#169038=CARTESIAN_POINT('Ctrl Pts',(0.232339728999104,-62.8965351787718,
40.0684393223556));
#169039=CARTESIAN_POINT('Ctrl Pts',(0.229175397308911,-62.8985027695519,
40.0715697951759));
#169040=CARTESIAN_POINT('Ctrl Pts',(0.211566610930123,-62.9094519648699,
40.0889901646418));
#169041=CARTESIAN_POINT('Ctrl Pts',(0.191177078584712,-62.9192690206957,
40.1045963098239));
#169042=CARTESIAN_POINT('Ctrl Pts',(0.168765047542055,-62.9274935913893,
40.1176634650721));
#169043=CARTESIAN_POINT('Ctrl Pts',(0.158706217640471,-62.9311848926133,
40.123528185306));
#169044=CARTESIAN_POINT('Ctrl Pts',(0.148239886921569,-62.9345557609575,
40.1288820140919));
#169045=CARTESIAN_POINT('Ctrl Pts',(0.137433186922152,-62.9375663198809,
40.1336621774101));
#169046=CARTESIAN_POINT('Ctrl Pts',(0.132736741273405,-62.9388746680683,
40.1357395717319));
#169047=CARTESIAN_POINT('Ctrl Pts',(0.127976140237891,-62.9401148076313,
40.1377083672884));
#169048=CARTESIAN_POINT('Ctrl Pts',(0.123156980417351,-62.9412833674838,
40.1395632548792));
#169049=CARTESIAN_POINT('Ctrl Pts',(0.10628992104546,-62.9453733269673,
40.146055361447));
#169050=CARTESIAN_POINT('Ctrl Pts',(0.0887055165508424,-62.9485864317704,
40.151152097463));
#169051=CARTESIAN_POINT('Ctrl Pts',(0.0706437212499514,-62.9507781643242,
40.1546258197409));
#169052=CARTESIAN_POINT('Ctrl Pts',(0.061612823599506,-62.9518740306011,
40.1563626808798));
#169053=CARTESIAN_POINT('Ctrl Pts',(0.052462578249927,-62.9527145544237,
40.1576937882008));
#169054=CARTESIAN_POINT('Ctrl Pts',(0.0432229794973055,-62.9532816790167,
40.1585906813668));
#169055=CARTESIAN_POINT('Ctrl Pts',(0.0386031801209948,-62.9535652413132,
40.1590391279498));
#169056=CARTESIAN_POINT('Ctrl Pts',(0.0339610423938992,-62.9537804539255,
40.1593790209175));
#169057=CARTESIAN_POINT('Ctrl Pts',(0.0293003156013867,-62.9539250604562,
40.1596068022931));
#169058=CARTESIAN_POINT('Ctrl Pts',(0.024639588808874,-62.9540696669868,
40.1598345836687));
#169059=CARTESIAN_POINT('Ctrl Pts',(0.0199602729505794,-62.9541436657296,
40.1599502506865));
#169060=CARTESIAN_POINT('Ctrl Pts',(0.0152661173106527,-62.9541448057648,
40.1599502534424));
#169061=CARTESIAN_POINT('',(-0.015266117311081,-62.9541448057648,40.1599502534424));
#169062=CARTESIAN_POINT('Origin',(-3.96846087890508E-17,1.55412650666996E-16,
40.1599502534424));
#169063=CARTESIAN_POINT('',(-0.318045750793257,-62.7644678366119,39.8576902534424));
#169064=CARTESIAN_POINT('Ctrl Pts',(-0.015266117311081,-62.9541448057648,
40.1599502534424));
#169065=CARTESIAN_POINT('Ctrl Pts',(-0.0190877352448612,-62.9541438736292,
40.1599502447858));
#169066=CARTESIAN_POINT('Ctrl Pts',(-0.022898872102436,-62.9540952129414,
40.1598744685927));
#169067=CARTESIAN_POINT('Ctrl Pts',(-0.0266975986405572,-62.9539999459718,
40.1597246934279));
#169068=CARTESIAN_POINT('Ctrl Pts',(-0.0486495517941837,-62.953449420412,
40.1588591777434));
#169069=CARTESIAN_POINT('Ctrl Pts',(-0.070189881249066,-62.9513443281451,
40.1555254706012));
#169070=CARTESIAN_POINT('Ctrl Pts',(-0.0909392844476108,-62.9479003565101,
40.150063182636));
#169071=CARTESIAN_POINT('Ctrl Pts',(-0.0993079960717487,-62.9465113235254,
40.1478601162465));
#169072=CARTESIAN_POINT('Ctrl Pts',(-0.107548428340522,-62.9449047668208,
40.1453112228298));
#169073=CARTESIAN_POINT('Ctrl Pts',(-0.115637319282431,-62.9430957254317,
40.1424401896328));
#169074=CARTESIAN_POINT('Ctrl Pts',(-0.118621628943688,-62.9424282989905,
40.1413809526905));
#169075=CARTESIAN_POINT('Ctrl Pts',(-0.121585194085774,-62.9417332466658,
40.1402777640512));
#169076=CARTESIAN_POINT('Ctrl Pts',(-0.124526788072995,-62.941011293136,
40.1391317641987));
#169077=CARTESIAN_POINT('Ctrl Pts',(-0.130042276799036,-62.9396576302675,
40.1369830144753));
#169078=CARTESIAN_POINT('Ctrl Pts',(-0.135480523183809,-62.938209392844,
40.134683756585));
#169079=CARTESIAN_POINT('Ctrl Pts',(-0.140833441493576,-62.9366713579026,
40.1322415082996));
#169080=CARTESIAN_POINT('Ctrl Pts',(-0.159568655577758,-62.9312882356078,
40.1236936393009));
#169081=CARTESIAN_POINT('Ctrl Pts',(-0.177258600739179,-62.9248050892389,
40.113394140767));
#169082=CARTESIAN_POINT('Ctrl Pts',(-0.193556601113859,-62.9174267595942,
40.101665321223));
#169083=CARTESIAN_POINT('Ctrl Pts',(-0.201705601301199,-62.9137375947718,
40.095800911451));
#169084=CARTESIAN_POINT('Ctrl Pts',(-0.209506615291615,-62.9098246351408,
40.0895791707949));
#169085=CARTESIAN_POINT('Ctrl Pts',(-0.216916308650606,-62.9057134946881,
40.0830403822906));
#169086=CARTESIAN_POINT('Ctrl Pts',(-0.220621155330102,-62.9036579244618,
40.0797709880385));
#169087=CARTESIAN_POINT('Ctrl Pts',(-0.224228171852759,-62.9015528091474,
40.0764223317514));
#169088=CARTESIAN_POINT('Ctrl Pts',(-0.227731941419747,-62.8994013510256,
40.0729994484778));
#169089=CARTESIAN_POINT('Ctrl Pts',(-0.231235710986736,-62.8972498929038,
40.0695765652042));
#169090=CARTESIAN_POINT('Ctrl Pts',(-0.23463611427696,-62.8950520414621,
40.0660793733488));
#169091=CARTESIAN_POINT('Ctrl Pts',(-0.237927978231146,-62.892811103745,
40.0625130768817));
#169092=CARTESIAN_POINT('Ctrl Pts',(-0.237956050936441,-62.8927919932396,
40.0624826638418));
#169093=CARTESIAN_POINT('Ctrl Pts',(-0.237984115711232,-62.8927728797351,
40.0624522459912));
#169094=CARTESIAN_POINT('Ctrl Pts',(-0.238012172553065,-62.8927537632335,
40.0624218233329));
#169095=CARTESIAN_POINT('Ctrl Pts',(-0.252341211296384,-62.8829906867849,
40.0468845275921));
#169096=CARTESIAN_POINT('Ctrl Pts',(-0.264702219189541,-62.8725309380422,
40.0302263329286));
#169097=CARTESIAN_POINT('Ctrl Pts',(-0.275152816745417,-62.8615664772848,
40.012751588482));
#169098=CARTESIAN_POINT('Ctrl Pts',(-0.285956846571237,-62.8502312057453,
39.9946858597818));
#169099=CARTESIAN_POINT('Ctrl Pts',(-0.294719332056317,-62.8383556508916,
39.9757460620621));
#169100=CARTESIAN_POINT('Ctrl Pts',(-0.301453885679313,-62.8261370346473,
39.9562444559289));
#169101=CARTESIAN_POINT('Ctrl Pts',(-0.308060333921541,-62.8141508421944,
39.9371138113796));
#169102=CARTESIAN_POINT('Ctrl Pts',(-0.312715155744977,-62.8018335935212,
39.9174410654562));
#169103=CARTESIAN_POINT('Ctrl Pts',(-0.315383336840583,-62.7893708783693,
39.8975196504379));
#169104=CARTESIAN_POINT('Ctrl Pts',(-0.317150913275331,-62.7811147664991,
39.8843224113931));
#169105=CARTESIAN_POINT('Ctrl Pts',(-0.318045664008668,-62.7727948225173,
39.871016044721));
#169106=CARTESIAN_POINT('Ctrl Pts',(-0.318045750793257,-62.7644678366119,
39.8576902534424));
#169107=CARTESIAN_POINT('',(-0.318048871877343,-62.4081695979768,39.2875012672119));
#169108=CARTESIAN_POINT('',(-0.318045750793259,-62.7644678366119,39.8576902534424));
#169109=CARTESIAN_POINT('',(-6.20712349654485,-62.0995362748658,39.2875012672119));
#169110=CARTESIAN_POINT('Origin',(5.53234440788222E-15,0.,39.2875012672119));
#169111=CARTESIAN_POINT('',(-6.24436990788081,-62.4538823482275,39.8576902534424));
#169112=CARTESIAN_POINT('',(-6.20712349654485,-62.0995362748658,39.2875012672119));
#169113=CARTESIAN_POINT('',(-6.56531752495323,-62.6108711573005,40.1599502534424));
#169114=CARTESIAN_POINT('Ctrl Pts',(-6.2443699078808,-62.4538823482275,
39.8576902534424));
#169115=CARTESIAN_POINT('Ctrl Pts',(-6.24565635961484,-62.4661208561118,
39.8773836120374));
#169116=CARTESIAN_POINT('Ctrl Pts',(-6.24887816048168,-62.4781153572978,
39.8969946442152));
#169117=CARTESIAN_POINT('Ctrl Pts',(-6.25393874389551,-62.4897034690595,
39.916252528827));
#169118=CARTESIAN_POINT('Ctrl Pts',(-6.25910101415687,-62.5015244311583,
39.9358973794102));
#169119=CARTESIAN_POINT('Ctrl Pts',(-6.26617675898623,-62.5129234357018,
39.9551762199786));
#169120=CARTESIAN_POINT('Ctrl Pts',(-6.27511683300914,-62.5237314369814,
39.9738152034297));
#169121=CARTESIAN_POINT('Ctrl Pts',(-6.28370959326059,-62.534119557209,
39.9917300792702));
#169122=CARTESIAN_POINT('Ctrl Pts',(-6.2940250923436,-62.543962460673,40.0090551158182));
#169123=CARTESIAN_POINT('Ctrl Pts',(-6.30606398948311,-62.5531007542797,
40.0255394551598));
#169124=CARTESIAN_POINT('Ctrl Pts',(-6.315311852504,-62.5601204743206,40.038202152619));
#169125=CARTESIAN_POINT('Ctrl Pts',(-6.32557753708339,-62.5667243349277,
40.0503687782142));
#169126=CARTESIAN_POINT('Ctrl Pts',(-6.33687803771711,-62.5728320301412,
40.0619155352442));
#169127=CARTESIAN_POINT('Ctrl Pts',(-6.33690765431396,-62.5728480373211,
40.0619457972351));
#169128=CARTESIAN_POINT('Ctrl Pts',(-6.33693727882117,-62.5728640408534,
40.0619760547304));
#169129=CARTESIAN_POINT('Ctrl Pts',(-6.33696691123597,-62.5728800407363,
40.0620063077269));
#169130=CARTESIAN_POINT('Ctrl Pts',(-6.34014410870348,-62.5745955535553,
40.06525004417));
#169131=CARTESIAN_POINT('Ctrl Pts',(-6.34341121944339,-62.5762674929177,
40.0684393223556));
#169132=CARTESIAN_POINT('Ctrl Pts',(-6.34676388583407,-62.5778935423007,
40.0715697951758));
#169133=CARTESIAN_POINT('Ctrl Pts',(-6.36542071199911,-62.586942137401,
40.0889901646417));
#169134=CARTESIAN_POINT('Ctrl Pts',(-6.38672471011203,-62.5945741278849,
40.1045963098237));
#169135=CARTESIAN_POINT('Ctrl Pts',(-6.40987366743906,-62.6004109483561,
40.1176634650718));
#169136=CARTESIAN_POINT('Ctrl Pts',(-6.42026324006253,-62.6030305942139,
40.1235281853058));
#169137=CARTESIAN_POINT('Ctrl Pts',(-6.43102458681472,-62.6052889671226,
40.1288820140918));
#169138=CARTESIAN_POINT('Ctrl Pts',(-6.44208677567884,-62.6071534261453,
40.1336621774101));
#169139=CARTESIAN_POINT('Ctrl Pts',(-6.44689425333237,-62.6079636948179,
40.1357395717319));
#169140=CARTESIAN_POINT('Ctrl Pts',(-6.45175840518007,-62.6086994224562,
40.1377083672884));
#169141=CARTESIAN_POINT('Ctrl Pts',(-6.45667331290448,-62.6093578414452,
40.1395632548792));
#169142=CARTESIAN_POINT('Ctrl Pts',(-6.47387548993995,-62.6116623079068,
40.146055361447));
#169143=CARTESIAN_POINT('Ctrl Pts',(-6.49169942613425,-62.6130197402063,
40.1511520974629));
#169144=CARTESIAN_POINT('Ctrl Pts',(-6.50989137546639,-62.6133114945132,
40.1546258197408));
#169145=CARTESIAN_POINT('Ctrl Pts',(-6.51898735013247,-62.6134573716666,
40.1563626808798));
#169146=CARTESIAN_POINT('Ctrl Pts',(-6.52817532814414,-62.6133368299269,
40.1576937882008));
#169147=CARTESIAN_POINT('Ctrl Pts',(-6.53742359207022,-62.6129350466932,
40.1585906813668));
#169148=CARTESIAN_POINT('Ctrl Pts',(-6.54204772403327,-62.6127341550763,
40.1590391279498));
#169149=CARTESIAN_POINT('Ctrl Pts',(-6.54668692748782,-62.6124629532086,
40.1593790209175));
#169150=CARTESIAN_POINT('Ctrl Pts',(-6.55133723782973,-62.6121195889602,
40.1596068022931));
#169151=CARTESIAN_POINT('Ctrl Pts',(-6.55598754817164,-62.6117762247118,
40.1598345836687));
#169152=CARTESIAN_POINT('Ctrl Pts',(-6.56064896522293,-62.6113606963859,
40.1599502506865));
#169153=CARTESIAN_POINT('Ctrl Pts',(-6.56531752495323,-62.6108711573005,
40.1599502534424));
#169154=CARTESIAN_POINT('',(-6.59568250079906,-62.6076796697354,40.1599502534424));
#169155=CARTESIAN_POINT('Origin',(-2.34395632424774E-17,1.54561283905546E-16,
40.1599502534424));
#169156=CARTESIAN_POINT('',(-6.87697683366585,-62.3873926810691,39.8576902534424));
#169157=CARTESIAN_POINT('Ctrl Pts',(-6.59568250079906,-62.6076796697354,
40.1599502534424));
#169158=CARTESIAN_POINT('Ctrl Pts',(-6.59948308607524,-62.6072792748563,
40.1599502447858));
#169159=CARTESIAN_POINT('Ctrl Pts',(-6.60326825869943,-62.6068325084578,
40.1598744685927));
#169160=CARTESIAN_POINT('Ctrl Pts',(-6.60703621730617,-62.6063406883232,
40.1597246934279));
#169161=CARTESIAN_POINT('Ctrl Pts',(-6.62881036976783,-62.6034985746718,
40.1588591777436));
#169162=CARTESIAN_POINT('Ctrl Pts',(-6.65001265697977,-62.5991534367857,
40.1555254706027));
#169163=CARTESIAN_POINT('Ctrl Pts',(-6.6702883997098,-62.5935594283595,
40.1500631826398));
#169164=CARTESIAN_POINT('Ctrl Pts',(-6.67846607317752,-62.5913032360762,
40.1478601162494));
#169165=CARTESIAN_POINT('Ctrl Pts',(-6.68649343259726,-62.5888441205342,
40.1453112228314));
#169166=CARTESIAN_POINT('Ctrl Pts',(-6.69434891543631,-62.586199469922,
40.1424401896328));
#169167=CARTESIAN_POINT('Ctrl Pts',(-6.69724711167674,-62.5852237544099,
40.1413809526905));
#169168=CARTESIAN_POINT('Ctrl Pts',(-6.7001217893475,-62.5842227327444,
40.1402777640511));
#169169=CARTESIAN_POINT('Ctrl Pts',(-6.70297180428205,-62.5831972538525,
40.1391317641987));
#169170=CARTESIAN_POINT('Ctrl Pts',(-6.70831558228433,-62.5812744809302,
40.1369830144753));
#169171=CARTESIAN_POINT('Ctrl Pts',(-6.71357265535406,-62.5792657255653,
40.1346837565849));
#169172=CARTESIAN_POINT('Ctrl Pts',(-6.71873548138837,-62.5771765838154,
40.1322415082996));
#169173=CARTESIAN_POINT('Ctrl Pts',(-6.73680537250844,-62.5698645876906,
40.1236936393008));
#169174=CARTESIAN_POINT('Ctrl Pts',(-6.75372073697224,-62.5615678538928,
40.113394140767));
#169175=CARTESIAN_POINT('Ctrl Pts',(-6.76915820973634,-62.5525263385764,
40.101665321223));
#169176=CARTESIAN_POINT('Ctrl Pts',(-6.77687694611839,-62.5480055809182,
40.095800911451));
#169177=CARTESIAN_POINT('Ctrl Pts',(-6.78422620968087,-62.5432986288851,
40.0895791707949));
#169178=CARTESIAN_POINT('Ctrl Pts',(-6.79116558077055,-62.5384354858298,
40.0830403822906));
#169179=CARTESIAN_POINT('Ctrl Pts',(-6.79463526631539,-62.5360039143022,
40.0797709880385));
#169180=CARTESIAN_POINT('Ctrl Pts',(-6.79800247875532,-62.5335332951358,
40.0764223317514));
#169181=CARTESIAN_POINT('Ctrl Pts',(-6.80126216569475,-62.5310273792782,
40.0729994484778));
#169182=CARTESIAN_POINT('Ctrl Pts',(-6.80452185263419,-62.5285214634206,
40.0695765652042));
#169183=CARTESIAN_POINT('Ctrl Pts',(-6.80767389012569,-62.5259802131086,
40.0660793733488));
#169184=CARTESIAN_POINT('Ctrl Pts',(-6.81071347912887,-62.5234074580024,
40.0625130768816));
#169185=CARTESIAN_POINT('Ctrl Pts',(-6.81073940045717,-62.5233855177896,
40.0624826638418));
#169186=CARTESIAN_POINT('Ctrl Pts',(-6.81076531358494,-62.5233635754231,
40.0624522459912));
#169187=CARTESIAN_POINT('Ctrl Pts',(-6.81079121850992,-62.5233416309051,
40.0624218233329));
#169188=CARTESIAN_POINT('Ctrl Pts',(-6.82402124190344,-62.5121342452095,
40.0468845275902));
#169189=CARTESIAN_POINT('Ctrl Pts',(-6.83522119344092,-62.5004397189038,
40.0302263329245));
#169190=CARTESIAN_POINT('Ctrl Pts',(-6.84446844329707,-62.4884429377054,
40.0127515884755));
#169191=CARTESIAN_POINT('Ctrl Pts',(-6.85402842900294,-62.476040433333,
39.994685859773));
#169192=CARTESIAN_POINT('Ctrl Pts',(-6.86150157917654,-62.4633140048676,
39.9757460620508));
#169193=CARTESIAN_POINT('Ctrl Pts',(-6.86692204703053,-62.450458370939,
39.9562444559149));
#169194=CARTESIAN_POINT('Ctrl Pts',(-6.8722394061801,-62.4378472782187,
39.9371138113634));
#169195=CARTESIAN_POINT('Ctrl Pts',(-6.87558122532622,-62.4251109433491,
39.9174410654378));
#169196=CARTESIAN_POINT('Ctrl Pts',(-6.87693208138238,-62.4124375993839,
39.8975196504171));
#169197=CARTESIAN_POINT('Ctrl Pts',(-6.87782697616072,-62.4040419533144,
39.8843224113792));
#169198=CARTESIAN_POINT('Ctrl Pts',(-6.87784715439656,-62.3956740599416,
39.871016044714));
#169199=CARTESIAN_POINT('Ctrl Pts',(-6.87697683366585,-62.3873926810691,
39.8576902534424));
#169200=CARTESIAN_POINT('',(-6.83973663030281,-62.0330459552232,39.2875012672119));
#169201=CARTESIAN_POINT('',(-6.87697683366585,-62.3873926810691,39.8576902534424));
#169202=CARTESIAN_POINT('',(-12.6642893210144,-61.1105274371641,39.2875012672119));
#169203=CARTESIAN_POINT('Origin',(5.53234440788222E-15,0.,39.2875012672119));
#169204=CARTESIAN_POINT('',(-12.7383709431253,-61.4590390555208,39.8576902534424));
#169205=CARTESIAN_POINT('',(-12.6642893210144,-61.1105274371641,39.2875012672119));
#169206=CARTESIAN_POINT('',(-13.0739701745327,-61.5816197022697,40.1599502534424));
#169207=CARTESIAN_POINT('Ctrl Pts',(-12.7383709431253,-61.4590390555208,
39.8576902534424));
#169208=CARTESIAN_POINT('Ctrl Pts',(-12.7409296199637,-61.4710760487551,
39.8773836120367));
#169209=CARTESIAN_POINT('Ctrl Pts',(-12.7453875382446,-61.4826680729147,
39.8969946442138));
#169210=CARTESIAN_POINT('Ctrl Pts',(-12.7516316867672,-61.4936637287798,
39.9162525288249));
#169211=CARTESIAN_POINT('Ctrl Pts',(-12.7580013045741,-61.5048803302338,
39.9358973794074));
#169212=CARTESIAN_POINT('Ctrl Pts',(-12.7662298081603,-61.5154772731038,
39.9551762199754));
#169213=CARTESIAN_POINT('Ctrl Pts',(-12.7762506512866,-61.5252915748223,
39.973815203426));
#169214=CARTESIAN_POINT('Ctrl Pts',(-12.7858821937415,-61.534724599816,
39.9917300792663));
#169215=CARTESIAN_POINT('Ctrl Pts',(-12.797170047014,-61.5434353195579,
40.0090551158141));
#169216=CARTESIAN_POINT('Ctrl Pts',(-12.8100982056025,-61.5512651452187,
40.0255394551555));
#169217=CARTESIAN_POINT('Ctrl Pts',(-12.8200291684115,-61.5572797455894,
40.0382021526163));
#169218=CARTESIAN_POINT('Ctrl Pts',(-12.8309289078987,-61.5627743733243,
40.0503687782129));
#169219=CARTESIAN_POINT('Ctrl Pts',(-12.8428059312037,-61.5676673859795,
40.0619155352442));
#169220=CARTESIAN_POINT('Ctrl Pts',(-12.8428370587636,-61.5676802096931,
40.0619457972351));
#169221=CARTESIAN_POINT('Ctrl Pts',(-12.8428681938093,-61.5676930289522,
40.0619760547305));
#169222=CARTESIAN_POINT('Ctrl Pts',(-12.8428993363378,-61.5677058437553,
40.0620063077269));
#169223=CARTESIAN_POINT('Ctrl Pts',(-12.8462384487039,-61.5690798512467,
40.06525004417));
#169224=CARTESIAN_POINT('Ctrl Pts',(-12.8496624271215,-61.5704011254854,
40.0684393223557));
#169225=CARTESIAN_POINT('Ctrl Pts',(-12.8531666956981,-61.5716678181341,
40.0715697951759));
#169226=CARTESIAN_POINT('Ctrl Pts',(-12.8726671535588,-61.5787166747155,
40.0889901646425));
#169227=CARTESIAN_POINT('Ctrl Pts',(-12.8946522063791,-61.5840799821729,
40.1045963098251));
#169228=CARTESIAN_POINT('Ctrl Pts',(-12.9182844651712,-61.5874651029952,
40.1176634650736));
#169229=CARTESIAN_POINT('Ctrl Pts',(-12.9288909501836,-61.5889843920983,
40.1235281853069));
#169230=CARTESIAN_POINT('Ctrl Pts',(-12.9398294094008,-61.5901055263651,
40.1288820140923));
#169231=CARTESIAN_POINT('Ctrl Pts',(-12.9510258874722,-61.5908034580837,
40.1336621774101));
#169232=CARTESIAN_POINT('Ctrl Pts',(-12.9558917253993,-61.5911067697685,
40.1357395717319));
#169233=CARTESIAN_POINT('Ctrl Pts',(-12.9608061353937,-61.591330024696,
40.1377083672884));
#169234=CARTESIAN_POINT('Ctrl Pts',(-12.9657629422644,-61.5914710890454,
40.1395632548792));
#169235=CARTESIAN_POINT('Ctrl Pts',(-12.9831117663121,-61.5919648142682,
40.146055361447));
#169236=CARTESIAN_POINT('Ctrl Pts',(-13.0009799514312,-61.5914517017517,
40.1511520974629));
#169237=CARTESIAN_POINT('Ctrl Pts',(-13.0191027399908,-61.5898402812905,
40.1546258197408));
#169238=CARTESIAN_POINT('Ctrl Pts',(-13.0281641342706,-61.5890345710599,
40.1563626808798));
#169239=CARTESIAN_POINT('Ctrl Pts',(-13.0372891795346,-61.5879542844383,
40.1576937882008));
#169240=CARTESIAN_POINT('Ctrl Pts',(-13.0464447827192,-61.5865879953991,
40.1585906813668));
#169241=CARTESIAN_POINT('Ctrl Pts',(-13.0510225843115,-61.5859048508795,
40.1590391279498));
#169242=CARTESIAN_POINT('Ctrl Pts',(-13.0556080254097,-61.585150205876,
40.1593790209175));
#169243=CARTESIAN_POINT('Ctrl Pts',(-13.0601969695277,-61.5843226328192,
40.1596068022931));
#169244=CARTESIAN_POINT('Ctrl Pts',(-13.0647859136458,-61.5834950597623,
40.1598345836687));
#169245=CARTESIAN_POINT('Ctrl Pts',(-13.0693783604294,-61.582594556983,
40.1599502506865));
#169246=CARTESIAN_POINT('Ctrl Pts',(-13.0739701745327,-61.5816197022697,
40.1599502534424));
#169247=CARTESIAN_POINT('',(-13.103835206573,-61.5752716937451,40.1599502534424));
#169248=CARTESIAN_POINT('Origin',(-7.37250181440781E-18,1.52016511373602E-16,
40.1599502534424));
#169249=CARTESIAN_POINT('',(-13.3605623192489,-61.3267881959112,39.8576902534424));
#169250=CARTESIAN_POINT('Ctrl Pts',(-13.103835206573,-61.5752716937451,
40.1599502534424));
#169251=CARTESIAN_POINT('Ctrl Pts',(-13.107573119184,-61.5744762229326,
40.1599502447859));
#169252=CARTESIAN_POINT('Ctrl Pts',(-13.1112908564314,-61.5736362456895,
40.1598744685927));
#169253=CARTESIAN_POINT('Ctrl Pts',(-13.1149867645638,-61.5727532608743,
40.1597246934279));
#169254=CARTESIAN_POINT('Ctrl Pts',(-13.1363445541706,-61.5676506979223,
40.1588591777434));
#169255=CARTESIAN_POINT('Ctrl Pts',(-13.1569765024517,-61.5611131206551,
40.1555254706018));
#169256=CARTESIAN_POINT('Ctrl Pts',(-13.1765564394397,-61.5534303645618,
40.1500631826374));
#169257=CARTESIAN_POINT('Ctrl Pts',(-13.1844534784414,-61.5503317322961,
40.1478601162476));
#169258=CARTESIAN_POINT('Ctrl Pts',(-13.192179815575,-61.5470470005032,
40.1453112228304));
#169259=CARTESIAN_POINT('Ctrl Pts',(-13.1997158239901,-61.5435957160156,
40.1424401896328));
#169260=CARTESIAN_POINT('Ctrl Pts',(-13.2024961535652,-61.5423224015759,
40.1413809526906));
#169261=CARTESIAN_POINT('Ctrl Pts',(-13.2052504481945,-61.5410263779725,
40.1402777640511));
#169262=CARTESIAN_POINT('Ctrl Pts',(-13.2079776587163,-61.5397086090799,
40.1391317641987));
#169263=CARTESIAN_POINT('Ctrl Pts',(-13.2130911784448,-61.5372377924062,
40.1369830144753));
#169264=CARTESIAN_POINT('Ctrl Pts',(-13.2181094806068,-61.5346905274442,
40.1346837565849));
#169265=CARTESIAN_POINT('Ctrl Pts',(-13.2230256493633,-61.5320731679598,
40.1322415082996));
#169266=CARTESIAN_POINT('Ctrl Pts',(-13.2402322400107,-61.5229124097647,
40.1236936393008));
#169267=CARTESIAN_POINT('Ctrl Pts',(-13.2561876955041,-61.5128929892897,
40.113394140767));
#169268=CARTESIAN_POINT('Ctrl Pts',(-13.2705955044755,-61.5022873490354,
40.101665321223));
#169269=CARTESIAN_POINT('Ctrl Pts',(-13.2777994089612,-61.4969845289083,
40.095800911451));
#169270=CARTESIAN_POINT('Ctrl Pts',(-13.2846164020262,-61.4915351548247,
40.0895791707949));
#169271=CARTESIAN_POINT('Ctrl Pts',(-13.2910094216448,-61.4859732907799,
40.0830403822906));
#169272=CARTESIAN_POINT('Ctrl Pts',(-13.2942059314541,-61.4831923587575,
40.0797709880385));
#169273=CARTESIAN_POINT('Ctrl Pts',(-13.2972964479272,-61.4803833043594,
40.0764223317514));
#169274=CARTESIAN_POINT('Ctrl Pts',(-13.3002763384268,-61.4775503861046,
40.0729994484778));
#169275=CARTESIAN_POINT('Ctrl Pts',(-13.3032562289264,-61.4747174678498,
40.0695765652042));
#169276=CARTESIAN_POINT('Ctrl Pts',(-13.3061253662369,-61.4718606611377,
40.0660793733488));
#169277=CARTESIAN_POINT('Ctrl Pts',(-13.3088793779158,-61.4689842762858,
40.0625130768817));
#169278=CARTESIAN_POINT('Ctrl Pts',(-13.3089028638677,-61.4689597467471,
40.0624826638418));
#169279=CARTESIAN_POINT('Ctrl Pts',(-13.3089263414387,-61.4689352159237,
40.0624522459912));
#169280=CARTESIAN_POINT('Ctrl Pts',(-13.3089498106271,-61.4689106838182,
40.0624218233329));
#169281=CARTESIAN_POINT('Ctrl Pts',(-13.3209358677635,-61.4563817793404,
40.046884527591));
#169282=CARTESIAN_POINT('Ctrl Pts',(-13.3308520539308,-61.4435806031513,
40.0302263329263));
#169283=CARTESIAN_POINT('Ctrl Pts',(-13.3387946412816,-61.4306829407593,
40.0127515884783));
#169284=CARTESIAN_POINT('Ctrl Pts',(-13.3470058416626,-61.4173490879895,
39.9946858597768));
#169285=CARTESIAN_POINT('Ctrl Pts',(-13.3531077791272,-61.4039112193281,
39.9757460620557));
#169286=CARTESIAN_POINT('Ctrl Pts',(-13.3571547734325,-61.390559416733,
39.956244455921));
#169287=CARTESIAN_POINT('Ctrl Pts',(-13.3611247853904,-61.3774615935182,
39.9371138113704));
#169288=CARTESIAN_POINT('Ctrl Pts',(-13.3631169881904,-61.3644457144043,
39.9174410654458));
#169289=CARTESIAN_POINT('Ctrl Pts',(-13.3631357189472,-61.3517005934362,
39.8975196504261));
#169290=CARTESIAN_POINT('Ctrl Pts',(-13.3631481274169,-61.3432573976163,
39.8843224113852));
#169291=CARTESIAN_POINT('Ctrl Pts',(-13.3622935120792,-61.3349332352371,
39.871016044717));
#169292=CARTESIAN_POINT('Ctrl Pts',(-13.3605623192489,-61.3267881959112,
39.8576902534424));
#169293=CARTESIAN_POINT('',(-13.2864868028998,-60.9782752797347,39.2875012672119));
#169294=CARTESIAN_POINT('',(-13.3605623192489,-61.3267881959112,39.8576902534424));
#169295=CARTESIAN_POINT('',(-18.9827025415099,-59.4519788726607,39.2875012672119));
#169296=CARTESIAN_POINT('Origin',(5.53234440788222E-15,0.,39.2875012672119));
#169297=CARTESIAN_POINT('',(-19.0928077206414,-59.7908376697911,39.8576902534424));
#169298=CARTESIAN_POINT('',(-18.9827025415099,-59.4519788726607,39.2875012672119));
#169299=CARTESIAN_POINT('',(-19.4393816709759,-59.8776671349984,40.1599502534424));
#169300=CARTESIAN_POINT('Ctrl Pts',(-19.0928077206414,-59.7908376697911,
39.8576902534424));
#169301=CARTESIAN_POINT('Ctrl Pts',(-19.0966105891856,-59.8025412685591,
39.8773836120369));
#169302=CARTESIAN_POINT('Ctrl Pts',(-19.1022557829954,-59.8136038110503,
39.8969946442141));
#169303=CARTESIAN_POINT('Ctrl Pts',(-19.1096150844294,-59.8238865403127,
39.9162525288254));
#169304=CARTESIAN_POINT('Ctrl Pts',(-19.1171222629167,-59.8343758896894,
39.9358973794081));
#169305=CARTESIAN_POINT('Ctrl Pts',(-19.1264133720529,-59.8440546685628,
39.9551762199762));
#169306=CARTESIAN_POINT('Ctrl Pts',(-19.1374051938288,-59.852767743177,
39.9738152034268));
#169307=CARTESIAN_POINT('Ctrl Pts',(-19.1479699932931,-59.8611423227411,
39.9917300792672));
#169308=CARTESIAN_POINT('Ctrl Pts',(-19.1601065286729,-59.8686254222926,
40.0090551158152));
#169309=CARTESIAN_POINT('Ctrl Pts',(-19.1737823051001,-59.875060994799,
40.0255394551566));
#169310=CARTESIAN_POINT('Ctrl Pts',(-19.1842875619894,-59.8800045782782,
40.038202152617));
#169311=CARTESIAN_POINT('Ctrl Pts',(-19.1957019365562,-59.8843297728487,
40.0503687782133));
#169312=CARTESIAN_POINT('Ctrl Pts',(-19.2080253553781,-59.8879544940744,
40.0619155352442));
#169313=CARTESIAN_POINT('Ctrl Pts',(-19.2080576528611,-59.8879639938223,
40.0619457972351));
#169314=CARTESIAN_POINT('Ctrl Pts',(-19.2080899573232,-59.8879734883576,
40.0619760547305));
#169315=CARTESIAN_POINT('Ctrl Pts',(-19.2081222687613,-59.8879829776792,
40.0620063077269));
#169316=CARTESIAN_POINT('Ctrl Pts',(-19.211586712012,-59.8890004259295,
40.06525004417));
#169317=CARTESIAN_POINT('Ctrl Pts',(-19.2151300442834,-59.8899565588874,
40.0684393223556));
#169318=CARTESIAN_POINT('Ctrl Pts',(-19.2187475215461,-59.8908500166521,
40.0715697951759));
#169319=CARTESIAN_POINT('Ctrl Pts',(-19.2388779600016,-59.8958219059657,
40.08899016464));
#169320=CARTESIAN_POINT('Ctrl Pts',(-19.2613031946851,-59.8988577688774,
40.1045963098206));
#169321=CARTESIAN_POINT('Ctrl Pts',(-19.2851598349646,-59.899754101959,
40.1176634650679));
#169322=CARTESIAN_POINT('Ctrl Pts',(-19.2958670255008,-59.9001563886589,
40.1235281853035));
#169323=CARTESIAN_POINT('Ctrl Pts',(-19.3068627531394,-59.9001280009024,
40.1288820140908));
#169324=CARTESIAN_POINT('Ctrl Pts',(-19.318070849466,-59.8996517586311,
40.1336621774101));
#169325=CARTESIAN_POINT('Ctrl Pts',(-19.3229417365282,-59.8994447901817,
40.1357395717319));
#169326=CARTESIAN_POINT('Ctrl Pts',(-19.3278525613648,-59.8991531263709,
40.1377083672884));
#169327=CARTESIAN_POINT('Ctrl Pts',(-19.3327969595686,-59.8987752905501,
40.1395632548792));
#169328=CARTESIAN_POINT('Ctrl Pts',(-19.3501023532817,-59.8974528651772,
40.146055361447));
#169329=CARTESIAN_POINT('Ctrl Pts',(-19.3678190197503,-59.8950748296129,
40.151152097463));
#169330=CARTESIAN_POINT('Ctrl Pts',(-19.3856740904735,-59.8915778894433,
40.1546258197409));
#169331=CARTESIAN_POINT('Ctrl Pts',(-19.3946016258351,-59.8898294193585,
40.1563626808798));
#169332=CARTESIAN_POINT('Ctrl Pts',(-19.4035637624458,-59.8878012237014,
40.1576937882008));
#169333=CARTESIAN_POINT('Ctrl Pts',(-19.4125263941846,-59.8854853982053,
40.1585906813668));
#169334=CARTESIAN_POINT('Ctrl Pts',(-19.417007710054,-59.8843274854573,
40.1590391279498));
#169335=CARTESIAN_POINT('Ctrl Pts',(-19.4214891497435,-59.8830976653667,
40.1593790209175));
#169336=CARTESIAN_POINT('Ctrl Pts',(-19.4259664502057,-59.881794950565,
40.1596068022931));
#169337=CARTESIAN_POINT('Ctrl Pts',(-19.4304437506678,-59.8804922357632,
40.1598345836687));
#169338=CARTESIAN_POINT('Ctrl Pts',(-19.4349169113758,-59.8791166246275,
40.1599502506865));
#169339=CARTESIAN_POINT('Ctrl Pts',(-19.4393816709759,-59.8776671349984,
40.1599502534424));
#169340=CARTESIAN_POINT('',(-19.4684195516699,-59.8682321556241,40.1599502534424));
#169341=CARTESIAN_POINT('Origin',(8.34054140790947E-18,1.4780621413155E-16,
40.1599502534424));
#169342=CARTESIAN_POINT('',(-19.6977666881848,-59.5942745858235,39.8576902534424));
#169343=CARTESIAN_POINT('Ctrl Pts',(-19.4684195516699,-59.8682321556241,
40.1599502534424));
#169344=CARTESIAN_POINT('Ctrl Pts',(-19.4720538382629,-59.8670503242229,
40.1599502447858));
#169345=CARTESIAN_POINT('Ctrl Pts',(-19.4756634078263,-59.8658263391018,
40.1598744685927));
#169346=CARTESIAN_POINT('Ctrl Pts',(-19.4792467723414,-59.8645618637723,
40.1597246934279));
#169347=CARTESIAN_POINT('Ctrl Pts',(-19.4999541986752,-59.8572547562686,
40.1588591777435));
#169348=CARTESIAN_POINT('Ctrl Pts',(-19.5197897600771,-59.848596366687,
40.1555254706027));
#169349=CARTESIAN_POINT('Ctrl Pts',(-19.5384593694314,-59.8389090368127,
40.1500631826396));
#169350=CARTESIAN_POINT('Ctrl Pts',(-19.5459892523608,-59.8350019138265,
40.1478601162493));
#169351=CARTESIAN_POINT('Ctrl Pts',(-19.553329915847,-59.8309275539895,
40.1453112228313));
#169352=CARTESIAN_POINT('Ctrl Pts',(-19.560463883758,-59.8267074486192,
40.1424401896328));
#169353=CARTESIAN_POINT('Ctrl Pts',(-19.5630958847952,-59.8251504859513,
40.1413809526906));
#169354=CARTESIAN_POINT('Ctrl Pts',(-19.5656996197547,-59.8235736599159,
40.1402777640511));
#169355=CARTESIAN_POINT('Ctrl Pts',(-19.5682741459747,-59.8219780387743,
40.1391317641987));
#169356=CARTESIAN_POINT('Ctrl Pts',(-19.5731013826371,-59.8189862491338,
40.1369830144753));
#169357=CARTESIAN_POINT('Ctrl Pts',(-19.5778259323228,-59.8159283829425,
40.134683756585));
#169358=CARTESIAN_POINT('Ctrl Pts',(-19.5824415812277,-59.812811482062,
40.1322415082996));
#169359=CARTESIAN_POINT('Ctrl Pts',(-19.5985963523948,-59.8019023289803,
40.1236936393009));
#169360=CARTESIAN_POINT('Ctrl Pts',(-19.6134170876084,-59.7902699966955,
40.113394140767));
#169361=CARTESIAN_POINT('Ctrl Pts',(-19.626637377817,-59.7782164291175,
40.101665321223));
#169362=CARTESIAN_POINT('Ctrl Pts',(-19.6332475229213,-59.7721896453284,
40.095800911451));
#169363=CARTESIAN_POINT('Ctrl Pts',(-19.6394575570863,-59.766057553677,
40.0895791707949));
#169364=CARTESIAN_POINT('Ctrl Pts',(-19.645234181973,-59.759857905589,40.0830403822906));
#169365=CARTESIAN_POINT('Ctrl Pts',(-19.6481224944163,-59.756758081545,
40.0797709880385));
#169366=CARTESIAN_POINT('Ctrl Pts',(-19.6509024545773,-59.7536413685032,
40.0764223317514));
#169367=CARTESIAN_POINT('Ctrl Pts',(-19.6535699003333,-59.7505124858964,
40.0729994484778));
#169368=CARTESIAN_POINT('Ctrl Pts',(-19.6562373460892,-59.7473836032895,
40.0695765652042));
#169369=CARTESIAN_POINT('Ctrl Pts',(-19.6587921483498,-59.7442425399496,
40.0660793733488));
#169370=CARTESIAN_POINT('Ctrl Pts',(-19.6612304091763,-59.7410940396262,
40.0625130768817));
#169371=CARTESIAN_POINT('Ctrl Pts',(-19.6612512024346,-59.7410671895124,
40.0624826638418));
#169372=CARTESIAN_POINT('Ctrl Pts',(-19.6612719872239,-59.7410403389971,
40.0624522459912));
#169373=CARTESIAN_POINT('Ctrl Pts',(-19.6612927635423,-59.7410134880828,
40.0624218233329));
#169374=CARTESIAN_POINT('Ctrl Pts',(-19.6719035326728,-59.7273003341207,
40.04688452759));
#169375=CARTESIAN_POINT('Ctrl Pts',(-19.6804273096601,-59.7135327604116,
40.0302263329241));
#169376=CARTESIAN_POINT('Ctrl Pts',(-19.686978213857,-59.6998755263127,
40.0127515884749));
#169377=CARTESIAN_POINT('Ctrl Pts',(-19.6937506652838,-59.6857564136253,
39.9946858597722));
#169378=CARTESIAN_POINT('Ctrl Pts',(-19.6984145359357,-59.6717543328675,
39.9757460620498));
#169379=CARTESIAN_POINT('Ctrl Pts',(-19.7010437169752,-59.6580526467476,
39.9562444559137));
#169380=CARTESIAN_POINT('Ctrl Pts',(-19.703622885459,-59.6446115955291,
39.937113811362));
#169381=CARTESIAN_POINT('Ctrl Pts',(-19.7042436449212,-59.6314587768652,
39.9174410654362));
#169382=CARTESIAN_POINT('Ctrl Pts',(-19.7029300451593,-59.6187815171056,
39.8975196504155));
#169383=CARTESIAN_POINT('Ctrl Pts',(-19.7020598313697,-59.6103832769599,
39.8843224113781));
#169384=CARTESIAN_POINT('Ctrl Pts',(-19.700339785803,-59.6021940468434,
39.8710160447134));
#169385=CARTESIAN_POINT('Ctrl Pts',(-19.6977666881848,-59.5942745858235,
39.8576902534424));
#169386=CARTESIAN_POINT('',(-19.5876674457081,-59.255413859757,39.2875012672119));
#169387=CARTESIAN_POINT('',(-19.6977666881848,-59.5942745858235,39.8576902534424));
#169388=CARTESIAN_POINT('',(-25.0931373005748,-57.142061986502,39.2875012672119));
#169389=CARTESIAN_POINT('Origin',(5.53234440788222E-15,0.,39.2875012672119));
#169390=CARTESIAN_POINT('',(-25.2380597013433,-57.4675553545139,39.8576902534424));
#169391=CARTESIAN_POINT('',(-25.0931373005748,-57.142061986502,39.2875012672119));
#169392=CARTESIAN_POINT('',(-25.5918112338797,-57.5176823163887,40.1599502534424));
#169393=CARTESIAN_POINT('Ctrl Pts',(-25.2380597013433,-57.4675553545139,
39.8576902534424));
#169394=CARTESIAN_POINT('Ctrl Pts',(-25.2430650965695,-57.478797331738,
39.8773836120361));
#169395=CARTESIAN_POINT('Ctrl Pts',(-25.2498357159831,-57.4892091890297,
39.8969946442126));
#169396=CARTESIAN_POINT('Ctrl Pts',(-25.2582295402814,-57.4986663319553,
39.9162525288231));
#169397=CARTESIAN_POINT('Ctrl Pts',(-25.2667920292299,-57.5083135057475,
39.9358973794049));
#169398=CARTESIAN_POINT('Ctrl Pts',(-25.2770439485794,-57.5169680778972,
39.9551762199722));
#169399=CARTESIAN_POINT('Ctrl Pts',(-25.2888863203044,-57.5244844631381,
39.9738152034221));
#169400=CARTESIAN_POINT('Ctrl Pts',(-25.3002686266233,-57.5317088436262,
39.9917300792616));
#169401=CARTESIAN_POINT('Ctrl Pts',(-25.313120873688,-57.5378823365827,
40.0090551158087));
#169402=CARTESIAN_POINT('Ctrl Pts',(-25.327394433284,-57.5428531464557,
40.0255394551494));
#169403=CARTESIAN_POINT('Ctrl Pts',(-25.3383588864627,-57.5466715501095,
40.0382021526124));
#169404=CARTESIAN_POINT('Ctrl Pts',(-25.3501628378352,-57.5497799237797,
40.0503687782111));
#169405=CARTESIAN_POINT('Ctrl Pts',(-25.3627976342212,-57.5520966403719,
40.0619155352442));
#169406=CARTESIAN_POINT('Ctrl Pts',(-25.3628307477693,-57.552102712073,
40.0619457972351));
#169407=CARTESIAN_POINT('Ctrl Pts',(-25.3628638677133,-57.5521087778605,
40.0619760547305));
#169408=CARTESIAN_POINT('Ctrl Pts',(-25.3628969940503,-57.5521148377336,
40.0620063077269));
#169409=CARTESIAN_POINT('Ctrl Pts',(-25.3664488110204,-57.5527645793669,
40.06525004417));
#169410=CARTESIAN_POINT('Ctrl Pts',(-25.3700726756556,-57.5533450954512,
40.0684393223557));
#169411=CARTESIAN_POINT('Ctrl Pts',(-25.3737637277665,-57.5538555294216,
40.0715697951759));
#169412=CARTESIAN_POINT('Ctrl Pts',(-25.3943035935255,-57.5566959784089,
40.0889901646418));
#169413=CARTESIAN_POINT('Ctrl Pts',(-25.4169233145145,-57.5573711352259,
40.1045963098239));
#169414=CARTESIAN_POINT('Ctrl Pts',(-25.4407429579447,-57.5557688601533,
40.1176634650721));
#169415=CARTESIAN_POINT('Ctrl Pts',(-25.451433543779,-57.5550497369119,
40.123528185306));
#169416=CARTESIAN_POINT('Ctrl Pts',(-25.46236606834,-57.5538721381541,40.1288820140919));
#169417=CARTESIAN_POINT('Ctrl Pts',(-25.4734629846668,-57.552226939703,
40.1336621774101));
#169418=CARTESIAN_POINT('Ctrl Pts',(-25.478285554406,-57.5515119587091,
40.1357395717319));
#169419=CARTESIAN_POINT('Ctrl Pts',(-25.4831389900605,-57.5507085716896,
40.1377083672884));
#169420=CARTESIAN_POINT('Ctrl Pts',(-25.4880168077358,-57.5498159753469,
40.1395632548792));
#169421=CARTESIAN_POINT('Ctrl Pts',(-25.5050891695995,-57.5466918881475,
40.146055361447));
#169422=CARTESIAN_POINT('Ctrl Pts',(-25.5224602099123,-57.5424749837906,
40.151152097463));
#169423=CARTESIAN_POINT('Ctrl Pts',(-25.5398519389078,-57.537130837121,
40.1546258197409));
#169424=CARTESIAN_POINT('Ctrl Pts',(-25.5485478034055,-57.5344587637861,
40.1563626808798));
#169425=CARTESIAN_POINT('Ctrl Pts',(-25.557248840319,-57.5315048804295,
40.1576937882008));
#169426=CARTESIAN_POINT('Ctrl Pts',(-25.565920304143,-57.5282648911454,
40.1585906813668));
#169427=CARTESIAN_POINT('Ctrl Pts',(-25.5702560360551,-57.5266448965033,
40.1590391279498));
#169428=CARTESIAN_POINT('Ctrl Pts',(-25.5745843747449,-57.5249533754918,
40.1593790209175));
#169429=CARTESIAN_POINT('Ctrl Pts',(-25.5789009773103,-57.5231897917612,
40.1596068022931));
#169430=CARTESIAN_POINT('Ctrl Pts',(-25.5832175798758,-57.5214262080305,
40.1598345836687));
#169431=CARTESIAN_POINT('Ctrl Pts',(-25.5875224456232,-57.5195905600218,
40.1599502506865));
#169432=CARTESIAN_POINT('Ctrl Pts',(-25.5918112338797,-57.5176823163887,
40.1599502534424));
#169433=CARTESIAN_POINT('',(-25.61970381813,-57.5052637377731,40.1599502534424));
#169434=CARTESIAN_POINT('Origin',(2.35274110347535E-17,1.4197652107703E-16,
40.1599502534424));
#169435=CARTESIAN_POINT('',(-25.8191582032623,-57.2088336324698,39.8576902534424));
#169436=CARTESIAN_POINT('Ctrl Pts',(-25.61970381813,-57.5052637377731,40.1599502534424));
#169437=CARTESIAN_POINT('Ctrl Pts',(-25.6231946607006,-57.5037084941753,
40.1599502447858));
#169438=CARTESIAN_POINT('Ctrl Pts',(-25.6266565153805,-57.5021139114132,
40.1598744685927));
#169439=CARTESIAN_POINT('Ctrl Pts',(-25.6300880761868,-57.5004817994258,
40.1597246934279));
#169440=CARTESIAN_POINT('Ctrl Pts',(-25.6499182643581,-57.4910502055668,
40.1588591777434));
#169441=CARTESIAN_POINT('Ctrl Pts',(-25.6687401163254,-57.4803658667955,
40.1555254706014));
#169442=CARTESIAN_POINT('Ctrl Pts',(-25.6862948499043,-57.4687800995496,
40.1500631826363));
#169443=CARTESIAN_POINT('Ctrl Pts',(-25.6933750777819,-57.4641072931028,
40.1478601162468));
#169444=CARTESIAN_POINT('Ctrl Pts',(-25.7002496417694,-57.4592879447641,
40.1453112228299));
#169445=CARTESIAN_POINT('Ctrl Pts',(-25.7069034079254,-57.4543452548723,
40.1424401896328));
#169446=CARTESIAN_POINT('Ctrl Pts',(-25.7093582436704,-57.4525217023851,
40.1413809526905));
#169447=CARTESIAN_POINT('Ctrl Pts',(-25.7117828918951,-57.4506813499536,
40.1402777640511));
#169448=CARTESIAN_POINT('Ctrl Pts',(-25.7141765267651,-57.4488253585221,
40.1391317641987));
#169449=CARTESIAN_POINT('Ctrl Pts',(-25.7186645921465,-57.4453453745882,
40.1369830144753));
#169450=CARTESIAN_POINT('Ctrl Pts',(-25.7230436262008,-57.4418104097895,
40.1346837565849));
#169451=CARTESIAN_POINT('Ctrl Pts',(-25.7273081852389,-57.4382281169312,
40.1322415082996));
#169452=CARTESIAN_POINT('Ctrl Pts',(-25.742234141872,-57.4256900919269,
40.1236936393009));
#169453=CARTESIAN_POINT('Ctrl Pts',(-25.7557577777295,-57.4125722940992,
40.113394140767));
#169454=CARTESIAN_POINT('Ctrl Pts',(-25.7676457049092,-57.399202860606,
40.101665321223));
#169455=CARTESIAN_POINT('Ctrl Pts',(-25.7735896684991,-57.3925181438595,
40.095800911451));
#169456=CARTESIAN_POINT('Ctrl Pts',(-25.7791247053302,-57.3857705191196,
40.0895791707949));
#169457=CARTESIAN_POINT('Ctrl Pts',(-25.7842216455739,-57.3790010116302,
40.0830403822906));
#169458=CARTESIAN_POINT('Ctrl Pts',(-25.7867701156958,-57.3756162578856,
40.0797709880385));
#169459=CARTESIAN_POINT('Ctrl Pts',(-25.7892090617194,-57.3722260335604,
40.0764223317514));
#169460=CARTESIAN_POINT('Ctrl Pts',(-25.7915348376378,-57.3688354672941,
40.0729994484778));
#169461=CARTESIAN_POINT('Ctrl Pts',(-25.7938606135562,-57.3654449010278,
40.0695765652042));
#169462=CARTESIAN_POINT('Ctrl Pts',(-25.7960730898187,-57.3620539952073,
40.0660793733488));
#169463=CARTESIAN_POINT('Ctrl Pts',(-25.7981688856969,-57.3586678750409,
40.0625130768817));
#169464=CARTESIAN_POINT('Ctrl Pts',(-25.7981867584464,-57.3586389985275,
40.0624826638418));
#169465=CARTESIAN_POINT('Ctrl Pts',(-25.7982046227313,-57.3586101225,40.0624522459912));
#169466=CARTESIAN_POINT('Ctrl Pts',(-25.7982224785501,-57.3585812469612,
40.0624218233329));
#169467=CARTESIAN_POINT('Ctrl Pts',(-25.8073417058667,-57.3438340877002,
40.0468845275903));
#169468=CARTESIAN_POINT('Ctrl Pts',(-25.8143796853889,-57.3292509568911,
40.0302263329247));
#169469=CARTESIAN_POINT('Ctrl Pts',(-25.8194671333544,-57.314983782601,
40.0127515884759));
#169470=CARTESIAN_POINT('Ctrl Pts',(-25.8247266354318,-57.3002341019502,
39.9946858597735));
#169471=CARTESIAN_POINT('Ctrl Pts',(-25.8279013409282,-57.2858212188239,
39.9757460620513));
#169472=CARTESIAN_POINT('Ctrl Pts',(-25.8290839028447,-57.2719197677207,
39.9562444559156));
#169473=CARTESIAN_POINT('Ctrl Pts',(-25.8302439699452,-57.2582827514691,
39.9371138113642));
#169474=CARTESIAN_POINT('Ctrl Pts',(-25.8294864848998,-57.2451370982896,
39.9174410654388));
#169475=CARTESIAN_POINT('Ctrl Pts',(-25.8268549466938,-57.23266659445,39.8975196504183));
#169476=CARTESIAN_POINT('Ctrl Pts',(-25.8251116448899,-57.2244053228521,
39.88432241138));
#169477=CARTESIAN_POINT('Ctrl Pts',(-25.8225450142732,-57.2164407479142,
39.8710160447144));
#169478=CARTESIAN_POINT('Ctrl Pts',(-25.8191582032623,-57.2088336324698,
39.8576902534424));
#169479=CARTESIAN_POINT('',(-25.6742415049982,-56.8833377255393,39.2875012672119));
#169480=CARTESIAN_POINT('',(-25.8191582032623,-57.2088336324698,39.8576902534424));
#169481=CARTESIAN_POINT('',(-30.9286463962981,-54.206084711474,39.2875012672119));
#169482=CARTESIAN_POINT('Origin',(5.53234440788222E-15,0.,39.2875012672119));
#169483=CARTESIAN_POINT('',(-31.1067982185537,-54.5146464769136,39.8576902534424));
#169484=CARTESIAN_POINT('',(-30.9286463962981,-54.206084711474,39.2875012672119));
#169485=CARTESIAN_POINT('',(-31.4638515574743,-54.5275217339718,40.1599502534424));
#169486=CARTESIAN_POINT('Ctrl Pts',(-31.1067982185537,-54.5146464769136,
39.8576902534424));
#169487=CARTESIAN_POINT('Ctrl Pts',(-31.1129513003034,-54.5253036631377,
39.8773836120333));
#169488=CARTESIAN_POINT('Ctrl Pts',(-31.1207731649965,-54.5349507607419,
39.896994644207));
#169489=CARTESIAN_POINT('Ctrl Pts',(-31.1301095476621,-54.5434787028934,
39.9162525288149));
#169490=CARTESIAN_POINT('Ctrl Pts',(-31.1396335346499,-54.5521780046457,
39.9358973793941));
#169491=CARTESIAN_POINT('Ctrl Pts',(-31.1507339420374,-54.559713548768,
39.9551762199589));
#169492=CARTESIAN_POINT('Ctrl Pts',(-31.1632971162072,-54.565950893546,
39.9738152034066));
#169493=CARTESIAN_POINT('Ctrl Pts',(-31.1753722224493,-54.5719459231339,
39.9917300792442));
#169494=CARTESIAN_POINT('Ctrl Pts',(-31.1887993692891,-54.576742171415,
40.0090551157898));
#169495=CARTESIAN_POINT('Ctrl Pts',(-31.2035143279466,-54.5801937574222,
40.0255394551292));
#169496=CARTESIAN_POINT('Ctrl Pts',(-31.2148178485749,-54.5828451460221,
40.0382021525994));
#169497=CARTESIAN_POINT('Ctrl Pts',(-31.2268820501958,-54.5847026428001,
40.050368778205));
#169498=CARTESIAN_POINT('Ctrl Pts',(-31.2396897946772,-54.5856859723271,
40.0619155352442));
#169499=CARTESIAN_POINT('Ctrl Pts',(-31.2397233614914,-54.5856885494584,
40.0619457972351));
#169500=CARTESIAN_POINT('Ctrl Pts',(-31.2397569340484,-54.58569112004,40.0619760547305));
#169501=CARTESIAN_POINT('Ctrl Pts',(-31.239790512345,-54.5856936840715,
40.0620063077269));
#169502=CARTESIAN_POINT('Ctrl Pts',(-31.2433907885846,-54.5859686003824,
40.06525004417));
#169503=CARTESIAN_POINT('Ctrl Pts',(-31.2470554817643,-54.5861671393375,
40.0684393223556));
#169504=CARTESIAN_POINT('Ctrl Pts',(-31.2507796687841,-54.5862889570922,
40.0715697951759));
#169505=CARTESIAN_POINT('Ctrl Pts',(-31.2715039227789,-54.5869668451993,
40.0889901646435));
#169506=CARTESIAN_POINT('Ctrl Pts',(-31.2940703036764,-54.5852738987617,
40.1045963098268));
#169507=CARTESIAN_POINT('Ctrl Pts',(-31.317591977259,-54.5811905703954,
40.1176634650757));
#169508=CARTESIAN_POINT('Ctrl Pts',(-31.328148830096,-54.5793579160778,
40.1235281853082));
#169509=CARTESIAN_POINT('Ctrl Pts',(-31.3388983725528,-54.5770440083377,
40.1288820140929));
#169510=CARTESIAN_POINT('Ctrl Pts',(-31.3497625287428,-54.5742478788458,
40.1336621774101));
#169511=CARTESIAN_POINT('Ctrl Pts',(-31.3544839440758,-54.5730327187887,
40.1357395717319));
#169512=CARTESIAN_POINT('Ctrl Pts',(-31.3592268152914,-54.5717264106368,
40.1377083672884));
#169513=CARTESIAN_POINT('Ctrl Pts',(-31.3639846100471,-54.5703288332446,
40.1395632548792));
#169514=CARTESIAN_POINT('Ctrl Pts',(-31.380636891692,-54.5654373123718,
40.146055361447));
#169515=CARTESIAN_POINT('Ctrl Pts',(-31.3974719850963,-54.559427740509,
40.1511520974629));
#169516=CARTESIAN_POINT('Ctrl Pts',(-31.4142098249418,-54.5522949389284,
40.1546258197409));
#169517=CARTESIAN_POINT('Ctrl Pts',(-31.4225787448645,-54.5487285381382,
40.1563626808798));
#169518=CARTESIAN_POINT('Ctrl Pts',(-31.4309233516994,-54.5448813304463,
40.1576937882008));
#169519=CARTESIAN_POINT('Ctrl Pts',(-31.4392086412365,-54.5407526753746,
40.1585906813668));
#169520=CARTESIAN_POINT('Ctrl Pts',(-31.443351286005,-54.5386883478388,
40.1590391279498));
#169521=CARTESIAN_POINT('Ctrl Pts',(-31.4474791015107,-54.5365536585646,
40.1593790209175));
#169522=CARTESIAN_POINT('Ctrl Pts',(-31.4515877125784,-54.5343485280975,
40.1596068022931));
#169523=CARTESIAN_POINT('Ctrl Pts',(-31.4556963236462,-54.5321433976303,
40.1598345836687));
#169524=CARTESIAN_POINT('Ctrl Pts',(-31.4597857294232,-54.5298678244923,
40.1599502506865));
#169525=CARTESIAN_POINT('Ctrl Pts',(-31.4638515574743,-54.5275217339718,
40.1599502534424));
#169526=CARTESIAN_POINT('',(-31.490293248291,-54.5122556166609,40.1599502534424));
#169527=CARTESIAN_POINT('Origin',(3.80217165444497E-17,1.34591303547096E-16,
40.1599502534424));
#169528=CARTESIAN_POINT('',(-31.6576696180587,-54.1966007261206,39.8576902534424));
#169529=CARTESIAN_POINT('Ctrl Pts',(-31.490293248291,-54.5122556166609,
40.1599502534424));
#169530=CARTESIAN_POINT('Ctrl Pts',(-31.4936024004374,-54.5103440004409,
40.1599502447858));
#169531=CARTESIAN_POINT('Ctrl Pts',(-31.4968786114295,-54.5083962906203,
40.1598744685927));
#169532=CARTESIAN_POINT('Ctrl Pts',(-31.5001207716287,-54.5064144237354,
40.1597246934279));
#169533=CARTESIAN_POINT('Ctrl Pts',(-31.5188564579439,-54.4949616780375,
40.1588591777433));
#169534=CARTESIAN_POINT('Ctrl Pts',(-31.5364583843255,-54.4823684499286,
40.1555254706007));
#169535=CARTESIAN_POINT('Ctrl Pts',(-31.5527059087924,-54.4690111814025,
40.1500631826348));
#169536=CARTESIAN_POINT('Ctrl Pts',(-31.5592589091622,-54.4636238877399,
40.1478601162456));
#169537=CARTESIAN_POINT('Ctrl Pts',(-31.5655920544915,-54.4581123526876,
40.1453112228293));
#169538=CARTESIAN_POINT('Ctrl Pts',(-31.57169271884,-54.4525012314183,40.1424401896328));
#169539=CARTESIAN_POINT('Ctrl Pts',(-31.5739434935988,-54.4504310683344,
40.1413809526906));
#169540=CARTESIAN_POINT('Ctrl Pts',(-31.5761624901353,-54.4483473527932,
40.1402777640512));
#169541=CARTESIAN_POINT('Ctrl Pts',(-31.5783490084909,-54.4462513257025,
40.1391317641987));
#169542=CARTESIAN_POINT('Ctrl Pts',(-31.5824487304078,-54.4423212749072,
40.1369830144753));
#169543=CARTESIAN_POINT('Ctrl Pts',(-31.5864342712172,-54.4383479413153,
40.134683756585));
#169544=CARTESIAN_POINT('Ctrl Pts',(-31.5903010169872,-54.4343395048293,
40.1322415082996));
#169545=CARTESIAN_POINT('Ctrl Pts',(-31.6038346271821,-54.4203099771282,
40.1236936393009));
#169546=CARTESIAN_POINT('Ctrl Pts',(-31.6159129958989,-54.4058504350956,
40.113394140767));
#169547=CARTESIAN_POINT('Ctrl Pts',(-31.6263383134319,-54.3913116139984,
40.101665321223));
#169548=CARTESIAN_POINT('Ctrl Pts',(-31.6315509721984,-54.3840422034499,
40.095800911451));
#169549=CARTESIAN_POINT('Ctrl Pts',(-31.6363503686739,-54.3767529740102,
40.0895791707949));
#169550=CARTESIAN_POINT('Ctrl Pts',(-31.6407117811307,-54.3694877752602,
40.0830403822906));
#169551=CARTESIAN_POINT('Ctrl Pts',(-31.6428924873591,-54.3658551758851,
40.0797709880385));
#169552=CARTESIAN_POINT('Ctrl Pts',(-31.6449636976424,-54.3622285842837,
40.0764223317514));
#169553=CARTESIAN_POINT('Ctrl Pts',(-31.6469223220355,-54.3586134821115,
40.0729994484778));
#169554=CARTESIAN_POINT('Ctrl Pts',(-31.6488809464287,-54.3549983799394,
40.0695765652042));
#169555=CARTESIAN_POINT('Ctrl Pts',(-31.6507268563402,-54.3513947831119,
40.0660793733488));
#169556=CARTESIAN_POINT('Ctrl Pts',(-31.6524572252919,-54.3478081421436,
40.0625130768817));
#169557=CARTESIAN_POINT('Ctrl Pts',(-31.6524719817151,-54.3477775556078,
40.0624826638418));
#169558=CARTESIAN_POINT('Ctrl Pts',(-31.6524867297707,-54.3477469704399,
40.0624522459912));
#169559=CARTESIAN_POINT('Ctrl Pts',(-31.6525014694577,-54.347716386643,
40.0624218233329));
#169560=CARTESIAN_POINT('Ctrl Pts',(-31.6600292427982,-54.3320967950452,
40.0468845275896));
#169561=CARTESIAN_POINT('Ctrl Pts',(-31.6655043152793,-54.3168578829677,
40.0302263329231));
#169562=CARTESIAN_POINT('Ctrl Pts',(-31.6690725678687,-54.3021370826328,
40.0127515884733));
#169563=CARTESIAN_POINT('Ctrl Pts',(-31.6727614963913,-54.2869184346054,
39.9946858597698));
#169564=CARTESIAN_POINT('Ctrl Pts',(-31.6744122539941,-54.2722526596734,
39.9757460620465));
#169565=CARTESIAN_POINT('Ctrl Pts',(-31.6741352403913,-54.2583037507934,
39.9562444559096));
#169566=CARTESIAN_POINT('Ctrl Pts',(-31.6738634961701,-54.2446201795118,
39.9371138113571));
#169567=CARTESIAN_POINT('Ctrl Pts',(-31.6717360657809,-54.2316257183431,
39.9174410654305));
#169568=CARTESIAN_POINT('Ctrl Pts',(-31.6678154208133,-54.2194985998727,
39.8975196504089));
#169569=CARTESIAN_POINT('Ctrl Pts',(-31.6652181309745,-54.2114648090456,
39.8843224113736));
#169570=CARTESIAN_POINT('Ctrl Pts',(-31.6618330358507,-54.2038121508387,
39.8710160447113));
#169571=CARTESIAN_POINT('Ctrl Pts',(-31.6576696180587,-54.1966007261206,
39.8576902534424));
#169572=CARTESIAN_POINT('',(-31.4795232016792,-53.8880358395969,39.2875012672119));
#169573=CARTESIAN_POINT('',(-31.6576696180587,-54.1966007261206,39.8576902534424));
#169574=CARTESIAN_POINT('',(-36.4252947698681,-50.6762142289946,39.2875012672119));
#169575=CARTESIAN_POINT('Origin',(5.53234440788222E-15,0.,39.2875012672119));
#169576=CARTESIAN_POINT('',(-36.6347241449657,-50.9644637245891,39.8576902534424));
#169577=CARTESIAN_POINT('',(-36.4252947698681,-50.6762142289946,39.2875012672119));
#169578=CARTESIAN_POINT('',(-36.991167339171,-50.93994621282,40.1599502534424));
#169579=CARTESIAN_POINT('Ctrl Pts',(-36.6347241449657,-50.9644637245891,
39.8576902534424));
#169580=CARTESIAN_POINT('Ctrl Pts',(-36.641957498789,-50.9744193574523,
39.8773836120336));
#169581=CARTESIAN_POINT('Ctrl Pts',(-36.6507449107767,-50.9831959997502,
39.8969946442077));
#169582=CARTESIAN_POINT('Ctrl Pts',(-36.6609215604495,-50.9907013072098,
39.9162525288159));
#169583=CARTESIAN_POINT('Ctrl Pts',(-36.6713026986838,-50.9983574255528,
39.9358973793952));
#169584=CARTESIAN_POINT('Ctrl Pts',(-36.6831299757253,-51.0046913806501,
39.9551762199601));
#169585=CARTESIAN_POINT('Ctrl Pts',(-36.6962763075769,-51.0095813473111,
39.9738152034078));
#169586=CARTESIAN_POINT('Ctrl Pts',(-36.7089119163533,-51.0142813432002,
39.9917300792449));
#169587=CARTESIAN_POINT('Ctrl Pts',(-36.7227668523395,-51.0176477981061,
40.0090551157899));
#169588=CARTESIAN_POINT('Ctrl Pts',(-36.7377619898945,-51.0195423439486,
40.0255394551289));
#169589=CARTESIAN_POINT('Ctrl Pts',(-36.74928073423,-51.0209976683236,40.0382021525992));
#169590=CARTESIAN_POINT('Ctrl Pts',(-36.7614730081759,-51.0215839370839,
40.0503687782048));
#169591=CARTESIAN_POINT('Ctrl Pts',(-36.7743133764174,-51.0212231059803,
40.0619155352442));
#169592=CARTESIAN_POINT('Ctrl Pts',(-36.7743470287326,-51.0212221603063,
40.0619457972351));
#169593=CARTESIAN_POINT('Ctrl Pts',(-36.7743806860745,-51.0212212075182,
40.0619760547305));
#169594=CARTESIAN_POINT('Ctrl Pts',(-36.77441434844,-51.0212202476159,40.0620063077269));
#169595=CARTESIAN_POINT('Ctrl Pts',(-36.7780236385692,-51.0211173265639,
40.06525004417));
#169596=CARTESIAN_POINT('Ctrl Pts',(-36.7816890091481,-51.0209317131554,
40.0684393223557));
#169597=CARTESIAN_POINT('Ctrl Pts',(-36.7854055281044,-51.0206635800336,
40.0715697951759));
#169598=CARTESIAN_POINT('Ctrl Pts',(-36.8060871110681,-51.0191714801764,
40.0889901646423));
#169599=CARTESIAN_POINT('Ctrl Pts',(-36.8283529098788,-51.0151289787601,
40.1045963098247));
#169600=CARTESIAN_POINT('Ctrl Pts',(-36.8513189052316,-51.0086093349016,
40.1176634650731));
#169601=CARTESIAN_POINT('Ctrl Pts',(-36.8616263619861,-51.0056832284519,
40.1235281853066));
#169602=CARTESIAN_POINT('Ctrl Pts',(-36.872075148106,-51.0022583633861,
40.1288820140922));
#169603=CARTESIAN_POINT('Ctrl Pts',(-36.8825875141943,-50.9983419378323,
40.1336621774101));
#169604=CARTESIAN_POINT('Ctrl Pts',(-36.8871560463067,-50.9966399122599,
40.1357395717319));
#169605=CARTESIAN_POINT('Ctrl Pts',(-36.8917363891939,-50.9948449951611,
40.1377083672884));
#169606=CARTESIAN_POINT('Ctrl Pts',(-36.896322033635,-50.9929577488697,
40.1395632548792));
#169607=CARTESIAN_POINT('Ctrl Pts',(-36.9123717891789,-50.9863523868499,
40.146055361447));
#169608=CARTESIAN_POINT('Ctrl Pts',(-36.9284864868683,-50.978615989608,
40.1511520974629));
#169609=CARTESIAN_POINT('Ctrl Pts',(-36.9443870542877,-50.9697726815834,
40.1546258197408));
#169610=CARTESIAN_POINT('Ctrl Pts',(-36.9523373379975,-50.9653510275711,
40.1563626808798));
#169611=CARTESIAN_POINT('Ctrl Pts',(-36.9602340894951,-50.9606526463564,
40.1576937882008));
#169612=CARTESIAN_POINT('Ctrl Pts',(-36.9680424293792,-50.9556805599062,
40.1585906813668));
#169613=CARTESIAN_POINT('Ctrl Pts',(-36.9719465993212,-50.953194516681,
40.1590391279498));
#169614=CARTESIAN_POINT('Ctrl Pts',(-36.9758286664323,-50.9506400472467,
40.1593790209175));
#169615=CARTESIAN_POINT('Ctrl Pts',(-36.9796842711996,-50.9480175299139,
40.1596068022931));
#169616=CARTESIAN_POINT('Ctrl Pts',(-36.983539875967,-50.9453950125811,
40.1598345836687));
#169617=CARTESIAN_POINT('Ctrl Pts',(-36.9873690173881,-50.9427044459692,
40.1599502506865));
#169618=CARTESIAN_POINT('Ctrl Pts',(-36.991167339171,-50.93994621282,40.1599502534424));
#169619=CARTESIAN_POINT('',(-37.0158684358562,-50.9219998155898,40.1599502534424));
#169620=CARTESIAN_POINT('Origin',(5.16646552926933E-17,1.25731475530457E-16,
40.1599502534424));
#169621=CARTESIAN_POINT('',(-37.1493329797263,-50.5905785208482,39.8576902534424));
#169622=CARTESIAN_POINT('Ctrl Pts',(-37.0158684358562,-50.9219998155898,
40.1599502534424));
#169623=CARTESIAN_POINT('Ctrl Pts',(-37.0189596418151,-50.9197527708149,
40.1599502447858));
#169624=CARTESIAN_POINT('Ctrl Pts',(-37.0220143142661,-50.9174732734521,
40.1598744685927));
#169625=CARTESIAN_POINT('Ctrl Pts',(-37.0250315520727,-50.9151633654181,
40.1597246934279));
#169626=CARTESIAN_POINT('Ctrl Pts',(-37.0424674644255,-50.9018149465641,
40.1588591777435));
#169627=CARTESIAN_POINT('Ctrl Pts',(-37.0586566148271,-50.8874508031651,
40.1555254706024));
#169628=CARTESIAN_POINT('Ctrl Pts',(-37.0734189188993,-50.8724683783931,
40.150063182639));
#169629=CARTESIAN_POINT('Ctrl Pts',(-37.0793728957238,-50.8664256218268,
40.1478601162488));
#169630=CARTESIAN_POINT('Ctrl Pts',(-37.0850952351349,-50.8602822855875,
40.145311222831));
#169631=CARTESIAN_POINT('Ctrl Pts',(-37.0905759575257,-50.8540642095544,
40.1424401896328));
#169632=CARTESIAN_POINT('Ctrl Pts',(-37.092598011339,-50.8517701170138,
40.1413809526905));
#169633=CARTESIAN_POINT('Ctrl Pts',(-37.0945870443968,-50.8494658679864,
40.1402777640511));
#169634=CARTESIAN_POINT('Ctrl Pts',(-37.0965424902854,-50.8471527697477,
40.1391317641987));
#169635=CARTESIAN_POINT('Ctrl Pts',(-37.1002089513264,-50.8428157105502,
40.1369830144753));
#169636=CARTESIAN_POINT('Ctrl Pts',(-37.1037573324719,-50.8384475408393,
40.1346837565849));
#169637=CARTESIAN_POINT('Ctrl Pts',(-37.107183900098,-50.8340568779946,
40.1322415082996));
#169638=CARTESIAN_POINT('Ctrl Pts',(-37.1191768867892,-50.8186895580381,
40.1236936393009));
#169639=CARTESIAN_POINT('Ctrl Pts',(-37.1296776552302,-50.8030466935689,
40.113394140767));
#169640=CARTESIAN_POINT('Ctrl Pts',(-37.1385261411559,-50.7874977752341,
40.101665321223));
#169641=CARTESIAN_POINT('Ctrl Pts',(-37.1429503841188,-50.7797233160668,
40.095800911451));
#169642=CARTESIAN_POINT('Ctrl Pts',(-37.1469615570465,-50.7719723442505,
40.0895791707949));
#169643=CARTESIAN_POINT('Ctrl Pts',(-37.1505396571688,-50.7642910532776,
40.0830403822906));
#169644=CARTESIAN_POINT('Ctrl Pts',(-37.1523287072299,-50.7604504077911,
40.0797709880385));
#169645=CARTESIAN_POINT('Ctrl Pts',(-37.1540094891596,-50.7566271826099,
40.0764223317514));
#169646=CARTESIAN_POINT('Ctrl Pts',(-37.1555795029288,-50.7528271523478,
40.0729994484778));
#169647=CARTESIAN_POINT('Ctrl Pts',(-37.1571495166979,-50.7490271220856,
40.0695765652042));
#169648=CARTESIAN_POINT('Ctrl Pts',(-37.1586086360832,-50.7452503160123,
40.0660793733488));
#169649=CARTESIAN_POINT('Ctrl Pts',(-37.159954619824,-50.7415024502311,
40.0625130768817));
#169650=CARTESIAN_POINT('Ctrl Pts',(-37.1599660982464,-50.7414704887852,
40.0624826638418));
#169651=CARTESIAN_POINT('Ctrl Pts',(-37.15997756849,-50.7414385295745,40.0624522459912));
#169652=CARTESIAN_POINT('Ctrl Pts',(-37.1599890305542,-50.741406572602,
40.0624218233329));
#169653=CARTESIAN_POINT('Ctrl Pts',(-37.1658428740573,-50.7250856801843,
40.0468845275916));
#169654=CARTESIAN_POINT('Ctrl Pts',(-37.1696950534569,-50.709357947551,
40.0302263329275));
#169655=CARTESIAN_POINT('Ctrl Pts',(-37.1717050161484,-50.6943448053427,
40.0127515884803));
#169656=CARTESIAN_POINT('Ctrl Pts',(-37.1737829544435,-50.6788239286339,
39.9946858597795));
#169657=CARTESIAN_POINT('Ctrl Pts',(-37.1738916781079,-50.6640659431977,
39.9757460620591));
#169658=CARTESIAN_POINT('Ctrl Pts',(-37.1721581240063,-50.6502224037077,
39.9562444559252));
#169659=CARTESIAN_POINT('Ctrl Pts',(-37.1704575457515,-50.6366421974684,
39.9371138113754));
#169660=CARTESIAN_POINT('Ctrl Pts',(-37.1669834785932,-50.6239412983478,
39.9174410654515));
#169661=CARTESIAN_POINT('Ctrl Pts',(-37.1618166822734,-50.6122904324954,
39.8975196504326));
#169662=CARTESIAN_POINT('Ctrl Pts',(-37.1583938608496,-50.6045721423254,
39.8843224113896));
#169663=CARTESIAN_POINT('Ctrl Pts',(-37.1542273890267,-50.5973152449674,
39.8710160447192));
#169664=CARTESIAN_POINT('Ctrl Pts',(-37.1493329797263,-50.5905785208482,
39.8576902534424));
#169665=CARTESIAN_POINT('',(-36.9399086546489,-50.3023253561993,39.2875012672119));
#169666=CARTESIAN_POINT('',(-37.1493329797263,-50.5905785208482,39.8576902534424));
#169667=CARTESIAN_POINT('',(-41.5228599914565,-46.5911245387428,39.2875012672119));
#169668=CARTESIAN_POINT('Origin',(5.53234440788222E-15,0.,39.2875012672119));
#169669=CARTESIAN_POINT('',(-41.7612723673365,-46.8559036426983,39.8576902534424));
#169670=CARTESIAN_POINT('',(-41.5228599914565,-46.5911245387428,39.2875012672119));
#169671=CARTESIAN_POINT('',(-42.1132001506003,-46.7942619810915,40.1599502534424));
#169672=CARTESIAN_POINT('Ctrl Pts',(-41.7612723673365,-46.8559036426983,
39.8576902534424));
#169673=CARTESIAN_POINT('Ctrl Pts',(-41.7695067430955,-46.8650486462049,
39.8773836120361));
#169674=CARTESIAN_POINT('Ctrl Pts',(-41.7791634256543,-46.8728586744677,
39.8969946442126));
#169675=CARTESIAN_POINT('Ctrl Pts',(-41.7900688448321,-46.8792591175168,
39.9162525288231));
#169676=CARTESIAN_POINT('Ctrl Pts',(-41.8011933963918,-46.8857881704164,
39.9358973794051));
#169677=CARTESIAN_POINT('Ctrl Pts',(-41.813617960967,-46.8908511403512,
39.9551762199724));
#169678=CARTESIAN_POINT('Ctrl Pts',(-41.8272034165403,-46.8943401533968,
39.9738152034225));
#169679=CARTESIAN_POINT('Ctrl Pts',(-41.8402610894803,-46.8976936214485,
39.9917300792623));
#169680=CARTESIAN_POINT('Ctrl Pts',(-41.8543920170388,-46.8995933993941,
40.0090551158097));
#169681=CARTESIAN_POINT('Ctrl Pts',(-41.8695030436303,-46.8999101480296,
40.0255394551508));
#169682=CARTESIAN_POINT('Ctrl Pts',(-41.8811108098936,-46.90015346334,40.0382021526132));
#169683=CARTESIAN_POINT('Ctrl Pts',(-41.893297575053,-46.8994620807992,
40.0503687782115));
#169684=CARTESIAN_POINT('Ctrl Pts',(-41.9060298852857,-46.897761042407,
40.0619155352442));
#169685=CARTESIAN_POINT('Ctrl Pts',(-41.9060632544001,-46.8977565842888,
40.0619457972351));
#169686=CARTESIAN_POINT('Ctrl Pts',(-41.9060966277702,-46.8977521185699,
40.0619760547305));
#169687=CARTESIAN_POINT('Ctrl Pts',(-41.9061300053926,-46.8977476452507,
40.0620063077269));
#169688=CARTESIAN_POINT('Ctrl Pts',(-41.9097087652733,-46.8972680144603,
40.06525004417));
#169689=CARTESIAN_POINT('Ctrl Pts',(-41.9133346546844,-46.8967002823075,
40.0684393223556));
#169690=CARTESIAN_POINT('Ctrl Pts',(-41.9170027866178,-46.8960451360318,
40.0715697951759));
#169691=CARTESIAN_POINT('Ctrl Pts',(-41.9374151067974,-46.8923993959692,
40.0889901646392));
#169692=CARTESIAN_POINT('Ctrl Pts',(-41.9591363747676,-46.8860516300672,
40.1045963098192));
#169693=CARTESIAN_POINT('Ctrl Pts',(-41.9812950716372,-46.8771671013007,
40.1176634650662));
#169694=CARTESIAN_POINT('Ctrl Pts',(-41.9912402016585,-46.8731796017523,
40.1235281853024));
#169695=CARTESIAN_POINT('Ctrl Pts',(-42.0012737523565,-46.8686813028981,
40.1288820140903));
#169696=CARTESIAN_POINT('Ctrl Pts',(-42.0113191526628,-46.8636874904588,
40.1336621774101));
#169697=CARTESIAN_POINT('Ctrl Pts',(-42.0156847477608,-46.8615172471195,
40.1357395717319));
#169698=CARTESIAN_POINT('Ctrl Pts',(-42.0200523791243,-46.8592533865611,
40.1377083672884));
#169699=CARTESIAN_POINT('Ctrl Pts',(-42.0244156319707,-46.8568971484358,
40.1395632548792));
#169700=CARTESIAN_POINT('Ctrl Pts',(-42.0396870169331,-46.8486503149974,
40.146055361447));
#169701=CARTESIAN_POINT('Ctrl Pts',(-42.0549047629075,-46.8392718539636,
40.151152097463));
#169702=CARTESIAN_POINT('Ctrl Pts',(-42.069793847957,-46.8288149286282,
40.1546258197409));
#169703=CARTESIAN_POINT('Ctrl Pts',(-42.0772383904817,-46.8235864659605,
40.1563626808798));
#169704=CARTESIAN_POINT('Ctrl Pts',(-42.0846007681801,-46.8180883876709,
40.1576937882008));
#169705=CARTESIAN_POINT('Ctrl Pts',(-42.0918466086054,-46.8123273450617,
40.1585906813668));
#169706=CARTESIAN_POINT('Ctrl Pts',(-42.095469528818,-46.8094468237571,
40.1590391279498));
#169707=CARTESIAN_POINT('Ctrl Pts',(-42.0990633147948,-46.8065005614642,
40.1593790209175));
#169708=CARTESIAN_POINT('Ctrl Pts',(-42.1026236704492,-46.8034893901144,
40.1596068022931));
#169709=CARTESIAN_POINT('Ctrl Pts',(-42.1061840261036,-46.8004782187647,
40.1598345836687));
#169710=CARTESIAN_POINT('Ctrl Pts',(-42.1097109502941,-46.7974021370899,
40.1599502506865));
#169711=CARTESIAN_POINT('Ctrl Pts',(-42.1132001506003,-46.7942619810915,
40.1599502534424));
#169712=CARTESIAN_POINT('',(-42.1358900227697,-46.7738319284255,40.1599502534424));
#169713=CARTESIAN_POINT('Origin',(6.43067523875937E-17,1.15494107156903E-16,
40.1599502534424));
#169714=CARTESIAN_POINT('',(-42.2339804752703,-46.4302753505423,39.8576902534424));
#169715=CARTESIAN_POINT('Ctrl Pts',(-42.1358900227697,-46.7738319284255,
40.1599502534424));
#169716=CARTESIAN_POINT('Ctrl Pts',(-42.1387294146417,-46.7712740741885,
40.1599502447858));
#169717=CARTESIAN_POINT('Ctrl Pts',(-42.141529080921,-46.7686877639337,
40.1598744685927));
#169718=CARTESIAN_POINT('Ctrl Pts',(-42.1442883388461,-46.7660751225864,
40.1597246934279));
#169719=CARTESIAN_POINT('Ctrl Pts',(-42.1602334457364,-46.750977278644,
40.1588591777436));
#169720=CARTESIAN_POINT('Ctrl Pts',(-42.1748324484421,-46.7349995965129,
40.1555254706026));
#169721=CARTESIAN_POINT('Ctrl Pts',(-42.1879477932303,-46.718556166073,
40.1500631826395));
#169722=CARTESIAN_POINT('Ctrl Pts',(-42.1932375134894,-46.7119241523112,
40.1478601162492));
#169723=CARTESIAN_POINT('Ctrl Pts',(-42.1982863518304,-46.7052163225652,
40.1453112228313));
#169724=CARTESIAN_POINT('Ctrl Pts',(-42.2030870843187,-46.6984594183137,
40.1424401896328));
#169725=CARTESIAN_POINT('Ctrl Pts',(-42.2048582631417,-46.6959665308743,
40.1413809526906));
#169726=CARTESIAN_POINT('Ctrl Pts',(-42.2065955404585,-46.6934669941952,
40.1402777640512));
#169727=CARTESIAN_POINT('Ctrl Pts',(-42.2082984896056,-46.690962167597,
40.1391317641987));
#169728=CARTESIAN_POINT('Ctrl Pts',(-42.2114915192564,-46.6862656177252,
40.1369830144753));
#169729=CARTESIAN_POINT('Ctrl Pts',(-42.2145638639316,-46.6815504704769,
40.134683756585));
#169730=CARTESIAN_POINT('Ctrl Pts',(-42.2175127112217,-46.6768256862944,
40.1322415082996));
#169731=CARTESIAN_POINT('Ctrl Pts',(-42.2278336767374,-46.6602889416557,
40.1236936393009));
#169732=CARTESIAN_POINT('Ctrl Pts',(-42.2366417962861,-46.6436341412465,
40.113394140767));
#169733=CARTESIAN_POINT('Ctrl Pts',(-42.2438165047411,-46.6272454828772,
40.101665321223));
#169734=CARTESIAN_POINT('Ctrl Pts',(-42.2474038589686,-46.6190511536926,
40.095800911451));
#169735=CARTESIAN_POINT('Ctrl Pts',(-42.2505828610986,-46.6109233607689,
40.0895791707949));
#169736=CARTESIAN_POINT('Ctrl Pts',(-42.2533384464727,-46.6029101354044,
40.0830403822907));
#169737=CARTESIAN_POINT('Ctrl Pts',(-42.2547162391598,-46.5989035227222,
40.0797709880385));
#169738=CARTESIAN_POINT('Ctrl Pts',(-42.2559881777373,-46.5949255520163,
40.0764223317514));
#169739=CARTESIAN_POINT('Ctrl Pts',(-42.2571523794831,-46.590982227591,
40.0729994484778));
#169740=CARTESIAN_POINT('Ctrl Pts',(-42.2583165812288,-46.5870389031656,
40.0695765652042));
#169741=CARTESIAN_POINT('Ctrl Pts',(-42.2593729236706,-46.5831302673241,
40.0660793733488));
#169742=CARTESIAN_POINT('Ctrl Pts',(-42.2603197753209,-46.5792622391317,
40.0625130768817));
#169743=CARTESIAN_POINT('Ctrl Pts',(-42.2603278499825,-46.5792292529522,
40.0624826638418));
#169744=CARTESIAN_POINT('Ctrl Pts',(-42.2603359167438,-46.5791962698504,
40.0624522459912));
#169745=CARTESIAN_POINT('Ctrl Pts',(-42.2603439756043,-46.5791632898296,
40.0624218233329));
#169746=CARTESIAN_POINT('Ctrl Pts',(-42.2644597533373,-46.5623199117001,
40.0468845275892));
#169747=CARTESIAN_POINT('Ctrl Pts',(-42.2666468343722,-46.5462756748365,
40.0302263329223));
#169748=CARTESIAN_POINT('Ctrl Pts',(-42.2670764855933,-46.5311346778787,
40.0127515884721));
#169749=CARTESIAN_POINT('Ctrl Pts',(-42.2675206673335,-46.5154816224575,
39.9946858597679));
#169750=CARTESIAN_POINT('Ctrl Pts',(-42.2660861658585,-46.5007931180901,
39.9757460620439));
#169751=CARTESIAN_POINT('Ctrl Pts',(-42.2629150644368,-46.4872066207025,
39.9562444559062));
#169752=CARTESIAN_POINT('Ctrl Pts',(-42.2598042840369,-46.4738785670839,
39.9371138113525));
#169753=CARTESIAN_POINT('Ctrl Pts',(-42.2550216427124,-46.4616103837176,
39.9174410654245));
#169754=CARTESIAN_POINT('Ctrl Pts',(-42.2486653035375,-46.4505634198058,
39.8975196504016));
#169755=CARTESIAN_POINT('Ctrl Pts',(-42.2444544516793,-46.4432451935069,
39.8843224113688));
#169756=CARTESIAN_POINT('Ctrl Pts',(-42.2395522518995,-46.4364635650945,
39.8710160447088));
#169757=CARTESIAN_POINT('Ctrl Pts',(-42.2339804752703,-46.4302753505423,
39.8576902534424));
#169758=CARTESIAN_POINT('',(-41.9955727382253,-46.165492069761,39.2875012672119));
#169759=CARTESIAN_POINT('',(-42.2339804752703,-46.4302753505423,39.8576902534424));
#169760=CARTESIAN_POINT('',(-46.1654920697614,-41.9955727382249,39.2875012672119));
#169761=CARTESIAN_POINT('Origin',(5.53234440788222E-15,0.,39.2875012672119));
#169762=CARTESIAN_POINT('',(-46.4302753505427,-42.2339804752699,39.8576902534424));
#169763=CARTESIAN_POINT('',(-46.1654920697614,-41.9955727382249,39.2875012672119));
#169764=CARTESIAN_POINT('',(-46.7738319284259,-42.1358900227692,40.1599502534424));
#169765=CARTESIAN_POINT('Ctrl Pts',(-46.4302753505427,-42.2339804752699,
39.8576902534424));
#169766=CARTESIAN_POINT('Ctrl Pts',(-46.4394205306938,-42.2422146548471,
39.8773836120379));
#169767=CARTESIAN_POINT('Ctrl Pts',(-46.4498406831885,-42.2489725007703,
39.8969946442163));
#169768=CARTESIAN_POINT('Ctrl Pts',(-46.4613553898164,-42.2541979548149,
39.9162525288286));
#169769=CARTESIAN_POINT('Ctrl Pts',(-46.4731014717862,-42.2595284086007,
39.9358973794123));
#169770=CARTESIAN_POINT('Ctrl Pts',(-46.4859871977651,-42.2632649224146,
39.9551762199814));
#169771=CARTESIAN_POINT('Ctrl Pts',(-46.499862931965,-42.2653147554874,
39.9738152034329));
#169772=CARTESIAN_POINT('Ctrl Pts',(-46.5131996064699,-42.2672849544035,
39.9917300792741));
#169773=CARTESIAN_POINT('Ctrl Pts',(-46.5274517041996,-42.2676972410238,
40.0090551158227));
#169774=CARTESIAN_POINT('Ctrl Pts',(-46.5425130602562,-42.2664327220881,
40.0255394551647));
#169775=CARTESIAN_POINT('Ctrl Pts',(-46.5540826713329,-42.2654613625219,
40.0382021526222));
#169776=CARTESIAN_POINT('Ctrl Pts',(-46.5661304069589,-42.263499903613,
40.0503687782157));
#169777=CARTESIAN_POINT('Ctrl Pts',(-46.5786151613303,-42.2604772948658,
40.0619155352442));
#169778=CARTESIAN_POINT('Ctrl Pts',(-46.578647881645,-42.2604693731473,
40.0619457972352));
#169779=CARTESIAN_POINT('Ctrl Pts',(-46.5786806053975,-42.260461443425,
40.0619760547305));
#169780=CARTESIAN_POINT('Ctrl Pts',(-46.5787133325846,-42.2604535056995,
40.062006307727));
#169781=CARTESIAN_POINT('Ctrl Pts',(-46.5822223525748,-42.259602420106,
40.06525004417));
#169782=CARTESIAN_POINT('Ctrl Pts',(-46.5857690348148,-42.2586587894012,
40.0684393223556));
#169783=CARTESIAN_POINT('Ctrl Pts',(-46.5893485909042,-42.2576238078913,
40.0715697951759));
#169784=CARTESIAN_POINT('Ctrl Pts',(-46.609268006654,-42.2518643711135,
40.0889901646411));
#169785=CARTESIAN_POINT('Ctrl Pts',(-46.6302067610331,-42.243280888175,
40.1045963098226));
#169786=CARTESIAN_POINT('Ctrl Pts',(-46.6513153841062,-42.2321288152531,
40.1176634650704));
#169787=CARTESIAN_POINT('Ctrl Pts',(-46.6607892264623,-42.2271236104873,
40.123528185305));
#169788=CARTESIAN_POINT('Ctrl Pts',(-46.6702976120509,-42.2216011621505,
40.1288820140914));
#169789=CARTESIAN_POINT('Ctrl Pts',(-46.6797659870608,-42.2155846760827,
40.1336621774101));
#169790=CARTESIAN_POINT('Ctrl Pts',(-46.6838808147709,-42.2129699926167,
40.1357395717319));
#169791=CARTESIAN_POINT('Ctrl Pts',(-46.6879878819276,-42.2102619919288,
40.1377083672884));
#169792=CARTESIAN_POINT('Ctrl Pts',(-46.692080938468,-42.2074625774076,
40.1395632548792));
#169793=CARTESIAN_POINT('Ctrl Pts',(-46.7064066363596,-42.1976646265836,
40.146055361447));
#169794=CARTESIAN_POINT('Ctrl Pts',(-46.7205607018097,-42.1867468541395,
40.151152097463));
#169795=CARTESIAN_POINT('Ctrl Pts',(-46.7342751765575,-42.1747908797555,
40.1546258197409));
#169796=CARTESIAN_POINT('Ctrl Pts',(-46.7411324139314,-42.1688128925635,
40.1563626808798));
#169797=CARTESIAN_POINT('Ctrl Pts',(-46.74787975408,-42.1625753552952,40.1576937882008));
#169798=CARTESIAN_POINT('Ctrl Pts',(-46.7544837081025,-42.1560884757155,
40.1585906813668));
#169799=CARTESIAN_POINT('Ctrl Pts',(-46.7577856851138,-42.1528450359257,
40.1590391279498));
#169800=CARTESIAN_POINT('Ctrl Pts',(-46.7610518156851,-42.1495392606404,
40.1593790209175));
#169801=CARTESIAN_POINT('Ctrl Pts',(-46.7642779142249,-42.1461724262971,
40.1596068022931));
#169802=CARTESIAN_POINT('Ctrl Pts',(-46.7675040127646,-42.1428055919538,
40.1598345836687));
#169803=CARTESIAN_POINT('Ctrl Pts',(-46.770690078005,-42.1393776974106,
40.1599502506865));
#169804=CARTESIAN_POINT('Ctrl Pts',(-46.773831928426,-42.1358900227693,
40.1599502534424));
#169805=CARTESIAN_POINT('',(-46.7942619810919,-42.1132001505999,40.1599502534424));
#169806=CARTESIAN_POINT('Origin',(7.58094983678529E-17,1.03991361176644E-16,
40.1599502534424));
#169807=CARTESIAN_POINT('',(-46.8559036426987,-41.761272367336,39.8576902534424));
#169808=CARTESIAN_POINT('Ctrl Pts',(-46.7942619810919,-42.1132001505999,
40.1599502534424));
#169809=CARTESIAN_POINT('Ctrl Pts',(-46.7968184499054,-42.1103595112869,
40.1599502447858));
#169810=CARTESIAN_POINT('Ctrl Pts',(-46.7993324362835,-42.1074947242965,
40.1598744685927));
#169811=CARTESIAN_POINT('Ctrl Pts',(-46.8018034833199,-42.1046079742812,
40.1597246934279));
#169812=CARTESIAN_POINT('Ctrl Pts',(-46.8160830868189,-42.0879261203894,
40.1588591777436));
#169813=CARTESIAN_POINT('Ctrl Pts',(-46.8289319920994,-42.0705099543564,
40.1555254706033));
#169814=CARTESIAN_POINT('Ctrl Pts',(-46.8402566831411,-42.0527856759149,
40.150063182641));
#169815=CARTESIAN_POINT('Ctrl Pts',(-46.8448241915534,-42.0456370666869,
40.1478601162504));
#169816=CARTESIAN_POINT('Ctrl Pts',(-46.8491442126956,-42.0384382358192,
40.1453112228319));
#169817=CARTESIAN_POINT('Ctrl Pts',(-46.8532123574521,-42.0312165334048,
40.1424401896328));
#169818=CARTESIAN_POINT('Ctrl Pts',(-46.8547132558792,-42.0285521636631,
40.1413809526905));
#169819=CARTESIAN_POINT('Ctrl Pts',(-46.8561797434811,-42.0258847247793,
40.1402777640511));
#169820=CARTESIAN_POINT('Ctrl Pts',(-46.8576115380195,-42.0232156132259,
40.1391317641987));
#169821=CARTESIAN_POINT('Ctrl Pts',(-46.860296152779,-42.0182110290632,
40.1369830144753));
#169822=CARTESIAN_POINT('Ctrl Pts',(-46.8628587997326,-42.0132005644173,
40.1346837565849));
#169823=CARTESIAN_POINT('Ctrl Pts',(-46.8652976184989,-42.0081934246213,
40.1322415082996));
#169824=CARTESIAN_POINT('Ctrl Pts',(-46.8738334841811,-41.9906684353352,
40.1236936393008));
#169825=CARTESIAN_POINT('Ctrl Pts',(-46.8808524512365,-41.9731841724646,
40.113394140767));
#169826=CARTESIAN_POINT('Ctrl Pts',(-46.8862747746135,-41.9561353316315,
40.101665321223));
#169827=CARTESIAN_POINT('Ctrl Pts',(-46.888985936302,-41.9476109112149,
40.095800911451));
#169828=CARTESIAN_POINT('Ctrl Pts',(-46.8912979378216,-41.9391953469839,
40.0895791707949));
#169829=CARTESIAN_POINT('Ctrl Pts',(-46.8932008176776,-41.9309379818018,
40.0830403822906));
#169830=CARTESIAN_POINT('Ctrl Pts',(-46.8941522576055,-41.9268092992108,
40.0797709880385));
#169831=CARTESIAN_POINT('Ctrl Pts',(-46.8950014172056,-41.9227201664598,
40.0764223317514));
#169832=CARTESIAN_POINT('Ctrl Pts',(-46.8957470516901,-41.9186767517589,
40.0729994484778));
#169833=CARTESIAN_POINT('Ctrl Pts',(-46.8964926861745,-41.9146333370579,
40.0695765652042));
#169834=CARTESIAN_POINT('Ctrl Pts',(-46.8971346781638,-41.9106356952803,
40.0660793733488));
#169835=CARTESIAN_POINT('Ctrl Pts',(-46.8976720238189,-41.9066898836032,
40.0625130768817));
#169836=CARTESIAN_POINT('Ctrl Pts',(-46.897676606252,-41.9066562340934,
40.0624826638418));
#169837=CARTESIAN_POINT('Ctrl Pts',(-46.8976811811498,-41.9066225884704,
40.0624522459912));
#169838=CARTESIAN_POINT('Ctrl Pts',(-46.8976857485122,-41.9065889467373,
40.0624218233329));
#169839=CARTESIAN_POINT('Ctrl Pts',(-46.9000183671518,-41.8894076224754,
40.0468845275905));
#169840=CARTESIAN_POINT('Ctrl Pts',(-46.9005163877045,-41.8732226654017,
40.0302263329251));
#169841=CARTESIAN_POINT('Ctrl Pts',(-46.8993610201074,-41.8581197016285,
40.0127515884765));
#169842=CARTESIAN_POINT('Ctrl Pts',(-46.8981665787455,-41.8425059656494,
39.9946858597745));
#169843=CARTESIAN_POINT('Ctrl Pts',(-46.8952045688313,-41.8280478726817,
39.9757460620529));
#169844=CARTESIAN_POINT('Ctrl Pts',(-46.8906306633432,-41.8148672739078,
39.9562444559176));
#169845=CARTESIAN_POINT('Ctrl Pts',(-46.886143763162,-41.8019373978574,
39.9371138113668));
#169846=CARTESIAN_POINT('Ctrl Pts',(-46.8801049472944,-41.7902363430322,
39.9174410654419));
#169847=CARTESIAN_POINT('Ctrl Pts',(-46.872628706651,-41.7799143139112,
39.897519650422));
#169848=CARTESIAN_POINT('Ctrl Pts',(-46.8676759593291,-41.7730763314914,
39.8843224113824));
#169849=CARTESIAN_POINT('Ctrl Pts',(-46.8620917411135,-41.7668442729553,
39.8710160447157));
#169850=CARTESIAN_POINT('Ctrl Pts',(-46.8559036426987,-41.761272367336,
39.8576902534424));
#169851=CARTESIAN_POINT('',(-46.5911245387432,-41.522859991456,39.2875012672119));
#169852=CARTESIAN_POINT('',(-46.8559036426987,-41.761272367336,39.8576902534424));
#169853=CARTESIAN_POINT('',(-50.3023253561997,-36.9399086546484,39.2875012672119));
#169854=CARTESIAN_POINT('Origin',(5.53234440788222E-15,0.,39.2875012672119));
#169855=CARTESIAN_POINT('',(-50.5905785208486,-37.1493329797258,39.8576902534424));
#169856=CARTESIAN_POINT('',(-50.3023253561997,-36.9399086546484,39.2875012672119));
#169857=CARTESIAN_POINT('',(-50.9219998155902,-37.0158684358557,40.1599502534424));
#169858=CARTESIAN_POINT('Ctrl Pts',(-50.5905785208486,-37.1493329797258,
39.8576902534424));
#169859=CARTESIAN_POINT('Ctrl Pts',(-50.6005343088827,-37.1565661199776,
39.8773836120365));
#169860=CARTESIAN_POINT('Ctrl Pts',(-50.6116037659404,-37.1621977431861,
39.8969946442134));
#169861=CARTESIAN_POINT('Ctrl Pts',(-50.6236016024807,-37.1661909570579,
39.9162525288243));
#169862=CARTESIAN_POINT('Ctrl Pts',(-50.6358405223261,-37.1702644101623,
39.9358973794066));
#169863=CARTESIAN_POINT('Ctrl Pts',(-50.6490462309955,-37.1726335298281,
39.9551762199742));
#169864=CARTESIAN_POINT('Ctrl Pts',(-50.6630602183712,-37.1732217245287,
39.9738152034244));
#169865=CARTESIAN_POINT('Ctrl Pts',(-50.6765297750414,-37.1737870683984,
39.9917300792642));
#169866=CARTESIAN_POINT('Ctrl Pts',(-50.6907468939737,-37.1727073465962,
40.0090551158116));
#169867=CARTESIAN_POINT('Ctrl Pts',(-50.7055935641233,-37.1698754144254,
40.0255394551526));
#169868=CARTESIAN_POINT('Ctrl Pts',(-50.7169982609406,-37.1677000224021,
40.0382021526144));
#169869=CARTESIAN_POINT('Ctrl Pts',(-50.7287749695284,-37.1644899772788,
40.0503687782121));
#169870=CARTESIAN_POINT('Ctrl Pts',(-50.7408753824655,-37.1601789145085,
40.0619155352442));
#169871=CARTESIAN_POINT('Ctrl Pts',(-50.7409070954898,-37.1601676159818,
40.0619457972351));
#169872=CARTESIAN_POINT('Ctrl Pts',(-50.7409388110965,-37.1601563091358,
40.0619760547305));
#169873=CARTESIAN_POINT('Ctrl Pts',(-50.7409705292823,-37.1601449939714,
40.0620063077269));
#169874=CARTESIAN_POINT('Ctrl Pts',(-50.7443713638247,-37.1589317782467,
40.06525004417));
#169875=CARTESIAN_POINT('Ctrl Pts',(-50.7477999807009,-37.1576225876054,
40.0684393223556));
#169876=CARTESIAN_POINT('Ctrl Pts',(-50.7512517425808,-37.1562191103353,
40.0715697951759));
#169877=CARTESIAN_POINT('Ctrl Pts',(-50.7704600126119,-37.148409078437,
40.0889901646418));
#169878=CARTESIAN_POINT('Ctrl Pts',(-50.7903868440233,-37.1376839208976,
40.1045963098238));
#169879=CARTESIAN_POINT('Ctrl Pts',(-50.8102141228066,-37.1243864882659,
40.1176634650719));
#169880=CARTESIAN_POINT('Ctrl Pts',(-50.8191128800998,-37.1184184163531,
40.1235281853059));
#169881=CARTESIAN_POINT('Ctrl Pts',(-50.8279919247184,-37.1119323236329,
40.1288820140919));
#169882=CARTESIAN_POINT('Ctrl Pts',(-50.8367795369357,-37.1049590818164,
40.1336621774102));
#169883=CARTESIAN_POINT('Ctrl Pts',(-50.8405985143444,-37.1019286052429,
40.135739571732));
#169884=CARTESIAN_POINT('Ctrl Pts',(-50.844400019407,-37.0988061338476,
40.1377083672884));
#169885=CARTESIAN_POINT('Ctrl Pts',(-50.8481780352575,-37.0955942139019,
40.1395632548792));
#169886=CARTESIAN_POINT('Ctrl Pts',(-50.8614010907343,-37.0843524940918,
40.146055361447));
#169887=CARTESIAN_POINT('Ctrl Pts',(-50.874336400757,-37.072015027637,40.151152097463));
#169888=CARTESIAN_POINT('Ctrl Pts',(-50.8867260065479,-37.0586909963618,
40.1546258197409));
#169889=CARTESIAN_POINT('Ctrl Pts',(-50.8929208094434,-37.0520289807242,
40.1563626808798));
#169890=CARTESIAN_POINT('Ctrl Pts',(-50.8989791867715,-37.0451203242408,
40.1576937882008));
#169891=CARTESIAN_POINT('Ctrl Pts',(-50.904868900089,-37.0379786793007,
40.1585906813668));
#169892=CARTESIAN_POINT('Ctrl Pts',(-50.9078137567478,-37.0344078568306,
40.1590391279498));
#169893=CARTESIAN_POINT('Ctrl Pts',(-50.9107164475036,-37.0307787873188,
40.1593790209175));
#169894=CARTESIAN_POINT('Ctrl Pts',(-50.913572943118,-37.0270931777236,
40.1596068022931));
#169895=CARTESIAN_POINT('Ctrl Pts',(-50.9164294387324,-37.0234075681284,
40.1598345836687));
#169896=CARTESIAN_POINT('Ctrl Pts',(-50.9192397378252,-37.0196654174467,
40.1599502506864));
#169897=CARTESIAN_POINT('Ctrl Pts',(-50.9219998155902,-37.0158684358557,
40.1599502534424));
#169898=CARTESIAN_POINT('',(-50.9399462128204,-36.9911673391705,40.1599502534424));
#169899=CARTESIAN_POINT('Origin',(8.60468667414046E-17,9.13492640817417E-17,
40.1599502534424));
#169900=CARTESIAN_POINT('',(-50.9644637245895,-36.6347241449652,39.8576902534424));
#169901=CARTESIAN_POINT('Ctrl Pts',(-50.9399462128204,-36.9911673391705,
40.1599502534424));
#169902=CARTESIAN_POINT('Ctrl Pts',(-50.9421917493682,-36.9880750374205,
40.1599502447858));
#169903=CARTESIAN_POINT('Ctrl Pts',(-50.9443925120841,-36.9849631609002,
40.1598744685927));
#169904=CARTESIAN_POINT('Ctrl Pts',(-50.9465482749233,-36.9818339300541,
40.1597246934279));
#169905=CARTESIAN_POINT('Ctrl Pts',(-50.9590059247108,-36.9637508360902,
40.1588591777435));
#169906=CARTESIAN_POINT('Ctrl Pts',(-50.969963957274,-36.94508700131,40.1555254706021));
#169907=CARTESIAN_POINT('Ctrl Pts',(-50.9793739188864,-36.9262760657652,
40.1500631826381));
#169908=CARTESIAN_POINT('Ctrl Pts',(-50.9831691728707,-36.9186891827346,
40.1478601162481));
#169909=CARTESIAN_POINT('Ctrl Pts',(-50.9867130457555,-36.9110782226479,
40.1453112228307));
#169910=CARTESIAN_POINT('Ctrl Pts',(-50.9900040313323,-36.9034708445586,
40.1424401896328));
#169911=CARTESIAN_POINT('Ctrl Pts',(-50.991218205206,-36.900664183907,40.1413809526906));
#169912=CARTESIAN_POINT('Ctrl Pts',(-50.9923978359481,-36.8978580678371,
40.1402777640512));
#169913=CARTESIAN_POINT('Ctrl Pts',(-50.9935427888372,-36.8950539146732,
40.1391317641987));
#169914=CARTESIAN_POINT('Ctrl Pts',(-50.9956895755044,-36.8897961274909,
40.1369830144753));
#169915=CARTESIAN_POINT('Ctrl Pts',(-50.9977144478401,-36.8845452411467,
40.1346837565849));
#169916=CARTESIAN_POINT('Ctrl Pts',(-50.9996165178738,-36.8793106050085,
40.1322415082996));
#169917=CARTESIAN_POINT('Ctrl Pts',(-51.0062737629917,-36.860989378525,
40.1236936393008));
#169918=CARTESIAN_POINT('Ctrl Pts',(-51.011426676282,-36.8428672144357,
40.113394140767));
#169919=CARTESIAN_POINT('Ctrl Pts',(-51.0150372064714,-36.8253449818066,
40.101665321223));
#169920=CARTESIAN_POINT('Ctrl Pts',(-51.0168424715662,-36.816583865492,
40.095800911451));
#169921=CARTESIAN_POINT('Ctrl Pts',(-51.0182621417029,-36.8079727326365,
40.0895791707949));
#169922=CARTESIAN_POINT('Ctrl Pts',(-51.0192914676908,-36.7995616970578,
40.0830403822907));
#169923=CARTESIAN_POINT('Ctrl Pts',(-51.0198061306847,-36.7953561792684,
40.0797709880385));
#169924=CARTESIAN_POINT('Ctrl Pts',(-51.0202232077371,-36.7912006858664,
40.0764223317514));
#169925=CARTESIAN_POINT('Ctrl Pts',(-51.0205421056328,-36.7871014813874,
40.0729994484778));
#169926=CARTESIAN_POINT('Ctrl Pts',(-51.0208610035285,-36.7830022769085,
40.0695765652043));
#169927=CARTESIAN_POINT('Ctrl Pts',(-51.0210816112668,-36.7789594281948,
40.0660793733488));
#169928=CARTESIAN_POINT('Ctrl Pts',(-51.0212035636552,-36.7749790641713,
40.0625130768817));
#169929=CARTESIAN_POINT('Ctrl Pts',(-51.0212046036537,-36.7749451200024,
40.0624826638418));
#169930=CARTESIAN_POINT('Ctrl Pts',(-51.0212056365645,-36.7749111804865,
40.0624522459912));
#169931=CARTESIAN_POINT('Ctrl Pts',(-51.0212066623877,-36.774877245627,
40.0624218233329));
#169932=CARTESIAN_POINT('Ctrl Pts',(-51.0217305652762,-36.7575462174171,
40.0468845275921));
#169933=CARTESIAN_POINT('Ctrl Pts',(-51.0205340689296,-36.7413978659102,
40.0302263329286));
#169934=CARTESIAN_POINT('Ctrl Pts',(-51.0178063409637,-36.7264984065536,
40.012751588482));
#169935=CARTESIAN_POINT('Ctrl Pts',(-51.0149863630493,-36.7110950573751,
39.9946858597819));
#169936=CARTESIAN_POINT('Ctrl Pts',(-51.0105292970966,-36.697025781699,
39.9757460620623));
#169937=CARTESIAN_POINT('Ctrl Pts',(-51.0046027002077,-36.6843954909367,
39.9562444559292));
#169938=CARTESIAN_POINT('Ctrl Pts',(-50.9987888396623,-36.6720054548815,
39.9371138113801));
#169939=CARTESIAN_POINT('Ctrl Pts',(-50.9915600117817,-36.6609997278017,
39.917441065457));
#169940=CARTESIAN_POINT('Ctrl Pts',(-50.9830457809264,-36.6515157237815,
39.8975196504388));
#169941=CARTESIAN_POINT('Ctrl Pts',(-50.9774054014764,-36.6452329036082,
39.8843224113937));
#169942=CARTESIAN_POINT('Ctrl Pts',(-50.9712003466883,-36.6396186946867,
39.8710160447213));
#169943=CARTESIAN_POINT('Ctrl Pts',(-50.9644637245895,-36.6347241449652,
39.8576902534424));
#169944=CARTESIAN_POINT('',(-50.676214228995,-36.4252947698676,39.2875012672119));
#169945=CARTESIAN_POINT('',(-50.9644637245895,-36.6347241449652,39.8576902534424));
#169946=CARTESIAN_POINT('',(-53.8880358395972,-31.4795232016787,39.2875012672119));
#169947=CARTESIAN_POINT('Origin',(5.53234440788222E-15,0.,39.2875012672119));
#169948=CARTESIAN_POINT('',(-54.1966007261209,-31.6576696180581,39.8576902534424));
#169949=CARTESIAN_POINT('',(-53.8880358395972,-31.4795232016787,39.2875012672119));
#169950=CARTESIAN_POINT('',(-54.5122556166612,-31.4902932482905,40.1599502534424));
#169951=CARTESIAN_POINT('Ctrl Pts',(-54.1966007261209,-31.6576696180581,
39.8576902534424));
#169952=CARTESIAN_POINT('Ctrl Pts',(-54.2072580443417,-31.6638224711871,
39.8773836120366));
#169953=CARTESIAN_POINT('Ctrl Pts',(-54.2188555266751,-31.668266170439,
39.8969946442136));
#169954=CARTESIAN_POINT('Ctrl Pts',(-54.2312050423211,-31.6709833936512,
39.9162525288247));
#169955=CARTESIAN_POINT('Ctrl Pts',(-54.2438027078763,-31.6737552164699,
39.9358973794071));
#169956=CARTESIAN_POINT('Ctrl Pts',(-54.25718371473,-31.6747309854166,39.9551762199749));
#169957=CARTESIAN_POINT('Ctrl Pts',(-54.2711824151049,-31.6738510973604,
39.9738152034253));
#169958=CARTESIAN_POINT('Ctrl Pts',(-54.2846372786604,-31.6730053921575,
39.9917300792653));
#169959=CARTESIAN_POINT('Ctrl Pts',(-54.2986636530671,-31.6704454915902,
40.0090551158128));
#169960=CARTESIAN_POINT('Ctrl Pts',(-54.3131329740864,-31.6660771734245,
40.025539455154));
#169961=CARTESIAN_POINT('Ctrl Pts',(-54.3242478043957,-31.662721582994,
40.0382021526153));
#169962=CARTESIAN_POINT('Ctrl Pts',(-54.3356244578575,-31.6582981215829,
40.0503687782125));
#169963=CARTESIAN_POINT('Ctrl Pts',(-54.3472079546995,-31.6527458376965,
40.0619155352442));
#169964=CARTESIAN_POINT('Ctrl Pts',(-54.347238312979,-31.6527312861506,
40.0619457972351));
#169965=CARTESIAN_POINT('Ctrl Pts',(-54.347268672957,-31.6527167260611,
40.0619760547305));
#169966=CARTESIAN_POINT('Ctrl Pts',(-54.3472990346306,-31.6527021574291,
40.0620063077269));
#169967=CARTESIAN_POINT('Ctrl Pts',(-54.3505544234702,-31.6511401038185,
40.06525004417));
#169968=CARTESIAN_POINT('Ctrl Pts',(-54.3538274103385,-31.6494796970074,
40.0684393223557));
#169969=CARTESIAN_POINT('Ctrl Pts',(-54.3571135597834,-31.6477231007677,
40.0715697951759));
#169970=CARTESIAN_POINT('Ctrl Pts',(-54.3754002342689,-31.6379480420931,
40.0889901646415));
#169971=CARTESIAN_POINT('Ctrl Pts',(-54.3940968201766,-31.6251987170239,
40.1045963098233));
#169972=CARTESIAN_POINT('Ctrl Pts',(-54.4124255228535,-31.6099016141378,
40.1176634650713));
#169973=CARTESIAN_POINT('Ctrl Pts',(-54.4206516984377,-31.6030360625224,
40.1235281853055));
#169974=CARTESIAN_POINT('Ctrl Pts',(-54.4288041214164,-31.5956573884072,
40.1288820140917));
#169975=CARTESIAN_POINT('Ctrl Pts',(-54.4368146919238,-31.5878037911379,
40.1336621774101));
#169976=CARTESIAN_POINT('Ctrl Pts',(-54.4402959775154,-31.5843907239923,
40.1357395717319));
#169977=CARTESIAN_POINT('Ctrl Pts',(-54.443750270399,-31.5808879923398,
40.1377083672884));
#169978=CARTESIAN_POINT('Ctrl Pts',(-54.4471718528273,-31.5772987574365,
40.1395632548792));
#169979=CARTESIAN_POINT('Ctrl Pts',(-54.4591473913264,-31.5647364352751,
40.146055361447));
#169980=CARTESIAN_POINT('Ctrl Pts',(-54.4707222239582,-31.5511144466739,
40.151152097463));
#169981=CARTESIAN_POINT('Ctrl Pts',(-54.4816512176786,-31.5365683393823,
40.1546258197409));
#169982=CARTESIAN_POINT('Ctrl Pts',(-54.4871157145388,-31.5292952857365,
40.1563626808798));
#169983=CARTESIAN_POINT('Ctrl Pts',(-54.4924187521965,-31.5217912027242,
40.1576937882008));
#169984=CARTESIAN_POINT('Ctrl Pts',(-54.4975296958774,-31.5140730377801,
40.1585906813668));
#169985=CARTESIAN_POINT('Ctrl Pts',(-54.5000851677179,-31.5102139553081,
40.1590391279498));
#169986=CARTESIAN_POINT('Ctrl Pts',(-54.5025926161709,-31.5063013524147,
40.1593790209175));
#169987=CARTESIAN_POINT('Ctrl Pts',(-54.5050482124962,-31.5023373478776,
40.1596068022931));
#169988=CARTESIAN_POINT('Ctrl Pts',(-54.5075038088216,-31.4983733433406,
40.1598345836687));
#169989=CARTESIAN_POINT('Ctrl Pts',(-54.5099075515418,-31.4943579363063,
40.1599502506865));
#169990=CARTESIAN_POINT('Ctrl Pts',(-54.5122556166612,-31.4902932482905,
40.1599502534424));
#169991=CARTESIAN_POINT('',(-54.5275217339721,-31.4638515574737,40.1599502534424));
#169992=CARTESIAN_POINT('Origin',(9.49066947580433E-17,7.77063253334978E-17,
40.1599502534424));
#169993=CARTESIAN_POINT('',(-54.514646476914,-31.1067982185532,39.8576902534424));
#169994=CARTESIAN_POINT('Ctrl Pts',(-54.5275217339721,-31.4638515574737,
40.1599502534424));
#169995=CARTESIAN_POINT('Ctrl Pts',(-54.5294317356859,-31.4605414731917,
40.1599502447858));
#169996=CARTESIAN_POINT('Ctrl Pts',(-54.5312951627229,-31.4572166015119,
40.1598744685927));
#169997=CARTESIAN_POINT('Ctrl Pts',(-54.5331120223761,-31.453879174343,
40.1597246934279));
#169998=CARTESIAN_POINT('Ctrl Pts',(-54.5436112298343,-31.4345929624664,
40.1588591777432));
#169999=CARTESIAN_POINT('Ctrl Pts',(-54.5525583311825,-31.414885943816,
40.1555254706002));
#170000=CARTESIAN_POINT('Ctrl Pts',(-54.5599504658566,-31.3951944477122,
40.1500631826335));
#170001=CARTESIAN_POINT('Ctrl Pts',(-54.5629318838159,-31.3872524143595,
40.1478601162446));
#170002=CARTESIAN_POINT('Ctrl Pts',(-54.5656607810303,-31.3793127123272,
40.1453112228287));
#170003=CARTESIAN_POINT('Ctrl Pts',(-54.5681385507009,-31.3714030065916,
40.1424401896328));
#170004=CARTESIAN_POINT('Ctrl Pts',(-54.5690526972783,-31.3684848053916,
40.1413809526906));
#170005=CARTESIAN_POINT('Ctrl Pts',(-54.5699325468791,-31.3655707565304,
40.1402777640511));
#170006=CARTESIAN_POINT('Ctrl Pts',(-54.5707781137755,-31.3626622846449,
40.1391317641987));
#170007=CARTESIAN_POINT('Ctrl Pts',(-54.5723635517064,-31.3572088998597,
40.1369830144753));
#170008=CARTESIAN_POINT('Ctrl Pts',(-54.5738284644993,-31.3517751216267,
40.134683756585));
#170009=CARTESIAN_POINT('Ctrl Pts',(-54.575172946323,-31.3463703409153,
40.1322415082996));
#170010=CARTESIAN_POINT('Ctrl Pts',(-54.5798786327061,-31.3274536084257,
40.1236936393009));
#170011=CARTESIAN_POINT('Ctrl Pts',(-54.5831090358349,-31.3088920933399,
40.113394140767));
#170012=CARTESIAN_POINT('Ctrl Pts',(-54.5848682151124,-31.2910884461622,
40.101665321223));
#170013=CARTESIAN_POINT('Ctrl Pts',(-54.5857478047512,-31.2821866225733,
40.095800911451));
#170014=CARTESIAN_POINT('Ctrl Pts',(-54.5862595893019,-31.2734742664669,
40.0895791707949));
#170015=CARTESIAN_POINT('Ctrl Pts',(-54.5864040839109,-31.2650017135574,
40.0830403822906));
#170016=CARTESIAN_POINT('Ctrl Pts',(-54.5864763312153,-31.2607654371026,
40.0797709880385));
#170017=CARTESIAN_POINT('Ctrl Pts',(-54.5864567561365,-31.256589111505,
40.0764223317514));
#170018=CARTESIAN_POINT('Ctrl Pts',(-54.5863454235314,-31.25247902899,40.0729994484778));
#170019=CARTESIAN_POINT('Ctrl Pts',(-54.5862340909262,-31.2483689464751,
40.0695765652042));
#170020=CARTESIAN_POINT('Ctrl Pts',(-54.586030897389,-31.2443251851218,
40.0660793733488));
#170021=CARTESIAN_POINT('Ctrl Pts',(-54.5857361203749,-31.2403538784532,
40.0625130768817));
#170022=CARTESIAN_POINT('Ctrl Pts',(-54.5857336065443,-31.2403200115245,
40.0624826638418));
#170023=CARTESIAN_POINT('Ctrl Pts',(-54.5857310861513,-31.2402861499643,
40.0624522459912));
#170024=CARTESIAN_POINT('Ctrl Pts',(-54.5857285591962,-31.2402522937758,
40.0624218233329));
#170025=CARTESIAN_POINT('Ctrl Pts',(-54.5844380063442,-31.2229614439868,
40.0468845275911));
#170026=CARTESIAN_POINT('Ctrl Pts',(-54.5815601021621,-31.2070266227626,
40.0302263329264));
#170027=CARTESIAN_POINT('Ctrl Pts',(-54.5772898993848,-31.1924939094151,
40.0127515884786));
#170028=CARTESIAN_POINT('Ctrl Pts',(-54.5728752811851,-31.177469709352,
39.9946858597769));
#170029=CARTESIAN_POINT('Ctrl Pts',(-54.5669719917396,-31.1639433968941,
39.9757460620557));
#170030=CARTESIAN_POINT('Ctrl Pts',(-54.5597576364835,-31.1520017942509,
39.9562444559208));
#170031=CARTESIAN_POINT('Ctrl Pts',(-54.5526805134449,-31.1402873460175,
39.9371138113699));
#170032=CARTESIAN_POINT('Ctrl Pts',(-54.5443408740998,-31.1300975277315,
39.917441065445));
#170033=CARTESIAN_POINT('Ctrl Pts',(-54.5348819367248,-31.1215554575449,
39.897519650425));
#170034=CARTESIAN_POINT('Ctrl Pts',(-54.5286157223278,-31.1158966355165,
39.8843224113845));
#170035=CARTESIAN_POINT('Ctrl Pts',(-54.5218578148503,-31.1109617866623,
39.8710160447167));
#170036=CARTESIAN_POINT('Ctrl Pts',(-54.514646476914,-31.1067982185532,
39.8576902534424));
#170037=CARTESIAN_POINT('',(-54.2060847114743,-30.9286463962975,39.2875012672119));
#170038=CARTESIAN_POINT('',(-54.514646476914,-31.1067982185532,39.8576902534424));
#170039=CARTESIAN_POINT('',(-56.8833377255396,-25.6742415049977,39.2875012672119));
#170040=CARTESIAN_POINT('Origin',(5.53234440788222E-15,0.,39.2875012672119));
#170041=CARTESIAN_POINT('',(-57.20883363247,-25.8191582032617,39.8576902534424));
#170042=CARTESIAN_POINT('',(-56.8833377255396,-25.6742415049977,39.2875012672119));
#170043=CARTESIAN_POINT('',(-57.5052637377733,-25.6197038181295,40.1599502534424));
#170044=CARTESIAN_POINT('Ctrl Pts',(-57.20883363247,-25.8191582032617,39.8576902534424));
#170045=CARTESIAN_POINT('Ctrl Pts',(-57.2200757170687,-25.8241633573214,
39.8773836120366));
#170046=CARTESIAN_POINT('Ctrl Pts',(-57.2320741602344,-25.8273704465178,
39.8969946442136));
#170047=CARTESIAN_POINT('Ctrl Pts',(-57.2446400511083,-25.8287819086044,
39.9162525288247));
#170048=CARTESIAN_POINT('Ctrl Pts',(-57.2574584397132,-25.8302217324664,
39.9358973794071));
#170049=CARTESIAN_POINT('Ctrl Pts',(-57.2708681396398,-25.8297934599654,
39.9551762199749));
#170050=CARTESIAN_POINT('Ctrl Pts',(-57.284698180323,-25.82745512939,39.9738152034254));
#170051=CARTESIAN_POINT('Ctrl Pts',(-57.2979909364631,-25.8252076408377,
39.9917300792656));
#170052=CARTESIAN_POINT('Ctrl Pts',(-57.311672890451,-25.8211956083115,
40.0090551158133));
#170053=CARTESIAN_POINT('Ctrl Pts',(-57.325606333431,-25.815338764359,40.0255394551547));
#170054=CARTESIAN_POINT('Ctrl Pts',(-57.3363095208257,-25.8108397400723,
40.0382021526157));
#170055=CARTESIAN_POINT('Ctrl Pts',(-57.3471614741657,-25.8052513267422,
40.0503687782127));
#170056=CARTESIAN_POINT('Ctrl Pts',(-57.3581011436975,-25.7985186537238,
40.0619155352442));
#170057=CARTESIAN_POINT('Ctrl Pts',(-57.3581298146204,-25.7985010085885,
40.0619457972351));
#170058=CARTESIAN_POINT('Ctrl Pts',(-57.3581584863395,-25.7984833547788,
40.0619760547305));
#170059=CARTESIAN_POINT('Ctrl Pts',(-57.358187158852,-25.7984656922963,
40.0620063077269));
#170060=CARTESIAN_POINT('Ctrl Pts',(-57.3612614352675,-25.796571914986,
40.06525004417));
#170061=CARTESIAN_POINT('Ctrl Pts',(-57.3643429325988,-25.7945784837695,
40.0684393223557));
#170062=CARTESIAN_POINT('Ctrl Pts',(-57.3674274658677,-25.7924880141963,
40.0715697951759));
#170063=CARTESIAN_POINT('Ctrl Pts',(-57.3845921921726,-25.7808550263355,
40.0889901646387));
#170064=CARTESIAN_POINT('Ctrl Pts',(-57.4018536888665,-25.7662212180126,
40.1045963098182));
#170065=CARTESIAN_POINT('Ctrl Pts',(-57.4184830023326,-25.7490920431358,
40.1176634650649));
#170066=CARTESIAN_POINT('Ctrl Pts',(-57.4259464685093,-25.7414042322357,
40.1235281853016));
#170067=CARTESIAN_POINT('Ctrl Pts',(-57.4332829501985,-25.7332138190206,
40.1288820140899));
#170068=CARTESIAN_POINT('Ctrl Pts',(-57.4404287135113,-25.7245659119508,
40.1336621774101));
#170069=CARTESIAN_POINT('Ctrl Pts',(-57.4435341655924,-25.720807648511,
40.1357395717319));
#170070=CARTESIAN_POINT('Ctrl Pts',(-57.4466034003413,-25.7169630332622,
40.1377083672884));
#170071=CARTESIAN_POINT('Ctrl Pts',(-57.4496310617744,-25.7130358078101,
40.1395632548792));
#170072=CARTESIAN_POINT('Ctrl Pts',(-57.46022787679,-25.6992905187278,40.146055361447));
#170073=CARTESIAN_POINT('Ctrl Pts',(-57.4703154157424,-25.6845332533378,
40.151152097463));
#170074=CARTESIAN_POINT('Ctrl Pts',(-57.4796640570499,-25.6689244402253,
40.1546258197409));
#170075=CARTESIAN_POINT('Ctrl Pts',(-57.4843383777036,-25.661120033669,
40.1563626808798));
#170076=CARTESIAN_POINT('Ctrl Pts',(-57.4888279745007,-25.6531027404317,
40.1576937882008));
#170077=CARTESIAN_POINT('Ctrl Pts',(-57.4931041519765,-25.6448926173139,
40.1585906813668));
#170078=CARTESIAN_POINT('Ctrl Pts',(-57.4952422407144,-25.6407875557551,
40.1590391279498));
#170079=CARTESIAN_POINT('Ctrl Pts',(-57.4973269747346,-25.6366342867762,
40.1593790209175));
#170080=CARTESIAN_POINT('Ctrl Pts',(-57.4993547677437,-25.6324353177604,
40.1596068022931));
#170081=CARTESIAN_POINT('Ctrl Pts',(-57.5013825607528,-25.6282363487447,
40.1598345836687));
#170082=CARTESIAN_POINT('Ctrl Pts',(-57.5033534111923,-25.6239916789977,
40.1599502506865));
#170083=CARTESIAN_POINT('Ctrl Pts',(-57.5052637377733,-25.6197038181295,
40.1599502534424));
#170084=CARTESIAN_POINT('',(-57.517682316389,-25.5918112338791,40.1599502534424));
#170085=CARTESIAN_POINT('Origin',(1.02291912287982E-16,6.3212019823805E-17,
40.1599502534424));
#170086=CARTESIAN_POINT('',(-57.4675553545142,-25.2380597013427,39.8576902534424));
#170087=CARTESIAN_POINT('Ctrl Pts',(-57.517682316389,-25.5918112338791,
40.1599502534424));
#170088=CARTESIAN_POINT('Ctrl Pts',(-57.5192358568902,-25.5883196330411,
40.1599502447858));
#170089=CARTESIAN_POINT('Ctrl Pts',(-57.5207415321516,-25.5848181941916,
40.1598744685927));
#170090=CARTESIAN_POINT('Ctrl Pts',(-57.5221995827244,-25.5813091362505,
40.1597246934279));
#170091=CARTESIAN_POINT('Ctrl Pts',(-57.5306253163328,-25.5610311102466,
40.1588591777435));
#170092=CARTESIAN_POINT('Ctrl Pts',(-57.5374634601467,-25.5404968219592,
40.1555254706026));
#170093=CARTESIAN_POINT('Ctrl Pts',(-57.5427567781056,-25.5201405094608,
40.1500631826394));
#170094=CARTESIAN_POINT('Ctrl Pts',(-57.5448916950062,-25.5119303403528,
40.1478601162491));
#170095=CARTESIAN_POINT('Ctrl Pts',(-57.5467757181857,-25.5037488853995,
40.1453112228312));
#170096=CARTESIAN_POINT('Ctrl Pts',(-57.5484131249909,-25.4956235123963,
40.1424401896328));
#170097=CARTESIAN_POINT('Ctrl Pts',(-57.5490172286907,-25.4926257430708,
40.1413809526906));
#170098=CARTESIAN_POINT('Ctrl Pts',(-57.549587657334,-25.4896356883475,
40.1402777640512));
#170099=CARTESIAN_POINT('Ctrl Pts',(-57.5501245740299,-25.4866547635671,
40.1391317641987));
#170100=CARTESIAN_POINT('Ctrl Pts',(-57.5511312928346,-25.4810655296038,
40.1369830144753));
#170101=CARTESIAN_POINT('Ctrl Pts',(-57.5520201961935,-25.4755083930934,
40.134683756585));
#170102=CARTESIAN_POINT('Ctrl Pts',(-57.5527923593831,-25.4699926837174,
40.1322415082996));
#170103=CARTESIAN_POINT('Ctrl Pts',(-57.5554949305467,-25.4506877009014,
40.1236936393009));
#170104=CARTESIAN_POINT('Ctrl Pts',(-57.5567674305412,-25.4318901986625,
40.113394140767));
#170105=CARTESIAN_POINT('Ctrl Pts',(-57.5566559849706,-25.4140001974204,
40.101665321223));
#170106=CARTESIAN_POINT('Ctrl Pts',(-57.5566002621852,-25.4050551967993,
40.095800911451));
#170107=CARTESIAN_POINT('Ctrl Pts',(-57.5561985539314,-25.3963370718386,
40.0895791707949));
#170108=CARTESIAN_POINT('Ctrl Pts',(-57.5554566340482,-25.387895828661,
40.0830403822906));
#170109=CARTESIAN_POINT('Ctrl Pts',(-57.5550856741066,-25.3836752070722,
40.0797709880385));
#170110=CARTESIAN_POINT('Ctrl Pts',(-57.5546296613653,-25.379523805976,
40.0764223317514));
#170111=CARTESIAN_POINT('Ctrl Pts',(-57.5540893180426,-25.3754478763493,
40.0729994484778));
#170112=CARTESIAN_POINT('Ctrl Pts',(-57.5535489747199,-25.3713719467226,
40.0695765652042));
#170113=CARTESIAN_POINT('Ctrl Pts',(-57.5529242061381,-25.3673715770253,
40.0660793733488));
#170114=CARTESIAN_POINT('Ctrl Pts',(-57.55221592936,-25.3634528381784,40.0625130768817));
#170115=CARTESIAN_POINT('Ctrl Pts',(-57.5522098892425,-25.3634194195431,
40.0624826638418));
#170116=CARTESIAN_POINT('Ctrl Pts',(-57.5522038431596,-25.3633860069329,
40.0624522459912));
#170117=CARTESIAN_POINT('Ctrl Pts',(-57.552197791112,-25.3633526003509,
40.0624218233329));
#170118=CARTESIAN_POINT('Ctrl Pts',(-57.5491069220861,-25.34629137115,40.0468845275888));
#170119=CARTESIAN_POINT('Ctrl Pts',(-57.5445791409883,-25.3307446654432,
40.0302263329214));
#170120=CARTESIAN_POINT('Ctrl Pts',(-57.5388132486341,-25.3167379215524,
40.0127515884706));
#170121=CARTESIAN_POINT('Ctrl Pts',(-57.5328523576292,-25.3022574788841,
39.9946858597662));
#170122=CARTESIAN_POINT('Ctrl Pts',(-57.5255675223644,-25.289422326754,
39.9757460620419));
#170123=CARTESIAN_POINT('Ctrl Pts',(-57.5171444507262,-25.2783002469273,
39.956244455904));
#170124=CARTESIAN_POINT('Ctrl Pts',(-57.5088816036346,-25.2673897324622,
39.9371138113505));
#170125=CARTESIAN_POINT('Ctrl Pts',(-57.4995225236582,-25.258127464752,
39.9174410654228));
#170126=CARTESIAN_POINT('Ctrl Pts',(-57.48922251386,-25.2506209171082,39.8975196504002));
#170127=CARTESIAN_POINT('Ctrl Pts',(-57.4823991184743,-25.2456480924645,
39.8843224113678));
#170128=CARTESIAN_POINT('Ctrl Pts',(-57.4751623993582,-25.2414466709153,
39.8710160447083));
#170129=CARTESIAN_POINT('Ctrl Pts',(-57.4675553545142,-25.2380597013427,
39.8576902534424));
#170130=CARTESIAN_POINT('',(-57.1420619865023,-25.0931373005743,39.2875012672119));
#170131=CARTESIAN_POINT('',(-57.4675553545142,-25.2380597013427,39.8576902534424));
#170132=CARTESIAN_POINT('',(-59.2554138597572,-19.5876674457075,39.2875012672119));
#170133=CARTESIAN_POINT('Origin',(5.53234440788222E-15,0.,39.2875012672119));
#170134=CARTESIAN_POINT('',(-59.5942745858237,-19.6977666881842,39.8576902534424));
#170135=CARTESIAN_POINT('',(-59.2554138597572,-19.5876674457075,39.2875012672119));
#170136=CARTESIAN_POINT('',(-59.8682321556243,-19.4684195516693,40.1599502534424));
#170137=CARTESIAN_POINT('Ctrl Pts',(-59.5942745858237,-19.6977666881842,
39.8576902534424));
#170138=CARTESIAN_POINT('Ctrl Pts',(-59.6059782661684,-19.7015693056588,
39.8773836120357));
#170139=CARTESIAN_POINT('Ctrl Pts',(-59.6182462127118,-19.7035046472592,
39.8969946442118));
#170140=CARTESIAN_POINT('Ctrl Pts',(-59.6308908042829,-19.7035948839463,
39.916252528822));
#170141=CARTESIAN_POINT('Ctrl Pts',(-59.6437894749888,-19.7036869338402,
39.9358973794034));
#170142=CARTESIAN_POINT('Ctrl Pts',(-59.6570809485089,-19.701859312135,
39.9551762199702));
#170143=CARTESIAN_POINT('Ctrl Pts',(-59.6705908046797,-19.6980881582803,
39.9738152034197));
#170144=CARTESIAN_POINT('Ctrl Pts',(-59.6835758151852,-19.6944635103343,
39.9917300792587));
#170145=CARTESIAN_POINT('Ctrl Pts',(-59.696763446402,-19.6890433025181,
40.0090551158054));
#170146=CARTESIAN_POINT('Ctrl Pts',(-59.7100083536245,-19.6817621015882,
40.0255394551458));
#170147=CARTESIAN_POINT('Ctrl Pts',(-59.7201826317462,-19.6761689356961,
40.03820215261));
#170148=CARTESIAN_POINT('Ctrl Pts',(-59.7303909886952,-19.6694767982716,
40.05036877821));
#170149=CARTESIAN_POINT('Ctrl Pts',(-59.7405669736108,-19.6616375006938,
40.0619155352442));
#170150=CARTESIAN_POINT('Ctrl Pts',(-59.7405936430525,-19.6616169552929,
40.0619457972351));
#170151=CARTESIAN_POINT('Ctrl Pts',(-59.7406203123794,-19.6615964011819,
40.0619760547305));
#170152=CARTESIAN_POINT('Ctrl Pts',(-59.7406469815886,-19.6615758383626,
40.0620063077269));
#170153=CARTESIAN_POINT('Ctrl Pts',(-59.7435064631642,-19.6593710859732,
40.06525004417));
#170154=CARTESIAN_POINT('Ctrl Pts',(-59.7463627094291,-19.6570664708009,
40.0684393223557));
#170155=CARTESIAN_POINT('Ctrl Pts',(-59.74921183173,-19.6546650315162,40.0715697951759));
#170156=CARTESIAN_POINT('Ctrl Pts',(-59.7650665495273,-19.6413015679142,
40.0889901646424));
#170157=CARTESIAN_POINT('Ctrl Pts',(-59.7807038364438,-19.6249436073972,
40.1045963098249));
#170158=CARTESIAN_POINT('Ctrl Pts',(-59.7954515664667,-19.6061700313457,
40.1176634650733));
#170159=CARTESIAN_POINT('Ctrl Pts',(-59.8020705519321,-19.5977441904316,
40.1235281853067));
#170160=CARTESIAN_POINT('Ctrl Pts',(-59.8085107122969,-19.5888317740044,
40.1288820140922));
#170161=CARTESIAN_POINT('Ctrl Pts',(-59.8147133779311,-19.5794843054209,
40.1336621774101));
#170162=CARTESIAN_POINT('Ctrl Pts',(-59.8174089725189,-19.5754220220077,
40.1357395717319));
#170163=CARTESIAN_POINT('Ctrl Pts',(-59.8200595219549,-19.5712776455717,
40.1377083672884));
#170164=CARTESIAN_POINT('Ctrl Pts',(-59.8226600907004,-19.5670554570747,
40.1395632548792));
#170165=CARTESIAN_POINT('Ctrl Pts',(-59.8317620813096,-19.552277797335,
40.146055361447));
#170166=CARTESIAN_POINT('Ctrl Pts',(-59.8402518053949,-19.5365469388441,
40.151152097463));
#170167=CARTESIAN_POINT('Ctrl Pts',(-59.8479176686191,-19.5200464333335,
40.1546258197409));
#170168=CARTESIAN_POINT('Ctrl Pts',(-59.8517506002312,-19.5117961805782,
40.1563626808798));
#170169=CARTESIAN_POINT('Ctrl Pts',(-59.8553775672056,-19.5033535162581,
40.1576937882008));
#170170=CARTESIAN_POINT('Ctrl Pts',(-59.858772127781,-19.4947413867936,
40.1585906813668));
#170171=CARTESIAN_POINT('Ctrl Pts',(-59.8604694080688,-19.4904353220614,
40.1590391279498));
#170172=CARTESIAN_POINT('Ctrl Pts',(-59.862108586874,-19.4860868910811,
40.1593790209175));
#170173=CARTESIAN_POINT('Ctrl Pts',(-59.8636863596423,-19.4816989623699,
40.1596068022931));
#170174=CARTESIAN_POINT('Ctrl Pts',(-59.8652641324106,-19.4773110336587,
40.1598345836687));
#170175=CARTESIAN_POINT('Ctrl Pts',(-59.8667804975193,-19.4728836066889,
40.1599502506864));
#170176=CARTESIAN_POINT('Ctrl Pts',(-59.8682321556243,-19.4684195516693,
40.1599502534424));
#170177=CARTESIAN_POINT('',(-59.8776671349986,-19.4393816709753,40.1599502534424));
#170178=CARTESIAN_POINT('Origin',(1.08121605342496E-16,4.80251501969578E-17,
40.1599502534424));
#170179=CARTESIAN_POINT('',(-59.7908376697913,-19.0928077206408,39.8576902534424));
#170180=CARTESIAN_POINT('Ctrl Pts',(-59.8776671349986,-19.4393816709753,
40.1599502534424));
#170181=CARTESIAN_POINT('Ctrl Pts',(-59.8788471933725,-19.4357468082908,
40.1599502447858));
#170182=CARTESIAN_POINT('Ctrl Pts',(-59.8799786203652,-19.4321071647684,
40.1598744685927));
#170183=CARTESIAN_POINT('Ctrl Pts',(-59.8810618871502,-19.4284649220281,
40.159724693428));
#170184=CARTESIAN_POINT('Ctrl Pts',(-59.8873218328122,-19.407417252186,
40.1588591777435));
#170185=CARTESIAN_POINT('Ctrl Pts',(-59.8919760989598,-19.3862806722135,
40.1555254706024));
#170186=CARTESIAN_POINT('Ctrl Pts',(-59.8951126055059,-19.3654825713326,
40.150063182639));
#170187=CARTESIAN_POINT('Ctrl Pts',(-59.8963776307481,-19.3570942188076,
40.1478601162488));
#170188=CARTESIAN_POINT('Ctrl Pts',(-59.897396138138,-19.3487606486732,
40.1453112228311));
#170189=CARTESIAN_POINT('Ctrl Pts',(-59.8981752423038,-19.3405086316968,
40.1424401896328));
#170190=CARTESIAN_POINT('Ctrl Pts',(-59.8984626844395,-19.337464138434,
40.1413809526905));
#170191=CARTESIAN_POINT('Ctrl Pts',(-59.8987174423897,-19.3344308375139,
40.1402777640511));
#170192=CARTESIAN_POINT('Ctrl Pts',(-59.8989398263133,-19.3314101194741,
40.1391317641987));
#170193=CARTESIAN_POINT('Ctrl Pts',(-59.8993567961701,-19.3257462731497,
40.1369830144753));
#170194=CARTESIAN_POINT('Ctrl Pts',(-59.8996599510837,-19.3201266635125,
40.1346837565849));
#170195=CARTESIAN_POINT('Ctrl Pts',(-59.8998513356577,-19.314560456738,
40.1322415082996));
#170196=CARTESIAN_POINT('Ctrl Pts',(-59.9005211816665,-19.2950787330271,
40.1236936393009));
#170197=CARTESIAN_POINT('Ctrl Pts',(-59.8998218367506,-19.2762511930034,
40.113394140767));
#170198=CARTESIAN_POINT('Ctrl Pts',(-59.8978409873528,-19.2584708442942,
40.101665321223));
#170199=CARTESIAN_POINT('Ctrl Pts',(-59.8968505626539,-19.2495806699396,
40.095800911451));
#170200=CARTESIAN_POINT('Ctrl Pts',(-59.8955397627952,-19.240952293726,
40.0895791707949));
#170201=CARTESIAN_POINT('Ctrl Pts',(-59.8939195570493,-19.2326348443071,
40.0830403822907));
#170202=CARTESIAN_POINT('Ctrl Pts',(-59.8931094541763,-19.2284761195976,
40.0797709880385));
#170203=CARTESIAN_POINT('Ctrl Pts',(-59.8922219999436,-19.2243951266221,
40.0764223317514));
#170204=CARTESIAN_POINT('Ctrl Pts',(-59.8912585660179,-19.2203980066215,
40.0729994484778));
#170205=CARTESIAN_POINT('Ctrl Pts',(-59.8902951320921,-19.2164008866209,
40.0695765652042));
#170206=CARTESIAN_POINT('Ctrl Pts',(-59.889255633561,-19.2124877374671,
40.0660793733488));
#170207=CARTESIAN_POINT('Ctrl Pts',(-59.8881416170477,-19.2086645009648,
40.0625130768817));
#170208=CARTESIAN_POINT('Ctrl Pts',(-59.8881321168199,-19.2086318967645,
40.0624826638418));
#170209=CARTESIAN_POINT('Ctrl Pts',(-59.8881226112893,-19.2085992991799,
40.0624522459912));
#170210=CARTESIAN_POINT('Ctrl Pts',(-59.8881131004568,-19.2085667082138,
40.0624218233329));
#170211=CARTESIAN_POINT('Ctrl Pts',(-59.8832557794653,-19.1919220260021,
40.0468845275897));
#170212=CARTESIAN_POINT('Ctrl Pts',(-59.8771277287702,-19.1769337687768,
40.0302263329234));
#170213=CARTESIAN_POINT('Ctrl Pts',(-59.8699293191639,-19.1636064551624,
40.0127515884738));
#170214=CARTESIAN_POINT('Ctrl Pts',(-59.8624874641246,-19.1498284206511,
39.9946858597706));
#170215=CARTESIAN_POINT('Ctrl Pts',(-59.8539008972224,-19.1378250534631,
39.9757460620477));
#170216=CARTESIAN_POINT('Ctrl Pts',(-59.8443613941402,-19.127644352288,
39.9562444559111));
#170217=CARTESIAN_POINT('Ctrl Pts',(-59.8350033524798,-19.1176573094716,
39.9371138113589));
#170218=CARTESIAN_POINT('Ctrl Pts',(-59.8247273719135,-19.1094240716805,
39.9174410654326));
#170219=CARTESIAN_POINT('Ctrl Pts',(-59.8136991387581,-19.1030352898857,
39.8975196504113));
#170220=CARTESIAN_POINT('Ctrl Pts',(-59.8063933209263,-19.098802945928,
39.8843224113753));
#170221=CARTESIAN_POINT('Ctrl Pts',(-59.7987570771745,-19.0953809833328,
39.8710160447121));
#170222=CARTESIAN_POINT('Ctrl Pts',(-59.7908376697913,-19.0928077206408,
39.8576902534424));
#170223=CARTESIAN_POINT('',(-59.4519788726609,-18.9827025415093,39.2875012672119));
#170224=CARTESIAN_POINT('',(-59.7908376697913,-19.0928077206408,39.8576902534424));
#170225=CARTESIAN_POINT('',(-60.9782752797349,-13.2864868028992,39.2875012672119));
#170226=CARTESIAN_POINT('Origin',(5.53234440788222E-15,0.,39.2875012672119));
#170227=CARTESIAN_POINT('',(-61.3267881959114,-13.3605623192483,39.8576902534424));
#170228=CARTESIAN_POINT('',(-60.9782752797349,-13.2864868028992,39.2875012672119));
#170229=CARTESIAN_POINT('',(-61.5752716937452,-13.1038352065724,40.1599502534424));
#170230=CARTESIAN_POINT('Ctrl Pts',(-61.3267881959114,-13.3605623192483,
39.8576902534424));
#170231=CARTESIAN_POINT('Ctrl Pts',(-61.3388252440322,-13.3631207378657,
39.8773836120366));
#170232=CARTESIAN_POINT('Ctrl Pts',(-61.3512282837647,-13.3637631278627,
39.8969946442137));
#170233=CARTESIAN_POINT('Ctrl Pts',(-61.363813039243,-13.3625311504981,
39.9162525288247));
#170234=CARTESIAN_POINT('Ctrl Pts',(-61.3766506715158,-13.3612744179057,
39.9358973794071));
#170235=CARTESIAN_POINT('Ctrl Pts',(-61.3896782944657,-13.3580674708013,
39.9551762199749));
#170236=CARTESIAN_POINT('Ctrl Pts',(-61.4027199493144,-13.3529048112168,
39.9738152034253));
#170237=CARTESIAN_POINT('Ctrl Pts',(-61.4152549476949,-13.3479427162771,
39.9917300792654));
#170238=CARTESIAN_POINT('Ctrl Pts',(-61.4278037696953,-13.3411737181002,
40.0090551158131));
#170239=CARTESIAN_POINT('Ctrl Pts',(-61.4402150271871,-13.3325479345514,
40.0255394551543));
#170240=CARTESIAN_POINT('Ctrl Pts',(-61.449748924511,-13.3259219069513,
40.0382021526155));
#170241=CARTESIAN_POINT('Ctrl Pts',(-61.4592018401694,-13.3181993658929,
40.0503687782126));
#170242=CARTESIAN_POINT('Ctrl Pts',(-61.4685026502439,-13.309339332744,
40.0619155352442));
#170243=CARTESIAN_POINT('Ctrl Pts',(-61.4685270260084,-13.3093161121772,
40.0619457972351));
#170244=CARTESIAN_POINT('Ctrl Pts',(-61.4685514007483,-13.30929288296,40.0619760547305));
#170245=CARTESIAN_POINT('Ctrl Pts',(-61.4685757744609,-13.3092696450946,
40.0620063077269));
#170246=CARTESIAN_POINT('Ctrl Pts',(-61.4711891321181,-13.3067780733547,
40.06525004417));
#170247=CARTESIAN_POINT('Ctrl Pts',(-61.4737888336847,-13.3041875240726,
40.0684393223557));
#170248=CARTESIAN_POINT('Ctrl Pts',(-61.4763713294375,-13.3015014257478,
40.0715697951759));
#170249=CARTESIAN_POINT('Ctrl Pts',(-61.490742331116,-13.2865538993123,
40.0889901646406));
#170250=CARTESIAN_POINT('Ctrl Pts',(-61.5045840828622,-13.2686510078457,
40.1045963098216));
#170251=CARTESIAN_POINT('Ctrl Pts',(-61.5172886502212,-13.2484387178548,
40.1176634650692));
#170252=CARTESIAN_POINT('Ctrl Pts',(-61.5229906359905,-13.2393671621978,
40.1235281853042));
#170253=CARTESIAN_POINT('Ctrl Pts',(-61.5284639152912,-13.2298303888521,
40.1288820140911));
#170254=CARTESIAN_POINT('Ctrl Pts',(-61.5336555255488,-13.2198857715702,
40.1336621774101));
#170255=CARTESIAN_POINT('Ctrl Pts',(-61.5359117291449,-13.2155639754107,
40.1357395717319));
#170256=CARTESIAN_POINT('Ctrl Pts',(-61.5381145532937,-13.2111652444432,
40.1377083672884));
#170257=CARTESIAN_POINT('Ctrl Pts',(-61.5402595369763,-13.2066943520819,
40.1395632548792));
#170258=CARTESIAN_POINT('Ctrl Pts',(-61.5477669798653,-13.1910462288175,
40.146055361447));
#170259=CARTESIAN_POINT('Ctrl Pts',(-61.5545658738899,-13.1745141278031,
40.151152097463));
#170260=CARTESIAN_POINT('Ctrl Pts',(-61.5604649702291,-13.1573027128857,
40.1546258197409));
#170261=CARTESIAN_POINT('Ctrl Pts',(-61.5634145183987,-13.148697005427,
40.1563626808798));
#170262=CARTESIAN_POINT('Ctrl Pts',(-61.5661391177411,-13.1399214696213,
40.1576937882008));
#170263=CARTESIAN_POINT('Ctrl Pts',(-61.5686148699002,-13.1310016901027,
40.1585906813668));
#170264=CARTESIAN_POINT('Ctrl Pts',(-61.5698527459798,-13.1265418003434,
40.1590391279498));
#170265=CARTESIAN_POINT('Ctrl Pts',(-61.571028410384,-13.1220458496815,
40.1593790209175));
#170266=CARTESIAN_POINT('Ctrl Pts',(-61.5721388765028,-13.11751703634,40.1596068022931));
#170267=CARTESIAN_POINT('Ctrl Pts',(-61.5732493426217,-13.1129882229985,
40.1598345836687));
#170268=CARTESIAN_POINT('Ctrl Pts',(-61.5742946087864,-13.1084265466224,
40.1599502506865));
#170269=CARTESIAN_POINT('Ctrl Pts',(-61.5752716937452,-13.1038352065724,
40.1599502534424));
#170270=CARTESIAN_POINT('',(-61.5816197022698,-13.0739701745321,40.1599502534424));
#170271=CARTESIAN_POINT('Origin',(1.12331902584552E-16,3.23121069746441E-17,
40.1599502534424));
#170272=CARTESIAN_POINT('',(-61.4590390555209,-12.7383709431247,39.8576902534424));
#170273=CARTESIAN_POINT('Ctrl Pts',(-61.5816197022698,-13.0739701745321,
40.1599502534424));
#170274=CARTESIAN_POINT('Ctrl Pts',(-61.5824133495499,-13.0702318743173,
40.1599502447858));
#170275=CARTESIAN_POINT('Ctrl Pts',(-61.5831581321229,-13.0664939028182,
40.1598744685927));
#170276=CARTESIAN_POINT('Ctrl Pts',(-61.5838547466226,-13.0627583804523,
40.1597246934279));
#170277=CARTESIAN_POINT('Ctrl Pts',(-61.5878803190634,-13.041171669447,
40.1588591777435));
#170278=CARTESIAN_POINT('Ctrl Pts',(-61.5902997144309,-13.0196643745825,
40.1555254706023));
#170279=CARTESIAN_POINT('Ctrl Pts',(-61.5912450453419,-12.9986523536645,
40.1500631826386));
#170280=CARTESIAN_POINT('Ctrl Pts',(-61.5916263190447,-12.9901777222684,
40.1478601162485));
#170281=CARTESIAN_POINT('Ctrl Pts',(-61.5917681516647,-12.9817833412915,
40.1453112228309));
#170282=CARTESIAN_POINT('Ctrl Pts',(-61.591680417163,-12.973495091167,40.1424401896328));
#170283=CARTESIAN_POINT('Ctrl Pts',(-61.5916480484584,-12.9704372300721,
40.1413809526906));
#170284=CARTESIAN_POINT('Ctrl Pts',(-61.5915843445341,-12.9673939164347,
40.1402777640511));
#170285=CARTESIAN_POINT('Ctrl Pts',(-61.5914897592007,-12.9643665007547,
40.1391317641987));
#170286=CARTESIAN_POINT('Ctrl Pts',(-61.5913124117005,-12.9586900963547,
40.1369830144753));
#170287=CARTESIAN_POINT('Ctrl Pts',(-61.5910264967403,-12.9530695832098,
40.134683756585));
#170288=CARTESIAN_POINT('Ctrl Pts',(-61.5906350058491,-12.9475138635629,
40.1322415082996));
#170289=CARTESIAN_POINT('Ctrl Pts',(-61.5892647877301,-12.9280688447991,
40.1236936393009));
#170290=CARTESIAN_POINT('Ctrl Pts',(-61.5866012600731,-12.9094175454589,
40.113394140767));
#170291=CARTESIAN_POINT('Ctrl Pts',(-61.5827727094485,-12.8919416545039,
40.101665321223));
#170292=CARTESIAN_POINT('Ctrl Pts',(-61.5808584341363,-12.8832037090263,
40.095800911451));
#170293=CARTESIAN_POINT('Ctrl Pts',(-61.5786529040703,-12.8747596158553,
40.0895791707949));
#170294=CARTESIAN_POINT('Ctrl Pts',(-61.5761721637749,-12.8666570879113,
40.0830403822907));
#170295=CARTESIAN_POINT('Ctrl Pts',(-61.5749317936272,-12.8626058239394,
40.0797709880385));
#170296=CARTESIAN_POINT('Ctrl Pts',(-61.5736226210372,-12.8586399512975,
40.0764223317514));
#170297=CARTESIAN_POINT('Ctrl Pts',(-61.5722466520922,-12.8547654342062,
40.0729994484778));
#170298=CARTESIAN_POINT('Ctrl Pts',(-61.5708706831472,-12.8508909171149,
40.0695765652042));
#170299=CARTESIAN_POINT('Ctrl Pts',(-61.5694278436302,-12.8471078617857,
40.0660793733488));
#170300=CARTESIAN_POINT('Ctrl Pts',(-61.5679202927796,-12.8434220158072,
40.0625130768817));
#170301=CARTESIAN_POINT('Ctrl Pts',(-61.5679074365281,-12.8433905832603,
40.0624826638418));
#170302=CARTESIAN_POINT('Ctrl Pts',(-61.5678945756944,-12.8433591578472,
40.0624522459912));
#170303=CARTESIAN_POINT('Ctrl Pts',(-61.5678817102796,-12.8433277395705,
40.0624218233329));
#170304=CARTESIAN_POINT('Ctrl Pts',(-61.5613111551479,-12.8272819669692,
40.0468845275905));
#170305=CARTESIAN_POINT('Ctrl Pts',(-61.5536499750613,-12.8130163727079,
40.0302263329252));
#170306=CARTESIAN_POINT('Ctrl Pts',(-61.545097915485,-12.8005145062065,
40.0127515884766));
#170307=CARTESIAN_POINT('Ctrl Pts',(-61.5362566309325,-12.7875898348815,
39.9946858597744));
#170308=CARTESIAN_POINT('Ctrl Pts',(-61.5264624086167,-12.7765497640383,
39.9757460620526));
#170309=CARTESIAN_POINT('Ctrl Pts',(-61.5159109908824,-12.767421983407,
39.9562444559172));
#170310=CARTESIAN_POINT('Ctrl Pts',(-61.5055602833158,-12.7584678323701,
39.937113811366));
#170311=CARTESIAN_POINT('Ctrl Pts',(-61.4944799879529,-12.7513538295741,
39.9174410654407));
#170312=CARTESIAN_POINT('Ctrl Pts',(-61.4828443590702,-12.7461528104584,
39.8975196504204));
#170313=CARTESIAN_POINT('Ctrl Pts',(-61.4751361628613,-12.7427073176334,
39.8843224113814));
#170314=CARTESIAN_POINT('Ctrl Pts',(-61.4671840587585,-12.7401023057311,
39.8710160447151));
#170315=CARTESIAN_POINT('Ctrl Pts',(-61.4590390555209,-12.7383709431247,
39.8576902534424));
#170316=CARTESIAN_POINT('',(-61.1105274371642,-12.6642893210138,39.2875012672119));
#170317=CARTESIAN_POINT('',(-61.4590390555209,-12.7383709431247,39.8576902534424));
#170318=CARTESIAN_POINT('',(-62.0330459552233,-6.83973663030219,39.2875012672119));
#170319=CARTESIAN_POINT('Origin',(5.53234440788222E-15,0.,39.2875012672119));
#170320=CARTESIAN_POINT('',(-62.3873926810692,-6.87697683366523,39.8576902534424));
#170321=CARTESIAN_POINT('',(-62.0330459552233,-6.83973663030219,39.2875012672119));
#170322=CARTESIAN_POINT('',(-62.6076796697355,-6.59568250079844,40.1599502534424));
#170323=CARTESIAN_POINT('Ctrl Pts',(-62.3873926810692,-6.87697683366523,
39.8576902534424));
#170324=CARTESIAN_POINT('Ctrl Pts',(-62.3996312165479,-6.87826302285553,
39.8773836120375));
#170325=CARTESIAN_POINT('Ctrl Pts',(-62.4120334591708,-6.87760542308973,
39.8969946442154));
#170326=CARTESIAN_POINT('Ctrl Pts',(-62.4244204973417,-6.87506472947493,
39.9162525288273));
#170327=CARTESIAN_POINT('Ctrl Pts',(-62.4370564393957,-6.87247298342148,
39.9358973794106));
#170328=CARTESIAN_POINT('Ctrl Pts',(-62.4496774784119,-6.8679218469014,
39.9551762199793));
#170329=CARTESIAN_POINT('Ctrl Pts',(-62.4621080448386,-6.86142424476579,
39.9738152034304));
#170330=CARTESIAN_POINT('Ctrl Pts',(-62.4740556950283,-6.85517906858289,
39.9917300792713));
#170331=CARTESIAN_POINT('Ctrl Pts',(-62.485828220292,-6.84713544260593,
40.0090551158197));
#170332=CARTESIAN_POINT('Ctrl Pts',(-62.4972698477183,-6.83725958232806,
40.0255394551615));
#170333=CARTESIAN_POINT('Ctrl Pts',(-62.5060589088708,-6.82967328916524,
40.0382021526201));
#170334=CARTESIAN_POINT('Ctrl Pts',(-62.5146528151171,-6.82100495424908,
40.0503687782148));
#170335=CARTESIAN_POINT('Ctrl Pts',(-62.5229765487298,-6.81122125790639,
40.0619155352442));
#170336=CARTESIAN_POINT('Ctrl Pts',(-62.5229983637511,-6.81119561658308,
40.0619457972351));
#170337=CARTESIAN_POINT('Ctrl Pts',(-62.5230201768492,-6.81116996676389,
40.0619760547305));
#170338=CARTESIAN_POINT('Ctrl Pts',(-62.5230419880218,-6.81114430845115,
40.0620063077269));
#170339=CARTESIAN_POINT('Ctrl Pts',(-62.5253805892672,-6.80839321554205,
40.06525004417));
#170340=CARTESIAN_POINT('Ctrl Pts',(-62.5276952632611,-6.80554511475028,
40.0684393223557));
#170341=CARTESIAN_POINT('Ctrl Pts',(-62.5299828381019,-6.80260378684076,
40.0715697951759));
#170342=CARTESIAN_POINT('Ctrl Pts',(-62.5427126719606,-6.78623596579932,
40.0889901646392));
#170343=CARTESIAN_POINT('Ctrl Pts',(-62.5546072354084,-6.76698429120816,
40.1045963098191));
#170344=CARTESIAN_POINT('Ctrl Pts',(-62.5651294462056,-6.74555473735616,
40.1176634650661));
#170345=CARTESIAN_POINT('Ctrl Pts',(-62.569851960129,-6.73593685681868,
40.1235281853023));
#170346=CARTESIAN_POINT('Ctrl Pts',(-62.5742983919715,-6.72588021343918,
40.1288820140902));
#170347=CARTESIAN_POINT('Ctrl Pts',(-62.5784220664834,-6.71544740276736,
40.1336621774101));
#170348=CARTESIAN_POINT('Ctrl Pts',(-62.580214159649,-6.71091344436472,
40.1357395717319));
#170349=CARTESIAN_POINT('Ctrl Pts',(-62.5819451239083,-6.70630855228255,
40.1377083672884));
#170350=CARTESIAN_POINT('Ctrl Pts',(-62.5836110216378,-6.70163794008936,
40.1395632548792));
#170351=CARTESIAN_POINT('Ctrl Pts',(-62.5894416636914,-6.68529079741317,
40.146055361447));
#170352=CARTESIAN_POINT('Ctrl Pts',(-62.5944752375494,-6.66813858303363,
40.151152097463));
#170353=CARTESIAN_POINT('Ctrl Pts',(-62.5985429352697,-6.65040483057297,
40.1546258197409));
#170354=CARTESIAN_POINT('Ctrl Pts',(-62.6005767841298,-6.64153795434265,
40.1563626808798));
#170355=CARTESIAN_POINT('Ctrl Pts',(-62.6023691645599,-6.63252569365801,
40.1576937882008));
#170356=CARTESIAN_POINT('Ctrl Pts',(-62.6038989834438,-6.62339599105629,
40.1585906813668));
#170357=CARTESIAN_POINT('Ctrl Pts',(-62.6046638928858,-6.61883113975543,
40.1590391279498));
#170358=CARTESIAN_POINT('Ctrl Pts',(-62.6053631620638,-6.61423692798816,
40.1593790209175));
#170359=CARTESIAN_POINT('Ctrl Pts',(-62.6059941550341,-6.6096168486431,
40.1596068022931));
#170360=CARTESIAN_POINT('Ctrl Pts',(-62.6066251480043,-6.60499676929804,
40.1598345836687));
#170361=CARTESIAN_POINT('Ctrl Pts',(-62.6071878630701,-6.60035082219649,
40.1599502506865));
#170362=CARTESIAN_POINT('Ctrl Pts',(-62.6076796697355,-6.59568250079845,
40.1599502534424));
#170363=CARTESIAN_POINT('',(-62.6108711573006,-6.56531752495261,40.1599502534424));
#170364=CARTESIAN_POINT('Origin',(1.148766751165E-16,1.62450455465728E-17,
40.1599502534424));
#170365=CARTESIAN_POINT('',(-62.4538823482276,-6.24436990788019,39.8576902534424));
#170366=CARTESIAN_POINT('Ctrl Pts',(-62.6108711573006,-6.56531752495261,
40.1599502534424));
#170367=CARTESIAN_POINT('Ctrl Pts',(-62.6112696981211,-6.56151674480702,
40.1599502447858));
#170368=CARTESIAN_POINT('Ctrl Pts',(-62.6116196762807,-6.557721399329,40.1598744685927));
#170369=CARTESIAN_POINT('Ctrl Pts',(-62.6119220062409,-6.55393352450239,
40.1597246934279));
#170370=CARTESIAN_POINT('Ctrl Pts',(-62.6136691004464,-6.53204428085628,
40.1588591777434));
#170371=CARTESIAN_POINT('Ctrl Pts',(-62.6138271176316,-6.51040190952224,
40.1555254706018));
#170372=CARTESIAN_POINT('Ctrl Pts',(-62.612570915664,-6.48940618066474,
40.1500631826375));
#170373=CARTESIAN_POINT('Ctrl Pts',(-62.6120642605129,-6.4809381202332,
40.1478601162477));
#170374=CARTESIAN_POINT('Ctrl Pts',(-62.6113278644156,-6.47257489900915,
40.1453112228304));
#170375=CARTESIAN_POINT('Ctrl Pts',(-62.610374252484,-6.46434122353989,
40.1424401896328));
#170376=CARTESIAN_POINT('Ctrl Pts',(-62.6100224275775,-6.46130349717896,
40.1413809526905));
#170377=CARTESIAN_POINT('Ctrl Pts',(-62.6096409597322,-6.45828351400542,
40.1402777640511));
#170378=CARTESIAN_POINT('Ctrl Pts',(-62.6092304414384,-6.45528256968482,
40.1391317641987));
#170379=CARTESIAN_POINT('Ctrl Pts',(-62.6084607196375,-6.4496557990837,
40.1369830144753));
#170380=CARTESIAN_POINT('Ctrl Pts',(-62.6075888673476,-6.44409596194931,
40.1346837565849));
#170381=CARTESIAN_POINT('Ctrl Pts',(-62.6066187902475,-6.43861159905725,
40.1322415082996));
#170382=CARTESIAN_POINT('Ctrl Pts',(-62.6032235203971,-6.41941632893507,
40.1236936393008));
#170383=CARTESIAN_POINT('Ctrl Pts',(-62.5986249921653,-6.40114561781709,
40.113394140767));
#170384=CARTESIAN_POINT('Ctrl Pts',(-62.5929906867159,-6.38416565413452,
40.101665321223));
#170385=CARTESIAN_POINT('Ctrl Pts',(-62.5901735339912,-6.37567567229323,
40.095800911451));
#170386=CARTESIAN_POINT('Ctrl Pts',(-62.5870974379668,-6.36750837741663,
40.0895791707949));
#170387=CARTESIAN_POINT('Ctrl Pts',(-62.5837833426318,-6.35970954393935,
40.0830403822907));
#170388=CARTESIAN_POINT('Ctrl Pts',(-62.5821262949642,-6.35581012720071,
40.0797709880385));
#170389=CARTESIAN_POINT('Ctrl Pts',(-62.580409747586,-6.35200282582317,
40.0764223317514));
#170390=CARTESIAN_POINT('Ctrl Pts',(-62.5786363190253,-6.34829336166122,
40.0729994484778));
#170391=CARTESIAN_POINT('Ctrl Pts',(-62.5768628904647,-6.34458389749927,
40.0695765652042));
#170392=CARTESIAN_POINT('Ctrl Pts',(-62.5750325180135,-6.34097238394038,
40.0660793733488));
#170393=CARTESIAN_POINT('Ctrl Pts',(-62.5731479498682,-6.33746431138553,
40.0625130768817));
#170394=CARTESIAN_POINT('Ctrl Pts',(-62.5731318784488,-6.33743439487368,
40.0624826638418));
#170395=CARTESIAN_POINT('Ctrl Pts',(-62.5731158032179,-6.33740448593541,
40.0624522459912));
#170396=CARTESIAN_POINT('Ctrl Pts',(-62.5730997241771,-6.33737458457336,
40.0624218233329));
#170397=CARTESIAN_POINT('Ctrl Pts',(-62.5648879232826,-6.32210352242532,
40.0468845275918));
#170398=CARTESIAN_POINT('Ctrl Pts',(-62.5557775512973,-6.3087168879643,
40.030226332928));
#170399=CARTESIAN_POINT('Ctrl Pts',(-62.5459655399057,-6.29717744164162,
40.012751588481));
#170400=CARTESIAN_POINT('Ctrl Pts',(-62.5358216928042,-6.28524773890675,
39.9946858597805));
#170401=CARTESIAN_POINT('Ctrl Pts',(-62.5249271226245,-6.27529192173462,
39.9757460620605));
#170402=CARTESIAN_POINT('Ctrl Pts',(-62.5134793937792,-6.26731706752176,
39.9562444559268));
#170403=CARTESIAN_POINT('Ctrl Pts',(-62.502249424825,-6.25949391181675,
39.9371138113773));
#170404=CARTESIAN_POINT('Ctrl Pts',(-62.4904862127005,-6.25357708651889,
39.9174410654536));
#170405=CARTESIAN_POINT('Ctrl Pts',(-62.4783706704757,-6.24962081353567,
39.8975196504349));
#170406=CARTESIAN_POINT('Ctrl Pts',(-62.4703445484992,-6.24699992138354,
39.8843224113911));
#170407=CARTESIAN_POINT('Ctrl Pts',(-62.4621637089609,-6.24524040122965,
39.87101604472));
#170408=CARTESIAN_POINT('Ctrl Pts',(-62.4538823482276,-6.24436990788019,
39.8576902534424));
#170409=CARTESIAN_POINT('',(-62.0995362748659,-6.20712349654422,39.2875012672119));
#170410=CARTESIAN_POINT('',(-62.4538823482276,-6.24436990788019,39.8576902534424));
#170411=CARTESIAN_POINT('',(-62.4081695979768,-0.318048871877127,39.2875012672119));
#170412=CARTESIAN_POINT('Origin',(5.53234440788222E-15,0.,39.2875012672119));
#170413=CARTESIAN_POINT('',(-62.7644678366119,-0.318045750793044,39.8576902534424));
#170414=CARTESIAN_POINT('',(-62.4081695979768,-0.318048871877129,39.2875012672119));
#170415=CARTESIAN_POINT('Ctrl Pts',(-62.7644678366119,-0.318045750793045,
39.8576902534424));
#170416=CARTESIAN_POINT('Ctrl Pts',(-62.7767737714912,-0.318045618798132,
39.8773836120357));
#170417=CARTESIAN_POINT('Ctrl Pts',(-62.7890393354372,-0.316095234070559,
39.8969946442117));
#170418=CARTESIAN_POINT('Ctrl Pts',(-62.8010929413166,-0.312273660577473,
39.9162525288219));
#170419=CARTESIAN_POINT('Ctrl Pts',(-62.8133887511246,-0.308375296775969,
39.9358973794033));
#170420=CARTESIAN_POINT('Ctrl Pts',(-62.8254649274609,-0.302529834045832,
39.9551762199702));
#170421=CARTESIAN_POINT('Ctrl Pts',(-62.8371482135769,-0.294768478449938,
39.9738152034198));
#170422=CARTESIAN_POINT('Ctrl Pts',(-62.8483776146185,-0.287308644483076,
39.9917300792591));
#170423=CARTESIAN_POINT('Ctrl Pts',(-62.8592448608937,-0.278078518358053,
40.0090551158061));
#170424=CARTESIAN_POINT('Ctrl Pts',(-62.8695915013888,-0.267060783346145,
40.0255394551467));
#170425=CARTESIAN_POINT('Ctrl Pts',(-62.8775394315818,-0.258597341632753,
40.0382021526107));
#170426=CARTESIAN_POINT('Ctrl Pts',(-62.8851801717857,-0.249078184945598,
40.0503687782103));
#170427=CARTESIAN_POINT('Ctrl Pts',(-62.8924356323738,-0.238478017627878,
40.0619155352442));
#170428=CARTESIAN_POINT('Ctrl Pts',(-62.892454647642,-0.23845023647977,
40.0619457972351));
#170429=CARTESIAN_POINT('Ctrl Pts',(-62.8924736601095,-0.238422447083347,
40.0619760547305));
#170430=CARTESIAN_POINT('Ctrl Pts',(-62.8924926697742,-0.238394649441185,
40.0620063077269));
#170431=CARTESIAN_POINT('Ctrl Pts',(-62.8945308924032,-0.23541417691252,
40.06525004417));
#170432=CARTESIAN_POINT('Ctrl Pts',(-62.8965351787718,-0.232339728999315,
40.0684393223557));
#170433=CARTESIAN_POINT('Ctrl Pts',(-62.8985027695519,-0.229175397309122,
40.0715697951759));
#170434=CARTESIAN_POINT('Ctrl Pts',(-62.9094519648694,-0.211566610931162,
40.088990164641));
#170435=CARTESIAN_POINT('Ctrl Pts',(-62.9192690206947,-0.191177078586841,
40.1045963098225));
#170436=CARTESIAN_POINT('Ctrl Pts',(-62.9274935913881,-0.168765047545427,
40.1176634650702));
#170437=CARTESIAN_POINT('Ctrl Pts',(-62.9311848926126,-0.158706217642862,
40.1235281853049));
#170438=CARTESIAN_POINT('Ctrl Pts',(-62.9345557609572,-0.148239886922884,
40.1288820140914));
#170439=CARTESIAN_POINT('Ctrl Pts',(-62.9375663198809,-0.137433186922322,
40.1336621774101));
#170440=CARTESIAN_POINT('Ctrl Pts',(-62.9388746680683,-0.132736741273575,
40.1357395717319));
#170441=CARTESIAN_POINT('Ctrl Pts',(-62.9401148076313,-0.127976140238065,
40.1377083672884));
#170442=CARTESIAN_POINT('Ctrl Pts',(-62.9412833674838,-0.123156980417526,
40.1395632548792));
#170443=CARTESIAN_POINT('Ctrl Pts',(-62.9453733269673,-0.106289921045641,
40.146055361447));
#170444=CARTESIAN_POINT('Ctrl Pts',(-62.9485864317704,-0.0887055165510291,
40.151152097463));
#170445=CARTESIAN_POINT('Ctrl Pts',(-62.9507781643242,-0.0706437212501446,
40.1546258197409));
#170446=CARTESIAN_POINT('Ctrl Pts',(-62.9518740306011,-0.0616128235997025,
40.1563626808798));
#170447=CARTESIAN_POINT('Ctrl Pts',(-62.9527145544237,-0.0524625782501274,
40.1576937882008));
#170448=CARTESIAN_POINT('Ctrl Pts',(-62.9532816790167,-0.0432229794975093,
40.1585906813668));
#170449=CARTESIAN_POINT('Ctrl Pts',(-62.9535652413132,-0.0386031801212003,
40.1590391279498));
#170450=CARTESIAN_POINT('Ctrl Pts',(-62.9537804539255,-0.0339610423941066,
40.1593790209175));
#170451=CARTESIAN_POINT('Ctrl Pts',(-62.9539250604562,-0.0293003156015957,
40.1596068022931));
#170452=CARTESIAN_POINT('Ctrl Pts',(-62.9540696669868,-0.0246395888090847,
40.1598345836687));
#170453=CARTESIAN_POINT('Ctrl Pts',(-62.9541436657296,-0.0199602729507917,
40.1599502506865));
#170454=CARTESIAN_POINT('Ctrl Pts',(-62.9541448057648,-0.0152661173108669,
40.1599502534424));
#170455=CARTESIAN_POINT('',(-62.2224557307631,-7.62005312457669E-15,38.989));
#170456=CARTESIAN_POINT('',(-62.7644678366119,0.318045750793044,39.8576902534424));
#170457=CARTESIAN_POINT('Ctrl Pts',(-62.9541448057648,0.0152661173108668,
40.1599502534424));
#170458=CARTESIAN_POINT('Ctrl Pts',(-62.9541438736292,0.0190877352446491,
40.1599502447858));
#170459=CARTESIAN_POINT('Ctrl Pts',(-62.9540952129414,0.0228988721022259,
40.1598744685927));
#170460=CARTESIAN_POINT('Ctrl Pts',(-62.9539999459718,0.0266975986403491,
40.1597246934279));
#170461=CARTESIAN_POINT('Ctrl Pts',(-62.953449420412,0.0486495517950492,
40.1588591777433));
#170462=CARTESIAN_POINT('Ctrl Pts',(-62.9513443281449,0.0701898812509633,
40.1555254706009));
#170463=CARTESIAN_POINT('Ctrl Pts',(-62.9479003565096,0.0909392844504461,
40.1500631826352));
#170464=CARTESIAN_POINT('Ctrl Pts',(-62.9465113235251,0.0993079960735539,
40.1478601162459));
#170465=CARTESIAN_POINT('Ctrl Pts',(-62.9449047668205,0.107548428341324,
40.1453112228295));
#170466=CARTESIAN_POINT('Ctrl Pts',(-62.9430957254317,0.115637319282268,
40.1424401896328));
#170467=CARTESIAN_POINT('Ctrl Pts',(-62.9424282989905,0.118621628943523,
40.1413809526906));
#170468=CARTESIAN_POINT('Ctrl Pts',(-62.9417332466658,0.121585194085607,
40.1402777640511));
#170469=CARTESIAN_POINT('Ctrl Pts',(-62.9410112931359,0.124526788072828,
40.1391317641987));
#170470=CARTESIAN_POINT('Ctrl Pts',(-62.9396576302675,0.130042276798866,
40.1369830144753));
#170471=CARTESIAN_POINT('Ctrl Pts',(-62.938209392844,0.135480523183637,
40.134683756585));
#170472=CARTESIAN_POINT('Ctrl Pts',(-62.9366713579026,0.140833441493401,
40.1322415082996));
#170473=CARTESIAN_POINT('Ctrl Pts',(-62.9312882356078,0.159568655577575,
40.1236936393009));
#170474=CARTESIAN_POINT('Ctrl Pts',(-62.9248050892389,0.177258600738988,
40.113394140767));
#170475=CARTESIAN_POINT('Ctrl Pts',(-62.9174267595942,0.193556601113662,
40.101665321223));
#170476=CARTESIAN_POINT('Ctrl Pts',(-62.9137375947718,0.201705601300999,
40.095800911451));
#170477=CARTESIAN_POINT('Ctrl Pts',(-62.9098246351408,0.209506615291412,
40.0895791707949));
#170478=CARTESIAN_POINT('Ctrl Pts',(-62.9057134946881,0.2169163086504,40.0830403822907));
#170479=CARTESIAN_POINT('Ctrl Pts',(-62.9036579244618,0.220621155329894,
40.0797709880385));
#170480=CARTESIAN_POINT('Ctrl Pts',(-62.9015528091474,0.22422817185255,
40.0764223317514));
#170481=CARTESIAN_POINT('Ctrl Pts',(-62.8994013510256,0.227731941419537,
40.0729994484778));
#170482=CARTESIAN_POINT('Ctrl Pts',(-62.8972498929038,0.231235710986524,
40.0695765652043));
#170483=CARTESIAN_POINT('Ctrl Pts',(-62.8950520414621,0.23463611427673,
40.0660793733488));
#170484=CARTESIAN_POINT('Ctrl Pts',(-62.8928111037451,0.237927978230917,
40.0625130768817));
#170485=CARTESIAN_POINT('Ctrl Pts',(-62.8927919932396,0.237956050936214,
40.0624826638418));
#170486=CARTESIAN_POINT('Ctrl Pts',(-62.8927728797351,0.237984115711007,
40.0624522459912));
#170487=CARTESIAN_POINT('Ctrl Pts',(-62.8927537632335,0.238012172552842,
40.0624218233329));
#170488=CARTESIAN_POINT('Ctrl Pts',(-62.8829906867849,0.25234121129618,
40.0468845275921));
#170489=CARTESIAN_POINT('Ctrl Pts',(-62.8725309380422,0.264702219189351,
40.0302263329286));
#170490=CARTESIAN_POINT('Ctrl Pts',(-62.8615664772848,0.275152816745237,
40.012751588482));
#170491=CARTESIAN_POINT('Ctrl Pts',(-62.8502312057452,0.285956846571069,
39.9946858597817));
#170492=CARTESIAN_POINT('Ctrl Pts',(-62.8383556508915,0.294719332056153,
39.975746062062));
#170493=CARTESIAN_POINT('Ctrl Pts',(-62.8261370346472,0.30145388567915,
39.9562444559287));
#170494=CARTESIAN_POINT('Ctrl Pts',(-62.8141508421943,0.308060333921374,
39.9371138113794));
#170495=CARTESIAN_POINT('Ctrl Pts',(-62.8018335935211,0.312715155744803,
39.9174410654561));
#170496=CARTESIAN_POINT('Ctrl Pts',(-62.7893708783692,0.315383336840398,
39.8975196504376));
#170497=CARTESIAN_POINT('Ctrl Pts',(-62.781114766499,0.317150913275127,
39.884322411393));
#170498=CARTESIAN_POINT('Ctrl Pts',(-62.7727948225173,0.318045664008455,
39.8710160447209));
#170499=CARTESIAN_POINT('Ctrl Pts',(-62.7644678366119,0.318045750793045,
39.8576902534424));
#170500=CARTESIAN_POINT('',(-62.4081695979768,0.318048871877127,39.2875012672119));
#170501=CARTESIAN_POINT('',(-62.7644678366119,0.318045750793045,39.8576902534424));
#170502=CARTESIAN_POINT('',(-62.0995362748658,6.20712349654507,39.2875012672119));
#170503=CARTESIAN_POINT('Origin',(5.53234440788222E-15,0.,39.2875012672119));
#170504=CARTESIAN_POINT('',(-62.4538823482275,6.24436990788103,39.8576902534424));
#170505=CARTESIAN_POINT('',(-62.0995362748658,6.20712349654507,39.2875012672119));
#170506=CARTESIAN_POINT('',(-62.6108711573005,6.56531752495345,40.1599502534424));
#170507=CARTESIAN_POINT('Ctrl Pts',(-62.4538823482275,6.24436990788103,
39.8576902534424));
#170508=CARTESIAN_POINT('Ctrl Pts',(-62.4661208561129,6.24565635961515,
39.8773836120393));
#170509=CARTESIAN_POINT('Ctrl Pts',(-62.4781153573,6.24887816048243,39.8969946442189));
#170510=CARTESIAN_POINT('Ctrl Pts',(-62.4897034690628,6.25393874389706,
39.9162525288325));
#170511=CARTESIAN_POINT('Ctrl Pts',(-62.5015244311627,6.25910101415925,
39.9358973794174));
#170512=CARTESIAN_POINT('Ctrl Pts',(-62.5129234357071,6.26617675898984,
39.9551762199877));
#170513=CARTESIAN_POINT('Ctrl Pts',(-62.5237314369876,6.27511683301435,
39.9738152034403));
#170514=CARTESIAN_POINT('Ctrl Pts',(-62.5341195572161,6.28370959326737,
39.9917300792824));
#170515=CARTESIAN_POINT('Ctrl Pts',(-62.5439624606807,6.29402509235232,
40.0090551158319));
#170516=CARTESIAN_POINT('Ctrl Pts',(-62.5531007542879,6.3060639894941,40.0255394551746));
#170517=CARTESIAN_POINT('Ctrl Pts',(-62.5601204743257,6.3153118525122,40.0382021526285));
#170518=CARTESIAN_POINT('Ctrl Pts',(-62.56672433493,6.32557753708801,40.0503687782188));
#170519=CARTESIAN_POINT('Ctrl Pts',(-62.5728320301412,6.33687803771732,
40.0619155352442));
#170520=CARTESIAN_POINT('Ctrl Pts',(-62.5728480373211,6.33690765431417,
40.0619457972352));
#170521=CARTESIAN_POINT('Ctrl Pts',(-62.5728640408534,6.33693727882138,
40.0619760547305));
#170522=CARTESIAN_POINT('Ctrl Pts',(-62.5728800407363,6.33696691123619,
40.062006307727));
#170523=CARTESIAN_POINT('Ctrl Pts',(-62.5745955535553,6.34014410870369,
40.06525004417));
#170524=CARTESIAN_POINT('Ctrl Pts',(-62.5762674929177,6.34341121944362,
40.0684393223557));
#170525=CARTESIAN_POINT('Ctrl Pts',(-62.5778935423007,6.3467638858343,40.0715697951759));
#170526=CARTESIAN_POINT('Ctrl Pts',(-62.586942137401,6.36542071199947,40.0889901646418));
#170527=CARTESIAN_POINT('Ctrl Pts',(-62.594574127885,6.38672471011255,40.1045963098239));
#170528=CARTESIAN_POINT('Ctrl Pts',(-62.6004109483562,6.40987366743977,
40.117663465072));
#170529=CARTESIAN_POINT('Ctrl Pts',(-62.603030594214,6.42026324006312,40.123528185306));
#170530=CARTESIAN_POINT('Ctrl Pts',(-62.6052889671226,6.43102458681517,
40.1288820140919));
#170531=CARTESIAN_POINT('Ctrl Pts',(-62.6071534261453,6.44208677567914,
40.1336621774101));
#170532=CARTESIAN_POINT('Ctrl Pts',(-62.6079636948179,6.44689425333267,
40.1357395717319));
#170533=CARTESIAN_POINT('Ctrl Pts',(-62.6086994224562,6.45175840518036,
40.1377083672884));
#170534=CARTESIAN_POINT('Ctrl Pts',(-62.6093578414452,6.45667331290478,
40.1395632548792));
#170535=CARTESIAN_POINT('Ctrl Pts',(-62.6116623079068,6.47387548994023,
40.146055361447));
#170536=CARTESIAN_POINT('Ctrl Pts',(-62.6130197402062,6.49169942613452,
40.151152097463));
#170537=CARTESIAN_POINT('Ctrl Pts',(-62.6133114945132,6.50989137546665,
40.1546258197409));
#170538=CARTESIAN_POINT('Ctrl Pts',(-62.6134573716666,6.51898735013272,
40.1563626808798));
#170539=CARTESIAN_POINT('Ctrl Pts',(-62.6133368299269,6.52817532814438,
40.1576937882008));
#170540=CARTESIAN_POINT('Ctrl Pts',(-62.6129350466932,6.53742359207046,
40.1585906813668));
#170541=CARTESIAN_POINT('Ctrl Pts',(-62.6127341550763,6.5420477240335,40.1590391279498));
#170542=CARTESIAN_POINT('Ctrl Pts',(-62.6124629532085,6.54668692748805,
40.1593790209175));
#170543=CARTESIAN_POINT('Ctrl Pts',(-62.6121195889601,6.55133723782996,
40.1596068022931));
#170544=CARTESIAN_POINT('Ctrl Pts',(-62.6117762247118,6.55598754817187,
40.1598345836687));
#170545=CARTESIAN_POINT('Ctrl Pts',(-62.6113606963859,6.56064896522315,
40.1599502506865));
#170546=CARTESIAN_POINT('Ctrl Pts',(-62.6108711573005,6.56531752495346,
40.1599502534424));
#170547=CARTESIAN_POINT('',(-62.6076796697354,6.59568250079929,40.1599502534424));
#170548=CARTESIAN_POINT('Origin',(1.14876675116497E-16,-1.62450455465748E-17,
40.1599502534424));
#170549=CARTESIAN_POINT('',(-62.3873926810691,6.87697683366608,39.8576902534424));
#170550=CARTESIAN_POINT('Ctrl Pts',(-62.6076796697354,6.59568250079929,
40.1599502534424));
#170551=CARTESIAN_POINT('Ctrl Pts',(-62.6072792748562,6.59948308607546,
40.1599502447858));
#170552=CARTESIAN_POINT('Ctrl Pts',(-62.6068325084578,6.60326825869965,
40.1598744685927));
#170553=CARTESIAN_POINT('Ctrl Pts',(-62.6063406883232,6.6070362173064,40.1597246934279));
#170554=CARTESIAN_POINT('Ctrl Pts',(-62.6034985746712,6.62881036977223,
40.1588591777434));
#170555=CARTESIAN_POINT('Ctrl Pts',(-62.5991534367841,6.65001265698812,
40.1555254706015));
#170556=CARTESIAN_POINT('Ctrl Pts',(-62.5935594283563,6.67028839972168,
40.1500631826366));
#170557=CARTESIAN_POINT('Ctrl Pts',(-62.5913032360739,6.67846607318537,
40.147860116247));
#170558=CARTESIAN_POINT('Ctrl Pts',(-62.588844120533,6.68649343260121,40.14531122283));
#170559=CARTESIAN_POINT('Ctrl Pts',(-62.586199469922,6.69434891543653,40.1424401896328));
#170560=CARTESIAN_POINT('Ctrl Pts',(-62.5852237544099,6.69724711167696,
40.1413809526905));
#170561=CARTESIAN_POINT('Ctrl Pts',(-62.5842227327444,6.70012178934772,
40.1402777640511));
#170562=CARTESIAN_POINT('Ctrl Pts',(-62.5831972538525,6.70297180428227,
40.1391317641987));
#170563=CARTESIAN_POINT('Ctrl Pts',(-62.5812744809302,6.70831558228455,
40.1369830144753));
#170564=CARTESIAN_POINT('Ctrl Pts',(-62.5792657255653,6.71357265535428,
40.1346837565849));
#170565=CARTESIAN_POINT('Ctrl Pts',(-62.5771765838154,6.71873548138859,
40.1322415082996));
#170566=CARTESIAN_POINT('Ctrl Pts',(-62.5698645876906,6.73680537250866,
40.1236936393008));
#170567=CARTESIAN_POINT('Ctrl Pts',(-62.5615678538927,6.75372073697247,
40.113394140767));
#170568=CARTESIAN_POINT('Ctrl Pts',(-62.5525263385764,6.76915820973656,
40.101665321223));
#170569=CARTESIAN_POINT('Ctrl Pts',(-62.5480055809182,6.77687694611861,
40.095800911451));
#170570=CARTESIAN_POINT('Ctrl Pts',(-62.5432986288851,6.78422620968109,
40.0895791707949));
#170571=CARTESIAN_POINT('Ctrl Pts',(-62.5384354858298,6.79116558077077,
40.0830403822906));
#170572=CARTESIAN_POINT('Ctrl Pts',(-62.5360039143022,6.79463526631561,
40.0797709880385));
#170573=CARTESIAN_POINT('Ctrl Pts',(-62.5335332951357,6.79800247875554,
40.0764223317514));
#170574=CARTESIAN_POINT('Ctrl Pts',(-62.5310273792782,6.80126216569498,
40.0729994484778));
#170575=CARTESIAN_POINT('Ctrl Pts',(-62.5285214634206,6.80452185263442,
40.0695765652042));
#170576=CARTESIAN_POINT('Ctrl Pts',(-62.5259802131085,6.80767389012592,
40.0660793733488));
#170577=CARTESIAN_POINT('Ctrl Pts',(-62.5234074580024,6.8107134791291,40.0625130768817));
#170578=CARTESIAN_POINT('Ctrl Pts',(-62.5233855177895,6.8107394004574,40.0624826638418));
#170579=CARTESIAN_POINT('Ctrl Pts',(-62.523363575423,6.81076531358517,40.0624522459912));
#170580=CARTESIAN_POINT('Ctrl Pts',(-62.5233416309051,6.81079121851015,
40.0624218233329));
#170581=CARTESIAN_POINT('Ctrl Pts',(-62.5121342452096,6.8240212419036,40.0468845275903));
#170582=CARTESIAN_POINT('Ctrl Pts',(-62.5004397189039,6.83522119344104,
40.0302263329247));
#170583=CARTESIAN_POINT('Ctrl Pts',(-62.4884429377056,6.84446844329716,
40.0127515884758));
#170584=CARTESIAN_POINT('Ctrl Pts',(-62.4760404333332,6.85402842900305,
39.9946858597733));
#170585=CARTESIAN_POINT('Ctrl Pts',(-62.4633140048678,6.86150157917666,
39.9757460620511));
#170586=CARTESIAN_POINT('Ctrl Pts',(-62.4504583709392,6.86692204703067,
39.9562444559153));
#170587=CARTESIAN_POINT('Ctrl Pts',(-62.4378472782189,6.87223940618026,
39.9371138113637));
#170588=CARTESIAN_POINT('Ctrl Pts',(-62.4251109433493,6.87558122532639,
39.9174410654381));
#170589=CARTESIAN_POINT('Ctrl Pts',(-62.4124375993841,6.87693208138258,
39.8975196504175));
#170590=CARTESIAN_POINT('Ctrl Pts',(-62.4040419533145,6.87782697616094,
39.8843224113794));
#170591=CARTESIAN_POINT('Ctrl Pts',(-62.3956740599416,6.87784715439679,
39.8710160447141));
#170592=CARTESIAN_POINT('Ctrl Pts',(-62.3873926810691,6.87697683366608,
39.8576902534424));
#170593=CARTESIAN_POINT('',(-62.0330459552232,6.83973663030303,39.2875012672119));
#170594=CARTESIAN_POINT('',(-62.3873926810691,6.87697683366608,39.8576902534424));
#170595=CARTESIAN_POINT('',(-61.110527437164,12.6642893210146,39.2875012672119));
#170596=CARTESIAN_POINT('Origin',(5.53234440788222E-15,0.,39.2875012672119));
#170597=CARTESIAN_POINT('',(-61.4590390555207,12.7383709431255,39.8576902534424));
#170598=CARTESIAN_POINT('',(-61.110527437164,12.6642893210146,39.2875012672119));
#170599=CARTESIAN_POINT('',(-61.5816197022697,13.0739701745329,40.1599502534424));
#170600=CARTESIAN_POINT('Ctrl Pts',(-61.4590390555208,12.7383709431255,
39.8576902534424));
#170601=CARTESIAN_POINT('Ctrl Pts',(-61.4710760487555,12.740929619964,39.8773836120375));
#170602=CARTESIAN_POINT('Ctrl Pts',(-61.4826680729155,12.7453875382452,
39.8969946442153));
#170603=CARTESIAN_POINT('Ctrl Pts',(-61.4936637287811,12.7516316867682,
39.9162525288271));
#170604=CARTESIAN_POINT('Ctrl Pts',(-61.5048803302354,12.7580013045755,
39.9358973794104));
#170605=CARTESIAN_POINT('Ctrl Pts',(-61.5154772731058,12.7662298081621,
39.955176219979));
#170606=CARTESIAN_POINT('Ctrl Pts',(-61.5252915748245,12.776250651289,39.9738152034302));
#170607=CARTESIAN_POINT('Ctrl Pts',(-61.5347245998185,12.7858821937447,
39.9917300792711));
#170608=CARTESIAN_POINT('Ctrl Pts',(-61.5434353195605,12.797170047018,40.0090551158196));
#170609=CARTESIAN_POINT('Ctrl Pts',(-61.5512651452214,12.8100982056074,
40.0255394551614));
#170610=CARTESIAN_POINT('Ctrl Pts',(-61.557279745591,12.8200291684151,40.0382021526201));
#170611=CARTESIAN_POINT('Ctrl Pts',(-61.562774373325,12.8309289079008,40.0503687782147));
#170612=CARTESIAN_POINT('Ctrl Pts',(-61.5676673859795,12.8428059312039,
40.0619155352442));
#170613=CARTESIAN_POINT('Ctrl Pts',(-61.5676802096931,12.8428370587639,
40.0619457972352));
#170614=CARTESIAN_POINT('Ctrl Pts',(-61.5676930289521,12.8428681938096,
40.0619760547305));
#170615=CARTESIAN_POINT('Ctrl Pts',(-61.5677058437552,12.8428993363381,
40.062006307727));
#170616=CARTESIAN_POINT('Ctrl Pts',(-61.5690798512467,12.8462384487041,
40.06525004417));
#170617=CARTESIAN_POINT('Ctrl Pts',(-61.5704011254853,12.8496624271217,
40.0684393223557));
#170618=CARTESIAN_POINT('Ctrl Pts',(-61.5716678181341,12.8531666956984,
40.0715697951759));
#170619=CARTESIAN_POINT('Ctrl Pts',(-61.5787166747147,12.8726671535572,
40.0889901646409));
#170620=CARTESIAN_POINT('Ctrl Pts',(-61.5840799821718,12.8946522063751,
40.1045963098221));
#170621=CARTESIAN_POINT('Ctrl Pts',(-61.5874651029941,12.9182844651646,
40.1176634650698));
#170622=CARTESIAN_POINT('Ctrl Pts',(-61.5889843920978,12.9288909501791,
40.1235281853046));
#170623=CARTESIAN_POINT('Ctrl Pts',(-61.5901055263649,12.9398294093986,
40.1288820140913));
#170624=CARTESIAN_POINT('Ctrl Pts',(-61.5908034580837,12.9510258874724,
40.1336621774101));
#170625=CARTESIAN_POINT('Ctrl Pts',(-61.5911067697684,12.9558917253995,
40.1357395717319));
#170626=CARTESIAN_POINT('Ctrl Pts',(-61.591330024696,12.9608061353938,40.1377083672884));
#170627=CARTESIAN_POINT('Ctrl Pts',(-61.5914710890454,12.9657629422646,
40.1395632548792));
#170628=CARTESIAN_POINT('Ctrl Pts',(-61.5919648142681,12.9831117663123,
40.146055361447));
#170629=CARTESIAN_POINT('Ctrl Pts',(-61.5914517017517,13.0009799514314,
40.151152097463));
#170630=CARTESIAN_POINT('Ctrl Pts',(-61.5898402812904,13.019102739991,40.1546258197409));
#170631=CARTESIAN_POINT('Ctrl Pts',(-61.5890345710598,13.0281641342708,
40.1563626808798));
#170632=CARTESIAN_POINT('Ctrl Pts',(-61.5879542844383,13.0372891795348,
40.1576937882008));
#170633=CARTESIAN_POINT('Ctrl Pts',(-61.5865879953991,13.0464447827194,
40.1585906813668));
#170634=CARTESIAN_POINT('Ctrl Pts',(-61.5859048508795,13.0510225843117,
40.1590391279498));
#170635=CARTESIAN_POINT('Ctrl Pts',(-61.585150205876,13.0556080254099,40.1593790209175));
#170636=CARTESIAN_POINT('Ctrl Pts',(-61.5843226328191,13.0601969695279,
40.1596068022931));
#170637=CARTESIAN_POINT('Ctrl Pts',(-61.5834950597622,13.064785913646,40.1598345836687));
#170638=CARTESIAN_POINT('Ctrl Pts',(-61.582594556983,13.0693783604296,40.1599502506865));
#170639=CARTESIAN_POINT('Ctrl Pts',(-61.5816197022697,13.0739701745329,
40.1599502534424));
#170640=CARTESIAN_POINT('',(-61.575271693745,13.1038352065732,40.1599502534424));
#170641=CARTESIAN_POINT('Origin',(1.12331902584553E-16,-3.23121069746461E-17,
40.1599502534424));
#170642=CARTESIAN_POINT('',(-61.3267881959112,13.3605623192491,39.8576902534424));
#170643=CARTESIAN_POINT('Ctrl Pts',(-61.575271693745,13.1038352065732,40.1599502534424));
#170644=CARTESIAN_POINT('Ctrl Pts',(-61.5744762229325,13.1075731191842,
40.1599502447858));
#170645=CARTESIAN_POINT('Ctrl Pts',(-61.5736362456895,13.1112908564316,
40.1598744685927));
#170646=CARTESIAN_POINT('Ctrl Pts',(-61.5727532608743,13.114986764564,40.1597246934279));
#170647=CARTESIAN_POINT('Ctrl Pts',(-61.567650697922,13.1363445541721,40.1588591777434));
#170648=CARTESIAN_POINT('Ctrl Pts',(-61.5611131206543,13.1569765024544,
40.1555254706014));
#170649=CARTESIAN_POINT('Ctrl Pts',(-61.5534303645603,13.1765564394435,
40.1500631826365));
#170650=CARTESIAN_POINT('Ctrl Pts',(-61.5503317322951,13.1844534784439,
40.1478601162469));
#170651=CARTESIAN_POINT('Ctrl Pts',(-61.5470470005027,13.1921798155763,
40.14531122283));
#170652=CARTESIAN_POINT('Ctrl Pts',(-61.5435957160156,13.1997158239902,
40.1424401896328));
#170653=CARTESIAN_POINT('Ctrl Pts',(-61.5423224015758,13.2024961535653,
40.1413809526906));
#170654=CARTESIAN_POINT('Ctrl Pts',(-61.5410263779725,13.2052504481946,
40.1402777640512));
#170655=CARTESIAN_POINT('Ctrl Pts',(-61.5397086090799,13.2079776587165,
40.1391317641987));
#170656=CARTESIAN_POINT('Ctrl Pts',(-61.5372377924062,13.213091178445,40.1369830144753));
#170657=CARTESIAN_POINT('Ctrl Pts',(-61.5346905274441,13.218109480607,40.134683756585));
#170658=CARTESIAN_POINT('Ctrl Pts',(-61.5320731679598,13.2230256493634,
40.1322415082996));
#170659=CARTESIAN_POINT('Ctrl Pts',(-61.5229124097646,13.2402322400109,
40.1236936393009));
#170660=CARTESIAN_POINT('Ctrl Pts',(-61.5128929892896,13.2561876955043,
40.113394140767));
#170661=CARTESIAN_POINT('Ctrl Pts',(-61.5022873490354,13.2705955044757,
40.101665321223));
#170662=CARTESIAN_POINT('Ctrl Pts',(-61.4969845289083,13.2777994089614,
40.095800911451));
#170663=CARTESIAN_POINT('Ctrl Pts',(-61.4915351548246,13.2846164020264,
40.0895791707949));
#170664=CARTESIAN_POINT('Ctrl Pts',(-61.4859732907798,13.291009421645,40.0830403822906));
#170665=CARTESIAN_POINT('Ctrl Pts',(-61.4831923587574,13.2942059314543,
40.0797709880385));
#170666=CARTESIAN_POINT('Ctrl Pts',(-61.4803833043594,13.2972964479274,
40.0764223317514));
#170667=CARTESIAN_POINT('Ctrl Pts',(-61.4775503861046,13.300276338427,40.0729994484778));
#170668=CARTESIAN_POINT('Ctrl Pts',(-61.4747174678497,13.3032562289267,
40.0695765652042));
#170669=CARTESIAN_POINT('Ctrl Pts',(-61.4718606611377,13.3061253662371,
40.0660793733488));
#170670=CARTESIAN_POINT('Ctrl Pts',(-61.4689842762857,13.3088793779161,
40.0625130768817));
#170671=CARTESIAN_POINT('Ctrl Pts',(-61.468959746747,13.3089028638679,40.0624826638418));
#170672=CARTESIAN_POINT('Ctrl Pts',(-61.4689352159237,13.308926341439,40.0624522459912));
#170673=CARTESIAN_POINT('Ctrl Pts',(-61.4689106838181,13.3089498106273,
40.0624218233329));
#170674=CARTESIAN_POINT('Ctrl Pts',(-61.4563817793395,13.3209358677646,
40.04688452759));
#170675=CARTESIAN_POINT('Ctrl Pts',(-61.4435806031494,13.3308520539325,
40.0302263329239));
#170676=CARTESIAN_POINT('Ctrl Pts',(-61.4306829407564,13.3387946412837,
40.0127515884746));
#170677=CARTESIAN_POINT('Ctrl Pts',(-61.4173490879857,13.347005841665,39.9946858597717));
#170678=CARTESIAN_POINT('Ctrl Pts',(-61.4039112193234,13.3531077791297,
39.9757460620491));
#170679=CARTESIAN_POINT('Ctrl Pts',(-61.3905594167273,13.3571547734346,
39.9562444559129));
#170680=CARTESIAN_POINT('Ctrl Pts',(-61.3774615935119,13.3611247853922,
39.9371138113612));
#170681=CARTESIAN_POINT('Ctrl Pts',(-61.3644457143974,13.3631169881916,
39.9174410654354));
#170682=CARTESIAN_POINT('Ctrl Pts',(-61.3517005934288,13.3631357189476,
39.8975196504146));
#170683=CARTESIAN_POINT('Ctrl Pts',(-61.3432573976115,13.3631481274168,
39.8843224113775));
#170684=CARTESIAN_POINT('Ctrl Pts',(-61.3349332352347,13.362293512079,39.8710160447132));
#170685=CARTESIAN_POINT('Ctrl Pts',(-61.3267881959112,13.3605623192491,
39.8576902534424));
#170686=CARTESIAN_POINT('',(-60.9782752797347,13.2864868029,39.2875012672119));
#170687=CARTESIAN_POINT('',(-61.3267881959112,13.3605623192491,39.8576902534424));
#170688=CARTESIAN_POINT('',(-59.4519788726606,18.9827025415101,39.2875012672119));
#170689=CARTESIAN_POINT('Origin',(5.53234440788222E-15,0.,39.2875012672119));
#170690=CARTESIAN_POINT('',(-59.790837669791,19.0928077206416,39.8576902534424));
#170691=CARTESIAN_POINT('',(-59.4519788726606,18.9827025415101,39.2875012672119));
#170692=CARTESIAN_POINT('',(-59.8776671349984,19.4393816709761,40.1599502534424));
#170693=CARTESIAN_POINT('Ctrl Pts',(-59.790837669791,19.0928077206416,39.8576902534424));
#170694=CARTESIAN_POINT('Ctrl Pts',(-59.8025412685589,19.0966105891859,
39.8773836120367));
#170695=CARTESIAN_POINT('Ctrl Pts',(-59.81360381105,19.1022557829957,39.8969946442138));
#170696=CARTESIAN_POINT('Ctrl Pts',(-59.8238865403123,19.1096150844297,
39.916252528825));
#170697=CARTESIAN_POINT('Ctrl Pts',(-59.8343758896888,19.1171222629168,
39.9358973794073));
#170698=CARTESIAN_POINT('Ctrl Pts',(-59.8440546685621,19.1264133720528,
39.9551762199751));
#170699=CARTESIAN_POINT('Ctrl Pts',(-59.8527677431762,19.1374051938284,
39.9738152034255));
#170700=CARTESIAN_POINT('Ctrl Pts',(-59.8611423227401,19.1479699932922,
39.9917300792653));
#170701=CARTESIAN_POINT('Ctrl Pts',(-59.8686254222915,19.1601065286715,
40.0090551158128));
#170702=CARTESIAN_POINT('Ctrl Pts',(-59.8750609947979,19.173782305098,40.0255394551538));
#170703=CARTESIAN_POINT('Ctrl Pts',(-59.8800045782775,19.1842875619879,
40.0382021526151));
#170704=CARTESIAN_POINT('Ctrl Pts',(-59.8843297728484,19.1957019365555,
40.0503687782124));
#170705=CARTESIAN_POINT('Ctrl Pts',(-59.8879544940743,19.2080253553783,
40.0619155352442));
#170706=CARTESIAN_POINT('Ctrl Pts',(-59.8879639938222,19.2080576528613,
40.0619457972351));
#170707=CARTESIAN_POINT('Ctrl Pts',(-59.8879734883575,19.2080899573234,
40.0619760547305));
#170708=CARTESIAN_POINT('Ctrl Pts',(-59.8879829776791,19.2081222687615,
40.0620063077269));
#170709=CARTESIAN_POINT('Ctrl Pts',(-59.8890004259295,19.2115867120122,
40.06525004417));
#170710=CARTESIAN_POINT('Ctrl Pts',(-59.8899565588874,19.2151300442836,
40.0684393223556));
#170711=CARTESIAN_POINT('Ctrl Pts',(-59.8908500166521,19.2187475215463,
40.0715697951759));
#170712=CARTESIAN_POINT('Ctrl Pts',(-59.8958219059662,19.2388779600043,
40.0889901646422));
#170713=CARTESIAN_POINT('Ctrl Pts',(-59.8988577688781,19.261303194691,40.1045963098246));
#170714=CARTESIAN_POINT('Ctrl Pts',(-59.8997541019592,19.2851598349738,
40.1176634650729));
#170715=CARTESIAN_POINT('Ctrl Pts',(-59.9001563886588,19.2958670255072,
40.1235281853065));
#170716=CARTESIAN_POINT('Ctrl Pts',(-59.9001280009022,19.3068627531428,
40.1288820140921));
#170717=CARTESIAN_POINT('Ctrl Pts',(-59.8996517586311,19.3180708494663,
40.1336621774102));
#170718=CARTESIAN_POINT('Ctrl Pts',(-59.8994447901816,19.3229417365284,
40.1357395717319));
#170719=CARTESIAN_POINT('Ctrl Pts',(-59.8991531263708,19.3278525613651,
40.1377083672884));
#170720=CARTESIAN_POINT('Ctrl Pts',(-59.89877529055,19.3327969595688,40.1395632548792));
#170721=CARTESIAN_POINT('Ctrl Pts',(-59.8974528651771,19.3501023532819,
40.146055361447));
#170722=CARTESIAN_POINT('Ctrl Pts',(-59.8950748296128,19.3678190197505,
40.151152097463));
#170723=CARTESIAN_POINT('Ctrl Pts',(-59.8915778894432,19.3856740904737,
40.1546258197409));
#170724=CARTESIAN_POINT('Ctrl Pts',(-59.8898294193584,19.3946016258353,
40.1563626808798));
#170725=CARTESIAN_POINT('Ctrl Pts',(-59.8878012237013,19.4035637624461,
40.1576937882008));
#170726=CARTESIAN_POINT('Ctrl Pts',(-59.8854853982053,19.4125263941848,
40.1585906813668));
#170727=CARTESIAN_POINT('Ctrl Pts',(-59.8843274854572,19.4170077100542,
40.1590391279498));
#170728=CARTESIAN_POINT('Ctrl Pts',(-59.8830976653666,19.4214891497437,
40.1593790209175));
#170729=CARTESIAN_POINT('Ctrl Pts',(-59.8817949505649,19.4259664502059,
40.1596068022931));
#170730=CARTESIAN_POINT('Ctrl Pts',(-59.8804922357632,19.430443750668,40.1598345836687));
#170731=CARTESIAN_POINT('Ctrl Pts',(-59.8791166246274,19.434916911376,40.1599502506865));
#170732=CARTESIAN_POINT('Ctrl Pts',(-59.8776671349984,19.4393816709761,
40.1599502534424));
#170733=CARTESIAN_POINT('',(-59.868232155624,19.4684195516701,40.1599502534424));
#170734=CARTESIAN_POINT('Origin',(1.08121605342496E-16,-4.80251501969599E-17,
40.1599502534424));
#170735=CARTESIAN_POINT('',(-59.5942745858234,19.697766688185,39.8576902534424));
#170736=CARTESIAN_POINT('Ctrl Pts',(-59.868232155624,19.4684195516701,40.1599502534424));
#170737=CARTESIAN_POINT('Ctrl Pts',(-59.8670503242228,19.4720538382631,
40.1599502447858));
#170738=CARTESIAN_POINT('Ctrl Pts',(-59.8658263391017,19.4756634078265,
40.1598744685927));
#170739=CARTESIAN_POINT('Ctrl Pts',(-59.8645618637722,19.4792467723416,
40.1597246934279));
#170740=CARTESIAN_POINT('Ctrl Pts',(-59.8572547562675,19.4999541986783,
40.1588591777434));
#170741=CARTESIAN_POINT('Ctrl Pts',(-59.8485963666845,19.5197897600828,
40.1555254706017));
#170742=CARTESIAN_POINT('Ctrl Pts',(-59.8389090368086,19.5384593694394,
40.1500631826373));
#170743=CARTESIAN_POINT('Ctrl Pts',(-59.8350019138236,19.545989252366,40.1478601162475));
#170744=CARTESIAN_POINT('Ctrl Pts',(-59.830927553988,19.5533299158496,40.1453112228304));
#170745=CARTESIAN_POINT('Ctrl Pts',(-59.8267074486192,19.5604638837582,
40.1424401896328));
#170746=CARTESIAN_POINT('Ctrl Pts',(-59.8251504859513,19.5630958847954,
40.1413809526906));
#170747=CARTESIAN_POINT('Ctrl Pts',(-59.8235736599158,19.5656996197549,
40.1402777640512));
#170748=CARTESIAN_POINT('Ctrl Pts',(-59.8219780387742,19.5682741459749,
40.1391317641987));
#170749=CARTESIAN_POINT('Ctrl Pts',(-59.8189862491337,19.5731013826373,
40.1369830144753));
#170750=CARTESIAN_POINT('Ctrl Pts',(-59.8159283829424,19.577825932323,40.134683756585));
#170751=CARTESIAN_POINT('Ctrl Pts',(-59.8128114820619,19.5824415812279,
40.1322415082996));
#170752=CARTESIAN_POINT('Ctrl Pts',(-59.8019023289802,19.5985963523949,
40.1236936393009));
#170753=CARTESIAN_POINT('Ctrl Pts',(-59.7902699966955,19.6134170876086,
40.113394140767));
#170754=CARTESIAN_POINT('Ctrl Pts',(-59.7782164291174,19.6266373778172,
40.101665321223));
#170755=CARTESIAN_POINT('Ctrl Pts',(-59.7721896453284,19.6332475229215,
40.095800911451));
#170756=CARTESIAN_POINT('Ctrl Pts',(-59.7660575536769,19.6394575570865,
40.0895791707949));
#170757=CARTESIAN_POINT('Ctrl Pts',(-59.7598579055889,19.6452341819732,
40.0830403822906));
#170758=CARTESIAN_POINT('Ctrl Pts',(-59.7567580815449,19.6481224944165,
40.0797709880385));
#170759=CARTESIAN_POINT('Ctrl Pts',(-59.7536413685032,19.6509024545775,
40.0764223317514));
#170760=CARTESIAN_POINT('Ctrl Pts',(-59.7505124858963,19.6535699003335,
40.0729994484778));
#170761=CARTESIAN_POINT('Ctrl Pts',(-59.7473836032895,19.6562373460894,
40.0695765652042));
#170762=CARTESIAN_POINT('Ctrl Pts',(-59.7442425399495,19.65879214835,40.0660793733488));
#170763=CARTESIAN_POINT('Ctrl Pts',(-59.7410940396261,19.6612304091765,
40.0625130768817));
#170764=CARTESIAN_POINT('Ctrl Pts',(-59.7410671895124,19.6612512024348,
40.0624826638418));
#170765=CARTESIAN_POINT('Ctrl Pts',(-59.741040338997,19.6612719872241,40.0624522459912));
#170766=CARTESIAN_POINT('Ctrl Pts',(-59.7410134880827,19.6612927635425,
40.0624218233329));
#170767=CARTESIAN_POINT('Ctrl Pts',(-59.7273003341234,19.6719035326708,
40.0468845275932));
#170768=CARTESIAN_POINT('Ctrl Pts',(-59.7135327604172,19.6804273096567,
40.030226332931));
#170769=CARTESIAN_POINT('Ctrl Pts',(-59.6998755263211,19.686978213853,40.0127515884857));
#170770=CARTESIAN_POINT('Ctrl Pts',(-59.6857564136365,19.6937506652793,
39.994685859787));
#170771=CARTESIAN_POINT('Ctrl Pts',(-59.6717543328814,19.6984145359315,
39.9757460620688));
#170772=CARTESIAN_POINT('Ctrl Pts',(-59.658052646764,19.7010437169722,39.9562444559372));
#170773=CARTESIAN_POINT('Ctrl Pts',(-59.6446115955477,19.7036228854571,
39.9371138113893));
#170774=CARTESIAN_POINT('Ctrl Pts',(-59.6314587768857,19.7042436449212,
39.9174410654674));
#170775=CARTESIAN_POINT('Ctrl Pts',(-59.6187815171278,19.7029300451618,
39.8975196504504));
#170776=CARTESIAN_POINT('Ctrl Pts',(-59.6103832769743,19.702059831373,39.8843224114016));
#170777=CARTESIAN_POINT('Ctrl Pts',(-59.6021940468503,19.7003397858055,
39.8710160447252));
#170778=CARTESIAN_POINT('Ctrl Pts',(-59.5942745858234,19.697766688185,39.8576902534424));
#170779=CARTESIAN_POINT('',(-59.255413859757,19.5876674457083,39.2875012672119));
#170780=CARTESIAN_POINT('',(-59.5942745858234,19.697766688185,39.8576902534424));
#170781=CARTESIAN_POINT('',(-57.1420619865019,25.093137300575,39.2875012672119));
#170782=CARTESIAN_POINT('Origin',(5.53234440788222E-15,0.,39.2875012672119));
#170783=CARTESIAN_POINT('',(-57.4675553545138,25.2380597013435,39.8576902534424));
#170784=CARTESIAN_POINT('',(-57.1420619865019,25.093137300575,39.2875012672119));
#170785=CARTESIAN_POINT('',(-57.5176823163886,25.5918112338799,40.1599502534424));
#170786=CARTESIAN_POINT('Ctrl Pts',(-57.4675553545138,25.2380597013435,
39.8576902534424));
#170787=CARTESIAN_POINT('Ctrl Pts',(-57.4787973317384,25.2430650965698,
39.8773836120369));
#170788=CARTESIAN_POINT('Ctrl Pts',(-57.4892091890305,25.2498357159837,
39.8969946442142));
#170789=CARTESIAN_POINT('Ctrl Pts',(-57.4986663319565,25.2582295402824,
39.9162525288255));
#170790=CARTESIAN_POINT('Ctrl Pts',(-57.508313505749,25.2667920292314,39.9358973794082));
#170791=CARTESIAN_POINT('Ctrl Pts',(-57.5169680778991,25.2770439485816,
39.9551762199763));
#170792=CARTESIAN_POINT('Ctrl Pts',(-57.5244844631401,25.2888863203075,
39.973815203427));
#170793=CARTESIAN_POINT('Ctrl Pts',(-57.5317088436283,25.3002686266273,
39.9917300792673));
#170794=CARTESIAN_POINT('Ctrl Pts',(-57.5378823365848,25.313120873693,40.0090551158152));
#170795=CARTESIAN_POINT('Ctrl Pts',(-57.5428531464578,25.3273944332903,
40.0255394551565));
#170796=CARTESIAN_POINT('Ctrl Pts',(-57.5466715501105,25.3383588864673,
40.0382021526169));
#170797=CARTESIAN_POINT('Ctrl Pts',(-57.54977992378,25.3501628378378,40.0503687782133));
#170798=CARTESIAN_POINT('Ctrl Pts',(-57.5520966403719,25.3627976342214,
40.0619155352442));
#170799=CARTESIAN_POINT('Ctrl Pts',(-57.5521027120729,25.3628307477695,
40.0619457972351));
#170800=CARTESIAN_POINT('Ctrl Pts',(-57.5521087778604,25.3628638677135,
40.0619760547305));
#170801=CARTESIAN_POINT('Ctrl Pts',(-57.5521148377335,25.3628969940505,
40.062006307727));
#170802=CARTESIAN_POINT('Ctrl Pts',(-57.5527645793668,25.3664488110206,
40.06525004417));
#170803=CARTESIAN_POINT('Ctrl Pts',(-57.5533450954511,25.3700726756558,
40.0684393223557));
#170804=CARTESIAN_POINT('Ctrl Pts',(-57.5538555294215,25.3737637277667,
40.0715697951759));
#170805=CARTESIAN_POINT('Ctrl Pts',(-57.5566959784093,25.3943035935289,
40.0889901646446));
#170806=CARTESIAN_POINT('Ctrl Pts',(-57.557371135226,25.4169233145218,40.1045963098288));
#170807=CARTESIAN_POINT('Ctrl Pts',(-57.5557688601525,25.4407429579562,
40.1176634650783));
#170808=CARTESIAN_POINT('Ctrl Pts',(-57.555049736911,25.4514335437868,40.1235281853097));
#170809=CARTESIAN_POINT('Ctrl Pts',(-57.5538721381535,25.4623660683441,
40.1288820140936));
#170810=CARTESIAN_POINT('Ctrl Pts',(-57.552226939703,25.473462984667,40.1336621774101));
#170811=CARTESIAN_POINT('Ctrl Pts',(-57.551511958709,25.4782855544062,40.1357395717319));
#170812=CARTESIAN_POINT('Ctrl Pts',(-57.5507085716895,25.4831389900607,
40.1377083672884));
#170813=CARTESIAN_POINT('Ctrl Pts',(-57.5498159753468,25.488016807736,40.1395632548792));
#170814=CARTESIAN_POINT('Ctrl Pts',(-57.5466918881474,25.5050891695996,
40.146055361447));
#170815=CARTESIAN_POINT('Ctrl Pts',(-57.5424749837905,25.5224602099125,
40.1511520974629));
#170816=CARTESIAN_POINT('Ctrl Pts',(-57.5371308371209,25.539851938908,40.1546258197408));
#170817=CARTESIAN_POINT('Ctrl Pts',(-57.534458763786,25.5485478034057,40.1563626808798));
#170818=CARTESIAN_POINT('Ctrl Pts',(-57.5315048804294,25.5572488403192,
40.1576937882008));
#170819=CARTESIAN_POINT('Ctrl Pts',(-57.5282648911453,25.5659203041432,
40.1585906813668));
#170820=CARTESIAN_POINT('Ctrl Pts',(-57.5266448965032,25.5702560360552,
40.1590391279498));
#170821=CARTESIAN_POINT('Ctrl Pts',(-57.5249533754917,25.5745843747451,
40.1593790209175));
#170822=CARTESIAN_POINT('Ctrl Pts',(-57.5231897917611,25.5789009773105,
40.1596068022931));
#170823=CARTESIAN_POINT('Ctrl Pts',(-57.5214262080304,25.583217579876,40.1598345836687));
#170824=CARTESIAN_POINT('Ctrl Pts',(-57.5195905600217,25.5875224456234,
40.1599502506865));
#170825=CARTESIAN_POINT('Ctrl Pts',(-57.5176823163886,25.5918112338799,
40.1599502534424));
#170826=CARTESIAN_POINT('',(-57.505263737773,25.6197038181302,40.1599502534424));
#170827=CARTESIAN_POINT('Origin',(1.02291912287982E-16,-6.32120198238069E-17,
40.1599502534424));
#170828=CARTESIAN_POINT('',(-57.2088336324697,25.8191582032625,39.8576902534424));
#170829=CARTESIAN_POINT('Ctrl Pts',(-57.505263737773,25.6197038181302,40.1599502534424));
#170830=CARTESIAN_POINT('Ctrl Pts',(-57.5037084941752,25.6231946607008,
40.1599502447858));
#170831=CARTESIAN_POINT('Ctrl Pts',(-57.5021139114131,25.6266565153807,
40.1598744685927));
#170832=CARTESIAN_POINT('Ctrl Pts',(-57.5004817994257,25.630088076187,40.1597246934279));
#170833=CARTESIAN_POINT('Ctrl Pts',(-57.4910502055662,25.6499182643595,
40.1588591777433));
#170834=CARTESIAN_POINT('Ctrl Pts',(-57.4803658667941,25.6687401163279,
40.155525470601));
#170835=CARTESIAN_POINT('Ctrl Pts',(-57.4687800995474,25.6862948499077,
40.1500631826354));
#170836=CARTESIAN_POINT('Ctrl Pts',(-57.4641072931013,25.6933750777842,
40.147860116246));
#170837=CARTESIAN_POINT('Ctrl Pts',(-57.4592879447633,25.7002496417706,
40.1453112228295));
#170838=CARTESIAN_POINT('Ctrl Pts',(-57.4543452548722,25.7069034079255,
40.1424401896328));
#170839=CARTESIAN_POINT('Ctrl Pts',(-57.452521702385,25.7093582436706,40.1413809526906));
#170840=CARTESIAN_POINT('Ctrl Pts',(-57.4506813499535,25.7117828918952,
40.1402777640512));
#170841=CARTESIAN_POINT('Ctrl Pts',(-57.4488253585221,25.7141765267653,
40.1391317641987));
#170842=CARTESIAN_POINT('Ctrl Pts',(-57.4453453745881,25.7186645921467,
40.1369830144753));
#170843=CARTESIAN_POINT('Ctrl Pts',(-57.4418104097894,25.723043626201,40.134683756585));
#170844=CARTESIAN_POINT('Ctrl Pts',(-57.4382281169311,25.727308185239,40.1322415082996));
#170845=CARTESIAN_POINT('Ctrl Pts',(-57.4256900919268,25.7422341418722,
40.1236936393009));
#170846=CARTESIAN_POINT('Ctrl Pts',(-57.4125722940991,25.7557577777296,
40.113394140767));
#170847=CARTESIAN_POINT('Ctrl Pts',(-57.399202860606,25.7676457049094,40.101665321223));
#170848=CARTESIAN_POINT('Ctrl Pts',(-57.3925181438594,25.7735896684993,
40.095800911451));
#170849=CARTESIAN_POINT('Ctrl Pts',(-57.3857705191195,25.7791247053304,
40.0895791707949));
#170850=CARTESIAN_POINT('Ctrl Pts',(-57.3790010116301,25.7842216455741,
40.0830403822906));
#170851=CARTESIAN_POINT('Ctrl Pts',(-57.3756162578855,25.786770115696,40.0797709880385));
#170852=CARTESIAN_POINT('Ctrl Pts',(-57.3722260335603,25.7892090617196,
40.0764223317514));
#170853=CARTESIAN_POINT('Ctrl Pts',(-57.368835467294,25.791534837638,40.0729994484778));
#170854=CARTESIAN_POINT('Ctrl Pts',(-57.3654449010277,25.7938606135564,
40.0695765652042));
#170855=CARTESIAN_POINT('Ctrl Pts',(-57.3620539952072,25.7960730898189,
40.0660793733488));
#170856=CARTESIAN_POINT('Ctrl Pts',(-57.3586678750408,25.7981688856971,
40.0625130768817));
#170857=CARTESIAN_POINT('Ctrl Pts',(-57.3586389985274,25.7981867584466,
40.0624826638418));
#170858=CARTESIAN_POINT('Ctrl Pts',(-57.3586101224999,25.7982046227315,
40.0624522459912));
#170859=CARTESIAN_POINT('Ctrl Pts',(-57.3585812469611,25.7982224785502,
40.0624218233329));
#170860=CARTESIAN_POINT('Ctrl Pts',(-57.3438340877015,25.807341705866,40.0468845275918));
#170861=CARTESIAN_POINT('Ctrl Pts',(-57.3292509568938,25.8143796853877,
40.0302263329279));
#170862=CARTESIAN_POINT('Ctrl Pts',(-57.3149837826051,25.819467133353,40.0127515884809));
#170863=CARTESIAN_POINT('Ctrl Pts',(-57.3002341019555,25.8247266354303,
39.9946858597802));
#170864=CARTESIAN_POINT('Ctrl Pts',(-57.2858212188304,25.8279013409269,
39.97574606206));
#170865=CARTESIAN_POINT('Ctrl Pts',(-57.2719197677283,25.8290839028441,
39.9562444559263));
#170866=CARTESIAN_POINT('Ctrl Pts',(-57.2582827514776,25.8302439699452,
39.9371138113765));
#170867=CARTESIAN_POINT('Ctrl Pts',(-57.2451370982986,25.8294864849006,
39.9174410654526));
#170868=CARTESIAN_POINT('Ctrl Pts',(-57.2326665944596,25.8268549466959,
39.8975196504337));
#170869=CARTESIAN_POINT('Ctrl Pts',(-57.2244053228583,25.8251116448919,
39.8843224113903));
#170870=CARTESIAN_POINT('Ctrl Pts',(-57.2164407479171,25.8225450142746,
39.8710160447196));
#170871=CARTESIAN_POINT('Ctrl Pts',(-57.2088336324697,25.8191582032625,
39.8576902534424));
#170872=CARTESIAN_POINT('',(-56.8833377255392,25.6742415049984,39.2875012672119));
#170873=CARTESIAN_POINT('',(-57.2088336324697,25.8191582032625,39.8576902534424));
#170874=CARTESIAN_POINT('',(-54.2060847114739,30.9286463962983,39.2875012672119));
#170875=CARTESIAN_POINT('Origin',(5.53234440788222E-15,0.,39.2875012672119));
#170876=CARTESIAN_POINT('',(-54.5146464769135,31.1067982185539,39.8576902534424));
#170877=CARTESIAN_POINT('',(-54.2060847114739,30.9286463962983,39.2875012672119));
#170878=CARTESIAN_POINT('',(-54.5275217339717,31.4638515574745,40.1599502534424));
#170879=CARTESIAN_POINT('Ctrl Pts',(-54.5146464769135,31.1067982185539,
39.8576902534424));
#170880=CARTESIAN_POINT('Ctrl Pts',(-54.5253036631391,31.1129513003049,
39.8773836120363));
#170881=CARTESIAN_POINT('Ctrl Pts',(-54.5349507607445,31.1207731649995,
39.896994644213));
#170882=CARTESIAN_POINT('Ctrl Pts',(-54.5434787028969,31.1301095476671,
39.9162525288237));
#170883=CARTESIAN_POINT('Ctrl Pts',(-54.5521780046501,31.1396335346567,
39.9358973794056));
#170884=CARTESIAN_POINT('Ctrl Pts',(-54.559713548773,31.1507339420464,39.955176219973));
#170885=CARTESIAN_POINT('Ctrl Pts',(-54.5659508935512,31.1632971162187,
39.973815203423));
#170886=CARTESIAN_POINT('Ctrl Pts',(-54.571945923139,31.175372222463,39.9917300792622));
#170887=CARTESIAN_POINT('Ctrl Pts',(-54.5767421714199,31.1887993693051,
40.0090551158092));
#170888=CARTESIAN_POINT('Ctrl Pts',(-54.5801937574264,31.2035143279653,
40.0255394551498));
#170889=CARTESIAN_POINT('Ctrl Pts',(-54.582845146024,31.2148178485882,40.0382021526126));
#170890=CARTESIAN_POINT('Ctrl Pts',(-54.5847026428005,31.2268820502029,
40.0503687782112));
#170891=CARTESIAN_POINT('Ctrl Pts',(-54.585685972327,31.2396897946774,40.0619155352442));
#170892=CARTESIAN_POINT('Ctrl Pts',(-54.5856885494583,31.2397233614916,
40.0619457972351));
#170893=CARTESIAN_POINT('Ctrl Pts',(-54.5856911200399,31.2397569340486,
40.0619760547305));
#170894=CARTESIAN_POINT('Ctrl Pts',(-54.5856936840714,31.2397905123452,
40.0620063077269));
#170895=CARTESIAN_POINT('Ctrl Pts',(-54.5859686003823,31.2433907885848,
40.06525004417));
#170896=CARTESIAN_POINT('Ctrl Pts',(-54.5861671393374,31.2470554817645,
40.0684393223557));
#170897=CARTESIAN_POINT('Ctrl Pts',(-54.5862889570921,31.2507796687843,
40.0715697951759));
#170898=CARTESIAN_POINT('Ctrl Pts',(-54.5869668451992,31.2715039227786,
40.0889901646431));
#170899=CARTESIAN_POINT('Ctrl Pts',(-54.5852738987616,31.2940703036755,
40.1045963098261));
#170900=CARTESIAN_POINT('Ctrl Pts',(-54.5811905703956,31.3175919772574,
40.1176634650748));
#170901=CARTESIAN_POINT('Ctrl Pts',(-54.5793579160779,31.328148830095,40.1235281853076));
#170902=CARTESIAN_POINT('Ctrl Pts',(-54.5770440083377,31.3388983725524,
40.1288820140926));
#170903=CARTESIAN_POINT('Ctrl Pts',(-54.5742478788457,31.349762528743,40.1336621774101));
#170904=CARTESIAN_POINT('Ctrl Pts',(-54.5730327187886,31.354483944076,40.1357395717319));
#170905=CARTESIAN_POINT('Ctrl Pts',(-54.5717264106366,31.3592268152916,
40.1377083672883));
#170906=CARTESIAN_POINT('Ctrl Pts',(-54.5703288332444,31.3639846100473,
40.1395632548791));
#170907=CARTESIAN_POINT('Ctrl Pts',(-54.5654373123716,31.3806368916922,
40.1460553614469));
#170908=CARTESIAN_POINT('Ctrl Pts',(-54.5594277405088,31.3974719850966,
40.1511520974629));
#170909=CARTESIAN_POINT('Ctrl Pts',(-54.5522949389283,31.414209824942,40.1546258197408));
#170910=CARTESIAN_POINT('Ctrl Pts',(-54.548728538138,31.4225787448647,40.1563626808798));
#170911=CARTESIAN_POINT('Ctrl Pts',(-54.5448813304462,31.4309233516996,
40.1576937882008));
#170912=CARTESIAN_POINT('Ctrl Pts',(-54.5407526753745,31.4392086412367,
40.1585906813668));
#170913=CARTESIAN_POINT('Ctrl Pts',(-54.5386883478386,31.4433512860052,
40.1590391279498));
#170914=CARTESIAN_POINT('Ctrl Pts',(-54.5365536585645,31.4474791015109,
40.1593790209175));
#170915=CARTESIAN_POINT('Ctrl Pts',(-54.5343485280974,31.4515877125786,
40.1596068022931));
#170916=CARTESIAN_POINT('Ctrl Pts',(-54.5321433976302,31.4556963236464,
40.1598345836687));
#170917=CARTESIAN_POINT('Ctrl Pts',(-54.5298678244922,31.4597857294234,
40.1599502506865));
#170918=CARTESIAN_POINT('Ctrl Pts',(-54.5275217339717,31.4638515574745,
40.1599502534424));
#170919=CARTESIAN_POINT('',(-54.5122556166608,31.4902932482912,40.1599502534424));
#170920=CARTESIAN_POINT('Origin',(9.49066947580418E-17,-7.7706325333499E-17,
40.1599502534424));
#170921=CARTESIAN_POINT('',(-54.1966007261205,31.6576696180589,39.8576902534424));
#170922=CARTESIAN_POINT('Ctrl Pts',(-54.5122556166608,31.4902932482912,
40.1599502534424));
#170923=CARTESIAN_POINT('Ctrl Pts',(-54.5103440004408,31.4936024004376,
40.1599502447858));
#170924=CARTESIAN_POINT('Ctrl Pts',(-54.5083962906202,31.4968786114297,
40.1598744685927));
#170925=CARTESIAN_POINT('Ctrl Pts',(-54.5064144237353,31.5001207716289,
40.1597246934279));
#170926=CARTESIAN_POINT('Ctrl Pts',(-54.494961678038,31.5188564579432,40.1588591777434));
#170927=CARTESIAN_POINT('Ctrl Pts',(-54.4823684499298,31.536458384324,40.1555254706011));
#170928=CARTESIAN_POINT('Ctrl Pts',(-54.4690111814043,31.5527059087901,
40.1500631826356));
#170929=CARTESIAN_POINT('Ctrl Pts',(-54.4636238877412,31.5592589091608,
40.1478601162462));
#170930=CARTESIAN_POINT('Ctrl Pts',(-54.4581123526882,31.565592054491,40.1453112228296));
#170931=CARTESIAN_POINT('Ctrl Pts',(-54.4525012314182,31.5716927188402,
40.1424401896328));
#170932=CARTESIAN_POINT('Ctrl Pts',(-54.4504310683343,31.573943493599,40.1413809526906));
#170933=CARTESIAN_POINT('Ctrl Pts',(-54.4483473527931,31.5761624901355,
40.1402777640512));
#170934=CARTESIAN_POINT('Ctrl Pts',(-54.4462513257023,31.5783490084911,
40.1391317641987));
#170935=CARTESIAN_POINT('Ctrl Pts',(-54.4423212749071,31.5824487304079,
40.1369830144753));
#170936=CARTESIAN_POINT('Ctrl Pts',(-54.4383479413152,31.5864342712174,
40.1346837565849));
#170937=CARTESIAN_POINT('Ctrl Pts',(-54.4343395048292,31.5903010169874,
40.1322415082996));
#170938=CARTESIAN_POINT('Ctrl Pts',(-54.4203099771281,31.6038346271822,
40.1236936393008));
#170939=CARTESIAN_POINT('Ctrl Pts',(-54.4058504350955,31.6159129958991,
40.113394140767));
#170940=CARTESIAN_POINT('Ctrl Pts',(-54.3913116139983,31.6263383134321,
40.101665321223));
#170941=CARTESIAN_POINT('Ctrl Pts',(-54.3840422034498,31.6315509721986,
40.095800911451));
#170942=CARTESIAN_POINT('Ctrl Pts',(-54.3767529740101,31.6363503686741,
40.0895791707949));
#170943=CARTESIAN_POINT('Ctrl Pts',(-54.36948777526,31.6407117811309,40.0830403822906));
#170944=CARTESIAN_POINT('Ctrl Pts',(-54.365855175885,31.6428924873593,40.0797709880385));
#170945=CARTESIAN_POINT('Ctrl Pts',(-54.3622285842836,31.6449636976426,
40.0764223317514));
#170946=CARTESIAN_POINT('Ctrl Pts',(-54.3586134821114,31.6469223220357,
40.0729994484778));
#170947=CARTESIAN_POINT('Ctrl Pts',(-54.3549983799392,31.6488809464288,
40.0695765652042));
#170948=CARTESIAN_POINT('Ctrl Pts',(-54.3513947831118,31.6507268563404,
40.0660793733488));
#170949=CARTESIAN_POINT('Ctrl Pts',(-54.3478081421435,31.652457225292,40.0625130768817));
#170950=CARTESIAN_POINT('Ctrl Pts',(-54.3477775556076,31.6524719817152,
40.0624826638418));
#170951=CARTESIAN_POINT('Ctrl Pts',(-54.3477469704398,31.6524867297709,
40.0624522459912));
#170952=CARTESIAN_POINT('Ctrl Pts',(-54.3477163866429,31.6525014694579,
40.0624218233329));
#170953=CARTESIAN_POINT('Ctrl Pts',(-54.3320967950451,31.6600292427984,
40.0468845275896));
#170954=CARTESIAN_POINT('Ctrl Pts',(-54.3168578829676,31.6655043152796,
40.0302263329231));
#170955=CARTESIAN_POINT('Ctrl Pts',(-54.3021370826326,31.6690725678691,
40.0127515884733));
#170956=CARTESIAN_POINT('Ctrl Pts',(-54.2869184346054,31.6727614963917,
39.9946858597701));
#170957=CARTESIAN_POINT('Ctrl Pts',(-54.2722526596735,31.6744122539946,
39.9757460620471));
#170958=CARTESIAN_POINT('Ctrl Pts',(-54.2583037507936,31.674135240392,39.9562444559105));
#170959=CARTESIAN_POINT('Ctrl Pts',(-54.2446201795125,31.6738634961709,
39.9371138113587));
#170960=CARTESIAN_POINT('Ctrl Pts',(-54.2316257183442,31.6717360657818,
39.9174410654328));
#170961=CARTESIAN_POINT('Ctrl Pts',(-54.2194985998742,31.6678154208145,
39.8975196504119));
#170962=CARTESIAN_POINT('Ctrl Pts',(-54.2114648090465,31.6652181309756,
39.8843224113757));
#170963=CARTESIAN_POINT('Ctrl Pts',(-54.203812150839,31.6618330358514,39.8710160447123));
#170964=CARTESIAN_POINT('Ctrl Pts',(-54.1966007261205,31.6576696180589,
39.8576902534424));
#170965=CARTESIAN_POINT('',(-53.8880358395968,31.4795232016794,39.2875012672119));
#170966=CARTESIAN_POINT('',(-54.1966007261205,31.6576696180589,39.8576902534424));
#170967=CARTESIAN_POINT('',(-50.6762142289945,36.4252947698683,39.2875012672119));
#170968=CARTESIAN_POINT('Origin',(5.53234440788222E-15,0.,39.2875012672119));
#170969=CARTESIAN_POINT('',(-50.964463724589,36.6347241449659,39.8576902534424));
#170970=CARTESIAN_POINT('',(-50.6762142289945,36.4252947698683,39.2875012672119));
#170971=CARTESIAN_POINT('',(-50.9399462128199,36.9911673391712,40.1599502534424));
#170972=CARTESIAN_POINT('Ctrl Pts',(-50.964463724589,36.6347241449659,39.8576902534424));
#170973=CARTESIAN_POINT('Ctrl Pts',(-50.9744193574544,36.6419574987908,
39.8773836120382));
#170974=CARTESIAN_POINT('Ctrl Pts',(-50.9831959997541,36.6507449107809,
39.8969946442167));
#170975=CARTESIAN_POINT('Ctrl Pts',(-50.9907013072149,36.6609215604566,
39.9162525288292));
#170976=CARTESIAN_POINT('Ctrl Pts',(-50.9983574255591,36.671302698694,39.9358973794129));
#170977=CARTESIAN_POINT('Ctrl Pts',(-51.0046913806569,36.6831299757391,
39.9551762199819));
#170978=CARTESIAN_POINT('Ctrl Pts',(-51.0095813473178,36.696276307595,39.9738152034334));
#170979=CARTESIAN_POINT('Ctrl Pts',(-51.0142813432067,36.7089119163756,
39.9917300792743));
#170980=CARTESIAN_POINT('Ctrl Pts',(-51.0176477981118,36.7227668523667,
40.0090551158226));
#170981=CARTESIAN_POINT('Ctrl Pts',(-51.0195423439525,36.7377619899269,
40.0255394551644));
#170982=CARTESIAN_POINT('Ctrl Pts',(-51.0209976683246,36.7492807342529,
40.0382021526219));
#170983=CARTESIAN_POINT('Ctrl Pts',(-51.0215839370835,36.761473008188,40.0503687782156));
#170984=CARTESIAN_POINT('Ctrl Pts',(-51.0212231059802,36.7743133764175,
40.0619155352442));
#170985=CARTESIAN_POINT('Ctrl Pts',(-51.0212221603062,36.7743470287327,
40.0619457972351));
#170986=CARTESIAN_POINT('Ctrl Pts',(-51.0212212075181,36.7743806860747,
40.0619760547305));
#170987=CARTESIAN_POINT('Ctrl Pts',(-51.0212202476158,36.7744143484402,
40.062006307727));
#170988=CARTESIAN_POINT('Ctrl Pts',(-51.0211173265637,36.7780236385693,
40.06525004417));
#170989=CARTESIAN_POINT('Ctrl Pts',(-51.0209317131552,36.7816890091483,
40.0684393223557));
#170990=CARTESIAN_POINT('Ctrl Pts',(-51.0206635800334,36.7854055281046,
40.0715697951759));
#170991=CARTESIAN_POINT('Ctrl Pts',(-51.0191714801765,36.8060871110647,
40.0889901646393));
#170992=CARTESIAN_POINT('Ctrl Pts',(-51.0151289787614,36.8283529098713,
40.1045963098193));
#170993=CARTESIAN_POINT('Ctrl Pts',(-51.0086093349049,36.8513189052198,
40.1176634650663));
#170994=CARTESIAN_POINT('Ctrl Pts',(-51.0056832284544,36.8616263619782,
40.1235281853025));
#170995=CARTESIAN_POINT('Ctrl Pts',(-51.0022583633875,36.8720751481021,
40.1288820140903));
#170996=CARTESIAN_POINT('Ctrl Pts',(-50.9983419378322,36.8825875141945,
40.1336621774101));
#170997=CARTESIAN_POINT('Ctrl Pts',(-50.9966399122598,36.8871560463069,
40.1357395717319));
#170998=CARTESIAN_POINT('Ctrl Pts',(-50.994844995161,36.891736389194,40.1377083672883));
#170999=CARTESIAN_POINT('Ctrl Pts',(-50.9929577488696,36.8963220336351,
40.1395632548791));
#171000=CARTESIAN_POINT('Ctrl Pts',(-50.9863523868498,36.912371789179,40.1460553614469));
#171001=CARTESIAN_POINT('Ctrl Pts',(-50.9786159896079,36.9284864868685,
40.1511520974629));
#171002=CARTESIAN_POINT('Ctrl Pts',(-50.9697726815833,36.9443870542879,
40.1546258197409));
#171003=CARTESIAN_POINT('Ctrl Pts',(-50.9653510275709,36.9523373379977,
40.1563626808798));
#171004=CARTESIAN_POINT('Ctrl Pts',(-50.9606526463563,36.9602340894953,
40.1576937882008));
#171005=CARTESIAN_POINT('Ctrl Pts',(-50.955680559906,36.9680424293794,40.1585906813668));
#171006=CARTESIAN_POINT('Ctrl Pts',(-50.9531945166809,36.9719465993214,
40.1590391279498));
#171007=CARTESIAN_POINT('Ctrl Pts',(-50.9506400472466,36.9758286664324,
40.1593790209175));
#171008=CARTESIAN_POINT('Ctrl Pts',(-50.9480175299137,36.9796842711998,
40.1596068022931));
#171009=CARTESIAN_POINT('Ctrl Pts',(-50.9453950125809,36.9835398759672,
40.1598345836687));
#171010=CARTESIAN_POINT('Ctrl Pts',(-50.9427044459691,36.9873690173883,
40.1599502506865));
#171011=CARTESIAN_POINT('Ctrl Pts',(-50.9399462128199,36.9911673391712,
40.1599502534424));
#171012=CARTESIAN_POINT('',(-50.9219998155897,37.0158684358564,40.1599502534424));
#171013=CARTESIAN_POINT('Origin',(8.60468667414046E-17,-9.13492640817437E-17,
40.1599502534424));
#171014=CARTESIAN_POINT('',(-50.5905785208481,37.1493329797265,39.8576902534424));
#171015=CARTESIAN_POINT('Ctrl Pts',(-50.9219998155897,37.0158684358564,
40.1599502534424));
#171016=CARTESIAN_POINT('Ctrl Pts',(-50.9197527708147,37.0189596418153,
40.1599502447858));
#171017=CARTESIAN_POINT('Ctrl Pts',(-50.917473273452,37.0220143142663,40.1598744685927));
#171018=CARTESIAN_POINT('Ctrl Pts',(-50.915163365418,37.0250315520728,40.1597246934279));
#171019=CARTESIAN_POINT('Ctrl Pts',(-50.9018149465622,37.0424674644279,
40.1588591777434));
#171020=CARTESIAN_POINT('Ctrl Pts',(-50.8874508031613,37.0586566148313,
40.1555254706016));
#171021=CARTESIAN_POINT('Ctrl Pts',(-50.8724683783873,37.0734189189051,
40.1500631826369));
#171022=CARTESIAN_POINT('Ctrl Pts',(-50.8664256218229,37.0793728957276,
40.1478601162472));
#171023=CARTESIAN_POINT('Ctrl Pts',(-50.8602822855854,37.0850952351368,
40.1453112228302));
#171024=CARTESIAN_POINT('Ctrl Pts',(-50.8540642095543,37.0905759575259,
40.1424401896328));
#171025=CARTESIAN_POINT('Ctrl Pts',(-50.8517701170137,37.0925980113392,
40.1413809526906));
#171026=CARTESIAN_POINT('Ctrl Pts',(-50.8494658679863,37.094587044397,40.1402777640512));
#171027=CARTESIAN_POINT('Ctrl Pts',(-50.8471527697476,37.0965424902856,
40.1391317641987));
#171028=CARTESIAN_POINT('Ctrl Pts',(-50.8428157105501,37.1002089513266,
40.1369830144753));
#171029=CARTESIAN_POINT('Ctrl Pts',(-50.8384475408392,37.1037573324721,
40.134683756585));
#171030=CARTESIAN_POINT('Ctrl Pts',(-50.8340568779945,37.1071839000981,
40.1322415082996));
#171031=CARTESIAN_POINT('Ctrl Pts',(-50.818689558038,37.1191768867893,40.1236936393009));
#171032=CARTESIAN_POINT('Ctrl Pts',(-50.8030466935688,37.1296776552303,
40.113394140767));
#171033=CARTESIAN_POINT('Ctrl Pts',(-50.787497775234,37.1385261411561,40.101665321223));
#171034=CARTESIAN_POINT('Ctrl Pts',(-50.7797233160666,37.142950384119,40.095800911451));
#171035=CARTESIAN_POINT('Ctrl Pts',(-50.7719723442504,37.1469615570466,
40.0895791707949));
#171036=CARTESIAN_POINT('Ctrl Pts',(-50.7642910532774,37.1505396571689,
40.0830403822907));
#171037=CARTESIAN_POINT('Ctrl Pts',(-50.760450407791,37.1523287072301,40.0797709880385));
#171038=CARTESIAN_POINT('Ctrl Pts',(-50.7566271826097,37.1540094891598,
40.0764223317514));
#171039=CARTESIAN_POINT('Ctrl Pts',(-50.7528271523476,37.155579502929,40.0729994484778));
#171040=CARTESIAN_POINT('Ctrl Pts',(-50.7490271220855,37.1571495166981,
40.0695765652042));
#171041=CARTESIAN_POINT('Ctrl Pts',(-50.7452503160122,37.1586086360834,
40.0660793733488));
#171042=CARTESIAN_POINT('Ctrl Pts',(-50.7415024502309,37.1599546198241,
40.0625130768817));
#171043=CARTESIAN_POINT('Ctrl Pts',(-50.7414704887851,37.1599660982465,
40.0624826638418));
#171044=CARTESIAN_POINT('Ctrl Pts',(-50.7414385295744,37.1599775684902,
40.0624522459912));
#171045=CARTESIAN_POINT('Ctrl Pts',(-50.7414065726019,37.1599890305544,
40.0624218233329));
#171046=CARTESIAN_POINT('Ctrl Pts',(-50.7250856801842,37.1658428740575,
40.0468845275916));
#171047=CARTESIAN_POINT('Ctrl Pts',(-50.7093579475509,37.1696950534571,
40.0302263329275));
#171048=CARTESIAN_POINT('Ctrl Pts',(-50.6943448053425,37.1717050161486,
40.0127515884802));
#171049=CARTESIAN_POINT('Ctrl Pts',(-50.6788239286337,37.1737829544436,
39.9946858597794));
#171050=CARTESIAN_POINT('Ctrl Pts',(-50.6640659431975,37.173891678108,39.975746062059));
#171051=CARTESIAN_POINT('Ctrl Pts',(-50.6502224037074,37.1721581240064,
39.956244455925));
#171052=CARTESIAN_POINT('Ctrl Pts',(-50.6366421974681,37.1704575457516,
39.937113811375));
#171053=CARTESIAN_POINT('Ctrl Pts',(-50.6239412983474,37.1669834785932,
39.917441065451));
#171054=CARTESIAN_POINT('Ctrl Pts',(-50.6122904324949,37.1618166822733,
39.8975196504319));
#171055=CARTESIAN_POINT('Ctrl Pts',(-50.604572142325,37.1583938608496,39.8843224113891));
#171056=CARTESIAN_POINT('Ctrl Pts',(-50.5973152449672,37.1542273890268,
39.871016044719));
#171057=CARTESIAN_POINT('Ctrl Pts',(-50.5905785208481,37.1493329797265,
39.8576902534424));
#171058=CARTESIAN_POINT('',(-50.3023253561992,36.939908654649,39.2875012672119));
#171059=CARTESIAN_POINT('',(-50.5905785208481,37.1493329797265,39.8576902534424));
#171060=CARTESIAN_POINT('',(-46.5911245387426,41.5228599914567,39.2875012672119));
#171061=CARTESIAN_POINT('Origin',(5.53234440788222E-15,0.,39.2875012672119));
#171062=CARTESIAN_POINT('',(-46.8559036426982,41.7612723673367,39.8576902534424));
#171063=CARTESIAN_POINT('',(-46.5911245387426,41.5228599914567,39.2875012672119));
#171064=CARTESIAN_POINT('',(-46.7942619810913,42.1132001506005,40.1599502534424));
#171065=CARTESIAN_POINT('Ctrl Pts',(-46.8559036426982,41.7612723673367,
39.8576902534424));
#171066=CARTESIAN_POINT('Ctrl Pts',(-46.865048646203,41.7695067430947,39.8773836120328));
#171067=CARTESIAN_POINT('Ctrl Pts',(-46.8728586744645,41.7791634256518,
39.8969946442061));
#171068=CARTESIAN_POINT('Ctrl Pts',(-46.8792591175129,41.7900688448274,
39.9162525288136));
#171069=CARTESIAN_POINT('Ctrl Pts',(-46.8857881704117,41.8011933963847,
39.9358973793919));
#171070=CARTESIAN_POINT('Ctrl Pts',(-46.8908511403464,41.8136179609569,
39.9551762199559));
#171071=CARTESIAN_POINT('Ctrl Pts',(-46.8943401533925,41.8272034165268,
39.9738152034029));
#171072=CARTESIAN_POINT('Ctrl Pts',(-46.8976936214446,41.8402610894628,
39.991730079239));
#171073=CARTESIAN_POINT('Ctrl Pts',(-46.8995933993913,41.8543920170169,
40.0090551157831));
#171074=CARTESIAN_POINT('Ctrl Pts',(-46.8999101480288,41.8695030436036,
40.0255394551213));
#171075=CARTESIAN_POINT('Ctrl Pts',(-46.9001534633409,41.8811108098749,
40.0382021525944));
#171076=CARTESIAN_POINT('Ctrl Pts',(-46.8994620808004,41.8932975750433,
40.0503687782025));
#171077=CARTESIAN_POINT('Ctrl Pts',(-46.8977610424069,41.9060298852858,
40.0619155352442));
#171078=CARTESIAN_POINT('Ctrl Pts',(-46.8977565842886,41.9060632544003,
40.0619457972351));
#171079=CARTESIAN_POINT('Ctrl Pts',(-46.8977521185698,41.9060966277703,
40.0619760547305));
#171080=CARTESIAN_POINT('Ctrl Pts',(-46.8977476452506,41.9061300053927,
40.0620063077269));
#171081=CARTESIAN_POINT('Ctrl Pts',(-46.8972680144601,41.9097087652735,
40.06525004417));
#171082=CARTESIAN_POINT('Ctrl Pts',(-46.8967002823074,41.9133346546845,
40.0684393223556));
#171083=CARTESIAN_POINT('Ctrl Pts',(-46.8960451360316,41.9170027866179,
40.0715697951759));
#171084=CARTESIAN_POINT('Ctrl Pts',(-46.8923993959675,41.9374151068061,
40.0889901646466));
#171085=CARTESIAN_POINT('Ctrl Pts',(-46.8860516300617,41.9591363747861,
40.1045963098324));
#171086=CARTESIAN_POINT('Ctrl Pts',(-46.8771671012894,41.9812950716655,
40.1176634650827));
#171087=CARTESIAN_POINT('Ctrl Pts',(-46.8731796017438,41.9912402016775,
40.1235281853125));
#171088=CARTESIAN_POINT('Ctrl Pts',(-46.8686813028933,42.0012737523661,
40.1288820140948));
#171089=CARTESIAN_POINT('Ctrl Pts',(-46.8636874904587,42.0113191526629,
40.1336621774101));
#171090=CARTESIAN_POINT('Ctrl Pts',(-46.8615172471194,42.0156847477609,
40.1357395717319));
#171091=CARTESIAN_POINT('Ctrl Pts',(-46.859253386561,42.0200523791244,40.1377083672884));
#171092=CARTESIAN_POINT('Ctrl Pts',(-46.8568971484357,42.0244156319708,
40.1395632548792));
#171093=CARTESIAN_POINT('Ctrl Pts',(-46.8486503149973,42.0396870169332,
40.146055361447));
#171094=CARTESIAN_POINT('Ctrl Pts',(-46.8392718539635,42.0549047629077,
40.1511520974629));
#171095=CARTESIAN_POINT('Ctrl Pts',(-46.8288149286281,42.0697938479571,
40.1546258197408));
#171096=CARTESIAN_POINT('Ctrl Pts',(-46.8235864659604,42.0772383904818,
40.1563626808798));
#171097=CARTESIAN_POINT('Ctrl Pts',(-46.8180883876708,42.0846007681803,
40.1576937882008));
#171098=CARTESIAN_POINT('Ctrl Pts',(-46.8123273450616,42.0918466086056,
40.1585906813668));
#171099=CARTESIAN_POINT('Ctrl Pts',(-46.809446823757,42.0954695288182,40.1590391279498));
#171100=CARTESIAN_POINT('Ctrl Pts',(-46.8065005614641,42.099063314795,40.1593790209175));
#171101=CARTESIAN_POINT('Ctrl Pts',(-46.8034893901143,42.1026236704494,
40.1596068022931));
#171102=CARTESIAN_POINT('Ctrl Pts',(-46.8004782187645,42.1061840261037,
40.1598345836687));
#171103=CARTESIAN_POINT('Ctrl Pts',(-46.7974021370897,42.1097109502942,
40.1599502506864));
#171104=CARTESIAN_POINT('Ctrl Pts',(-46.7942619810913,42.1132001506005,
40.1599502534424));
#171105=CARTESIAN_POINT('',(-46.7738319284254,42.1358900227699,40.1599502534424));
#171106=CARTESIAN_POINT('Origin',(7.58094983678529E-17,-1.03991361176645E-16,
40.1599502534424));
#171107=CARTESIAN_POINT('',(-46.4302753505421,42.2339804752705,39.8576902534424));
#171108=CARTESIAN_POINT('Ctrl Pts',(-46.7738319284254,42.1358900227699,
40.1599502534424));
#171109=CARTESIAN_POINT('Ctrl Pts',(-46.7712740741883,42.1387294146419,
40.1599502447858));
#171110=CARTESIAN_POINT('Ctrl Pts',(-46.7686877639335,42.1415290809212,
40.1598744685927));
#171111=CARTESIAN_POINT('Ctrl Pts',(-46.7660751225862,42.1442883388463,
40.1597246934279));
#171112=CARTESIAN_POINT('Ctrl Pts',(-46.7509772786444,42.1602334457359,
40.1588591777436));
#171113=CARTESIAN_POINT('Ctrl Pts',(-46.734999596514,42.1748324484411,40.1555254706029));
#171114=CARTESIAN_POINT('Ctrl Pts',(-46.7185561660749,42.1879477932289,
40.1500631826401));
#171115=CARTESIAN_POINT('Ctrl Pts',(-46.7119241523125,42.1932375134885,
40.1478601162497));
#171116=CARTESIAN_POINT('Ctrl Pts',(-46.7052163225658,42.1982863518301,
40.1453112228316));
#171117=CARTESIAN_POINT('Ctrl Pts',(-46.6984594183135,42.2030870843188,
40.1424401896328));
#171118=CARTESIAN_POINT('Ctrl Pts',(-46.6959665308742,42.2048582631419,
40.1413809526906));
#171119=CARTESIAN_POINT('Ctrl Pts',(-46.6934669941951,42.2065955404587,
40.1402777640512));
#171120=CARTESIAN_POINT('Ctrl Pts',(-46.6909621675968,42.2082984896058,
40.1391317641987));
#171121=CARTESIAN_POINT('Ctrl Pts',(-46.6862656177251,42.2114915192566,
40.1369830144753));
#171122=CARTESIAN_POINT('Ctrl Pts',(-46.6815504704768,42.2145638639317,
40.134683756585));
#171123=CARTESIAN_POINT('Ctrl Pts',(-46.6768256862943,42.2175127112219,
40.1322415082996));
#171124=CARTESIAN_POINT('Ctrl Pts',(-46.6602889416556,42.2278336767376,
40.1236936393009));
#171125=CARTESIAN_POINT('Ctrl Pts',(-46.6436341412463,42.2366417962863,
40.113394140767));
#171126=CARTESIAN_POINT('Ctrl Pts',(-46.6272454828771,42.2438165047413,
40.101665321223));
#171127=CARTESIAN_POINT('Ctrl Pts',(-46.6190511536924,42.2474038589688,
40.095800911451));
#171128=CARTESIAN_POINT('Ctrl Pts',(-46.6109233607687,42.2505828610987,
40.0895791707949));
#171129=CARTESIAN_POINT('Ctrl Pts',(-46.6029101354043,42.2533384464729,
40.0830403822906));
#171130=CARTESIAN_POINT('Ctrl Pts',(-46.598903522722,42.25471623916,40.0797709880385));
#171131=CARTESIAN_POINT('Ctrl Pts',(-46.5949255520162,42.2559881777374,
40.0764223317514));
#171132=CARTESIAN_POINT('Ctrl Pts',(-46.5909822275908,42.2571523794832,
40.0729994484778));
#171133=CARTESIAN_POINT('Ctrl Pts',(-46.5870389031655,42.258316581229,40.0695765652042));
#171134=CARTESIAN_POINT('Ctrl Pts',(-46.5831302673239,42.2593729236707,
40.0660793733488));
#171135=CARTESIAN_POINT('Ctrl Pts',(-46.5792622391316,42.2603197753211,
40.0625130768817));
#171136=CARTESIAN_POINT('Ctrl Pts',(-46.579229252952,42.2603278499826,40.0624826638418));
#171137=CARTESIAN_POINT('Ctrl Pts',(-46.5791962698503,42.260335916744,40.0624522459912));
#171138=CARTESIAN_POINT('Ctrl Pts',(-46.5791632898295,42.2603439756045,
40.0624218233329));
#171139=CARTESIAN_POINT('Ctrl Pts',(-46.5623199116986,42.2644597533378,
40.046884527588));
#171140=CARTESIAN_POINT('Ctrl Pts',(-46.5462756748339,42.2666468343728,
40.0302263329197));
#171141=CARTESIAN_POINT('Ctrl Pts',(-46.531134677875,42.2670764855937,40.012751588468));
#171142=CARTESIAN_POINT('Ctrl Pts',(-46.5154816224528,42.2675206673337,
39.9946858597626));
#171143=CARTESIAN_POINT('Ctrl Pts',(-46.5007931180847,42.2660861658582,
39.9757460620372));
#171144=CARTESIAN_POINT('Ctrl Pts',(-46.4872066206965,42.262915064436,39.9562444558982));
#171145=CARTESIAN_POINT('Ctrl Pts',(-46.4738785670777,42.2598042840354,
39.9371138113436));
#171146=CARTESIAN_POINT('Ctrl Pts',(-46.4616103837113,42.2550216427103,
39.9174410654147));
#171147=CARTESIAN_POINT('Ctrl Pts',(-46.4505634197995,42.2486653035344,
39.897519650391));
#171148=CARTESIAN_POINT('Ctrl Pts',(-46.4432451935029,42.244454451677,39.8843224113616));
#171149=CARTESIAN_POINT('Ctrl Pts',(-46.4364635650926,42.2395522518983,
39.8710160447052));
#171150=CARTESIAN_POINT('Ctrl Pts',(-46.4302753505421,42.2339804752705,
39.8576902534424));
#171151=CARTESIAN_POINT('',(-46.1654920697608,41.9955727382255,39.2875012672119));
#171152=CARTESIAN_POINT('',(-46.4302753505421,42.2339804752705,39.8576902534424));
#171153=CARTESIAN_POINT('',(-41.9955727382247,46.1654920697616,39.2875012672119));
#171154=CARTESIAN_POINT('Origin',(5.53234440788222E-15,0.,39.2875012672119));
#171155=CARTESIAN_POINT('',(-42.2339804752697,46.4302753505428,39.8576902534424));
#171156=CARTESIAN_POINT('',(-41.9955727382247,46.1654920697616,39.2875012672119));
#171157=CARTESIAN_POINT('',(-42.1358900227691,46.7738319284261,40.1599502534424));
#171158=CARTESIAN_POINT('Ctrl Pts',(-42.2339804752697,46.4302753505428,
39.8576902534424));
#171159=CARTESIAN_POINT('Ctrl Pts',(-42.2422146548469,46.4394205306943,
39.8773836120384));
#171160=CARTESIAN_POINT('Ctrl Pts',(-42.2489725007701,46.4498406831895,
39.8969946442172));
#171161=CARTESIAN_POINT('Ctrl Pts',(-42.2541979548148,46.4613553898177,
39.91625252883));
#171162=CARTESIAN_POINT('Ctrl Pts',(-42.2595284086006,46.4731014717878,
39.935897379414));
#171163=CARTESIAN_POINT('Ctrl Pts',(-42.2632649224145,46.4859871977669,
39.9551762199833));
#171164=CARTESIAN_POINT('Ctrl Pts',(-42.2653147554872,46.499862931967,39.9738152034351));
#171165=CARTESIAN_POINT('Ctrl Pts',(-42.2672849544032,46.5131996064718,
39.9917300792761));
#171166=CARTESIAN_POINT('Ctrl Pts',(-42.2676972410234,46.5274517042014,
40.0090551158245));
#171167=CARTESIAN_POINT('Ctrl Pts',(-42.2664327220877,46.5425130602579,
40.0255394551664));
#171168=CARTESIAN_POINT('Ctrl Pts',(-42.2654613625215,46.5540826713342,
40.0382021526232));
#171169=CARTESIAN_POINT('Ctrl Pts',(-42.2634999036127,46.5661304069596,
40.0503687782163));
#171170=CARTESIAN_POINT('Ctrl Pts',(-42.2604772948656,46.5786151613304,
40.0619155352442));
#171171=CARTESIAN_POINT('Ctrl Pts',(-42.2604693731471,46.5786478816451,
40.0619457972352));
#171172=CARTESIAN_POINT('Ctrl Pts',(-42.2604614434249,46.5786806053976,
40.0619760547305));
#171173=CARTESIAN_POINT('Ctrl Pts',(-42.2604535056994,46.5787133325847,
40.062006307727));
#171174=CARTESIAN_POINT('Ctrl Pts',(-42.2596024201058,46.5822223525749,
40.06525004417));
#171175=CARTESIAN_POINT('Ctrl Pts',(-42.2586587894011,46.5857690348149,
40.0684393223556));
#171176=CARTESIAN_POINT('Ctrl Pts',(-42.2576238078912,46.5893485909044,
40.0715697951759));
#171177=CARTESIAN_POINT('Ctrl Pts',(-42.2518643711132,46.609268006655,40.0889901646418));
#171178=CARTESIAN_POINT('Ctrl Pts',(-42.2432808881741,46.6302067610349,
40.1045963098239));
#171179=CARTESIAN_POINT('Ctrl Pts',(-42.2321288152516,46.651315384109,40.117663465072));
#171180=CARTESIAN_POINT('Ctrl Pts',(-42.2271236104862,46.6607892264642,
40.123528185306));
#171181=CARTESIAN_POINT('Ctrl Pts',(-42.2216011621498,46.6702976120519,
40.1288820140919));
#171182=CARTESIAN_POINT('Ctrl Pts',(-42.2155846760826,46.679765987061,40.1336621774101));
#171183=CARTESIAN_POINT('Ctrl Pts',(-42.2129699926165,46.683880814771,40.1357395717319));
#171184=CARTESIAN_POINT('Ctrl Pts',(-42.2102619919286,46.6879878819277,
40.1377083672884));
#171185=CARTESIAN_POINT('Ctrl Pts',(-42.2074625774074,46.6920809384682,
40.1395632548792));
#171186=CARTESIAN_POINT('Ctrl Pts',(-42.1976646265834,46.7064066363598,
40.146055361447));
#171187=CARTESIAN_POINT('Ctrl Pts',(-42.1867468541393,46.7205607018098,
40.151152097463));
#171188=CARTESIAN_POINT('Ctrl Pts',(-42.1747908797553,46.7342751765576,
40.1546258197409));
#171189=CARTESIAN_POINT('Ctrl Pts',(-42.1688128925634,46.7411324139316,
40.1563626808798));
#171190=CARTESIAN_POINT('Ctrl Pts',(-42.1625753552951,46.7478797540802,
40.1576937882008));
#171191=CARTESIAN_POINT('Ctrl Pts',(-42.1560884757154,46.7544837081027,
40.1585906813668));
#171192=CARTESIAN_POINT('Ctrl Pts',(-42.1528450359255,46.7577856851139,
40.1590391279498));
#171193=CARTESIAN_POINT('Ctrl Pts',(-42.1495392606402,46.7610518156853,
40.1593790209175));
#171194=CARTESIAN_POINT('Ctrl Pts',(-42.1461724262969,46.764277914225,40.1596068022931));
#171195=CARTESIAN_POINT('Ctrl Pts',(-42.1428055919536,46.7675040127647,
40.1598345836687));
#171196=CARTESIAN_POINT('Ctrl Pts',(-42.1393776974104,46.7706900780051,
40.1599502506865));
#171197=CARTESIAN_POINT('Ctrl Pts',(-42.1358900227691,46.7738319284261,
40.1599502534424));
#171198=CARTESIAN_POINT('',(-42.1132001505997,46.794261981092,40.1599502534424));
#171199=CARTESIAN_POINT('Origin',(6.43067523875891E-17,-1.15494107156905E-16,
40.1599502534424));
#171200=CARTESIAN_POINT('',(-41.7612723673359,46.8559036426989,39.8576902534424));
#171201=CARTESIAN_POINT('Ctrl Pts',(-42.1132001505997,46.794261981092,40.1599502534424));
#171202=CARTESIAN_POINT('Ctrl Pts',(-42.1103595112868,46.7968184499056,
40.1599502447859));
#171203=CARTESIAN_POINT('Ctrl Pts',(-42.1074947242963,46.7993324362836,
40.1598744685926));
#171204=CARTESIAN_POINT('Ctrl Pts',(-42.104607974281,46.80180348332,40.1597246934279));
#171205=CARTESIAN_POINT('Ctrl Pts',(-42.0879261203839,46.8160830868235,
40.1588591777433));
#171206=CARTESIAN_POINT('Ctrl Pts',(-42.0705099543453,46.8289319921076,
40.1555254706011));
#171207=CARTESIAN_POINT('Ctrl Pts',(-42.052785675898,46.8402566831519,40.1500631826359));
#171208=CARTESIAN_POINT('Ctrl Pts',(-42.0456370666755,46.8448241915603,
40.1478601162464));
#171209=CARTESIAN_POINT('Ctrl Pts',(-42.0384382358134,46.849144212699,40.1453112228297));
#171210=CARTESIAN_POINT('Ctrl Pts',(-42.0312165334047,46.8532123574523,
40.1424401896328));
#171211=CARTESIAN_POINT('Ctrl Pts',(-42.028552163663,46.8547132558793,40.1413809526906));
#171212=CARTESIAN_POINT('Ctrl Pts',(-42.0258847247792,46.8561797434812,
40.1402777640511));
#171213=CARTESIAN_POINT('Ctrl Pts',(-42.0232156132258,46.8576115380197,
40.1391317641987));
#171214=CARTESIAN_POINT('Ctrl Pts',(-42.0182110290631,46.8602961527792,
40.1369830144753));
#171215=CARTESIAN_POINT('Ctrl Pts',(-42.0132005644172,46.8628587997327,
40.1346837565849));
#171216=CARTESIAN_POINT('Ctrl Pts',(-42.0081934246212,46.8652976184991,
40.1322415082996));
#171217=CARTESIAN_POINT('Ctrl Pts',(-41.9906684353351,46.8738334841812,
40.1236936393008));
#171218=CARTESIAN_POINT('Ctrl Pts',(-41.9731841724644,46.8808524512366,
40.113394140767));
#171219=CARTESIAN_POINT('Ctrl Pts',(-41.9561353316313,46.8862747746137,
40.101665321223));
#171220=CARTESIAN_POINT('Ctrl Pts',(-41.9476109112147,46.8889859363022,
40.095800911451));
#171221=CARTESIAN_POINT('Ctrl Pts',(-41.9391953469837,46.8912979378217,
40.0895791707949));
#171222=CARTESIAN_POINT('Ctrl Pts',(-41.9309379818017,46.8932008176777,
40.0830403822906));
#171223=CARTESIAN_POINT('Ctrl Pts',(-41.9268092992106,46.8941522576057,
40.0797709880385));
#171224=CARTESIAN_POINT('Ctrl Pts',(-41.9227201664597,46.8950014172057,
40.0764223317514));
#171225=CARTESIAN_POINT('Ctrl Pts',(-41.9186767517587,46.8957470516902,
40.0729994484778));
#171226=CARTESIAN_POINT('Ctrl Pts',(-41.9146333370577,46.8964926861746,
40.0695765652042));
#171227=CARTESIAN_POINT('Ctrl Pts',(-41.9106356952802,46.897134678164,40.0660793733488));
#171228=CARTESIAN_POINT('Ctrl Pts',(-41.9066898836031,46.8976720238191,
40.0625130768817));
#171229=CARTESIAN_POINT('Ctrl Pts',(-41.9066562340933,46.8976766062522,
40.0624826638418));
#171230=CARTESIAN_POINT('Ctrl Pts',(-41.9066225884702,46.89768118115,40.0624522459912));
#171231=CARTESIAN_POINT('Ctrl Pts',(-41.9065889467371,46.8976857485123,
40.0624218233329));
#171232=CARTESIAN_POINT('Ctrl Pts',(-41.8894076224742,46.9000183671521,
40.0468845275896));
#171233=CARTESIAN_POINT('Ctrl Pts',(-41.8732226653996,46.9005163877047,
40.0302263329231));
#171234=CARTESIAN_POINT('Ctrl Pts',(-41.8581197016257,46.8993610201073,
40.0127515884734));
#171235=CARTESIAN_POINT('Ctrl Pts',(-41.8425059656456,46.898166578745,39.9946858597699));
#171236=CARTESIAN_POINT('Ctrl Pts',(-41.8280478726772,46.8952045688303,
39.9757460620467));
#171237=CARTESIAN_POINT('Ctrl Pts',(-41.8148672739026,46.8906306633413,
39.9562444559099));
#171238=CARTESIAN_POINT('Ctrl Pts',(-41.8019373978516,46.8861437631592,
39.9371138113573));
#171239=CARTESIAN_POINT('Ctrl Pts',(-41.7902363430259,46.8801049472907,
39.9174410654306));
#171240=CARTESIAN_POINT('Ctrl Pts',(-41.7799143139045,46.872628706646,39.897519650409));
#171241=CARTESIAN_POINT('Ctrl Pts',(-41.7730763314874,46.8676759593254,
39.8843224113737));
#171242=CARTESIAN_POINT('Ctrl Pts',(-41.7668442729534,46.8620917411115,
39.8710160447113));
#171243=CARTESIAN_POINT('Ctrl Pts',(-41.7612723673359,46.8559036426989,
39.8576902534424));
#171244=CARTESIAN_POINT('',(-41.5228599914559,46.5911245387433,39.2875012672119));
#171245=CARTESIAN_POINT('',(-41.7612723673359,46.8559036426989,39.8576902534424));
#171246=CARTESIAN_POINT('',(-36.9399086546482,50.3023253561999,39.2875012672119));
#171247=CARTESIAN_POINT('Origin',(5.53234440788222E-15,0.,39.2875012672119));
#171248=CARTESIAN_POINT('',(-37.1493329797256,50.5905785208487,39.8576902534424));
#171249=CARTESIAN_POINT('',(-36.9399086546482,50.3023253561999,39.2875012672119));
#171250=CARTESIAN_POINT('',(-37.0158684358555,50.9219998155903,40.1599502534424));
#171251=CARTESIAN_POINT('Ctrl Pts',(-37.1493329797256,50.5905785208487,
39.8576902534424));
#171252=CARTESIAN_POINT('Ctrl Pts',(-37.1565661199767,50.6005343088816,
39.8773836120343));
#171253=CARTESIAN_POINT('Ctrl Pts',(-37.1621977431848,50.6116037659379,
39.8969946442089));
#171254=CARTESIAN_POINT('Ctrl Pts',(-37.1661909570565,50.6236016024766,
39.9162525288178));
#171255=CARTESIAN_POINT('Ctrl Pts',(-37.1702644101608,50.6358405223205,
39.9358973793979));
#171256=CARTESIAN_POINT('Ctrl Pts',(-37.1726335298269,50.6490462309881,
39.9551762199636));
#171257=CARTESIAN_POINT('Ctrl Pts',(-37.1732217245282,50.663060218362,39.9738152034121));
#171258=CARTESIAN_POINT('Ctrl Pts',(-37.1737870683986,50.6765297750304,
39.9917300792502));
#171259=CARTESIAN_POINT('Ctrl Pts',(-37.1727073465975,50.6907468939608,
40.0090551157961));
#171260=CARTESIAN_POINT('Ctrl Pts',(-37.1698754144281,50.7055935641083,
40.0255394551359));
#171261=CARTESIAN_POINT('Ctrl Pts',(-37.1677000224047,50.7169982609304,
40.0382021526037));
#171262=CARTESIAN_POINT('Ctrl Pts',(-37.1644899772806,50.7287749695232,
40.050368778207));
#171263=CARTESIAN_POINT('Ctrl Pts',(-37.1601789145083,50.7408753824656,
40.0619155352442));
#171264=CARTESIAN_POINT('Ctrl Pts',(-37.1601676159816,50.7409070954899,
40.0619457972351));
#171265=CARTESIAN_POINT('Ctrl Pts',(-37.1601563091356,50.7409388110966,
40.0619760547305));
#171266=CARTESIAN_POINT('Ctrl Pts',(-37.1601449939713,50.7409705292825,
40.0620063077269));
#171267=CARTESIAN_POINT('Ctrl Pts',(-37.1589317782465,50.7443713638249,
40.06525004417));
#171268=CARTESIAN_POINT('Ctrl Pts',(-37.1576225876053,50.747799980701,40.0684393223557));
#171269=CARTESIAN_POINT('Ctrl Pts',(-37.1562191103351,50.7512517425809,
40.0715697951759));
#171270=CARTESIAN_POINT('Ctrl Pts',(-37.1484090784357,50.7704600126149,
40.0889901646443));
#171271=CARTESIAN_POINT('Ctrl Pts',(-37.1376839208943,50.7903868440293,
40.1045963098283));
#171272=CARTESIAN_POINT('Ctrl Pts',(-37.1243864882599,50.8102141228154,
40.1176634650776));
#171273=CARTESIAN_POINT('Ctrl Pts',(-37.1184184163487,50.8191128801057,
40.1235281853093));
#171274=CARTESIAN_POINT('Ctrl Pts',(-37.1119323236304,50.8279919247214,
40.1288820140934));
#171275=CARTESIAN_POINT('Ctrl Pts',(-37.1049590818163,50.8367795369358,
40.1336621774101));
#171276=CARTESIAN_POINT('Ctrl Pts',(-37.1019286052427,50.8405985143445,
40.1357395717319));
#171277=CARTESIAN_POINT('Ctrl Pts',(-37.0988061338475,50.8444000194071,
40.1377083672884));
#171278=CARTESIAN_POINT('Ctrl Pts',(-37.0955942139017,50.8481780352576,
40.1395632548792));
#171279=CARTESIAN_POINT('Ctrl Pts',(-37.0843524940916,50.8614010907344,
40.146055361447));
#171280=CARTESIAN_POINT('Ctrl Pts',(-37.0720150276368,50.8743364007571,
40.1511520974629));
#171281=CARTESIAN_POINT('Ctrl Pts',(-37.0586909963616,50.886726006548,40.1546258197408));
#171282=CARTESIAN_POINT('Ctrl Pts',(-37.052028980724,50.8929208094435,40.1563626808798));
#171283=CARTESIAN_POINT('Ctrl Pts',(-37.0451203242406,50.8989791867716,
40.1576937882008));
#171284=CARTESIAN_POINT('Ctrl Pts',(-37.0379786793005,50.9048689000891,
40.1585906813668));
#171285=CARTESIAN_POINT('Ctrl Pts',(-37.0344078568305,50.9078137567479,
40.1590391279498));
#171286=CARTESIAN_POINT('Ctrl Pts',(-37.0307787873186,50.9107164475037,
40.1593790209175));
#171287=CARTESIAN_POINT('Ctrl Pts',(-37.0270931777235,50.9135729431181,
40.1596068022931));
#171288=CARTESIAN_POINT('Ctrl Pts',(-37.0234075681283,50.9164294387325,
40.1598345836687));
#171289=CARTESIAN_POINT('Ctrl Pts',(-37.0196654174466,50.9192397378253,
40.1599502506865));
#171290=CARTESIAN_POINT('Ctrl Pts',(-37.0158684358555,50.9219998155903,
40.1599502534424));
#171291=CARTESIAN_POINT('',(-36.9911673391703,50.9399462128205,40.1599502534424));
#171292=CARTESIAN_POINT('Origin',(5.16646552926871E-17,-1.25731475530457E-16,
40.1599502534424));
#171293=CARTESIAN_POINT('',(-36.634724144965,50.9644637245896,39.8576902534424));
#171294=CARTESIAN_POINT('Ctrl Pts',(-36.9911673391703,50.9399462128205,
40.1599502534424));
#171295=CARTESIAN_POINT('Ctrl Pts',(-36.9880750374203,50.9421917493683,
40.1599502447858));
#171296=CARTESIAN_POINT('Ctrl Pts',(-36.9849631609,50.9443925120842,40.1598744685927));
#171297=CARTESIAN_POINT('Ctrl Pts',(-36.9818339300539,50.9465482749234,
40.1597246934279));
#171298=CARTESIAN_POINT('Ctrl Pts',(-36.9637508360915,50.9590059247098,
40.1588591777435));
#171299=CARTESIAN_POINT('Ctrl Pts',(-36.9450870013129,50.9699639572724,
40.1555254706026));
#171300=CARTESIAN_POINT('Ctrl Pts',(-36.9262760657698,50.9793739188842,
40.1500631826394));
#171301=CARTESIAN_POINT('Ctrl Pts',(-36.9186891827376,50.9831691728694,
40.1478601162492));
#171302=CARTESIAN_POINT('Ctrl Pts',(-36.9110782226493,50.9867130457549,
40.1453112228313));
#171303=CARTESIAN_POINT('Ctrl Pts',(-36.9034708445584,50.9900040313324,
40.1424401896328));
#171304=CARTESIAN_POINT('Ctrl Pts',(-36.9006641839068,50.9912182052062,
40.1413809526906));
#171305=CARTESIAN_POINT('Ctrl Pts',(-36.8978580678369,50.9923978359482,
40.1402777640512));
#171306=CARTESIAN_POINT('Ctrl Pts',(-36.895053914673,50.9935427888373,40.1391317641987));
#171307=CARTESIAN_POINT('Ctrl Pts',(-36.8897961274908,50.9956895755045,
40.1369830144753));
#171308=CARTESIAN_POINT('Ctrl Pts',(-36.8845452411465,50.9977144478402,
40.1346837565849));
#171309=CARTESIAN_POINT('Ctrl Pts',(-36.8793106050083,50.9996165178739,
40.1322415082996));
#171310=CARTESIAN_POINT('Ctrl Pts',(-36.8609893785248,51.0062737629919,
40.1236936393009));
#171311=CARTESIAN_POINT('Ctrl Pts',(-36.8428672144356,51.0114266762821,
40.113394140767));
#171312=CARTESIAN_POINT('Ctrl Pts',(-36.8253449818064,51.0150372064716,
40.101665321223));
#171313=CARTESIAN_POINT('Ctrl Pts',(-36.8165838654919,51.0168424715663,
40.095800911451));
#171314=CARTESIAN_POINT('Ctrl Pts',(-36.8079727326363,51.018262141703,40.0895791707949));
#171315=CARTESIAN_POINT('Ctrl Pts',(-36.7995616970576,51.0192914676909,
40.0830403822907));
#171316=CARTESIAN_POINT('Ctrl Pts',(-36.7953561792682,51.0198061306849,
40.0797709880385));
#171317=CARTESIAN_POINT('Ctrl Pts',(-36.7912006858663,51.0202232077372,
40.0764223317514));
#171318=CARTESIAN_POINT('Ctrl Pts',(-36.7871014813873,51.0205421056329,
40.0729994484778));
#171319=CARTESIAN_POINT('Ctrl Pts',(-36.7830022769083,51.0208610035286,
40.0695765652042));
#171320=CARTESIAN_POINT('Ctrl Pts',(-36.7789594281946,51.0210816112669,
40.0660793733488));
#171321=CARTESIAN_POINT('Ctrl Pts',(-36.7749790641711,51.0212035636554,
40.0625130768817));
#171322=CARTESIAN_POINT('Ctrl Pts',(-36.7749451200022,51.0212046036538,
40.0624826638418));
#171323=CARTESIAN_POINT('Ctrl Pts',(-36.7749111804864,51.0212056365646,
40.0624522459912));
#171324=CARTESIAN_POINT('Ctrl Pts',(-36.7748772456268,51.0212066623878,
40.0624218233329));
#171325=CARTESIAN_POINT('Ctrl Pts',(-36.7575462174132,51.0217305652765,
40.0468845275888));
#171326=CARTESIAN_POINT('Ctrl Pts',(-36.7413978659031,51.0205340689293,
40.0302263329216));
#171327=CARTESIAN_POINT('Ctrl Pts',(-36.7264984065438,51.0178063409622,
40.0127515884709));
#171328=CARTESIAN_POINT('Ctrl Pts',(-36.7110950573628,51.0149863630466,
39.9946858597669));
#171329=CARTESIAN_POINT('Ctrl Pts',(-36.6970257816846,51.0105292970922,
39.9757460620431));
#171330=CARTESIAN_POINT('Ctrl Pts',(-36.684395490921,51.0046027002009,39.9562444559056));
#171331=CARTESIAN_POINT('Ctrl Pts',(-36.6720054548649,50.9987888396535,
39.9371138113531));
#171332=CARTESIAN_POINT('Ctrl Pts',(-36.6609997277847,50.9915600117704,
39.9174410654264));
#171333=CARTESIAN_POINT('Ctrl Pts',(-36.6515157237649,50.9830457809122,
39.8975196504048));
#171334=CARTESIAN_POINT('Ctrl Pts',(-36.6452329035982,50.977405401466,39.8843224113709));
#171335=CARTESIAN_POINT('Ctrl Pts',(-36.6396186946822,50.9712003466828,
39.8710160447099));
#171336=CARTESIAN_POINT('Ctrl Pts',(-36.634724144965,50.9644637245896,39.8576902534424));
#171337=CARTESIAN_POINT('',(-36.4252947698674,50.6762142289951,39.2875012672119));
#171338=CARTESIAN_POINT('',(-36.634724144965,50.9644637245896,39.8576902534424));
#171339=CARTESIAN_POINT('',(-31.4795232016785,53.8880358395973,39.2875012672119));
#171340=CARTESIAN_POINT('Origin',(5.53234440788222E-15,0.,39.2875012672119));
#171341=CARTESIAN_POINT('',(-31.6576696180579,54.196600726121,39.8576902534424));
#171342=CARTESIAN_POINT('',(-31.4795232016785,53.8880358395973,39.2875012672119));
#171343=CARTESIAN_POINT('',(-31.4902932482903,54.5122556166614,40.1599502534424));
#171344=CARTESIAN_POINT('Ctrl Pts',(-31.6576696180579,54.196600726121,39.8576902534424));
#171345=CARTESIAN_POINT('Ctrl Pts',(-31.6638224711875,54.2072580443428,
39.8773836120385));
#171346=CARTESIAN_POINT('Ctrl Pts',(-31.6682661704396,54.2188555266773,
39.8969946442173));
#171347=CARTESIAN_POINT('Ctrl Pts',(-31.6709833936518,54.2312050423246,
39.91625252883));
#171348=CARTESIAN_POINT('Ctrl Pts',(-31.6737552164704,54.2438027078811,
39.9358973794142));
#171349=CARTESIAN_POINT('Ctrl Pts',(-31.6747309854168,54.2571837147363,
39.9551762199837));
#171350=CARTESIAN_POINT('Ctrl Pts',(-31.6738510973598,54.2711824151128,
39.9738152034356));
#171351=CARTESIAN_POINT('Ctrl Pts',(-31.6730053921561,54.2846372786697,
39.9917300792771));
#171352=CARTESIAN_POINT('Ctrl Pts',(-31.6704454915877,54.2986636530781,
40.009055115826));
#171353=CARTESIAN_POINT('Ctrl Pts',(-31.6660771734206,54.313132974099,40.0255394551682));
#171354=CARTESIAN_POINT('Ctrl Pts',(-31.6627215829905,54.3242478044044,
40.0382021526244));
#171355=CARTESIAN_POINT('Ctrl Pts',(-31.6582981215806,54.335624457862,40.0503687782168));
#171356=CARTESIAN_POINT('Ctrl Pts',(-31.6527458376963,54.3472079546997,
40.0619155352442));
#171357=CARTESIAN_POINT('Ctrl Pts',(-31.6527312861504,54.3472383129791,
40.0619457972352));
#171358=CARTESIAN_POINT('Ctrl Pts',(-31.6527167260609,54.3472686729571,
40.0619760547305));
#171359=CARTESIAN_POINT('Ctrl Pts',(-31.6527021574289,54.3472990346307,
40.0620063077269));
#171360=CARTESIAN_POINT('Ctrl Pts',(-31.6511401038183,54.3505544234703,
40.06525004417));
#171361=CARTESIAN_POINT('Ctrl Pts',(-31.6494796970072,54.3538274103386,
40.0684393223556));
#171362=CARTESIAN_POINT('Ctrl Pts',(-31.6477231007675,54.3571135597835,
40.0715697951759));
#171363=CARTESIAN_POINT('Ctrl Pts',(-31.6379480420933,54.3754002342682,
40.0889901646408));
#171364=CARTESIAN_POINT('Ctrl Pts',(-31.6251987170247,54.3940968201752,
40.104596309822));
#171365=CARTESIAN_POINT('Ctrl Pts',(-31.6099016141394,54.4124255228513,
40.1176634650697));
#171366=CARTESIAN_POINT('Ctrl Pts',(-31.6030360625235,54.4206516984363,
40.1235281853045));
#171367=CARTESIAN_POINT('Ctrl Pts',(-31.5956573884077,54.4288041214158,
40.1288820140912));
#171368=CARTESIAN_POINT('Ctrl Pts',(-31.5878037911377,54.4368146919238,
40.1336621774101));
#171369=CARTESIAN_POINT('Ctrl Pts',(-31.5843907239921,54.4402959775155,
40.1357395717319));
#171370=CARTESIAN_POINT('Ctrl Pts',(-31.5808879923396,54.4437502703991,
40.1377083672884));
#171371=CARTESIAN_POINT('Ctrl Pts',(-31.5772987574364,54.4471718528274,
40.1395632548792));
#171372=CARTESIAN_POINT('Ctrl Pts',(-31.5647364352749,54.4591473913265,
40.146055361447));
#171373=CARTESIAN_POINT('Ctrl Pts',(-31.5511144466737,54.4707222239583,
40.151152097463));
#171374=CARTESIAN_POINT('Ctrl Pts',(-31.5365683393821,54.4816512176787,
40.1546258197409));
#171375=CARTESIAN_POINT('Ctrl Pts',(-31.5292952857363,54.4871157145389,
40.1563626808798));
#171376=CARTESIAN_POINT('Ctrl Pts',(-31.521791202724,54.4924187521965,40.1576937882008));
#171377=CARTESIAN_POINT('Ctrl Pts',(-31.51407303778,54.4975296958775,40.1585906813668));
#171378=CARTESIAN_POINT('Ctrl Pts',(-31.5102139553079,54.500085167718,40.1590391279498));
#171379=CARTESIAN_POINT('Ctrl Pts',(-31.5063013524145,54.502592616171,40.1593790209175));
#171380=CARTESIAN_POINT('Ctrl Pts',(-31.5023373478775,54.5050482124963,
40.1596068022931));
#171381=CARTESIAN_POINT('Ctrl Pts',(-31.4983733433404,54.5075038088217,
40.1598345836687));
#171382=CARTESIAN_POINT('Ctrl Pts',(-31.4943579363062,54.509907551542,40.1599502506865));
#171383=CARTESIAN_POINT('Ctrl Pts',(-31.4902932482903,54.5122556166614,
40.1599502534424));
#171384=CARTESIAN_POINT('',(-31.4638515574735,54.5275217339722,40.1599502534424));
#171385=CARTESIAN_POINT('Origin',(3.80217165444466E-17,-1.34591303547096E-16,
40.1599502534424));
#171386=CARTESIAN_POINT('',(-31.106798218553,54.5146464769141,39.8576902534424));
#171387=CARTESIAN_POINT('Ctrl Pts',(-31.4638515574735,54.5275217339722,
40.1599502534424));
#171388=CARTESIAN_POINT('Ctrl Pts',(-31.4605414731915,54.529431735686,40.1599502447858));
#171389=CARTESIAN_POINT('Ctrl Pts',(-31.4572166015116,54.531295162723,40.1598744685927));
#171390=CARTESIAN_POINT('Ctrl Pts',(-31.4538791743428,54.5331120223762,
40.1597246934279));
#171391=CARTESIAN_POINT('Ctrl Pts',(-31.4345929624705,54.5436112298321,
40.1588591777434));
#171392=CARTESIAN_POINT('Ctrl Pts',(-31.4148859438247,54.5525583311786,
40.1555254706017));
#171393=CARTESIAN_POINT('Ctrl Pts',(-31.3951944477252,54.5599504658517,
40.1500631826372));
#171394=CARTESIAN_POINT('Ctrl Pts',(-31.3872524143681,54.562931883813,40.1478601162474));
#171395=CARTESIAN_POINT('Ctrl Pts',(-31.3793127123314,54.565660781029,40.1453112228303));
#171396=CARTESIAN_POINT('Ctrl Pts',(-31.3714030065914,54.568138550701,40.1424401896328));
#171397=CARTESIAN_POINT('Ctrl Pts',(-31.3684848053913,54.5690526972784,
40.1413809526905));
#171398=CARTESIAN_POINT('Ctrl Pts',(-31.3655707565302,54.5699325468792,
40.1402777640511));
#171399=CARTESIAN_POINT('Ctrl Pts',(-31.3626622846447,54.5707781137757,
40.1391317641987));
#171400=CARTESIAN_POINT('Ctrl Pts',(-31.3572088998595,54.5723635517065,
40.1369830144753));
#171401=CARTESIAN_POINT('Ctrl Pts',(-31.3517751216264,54.5738284644994,
40.1346837565849));
#171402=CARTESIAN_POINT('Ctrl Pts',(-31.3463703409151,54.5751729463231,
40.1322415082996));
#171403=CARTESIAN_POINT('Ctrl Pts',(-31.3274536084255,54.5798786327062,
40.1236936393009));
#171404=CARTESIAN_POINT('Ctrl Pts',(-31.3088920933397,54.583109035835,40.113394140767));
#171405=CARTESIAN_POINT('Ctrl Pts',(-31.291088446162,54.5848682151125,40.101665321223));
#171406=CARTESIAN_POINT('Ctrl Pts',(-31.2821866225731,54.5857478047513,
40.095800911451));
#171407=CARTESIAN_POINT('Ctrl Pts',(-31.2734742664666,54.5862595893021,
40.0895791707949));
#171408=CARTESIAN_POINT('Ctrl Pts',(-31.2650017135572,54.586404083911,40.0830403822906));
#171409=CARTESIAN_POINT('Ctrl Pts',(-31.2607654371024,54.5864763312154,
40.0797709880385));
#171410=CARTESIAN_POINT('Ctrl Pts',(-31.2565891115048,54.5864567561367,
40.0764223317514));
#171411=CARTESIAN_POINT('Ctrl Pts',(-31.2524790289898,54.5863454235315,
40.0729994484778));
#171412=CARTESIAN_POINT('Ctrl Pts',(-31.2483689464749,54.5862340909263,
40.0695765652042));
#171413=CARTESIAN_POINT('Ctrl Pts',(-31.2443251851216,54.5860308973891,
40.0660793733488));
#171414=CARTESIAN_POINT('Ctrl Pts',(-31.240353878453,54.585736120375,40.0625130768817));
#171415=CARTESIAN_POINT('Ctrl Pts',(-31.2403200115243,54.5857336065444,
40.0624826638418));
#171416=CARTESIAN_POINT('Ctrl Pts',(-31.2402861499641,54.5857310861514,
40.0624522459912));
#171417=CARTESIAN_POINT('Ctrl Pts',(-31.2402522937756,54.5857285591963,
40.0624218233329));
#171418=CARTESIAN_POINT('Ctrl Pts',(-31.2229614439845,54.5844380063441,
40.0468845275892));
#171419=CARTESIAN_POINT('Ctrl Pts',(-31.2070266227585,54.5815601021615,
40.0302263329224));
#171420=CARTESIAN_POINT('Ctrl Pts',(-31.1924939094095,54.5772898993835,
40.0127515884722));
#171421=CARTESIAN_POINT('Ctrl Pts',(-31.177469709345,54.5728752811829,39.9946858597683));
#171422=CARTESIAN_POINT('Ctrl Pts',(-31.1639433968861,54.5669719917362,
39.9757460620447));
#171423=CARTESIAN_POINT('Ctrl Pts',(-31.1520017942423,54.5597576364788,
39.9562444559074));
#171424=CARTESIAN_POINT('Ctrl Pts',(-31.1402873460085,54.5526805134389,
39.9371138113545));
#171425=CARTESIAN_POINT('Ctrl Pts',(-31.1300975277224,54.5443408740924,
39.9174410654274));
#171426=CARTESIAN_POINT('Ctrl Pts',(-31.1215554575362,54.5348819367158,
39.8975196504055));
#171427=CARTESIAN_POINT('Ctrl Pts',(-31.1158966355113,54.5286157223213,
39.8843224113713));
#171428=CARTESIAN_POINT('Ctrl Pts',(-31.11096178666,54.5218578148469,39.8710160447101));
#171429=CARTESIAN_POINT('Ctrl Pts',(-31.106798218553,54.5146464769141,39.8576902534424));
#171430=CARTESIAN_POINT('',(-30.9286463962973,54.2060847114744,39.2875012672119));
#171431=CARTESIAN_POINT('',(-31.106798218553,54.5146464769141,39.8576902534424));
#171432=CARTESIAN_POINT('',(-25.6742415049975,56.8833377255397,39.2875012672119));
#171433=CARTESIAN_POINT('Origin',(5.53234440788222E-15,0.,39.2875012672119));
#171434=CARTESIAN_POINT('',(-25.8191582032616,57.2088336324701,39.8576902534424));
#171435=CARTESIAN_POINT('',(-25.6742415049975,56.8833377255397,39.2875012672119));
#171436=CARTESIAN_POINT('',(-25.6197038181293,57.5052637377734,40.1599502534424));
#171437=CARTESIAN_POINT('Ctrl Pts',(-25.8191582032616,57.2088336324701,
39.8576902534424));
#171438=CARTESIAN_POINT('Ctrl Pts',(-25.8241633573205,57.2200757170674,
39.8773836120341));
#171439=CARTESIAN_POINT('Ctrl Pts',(-25.8273704465167,57.2320741602315,
39.8969946442087));
#171440=CARTESIAN_POINT('Ctrl Pts',(-25.8287819086036,57.2446400511037,
39.9162525288174));
#171441=CARTESIAN_POINT('Ctrl Pts',(-25.8302217324658,57.2574584397068,
39.9358973793973));
#171442=CARTESIAN_POINT('Ctrl Pts',(-25.8297934599656,57.2708681396314,
39.9551762199628));
#171443=CARTESIAN_POINT('Ctrl Pts',(-25.8274551293915,57.2846981803126,
39.9738152034111));
#171444=CARTESIAN_POINT('Ctrl Pts',(-25.8252076408405,57.2979909364506,
39.9917300792492));
#171445=CARTESIAN_POINT('Ctrl Pts',(-25.821195608316,57.3116728904364,40.0090551157951));
#171446=CARTESIAN_POINT('Ctrl Pts',(-25.8153387643658,57.3256063334144,
40.0255394551348));
#171447=CARTESIAN_POINT('Ctrl Pts',(-25.8108397400779,57.3363095208145,
40.038202152603));
#171448=CARTESIAN_POINT('Ctrl Pts',(-25.8052513267455,57.34716147416,40.0503687782067));
#171449=CARTESIAN_POINT('Ctrl Pts',(-25.7985186537236,57.3581011436976,
40.0619155352442));
#171450=CARTESIAN_POINT('Ctrl Pts',(-25.7985010085883,57.3581298146205,
40.0619457972351));
#171451=CARTESIAN_POINT('Ctrl Pts',(-25.7984833547786,57.3581584863396,
40.0619760547305));
#171452=CARTESIAN_POINT('Ctrl Pts',(-25.7984656922961,57.3581871588521,
40.0620063077269));
#171453=CARTESIAN_POINT('Ctrl Pts',(-25.7965719149858,57.3612614352675,
40.06525004417));
#171454=CARTESIAN_POINT('Ctrl Pts',(-25.7945784837693,57.3643429325989,
40.0684393223557));
#171455=CARTESIAN_POINT('Ctrl Pts',(-25.7924880141961,57.3674274658678,
40.0715697951759));
#171456=CARTESIAN_POINT('Ctrl Pts',(-25.7808550263345,57.3845921921739,
40.0889901646399));
#171457=CARTESIAN_POINT('Ctrl Pts',(-25.7662212180103,57.4018536888691,
40.1045963098205));
#171458=CARTESIAN_POINT('Ctrl Pts',(-25.7490920431318,57.4184830023364,
40.1176634650677));
#171459=CARTESIAN_POINT('Ctrl Pts',(-25.7414042322328,57.4259464685117,
40.1235281853033));
#171460=CARTESIAN_POINT('Ctrl Pts',(-25.7332138190191,57.4332829501997,
40.1288820140907));
#171461=CARTESIAN_POINT('Ctrl Pts',(-25.7245659119506,57.4404287135114,
40.1336621774101));
#171462=CARTESIAN_POINT('Ctrl Pts',(-25.7208076485109,57.4435341655925,
40.1357395717319));
#171463=CARTESIAN_POINT('Ctrl Pts',(-25.716963033262,57.4466034003414,40.1377083672884));
#171464=CARTESIAN_POINT('Ctrl Pts',(-25.7130358078099,57.4496310617744,
40.1395632548792));
#171465=CARTESIAN_POINT('Ctrl Pts',(-25.6992905187276,57.46022787679,40.146055361447));
#171466=CARTESIAN_POINT('Ctrl Pts',(-25.6845332533377,57.4703154157424,
40.1511520974629));
#171467=CARTESIAN_POINT('Ctrl Pts',(-25.6689244402251,57.4796640570499,
40.1546258197408));
#171468=CARTESIAN_POINT('Ctrl Pts',(-25.6611200336689,57.4843383777037,
40.1563626808798));
#171469=CARTESIAN_POINT('Ctrl Pts',(-25.6531027404315,57.4888279745008,
40.1576937882008));
#171470=CARTESIAN_POINT('Ctrl Pts',(-25.6448926173138,57.4931041519766,
40.1585906813668));
#171471=CARTESIAN_POINT('Ctrl Pts',(-25.6407875557549,57.4952422407145,
40.1590391279498));
#171472=CARTESIAN_POINT('Ctrl Pts',(-25.636634286776,57.4973269747347,40.1593790209175));
#171473=CARTESIAN_POINT('Ctrl Pts',(-25.6324353177602,57.4993547677438,
40.1596068022931));
#171474=CARTESIAN_POINT('Ctrl Pts',(-25.6282363487445,57.5013825607529,
40.1598345836687));
#171475=CARTESIAN_POINT('Ctrl Pts',(-25.6239916789975,57.5033534111924,
40.1599502506865));
#171476=CARTESIAN_POINT('Ctrl Pts',(-25.6197038181293,57.5052637377734,
40.1599502534424));
#171477=CARTESIAN_POINT('',(-25.5918112338789,57.5176823163891,40.1599502534424));
#171478=CARTESIAN_POINT('Origin',(2.35274110347535E-17,-1.41976521077031E-16,
40.1599502534424));
#171479=CARTESIAN_POINT('',(-25.2380597013425,57.4675553545143,39.8576902534424));
#171480=CARTESIAN_POINT('Ctrl Pts',(-25.5918112338789,57.5176823163891,
40.1599502534424));
#171481=CARTESIAN_POINT('Ctrl Pts',(-25.5883196330409,57.5192358568903,
40.1599502447858));
#171482=CARTESIAN_POINT('Ctrl Pts',(-25.5848181941914,57.5207415321517,
40.1598744685927));
#171483=CARTESIAN_POINT('Ctrl Pts',(-25.5813091362503,57.5221995827245,
40.1597246934279));
#171484=CARTESIAN_POINT('Ctrl Pts',(-25.5610311102455,57.5306253163333,
40.1588591777435));
#171485=CARTESIAN_POINT('Ctrl Pts',(-25.5404968219571,57.5374634601474,
40.1555254706023));
#171486=CARTESIAN_POINT('Ctrl Pts',(-25.5201405094577,57.5427567781065,
40.1500631826386));
#171487=CARTESIAN_POINT('Ctrl Pts',(-25.5119303403506,57.5448916950067,
40.1478601162485));
#171488=CARTESIAN_POINT('Ctrl Pts',(-25.5037488853983,57.546775718186,40.1453112228309));
#171489=CARTESIAN_POINT('Ctrl Pts',(-25.4956235123961,57.548413124991,40.1424401896328));
#171490=CARTESIAN_POINT('Ctrl Pts',(-25.4926257430706,57.5490172286908,
40.1413809526906));
#171491=CARTESIAN_POINT('Ctrl Pts',(-25.4896356883473,57.5495876573341,
40.1402777640512));
#171492=CARTESIAN_POINT('Ctrl Pts',(-25.4866547635669,57.55012457403,40.1391317641987));
#171493=CARTESIAN_POINT('Ctrl Pts',(-25.4810655296036,57.5511312928347,
40.1369830144753));
#171494=CARTESIAN_POINT('Ctrl Pts',(-25.4755083930932,57.5520201961936,
40.134683756585));
#171495=CARTESIAN_POINT('Ctrl Pts',(-25.4699926837172,57.5527923593832,
40.1322415082996));
#171496=CARTESIAN_POINT('Ctrl Pts',(-25.4506877009012,57.5554949305467,
40.1236936393009));
#171497=CARTESIAN_POINT('Ctrl Pts',(-25.4318901986623,57.5567674305413,
40.113394140767));
#171498=CARTESIAN_POINT('Ctrl Pts',(-25.4140001974202,57.5566559849707,
40.101665321223));
#171499=CARTESIAN_POINT('Ctrl Pts',(-25.4050551967992,57.5566002621853,
40.095800911451));
#171500=CARTESIAN_POINT('Ctrl Pts',(-25.3963370718384,57.5561985539315,
40.0895791707949));
#171501=CARTESIAN_POINT('Ctrl Pts',(-25.3878958286608,57.5554566340483,
40.0830403822907));
#171502=CARTESIAN_POINT('Ctrl Pts',(-25.383675207072,57.5550856741067,40.0797709880385));
#171503=CARTESIAN_POINT('Ctrl Pts',(-25.3795238059759,57.5546296613654,
40.0764223317514));
#171504=CARTESIAN_POINT('Ctrl Pts',(-25.3754478763491,57.5540893180427,
40.0729994484778));
#171505=CARTESIAN_POINT('Ctrl Pts',(-25.3713719467224,57.55354897472,40.0695765652042));
#171506=CARTESIAN_POINT('Ctrl Pts',(-25.3673715770251,57.5529242061382,
40.0660793733488));
#171507=CARTESIAN_POINT('Ctrl Pts',(-25.3634528381782,57.5522159293601,
40.0625130768817));
#171508=CARTESIAN_POINT('Ctrl Pts',(-25.363419419543,57.5522098892426,40.0624826638418));
#171509=CARTESIAN_POINT('Ctrl Pts',(-25.3633860069328,57.5522038431596,
40.0624522459912));
#171510=CARTESIAN_POINT('Ctrl Pts',(-25.3633526003507,57.5521977911121,
40.0624218233329));
#171511=CARTESIAN_POINT('Ctrl Pts',(-25.346291371152,57.5491069220866,40.0468845275908));
#171512=CARTESIAN_POINT('Ctrl Pts',(-25.3307446654471,57.5445791409896,
40.0302263329257));
#171513=CARTESIAN_POINT('Ctrl Pts',(-25.3167379215577,57.5388132486365,
40.0127515884774));
#171514=CARTESIAN_POINT('Ctrl Pts',(-25.3022574788908,57.5328523576327,
39.9946858597756));
#171515=CARTESIAN_POINT('Ctrl Pts',(-25.2894223267617,57.5255675223694,
39.9757460620541));
#171516=CARTESIAN_POINT('Ctrl Pts',(-25.2783002469356,57.5171444507329,
39.9562444559191));
#171517=CARTESIAN_POINT('Ctrl Pts',(-25.267389732471,57.5088816036429,39.9371138113683));
#171518=CARTESIAN_POINT('Ctrl Pts',(-25.2581274647609,57.4995225236683,
39.9174410654434));
#171519=CARTESIAN_POINT('Ctrl Pts',(-25.2506209171167,57.4892225138723,
39.8975196504236));
#171520=CARTESIAN_POINT('Ctrl Pts',(-25.2456480924691,57.482399118483,39.8843224113835));
#171521=CARTESIAN_POINT('Ctrl Pts',(-25.2414466709171,57.4751623993628,
39.8710160447162));
#171522=CARTESIAN_POINT('Ctrl Pts',(-25.2380597013425,57.4675553545143,
39.8576902534424));
#171523=CARTESIAN_POINT('',(-25.0931373005741,57.1420619865023,39.2875012672119));
#171524=CARTESIAN_POINT('',(-25.2380597013425,57.4675553545143,39.8576902534424));
#171525=CARTESIAN_POINT('',(-19.5876674457073,59.2554138597573,39.2875012672119));
#171526=CARTESIAN_POINT('Origin',(5.53234440788222E-15,0.,39.2875012672119));
#171527=CARTESIAN_POINT('',(-19.697766688184,59.5942745858238,39.8576902534424));
#171528=CARTESIAN_POINT('',(-19.5876674457073,59.2554138597573,39.2875012672119));
#171529=CARTESIAN_POINT('',(-19.4684195516691,59.8682321556243,40.1599502534424));
#171530=CARTESIAN_POINT('Ctrl Pts',(-19.697766688184,59.5942745858238,39.8576902534424));
#171531=CARTESIAN_POINT('Ctrl Pts',(-19.7015693056583,59.6059782661673,
39.8773836120336));
#171532=CARTESIAN_POINT('Ctrl Pts',(-19.7035046472587,59.6182462127092,
39.8969946442077));
#171533=CARTESIAN_POINT('Ctrl Pts',(-19.7035948839462,59.630890804279,39.9162525288159));
#171534=CARTESIAN_POINT('Ctrl Pts',(-19.7036869338405,59.6437894749834,
39.9358973793953));
#171535=CARTESIAN_POINT('Ctrl Pts',(-19.7018593121361,59.657080948502,39.9551762199603));
#171536=CARTESIAN_POINT('Ctrl Pts',(-19.6980881582825,59.6705908046714,
39.9738152034081));
#171537=CARTESIAN_POINT('Ctrl Pts',(-19.6944635103376,59.6835758151756,
39.9917300792457));
#171538=CARTESIAN_POINT('Ctrl Pts',(-19.6890433025229,59.696763446391,40.0090551157911));
#171539=CARTESIAN_POINT('Ctrl Pts',(-19.6817621015947,59.7100083536123,
40.0255394551304));
#171540=CARTESIAN_POINT('Ctrl Pts',(-19.6761689357012,59.7201826317381,
40.0382021526002));
#171541=CARTESIAN_POINT('Ctrl Pts',(-19.6694767982745,59.7303909886912,
40.0503687782053));
#171542=CARTESIAN_POINT('Ctrl Pts',(-19.6616375006935,59.7405669736109,
40.0619155352442));
#171543=CARTESIAN_POINT('Ctrl Pts',(-19.6616169552927,59.7405936430526,
40.0619457972351));
#171544=CARTESIAN_POINT('Ctrl Pts',(-19.6615964011817,59.7406203123794,
40.0619760547305));
#171545=CARTESIAN_POINT('Ctrl Pts',(-19.6615758383624,59.7406469815887,
40.0620063077269));
#171546=CARTESIAN_POINT('Ctrl Pts',(-19.659371085973,59.7435064631643,40.06525004417));
#171547=CARTESIAN_POINT('Ctrl Pts',(-19.6570664708007,59.7463627094292,
40.0684393223557));
#171548=CARTESIAN_POINT('Ctrl Pts',(-19.654665031516,59.7492118317301,40.0715697951759));
#171549=CARTESIAN_POINT('Ctrl Pts',(-19.6413015679145,59.7650665495268,
40.0889901646418));
#171550=CARTESIAN_POINT('Ctrl Pts',(-19.6249436073982,59.7807038364427,
40.1045963098238));
#171551=CARTESIAN_POINT('Ctrl Pts',(-19.6061700313475,59.7954515664652,
40.1176634650719));
#171552=CARTESIAN_POINT('Ctrl Pts',(-19.5977441904328,59.8020705519311,
40.1235281853059));
#171553=CARTESIAN_POINT('Ctrl Pts',(-19.588831774005,59.8085107122964,40.1288820140919));
#171554=CARTESIAN_POINT('Ctrl Pts',(-19.5794843054207,59.8147133779312,
40.1336621774101));
#171555=CARTESIAN_POINT('Ctrl Pts',(-19.5754220220075,59.817408972519,40.1357395717319));
#171556=CARTESIAN_POINT('Ctrl Pts',(-19.5712776455715,59.820059521955,40.1377083672884));
#171557=CARTESIAN_POINT('Ctrl Pts',(-19.5670554570745,59.8226600907005,
40.1395632548792));
#171558=CARTESIAN_POINT('Ctrl Pts',(-19.5522777973348,59.8317620813097,
40.146055361447));
#171559=CARTESIAN_POINT('Ctrl Pts',(-19.5365469388439,59.840251805395,40.151152097463));
#171560=CARTESIAN_POINT('Ctrl Pts',(-19.5200464333333,59.8479176686192,
40.1546258197409));
#171561=CARTESIAN_POINT('Ctrl Pts',(-19.5117961805779,59.8517506002313,
40.1563626808798));
#171562=CARTESIAN_POINT('Ctrl Pts',(-19.5033535162579,59.8553775672056,
40.1576937882008));
#171563=CARTESIAN_POINT('Ctrl Pts',(-19.4947413867934,59.8587721277811,
40.1585906813668));
#171564=CARTESIAN_POINT('Ctrl Pts',(-19.4904353220612,59.8604694080688,
40.1590391279498));
#171565=CARTESIAN_POINT('Ctrl Pts',(-19.4860868910809,59.862108586874,40.1593790209175));
#171566=CARTESIAN_POINT('Ctrl Pts',(-19.4816989623697,59.8636863596423,
40.1596068022931));
#171567=CARTESIAN_POINT('Ctrl Pts',(-19.4773110336584,59.8652641324106,
40.1598345836687));
#171568=CARTESIAN_POINT('Ctrl Pts',(-19.4728836066887,59.8667804975194,
40.1599502506865));
#171569=CARTESIAN_POINT('Ctrl Pts',(-19.4684195516691,59.8682321556243,
40.1599502534424));
#171570=CARTESIAN_POINT('',(-19.4393816709751,59.8776671349987,40.1599502534424));
#171571=CARTESIAN_POINT('Origin',(8.34054140790793E-18,-1.47806214131551E-16,
40.1599502534424));
#171572=CARTESIAN_POINT('',(-19.0928077206406,59.7908376697913,39.8576902534424));
#171573=CARTESIAN_POINT('Ctrl Pts',(-19.4393816709751,59.8776671349987,
40.1599502534424));
#171574=CARTESIAN_POINT('Ctrl Pts',(-19.4357468082906,59.8788471933726,
40.1599502447858));
#171575=CARTESIAN_POINT('Ctrl Pts',(-19.4321071647682,59.8799786203652,
40.1598744685927));
#171576=CARTESIAN_POINT('Ctrl Pts',(-19.4284649220279,59.8810618871503,
40.1597246934279));
#171577=CARTESIAN_POINT('Ctrl Pts',(-19.4074172521851,59.8873218328125,
40.1588591777435));
#171578=CARTESIAN_POINT('Ctrl Pts',(-19.3862806722119,59.8919760989602,
40.1555254706022));
#171579=CARTESIAN_POINT('Ctrl Pts',(-19.3654825713304,59.8951126055063,
40.1500631826385));
#171580=CARTESIAN_POINT('Ctrl Pts',(-19.3570942188061,59.8963776307484,
40.1478601162485));
#171581=CARTESIAN_POINT('Ctrl Pts',(-19.3487606486724,59.8973961381381,
40.1453112228309));
#171582=CARTESIAN_POINT('Ctrl Pts',(-19.3405086316967,59.8981752423038,
40.1424401896328));
#171583=CARTESIAN_POINT('Ctrl Pts',(-19.3374641384338,59.8984626844396,
40.1413809526906));
#171584=CARTESIAN_POINT('Ctrl Pts',(-19.3344308375137,59.8987174423898,
40.1402777640512));
#171585=CARTESIAN_POINT('Ctrl Pts',(-19.331410119474,59.8989398263134,40.1391317641987));
#171586=CARTESIAN_POINT('Ctrl Pts',(-19.3257462731495,59.8993567961702,
40.1369830144753));
#171587=CARTESIAN_POINT('Ctrl Pts',(-19.3201266635123,59.8996599510838,
40.134683756585));
#171588=CARTESIAN_POINT('Ctrl Pts',(-19.3145604567378,59.8998513356578,
40.1322415082996));
#171589=CARTESIAN_POINT('Ctrl Pts',(-19.295078733027,59.9005211816666,40.1236936393009));
#171590=CARTESIAN_POINT('Ctrl Pts',(-19.2762511930033,59.8998218367507,
40.113394140767));
#171591=CARTESIAN_POINT('Ctrl Pts',(-19.258470844294,59.8978409873529,40.101665321223));
#171592=CARTESIAN_POINT('Ctrl Pts',(-19.2495806699394,59.896850562654,40.095800911451));
#171593=CARTESIAN_POINT('Ctrl Pts',(-19.2409522937258,59.8955397627953,
40.0895791707949));
#171594=CARTESIAN_POINT('Ctrl Pts',(-19.2326348443069,59.8939195570494,
40.0830403822906));
#171595=CARTESIAN_POINT('Ctrl Pts',(-19.2284761195974,59.8931094541764,
40.0797709880385));
#171596=CARTESIAN_POINT('Ctrl Pts',(-19.2243951266219,59.8922219999437,
40.0764223317514));
#171597=CARTESIAN_POINT('Ctrl Pts',(-19.2203980066213,59.891258566018,40.0729994484778));
#171598=CARTESIAN_POINT('Ctrl Pts',(-19.2164008866207,59.8902951320922,
40.0695765652043));
#171599=CARTESIAN_POINT('Ctrl Pts',(-19.2124877374669,59.8892556335611,
40.0660793733488));
#171600=CARTESIAN_POINT('Ctrl Pts',(-19.2086645009646,59.8881416170477,
40.0625130768816));
#171601=CARTESIAN_POINT('Ctrl Pts',(-19.2086318967643,59.88813211682,40.0624826638418));
#171602=CARTESIAN_POINT('Ctrl Pts',(-19.2085992991797,59.8881226112893,
40.0624522459912));
#171603=CARTESIAN_POINT('Ctrl Pts',(-19.2085667082136,59.8881131004569,
40.0624218233329));
#171604=CARTESIAN_POINT('Ctrl Pts',(-19.1919220260049,59.8832557794662,
40.0468845275925));
#171605=CARTESIAN_POINT('Ctrl Pts',(-19.1769337687821,59.8771277287725,
40.0302263329295));
#171606=CARTESIAN_POINT('Ctrl Pts',(-19.1636064551696,59.8699293191679,
40.0127515884834));
#171607=CARTESIAN_POINT('Ctrl Pts',(-19.1498284206602,59.8624874641303,
39.9946858597837));
#171608=CARTESIAN_POINT('Ctrl Pts',(-19.1378250534734,59.8539008972302,
39.9757460620646));
#171609=CARTESIAN_POINT('Ctrl Pts',(-19.1276443522988,59.8443613941504,
39.956244455932));
#171610=CARTESIAN_POINT('Ctrl Pts',(-19.1176573094827,59.8350033524921,
39.9371138113831));
#171611=CARTESIAN_POINT('Ctrl Pts',(-19.1094240716913,59.8247273719282,
39.9174410654602));
#171612=CARTESIAN_POINT('Ctrl Pts',(-19.1030352898955,59.8136991387752,
39.8975196504422));
#171613=CARTESIAN_POINT('Ctrl Pts',(-19.0988029459332,59.8063933209382,
39.8843224113961));
#171614=CARTESIAN_POINT('Ctrl Pts',(-19.0953809833347,59.7987570771807,
39.8710160447225));
#171615=CARTESIAN_POINT('Ctrl Pts',(-19.0928077206406,59.7908376697913,
39.8576902534424));
#171616=CARTESIAN_POINT('',(-18.9827025415091,59.4519788726609,39.2875012672119));
#171617=CARTESIAN_POINT('',(-19.0928077206406,59.7908376697913,39.8576902534424));
#171618=CARTESIAN_POINT('',(-13.2864868028989,60.9782752797349,39.2875012672119));
#171619=CARTESIAN_POINT('Origin',(5.53234440788222E-15,0.,39.2875012672119));
#171620=CARTESIAN_POINT('',(-13.360562319248,61.3267881959114,39.8576902534424));
#171621=CARTESIAN_POINT('',(-13.2864868028989,60.9782752797349,39.2875012672119));
#171622=CARTESIAN_POINT('',(-13.1038352065721,61.5752716937453,40.1599502534424));
#171623=CARTESIAN_POINT('Ctrl Pts',(-13.360562319248,61.3267881959114,39.8576902534424));
#171624=CARTESIAN_POINT('Ctrl Pts',(-13.3631207378653,61.338825244031,39.8773836120346));
#171625=CARTESIAN_POINT('Ctrl Pts',(-13.3637631278625,61.3512282837622,
39.8969946442097));
#171626=CARTESIAN_POINT('Ctrl Pts',(-13.3625311504983,61.3638130392393,
39.9162525288189));
#171627=CARTESIAN_POINT('Ctrl Pts',(-13.3612744179065,61.3766506715107,
39.9358973793994));
#171628=CARTESIAN_POINT('Ctrl Pts',(-13.3580674708029,61.3896782944593,
39.9551762199655));
#171629=CARTESIAN_POINT('Ctrl Pts',(-13.3529048112197,61.4027199493068,
39.9738152034143));
#171630=CARTESIAN_POINT('Ctrl Pts',(-13.3479427162811,61.415254947686,39.991730079253));
#171631=CARTESIAN_POINT('Ctrl Pts',(-13.3411737181058,61.4278037696853,
40.0090551157994));
#171632=CARTESIAN_POINT('Ctrl Pts',(-13.3325479345589,61.440215027176,40.0255394551395));
#171633=CARTESIAN_POINT('Ctrl Pts',(-13.325921906957,61.4497489245037,40.038202152606));
#171634=CARTESIAN_POINT('Ctrl Pts',(-13.3181993658961,61.4592018401658,
40.0503687782081));
#171635=CARTESIAN_POINT('Ctrl Pts',(-13.3093393327438,61.468502650244,40.0619155352442));
#171636=CARTESIAN_POINT('Ctrl Pts',(-13.309316112177,61.4685270260085,40.0619457972351));
#171637=CARTESIAN_POINT('Ctrl Pts',(-13.3092928829598,61.4685514007483,
40.0619760547305));
#171638=CARTESIAN_POINT('Ctrl Pts',(-13.3092696450943,61.468575774461,40.0620063077269));
#171639=CARTESIAN_POINT('Ctrl Pts',(-13.3067780733544,61.4711891321182,
40.06525004417));
#171640=CARTESIAN_POINT('Ctrl Pts',(-13.3041875240723,61.4737888336848,
40.0684393223556));
#171641=CARTESIAN_POINT('Ctrl Pts',(-13.3015014257475,61.4763713294375,
40.0715697951759));
#171642=CARTESIAN_POINT('Ctrl Pts',(-13.2865538993096,61.4907423311184,
40.0889901646434));
#171643=CARTESIAN_POINT('Ctrl Pts',(-13.2686510078396,61.5045840828668,
40.1045963098267));
#171644=CARTESIAN_POINT('Ctrl Pts',(-13.2484387178445,61.5172886502275,
40.1176634650756));
#171645=CARTESIAN_POINT('Ctrl Pts',(-13.2393671621905,61.5229906359946,
40.1235281853082));
#171646=CARTESIAN_POINT('Ctrl Pts',(-13.2298303888482,61.5284639152932,
40.1288820140929));
#171647=CARTESIAN_POINT('Ctrl Pts',(-13.2198857715699,61.5336555255489,
40.1336621774101));
#171648=CARTESIAN_POINT('Ctrl Pts',(-13.2155639754105,61.535911729145,40.1357395717319));
#171649=CARTESIAN_POINT('Ctrl Pts',(-13.2111652444429,61.5381145532938,
40.1377083672884));
#171650=CARTESIAN_POINT('Ctrl Pts',(-13.2066943520817,61.5402595369764,
40.1395632548792));
#171651=CARTESIAN_POINT('Ctrl Pts',(-13.1910462288172,61.5477669798654,
40.146055361447));
#171652=CARTESIAN_POINT('Ctrl Pts',(-13.1745141278029,61.5545658738899,
40.1511520974629));
#171653=CARTESIAN_POINT('Ctrl Pts',(-13.1573027128854,61.5604649702291,
40.1546258197408));
#171654=CARTESIAN_POINT('Ctrl Pts',(-13.1486970054267,61.5634145183987,
40.1563626808798));
#171655=CARTESIAN_POINT('Ctrl Pts',(-13.1399214696211,61.5661391177412,
40.1576937882008));
#171656=CARTESIAN_POINT('Ctrl Pts',(-13.1310016901025,61.5686148699003,
40.1585906813668));
#171657=CARTESIAN_POINT('Ctrl Pts',(-13.1265418003432,61.5698527459798,
40.1590391279498));
#171658=CARTESIAN_POINT('Ctrl Pts',(-13.1220458496812,61.571028410384,40.1593790209175));
#171659=CARTESIAN_POINT('Ctrl Pts',(-13.1175170363398,61.5721388765029,
40.1596068022931));
#171660=CARTESIAN_POINT('Ctrl Pts',(-13.1129882229983,61.5732493426218,
40.1598345836687));
#171661=CARTESIAN_POINT('Ctrl Pts',(-13.1084265466222,61.5742946087865,
40.1599502506865));
#171662=CARTESIAN_POINT('Ctrl Pts',(-13.1038352065721,61.5752716937453,
40.1599502534424));
#171663=CARTESIAN_POINT('',(-13.0739701745318,61.5816197022699,40.1599502534424));
#171664=CARTESIAN_POINT('Origin',(-7.37250181440935E-18,-1.52016511373604E-16,
40.1599502534424));
#171665=CARTESIAN_POINT('',(-12.7383709431244,61.459039055521,39.8576902534424));
#171666=CARTESIAN_POINT('Ctrl Pts',(-13.0739701745318,61.5816197022699,
40.1599502534424));
#171667=CARTESIAN_POINT('Ctrl Pts',(-13.0702318743171,61.5824133495499,
40.1599502447858));
#171668=CARTESIAN_POINT('Ctrl Pts',(-13.0664939028179,61.5831581321229,
40.1598744685927));
#171669=CARTESIAN_POINT('Ctrl Pts',(-13.0627583804521,61.5838547466227,
40.1597246934279));
#171670=CARTESIAN_POINT('Ctrl Pts',(-13.0411716694483,61.5878803190632,
40.1588591777436));
#171671=CARTESIAN_POINT('Ctrl Pts',(-13.0196643745853,61.5902997144306,
40.1555254706027));
#171672=CARTESIAN_POINT('Ctrl Pts',(-12.9986523536687,61.5912450453417,
40.1500631826397));
#171673=CARTESIAN_POINT('Ctrl Pts',(-12.9901777222711,61.5916263190447,
40.1478601162494));
#171674=CARTESIAN_POINT('Ctrl Pts',(-12.9817833412928,61.5917681516648,
40.1453112228314));
#171675=CARTESIAN_POINT('Ctrl Pts',(-12.9734950911668,61.591680417163,40.1424401896328));
#171676=CARTESIAN_POINT('Ctrl Pts',(-12.9704372300719,61.5916480484585,
40.1413809526906));
#171677=CARTESIAN_POINT('Ctrl Pts',(-12.9673939164345,61.5915843445342,
40.1402777640511));
#171678=CARTESIAN_POINT('Ctrl Pts',(-12.9643665007545,61.5914897592007,
40.1391317641987));
#171679=CARTESIAN_POINT('Ctrl Pts',(-12.9586900963545,61.5913124117005,
40.1369830144753));
#171680=CARTESIAN_POINT('Ctrl Pts',(-12.9530695832096,61.5910264967403,
40.134683756585));
#171681=CARTESIAN_POINT('Ctrl Pts',(-12.9475138635627,61.5906350058492,
40.1322415082996));
#171682=CARTESIAN_POINT('Ctrl Pts',(-12.9280688447989,61.5892647877302,
40.1236936393009));
#171683=CARTESIAN_POINT('Ctrl Pts',(-12.9094175454587,61.5866012600731,
40.113394140767));
#171684=CARTESIAN_POINT('Ctrl Pts',(-12.8919416545036,61.5827727094486,
40.101665321223));
#171685=CARTESIAN_POINT('Ctrl Pts',(-12.8832037090261,61.5808584341363,
40.095800911451));
#171686=CARTESIAN_POINT('Ctrl Pts',(-12.8747596158551,61.5786529040703,
40.0895791707949));
#171687=CARTESIAN_POINT('Ctrl Pts',(-12.8666570879111,61.5761721637749,
40.0830403822906));
#171688=CARTESIAN_POINT('Ctrl Pts',(-12.8626058239391,61.5749317936273,
40.0797709880385));
#171689=CARTESIAN_POINT('Ctrl Pts',(-12.8586399512973,61.5736226210373,
40.0764223317514));
#171690=CARTESIAN_POINT('Ctrl Pts',(-12.854765434206,61.5722466520923,40.0729994484778));
#171691=CARTESIAN_POINT('Ctrl Pts',(-12.8508909171147,61.5708706831473,
40.0695765652042));
#171692=CARTESIAN_POINT('Ctrl Pts',(-12.8471078617854,61.5694278436303,
40.0660793733488));
#171693=CARTESIAN_POINT('Ctrl Pts',(-12.8434220158069,61.5679202927797,
40.0625130768816));
#171694=CARTESIAN_POINT('Ctrl Pts',(-12.8433905832601,61.5679074365282,
40.0624826638418));
#171695=CARTESIAN_POINT('Ctrl Pts',(-12.8433591578469,61.5678945756944,
40.0624522459912));
#171696=CARTESIAN_POINT('Ctrl Pts',(-12.8433277395702,61.5678817102797,
40.0624218233329));
#171697=CARTESIAN_POINT('Ctrl Pts',(-12.827281966969,61.561311155148,40.0468845275905));
#171698=CARTESIAN_POINT('Ctrl Pts',(-12.8130163727078,61.5536499750614,
40.0302263329252));
#171699=CARTESIAN_POINT('Ctrl Pts',(-12.8005145062063,61.5450979154851,
40.0127515884767));
#171700=CARTESIAN_POINT('Ctrl Pts',(-12.7875898348814,61.5362566309327,
39.9946858597746));
#171701=CARTESIAN_POINT('Ctrl Pts',(-12.7765497640382,61.5264624086169,
39.9757460620528));
#171702=CARTESIAN_POINT('Ctrl Pts',(-12.7674219834069,61.5159109908826,
39.9562444559174));
#171703=CARTESIAN_POINT('Ctrl Pts',(-12.75846783237,61.505560283316,39.9371138113663));
#171704=CARTESIAN_POINT('Ctrl Pts',(-12.751353829574,61.4944799879532,39.917441065441));
#171705=CARTESIAN_POINT('Ctrl Pts',(-12.7461528104583,61.4828443590704,
39.8975196504208));
#171706=CARTESIAN_POINT('Ctrl Pts',(-12.7427073176332,61.4751361628615,
39.8843224113816));
#171707=CARTESIAN_POINT('Ctrl Pts',(-12.7401023057309,61.4671840587587,
39.8710160447152));
#171708=CARTESIAN_POINT('Ctrl Pts',(-12.7383709431244,61.459039055521,39.8576902534424));
#171709=CARTESIAN_POINT('',(-12.6642893210135,61.1105274371642,39.2875012672119));
#171710=CARTESIAN_POINT('',(-12.7383709431244,61.459039055521,39.8576902534424));
#171711=CARTESIAN_POINT('',(-6.83973663030197,62.0330459552233,39.2875012672119));
#171712=CARTESIAN_POINT('Origin',(5.53234440788222E-15,0.,39.2875012672119));
#171713=CARTESIAN_POINT('',(-6.87697683366501,62.3873926810692,39.8576902534424));
#171714=CARTESIAN_POINT('',(-6.83973663030197,62.0330459552233,39.2875012672119));
#171715=CARTESIAN_POINT('',(-6.59568250079822,62.6076796697355,40.1599502534424));
#171716=CARTESIAN_POINT('Ctrl Pts',(-6.87697683366501,62.3873926810692,
39.8576902534424));
#171717=CARTESIAN_POINT('Ctrl Pts',(-6.87826302285531,62.3996312165479,
39.8773836120375));
#171718=CARTESIAN_POINT('Ctrl Pts',(-6.87760542308951,62.4120334591708,
39.8969946442153));
#171719=CARTESIAN_POINT('Ctrl Pts',(-6.87506472947472,62.4244204973417,
39.9162525288272));
#171720=CARTESIAN_POINT('Ctrl Pts',(-6.87247298342128,62.4370564393956,
39.9358973794105));
#171721=CARTESIAN_POINT('Ctrl Pts',(-6.86792184690122,62.4496774784119,
39.9551762199791));
#171722=CARTESIAN_POINT('Ctrl Pts',(-6.86142424476564,62.4621080448385,
39.9738152034302));
#171723=CARTESIAN_POINT('Ctrl Pts',(-6.85517906858276,62.4740556950282,
39.9917300792711));
#171724=CARTESIAN_POINT('Ctrl Pts',(-6.84713544260583,62.4858282202919,
40.0090551158194));
#171725=CARTESIAN_POINT('Ctrl Pts',(-6.83725958232801,62.4972698477182,
40.0255394551612));
#171726=CARTESIAN_POINT('Ctrl Pts',(-6.82967328916514,62.5060589088707,
40.0382021526199));
#171727=CARTESIAN_POINT('Ctrl Pts',(-6.82100495424893,62.5146528151171,
40.0503687782147));
#171728=CARTESIAN_POINT('Ctrl Pts',(-6.81122125790617,62.5229765487298,
40.0619155352442));
#171729=CARTESIAN_POINT('Ctrl Pts',(-6.81119561658286,62.5229983637512,
40.0619457972351));
#171730=CARTESIAN_POINT('Ctrl Pts',(-6.81116996676367,62.5230201768493,
40.0619760547305));
#171731=CARTESIAN_POINT('Ctrl Pts',(-6.81114430845093,62.5230419880218,
40.0620063077269));
#171732=CARTESIAN_POINT('Ctrl Pts',(-6.80839321554184,62.5253805892672,
40.06525004417));
#171733=CARTESIAN_POINT('Ctrl Pts',(-6.80554511475005,62.5276952632612,
40.0684393223556));
#171734=CARTESIAN_POINT('Ctrl Pts',(-6.80260378684053,62.5299828381019,
40.0715697951759));
#171735=CARTESIAN_POINT('Ctrl Pts',(-6.78623596579978,62.5427126719601,
40.0889901646384));
#171736=CARTESIAN_POINT('Ctrl Pts',(-6.76698429120954,62.5546072354075,
40.1045963098178));
#171737=CARTESIAN_POINT('Ctrl Pts',(-6.74555473735862,62.5651294462044,
40.1176634650644));
#171738=CARTESIAN_POINT('Ctrl Pts',(-6.73593685682031,62.5698519601282,
40.1235281853013));
#171739=CARTESIAN_POINT('Ctrl Pts',(-6.72588021343989,62.5742983919711,
40.1288820140898));
#171740=CARTESIAN_POINT('Ctrl Pts',(-6.71544740276709,62.5784220664834,
40.1336621774101));
#171741=CARTESIAN_POINT('Ctrl Pts',(-6.71091344436445,62.580214159649,40.1357395717319));
#171742=CARTESIAN_POINT('Ctrl Pts',(-6.70630855228228,62.5819451239083,
40.1377083672884));
#171743=CARTESIAN_POINT('Ctrl Pts',(-6.70163794008908,62.5836110216379,
40.1395632548792));
#171744=CARTESIAN_POINT('Ctrl Pts',(-6.6852907974129,62.5894416636914,40.146055361447));
#171745=CARTESIAN_POINT('Ctrl Pts',(-6.66813858303337,62.5944752375495,
40.151152097463));
#171746=CARTESIAN_POINT('Ctrl Pts',(-6.65040483057272,62.5985429352697,
40.1546258197409));
#171747=CARTESIAN_POINT('Ctrl Pts',(-6.6415379543424,62.6005767841298,40.1563626808798));
#171748=CARTESIAN_POINT('Ctrl Pts',(-6.63252569365777,62.6023691645599,
40.1576937882008));
#171749=CARTESIAN_POINT('Ctrl Pts',(-6.62339599105606,62.6038989834438,
40.1585906813668));
#171750=CARTESIAN_POINT('Ctrl Pts',(-6.6188311397552,62.6046638928858,40.1590391279498));
#171751=CARTESIAN_POINT('Ctrl Pts',(-6.61423692798793,62.6053631620638,
40.1593790209175));
#171752=CARTESIAN_POINT('Ctrl Pts',(-6.60961684864287,62.6059941550341,
40.1596068022931));
#171753=CARTESIAN_POINT('Ctrl Pts',(-6.60499676929781,62.6066251480043,
40.1598345836687));
#171754=CARTESIAN_POINT('Ctrl Pts',(-6.60035082219627,62.6071878630701,
40.1599502506865));
#171755=CARTESIAN_POINT('Ctrl Pts',(-6.59568250079822,62.6076796697355,
40.1599502534424));
#171756=CARTESIAN_POINT('',(-6.56531752495238,62.6108711573006,40.1599502534424));
#171757=CARTESIAN_POINT('Origin',(-2.34395632424767E-17,-1.54561283905549E-16,
40.1599502534424));
#171758=CARTESIAN_POINT('',(-6.24436990787996,62.4538823482276,39.8576902534424));
#171759=CARTESIAN_POINT('Ctrl Pts',(-6.56531752495238,62.6108711573006,
40.1599502534424));
#171760=CARTESIAN_POINT('Ctrl Pts',(-6.5615167448068,62.6112696981211,40.1599502447858));
#171761=CARTESIAN_POINT('Ctrl Pts',(-6.55772139932878,62.6116196762807,
40.1598744685927));
#171762=CARTESIAN_POINT('Ctrl Pts',(-6.55393352450217,62.6119220062409,
40.1597246934279));
#171763=CARTESIAN_POINT('Ctrl Pts',(-6.5320442808587,62.6136691004462,40.1588591777436));
#171764=CARTESIAN_POINT('Ctrl Pts',(-6.51040190952723,62.6138271176316,
40.1555254706026));
#171765=CARTESIAN_POINT('Ctrl Pts',(-6.48940618067211,62.6125709156645,
40.1500631826395));
#171766=CARTESIAN_POINT('Ctrl Pts',(-6.48093812023799,62.6120642605134,
40.1478601162492));
#171767=CARTESIAN_POINT('Ctrl Pts',(-6.47257489901142,62.6113278644159,
40.1453112228313));
#171768=CARTESIAN_POINT('Ctrl Pts',(-6.46434122353972,62.6103742524841,
40.1424401896328));
#171769=CARTESIAN_POINT('Ctrl Pts',(-6.4613034971788,62.6100224275775,40.1413809526906));
#171770=CARTESIAN_POINT('Ctrl Pts',(-6.45828351400525,62.6096409597322,
40.1402777640512));
#171771=CARTESIAN_POINT('Ctrl Pts',(-6.45528256968465,62.6092304414384,
40.1391317641987));
#171772=CARTESIAN_POINT('Ctrl Pts',(-6.44965579908353,62.6084607196376,
40.1369830144753));
#171773=CARTESIAN_POINT('Ctrl Pts',(-6.44409596194913,62.6075888673476,
40.134683756585));
#171774=CARTESIAN_POINT('Ctrl Pts',(-6.43861159905708,62.6066187902475,
40.1322415082996));
#171775=CARTESIAN_POINT('Ctrl Pts',(-6.41941632893489,62.6032235203971,
40.1236936393009));
#171776=CARTESIAN_POINT('Ctrl Pts',(-6.4011456178169,62.5986249921653,40.113394140767));
#171777=CARTESIAN_POINT('Ctrl Pts',(-6.38416565413432,62.5929906867159,
40.101665321223));
#171778=CARTESIAN_POINT('Ctrl Pts',(-6.37567567229303,62.5901735339912,
40.095800911451));
#171779=CARTESIAN_POINT('Ctrl Pts',(-6.36750837741642,62.5870974379669,
40.0895791707949));
#171780=CARTESIAN_POINT('Ctrl Pts',(-6.35970954393914,62.5837833426318,
40.0830403822907));
#171781=CARTESIAN_POINT('Ctrl Pts',(-6.3558101272005,62.5821262949643,40.0797709880385));
#171782=CARTESIAN_POINT('Ctrl Pts',(-6.35200282582295,62.580409747586,40.0764223317514));
#171783=CARTESIAN_POINT('Ctrl Pts',(-6.348293361661,62.5786363190253,40.0729994484778));
#171784=CARTESIAN_POINT('Ctrl Pts',(-6.34458389749904,62.5768628904647,
40.0695765652042));
#171785=CARTESIAN_POINT('Ctrl Pts',(-6.34097238394016,62.5750325180135,
40.0660793733488));
#171786=CARTESIAN_POINT('Ctrl Pts',(-6.33746431138531,62.5731479498682,
40.0625130768817));
#171787=CARTESIAN_POINT('Ctrl Pts',(-6.33743439487346,62.5731318784489,
40.0624826638418));
#171788=CARTESIAN_POINT('Ctrl Pts',(-6.33740448593519,62.5731158032179,
40.0624522459912));
#171789=CARTESIAN_POINT('Ctrl Pts',(-6.33737458457314,62.5730997241771,
40.0624218233329));
#171790=CARTESIAN_POINT('Ctrl Pts',(-6.32210352242488,62.5648879232825,
40.0468845275916));
#171791=CARTESIAN_POINT('Ctrl Pts',(-6.30871688796368,62.555777551297,40.0302263329275));
#171792=CARTESIAN_POINT('Ctrl Pts',(-6.29717744164088,62.5459655399053,
40.0127515884803));
#171793=CARTESIAN_POINT('Ctrl Pts',(-6.28524773890592,62.5358216928037,
39.9946858597795));
#171794=CARTESIAN_POINT('Ctrl Pts',(-6.27529192173375,62.5249271226238,
39.9757460620592));
#171795=CARTESIAN_POINT('Ctrl Pts',(-6.26731706752089,62.5134793937784,
39.9562444559254));
#171796=CARTESIAN_POINT('Ctrl Pts',(-6.25949391181591,62.502249424824,39.9371138113756));
#171797=CARTESIAN_POINT('Ctrl Pts',(-6.25357708651812,62.4904862126995,
39.9174410654517));
#171798=CARTESIAN_POINT('Ctrl Pts',(-6.24962081353501,62.4783706704745,
39.8975196504329));
#171799=CARTESIAN_POINT('Ctrl Pts',(-6.24699992138311,62.4703445484983,
39.8843224113898));
#171800=CARTESIAN_POINT('Ctrl Pts',(-6.24524040122936,62.4621637089605,
39.8710160447193));
#171801=CARTESIAN_POINT('Ctrl Pts',(-6.24436990787996,62.4538823482276,
39.8576902534424));
#171802=CARTESIAN_POINT('',(-6.207123496544,62.0995362748659,39.2875012672119));
#171803=CARTESIAN_POINT('',(-6.24436990787996,62.4538823482276,39.8576902534424));
#171804=CARTESIAN_POINT('',(-0.318048871876471,62.4081695979768,39.2875012672119));
#171805=CARTESIAN_POINT('Origin',(5.53234440788222E-15,0.,39.2875012672119));
#171806=CARTESIAN_POINT('',(-0.318045750792381,62.7644678366119,39.8576902534424));
#171807=CARTESIAN_POINT('',(-0.31804887187647,62.4081695979768,39.2875012672119));
#171808=CARTESIAN_POINT('Ctrl Pts',(-0.318045750792382,62.7644678366119,
39.8576902534424));
#171809=CARTESIAN_POINT('Ctrl Pts',(-0.318045618797467,62.7767737714913,
39.8773836120359));
#171810=CARTESIAN_POINT('Ctrl Pts',(-0.316095234069849,62.7890393354375,
39.8969946442122));
#171811=CARTESIAN_POINT('Ctrl Pts',(-0.312273660576672,62.8010929413171,
39.9162525288225));
#171812=CARTESIAN_POINT('Ctrl Pts',(-0.308375296775076,62.8133887511252,
39.9358973794042));
#171813=CARTESIAN_POINT('Ctrl Pts',(-0.302529834044801,62.8254649274616,
39.9551762199713));
#171814=CARTESIAN_POINT('Ctrl Pts',(-0.294768478448722,62.8371482135778,
39.9738152034211));
#171815=CARTESIAN_POINT('Ctrl Pts',(-0.287308644481687,62.8483776146195,
39.9917300792606));
#171816=CARTESIAN_POINT('Ctrl Pts',(-0.278078518356449,62.8592448608948,
40.0090551158078));
#171817=CARTESIAN_POINT('Ctrl Pts',(-0.267060783344285,62.8695915013899,
40.0255394551485));
#171818=CARTESIAN_POINT('Ctrl Pts',(-0.258597341631192,62.8775394315825,
40.0382021526118));
#171819=CARTESIAN_POINT('Ctrl Pts',(-0.249078184944433,62.8851801717861,
40.0503687782108));
#171820=CARTESIAN_POINT('Ctrl Pts',(-0.238478017627214,62.8924356323738,
40.0619155352442));
#171821=CARTESIAN_POINT('Ctrl Pts',(-0.238450236479103,62.892454647642,
40.0619457972351));
#171822=CARTESIAN_POINT('Ctrl Pts',(-0.238422447082677,62.8924736601095,
40.0619760547305));
#171823=CARTESIAN_POINT('Ctrl Pts',(-0.238394649440512,62.8924926697742,
40.0620063077269));
#171824=CARTESIAN_POINT('Ctrl Pts',(-0.235414176911847,62.8945308924032,
40.06525004417));
#171825=CARTESIAN_POINT('Ctrl Pts',(-0.232339728998654,62.8965351787718,
40.0684393223557));
#171826=CARTESIAN_POINT('Ctrl Pts',(-0.229175397308462,62.8985027695519,
40.0715697951759));
#171827=CARTESIAN_POINT('Ctrl Pts',(-0.211566610930674,62.9094519648693,
40.0889901646409));
#171828=CARTESIAN_POINT('Ctrl Pts',(-0.191177078586578,62.9192690206945,
40.1045963098222));
#171829=CARTESIAN_POINT('Ctrl Pts',(-0.168765047545422,62.9274935913879,
40.1176634650699));
#171830=CARTESIAN_POINT('Ctrl Pts',(-0.158706217642669,62.9311848926124,
40.1235281853046));
#171831=CARTESIAN_POINT('Ctrl Pts',(-0.148239886922486,62.9345557609571,
40.1288820140913));
#171832=CARTESIAN_POINT('Ctrl Pts',(-0.137433186921703,62.9375663198809,
40.1336621774101));
#171833=CARTESIAN_POINT('Ctrl Pts',(-0.132736741272955,62.9388746680683,
40.1357395717319));
#171834=CARTESIAN_POINT('Ctrl Pts',(-0.127976140237443,62.9401148076313,
40.1377083672884));
#171835=CARTESIAN_POINT('Ctrl Pts',(-0.123156980416903,62.9412833674838,
40.1395632548792));
#171836=CARTESIAN_POINT('Ctrl Pts',(-0.106289921045012,62.9453733269673,
40.146055361447));
#171837=CARTESIAN_POINT('Ctrl Pts',(-0.0887055165503932,62.9485864317703,
40.1511520974629));
#171838=CARTESIAN_POINT('Ctrl Pts',(-0.0706437212495017,62.9507781643242,
40.1546258197408));
#171839=CARTESIAN_POINT('Ctrl Pts',(-0.0616128235990559,62.9518740306011,
40.1563626808798));
#171840=CARTESIAN_POINT('Ctrl Pts',(-0.0524625782494773,62.9527145544237,
40.1576937882008));
#171841=CARTESIAN_POINT('Ctrl Pts',(-0.0432229794968555,62.9532816790167,
40.1585906813668));
#171842=CARTESIAN_POINT('Ctrl Pts',(-0.0386031801205446,62.9535652413132,
40.1590391279498));
#171843=CARTESIAN_POINT('Ctrl Pts',(-0.0339610423934489,62.9537804539255,
40.1593790209175));
#171844=CARTESIAN_POINT('Ctrl Pts',(-0.0293003156009363,62.9539250604562,
40.1596068022931));
#171845=CARTESIAN_POINT('Ctrl Pts',(-0.0246395888084235,62.9540696669868,
40.1598345836687));
#171846=CARTESIAN_POINT('Ctrl Pts',(-0.0199602729501285,62.9541436657296,
40.1599502506865));
#171847=CARTESIAN_POINT('Ctrl Pts',(-0.0152661173102018,62.9541448057648,
40.1599502534424));
#171848=CARTESIAN_POINT('',(0.318045750793707,62.7644678366119,39.8576902534424));
#171849=CARTESIAN_POINT('Ctrl Pts',(0.0152661173115319,62.9541448057648,
40.1599502534424));
#171850=CARTESIAN_POINT('Ctrl Pts',(0.0190877352453135,62.9541438736292,
40.1599502447858));
#171851=CARTESIAN_POINT('Ctrl Pts',(0.0228988721028898,62.9540952129414,
40.1598744685927));
#171852=CARTESIAN_POINT('Ctrl Pts',(0.0266975986410124,62.9539999459718,
40.1597246934279));
#171853=CARTESIAN_POINT('Ctrl Pts',(0.0486495517936765,62.953449420412,
40.1588591777434));
#171854=CARTESIAN_POINT('Ctrl Pts',(0.0701898812476337,62.9513443281453,
40.1555254706015));
#171855=CARTESIAN_POINT('Ctrl Pts',(0.0909392844453373,62.9479003565106,
40.1500631826367));
#171856=CARTESIAN_POINT('Ctrl Pts',(0.0993079960704183,62.9465113235258,
40.1478601162471));
#171857=CARTESIAN_POINT('Ctrl Pts',(0.107548428340109,62.9449047668209,
40.1453112228301));
#171858=CARTESIAN_POINT('Ctrl Pts',(0.115637319282903,62.9430957254317,
40.1424401896328));
#171859=CARTESIAN_POINT('Ctrl Pts',(0.118621628944159,62.9424282989905,
40.1413809526905));
#171860=CARTESIAN_POINT('Ctrl Pts',(0.121585194086244,62.9417332466658,
40.1402777640511));
#171861=CARTESIAN_POINT('Ctrl Pts',(0.124526788073465,62.941011293136,40.1391317641987));
#171862=CARTESIAN_POINT('Ctrl Pts',(0.130042276799505,62.9396576302675,
40.1369830144753));
#171863=CARTESIAN_POINT('Ctrl Pts',(0.135480523184277,62.938209392844,40.134683756585));
#171864=CARTESIAN_POINT('Ctrl Pts',(0.140833441494043,62.9366713579026,
40.1322415082996));
#171865=CARTESIAN_POINT('Ctrl Pts',(0.159568655578222,62.9312882356078,
40.1236936393009));
#171866=CARTESIAN_POINT('Ctrl Pts',(0.177258600739639,62.9248050892389,
40.113394140767));
#171867=CARTESIAN_POINT('Ctrl Pts',(0.193556601114317,62.9174267595942,
40.101665321223));
#171868=CARTESIAN_POINT('Ctrl Pts',(0.201705601301656,62.9137375947719,
40.095800911451));
#171869=CARTESIAN_POINT('Ctrl Pts',(0.20950661529207,62.9098246351409,40.0895791707949));
#171870=CARTESIAN_POINT('Ctrl Pts',(0.21691630865106,62.9057134946881,40.0830403822907));
#171871=CARTESIAN_POINT('Ctrl Pts',(0.220621155330555,62.9036579244618,
40.0797709880385));
#171872=CARTESIAN_POINT('Ctrl Pts',(0.224228171853212,62.9015528091475,
40.0764223317514));
#171873=CARTESIAN_POINT('Ctrl Pts',(0.227731941420199,62.8994013510256,
40.0729994484778));
#171874=CARTESIAN_POINT('Ctrl Pts',(0.231235710987187,62.8972498929038,
40.0695765652043));
#171875=CARTESIAN_POINT('Ctrl Pts',(0.234636114277394,62.8950520414621,
40.0660793733488));
#171876=CARTESIAN_POINT('Ctrl Pts',(0.237927978231581,62.8928111037451,
40.0625130768817));
#171877=CARTESIAN_POINT('Ctrl Pts',(0.237956050936881,62.8927919932396,
40.0624826638418));
#171878=CARTESIAN_POINT('Ctrl Pts',(0.237984115711677,62.8927728797351,
40.0624522459912));
#171879=CARTESIAN_POINT('Ctrl Pts',(0.238012172553515,62.8927537632335,
40.0624218233329));
#171880=CARTESIAN_POINT('Ctrl Pts',(0.252341211296938,62.8829906867849,
40.046884527592));
#171881=CARTESIAN_POINT('Ctrl Pts',(0.264702219190169,62.8725309380421,
40.0302263329284));
#171882=CARTESIAN_POINT('Ctrl Pts',(0.275152816746093,62.8615664772846,
40.0127515884816));
#171883=CARTESIAN_POINT('Ctrl Pts',(0.285956846571966,62.8502312057449,
39.9946858597813));
#171884=CARTESIAN_POINT('Ctrl Pts',(0.294719332057067,62.8383556508911,
39.9757460620614));
#171885=CARTESIAN_POINT('Ctrl Pts',(0.301453885680055,62.8261370346467,
39.956244455928));
#171886=CARTESIAN_POINT('Ctrl Pts',(0.308060333922269,62.8141508421938,
39.9371138113786));
#171887=CARTESIAN_POINT('Ctrl Pts',(0.312715155745665,62.8018335935204,
39.9174410654551));
#171888=CARTESIAN_POINT('Ctrl Pts',(0.315383336841203,62.7893708783685,
39.8975196504365));
#171889=CARTESIAN_POINT('Ctrl Pts',(0.317150913275835,62.7811147664985,
39.8843224113922));
#171890=CARTESIAN_POINT('Ctrl Pts',(0.318045664009114,62.7727948225171,
39.8710160447206));
#171891=CARTESIAN_POINT('Ctrl Pts',(0.318045750793707,62.7644678366119,
39.8576902534424));
#171892=CARTESIAN_POINT('',(0.318048871877787,62.4081695979768,39.2875012672119));
#171893=CARTESIAN_POINT('',(0.318045750793708,62.7644678366119,39.8576902534424));
#171894=CARTESIAN_POINT('',(6.20712349654526,62.0995362748658,39.2875012672119));
#171895=CARTESIAN_POINT('Origin',(5.53234440788222E-15,0.,39.2875012672119));
#171896=CARTESIAN_POINT('',(6.24436990788123,62.4538823482275,39.8576902534424));
#171897=CARTESIAN_POINT('',(6.20712349654526,62.0995362748658,39.2875012672119));
#171898=CARTESIAN_POINT('',(6.56531752495365,62.6108711573005,40.1599502534424));
#171899=CARTESIAN_POINT('Ctrl Pts',(6.24436990788122,62.4538823482275,39.8576902534424));
#171900=CARTESIAN_POINT('Ctrl Pts',(6.24565635961526,62.4661208561117,39.8773836120374));
#171901=CARTESIAN_POINT('Ctrl Pts',(6.24887816048211,62.4781153572978,39.8969946442152));
#171902=CARTESIAN_POINT('Ctrl Pts',(6.25393874389594,62.4897034690595,39.9162525288271));
#171903=CARTESIAN_POINT('Ctrl Pts',(6.2591010141573,62.5015244311583,39.9358973794102));
#171904=CARTESIAN_POINT('Ctrl Pts',(6.26617675898668,62.5129234357018,39.9551762199787));
#171905=CARTESIAN_POINT('Ctrl Pts',(6.27511683300959,62.5237314369814,39.9738152034297));
#171906=CARTESIAN_POINT('Ctrl Pts',(6.28370959326105,62.534119557209,39.9917300792702));
#171907=CARTESIAN_POINT('Ctrl Pts',(6.29402509234407,62.543962460673,40.0090551158183));
#171908=CARTESIAN_POINT('Ctrl Pts',(6.30606398948359,62.5531007542797,40.0255394551599));
#171909=CARTESIAN_POINT('Ctrl Pts',(6.31531185250446,62.5601204743206,40.038202152619));
#171910=CARTESIAN_POINT('Ctrl Pts',(6.32557753708383,62.5667243349276,40.0503687782142));
#171911=CARTESIAN_POINT('Ctrl Pts',(6.33687803771753,62.5728320301412,40.0619155352442));
#171912=CARTESIAN_POINT('Ctrl Pts',(6.33690765431437,62.5728480373211,40.0619457972351));
#171913=CARTESIAN_POINT('Ctrl Pts',(6.33693727882158,62.5728640408534,40.0619760547304));
#171914=CARTESIAN_POINT('Ctrl Pts',(6.33696691123639,62.5728800407363,40.0620063077269));
#171915=CARTESIAN_POINT('Ctrl Pts',(6.34014410870389,62.5745955535552,40.06525004417));
#171916=CARTESIAN_POINT('Ctrl Pts',(6.34341121944381,62.5762674929177,40.0684393223556));
#171917=CARTESIAN_POINT('Ctrl Pts',(6.34676388583449,62.5778935423007,40.0715697951759));
#171918=CARTESIAN_POINT('Ctrl Pts',(6.36542071199982,62.5869421374011,40.088990164642));
#171919=CARTESIAN_POINT('Ctrl Pts',(6.38672471011312,62.5945741278851,40.1045963098242));
#171920=CARTESIAN_POINT('Ctrl Pts',(6.40987366744057,62.6004109483563,40.1176634650724));
#171921=CARTESIAN_POINT('Ctrl Pts',(6.4202632400637,62.603030594214,40.1235281853061));
#171922=CARTESIAN_POINT('Ctrl Pts',(6.43102458681551,62.6052889671226,40.1288820140919));
#171923=CARTESIAN_POINT('Ctrl Pts',(6.44208677567923,62.6071534261452,40.1336621774101));
#171924=CARTESIAN_POINT('Ctrl Pts',(6.44689425333276,62.6079636948179,40.1357395717319));
#171925=CARTESIAN_POINT('Ctrl Pts',(6.45175840518046,62.6086994224562,40.1377083672883));
#171926=CARTESIAN_POINT('Ctrl Pts',(6.45667331290488,62.6093578414452,40.1395632548791));
#171927=CARTESIAN_POINT('Ctrl Pts',(6.47387548994035,62.6116623079067,40.1460553614469));
#171928=CARTESIAN_POINT('Ctrl Pts',(6.49169942613465,62.6130197402062,40.1511520974629));
#171929=CARTESIAN_POINT('Ctrl Pts',(6.5098913754668,62.6133114945131,40.1546258197408));
#171930=CARTESIAN_POINT('Ctrl Pts',(6.51898735013287,62.6134573716666,40.1563626808798));
#171931=CARTESIAN_POINT('Ctrl Pts',(6.52817532814455,62.6133368299269,40.1576937882008));
#171932=CARTESIAN_POINT('Ctrl Pts',(6.53742359207063,62.6129350466932,40.1585906813668));
#171933=CARTESIAN_POINT('Ctrl Pts',(6.54204772403368,62.6127341550763,40.1590391279498));
#171934=CARTESIAN_POINT('Ctrl Pts',(6.54668692748823,62.6124629532085,40.1593790209175));
#171935=CARTESIAN_POINT('Ctrl Pts',(6.55133723783015,62.6121195889601,40.1596068022931));
#171936=CARTESIAN_POINT('Ctrl Pts',(6.55598754817206,62.6117762247117,40.1598345836687));
#171937=CARTESIAN_POINT('Ctrl Pts',(6.56064896522335,62.6113606963859,40.1599502506865));
#171938=CARTESIAN_POINT('Ctrl Pts',(6.56531752495365,62.6108711573005,40.1599502534424));
#171939=CARTESIAN_POINT('',(6.59568250079948,62.6076796697353,40.1599502534424));
#171940=CARTESIAN_POINT('Origin',(5.63895492999586E-15,5.54032330042594E-15,
40.1599502534424));
#171941=CARTESIAN_POINT('',(6.87697683366627,62.387392681069,39.8576902534424));
#171942=CARTESIAN_POINT('Ctrl Pts',(6.59568250079949,62.6076796697354,40.1599502534424));
#171943=CARTESIAN_POINT('Ctrl Pts',(6.59948308607566,62.6072792748562,40.1599502447858));
#171944=CARTESIAN_POINT('Ctrl Pts',(6.60326825869985,62.6068325084577,40.1598744685927));
#171945=CARTESIAN_POINT('Ctrl Pts',(6.60703621730659,62.6063406883232,40.1597246934279));
#171946=CARTESIAN_POINT('Ctrl Pts',(6.62881036977204,62.6034985746713,40.1588591777434));
#171947=CARTESIAN_POINT('Ctrl Pts',(6.65001265698756,62.5991534367842,40.1555254706016));
#171948=CARTESIAN_POINT('Ctrl Pts',(6.67028839972079,62.5935594283565,40.1500631826369));
#171949=CARTESIAN_POINT('Ctrl Pts',(6.67846607318486,62.5913032360741,40.1478601162472));
#171950=CARTESIAN_POINT('Ctrl Pts',(6.68649343260107,62.588844120533,40.1453112228302));
#171951=CARTESIAN_POINT('Ctrl Pts',(6.69434891543673,62.586199469922,40.1424401896328));
#171952=CARTESIAN_POINT('Ctrl Pts',(6.69724711167717,62.5852237544098,40.1413809526905));
#171953=CARTESIAN_POINT('Ctrl Pts',(6.70012178934792,62.5842227327444,40.1402777640511));
#171954=CARTESIAN_POINT('Ctrl Pts',(6.70297180428247,62.5831972538525,40.1391317641987));
#171955=CARTESIAN_POINT('Ctrl Pts',(6.70831558228476,62.5812744809302,40.1369830144753));
#171956=CARTESIAN_POINT('Ctrl Pts',(6.71357265535449,62.5792657255653,40.1346837565849));
#171957=CARTESIAN_POINT('Ctrl Pts',(6.7187354813888,62.5771765838154,40.1322415082996));
#171958=CARTESIAN_POINT('Ctrl Pts',(6.73680537250886,62.5698645876905,40.1236936393009));
#171959=CARTESIAN_POINT('Ctrl Pts',(6.75372073697266,62.5615678538927,40.113394140767));
#171960=CARTESIAN_POINT('Ctrl Pts',(6.76915820973676,62.5525263385763,40.101665321223));
#171961=CARTESIAN_POINT('Ctrl Pts',(6.7768769461188,62.5480055809181,40.095800911451));
#171962=CARTESIAN_POINT('Ctrl Pts',(6.78422620968128,62.5432986288851,40.0895791707949));
#171963=CARTESIAN_POINT('Ctrl Pts',(6.79116558077096,62.5384354858298,40.0830403822906));
#171964=CARTESIAN_POINT('Ctrl Pts',(6.7946352663158,62.5360039143022,40.0797709880385));
#171965=CARTESIAN_POINT('Ctrl Pts',(6.79800247875573,62.5335332951357,40.0764223317514));
#171966=CARTESIAN_POINT('Ctrl Pts',(6.80126216569517,62.5310273792781,40.0729994484778));
#171967=CARTESIAN_POINT('Ctrl Pts',(6.8045218526346,62.5285214634205,40.0695765652042));
#171968=CARTESIAN_POINT('Ctrl Pts',(6.80767389012611,62.5259802131085,40.0660793733488));
#171969=CARTESIAN_POINT('Ctrl Pts',(6.81071347912929,62.5234074580024,40.0625130768817));
#171970=CARTESIAN_POINT('Ctrl Pts',(6.8107394004576,62.5233855177895,40.0624826638418));
#171971=CARTESIAN_POINT('Ctrl Pts',(6.81076531358536,62.523363575423,40.0624522459912));
#171972=CARTESIAN_POINT('Ctrl Pts',(6.81079121851035,62.5233416309051,40.0624218233329));
#171973=CARTESIAN_POINT('Ctrl Pts',(6.82402124190388,62.5121342452095,40.0468845275902));
#171974=CARTESIAN_POINT('Ctrl Pts',(6.83522119344137,62.5004397189038,40.0302263329244));
#171975=CARTESIAN_POINT('Ctrl Pts',(6.84446844329752,62.4884429377053,40.0127515884755));
#171976=CARTESIAN_POINT('Ctrl Pts',(6.85402842900344,62.4760404333329,39.9946858597728));
#171977=CARTESIAN_POINT('Ctrl Pts',(6.86150157917705,62.4633140048674,39.9757460620505));
#171978=CARTESIAN_POINT('Ctrl Pts',(6.86692204703104,62.4504583709387,39.9562444559146));
#171979=CARTESIAN_POINT('Ctrl Pts',(6.87223940618061,62.4378472782183,39.9371138113629));
#171980=CARTESIAN_POINT('Ctrl Pts',(6.87558122532671,62.4251109433487,39.9174410654371));
#171981=CARTESIAN_POINT('Ctrl Pts',(6.87693208138284,62.4124375993835,39.8975196504164));
#171982=CARTESIAN_POINT('Ctrl Pts',(6.87782697616113,62.404041953314,39.8843224113787));
#171983=CARTESIAN_POINT('Ctrl Pts',(6.87784715439695,62.3956740599414,39.8710160447138));
#171984=CARTESIAN_POINT('Ctrl Pts',(6.87697683366627,62.3873926810691,39.8576902534424));
#171985=CARTESIAN_POINT('',(6.83973663030322,62.0330459552232,39.2875012672119));
#171986=CARTESIAN_POINT('',(6.87697683366627,62.387392681069,39.8576902534424));
#171987=CARTESIAN_POINT('',(12.6642893210148,61.110527437164,39.2875012672119));
#171988=CARTESIAN_POINT('Origin',(5.53234440788222E-15,0.,39.2875012672119));
#171989=CARTESIAN_POINT('',(12.7383709431257,61.4590390555207,39.8576902534424));
#171990=CARTESIAN_POINT('',(12.6642893210148,61.110527437164,39.2875012672119));
#171991=CARTESIAN_POINT('',(13.0739701745332,61.5816197022696,40.1599502534424));
#171992=CARTESIAN_POINT('Ctrl Pts',(12.7383709431257,61.4590390555207,39.8576902534424));
#171993=CARTESIAN_POINT('Ctrl Pts',(12.7409296199642,61.4710760487551,39.8773836120368));
#171994=CARTESIAN_POINT('Ctrl Pts',(12.7453875382452,61.4826680729147,39.896994644214));
#171995=CARTESIAN_POINT('Ctrl Pts',(12.7516316867679,61.4936637287799,39.9162525288252));
#171996=CARTESIAN_POINT('Ctrl Pts',(12.7580013045749,61.5048803302339,39.9358973794079));
#171997=CARTESIAN_POINT('Ctrl Pts',(12.7662298081611,61.515477273104,39.9551762199759));
#171998=CARTESIAN_POINT('Ctrl Pts',(12.7762506512874,61.5252915748225,39.9738152034265));
#171999=CARTESIAN_POINT('Ctrl Pts',(12.7858821937424,61.5347245998162,39.9917300792667));
#172000=CARTESIAN_POINT('Ctrl Pts',(12.7971700470149,61.543435319558,40.0090551158146));
#172001=CARTESIAN_POINT('Ctrl Pts',(12.8100982056033,61.5512651452188,40.025539455156));
#172002=CARTESIAN_POINT('Ctrl Pts',(12.8200291684122,61.5572797455894,40.0382021526165));
#172003=CARTESIAN_POINT('Ctrl Pts',(12.8309289078993,61.5627743733242,40.050368778213));
#172004=CARTESIAN_POINT('Ctrl Pts',(12.8428059312041,61.5676673859794,40.0619155352442));
#172005=CARTESIAN_POINT('Ctrl Pts',(12.8428370587641,61.567680209693,40.0619457972351));
#172006=CARTESIAN_POINT('Ctrl Pts',(12.8428681938098,61.5676930289521,40.0619760547304));
#172007=CARTESIAN_POINT('Ctrl Pts',(12.8428993363383,61.5677058437551,40.0620063077269));
#172008=CARTESIAN_POINT('Ctrl Pts',(12.8462384487043,61.5690798512466,40.06525004417));
#172009=CARTESIAN_POINT('Ctrl Pts',(12.849662427122,61.5704011254853,40.0684393223556));
#172010=CARTESIAN_POINT('Ctrl Pts',(12.8531666956986,61.571667818134,40.0715697951759));
#172011=CARTESIAN_POINT('Ctrl Pts',(12.8726671535569,61.5787166747145,40.0889901646404));
#172012=CARTESIAN_POINT('Ctrl Pts',(12.8946522063743,61.5840799821715,40.1045963098214));
#172013=CARTESIAN_POINT('Ctrl Pts',(12.9182844651632,61.5874651029938,40.1176634650689));
#172014=CARTESIAN_POINT('Ctrl Pts',(12.9288909501782,61.5889843920976,40.123528185304));
#172015=CARTESIAN_POINT('Ctrl Pts',(12.9398294093983,61.5901055263648,40.128882014091));
#172016=CARTESIAN_POINT('Ctrl Pts',(12.9510258874727,61.5908034580836,40.1336621774101));
#172017=CARTESIAN_POINT('Ctrl Pts',(12.9558917253998,61.5911067697684,40.1357395717319));
#172018=CARTESIAN_POINT('Ctrl Pts',(12.9608061353941,61.591330024696,40.1377083672884));
#172019=CARTESIAN_POINT('Ctrl Pts',(12.9657629422649,61.5914710890453,40.1395632548792));
#172020=CARTESIAN_POINT('Ctrl Pts',(12.9831117663125,61.5919648142681,40.146055361447));
#172021=CARTESIAN_POINT('Ctrl Pts',(13.0009799514316,61.5914517017516,40.1511520974629));
#172022=CARTESIAN_POINT('Ctrl Pts',(13.0191027399912,61.5898402812904,40.1546258197408));
#172023=CARTESIAN_POINT('Ctrl Pts',(13.028164134271,61.5890345710598,40.1563626808798));
#172024=CARTESIAN_POINT('Ctrl Pts',(13.037289179535,61.5879542844382,40.1576937882008));
#172025=CARTESIAN_POINT('Ctrl Pts',(13.0464447827196,61.586587995399,40.1585906813668));
#172026=CARTESIAN_POINT('Ctrl Pts',(13.051022584312,61.5859048508794,40.1590391279498));
#172027=CARTESIAN_POINT('Ctrl Pts',(13.0556080254101,61.5851502058759,40.1593790209175));
#172028=CARTESIAN_POINT('Ctrl Pts',(13.0601969695282,61.5843226328191,40.1596068022931));
#172029=CARTESIAN_POINT('Ctrl Pts',(13.0647859136462,61.5834950597622,40.1598345836687));
#172030=CARTESIAN_POINT('Ctrl Pts',(13.0693783604298,61.582594556983,40.1599502506865));
#172031=CARTESIAN_POINT('Ctrl Pts',(13.0739701745332,61.5816197022696,40.1599502534424));
#172032=CARTESIAN_POINT('',(13.1038352065734,61.575271693745,40.1599502534424));
#172033=CARTESIAN_POINT('Origin',(5.62288786856779E-15,5.54286807295788E-15,
40.1599502534424));
#172034=CARTESIAN_POINT('',(13.3605623192493,61.3267881959111,39.8576902534424));
#172035=CARTESIAN_POINT('Ctrl Pts',(13.1038352065734,61.575271693745,40.1599502534424));
#172036=CARTESIAN_POINT('Ctrl Pts',(13.1075731191844,61.5744762229325,40.1599502447858));
#172037=CARTESIAN_POINT('Ctrl Pts',(13.1112908564318,61.5736362456894,40.1598744685927));
#172038=CARTESIAN_POINT('Ctrl Pts',(13.1149867645642,61.5727532608742,40.1597246934279));
#172039=CARTESIAN_POINT('Ctrl Pts',(13.1363445541734,61.5676506979217,40.1588591777433));
#172040=CARTESIAN_POINT('Ctrl Pts',(13.1569765024567,61.5611131206536,40.1555254706011));
#172041=CARTESIAN_POINT('Ctrl Pts',(13.1765564394468,61.5534303645591,40.1500631826356));
#172042=CARTESIAN_POINT('Ctrl Pts',(13.1844534784461,61.5503317322942,40.1478601162462));
#172043=CARTESIAN_POINT('Ctrl Pts',(13.1921798155775,61.5470470005022,40.1453112228296));
#172044=CARTESIAN_POINT('Ctrl Pts',(13.1997158239904,61.5435957160156,40.1424401896328));
#172045=CARTESIAN_POINT('Ctrl Pts',(13.2024961535655,61.5423224015758,40.1413809526906));
#172046=CARTESIAN_POINT('Ctrl Pts',(13.2052504481948,61.5410263779725,40.1402777640512));
#172047=CARTESIAN_POINT('Ctrl Pts',(13.2079776587167,61.5397086090799,40.1391317641987));
#172048=CARTESIAN_POINT('Ctrl Pts',(13.2130911784452,61.5372377924062,40.1369830144753));
#172049=CARTESIAN_POINT('Ctrl Pts',(13.2181094806072,61.5346905274441,40.134683756585));
#172050=CARTESIAN_POINT('Ctrl Pts',(13.2230256493636,61.5320731679598,40.1322415082996));
#172051=CARTESIAN_POINT('Ctrl Pts',(13.2402322400111,61.5229124097646,40.1236936393009));
#172052=CARTESIAN_POINT('Ctrl Pts',(13.2561876955045,61.5128929892896,40.113394140767));
#172053=CARTESIAN_POINT('Ctrl Pts',(13.2705955044759,61.5022873490354,40.101665321223));
#172054=CARTESIAN_POINT('Ctrl Pts',(13.2777994089616,61.4969845289083,40.095800911451));
#172055=CARTESIAN_POINT('Ctrl Pts',(13.2846164020267,61.4915351548246,40.0895791707949));
#172056=CARTESIAN_POINT('Ctrl Pts',(13.2910094216452,61.4859732907798,40.0830403822906));
#172057=CARTESIAN_POINT('Ctrl Pts',(13.2942059314545,61.4831923587574,40.0797709880385));
#172058=CARTESIAN_POINT('Ctrl Pts',(13.2972964479276,61.4803833043593,40.0764223317514));
#172059=CARTESIAN_POINT('Ctrl Pts',(13.3002763384272,61.4775503861045,40.0729994484778));
#172060=CARTESIAN_POINT('Ctrl Pts',(13.3032562289269,61.4747174678497,40.0695765652042));
#172061=CARTESIAN_POINT('Ctrl Pts',(13.3061253662373,61.4718606611376,40.0660793733488));
#172062=CARTESIAN_POINT('Ctrl Pts',(13.3088793779163,61.4689842762857,40.0625130768816));
#172063=CARTESIAN_POINT('Ctrl Pts',(13.3089028638681,61.468959746747,40.0624826638418));
#172064=CARTESIAN_POINT('Ctrl Pts',(13.3089263414392,61.4689352159237,40.0624522459912));
#172065=CARTESIAN_POINT('Ctrl Pts',(13.3089498106276,61.4689106838181,40.0624218233329));
#172066=CARTESIAN_POINT('Ctrl Pts',(13.320935867764,61.4563817793403,40.046884527591));
#172067=CARTESIAN_POINT('Ctrl Pts',(13.3308520539314,61.443580603151,40.0302263329261));
#172068=CARTESIAN_POINT('Ctrl Pts',(13.3387946412822,61.430682940759,40.0127515884781));
#172069=CARTESIAN_POINT('Ctrl Pts',(13.3470058416633,61.4173490879891,39.9946858597764));
#172070=CARTESIAN_POINT('Ctrl Pts',(13.3531077791279,61.4039112193276,39.9757460620551));
#172071=CARTESIAN_POINT('Ctrl Pts',(13.3571547734332,61.3905594167323,39.9562444559201));
#172072=CARTESIAN_POINT('Ctrl Pts',(13.361124785391,61.3774615935173,39.9371138113694));
#172073=CARTESIAN_POINT('Ctrl Pts',(13.3631169881909,61.3644457144034,39.9174410654445));
#172074=CARTESIAN_POINT('Ctrl Pts',(13.3631357189476,61.3517005934352,39.8975196504246));
#172075=CARTESIAN_POINT('Ctrl Pts',(13.3631481274173,61.3432573976156,39.8843224113842));
#172076=CARTESIAN_POINT('Ctrl Pts',(13.3622935120796,61.3349332352367,39.8710160447165));
#172077=CARTESIAN_POINT('Ctrl Pts',(13.3605623192493,61.3267881959111,39.8576902534424));
#172078=CARTESIAN_POINT('',(13.2864868029002,60.9782752797346,39.2875012672119));
#172079=CARTESIAN_POINT('',(13.3605623192493,61.3267881959111,39.8576902534424));
#172080=CARTESIAN_POINT('',(18.9827025415103,59.4519788726605,39.2875012672119));
#172081=CARTESIAN_POINT('Origin',(5.53234440788222E-15,0.,39.2875012672119));
#172082=CARTESIAN_POINT('',(19.0928077206418,59.7908376697909,39.8576902534424));
#172083=CARTESIAN_POINT('',(18.9827025415103,59.4519788726606,39.2875012672119));
#172084=CARTESIAN_POINT('',(19.4393816709763,59.8776671349983,40.1599502534424));
#172085=CARTESIAN_POINT('Ctrl Pts',(19.0928077206418,59.7908376697909,39.8576902534424));
#172086=CARTESIAN_POINT('Ctrl Pts',(19.0966105891856,59.8025412685583,39.8773836120355));
#172087=CARTESIAN_POINT('Ctrl Pts',(19.1022557829948,59.8136038110487,39.8969946442114));
#172088=CARTESIAN_POINT('Ctrl Pts',(19.1096150844281,59.8238865403105,39.9162525288214));
#172089=CARTESIAN_POINT('Ctrl Pts',(19.1171222629146,59.8343758896866,39.9358973794029));
#172090=CARTESIAN_POINT('Ctrl Pts',(19.1264133720499,59.8440546685596,39.9551762199699));
#172091=CARTESIAN_POINT('Ctrl Pts',(19.1374051938247,59.8527677431735,39.9738152034195));
#172092=CARTESIAN_POINT('Ctrl Pts',(19.147969993288,59.8611423227373,39.991730079259));
#172093=CARTESIAN_POINT('Ctrl Pts',(19.1601065286666,59.8686254222887,40.0090551158061));
#172094=CARTESIAN_POINT('Ctrl Pts',(19.1737823050924,59.8750609947952,40.0255394551469));
#172095=CARTESIAN_POINT('Ctrl Pts',(19.1842875619839,59.8800045782759,40.0382021526108));
#172096=CARTESIAN_POINT('Ctrl Pts',(19.1957019365535,59.8843297728477,40.0503687782103));
#172097=CARTESIAN_POINT('Ctrl Pts',(19.2080253553785,59.8879544940742,40.0619155352442));
#172098=CARTESIAN_POINT('Ctrl Pts',(19.2080576528615,59.8879639938221,40.0619457972351));
#172099=CARTESIAN_POINT('Ctrl Pts',(19.2080899573236,59.8879734883575,40.0619760547305));
#172100=CARTESIAN_POINT('Ctrl Pts',(19.2081222687617,59.8879829776791,40.0620063077269));
#172101=CARTESIAN_POINT('Ctrl Pts',(19.2115867120124,59.8890004259294,40.06525004417));
#172102=CARTESIAN_POINT('Ctrl Pts',(19.2151300442838,59.8899565588873,40.0684393223556));
#172103=CARTESIAN_POINT('Ctrl Pts',(19.2187475215465,59.890850016652,40.0715697951759));
#172104=CARTESIAN_POINT('Ctrl Pts',(19.2388779600064,59.8958219059666,40.0889901646438));
#172105=CARTESIAN_POINT('Ctrl Pts',(19.2613031946953,59.8988577688785,40.1045963098274));
#172106=CARTESIAN_POINT('Ctrl Pts',(19.2851598349806,59.8997541019594,40.1176634650765));
#172107=CARTESIAN_POINT('Ctrl Pts',(19.2958670255119,59.9001563886587,40.1235281853086));
#172108=CARTESIAN_POINT('Ctrl Pts',(19.3068627531452,59.9001280009021,40.1288820140931));
#172109=CARTESIAN_POINT('Ctrl Pts',(19.3180708494664,59.899651758631,40.1336621774101));
#172110=CARTESIAN_POINT('Ctrl Pts',(19.3229417365285,59.8994447901816,40.1357395717319));
#172111=CARTESIAN_POINT('Ctrl Pts',(19.3278525613652,59.8991531263707,40.1377083672884));
#172112=CARTESIAN_POINT('Ctrl Pts',(19.332796959569,59.8987752905499,40.1395632548792));
#172113=CARTESIAN_POINT('Ctrl Pts',(19.3501023532821,59.8974528651771,40.146055361447));
#172114=CARTESIAN_POINT('Ctrl Pts',(19.3678190197507,59.8950748296128,40.1511520974629));
#172115=CARTESIAN_POINT('Ctrl Pts',(19.3856740904739,59.8915778894432,40.1546258197408));
#172116=CARTESIAN_POINT('Ctrl Pts',(19.3946016258354,59.8898294193584,40.1563626808798));
#172117=CARTESIAN_POINT('Ctrl Pts',(19.4035637624462,59.8878012237013,40.1576937882008));
#172118=CARTESIAN_POINT('Ctrl Pts',(19.412526394185,59.8854853982052,40.1585906813668));
#172119=CARTESIAN_POINT('Ctrl Pts',(19.4170077100544,59.8843274854572,40.1590391279498));
#172120=CARTESIAN_POINT('Ctrl Pts',(19.4214891497439,59.8830976653666,40.1593790209175));
#172121=CARTESIAN_POINT('Ctrl Pts',(19.4259664502061,59.8817949505648,40.1596068022931));
#172122=CARTESIAN_POINT('Ctrl Pts',(19.4304437506682,59.8804922357631,40.1598345836687));
#172123=CARTESIAN_POINT('Ctrl Pts',(19.4349169113761,59.8791166246274,40.1599502506865));
#172124=CARTESIAN_POINT('Ctrl Pts',(19.4393816709763,59.8776671349983,40.1599502534424));
#172125=CARTESIAN_POINT('',(19.4684195516703,59.868232155624,40.1599502534424));
#172126=CARTESIAN_POINT('Origin',(5.60717482534548E-15,5.54707837019994E-15,
40.1599502534424));
#172127=CARTESIAN_POINT('',(19.6977666881852,59.5942745858234,39.8576902534424));
#172128=CARTESIAN_POINT('Ctrl Pts',(19.4684195516703,59.868232155624,40.1599502534424));
#172129=CARTESIAN_POINT('Ctrl Pts',(19.4720538382633,59.8670503242228,40.1599502447858));
#172130=CARTESIAN_POINT('Ctrl Pts',(19.4756634078267,59.8658263391016,40.1598744685927));
#172131=CARTESIAN_POINT('Ctrl Pts',(19.4792467723418,59.8645618637721,40.1597246934279));
#172132=CARTESIAN_POINT('Ctrl Pts',(19.4999541986819,59.8572547562663,40.1588591777433));
#172133=CARTESIAN_POINT('Ctrl Pts',(19.5197897600895,59.8485963666816,40.1555254706007));
#172134=CARTESIAN_POINT('Ctrl Pts',(19.5384593694488,59.8389090368037,40.1500631826346));
#172135=CARTESIAN_POINT('Ctrl Pts',(19.5459892523722,59.8350019138202,40.1478601162455));
#172136=CARTESIAN_POINT('Ctrl Pts',(19.5533299158528,59.8309275539862,40.1453112228292));
#172137=CARTESIAN_POINT('Ctrl Pts',(19.5604638837584,59.8267074486191,40.1424401896328));
#172138=CARTESIAN_POINT('Ctrl Pts',(19.5630958847956,59.8251504859512,40.1413809526905));
#172139=CARTESIAN_POINT('Ctrl Pts',(19.5656996197551,59.8235736599158,40.1402777640511));
#172140=CARTESIAN_POINT('Ctrl Pts',(19.5682741459751,59.8219780387742,40.1391317641987));
#172141=CARTESIAN_POINT('Ctrl Pts',(19.5731013826375,59.8189862491337,40.1369830144753));
#172142=CARTESIAN_POINT('Ctrl Pts',(19.5778259323232,59.8159283829423,40.1346837565849));
#172143=CARTESIAN_POINT('Ctrl Pts',(19.5824415812281,59.8128114820619,40.1322415082996));
#172144=CARTESIAN_POINT('Ctrl Pts',(19.5985963523951,59.8019023289801,40.1236936393009));
#172145=CARTESIAN_POINT('Ctrl Pts',(19.6134170876088,59.7902699966954,40.113394140767));
#172146=CARTESIAN_POINT('Ctrl Pts',(19.6266373778174,59.7782164291174,40.101665321223));
#172147=CARTESIAN_POINT('Ctrl Pts',(19.6332475229217,59.7721896453283,40.095800911451));
#172148=CARTESIAN_POINT('Ctrl Pts',(19.6394575570867,59.7660575536769,40.0895791707949));
#172149=CARTESIAN_POINT('Ctrl Pts',(19.6452341819734,59.7598579055889,40.0830403822906));
#172150=CARTESIAN_POINT('Ctrl Pts',(19.6481224944167,59.7567580815449,40.0797709880385));
#172151=CARTESIAN_POINT('Ctrl Pts',(19.6509024545777,59.7536413685031,40.0764223317514));
#172152=CARTESIAN_POINT('Ctrl Pts',(19.6535699003337,59.7505124858963,40.0729994484778));
#172153=CARTESIAN_POINT('Ctrl Pts',(19.6562373460896,59.7473836032894,40.0695765652042));
#172154=CARTESIAN_POINT('Ctrl Pts',(19.6587921483502,59.7442425399495,40.0660793733488));
#172155=CARTESIAN_POINT('Ctrl Pts',(19.6612304091767,59.7410940396261,40.0625130768816));
#172156=CARTESIAN_POINT('Ctrl Pts',(19.661251202435,59.7410671895123,40.0624826638418));
#172157=CARTESIAN_POINT('Ctrl Pts',(19.6612719872243,59.741040338997,40.0624522459912));
#172158=CARTESIAN_POINT('Ctrl Pts',(19.6612927635427,59.7410134880826,40.0624218233329));
#172159=CARTESIAN_POINT('Ctrl Pts',(19.6719035326713,59.7273003341229,40.0468845275927));
#172160=CARTESIAN_POINT('Ctrl Pts',(19.6804273096575,59.7135327604163,40.0302263329299));
#172161=CARTESIAN_POINT('Ctrl Pts',(19.6869782138539,59.6998755263197,40.0127515884841));
#172162=CARTESIAN_POINT('Ctrl Pts',(19.6937506652803,59.6857564136346,39.9946858597846));
#172163=CARTESIAN_POINT('Ctrl Pts',(19.6984145359325,59.671754332879,39.9757460620657));
#172164=CARTESIAN_POINT('Ctrl Pts',(19.7010437169729,59.6580526467613,39.9562444559333));
#172165=CARTESIAN_POINT('Ctrl Pts',(19.7036228854577,59.6446115955445,39.9371138113848));
#172166=CARTESIAN_POINT('Ctrl Pts',(19.7042436449215,59.6314587768822,39.9174410654622));
#172167=CARTESIAN_POINT('Ctrl Pts',(19.7029300451616,59.618781517124,39.8975196504446));
#172168=CARTESIAN_POINT('Ctrl Pts',(19.7020598313727,59.6103832769719,39.8843224113977));
#172169=CARTESIAN_POINT('Ctrl Pts',(19.7003397858053,59.6021940468491,39.8710160447233));
#172170=CARTESIAN_POINT('Ctrl Pts',(19.6977666881852,59.5942745858234,39.8576902534424));
#172171=CARTESIAN_POINT('',(19.5876674457085,59.2554138597569,39.2875012672119));
#172172=CARTESIAN_POINT('',(19.6977666881852,59.5942745858234,39.8576902534424));
#172173=CARTESIAN_POINT('',(25.0931373005752,57.1420619865018,39.2875012672119));
#172174=CARTESIAN_POINT('Origin',(5.53234440788222E-15,0.,39.2875012672119));
#172175=CARTESIAN_POINT('',(25.2380597013437,57.4675553545137,39.8576902534424));
#172176=CARTESIAN_POINT('',(25.0931373005752,57.1420619865019,39.2875012672119));
#172177=CARTESIAN_POINT('',(25.5918112338801,57.5176823163886,40.1599502534424));
#172178=CARTESIAN_POINT('Ctrl Pts',(25.2380597013437,57.4675553545137,39.8576902534424));
#172179=CARTESIAN_POINT('Ctrl Pts',(25.24306509657,57.4787973317381,39.8773836120366));
#172180=CARTESIAN_POINT('Ctrl Pts',(25.2498357159838,57.4892091890301,39.8969946442136));
#172181=CARTESIAN_POINT('Ctrl Pts',(25.2582295402824,57.498666331956,39.9162525288247));
#172182=CARTESIAN_POINT('Ctrl Pts',(25.2667920292312,57.5083135057483,39.9358973794071));
#172183=CARTESIAN_POINT('Ctrl Pts',(25.2770439485812,57.5169680778983,39.9551762199749));
#172184=CARTESIAN_POINT('Ctrl Pts',(25.2888863203068,57.5244844631393,39.9738152034253));
#172185=CARTESIAN_POINT('Ctrl Pts',(25.3002686266262,57.5317088436274,39.9917300792652));
#172186=CARTESIAN_POINT('Ctrl Pts',(25.3131208736915,57.5378823365839,40.0090551158128));
#172187=CARTESIAN_POINT('Ctrl Pts',(25.3273944332882,57.5428531464569,40.0255394551538));
#172188=CARTESIAN_POINT('Ctrl Pts',(25.3383588864659,57.54667155011,40.0382021526152));
#172189=CARTESIAN_POINT('Ctrl Pts',(25.3501628378371,57.5497799237798,40.0503687782124));
#172190=CARTESIAN_POINT('Ctrl Pts',(25.3627976342216,57.5520966403718,40.0619155352442));
#172191=CARTESIAN_POINT('Ctrl Pts',(25.3628307477697,57.5521027120728,40.0619457972351));
#172192=CARTESIAN_POINT('Ctrl Pts',(25.3628638677137,57.5521087778603,40.0619760547305));
#172193=CARTESIAN_POINT('Ctrl Pts',(25.3628969940507,57.5521148377334,40.0620063077269));
#172194=CARTESIAN_POINT('Ctrl Pts',(25.3664488110208,57.5527645793667,40.06525004417));
#172195=CARTESIAN_POINT('Ctrl Pts',(25.370072675656,57.553345095451,40.0684393223556));
#172196=CARTESIAN_POINT('Ctrl Pts',(25.3737637277669,57.5538555294214,40.0715697951759));
#172197=CARTESIAN_POINT('Ctrl Pts',(25.3943035935321,57.5566959784096,40.0889901646471));
#172198=CARTESIAN_POINT('Ctrl Pts',(25.4169233145287,57.5573711352261,40.1045963098334));
#172199=CARTESIAN_POINT('Ctrl Pts',(25.4407429579668,57.5557688601517,40.117663465084));
#172200=CARTESIAN_POINT('Ctrl Pts',(25.4514335437942,57.5550497369101,40.1235281853132));
#172201=CARTESIAN_POINT('Ctrl Pts',(25.462366068348,57.5538721381528,40.1288820140951));
#172202=CARTESIAN_POINT('Ctrl Pts',(25.4734629846673,57.5522269397028,40.1336621774101));
#172203=CARTESIAN_POINT('Ctrl Pts',(25.4782855544065,57.5515119587089,40.1357395717319));
#172204=CARTESIAN_POINT('Ctrl Pts',(25.483138990061,57.5507085716893,40.1377083672884));
#172205=CARTESIAN_POINT('Ctrl Pts',(25.4880168077363,57.5498159753467,40.1395632548792));
#172206=CARTESIAN_POINT('Ctrl Pts',(25.5050891695999,57.5466918881473,40.146055361447));
#172207=CARTESIAN_POINT('Ctrl Pts',(25.5224602099128,57.5424749837905,40.1511520974629));
#172208=CARTESIAN_POINT('Ctrl Pts',(25.5398519389082,57.5371308371208,40.1546258197408));
#172209=CARTESIAN_POINT('Ctrl Pts',(25.5485478034059,57.5344587637859,40.1563626808798));
#172210=CARTESIAN_POINT('Ctrl Pts',(25.5572488403194,57.5315048804294,40.1576937882008));
#172211=CARTESIAN_POINT('Ctrl Pts',(25.5659203041434,57.5282648911452,40.1585906813668));
#172212=CARTESIAN_POINT('Ctrl Pts',(25.5702560360555,57.5266448965031,40.1590391279498));
#172213=CARTESIAN_POINT('Ctrl Pts',(25.5745843747453,57.5249533754917,40.1593790209175));
#172214=CARTESIAN_POINT('Ctrl Pts',(25.5789009773107,57.523189791761,40.1596068022931));
#172215=CARTESIAN_POINT('Ctrl Pts',(25.5832175798762,57.5214262080303,40.1598345836687));
#172216=CARTESIAN_POINT('Ctrl Pts',(25.5875224456236,57.5195905600216,40.1599502506864));
#172217=CARTESIAN_POINT('Ctrl Pts',(25.5918112338801,57.5176823163886,40.1599502534424));
#172218=CARTESIAN_POINT('',(25.6197038181304,57.5052637377729,40.1599502534424));
#172219=CARTESIAN_POINT('Origin',(5.59198795571863E-15,5.55290806325446E-15,
40.1599502534424));
#172220=CARTESIAN_POINT('',(25.8191582032627,57.2088336324696,39.8576902534424));
#172221=CARTESIAN_POINT('Ctrl Pts',(25.6197038181304,57.5052637377729,40.1599502534424));
#172222=CARTESIAN_POINT('Ctrl Pts',(25.623194660701,57.5037084941751,40.1599502447858));
#172223=CARTESIAN_POINT('Ctrl Pts',(25.6266565153809,57.502113911413,40.1598744685927));
#172224=CARTESIAN_POINT('Ctrl Pts',(25.6300880761872,57.5004817994256,40.1597246934279));
#172225=CARTESIAN_POINT('Ctrl Pts',(25.6499182643587,57.4910502055666,40.1588591777434));
#172226=CARTESIAN_POINT('Ctrl Pts',(25.6687401163261,57.4803658667952,40.1555254706013));
#172227=CARTESIAN_POINT('Ctrl Pts',(25.6862948499051,57.4687800995491,40.1500631826362));
#172228=CARTESIAN_POINT('Ctrl Pts',(25.6933750777826,57.4641072931025,40.1478601162467));
#172229=CARTESIAN_POINT('Ctrl Pts',(25.7002496417699,57.4592879447638,40.1453112228299));
#172230=CARTESIAN_POINT('Ctrl Pts',(25.7069034079257,57.4543452548722,40.1424401896328));
#172231=CARTESIAN_POINT('Ctrl Pts',(25.7093582436707,57.4525217023849,40.1413809526906));
#172232=CARTESIAN_POINT('Ctrl Pts',(25.7117828918954,57.4506813499534,40.1402777640512));
#172233=CARTESIAN_POINT('Ctrl Pts',(25.7141765267655,57.448825358522,40.1391317641987));
#172234=CARTESIAN_POINT('Ctrl Pts',(25.7186645921469,57.445345374588,40.1369830144753));
#172235=CARTESIAN_POINT('Ctrl Pts',(25.7230436262012,57.4418104097894,40.1346837565849));
#172236=CARTESIAN_POINT('Ctrl Pts',(25.7273081852392,57.438228116931,40.1322415082996));
#172237=CARTESIAN_POINT('Ctrl Pts',(25.7422341418723,57.4256900919268,40.1236936393008));
#172238=CARTESIAN_POINT('Ctrl Pts',(25.7557577777298,57.412572294099,40.113394140767));
#172239=CARTESIAN_POINT('Ctrl Pts',(25.7676457049096,57.3992028606059,40.101665321223));
#172240=CARTESIAN_POINT('Ctrl Pts',(25.7735896684995,57.3925181438593,40.095800911451));
#172241=CARTESIAN_POINT('Ctrl Pts',(25.7791247053306,57.3857705191194,40.0895791707949));
#172242=CARTESIAN_POINT('Ctrl Pts',(25.7842216455743,57.3790010116301,40.0830403822906));
#172243=CARTESIAN_POINT('Ctrl Pts',(25.7867701156962,57.3756162578854,40.0797709880385));
#172244=CARTESIAN_POINT('Ctrl Pts',(25.7892090617198,57.3722260335602,40.0764223317514));
#172245=CARTESIAN_POINT('Ctrl Pts',(25.7915348376382,57.3688354672939,40.0729994484778));
#172246=CARTESIAN_POINT('Ctrl Pts',(25.7938606135566,57.3654449010277,40.0695765652042));
#172247=CARTESIAN_POINT('Ctrl Pts',(25.7960730898191,57.3620539952071,40.0660793733488));
#172248=CARTESIAN_POINT('Ctrl Pts',(25.7981688856973,57.3586678750407,40.0625130768817));
#172249=CARTESIAN_POINT('Ctrl Pts',(25.7981867584468,57.3586389985273,40.0624826638418));
#172250=CARTESIAN_POINT('Ctrl Pts',(25.7982046227317,57.3586101224998,40.0624522459912));
#172251=CARTESIAN_POINT('Ctrl Pts',(25.7982224785504,57.358581246961,40.0624218233329));
#172252=CARTESIAN_POINT('Ctrl Pts',(25.8073417058668,57.3438340877005,40.0468845275908));
#172253=CARTESIAN_POINT('Ctrl Pts',(25.8143796853889,57.3292509568918,40.0302263329258));
#172254=CARTESIAN_POINT('Ctrl Pts',(25.8194671333542,57.3149837826022,40.0127515884775));
#172255=CARTESIAN_POINT('Ctrl Pts',(25.8247266354315,57.3002341019519,39.9946858597757));
#172256=CARTESIAN_POINT('Ctrl Pts',(25.827901340928,57.285821218826,39.9757460620543));
#172257=CARTESIAN_POINT('Ctrl Pts',(25.8290839028447,57.2719197677231,39.9562444559192));
#172258=CARTESIAN_POINT('Ctrl Pts',(25.8302439699455,57.2582827514719,39.9371138113683));
#172259=CARTESIAN_POINT('Ctrl Pts',(25.8294864849003,57.2451370982925,39.9174410654434));
#172260=CARTESIAN_POINT('Ctrl Pts',(25.8268549466948,57.2326665944531,39.8975196504234));
#172261=CARTESIAN_POINT('Ctrl Pts',(25.8251116448908,57.224405322854,39.8843224113834));
#172262=CARTESIAN_POINT('Ctrl Pts',(25.8225450142739,57.216440747915,39.8710160447161));
#172263=CARTESIAN_POINT('Ctrl Pts',(25.8191582032627,57.2088336324696,39.8576902534424));
#172264=CARTESIAN_POINT('',(25.6742415049986,56.8833377255391,39.2875012672119));
#172265=CARTESIAN_POINT('',(25.8191582032627,57.2088336324696,39.8576902534424));
#172266=CARTESIAN_POINT('',(30.9286463962985,54.2060847114738,39.2875012672119));
#172267=CARTESIAN_POINT('Origin',(5.53234440788222E-15,0.,39.2875012672119));
#172268=CARTESIAN_POINT('',(31.1067982185541,54.5146464769134,39.8576902534424));
#172269=CARTESIAN_POINT('',(30.9286463962985,54.2060847114738,39.2875012672119));
#172270=CARTESIAN_POINT('',(31.4638515574747,54.5275217339716,40.1599502534424));
#172271=CARTESIAN_POINT('Ctrl Pts',(31.1067982185541,54.5146464769134,39.8576902534424));
#172272=CARTESIAN_POINT('Ctrl Pts',(31.1129513003045,54.5253036631383,39.8773836120348));
#172273=CARTESIAN_POINT('Ctrl Pts',(31.1207731649983,54.5349507607431,39.8969946442101));
#172274=CARTESIAN_POINT('Ctrl Pts',(31.130109547665,54.5434787028951,39.9162525288194));
#172275=CARTESIAN_POINT('Ctrl Pts',(31.1396335346537,54.5521780046478,39.9358973794001));
#172276=CARTESIAN_POINT('Ctrl Pts',(31.1507339420424,54.5597135487704,39.9551762199662));
#172277=CARTESIAN_POINT('Ctrl Pts',(31.1632971162134,54.5659508935486,39.9738152034151));
#172278=CARTESIAN_POINT('Ctrl Pts',(31.1753722224568,54.5719459231365,39.9917300792537));
#172279=CARTESIAN_POINT('Ctrl Pts',(31.1887993692979,54.5767421714175,40.0090551158002));
#172280=CARTESIAN_POINT('Ctrl Pts',(31.203514327957,54.5801937574243,40.0255394551403));
#172281=CARTESIAN_POINT('Ctrl Pts',(31.2148178485824,54.582845146023,40.0382021526065));
#172282=CARTESIAN_POINT('Ctrl Pts',(31.2268820502,54.5847026428002,40.0503687782083));
#172283=CARTESIAN_POINT('Ctrl Pts',(31.2396897946776,54.5856859723269,40.0619155352442));
#172284=CARTESIAN_POINT('Ctrl Pts',(31.2397233614918,54.5856885494582,40.0619457972351));
#172285=CARTESIAN_POINT('Ctrl Pts',(31.2397569340488,54.5856911200398,40.0619760547304));
#172286=CARTESIAN_POINT('Ctrl Pts',(31.2397905123454,54.5856936840712,40.0620063077269));
#172287=CARTESIAN_POINT('Ctrl Pts',(31.243390788585,54.5859686003822,40.06525004417));
#172288=CARTESIAN_POINT('Ctrl Pts',(31.2470554817647,54.5861671393373,40.0684393223556));
#172289=CARTESIAN_POINT('Ctrl Pts',(31.2507796687845,54.586288957092,40.0715697951759));
#172290=CARTESIAN_POINT('Ctrl Pts',(31.2715039227771,54.586966845199,40.0889901646416));
#172291=CARTESIAN_POINT('Ctrl Pts',(31.294070303672,54.5852738987618,40.1045963098235));
#172292=CARTESIAN_POINT('Ctrl Pts',(31.3175919772518,54.5811905703965,40.1176634650715));
#172293=CARTESIAN_POINT('Ctrl Pts',(31.3281488300912,54.5793579160787,40.1235281853056));
#172294=CARTESIAN_POINT('Ctrl Pts',(31.3388983725506,54.5770440083381,40.1288820140917));
#172295=CARTESIAN_POINT('Ctrl Pts',(31.3497625287432,54.5742478788456,40.1336621774101));
#172296=CARTESIAN_POINT('Ctrl Pts',(31.3544839440762,54.5730327187885,40.1357395717319));
#172297=CARTESIAN_POINT('Ctrl Pts',(31.3592268152918,54.5717264106366,40.1377083672883));
#172298=CARTESIAN_POINT('Ctrl Pts',(31.3639846100475,54.5703288332443,40.1395632548791));
#172299=CARTESIAN_POINT('Ctrl Pts',(31.3806368916924,54.5654373123716,40.1460553614469));
#172300=CARTESIAN_POINT('Ctrl Pts',(31.3974719850968,54.5594277405088,40.1511520974629));
#172301=CARTESIAN_POINT('Ctrl Pts',(31.4142098249422,54.5522949389282,40.1546258197409));
#172302=CARTESIAN_POINT('Ctrl Pts',(31.4225787448649,54.548728538138,40.1563626808798));
#172303=CARTESIAN_POINT('Ctrl Pts',(31.4309233516999,54.5448813304461,40.1576937882008));
#172304=CARTESIAN_POINT('Ctrl Pts',(31.4392086412369,54.5407526753744,40.1585906813668));
#172305=CARTESIAN_POINT('Ctrl Pts',(31.4433512860054,54.5386883478385,40.1590391279498));
#172306=CARTESIAN_POINT('Ctrl Pts',(31.4474791015111,54.5365536585644,40.1593790209175));
#172307=CARTESIAN_POINT('Ctrl Pts',(31.4515877125788,54.5343485280973,40.1596068022931));
#172308=CARTESIAN_POINT('Ctrl Pts',(31.4556963236466,54.5321433976301,40.1598345836687));
#172309=CARTESIAN_POINT('Ctrl Pts',(31.4597857294236,54.529867824492,40.1599502506864));
#172310=CARTESIAN_POINT('Ctrl Pts',(31.4638515574747,54.5275217339716,40.1599502534424));
#172311=CARTESIAN_POINT('',(31.4902932482914,54.5122556166607,40.1599502534424));
#172312=CARTESIAN_POINT('Origin',(5.57749365020894E-15,5.56029328078439E-15,
40.1599502534424));
#172313=CARTESIAN_POINT('',(31.6576696180591,54.1966007261204,39.8576902534424));
#172314=CARTESIAN_POINT('Ctrl Pts',(31.4902932482914,54.5122556166607,40.1599502534424));
#172315=CARTESIAN_POINT('Ctrl Pts',(31.4936024004378,54.5103440004407,40.1599502447858));
#172316=CARTESIAN_POINT('Ctrl Pts',(31.4968786114299,54.5083962906201,40.1598744685927));
#172317=CARTESIAN_POINT('Ctrl Pts',(31.5001207716291,54.5064144237352,40.1597246934279));
#172318=CARTESIAN_POINT('Ctrl Pts',(31.5188564579433,54.4949616780379,40.1588591777433));
#172319=CARTESIAN_POINT('Ctrl Pts',(31.536458384324,54.4823684499298,40.1555254706011));
#172320=CARTESIAN_POINT('Ctrl Pts',(31.5527059087901,54.4690111814044,40.1500631826357));
#172321=CARTESIAN_POINT('Ctrl Pts',(31.5592589091609,54.4636238877412,40.1478601162463));
#172322=CARTESIAN_POINT('Ctrl Pts',(31.5655920544911,54.4581123526882,40.1453112228296));
#172323=CARTESIAN_POINT('Ctrl Pts',(31.5716927188405,54.4525012314181,40.1424401896328));
#172324=CARTESIAN_POINT('Ctrl Pts',(31.5739434935993,54.4504310683342,40.1413809526905));
#172325=CARTESIAN_POINT('Ctrl Pts',(31.5761624901357,54.448347352793,40.1402777640511));
#172326=CARTESIAN_POINT('Ctrl Pts',(31.5783490084914,54.4462513257022,40.1391317641987));
#172327=CARTESIAN_POINT('Ctrl Pts',(31.5824487304082,54.442321274907,40.1369830144753));
#172328=CARTESIAN_POINT('Ctrl Pts',(31.5864342712177,54.4383479413151,40.134683756585));
#172329=CARTESIAN_POINT('Ctrl Pts',(31.5903010169876,54.4343395048291,40.1322415082996));
#172330=CARTESIAN_POINT('Ctrl Pts',(31.6038346271825,54.420309977128,40.1236936393009));
#172331=CARTESIAN_POINT('Ctrl Pts',(31.6159129958993,54.4058504350953,40.113394140767));
#172332=CARTESIAN_POINT('Ctrl Pts',(31.6263383134323,54.3913116139982,40.101665321223));
#172333=CARTESIAN_POINT('Ctrl Pts',(31.6315509721988,54.3840422034496,40.095800911451));
#172334=CARTESIAN_POINT('Ctrl Pts',(31.6363503686743,54.37675297401,40.0895791707949));
#172335=CARTESIAN_POINT('Ctrl Pts',(31.6407117811311,54.3694877752599,40.0830403822906));
#172336=CARTESIAN_POINT('Ctrl Pts',(31.6428924873595,54.3658551758849,40.0797709880385));
#172337=CARTESIAN_POINT('Ctrl Pts',(31.6449636976428,54.3622285842835,40.0764223317514));
#172338=CARTESIAN_POINT('Ctrl Pts',(31.6469223220359,54.3586134821113,40.0729994484778));
#172339=CARTESIAN_POINT('Ctrl Pts',(31.648880946429,54.3549983799391,40.0695765652042));
#172340=CARTESIAN_POINT('Ctrl Pts',(31.6507268563406,54.3513947831117,40.0660793733488));
#172341=CARTESIAN_POINT('Ctrl Pts',(31.6524572252922,54.3478081421434,40.0625130768817));
#172342=CARTESIAN_POINT('Ctrl Pts',(31.6524719817154,54.3477775556075,40.0624826638418));
#172343=CARTESIAN_POINT('Ctrl Pts',(31.6524867297711,54.3477469704397,40.0624522459912));
#172344=CARTESIAN_POINT('Ctrl Pts',(31.6525014694581,54.3477163866428,40.0624218233329));
#172345=CARTESIAN_POINT('Ctrl Pts',(31.660029242797,54.3320967950481,40.0468845275927));
#172346=CARTESIAN_POINT('Ctrl Pts',(31.6655043152774,54.3168578829737,40.0302263329298));
#172347=CARTESIAN_POINT('Ctrl Pts',(31.6690725678669,54.3021370826415,40.0127515884839));
#172348=CARTESIAN_POINT('Ctrl Pts',(31.6727614963895,54.286918434617,39.9946858597844));
#172349=CARTESIAN_POINT('Ctrl Pts',(31.6744122539932,54.2722526596876,39.9757460620654));
#172350=CARTESIAN_POINT('Ctrl Pts',(31.674135240392,54.2583037508099,39.956244455933));
#172351=CARTESIAN_POINT('Ctrl Pts',(31.6738634961724,54.2446201795303,39.9371138113845));
#172352=CARTESIAN_POINT('Ctrl Pts',(31.6717360657854,54.2316257183632,39.9174410654619));
#172353=CARTESIAN_POINT('Ctrl Pts',(31.6678154208207,54.219498599894,39.8975196504443));
#172354=CARTESIAN_POINT('Ctrl Pts',(31.665218130981,54.2114648090591,39.8843224113974));
#172355=CARTESIAN_POINT('Ctrl Pts',(31.6618330358548,54.2038121508449,39.8710160447231));
#172356=CARTESIAN_POINT('Ctrl Pts',(31.6576696180591,54.1966007261204,39.8576902534424));
#172357=CARTESIAN_POINT('',(31.4795232016796,53.8880358395967,39.2875012672119));
#172358=CARTESIAN_POINT('',(31.6576696180591,54.1966007261204,39.8576902534424));
#172359=CARTESIAN_POINT('',(36.4252947698685,50.6762142289944,39.2875012672119));
#172360=CARTESIAN_POINT('Origin',(5.53234440788222E-15,0.,39.2875012672119));
#172361=CARTESIAN_POINT('',(36.634724144966,50.9644637245889,39.8576902534424));
#172362=CARTESIAN_POINT('',(36.4252947698685,50.6762142289944,39.2875012672119));
#172363=CARTESIAN_POINT('',(36.9911673391713,50.9399462128198,40.1599502534424));
#172364=CARTESIAN_POINT('Ctrl Pts',(36.634724144966,50.9644637245889,39.8576902534424));
#172365=CARTESIAN_POINT('Ctrl Pts',(36.6419574987908,50.9744193574547,39.8773836120385));
#172366=CARTESIAN_POINT('Ctrl Pts',(36.6507449107808,50.9831959997547,39.8969946442174));
#172367=CARTESIAN_POINT('Ctrl Pts',(36.6609215604567,50.9907013072156,39.9162525288302));
#172368=CARTESIAN_POINT('Ctrl Pts',(36.6713026986945,50.9983574255601,39.9358973794146));
#172369=CARTESIAN_POINT('Ctrl Pts',(36.6831299757402,51.004691380658,39.9551762199843));
#172370=CARTESIAN_POINT('Ctrl Pts',(36.6962763075968,51.0095813473188,39.9738152034364));
#172371=CARTESIAN_POINT('Ctrl Pts',(36.7089119163785,51.0142813432078,39.9917300792784));
#172372=CARTESIAN_POINT('Ctrl Pts',(36.7227668523708,51.0176477981128,40.0090551158278));
#172373=CARTESIAN_POINT('Ctrl Pts',(36.7377619899324,51.0195423439532,40.0255394551704));
#172374=CARTESIAN_POINT('Ctrl Pts',(36.7492807342569,51.0209976683247,40.0382021526258));
#172375=CARTESIAN_POINT('Ctrl Pts',(36.7614730081902,51.0215839370833,40.0503687782175));
#172376=CARTESIAN_POINT('Ctrl Pts',(36.7743133764177,51.0212231059801,40.0619155352442));
#172377=CARTESIAN_POINT('Ctrl Pts',(36.7743470287329,51.0212221603061,40.0619457972352));
#172378=CARTESIAN_POINT('Ctrl Pts',(36.7743806860749,51.021221207518,40.0619760547305));
#172379=CARTESIAN_POINT('Ctrl Pts',(36.7744143484403,51.0212202476157,40.062006307727));
#172380=CARTESIAN_POINT('Ctrl Pts',(36.7780236385695,51.0211173265636,40.06525004417));
#172381=CARTESIAN_POINT('Ctrl Pts',(36.7816890091485,51.0209317131551,40.0684393223556));
#172382=CARTESIAN_POINT('Ctrl Pts',(36.7854055281047,51.0206635800333,40.0715697951759));
#172383=CARTESIAN_POINT('Ctrl Pts',(36.8060871110678,51.0191714801762,40.0889901646418));
#172384=CARTESIAN_POINT('Ctrl Pts',(36.8283529098778,51.0151289787602,40.1045963098238));
#172385=CARTESIAN_POINT('Ctrl Pts',(36.8513189052297,51.008609334902,40.1176634650719));
#172386=CARTESIAN_POINT('Ctrl Pts',(36.861626361985,51.0056832284521,40.1235281853059));
#172387=CARTESIAN_POINT('Ctrl Pts',(36.8720751481056,51.0022583633862,40.1288820140918));
#172388=CARTESIAN_POINT('Ctrl Pts',(36.8825875141947,50.9983419378321,40.1336621774101));
#172389=CARTESIAN_POINT('Ctrl Pts',(36.8871560463071,50.9966399122597,40.1357395717319));
#172390=CARTESIAN_POINT('Ctrl Pts',(36.8917363891942,50.9948449951609,40.1377083672884));
#172391=CARTESIAN_POINT('Ctrl Pts',(36.8963220336353,50.9929577488695,40.1395632548792));
#172392=CARTESIAN_POINT('Ctrl Pts',(36.9123717891792,50.9863523868496,40.146055361447));
#172393=CARTESIAN_POINT('Ctrl Pts',(36.9284864868686,50.9786159896077,40.1511520974629));
#172394=CARTESIAN_POINT('Ctrl Pts',(36.9443870542881,50.9697726815831,40.1546258197408));
#172395=CARTESIAN_POINT('Ctrl Pts',(36.9523373379978,50.9653510275708,40.1563626808798));
#172396=CARTESIAN_POINT('Ctrl Pts',(36.9602340894955,50.9606526463562,40.1576937882008));
#172397=CARTESIAN_POINT('Ctrl Pts',(36.9680424293795,50.9556805599059,40.1585906813668));
#172398=CARTESIAN_POINT('Ctrl Pts',(36.9719465993215,50.9531945166808,40.1590391279498));
#172399=CARTESIAN_POINT('Ctrl Pts',(36.9758286664326,50.9506400472465,40.1593790209175));
#172400=CARTESIAN_POINT('Ctrl Pts',(36.9796842712,50.9480175299136,40.1596068022931));
#172401=CARTESIAN_POINT('Ctrl Pts',(36.9835398759674,50.9453950125808,40.1598345836687));
#172402=CARTESIAN_POINT('Ctrl Pts',(36.9873690173885,50.942704445969,40.1599502506864));
#172403=CARTESIAN_POINT('Ctrl Pts',(36.9911673391713,50.9399462128198,40.1599502534424));
#172404=CARTESIAN_POINT('',(37.0158684358566,50.9219998155896,40.1599502534424));
#172405=CARTESIAN_POINT('Origin',(5.56385071146069E-15,5.56915310880103E-15,
40.1599502534424));
#172406=CARTESIAN_POINT('',(37.1493329797267,50.590578520848,39.8576902534424));
#172407=CARTESIAN_POINT('Ctrl Pts',(37.0158684358566,50.9219998155896,40.1599502534424));
#172408=CARTESIAN_POINT('Ctrl Pts',(37.0189596418154,50.9197527708146,40.1599502447858));
#172409=CARTESIAN_POINT('Ctrl Pts',(37.0220143142664,50.9174732734519,40.1598744685927));
#172410=CARTESIAN_POINT('Ctrl Pts',(37.025031552073,50.9151633654179,40.1597246934279));
#172411=CARTESIAN_POINT('Ctrl Pts',(37.0424674644282,50.901814946562,40.1588591777434));
#172412=CARTESIAN_POINT('Ctrl Pts',(37.0586566148318,50.8874508031609,40.1555254706015));
#172413=CARTESIAN_POINT('Ctrl Pts',(37.0734189189057,50.8724683783868,40.1500631826367));
#172414=CARTESIAN_POINT('Ctrl Pts',(37.079372895728,50.8664256218225,40.1478601162471));
#172415=CARTESIAN_POINT('Ctrl Pts',(37.085095235137,50.8602822855852,40.1453112228301));
#172416=CARTESIAN_POINT('Ctrl Pts',(37.090575957526,50.8540642095543,40.1424401896328));
#172417=CARTESIAN_POINT('Ctrl Pts',(37.0925980113393,50.8517701170137,40.1413809526906));
#172418=CARTESIAN_POINT('Ctrl Pts',(37.0945870443971,50.8494658679862,40.1402777640511));
#172419=CARTESIAN_POINT('Ctrl Pts',(37.0965424902857,50.8471527697475,40.1391317641987));
#172420=CARTESIAN_POINT('Ctrl Pts',(37.1002089513267,50.84281571055,40.1369830144753));
#172421=CARTESIAN_POINT('Ctrl Pts',(37.1037573324722,50.8384475408391,40.1346837565849));
#172422=CARTESIAN_POINT('Ctrl Pts',(37.1071839000983,50.8340568779944,40.1322415082996));
#172423=CARTESIAN_POINT('Ctrl Pts',(37.1191768867895,50.8186895580379,40.1236936393008));
#172424=CARTESIAN_POINT('Ctrl Pts',(37.1296776552305,50.8030466935687,40.113394140767));
#172425=CARTESIAN_POINT('Ctrl Pts',(37.1385261411562,50.7874977752339,40.101665321223));
#172426=CARTESIAN_POINT('Ctrl Pts',(37.1429503841191,50.7797233160665,40.095800911451));
#172427=CARTESIAN_POINT('Ctrl Pts',(37.1469615570468,50.7719723442503,40.0895791707949));
#172428=CARTESIAN_POINT('Ctrl Pts',(37.1505396571691,50.7642910532773,40.0830403822906));
#172429=CARTESIAN_POINT('Ctrl Pts',(37.1523287072303,50.7604504077909,40.0797709880385));
#172430=CARTESIAN_POINT('Ctrl Pts',(37.1540094891599,50.7566271826096,40.0764223317514));
#172431=CARTESIAN_POINT('Ctrl Pts',(37.1555795029291,50.7528271523475,40.0729994484778));
#172432=CARTESIAN_POINT('Ctrl Pts',(37.1571495166982,50.7490271220854,40.0695765652042));
#172433=CARTESIAN_POINT('Ctrl Pts',(37.1586086360836,50.7452503160121,40.0660793733488));
#172434=CARTESIAN_POINT('Ctrl Pts',(37.1599546198243,50.7415024502308,40.0625130768817));
#172435=CARTESIAN_POINT('Ctrl Pts',(37.1599660982467,50.741470488785,40.0624826638418));
#172436=CARTESIAN_POINT('Ctrl Pts',(37.1599775684904,50.7414385295743,40.0624522459912));
#172437=CARTESIAN_POINT('Ctrl Pts',(37.1599890305545,50.7414065726018,40.0624218233329));
#172438=CARTESIAN_POINT('Ctrl Pts',(37.1658428740582,50.7250856801826,40.0468845275902));
#172439=CARTESIAN_POINT('Ctrl Pts',(37.1696950534579,50.709357947548,40.0302263329246));
#172440=CARTESIAN_POINT('Ctrl Pts',(37.1717050161492,50.6943448053385,40.0127515884756));
#172441=CARTESIAN_POINT('Ctrl Pts',(37.1737829544441,50.6788239286284,39.9946858597729));
#172442=CARTESIAN_POINT('Ctrl Pts',(37.1738916781079,50.664065943191,39.9757460620504));
#172443=CARTESIAN_POINT('Ctrl Pts',(37.1721581240054,50.6502224036999,39.9562444559144));
#172444=CARTESIAN_POINT('Ctrl Pts',(37.1704575457498,50.6366421974596,39.9371138113623));
#172445=CARTESIAN_POINT('Ctrl Pts',(37.1669834785902,50.6239412983381,39.9174410654362));
#172446=CARTESIAN_POINT('Ctrl Pts',(37.1618166822689,50.612290432485,39.897519650415));
#172447=CARTESIAN_POINT('Ctrl Pts',(37.158393860846,50.6045721423189,39.8843224113778));
#172448=CARTESIAN_POINT('Ctrl Pts',(37.1542273890247,50.5973152449643,39.8710160447133));
#172449=CARTESIAN_POINT('Ctrl Pts',(37.1493329797266,50.590578520848,39.8576902534424));
#172450=CARTESIAN_POINT('',(36.9399086546492,50.3023253561991,39.2875012672119));
#172451=CARTESIAN_POINT('',(37.1493329797266,50.590578520848,39.8576902534424));
#172452=CARTESIAN_POINT('',(41.5228599914568,46.5911245387425,39.2875012672119));
#172453=CARTESIAN_POINT('Origin',(5.53234440788222E-15,0.,39.2875012672119));
#172454=CARTESIAN_POINT('',(41.7612723673368,46.855903642698,39.8576902534424));
#172455=CARTESIAN_POINT('',(41.5228599914568,46.5911245387425,39.2875012672119));
#172456=CARTESIAN_POINT('',(42.1132001506006,46.7942619810912,40.1599502534424));
#172457=CARTESIAN_POINT('Ctrl Pts',(41.7612723673368,46.855903642698,39.8576902534424));
#172458=CARTESIAN_POINT('Ctrl Pts',(41.7695067430961,46.8650486462045,39.8773836120362));
#172459=CARTESIAN_POINT('Ctrl Pts',(41.779163425655,46.8728586744673,39.8969946442129));
#172460=CARTESIAN_POINT('Ctrl Pts',(41.7900688448329,46.8792591175164,39.9162525288236));
#172461=CARTESIAN_POINT('Ctrl Pts',(41.8011933963927,46.885788170416,39.9358973794055));
#172462=CARTESIAN_POINT('Ctrl Pts',(41.8136179609679,46.8908511403508,39.9551762199728));
#172463=CARTESIAN_POINT('Ctrl Pts',(41.8272034165412,46.8943401533964,39.9738152034229));
#172464=CARTESIAN_POINT('Ctrl Pts',(41.8402610894808,46.897693621448,39.9917300792622));
#172465=CARTESIAN_POINT('Ctrl Pts',(41.8543920170388,46.8995933993937,40.0090551158092));
#172466=CARTESIAN_POINT('Ctrl Pts',(41.8695030436299,46.8999101480293,40.0255394551499));
#172467=CARTESIAN_POINT('Ctrl Pts',(41.8811108098934,46.9001534633397,40.0382021526126));
#172468=CARTESIAN_POINT('Ctrl Pts',(41.893297575053,46.899462080799,40.0503687782112));
#172469=CARTESIAN_POINT('Ctrl Pts',(41.906029885286,46.8977610424068,40.0619155352442));
#172470=CARTESIAN_POINT('Ctrl Pts',(41.9060632544005,46.8977565842885,40.0619457972351));
#172471=CARTESIAN_POINT('Ctrl Pts',(41.9060966277705,46.8977521185696,40.0619760547305));
#172472=CARTESIAN_POINT('Ctrl Pts',(41.9061300053929,46.8977476452504,40.0620063077269));
#172473=CARTESIAN_POINT('Ctrl Pts',(41.9097087652737,46.89726801446,40.06525004417));
#172474=CARTESIAN_POINT('Ctrl Pts',(41.9133346546847,46.8967002823072,40.0684393223556));
#172475=CARTESIAN_POINT('Ctrl Pts',(41.9170027866181,46.8960451360315,40.0715697951759));
#172476=CARTESIAN_POINT('Ctrl Pts',(41.9374151068048,46.8923993959677,40.0889901646453));
#172477=CARTESIAN_POINT('Ctrl Pts',(41.959136374783,46.8860516300625,40.10459630983));
#172478=CARTESIAN_POINT('Ctrl Pts',(41.9812950716606,46.8771671012912,40.1176634650798));
#172479=CARTESIAN_POINT('Ctrl Pts',(41.9912402016744,46.8731796017451,40.1235281853107));
#172480=CARTESIAN_POINT('Ctrl Pts',(42.0012737523646,46.8686813028939,40.128882014094));
#172481=CARTESIAN_POINT('Ctrl Pts',(42.0113191526632,46.8636874904585,40.1336621774102));
#172482=CARTESIAN_POINT('Ctrl Pts',(42.0156847477611,46.8615172471192,40.135739571732));
#172483=CARTESIAN_POINT('Ctrl Pts',(42.0200523791246,46.8592533865608,40.1377083672884));
#172484=CARTESIAN_POINT('Ctrl Pts',(42.024415631971,46.8568971484355,40.1395632548792));
#172485=CARTESIAN_POINT('Ctrl Pts',(42.0396870169335,46.8486503149971,40.146055361447));
#172486=CARTESIAN_POINT('Ctrl Pts',(42.0549047629079,46.8392718539633,40.151152097463));
#172487=CARTESIAN_POINT('Ctrl Pts',(42.0697938479573,46.8288149286279,40.1546258197409));
#172488=CARTESIAN_POINT('Ctrl Pts',(42.077238390482,46.8235864659602,40.1563626808798));
#172489=CARTESIAN_POINT('Ctrl Pts',(42.0846007681805,46.8180883876706,40.1576937882008));
#172490=CARTESIAN_POINT('Ctrl Pts',(42.0918466086057,46.8123273450614,40.1585906813668));
#172491=CARTESIAN_POINT('Ctrl Pts',(42.0954695288184,46.8094468237568,40.1590391279498));
#172492=CARTESIAN_POINT('Ctrl Pts',(42.0990633147952,46.8065005614639,40.1593790209175));
#172493=CARTESIAN_POINT('Ctrl Pts',(42.1026236704495,46.8034893901141,40.1596068022931));
#172494=CARTESIAN_POINT('Ctrl Pts',(42.1061840261039,46.8004782187644,40.1598345836687));
#172495=CARTESIAN_POINT('Ctrl Pts',(42.1097109502944,46.7974021370896,40.1599502506864));
#172496=CARTESIAN_POINT('Ctrl Pts',(42.1132001506006,46.7942619810912,40.1599502534424));
#172497=CARTESIAN_POINT('',(42.1358900227701,46.7738319284252,40.1599502534424));
#172498=CARTESIAN_POINT('Origin',(5.55120861436579E-15,5.57939047717458E-15,
40.1599502534424));
#172499=CARTESIAN_POINT('',(42.2339804752707,46.430275350542,39.8576902534424));
#172500=CARTESIAN_POINT('Ctrl Pts',(42.1358900227701,46.7738319284252,40.1599502534424));
#172501=CARTESIAN_POINT('Ctrl Pts',(42.138729414642,46.7712740741881,40.1599502447857));
#172502=CARTESIAN_POINT('Ctrl Pts',(42.1415290809214,46.7686877639334,40.1598744685927));
#172503=CARTESIAN_POINT('Ctrl Pts',(42.1442883388465,46.766075122586,40.1597246934279));
#172504=CARTESIAN_POINT('Ctrl Pts',(42.1602334457308,46.7509772786493,40.1588591777438));
#172505=CARTESIAN_POINT('Ctrl Pts',(42.1748324484317,46.7349995965244,40.1555254706051));
#172506=CARTESIAN_POINT('Ctrl Pts',(42.1879477932161,46.718556166091,40.1500631826455));
#172507=CARTESIAN_POINT('Ctrl Pts',(42.1932375134805,46.7119241523232,40.1478601162538));
#172508=CARTESIAN_POINT('Ctrl Pts',(42.1982863518264,46.705216322571,40.1453112228339));
#172509=CARTESIAN_POINT('Ctrl Pts',(42.2030870843191,46.6984594183133,40.1424401896328));
#172510=CARTESIAN_POINT('Ctrl Pts',(42.2048582631421,46.6959665308739,40.1413809526905));
#172511=CARTESIAN_POINT('Ctrl Pts',(42.2065955404589,46.6934669941948,40.1402777640511));
#172512=CARTESIAN_POINT('Ctrl Pts',(42.208298489606,46.6909621675966,40.1391317641986));
#172513=CARTESIAN_POINT('Ctrl Pts',(42.2114915192568,46.6862656177249,40.1369830144753));
#172514=CARTESIAN_POINT('Ctrl Pts',(42.214563863932,46.6815504704765,40.1346837565849));
#172515=CARTESIAN_POINT('Ctrl Pts',(42.2175127112221,46.676825686294,40.1322415082996));
#172516=CARTESIAN_POINT('Ctrl Pts',(42.2278336767378,46.6602889416554,40.1236936393008));
#172517=CARTESIAN_POINT('Ctrl Pts',(42.2366417962865,46.6436341412461,40.113394140767));
#172518=CARTESIAN_POINT('Ctrl Pts',(42.2438165047415,46.6272454828769,40.101665321223));
#172519=CARTESIAN_POINT('Ctrl Pts',(42.247403858969,46.6190511536923,40.095800911451));
#172520=CARTESIAN_POINT('Ctrl Pts',(42.2505828610989,46.6109233607685,40.0895791707949));
#172521=CARTESIAN_POINT('Ctrl Pts',(42.253338446473,46.6029101354041,40.0830403822906));
#172522=CARTESIAN_POINT('Ctrl Pts',(42.2547162391601,46.5989035227218,40.0797709880385));
#172523=CARTESIAN_POINT('Ctrl Pts',(42.2559881777376,46.594925552016,40.0764223317514));
#172524=CARTESIAN_POINT('Ctrl Pts',(42.2571523794834,46.5909822275907,40.0729994484778));
#172525=CARTESIAN_POINT('Ctrl Pts',(42.2583165812292,46.5870389031653,40.0695765652042));
#172526=CARTESIAN_POINT('Ctrl Pts',(42.2593729236709,46.5831302673238,40.0660793733488));
#172527=CARTESIAN_POINT('Ctrl Pts',(42.2603197753212,46.5792622391315,40.0625130768816));
#172528=CARTESIAN_POINT('Ctrl Pts',(42.2603278499828,46.5792292529519,40.0624826638418));
#172529=CARTESIAN_POINT('Ctrl Pts',(42.2603359167441,46.5791962698501,40.0624522459912));
#172530=CARTESIAN_POINT('Ctrl Pts',(42.2603439756046,46.5791632898293,40.0624218233329));
#172531=CARTESIAN_POINT('Ctrl Pts',(42.2644597533381,46.5623199116979,40.0468845275875));
#172532=CARTESIAN_POINT('Ctrl Pts',(42.2666468343731,46.5462756748327,40.0302263329187));
#172533=CARTESIAN_POINT('Ctrl Pts',(42.267076485594,46.5311346778733,40.0127515884664));
#172534=CARTESIAN_POINT('Ctrl Pts',(42.2675206673339,46.515481622451,39.9946858597607));
#172535=CARTESIAN_POINT('Ctrl Pts',(42.2660861658584,46.5007931180827,39.975746062035));
#172536=CARTESIAN_POINT('Ctrl Pts',(42.2629150644359,46.4872066206944,39.9562444558956));
#172537=CARTESIAN_POINT('Ctrl Pts',(42.2598042840353,46.4738785670757,39.937113811341));
#172538=CARTESIAN_POINT('Ctrl Pts',(42.25502164271,46.4616103837094,39.9174410654122));
#172539=CARTESIAN_POINT('Ctrl Pts',(42.248665303534,46.4505634197978,39.8975196503884));
#172540=CARTESIAN_POINT('Ctrl Pts',(42.2444544516767,46.4432451935018,39.8843224113599));
#172541=CARTESIAN_POINT('Ctrl Pts',(42.2395522518982,46.4364635650919,39.8710160447043));
#172542=CARTESIAN_POINT('Ctrl Pts',(42.2339804752707,46.430275350542,39.8576902534424));
#172543=CARTESIAN_POINT('',(41.9955727382256,46.1654920697607,39.2875012672119));
#172544=CARTESIAN_POINT('',(42.2339804752707,46.430275350542,39.8576902534424));
#172545=CARTESIAN_POINT('',(46.1654920697617,41.9955727382246,39.2875012672119));
#172546=CARTESIAN_POINT('Origin',(5.53234440788222E-15,0.,39.2875012672119));
#172547=CARTESIAN_POINT('',(46.430275350543,42.2339804752696,39.8576902534424));
#172548=CARTESIAN_POINT('',(46.1654920697617,41.9955727382246,39.2875012672119));
#172549=CARTESIAN_POINT('',(46.7738319284262,42.1358900227689,40.1599502534424));
#172550=CARTESIAN_POINT('Ctrl Pts',(46.430275350543,42.2339804752696,39.8576902534424));
#172551=CARTESIAN_POINT('Ctrl Pts',(46.4394205306927,42.2422146548452,39.8773836120346));
#172552=CARTESIAN_POINT('Ctrl Pts',(46.4498406831856,42.2489725007674,39.8969946442096));
#172553=CARTESIAN_POINT('Ctrl Pts',(46.4613553898112,42.2541979548116,39.9162525288188));
#172554=CARTESIAN_POINT('Ctrl Pts',(46.4731014717785,42.2595284085969,39.935897379399));
#172555=CARTESIAN_POINT('Ctrl Pts',(46.4859871977545,42.2632649224109,39.9551762199648));
#172556=CARTESIAN_POINT('Ctrl Pts',(46.4998629319511,42.2653147554846,39.9738152034134));
#172557=CARTESIAN_POINT('Ctrl Pts',(46.5131996064525,42.2672849544014,39.9917300792513));
#172558=CARTESIAN_POINT('Ctrl Pts',(46.5274517041783,42.2676972410233,40.009055115797));
#172559=CARTESIAN_POINT('Ctrl Pts',(46.5425130602309,42.2664327220898,40.0255394551366));
#172560=CARTESIAN_POINT('Ctrl Pts',(46.5540826713154,42.2654613625244,40.0382021526041));
#172561=CARTESIAN_POINT('Ctrl Pts',(46.56613040695,42.2634999036149,40.0503687782072));
#172562=CARTESIAN_POINT('Ctrl Pts',(46.5786151613306,42.2604772948654,40.0619155352442));
#172563=CARTESIAN_POINT('Ctrl Pts',(46.5786478816453,42.260469373147,40.0619457972351));
#172564=CARTESIAN_POINT('Ctrl Pts',(46.5786806053978,42.2604614434247,40.0619760547305));
#172565=CARTESIAN_POINT('Ctrl Pts',(46.5787133325848,42.2604535056992,40.0620063077269));
#172566=CARTESIAN_POINT('Ctrl Pts',(46.5822223525751,42.2596024201057,40.06525004417));
#172567=CARTESIAN_POINT('Ctrl Pts',(46.5857690348151,42.2586587894009,40.0684393223556));
#172568=CARTESIAN_POINT('Ctrl Pts',(46.5893485909045,42.257623807891,40.0715697951758));
#172569=CARTESIAN_POINT('Ctrl Pts',(46.6092680066565,42.2518643711126,40.088990164643));
#172570=CARTESIAN_POINT('Ctrl Pts',(46.630206761038,42.2432808881728,40.104596309826));
#172571=CARTESIAN_POINT('Ctrl Pts',(46.6513153841135,42.2321288152491,40.1176634650747));
#172572=CARTESIAN_POINT('Ctrl Pts',(46.6607892264673,42.2271236104843,40.1235281853076));
#172573=CARTESIAN_POINT('Ctrl Pts',(46.6702976120535,42.2216011621487,40.1288820140926));
#172574=CARTESIAN_POINT('Ctrl Pts',(46.6797659870611,42.2155846760824,40.1336621774101));
#172575=CARTESIAN_POINT('Ctrl Pts',(46.6838808147711,42.2129699926164,40.1357395717319));
#172576=CARTESIAN_POINT('Ctrl Pts',(46.6879878819278,42.2102619919285,40.1377083672883));
#172577=CARTESIAN_POINT('Ctrl Pts',(46.6920809384683,42.2074625774073,40.1395632548791));
#172578=CARTESIAN_POINT('Ctrl Pts',(46.7064066363599,42.1976646265833,40.1460553614469));
#172579=CARTESIAN_POINT('Ctrl Pts',(46.72056070181,42.1867468541392,40.1511520974629));
#172580=CARTESIAN_POINT('Ctrl Pts',(46.7342751765578,42.1747908797552,40.1546258197408));
#172581=CARTESIAN_POINT('Ctrl Pts',(46.7411324139317,42.1688128925632,40.1563626808798));
#172582=CARTESIAN_POINT('Ctrl Pts',(46.7478797540803,42.1625753552949,40.1576937882008));
#172583=CARTESIAN_POINT('Ctrl Pts',(46.7544837081028,42.1560884757152,40.1585906813668));
#172584=CARTESIAN_POINT('Ctrl Pts',(46.7577856851141,42.1528450359254,40.1590391279498));
#172585=CARTESIAN_POINT('Ctrl Pts',(46.7610518156854,42.1495392606401,40.1593790209175));
#172586=CARTESIAN_POINT('Ctrl Pts',(46.7642779142251,42.1461724262968,40.1596068022931));
#172587=CARTESIAN_POINT('Ctrl Pts',(46.7675040127649,42.1428055919535,40.1598345836686));
#172588=CARTESIAN_POINT('Ctrl Pts',(46.7706900780053,42.1393776974103,40.1599502506865));
#172589=CARTESIAN_POINT('Ctrl Pts',(46.7738319284262,42.1358900227689,40.1599502534424));
#172590=CARTESIAN_POINT('',(46.7942619810922,42.1132001505995,40.1599502534424));
#172591=CARTESIAN_POINT('Origin',(5.53970586838553E-15,5.59089322315484E-15,
40.1599502534424));
#172592=CARTESIAN_POINT('',(46.855903642699,41.7612723673357,39.8576902534424));
#172593=CARTESIAN_POINT('Ctrl Pts',(46.7942619810922,42.1132001505995,40.1599502534424));
#172594=CARTESIAN_POINT('Ctrl Pts',(46.7968184499057,42.1103595112866,40.1599502447858));
#172595=CARTESIAN_POINT('Ctrl Pts',(46.7993324362838,42.1074947242962,40.1598744685927));
#172596=CARTESIAN_POINT('Ctrl Pts',(46.8018034833201,42.1046079742808,40.1597246934279));
#172597=CARTESIAN_POINT('Ctrl Pts',(46.8160830868243,42.087926120383,40.1588591777433));
#172598=CARTESIAN_POINT('Ctrl Pts',(46.828931992109,42.0705099543436,40.1555254706008));
#172599=CARTESIAN_POINT('Ctrl Pts',(46.8402566831536,42.0527856758954,40.1500631826351));
#172600=CARTESIAN_POINT('Ctrl Pts',(46.8448241915615,42.0456370666737,40.1478601162458));
#172601=CARTESIAN_POINT('Ctrl Pts',(46.8491442126995,42.0384382358125,40.1453112228294));
#172602=CARTESIAN_POINT('Ctrl Pts',(46.8532123574524,42.0312165334046,40.1424401896328));
#172603=CARTESIAN_POINT('Ctrl Pts',(46.8547132558794,42.0285521636629,40.1413809526906));
#172604=CARTESIAN_POINT('Ctrl Pts',(46.8561797434814,42.0258847247791,40.1402777640512));
#172605=CARTESIAN_POINT('Ctrl Pts',(46.8576115380198,42.0232156132257,40.1391317641987));
#172606=CARTESIAN_POINT('Ctrl Pts',(46.8602961527793,42.018211029063,40.1369830144753));
#172607=CARTESIAN_POINT('Ctrl Pts',(46.8628587997329,42.0132005644171,40.134683756585));
#172608=CARTESIAN_POINT('Ctrl Pts',(46.8652976184992,42.0081934246211,40.1322415082996));
#172609=CARTESIAN_POINT('Ctrl Pts',(46.8738334841813,41.990668435335,40.1236936393009));
#172610=CARTESIAN_POINT('Ctrl Pts',(46.8808524512367,41.9731841724643,40.113394140767));
#172611=CARTESIAN_POINT('Ctrl Pts',(46.8862747746138,41.9561353316312,40.101665321223));
#172612=CARTESIAN_POINT('Ctrl Pts',(46.8889859363023,41.9476109112146,40.095800911451));
#172613=CARTESIAN_POINT('Ctrl Pts',(46.8912979378218,41.9391953469836,40.0895791707949));
#172614=CARTESIAN_POINT('Ctrl Pts',(46.8932008176778,41.9309379818015,40.0830403822906));
#172615=CARTESIAN_POINT('Ctrl Pts',(46.8941522576058,41.9268092992105,40.0797709880385));
#172616=CARTESIAN_POINT('Ctrl Pts',(46.8950014172059,41.9227201664596,40.0764223317514));
#172617=CARTESIAN_POINT('Ctrl Pts',(46.8957470516903,41.9186767517586,40.0729994484778));
#172618=CARTESIAN_POINT('Ctrl Pts',(46.8964926861748,41.9146333370576,40.0695765652042));
#172619=CARTESIAN_POINT('Ctrl Pts',(46.8971346781641,41.91063569528,40.0660793733488));
#172620=CARTESIAN_POINT('Ctrl Pts',(46.8976720238192,41.9066898836029,40.0625130768817));
#172621=CARTESIAN_POINT('Ctrl Pts',(46.8976766062523,41.9066562340931,40.0624826638418));
#172622=CARTESIAN_POINT('Ctrl Pts',(46.8976811811501,41.9066225884701,40.0624522459912));
#172623=CARTESIAN_POINT('Ctrl Pts',(46.8976857485125,41.906588946737,40.0624218233329));
#172624=CARTESIAN_POINT('Ctrl Pts',(46.9000183671521,41.889407622475,40.0468845275904));
#172625=CARTESIAN_POINT('Ctrl Pts',(46.9005163877048,41.8732226654012,40.030226332925));
#172626=CARTESIAN_POINT('Ctrl Pts',(46.8993610201077,41.858119701628,40.0127515884763));
#172627=CARTESIAN_POINT('Ctrl Pts',(46.8981665787457,41.8425059656487,39.994685859774));
#172628=CARTESIAN_POINT('Ctrl Pts',(46.8952045688315,41.8280478726808,39.9757460620521));
#172629=CARTESIAN_POINT('Ctrl Pts',(46.8906306633432,41.8148672739068,39.9562444559166));
#172630=CARTESIAN_POINT('Ctrl Pts',(46.8861437631619,41.8019373978563,39.9371138113654));
#172631=CARTESIAN_POINT('Ctrl Pts',(46.8801049472942,41.7902363430309,39.9174410654402));
#172632=CARTESIAN_POINT('Ctrl Pts',(46.8726287066505,41.7799143139099,39.8975196504199));
#172633=CARTESIAN_POINT('Ctrl Pts',(46.8676759593288,41.7730763314905,39.8843224113811));
#172634=CARTESIAN_POINT('Ctrl Pts',(46.8620917411135,41.7668442729547,39.871016044715));
#172635=CARTESIAN_POINT('Ctrl Pts',(46.855903642699,41.7612723673357,39.8576902534424));
#172636=CARTESIAN_POINT('',(46.5911245387435,41.5228599914557,39.2875012672119));
#172637=CARTESIAN_POINT('',(46.855903642699,41.7612723673357,39.8576902534424));
#172638=CARTESIAN_POINT('',(50.3023253562,36.939908654648,39.2875012672119));
#172639=CARTESIAN_POINT('Origin',(5.53234440788222E-15,0.,39.2875012672119));
#172640=CARTESIAN_POINT('',(50.5905785208489,37.1493329797255,39.8576902534424));
#172641=CARTESIAN_POINT('',(50.3023253562,36.939908654648,39.2875012672119));
#172642=CARTESIAN_POINT('',(50.9219998155904,37.0158684358554,40.1599502534424));
#172643=CARTESIAN_POINT('Ctrl Pts',(50.5905785208489,37.1493329797255,39.8576902534424));
#172644=CARTESIAN_POINT('Ctrl Pts',(50.6005343088819,37.1565661199767,39.8773836120345));
#172645=CARTESIAN_POINT('Ctrl Pts',(50.6116037659383,37.1621977431848,39.8969946442095));
#172646=CARTESIAN_POINT('Ctrl Pts',(50.6236016024772,37.1661909570565,39.9162525288185));
#172647=CARTESIAN_POINT('Ctrl Pts',(50.6358405223212,37.1702644101609,39.9358973793989));
#172648=CARTESIAN_POINT('Ctrl Pts',(50.6490462309891,37.1726335298269,39.9551762199648));
#172649=CARTESIAN_POINT('Ctrl Pts',(50.6630602183632,37.1732217245281,39.9738152034136));
#172650=CARTESIAN_POINT('Ctrl Pts',(50.6765297750321,37.1737870683984,39.9917300792521));
#172651=CARTESIAN_POINT('Ctrl Pts',(50.690746893963,37.1727073465971,40.0090551157985));
#172652=CARTESIAN_POINT('Ctrl Pts',(50.7055935641109,37.1698754144274,40.0255394551386));
#172653=CARTESIAN_POINT('Ctrl Pts',(50.7169982609322,37.1677000224041,40.0382021526055));
#172654=CARTESIAN_POINT('Ctrl Pts',(50.7287749695242,37.1644899772801,40.0503687782078));
#172655=CARTESIAN_POINT('Ctrl Pts',(50.7408753824657,37.1601789145081,40.0619155352442));
#172656=CARTESIAN_POINT('Ctrl Pts',(50.7409070954901,37.1601676159814,40.0619457972351));
#172657=CARTESIAN_POINT('Ctrl Pts',(50.7409388110967,37.1601563091354,40.0619760547305));
#172658=CARTESIAN_POINT('Ctrl Pts',(50.7409705292826,37.1601449939711,40.0620063077269));
#172659=CARTESIAN_POINT('Ctrl Pts',(50.744371363825,37.1589317782463,40.06525004417));
#172660=CARTESIAN_POINT('Ctrl Pts',(50.7477999807011,37.1576225876051,40.0684393223556));
#172661=CARTESIAN_POINT('Ctrl Pts',(50.751251742581,37.1562191103349,40.0715697951759));
#172662=CARTESIAN_POINT('Ctrl Pts',(50.7704600126123,37.1484090784366,40.0889901646418));
#172663=CARTESIAN_POINT('Ctrl Pts',(50.7903868440238,37.1376839208971,40.1045963098239));
#172664=CARTESIAN_POINT('Ctrl Pts',(50.8102141228071,37.1243864882653,40.117663465072));
#172665=CARTESIAN_POINT('Ctrl Pts',(50.8191128801002,37.1184184163527,40.1235281853059));
#172666=CARTESIAN_POINT('Ctrl Pts',(50.8279919247187,37.1119323236325,40.1288820140919));
#172667=CARTESIAN_POINT('Ctrl Pts',(50.8367795369359,37.1049590818162,40.1336621774101));
#172668=CARTESIAN_POINT('Ctrl Pts',(50.8405985143445,37.1019286052426,40.1357395717319));
#172669=CARTESIAN_POINT('Ctrl Pts',(50.8444000194072,37.0988061338473,40.1377083672883));
#172670=CARTESIAN_POINT('Ctrl Pts',(50.8481780352577,37.0955942139016,40.1395632548791));
#172671=CARTESIAN_POINT('Ctrl Pts',(50.8614010907345,37.0843524940915,40.1460553614469));
#172672=CARTESIAN_POINT('Ctrl Pts',(50.8743364007572,37.0720150276367,40.1511520974629));
#172673=CARTESIAN_POINT('Ctrl Pts',(50.8867260065482,37.0586909963615,40.1546258197408));
#172674=CARTESIAN_POINT('Ctrl Pts',(50.8929208094437,37.0520289807239,40.1563626808798));
#172675=CARTESIAN_POINT('Ctrl Pts',(50.8989791867717,37.0451203242405,40.1576937882008));
#172676=CARTESIAN_POINT('Ctrl Pts',(50.9048689000892,37.0379786793004,40.1585906813668));
#172677=CARTESIAN_POINT('Ctrl Pts',(50.907813756748,37.0344078568303,40.1590391279498));
#172678=CARTESIAN_POINT('Ctrl Pts',(50.9107164475038,37.0307787873185,40.1593790209175));
#172679=CARTESIAN_POINT('Ctrl Pts',(50.9135729431182,37.0270931777233,40.1596068022931));
#172680=CARTESIAN_POINT('Ctrl Pts',(50.9164294387326,37.0234075681281,40.1598345836687));
#172681=CARTESIAN_POINT('Ctrl Pts',(50.9192397378254,37.0196654174464,40.1599502506864));
#172682=CARTESIAN_POINT('Ctrl Pts',(50.9219998155904,37.0158684358554,40.1599502534424));
#172683=CARTESIAN_POINT('',(50.9399462128206,36.9911673391701,40.1599502534424));
#172684=CARTESIAN_POINT('Origin',(5.52946850001198E-15,5.60353532024975E-15,
40.1599502534424));
#172685=CARTESIAN_POINT('',(50.9644637245897,36.6347241449648,39.8576902534424));
#172686=CARTESIAN_POINT('Ctrl Pts',(50.9399462128206,36.9911673391701,40.1599502534424));
#172687=CARTESIAN_POINT('Ctrl Pts',(50.9421917493684,36.9880750374201,40.1599502447858));
#172688=CARTESIAN_POINT('Ctrl Pts',(50.9443925120844,36.9849631608998,40.1598744685927));
#172689=CARTESIAN_POINT('Ctrl Pts',(50.9465482749236,36.9818339300537,40.1597246934279));
#172690=CARTESIAN_POINT('Ctrl Pts',(50.9590059247076,36.9637508360949,40.1588591777437));
#172691=CARTESIAN_POINT('Ctrl Pts',(50.9699639572682,36.94508700132,40.1555254706039));
#172692=CARTESIAN_POINT('Ctrl Pts',(50.9793739188788,36.9262760657806,40.1500631826426));
#172693=CARTESIAN_POINT('Ctrl Pts',(50.9831691728661,36.9186891827448,40.1478601162516));
#172694=CARTESIAN_POINT('Ctrl Pts',(50.9867130457535,36.9110782226527,40.1453112228326));
#172695=CARTESIAN_POINT('Ctrl Pts',(50.9900040313326,36.9034708445582,40.1424401896328));
#172696=CARTESIAN_POINT('Ctrl Pts',(50.9912182052063,36.9006641839067,40.1413809526905));
#172697=CARTESIAN_POINT('Ctrl Pts',(50.9923978359483,36.8978580678368,40.1402777640511));
#172698=CARTESIAN_POINT('Ctrl Pts',(50.9935427888375,36.8950539146729,40.1391317641987));
#172699=CARTESIAN_POINT('Ctrl Pts',(50.9956895755046,36.8897961274906,40.1369830144753));
#172700=CARTESIAN_POINT('Ctrl Pts',(50.9977144478404,36.8845452411463,40.1346837565849));
#172701=CARTESIAN_POINT('Ctrl Pts',(50.9996165178741,36.8793106050082,40.1322415082996));
#172702=CARTESIAN_POINT('Ctrl Pts',(51.006273762992,36.8609893785247,40.1236936393009));
#172703=CARTESIAN_POINT('Ctrl Pts',(51.0114266762823,36.8428672144354,40.113394140767));
#172704=CARTESIAN_POINT('Ctrl Pts',(51.0150372064717,36.8253449818063,40.101665321223));
#172705=CARTESIAN_POINT('Ctrl Pts',(51.0168424715664,36.8165838654917,40.095800911451));
#172706=CARTESIAN_POINT('Ctrl Pts',(51.0182621417031,36.8079727326361,40.0895791707949));
#172707=CARTESIAN_POINT('Ctrl Pts',(51.019291467691,36.7995616970574,40.0830403822906));
#172708=CARTESIAN_POINT('Ctrl Pts',(51.019806130685,36.795356179268,40.0797709880385));
#172709=CARTESIAN_POINT('Ctrl Pts',(51.0202232077374,36.7912006858661,40.0764223317514));
#172710=CARTESIAN_POINT('Ctrl Pts',(51.0205421056331,36.7871014813871,40.0729994484778));
#172711=CARTESIAN_POINT('Ctrl Pts',(51.0208610035287,36.7830022769081,40.0695765652042));
#172712=CARTESIAN_POINT('Ctrl Pts',(51.0210816112671,36.7789594281944,40.0660793733488));
#172713=CARTESIAN_POINT('Ctrl Pts',(51.0212035636555,36.7749790641709,40.0625130768816));
#172714=CARTESIAN_POINT('Ctrl Pts',(51.021204603654,36.774945120002,40.0624826638418));
#172715=CARTESIAN_POINT('Ctrl Pts',(51.0212056365647,36.7749111804862,40.0624522459912));
#172716=CARTESIAN_POINT('Ctrl Pts',(51.021206662388,36.7748772456266,40.0624218233329));
#172717=CARTESIAN_POINT('Ctrl Pts',(51.0217305652767,36.7575462174121,40.0468845275879));
#172718=CARTESIAN_POINT('Ctrl Pts',(51.0205340689293,36.7413978659011,40.0302263329196));
#172719=CARTESIAN_POINT('Ctrl Pts',(51.017806340962,36.726498406541,40.0127515884679));
#172720=CARTESIAN_POINT('Ctrl Pts',(51.0149863630461,36.7110950573594,39.994685859763));
#172721=CARTESIAN_POINT('Ctrl Pts',(51.0105292970913,36.6970257816808,39.9757460620383));
#172722=CARTESIAN_POINT('Ctrl Pts',(51.0046027001994,36.6843954909168,39.9562444558998));
#172723=CARTESIAN_POINT('Ctrl Pts',(50.9987888396517,36.6720054548607,39.9371138113467));
#172724=CARTESIAN_POINT('Ctrl Pts',(50.9915600117681,36.6609997277806,39.9174410654195));
#172725=CARTESIAN_POINT('Ctrl Pts',(50.9830457809093,36.651515723761,39.8975196503974));
#172726=CARTESIAN_POINT('Ctrl Pts',(50.977405401464,36.6452329035958,39.8843224113659));
#172727=CARTESIAN_POINT('Ctrl Pts',(50.9712003466817,36.639618694681,39.8710160447074));
#172728=CARTESIAN_POINT('Ctrl Pts',(50.9644637245897,36.6347241449648,39.8576902534424));
#172729=CARTESIAN_POINT('',(50.6762142289952,36.4252947698673,39.2875012672119));
#172730=CARTESIAN_POINT('',(50.9644637245897,36.6347241449648,39.8576902534424));
#172731=CARTESIAN_POINT('',(53.8880358395974,31.4795232016783,39.2875012672119));
#172732=CARTESIAN_POINT('Origin',(5.53234440788222E-15,0.,39.2875012672119));
#172733=CARTESIAN_POINT('',(54.1966007261211,31.6576696180577,39.8576902534424));
#172734=CARTESIAN_POINT('',(53.8880358395974,31.4795232016783,39.2875012672119));
#172735=CARTESIAN_POINT('',(54.5122556166615,31.4902932482901,40.1599502534424));
#172736=CARTESIAN_POINT('Ctrl Pts',(54.1966007261211,31.6576696180577,39.8576902534424));
#172737=CARTESIAN_POINT('Ctrl Pts',(54.207258044343,31.6638224711873,39.8773836120385));
#172738=CARTESIAN_POINT('Ctrl Pts',(54.2188555266776,31.6682661704395,39.8969946442175));
#172739=CARTESIAN_POINT('Ctrl Pts',(54.231205042325,31.6709833936517,39.9162525288304));
#172740=CARTESIAN_POINT('Ctrl Pts',(54.2438027078816,31.6737552164703,39.9358973794147));
#172741=CARTESIAN_POINT('Ctrl Pts',(54.2571837147368,31.6747309854166,39.9551762199842));
#172742=CARTESIAN_POINT('Ctrl Pts',(54.2711824151134,31.6738510973596,39.9738152034363));
#172743=CARTESIAN_POINT('Ctrl Pts',(54.2846372786704,31.6730053921559,39.9917300792778));
#172744=CARTESIAN_POINT('Ctrl Pts',(54.2986636530789,31.6704454915874,40.0090551158268));
#172745=CARTESIAN_POINT('Ctrl Pts',(54.3131329740999,31.6660771734201,40.0255394551691));
#172746=CARTESIAN_POINT('Ctrl Pts',(54.324247804405,31.6627215829901,40.038202152625));
#172747=CARTESIAN_POINT('Ctrl Pts',(54.3356244578624,31.6582981215803,40.0503687782171));
#172748=CARTESIAN_POINT('Ctrl Pts',(54.3472079546998,31.6527458376961,40.0619155352442));
#172749=CARTESIAN_POINT('Ctrl Pts',(54.3472383129792,31.6527312861502,40.0619457972351));
#172750=CARTESIAN_POINT('Ctrl Pts',(54.3472686729572,31.6527167260607,40.0619760547305));
#172751=CARTESIAN_POINT('Ctrl Pts',(54.3472990346308,31.6527021574288,40.0620063077269));
#172752=CARTESIAN_POINT('Ctrl Pts',(54.3505544234704,31.6511401038181,40.06525004417));
#172753=CARTESIAN_POINT('Ctrl Pts',(54.3538274103387,31.649479697007,40.0684393223556));
#172754=CARTESIAN_POINT('Ctrl Pts',(54.3571135597836,31.6477231007673,40.0715697951759));
#172755=CARTESIAN_POINT('Ctrl Pts',(54.3754002342679,31.6379480420934,40.0889901646403));
#172756=CARTESIAN_POINT('Ctrl Pts',(54.3940968201743,31.6251987170252,40.1045963098211));
#172757=CARTESIAN_POINT('Ctrl Pts',(54.4124255228499,31.6099016141405,40.1176634650686));
#172758=CARTESIAN_POINT('Ctrl Pts',(54.4206516984354,31.6030360625242,40.1235281853038));
#172759=CARTESIAN_POINT('Ctrl Pts',(54.4288041214155,31.595657388408,40.1288820140909));
#172760=CARTESIAN_POINT('Ctrl Pts',(54.436814691924,31.5878037911375,40.1336621774101));
#172761=CARTESIAN_POINT('Ctrl Pts',(54.4402959775156,31.5843907239919,40.1357395717319));
#172762=CARTESIAN_POINT('Ctrl Pts',(54.4437502703992,31.5808879923394,40.1377083672884));
#172763=CARTESIAN_POINT('Ctrl Pts',(54.4471718528276,31.5772987574361,40.1395632548792));
#172764=CARTESIAN_POINT('Ctrl Pts',(54.4591473913267,31.5647364352747,40.146055361447));
#172765=CARTESIAN_POINT('Ctrl Pts',(54.4707222239585,31.5511144466735,40.151152097463));
#172766=CARTESIAN_POINT('Ctrl Pts',(54.4816512176788,31.5365683393819,40.1546258197409));
#172767=CARTESIAN_POINT('Ctrl Pts',(54.487115714539,31.5292952857361,40.1563626808798));
#172768=CARTESIAN_POINT('Ctrl Pts',(54.4924187521967,31.5217912027238,40.1576937882008));
#172769=CARTESIAN_POINT('Ctrl Pts',(54.4975296958776,31.5140730377798,40.1585906813668));
#172770=CARTESIAN_POINT('Ctrl Pts',(54.5000851677181,31.5102139553077,40.1590391279498));
#172771=CARTESIAN_POINT('Ctrl Pts',(54.5025926161711,31.5063013524143,40.1593790209175));
#172772=CARTESIAN_POINT('Ctrl Pts',(54.5050482124964,31.5023373478773,40.1596068022931));
#172773=CARTESIAN_POINT('Ctrl Pts',(54.5075038088218,31.4983733433402,40.1598345836687));
#172774=CARTESIAN_POINT('Ctrl Pts',(54.5099075515421,31.494357936306,40.1599502506865));
#172775=CARTESIAN_POINT('Ctrl Pts',(54.5122556166615,31.4902932482901,40.1599502534424));
#172776=CARTESIAN_POINT('',(54.5275217339723,31.4638515574734,40.1599502534424));
#172777=CARTESIAN_POINT('Origin',(5.52060867199534E-15,5.61717825899799E-15,
40.1599502534424));
#172778=CARTESIAN_POINT('',(54.5146464769142,31.1067982185528,39.8576902534424));
#172779=CARTESIAN_POINT('Ctrl Pts',(54.5275217339724,31.4638515574734,40.1599502534424));
#172780=CARTESIAN_POINT('Ctrl Pts',(54.5294317356861,31.4605414731913,40.1599502447858));
#172781=CARTESIAN_POINT('Ctrl Pts',(54.5312951627231,31.4572166015115,40.1598744685927));
#172782=CARTESIAN_POINT('Ctrl Pts',(54.5331120223763,31.4538791743426,40.1597246934279));
#172783=CARTESIAN_POINT('Ctrl Pts',(54.543611229832,31.4345929624707,40.1588591777434));
#172784=CARTESIAN_POINT('Ctrl Pts',(54.5525583311783,31.4148859438253,40.1555254706018));
#172785=CARTESIAN_POINT('Ctrl Pts',(54.5599504658514,31.3951944477263,40.1500631826375));
#172786=CARTESIAN_POINT('Ctrl Pts',(54.5629318838128,31.3872524143687,40.1478601162477));
#172787=CARTESIAN_POINT('Ctrl Pts',(54.565660781029,31.3793127123316,40.1453112228304));
#172788=CARTESIAN_POINT('Ctrl Pts',(54.5681385507011,31.3714030065912,40.1424401896328));
#172789=CARTESIAN_POINT('Ctrl Pts',(54.5690526972785,31.3684848053912,40.1413809526905));
#172790=CARTESIAN_POINT('Ctrl Pts',(54.5699325468794,31.36557075653,40.1402777640511));
#172791=CARTESIAN_POINT('Ctrl Pts',(54.5707781137758,31.3626622846446,40.1391317641987));
#172792=CARTESIAN_POINT('Ctrl Pts',(54.5723635517066,31.3572088998593,40.1369830144753));
#172793=CARTESIAN_POINT('Ctrl Pts',(54.5738284644995,31.3517751216263,40.1346837565849));
#172794=CARTESIAN_POINT('Ctrl Pts',(54.5751729463232,31.3463703409149,40.1322415082996));
#172795=CARTESIAN_POINT('Ctrl Pts',(54.5798786327064,31.3274536084253,40.1236936393008));
#172796=CARTESIAN_POINT('Ctrl Pts',(54.5831090358351,31.3088920933395,40.113394140767));
#172797=CARTESIAN_POINT('Ctrl Pts',(54.5848682151126,31.2910884461618,40.101665321223));
#172798=CARTESIAN_POINT('Ctrl Pts',(54.5857478047514,31.282186622573,40.095800911451));
#172799=CARTESIAN_POINT('Ctrl Pts',(54.5862595893022,31.2734742664665,40.0895791707949));
#172800=CARTESIAN_POINT('Ctrl Pts',(54.5864040839111,31.265001713557,40.0830403822906));
#172801=CARTESIAN_POINT('Ctrl Pts',(54.5864763312156,31.2607654371022,40.0797709880385));
#172802=CARTESIAN_POINT('Ctrl Pts',(54.5864567561368,31.2565891115046,40.0764223317514));
#172803=CARTESIAN_POINT('Ctrl Pts',(54.5863454235316,31.2524790289897,40.0729994484778));
#172804=CARTESIAN_POINT('Ctrl Pts',(54.5862340909265,31.2483689464747,40.0695765652042));
#172805=CARTESIAN_POINT('Ctrl Pts',(54.5860308973893,31.2443251851214,40.0660793733488));
#172806=CARTESIAN_POINT('Ctrl Pts',(54.5857361203751,31.2403538784528,40.0625130768817));
#172807=CARTESIAN_POINT('Ctrl Pts',(54.5857336065446,31.2403200115241,40.0624826638418));
#172808=CARTESIAN_POINT('Ctrl Pts',(54.5857310861515,31.2402861499639,40.0624522459912));
#172809=CARTESIAN_POINT('Ctrl Pts',(54.5857285591964,31.2402522937754,40.0624218233329));
#172810=CARTESIAN_POINT('Ctrl Pts',(54.5844380063443,31.2229614439847,40.0468845275895));
#172811=CARTESIAN_POINT('Ctrl Pts',(54.5815601021618,31.207026622759,40.030226332923));
#172812=CARTESIAN_POINT('Ctrl Pts',(54.5772898993838,31.1924939094102,40.0127515884733));
#172813=CARTESIAN_POINT('Ctrl Pts',(54.5728752811835,31.1774697093461,39.9946858597698));
#172814=CARTESIAN_POINT('Ctrl Pts',(54.566971991737,31.1639433968874,39.9757460620467));
#172815=CARTESIAN_POINT('Ctrl Pts',(54.5597576364798,31.1520017942437,39.9562444559099));
#172816=CARTESIAN_POINT('Ctrl Pts',(54.5526805134402,31.14028734601,39.9371138113575));
#172817=CARTESIAN_POINT('Ctrl Pts',(54.544340874094,31.130097527724,39.9174410654309));
#172818=CARTESIAN_POINT('Ctrl Pts',(54.5348819367177,31.1215554575377,39.8975196504094));
#172819=CARTESIAN_POINT('Ctrl Pts',(54.5286157223228,31.1158966355121,39.884322411374));
#172820=CARTESIAN_POINT('Ctrl Pts',(54.5218578148477,31.1109617866602,39.8710160447114));
#172821=CARTESIAN_POINT('Ctrl Pts',(54.5146464769142,31.1067982185528,39.8576902534424));
#172822=CARTESIAN_POINT('',(54.2060847114746,30.9286463962971,39.2875012672119));
#172823=CARTESIAN_POINT('',(54.5146464769142,31.1067982185528,39.8576902534424));
#172824=CARTESIAN_POINT('',(56.8833377255397,25.6742415049973,39.2875012672119));
#172825=CARTESIAN_POINT('Origin',(5.53234440788222E-15,0.,39.2875012672119));
#172826=CARTESIAN_POINT('',(57.2088336324702,25.8191582032614,39.8576902534424));
#172827=CARTESIAN_POINT('',(56.8833377255398,25.6742415049973,39.2875012672119));
#172828=CARTESIAN_POINT('',(57.5052637377735,25.6197038181291,40.1599502534424));
#172829=CARTESIAN_POINT('Ctrl Pts',(57.2088336324702,25.8191582032614,39.8576902534424));
#172830=CARTESIAN_POINT('Ctrl Pts',(57.2200757170675,25.8241633573202,39.8773836120341));
#172831=CARTESIAN_POINT('Ctrl Pts',(57.2320741602317,25.8273704465163,39.8969946442086));
#172832=CARTESIAN_POINT('Ctrl Pts',(57.2446400511038,25.8287819086031,39.9162525288172));
#172833=CARTESIAN_POINT('Ctrl Pts',(57.2574584397068,25.8302217324653,39.935897379397));
#172834=CARTESIAN_POINT('Ctrl Pts',(57.2708681396313,25.8297934599651,39.9551762199623));
#172835=CARTESIAN_POINT('Ctrl Pts',(57.2846981803123,25.8274551293912,39.9738152034104));
#172836=CARTESIAN_POINT('Ctrl Pts',(57.29799093645,25.8252076408403,39.9917300792482));
#172837=CARTESIAN_POINT('Ctrl Pts',(57.3116728904355,25.821195608316,40.0090551157937));
#172838=CARTESIAN_POINT('Ctrl Pts',(57.3256063334131,25.8153387643661,40.0255394551332));
#172839=CARTESIAN_POINT('Ctrl Pts',(57.3363095208137,25.8108397400781,40.0382021526019));
#172840=CARTESIAN_POINT('Ctrl Pts',(57.3471614741597,25.8052513267456,40.0503687782061));
#172841=CARTESIAN_POINT('Ctrl Pts',(57.3581011436977,25.7985186537234,40.0619155352442));
#172842=CARTESIAN_POINT('Ctrl Pts',(57.3581298146206,25.7985010085881,40.0619457972351));
#172843=CARTESIAN_POINT('Ctrl Pts',(57.3581584863397,25.7984833547784,40.0619760547304));
#172844=CARTESIAN_POINT('Ctrl Pts',(57.3581871588522,25.7984656922959,40.0620063077269));
#172845=CARTESIAN_POINT('Ctrl Pts',(57.3612614352676,25.7965719149857,40.06525004417));
#172846=CARTESIAN_POINT('Ctrl Pts',(57.364342932599,25.7945784837691,40.0684393223556));
#172847=CARTESIAN_POINT('Ctrl Pts',(57.3674274658679,25.7924880141959,40.0715697951759));
#172848=CARTESIAN_POINT('Ctrl Pts',(57.3845921921748,25.7808550263338,40.0889901646407));
#172849=CARTESIAN_POINT('Ctrl Pts',(57.4018536888708,25.7662212180087,40.104596309822));
#172850=CARTESIAN_POINT('Ctrl Pts',(57.4184830023389,25.7490920431292,40.1176634650696));
#172851=CARTESIAN_POINT('Ctrl Pts',(57.4259464685134,25.7414042322309,40.1235281853045));
#172852=CARTESIAN_POINT('Ctrl Pts',(57.4332829502005,25.733213819018,40.1288820140912));
#172853=CARTESIAN_POINT('Ctrl Pts',(57.4404287135114,25.7245659119504,40.1336621774101));
#172854=CARTESIAN_POINT('Ctrl Pts',(57.4435341655926,25.7208076485107,40.1357395717319));
#172855=CARTESIAN_POINT('Ctrl Pts',(57.4466034003415,25.7169630332619,40.1377083672884));
#172856=CARTESIAN_POINT('Ctrl Pts',(57.4496310617745,25.7130358078098,40.1395632548792));
#172857=CARTESIAN_POINT('Ctrl Pts',(57.4602278767901,25.6992905187274,40.146055361447));
#172858=CARTESIAN_POINT('Ctrl Pts',(57.4703154157425,25.6845332533375,40.1511520974629));
#172859=CARTESIAN_POINT('Ctrl Pts',(57.4796640570501,25.668924440225,40.1546258197408));
#172860=CARTESIAN_POINT('Ctrl Pts',(57.4843383777038,25.6611200336687,40.1563626808798));
#172861=CARTESIAN_POINT('Ctrl Pts',(57.4888279745008,25.6531027404313,40.1576937882008));
#172862=CARTESIAN_POINT('Ctrl Pts',(57.4931041519767,25.6448926173136,40.1585906813668));
#172863=CARTESIAN_POINT('Ctrl Pts',(57.4952422407146,25.6407875557547,40.1590391279498));
#172864=CARTESIAN_POINT('Ctrl Pts',(57.4973269747348,25.6366342867758,40.1593790209175));
#172865=CARTESIAN_POINT('Ctrl Pts',(57.4993547677439,25.63243531776,40.1596068022931));
#172866=CARTESIAN_POINT('Ctrl Pts',(57.501382560753,25.6282363487443,40.1598345836687));
#172867=CARTESIAN_POINT('Ctrl Pts',(57.5033534111924,25.6239916789973,40.1599502506864));
#172868=CARTESIAN_POINT('Ctrl Pts',(57.5052637377735,25.6197038181291,40.1599502534424));
#172869=CARTESIAN_POINT('',(57.5176823163891,25.5918112338787,40.1599502534424));
#172870=CARTESIAN_POINT('Origin',(5.5132234544654E-15,5.63167256450768E-15,
40.1599502534424));
#172871=CARTESIAN_POINT('',(57.4675553545144,25.2380597013423,39.8576902534424));
#172872=CARTESIAN_POINT('Ctrl Pts',(57.5176823163891,25.5918112338787,40.1599502534424));
#172873=CARTESIAN_POINT('Ctrl Pts',(57.5192358568904,25.5883196330407,40.1599502447858));
#172874=CARTESIAN_POINT('Ctrl Pts',(57.5207415321518,25.5848181941912,40.1598744685927));
#172875=CARTESIAN_POINT('Ctrl Pts',(57.5221995827245,25.5813091362501,40.1597246934279));
#172876=CARTESIAN_POINT('Ctrl Pts',(57.530625316332,25.5610311102486,40.1588591777436));
#172877=CARTESIAN_POINT('Ctrl Pts',(57.5374634601452,25.5404968219637,40.1555254706034));
#172878=CARTESIAN_POINT('Ctrl Pts',(57.5427567781039,25.5201405094677,40.1500631826413));
#172879=CARTESIAN_POINT('Ctrl Pts',(57.5448916950053,25.5119303403572,40.1478601162506));
#172880=CARTESIAN_POINT('Ctrl Pts',(57.5467757181854,25.5037488854015,40.1453112228321));
#172881=CARTESIAN_POINT('Ctrl Pts',(57.548413124991,25.4956235123959,40.1424401896328));
#172882=CARTESIAN_POINT('Ctrl Pts',(57.5490172286909,25.4926257430704,40.1413809526905));
#172883=CARTESIAN_POINT('Ctrl Pts',(57.5495876573342,25.4896356883471,40.1402777640512));
#172884=CARTESIAN_POINT('Ctrl Pts',(57.5501245740301,25.4866547635667,40.1391317641987));
#172885=CARTESIAN_POINT('Ctrl Pts',(57.5511312928348,25.4810655296034,40.1369830144753));
#172886=CARTESIAN_POINT('Ctrl Pts',(57.5520201961937,25.475508393093,40.1346837565849));
#172887=CARTESIAN_POINT('Ctrl Pts',(57.5527923593833,25.469992683717,40.1322415082996));
#172888=CARTESIAN_POINT('Ctrl Pts',(57.5554949305468,25.450687700901,40.1236936393008));
#172889=CARTESIAN_POINT('Ctrl Pts',(57.5567674305414,25.4318901986622,40.113394140767));
#172890=CARTESIAN_POINT('Ctrl Pts',(57.5566559849708,25.41400019742,40.101665321223));
#172891=CARTESIAN_POINT('Ctrl Pts',(57.5566002621854,25.405055196799,40.095800911451));
#172892=CARTESIAN_POINT('Ctrl Pts',(57.5561985539316,25.3963370718382,40.0895791707949));
#172893=CARTESIAN_POINT('Ctrl Pts',(57.5554566340484,25.3878958286606,40.0830403822906));
#172894=CARTESIAN_POINT('Ctrl Pts',(57.5550856741068,25.3836752070718,40.0797709880385));
#172895=CARTESIAN_POINT('Ctrl Pts',(57.5546296613655,25.3795238059757,40.0764223317514));
#172896=CARTESIAN_POINT('Ctrl Pts',(57.5540893180428,25.3754478763489,40.0729994484778));
#172897=CARTESIAN_POINT('Ctrl Pts',(57.5535489747201,25.3713719467222,40.0695765652042));
#172898=CARTESIAN_POINT('Ctrl Pts',(57.5529242061383,25.3673715770249,40.0660793733488));
#172899=CARTESIAN_POINT('Ctrl Pts',(57.5522159293602,25.363452838178,40.0625130768817));
#172900=CARTESIAN_POINT('Ctrl Pts',(57.5522098892427,25.3634194195428,40.0624826638418));
#172901=CARTESIAN_POINT('Ctrl Pts',(57.5522038431597,25.3633860069326,40.0624522459912));
#172902=CARTESIAN_POINT('Ctrl Pts',(57.5521977911122,25.3633526003505,40.0624218233329));
#172903=CARTESIAN_POINT('Ctrl Pts',(57.549106922086,25.3462913711479,40.0468845275872));
#172904=CARTESIAN_POINT('Ctrl Pts',(57.5445791409876,25.3307446654397,40.030226332918));
#172905=CARTESIAN_POINT('Ctrl Pts',(57.5388132486326,25.3167379215479,40.0127515884654));
#172906=CARTESIAN_POINT('Ctrl Pts',(57.5328523576269,25.3022574788784,39.994685859759));
#172907=CARTESIAN_POINT('Ctrl Pts',(57.525567522361,25.2894223267475,39.9757460620327));
#172908=CARTESIAN_POINT('Ctrl Pts',(57.5171444507216,25.2783002469205,39.9562444558927));
#172909=CARTESIAN_POINT('Ctrl Pts',(57.5088816036288,25.2673897324551,39.9371138113373));
#172910=CARTESIAN_POINT('Ctrl Pts',(57.499522523651,25.258127464745,39.9174410654078));
#172911=CARTESIAN_POINT('Ctrl Pts',(57.4892225138515,25.2506209171015,39.8975196503834));
#172912=CARTESIAN_POINT('Ctrl Pts',(57.4823991184684,25.2456480924605,39.8843224113565));
#172913=CARTESIAN_POINT('Ctrl Pts',(57.4751623993551,25.2414466709135,39.8710160447026));
#172914=CARTESIAN_POINT('Ctrl Pts',(57.4675553545144,25.2380597013423,39.8576902534424));
#172915=CARTESIAN_POINT('',(57.1420619865024,25.0931373005739,39.2875012672119));
#172916=CARTESIAN_POINT('',(57.4675553545144,25.2380597013423,39.8576902534424));
#172917=CARTESIAN_POINT('',(59.2554138597574,19.5876674457071,39.2875012672119));
#172918=CARTESIAN_POINT('Origin',(5.53234440788222E-15,0.,39.2875012672119));
#172919=CARTESIAN_POINT('',(59.5942745858238,19.6977666881838,39.8576902534424));
#172920=CARTESIAN_POINT('',(59.2554138597574,19.5876674457071,39.2875012672119));
#172921=CARTESIAN_POINT('',(59.8682321556244,19.4684195516689,40.1599502534424));
#172922=CARTESIAN_POINT('Ctrl Pts',(59.5942745858238,19.6977666881838,39.8576902534424));
#172923=CARTESIAN_POINT('Ctrl Pts',(59.6059782661682,19.7015693056585,39.877383612035));
#172924=CARTESIAN_POINT('Ctrl Pts',(59.618246212711,19.7035046472589,39.8969946442105));
#172925=CARTESIAN_POINT('Ctrl Pts',(59.6308908042817,19.7035948839462,39.91625252882));
#172926=CARTESIAN_POINT('Ctrl Pts',(59.6437894749872,19.7036869338402,39.9358973794009));
#172927=CARTESIAN_POINT('Ctrl Pts',(59.657080948507,19.7018593121352,39.9551762199673));
#172928=CARTESIAN_POINT('Ctrl Pts',(59.6705908046774,19.6980881582808,39.9738152034164));
#172929=CARTESIAN_POINT('Ctrl Pts',(59.6835758151828,19.6944635103349,39.9917300792554));
#172930=CARTESIAN_POINT('Ctrl Pts',(59.6967634463995,19.689043302519,40.009055115802));
#172931=CARTESIAN_POINT('Ctrl Pts',(59.710008353622,19.6817621015893,40.0255394551424));
#172932=CARTESIAN_POINT('Ctrl Pts',(59.7201826317446,19.6761689356968,40.0382021526078));
#172933=CARTESIAN_POINT('Ctrl Pts',(59.7303909886945,19.6694767982719,40.0503687782089));
#172934=CARTESIAN_POINT('Ctrl Pts',(59.740566973611,19.6616375006933,40.0619155352442));
#172935=CARTESIAN_POINT('Ctrl Pts',(59.7405936430527,19.6616169552925,40.0619457972351));
#172936=CARTESIAN_POINT('Ctrl Pts',(59.7406203123795,19.6615964011814,40.0619760547304));
#172937=CARTESIAN_POINT('Ctrl Pts',(59.7406469815888,19.6615758383622,40.0620063077269));
#172938=CARTESIAN_POINT('Ctrl Pts',(59.7435064631644,19.6593710859728,40.06525004417));
#172939=CARTESIAN_POINT('Ctrl Pts',(59.7463627094293,19.6570664708005,40.0684393223556));
#172940=CARTESIAN_POINT('Ctrl Pts',(59.7492118317302,19.6546650315158,40.0715697951759));
#172941=CARTESIAN_POINT('Ctrl Pts',(59.7650665495264,19.6413015679147,40.0889901646412));
#172942=CARTESIAN_POINT('Ctrl Pts',(59.7807038364419,19.6249436073989,40.1045963098228));
#172943=CARTESIAN_POINT('Ctrl Pts',(59.795451566464,19.606170031349,40.1176634650707));
#172944=CARTESIAN_POINT('Ctrl Pts',(59.8020705519303,19.5977441904338,40.1235281853051));
#172945=CARTESIAN_POINT('Ctrl Pts',(59.8085107122961,19.5888317740054,40.1288820140915));
#172946=CARTESIAN_POINT('Ctrl Pts',(59.8147133779312,19.5794843054205,40.1336621774101));
#172947=CARTESIAN_POINT('Ctrl Pts',(59.817408972519,19.5754220220073,40.1357395717319));
#172948=CARTESIAN_POINT('Ctrl Pts',(59.820059521955,19.5712776455713,40.1377083672884));
#172949=CARTESIAN_POINT('Ctrl Pts',(59.8226600907005,19.5670554570743,40.1395632548792));
#172950=CARTESIAN_POINT('Ctrl Pts',(59.8317620813098,19.5522777973346,40.146055361447));
#172951=CARTESIAN_POINT('Ctrl Pts',(59.8402518053951,19.5365469388437,40.1511520974629));
#172952=CARTESIAN_POINT('Ctrl Pts',(59.8479176686193,19.5200464333331,40.1546258197408));
#172953=CARTESIAN_POINT('Ctrl Pts',(59.8517506002314,19.5117961805777,40.1563626808798));
#172954=CARTESIAN_POINT('Ctrl Pts',(59.8553775672057,19.5033535162577,40.1576937882008));
#172955=CARTESIAN_POINT('Ctrl Pts',(59.8587721277812,19.4947413867932,40.1585906813668));
#172956=CARTESIAN_POINT('Ctrl Pts',(59.8604694080689,19.490435322061,40.1590391279498));
#172957=CARTESIAN_POINT('Ctrl Pts',(59.8621085868741,19.4860868910807,40.1593790209175));
#172958=CARTESIAN_POINT('Ctrl Pts',(59.8636863596424,19.4816989623695,40.1596068022931));
#172959=CARTESIAN_POINT('Ctrl Pts',(59.8652641324107,19.4773110336582,40.1598345836686));
#172960=CARTESIAN_POINT('Ctrl Pts',(59.8667804975195,19.4728836066885,40.1599502506864));
#172961=CARTESIAN_POINT('Ctrl Pts',(59.8682321556244,19.4684195516689,40.1599502534424));
#172962=CARTESIAN_POINT('',(59.8776671349988,19.4393816709748,40.1599502534424));
#172963=CARTESIAN_POINT('Origin',(5.50739376141089E-15,5.64685943413453E-15,
40.1599502534424));
#172964=CARTESIAN_POINT('',(59.7908376697914,19.0928077206404,39.8576902534424));
#172965=CARTESIAN_POINT('Ctrl Pts',(59.8776671349988,19.4393816709748,40.1599502534424));
#172966=CARTESIAN_POINT('Ctrl Pts',(59.8788471933727,19.4357468082904,40.1599502447858));
#172967=CARTESIAN_POINT('Ctrl Pts',(59.8799786203653,19.432107164768,40.1598744685927));
#172968=CARTESIAN_POINT('Ctrl Pts',(59.8810618871504,19.4284649220277,40.1597246934279));
#172969=CARTESIAN_POINT('Ctrl Pts',(59.8873218328124,19.4074172521853,40.1588591777435));
#172970=CARTESIAN_POINT('Ctrl Pts',(59.8919760989601,19.3862806722125,40.1555254706023));
#172971=CARTESIAN_POINT('Ctrl Pts',(59.8951126055062,19.3654825713314,40.1500631826388));
#172972=CARTESIAN_POINT('Ctrl Pts',(59.8963776307484,19.3570942188066,40.1478601162487));
#172973=CARTESIAN_POINT('Ctrl Pts',(59.8973961381381,19.3487606486725,40.1453112228309));
#172974=CARTESIAN_POINT('Ctrl Pts',(59.8981752423039,19.3405086316964,40.1424401896328));
#172975=CARTESIAN_POINT('Ctrl Pts',(59.8984626844396,19.3374641384336,40.1413809526905));
#172976=CARTESIAN_POINT('Ctrl Pts',(59.8987174423899,19.3344308375134,40.1402777640511));
#172977=CARTESIAN_POINT('Ctrl Pts',(59.8989398263135,19.3314101194737,40.1391317641986));
#172978=CARTESIAN_POINT('Ctrl Pts',(59.8993567961703,19.3257462731493,40.1369830144753));
#172979=CARTESIAN_POINT('Ctrl Pts',(59.8996599510839,19.320126663512,40.1346837565849));
#172980=CARTESIAN_POINT('Ctrl Pts',(59.8998513356578,19.3145604567375,40.1322415082996));
#172981=CARTESIAN_POINT('Ctrl Pts',(59.9005211816666,19.2950787330267,40.1236936393008));
#172982=CARTESIAN_POINT('Ctrl Pts',(59.8998218367508,19.276251193003,40.113394140767));
#172983=CARTESIAN_POINT('Ctrl Pts',(59.8978409873529,19.2584708442938,40.101665321223));
#172984=CARTESIAN_POINT('Ctrl Pts',(59.896850562654,19.2495806699392,40.095800911451));
#172985=CARTESIAN_POINT('Ctrl Pts',(59.8955397627954,19.2409522937256,40.0895791707949));
#172986=CARTESIAN_POINT('Ctrl Pts',(59.8939195570494,19.2326348443066,40.0830403822906));
#172987=CARTESIAN_POINT('Ctrl Pts',(59.8931094541765,19.2284761195972,40.0797709880385));
#172988=CARTESIAN_POINT('Ctrl Pts',(59.8922219999437,19.2243951266217,40.0764223317514));
#172989=CARTESIAN_POINT('Ctrl Pts',(59.891258566018,19.2203980066211,40.0729994484778));
#172990=CARTESIAN_POINT('Ctrl Pts',(59.8902951320923,19.2164008866205,40.0695765652042));
#172991=CARTESIAN_POINT('Ctrl Pts',(59.8892556335612,19.2124877374667,40.0660793733488));
#172992=CARTESIAN_POINT('Ctrl Pts',(59.8881416170478,19.2086645009644,40.0625130768817));
#172993=CARTESIAN_POINT('Ctrl Pts',(59.8881321168201,19.2086318967641,40.0624826638418));
#172994=CARTESIAN_POINT('Ctrl Pts',(59.8881226112894,19.2085992991795,40.0624522459912));
#172995=CARTESIAN_POINT('Ctrl Pts',(59.888113100457,19.2085667082134,40.0624218233329));
#172996=CARTESIAN_POINT('Ctrl Pts',(59.883255779466,19.1919220260038,40.0468845275916));
#172997=CARTESIAN_POINT('Ctrl Pts',(59.8771277287718,19.1769337687802,40.0302263329276));
#172998=CARTESIAN_POINT('Ctrl Pts',(59.8699293191667,19.1636064551671,40.0127515884804));
#172999=CARTESIAN_POINT('Ctrl Pts',(59.8624874641286,19.1498284206571,39.9946858597795));
#173000=CARTESIAN_POINT('Ctrl Pts',(59.8539008972278,19.1378250534699,39.9757460620591));
#173001=CARTESIAN_POINT('Ctrl Pts',(59.8443613941471,19.1276443522951,39.9562444559251));
#173002=CARTESIAN_POINT('Ctrl Pts',(59.8350033524881,19.1176573094789,39.937113811375));
#173003=CARTESIAN_POINT('Ctrl Pts',(59.8247273719232,19.1094240716875,39.9174410654508));
#173004=CARTESIAN_POINT('Ctrl Pts',(59.8136991387694,19.103035289892,39.8975196504315));
#173005=CARTESIAN_POINT('Ctrl Pts',(59.8063933209342,19.0988029459312,39.8843224113889));
#173006=CARTESIAN_POINT('Ctrl Pts',(59.7987570771787,19.0953809833338,39.8710160447189));
#173007=CARTESIAN_POINT('Ctrl Pts',(59.7908376697914,19.0928077206404,39.8576902534424));
#173008=CARTESIAN_POINT('',(59.451978872661,18.9827025415089,39.2875012672119));
#173009=CARTESIAN_POINT('',(59.7908376697914,19.0928077206404,39.8576902534424));
#173010=CARTESIAN_POINT('',(60.978275279735,13.2864868028988,39.2875012672119));
#173011=CARTESIAN_POINT('Origin',(5.53234440788222E-15,0.,39.2875012672119));
#173012=CARTESIAN_POINT('',(61.3267881959115,13.3605623192479,39.8576902534424));
#173013=CARTESIAN_POINT('',(60.978275279735,13.2864868028988,39.2875012672119));
#173014=CARTESIAN_POINT('',(61.5752716937453,13.103835206572,40.1599502534424));
#173015=CARTESIAN_POINT('Ctrl Pts',(61.3267881959115,13.3605623192479,39.8576902534424));
#173016=CARTESIAN_POINT('Ctrl Pts',(61.3388252440299,13.3631207378648,39.8773836120328));
#173017=CARTESIAN_POINT('Ctrl Pts',(61.35122828376,13.363763127862,39.896994644206));
#173018=CARTESIAN_POINT('Ctrl Pts',(61.3638130392359,13.3625311504982,39.9162525288135));
#173019=CARTESIAN_POINT('Ctrl Pts',(61.376650671506,13.3612744179069,39.9358973793921));
#173020=CARTESIAN_POINT('Ctrl Pts',(61.3896782944532,13.3580674708042,39.9551762199564));
#173021=CARTESIAN_POINT('Ctrl Pts',(61.4027199492994,13.3529048112222,39.9738152034036));
#173022=CARTESIAN_POINT('Ctrl Pts',(61.4152549476772,13.347942716285,39.9917300792404));
#173023=CARTESIAN_POINT('Ctrl Pts',(61.427803769675,13.3411737181114,40.0090551157852));
#173024=CARTESIAN_POINT('Ctrl Pts',(61.4402150271644,13.3325479345667,40.025539455124));
#173025=CARTESIAN_POINT('Ctrl Pts',(61.4497489244961,13.3259219069631,40.0382021525961));
#173026=CARTESIAN_POINT('Ctrl Pts',(61.4592018401621,13.3181993658996,40.0503687782034));
#173027=CARTESIAN_POINT('Ctrl Pts',(61.468502650244,13.3093393327436,40.0619155352442));
#173028=CARTESIAN_POINT('Ctrl Pts',(61.4685270260085,13.3093161121768,40.0619457972351));
#173029=CARTESIAN_POINT('Ctrl Pts',(61.4685514007484,13.3092928829596,40.0619760547305));
#173030=CARTESIAN_POINT('Ctrl Pts',(61.468575774461,13.3092696450942,40.0620063077269));
#173031=CARTESIAN_POINT('Ctrl Pts',(61.4711891321182,13.3067780733542,40.06525004417));
#173032=CARTESIAN_POINT('Ctrl Pts',(61.4737888336848,13.3041875240722,40.0684393223556));
#173033=CARTESIAN_POINT('Ctrl Pts',(61.4763713294376,13.3015014257474,40.0715697951759));
#173034=CARTESIAN_POINT('Ctrl Pts',(61.4907423311191,13.2865538993088,40.0889901646442));
#173035=CARTESIAN_POINT('Ctrl Pts',(61.504584082868,13.2686510078378,40.1045963098281));
#173036=CARTESIAN_POINT('Ctrl Pts',(61.5172886502292,13.2484387178417,40.1176634650774));
#173037=CARTESIAN_POINT('Ctrl Pts',(61.5229906359957,13.2393671621885,40.1235281853092));
#173038=CARTESIAN_POINT('Ctrl Pts',(61.5284639152937,13.229830388847,40.1288820140933));
#173039=CARTESIAN_POINT('Ctrl Pts',(61.5336555255489,13.2198857715698,40.1336621774101));
#173040=CARTESIAN_POINT('Ctrl Pts',(61.535911729145,13.2155639754103,40.1357395717319));
#173041=CARTESIAN_POINT('Ctrl Pts',(61.5381145532938,13.2111652444428,40.1377083672884));
#173042=CARTESIAN_POINT('Ctrl Pts',(61.5402595369764,13.2066943520815,40.1395632548792));
#173043=CARTESIAN_POINT('Ctrl Pts',(61.5477669798654,13.1910462288171,40.146055361447));
#173044=CARTESIAN_POINT('Ctrl Pts',(61.5545658738899,13.1745141278027,40.1511520974629));
#173045=CARTESIAN_POINT('Ctrl Pts',(61.5604649702291,13.1573027128853,40.1546258197408));
#173046=CARTESIAN_POINT('Ctrl Pts',(61.5634145183987,13.1486970054266,40.1563626808798));
#173047=CARTESIAN_POINT('Ctrl Pts',(61.5661391177413,13.1399214696209,40.1576937882008));
#173048=CARTESIAN_POINT('Ctrl Pts',(61.5686148699003,13.1310016901023,40.1585906813668));
#173049=CARTESIAN_POINT('Ctrl Pts',(61.5698527459799,13.126541800343,40.1590391279498));
#173050=CARTESIAN_POINT('Ctrl Pts',(61.5710284103841,13.1220458496811,40.1593790209175));
#173051=CARTESIAN_POINT('Ctrl Pts',(61.5721388765029,13.1175170363396,40.1596068022931));
#173052=CARTESIAN_POINT('Ctrl Pts',(61.5732493426218,13.1129882229981,40.1598345836687));
#173053=CARTESIAN_POINT('Ctrl Pts',(61.5742946087865,13.108426546622,40.1599502506865));
#173054=CARTESIAN_POINT('Ctrl Pts',(61.5752716937453,13.103835206572,40.1599502534424));
#173055=CARTESIAN_POINT('',(61.5816197022699,13.0739701745317,40.1599502534424));
#173056=CARTESIAN_POINT('Origin',(5.50318346416883E-15,5.66257247735684E-15,
40.1599502534424));
#173057=CARTESIAN_POINT('',(61.459039055521,12.7383709431243,39.8576902534424));
#173058=CARTESIAN_POINT('Ctrl Pts',(61.5816197022699,13.0739701745317,40.1599502534424));
#173059=CARTESIAN_POINT('Ctrl Pts',(61.58241334955,13.070231874317,40.1599502447858));
#173060=CARTESIAN_POINT('Ctrl Pts',(61.5831581321229,13.0664939028178,40.1598744685927));
#173061=CARTESIAN_POINT('Ctrl Pts',(61.5838547466227,13.0627583804519,40.1597246934279));
#173062=CARTESIAN_POINT('Ctrl Pts',(61.5878803190637,13.041171669446,40.1588591777435));
#173063=CARTESIAN_POINT('Ctrl Pts',(61.5902997144311,13.0196643745808,40.155525470602));
#173064=CARTESIAN_POINT('Ctrl Pts',(61.5912450453421,12.9986523536622,40.150063182638));
#173065=CARTESIAN_POINT('Ctrl Pts',(61.5916263190448,12.9901777222667,40.1478601162481));
#173066=CARTESIAN_POINT('Ctrl Pts',(61.5917681516648,12.9817833412905,40.1453112228306));
#173067=CARTESIAN_POINT('Ctrl Pts',(61.5916804171631,12.9734950911666,40.1424401896328));
#173068=CARTESIAN_POINT('Ctrl Pts',(61.5916480484585,12.9704372300717,40.1413809526905));
#173069=CARTESIAN_POINT('Ctrl Pts',(61.5915843445342,12.9673939164343,40.1402777640511));
#173070=CARTESIAN_POINT('Ctrl Pts',(61.5914897592008,12.9643665007543,40.1391317641987));
#173071=CARTESIAN_POINT('Ctrl Pts',(61.5913124117006,12.9586900963543,40.1369830144753));
#173072=CARTESIAN_POINT('Ctrl Pts',(61.5910264967404,12.9530695832094,40.134683756585));
#173073=CARTESIAN_POINT('Ctrl Pts',(61.5906350058492,12.9475138635626,40.1322415082996));
#173074=CARTESIAN_POINT('Ctrl Pts',(61.5892647877302,12.9280688447987,40.1236936393009));
#173075=CARTESIAN_POINT('Ctrl Pts',(61.5866012600732,12.9094175454586,40.113394140767));
#173076=CARTESIAN_POINT('Ctrl Pts',(61.5827727094486,12.8919416545035,40.101665321223));
#173077=CARTESIAN_POINT('Ctrl Pts',(61.5808584341364,12.8832037090259,40.095800911451));
#173078=CARTESIAN_POINT('Ctrl Pts',(61.5786529040704,12.8747596158549,40.0895791707949));
#173079=CARTESIAN_POINT('Ctrl Pts',(61.576172163775,12.8666570879109,40.0830403822906));
#173080=CARTESIAN_POINT('Ctrl Pts',(61.5749317936273,12.862605823939,40.0797709880385));
#173081=CARTESIAN_POINT('Ctrl Pts',(61.5736226210374,12.8586399512971,40.0764223317514));
#173082=CARTESIAN_POINT('Ctrl Pts',(61.5722466520923,12.8547654342058,40.0729994484778));
#173083=CARTESIAN_POINT('Ctrl Pts',(61.5708706831473,12.8508909171145,40.0695765652042));
#173084=CARTESIAN_POINT('Ctrl Pts',(61.5694278436303,12.8471078617853,40.0660793733488));
#173085=CARTESIAN_POINT('Ctrl Pts',(61.5679202927797,12.8434220158068,40.0625130768817));
#173086=CARTESIAN_POINT('Ctrl Pts',(61.5679074365282,12.8433905832599,40.0624826638418));
#173087=CARTESIAN_POINT('Ctrl Pts',(61.5678945756945,12.8433591578468,40.0624522459912));
#173088=CARTESIAN_POINT('Ctrl Pts',(61.5678817102797,12.8433277395701,40.0624218233329));
#173089=CARTESIAN_POINT('Ctrl Pts',(61.5613111551481,12.8272819669691,40.0468845275908));
#173090=CARTESIAN_POINT('Ctrl Pts',(61.5536499750617,12.813016372708,40.0302263329257));
#173091=CARTESIAN_POINT('Ctrl Pts',(61.5450979154855,12.8005145062067,40.0127515884775));
#173092=CARTESIAN_POINT('Ctrl Pts',(61.5362566309333,12.7875898348819,39.9946858597757));
#173093=CARTESIAN_POINT('Ctrl Pts',(61.5264624086177,12.7765497640387,39.9757460620543));
#173094=CARTESIAN_POINT('Ctrl Pts',(61.5159109908837,12.7674219834074,39.9562444559193));
#173095=CARTESIAN_POINT('Ctrl Pts',(61.5055602833174,12.7584678323706,39.9371138113686));
#173096=CARTESIAN_POINT('Ctrl Pts',(61.4944799879548,12.7513538295746,39.9174410654438));
#173097=CARTESIAN_POINT('Ctrl Pts',(61.4828443590724,12.7461528104588,39.897519650424));
#173098=CARTESIAN_POINT('Ctrl Pts',(61.4751361628629,12.7427073176333,39.8843224113838));
#173099=CARTESIAN_POINT('Ctrl Pts',(61.4671840587594,12.7401023057308,39.8710160447164));
#173100=CARTESIAN_POINT('Ctrl Pts',(61.459039055521,12.7383709431243,39.8576902534424));
#173101=CARTESIAN_POINT('',(61.1105274371643,12.6642893210133,39.2875012672119));
#173102=CARTESIAN_POINT('',(61.459039055521,12.7383709431243,39.8576902534424));
#173103=CARTESIAN_POINT('',(62.0330459552233,6.83973663030176,39.2875012672119));
#173104=CARTESIAN_POINT('Origin',(5.53234440788222E-15,0.,39.2875012672119));
#173105=CARTESIAN_POINT('',(62.3873926810692,6.8769768336648,39.8576902534424));
#173106=CARTESIAN_POINT('',(62.0330459552233,6.83973663030176,39.2875012672119));
#173107=CARTESIAN_POINT('',(62.6076796697355,6.59568250079801,40.1599502534424));
#173108=CARTESIAN_POINT('Ctrl Pts',(62.3873926810692,6.8769768336648,39.8576902534424));
#173109=CARTESIAN_POINT('Ctrl Pts',(62.3996312165469,6.87826302285496,39.8773836120357));
#173110=CARTESIAN_POINT('Ctrl Pts',(62.4120334591686,6.87760542308938,39.8969946442118));
#173111=CARTESIAN_POINT('Ctrl Pts',(62.4244204973384,6.87506472947515,39.9162525288219));
#173112=CARTESIAN_POINT('Ctrl Pts',(62.4370564393911,6.87247298342229,39.9358973794034));
#173113=CARTESIAN_POINT('Ctrl Pts',(62.4496774784062,6.86792184690318,39.9551762199703));
#173114=CARTESIAN_POINT('Ctrl Pts',(62.4621080448317,6.86142424476893,39.97381520342));
#173115=CARTESIAN_POINT('Ctrl Pts',(62.4740556950203,6.85517906858736,39.9917300792593));
#173116=CARTESIAN_POINT('Ctrl Pts',(62.4858282202829,6.8471354426121,40.0090551158062));
#173117=CARTESIAN_POINT('Ctrl Pts',(62.4972698477083,6.83725958233632,40.0255394551469));
#173118=CARTESIAN_POINT('Ctrl Pts',(62.5060589088643,6.82967328917143,40.0382021526107));
#173119=CARTESIAN_POINT('Ctrl Pts',(62.514652815114,6.82100495425239,40.0503687782103));
#173120=CARTESIAN_POINT('Ctrl Pts',(62.5229765487298,6.81122125790595,40.0619155352442));
#173121=CARTESIAN_POINT('Ctrl Pts',(62.5229983637512,6.81119561658265,40.0619457972351));
#173122=CARTESIAN_POINT('Ctrl Pts',(62.5230201768493,6.81116996676345,40.0619760547305));
#173123=CARTESIAN_POINT('Ctrl Pts',(62.5230419880218,6.81114430845071,40.0620063077269));
#173124=CARTESIAN_POINT('Ctrl Pts',(62.5253805892672,6.80839321554162,40.06525004417));
#173125=CARTESIAN_POINT('Ctrl Pts',(62.5276952632612,6.80554511474983,40.0684393223556));
#173126=CARTESIAN_POINT('Ctrl Pts',(62.5299828381019,6.80260378684031,40.0715697951759));
#173127=CARTESIAN_POINT('Ctrl Pts',(62.5427126719621,6.78623596579693,40.0889901646412));
#173128=CARTESIAN_POINT('Ctrl Pts',(62.5546072354113,6.76698429120314,40.1045963098228));
#173129=CARTESIAN_POINT('Ctrl Pts',(62.5651294462094,6.74555473734808,40.1176634650707));
#173130=CARTESIAN_POINT('Ctrl Pts',(62.5698519601314,6.7359368568129,40.1235281853051));
#173131=CARTESIAN_POINT('Ctrl Pts',(62.5742983919726,6.72588021343593,40.1288820140915));
#173132=CARTESIAN_POINT('Ctrl Pts',(62.5784220664835,6.71544740276686,40.1336621774101));
#173133=CARTESIAN_POINT('Ctrl Pts',(62.5802141596491,6.71091344436422,40.1357395717319));
#173134=CARTESIAN_POINT('Ctrl Pts',(62.5819451239083,6.70630855228205,40.1377083672884));
#173135=CARTESIAN_POINT('Ctrl Pts',(62.5836110216379,6.70163794008886,40.1395632548791));
#173136=CARTESIAN_POINT('Ctrl Pts',(62.5894416636914,6.68529079741268,40.1460553614469));
#173137=CARTESIAN_POINT('Ctrl Pts',(62.5944752375495,6.66813858303315,40.1511520974629));
#173138=CARTESIAN_POINT('Ctrl Pts',(62.5985429352697,6.6504048305725,40.1546258197408));
#173139=CARTESIAN_POINT('Ctrl Pts',(62.6005767841298,6.64153795434218,40.1563626808798));
#173140=CARTESIAN_POINT('Ctrl Pts',(62.6023691645599,6.63252569365755,40.1576937882008));
#173141=CARTESIAN_POINT('Ctrl Pts',(62.6038989834439,6.62339599105584,40.1585906813668));
#173142=CARTESIAN_POINT('Ctrl Pts',(62.6046638928858,6.61883113975498,40.1590391279498));
#173143=CARTESIAN_POINT('Ctrl Pts',(62.6053631620638,6.61423692798771,40.1593790209175));
#173144=CARTESIAN_POINT('Ctrl Pts',(62.6059941550341,6.60961684864265,40.1596068022931));
#173145=CARTESIAN_POINT('Ctrl Pts',(62.6066251480044,6.6049967692976,40.1598345836687));
#173146=CARTESIAN_POINT('Ctrl Pts',(62.6071878630701,6.60035082219605,40.1599502506865));
#173147=CARTESIAN_POINT('Ctrl Pts',(62.6076796697355,6.59568250079801,40.1599502534424));
#173148=CARTESIAN_POINT('',(62.6108711573006,6.56531752495217,40.1599502534424));
#173149=CARTESIAN_POINT('Origin',(5.50063869163689E-15,5.67863953878492E-15,
40.1599502534424));
#173150=CARTESIAN_POINT('',(62.4538823482276,6.24436990787975,39.8576902534424));
#173151=CARTESIAN_POINT('Ctrl Pts',(62.6108711573006,6.56531752495217,40.1599502534424));
#173152=CARTESIAN_POINT('Ctrl Pts',(62.6112696981211,6.56151674480659,40.1599502447858));
#173153=CARTESIAN_POINT('Ctrl Pts',(62.6116196762807,6.55772139932857,40.1598744685927));
#173154=CARTESIAN_POINT('Ctrl Pts',(62.6119220062409,6.55393352450196,40.1597246934279));
#173155=CARTESIAN_POINT('Ctrl Pts',(62.6136691004464,6.53204428085642,40.1588591777434));
#173156=CARTESIAN_POINT('Ctrl Pts',(62.6138271176316,6.51040190952294,40.155525470602));
#173157=CARTESIAN_POINT('Ctrl Pts',(62.6125709156641,6.48940618066597,40.150063182638));
#173158=CARTESIAN_POINT('Ctrl Pts',(62.6120642605131,6.48093812023388,40.147860116248));
#173159=CARTESIAN_POINT('Ctrl Pts',(62.6113278644157,6.47257489900929,40.1453112228306));
#173160=CARTESIAN_POINT('Ctrl Pts',(62.6103742524841,6.46434122353952,40.1424401896328));
#173161=CARTESIAN_POINT('Ctrl Pts',(62.6100224275775,6.46130349717859,40.1413809526906));
#173162=CARTESIAN_POINT('Ctrl Pts',(62.6096409597323,6.45828351400505,40.1402777640512));
#173163=CARTESIAN_POINT('Ctrl Pts',(62.6092304414385,6.45528256968445,40.1391317641987));
#173164=CARTESIAN_POINT('Ctrl Pts',(62.6084607196376,6.44965579908332,40.1369830144753));
#173165=CARTESIAN_POINT('Ctrl Pts',(62.6075888673476,6.44409596194893,40.134683756585));
#173166=CARTESIAN_POINT('Ctrl Pts',(62.6066187902475,6.43861159905687,40.1322415082996));
#173167=CARTESIAN_POINT('Ctrl Pts',(62.6032235203971,6.41941632893468,40.1236936393009));
#173168=CARTESIAN_POINT('Ctrl Pts',(62.5986249921653,6.40114561781669,40.113394140767));
#173169=CARTESIAN_POINT('Ctrl Pts',(62.592990686716,6.38416565413411,40.101665321223));
#173170=CARTESIAN_POINT('Ctrl Pts',(62.5901735339913,6.37567567229282,40.095800911451));
#173171=CARTESIAN_POINT('Ctrl Pts',(62.5870974379669,6.36750837741621,40.0895791707949));
#173172=CARTESIAN_POINT('Ctrl Pts',(62.5837833426318,6.35970954393893,40.0830403822906));
#173173=CARTESIAN_POINT('Ctrl Pts',(62.5821262949643,6.35581012720029,40.0797709880385));
#173174=CARTESIAN_POINT('Ctrl Pts',(62.580409747586,6.35200282582274,40.0764223317514));
#173175=CARTESIAN_POINT('Ctrl Pts',(62.5786363190254,6.34829336166079,40.0729994484778));
#173176=CARTESIAN_POINT('Ctrl Pts',(62.5768628904648,6.34458389749884,40.0695765652042));
#173177=CARTESIAN_POINT('Ctrl Pts',(62.5750325180136,6.34097238393994,40.0660793733488));
#173178=CARTESIAN_POINT('Ctrl Pts',(62.5731479498683,6.33746431138509,40.0625130768817));
#173179=CARTESIAN_POINT('Ctrl Pts',(62.5731318784489,6.33743439487324,40.0624826638418));
#173180=CARTESIAN_POINT('Ctrl Pts',(62.573115803218,6.33740448593497,40.0624522459912));
#173181=CARTESIAN_POINT('Ctrl Pts',(62.5730997241772,6.33737458457292,40.0624218233329));
#173182=CARTESIAN_POINT('Ctrl Pts',(62.5648879232826,6.32210352242476,40.0468845275917));
#173183=CARTESIAN_POINT('Ctrl Pts',(62.5557775512972,6.30871688796365,40.0302263329277));
#173184=CARTESIAN_POINT('Ctrl Pts',(62.5459655399055,6.2971774416409,40.0127515884806));
#173185=CARTESIAN_POINT('Ctrl Pts',(62.535821692804,6.28524773890599,39.99468585978));
#173186=CARTESIAN_POINT('Ctrl Pts',(62.5249271226242,6.27529192173385,39.9757460620598));
#173187=CARTESIAN_POINT('Ctrl Pts',(62.5134793937788,6.26731706752099,39.9562444559261));
#173188=CARTESIAN_POINT('Ctrl Pts',(62.5022494248245,6.25949391181599,39.9371138113764));
#173189=CARTESIAN_POINT('Ctrl Pts',(62.4904862127,6.25357708651817,39.9174410654527));
#173190=CARTESIAN_POINT('Ctrl Pts',(62.4783706704752,6.24962081353501,39.8975196504339));
#173191=CARTESIAN_POINT('Ctrl Pts',(62.4703445484988,6.24699992138299,39.8843224113905));
#173192=CARTESIAN_POINT('Ctrl Pts',(62.4621637089607,6.24524040122917,39.8710160447197));
#173193=CARTESIAN_POINT('Ctrl Pts',(62.4538823482276,6.24436990787975,39.8576902534424));
#173194=CARTESIAN_POINT('',(62.099536274866,6.20712349654379,39.2875012672119));
#173195=CARTESIAN_POINT('',(62.4538823482276,6.24436990787975,39.8576902534424));
#173196=CARTESIAN_POINT('',(62.4081695979768,0.318048871877121,39.2875012672119));
#173197=CARTESIAN_POINT('Origin',(5.53234440788222E-15,0.,39.2875012672119));
#173198=CARTESIAN_POINT('',(62.7644678366119,0.318045750793045,39.8576902534424));
#173199=CARTESIAN_POINT('',(62.4081695979768,0.318048871877129,39.2875012672119));
#173200=CARTESIAN_POINT('Ctrl Pts',(62.7644678366119,0.318045750793045,
39.8576902534424));
#173201=CARTESIAN_POINT('Ctrl Pts',(62.77677377149,0.318045618798131,39.8773836120337));
#173202=CARTESIAN_POINT('Ctrl Pts',(62.7890393354348,0.316095234070915,
39.8969946442079));
#173203=CARTESIAN_POINT('Ctrl Pts',(62.8010929413131,0.312273660578547,
39.9162525288162));
#173204=CARTESIAN_POINT('Ctrl Pts',(62.8133887511199,0.308375296777785,
39.9358973793958));
#173205=CARTESIAN_POINT('Ctrl Pts',(62.8254649274551,0.302529834048776,
39.9551762199609));
#173206=CARTESIAN_POINT('Ctrl Pts',(62.8371482135701,0.294768478454403,
39.9738152034089));
#173207=CARTESIAN_POINT('Ctrl Pts',(62.8483776146108,0.287308644488986,
39.9917300792467));
#173208=CARTESIAN_POINT('Ctrl Pts',(62.8592448608851,0.278078518365762,
40.0090551157924));
#173209=CARTESIAN_POINT('Ctrl Pts',(62.8695915013795,0.267060783356013,
40.0255394551319));
#173210=CARTESIAN_POINT('Ctrl Pts',(62.8775394315759,0.258597341640156,
40.0382021526012));
#173211=CARTESIAN_POINT('Ctrl Pts',(62.8851801717829,0.24907818494972,40.0503687782058));
#173212=CARTESIAN_POINT('Ctrl Pts',(62.8924356323738,0.238478017627863,
40.0619155352442));
#173213=CARTESIAN_POINT('Ctrl Pts',(62.892454647642,0.238450236479755,40.0619457972351));
#173214=CARTESIAN_POINT('Ctrl Pts',(62.8924736601095,0.238422447083332,
40.0619760547304));
#173215=CARTESIAN_POINT('Ctrl Pts',(62.8924926697742,0.238394649441168,
40.0620063077269));
#173216=CARTESIAN_POINT('Ctrl Pts',(62.8945308924032,0.235414176912503,
40.06525004417));
#173217=CARTESIAN_POINT('Ctrl Pts',(62.8965351787718,0.232339728999319,
40.0684393223556));
#173218=CARTESIAN_POINT('Ctrl Pts',(62.8985027695519,0.229175397309127,
40.0715697951759));
#173219=CARTESIAN_POINT('Ctrl Pts',(62.9094519648687,0.211566610932373,
40.0889901646398));
#173220=CARTESIAN_POINT('Ctrl Pts',(62.9192690206934,0.191177078589634,
40.1045963098203));
#173221=CARTESIAN_POINT('Ctrl Pts',(62.9274935913864,0.168765047550033,
40.1176634650675));
#173222=CARTESIAN_POINT('Ctrl Pts',(62.9311848926116,0.158706217646069,
40.1235281853032));
#173223=CARTESIAN_POINT('Ctrl Pts',(62.9345557609568,0.14823988692456,40.1288820140906));
#173224=CARTESIAN_POINT('Ctrl Pts',(62.9375663198809,0.137433186922361,
40.1336621774101));
#173225=CARTESIAN_POINT('Ctrl Pts',(62.9388746680683,0.132736741273613,
40.1357395717319));
#173226=CARTESIAN_POINT('Ctrl Pts',(62.9401148076313,0.127976140238101,
40.1377083672884));
#173227=CARTESIAN_POINT('Ctrl Pts',(62.9412833674838,0.123156980417561,
40.1395632548791));
#173228=CARTESIAN_POINT('Ctrl Pts',(62.9453733269673,0.106289921045671,
40.1460553614469));
#173229=CARTESIAN_POINT('Ctrl Pts',(62.9485864317704,0.0887055165510538,
40.151152097463));
#173230=CARTESIAN_POINT('Ctrl Pts',(62.9507781643242,0.0706437212501634,
40.1546258197409));
#173231=CARTESIAN_POINT('Ctrl Pts',(62.9518740306011,0.0616128235997182,
40.1563626808798));
#173232=CARTESIAN_POINT('Ctrl Pts',(62.9527145544238,0.05246257825014,40.1576937882008));
#173233=CARTESIAN_POINT('Ctrl Pts',(62.9532816790167,0.0432229794975189,
40.1585906813668));
#173234=CARTESIAN_POINT('Ctrl Pts',(62.9535652413132,0.0386031801212083,
40.1590391279498));
#173235=CARTESIAN_POINT('Ctrl Pts',(62.9537804539255,0.0339610423941129,
40.1593790209175));
#173236=CARTESIAN_POINT('Ctrl Pts',(62.9539250604562,0.0293003156016006,
40.1596068022931));
#173237=CARTESIAN_POINT('Ctrl Pts',(62.9540696669868,0.024639588809088,
40.1598345836686));
#173238=CARTESIAN_POINT('Ctrl Pts',(62.9541436657296,0.0199602729507933,
40.1599502506865));
#173239=CARTESIAN_POINT('Ctrl Pts',(62.9541448057648,0.0152661173108668,
40.1599502534424));
#173240=CARTESIAN_POINT('Origin',(5.71385722241845E-15,0.,40.5765));
#173241=CARTESIAN_POINT('',(-59.1088767419348,-0.316922544675689,39.8576902534424));
#173242=CARTESIAN_POINT('Ctrl Pts',(-58.9208513795073,-0.0152121934559198,
40.1599502534424));
#173243=CARTESIAN_POINT('Ctrl Pts',(-58.9208504012364,-0.0190220008285423,
40.1599502448875));
#173244=CARTESIAN_POINT('Ctrl Pts',(-58.9208964366351,-0.0228214099817212,
40.1598743450437));
#173245=CARTESIAN_POINT('Ctrl Pts',(-58.9209883940807,-0.0266084895330029,
40.1597243308499));
#173246=CARTESIAN_POINT('Ctrl Pts',(-58.9215313038856,-0.048967120813079,
40.1588386583938));
#173247=CARTESIAN_POINT('Ctrl Pts',(-58.9236732325286,-0.0708986527603139,
40.1553722553618));
#173248=CARTESIAN_POINT('Ctrl Pts',(-58.9271900305696,-0.0919988953507848,
40.1496902177788));
#173249=CARTESIAN_POINT('Ctrl Pts',(-58.9285037892487,-0.0998812435867534,
40.1475675976844));
#173250=CARTESIAN_POINT('Ctrl Pts',(-58.9300091878196,-0.107647933246467,
40.1451361443096));
#173251=CARTESIAN_POINT('Ctrl Pts',(-58.9316938830317,-0.115279202946911,
40.1424159447501));
#173252=CARTESIAN_POINT('Ctrl Pts',(-58.933008366749,-0.121233502390215,
40.1402935085949));
#173253=CARTESIAN_POINT('Ctrl Pts',(-58.9344322364591,-0.127104908280006,
40.1379949176048));
#173254=CARTESIAN_POINT('Ctrl Pts',(-58.9359598525093,-0.132883578273067,
40.1355293609261));
#173255=CARTESIAN_POINT('Ctrl Pts',(-58.9413065086849,-0.153108923248783,
40.1268999125509));
#173256=CARTESIAN_POINT('Ctrl Pts',(-58.9479240485795,-0.172198253417716,
40.1162251288835));
#173257=CARTESIAN_POINT('Ctrl Pts',(-58.9555707636545,-0.189729578870775,
40.1038990521418));
#173258=CARTESIAN_POINT('Ctrl Pts',(-58.959394121192,-0.198495241597304,
40.097736013771));
#173259=CARTESIAN_POINT('Ctrl Pts',(-58.9634747743348,-0.20687140316055,
40.0911601532641));
#173260=CARTESIAN_POINT('Ctrl Pts',(-58.9677825146336,-0.214805314863214,
40.084220729064));
#173261=CARTESIAN_POINT('Ctrl Pts',(-58.9720718502312,-0.222705329147628,
40.0773109533618));
#173262=CARTESIAN_POINT('Ctrl Pts',(-58.9765861722458,-0.230167055079178,
40.0700409753048));
#173263=CARTESIAN_POINT('Ctrl Pts',(-58.9812961520165,-0.237137844566648,
40.0624586415899));
#173264=CARTESIAN_POINT('Ctrl Pts',(-58.9813163616197,-0.237167754862791,
40.062426107277));
#173265=CARTESIAN_POINT('Ctrl Pts',(-58.9813365744745,-0.2371976565367,
40.0623935677889));
#173266=CARTESIAN_POINT('Ctrl Pts',(-58.9813567905789,-0.237227549587953,
40.0623610231289));
#173267=CARTESIAN_POINT('Ctrl Pts',(-58.9908903168209,-0.251324537972149,
40.0470135870235));
#173268=CARTESIAN_POINT('Ctrl Pts',(-59.0011093202327,-0.263501580512048,
40.0305755292096));
#173269=CARTESIAN_POINT('Ctrl Pts',(-59.0118294103842,-0.273820596508944,
40.0133447567344));
#173270=CARTESIAN_POINT('Ctrl Pts',(-59.0229394763222,-0.284514998003796,
39.9954871626604));
#173271=CARTESIAN_POINT('Ctrl Pts',(-59.034588573655,-0.293214009568305,
39.9767767954325));
#173272=CARTESIAN_POINT('Ctrl Pts',(-59.0465875206388,-0.299936893972227,
39.9575197577489));
#173273=CARTESIAN_POINT('Ctrl Pts',(-59.0584152157261,-0.306563827731033,
39.9385375612016));
#173274=CARTESIAN_POINT('Ctrl Pts',(-59.0705837677952,-0.311270560393244,
39.9190226977119));
#173275=CARTESIAN_POINT('Ctrl Pts',(-59.0829139906028,-0.314027284735643,
39.8992655451885));
#173276=CARTESIAN_POINT('Ctrl Pts',(-59.0915108413207,-0.315949321994157,
39.8854905069345));
#173277=CARTESIAN_POINT('Ctrl Pts',(-59.100186339707,-0.316922445687725,
39.8715976051485));
#173278=CARTESIAN_POINT('Ctrl Pts',(-59.1088767419348,-0.316922544675689,
39.8576902534424));
#173279=CARTESIAN_POINT('',(-59.4651754363832,-0.316925998273048,39.2875012672119));
#173280=CARTESIAN_POINT('',(-59.1088767419348,-0.316922544675689,39.8576902534424));
#173281=CARTESIAN_POINT('',(-59.1725467709678,-5.90061356181218,39.2875012672119));
#173282=CARTESIAN_POINT('Origin',(5.53234440788222E-15,0.,39.2875012672119));
#173283=CARTESIAN_POINT('',(-58.8181995570485,-5.86337364149541,39.8576902534424));
#173284=CARTESIAN_POINT('',(-59.1725467709678,-5.90061356181218,39.2875012672119));
#173285=CARTESIAN_POINT('',(-58.5996668978649,-6.14377718965283,40.1599502534424));
#173286=CARTESIAN_POINT('Ctrl Pts',(-58.8181995570485,-5.86337364149541,
39.8576902534424));
#173287=CARTESIAN_POINT('Ctrl Pts',(-58.8060365798455,-5.86209540502828,
39.8772619994052));
#173288=CARTESIAN_POINT('Ctrl Pts',(-58.7937272422247,-5.86273454612488,
39.8967644650367));
#173289=CARTESIAN_POINT('Ctrl Pts',(-58.7814443761802,-5.86523378400431,
39.9159282836043));
#173290=CARTESIAN_POINT('Ctrl Pts',(-58.7689396367198,-5.86777816724666,
39.9354382707185));
#173291=CARTESIAN_POINT('Ctrl Pts',(-58.7564614161384,-5.87225032431021,
39.9545987622356));
#173292=CARTESIAN_POINT('Ctrl Pts',(-58.7441787427588,-5.87864135443934,
39.9731387498235));
#173293=CARTESIAN_POINT('Ctrl Pts',(-58.7324160859241,-5.88476180492315,
39.9908938024065));
#173294=CARTESIAN_POINT('Ctrl Pts',(-58.7208319573121,-5.89264238981923,
40.0080810366197));
#173295=CARTESIAN_POINT('Ctrl Pts',(-58.709575439463,-5.90232005415971,
40.024454274256));
#173296=CARTESIAN_POINT('Ctrl Pts',(-58.7006223753283,-5.91001735013313,
40.0374770090498));
#173297=CARTESIAN_POINT('Ctrl Pts',(-58.6918764318948,-5.91885232406574,
40.0499848770044));
#173298=CARTESIAN_POINT('Ctrl Pts',(-58.6834178317481,-5.92886364759513,
40.0618424270193));
#173299=CARTESIAN_POINT('Ctrl Pts',(-58.6833947425173,-5.92889097525637,
40.0618747942791));
#173300=CARTESIAN_POINT('Ctrl Pts',(-58.683371655605,-5.92891831167191,
40.0619071564124));
#173301=CARTESIAN_POINT('Ctrl Pts',(-58.6833485710132,-5.9289456568414,
40.0619395134161));
#173302=CARTESIAN_POINT('Ctrl Pts',(-58.6787531612542,-5.9343892124318,
40.0683807661799));
#173303=CARTESIAN_POINT('Ctrl Pts',(-58.6742527563956,-5.94021607194738,
40.0746073439084));
#173304=CARTESIAN_POINT('Ctrl Pts',(-58.6698707672381,-5.94639317576837,
40.0805869293669));
#173305=CARTESIAN_POINT('Ctrl Pts',(-58.6611744062938,-5.95865206607742,
40.092453830807));
#173306=CARTESIAN_POINT('Ctrl Pts',(-58.6529445485198,-5.97229179622479,
40.1033475319609));
#173307=CARTESIAN_POINT('Ctrl Pts',(-58.6453649253901,-5.98706231729999,
40.1130129263075));
#173308=CARTESIAN_POINT('Ctrl Pts',(-58.6396802080428,-5.99814020810639,
40.1202619720674));
#173309=CARTESIAN_POINT('Ctrl Pts',(-58.6343612468744,-6.0098541687323,
40.1268200947266));
#173310=CARTESIAN_POINT('Ctrl Pts',(-58.6294855649109,-6.02209871088753,
40.1325796782703));
#173311=CARTESIAN_POINT('Ctrl Pts',(-58.6276571841746,-6.02669041419573,
40.1347395220992));
#173312=CARTESIAN_POINT('Ctrl Pts',(-58.6258911397672,-6.03135673055,40.1367870714852));
#173313=CARTESIAN_POINT('Ctrl Pts',(-58.624191520627,-6.0360920971711,40.1387166518767));
#173314=CARTESIAN_POINT('Ctrl Pts',(-58.6182428536363,-6.05266588034495,
40.1454701832469));
#173315=CARTESIAN_POINT('Ctrl Pts',(-58.6131078911177,-6.07008552874929,
40.1507785912492));
#173316=CARTESIAN_POINT('Ctrl Pts',(-58.608961992561,-6.08811254303222,
40.1543986087265));
#173317=CARTESIAN_POINT('Ctrl Pts',(-58.6068890432827,-6.09712605017368,
40.1562086174652));
#173318=CARTESIAN_POINT('Ctrl Pts',(-58.6050633610079,-6.10629139889362,
40.1575965292115));
#173319=CARTESIAN_POINT('Ctrl Pts',(-58.6035068699781,-6.11557877725374,
40.1585319382567));
#173320=CARTESIAN_POINT('Ctrl Pts',(-58.6027286244632,-6.1202224664338,
40.1589996427793));
#173321=CARTESIAN_POINT('Ctrl Pts',(-58.6020176767849,-6.12489666302693,
40.159354221642));
#173322=CARTESIAN_POINT('Ctrl Pts',(-58.6013767677628,-6.1295976405732,
40.159591874311));
#173323=CARTESIAN_POINT('Ctrl Pts',(-58.6007358587407,-6.13429861811947,
40.1598295269801));
#173324=CARTESIAN_POINT('Ctrl Pts',(-58.600164990065,-6.13902637679605,
40.1599502506896));
#173325=CARTESIAN_POINT('Ctrl Pts',(-58.5996668978649,-6.14377718965283,
40.1599502534424));
#173326=CARTESIAN_POINT('',(-58.5964866834551,-6.17403490858981,40.1599502534424));
#173327=CARTESIAN_POINT('Origin',(3.34731138317026E-16,-7.12196207432512E-18,
40.1599502534424));
#173328=CARTESIAN_POINT('',(-58.7519447039089,-6.49374646112701,39.8576902534424));
#173329=CARTESIAN_POINT('Ctrl Pts',(-58.5964866834551,-6.17403490858982,
40.1599502534424));
#173330=CARTESIAN_POINT('Ctrl Pts',(-58.5960874772333,-6.17782374318187,
40.1599502448875));
#173331=CARTESIAN_POINT('Ctrl Pts',(-58.5957361140451,-6.18160715078365,
40.1598743450437));
#173332=CARTESIAN_POINT('Ctrl Pts',(-58.5954317101325,-6.18538309648738,
40.1597243308499));
#173333=CARTESIAN_POINT('Ctrl Pts',(-58.5936345324521,-6.20767599437444,
40.1588386583938));
#173334=CARTESIAN_POINT('Ctrl Pts',(-58.5934722580544,-6.22971127560536,
40.1553722553615));
#173335=CARTESIAN_POINT('Ctrl Pts',(-58.5947642147754,-6.25106353435488,
40.149690217778));
#173336=CARTESIAN_POINT('Ctrl Pts',(-58.5952468467989,-6.25904002743736,
40.1475675976838));
#173337=CARTESIAN_POINT('Ctrl Pts',(-58.595932158504,-6.26692152735676,
40.1451361443093));
#173338=CARTESIAN_POINT('Ctrl Pts',(-58.5968099398848,-6.27468709076401,
40.1424159447501));
#173339=CARTESIAN_POINT('Ctrl Pts',(-58.5974948289521,-6.28074617289492,
40.1402935085949));
#173340=CARTESIAN_POINT('Ctrl Pts',(-58.5982971695201,-6.2867342495216,
40.1379949176048));
#173341=CARTESIAN_POINT('Ctrl Pts',(-58.5992123816356,-6.292640942714,40.1355293609261));
#173342=CARTESIAN_POINT('Ctrl Pts',(-58.6024156240399,-6.31331436888738,
40.1268999125509));
#173343=CARTESIAN_POINT('Ctrl Pts',(-58.6070015340112,-6.33299084698409,
40.1162251288835));
#173344=CARTESIAN_POINT('Ctrl Pts',(-58.6127738370723,-6.35122543337782,
40.1038990521418));
#173345=CARTESIAN_POINT('Ctrl Pts',(-58.6156599886028,-6.36034272657469,
40.097736013771));
#173346=CARTESIAN_POINT('Ctrl Pts',(-58.6188427402045,-6.36909954705062,
40.0911601532641));
#173347=CARTESIAN_POINT('Ctrl Pts',(-58.6222975626532,-6.37744027742843,
40.084220729064));
#173348=CARTESIAN_POINT('Ctrl Pts',(-58.6257376244687,-6.38574537226646,
40.0773109533619));
#173349=CARTESIAN_POINT('Ctrl Pts',(-58.6294472538099,-6.3936380972255,
40.0700409753048));
#173350=CARTESIAN_POINT('Ctrl Pts',(-58.6334027859057,-6.40106302694625,
40.0624586415899));
#173351=CARTESIAN_POINT('Ctrl Pts',(-58.6334197583214,-6.40109488586943,
40.0624261072769));
#173352=CARTESIAN_POINT('Ctrl Pts',(-58.633436734872,-6.40112673655749,
40.0623935677889));
#173353=CARTESIAN_POINT('Ctrl Pts',(-58.6334537155557,-6.4011585790098,
40.0623610231289));
#173354=CARTESIAN_POINT('Ctrl Pts',(-58.6414614796112,-6.41617486746464,
40.0470135870231));
#173355=CARTESIAN_POINT('Ctrl Pts',(-58.6503516547095,-6.42935337961447,
40.0305755292087));
#173356=CARTESIAN_POINT('Ctrl Pts',(-58.6599343882012,-6.44073642151188,
40.013344756733));
#173357=CARTESIAN_POINT('Ctrl Pts',(-58.6698657226821,-6.45253355607591,
39.9954871626584));
#173358=CARTESIAN_POINT('Ctrl Pts',(-58.6805417107304,-6.46240257578764,
39.9767767954299));
#173359=CARTESIAN_POINT('Ctrl Pts',(-58.691772193452,-6.47034286301642,
39.9575197577457));
#173360=CARTESIAN_POINT('Ctrl Pts',(-58.7028423919865,-6.47816982453019,
39.9385375611978));
#173361=CARTESIAN_POINT('Ctrl Pts',(-58.7144522959223,-6.48412273326628,
39.9190226977075));
#173362=CARTESIAN_POINT('Ctrl Pts',(-58.7264268163205,-6.48815321522591,
39.8992655451835));
#173363=CARTESIAN_POINT('Ctrl Pts',(-58.7347756649887,-6.49096333895714,
39.8854905069312));
#173364=CARTESIAN_POINT('Ctrl Pts',(-58.7433019189619,-6.49283796829136,
39.8715976051468));
#173365=CARTESIAN_POINT('Ctrl Pts',(-58.7519447039089,-6.49374646112702,
39.8576902534424));
#173366=CARTESIAN_POINT('',(-59.1062911958297,-6.53099325080016,39.2875012672119));
#173367=CARTESIAN_POINT('',(-58.7519447039089,-6.49374646112701,39.8576902534424));
#173368=CARTESIAN_POINT('',(-58.2316113004782,-12.0535047649318,39.2875012672119));
#173369=CARTESIAN_POINT('Origin',(5.53234440788222E-15,0.,39.2875012672119));
#173370=CARTESIAN_POINT('',(-57.8830978693156,-11.9794294790609,39.8576902534424));
#173371=CARTESIAN_POINT('',(-58.2316113004781,-12.0535047649318,39.2875012672119));
#173372=CARTESIAN_POINT('',(-57.6364522029208,-12.2354540642041,40.1599502534424));
#173373=CARTESIAN_POINT('Ctrl Pts',(-57.8830978693156,-11.9794294790609,
39.8576902534424));
#173374=CARTESIAN_POINT('Ctrl Pts',(-57.8711351342687,-11.9768868675911,
39.877261999404));
#173375=CARTESIAN_POINT('Ctrl Pts',(-57.8588264200515,-11.9762358312605,
39.8967644650343));
#173376=CARTESIAN_POINT('Ctrl Pts',(-57.8463495993382,-11.9774374689408,
39.9159282836008));
#173377=CARTESIAN_POINT('Ctrl Pts',(-57.8336474016795,-11.9786608125859,
39.9354382707139));
#173378=CARTESIAN_POINT('Ctrl Pts',(-57.8207700703914,-11.9818041414829,
39.95459876223));
#173379=CARTESIAN_POINT('Ctrl Pts',(-57.8078866382244,-11.9868762719064,
39.973138749817));
#173380=CARTESIAN_POINT('Ctrl Pts',(-57.7955486571718,-11.9917336614785,
39.9908938023992));
#173381=CARTESIAN_POINT('Ctrl Pts',(-57.7832042422001,-11.998360204543,
40.0080810366116));
#173382=CARTESIAN_POINT('Ctrl Pts',(-57.7709977973527,-12.006808227112,
40.0244542742473));
#173383=CARTESIAN_POINT('Ctrl Pts',(-57.7612891925185,-12.0135275064582,
40.0374770090442));
#173384=CARTESIAN_POINT('Ctrl Pts',(-57.7516676540278,-12.0213998814537,
40.0499848770018));
#173385=CARTESIAN_POINT('Ctrl Pts',(-57.7422089227118,-12.0304721974326,
40.0618424270193));
#173386=CARTESIAN_POINT('Ctrl Pts',(-57.7421831034479,-12.0304969619082,
40.0618747942791));
#173387=CARTESIAN_POINT('Ctrl Pts',(-57.7421572855746,-12.0305217353326,
40.0619071564124));
#173388=CARTESIAN_POINT('Ctrl Pts',(-57.7421314690941,-12.0305465177055,
40.0619395134162));
#173389=CARTESIAN_POINT('Ctrl Pts',(-57.7369922269699,-12.0354799018086,
40.0683807661799));
#173390=CARTESIAN_POINT('Ctrl Pts',(-57.7319074031292,-12.0408044207741,
40.0746073439084));
#173391=CARTESIAN_POINT('Ctrl Pts',(-57.726903735797,-12.0464896431813,
40.0805869293669));
#173392=CARTESIAN_POINT('Ctrl Pts',(-57.7169736114625,-12.0577723607611,
40.092453830807));
#173393=CARTESIAN_POINT('Ctrl Pts',(-57.7073630976788,-12.0704771166535,
40.1033475319609));
#173394=CARTESIAN_POINT('Ctrl Pts',(-57.698281056648,-12.0843744369109,
40.1130129263075));
#173395=CARTESIAN_POINT('Ctrl Pts',(-57.6914695258749,-12.094797427104,
40.1202619720674));
#173396=CARTESIAN_POINT('Ctrl Pts',(-57.6849552602293,-12.1058912345908,
40.1268200947266));
#173397=CARTESIAN_POINT('Ctrl Pts',(-57.6788263845868,-12.1175590523199,
40.1325796782703));
#173398=CARTESIAN_POINT('Ctrl Pts',(-57.6765280562209,-12.1219344839683,
40.1347395220992));
#173399=CARTESIAN_POINT('Ctrl Pts',(-57.674283923512,-12.1263906358454,
40.1367870714852));
#173400=CARTESIAN_POINT('Ctrl Pts',(-57.6720986344674,-12.1309224030558,
40.1387166518767));
#173401=CARTESIAN_POINT('Ctrl Pts',(-57.6644501228112,-12.1467835882923,
40.1454701832469));
#173402=CARTESIAN_POINT('Ctrl Pts',(-57.6575224410761,-12.163571060299,
40.1507785912492));
#173403=CARTESIAN_POINT('Ctrl Pts',(-57.6515149180852,-12.1810659563065,
40.1543986087265));
#173404=CARTESIAN_POINT('Ctrl Pts',(-57.6485111565898,-12.1898134043102,
40.1562086174652));
#173405=CARTESIAN_POINT('Ctrl Pts',(-57.6457374357765,-12.1987377085283,
40.1575965292115));
#173406=CARTESIAN_POINT('Ctrl Pts',(-57.6432186759796,-12.2078115120426,
40.1585319382567));
#173407=CARTESIAN_POINT('Ctrl Pts',(-57.6419592960812,-12.2123484137997,
40.1589996427793));
#173408=CARTESIAN_POINT('Ctrl Pts',(-57.6407636564618,-12.2169226903865,
40.159354221642));
#173409=CARTESIAN_POINT('Ctrl Pts',(-57.6396348724476,-12.2215309222508,
40.1595918743111));
#173410=CARTESIAN_POINT('Ctrl Pts',(-57.6385060884334,-12.226139154115,
40.1598295269801));
#173411=CARTESIAN_POINT('Ctrl Pts',(-57.637444161687,-12.2307813416095,
40.1599502506896));
#173412=CARTESIAN_POINT('Ctrl Pts',(-57.6364522029208,-12.2354540642041,
40.1599502534424));
#173413=CARTESIAN_POINT('',(-57.6301266171958,-12.2652136052657,40.1599502534424));
#173414=CARTESIAN_POINT('Origin',(3.35846787602729E-16,-1.41658944417981E-17,
40.1599502534424));
#173415=CARTESIAN_POINT('',(-57.7513140650721,-12.5994235324468,39.8576902534424));
#173416=CARTESIAN_POINT('Ctrl Pts',(-57.6301266171958,-12.2652136052657,
40.1599502534424));
#173417=CARTESIAN_POINT('Ctrl Pts',(-57.62933355681,-12.2689399558126,40.1599502448875));
#173418=CARTESIAN_POINT('Ctrl Pts',(-57.6285886446436,-12.2726659100575,
40.1598743450437));
#173419=CARTESIAN_POINT('Ctrl Pts',(-57.6278912144856,-12.2763893518624,
40.1597243308499));
#173420=CARTESIAN_POINT('Ctrl Pts',(-57.6237736395752,-12.2983722706985,
40.1588386583939));
#173421=CARTESIAN_POINT('Ctrl Pts',(-57.621308940049,-12.3202698780571,
40.1553722553623));
#173422=CARTESIAN_POINT('Ctrl Pts',(-57.6203619005013,-12.3416402131472,
40.1496902177801));
#173423=CARTESIAN_POINT('Ctrl Pts',(-57.6200081180517,-12.3496234589524,
40.1475675976854));
#173424=CARTESIAN_POINT('Ctrl Pts',(-57.6198658344726,-12.3575334177726,
40.1451361443101));
#173425=CARTESIAN_POINT('Ctrl Pts',(-57.6199270848658,-12.3653481937524,
40.1424159447501));
#173426=CARTESIAN_POINT('Ctrl Pts',(-57.6199748754952,-12.3714456739991,
40.1402935085949));
#173427=CARTESIAN_POINT('Ctrl Pts',(-57.6201468963099,-12.3774848147421,
40.1379949176048));
#173428=CARTESIAN_POINT('Ctrl Pts',(-57.6204396772352,-12.3834548161672,
40.1355293609261));
#173429=CARTESIAN_POINT('Ctrl Pts',(-57.6214644104741,-12.4043498211549,
40.1268999125509));
#173430=CARTESIAN_POINT('Ctrl Pts',(-57.6239684463328,-12.4243978675678,
40.1162251288835));
#173431=CARTESIAN_POINT('Ctrl Pts',(-57.6278030948197,-12.4431359329578,
40.1038990521418));
#173432=CARTESIAN_POINT('Ctrl Pts',(-57.6297204190631,-12.4525049656528,
40.097736013771));
#173433=CARTESIAN_POINT('Ctrl Pts',(-57.631970398231,-12.4615465034838,
40.0911601532641));
#173434=CARTESIAN_POINT('Ctrl Pts',(-57.634534451072,-12.4702026697494,
40.084220729064));
#173435=CARTESIAN_POINT('Ctrl Pts',(-57.6370875490682,-12.478821852784,
40.0773109533619));
#173436=CARTESIAN_POINT('Ctrl Pts',(-57.6399518422608,-12.4870591024242,
40.0700409753048));
#173437=CARTESIAN_POINT('Ctrl Pts',(-57.6431095890443,-12.4948568232945,
40.0624586415899));
#173438=CARTESIAN_POINT('Ctrl Pts',(-57.643123138319,-12.4948902817916,
40.062426107277));
#173439=CARTESIAN_POINT('Ctrl Pts',(-57.6431366925668,-12.4949237325311,
40.0623935677889));
#173440=CARTESIAN_POINT('Ctrl Pts',(-57.643150251786,-12.4949571755119,
40.0623610231289));
#173441=CARTESIAN_POINT('Ctrl Pts',(-57.6495445189164,-12.5107282424396,
40.0470135870218));
#173442=CARTESIAN_POINT('Ctrl Pts',(-57.6570084630829,-12.5247638376633,
40.0305755292059));
#173443=CARTESIAN_POINT('Ctrl Pts',(-57.6653488494819,-12.5370861904728,
40.0133447567286));
#173444=CARTESIAN_POINT('Ctrl Pts',(-57.6739926427273,-12.5498568062315,
39.9954871626524));
#173445=CARTESIAN_POINT('Ctrl Pts',(-57.6835785531326,-12.5607877070457,
39.9767767954222));
#173446=CARTESIAN_POINT('Ctrl Pts',(-57.693917528074,-12.569858401651,39.9575197577362));
#173447=CARTESIAN_POINT('Ctrl Pts',(-57.7041089426444,-12.5787996370916,
39.9385375611868));
#173448=CARTESIAN_POINT('Ctrl Pts',(-57.7150329979106,-12.5859335005876,
39.919022697695));
#173449=CARTESIAN_POINT('Ctrl Pts',(-57.7265206205487,-12.5911935813604,
39.8992655451695));
#173450=CARTESIAN_POINT('Ctrl Pts',(-57.7345299954327,-12.5948610032592,
39.8854905069218));
#173451=CARTESIAN_POINT('Ctrl Pts',(-57.7428135895682,-12.5976165994018,
39.8715976051421));
#173452=CARTESIAN_POINT('Ctrl Pts',(-57.7513140650721,-12.5994235324468,
39.8576902534424));
#173453=CARTESIAN_POINT('',(-58.0998260601481,-12.6735055745737,39.2875012672119));
#173454=CARTESIAN_POINT('',(-57.7513140650721,-12.5994235324468,39.8576902534424));
#173455=CARTESIAN_POINT('',(-56.6526781108324,-18.0743352474888,39.2875012672119));
#173456=CARTESIAN_POINT('Origin',(5.53234440788222E-15,0.,39.2875012672119));
#173457=CARTESIAN_POINT('',(-56.3138168485096,-17.9642361803969,39.8576902534424));
#173458=CARTESIAN_POINT('',(-56.6526781108324,-18.0743352474888,39.2875012672119));
#173459=CARTESIAN_POINT('',(-56.0417604764384,-18.1930767435946,40.1599502534424));
#173460=CARTESIAN_POINT('Ctrl Pts',(-56.3138168485096,-17.9642361803969,
39.8576902534424));
#173461=CARTESIAN_POINT('Ctrl Pts',(-56.3021854218462,-17.960457051308,
39.8772619994045));
#173462=CARTESIAN_POINT('Ctrl Pts',(-56.2900121878802,-17.9585229704407,
39.8967644650352));
#173463=CARTESIAN_POINT('Ctrl Pts',(-56.2774781111558,-17.9584138425286,
39.9159282836022));
#173464=CARTESIAN_POINT('Ctrl Pts',(-56.2647176232334,-17.9583027433679,
39.9354382707156));
#173465=CARTESIAN_POINT('Ctrl Pts',(-56.2515822679742,-17.9600828051299,
39.9545987622319));
#173466=CARTESIAN_POINT('Ctrl Pts',(-56.2382392305977,-17.9637804645263,
39.9731387498191));
#173467=CARTESIAN_POINT('Ctrl Pts',(-56.2254611028288,-17.967321574611,
39.9908938024012));
#173468=CARTESIAN_POINT('Ctrl Pts',(-56.2124916494907,-17.9726214740523,
40.0080810366136));
#173469=CARTESIAN_POINT('Ctrl Pts',(-56.1994690140086,-17.979747296548,
40.0244542742491));
#173470=CARTESIAN_POINT('Ctrl Pts',(-56.1891112379837,-17.9854149414348,
40.0374770090454));
#173471=CARTESIAN_POINT('Ctrl Pts',(-56.1787195200275,-17.9922384661035,
40.0499848770023));
#173472=CARTESIAN_POINT('Ctrl Pts',(-56.1683642893843,-18.0002723763369,
40.0618424270193));
#173473=CARTESIAN_POINT('Ctrl Pts',(-56.1683360229684,-18.0002943063021,
40.0618747942791));
#173474=CARTESIAN_POINT('Ctrl Pts',(-56.1683077570002,-18.0003162453124,
40.0619071564124));
#173475=CARTESIAN_POINT('Ctrl Pts',(-56.1682794914817,-18.0003381933678,
40.0619395134161));
#173476=CARTESIAN_POINT('Ctrl Pts',(-56.1626527236046,-18.004707354795,
40.0683807661799));
#173477=CARTESIAN_POINT('Ctrl Pts',(-56.1570391911758,-18.0094711966665,
40.0746073439084));
#173478=CARTESIAN_POINT('Ctrl Pts',(-56.1514686668952,-18.0146022491736,
40.0805869293669));
#173479=CARTESIAN_POINT('Ctrl Pts',(-56.1404135756907,-18.0247851782092,
40.092453830807));
#173480=CARTESIAN_POINT('Ctrl Pts',(-56.1295277006975,-18.0364157638825,
40.1033475319609));
#173481=CARTESIAN_POINT('Ctrl Pts',(-56.1190427465077,-18.0492876213731,
40.1130129263075));
#173482=CARTESIAN_POINT('Ctrl Pts',(-56.1111790308653,-18.0589415144911,
40.1202619720674));
#173483=CARTESIAN_POINT('Ctrl Pts',(-56.1035408324002,-18.0692936227625,
40.1268200947266));
#173484=CARTESIAN_POINT('Ctrl Pts',(-56.0962259123228,-18.0802568810128,
40.1325796782703));
#173485=CARTESIAN_POINT('Ctrl Pts',(-56.0934828172938,-18.0843681028567,
40.1347395220992));
#173486=CARTESIAN_POINT('Ctrl Pts',(-56.0907851834709,-18.0885652677241,
40.1367870714852));
#173487=CARTESIAN_POINT('Ctrl Pts',(-56.0881381670059,-18.0928437845339,
40.1387166518767));
#173488=CARTESIAN_POINT('Ctrl Pts',(-56.0788736093784,-18.1078185933684,
40.1454701832469));
#173489=CARTESIAN_POINT('Ctrl Pts',(-56.0702291095578,-18.1237899619212,
40.1507785912492));
#173490=CARTESIAN_POINT('Ctrl Pts',(-56.0624257818118,-18.1405610619115,
40.1543986087265));
#173491=CARTESIAN_POINT('Ctrl Pts',(-56.0585241179387,-18.1489466119067,
40.1562086174652));
#173492=CARTESIAN_POINT('Ctrl Pts',(-56.0548327480526,-18.1575320950784,
40.1575965292115));
#173493=CARTESIAN_POINT('Ctrl Pts',(-56.0513793155481,-18.1662929092567,
40.1585319382567));
#173494=CARTESIAN_POINT('Ctrl Pts',(-56.0496525992959,-18.1706733163458,
40.1589996427793));
#173495=CARTESIAN_POINT('Ctrl Pts',(-56.0479853674132,-18.1750975561949,
40.159354221642));
#173496=CARTESIAN_POINT('Ctrl Pts',(-56.0463810756008,-18.1795625536244,
40.159591874311));
#173497=CARTESIAN_POINT('Ctrl Pts',(-56.0447767837884,-18.1840275510539,
40.1598295269801));
#173498=CARTESIAN_POINT('Ctrl Pts',(-56.0432354336628,-18.1885333065887,
40.1599502506896));
#173499=CARTESIAN_POINT('Ctrl Pts',(-56.0417604764384,-18.1930767435946,
40.1599502534424));
#173500=CARTESIAN_POINT('',(-56.0323588238392,-18.2220120550214,40.1599502534424));
#173501=CARTESIAN_POINT('Origin',(3.37692616670652E-16,-2.10546223053625E-17,
40.1599502534424));
#173502=CARTESIAN_POINT('',(-56.1179479440989,-18.5670586829462,39.8576902534424));
#173503=CARTESIAN_POINT('Ctrl Pts',(-56.0323588238392,-18.2220120550214,
40.1599502534424));
#173504=CARTESIAN_POINT('Ctrl Pts',(-56.0311805982249,-18.2256350948466,
40.1599502448875));
#173505=CARTESIAN_POINT('Ctrl Pts',(-56.0300502984939,-18.2292627734003,
40.1598743450437));
#173506=CARTESIAN_POINT('Ctrl Pts',(-56.0289674832814,-18.2328929164988,
40.1597243308499));
#173507=CARTESIAN_POINT('Ctrl Pts',(-56.0225746241534,-18.2543250068264,
40.1588386583939));
#173508=CARTESIAN_POINT('Ctrl Pts',(-56.0178345032628,-18.2758450255457,
40.1553722553627));
#173509=CARTESIAN_POINT('Ctrl Pts',(-56.0146588434103,-18.2969992991145,
40.149690217781));
#173510=CARTESIAN_POINT('Ctrl Pts',(-56.0134725226018,-18.3049018315292,
40.1475675976861));
#173511=CARTESIAN_POINT('Ctrl Pts',(-56.0125042026269,-18.3127535860847,
40.1451361443106));
#173512=CARTESIAN_POINT('Ctrl Pts',(-56.01174825096,-18.3205319543145,40.1424159447501));
#173513=CARTESIAN_POINT('Ctrl Pts',(-56.0111584195474,-18.3266010274075,
40.1402935085949));
#173514=CARTESIAN_POINT('Ctrl Pts',(-56.0106982359127,-18.332625066177,
40.1379949176048));
#173515=CARTESIAN_POINT('Ctrl Pts',(-56.0103653778789,-18.3385929672498,
40.1355293609261));
#173516=CARTESIAN_POINT('Ctrl Pts',(-56.0092003747605,-18.3594806210046,
40.1268999125509));
#173517=CARTESIAN_POINT('Ctrl Pts',(-56.0095951017657,-18.3796805851419,
40.1162251288835));
#173518=CARTESIAN_POINT('Ctrl Pts',(-56.0114500824671,-18.3987168313627,
40.1038990521418));
#173519=CARTESIAN_POINT('Ctrl Pts',(-56.0123775728178,-18.408234954473,
40.097736013771));
#173520=CARTESIAN_POINT('Ctrl Pts',(-56.0136701283094,-18.4174621486786,
40.0911601532641));
#173521=CARTESIAN_POINT('Ctrl Pts',(-56.0153153192431,-18.4263389120628,
40.084220729064));
#173522=CARTESIAN_POINT('Ctrl Pts',(-56.016953481144,-18.4351777497211,
40.0773109533618));
#173523=CARTESIAN_POINT('Ctrl Pts',(-56.0189410563924,-18.4436692750117,
40.0700409753048));
#173524=CARTESIAN_POINT('Ctrl Pts',(-56.0212664209291,-18.4517543535697,
40.0624586415899));
#173525=CARTESIAN_POINT('Ctrl Pts',(-56.0212763986141,-18.4517890450626,
40.0624261072769));
#173526=CARTESIAN_POINT('Ctrl Pts',(-56.021286382056,-18.4518237293601,
40.0623935677888));
#173527=CARTESIAN_POINT('Ctrl Pts',(-56.021296371253,-18.4518584064611,
40.0623610231288));
#173528=CARTESIAN_POINT('Ctrl Pts',(-56.0260070845288,-18.4682114607502,
40.0470135870224));
#173529=CARTESIAN_POINT('Ctrl Pts',(-56.031963021228,-18.4829503621277,
40.0305755292074));
#173530=CARTESIAN_POINT('Ctrl Pts',(-56.0389696815142,-18.4960770195721,
40.0133447567309));
#173531=CARTESIAN_POINT('Ctrl Pts',(-56.0462312303151,-18.5096811989857,
39.9954871626557));
#173532=CARTESIAN_POINT('Ctrl Pts',(-56.0546220378354,-18.5215542196648,
39.9767767954265));
#173533=CARTESIAN_POINT('Ctrl Pts',(-56.0639562290217,-18.5316559412182,
39.9575197577416));
#173534=CARTESIAN_POINT('Ctrl Pts',(-56.0731572003559,-18.5416134885389,
39.9385375611932));
#173535=CARTESIAN_POINT('Ctrl Pts',(-56.0832757207152,-18.5498501466939,
39.9190226977025));
#173536=CARTESIAN_POINT('Ctrl Pts',(-56.094150584794,-18.5562821957351,
39.899265545178));
#173537=CARTESIAN_POINT('Ctrl Pts',(-56.1017327335105,-18.5607667347627,
39.8854905069275));
#173538=CARTESIAN_POINT('Ctrl Pts',(-56.109682911022,-18.5643731068275,
39.8715976051449));
#173539=CARTESIAN_POINT('Ctrl Pts',(-56.1179479440989,-18.5670586829462,
39.8576902534424));
#173540=CARTESIAN_POINT('',(-56.4568070719812,-18.6771643191707,39.2875012672119));
#173541=CARTESIAN_POINT('',(-56.1179479440989,-18.5670586829462,39.8576902534424));
#173542=CARTESIAN_POINT('',(-54.4530463244694,-23.8971395307765,39.2875012672119));
#173543=CARTESIAN_POINT('Origin',(5.53234440788222E-15,0.,39.2875012672119));
#173544=CARTESIAN_POINT('',(-54.1275498658875,-23.7522229508825,39.8576902534424));
#173545=CARTESIAN_POINT('',(-54.4530463244694,-23.8971395307765,39.2875012672119));
#173546=CARTESIAN_POINT('',(-53.8330634946839,-23.9513722670362,40.1599502534424));
#173547=CARTESIAN_POINT('Ctrl Pts',(-54.1275498658875,-23.7522229508825,
39.8576902534424));
#173548=CARTESIAN_POINT('Ctrl Pts',(-54.1163771839516,-23.747248709103,
39.8772619994063));
#173549=CARTESIAN_POINT('Ctrl Pts',(-54.1044728027347,-23.7440527738934,
39.8967644650387));
#173550=CARTESIAN_POINT('Ctrl Pts',(-54.0920187959658,-23.7426340760171,
39.9159282836073));
#173551=CARTESIAN_POINT('Ctrl Pts',(-54.0793398243547,-23.7411897512764,
39.9354382707224));
#173552=CARTESIAN_POINT('Ctrl Pts',(-54.0660903588241,-23.7415870431746,
39.9545987622403));
#173553=CARTESIAN_POINT('Ctrl Pts',(-54.0524339053468,-23.7438697192145,
39.9731387498289));
#173554=CARTESIAN_POINT('Ctrl Pts',(-54.0393556307021,-23.7460557526693,
39.9908938024123));
#173555=CARTESIAN_POINT('Ctrl Pts',(-54.0259032350411,-23.7499709416813,
40.0080810366259));
#173556=CARTESIAN_POINT('Ctrl Pts',(-54.0122070876424,-23.7556964921025,
40.0244542742624));
#173557=CARTESIAN_POINT('Ctrl Pts',(-54.0013136223915,-23.7602504066262,
40.0374770090539));
#173558=CARTESIAN_POINT('Ctrl Pts',(-53.9902655788097,-23.7659503210025,
40.0499848770064));
#173559=CARTESIAN_POINT('Ctrl Pts',(-53.9791273029165,-23.7728578042868,
40.0618424270193));
#173560=CARTESIAN_POINT('Ctrl Pts',(-53.9790968990413,-23.7728766594724,
40.0618747942791));
#173561=CARTESIAN_POINT('Ctrl Pts',(-53.979066494666,-23.7728955237003,
40.0619071564124));
#173562=CARTESIAN_POINT('Ctrl Pts',(-53.9790360897925,-23.7729143969707,
40.0619395134162));
#173563=CARTESIAN_POINT('Ctrl Pts',(-53.9729834442088,-23.7766714662751,
40.0683807661799));
#173564=CARTESIAN_POINT('Ctrl Pts',(-53.966902706228,-23.7808224374041,
40.0746073439084));
#173565=CARTESIAN_POINT('Ctrl Pts',(-53.9608263568287,-23.7853431031261,
40.0805869293669));
#173566=CARTESIAN_POINT('Ctrl Pts',(-53.9487674206469,-23.794314677316,
40.092453830807));
#173567=CARTESIAN_POINT('Ctrl Pts',(-53.9367254523686,-23.8047436656398,
40.1033475319609));
#173568=CARTESIAN_POINT('Ctrl Pts',(-53.924952460372,-23.8164490335994,
40.1130129263075));
#173569=CARTESIAN_POINT('Ctrl Pts',(-53.9161227163745,-23.8252280595691,
40.1202619720674));
#173570=CARTESIAN_POINT('Ctrl Pts',(-53.9074442707905,-23.8347250487605,
40.1268200947266));
#173571=CARTESIAN_POINT('Ctrl Pts',(-53.8990234500734,-23.8448636317804,
40.1325796782703));
#173572=CARTESIAN_POINT('Ctrl Pts',(-53.8958656423045,-23.8486656004128,
40.1347395220992));
#173573=CARTESIAN_POINT('Ctrl Pts',(-53.8927440632083,-23.852557793254,
40.1367870714852));
#173574=CARTESIAN_POINT('Ctrl Pts',(-53.8896643205893,-23.8565361833377,
40.1387166518767));
#173575=CARTESIAN_POINT('Ctrl Pts',(-53.8788852214227,-23.8704605486309,
40.1454701832469));
#173576=CARTESIAN_POINT('Ctrl Pts',(-53.8686186144654,-23.8854408280736,
40.1507785912492));
#173577=CARTESIAN_POINT('Ctrl Pts',(-53.8591049768559,-23.9013043843658,
40.1543986087265));
#173578=CARTESIAN_POINT('Ctrl Pts',(-53.8543481580512,-23.9092361625119,
40.1562086174652));
#173579=CARTESIAN_POINT('Ctrl Pts',(-53.8497795825132,-23.9173887602869,
40.1575965292115));
#173580=CARTESIAN_POINT('Ctrl Pts',(-53.8454293138303,-23.9257405998158,
40.1585319382567));
#173581=CARTESIAN_POINT('Ctrl Pts',(-53.8432541794888,-23.9299165195802,
40.1589996427793));
#173582=CARTESIAN_POINT('Ctrl Pts',(-53.8411336218843,-23.9341422497938,
40.159354221642));
#173583=CARTESIAN_POINT('Ctrl Pts',(-53.8390713992305,-23.9384150933425,
40.1595918743111));
#173584=CARTESIAN_POINT('Ctrl Pts',(-53.8370091765767,-23.9426879368912,
40.1598295269801));
#173585=CARTESIAN_POINT('Ctrl Pts',(-53.8350052904264,-23.9470078944656,
40.1599502506896));
#173586=CARTESIAN_POINT('Ctrl Pts',(-53.8330634946839,-23.9513722670362,
40.1599502534424));
#173587=CARTESIAN_POINT('',(-53.8206887816837,-23.9791663275011,40.1599502534424));
#173588=CARTESIAN_POINT('Origin',(3.40248402231255E-16,-2.77126713209864E-17,
40.1599502534424));
#173589=CARTESIAN_POINT('',(-53.8697418420146,-24.3312692531085,39.8576902534424));
#173590=CARTESIAN_POINT('Ctrl Pts',(-53.8206887816837,-23.9791663275011,
40.1599502534424));
#173591=CARTESIAN_POINT('Ctrl Pts',(-53.8191382997273,-23.9826463618222,
40.1599502448875));
#173592=CARTESIAN_POINT('Ctrl Pts',(-53.817634996232,-23.9861360190793,
40.1598743450437));
#173593=CARTESIAN_POINT('Ctrl Pts',(-53.816178659515,-23.9896330908639,
40.1597243308499));
#173594=CARTESIAN_POINT('Ctrl Pts',(-53.8075805576699,-24.010279538222,
40.1588386583938));
#173595=CARTESIAN_POINT('Ctrl Pts',(-53.8006169491702,-24.0311861904791,
40.1553722553612));
#173596=CARTESIAN_POINT('Ctrl Pts',(-53.7952474622065,-24.0518926318839,
40.1496902177775));
#173597=CARTESIAN_POINT('Ctrl Pts',(-53.7932416006197,-24.0596278691038,
40.1475675976834));
#173598=CARTESIAN_POINT('Ctrl Pts',(-53.7914578533664,-24.0673353939229,
40.145136144309));
#173599=CARTESIAN_POINT('Ctrl Pts',(-53.7898929820049,-24.0749921329674,
40.1424159447501));
#173600=CARTESIAN_POINT('Ctrl Pts',(-53.7886719908666,-24.0809663048718,
40.1402935085949));
#173601=CARTESIAN_POINT('Ctrl Pts',(-53.7875846446508,-24.0869092410385,
40.1379949176048));
#173602=CARTESIAN_POINT('Ctrl Pts',(-53.78662979452,-24.092809656186,40.1355293609262));
#173603=CARTESIAN_POINT('Ctrl Pts',(-53.7832878190623,-24.1134611092024,
40.1268999125509));
#173604=CARTESIAN_POINT('Ctrl Pts',(-53.7815689125023,-24.1335916760299,
40.1162251288835));
#173605=CARTESIAN_POINT('Ctrl Pts',(-53.7814239018616,-24.1527175379841,
40.1038990521418));
#173606=CARTESIAN_POINT('Ctrl Pts',(-53.7813513965412,-24.1622804689613,
40.097736013771));
#173607=CARTESIAN_POINT('Ctrl Pts',(-53.7816723668479,-24.1715922244707,
40.0911601532641));
#173608=CARTESIAN_POINT('Ctrl Pts',(-53.7823806708182,-24.1805923292964,
40.0842207290641));
#173609=CARTESIAN_POINT('Ctrl Pts',(-53.7830859485794,-24.1895539814232,
40.0773109533619));
#173610=CARTESIAN_POINT('Ctrl Pts',(-53.7841750295932,-24.1982067474361,
40.0700409753048));
#173611=CARTESIAN_POINT('Ctrl Pts',(-53.7856425347026,-24.2064906018695,
40.0624586415899));
#173612=CARTESIAN_POINT('Ctrl Pts',(-53.7856488314803,-24.2065261462708,
40.0624261072769));
#173613=CARTESIAN_POINT('Ctrl Pts',(-53.7856551347355,-24.2065616841179,
40.0623935677889));
#173614=CARTESIAN_POINT('Ctrl Pts',(-53.7856614444665,-24.2065972154095,
40.0623610231288));
#173615=CARTESIAN_POINT('Ctrl Pts',(-53.7886369923274,-24.2233530895747,
40.0470135870235));
#173616=CARTESIAN_POINT('Ctrl Pts',(-53.7930196670706,-24.2386338146178,
40.0305755292097));
#173617=CARTESIAN_POINT('Ctrl Pts',(-53.7986158348076,-24.2524209582908,
40.0133447567345));
#173618=CARTESIAN_POINT('Ctrl Pts',(-53.8044155801157,-24.2667096511226,
39.9954871626604));
#173619=CARTESIAN_POINT('Ctrl Pts',(-53.8115193533079,-24.2793947083673,
39.9767767954325));
#173620=CARTESIAN_POINT('Ctrl Pts',(-53.8197464933872,-24.2904167802934,
39.9575197577489));
#173621=CARTESIAN_POINT('Ctrl Pts',(-53.8278562137176,-24.3012815425221,
39.9385375612015));
#173622=CARTESIAN_POINT('Ctrl Pts',(-53.8370583385436,-24.3105307527857,
39.9190226977117));
#173623=CARTESIAN_POINT('Ctrl Pts',(-53.8472012967764,-24.3180642992198,
39.8992655451882));
#173624=CARTESIAN_POINT('Ctrl Pts',(-53.8542731477173,-24.3233168218288,
39.8854905069344));
#173625=CARTESIAN_POINT('Ctrl Pts',(-53.8618028047964,-24.3277344576494,
39.8715976051484));
#173626=CARTESIAN_POINT('Ctrl Pts',(-53.8697418420146,-24.3312692531085,
39.8576902534424));
#173627=CARTESIAN_POINT('',(-54.1952354911873,-24.4761921430389,39.2875012672119));
#173628=CARTESIAN_POINT('',(-53.8697418420146,-24.3312692531085,39.8576902534424));
#173629=CARTESIAN_POINT('',(-51.6568155675429,-29.4581217525671,39.2875012672119));
#173630=CARTESIAN_POINT('Origin',(5.53234440788222E-15,0.,39.2875012672119));
#173631=CARTESIAN_POINT('',(-51.3482501200167,-29.279975396246,39.8576902534424));
#173632=CARTESIAN_POINT('',(-51.6568155675429,-29.4581217525671,39.2875012672119));
#173633=CARTESIAN_POINT('',(-51.0345602039888,-29.4472515437732,40.1599502534424));
#173634=CARTESIAN_POINT('Ctrl Pts',(-51.3482501200167,-29.2799753962459,
39.8576902534424));
#173635=CARTESIAN_POINT('Ctrl Pts',(-51.3376585930521,-29.2738605406108,
39.8772619994035));
#173636=CARTESIAN_POINT('Ctrl Pts',(-51.326153491479,-29.2694377663943,
39.8967644650332));
#173637=CARTESIAN_POINT('Ctrl Pts',(-51.3139160033731,-29.2667250421043,
39.9159282835992));
#173638=CARTESIAN_POINT('Ctrl Pts',(-51.3014574615426,-29.2639633161072,
39.9354382707117));
#173639=CARTESIAN_POINT('Ctrl Pts',(-51.288239049661,-29.2629734853272,
39.9545987622272));
#173640=CARTESIAN_POINT('Ctrl Pts',(-51.2744188030484,-29.2638161685322,
39.9731387498136));
#173641=CARTESIAN_POINT('Ctrl Pts',(-51.2611836698449,-29.2646231747151,
39.9908938023951));
#173642=CARTESIAN_POINT('Ctrl Pts',(-51.2473957191261,-29.2671107576648,
40.0080810366069));
#173643=CARTESIAN_POINT('Ctrl Pts',(-51.2331761176712,-29.2713733056795,
40.024454274242));
#173644=CARTESIAN_POINT('Ctrl Pts',(-51.2218663142702,-29.2747635962011,
40.0374770090408));
#173645=CARTESIAN_POINT('Ctrl Pts',(-51.2102829897306,-29.2792774508342,
40.0499848770002));
#173646=CARTESIAN_POINT('Ctrl Pts',(-51.1984837018592,-29.2849828273427,
40.0618424270193));
#173647=CARTESIAN_POINT('Ctrl Pts',(-51.1984514936361,-29.2849984011672,
40.0618747942791));
#173648=CARTESIAN_POINT('Ctrl Pts',(-51.1984192839704,-29.2850139839323,
40.0619071564124));
#173649=CARTESIAN_POINT('Ctrl Pts',(-51.198387072864,-29.2850295756383,
40.0619395134161));
#173650=CARTESIAN_POINT('Ctrl Pts',(-51.1919748636254,-29.2881333895824,
40.0683807661799));
#173651=CARTESIAN_POINT('Ctrl Pts',(-51.1854935419303,-29.2916260110605,
40.0746073439084));
#173652=CARTESIAN_POINT('Ctrl Pts',(-51.1789779411679,-29.2954867606376,
40.0805869293669));
#173653=CARTESIAN_POINT('Ctrl Pts',(-51.1660472802371,-29.3031486855377,
40.092453830807));
#173654=CARTESIAN_POINT('Ctrl Pts',(-51.152981152998,-29.3122618143334,
40.1033475319609));
#173655=CARTESIAN_POINT('Ctrl Pts',(-51.1400491105586,-29.3226724463011,
40.1130129263075));
#173656=CARTESIAN_POINT('Ctrl Pts',(-51.1303500787291,-29.3304804202768,
40.1202619720674));
#173657=CARTESIAN_POINT('Ctrl Pts',(-51.1207264688922,-29.3390182393874,
40.1268200947266));
#173658=CARTESIAN_POINT('Ctrl Pts',(-51.1112920078093,-29.3482210667396,
40.1325796782703));
#173659=CARTESIAN_POINT('Ctrl Pts',(-51.1077540849032,-29.3516721269967,
40.1347395220992));
#173660=CARTESIAN_POINT('Ctrl Pts',(-51.1042427612074,-29.3552167041323,
40.1367870714852));
#173661=CARTESIAN_POINT('Ctrl Pts',(-51.100764034739,-29.3588513794157,
40.1387166518767));
#173662=CARTESIAN_POINT('Ctrl Pts',(-51.0885884920994,-29.3715727429076,
40.1454701832469));
#173663=CARTESIAN_POINT('Ctrl Pts',(-51.0768122610998,-29.3853978061639,
40.1507785912492));
#173664=CARTESIAN_POINT('Ctrl Pts',(-51.0656925470314,-29.4001800143155,
40.1543986087265));
#173665=CARTESIAN_POINT('Ctrl Pts',(-51.0601326899972,-29.4075711183913,
40.1562086174652));
#173666=CARTESIAN_POINT('Ctrl Pts',(-51.0547369630769,-29.4152015092023,
40.1575965292115));
#173667=CARTESIAN_POINT('Ctrl Pts',(-51.0495375206696,-29.4230528695802,
40.1585319382567));
#173668=CARTESIAN_POINT('Ctrl Pts',(-51.046937799466,-29.4269785497691,
40.1589996427793));
#173669=CARTESIAN_POINT('Ctrl Pts',(-51.0443871494124,-29.4309594723628,
40.159354221642));
#173670=CARTESIAN_POINT('Ctrl Pts',(-51.0418895900602,-29.4349933478625,
40.159591874311));
#173671=CARTESIAN_POINT('Ctrl Pts',(-51.039392030708,-29.4390272233622,
40.1598295269801));
#173672=CARTESIAN_POINT('Ctrl Pts',(-51.0369475635291,-29.4431140526173,
40.1599502506895));
#173673=CARTESIAN_POINT('Ctrl Pts',(-51.0345602039888,-29.4472515437732,
40.1599502534424));
#173674=CARTESIAN_POINT('',(-51.0193480105329,-29.4735998357335,40.1599502534424));
#173675=CARTESIAN_POINT('Origin',(3.434861425631E-16,-3.40670945103686E-17,
40.1599502534424));
#173676=CARTESIAN_POINT('',(-51.031327575341,-29.8289013456883,39.8576902534424));
#173677=CARTESIAN_POINT('Ctrl Pts',(-51.0193480105329,-29.4735998357335,
40.1599502534424));
#173678=CARTESIAN_POINT('Ctrl Pts',(-51.0174422596392,-29.4768987365662,
40.1599502448875));
#173679=CARTESIAN_POINT('Ctrl Pts',(-51.0155824228873,-29.4802121391116,
40.1598743450437));
#173680=CARTESIAN_POINT('Ctrl Pts',(-51.0137685205956,-29.483537824932,
40.1597243308499));
#173681=CARTESIAN_POINT('Ctrl Pts',(-51.0030593786376,-29.5031724225186,
40.1588386583938));
#173682=CARTESIAN_POINT('Ctrl Pts',(-50.9939485772813,-29.5232366506522,
40.1553722553611));
#173683=CARTESIAN_POINT('Ctrl Pts',(-50.9864440924291,-29.5432683957839,
40.1496902177772));
#173684=CARTESIAN_POINT('Ctrl Pts',(-50.9836406667025,-29.5507515889354,
40.1475675976832));
#173685=CARTESIAN_POINT('Ctrl Pts',(-50.9810610352785,-29.5582304387676,
40.1451361443089));
#173686=CARTESIAN_POINT('Ctrl Pts',(-50.9787043892801,-29.5656816597956,
40.1424159447501));
#173687=CARTESIAN_POINT('Ctrl Pts',(-50.9768656158505,-29.5714954762339,
40.1402935085949));
#173688=CARTESIAN_POINT('Ctrl Pts',(-50.9751630202463,-29.5772921977454,
40.1379949176048));
#173689=CARTESIAN_POINT('Ctrl Pts',(-50.9735966395564,-29.5830604807846,
40.1355293609261));
#173690=CARTESIAN_POINT('Ctrl Pts',(-50.9681143071419,-29.6032494714217,
40.1268999125509));
#173691=CARTESIAN_POINT('Ctrl Pts',(-50.9643005997168,-29.6230900862365,
40.1162251288835));
#173692=CARTESIAN_POINT('Ctrl Pts',(-50.9621571865007,-29.6420960169784,
40.1038990521418));
#173693=CARTESIAN_POINT('Ctrl Pts',(-50.9610854798927,-29.6515989823493,
40.0977360137709));
#173694=CARTESIAN_POINT('Ctrl Pts',(-50.9604313483968,-29.6608932776207,
40.0911601532641));
#173695=CARTESIAN_POINT('Ctrl Pts',(-50.9601950050771,-29.669918116856,
40.084220729064));
#173696=CARTESIAN_POINT('Ctrl Pts',(-50.9599596715278,-29.6789043977153,
40.0773109533619));
#173697=CARTESIAN_POINT('Ctrl Pts',(-50.9601383261075,-29.6876236029354,
40.0700409753048));
#173698=CARTESIAN_POINT('Ctrl Pts',(-50.9607318934965,-29.6960154736014,
40.0624586415899));
#173699=CARTESIAN_POINT('Ctrl Pts',(-50.9607344403782,-29.6960514814793,
40.0624261072769));
#173700=CARTESIAN_POINT('Ctrl Pts',(-50.960736994387,-29.6960874835159,
40.0623935677889));
#173701=CARTESIAN_POINT('Ctrl Pts',(-50.9607395555213,-29.6961234797099,
40.0623610231289));
#173702=CARTESIAN_POINT('Ctrl Pts',(-50.9619473372424,-29.7130985928884,
40.0470135870235));
#173703=CARTESIAN_POINT('Ctrl Pts',(-50.9647087325285,-29.7287537227769,
40.0305755292096));
#173704=CARTESIAN_POINT('Ctrl Pts',(-50.9688330949321,-29.743050297848,
40.0133447567344));
#173705=CARTESIAN_POINT('Ctrl Pts',(-50.9731074935248,-29.7578669541898,
39.9954871626603));
#173706=CARTESIAN_POINT('Ctrl Pts',(-50.9788464019639,-29.7712250678589,
39.9767767954323));
#173707=CARTESIAN_POINT('Ctrl Pts',(-50.9858763526686,-29.7830467300313,
39.9575197577486));
#173708=CARTESIAN_POINT('Ctrl Pts',(-50.992805970203,-29.7946996705593,
39.9385375612012));
#173709=CARTESIAN_POINT('Ctrl Pts',(-51.0009908790911,-29.8048600966482,
39.9190226977114));
#173710=CARTESIAN_POINT('Ctrl Pts',(-51.0102908031057,-29.8134126013638,
39.8992655451879));
#173711=CARTESIAN_POINT('Ctrl Pts',(-51.0167748755906,-29.8193755598155,
39.8854905069341));
#173712=CARTESIAN_POINT('Ctrl Pts',(-51.0238015157368,-29.8245560588483,
39.8715976051482));
#173713=CARTESIAN_POINT('Ctrl Pts',(-51.0313275753411,-29.8289013456882,
39.8576902534424));
#173714=CARTESIAN_POINT('',(-51.3398895692699,-30.0070536838155,39.2875012672119));
#173715=CARTESIAN_POINT('',(-51.031327575341,-29.8289013456883,39.8576902534424));
#173716=CARTESIAN_POINT('',(-48.2946219293748,-34.6963546279283,39.2875012672119));
#173717=CARTESIAN_POINT('Origin',(5.53234440788222E-15,0.,39.2875012672119));
#173718=CARTESIAN_POINT('',(-48.0063682005189,-34.4869303039394,39.8576902534424));
#173719=CARTESIAN_POINT('',(-48.2946219293748,-34.6963546279283,39.2875012672119));
#173720=CARTESIAN_POINT('',(-47.6769115920306,-34.6205005703632,40.1599502534424));
#173721=CARTESIAN_POINT('Ctrl Pts',(-48.0063682005189,-34.4869303039394,
39.8576902534424));
#173722=CARTESIAN_POINT('Ctrl Pts',(-47.9964738715087,-34.4797418300851,
39.8772619994058));
#173723=CARTESIAN_POINT('Ctrl Pts',(-47.9854941018767,-34.4741406737008,
39.8967644650379));
#173724=CARTESIAN_POINT('Ctrl Pts',(-47.9736072089107,-34.4701636441721,
39.9159282836061));
#173725=CARTESIAN_POINT('Ctrl Pts',(-47.9615055952487,-34.4661147749668,
39.9354382707209));
#173726=CARTESIAN_POINT('Ctrl Pts',(-47.9484630606988,-34.4637486663029,
39.9545987622386));
#173727=CARTESIAN_POINT('Ctrl Pts',(-47.9346304384606,-34.4631421240615,
39.9731387498271));
#173728=CARTESIAN_POINT('Ctrl Pts',(-47.9213834535833,-34.462561261246,
39.9908938024107));
#173729=CARTESIAN_POINT('Ctrl Pts',(-47.9074110114758,-34.463593983657,
40.0080810366245));
#173730=CARTESIAN_POINT('Ctrl Pts',(-47.8928237488894,-34.4663468279011,
40.0244542742612));
#173731=CARTESIAN_POINT('Ctrl Pts',(-47.8812215199217,-34.4685363496872,
40.0374770090531));
#173732=CARTESIAN_POINT('Ctrl Pts',(-47.8692298237635,-34.4718146898375,
40.049984877006));
#173733=CARTESIAN_POINT('Ctrl Pts',(-47.8568987993929,-34.4762554502655,
40.0618424270192));
#173734=CARTESIAN_POINT('Ctrl Pts',(-47.8568651397019,-34.476267572099,
40.0618747942791));
#173735=CARTESIAN_POINT('Ctrl Pts',(-47.8568314776416,-34.4762797026732,
40.0619071564124));
#173736=CARTESIAN_POINT('Ctrl Pts',(-47.8567978132139,-34.4762918419887,
40.0619395134162));
#173737=CARTESIAN_POINT('Ctrl Pts',(-47.8500962938266,-34.4787083945374,
40.0683807661799));
#173738=CARTESIAN_POINT('Ctrl Pts',(-47.843285399134,-34.4815044004729,
40.0746073439084));
#173739=CARTESIAN_POINT('Ctrl Pts',(-47.836401933294,-34.4846629347249,
40.0805869293669));
#173740=CARTESIAN_POINT('Ctrl Pts',(-47.8227412186412,-34.4909312646827,
40.092453830807));
#173741=CARTESIAN_POINT('Ctrl Pts',(-47.8087940876657,-34.4986286886041,
40.1033475319609));
#173742=CARTESIAN_POINT('Ctrl Pts',(-47.7948446809467,-34.5076305235174,
40.1130129263075));
#173743=CARTESIAN_POINT('Ctrl Pts',(-47.7843826259074,-34.5143818997025,
40.1202619720674));
#173744=CARTESIAN_POINT('Ctrl Pts',(-47.7739192901009,-34.5218670065993,
40.1268200947266));
#173745=CARTESIAN_POINT('Ctrl Pts',(-47.763574554582,-34.5300332501816,
40.1325796782703));
#173746=CARTESIAN_POINT('Ctrl Pts',(-47.7596952787625,-34.533095591525,
40.1347395220992));
#173747=CARTESIAN_POINT('Ctrl Pts',(-47.7558326812644,-34.5362537178262,
40.1367870714852));
#173748=CARTESIAN_POINT('Ctrl Pts',(-47.7519930846017,-34.5395048560462,
40.1387166518767));
#173749=CARTESIAN_POINT('Ctrl Pts',(-47.7385544962822,-34.5508838398163,
40.1454701832469));
#173750=CARTESIAN_POINT('Ctrl Pts',(-47.7253976640914,-34.5634022166001,
40.1507785912492));
#173751=CARTESIAN_POINT('Ctrl Pts',(-47.7127937034783,-34.5769411196452,
40.1543986087265));
#173752=CARTESIAN_POINT('Ctrl Pts',(-47.7064917231718,-34.5837105711677,
40.1562086174652));
#173753=CARTESIAN_POINT('Ctrl Pts',(-47.7003279615826,-34.5907351548563,
40.1575965292115));
#173754=CARTESIAN_POINT('Ctrl Pts',(-47.69433631163,-34.5980000149358,40.1585319382567));
#173755=CARTESIAN_POINT('Ctrl Pts',(-47.6913404866536,-34.6016324449756,
40.1589996427793));
#173756=CARTESIAN_POINT('Ctrl Pts',(-47.6883876896069,-34.6053249441283,
40.159354221642));
#173757=CARTESIAN_POINT('Ctrl Pts',(-47.6854821573391,-34.609075655595,
40.159591874311));
#173758=CARTESIAN_POINT('Ctrl Pts',(-47.6825766250713,-34.6128263670616,
40.1598295269801));
#173759=CARTESIAN_POINT('Ctrl Pts',(-47.6797183589577,-34.6166352918407,
40.1599502506896));
#173760=CARTESIAN_POINT('Ctrl Pts',(-47.6769115920305,-34.6205005703632,
40.1599502534424));
#173761=CARTESIAN_POINT('',(-47.6590285860937,-34.6451144164183,40.1599502534424));
#173762=CARTESIAN_POINT('Origin',(3.4737036430558E-16,-4.00482714832972E-17,
40.1599502534424));
#173763=CARTESIAN_POINT('',(-47.6338034047601,-34.9997217530258,39.8576902534424));
#173764=CARTESIAN_POINT('Ctrl Pts',(-47.6590285860937,-34.6451144164183,
40.1599502534424));
#173765=CARTESIAN_POINT('Ctrl Pts',(-47.6567884460683,-34.6481960403149,
40.1599502448875));
#173766=CARTESIAN_POINT('Ctrl Pts',(-47.6545924528205,-34.6512968858168,
40.1598743450437));
#173767=CARTESIAN_POINT('Ctrl Pts',(-47.6524408584472,-34.6544147487632,
40.1597243308499));
#173768=CARTESIAN_POINT('Ctrl Pts',(-47.6397380079794,-34.6728223758142,
40.1588386583939));
#173769=CARTESIAN_POINT('Ctrl Pts',(-47.6285798336148,-34.6918243519377,
40.1553722553626));
#173770=CARTESIAN_POINT('Ctrl Pts',(-47.619022571582,-34.7109619288003,
40.1496902177808));
#173771=CARTESIAN_POINT('Ctrl Pts',(-47.6154522966321,-34.7181110904577,
40.1475675976859));
#173772=CARTESIAN_POINT('Ctrl Pts',(-47.6121050440169,-34.7252793254635,
40.1451361443104));
#173773=CARTESIAN_POINT('Ctrl Pts',(-47.6089824432867,-34.7324433913424,
40.1424159447501));
#173774=CARTESIAN_POINT('Ctrl Pts',(-47.6065460335523,-34.738033154925,
40.1402935085949));
#173775=CARTESIAN_POINT('Ctrl Pts',(-47.6042468425534,-34.7436201516875,
40.1379949176048));
#173776=CARTESIAN_POINT('Ctrl Pts',(-47.602086092899,-34.7491931041022,
40.1355293609261));
#173777=CARTESIAN_POINT('Ctrl Pts',(-47.5945234691089,-34.7686984375538,
40.1268999125509));
#173778=CARTESIAN_POINT('Ctrl Pts',(-47.5886567445952,-34.7880317224282,
40.1162251288835));
#173779=CARTESIAN_POINT('Ctrl Pts',(-47.5845384124876,-34.8067094890032,
40.1038990521418));
#173780=CARTESIAN_POINT('Ctrl Pts',(-47.5824792464338,-34.8160483722907,
40.097736013771));
#173781=CARTESIAN_POINT('Ctrl Pts',(-47.5808571799368,-34.8252233770801,
40.0911601532641));
#173782=CARTESIAN_POINT('Ctrl Pts',(-47.5796787787541,-34.8341740726978,
40.0842207290641));
#173783=CARTESIAN_POINT('Ctrl Pts',(-47.5785054122578,-34.8430865267161,
40.0773109533619));
#173784=CARTESIAN_POINT('Ctrl Pts',(-47.5777716830264,-34.8517766417063,
40.0700409753048));
#173785=CARTESIAN_POINT('Ctrl Pts',(-47.5774848094465,-34.8601845855137,
40.0624586415899));
#173786=CARTESIAN_POINT('Ctrl Pts',(-47.577483578528,-34.8602206623583,
40.0624261072769));
#173787=CARTESIAN_POINT('Ctrl Pts',(-47.5774823553081,-34.8602567341386,
40.0623935677888));
#173788=CARTESIAN_POINT('Ctrl Pts',(-47.5774811397854,-34.8602928008531,
40.0623610231288));
#173789=CARTESIAN_POINT('Ctrl Pts',(-47.5769079226575,-34.8773011701534,
40.047013587023));
#173790=CARTESIAN_POINT('Ctrl Pts',(-47.5780177840619,-34.8931591840084,
40.0305755292085));
#173791=CARTESIAN_POINT('Ctrl Pts',(-47.5806251537548,-34.9078085542098,
40.0133447567327));
#173792=CARTESIAN_POINT('Ctrl Pts',(-47.5833273744267,-34.9229908396747,
39.9954871626579));
#173793=CARTESIAN_POINT('Ctrl Pts',(-47.5876385414313,-34.9368756554797,
39.9767767954292));
#173794=CARTESIAN_POINT('Ctrl Pts',(-47.5933942811507,-34.949367387294,
39.9575197577448));
#173795=CARTESIAN_POINT('Ctrl Pts',(-47.5990678735498,-34.9616808340667,
39.9385375611966));
#173796=CARTESIAN_POINT('Ctrl Pts',(-47.6061458909259,-34.9726411562266,
39.9190226977059));
#173797=CARTESIAN_POINT('Ctrl Pts',(-47.6145008888092,-34.9821189161924,
39.8992655451816));
#173798=CARTESIAN_POINT('Ctrl Pts',(-47.6203261419824,-34.9887269790652,
39.8854905069299));
#173799=CARTESIAN_POINT('Ctrl Pts',(-47.6267727798548,-34.9946135826776,
39.8715976051461));
#173800=CARTESIAN_POINT('Ctrl Pts',(-47.6338034047601,-34.9997217530258,
39.8576902534424));
#173801=CARTESIAN_POINT('',(-47.9220530736689,-35.2091516650525,39.2875012672119));
#173802=CARTESIAN_POINT('',(-47.6338034047601,-34.9997217530258,39.8576902534424));
#173803=CARTESIAN_POINT('',(-44.4033023070491,-39.5544469813068,39.2875012672119));
#173804=CARTESIAN_POINT('Origin',(5.53234440788222E-15,0.,39.2875012672119));
#173805=CARTESIAN_POINT('',(-44.1385184650378,-39.3160391863688,39.8576902534424));
#173806=CARTESIAN_POINT('',(-44.4033023070491,-39.5544469813068,39.2875012672119));
#173807=CARTESIAN_POINT('',(-43.7969047596348,-39.4144401478987,40.1599502534424));
#173808=CARTESIAN_POINT('Ctrl Pts',(-44.1385184650378,-39.3160391863687,
39.8576902534424));
#173809=CARTESIAN_POINT('Ctrl Pts',(-44.1294297383233,-39.3078558527208,
39.8772619994037));
#173810=CARTESIAN_POINT('Ctrl Pts',(-44.1190955972887,-39.3011376816112,
39.8967644650337));
#173811=CARTESIAN_POINT('Ctrl Pts',(-44.1076895347526,-39.2959399200119,
39.9159282835999));
#173812=CARTESIAN_POINT('Ctrl Pts',(-44.096077437074,-39.2906482678568,
39.9354382707126));
#173813=CARTESIAN_POINT('Ctrl Pts',(-44.0833536765974,-39.2869318048901,
39.9545987622283));
#173814=CARTESIAN_POINT('Ctrl Pts',(-44.0696602318415,-39.2848826826045,
39.9731387498149));
#173815=CARTESIAN_POINT('Ctrl Pts',(-44.0565465320329,-39.2829203148436,
39.9908938023966));
#173816=CARTESIAN_POINT('Ctrl Pts',(-44.042542683541,-39.2824868619907,
40.0080810366086));
#173817=CARTESIAN_POINT('Ctrl Pts',(-44.0277475809293,-39.2836998417232,
40.0244542742438));
#173818=CARTESIAN_POINT('Ctrl Pts',(-44.0159800428336,-39.2846646059149,
40.037477009042));
#173819=CARTESIAN_POINT('Ctrl Pts',(-44.0037113585784,-39.2866715134039,
40.0499848770007));
#173820=CARTESIAN_POINT('Ctrl Pts',(-43.9909836989806,-39.289799003855,
40.0618424270193));
#173821=CARTESIAN_POINT('Ctrl Pts',(-43.9909489566042,-39.289807540888,
40.0618747942791));
#173822=CARTESIAN_POINT('Ctrl Pts',(-43.990914210958,-39.2898160863662,
40.0619071564124));
#173823=CARTESIAN_POINT('Ctrl Pts',(-43.9908794620435,-39.2898246402904,
40.0619395134161));
#173824=CARTESIAN_POINT('Ctrl Pts',(-43.9839620557563,-39.2915274551883,
40.0683807661799));
#173825=CARTESIAN_POINT('Ctrl Pts',(-43.9768962096537,-39.293596211955,
40.0746073439084));
#173826=CARTESIAN_POINT('Ctrl Pts',(-43.9697202954283,-39.2960179253197,
40.0805869293669));
#173827=CARTESIAN_POINT('Ctrl Pts',(-43.955479196702,-39.3008239832003,
40.092453830807));
#173828=CARTESIAN_POINT('Ctrl Pts',(-43.9408038696757,-39.3070213676602,
40.1033475319609));
#173829=CARTESIAN_POINT('Ctrl Pts',(-43.9259899312961,-39.3145157795322,
40.1130129263075));
#173830=CARTESIAN_POINT('Ctrl Pts',(-43.9148794775114,-39.3201365884362,
40.1202619720674));
#173831=CARTESIAN_POINT('Ctrl Pts',(-43.9036910542319,-39.3264869747217,
40.1268200947266));
#173832=CARTESIAN_POINT('Ctrl Pts',(-43.8925493833643,-39.3335271634606,
40.1325796782703));
#173833=CARTESIAN_POINT('Ctrl Pts',(-43.888371256789,-39.3361672342377,
40.1347395220992));
#173834=CARTESIAN_POINT('Ctrl Pts',(-43.8841997049151,-39.3389043086119,
40.1367870714852));
#173835=CARTESIAN_POINT('Ctrl Pts',(-43.8800413054826,-39.3417362896178,
40.1387166518767));
#173836=CARTESIAN_POINT('Ctrl Pts',(-43.865486907469,-39.3516482231386,
40.1454701832469));
#173837=CARTESIAN_POINT('Ctrl Pts',(-43.8510936230937,-39.3627227594942,
40.1507785912492));
#173838=CARTESIAN_POINT('Ctrl Pts',(-43.8371435075661,-39.3748700223779,
40.1543986087265));
#173839=CARTESIAN_POINT('Ctrl Pts',(-43.8301684498022,-39.3809436538197,
40.1562086174652));
#173840=CARTESIAN_POINT('Ctrl Pts',(-43.8233041850059,-39.387285467577,
40.1575965292115));
#173841=CARTESIAN_POINT('Ctrl Pts',(-43.8165859732786,-39.3938842320308,
40.1585319382567));
#173842=CARTESIAN_POINT('Ctrl Pts',(-43.813226867415,-39.3971836142578,
40.1589996427793));
#173843=CARTESIAN_POINT('Ctrl Pts',(-43.8099042748374,-39.4005472341762,
40.159354221642));
#173844=CARTESIAN_POINT('Ctrl Pts',(-43.8066226032736,-39.4039736880301,
40.159591874311));
#173845=CARTESIAN_POINT('Ctrl Pts',(-43.8033409317098,-39.4074001418839,
40.1598295269801));
#173846=CARTESIAN_POINT('Ctrl Pts',(-43.8001001824232,-39.4108894308101,
40.1599502506895));
#173847=CARTESIAN_POINT('Ctrl Pts',(-43.7969047596348,-39.4144401478987,
40.1599502534424));
#173848=CARTESIAN_POINT('',(-43.7765468711724,-39.4370498736006,40.1599502534424));
#173849=CARTESIAN_POINT('Origin',(3.51858511112454E-16,-4.55906712132145E-17,
40.1599502534424));
#173850=CARTESIAN_POINT('',(-43.7143933160625,-39.7870778846745,39.8576902534424));
#173851=CARTESIAN_POINT('Ctrl Pts',(-43.7765468711724,-39.4370498736006,
40.1599502534424));
#173852=CARTESIAN_POINT('Ctrl Pts',(-43.7739968854581,-39.4398804576446,
40.1599502448875));
#173853=CARTESIAN_POINT('Ctrl Pts',(-43.771488795476,-39.4427347725909,
40.1598743450437));
#173854=CARTESIAN_POINT('Ctrl Pts',(-43.7690230823394,-39.4456106527045,
40.1597243308499));
#173855=CARTESIAN_POINT('Ctrl Pts',(-43.7544656984485,-39.4625896314089,
40.158838658394));
#173856=CARTESIAN_POINT('Ctrl Pts',(-43.7413824023679,-39.4803211658986,
40.155372255363));
#173857=CARTESIAN_POINT('Ctrl Pts',(-43.7298770745169,-39.4983548991982,
40.1496902177819));
#173858=CARTESIAN_POINT('Ctrl Pts',(-43.7255790670243,-39.5050917016472,
40.1475675976867));
#173859=CARTESIAN_POINT('Ctrl Pts',(-43.721500866419,-39.5118707851407,
40.1451361443109));
#173860=CARTESIAN_POINT('Ctrl Pts',(-43.7176465228246,-39.5186692048625,
40.1424159447501));
#173861=CARTESIAN_POINT('Ctrl Pts',(-43.7146391706004,-39.5239736729699,
40.1402935085949));
#173862=CARTESIAN_POINT('Ctrl Pts',(-43.7117685746243,-39.5292897326777,
40.1379949176048));
#173863=CARTESIAN_POINT('Ctrl Pts',(-43.7090371296309,-39.5346062960351,
40.1355293609261));
#173864=CARTESIAN_POINT('Ctrl Pts',(-43.699477072154,-39.5532142677861,
40.1268999125509));
#173865=CARTESIAN_POINT('Ctrl Pts',(-43.6916216076132,-39.5718284032053,
40.1162251288835));
#173866=CARTESIAN_POINT('Ctrl Pts',(-43.6855734779224,-39.5899733680943,
40.1038990521418));
#173867=CARTESIAN_POINT('Ctrl Pts',(-43.682549413077,-39.5990458505388,
40.097736013771));
#173868=CARTESIAN_POINT('Ctrl Pts',(-43.6799771832789,-39.6080010415737,
40.0911601532641));
#173869=CARTESIAN_POINT('Ctrl Pts',(-43.677869635043,-39.6167795278795,
40.084220729064));
#173870=CARTESIAN_POINT('Ctrl Pts',(-43.6757710912487,-39.6255205083455,
40.0773109533619));
#173871=CARTESIAN_POINT('Ctrl Pts',(-43.6741330170974,-39.6340863223875,
40.0700409753048));
#173872=CARTESIAN_POINT('Ctrl Pts',(-43.6729688455955,-39.6424182201445,
40.0624586415899));
#173873=CARTESIAN_POINT('Ctrl Pts',(-43.672963850363,-39.6424539706904,
40.0624261072769));
#173874=CARTESIAN_POINT('Ctrl Pts',(-43.6729588633162,-39.6424897170044,
40.0623935677889));
#173875=CARTESIAN_POINT('Ctrl Pts',(-43.6729538844541,-39.6425254590849,
40.0623610231289));
#173876=CARTESIAN_POINT('Ctrl Pts',(-43.6706059487639,-39.6593807372529,
40.0470135870232));
#173877=CARTESIAN_POINT('Ctrl Pts',(-43.6700521164126,-39.6752678913557,
40.0305755292089));
#173878=CARTESIAN_POINT('Ctrl Pts',(-43.6711139265064,-39.6901095551213,
40.0133447567333));
#173879=CARTESIAN_POINT('Ctrl Pts',(-43.6722143631621,-39.7054911294118,
39.995487162659));
#173880=CARTESIAN_POINT('Ctrl Pts',(-43.6750505546837,-39.7197505224047,
39.9767767954308));
#173881=CARTESIAN_POINT('Ctrl Pts',(-43.6794690223284,-39.7327754618328,
39.9575197577469));
#173882=CARTESIAN_POINT('Ctrl Pts',(-43.6838244285256,-39.74561450615,39.9385375611994));
#173883=CARTESIAN_POINT('Ctrl Pts',(-43.6897180061492,-39.7572546407973,
39.9190226977096));
#173884=CARTESIAN_POINT('Ctrl Pts',(-43.6970365387951,-39.7675538156914,
39.899265545186));
#173885=CARTESIAN_POINT('Ctrl Pts',(-43.7021391499651,-39.7747345836676,
39.8854905069329));
#173886=CARTESIAN_POINT('Ctrl Pts',(-43.7079351548518,-39.7812627970003,
39.8715976051476));
#173887=CARTESIAN_POINT('Ctrl Pts',(-43.7143933160625,-39.7870778846745,
39.8576902534424));
#173888=CARTESIAN_POINT('',(-43.9791725362585,-40.0254908126586,39.2875012672119));
#173889=CARTESIAN_POINT('',(-43.7143933160625,-39.7870778846745,39.8576902534424));
#173890=CARTESIAN_POINT('',(-40.025490812659,-43.9791725362581,39.2875012672119));
#173891=CARTESIAN_POINT('Origin',(5.53234440788222E-15,0.,39.2875012672119));
#173892=CARTESIAN_POINT('',(-39.7870778846749,-43.7143933160621,39.8576902534424));
#173893=CARTESIAN_POINT('',(-40.025490812659,-43.9791725362581,39.2875012672119));
#173894=CARTESIAN_POINT('',(-39.437049873601,-43.776546871172,40.1599502534424));
#173895=CARTESIAN_POINT('Ctrl Pts',(-39.7870778846749,-43.7143933160621,
39.8576902534424));
#173896=CARTESIAN_POINT('Ctrl Pts',(-39.778894338246,-43.7053047809342,
39.8772619994065));
#173897=CARTESIAN_POINT('Ctrl Pts',(-39.7693190488178,-43.6975432007863,
39.8967644650393));
#173898=CARTESIAN_POINT('Ctrl Pts',(-39.7585187839162,-43.6911816548796,
39.9159282836082));
#173899=CARTESIAN_POINT('Ctrl Pts',(-39.7475234267896,-43.6847051962224,
39.9354382707237));
#173900=CARTESIAN_POINT('Ctrl Pts',(-39.7352578445645,-43.6796790972989,
39.9545987622422));
#173901=CARTESIAN_POINT('Ctrl Pts',(-39.7218536055326,-43.6762098455828,
39.9731387498312));
#173902=CARTESIAN_POINT('Ctrl Pts',(-39.7090168672273,-43.6728874729895,
39.9908938024155));
#173903=CARTESIAN_POINT('Ctrl Pts',(-39.69513504144,-43.6709925938748,40.0080810366299));
#173904=CARTESIAN_POINT('Ctrl Pts',(-39.6802941970377,-43.670652419439,
40.0244542742671));
#173905=CARTESIAN_POINT('Ctrl Pts',(-39.6684902774348,-43.6703818558793,
40.0374770090569));
#173906=CARTESIAN_POINT('Ctrl Pts',(-39.6560790233668,-43.6710953426078,
40.0499848770078));
#173907=CARTESIAN_POINT('Ctrl Pts',(-39.643094175457,-43.6728752976392,
40.0618424270193));
#173908=CARTESIAN_POINT('Ctrl Pts',(-39.6430587310401,-43.6728801563383,
40.0618747942791));
#173909=CARTESIAN_POINT('Ctrl Pts',(-39.6430232824884,-43.6728850230944,
40.0619071564124));
#173910=CARTESIAN_POINT('Ctrl Pts',(-39.6429878298037,-43.6728898979087,
40.0619395134161));
#173911=CARTESIAN_POINT('Ctrl Pts',(-39.6359303251673,-43.6738603187594,
40.0683807661799));
#173912=CARTESIAN_POINT('Ctrl Pts',(-39.6286869425433,-43.6751791606253,
40.0746073439084));
#173913=CARTESIAN_POINT('Ctrl Pts',(-39.6212972007503,-43.6768375203043,
40.0805869293669));
#173914=CARTESIAN_POINT('Ctrl Pts',(-39.6066317464083,-43.6801286499318,
40.092453830807));
#173915=CARTESIAN_POINT('Ctrl Pts',(-39.5913890092851,-43.6847580950892,
40.1033475319609));
#173916=CARTESIAN_POINT('Ctrl Pts',(-39.5758728438539,-43.6906629735751,
40.1130129263075));
#173917=CARTESIAN_POINT('Ctrl Pts',(-39.5642357197805,-43.6950916324395,
40.1202619720674));
#173918=CARTESIAN_POINT('Ctrl Pts',(-39.5524447917348,-43.7002377219526,
40.1268200947266));
#173919=CARTESIAN_POINT('Ctrl Pts',(-39.540628255996,-43.706074722067,40.1325796782703));
#173920=CARTESIAN_POINT('Ctrl Pts',(-39.5361970550939,-43.7082635971098,
40.1347395220992));
#173921=CARTESIAN_POINT('Ctrl Pts',(-39.5317622532395,-43.7105496315974,
40.1367870714852));
#173922=CARTESIAN_POINT('Ctrl Pts',(-39.5273306113316,-43.7129314276128,
40.1387166518767));
#173923=CARTESIAN_POINT('Ctrl Pts',(-39.5118198646542,-43.7212677136665,
40.1454701832469));
#173924=CARTESIAN_POINT('Ctrl Pts',(-39.4963478239301,-43.7307770746561,
40.1507785912492));
#173925=CARTESIAN_POINT('Ctrl Pts',(-39.4812043938728,-43.7413996094241,
40.1543986087265));
#173926=CARTESIAN_POINT('Ctrl Pts',(-39.4736326788442,-43.7467108768082,
40.1562086174652));
#173927=CARTESIAN_POINT('Ctrl Pts',(-39.4661431171622,-43.7523004383955,
40.1575965292115));
#173928=CARTESIAN_POINT('Ctrl Pts',(-39.4587719497939,-43.7581608097795,
40.1585319382567));
#173929=CARTESIAN_POINT('Ctrl Pts',(-39.4550863661098,-43.7610909954715,
40.1589996427793));
#173930=CARTESIAN_POINT('Ctrl Pts',(-39.4514303810208,-43.7640888836318,
40.159354221642));
#173931=CARTESIAN_POINT('Ctrl Pts',(-39.4478085248414,-43.7671535389275,
40.159591874311));
#173932=CARTESIAN_POINT('Ctrl Pts',(-39.4441866686621,-43.7702181942231,
40.1598295269801));
#173933=CARTESIAN_POINT('Ctrl Pts',(-39.4405989425298,-43.7733496179167,
40.1599502506895));
#173934=CARTESIAN_POINT('Ctrl Pts',(-39.437049873601,-43.776546871172,40.1599502534424));
#173935=CARTESIAN_POINT('',(-39.4144401478992,-43.7969047596345,40.1599502534424));
#173936=CARTESIAN_POINT('Origin',(3.56901409908097E-16,-5.06335700088594E-17,
40.1599502534424));
#173937=CARTESIAN_POINT('',(-39.3160391863692,-44.1385184650374,39.8576902534424));
#173938=CARTESIAN_POINT('Ctrl Pts',(-39.4144401478992,-43.7969047596345,
40.1599502534424));
#173939=CARTESIAN_POINT('Ctrl Pts',(-39.4116082546731,-43.7994532913549,
40.1599502448875));
#173940=CARTESIAN_POINT('Ctrl Pts',(-39.4088155471153,-43.8020298032736,
40.1598743450437));
#173941=CARTESIAN_POINT('Ctrl Pts',(-39.4060627300845,-43.80463219181,40.1597243308499));
#173942=CARTESIAN_POINT('Ctrl Pts',(-39.3898103065094,-43.8199964969294,
40.1588386583938));
#173943=CARTESIAN_POINT('Ctrl Pts',(-39.3749452320384,-43.8362633193889,
40.1553722553611));
#173944=CARTESIAN_POINT('Ctrl Pts',(-39.3616178931456,-43.8529956277758,
40.1496902177772));
#173945=CARTESIAN_POINT('Ctrl Pts',(-39.3566392429844,-43.8592462611932,
40.1475675976832));
#173946=CARTESIAN_POINT('Ctrl Pts',(-39.3518747760124,-43.8655619201113,
40.1451361443089));
#173947=CARTESIAN_POINT('Ctrl Pts',(-39.3473309185527,-43.871920208761,
40.1424159447501));
#173948=CARTESIAN_POINT('Ctrl Pts',(-39.3437855730188,-43.8768812645307,
40.1402935085949));
#173949=CARTESIAN_POINT('Ctrl Pts',(-39.3403750229161,-43.8818681433211,
40.1379949176048));
#173950=CARTESIAN_POINT('Ctrl Pts',(-39.3371028088665,-43.8868700682405,
40.1355293609261));
#173951=CARTESIAN_POINT('Ctrl Pts',(-39.3256500596931,-43.9043768054584,
40.1268999125509));
#173952=CARTESIAN_POINT('Ctrl Pts',(-39.3158919212385,-43.9220678510595,
40.1162251288835));
#173953=CARTESIAN_POINT('Ctrl Pts',(-39.3079802585391,-43.93948121423,40.1038990521418));
#173954=CARTESIAN_POINT('Ctrl Pts',(-39.3040244271894,-43.9481878958153,
40.097736013771));
#173955=CARTESIAN_POINT('Ctrl Pts',(-39.3005302159781,-43.9568251581487,
40.0911601532641));
#173956=CARTESIAN_POINT('Ctrl Pts',(-39.2975166114287,-43.9653352562097,
40.084220729064));
#173957=CARTESIAN_POINT('Ctrl Pts',(-39.2945158824213,-43.9738089951121,
40.0773109533619));
#173958=CARTESIAN_POINT('Ctrl Pts',(-39.2919914104331,-43.9821566593549,
40.0700409753048));
#173959=CARTESIAN_POINT('Ctrl Pts',(-39.2899626959158,-43.9903212250461,
40.0624586415899));
#173960=CARTESIAN_POINT('Ctrl Pts',(-39.2899539910981,-43.9903562576028,
40.0624261072769));
#173961=CARTESIAN_POINT('Ctrl Pts',(-39.2899452948636,-43.9903912868064,
40.0623935677888));
#173962=CARTESIAN_POINT('Ctrl Pts',(-39.2899366072115,-43.9904263126553,
40.0623610231288));
#173963=CARTESIAN_POINT('Ctrl Pts',(-39.2858396774348,-44.0069438297326,
40.0470135870265));
#173964=CARTESIAN_POINT('Ctrl Pts',(-39.2836282192311,-44.022686061095,
40.0305755292161));
#173965=CARTESIAN_POINT('Ctrl Pts',(-39.2831328363118,-44.0375574100482,
40.0133447567446));
#173966=CARTESIAN_POINT('Ctrl Pts',(-39.2826194323365,-44.052969749415,
39.9954871626743));
#173967=CARTESIAN_POINT('Ctrl Pts',(-39.2839495744662,-44.0674474907,39.9767767954504));
#173968=CARTESIAN_POINT('Ctrl Pts',(-39.2869823603782,-44.0808629337781,
39.9575197577708));
#173969=CARTESIAN_POINT('Ctrl Pts',(-39.2899718616304,-44.0940869083826,
39.9385375612269));
#173970=CARTESIAN_POINT('Ctrl Pts',(-39.2946164282299,-44.1062793237656,
39.9190226977407));
#173971=CARTESIAN_POINT('Ctrl Pts',(-39.3008183122606,-44.1172870736725,
39.8992655452207));
#173972=CARTESIAN_POINT('Ctrl Pts',(-39.3051423761534,-44.124961872762,
39.8854905069562));
#173973=CARTESIAN_POINT('Ctrl Pts',(-39.310224245815,-44.1320601713495,
39.8715976051593));
#173974=CARTESIAN_POINT('Ctrl Pts',(-39.3160391863692,-44.1385184650374,
39.8576902534424));
#173975=CARTESIAN_POINT('',(-39.5544469813073,-44.4033023070487,39.2875012672119));
#173976=CARTESIAN_POINT('',(-39.3160391863692,-44.1385184650374,39.8576902534424));
#173977=CARTESIAN_POINT('',(-35.209151665053,-47.9220530736685,39.2875012672119));
#173978=CARTESIAN_POINT('Origin',(5.53234440788222E-15,0.,39.2875012672119));
#173979=CARTESIAN_POINT('',(-34.9997217530263,-47.6338034047598,39.8576902534424));
#173980=CARTESIAN_POINT('',(-35.209151665053,-47.9220530736685,39.2875012672119));
#173981=CARTESIAN_POINT('',(-34.6451144164188,-47.6590285860934,40.1599502534424));
#173982=CARTESIAN_POINT('Ctrl Pts',(-34.9997217530263,-47.6338034047598,
39.8576902534424));
#173983=CARTESIAN_POINT('Ctrl Pts',(-34.9925330475314,-47.6239092440462,
39.8772619994059));
#173984=CARTESIAN_POINT('Ctrl Pts',(-34.9838215185863,-47.6151892923575,
39.8967644650381));
#173985=CARTESIAN_POINT('Ctrl Pts',(-34.9737453812839,-47.6077336605719,
39.9159282836064));
#173986=CARTESIAN_POINT('Ctrl Pts',(-34.9634872321454,-47.6001433528495,
39.9354382707214));
#173987=CARTESIAN_POINT('Ctrl Pts',(-34.9518142124603,-47.5938626849608,
39.9545987622393));
#173988=CARTESIAN_POINT('Ctrl Pts',(-34.9388460388034,-47.5890113136614,
39.9731387498278));
#173989=CARTESIAN_POINT('Ctrl Pts',(-34.9264269039957,-47.5843653368443,
39.9908938024117));
#173990=CARTESIAN_POINT('Ctrl Pts',(-34.9128191931051,-47.5810297921587,
40.0080810366257));
#173991=CARTESIAN_POINT('Ctrl Pts',(-34.8980952063128,-47.5791401905748,
40.0244542742626));
#173992=CARTESIAN_POINT('Ctrl Pts',(-34.8863842314085,-47.5776372636136,
40.037477009054));
#173993=CARTESIAN_POINT('Ctrl Pts',(-34.8739663878163,-47.577049512472,
40.0499848770064));
#173994=CARTESIAN_POINT('Ctrl Pts',(-34.8608666162964,-47.5774624305258,
40.0618424270193));
#173995=CARTESIAN_POINT('Ctrl Pts',(-34.8608308581753,-47.5774635576579,
40.0618747942791));
#173996=CARTESIAN_POINT('Ctrl Pts',(-34.8607950951,-47.5774646923709,40.0619071564124));
#173997=CARTESIAN_POINT('Ctrl Pts',(-34.8607593270719,-47.5774658346658,
40.0619395134162));
#173998=CARTESIAN_POINT('Ctrl Pts',(-34.8536390475841,-47.5776932293353,
40.0683807661799));
#173999=CARTESIAN_POINT('Ctrl Pts',(-34.8462974884545,-47.578247706793,
40.0746073439084));
#174000=CARTESIAN_POINT('Ctrl Pts',(-34.8387748826515,-47.5791245434505,
40.0805869293669));
#174001=CARTESIAN_POINT('Ctrl Pts',(-34.8238457504804,-47.5808646865201,
40.092453830807));
#174002=CARTESIAN_POINT('Ctrl Pts',(-34.808202605878,-47.583875471205,40.1033475319609));
#174003=CARTESIAN_POINT('Ctrl Pts',(-34.7921542117506,-47.5881261212204,
40.1130129263075));
#174004=CARTESIAN_POINT('Ctrl Pts',(-34.780117916155,-47.5913141087319,
40.1202619720674));
#174005=CARTESIAN_POINT('Ctrl Pts',(-34.7678536672182,-47.5951995198392,
40.1268200947267));
#174006=CARTESIAN_POINT('Ctrl Pts',(-34.7554917310465,-47.5997693799342,
40.1325796782703));
#174007=CARTESIAN_POINT('Ctrl Pts',(-34.7508560049821,-47.6014830774699,
40.1347395220992));
#174008=CARTESIAN_POINT('Ctrl Pts',(-34.7462065417643,-47.6032930257986,
40.1367870714852));
#174009=CARTESIAN_POINT('Ctrl Pts',(-34.7415502113773,-47.6051985413678,
40.1387166518767));
#174010=CARTESIAN_POINT('Ctrl Pts',(-34.7252530550225,-47.6118678458599,
40.1454701832469));
#174011=CARTESIAN_POINT('Ctrl Pts',(-34.7088717728655,-47.6197078449345,
40.1507785912492));
#174012=CARTESIAN_POINT('Ctrl Pts',(-34.6927009428672,-47.6286892688732,
40.1543986087265));
#174013=CARTESIAN_POINT('Ctrl Pts',(-34.684615527868,-47.6331799808425,
40.1562086174652));
#174014=CARTESIAN_POINT('Ctrl Pts',(-34.6765827265055,-47.6379560498535,
40.1575965292115));
#174015=CARTESIAN_POINT('Ctrl Pts',(-34.6686393635484,-47.6430138207123,
40.1585319382567));
#174016=CARTESIAN_POINT('Ctrl Pts',(-34.6646676820698,-47.6455427061418,
40.1589996427793));
#174017=CARTESIAN_POINT('Ctrl Pts',(-34.6607183602073,-47.6481420170541,
40.159354221642));
#174018=CARTESIAN_POINT('Ctrl Pts',(-34.6567960012265,-47.6508112967867,
40.1595918743111));
#174019=CARTESIAN_POINT('Ctrl Pts',(-34.6528736422457,-47.6534805765194,
40.1598295269801));
#174020=CARTESIAN_POINT('Ctrl Pts',(-34.6489782471461,-47.656219826447,
40.1599502506896));
#174021=CARTESIAN_POINT('Ctrl Pts',(-34.6451144164188,-47.6590285860934,
40.1599502534424));
#174022=CARTESIAN_POINT('',(-34.6205005703637,-47.6769115920302,40.1599502534424));
#174023=CARTESIAN_POINT('Origin',(3.62443809638014E-16,-5.51217168157313E-17,
40.1599502534424));
#174024=CARTESIAN_POINT('',(-34.4869303039399,-48.0063682005185,39.8576902534424));
#174025=CARTESIAN_POINT('Ctrl Pts',(-34.6205005703637,-47.6769115920302,
40.1599502534424));
#174026=CARTESIAN_POINT('Ctrl Pts',(-34.6174177964407,-47.6791501491801,
40.1599502448875));
#174027=CARTESIAN_POINT('Ctrl Pts',(-34.6143710687956,-47.6814206292677,
40.1598743450437));
#174028=CARTESIAN_POINT('Ctrl Pts',(-34.61136130831,-47.6837210139134,40.1597243308499));
#174029=CARTESIAN_POINT('Ctrl Pts',(-34.5935919100082,-47.6973023109013,
40.1588386583937));
#174030=CARTESIAN_POINT('Ctrl Pts',(-34.5771079220164,-47.7119261986147,
40.155372255361));
#174031=CARTESIAN_POINT('Ctrl Pts',(-34.5621045891978,-47.7271737594119,
40.1496902177769));
#174032=CARTESIAN_POINT('Ctrl Pts',(-34.5564998434977,-47.7328697405547,
40.147567597683));
#174033=CARTESIAN_POINT('Ctrl Pts',(-34.5511013106533,-47.7386527792213,
40.1451361443088));
#174034=CARTESIAN_POINT('Ctrl Pts',(-34.5459177227788,-47.7445012740628,
40.1424159447501));
#174035=CARTESIAN_POINT('Ctrl Pts',(-34.5418732274829,-47.7490645631294,
40.1402935085949));
#174036=CARTESIAN_POINT('Ctrl Pts',(-34.537960089954,-47.7536676237149,
40.1379949176048));
#174037=CARTESIAN_POINT('Ctrl Pts',(-34.5341829579102,-47.7583001080602,
40.1355293609261));
#174038=CARTESIAN_POINT('Ctrl Pts',(-34.5209629957568,-47.7745138032686,
40.1268999125509));
#174039=CARTESIAN_POINT('Ctrl Pts',(-34.5094090955954,-47.7910879322537,
40.1162251288835));
#174040=CARTESIAN_POINT('Ctrl Pts',(-34.4997205817196,-47.807578909255,
40.1038990521418));
#174041=CARTESIAN_POINT('Ctrl Pts',(-34.4948763247817,-47.8158243977557,
40.097736013771));
#174042=CARTESIAN_POINT('Ctrl Pts',(-34.4904984154664,-47.824049099734,
40.0911601532641));
#174043=CARTESIAN_POINT('Ctrl Pts',(-34.4866117722854,-47.832197571135,
40.084220729064));
#174044=CARTESIAN_POINT('Ctrl Pts',(-34.4827417346799,-47.8403112284173,
40.0773109533619));
#174045=CARTESIAN_POINT('Ctrl Pts',(-34.4793585234982,-47.8483492841043,
40.0700409753048));
#174046=CARTESIAN_POINT('Ctrl Pts',(-34.4764874929864,-47.8562570650396,
40.0624586415899));
#174047=CARTESIAN_POINT('Ctrl Pts',(-34.4764751739553,-47.856290995783,
40.062426107277));
#174048=CARTESIAN_POINT('Ctrl Pts',(-34.4764628638109,-47.856324924089,
40.0623935677889));
#174049=CARTESIAN_POINT('Ctrl Pts',(-34.4764505625524,-47.8563588499556,
40.0623610231289));
#174050=CARTESIAN_POINT('Ctrl Pts',(-34.4706495255073,-47.872357636576,
40.0470135870232));
#174051=CARTESIAN_POINT('Ctrl Pts',(-34.4668046706499,-47.8877824700235,
40.030575529209));
#174052=CARTESIAN_POINT('Ctrl Pts',(-34.4647575222376,-47.9025205705587,
40.0133447567334));
#174053=CARTESIAN_POINT('Ctrl Pts',(-34.462635902594,-47.9177948141924,
39.9954871626587));
#174054=CARTESIAN_POINT('Ctrl Pts',(-34.462445422019,-47.9323322826113,
39.9767767954302));
#174055=CARTESIAN_POINT('Ctrl Pts',(-34.4640592983654,-47.9459912469416,
39.9575197577459));
#174056=CARTESIAN_POINT('Ctrl Pts',(-34.4656501410751,-47.9594552672033,
39.9385375611976));
#174057=CARTESIAN_POINT('Ctrl Pts',(-34.4689948098118,-47.9720663806699,
39.919022697707));
#174058=CARTESIAN_POINT('Ctrl Pts',(-34.4740120960943,-47.9836621023791,
39.8992655451827));
#174059=CARTESIAN_POINT('Ctrl Pts',(-34.4775102373562,-47.9917468458617,
39.8854905069307));
#174060=CARTESIAN_POINT('Ctrl Pts',(-34.4818222937577,-47.9993374592455,
39.8715976051465));
#174061=CARTESIAN_POINT('Ctrl Pts',(-34.4869303039399,-48.0063682005185,
39.8576902534424));
#174062=CARTESIAN_POINT('',(-34.6963546279287,-48.2946219293745,39.2875012672119));
#174063=CARTESIAN_POINT('',(-34.4869303039399,-48.0063682005185,39.8576902534424));
#174064=CARTESIAN_POINT('',(-30.007053683816,-51.3398895692696,39.2875012672119));
#174065=CARTESIAN_POINT('Origin',(5.53234440788222E-15,0.,39.2875012672119));
#174066=CARTESIAN_POINT('',(-29.8289013456888,-51.0313275753407,39.8576902534424));
#174067=CARTESIAN_POINT('',(-30.007053683816,-51.3398895692696,39.2875012672119));
#174068=CARTESIAN_POINT('',(-29.473599835734,-51.0193480105326,40.1599502534424));
#174069=CARTESIAN_POINT('Ctrl Pts',(-29.8289013456888,-51.0313275753407,
39.8576902534424));
#174070=CARTESIAN_POINT('Ctrl Pts',(-29.822786242089,-51.0207361915361,
39.877261999407));
#174071=CARTESIAN_POINT('Ctrl Pts',(-29.8150339189602,-51.0111534059212,
39.8967644650402));
#174072=CARTESIAN_POINT('Ctrl Pts',(-29.8057923055248,-51.0026853737185,
39.9159282836095));
#174073=CARTESIAN_POINT('Ctrl Pts',(-29.7963837548019,-50.9940643779303,
39.9354382707254));
#174074=CARTESIAN_POINT('Ctrl Pts',(-29.7854311897019,-50.9865979533879,
39.9545987622442));
#174075=CARTESIAN_POINT('Ctrl Pts',(-29.7730411634431,-50.9804176151442,
39.9731387498335));
#174076=CARTESIAN_POINT('Ctrl Pts',(-29.7611756987718,-50.9744989363977,
39.9908938024178));
#174077=CARTESIAN_POINT('Ctrl Pts',(-29.7479911917047,-50.969759271067,
40.0080810366322));
#174078=CARTESIAN_POINT('Ctrl Pts',(-29.7335453816016,-50.966340945206,
40.0244542742694));
#174079=CARTESIAN_POINT('Ctrl Pts',(-29.7220556592906,-50.9636221212266,
40.0374770090583));
#174080=CARTESIAN_POINT('Ctrl Pts',(-29.7097672786705,-50.9617395717399,
40.0499848770085));
#174081=CARTESIAN_POINT('Ctrl Pts',(-29.6966961073823,-50.9607809287994,
40.0618424270193));
#174082=CARTESIAN_POINT('Ctrl Pts',(-29.6966604273306,-50.9607783120156,
40.0618747942791));
#174083=CARTESIAN_POINT('Ctrl Pts',(-29.6966247415593,-50.9607757022531,
40.0619071564124));
#174084=CARTESIAN_POINT('Ctrl Pts',(-29.6965890500698,-50.9607730995134,
40.0619395134161));
#174085=CARTESIAN_POINT('Ctrl Pts',(-29.6894840070028,-50.9602549766183,
40.0683807661799));
#174086=CARTESIAN_POINT('Ctrl Pts',(-29.6821247070256,-50.9600390146966,
40.0746073439084));
#174087=CARTESIAN_POINT('Ctrl Pts',(-29.6745516564559,-50.9601247215269,
40.0805869293669));
#174088=CARTESIAN_POINT('Ctrl Pts',(-29.6595224131521,-50.9602948126669,
40.092453830807));
#174089=CARTESIAN_POINT('Ctrl Pts',(-29.6436502506361,-50.9616539500923,
40.1033475319609));
#174090=CARTESIAN_POINT('Ctrl Pts',(-29.6272454573769,-50.9642038006261,
40.1130129263075));
#174091=CARTESIAN_POINT('Ctrl Pts',(-29.6149418624325,-50.9661161885264,
40.1202619720674));
#174092=CARTESIAN_POINT('Ctrl Pts',(-29.6023386622824,-50.9686983518506,
40.1268200947266));
#174093=CARTESIAN_POINT('Ctrl Pts',(-29.5895667656375,-50.9719510035828,
40.1325796782703));
#174094=CARTESIAN_POINT('Ctrl Pts',(-29.5847773043956,-50.9731707479824,
40.1347395220992));
#174095=CARTESIAN_POINT('Ctrl Pts',(-29.5799641203064,-50.9744847799796,
40.1367870714852));
#174096=CARTESIAN_POINT('Ctrl Pts',(-29.5751341171702,-50.9758931378753,
40.1387166518767));
#174097=CARTESIAN_POINT('Ctrl Pts',(-29.5582291061935,-50.9808223905103,
40.1454701832469));
#174098=CARTESIAN_POINT('Ctrl Pts',(-29.5411180593589,-50.9869071309994,
40.1507785912492));
#174099=CARTESIAN_POINT('Ctrl Pts',(-29.524097000417,-50.9941490417485,
40.1543986087265));
#174100=CARTESIAN_POINT('Ctrl Pts',(-29.5155864709461,-50.997769997123,
40.1562086174652));
#174101=CARTESIAN_POINT('Ctrl Pts',(-29.5070984389558,-51.0016802459461,
40.1575965292115));
#174102=CARTESIAN_POINT('Ctrl Pts',(-29.4986699095566,-51.0058800022839,
40.1585319382567));
#174103=CARTESIAN_POINT('Ctrl Pts',(-29.494455644857,-51.0079798804528,
40.1589996427793));
#174104=CARTESIAN_POINT('Ctrl Pts',(-29.4902562558177,-51.0101521355227,
40.159354221642));
#174105=CARTESIAN_POINT('Ctrl Pts',(-29.4860763682213,-51.012396794505,
40.1595918743111));
#174106=CARTESIAN_POINT('Ctrl Pts',(-29.481896480625,-51.0146414534874,
40.1598295269801));
#174107=CARTESIAN_POINT('Ctrl Pts',(-29.4777360953218,-51.0169585178537,
40.1599502506895));
#174108=CARTESIAN_POINT('Ctrl Pts',(-29.473599835734,-51.0193480105326,
40.1599502534424));
#174109=CARTESIAN_POINT('',(-29.4472515437738,-51.0345602039885,40.1599502534424));
#174110=CARTESIAN_POINT('Origin',(3.68424986610942E-16,-5.90059385582098E-17,
40.1599502534424));
#174111=CARTESIAN_POINT('',(-29.2799753962465,-51.3482501200164,39.8576902534424));
#174112=CARTESIAN_POINT('Ctrl Pts',(-29.4472515437738,-51.0345602039885,
40.1599502534424));
#174113=CARTESIAN_POINT('Ctrl Pts',(-29.4439516646701,-51.0364642604674,
40.1599502448875));
#174114=CARTESIAN_POINT('Ctrl Pts',(-29.4406842975234,-51.0384038328687,
40.1598743450437));
#174115=CARTESIAN_POINT('Ctrl Pts',(-29.4374505691487,-51.0403770101283,
40.1597243308499));
#174116=CARTESIAN_POINT('Ctrl Pts',(-29.4183588813689,-51.0520264994513,
40.1588386583938));
#174117=CARTESIAN_POINT('Ctrl Pts',(-29.4004365818804,-51.0648472300426,
40.1553722553618));
#174118=CARTESIAN_POINT('Ctrl Pts',(-29.3839216347917,-51.0784429877812,
40.149690217779));
#174119=CARTESIAN_POINT('Ctrl Pts',(-29.3777522003172,-51.0835219102899,
40.1475675976845));
#174120=CARTESIAN_POINT('Ctrl Pts',(-29.3717787490539,-51.088708968525,
40.1451361443097));
#174121=CARTESIAN_POINT('Ctrl Pts',(-29.3660122232361,-51.0939835922267,
40.1424159447501));
#174122=CARTESIAN_POINT('Ctrl Pts',(-29.3615128905151,-51.0980991182404,
40.1402935085949));
#174123=CARTESIAN_POINT('Ctrl Pts',(-29.3571400387136,-51.102267928526,
40.1379949176048));
#174124=CARTESIAN_POINT('Ctrl Pts',(-29.3528993717246,-51.1064802178292,
40.1355293609261));
#174125=CARTESIAN_POINT('Ctrl Pts',(-29.3380570372632,-51.1212232303904,
40.1268999125509));
#174126=CARTESIAN_POINT('Ctrl Pts',(-29.3248339623429,-51.1364988531342,
40.1162251288835));
#174127=CARTESIAN_POINT('Ctrl Pts',(-29.3134747466761,-51.1518867653712,
40.1038990521418));
#174128=CARTESIAN_POINT('Ctrl Pts',(-29.3077951388427,-51.1595807214897,
40.097736013771));
#174129=CARTESIAN_POINT('Ctrl Pts',(-29.3025814967141,-51.167302751557,
40.0911601532641));
#174130=CARTESIAN_POINT('Ctrl Pts',(-29.2978643977776,-51.17500031994,40.084220729064));
#174131=CARTESIAN_POINT('Ctrl Pts',(-29.2931674525158,-51.1826650006751,
40.0773109533619));
#174132=CARTESIAN_POINT('Ctrl Pts',(-29.2889625693103,-51.1903053811864,
40.0700409753048));
#174133=CARTESIAN_POINT('Ctrl Pts',(-29.2852806784151,-51.1978697380628,
40.0624586415899));
#174134=CARTESIAN_POINT('Ctrl Pts',(-29.2852648801404,-51.1979021952407,
40.0624261072769));
#174135=CARTESIAN_POINT('Ctrl Pts',(-29.2852490909586,-51.1979346509234,
40.0623935677888));
#174136=CARTESIAN_POINT('Ctrl Pts',(-29.285233310869,-51.197967105109,40.0623610231288));
#174137=CARTESIAN_POINT('Ctrl Pts',(-29.2777917239326,-51.2132718752139,
40.0470135870239));
#174138=CARTESIAN_POINT('Ctrl Pts',(-29.2723555974561,-51.2282103130394,
40.0305755292105));
#174139=CARTESIAN_POINT('Ctrl Pts',(-29.2687791125364,-51.2426536914396,
40.0133447567357));
#174140=CARTESIAN_POINT('Ctrl Pts',(-29.2650725221326,-51.2576224915267,
39.9954871626622));
#174141=CARTESIAN_POINT('Ctrl Pts',(-29.2633635057962,-51.27206041153,39.976776795435));
#174142=CARTESIAN_POINT('Ctrl Pts',(-29.2635407906074,-51.2858132466382,
39.957519757752));
#174143=CARTESIAN_POINT('Ctrl Pts',(-29.2637155451665,-51.2993697979311,
39.9385375612053));
#174144=CARTESIAN_POINT('Ctrl Pts',(-29.2657236711464,-51.312261439481,
39.9190226977163));
#174145=CARTESIAN_POINT('Ctrl Pts',(-29.2695013892381,-51.3243180878377,
39.8992655451936));
#174146=CARTESIAN_POINT('Ctrl Pts',(-29.2721352815043,-51.3327241975823,
39.885490506938));
#174147=CARTESIAN_POINT('Ctrl Pts',(-29.2756302808581,-51.3407239614232,
39.8715976051502));
#174148=CARTESIAN_POINT('Ctrl Pts',(-29.2799753962465,-51.3482501200164,
39.8576902534424));
#174149=CARTESIAN_POINT('',(-29.4581217525676,-51.6568155675426,39.2875012672119));
#174150=CARTESIAN_POINT('',(-29.2799753962465,-51.3482501200164,39.8576902534424));
#174151=CARTESIAN_POINT('',(-24.4761921430394,-54.1952354911871,39.2875012672119));
#174152=CARTESIAN_POINT('Origin',(5.53234440788222E-15,0.,39.2875012672119));
#174153=CARTESIAN_POINT('',(-24.331269253109,-53.8697418420144,39.8576902534424));
#174154=CARTESIAN_POINT('',(-24.4761921430394,-54.1952354911871,39.2875012672119));
#174155=CARTESIAN_POINT('',(-23.9791663275016,-53.8206887816835,40.1599502534424));
#174156=CARTESIAN_POINT('Ctrl Pts',(-24.331269253109,-53.8697418420144,
39.8576902534424));
#174157=CARTESIAN_POINT('Ctrl Pts',(-24.3262947497604,-53.858569276538,
39.877261999404));
#174158=CARTESIAN_POINT('Ctrl Pts',(-24.3195865685243,-53.8482286480035,
39.8967644650344));
#174159=CARTESIAN_POINT('Ctrl Pts',(-24.311280732009,-53.8388409929178,
39.9159282836009));
#174160=CARTESIAN_POINT('Ctrl Pts',(-24.3028248617547,-53.8292837624991,
39.935438270714));
#174161=CARTESIAN_POINT('Ctrl Pts',(-24.2927127498381,-53.8207133850136,
39.95459876223));
#174162=CARTESIAN_POINT('Ctrl Pts',(-24.2810366187012,-53.8132717929053,
39.973138749817));
#174163=CARTESIAN_POINT('Ctrl Pts',(-24.2698548246833,-53.8061452585126,
39.990893802399));
#174164=CARTESIAN_POINT('Ctrl Pts',(-24.2572379736618,-53.8000534013019,
40.0080810366113));
#174165=CARTESIAN_POINT('Ctrl Pts',(-24.2432286115706,-53.7951438030566,
40.0244542742468));
#174166=CARTESIAN_POINT('Ctrl Pts',(-24.2320860256476,-53.7912388700597,
40.0374770090439));
#174167=CARTESIAN_POINT('Ctrl Pts',(-24.2200617420608,-53.7880821478315,
40.0499848770016));
#174168=CARTESIAN_POINT('Ctrl Pts',(-24.2071623814825,-53.7857624469882,
40.0618424270193));
#174169=CARTESIAN_POINT('Ctrl Pts',(-24.2071271704182,-53.7857561149584,
40.0618747942791));
#174170=CARTESIAN_POINT('Ctrl Pts',(-24.2070919529318,-53.7857497893136,
40.0619071564124));
#174171=CARTESIAN_POINT('Ctrl Pts',(-24.2070567290244,-53.7857434700554,
40.0619395134162));
#174172=CARTESIAN_POINT('Ctrl Pts',(-24.2000447667167,-53.7844855062585,
40.0683807661799));
#174173=CARTESIAN_POINT('Ctrl Pts',(-24.1927483559227,-53.7835014710815,
40.0746073439084));
#174174=CARTESIAN_POINT('Ctrl Pts',(-24.1852078325131,-53.7827951090624,
40.0805869293669));
#174175=CARTESIAN_POINT('Ctrl Pts',(-24.1702431416111,-53.7813932847187,
40.092453830807));
#174176=CARTESIAN_POINT('Ctrl Pts',(-24.1543158599158,-53.7810858838906,
40.1033475319609));
#174177=CARTESIAN_POINT('Ctrl Pts',(-24.1377344018726,-53.7819069982468,
40.1130129263075));
#174178=CARTESIAN_POINT('Ctrl Pts',(-24.1252983083403,-53.7825228340139,
40.1202619720675));
#174179=CARTESIAN_POINT('Ctrl Pts',(-24.1124942402751,-53.7837734588333,
40.1268200947266));
#174180=CARTESIAN_POINT('Ctrl Pts',(-24.0994523147292,-53.7856732654697,
40.1325796782703));
#174181=CARTESIAN_POINT('Ctrl Pts',(-24.0945615926495,-53.7863856929583,
40.1347395220992));
#174182=CARTESIAN_POINT('Ctrl Pts',(-24.089637421941,-53.7871894118145,
40.1367870714852));
#174183=CARTESIAN_POINT('Ctrl Pts',(-24.0846866645808,-53.7880851817729,
40.1387166518767));
#174184=CARTESIAN_POINT('Ctrl Pts',(-24.06735901382,-53.7912203766272,40.1454701832469));
#174185=CARTESIAN_POINT('Ctrl Pts',(-24.0497056745176,-53.7954831928408,
40.1507785912492));
#174186=CARTESIAN_POINT('Ctrl Pts',(-24.0320208729158,-53.8009062465107,
40.1543986087265));
#174187=CARTESIAN_POINT('Ctrl Pts',(-24.023178472115,-53.8036177733456,
40.1562086174652));
#174188=CARTESIAN_POINT('Ctrl Pts',(-24.0143282061515,-53.8066193604763,
40.1575965292115));
#174189=CARTESIAN_POINT('Ctrl Pts',(-24.0055068550422,-53.8099150888838,
40.1585319382567));
#174190=CARTESIAN_POINT('Ctrl Pts',(-24.0010961794876,-53.8115629530876,
40.1589996427793));
#174191=CARTESIAN_POINT('Ctrl Pts',(-23.9966927326565,-53.8132843526339,
40.159354221642));
#174192=CARTESIAN_POINT('Ctrl Pts',(-23.9923011121677,-53.8150797979124,
40.159591874311));
#174193=CARTESIAN_POINT('Ctrl Pts',(-23.987909491679,-53.8168752431909,
40.1598295269801));
#174194=CARTESIAN_POINT('Ctrl Pts',(-23.9835296982243,-53.8187447357539,
40.1599502506895));
#174195=CARTESIAN_POINT('Ctrl Pts',(-23.9791663275016,-53.8206887816835,
40.1599502534424));
#174196=CARTESIAN_POINT('',(-23.9513722670367,-53.8330634946837,40.1599502534424));
#174197=CARTESIAN_POINT('Origin',(3.74779409800327E-16,-6.22436788900567E-17,
40.1599502534424));
#174198=CARTESIAN_POINT('',(-23.752222950883,-54.1275498658872,39.8576902534424));
#174199=CARTESIAN_POINT('Ctrl Pts',(-23.9513722670367,-53.8330634946837,
40.1599502534424));
#174200=CARTESIAN_POINT('Ctrl Pts',(-23.9478914369183,-53.8346121892502,
40.1599502448875));
#174201=CARTESIAN_POINT('Ctrl Pts',(-23.9444392282283,-53.8361996036042,
40.1598743450437));
#174202=CARTESIAN_POINT('Ctrl Pts',(-23.9410169613692,-53.8378239549347,
40.1597243308499));
#174203=CARTESIAN_POINT('Ctrl Pts',(-23.920812156637,-53.8474140023509,
40.1588386583939));
#174204=CARTESIAN_POINT('Ctrl Pts',(-23.9016479061145,-53.8582911092143,
40.1553722553622));
#174205=CARTESIAN_POINT('Ctrl Pts',(-23.8838022859714,-53.8700861059286,
40.1496902177798));
#174206=CARTESIAN_POINT('Ctrl Pts',(-23.8771357563386,-53.874492324064,
40.1475675976852));
#174207=CARTESIAN_POINT('Ctrl Pts',(-23.8706528330392,-53.8790265713711,
40.1451361443101));
#174208=CARTESIAN_POINT('Ctrl Pts',(-23.8643665485424,-53.8836695340508,
40.1424159447502));
#174209=CARTESIAN_POINT('Ctrl Pts',(-23.8594616740271,-53.8872922064473,
40.1402935085949));
#174210=CARTESIAN_POINT('Ctrl Pts',(-23.8546770178326,-53.890981092075,
40.1379949176048));
#174211=CARTESIAN_POINT('Ctrl Pts',(-23.8500192775334,-53.8947270356131,
40.1355293609261));
#174212=CARTESIAN_POINT('Ctrl Pts',(-23.8337171864861,-53.9078378379964,
40.1268999125509));
#174213=CARTESIAN_POINT('Ctrl Pts',(-23.818969811583,-53.9216475915793,
40.1162251288835));
#174214=CARTESIAN_POINT('Ctrl Pts',(-23.806064348069,-53.9357638458655,
40.1038990521418));
#174215=CARTESIAN_POINT('Ctrl Pts',(-23.7996116163121,-53.9428219730085,
40.097736013771));
#174216=CARTESIAN_POINT('Ctrl Pts',(-23.7936193631243,-53.9499567269874,
40.0911601532641));
#174217=CARTESIAN_POINT('Ctrl Pts',(-23.7881234899554,-53.9571190561825,
40.084220729064));
#174218=CARTESIAN_POINT('Ctrl Pts',(-23.7826510977526,-53.9642507845243,
40.0773109533619));
#174219=CARTESIAN_POINT('Ctrl Pts',(-23.7776706121036,-53.971409780252,
40.0700409753048));
#174220=CARTESIAN_POINT('Ctrl Pts',(-23.773218200392,-53.9785478363928,
40.0624586415899));
#174221=CARTESIAN_POINT('Ctrl Pts',(-23.773199095963,-53.9785784643975,
40.0624261072769));
#174222=CARTESIAN_POINT('Ctrl Pts',(-23.7731800007333,-53.9786090918657,
40.0623935677888));
#174223=CARTESIAN_POINT('Ctrl Pts',(-23.7731609147026,-53.9786397187953,
40.0623610231288));
#174224=CARTESIAN_POINT('Ctrl Pts',(-23.7641603094579,-53.9930827901221,
40.0470135870232));
#174225=CARTESIAN_POINT('Ctrl Pts',(-23.7571924707012,-54.0073711636762,
40.030575529209));
#174226=CARTESIAN_POINT('Ctrl Pts',(-23.7521258339916,-54.0213615752664,
40.0133447567334));
#174227=CARTESIAN_POINT('Ctrl Pts',(-23.7468748830077,-54.0358609305021,
39.9954871626591));
#174228=CARTESIAN_POINT('Ctrl Pts',(-23.743666055251,-54.0500411172181,
39.976776795431));
#174229=CARTESIAN_POINT('Ctrl Pts',(-23.7424048061582,-54.0637371441659,
39.9575197577471));
#174230=CARTESIAN_POINT('Ctrl Pts',(-23.74116155792,-54.0772376980782,39.9385375611998));
#174231=CARTESIAN_POINT('Ctrl Pts',(-23.7418111396959,-54.0902686241898,
39.9190226977101));
#174232=CARTESIAN_POINT('Ctrl Pts',(-23.7443079001282,-54.1026541040323,
39.8992655451867));
#174233=CARTESIAN_POINT('Ctrl Pts',(-23.7460486859234,-54.1112894809377,
39.8854905069334));
#174234=CARTESIAN_POINT('Ctrl Pts',(-23.748688336284,-54.1196107481453,
39.8715976051479));
#174235=CARTESIAN_POINT('Ctrl Pts',(-23.7522229508831,-54.1275498658872,
39.8576902534424));
#174236=CARTESIAN_POINT('',(-23.8971395307771,-54.4530463244691,39.2875012672119));
#174237=CARTESIAN_POINT('',(-23.752222950883,-54.1275498658872,39.8576902534424));
#174238=CARTESIAN_POINT('',(-18.6771643191712,-56.456807071981,39.2875012672119));
#174239=CARTESIAN_POINT('Origin',(5.53234440788222E-15,0.,39.2875012672119));
#174240=CARTESIAN_POINT('',(-18.5670586829468,-56.1179479440987,39.8576902534424));
#174241=CARTESIAN_POINT('',(-18.6771643191712,-56.456807071981,39.2875012672119));
#174242=CARTESIAN_POINT('',(-18.2220120550219,-56.032358823839,40.1599502534424));
#174243=CARTESIAN_POINT('Ctrl Pts',(-18.5670586829468,-56.1179479440987,
39.8576902534424));
#174244=CARTESIAN_POINT('Ctrl Pts',(-18.5632792815475,-56.1063166059131,
39.8772619994065));
#174245=CARTESIAN_POINT('Ctrl Pts',(-18.557688738439,-56.0953314285464,
39.8967644650392));
#174246=CARTESIAN_POINT('Ctrl Pts',(-18.5504096793237,-56.0851270036894,
39.915928283608));
#174247=CARTESIAN_POINT('Ctrl Pts',(-18.5429991338188,-56.0747382496545,
39.9354382707233));
#174248=CARTESIAN_POINT('Ctrl Pts',(-18.5338382654958,-56.0651578180738,
39.9545987622416));
#174249=CARTESIAN_POINT('Ctrl Pts',(-18.5230039556122,-56.0565365037404,
39.9731387498305));
#174250=CARTESIAN_POINT('Ctrl Pts',(-18.5126283423185,-56.048280193503,
39.9908938024142));
#174251=CARTESIAN_POINT('Ctrl Pts',(-18.5007173801975,-56.0409028880747,
40.0080810366281));
#174252=CARTESIAN_POINT('Ctrl Pts',(-18.4872979556147,-56.0345558080315,
40.0244542742649));
#174253=CARTESIAN_POINT('Ctrl Pts',(-18.4766245865927,-56.0295075492857,
40.0374770090555));
#174254=CARTESIAN_POINT('Ctrl Pts',(-18.464996140618,-56.0251112400294,
40.0499848770071));
#174255=CARTESIAN_POINT('Ctrl Pts',(-18.4524099188568,-56.0214558964133,
40.0618424270193));
#174256=CARTESIAN_POINT('Ctrl Pts',(-18.4523755625598,-56.0214459185126,
40.0618747942791));
#174257=CARTESIAN_POINT('Ctrl Pts',(-18.4523411992083,-56.0214359462906,
40.0619071564124));
#174258=CARTESIAN_POINT('Ctrl Pts',(-18.4523068288036,-56.0214259797491,
40.0619395134162));
#174259=CARTESIAN_POINT('Ctrl Pts',(-18.4454647717816,-56.0194419575649,
40.0683807661799));
#174260=CARTESIAN_POINT('Ctrl Pts',(-18.4383111911741,-56.0177006304279,
40.0746073439084));
#174261=CARTESIAN_POINT('Ctrl Pts',(-18.4308858104772,-56.0162099386097,
40.0805869293669));
#174262=CARTESIAN_POINT('Ctrl Pts',(-18.4161496282621,-56.0132515574632,
40.092453830807));
#174263=CARTESIAN_POINT('Ctrl Pts',(-18.4003417300186,-56.0112809863293,
40.1033475319609));
#174264=CARTESIAN_POINT('Ctrl Pts',(-18.3837652771157,-56.0103643682071,
40.1130129263075));
#174265=CARTESIAN_POINT('Ctrl Pts',(-18.3713329374386,-56.0096769046155,
40.1202619720674));
#174266=CARTESIAN_POINT('Ctrl Pts',(-18.3584682855075,-56.0095822888228,
40.1268200947266));
#174267=CARTESIAN_POINT('Ctrl Pts',(-18.3452992211262,-56.0101084356843,
40.1325796782703));
#174268=CARTESIAN_POINT('Ctrl Pts',(-18.3403608219831,-56.0103057407574,
40.1347395220992));
#174269=CARTESIAN_POINT('Ctrl Pts',(-18.3353796149,-56.0105903407606,40.1367870714852));
#174270=CARTESIAN_POINT('Ctrl Pts',(-18.3303623448495,-56.0109637085385,
40.1387166518767));
#174271=CARTESIAN_POINT('Ctrl Pts',(-18.3128018996725,-56.0122704957613,
40.1454701832469));
#174272=CARTESIAN_POINT('Ctrl Pts',(-18.2947996815818,-56.0146646833928,
40.1507785912492));
#174273=CARTESIAN_POINT('Ctrl Pts',(-18.2766448957073,-56.0182094638726,
40.1543986087265));
#174274=CARTESIAN_POINT('Ctrl Pts',(-18.2675675027701,-56.0199818541126,
40.1562086174652));
#174275=CARTESIAN_POINT('Ctrl Pts',(-18.2584519681994,-56.0220418935342,
40.1575965292115));
#174276=CARTESIAN_POINT('Ctrl Pts',(-18.2493344439487,-56.0243974853213,
40.1585319382567));
#174277=CARTESIAN_POINT('Ctrl Pts',(-18.2447756818233,-56.0255752812148,
40.1589996427793));
#174278=CARTESIAN_POINT('Ctrl Pts',(-18.2402164222855,-56.026826965224,
40.159354221642));
#174279=CARTESIAN_POINT('Ctrl Pts',(-18.2356611844174,-56.0281535255244,
40.159591874311));
#174280=CARTESIAN_POINT('Ctrl Pts',(-18.2311059465494,-56.0294800858249,
40.1598295269801));
#174281=CARTESIAN_POINT('Ctrl Pts',(-18.2265547308768,-56.0308815240328,
40.1599502506895));
#174282=CARTESIAN_POINT('Ctrl Pts',(-18.2220120550219,-56.032358823839,
40.1599502534424));
#174283=CARTESIAN_POINT('',(-18.1930767435952,-56.0417604764382,40.1599502534424));
#174284=CARTESIAN_POINT('Origin',(3.81437458815951E-16,-6.47994644506575E-17,
40.1599502534424));
#174285=CARTESIAN_POINT('',(-17.9642361803975,-56.3138168485094,39.8576902534424));
#174286=CARTESIAN_POINT('Ctrl Pts',(-18.1930767435952,-56.0417604764382,
40.1599502534424));
#174287=CARTESIAN_POINT('Ctrl Pts',(-18.1894530991653,-56.0429368412708,
40.1599502448875));
#174288=CARTESIAN_POINT('Ctrl Pts',(-18.1858538720526,-56.0441547055336,
40.1598743450437));
#174289=CARTESIAN_POINT('Ctrl Pts',(-18.1822805617811,-56.0454124342019,
40.1597243308499));
#174290=CARTESIAN_POINT('Ctrl Pts',(-18.1611840081625,-56.0528379691462,
40.1588386583938));
#174291=CARTESIAN_POINT('Ctrl Pts',(-18.1409877741429,-56.0616522804241,
40.1553722553617));
#174292=CARTESIAN_POINT('Ctrl Pts',(-18.122007001292,-56.0715172876635,
40.1496902177785));
#174293=CARTESIAN_POINT('Ctrl Pts',(-18.1149164163972,-56.0752025259765,
40.1475675976842));
#174294=CARTESIAN_POINT('Ctrl Pts',(-18.1079950493283,-56.0790342841916,
40.1451361443095));
#174295=CARTESIAN_POINT('Ctrl Pts',(-18.1012578800032,-56.082994716577,
40.1424159447502));
#174296=CARTESIAN_POINT('Ctrl Pts',(-18.0960012025252,-56.0860848445995,
40.1402935085949));
#174297=CARTESIAN_POINT('Ctrl Pts',(-18.0908571636321,-56.0892533893665,
40.1379949176048));
#174298=CARTESIAN_POINT('Ctrl Pts',(-18.0858333812,-56.0924919457981,40.1355293609261));
#174299=CARTESIAN_POINT('Ctrl Pts',(-18.0682501426879,-56.1038268933089,
40.1268999125509));
#174300=CARTESIAN_POINT('Ctrl Pts',(-18.0521400431274,-56.116019475181,
40.1162251288835));
#174301=CARTESIAN_POINT('Ctrl Pts',(-18.0378297267253,-56.1287094108802,
40.1038990521418));
#174302=CARTESIAN_POINT('Ctrl Pts',(-18.0306745685242,-56.1350543787299,
40.097736013771));
#174303=CARTESIAN_POINT('Ctrl Pts',(-18.0239693566573,-56.1415236867628,
40.0911601532641));
#174304=CARTESIAN_POINT('Ctrl Pts',(-18.0177549231924,-56.1480723047925,
40.0842207290641));
#174305=CARTESIAN_POINT('Ctrl Pts',(-18.0115670407226,-56.1545929440328,
40.0773109533619));
#174306=CARTESIAN_POINT('Ctrl Pts',(-18.0058655198732,-56.1611921195216,
40.0700409753048));
#174307=CARTESIAN_POINT('Ctrl Pts',(-18.0006913688997,-56.16782566889,40.0624586415899));
#174308=CARTESIAN_POINT('Ctrl Pts',(-18.0006691676285,-56.1678541321547,
40.0624261072769));
#174309=CARTESIAN_POINT('Ctrl Pts',(-18.0006469755623,-56.1678825958473,
40.0623935677888));
#174310=CARTESIAN_POINT('Ctrl Pts',(-18.000624792701,-56.167911059966,40.0623610231288));
#174311=CARTESIAN_POINT('Ctrl Pts',(-17.9901637816642,-56.1813341912006,
40.047013587025));
#174312=CARTESIAN_POINT('Ctrl Pts',(-17.9817405717279,-56.1948159540701,
40.0305755292129));
#174313=CARTESIAN_POINT('Ctrl Pts',(-17.9752392943607,-56.2082001169709,
40.0133447567395));
#174314=CARTESIAN_POINT('Ctrl Pts',(-17.9685015133149,-56.222071169383,
39.9954871626674));
#174315=CARTESIAN_POINT('Ctrl Pts',(-17.963828030726,-56.2358382617167,
39.9767767954415));
#174316=CARTESIAN_POINT('Ctrl Pts',(-17.9611420662374,-56.2493274239651,
39.9575197577599));
#174317=CARTESIAN_POINT('Ctrl Pts',(-17.9584944364888,-56.2626240656018,
39.9385375612143));
#174318=CARTESIAN_POINT('Ctrl Pts',(-17.9577783571054,-56.2756515067207,
39.9190226977264));
#174319=CARTESIAN_POINT('Ctrl Pts',(-17.9589668048467,-56.2882301201392,
39.8992655452047));
#174320=CARTESIAN_POINT('Ctrl Pts',(-17.959795411757,-56.2970001532144,
39.8854905069454));
#174321=CARTESIAN_POINT('Ctrl Pts',(-17.9615507925633,-56.3055517542492,
39.8715976051539));
#174322=CARTESIAN_POINT('Ctrl Pts',(-17.9642361803975,-56.3138168485094,
39.8576902534424));
#174323=CARTESIAN_POINT('',(-18.0743352474894,-56.6526781108323,39.2875012672119));
#174324=CARTESIAN_POINT('',(-17.9642361803975,-56.3138168485094,39.8576902534424));
#174325=CARTESIAN_POINT('',(-12.6735055745743,-58.0998260601479,39.2875012672119));
#174326=CARTESIAN_POINT('Origin',(5.53234440788222E-15,0.,39.2875012672119));
#174327=CARTESIAN_POINT('',(-12.5994235324474,-57.751314065072,39.8576902534424));
#174328=CARTESIAN_POINT('',(-12.6735055745743,-58.0998260601479,39.2875012672119));
#174329=CARTESIAN_POINT('',(-12.2652136052663,-57.6301266171957,40.1599502534424));
#174330=CARTESIAN_POINT('Ctrl Pts',(-12.5994235324474,-57.751314065072,
39.8576902534424));
#174331=CARTESIAN_POINT('Ctrl Pts',(-12.5968806409107,-57.7393513895537,
39.8772619994062));
#174332=CARTESIAN_POINT('Ctrl Pts',(-12.5924689870913,-57.7278420192582,
39.8967644650387));
#174333=CARTESIAN_POINT('Ctrl Pts',(-12.5862964562724,-57.716932626445,
39.9159282836073));
#174334=CARTESIAN_POINT('Ctrl Pts',(-12.5800124270059,-57.7058261701582,
39.9354382707225));
#174335=CARTESIAN_POINT('Ctrl Pts',(-12.5719031706688,-57.6953406496962,
39.9545987622405));
#174336=CARTESIAN_POINT('Ctrl Pts',(-12.5620293850071,-57.6856340700621,
39.9731387498292));
#174337=CARTESIAN_POINT('Ctrl Pts',(-12.5525736298301,-57.676338441843,
39.990893802413));
#174338=CARTESIAN_POINT('Ctrl Pts',(-12.5414990556053,-57.6677565154992,
40.0080810366269));
#174339=CARTESIAN_POINT('Ctrl Pts',(-12.5288165945578,-57.660041493595,
40.0244542742637));
#174340=CARTESIAN_POINT('Ctrl Pts',(-12.5187293820967,-57.6539052188769,
40.0374770090547));
#174341=CARTESIAN_POINT('Ctrl Pts',(-12.507624177416,-57.6483174894745,
40.0499848770067));
#174342=CARTESIAN_POINT('Ctrl Pts',(-12.495488991745,-57.643366551794,40.0618424270193));
#174343=CARTESIAN_POINT('Ctrl Pts',(-12.49545586663,-57.6433530373423,40.0618747942791));
#174344=CARTESIAN_POINT('Ctrl Pts',(-12.4954227339057,-57.643339527801,
40.0619071564124));
#174345=CARTESIAN_POINT('Ctrl Pts',(-12.4953895935729,-57.6433260231716,
40.0619395134161));
#174346=CARTESIAN_POINT('Ctrl Pts',(-12.4887924048451,-57.6406376799625,
40.0683807661799));
#174347=CARTESIAN_POINT('Ctrl Pts',(-12.4818600305505,-57.6381581392099,
40.0746073439084));
#174348=CARTESIAN_POINT('Ctrl Pts',(-12.4746311465908,-57.635899449924,
40.0805869293669));
#174349=CARTESIAN_POINT('Ctrl Pts',(-12.4602849257588,-57.6314169246176,
40.092453830807));
#174350=CARTESIAN_POINT('Ctrl Pts',(-12.4447696056082,-57.6278047731677,
40.1033475319609));
#174351=CARTESIAN_POINT('Ctrl Pts',(-12.4283797729326,-57.6251604652271,
40.1130129263075));
#174352=CARTESIAN_POINT('Ctrl Pts',(-12.4160873984258,-57.6231772342717,
40.1202619720674));
#174353=CARTESIAN_POINT('Ctrl Pts',(-12.4033031104474,-57.6217384144974,
40.1268200947266));
#174354=CARTESIAN_POINT('Ctrl Pts',(-12.3901511902558,-57.6208851370089,
40.1325796782703));
#174355=CARTESIAN_POINT('Ctrl Pts',(-12.3852192201839,-57.6205651579507,
40.1347395220992));
#174356=CARTESIAN_POINT('Ctrl Pts',(-12.3802355518734,-57.6203275209637,
40.1367870714852));
#174357=CARTESIAN_POINT('Ctrl Pts',(-12.3752067393931,-57.6201743958657,
40.1387166518767));
#174358=CARTESIAN_POINT('Ctrl Pts',(-12.3576058957119,-57.6196384580227,
40.1454701832469));
#174359=CARTESIAN_POINT('Ctrl Pts',(-12.3394520349016,-57.6201377858514,
40.1507785912492));
#174360=CARTESIAN_POINT('Ctrl Pts',(-12.3210261723876,-57.6217654557844,
40.1543986087265));
#174361=CARTESIAN_POINT('Ctrl Pts',(-12.3118132411305,-57.622579290751,
40.1562086174652));
#174362=CARTESIAN_POINT('Ctrl Pts',(-12.302532309657,-57.6236752122406,
40.1575965292115));
#174363=CARTESIAN_POINT('Ctrl Pts',(-12.2932185057685,-57.6250648590507,
40.1585319382567));
#174364=CARTESIAN_POINT('Ctrl Pts',(-12.2885616038243,-57.6257596824557,
40.1589996427793));
#174365=CARTESIAN_POINT('Ctrl Pts',(-12.2838964837812,-57.6265279372158,
40.159354221642));
#174366=CARTESIAN_POINT('Ctrl Pts',(-12.2792275366732,-57.6273710784659,
40.159591874311));
#174367=CARTESIAN_POINT('Ctrl Pts',(-12.2745585895652,-57.6282142197161,
40.1598295269801));
#174368=CARTESIAN_POINT('Ctrl Pts',(-12.2698858157461,-57.6291322491186,
40.1599502506895));
#174369=CARTESIAN_POINT('Ctrl Pts',(-12.2652136052663,-57.6301266171957,
40.1599502534424));
#174370=CARTESIAN_POINT('',(-12.2354540642047,-57.6364522029206,40.1599502534424));
#174371=CARTESIAN_POINT('Origin',(3.88326186679512E-16,-6.6645293518578E-17,
40.1599502534424));
#174372=CARTESIAN_POINT('',(-11.9794294790614,-57.8830978693155,39.8576902534424));
#174373=CARTESIAN_POINT('Ctrl Pts',(-12.2354540642047,-57.6364522029206,
40.1599502534424));
#174374=CARTESIAN_POINT('Ctrl Pts',(-12.2317273068699,-57.6372433495199,
40.1599502448875));
#174375=CARTESIAN_POINT('Ctrl Pts',(-12.2280204952201,-57.6380783205158,
40.1598743450437));
#174376=CARTESIAN_POINT('Ctrl Pts',(-12.2243352914712,-57.6389556465833,
40.1597243308499));
#174377=CARTESIAN_POINT('Ctrl Pts',(-12.2025781272236,-57.6441353133404,
40.1588386583938));
#174378=CARTESIAN_POINT('Ctrl Pts',(-12.181571183874,-57.6507902575932,
40.1553722553615));
#174379=CARTESIAN_POINT('Ctrl Pts',(-12.1616632156355,-57.6586171922733,
40.1496902177781));
#174380=CARTESIAN_POINT('Ctrl Pts',(-12.1542262614095,-57.6615410745223,
40.1475675976839));
#174381=CARTESIAN_POINT('Ctrl Pts',(-12.1469422825162,-57.6646283621014,
40.1451361443093));
#174382=CARTESIAN_POINT('Ctrl Pts',(-12.139828042199,-57.6678628728673,
40.1424159447501));
#174383=CARTESIAN_POINT('Ctrl Pts',(-12.1342771550167,-57.6703866004265,
40.1402935085949));
#174384=CARTESIAN_POINT('Ctrl Pts',(-12.1288300925916,-57.6730000890932,
40.1379949176048));
#174385=CARTESIAN_POINT('Ctrl Pts',(-12.1234953096383,-57.6756957761164,
40.1355293609261));
#174386=CARTESIAN_POINT('Ctrl Pts',(-12.104823569302,-57.6851306806978,
40.1268999125509));
#174387=CARTESIAN_POINT('Ctrl Pts',(-12.0875272507062,-57.6955725063805,
40.1162251288835));
#174388=CARTESIAN_POINT('Ctrl Pts',(-12.071968868237,-57.7066970899019,
40.1038990521418));
#174389=CARTESIAN_POINT('Ctrl Pts',(-12.0641896770024,-57.7122593816626,
40.097736013771));
#174390=CARTESIAN_POINT('Ctrl Pts',(-12.0568449701605,-57.7179923646568,
40.0911601532641));
#174391=CARTESIAN_POINT('Ctrl Pts',(-12.0499800630333,-57.7238555234916,
40.084220729064));
#174392=CARTESIAN_POINT('Ctrl Pts',(-12.0431444860318,-57.7296936321424,
40.0773109533618));
#174393=CARTESIAN_POINT('Ctrl Pts',(-12.0367843970375,-57.7356606854448,
40.0700409753047));
#174394=CARTESIAN_POINT('Ctrl Pts',(-12.0309451958829,-57.7417170494856,
40.0624586415899));
#174395=CARTESIAN_POINT('Ctrl Pts',(-12.0309201410113,-57.7417430361608,
40.0624261072769));
#174396=CARTESIAN_POINT('Ctrl Pts',(-12.0308950952495,-57.7417690242238,
40.0623935677888));
#174397=CARTESIAN_POINT('Ctrl Pts',(-12.0308700585976,-57.7417950136726,
40.0623610231288));
#174398=CARTESIAN_POINT('Ctrl Pts',(-12.0190632547924,-57.7540511381832,
40.0470135870234));
#174399=CARTESIAN_POINT('Ctrl Pts',(-12.0092769601257,-57.7665785813561,
40.0305755292095));
#174400=CARTESIAN_POINT('Ctrl Pts',(-12.0014122714555,-57.7792098558809,
40.0133447567342));
#174401=CARTESIAN_POINT('Ctrl Pts',(-11.9932614808863,-57.7923006313193,
39.9954871626601));
#174402=CARTESIAN_POINT('Ctrl Pts',(-11.9871745471187,-57.805503794129,
39.9767767954322));
#174403=CARTESIAN_POINT('Ctrl Pts',(-11.9830932952244,-57.8186383015961,
39.9575197577485));
#174404=CARTESIAN_POINT('Ctrl Pts',(-11.9790702919521,-57.8315853501706,
39.9385375612013));
#174405=CARTESIAN_POINT('Ctrl Pts',(-11.9769963969268,-57.8444665749274,
39.9190226977116));
#174406=CARTESIAN_POINT('Ctrl Pts',(-11.9768635110975,-57.8571005080023,
39.8992655451883));
#174407=CARTESIAN_POINT('Ctrl Pts',(-11.9767708607331,-57.8659091109221,
39.8854905069344));
#174408=CARTESIAN_POINT('Ctrl Pts',(-11.9776227396652,-57.8745973526463,
39.8715976051484));
#174409=CARTESIAN_POINT('Ctrl Pts',(-11.9794294790615,-57.8830978693155,
39.8576902534424));
#174410=CARTESIAN_POINT('',(-12.0535047649324,-58.2316113004781,39.2875012672119));
#174411=CARTESIAN_POINT('',(-11.9794294790614,-57.8830978693155,39.8576902534424));
#174412=CARTESIAN_POINT('',(-6.53099325080075,-59.1062911958296,39.2875012672119));
#174413=CARTESIAN_POINT('Origin',(5.53234440788222E-15,0.,39.2875012672119));
#174414=CARTESIAN_POINT('',(-6.4937464611276,-58.7519447039088,39.8576902534424));
#174415=CARTESIAN_POINT('',(-6.53099325080075,-59.1062911958296,39.2875012672119));
#174416=CARTESIAN_POINT('',(-6.1740349085904,-58.5964866834551,40.1599502534424));
#174417=CARTESIAN_POINT('Ctrl Pts',(-6.4937464611276,-58.7519447039088,
39.8576902534424));
#174418=CARTESIAN_POINT('Ctrl Pts',(-6.49246793990533,-58.739781756634,
39.8772619994064));
#174419=CARTESIAN_POINT('Ctrl Pts',(-6.48928351037725,-58.7278742924789,
39.8967644650391));
#174420=CARTESIAN_POINT('Ctrl Pts',(-6.48428513539387,-58.7163794572999,
39.915928283608));
#174421=CARTESIAN_POINT('Ctrl Pts',(-6.47919647150502,-58.7046769834202,
39.9354382707233));
#174422=CARTESIAN_POINT('Ctrl Pts',(-6.47222767386294,-58.6934012556331,
39.9545987622416));
#174423=CARTESIAN_POINT('Ctrl Pts',(-6.46342259168479,-58.682715758016,
39.9731387498305));
#174424=CARTESIAN_POINT('Ctrl Pts',(-6.45499029385669,-58.6724826566631,
39.9908938024145));
#174425=CARTESIAN_POINT('Ctrl Pts',(-6.44487344288068,-58.6627901347846,
40.0080810366285));
#174426=CARTESIAN_POINT('Ctrl Pts',(-6.43306689706524,-58.6537916984138,
40.0244542742654));
#174427=CARTESIAN_POINT('Ctrl Pts',(-6.42367635877621,-58.6466346380338,
40.0374770090558));
#174428=CARTESIAN_POINT('Ctrl Pts',(-6.41321606633668,-58.6399167088185,
40.0499848770073));
#174429=CARTESIAN_POINT('Ctrl Pts',(-6.40166487239057,-58.6337244205833,
40.0618424270192));
#174430=CARTESIAN_POINT('Ctrl Pts',(-6.40163334138329,-58.6337075176478,
40.0618747942791));
#174431=CARTESIAN_POINT('Ctrl Pts',(-6.40160180229505,-58.6336906188004,
40.0619071564124));
#174432=CARTESIAN_POINT('Ctrl Pts',(-6.40157025512661,-58.6336737240427,
40.0619395134161));
#174433=CARTESIAN_POINT('Ctrl Pts',(-6.3952902148734,-58.6303105138594,
40.0683807661799));
#174434=CARTESIAN_POINT('Ctrl Pts',(-6.38865499943491,-58.6271199258587,
40.0746073439084));
#174435=CARTESIAN_POINT('Ctrl Pts',(-6.38170181337804,-58.6241179857776,
40.0805869293668));
#174436=CARTESIAN_POINT('Ctrl Pts',(-6.36790273412669,-58.6181604277965,
40.092453830807));
#174437=CARTESIAN_POINT('Ctrl Pts',(-6.35284998116341,-58.6129462715178,
40.1033475319609));
#174438=CARTESIAN_POINT('Ctrl Pts',(-6.33682633915145,-58.60860324535,40.1130129263075));
#174439=CARTESIAN_POINT('Ctrl Pts',(-6.32480860764249,-58.6053459757241,
40.1202619720674));
#174440=CARTESIAN_POINT('Ctrl Pts',(-6.31224475095125,-58.6025787159788,
40.1268200947266));
#174441=CARTESIAN_POINT('Ctrl Pts',(-6.2992540701391,-58.600355362827,40.1325796782703));
#174442=CARTESIAN_POINT('Ctrl Pts',(-6.29438256483455,-58.5995216053951,
40.1347395220992));
#174443=CARTESIAN_POINT('Ctrl Pts',(-6.28945103740957,-58.5987643350184,
40.1367870714852));
#174444=CARTESIAN_POINT('Ctrl Pts',(-6.28446577922136,-58.598086394715,
40.1387166518767));
#174445=CARTESIAN_POINT('Ctrl Pts',(-6.26701737556263,-58.5957136036534,
40.1454701832469));
#174446=CARTESIAN_POINT('Ctrl Pts',(-6.24891076953076,-58.5943126009392,
40.1507785912492));
#174447=CARTESIAN_POINT('Ctrl Pts',(-6.23041570798265,-58.5940053272331,
40.1543986087265));
#174448=CARTESIAN_POINT('Ctrl Pts',(-6.2211681772086,-58.59385169038,40.1562086174652));
#174449=CARTESIAN_POINT('Ctrl Pts',(-6.21182353265963,-58.5939714867925,
40.1575965292115));
#174450=CARTESIAN_POINT('Ctrl Pts',(-6.20241549311782,-58.5943799633642,
40.1585319382567));
#174451=CARTESIAN_POINT('Ctrl Pts',(-6.19771147334692,-58.5945842016501,
40.1589996427793));
#174452=CARTESIAN_POINT('Ctrl Pts',(-6.19299160483011,-58.5948606100012,
40.159354221642));
#174453=CARTESIAN_POINT('Ctrl Pts',(-6.18826010244368,-58.5952110945691,
40.159591874311));
#174454=CARTESIAN_POINT('Ctrl Pts',(-6.18352860005725,-58.595561579137,
40.1598295269801));
#174455=CARTESIAN_POINT('Ctrl Pts',(-6.17878546397932,-58.5959861416118,
40.1599502506895));
#174456=CARTESIAN_POINT('Ctrl Pts',(-6.1740349085904,-58.5964866834551,
40.1599502534424));
#174457=CARTESIAN_POINT('',(-6.14377718965342,-58.5996668978648,40.1599502534424));
#174458=CARTESIAN_POINT('Origin',(3.95370119046986E-16,-6.77609428042844E-17,
40.1599502534424));
#174459=CARTESIAN_POINT('',(-5.86337364149601,-58.8181995570485,39.8576902534424));
#174460=CARTESIAN_POINT('Ctrl Pts',(-6.14377718965342,-58.5996668978648,
40.1599502534424));
#174461=CARTESIAN_POINT('Ctrl Pts',(-6.13998815054705,-58.600064158263,
40.1599502448875));
#174462=CARTESIAN_POINT('Ctrl Pts',(-6.13621436696423,-58.6005070878751,
40.1598743450437));
#174463=CARTESIAN_POINT('Ctrl Pts',(-6.13245764560146,-58.6009943991739,
40.1597243308499));
#174464=CARTESIAN_POINT('Ctrl Pts',(-6.11027824676966,-58.6038714482307,
40.1588386583938));
#174465=CARTESIAN_POINT('Ctrl Pts',(-6.08869075055779,-58.6082941124963,
40.1553722553615));
#174466=CARTESIAN_POINT('Ctrl Pts',(-6.06807370279808,-58.6139972210825,
40.1496902177781));
#174467=CARTESIAN_POINT('Ctrl Pts',(-6.06037186006718,-58.616127712602,
40.1475675976838));
#174468=CARTESIAN_POINT('Ctrl Pts',(-6.05280507414612,-58.6184367045765,
40.1451361443093));
#174469=CARTESIAN_POINT('Ctrl Pts',(-6.04539170794196,-58.6209098557463,
40.1424159447501));
#174470=CARTESIAN_POINT('Ctrl Pts',(-6.03960742773698,-58.6228395323549,
40.1402935085949));
#174471=CARTESIAN_POINT('Ctrl Pts',(-6.03391702093568,-58.6248693309927,
40.1379949176048));
#174472=CARTESIAN_POINT('Ctrl Pts',(-6.02832968645966,-58.6269926140964,
40.1355293609261));
#174473=CARTESIAN_POINT('Ctrl Pts',(-6.00877401579359,-58.6344241049594,
40.1268999125508));
#174474=CARTESIAN_POINT('Ctrl Pts',(-5.99048098024847,-58.6430007716254,
40.1162251288835));
#174475=CARTESIAN_POINT('Ctrl Pts',(-5.97384499260642,-58.6524381197038,
40.1038990521418));
#174476=CARTESIAN_POINT('Ctrl Pts',(-5.96552699878539,-58.657156793743,
40.0977360137709));
#174477=CARTESIAN_POINT('Ctrl Pts',(-5.95762326711375,-58.6620906399372,
40.0911601532641));
#174478=CARTESIAN_POINT('Ctrl Pts',(-5.95018309968312,-58.667204101582,
40.084220729064));
#174479=CARTESIAN_POINT('Ctrl Pts',(-5.942774720162,-58.6722957161033,40.0773109533618));
#174480=CARTESIAN_POINT('Ctrl Pts',(-5.93582574548873,-58.6775652709344,
40.0700409753047));
#174481=CARTESIAN_POINT('Ctrl Pts',(-5.92938546966289,-58.682978094856,
40.0624586415899));
#174482=CARTESIAN_POINT('Ctrl Pts',(-5.92935783569725,-58.6830013202262,
40.0624261072769));
#174483=CARTESIAN_POINT('Ctrl Pts',(-5.92933021064649,-58.6830245479289,
40.0623935677888));
#174484=CARTESIAN_POINT('Ctrl Pts',(-5.92930259451082,-58.6830477779621,
40.0623610231288));
#174485=CARTESIAN_POINT('Ctrl Pts',(-5.91627935575207,-58.6940026150819,
40.047013587024));
#174486=CARTESIAN_POINT('Ctrl Pts',(-5.90523719704842,-58.7054384852672,
40.0305755292109));
#174487=CARTESIAN_POINT('Ctrl Pts',(-5.89609526425068,-58.7171784805273,
40.0133447567363));
#174488=CARTESIAN_POINT('Ctrl Pts',(-5.88662076592572,-58.729345553715,
39.995487162663));
#174489=CARTESIAN_POINT('Ctrl Pts',(-5.87918707069946,-58.741840130384,
39.976776795436));
#174490=CARTESIAN_POINT('Ctrl Pts',(-5.87375524644868,-58.7544760786557,
39.9575197577532));
#174491=CARTESIAN_POINT('Ctrl Pts',(-5.86840094651777,-58.7669316835932,
39.9385375612066));
#174492=CARTESIAN_POINT('Ctrl Pts',(-5.86499195787729,-58.7795255625926,
39.9190226977177));
#174493=CARTESIAN_POINT('Ctrl Pts',(-5.86353919440072,-58.7920763953083,
39.8992655451951));
#174494=CARTESIAN_POINT('Ctrl Pts',(-5.86252630185744,-58.8008270591809,
39.885490506939));
#174495=CARTESIAN_POINT('Ctrl Pts',(-5.86246534555152,-58.8095567514049,
39.8715976051507));
#174496=CARTESIAN_POINT('Ctrl Pts',(-5.86337364149604,-58.8181995570485,
39.8576902534424));
#174497=CARTESIAN_POINT('',(-5.90061356181277,-59.1725467709677,39.2875012672119));
#174498=CARTESIAN_POINT('',(-5.863373641496,-58.8181995570485,39.8576902534424));
#174499=CARTESIAN_POINT('',(-0.316925998273249,-59.4651754363832,39.2875012672119));
#174500=CARTESIAN_POINT('Origin',(5.53234440788222E-15,0.,39.2875012672119));
#174501=CARTESIAN_POINT('',(-0.316922544675889,-59.1088767419348,39.8576902534424));
#174502=CARTESIAN_POINT('',(-0.316925998273249,-59.4651754363832,39.2875012672119));
#174503=CARTESIAN_POINT('',(-0.0152121934561199,-58.9208513795073,40.1599502534424));
#174504=CARTESIAN_POINT('Ctrl Pts',(-0.316922544675889,-59.1088767419348,
39.8576902534424));
#174505=CARTESIAN_POINT('Ctrl Pts',(-0.316922401514067,-59.0966467826991,
39.8772619994066));
#174506=CARTESIAN_POINT('Ctrl Pts',(-0.31500008555365,-59.0844716853535,
39.8967644650393));
#174507=CARTESIAN_POINT('Ctrl Pts',(-0.311230629648154,-59.0725173476285,
39.9159282836083));
#174508=CARTESIAN_POINT('Ctrl Pts',(-0.307393083603557,-59.0603470709087,
39.9354382707237));
#174509=CARTESIAN_POINT('Ctrl Pts',(-0.30164109626188,-59.0484046750299,
39.954598762242));
#174510=CARTESIAN_POINT('Ctrl Pts',(-0.294001187890306,-59.0368573319776,
39.973138749831));
#174511=CARTESIAN_POINT('Ctrl Pts',(-0.286684733430826,-59.0257988734909,
39.990893802415));
#174512=CARTESIAN_POINT('Ctrl Pts',(-0.2776364480401,-59.0151019493757,
40.0080810366291));
#174513=CARTESIAN_POINT('Ctrl Pts',(-0.266835172443557,-59.0049186872903,
40.024454274266));
#174514=CARTESIAN_POINT('Ctrl Pts',(-0.258244193028963,-58.9968192554994,
40.0374770090562));
#174515=CARTESIAN_POINT('Ctrl Pts',(-0.248543417983242,-58.9890447295094,
40.0499848770074));
#174516=CARTESIAN_POINT('Ctrl Pts',(-0.237702773059699,-58.981678934725,
40.0618424270193));
#174517=CARTESIAN_POINT('Ctrl Pts',(-0.23767318162044,-58.9816588284979,
40.0618747942791));
#174518=CARTESIAN_POINT('Ctrl Pts',(-0.23764358171718,-58.9816387254916,
40.0619071564124));
#174519=CARTESIAN_POINT('Ctrl Pts',(-0.237613973350494,-58.9816186257082,
40.0619395134161));
#174520=CARTESIAN_POINT('Ctrl Pts',(-0.231719887006989,-58.9776173965852,
40.0683807661799));
#174521=CARTESIAN_POINT('Ctrl Pts',(-0.225454527233562,-58.9737507180862,
40.0746073439084));
#174522=CARTESIAN_POINT('Ctrl Pts',(-0.218853219640932,-58.9700384170936,
40.0805869293669));
#174523=CARTESIAN_POINT('Ctrl Pts',(-0.205752467570129,-58.9626710986899,
40.092453830807));
#174524=CARTESIAN_POINT('Ctrl Pts',(-0.191327202905632,-58.9559120649696,
40.1033475319609));
#174525=CARTESIAN_POINT('Ctrl Pts',(-0.17584530993245,-58.9499179036781,
40.1130129263075));
#174526=CARTESIAN_POINT('Ctrl Pts',(-0.164233890202564,-58.9454222827095,
40.1202619720674));
#174527=CARTESIAN_POINT('Ctrl Pts',(-0.152028117041501,-58.9413569016699,
40.1268200947266));
#174528=CARTESIAN_POINT('Ctrl Pts',(-0.139341004226341,-58.9377878323772,
40.1325796782703));
#174529=CARTESIAN_POINT('Ctrl Pts',(-0.134583336920656,-58.9364494313924,
40.1347395220992));
#174530=CARTESIAN_POINT('Ctrl Pts',(-0.129757981227665,-58.9351808244388,
40.1367870714852));
#174531=CARTESIAN_POINT('Ctrl Pts',(-0.124870896863519,-58.933985496586,
40.1387166518767));
#174532=CARTESIAN_POINT('Ctrl Pts',(-0.10776610158901,-58.9298018491012,
40.1454701832469));
#174533=CARTESIAN_POINT('Ctrl Pts',(-0.089905130100263,-58.9265158655229,
40.1507785912492));
#174534=CARTESIAN_POINT('Ctrl Pts',(-0.0715435052827867,-58.9242770147326,
40.1543986087265));
#174535=CARTESIAN_POINT('Ctrl Pts',(-0.0623626928740485,-58.9231575893375,
40.1562086174652));
#174536=CARTESIAN_POINT('Ctrl Pts',(-0.0530567171307724,-58.9222999481582,
40.1575965292115));
#174537=CARTESIAN_POINT('Ctrl Pts',(-0.0436575183856271,-58.9217227791368,
40.1585319382567));
#174538=CARTESIAN_POINT('Ctrl Pts',(-0.0389579190130544,-58.9214341946262,
40.1589996427793));
#174539=CARTESIAN_POINT('Ctrl Pts',(-0.0342350138896586,-58.9212157281805,
40.159354221642));
#174540=CARTESIAN_POINT('Ctrl Pts',(-0.0294927955550829,-58.9210697160839,
40.159591874311));
#174541=CARTESIAN_POINT('Ctrl Pts',(-0.0247505772205073,-58.9209237039872,
40.1598295269801));
#174542=CARTESIAN_POINT('Ctrl Pts',(-0.0199890456752399,-58.9208501479391,
40.1599502506895));
#174543=CARTESIAN_POINT('Ctrl Pts',(-0.0152121934561203,-58.9208513795073,
40.1599502534424));
#174544=CARTESIAN_POINT('',(0.0152121934557198,-58.9208513795073,40.1599502534424));
#174545=CARTESIAN_POINT('Origin',(4.02492081121313E-16,-6.81341890207372E-17,
40.1599502534424));
#174546=CARTESIAN_POINT('',(0.316922544675488,-59.1088767419348,39.8576902534424));
#174547=CARTESIAN_POINT('Ctrl Pts',(0.0152121934557198,-58.9208513795073,
40.1599502534424));
#174548=CARTESIAN_POINT('Ctrl Pts',(0.0190220008283426,-58.9208504012364,
40.1599502448875));
#174549=CARTESIAN_POINT('Ctrl Pts',(0.0228214099815219,-58.9208964366351,
40.1598743450437));
#174550=CARTESIAN_POINT('Ctrl Pts',(0.0266084895328039,-58.9209883940807,
40.1597243308499));
#174551=CARTESIAN_POINT('Ctrl Pts',(0.0489671208138393,-58.9215313038857,
40.1588386583938));
#174552=CARTESIAN_POINT('Ctrl Pts',(0.0708986527619951,-58.9236732325288,
40.1553722553614));
#174553=CARTESIAN_POINT('Ctrl Pts',(0.0919988953533014,-58.9271900305701,
40.149690217778));
#174554=CARTESIAN_POINT('Ctrl Pts',(0.0998812435883289,-58.9285037892491,
40.1475675976838));
#174555=CARTESIAN_POINT('Ctrl Pts',(0.107647933247126,-58.9300091878198,
40.1451361443093));
#174556=CARTESIAN_POINT('Ctrl Pts',(0.115279202946685,-58.9316938830317,
40.1424159447501));
#174557=CARTESIAN_POINT('Ctrl Pts',(0.12123350238999,-58.933008366749,40.1402935085949));
#174558=CARTESIAN_POINT('Ctrl Pts',(0.127104908279783,-58.9344322364591,
40.1379949176048));
#174559=CARTESIAN_POINT('Ctrl Pts',(0.132883578272846,-58.9359598525093,
40.1355293609261));
#174560=CARTESIAN_POINT('Ctrl Pts',(0.153108923248566,-58.9413065086849,
40.1268999125509));
#174561=CARTESIAN_POINT('Ctrl Pts',(0.172198253417505,-58.9479240485795,
40.1162251288835));
#174562=CARTESIAN_POINT('Ctrl Pts',(0.189729578870567,-58.9555707636545,
40.1038990521418));
#174563=CARTESIAN_POINT('Ctrl Pts',(0.198495241597098,-58.959394121192,
40.097736013771));
#174564=CARTESIAN_POINT('Ctrl Pts',(0.206871403160346,-58.9634747743348,
40.0911601532641));
#174565=CARTESIAN_POINT('Ctrl Pts',(0.214805314863011,-58.9677825146336,
40.0842207290641));
#174566=CARTESIAN_POINT('Ctrl Pts',(0.222705329147431,-58.9720718502312,
40.0773109533619));
#174567=CARTESIAN_POINT('Ctrl Pts',(0.230167055078978,-58.9765861722458,
40.0700409753048));
#174568=CARTESIAN_POINT('Ctrl Pts',(0.237137844566452,-58.9812961520165,
40.0624586415899));
#174569=CARTESIAN_POINT('Ctrl Pts',(0.237167754862592,-58.9813163616197,
40.0624261072769));
#174570=CARTESIAN_POINT('Ctrl Pts',(0.237197656536499,-58.9813365744745,
40.0623935677888));
#174571=CARTESIAN_POINT('Ctrl Pts',(0.237227549587748,-58.9813567905789,
40.0623610231288));
#174572=CARTESIAN_POINT('Ctrl Pts',(0.251324537972111,-58.990890316821,
40.0470135870233));
#174573=CARTESIAN_POINT('Ctrl Pts',(0.263501580512134,-59.0011093202329,
40.0305755292092));
#174574=CARTESIAN_POINT('Ctrl Pts',(0.273820596509111,-59.0118294103846,
40.0133447567338));
#174575=CARTESIAN_POINT('Ctrl Pts',(0.284514998004039,-59.0229394763227,
39.9954871626595));
#174576=CARTESIAN_POINT('Ctrl Pts',(0.29321400956858,-59.0345885736557,
39.9767767954314));
#174577=CARTESIAN_POINT('Ctrl Pts',(0.299936893972488,-59.0465875206396,
39.9575197577476));
#174578=CARTESIAN_POINT('Ctrl Pts',(0.306563827731274,-59.058415215727,
39.9385375612));
#174579=CARTESIAN_POINT('Ctrl Pts',(0.311270560393424,-59.0705837677963,
39.9190226977101));
#174580=CARTESIAN_POINT('Ctrl Pts',(0.314027284735721,-59.082913990604,
39.8992655451865));
#174581=CARTESIAN_POINT('Ctrl Pts',(0.315949321994053,-59.0915108413215,
39.8854905069332));
#174582=CARTESIAN_POINT('Ctrl Pts',(0.316922445687527,-59.1001863397074,
39.8715976051478));
#174583=CARTESIAN_POINT('Ctrl Pts',(0.316922544675488,-59.1088767419348,
39.8576902534424));
#174584=CARTESIAN_POINT('',(0.316925998272844,-59.4651754363832,39.2875012672119));
#174585=CARTESIAN_POINT('',(0.316922544675488,-59.1088767419348,39.8576902534424));
#174586=CARTESIAN_POINT('',(5.90061356181238,-59.1725467709678,39.2875012672119));
#174587=CARTESIAN_POINT('Origin',(5.53234440788222E-15,0.,39.2875012672119));
#174588=CARTESIAN_POINT('',(5.86337364149561,-58.8181995570485,39.8576902534424));
#174589=CARTESIAN_POINT('',(5.90061356181238,-59.1725467709677,39.2875012672119));
#174590=CARTESIAN_POINT('',(6.14377718965303,-58.5996668978649,40.1599502534424));
#174591=CARTESIAN_POINT('Ctrl Pts',(5.86337364149561,-58.8181995570485,
39.8576902534424));
#174592=CARTESIAN_POINT('Ctrl Pts',(5.86209540502861,-58.8060365798462,
39.8772619994041));
#174593=CARTESIAN_POINT('Ctrl Pts',(5.8627345461251,-58.7937272422261,39.8967644650344));
#174594=CARTESIAN_POINT('Ctrl Pts',(5.86523378400419,-58.7814443761823,
39.915928283601));
#174595=CARTESIAN_POINT('Ctrl Pts',(5.86777816724618,-58.7689396367226,
39.935438270714));
#174596=CARTESIAN_POINT('Ctrl Pts',(5.87225032430913,-58.756461416142,39.9545987622301));
#174597=CARTESIAN_POINT('Ctrl Pts',(5.8786413544374,-58.7441787427631,39.973138749817));
#174598=CARTESIAN_POINT('Ctrl Pts',(5.88476180492035,-58.7324160859292,
39.9908938023989));
#174599=CARTESIAN_POINT('Ctrl Pts',(5.8926423898153,-58.7208319573178,40.0080810366112));
#174600=CARTESIAN_POINT('Ctrl Pts',(5.90232005415442,-58.7095754394694,
40.0244542742466));
#174601=CARTESIAN_POINT('Ctrl Pts',(5.91001735012912,-58.7006223753325,
40.0374770090438));
#174602=CARTESIAN_POINT('Ctrl Pts',(5.91885232406354,-58.6918764318968,
40.0499848770016));
#174603=CARTESIAN_POINT('Ctrl Pts',(5.92886364759533,-58.683417831748,40.0618424270192));
#174604=CARTESIAN_POINT('Ctrl Pts',(5.92889097525656,-58.6833947425173,
40.0618747942791));
#174605=CARTESIAN_POINT('Ctrl Pts',(5.92891831167211,-58.683371655605,40.0619071564124));
#174606=CARTESIAN_POINT('Ctrl Pts',(5.92894565684159,-58.6833485710132,
40.0619395134162));
#174607=CARTESIAN_POINT('Ctrl Pts',(5.93438921243199,-58.6787531612542,
40.0683807661799));
#174608=CARTESIAN_POINT('Ctrl Pts',(5.94021607194758,-58.6742527563956,
40.0746073439084));
#174609=CARTESIAN_POINT('Ctrl Pts',(5.94639317576857,-58.6698707672381,
40.0805869293669));
#174610=CARTESIAN_POINT('Ctrl Pts',(5.95865206607762,-58.6611744062938,
40.092453830807));
#174611=CARTESIAN_POINT('Ctrl Pts',(5.97229179622499,-58.6529445485198,
40.1033475319609));
#174612=CARTESIAN_POINT('Ctrl Pts',(5.98706231730019,-58.6453649253901,
40.1130129263075));
#174613=CARTESIAN_POINT('Ctrl Pts',(5.99814020810659,-58.6396802080428,
40.1202619720674));
#174614=CARTESIAN_POINT('Ctrl Pts',(6.0098541687325,-58.6343612468744,40.1268200947266));
#174615=CARTESIAN_POINT('Ctrl Pts',(6.02209871088773,-58.6294855649109,
40.1325796782703));
#174616=CARTESIAN_POINT('Ctrl Pts',(6.02669041419593,-58.6276571841746,
40.1347395220992));
#174617=CARTESIAN_POINT('Ctrl Pts',(6.0313567305502,-58.6258911397672,40.1367870714852));
#174618=CARTESIAN_POINT('Ctrl Pts',(6.0360920971713,-58.624191520627,40.1387166518767));
#174619=CARTESIAN_POINT('Ctrl Pts',(6.05266588034515,-58.6182428536363,
40.1454701832469));
#174620=CARTESIAN_POINT('Ctrl Pts',(6.07008552874949,-58.6131078911177,
40.1507785912492));
#174621=CARTESIAN_POINT('Ctrl Pts',(6.08811254303242,-58.608961992561,40.1543986087265));
#174622=CARTESIAN_POINT('Ctrl Pts',(6.09712605017388,-58.6068890432827,
40.1562086174652));
#174623=CARTESIAN_POINT('Ctrl Pts',(6.10629139889382,-58.6050633610079,
40.1575965292115));
#174624=CARTESIAN_POINT('Ctrl Pts',(6.11557877725394,-58.6035068699781,
40.1585319382567));
#174625=CARTESIAN_POINT('Ctrl Pts',(6.120222466434,-58.6027286244632,40.1589996427793));
#174626=CARTESIAN_POINT('Ctrl Pts',(6.12489666302713,-58.6020176767849,
40.159354221642));
#174627=CARTESIAN_POINT('Ctrl Pts',(6.1295976405734,-58.6013767677628,40.159591874311));
#174628=CARTESIAN_POINT('Ctrl Pts',(6.13429861811967,-58.6007358587407,
40.1598295269801));
#174629=CARTESIAN_POINT('Ctrl Pts',(6.13902637679625,-58.6001649900651,
40.1599502506895));
#174630=CARTESIAN_POINT('Ctrl Pts',(6.14377718965303,-58.5996668978649,
40.1599502534424));
#174631=CARTESIAN_POINT('',(6.17403490859001,-58.5964866834551,40.1599502534424));
#174632=CARTESIAN_POINT('Origin',(5.66232193761676E-15,5.18494695161684E-15,
40.1599502534424));
#174633=CARTESIAN_POINT('',(6.4937464611272,-58.7519447039089,39.8576902534424));
#174634=CARTESIAN_POINT('Ctrl Pts',(6.17403490859001,-58.5964866834551,
40.1599502534424));
#174635=CARTESIAN_POINT('Ctrl Pts',(6.17782374318207,-58.5960874772333,
40.1599502448875));
#174636=CARTESIAN_POINT('Ctrl Pts',(6.18160715078385,-58.5957361140451,
40.1598743450437));
#174637=CARTESIAN_POINT('Ctrl Pts',(6.18538309648758,-58.5954317101325,
40.1597243308499));
#174638=CARTESIAN_POINT('Ctrl Pts',(6.20767599437374,-58.5936345324522,
40.1588386583938));
#174639=CARTESIAN_POINT('Ctrl Pts',(6.22971127560378,-58.5934722580544,
40.1553722553617));
#174640=CARTESIAN_POINT('Ctrl Pts',(6.25106353435248,-58.5947642147752,
40.1496902177787));
#174641=CARTESIAN_POINT('Ctrl Pts',(6.25904002743583,-58.5952468467988,
40.1475675976843));
#174642=CARTESIAN_POINT('Ctrl Pts',(6.26692152735609,-58.5959321585039,
40.1451361443095));
#174643=CARTESIAN_POINT('Ctrl Pts',(6.27468709076417,-58.5968099398848,
40.1424159447501));
#174644=CARTESIAN_POINT('Ctrl Pts',(6.28074617289508,-58.5974948289521,
40.1402935085949));
#174645=CARTESIAN_POINT('Ctrl Pts',(6.28673424952176,-58.5982971695201,
40.1379949176048));
#174646=CARTESIAN_POINT('Ctrl Pts',(6.29264094271416,-58.5992123816356,
40.1355293609261));
#174647=CARTESIAN_POINT('Ctrl Pts',(6.31331436888755,-58.6024156240399,
40.1268999125509));
#174648=CARTESIAN_POINT('Ctrl Pts',(6.33299084698427,-58.6070015340112,
40.1162251288835));
#174649=CARTESIAN_POINT('Ctrl Pts',(6.35122543337801,-58.6127738370723,
40.1038990521418));
#174650=CARTESIAN_POINT('Ctrl Pts',(6.36034272657487,-58.6156599886028,
40.097736013771));
#174651=CARTESIAN_POINT('Ctrl Pts',(6.36909954705081,-58.6188427402045,
40.0911601532641));
#174652=CARTESIAN_POINT('Ctrl Pts',(6.37744027742862,-58.6222975626532,
40.084220729064));
#174653=CARTESIAN_POINT('Ctrl Pts',(6.38574537226665,-58.6257376244687,
40.0773109533618));
#174654=CARTESIAN_POINT('Ctrl Pts',(6.39363809722571,-58.6294472538099,
40.0700409753047));
#174655=CARTESIAN_POINT('Ctrl Pts',(6.40106302694645,-58.6334027859057,
40.0624586415899));
#174656=CARTESIAN_POINT('Ctrl Pts',(6.40109488586963,-58.6334197583214,
40.0624261072769));
#174657=CARTESIAN_POINT('Ctrl Pts',(6.40112673655769,-58.633436734872,40.0623935677888));
#174658=CARTESIAN_POINT('Ctrl Pts',(6.40115857901001,-58.6334537155557,
40.0623610231288));
#174659=CARTESIAN_POINT('Ctrl Pts',(6.41617486746476,-58.6414614796111,
40.0470135870231));
#174660=CARTESIAN_POINT('Ctrl Pts',(6.42935337961453,-58.6503516547094,
40.0305755292089));
#174661=CARTESIAN_POINT('Ctrl Pts',(6.4407364215119,-58.659934388201,40.0133447567333));
#174662=CARTESIAN_POINT('Ctrl Pts',(6.45253355607587,-58.6698657226818,
39.9954871626588));
#174663=CARTESIAN_POINT('Ctrl Pts',(6.46240257578758,-58.68054171073,39.9767767954305));
#174664=CARTESIAN_POINT('Ctrl Pts',(6.47034286301635,-58.6917721934516,
39.9575197577464));
#174665=CARTESIAN_POINT('Ctrl Pts',(6.47816982453009,-58.7028423919859,
39.9385375611987));
#174666=CARTESIAN_POINT('Ctrl Pts',(6.48412273326619,-58.7144522959216,
39.9190226977086));
#174667=CARTESIAN_POINT('Ctrl Pts',(6.48815321522585,-58.7264268163197,
39.8992655451849));
#174668=CARTESIAN_POINT('Ctrl Pts',(6.49096333895723,-58.7347756649882,
39.8854905069321));
#174669=CARTESIAN_POINT('Ctrl Pts',(6.49283796829152,-58.7433019189616,
39.8715976051472));
#174670=CARTESIAN_POINT('Ctrl Pts',(6.49374646112718,-58.7519447039089,
39.8576902534424));
#174671=CARTESIAN_POINT('',(6.53099325080036,-59.1062911958297,39.2875012672119));
#174672=CARTESIAN_POINT('',(6.49374646112721,-58.7519447039089,39.8576902534424));
#174673=CARTESIAN_POINT('',(12.053504764932,-58.2316113004781,39.2875012672119));
#174674=CARTESIAN_POINT('Origin',(5.53234440788222E-15,0.,39.2875012672119));
#174675=CARTESIAN_POINT('',(11.9794294790611,-57.8830978693156,39.8576902534424));
#174676=CARTESIAN_POINT('',(12.053504764932,-58.2316113004781,39.2875012672119));
#174677=CARTESIAN_POINT('',(12.2354540642043,-57.6364522029207,40.1599502534424));
#174678=CARTESIAN_POINT('Ctrl Pts',(11.9794294790611,-57.8830978693156,
39.8576902534424));
#174679=CARTESIAN_POINT('Ctrl Pts',(11.9768868675911,-57.8711351342675,
39.877261999406));
#174680=CARTESIAN_POINT('Ctrl Pts',(11.9762358312606,-57.858826420049,39.8967644650382));
#174681=CARTESIAN_POINT('Ctrl Pts',(11.9774374689414,-57.8463495993344,
39.9159282836066));
#174682=CARTESIAN_POINT('Ctrl Pts',(11.978660812587,-57.8336474016744,39.9354382707216));
#174683=CARTESIAN_POINT('Ctrl Pts',(11.9818041414849,-57.820770070385,39.9545987622394));
#174684=CARTESIAN_POINT('Ctrl Pts',(11.9868762719096,-57.8078866382167,
39.973138749828));
#174685=CARTESIAN_POINT('Ctrl Pts',(11.9917336614829,-57.7955486571629,
39.9908938024116));
#174686=CARTESIAN_POINT('Ctrl Pts',(11.9983602045489,-57.7832042421901,
40.0080810366254));
#174687=CARTESIAN_POINT('Ctrl Pts',(12.0068082271198,-57.7709977973416,
40.0244542742621));
#174688=CARTESIAN_POINT('Ctrl Pts',(12.0135275064643,-57.7612891925112,
40.0374770090537));
#174689=CARTESIAN_POINT('Ctrl Pts',(12.0213998814573,-57.7516676540242,
40.0499848770063));
#174690=CARTESIAN_POINT('Ctrl Pts',(12.0304721974328,-57.7422089227118,
40.0618424270193));
#174691=CARTESIAN_POINT('Ctrl Pts',(12.0304969619084,-57.7421831034478,
40.0618747942791));
#174692=CARTESIAN_POINT('Ctrl Pts',(12.0305217353328,-57.7421572855745,
40.0619071564124));
#174693=CARTESIAN_POINT('Ctrl Pts',(12.0305465177056,-57.742131469094,40.0619395134162));
#174694=CARTESIAN_POINT('Ctrl Pts',(12.0354799018087,-57.7369922269699,
40.0683807661799));
#174695=CARTESIAN_POINT('Ctrl Pts',(12.0408044207743,-57.7319074031292,
40.0746073439084));
#174696=CARTESIAN_POINT('Ctrl Pts',(12.0464896431815,-57.7269037357969,
40.0805869293669));
#174697=CARTESIAN_POINT('Ctrl Pts',(12.0577723607613,-57.7169736114624,
40.092453830807));
#174698=CARTESIAN_POINT('Ctrl Pts',(12.0704771166537,-57.7073630976788,
40.1033475319609));
#174699=CARTESIAN_POINT('Ctrl Pts',(12.0843744369111,-57.698281056648,40.1130129263075));
#174700=CARTESIAN_POINT('Ctrl Pts',(12.0947974271042,-57.6914695258749,
40.1202619720674));
#174701=CARTESIAN_POINT('Ctrl Pts',(12.105891234591,-57.6849552602293,40.1268200947266));
#174702=CARTESIAN_POINT('Ctrl Pts',(12.1175590523201,-57.6788263845868,
40.1325796782703));
#174703=CARTESIAN_POINT('Ctrl Pts',(12.1219344839685,-57.6765280562208,
40.1347395220992));
#174704=CARTESIAN_POINT('Ctrl Pts',(12.1263906358456,-57.6742839235119,
40.1367870714852));
#174705=CARTESIAN_POINT('Ctrl Pts',(12.130922403056,-57.6720986344673,40.1387166518767));
#174706=CARTESIAN_POINT('Ctrl Pts',(12.1467835882925,-57.6644501228111,
40.1454701832469));
#174707=CARTESIAN_POINT('Ctrl Pts',(12.1635710602992,-57.657522441076,40.1507785912492));
#174708=CARTESIAN_POINT('Ctrl Pts',(12.1810659563067,-57.6515149180852,
40.1543986087265));
#174709=CARTESIAN_POINT('Ctrl Pts',(12.1898134043104,-57.6485111565898,
40.1562086174652));
#174710=CARTESIAN_POINT('Ctrl Pts',(12.1987377085285,-57.6457374357764,
40.1575965292115));
#174711=CARTESIAN_POINT('Ctrl Pts',(12.2078115120428,-57.6432186759796,
40.1585319382567));
#174712=CARTESIAN_POINT('Ctrl Pts',(12.2123484137999,-57.6419592960811,
40.1589996427793));
#174713=CARTESIAN_POINT('Ctrl Pts',(12.2169226903867,-57.6407636564617,
40.159354221642));
#174714=CARTESIAN_POINT('Ctrl Pts',(12.221530922251,-57.6396348724475,40.159591874311));
#174715=CARTESIAN_POINT('Ctrl Pts',(12.2261391541152,-57.6385060884334,
40.1598295269801));
#174716=CARTESIAN_POINT('Ctrl Pts',(12.2307813416097,-57.6374441616869,
40.1599502506895));
#174717=CARTESIAN_POINT('Ctrl Pts',(12.2354540642043,-57.6364522029207,
40.1599502534424));
#174718=CARTESIAN_POINT('',(12.2652136052659,-57.6301266171958,40.1599502534424));
#174719=CARTESIAN_POINT('Origin',(5.66936586998423E-15,5.18606260090255E-15,
40.1599502534424));
#174720=CARTESIAN_POINT('',(12.599423532447,-57.751314065072,39.8576902534424));
#174721=CARTESIAN_POINT('Ctrl Pts',(12.2652136052659,-57.6301266171958,
40.1599502534424));
#174722=CARTESIAN_POINT('Ctrl Pts',(12.2689399558127,-57.6293335568099,
40.1599502448875));
#174723=CARTESIAN_POINT('Ctrl Pts',(12.2726659100577,-57.6285886446436,
40.1598743450437));
#174724=CARTESIAN_POINT('Ctrl Pts',(12.2763893518626,-57.6278912144856,
40.1597243308499));
#174725=CARTESIAN_POINT('Ctrl Pts',(12.2983722707009,-57.6237736395748,
40.1588386583938));
#174726=CARTESIAN_POINT('Ctrl Pts',(12.3202698780618,-57.6213089400485,
40.1553722553616));
#174727=CARTESIAN_POINT('Ctrl Pts',(12.341640213154,-57.6203619005009,40.1496902177784));
#174728=CARTESIAN_POINT('Ctrl Pts',(12.349623458957,-57.6200081180515,40.1475675976841));
#174729=CARTESIAN_POINT('Ctrl Pts',(12.357533417775,-57.6198658344726,40.1451361443094));
#174730=CARTESIAN_POINT('Ctrl Pts',(12.3653481937526,-57.6199270848658,
40.1424159447501));
#174731=CARTESIAN_POINT('Ctrl Pts',(12.3714456739993,-57.6199748754952,
40.1402935085949));
#174732=CARTESIAN_POINT('Ctrl Pts',(12.3774848147423,-57.6201468963098,
40.1379949176048));
#174733=CARTESIAN_POINT('Ctrl Pts',(12.3834548161673,-57.6204396772352,
40.1355293609261));
#174734=CARTESIAN_POINT('Ctrl Pts',(12.404349821155,-57.621464410474,40.1268999125509));
#174735=CARTESIAN_POINT('Ctrl Pts',(12.4243978675679,-57.6239684463327,
40.1162251288835));
#174736=CARTESIAN_POINT('Ctrl Pts',(12.443135932958,-57.6278030948196,40.1038990521418));
#174737=CARTESIAN_POINT('Ctrl Pts',(12.452504965653,-57.6297204190631,40.097736013771));
#174738=CARTESIAN_POINT('Ctrl Pts',(12.461546503484,-57.631970398231,40.0911601532641));
#174739=CARTESIAN_POINT('Ctrl Pts',(12.4702026697495,-57.6345344510719,
40.084220729064));
#174740=CARTESIAN_POINT('Ctrl Pts',(12.4788218527842,-57.6370875490681,
40.0773109533619));
#174741=CARTESIAN_POINT('Ctrl Pts',(12.4870591024244,-57.6399518422607,
40.0700409753048));
#174742=CARTESIAN_POINT('Ctrl Pts',(12.4948568232946,-57.6431095890442,
40.0624586415899));
#174743=CARTESIAN_POINT('Ctrl Pts',(12.4948902817918,-57.6431231383189,
40.0624261072769));
#174744=CARTESIAN_POINT('Ctrl Pts',(12.4949237325312,-57.6431366925668,
40.0623935677889));
#174745=CARTESIAN_POINT('Ctrl Pts',(12.494957175512,-57.6431502517859,40.0623610231289));
#174746=CARTESIAN_POINT('Ctrl Pts',(12.5107282424386,-57.6495445189159,
40.0470135870229));
#174747=CARTESIAN_POINT('Ctrl Pts',(12.5247638376614,-57.6570084630818,
40.0305755292084));
#174748=CARTESIAN_POINT('Ctrl Pts',(12.5370861904701,-57.66534884948,40.0133447567324));
#174749=CARTESIAN_POINT('Ctrl Pts',(12.5498568062282,-57.6739926427246,
39.9954871626576));
#174750=CARTESIAN_POINT('Ctrl Pts',(12.560787707042,-57.683578553129,39.976776795429));
#174751=CARTESIAN_POINT('Ctrl Pts',(12.5698584016472,-57.6939175280694,
39.9575197577446));
#174752=CARTESIAN_POINT('Ctrl Pts',(12.5787996370877,-57.7041089426389,
39.9385375611966));
#174753=CARTESIAN_POINT('Ctrl Pts',(12.5859335005839,-57.7150329979042,
39.9190226977063));
#174754=CARTESIAN_POINT('Ctrl Pts',(12.5911935813571,-57.7265206205413,
39.8992655451822));
#174755=CARTESIAN_POINT('Ctrl Pts',(12.5948610032577,-57.7345299954275,
39.8854905069303));
#174756=CARTESIAN_POINT('Ctrl Pts',(12.5976165994014,-57.7428135895655,
39.8715976051464));
#174757=CARTESIAN_POINT('Ctrl Pts',(12.599423532447,-57.751314065072,39.8576902534424));
#174758=CARTESIAN_POINT('',(12.6735055745739,-58.099826060148,39.2875012672119));
#174759=CARTESIAN_POINT('',(12.599423532447,-57.751314065072,39.8576902534424));
#174760=CARTESIAN_POINT('',(18.074335247489,-56.6526781108324,39.2875012672119));
#174761=CARTESIAN_POINT('Origin',(5.53234440788222E-15,0.,39.2875012672119));
#174762=CARTESIAN_POINT('',(17.9642361803971,-56.3138168485095,39.8576902534424));
#174763=CARTESIAN_POINT('',(18.074335247489,-56.6526781108324,39.2875012672119));
#174764=CARTESIAN_POINT('',(18.1930767435948,-56.0417604764384,40.1599502534424));
#174765=CARTESIAN_POINT('Ctrl Pts',(17.9642361803971,-56.3138168485095,
39.8576902534424));
#174766=CARTESIAN_POINT('Ctrl Pts',(17.9604570513081,-56.3021854218454,
39.8772619994058));
#174767=CARTESIAN_POINT('Ctrl Pts',(17.9585229704408,-56.2900121878784,
39.8967644650379));
#174768=CARTESIAN_POINT('Ctrl Pts',(17.958413842529,-56.2774781111531,39.9159282836061));
#174769=CARTESIAN_POINT('Ctrl Pts',(17.9583027433685,-56.2647176232298,
39.9354382707207));
#174770=CARTESIAN_POINT('Ctrl Pts',(17.960082805131,-56.2515822679697,39.9545987622382));
#174771=CARTESIAN_POINT('Ctrl Pts',(17.9637804645281,-56.2382392305924,
39.9731387498264));
#174772=CARTESIAN_POINT('Ctrl Pts',(17.9673215746134,-56.2254611028227,
39.9908938024093));
#174773=CARTESIAN_POINT('Ctrl Pts',(17.9726214740556,-56.2124916494839,
40.0080810366224));
#174774=CARTESIAN_POINT('Ctrl Pts',(17.9797472965523,-56.1994690140011,
40.0244542742585));
#174775=CARTESIAN_POINT('Ctrl Pts',(17.9854149414383,-56.1891112379787,
40.0374770090514));
#174776=CARTESIAN_POINT('Ctrl Pts',(17.9922384661056,-56.178719520025,40.0499848770052));
#174777=CARTESIAN_POINT('Ctrl Pts',(18.0002723763371,-56.1683642893843,
40.0618424270193));
#174778=CARTESIAN_POINT('Ctrl Pts',(18.0002943063023,-56.1683360229683,
40.0618747942791));
#174779=CARTESIAN_POINT('Ctrl Pts',(18.0003162453126,-56.1683077570001,
40.0619071564124));
#174780=CARTESIAN_POINT('Ctrl Pts',(18.000338193368,-56.1682794914816,40.0619395134161));
#174781=CARTESIAN_POINT('Ctrl Pts',(18.0047073547952,-56.1626527236046,
40.0683807661799));
#174782=CARTESIAN_POINT('Ctrl Pts',(18.0094711966667,-56.1570391911758,
40.0746073439084));
#174783=CARTESIAN_POINT('Ctrl Pts',(18.0146022491738,-56.1514686668951,
40.0805869293669));
#174784=CARTESIAN_POINT('Ctrl Pts',(18.0247851782094,-56.1404135756907,
40.092453830807));
#174785=CARTESIAN_POINT('Ctrl Pts',(18.0364157638827,-56.1295277006974,
40.1033475319609));
#174786=CARTESIAN_POINT('Ctrl Pts',(18.0492876213734,-56.1190427465076,
40.1130129263075));
#174787=CARTESIAN_POINT('Ctrl Pts',(18.0589415144913,-56.1111790308653,
40.1202619720674));
#174788=CARTESIAN_POINT('Ctrl Pts',(18.0692936227627,-56.1035408324001,
40.1268200947266));
#174789=CARTESIAN_POINT('Ctrl Pts',(18.080256881013,-56.0962259123227,40.1325796782703));
#174790=CARTESIAN_POINT('Ctrl Pts',(18.0843681028569,-56.0934828172937,
40.1347395220992));
#174791=CARTESIAN_POINT('Ctrl Pts',(18.0885652677243,-56.0907851834708,
40.1367870714852));
#174792=CARTESIAN_POINT('Ctrl Pts',(18.0928437845341,-56.0881381670059,
40.1387166518767));
#174793=CARTESIAN_POINT('Ctrl Pts',(18.1078185933686,-56.0788736093784,
40.1454701832469));
#174794=CARTESIAN_POINT('Ctrl Pts',(18.1237899619214,-56.0702291095577,
40.1507785912492));
#174795=CARTESIAN_POINT('Ctrl Pts',(18.1405610619117,-56.0624257818117,
40.1543986087265));
#174796=CARTESIAN_POINT('Ctrl Pts',(18.1489466119069,-56.0585241179387,
40.1562086174652));
#174797=CARTESIAN_POINT('Ctrl Pts',(18.1575320950786,-56.0548327480525,
40.1575965292115));
#174798=CARTESIAN_POINT('Ctrl Pts',(18.1662929092569,-56.0513793155481,
40.1585319382567));
#174799=CARTESIAN_POINT('Ctrl Pts',(18.170673316346,-56.0496525992958,40.1589996427793));
#174800=CARTESIAN_POINT('Ctrl Pts',(18.1750975561951,-56.0479853674131,
40.159354221642));
#174801=CARTESIAN_POINT('Ctrl Pts',(18.1795625536246,-56.0463810756007,
40.1595918743111));
#174802=CARTESIAN_POINT('Ctrl Pts',(18.1840275510542,-56.0447767837883,
40.1598295269801));
#174803=CARTESIAN_POINT('Ctrl Pts',(18.1885333065889,-56.0432354336628,
40.1599502506895));
#174804=CARTESIAN_POINT('Ctrl Pts',(18.1930767435948,-56.0417604764383,
40.1599502534424));
#174805=CARTESIAN_POINT('',(18.2220120550216,-56.0323588238392,40.1599502534424));
#174806=CARTESIAN_POINT('Origin',(5.6762545978478E-15,5.18790842997046E-15,
40.1599502534424));
#174807=CARTESIAN_POINT('',(18.5670586829464,-56.1179479440989,39.8576902534424));
#174808=CARTESIAN_POINT('Ctrl Pts',(18.2220120550216,-56.0323588238392,
40.1599502534424));
#174809=CARTESIAN_POINT('Ctrl Pts',(18.2256350948468,-56.0311805982248,
40.1599502448875));
#174810=CARTESIAN_POINT('Ctrl Pts',(18.2292627734005,-56.0300502984938,
40.1598743450437));
#174811=CARTESIAN_POINT('Ctrl Pts',(18.232892916499,-56.0289674832813,40.1597243308499));
#174812=CARTESIAN_POINT('Ctrl Pts',(18.2543250068277,-56.022574624153,40.1588386583939));
#174813=CARTESIAN_POINT('Ctrl Pts',(18.2758450255481,-56.0178345032623,
40.1553722553623));
#174814=CARTESIAN_POINT('Ctrl Pts',(18.296999299118,-56.0146588434098,40.1496902177801));
#174815=CARTESIAN_POINT('Ctrl Pts',(18.3049018315316,-56.0134725226015,
40.1475675976854));
#174816=CARTESIAN_POINT('Ctrl Pts',(18.3127535860859,-56.0125042026268,
40.1451361443102));
#174817=CARTESIAN_POINT('Ctrl Pts',(18.3205319543147,-56.01174825096,40.1424159447501));
#174818=CARTESIAN_POINT('Ctrl Pts',(18.3266010274077,-56.0111584195473,
40.1402935085949));
#174819=CARTESIAN_POINT('Ctrl Pts',(18.3326250661772,-56.0106982359126,
40.1379949176048));
#174820=CARTESIAN_POINT('Ctrl Pts',(18.33859296725,-56.0103653778788,40.1355293609261));
#174821=CARTESIAN_POINT('Ctrl Pts',(18.3594806210048,-56.0092003747604,
40.1268999125509));
#174822=CARTESIAN_POINT('Ctrl Pts',(18.3796805851421,-56.0095951017656,
40.1162251288835));
#174823=CARTESIAN_POINT('Ctrl Pts',(18.3987168313629,-56.011450082467,40.1038990521418));
#174824=CARTESIAN_POINT('Ctrl Pts',(18.4082349544732,-56.0123775728178,
40.097736013771));
#174825=CARTESIAN_POINT('Ctrl Pts',(18.4174621486788,-56.0136701283093,
40.0911601532641));
#174826=CARTESIAN_POINT('Ctrl Pts',(18.426338912063,-56.015315319243,40.0842207290641));
#174827=CARTESIAN_POINT('Ctrl Pts',(18.4351777497213,-56.016953481144,40.0773109533619));
#174828=CARTESIAN_POINT('Ctrl Pts',(18.4436692750118,-56.0189410563924,
40.0700409753047));
#174829=CARTESIAN_POINT('Ctrl Pts',(18.4517543535699,-56.0212664209291,
40.0624586415899));
#174830=CARTESIAN_POINT('Ctrl Pts',(18.4517890450628,-56.0212763986141,
40.0624261072769));
#174831=CARTESIAN_POINT('Ctrl Pts',(18.4518237293603,-56.021286382056,40.0623935677888));
#174832=CARTESIAN_POINT('Ctrl Pts',(18.4518584064613,-56.0212963712529,
40.0623610231288));
#174833=CARTESIAN_POINT('Ctrl Pts',(18.4682114607472,-56.0260070845278,
40.0470135870254));
#174834=CARTESIAN_POINT('Ctrl Pts',(18.4829503621221,-56.0319630212257,
40.0305755292138));
#174835=CARTESIAN_POINT('Ctrl Pts',(18.4960770195644,-56.0389696815101,
40.013344756741));
#174836=CARTESIAN_POINT('Ctrl Pts',(18.5096811989761,-56.0462312303092,
39.9954871626695));
#174837=CARTESIAN_POINT('Ctrl Pts',(18.5215542196539,-56.0546220378273,
39.9767767954443));
#174838=CARTESIAN_POINT('Ctrl Pts',(18.5316559412067,-56.0639562290112,
39.9575197577634));
#174839=CARTESIAN_POINT('Ctrl Pts',(18.5416134885271,-56.0731572003431,
39.9385375612185));
#174840=CARTESIAN_POINT('Ctrl Pts',(18.5498501466824,-56.0832757207001,
39.9190226977313));
#174841=CARTESIAN_POINT('Ctrl Pts',(18.5562821957245,-56.0941505847762,
39.8992655452103));
#174842=CARTESIAN_POINT('Ctrl Pts',(18.5607667347571,-56.101732733498,39.8854905069492));
#174843=CARTESIAN_POINT('Ctrl Pts',(18.5643731068255,-56.1096829110155,
39.8715976051558));
#174844=CARTESIAN_POINT('Ctrl Pts',(18.5670586829464,-56.1179479440989,
39.8576902534424));
#174845=CARTESIAN_POINT('',(18.6771643191709,-56.4568070719812,39.2875012672119));
#174846=CARTESIAN_POINT('',(18.5670586829464,-56.1179479440989,39.8576902534424));
#174847=CARTESIAN_POINT('',(23.8971395307767,-54.4530463244693,39.2875012672119));
#174848=CARTESIAN_POINT('Origin',(5.53234440788222E-15,0.,39.2875012672119));
#174849=CARTESIAN_POINT('',(23.7522229508827,-54.1275498658874,39.8576902534424));
#174850=CARTESIAN_POINT('',(23.8971395307767,-54.4530463244693,39.2875012672119));
#174851=CARTESIAN_POINT('',(23.9513722670364,-53.8330634946838,40.1599502534424));
#174852=CARTESIAN_POINT('Ctrl Pts',(23.7522229508827,-54.1275498658874,
39.8576902534424));
#174853=CARTESIAN_POINT('Ctrl Pts',(23.7472487091037,-54.116377183953,39.8772619994037));
#174854=CARTESIAN_POINT('Ctrl Pts',(23.7440527738942,-54.1044728027377,
39.8967644650337));
#174855=CARTESIAN_POINT('Ctrl Pts',(23.7426340760177,-54.0920187959705,
39.9159282836));
#174856=CARTESIAN_POINT('Ctrl Pts',(23.7411897512766,-54.0793398243611,
39.9354382707127));
#174857=CARTESIAN_POINT('Ctrl Pts',(23.7415870431742,-54.0660903588324,
39.9545987622285));
#174858=CARTESIAN_POINT('Ctrl Pts',(23.7438697192129,-54.0524339053569,
39.9731387498152));
#174859=CARTESIAN_POINT('Ctrl Pts',(23.7460557526666,-54.0393556307138,
39.990893802397));
#174860=CARTESIAN_POINT('Ctrl Pts',(23.7499709416771,-54.0259032350543,
40.0080810366091));
#174861=CARTESIAN_POINT('Ctrl Pts',(23.7556964920965,-54.0122070876573,
40.0244542742445));
#174862=CARTESIAN_POINT('Ctrl Pts',(23.7602504066211,-54.0013136224016,
40.0374770090424));
#174863=CARTESIAN_POINT('Ctrl Pts',(23.7659503209996,-53.9902655788147,
40.0499848770009));
#174864=CARTESIAN_POINT('Ctrl Pts',(23.772857804287,-53.9791273029164,40.0618424270192));
#174865=CARTESIAN_POINT('Ctrl Pts',(23.7728766594726,-53.9790968990413,
40.0618747942791));
#174866=CARTESIAN_POINT('Ctrl Pts',(23.7728955237005,-53.9790664946659,
40.0619071564124));
#174867=CARTESIAN_POINT('Ctrl Pts',(23.772914396971,-53.9790360897924,40.0619395134161));
#174868=CARTESIAN_POINT('Ctrl Pts',(23.7766714662754,-53.9729834442088,
40.0683807661799));
#174869=CARTESIAN_POINT('Ctrl Pts',(23.7808224374043,-53.9669027062279,
40.0746073439084));
#174870=CARTESIAN_POINT('Ctrl Pts',(23.7853431031263,-53.9608263568286,
40.0805869293668));
#174871=CARTESIAN_POINT('Ctrl Pts',(23.7943146773162,-53.9487674206468,
40.092453830807));
#174872=CARTESIAN_POINT('Ctrl Pts',(23.8047436656399,-53.9367254523685,
40.1033475319609));
#174873=CARTESIAN_POINT('Ctrl Pts',(23.8164490335995,-53.9249524603719,
40.1130129263075));
#174874=CARTESIAN_POINT('Ctrl Pts',(23.8252280595692,-53.9161227163744,
40.1202619720674));
#174875=CARTESIAN_POINT('Ctrl Pts',(23.8347250487607,-53.9074442707905,
40.1268200947266));
#174876=CARTESIAN_POINT('Ctrl Pts',(23.8448636317806,-53.8990234500734,
40.1325796782703));
#174877=CARTESIAN_POINT('Ctrl Pts',(23.848665600413,-53.8958656423044,40.1347395220992));
#174878=CARTESIAN_POINT('Ctrl Pts',(23.8525577932542,-53.8927440632082,
40.1367870714852));
#174879=CARTESIAN_POINT('Ctrl Pts',(23.8565361833379,-53.8896643205892,
40.1387166518767));
#174880=CARTESIAN_POINT('Ctrl Pts',(23.8704605486311,-53.8788852214226,
40.1454701832469));
#174881=CARTESIAN_POINT('Ctrl Pts',(23.8854408280738,-53.8686186144653,
40.1507785912492));
#174882=CARTESIAN_POINT('Ctrl Pts',(23.901304384366,-53.8591049768559,40.1543986087265));
#174883=CARTESIAN_POINT('Ctrl Pts',(23.9092361625121,-53.8543481580511,
40.1562086174652));
#174884=CARTESIAN_POINT('Ctrl Pts',(23.9173887602871,-53.8497795825131,
40.1575965292115));
#174885=CARTESIAN_POINT('Ctrl Pts',(23.9257405998159,-53.8454293138302,
40.1585319382567));
#174886=CARTESIAN_POINT('Ctrl Pts',(23.9299165195804,-53.8432541794887,
40.1589996427793));
#174887=CARTESIAN_POINT('Ctrl Pts',(23.934142249794,-53.8411336218842,40.159354221642));
#174888=CARTESIAN_POINT('Ctrl Pts',(23.9384150933427,-53.8390713992304,
40.159591874311));
#174889=CARTESIAN_POINT('Ctrl Pts',(23.9426879368913,-53.8370091765766,
40.1598295269801));
#174890=CARTESIAN_POINT('Ctrl Pts',(23.9470078944659,-53.8350052904264,
40.1599502506895));
#174891=CARTESIAN_POINT('Ctrl Pts',(23.9513722670364,-53.8330634946838,
40.1599502534424));
#174892=CARTESIAN_POINT('',(23.9791663275012,-53.8206887816837,40.1599502534424));
#174893=CARTESIAN_POINT('Origin',(5.68291264686342E-15,5.19046421553107E-15,
40.1599502534424));
#174894=CARTESIAN_POINT('',(24.3312692531087,-53.8697418420146,39.8576902534424));
#174895=CARTESIAN_POINT('Ctrl Pts',(23.9791663275012,-53.8206887816837,
40.1599502534424));
#174896=CARTESIAN_POINT('Ctrl Pts',(23.9826463618224,-53.8191382997272,
40.1599502448875));
#174897=CARTESIAN_POINT('Ctrl Pts',(23.9861360190795,-53.8176349962319,
40.1598743450437));
#174898=CARTESIAN_POINT('Ctrl Pts',(23.9896330908641,-53.8161786595149,
40.1597243308499));
#174899=CARTESIAN_POINT('Ctrl Pts',(24.0102795382215,-53.8075805576701,
40.1588386583938));
#174900=CARTESIAN_POINT('Ctrl Pts',(24.0311861904778,-53.8006169491706,
40.1553722553615));
#174901=CARTESIAN_POINT('Ctrl Pts',(24.0518926318819,-53.795247462207,40.1496902177781));
#174902=CARTESIAN_POINT('Ctrl Pts',(24.0596278691025,-53.7932416006199,
40.1475675976838));
#174903=CARTESIAN_POINT('Ctrl Pts',(24.0673353939224,-53.7914578533665,
40.1451361443093));
#174904=CARTESIAN_POINT('Ctrl Pts',(24.0749921329677,-53.7898929820048,
40.1424159447501));
#174905=CARTESIAN_POINT('Ctrl Pts',(24.0809663048721,-53.7886719908665,
40.1402935085949));
#174906=CARTESIAN_POINT('Ctrl Pts',(24.0869092410388,-53.7875846446507,
40.1379949176048));
#174907=CARTESIAN_POINT('Ctrl Pts',(24.0928096561863,-53.7866297945199,
40.1355293609261));
#174908=CARTESIAN_POINT('Ctrl Pts',(24.1134611092026,-53.7832878190622,
40.1268999125509));
#174909=CARTESIAN_POINT('Ctrl Pts',(24.1335916760301,-53.7815689125023,
40.1162251288835));
#174910=CARTESIAN_POINT('Ctrl Pts',(24.1527175379843,-53.7814239018615,
40.1038990521418));
#174911=CARTESIAN_POINT('Ctrl Pts',(24.1622804689615,-53.7813513965411,
40.0977360137709));
#174912=CARTESIAN_POINT('Ctrl Pts',(24.1715922244709,-53.7816723668478,
40.0911601532641));
#174913=CARTESIAN_POINT('Ctrl Pts',(24.1805923292966,-53.7823806708181,
40.084220729064));
#174914=CARTESIAN_POINT('Ctrl Pts',(24.1895539814234,-53.7830859485793,
40.0773109533618));
#174915=CARTESIAN_POINT('Ctrl Pts',(24.1982067474363,-53.7841750295931,
40.0700409753047));
#174916=CARTESIAN_POINT('Ctrl Pts',(24.2064906018697,-53.7856425347025,
40.0624586415899));
#174917=CARTESIAN_POINT('Ctrl Pts',(24.206526146271,-53.7856488314803,40.0624261072769));
#174918=CARTESIAN_POINT('Ctrl Pts',(24.2065616841181,-53.7856551347355,
40.0623935677888));
#174919=CARTESIAN_POINT('Ctrl Pts',(24.2065972154097,-53.7856614444665,
40.0623610231288));
#174920=CARTESIAN_POINT('Ctrl Pts',(24.2233530895738,-53.7886369923271,
40.0470135870244));
#174921=CARTESIAN_POINT('Ctrl Pts',(24.2386338146162,-53.79301966707,40.0305755292117));
#174922=CARTESIAN_POINT('Ctrl Pts',(24.2524209582886,-53.7986158348064,
40.0133447567377));
#174923=CARTESIAN_POINT('Ctrl Pts',(24.2667096511195,-53.8044155801139,
39.9954871626651));
#174924=CARTESIAN_POINT('Ctrl Pts',(24.2793947083637,-53.8115193533052,
39.9767767954389));
#174925=CARTESIAN_POINT('Ctrl Pts',(24.2904167802894,-53.8197464933835,
39.9575197577569));
#174926=CARTESIAN_POINT('Ctrl Pts',(24.3012815425175,-53.8278562137128,
39.9385375612115));
#174927=CARTESIAN_POINT('Ctrl Pts',(24.3105307527809,-53.8370583385375,
39.9190226977238));
#174928=CARTESIAN_POINT('Ctrl Pts',(24.318064299215,-53.8472012967688,39.8992655452024));
#174929=CARTESIAN_POINT('Ctrl Pts',(24.3233168218262,-53.8542731477119,
39.8854905069439));
#174930=CARTESIAN_POINT('Ctrl Pts',(24.3277344576485,-53.8618028047936,
39.8715976051531));
#174931=CARTESIAN_POINT('Ctrl Pts',(24.3312692531087,-53.8697418420146,
39.8576902534424));
#174932=CARTESIAN_POINT('',(24.4761921430391,-54.1952354911873,39.2875012672119));
#174933=CARTESIAN_POINT('',(24.3312692531087,-53.8697418420146,39.8576902534424));
#174934=CARTESIAN_POINT('',(29.4581217525673,-51.6568155675428,39.2875012672119));
#174935=CARTESIAN_POINT('Origin',(5.53234440788222E-15,0.,39.2875012672119));
#174936=CARTESIAN_POINT('',(29.2799753962461,-51.3482501200166,39.8576902534424));
#174937=CARTESIAN_POINT('',(29.4581217525673,-51.6568155675428,39.2875012672119));
#174938=CARTESIAN_POINT('',(29.4472515437734,-51.0345602039887,40.1599502534424));
#174939=CARTESIAN_POINT('Ctrl Pts',(29.2799753962461,-51.3482501200166,
39.8576902534424));
#174940=CARTESIAN_POINT('Ctrl Pts',(29.273860540611,-51.337658593052,39.8772619994036));
#174941=CARTESIAN_POINT('Ctrl Pts',(29.2694377663945,-51.3261534914788,
39.8967644650335));
#174942=CARTESIAN_POINT('Ctrl Pts',(29.2667250421045,-51.3139160033728,
39.9159282835996));
#174943=CARTESIAN_POINT('Ctrl Pts',(29.2639633161073,-51.3014574615422,
39.9354382707121));
#174944=CARTESIAN_POINT('Ctrl Pts',(29.2629734853274,-51.2882390496606,
39.9545987622277));
#174945=CARTESIAN_POINT('Ctrl Pts',(29.2638161685324,-51.2744188030479,
39.9731387498142));
#174946=CARTESIAN_POINT('Ctrl Pts',(29.2646231747154,-51.2611836698443,
39.9908938023957));
#174947=CARTESIAN_POINT('Ctrl Pts',(29.2671107576651,-51.2473957191255,
40.0080810366075));
#174948=CARTESIAN_POINT('Ctrl Pts',(29.2713733056799,-51.2331761176706,
40.0244542742427));
#174949=CARTESIAN_POINT('Ctrl Pts',(29.2747635962015,-51.2218663142697,
40.0374770090412));
#174950=CARTESIAN_POINT('Ctrl Pts',(29.2792774508344,-51.2102829897303,
40.0499848770004));
#174951=CARTESIAN_POINT('Ctrl Pts',(29.2849828273429,-51.1984837018591,
40.0618424270193));
#174952=CARTESIAN_POINT('Ctrl Pts',(29.2849984011674,-51.1984514936361,
40.0618747942791));
#174953=CARTESIAN_POINT('Ctrl Pts',(29.2850139839325,-51.1984192839703,
40.0619071564124));
#174954=CARTESIAN_POINT('Ctrl Pts',(29.2850295756385,-51.1983870728639,
40.0619395134161));
#174955=CARTESIAN_POINT('Ctrl Pts',(29.2881333895826,-51.1919748636253,
40.0683807661799));
#174956=CARTESIAN_POINT('Ctrl Pts',(29.2916260110607,-51.1854935419302,
40.0746073439084));
#174957=CARTESIAN_POINT('Ctrl Pts',(29.2954867606378,-51.1789779411678,
40.0805869293669));
#174958=CARTESIAN_POINT('Ctrl Pts',(29.3031486855379,-51.166047280237,40.092453830807));
#174959=CARTESIAN_POINT('Ctrl Pts',(29.3122618143336,-51.1529811529979,
40.1033475319609));
#174960=CARTESIAN_POINT('Ctrl Pts',(29.3226724463013,-51.1400491105585,
40.1130129263075));
#174961=CARTESIAN_POINT('Ctrl Pts',(29.330480420277,-51.130350078729,40.1202619720674));
#174962=CARTESIAN_POINT('Ctrl Pts',(29.3390182393876,-51.1207264688921,
40.1268200947266));
#174963=CARTESIAN_POINT('Ctrl Pts',(29.3482210667398,-51.1112920078092,
40.1325796782703));
#174964=CARTESIAN_POINT('Ctrl Pts',(29.3516721269969,-51.1077540849031,
40.1347395220992));
#174965=CARTESIAN_POINT('Ctrl Pts',(29.3552167041325,-51.1042427612073,
40.1367870714852));
#174966=CARTESIAN_POINT('Ctrl Pts',(29.3588513794159,-51.1007640347389,
40.1387166518767));
#174967=CARTESIAN_POINT('Ctrl Pts',(29.3715727429078,-51.0885884920993,
40.1454701832469));
#174968=CARTESIAN_POINT('Ctrl Pts',(29.3853978061641,-51.0768122610997,
40.1507785912492));
#174969=CARTESIAN_POINT('Ctrl Pts',(29.4001800143157,-51.0656925470313,
40.1543986087265));
#174970=CARTESIAN_POINT('Ctrl Pts',(29.4075711183915,-51.0601326899971,
40.1562086174652));
#174971=CARTESIAN_POINT('Ctrl Pts',(29.4152015092025,-51.0547369630768,
40.1575965292115));
#174972=CARTESIAN_POINT('Ctrl Pts',(29.4230528695803,-51.0495375206695,
40.1585319382567));
#174973=CARTESIAN_POINT('Ctrl Pts',(29.4269785497693,-51.0469377994658,
40.1589996427793));
#174974=CARTESIAN_POINT('Ctrl Pts',(29.430959472363,-51.0443871494123,40.159354221642));
#174975=CARTESIAN_POINT('Ctrl Pts',(29.4349933478627,-51.0418895900601,
40.159591874311));
#174976=CARTESIAN_POINT('Ctrl Pts',(29.4390272233624,-51.0393920307079,
40.1598295269801));
#174977=CARTESIAN_POINT('Ctrl Pts',(29.4431140526175,-51.036947563529,40.1599502506895));
#174978=CARTESIAN_POINT('Ctrl Pts',(29.4472515437734,-51.0345602039887,
40.1599502534424));
#174979=CARTESIAN_POINT('',(29.4735998357337,-51.0193480105328,40.1599502534424));
#174980=CARTESIAN_POINT('Origin',(5.68926707005281E-15,5.19370195586291E-15,
40.1599502534424));
#174981=CARTESIAN_POINT('',(29.8289013456884,-51.0313275753409,39.8576902534424));
#174982=CARTESIAN_POINT('Ctrl Pts',(29.4735998357337,-51.0193480105328,
40.1599502534424));
#174983=CARTESIAN_POINT('Ctrl Pts',(29.4768987365664,-51.0174422596391,
40.1599502448875));
#174984=CARTESIAN_POINT('Ctrl Pts',(29.4802121391118,-51.0155824228872,
40.1598743450437));
#174985=CARTESIAN_POINT('Ctrl Pts',(29.4835378249322,-51.0137685205955,
40.1597243308499));
#174986=CARTESIAN_POINT('Ctrl Pts',(29.5031724225184,-51.0030593786378,
40.1588386583938));
#174987=CARTESIAN_POINT('Ctrl Pts',(29.5232366506516,-50.9939485772816,
40.1553722553613));
#174988=CARTESIAN_POINT('Ctrl Pts',(29.5432683957828,-50.9864440924295,
40.1496902177776));
#174989=CARTESIAN_POINT('Ctrl Pts',(29.5507515889348,-50.9836406667027,
40.1475675976835));
#174990=CARTESIAN_POINT('Ctrl Pts',(29.5582304387674,-50.9810610352785,
40.1451361443091));
#174991=CARTESIAN_POINT('Ctrl Pts',(29.5656816597957,-50.9787043892801,
40.1424159447501));
#174992=CARTESIAN_POINT('Ctrl Pts',(29.571495476234,-50.9768656158505,40.1402935085949));
#174993=CARTESIAN_POINT('Ctrl Pts',(29.5772921977456,-50.9751630202462,
40.1379949176048));
#174994=CARTESIAN_POINT('Ctrl Pts',(29.5830604807847,-50.9735966395564,
40.1355293609261));
#174995=CARTESIAN_POINT('Ctrl Pts',(29.6032494714218,-50.9681143071419,
40.1268999125509));
#174996=CARTESIAN_POINT('Ctrl Pts',(29.6230900862367,-50.9643005997167,
40.1162251288835));
#174997=CARTESIAN_POINT('Ctrl Pts',(29.6420960169785,-50.9621571865006,
40.1038990521418));
#174998=CARTESIAN_POINT('Ctrl Pts',(29.6515989823495,-50.9610854798926,
40.097736013771));
#174999=CARTESIAN_POINT('Ctrl Pts',(29.6608932776208,-50.9604313483967,
40.0911601532641));
#175000=CARTESIAN_POINT('Ctrl Pts',(29.6699181168562,-50.960195005077,40.084220729064));
#175001=CARTESIAN_POINT('Ctrl Pts',(29.6789043977155,-50.9599596715277,
40.0773109533618));
#175002=CARTESIAN_POINT('Ctrl Pts',(29.6876236029356,-50.9601383261074,
40.0700409753048));
#175003=CARTESIAN_POINT('Ctrl Pts',(29.6960154736015,-50.9607318934964,
40.0624586415899));
#175004=CARTESIAN_POINT('Ctrl Pts',(29.6960514814794,-50.9607344403781,
40.0624261072769));
#175005=CARTESIAN_POINT('Ctrl Pts',(29.6960874835161,-50.9607369943869,
40.0623935677888));
#175006=CARTESIAN_POINT('Ctrl Pts',(29.69612347971,-50.9607395555212,40.0623610231288));
#175007=CARTESIAN_POINT('Ctrl Pts',(29.7130985928867,-50.9619473372422,
40.0470135870252));
#175008=CARTESIAN_POINT('Ctrl Pts',(29.7287537227735,-50.9647087325278,
40.0305755292133));
#175009=CARTESIAN_POINT('Ctrl Pts',(29.7430502978434,-50.9688330949306,
40.0133447567401));
#175010=CARTESIAN_POINT('Ctrl Pts',(29.7578669541839,-50.9731074935224,
39.9954871626683));
#175011=CARTESIAN_POINT('Ctrl Pts',(29.7712250678519,-50.9788464019604,
39.9767767954429));
#175012=CARTESIAN_POINT('Ctrl Pts',(29.7830467300236,-50.9858763526636,
39.9575197577617));
#175013=CARTESIAN_POINT('Ctrl Pts',(29.794699670551,-50.9928059701967,39.9385375612167));
#175014=CARTESIAN_POINT('Ctrl Pts',(29.8048600966396,-51.0009908790831,
39.9190226977294));
#175015=CARTESIAN_POINT('Ctrl Pts',(29.8134126013553,-51.0102908030958,
39.8992655452084));
#175016=CARTESIAN_POINT('Ctrl Pts',(29.8193755598108,-51.0167748755835,
39.8854905069479));
#175017=CARTESIAN_POINT('Ctrl Pts',(29.8245560588464,-51.0238015157329,
39.8715976051552));
#175018=CARTESIAN_POINT('Ctrl Pts',(29.8289013456884,-51.0313275753409,
39.8576902534424));
#175019=CARTESIAN_POINT('',(30.0070536838157,-51.3398895692698,39.2875012672119));
#175020=CARTESIAN_POINT('',(29.8289013456884,-51.0313275753409,39.8576902534424));
#175021=CARTESIAN_POINT('',(34.6963546279284,-48.2946219293747,39.2875012672119));
#175022=CARTESIAN_POINT('Origin',(5.53234440788222E-15,0.,39.2875012672119));
#175023=CARTESIAN_POINT('',(34.4869303039396,-48.0063682005188,39.8576902534424));
#175024=CARTESIAN_POINT('',(34.6963546279284,-48.2946219293747,39.2875012672119));
#175025=CARTESIAN_POINT('',(34.6205005703634,-47.6769115920305,40.1599502534424));
#175026=CARTESIAN_POINT('Ctrl Pts',(34.4869303039396,-48.0063682005188,
39.8576902534424));
#175027=CARTESIAN_POINT('Ctrl Pts',(34.4797418300849,-47.9964738715081,
39.8772619994068));
#175028=CARTESIAN_POINT('Ctrl Pts',(34.4741406737004,-47.9854941018754,
39.8967644650398));
#175029=CARTESIAN_POINT('Ctrl Pts',(34.4701636441718,-47.9736072089088,
39.9159282836089));
#175030=CARTESIAN_POINT('Ctrl Pts',(34.4661147749664,-47.9615055952461,
39.9354382707247));
#175031=CARTESIAN_POINT('Ctrl Pts',(34.4637486663026,-47.9484630606955,
39.9545987622433));
#175032=CARTESIAN_POINT('Ctrl Pts',(34.4631421240615,-47.9346304384564,
39.9731387498325));
#175033=CARTESIAN_POINT('Ctrl Pts',(34.4625612612463,-47.9213834535785,
39.9908938024167));
#175034=CARTESIAN_POINT('Ctrl Pts',(34.4635939836577,-47.9074110114703,
40.0080810366309));
#175035=CARTESIAN_POINT('Ctrl Pts',(34.4663468279024,-47.8928237488832,
40.024454274268));
#175036=CARTESIAN_POINT('Ctrl Pts',(34.4685363496885,-47.8812215199175,
40.0374770090575));
#175037=CARTESIAN_POINT('Ctrl Pts',(34.4718146898385,-47.8692298237612,
40.0499848770081));
#175038=CARTESIAN_POINT('Ctrl Pts',(34.4762554502657,-47.8568987993928,
40.0618424270193));
#175039=CARTESIAN_POINT('Ctrl Pts',(34.4762675720991,-47.8568651397018,
40.0618747942791));
#175040=CARTESIAN_POINT('Ctrl Pts',(34.4762797026733,-47.8568314776415,
40.0619071564124));
#175041=CARTESIAN_POINT('Ctrl Pts',(34.4762918419889,-47.8567978132139,
40.0619395134161));
#175042=CARTESIAN_POINT('Ctrl Pts',(34.4787083945375,-47.8500962938265,
40.0683807661799));
#175043=CARTESIAN_POINT('Ctrl Pts',(34.4815044004731,-47.8432853991339,
40.0746073439084));
#175044=CARTESIAN_POINT('Ctrl Pts',(34.4846629347251,-47.8364019332939,
40.0805869293669));
#175045=CARTESIAN_POINT('Ctrl Pts',(34.4909312646828,-47.8227412186411,
40.092453830807));
#175046=CARTESIAN_POINT('Ctrl Pts',(34.4986286886042,-47.8087940876656,
40.1033475319609));
#175047=CARTESIAN_POINT('Ctrl Pts',(34.5076305235176,-47.7948446809466,
40.1130129263075));
#175048=CARTESIAN_POINT('Ctrl Pts',(34.5143818997026,-47.7843826259073,
40.1202619720674));
#175049=CARTESIAN_POINT('Ctrl Pts',(34.5218670065994,-47.7739192901008,
40.1268200947266));
#175050=CARTESIAN_POINT('Ctrl Pts',(34.5300332501818,-47.763574554582,40.1325796782703));
#175051=CARTESIAN_POINT('Ctrl Pts',(34.5330955915252,-47.7596952787624,
40.1347395220992));
#175052=CARTESIAN_POINT('Ctrl Pts',(34.5362537178264,-47.7558326812643,
40.1367870714852));
#175053=CARTESIAN_POINT('Ctrl Pts',(34.5395048560464,-47.7519930846016,
40.1387166518767));
#175054=CARTESIAN_POINT('Ctrl Pts',(34.5508838398164,-47.7385544962821,
40.1454701832469));
#175055=CARTESIAN_POINT('Ctrl Pts',(34.5634022166003,-47.7253976640913,
40.1507785912492));
#175056=CARTESIAN_POINT('Ctrl Pts',(34.5769411196453,-47.7127937034783,
40.1543986087265));
#175057=CARTESIAN_POINT('Ctrl Pts',(34.5837105711679,-47.7064917231718,
40.1562086174652));
#175058=CARTESIAN_POINT('Ctrl Pts',(34.5907351548565,-47.7003279615825,
40.1575965292115));
#175059=CARTESIAN_POINT('Ctrl Pts',(34.598000014936,-47.6943363116299,40.1585319382567));
#175060=CARTESIAN_POINT('Ctrl Pts',(34.6016324449757,-47.6913404866536,
40.1589996427793));
#175061=CARTESIAN_POINT('Ctrl Pts',(34.6053249441285,-47.6883876896068,
40.159354221642));
#175062=CARTESIAN_POINT('Ctrl Pts',(34.6090756555951,-47.685482157339,40.159591874311));
#175063=CARTESIAN_POINT('Ctrl Pts',(34.6128263670618,-47.6825766250712,
40.1598295269801));
#175064=CARTESIAN_POINT('Ctrl Pts',(34.6166352918409,-47.6797183589577,
40.1599502506895));
#175065=CARTESIAN_POINT('Ctrl Pts',(34.6205005703634,-47.6769115920305,
40.1599502534424));
#175066=CARTESIAN_POINT('',(34.6451144164185,-47.6590285860936,40.1599502534424));
#175067=CARTESIAN_POINT('Origin',(5.69524824702573E-15,5.19758617760539E-15,
40.1599502534424));
#175068=CARTESIAN_POINT('',(34.9997217530259,-47.63380340476,39.8576902534424));
#175069=CARTESIAN_POINT('Ctrl Pts',(34.6451144164185,-47.6590285860936,
40.1599502534424));
#175070=CARTESIAN_POINT('Ctrl Pts',(34.648196040315,-47.6567884460682,40.1599502448875));
#175071=CARTESIAN_POINT('Ctrl Pts',(34.651296885817,-47.6545924528204,40.1598743450437));
#175072=CARTESIAN_POINT('Ctrl Pts',(34.6544147487634,-47.6524408584472,
40.1597243308499));
#175073=CARTESIAN_POINT('Ctrl Pts',(34.6728223758152,-47.6397380079788,
40.1588386583939));
#175074=CARTESIAN_POINT('Ctrl Pts',(34.6918243519396,-47.6285798336136,
40.1553722553623));
#175075=CARTESIAN_POINT('Ctrl Pts',(34.7109619288031,-47.6190225715805,
40.14969021778));
#175076=CARTESIAN_POINT('Ctrl Pts',(34.7181110904596,-47.6154522966311,
40.1475675976853));
#175077=CARTESIAN_POINT('Ctrl Pts',(34.7252793254645,-47.6121050440165,
40.1451361443101));
#175078=CARTESIAN_POINT('Ctrl Pts',(34.7324433913425,-47.6089824432866,
40.1424159447501));
#175079=CARTESIAN_POINT('Ctrl Pts',(34.7380331549251,-47.6065460335523,
40.1402935085949));
#175080=CARTESIAN_POINT('Ctrl Pts',(34.7436201516876,-47.6042468425533,
40.1379949176048));
#175081=CARTESIAN_POINT('Ctrl Pts',(34.7491931041024,-47.6020860928989,
40.1355293609261));
#175082=CARTESIAN_POINT('Ctrl Pts',(34.7686984375539,-47.5945234691088,
40.1268999125509));
#175083=CARTESIAN_POINT('Ctrl Pts',(34.7880317224283,-47.5886567445951,
40.1162251288835));
#175084=CARTESIAN_POINT('Ctrl Pts',(34.8067094890034,-47.5845384124875,
40.1038990521418));
#175085=CARTESIAN_POINT('Ctrl Pts',(34.8160483722909,-47.5824792464336,
40.097736013771));
#175086=CARTESIAN_POINT('Ctrl Pts',(34.8252233770802,-47.5808571799366,
40.0911601532641));
#175087=CARTESIAN_POINT('Ctrl Pts',(34.8341740726979,-47.5796787787539,
40.084220729064));
#175088=CARTESIAN_POINT('Ctrl Pts',(34.8430865267162,-47.5785054122577,
40.0773109533618));
#175089=CARTESIAN_POINT('Ctrl Pts',(34.8517766417065,-47.5777716830263,
40.0700409753048));
#175090=CARTESIAN_POINT('Ctrl Pts',(34.8601845855138,-47.5774848094464,
40.0624586415899));
#175091=CARTESIAN_POINT('Ctrl Pts',(34.8602206623585,-47.5774835785279,
40.0624261072769));
#175092=CARTESIAN_POINT('Ctrl Pts',(34.8602567341388,-47.577482355308,40.0623935677889));
#175093=CARTESIAN_POINT('Ctrl Pts',(34.8602928008533,-47.5774811397853,
40.0623610231288));
#175094=CARTESIAN_POINT('Ctrl Pts',(34.8773011701546,-47.5769079226574,
40.047013587022));
#175095=CARTESIAN_POINT('Ctrl Pts',(34.8931591840106,-47.5780177840619,
40.0305755292066));
#175096=CARTESIAN_POINT('Ctrl Pts',(34.9078085542128,-47.580625153755,40.0133447567296));
#175097=CARTESIAN_POINT('Ctrl Pts',(34.9229908396783,-47.5833273744273,
39.9954871626538));
#175098=CARTESIAN_POINT('Ctrl Pts',(34.9368756554839,-47.5876385414323,
39.976776795424));
#175099=CARTESIAN_POINT('Ctrl Pts',(34.9493673872986,-47.5933942811523,
39.9575197577385));
#175100=CARTESIAN_POINT('Ctrl Pts',(34.9616808340714,-47.5990678735518,
39.9385375611895));
#175101=CARTESIAN_POINT('Ctrl Pts',(34.9726411562313,-47.6061458909284,
39.9190226976982));
#175102=CARTESIAN_POINT('Ctrl Pts',(34.9821189161968,-47.6145008888124,
39.8992655451732));
#175103=CARTESIAN_POINT('Ctrl Pts',(34.9887269790679,-47.6203261419847,
39.8854905069243));
#175104=CARTESIAN_POINT('Ctrl Pts',(34.9946135826789,-47.626772779856,39.8715976051433));
#175105=CARTESIAN_POINT('Ctrl Pts',(34.9997217530259,-47.6338034047601,
39.8576902534424));
#175106=CARTESIAN_POINT('',(35.2091516650527,-47.9220530736688,39.2875012672119));
#175107=CARTESIAN_POINT('',(34.9997217530259,-47.63380340476,39.8576902534424));
#175108=CARTESIAN_POINT('',(39.554446981307,-44.403302307049,39.2875012672119));
#175109=CARTESIAN_POINT('Origin',(5.53234440788222E-15,0.,39.2875012672119));
#175110=CARTESIAN_POINT('',(39.3160391863689,-44.1385184650376,39.8576902534424));
#175111=CARTESIAN_POINT('',(39.554446981307,-44.403302307049,39.2875012672119));
#175112=CARTESIAN_POINT('',(39.4144401478989,-43.7969047596347,40.1599502534424));
#175113=CARTESIAN_POINT('Ctrl Pts',(39.3160391863689,-44.1385184650377,
39.8576902534424));
#175114=CARTESIAN_POINT('Ctrl Pts',(39.3078558527209,-44.1294297383233,
39.8772619994037));
#175115=CARTESIAN_POINT('Ctrl Pts',(39.3011376816113,-44.1190955972887,
39.8967644650336));
#175116=CARTESIAN_POINT('Ctrl Pts',(39.2959399200121,-44.1076895347526,
39.9159282835998));
#175117=CARTESIAN_POINT('Ctrl Pts',(39.2906482678569,-44.0960774370739,
39.9354382707125));
#175118=CARTESIAN_POINT('Ctrl Pts',(39.2869318048902,-44.0833536765974,
39.9545987622282));
#175119=CARTESIAN_POINT('Ctrl Pts',(39.2848826826046,-44.0696602318415,
39.9731387498148));
#175120=CARTESIAN_POINT('Ctrl Pts',(39.2829203148437,-44.0565465320328,
39.9908938023966));
#175121=CARTESIAN_POINT('Ctrl Pts',(39.2824868619908,-44.0425426835408,
40.0080810366086));
#175122=CARTESIAN_POINT('Ctrl Pts',(39.2836998417234,-44.0277475809291,
40.0244542742439));
#175123=CARTESIAN_POINT('Ctrl Pts',(39.284664605915,-44.0159800428334,40.037477009042));
#175124=CARTESIAN_POINT('Ctrl Pts',(39.286671513404,-44.0037113585782,40.0499848770007));
#175125=CARTESIAN_POINT('Ctrl Pts',(39.2897990038552,-43.9909836989804,
40.0618424270192));
#175126=CARTESIAN_POINT('Ctrl Pts',(39.2898075408882,-43.9909489566041,
40.0618747942791));
#175127=CARTESIAN_POINT('Ctrl Pts',(39.2898160863664,-43.9909142109578,
40.0619071564124));
#175128=CARTESIAN_POINT('Ctrl Pts',(39.2898246402906,-43.9908794620434,
40.0619395134161));
#175129=CARTESIAN_POINT('Ctrl Pts',(39.2915274551884,-43.9839620557562,
40.0683807661799));
#175130=CARTESIAN_POINT('Ctrl Pts',(39.2935962119552,-43.9768962096536,
40.0746073439084));
#175131=CARTESIAN_POINT('Ctrl Pts',(39.2960179253199,-43.9697202954281,
40.0805869293669));
#175132=CARTESIAN_POINT('Ctrl Pts',(39.3008239832004,-43.9554791967018,
40.092453830807));
#175133=CARTESIAN_POINT('Ctrl Pts',(39.3070213676603,-43.9408038696755,
40.1033475319609));
#175134=CARTESIAN_POINT('Ctrl Pts',(39.3145157795323,-43.925989931296,40.1130129263075));
#175135=CARTESIAN_POINT('Ctrl Pts',(39.3201365884364,-43.9148794775113,
40.1202619720674));
#175136=CARTESIAN_POINT('Ctrl Pts',(39.3264869747219,-43.9036910542318,
40.1268200947266));
#175137=CARTESIAN_POINT('Ctrl Pts',(39.3335271634607,-43.8925493833642,
40.1325796782703));
#175138=CARTESIAN_POINT('Ctrl Pts',(39.3361672342378,-43.8883712567889,
40.1347395220992));
#175139=CARTESIAN_POINT('Ctrl Pts',(39.338904308612,-43.8841997049149,40.1367870714852));
#175140=CARTESIAN_POINT('Ctrl Pts',(39.341736289618,-43.8800413054825,40.1387166518767));
#175141=CARTESIAN_POINT('Ctrl Pts',(39.3516482231388,-43.8654869074688,
40.1454701832469));
#175142=CARTESIAN_POINT('Ctrl Pts',(39.3627227594944,-43.8510936230936,
40.1507785912492));
#175143=CARTESIAN_POINT('Ctrl Pts',(39.374870022378,-43.8371435075659,40.1543986087265));
#175144=CARTESIAN_POINT('Ctrl Pts',(39.3809436538198,-43.8301684498021,
40.1562086174652));
#175145=CARTESIAN_POINT('Ctrl Pts',(39.3872854675771,-43.8233041850057,
40.1575965292115));
#175146=CARTESIAN_POINT('Ctrl Pts',(39.393884232031,-43.8165859732785,40.1585319382567));
#175147=CARTESIAN_POINT('Ctrl Pts',(39.3971836142579,-43.8132268674149,
40.1589996427793));
#175148=CARTESIAN_POINT('Ctrl Pts',(39.4005472341764,-43.8099042748372,
40.159354221642));
#175149=CARTESIAN_POINT('Ctrl Pts',(39.4039736880302,-43.8066226032735,
40.1595918743111));
#175150=CARTESIAN_POINT('Ctrl Pts',(39.4074001418841,-43.8033409317097,
40.1598295269801));
#175151=CARTESIAN_POINT('Ctrl Pts',(39.4108894308102,-43.8001001824231,
40.1599502506895));
#175152=CARTESIAN_POINT('Ctrl Pts',(39.4144401478989,-43.7969047596347,
40.1599502534424));
#175153=CARTESIAN_POINT('',(39.4370498736007,-43.7765468711723,40.1599502534424));
#175154=CARTESIAN_POINT('Origin',(5.70079064675565E-15,5.20207432441226E-15,
40.1599502534424));
#175155=CARTESIAN_POINT('',(39.7870778846746,-43.7143933160624,39.8576902534424));
#175156=CARTESIAN_POINT('Ctrl Pts',(39.4370498736007,-43.7765468711723,
40.1599502534424));
#175157=CARTESIAN_POINT('Ctrl Pts',(39.4398804576448,-43.773996885458,40.1599502448875));
#175158=CARTESIAN_POINT('Ctrl Pts',(39.4427347725911,-43.7714887954758,
40.1598743450437));
#175159=CARTESIAN_POINT('Ctrl Pts',(39.4456106527046,-43.7690230823392,
40.1597243308499));
#175160=CARTESIAN_POINT('Ctrl Pts',(39.4625896314128,-43.7544656984451,
40.1588386583938));
#175161=CARTESIAN_POINT('Ctrl Pts',(39.4803211659066,-43.741382402362,40.1553722553615));
#175162=CARTESIAN_POINT('Ctrl Pts',(39.4983548992104,-43.7298770745092,
40.1496902177781));
#175163=CARTESIAN_POINT('Ctrl Pts',(39.5050917016554,-43.7255790670193,
40.1475675976838));
#175164=CARTESIAN_POINT('Ctrl Pts',(39.5118707851449,-43.7215008664166,
40.1451361443093));
#175165=CARTESIAN_POINT('Ctrl Pts',(39.5186692048627,-43.7176465228244,
40.1424159447501));
#175166=CARTESIAN_POINT('Ctrl Pts',(39.5239736729701,-43.7146391706002,
40.1402935085949));
#175167=CARTESIAN_POINT('Ctrl Pts',(39.5292897326779,-43.7117685746242,
40.1379949176048));
#175168=CARTESIAN_POINT('Ctrl Pts',(39.5346062960353,-43.7090371296308,
40.1355293609261));
#175169=CARTESIAN_POINT('Ctrl Pts',(39.5532142677863,-43.6994770721539,
40.1268999125508));
#175170=CARTESIAN_POINT('Ctrl Pts',(39.5718284032055,-43.691621607613,40.1162251288835));
#175171=CARTESIAN_POINT('Ctrl Pts',(39.5899733680945,-43.6855734779223,
40.1038990521418));
#175172=CARTESIAN_POINT('Ctrl Pts',(39.599045850539,-43.6825494130769,40.0977360137709));
#175173=CARTESIAN_POINT('Ctrl Pts',(39.6080010415738,-43.6799771832788,
40.0911601532641));
#175174=CARTESIAN_POINT('Ctrl Pts',(39.6167795278797,-43.6778696350429,
40.084220729064));
#175175=CARTESIAN_POINT('Ctrl Pts',(39.6255205083456,-43.6757710912486,
40.0773109533618));
#175176=CARTESIAN_POINT('Ctrl Pts',(39.6340863223877,-43.6741330170972,
40.0700409753048));
#175177=CARTESIAN_POINT('Ctrl Pts',(39.6424182201447,-43.6729688455953,
40.0624586415899));
#175178=CARTESIAN_POINT('Ctrl Pts',(39.6424539706906,-43.6729638503628,
40.0624261072769));
#175179=CARTESIAN_POINT('Ctrl Pts',(39.6424897170046,-43.6729588633161,
40.0623935677889));
#175180=CARTESIAN_POINT('Ctrl Pts',(39.6425254590851,-43.6729538844539,
40.0623610231289));
#175181=CARTESIAN_POINT('Ctrl Pts',(39.6593807372547,-43.6706059487636,
40.0470135870217));
#175182=CARTESIAN_POINT('Ctrl Pts',(39.6752678913589,-43.6700521164124,
40.0305755292057));
#175183=CARTESIAN_POINT('Ctrl Pts',(39.6901095551258,-43.6711139265066,
40.0133447567283));
#175184=CARTESIAN_POINT('Ctrl Pts',(39.7054911294178,-43.6722143631629,
39.9954871626517));
#175185=CARTESIAN_POINT('Ctrl Pts',(39.7197505224119,-43.6750505546854,
39.9767767954212));
#175186=CARTESIAN_POINT('Ctrl Pts',(39.7327754618409,-43.6794690223312,
39.9575197577348));
#175187=CARTESIAN_POINT('Ctrl Pts',(39.7456145061592,-43.6838244285297,
39.9385375611848));
#175188=CARTESIAN_POINT('Ctrl Pts',(39.7572546408072,-43.6897180061549,
39.9190226976923));
#175189=CARTESIAN_POINT('Ctrl Pts',(39.7675538157017,-43.6970365388026,
39.8992655451661));
#175190=CARTESIAN_POINT('Ctrl Pts',(39.7747345836738,-43.7021391499707,
39.8854905069195));
#175191=CARTESIAN_POINT('Ctrl Pts',(39.7812627970031,-43.707935154855,39.8715976051409));
#175192=CARTESIAN_POINT('Ctrl Pts',(39.7870778846746,-43.7143933160624,
39.8576902534424));
#175193=CARTESIAN_POINT('',(40.0254908126588,-43.9791725362583,39.2875012672119));
#175194=CARTESIAN_POINT('',(39.7870778846746,-43.7143933160624,39.8576902534424));
#175195=CARTESIAN_POINT('',(43.9791725362582,-40.0254908126589,39.2875012672119));
#175196=CARTESIAN_POINT('Origin',(5.53234440788222E-15,0.,39.2875012672119));
#175197=CARTESIAN_POINT('',(43.7143933160623,-39.7870778846748,39.8576902534424));
#175198=CARTESIAN_POINT('',(43.9791725362582,-40.0254908126589,39.2875012672119));
#175199=CARTESIAN_POINT('',(43.7765468711722,-39.4370498736009,40.1599502534424));
#175200=CARTESIAN_POINT('Ctrl Pts',(43.7143933160623,-39.7870778846748,
39.8576902534424));
#175201=CARTESIAN_POINT('Ctrl Pts',(43.7053047809348,-39.7788943382461,
39.8772619994057));
#175202=CARTESIAN_POINT('Ctrl Pts',(43.6975432007873,-39.7693190488183,
39.8967644650376));
#175203=CARTESIAN_POINT('Ctrl Pts',(43.6911816548807,-39.7585187839172,
39.9159282836057));
#175204=CARTESIAN_POINT('Ctrl Pts',(43.6847051962237,-39.7475234267912,
39.9354382707203));
#175205=CARTESIAN_POINT('Ctrl Pts',(43.6796790973003,-39.735257844567,39.9545987622378));
#175206=CARTESIAN_POINT('Ctrl Pts',(43.6762098455841,-39.7218536055359,
39.9731387498261));
#175207=CARTESIAN_POINT('Ctrl Pts',(43.6728874729907,-39.7090168672317,
39.9908938024093));
#175208=CARTESIAN_POINT('Ctrl Pts',(43.6709925938757,-39.6951350414458,
40.0080810366227));
#175209=CARTESIAN_POINT('Ctrl Pts',(43.6706524194394,-39.6802941970447,
40.024454274259));
#175210=CARTESIAN_POINT('Ctrl Pts',(43.6703818558792,-39.6684902774397,
40.0374770090517));
#175211=CARTESIAN_POINT('Ctrl Pts',(43.6710953426076,-39.6560790233694,
40.0499848770053));
#175212=CARTESIAN_POINT('Ctrl Pts',(43.6728752976393,-39.6430941754569,
40.0618424270193));
#175213=CARTESIAN_POINT('Ctrl Pts',(43.6728801563384,-39.64305873104,40.0618747942791));
#175214=CARTESIAN_POINT('Ctrl Pts',(43.6728850230945,-39.6430232824883,
40.0619071564124));
#175215=CARTESIAN_POINT('Ctrl Pts',(43.6728898979088,-39.6429878298035,
40.0619395134161));
#175216=CARTESIAN_POINT('Ctrl Pts',(43.6738603187595,-39.6359303251672,
40.0683807661799));
#175217=CARTESIAN_POINT('Ctrl Pts',(43.6751791606254,-39.6286869425432,
40.0746073439084));
#175218=CARTESIAN_POINT('Ctrl Pts',(43.6768375203044,-39.6212972007502,
40.0805869293669));
#175219=CARTESIAN_POINT('Ctrl Pts',(43.6801286499319,-39.6066317464081,
40.092453830807));
#175220=CARTESIAN_POINT('Ctrl Pts',(43.6847580950893,-39.5913890092849,
40.1033475319609));
#175221=CARTESIAN_POINT('Ctrl Pts',(43.6906629735752,-39.5758728438537,
40.1130129263075));
#175222=CARTESIAN_POINT('Ctrl Pts',(43.6950916324396,-39.5642357197803,
40.1202619720674));
#175223=CARTESIAN_POINT('Ctrl Pts',(43.7002377219528,-39.5524447917346,
40.1268200947266));
#175224=CARTESIAN_POINT('Ctrl Pts',(43.7060747220671,-39.5406282559958,
40.1325796782703));
#175225=CARTESIAN_POINT('Ctrl Pts',(43.70826359711,-39.5361970550938,40.1347395220992));
#175226=CARTESIAN_POINT('Ctrl Pts',(43.7105496315975,-39.5317622532393,
40.1367870714852));
#175227=CARTESIAN_POINT('Ctrl Pts',(43.7129314276129,-39.5273306113315,
40.1387166518767));
#175228=CARTESIAN_POINT('Ctrl Pts',(43.7212677136666,-39.5118198646541,
40.1454701832469));
#175229=CARTESIAN_POINT('Ctrl Pts',(43.7307770746562,-39.49634782393,40.1507785912491));
#175230=CARTESIAN_POINT('Ctrl Pts',(43.7413996094243,-39.4812043938727,
40.1543986087265));
#175231=CARTESIAN_POINT('Ctrl Pts',(43.7467108768083,-39.473632678844,40.1562086174652));
#175232=CARTESIAN_POINT('Ctrl Pts',(43.7523004383956,-39.4661431171621,
40.1575965292115));
#175233=CARTESIAN_POINT('Ctrl Pts',(43.7581608097796,-39.4587719497938,
40.1585319382567));
#175234=CARTESIAN_POINT('Ctrl Pts',(43.7610909954716,-39.4550863661096,
40.1589996427793));
#175235=CARTESIAN_POINT('Ctrl Pts',(43.764088883632,-39.4514303810207,40.159354221642));
#175236=CARTESIAN_POINT('Ctrl Pts',(43.7671535389276,-39.4478085248413,
40.159591874311));
#175237=CARTESIAN_POINT('Ctrl Pts',(43.7702181942232,-39.4441866686619,
40.1598295269801));
#175238=CARTESIAN_POINT('Ctrl Pts',(43.7733496179168,-39.4405989425296,
40.1599502506895));
#175239=CARTESIAN_POINT('Ctrl Pts',(43.7765468711722,-39.4370498736009,
40.1599502534424));
#175240=CARTESIAN_POINT('',(43.7969047596346,-39.414440147899,40.1599502534424));
#175241=CARTESIAN_POINT('Origin',(5.7058335455513E-15,5.20711722320791E-15,
40.1599502534424));
#175242=CARTESIAN_POINT('',(44.1385184650375,-39.3160391863691,39.8576902534424));
#175243=CARTESIAN_POINT('Ctrl Pts',(43.7969047596346,-39.414440147899,40.1599502534424));
#175244=CARTESIAN_POINT('Ctrl Pts',(43.799453291355,-39.411608254673,40.1599502448875));
#175245=CARTESIAN_POINT('Ctrl Pts',(43.8020298032738,-39.4088155471152,
40.1598743450437));
#175246=CARTESIAN_POINT('Ctrl Pts',(43.8046321918101,-39.4060627300843,
40.1597243308499));
#175247=CARTESIAN_POINT('Ctrl Pts',(43.8199964969274,-39.3898103065115,
40.1588386583939));
#175248=CARTESIAN_POINT('Ctrl Pts',(43.8362633193845,-39.3749452320424,
40.1553722553621));
#175249=CARTESIAN_POINT('Ctrl Pts',(43.8529956277689,-39.3616178931511,
40.1496902177795));
#175250=CARTESIAN_POINT('Ctrl Pts',(43.8592462611886,-39.3566392429878,
40.147567597685));
#175251=CARTESIAN_POINT('Ctrl Pts',(43.865561920109,-39.351874776014,40.1451361443099));
#175252=CARTESIAN_POINT('Ctrl Pts',(43.8719202087611,-39.3473309185525,
40.1424159447501));
#175253=CARTESIAN_POINT('Ctrl Pts',(43.8768812645308,-39.3437855730187,
40.1402935085949));
#175254=CARTESIAN_POINT('Ctrl Pts',(43.8818681433212,-39.3403750229159,
40.1379949176048));
#175255=CARTESIAN_POINT('Ctrl Pts',(43.8868700682406,-39.3371028088664,
40.1355293609261));
#175256=CARTESIAN_POINT('Ctrl Pts',(43.9043768054585,-39.325650059693,40.1268999125508));
#175257=CARTESIAN_POINT('Ctrl Pts',(43.9220678510596,-39.3158919212384,
40.1162251288835));
#175258=CARTESIAN_POINT('Ctrl Pts',(43.9394812142301,-39.307980258539,40.1038990521418));
#175259=CARTESIAN_POINT('Ctrl Pts',(43.9481878958154,-39.3040244271893,
40.0977360137709));
#175260=CARTESIAN_POINT('Ctrl Pts',(43.9568251581488,-39.300530215978,40.0911601532641));
#175261=CARTESIAN_POINT('Ctrl Pts',(43.9653352562098,-39.2975166114285,
40.084220729064));
#175262=CARTESIAN_POINT('Ctrl Pts',(43.9738089951123,-39.2945158824212,
40.0773109533618));
#175263=CARTESIAN_POINT('Ctrl Pts',(43.982156659355,-39.2919914104329,40.0700409753048));
#175264=CARTESIAN_POINT('Ctrl Pts',(43.9903212250463,-39.2899626959157,
40.0624586415899));
#175265=CARTESIAN_POINT('Ctrl Pts',(43.9903562576029,-39.2899539910979,
40.0624261072769));
#175266=CARTESIAN_POINT('Ctrl Pts',(43.9903912868066,-39.2899452948635,
40.0623935677889));
#175267=CARTESIAN_POINT('Ctrl Pts',(43.9904263126554,-39.2899366072113,
40.0623610231288));
#175268=CARTESIAN_POINT('Ctrl Pts',(44.006943829738,-39.2858396774333,40.0470135870217));
#175269=CARTESIAN_POINT('Ctrl Pts',(44.0226860611052,-39.2836282192294,
40.0305755292057));
#175270=CARTESIAN_POINT('Ctrl Pts',(44.0375574100625,-39.283132836311,40.0133447567283));
#175271=CARTESIAN_POINT('Ctrl Pts',(44.0529697494336,-39.2826194323366,
39.995487162652));
#175272=CARTESIAN_POINT('Ctrl Pts',(44.0674474907222,-39.2839495744683,
39.9767767954217));
#175273=CARTESIAN_POINT('Ctrl Pts',(44.080862933803,-39.2869823603832,39.9575197577357));
#175274=CARTESIAN_POINT('Ctrl Pts',(44.0940869084097,-39.2899718616383,
39.9385375611862));
#175275=CARTESIAN_POINT('Ctrl Pts',(44.1062793237942,-39.2946164282413,
39.9190226976944));
#175276=CARTESIAN_POINT('Ctrl Pts',(44.1172870737017,-39.3008183122765,
39.8992655451689));
#175277=CARTESIAN_POINT('Ctrl Pts',(44.1249618727802,-39.3051423761658,
39.8854905069213));
#175278=CARTESIAN_POINT('Ctrl Pts',(44.1320601713578,-39.310224245822,39.8715976051418));
#175279=CARTESIAN_POINT('Ctrl Pts',(44.1385184650375,-39.3160391863691,
39.8576902534424));
#175280=CARTESIAN_POINT('',(44.4033023070489,-39.5544469813072,39.2875012672119));
#175281=CARTESIAN_POINT('',(44.1385184650375,-39.3160391863691,39.8576902534424));
#175282=CARTESIAN_POINT('',(47.9220530736687,-35.2091516650529,39.2875012672119));
#175283=CARTESIAN_POINT('Origin',(5.53234440788222E-15,0.,39.2875012672119));
#175284=CARTESIAN_POINT('',(47.6338034047599,-34.9997217530261,39.8576902534424));
#175285=CARTESIAN_POINT('',(47.9220530736687,-35.2091516650529,39.2875012672119));
#175286=CARTESIAN_POINT('',(47.6590285860935,-34.6451144164186,40.1599502534424));
#175287=CARTESIAN_POINT('Ctrl Pts',(47.6338034047599,-34.9997217530261,
39.8576902534424));
#175288=CARTESIAN_POINT('Ctrl Pts',(47.6239092440476,-34.9925330475317,
39.8772619994039));
#175289=CARTESIAN_POINT('Ctrl Pts',(47.6151892923597,-34.9838215185875,
39.8967644650341));
#175290=CARTESIAN_POINT('Ctrl Pts',(47.6077336605747,-34.9737453812864,
39.9159282836005));
#175291=CARTESIAN_POINT('Ctrl Pts',(47.600143352853,-34.9634872321492,39.9354382707132));
#175292=CARTESIAN_POINT('Ctrl Pts',(47.5938626849646,-34.951814212466,39.954598762229));
#175293=CARTESIAN_POINT('Ctrl Pts',(47.589011313665,-34.9388460388113,39.9731387498156));
#175294=CARTESIAN_POINT('Ctrl Pts',(47.584365336848,-34.9264269040061,39.990893802397));
#175295=CARTESIAN_POINT('Ctrl Pts',(47.581029792162,-34.9128191931185,40.0080810366088));
#175296=CARTESIAN_POINT('Ctrl Pts',(47.5791401905773,-34.8980952063294,
40.0244542742438));
#175297=CARTESIAN_POINT('Ctrl Pts',(47.5776372636143,-34.8863842314202,
40.037477009042));
#175298=CARTESIAN_POINT('Ctrl Pts',(47.5770495124719,-34.8739663878225,
40.0499848770007));
#175299=CARTESIAN_POINT('Ctrl Pts',(47.5774624305259,-34.8608666162962,
40.0618424270193));
#175300=CARTESIAN_POINT('Ctrl Pts',(47.5774635576581,-34.8608308581752,
40.0618747942791));
#175301=CARTESIAN_POINT('Ctrl Pts',(47.577464692371,-34.8607950950998,40.0619071564124));
#175302=CARTESIAN_POINT('Ctrl Pts',(47.5774658346659,-34.8607593270717,
40.0619395134161));
#175303=CARTESIAN_POINT('Ctrl Pts',(47.5776932293355,-34.853639047584,40.0683807661799));
#175304=CARTESIAN_POINT('Ctrl Pts',(47.5782477067931,-34.8462974884544,
40.0746073439084));
#175305=CARTESIAN_POINT('Ctrl Pts',(47.5791245434507,-34.8387748826513,
40.0805869293668));
#175306=CARTESIAN_POINT('Ctrl Pts',(47.5808646865202,-34.8238457504803,
40.092453830807));
#175307=CARTESIAN_POINT('Ctrl Pts',(47.5838754712052,-34.8082026058778,
40.1033475319609));
#175308=CARTESIAN_POINT('Ctrl Pts',(47.5881261212205,-34.7921542117504,
40.1130129263075));
#175309=CARTESIAN_POINT('Ctrl Pts',(47.591314108732,-34.7801179161549,40.1202619720674));
#175310=CARTESIAN_POINT('Ctrl Pts',(47.5951995198393,-34.7678536672181,
40.1268200947266));
#175311=CARTESIAN_POINT('Ctrl Pts',(47.5997693799344,-34.7554917310464,
40.1325796782703));
#175312=CARTESIAN_POINT('Ctrl Pts',(47.60148307747,-34.750856004982,40.1347395220992));
#175313=CARTESIAN_POINT('Ctrl Pts',(47.6032930257987,-34.7462065417642,
40.1367870714852));
#175314=CARTESIAN_POINT('Ctrl Pts',(47.6051985413679,-34.7415502113771,
40.1387166518767));
#175315=CARTESIAN_POINT('Ctrl Pts',(47.6118678458601,-34.7252530550223,
40.1454701832469));
#175316=CARTESIAN_POINT('Ctrl Pts',(47.6197078449347,-34.7088717728653,
40.1507785912492));
#175317=CARTESIAN_POINT('Ctrl Pts',(47.6286892688733,-34.692700942867,40.1543986087265));
#175318=CARTESIAN_POINT('Ctrl Pts',(47.6331799808426,-34.6846155278679,
40.1562086174652));
#175319=CARTESIAN_POINT('Ctrl Pts',(47.6379560498536,-34.6765827265054,
40.1575965292115));
#175320=CARTESIAN_POINT('Ctrl Pts',(47.6430138207125,-34.6686393635482,
40.1585319382567));
#175321=CARTESIAN_POINT('Ctrl Pts',(47.6455427061419,-34.6646676820696,
40.1589996427793));
#175322=CARTESIAN_POINT('Ctrl Pts',(47.6481420170542,-34.6607183602071,
40.159354221642));
#175323=CARTESIAN_POINT('Ctrl Pts',(47.6508112967868,-34.6567960012263,
40.159591874311));
#175324=CARTESIAN_POINT('Ctrl Pts',(47.6534805765195,-34.6528736422456,
40.1598295269801));
#175325=CARTESIAN_POINT('Ctrl Pts',(47.6562198264472,-34.6489782471459,
40.1599502506895));
#175326=CARTESIAN_POINT('Ctrl Pts',(47.6590285860935,-34.6451144164186,
40.1599502534424));
#175327=CARTESIAN_POINT('',(47.6769115920304,-34.6205005703635,40.1599502534424));
#175328=CARTESIAN_POINT('Origin',(5.71032169235817E-15,5.21265962293783E-15,
40.1599502534424));
#175329=CARTESIAN_POINT('',(48.0063682005187,-34.4869303039397,39.8576902534424));
#175330=CARTESIAN_POINT('Ctrl Pts',(47.6769115920304,-34.6205005703635,
40.1599502534424));
#175331=CARTESIAN_POINT('Ctrl Pts',(47.6791501491803,-34.6174177964406,
40.1599502448875));
#175332=CARTESIAN_POINT('Ctrl Pts',(47.6814206292678,-34.6143710687955,
40.1598743450437));
#175333=CARTESIAN_POINT('Ctrl Pts',(47.6837210139136,-34.6113613083098,
40.1597243308499));
#175334=CARTESIAN_POINT('Ctrl Pts',(47.6973023109009,-34.5935919100088,
40.1588386583938));
#175335=CARTESIAN_POINT('Ctrl Pts',(47.7119261986137,-34.5771079220176,
40.1553722553613));
#175336=CARTESIAN_POINT('Ctrl Pts',(47.7271737594101,-34.5621045891995,
40.1496902177776));
#175337=CARTESIAN_POINT('Ctrl Pts',(47.7328697405536,-34.5564998434987,
40.1475675976835));
#175338=CARTESIAN_POINT('Ctrl Pts',(47.7386527792208,-34.5511013106537,
40.1451361443091));
#175339=CARTESIAN_POINT('Ctrl Pts',(47.7445012740629,-34.5459177227786,
40.1424159447501));
#175340=CARTESIAN_POINT('Ctrl Pts',(47.7490645631296,-34.5418732274828,
40.1402935085949));
#175341=CARTESIAN_POINT('Ctrl Pts',(47.7536676237151,-34.5379600899538,
40.1379949176048));
#175342=CARTESIAN_POINT('Ctrl Pts',(47.7583001080603,-34.53418295791,40.1355293609261));
#175343=CARTESIAN_POINT('Ctrl Pts',(47.7745138032687,-34.5209629957567,
40.1268999125509));
#175344=CARTESIAN_POINT('Ctrl Pts',(47.7910879322539,-34.5094090955953,
40.1162251288835));
#175345=CARTESIAN_POINT('Ctrl Pts',(47.8075789092552,-34.4997205817194,
40.1038990521418));
#175346=CARTESIAN_POINT('Ctrl Pts',(47.8158243977558,-34.4948763247815,
40.0977360137709));
#175347=CARTESIAN_POINT('Ctrl Pts',(47.8240490997342,-34.4904984154663,
40.0911601532641));
#175348=CARTESIAN_POINT('Ctrl Pts',(47.8321975711351,-34.4866117722853,
40.084220729064));
#175349=CARTESIAN_POINT('Ctrl Pts',(47.8403112284174,-34.4827417346798,
40.0773109533618));
#175350=CARTESIAN_POINT('Ctrl Pts',(47.8483492841045,-34.479358523498,40.0700409753047));
#175351=CARTESIAN_POINT('Ctrl Pts',(47.8562570650397,-34.4764874929863,
40.0624586415899));
#175352=CARTESIAN_POINT('Ctrl Pts',(47.8562909957831,-34.4764751739551,
40.0624261072769));
#175353=CARTESIAN_POINT('Ctrl Pts',(47.8563249240891,-34.4764628638107,
40.0623935677888));
#175354=CARTESIAN_POINT('Ctrl Pts',(47.8563588499558,-34.4764505625523,
40.0623610231288));
#175355=CARTESIAN_POINT('Ctrl Pts',(47.8723576365755,-34.4706495255074,
40.0470135870237));
#175356=CARTESIAN_POINT('Ctrl Pts',(47.8877824700225,-34.4668046706501,
40.0305755292102));
#175357=CARTESIAN_POINT('Ctrl Pts',(47.9025205705571,-34.4647575222378,
40.0133447567353));
#175358=CARTESIAN_POINT('Ctrl Pts',(47.9177948141903,-34.4626359025942,
39.9954871626613));
#175359=CARTESIAN_POINT('Ctrl Pts',(47.9323322826087,-34.462445422019,39.9767767954335));
#175360=CARTESIAN_POINT('Ctrl Pts',(47.9459912469386,-34.464059298365,39.95751975775));
#175361=CARTESIAN_POINT('Ctrl Pts',(47.9594552672001,-34.4656501410745,
39.9385375612023));
#175362=CARTESIAN_POINT('Ctrl Pts',(47.9720663806666,-34.4689948098108,
39.9190226977123));
#175363=CARTESIAN_POINT('Ctrl Pts',(47.9836621023758,-34.4740120960928,
39.8992655451885));
#175364=CARTESIAN_POINT('Ctrl Pts',(47.9917468458596,-34.4775102373549,
39.8854905069345));
#175365=CARTESIAN_POINT('Ctrl Pts',(47.9993374592446,-34.4818222937569,
39.8715976051484));
#175366=CARTESIAN_POINT('Ctrl Pts',(48.0063682005187,-34.4869303039397,
39.8576902534424));
#175367=CARTESIAN_POINT('',(48.2946219293746,-34.6963546279286,39.2875012672119));
#175368=CARTESIAN_POINT('',(48.0063682005187,-34.4869303039397,39.8576902534424));
#175369=CARTESIAN_POINT('',(51.3398895692697,-30.0070536838158,39.2875012672119));
#175370=CARTESIAN_POINT('Origin',(5.53234440788222E-15,0.,39.2875012672119));
#175371=CARTESIAN_POINT('',(51.0313275753408,-29.8289013456886,39.8576902534424));
#175372=CARTESIAN_POINT('',(51.3398895692697,-30.0070536838158,39.2875012672119));
#175373=CARTESIAN_POINT('',(51.0193480105327,-29.4735998357338,40.1599502534424));
#175374=CARTESIAN_POINT('Ctrl Pts',(51.0313275753408,-29.8289013456886,
39.8576902534424));
#175375=CARTESIAN_POINT('Ctrl Pts',(51.0207361915351,-29.8227862420882,
39.8772619994089));
#175376=CARTESIAN_POINT('Ctrl Pts',(51.0111534059195,-29.8150339189585,
39.8967644650441));
#175377=CARTESIAN_POINT('Ctrl Pts',(51.0026853737161,-29.8057923055218,
39.9159282836152));
#175378=CARTESIAN_POINT('Ctrl Pts',(50.9940643779273,-29.7963837547977,
39.935438270733));
#175379=CARTESIAN_POINT('Ctrl Pts',(50.9865979533845,-29.7854311896963,
39.9545987622535));
#175380=CARTESIAN_POINT('Ctrl Pts',(50.9804176151407,-29.7730411634356,
39.9731387498444));
#175381=CARTESIAN_POINT('Ctrl Pts',(50.9744989363941,-29.7611756987626,
39.9908938024301));
#175382=CARTESIAN_POINT('Ctrl Pts',(50.9697592710636,-29.7479911916937,
40.0080810366458));
#175383=CARTESIAN_POINT('Ctrl Pts',(50.9663409452031,-29.7335453815885,
40.024454274284));
#175384=CARTESIAN_POINT('Ctrl Pts',(50.9636221212252,-29.7220556592812,
40.0374770090677));
#175385=CARTESIAN_POINT('Ctrl Pts',(50.9617395717397,-29.7097672786655,
40.0499848770129));
#175386=CARTESIAN_POINT('Ctrl Pts',(50.9607809287995,-29.6966961073821,
40.0618424270193));
#175387=CARTESIAN_POINT('Ctrl Pts',(50.9607783120157,-29.6966604273304,
40.0618747942791));
#175388=CARTESIAN_POINT('Ctrl Pts',(50.9607757022532,-29.6966247415591,
40.0619071564124));
#175389=CARTESIAN_POINT('Ctrl Pts',(50.9607730995135,-29.6965890500697,
40.0619395134161));
#175390=CARTESIAN_POINT('Ctrl Pts',(50.9602549766184,-29.6894840070026,
40.0683807661799));
#175391=CARTESIAN_POINT('Ctrl Pts',(50.9600390146967,-29.6821247070255,
40.0746073439084));
#175392=CARTESIAN_POINT('Ctrl Pts',(50.960124721527,-29.6745516564558,40.0805869293669));
#175393=CARTESIAN_POINT('Ctrl Pts',(50.960294812667,-29.6595224131519,40.092453830807));
#175394=CARTESIAN_POINT('Ctrl Pts',(50.9616539500924,-29.643650250636,40.1033475319609));
#175395=CARTESIAN_POINT('Ctrl Pts',(50.9642038006262,-29.6272454573768,
40.1130129263075));
#175396=CARTESIAN_POINT('Ctrl Pts',(50.9661161885265,-29.6149418624324,
40.1202619720674));
#175397=CARTESIAN_POINT('Ctrl Pts',(50.9686983518507,-29.6023386622823,
40.1268200947266));
#175398=CARTESIAN_POINT('Ctrl Pts',(50.9719510035829,-29.5895667656373,
40.1325796782703));
#175399=CARTESIAN_POINT('Ctrl Pts',(50.9731707479825,-29.5847773043955,
40.1347395220992));
#175400=CARTESIAN_POINT('Ctrl Pts',(50.9744847799797,-29.5799641203062,
40.1367870714852));
#175401=CARTESIAN_POINT('Ctrl Pts',(50.9758931378754,-29.57513411717,40.1387166518767));
#175402=CARTESIAN_POINT('Ctrl Pts',(50.9808223905104,-29.5582291061934,
40.1454701832469));
#175403=CARTESIAN_POINT('Ctrl Pts',(50.9869071309995,-29.5411180593587,
40.1507785912492));
#175404=CARTESIAN_POINT('Ctrl Pts',(50.9941490417486,-29.5240970004169,
40.1543986087265));
#175405=CARTESIAN_POINT('Ctrl Pts',(50.9977699971231,-29.515586470946,40.1562086174652));
#175406=CARTESIAN_POINT('Ctrl Pts',(51.0016802459462,-29.5070984389556,
40.1575965292115));
#175407=CARTESIAN_POINT('Ctrl Pts',(51.005880002284,-29.4986699095565,40.1585319382567));
#175408=CARTESIAN_POINT('Ctrl Pts',(51.0079798804529,-29.4944556448569,
40.1589996427793));
#175409=CARTESIAN_POINT('Ctrl Pts',(51.0101521355228,-29.4902562558175,
40.159354221642));
#175410=CARTESIAN_POINT('Ctrl Pts',(51.0123967945051,-29.4860763682211,
40.159591874311));
#175411=CARTESIAN_POINT('Ctrl Pts',(51.0146414534875,-29.4818964806248,
40.1598295269801));
#175412=CARTESIAN_POINT('Ctrl Pts',(51.0169585178538,-29.4777360953216,
40.1599502506895));
#175413=CARTESIAN_POINT('Ctrl Pts',(51.0193480105327,-29.4735998357338,
40.1599502534424));
#175414=CARTESIAN_POINT('',(51.0345602039887,-29.4472515437736,40.1599502534424));
#175415=CARTESIAN_POINT('Origin',(5.71420591410065E-15,5.21864079991075E-15,
40.1599502534424));
#175416=CARTESIAN_POINT('',(51.3482501200165,-29.2799753962463,39.8576902534424));
#175417=CARTESIAN_POINT('Ctrl Pts',(51.0345602039887,-29.4472515437736,
40.1599502534424));
#175418=CARTESIAN_POINT('Ctrl Pts',(51.0364642604675,-29.4439516646699,
40.1599502448875));
#175419=CARTESIAN_POINT('Ctrl Pts',(51.0384038328688,-29.4406842975233,
40.1598743450437));
#175420=CARTESIAN_POINT('Ctrl Pts',(51.0403770101285,-29.4374505691485,
40.1597243308499));
#175421=CARTESIAN_POINT('Ctrl Pts',(51.0520264994549,-29.4183588813631,
40.1588386583936));
#175422=CARTESIAN_POINT('Ctrl Pts',(51.0648472300504,-29.4004365818696,
40.1553722553598));
#175423=CARTESIAN_POINT('Ctrl Pts',(51.0784429877935,-29.3839216347767,
40.1496902177739));
#175424=CARTESIAN_POINT('Ctrl Pts',(51.0835219102983,-29.3777522003075,
40.1475675976806));
#175425=CARTESIAN_POINT('Ctrl Pts',(51.0887089685294,-29.371778749049,40.1451361443075));
#175426=CARTESIAN_POINT('Ctrl Pts',(51.0939835922269,-29.3660122232358,
40.1424159447501));
#175427=CARTESIAN_POINT('Ctrl Pts',(51.0980991182406,-29.3615128905148,
40.1402935085949));
#175428=CARTESIAN_POINT('Ctrl Pts',(51.1022679285261,-29.3571400387134,
40.1379949176048));
#175429=CARTESIAN_POINT('Ctrl Pts',(51.1064802178293,-29.3528993717244,
40.1355293609261));
#175430=CARTESIAN_POINT('Ctrl Pts',(51.1212232303906,-29.3380570372629,
40.1268999125508));
#175431=CARTESIAN_POINT('Ctrl Pts',(51.1364988531343,-29.3248339623427,
40.1162251288835));
#175432=CARTESIAN_POINT('Ctrl Pts',(51.1518867653713,-29.3134747466759,
40.1038990521418));
#175433=CARTESIAN_POINT('Ctrl Pts',(51.1595807214898,-29.3077951388425,
40.0977360137709));
#175434=CARTESIAN_POINT('Ctrl Pts',(51.1673027515571,-29.3025814967139,
40.0911601532641));
#175435=CARTESIAN_POINT('Ctrl Pts',(51.1750003199402,-29.2978643977774,
40.084220729064));
#175436=CARTESIAN_POINT('Ctrl Pts',(51.1826650006752,-29.2931674525157,
40.0773109533619));
#175437=CARTESIAN_POINT('Ctrl Pts',(51.1903053811865,-29.2889625693101,
40.0700409753048));
#175438=CARTESIAN_POINT('Ctrl Pts',(51.1978697380629,-29.2852806784149,
40.0624586415899));
#175439=CARTESIAN_POINT('Ctrl Pts',(51.1979021952408,-29.2852648801402,
40.0624261072769));
#175440=CARTESIAN_POINT('Ctrl Pts',(51.1979346509235,-29.2852490909584,
40.0623935677889));
#175441=CARTESIAN_POINT('Ctrl Pts',(51.1979671051091,-29.2852333108688,
40.0623610231288));
#175442=CARTESIAN_POINT('Ctrl Pts',(51.2132718752132,-29.2777917239328,
40.0470135870247));
#175443=CARTESIAN_POINT('Ctrl Pts',(51.228210313038,-29.2723555974564,40.0305755292122));
#175444=CARTESIAN_POINT('Ctrl Pts',(51.2426536914375,-29.2687791125368,
40.0133447567384));
#175445=CARTESIAN_POINT('Ctrl Pts',(51.2576224915239,-29.265072522133,39.995487162666));
#175446=CARTESIAN_POINT('Ctrl Pts',(51.2720604115264,-29.2633635057963,
39.9767767954398));
#175447=CARTESIAN_POINT('Ctrl Pts',(51.2858132466341,-29.263540790607,39.9575197577579));
#175448=CARTESIAN_POINT('Ctrl Pts',(51.2993697979264,-29.2637155451657,
39.9385375612124));
#175449=CARTESIAN_POINT('Ctrl Pts',(51.3122614394758,-29.265723671145,39.9190226977245));
#175450=CARTESIAN_POINT('Ctrl Pts',(51.3243180878321,-29.269501389236,39.899265545203));
#175451=CARTESIAN_POINT('Ctrl Pts',(51.3327241975788,-29.2721352815024,
39.8854905069443));
#175452=CARTESIAN_POINT('Ctrl Pts',(51.3407239614216,-29.2756302808569,
39.8715976051533));
#175453=CARTESIAN_POINT('Ctrl Pts',(51.3482501200165,-29.2799753962463,
39.8576902534424));
#175454=CARTESIAN_POINT('',(51.6568155675427,-29.4581217525674,39.2875012672119));
#175455=CARTESIAN_POINT('',(51.3482501200165,-29.2799753962463,39.8576902534424));
#175456=CARTESIAN_POINT('',(54.1952354911872,-24.4761921430393,39.2875012672119));
#175457=CARTESIAN_POINT('Origin',(5.53234440788222E-15,0.,39.2875012672119));
#175458=CARTESIAN_POINT('',(53.8697418420145,-24.3312692531089,39.8576902534424));
#175459=CARTESIAN_POINT('',(54.1952354911872,-24.4761921430393,39.2875012672119));
#175460=CARTESIAN_POINT('',(53.8206887816836,-23.9791663275014,40.1599502534424));
#175461=CARTESIAN_POINT('Ctrl Pts',(53.8697418420145,-24.3312692531089,
39.8576902534424));
#175462=CARTESIAN_POINT('Ctrl Pts',(53.8585692765391,-24.3262947497603,
39.8772619994026));
#175463=CARTESIAN_POINT('Ctrl Pts',(53.8482286480054,-24.3195865685246,
39.8967644650314));
#175464=CARTESIAN_POINT('Ctrl Pts',(53.8388409929203,-24.3112807320101,
39.9159282835966));
#175465=CARTESIAN_POINT('Ctrl Pts',(53.8292837625023,-24.3028248617567,
39.9354382707079));
#175466=CARTESIAN_POINT('Ctrl Pts',(53.8207133850174,-24.2927127498415,
39.9545987622223));
#175467=CARTESIAN_POINT('Ctrl Pts',(53.8132717929093,-24.2810366187063,
39.9731387498077));
#175468=CARTESIAN_POINT('Ctrl Pts',(53.8061452585171,-24.2698548246904,
39.9908938023878));
#175469=CARTESIAN_POINT('Ctrl Pts',(53.8000534013066,-24.2572379736713,
40.0080810365982));
#175470=CARTESIAN_POINT('Ctrl Pts',(53.7951438030611,-24.2432286115827,
40.0244542742322));
#175471=CARTESIAN_POINT('Ctrl Pts',(53.7912388700622,-24.2320860256563,
40.0374770090346));
#175472=CARTESIAN_POINT('Ctrl Pts',(53.7880821478325,-24.2200617420654,
40.0499848769972));
#175473=CARTESIAN_POINT('Ctrl Pts',(53.7857624469883,-24.2071623814823,
40.0618424270193));
#175474=CARTESIAN_POINT('Ctrl Pts',(53.7857561149585,-24.207127170418,40.0618747942791));
#175475=CARTESIAN_POINT('Ctrl Pts',(53.7857497893137,-24.2070919529316,
40.0619071564124));
#175476=CARTESIAN_POINT('Ctrl Pts',(53.7857434700555,-24.2070567290242,
40.0619395134162));
#175477=CARTESIAN_POINT('Ctrl Pts',(53.7844855062586,-24.2000447667165,
40.0683807661799));
#175478=CARTESIAN_POINT('Ctrl Pts',(53.7835014710816,-24.1927483559225,
40.0746073439084));
#175479=CARTESIAN_POINT('Ctrl Pts',(53.7827951090625,-24.1852078325129,
40.0805869293669));
#175480=CARTESIAN_POINT('Ctrl Pts',(53.7813932847188,-24.1702431416109,
40.092453830807));
#175481=CARTESIAN_POINT('Ctrl Pts',(53.7810858838907,-24.1543158599156,
40.1033475319609));
#175482=CARTESIAN_POINT('Ctrl Pts',(53.7819069982469,-24.1377344018724,
40.1130129263075));
#175483=CARTESIAN_POINT('Ctrl Pts',(53.782522834014,-24.1252983083401,40.1202619720674));
#175484=CARTESIAN_POINT('Ctrl Pts',(53.7837734588334,-24.1124942402749,
40.1268200947266));
#175485=CARTESIAN_POINT('Ctrl Pts',(53.7856732654698,-24.099452314729,40.1325796782703));
#175486=CARTESIAN_POINT('Ctrl Pts',(53.7863856929585,-24.0945615926493,
40.1347395220992));
#175487=CARTESIAN_POINT('Ctrl Pts',(53.7871894118146,-24.0896374219408,
40.1367870714852));
#175488=CARTESIAN_POINT('Ctrl Pts',(53.788085181773,-24.0846866645806,40.1387166518767));
#175489=CARTESIAN_POINT('Ctrl Pts',(53.7912203766273,-24.0673590138199,
40.1454701832468));
#175490=CARTESIAN_POINT('Ctrl Pts',(53.7954831928409,-24.0497056745174,
40.1507785912492));
#175491=CARTESIAN_POINT('Ctrl Pts',(53.8009062465108,-24.0320208729156,
40.1543986087265));
#175492=CARTESIAN_POINT('Ctrl Pts',(53.8036177733457,-24.0231784721148,
40.1562086174652));
#175493=CARTESIAN_POINT('Ctrl Pts',(53.8066193604764,-24.0143282061514,
40.1575965292115));
#175494=CARTESIAN_POINT('Ctrl Pts',(53.8099150888839,-24.005506855042,40.1585319382567));
#175495=CARTESIAN_POINT('Ctrl Pts',(53.8115629530877,-24.0010961794874,
40.1589996427793));
#175496=CARTESIAN_POINT('Ctrl Pts',(53.813284352634,-23.9966927326563,40.159354221642));
#175497=CARTESIAN_POINT('Ctrl Pts',(53.8150797979125,-23.9923011121675,
40.159591874311));
#175498=CARTESIAN_POINT('Ctrl Pts',(53.816875243191,-23.9879094916788,40.1598295269801));
#175499=CARTESIAN_POINT('Ctrl Pts',(53.818744735754,-23.9835296982241,40.1599502506895));
#175500=CARTESIAN_POINT('Ctrl Pts',(53.8206887816836,-23.9791663275014,
40.1599502534424));
#175501=CARTESIAN_POINT('',(53.8330634946837,-23.9513722670365,40.1599502534424));
#175502=CARTESIAN_POINT('Origin',(5.71744365443249E-15,5.22499522310014E-15,
40.1599502534424));
#175503=CARTESIAN_POINT('',(54.1275498658873,-23.7522229508829,39.8576902534424));
#175504=CARTESIAN_POINT('Ctrl Pts',(53.8330634946837,-23.9513722670365,
40.1599502534424));
#175505=CARTESIAN_POINT('Ctrl Pts',(53.8346121892503,-23.9478914369182,
40.1599502448875));
#175506=CARTESIAN_POINT('Ctrl Pts',(53.8361996036043,-23.9444392282281,
40.1598743450437));
#175507=CARTESIAN_POINT('Ctrl Pts',(53.8378239549348,-23.941016961369,40.1597243308498));
#175508=CARTESIAN_POINT('Ctrl Pts',(53.8474140023521,-23.9208121566345,
40.1588386583938));
#175509=CARTESIAN_POINT('Ctrl Pts',(53.8582911092169,-23.90164790611,40.1553722553614));
#175510=CARTESIAN_POINT('Ctrl Pts',(53.8700861059327,-23.8838022859651,
40.1496902177779));
#175511=CARTESIAN_POINT('Ctrl Pts',(53.8744923240669,-23.8771357563345,
40.1475675976837));
#175512=CARTESIAN_POINT('Ctrl Pts',(53.8790265713726,-23.8706528330371,
40.1451361443092));
#175513=CARTESIAN_POINT('Ctrl Pts',(53.8836695340509,-23.8643665485423,
40.1424159447501));
#175514=CARTESIAN_POINT('Ctrl Pts',(53.8872922064474,-23.8594616740269,
40.1402935085949));
#175515=CARTESIAN_POINT('Ctrl Pts',(53.8909810920751,-23.8546770178324,
40.1379949176048));
#175516=CARTESIAN_POINT('Ctrl Pts',(53.8947270356132,-23.8500192775332,
40.1355293609261));
#175517=CARTESIAN_POINT('Ctrl Pts',(53.9078378379964,-23.8337171864859,
40.1268999125509));
#175518=CARTESIAN_POINT('Ctrl Pts',(53.9216475915794,-23.8189698115828,
40.1162251288835));
#175519=CARTESIAN_POINT('Ctrl Pts',(53.9357638458656,-23.8060643480688,
40.1038990521418));
#175520=CARTESIAN_POINT('Ctrl Pts',(53.9428219730086,-23.7996116163119,
40.097736013771));
#175521=CARTESIAN_POINT('Ctrl Pts',(53.9499567269876,-23.7936193631242,
40.0911601532641));
#175522=CARTESIAN_POINT('Ctrl Pts',(53.9571190561826,-23.7881234899552,
40.084220729064));
#175523=CARTESIAN_POINT('Ctrl Pts',(53.9642507845244,-23.7826510977524,
40.0773109533618));
#175524=CARTESIAN_POINT('Ctrl Pts',(53.9714097802521,-23.7776706121034,
40.0700409753047));
#175525=CARTESIAN_POINT('Ctrl Pts',(53.9785478363929,-23.7732182003918,
40.0624586415899));
#175526=CARTESIAN_POINT('Ctrl Pts',(53.9785784643976,-23.7731990959628,
40.0624261072769));
#175527=CARTESIAN_POINT('Ctrl Pts',(53.9786090918658,-23.7731800007332,
40.0623935677888));
#175528=CARTESIAN_POINT('Ctrl Pts',(53.9786397187954,-23.7731609147024,
40.0623610231288));
#175529=CARTESIAN_POINT('Ctrl Pts',(53.9930827901212,-23.7641603094583,
40.0470135870242));
#175530=CARTESIAN_POINT('Ctrl Pts',(54.0073711636744,-23.757192470702,40.0305755292112));
#175531=CARTESIAN_POINT('Ctrl Pts',(54.0213615752636,-23.7521258339925,
40.0133447567369));
#175532=CARTESIAN_POINT('Ctrl Pts',(54.0358609304984,-23.7468748830087,
39.9954871626638));
#175533=CARTESIAN_POINT('Ctrl Pts',(54.0500411172136,-23.7436660552518,
39.976776795437));
#175534=CARTESIAN_POINT('Ctrl Pts',(54.0637371441607,-23.7424048061586,
39.9575197577545));
#175535=CARTESIAN_POINT('Ctrl Pts',(54.0772376980724,-23.74116155792,39.9385375612083));
#175536=CARTESIAN_POINT('Ctrl Pts',(54.0902686241836,-23.7418111396953,
39.9190226977197));
#175537=CARTESIAN_POINT('Ctrl Pts',(54.1026541040257,-23.7443079001268,
39.8992655451974));
#175538=CARTESIAN_POINT('Ctrl Pts',(54.1112894809334,-23.7460486859219,
39.8854905069405));
#175539=CARTESIAN_POINT('Ctrl Pts',(54.1196107481433,-23.7486883362829,
39.8715976051514));
#175540=CARTESIAN_POINT('Ctrl Pts',(54.1275498658873,-23.7522229508829,
39.8576902534424));
#175541=CARTESIAN_POINT('',(54.4530463244692,-23.8971395307769,39.2875012672119));
#175542=CARTESIAN_POINT('',(54.1275498658873,-23.7522229508828,39.8576902534424));
#175543=CARTESIAN_POINT('',(56.4568070719811,-18.6771643191711,39.2875012672119));
#175544=CARTESIAN_POINT('Origin',(5.53234440788222E-15,0.,39.2875012672119));
#175545=CARTESIAN_POINT('',(56.1179479440988,-18.5670586829466,39.8576902534424));
#175546=CARTESIAN_POINT('',(56.4568070719811,-18.677164319171,39.2875012672119));
#175547=CARTESIAN_POINT('',(56.0323588238391,-18.2220120550218,40.1599502534424));
#175548=CARTESIAN_POINT('Ctrl Pts',(56.1179479440988,-18.5670586829466,
39.8576902534424));
#175549=CARTESIAN_POINT('Ctrl Pts',(56.1063166059129,-18.563279281547,39.877261999407));
#175550=CARTESIAN_POINT('Ctrl Pts',(56.095331428546,-18.5576887384383,39.8967644650402));
#175551=CARTESIAN_POINT('Ctrl Pts',(56.0851270036887,-18.5504096793227,
39.9159282836095));
#175552=CARTESIAN_POINT('Ctrl Pts',(56.0747382496537,-18.5429991338175,
39.9354382707253));
#175553=CARTESIAN_POINT('Ctrl Pts',(56.0651578180728,-18.5338382654942,
39.9545987622439));
#175554=CARTESIAN_POINT('Ctrl Pts',(56.0565365037393,-18.5230039556103,
39.9731387498331));
#175555=CARTESIAN_POINT('Ctrl Pts',(56.0482801935019,-18.5126283423164,
39.990893802417));
#175556=CARTESIAN_POINT('Ctrl Pts',(56.0409028880736,-18.5007173801951,
40.008081036631));
#175557=CARTESIAN_POINT('Ctrl Pts',(56.0345558080305,-18.4872979556121,
40.0244542742679));
#175558=CARTESIAN_POINT('Ctrl Pts',(56.0295075492851,-18.4766245865907,
40.0374770090574));
#175559=CARTESIAN_POINT('Ctrl Pts',(56.0251112400292,-18.4649961406168,
40.049984877008));
#175560=CARTESIAN_POINT('Ctrl Pts',(56.0214558964133,-18.4524099188566,
40.0618424270193));
#175561=CARTESIAN_POINT('Ctrl Pts',(56.0214459185126,-18.4523755625596,
40.0618747942791));
#175562=CARTESIAN_POINT('Ctrl Pts',(56.0214359462907,-18.4523411992081,
40.0619071564124));
#175563=CARTESIAN_POINT('Ctrl Pts',(56.0214259797492,-18.4523068288034,
40.0619395134161));
#175564=CARTESIAN_POINT('Ctrl Pts',(56.019441957565,-18.4454647717814,40.0683807661799));
#175565=CARTESIAN_POINT('Ctrl Pts',(56.017700630428,-18.438311191174,40.0746073439084));
#175566=CARTESIAN_POINT('Ctrl Pts',(56.0162099386098,-18.430885810477,40.0805869293668));
#175567=CARTESIAN_POINT('Ctrl Pts',(56.0132515574632,-18.4161496282619,
40.092453830807));
#175568=CARTESIAN_POINT('Ctrl Pts',(56.0112809863294,-18.4003417300184,
40.1033475319609));
#175569=CARTESIAN_POINT('Ctrl Pts',(56.0103643682072,-18.3837652771156,
40.1130129263075));
#175570=CARTESIAN_POINT('Ctrl Pts',(56.0096769046155,-18.3713329374384,
40.1202619720674));
#175571=CARTESIAN_POINT('Ctrl Pts',(56.0095822888229,-18.3584682855073,
40.1268200947266));
#175572=CARTESIAN_POINT('Ctrl Pts',(56.0101084356844,-18.345299221126,40.1325796782703));
#175573=CARTESIAN_POINT('Ctrl Pts',(56.0103057407575,-18.340360821983,40.1347395220992));
#175574=CARTESIAN_POINT('Ctrl Pts',(56.0105903407606,-18.3353796148998,
40.1367870714852));
#175575=CARTESIAN_POINT('Ctrl Pts',(56.0109637085386,-18.3303623448493,
40.1387166518767));
#175576=CARTESIAN_POINT('Ctrl Pts',(56.0122704957614,-18.3128018996723,
40.1454701832469));
#175577=CARTESIAN_POINT('Ctrl Pts',(56.0146646833929,-18.2947996815816,
40.1507785912491));
#175578=CARTESIAN_POINT('Ctrl Pts',(56.0182094638727,-18.2766448957071,
40.1543986087265));
#175579=CARTESIAN_POINT('Ctrl Pts',(56.0199818541126,-18.2675675027699,
40.1562086174652));
#175580=CARTESIAN_POINT('Ctrl Pts',(56.0220418935343,-18.2584519681993,
40.1575965292115));
#175581=CARTESIAN_POINT('Ctrl Pts',(56.0243974853213,-18.2493344439485,
40.1585319382567));
#175582=CARTESIAN_POINT('Ctrl Pts',(56.0255752812149,-18.2447756818231,
40.1589996427793));
#175583=CARTESIAN_POINT('Ctrl Pts',(56.0268269652241,-18.2402164222853,
40.159354221642));
#175584=CARTESIAN_POINT('Ctrl Pts',(56.0281535255245,-18.2356611844172,
40.159591874311));
#175585=CARTESIAN_POINT('Ctrl Pts',(56.029480085825,-18.2311059465492,40.1598295269801));
#175586=CARTESIAN_POINT('Ctrl Pts',(56.0308815240329,-18.2265547308766,
40.1599502506895));
#175587=CARTESIAN_POINT('Ctrl Pts',(56.0323588238391,-18.2220120550218,
40.1599502534424));
#175588=CARTESIAN_POINT('',(56.0417604764383,-18.193076743595,40.1599502534424));
#175589=CARTESIAN_POINT('Origin',(5.71999943999309E-15,5.23165327211576E-15,
40.1599502534424));
#175590=CARTESIAN_POINT('',(56.3138168485095,-17.9642361803973,39.8576902534424));
#175591=CARTESIAN_POINT('Ctrl Pts',(56.0417604764383,-18.193076743595,40.1599502534424));
#175592=CARTESIAN_POINT('Ctrl Pts',(56.0429368412708,-18.1894530991651,
40.1599502448875));
#175593=CARTESIAN_POINT('Ctrl Pts',(56.0441547055336,-18.1858538720524,
40.1598743450437));
#175594=CARTESIAN_POINT('Ctrl Pts',(56.0454124342019,-18.1822805617809,
40.1597243308499));
#175595=CARTESIAN_POINT('Ctrl Pts',(56.0528379691473,-18.1611840081594,
40.1588386583937));
#175596=CARTESIAN_POINT('Ctrl Pts',(56.0616522804266,-18.1409877741371,
40.1553722553607));
#175597=CARTESIAN_POINT('Ctrl Pts',(56.0715172876677,-18.1220070012839,
40.1496902177761));
#175598=CARTESIAN_POINT('Ctrl Pts',(56.0752025259794,-18.1149164163918,
40.1475675976823));
#175599=CARTESIAN_POINT('Ctrl Pts',(56.0790342841932,-18.1079950493255,
40.1451361443084));
#175600=CARTESIAN_POINT('Ctrl Pts',(56.0829947165771,-18.101257880003,40.1424159447501));
#175601=CARTESIAN_POINT('Ctrl Pts',(56.0860848445996,-18.096001202525,40.1402935085949));
#175602=CARTESIAN_POINT('Ctrl Pts',(56.0892533893665,-18.0908571636319,
40.1379949176048));
#175603=CARTESIAN_POINT('Ctrl Pts',(56.0924919457982,-18.0858333811998,
40.1355293609261));
#175604=CARTESIAN_POINT('Ctrl Pts',(56.103826893309,-18.0682501426877,40.1268999125509));
#175605=CARTESIAN_POINT('Ctrl Pts',(56.1160194751811,-18.0521400431272,
40.1162251288835));
#175606=CARTESIAN_POINT('Ctrl Pts',(56.1287094108803,-18.0378297267251,
40.1038990521418));
#175607=CARTESIAN_POINT('Ctrl Pts',(56.13505437873,-18.0306745685241,40.097736013771));
#175608=CARTESIAN_POINT('Ctrl Pts',(56.1415236867628,-18.0239693566571,
40.0911601532641));
#175609=CARTESIAN_POINT('Ctrl Pts',(56.1480723047925,-18.0177549231922,
40.084220729064));
#175610=CARTESIAN_POINT('Ctrl Pts',(56.1545929440329,-18.0115670407224,
40.0773109533618));
#175611=CARTESIAN_POINT('Ctrl Pts',(56.1611921195217,-18.005865519873,40.0700409753047));
#175612=CARTESIAN_POINT('Ctrl Pts',(56.1678256688901,-18.0006913688995,
40.0624586415899));
#175613=CARTESIAN_POINT('Ctrl Pts',(56.1678541321547,-18.0006691676283,
40.0624261072769));
#175614=CARTESIAN_POINT('Ctrl Pts',(56.1678825958474,-18.0006469755621,
40.0623935677888));
#175615=CARTESIAN_POINT('Ctrl Pts',(56.167911059966,-18.0006247927008,40.0623610231288));
#175616=CARTESIAN_POINT('Ctrl Pts',(56.1813341912004,-17.9901637816641,
40.0470135870252));
#175617=CARTESIAN_POINT('Ctrl Pts',(56.1948159540698,-17.9817405717279,
40.0305755292134));
#175618=CARTESIAN_POINT('Ctrl Pts',(56.2082001169704,-17.9752392943607,
40.0133447567403));
#175619=CARTESIAN_POINT('Ctrl Pts',(56.2220711693822,-17.9685015133149,
39.9954871626685));
#175620=CARTESIAN_POINT('Ctrl Pts',(56.2358382617157,-17.963828030726,39.9767767954431));
#175621=CARTESIAN_POINT('Ctrl Pts',(56.2493274239639,-17.9611420662373,
39.957519757762));
#175622=CARTESIAN_POINT('Ctrl Pts',(56.2626240656001,-17.9584944364886,
39.938537561217));
#175623=CARTESIAN_POINT('Ctrl Pts',(56.2756515067187,-17.9577783571049,
39.9190226977296));
#175624=CARTESIAN_POINT('Ctrl Pts',(56.2882301201368,-17.9589668048461,
39.8992655452086));
#175625=CARTESIAN_POINT('Ctrl Pts',(56.2970001532129,-17.9597954117562,
39.885490506948));
#175626=CARTESIAN_POINT('Ctrl Pts',(56.3055517542485,-17.9615507925628,
39.8715976051552));
#175627=CARTESIAN_POINT('Ctrl Pts',(56.3138168485095,-17.9642361803973,
39.8576902534424));
#175628=CARTESIAN_POINT('',(56.6526781108323,-18.0743352474892,39.2875012672119));
#175629=CARTESIAN_POINT('',(56.3138168485095,-17.9642361803973,39.8576902534424));
#175630=CARTESIAN_POINT('',(58.099826060148,-12.6735055745741,39.2875012672119));
#175631=CARTESIAN_POINT('Origin',(5.53234440788222E-15,0.,39.2875012672119));
#175632=CARTESIAN_POINT('',(57.751314065072,-12.5994235324472,39.8576902534424));
#175633=CARTESIAN_POINT('',(58.099826060148,-12.6735055745741,39.2875012672119));
#175634=CARTESIAN_POINT('',(57.6301266171957,-12.2652136052661,40.1599502534424));
#175635=CARTESIAN_POINT('Ctrl Pts',(57.751314065072,-12.5994235324472,39.8576902534424));
#175636=CARTESIAN_POINT('Ctrl Pts',(57.7393513895544,-12.5968806409106,
39.8772619994052));
#175637=CARTESIAN_POINT('Ctrl Pts',(57.7278420192595,-12.5924689870915,
39.8967644650367));
#175638=CARTESIAN_POINT('Ctrl Pts',(57.7169326264468,-12.5862964562731,
39.9159282836043));
#175639=CARTESIAN_POINT('Ctrl Pts',(57.7058261701605,-12.580012427007,39.9354382707184));
#175640=CARTESIAN_POINT('Ctrl Pts',(57.695340649699,-12.5719031706707,39.9545987622355));
#175641=CARTESIAN_POINT('Ctrl Pts',(57.6856340700653,-12.5620293850099,
39.9731387498233));
#175642=CARTESIAN_POINT('Ctrl Pts',(57.6763384418466,-12.5525736298339,
39.9908938024062));
#175643=CARTESIAN_POINT('Ctrl Pts',(57.667756515503,-12.5414990556102,40.0080810366192));
#175644=CARTESIAN_POINT('Ctrl Pts',(57.660041493599,-12.528816594564,40.0244542742554));
#175645=CARTESIAN_POINT('Ctrl Pts',(57.6539052188793,-12.5187293821012,
40.0374770090494));
#175646=CARTESIAN_POINT('Ctrl Pts',(57.6483174894756,-12.5076241774183,
40.0499848770042));
#175647=CARTESIAN_POINT('Ctrl Pts',(57.643366551794,-12.4954889917448,40.0618424270193));
#175648=CARTESIAN_POINT('Ctrl Pts',(57.6433530373424,-12.4954558666298,
40.0618747942791));
#175649=CARTESIAN_POINT('Ctrl Pts',(57.643339527801,-12.4954227339055,40.0619071564124));
#175650=CARTESIAN_POINT('Ctrl Pts',(57.6433260231716,-12.4953895935727,
40.0619395134161));
#175651=CARTESIAN_POINT('Ctrl Pts',(57.6406376799625,-12.4887924048449,
40.0683807661799));
#175652=CARTESIAN_POINT('Ctrl Pts',(57.63815813921,-12.4818600305503,40.0746073439084));
#175653=CARTESIAN_POINT('Ctrl Pts',(57.6358994499241,-12.4746311465906,
40.0805869293669));
#175654=CARTESIAN_POINT('Ctrl Pts',(57.6314169246176,-12.4602849257587,
40.092453830807));
#175655=CARTESIAN_POINT('Ctrl Pts',(57.6278047731677,-12.444769605608,40.1033475319609));
#175656=CARTESIAN_POINT('Ctrl Pts',(57.6251604652272,-12.4283797729324,
40.1130129263075));
#175657=CARTESIAN_POINT('Ctrl Pts',(57.6231772342717,-12.4160873984256,
40.1202619720674));
#175658=CARTESIAN_POINT('Ctrl Pts',(57.6217384144975,-12.4033031104472,
40.1268200947266));
#175659=CARTESIAN_POINT('Ctrl Pts',(57.620885137009,-12.3901511902556,40.1325796782703));
#175660=CARTESIAN_POINT('Ctrl Pts',(57.6205651579508,-12.3852192201837,
40.1347395220992));
#175661=CARTESIAN_POINT('Ctrl Pts',(57.6203275209637,-12.3802355518732,
40.1367870714852));
#175662=CARTESIAN_POINT('Ctrl Pts',(57.6201743958657,-12.3752067393928,
40.1387166518767));
#175663=CARTESIAN_POINT('Ctrl Pts',(57.6196384580227,-12.3576058957117,
40.1454701832469));
#175664=CARTESIAN_POINT('Ctrl Pts',(57.6201377858514,-12.3394520349014,
40.1507785912492));
#175665=CARTESIAN_POINT('Ctrl Pts',(57.6217654557845,-12.3210261723874,
40.1543986087265));
#175666=CARTESIAN_POINT('Ctrl Pts',(57.622579290751,-12.3118132411303,40.1562086174652));
#175667=CARTESIAN_POINT('Ctrl Pts',(57.6236752122407,-12.3025323096568,
40.1575965292115));
#175668=CARTESIAN_POINT('Ctrl Pts',(57.6250648590507,-12.2932185057683,
40.1585319382567));
#175669=CARTESIAN_POINT('Ctrl Pts',(57.6257596824557,-12.2885616038241,
40.1589996427793));
#175670=CARTESIAN_POINT('Ctrl Pts',(57.6265279372158,-12.2838964837811,
40.159354221642));
#175671=CARTESIAN_POINT('Ctrl Pts',(57.627371078466,-12.279227536673,40.159591874311));
#175672=CARTESIAN_POINT('Ctrl Pts',(57.6282142197162,-12.274558589565,40.1598295269801));
#175673=CARTESIAN_POINT('Ctrl Pts',(57.6291322491186,-12.2698858157459,
40.1599502506895));
#175674=CARTESIAN_POINT('Ctrl Pts',(57.6301266171957,-12.2652136052661,
40.1599502534424));
#175675=CARTESIAN_POINT('',(57.6364522029207,-12.2354540642045,40.1599502534424));
#175676=CARTESIAN_POINT('Origin',(5.72184526906101E-15,5.23854199997932E-15,
40.1599502534424));
#175677=CARTESIAN_POINT('',(57.8830978693156,-11.9794294790612,39.8576902534424));
#175678=CARTESIAN_POINT('Ctrl Pts',(57.6364522029207,-12.2354540642045,
40.1599502534424));
#175679=CARTESIAN_POINT('Ctrl Pts',(57.6372433495199,-12.2317273068698,
40.1599502448874));
#175680=CARTESIAN_POINT('Ctrl Pts',(57.6380783205158,-12.2280204952199,
40.1598743450437));
#175681=CARTESIAN_POINT('Ctrl Pts',(57.6389556465834,-12.2243352914711,
40.1597243308498));
#175682=CARTESIAN_POINT('Ctrl Pts',(57.6441353133399,-12.2025781272258,
40.1588386583939));
#175683=CARTESIAN_POINT('Ctrl Pts',(57.6507902575918,-12.1815711838785,
40.1553722553622));
#175684=CARTESIAN_POINT('Ctrl Pts',(57.6586171922707,-12.161663215642,40.14969021778));
#175685=CARTESIAN_POINT('Ctrl Pts',(57.6615410745205,-12.1542262614136,
40.1475675976853));
#175686=CARTESIAN_POINT('Ctrl Pts',(57.6646283621005,-12.1469422825181,
40.1451361443101));
#175687=CARTESIAN_POINT('Ctrl Pts',(57.6678628728673,-12.1398280421987,
40.1424159447501));
#175688=CARTESIAN_POINT('Ctrl Pts',(57.6703866004265,-12.1342771550164,
40.1402935085949));
#175689=CARTESIAN_POINT('Ctrl Pts',(57.6730000890933,-12.1288300925913,
40.1379949176047));
#175690=CARTESIAN_POINT('Ctrl Pts',(57.6756957761165,-12.1234953096381,
40.1355293609261));
#175691=CARTESIAN_POINT('Ctrl Pts',(57.6851306806979,-12.1048235693018,
40.1268999125508));
#175692=CARTESIAN_POINT('Ctrl Pts',(57.6955725063806,-12.087527250706,40.1162251288835));
#175693=CARTESIAN_POINT('Ctrl Pts',(57.7066970899019,-12.0719688682368,
40.1038990521418));
#175694=CARTESIAN_POINT('Ctrl Pts',(57.7122593816626,-12.0641896770022,
40.0977360137709));
#175695=CARTESIAN_POINT('Ctrl Pts',(57.7179923646568,-12.0568449701604,
40.0911601532641));
#175696=CARTESIAN_POINT('Ctrl Pts',(57.7238555234916,-12.0499800630331,
40.084220729064));
#175697=CARTESIAN_POINT('Ctrl Pts',(57.7296936321425,-12.0431444860316,
40.0773109533618));
#175698=CARTESIAN_POINT('Ctrl Pts',(57.7356606854448,-12.0367843970373,
40.0700409753048));
#175699=CARTESIAN_POINT('Ctrl Pts',(57.7417170494857,-12.0309451958827,
40.0624586415899));
#175700=CARTESIAN_POINT('Ctrl Pts',(57.7417430361609,-12.0309201410111,
40.0624261072769));
#175701=CARTESIAN_POINT('Ctrl Pts',(57.7417690242238,-12.0308950952493,
40.0623935677888));
#175702=CARTESIAN_POINT('Ctrl Pts',(57.7417950136727,-12.0308700585974,
40.0623610231288));
#175703=CARTESIAN_POINT('Ctrl Pts',(57.7540511381846,-12.0190632547909,
40.0470135870217));
#175704=CARTESIAN_POINT('Ctrl Pts',(57.7665785813589,-12.0092769601233,
40.0305755292058));
#175705=CARTESIAN_POINT('Ctrl Pts',(57.7792098558853,-12.0014122714526,
40.0133447567283));
#175706=CARTESIAN_POINT('Ctrl Pts',(57.7923006313251,-11.993261480883,39.9954871626521));
#175707=CARTESIAN_POINT('Ctrl Pts',(57.8055037941362,-11.9871745471154,
39.9767767954219));
#175708=CARTESIAN_POINT('Ctrl Pts',(57.8186383016047,-11.9830932952215,
39.9575197577359));
#175709=CARTESIAN_POINT('Ctrl Pts',(57.8315853501805,-11.9790702919497,
39.9385375611865));
#175710=CARTESIAN_POINT('Ctrl Pts',(57.8444665749385,-11.9769963969252,
39.9190226976948));
#175711=CARTESIAN_POINT('Ctrl Pts',(57.8571005080145,-11.9768635110972,
39.8992655451694));
#175712=CARTESIAN_POINT('Ctrl Pts',(57.8659091109301,-11.9767708607337,
39.8854905069217));
#175713=CARTESIAN_POINT('Ctrl Pts',(57.8745973526502,-11.9776227396658,
39.871597605142));
#175714=CARTESIAN_POINT('Ctrl Pts',(57.8830978693156,-11.9794294790612,
39.8576902534424));
#175715=CARTESIAN_POINT('',(58.2316113004781,-12.0535047649322,39.2875012672119));
#175716=CARTESIAN_POINT('',(57.8830978693156,-11.9794294790612,39.8576902534424));
#175717=CARTESIAN_POINT('',(59.1062911958296,-6.53099325080055,39.2875012672119));
#175718=CARTESIAN_POINT('Origin',(5.53234440788222E-15,0.,39.2875012672119));
#175719=CARTESIAN_POINT('',(58.7519447039088,-6.4937464611274,39.8576902534424));
#175720=CARTESIAN_POINT('',(59.1062911958296,-6.53099325080055,39.2875012672119));
#175721=CARTESIAN_POINT('',(58.5964866834551,-6.1740349085902,40.1599502534424));
#175722=CARTESIAN_POINT('Ctrl Pts',(58.7519447039088,-6.49374646112741,
39.8576902534424));
#175723=CARTESIAN_POINT('Ctrl Pts',(58.7397817566352,-6.49246793990524,
39.8772619994045));
#175724=CARTESIAN_POINT('Ctrl Pts',(58.7278742924813,-6.48928351037763,
39.8967644650353));
#175725=CARTESIAN_POINT('Ctrl Pts',(58.7163794573033,-6.48428513539508,
39.9159282836023));
#175726=CARTESIAN_POINT('Ctrl Pts',(58.7046769834247,-6.47919647150708,
39.9354382707158));
#175727=CARTESIAN_POINT('Ctrl Pts',(58.6934012556386,-6.47222767386624,
39.9545987622323));
#175728=CARTESIAN_POINT('Ctrl Pts',(58.6827157580223,-6.4634225916897,39.9731387498196));
#175729=CARTESIAN_POINT('Ctrl Pts',(58.6724826566703,-6.4549902938632,39.9908938024019));
#175730=CARTESIAN_POINT('Ctrl Pts',(58.6627901347925,-6.44487344288915,
40.0080810366144));
#175731=CARTESIAN_POINT('Ctrl Pts',(58.6537916984223,-6.43306689707603,
40.0244542742501));
#175732=CARTESIAN_POINT('Ctrl Pts',(58.6466346380391,-6.42367635878418,
40.037477009046));
#175733=CARTESIAN_POINT('Ctrl Pts',(58.639916708821,-6.413216066341,40.0499848770026));
#175734=CARTESIAN_POINT('Ctrl Pts',(58.6337244205833,-6.40166487239037,
40.0618424270193));
#175735=CARTESIAN_POINT('Ctrl Pts',(58.6337075176478,-6.40163334138309,
40.0618747942791));
#175736=CARTESIAN_POINT('Ctrl Pts',(58.6336906188004,-6.40160180229485,
40.0619071564124));
#175737=CARTESIAN_POINT('Ctrl Pts',(58.6336737240427,-6.40157025512642,
40.0619395134161));
#175738=CARTESIAN_POINT('Ctrl Pts',(58.6303105138594,-6.39529021487321,
40.0683807661799));
#175739=CARTESIAN_POINT('Ctrl Pts',(58.6271199258587,-6.38865499943471,
40.0746073439084));
#175740=CARTESIAN_POINT('Ctrl Pts',(58.6241179857776,-6.38170181337784,
40.0805869293669));
#175741=CARTESIAN_POINT('Ctrl Pts',(58.6181604277966,-6.36790273412649,
40.092453830807));
#175742=CARTESIAN_POINT('Ctrl Pts',(58.6129462715178,-6.35284998116321,
40.1033475319609));
#175743=CARTESIAN_POINT('Ctrl Pts',(58.60860324535,-6.33682633915125,40.1130129263075));
#175744=CARTESIAN_POINT('Ctrl Pts',(58.6053459757242,-6.32480860764228,
40.1202619720674));
#175745=CARTESIAN_POINT('Ctrl Pts',(58.6025787159788,-6.31224475095104,
40.1268200947266));
#175746=CARTESIAN_POINT('Ctrl Pts',(58.600355362827,-6.2992540701389,40.1325796782703));
#175747=CARTESIAN_POINT('Ctrl Pts',(58.5995216053951,-6.29438256483434,
40.1347395220992));
#175748=CARTESIAN_POINT('Ctrl Pts',(58.5987643350184,-6.28945103740937,
40.1367870714852));
#175749=CARTESIAN_POINT('Ctrl Pts',(58.5980863947151,-6.28446577922116,
40.1387166518766));
#175750=CARTESIAN_POINT('Ctrl Pts',(58.5957136036535,-6.26701737556243,
40.1454701832468));
#175751=CARTESIAN_POINT('Ctrl Pts',(58.5943126009392,-6.24891076953056,
40.1507785912491));
#175752=CARTESIAN_POINT('Ctrl Pts',(58.5940053272331,-6.23041570798245,
40.1543986087265));
#175753=CARTESIAN_POINT('Ctrl Pts',(58.59385169038,-6.2211681772084,40.1562086174652));
#175754=CARTESIAN_POINT('Ctrl Pts',(58.5939714867925,-6.21182353265943,
40.1575965292115));
#175755=CARTESIAN_POINT('Ctrl Pts',(58.5943799633642,-6.20241549311763,
40.1585319382567));
#175756=CARTESIAN_POINT('Ctrl Pts',(58.5945842016501,-6.19771147334672,
40.1589996427793));
#175757=CARTESIAN_POINT('Ctrl Pts',(58.5948606100012,-6.19299160482992,
40.159354221642));
#175758=CARTESIAN_POINT('Ctrl Pts',(58.5952110945691,-6.18826010244349,
40.159591874311));
#175759=CARTESIAN_POINT('Ctrl Pts',(58.595561579137,-6.18352860005705,40.1598295269801));
#175760=CARTESIAN_POINT('Ctrl Pts',(58.5959861416119,-6.17878546397913,
40.1599502506895));
#175761=CARTESIAN_POINT('Ctrl Pts',(58.5964866834551,-6.1740349085902,40.1599502534424));
#175762=CARTESIAN_POINT('',(58.5996668978648,-6.14377718965322,40.1599502534424));
#175763=CARTESIAN_POINT('Origin',(5.72296091834672E-15,5.2455859323468E-15,
40.1599502534424));
#175764=CARTESIAN_POINT('',(58.8181995570485,-5.86337364149581,39.8576902534424));
#175765=CARTESIAN_POINT('Ctrl Pts',(58.5996668978648,-6.14377718965322,
40.1599502534424));
#175766=CARTESIAN_POINT('Ctrl Pts',(58.600064158263,-6.13998815054686,40.1599502448875));
#175767=CARTESIAN_POINT('Ctrl Pts',(58.6005070878751,-6.13621436696404,
40.1598743450437));
#175768=CARTESIAN_POINT('Ctrl Pts',(58.600994399174,-6.13245764560126,40.1597243308498));
#175769=CARTESIAN_POINT('Ctrl Pts',(58.6038714482307,-6.11027824676979,
40.1588386583938));
#175770=CARTESIAN_POINT('Ctrl Pts',(58.6082941124962,-6.08869075055824,
40.1553722553616));
#175771=CARTESIAN_POINT('Ctrl Pts',(58.6139972210823,-6.0680737027988,40.1496902177783));
#175772=CARTESIAN_POINT('Ctrl Pts',(58.6161277126018,-6.06037186006759,
40.147567597684));
#175773=CARTESIAN_POINT('Ctrl Pts',(58.6184367045765,-6.05280507414621,
40.1451361443094));
#175774=CARTESIAN_POINT('Ctrl Pts',(58.6209098557463,-6.04539170794176,
40.1424159447501));
#175775=CARTESIAN_POINT('Ctrl Pts',(58.6228395323549,-6.03960742773678,
40.1402935085949));
#175776=CARTESIAN_POINT('Ctrl Pts',(58.6248693309927,-6.03391702093548,
40.1379949176048));
#175777=CARTESIAN_POINT('Ctrl Pts',(58.6269926140964,-6.02832968645946,
40.1355293609261));
#175778=CARTESIAN_POINT('Ctrl Pts',(58.6344241049594,-6.0087740157934,40.1268999125508));
#175779=CARTESIAN_POINT('Ctrl Pts',(58.6430007716254,-5.99048098024828,
40.1162251288835));
#175780=CARTESIAN_POINT('Ctrl Pts',(58.6524381197038,-5.97384499260622,
40.1038990521418));
#175781=CARTESIAN_POINT('Ctrl Pts',(58.657156793743,-5.9655269987852,40.0977360137709));
#175782=CARTESIAN_POINT('Ctrl Pts',(58.6620906399372,-5.95762326711356,
40.0911601532641));
#175783=CARTESIAN_POINT('Ctrl Pts',(58.667204101582,-5.95018309968293,40.084220729064));
#175784=CARTESIAN_POINT('Ctrl Pts',(58.6722957161033,-5.94277472016181,
40.0773109533618));
#175785=CARTESIAN_POINT('Ctrl Pts',(58.6775652709345,-5.93582574548853,
40.0700409753048));
#175786=CARTESIAN_POINT('Ctrl Pts',(58.682978094856,-5.92938546966269,40.0624586415899));
#175787=CARTESIAN_POINT('Ctrl Pts',(58.6830013202262,-5.92935783569705,
40.0624261072769));
#175788=CARTESIAN_POINT('Ctrl Pts',(58.6830245479289,-5.92933021064629,
40.0623935677888));
#175789=CARTESIAN_POINT('Ctrl Pts',(58.6830477779621,-5.92930259451062,
40.0623610231288));
#175790=CARTESIAN_POINT('Ctrl Pts',(58.6940026150818,-5.91627935575194,
40.0470135870241));
#175791=CARTESIAN_POINT('Ctrl Pts',(58.7054384852671,-5.90523719704834,
40.030575529211));
#175792=CARTESIAN_POINT('Ctrl Pts',(58.7171784805271,-5.89609526425064,
40.0133447567366));
#175793=CARTESIAN_POINT('Ctrl Pts',(58.7293455537148,-5.8866207659257,39.9954871626633));
#175794=CARTESIAN_POINT('Ctrl Pts',(58.7418401303837,-5.87918707069946,
39.9767767954363));
#175795=CARTESIAN_POINT('Ctrl Pts',(58.7544760786554,-5.87375524644868,
39.9575197577536));
#175796=CARTESIAN_POINT('Ctrl Pts',(58.7669316835929,-5.86840094651774,
39.938537561207));
#175797=CARTESIAN_POINT('Ctrl Pts',(58.7795255625923,-5.86499195787722,
39.9190226977181));
#175798=CARTESIAN_POINT('Ctrl Pts',(58.792076395308,-5.86353919440062,39.8992655451955));
#175799=CARTESIAN_POINT('Ctrl Pts',(58.8008270591807,-5.86252630185729,
39.8854905069393));
#175800=CARTESIAN_POINT('Ctrl Pts',(58.8095567514049,-5.86246534555135,
39.8715976051508));
#175801=CARTESIAN_POINT('Ctrl Pts',(58.8181995570485,-5.86337364149584,
39.8576902534424));
#175802=CARTESIAN_POINT('',(59.1725467709677,-5.90061356181257,39.2875012672119));
#175803=CARTESIAN_POINT('',(58.8181995570485,-5.8633736414958,39.8576902534424));
#175804=CARTESIAN_POINT('',(59.4651754363832,-0.316925998273047,39.2875012672119));
#175805=CARTESIAN_POINT('Origin',(5.53234440788222E-15,0.,39.2875012672119));
#175806=CARTESIAN_POINT('',(59.1088767419348,-0.316922544675689,39.8576902534424));
#175807=CARTESIAN_POINT('',(59.4651754363832,-0.316925998273047,39.2875012672119));
#175808=CARTESIAN_POINT('',(58.9208513795073,-0.0152121934559198,40.1599502534424));
#175809=CARTESIAN_POINT('Ctrl Pts',(59.1088767419348,-0.316922544675689,
39.8576902534424));
#175810=CARTESIAN_POINT('Ctrl Pts',(59.0966467826998,-0.316922401513862,
39.8772619994055));
#175811=CARTESIAN_POINT('Ctrl Pts',(59.0844716853548,-0.315000085553629,
39.8967644650373));
#175812=CARTESIAN_POINT('Ctrl Pts',(59.0725173476303,-0.311230629648508,
39.9159282836053));
#175813=CARTESIAN_POINT('Ctrl Pts',(59.0603470709112,-0.307393083604294,
39.9354382707198));
#175814=CARTESIAN_POINT('Ctrl Pts',(59.0484046750329,-0.301641096263203,
39.9545987622372));
#175815=CARTESIAN_POINT('Ctrl Pts',(59.0368573319812,-0.294001187892417,
39.9731387498253));
#175816=CARTESIAN_POINT('Ctrl Pts',(59.0257988734949,-0.286684733433703,
39.9908938024085));
#175817=CARTESIAN_POINT('Ctrl Pts',(59.0151019493803,-0.277636448043934,
40.0080810366218));
#175818=CARTESIAN_POINT('Ctrl Pts',(59.0049186872952,-0.266835172448542,
40.0244542742581));
#175819=CARTESIAN_POINT('Ctrl Pts',(58.9968192555025,-0.258244193032669,
40.0374770090511));
#175820=CARTESIAN_POINT('Ctrl Pts',(58.9890447295109,-0.248543417985227,
40.049984877005));
#175821=CARTESIAN_POINT('Ctrl Pts',(58.981678934725,-0.237702773059495,
40.0618424270192));
#175822=CARTESIAN_POINT('Ctrl Pts',(58.9816588284979,-0.237673181620236,
40.0618747942791));
#175823=CARTESIAN_POINT('Ctrl Pts',(58.9816387254916,-0.237643581716976,
40.0619071564124));
#175824=CARTESIAN_POINT('Ctrl Pts',(58.9816186257082,-0.237613973350289,
40.0619395134161));
#175825=CARTESIAN_POINT('Ctrl Pts',(58.9776173965852,-0.231719887006783,
40.0683807661799));
#175826=CARTESIAN_POINT('Ctrl Pts',(58.9737507180862,-0.225454527233356,
40.0746073439084));
#175827=CARTESIAN_POINT('Ctrl Pts',(58.9700384170936,-0.218853219640725,
40.0805869293669));
#175828=CARTESIAN_POINT('Ctrl Pts',(58.9626710986899,-0.205752467569922,
40.092453830807));
#175829=CARTESIAN_POINT('Ctrl Pts',(58.9559120649696,-0.191327202905425,
40.1033475319609));
#175830=CARTESIAN_POINT('Ctrl Pts',(58.9499179036781,-0.175845309932244,
40.1130129263075));
#175831=CARTESIAN_POINT('Ctrl Pts',(58.9454222827095,-0.164233890202358,
40.1202619720674));
#175832=CARTESIAN_POINT('Ctrl Pts',(58.9413569016699,-0.152028117041295,
40.1268200947266));
#175833=CARTESIAN_POINT('Ctrl Pts',(58.9377878323772,-0.139341004226136,
40.1325796782703));
#175834=CARTESIAN_POINT('Ctrl Pts',(58.9364494313924,-0.134583336920451,
40.1347395220992));
#175835=CARTESIAN_POINT('Ctrl Pts',(58.9351808244388,-0.12975798122746,
40.1367870714852));
#175836=CARTESIAN_POINT('Ctrl Pts',(58.933985496586,-0.124870896863315,
40.1387166518767));
#175837=CARTESIAN_POINT('Ctrl Pts',(58.9298018491012,-0.107766101588806,
40.1454701832469));
#175838=CARTESIAN_POINT('Ctrl Pts',(58.9265158655229,-0.0899051301000603,
40.1507785912492));
#175839=CARTESIAN_POINT('Ctrl Pts',(58.9242770147326,-0.0715435052825847,
40.1543986087265));
#175840=CARTESIAN_POINT('Ctrl Pts',(58.9231575893375,-0.0623626928738469,
40.1562086174652));
#175841=CARTESIAN_POINT('Ctrl Pts',(58.9222999481582,-0.0530567171305711,
40.1575965292115));
#175842=CARTESIAN_POINT('Ctrl Pts',(58.9217227791368,-0.043657518385426,
40.1585319382567));
#175843=CARTESIAN_POINT('Ctrl Pts',(58.9214341946262,-0.0389579190128535,
40.1589996427793));
#175844=CARTESIAN_POINT('Ctrl Pts',(58.9212157281805,-0.0342350138894578,
40.159354221642));
#175845=CARTESIAN_POINT('Ctrl Pts',(58.9210697160839,-0.0294927955548823,
40.159591874311));
#175846=CARTESIAN_POINT('Ctrl Pts',(58.9209237039872,-0.0247505772203069,
40.1598295269801));
#175847=CARTESIAN_POINT('Ctrl Pts',(58.9208501479391,-0.0199890456750397,
40.1599502506895));
#175848=CARTESIAN_POINT('Ctrl Pts',(58.9208513795073,-0.0152121934559204,
40.1599502534424));
#175849=CARTESIAN_POINT('',(58.9208533432504,-7.21572344498422E-15,40.1599502534424));
#175850=CARTESIAN_POINT('Origin',(4.7062627014205E-16,0.,40.1599502534424));
#175851=CARTESIAN_POINT('',(58.6605641730809,-7.18384721507414E-15,40.5765));
#175852=CARTESIAN_POINT('',(58.9208513795073,0.0152121934559198,40.1599502534424));
#175853=CARTESIAN_POINT('Origin',(4.7062627014205E-16,0.,40.1599502534424));
#175854=CARTESIAN_POINT('',(59.1088767419348,0.316922544675676,39.8576902534424));
#175855=CARTESIAN_POINT('Ctrl Pts',(58.9208513795073,0.0152121934559198,
40.1599502534424));
#175856=CARTESIAN_POINT('Ctrl Pts',(58.9208504012364,0.0190220008285439,
40.1599502448875));
#175857=CARTESIAN_POINT('Ctrl Pts',(58.9208964366351,0.0228214099817244,
40.1598743450437));
#175858=CARTESIAN_POINT('Ctrl Pts',(58.9209883940807,0.0266084895330077,
40.1597243308498));
#175859=CARTESIAN_POINT('Ctrl Pts',(58.9215313038857,0.0489671208154066,
40.1588386583937));
#175860=CARTESIAN_POINT('Ctrl Pts',(58.9236732325291,0.0708986527648728,
40.155372255361));
#175861=CARTESIAN_POINT('Ctrl Pts',(58.9271900305707,0.0919988953573648,
40.149690217777));
#175862=CARTESIAN_POINT('Ctrl Pts',(58.9285037892496,0.0998812435910838,
40.147567597683));
#175863=CARTESIAN_POINT('Ctrl Pts',(58.93000918782,0.107647933248606,40.1451361443088));
#175864=CARTESIAN_POINT('Ctrl Pts',(58.9316938830317,0.115279202946934,
40.1424159447501));
#175865=CARTESIAN_POINT('Ctrl Pts',(58.933008366749,0.121233502390237,40.1402935085949));
#175866=CARTESIAN_POINT('Ctrl Pts',(58.9344322364591,0.127104908280027,
40.1379949176047));
#175867=CARTESIAN_POINT('Ctrl Pts',(58.9359598525093,0.132883578273087,
40.1355293609261));
#175868=CARTESIAN_POINT('Ctrl Pts',(58.9413065086849,0.153108923248799,
40.1268999125508));
#175869=CARTESIAN_POINT('Ctrl Pts',(58.9479240485795,0.172198253417729,
40.1162251288835));
#175870=CARTESIAN_POINT('Ctrl Pts',(58.9555707636545,0.189729578870784,
40.1038990521418));
#175871=CARTESIAN_POINT('Ctrl Pts',(58.959394121192,0.198495241597312,40.0977360137709));
#175872=CARTESIAN_POINT('Ctrl Pts',(58.9634747743348,0.206871403160556,
40.0911601532641));
#175873=CARTESIAN_POINT('Ctrl Pts',(58.9677825146337,0.214805314863219,
40.084220729064));
#175874=CARTESIAN_POINT('Ctrl Pts',(58.9720718502312,0.222705329147635,
40.0773109533618));
#175875=CARTESIAN_POINT('Ctrl Pts',(58.9765861722458,0.230167055079184,
40.0700409753048));
#175876=CARTESIAN_POINT('Ctrl Pts',(58.9812961520165,0.237137844566655,
40.0624586415899));
#175877=CARTESIAN_POINT('Ctrl Pts',(58.9813163616197,0.237167754862796,
40.0624261072769));
#175878=CARTESIAN_POINT('Ctrl Pts',(58.9813365744745,0.237197656536702,
40.0623935677888));
#175879=CARTESIAN_POINT('Ctrl Pts',(58.9813567905789,0.237227549587952,
40.0623610231288));
#175880=CARTESIAN_POINT('Ctrl Pts',(58.9908903168209,0.251324537972177,
40.0470135870234));
#175881=CARTESIAN_POINT('Ctrl Pts',(59.0011093202327,0.263501580512099,
40.0305755292095));
#175882=CARTESIAN_POINT('Ctrl Pts',(59.0118294103843,0.27382059650901,40.0133447567343));
#175883=CARTESIAN_POINT('Ctrl Pts',(59.0229394763223,0.284514998003889,
39.9954871626602));
#175884=CARTESIAN_POINT('Ctrl Pts',(59.0345885736552,0.293214009568411,
39.9767767954322));
#175885=CARTESIAN_POINT('Ctrl Pts',(59.046587520639,0.299936893972332,39.9575197577486));
#175886=CARTESIAN_POINT('Ctrl Pts',(59.0584152157263,0.306563827731132,
39.9385375612012));
#175887=CARTESIAN_POINT('Ctrl Pts',(59.0705837677954,0.311270560393325,
39.9190226977114));
#175888=CARTESIAN_POINT('Ctrl Pts',(59.0829139906031,0.314027284735693,
39.899265545188));
#175889=CARTESIAN_POINT('Ctrl Pts',(59.0915108413209,0.315949321994159,
39.8854905069342));
#175890=CARTESIAN_POINT('Ctrl Pts',(59.1001863397071,0.316922445687698,
39.8715976051483));
#175891=CARTESIAN_POINT('Ctrl Pts',(59.1088767419348,0.316922544675652,
39.8576902534424));
#175892=CARTESIAN_POINT('',(59.4651754363832,0.316925998273047,39.2875012672119));
#175893=CARTESIAN_POINT('',(59.1088767419348,0.316922544675689,39.8576902534424));
#175894=CARTESIAN_POINT('',(59.1725467709678,5.90061356181176,39.2875012672119));
#175895=CARTESIAN_POINT('Origin',(5.53234440788222E-15,0.,39.2875012672119));
#175896=CARTESIAN_POINT('',(58.8181995570486,5.863373641495,39.8576902534424));
#175897=CARTESIAN_POINT('',(59.1725467709678,5.90061356181176,39.2875012672119));
#175898=CARTESIAN_POINT('',(58.5996668978649,6.14377718965242,40.1599502534424));
#175899=CARTESIAN_POINT('Ctrl Pts',(58.8181995570486,5.863373641495,39.8576902534424));
#175900=CARTESIAN_POINT('Ctrl Pts',(58.806036579845,5.86209540502784,39.877261999406));
#175901=CARTESIAN_POINT('Ctrl Pts',(58.7937272422237,5.86273454612455,39.8967644650383));
#175902=CARTESIAN_POINT('Ctrl Pts',(58.7814443761786,5.86523378400424,39.9159282836067));
#175903=CARTESIAN_POINT('Ctrl Pts',(58.7689396367178,5.86777816724686,39.9354382707217));
#175904=CARTESIAN_POINT('Ctrl Pts',(58.7564614161358,5.87225032431083,39.9545987622396));
#175905=CARTESIAN_POINT('Ctrl Pts',(58.7441787427557,5.87864135444053,39.9731387498282));
#175906=CARTESIAN_POINT('Ctrl Pts',(58.7324160859207,5.88476180492487,39.9908938024117));
#175907=CARTESIAN_POINT('Ctrl Pts',(58.7208319573083,5.8926423898216,40.0080810366254));
#175908=CARTESIAN_POINT('Ctrl Pts',(58.7095754394589,5.90232005416288,40.024454274262));
#175909=CARTESIAN_POINT('Ctrl Pts',(58.7006223753257,5.91001735013546,40.0374770090537));
#175910=CARTESIAN_POINT('Ctrl Pts',(58.6918764318935,5.91885232406688,40.0499848770062));
#175911=CARTESIAN_POINT('Ctrl Pts',(58.6834178317481,5.92886364759471,40.0618424270193));
#175912=CARTESIAN_POINT('Ctrl Pts',(58.6833947425173,5.92889097525594,40.0618747942791));
#175913=CARTESIAN_POINT('Ctrl Pts',(58.6833716556051,5.92891831167149,40.0619071564124));
#175914=CARTESIAN_POINT('Ctrl Pts',(58.6833485710133,5.92894565684097,40.0619395134161));
#175915=CARTESIAN_POINT('Ctrl Pts',(58.6787531612542,5.93438921243137,40.0683807661799));
#175916=CARTESIAN_POINT('Ctrl Pts',(58.6742527563957,5.94021607194697,40.0746073439084));
#175917=CARTESIAN_POINT('Ctrl Pts',(58.6698707672382,5.94639317576796,40.0805869293669));
#175918=CARTESIAN_POINT('Ctrl Pts',(58.6611744062939,5.95865206607701,40.092453830807));
#175919=CARTESIAN_POINT('Ctrl Pts',(58.6529445485199,5.97229179622438,40.1033475319609));
#175920=CARTESIAN_POINT('Ctrl Pts',(58.6453649253902,5.98706231729958,40.1130129263075));
#175921=CARTESIAN_POINT('Ctrl Pts',(58.6396802080429,5.99814020810598,40.1202619720674));
#175922=CARTESIAN_POINT('Ctrl Pts',(58.6343612468745,6.00985416873189,40.1268200947266));
#175923=CARTESIAN_POINT('Ctrl Pts',(58.629485564911,6.02209871088711,40.1325796782703));
#175924=CARTESIAN_POINT('Ctrl Pts',(58.6276571841746,6.02669041419532,40.1347395220992));
#175925=CARTESIAN_POINT('Ctrl Pts',(58.6258911397673,6.03135673054958,40.1367870714852));
#175926=CARTESIAN_POINT('Ctrl Pts',(58.6241915206271,6.03609209717068,40.1387166518767));
#175927=CARTESIAN_POINT('Ctrl Pts',(58.6182428536364,6.05266588034453,40.1454701832469));
#175928=CARTESIAN_POINT('Ctrl Pts',(58.6131078911178,6.07008552874888,40.1507785912492));
#175929=CARTESIAN_POINT('Ctrl Pts',(58.6089619925611,6.0881125430318,40.1543986087265));
#175930=CARTESIAN_POINT('Ctrl Pts',(58.6068890432828,6.09712605017327,40.1562086174652));
#175931=CARTESIAN_POINT('Ctrl Pts',(58.6050633610079,6.10629139889321,40.1575965292115));
#175932=CARTESIAN_POINT('Ctrl Pts',(58.6035068699781,6.11557877725333,40.1585319382567));
#175933=CARTESIAN_POINT('Ctrl Pts',(58.6027286244632,6.12022246643339,40.1589996427793));
#175934=CARTESIAN_POINT('Ctrl Pts',(58.6020176767849,6.12489666302651,40.159354221642));
#175935=CARTESIAN_POINT('Ctrl Pts',(58.6013767677628,6.12959764057279,40.159591874311));
#175936=CARTESIAN_POINT('Ctrl Pts',(58.6007358587407,6.13429861811906,40.1598295269801));
#175937=CARTESIAN_POINT('Ctrl Pts',(58.6001649900651,6.13902637679564,40.1599502506895));
#175938=CARTESIAN_POINT('Ctrl Pts',(58.5996668978649,6.14377718965242,40.1599502534424));
#175939=CARTESIAN_POINT('',(58.5964866834552,6.17403490858941,40.1599502534424));
#175940=CARTESIAN_POINT('Origin',(5.72296091834672E-15,5.25982985649545E-15,
40.1599502534424));
#175941=CARTESIAN_POINT('',(58.7519447039089,6.49374646112659,39.8576902534424));
#175942=CARTESIAN_POINT('Ctrl Pts',(58.5964866834552,6.17403490858941,40.1599502534424));
#175943=CARTESIAN_POINT('Ctrl Pts',(58.5960874772333,6.17782374318146,40.1599502448875));
#175944=CARTESIAN_POINT('Ctrl Pts',(58.5957361140452,6.18160715078324,40.1598743450437));
#175945=CARTESIAN_POINT('Ctrl Pts',(58.5954317101325,6.18538309648697,40.1597243308499));
#175946=CARTESIAN_POINT('Ctrl Pts',(58.5936345324522,6.20767599437318,40.1588386583938));
#175947=CARTESIAN_POINT('Ctrl Pts',(58.5934722580545,6.22971127560327,40.1553722553617));
#175948=CARTESIAN_POINT('Ctrl Pts',(58.5947642147753,6.25106353435202,40.1496902177787));
#175949=CARTESIAN_POINT('Ctrl Pts',(58.5952468467988,6.25904002743534,40.1475675976843));
#175950=CARTESIAN_POINT('Ctrl Pts',(58.595932158504,6.26692152735556,40.1451361443095));
#175951=CARTESIAN_POINT('Ctrl Pts',(58.5968099398849,6.27468709076361,40.1424159447501));
#175952=CARTESIAN_POINT('Ctrl Pts',(58.5974948289522,6.28074617289452,40.1402935085949));
#175953=CARTESIAN_POINT('Ctrl Pts',(58.5982971695202,6.2867342495212,40.1379949176048));
#175954=CARTESIAN_POINT('Ctrl Pts',(58.5992123816357,6.29264094271359,40.1355293609261));
#175955=CARTESIAN_POINT('Ctrl Pts',(58.6024156240399,6.31331436888697,40.1268999125508));
#175956=CARTESIAN_POINT('Ctrl Pts',(58.6070015340113,6.33299084698369,40.1162251288835));
#175957=CARTESIAN_POINT('Ctrl Pts',(58.6127738370723,6.35122543337742,40.1038990521418));
#175958=CARTESIAN_POINT('Ctrl Pts',(58.6156599886029,6.36034272657428,40.097736013771));
#175959=CARTESIAN_POINT('Ctrl Pts',(58.6188427402045,6.36909954705021,40.0911601532641));
#175960=CARTESIAN_POINT('Ctrl Pts',(58.6222975626533,6.37744027742802,40.084220729064));
#175961=CARTESIAN_POINT('Ctrl Pts',(58.6257376244687,6.38574537226605,40.0773109533618));
#175962=CARTESIAN_POINT('Ctrl Pts',(58.62944725381,6.3936380972251,40.0700409753048));
#175963=CARTESIAN_POINT('Ctrl Pts',(58.6334027859058,6.40106302694584,40.0624586415899));
#175964=CARTESIAN_POINT('Ctrl Pts',(58.6334197583214,6.40109488586902,40.0624261072769));
#175965=CARTESIAN_POINT('Ctrl Pts',(58.6334367348721,6.40112673655708,40.0623935677888));
#175966=CARTESIAN_POINT('Ctrl Pts',(58.6334537155558,6.40115857900939,40.0623610231288));
#175967=CARTESIAN_POINT('Ctrl Pts',(58.6414614796113,6.41617486746432,40.047013587023));
#175968=CARTESIAN_POINT('Ctrl Pts',(58.6503516547097,6.42935337961424,40.0305755292085));
#175969=CARTESIAN_POINT('Ctrl Pts',(58.6599343882014,6.44073642151171,40.0133447567327));
#175970=CARTESIAN_POINT('Ctrl Pts',(58.6698657226823,6.45253355607577,39.995487162658));
#175971=CARTESIAN_POINT('Ctrl Pts',(58.6805417107307,6.46240257578753,39.9767767954295));
#175972=CARTESIAN_POINT('Ctrl Pts',(58.6917721934523,6.47034286301631,39.9575197577452));
#175973=CARTESIAN_POINT('Ctrl Pts',(58.7028423919867,6.47816982453002,39.9385375611974));
#175974=CARTESIAN_POINT('Ctrl Pts',(58.7144522959225,6.48412273326606,39.9190226977072));
#175975=CARTESIAN_POINT('Ctrl Pts',(58.7264268163207,6.48815321522562,39.8992655451833));
#175976=CARTESIAN_POINT('Ctrl Pts',(58.7347756649889,6.49096333895681,39.885490506931));
#175977=CARTESIAN_POINT('Ctrl Pts',(58.743301918962,6.49283796829098,39.8715976051467));
#175978=CARTESIAN_POINT('Ctrl Pts',(58.7519447039089,6.49374646112657,39.8576902534424));
#175979=CARTESIAN_POINT('',(59.1062911958297,6.53099325079975,39.2875012672119));
#175980=CARTESIAN_POINT('',(58.7519447039089,6.49374646112661,39.8576902534424));
#175981=CARTESIAN_POINT('',(58.2316113004783,12.0535047649314,39.2875012672119));
#175982=CARTESIAN_POINT('Origin',(5.53234440788222E-15,0.,39.2875012672119));
#175983=CARTESIAN_POINT('',(57.8830978693157,11.9794294790605,39.8576902534424));
#175984=CARTESIAN_POINT('',(58.2316113004783,12.0535047649314,39.2875012672119));
#175985=CARTESIAN_POINT('',(57.6364522029208,12.2354540642037,40.1599502534424));
#175986=CARTESIAN_POINT('Ctrl Pts',(57.8830978693157,11.9794294790605,39.8576902534424));
#175987=CARTESIAN_POINT('Ctrl Pts',(57.8711351342687,11.9768868675908,39.8772619994041));
#175988=CARTESIAN_POINT('Ctrl Pts',(57.8588264200514,11.9762358312602,39.8967644650345));
#175989=CARTESIAN_POINT('Ctrl Pts',(57.8463495993381,11.9774374689406,39.9159282836011));
#175990=CARTESIAN_POINT('Ctrl Pts',(57.8336474016793,11.9786608125857,39.9354382707143));
#175991=CARTESIAN_POINT('Ctrl Pts',(57.8207700703912,11.9818041414828,39.9545987622304));
#175992=CARTESIAN_POINT('Ctrl Pts',(57.8078866382242,11.9868762719063,39.9731387498174));
#175993=CARTESIAN_POINT('Ctrl Pts',(57.7955486571716,11.9917336614784,39.9908938023995));
#175994=CARTESIAN_POINT('Ctrl Pts',(57.7832042422,11.9983602045428,40.0080810366118));
#175995=CARTESIAN_POINT('Ctrl Pts',(57.7709977973527,12.0068082271118,40.0244542742474));
#175996=CARTESIAN_POINT('Ctrl Pts',(57.7612891925185,12.0135275064579,40.0374770090443));
#175997=CARTESIAN_POINT('Ctrl Pts',(57.7516676540279,12.0213998814534,40.0499848770018));
#175998=CARTESIAN_POINT('Ctrl Pts',(57.7422089227119,12.0304721974322,40.0618424270192));
#175999=CARTESIAN_POINT('Ctrl Pts',(57.7421831034479,12.0304969619079,40.0618747942791));
#176000=CARTESIAN_POINT('Ctrl Pts',(57.7421572855747,12.0305217353322,40.0619071564124));
#176001=CARTESIAN_POINT('Ctrl Pts',(57.7421314690942,12.0305465177051,40.0619395134161));
#176002=CARTESIAN_POINT('Ctrl Pts',(57.73699222697,12.0354799018082,40.0683807661799));
#176003=CARTESIAN_POINT('Ctrl Pts',(57.7319074031293,12.0408044207737,40.0746073439084));
#176004=CARTESIAN_POINT('Ctrl Pts',(57.726903735797,12.046489643181,40.0805869293669));
#176005=CARTESIAN_POINT('Ctrl Pts',(57.7169736114626,12.0577723607607,40.092453830807));
#176006=CARTESIAN_POINT('Ctrl Pts',(57.7073630976789,12.0704771166532,40.1033475319609));
#176007=CARTESIAN_POINT('Ctrl Pts',(57.6982810566481,12.0843744369106,40.1130129263075));
#176008=CARTESIAN_POINT('Ctrl Pts',(57.691469525875,12.0947974271036,40.1202619720674));
#176009=CARTESIAN_POINT('Ctrl Pts',(57.6849552602294,12.1058912345904,40.1268200947266));
#176010=CARTESIAN_POINT('Ctrl Pts',(57.6788263845869,12.1175590523195,40.1325796782703));
#176011=CARTESIAN_POINT('Ctrl Pts',(57.676528056221,12.1219344839679,40.1347395220992));
#176012=CARTESIAN_POINT('Ctrl Pts',(57.6742839235121,12.126390635845,40.1367870714852));
#176013=CARTESIAN_POINT('Ctrl Pts',(57.6720986344674,12.1309224030554,40.1387166518767));
#176014=CARTESIAN_POINT('Ctrl Pts',(57.6644501228112,12.1467835882919,40.1454701832469));
#176015=CARTESIAN_POINT('Ctrl Pts',(57.6575224410762,12.1635710602986,40.1507785912492));
#176016=CARTESIAN_POINT('Ctrl Pts',(57.6515149180853,12.1810659563061,40.1543986087265));
#176017=CARTESIAN_POINT('Ctrl Pts',(57.6485111565899,12.1898134043099,40.1562086174652));
#176018=CARTESIAN_POINT('Ctrl Pts',(57.6457374357766,12.1987377085279,40.1575965292115));
#176019=CARTESIAN_POINT('Ctrl Pts',(57.6432186759797,12.2078115120422,40.1585319382567));
#176020=CARTESIAN_POINT('Ctrl Pts',(57.6419592960813,12.2123484137993,40.1589996427793));
#176021=CARTESIAN_POINT('Ctrl Pts',(57.6407636564618,12.2169226903862,40.159354221642));
#176022=CARTESIAN_POINT('Ctrl Pts',(57.6396348724477,12.2215309222504,40.159591874311));
#176023=CARTESIAN_POINT('Ctrl Pts',(57.6385060884335,12.2261391541146,40.1598295269801));
#176024=CARTESIAN_POINT('Ctrl Pts',(57.6374441616871,12.2307813416091,40.1599502506895));
#176025=CARTESIAN_POINT('Ctrl Pts',(57.6364522029208,12.2354540642037,40.1599502534424));
#176026=CARTESIAN_POINT('',(57.6301266171959,12.2652136052653,40.1599502534424));
#176027=CARTESIAN_POINT('Origin',(5.72184526906101E-15,5.26687378886292E-15,
40.1599502534424));
#176028=CARTESIAN_POINT('',(57.7513140650722,12.5994235324464,39.8576902534424));
#176029=CARTESIAN_POINT('Ctrl Pts',(57.6301266171959,12.2652136052653,40.1599502534424));
#176030=CARTESIAN_POINT('Ctrl Pts',(57.6293335568101,12.2689399558122,40.1599502448875));
#176031=CARTESIAN_POINT('Ctrl Pts',(57.6285886446437,12.2726659100571,40.1598743450437));
#176032=CARTESIAN_POINT('Ctrl Pts',(57.6278912144857,12.276389351862,40.1597243308498));
#176033=CARTESIAN_POINT('Ctrl Pts',(57.6237736395748,12.2983722707006,40.1588386583938));
#176034=CARTESIAN_POINT('Ctrl Pts',(57.6213089400485,12.3202698780618,40.1553722553615));
#176035=CARTESIAN_POINT('Ctrl Pts',(57.620361900501,12.3416402131543,40.1496902177781));
#176036=CARTESIAN_POINT('Ctrl Pts',(57.6200081180517,12.349623458957,40.1475675976839));
#176037=CARTESIAN_POINT('Ctrl Pts',(57.6198658344727,12.3575334177747,40.1451361443093));
#176038=CARTESIAN_POINT('Ctrl Pts',(57.6199270848659,12.365348193752,40.1424159447501));
#176039=CARTESIAN_POINT('Ctrl Pts',(57.6199748754953,12.3714456739988,40.1402935085949));
#176040=CARTESIAN_POINT('Ctrl Pts',(57.62014689631,12.3774848147417,40.1379949176047));
#176041=CARTESIAN_POINT('Ctrl Pts',(57.6204396772353,12.3834548161668,40.1355293609261));
#176042=CARTESIAN_POINT('Ctrl Pts',(57.6214644104742,12.4043498211545,40.1268999125508));
#176043=CARTESIAN_POINT('Ctrl Pts',(57.6239684463329,12.4243978675674,40.1162251288835));
#176044=CARTESIAN_POINT('Ctrl Pts',(57.6278030948198,12.4431359329574,40.1038990521418));
#176045=CARTESIAN_POINT('Ctrl Pts',(57.6297204190632,12.4525049656524,40.0977360137709));
#176046=CARTESIAN_POINT('Ctrl Pts',(57.6319703982311,12.4615465034834,40.0911601532641));
#176047=CARTESIAN_POINT('Ctrl Pts',(57.6345344510721,12.470202669749,40.084220729064));
#176048=CARTESIAN_POINT('Ctrl Pts',(57.6370875490682,12.4788218527836,40.0773109533618));
#176049=CARTESIAN_POINT('Ctrl Pts',(57.6399518422609,12.4870591024238,40.0700409753048));
#176050=CARTESIAN_POINT('Ctrl Pts',(57.6431095890444,12.4948568232941,40.0624586415899));
#176051=CARTESIAN_POINT('Ctrl Pts',(57.6431231383191,12.4948902817913,40.0624261072769));
#176052=CARTESIAN_POINT('Ctrl Pts',(57.6431366925669,12.4949237325307,40.0623935677888));
#176053=CARTESIAN_POINT('Ctrl Pts',(57.6431502517861,12.4949571755115,40.0623610231288));
#176054=CARTESIAN_POINT('Ctrl Pts',(57.6495445189161,12.5107282424382,40.0470135870228));
#176055=CARTESIAN_POINT('Ctrl Pts',(57.657008463082,12.524763837661,40.0305755292082));
#176056=CARTESIAN_POINT('Ctrl Pts',(57.6653488494803,12.5370861904698,40.0133447567321));
#176057=CARTESIAN_POINT('Ctrl Pts',(57.673992642725,12.549856806228,39.9954871626571));
#176058=CARTESIAN_POINT('Ctrl Pts',(57.6835785531295,12.5607877070418,39.9767767954283));
#176059=CARTESIAN_POINT('Ctrl Pts',(57.69391752807,12.569858401647,39.9575197577437));
#176060=CARTESIAN_POINT('Ctrl Pts',(57.7041089426397,12.5787996370875,39.9385375611954));
#176061=CARTESIAN_POINT('Ctrl Pts',(57.7150329979052,12.5859335005837,39.9190226977048));
#176062=CARTESIAN_POINT('Ctrl Pts',(57.7265206205425,12.591193581357,39.8992655451805));
#176063=CARTESIAN_POINT('Ctrl Pts',(57.7345299954284,12.5948610032573,39.8854905069291));
#176064=CARTESIAN_POINT('Ctrl Pts',(57.742813589566,12.5976165994009,39.8715976051458));
#176065=CARTESIAN_POINT('Ctrl Pts',(57.7513140650722,12.5994235324464,39.8576902534424));
#176066=CARTESIAN_POINT('',(58.0998260601482,12.6735055745733,39.2875012672119));
#176067=CARTESIAN_POINT('',(57.7513140650722,12.5994235324464,39.8576902534424));
#176068=CARTESIAN_POINT('',(56.6526781108326,18.0743352474884,39.2875012672119));
#176069=CARTESIAN_POINT('Origin',(5.53234440788222E-15,0.,39.2875012672119));
#176070=CARTESIAN_POINT('',(56.3138168485097,17.9642361803965,39.8576902534424));
#176071=CARTESIAN_POINT('',(56.6526781108326,18.0743352474884,39.2875012672119));
#176072=CARTESIAN_POINT('',(56.0417604764386,18.1930767435942,40.1599502534424));
#176073=CARTESIAN_POINT('Ctrl Pts',(56.3138168485097,17.9642361803965,39.8576902534424));
#176074=CARTESIAN_POINT('Ctrl Pts',(56.302185421847,17.9604570513077,39.8772619994036));
#176075=CARTESIAN_POINT('Ctrl Pts',(56.2900121878815,17.9585229704403,39.8967644650334));
#176076=CARTESIAN_POINT('Ctrl Pts',(56.2774781111578,17.9584138425281,39.9159282835995));
#176077=CARTESIAN_POINT('Ctrl Pts',(56.2647176232359,17.9583027433672,39.935438270712));
#176078=CARTESIAN_POINT('Ctrl Pts',(56.2515822679773,17.9600828051289,39.9545987622276));
#176079=CARTESIAN_POINT('Ctrl Pts',(56.2382392306015,17.9637804645249,39.9731387498141));
#176080=CARTESIAN_POINT('Ctrl Pts',(56.225461102833,17.9673215746091,39.9908938023957));
#176081=CARTESIAN_POINT('Ctrl Pts',(56.2124916494954,17.9726214740499,40.0080810366076));
#176082=CARTESIAN_POINT('Ctrl Pts',(56.1994690140138,17.9797472965448,40.0244542742428));
#176083=CARTESIAN_POINT('Ctrl Pts',(56.1891112379872,17.9854149414322,40.0374770090413));
#176084=CARTESIAN_POINT('Ctrl Pts',(56.1787195200293,17.9922384661018,40.0499848770004));
#176085=CARTESIAN_POINT('Ctrl Pts',(56.1683642893845,18.0002723763365,40.0618424270192));
#176086=CARTESIAN_POINT('Ctrl Pts',(56.1683360229685,18.0002943063017,40.0618747942791));
#176087=CARTESIAN_POINT('Ctrl Pts',(56.1683077570003,18.000316245312,40.0619071564124));
#176088=CARTESIAN_POINT('Ctrl Pts',(56.1682794914818,18.0003381933675,40.0619395134161));
#176089=CARTESIAN_POINT('Ctrl Pts',(56.1626527236048,18.0047073547947,40.0683807661799));
#176090=CARTESIAN_POINT('Ctrl Pts',(56.157039191176,18.0094711966661,40.0746073439084));
#176091=CARTESIAN_POINT('Ctrl Pts',(56.1514686668953,18.0146022491732,40.0805869293669));
#176092=CARTESIAN_POINT('Ctrl Pts',(56.1404135756909,18.0247851782088,40.092453830807));
#176093=CARTESIAN_POINT('Ctrl Pts',(56.1295277006976,18.0364157638821,40.1033475319609));
#176094=CARTESIAN_POINT('Ctrl Pts',(56.1190427465078,18.0492876213728,40.1130129263075));
#176095=CARTESIAN_POINT('Ctrl Pts',(56.1111790308655,18.0589415144907,40.1202619720674));
#176096=CARTESIAN_POINT('Ctrl Pts',(56.1035408324003,18.0692936227621,40.1268200947266));
#176097=CARTESIAN_POINT('Ctrl Pts',(56.096225912323,18.0802568810124,40.1325796782703));
#176098=CARTESIAN_POINT('Ctrl Pts',(56.0934828172939,18.0843681028563,40.1347395220992));
#176099=CARTESIAN_POINT('Ctrl Pts',(56.090785183471,18.0885652677237,40.1367870714852));
#176100=CARTESIAN_POINT('Ctrl Pts',(56.088138167006,18.0928437845335,40.1387166518767));
#176101=CARTESIAN_POINT('Ctrl Pts',(56.0788736093786,18.107818593368,40.1454701832469));
#176102=CARTESIAN_POINT('Ctrl Pts',(56.0702291095579,18.1237899619208,40.1507785912492));
#176103=CARTESIAN_POINT('Ctrl Pts',(56.0624257818119,18.1405610619111,40.1543986087265));
#176104=CARTESIAN_POINT('Ctrl Pts',(56.0585241179389,18.1489466119063,40.1562086174652));
#176105=CARTESIAN_POINT('Ctrl Pts',(56.0548327480527,18.157532095078,40.1575965292115));
#176106=CARTESIAN_POINT('Ctrl Pts',(56.0513793155483,18.1662929092563,40.1585319382567));
#176107=CARTESIAN_POINT('Ctrl Pts',(56.049652599296,18.1706733163454,40.1589996427793));
#176108=CARTESIAN_POINT('Ctrl Pts',(56.0479853674133,18.1750975561945,40.159354221642));
#176109=CARTESIAN_POINT('Ctrl Pts',(56.0463810756009,18.179562553624,40.159591874311));
#176110=CARTESIAN_POINT('Ctrl Pts',(56.0447767837886,18.1840275510536,40.1598295269801));
#176111=CARTESIAN_POINT('Ctrl Pts',(56.043235433663,18.1885333065883,40.1599502506895));
#176112=CARTESIAN_POINT('Ctrl Pts',(56.0417604764386,18.1930767435942,40.1599502534424));
#176113=CARTESIAN_POINT('',(56.0323588238394,18.222012055021,40.1599502534424));
#176114=CARTESIAN_POINT('Origin',(5.71999943999309E-15,5.27376251672649E-15,
40.1599502534424));
#176115=CARTESIAN_POINT('',(56.1179479440991,18.5670586829459,39.8576902534424));
#176116=CARTESIAN_POINT('Ctrl Pts',(56.0323588238394,18.222012055021,40.1599502534424));
#176117=CARTESIAN_POINT('Ctrl Pts',(56.031180598225,18.2256350948462,40.1599502448875));
#176118=CARTESIAN_POINT('Ctrl Pts',(56.030050298494,18.2292627734,40.1598743450437));
#176119=CARTESIAN_POINT('Ctrl Pts',(56.0289674832815,18.2328929164984,40.1597243308499));
#176120=CARTESIAN_POINT('Ctrl Pts',(56.0225746241526,18.2543250068291,40.1588386583938));
#176121=CARTESIAN_POINT('Ctrl Pts',(56.0178345032616,18.2758450255515,40.1553722553616));
#176122=CARTESIAN_POINT('Ctrl Pts',(56.0146588434091,18.2969992991233,40.1496902177785));
#176123=CARTESIAN_POINT('Ctrl Pts',(56.0134725226012,18.3049018315349,40.1475675976842));
#176124=CARTESIAN_POINT('Ctrl Pts',(56.0125042026268,18.3127535860873,40.1451361443095));
#176125=CARTESIAN_POINT('Ctrl Pts',(56.0117482509602,18.3205319543142,40.1424159447501));
#176126=CARTESIAN_POINT('Ctrl Pts',(56.0111584195475,18.3266010274072,40.1402935085949));
#176127=CARTESIAN_POINT('Ctrl Pts',(56.0106982359128,18.3326250661767,40.1379949176047));
#176128=CARTESIAN_POINT('Ctrl Pts',(56.010365377879,18.3385929672495,40.1355293609261));
#176129=CARTESIAN_POINT('Ctrl Pts',(56.0092003747606,18.3594806210043,40.1268999125508));
#176130=CARTESIAN_POINT('Ctrl Pts',(56.0095951017658,18.3796805851416,40.1162251288835));
#176131=CARTESIAN_POINT('Ctrl Pts',(56.0114500824673,18.3987168313623,40.1038990521418));
#176132=CARTESIAN_POINT('Ctrl Pts',(56.012377572818,18.4082349544727,40.0977360137709));
#176133=CARTESIAN_POINT('Ctrl Pts',(56.0136701283095,18.4174621486782,40.0911601532641));
#176134=CARTESIAN_POINT('Ctrl Pts',(56.0153153192432,18.4263389120624,40.084220729064));
#176135=CARTESIAN_POINT('Ctrl Pts',(56.0169534811442,18.4351777497207,40.0773109533618));
#176136=CARTESIAN_POINT('Ctrl Pts',(56.0189410563926,18.4436692750113,40.0700409753048));
#176137=CARTESIAN_POINT('Ctrl Pts',(56.0212664209293,18.4517543535694,40.0624586415899));
#176138=CARTESIAN_POINT('Ctrl Pts',(56.0212763986143,18.4517890450622,40.0624261072769));
#176139=CARTESIAN_POINT('Ctrl Pts',(56.0212863820562,18.4518237293597,40.0623935677888));
#176140=CARTESIAN_POINT('Ctrl Pts',(56.0212963712531,18.4518584064607,40.0623610231288));
#176141=CARTESIAN_POINT('Ctrl Pts',(56.0260070845284,18.4682114607482,40.047013587024));
#176142=CARTESIAN_POINT('Ctrl Pts',(56.031963021227,18.4829503621244,40.0305755292107));
#176143=CARTESIAN_POINT('Ctrl Pts',(56.0389696815123,18.4960770195677,40.0133447567361));
#176144=CARTESIAN_POINT('Ctrl Pts',(56.0462312303122,18.5096811989804,39.9954871626627));
#176145=CARTESIAN_POINT('Ctrl Pts',(56.0546220378314,18.5215542196589,39.9767767954356));
#176146=CARTESIAN_POINT('Ctrl Pts',(56.0639562290165,18.531655941212,39.9575197577527));
#176147=CARTESIAN_POINT('Ctrl Pts',(56.0731572003495,18.5416134885325,39.9385375612061));
#176148=CARTESIAN_POINT('Ctrl Pts',(56.0832757207076,18.5498501466877,39.9190226977172));
#176149=CARTESIAN_POINT('Ctrl Pts',(56.0941505847851,18.5562821957293,39.8992655451945));
#176150=CARTESIAN_POINT('Ctrl Pts',(56.1017327335043,18.5607667347594,39.8854905069386));
#176151=CARTESIAN_POINT('Ctrl Pts',(56.1096829110188,18.564373106826,39.8715976051505));
#176152=CARTESIAN_POINT('Ctrl Pts',(56.1179479440991,18.5670586829458,39.8576902534424));
#176153=CARTESIAN_POINT('',(56.4568070719814,18.6771643191703,39.2875012672119));
#176154=CARTESIAN_POINT('',(56.1179479440991,18.5670586829459,39.8576902534424));
#176155=CARTESIAN_POINT('',(54.4530463244696,23.8971395307762,39.2875012672119));
#176156=CARTESIAN_POINT('Origin',(5.53234440788222E-15,0.,39.2875012672119));
#176157=CARTESIAN_POINT('',(54.1275498658877,23.7522229508821,39.8576902534424));
#176158=CARTESIAN_POINT('',(54.4530463244695,23.8971395307762,39.2875012672119));
#176159=CARTESIAN_POINT('',(53.8330634946841,23.9513722670358,40.1599502534424));
#176160=CARTESIAN_POINT('Ctrl Pts',(54.1275498658877,23.7522229508821,39.8576902534424));
#176161=CARTESIAN_POINT('Ctrl Pts',(54.1163771839515,23.7472487091024,39.8772619994067));
#176162=CARTESIAN_POINT('Ctrl Pts',(54.1044728027344,23.7440527738927,39.8967644650396));
#176163=CARTESIAN_POINT('Ctrl Pts',(54.0920187959652,23.7426340760165,39.9159282836086));
#176164=CARTESIAN_POINT('Ctrl Pts',(54.0793398243537,23.7411897512758,39.9354382707242));
#176165=CARTESIAN_POINT('Ctrl Pts',(54.0660903588227,23.7415870431742,39.9545987622426));
#176166=CARTESIAN_POINT('Ctrl Pts',(54.052433905345,23.7438697192144,39.9731387498317));
#176167=CARTESIAN_POINT('Ctrl Pts',(54.0393556306996,23.7460557526694,39.9908938024159));
#176168=CARTESIAN_POINT('Ctrl Pts',(54.0259032350379,23.7499709416819,40.0080810366301));
#176169=CARTESIAN_POINT('Ctrl Pts',(54.0122070876386,23.7556964921038,40.0244542742672));
#176170=CARTESIAN_POINT('Ctrl Pts',(54.001313622389,23.7602504066272,40.0374770090569));
#176171=CARTESIAN_POINT('Ctrl Pts',(53.9902655788085,23.765950321003,40.0499848770078));
#176172=CARTESIAN_POINT('Ctrl Pts',(53.9791273029166,23.7728578042865,40.0618424270193));
#176173=CARTESIAN_POINT('Ctrl Pts',(53.9790968990415,23.7728766594721,40.0618747942791));
#176174=CARTESIAN_POINT('Ctrl Pts',(53.9790664946662,23.7728955236999,40.0619071564124));
#176175=CARTESIAN_POINT('Ctrl Pts',(53.9790360897926,23.7729143969704,40.0619395134161));
#176176=CARTESIAN_POINT('Ctrl Pts',(53.972983444209,23.7766714662748,40.0683807661799));
#176177=CARTESIAN_POINT('Ctrl Pts',(53.9669027062282,23.7808224374038,40.0746073439084));
#176178=CARTESIAN_POINT('Ctrl Pts',(53.9608263568289,23.7853431031257,40.0805869293668));
#176179=CARTESIAN_POINT('Ctrl Pts',(53.9487674206471,23.7943146773157,40.092453830807));
#176180=CARTESIAN_POINT('Ctrl Pts',(53.9367254523687,23.8047436656394,40.1033475319609));
#176181=CARTESIAN_POINT('Ctrl Pts',(53.9249524603721,23.816449033599,40.1130129263075));
#176182=CARTESIAN_POINT('Ctrl Pts',(53.9161227163747,23.8252280595687,40.1202619720674));
#176183=CARTESIAN_POINT('Ctrl Pts',(53.9074442707907,23.8347250487601,40.1268200947266));
#176184=CARTESIAN_POINT('Ctrl Pts',(53.8990234500736,23.84486363178,40.1325796782703));
#176185=CARTESIAN_POINT('Ctrl Pts',(53.8958656423047,23.8486656004125,40.1347395220992));
#176186=CARTESIAN_POINT('Ctrl Pts',(53.8927440632084,23.8525577932536,40.1367870714852));
#176187=CARTESIAN_POINT('Ctrl Pts',(53.8896643205894,23.8565361833374,40.1387166518767));
#176188=CARTESIAN_POINT('Ctrl Pts',(53.8788852214228,23.8704605486305,40.1454701832469));
#176189=CARTESIAN_POINT('Ctrl Pts',(53.8686186144656,23.8854408280733,40.1507785912491));
#176190=CARTESIAN_POINT('Ctrl Pts',(53.8591049768561,23.9013043843655,40.1543986087265));
#176191=CARTESIAN_POINT('Ctrl Pts',(53.8543481580514,23.9092361625115,40.1562086174652));
#176192=CARTESIAN_POINT('Ctrl Pts',(53.8497795825134,23.9173887602865,40.1575965292115));
#176193=CARTESIAN_POINT('Ctrl Pts',(53.8454293138304,23.9257405998154,40.1585319382567));
#176194=CARTESIAN_POINT('Ctrl Pts',(53.843254179489,23.9299165195798,40.1589996427793));
#176195=CARTESIAN_POINT('Ctrl Pts',(53.8411336218844,23.9341422497935,40.159354221642));
#176196=CARTESIAN_POINT('Ctrl Pts',(53.8390713992307,23.9384150933421,40.159591874311));
#176197=CARTESIAN_POINT('Ctrl Pts',(53.8370091765769,23.9426879368908,40.1598295269801));
#176198=CARTESIAN_POINT('Ctrl Pts',(53.8350052904266,23.9470078944653,40.1599502506895));
#176199=CARTESIAN_POINT('Ctrl Pts',(53.8330634946841,23.9513722670358,40.1599502534424));
#176200=CARTESIAN_POINT('',(53.8206887816839,23.9791663275007,40.1599502534424));
#176201=CARTESIAN_POINT('Origin',(5.71744365443249E-15,5.28042056574211E-15,
40.1599502534424));
#176202=CARTESIAN_POINT('',(53.8697418420148,24.3312692531081,39.8576902534424));
#176203=CARTESIAN_POINT('Ctrl Pts',(53.8206887816839,23.9791663275007,40.1599502534424));
#176204=CARTESIAN_POINT('Ctrl Pts',(53.8191382997274,23.9826463618218,40.1599502448875));
#176205=CARTESIAN_POINT('Ctrl Pts',(53.8176349962322,23.986136019079,40.1598743450437));
#176206=CARTESIAN_POINT('Ctrl Pts',(53.8161786595152,23.9896330908635,40.1597243308499));
#176207=CARTESIAN_POINT('Ctrl Pts',(53.8075805576712,24.010279538219,40.1588386583939));
#176208=CARTESIAN_POINT('Ctrl Pts',(53.8006169491721,24.0311861904735,40.1553722553621));
#176209=CARTESIAN_POINT('Ctrl Pts',(53.7952474622087,24.0518926318757,40.1496902177796));
#176210=CARTESIAN_POINT('Ctrl Pts',(53.7932416006211,24.0596278690982,40.147567597685));
#176211=CARTESIAN_POINT('Ctrl Pts',(53.7914578533671,24.06733539392,40.1451361443099));
#176212=CARTESIAN_POINT('Ctrl Pts',(53.7898929820051,24.0749921329672,40.1424159447501));
#176213=CARTESIAN_POINT('Ctrl Pts',(53.7886719908667,24.0809663048716,40.1402935085949));
#176214=CARTESIAN_POINT('Ctrl Pts',(53.7875846446509,24.0869092410382,40.1379949176048));
#176215=CARTESIAN_POINT('Ctrl Pts',(53.7866297945202,24.0928096561858,40.1355293609261));
#176216=CARTESIAN_POINT('Ctrl Pts',(53.7832878190625,24.1134611092021,40.1268999125508));
#176217=CARTESIAN_POINT('Ctrl Pts',(53.7815689125025,24.1335916760296,40.1162251288835));
#176218=CARTESIAN_POINT('Ctrl Pts',(53.7814239018617,24.1527175379838,40.1038990521418));
#176219=CARTESIAN_POINT('Ctrl Pts',(53.7813513965413,24.1622804689609,40.0977360137709));
#176220=CARTESIAN_POINT('Ctrl Pts',(53.7816723668481,24.1715922244704,40.0911601532641));
#176221=CARTESIAN_POINT('Ctrl Pts',(53.7823806708184,24.1805923292961,40.084220729064));
#176222=CARTESIAN_POINT('Ctrl Pts',(53.7830859485795,24.1895539814229,40.0773109533618));
#176223=CARTESIAN_POINT('Ctrl Pts',(53.7841750295933,24.1982067474358,40.0700409753048));
#176224=CARTESIAN_POINT('Ctrl Pts',(53.7856425347027,24.2064906018692,40.0624586415899));
#176225=CARTESIAN_POINT('Ctrl Pts',(53.7856488314805,24.2065261462705,40.0624261072769));
#176226=CARTESIAN_POINT('Ctrl Pts',(53.7856551347357,24.2065616841176,40.0623935677888));
#176227=CARTESIAN_POINT('Ctrl Pts',(53.7856614444667,24.2065972154092,40.0623610231288));
#176228=CARTESIAN_POINT('Ctrl Pts',(53.7886369923277,24.2233530895755,40.0470135870225));
#176229=CARTESIAN_POINT('Ctrl Pts',(53.7930196670713,24.2386338146195,40.0305755292075));
#176230=CARTESIAN_POINT('Ctrl Pts',(53.7986158348088,24.2524209582933,40.013344756731));
#176231=CARTESIAN_POINT('Ctrl Pts',(53.8044155801174,24.2667096511258,39.9954871626558));
#176232=CARTESIAN_POINT('Ctrl Pts',(53.8115193533103,24.279394708371,39.9767767954267));
#176233=CARTESIAN_POINT('Ctrl Pts',(53.8197464933903,24.2904167802974,39.9575197577417));
#176234=CARTESIAN_POINT('Ctrl Pts',(53.8278562137214,24.3012815425261,39.9385375611934));
#176235=CARTESIAN_POINT('Ctrl Pts',(53.837058338548,24.3105307527896,39.9190226977027));
#176236=CARTESIAN_POINT('Ctrl Pts',(53.8472012967816,24.3180642992234,39.8992655451783));
#176237=CARTESIAN_POINT('Ctrl Pts',(53.8542731477211,24.3233168218307,39.8854905069277));
#176238=CARTESIAN_POINT('Ctrl Pts',(53.8618028047985,24.32773445765,39.871597605145));
#176239=CARTESIAN_POINT('Ctrl Pts',(53.8697418420148,24.3312692531081,39.8576902534424));
#176240=CARTESIAN_POINT('',(54.1952354911875,24.4761921430385,39.2875012672119));
#176241=CARTESIAN_POINT('',(53.8697418420148,24.3312692531081,39.8576902534424));
#176242=CARTESIAN_POINT('',(51.6568155675431,29.4581217525667,39.2875012672119));
#176243=CARTESIAN_POINT('Origin',(5.53234440788222E-15,0.,39.2875012672119));
#176244=CARTESIAN_POINT('',(51.3482501200169,29.2799753962456,39.8576902534424));
#176245=CARTESIAN_POINT('',(51.6568155675431,29.4581217525667,39.2875012672119));
#176246=CARTESIAN_POINT('',(51.0345602039891,29.4472515437729,40.1599502534424));
#176247=CARTESIAN_POINT('Ctrl Pts',(51.3482501200169,29.2799753962456,39.8576902534424));
#176248=CARTESIAN_POINT('Ctrl Pts',(51.3376585930516,29.2738605406101,39.8772619994048));
#176249=CARTESIAN_POINT('Ctrl Pts',(51.3261534914777,29.2694377663934,39.8967644650358));
#176250=CARTESIAN_POINT('Ctrl Pts',(51.3139160033709,29.2667250421034,39.915928283603));
#176251=CARTESIAN_POINT('Ctrl Pts',(51.3014574615395,29.2639633161063,39.9354382707168));
#176252=CARTESIAN_POINT('Ctrl Pts',(51.2882390496569,29.2629734853266,39.9545987622334));
#176253=CARTESIAN_POINT('Ctrl Pts',(51.2744188030431,29.2638161685321,39.9731387498209));
#176254=CARTESIAN_POINT('Ctrl Pts',(51.2611836698386,29.2646231747156,39.9908938024034));
#176255=CARTESIAN_POINT('Ctrl Pts',(51.2473957191187,29.267110757666,40.0080810366162));
#176256=CARTESIAN_POINT('Ctrl Pts',(51.2331761176627,29.2713733056818,40.0244542742521));
#176257=CARTESIAN_POINT('Ctrl Pts',(51.2218663142644,29.2747635962031,40.0374770090473));
#176258=CARTESIAN_POINT('Ctrl Pts',(51.2102829897278,29.2792774508353,40.0499848770032));
#176259=CARTESIAN_POINT('Ctrl Pts',(51.1984837018595,29.2849828273423,40.0618424270193));
#176260=CARTESIAN_POINT('Ctrl Pts',(51.1984514936364,29.2849984011669,40.0618747942791));
#176261=CARTESIAN_POINT('Ctrl Pts',(51.1984192839706,29.2850139839319,40.0619071564124));
#176262=CARTESIAN_POINT('Ctrl Pts',(51.1983870728642,29.2850295756379,40.0619395134161));
#176263=CARTESIAN_POINT('Ctrl Pts',(51.1919748636256,29.288133389582,40.0683807661799));
#176264=CARTESIAN_POINT('Ctrl Pts',(51.1854935419305,29.2916260110601,40.0746073439084));
#176265=CARTESIAN_POINT('Ctrl Pts',(51.1789779411681,29.2954867606373,40.0805869293669));
#176266=CARTESIAN_POINT('Ctrl Pts',(51.1660472802373,29.3031486855374,40.092453830807));
#176267=CARTESIAN_POINT('Ctrl Pts',(51.1529811529982,29.312261814333,40.1033475319609));
#176268=CARTESIAN_POINT('Ctrl Pts',(51.1400491105588,29.3226724463007,40.1130129263075));
#176269=CARTESIAN_POINT('Ctrl Pts',(51.1303500787293,29.3304804202765,40.1202619720674));
#176270=CARTESIAN_POINT('Ctrl Pts',(51.1207264688924,29.339018239387,40.1268200947266));
#176271=CARTESIAN_POINT('Ctrl Pts',(51.1112920078095,29.3482210667393,40.1325796782703));
#176272=CARTESIAN_POINT('Ctrl Pts',(51.1077540849034,29.3516721269964,40.1347395220992));
#176273=CARTESIAN_POINT('Ctrl Pts',(51.1042427612076,29.355216704132,40.1367870714852));
#176274=CARTESIAN_POINT('Ctrl Pts',(51.1007640347392,29.3588513794154,40.1387166518767));
#176275=CARTESIAN_POINT('Ctrl Pts',(51.0885884920996,29.3715727429072,40.1454701832469));
#176276=CARTESIAN_POINT('Ctrl Pts',(51.0768122611,29.3853978061636,40.1507785912491));
#176277=CARTESIAN_POINT('Ctrl Pts',(51.0656925470316,29.4001800143151,40.1543986087265));
#176278=CARTESIAN_POINT('Ctrl Pts',(51.0601326899974,29.4075711183909,40.1562086174652));
#176279=CARTESIAN_POINT('Ctrl Pts',(51.0547369630771,29.4152015092019,40.1575965292115));
#176280=CARTESIAN_POINT('Ctrl Pts',(51.0495375206698,29.4230528695798,40.1585319382567));
#176281=CARTESIAN_POINT('Ctrl Pts',(51.0469377994662,29.4269785497687,40.1589996427792));
#176282=CARTESIAN_POINT('Ctrl Pts',(51.0443871494127,29.4309594723624,40.159354221642));
#176283=CARTESIAN_POINT('Ctrl Pts',(51.0418895900604,29.4349933478621,40.159591874311));
#176284=CARTESIAN_POINT('Ctrl Pts',(51.0393920307082,29.4390272233619,40.1598295269801));
#176285=CARTESIAN_POINT('Ctrl Pts',(51.0369475635293,29.4431140526169,40.1599502506895));
#176286=CARTESIAN_POINT('Ctrl Pts',(51.0345602039891,29.4472515437729,40.1599502534424));
#176287=CARTESIAN_POINT('',(51.0193480105331,29.4735998357331,40.1599502534424));
#176288=CARTESIAN_POINT('Origin',(5.71420591410065E-15,5.28677498893149E-15,
40.1599502534424));
#176289=CARTESIAN_POINT('',(51.0313275753413,29.8289013456879,39.8576902534424));
#176290=CARTESIAN_POINT('Ctrl Pts',(51.0193480105331,29.4735998357331,40.1599502534424));
#176291=CARTESIAN_POINT('Ctrl Pts',(51.0174422596394,29.4768987365659,40.1599502448875));
#176292=CARTESIAN_POINT('Ctrl Pts',(51.0155824228875,29.4802121391113,40.1598743450437));
#176293=CARTESIAN_POINT('Ctrl Pts',(51.0137685205959,29.4835378249316,40.1597243308499));
#176294=CARTESIAN_POINT('Ctrl Pts',(51.0030593786379,29.5031724225183,40.1588386583937));
#176295=CARTESIAN_POINT('Ctrl Pts',(50.9939485772815,29.5232366506519,40.1553722553611));
#176296=CARTESIAN_POINT('Ctrl Pts',(50.9864440924293,29.5432683957836,40.1496902177772));
#176297=CARTESIAN_POINT('Ctrl Pts',(50.9836406667027,29.5507515889351,40.1475675976832));
#176298=CARTESIAN_POINT('Ctrl Pts',(50.9810610352787,29.5582304387673,40.1451361443089));
#176299=CARTESIAN_POINT('Ctrl Pts',(50.9787043892804,29.5656816597952,40.1424159447501));
#176300=CARTESIAN_POINT('Ctrl Pts',(50.9768656158508,29.5714954762335,40.1402935085949));
#176301=CARTESIAN_POINT('Ctrl Pts',(50.9751630202465,29.5772921977451,40.1379949176048));
#176302=CARTESIAN_POINT('Ctrl Pts',(50.9735966395567,29.5830604807842,40.1355293609261));
#176303=CARTESIAN_POINT('Ctrl Pts',(50.9681143071422,29.6032494714213,40.1268999125509));
#176304=CARTESIAN_POINT('Ctrl Pts',(50.964300599717,29.6230900862361,40.1162251288835));
#176305=CARTESIAN_POINT('Ctrl Pts',(50.9621571865009,29.642096016978,40.1038990521418));
#176306=CARTESIAN_POINT('Ctrl Pts',(50.9610854798929,29.6515989823489,40.0977360137709));
#176307=CARTESIAN_POINT('Ctrl Pts',(50.960431348397,29.6608932776203,40.0911601532641));
#176308=CARTESIAN_POINT('Ctrl Pts',(50.9601950050774,29.6699181168556,40.084220729064));
#176309=CARTESIAN_POINT('Ctrl Pts',(50.959959671528,29.678904397715,40.0773109533618));
#176310=CARTESIAN_POINT('Ctrl Pts',(50.9601383261077,29.6876236029351,40.0700409753048));
#176311=CARTESIAN_POINT('Ctrl Pts',(50.9607318934967,29.696015473601,40.0624586415899));
#176312=CARTESIAN_POINT('Ctrl Pts',(50.9607344403784,29.6960514814789,40.0624261072769));
#176313=CARTESIAN_POINT('Ctrl Pts',(50.9607369943872,29.6960874835155,40.0623935677888));
#176314=CARTESIAN_POINT('Ctrl Pts',(50.9607395555215,29.6961234797095,40.0623610231288));
#176315=CARTESIAN_POINT('Ctrl Pts',(50.9619473372426,29.7130985928882,40.0470135870233));
#176316=CARTESIAN_POINT('Ctrl Pts',(50.9647087325287,29.7287537227769,40.0305755292093));
#176317=CARTESIAN_POINT('Ctrl Pts',(50.9688330949324,29.7430502978482,40.0133447567338));
#176318=CARTESIAN_POINT('Ctrl Pts',(50.9731074935251,29.7578669541901,39.9954871626596));
#176319=CARTESIAN_POINT('Ctrl Pts',(50.9788464019642,29.7712250678592,39.9767767954316));
#176320=CARTESIAN_POINT('Ctrl Pts',(50.9858763526689,29.7830467300316,39.9575197577479));
#176321=CARTESIAN_POINT('Ctrl Pts',(50.9928059702033,29.7946996705595,39.9385375612006));
#176322=CARTESIAN_POINT('Ctrl Pts',(51.0009908790913,29.8048600966483,39.919022697711));
#176323=CARTESIAN_POINT('Ctrl Pts',(51.0102908031059,29.8134126013637,39.8992655451877));
#176324=CARTESIAN_POINT('Ctrl Pts',(51.0167748755908,29.8193755598154,39.885490506934));
#176325=CARTESIAN_POINT('Ctrl Pts',(51.023801515737,29.8245560588481,39.8715976051482));
#176326=CARTESIAN_POINT('Ctrl Pts',(51.0313275753413,29.8289013456879,39.8576902534424));
#176327=CARTESIAN_POINT('',(51.3398895692701,30.0070536838151,39.2875012672119));
#176328=CARTESIAN_POINT('',(51.0313275753413,29.8289013456879,39.8576902534424));
#176329=CARTESIAN_POINT('',(48.2946219293751,34.6963546279279,39.2875012672119));
#176330=CARTESIAN_POINT('Origin',(5.53234440788222E-15,0.,39.2875012672119));
#176331=CARTESIAN_POINT('',(48.0063682005191,34.4869303039391,39.8576902534424));
#176332=CARTESIAN_POINT('',(48.2946219293751,34.6963546279279,39.2875012672119));
#176333=CARTESIAN_POINT('',(47.6769115920308,34.6205005703629,40.1599502534424));
#176334=CARTESIAN_POINT('Ctrl Pts',(48.0063682005191,34.4869303039391,39.8576902534424));
#176335=CARTESIAN_POINT('Ctrl Pts',(47.9964738715094,34.4797418300848,39.8772619994052));
#176336=CARTESIAN_POINT('Ctrl Pts',(47.9854941018778,34.4741406737006,39.8967644650366));
#176337=CARTESIAN_POINT('Ctrl Pts',(47.9736072089122,34.470163644172,39.9159282836043));
#176338=CARTESIAN_POINT('Ctrl Pts',(47.9615055952506,34.4661147749665,39.9354382707186));
#176339=CARTESIAN_POINT('Ctrl Pts',(47.9484630607011,34.4637486663026,39.954598762236));
#176340=CARTESIAN_POINT('Ctrl Pts',(47.9346304384632,34.4631421240611,39.973138749824));
#176341=CARTESIAN_POINT('Ctrl Pts',(47.9213834535862,34.4625612612454,39.9908938024074));
#176342=CARTESIAN_POINT('Ctrl Pts',(47.907411011479,34.4635939836562,40.008081036621));
#176343=CARTESIAN_POINT('Ctrl Pts',(47.8928237488929,34.4663468279001,40.0244542742576));
#176344=CARTESIAN_POINT('Ctrl Pts',(47.8812215199242,34.4685363496862,40.0374770090508));
#176345=CARTESIAN_POINT('Ctrl Pts',(47.8692298237649,34.4718146898368,40.0499848770049));
#176346=CARTESIAN_POINT('Ctrl Pts',(47.8568987993932,34.4762554502652,40.0618424270193));
#176347=CARTESIAN_POINT('Ctrl Pts',(47.8568651397022,34.4762675720986,40.0618747942791));
#176348=CARTESIAN_POINT('Ctrl Pts',(47.8568314776419,34.4762797026728,40.0619071564124));
#176349=CARTESIAN_POINT('Ctrl Pts',(47.8567978132142,34.4762918419884,40.0619395134162));
#176350=CARTESIAN_POINT('Ctrl Pts',(47.8500962938269,34.4787083945371,40.0683807661799));
#176351=CARTESIAN_POINT('Ctrl Pts',(47.8432853991343,34.4815044004726,40.0746073439084));
#176352=CARTESIAN_POINT('Ctrl Pts',(47.8364019332942,34.4846629347246,40.0805869293669));
#176353=CARTESIAN_POINT('Ctrl Pts',(47.8227412186415,34.4909312646823,40.092453830807));
#176354=CARTESIAN_POINT('Ctrl Pts',(47.808794087666,34.4986286886037,40.1033475319609));
#176355=CARTESIAN_POINT('Ctrl Pts',(47.7948446809469,34.5076305235171,40.1130129263075));
#176356=CARTESIAN_POINT('Ctrl Pts',(47.7843826259076,34.5143818997022,40.1202619720674));
#176357=CARTESIAN_POINT('Ctrl Pts',(47.7739192901011,34.5218670065989,40.1268200947266));
#176358=CARTESIAN_POINT('Ctrl Pts',(47.7635745545823,34.5300332501813,40.1325796782703));
#176359=CARTESIAN_POINT('Ctrl Pts',(47.7596952787628,34.5330955915247,40.1347395220992));
#176360=CARTESIAN_POINT('Ctrl Pts',(47.7558326812647,34.5362537178259,40.1367870714852));
#176361=CARTESIAN_POINT('Ctrl Pts',(47.751993084602,34.5395048560459,40.1387166518767));
#176362=CARTESIAN_POINT('Ctrl Pts',(47.7385544962824,34.5508838398159,40.1454701832469));
#176363=CARTESIAN_POINT('Ctrl Pts',(47.7253976640916,34.5634022165997,40.1507785912491));
#176364=CARTESIAN_POINT('Ctrl Pts',(47.7127937034786,34.5769411196448,40.1543986087265));
#176365=CARTESIAN_POINT('Ctrl Pts',(47.7064917231721,34.5837105711674,40.1562086174652));
#176366=CARTESIAN_POINT('Ctrl Pts',(47.7003279615829,34.590735154856,40.1575965292115));
#176367=CARTESIAN_POINT('Ctrl Pts',(47.6943363116302,34.5980000149355,40.1585319382567));
#176368=CARTESIAN_POINT('Ctrl Pts',(47.6913404866539,34.6016324449753,40.1589996427793));
#176369=CARTESIAN_POINT('Ctrl Pts',(47.6883876896072,34.605324944128,40.159354221642));
#176370=CARTESIAN_POINT('Ctrl Pts',(47.6854821573394,34.6090756555947,40.159591874311));
#176371=CARTESIAN_POINT('Ctrl Pts',(47.6825766250716,34.6128263670613,40.1598295269801));
#176372=CARTESIAN_POINT('Ctrl Pts',(47.679718358958,34.6166352918404,40.1599502506895));
#176373=CARTESIAN_POINT('Ctrl Pts',(47.6769115920308,34.6205005703629,40.1599502534424));
#176374=CARTESIAN_POINT('',(47.659028586094,34.645114416418,40.1599502534424));
#176375=CARTESIAN_POINT('Origin',(5.71032169235817E-15,5.29275616590442E-15,
40.1599502534424));
#176376=CARTESIAN_POINT('',(47.6338034047604,34.9997217530255,39.8576902534424));
#176377=CARTESIAN_POINT('Ctrl Pts',(47.659028586094,34.645114416418,40.1599502534424));
#176378=CARTESIAN_POINT('Ctrl Pts',(47.6567884460685,34.6481960403145,40.1599502448875));
#176379=CARTESIAN_POINT('Ctrl Pts',(47.6545924528207,34.6512968858165,40.1598743450437));
#176380=CARTESIAN_POINT('Ctrl Pts',(47.6524408584475,34.6544147487629,40.1597243308499));
#176381=CARTESIAN_POINT('Ctrl Pts',(47.6397380079776,34.6728223758169,40.1588386583938));
#176382=CARTESIAN_POINT('Ctrl Pts',(47.6285798336113,34.6918243519436,40.1553722553614));
#176383=CARTESIAN_POINT('Ctrl Pts',(47.6190225715775,34.7109619288094,40.149690217778));
#176384=CARTESIAN_POINT('Ctrl Pts',(47.6154522966294,34.7181110904637,40.1475675976838));
#176385=CARTESIAN_POINT('Ctrl Pts',(47.6121050440158,34.7252793254663,40.1451361443092));
#176386=CARTESIAN_POINT('Ctrl Pts',(47.608982443287,34.732443391342,40.1424159447501));
#176387=CARTESIAN_POINT('Ctrl Pts',(47.6065460335526,34.7380331549247,40.1402935085949));
#176388=CARTESIAN_POINT('Ctrl Pts',(47.6042468425536,34.7436201516872,40.1379949176048));
#176389=CARTESIAN_POINT('Ctrl Pts',(47.6020860928993,34.7491931041019,40.1355293609261));
#176390=CARTESIAN_POINT('Ctrl Pts',(47.5945234691092,34.7686984375535,40.1268999125509));
#176391=CARTESIAN_POINT('Ctrl Pts',(47.5886567445954,34.7880317224279,40.1162251288835));
#176392=CARTESIAN_POINT('Ctrl Pts',(47.5845384124878,34.8067094890029,40.1038990521418));
#176393=CARTESIAN_POINT('Ctrl Pts',(47.582479246434,34.8160483722904,40.097736013771));
#176394=CARTESIAN_POINT('Ctrl Pts',(47.580857179937,34.8252233770798,40.0911601532641));
#176395=CARTESIAN_POINT('Ctrl Pts',(47.5796787787543,34.8341740726974,40.084220729064));
#176396=CARTESIAN_POINT('Ctrl Pts',(47.578505412258,34.8430865267157,40.0773109533619));
#176397=CARTESIAN_POINT('Ctrl Pts',(47.5777716830267,34.851776641706,40.0700409753047));
#176398=CARTESIAN_POINT('Ctrl Pts',(47.5774848094468,34.8601845855133,40.0624586415899));
#176399=CARTESIAN_POINT('Ctrl Pts',(47.5774835785283,34.860220662358,40.0624261072769));
#176400=CARTESIAN_POINT('Ctrl Pts',(47.5774823553084,34.8602567341383,40.0623935677888));
#176401=CARTESIAN_POINT('Ctrl Pts',(47.5774811397857,34.8602928008528,40.0623610231288));
#176402=CARTESIAN_POINT('Ctrl Pts',(47.5769079226579,34.8773011701495,40.0470135870261));
#176403=CARTESIAN_POINT('Ctrl Pts',(47.5780177840617,34.8931591840015,40.0305755292153));
#176404=CARTESIAN_POINT('Ctrl Pts',(47.5806251537534,34.9078085542004,40.0133447567433));
#176405=CARTESIAN_POINT('Ctrl Pts',(47.5833273744242,34.9229908396626,39.9954871626726));
#176406=CARTESIAN_POINT('Ctrl Pts',(47.587638541427,34.9368756554655,39.9767767954483));
#176407=CARTESIAN_POINT('Ctrl Pts',(47.593394281144,34.9493673872784,39.9575197577683));
#176408=CARTESIAN_POINT('Ctrl Pts',(47.5990678735408,34.96168083405,39.938537561224));
#176409=CARTESIAN_POINT('Ctrl Pts',(47.6061458909142,34.9726411562093,39.9190226977374));
#176410=CARTESIAN_POINT('Ctrl Pts',(47.6145008887944,34.982118916175,39.8992655452171));
#176411=CARTESIAN_POINT('Ctrl Pts',(47.6203261419715,34.9887269790548,39.8854905069538));
#176412=CARTESIAN_POINT('Ctrl Pts',(47.626772779849,34.9946135826729,39.8715976051581));
#176413=CARTESIAN_POINT('Ctrl Pts',(47.6338034047604,34.9997217530255,39.8576902534424));
#176414=CARTESIAN_POINT('',(47.9220530736691,35.2091516650522,39.2875012672119));
#176415=CARTESIAN_POINT('',(47.6338034047604,34.9997217530255,39.8576902534424));
#176416=CARTESIAN_POINT('',(44.4033023070494,39.5544469813066,39.2875012672119));
#176417=CARTESIAN_POINT('Origin',(5.53234440788222E-15,0.,39.2875012672119));
#176418=CARTESIAN_POINT('',(44.1385184650381,39.3160391863685,39.8576902534424));
#176419=CARTESIAN_POINT('',(44.4033023070494,39.5544469813066,39.2875012672119));
#176420=CARTESIAN_POINT('',(43.7969047596351,39.4144401478985,40.1599502534424));
#176421=CARTESIAN_POINT('Ctrl Pts',(44.1385184650381,39.3160391863685,39.8576902534424));
#176422=CARTESIAN_POINT('Ctrl Pts',(44.1294297383225,39.3078558527197,39.877261999406));
#176423=CARTESIAN_POINT('Ctrl Pts',(44.1190955972865,39.3011376816095,39.8967644650382));
#176424=CARTESIAN_POINT('Ctrl Pts',(44.1076895347488,39.29593992001,39.9159282836065));
#176425=CARTESIAN_POINT('Ctrl Pts',(44.0960774370686,39.2906482678547,39.9354382707213));
#176426=CARTESIAN_POINT('Ctrl Pts',(44.0833536765903,39.286931804888,39.954598762239));
#176427=CARTESIAN_POINT('Ctrl Pts',(44.0696602318325,39.2848826826029,39.9731387498273));
#176428=CARTESIAN_POINT('Ctrl Pts',(44.0565465320223,39.2829203148425,39.9908938024105));
#176429=CARTESIAN_POINT('Ctrl Pts',(44.0425426835285,39.2824868619904,40.0080810366238));
#176430=CARTESIAN_POINT('Ctrl Pts',(44.0277475809149,39.2836998417242,40.0244542742601));
#176431=CARTESIAN_POINT('Ctrl Pts',(44.0159800428236,39.2846646059163,40.0374770090524));
#176432=CARTESIAN_POINT('Ctrl Pts',(44.0037113585733,39.2866715134049,40.0499848770057));
#176433=CARTESIAN_POINT('Ctrl Pts',(43.9909836989809,39.2897990038547,40.0618424270193));
#176434=CARTESIAN_POINT('Ctrl Pts',(43.9909489566045,39.2898075408878,40.0618747942791));
#176435=CARTESIAN_POINT('Ctrl Pts',(43.9909142109582,39.2898160863659,40.0619071564124));
#176436=CARTESIAN_POINT('Ctrl Pts',(43.9908794620438,39.2898246402901,40.0619395134161));
#176437=CARTESIAN_POINT('Ctrl Pts',(43.9839620557566,39.291527455188,40.0683807661799));
#176438=CARTESIAN_POINT('Ctrl Pts',(43.976896209654,39.2935962119547,40.0746073439084));
#176439=CARTESIAN_POINT('Ctrl Pts',(43.9697202954285,39.2960179253194,40.0805869293669));
#176440=CARTESIAN_POINT('Ctrl Pts',(43.9554791967022,39.3008239832,40.092453830807));
#176441=CARTESIAN_POINT('Ctrl Pts',(43.9408038696759,39.3070213676599,40.1033475319609));
#176442=CARTESIAN_POINT('Ctrl Pts',(43.9259899312964,39.3145157795319,40.1130129263075));
#176443=CARTESIAN_POINT('Ctrl Pts',(43.9148794775117,39.3201365884359,40.1202619720674));
#176444=CARTESIAN_POINT('Ctrl Pts',(43.9036910542322,39.3264869747214,40.1268200947266));
#176445=CARTESIAN_POINT('Ctrl Pts',(43.8925493833646,39.3335271634603,40.1325796782703));
#176446=CARTESIAN_POINT('Ctrl Pts',(43.8883712567893,39.3361672342374,40.1347395220992));
#176447=CARTESIAN_POINT('Ctrl Pts',(43.8841997049153,39.3389043086116,40.1367870714852));
#176448=CARTESIAN_POINT('Ctrl Pts',(43.8800413054829,39.3417362896176,40.1387166518767));
#176449=CARTESIAN_POINT('Ctrl Pts',(43.8654869074692,39.3516482231383,40.1454701832469));
#176450=CARTESIAN_POINT('Ctrl Pts',(43.851093623094,39.362722759494,40.1507785912492));
#176451=CARTESIAN_POINT('Ctrl Pts',(43.8371435075663,39.3748700223776,40.1543986087265));
#176452=CARTESIAN_POINT('Ctrl Pts',(43.8301684498025,39.3809436538194,40.1562086174652));
#176453=CARTESIAN_POINT('Ctrl Pts',(43.8233041850061,39.3872854675767,40.1575965292115));
#176454=CARTESIAN_POINT('Ctrl Pts',(43.8165859732789,39.3938842320306,40.1585319382567));
#176455=CARTESIAN_POINT('Ctrl Pts',(43.8132268674153,39.3971836142575,40.1589996427793));
#176456=CARTESIAN_POINT('Ctrl Pts',(43.8099042748376,39.4005472341759,40.159354221642));
#176457=CARTESIAN_POINT('Ctrl Pts',(43.8066226032738,39.4039736880298,40.159591874311));
#176458=CARTESIAN_POINT('Ctrl Pts',(43.8033409317101,39.4074001418836,40.1598295269801));
#176459=CARTESIAN_POINT('Ctrl Pts',(43.8001001824235,39.4108894308098,40.1599502506895));
#176460=CARTESIAN_POINT('Ctrl Pts',(43.7969047596351,39.4144401478985,40.1599502534424));
#176461=CARTESIAN_POINT('',(43.7765468711727,39.4370498736003,40.1599502534424));
#176462=CARTESIAN_POINT('Origin',(5.7058335455513E-15,5.29829856563434E-15,
40.1599502534424));
#176463=CARTESIAN_POINT('',(43.7143933160628,39.7870778846742,39.8576902534424));
#176464=CARTESIAN_POINT('Ctrl Pts',(43.7765468711727,39.4370498736003,40.1599502534424));
#176465=CARTESIAN_POINT('Ctrl Pts',(43.7739968854584,39.4398804576443,40.1599502448875));
#176466=CARTESIAN_POINT('Ctrl Pts',(43.7714887954763,39.4427347725906,40.1598743450437));
#176467=CARTESIAN_POINT('Ctrl Pts',(43.7690230823397,39.4456106527042,40.1597243308499));
#176468=CARTESIAN_POINT('Ctrl Pts',(43.7544656984424,39.4625896314159,40.1588386583936));
#176469=CARTESIAN_POINT('Ctrl Pts',(43.7413824023569,39.4803211659136,40.15537225536));
#176470=CARTESIAN_POINT('Ctrl Pts',(43.7298770745023,39.4983548992213,40.1496902177745));
#176471=CARTESIAN_POINT('Ctrl Pts',(43.7255790670151,39.5050917016626,40.1475675976811));
#176472=CARTESIAN_POINT('Ctrl Pts',(43.7215008664148,39.5118707851483,40.1451361443077));
#176473=CARTESIAN_POINT('Ctrl Pts',(43.7176465228248,39.5186692048623,40.1424159447501));
#176474=CARTESIAN_POINT('Ctrl Pts',(43.7146391706006,39.5239736729698,40.1402935085948));
#176475=CARTESIAN_POINT('Ctrl Pts',(43.7117685746245,39.5292897326775,40.1379949176047));
#176476=CARTESIAN_POINT('Ctrl Pts',(43.7090371296311,39.534606296035,40.1355293609261));
#176477=CARTESIAN_POINT('Ctrl Pts',(43.6994770721542,39.5532142677859,40.1268999125508));
#176478=CARTESIAN_POINT('Ctrl Pts',(43.6916216076134,39.5718284032051,40.1162251288835));
#176479=CARTESIAN_POINT('Ctrl Pts',(43.6855734779227,39.5899733680941,40.1038990521418));
#176480=CARTESIAN_POINT('Ctrl Pts',(43.6825494130773,39.5990458505386,40.0977360137709));
#176481=CARTESIAN_POINT('Ctrl Pts',(43.6799771832791,39.6080010415734,40.0911601532641));
#176482=CARTESIAN_POINT('Ctrl Pts',(43.6778696350433,39.6167795278792,40.084220729064));
#176483=CARTESIAN_POINT('Ctrl Pts',(43.675771091249,39.6255205083452,40.0773109533618));
#176484=CARTESIAN_POINT('Ctrl Pts',(43.6741330170976,39.6340863223872,40.0700409753048));
#176485=CARTESIAN_POINT('Ctrl Pts',(43.6729688455957,39.6424182201442,40.0624586415899));
#176486=CARTESIAN_POINT('Ctrl Pts',(43.6729638503632,39.6424539706901,40.0624261072769));
#176487=CARTESIAN_POINT('Ctrl Pts',(43.6729588633165,39.6424897170041,40.0623935677889));
#176488=CARTESIAN_POINT('Ctrl Pts',(43.6729538844543,39.6425254590847,40.0623610231289));
#176489=CARTESIAN_POINT('Ctrl Pts',(43.6706059487643,39.6593807372514,40.0470135870242));
#176490=CARTESIAN_POINT('Ctrl Pts',(43.670052116413,39.6752678913532,40.0305755292112));
#176491=CARTESIAN_POINT('Ctrl Pts',(43.6711139265065,39.690109555118,40.0133447567368));
#176492=CARTESIAN_POINT('Ctrl Pts',(43.672214363162,39.7054911294078,39.9954871626635));
#176493=CARTESIAN_POINT('Ctrl Pts',(43.6750505546831,39.7197505224001,39.9767767954365));
#176494=CARTESIAN_POINT('Ctrl Pts',(43.6794690223272,39.7327754618278,39.9575197577537));
#176495=CARTESIAN_POINT('Ctrl Pts',(43.6838244285239,39.7456145061448,39.938537561207));
#176496=CARTESIAN_POINT('Ctrl Pts',(43.6897180061469,39.7572546407921,39.919022697718));
#176497=CARTESIAN_POINT('Ctrl Pts',(43.697036538792,39.7675538156862,39.8992655451953));
#176498=CARTESIAN_POINT('Ctrl Pts',(43.7021391499628,39.7747345836643,39.8854905069391));
#176499=CARTESIAN_POINT('Ctrl Pts',(43.7079351548507,39.7812627969986,39.8715976051507));
#176500=CARTESIAN_POINT('Ctrl Pts',(43.7143933160628,39.7870778846742,39.8576902534424));
#176501=CARTESIAN_POINT('',(43.9791725362587,40.0254908126583,39.2875012672119));
#176502=CARTESIAN_POINT('',(43.7143933160628,39.7870778846742,39.8576902534424));
#176503=CARTESIAN_POINT('',(40.0254908126594,43.9791725362578,39.2875012672119));
#176504=CARTESIAN_POINT('Origin',(5.53234440788222E-15,0.,39.2875012672119));
#176505=CARTESIAN_POINT('',(39.7870778846752,43.7143933160618,39.8576902534424));
#176506=CARTESIAN_POINT('',(40.0254908126594,43.9791725362578,39.2875012672119));
#176507=CARTESIAN_POINT('',(39.4370498736014,43.7765468711718,40.1599502534424));
#176508=CARTESIAN_POINT('Ctrl Pts',(39.7870778846752,43.7143933160618,39.8576902534424));
#176509=CARTESIAN_POINT('Ctrl Pts',(39.7788943382462,43.7053047809343,39.8772619994062));
#176510=CARTESIAN_POINT('Ctrl Pts',(39.7693190488181,43.6975432007866,39.8967644650386));
#176511=CARTESIAN_POINT('Ctrl Pts',(39.7585187839167,43.69118165488,39.9159282836071));
#176512=CARTESIAN_POINT('Ctrl Pts',(39.7475234267904,43.684705196223,39.9354382707221));
#176513=CARTESIAN_POINT('Ctrl Pts',(39.7352578445659,43.6796790972996,39.9545987622399));
#176514=CARTESIAN_POINT('Ctrl Pts',(39.7218536055345,43.6762098455834,39.9731387498284));
#176515=CARTESIAN_POINT('Ctrl Pts',(39.7090168672302,43.67288747299,39.9908938024117));
#176516=CARTESIAN_POINT('Ctrl Pts',(39.6951350414442,43.6709925938752,40.008081036625));
#176517=CARTESIAN_POINT('Ctrl Pts',(39.680294197043,43.670652419439,40.0244542742614));
#176518=CARTESIAN_POINT('Ctrl Pts',(39.6684902774386,43.6703818558789,40.0374770090532));
#176519=CARTESIAN_POINT('Ctrl Pts',(39.656079023369,43.6710953426073,40.049984877006));
#176520=CARTESIAN_POINT('Ctrl Pts',(39.6430941754573,43.6728752976389,40.0618424270193));
#176521=CARTESIAN_POINT('Ctrl Pts',(39.6430587310404,43.672880156338,40.0618747942791));
#176522=CARTESIAN_POINT('Ctrl Pts',(39.6430232824887,43.6728850230941,40.0619071564124));
#176523=CARTESIAN_POINT('Ctrl Pts',(39.642987829804,43.6728898979084,40.0619395134161));
#176524=CARTESIAN_POINT('Ctrl Pts',(39.6359303251676,43.6738603187591,40.0683807661799));
#176525=CARTESIAN_POINT('Ctrl Pts',(39.6286869425436,43.675179160625,40.0746073439084));
#176526=CARTESIAN_POINT('Ctrl Pts',(39.6212972007506,43.676837520304,40.0805869293668));
#176527=CARTESIAN_POINT('Ctrl Pts',(39.6066317464086,43.6801286499315,40.092453830807));
#176528=CARTESIAN_POINT('Ctrl Pts',(39.5913890092854,43.6847580950889,40.1033475319609));
#176529=CARTESIAN_POINT('Ctrl Pts',(39.5758728438542,43.6906629735748,40.1130129263075));
#176530=CARTESIAN_POINT('Ctrl Pts',(39.5642357197808,43.6950916324392,40.1202619720674));
#176531=CARTESIAN_POINT('Ctrl Pts',(39.5524447917351,43.7002377219523,40.1268200947266));
#176532=CARTESIAN_POINT('Ctrl Pts',(39.5406282559963,43.7060747220667,40.1325796782703));
#176533=CARTESIAN_POINT('Ctrl Pts',(39.5361970550943,43.7082635971095,40.1347395220992));
#176534=CARTESIAN_POINT('Ctrl Pts',(39.5317622532398,43.7105496315971,40.1367870714852));
#176535=CARTESIAN_POINT('Ctrl Pts',(39.527330611332,43.7129314276125,40.1387166518767));
#176536=CARTESIAN_POINT('Ctrl Pts',(39.5118198646546,43.7212677136662,40.1454701832469));
#176537=CARTESIAN_POINT('Ctrl Pts',(39.4963478239305,43.7307770746558,40.1507785912492));
#176538=CARTESIAN_POINT('Ctrl Pts',(39.4812043938732,43.7413996094238,40.1543986087265));
#176539=CARTESIAN_POINT('Ctrl Pts',(39.4736326788445,43.7467108768079,40.1562086174652));
#176540=CARTESIAN_POINT('Ctrl Pts',(39.4661431171625,43.7523004383952,40.1575965292115));
#176541=CARTESIAN_POINT('Ctrl Pts',(39.4587719497942,43.7581608097792,40.1585319382567));
#176542=CARTESIAN_POINT('Ctrl Pts',(39.4550863661101,43.7610909954712,40.1589996427793));
#176543=CARTESIAN_POINT('Ctrl Pts',(39.4514303810211,43.7640888836316,40.159354221642));
#176544=CARTESIAN_POINT('Ctrl Pts',(39.4478085248418,43.7671535389272,40.159591874311));
#176545=CARTESIAN_POINT('Ctrl Pts',(39.4441866686624,43.7702181942228,40.1598295269801));
#176546=CARTESIAN_POINT('Ctrl Pts',(39.4405989425301,43.7733496179164,40.1599502506895));
#176547=CARTESIAN_POINT('Ctrl Pts',(39.4370498736014,43.7765468711718,40.1599502534424));
#176548=CARTESIAN_POINT('',(39.4144401478995,43.7969047596342,40.1599502534424));
#176549=CARTESIAN_POINT('Origin',(5.70079064675565E-15,5.30334146442998E-15,
40.1599502534424));
#176550=CARTESIAN_POINT('',(39.3160391863695,44.1385184650371,39.8576902534424));
#176551=CARTESIAN_POINT('Ctrl Pts',(39.4144401478995,43.7969047596342,40.1599502534424));
#176552=CARTESIAN_POINT('Ctrl Pts',(39.4116082546735,43.7994532913546,40.1599502448875));
#176553=CARTESIAN_POINT('Ctrl Pts',(39.4088155471156,43.8020298032734,40.1598743450437));
#176554=CARTESIAN_POINT('Ctrl Pts',(39.4060627300848,43.8046321918097,40.1597243308499));
#176555=CARTESIAN_POINT('Ctrl Pts',(39.3898103065136,43.8199964969255,40.1588386583939));
#176556=CARTESIAN_POINT('Ctrl Pts',(39.3749452320458,43.8362633193808,40.1553722553627));
#176557=CARTESIAN_POINT('Ctrl Pts',(39.3616178931555,43.8529956277635,40.1496902177812));
#176558=CARTESIAN_POINT('Ctrl Pts',(39.3566392429908,43.8592462611849,40.1475675976862));
#176559=CARTESIAN_POINT('Ctrl Pts',(39.3518747760156,43.865561920107,40.1451361443106));
#176560=CARTESIAN_POINT('Ctrl Pts',(39.347330918553,43.8719202087608,40.1424159447501));
#176561=CARTESIAN_POINT('Ctrl Pts',(39.3437855730191,43.8768812645304,40.1402935085949));
#176562=CARTESIAN_POINT('Ctrl Pts',(39.3403750229164,43.8818681433209,40.1379949176048));
#176563=CARTESIAN_POINT('Ctrl Pts',(39.3371028088668,43.8868700682403,40.1355293609261));
#176564=CARTESIAN_POINT('Ctrl Pts',(39.3256500596934,43.9043768054582,40.1268999125508));
#176565=CARTESIAN_POINT('Ctrl Pts',(39.3158919212388,43.9220678510592,40.1162251288835));
#176566=CARTESIAN_POINT('Ctrl Pts',(39.3079802585394,43.9394812142298,40.1038990521418));
#176567=CARTESIAN_POINT('Ctrl Pts',(39.3040244271897,43.948187895815,40.0977360137709));
#176568=CARTESIAN_POINT('Ctrl Pts',(39.3005302159784,43.9568251581485,40.0911601532641));
#176569=CARTESIAN_POINT('Ctrl Pts',(39.297516611429,43.9653352562094,40.084220729064));
#176570=CARTESIAN_POINT('Ctrl Pts',(39.2945158824216,43.9738089951119,40.0773109533619));
#176571=CARTESIAN_POINT('Ctrl Pts',(39.2919914104334,43.9821566593546,40.0700409753047));
#176572=CARTESIAN_POINT('Ctrl Pts',(39.2899626959162,43.9903212250458,40.0624586415899));
#176573=CARTESIAN_POINT('Ctrl Pts',(39.2899539910984,43.9903562576025,40.0624261072769));
#176574=CARTESIAN_POINT('Ctrl Pts',(39.289945294864,43.9903912868061,40.0623935677888));
#176575=CARTESIAN_POINT('Ctrl Pts',(39.2899366072118,43.990426312655,40.0623610231288));
#176576=CARTESIAN_POINT('Ctrl Pts',(39.2858396774346,44.0069438297345,40.0470135870245));
#176577=CARTESIAN_POINT('Ctrl Pts',(39.2836282192308,44.0226860610988,40.0305755292119));
#176578=CARTESIAN_POINT('Ctrl Pts',(39.2831328363119,44.0375574100537,40.013344756738));
#176579=CARTESIAN_POINT('Ctrl Pts',(39.282619432337,44.0529697494221,39.9954871626652));
#176580=CARTESIAN_POINT('Ctrl Pts',(39.2839495744675,44.0674474907085,39.9767767954388));
#176581=CARTESIAN_POINT('Ctrl Pts',(39.2869823603807,44.0808629337877,39.9575197577567));
#176582=CARTESIAN_POINT('Ctrl Pts',(39.2899718616341,44.094086908393,39.9385375612105));
#176583=CARTESIAN_POINT('Ctrl Pts',(39.294616428235,44.1062793237767,39.919022697722));
#176584=CARTESIAN_POINT('Ctrl Pts',(39.3008183122675,44.1172870736838,39.8992655451998));
#176585=CARTESIAN_POINT('Ctrl Pts',(39.3051423761588,44.1249618727689,39.8854905069421));
#176586=CARTESIAN_POINT('Ctrl Pts',(39.3102242458182,44.1320601713525,39.8715976051522));
#176587=CARTESIAN_POINT('Ctrl Pts',(39.3160391863696,44.1385184650371,39.8576902534424));
#176588=CARTESIAN_POINT('',(39.5544469813076,44.4033023070484,39.2875012672119));
#176589=CARTESIAN_POINT('',(39.3160391863695,44.1385184650371,39.8576902534424));
#176590=CARTESIAN_POINT('',(35.2091516650533,47.9220530736683,39.2875012672119));
#176591=CARTESIAN_POINT('Origin',(5.53234440788222E-15,0.,39.2875012672119));
#176592=CARTESIAN_POINT('',(34.9997217530266,47.6338034047596,39.8576902534424));
#176593=CARTESIAN_POINT('',(35.2091516650533,47.9220530736683,39.2875012672119));
#176594=CARTESIAN_POINT('',(34.6451144164191,47.6590285860932,40.1599502534424));
#176595=CARTESIAN_POINT('Ctrl Pts',(34.9997217530266,47.6338034047596,39.8576902534424));
#176596=CARTESIAN_POINT('Ctrl Pts',(34.9925330475319,47.6239092440465,39.8772619994051));
#176597=CARTESIAN_POINT('Ctrl Pts',(34.9838215185872,47.6151892923581,39.8967644650364));
#176598=CARTESIAN_POINT('Ctrl Pts',(34.9737453812853,47.6077336605728,39.915928283604));
#176599=CARTESIAN_POINT('Ctrl Pts',(34.9634872321473,47.6001433528506,39.9354382707181));
#176600=CARTESIAN_POINT('Ctrl Pts',(34.951814212463,47.5938626849621,39.9545987622351));
#176601=CARTESIAN_POINT('Ctrl Pts',(34.9388460388069,47.5890113136625,39.9731387498229));
#176602=CARTESIAN_POINT('Ctrl Pts',(34.9264269040003,47.5843653368455,39.9908938024059));
#176603=CARTESIAN_POINT('Ctrl Pts',(34.9128191931108,47.5810297921597,40.008081036619));
#176604=CARTESIAN_POINT('Ctrl Pts',(34.8980952063197,47.5791401905755,40.0244542742552));
#176605=CARTESIAN_POINT('Ctrl Pts',(34.8863842314135,47.5776372636136,40.0374770090492));
#176606=CARTESIAN_POINT('Ctrl Pts',(34.8739663878191,47.5770495124717,40.0499848770041));
#176607=CARTESIAN_POINT('Ctrl Pts',(34.8608666162967,47.5774624305256,40.0618424270192));
#176608=CARTESIAN_POINT('Ctrl Pts',(34.8608308581757,47.5774635576577,40.0618747942791));
#176609=CARTESIAN_POINT('Ctrl Pts',(34.8607950951003,47.5774646923706,40.0619071564124));
#176610=CARTESIAN_POINT('Ctrl Pts',(34.8607593270722,47.5774658346655,40.0619395134161));
#176611=CARTESIAN_POINT('Ctrl Pts',(34.8536390475845,47.5776932293351,40.0683807661799));
#176612=CARTESIAN_POINT('Ctrl Pts',(34.8462974884548,47.5782477067928,40.0746073439084));
#176613=CARTESIAN_POINT('Ctrl Pts',(34.8387748826518,47.5791245434503,40.0805869293669));
#176614=CARTESIAN_POINT('Ctrl Pts',(34.8238457504807,47.5808646865199,40.092453830807));
#176615=CARTESIAN_POINT('Ctrl Pts',(34.8082026058783,47.5838754712048,40.1033475319609));
#176616=CARTESIAN_POINT('Ctrl Pts',(34.7921542117509,47.5881261212202,40.1130129263075));
#176617=CARTESIAN_POINT('Ctrl Pts',(34.7801179161553,47.5913141087317,40.1202619720674));
#176618=CARTESIAN_POINT('Ctrl Pts',(34.7678536672185,47.595199519839,40.1268200947266));
#176619=CARTESIAN_POINT('Ctrl Pts',(34.7554917310469,47.599769379934,40.1325796782703));
#176620=CARTESIAN_POINT('Ctrl Pts',(34.7508560049825,47.6014830774696,40.1347395220992));
#176621=CARTESIAN_POINT('Ctrl Pts',(34.7462065417646,47.6032930257984,40.1367870714852));
#176622=CARTESIAN_POINT('Ctrl Pts',(34.7415502113776,47.6051985413675,40.1387166518767));
#176623=CARTESIAN_POINT('Ctrl Pts',(34.7252530550228,47.6118678458597,40.1454701832469));
#176624=CARTESIAN_POINT('Ctrl Pts',(34.7088717728658,47.6197078449343,40.1507785912492));
#176625=CARTESIAN_POINT('Ctrl Pts',(34.6927009428675,47.628689268873,40.1543986087265));
#176626=CARTESIAN_POINT('Ctrl Pts',(34.6846155278684,47.6331799808423,40.1562086174652));
#176627=CARTESIAN_POINT('Ctrl Pts',(34.6765827265058,47.6379560498532,40.1575965292115));
#176628=CARTESIAN_POINT('Ctrl Pts',(34.6686393635487,47.6430138207121,40.1585319382567));
#176629=CARTESIAN_POINT('Ctrl Pts',(34.6646676820701,47.6455427061416,40.1589996427793));
#176630=CARTESIAN_POINT('Ctrl Pts',(34.6607183602076,47.6481420170538,40.159354221642));
#176631=CARTESIAN_POINT('Ctrl Pts',(34.6567960012268,47.6508112967865,40.159591874311));
#176632=CARTESIAN_POINT('Ctrl Pts',(34.6528736422461,47.6534805765192,40.1598295269801));
#176633=CARTESIAN_POINT('Ctrl Pts',(34.6489782471464,47.6562198264468,40.1599502506894));
#176634=CARTESIAN_POINT('Ctrl Pts',(34.6451144164191,47.6590285860932,40.1599502534424));
#176635=CARTESIAN_POINT('',(34.620500570364,47.67691159203,40.1599502534424));
#176636=CARTESIAN_POINT('Origin',(5.69524824702573E-15,5.30782961123685E-15,
40.1599502534424));
#176637=CARTESIAN_POINT('',(34.4869303039402,48.0063682005183,39.8576902534424));
#176638=CARTESIAN_POINT('Ctrl Pts',(34.620500570364,47.67691159203,40.1599502534424));
#176639=CARTESIAN_POINT('Ctrl Pts',(34.617417796441,47.6791501491799,40.1599502448875));
#176640=CARTESIAN_POINT('Ctrl Pts',(34.614371068796,47.6814206292675,40.1598743450437));
#176641=CARTESIAN_POINT('Ctrl Pts',(34.6113613083103,47.6837210139132,40.1597243308499));
#176642=CARTESIAN_POINT('Ctrl Pts',(34.5935919100098,47.6973023109002,40.1588386583938));
#176643=CARTESIAN_POINT('Ctrl Pts',(34.5771079220191,47.7119261986124,40.1553722553615));
#176644=CARTESIAN_POINT('Ctrl Pts',(34.5621045892013,47.7271737594084,40.1496902177782));
#176645=CARTESIAN_POINT('Ctrl Pts',(34.5564998435001,47.7328697405523,40.1475675976839));
#176646=CARTESIAN_POINT('Ctrl Pts',(34.5511013106546,47.73865277922,40.1451361443093));
#176647=CARTESIAN_POINT('Ctrl Pts',(34.5459177227791,47.7445012740626,40.1424159447501));
#176648=CARTESIAN_POINT('Ctrl Pts',(34.5418732274832,47.7490645631293,40.1402935085949));
#176649=CARTESIAN_POINT('Ctrl Pts',(34.5379600899543,47.7536676237148,40.1379949176048));
#176650=CARTESIAN_POINT('Ctrl Pts',(34.5341829579105,47.75830010806,40.1355293609261));
#176651=CARTESIAN_POINT('Ctrl Pts',(34.5209629957571,47.7745138032684,40.1268999125509));
#176652=CARTESIAN_POINT('Ctrl Pts',(34.5094090955958,47.7910879322535,40.1162251288835));
#176653=CARTESIAN_POINT('Ctrl Pts',(34.4997205817199,47.8075789092548,40.1038990521418));
#176654=CARTESIAN_POINT('Ctrl Pts',(34.494876324782,47.8158243977555,40.097736013771));
#176655=CARTESIAN_POINT('Ctrl Pts',(34.4904984154667,47.8240490997338,40.0911601532641));
#176656=CARTESIAN_POINT('Ctrl Pts',(34.4866117722857,47.8321975711347,40.084220729064));
#176657=CARTESIAN_POINT('Ctrl Pts',(34.4827417346802,47.840311228417,40.0773109533618));
#176658=CARTESIAN_POINT('Ctrl Pts',(34.4793585234985,47.8483492841041,40.0700409753047));
#176659=CARTESIAN_POINT('Ctrl Pts',(34.4764874929868,47.8562570650393,40.0624586415899));
#176660=CARTESIAN_POINT('Ctrl Pts',(34.4764751739556,47.8562909957828,40.0624261072769));
#176661=CARTESIAN_POINT('Ctrl Pts',(34.4764628638112,47.8563249240887,40.0623935677888));
#176662=CARTESIAN_POINT('Ctrl Pts',(34.4764505625528,47.8563588499554,40.0623610231288));
#176663=CARTESIAN_POINT('Ctrl Pts',(34.4706495255091,47.8723576365719,40.0470135870269));
#176664=CARTESIAN_POINT('Ctrl Pts',(34.4668046706522,47.8877824700158,40.0305755292169));
#176665=CARTESIAN_POINT('Ctrl Pts',(34.4647575222394,47.9025205705478,40.0133447567459));
#176666=CARTESIAN_POINT('Ctrl Pts',(34.4626359025954,47.9177948141779,39.9954871626762));
#176667=CARTESIAN_POINT('Ctrl Pts',(34.462445422019,47.9323322825936,39.9767767954531));
#176668=CARTESIAN_POINT('Ctrl Pts',(34.4640592983631,47.9459912469213,39.9575197577743));
#176669=CARTESIAN_POINT('Ctrl Pts',(34.4656501410707,47.9594552671806,39.9385375612313));
#176670=CARTESIAN_POINT('Ctrl Pts',(34.4689948098043,47.9720663806451,39.9190226977461));
#176671=CARTESIAN_POINT('Ctrl Pts',(34.4740120960831,47.983662102353,39.8992655452271));
#176672=CARTESIAN_POINT('Ctrl Pts',(34.477510237347,47.9917468458453,39.8854905069605));
#176673=CARTESIAN_POINT('Ctrl Pts',(34.4818222937524,47.9993374592379,39.8715976051615));
#176674=CARTESIAN_POINT('Ctrl Pts',(34.4869303039402,48.0063682005183,39.8576902534424));
#176675=CARTESIAN_POINT('',(34.6963546279291,48.2946219293742,39.2875012672119));
#176676=CARTESIAN_POINT('',(34.4869303039402,48.0063682005183,39.8576902534424));
#176677=CARTESIAN_POINT('',(30.0070536838164,51.3398895692693,39.2875012672119));
#176678=CARTESIAN_POINT('Origin',(5.53234440788222E-15,0.,39.2875012672119));
#176679=CARTESIAN_POINT('',(29.8289013456892,51.0313275753405,39.8576902534424));
#176680=CARTESIAN_POINT('',(30.0070536838164,51.3398895692693,39.2875012672119));
#176681=CARTESIAN_POINT('',(29.4735998357344,51.0193480105324,40.1599502534424));
#176682=CARTESIAN_POINT('Ctrl Pts',(29.8289013456892,51.0313275753405,39.8576902534424));
#176683=CARTESIAN_POINT('Ctrl Pts',(29.82278624209,51.020736191537,39.8772619994049));
#176684=CARTESIAN_POINT('Ctrl Pts',(29.8150339189622,51.0111534059232,39.896764465036));
#176685=CARTESIAN_POINT('Ctrl Pts',(29.8057923055281,51.0026853737211,39.9159282836033));
#176686=CARTESIAN_POINT('Ctrl Pts',(29.7963837548065,50.9940643779337,39.935438270717));
#176687=CARTESIAN_POINT('Ctrl Pts',(29.7854311897083,50.9865979533917,39.9545987622337));
#176688=CARTESIAN_POINT('Ctrl Pts',(29.7730411634515,50.9804176151481,39.9731387498212));
#176689=CARTESIAN_POINT('Ctrl Pts',(29.7611756987822,50.9744989364018,39.9908938024036));
#176690=CARTESIAN_POINT('Ctrl Pts',(29.7479911917175,50.969759271071,40.0080810366163));
#176691=CARTESIAN_POINT('Ctrl Pts',(29.7335453816171,50.9663409452095,40.0244542742521));
#176692=CARTESIAN_POINT('Ctrl Pts',(29.7220556593017,50.963622121228,40.0374770090473));
#176693=CARTESIAN_POINT('Ctrl Pts',(29.7097672786766,50.9617395717401,40.0499848770032));
#176694=CARTESIAN_POINT('Ctrl Pts',(29.6966961073826,50.9607809287992,40.0618424270192));
#176695=CARTESIAN_POINT('Ctrl Pts',(29.6966604273309,50.9607783120154,40.0618747942791));
#176696=CARTESIAN_POINT('Ctrl Pts',(29.6966247415596,50.9607757022529,40.0619071564124));
#176697=CARTESIAN_POINT('Ctrl Pts',(29.6965890500702,50.9607730995132,40.0619395134161));
#176698=CARTESIAN_POINT('Ctrl Pts',(29.6894840070031,50.9602549766181,40.0683807661799));
#176699=CARTESIAN_POINT('Ctrl Pts',(29.682124707026,50.9600390146964,40.0746073439084));
#176700=CARTESIAN_POINT('Ctrl Pts',(29.6745516564563,50.9601247215267,40.0805869293668));
#176701=CARTESIAN_POINT('Ctrl Pts',(29.6595224131525,50.9602948126666,40.092453830807));
#176702=CARTESIAN_POINT('Ctrl Pts',(29.6436502506365,50.9616539500921,40.1033475319609));
#176703=CARTESIAN_POINT('Ctrl Pts',(29.6272454573773,50.9642038006258,40.1130129263075));
#176704=CARTESIAN_POINT('Ctrl Pts',(29.6149418624329,50.9661161885262,40.1202619720674));
#176705=CARTESIAN_POINT('Ctrl Pts',(29.6023386622828,50.9686983518504,40.1268200947266));
#176706=CARTESIAN_POINT('Ctrl Pts',(29.5895667656379,50.9719510035826,40.1325796782703));
#176707=CARTESIAN_POINT('Ctrl Pts',(29.584777304396,50.9731707479822,40.1347395220992));
#176708=CARTESIAN_POINT('Ctrl Pts',(29.5799641203068,50.9744847799794,40.1367870714852));
#176709=CARTESIAN_POINT('Ctrl Pts',(29.5751341171706,50.9758931378751,40.1387166518767));
#176710=CARTESIAN_POINT('Ctrl Pts',(29.5582291061939,50.9808223905101,40.1454701832469));
#176711=CARTESIAN_POINT('Ctrl Pts',(29.5411180593592,50.9869071309992,40.1507785912492));
#176712=CARTESIAN_POINT('Ctrl Pts',(29.5240970004174,50.9941490417483,40.1543986087265));
#176713=CARTESIAN_POINT('Ctrl Pts',(29.5155864709465,50.9977699971228,40.1562086174652));
#176714=CARTESIAN_POINT('Ctrl Pts',(29.5070984389562,51.0016802459459,40.1575965292115));
#176715=CARTESIAN_POINT('Ctrl Pts',(29.498669909557,51.0058800022837,40.1585319382567));
#176716=CARTESIAN_POINT('Ctrl Pts',(29.4944556448574,51.0079798804526,40.1589996427793));
#176717=CARTESIAN_POINT('Ctrl Pts',(29.490256255818,51.0101521355225,40.159354221642));
#176718=CARTESIAN_POINT('Ctrl Pts',(29.4860763682217,51.0123967945048,40.159591874311));
#176719=CARTESIAN_POINT('Ctrl Pts',(29.4818964806253,51.0146414534872,40.1598295269801));
#176720=CARTESIAN_POINT('Ctrl Pts',(29.4777360953222,51.0169585178535,40.1599502506895));
#176721=CARTESIAN_POINT('Ctrl Pts',(29.4735998357344,51.0193480105324,40.1599502534424));
#176722=CARTESIAN_POINT('',(29.4472515437741,51.0345602039883,40.1599502534424));
#176723=CARTESIAN_POINT('Origin',(5.68926707005281E-15,5.31171383297933E-15,
40.1599502534424));
#176724=CARTESIAN_POINT('',(29.2799753962469,51.3482501200162,39.8576902534424));
#176725=CARTESIAN_POINT('Ctrl Pts',(29.4472515437741,51.0345602039883,40.1599502534424));
#176726=CARTESIAN_POINT('Ctrl Pts',(29.4439516646705,51.0364642604672,40.1599502448875));
#176727=CARTESIAN_POINT('Ctrl Pts',(29.4406842975238,51.0384038328685,40.1598743450437));
#176728=CARTESIAN_POINT('Ctrl Pts',(29.4374505691491,51.0403770101281,40.1597243308499));
#176729=CARTESIAN_POINT('Ctrl Pts',(29.4183588813694,51.052026499451,40.1588386583938));
#176730=CARTESIAN_POINT('Ctrl Pts',(29.4004365818809,51.0648472300424,40.1553722553619));
#176731=CARTESIAN_POINT('Ctrl Pts',(29.3839216347922,51.0784429877809,40.149690217779));
#176732=CARTESIAN_POINT('Ctrl Pts',(29.3777522003177,51.0835219102896,40.1475675976846));
#176733=CARTESIAN_POINT('Ctrl Pts',(29.3717787490543,51.0887089685248,40.1451361443097));
#176734=CARTESIAN_POINT('Ctrl Pts',(29.3660122232364,51.0939835922265,40.1424159447501));
#176735=CARTESIAN_POINT('Ctrl Pts',(29.3615128905155,51.0980991182402,40.1402935085949));
#176736=CARTESIAN_POINT('Ctrl Pts',(29.357140038714,51.1022679285257,40.1379949176048));
#176737=CARTESIAN_POINT('Ctrl Pts',(29.352899371725,51.1064802178289,40.1355293609261));
#176738=CARTESIAN_POINT('Ctrl Pts',(29.3380570372635,51.1212232303902,40.1268999125509));
#176739=CARTESIAN_POINT('Ctrl Pts',(29.3248339623433,51.136498853134,40.1162251288835));
#176740=CARTESIAN_POINT('Ctrl Pts',(29.3134747466765,51.151886765371,40.1038990521418));
#176741=CARTESIAN_POINT('Ctrl Pts',(29.307795138843,51.1595807214895,40.097736013771));
#176742=CARTESIAN_POINT('Ctrl Pts',(29.3025814967144,51.1673027515568,40.0911601532641));
#176743=CARTESIAN_POINT('Ctrl Pts',(29.297864397778,51.1750003199398,40.084220729064));
#176744=CARTESIAN_POINT('Ctrl Pts',(29.2931674525162,51.1826650006749,40.0773109533618));
#176745=CARTESIAN_POINT('Ctrl Pts',(29.2889625693107,51.1903053811861,40.0700409753048));
#176746=CARTESIAN_POINT('Ctrl Pts',(29.2852806784154,51.1978697380626,40.0624586415899));
#176747=CARTESIAN_POINT('Ctrl Pts',(29.2852648801407,51.1979021952405,40.0624261072769));
#176748=CARTESIAN_POINT('Ctrl Pts',(29.2852490909589,51.1979346509232,40.0623935677889));
#176749=CARTESIAN_POINT('Ctrl Pts',(29.2852333108693,51.1979671051088,40.0623610231288));
#176750=CARTESIAN_POINT('Ctrl Pts',(29.2777917239323,51.2132718752149,40.0470135870226));
#176751=CARTESIAN_POINT('Ctrl Pts',(29.2723555974555,51.2282103130417,40.0305755292077));
#176752=CARTESIAN_POINT('Ctrl Pts',(29.2687791125359,51.242653691443,40.0133447567315));
#176753=CARTESIAN_POINT('Ctrl Pts',(29.2650725221321,51.2576224915312,39.9954871626564));
#176754=CARTESIAN_POINT('Ctrl Pts',(29.263363505796,51.2720604115355,39.9767767954275));
#176755=CARTESIAN_POINT('Ctrl Pts',(29.2635407906077,51.2858132466446,39.9575197577428));
#176756=CARTESIAN_POINT('Ctrl Pts',(29.2637155451674,51.2993697979382,39.9385375611947));
#176757=CARTESIAN_POINT('Ctrl Pts',(29.2657236711482,51.3122614394886,39.9190226977042));
#176758=CARTESIAN_POINT('Ctrl Pts',(29.2695013892409,51.3243180878457,39.8992655451801));
#176759=CARTESIAN_POINT('Ctrl Pts',(29.2721352815069,51.3327241975874,39.8854905069289));
#176760=CARTESIAN_POINT('Ctrl Pts',(29.2756302808599,51.3407239614254,39.8715976051456));
#176761=CARTESIAN_POINT('Ctrl Pts',(29.2799753962468,51.3482501200162,39.8576902534424));
#176762=CARTESIAN_POINT('',(29.458121752568,51.6568155675424,39.2875012672119));
#176763=CARTESIAN_POINT('',(29.2799753962469,51.3482501200162,39.8576902534424));
#176764=CARTESIAN_POINT('',(24.4761921430398,54.1952354911869,39.2875012672119));
#176765=CARTESIAN_POINT('Origin',(5.53234440788222E-15,0.,39.2875012672119));
#176766=CARTESIAN_POINT('',(24.3312692531094,53.8697418420142,39.8576902534424));
#176767=CARTESIAN_POINT('',(24.4761921430398,54.1952354911869,39.2875012672119));
#176768=CARTESIAN_POINT('',(23.979166327502,53.8206887816833,40.1599502534424));
#176769=CARTESIAN_POINT('Ctrl Pts',(24.3312692531094,53.8697418420142,39.8576902534424));
#176770=CARTESIAN_POINT('Ctrl Pts',(24.3262947497605,53.8585692765376,39.8772619994046));
#176771=CARTESIAN_POINT('Ctrl Pts',(24.3195865685239,53.8482286480028,39.8967644650355));
#176772=CARTESIAN_POINT('Ctrl Pts',(24.3112807320083,53.8388409929169,39.9159282836026));
#176773=CARTESIAN_POINT('Ctrl Pts',(24.3028248617536,53.8292837624981,39.9354382707161));
#176774=CARTESIAN_POINT('Ctrl Pts',(24.2927127498367,53.8207133850125,39.9545987622325));
#176775=CARTESIAN_POINT('Ctrl Pts',(24.2810366186995,53.8132717929041,39.9731387498198));
#176776=CARTESIAN_POINT('Ctrl Pts',(24.2698548246814,53.8061452585114,39.9908938024019));
#176777=CARTESIAN_POINT('Ctrl Pts',(24.2572379736598,53.8000534013008,40.0080810366143));
#176778=CARTESIAN_POINT('Ctrl Pts',(24.2432286115683,53.7951438030556,40.0244542742498));
#176779=CARTESIAN_POINT('Ctrl Pts',(24.2320860256461,53.791238870059,40.0374770090458));
#176780=CARTESIAN_POINT('Ctrl Pts',(24.2200617420602,53.7880821478312,40.0499848770025));
#176781=CARTESIAN_POINT('Ctrl Pts',(24.2071623814828,53.785762446988,40.0618424270193));
#176782=CARTESIAN_POINT('Ctrl Pts',(24.2071271704186,53.7857561149582,40.0618747942791));
#176783=CARTESIAN_POINT('Ctrl Pts',(24.2070919529321,53.7857497893135,40.0619071564124));
#176784=CARTESIAN_POINT('Ctrl Pts',(24.2070567290248,53.7857434700553,40.0619395134161));
#176785=CARTESIAN_POINT('Ctrl Pts',(24.2000447667171,53.7844855062584,40.0683807661799));
#176786=CARTESIAN_POINT('Ctrl Pts',(24.192748355923,53.7835014710813,40.0746073439084));
#176787=CARTESIAN_POINT('Ctrl Pts',(24.1852078325135,53.7827951090623,40.0805869293669));
#176788=CARTESIAN_POINT('Ctrl Pts',(24.1702431416115,53.7813932847186,40.092453830807));
#176789=CARTESIAN_POINT('Ctrl Pts',(24.1543158599161,53.7810858838905,40.1033475319609));
#176790=CARTESIAN_POINT('Ctrl Pts',(24.137734401873,53.7819069982466,40.1130129263075));
#176791=CARTESIAN_POINT('Ctrl Pts',(24.1252983083407,53.7825228340137,40.1202619720674));
#176792=CARTESIAN_POINT('Ctrl Pts',(24.1124942402755,53.7837734588331,40.1268200947266));
#176793=CARTESIAN_POINT('Ctrl Pts',(24.0994523147296,53.7856732654695,40.1325796782703));
#176794=CARTESIAN_POINT('Ctrl Pts',(24.0945615926499,53.7863856929582,40.1347395220992));
#176795=CARTESIAN_POINT('Ctrl Pts',(24.0896374219413,53.7871894118144,40.1367870714852));
#176796=CARTESIAN_POINT('Ctrl Pts',(24.0846866645811,53.7880851817728,40.1387166518767));
#176797=CARTESIAN_POINT('Ctrl Pts',(24.0673590138204,53.7912203766271,40.1454701832469));
#176798=CARTESIAN_POINT('Ctrl Pts',(24.0497056745179,53.7954831928406,40.1507785912491));
#176799=CARTESIAN_POINT('Ctrl Pts',(24.0320208729162,53.8009062465105,40.1543986087265));
#176800=CARTESIAN_POINT('Ctrl Pts',(24.0231784721154,53.8036177733455,40.1562086174652));
#176801=CARTESIAN_POINT('Ctrl Pts',(24.0143282061519,53.8066193604762,40.1575965292115));
#176802=CARTESIAN_POINT('Ctrl Pts',(24.0055068550426,53.8099150888837,40.1585319382567));
#176803=CARTESIAN_POINT('Ctrl Pts',(24.0010961794879,53.8115629530874,40.1589996427793));
#176804=CARTESIAN_POINT('Ctrl Pts',(23.9966927326568,53.8132843526338,40.159354221642));
#176805=CARTESIAN_POINT('Ctrl Pts',(23.9923011121681,53.8150797979123,40.159591874311));
#176806=CARTESIAN_POINT('Ctrl Pts',(23.9879094916794,53.8168752431908,40.1598295269801));
#176807=CARTESIAN_POINT('Ctrl Pts',(23.9835296982247,53.8187447357538,40.1599502506895));
#176808=CARTESIAN_POINT('Ctrl Pts',(23.979166327502,53.8206887816833,40.1599502534424));
#176809=CARTESIAN_POINT('',(23.9513722670371,53.8330634946835,40.1599502534424));
#176810=CARTESIAN_POINT('Origin',(5.68291264686342E-15,5.31495157331118E-15,
40.1599502534424));
#176811=CARTESIAN_POINT('',(23.7522229508834,54.1275498658871,39.8576902534424));
#176812=CARTESIAN_POINT('Ctrl Pts',(23.9513722670371,53.8330634946835,40.1599502534424));
#176813=CARTESIAN_POINT('Ctrl Pts',(23.9478914369187,53.8346121892501,40.1599502448875));
#176814=CARTESIAN_POINT('Ctrl Pts',(23.9444392282286,53.8361996036041,40.1598743450437));
#176815=CARTESIAN_POINT('Ctrl Pts',(23.9410169613696,53.8378239549346,40.1597243308499));
#176816=CARTESIAN_POINT('Ctrl Pts',(23.9208121566336,53.8474140023525,40.1588386583937));
#176817=CARTESIAN_POINT('Ctrl Pts',(23.9016479061078,53.8582911092182,40.1553722553609));
#176818=CARTESIAN_POINT('Ctrl Pts',(23.8838022859618,53.8700861059349,40.1496902177767));
#176819=CARTESIAN_POINT('Ctrl Pts',(23.8771357563326,53.8744923240684,40.1475675976828));
#176820=CARTESIAN_POINT('Ctrl Pts',(23.8706528330364,53.8790265713733,40.1451361443087));
#176821=CARTESIAN_POINT('Ctrl Pts',(23.8643665485428,53.8836695340507,40.1424159447501));
#176822=CARTESIAN_POINT('Ctrl Pts',(23.8594616740274,53.8872922064472,40.1402935085949));
#176823=CARTESIAN_POINT('Ctrl Pts',(23.8546770178329,53.8909810920749,40.1379949176048));
#176824=CARTESIAN_POINT('Ctrl Pts',(23.8500192775337,53.894727035613,40.1355293609261));
#176825=CARTESIAN_POINT('Ctrl Pts',(23.8337171864864,53.9078378379962,40.1268999125508));
#176826=CARTESIAN_POINT('Ctrl Pts',(23.8189698115833,53.9216475915792,40.1162251288835));
#176827=CARTESIAN_POINT('Ctrl Pts',(23.8060643480694,53.9357638458653,40.1038990521418));
#176828=CARTESIAN_POINT('Ctrl Pts',(23.7996116163124,53.9428219730084,40.0977360137709));
#176829=CARTESIAN_POINT('Ctrl Pts',(23.7936193631247,53.9499567269873,40.0911601532641));
#176830=CARTESIAN_POINT('Ctrl Pts',(23.7881234899558,53.9571190561824,40.084220729064));
#176831=CARTESIAN_POINT('Ctrl Pts',(23.7826510977529,53.9642507845242,40.0773109533618));
#176832=CARTESIAN_POINT('Ctrl Pts',(23.7776706121039,53.9714097802518,40.0700409753047));
#176833=CARTESIAN_POINT('Ctrl Pts',(23.7732182003924,53.9785478363927,40.0624586415899));
#176834=CARTESIAN_POINT('Ctrl Pts',(23.7731990959634,53.9785784643974,40.0624261072769));
#176835=CARTESIAN_POINT('Ctrl Pts',(23.7731800007337,53.9786090918655,40.0623935677888));
#176836=CARTESIAN_POINT('Ctrl Pts',(23.7731609147029,53.9786397187951,40.0623610231288));
#176837=CARTESIAN_POINT('Ctrl Pts',(23.7641603094588,53.9930827901211,40.0470135870241));
#176838=CARTESIAN_POINT('Ctrl Pts',(23.7571924707025,54.0073711636743,40.0305755292109));
#176839=CARTESIAN_POINT('Ctrl Pts',(23.7521258339929,54.0213615752637,40.0133447567365));
#176840=CARTESIAN_POINT('Ctrl Pts',(23.7468748830091,54.0358609304986,39.9954871626633));
#176841=CARTESIAN_POINT('Ctrl Pts',(23.7436660552522,54.0500411172139,39.9767767954363));
#176842=CARTESIAN_POINT('Ctrl Pts',(23.7424048061591,54.0637371441611,39.9575197577536));
#176843=CARTESIAN_POINT('Ctrl Pts',(23.7411615579205,54.0772376980728,39.9385375612074));
#176844=CARTESIAN_POINT('Ctrl Pts',(23.7418111396958,54.090268624184,39.9190226977187));
#176845=CARTESIAN_POINT('Ctrl Pts',(23.7443079001274,54.1026541040261,39.8992655451964));
#176846=CARTESIAN_POINT('Ctrl Pts',(23.7460486859225,54.1112894809336,39.8854905069398));
#176847=CARTESIAN_POINT('Ctrl Pts',(23.7486883362836,54.1196107481433,39.8715976051511));
#176848=CARTESIAN_POINT('Ctrl Pts',(23.7522229508834,54.1275498658871,39.8576902534424));
#176849=CARTESIAN_POINT('',(23.8971395307774,54.453046324469,39.2875012672119));
#176850=CARTESIAN_POINT('',(23.7522229508834,54.1275498658871,39.8576902534424));
#176851=CARTESIAN_POINT('',(18.6771643191716,56.4568070719809,39.2875012672119));
#176852=CARTESIAN_POINT('Origin',(5.53234440788222E-15,0.,39.2875012672119));
#176853=CARTESIAN_POINT('',(18.5670586829472,56.1179479440986,39.8576902534424));
#176854=CARTESIAN_POINT('',(18.6771643191716,56.4568070719809,39.2875012672119));
#176855=CARTESIAN_POINT('',(18.2220120550223,56.0323588238389,40.1599502534424));
#176856=CARTESIAN_POINT('Ctrl Pts',(18.5670586829472,56.1179479440986,39.8576902534424));
#176857=CARTESIAN_POINT('Ctrl Pts',(18.5632792815478,56.106316605913,39.8772619994065));
#176858=CARTESIAN_POINT('Ctrl Pts',(18.5576887384393,56.0953314285463,39.8967644650392));
#176859=CARTESIAN_POINT('Ctrl Pts',(18.5504096793239,56.0851270036893,39.915928283608));
#176860=CARTESIAN_POINT('Ctrl Pts',(18.5429991338191,56.0747382496544,39.9354382707233));
#176861=CARTESIAN_POINT('Ctrl Pts',(18.5338382654961,56.0651578180737,39.9545987622415));
#176862=CARTESIAN_POINT('Ctrl Pts',(18.5230039556125,56.0565365037403,39.9731387498304));
#176863=CARTESIAN_POINT('Ctrl Pts',(18.512628342319,56.048280193503,39.990893802414));
#176864=CARTESIAN_POINT('Ctrl Pts',(18.5007173801981,56.0409028880748,40.0080810366277));
#176865=CARTESIAN_POINT('Ctrl Pts',(18.4872979556155,56.0345558080316,40.0244542742644));
#176866=CARTESIAN_POINT('Ctrl Pts',(18.4766245865934,56.0295075492857,40.0374770090551));
#176867=CARTESIAN_POINT('Ctrl Pts',(18.4649961406185,56.0251112400293,40.049984877007));
#176868=CARTESIAN_POINT('Ctrl Pts',(18.4524099188571,56.0214558964132,40.0618424270193));
#176869=CARTESIAN_POINT('Ctrl Pts',(18.4523755625601,56.0214459185124,40.0618747942791));
#176870=CARTESIAN_POINT('Ctrl Pts',(18.4523411992087,56.0214359462905,40.0619071564124));
#176871=CARTESIAN_POINT('Ctrl Pts',(18.4523068288039,56.021425979749,40.0619395134162));
#176872=CARTESIAN_POINT('Ctrl Pts',(18.445464771782,56.0194419575648,40.0683807661799));
#176873=CARTESIAN_POINT('Ctrl Pts',(18.4383111911745,56.0177006304278,40.0746073439084));
#176874=CARTESIAN_POINT('Ctrl Pts',(18.4308858104775,56.0162099386096,40.0805869293669));
#176875=CARTESIAN_POINT('Ctrl Pts',(18.4161496282625,56.0132515574631,40.092453830807));
#176876=CARTESIAN_POINT('Ctrl Pts',(18.4003417300189,56.0112809863292,40.1033475319609));
#176877=CARTESIAN_POINT('Ctrl Pts',(18.3837652771161,56.010364368207,40.1130129263075));
#176878=CARTESIAN_POINT('Ctrl Pts',(18.371332937439,56.0096769046154,40.1202619720674));
#176879=CARTESIAN_POINT('Ctrl Pts',(18.3584682855079,56.0095822888227,40.1268200947266));
#176880=CARTESIAN_POINT('Ctrl Pts',(18.3452992211265,56.0101084356842,40.1325796782703));
#176881=CARTESIAN_POINT('Ctrl Pts',(18.3403608219835,56.0103057407573,40.1347395220992));
#176882=CARTESIAN_POINT('Ctrl Pts',(18.3353796149004,56.0105903407604,40.1367870714852));
#176883=CARTESIAN_POINT('Ctrl Pts',(18.3303623448498,56.0109637085384,40.1387166518767));
#176884=CARTESIAN_POINT('Ctrl Pts',(18.3128018996728,56.0122704957612,40.1454701832468));
#176885=CARTESIAN_POINT('Ctrl Pts',(18.2947996815822,56.0146646833927,40.1507785912492));
#176886=CARTESIAN_POINT('Ctrl Pts',(18.2766448957077,56.0182094638725,40.1543986087265));
#176887=CARTESIAN_POINT('Ctrl Pts',(18.2675675027704,56.0199818541124,40.1562086174652));
#176888=CARTESIAN_POINT('Ctrl Pts',(18.2584519681998,56.0220418935341,40.1575965292115));
#176889=CARTESIAN_POINT('Ctrl Pts',(18.2493344439491,56.0243974853212,40.1585319382567));
#176890=CARTESIAN_POINT('Ctrl Pts',(18.2447756818237,56.0255752812147,40.1589996427793));
#176891=CARTESIAN_POINT('Ctrl Pts',(18.2402164222858,56.0268269652239,40.159354221642));
#176892=CARTESIAN_POINT('Ctrl Pts',(18.2356611844178,56.0281535255243,40.159591874311));
#176893=CARTESIAN_POINT('Ctrl Pts',(18.2311059465498,56.0294800858248,40.1598295269801));
#176894=CARTESIAN_POINT('Ctrl Pts',(18.2265547308772,56.0308815240327,40.1599502506895));
#176895=CARTESIAN_POINT('Ctrl Pts',(18.2220120550223,56.0323588238389,40.1599502534424));
#176896=CARTESIAN_POINT('',(18.1930767435955,56.0417604764381,40.1599502534424));
#176897=CARTESIAN_POINT('Origin',(5.6762545978478E-15,5.31750735887178E-15,
40.1599502534424));
#176898=CARTESIAN_POINT('',(17.9642361803979,56.3138168485093,39.8576902534424));
#176899=CARTESIAN_POINT('Ctrl Pts',(18.1930767435955,56.0417604764381,40.1599502534424));
#176900=CARTESIAN_POINT('Ctrl Pts',(18.1894530991656,56.0429368412706,40.1599502448875));
#176901=CARTESIAN_POINT('Ctrl Pts',(18.185853872053,56.0441547055335,40.1598743450437));
#176902=CARTESIAN_POINT('Ctrl Pts',(18.1822805617814,56.0454124342017,40.1597243308498));
#176903=CARTESIAN_POINT('Ctrl Pts',(18.1611840081625,56.0528379691462,40.1588386583938));
#176904=CARTESIAN_POINT('Ctrl Pts',(18.1409877741425,56.0616522804243,40.1553722553615));
#176905=CARTESIAN_POINT('Ctrl Pts',(18.1220070012914,56.071517287664,40.1496902177782));
#176906=CARTESIAN_POINT('Ctrl Pts',(18.1149164163968,56.0752025259768,40.1475675976839));
#176907=CARTESIAN_POINT('Ctrl Pts',(18.1079950493283,56.0790342841917,40.1451361443093));
#176908=CARTESIAN_POINT('Ctrl Pts',(18.1012578800035,56.0829947165769,40.1424159447501));
#176909=CARTESIAN_POINT('Ctrl Pts',(18.0960012025255,56.0860848445994,40.1402935085949));
#176910=CARTESIAN_POINT('Ctrl Pts',(18.0908571636324,56.0892533893664,40.1379949176048));
#176911=CARTESIAN_POINT('Ctrl Pts',(18.0858333812004,56.0924919457981,40.1355293609261));
#176912=CARTESIAN_POINT('Ctrl Pts',(18.0682501426882,56.1038268933088,40.1268999125509));
#176913=CARTESIAN_POINT('Ctrl Pts',(18.0521400431277,56.1160194751809,40.1162251288835));
#176914=CARTESIAN_POINT('Ctrl Pts',(18.0378297267256,56.1287094108802,40.1038990521418));
#176915=CARTESIAN_POINT('Ctrl Pts',(18.0306745685246,56.1350543787298,40.0977360137709));
#176916=CARTESIAN_POINT('Ctrl Pts',(18.0239693566576,56.1415236867627,40.0911601532641));
#176917=CARTESIAN_POINT('Ctrl Pts',(18.0177549231928,56.1480723047924,40.084220729064));
#176918=CARTESIAN_POINT('Ctrl Pts',(18.011567040723,56.1545929440327,40.0773109533618));
#176919=CARTESIAN_POINT('Ctrl Pts',(18.0058655198736,56.1611921195215,40.0700409753047));
#176920=CARTESIAN_POINT('Ctrl Pts',(18.0006913689001,56.1678256688899,40.0624586415899));
#176921=CARTESIAN_POINT('Ctrl Pts',(18.0006691676289,56.1678541321546,40.0624261072769));
#176922=CARTESIAN_POINT('Ctrl Pts',(18.0006469755627,56.1678825958472,40.0623935677888));
#176923=CARTESIAN_POINT('Ctrl Pts',(18.0006247927013,56.1679110599659,40.0623610231288));
#176924=CARTESIAN_POINT('Ctrl Pts',(17.9901637816636,56.1813341912017,40.0470135870236));
#176925=CARTESIAN_POINT('Ctrl Pts',(17.9817405717267,56.1948159540725,40.0305755292099));
#176926=CARTESIAN_POINT('Ctrl Pts',(17.9752392943591,56.2082001169745,40.0133447567349));
#176927=CARTESIAN_POINT('Ctrl Pts',(17.9685015133131,56.2220711693878,39.995487162661));
#176928=CARTESIAN_POINT('Ctrl Pts',(17.9638280307243,56.2358382617226,39.9767767954334));
#176929=CARTESIAN_POINT('Ctrl Pts',(17.9611420662362,56.2493274239721,39.95751975775));
#176930=CARTESIAN_POINT('Ctrl Pts',(17.958494436488,56.2626240656095,39.938537561203));
#176931=CARTESIAN_POINT('Ctrl Pts',(17.9577783571053,56.2756515067291,39.9190226977136));
#176932=CARTESIAN_POINT('Ctrl Pts',(17.9589668048477,56.2882301201481,39.8992655451906));
#176933=CARTESIAN_POINT('Ctrl Pts',(17.9597954117583,56.2970001532202,39.8854905069359));
#176934=CARTESIAN_POINT('Ctrl Pts',(17.9615507925645,56.305551754252,39.8715976051492));
#176935=CARTESIAN_POINT('Ctrl Pts',(17.9642361803979,56.3138168485093,39.8576902534424));
#176936=CARTESIAN_POINT('',(18.0743352474898,56.6526781108321,39.2875012672119));
#176937=CARTESIAN_POINT('',(17.9642361803979,56.3138168485093,39.8576902534424));
#176938=CARTESIAN_POINT('',(12.6735055745747,58.0998260601478,39.2875012672119));
#176939=CARTESIAN_POINT('Origin',(5.53234440788222E-15,0.,39.2875012672119));
#176940=CARTESIAN_POINT('',(12.5994235324478,57.7513140650719,39.8576902534424));
#176941=CARTESIAN_POINT('',(12.6735055745747,58.0998260601478,39.2875012672119));
#176942=CARTESIAN_POINT('',(12.2652136052667,57.6301266171956,40.1599502534424));
#176943=CARTESIAN_POINT('Ctrl Pts',(12.5994235324478,57.7513140650719,39.8576902534424));
#176944=CARTESIAN_POINT('Ctrl Pts',(12.5968806409115,57.739351389555,39.8772619994039));
#176945=CARTESIAN_POINT('Ctrl Pts',(12.5924689870928,57.7278420192608,39.8967644650342));
#176946=CARTESIAN_POINT('Ctrl Pts',(12.5862964562751,57.7169326264487,39.9159282836006));
#176947=CARTESIAN_POINT('Ctrl Pts',(12.5800124270096,57.7058261701631,39.9354382707136));
#176948=CARTESIAN_POINT('Ctrl Pts',(12.571903170674,57.695340649702,39.9545987622296));
#176949=CARTESIAN_POINT('Ctrl Pts',(12.5620293850143,57.6856340700687,39.9731387498165));
#176950=CARTESIAN_POINT('Ctrl Pts',(12.5525736298391,57.6763384418503,39.9908938023985));
#176951=CARTESIAN_POINT('Ctrl Pts',(12.5414990556166,57.6677565155071,40.0080810366108));
#176952=CARTESIAN_POINT('Ctrl Pts',(12.5288165945717,57.6600414936031,40.0244542742463));
#176953=CARTESIAN_POINT('Ctrl Pts',(12.518729382107,57.6539052188818,40.0374770090436));
#176954=CARTESIAN_POINT('Ctrl Pts',(12.5076241774218,57.6483174894766,40.0499848770015));
#176955=CARTESIAN_POINT('Ctrl Pts',(12.4954889917454,57.6433665517939,40.0618424270192));
#176956=CARTESIAN_POINT('Ctrl Pts',(12.4954558666304,57.6433530373422,40.0618747942791));
#176957=CARTESIAN_POINT('Ctrl Pts',(12.4954227339061,57.6433395278008,40.0619071564124));
#176958=CARTESIAN_POINT('Ctrl Pts',(12.4953895935733,57.6433260231715,40.0619395134161));
#176959=CARTESIAN_POINT('Ctrl Pts',(12.4887924048456,57.6406376799624,40.0683807661799));
#176960=CARTESIAN_POINT('Ctrl Pts',(12.4818600305509,57.6381581392098,40.0746073439084));
#176961=CARTESIAN_POINT('Ctrl Pts',(12.4746311465912,57.6358994499239,40.0805869293669));
#176962=CARTESIAN_POINT('Ctrl Pts',(12.4602849257593,57.6314169246175,40.092453830807));
#176963=CARTESIAN_POINT('Ctrl Pts',(12.4447696056087,57.6278047731676,40.1033475319609));
#176964=CARTESIAN_POINT('Ctrl Pts',(12.428379772933,57.625160465227,40.1130129263075));
#176965=CARTESIAN_POINT('Ctrl Pts',(12.4160873984262,57.6231772342716,40.1202619720674));
#176966=CARTESIAN_POINT('Ctrl Pts',(12.4033031104478,57.6217384144973,40.1268200947266));
#176967=CARTESIAN_POINT('Ctrl Pts',(12.3901511902562,57.6208851370088,40.1325796782703));
#176968=CARTESIAN_POINT('Ctrl Pts',(12.3852192201843,57.6205651579506,40.1347395220992));
#176969=CARTESIAN_POINT('Ctrl Pts',(12.3802355518738,57.6203275209636,40.1367870714852));
#176970=CARTESIAN_POINT('Ctrl Pts',(12.3752067393935,57.6201743958656,40.1387166518767));
#176971=CARTESIAN_POINT('Ctrl Pts',(12.3576058957123,57.6196384580226,40.1454701832469));
#176972=CARTESIAN_POINT('Ctrl Pts',(12.339452034902,57.6201377858513,40.1507785912492));
#176973=CARTESIAN_POINT('Ctrl Pts',(12.321026172388,57.6217654557844,40.1543986087265));
#176974=CARTESIAN_POINT('Ctrl Pts',(12.3118132411309,57.6225792907509,40.1562086174652));
#176975=CARTESIAN_POINT('Ctrl Pts',(12.3025323096575,57.6236752122406,40.1575965292115));
#176976=CARTESIAN_POINT('Ctrl Pts',(12.293218505769,57.6250648590506,40.1585319382567));
#176977=CARTESIAN_POINT('Ctrl Pts',(12.2885616038247,57.6257596824556,40.1589996427793));
#176978=CARTESIAN_POINT('Ctrl Pts',(12.2838964837817,57.6265279372157,40.159354221642));
#176979=CARTESIAN_POINT('Ctrl Pts',(12.2792275366736,57.6273710784659,40.159591874311));
#176980=CARTESIAN_POINT('Ctrl Pts',(12.2745585895656,57.628214219716,40.1598295269801));
#176981=CARTESIAN_POINT('Ctrl Pts',(12.2698858157465,57.6291322491185,40.1599502506895));
#176982=CARTESIAN_POINT('Ctrl Pts',(12.2652136052667,57.6301266171956,40.1599502534424));
#176983=CARTESIAN_POINT('',(12.2354540642051,57.6364522029206,40.1599502534424));
#176984=CARTESIAN_POINT('Origin',(5.66936586998424E-15,5.3193531879397E-15,
40.1599502534424));
#176985=CARTESIAN_POINT('',(11.9794294790618,57.8830978693155,39.8576902534424));
#176986=CARTESIAN_POINT('Ctrl Pts',(12.2354540642051,57.6364522029206,40.1599502534424));
#176987=CARTESIAN_POINT('Ctrl Pts',(12.2317273068703,57.6372433495198,40.1599502448875));
#176988=CARTESIAN_POINT('Ctrl Pts',(12.2280204952205,57.6380783205157,40.1598743450437));
#176989=CARTESIAN_POINT('Ctrl Pts',(12.2243352914717,57.6389556465833,40.1597243308499));
#176990=CARTESIAN_POINT('Ctrl Pts',(12.202578127225,57.6441353133401,40.1588386583938));
#176991=CARTESIAN_POINT('Ctrl Pts',(12.1815711838763,57.6507902575925,40.1553722553618));
#176992=CARTESIAN_POINT('Ctrl Pts',(12.1616632156387,57.6586171922721,40.1496902177789));
#176993=CARTESIAN_POINT('Ctrl Pts',(12.1542262614116,57.6615410745215,40.1475675976844));
#176994=CARTESIAN_POINT('Ctrl Pts',(12.1469422825174,57.664628362101,40.1451361443096));
#176995=CARTESIAN_POINT('Ctrl Pts',(12.1398280421993,57.6678628728672,40.1424159447501));
#176996=CARTESIAN_POINT('Ctrl Pts',(12.134277155017,57.6703866004264,40.1402935085949));
#176997=CARTESIAN_POINT('Ctrl Pts',(12.1288300925919,57.6730000890931,40.1379949176047));
#176998=CARTESIAN_POINT('Ctrl Pts',(12.1234953096386,57.6756957761164,40.1355293609261));
#176999=CARTESIAN_POINT('Ctrl Pts',(12.1048235693023,57.6851306806978,40.1268999125508));
#177000=CARTESIAN_POINT('Ctrl Pts',(12.0875272507065,57.6955725063805,40.1162251288835));
#177001=CARTESIAN_POINT('Ctrl Pts',(12.0719688682374,57.7066970899018,40.1038990521418));
#177002=CARTESIAN_POINT('Ctrl Pts',(12.0641896770028,57.7122593816625,40.0977360137709));
#177003=CARTESIAN_POINT('Ctrl Pts',(12.0568449701609,57.7179923646567,40.0911601532641));
#177004=CARTESIAN_POINT('Ctrl Pts',(12.0499800630337,57.7238555234915,40.084220729064));
#177005=CARTESIAN_POINT('Ctrl Pts',(12.0431444860322,57.7296936321424,40.0773109533619));
#177006=CARTESIAN_POINT('Ctrl Pts',(12.0367843970379,57.7356606854447,40.0700409753048));
#177007=CARTESIAN_POINT('Ctrl Pts',(12.0309451958833,57.7417170494856,40.0624586415899));
#177008=CARTESIAN_POINT('Ctrl Pts',(12.0309201410117,57.7417430361607,40.0624261072769));
#177009=CARTESIAN_POINT('Ctrl Pts',(12.0308950952499,57.7417690242237,40.0623935677889));
#177010=CARTESIAN_POINT('Ctrl Pts',(12.030870058598,57.7417950136726,40.0623610231289));
#177011=CARTESIAN_POINT('Ctrl Pts',(12.0190632547928,57.7540511381831,40.0470135870234));
#177012=CARTESIAN_POINT('Ctrl Pts',(12.0092769601261,57.766578581356,40.0305755292094));
#177013=CARTESIAN_POINT('Ctrl Pts',(12.0014122714559,57.7792098558809,40.0133447567341));
#177014=CARTESIAN_POINT('Ctrl Pts',(11.9932614808867,57.7923006313193,39.99548716266));
#177015=CARTESIAN_POINT('Ctrl Pts',(11.9871745471191,57.805503794129,39.976776795432));
#177016=CARTESIAN_POINT('Ctrl Pts',(11.9830932952248,57.8186383015961,39.9575197577483));
#177017=CARTESIAN_POINT('Ctrl Pts',(11.9790702919525,57.8315853501707,39.9385375612009));
#177018=CARTESIAN_POINT('Ctrl Pts',(11.9769963969272,57.8444665749276,39.9190226977112));
#177019=CARTESIAN_POINT('Ctrl Pts',(11.976863511098,57.8571005080025,39.8992655451878));
#177020=CARTESIAN_POINT('Ctrl Pts',(11.9767708607335,57.8659091109222,39.8854905069341));
#177021=CARTESIAN_POINT('Ctrl Pts',(11.9776227396656,57.8745973526463,39.8715976051482));
#177022=CARTESIAN_POINT('Ctrl Pts',(11.9794294790618,57.8830978693154,39.8576902534424));
#177023=CARTESIAN_POINT('',(12.0535047649328,58.231611300478,39.2875012672119));
#177024=CARTESIAN_POINT('',(11.9794294790618,57.8830978693155,39.8576902534424));
#177025=CARTESIAN_POINT('',(6.53099325080115,59.1062911958296,39.2875012672119));
#177026=CARTESIAN_POINT('Origin',(5.53234440788222E-15,0.,39.2875012672119));
#177027=CARTESIAN_POINT('',(6.493746461128,58.7519447039088,39.8576902534424));
#177028=CARTESIAN_POINT('',(6.53099325080115,59.1062911958296,39.2875012672119));
#177029=CARTESIAN_POINT('',(6.17403490859079,58.596486683455,40.1599502534424));
#177030=CARTESIAN_POINT('Ctrl Pts',(6.493746461128,58.7519447039088,39.8576902534424));
#177031=CARTESIAN_POINT('Ctrl Pts',(6.49246793990594,58.7397817566363,39.8772619994027));
#177032=CARTESIAN_POINT('Ctrl Pts',(6.48928351037877,58.7278742924834,39.8967644650317));
#177033=CARTESIAN_POINT('Ctrl Pts',(6.484285135397,58.7163794573064,39.915928283597));
#177034=CARTESIAN_POINT('Ctrl Pts',(6.47919647150981,58.7046769834289,39.9354382707087));
#177035=CARTESIAN_POINT('Ctrl Pts',(6.47222767387013,58.6934012556437,39.9545987622235));
#177036=CARTESIAN_POINT('Ctrl Pts',(6.4634225916951,58.6827157580282,39.9731387498093));
#177037=CARTESIAN_POINT('Ctrl Pts',(6.45499029387005,58.672482656677,39.9908938023901));
#177038=CARTESIAN_POINT('Ctrl Pts',(6.4448734428978,58.6627901347998,40.0080810366013));
#177039=CARTESIAN_POINT('Ctrl Pts',(6.4330668970868,58.65379169843,40.024454274236));
#177040=CARTESIAN_POINT('Ctrl Pts',(6.42367635879233,58.6466346380439,40.0374770090369));
#177041=CARTESIAN_POINT('Ctrl Pts',(6.41321606634576,58.6399167088232,40.0499848769983));
#177042=CARTESIAN_POINT('Ctrl Pts',(6.40166487239094,58.6337244205832,40.0618424270192));
#177043=CARTESIAN_POINT('Ctrl Pts',(6.40163334138366,58.6337075176478,40.0618747942791));
#177044=CARTESIAN_POINT('Ctrl Pts',(6.40160180229542,58.6336906188003,40.0619071564124));
#177045=CARTESIAN_POINT('Ctrl Pts',(6.40157025512699,58.6336737240427,40.0619395134161));
#177046=CARTESIAN_POINT('Ctrl Pts',(6.39529021487377,58.6303105138593,40.0683807661799));
#177047=CARTESIAN_POINT('Ctrl Pts',(6.38865499943531,58.6271199258587,40.0746073439084));
#177048=CARTESIAN_POINT('Ctrl Pts',(6.38170181337843,58.6241179857776,40.0805869293669));
#177049=CARTESIAN_POINT('Ctrl Pts',(6.36790273412708,58.6181604277965,40.092453830807));
#177050=CARTESIAN_POINT('Ctrl Pts',(6.3528499811638,58.6129462715177,40.1033475319609));
#177051=CARTESIAN_POINT('Ctrl Pts',(6.33682633915184,58.6086032453499,40.1130129263075));
#177052=CARTESIAN_POINT('Ctrl Pts',(6.32480860764288,58.6053459757241,40.1202619720674));
#177053=CARTESIAN_POINT('Ctrl Pts',(6.31224475095164,58.6025787159787,40.1268200947266));
#177054=CARTESIAN_POINT('Ctrl Pts',(6.29925407013949,58.6003553628269,40.1325796782703));
#177055=CARTESIAN_POINT('Ctrl Pts',(6.29438256483494,58.599521605395,40.1347395220992));
#177056=CARTESIAN_POINT('Ctrl Pts',(6.28945103740996,58.5987643350183,40.1367870714852));
#177057=CARTESIAN_POINT('Ctrl Pts',(6.28446577922175,58.598086394715,40.1387166518767));
#177058=CARTESIAN_POINT('Ctrl Pts',(6.26701737556302,58.5957136036534,40.1454701832469));
#177059=CARTESIAN_POINT('Ctrl Pts',(6.24891076953115,58.5943126009391,40.1507785912491));
#177060=CARTESIAN_POINT('Ctrl Pts',(6.23041570798304,58.594005327233,40.1543986087265));
#177061=CARTESIAN_POINT('Ctrl Pts',(6.22116817720899,58.59385169038,40.1562086174652));
#177062=CARTESIAN_POINT('Ctrl Pts',(6.21182353266002,58.5939714867924,40.1575965292115));
#177063=CARTESIAN_POINT('Ctrl Pts',(6.20241549311822,58.5943799633642,40.1585319382567));
#177064=CARTESIAN_POINT('Ctrl Pts',(6.19771147334731,58.59458420165,40.1589996427793));
#177065=CARTESIAN_POINT('Ctrl Pts',(6.19299160483051,58.5948606100011,40.159354221642));
#177066=CARTESIAN_POINT('Ctrl Pts',(6.18826010244408,58.595211094569,40.159591874311));
#177067=CARTESIAN_POINT('Ctrl Pts',(6.18352860005764,58.5955615791369,40.1598295269801));
#177068=CARTESIAN_POINT('Ctrl Pts',(6.17878546397972,58.5959861416118,40.1599502506895));
#177069=CARTESIAN_POINT('Ctrl Pts',(6.17403490859079,58.596486683455,40.1599502534424));
#177070=CARTESIAN_POINT('',(6.14377718965381,58.5996668978648,40.1599502534424));
#177071=CARTESIAN_POINT('Origin',(5.66232193761676E-15,5.32046883722541E-15,
40.1599502534424));
#177072=CARTESIAN_POINT('',(5.86337364149639,58.8181995570484,39.8576902534424));
#177073=CARTESIAN_POINT('Ctrl Pts',(6.14377718965381,58.5996668978648,40.1599502534424));
#177074=CARTESIAN_POINT('Ctrl Pts',(6.13998815054745,58.6000641582629,40.1599502448875));
#177075=CARTESIAN_POINT('Ctrl Pts',(6.13621436696463,58.600507087875,40.1598743450437));
#177076=CARTESIAN_POINT('Ctrl Pts',(6.13245764560186,58.6009943991739,40.1597243308499));
#177077=CARTESIAN_POINT('Ctrl Pts',(6.11027824677019,58.6038714482306,40.1588386583938));
#177078=CARTESIAN_POINT('Ctrl Pts',(6.08869075055846,58.6082941124962,40.1553722553615));
#177079=CARTESIAN_POINT('Ctrl Pts',(6.06807370279885,58.6139972210824,40.1496902177782));
#177080=CARTESIAN_POINT('Ctrl Pts',(6.06037186006783,58.6161277126019,40.1475675976839));
#177081=CARTESIAN_POINT('Ctrl Pts',(6.05280507414665,58.6184367045764,40.1451361443093));
#177082=CARTESIAN_POINT('Ctrl Pts',(6.04539170794238,58.6209098557462,40.1424159447501));
#177083=CARTESIAN_POINT('Ctrl Pts',(6.0396074277374,58.6228395323549,40.1402935085949));
#177084=CARTESIAN_POINT('Ctrl Pts',(6.0339170209361,58.6248693309926,40.1379949176048));
#177085=CARTESIAN_POINT('Ctrl Pts',(6.02832968646008,58.6269926140963,40.1355293609261));
#177086=CARTESIAN_POINT('Ctrl Pts',(6.00877401579401,58.6344241049593,40.1268999125508));
#177087=CARTESIAN_POINT('Ctrl Pts',(5.99048098024888,58.6430007716254,40.1162251288835));
#177088=CARTESIAN_POINT('Ctrl Pts',(5.97384499260683,58.6524381197038,40.1038990521418));
#177089=CARTESIAN_POINT('Ctrl Pts',(5.9655269987858,58.657156793743,40.097736013771));
#177090=CARTESIAN_POINT('Ctrl Pts',(5.95762326711415,58.6620906399372,40.0911601532641));
#177091=CARTESIAN_POINT('Ctrl Pts',(5.95018309968352,58.6672041015819,40.084220729064));
#177092=CARTESIAN_POINT('Ctrl Pts',(5.9427747201624,58.6722957161032,40.0773109533618));
#177093=CARTESIAN_POINT('Ctrl Pts',(5.93582574548912,58.6775652709344,40.0700409753048));
#177094=CARTESIAN_POINT('Ctrl Pts',(5.92938546966327,58.682978094856,40.0624586415899));
#177095=CARTESIAN_POINT('Ctrl Pts',(5.92935783569764,58.6830013202262,40.0624261072769));
#177096=CARTESIAN_POINT('Ctrl Pts',(5.92933021064688,58.6830245479289,40.0623935677889));
#177097=CARTESIAN_POINT('Ctrl Pts',(5.92930259451122,58.683047777962,40.0623610231289));
#177098=CARTESIAN_POINT('Ctrl Pts',(5.91627935575158,58.6940026150826,40.047013587023));
#177099=CARTESIAN_POINT('Ctrl Pts',(5.90523719704731,58.7054384852687,40.0305755292086));
#177100=CARTESIAN_POINT('Ctrl Pts',(5.8960952642492,58.7171784805296,40.0133447567329));
#177101=CARTESIAN_POINT('Ctrl Pts',(5.88662076592385,58.7293455537182,39.9954871626582));
#177102=CARTESIAN_POINT('Ctrl Pts',(5.87918707069749,58.7418401303881,39.9767767954297));
#177103=CARTESIAN_POINT('Ctrl Pts',(5.87375524644688,58.7544760786607,39.9575197577455));
#177104=CARTESIAN_POINT('Ctrl Pts',(5.86840094651616,58.766931683599,39.9385375611976));
#177105=CARTESIAN_POINT('Ctrl Pts',(5.86499195787612,58.7795255625992,39.9190226977074));
#177106=CARTESIAN_POINT('Ctrl Pts',(5.86353919440024,58.7920763953157,39.8992655451834));
#177107=CARTESIAN_POINT('Ctrl Pts',(5.86252630185778,58.8008270591857,39.8854905069311));
#177108=CARTESIAN_POINT('Ctrl Pts',(5.86246534555215,58.8095567514073,39.8715976051467));
#177109=CARTESIAN_POINT('Ctrl Pts',(5.86337364149639,58.8181995570484,39.8576902534424));
#177110=CARTESIAN_POINT('',(5.90061356181316,59.1725467709677,39.2875012672119));
#177111=CARTESIAN_POINT('',(5.86337364149639,58.8181995570484,39.8576902534424));
#177112=CARTESIAN_POINT('',(0.316925998273675,59.4651754363832,39.2875012672119));
#177113=CARTESIAN_POINT('Origin',(5.53234440788222E-15,0.,39.2875012672119));
#177114=CARTESIAN_POINT('',(0.316922544676313,59.1088767419348,39.8576902534424));
#177115=CARTESIAN_POINT('',(0.316925998273675,59.4651754363832,39.2875012672119));
#177116=CARTESIAN_POINT('Ctrl Pts',(0.316922544676314,59.1088767419348,
39.8576902534424));
#177117=CARTESIAN_POINT('Ctrl Pts',(0.316922401514489,59.0966467826992,
39.8772619994065));
#177118=CARTESIAN_POINT('Ctrl Pts',(0.31500008555408,59.0844716853536,39.8967644650393));
#177119=CARTESIAN_POINT('Ctrl Pts',(0.311230629648603,59.0725173476285,
39.9159282836081));
#177120=CARTESIAN_POINT('Ctrl Pts',(0.307393083604025,59.0603470709089,
39.9354382707235));
#177121=CARTESIAN_POINT('Ctrl Pts',(0.301641096262377,59.04840467503,39.9545987622418));
#177122=CARTESIAN_POINT('Ctrl Pts',(0.294001187890843,59.0368573319778,
39.9731387498307));
#177123=CARTESIAN_POINT('Ctrl Pts',(0.2866847334314,59.0257988734911,39.9908938024147));
#177124=CARTESIAN_POINT('Ctrl Pts',(0.27763644804072,59.0151019493759,40.0080810366287));
#177125=CARTESIAN_POINT('Ctrl Pts',(0.266835172444231,59.0049186872905,
40.0244542742656));
#177126=CARTESIAN_POINT('Ctrl Pts',(0.258244193029575,58.9968192554995,
40.0374770090559));
#177127=CARTESIAN_POINT('Ctrl Pts',(0.24854341798377,58.9890447295094,40.0499848770073));
#177128=CARTESIAN_POINT('Ctrl Pts',(0.237702773060119,58.981678934725,40.0618424270193));
#177129=CARTESIAN_POINT('Ctrl Pts',(0.237673181620862,58.9816588284979,
40.0618747942791));
#177130=CARTESIAN_POINT('Ctrl Pts',(0.237643581717602,58.9816387254916,
40.0619071564124));
#177131=CARTESIAN_POINT('Ctrl Pts',(0.237613973350917,58.9816186257082,
40.0619395134161));
#177132=CARTESIAN_POINT('Ctrl Pts',(0.231719887007412,58.9776173965852,
40.0683807661799));
#177133=CARTESIAN_POINT('Ctrl Pts',(0.225454527233989,58.9737507180862,
40.0746073439084));
#177134=CARTESIAN_POINT('Ctrl Pts',(0.218853219641359,58.9700384170936,
40.0805869293669));
#177135=CARTESIAN_POINT('Ctrl Pts',(0.205752467570556,58.9626710986899,
40.092453830807));
#177136=CARTESIAN_POINT('Ctrl Pts',(0.191327202906059,58.9559120649696,
40.1033475319609));
#177137=CARTESIAN_POINT('Ctrl Pts',(0.175845309932877,58.9499179036781,
40.1130129263075));
#177138=CARTESIAN_POINT('Ctrl Pts',(0.16423389020299,58.9454222827095,40.1202619720674));
#177139=CARTESIAN_POINT('Ctrl Pts',(0.152028117041927,58.9413569016699,
40.1268200947266));
#177140=CARTESIAN_POINT('Ctrl Pts',(0.139341004226766,58.9377878323772,
40.1325796782703));
#177141=CARTESIAN_POINT('Ctrl Pts',(0.134583336921081,58.9364494313924,
40.1347395220992));
#177142=CARTESIAN_POINT('Ctrl Pts',(0.12975798122809,58.9351808244388,40.1367870714852));
#177143=CARTESIAN_POINT('Ctrl Pts',(0.124870896863944,58.933985496586,40.1387166518767));
#177144=CARTESIAN_POINT('Ctrl Pts',(0.107766101589435,58.9298018491012,
40.1454701832469));
#177145=CARTESIAN_POINT('Ctrl Pts',(0.0899051301006875,58.9265158655229,
40.1507785912492));
#177146=CARTESIAN_POINT('Ctrl Pts',(0.0715435052832107,58.9242770147326,
40.1543986087265));
#177147=CARTESIAN_POINT('Ctrl Pts',(0.0623626928744723,58.9231575893375,
40.1562086174652));
#177148=CARTESIAN_POINT('Ctrl Pts',(0.053056717131196,58.9222999481582,
40.1575965292115));
#177149=CARTESIAN_POINT('Ctrl Pts',(0.0436575183860504,58.9217227791369,
40.1585319382567));
#177150=CARTESIAN_POINT('Ctrl Pts',(0.0389579190134777,58.9214341946262,
40.1589996427793));
#177151=CARTESIAN_POINT('Ctrl Pts',(0.0342350138900817,58.9212157281805,
40.159354221642));
#177152=CARTESIAN_POINT('Ctrl Pts',(0.029492795555506,58.9210697160839,
40.159591874311));
#177153=CARTESIAN_POINT('Ctrl Pts',(0.0247505772209303,58.9209237039872,
40.1598295269801));
#177154=CARTESIAN_POINT('Ctrl Pts',(0.0199890456756627,58.9208501479391,
40.1599502506895));
#177155=CARTESIAN_POINT('Ctrl Pts',(0.0152121934565431,58.9208513795073,
40.1599502534424));
#177156=CARTESIAN_POINT('',(-0.316922544675064,59.1088767419348,39.8576902534424));
#177157=CARTESIAN_POINT('Ctrl Pts',(-0.015212193455297,58.9208513795073,
40.1599502534424));
#177158=CARTESIAN_POINT('Ctrl Pts',(-0.0190220008279198,58.9208504012364,
40.1599502448875));
#177159=CARTESIAN_POINT('Ctrl Pts',(-0.0228214099810991,58.9208964366351,
40.1598743450437));
#177160=CARTESIAN_POINT('Ctrl Pts',(-0.0266084895323811,58.9209883940807,
40.1597243308499));
#177161=CARTESIAN_POINT('Ctrl Pts',(-0.0489671208125404,58.9215313038856,
40.1588386583938));
#177162=CARTESIAN_POINT('Ctrl Pts',(-0.0708986527598547,58.9236732325286,
40.1553722553617));
#177163=CARTESIAN_POINT('Ctrl Pts',(-0.0919988953503987,58.9271900305696,
40.1496902177787));
#177164=CARTESIAN_POINT('Ctrl Pts',(-0.0998812435862781,58.9285037892488,
40.1475675976843));
#177165=CARTESIAN_POINT('Ctrl Pts',(-0.107647933245904,58.9300091878196,
40.1451361443095));
#177166=CARTESIAN_POINT('Ctrl Pts',(-0.115279202946265,58.9316938830317,
40.1424159447501));
#177167=CARTESIAN_POINT('Ctrl Pts',(-0.12123350238957,58.933008366749,40.1402935085949));
#177168=CARTESIAN_POINT('Ctrl Pts',(-0.127104908279362,58.9344322364591,
40.1379949176048));
#177169=CARTESIAN_POINT('Ctrl Pts',(-0.132883578272425,58.9359598525093,
40.1355293609261));
#177170=CARTESIAN_POINT('Ctrl Pts',(-0.153108923248145,58.9413065086849,
40.1268999125509));
#177171=CARTESIAN_POINT('Ctrl Pts',(-0.172198253417083,58.9479240485795,
40.1162251288835));
#177172=CARTESIAN_POINT('Ctrl Pts',(-0.189729578870145,58.9555707636545,
40.1038990521418));
#177173=CARTESIAN_POINT('Ctrl Pts',(-0.198495241596676,58.959394121192,
40.097736013771));
#177174=CARTESIAN_POINT('Ctrl Pts',(-0.206871403159924,58.9634747743348,
40.0911601532641));
#177175=CARTESIAN_POINT('Ctrl Pts',(-0.214805314862589,58.9677825146336,
40.084220729064));
#177176=CARTESIAN_POINT('Ctrl Pts',(-0.222705329147007,58.9720718502312,
40.0773109533618));
#177177=CARTESIAN_POINT('Ctrl Pts',(-0.230167055078556,58.9765861722458,
40.0700409753047));
#177178=CARTESIAN_POINT('Ctrl Pts',(-0.237137844566028,58.9812961520165,
40.0624586415899));
#177179=CARTESIAN_POINT('Ctrl Pts',(-0.23716775486217,58.9813163616197,
40.0624261072769));
#177180=CARTESIAN_POINT('Ctrl Pts',(-0.237197656536078,58.9813365744745,
40.0623935677888));
#177181=CARTESIAN_POINT('Ctrl Pts',(-0.237227549587329,58.9813567905789,
40.0623610231288));
#177182=CARTESIAN_POINT('Ctrl Pts',(-0.251324537971654,58.990890316821,
40.0470135870233));
#177183=CARTESIAN_POINT('Ctrl Pts',(-0.263501580511648,59.0011093202329,
40.0305755292093));
#177184=CARTESIAN_POINT('Ctrl Pts',(-0.273820596508607,59.0118294103845,
40.0133447567339));
#177185=CARTESIAN_POINT('Ctrl Pts',(-0.284514998003514,59.0229394763226,
39.9954871626597));
#177186=CARTESIAN_POINT('Ctrl Pts',(-0.293214009568045,59.0345885736555,
39.9767767954317));
#177187=CARTESIAN_POINT('Ctrl Pts',(-0.299936893971955,59.0465875206394,
39.9575197577479));
#177188=CARTESIAN_POINT('Ctrl Pts',(-0.306563827730748,59.0584152157268,
39.9385375612004));
#177189=CARTESIAN_POINT('Ctrl Pts',(-0.311270560392914,59.070583767796,
39.9190226977105));
#177190=CARTESIAN_POINT('Ctrl Pts',(-0.314027284735234,59.0829139906038,
39.899265545187));
#177191=CARTESIAN_POINT('Ctrl Pts',(-0.315949321993608,59.0915108413214,
39.8854905069335));
#177192=CARTESIAN_POINT('Ctrl Pts',(-0.316922445687103,59.1001863397073,
39.8715976051479));
#177193=CARTESIAN_POINT('Ctrl Pts',(-0.316922544675064,59.1088767419348,
39.8576902534424));
#177194=CARTESIAN_POINT('',(-0.316925998272418,59.4651754363832,39.2875012672119));
#177195=CARTESIAN_POINT('',(-0.316922544675064,59.1088767419348,39.8576902534424));
#177196=CARTESIAN_POINT('',(-5.90061356181196,59.1725467709678,39.2875012672119));
#177197=CARTESIAN_POINT('Origin',(5.53234440788222E-15,0.,39.2875012672119));
#177198=CARTESIAN_POINT('',(-5.8633736414952,58.8181995570485,39.8576902534424));
#177199=CARTESIAN_POINT('',(-5.90061356181196,59.1725467709678,39.2875012672119));
#177200=CARTESIAN_POINT('',(-6.14377718965262,58.5996668978649,40.1599502534424));
#177201=CARTESIAN_POINT('Ctrl Pts',(-5.8633736414952,58.8181995570485,39.8576902534424));
#177202=CARTESIAN_POINT('Ctrl Pts',(-5.86209540502807,58.8060365798455,
39.8772619994052));
#177203=CARTESIAN_POINT('Ctrl Pts',(-5.86273454612467,58.7937272422247,
39.8967644650367));
#177204=CARTESIAN_POINT('Ctrl Pts',(-5.8652337840041,58.7814443761802,39.9159282836043));
#177205=CARTESIAN_POINT('Ctrl Pts',(-5.86777816724645,58.7689396367198,
39.9354382707185));
#177206=CARTESIAN_POINT('Ctrl Pts',(-5.87225032431001,58.7564614161383,
39.9545987622357));
#177207=CARTESIAN_POINT('Ctrl Pts',(-5.87864135443915,58.7441787427587,
39.9731387498236));
#177208=CARTESIAN_POINT('Ctrl Pts',(-5.88476180492296,58.7324160859241,
39.9908938024066));
#177209=CARTESIAN_POINT('Ctrl Pts',(-5.89264238981903,58.7208319573121,
40.0080810366197));
#177210=CARTESIAN_POINT('Ctrl Pts',(-5.9023200541595,58.709575439463,40.024454274256));
#177211=CARTESIAN_POINT('Ctrl Pts',(-5.91001735013293,58.7006223753283,
40.0374770090498));
#177212=CARTESIAN_POINT('Ctrl Pts',(-5.91885232406554,58.6918764318948,
40.0499848770044));
#177213=CARTESIAN_POINT('Ctrl Pts',(-5.92886364759493,58.6834178317481,
40.0618424270193));
#177214=CARTESIAN_POINT('Ctrl Pts',(-5.92889097525616,58.6833947425173,
40.0618747942791));
#177215=CARTESIAN_POINT('Ctrl Pts',(-5.9289183116717,58.683371655605,40.0619071564124));
#177216=CARTESIAN_POINT('Ctrl Pts',(-5.92894565684118,58.6833485710132,
40.0619395134161));
#177217=CARTESIAN_POINT('Ctrl Pts',(-5.93438921243158,58.6787531612542,
40.0683807661799));
#177218=CARTESIAN_POINT('Ctrl Pts',(-5.94021607194716,58.6742527563957,
40.0746073439084));
#177219=CARTESIAN_POINT('Ctrl Pts',(-5.94639317576815,58.6698707672381,
40.0805869293669));
#177220=CARTESIAN_POINT('Ctrl Pts',(-5.95865206607721,58.6611744062939,
40.092453830807));
#177221=CARTESIAN_POINT('Ctrl Pts',(-5.97229179622457,58.6529445485199,
40.1033475319609));
#177222=CARTESIAN_POINT('Ctrl Pts',(-5.98706231729977,58.6453649253901,
40.1130129263075));
#177223=CARTESIAN_POINT('Ctrl Pts',(-5.99814020810617,58.6396802080428,
40.1202619720675));
#177224=CARTESIAN_POINT('Ctrl Pts',(-6.00985416873208,58.6343612468744,
40.1268200947266));
#177225=CARTESIAN_POINT('Ctrl Pts',(-6.02209871088731,58.6294855649109,
40.1325796782703));
#177226=CARTESIAN_POINT('Ctrl Pts',(-6.02669041419551,58.6276571841746,
40.1347395220992));
#177227=CARTESIAN_POINT('Ctrl Pts',(-6.03135673054978,58.6258911397673,
40.1367870714852));
#177228=CARTESIAN_POINT('Ctrl Pts',(-6.03609209717088,58.6241915206271,
40.1387166518767));
#177229=CARTESIAN_POINT('Ctrl Pts',(-6.05266588034473,58.6182428536364,
40.1454701832469));
#177230=CARTESIAN_POINT('Ctrl Pts',(-6.07008552874908,58.6131078911177,
40.1507785912492));
#177231=CARTESIAN_POINT('Ctrl Pts',(-6.088112543032,58.6089619925611,40.1543986087265));
#177232=CARTESIAN_POINT('Ctrl Pts',(-6.09712605017347,58.6068890432828,
40.1562086174652));
#177233=CARTESIAN_POINT('Ctrl Pts',(-6.10629139889341,58.6050633610079,
40.1575965292115));
#177234=CARTESIAN_POINT('Ctrl Pts',(-6.11557877725353,58.6035068699781,
40.1585319382567));
#177235=CARTESIAN_POINT('Ctrl Pts',(-6.12022246643359,58.6027286244632,
40.1589996427793));
#177236=CARTESIAN_POINT('Ctrl Pts',(-6.12489666302671,58.6020176767849,
40.159354221642));
#177237=CARTESIAN_POINT('Ctrl Pts',(-6.12959764057299,58.6013767677628,
40.159591874311));
#177238=CARTESIAN_POINT('Ctrl Pts',(-6.13429861811926,58.6007358587407,
40.1598295269801));
#177239=CARTESIAN_POINT('Ctrl Pts',(-6.13902637679584,58.6001649900651,
40.1599502506895));
#177240=CARTESIAN_POINT('Ctrl Pts',(-6.14377718965262,58.5996668978649,
40.1599502534424));
#177241=CARTESIAN_POINT('',(-6.17403490858961,58.5964866834551,40.1599502534424));
#177242=CARTESIAN_POINT('Origin',(3.95370119046988E-16,6.77609428042844E-17,
40.1599502534424));
#177243=CARTESIAN_POINT('',(-6.49374646112681,58.7519447039089,39.8576902534424));
#177244=CARTESIAN_POINT('Ctrl Pts',(-6.17403490858961,58.5964866834551,
40.1599502534424));
#177245=CARTESIAN_POINT('Ctrl Pts',(-6.17782374318166,58.5960874772333,
40.1599502448875));
#177246=CARTESIAN_POINT('Ctrl Pts',(-6.18160715078344,58.5957361140451,
40.1598743450437));
#177247=CARTESIAN_POINT('Ctrl Pts',(-6.18538309648717,58.5954317101325,
40.1597243308499));
#177248=CARTESIAN_POINT('Ctrl Pts',(-6.20767599437464,58.5936345324521,
40.1588386583938));
#177249=CARTESIAN_POINT('Ctrl Pts',(-6.22971127560594,58.5934722580544,
40.1553722553613));
#177250=CARTESIAN_POINT('Ctrl Pts',(-6.25106353435582,58.5947642147755,
40.1496902177777));
#177251=CARTESIAN_POINT('Ctrl Pts',(-6.2590400274379,58.595246846799,40.1475675976836));
#177252=CARTESIAN_POINT('Ctrl Pts',(-6.26692152735692,58.5959321585041,
40.1451361443091));
#177253=CARTESIAN_POINT('Ctrl Pts',(-6.2746870907638,58.5968099398849,40.1424159447501));
#177254=CARTESIAN_POINT('Ctrl Pts',(-6.2807461728947,58.5974948289522,40.1402935085949));
#177255=CARTESIAN_POINT('Ctrl Pts',(-6.28673424952138,58.5982971695202,
40.1379949176048));
#177256=CARTESIAN_POINT('Ctrl Pts',(-6.29264094271378,58.5992123816357,
40.1355293609261));
#177257=CARTESIAN_POINT('Ctrl Pts',(-6.31331436888716,58.6024156240399,
40.1268999125509));
#177258=CARTESIAN_POINT('Ctrl Pts',(-6.33299084698388,58.6070015340112,
40.1162251288835));
#177259=CARTESIAN_POINT('Ctrl Pts',(-6.35122543337761,58.6127738370723,
40.1038990521418));
#177260=CARTESIAN_POINT('Ctrl Pts',(-6.36034272657447,58.6156599886029,
40.097736013771));
#177261=CARTESIAN_POINT('Ctrl Pts',(-6.36909954705041,58.6188427402045,
40.0911601532641));
#177262=CARTESIAN_POINT('Ctrl Pts',(-6.37744027742822,58.6222975626533,
40.084220729064));
#177263=CARTESIAN_POINT('Ctrl Pts',(-6.38574537226625,58.6257376244687,
40.0773109533618));
#177264=CARTESIAN_POINT('Ctrl Pts',(-6.3936380972253,58.62944725381,40.0700409753048));
#177265=CARTESIAN_POINT('Ctrl Pts',(-6.40106302694604,58.6334027859058,
40.0624586415899));
#177266=CARTESIAN_POINT('Ctrl Pts',(-6.40109488586922,58.6334197583214,
40.0624261072769));
#177267=CARTESIAN_POINT('Ctrl Pts',(-6.40112673655728,58.633436734872,40.0623935677888));
#177268=CARTESIAN_POINT('Ctrl Pts',(-6.40115857900959,58.6334537155558,
40.0623610231288));
#177269=CARTESIAN_POINT('Ctrl Pts',(-6.41617486746443,58.6414614796112,
40.0470135870231));
#177270=CARTESIAN_POINT('Ctrl Pts',(-6.42935337961428,58.6503516547095,
40.0305755292087));
#177271=CARTESIAN_POINT('Ctrl Pts',(-6.44073642151171,58.6599343882012,
40.013344756733));
#177272=CARTESIAN_POINT('Ctrl Pts',(-6.45253355607573,58.6698657226821,
39.9954871626584));
#177273=CARTESIAN_POINT('Ctrl Pts',(-6.46240257578747,58.6805417107303,
39.97677679543));
#177274=CARTESIAN_POINT('Ctrl Pts',(-6.47034286301626,58.6917721934519,
39.9575197577459));
#177275=CARTESIAN_POINT('Ctrl Pts',(-6.47816982452998,58.7028423919863,
39.9385375611982));
#177276=CARTESIAN_POINT('Ctrl Pts',(-6.48412273326605,58.714452295922,39.9190226977081));
#177277=CARTESIAN_POINT('Ctrl Pts',(-6.48815321522567,58.7264268163201,
39.8992655451843));
#177278=CARTESIAN_POINT('Ctrl Pts',(-6.49096333895696,58.7347756649885,
39.8854905069317));
#177279=CARTESIAN_POINT('Ctrl Pts',(-6.4928379682912,58.7433019189617,39.871597605147));
#177280=CARTESIAN_POINT('Ctrl Pts',(-6.49374646112681,58.7519447039089,
39.8576902534424));
#177281=CARTESIAN_POINT('',(-6.53099325079995,59.1062911958297,39.2875012672119));
#177282=CARTESIAN_POINT('',(-6.49374646112681,58.7519447039089,39.8576902534424));
#177283=CARTESIAN_POINT('',(-12.0535047649316,58.2316113004782,39.2875012672119));
#177284=CARTESIAN_POINT('Origin',(5.53234440788222E-15,0.,39.2875012672119));
#177285=CARTESIAN_POINT('',(-11.9794294790606,57.8830978693157,39.8576902534424));
#177286=CARTESIAN_POINT('',(-12.0535047649316,58.2316113004782,39.2875012672119));
#177287=CARTESIAN_POINT('',(-12.2354540642039,57.6364522029208,40.1599502534424));
#177288=CARTESIAN_POINT('Ctrl Pts',(-11.9794294790606,57.8830978693157,
39.8576902534424));
#177289=CARTESIAN_POINT('Ctrl Pts',(-11.9768868675907,57.8711351342676,
39.877261999406));
#177290=CARTESIAN_POINT('Ctrl Pts',(-11.9762358312602,57.858826420049,39.8967644650382));
#177291=CARTESIAN_POINT('Ctrl Pts',(-11.9774374689411,57.8463495993345,
39.9159282836066));
#177292=CARTESIAN_POINT('Ctrl Pts',(-11.9786608125867,57.8336474016745,
39.9354382707215));
#177293=CARTESIAN_POINT('Ctrl Pts',(-11.9818041414845,57.8207700703852,
39.9545987622393));
#177294=CARTESIAN_POINT('Ctrl Pts',(-11.9868762719092,57.8078866382169,
39.9731387498279));
#177295=CARTESIAN_POINT('Ctrl Pts',(-11.9917336614825,57.7955486571631,
39.9908938024114));
#177296=CARTESIAN_POINT('Ctrl Pts',(-11.9983602045484,57.7832042421904,
40.0080810366251));
#177297=CARTESIAN_POINT('Ctrl Pts',(-12.0068082271193,57.770997797342,40.0244542742617));
#177298=CARTESIAN_POINT('Ctrl Pts',(-12.0135275064638,57.7612891925114,
40.0374770090534));
#177299=CARTESIAN_POINT('Ctrl Pts',(-12.0213998814569,57.7516676540244,
40.0499848770061));
#177300=CARTESIAN_POINT('Ctrl Pts',(-12.0304721974324,57.7422089227119,
40.0618424270193));
#177301=CARTESIAN_POINT('Ctrl Pts',(-12.030496961908,57.7421831034479,40.0618747942791));
#177302=CARTESIAN_POINT('Ctrl Pts',(-12.0305217353323,57.7421572855746,
40.0619071564124));
#177303=CARTESIAN_POINT('Ctrl Pts',(-12.0305465177052,57.7421314690941,
40.0619395134161));
#177304=CARTESIAN_POINT('Ctrl Pts',(-12.0354799018083,57.73699222697,40.0683807661799));
#177305=CARTESIAN_POINT('Ctrl Pts',(-12.0408044207739,57.7319074031293,
40.0746073439084));
#177306=CARTESIAN_POINT('Ctrl Pts',(-12.0464896431811,57.726903735797,40.0805869293669));
#177307=CARTESIAN_POINT('Ctrl Pts',(-12.0577723607609,57.7169736114625,
40.092453830807));
#177308=CARTESIAN_POINT('Ctrl Pts',(-12.0704771166533,57.7073630976789,
40.1033475319609));
#177309=CARTESIAN_POINT('Ctrl Pts',(-12.0843744369107,57.698281056648,40.1130129263075));
#177310=CARTESIAN_POINT('Ctrl Pts',(-12.0947974271037,57.6914695258749,
40.1202619720674));
#177311=CARTESIAN_POINT('Ctrl Pts',(-12.1058912345906,57.6849552602294,
40.1268200947266));
#177312=CARTESIAN_POINT('Ctrl Pts',(-12.1175590523197,57.6788263845869,
40.1325796782703));
#177313=CARTESIAN_POINT('Ctrl Pts',(-12.1219344839681,57.6765280562209,
40.1347395220992));
#177314=CARTESIAN_POINT('Ctrl Pts',(-12.1263906358452,57.674283923512,40.1367870714852));
#177315=CARTESIAN_POINT('Ctrl Pts',(-12.1309224030556,57.6720986344674,
40.1387166518767));
#177316=CARTESIAN_POINT('Ctrl Pts',(-12.146783588292,57.6644501228112,40.1454701832469));
#177317=CARTESIAN_POINT('Ctrl Pts',(-12.1635710602988,57.6575224410761,
40.1507785912492));
#177318=CARTESIAN_POINT('Ctrl Pts',(-12.1810659563062,57.6515149180853,
40.1543986087265));
#177319=CARTESIAN_POINT('Ctrl Pts',(-12.18981340431,57.6485111565899,40.1562086174652));
#177320=CARTESIAN_POINT('Ctrl Pts',(-12.1987377085281,57.6457374357765,
40.1575965292115));
#177321=CARTESIAN_POINT('Ctrl Pts',(-12.2078115120423,57.6432186759797,
40.1585319382567));
#177322=CARTESIAN_POINT('Ctrl Pts',(-12.2123484137995,57.6419592960812,
40.1589996427793));
#177323=CARTESIAN_POINT('Ctrl Pts',(-12.2169226903863,57.6407636564618,
40.159354221642));
#177324=CARTESIAN_POINT('Ctrl Pts',(-12.2215309222505,57.6396348724476,
40.159591874311));
#177325=CARTESIAN_POINT('Ctrl Pts',(-12.2261391541148,57.6385060884334,
40.1598295269801));
#177326=CARTESIAN_POINT('Ctrl Pts',(-12.2307813416093,57.637444161687,40.1599502506895));
#177327=CARTESIAN_POINT('Ctrl Pts',(-12.2354540642039,57.6364522029208,
40.1599502534424));
#177328=CARTESIAN_POINT('',(-12.2652136052655,57.6301266171959,40.1599502534424));
#177329=CARTESIAN_POINT('Origin',(3.88326186679512E-16,6.66452935185788E-17,
40.1599502534424));
#177330=CARTESIAN_POINT('',(-12.5994235324466,57.7513140650721,39.8576902534424));
#177331=CARTESIAN_POINT('Ctrl Pts',(-12.2652136052655,57.6301266171959,
40.1599502534424));
#177332=CARTESIAN_POINT('Ctrl Pts',(-12.2689399558123,57.62933355681,40.1599502448875));
#177333=CARTESIAN_POINT('Ctrl Pts',(-12.2726659100573,57.6285886446436,
40.1598743450437));
#177334=CARTESIAN_POINT('Ctrl Pts',(-12.2763893518622,57.6278912144857,
40.1597243308499));
#177335=CARTESIAN_POINT('Ctrl Pts',(-12.2983722706983,57.6237736395753,
40.1588386583939));
#177336=CARTESIAN_POINT('Ctrl Pts',(-12.3202698780569,57.6213089400491,
40.1553722553623));
#177337=CARTESIAN_POINT('Ctrl Pts',(-12.3416402131471,57.6203619005013,
40.1496902177801));
#177338=CARTESIAN_POINT('Ctrl Pts',(-12.3496234589522,57.6200081180517,
40.1475675976854));
#177339=CARTESIAN_POINT('Ctrl Pts',(-12.3575334177724,57.6198658344726,
40.1451361443101));
#177340=CARTESIAN_POINT('Ctrl Pts',(-12.3653481937521,57.6199270848659,
40.1424159447501));
#177341=CARTESIAN_POINT('Ctrl Pts',(-12.3714456739989,57.6199748754953,
40.1402935085949));
#177342=CARTESIAN_POINT('Ctrl Pts',(-12.3774848147418,57.6201468963099,
40.1379949176048));
#177343=CARTESIAN_POINT('Ctrl Pts',(-12.3834548161669,57.6204396772353,
40.1355293609261));
#177344=CARTESIAN_POINT('Ctrl Pts',(-12.4043498211546,57.6214644104741,
40.1268999125509));
#177345=CARTESIAN_POINT('Ctrl Pts',(-12.4243978675675,57.6239684463328,
40.1162251288835));
#177346=CARTESIAN_POINT('Ctrl Pts',(-12.4431359329575,57.6278030948197,
40.1038990521418));
#177347=CARTESIAN_POINT('Ctrl Pts',(-12.4525049656526,57.6297204190632,
40.0977360137709));
#177348=CARTESIAN_POINT('Ctrl Pts',(-12.4615465034836,57.6319703982311,
40.0911601532641));
#177349=CARTESIAN_POINT('Ctrl Pts',(-12.4702026697491,57.634534451072,40.084220729064));
#177350=CARTESIAN_POINT('Ctrl Pts',(-12.4788218527838,57.6370875490682,
40.0773109533618));
#177351=CARTESIAN_POINT('Ctrl Pts',(-12.487059102424,57.6399518422609,40.0700409753047));
#177352=CARTESIAN_POINT('Ctrl Pts',(-12.4948568232942,57.6431095890444,
40.0624586415899));
#177353=CARTESIAN_POINT('Ctrl Pts',(-12.4948902817914,57.6431231383191,
40.0624261072769));
#177354=CARTESIAN_POINT('Ctrl Pts',(-12.4949237325308,57.6431366925669,
40.0623935677888));
#177355=CARTESIAN_POINT('Ctrl Pts',(-12.4949571755116,57.6431502517861,
40.0623610231288));
#177356=CARTESIAN_POINT('Ctrl Pts',(-12.5107282424363,57.6495445189153,
40.0470135870247));
#177357=CARTESIAN_POINT('Ctrl Pts',(-12.5247638376576,57.6570084630801,
40.0305755292122));
#177358=CARTESIAN_POINT('Ctrl Pts',(-12.5370861904653,57.6653488494772,
40.0133447567385));
#177359=CARTESIAN_POINT('Ctrl Pts',(-12.5498568062223,57.6739926427205,
39.995487162666));
#177360=CARTESIAN_POINT('Ctrl Pts',(-12.5607877070354,57.6835785531235,
39.9767767954399));
#177361=CARTESIAN_POINT('Ctrl Pts',(-12.5698584016403,57.6939175280623,
39.9575197577581));
#177362=CARTESIAN_POINT('Ctrl Pts',(-12.5787996370807,57.7041089426304,
39.9385375612124));
#177363=CARTESIAN_POINT('Ctrl Pts',(-12.5859335005772,57.715032997894,39.9190226977244));
#177364=CARTESIAN_POINT('Ctrl Pts',(-12.5911935813512,57.7265206205295,
39.8992655452027));
#177365=CARTESIAN_POINT('Ctrl Pts',(-12.5948610032545,57.7345299954194,
39.8854905069441));
#177366=CARTESIAN_POINT('Ctrl Pts',(-12.5976165994001,57.7428135895614,
39.8715976051532));
#177367=CARTESIAN_POINT('Ctrl Pts',(-12.5994235324466,57.7513140650721,
39.8576902534424));
#177368=CARTESIAN_POINT('',(-12.6735055745735,58.0998260601481,39.2875012672119));
#177369=CARTESIAN_POINT('',(-12.5994235324466,57.7513140650721,39.8576902534424));
#177370=CARTESIAN_POINT('',(-18.0743352474886,56.6526781108325,39.2875012672119));
#177371=CARTESIAN_POINT('Origin',(5.53234440788222E-15,0.,39.2875012672119));
#177372=CARTESIAN_POINT('',(-17.9642361803967,56.3138168485097,39.8576902534424));
#177373=CARTESIAN_POINT('',(-18.0743352474886,56.6526781108325,39.2875012672119));
#177374=CARTESIAN_POINT('',(-18.1930767435944,56.0417604764385,40.1599502534424));
#177375=CARTESIAN_POINT('Ctrl Pts',(-17.9642361803967,56.3138168485097,
39.8576902534424));
#177376=CARTESIAN_POINT('Ctrl Pts',(-17.9604570513079,56.3021854218463,
39.8772619994045));
#177377=CARTESIAN_POINT('Ctrl Pts',(-17.9585229704406,56.2900121878802,
39.8967644650353));
#177378=CARTESIAN_POINT('Ctrl Pts',(-17.9584138425285,56.2774781111558,
39.9159282836022));
#177379=CARTESIAN_POINT('Ctrl Pts',(-17.9583027433679,56.2647176232334,
39.9354382707156));
#177380=CARTESIAN_POINT('Ctrl Pts',(-17.9600828051299,56.2515822679742,
39.9545987622319));
#177381=CARTESIAN_POINT('Ctrl Pts',(-17.9637804645262,56.2382392305978,
39.973138749819));
#177382=CARTESIAN_POINT('Ctrl Pts',(-17.9673215746108,56.225461102829,39.990893802401));
#177383=CARTESIAN_POINT('Ctrl Pts',(-17.9726214740521,56.212491649491,40.0080810366132));
#177384=CARTESIAN_POINT('Ctrl Pts',(-17.9797472965476,56.199469014009,40.0244542742487));
#177385=CARTESIAN_POINT('Ctrl Pts',(-17.9854149414345,56.189111237984,40.0374770090451));
#177386=CARTESIAN_POINT('Ctrl Pts',(-17.9922384661032,56.1787195200277,
40.0499848770022));
#177387=CARTESIAN_POINT('Ctrl Pts',(-18.0002723763367,56.1683642893844,
40.0618424270193));
#177388=CARTESIAN_POINT('Ctrl Pts',(-18.0002943063019,56.1683360229685,
40.0618747942791));
#177389=CARTESIAN_POINT('Ctrl Pts',(-18.0003162453122,56.1683077570002,
40.0619071564124));
#177390=CARTESIAN_POINT('Ctrl Pts',(-18.0003381933676,56.1682794914817,
40.0619395134161));
#177391=CARTESIAN_POINT('Ctrl Pts',(-18.0047073547949,56.1626527236047,
40.0683807661799));
#177392=CARTESIAN_POINT('Ctrl Pts',(-18.0094711966663,56.1570391911759,
40.0746073439084));
#177393=CARTESIAN_POINT('Ctrl Pts',(-18.0146022491734,56.1514686668952,
40.0805869293669));
#177394=CARTESIAN_POINT('Ctrl Pts',(-18.024785178209,56.1404135756908,40.092453830807));
#177395=CARTESIAN_POINT('Ctrl Pts',(-18.0364157638823,56.1295277006976,
40.1033475319609));
#177396=CARTESIAN_POINT('Ctrl Pts',(-18.049287621373,56.1190427465077,40.1130129263075));
#177397=CARTESIAN_POINT('Ctrl Pts',(-18.0589415144909,56.1111790308654,
40.1202619720674));
#177398=CARTESIAN_POINT('Ctrl Pts',(-18.0692936227623,56.1035408324002,
40.1268200947266));
#177399=CARTESIAN_POINT('Ctrl Pts',(-18.0802568810126,56.0962259123229,
40.1325796782703));
#177400=CARTESIAN_POINT('Ctrl Pts',(-18.0843681028565,56.0934828172939,
40.1347395220992));
#177401=CARTESIAN_POINT('Ctrl Pts',(-18.0885652677239,56.0907851834709,
40.1367870714852));
#177402=CARTESIAN_POINT('Ctrl Pts',(-18.0928437845337,56.088138167006,40.1387166518767));
#177403=CARTESIAN_POINT('Ctrl Pts',(-18.1078185933682,56.0788736093785,
40.1454701832469));
#177404=CARTESIAN_POINT('Ctrl Pts',(-18.1237899619209,56.0702291095579,
40.1507785912491));
#177405=CARTESIAN_POINT('Ctrl Pts',(-18.1405610619113,56.0624257818118,
40.1543986087265));
#177406=CARTESIAN_POINT('Ctrl Pts',(-18.1489466119065,56.0585241179388,
40.1562086174652));
#177407=CARTESIAN_POINT('Ctrl Pts',(-18.1575320950781,56.0548327480527,
40.1575965292115));
#177408=CARTESIAN_POINT('Ctrl Pts',(-18.1662929092565,56.0513793155482,
40.1585319382567));
#177409=CARTESIAN_POINT('Ctrl Pts',(-18.1706733163456,56.0496525992959,
40.1589996427793));
#177410=CARTESIAN_POINT('Ctrl Pts',(-18.1750975561947,56.0479853674133,
40.159354221642));
#177411=CARTESIAN_POINT('Ctrl Pts',(-18.1795625536242,56.0463810756009,
40.1595918743111));
#177412=CARTESIAN_POINT('Ctrl Pts',(-18.1840275510537,56.0447767837885,
40.1598295269801));
#177413=CARTESIAN_POINT('Ctrl Pts',(-18.1885333065885,56.0432354336629,
40.1599502506895));
#177414=CARTESIAN_POINT('Ctrl Pts',(-18.1930767435944,56.0417604764385,
40.1599502534424));
#177415=CARTESIAN_POINT('',(-18.2220120550212,56.0323588238393,40.1599502534424));
#177416=CARTESIAN_POINT('Origin',(3.81437458815951E-16,6.47994644506575E-17,
40.1599502534424));
#177417=CARTESIAN_POINT('',(-18.567058682946,56.117947944099,39.8576902534424));
#177418=CARTESIAN_POINT('Ctrl Pts',(-18.2220120550212,56.0323588238393,
40.1599502534424));
#177419=CARTESIAN_POINT('Ctrl Pts',(-18.2256350948464,56.0311805982249,
40.1599502448875));
#177420=CARTESIAN_POINT('Ctrl Pts',(-18.2292627734001,56.0300502984939,
40.1598743450437));
#177421=CARTESIAN_POINT('Ctrl Pts',(-18.2328929164986,56.0289674832814,
40.1597243308499));
#177422=CARTESIAN_POINT('Ctrl Pts',(-18.2543250068315,56.0225746241519,
40.1588386583937));
#177423=CARTESIAN_POINT('Ctrl Pts',(-18.2758450255561,56.0178345032605,
40.155372255361));
#177424=CARTESIAN_POINT('Ctrl Pts',(-18.2969992991299,56.014658843408,40.1496902177768));
#177425=CARTESIAN_POINT('Ctrl Pts',(-18.3049018315393,56.0134725226006,
40.1475675976829));
#177426=CARTESIAN_POINT('Ctrl Pts',(-18.3127535860896,56.0125042026265,
40.1451361443088));
#177427=CARTESIAN_POINT('Ctrl Pts',(-18.3205319543143,56.0117482509601,
40.1424159447501));
#177428=CARTESIAN_POINT('Ctrl Pts',(-18.3266010274073,56.0111584195474,
40.1402935085949));
#177429=CARTESIAN_POINT('Ctrl Pts',(-18.3326250661768,56.0106982359128,
40.1379949176048));
#177430=CARTESIAN_POINT('Ctrl Pts',(-18.3385929672496,56.0103653778789,
40.1355293609261));
#177431=CARTESIAN_POINT('Ctrl Pts',(-18.3594806210044,56.0092003747605,
40.1268999125509));
#177432=CARTESIAN_POINT('Ctrl Pts',(-18.3796805851417,56.0095951017657,
40.1162251288835));
#177433=CARTESIAN_POINT('Ctrl Pts',(-18.3987168313625,56.0114500824672,
40.1038990521418));
#177434=CARTESIAN_POINT('Ctrl Pts',(-18.4082349544728,56.0123775728179,
40.097736013771));
#177435=CARTESIAN_POINT('Ctrl Pts',(-18.4174621486784,56.0136701283094,
40.0911601532641));
#177436=CARTESIAN_POINT('Ctrl Pts',(-18.4263389120626,56.0153153192431,
40.0842207290641));
#177437=CARTESIAN_POINT('Ctrl Pts',(-18.4351777497209,56.0169534811441,
40.0773109533619));
#177438=CARTESIAN_POINT('Ctrl Pts',(-18.4436692750114,56.0189410563925,
40.0700409753048));
#177439=CARTESIAN_POINT('Ctrl Pts',(-18.4517543535695,56.0212664209292,
40.0624586415899));
#177440=CARTESIAN_POINT('Ctrl Pts',(-18.4517890450624,56.0212763986142,
40.0624261072769));
#177441=CARTESIAN_POINT('Ctrl Pts',(-18.4518237293599,56.0212863820561,
40.0623935677888));
#177442=CARTESIAN_POINT('Ctrl Pts',(-18.4518584064609,56.021296371253,40.0623610231288));
#177443=CARTESIAN_POINT('Ctrl Pts',(-18.4682114607453,56.0260070845275,
40.0470135870268));
#177444=CARTESIAN_POINT('Ctrl Pts',(-18.482950362119,56.0319630212247,40.0305755292168));
#177445=CARTESIAN_POINT('Ctrl Pts',(-18.4960770195605,56.0389696815083,
40.0133447567458));
#177446=CARTESIAN_POINT('Ctrl Pts',(-18.5096811989713,56.0462312303064,
39.9954871626761));
#177447=CARTESIAN_POINT('Ctrl Pts',(-18.5215542196485,56.0546220378234,
39.976776795453));
#177448=CARTESIAN_POINT('Ctrl Pts',(-18.531655941201,56.063956229006,39.9575197577742));
#177449=CARTESIAN_POINT('Ctrl Pts',(-18.541613488521,56.0731572003366,39.9385375612315));
#177450=CARTESIAN_POINT('Ctrl Pts',(-18.5498501466764,56.0832757206921,
39.9190226977465));
#177451=CARTESIAN_POINT('Ctrl Pts',(-18.5562821957188,56.0941505847667,
39.8992655452277));
#177452=CARTESIAN_POINT('Ctrl Pts',(-18.5607667347539,56.1017327334914,
39.8854905069609));
#177453=CARTESIAN_POINT('Ctrl Pts',(-18.5643731068241,56.1096829110121,
39.8715976051617));
#177454=CARTESIAN_POINT('Ctrl Pts',(-18.567058682946,56.117947944099,39.8576902534424));
#177455=CARTESIAN_POINT('',(-18.6771643191705,56.4568070719813,39.2875012672119));
#177456=CARTESIAN_POINT('',(-18.567058682946,56.117947944099,39.8576902534424));
#177457=CARTESIAN_POINT('',(-23.8971395307763,54.4530463244695,39.2875012672119));
#177458=CARTESIAN_POINT('Origin',(5.53234440788222E-15,0.,39.2875012672119));
#177459=CARTESIAN_POINT('',(-23.7522229508823,54.1275498658876,39.8576902534424));
#177460=CARTESIAN_POINT('',(-23.8971395307763,54.4530463244694,39.2875012672119));
#177461=CARTESIAN_POINT('',(-23.951372267036,53.833063494684,40.1599502534424));
#177462=CARTESIAN_POINT('Ctrl Pts',(-23.7522229508823,54.1275498658876,
39.8576902534424));
#177463=CARTESIAN_POINT('Ctrl Pts',(-23.7472487091031,54.1163771839524,
39.8772619994049));
#177464=CARTESIAN_POINT('Ctrl Pts',(-23.7440527738935,54.1044728027364,
39.8967644650361));
#177465=CARTESIAN_POINT('Ctrl Pts',(-23.7426340760171,54.0920187959684,
39.9159282836035));
#177466=CARTESIAN_POINT('Ctrl Pts',(-23.7411897512762,54.0793398243582,
39.9354382707173));
#177467=CARTESIAN_POINT('Ctrl Pts',(-23.7415870431741,54.0660903588286,
39.9545987622342));
#177468=CARTESIAN_POINT('Ctrl Pts',(-23.7438697192134,54.0524339053522,
39.9731387498218));
#177469=CARTESIAN_POINT('Ctrl Pts',(-23.7460557526676,54.0393556307082,
39.9908938024045));
#177470=CARTESIAN_POINT('Ctrl Pts',(-23.7499709416789,54.0259032350479,
40.0080810366174));
#177471=CARTESIAN_POINT('Ctrl Pts',(-23.7556964920992,54.01220708765,40.0244542742534));
#177472=CARTESIAN_POINT('Ctrl Pts',(-23.7602504066234,54.0013136223967,
40.0374770090481));
#177473=CARTESIAN_POINT('Ctrl Pts',(-23.7659503210008,53.9902655788123,
40.0499848770036));
#177474=CARTESIAN_POINT('Ctrl Pts',(-23.7728578042866,53.9791273029165,
40.0618424270192));
#177475=CARTESIAN_POINT('Ctrl Pts',(-23.7728766594722,53.9790968990414,
40.0618747942791));
#177476=CARTESIAN_POINT('Ctrl Pts',(-23.7728955237001,53.9790664946661,
40.0619071564124));
#177477=CARTESIAN_POINT('Ctrl Pts',(-23.7729143969706,53.9790360897925,
40.0619395134161));
#177478=CARTESIAN_POINT('Ctrl Pts',(-23.776671466275,53.9729834442089,40.0683807661799));
#177479=CARTESIAN_POINT('Ctrl Pts',(-23.780822437404,53.966902706228,40.0746073439084));
#177480=CARTESIAN_POINT('Ctrl Pts',(-23.7853431031259,53.9608263568287,
40.0805869293669));
#177481=CARTESIAN_POINT('Ctrl Pts',(-23.7943146773159,53.9487674206469,
40.092453830807));
#177482=CARTESIAN_POINT('Ctrl Pts',(-23.8047436656396,53.9367254523686,
40.1033475319609));
#177483=CARTESIAN_POINT('Ctrl Pts',(-23.8164490335992,53.924952460372,40.1130129263075));
#177484=CARTESIAN_POINT('Ctrl Pts',(-23.8252280595689,53.9161227163746,
40.1202619720674));
#177485=CARTESIAN_POINT('Ctrl Pts',(-23.8347250487603,53.9074442707906,
40.1268200947266));
#177486=CARTESIAN_POINT('Ctrl Pts',(-23.8448636317802,53.8990234500735,
40.1325796782703));
#177487=CARTESIAN_POINT('Ctrl Pts',(-23.8486656004127,53.8958656423046,
40.1347395220992));
#177488=CARTESIAN_POINT('Ctrl Pts',(-23.8525577932538,53.8927440632083,
40.1367870714852));
#177489=CARTESIAN_POINT('Ctrl Pts',(-23.8565361833376,53.8896643205893,
40.1387166518767));
#177490=CARTESIAN_POINT('Ctrl Pts',(-23.8704605486307,53.8788852214227,
40.1454701832469));
#177491=CARTESIAN_POINT('Ctrl Pts',(-23.8854408280735,53.8686186144655,
40.1507785912492));
#177492=CARTESIAN_POINT('Ctrl Pts',(-23.9013043843657,53.859104976856,40.1543986087265));
#177493=CARTESIAN_POINT('Ctrl Pts',(-23.9092361625117,53.8543481580513,
40.1562086174652));
#177494=CARTESIAN_POINT('Ctrl Pts',(-23.9173887602867,53.8497795825133,
40.1575965292115));
#177495=CARTESIAN_POINT('Ctrl Pts',(-23.9257405998156,53.8454293138304,
40.1585319382567));
#177496=CARTESIAN_POINT('Ctrl Pts',(-23.92991651958,53.8432541794889,40.1589996427793));
#177497=CARTESIAN_POINT('Ctrl Pts',(-23.9341422497936,53.8411336218844,
40.159354221642));
#177498=CARTESIAN_POINT('Ctrl Pts',(-23.9384150933423,53.8390713992306,
40.1595918743111));
#177499=CARTESIAN_POINT('Ctrl Pts',(-23.942687936891,53.8370091765768,40.1598295269801));
#177500=CARTESIAN_POINT('Ctrl Pts',(-23.9470078944655,53.8350052904266,
40.1599502506895));
#177501=CARTESIAN_POINT('Ctrl Pts',(-23.951372267036,53.833063494684,40.1599502534424));
#177502=CARTESIAN_POINT('',(-23.9791663275009,53.8206887816838,40.1599502534424));
#177503=CARTESIAN_POINT('Origin',(3.74779409800327E-16,6.22436788900575E-17,
40.1599502534424));
#177504=CARTESIAN_POINT('',(-24.3312692531083,53.8697418420147,39.8576902534424));
#177505=CARTESIAN_POINT('Ctrl Pts',(-23.9791663275009,53.8206887816838,
40.1599502534424));
#177506=CARTESIAN_POINT('Ctrl Pts',(-23.982646361822,53.8191382997274,40.1599502448875));
#177507=CARTESIAN_POINT('Ctrl Pts',(-23.9861360190791,53.8176349962321,
40.1598743450437));
#177508=CARTESIAN_POINT('Ctrl Pts',(-23.9896330908637,53.8161786595151,
40.1597243308499));
#177509=CARTESIAN_POINT('Ctrl Pts',(-24.0102795382188,53.8075805576713,
40.1588386583939));
#177510=CARTESIAN_POINT('Ctrl Pts',(-24.0311861904727,53.8006169491723,
40.1553722553623));
#177511=CARTESIAN_POINT('Ctrl Pts',(-24.0518926318745,53.7952474622089,
40.14969021778));
#177512=CARTESIAN_POINT('Ctrl Pts',(-24.0596278690975,53.7932416006212,
40.1475675976853));
#177513=CARTESIAN_POINT('Ctrl Pts',(-24.0673353939197,53.7914578533671,
40.1451361443101));
#177514=CARTESIAN_POINT('Ctrl Pts',(-24.0749921329673,53.789892982005,40.1424159447501));
#177515=CARTESIAN_POINT('Ctrl Pts',(-24.0809663048717,53.7886719908666,
40.1402935085949));
#177516=CARTESIAN_POINT('Ctrl Pts',(-24.0869092410384,53.7875846446508,
40.1379949176048));
#177517=CARTESIAN_POINT('Ctrl Pts',(-24.0928096561859,53.7866297945201,
40.1355293609261));
#177518=CARTESIAN_POINT('Ctrl Pts',(-24.1134611092023,53.7832878190624,
40.1268999125509));
#177519=CARTESIAN_POINT('Ctrl Pts',(-24.1335916760297,53.7815689125024,
40.1162251288835));
#177520=CARTESIAN_POINT('Ctrl Pts',(-24.152717537984,53.7814239018616,40.1038990521418));
#177521=CARTESIAN_POINT('Ctrl Pts',(-24.1622804689611,53.7813513965412,
40.097736013771));
#177522=CARTESIAN_POINT('Ctrl Pts',(-24.1715922244705,53.781672366848,40.0911601532641));
#177523=CARTESIAN_POINT('Ctrl Pts',(-24.1805923292962,53.7823806708183,
40.084220729064));
#177524=CARTESIAN_POINT('Ctrl Pts',(-24.1895539814231,53.7830859485794,
40.0773109533619));
#177525=CARTESIAN_POINT('Ctrl Pts',(-24.198206747436,53.7841750295932,40.0700409753048));
#177526=CARTESIAN_POINT('Ctrl Pts',(-24.2064906018693,53.7856425347026,
40.0624586415899));
#177527=CARTESIAN_POINT('Ctrl Pts',(-24.2065261462707,53.7856488314804,
40.062426107277));
#177528=CARTESIAN_POINT('Ctrl Pts',(-24.2065616841178,53.7856551347356,
40.0623935677889));
#177529=CARTESIAN_POINT('Ctrl Pts',(-24.2065972154094,53.7856614444666,
40.0623610231289));
#177530=CARTESIAN_POINT('Ctrl Pts',(-24.2233530895771,53.7886369923279,
40.0470135870212));
#177531=CARTESIAN_POINT('Ctrl Pts',(-24.2386338146223,53.793019667072,40.0305755292047));
#177532=CARTESIAN_POINT('Ctrl Pts',(-24.252420958297,53.7986158348102,40.0133447567266));
#177533=CARTESIAN_POINT('Ctrl Pts',(-24.2667096511305,53.8044155801195,
39.9954871626496));
#177534=CARTESIAN_POINT('Ctrl Pts',(-24.2793947083764,53.8115193533133,
39.9767767954186));
#177535=CARTESIAN_POINT('Ctrl Pts',(-24.2904167803032,53.8197464933945,
39.9575197577317));
#177536=CARTESIAN_POINT('Ctrl Pts',(-24.3012815425323,53.8278562137268,
39.9385375611815));
#177537=CARTESIAN_POINT('Ctrl Pts',(-24.3105307527959,53.8370583385547,
39.9190226976888));
#177538=CARTESIAN_POINT('Ctrl Pts',(-24.3180642992295,53.8472012967897,
39.8992655451625));
#177539=CARTESIAN_POINT('Ctrl Pts',(-24.3233168218341,53.8542731477268,
39.885490506917));
#177540=CARTESIAN_POINT('Ctrl Pts',(-24.3277344576514,53.8618028048015,
39.8715976051397));
#177541=CARTESIAN_POINT('Ctrl Pts',(-24.3312692531083,53.8697418420147,
39.8576902534424));
#177542=CARTESIAN_POINT('',(-24.4761921430387,54.1952354911874,39.2875012672119));
#177543=CARTESIAN_POINT('',(-24.3312692531083,53.8697418420147,39.8576902534424));
#177544=CARTESIAN_POINT('',(-29.4581217525669,51.656815567543,39.2875012672119));
#177545=CARTESIAN_POINT('Origin',(5.53234440788222E-15,0.,39.2875012672119));
#177546=CARTESIAN_POINT('',(-29.2799753962458,51.3482501200168,39.8576902534424));
#177547=CARTESIAN_POINT('',(-29.4581217525669,51.656815567543,39.2875012672119));
#177548=CARTESIAN_POINT('',(-29.4472515437731,51.0345602039889,40.1599502534424));
#177549=CARTESIAN_POINT('Ctrl Pts',(-29.2799753962458,51.3482501200168,
39.8576902534424));
#177550=CARTESIAN_POINT('Ctrl Pts',(-29.2738605406099,51.3376585930511,
39.8772619994057));
#177551=CARTESIAN_POINT('Ctrl Pts',(-29.269437766393,51.3261534914766,39.8967644650376));
#177552=CARTESIAN_POINT('Ctrl Pts',(-29.266725042103,51.3139160033692,39.9159282836057));
#177553=CARTESIAN_POINT('Ctrl Pts',(-29.2639633161059,51.3014574615371,
39.9354382707205));
#177554=CARTESIAN_POINT('Ctrl Pts',(-29.2629734853264,51.2882390496537,
39.9545987622381));
#177555=CARTESIAN_POINT('Ctrl Pts',(-29.2638161685324,51.2744188030391,
39.9731387498264));
#177556=CARTESIAN_POINT('Ctrl Pts',(-29.2646231747162,51.2611836698336,
39.99089380241));
#177557=CARTESIAN_POINT('Ctrl Pts',(-29.2671107576673,51.2473957191126,
40.0080810366237));
#177558=CARTESIAN_POINT('Ctrl Pts',(-29.271373305684,51.2331761176555,40.0244542742603));
#177559=CARTESIAN_POINT('Ctrl Pts',(-29.2747635962052,51.2218663142594,
40.0374770090526));
#177560=CARTESIAN_POINT('Ctrl Pts',(-29.2792774508366,51.2102829897252,
40.0499848770057));
#177561=CARTESIAN_POINT('Ctrl Pts',(-29.2849828273425,51.1984837018593,
40.0618424270193));
#177562=CARTESIAN_POINT('Ctrl Pts',(-29.2849984011671,51.1984514936363,
40.0618747942791));
#177563=CARTESIAN_POINT('Ctrl Pts',(-29.2850139839321,51.1984192839705,
40.0619071564124));
#177564=CARTESIAN_POINT('Ctrl Pts',(-29.2850295756381,51.1983870728641,
40.0619395134162));
#177565=CARTESIAN_POINT('Ctrl Pts',(-29.2881333895822,51.1919748636255,
40.0683807661799));
#177566=CARTESIAN_POINT('Ctrl Pts',(-29.2916260110603,51.1854935419304,
40.0746073439084));
#177567=CARTESIAN_POINT('Ctrl Pts',(-29.2954867606374,51.178977941168,40.0805869293669));
#177568=CARTESIAN_POINT('Ctrl Pts',(-29.3031486855376,51.1660472802372,
40.092453830807));
#177569=CARTESIAN_POINT('Ctrl Pts',(-29.3122618143332,51.1529811529981,
40.1033475319609));
#177570=CARTESIAN_POINT('Ctrl Pts',(-29.3226724463009,51.1400491105587,
40.1130129263075));
#177571=CARTESIAN_POINT('Ctrl Pts',(-29.3304804202767,51.1303500787292,
40.1202619720674));
#177572=CARTESIAN_POINT('Ctrl Pts',(-29.3390182393872,51.1207264688923,
40.1268200947266));
#177573=CARTESIAN_POINT('Ctrl Pts',(-29.3482210667394,51.1112920078094,
40.1325796782703));
#177574=CARTESIAN_POINT('Ctrl Pts',(-29.3516721269965,51.1077540849033,
40.1347395220992));
#177575=CARTESIAN_POINT('Ctrl Pts',(-29.3552167041322,51.1042427612075,
40.1367870714852));
#177576=CARTESIAN_POINT('Ctrl Pts',(-29.3588513794155,51.1007640347391,
40.1387166518767));
#177577=CARTESIAN_POINT('Ctrl Pts',(-29.3715727429074,51.0885884920995,
40.1454701832469));
#177578=CARTESIAN_POINT('Ctrl Pts',(-29.3853978061637,51.0768122610999,
40.1507785912492));
#177579=CARTESIAN_POINT('Ctrl Pts',(-29.4001800143153,51.0656925470315,
40.1543986087265));
#177580=CARTESIAN_POINT('Ctrl Pts',(-29.4075711183911,51.0601326899973,
40.1562086174652));
#177581=CARTESIAN_POINT('Ctrl Pts',(-29.4152015092021,51.054736963077,40.1575965292115));
#177582=CARTESIAN_POINT('Ctrl Pts',(-29.42305286958,51.0495375206697,40.1585319382567));
#177583=CARTESIAN_POINT('Ctrl Pts',(-29.4269785497689,51.0469377994661,
40.1589996427793));
#177584=CARTESIAN_POINT('Ctrl Pts',(-29.4309594723626,51.0443871494125,
40.159354221642));
#177585=CARTESIAN_POINT('Ctrl Pts',(-29.4349933478623,51.0418895900603,
40.1595918743111));
#177586=CARTESIAN_POINT('Ctrl Pts',(-29.439027223362,51.0393920307081,40.1598295269801));
#177587=CARTESIAN_POINT('Ctrl Pts',(-29.4431140526171,51.0369475635292,
40.1599502506895));
#177588=CARTESIAN_POINT('Ctrl Pts',(-29.4472515437731,51.034560203989,40.1599502534424));
#177589=CARTESIAN_POINT('',(-29.4735998357333,51.019348010533,40.1599502534424));
#177590=CARTESIAN_POINT('Origin',(3.68424986610945E-16,5.90059385582091E-17,
40.1599502534424));
#177591=CARTESIAN_POINT('',(-29.8289013456881,51.0313275753412,39.8576902534424));
#177592=CARTESIAN_POINT('Ctrl Pts',(-29.4735998357333,51.019348010533,40.1599502534424));
#177593=CARTESIAN_POINT('Ctrl Pts',(-29.476898736566,51.0174422596393,40.1599502448875));
#177594=CARTESIAN_POINT('Ctrl Pts',(-29.4802121391114,51.0155824228874,
40.1598743450438));
#177595=CARTESIAN_POINT('Ctrl Pts',(-29.4835378249318,51.0137685205958,
40.1597243308499));
#177596=CARTESIAN_POINT('Ctrl Pts',(-29.5031724225167,51.0030593786387,
40.1588386583938));
#177597=CARTESIAN_POINT('Ctrl Pts',(-29.5232366506486,50.9939485772829,
40.1553722553617));
#177598=CARTESIAN_POINT('Ctrl Pts',(-29.5432683957785,50.9864440924311,
40.1496902177787));
#177599=CARTESIAN_POINT('Ctrl Pts',(-29.5507515889318,50.9836406667038,
40.1475675976843));
#177600=CARTESIAN_POINT('Ctrl Pts',(-29.5582304387657,50.9810610352791,
40.1451361443096));
#177601=CARTESIAN_POINT('Ctrl Pts',(-29.5656816597953,50.9787043892803,
40.1424159447501));
#177602=CARTESIAN_POINT('Ctrl Pts',(-29.5714954762336,50.9768656158507,
40.1402935085949));
#177603=CARTESIAN_POINT('Ctrl Pts',(-29.5772921977452,50.9751630202464,
40.1379949176048));
#177604=CARTESIAN_POINT('Ctrl Pts',(-29.5830604807844,50.9735966395566,
40.1355293609262));
#177605=CARTESIAN_POINT('Ctrl Pts',(-29.6032494714214,50.9681143071421,
40.1268999125509));
#177606=CARTESIAN_POINT('Ctrl Pts',(-29.6230900862363,50.9643005997169,
40.1162251288835));
#177607=CARTESIAN_POINT('Ctrl Pts',(-29.6420960169782,50.9621571865008,
40.1038990521418));
#177608=CARTESIAN_POINT('Ctrl Pts',(-29.6515989823491,50.9610854798928,
40.097736013771));
#177609=CARTESIAN_POINT('Ctrl Pts',(-29.6608932776205,50.9604313483969,
40.0911601532641));
#177610=CARTESIAN_POINT('Ctrl Pts',(-29.6699181168558,50.9601950050772,
40.084220729064));
#177611=CARTESIAN_POINT('Ctrl Pts',(-29.6789043977152,50.9599596715279,
40.0773109533619));
#177612=CARTESIAN_POINT('Ctrl Pts',(-29.6876236029352,50.9601383261076,
40.0700409753048));
#177613=CARTESIAN_POINT('Ctrl Pts',(-29.6960154736012,50.9607318934966,
40.0624586415899));
#177614=CARTESIAN_POINT('Ctrl Pts',(-29.6960514814791,50.9607344403783,
40.0624261072769));
#177615=CARTESIAN_POINT('Ctrl Pts',(-29.6960874835157,50.9607369943871,
40.0623935677888));
#177616=CARTESIAN_POINT('Ctrl Pts',(-29.6961234797097,50.9607395555214,
40.0623610231288));
#177617=CARTESIAN_POINT('Ctrl Pts',(-29.7130985928884,50.9619473372425,
40.0470135870233));
#177618=CARTESIAN_POINT('Ctrl Pts',(-29.728753722777,50.9647087325286,40.0305755292094));
#177619=CARTESIAN_POINT('Ctrl Pts',(-29.7430502978482,50.9688330949322,
40.013344756734));
#177620=CARTESIAN_POINT('Ctrl Pts',(-29.7578669541901,50.9731074935248,
39.9954871626599));
#177621=CARTESIAN_POINT('Ctrl Pts',(-29.7712250678592,50.9788464019639,
39.9767767954321));
#177622=CARTESIAN_POINT('Ctrl Pts',(-29.7830467300316,50.9858763526685,
39.9575197577485));
#177623=CARTESIAN_POINT('Ctrl Pts',(-29.7946996705594,50.9928059702028,
39.9385375612016));
#177624=CARTESIAN_POINT('Ctrl Pts',(-29.804860096648,51.0009908790906,39.9190226977123));
#177625=CARTESIAN_POINT('Ctrl Pts',(-29.8134126013634,51.010290803105,39.8992655451893));
#177626=CARTESIAN_POINT('Ctrl Pts',(-29.8193755598153,51.0167748755901,
39.8854905069351));
#177627=CARTESIAN_POINT('Ctrl Pts',(-29.8245560588482,51.0238015157365,
39.8715976051487));
#177628=CARTESIAN_POINT('Ctrl Pts',(-29.8289013456881,51.0313275753412,
39.8576902534424));
#177629=CARTESIAN_POINT('',(-30.0070536838153,51.33988956927,39.2875012672119));
#177630=CARTESIAN_POINT('',(-29.8289013456881,51.0313275753412,39.8576902534424));
#177631=CARTESIAN_POINT('',(-34.6963546279281,48.2946219293749,39.2875012672119));
#177632=CARTESIAN_POINT('Origin',(5.53234440788222E-15,0.,39.2875012672119));
#177633=CARTESIAN_POINT('',(-34.4869303039392,48.006368200519,39.8576902534424));
#177634=CARTESIAN_POINT('',(-34.6963546279281,48.2946219293749,39.2875012672119));
#177635=CARTESIAN_POINT('',(-34.620500570363,47.6769115920307,40.1599502534424));
#177636=CARTESIAN_POINT('Ctrl Pts',(-34.4869303039393,48.006368200519,39.8576902534424));
#177637=CARTESIAN_POINT('Ctrl Pts',(-34.4797418300853,47.9964738715094,
39.8772619994048));
#177638=CARTESIAN_POINT('Ctrl Pts',(-34.4741406737012,47.9854941018779,
39.8967644650359));
#177639=CARTESIAN_POINT('Ctrl Pts',(-34.4701636441726,47.9736072089126,
39.9159282836032));
#177640=CARTESIAN_POINT('Ctrl Pts',(-34.4661147749673,47.9615055952513,
39.935438270717));
#177641=CARTESIAN_POINT('Ctrl Pts',(-34.4637486663033,47.9484630607023,
39.9545987622339));
#177642=CARTESIAN_POINT('Ctrl Pts',(-34.4631421240615,47.9346304384649,
39.9731387498215));
#177643=CARTESIAN_POINT('Ctrl Pts',(-34.4625612612457,47.9213834535885,
39.9908938024042));
#177644=CARTESIAN_POINT('Ctrl Pts',(-34.4635939836562,47.907411011482,40.0080810366171));
#177645=CARTESIAN_POINT('Ctrl Pts',(-34.4663468278996,47.8928237488966,
40.0244542742532));
#177646=CARTESIAN_POINT('Ctrl Pts',(-34.4685363496856,47.8812215199268,
40.037477009048));
#177647=CARTESIAN_POINT('Ctrl Pts',(-34.4718146898364,47.8692298237661,
40.0499848770036));
#177648=CARTESIAN_POINT('Ctrl Pts',(-34.4762554502654,47.8568987993931,
40.0618424270193));
#177649=CARTESIAN_POINT('Ctrl Pts',(-34.4762675720988,47.856865139702,40.0618747942791));
#177650=CARTESIAN_POINT('Ctrl Pts',(-34.476279702673,47.8568314776417,40.0619071564124));
#177651=CARTESIAN_POINT('Ctrl Pts',(-34.4762918419885,47.8567978132141,
40.0619395134161));
#177652=CARTESIAN_POINT('Ctrl Pts',(-34.4787083945372,47.8500962938268,
40.0683807661799));
#177653=CARTESIAN_POINT('Ctrl Pts',(-34.4815044004727,47.8432853991342,
40.0746073439084));
#177654=CARTESIAN_POINT('Ctrl Pts',(-34.4846629347248,47.8364019332941,
40.0805869293668));
#177655=CARTESIAN_POINT('Ctrl Pts',(-34.4909312646825,47.8227412186414,
40.092453830807));
#177656=CARTESIAN_POINT('Ctrl Pts',(-34.4986286886039,47.8087940876659,
40.1033475319609));
#177657=CARTESIAN_POINT('Ctrl Pts',(-34.5076305235172,47.7948446809468,
40.1130129263075));
#177658=CARTESIAN_POINT('Ctrl Pts',(-34.5143818997023,47.7843826259075,
40.1202619720674));
#177659=CARTESIAN_POINT('Ctrl Pts',(-34.5218670065991,47.773919290101,40.1268200947266));
#177660=CARTESIAN_POINT('Ctrl Pts',(-34.5300332501814,47.7635745545822,
40.1325796782703));
#177661=CARTESIAN_POINT('Ctrl Pts',(-34.5330955915248,47.7596952787626,
40.1347395220992));
#177662=CARTESIAN_POINT('Ctrl Pts',(-34.5362537178261,47.7558326812646,
40.1367870714852));
#177663=CARTESIAN_POINT('Ctrl Pts',(-34.5395048560461,47.7519930846018,
40.1387166518767));
#177664=CARTESIAN_POINT('Ctrl Pts',(-34.5508838398161,47.7385544962823,
40.1454701832469));
#177665=CARTESIAN_POINT('Ctrl Pts',(-34.5634022165999,47.7253976640915,
40.1507785912492));
#177666=CARTESIAN_POINT('Ctrl Pts',(-34.576941119645,47.7127937034785,40.1543986087265));
#177667=CARTESIAN_POINT('Ctrl Pts',(-34.5837105711675,47.706491723172,40.1562086174652));
#177668=CARTESIAN_POINT('Ctrl Pts',(-34.5907351548561,47.7003279615827,
40.1575965292115));
#177669=CARTESIAN_POINT('Ctrl Pts',(-34.5980000149356,47.6943363116301,
40.1585319382567));
#177670=CARTESIAN_POINT('Ctrl Pts',(-34.6016324449754,47.6913404866538,
40.1589996427793));
#177671=CARTESIAN_POINT('Ctrl Pts',(-34.6053249441282,47.688387689607,40.159354221642));
#177672=CARTESIAN_POINT('Ctrl Pts',(-34.6090756555948,47.6854821573393,
40.159591874311));
#177673=CARTESIAN_POINT('Ctrl Pts',(-34.6128263670615,47.6825766250715,
40.1598295269801));
#177674=CARTESIAN_POINT('Ctrl Pts',(-34.6166352918406,47.6797183589579,
40.1599502506895));
#177675=CARTESIAN_POINT('Ctrl Pts',(-34.620500570363,47.6769115920307,40.1599502534424));
#177676=CARTESIAN_POINT('',(-34.6451144164181,47.6590285860939,40.1599502534424));
#177677=CARTESIAN_POINT('Origin',(3.62443809638016E-16,5.51217168157321E-17,
40.1599502534424));
#177678=CARTESIAN_POINT('',(-34.9997217530256,47.6338034047603,39.8576902534424));
#177679=CARTESIAN_POINT('Ctrl Pts',(-34.6451144164181,47.6590285860939,
40.1599502534424));
#177680=CARTESIAN_POINT('Ctrl Pts',(-34.6481960403147,47.6567884460684,
40.1599502448875));
#177681=CARTESIAN_POINT('Ctrl Pts',(-34.6512968858166,47.6545924528206,
40.1598743450437));
#177682=CARTESIAN_POINT('Ctrl Pts',(-34.654414748763,47.6524408584474,40.1597243308499));
#177683=CARTESIAN_POINT('Ctrl Pts',(-34.672822375821,47.6397380079748,40.1588386583936));
#177684=CARTESIAN_POINT('Ctrl Pts',(-34.6918243519518,47.6285798336065,
40.15537225536));
#177685=CARTESIAN_POINT('Ctrl Pts',(-34.7109619288217,47.6190225715713,
40.1496902177744));
#177686=CARTESIAN_POINT('Ctrl Pts',(-34.718111090472,47.6154522966254,40.147567597681));
#177687=CARTESIAN_POINT('Ctrl Pts',(-34.7252793254705,47.6121050440139,
40.1451361443077));
#177688=CARTESIAN_POINT('Ctrl Pts',(-34.7324433913422,47.6089824432868,
40.1424159447501));
#177689=CARTESIAN_POINT('Ctrl Pts',(-34.7380331549248,47.6065460335525,
40.1402935085949));
#177690=CARTESIAN_POINT('Ctrl Pts',(-34.7436201516873,47.6042468425535,
40.1379949176048));
#177691=CARTESIAN_POINT('Ctrl Pts',(-34.7491931041021,47.6020860928991,
40.1355293609261));
#177692=CARTESIAN_POINT('Ctrl Pts',(-34.7686984375536,47.594523469109,40.1268999125509));
#177693=CARTESIAN_POINT('Ctrl Pts',(-34.788031722428,47.5886567445953,40.1162251288835));
#177694=CARTESIAN_POINT('Ctrl Pts',(-34.806709489003,47.5845384124877,40.1038990521418));
#177695=CARTESIAN_POINT('Ctrl Pts',(-34.8160483722906,47.5824792464339,
40.097736013771));
#177696=CARTESIAN_POINT('Ctrl Pts',(-34.8252233770799,47.5808571799369,
40.0911601532641));
#177697=CARTESIAN_POINT('Ctrl Pts',(-34.8341740726976,47.5796787787542,
40.084220729064));
#177698=CARTESIAN_POINT('Ctrl Pts',(-34.8430865267159,47.5785054122579,
40.0773109533619));
#177699=CARTESIAN_POINT('Ctrl Pts',(-34.8517766417061,47.5777716830265,
40.0700409753048));
#177700=CARTESIAN_POINT('Ctrl Pts',(-34.8601845855135,47.5774848094466,
40.0624586415899));
#177701=CARTESIAN_POINT('Ctrl Pts',(-34.8602206623581,47.5774835785281,
40.0624261072769));
#177702=CARTESIAN_POINT('Ctrl Pts',(-34.8602567341385,47.5774823553082,
40.0623935677889));
#177703=CARTESIAN_POINT('Ctrl Pts',(-34.8602928008529,47.5774811397856,
40.0623610231288));
#177704=CARTESIAN_POINT('Ctrl Pts',(-34.8773011701497,47.5769079226578,
40.0470135870262));
#177705=CARTESIAN_POINT('Ctrl Pts',(-34.8931591840017,47.5780177840616,
40.0305755292153));
#177706=CARTESIAN_POINT('Ctrl Pts',(-34.9078085542006,47.5806251537532,
40.0133447567434));
#177707=CARTESIAN_POINT('Ctrl Pts',(-34.9229908396628,47.583327374424,39.9954871626726));
#177708=CARTESIAN_POINT('Ctrl Pts',(-34.9368756554658,47.5876385414267,
39.9767767954483));
#177709=CARTESIAN_POINT('Ctrl Pts',(-34.9493673872787,47.5933942811437,
39.9575197577683));
#177710=CARTESIAN_POINT('Ctrl Pts',(-34.9616808340502,47.5990678735405,
39.9385375612242));
#177711=CARTESIAN_POINT('Ctrl Pts',(-34.9726411562094,47.6061458909138,
39.9190226977378));
#177712=CARTESIAN_POINT('Ctrl Pts',(-34.9821189161751,47.6145008887939,
39.8992655452176));
#177713=CARTESIAN_POINT('Ctrl Pts',(-34.9887269790549,47.6203261419712,
39.8854905069541));
#177714=CARTESIAN_POINT('Ctrl Pts',(-34.9946135826731,47.6267727798487,
39.8715976051582));
#177715=CARTESIAN_POINT('Ctrl Pts',(-34.9997217530256,47.6338034047603,
39.8576902534424));
#177716=CARTESIAN_POINT('',(-35.2091516650524,47.922053073669,39.2875012672119));
#177717=CARTESIAN_POINT('',(-34.9997217530256,47.6338034047603,39.8576902534424));
#177718=CARTESIAN_POINT('',(-39.5544469813067,44.4033023070493,39.2875012672119));
#177719=CARTESIAN_POINT('Origin',(5.53234440788222E-15,0.,39.2875012672119));
#177720=CARTESIAN_POINT('',(-39.3160391863686,44.1385184650379,39.8576902534424));
#177721=CARTESIAN_POINT('',(-39.5544469813067,44.4033023070493,39.2875012672119));
#177722=CARTESIAN_POINT('',(-39.4144401478986,43.796904759635,40.1599502534424));
#177723=CARTESIAN_POINT('Ctrl Pts',(-39.3160391863686,44.1385184650379,
39.8576902534424));
#177724=CARTESIAN_POINT('Ctrl Pts',(-39.3078558527195,44.1294297383223,
39.8772619994063));
#177725=CARTESIAN_POINT('Ctrl Pts',(-39.3011376816091,44.1190955972862,
39.8967644650388));
#177726=CARTESIAN_POINT('Ctrl Pts',(-39.2959399200096,44.1076895347483,
39.9159282836075));
#177727=CARTESIAN_POINT('Ctrl Pts',(-39.2906482678542,44.0960774370678,
39.9354382707228));
#177728=CARTESIAN_POINT('Ctrl Pts',(-39.2869318048875,44.0833536765891,
39.9545987622409));
#177729=CARTESIAN_POINT('Ctrl Pts',(-39.2848826826026,44.0696602318308,
39.9731387498297));
#177730=CARTESIAN_POINT('Ctrl Pts',(-39.2829203148423,44.0565465320198,
39.9908938024137));
#177731=CARTESIAN_POINT('Ctrl Pts',(-39.2824868619904,44.0425426835252,
40.0080810366277));
#177732=CARTESIAN_POINT('Ctrl Pts',(-39.2836998417246,44.0277475809106,
40.0244542742647));
#177733=CARTESIAN_POINT('Ctrl Pts',(-39.2846646059168,44.0159800428206,
40.0374770090554));
#177734=CARTESIAN_POINT('Ctrl Pts',(-39.2866715134054,44.0037113585717,
40.049984877007));
#177735=CARTESIAN_POINT('Ctrl Pts',(-39.2897990038549,43.9909836989807,
40.0618424270193));
#177736=CARTESIAN_POINT('Ctrl Pts',(-39.2898075408879,43.9909489566044,
40.0618747942791));
#177737=CARTESIAN_POINT('Ctrl Pts',(-39.2898160863661,43.9909142109581,
40.0619071564124));
#177738=CARTESIAN_POINT('Ctrl Pts',(-39.2898246402903,43.9908794620437,
40.0619395134162));
#177739=CARTESIAN_POINT('Ctrl Pts',(-39.2915274551881,43.9839620557564,
40.0683807661799));
#177740=CARTESIAN_POINT('Ctrl Pts',(-39.2935962119549,43.9768962096539,
40.0746073439084));
#177741=CARTESIAN_POINT('Ctrl Pts',(-39.2960179253196,43.9697202954284,
40.0805869293669));
#177742=CARTESIAN_POINT('Ctrl Pts',(-39.3008239832001,43.9554791967021,
40.092453830807));
#177743=CARTESIAN_POINT('Ctrl Pts',(-39.30702136766,43.9408038696758,40.1033475319609));
#177744=CARTESIAN_POINT('Ctrl Pts',(-39.314515779532,43.9259899312962,40.1130129263075));
#177745=CARTESIAN_POINT('Ctrl Pts',(-39.320136588436,43.9148794775116,40.1202619720674));
#177746=CARTESIAN_POINT('Ctrl Pts',(-39.3264869747216,43.9036910542321,
40.1268200947266));
#177747=CARTESIAN_POINT('Ctrl Pts',(-39.3335271634604,43.8925493833645,
40.1325796782703));
#177748=CARTESIAN_POINT('Ctrl Pts',(-39.3361672342375,43.8883712567891,
40.1347395220992));
#177749=CARTESIAN_POINT('Ctrl Pts',(-39.3389043086117,43.8841997049152,
40.1367870714852));
#177750=CARTESIAN_POINT('Ctrl Pts',(-39.3417362896176,43.8800413054828,
40.1387166518767));
#177751=CARTESIAN_POINT('Ctrl Pts',(-39.3516482231384,43.8654869074691,
40.1454701832469));
#177752=CARTESIAN_POINT('Ctrl Pts',(-39.3627227594941,43.8510936230939,
40.1507785912492));
#177753=CARTESIAN_POINT('Ctrl Pts',(-39.3748700223777,43.8371435075662,
40.1543986087265));
#177754=CARTESIAN_POINT('Ctrl Pts',(-39.3809436538195,43.8301684498024,
40.1562086174652));
#177755=CARTESIAN_POINT('Ctrl Pts',(-39.3872854675768,43.823304185006,40.1575965292115));
#177756=CARTESIAN_POINT('Ctrl Pts',(-39.3938842320307,43.8165859732788,
40.1585319382567));
#177757=CARTESIAN_POINT('Ctrl Pts',(-39.3971836142576,43.8132268674151,
40.1589996427793));
#177758=CARTESIAN_POINT('Ctrl Pts',(-39.400547234176,43.8099042748375,40.159354221642));
#177759=CARTESIAN_POINT('Ctrl Pts',(-39.4039736880299,43.8066226032737,
40.1595918743111));
#177760=CARTESIAN_POINT('Ctrl Pts',(-39.4074001418838,43.8033409317099,
40.1598295269801));
#177761=CARTESIAN_POINT('Ctrl Pts',(-39.4108894308099,43.8001001824233,
40.1599502506895));
#177762=CARTESIAN_POINT('Ctrl Pts',(-39.4144401478986,43.796904759635,40.1599502534424));
#177763=CARTESIAN_POINT('',(-39.4370498736004,43.7765468711726,40.1599502534424));
#177764=CARTESIAN_POINT('Origin',(3.56901409908096E-16,5.06335700088602E-17,
40.1599502534424));
#177765=CARTESIAN_POINT('',(-39.7870778846743,43.7143933160627,39.8576902534424));
#177766=CARTESIAN_POINT('Ctrl Pts',(-39.4370498736004,43.7765468711726,
40.1599502534424));
#177767=CARTESIAN_POINT('Ctrl Pts',(-39.4398804576445,43.7739968854583,
40.1599502448875));
#177768=CARTESIAN_POINT('Ctrl Pts',(-39.4427347725908,43.7714887954761,
40.1598743450437));
#177769=CARTESIAN_POINT('Ctrl Pts',(-39.4456106527043,43.7690230823395,
40.1597243308499));
#177770=CARTESIAN_POINT('Ctrl Pts',(-39.4625896314139,43.7544656984441,
40.1588386583937));
#177771=CARTESIAN_POINT('Ctrl Pts',(-39.4803211659092,43.7413824023601,
40.1553722553609));
#177772=CARTESIAN_POINT('Ctrl Pts',(-39.4983548992145,43.7298770745066,
40.1496902177767));
#177773=CARTESIAN_POINT('Ctrl Pts',(-39.505091701658,43.7255790670178,40.1475675976828));
#177774=CARTESIAN_POINT('Ctrl Pts',(-39.511870785146,43.721500866416,40.1451361443087));
#177775=CARTESIAN_POINT('Ctrl Pts',(-39.5186692048623,43.7176465228247,
40.1424159447502));
#177776=CARTESIAN_POINT('Ctrl Pts',(-39.5239736729698,43.7146391706005,
40.1402935085949));
#177777=CARTESIAN_POINT('Ctrl Pts',(-39.5292897326775,43.7117685746245,
40.1379949176048));
#177778=CARTESIAN_POINT('Ctrl Pts',(-39.534606296035,43.7090371296311,40.1355293609261));
#177779=CARTESIAN_POINT('Ctrl Pts',(-39.5532142677859,43.6994770721542,
40.1268999125509));
#177780=CARTESIAN_POINT('Ctrl Pts',(-39.5718284032051,43.6916216076133,
40.1162251288835));
#177781=CARTESIAN_POINT('Ctrl Pts',(-39.5899733680941,43.6855734779225,
40.1038990521418));
#177782=CARTESIAN_POINT('Ctrl Pts',(-39.5990458505387,43.6825494130771,
40.097736013771));
#177783=CARTESIAN_POINT('Ctrl Pts',(-39.6080010415735,43.679977183279,40.0911601532641));
#177784=CARTESIAN_POINT('Ctrl Pts',(-39.6167795278793,43.6778696350432,
40.084220729064));
#177785=CARTESIAN_POINT('Ctrl Pts',(-39.6255205083453,43.6757710912489,
40.0773109533619));
#177786=CARTESIAN_POINT('Ctrl Pts',(-39.6340863223874,43.6741330170974,
40.0700409753048));
#177787=CARTESIAN_POINT('Ctrl Pts',(-39.6424182201444,43.6729688455956,
40.0624586415899));
#177788=CARTESIAN_POINT('Ctrl Pts',(-39.6424539706902,43.6729638503631,
40.0624261072769));
#177789=CARTESIAN_POINT('Ctrl Pts',(-39.6424897170043,43.6729588633163,
40.0623935677889));
#177790=CARTESIAN_POINT('Ctrl Pts',(-39.6425254590848,43.6729538844542,
40.0623610231289));
#177791=CARTESIAN_POINT('Ctrl Pts',(-39.6593807372525,43.6706059487641,
40.0470135870233));
#177792=CARTESIAN_POINT('Ctrl Pts',(-39.6752678913551,43.6700521164128,
40.0305755292093));
#177793=CARTESIAN_POINT('Ctrl Pts',(-39.6901095551207,43.6711139265065,
40.0133447567339));
#177794=CARTESIAN_POINT('Ctrl Pts',(-39.7054911294111,43.6722143631623,
39.9954871626596));
#177795=CARTESIAN_POINT('Ctrl Pts',(-39.719750522404,43.6750505546838,39.9767767954314));
#177796=CARTESIAN_POINT('Ctrl Pts',(-39.7327754618321,43.6794690223284,
39.9575197577475));
#177797=CARTESIAN_POINT('Ctrl Pts',(-39.7456145061495,43.6838244285257,
39.9385375611999));
#177798=CARTESIAN_POINT('Ctrl Pts',(-39.7572546407969,43.6897180061494,
39.9190226977099));
#177799=CARTESIAN_POINT('Ctrl Pts',(-39.7675538156911,43.6970365387953,
39.8992655451861));
#177800=CARTESIAN_POINT('Ctrl Pts',(-39.7747345836673,43.7021391499652,
39.885490506933));
#177801=CARTESIAN_POINT('Ctrl Pts',(-39.7812627970001,43.707935154852,39.8715976051477));
#177802=CARTESIAN_POINT('Ctrl Pts',(-39.7870778846743,43.7143933160627,
39.8576902534424));
#177803=CARTESIAN_POINT('',(-40.0254908126585,43.9791725362586,39.2875012672119));
#177804=CARTESIAN_POINT('',(-39.7870778846743,43.7143933160627,39.8576902534424));
#177805=CARTESIAN_POINT('',(-43.9791725362579,40.0254908126592,39.2875012672119));
#177806=CARTESIAN_POINT('Origin',(5.53234440788222E-15,0.,39.2875012672119));
#177807=CARTESIAN_POINT('',(-43.714393316062,39.7870778846751,39.8576902534424));
#177808=CARTESIAN_POINT('',(-43.9791725362579,40.0254908126592,39.2875012672119));
#177809=CARTESIAN_POINT('',(-43.7765468711719,39.4370498736012,40.1599502534424));
#177810=CARTESIAN_POINT('Ctrl Pts',(-43.714393316062,39.7870778846751,39.8576902534424));
#177811=CARTESIAN_POINT('Ctrl Pts',(-43.7053047809354,39.7788943382471,
39.8772619994039));
#177812=CARTESIAN_POINT('Ctrl Pts',(-43.6975432007884,39.7693190488203,
39.896764465034));
#177813=CARTESIAN_POINT('Ctrl Pts',(-43.6911816548822,39.7585187839205,
39.9159282836004));
#177814=CARTESIAN_POINT('Ctrl Pts',(-43.6847051962256,39.7475234267957,
39.9354382707133));
#177815=CARTESIAN_POINT('Ctrl Pts',(-43.6796790973022,39.7352578445729,
39.9545987622292));
#177816=CARTESIAN_POINT('Ctrl Pts',(-43.6762098455857,39.7218536055436,
39.9731387498159));
#177817=CARTESIAN_POINT('Ctrl Pts',(-43.6728874729921,39.7090168672409,
39.9908938023977));
#177818=CARTESIAN_POINT('Ctrl Pts',(-43.6709925938766,39.6951350414567,
40.0080810366098));
#177819=CARTESIAN_POINT('Ctrl Pts',(-43.6706524194394,39.6802941970576,
40.0244542742451));
#177820=CARTESIAN_POINT('Ctrl Pts',(-43.6703818558784,39.6684902774488,
40.0374770090428));
#177821=CARTESIAN_POINT('Ctrl Pts',(-43.6710953426067,39.6560790233743,
40.0499848770011));
#177822=CARTESIAN_POINT('Ctrl Pts',(-43.6728752976391,39.6430941754572,
40.0618424270193));
#177823=CARTESIAN_POINT('Ctrl Pts',(-43.6728801563381,39.6430587310403,
40.0618747942791));
#177824=CARTESIAN_POINT('Ctrl Pts',(-43.6728850230943,39.6430232824886,
40.0619071564124));
#177825=CARTESIAN_POINT('Ctrl Pts',(-43.6728898979086,39.6429878298038,
40.0619395134161));
#177826=CARTESIAN_POINT('Ctrl Pts',(-43.6738603187593,39.6359303251675,
40.0683807661799));
#177827=CARTESIAN_POINT('Ctrl Pts',(-43.6751791606252,39.6286869425435,
40.0746073439084));
#177828=CARTESIAN_POINT('Ctrl Pts',(-43.6768375203041,39.6212972007505,
40.0805869293669));
#177829=CARTESIAN_POINT('Ctrl Pts',(-43.6801286499317,39.6066317464085,
40.092453830807));
#177830=CARTESIAN_POINT('Ctrl Pts',(-43.684758095089,39.5913890092852,40.1033475319609));
#177831=CARTESIAN_POINT('Ctrl Pts',(-43.6906629735749,39.575872843854,40.1130129263075));
#177832=CARTESIAN_POINT('Ctrl Pts',(-43.6950916324393,39.5642357197806,
40.1202619720674));
#177833=CARTESIAN_POINT('Ctrl Pts',(-43.7002377219525,39.5524447917349,
40.1268200947266));
#177834=CARTESIAN_POINT('Ctrl Pts',(-43.7060747220668,39.5406282559961,
40.1325796782703));
#177835=CARTESIAN_POINT('Ctrl Pts',(-43.7082635971097,39.5361970550941,
40.1347395220992));
#177836=CARTESIAN_POINT('Ctrl Pts',(-43.7105496315973,39.5317622532396,
40.1367870714852));
#177837=CARTESIAN_POINT('Ctrl Pts',(-43.7129314276126,39.5273306113318,
40.1387166518767));
#177838=CARTESIAN_POINT('Ctrl Pts',(-43.7212677136663,39.5118198646544,
40.1454701832469));
#177839=CARTESIAN_POINT('Ctrl Pts',(-43.7307770746559,39.4963478239303,
40.1507785912492));
#177840=CARTESIAN_POINT('Ctrl Pts',(-43.741399609424,39.481204393873,40.1543986087265));
#177841=CARTESIAN_POINT('Ctrl Pts',(-43.746710876808,39.4736326788443,40.1562086174652));
#177842=CARTESIAN_POINT('Ctrl Pts',(-43.7523004383954,39.4661431171624,
40.1575965292115));
#177843=CARTESIAN_POINT('Ctrl Pts',(-43.7581608097794,39.4587719497941,
40.1585319382567));
#177844=CARTESIAN_POINT('Ctrl Pts',(-43.7610909954714,39.4550863661099,
40.1589996427793));
#177845=CARTESIAN_POINT('Ctrl Pts',(-43.7640888836317,39.451430381021,40.159354221642));
#177846=CARTESIAN_POINT('Ctrl Pts',(-43.7671535389273,39.4478085248416,
40.159591874311));
#177847=CARTESIAN_POINT('Ctrl Pts',(-43.7702181942229,39.4441866686622,
40.1598295269801));
#177848=CARTESIAN_POINT('Ctrl Pts',(-43.7733496179165,39.4405989425299,
40.1599502506895));
#177849=CARTESIAN_POINT('Ctrl Pts',(-43.7765468711719,39.4370498736012,
40.1599502534424));
#177850=CARTESIAN_POINT('',(-43.7969047596343,39.4144401478993,40.1599502534424));
#177851=CARTESIAN_POINT('Origin',(3.51858511112452E-16,4.55906712132165E-17,
40.1599502534424));
#177852=CARTESIAN_POINT('',(-44.1385184650372,39.3160391863694,39.8576902534424));
#177853=CARTESIAN_POINT('Ctrl Pts',(-43.7969047596343,39.4144401478993,
40.1599502534424));
#177854=CARTESIAN_POINT('Ctrl Pts',(-43.7994532913547,39.4116082546733,
40.1599502448875));
#177855=CARTESIAN_POINT('Ctrl Pts',(-43.8020298032735,39.4088155471155,
40.1598743450437));
#177856=CARTESIAN_POINT('Ctrl Pts',(-43.8046321918099,39.4060627300846,
40.1597243308499));
#177857=CARTESIAN_POINT('Ctrl Pts',(-43.8199964969272,39.3898103065117,
40.1588386583939));
#177858=CARTESIAN_POINT('Ctrl Pts',(-43.8362633193843,39.3749452320426,
40.1553722553621));
#177859=CARTESIAN_POINT('Ctrl Pts',(-43.8529956277688,39.3616178931512,
40.1496902177795));
#177860=CARTESIAN_POINT('Ctrl Pts',(-43.8592462611885,39.356639242988,40.1475675976849));
#177861=CARTESIAN_POINT('Ctrl Pts',(-43.8655619201088,39.3518747760142,
40.1451361443099));
#177862=CARTESIAN_POINT('Ctrl Pts',(-43.8719202087609,39.3473309185528,
40.1424159447501));
#177863=CARTESIAN_POINT('Ctrl Pts',(-43.8768812645305,39.343785573019,40.1402935085949));
#177864=CARTESIAN_POINT('Ctrl Pts',(-43.881868143321,39.3403750229162,40.1379949176048));
#177865=CARTESIAN_POINT('Ctrl Pts',(-43.8868700682404,39.3371028088667,
40.1355293609261));
#177866=CARTESIAN_POINT('Ctrl Pts',(-43.9043768054583,39.3256500596932,
40.1268999125509));
#177867=CARTESIAN_POINT('Ctrl Pts',(-43.9220678510593,39.3158919212387,
40.1162251288835));
#177868=CARTESIAN_POINT('Ctrl Pts',(-43.9394812142299,39.3079802585393,
40.1038990521418));
#177869=CARTESIAN_POINT('Ctrl Pts',(-43.9481878958152,39.3040244271896,
40.097736013771));
#177870=CARTESIAN_POINT('Ctrl Pts',(-43.9568251581486,39.3005302159783,
40.0911601532641));
#177871=CARTESIAN_POINT('Ctrl Pts',(-43.9653352562096,39.2975166114288,
40.084220729064));
#177872=CARTESIAN_POINT('Ctrl Pts',(-43.973808995112,39.2945158824214,40.0773109533619));
#177873=CARTESIAN_POINT('Ctrl Pts',(-43.9821566593547,39.2919914104332,
40.0700409753048));
#177874=CARTESIAN_POINT('Ctrl Pts',(-43.990321225046,39.289962695916,40.0624586415899));
#177875=CARTESIAN_POINT('Ctrl Pts',(-43.9903562576026,39.2899539910983,
40.0624261072769));
#177876=CARTESIAN_POINT('Ctrl Pts',(-43.9903912868063,39.2899452948638,
40.0623935677888));
#177877=CARTESIAN_POINT('Ctrl Pts',(-43.9904263126551,39.2899366072116,
40.0623610231288));
#177878=CARTESIAN_POINT('Ctrl Pts',(-44.0069438297354,39.2858396774342,
40.0470135870238));
#177879=CARTESIAN_POINT('Ctrl Pts',(-44.0226860611005,39.2836282192304,
40.0305755292104));
#177880=CARTESIAN_POINT('Ctrl Pts',(-44.037557410056,39.2831328363114,40.0133447567356));
#177881=CARTESIAN_POINT('Ctrl Pts',(-44.052969749425,39.2826194323366,39.9954871626623));
#177882=CARTESIAN_POINT('Ctrl Pts',(-44.0674474907118,39.2839495744672,
39.9767767954353));
#177883=CARTESIAN_POINT('Ctrl Pts',(-44.0808629337912,39.2869823603807,
39.9575197577525));
#177884=CARTESIAN_POINT('Ctrl Pts',(-44.0940869083964,39.2899718616342,
39.9385375612064));
#177885=CARTESIAN_POINT('Ctrl Pts',(-44.1062793237798,39.2946164282353,
39.919022697718));
#177886=CARTESIAN_POINT('Ctrl Pts',(-44.1172870736866,39.3008183122681,
39.8992655451958));
#177887=CARTESIAN_POINT('Ctrl Pts',(-44.1249618727708,39.3051423761592,
39.8854905069395));
#177888=CARTESIAN_POINT('Ctrl Pts',(-44.1320601713535,39.3102242458184,
39.8715976051509));
#177889=CARTESIAN_POINT('Ctrl Pts',(-44.1385184650372,39.3160391863694,
39.8576902534424));
#177890=CARTESIAN_POINT('',(-44.4033023070486,39.5544469813075,39.2875012672119));
#177891=CARTESIAN_POINT('',(-44.1385184650372,39.3160391863694,39.8576902534424));
#177892=CARTESIAN_POINT('',(-47.9220530736684,35.2091516650532,39.2875012672119));
#177893=CARTESIAN_POINT('Origin',(5.53234440788222E-15,0.,39.2875012672119));
#177894=CARTESIAN_POINT('',(-47.6338034047597,34.9997217530264,39.8576902534424));
#177895=CARTESIAN_POINT('',(-47.9220530736684,35.2091516650532,39.2875012672119));
#177896=CARTESIAN_POINT('',(-47.6590285860933,34.645114416419,40.1599502534424));
#177897=CARTESIAN_POINT('Ctrl Pts',(-47.6338034047597,34.9997217530264,
39.8576902534424));
#177898=CARTESIAN_POINT('Ctrl Pts',(-47.6239092440465,34.9925330475316,
39.8772619994054));
#177899=CARTESIAN_POINT('Ctrl Pts',(-47.615189292358,34.9838215185866,39.8967644650371));
#177900=CARTESIAN_POINT('Ctrl Pts',(-47.6077336605726,34.9737453812845,
39.9159282836049));
#177901=CARTESIAN_POINT('Ctrl Pts',(-47.6001433528505,34.9634872321464,
39.9354382707192));
#177902=CARTESIAN_POINT('Ctrl Pts',(-47.5938626849619,34.9518142124619,
39.9545987622365));
#177903=CARTESIAN_POINT('Ctrl Pts',(-47.5890113136624,34.9388460388056,
39.9731387498244));
#177904=CARTESIAN_POINT('Ctrl Pts',(-47.5843653368453,34.9264269039989,
39.9908938024073));
#177905=CARTESIAN_POINT('Ctrl Pts',(-47.5810297921596,34.9128191931094,
40.0080810366204));
#177906=CARTESIAN_POINT('Ctrl Pts',(-47.5791401905755,34.8980952063184,
40.0244542742565));
#177907=CARTESIAN_POINT('Ctrl Pts',(-47.5776372636137,34.8863842314125,
40.0374770090501));
#177908=CARTESIAN_POINT('Ctrl Pts',(-47.5770495124718,34.8739663878185,
40.0499848770046));
#177909=CARTESIAN_POINT('Ctrl Pts',(-47.5774624305257,34.8608666162966,
40.0618424270193));
#177910=CARTESIAN_POINT('Ctrl Pts',(-47.5774635576578,34.8608308581755,
40.0618747942791));
#177911=CARTESIAN_POINT('Ctrl Pts',(-47.5774646923707,34.8607950951002,
40.0619071564124));
#177912=CARTESIAN_POINT('Ctrl Pts',(-47.5774658346656,34.860759327072,40.0619395134161));
#177913=CARTESIAN_POINT('Ctrl Pts',(-47.5776932293352,34.8536390475843,
40.0683807661799));
#177914=CARTESIAN_POINT('Ctrl Pts',(-47.5782477067929,34.8462974884547,
40.0746073439084));
#177915=CARTESIAN_POINT('Ctrl Pts',(-47.5791245434504,34.8387748826516,
40.0805869293669));
#177916=CARTESIAN_POINT('Ctrl Pts',(-47.58086468652,34.8238457504806,40.092453830807));
#177917=CARTESIAN_POINT('Ctrl Pts',(-47.5838754712049,34.8082026058781,
40.1033475319609));
#177918=CARTESIAN_POINT('Ctrl Pts',(-47.5881261212203,34.7921542117507,
40.1130129263075));
#177919=CARTESIAN_POINT('Ctrl Pts',(-47.5913141087318,34.7801179161552,
40.1202619720674));
#177920=CARTESIAN_POINT('Ctrl Pts',(-47.5951995198391,34.7678536672184,
40.1268200947266));
#177921=CARTESIAN_POINT('Ctrl Pts',(-47.5997693799341,34.7554917310467,
40.1325796782703));
#177922=CARTESIAN_POINT('Ctrl Pts',(-47.6014830774698,34.7508560049823,
40.1347395220992));
#177923=CARTESIAN_POINT('Ctrl Pts',(-47.6032930257985,34.7462065417645,
40.1367870714852));
#177924=CARTESIAN_POINT('Ctrl Pts',(-47.6051985413677,34.7415502113774,
40.1387166518767));
#177925=CARTESIAN_POINT('Ctrl Pts',(-47.6118678458598,34.7252530550227,
40.1454701832469));
#177926=CARTESIAN_POINT('Ctrl Pts',(-47.6197078449344,34.7088717728656,
40.1507785912492));
#177927=CARTESIAN_POINT('Ctrl Pts',(-47.6286892688731,34.6927009428673,
40.1543986087265));
#177928=CARTESIAN_POINT('Ctrl Pts',(-47.6331799808424,34.6846155278682,
40.1562086174652));
#177929=CARTESIAN_POINT('Ctrl Pts',(-47.6379560498533,34.6765827265057,
40.1575965292115));
#177930=CARTESIAN_POINT('Ctrl Pts',(-47.6430138207122,34.6686393635485,
40.1585319382567));
#177931=CARTESIAN_POINT('Ctrl Pts',(-47.6455427061417,34.66466768207,40.1589996427793));
#177932=CARTESIAN_POINT('Ctrl Pts',(-47.6481420170539,34.6607183602074,
40.159354221642));
#177933=CARTESIAN_POINT('Ctrl Pts',(-47.6508112967866,34.6567960012267,
40.159591874311));
#177934=CARTESIAN_POINT('Ctrl Pts',(-47.6534805765192,34.6528736422459,
40.1598295269801));
#177935=CARTESIAN_POINT('Ctrl Pts',(-47.6562198264469,34.6489782471462,
40.1599502506895));
#177936=CARTESIAN_POINT('Ctrl Pts',(-47.6590285860933,34.645114416419,40.1599502534424));
#177937=CARTESIAN_POINT('',(-47.6769115920301,34.6205005703638,40.1599502534424));
#177938=CARTESIAN_POINT('Origin',(3.4737036430558E-16,4.0048271483298E-17,
40.1599502534424));
#177939=CARTESIAN_POINT('',(-48.0063682005184,34.4869303039401,39.8576902534424));
#177940=CARTESIAN_POINT('Ctrl Pts',(-47.6769115920301,34.6205005703638,
40.1599502534424));
#177941=CARTESIAN_POINT('Ctrl Pts',(-47.67915014918,34.6174177964409,40.1599502448875));
#177942=CARTESIAN_POINT('Ctrl Pts',(-47.6814206292676,34.6143710687958,
40.1598743450437));
#177943=CARTESIAN_POINT('Ctrl Pts',(-47.6837210139133,34.6113613083102,
40.1597243308499));
#177944=CARTESIAN_POINT('Ctrl Pts',(-47.6973023108995,34.5935919100107,
40.1588386583939));
#177945=CARTESIAN_POINT('Ctrl Pts',(-47.7119261986107,34.5771079220209,
40.1553722553619));
#177946=CARTESIAN_POINT('Ctrl Pts',(-47.7271737594057,34.5621045892039,
40.1496902177792));
#177947=CARTESIAN_POINT('Ctrl Pts',(-47.7328697405506,34.5564998435016,
40.1475675976847));
#177948=CARTESIAN_POINT('Ctrl Pts',(-47.7386527792192,34.5511013106553,
40.1451361443098));
#177949=CARTESIAN_POINT('Ctrl Pts',(-47.7445012740627,34.5459177227789,
40.1424159447501));
#177950=CARTESIAN_POINT('Ctrl Pts',(-47.7490645631294,34.5418732274831,
40.1402935085949));
#177951=CARTESIAN_POINT('Ctrl Pts',(-47.7536676237148,34.5379600899542,
40.1379949176048));
#177952=CARTESIAN_POINT('Ctrl Pts',(-47.7583001080601,34.5341829579103,
40.1355293609261));
#177953=CARTESIAN_POINT('Ctrl Pts',(-47.7745138032685,34.520962995757,40.1268999125509));
#177954=CARTESIAN_POINT('Ctrl Pts',(-47.7910879322536,34.5094090955956,
40.1162251288835));
#177955=CARTESIAN_POINT('Ctrl Pts',(-47.8075789092549,34.4997205817197,
40.1038990521418));
#177956=CARTESIAN_POINT('Ctrl Pts',(-47.8158243977556,34.4948763247818,
40.0977360137709));
#177957=CARTESIAN_POINT('Ctrl Pts',(-47.8240490997339,34.4904984154666,
40.0911601532641));
#177958=CARTESIAN_POINT('Ctrl Pts',(-47.8321975711348,34.4866117722856,
40.084220729064));
#177959=CARTESIAN_POINT('Ctrl Pts',(-47.8403112284171,34.4827417346801,
40.0773109533618));
#177960=CARTESIAN_POINT('Ctrl Pts',(-47.8483492841042,34.4793585234984,
40.0700409753048));
#177961=CARTESIAN_POINT('Ctrl Pts',(-47.8562570650395,34.4764874929866,
40.0624586415899));
#177962=CARTESIAN_POINT('Ctrl Pts',(-47.8562909957829,34.4764751739554,
40.0624261072769));
#177963=CARTESIAN_POINT('Ctrl Pts',(-47.8563249240888,34.4764628638111,
40.0623935677888));
#177964=CARTESIAN_POINT('Ctrl Pts',(-47.8563588499555,34.4764505625526,
40.0623610231288));
#177965=CARTESIAN_POINT('Ctrl Pts',(-47.8723576365755,34.4706495255077,
40.0470135870235));
#177966=CARTESIAN_POINT('Ctrl Pts',(-47.8877824700227,34.4668046706503,
40.0305755292097));
#177967=CARTESIAN_POINT('Ctrl Pts',(-47.9025205705575,34.464757522238,40.0133447567346));
#177968=CARTESIAN_POINT('Ctrl Pts',(-47.9177948141909,34.4626359025944,
39.9954871626604));
#177969=CARTESIAN_POINT('Ctrl Pts',(-47.9323322826094,34.4624454220193,
39.9767767954324));
#177970=CARTESIAN_POINT('Ctrl Pts',(-47.9459912469394,34.4640592983654,
39.9575197577486));
#177971=CARTESIAN_POINT('Ctrl Pts',(-47.959455267201,34.465650141075,39.9385375612008));
#177972=CARTESIAN_POINT('Ctrl Pts',(-47.9720663806674,34.4689948098114,
39.9190226977106));
#177973=CARTESIAN_POINT('Ctrl Pts',(-47.9836621023766,34.4740120960936,
39.8992655451867));
#177974=CARTESIAN_POINT('Ctrl Pts',(-47.9917468458601,34.4775102373556,
39.8854905069333));
#177975=CARTESIAN_POINT('Ctrl Pts',(-47.9993374592447,34.4818222937574,
39.8715976051478));
#177976=CARTESIAN_POINT('Ctrl Pts',(-48.0063682005184,34.4869303039401,
39.8576902534424));
#177977=CARTESIAN_POINT('',(-48.2946219293743,34.6963546279289,39.2875012672119));
#177978=CARTESIAN_POINT('',(-48.0063682005184,34.4869303039401,39.8576902534424));
#177979=CARTESIAN_POINT('',(-51.3398895692695,30.0070536838162,39.2875012672119));
#177980=CARTESIAN_POINT('Origin',(5.53234440788222E-15,0.,39.2875012672119));
#177981=CARTESIAN_POINT('',(-51.0313275753406,29.828901345689,39.8576902534424));
#177982=CARTESIAN_POINT('',(-51.3398895692695,30.0070536838162,39.2875012672119));
#177983=CARTESIAN_POINT('',(-51.0193480105325,29.4735998357342,40.1599502534424));
#177984=CARTESIAN_POINT('Ctrl Pts',(-51.0313275753406,29.828901345689,39.8576902534424));
#177985=CARTESIAN_POINT('Ctrl Pts',(-51.020736191538,29.8227862420905,39.8772619994031));
#177986=CARTESIAN_POINT('Ctrl Pts',(-51.0111534059249,29.8150339189635,
39.8967644650325));
#177987=CARTESIAN_POINT('Ctrl Pts',(-51.0026853737234,29.8057923055305,
39.9159282835982));
#177988=CARTESIAN_POINT('Ctrl Pts',(-50.9940643779364,29.79638375481,39.9354382707104));
#177989=CARTESIAN_POINT('Ctrl Pts',(-50.9865979533948,29.7854311897131,
39.9545987622257));
#177990=CARTESIAN_POINT('Ctrl Pts',(-50.9804176151513,29.7730411634577,
39.9731387498119));
#177991=CARTESIAN_POINT('Ctrl Pts',(-50.974498936405,29.7611756987897,39.9908938023933));
#177992=CARTESIAN_POINT('Ctrl Pts',(-50.969759271074,29.7479911917264,40.0080810366051));
#177993=CARTESIAN_POINT('Ctrl Pts',(-50.966340945212,29.7335453816275,40.0244542742402));
#177994=CARTESIAN_POINT('Ctrl Pts',(-50.9636221212293,29.7220556593091,
40.0374770090397));
#177995=CARTESIAN_POINT('Ctrl Pts',(-50.9617395717405,29.7097672786805,
40.0499848769996));
#177996=CARTESIAN_POINT('Ctrl Pts',(-50.9607809287993,29.6966961073824,
40.0618424270193));
#177997=CARTESIAN_POINT('Ctrl Pts',(-50.9607783120155,29.6966604273307,
40.0618747942791));
#177998=CARTESIAN_POINT('Ctrl Pts',(-50.960775702253,29.6966247415594,40.0619071564124));
#177999=CARTESIAN_POINT('Ctrl Pts',(-50.9607730995133,29.69658905007,40.0619395134161));
#178000=CARTESIAN_POINT('Ctrl Pts',(-50.9602549766182,29.6894840070029,
40.0683807661799));
#178001=CARTESIAN_POINT('Ctrl Pts',(-50.9600390146965,29.6821247070258,
40.0746073439084));
#178002=CARTESIAN_POINT('Ctrl Pts',(-50.9601247215268,29.6745516564561,
40.0805869293669));
#178003=CARTESIAN_POINT('Ctrl Pts',(-50.9602948126668,29.6595224131522,
40.092453830807));
#178004=CARTESIAN_POINT('Ctrl Pts',(-50.9616539500922,29.6436502506363,
40.1033475319609));
#178005=CARTESIAN_POINT('Ctrl Pts',(-50.964203800626,29.6272454573771,40.1130129263075));
#178006=CARTESIAN_POINT('Ctrl Pts',(-50.9661161885263,29.6149418624327,
40.1202619720674));
#178007=CARTESIAN_POINT('Ctrl Pts',(-50.9686983518505,29.6023386622826,
40.1268200947266));
#178008=CARTESIAN_POINT('Ctrl Pts',(-50.9719510035827,29.5895667656377,
40.1325796782703));
#178009=CARTESIAN_POINT('Ctrl Pts',(-50.9731707479823,29.5847773043958,
40.1347395220992));
#178010=CARTESIAN_POINT('Ctrl Pts',(-50.9744847799795,29.5799641203066,
40.1367870714852));
#178011=CARTESIAN_POINT('Ctrl Pts',(-50.9758931378752,29.5751341171704,
40.1387166518767));
#178012=CARTESIAN_POINT('Ctrl Pts',(-50.9808223905102,29.5582291061937,
40.1454701832469));
#178013=CARTESIAN_POINT('Ctrl Pts',(-50.9869071309993,29.541118059359,40.1507785912492));
#178014=CARTESIAN_POINT('Ctrl Pts',(-50.9941490417484,29.5240970004172,
40.1543986087265));
#178015=CARTESIAN_POINT('Ctrl Pts',(-50.9977699971229,29.5155864709463,
40.1562086174652));
#178016=CARTESIAN_POINT('Ctrl Pts',(-51.001680245946,29.507098438956,40.1575965292115));
#178017=CARTESIAN_POINT('Ctrl Pts',(-51.0058800022838,29.4986699095568,
40.1585319382567));
#178018=CARTESIAN_POINT('Ctrl Pts',(-51.0079798804527,29.4944556448572,
40.1589996427793));
#178019=CARTESIAN_POINT('Ctrl Pts',(-51.0101521355226,29.4902562558179,
40.159354221642));
#178020=CARTESIAN_POINT('Ctrl Pts',(-51.0123967945049,29.4860763682215,
40.159591874311));
#178021=CARTESIAN_POINT('Ctrl Pts',(-51.0146414534873,29.4818964806251,
40.1598295269801));
#178022=CARTESIAN_POINT('Ctrl Pts',(-51.0169585178536,29.477736095322,40.1599502506896));
#178023=CARTESIAN_POINT('Ctrl Pts',(-51.0193480105325,29.4735998357342,
40.1599502534424));
#178024=CARTESIAN_POINT('',(-51.0345602039884,29.447251543774,40.1599502534424));
#178025=CARTESIAN_POINT('Origin',(3.43486142563102E-16,3.40670945103694E-17,
40.1599502534424));
#178026=CARTESIAN_POINT('',(-51.3482501200163,29.2799753962467,39.8576902534424));
#178027=CARTESIAN_POINT('Ctrl Pts',(-51.0345602039884,29.447251543774,40.1599502534424));
#178028=CARTESIAN_POINT('Ctrl Pts',(-51.0364642604673,29.4439516646703,
40.1599502448875));
#178029=CARTESIAN_POINT('Ctrl Pts',(-51.0384038328686,29.4406842975236,
40.1598743450437));
#178030=CARTESIAN_POINT('Ctrl Pts',(-51.0403770101282,29.4374505691489,
40.1597243308499));
#178031=CARTESIAN_POINT('Ctrl Pts',(-51.0520264994498,29.4183588813712,
40.158838658394));
#178032=CARTESIAN_POINT('Ctrl Pts',(-51.0648472300397,29.4004365818846,
40.1553722553626));
#178033=CARTESIAN_POINT('Ctrl Pts',(-51.0784429877766,29.3839216347975,
40.1496902177808));
#178034=CARTESIAN_POINT('Ctrl Pts',(-51.0835219102867,29.377752200321,40.1475675976859));
#178035=CARTESIAN_POINT('Ctrl Pts',(-51.0887089685234,29.3717787490558,
40.1451361443104));
#178036=CARTESIAN_POINT('Ctrl Pts',(-51.0939835922267,29.3660122232363,
40.14241594475));
#178037=CARTESIAN_POINT('Ctrl Pts',(-51.0980991182404,29.3615128905153,
40.1402935085948));
#178038=CARTESIAN_POINT('Ctrl Pts',(-51.1022679285259,29.3571400387138,
40.1379949176048));
#178039=CARTESIAN_POINT('Ctrl Pts',(-51.1064802178291,29.3528993717248,
40.1355293609261));
#178040=CARTESIAN_POINT('Ctrl Pts',(-51.1212232303903,29.3380570372633,
40.1268999125509));
#178041=CARTESIAN_POINT('Ctrl Pts',(-51.1364988531341,29.3248339623431,
40.1162251288835));
#178042=CARTESIAN_POINT('Ctrl Pts',(-51.1518867653711,29.3134747466763,
40.1038990521418));
#178043=CARTESIAN_POINT('Ctrl Pts',(-51.1595807214896,29.3077951388428,
40.0977360137709));
#178044=CARTESIAN_POINT('Ctrl Pts',(-51.1673027515569,29.3025814967143,
40.0911601532641));
#178045=CARTESIAN_POINT('Ctrl Pts',(-51.1750003199399,29.2978643977778,
40.084220729064));
#178046=CARTESIAN_POINT('Ctrl Pts',(-51.182665000675,29.293167452516,40.0773109533618));
#178047=CARTESIAN_POINT('Ctrl Pts',(-51.1903053811862,29.2889625693105,
40.0700409753047));
#178048=CARTESIAN_POINT('Ctrl Pts',(-51.1978697380627,29.2852806784153,
40.0624586415899));
#178049=CARTESIAN_POINT('Ctrl Pts',(-51.1979021952406,29.2852648801406,
40.0624261072769));
#178050=CARTESIAN_POINT('Ctrl Pts',(-51.1979346509233,29.2852490909588,
40.0623935677888));
#178051=CARTESIAN_POINT('Ctrl Pts',(-51.1979671051088,29.2852333108692,
40.0623610231288));
#178052=CARTESIAN_POINT('Ctrl Pts',(-51.2132718752125,29.2777917239334,
40.0470135870251));
#178053=CARTESIAN_POINT('Ctrl Pts',(-51.228210313037,29.2723555974571,40.030575529213));
#178054=CARTESIAN_POINT('Ctrl Pts',(-51.2426536914361,29.2687791125375,
40.0133447567398));
#178055=CARTESIAN_POINT('Ctrl Pts',(-51.2576224915221,29.2650725221337,
39.9954871626678));
#178056=CARTESIAN_POINT('Ctrl Pts',(-51.2720604115243,29.2633635057969,
39.9767767954423));
#178057=CARTESIAN_POINT('Ctrl Pts',(-51.2858132466317,29.2635407906075,
39.957519757761));
#178058=CARTESIAN_POINT('Ctrl Pts',(-51.2993697979237,29.263715545166,39.9385375612159));
#178059=CARTESIAN_POINT('Ctrl Pts',(-51.312261439473,29.265723671145,39.9190226977285));
#178060=CARTESIAN_POINT('Ctrl Pts',(-51.3243180878291,29.2695013892356,
39.8992655452074));
#178061=CARTESIAN_POINT('Ctrl Pts',(-51.3327241975769,29.2721352815021,
39.8854905069473));
#178062=CARTESIAN_POINT('Ctrl Pts',(-51.3407239614206,29.2756302808568,
39.8715976051548));
#178063=CARTESIAN_POINT('Ctrl Pts',(-51.3482501200163,29.2799753962467,
39.8576902534424));
#178064=CARTESIAN_POINT('',(-51.6568155675425,29.4581217525678,39.2875012672119));
#178065=CARTESIAN_POINT('',(-51.3482501200163,29.2799753962467,39.8576902534424));
#178066=CARTESIAN_POINT('',(-54.195235491187,24.4761921430396,39.2875012672119));
#178067=CARTESIAN_POINT('Origin',(5.53234440788222E-15,0.,39.2875012672119));
#178068=CARTESIAN_POINT('',(-53.8697418420143,24.3312692531092,39.8576902534424));
#178069=CARTESIAN_POINT('',(-54.195235491187,24.4761921430396,39.2875012672119));
#178070=CARTESIAN_POINT('',(-53.8206887816834,23.9791663275018,40.1599502534424));
#178071=CARTESIAN_POINT('Ctrl Pts',(-53.8697418420143,24.3312692531092,
39.8576902534424));
#178072=CARTESIAN_POINT('Ctrl Pts',(-53.8585692765373,24.3262947497602,
39.8772619994052));
#178073=CARTESIAN_POINT('Ctrl Pts',(-53.8482286480022,24.3195865685235,
39.8967644650367));
#178074=CARTESIAN_POINT('Ctrl Pts',(-53.838840992916,24.3112807320075,39.9159282836044));
#178075=CARTESIAN_POINT('Ctrl Pts',(-53.8292837624968,24.3028248617525,
39.9354382707186));
#178076=CARTESIAN_POINT('Ctrl Pts',(-53.8207133850111,24.2927127498351,
39.9545987622357));
#178077=CARTESIAN_POINT('Ctrl Pts',(-53.8132717929025,24.2810366186971,
39.9731387498236));
#178078=CARTESIAN_POINT('Ctrl Pts',(-53.8061452585097,24.2698548246783,
39.9908938024065));
#178079=CARTESIAN_POINT('Ctrl Pts',(-53.800053401299,24.2572379736556,40.0080810366196));
#178080=CARTESIAN_POINT('Ctrl Pts',(-53.7951438030538,24.2432286115631,
40.0244542742558));
#178081=CARTESIAN_POINT('Ctrl Pts',(-53.7912388700581,24.2320860256422,
40.0374770090497));
#178082=CARTESIAN_POINT('Ctrl Pts',(-53.7880821478309,24.220061742058,40.0499848770043));
#178083=CARTESIAN_POINT('Ctrl Pts',(-53.7857624469881,24.2071623814826,
40.0618424270193));
#178084=CARTESIAN_POINT('Ctrl Pts',(-53.7857561149583,24.2071271704184,
40.0618747942791));
#178085=CARTESIAN_POINT('Ctrl Pts',(-53.7857497893135,24.207091952932,40.0619071564124));
#178086=CARTESIAN_POINT('Ctrl Pts',(-53.7857434700554,24.2070567290246,
40.0619395134161));
#178087=CARTESIAN_POINT('Ctrl Pts',(-53.7844855062584,24.2000447667169,
40.0683807661799));
#178088=CARTESIAN_POINT('Ctrl Pts',(-53.7835014710814,24.1927483559228,
40.0746073439084));
#178089=CARTESIAN_POINT('Ctrl Pts',(-53.7827951090624,24.1852078325133,
40.0805869293669));
#178090=CARTESIAN_POINT('Ctrl Pts',(-53.7813932847187,24.1702431416113,
40.092453830807));
#178091=CARTESIAN_POINT('Ctrl Pts',(-53.7810858838905,24.1543158599159,
40.1033475319609));
#178092=CARTESIAN_POINT('Ctrl Pts',(-53.7819069982467,24.1377344018728,
40.1130129263075));
#178093=CARTESIAN_POINT('Ctrl Pts',(-53.7825228340138,24.1252983083405,
40.1202619720674));
#178094=CARTESIAN_POINT('Ctrl Pts',(-53.7837734588332,24.1124942402753,
40.1268200947266));
#178095=CARTESIAN_POINT('Ctrl Pts',(-53.7856732654696,24.0994523147294,
40.1325796782703));
#178096=CARTESIAN_POINT('Ctrl Pts',(-53.7863856929583,24.0945615926497,
40.1347395220992));
#178097=CARTESIAN_POINT('Ctrl Pts',(-53.7871894118144,24.0896374219411,
40.1367870714852));
#178098=CARTESIAN_POINT('Ctrl Pts',(-53.7880851817728,24.0846866645809,
40.1387166518767));
#178099=CARTESIAN_POINT('Ctrl Pts',(-53.7912203766271,24.0673590138202,
40.1454701832469));
#178100=CARTESIAN_POINT('Ctrl Pts',(-53.7954831928407,24.0497056745177,
40.1507785912492));
#178101=CARTESIAN_POINT('Ctrl Pts',(-53.8009062465106,24.032020872916,40.1543986087265));
#178102=CARTESIAN_POINT('Ctrl Pts',(-53.8036177733455,24.0231784721152,
40.1562086174652));
#178103=CARTESIAN_POINT('Ctrl Pts',(-53.8066193604763,24.0143282061517,
40.1575965292115));
#178104=CARTESIAN_POINT('Ctrl Pts',(-53.8099150888837,24.0055068550424,
40.1585319382567));
#178105=CARTESIAN_POINT('Ctrl Pts',(-53.8115629530875,24.0010961794877,
40.1589996427793));
#178106=CARTESIAN_POINT('Ctrl Pts',(-53.8132843526339,23.9966927326566,
40.159354221642));
#178107=CARTESIAN_POINT('Ctrl Pts',(-53.8150797979123,23.9923011121679,
40.159591874311));
#178108=CARTESIAN_POINT('Ctrl Pts',(-53.8168752431908,23.9879094916792,
40.1598295269801));
#178109=CARTESIAN_POINT('Ctrl Pts',(-53.8187447357538,23.9835296982245,
40.1599502506895));
#178110=CARTESIAN_POINT('Ctrl Pts',(-53.8206887816834,23.9791663275018,
40.1599502534424));
#178111=CARTESIAN_POINT('',(-53.8330634946836,23.9513722670369,40.1599502534424));
#178112=CARTESIAN_POINT('Origin',(3.40248402231257E-16,2.77126713209872E-17,
40.1599502534424));
#178113=CARTESIAN_POINT('',(-54.1275498658872,23.7522229508832,39.8576902534424));
#178114=CARTESIAN_POINT('Ctrl Pts',(-53.8330634946836,23.9513722670369,
40.1599502534424));
#178115=CARTESIAN_POINT('Ctrl Pts',(-53.8346121892501,23.9478914369185,
40.1599502448875));
#178116=CARTESIAN_POINT('Ctrl Pts',(-53.8361996036041,23.9444392282284,
40.1598743450437));
#178117=CARTESIAN_POINT('Ctrl Pts',(-53.8378239549346,23.9410169613694,
40.1597243308499));
#178118=CARTESIAN_POINT('Ctrl Pts',(-53.8474140023496,23.9208121566398,
40.158838658394));
#178119=CARTESIAN_POINT('Ctrl Pts',(-53.8582911092114,23.9016479061198,
40.1553722553631));
#178120=CARTESIAN_POINT('Ctrl Pts',(-53.8700861059238,23.8838022859786,
40.1496902177821));
#178121=CARTESIAN_POINT('Ctrl Pts',(-53.8744923240608,23.8771357563434,
40.1475675976869));
#178122=CARTESIAN_POINT('Ctrl Pts',(-53.8790265713694,23.8706528330416,
40.145136144311));
#178123=CARTESIAN_POINT('Ctrl Pts',(-53.8836695340507,23.8643665485426,
40.1424159447501));
#178124=CARTESIAN_POINT('Ctrl Pts',(-53.8872922064473,23.8594616740273,
40.1402935085949));
#178125=CARTESIAN_POINT('Ctrl Pts',(-53.8909810920749,23.8546770178327,
40.1379949176048));
#178126=CARTESIAN_POINT('Ctrl Pts',(-53.894727035613,23.8500192775335,40.1355293609261));
#178127=CARTESIAN_POINT('Ctrl Pts',(-53.9078378379963,23.8337171864862,
40.1268999125509));
#178128=CARTESIAN_POINT('Ctrl Pts',(-53.9216475915793,23.8189698115831,
40.1162251288835));
#178129=CARTESIAN_POINT('Ctrl Pts',(-53.9357638458654,23.8060643480692,
40.1038990521418));
#178130=CARTESIAN_POINT('Ctrl Pts',(-53.9428219730085,23.7996116163122,
40.097736013771));
#178131=CARTESIAN_POINT('Ctrl Pts',(-53.9499567269874,23.7936193631245,
40.0911601532641));
#178132=CARTESIAN_POINT('Ctrl Pts',(-53.9571190561825,23.7881234899556,
40.084220729064));
#178133=CARTESIAN_POINT('Ctrl Pts',(-53.9642507845243,23.7826510977527,
40.0773109533619));
#178134=CARTESIAN_POINT('Ctrl Pts',(-53.9714097802519,23.7776706121038,
40.0700409753048));
#178135=CARTESIAN_POINT('Ctrl Pts',(-53.9785478363928,23.7732182003922,
40.0624586415899));
#178136=CARTESIAN_POINT('Ctrl Pts',(-53.9785784643974,23.7731990959632,
40.0624261072769));
#178137=CARTESIAN_POINT('Ctrl Pts',(-53.9786090918656,23.7731800007335,
40.0623935677888));
#178138=CARTESIAN_POINT('Ctrl Pts',(-53.9786397187952,23.7731609147028,
40.0623610231288));
#178139=CARTESIAN_POINT('Ctrl Pts',(-53.9930827901223,23.764160309458,40.0470135870229));
#178140=CARTESIAN_POINT('Ctrl Pts',(-54.0073711636766,23.7571924707013,
40.0305755292085));
#178141=CARTESIAN_POINT('Ctrl Pts',(-54.0213615752669,23.7521258339916,
40.0133447567326));
#178142=CARTESIAN_POINT('Ctrl Pts',(-54.0358609305028,23.7468748830077,
39.995487162658));
#178143=CARTESIAN_POINT('Ctrl Pts',(-54.050041117219,23.7436660552511,39.9767767954295));
#178144=CARTESIAN_POINT('Ctrl Pts',(-54.0637371441671,23.7424048061585,
39.9575197577452));
#178145=CARTESIAN_POINT('Ctrl Pts',(-54.0772376980797,23.7411615579204,
39.9385375611974));
#178146=CARTESIAN_POINT('Ctrl Pts',(-54.0902686241916,23.7418111396964,
39.9190226977072));
#178147=CARTESIAN_POINT('Ctrl Pts',(-54.1026541040343,23.744307900129,39.8992655451833));
#178148=CARTESIAN_POINT('Ctrl Pts',(-54.1112894809389,23.7460486859241,
39.885490506931));
#178149=CARTESIAN_POINT('Ctrl Pts',(-54.1196107481458,23.7486883362846,
39.8715976051467));
#178150=CARTESIAN_POINT('Ctrl Pts',(-54.1275498658872,23.7522229508832,
39.8576902534424));
#178151=CARTESIAN_POINT('',(-54.4530463244691,23.8971395307772,39.2875012672119));
#178152=CARTESIAN_POINT('',(-54.1275498658872,23.7522229508832,39.8576902534424));
#178153=CARTESIAN_POINT('',(-56.456807071981,18.6771643191714,39.2875012672119));
#178154=CARTESIAN_POINT('Origin',(5.53234440788222E-15,0.,39.2875012672119));
#178155=CARTESIAN_POINT('',(-56.1179479440987,18.567058682947,39.8576902534424));
#178156=CARTESIAN_POINT('',(-56.456807071981,18.6771643191714,39.2875012672119));
#178157=CARTESIAN_POINT('',(-56.032358823839,18.2220120550221,40.1599502534424));
#178158=CARTESIAN_POINT('Ctrl Pts',(-56.1179479440987,18.567058682947,39.8576902534424));
#178159=CARTESIAN_POINT('Ctrl Pts',(-56.1063166059142,18.563279281548,39.8772619994045));
#178160=CARTESIAN_POINT('Ctrl Pts',(-56.0953314285486,18.5576887384402,
39.8967644650353));
#178161=CARTESIAN_POINT('Ctrl Pts',(-56.0851270036924,18.5504096793259,
39.9159282836023));
#178162=CARTESIAN_POINT('Ctrl Pts',(-56.0747382496585,18.5429991338221,
39.9354382707157));
#178163=CARTESIAN_POINT('Ctrl Pts',(-56.0651578180785,18.5338382655006,
39.9545987622321));
#178164=CARTESIAN_POINT('Ctrl Pts',(-56.0565365037455,18.5230039556188,
39.9731387498193));
#178165=CARTESIAN_POINT('Ctrl Pts',(-56.0482801935087,18.5126283423269,
39.9908938024014));
#178166=CARTESIAN_POINT('Ctrl Pts',(-56.0409028880807,18.500717380208,40.0080810366137));
#178167=CARTESIAN_POINT('Ctrl Pts',(-56.0345558080376,18.4872979556277,
40.0244542742492));
#178168=CARTESIAN_POINT('Ctrl Pts',(-56.0295075492892,18.4766245866022,
40.0374770090455));
#178169=CARTESIAN_POINT('Ctrl Pts',(-56.0251112400308,18.4649961406232,
40.0499848770024));
#178170=CARTESIAN_POINT('Ctrl Pts',(-56.0214558964132,18.452409918857,40.0618424270193));
#178171=CARTESIAN_POINT('Ctrl Pts',(-56.0214459185125,18.45237556256,40.0618747942791));
#178172=CARTESIAN_POINT('Ctrl Pts',(-56.0214359462906,18.4523411992085,
40.0619071564124));
#178173=CARTESIAN_POINT('Ctrl Pts',(-56.021425979749,18.4523068288038,40.0619395134161));
#178174=CARTESIAN_POINT('Ctrl Pts',(-56.0194419575649,18.4454647717818,
40.0683807661799));
#178175=CARTESIAN_POINT('Ctrl Pts',(-56.0177006304278,18.4383111911743,
40.0746073439084));
#178176=CARTESIAN_POINT('Ctrl Pts',(-56.0162099386096,18.4308858104773,
40.0805869293669));
#178177=CARTESIAN_POINT('Ctrl Pts',(-56.0132515574631,18.4161496282623,
40.092453830807));
#178178=CARTESIAN_POINT('Ctrl Pts',(-56.0112809863292,18.4003417300187,
40.1033475319609));
#178179=CARTESIAN_POINT('Ctrl Pts',(-56.010364368207,18.3837652771159,40.1130129263075));
#178180=CARTESIAN_POINT('Ctrl Pts',(-56.0096769046154,18.3713329374388,
40.1202619720674));
#178181=CARTESIAN_POINT('Ctrl Pts',(-56.0095822888227,18.3584682855077,
40.1268200947267));
#178182=CARTESIAN_POINT('Ctrl Pts',(-56.0101084356843,18.3452992211263,
40.1325796782703));
#178183=CARTESIAN_POINT('Ctrl Pts',(-56.0103057407573,18.3403608219833,
40.1347395220992));
#178184=CARTESIAN_POINT('Ctrl Pts',(-56.0105903407605,18.3353796149002,
40.1367870714852));
#178185=CARTESIAN_POINT('Ctrl Pts',(-56.0109637085384,18.3303623448496,
40.1387166518767));
#178186=CARTESIAN_POINT('Ctrl Pts',(-56.0122704957612,18.3128018996726,
40.1454701832469));
#178187=CARTESIAN_POINT('Ctrl Pts',(-56.0146646833927,18.294799681582,40.1507785912492));
#178188=CARTESIAN_POINT('Ctrl Pts',(-56.0182094638726,18.2766448957075,
40.1543986087265));
#178189=CARTESIAN_POINT('Ctrl Pts',(-56.0199818541125,18.2675675027702,
40.1562086174652));
#178190=CARTESIAN_POINT('Ctrl Pts',(-56.0220418935342,18.2584519681996,
40.1575965292115));
#178191=CARTESIAN_POINT('Ctrl Pts',(-56.0243974853212,18.2493344439489,
40.1585319382567));
#178192=CARTESIAN_POINT('Ctrl Pts',(-56.0255752812147,18.2447756818235,
40.1589996427793));
#178193=CARTESIAN_POINT('Ctrl Pts',(-56.0268269652239,18.2402164222857,
40.159354221642));
#178194=CARTESIAN_POINT('Ctrl Pts',(-56.0281535255244,18.2356611844176,
40.1595918743111));
#178195=CARTESIAN_POINT('Ctrl Pts',(-56.0294800858248,18.2311059465496,
40.1598295269801));
#178196=CARTESIAN_POINT('Ctrl Pts',(-56.0308815240327,18.226554730877,40.1599502506896));
#178197=CARTESIAN_POINT('Ctrl Pts',(-56.032358823839,18.2220120550221,40.1599502534424));
#178198=CARTESIAN_POINT('',(-56.0417604764382,18.1930767435953,40.1599502534424));
#178199=CARTESIAN_POINT('Origin',(3.37692616670652E-16,2.10546223053637E-17,
40.1599502534424));
#178200=CARTESIAN_POINT('',(-56.3138168485094,17.9642361803977,39.8576902534424));
#178201=CARTESIAN_POINT('Ctrl Pts',(-56.0417604764382,18.1930767435953,
40.1599502534424));
#178202=CARTESIAN_POINT('Ctrl Pts',(-56.0429368412707,18.1894530991654,
40.1599502448875));
#178203=CARTESIAN_POINT('Ctrl Pts',(-56.0441547055335,18.1858538720528,
40.1598743450437));
#178204=CARTESIAN_POINT('Ctrl Pts',(-56.0454124342018,18.1822805617813,
40.1597243308499));
#178205=CARTESIAN_POINT('Ctrl Pts',(-56.0528379691453,18.1611840081651,
40.1588386583939));
#178206=CARTESIAN_POINT('Ctrl Pts',(-56.0616522804221,18.1409877741476,
40.1553722553624));
#178207=CARTESIAN_POINT('Ctrl Pts',(-56.0715172876601,18.1220070012986,
40.1496902177804));
#178208=CARTESIAN_POINT('Ctrl Pts',(-56.0752025259741,18.1149164164015,
40.1475675976856));
#178209=CARTESIAN_POINT('Ctrl Pts',(-56.0790342841904,18.1079950493304,
40.1451361443103));
#178210=CARTESIAN_POINT('Ctrl Pts',(-56.082994716577,18.1012578800034,40.1424159447501));
#178211=CARTESIAN_POINT('Ctrl Pts',(-56.0860848445995,18.0960012025253,
40.1402935085949));
#178212=CARTESIAN_POINT('Ctrl Pts',(-56.0892533893664,18.0908571636322,
40.1379949176048));
#178213=CARTESIAN_POINT('Ctrl Pts',(-56.0924919457981,18.0858333812002,
40.1355293609261));
#178214=CARTESIAN_POINT('Ctrl Pts',(-56.1038268933089,18.068250142688,40.1268999125509));
#178215=CARTESIAN_POINT('Ctrl Pts',(-56.1160194751809,18.0521400431276,
40.1162251288835));
#178216=CARTESIAN_POINT('Ctrl Pts',(-56.1287094108802,18.0378297267255,
40.1038990521418));
#178217=CARTESIAN_POINT('Ctrl Pts',(-56.1350543787298,18.0306745685244,
40.097736013771));
#178218=CARTESIAN_POINT('Ctrl Pts',(-56.1415236867627,18.0239693566574,
40.0911601532641));
#178219=CARTESIAN_POINT('Ctrl Pts',(-56.1480723047924,18.0177549231926,
40.084220729064));
#178220=CARTESIAN_POINT('Ctrl Pts',(-56.1545929440328,18.0115670407228,
40.0773109533618));
#178221=CARTESIAN_POINT('Ctrl Pts',(-56.1611921195216,18.0058655198734,
40.0700409753047));
#178222=CARTESIAN_POINT('Ctrl Pts',(-56.1678256688899,18.0006913688999,
40.0624586415899));
#178223=CARTESIAN_POINT('Ctrl Pts',(-56.1678541321546,18.0006691676287,
40.0624261072769));
#178224=CARTESIAN_POINT('Ctrl Pts',(-56.1678825958473,18.0006469755625,
40.0623935677888));
#178225=CARTESIAN_POINT('Ctrl Pts',(-56.1679110599659,18.0006247927011,
40.0623610231288));
#178226=CARTESIAN_POINT('Ctrl Pts',(-56.1813341912027,17.9901637816626,
40.0470135870225));
#178227=CARTESIAN_POINT('Ctrl Pts',(-56.1948159540745,17.9817405717252,
40.0305755292076));
#178228=CARTESIAN_POINT('Ctrl Pts',(-56.2082001169775,17.9752392943574,
40.0133447567312));
#178229=CARTESIAN_POINT('Ctrl Pts',(-56.2220711693916,17.9685015133111,
39.9954871626562));
#178230=CARTESIAN_POINT('Ctrl Pts',(-56.2358382617272,17.9638280307224,
39.9767767954273));
#178231=CARTESIAN_POINT('Ctrl Pts',(-56.2493274239774,17.9611420662345,
39.9575197577427));
#178232=CARTESIAN_POINT('Ctrl Pts',(-56.2626240656151,17.9584944364867,
39.938537561195));
#178233=CARTESIAN_POINT('Ctrl Pts',(-56.275651506735,17.9577783571046,39.9190226977049));
#178234=CARTESIAN_POINT('Ctrl Pts',(-56.2882301201542,17.9589668048477,
39.8992655451812));
#178235=CARTESIAN_POINT('Ctrl Pts',(-56.2970001532242,17.9597954117587,
39.8854905069296));
#178236=CARTESIAN_POINT('Ctrl Pts',(-56.3055517542539,17.9615507925648,
39.871597605146));
#178237=CARTESIAN_POINT('Ctrl Pts',(-56.3138168485093,17.9642361803977,
39.8576902534424));
#178238=CARTESIAN_POINT('',(-56.6526781108322,18.0743352474896,39.2875012672119));
#178239=CARTESIAN_POINT('',(-56.3138168485094,17.9642361803977,39.8576902534424));
#178240=CARTESIAN_POINT('',(-58.0998260601479,12.6735055745745,39.2875012672119));
#178241=CARTESIAN_POINT('Origin',(5.53234440788222E-15,0.,39.2875012672119));
#178242=CARTESIAN_POINT('',(-57.7513140650719,12.5994235324476,39.8576902534424));
#178243=CARTESIAN_POINT('',(-58.0998260601479,12.6735055745745,39.2875012672119));
#178244=CARTESIAN_POINT('',(-57.6301266171956,12.2652136052665,40.1599502534424));
#178245=CARTESIAN_POINT('Ctrl Pts',(-57.7513140650719,12.5994235324476,
39.8576902534424));
#178246=CARTESIAN_POINT('Ctrl Pts',(-57.7393513895531,12.5968806409109,
39.8772619994072));
#178247=CARTESIAN_POINT('Ctrl Pts',(-57.727842019257,12.5924689870912,39.8967644650405));
#178248=CARTESIAN_POINT('Ctrl Pts',(-57.7169326264434,12.5862964562719,
39.91592828361));
#178249=CARTESIAN_POINT('Ctrl Pts',(-57.7058261701561,12.5800124270049,
39.9354382707261));
#178250=CARTESIAN_POINT('Ctrl Pts',(-57.6953406496936,12.5719031706671,
39.9545987622451));
#178251=CARTESIAN_POINT('Ctrl Pts',(-57.6856340700592,12.5620293850045,
39.9731387498347));
#178252=CARTESIAN_POINT('Ctrl Pts',(-57.6763384418397,12.5525736298267,
39.9908938024193));
#178253=CARTESIAN_POINT('Ctrl Pts',(-57.6677565154956,12.5414990556008,
40.008081036634));
#178254=CARTESIAN_POINT('Ctrl Pts',(-57.6600414935913,12.5288165945521,
40.0244542742715));
#178255=CARTESIAN_POINT('Ctrl Pts',(-57.6539052188746,12.5187293820925,
40.0374770090597));
#178256=CARTESIAN_POINT('Ctrl Pts',(-57.6483174894735,12.5076241774138,
40.0499848770091));
#178257=CARTESIAN_POINT('Ctrl Pts',(-57.6433665517939,12.4954889917452,
40.0618424270193));
#178258=CARTESIAN_POINT('Ctrl Pts',(-57.6433530373423,12.4954558666302,
40.0618747942791));
#178259=CARTESIAN_POINT('Ctrl Pts',(-57.6433395278009,12.4954227339059,
40.0619071564124));
#178260=CARTESIAN_POINT('Ctrl Pts',(-57.6433260231715,12.4953895935731,
40.0619395134162));
#178261=CARTESIAN_POINT('Ctrl Pts',(-57.6406376799624,12.4887924048454,
40.0683807661799));
#178262=CARTESIAN_POINT('Ctrl Pts',(-57.6381581392099,12.4818600305507,
40.0746073439084));
#178263=CARTESIAN_POINT('Ctrl Pts',(-57.635899449924,12.474631146591,40.0805869293669));
#178264=CARTESIAN_POINT('Ctrl Pts',(-57.6314169246175,12.460284925759,40.092453830807));
#178265=CARTESIAN_POINT('Ctrl Pts',(-57.6278047731676,12.4447696056084,
40.1033475319609));
#178266=CARTESIAN_POINT('Ctrl Pts',(-57.6251604652271,12.4283797729328,
40.1130129263075));
#178267=CARTESIAN_POINT('Ctrl Pts',(-57.6231772342716,12.416087398426,40.1202619720674));
#178268=CARTESIAN_POINT('Ctrl Pts',(-57.6217384144973,12.4033031104476,
40.1268200947266));
#178269=CARTESIAN_POINT('Ctrl Pts',(-57.6208851370088,12.390151190256,40.1325796782703));
#178270=CARTESIAN_POINT('Ctrl Pts',(-57.6205651579507,12.3852192201841,
40.1347395220992));
#178271=CARTESIAN_POINT('Ctrl Pts',(-57.6203275209636,12.3802355518736,
40.1367870714852));
#178272=CARTESIAN_POINT('Ctrl Pts',(-57.6201743958656,12.3752067393933,
40.1387166518767));
#178273=CARTESIAN_POINT('Ctrl Pts',(-57.6196384580226,12.3576058957121,
40.1454701832469));
#178274=CARTESIAN_POINT('Ctrl Pts',(-57.6201377858513,12.3394520349018,
40.1507785912492));
#178275=CARTESIAN_POINT('Ctrl Pts',(-57.6217654557844,12.3210261723878,
40.1543986087265));
#178276=CARTESIAN_POINT('Ctrl Pts',(-57.6225792907509,12.3118132411307,
40.1562086174652));
#178277=CARTESIAN_POINT('Ctrl Pts',(-57.6236752122406,12.3025323096572,
40.1575965292115));
#178278=CARTESIAN_POINT('Ctrl Pts',(-57.6250648590506,12.2932185057687,
40.1585319382567));
#178279=CARTESIAN_POINT('Ctrl Pts',(-57.6257596824556,12.2885616038245,
40.1589996427793));
#178280=CARTESIAN_POINT('Ctrl Pts',(-57.6265279372157,12.2838964837814,
40.159354221642));
#178281=CARTESIAN_POINT('Ctrl Pts',(-57.6273710784659,12.2792275366734,
40.159591874311));
#178282=CARTESIAN_POINT('Ctrl Pts',(-57.6282142197161,12.2745585895654,
40.1598295269801));
#178283=CARTESIAN_POINT('Ctrl Pts',(-57.6291322491185,12.2698858157463,
40.1599502506896));
#178284=CARTESIAN_POINT('Ctrl Pts',(-57.6301266171956,12.2652136052665,
40.1599502534424));
#178285=CARTESIAN_POINT('',(-57.6364522029206,12.2354540642049,40.1599502534424));
#178286=CARTESIAN_POINT('Origin',(3.35846787602732E-16,1.4165894441799E-17,
40.1599502534424));
#178287=CARTESIAN_POINT('',(-57.8830978693155,11.9794294790617,39.8576902534424));
#178288=CARTESIAN_POINT('Ctrl Pts',(-57.6364522029206,12.2354540642049,
40.1599502534424));
#178289=CARTESIAN_POINT('Ctrl Pts',(-57.6372433495198,12.2317273068701,
40.1599502448875));
#178290=CARTESIAN_POINT('Ctrl Pts',(-57.6380783205157,12.2280204952203,
40.1598743450438));
#178291=CARTESIAN_POINT('Ctrl Pts',(-57.6389556465833,12.2243352914715,
40.1597243308499));
#178292=CARTESIAN_POINT('Ctrl Pts',(-57.6441353133406,12.2025781272228,
40.1588386583938));
#178293=CARTESIAN_POINT('Ctrl Pts',(-57.6507902575938,12.1815711838723,
40.1553722553612));
#178294=CARTESIAN_POINT('Ctrl Pts',(-57.6586171922743,12.161663215633,40.1496902177773));
#178295=CARTESIAN_POINT('Ctrl Pts',(-57.661541074523,12.1542262614079,40.1475675976833));
#178296=CARTESIAN_POINT('Ctrl Pts',(-57.6646283621018,12.1469422825155,
40.145136144309));
#178297=CARTESIAN_POINT('Ctrl Pts',(-57.6678628728672,12.1398280421991,
40.1424159447501));
#178298=CARTESIAN_POINT('Ctrl Pts',(-57.6703866004264,12.1342771550168,
40.1402935085949));
#178299=CARTESIAN_POINT('Ctrl Pts',(-57.6730000890932,12.1288300925917,
40.1379949176048));
#178300=CARTESIAN_POINT('Ctrl Pts',(-57.6756957761164,12.1234953096385,
40.1355293609261));
#178301=CARTESIAN_POINT('Ctrl Pts',(-57.6851306806978,12.1048235693021,
40.1268999125508));
#178302=CARTESIAN_POINT('Ctrl Pts',(-57.6955725063805,12.0875272507063,
40.1162251288835));
#178303=CARTESIAN_POINT('Ctrl Pts',(-57.7066970899018,12.0719688682372,
40.1038990521418));
#178304=CARTESIAN_POINT('Ctrl Pts',(-57.7122593816625,12.0641896770026,
40.097736013771));
#178305=CARTESIAN_POINT('Ctrl Pts',(-57.7179923646568,12.0568449701607,
40.0911601532641));
#178306=CARTESIAN_POINT('Ctrl Pts',(-57.7238555234915,12.0499800630335,
40.084220729064));
#178307=CARTESIAN_POINT('Ctrl Pts',(-57.7296936321424,12.043144486032,40.0773109533618));
#178308=CARTESIAN_POINT('Ctrl Pts',(-57.7356606854447,12.0367843970377,
40.0700409753048));
#178309=CARTESIAN_POINT('Ctrl Pts',(-57.7417170494856,12.0309451958831,
40.0624586415899));
#178310=CARTESIAN_POINT('Ctrl Pts',(-57.7417430361607,12.0309201410115,
40.0624261072769));
#178311=CARTESIAN_POINT('Ctrl Pts',(-57.7417690242238,12.0308950952497,
40.0623935677889));
#178312=CARTESIAN_POINT('Ctrl Pts',(-57.7417950136726,12.0308700585978,
40.0623610231289));
#178313=CARTESIAN_POINT('Ctrl Pts',(-57.7540511381833,12.0190632547925,
40.0470135870233));
#178314=CARTESIAN_POINT('Ctrl Pts',(-57.7665785813563,12.0092769601257,
40.0305755292092));
#178315=CARTESIAN_POINT('Ctrl Pts',(-57.7792098558813,12.0014122714555,
40.0133447567337));
#178316=CARTESIAN_POINT('Ctrl Pts',(-57.7923006313198,11.9932614808862,
39.9954871626594));
#178317=CARTESIAN_POINT('Ctrl Pts',(-57.8055037941296,11.9871745471185,
39.9767767954313));
#178318=CARTESIAN_POINT('Ctrl Pts',(-57.8186383015968,11.9830932952243,
39.9575197577474));
#178319=CARTESIAN_POINT('Ctrl Pts',(-57.8315853501714,11.9790702919521,
39.9385375612));
#178320=CARTESIAN_POINT('Ctrl Pts',(-57.8444665749283,11.9769963969268,
39.9190226977102));
#178321=CARTESIAN_POINT('Ctrl Pts',(-57.8571005080032,11.9768635110977,
39.8992655451868));
#178322=CARTESIAN_POINT('Ctrl Pts',(-57.8659091109227,11.9767708607333,
39.8854905069334));
#178323=CARTESIAN_POINT('Ctrl Pts',(-57.8745973526466,11.9776227396654,
39.8715976051479));
#178324=CARTESIAN_POINT('Ctrl Pts',(-57.8830978693155,11.9794294790617,
39.8576902534424));
#178325=CARTESIAN_POINT('',(-58.231611300478,12.0535047649326,39.2875012672119));
#178326=CARTESIAN_POINT('',(-57.8830978693155,11.9794294790616,39.8576902534424));
#178327=CARTESIAN_POINT('',(-59.1062911958296,6.53099325080096,39.2875012672119));
#178328=CARTESIAN_POINT('Origin',(5.53234440788222E-15,0.,39.2875012672119));
#178329=CARTESIAN_POINT('',(-58.7519447039088,6.49374646112781,39.8576902534424));
#178330=CARTESIAN_POINT('',(-59.1062911958296,6.53099325080096,39.2875012672119));
#178331=CARTESIAN_POINT('',(-58.596486683455,6.17403490859061,40.1599502534424));
#178332=CARTESIAN_POINT('Ctrl Pts',(-58.7519447039088,6.49374646112781,
39.8576902534424));
#178333=CARTESIAN_POINT('Ctrl Pts',(-58.7397817566348,6.4924679399056,39.8772619994052));
#178334=CARTESIAN_POINT('Ctrl Pts',(-58.7278742924804,6.48928351037781,
39.8967644650367));
#178335=CARTESIAN_POINT('Ctrl Pts',(-58.716379457302,6.48428513539496,39.9159282836043));
#178336=CARTESIAN_POINT('Ctrl Pts',(-58.7046769834231,6.47919647150667,
39.9354382707185));
#178337=CARTESIAN_POINT('Ctrl Pts',(-58.6934012556367,6.47222767386539,
39.9545987622356));
#178338=CARTESIAN_POINT('Ctrl Pts',(-58.6827157580201,6.4634225916883,39.9731387498234));
#178339=CARTESIAN_POINT('Ctrl Pts',(-58.6724826566677,6.45499029386124,
39.9908938024063));
#178340=CARTESIAN_POINT('Ctrl Pts',(-58.6627901347897,6.44487344288651,
40.0080810366194));
#178341=CARTESIAN_POINT('Ctrl Pts',(-58.6537916984193,6.43306689707259,
40.0244542742555));
#178342=CARTESIAN_POINT('Ctrl Pts',(-58.6466346380372,6.42367635878173,
40.0374770090495));
#178343=CARTESIAN_POINT('Ctrl Pts',(-58.6399167088201,6.41321606633983,
40.0499848770043));
#178344=CARTESIAN_POINT('Ctrl Pts',(-58.6337244205832,6.40166487239078,
40.0618424270193));
#178345=CARTESIAN_POINT('Ctrl Pts',(-58.6337075176478,6.4016333413835,40.0618747942791));
#178346=CARTESIAN_POINT('Ctrl Pts',(-58.6336906188003,6.40160180229526,
40.0619071564124));
#178347=CARTESIAN_POINT('Ctrl Pts',(-58.6336737240427,6.40157025512682,
40.0619395134162));
#178348=CARTESIAN_POINT('Ctrl Pts',(-58.6303105138593,6.39529021487361,
40.0683807661799));
#178349=CARTESIAN_POINT('Ctrl Pts',(-58.6271199258587,6.38865499943512,
40.0746073439084));
#178350=CARTESIAN_POINT('Ctrl Pts',(-58.6241179857776,6.38170181337825,
40.0805869293669));
#178351=CARTESIAN_POINT('Ctrl Pts',(-58.6181604277965,6.3679027341269,40.092453830807));
#178352=CARTESIAN_POINT('Ctrl Pts',(-58.6129462715177,6.35284998116362,
40.1033475319609));
#178353=CARTESIAN_POINT('Ctrl Pts',(-58.6086032453499,6.33682633915166,
40.1130129263075));
#178354=CARTESIAN_POINT('Ctrl Pts',(-58.6053459757241,6.3248086076427,40.1202619720674));
#178355=CARTESIAN_POINT('Ctrl Pts',(-58.6025787159787,6.31224475095145,
40.1268200947266));
#178356=CARTESIAN_POINT('Ctrl Pts',(-58.600355362827,6.29925407013931,40.1325796782703));
#178357=CARTESIAN_POINT('Ctrl Pts',(-58.599521605395,6.29438256483475,40.1347395220992));
#178358=CARTESIAN_POINT('Ctrl Pts',(-58.5987643350183,6.28945103740978,
40.1367870714852));
#178359=CARTESIAN_POINT('Ctrl Pts',(-58.598086394715,6.28446577922157,40.1387166518767));
#178360=CARTESIAN_POINT('Ctrl Pts',(-58.5957136036534,6.26701737556284,
40.1454701832469));
#178361=CARTESIAN_POINT('Ctrl Pts',(-58.5943126009392,6.24891076953097,
40.1507785912492));
#178362=CARTESIAN_POINT('Ctrl Pts',(-58.594005327233,6.23041570798286,40.1543986087265));
#178363=CARTESIAN_POINT('Ctrl Pts',(-58.59385169038,6.22116817720881,40.1562086174652));
#178364=CARTESIAN_POINT('Ctrl Pts',(-58.5939714867924,6.21182353265984,
40.1575965292115));
#178365=CARTESIAN_POINT('Ctrl Pts',(-58.5943799633642,6.20241549311804,
40.1585319382567));
#178366=CARTESIAN_POINT('Ctrl Pts',(-58.5945842016501,6.19771147334713,
40.1589996427793));
#178367=CARTESIAN_POINT('Ctrl Pts',(-58.5948606100011,6.19299160483032,
40.159354221642));
#178368=CARTESIAN_POINT('Ctrl Pts',(-58.595211094569,6.18826010244389,40.159591874311));
#178369=CARTESIAN_POINT('Ctrl Pts',(-58.5955615791369,6.18352860005746,
40.1598295269801));
#178370=CARTESIAN_POINT('Ctrl Pts',(-58.5959861416118,6.17878546397953,
40.1599502506895));
#178371=CARTESIAN_POINT('Ctrl Pts',(-58.596486683455,6.17403490859061,40.1599502534424));
#178372=CARTESIAN_POINT('',(-58.5996668978648,6.14377718965363,40.1599502534424));
#178373=CARTESIAN_POINT('Origin',(3.34731138317027E-16,7.12196207432608E-18,
40.1599502534424));
#178374=CARTESIAN_POINT('',(-58.8181995570484,5.86337364149622,39.8576902534424));
#178375=CARTESIAN_POINT('Ctrl Pts',(-58.5996668978648,6.14377718965363,
40.1599502534424));
#178376=CARTESIAN_POINT('Ctrl Pts',(-58.600064158263,6.13998815054726,40.1599502448875));
#178377=CARTESIAN_POINT('Ctrl Pts',(-58.600507087875,6.13621436696444,40.1598743450437));
#178378=CARTESIAN_POINT('Ctrl Pts',(-58.6009943991739,6.13245764560167,
40.1597243308499));
#178379=CARTESIAN_POINT('Ctrl Pts',(-58.6038714482307,6.11027824676932,
40.1588386583938));
#178380=CARTESIAN_POINT('Ctrl Pts',(-58.6082941124965,6.08869075055693,
40.1553722553613));
#178381=CARTESIAN_POINT('Ctrl Pts',(-58.6139972210829,6.06807370279675,
40.1496902177777));
#178382=CARTESIAN_POINT('Ctrl Pts',(-58.6161277126023,6.0603718600664,40.1475675976835));
#178383=CARTESIAN_POINT('Ctrl Pts',(-58.6184367045766,6.05280507414586,
40.1451361443091));
#178384=CARTESIAN_POINT('Ctrl Pts',(-58.6209098557462,6.04539170794222,
40.1424159447501));
#178385=CARTESIAN_POINT('Ctrl Pts',(-58.6228395323549,6.03960742773723,
40.1402935085949));
#178386=CARTESIAN_POINT('Ctrl Pts',(-58.6248693309926,6.03391702093593,
40.1379949176048));
#178387=CARTESIAN_POINT('Ctrl Pts',(-58.6269926140963,6.02832968645991,
40.1355293609261));
#178388=CARTESIAN_POINT('Ctrl Pts',(-58.6344241049593,6.00877401579383,
40.1268999125509));
#178389=CARTESIAN_POINT('Ctrl Pts',(-58.6430007716254,5.9904809802487,40.1162251288835));
#178390=CARTESIAN_POINT('Ctrl Pts',(-58.6524381197038,5.97384499260664,
40.1038990521418));
#178391=CARTESIAN_POINT('Ctrl Pts',(-58.657156793743,5.96552699878561,40.097736013771));
#178392=CARTESIAN_POINT('Ctrl Pts',(-58.6620906399372,5.95762326711397,
40.0911601532641));
#178393=CARTESIAN_POINT('Ctrl Pts',(-58.6672041015819,5.95018309968334,
40.084220729064));
#178394=CARTESIAN_POINT('Ctrl Pts',(-58.6722957161032,5.94277472016222,
40.0773109533619));
#178395=CARTESIAN_POINT('Ctrl Pts',(-58.6775652709344,5.93582574548894,
40.0700409753048));
#178396=CARTESIAN_POINT('Ctrl Pts',(-58.682978094856,5.9293854696631,40.0624586415899));
#178397=CARTESIAN_POINT('Ctrl Pts',(-58.6830013202262,5.92935783569746,
40.0624261072769));
#178398=CARTESIAN_POINT('Ctrl Pts',(-58.6830245479289,5.9293302106467,40.0623935677888));
#178399=CARTESIAN_POINT('Ctrl Pts',(-58.683047777962,5.92930259451103,40.0623610231288));
#178400=CARTESIAN_POINT('Ctrl Pts',(-58.6940026150817,5.91627935575239,
40.0470135870242));
#178401=CARTESIAN_POINT('Ctrl Pts',(-58.7054384852669,5.90523719704883,
40.0305755292111));
#178402=CARTESIAN_POINT('Ctrl Pts',(-58.7171784805269,5.89609526425114,
40.0133447567368));
#178403=CARTESIAN_POINT('Ctrl Pts',(-58.7293455537145,5.88662076592623,
39.9954871626637));
#178404=CARTESIAN_POINT('Ctrl Pts',(-58.7418401303834,5.87918707069999,
39.9767767954368));
#178405=CARTESIAN_POINT('Ctrl Pts',(-58.754476078655,5.87375524644919,39.9575197577541));
#178406=CARTESIAN_POINT('Ctrl Pts',(-58.7669316835925,5.86840094651825,
39.9385375612077));
#178407=CARTESIAN_POINT('Ctrl Pts',(-58.7795255625917,5.86499195787771,
39.919022697719));
#178408=CARTESIAN_POINT('Ctrl Pts',(-58.7920763953073,5.86353919440106,
39.8992655451965));
#178409=CARTESIAN_POINT('Ctrl Pts',(-58.8008270591802,5.86252630185767,
39.8854905069399));
#178410=CARTESIAN_POINT('Ctrl Pts',(-58.8095567514046,5.86246534555171,
39.8715976051512));
#178411=CARTESIAN_POINT('Ctrl Pts',(-58.8181995570484,5.86337364149624,
39.8576902534424));
#178412=CARTESIAN_POINT('',(-59.1725467709677,5.90061356181298,39.2875012672119));
#178413=CARTESIAN_POINT('',(-58.8181995570484,5.8633736414962,39.8576902534424));
#178414=CARTESIAN_POINT('',(-59.4651754363832,0.316925998273044,39.2875012672119));
#178415=CARTESIAN_POINT('Origin',(5.53234440788222E-15,0.,39.2875012672119));
#178416=CARTESIAN_POINT('',(-59.1088767419348,0.316922544675689,39.8576902534424));
#178417=CARTESIAN_POINT('',(-59.4651754363832,0.316925998273047,39.2875012672119));
#178418=CARTESIAN_POINT('Ctrl Pts',(-59.1088767419348,0.316922544675689,
39.8576902534424));
#178419=CARTESIAN_POINT('Ctrl Pts',(-59.096646782701,0.316922401513864,
39.8772619994035));
#178420=CARTESIAN_POINT('Ctrl Pts',(-59.0844716853573,0.315000085554014,
39.8967644650332));
#178421=CARTESIAN_POINT('Ctrl Pts',(-59.0725173476341,0.311230629649666,
39.9159282835992));
#178422=CARTESIAN_POINT('Ctrl Pts',(-59.0603470709162,0.307393083606243,
39.9354382707117));
#178423=CARTESIAN_POINT('Ctrl Pts',(-59.0484046750391,0.30164109626635,
39.9545987622272));
#178424=CARTESIAN_POINT('Ctrl Pts',(-59.0368573319885,0.294001187897179,
39.9731387498136));
#178425=CARTESIAN_POINT('Ctrl Pts',(-59.0257988735033,0.286684733440014,
39.9908938023951));
#178426=CARTESIAN_POINT('Ctrl Pts',(-59.0151019493895,0.27763644805218,
40.0080810366069));
#178427=CARTESIAN_POINT('Ctrl Pts',(-59.0049186873052,0.266835172459114,
40.0244542742421));
#178428=CARTESIAN_POINT('Ctrl Pts',(-58.9968192555089,0.258244193040634,
40.0374770090409));
#178429=CARTESIAN_POINT('Ctrl Pts',(-58.9890447295139,0.248543417989683,
40.0499848770002));
#178430=CARTESIAN_POINT('Ctrl Pts',(-58.981678934725,0.23770277305949,40.0618424270193));
#178431=CARTESIAN_POINT('Ctrl Pts',(-58.9816588284979,0.23767318162023,
40.0618747942791));
#178432=CARTESIAN_POINT('Ctrl Pts',(-58.9816387254916,0.237643581716968,
40.0619071564124));
#178433=CARTESIAN_POINT('Ctrl Pts',(-58.9816186257082,0.23761397335028,
40.0619395134162));
#178434=CARTESIAN_POINT('Ctrl Pts',(-58.9776173965852,0.231719887006775,
40.0683807661799));
#178435=CARTESIAN_POINT('Ctrl Pts',(-58.9737507180862,0.22545452723336,
40.0746073439084));
#178436=CARTESIAN_POINT('Ctrl Pts',(-58.9700384170936,0.218853219640731,
40.0805869293669));
#178437=CARTESIAN_POINT('Ctrl Pts',(-58.9626710986899,0.205752467569928,
40.092453830807));
#178438=CARTESIAN_POINT('Ctrl Pts',(-58.9559120649696,0.191327202905431,
40.1033475319609));
#178439=CARTESIAN_POINT('Ctrl Pts',(-58.9499179036781,0.175845309932249,
40.1130129263075));
#178440=CARTESIAN_POINT('Ctrl Pts',(-58.9454222827095,0.164233890202363,
40.1202619720674));
#178441=CARTESIAN_POINT('Ctrl Pts',(-58.9413569016699,0.1520281170413,40.1268200947267));
#178442=CARTESIAN_POINT('Ctrl Pts',(-58.9377878323772,0.139341004226139,
40.1325796782703));
#178443=CARTESIAN_POINT('Ctrl Pts',(-58.9364494313924,0.134583336920454,
40.1347395220992));
#178444=CARTESIAN_POINT('Ctrl Pts',(-58.9351808244388,0.129757981227463,
40.1367870714852));
#178445=CARTESIAN_POINT('Ctrl Pts',(-58.933985496586,0.124870896863318,
40.1387166518767));
#178446=CARTESIAN_POINT('Ctrl Pts',(-58.9298018491012,0.107766101588809,
40.1454701832469));
#178447=CARTESIAN_POINT('Ctrl Pts',(-58.9265158655229,0.089905130100062,
40.1507785912492));
#178448=CARTESIAN_POINT('Ctrl Pts',(-58.9242770147326,0.0715435052825858,
40.1543986087265));
#178449=CARTESIAN_POINT('Ctrl Pts',(-58.9231575893375,0.0623626928738478,
40.1562086174652));
#178450=CARTESIAN_POINT('Ctrl Pts',(-58.9222999481582,0.0530567171305718,
40.1575965292115));
#178451=CARTESIAN_POINT('Ctrl Pts',(-58.9217227791368,0.0436575183854266,
40.1585319382567));
#178452=CARTESIAN_POINT('Ctrl Pts',(-58.9214341946262,0.038957919012854,
40.1589996427793));
#178453=CARTESIAN_POINT('Ctrl Pts',(-58.9212157281805,0.034235013889458,
40.159354221642));
#178454=CARTESIAN_POINT('Ctrl Pts',(-58.9210697160839,0.0294927955548825,
40.1595918743111));
#178455=CARTESIAN_POINT('Ctrl Pts',(-58.9209237039872,0.024750577220307,
40.1598295269801));
#178456=CARTESIAN_POINT('Ctrl Pts',(-58.9208501479391,0.0199890456750398,
40.1599502506895));
#178457=CARTESIAN_POINT('Ctrl Pts',(-58.9208513795073,0.0152121934559205,
40.1599502534424));
#178458=CARTESIAN_POINT('Origin',(5.49031038273072E-15,0.,38.989));
#178459=CARTESIAN_POINT('',(56.875,6.96517867015057E-15,38.989));
#178460=CARTESIAN_POINT('',(-56.875,-6.96517867015057E-15,38.989));
#178461=CARTESIAN_POINT('Origin',(5.49031038273072E-15,0.,38.989));
#178462=CARTESIAN_POINT('',(-56.875,-6.96517867015057E-15,38.989));
#178463=CARTESIAN_POINT('Origin',(5.49031038273072E-15,0.,38.989));
#178464=CARTESIAN_POINT('Origin',(0.,0.,0.));
#178465=CARTESIAN_POINT('',(56.875,-6.96517867015057E-15,38.6715));
#178466=CARTESIAN_POINT('',(56.875,-6.96517867015057E-15,-8.00896157936366E-15));
#178467=CARTESIAN_POINT('Origin',(5.44560101479317E-15,0.,38.6715));
#178468=CARTESIAN_POINT('Origin',(60.4792282238308,0.,38.989));
#178469=CARTESIAN_POINT('',(60.1802756340597,6.00595296980781,38.989));
#178470=CARTESIAN_POINT('',(60.1803330762808,6.00537737563911,38.9889999997818));
#178471=CARTESIAN_POINT('Origin',(5.49031038273072E-15,0.,38.989));
#178472=CARTESIAN_POINT('',(59.7081718144893,5.95633285891129,38.989));
#178473=CARTESIAN_POINT('',(59.70870646733,5.95638905318924,38.989));
#178474=CARTESIAN_POINT('',(60.0036905223731,0.3175,38.989));
#178475=CARTESIAN_POINT('Origin',(5.49031038273072E-15,0.,38.989));
#178476=CARTESIAN_POINT('',(60.4783948217626,0.317500000025261,38.989));
#178477=CARTESIAN_POINT('',(60.4792282238308,0.3175,38.989));
#178478=CARTESIAN_POINT('',(60.4783917836883,0.318078445377853,38.9889999995776));
#178479=CARTESIAN_POINT('Origin',(5.49031038273072E-15,0.,38.989));
#178480=CARTESIAN_POINT('Origin',(5.49031038273072E-15,0.,38.989));
#178481=CARTESIAN_POINT('Origin',(5.49031038273072E-15,0.,38.989));
#178482=CARTESIAN_POINT('',(60.6410923272405,0.318076890623366,39.2708017080178));
#178483=CARTESIAN_POINT('',(60.3421421673489,6.02238575973002,39.2708017078546));
#178484=CARTESIAN_POINT('Origin',(5.52999282761009E-15,0.,39.2708017080178));
#178485=CARTESIAN_POINT('',(60.3421421670676,6.02238575970194,39.2708017080178));
#178486=CARTESIAN_POINT('',(60.4783917829566,0.318078445374005,38.989));
#178487=CARTESIAN_POINT('Origin',(60.71525,0.,39.3978017080178));
#178488=CARTESIAN_POINT('',(61.0122769227456,0.3175,39.3978017080178));
#178489=CARTESIAN_POINT('',(60.7112330730305,6.06175884541488,39.3978017080178));
#178490=CARTESIAN_POINT('Origin',(5.5478765747851E-15,0.,39.3978017080178));
#178491=CARTESIAN_POINT('',(60.5608532912344,6.04595329344978,39.3978017080178));
#178492=CARTESIAN_POINT('',(60.561380412237,6.04600869609965,39.3978017080178));
#178493=CARTESIAN_POINT('',(60.8610688070707,0.3175,39.3978017080178));
#178494=CARTESIAN_POINT('Origin',(5.5478765747851E-15,0.,39.3978017080178));
#178495=CARTESIAN_POINT('',(60.71525,0.3175,39.3978017080178));
#178496=CARTESIAN_POINT('Origin',(5.5478765747851E-15,0.,39.3978017080178));
#178497=CARTESIAN_POINT('',(61.0917542093525,6.10232411256005,38.9890000005754));
#178498=CARTESIAN_POINT('',(61.0918106390013,6.1017591594455,38.989));
#178499=CARTESIAN_POINT('Origin',(5.49031038273072E-15,0.,38.989));
#178500=CARTESIAN_POINT('',(60.9299448846691,6.08531878138237,39.2708017080178));
#178501=CARTESIAN_POINT('',(61.0917542096815,6.10232411260841,38.989));
#178502=CARTESIAN_POINT('',(61.2322532923707,0.316930737397327,39.2708017081757));
#178503=CARTESIAN_POINT('Origin',(5.52999282761008E-15,0.,39.2708017080178));
#178504=CARTESIAN_POINT('',(61.3949537495049,0.31693224325326,38.9890000005756));
#178505=CARTESIAN_POINT('',(61.2322532920972,0.316930737395914,39.2708017080178));
#178506=CARTESIAN_POINT('',(61.3949508163454,0.3175,38.989));
#178507=CARTESIAN_POINT('Origin',(5.49031038273072E-15,0.,38.989));
#178508=CARTESIAN_POINT('Origin',(5.49031038273072E-15,0.,38.989));
#178509=CARTESIAN_POINT('Origin',(62.2224557307631,0.,38.989));
#178510=CARTESIAN_POINT('',(61.8696548221181,0.3175,38.989));
#178511=CARTESIAN_POINT('',(61.5639141665613,6.15137923967592,38.989));
#178512=CARTESIAN_POINT('Origin',(5.49031038273072E-15,0.,38.989));
#178513=CARTESIAN_POINT('',(61.0923331762718,6.10181408032572,38.989));
#178514=CARTESIAN_POINT('',(62.2224557307631,0.3175,38.989));
#178515=CARTESIAN_POINT('Origin',(5.57972911860581E-15,0.,39.624));
#178516=CARTESIAN_POINT('Origin',(59.7081714060831,5.95632779542214,39.6240070731883));
#178517=CARTESIAN_POINT('Origin',(60.0036895869254,0.317504993060516,39.6240070731883));
#178518=CARTESIAN_POINT('Origin',(5.57972911860581E-15,0.,39.624));
#178519=CARTESIAN_POINT('Origin',(61.6018378049617,6.15533145331002,39.555211759881));
#178520=CARTESIAN_POINT('Origin',(61.9077842377873,0.31753353701155,39.5552135207987));
#178521=CARTESIAN_POINT('Origin',(5.51210908043506E-15,0.,39.1438017080178));
#178522=CARTESIAN_POINT('Origin',(60.7269085901936,6.06344346747426,39.1712173702614));
#178523=CARTESIAN_POINT('Origin',(61.0281367271395,0.31746290747849,39.1711625381338));
#178524=CARTESIAN_POINT('Origin',(5.51210908043507E-15,0.,39.1438017080178));
#178525=CARTESIAN_POINT('Origin',(60.5450849487961,6.04425010054726,39.1711627526728));
#178526=CARTESIAN_POINT('Origin',(60.845302880269,0.317545368445466,39.171217585939));
#178527=CARTESIAN_POINT('Origin',(60.4792282238308,0.,38.989));
#178528=CARTESIAN_POINT('',(58.7584778814678,12.1649068885784,38.989));
#178529=CARTESIAN_POINT('',(59.6417962403144,6.58785426247015,38.989));
#178530=CARTESIAN_POINT('Origin',(5.49031038273072E-15,0.,38.989));
#178531=CARTESIAN_POINT('',(60.1139000598801,6.637474373417,38.989));
#178532=CARTESIAN_POINT('',(59.7852323155142,6.60293000146354,38.989));
#178533=CARTESIAN_POINT('',(60.1138365744453,6.63804933242023,38.9889999995773));
#178534=CARTESIAN_POINT('Origin',(5.49031038273072E-15,0.,38.989));
#178535=CARTESIAN_POINT('',(59.2229260464988,12.2630370254216,38.9889999997818));
#178536=CARTESIAN_POINT('Origin',(5.49031038273072E-15,0.,38.989));
#178537=CARTESIAN_POINT('',(59.2228087529784,12.2636034620781,38.989));
#178538=CARTESIAN_POINT('Origin',(5.49031038273072E-15,0.,38.989));
#178539=CARTESIAN_POINT('',(58.7590037315227,12.165018661458,38.989));
#178540=CARTESIAN_POINT('Origin',(5.49031038273072E-15,0.,38.989));
#178541=CARTESIAN_POINT('',(60.275645989912,6.65505462397314,39.2708017080178));
#178542=CARTESIAN_POINT('',(60.1138365737176,6.63804933233988,38.989));
#178543=CARTESIAN_POINT('',(59.3820708701841,12.2968658914369,39.2708017078546));
#178544=CARTESIAN_POINT('Origin',(5.52999282761009E-15,0.,39.2708017080178));
#178545=CARTESIAN_POINT('',(59.3820708699072,12.2968658913796,39.2708017080178));
#178546=CARTESIAN_POINT('Origin',(60.71525,0.,39.3978017080178));
#178547=CARTESIAN_POINT('',(59.5971203935661,12.3431658574203,39.3978017080178));
#178548=CARTESIAN_POINT('',(60.4944777170595,6.67747469700864,39.3978017080178));
#178549=CARTESIAN_POINT('Origin',(5.5478765747851E-15,0.,39.3978017080178));
#178550=CARTESIAN_POINT('',(60.6448574988555,6.69328024897373,39.3978017080178));
#178551=CARTESIAN_POINT('',(60.0186752706393,6.62746584474012,39.3978017080178));
#178552=CARTESIAN_POINT('',(59.7450242491249,12.3746037924156,39.3978017080178));
#178553=CARTESIAN_POINT('Origin',(5.5478765747851E-15,0.,39.3978017080178));
#178554=CARTESIAN_POINT('',(59.5976388357908,12.343276055717,39.3978017080178));
#178555=CARTESIAN_POINT('Origin',(5.5478765747851E-15,0.,39.3978017080178));
#178556=CARTESIAN_POINT('',(59.9600752506739,12.4208962741579,39.2708017080178));
#178557=CARTESIAN_POINT('',(60.8636883190564,6.71570789672327,39.2708017081757));
#178558=CARTESIAN_POINT('Origin',(5.52999282761008E-15,0.,39.2708017080178));
#178559=CARTESIAN_POINT('',(61.025497328658,6.73271622308714,38.9890000005756));
#178560=CARTESIAN_POINT('',(60.8636883187846,6.71570789669327,39.2708017080178));
#178561=CARTESIAN_POINT('',(61.0254350648263,6.73328056300436,38.989));
#178562=CARTESIAN_POINT('Origin',(5.49031038273072E-15,0.,38.989));
#178563=CARTESIAN_POINT('',(60.119335800013,12.4541661686658,38.989));
#178564=CARTESIAN_POINT('Origin',(5.49031038273072E-15,0.,38.989));
#178565=CARTESIAN_POINT('',(60.1192206258109,12.4547221284036,38.9890000005754));
#178566=CARTESIAN_POINT('Origin',(5.49031038273072E-15,0.,38.989));
#178567=CARTESIAN_POINT('',(60.1192206261331,12.4547221284861,38.989));
#178568=CARTESIAN_POINT('Origin',(62.2224557307631,0.,38.989));
#178569=CARTESIAN_POINT('',(61.4975385923863,6.78290064323477,38.989));
#178570=CARTESIAN_POINT('',(61.5094129706999,6.78414869068668,38.989));
#178571=CARTESIAN_POINT('',(60.5836663843183,12.5528626811439,38.989));
#178572=CARTESIAN_POINT('Origin',(5.49031038273072E-15,0.,38.989));
#178573=CARTESIAN_POINT('',(60.1198497339745,12.4542754087016,38.989));
#178574=CARTESIAN_POINT('Origin',(5.57972911860581E-15,0.,39.624));
#178575=CARTESIAN_POINT('Origin',(59.6417947880742,6.58785913039734,39.6240070731883));
#178576=CARTESIAN_POINT('Origin',(58.7584780045776,12.1649018101376,39.6240070731883));
#178577=CARTESIAN_POINT('Origin',(5.57972911860581E-15,0.,39.624));
#178578=CARTESIAN_POINT('Origin',(61.535455625554,6.78691960575244,39.5552135207993));
#178579=CARTESIAN_POINT('Origin',(60.6209691542404,12.5607573437818,39.5552117598835));
#178580=CARTESIAN_POINT('Origin',(5.51210908043506E-15,0.,39.1438017080178));
#178581=CARTESIAN_POINT('Origin',(60.6606342988042,6.69490116062979,39.1711625381311));
#178582=CARTESIAN_POINT('Origin',(59.7604378032078,12.3779177236587,39.1712173702578));
#178583=CARTESIAN_POINT('Origin',(5.51210908043507E-15,0.,39.1438017080178));
#178584=CARTESIAN_POINT('Origin',(60.4787934153619,6.67587182882045,39.1712175859371));
#178585=CARTESIAN_POINT('Origin',(59.5816164638931,12.3398237541811,39.1711627526761));
#178586=CARTESIAN_POINT('Origin',(60.4792282238308,0.,38.989));
#178587=CARTESIAN_POINT('',(57.1650137687749,18.2401996527038,38.989));
#178588=CARTESIAN_POINT('',(58.6264539577985,12.7860306150444,38.989));
#178589=CARTESIAN_POINT('Origin',(5.49031038273072E-15,0.,38.989));
#178590=CARTESIAN_POINT('',(59.0907848292992,12.8847271885936,38.989));
#178591=CARTESIAN_POINT('',(57.7988642628865,12.6101209950203,38.989));
#178592=CARTESIAN_POINT('',(59.0906615920642,12.8852923618765,38.9889999995768));
#178593=CARTESIAN_POINT('Origin',(5.49031038273072E-15,0.,38.989));
#178594=CARTESIAN_POINT('',(57.6166602457575,18.386340275348,38.9889999997818));
#178595=CARTESIAN_POINT('Origin',(5.49031038273072E-15,0.,38.989));
#178596=CARTESIAN_POINT('',(57.6164843860299,18.3868913484938,38.989));
#178597=CARTESIAN_POINT('Origin',(5.49031038273072E-15,0.,38.989));
#178598=CARTESIAN_POINT('',(57.1655250547209,18.240365779578,38.989));
#178599=CARTESIAN_POINT('Origin',(5.49031038273072E-15,0.,38.989));
#178600=CARTESIAN_POINT('',(59.2498070616281,12.9191181862038,39.2708017080178));
#178601=CARTESIAN_POINT('',(59.0906615913479,12.8852923617204,38.989));
#178602=CARTESIAN_POINT('',(57.7713971780683,18.4366189871525,39.2708017078546));
#178603=CARTESIAN_POINT('Origin',(5.52999282761009E-15,0.,39.2708017080178));
#178604=CARTESIAN_POINT('',(57.771397177799,18.4366189870665,39.2708017080178));
#178605=CARTESIAN_POINT('Origin',(60.71525,0.,39.3978017080178));
#178606=CARTESIAN_POINT('',(57.9804289733666,18.5051441132834,39.3978017080178));
#178607=CARTESIAN_POINT('',(59.4650964698968,12.9642895838863,39.3978017080178));
#178608=CARTESIAN_POINT('Origin',(5.5478765747851E-15,0.,39.3978017080178));
#178609=CARTESIAN_POINT('',(59.6130003254557,12.9957275188816,39.3978017080178));
#178610=CARTESIAN_POINT('',(58.0246834617332,12.6581203474863,39.3978017080178));
#178611=CARTESIAN_POINT('',(58.1242364370959,18.5518699907143,39.3978017080178));
#178612=CARTESIAN_POINT('Origin',(5.5478765747851E-15,0.,39.3978017080178));
#178613=CARTESIAN_POINT('',(57.9809330566519,18.5053078998713,39.3978017080178));
#178614=CARTESIAN_POINT('Origin',(5.5478765747851E-15,0.,39.3978017080178));
#178615=CARTESIAN_POINT('',(58.3332704847798,18.620387828114,39.2708017080178));
#178616=CARTESIAN_POINT('',(59.8282880399729,13.0409063549813,39.2708017081757));
#178617=CARTESIAN_POINT('Origin',(5.52999282761008E-15,0.,39.2708017080178));
#178618=CARTESIAN_POINT('',(59.9874327886719,13.0747351550703,38.9890000005756));
#178619=CARTESIAN_POINT('',(59.8282880397057,13.0409063549231,39.2708017080178));
#178620=CARTESIAN_POINT('',(59.9873118763437,13.0752898951317,38.989));
#178621=CARTESIAN_POINT('Origin',(5.49031038273072E-15,0.,38.989));
#178622=CARTESIAN_POINT('',(58.48818093722,18.6701227271403,38.989));
#178623=CARTESIAN_POINT('Origin',(5.49031038273072E-15,0.,38.989));
#178624=CARTESIAN_POINT('',(58.4880082803372,18.6706636022901,38.9890000005754));
#178625=CARTESIAN_POINT('Origin',(5.49031038273072E-15,0.,38.989));
#178626=CARTESIAN_POINT('',(58.488008280649,18.6706636024058,38.989));
#178627=CARTESIAN_POINT('Origin',(62.2224557307631,0.,38.989));
#178628=CARTESIAN_POINT('',(60.4516424606491,13.1739864076099,38.989));
#178629=CARTESIAN_POINT('',(59.4667368016504,12.9646382471638,38.989));
#178630=CARTESIAN_POINT('',(58.9396512752216,18.8168143322219,38.989));
#178631=CARTESIAN_POINT('Origin',(5.49031038273072E-15,0.,38.989));
#178632=CARTESIAN_POINT('',(58.4886806371044,18.6702850894749,38.989));
#178633=CARTESIAN_POINT('Origin',(5.57972911860581E-15,0.,39.624));
#178634=CARTESIAN_POINT('Origin',(58.626452004677,12.7860353045041,39.6240070731883));
#178635=CARTESIAN_POINT('Origin',(57.165014422052,18.2401946149516,39.6240070731883));
#178636=CARTESIAN_POINT('Origin',(5.57972911860581E-15,0.,39.624));
#178637=CARTESIAN_POINT('Origin',(60.4889316843632,13.1819467630385,39.5552135208047));
#178638=CARTESIAN_POINT('Origin',(58.975924479715,18.8285649482875,39.5552117598805));
#178639=CARTESIAN_POINT('Origin',(5.51210908043506E-15,0.,39.1438017080178));
#178640=CARTESIAN_POINT('Origin',(59.6285212670419,12.9989886756685,39.1711625381368));
#178641=CARTESIAN_POINT('Origin',(58.1392191539782,18.5567769230176,39.1712173702607));
#178642=CARTESIAN_POINT('Origin',(5.51210908043507E-15,0.,39.1438017080178));
#178643=CARTESIAN_POINT('Origin',(59.4496656337923,12.9610560404236,39.1712175859393));
#178644=CARTESIAN_POINT('Origin',(57.9653593207591,18.5001997164918,39.1711627526745));
#178645=CARTESIAN_POINT('Origin',(60.4792282238308,0.,38.989));
#178646=CARTESIAN_POINT('',(54.9452378026832,24.115648972427,38.989));
#178647=CARTESIAN_POINT('',(56.9687879773468,18.8441205405512,38.989));
#178648=CARTESIAN_POINT('Origin',(5.49031038273072E-15,0.,38.989));
#178649=CARTESIAN_POINT('',(57.4202585945868,18.9908122363895,38.989));
#178650=CARTESIAN_POINT('',(54.6058629360818,18.0763596539223,38.989));
#178651=CARTESIAN_POINT('',(57.4200769557624,18.9913614317948,38.9889999995774));
#178652=CARTESIAN_POINT('Origin',(5.49031038273072E-15,0.,38.989));
#178653=CARTESIAN_POINT('',(55.3791342583023,24.3081989336286,38.9889999997818));
#178654=CARTESIAN_POINT('Origin',(5.49031038273072E-15,0.,38.989));
#178655=CARTESIAN_POINT('',(55.3789017591236,24.308728605591,38.989));
#178656=CARTESIAN_POINT('Origin',(5.49031038273072E-15,0.,38.989));
#178657=CARTESIAN_POINT('',(54.9457289227643,24.1158676331751,38.989));
#178658=CARTESIAN_POINT('Origin',(5.49031038273072E-15,0.,38.989));
#178659=CARTESIAN_POINT('',(57.5748148483578,19.041637186087,39.2708017080178));
#178660=CARTESIAN_POINT('',(57.4200769550675,18.991361431565,38.989));
#178661=CARTESIAN_POINT('',(55.5277679690275,24.3743766271344,39.2708017078546));
#178662=CARTESIAN_POINT('Origin',(5.52999282761009E-15,0.,39.2708017080178));
#178663=CARTESIAN_POINT('',(55.5277679687686,24.3743766270207,39.2708017080178));
#178664=CARTESIAN_POINT('Origin',(60.71525,0.,39.3978017080178));
#178665=CARTESIAN_POINT('',(55.7284918401501,24.464376137791,39.3978017080178));
#178666=CARTESIAN_POINT('',(57.7842031819385,19.1090650011308,39.3978017080178));
#178667=CARTESIAN_POINT('Origin',(5.5478765747851E-15,0.,39.3978017080178));
#178668=CARTESIAN_POINT('',(57.9280106456678,19.1557908785618,39.3978017080178));
#178669=CARTESIAN_POINT('',(54.8193466381482,18.1457247135484,39.3978017080178));
#178670=CARTESIAN_POINT('',(55.8666273273836,24.5258780191664,39.3978017080178));
#178671=CARTESIAN_POINT('Origin',(5.5478765747851E-15,0.,39.3978017080178));
#178672=CARTESIAN_POINT('',(55.7289760416541,24.4645917181901,39.3978017080178));
#178673=CARTESIAN_POINT('Origin',(5.5478765747851E-15,0.,39.3978017080178));
#178674=CARTESIAN_POINT('',(56.0673542004329,24.6158705164587,39.2708017080178));
#178675=CARTESIAN_POINT('',(58.1373965172492,19.2232259142291,39.2708017081757));
#178676=CARTESIAN_POINT('Origin',(5.52999282761008E-15,0.,39.2708017080178));
#178677=CARTESIAN_POINT('',(58.2921333818759,19.2735045526302,38.9890000005756));
#178678=CARTESIAN_POINT('',(58.1373965169896,19.2232259141432,39.2708017080178));
#178679=CARTESIAN_POINT('',(58.2919551457919,19.2740436149877,38.989));
#178680=CARTESIAN_POINT('Origin',(5.49031038273072E-15,0.,38.989));
#178681=CARTESIAN_POINT('',(56.2162173246401,24.6815255140419,38.989));
#178682=CARTESIAN_POINT('Origin',(5.49031038273072E-15,0.,38.989));
#178683=CARTESIAN_POINT('',(56.2159890767415,24.6820453786625,38.9890000005754));
#178684=CARTESIAN_POINT('Origin',(5.49031038273072E-15,0.,38.989));
#178685=CARTESIAN_POINT('',(56.2159890770395,24.6820453788101,38.989));
#178686=CARTESIAN_POINT('Origin',(62.2224557307631,0.,38.989));
#178687=CARTESIAN_POINT('',(58.7434254837935,19.4207352200693,38.989));
#178688=CARTESIAN_POINT('',(56.182627028633,18.588681363905,38.989));
#178689=CARTESIAN_POINT('',(56.6498810128385,24.8746050278046,38.989));
#178690=CARTESIAN_POINT('Origin',(5.49031038273072E-15,0.,38.989));
#178691=CARTESIAN_POINT('',(56.2166973156309,24.6817392197998,38.989));
#178692=CARTESIAN_POINT('Origin',(5.57972911860581E-15,0.,39.624));
#178693=CARTESIAN_POINT('Origin',(56.9687855447427,18.8441250001648,39.6240070731883));
#178694=CARTESIAN_POINT('Origin',(54.94523897897,24.1156440305582,39.6240070731883));
#178695=CARTESIAN_POINT('Origin',(5.57972911860581E-15,0.,39.624));
#178696=CARTESIAN_POINT('Origin',(58.77967834952,19.4325497530897,39.5552135208021));
#178697=CARTESIAN_POINT('Origin',(56.6847272350833,24.8900828550895,39.555211759879));
#178698=CARTESIAN_POINT('Origin',(5.51210908043506E-15,0.,39.1438017080178));
#178699=CARTESIAN_POINT('Origin',(57.9431056782062,19.1606565505636,39.1711625381395));
#178700=CARTESIAN_POINT('Origin',(55.8810150532815,24.5323241911521,39.171217370259));
#178701=CARTESIAN_POINT('Origin',(5.51210908043507E-15,0.,39.1438017080178));
#178702=CARTESIAN_POINT('Origin',(57.7691948748958,19.1042362097737,39.1712175859413));
#178703=CARTESIAN_POINT('Origin',(55.7140215708744,24.4578836192922,39.1711627526757));
#178704=CARTESIAN_POINT('Origin',(60.4792282238308,0.,38.989));
#178705=CARTESIAN_POINT('',(52.123470313195,29.7268821954843,38.989));
#178706=CARTESIAN_POINT('',(54.68696003433,24.6957503380301,38.989));
#178707=CARTESIAN_POINT('Origin',(5.49031038273072E-15,0.,38.989));
#178708=CARTESIAN_POINT('',(55.1206239907505,24.8888299712405,38.989));
#178709=CARTESIAN_POINT('',(50.3447265545032,22.7624634345041,38.989));
#178710=CARTESIAN_POINT('',(55.1203859404108,24.8893571716688,38.9889999995774));
#178711=CARTESIAN_POINT('Origin',(5.49031038273072E-15,0.,38.989));
#178712=CARTESIAN_POINT('',(52.5348628870842,29.9637318775748,38.9889999997818));
#178713=CARTESIAN_POINT('Origin',(5.49031038273072E-15,0.,38.989));
#178714=CARTESIAN_POINT('',(52.5345762957642,29.9642343451569,38.989));
#178715=CARTESIAN_POINT('Origin',(5.49031038273072E-15,0.,38.989));
#178716=CARTESIAN_POINT('',(52.123935886597,29.7271509944133,38.989));
#178717=CARTESIAN_POINT('Origin',(5.49031038273072E-15,0.,38.989));
#178718=CARTESIAN_POINT('',(55.2690209153043,24.9555320242408,39.2708017080178));
#178719=CARTESIAN_POINT('',(55.1203859397437,24.8893571713676,38.989));
#178720=CARTESIAN_POINT('',(52.6757649141856,30.0450834961231,39.2708017078546));
#178721=CARTESIAN_POINT('Origin',(5.52999282761009E-15,0.,39.2708017080178));
#178722=CARTESIAN_POINT('',(52.67576491394,30.045083495983,39.2708017080178));
#178723=CARTESIAN_POINT('Origin',(60.71525,0.,39.3978017080178));
#178724=CARTESIAN_POINT('',(52.8659816883963,30.1555713378331,39.3978017080178));
#178725=CARTESIAN_POINT('',(55.470214071797,25.0444775033941,39.3978017080178));
#178726=CARTESIAN_POINT('Origin',(5.5478765747851E-15,0.,39.3978017080178));
#178727=CARTESIAN_POINT('',(55.6083495590305,25.1059793847695,39.3978017080178));
#178728=CARTESIAN_POINT('',(50.5417021396889,22.8501626153342,39.3978017080178));
#178729=CARTESIAN_POINT('',(52.9969317578291,30.2311753956706,39.3978017080178));
#178730=CARTESIAN_POINT('Origin',(5.5478765747851E-15,0.,39.3978017080178));
#178731=CARTESIAN_POINT('',(52.866440703106,30.1558363500993,39.3978017080178));
#178732=CARTESIAN_POINT('Origin',(5.5478765747851E-15,0.,39.3978017080178));
#178733=CARTESIAN_POINT('',(53.1871522506179,30.3416565762229,39.2708017080178));
#178734=CARTESIAN_POINT('',(55.8095395122503,25.1949317876419,39.2708017081757));
#178735=CARTESIAN_POINT('Origin',(5.52999282761008E-15,0.,39.2708017080178));
#178736=CARTESIAN_POINT('',(55.9581731633348,25.2611094010714,38.9890000005756));
#178737=CARTESIAN_POINT('',(55.809539512001,25.1949317875294,39.2708017080178));
#178738=CARTESIAN_POINT('',(55.9579395562869,25.261626879645,38.989));
#178739=CARTESIAN_POINT('Origin',(5.49031038273072E-15,0.,38.989));
#178740=CARTESIAN_POINT('',(53.3283370710516,30.4225123424704,38.989));
#178741=CARTESIAN_POINT('Origin',(5.49031038273072E-15,0.,38.989));
#178742=CARTESIAN_POINT('',(53.328055732869,30.4230055008161,38.9890000005754));
#178743=CARTESIAN_POINT('Origin',(5.49031038273072E-15,0.,38.989));
#178744=CARTESIAN_POINT('',(53.32805573315,30.4230055009941,38.989));
#178745=CARTESIAN_POINT('Origin',(62.2224557307631,0.,38.989));
#178746=CARTESIAN_POINT('',(56.3916032444854,25.4547063934076,38.989));
#178747=CARTESIAN_POINT('',(51.7995637473369,23.4101986852074,38.989));
#178748=CARTESIAN_POINT('',(53.7394427993291,30.6598643453568,38.989));
#178749=CARTESIAN_POINT('Origin',(5.49031038273072E-15,0.,38.989));
#178750=CARTESIAN_POINT('',(53.3287920942672,30.4227750502464,38.989));
#178751=CARTESIAN_POINT('Origin',(5.57972911860581E-15,0.,39.624));
#178752=CARTESIAN_POINT('Origin',(54.6869571488954,24.6957545189371,39.6240070731883));
#178753=CARTESIAN_POINT('Origin',(52.1234719996039,29.7268774036431,39.6240070731883));
#178754=CARTESIAN_POINT('Origin',(5.57972911860581E-15,0.,39.624));
#178755=CARTESIAN_POINT('Origin',(56.4264225582409,25.4702456615226,39.5552135207995));
#178756=CARTESIAN_POINT('Origin',(53.7724802568187,30.6788998055464,39.5552117598838));
#178757=CARTESIAN_POINT('Origin',(5.51210908043506E-15,0.,39.1438017080178));
#178758=CARTESIAN_POINT('Origin',(55.6228532981798,25.1123962626632,39.1711625381312));
#178759=CARTESIAN_POINT('Origin',(53.0105668578091,30.2390901817305,39.1712173702627));
#178760=CARTESIAN_POINT('Origin',(5.51210908043507E-15,0.,39.1438017080178));
#178761=CARTESIAN_POINT('Origin',(55.4557927279734,25.03810636939,39.1712175859376));
#178762=CARTESIAN_POINT('Origin',(52.8522693417516,30.1476018310223,39.1711627526727));
#178763=CARTESIAN_POINT('Origin',(60.4792282238308,0.,38.989));
#178764=CARTESIAN_POINT('',(48.7306271754181,35.0124214764579,38.989));
#178765=CARTESIAN_POINT('',(51.805970313195,30.2768083268874,38.989));
#178766=CARTESIAN_POINT('Origin',(5.49031038273072E-15,0.,38.989));
#178767=CARTESIAN_POINT('',(52.2170762957395,30.5141604766041,38.989));
#178768=CARTESIAN_POINT('',(45.2006711678738,26.4632370872583,38.989));
#178769=CARTESIAN_POINT('',(52.2167844420139,30.5146599059371,38.9889999995774));
#178770=CARTESIAN_POINT('Origin',(5.49031038273072E-15,0.,38.989));
#178771=CARTESIAN_POINT('',(49.1150085644485,35.2909759047562,38.9889999997818));
#178772=CARTESIAN_POINT('Origin',(5.49031038273072E-15,0.,38.989));
#178773=CARTESIAN_POINT('',(49.1146710209415,35.2914456628181,38.989));
#178774=CARTESIAN_POINT('Origin',(5.49031038273072E-15,0.,38.989));
#178775=CARTESIAN_POINT('',(48.7310621012213,35.0127374685504,38.989));
#178776=CARTESIAN_POINT('Origin',(5.49031038273072E-15,0.,38.989));
#178777=CARTESIAN_POINT('',(52.3576880233166,30.5960088312562,39.2708017080178));
#178778=CARTESIAN_POINT('',(52.2167844413819,30.5146599055678,38.989));
#178779=CARTESIAN_POINT('',(49.2466351558313,35.3866101429904,39.2708017078546));
#178780=CARTESIAN_POINT('Origin',(5.52999282761009E-15,0.,39.2708017080178));
#178781=CARTESIAN_POINT('',(49.2466351556017,35.3866101428254,39.2708017080178));
#178782=CARTESIAN_POINT('Origin',(60.71525,0.,39.3978017080178));
#178783=CARTESIAN_POINT('',(49.4242607783465,35.516375787839,39.3978017080178));
#178784=CARTESIAN_POINT('',(52.5484816883963,30.7054974692362,39.3978017080178));
#178785=CARTESIAN_POINT('Origin',(5.5478765747851E-15,0.,39.3978017080178));
#178786=CARTESIAN_POINT('',(52.6794317578291,30.7811015270737,39.3978017080178));
#178787=CARTESIAN_POINT('',(45.3776875000007,26.5654375142627,39.3978017080178));
#178788=CARTESIAN_POINT('',(49.5465907136149,35.6052536882596,39.3978017080178));
#178789=CARTESIAN_POINT('Origin',(5.5478765747851E-15,0.,39.3978017080178));
#178790=CARTESIAN_POINT('',(49.4246895772007,35.5166873284425,39.3978017080178));
#178791=CARTESIAN_POINT('Origin',(5.5478765747851E-15,0.,39.3978017080178));
#178792=CARTESIAN_POINT('',(49.7242207306179,35.7350130971383,39.2708017080178));
#178793=CARTESIAN_POINT('',(52.8702215134581,30.8905967160109,39.2708017081757));
#178794=CARTESIAN_POINT('Origin',(5.52999282761008E-15,0.,39.2708017080178));
#178795=CARTESIAN_POINT('',(53.0111234896157,30.9719482486875,38.9890000005756));
#178796=CARTESIAN_POINT('',(52.870221513222,30.8905967158729,39.2708017080178));
#178797=CARTESIAN_POINT('',(53.0108370710516,30.9724384738736,38.989));
#178798=CARTESIAN_POINT('Origin',(5.49031038273072E-15,0.,38.989));
#178799=CARTESIAN_POINT('',(49.8561803968407,35.8301837593549,38.989));
#178800=CARTESIAN_POINT('Origin',(5.49031038273072E-15,0.,38.989));
#178801=CARTESIAN_POINT('',(49.8558490507741,35.8306448082797,38.9890000005754));
#178802=CARTESIAN_POINT('Origin',(5.49031038273072E-15,0.,38.989));
#178803=CARTESIAN_POINT('',(49.8558490510349,35.830644808486,38.989));
#178804=CARTESIAN_POINT('Origin',(62.2224557307631,0.,38.989));
#178805=CARTESIAN_POINT('',(53.4219427993291,31.2097904767599,38.989));
#178806=CARTESIAN_POINT('',(46.508091798073,27.2180767400479,38.989));
#178807=CARTESIAN_POINT('',(50.2402240048087,36.1092077731522,38.989));
#178808=CARTESIAN_POINT('Origin',(5.49031038273072E-15,0.,38.989));
#178809=CARTESIAN_POINT('',(49.8566054669514,35.8304925908676,38.989));
#178810=CARTESIAN_POINT('Origin',(5.57972911860581E-15,0.,39.624));
#178811=CARTESIAN_POINT('Origin',(51.8059670065433,30.2768121832809,39.6240070731883));
#178812=CARTESIAN_POINT('Origin',(48.7306293534724,35.0124168871446,39.6240070731883));
#178813=CARTESIAN_POINT('Origin',(5.57972911860581E-15,0.,39.624));
#178814=CARTESIAN_POINT('Origin',(53.454947073427,31.2288842284962,39.5552135207965));
#178815=CARTESIAN_POINT('Origin',(50.271090732248,36.1315923097651,39.5552117598796));
#178816=CARTESIAN_POINT('Origin',(5.51210908043506E-15,0.,39.1438017080178));
#178817=CARTESIAN_POINT('Origin',(52.6931852975962,30.7889993062059,39.1711625381385));
#178818=CARTESIAN_POINT('Origin',(49.5593237986654,35.6145503723399,39.1712173702604));
#178819=CARTESIAN_POINT('Origin',(5.51210908043507E-15,0.,39.1438017080178));
#178820=CARTESIAN_POINT('Origin',(52.5348053110498,30.6976537960598,39.1712175859399));
#178821=CARTESIAN_POINT('Origin',(49.4114565896725,35.507016608296,39.171162752673));
#178822=CARTESIAN_POINT('Origin',(60.4792282238308,0.,38.989));
#178823=CARTESIAN_POINT('',(44.8038810887679,39.9143573409152,38.989));
#178824=CARTESIAN_POINT('',(48.3573835402124,35.526147267886,38.989));
#178825=CARTESIAN_POINT('Origin',(5.49031038273072E-15,0.,38.989));
#178826=CARTESIAN_POINT('',(48.7414273857065,35.8051714542874,38.989));
#178827=CARTESIAN_POINT('',(39.3975469582356,29.0164449471018,38.989));
#178828=CARTESIAN_POINT('',(48.7410849262056,35.805637640673,38.9889999995773));
#178829=CARTESIAN_POINT('Origin',(5.49031038273072E-15,0.,38.989));
#178830=CARTESIAN_POINT('',(45.1570399300043,40.2315646148137,38.9889999997818));
#178831=CARTESIAN_POINT('Origin',(5.49031038273072E-15,0.,38.989));
#178832=CARTESIAN_POINT('',(45.1566551325076,40.2319965165876,38.989));
#178833=CARTESIAN_POINT('Origin',(5.49031038273072E-15,0.,38.989));
#178834=CARTESIAN_POINT('',(44.8042806018342,39.9147170640958,38.989));
#178835=CARTESIAN_POINT('Origin',(5.49031038273072E-15,0.,38.989));
#178836=CARTESIAN_POINT('',(48.8727133447948,35.9012693628899,39.2708017080178));
#178837=CARTESIAN_POINT('',(48.7410849256156,35.8056376402395,38.989));
#178838=CARTESIAN_POINT('',(45.2779489571888,40.3404336840068,39.2708017078546));
#178839=CARTESIAN_POINT('Origin',(5.52999282761009E-15,0.,39.2708017080178));
#178840=CARTESIAN_POINT('',(45.2779489569777,40.3404336838187,39.2708017080178));
#178841=CARTESIAN_POINT('Origin',(60.71525,0.,39.3978017080178));
#178842=CARTESIAN_POINT('',(45.4410373245177,40.4880553924338,39.3978017080178));
#178843=CARTESIAN_POINT('',(49.0510171431408,36.0301015792671,39.3978017080178));
#178844=CARTESIAN_POINT('Origin',(5.5478765747851E-15,0.,39.3978017080178));
#178845=CARTESIAN_POINT('',(49.1733470784092,36.1189794796877,39.3978017080178));
#178846=CARTESIAN_POINT('',(39.5520252162596,29.1286799712085,39.3978017080178));
#178847=CARTESIAN_POINT('',(45.5534068532516,40.5892333705617,39.3978017080178));
#178848=CARTESIAN_POINT('Origin',(5.5478765747851E-15,0.,39.3978017080178));
#178849=CARTESIAN_POINT('',(45.4414312095063,40.4884100480706,39.3978017080178));
#178850=CARTESIAN_POINT('Origin',(5.5478765747851E-15,0.,39.3978017080178));
#178851=CARTESIAN_POINT('',(45.7165002428312,40.7368493365292,39.2708017080178));
#178852=CARTESIAN_POINT('',(49.3516463039594,36.2478178024864,39.2708017081757));
#178853=CARTESIAN_POINT('Origin',(5.52999282761008E-15,0.,39.2708017080178));
#178854=CARTESIAN_POINT('',(49.4832728536536,36.3434519499941,38.9890000005756));
#178855=CARTESIAN_POINT('',(49.351646303739,36.2478178023245,39.2708017080178));
#178856=CARTESIAN_POINT('',(49.482936761635,36.343909550783,38.989));
#178857=CARTESIAN_POINT('Origin',(5.49031038273072E-15,0.,38.989));
#178858=CARTESIAN_POINT('',(45.8377889771256,40.8452921850238,38.989));
#178859=CARTESIAN_POINT('Origin',(5.49031038273072E-15,0.,38.989));
#178860=CARTESIAN_POINT('',(45.8374112534718,40.8457160731792,38.9890000005754));
#178861=CARTESIAN_POINT('Origin',(5.49031038273072E-15,0.,38.989));
#178862=CARTESIAN_POINT('',(45.8374112537096,40.8457160734117,38.989));
#178863=CARTESIAN_POINT('Origin',(62.2224557307631,0.,38.989));
#178864=CARTESIAN_POINT('',(49.866980369603,36.6229335645803,38.989));
#178865=CARTESIAN_POINT('',(40.5385041740537,29.8453988870283,38.989));
#178866=CARTESIAN_POINT('',(46.190562802649,41.1629311642475,38.989));
#178867=CARTESIAN_POINT('Origin',(5.49031038273072E-15,0.,38.989));
#178868=CARTESIAN_POINT('',(45.8381794369742,40.8456437566507,38.989));
#178869=CARTESIAN_POINT('Origin',(5.57972911860581E-15,0.,39.624));
#178870=CARTESIAN_POINT('Origin',(48.3573798485719,35.5261507575145,39.6240070731883));
#178871=CARTESIAN_POINT('Origin',(44.8038837346046,39.9143530044112,39.6240070731883));
#178872=CARTESIAN_POINT('Origin',(5.57972911860581E-15,0.,39.624));
#178873=CARTESIAN_POINT('Origin',(49.8978080023047,36.6453726047993,39.5552135208004));
#178874=CARTESIAN_POINT('Origin',(46.2189206177148,41.1884195276092,39.5552117598801));
#178875=CARTESIAN_POINT('Origin',(5.51210908043506E-15,0.,39.1438017080178));
#178876=CARTESIAN_POINT('Origin',(49.18619973213,36.1282716303355,39.1711625381374));
#178877=CARTESIAN_POINT('Origin',(45.5650984170279,40.5998100962455,39.1712173702563));
#178878=CARTESIAN_POINT('Origin',(5.51210908043507E-15,0.,39.1438017080178));
#178879=CARTESIAN_POINT('Origin',(49.0382355735257,36.0208713038458,39.1712175859374));
#178880=CARTESIAN_POINT('Origin',(45.4292815791832,40.4774090812886,39.1711627526757));
#178881=CARTESIAN_POINT('Origin',(60.4792282238308,0.,38.989));
#178882=CARTESIAN_POINT('',(40.3862543050944,44.3789831537291,38.989));
#178883=CARTESIAN_POINT('',(44.37898315373,40.3862543050933,38.989));
#178884=CARTESIAN_POINT('Origin',(5.49031038273072E-15,0.,38.989));
#178885=CARTESIAN_POINT('',(44.7317571974364,40.7038934808038,38.989));
#178886=CARTESIAN_POINT('',(33.1880655373225,30.3099068238763,38.989));
#178887=CARTESIAN_POINT('',(44.731367884218,40.7043213166062,38.9889999995773));
#178888=CARTESIAN_POINT('Origin',(5.49031038273072E-15,0.,38.989));
#178889=CARTESIAN_POINT('',(40.7043213163689,44.7313678839551,38.9889999997818));
#178890=CARTESIAN_POINT('Origin',(5.49031038273072E-15,0.,38.989));
#178891=CARTESIAN_POINT('',(40.7038934808044,44.7317571974349,38.989));
#178892=CARTESIAN_POINT('Origin',(5.49031038273072E-15,0.,38.989));
#178893=CARTESIAN_POINT('',(40.386614028275,44.3793826667954,38.989));
#178894=CARTESIAN_POINT('Origin',(5.49031038273072E-15,0.,38.989));
#178895=CARTESIAN_POINT('',(44.8522789915946,40.8131880745601,39.2708017080178));
#178896=CARTESIAN_POINT('',(44.7313678836765,40.7043213161134,38.989));
#178897=CARTESIAN_POINT('',(40.8131880747515,44.8522789918028,39.2708017078546));
#178898=CARTESIAN_POINT('Origin',(5.52999282761009E-15,0.,39.2708017080178));
#178899=CARTESIAN_POINT('',(40.8131880745612,44.8522789915937,39.2708017080178));
#178900=CARTESIAN_POINT('Origin',(60.71525,0.,39.3978017080178));
#178901=CARTESIAN_POINT('',(40.959952356613,45.0161393894788,39.3978017080178));
#178902=CARTESIAN_POINT('',(45.0161393894798,40.959952356612,39.3978017080178));
#178903=CARTESIAN_POINT('Origin',(5.5478765747851E-15,0.,39.3978017080178));
#178904=CARTESIAN_POINT('',(45.1285089182138,41.0611303347399,39.3978017080178));
#178905=CARTESIAN_POINT('',(33.3184119221875,30.4272712359683,39.3978017080178));
#178906=CARTESIAN_POINT('',(41.0611303347409,45.1285089182128,39.3978017080178));
#178907=CARTESIAN_POINT('Origin',(5.5478765747851E-15,0.,39.3978017080178));
#178908=CARTESIAN_POINT('',(40.9603070122498,45.0165332744675,39.3978017080178));
#178909=CARTESIAN_POINT('Origin',(5.5478765747851E-15,0.,39.3978017080178));
#178910=CARTESIAN_POINT('',(41.2079002115913,45.2923641298552,39.2708017080178));
#178911=CARTESIAN_POINT('',(45.2923641300585,41.2079002117742,39.2708017081757));
#178912=CARTESIAN_POINT('Origin',(5.52999282761008E-15,0.,39.2708017080178));
#178913=CARTESIAN_POINT('',(45.4132731252663,41.3167691863804,38.9890000005756));
#178914=CARTESIAN_POINT('',(45.2923641298562,41.2079002115902,39.2708017080178));
#178915=CARTESIAN_POINT('',(45.4128910420877,41.317189149202,38.989));
#178916=CARTESIAN_POINT('Origin',(5.49031038273072E-15,0.,38.989));
#178917=CARTESIAN_POINT('',(41.3171891492031,45.4128910420867,38.989));
#178918=CARTESIAN_POINT('Origin',(5.49031038273072E-15,0.,38.989));
#178919=CARTESIAN_POINT('',(41.3167691863815,45.4132731252654,38.9890000005754));
#178920=CARTESIAN_POINT('Origin',(5.49031038273072E-15,0.,38.989));
#178921=CARTESIAN_POINT('',(41.3167691865937,45.4132731255215,38.989));
#178922=CARTESIAN_POINT('Origin',(62.2224557307631,0.,38.989));
#178923=CARTESIAN_POINT('',(45.7656648676111,41.6348281284257,38.989));
#178924=CARTESIAN_POINT('',(34.1507877370015,31.1767457860025,38.989));
#178925=CARTESIAN_POINT('',(41.6348281284267,45.7656648676101,38.989));
#178926=CARTESIAN_POINT('Origin',(5.49031038273072E-15,0.,38.989));
#178927=CARTESIAN_POINT('',(41.3175407208299,45.4132815019354,38.989));
#178928=CARTESIAN_POINT('Origin',(5.57972911860581E-15,0.,39.624));
#178929=CARTESIAN_POINT('Origin',(44.3789791175472,40.3862573897239,39.6240070731883));
#178930=CARTESIAN_POINT('Origin',(40.386257389725,44.3789791175462,39.6240070731883));
#178931=CARTESIAN_POINT('Origin',(5.57972911860581E-15,0.,39.624));
#178932=CARTESIAN_POINT('Origin',(45.7939781049223,41.6603666103081,39.5552135208011));
#178933=CARTESIAN_POINT('Origin',(41.6603663369573,45.7939778018841,39.5552117598806));
#178934=CARTESIAN_POINT('Origin',(5.51210908043506E-15,0.,39.1438017080178));
#178935=CARTESIAN_POINT('Origin',(45.1403198695228,41.0717150501545,39.1711625381326));
#178936=CARTESIAN_POINT('Origin',(41.0716522820274,45.1402498046835,39.1712173702617));
#178937=CARTESIAN_POINT('Origin',(5.51210908043507E-15,0.,39.1438017080178));
#178938=CARTESIAN_POINT('Origin',(45.0043926651423,40.949436607778,39.171217585939));
#178939=CARTESIAN_POINT('Origin',(40.9493738530264,45.0043225899457,39.1711627526739));
#178940=CARTESIAN_POINT('Origin',(60.4792282238308,0.,38.989));
#178941=CARTESIAN_POINT('',(35.5261472678871,48.3573835402115,38.989));
#178942=CARTESIAN_POINT('',(39.9143573409162,44.803881088767,38.989));
#178943=CARTESIAN_POINT('Origin',(5.49031038273072E-15,0.,38.989));
#178944=CARTESIAN_POINT('',(40.2319965165892,45.1566551325071,38.989));
#178945=CARTESIAN_POINT('',(26.8427652369017,30.2864073093063,38.989));
#178946=CARTESIAN_POINT('',(40.2315646150503,45.1570399302677,38.9889999995773));
#178947=CARTESIAN_POINT('Origin',(5.49031038273072E-15,0.,38.989));
#178948=CARTESIAN_POINT('',(35.8056376404645,48.7410849259194,38.9889999997818));
#178949=CARTESIAN_POINT('Origin',(5.49031038273072E-15,0.,38.989));
#178950=CARTESIAN_POINT('',(35.8051714542882,48.7414273857052,38.989));
#178951=CARTESIAN_POINT('Origin',(5.49031038273072E-15,0.,38.989));
#178952=CARTESIAN_POINT('',(35.5264632599797,48.3578184660147,38.989));
#178953=CARTESIAN_POINT('Origin',(5.49031038273072E-15,0.,38.989));
#178954=CARTESIAN_POINT('',(40.3404336838198,45.2779489569768,39.2708017080178));
#178955=CARTESIAN_POINT('',(40.2315646145633,45.1570399297211,38.989));
#178956=CARTESIAN_POINT('',(35.9012693630584,48.8727133450218,39.2708017078546));
#178957=CARTESIAN_POINT('Origin',(5.52999282761009E-15,0.,39.2708017080178));
#178958=CARTESIAN_POINT('',(35.901269362891,48.8727133447939,39.2708017080178));
#178959=CARTESIAN_POINT('Origin',(60.71525,0.,39.3978017080178));
#178960=CARTESIAN_POINT('',(36.0301015792682,49.0510171431399,39.3978017080178));
#178961=CARTESIAN_POINT('',(40.4880553924349,45.4410373245167,39.3978017080178));
#178962=CARTESIAN_POINT('Origin',(5.5478765747851E-15,0.,39.3978017080178));
#178963=CARTESIAN_POINT('',(40.5892333705628,45.5534068532507,39.3978017080178));
#178964=CARTESIAN_POINT('',(26.948440628206,30.4037717213983,39.3978017080178));
#178965=CARTESIAN_POINT('',(36.1189794796889,49.1733470784083,39.3978017080178));
#178966=CARTESIAN_POINT('Origin',(5.5478765747851E-15,0.,39.3978017080178));
#178967=CARTESIAN_POINT('',(36.0304131198717,49.0514459419941,39.3978017080178));
#178968=CARTESIAN_POINT('Origin',(5.5478765747851E-15,0.,39.3978017080178));
#178969=CARTESIAN_POINT('',(36.2478178023256,49.3516463037381,39.2708017080178));
#178970=CARTESIAN_POINT('',(40.7368493367122,45.7165002430344,39.2708017081757));
#178971=CARTESIAN_POINT('Origin',(5.52999282761008E-15,0.,39.2708017080178));
#178972=CARTESIAN_POINT('',(40.8457160731802,45.8374112534707,38.9890000005756));
#178973=CARTESIAN_POINT('',(40.7368493365303,45.7165002428302,39.2708017080178));
#178974=CARTESIAN_POINT('',(40.8452921850249,45.8377889771246,38.989));
#178975=CARTESIAN_POINT('Origin',(5.49031038273072E-15,0.,38.989));
#178976=CARTESIAN_POINT('',(36.3439095507841,49.4829367616342,38.989));
#178977=CARTESIAN_POINT('Origin',(5.49031038273072E-15,0.,38.989));
#178978=CARTESIAN_POINT('',(36.3434519499953,49.4832728536528,38.9890000005754));
#178979=CARTESIAN_POINT('Origin',(5.49031038273072E-15,0.,38.989));
#178980=CARTESIAN_POINT('',(36.3434519501796,49.4832728539297,38.989));
#178981=CARTESIAN_POINT('Origin',(62.2224557307631,0.,38.989));
#178982=CARTESIAN_POINT('',(41.1629311642486,46.190562802648,38.989));
#178983=CARTESIAN_POINT('',(27.6232705441551,31.1532462714325,38.989));
#178984=CARTESIAN_POINT('',(36.6229335645815,49.8669803696022,38.989));
#178985=CARTESIAN_POINT('Origin',(5.49031038273072E-15,0.,38.989));
#178986=CARTESIAN_POINT('',(36.3442183822969,49.4833618317448,38.989));
#178987=CARTESIAN_POINT('Origin',(5.57972911860581E-15,0.,39.624));
#178988=CARTESIAN_POINT('Origin',(39.9143530044124,44.8038837346035,39.6240070731883));
#178989=CARTESIAN_POINT('Origin',(35.5261507575157,48.357379848571,39.6240070731883));
#178990=CARTESIAN_POINT('Origin',(5.57972911860581E-15,0.,39.624));
#178991=CARTESIAN_POINT('Origin',(41.1884198004163,46.2189209212438,39.5552135207988));
#178992=CARTESIAN_POINT('Origin',(36.6453723646245,49.8978076723501,39.5552117598822));
#178993=CARTESIAN_POINT('Origin',(5.51210908043506E-15,0.,39.1438017080178));
#178994=CARTESIAN_POINT('Origin',(40.5998732162095,45.5651681650781,39.1711625381354));
#178995=CARTESIAN_POINT('Origin',(36.1282165298278,49.1861234900562,39.1712173702643));
#178996=CARTESIAN_POINT('Origin',(5.51210908043507E-15,0.,39.1438017080178));
#178997=CARTESIAN_POINT('Origin',(40.4774722129479,45.4293513150122,39.1712175859383));
#178998=CARTESIAN_POINT('Origin',(36.0208162177228,49.0381593225517,39.1711627526726));
#178999=CARTESIAN_POINT('Origin',(60.4792282238308,0.,38.989));
#179000=CARTESIAN_POINT('',(30.2768083268887,51.8059703131943,38.989));
#179001=CARTESIAN_POINT('',(35.012421476459,48.7306271754172,38.989));
#179002=CARTESIAN_POINT('Origin',(5.49031038273072E-15,0.,38.989));
#179003=CARTESIAN_POINT('',(35.2914456628196,49.1146710209411,38.989));
#179004=CARTESIAN_POINT('',(20.6381965522797,28.9462038689911,38.989));
#179005=CARTESIAN_POINT('',(35.2909759049641,49.1150085647353,38.9889999995772));
#179006=CARTESIAN_POINT('Origin',(5.49031038273072E-15,0.,38.989));
#179007=CARTESIAN_POINT('',(30.5146599057598,52.2167844417075,38.9889999997818));
#179008=CARTESIAN_POINT('Origin',(5.49031038273072E-15,0.,38.989));
#179009=CARTESIAN_POINT('',(30.5141604766051,52.2170762957381,38.989));
#179010=CARTESIAN_POINT('Origin',(5.49031038273072E-15,0.,38.989));
#179011=CARTESIAN_POINT('',(30.2770771258177,51.8064358865963,38.989));
#179012=CARTESIAN_POINT('Origin',(5.49031038273072E-15,0.,38.989));
#179013=CARTESIAN_POINT('',(35.3866101428265,49.2466351556009,39.2708017080178));
#179014=CARTESIAN_POINT('',(35.2909759045368,49.1150085641407,38.989));
#179015=CARTESIAN_POINT('',(30.5960088314001,52.35768802356,39.2708017078546));
#179016=CARTESIAN_POINT('Origin',(5.52999282761009E-15,0.,39.2708017080178));
#179017=CARTESIAN_POINT('',(30.5960088312575,52.3576880233159,39.2708017080178));
#179018=CARTESIAN_POINT('Origin',(60.71525,0.,39.3978017080178));
#179019=CARTESIAN_POINT('',(30.7054974692375,52.5484816883955,39.3978017080178));
#179020=CARTESIAN_POINT('',(35.5163757878401,49.4242607783457,39.3978017080178));
#179021=CARTESIAN_POINT('Origin',(5.5478765747851E-15,0.,39.3978017080178));
#179022=CARTESIAN_POINT('',(35.6052536882608,49.5465907136141,39.3978017080178));
#179023=CARTESIAN_POINT('',(20.7197400704249,29.0584388930977,39.3978017080178));
#179024=CARTESIAN_POINT('',(30.781101527075,52.6794317578284,39.3978017080178));
#179025=CARTESIAN_POINT('Origin',(5.5478765747851E-15,0.,39.3978017080178));
#179026=CARTESIAN_POINT('',(30.7057624815037,52.5489407031053,39.3978017080178));
#179027=CARTESIAN_POINT('Origin',(5.5478765747851E-15,0.,39.3978017080178));
#179028=CARTESIAN_POINT('',(30.8905967158742,52.8702215132212,39.2708017080178));
#179029=CARTESIAN_POINT('',(35.7350130972991,49.7242207308392,39.2708017081757));
#179030=CARTESIAN_POINT('Origin',(5.52999282761008E-15,0.,39.2708017080178));
#179031=CARTESIAN_POINT('',(35.8306448082808,49.8558490507732,38.9890000005756));
#179032=CARTESIAN_POINT('',(35.7350130971395,49.7242207306171,39.2708017080178));
#179033=CARTESIAN_POINT('',(35.8301837593561,49.8561803968399,38.989));
#179034=CARTESIAN_POINT('Origin',(5.49031038273072E-15,0.,38.989));
#179035=CARTESIAN_POINT('',(30.9724384738749,53.0108370710509,38.989));
#179036=CARTESIAN_POINT('Origin',(5.49031038273072E-15,0.,38.989));
#179037=CARTESIAN_POINT('',(30.9719482486888,53.011123489615,38.9890000005754));
#179038=CARTESIAN_POINT('Origin',(5.49031038273072E-15,0.,38.989));
#179039=CARTESIAN_POINT('',(30.9719482488431,53.0111234899096,38.989));
#179040=CARTESIAN_POINT('Origin',(62.2224557307631,0.,38.989));
#179041=CARTESIAN_POINT('',(36.1092077731534,50.2402240048079,38.989));
#179042=CARTESIAN_POINT('',(21.2404668433939,29.7751578089176,38.989));
#179043=CARTESIAN_POINT('',(31.2097904767612,53.4219427993283,38.989));
#179044=CARTESIAN_POINT('Origin',(5.49031038273072E-15,0.,38.989));
#179045=CARTESIAN_POINT('',(30.9727011816508,53.0112920942664,38.989));
#179046=CARTESIAN_POINT('Origin',(5.57972911860581E-15,0.,39.624));
#179047=CARTESIAN_POINT('Origin',(35.0124168871459,48.7306293534715,39.6240070731883));
#179048=CARTESIAN_POINT('Origin',(30.2768121832823,51.8059670065424,39.6240070731883));
#179049=CARTESIAN_POINT('Origin',(5.57972911860581E-15,0.,39.624));
#179050=CARTESIAN_POINT('Origin',(36.131592549347,50.2710910626322,39.5552135207999));
#179051=CARTESIAN_POINT('Origin',(31.22888402413,53.4549467201701,39.5552117598832));
#179052=CARTESIAN_POINT('Origin',(5.51210908043506E-15,0.,39.1438017080178));
#179053=CARTESIAN_POINT('Origin',(35.6146058558682,49.5593997624593,39.1711625381345));
#179054=CARTESIAN_POINT('Origin',(30.7889524770109,52.6931037136121,39.1712173702631));
#179055=CARTESIAN_POINT('Origin',(5.51210908043507E-15,0.,39.1438017080178));
#179056=CARTESIAN_POINT('Origin',(35.5070721047336,49.411532542537,39.1712175859357));
#179057=CARTESIAN_POINT('Origin',(30.6976069821061,52.5347237197182,39.1711627526718));
#179058=CARTESIAN_POINT('Origin',(60.4792282238308,0.,38.989));
#179059=CARTESIAN_POINT('',(24.6957503380314,54.6869600343295,38.989));
#179060=CARTESIAN_POINT('',(29.7268821954856,52.1234703131943,38.989));
#179061=CARTESIAN_POINT('Origin',(5.49031038273072E-15,0.,38.989));
#179062=CARTESIAN_POINT('',(29.9642343451585,52.534576295764,38.989));
#179063=CARTESIAN_POINT('',(14.8448439902567,26.3470240215575,38.989));
#179064=CARTESIAN_POINT('',(29.9637318777514,52.534862887391,38.9889999995774));
#179065=CARTESIAN_POINT('Origin',(5.49031038273072E-15,0.,38.989));
#179066=CARTESIAN_POINT('',(24.8893571715245,55.1203859400877,38.9889999997818));
#179067=CARTESIAN_POINT('Origin',(5.49031038273072E-15,0.,38.989));
#179068=CARTESIAN_POINT('',(24.8888299712416,55.1206239907494,38.989));
#179069=CARTESIAN_POINT('Origin',(5.49031038273072E-15,0.,38.989));
#179070=CARTESIAN_POINT('',(24.6959689987794,54.6874511544106,38.989));
#179071=CARTESIAN_POINT('Origin',(5.49031038273072E-15,0.,38.989));
#179072=CARTESIAN_POINT('',(30.0450834959843,52.6757649139392,39.2708017080178));
#179073=CARTESIAN_POINT('',(29.9637318773888,52.5348628867551,38.989));
#179074=CARTESIAN_POINT('',(24.9555320243585,55.2690209155614,39.2708017078546));
#179075=CARTESIAN_POINT('Origin',(5.52999282761009E-15,0.,39.2708017080178));
#179076=CARTESIAN_POINT('',(24.9555320242422,55.2690209153037,39.2708017080178));
#179077=CARTESIAN_POINT('Origin',(60.71525,0.,39.3978017080178));
#179078=CARTESIAN_POINT('',(25.0444775033954,55.4702140717964,39.3978017080178));
#179079=CARTESIAN_POINT('',(30.1555713378344,52.8659816883956,39.3978017080178));
#179080=CARTESIAN_POINT('Origin',(5.5478765747851E-15,0.,39.3978017080178));
#179081=CARTESIAN_POINT('',(30.2311753956719,52.9969317578284,39.3978017080178));
#179082=CARTESIAN_POINT('',(14.9038494342991,26.4492244485619,39.3978017080178));
#179083=CARTESIAN_POINT('',(25.1059793847708,55.6083495590299,39.3978017080178));
#179084=CARTESIAN_POINT('Origin',(5.5478765747851E-15,0.,39.3978017080178));
#179085=CARTESIAN_POINT('',(25.0446930837944,55.4706982733004,39.3978017080178));
#179086=CARTESIAN_POINT('Origin',(5.5478765747851E-15,0.,39.3978017080178));
#179087=CARTESIAN_POINT('',(25.1949317875307,55.8095395120004,39.2708017080178));
#179088=CARTESIAN_POINT('',(30.3416565763598,53.1871522508547,39.2708017081757));
#179089=CARTESIAN_POINT('Origin',(5.52999282761008E-15,0.,39.2708017080178));
#179090=CARTESIAN_POINT('',(30.4230055008174,53.3280557328682,38.9890000005756));
#179091=CARTESIAN_POINT('',(30.3416565762242,53.1871522506171,39.2708017080178));
#179092=CARTESIAN_POINT('',(30.4225123424717,53.3283370710509,38.989));
#179093=CARTESIAN_POINT('Origin',(5.49031038273072E-15,0.,38.989));
#179094=CARTESIAN_POINT('',(25.2616268796463,55.9579395562863,38.989));
#179095=CARTESIAN_POINT('Origin',(5.49031038273072E-15,0.,38.989));
#179096=CARTESIAN_POINT('',(25.2611094010728,55.9581731633343,38.9890000005754));
#179097=CARTESIAN_POINT('Origin',(5.49031038273072E-15,0.,38.989));
#179098=CARTESIAN_POINT('',(25.2611094011954,55.9581731636434,38.989));
#179099=CARTESIAN_POINT('Origin',(62.2224557307631,0.,38.989));
#179100=CARTESIAN_POINT('',(30.6598643453581,53.7394427993283,38.989));
#179101=CARTESIAN_POINT('',(15.2806508669898,27.1018636743471,38.989));
#179102=CARTESIAN_POINT('',(25.454706393409,56.3916032444848,38.989));
#179103=CARTESIAN_POINT('Origin',(5.49031038273072E-15,0.,38.989));
#179104=CARTESIAN_POINT('',(25.2618405854041,55.9584195472772,38.989));
#179105=CARTESIAN_POINT('Origin',(5.57972911860581E-15,0.,39.624));
#179106=CARTESIAN_POINT('Origin',(29.7268774036444,52.1234719996031,39.6240070731883));
#179107=CARTESIAN_POINT('Origin',(24.6957545189384,54.6869571488947,39.6240070731883));
#179108=CARTESIAN_POINT('Origin',(5.57972911860581E-15,0.,39.624));
#179109=CARTESIAN_POINT('Origin',(30.6789000092884,53.7724806104368,39.5552135207961));
#179110=CARTESIAN_POINT('Origin',(25.4702454952004,56.4264221855602,39.5552117598815));
#179111=CARTESIAN_POINT('Origin',(5.51210908043506E-15,0.,39.1438017080178));
#179112=CARTESIAN_POINT('Origin',(30.2391374209353,53.0106482050728,39.1711625381366));
#179113=CARTESIAN_POINT('Origin',(25.112358217853,55.6227672661399,39.1712173702603));
#179114=CARTESIAN_POINT('Origin',(5.51210908043507E-15,0.,39.1438017080178));
#179115=CARTESIAN_POINT('Origin',(30.1476490842099,52.8523506794944,39.1712175859362));
#179116=CARTESIAN_POINT('Origin',(25.038068340494,55.4557066902169,39.171162752677));
#179117=CARTESIAN_POINT('Origin',(60.4792282238308,0.,38.989));
#179118=CARTESIAN_POINT('',(18.8441205405526,56.9687879773464,38.989));
#179119=CARTESIAN_POINT('',(24.1156489724283,54.9452378026826,38.989));
#179120=CARTESIAN_POINT('Origin',(5.49031038273072E-15,0.,38.989));
#179121=CARTESIAN_POINT('',(24.3087286055926,55.3789017591236,38.989));
#179122=CARTESIAN_POINT('',(9.71531210235053,22.6015516358801,38.989));
#179123=CARTESIAN_POINT('',(24.3081989337721,55.3791342586255,38.9889999995776));
#179124=CARTESIAN_POINT('Origin',(5.49031038273072E-15,0.,38.989));
#179125=CARTESIAN_POINT('',(18.9913614316851,57.4200769554259,38.9889999997818));
#179126=CARTESIAN_POINT('Origin',(5.49031038273072E-15,0.,38.989));
#179127=CARTESIAN_POINT('',(18.9908122363906,57.4202585945858,38.989));
#179128=CARTESIAN_POINT('Origin',(5.49031038273072E-15,0.,38.989));
#179129=CARTESIAN_POINT('',(18.8442866674268,56.9692992632924,38.989));
#179130=CARTESIAN_POINT('Origin',(5.49031038273072E-15,0.,38.989));
#179131=CARTESIAN_POINT('',(24.374376627022,55.527767968768,39.2708017080178));
#179132=CARTESIAN_POINT('',(24.308198933478,55.3791342579555,38.989));
#179133=CARTESIAN_POINT('',(19.0416371861772,57.5748148486258,39.2708017078546));
#179134=CARTESIAN_POINT('Origin',(5.52999282761009E-15,0.,39.2708017080178));
#179135=CARTESIAN_POINT('',(19.0416371860884,57.5748148483574,39.2708017080178));
#179136=CARTESIAN_POINT('Origin',(60.71525,0.,39.3978017080178));
#179137=CARTESIAN_POINT('',(19.1090650011322,57.7842031819381,39.3978017080178));
#179138=CARTESIAN_POINT('',(24.4643761377923,55.7284918401495,39.3978017080178));
#179139=CARTESIAN_POINT('Origin',(5.5478765747851E-15,0.,39.3978017080178));
#179140=CARTESIAN_POINT('',(24.5258780191677,55.866627327383,39.3978017080178));
#179141=CARTESIAN_POINT('',(9.75435829333414,22.6892508167102,39.3978017080178));
#179142=CARTESIAN_POINT('',(19.1557908785631,57.9280106456674,39.3978017080178));
#179143=CARTESIAN_POINT('Origin',(5.5478765747851E-15,0.,39.3978017080178));
#179144=CARTESIAN_POINT('',(19.1092287877201,57.7847072652234,39.3978017080178));
#179145=CARTESIAN_POINT('Origin',(5.5478765747851E-15,0.,39.3978017080178));
#179146=CARTESIAN_POINT('',(19.2232259141446,58.1373965169891,39.2708017080178));
#179147=CARTESIAN_POINT('',(24.6158705165699,56.0673542006827,39.2708017081757));
#179148=CARTESIAN_POINT('Origin',(5.52999282761008E-15,0.,39.2708017080178));
#179149=CARTESIAN_POINT('',(24.6820453786638,56.2159890767408,38.9890000005756));
#179150=CARTESIAN_POINT('',(24.61587051646,56.0673542004323,39.2708017080178));
#179151=CARTESIAN_POINT('',(24.6815255140433,56.2162173246395,38.989));
#179152=CARTESIAN_POINT('Origin',(5.49031038273072E-15,0.,38.989));
#179153=CARTESIAN_POINT('',(19.2740436149891,58.2919551457914,38.989));
#179154=CARTESIAN_POINT('Origin',(5.49031038273072E-15,0.,38.989));
#179155=CARTESIAN_POINT('',(19.2735045526316,58.2921333818755,38.9890000005754));
#179156=CARTESIAN_POINT('Origin',(5.49031038273072E-15,0.,38.989));
#179157=CARTESIAN_POINT('',(19.2735045527213,58.2921333821957,38.989));
#179158=CARTESIAN_POINT('Origin',(62.2224557307631,0.,38.989));
#179159=CARTESIAN_POINT('',(24.8746050278059,56.6498810128379,38.989));
#179160=CARTESIAN_POINT('',(10.0037024164492,23.2492868865834,38.989));
#179161=CARTESIAN_POINT('',(19.4207352200707,58.743425483793,38.989));
#179162=CARTESIAN_POINT('Origin',(5.49031038273072E-15,0.,38.989));
#179163=CARTESIAN_POINT('',(19.2742059773237,58.2924548456759,38.989));
#179164=CARTESIAN_POINT('Origin',(5.57972911860581E-15,0.,39.624));
#179165=CARTESIAN_POINT('Origin',(24.1156440305597,54.9452389789693,39.6240070731883));
#179166=CARTESIAN_POINT('Origin',(18.8441250001663,56.9687855447422,39.6240070731883));
#179167=CARTESIAN_POINT('Origin',(5.57972911860581E-15,0.,39.624));
#179168=CARTESIAN_POINT('Origin',(24.8900830207503,56.6847276080573,39.5552135207989));
#179169=CARTESIAN_POINT('Origin',(19.4325496266321,58.7796779614968,39.5552117598826));
#179170=CARTESIAN_POINT('Origin',(5.51210908043506E-15,0.,39.1438017080178));
#179171=CARTESIAN_POINT('Origin',(24.5323626684704,55.8811008927563,39.1711625381296));
#179172=CARTESIAN_POINT('Origin',(19.1606277069624,57.9430161406894,39.1712173702622));
#179173=CARTESIAN_POINT('Origin',(5.51210908043507E-15,0.,39.1438017080178));
#179174=CARTESIAN_POINT('Origin',(24.4579221115139,55.7141074023442,39.1712175859374));
#179175=CARTESIAN_POINT('Origin',(19.1042073826023,57.769105333365,39.171162752673));
#179176=CARTESIAN_POINT('Origin',(60.4792282238308,0.,38.989));
#179177=CARTESIAN_POINT('',(12.7860306150458,58.6264539577982,38.989));
#179178=CARTESIAN_POINT('',(18.2401996527051,57.1650137687745,38.989));
#179179=CARTESIAN_POINT('Origin',(5.49031038273072E-15,0.,38.989));
#179180=CARTESIAN_POINT('',(18.3868913484954,57.6164843860301,38.989));
#179181=CARTESIAN_POINT('',(5.47329194811204,17.8725121057138,38.989));
#179182=CARTESIAN_POINT('',(18.3863402754571,57.6166602460946,38.9889999995772));
#179183=CARTESIAN_POINT('Origin',(5.49031038273072E-15,0.,38.989));
#179184=CARTESIAN_POINT('',(12.8852923618023,59.0906615917169,38.9889999997818));
#179185=CARTESIAN_POINT('Origin',(5.49031038273072E-15,0.,38.989));
#179186=CARTESIAN_POINT('',(12.8847271885949,59.0907848292983,38.989));
#179187=CARTESIAN_POINT('Origin',(5.49031038273072E-15,0.,38.989));
#179188=CARTESIAN_POINT('',(12.7861423879254,58.6269798078531,38.989));
#179189=CARTESIAN_POINT('Origin',(5.49031038273072E-15,0.,38.989));
#179190=CARTESIAN_POINT('',(18.4366189870679,57.7713971777985,39.2708017080178));
#179191=CARTESIAN_POINT('',(18.3863402752344,57.6166602453969,38.989));
#179192=CARTESIAN_POINT('',(12.9191181862654,59.249807061904,39.2708017078546));
#179193=CARTESIAN_POINT('Origin',(5.52999282761009E-15,0.,39.2708017080178));
#179194=CARTESIAN_POINT('',(12.9191181862052,59.2498070616278,39.2708017080178));
#179195=CARTESIAN_POINT('Origin',(60.71525,0.,39.3978017080178));
#179196=CARTESIAN_POINT('',(12.9642895838877,59.4650964698965,39.3978017080178));
#179197=CARTESIAN_POINT('',(18.5051441132848,57.9804289733662,39.3978017080178));
#179198=CARTESIAN_POINT('Origin',(5.5478765747851E-15,0.,39.3978017080178));
#179199=CARTESIAN_POINT('',(18.5518699907157,58.1242364370955,39.3978017080178));
#179200=CARTESIAN_POINT('',(5.49583002221492,17.9418771653399,39.3978017080178));
#179201=CARTESIAN_POINT('',(12.995727518883,59.6130003254554,39.3978017080178));
#179202=CARTESIAN_POINT('Origin',(5.5478765747851E-15,0.,39.3978017080178));
#179203=CARTESIAN_POINT('',(12.9643997821844,59.4656149121212,39.3978017080178));
#179204=CARTESIAN_POINT('Origin',(5.5478765747851E-15,0.,39.3978017080178));
#179205=CARTESIAN_POINT('',(13.0409063549245,59.8282880397053,39.2708017080178));
#179206=CARTESIAN_POINT('',(18.6203878281985,58.3332704850399,39.2708017081757));
#179207=CARTESIAN_POINT('Origin',(5.52999282761008E-15,0.,39.2708017080178));
#179208=CARTESIAN_POINT('',(18.6706636022915,58.4880082803367,38.9890000005756));
#179209=CARTESIAN_POINT('',(18.6203878281154,58.3332704847794,39.2708017080178));
#179210=CARTESIAN_POINT('',(18.6701227271417,58.4881809372196,38.989));
#179211=CARTESIAN_POINT('Origin',(5.49031038273072E-15,0.,38.989));
#179212=CARTESIAN_POINT('',(13.0752898951332,59.9873118763434,38.989));
#179213=CARTESIAN_POINT('Origin',(5.49031038273072E-15,0.,38.989));
#179214=CARTESIAN_POINT('',(13.0747351550717,59.9874327886717,38.9890000005754));
#179215=CARTESIAN_POINT('Origin',(5.49031038273072E-15,0.,38.989));
#179216=CARTESIAN_POINT('',(13.0747351551274,59.9874327889996,38.989));
#179217=CARTESIAN_POINT('Origin',(62.2224557307631,0.,38.989));
#179218=CARTESIAN_POINT('',(18.8168143322233,58.9396512752211,38.989));
#179219=CARTESIAN_POINT('',(5.63975536249314,18.3848338156965,38.989));
#179220=CARTESIAN_POINT('',(13.1739864076113,60.4516424606487,38.989));
#179221=CARTESIAN_POINT('Origin',(5.49031038273072E-15,0.,38.989));
#179222=CARTESIAN_POINT('',(13.075399135169,59.9878258103049,38.989));
#179223=CARTESIAN_POINT('Origin',(5.57972911860581E-15,0.,39.624));
#179224=CARTESIAN_POINT('Origin',(18.2401946149532,57.1650144220515,39.6240070731883));
#179225=CARTESIAN_POINT('Origin',(12.7860353045056,58.6264520046766,39.6240070731883));
#179226=CARTESIAN_POINT('Origin',(5.57972911860581E-15,0.,39.624));
#179227=CARTESIAN_POINT('Origin',(18.8285650740585,58.9759248679615,39.5552135207994));
#179228=CARTESIAN_POINT('Origin',(13.1819466778345,60.4889312852505,39.555211759879));
#179229=CARTESIAN_POINT('Origin',(5.51210908043506E-15,0.,39.1438017080178));
#179230=CARTESIAN_POINT('Origin',(18.5568062168849,58.1393085451912,39.1711625381331));
#179231=CARTESIAN_POINT('Origin',(12.9989693492948,59.6284292050442,39.1712173702602));
#179232=CARTESIAN_POINT('Origin',(5.51210908043507E-15,0.,39.1438017080178));
#179233=CARTESIAN_POINT('Origin',(18.5002290260147,57.9654487055675,39.1712175859381));
#179234=CARTESIAN_POINT('Origin',(12.9610367308112,59.4495735695181,39.1711627526717));
#179235=CARTESIAN_POINT('Origin',(60.4792282238308,0.,38.989));
#179236=CARTESIAN_POINT('',(6.58785426247156,59.6417962403142,38.989));
#179237=CARTESIAN_POINT('',(12.1649068885798,58.7584778814675,38.989));
#179238=CARTESIAN_POINT('Origin',(5.49031038273072E-15,0.,38.989));
#179239=CARTESIAN_POINT('',(12.2636034620796,59.2228087529787,38.989));
#179240=CARTESIAN_POINT('',(2.30379013587727,12.3655710936233,38.989));
#179241=CARTESIAN_POINT('',(12.2630370254948,59.2229260468454,38.9889999995773));
#179242=CARTESIAN_POINT('Origin',(5.49031038273072E-15,0.,38.989));
#179243=CARTESIAN_POINT('',(6.63804933238279,60.1138365740932,38.9889999997818));
#179244=CARTESIAN_POINT('Origin',(5.49031038273072E-15,0.,38.989));
#179245=CARTESIAN_POINT('',(6.63747437341838,60.1139000598793,38.989));
#179246=CARTESIAN_POINT('Origin',(5.49031038273072E-15,0.,38.989));
#179247=CARTESIAN_POINT('',(6.58791045674951,59.6423308931549,38.989));
#179248=CARTESIAN_POINT('Origin',(5.49031038273072E-15,0.,38.989));
#179249=CARTESIAN_POINT('',(12.296865891381,59.3820708699069,39.2708017080178));
#179250=CARTESIAN_POINT('',(12.2630370253463,59.2229260461284,38.989));
#179251=CARTESIAN_POINT('',(6.65505462400558,60.2756459901928,39.2708017078546));
#179252=CARTESIAN_POINT('Origin',(5.52999282761009E-15,0.,39.2708017080178));
#179253=CARTESIAN_POINT('',(6.65505462397456,60.2756459899118,39.2708017080178));
#179254=CARTESIAN_POINT('Origin',(60.71525,0.,39.3978017080178));
#179255=CARTESIAN_POINT('',(6.67747469701007,60.4944777170593,39.3978017080178));
#179256=CARTESIAN_POINT('',(12.3431658574217,59.5971203935658,39.3978017080178));
#179257=CARTESIAN_POINT('Origin',(5.5478765747851E-15,0.,39.3978017080178));
#179258=CARTESIAN_POINT('',(12.3746037924171,59.7450242491246,39.3978017080178));
#179259=CARTESIAN_POINT('',(2.31399271319981,12.4135704460892,39.3978017080178));
#179260=CARTESIAN_POINT('',(6.69328024897516,60.6448574988554,39.3978017080178));
#179261=CARTESIAN_POINT('Origin',(5.5478765747851E-15,0.,39.3978017080178));
#179262=CARTESIAN_POINT('',(6.67753009965994,60.4950048380619,39.3978017080178));
#179263=CARTESIAN_POINT('Origin',(5.5478765747851E-15,0.,39.3978017080178));
#179264=CARTESIAN_POINT('',(6.71570789669471,60.8636883187844,39.2708017080178));
#179265=CARTESIAN_POINT('',(12.4208962742148,59.9600752509413,39.2708017081757));
#179266=CARTESIAN_POINT('Origin',(5.52999282761008E-15,0.,39.2708017080178));
#179267=CARTESIAN_POINT('',(12.454722128405,60.1192206258105,38.9890000005756));
#179268=CARTESIAN_POINT('',(12.4208962741593,59.9600752506736,39.2708017080178));
#179269=CARTESIAN_POINT('',(12.4541661686672,60.1193358000127,38.989));
#179270=CARTESIAN_POINT('Origin',(5.49031038273072E-15,0.,38.989));
#179271=CARTESIAN_POINT('',(6.7332805630058,61.0254350648261,38.989));
#179272=CARTESIAN_POINT('Origin',(5.49031038273072E-15,0.,38.989));
#179273=CARTESIAN_POINT('',(6.73271622308859,61.0254973286579,38.9890000005754));
#179274=CARTESIAN_POINT('Origin',(5.49031038273072E-15,0.,38.989));
#179275=CARTESIAN_POINT('',(6.7327162231097,61.0254973289898,38.989));
#179276=CARTESIAN_POINT('Origin',(62.2224557307631,0.,38.989));
#179277=CARTESIAN_POINT('',(12.5528626811454,60.583666384318,38.989));
#179278=CARTESIAN_POINT('',(2.3791451040456,12.7200883457668,38.989));
#179279=CARTESIAN_POINT('',(6.78290064323623,61.4975385923861,38.989));
#179280=CARTESIAN_POINT('Origin',(5.49031038273072E-15,0.,38.989));
#179281=CARTESIAN_POINT('',(6.73333548388602,61.0259576020967,38.989));
#179282=CARTESIAN_POINT('Origin',(5.57972911860581E-15,0.,39.624));
#179283=CARTESIAN_POINT('Origin',(12.1649018101392,58.7584780045773,39.6240070731883));
#179284=CARTESIAN_POINT('Origin',(6.58785913039885,59.6417947880741,39.6240070731883));
#179285=CARTESIAN_POINT('Origin',(5.57972911860581E-15,0.,39.624));
#179286=CARTESIAN_POINT('Origin',(12.5607574282786,60.6209695535089,39.5552135207989));
#179287=CARTESIAN_POINT('Origin',(6.78691956273318,61.5354552197195,39.5552117598775));
#179288=CARTESIAN_POINT('Origin',(5.51210908043506E-15,0.,39.1438017080178));
#179289=CARTESIAN_POINT('Origin',(12.3779375131252,59.7605297667703,39.1711625381316));
#179290=CARTESIAN_POINT('Origin',(6.69489156322753,60.6605407209802,39.1712173702623));
#179291=CARTESIAN_POINT('Origin',(5.51210908043507E-15,0.,39.1438017080178));
#179292=CARTESIAN_POINT('Origin',(12.3398435598877,59.5817084227229,39.171217585937));
#179293=CARTESIAN_POINT('Origin',(6.67586224832399,60.4786998370191,39.1711627526734));
#179294=CARTESIAN_POINT('Origin',(60.4792282238308,0.,38.989));
#179295=CARTESIAN_POINT('',(0.317500000000634,60.0036905223731,38.989));
#179296=CARTESIAN_POINT('',(5.95633285891271,59.7081718144892,38.989));
#179297=CARTESIAN_POINT('Origin',(5.49031038273072E-15,0.,38.989));
#179298=CARTESIAN_POINT('',(6.00595296980932,60.1802756340602,38.989));
#179299=CARTESIAN_POINT('',(0.34504741944992,6.32035708677299,38.989));
#179300=CARTESIAN_POINT('',(6.00537737567573,60.1803330766332,38.9889999995772));
#179301=CARTESIAN_POINT('Origin',(5.49031038273072E-15,0.,38.989));
#179302=CARTESIAN_POINT('',(0.31807844537663,60.4783917833346,38.9889999997818));
#179303=CARTESIAN_POINT('Origin',(5.49031038273072E-15,0.,38.989));
#179304=CARTESIAN_POINT('',(0.317500000025924,60.478394821762,38.989));
#179305=CARTESIAN_POINT('Origin',(5.49031038273072E-15,0.,38.989));
#179306=CARTESIAN_POINT('',(0.317500000000634,60.004228120231,38.989));
#179307=CARTESIAN_POINT('Origin',(5.49031038273072E-15,0.,38.989));
#179308=CARTESIAN_POINT('',(6.02238575970337,60.3421421670675,39.2708017080178));
#179309=CARTESIAN_POINT('',(6.00537737560301,60.1803330759045,38.989));
#179310=CARTESIAN_POINT('',(0.318076890625489,60.6410923275232,39.2708017078546));
#179311=CARTESIAN_POINT('Origin',(5.52999282761009E-15,0.,39.2708017080178));
#179312=CARTESIAN_POINT('',(0.318076890624007,60.6410923272405,39.2708017080178));
#179313=CARTESIAN_POINT('Origin',(60.71525,0.,39.3978017080178));
#179314=CARTESIAN_POINT('',(0.317500000000643,60.8610688070707,39.3978017080178));
#179315=CARTESIAN_POINT('',(6.04595329345123,60.5608532912343,39.3978017080178));
#179316=CARTESIAN_POINT('Origin',(5.5478765747851E-15,0.,39.3978017080178));
#179317=CARTESIAN_POINT('',(6.06175884541631,60.7112330730303,39.3978017080178));
#179318=CARTESIAN_POINT('',(0.347626240494121,6.34489293004957,39.3978017080178));
#179319=CARTESIAN_POINT('',(0.317500000000645,61.0122769227456,39.3978017080178));
#179320=CARTESIAN_POINT('Origin',(5.5478765747851E-15,0.,39.3978017080178));
#179321=CARTESIAN_POINT('',(0.317500000000643,60.8615988316031,39.3978017080178));
#179322=CARTESIAN_POINT('Origin',(5.5478765747851E-15,0.,39.3978017080178));
#179323=CARTESIAN_POINT('',(0.316930737396561,61.2322532920972,39.2708017080178));
#179324=CARTESIAN_POINT('',(6.08531878141099,60.9299448849411,39.2708017081757));
#179325=CARTESIAN_POINT('Origin',(5.52999282761008E-15,0.,39.2708017080178));
#179326=CARTESIAN_POINT('',(6.10232411256148,61.0917542093523,38.9890000005756));
#179327=CARTESIAN_POINT('',(6.08531878138382,60.929944884669,39.2708017080178));
#179328=CARTESIAN_POINT('',(6.10175915944695,61.0918106390011,38.989));
#179329=CARTESIAN_POINT('Origin',(5.49031038273072E-15,0.,38.989));
#179330=CARTESIAN_POINT('',(0.317500000000649,61.3949508163454,38.989));
#179331=CARTESIAN_POINT('Origin',(5.49031038273072E-15,0.,38.989));
#179332=CARTESIAN_POINT('',(0.316932243253905,61.394953749505,38.9890000005754));
#179333=CARTESIAN_POINT('Origin',(5.49031038273072E-15,0.,38.989));
#179334=CARTESIAN_POINT('',(0.316932243240209,61.3949537498373,38.989));
#179335=CARTESIAN_POINT('Origin',(62.2224557307631,0.,38.989));
#179336=CARTESIAN_POINT('',(6.15137923967738,61.5639141665611,38.989));
#179337=CARTESIAN_POINT('',(0.364094271196581,6.50157577599617,38.989));
#179338=CARTESIAN_POINT('',(0.317500000000654,61.8696548221181,38.989));
#179339=CARTESIAN_POINT('Origin',(5.49031038273072E-15,0.,38.989));
#179340=CARTESIAN_POINT('',(0.317500000000649,61.3954762318973,38.989));
#179341=CARTESIAN_POINT('Origin',(5.57972911860581E-15,0.,39.624));
#179342=CARTESIAN_POINT('Origin',(5.95632779542376,59.7081714060829,39.6240070731883));
#179343=CARTESIAN_POINT('Origin',(0.317504993061332,60.0036895869254,39.6240070731883));
#179344=CARTESIAN_POINT('Origin',(5.57972911860581E-15,0.,39.624));
#179345=CARTESIAN_POINT('Origin',(6.15533149561049,61.6018382108738,39.5552135207989));
#179346=CARTESIAN_POINT('Origin',(0.31753353664925,61.907783829676,39.5552117598823));
#179347=CARTESIAN_POINT('Origin',(5.51210908043506E-15,0.,39.1438017080178));
#179348=CARTESIAN_POINT('Origin',(6.06345353572217,60.7270021185324,39.1711625381353));
#179349=CARTESIAN_POINT('Origin',(0.317463144197165,61.0280426587396,39.1712173702592));
#179350=CARTESIAN_POINT('Origin',(5.51210908043507E-15,0.,39.1438017080178));
#179351=CARTESIAN_POINT('Origin',(6.04426018543824,60.545178474123,39.1712175859392));
#179352=CARTESIAN_POINT('Origin',(0.317545622031397,60.845208813123,39.1711627526774));
#179353=CARTESIAN_POINT('Origin',(60.4792282238308,0.,38.989));
#179354=CARTESIAN_POINT('',(-5.9563328589115,59.7081718144893,38.989));
#179355=CARTESIAN_POINT('',(-0.317499999999366,60.0036905223731,38.989));
#179356=CARTESIAN_POINT('Origin',(5.49031038273072E-15,0.,38.989));
#179357=CARTESIAN_POINT('',(-0.317500000024619,60.4783948217626,38.989));
#179358=CARTESIAN_POINT('',(-0.317499999999991,6.36811926168668E-13,38.989));
#179359=CARTESIAN_POINT('',(-0.318078445377217,60.4783917836887,38.9889999995774));
#179360=CARTESIAN_POINT('Origin',(5.49031038273072E-15,0.,38.989));
#179361=CARTESIAN_POINT('',(-6.00537737563932,60.1803330762807,38.9889999997818));
#179362=CARTESIAN_POINT('Origin',(5.49031038273072E-15,0.,38.989));
#179363=CARTESIAN_POINT('',(-6.00595296980802,60.1802756340597,38.989));
#179364=CARTESIAN_POINT('Origin',(5.49031038273072E-15,0.,38.989));
#179365=CARTESIAN_POINT('',(-5.95638905318945,59.7087064673299,38.989));
#179366=CARTESIAN_POINT('Origin',(5.49031038273072E-15,0.,38.989));
#179367=CARTESIAN_POINT('',(-0.318076890622726,60.6410923272405,39.2708017080178));
#179368=CARTESIAN_POINT('',(-0.318078445373366,60.4783917829566,38.989));
#179369=CARTESIAN_POINT('',(-6.02238575973022,60.3421421673489,39.2708017078546));
#179370=CARTESIAN_POINT('Origin',(5.52999282761009E-15,0.,39.2708017080178));
#179371=CARTESIAN_POINT('',(-6.02238575970214,60.3421421670676,39.2708017080178));
#179372=CARTESIAN_POINT('Origin',(60.71525,0.,39.3978017080178));
#179373=CARTESIAN_POINT('',(-6.04595329344999,60.5608532912344,39.3978017080178));
#179374=CARTESIAN_POINT('',(-0.317499999999354,60.8610688070707,39.3978017080178));
#179375=CARTESIAN_POINT('Origin',(5.5478765747851E-15,0.,39.3978017080178));
#179376=CARTESIAN_POINT('',(-0.317499999999355,61.0122769227456,39.3978017080178));
#179377=CARTESIAN_POINT('',(-0.317499999999991,6.39284123049835E-13,39.3978017080178));
#179378=CARTESIAN_POINT('',(-6.06175884541508,60.7112330730304,39.3978017080178));
#179379=CARTESIAN_POINT('Origin',(5.5478765747851E-15,0.,39.3978017080178));
#179380=CARTESIAN_POINT('',(-6.04600869609986,60.561380412237,39.3978017080178));
#179381=CARTESIAN_POINT('Origin',(5.5478765747851E-15,0.,39.3978017080178));
#179382=CARTESIAN_POINT('',(-6.08531878138258,60.9299448846691,39.2708017080178));
#179383=CARTESIAN_POINT('',(-0.316930737396683,61.2322532923707,39.2708017081757));
#179384=CARTESIAN_POINT('Origin',(5.52999282761008E-15,0.,39.2708017080178));
#179385=CARTESIAN_POINT('',(-0.316932243252611,61.3949537495049,38.9890000005756));
#179386=CARTESIAN_POINT('',(-0.316930737395267,61.2322532920972,39.2708017080178));
#179387=CARTESIAN_POINT('',(-0.317499999999355,61.3949508163454,38.989));
#179388=CARTESIAN_POINT('Origin',(5.49031038273072E-15,0.,38.989));
#179389=CARTESIAN_POINT('',(-6.10175915944571,61.0918106390012,38.989));
#179390=CARTESIAN_POINT('Origin',(5.49031038273072E-15,0.,38.989));
#179391=CARTESIAN_POINT('',(-6.10232411256026,61.0917542093525,38.9890000005754));
#179392=CARTESIAN_POINT('Origin',(5.49031038273072E-15,0.,38.989));
#179393=CARTESIAN_POINT('',(-6.10232411260861,61.0917542096815,38.989));
#179394=CARTESIAN_POINT('Origin',(62.2224557307631,0.,38.989));
#179395=CARTESIAN_POINT('',(-0.317499999999346,61.8696548221181,38.989));
#179396=CARTESIAN_POINT('',(-0.317499999999998,6.55071265098105E-13,38.989));
#179397=CARTESIAN_POINT('',(-6.15137923967613,61.5639141665612,38.989));
#179398=CARTESIAN_POINT('Origin',(5.49031038273072E-15,0.,38.989));
#179399=CARTESIAN_POINT('',(-6.10181408032593,61.0923331762718,38.989));
#179400=CARTESIAN_POINT('Origin',(5.57972911860581E-15,0.,39.624));
#179401=CARTESIAN_POINT('Origin',(-0.317504993059919,60.0036895869254,39.6240070731883));
#179402=CARTESIAN_POINT('Origin',(-5.95632779542241,59.7081714060831,39.6240070731883));
#179403=CARTESIAN_POINT('Origin',(5.57972911860581E-15,0.,39.624));
#179404=CARTESIAN_POINT('Origin',(-0.317533537010864,61.9077842377891,39.5552135207949));
#179405=CARTESIAN_POINT('Origin',(-6.15533145331129,61.6018378049591,39.5552117598854));
#179406=CARTESIAN_POINT('Origin',(5.51210908043506E-15,0.,39.1438017080178));
#179407=CARTESIAN_POINT('Origin',(-0.317462907477851,61.0281367271385,39.1711625381323));
#179408=CARTESIAN_POINT('Origin',(-6.06344346747441,60.7269085901931,39.1712173702603));
#179409=CARTESIAN_POINT('Origin',(5.51210908043507E-15,0.,39.1438017080178));
#179410=CARTESIAN_POINT('Origin',(-0.317545368444817,60.8453028802704,39.1712175859369));
#179411=CARTESIAN_POINT('Origin',(-6.04425010054706,60.5450849487948,39.1711627526752));
#179412=CARTESIAN_POINT('Origin',(60.4792282238308,0.,38.989));
#179413=CARTESIAN_POINT('',(-12.1649068885786,58.7584778814678,38.989));
#179414=CARTESIAN_POINT('',(-6.58785426247035,59.6417962403143,38.989));
#179415=CARTESIAN_POINT('Origin',(5.49031038273072E-15,0.,38.989));
#179416=CARTESIAN_POINT('',(-6.63747437341721,60.1139000598801,38.989));
#179417=CARTESIAN_POINT('',(0.345047419449671,-6.32035708677179,38.989));
#179418=CARTESIAN_POINT('',(-6.6380493324205,60.1138365744458,38.988999999577));
#179419=CARTESIAN_POINT('Origin',(5.49031038273072E-15,0.,38.989));
#179420=CARTESIAN_POINT('',(-12.2630370254217,59.2229260464988,38.9889999997818));
#179421=CARTESIAN_POINT('Origin',(5.49031038273072E-15,0.,38.989));
#179422=CARTESIAN_POINT('',(-12.2636034620782,59.2228087529783,38.989));
#179423=CARTESIAN_POINT('Origin',(5.49031038273072E-15,0.,38.989));
#179424=CARTESIAN_POINT('',(-12.1650186614582,58.7590037315227,38.989));
#179425=CARTESIAN_POINT('Origin',(5.49031038273072E-15,0.,38.989));
#179426=CARTESIAN_POINT('',(-6.65505462397334,60.275645989912,39.2708017080178));
#179427=CARTESIAN_POINT('',(-6.63804933234009,60.1138365737176,38.989));
#179428=CARTESIAN_POINT('',(-12.296865891437,59.3820708701841,39.2708017078546));
#179429=CARTESIAN_POINT('Origin',(5.52999282761009E-15,0.,39.2708017080178));
#179430=CARTESIAN_POINT('',(-12.2968658913797,59.3820708699072,39.2708017080178));
#179431=CARTESIAN_POINT('Origin',(60.71525,0.,39.3978017080178));
#179432=CARTESIAN_POINT('',(-12.3431658574205,59.597120393566,39.3978017080178));
#179433=CARTESIAN_POINT('',(-6.67747469700884,60.4944777170594,39.3978017080178));
#179434=CARTESIAN_POINT('Origin',(5.5478765747851E-15,0.,39.3978017080178));
#179435=CARTESIAN_POINT('',(-6.69328024897394,60.6448574988555,39.3978017080178));
#179436=CARTESIAN_POINT('',(0.347626240493851,-6.34489293004837,39.3978017080178));
#179437=CARTESIAN_POINT('',(-12.3746037924158,59.7450242491249,39.3978017080178));
#179438=CARTESIAN_POINT('Origin',(5.5478765747851E-15,0.,39.3978017080178));
#179439=CARTESIAN_POINT('',(-12.3432760557172,59.5976388357908,39.3978017080178));
#179440=CARTESIAN_POINT('Origin',(5.5478765747851E-15,0.,39.3978017080178));
#179441=CARTESIAN_POINT('',(-12.420896274158,59.9600752506738,39.2708017080178));
#179442=CARTESIAN_POINT('',(-6.71570789672347,60.8636883190564,39.2708017081757));
#179443=CARTESIAN_POINT('Origin',(5.52999282761008E-15,0.,39.2708017080178));
#179444=CARTESIAN_POINT('',(-6.73271622308735,61.0254973286579,38.9890000005756));
#179445=CARTESIAN_POINT('',(-6.71570789669348,60.8636883187845,39.2708017080178));
#179446=CARTESIAN_POINT('',(-6.73328056300457,61.0254350648263,38.989));
#179447=CARTESIAN_POINT('Origin',(5.49031038273072E-15,0.,38.989));
#179448=CARTESIAN_POINT('',(-12.4541661686659,60.119335800013,38.989));
#179449=CARTESIAN_POINT('Origin',(5.49031038273072E-15,0.,38.989));
#179450=CARTESIAN_POINT('',(-12.4547221284037,60.1192206258109,38.9890000005754));
#179451=CARTESIAN_POINT('Origin',(5.49031038273072E-15,0.,38.989));
#179452=CARTESIAN_POINT('',(-12.4547221284862,60.119220626133,38.989));
#179453=CARTESIAN_POINT('Origin',(62.2224557307631,0.,38.989));
#179454=CARTESIAN_POINT('',(-6.78290064323498,61.4975385923863,38.989));
#179455=CARTESIAN_POINT('',(0.364094271196325,-6.50157577599494,38.989));
#179456=CARTESIAN_POINT('',(-12.5528626811441,60.5836663843183,38.989));
#179457=CARTESIAN_POINT('Origin',(5.49031038273072E-15,0.,38.989));
#179458=CARTESIAN_POINT('',(-12.4542754087017,60.1198497339745,38.989));
#179459=CARTESIAN_POINT('Origin',(5.57972911860581E-15,0.,39.624));
#179460=CARTESIAN_POINT('Origin',(-6.58785913039747,59.6417947880742,39.6240070731883));
#179461=CARTESIAN_POINT('Origin',(-12.1649018101377,58.7584780045776,39.6240070731883));
#179462=CARTESIAN_POINT('Origin',(5.57972911860581E-15,0.,39.624));
#179463=CARTESIAN_POINT('Origin',(-6.78691960575238,61.5354556255527,39.5552135208018));
#179464=CARTESIAN_POINT('Origin',(-12.5607573437817,60.620969154241,39.5552117598825));
#179465=CARTESIAN_POINT('Origin',(5.51210908043506E-15,0.,39.1438017080178));
#179466=CARTESIAN_POINT('Origin',(-6.69490116062997,60.6606342988039,39.1711625381309));
#179467=CARTESIAN_POINT('Origin',(-12.3779177236594,59.7604378032104,39.1712173702625));
#179468=CARTESIAN_POINT('Origin',(5.51210908043507E-15,0.,39.1438017080178));
#179469=CARTESIAN_POINT('Origin',(-6.67587182882098,60.4787934153615,39.1712175859378));
#179470=CARTESIAN_POINT('Origin',(-12.3398237541834,59.5816164638937,39.1711627526742));
#179471=CARTESIAN_POINT('Origin',(60.4792282238308,0.,38.989));
#179472=CARTESIAN_POINT('',(-18.240199652704,57.1650137687749,38.989));
#179473=CARTESIAN_POINT('',(-12.7860306150445,58.6264539577985,38.989));
#179474=CARTESIAN_POINT('Origin',(5.49031038273072E-15,0.,38.989));
#179475=CARTESIAN_POINT('',(-12.8847271885938,59.0907848292992,38.989));
#179476=CARTESIAN_POINT('',(2.30379013587678,-12.3655710936221,38.989));
#179477=CARTESIAN_POINT('',(-12.8852923618764,59.0906615920626,38.9889999995776));
#179478=CARTESIAN_POINT('Origin',(5.49031038273072E-15,0.,38.989));
#179479=CARTESIAN_POINT('',(-18.3863402753482,57.6166602457574,38.9889999997818));
#179480=CARTESIAN_POINT('Origin',(5.49031038273072E-15,0.,38.989));
#179481=CARTESIAN_POINT('',(-18.386891348494,57.6164843860299,38.989));
#179482=CARTESIAN_POINT('Origin',(5.49031038273072E-15,0.,38.989));
#179483=CARTESIAN_POINT('',(-18.2403657795782,57.1655250547208,38.989));
#179484=CARTESIAN_POINT('Origin',(5.49031038273072E-15,0.,38.989));
#179485=CARTESIAN_POINT('',(-12.9191181862039,59.2498070616281,39.2708017080178));
#179486=CARTESIAN_POINT('',(-12.8852923617205,59.0906615913479,38.989));
#179487=CARTESIAN_POINT('',(-18.4366189871527,57.7713971780682,39.2708017078546));
#179488=CARTESIAN_POINT('Origin',(5.52999282761009E-15,0.,39.2708017080178));
#179489=CARTESIAN_POINT('',(-18.4366189870667,57.7713971777989,39.2708017080178));
#179490=CARTESIAN_POINT('Origin',(60.71525,0.,39.3978017080178));
#179491=CARTESIAN_POINT('',(-18.5051441132836,57.9804289733665,39.3978017080178));
#179492=CARTESIAN_POINT('',(-12.9642895838864,59.4650964698968,39.3978017080178));
#179493=CARTESIAN_POINT('Origin',(5.5478765747851E-15,0.,39.3978017080178));
#179494=CARTESIAN_POINT('',(-12.9957275188818,59.6130003254556,39.3978017080178));
#179495=CARTESIAN_POINT('',(2.31399271319931,-12.4135704460881,39.3978017080178));
#179496=CARTESIAN_POINT('',(-18.5518699907145,58.1242364370958,39.3978017080178));
#179497=CARTESIAN_POINT('Origin',(5.5478765747851E-15,0.,39.3978017080178));
#179498=CARTESIAN_POINT('',(-18.5053078998715,57.9809330566519,39.3978017080178));
#179499=CARTESIAN_POINT('Origin',(5.5478765747851E-15,0.,39.3978017080178));
#179500=CARTESIAN_POINT('',(-18.6203878281142,58.3332704847798,39.2708017080178));
#179501=CARTESIAN_POINT('',(-13.0409063549815,59.8282880399728,39.2708017081757));
#179502=CARTESIAN_POINT('Origin',(5.52999282761008E-15,0.,39.2708017080178));
#179503=CARTESIAN_POINT('',(-13.0747351550704,59.9874327886719,38.9890000005756));
#179504=CARTESIAN_POINT('',(-13.0409063549232,59.8282880397056,39.2708017080178));
#179505=CARTESIAN_POINT('',(-13.0752898951319,59.9873118763437,38.989));
#179506=CARTESIAN_POINT('Origin',(5.49031038273072E-15,0.,38.989));
#179507=CARTESIAN_POINT('',(-18.6701227271405,58.4881809372199,38.989));
#179508=CARTESIAN_POINT('Origin',(5.49031038273072E-15,0.,38.989));
#179509=CARTESIAN_POINT('',(-18.6706636022903,58.4880082803371,38.9890000005754));
#179510=CARTESIAN_POINT('Origin',(5.49031038273072E-15,0.,38.989));
#179511=CARTESIAN_POINT('',(-18.670663602406,58.4880082806489,38.989));
#179512=CARTESIAN_POINT('Origin',(62.2224557307631,0.,38.989));
#179513=CARTESIAN_POINT('',(-13.1739864076101,60.451642460649,38.989));
#179514=CARTESIAN_POINT('',(2.3791451040451,-12.7200883457656,38.989));
#179515=CARTESIAN_POINT('',(-18.8168143322221,58.9396512752215,38.989));
#179516=CARTESIAN_POINT('Origin',(5.49031038273072E-15,0.,38.989));
#179517=CARTESIAN_POINT('',(-18.6702850894751,58.4886806371044,38.989));
#179518=CARTESIAN_POINT('Origin',(5.57972911860581E-15,0.,39.624));
#179519=CARTESIAN_POINT('Origin',(-12.7860353045041,58.626452004677,39.6240070731883));
#179520=CARTESIAN_POINT('Origin',(-18.2401946149518,57.1650144220519,39.6240070731883));
#179521=CARTESIAN_POINT('Origin',(5.57972911860581E-15,0.,39.624));
#179522=CARTESIAN_POINT('Origin',(-13.1819467630411,60.4889316843654,39.5552135207998));
#179523=CARTESIAN_POINT('Origin',(-18.8285649482859,58.9759244797165,39.5552117598789));
#179524=CARTESIAN_POINT('Origin',(5.51210908043506E-15,0.,39.1438017080178));
#179525=CARTESIAN_POINT('Origin',(-12.9989886756678,59.6285212670377,39.1711625381293));
#179526=CARTESIAN_POINT('Origin',(-18.5567769230181,58.1392191539792,39.1712173702626));
#179527=CARTESIAN_POINT('Origin',(5.51210908043507E-15,0.,39.1438017080178));
#179528=CARTESIAN_POINT('Origin',(-12.9610560404226,59.4496656337912,39.1712175859416));
#179529=CARTESIAN_POINT('Origin',(-18.5001997164926,57.9653593207583,39.1711627526753));
#179530=CARTESIAN_POINT('Origin',(60.4792282238308,0.,38.989));
#179531=CARTESIAN_POINT('',(-24.1156489724272,54.9452378026831,38.989));
#179532=CARTESIAN_POINT('',(-18.8441205405514,56.9687879773468,38.989));
#179533=CARTESIAN_POINT('Origin',(5.49031038273072E-15,0.,38.989));
#179534=CARTESIAN_POINT('',(-18.9908122363897,57.4202585945868,38.989));
#179535=CARTESIAN_POINT('',(5.47329194811131,-17.8725121057128,38.989));
#179536=CARTESIAN_POINT('',(-18.9913614317952,57.4200769557627,38.9889999995772));
#179537=CARTESIAN_POINT('Origin',(5.49031038273072E-15,0.,38.989));
#179538=CARTESIAN_POINT('',(-24.3081989336288,55.3791342583022,38.9889999997818));
#179539=CARTESIAN_POINT('Origin',(5.49031038273072E-15,0.,38.989));
#179540=CARTESIAN_POINT('',(-24.3087286055912,55.3789017591235,38.989));
#179541=CARTESIAN_POINT('Origin',(5.49031038273072E-15,0.,38.989));
#179542=CARTESIAN_POINT('',(-24.1158676331753,54.9457289227642,38.989));
#179543=CARTESIAN_POINT('Origin',(5.49031038273072E-15,0.,38.989));
#179544=CARTESIAN_POINT('',(-19.0416371860872,57.5748148483578,39.2708017080178));
#179545=CARTESIAN_POINT('',(-18.9913614315652,57.4200769550674,38.989));
#179546=CARTESIAN_POINT('',(-24.3743766271346,55.5277679690274,39.2708017078546));
#179547=CARTESIAN_POINT('Origin',(5.52999282761009E-15,0.,39.2708017080178));
#179548=CARTESIAN_POINT('',(-24.3743766270209,55.5277679687685,39.2708017080178));
#179549=CARTESIAN_POINT('Origin',(60.71525,0.,39.3978017080178));
#179550=CARTESIAN_POINT('',(-24.4643761377912,55.72849184015,39.3978017080178));
#179551=CARTESIAN_POINT('',(-19.109065001131,57.7842031819385,39.3978017080178));
#179552=CARTESIAN_POINT('Origin',(5.5478765747851E-15,0.,39.3978017080178));
#179553=CARTESIAN_POINT('',(-19.155790878562,57.9280106456677,39.3978017080178));
#179554=CARTESIAN_POINT('',(5.4958300222142,-17.9418771653389,39.3978017080178));
#179555=CARTESIAN_POINT('',(-24.5258780191666,55.8666273273835,39.3978017080178));
#179556=CARTESIAN_POINT('Origin',(5.5478765747851E-15,0.,39.3978017080178));
#179557=CARTESIAN_POINT('',(-24.4645917181903,55.7289760416541,39.3978017080178));
#179558=CARTESIAN_POINT('Origin',(5.5478765747851E-15,0.,39.3978017080178));
#179559=CARTESIAN_POINT('',(-24.6158705164589,56.0673542004328,39.2708017080178));
#179560=CARTESIAN_POINT('',(-19.2232259142293,58.1373965172492,39.2708017081757));
#179561=CARTESIAN_POINT('Origin',(5.52999282761008E-15,0.,39.2708017080178));
#179562=CARTESIAN_POINT('',(-19.2735045526304,58.2921333818758,38.9890000005756));
#179563=CARTESIAN_POINT('',(-19.2232259141434,58.1373965169895,39.2708017080178));
#179564=CARTESIAN_POINT('',(-19.2740436149879,58.2919551457918,38.989));
#179565=CARTESIAN_POINT('Origin',(5.49031038273072E-15,0.,38.989));
#179566=CARTESIAN_POINT('',(-24.6815255140421,56.21621732464,38.989));
#179567=CARTESIAN_POINT('Origin',(5.49031038273072E-15,0.,38.989));
#179568=CARTESIAN_POINT('',(-24.6820453786627,56.2159890767414,38.9890000005754));
#179569=CARTESIAN_POINT('Origin',(5.49031038273072E-15,0.,38.989));
#179570=CARTESIAN_POINT('',(-24.6820453788103,56.2159890770394,38.989));
#179571=CARTESIAN_POINT('Origin',(62.2224557307631,0.,38.989));
#179572=CARTESIAN_POINT('',(-19.4207352200695,58.7434254837934,38.989));
#179573=CARTESIAN_POINT('',(5.6397553624924,-18.3848338156955,38.989));
#179574=CARTESIAN_POINT('',(-24.8746050278048,56.6498810128384,38.989));
#179575=CARTESIAN_POINT('Origin',(5.49031038273072E-15,0.,38.989));
#179576=CARTESIAN_POINT('',(-24.6817392197999,56.2166973156308,38.989));
#179577=CARTESIAN_POINT('Origin',(5.57972911860581E-15,0.,39.624));
#179578=CARTESIAN_POINT('Origin',(-18.8441250001649,56.9687855447426,39.6240070731883));
#179579=CARTESIAN_POINT('Origin',(-24.1156440305584,54.9452389789698,39.6240070731883));
#179580=CARTESIAN_POINT('Origin',(5.57972911860581E-15,0.,39.624));
#179581=CARTESIAN_POINT('Origin',(-19.4325497530907,58.7796783495197,39.5552135208017));
#179582=CARTESIAN_POINT('Origin',(-24.8900828550914,56.6847272350837,39.5552117598772));
#179583=CARTESIAN_POINT('Origin',(5.51210908043506E-15,0.,39.1438017080178));
#179584=CARTESIAN_POINT('Origin',(-19.1606565505623,57.9431056782018,39.1711625381312));
#179585=CARTESIAN_POINT('Origin',(-24.5323241911529,55.8810150532827,39.1712173702612));
#179586=CARTESIAN_POINT('Origin',(5.51210908043507E-15,0.,39.1438017080178));
#179587=CARTESIAN_POINT('Origin',(-19.1042362097708,57.7691948748993,39.1712175859379));
#179588=CARTESIAN_POINT('Origin',(-24.4578836192968,55.7140215708741,39.171162752673));
#179589=CARTESIAN_POINT('Origin',(60.4792282238308,0.,38.989));
#179590=CARTESIAN_POINT('',(-29.7268821954845,52.1234703131949,38.989));
#179591=CARTESIAN_POINT('',(-24.6957503380303,54.6869600343299,38.989));
#179592=CARTESIAN_POINT('Origin',(5.49031038273072E-15,0.,38.989));
#179593=CARTESIAN_POINT('',(-24.8888299712407,55.1206239907504,38.989));
#179594=CARTESIAN_POINT('',(9.71531210234964,-22.6015516358793,38.989));
#179595=CARTESIAN_POINT('',(-24.8893571716693,55.1203859404114,38.988999999577));
#179596=CARTESIAN_POINT('Origin',(5.49031038273072E-15,0.,38.989));
#179597=CARTESIAN_POINT('',(-29.963731877575,52.5348628870841,38.9889999997818));
#179598=CARTESIAN_POINT('Origin',(5.49031038273072E-15,0.,38.989));
#179599=CARTESIAN_POINT('',(-29.964234345157,52.5345762957641,38.989));
#179600=CARTESIAN_POINT('Origin',(5.49031038273072E-15,0.,38.989));
#179601=CARTESIAN_POINT('',(-29.7271509944135,52.1239358865969,38.989));
#179602=CARTESIAN_POINT('Origin',(5.49031038273072E-15,0.,38.989));
#179603=CARTESIAN_POINT('',(-24.955532024241,55.2690209153042,39.2708017080178));
#179604=CARTESIAN_POINT('',(-24.8893571713678,55.1203859397437,38.989));
#179605=CARTESIAN_POINT('',(-30.0450834961232,52.6757649141855,39.2708017078546));
#179606=CARTESIAN_POINT('Origin',(5.52999282761009E-15,0.,39.2708017080178));
#179607=CARTESIAN_POINT('',(-30.0450834959832,52.6757649139399,39.2708017080178));
#179608=CARTESIAN_POINT('Origin',(60.71525,0.,39.3978017080178));
#179609=CARTESIAN_POINT('',(-30.1555713378333,52.8659816883962,39.3978017080178));
#179610=CARTESIAN_POINT('',(-25.0444775033943,55.4702140717969,39.3978017080178));
#179611=CARTESIAN_POINT('Origin',(5.5478765747851E-15,0.,39.3978017080178));
#179612=CARTESIAN_POINT('',(-25.1059793847697,55.6083495590304,39.3978017080178));
#179613=CARTESIAN_POINT('',(9.75435829333326,-22.6892508167094,39.3978017080178));
#179614=CARTESIAN_POINT('',(-30.2311753956707,52.996931757829,39.3978017080178));
#179615=CARTESIAN_POINT('Origin',(5.5478765747851E-15,0.,39.3978017080178));
#179616=CARTESIAN_POINT('',(-30.1558363500995,52.8664407031059,39.3978017080178));
#179617=CARTESIAN_POINT('Origin',(5.5478765747851E-15,0.,39.3978017080178));
#179618=CARTESIAN_POINT('',(-30.3416565762231,53.1871522506178,39.2708017080178));
#179619=CARTESIAN_POINT('',(-25.1949317876421,55.8095395122502,39.2708017081757));
#179620=CARTESIAN_POINT('Origin',(5.52999282761008E-15,0.,39.2708017080178));
#179621=CARTESIAN_POINT('',(-25.2611094010716,55.9581731633347,38.9890000005756));
#179622=CARTESIAN_POINT('',(-25.1949317875296,55.8095395120009,39.2708017080178));
#179623=CARTESIAN_POINT('',(-25.2616268796452,55.9579395562868,38.989));
#179624=CARTESIAN_POINT('Origin',(5.49031038273072E-15,0.,38.989));
#179625=CARTESIAN_POINT('',(-30.4225123424706,53.3283370710515,38.989));
#179626=CARTESIAN_POINT('Origin',(5.49031038273072E-15,0.,38.989));
#179627=CARTESIAN_POINT('',(-30.4230055008163,53.3280557328689,38.9890000005754));
#179628=CARTESIAN_POINT('Origin',(5.49031038273072E-15,0.,38.989));
#179629=CARTESIAN_POINT('',(-30.4230055009943,53.3280557331498,38.989));
#179630=CARTESIAN_POINT('Origin',(62.2224557307631,0.,38.989));
#179631=CARTESIAN_POINT('',(-25.4547063934078,56.3916032444853,38.989));
#179632=CARTESIAN_POINT('',(10.0037024164483,-23.2492868865826,38.989));
#179633=CARTESIAN_POINT('',(-30.659864345357,53.7394427993289,38.989));
#179634=CARTESIAN_POINT('Origin',(5.49031038273072E-15,0.,38.989));
#179635=CARTESIAN_POINT('',(-30.4227750502466,53.328792094267,38.989));
#179636=CARTESIAN_POINT('Origin',(5.57972911860581E-15,0.,39.624));
#179637=CARTESIAN_POINT('Origin',(-24.6957545189371,54.6869571488953,39.6240070731883));
#179638=CARTESIAN_POINT('Origin',(-29.7268774036432,52.1234719996038,39.6240070731883));
#179639=CARTESIAN_POINT('Origin',(5.57972911860581E-15,0.,39.624));
#179640=CARTESIAN_POINT('Origin',(-25.4702456615205,56.4264225582429,39.5552135207977));
#179641=CARTESIAN_POINT('Origin',(-30.6788998055462,53.7724802568187,39.5552117598843));
#179642=CARTESIAN_POINT('Origin',(5.51210908043506E-15,0.,39.1438017080178));
#179643=CARTESIAN_POINT('Origin',(-25.112396262664,55.6228532981809,39.1711625381333));
#179644=CARTESIAN_POINT('Origin',(-30.2390901817291,53.0105668578062,39.1712173702566));
#179645=CARTESIAN_POINT('Origin',(5.51210908043507E-15,0.,39.1438017080178));
#179646=CARTESIAN_POINT('Origin',(-25.0381063693886,55.4557927279736,39.171217585938));
#179647=CARTESIAN_POINT('Origin',(-30.147601831023,52.8522693417483,39.1711627526774));
#179648=CARTESIAN_POINT('Origin',(60.4792282238308,0.,38.989));
#179649=CARTESIAN_POINT('',(-35.0124214764581,48.7306271754179,38.989));
#179650=CARTESIAN_POINT('',(-30.2768083268876,51.8059703131949,38.989));
#179651=CARTESIAN_POINT('Origin',(5.49031038273072E-15,0.,38.989));
#179652=CARTESIAN_POINT('',(-30.5141604766043,52.2170762957393,38.989));
#179653=CARTESIAN_POINT('',(14.8448439902557,-26.3470240215568,38.989));
#179654=CARTESIAN_POINT('',(-30.5146599059373,52.2167844420138,38.9889999995774));
#179655=CARTESIAN_POINT('Origin',(5.49031038273072E-15,0.,38.989));
#179656=CARTESIAN_POINT('',(-35.2909759047564,49.1150085644483,38.9889999997818));
#179657=CARTESIAN_POINT('Origin',(5.49031038273072E-15,0.,38.989));
#179658=CARTESIAN_POINT('',(-35.2914456628182,49.1146710209413,38.989));
#179659=CARTESIAN_POINT('Origin',(5.49031038273072E-15,0.,38.989));
#179660=CARTESIAN_POINT('',(-35.0127374685506,48.7310621012212,38.989));
#179661=CARTESIAN_POINT('Origin',(5.49031038273072E-15,0.,38.989));
#179662=CARTESIAN_POINT('',(-30.5960088312564,52.3576880233165,39.2708017080178));
#179663=CARTESIAN_POINT('',(-30.514659905568,52.2167844413818,38.989));
#179664=CARTESIAN_POINT('',(-35.3866101429905,49.2466351558312,39.2708017078546));
#179665=CARTESIAN_POINT('Origin',(5.52999282761009E-15,0.,39.2708017080178));
#179666=CARTESIAN_POINT('',(-35.3866101428255,49.2466351556016,39.2708017080178));
#179667=CARTESIAN_POINT('Origin',(60.71525,0.,39.3978017080178));
#179668=CARTESIAN_POINT('',(-35.5163757878391,49.4242607783464,39.3978017080178));
#179669=CARTESIAN_POINT('',(-30.7054974692364,52.5484816883962,39.3978017080178));
#179670=CARTESIAN_POINT('Origin',(5.5478765747851E-15,0.,39.3978017080178));
#179671=CARTESIAN_POINT('',(-30.7811015270739,52.679431757829,39.3978017080178));
#179672=CARTESIAN_POINT('',(14.903849434298,-26.4492244485613,39.3978017080178));
#179673=CARTESIAN_POINT('',(-35.6052536882598,49.5465907136148,39.3978017080178));
#179674=CARTESIAN_POINT('Origin',(5.5478765747851E-15,0.,39.3978017080178));
#179675=CARTESIAN_POINT('',(-35.5166873284426,49.4246895772005,39.3978017080178));
#179676=CARTESIAN_POINT('Origin',(5.5478765747851E-15,0.,39.3978017080178));
#179677=CARTESIAN_POINT('',(-35.7350130971385,49.7242207306178,39.2708017080178));
#179678=CARTESIAN_POINT('',(-30.8905967160111,52.870221513458,39.2708017081757));
#179679=CARTESIAN_POINT('Origin',(5.52999282761008E-15,0.,39.2708017080178));
#179680=CARTESIAN_POINT('',(-30.9719482486877,53.0111234896156,38.9890000005756));
#179681=CARTESIAN_POINT('',(-30.8905967158731,52.8702215132219,39.2708017080178));
#179682=CARTESIAN_POINT('',(-30.9724384738737,53.0108370710515,38.989));
#179683=CARTESIAN_POINT('Origin',(5.49031038273072E-15,0.,38.989));
#179684=CARTESIAN_POINT('',(-35.830183759355,49.8561803968406,38.989));
#179685=CARTESIAN_POINT('Origin',(5.49031038273072E-15,0.,38.989));
#179686=CARTESIAN_POINT('',(-35.8306448082798,49.855849050774,38.9890000005754));
#179687=CARTESIAN_POINT('Origin',(5.49031038273072E-15,0.,38.989));
#179688=CARTESIAN_POINT('',(-35.8306448084862,49.8558490510348,38.989));
#179689=CARTESIAN_POINT('Origin',(62.2224557307631,0.,38.989));
#179690=CARTESIAN_POINT('',(-31.2097904767601,53.4219427993289,38.989));
#179691=CARTESIAN_POINT('',(15.2806508669887,-27.1018636743464,38.989));
#179692=CARTESIAN_POINT('',(-36.1092077731524,50.2402240048086,38.989));
#179693=CARTESIAN_POINT('Origin',(5.49031038273072E-15,0.,38.989));
#179694=CARTESIAN_POINT('',(-35.8304925908678,49.8566054669512,38.989));
#179695=CARTESIAN_POINT('Origin',(5.57972911860581E-15,0.,39.624));
#179696=CARTESIAN_POINT('Origin',(-30.2768121832811,51.8059670065432,39.6240070731883));
#179697=CARTESIAN_POINT('Origin',(-35.0124168871447,48.7306293534723,39.6240070731883));
#179698=CARTESIAN_POINT('Origin',(5.57972911860581E-15,0.,39.624));
#179699=CARTESIAN_POINT('Origin',(-31.2288842284945,53.4549470734247,39.5552135208013));
#179700=CARTESIAN_POINT('Origin',(-36.1315923097633,50.2710907322474,39.5552117598819));
#179701=CARTESIAN_POINT('Origin',(5.51210908043506E-15,0.,39.1438017080178));
#179702=CARTESIAN_POINT('Origin',(-30.7889993062062,52.6931852975962,39.1711625381386));
#179703=CARTESIAN_POINT('Origin',(-35.614550372342,49.5593237986677,39.1712173702654));
#179704=CARTESIAN_POINT('Origin',(5.51210908043507E-15,0.,39.1438017080178));
#179705=CARTESIAN_POINT('Origin',(-30.6976537960621,52.5348053110493,39.1712175859384));
#179706=CARTESIAN_POINT('Origin',(-35.5070166083006,49.4114565896685,39.1711627526738));
#179707=CARTESIAN_POINT('Origin',(60.4792282238308,0.,38.989));
#179708=CARTESIAN_POINT('',(-39.9143573409153,44.8038810887678,38.989));
#179709=CARTESIAN_POINT('',(-35.5261472678861,48.3573835402122,38.989));
#179710=CARTESIAN_POINT('Origin',(5.49031038273072E-15,0.,38.989));
#179711=CARTESIAN_POINT('',(-35.8051714542876,48.7414273857064,38.989));
#179712=CARTESIAN_POINT('',(20.6381965522785,-28.9462038689907,38.989));
#179713=CARTESIAN_POINT('',(-35.8056376406732,48.7410849262056,38.9889999995772));
#179714=CARTESIAN_POINT('Origin',(5.49031038273072E-15,0.,38.989));
#179715=CARTESIAN_POINT('',(-40.2315646148138,45.1570399300041,38.9889999997818));
#179716=CARTESIAN_POINT('Origin',(5.49031038273072E-15,0.,38.989));
#179717=CARTESIAN_POINT('',(-40.2319965165878,45.1566551325075,38.989));
#179718=CARTESIAN_POINT('Origin',(5.49031038273072E-15,0.,38.989));
#179719=CARTESIAN_POINT('',(-39.914717064096,44.8042806018341,38.989));
#179720=CARTESIAN_POINT('Origin',(5.49031038273072E-15,0.,38.989));
#179721=CARTESIAN_POINT('',(-35.90126936289,48.8727133447947,39.2708017080178));
#179722=CARTESIAN_POINT('',(-35.8056376402397,48.7410849256154,38.989));
#179723=CARTESIAN_POINT('',(-40.3404336840069,45.2779489571887,39.2708017078546));
#179724=CARTESIAN_POINT('Origin',(5.52999282761009E-15,0.,39.2708017080178));
#179725=CARTESIAN_POINT('',(-40.3404336838189,45.2779489569776,39.2708017080178));
#179726=CARTESIAN_POINT('Origin',(60.71525,0.,39.3978017080178));
#179727=CARTESIAN_POINT('',(-40.4880553924339,45.4410373245175,39.3978017080178));
#179728=CARTESIAN_POINT('',(-36.0301015792672,49.0510171431407,39.3978017080178));
#179729=CARTESIAN_POINT('Origin',(5.5478765747851E-15,0.,39.3978017080178));
#179730=CARTESIAN_POINT('',(-36.1189794796879,49.1733470784091,39.3978017080178));
#179731=CARTESIAN_POINT('',(20.7197400704237,-29.0584388930974,39.3978017080178));
#179732=CARTESIAN_POINT('',(-40.5892333705619,45.5534068532515,39.3978017080178));
#179733=CARTESIAN_POINT('Origin',(5.5478765747851E-15,0.,39.3978017080178));
#179734=CARTESIAN_POINT('',(-40.4884100480707,45.4414312095062,39.3978017080178));
#179735=CARTESIAN_POINT('Origin',(5.5478765747851E-15,0.,39.3978017080178));
#179736=CARTESIAN_POINT('',(-40.7368493365293,45.716500242831,39.2708017080178));
#179737=CARTESIAN_POINT('',(-36.2478178024865,49.3516463039592,39.2708017081757));
#179738=CARTESIAN_POINT('Origin',(5.52999282761008E-15,0.,39.2708017080178));
#179739=CARTESIAN_POINT('',(-36.3434519499943,49.4832728536535,38.9890000005756));
#179740=CARTESIAN_POINT('',(-36.2478178023246,49.3516463037388,39.2708017080178));
#179741=CARTESIAN_POINT('',(-36.3439095507831,49.4829367616349,38.989));
#179742=CARTESIAN_POINT('Origin',(5.49031038273072E-15,0.,38.989));
#179743=CARTESIAN_POINT('',(-40.845292185024,45.8377889771254,38.989));
#179744=CARTESIAN_POINT('Origin',(5.49031038273072E-15,0.,38.989));
#179745=CARTESIAN_POINT('',(-40.8457160731793,45.8374112534716,38.9890000005754));
#179746=CARTESIAN_POINT('Origin',(5.49031038273072E-15,0.,38.989));
#179747=CARTESIAN_POINT('',(-40.8457160734119,45.8374112537094,38.989));
#179748=CARTESIAN_POINT('Origin',(62.2224557307631,0.,38.989));
#179749=CARTESIAN_POINT('',(-36.6229335645805,49.8669803696029,38.989));
#179750=CARTESIAN_POINT('',(21.2404668433927,-29.7751578089171,38.989));
#179751=CARTESIAN_POINT('',(-41.1629311642477,46.1905628026488,38.989));
#179752=CARTESIAN_POINT('Origin',(5.49031038273072E-15,0.,38.989));
#179753=CARTESIAN_POINT('',(-40.8456437566508,45.8381794369741,38.989));
#179754=CARTESIAN_POINT('Origin',(5.57972911860581E-15,0.,39.624));
#179755=CARTESIAN_POINT('Origin',(-35.5261507575146,48.3573798485718,39.6240070731883));
#179756=CARTESIAN_POINT('Origin',(-39.9143530044114,44.8038837346044,39.6240070731883));
#179757=CARTESIAN_POINT('Origin',(5.57972911860581E-15,0.,39.624));
#179758=CARTESIAN_POINT('Origin',(-36.6453726048013,49.8978080023008,39.555213520804));
#179759=CARTESIAN_POINT('Origin',(-41.1884195276088,46.218920617714,39.5552117598819));
#179760=CARTESIAN_POINT('Origin',(5.51210908043506E-15,0.,39.1438017080178));
#179761=CARTESIAN_POINT('Origin',(-36.1282716303341,49.1861997321277,39.1711625381329));
#179762=CARTESIAN_POINT('Origin',(-40.5998100962482,45.5650984170306,39.1712173702632));
#179763=CARTESIAN_POINT('Origin',(5.51210908043507E-15,0.,39.1438017080178));
#179764=CARTESIAN_POINT('Origin',(-36.0208713038459,49.0382355735241,39.1712175859398));
#179765=CARTESIAN_POINT('Origin',(-40.4774090812904,45.4292815791817,39.1711627526756));
#179766=CARTESIAN_POINT('Origin',(60.4792282238308,0.,38.989));
#179767=CARTESIAN_POINT('',(-44.3789831537292,40.3862543050942,38.989));
#179768=CARTESIAN_POINT('',(-40.3862543050934,44.3789831537299,38.989));
#179769=CARTESIAN_POINT('Origin',(5.49031038273072E-15,0.,38.989));
#179770=CARTESIAN_POINT('',(-40.7038934808039,44.7317571974363,38.989));
#179771=CARTESIAN_POINT('',(26.8427652369004,-30.2864073093061,38.989));
#179772=CARTESIAN_POINT('',(-40.7043213166062,44.7313678842177,38.9889999995774));
#179773=CARTESIAN_POINT('Origin',(5.49031038273072E-15,0.,38.989));
#179774=CARTESIAN_POINT('',(-44.7313678839552,40.7043213163687,38.9889999997818));
#179775=CARTESIAN_POINT('Origin',(5.49031038273072E-15,0.,38.989));
#179776=CARTESIAN_POINT('',(-44.7317571974351,40.7038934808043,38.989));
#179777=CARTESIAN_POINT('Origin',(5.49031038273072E-15,0.,38.989));
#179778=CARTESIAN_POINT('',(-44.3793826667955,40.3866140282749,38.989));
#179779=CARTESIAN_POINT('Origin',(5.49031038273072E-15,0.,38.989));
#179780=CARTESIAN_POINT('',(-40.8131880745603,44.8522789915945,39.2708017080178));
#179781=CARTESIAN_POINT('',(-40.7043213161135,44.7313678836763,38.989));
#179782=CARTESIAN_POINT('',(-44.8522789918029,40.8131880747513,39.2708017078546));
#179783=CARTESIAN_POINT('Origin',(5.52999282761009E-15,0.,39.2708017080178));
#179784=CARTESIAN_POINT('',(-44.8522789915938,40.813188074561,39.2708017080178));
#179785=CARTESIAN_POINT('Origin',(60.71525,0.,39.3978017080178));
#179786=CARTESIAN_POINT('',(-45.016139389479,40.9599523566129,39.3978017080178));
#179787=CARTESIAN_POINT('',(-40.9599523566121,45.0161393894797,39.3978017080178));
#179788=CARTESIAN_POINT('Origin',(5.5478765747851E-15,0.,39.3978017080178));
#179789=CARTESIAN_POINT('',(-41.06113033474,45.1285089182136,39.3978017080178));
#179790=CARTESIAN_POINT('',(26.9484406282047,-30.4037717213982,39.3978017080178));
#179791=CARTESIAN_POINT('',(-45.1285089182129,41.0611303347408,39.3978017080178));
#179792=CARTESIAN_POINT('Origin',(5.5478765747851E-15,0.,39.3978017080178));
#179793=CARTESIAN_POINT('',(-45.0165332744676,40.9603070122496,39.3978017080178));
#179794=CARTESIAN_POINT('Origin',(5.5478765747851E-15,0.,39.3978017080178));
#179795=CARTESIAN_POINT('',(-45.2923641298554,41.2079002115911,39.2708017080178));
#179796=CARTESIAN_POINT('',(-41.2079002117744,45.2923641300583,39.2708017081757));
#179797=CARTESIAN_POINT('Origin',(5.52999282761008E-15,0.,39.2708017080178));
#179798=CARTESIAN_POINT('',(-41.3167691863805,45.4132731252661,38.9890000005756));
#179799=CARTESIAN_POINT('',(-41.2079002115903,45.2923641298561,39.2708017080178));
#179800=CARTESIAN_POINT('',(-41.3171891492021,45.4128910420876,38.989));
#179801=CARTESIAN_POINT('Origin',(5.49031038273072E-15,0.,38.989));
#179802=CARTESIAN_POINT('',(-45.4128910420869,41.3171891492029,38.989));
#179803=CARTESIAN_POINT('Origin',(5.49031038273072E-15,0.,38.989));
#179804=CARTESIAN_POINT('',(-45.4132731252655,41.3167691863813,38.9890000005754));
#179805=CARTESIAN_POINT('Origin',(5.49031038273072E-15,0.,38.989));
#179806=CARTESIAN_POINT('',(-45.4132731255216,41.3167691865935,38.989));
#179807=CARTESIAN_POINT('Origin',(62.2224557307631,0.,38.989));
#179808=CARTESIAN_POINT('',(-41.6348281284258,45.765664867611,38.989));
#179809=CARTESIAN_POINT('',(27.6232705441538,-31.1532462714324,38.989));
#179810=CARTESIAN_POINT('',(-45.7656648676103,41.6348281284266,38.989));
#179811=CARTESIAN_POINT('Origin',(5.49031038273072E-15,0.,38.989));
#179812=CARTESIAN_POINT('',(-45.4132815019355,41.3175407208297,38.989));
#179813=CARTESIAN_POINT('Origin',(5.57972911860581E-15,0.,39.624));
#179814=CARTESIAN_POINT('Origin',(-40.3862573897239,44.3789791175472,39.6240070731883));
#179815=CARTESIAN_POINT('Origin',(-44.3789791175464,40.3862573897248,39.6240070731883));
#179816=CARTESIAN_POINT('Origin',(5.57972911860581E-15,0.,39.624));
#179817=CARTESIAN_POINT('Origin',(-41.6603666103049,45.7939781049238,39.5552135208033));
#179818=CARTESIAN_POINT('Origin',(-45.7939778018808,41.6603663369617,39.5552117598793));
#179819=CARTESIAN_POINT('Origin',(5.51210908043506E-15,0.,39.1438017080178));
#179820=CARTESIAN_POINT('Origin',(-41.0717150501544,45.1403198695223,39.1711625381314));
#179821=CARTESIAN_POINT('Origin',(-45.1402498046847,41.0716522820281,39.1712173702639));
#179822=CARTESIAN_POINT('Origin',(5.51210908043507E-15,0.,39.1438017080178));
#179823=CARTESIAN_POINT('Origin',(-40.9494366077754,45.0043926651436,39.1712175859396));
#179824=CARTESIAN_POINT('Origin',(-45.0043225899482,40.9493738530245,39.1711627526731));
#179825=CARTESIAN_POINT('Origin',(60.4792282238308,0.,38.989));
#179826=CARTESIAN_POINT('',(-48.3573835402116,35.526147267887,38.989));
#179827=CARTESIAN_POINT('',(-44.8038810887671,39.9143573409161,38.989));
#179828=CARTESIAN_POINT('Origin',(5.49031038273072E-15,0.,38.989));
#179829=CARTESIAN_POINT('',(-45.1566551325072,40.231996516589,38.989));
#179830=CARTESIAN_POINT('',(33.1880655373213,-30.3099068238764,38.989));
#179831=CARTESIAN_POINT('',(-45.1570399302679,40.2315646150502,38.9889999995773));
#179832=CARTESIAN_POINT('Origin',(5.49031038273072E-15,0.,38.989));
#179833=CARTESIAN_POINT('',(-48.7410849259195,35.8056376404643,38.9889999997818));
#179834=CARTESIAN_POINT('Origin',(5.49031038273072E-15,0.,38.989));
#179835=CARTESIAN_POINT('',(-48.7414273857053,35.8051714542881,38.989));
#179836=CARTESIAN_POINT('Origin',(5.49031038273072E-15,0.,38.989));
#179837=CARTESIAN_POINT('',(-48.3578184660148,35.5264632599795,38.989));
#179838=CARTESIAN_POINT('Origin',(5.49031038273072E-15,0.,38.989));
#179839=CARTESIAN_POINT('',(-45.2779489569769,40.3404336838196,39.2708017080178));
#179840=CARTESIAN_POINT('',(-45.1570399297212,40.2315646145632,38.989));
#179841=CARTESIAN_POINT('',(-48.8727133450219,35.9012693630583,39.2708017078546));
#179842=CARTESIAN_POINT('Origin',(5.52999282761009E-15,0.,39.2708017080178));
#179843=CARTESIAN_POINT('',(-48.8727133447941,35.9012693628909,39.2708017080178));
#179844=CARTESIAN_POINT('Origin',(60.71525,0.,39.3978017080178));
#179845=CARTESIAN_POINT('',(-49.05101714314,36.0301015792681,39.3978017080178));
#179846=CARTESIAN_POINT('',(-45.4410373245168,40.4880553924347,39.3978017080178));
#179847=CARTESIAN_POINT('Origin',(5.5478765747851E-15,0.,39.3978017080178));
#179848=CARTESIAN_POINT('',(-45.5534068532508,40.5892333705626,39.3978017080178));
#179849=CARTESIAN_POINT('',(33.3184119221863,-30.4272712359684,39.3978017080178));
#179850=CARTESIAN_POINT('',(-49.1733470784084,36.1189794796887,39.3978017080178));
#179851=CARTESIAN_POINT('Origin',(5.5478765747851E-15,0.,39.3978017080178));
#179852=CARTESIAN_POINT('',(-49.0514459419942,36.0304131198716,39.3978017080178));
#179853=CARTESIAN_POINT('Origin',(5.5478765747851E-15,0.,39.3978017080178));
#179854=CARTESIAN_POINT('',(-49.3516463037382,36.2478178023255,39.2708017080178));
#179855=CARTESIAN_POINT('',(-45.7165002430345,40.736849336712,39.2708017081757));
#179856=CARTESIAN_POINT('Origin',(5.52999282761008E-15,0.,39.2708017080178));
#179857=CARTESIAN_POINT('',(-45.8374112534709,40.84571607318,38.9890000005756));
#179858=CARTESIAN_POINT('',(-45.7165002428303,40.7368493365301,39.2708017080178));
#179859=CARTESIAN_POINT('',(-45.8377889771247,40.8452921850248,38.989));
#179860=CARTESIAN_POINT('Origin',(5.49031038273072E-15,0.,38.989));
#179861=CARTESIAN_POINT('',(-49.4829367616343,36.343909550784,38.989));
#179862=CARTESIAN_POINT('Origin',(5.49031038273072E-15,0.,38.989));
#179863=CARTESIAN_POINT('',(-49.4832728536529,36.3434519499952,38.9890000005754));
#179864=CARTESIAN_POINT('Origin',(5.49031038273072E-15,0.,38.989));
#179865=CARTESIAN_POINT('',(-49.4832728539298,36.3434519501794,38.989));
#179866=CARTESIAN_POINT('Origin',(62.2224557307631,0.,38.989));
#179867=CARTESIAN_POINT('',(-46.1905628026481,41.1629311642484,38.989));
#179868=CARTESIAN_POINT('',(34.1507877370002,-31.1767457860026,38.989));
#179869=CARTESIAN_POINT('',(-49.8669803696023,36.6229335645814,38.989));
#179870=CARTESIAN_POINT('Origin',(5.49031038273072E-15,0.,38.989));
#179871=CARTESIAN_POINT('',(-49.4833618317449,36.3442183822967,38.989));
#179872=CARTESIAN_POINT('Origin',(5.57972911860581E-15,0.,39.624));
#179873=CARTESIAN_POINT('Origin',(-44.8038837346036,39.9143530044123,39.6240070731883));
#179874=CARTESIAN_POINT('Origin',(-48.3573798485711,35.5261507575156,39.6240070731883));
#179875=CARTESIAN_POINT('Origin',(5.57972911860581E-15,0.,39.624));
#179876=CARTESIAN_POINT('Origin',(-46.2189209212417,41.1884198004172,39.5552135208006));
#179877=CARTESIAN_POINT('Origin',(-49.897807672349,36.6453723646258,39.5552117598824));
#179878=CARTESIAN_POINT('Origin',(5.51210908043506E-15,0.,39.1438017080178));
#179879=CARTESIAN_POINT('Origin',(-45.5651681650772,40.5998732162083,39.1711625381327));
#179880=CARTESIAN_POINT('Origin',(-49.1861234900541,36.1282165298261,39.1712173702595));
#179881=CARTESIAN_POINT('Origin',(5.51210908043507E-15,0.,39.1438017080178));
#179882=CARTESIAN_POINT('Origin',(-45.4293513150125,40.4774722129461,39.1712175859399));
#179883=CARTESIAN_POINT('Origin',(-49.0381593225488,36.0208162177226,39.171162752677));
#179884=CARTESIAN_POINT('Origin',(60.4792282238308,0.,38.989));
#179885=CARTESIAN_POINT('',(-51.8059703131944,30.2768083268885,38.989));
#179886=CARTESIAN_POINT('',(-48.7306271754173,35.0124214764589,38.989));
#179887=CARTESIAN_POINT('Origin',(5.49031038273072E-15,0.,38.989));
#179888=CARTESIAN_POINT('',(-49.1146710209412,35.2914456628195,38.989));
#179889=CARTESIAN_POINT('',(39.3975469582344,-29.0164449471022,38.989));
#179890=CARTESIAN_POINT('',(-49.115008564735,35.2909759049636,38.9889999995775));
#179891=CARTESIAN_POINT('Origin',(5.49031038273072E-15,0.,38.989));
#179892=CARTESIAN_POINT('',(-52.2167844417076,30.5146599057596,38.9889999997818));
#179893=CARTESIAN_POINT('Origin',(5.49031038273072E-15,0.,38.989));
#179894=CARTESIAN_POINT('',(-52.2170762957382,30.5141604766049,38.989));
#179895=CARTESIAN_POINT('Origin',(5.49031038273072E-15,0.,38.989));
#179896=CARTESIAN_POINT('',(-51.8064358865964,30.2770771258175,38.989));
#179897=CARTESIAN_POINT('Origin',(5.49031038273072E-15,0.,38.989));
#179898=CARTESIAN_POINT('',(-49.246635155601,35.3866101428264,39.2708017080178));
#179899=CARTESIAN_POINT('',(-49.1150085641408,35.2909759045367,38.989));
#179900=CARTESIAN_POINT('',(-52.3576880235601,30.5960088313999,39.2708017078546));
#179901=CARTESIAN_POINT('Origin',(5.52999282761009E-15,0.,39.2708017080178));
#179902=CARTESIAN_POINT('',(-52.357688023316,30.5960088312573,39.2708017080178));
#179903=CARTESIAN_POINT('Origin',(60.71525,0.,39.3978017080178));
#179904=CARTESIAN_POINT('',(-52.5484816883957,30.7054974692373,39.3978017080178));
#179905=CARTESIAN_POINT('',(-49.4242607783458,35.51637578784,39.3978017080178));
#179906=CARTESIAN_POINT('Origin',(5.5478765747851E-15,0.,39.3978017080178));
#179907=CARTESIAN_POINT('',(-49.5465907136142,35.6052536882606,39.3978017080178));
#179908=CARTESIAN_POINT('',(39.5520252162584,-29.1286799712089,39.3978017080178));
#179909=CARTESIAN_POINT('',(-52.6794317578285,30.7811015270748,39.3978017080178));
#179910=CARTESIAN_POINT('Origin',(5.5478765747851E-15,0.,39.3978017080178));
#179911=CARTESIAN_POINT('',(-52.5489407031054,30.7057624815036,39.3978017080178));
#179912=CARTESIAN_POINT('Origin',(5.5478765747851E-15,0.,39.3978017080178));
#179913=CARTESIAN_POINT('',(-52.8702215132213,30.8905967158741,39.2708017080178));
#179914=CARTESIAN_POINT('',(-49.7242207308393,35.7350130972989,39.2708017081757));
#179915=CARTESIAN_POINT('Origin',(5.52999282761008E-15,0.,39.2708017080178));
#179916=CARTESIAN_POINT('',(-49.8558490507733,35.8306448082806,38.9890000005756));
#179917=CARTESIAN_POINT('',(-49.7242207306172,35.7350130971393,39.2708017080178));
#179918=CARTESIAN_POINT('',(-49.85618039684,35.8301837593559,38.989));
#179919=CARTESIAN_POINT('Origin',(5.49031038273072E-15,0.,38.989));
#179920=CARTESIAN_POINT('',(-53.010837071051,30.9724384738747,38.989));
#179921=CARTESIAN_POINT('Origin',(5.49031038273072E-15,0.,38.989));
#179922=CARTESIAN_POINT('',(-53.0111234896151,30.9719482486886,38.9890000005754));
#179923=CARTESIAN_POINT('Origin',(5.49031038273072E-15,0.,38.989));
#179924=CARTESIAN_POINT('',(-53.0111234899097,30.9719482488429,38.989));
#179925=CARTESIAN_POINT('Origin',(62.2224557307631,0.,38.989));
#179926=CARTESIAN_POINT('',(-50.240224004808,36.1092077731533,38.989));
#179927=CARTESIAN_POINT('',(40.5385041740525,-29.8453988870287,38.989));
#179928=CARTESIAN_POINT('',(-53.4219427993284,31.209790476761,38.989));
#179929=CARTESIAN_POINT('Origin',(5.49031038273072E-15,0.,38.989));
#179930=CARTESIAN_POINT('',(-53.0112920942665,30.9727011816506,38.989));
#179931=CARTESIAN_POINT('Origin',(5.57972911860581E-15,0.,39.624));
#179932=CARTESIAN_POINT('Origin',(-48.7306293534716,35.0124168871457,39.6240070731883));
#179933=CARTESIAN_POINT('Origin',(-51.8059670065426,30.2768121832821,39.6240070731883));
#179934=CARTESIAN_POINT('Origin',(5.57972911860581E-15,0.,39.624));
#179935=CARTESIAN_POINT('Origin',(-50.2710910626268,36.1315925493537,39.5552135208003));
#179936=CARTESIAN_POINT('Origin',(-53.4549467201713,31.2288840241332,39.5552117598781));
#179937=CARTESIAN_POINT('Origin',(5.51210908043506E-15,0.,39.1438017080178));
#179938=CARTESIAN_POINT('Origin',(-49.5593997624591,35.6146058558679,39.1711625381343));
#179939=CARTESIAN_POINT('Origin',(-52.6931037136118,30.7889524770105,39.171217370262));
#179940=CARTESIAN_POINT('Origin',(5.51210908043507E-15,0.,39.1438017080178));
#179941=CARTESIAN_POINT('Origin',(-49.4115325425356,35.5070721047332,39.1712175859377));
#179942=CARTESIAN_POINT('Origin',(-52.5347237197191,30.697606982104,39.1711627526724));
#179943=CARTESIAN_POINT('Origin',(60.4792282238308,0.,38.989));
#179944=CARTESIAN_POINT('',(-54.6869600343295,24.6957503380312,38.989));
#179945=CARTESIAN_POINT('',(-52.1234703131944,29.7268821954854,38.989));
#179946=CARTESIAN_POINT('Origin',(5.49031038273072E-15,0.,38.989));
#179947=CARTESIAN_POINT('',(-52.5345762957641,29.9642343451583,38.989));
#179948=CARTESIAN_POINT('',(45.2006711678726,-26.4632370872589,38.989));
#179949=CARTESIAN_POINT('',(-52.5348628873914,29.9637318777514,38.9889999995772));
#179950=CARTESIAN_POINT('Origin',(5.49031038273072E-15,0.,38.989));
#179951=CARTESIAN_POINT('',(-55.1203859400878,24.8893571715243,38.9889999997818));
#179952=CARTESIAN_POINT('Origin',(5.49031038273072E-15,0.,38.989));
#179953=CARTESIAN_POINT('',(-55.1206239907494,24.8888299712414,38.989));
#179954=CARTESIAN_POINT('Origin',(5.49031038273072E-15,0.,38.989));
#179955=CARTESIAN_POINT('',(-54.6874511544107,24.6959689987792,38.989));
#179956=CARTESIAN_POINT('Origin',(5.49031038273072E-15,0.,38.989));
#179957=CARTESIAN_POINT('',(-52.6757649139393,30.0450834959841,39.2708017080178));
#179958=CARTESIAN_POINT('',(-52.5348628867552,29.9637318773886,38.989));
#179959=CARTESIAN_POINT('',(-55.2690209155615,24.9555320243583,39.2708017078546));
#179960=CARTESIAN_POINT('Origin',(5.52999282761009E-15,0.,39.2708017080178));
#179961=CARTESIAN_POINT('',(-55.2690209153038,24.9555320242419,39.2708017080178));
#179962=CARTESIAN_POINT('Origin',(60.71525,0.,39.3978017080178));
#179963=CARTESIAN_POINT('',(-55.4702140717965,25.0444775033952,39.3978017080178));
#179964=CARTESIAN_POINT('',(-52.8659816883957,30.1555713378342,39.3978017080178));
#179965=CARTESIAN_POINT('Origin',(5.5478765747851E-15,0.,39.3978017080178));
#179966=CARTESIAN_POINT('',(-52.9969317578285,30.2311753956717,39.3978017080178));
#179967=CARTESIAN_POINT('',(45.3776874999996,-26.5654375142634,39.3978017080178));
#179968=CARTESIAN_POINT('',(-55.6083495590299,25.1059793847706,39.3978017080178));
#179969=CARTESIAN_POINT('Origin',(5.5478765747851E-15,0.,39.3978017080178));
#179970=CARTESIAN_POINT('',(-55.4706982733005,25.0446930837942,39.3978017080178));
#179971=CARTESIAN_POINT('Origin',(5.5478765747851E-15,0.,39.3978017080178));
#179972=CARTESIAN_POINT('',(-55.8095395120005,25.1949317875305,39.2708017080178));
#179973=CARTESIAN_POINT('',(-53.1871522508548,30.3416565763596,39.2708017081757));
#179974=CARTESIAN_POINT('Origin',(5.52999282761008E-15,0.,39.2708017080178));
#179975=CARTESIAN_POINT('',(-53.3280557328683,30.4230055008172,38.9890000005756));
#179976=CARTESIAN_POINT('',(-53.1871522506172,30.3416565762241,39.2708017080178));
#179977=CARTESIAN_POINT('',(-53.328337071051,30.4225123424716,38.989));
#179978=CARTESIAN_POINT('Origin',(5.49031038273072E-15,0.,38.989));
#179979=CARTESIAN_POINT('',(-55.9579395562864,25.2616268796461,38.989));
#179980=CARTESIAN_POINT('Origin',(5.49031038273072E-15,0.,38.989));
#179981=CARTESIAN_POINT('',(-55.9581731633343,25.2611094010726,38.9890000005754));
#179982=CARTESIAN_POINT('Origin',(5.49031038273072E-15,0.,38.989));
#179983=CARTESIAN_POINT('',(-55.9581731636435,25.2611094011952,38.989));
#179984=CARTESIAN_POINT('Origin',(62.2224557307631,0.,38.989));
#179985=CARTESIAN_POINT('',(-53.7394427993284,30.6598643453579,38.989));
#179986=CARTESIAN_POINT('',(46.5080917980719,-27.2180767400485,38.989));
#179987=CARTESIAN_POINT('',(-56.3916032444849,25.4547063934088,38.989));
#179988=CARTESIAN_POINT('Origin',(5.49031038273072E-15,0.,38.989));
#179989=CARTESIAN_POINT('',(-55.9584195472773,25.2618405854039,38.989));
#179990=CARTESIAN_POINT('Origin',(5.57972911860581E-15,0.,39.624));
#179991=CARTESIAN_POINT('Origin',(-52.1234719996032,29.7268774036442,39.6240070731883));
#179992=CARTESIAN_POINT('Origin',(-54.6869571488948,24.6957545189383,39.6240070731883));
#179993=CARTESIAN_POINT('Origin',(5.57972911860581E-15,0.,39.624));
#179994=CARTESIAN_POINT('Origin',(-53.7724806104361,30.6789000092871,39.5552135207983));
#179995=CARTESIAN_POINT('Origin',(-56.4264221855586,25.4702454951994,39.5552117598846));
#179996=CARTESIAN_POINT('Origin',(5.51210908043506E-15,0.,39.1438017080178));
#179997=CARTESIAN_POINT('Origin',(-53.0106482050727,30.239137420935,39.1711625381359));
#179998=CARTESIAN_POINT('Origin',(-55.6227672661403,25.112358217853,39.1712173702612));
#179999=CARTESIAN_POINT('Origin',(5.51210908043507E-15,0.,39.1438017080178));
#180000=CARTESIAN_POINT('Origin',(-52.8523506794951,30.1476490842054,39.1712175859386));
#180001=CARTESIAN_POINT('Origin',(-55.4557066902174,25.0380683404998,39.1711627526719));
#180002=CARTESIAN_POINT('Origin',(60.4792282238308,0.,38.989));
#180003=CARTESIAN_POINT('',(-56.9687879773465,18.8441205405524,38.989));
#180004=CARTESIAN_POINT('',(-54.9452378026827,24.1156489724281,38.989));
#180005=CARTESIAN_POINT('Origin',(5.49031038273072E-15,0.,38.989));
#180006=CARTESIAN_POINT('',(-55.3789017591237,24.3087286055924,38.989));
#180007=CARTESIAN_POINT('',(50.3447265545023,-22.7624634345049,38.989));
#180008=CARTESIAN_POINT('',(-55.3791342586262,24.3081989337722,38.9889999995772));
#180009=CARTESIAN_POINT('Origin',(5.49031038273072E-15,0.,38.989));
#180010=CARTESIAN_POINT('',(-57.420076955426,18.9913614316849,38.9889999997818));
#180011=CARTESIAN_POINT('Origin',(5.49031038273072E-15,0.,38.989));
#180012=CARTESIAN_POINT('',(-57.4202585945858,18.9908122363905,38.989));
#180013=CARTESIAN_POINT('Origin',(5.49031038273072E-15,0.,38.989));
#180014=CARTESIAN_POINT('',(-56.9692992632924,18.8442866674266,38.989));
#180015=CARTESIAN_POINT('Origin',(5.49031038273072E-15,0.,38.989));
#180016=CARTESIAN_POINT('',(-55.5277679687681,24.3743766270218,39.2708017080178));
#180017=CARTESIAN_POINT('',(-55.3791342579556,24.3081989334778,38.989));
#180018=CARTESIAN_POINT('',(-57.5748148486259,19.041637186177,39.2708017078546));
#180019=CARTESIAN_POINT('Origin',(5.52999282761009E-15,0.,39.2708017080178));
#180020=CARTESIAN_POINT('',(-57.5748148483574,19.0416371860882,39.2708017080178));
#180021=CARTESIAN_POINT('Origin',(60.71525,0.,39.3978017080178));
#180022=CARTESIAN_POINT('',(-57.7842031819381,19.109065001132,39.3978017080178));
#180023=CARTESIAN_POINT('',(-55.7284918401496,24.4643761377921,39.3978017080178));
#180024=CARTESIAN_POINT('Origin',(5.5478765747851E-15,0.,39.3978017080178));
#180025=CARTESIAN_POINT('',(-55.8666273273831,24.5258780191675,39.3978017080178));
#180026=CARTESIAN_POINT('',(50.541702139688,-22.850162615335,39.3978017080178));
#180027=CARTESIAN_POINT('',(-57.9280106456674,19.1557908785629,39.3978017080178));
#180028=CARTESIAN_POINT('Origin',(5.5478765747851E-15,0.,39.3978017080178));
#180029=CARTESIAN_POINT('',(-57.7847072652235,19.1092287877199,39.3978017080178));
#180030=CARTESIAN_POINT('Origin',(5.5478765747851E-15,0.,39.3978017080178));
#180031=CARTESIAN_POINT('',(-58.1373965169892,19.2232259141444,39.2708017080178));
#180032=CARTESIAN_POINT('',(-56.0673542006828,24.6158705165698,39.2708017081757));
#180033=CARTESIAN_POINT('Origin',(5.52999282761008E-15,0.,39.2708017080178));
#180034=CARTESIAN_POINT('',(-56.2159890767409,24.6820453786636,38.9890000005756));
#180035=CARTESIAN_POINT('',(-56.0673542004324,24.6158705164598,39.2708017080178));
#180036=CARTESIAN_POINT('',(-56.2162173246396,24.6815255140431,38.989));
#180037=CARTESIAN_POINT('Origin',(5.49031038273072E-15,0.,38.989));
#180038=CARTESIAN_POINT('',(-58.2919551457915,19.2740436149889,38.989));
#180039=CARTESIAN_POINT('Origin',(5.49031038273072E-15,0.,38.989));
#180040=CARTESIAN_POINT('',(-58.2921333818755,19.2735045526314,38.9890000005754));
#180041=CARTESIAN_POINT('Origin',(5.49031038273072E-15,0.,38.989));
#180042=CARTESIAN_POINT('',(-58.2921333821958,19.2735045527211,38.989));
#180043=CARTESIAN_POINT('Origin',(62.2224557307631,0.,38.989));
#180044=CARTESIAN_POINT('',(-56.649881012838,24.8746050278057,38.989));
#180045=CARTESIAN_POINT('',(51.799563747336,-23.4101986852082,38.989));
#180046=CARTESIAN_POINT('',(-58.7434254837931,19.4207352200705,38.989));
#180047=CARTESIAN_POINT('Origin',(5.49031038273072E-15,0.,38.989));
#180048=CARTESIAN_POINT('',(-58.2924548456759,19.2742059773236,38.989));
#180049=CARTESIAN_POINT('Origin',(5.57972911860581E-15,0.,39.624));
#180050=CARTESIAN_POINT('Origin',(-54.9452389789694,24.1156440305594,39.6240070731884));
#180051=CARTESIAN_POINT('Origin',(-56.9687855447422,18.8441250001661,39.6240070731883));
#180052=CARTESIAN_POINT('Origin',(5.57972911860581E-15,0.,39.624));
#180053=CARTESIAN_POINT('Origin',(-56.6847276080567,24.8900830207528,39.5552135207981));
#180054=CARTESIAN_POINT('Origin',(-58.7796779614985,19.4325496266337,39.5552117598791));
#180055=CARTESIAN_POINT('Origin',(5.51210908043506E-15,0.,39.1438017080178));
#180056=CARTESIAN_POINT('Origin',(-55.8811008927611,24.5323626684723,39.1711625381393));
#180057=CARTESIAN_POINT('Origin',(-57.94301614069,19.1606277069624,39.171217370263));
#180058=CARTESIAN_POINT('Origin',(5.51210908043507E-15,0.,39.1438017080178));
#180059=CARTESIAN_POINT('Origin',(-55.7141074023455,24.4579221115113,39.1712175859368));
#180060=CARTESIAN_POINT('Origin',(-57.7691053333631,19.1042073826016,39.1711627526768));
#180061=CARTESIAN_POINT('Origin',(60.4792282238308,0.,38.989));
#180062=CARTESIAN_POINT('',(-58.6264539577983,12.7860306150456,38.989));
#180063=CARTESIAN_POINT('',(-57.1650137687745,18.240199652705,38.989));
#180064=CARTESIAN_POINT('Origin',(5.49031038273072E-15,0.,38.989));
#180065=CARTESIAN_POINT('',(-57.6164843860301,18.3868913484952,38.989));
#180066=CARTESIAN_POINT('',(54.6058629360811,-18.0763596539233,38.989));
#180067=CARTESIAN_POINT('',(-57.616660246095,18.386340275457,38.988999999577));
#180068=CARTESIAN_POINT('Origin',(5.49031038273072E-15,0.,38.989));
#180069=CARTESIAN_POINT('',(-59.090661591717,12.8852923618021,38.9889999997818));
#180070=CARTESIAN_POINT('Origin',(5.49031038273072E-15,0.,38.989));
#180071=CARTESIAN_POINT('',(-59.0907848292983,12.8847271885947,38.989));
#180072=CARTESIAN_POINT('Origin',(5.49031038273072E-15,0.,38.989));
#180073=CARTESIAN_POINT('',(-58.6269798078532,12.7861423879252,38.989));
#180074=CARTESIAN_POINT('Origin',(5.49031038273072E-15,0.,38.989));
#180075=CARTESIAN_POINT('',(-57.7713971777986,18.4366189870677,39.2708017080178));
#180076=CARTESIAN_POINT('',(-57.616660245397,18.3863402752342,38.989));
#180077=CARTESIAN_POINT('',(-59.2498070619041,12.9191181862652,39.2708017078546));
#180078=CARTESIAN_POINT('Origin',(5.52999282761009E-15,0.,39.2708017080178));
#180079=CARTESIAN_POINT('',(-59.2498070616278,12.919118186205,39.2708017080178));
#180080=CARTESIAN_POINT('Origin',(60.71525,0.,39.3978017080178));
#180081=CARTESIAN_POINT('',(-59.4650964698965,12.9642895838875,39.3978017080178));
#180082=CARTESIAN_POINT('',(-57.9804289733662,18.5051441132846,39.3978017080178));
#180083=CARTESIAN_POINT('Origin',(5.5478765747851E-15,0.,39.3978017080178));
#180084=CARTESIAN_POINT('',(-58.1242364370955,18.5518699907155,39.3978017080178));
#180085=CARTESIAN_POINT('',(54.8193466381475,-18.1457247135494,39.3978017080178));
#180086=CARTESIAN_POINT('',(-59.6130003254554,12.9957275188828,39.3978017080178));
#180087=CARTESIAN_POINT('Origin',(5.5478765747851E-15,0.,39.3978017080178));
#180088=CARTESIAN_POINT('',(-59.4656149121213,12.9643997821842,39.3978017080178));
#180089=CARTESIAN_POINT('Origin',(5.5478765747851E-15,0.,39.3978017080178));
#180090=CARTESIAN_POINT('',(-59.8282880397054,13.0409063549243,39.2708017080178));
#180091=CARTESIAN_POINT('',(-58.33327048504,18.6203878281983,39.2708017081757));
#180092=CARTESIAN_POINT('Origin',(5.52999282761008E-15,0.,39.2708017080178));
#180093=CARTESIAN_POINT('',(-58.4880082803367,18.6706636022913,38.9890000005756));
#180094=CARTESIAN_POINT('',(-58.3332704847794,18.6203878281152,39.2708017080178));
#180095=CARTESIAN_POINT('',(-58.4881809372196,18.6701227271415,38.989));
#180096=CARTESIAN_POINT('Origin',(5.49031038273072E-15,0.,38.989));
#180097=CARTESIAN_POINT('',(-59.9873118763435,13.075289895133,38.989));
#180098=CARTESIAN_POINT('Origin',(5.49031038273072E-15,0.,38.989));
#180099=CARTESIAN_POINT('',(-59.9874327886717,13.0747351550715,38.9890000005754));
#180100=CARTESIAN_POINT('Origin',(5.49031038273072E-15,0.,38.989));
#180101=CARTESIAN_POINT('',(-59.9874327889996,13.0747351551272,38.989));
#180102=CARTESIAN_POINT('Origin',(62.2224557307631,0.,38.989));
#180103=CARTESIAN_POINT('',(-58.9396512752212,18.8168143322231,38.989));
#180104=CARTESIAN_POINT('',(56.1826270286323,-18.588681363906,38.989));
#180105=CARTESIAN_POINT('',(-60.4516424606488,13.1739864076111,38.989));
#180106=CARTESIAN_POINT('Origin',(5.49031038273072E-15,0.,38.989));
#180107=CARTESIAN_POINT('',(-59.987825810305,13.0753991351687,38.989));
#180108=CARTESIAN_POINT('Origin',(5.57972911860581E-15,0.,39.624));
#180109=CARTESIAN_POINT('Origin',(-57.1650144220515,18.2401946149529,39.6240070731884));
#180110=CARTESIAN_POINT('Origin',(-58.6264520046767,12.7860353045054,39.6240070731884));
#180111=CARTESIAN_POINT('Origin',(5.57972911860581E-15,0.,39.624));
#180112=CARTESIAN_POINT('Origin',(-58.9759248679604,18.8285650740589,39.5552135208012));
#180113=CARTESIAN_POINT('Origin',(-60.4889312852515,13.1819466778347,39.5552117598777));
#180114=CARTESIAN_POINT('Origin',(5.51210908043506E-15,0.,39.1438017080178));
#180115=CARTESIAN_POINT('Origin',(-58.1393085451906,18.5568062168846,39.1711625381322));
#180116=CARTESIAN_POINT('Origin',(-59.6284292050461,12.998969349295,39.171217370263));
#180117=CARTESIAN_POINT('Origin',(5.51210908043507E-15,0.,39.1438017080178));
#180118=CARTESIAN_POINT('Origin',(-57.9654487055671,18.5002290260152,39.1712175859384));
#180119=CARTESIAN_POINT('Origin',(-59.4495735695152,12.9610367308092,39.1711627526779));
#180120=CARTESIAN_POINT('Origin',(60.4792282238308,0.,38.989));
#180121=CARTESIAN_POINT('',(-59.6417962403142,6.58785426247137,38.989));
#180122=CARTESIAN_POINT('',(-58.7584778814675,12.1649068885796,38.989));
#180123=CARTESIAN_POINT('Origin',(5.49031038273072E-15,0.,38.989));
#180124=CARTESIAN_POINT('',(-59.2228087529787,12.2636034620794,38.989));
#180125=CARTESIAN_POINT('',(57.7988642628859,-12.6101209950214,38.989));
#180126=CARTESIAN_POINT('',(-59.2229260468456,12.2630370254946,38.9889999995771));
#180127=CARTESIAN_POINT('Origin',(5.49031038273072E-15,0.,38.989));
#180128=CARTESIAN_POINT('',(-60.1138365740932,6.6380493323826,38.9889999997818));
#180129=CARTESIAN_POINT('Origin',(5.49031038273072E-15,0.,38.989));
#180130=CARTESIAN_POINT('',(-60.1139000598793,6.63747437341819,38.989));
#180131=CARTESIAN_POINT('Origin',(5.49031038273072E-15,0.,38.989));
#180132=CARTESIAN_POINT('',(-59.6423308931549,6.58791045674932,38.989));
#180133=CARTESIAN_POINT('Origin',(5.49031038273072E-15,0.,38.989));
#180134=CARTESIAN_POINT('',(-59.382070869907,12.2968658913807,39.2708017080178));
#180135=CARTESIAN_POINT('',(-59.2229260461284,12.2630370253461,38.989));
#180136=CARTESIAN_POINT('',(-60.2756459901929,6.6550546240054,39.2708017078546));
#180137=CARTESIAN_POINT('Origin',(5.52999282761009E-15,0.,39.2708017080178));
#180138=CARTESIAN_POINT('',(-60.2756459899118,6.65505462397437,39.2708017080178));
#180139=CARTESIAN_POINT('Origin',(60.71525,0.,39.3978017080178));
#180140=CARTESIAN_POINT('',(-60.4944777170593,6.67747469700988,39.3978017080178));
#180141=CARTESIAN_POINT('',(-59.5971203935658,12.3431658574215,39.3978017080178));
#180142=CARTESIAN_POINT('Origin',(5.5478765747851E-15,0.,39.3978017080178));
#180143=CARTESIAN_POINT('',(-59.7450242491247,12.3746037924168,39.3978017080178));
#180144=CARTESIAN_POINT('',(58.0246834617327,-12.6581203474874,39.3978017080178));
#180145=CARTESIAN_POINT('',(-60.6448574988554,6.69328024897497,39.3978017080178));
#180146=CARTESIAN_POINT('Origin',(5.5478765747851E-15,0.,39.3978017080178));
#180147=CARTESIAN_POINT('',(-60.4950048380619,6.67753009965975,39.3978017080178));
#180148=CARTESIAN_POINT('Origin',(5.5478765747851E-15,0.,39.3978017080178));
#180149=CARTESIAN_POINT('',(-60.8636883187844,6.71570789669452,39.2708017080178));
#180150=CARTESIAN_POINT('',(-59.9600752509414,12.4208962742145,39.2708017081757));
#180151=CARTESIAN_POINT('Origin',(5.52999282761008E-15,0.,39.2708017080178));
#180152=CARTESIAN_POINT('',(-60.1192206258105,12.4547221284048,38.9890000005756));
#180153=CARTESIAN_POINT('',(-59.9600752506736,12.4208962741591,39.2708017080178));
#180154=CARTESIAN_POINT('',(-60.1193358000127,12.454166168667,38.989));
#180155=CARTESIAN_POINT('Origin',(5.49031038273072E-15,0.,38.989));
#180156=CARTESIAN_POINT('',(-61.0254350648262,6.73328056300561,38.989));
#180157=CARTESIAN_POINT('Origin',(5.49031038273072E-15,0.,38.989));
#180158=CARTESIAN_POINT('',(-61.0254973286579,6.7327162230884,38.9890000005754));
#180159=CARTESIAN_POINT('Origin',(5.49031038273072E-15,0.,38.989));
#180160=CARTESIAN_POINT('',(-61.0254973289898,6.73271622310951,38.989));
#180161=CARTESIAN_POINT('Origin',(62.2224557307631,0.,38.989));
#180162=CARTESIAN_POINT('',(-60.5836663843181,12.5528626811452,38.989));
#180163=CARTESIAN_POINT('',(59.4667368016499,-12.964638247165,38.989));
#180164=CARTESIAN_POINT('',(-61.4975385923862,6.78290064323603,38.989));
#180165=CARTESIAN_POINT('Origin',(5.49031038273072E-15,0.,38.989));
#180166=CARTESIAN_POINT('',(-61.0259576020967,6.73333548388583,38.989));
#180167=CARTESIAN_POINT('Origin',(5.57972911860581E-15,0.,39.624));
#180168=CARTESIAN_POINT('Origin',(-58.7584780045773,12.1649018101389,39.6240070731883));
#180169=CARTESIAN_POINT('Origin',(-59.6417947880741,6.58785913039868,39.6240070731883));
#180170=CARTESIAN_POINT('Origin',(5.57972911860581E-15,0.,39.624));
#180171=CARTESIAN_POINT('Origin',(-60.620969553508,12.5607574282799,39.5552135208001));
#180172=CARTESIAN_POINT('Origin',(-61.5354552197157,6.78691956273326,39.5552117598845));
#180173=CARTESIAN_POINT('Origin',(5.51210908043506E-15,0.,39.1438017080178));
#180174=CARTESIAN_POINT('Origin',(-59.7605297667705,12.3779375131251,39.1711625381321));
#180175=CARTESIAN_POINT('Origin',(-60.6605407209825,6.6948915632276,39.1712173702665));
#180176=CARTESIAN_POINT('Origin',(5.51210908043507E-15,0.,39.1438017080178));
#180177=CARTESIAN_POINT('Origin',(-59.5817084227212,12.339843559887,39.17121758594));
#180178=CARTESIAN_POINT('Origin',(-60.4786998370186,6.67586224832373,39.1711627526745));
#180179=CARTESIAN_POINT('Origin',(60.4792282238308,0.,38.989));
#180180=CARTESIAN_POINT('',(-60.003690522373,0.3175,38.989));
#180181=CARTESIAN_POINT('',(-59.7081718144892,5.95633285891252,38.989));
#180182=CARTESIAN_POINT('Origin',(5.49031038273072E-15,0.,38.989));
#180183=CARTESIAN_POINT('',(-60.1802756340603,6.00595296980914,38.989));
#180184=CARTESIAN_POINT('',(59.785232315514,-6.60293000146475,38.989));
#180185=CARTESIAN_POINT('',(-60.1803330766331,6.00537737567553,38.9889999995772));
#180186=CARTESIAN_POINT('Origin',(5.49031038273072E-15,0.,38.989));
#180187=CARTESIAN_POINT('',(-60.4783917833346,0.318078445375988,38.9889999997818));
#180188=CARTESIAN_POINT('Origin',(5.49031038273072E-15,0.,38.989));
#180189=CARTESIAN_POINT('',(-60.478394821762,0.317500000025284,38.989));
#180190=CARTESIAN_POINT('Origin',(5.49031038273072E-15,0.,38.989));
#180191=CARTESIAN_POINT('',(-60.004228120231,0.3175,38.989));
#180192=CARTESIAN_POINT('Origin',(5.49031038273072E-15,0.,38.989));
#180193=CARTESIAN_POINT('',(-60.3421421670675,6.02238575970318,39.2708017080178));
#180194=CARTESIAN_POINT('',(-60.1803330759045,6.00537737560282,38.989));
#180195=CARTESIAN_POINT('',(-60.6410923275232,0.31807689062485,39.2708017078546));
#180196=CARTESIAN_POINT('Origin',(5.52999282761009E-15,0.,39.2708017080178));
#180197=CARTESIAN_POINT('',(-60.6410923272405,0.318076890623367,39.2708017080178));
#180198=CARTESIAN_POINT('Origin',(60.71525,0.,39.3978017080178));
#180199=CARTESIAN_POINT('',(-60.8610688070707,0.3175,39.3978017080178));
#180200=CARTESIAN_POINT('',(-60.5608532912343,6.04595329345103,39.3978017080178));
#180201=CARTESIAN_POINT('Origin',(5.5478765747851E-15,0.,39.3978017080178));
#180202=CARTESIAN_POINT('',(-60.7112330730303,6.06175884541612,39.3978017080178));
#180203=CARTESIAN_POINT('',(60.0186752706391,-6.62746584474133,39.3978017080178));
#180204=CARTESIAN_POINT('',(-61.0122769227456,0.3175,39.3978017080178));
#180205=CARTESIAN_POINT('Origin',(5.5478765747851E-15,0.,39.3978017080178));
#180206=CARTESIAN_POINT('',(-60.8615988316031,0.3175,39.3978017080178));
#180207=CARTESIAN_POINT('Origin',(5.5478765747851E-15,0.,39.3978017080178));
#180208=CARTESIAN_POINT('',(-61.2322532920972,0.316930737395914,39.2708017080178));
#180209=CARTESIAN_POINT('',(-60.9299448849411,6.0853187814108,39.2708017081757));
#180210=CARTESIAN_POINT('Origin',(5.52999282761008E-15,0.,39.2708017080178));
#180211=CARTESIAN_POINT('',(-61.0917542093523,6.10232411256129,38.9890000005756));
#180212=CARTESIAN_POINT('',(-60.929944884669,6.08531878138362,39.2708017080178));
#180213=CARTESIAN_POINT('',(-61.0918106390011,6.10175915944675,38.989));
#180214=CARTESIAN_POINT('Origin',(5.49031038273072E-15,0.,38.989));
#180215=CARTESIAN_POINT('',(-61.3949508163453,0.3175,38.989));
#180216=CARTESIAN_POINT('Origin',(5.49031038273072E-15,0.,38.989));
#180217=CARTESIAN_POINT('',(-61.394953749505,0.316932243253257,38.9890000005754));
#180218=CARTESIAN_POINT('Origin',(5.49031038273072E-15,0.,38.989));
#180219=CARTESIAN_POINT('',(-61.3949537498373,0.31693224323956,38.989));
#180220=CARTESIAN_POINT('Origin',(62.2224557307631,0.,38.989));
#180221=CARTESIAN_POINT('',(-61.5639141665611,6.15137923967718,38.989));
#180222=CARTESIAN_POINT('',(61.5094129706996,-6.78414869068793,38.989));
#180223=CARTESIAN_POINT('',(-61.8696548221181,0.3175,38.989));
#180224=CARTESIAN_POINT('Origin',(5.49031038273072E-15,0.,38.989));
#180225=CARTESIAN_POINT('',(-61.3954762318973,0.3175,38.989));
#180226=CARTESIAN_POINT('Origin',(5.57972911860581E-15,0.,39.624));
#180227=CARTESIAN_POINT('Origin',(-59.7081714060829,5.95632779542356,39.6240070731883));
#180228=CARTESIAN_POINT('Origin',(-60.0036895869254,0.317504993060722,39.6240070731883));
#180229=CARTESIAN_POINT('Origin',(5.57972911860581E-15,0.,39.624));
#180230=CARTESIAN_POINT('Origin',(-61.6018382108737,6.15533149561012,39.5552135207994));
#180231=CARTESIAN_POINT('Origin',(-61.9077838296762,0.317533536648604,39.5552117598821));
#180232=CARTESIAN_POINT('Origin',(5.51210908043506E-15,0.,39.1438017080178));
#180233=CARTESIAN_POINT('Origin',(-60.7270021185293,6.06345353572164,39.17116253813));
#180234=CARTESIAN_POINT('Origin',(-61.0280426587373,0.317463144196525,39.1712173702556));
#180235=CARTESIAN_POINT('Origin',(5.51210908043507E-15,0.,39.1438017080178));
#180236=CARTESIAN_POINT('Origin',(-60.5451784741237,6.04426018543771,39.1712175859386));
#180237=CARTESIAN_POINT('Origin',(-60.8452088131251,0.317545622030734,39.1711627526739));
#180238=CARTESIAN_POINT('Origin',(60.4792282238308,0.,38.989));
#180239=CARTESIAN_POINT('',(-59.7081718144893,-5.95633285891171,38.989));
#180240=CARTESIAN_POINT('',(-60.003690522373,-0.3175,38.989));
#180241=CARTESIAN_POINT('Origin',(5.49031038273072E-15,0.,38.989));
#180242=CARTESIAN_POINT('',(-60.4783948217626,-0.317500000025261,38.989));
#180243=CARTESIAN_POINT('',(60.4792282238308,-0.3175,38.989));
#180244=CARTESIAN_POINT('',(-60.4783917836889,-0.318078445377852,38.9889999995772));
#180245=CARTESIAN_POINT('Origin',(5.49031038273072E-15,0.,38.989));
#180246=CARTESIAN_POINT('',(-60.1803330762807,-6.00537737563954,38.9889999997818));
#180247=CARTESIAN_POINT('Origin',(5.49031038273072E-15,0.,38.989));
#180248=CARTESIAN_POINT('',(-60.1802756340597,-6.00595296980823,38.989));
#180249=CARTESIAN_POINT('Origin',(5.49031038273072E-15,0.,38.989));
#180250=CARTESIAN_POINT('',(-59.7087064673299,-5.95638905318966,38.989));
#180251=CARTESIAN_POINT('Origin',(5.49031038273072E-15,0.,38.989));
#180252=CARTESIAN_POINT('',(-60.6410923272405,-0.318076890623366,39.2708017080178));
#180253=CARTESIAN_POINT('',(-60.4783917829566,-0.318078445374005,38.989));
#180254=CARTESIAN_POINT('',(-60.3421421673489,-6.02238575973044,39.2708017078546));
#180255=CARTESIAN_POINT('Origin',(5.52999282761009E-15,0.,39.2708017080178));
#180256=CARTESIAN_POINT('',(-60.3421421670675,-6.02238575970236,39.2708017080178));
#180257=CARTESIAN_POINT('Origin',(60.71525,0.,39.3978017080178));
#180258=CARTESIAN_POINT('',(-60.5608532912344,-6.04595329345021,39.3978017080178));
#180259=CARTESIAN_POINT('',(-60.8610688070707,-0.3175,39.3978017080178));
#180260=CARTESIAN_POINT('Origin',(5.5478765747851E-15,0.,39.3978017080178));
#180261=CARTESIAN_POINT('',(-61.0122769227456,-0.3175,39.3978017080178));
#180262=CARTESIAN_POINT('',(60.71525,-0.3175,39.3978017080178));
#180263=CARTESIAN_POINT('',(-60.7112330730304,-6.0617588454153,39.3978017080178));
#180264=CARTESIAN_POINT('Origin',(5.5478765747851E-15,0.,39.3978017080178));
#180265=CARTESIAN_POINT('',(-60.5613804122369,-6.04600869610007,39.3978017080178));
#180266=CARTESIAN_POINT('Origin',(5.5478765747851E-15,0.,39.3978017080178));
#180267=CARTESIAN_POINT('',(-60.9299448846691,-6.0853187813828,39.2708017080178));
#180268=CARTESIAN_POINT('',(-61.2322532923707,-0.31693073739733,39.2708017081757));
#180269=CARTESIAN_POINT('Origin',(5.52999282761008E-15,0.,39.2708017080178));
#180270=CARTESIAN_POINT('',(-61.3949537495049,-0.31693224325326,38.9890000005756));
#180271=CARTESIAN_POINT('',(-61.2322532920972,-0.316930737395914,39.2708017080178));
#180272=CARTESIAN_POINT('',(-61.3949508163453,-0.3175,38.989));
#180273=CARTESIAN_POINT('Origin',(5.49031038273072E-15,0.,38.989));
#180274=CARTESIAN_POINT('',(-61.0918106390012,-6.10175915944593,38.989));
#180275=CARTESIAN_POINT('Origin',(5.49031038273072E-15,0.,38.989));
#180276=CARTESIAN_POINT('',(-61.0917542093524,-6.10232411256048,38.9890000005754));
#180277=CARTESIAN_POINT('Origin',(5.49031038273072E-15,0.,38.989));
#180278=CARTESIAN_POINT('',(-61.0917542096815,-6.10232411260883,38.989));
#180279=CARTESIAN_POINT('Origin',(62.2224557307631,0.,38.989));
#180280=CARTESIAN_POINT('',(-61.8696548221181,-0.3175,38.989));
#180281=CARTESIAN_POINT('',(62.2224557307631,-0.3175,38.989));
#180282=CARTESIAN_POINT('',(-61.5639141665612,-6.15137923967635,38.989));
#180283=CARTESIAN_POINT('Origin',(5.49031038273072E-15,0.,38.989));
#180284=CARTESIAN_POINT('',(-61.0923331762718,-6.10181408032615,38.989));
#180285=CARTESIAN_POINT('Origin',(5.57972911860581E-15,0.,39.624));
#180286=CARTESIAN_POINT('Origin',(-60.0036895869254,-0.317504993060547,
39.6240070731883));
#180287=CARTESIAN_POINT('Origin',(-59.708171406083,-5.95632779542259,39.6240070731883));
#180288=CARTESIAN_POINT('Origin',(5.57972911860581E-15,0.,39.624));
#180289=CARTESIAN_POINT('Origin',(-61.9077842377874,-0.317533537011564,
39.5552135207981));
#180290=CARTESIAN_POINT('Origin',(-61.6018378049611,-6.15533145331103,39.5552117598819));
#180291=CARTESIAN_POINT('Origin',(5.51210908043506E-15,0.,39.1438017080178));
#180292=CARTESIAN_POINT('Origin',(-61.028136727137,-0.317462907478496,39.1711625381301));
#180293=CARTESIAN_POINT('Origin',(-60.726908590193,-6.0634434674746,39.1712173702598));
#180294=CARTESIAN_POINT('Origin',(5.51210908043507E-15,0.,39.1438017080178));
#180295=CARTESIAN_POINT('Origin',(-60.845302880271,-0.31754536844547,39.1712175859354));
#180296=CARTESIAN_POINT('Origin',(-60.5450849487951,-6.04425010054802,39.1711627526745));
#180297=CARTESIAN_POINT('Origin',(60.4792282238308,0.,38.989));
#180298=CARTESIAN_POINT('',(-58.7584778814677,-12.1649068885788,38.989));
#180299=CARTESIAN_POINT('',(-59.6417962403143,-6.58785426247057,38.989));
#180300=CARTESIAN_POINT('Origin',(5.49031038273072E-15,0.,38.989));
#180301=CARTESIAN_POINT('',(-60.1139000598801,-6.63747437341743,38.989));
#180302=CARTESIAN_POINT('',(59.8516078896891,5.9714085979051,38.989));
#180303=CARTESIAN_POINT('',(-60.1138365744455,-6.63804933242069,38.9889999995772));
#180304=CARTESIAN_POINT('Origin',(5.49031038273072E-15,0.,38.989));
#180305=CARTESIAN_POINT('',(-59.2229260464987,-12.2630370254219,38.9889999997818));
#180306=CARTESIAN_POINT('Origin',(5.49031038273072E-15,0.,38.989));
#180307=CARTESIAN_POINT('',(-59.2228087529783,-12.2636034620785,38.989));
#180308=CARTESIAN_POINT('Origin',(5.49031038273072E-15,0.,38.989));
#180309=CARTESIAN_POINT('',(-58.7590037315226,-12.1650186614584,38.989));
#180310=CARTESIAN_POINT('Origin',(5.49031038273072E-15,0.,38.989));
#180311=CARTESIAN_POINT('',(-60.2756459899119,-6.65505462397356,39.2708017080178));
#180312=CARTESIAN_POINT('',(-60.1138365737176,-6.6380493323403,38.989));
#180313=CARTESIAN_POINT('',(-59.382070870184,-12.2968658914373,39.2708017078546));
#180314=CARTESIAN_POINT('Origin',(5.52999282761009E-15,0.,39.2708017080178));
#180315=CARTESIAN_POINT('',(-59.3820708699071,-12.2968658913799,39.2708017080178));
#180316=CARTESIAN_POINT('Origin',(60.71525,0.,39.3978017080178));
#180317=CARTESIAN_POINT('',(-59.597120393566,-12.3431658574207,39.3978017080178));
#180318=CARTESIAN_POINT('',(-60.4944777170594,-6.67747469700906,39.3978017080178));
#180319=CARTESIAN_POINT('Origin',(5.5478765747851E-15,0.,39.3978017080178));
#180320=CARTESIAN_POINT('',(-60.6448574988555,-6.69328024897415,39.3978017080178));
#180321=CARTESIAN_POINT('',(60.0850508448142,5.99594444118168,39.3978017080178));
#180322=CARTESIAN_POINT('',(-59.7450242491248,-12.374603792416,39.3978017080178));
#180323=CARTESIAN_POINT('Origin',(5.5478765747851E-15,0.,39.3978017080178));
#180324=CARTESIAN_POINT('',(-59.5976388357907,-12.3432760557174,39.3978017080178));
#180325=CARTESIAN_POINT('Origin',(5.5478765747851E-15,0.,39.3978017080178));
#180326=CARTESIAN_POINT('',(-59.9600752506738,-12.4208962741583,39.2708017080178));
#180327=CARTESIAN_POINT('',(-60.8636883190563,-6.71570789672369,39.2708017081757));
#180328=CARTESIAN_POINT('Origin',(5.52999282761008E-15,0.,39.2708017080178));
#180329=CARTESIAN_POINT('',(-61.0254973286579,-6.73271622308757,38.9890000005756));
#180330=CARTESIAN_POINT('',(-60.8636883187845,-6.7157078966937,39.2708017080178));
#180331=CARTESIAN_POINT('',(-61.0254350648263,-6.73328056300478,38.989));
#180332=CARTESIAN_POINT('Origin',(5.49031038273072E-15,0.,38.989));
#180333=CARTESIAN_POINT('',(-60.1193358000129,-12.4541661686662,38.989));
#180334=CARTESIAN_POINT('Origin',(5.49031038273072E-15,0.,38.989));
#180335=CARTESIAN_POINT('',(-60.1192206258108,-12.454722128404,38.9890000005754));
#180336=CARTESIAN_POINT('Origin',(5.49031038273072E-15,0.,38.989));
#180337=CARTESIAN_POINT('',(-60.119220626133,-12.4547221284865,38.989));
#180338=CARTESIAN_POINT('Origin',(62.2224557307631,0.,38.989));
#180339=CARTESIAN_POINT('',(-61.4975385923863,-6.7829006432352,38.989));
#180340=CARTESIAN_POINT('',(61.5757885448748,6.15262728712825,38.989));
#180341=CARTESIAN_POINT('',(-60.5836663843182,-12.5528626811443,38.989));
#180342=CARTESIAN_POINT('Origin',(5.49031038273072E-15,0.,38.989));
#180343=CARTESIAN_POINT('',(-60.1198497339744,-12.454275408702,38.989));
#180344=CARTESIAN_POINT('Origin',(5.57972911860581E-15,0.,39.624));
#180345=CARTESIAN_POINT('Origin',(-59.6417947880742,-6.58785913039772,39.6240070731883));
#180346=CARTESIAN_POINT('Origin',(-58.7584780045775,-12.1649018101379,39.6240070731883));
#180347=CARTESIAN_POINT('Origin',(5.57972911860581E-15,0.,39.624));
#180348=CARTESIAN_POINT('Origin',(-61.5354556255515,-6.78691960575365,39.555213520804));
#180349=CARTESIAN_POINT('Origin',(-60.620969154242,-12.5607573437815,39.555211759881));
#180350=CARTESIAN_POINT('Origin',(5.51210908043506E-15,0.,39.1438017080178));
#180351=CARTESIAN_POINT('Origin',(-60.6606342988047,-6.69490116063027,39.1711625381324));
#180352=CARTESIAN_POINT('Origin',(-59.7604378032096,-12.3779177236595,39.171217370261));
#180353=CARTESIAN_POINT('Origin',(5.51210908043507E-15,0.,39.1438017080178));
#180354=CARTESIAN_POINT('Origin',(-60.478793415361,-6.67587182882111,39.1712175859386));
#180355=CARTESIAN_POINT('Origin',(-59.5816164638925,-12.3398237541832,39.1711627526759));
#180356=CARTESIAN_POINT('Origin',(60.4792282238308,0.,38.989));
#180357=CARTESIAN_POINT('',(-57.1650137687748,-18.2401996527042,38.989));
#180358=CARTESIAN_POINT('',(-58.6264539577984,-12.7860306150448,38.989));
#180359=CARTESIAN_POINT('Origin',(5.49031038273072E-15,0.,38.989));
#180360=CARTESIAN_POINT('',(-59.0907848292991,-12.884727188594,38.989));
#180361=CARTESIAN_POINT('',(57.9308881865556,11.9889972685547,38.989));
#180362=CARTESIAN_POINT('',(-59.0906615920626,-12.8852923618766,38.9889999995776));
#180363=CARTESIAN_POINT('Origin',(5.49031038273072E-15,0.,38.989));
#180364=CARTESIAN_POINT('',(-57.6166602457573,-18.3863402753484,38.9889999997818));
#180365=CARTESIAN_POINT('Origin',(5.49031038273072E-15,0.,38.989));
#180366=CARTESIAN_POINT('',(-57.6164843860298,-18.3868913484942,38.989));
#180367=CARTESIAN_POINT('Origin',(5.49031038273072E-15,0.,38.989));
#180368=CARTESIAN_POINT('',(-57.1655250547207,-18.2403657795784,38.989));
#180369=CARTESIAN_POINT('Origin',(5.49031038273072E-15,0.,38.989));
#180370=CARTESIAN_POINT('',(-59.249807061628,-12.9191181862042,39.2708017080178));
#180371=CARTESIAN_POINT('',(-59.0906615913478,-12.8852923617207,38.989));
#180372=CARTESIAN_POINT('',(-57.7713971780681,-18.4366189871529,39.2708017078546));
#180373=CARTESIAN_POINT('Origin',(5.52999282761009E-15,0.,39.2708017080178));
#180374=CARTESIAN_POINT('',(-57.7713971777988,-18.4366189870669,39.2708017080178));
#180375=CARTESIAN_POINT('Origin',(60.71525,0.,39.3978017080178));
#180376=CARTESIAN_POINT('',(-57.9804289733665,-18.5051441132838,39.3978017080178));
#180377=CARTESIAN_POINT('',(-59.4650964698967,-12.9642895838867,39.3978017080178));
#180378=CARTESIAN_POINT('Origin',(5.5478765747851E-15,0.,39.3978017080178));
#180379=CARTESIAN_POINT('',(-59.6130003254556,-12.995727518882,39.3978017080178));
#180380=CARTESIAN_POINT('',(58.1567073854023,12.0369966210207,39.3978017080178));
#180381=CARTESIAN_POINT('',(-58.1242364370958,-18.5518699907147,39.3978017080178));
#180382=CARTESIAN_POINT('Origin',(5.5478765747851E-15,0.,39.3978017080178));
#180383=CARTESIAN_POINT('',(-57.9809330566518,-18.5053078998717,39.3978017080178));
#180384=CARTESIAN_POINT('Origin',(5.5478765747851E-15,0.,39.3978017080178));
#180385=CARTESIAN_POINT('',(-58.3332704847797,-18.6203878281144,39.2708017080178));
#180386=CARTESIAN_POINT('',(-59.8282880399728,-13.0409063549817,39.2708017081757));
#180387=CARTESIAN_POINT('Origin',(5.52999282761008E-15,0.,39.2708017080178));
#180388=CARTESIAN_POINT('',(-59.9874327886718,-13.0747351550707,38.9890000005756));
#180389=CARTESIAN_POINT('',(-59.8282880397056,-13.0409063549235,39.2708017080178));
#180390=CARTESIAN_POINT('',(-59.9873118763436,-13.0752898951321,38.989));
#180391=CARTESIAN_POINT('Origin',(5.49031038273072E-15,0.,38.989));
#180392=CARTESIAN_POINT('',(-58.4881809372199,-18.6701227271407,38.989));
#180393=CARTESIAN_POINT('Origin',(5.49031038273072E-15,0.,38.989));
#180394=CARTESIAN_POINT('',(-58.488008280337,-18.6706636022905,38.9890000005754));
#180395=CARTESIAN_POINT('Origin',(5.49031038273072E-15,0.,38.989));
#180396=CARTESIAN_POINT('',(-58.4880082806488,-18.6706636024062,38.989));
#180397=CARTESIAN_POINT('Origin',(62.2224557307631,0.,38.989));
#180398=CARTESIAN_POINT('',(-60.451642460649,-13.1739864076103,38.989));
#180399=CARTESIAN_POINT('',(59.5987607253196,12.3435145206982,38.989));
#180400=CARTESIAN_POINT('',(-58.9396512752214,-18.8168143322223,38.989));
#180401=CARTESIAN_POINT('Origin',(5.49031038273072E-15,0.,38.989));
#180402=CARTESIAN_POINT('',(-58.4886806371043,-18.6702850894754,38.989));
#180403=CARTESIAN_POINT('Origin',(5.57972911860581E-15,0.,39.624));
#180404=CARTESIAN_POINT('Origin',(-58.6264520046769,-12.7860353045044,39.6240070731883));
#180405=CARTESIAN_POINT('Origin',(-57.1650144220518,-18.240194614952,39.6240070731883));
#180406=CARTESIAN_POINT('Origin',(5.57972911860581E-15,0.,39.624));
#180407=CARTESIAN_POINT('Origin',(-60.488931684366,-13.1819467630401,39.5552135207985));
#180408=CARTESIAN_POINT('Origin',(-58.9759244797144,-18.8285649482878,39.5552117598814));
#180409=CARTESIAN_POINT('Origin',(5.51210908043506E-15,0.,39.1438017080178));
#180410=CARTESIAN_POINT('Origin',(-59.6285212670397,-12.9989886756685,39.1711625381335));
#180411=CARTESIAN_POINT('Origin',(-58.139219153978,-18.556776923018,39.171217370261));
#180412=CARTESIAN_POINT('Origin',(5.51210908043507E-15,0.,39.1438017080178));
#180413=CARTESIAN_POINT('Origin',(-59.4496656337937,-12.9610560404249,39.1712175859361));
#180414=CARTESIAN_POINT('Origin',(-57.9653593207593,-18.5001997164937,39.1711627526731));
#180415=CARTESIAN_POINT('Origin',(60.4792282238308,0.,38.989));
#180416=CARTESIAN_POINT('',(-54.945237802683,-24.1156489724274,38.989));
#180417=CARTESIAN_POINT('',(-56.9687879773467,-18.8441205405516,38.989));
#180418=CARTESIAN_POINT('Origin',(5.49031038273072E-15,0.,38.989));
#180419=CARTESIAN_POINT('',(-57.4202585945867,-18.9908122363899,38.989));
#180420=CARTESIAN_POINT('',(54.8020887275097,17.4724387660752,38.989));
#180421=CARTESIAN_POINT('',(-57.4200769557628,-18.9913614317954,38.9889999995771));
#180422=CARTESIAN_POINT('Origin',(5.49031038273072E-15,0.,38.989));
#180423=CARTESIAN_POINT('',(-55.3791342583021,-24.308198933629,38.9889999997818));
#180424=CARTESIAN_POINT('Origin',(5.49031038273072E-15,0.,38.989));
#180425=CARTESIAN_POINT('',(-55.3789017591235,-24.3087286055914,38.989));
#180426=CARTESIAN_POINT('Origin',(5.49031038273072E-15,0.,38.989));
#180427=CARTESIAN_POINT('',(-54.9457289227642,-24.1158676331754,38.989));
#180428=CARTESIAN_POINT('Origin',(5.49031038273072E-15,0.,38.989));
#180429=CARTESIAN_POINT('',(-57.5748148483577,-19.0416371860875,39.2708017080178));
#180430=CARTESIAN_POINT('',(-57.4200769550674,-18.9913614315654,38.989));
#180431=CARTESIAN_POINT('',(-55.5277679690273,-24.3743766271347,39.2708017078546));
#180432=CARTESIAN_POINT('Origin',(5.52999282761009E-15,0.,39.2708017080178));
#180433=CARTESIAN_POINT('',(-55.5277679687684,-24.3743766270211,39.2708017080178));
#180434=CARTESIAN_POINT('Origin',(60.71525,0.,39.3978017080178));
#180435=CARTESIAN_POINT('',(-55.7284918401499,-24.4643761377914,39.3978017080178));
#180436=CARTESIAN_POINT('',(-57.7842031819384,-19.1090650011312,39.3978017080178));
#180437=CARTESIAN_POINT('Origin',(5.5478765747851E-15,0.,39.3978017080178));
#180438=CARTESIAN_POINT('',(-57.9280106456677,-19.1557908785622,39.3978017080178));
#180439=CARTESIAN_POINT('',(55.0155724295761,17.5418038257013,39.3978017080178));
#180440=CARTESIAN_POINT('',(-55.8666273273834,-24.5258780191668,39.3978017080178));
#180441=CARTESIAN_POINT('Origin',(5.5478765747851E-15,0.,39.3978017080178));
#180442=CARTESIAN_POINT('',(-55.728976041654,-24.4645917181904,39.3978017080178));
#180443=CARTESIAN_POINT('Origin',(5.5478765747851E-15,0.,39.3978017080178));
#180444=CARTESIAN_POINT('',(-56.0673542004327,-24.6158705164591,39.2708017080178));
#180445=CARTESIAN_POINT('',(-58.1373965172491,-19.2232259142295,39.2708017081757));
#180446=CARTESIAN_POINT('Origin',(5.52999282761008E-15,0.,39.2708017080178));
#180447=CARTESIAN_POINT('',(-58.2921333818757,-19.2735045526306,38.9890000005756));
#180448=CARTESIAN_POINT('',(-58.1373965169894,-19.2232259141436,39.2708017080178));
#180449=CARTESIAN_POINT('',(-58.2919551457918,-19.2740436149881,38.989));
#180450=CARTESIAN_POINT('Origin',(5.49031038273072E-15,0.,38.989));
#180451=CARTESIAN_POINT('',(-56.2162173246399,-24.6815255140423,38.989));
#180452=CARTESIAN_POINT('Origin',(5.49031038273072E-15,0.,38.989));
#180453=CARTESIAN_POINT('',(-56.2159890767413,-24.6820453786628,38.9890000005754));
#180454=CARTESIAN_POINT('Origin',(5.49031038273072E-15,0.,38.989));
#180455=CARTESIAN_POINT('',(-56.2159890770393,-24.6820453788105,38.989));
#180456=CARTESIAN_POINT('Origin',(62.2224557307631,0.,38.989));
#180457=CARTESIAN_POINT('',(-58.7434254837933,-19.4207352200698,38.989));
#180458=CARTESIAN_POINT('',(56.3788528200609,17.9847604760579,38.989));
#180459=CARTESIAN_POINT('',(-56.6498810128383,-24.8746050278049,38.989));
#180460=CARTESIAN_POINT('Origin',(5.49031038273072E-15,0.,38.989));
#180461=CARTESIAN_POINT('',(-56.2166973156307,-24.6817392198001,38.989));
#180462=CARTESIAN_POINT('Origin',(5.57972911860581E-15,0.,39.624));
#180463=CARTESIAN_POINT('Origin',(-56.9687855447425,-18.8441250001651,39.6240070731883));
#180464=CARTESIAN_POINT('Origin',(-54.9452389789698,-24.1156440305586,39.6240070731883));
#180465=CARTESIAN_POINT('Origin',(5.57972911860581E-15,0.,39.624));
#180466=CARTESIAN_POINT('Origin',(-58.7796783495205,-19.4325497530928,39.5552135207989));
#180467=CARTESIAN_POINT('Origin',(-56.6847272350812,-24.8900828550894,39.5552117598828));
#180468=CARTESIAN_POINT('Origin',(5.51210908043506E-15,0.,39.1438017080178));
#180469=CARTESIAN_POINT('Origin',(-57.9431056782044,-19.1606565505634,39.1711625381365));
#180470=CARTESIAN_POINT('Origin',(-55.8810150532827,-24.5323241911531,39.1712173702617));
#180471=CARTESIAN_POINT('Origin',(5.51210908043507E-15,0.,39.1438017080178));
#180472=CARTESIAN_POINT('Origin',(-57.7691948748979,-19.1042362097727,39.171217585939));
#180473=CARTESIAN_POINT('Origin',(-55.7140215708744,-24.4578836192969,39.1711627526724));
#180474=CARTESIAN_POINT('Origin',(60.4792282238308,0.,38.989));
#180475=CARTESIAN_POINT('',(-52.1234703131948,-29.7268821954847,38.989));
#180476=CARTESIAN_POINT('',(-54.6869600343299,-24.6957503380304,38.989));
#180477=CARTESIAN_POINT('Origin',(5.49031038273072E-15,0.,38.989));
#180478=CARTESIAN_POINT('',(-55.1206239907504,-24.8888299712409,38.989));
#180479=CARTESIAN_POINT('',(50.603004322856,22.1823620689013,38.989));
#180480=CARTESIAN_POINT('',(-55.1203859404106,-24.8893571716692,38.9889999995774));
#180481=CARTESIAN_POINT('Origin',(5.49031038273072E-15,0.,38.989));
#180482=CARTESIAN_POINT('',(-52.534862887084,-29.9637318775751,38.9889999997818));
#180483=CARTESIAN_POINT('Origin',(5.49031038273072E-15,0.,38.989));
#180484=CARTESIAN_POINT('',(-52.5345762957639,-29.9642343451572,38.989));
#180485=CARTESIAN_POINT('Origin',(5.49031038273072E-15,0.,38.989));
#180486=CARTESIAN_POINT('',(-52.1239358865968,-29.7271509944136,38.989));
#180487=CARTESIAN_POINT('Origin',(5.49031038273072E-15,0.,38.989));
#180488=CARTESIAN_POINT('',(-55.2690209153042,-24.9555320242412,39.2708017080178));
#180489=CARTESIAN_POINT('',(-55.1203859397436,-24.889357171368,38.989));
#180490=CARTESIAN_POINT('',(-52.6757649141853,-30.0450834961234,39.2708017078546));
#180491=CARTESIAN_POINT('Origin',(5.52999282761009E-15,0.,39.2708017080178));
#180492=CARTESIAN_POINT('',(-52.6757649139398,-30.0450834959834,39.2708017080178));
#180493=CARTESIAN_POINT('Origin',(60.71525,0.,39.3978017080178));
#180494=CARTESIAN_POINT('',(-52.8659816883961,-30.1555713378335,39.3978017080178));
#180495=CARTESIAN_POINT('',(-55.4702140717968,-25.0444775033944,39.3978017080178));
#180496=CARTESIAN_POINT('Origin',(5.5478765747851E-15,0.,39.3978017080178));
#180497=CARTESIAN_POINT('',(-55.6083495590303,-25.1059793847698,39.3978017080178));
#180498=CARTESIAN_POINT('',(50.7999799080417,22.2700612497314,39.3978017080178));
#180499=CARTESIAN_POINT('',(-52.9969317578289,-30.2311753956709,39.3978017080178));
#180500=CARTESIAN_POINT('Origin',(5.5478765747851E-15,0.,39.3978017080178));
#180501=CARTESIAN_POINT('',(-52.8664407031058,-30.1558363500997,39.3978017080178));
#180502=CARTESIAN_POINT('Origin',(5.5478765747851E-15,0.,39.3978017080178));
#180503=CARTESIAN_POINT('',(-53.1871522506177,-30.3416565762233,39.2708017080178));
#180504=CARTESIAN_POINT('',(-55.8095395122501,-25.1949317876423,39.2708017081757));
#180505=CARTESIAN_POINT('Origin',(5.52999282761008E-15,0.,39.2708017080178));
#180506=CARTESIAN_POINT('',(-55.9581731633346,-25.2611094010718,38.9890000005756));
#180507=CARTESIAN_POINT('',(-55.8095395120008,-25.1949317875298,39.2708017080178));
#180508=CARTESIAN_POINT('',(-55.9579395562868,-25.2616268796454,38.989));
#180509=CARTESIAN_POINT('Origin',(5.49031038273072E-15,0.,38.989));
#180510=CARTESIAN_POINT('',(-53.3283370710514,-30.4225123424708,38.989));
#180511=CARTESIAN_POINT('Origin',(5.49031038273072E-15,0.,38.989));
#180512=CARTESIAN_POINT('',(-53.3280557328688,-30.4230055008165,38.9890000005754));
#180513=CARTESIAN_POINT('Origin',(5.49031038273072E-15,0.,38.989));
#180514=CARTESIAN_POINT('',(-53.3280557331497,-30.4230055009945,38.989));
#180515=CARTESIAN_POINT('Origin',(62.2224557307631,0.,38.989));
#180516=CARTESIAN_POINT('',(-56.3916032444852,-25.454706393408,38.989));
#180517=CARTESIAN_POINT('',(52.0578415156897,22.8300973196046,38.989));
#180518=CARTESIAN_POINT('',(-53.7394427993288,-30.6598643453572,38.989));
#180519=CARTESIAN_POINT('Origin',(5.49031038273072E-15,0.,38.989));
#180520=CARTESIAN_POINT('',(-53.3287920942669,-30.4227750502468,38.989));
#180521=CARTESIAN_POINT('Origin',(5.57972911860581E-15,0.,39.624));
#180522=CARTESIAN_POINT('Origin',(-54.6869571488952,-24.6957545189373,39.6240070731883));
#180523=CARTESIAN_POINT('Origin',(-52.1234719996037,-29.7268774036434,39.6240070731883));
#180524=CARTESIAN_POINT('Origin',(5.57972911860581E-15,0.,39.624));
#180525=CARTESIAN_POINT('Origin',(-56.4264225582403,-25.4702456615252,39.5552135207993));
#180526=CARTESIAN_POINT('Origin',(-53.7724802568185,-30.6788998055495,39.5552117598812));
#180527=CARTESIAN_POINT('Origin',(5.51210908043506E-15,0.,39.1438017080178));
#180528=CARTESIAN_POINT('Origin',(-55.6228532981808,-25.1123962626642,39.1711625381337));
#180529=CARTESIAN_POINT('Origin',(-53.0105668578087,-30.2390901817308,39.1712173702625));
#180530=CARTESIAN_POINT('Origin',(5.51210908043507E-15,0.,39.1438017080178));
#180531=CARTESIAN_POINT('Origin',(-55.4557927279719,-25.0381063693876,39.1712175859413));
#180532=CARTESIAN_POINT('Origin',(-52.852269341752,-30.1476018310227,39.1711627526721));
#180533=CARTESIAN_POINT('Origin',(60.4792282238308,0.,38.989));
#180534=CARTESIAN_POINT('',(-48.7306271754178,-35.0124214764582,38.989));
#180535=CARTESIAN_POINT('',(-51.8059703131948,-30.2768083268878,38.989));
#180536=CARTESIAN_POINT('Origin',(5.49031038273072E-15,0.,38.989));
#180537=CARTESIAN_POINT('',(-52.2170762957392,-30.5141604766044,38.989));
#180538=CARTESIAN_POINT('',(45.5181711678734,25.9133109558554,38.989));
#180539=CARTESIAN_POINT('',(-52.2167844420139,-30.5146599059376,38.9889999995773));
#180540=CARTESIAN_POINT('Origin',(5.49031038273072E-15,0.,38.989));
#180541=CARTESIAN_POINT('',(-49.1150085644482,-35.2909759047566,38.9889999997818));
#180542=CARTESIAN_POINT('Origin',(5.49031038273072E-15,0.,38.989));
#180543=CARTESIAN_POINT('',(-49.1146710209412,-35.2914456628184,38.989));
#180544=CARTESIAN_POINT('Origin',(5.49031038273072E-15,0.,38.989));
#180545=CARTESIAN_POINT('',(-48.731062101221,-35.0127374685508,38.989));
#180546=CARTESIAN_POINT('Origin',(5.49031038273072E-15,0.,38.989));
#180547=CARTESIAN_POINT('',(-52.3576880233164,-30.5960088312566,39.2708017080178));
#180548=CARTESIAN_POINT('',(-52.2167844413817,-30.5146599055682,38.989));
#180549=CARTESIAN_POINT('',(-49.2466351558311,-35.3866101429907,39.2708017078546));
#180550=CARTESIAN_POINT('Origin',(5.52999282761009E-15,0.,39.2708017080178));
#180551=CARTESIAN_POINT('',(-49.2466351556015,-35.3866101428257,39.2708017080178));
#180552=CARTESIAN_POINT('Origin',(60.71525,0.,39.3978017080178));
#180553=CARTESIAN_POINT('',(-49.4242607783462,-35.5163757878393,39.3978017080178));
#180554=CARTESIAN_POINT('',(-52.5484816883961,-30.7054974692366,39.3978017080178));
#180555=CARTESIAN_POINT('Origin',(5.5478765747851E-15,0.,39.3978017080178));
#180556=CARTESIAN_POINT('',(-52.6794317578289,-30.781101527074,39.3978017080178));
#180557=CARTESIAN_POINT('',(45.6951875000003,26.0155113828598,39.3978017080178));
#180558=CARTESIAN_POINT('',(-49.5465907136146,-35.6052536882599,39.3978017080178));
#180559=CARTESIAN_POINT('Origin',(5.5478765747851E-15,0.,39.3978017080178));
#180560=CARTESIAN_POINT('',(-49.4246895772004,-35.5166873284428,39.3978017080178));
#180561=CARTESIAN_POINT('Origin',(5.5478765747851E-15,0.,39.3978017080178));
#180562=CARTESIAN_POINT('',(-49.7242207306177,-35.7350130971387,39.2708017080178));
#180563=CARTESIAN_POINT('',(-52.8702215134579,-30.8905967160113,39.2708017081757));
#180564=CARTESIAN_POINT('Origin',(5.52999282761008E-15,0.,39.2708017080178));
#180565=CARTESIAN_POINT('',(-53.0111234896155,-30.9719482486879,38.9890000005756));
#180566=CARTESIAN_POINT('',(-52.8702215132218,-30.8905967158733,39.2708017080178));
#180567=CARTESIAN_POINT('',(-53.0108370710514,-30.9724384738739,38.989));
#180568=CARTESIAN_POINT('Origin',(5.49031038273072E-15,0.,38.989));
#180569=CARTESIAN_POINT('',(-49.8561803968405,-35.8301837593552,38.989));
#180570=CARTESIAN_POINT('Origin',(5.49031038273072E-15,0.,38.989));
#180571=CARTESIAN_POINT('',(-49.8558490507739,-35.83064480828,38.9890000005754));
#180572=CARTESIAN_POINT('Origin',(5.49031038273072E-15,0.,38.989));
#180573=CARTESIAN_POINT('',(-49.8558490510346,-35.8306448084864,38.989));
#180574=CARTESIAN_POINT('Origin',(62.2224557307631,0.,38.989));
#180575=CARTESIAN_POINT('',(-53.4219427993288,-31.2097904767603,38.989));
#180576=CARTESIAN_POINT('',(46.8255917980726,26.668150608645,38.989));
#180577=CARTESIAN_POINT('',(-50.2402240048085,-36.1092077731526,38.989));
#180578=CARTESIAN_POINT('Origin',(5.49031038273072E-15,0.,38.989));
#180579=CARTESIAN_POINT('',(-49.8566054669511,-35.830492590868,38.989));
#180580=CARTESIAN_POINT('Origin',(5.57972911860581E-15,0.,39.624));
#180581=CARTESIAN_POINT('Origin',(-51.8059670065431,-30.2768121832812,39.6240070731883));
#180582=CARTESIAN_POINT('Origin',(-48.7306293534723,-35.0124168871448,39.6240070731883));
#180583=CARTESIAN_POINT('Origin',(5.57972911860581E-15,0.,39.624));
#180584=CARTESIAN_POINT('Origin',(-53.4549470734238,-31.2288842284974,39.5552135208002));
#180585=CARTESIAN_POINT('Origin',(-50.2710907322476,-36.1315923097635,39.5552117598819));
#180586=CARTESIAN_POINT('Origin',(5.51210908043506E-15,0.,39.1438017080178));
#180587=CARTESIAN_POINT('Origin',(-52.6931852975955,-30.788999306206,39.1711625381373));
#180588=CARTESIAN_POINT('Origin',(-49.559323798665,-35.6145503723402,39.1712173702594));
#180589=CARTESIAN_POINT('Origin',(5.51210908043507E-15,0.,39.1438017080178));
#180590=CARTESIAN_POINT('Origin',(-52.5348053110496,-30.6976537960616,39.1712175859388));
#180591=CARTESIAN_POINT('Origin',(-49.4114565896704,-35.5070166082983,39.1711627526735));
#180592=CARTESIAN_POINT('Origin',(60.4792282238308,0.,38.989));
#180593=CARTESIAN_POINT('',(-44.8038810887676,-39.9143573409155,38.989));
#180594=CARTESIAN_POINT('',(-48.3573835402121,-35.5261472678863,38.989));
#180595=CARTESIAN_POINT('Origin',(5.49031038273072E-15,0.,38.989));
#180596=CARTESIAN_POINT('',(-48.7414273857063,-35.8051714542878,38.989));
#180597=CARTESIAN_POINT('',(39.7707905934409,28.5027191556738,38.989));
#180598=CARTESIAN_POINT('',(-48.7410849262056,-35.8056376406735,38.9889999995771));
#180599=CARTESIAN_POINT('Origin',(5.49031038273072E-15,0.,38.989));
#180600=CARTESIAN_POINT('',(-45.157039930004,-40.231564614814,38.9889999997818));
#180601=CARTESIAN_POINT('Origin',(5.49031038273072E-15,0.,38.989));
#180602=CARTESIAN_POINT('',(-45.1566551325073,-40.231996516588,38.989));
#180603=CARTESIAN_POINT('Origin',(5.49031038273072E-15,0.,38.989));
#180604=CARTESIAN_POINT('',(-44.804280601834,-39.9147170640961,38.989));
#180605=CARTESIAN_POINT('Origin',(5.49031038273072E-15,0.,38.989));
#180606=CARTESIAN_POINT('',(-48.8727133447945,-35.9012693628902,39.2708017080178));
#180607=CARTESIAN_POINT('',(-48.7410849256153,-35.8056376402399,38.989));
#180608=CARTESIAN_POINT('',(-45.2779489571886,-40.3404336840071,39.2708017078546));
#180609=CARTESIAN_POINT('Origin',(5.52999282761009E-15,0.,39.2708017080178));
#180610=CARTESIAN_POINT('',(-45.2779489569775,-40.340433683819,39.2708017080178));
#180611=CARTESIAN_POINT('Origin',(60.71525,0.,39.3978017080178));
#180612=CARTESIAN_POINT('',(-45.4410373245174,-40.4880553924341,39.3978017080178));
#180613=CARTESIAN_POINT('',(-49.0510171431405,-36.0301015792674,39.3978017080178));
#180614=CARTESIAN_POINT('Origin',(5.5478765747851E-15,0.,39.3978017080178));
#180615=CARTESIAN_POINT('',(-49.1733470784089,-36.118979479688,39.3978017080178));
#180616=CARTESIAN_POINT('',(39.9252688514649,28.6149541797805,39.3978017080178));
#180617=CARTESIAN_POINT('',(-45.5534068532513,-40.589233370562,39.3978017080178));
#180618=CARTESIAN_POINT('Origin',(5.5478765747851E-15,0.,39.3978017080178));
#180619=CARTESIAN_POINT('',(-45.441431209506,-40.4884100480709,39.3978017080178));
#180620=CARTESIAN_POINT('Origin',(5.5478765747851E-15,0.,39.3978017080178));
#180621=CARTESIAN_POINT('',(-45.7165002428309,-40.7368493365295,39.2708017080178));
#180622=CARTESIAN_POINT('',(-49.3516463039591,-36.2478178024867,39.2708017081757));
#180623=CARTESIAN_POINT('Origin',(5.52999282761008E-15,0.,39.2708017080178));
#180624=CARTESIAN_POINT('',(-49.4832728536533,-36.3434519499945,38.9890000005756));
#180625=CARTESIAN_POINT('',(-49.3516463037387,-36.2478178023248,39.2708017080178));
#180626=CARTESIAN_POINT('',(-49.4829367616348,-36.3439095507833,38.989));
#180627=CARTESIAN_POINT('Origin',(5.49031038273072E-15,0.,38.989));
#180628=CARTESIAN_POINT('',(-45.8377889771253,-40.8452921850241,38.989));
#180629=CARTESIAN_POINT('Origin',(5.49031038273072E-15,0.,38.989));
#180630=CARTESIAN_POINT('',(-45.8374112534715,-40.8457160731795,38.9890000005754));
#180631=CARTESIAN_POINT('Origin',(5.49031038273072E-15,0.,38.989));
#180632=CARTESIAN_POINT('',(-45.8374112537093,-40.845716073412,38.989));
#180633=CARTESIAN_POINT('Origin',(62.2224557307631,0.,38.989));
#180634=CARTESIAN_POINT('',(-49.8669803696028,-36.6229335645807,38.989));
#180635=CARTESIAN_POINT('',(40.911747809259,29.3316730956003,38.989));
#180636=CARTESIAN_POINT('',(-46.1905628026487,-41.1629311642478,38.989));
#180637=CARTESIAN_POINT('Origin',(5.49031038273072E-15,0.,38.989));
#180638=CARTESIAN_POINT('',(-45.838179436974,-40.845643756651,38.989));
#180639=CARTESIAN_POINT('Origin',(5.57972911860581E-15,0.,39.624));
#180640=CARTESIAN_POINT('Origin',(-48.3573798485717,-35.5261507575148,39.6240070731883));
#180641=CARTESIAN_POINT('Origin',(-44.8038837346043,-39.9143530044115,39.6240070731883));
#180642=CARTESIAN_POINT('Origin',(5.57972911860581E-15,0.,39.624));
#180643=CARTESIAN_POINT('Origin',(-49.8978080023051,-36.6453726047975,39.5552135208017));
#180644=CARTESIAN_POINT('Origin',(-46.2189206177146,-41.188419527607,39.5552117598829));
#180645=CARTESIAN_POINT('Origin',(5.51210908043506E-15,0.,39.1438017080178));
#180646=CARTESIAN_POINT('Origin',(-49.1861997321292,-36.1282716303355,39.1711625381366));
#180647=CARTESIAN_POINT('Origin',(-45.5650984170296,-40.5998100962475,39.1712173702608));
#180648=CARTESIAN_POINT('Origin',(5.51210908043507E-15,0.,39.1438017080178));
#180649=CARTESIAN_POINT('Origin',(-49.0382355735267,-36.0208713038452,39.1712175859367));
#180650=CARTESIAN_POINT('Origin',(-45.4292815791796,-40.4774090812932,39.1711627526754));
#180651=CARTESIAN_POINT('Origin',(60.4792282238308,0.,38.989));
#180652=CARTESIAN_POINT('',(-40.386254305094,-44.3789831537294,38.989));
#180653=CARTESIAN_POINT('',(-44.3789831537298,-40.3862543050936,38.989));
#180654=CARTESIAN_POINT('Origin',(5.49031038273072E-15,0.,38.989));
#180655=CARTESIAN_POINT('',(-44.7317571974361,-40.7038934808041,38.989));
#180656=CARTESIAN_POINT('',(33.61296347236,29.8380098596982,38.989));
#180657=CARTESIAN_POINT('',(-44.7313678842178,-40.7043213166066,38.9889999995772));
#180658=CARTESIAN_POINT('Origin',(5.49031038273072E-15,0.,38.989));
#180659=CARTESIAN_POINT('',(-40.7043213163686,-44.7313678839554,38.9889999997818));
#180660=CARTESIAN_POINT('Origin',(5.49031038273072E-15,0.,38.989));
#180661=CARTESIAN_POINT('',(-40.7038934808041,-44.7317571974352,38.989));
#180662=CARTESIAN_POINT('Origin',(5.49031038273072E-15,0.,38.989));
#180663=CARTESIAN_POINT('',(-40.3866140282747,-44.3793826667957,38.989));
#180664=CARTESIAN_POINT('Origin',(5.49031038273072E-15,0.,38.989));
#180665=CARTESIAN_POINT('',(-44.8522789915944,-40.8131880745604,39.2708017080178));
#180666=CARTESIAN_POINT('',(-44.7313678836762,-40.7043213161137,38.989));
#180667=CARTESIAN_POINT('',(-40.8131880747511,-44.8522789918031,39.2708017078546));
#180668=CARTESIAN_POINT('Origin',(5.52999282761009E-15,0.,39.2708017080178));
#180669=CARTESIAN_POINT('',(-40.8131880745609,-44.8522789915939,39.2708017080178));
#180670=CARTESIAN_POINT('Origin',(60.71525,0.,39.3978017080178));
#180671=CARTESIAN_POINT('',(-40.9599523566127,-45.0161393894791,39.3978017080178));
#180672=CARTESIAN_POINT('',(-45.0161393894795,-40.9599523566123,39.3978017080178));
#180673=CARTESIAN_POINT('Origin',(5.5478765747851E-15,0.,39.3978017080178));
#180674=CARTESIAN_POINT('',(-45.1285089182135,-41.0611303347402,39.3978017080178));
#180675=CARTESIAN_POINT('',(33.743309857225,29.9553742717902,39.3978017080178));
#180676=CARTESIAN_POINT('',(-41.0611303347406,-45.1285089182131,39.3978017080178));
#180677=CARTESIAN_POINT('Origin',(5.5478765747851E-15,0.,39.3978017080178));
#180678=CARTESIAN_POINT('',(-40.9603070122495,-45.0165332744677,39.3978017080178));
#180679=CARTESIAN_POINT('Origin',(5.5478765747851E-15,0.,39.3978017080178));
#180680=CARTESIAN_POINT('',(-41.2079002115909,-45.2923641298555,39.2708017080178));
#180681=CARTESIAN_POINT('',(-45.2923641300582,-41.2079002117745,39.2708017081757));
#180682=CARTESIAN_POINT('Origin',(5.52999282761008E-15,0.,39.2708017080178));
#180683=CARTESIAN_POINT('',(-45.413273125266,-41.3167691863806,38.9890000005756));
#180684=CARTESIAN_POINT('',(-45.2923641298559,-41.2079002115905,39.2708017080178));
#180685=CARTESIAN_POINT('',(-45.4128910420874,-41.3171891492023,38.989));
#180686=CARTESIAN_POINT('Origin',(5.49031038273072E-15,0.,38.989));
#180687=CARTESIAN_POINT('',(-41.3171891492027,-45.412891042087,38.989));
#180688=CARTESIAN_POINT('Origin',(5.49031038273072E-15,0.,38.989));
#180689=CARTESIAN_POINT('',(-41.3167691863812,-45.4132731252656,38.9890000005754));
#180690=CARTESIAN_POINT('Origin',(5.49031038273072E-15,0.,38.989));
#180691=CARTESIAN_POINT('',(-41.3167691865933,-45.4132731255218,38.989));
#180692=CARTESIAN_POINT('Origin',(62.2224557307631,0.,38.989));
#180693=CARTESIAN_POINT('',(-45.7656648676108,-41.634828128426,38.989));
#180694=CARTESIAN_POINT('',(34.5756856720389,30.7048488218244,38.989));
#180695=CARTESIAN_POINT('',(-41.6348281284264,-45.7656648676104,38.989));
#180696=CARTESIAN_POINT('Origin',(5.49031038273072E-15,0.,38.989));
#180697=CARTESIAN_POINT('',(-41.3175407208296,-45.4132815019357,38.989));
#180698=CARTESIAN_POINT('Origin',(5.57972911860581E-15,0.,39.624));
#180699=CARTESIAN_POINT('Origin',(-44.378979117547,-40.386257389724,39.6240070731883));
#180700=CARTESIAN_POINT('Origin',(-40.3862573897246,-44.3789791175465,39.6240070731883));
#180701=CARTESIAN_POINT('Origin',(5.57972911860581E-15,0.,39.624));
#180702=CARTESIAN_POINT('Origin',(-45.7939781049219,-41.6603666103106,39.5552135207989));
#180703=CARTESIAN_POINT('Origin',(-41.6603663369578,-45.7939778018852,39.5552117598784));
#180704=CARTESIAN_POINT('Origin',(5.51210908043506E-15,0.,39.1438017080178));
#180705=CARTESIAN_POINT('Origin',(-45.1403198695221,-41.0717150501546,39.1711625381318));
#180706=CARTESIAN_POINT('Origin',(-41.0716522820273,-45.1402498046841,39.1712173702621));
#180707=CARTESIAN_POINT('Origin',(5.51210908043507E-15,0.,39.1438017080178));
#180708=CARTESIAN_POINT('Origin',(-45.0043926651424,-40.9494366077789,39.1712175859375));
#180709=CARTESIAN_POINT('Origin',(-40.9493738530243,-45.0043225899483,39.1711627526731));
#180710=CARTESIAN_POINT('Origin',(60.4792282238308,0.,38.989));
#180711=CARTESIAN_POINT('',(-35.5261472678868,-48.3573835402117,38.989));
#180712=CARTESIAN_POINT('',(-39.9143573409159,-44.8038810887672,38.989));
#180713=CARTESIAN_POINT('Origin',(5.49031038273072E-15,0.,38.989));
#180714=CARTESIAN_POINT('',(-40.2319965165888,-45.1566551325074,38.989));
#180715=CARTESIAN_POINT('',(27.3146622010794,29.8615093742684,38.989));
#180716=CARTESIAN_POINT('',(-40.2315646150499,-45.1570399302679,38.9889999995774));
#180717=CARTESIAN_POINT('Origin',(5.49031038273072E-15,0.,38.989));
#180718=CARTESIAN_POINT('',(-35.8056376404641,-48.7410849259196,38.9889999997818));
#180719=CARTESIAN_POINT('Origin',(5.49031038273072E-15,0.,38.989));
#180720=CARTESIAN_POINT('',(-35.8051714542879,-48.7414273857054,38.989));
#180721=CARTESIAN_POINT('Origin',(5.49031038273072E-15,0.,38.989));
#180722=CARTESIAN_POINT('',(-35.5264632599794,-48.357818466015,38.989));
#180723=CARTESIAN_POINT('Origin',(5.49031038273072E-15,0.,38.989));
#180724=CARTESIAN_POINT('',(-40.3404336838195,-45.2779489569771,39.2708017080178));
#180725=CARTESIAN_POINT('',(-40.231564614563,-45.1570399297214,38.989));
#180726=CARTESIAN_POINT('',(-35.9012693630581,-48.872713345022,39.2708017078546));
#180727=CARTESIAN_POINT('Origin',(5.52999282761009E-15,0.,39.2708017080178));
#180728=CARTESIAN_POINT('',(-35.9012693628907,-48.8727133447942,39.2708017080178));
#180729=CARTESIAN_POINT('Origin',(60.71525,0.,39.3978017080178));
#180730=CARTESIAN_POINT('',(-36.0301015792679,-49.0510171431402,39.3978017080178));
#180731=CARTESIAN_POINT('',(-40.4880553924345,-45.441037324517,39.3978017080178));
#180732=CARTESIAN_POINT('Origin',(5.5478765747851E-15,0.,39.3978017080178));
#180733=CARTESIAN_POINT('',(-40.5892333705625,-45.5534068532509,39.3978017080178));
#180734=CARTESIAN_POINT('',(27.4203375923837,29.9788737863604,39.3978017080178));
#180735=CARTESIAN_POINT('',(-36.1189794796885,-49.1733470784086,39.3978017080178));
#180736=CARTESIAN_POINT('Origin',(5.5478765747851E-15,0.,39.3978017080178));
#180737=CARTESIAN_POINT('',(-36.0304131198714,-49.0514459419943,39.3978017080178));
#180738=CARTESIAN_POINT('Origin',(5.5478765747851E-15,0.,39.3978017080178));
#180739=CARTESIAN_POINT('',(-36.2478178023253,-49.3516463037383,39.2708017080178));
#180740=CARTESIAN_POINT('',(-40.7368493367119,-45.7165002430347,39.2708017081757));
#180741=CARTESIAN_POINT('Origin',(5.52999282761008E-15,0.,39.2708017080178));
#180742=CARTESIAN_POINT('',(-40.8457160731799,-45.837411253471,38.9890000005756));
#180743=CARTESIAN_POINT('',(-40.7368493365299,-45.7165002428305,39.2708017080178));
#180744=CARTESIAN_POINT('',(-40.8452921850246,-45.8377889771249,38.989));
#180745=CARTESIAN_POINT('Origin',(5.49031038273072E-15,0.,38.989));
#180746=CARTESIAN_POINT('',(-36.3439095507838,-49.4829367616344,38.989));
#180747=CARTESIAN_POINT('Origin',(5.49031038273072E-15,0.,38.989));
#180748=CARTESIAN_POINT('',(-36.343451949995,-49.483272853653,38.9890000005754));
#180749=CARTESIAN_POINT('Origin',(5.49031038273072E-15,0.,38.989));
#180750=CARTESIAN_POINT('',(-36.3434519501792,-49.4832728539299,38.989));
#180751=CARTESIAN_POINT('Origin',(62.2224557307631,0.,38.989));
#180752=CARTESIAN_POINT('',(-41.1629311642483,-46.1905628026483,38.989));
#180753=CARTESIAN_POINT('',(28.0951675083328,30.7283483363946,38.989));
#180754=CARTESIAN_POINT('',(-36.6229335645812,-49.8669803696024,38.989));
#180755=CARTESIAN_POINT('Origin',(5.49031038273072E-15,0.,38.989));
#180756=CARTESIAN_POINT('',(-36.3442183822966,-49.483361831745,38.989));
#180757=CARTESIAN_POINT('Origin',(5.57972911860581E-15,0.,39.624));
#180758=CARTESIAN_POINT('Origin',(-39.9143530044121,-44.8038837346038,39.6240070731883));
#180759=CARTESIAN_POINT('Origin',(-35.5261507575154,-48.3573798485712,39.6240070731883));
#180760=CARTESIAN_POINT('Origin',(5.57972911860581E-15,0.,39.624));
#180761=CARTESIAN_POINT('Origin',(-41.1884198004145,-46.2189209212423,39.555213520803));
#180762=CARTESIAN_POINT('Origin',(-36.6453723646293,-49.8978076723474,39.5552117598808));
#180763=CARTESIAN_POINT('Origin',(5.51210908043506E-15,0.,39.1438017080178));
#180764=CARTESIAN_POINT('Origin',(-40.5998732162091,-45.5651681650783,39.1711625381351));
#180765=CARTESIAN_POINT('Origin',(-36.1282165298269,-49.1861234900555,39.1712173702626));
#180766=CARTESIAN_POINT('Origin',(5.51210908043507E-15,0.,39.1438017080178));
#180767=CARTESIAN_POINT('Origin',(-40.4774722129479,-45.4293513150148,39.1712175859345));
#180768=CARTESIAN_POINT('Origin',(-36.0208162177223,-49.03815932255,39.1711627526757));
#180769=CARTESIAN_POINT('Origin',(60.4792282238308,0.,38.989));
#180770=CARTESIAN_POINT('',(-30.2768083268883,-51.8059703131945,38.989));
#180771=CARTESIAN_POINT('',(-35.0124214764587,-48.7306271754175,38.989));
#180772=CARTESIAN_POINT('Origin',(5.49031038273072E-15,0.,38.989));
#180773=CARTESIAN_POINT('',(-35.2914456628193,-49.1146710209414,38.989));
#180774=CARTESIAN_POINT('',(21.1519223437074,28.5729602337852,38.989));
#180775=CARTESIAN_POINT('',(-35.2909759049637,-49.1150085647354,38.9889999995773));
#180776=CARTESIAN_POINT('Origin',(5.49031038273072E-15,0.,38.989));
#180777=CARTESIAN_POINT('',(-30.5146599057594,-52.2167844417077,38.9889999997818));
#180778=CARTESIAN_POINT('Origin',(5.49031038273072E-15,0.,38.989));
#180779=CARTESIAN_POINT('',(-30.5141604766047,-52.2170762957384,38.989));
#180780=CARTESIAN_POINT('Origin',(5.49031038273072E-15,0.,38.989));
#180781=CARTESIAN_POINT('',(-30.2770771258173,-51.8064358865965,38.989));
#180782=CARTESIAN_POINT('Origin',(5.49031038273072E-15,0.,38.989));
#180783=CARTESIAN_POINT('',(-35.3866101428262,-49.2466351556011,39.2708017080178));
#180784=CARTESIAN_POINT('',(-35.2909759045365,-49.1150085641409,38.989));
#180785=CARTESIAN_POINT('',(-30.5960088313997,-52.3576880235602,39.2708017078546));
#180786=CARTESIAN_POINT('Origin',(5.52999282761009E-15,0.,39.2708017080178));
#180787=CARTESIAN_POINT('',(-30.5960088312571,-52.3576880233161,39.2708017080178));
#180788=CARTESIAN_POINT('Origin',(60.71525,0.,39.3978017080178));
#180789=CARTESIAN_POINT('',(-30.7054974692372,-52.5484816883958,39.3978017080178));
#180790=CARTESIAN_POINT('',(-35.5163757878398,-49.4242607783459,39.3978017080178));
#180791=CARTESIAN_POINT('Origin',(5.5478765747851E-15,0.,39.3978017080178));
#180792=CARTESIAN_POINT('',(-35.6052536882604,-49.5465907136143,39.3978017080178));
#180793=CARTESIAN_POINT('',(21.2334658618526,28.6851952578919,39.3978017080178));
#180794=CARTESIAN_POINT('',(-30.7811015270746,-52.6794317578286,39.3978017080178));
#180795=CARTESIAN_POINT('Origin',(5.5478765747851E-15,0.,39.3978017080178));
#180796=CARTESIAN_POINT('',(-30.7057624815034,-52.5489407031055,39.3978017080178));
#180797=CARTESIAN_POINT('Origin',(5.5478765747851E-15,0.,39.3978017080178));
#180798=CARTESIAN_POINT('',(-30.8905967158739,-52.8702215132214,39.2708017080178));
#180799=CARTESIAN_POINT('',(-35.7350130972987,-49.7242207308394,39.2708017081757));
#180800=CARTESIAN_POINT('Origin',(5.52999282761008E-15,0.,39.2708017080178));
#180801=CARTESIAN_POINT('',(-35.8306448082804,-49.8558490507735,38.9890000005756));
#180802=CARTESIAN_POINT('',(-35.7350130971392,-49.7242207306173,39.2708017080178));
#180803=CARTESIAN_POINT('',(-35.8301837593557,-49.8561803968401,38.989));
#180804=CARTESIAN_POINT('Origin',(5.49031038273072E-15,0.,38.989));
#180805=CARTESIAN_POINT('',(-30.9724384738745,-53.0108370710511,38.989));
#180806=CARTESIAN_POINT('Origin',(5.49031038273072E-15,0.,38.989));
#180807=CARTESIAN_POINT('',(-30.9719482486884,-53.0111234896152,38.9890000005754));
#180808=CARTESIAN_POINT('Origin',(5.49031038273072E-15,0.,38.989));
#180809=CARTESIAN_POINT('',(-30.9719482488427,-53.0111234899098,38.989));
#180810=CARTESIAN_POINT('Origin',(62.2224557307631,0.,38.989));
#180811=CARTESIAN_POINT('',(-36.1092077731531,-50.2402240048081,38.989));
#180812=CARTESIAN_POINT('',(21.7541926348216,29.4019141737117,38.989));
#180813=CARTESIAN_POINT('',(-31.2097904767608,-53.4219427993285,38.989));
#180814=CARTESIAN_POINT('Origin',(5.49031038273072E-15,0.,38.989));
#180815=CARTESIAN_POINT('',(-30.9727011816504,-53.0112920942666,38.989));
#180816=CARTESIAN_POINT('Origin',(5.57972911860581E-15,0.,39.624));
#180817=CARTESIAN_POINT('Origin',(-35.0124168871455,-48.7306293534718,39.6240070731883));
#180818=CARTESIAN_POINT('Origin',(-30.276812183282,-51.8059670065426,39.6240070731883));
#180819=CARTESIAN_POINT('Origin',(5.57972911860581E-15,0.,39.624));
#180820=CARTESIAN_POINT('Origin',(-36.1315925493512,-50.2710910626307,39.5552135207972));
#180821=CARTESIAN_POINT('Origin',(-31.2288840241297,-53.4549467201703,39.5552117598825));
#180822=CARTESIAN_POINT('Origin',(5.51210908043506E-15,0.,39.1438017080178));
#180823=CARTESIAN_POINT('Origin',(-35.6146058558682,-49.55939976246,39.171162538136));
#180824=CARTESIAN_POINT('Origin',(-30.7889524770111,-52.6931037136134,39.1712173702653));
#180825=CARTESIAN_POINT('Origin',(5.51210908043507E-15,0.,39.1438017080178));
#180826=CARTESIAN_POINT('Origin',(-35.5070721047369,-49.4115325425342,39.171217585936));
#180827=CARTESIAN_POINT('Origin',(-30.6976069821036,-52.534723719719,39.1711627526727));
#180828=CARTESIAN_POINT('Origin',(60.4792282238308,0.,38.989));
#180829=CARTESIAN_POINT('',(-24.695750338031,-54.6869600343296,38.989));
#180830=CARTESIAN_POINT('',(-29.7268821954852,-52.1234703131945,38.989));
#180831=CARTESIAN_POINT('Origin',(5.49031038273072E-15,0.,38.989));
#180832=CARTESIAN_POINT('',(-29.9642343451581,-52.5345762957642,38.989));
#180833=CARTESIAN_POINT('',(15.3947701216595,26.0295240215573,38.989));
#180834=CARTESIAN_POINT('',(-29.9637318777512,-52.5348628873915,38.9889999995772));
#180835=CARTESIAN_POINT('Origin',(5.49031038273072E-15,0.,38.989));
#180836=CARTESIAN_POINT('',(-24.8893571715241,-55.1203859400878,38.9889999997818));
#180837=CARTESIAN_POINT('Origin',(5.49031038273072E-15,0.,38.989));
#180838=CARTESIAN_POINT('',(-24.8888299712412,-55.1206239907495,38.989));
#180839=CARTESIAN_POINT('Origin',(5.49031038273072E-15,0.,38.989));
#180840=CARTESIAN_POINT('',(-24.6959689987791,-54.6874511544108,38.989));
#180841=CARTESIAN_POINT('Origin',(5.49031038273072E-15,0.,38.989));
#180842=CARTESIAN_POINT('',(-30.0450834959839,-52.6757649139395,39.2708017080178));
#180843=CARTESIAN_POINT('',(-29.9637318773884,-52.5348628867553,38.989));
#180844=CARTESIAN_POINT('',(-24.9555320243581,-55.2690209155616,39.2708017078546));
#180845=CARTESIAN_POINT('Origin',(5.52999282761009E-15,0.,39.2708017080178));
#180846=CARTESIAN_POINT('',(-24.9555320242418,-55.2690209153039,39.2708017080178));
#180847=CARTESIAN_POINT('Origin',(60.71525,0.,39.3978017080178));
#180848=CARTESIAN_POINT('',(-25.044477503395,-55.4702140717966,39.3978017080178));
#180849=CARTESIAN_POINT('',(-30.155571337834,-52.8659816883958,39.3978017080178));
#180850=CARTESIAN_POINT('Origin',(5.5478765747851E-15,0.,39.3978017080178));
#180851=CARTESIAN_POINT('',(-30.2311753956715,-52.9969317578286,39.3978017080178));
#180852=CARTESIAN_POINT('',(15.4537755657018,26.1317244485617,39.3978017080178));
#180853=CARTESIAN_POINT('',(-25.1059793847704,-55.60834955903,39.3978017080178));
#180854=CARTESIAN_POINT('Origin',(5.5478765747851E-15,0.,39.3978017080178));
#180855=CARTESIAN_POINT('',(-25.0446930837941,-55.4706982733006,39.3978017080178));
#180856=CARTESIAN_POINT('Origin',(5.5478765747851E-15,0.,39.3978017080178));
#180857=CARTESIAN_POINT('',(-25.1949317875303,-55.8095395120006,39.2708017080178));
#180858=CARTESIAN_POINT('',(-30.3416565763594,-53.1871522508549,39.2708017081757));
#180859=CARTESIAN_POINT('Origin',(5.52999282761008E-15,0.,39.2708017080178));
#180860=CARTESIAN_POINT('',(-30.423005500817,-53.3280557328684,38.9890000005756));
#180861=CARTESIAN_POINT('',(-30.3416565762239,-53.1871522506173,39.2708017080178));
#180862=CARTESIAN_POINT('',(-30.4225123424714,-53.3283370710511,38.989));
#180863=CARTESIAN_POINT('Origin',(5.49031038273072E-15,0.,38.989));
#180864=CARTESIAN_POINT('',(-25.2616268796459,-55.9579395562865,38.989));
#180865=CARTESIAN_POINT('Origin',(5.49031038273072E-15,0.,38.989));
#180866=CARTESIAN_POINT('',(-25.2611094010724,-55.9581731633344,38.9890000005754));
#180867=CARTESIAN_POINT('Origin',(5.49031038273072E-15,0.,38.989));
#180868=CARTESIAN_POINT('',(-25.261109401195,-55.9581731636436,38.989));
#180869=CARTESIAN_POINT('Origin',(62.2224557307631,0.,38.989));
#180870=CARTESIAN_POINT('',(-30.6598643453577,-53.7394427993285,38.989));
#180871=CARTESIAN_POINT('',(15.8305769983926,26.7843636743469,38.989));
#180872=CARTESIAN_POINT('',(-25.4547063934086,-56.3916032444849,38.989));
#180873=CARTESIAN_POINT('Origin',(5.49031038273072E-15,0.,38.989));
#180874=CARTESIAN_POINT('',(-25.2618405854037,-55.9584195472774,38.989));
#180875=CARTESIAN_POINT('Origin',(5.57972911860581E-15,0.,39.624));
#180876=CARTESIAN_POINT('Origin',(-29.7268774036441,-52.1234719996033,39.6240070731883));
#180877=CARTESIAN_POINT('Origin',(-24.6957545189381,-54.6869571488949,39.6240070731883));
#180878=CARTESIAN_POINT('Origin',(5.57972911860581E-15,0.,39.624));
#180879=CARTESIAN_POINT('Origin',(-30.6789000092878,-53.7724806104346,39.5552135207999));
#180880=CARTESIAN_POINT('Origin',(-25.4702454952,-56.4264221855589,39.5552117598839));
#180881=CARTESIAN_POINT('Origin',(5.51210908043506E-15,0.,39.1438017080178));
#180882=CARTESIAN_POINT('Origin',(-30.2391374209327,-53.0106482050692,39.1711625381285));
#180883=CARTESIAN_POINT('Origin',(-25.1123582178529,-55.6227672661409,39.1712173702621));
#180884=CARTESIAN_POINT('Origin',(5.51210908043507E-15,0.,39.1438017080178));
#180885=CARTESIAN_POINT('Origin',(-30.1476490842061,-52.8523506794962,39.1712175859364));
#180886=CARTESIAN_POINT('Origin',(-25.0380683404975,-55.4557066902184,39.1711627526722));
#180887=CARTESIAN_POINT('Origin',(60.4792282238308,0.,38.989));
#180888=CARTESIAN_POINT('',(-18.8441205405522,-56.9687879773465,38.989));
#180889=CARTESIAN_POINT('',(-24.1156489724279,-54.9452378026827,38.989));
#180890=CARTESIAN_POINT('Origin',(5.49031038273072E-15,0.,38.989));
#180891=CARTESIAN_POINT('',(-24.3087286055922,-55.3789017591238,38.989));
#180892=CARTESIAN_POINT('',(10.2954134679533,22.3432738675267,38.989));
#180893=CARTESIAN_POINT('',(-24.3081989337718,-55.3791342586258,38.9889999995775));
#180894=CARTESIAN_POINT('Origin',(5.49031038273072E-15,0.,38.989));
#180895=CARTESIAN_POINT('',(-18.9913614316847,-57.420076955426,38.9889999997818));
#180896=CARTESIAN_POINT('Origin',(5.49031038273072E-15,0.,38.989));
#180897=CARTESIAN_POINT('',(-18.9908122363903,-57.4202585945859,38.989));
#180898=CARTESIAN_POINT('Origin',(5.49031038273072E-15,0.,38.989));
#180899=CARTESIAN_POINT('',(-18.8442866674264,-56.9692992632925,38.989));
#180900=CARTESIAN_POINT('Origin',(5.49031038273072E-15,0.,38.989));
#180901=CARTESIAN_POINT('',(-24.3743766270217,-55.5277679687682,39.2708017080178));
#180902=CARTESIAN_POINT('',(-24.3081989334776,-55.3791342579557,38.989));
#180903=CARTESIAN_POINT('',(-19.0416371861768,-57.5748148486259,39.2708017078546));
#180904=CARTESIAN_POINT('Origin',(5.52999282761009E-15,0.,39.2708017080178));
#180905=CARTESIAN_POINT('',(-19.041637186088,-57.5748148483575,39.2708017080178));
#180906=CARTESIAN_POINT('Origin',(60.71525,0.,39.3978017080178));
#180907=CARTESIAN_POINT('',(-19.1090650011318,-57.7842031819382,39.3978017080178));
#180908=CARTESIAN_POINT('',(-24.464376137792,-55.7284918401497,39.3978017080178));
#180909=CARTESIAN_POINT('Origin',(5.5478765747851E-15,0.,39.3978017080178));
#180910=CARTESIAN_POINT('',(-24.5258780191674,-55.8666273273832,39.3978017080178));
#180911=CARTESIAN_POINT('',(10.3344596589369,22.4309730483568,39.3978017080178));
#180912=CARTESIAN_POINT('',(-19.1557908785628,-57.9280106456675,39.3978017080178));
#180913=CARTESIAN_POINT('Origin',(5.5478765747851E-15,0.,39.3978017080178));
#180914=CARTESIAN_POINT('',(-19.1092287877198,-57.7847072652235,39.3978017080178));
#180915=CARTESIAN_POINT('Origin',(5.5478765747851E-15,0.,39.3978017080178));
#180916=CARTESIAN_POINT('',(-19.2232259141442,-58.1373965169892,39.2708017080178));
#180917=CARTESIAN_POINT('',(-24.6158705165696,-56.0673542006829,39.2708017081757));
#180918=CARTESIAN_POINT('Origin',(5.52999282761008E-15,0.,39.2708017080178));
#180919=CARTESIAN_POINT('',(-24.6820453786634,-56.215989076741,38.9890000005756));
#180920=CARTESIAN_POINT('',(-24.6158705164596,-56.0673542004325,39.2708017080178));
#180921=CARTESIAN_POINT('',(-24.6815255140429,-56.2162173246396,38.989));
#180922=CARTESIAN_POINT('Origin',(5.49031038273072E-15,0.,38.989));
#180923=CARTESIAN_POINT('',(-19.2740436149887,-58.2919551457916,38.989));
#180924=CARTESIAN_POINT('Origin',(5.49031038273072E-15,0.,38.989));
#180925=CARTESIAN_POINT('',(-19.2735045526312,-58.2921333818756,38.9890000005754));
#180926=CARTESIAN_POINT('Origin',(5.49031038273072E-15,0.,38.989));
#180927=CARTESIAN_POINT('',(-19.2735045527209,-58.2921333821958,38.989));
#180928=CARTESIAN_POINT('Origin',(62.2224557307631,0.,38.989));
#180929=CARTESIAN_POINT('',(-24.8746050278055,-56.6498810128381,38.989));
#180930=CARTESIAN_POINT('',(10.5838037820519,22.99100911823,38.989));
#180931=CARTESIAN_POINT('',(-19.4207352200703,-58.7434254837931,38.989));
#180932=CARTESIAN_POINT('Origin',(5.49031038273072E-15,0.,38.989));
#180933=CARTESIAN_POINT('',(-19.2742059773234,-58.292454845676,38.989));
#180934=CARTESIAN_POINT('Origin',(5.57972911860581E-15,0.,39.624));
#180935=CARTESIAN_POINT('Origin',(-24.1156440305593,-54.9452389789695,39.6240070731883));
#180936=CARTESIAN_POINT('Origin',(-18.844125000166,-56.9687855447423,39.6240070731883));
#180937=CARTESIAN_POINT('Origin',(5.57972911860581E-15,0.,39.624));
#180938=CARTESIAN_POINT('Origin',(-24.8900830207539,-56.6847276080563,39.5552135207985));
#180939=CARTESIAN_POINT('Origin',(-19.432549626632,-58.779677961498,39.5552117598806));
#180940=CARTESIAN_POINT('Origin',(5.51210908043506E-15,0.,39.1438017080178));
#180941=CARTESIAN_POINT('Origin',(-24.5323626684707,-55.8811008927581,39.171162538133));
#180942=CARTESIAN_POINT('Origin',(-19.1606277069624,-57.9430161406907,39.1712173702639));
#180943=CARTESIAN_POINT('Origin',(5.51210908043507E-15,0.,39.1438017080178));
#180944=CARTESIAN_POINT('Origin',(-24.4579221115101,-55.7141074023459,39.1712175859372));
#180945=CARTESIAN_POINT('Origin',(-19.1042073826023,-57.7691053333654,39.1711627526724));
#180946=CARTESIAN_POINT('Origin',(60.4792282238308,0.,38.989));
#180947=CARTESIAN_POINT('',(-12.7860306150453,-58.6264539577983,38.989));
#180948=CARTESIAN_POINT('',(-18.2401996527048,-57.1650137687746,38.989));
#180949=CARTESIAN_POINT('Origin',(5.49031038273072E-15,0.,38.989));
#180950=CARTESIAN_POINT('',(-18.386891348495,-57.6164843860302,38.989));
#180951=CARTESIAN_POINT('',(6.07721283595923,17.6762863142854,38.989));
#180952=CARTESIAN_POINT('',(-18.3863402754567,-57.6166602460949,38.988999999577));
#180953=CARTESIAN_POINT('Origin',(5.49031038273072E-15,0.,38.989));
#180954=CARTESIAN_POINT('',(-12.8852923618019,-59.090661591717,38.9889999997818));
#180955=CARTESIAN_POINT('Origin',(5.49031038273072E-15,0.,38.989));
#180956=CARTESIAN_POINT('',(-12.8847271885945,-59.0907848292984,38.989));
#180957=CARTESIAN_POINT('Origin',(5.49031038273072E-15,0.,38.989));
#180958=CARTESIAN_POINT('',(-12.786142387925,-58.6269798078532,38.989));
#180959=CARTESIAN_POINT('Origin',(5.49031038273072E-15,0.,38.989));
#180960=CARTESIAN_POINT('',(-18.4366189870675,-57.7713971777986,39.2708017080178));
#180961=CARTESIAN_POINT('',(-18.386340275234,-57.616660245397,38.989));
#180962=CARTESIAN_POINT('',(-12.919118186265,-59.2498070619041,39.2708017078546));
#180963=CARTESIAN_POINT('Origin',(5.52999282761009E-15,0.,39.2708017080178));
#180964=CARTESIAN_POINT('',(-12.9191181862048,-59.2498070616279,39.2708017080178));
#180965=CARTESIAN_POINT('Origin',(60.71525,0.,39.3978017080178));
#180966=CARTESIAN_POINT('',(-12.9642895838873,-59.4650964698966,39.3978017080178));
#180967=CARTESIAN_POINT('',(-18.5051441132844,-57.9804289733663,39.3978017080178));
#180968=CARTESIAN_POINT('Origin',(5.5478765747851E-15,0.,39.3978017080178));
#180969=CARTESIAN_POINT('',(-18.5518699907153,-58.1242364370956,39.3978017080178));
#180970=CARTESIAN_POINT('',(6.0997509100621,17.7456513739115,39.3978017080178));
#180971=CARTESIAN_POINT('',(-12.9957275188826,-59.6130003254554,39.3978017080178));
#180972=CARTESIAN_POINT('Origin',(5.5478765747851E-15,0.,39.3978017080178));
#180973=CARTESIAN_POINT('',(-12.964399782184,-59.4656149121213,39.3978017080178));
#180974=CARTESIAN_POINT('Origin',(5.5478765747851E-15,0.,39.3978017080178));
#180975=CARTESIAN_POINT('',(-13.0409063549241,-59.8282880397054,39.2708017080178));
#180976=CARTESIAN_POINT('',(-18.6203878281982,-58.33327048504,39.2708017081757));
#180977=CARTESIAN_POINT('Origin',(5.52999282761008E-15,0.,39.2708017080178));
#180978=CARTESIAN_POINT('',(-18.6706636022911,-58.4880082803368,38.9890000005756));
#180979=CARTESIAN_POINT('',(-18.620387828115,-58.3332704847795,39.2708017080178));
#180980=CARTESIAN_POINT('',(-18.6701227271413,-58.4881809372197,38.989));
#180981=CARTESIAN_POINT('Origin',(5.49031038273072E-15,0.,38.989));
#180982=CARTESIAN_POINT('',(-13.0752898951327,-59.9873118763435,38.989));
#180983=CARTESIAN_POINT('Origin',(5.49031038273072E-15,0.,38.989));
#180984=CARTESIAN_POINT('',(-13.0747351550713,-59.9874327886718,38.9890000005754));
#180985=CARTESIAN_POINT('Origin',(5.49031038273072E-15,0.,38.989));
#180986=CARTESIAN_POINT('',(-13.074735155127,-59.9874327889997,38.989));
#180987=CARTESIAN_POINT('Origin',(62.2224557307631,0.,38.989));
#180988=CARTESIAN_POINT('',(-18.8168143322229,-58.9396512752212,38.989));
#180989=CARTESIAN_POINT('',(6.24367625034032,18.1886080242681,38.989));
#180990=CARTESIAN_POINT('',(-13.1739864076109,-60.4516424606488,38.989));
#180991=CARTESIAN_POINT('Origin',(5.49031038273072E-15,0.,38.989));
#180992=CARTESIAN_POINT('',(-13.0753991351685,-59.987825810305,38.989));
#180993=CARTESIAN_POINT('Origin',(5.57972911860581E-15,0.,39.624));
#180994=CARTESIAN_POINT('Origin',(-18.2401946149528,-57.1650144220516,39.6240070731883));
#180995=CARTESIAN_POINT('Origin',(-12.7860353045052,-58.6264520046767,39.6240070731883));
#180996=CARTESIAN_POINT('Origin',(5.57972911860581E-15,0.,39.624));
#180997=CARTESIAN_POINT('Origin',(-18.8285650740579,-58.9759248679608,39.5552135208012));
#180998=CARTESIAN_POINT('Origin',(-13.1819466778331,-60.488931285249,39.5552117598823));
#180999=CARTESIAN_POINT('Origin',(5.51210908043506E-15,0.,39.1438017080178));
#181000=CARTESIAN_POINT('Origin',(-18.5568062168851,-58.139308545193,39.1711625381365));
#181001=CARTESIAN_POINT('Origin',(-12.9989693492948,-59.6284292050461,39.1712173702627));
#181002=CARTESIAN_POINT('Origin',(5.51210908043507E-15,0.,39.1438017080178));
#181003=CARTESIAN_POINT('Origin',(-18.5002290260138,-57.9654487055683,39.1712175859374));
#181004=CARTESIAN_POINT('Origin',(-12.961036730811,-59.4495735695164,39.1711627526749));
#181005=CARTESIAN_POINT('Origin',(60.4792282238308,0.,38.989));
#181006=CARTESIAN_POINT('',(-6.58785426247116,-59.6417962403142,38.989));
#181007=CARTESIAN_POINT('',(-12.1649068885794,-58.7584778814676,38.989));
#181008=CARTESIAN_POINT('Origin',(5.49031038273072E-15,0.,38.989));
#181009=CARTESIAN_POINT('',(-12.2636034620792,-59.2228087529788,38.989));
#181010=CARTESIAN_POINT('',(2.92491386234308,12.2335471699536,38.989));
#181011=CARTESIAN_POINT('',(-12.2630370254944,-59.2229260468456,38.9889999995772));
#181012=CARTESIAN_POINT('Origin',(5.49031038273072E-15,0.,38.989));
#181013=CARTESIAN_POINT('',(-6.63804933238239,-60.1138365740932,38.9889999997818));
#181014=CARTESIAN_POINT('Origin',(5.49031038273072E-15,0.,38.989));
#181015=CARTESIAN_POINT('',(-6.63747437341798,-60.1139000598793,38.989));
#181016=CARTESIAN_POINT('Origin',(5.49031038273072E-15,0.,38.989));
#181017=CARTESIAN_POINT('',(-6.58791045674911,-59.6423308931549,38.989));
#181018=CARTESIAN_POINT('Origin',(5.49031038273072E-15,0.,38.989));
#181019=CARTESIAN_POINT('',(-12.2968658913805,-59.382070869907,39.2708017080178));
#181020=CARTESIAN_POINT('',(-12.2630370253459,-59.2229260461285,38.989));
#181021=CARTESIAN_POINT('',(-6.65505462400518,-60.2756459901929,39.2708017078546));
#181022=CARTESIAN_POINT('Origin',(5.52999282761009E-15,0.,39.2708017080178));
#181023=CARTESIAN_POINT('',(-6.65505462397415,-60.2756459899119,39.2708017080178));
#181024=CARTESIAN_POINT('Origin',(60.71525,0.,39.3978017080178));
#181025=CARTESIAN_POINT('',(-6.67747469700966,-60.4944777170594,39.3978017080178));
#181026=CARTESIAN_POINT('',(-12.3431658574213,-59.5971203935659,39.3978017080178));
#181027=CARTESIAN_POINT('Origin',(5.5478765747851E-15,0.,39.3978017080178));
#181028=CARTESIAN_POINT('',(-12.3746037924166,-59.7450242491247,39.3978017080178));
#181029=CARTESIAN_POINT('',(2.93511643966565,12.2815465224196,39.3978017080178));
#181030=CARTESIAN_POINT('',(-6.69328024897475,-60.6448574988554,39.3978017080178));
#181031=CARTESIAN_POINT('Origin',(5.5478765747851E-15,0.,39.3978017080178));
#181032=CARTESIAN_POINT('',(-6.67753009965953,-60.4950048380619,39.3978017080178));
#181033=CARTESIAN_POINT('Origin',(5.5478765747851E-15,0.,39.3978017080178));
#181034=CARTESIAN_POINT('',(-6.7157078966943,-60.8636883187844,39.2708017080178));
#181035=CARTESIAN_POINT('',(-12.4208962742143,-59.9600752509414,39.2708017081757));
#181036=CARTESIAN_POINT('Origin',(5.52999282761008E-15,0.,39.2708017080178));
#181037=CARTESIAN_POINT('',(-12.4547221284046,-60.1192206258106,38.9890000005756));
#181038=CARTESIAN_POINT('',(-12.4208962741589,-59.9600752506736,39.2708017080178));
#181039=CARTESIAN_POINT('',(-12.4541661686668,-60.1193358000128,38.989));
#181040=CARTESIAN_POINT('Origin',(5.49031038273072E-15,0.,38.989));
#181041=CARTESIAN_POINT('',(-6.73328056300539,-61.0254350648262,38.989));
#181042=CARTESIAN_POINT('Origin',(5.49031038273072E-15,0.,38.989));
#181043=CARTESIAN_POINT('',(-6.73271622308818,-61.0254973286579,38.9890000005754));
#181044=CARTESIAN_POINT('Origin',(5.49031038273072E-15,0.,38.989));
#181045=CARTESIAN_POINT('',(-6.73271622310929,-61.0254973289898,38.989));
#181046=CARTESIAN_POINT('Origin',(62.2224557307631,0.,38.989));
#181047=CARTESIAN_POINT('',(-12.5528626811449,-60.5836663843181,38.989));
#181048=CARTESIAN_POINT('',(3.00026883051142,12.5880644220972,38.989));
#181049=CARTESIAN_POINT('',(-6.78290064323581,-61.4975385923862,38.989));
#181050=CARTESIAN_POINT('Origin',(5.49031038273072E-15,0.,38.989));
#181051=CARTESIAN_POINT('',(-6.73333548388561,-61.0259576020968,38.989));
#181052=CARTESIAN_POINT('Origin',(5.57972911860581E-15,0.,39.624));
#181053=CARTESIAN_POINT('Origin',(-12.1649018101387,-58.7584780045774,39.6240070731883));
#181054=CARTESIAN_POINT('Origin',(-6.58785913039844,-59.6417947880741,39.6240070731883));
#181055=CARTESIAN_POINT('Origin',(5.57972911860581E-15,0.,39.624));
#181056=CARTESIAN_POINT('Origin',(-12.560757428279,-60.6209695535074,39.5552135208015));
#181057=CARTESIAN_POINT('Origin',(-6.78691956273258,-61.5354552197177,39.5552117598811));
#181058=CARTESIAN_POINT('Origin',(5.51210908043506E-15,0.,39.1438017080178));
#181059=CARTESIAN_POINT('Origin',(-12.3779375131254,-59.7605297667732,39.1711625381368));
#181060=CARTESIAN_POINT('Origin',(-6.69489156322713,-60.6605407209803,39.1712173702631));
#181061=CARTESIAN_POINT('Origin',(5.51210908043507E-15,0.,39.1438017080178));
#181062=CARTESIAN_POINT('Origin',(-12.3398435598864,-59.581708422721,39.1712175859406));
#181063=CARTESIAN_POINT('Origin',(-6.67586224832375,-60.4786998370192,39.1711627526733));
#181064=CARTESIAN_POINT('Origin',(60.4792282238308,0.,38.989));
#181065=CARTESIAN_POINT('',(-0.317500000000204,-60.0036905223731,38.989));
#181066=CARTESIAN_POINT('',(-5.9563328589123,-59.7081718144892,38.989));
#181067=CARTESIAN_POINT('Origin',(5.49031038273072E-15,0.,38.989));
#181068=CARTESIAN_POINT('',(-6.00595296980892,-60.1802756340603,38.989));
#181069=CARTESIAN_POINT('',(0.9765688230087,6.25398151259764,38.989));
#181070=CARTESIAN_POINT('',(-6.00537737567531,-60.1803330766331,38.9889999995773));
#181071=CARTESIAN_POINT('Origin',(5.49031038273072E-15,0.,38.989));
#181072=CARTESIAN_POINT('',(-0.3180784453762,-60.4783917833346,38.9889999997818));
#181073=CARTESIAN_POINT('Origin',(5.49031038273072E-15,0.,38.989));
#181074=CARTESIAN_POINT('',(-0.31750000002549,-60.478394821762,38.989));
#181075=CARTESIAN_POINT('Origin',(5.49031038273072E-15,0.,38.989));
#181076=CARTESIAN_POINT('',(-0.317500000000204,-60.004228120231,38.989));
#181077=CARTESIAN_POINT('Origin',(5.49031038273072E-15,0.,38.989));
#181078=CARTESIAN_POINT('',(-6.02238575970296,-60.3421421670675,39.2708017080178));
#181079=CARTESIAN_POINT('',(-6.0053773756026,-60.1803330759045,38.989));
#181080=CARTESIAN_POINT('',(-0.318076890625054,-60.6410923275232,39.2708017078546));
#181081=CARTESIAN_POINT('Origin',(5.52999282761009E-15,0.,39.2708017080178));
#181082=CARTESIAN_POINT('',(-0.318076890623573,-60.6410923272405,39.2708017080178));
#181083=CARTESIAN_POINT('Origin',(60.71525,0.,39.3978017080178));
#181084=CARTESIAN_POINT('',(-0.317500000000207,-60.8610688070707,39.3978017080178));
#181085=CARTESIAN_POINT('',(-6.04595329345081,-60.5608532912343,39.3978017080178));
#181086=CARTESIAN_POINT('Origin',(5.5478765747851E-15,0.,39.3978017080178));
#181087=CARTESIAN_POINT('',(-6.0617588454159,-60.7112330730304,39.3978017080178));
#181088=CARTESIAN_POINT('',(0.97914764405288,6.27851735587422,39.3978017080178));
#181089=CARTESIAN_POINT('',(-0.317500000000208,-61.0122769227456,39.3978017080178));
#181090=CARTESIAN_POINT('Origin',(5.5478765747851E-15,0.,39.3978017080178));
#181091=CARTESIAN_POINT('',(-0.317500000000207,-60.8615988316031,39.3978017080178));
#181092=CARTESIAN_POINT('Origin',(5.5478765747851E-15,0.,39.3978017080178));
#181093=CARTESIAN_POINT('',(-0.316930737396123,-61.2322532920972,39.2708017080178));
#181094=CARTESIAN_POINT('',(-6.08531878141059,-60.9299448849411,39.2708017081757));
#181095=CARTESIAN_POINT('Origin',(5.52999282761008E-15,0.,39.2708017080178));
#181096=CARTESIAN_POINT('',(-6.10232411256107,-61.0917542093523,38.9890000005756));
#181097=CARTESIAN_POINT('',(-6.08531878138341,-60.929944884669,39.2708017080178));
#181098=CARTESIAN_POINT('',(-6.10175915944654,-61.0918106390012,38.989));
#181099=CARTESIAN_POINT('Origin',(5.49031038273072E-15,0.,38.989));
#181100=CARTESIAN_POINT('',(-0.317500000000209,-61.3949508163454,38.989));
#181101=CARTESIAN_POINT('Origin',(5.49031038273072E-15,0.,38.989));
#181102=CARTESIAN_POINT('',(-0.316932243253465,-61.394953749505,38.9890000005754));
#181103=CARTESIAN_POINT('Origin',(5.49031038273072E-15,0.,38.989));
#181104=CARTESIAN_POINT('',(-0.316932243239769,-61.3949537498373,38.989));
#181105=CARTESIAN_POINT('Origin',(62.2224557307631,0.,38.989));
#181106=CARTESIAN_POINT('',(-6.15137923967696,-61.5639141665612,38.989));
#181107=CARTESIAN_POINT('',(0.995615674755347,6.43520020182081,38.989));
#181108=CARTESIAN_POINT('',(-0.317500000000211,-61.8696548221181,38.989));
#181109=CARTESIAN_POINT('Origin',(5.49031038273072E-15,0.,38.989));
#181110=CARTESIAN_POINT('',(-0.317500000000209,-61.3954762318973,38.989));
#181111=CARTESIAN_POINT('Origin',(5.57972911860581E-15,0.,39.624));
#181112=CARTESIAN_POINT('Origin',(-5.95632779542335,-59.708171406083,39.6240070731883));
#181113=CARTESIAN_POINT('Origin',(-0.317504993060902,-60.0036895869254,
39.6240070731883));
#181114=CARTESIAN_POINT('Origin',(5.57972911860581E-15,0.,39.624));
#181115=CARTESIAN_POINT('Origin',(-6.15533149561007,-61.6018382108724,39.5552135208017));
#181116=CARTESIAN_POINT('Origin',(-0.317533536648827,-61.9077838296766,
39.5552117598813));
#181117=CARTESIAN_POINT('Origin',(5.51210908043506E-15,0.,39.1438017080178));
#181118=CARTESIAN_POINT('Origin',(-6.06345353572162,-60.7270021185312,39.1711625381328));
#181119=CARTESIAN_POINT('Origin',(-0.317463144196724,-61.0280426587412,
39.1712173702625));
#181120=CARTESIAN_POINT('Origin',(5.51210908043507E-15,0.,39.1438017080178));
#181121=CARTESIAN_POINT('Origin',(-6.04426018543789,-60.5451784741235,39.1712175859388));
#181122=CARTESIAN_POINT('Origin',(-0.317545622030958,-60.8452088131237,
39.171162752676));
#181123=CARTESIAN_POINT('Origin',(60.4792282238308,0.,38.989));
#181124=CARTESIAN_POINT('',(5.95633285891191,-59.7081718144893,38.989));
#181125=CARTESIAN_POINT('',(0.317499999999796,-60.0036905223731,38.989));
#181126=CARTESIAN_POINT('Origin',(5.49031038273072E-15,0.,38.989));
#181127=CARTESIAN_POINT('',(0.317500000025055,-60.4783948217626,38.989));
#181128=CARTESIAN_POINT('',(0.317500000000005,2.10053551406057E-13,38.989));
#181129=CARTESIAN_POINT('',(0.318078445377651,-60.4783917836887,38.9889999995774));
#181130=CARTESIAN_POINT('Origin',(5.49031038273072E-15,0.,38.989));
#181131=CARTESIAN_POINT('',(6.00537737563974,-60.1803330762807,38.9889999997818));
#181132=CARTESIAN_POINT('Origin',(5.49031038273072E-15,0.,38.989));
#181133=CARTESIAN_POINT('',(6.00595296980844,-60.1802756340597,38.989));
#181134=CARTESIAN_POINT('Origin',(5.49031038273072E-15,0.,38.989));
#181135=CARTESIAN_POINT('',(5.95638905318986,-59.7087064673299,38.989));
#181136=CARTESIAN_POINT('Origin',(5.49031038273072E-15,0.,38.989));
#181137=CARTESIAN_POINT('',(0.31807689062316,-60.6410923272405,39.2708017080178));
#181138=CARTESIAN_POINT('',(0.318078445373799,-60.4783917829566,38.989));
#181139=CARTESIAN_POINT('',(6.02238575973065,-60.3421421673489,39.2708017078546));
#181140=CARTESIAN_POINT('Origin',(5.52999282761009E-15,0.,39.2708017080178));
#181141=CARTESIAN_POINT('',(6.02238575970257,-60.3421421670675,39.2708017080178));
#181142=CARTESIAN_POINT('Origin',(60.71525,0.,39.3978017080178));
#181143=CARTESIAN_POINT('',(6.04595329345041,-60.5608532912344,39.3978017080178));
#181144=CARTESIAN_POINT('',(0.317499999999793,-60.8610688070707,39.3978017080178));
#181145=CARTESIAN_POINT('Origin',(5.5478765747851E-15,0.,39.3978017080178));
#181146=CARTESIAN_POINT('',(0.317499999999792,-61.0122769227456,39.3978017080178));
#181147=CARTESIAN_POINT('',(0.317500000000005,2.10877617033113E-13,39.3978017080178));
#181148=CARTESIAN_POINT('',(6.0617588454155,-60.7112330730304,39.3978017080178));
#181149=CARTESIAN_POINT('Origin',(5.5478765747851E-15,0.,39.3978017080178));
#181150=CARTESIAN_POINT('',(6.04600869610028,-60.5613804122369,39.3978017080178));
#181151=CARTESIAN_POINT('Origin',(5.5478765747851E-15,0.,39.3978017080178));
#181152=CARTESIAN_POINT('',(6.08531878138301,-60.929944884669,39.2708017080178));
#181153=CARTESIAN_POINT('',(0.316930737397122,-61.2322532923707,39.2708017081757));
#181154=CARTESIAN_POINT('Origin',(5.52999282761008E-15,0.,39.2708017080178));
#181155=CARTESIAN_POINT('',(0.316932243253051,-61.3949537495049,38.9890000005756));
#181156=CARTESIAN_POINT('',(0.316930737395706,-61.2322532920972,39.2708017080178));
#181157=CARTESIAN_POINT('',(0.317499999999791,-61.3949508163454,38.989));
#181158=CARTESIAN_POINT('Origin',(5.49031038273072E-15,0.,38.989));
#181159=CARTESIAN_POINT('',(6.10175915944613,-61.0918106390012,38.989));
#181160=CARTESIAN_POINT('Origin',(5.49031038273072E-15,0.,38.989));
#181161=CARTESIAN_POINT('',(6.10232411256069,-61.0917542093524,38.9890000005754));
#181162=CARTESIAN_POINT('Origin',(5.49031038273072E-15,0.,38.989));
#181163=CARTESIAN_POINT('',(6.10232411260904,-61.0917542096815,38.989));
#181164=CARTESIAN_POINT('Origin',(62.2224557307631,0.,38.989));
#181165=CARTESIAN_POINT('',(0.31749999999979,-61.8696548221181,38.989));
#181166=CARTESIAN_POINT('',(0.317500000000005,2.1613999771587E-13,38.989));
#181167=CARTESIAN_POINT('',(6.15137923967656,-61.5639141665612,38.989));
#181168=CARTESIAN_POINT('Origin',(5.49031038273072E-15,0.,38.989));
#181169=CARTESIAN_POINT('',(6.10181408032636,-61.0923331762718,38.989));
#181170=CARTESIAN_POINT('Origin',(5.57972911860581E-15,0.,39.624));
#181171=CARTESIAN_POINT('Origin',(0.317504993060349,-60.0036895869254,39.6240070731883));
#181172=CARTESIAN_POINT('Origin',(5.95632779542281,-59.708171406083,39.6240070731883));
#181173=CARTESIAN_POINT('Origin',(5.57972911860581E-15,0.,39.624));
#181174=CARTESIAN_POINT('Origin',(0.31753353701135,-61.9077842377855,39.5552135208018));
#181175=CARTESIAN_POINT('Origin',(6.15533145331131,-61.6018378049618,39.5552117598803));
#181176=CARTESIAN_POINT('Origin',(5.51210908043506E-15,0.,39.1438017080178));
#181177=CARTESIAN_POINT('Origin',(0.317462907478285,-61.0281367271401,39.1711625381349));
#181178=CARTESIAN_POINT('Origin',(6.06344346747477,-60.7269085901925,39.1712173702593));
#181179=CARTESIAN_POINT('Origin',(5.51210908043507E-15,0.,39.1438017080178));
#181180=CARTESIAN_POINT('Origin',(0.317545368445239,-60.8453028802699,39.1712175859377));
#181181=CARTESIAN_POINT('Origin',(6.04425010054675,-60.5450849487952,39.1711627526747));
#181182=CARTESIAN_POINT('Origin',(60.4792282238308,0.,38.989));
#181183=CARTESIAN_POINT('',(12.164906888579,-58.7584778814677,38.989));
#181184=CARTESIAN_POINT('',(6.58785426247077,-59.6417962403143,38.989));
#181185=CARTESIAN_POINT('Origin',(5.49031038273072E-15,0.,38.989));
#181186=CARTESIAN_POINT('',(6.63747437341763,-60.1139000598801,38.989));
#181187=CARTESIAN_POINT('',(0.976568823008617,-6.25398151259724,38.989));
#181188=CARTESIAN_POINT('',(6.63804933242089,-60.1138365744455,38.9889999995772));
#181189=CARTESIAN_POINT('Origin',(5.49031038273072E-15,0.,38.989));
#181190=CARTESIAN_POINT('',(12.2630370254221,-59.2229260464987,38.9889999997818));
#181191=CARTESIAN_POINT('Origin',(5.49031038273072E-15,0.,38.989));
#181192=CARTESIAN_POINT('',(12.2636034620787,-59.2228087529783,38.989));
#181193=CARTESIAN_POINT('Origin',(5.49031038273072E-15,0.,38.989));
#181194=CARTESIAN_POINT('',(12.1650186614586,-58.7590037315226,38.989));
#181195=CARTESIAN_POINT('Origin',(5.49031038273072E-15,0.,38.989));
#181196=CARTESIAN_POINT('',(6.65505462397376,-60.2756459899119,39.2708017080178));
#181197=CARTESIAN_POINT('',(6.6380493323405,-60.1138365737175,38.989));
#181198=CARTESIAN_POINT('',(12.2968658914375,-59.382070870184,39.2708017078546));
#181199=CARTESIAN_POINT('Origin',(5.52999282761009E-15,0.,39.2708017080178));
#181200=CARTESIAN_POINT('',(12.2968658913801,-59.3820708699071,39.2708017080178));
#181201=CARTESIAN_POINT('Origin',(60.71525,0.,39.3978017080178));
#181202=CARTESIAN_POINT('',(12.3431658574209,-59.5971203935659,39.3978017080178));
#181203=CARTESIAN_POINT('',(6.67747469700926,-60.4944777170594,39.3978017080178));
#181204=CARTESIAN_POINT('Origin',(5.5478765747851E-15,0.,39.3978017080178));
#181205=CARTESIAN_POINT('',(6.69328024897435,-60.6448574988554,39.3978017080178));
#181206=CARTESIAN_POINT('',(0.979147644052797,-6.27851735587382,39.3978017080178));
#181207=CARTESIAN_POINT('',(12.3746037924162,-59.7450242491248,39.3978017080178));
#181208=CARTESIAN_POINT('Origin',(5.5478765747851E-15,0.,39.3978017080178));
#181209=CARTESIAN_POINT('',(12.3432760557176,-59.5976388357907,39.3978017080178));
#181210=CARTESIAN_POINT('Origin',(5.5478765747851E-15,0.,39.3978017080178));
#181211=CARTESIAN_POINT('',(12.4208962741585,-59.9600752506737,39.2708017080178));
#181212=CARTESIAN_POINT('',(6.7157078967239,-60.8636883190563,39.2708017081757));
#181213=CARTESIAN_POINT('Origin',(5.52999282761008E-15,0.,39.2708017080178));
#181214=CARTESIAN_POINT('',(6.73271622308777,-61.0254973286579,38.9890000005756));
#181215=CARTESIAN_POINT('',(6.7157078966939,-60.8636883187845,39.2708017080178));
#181216=CARTESIAN_POINT('',(6.73328056300499,-61.0254350648262,38.989));
#181217=CARTESIAN_POINT('Origin',(5.49031038273072E-15,0.,38.989));
#181218=CARTESIAN_POINT('',(12.4541661686664,-60.1193358000129,38.989));
#181219=CARTESIAN_POINT('Origin',(5.49031038273072E-15,0.,38.989));
#181220=CARTESIAN_POINT('',(12.4547221284042,-60.1192206258107,38.9890000005754));
#181221=CARTESIAN_POINT('Origin',(5.49031038273072E-15,0.,38.989));
#181222=CARTESIAN_POINT('',(12.4547221284867,-60.1192206261329,38.989));
#181223=CARTESIAN_POINT('Origin',(62.2224557307631,0.,38.989));
#181224=CARTESIAN_POINT('',(6.78290064323541,-61.4975385923862,38.989));
#181225=CARTESIAN_POINT('',(0.995615674755264,-6.4352002018204,38.989));
#181226=CARTESIAN_POINT('',(12.5528626811445,-60.5836663843182,38.989));
#181227=CARTESIAN_POINT('Origin',(5.49031038273072E-15,0.,38.989));
#181228=CARTESIAN_POINT('',(12.4542754087022,-60.1198497339744,38.989));
#181229=CARTESIAN_POINT('Origin',(5.57972911860581E-15,0.,39.624));
#181230=CARTESIAN_POINT('Origin',(6.5878591303979,-59.6417947880742,39.6240070731883));
#181231=CARTESIAN_POINT('Origin',(12.1649018101382,-58.7584780045775,39.6240070731883));
#181232=CARTESIAN_POINT('Origin',(5.57972911860581E-15,0.,39.624));
#181233=CARTESIAN_POINT('Origin',(6.78691960575346,-61.5354556255537,39.5552135208006));
#181234=CARTESIAN_POINT('Origin',(12.5607573437828,-60.6209691542412,39.5552117598815));
#181235=CARTESIAN_POINT('Origin',(5.51210908043506E-15,0.,39.1438017080178));
#181236=CARTESIAN_POINT('Origin',(6.69490116063052,-60.6606342988051,39.1711625381332));
#181237=CARTESIAN_POINT('Origin',(12.3779177236596,-59.7604378032094,39.1712173702605));
#181238=CARTESIAN_POINT('Origin',(5.51210908043507E-15,0.,39.1438017080178));
#181239=CARTESIAN_POINT('Origin',(6.67587182882202,-60.4787934153613,39.1712175859376));
#181240=CARTESIAN_POINT('Origin',(12.3398237541815,-59.5816164638928,39.171162752676));
#181241=CARTESIAN_POINT('Origin',(60.4792282238308,0.,38.989));
#181242=CARTESIAN_POINT('',(18.2401996527044,-57.1650137687747,38.989));
#181243=CARTESIAN_POINT('',(12.786030615045,-58.6264539577984,38.989));
#181244=CARTESIAN_POINT('Origin',(5.49031038273072E-15,0.,38.989));
#181245=CARTESIAN_POINT('',(12.8847271885942,-59.0907848292991,38.989));
#181246=CARTESIAN_POINT('',(2.92491386234291,-12.2335471699533,38.989));
#181247=CARTESIAN_POINT('',(12.885292361877,-59.0906615920632,38.9889999995772));
#181248=CARTESIAN_POINT('Origin',(5.49031038273072E-15,0.,38.989));
#181249=CARTESIAN_POINT('',(18.3863402753486,-57.6166602457573,38.9889999997818));
#181250=CARTESIAN_POINT('Origin',(5.49031038273072E-15,0.,38.989));
#181251=CARTESIAN_POINT('',(18.3868913484944,-57.6164843860297,38.989));
#181252=CARTESIAN_POINT('Origin',(5.49031038273072E-15,0.,38.989));
#181253=CARTESIAN_POINT('',(18.2403657795786,-57.1655250547207,38.989));
#181254=CARTESIAN_POINT('Origin',(5.49031038273072E-15,0.,38.989));
#181255=CARTESIAN_POINT('',(12.9191181862044,-59.249807061628,39.2708017080178));
#181256=CARTESIAN_POINT('',(12.8852923617209,-59.0906615913478,38.989));
#181257=CARTESIAN_POINT('',(18.4366189871531,-57.7713971780681,39.2708017078546));
#181258=CARTESIAN_POINT('Origin',(5.52999282761009E-15,0.,39.2708017080178));
#181259=CARTESIAN_POINT('',(18.4366189870671,-57.7713971777987,39.2708017080178));
#181260=CARTESIAN_POINT('Origin',(60.71525,0.,39.3978017080178));
#181261=CARTESIAN_POINT('',(18.505144113284,-57.9804289733664,39.3978017080178));
#181262=CARTESIAN_POINT('',(12.9642895838869,-59.4650964698967,39.3978017080178));
#181263=CARTESIAN_POINT('Origin',(5.5478765747851E-15,0.,39.3978017080178));
#181264=CARTESIAN_POINT('',(12.9957275188822,-59.6130003254555,39.3978017080178));
#181265=CARTESIAN_POINT('',(2.93511643966547,-12.2815465224192,39.3978017080178));
#181266=CARTESIAN_POINT('',(18.5518699907149,-58.1242364370957,39.3978017080178));
#181267=CARTESIAN_POINT('Origin',(5.5478765747851E-15,0.,39.3978017080178));
#181268=CARTESIAN_POINT('',(18.505307899872,-57.9809330566518,39.3978017080178));
#181269=CARTESIAN_POINT('Origin',(5.5478765747851E-15,0.,39.3978017080178));
#181270=CARTESIAN_POINT('',(18.6203878281146,-58.3332704847796,39.2708017080178));
#181271=CARTESIAN_POINT('',(13.0409063549819,-59.8282880399727,39.2708017081757));
#181272=CARTESIAN_POINT('Origin',(5.52999282761008E-15,0.,39.2708017080178));
#181273=CARTESIAN_POINT('',(13.0747351550709,-59.9874327886718,38.9890000005756));
#181274=CARTESIAN_POINT('',(13.0409063549237,-59.8282880397055,39.2708017080178));
#181275=CARTESIAN_POINT('',(13.0752898951324,-59.9873118763436,38.989));
#181276=CARTESIAN_POINT('Origin',(5.49031038273072E-15,0.,38.989));
#181277=CARTESIAN_POINT('',(18.6701227271409,-58.4881809372198,38.989));
#181278=CARTESIAN_POINT('Origin',(5.49031038273072E-15,0.,38.989));
#181279=CARTESIAN_POINT('',(18.6706636022907,-58.488008280337,38.9890000005754));
#181280=CARTESIAN_POINT('Origin',(5.49031038273072E-15,0.,38.989));
#181281=CARTESIAN_POINT('',(18.6706636024065,-58.4880082806488,38.989));
#181282=CARTESIAN_POINT('Origin',(62.2224557307631,0.,38.989));
#181283=CARTESIAN_POINT('',(13.1739864076105,-60.4516424606489,38.989));
#181284=CARTESIAN_POINT('',(3.00026883051124,-12.5880644220968,38.989));
#181285=CARTESIAN_POINT('',(18.8168143322225,-58.9396512752214,38.989));
#181286=CARTESIAN_POINT('Origin',(5.49031038273072E-15,0.,38.989));
#181287=CARTESIAN_POINT('',(18.6702850894756,-58.4886806371042,38.989));
#181288=CARTESIAN_POINT('Origin',(5.57972911860581E-15,0.,39.624));
#181289=CARTESIAN_POINT('Origin',(12.7860353045047,-58.6264520046768,39.6240070731883));
#181290=CARTESIAN_POINT('Origin',(18.2401946149522,-57.1650144220518,39.6240070731883));
#181291=CARTESIAN_POINT('Origin',(5.57972911860581E-15,0.,39.624));
#181292=CARTESIAN_POINT('Origin',(13.18194676304,-60.4889316843658,39.5552135207995));
#181293=CARTESIAN_POINT('Origin',(18.8285649482889,-58.9759244797131,39.5552117598831));
#181294=CARTESIAN_POINT('Origin',(5.51210908043506E-15,0.,39.1438017080178));
#181295=CARTESIAN_POINT('Origin',(12.9989886756685,-59.6285212670386,39.1711625381305));
#181296=CARTESIAN_POINT('Origin',(18.5567769230188,-58.1392191539798,39.1712173702638));
#181297=CARTESIAN_POINT('Origin',(5.51210908043507E-15,0.,39.1438017080178));
#181298=CARTESIAN_POINT('Origin',(12.9610560404262,-59.4496656337931,39.171217585937));
#181299=CARTESIAN_POINT('Origin',(18.5001997164958,-57.9653593207584,39.1711627526739));
#181300=CARTESIAN_POINT('Origin',(60.4792282238308,0.,38.989));
#181301=CARTESIAN_POINT('',(24.1156489724276,-54.9452378026829,38.989));
#181302=CARTESIAN_POINT('',(18.8441205405518,-56.9687879773467,38.989));
#181303=CARTESIAN_POINT('Origin',(5.49031038273072E-15,0.,38.989));
#181304=CARTESIAN_POINT('',(18.9908122363901,-57.4202585945866,38.989));
#181305=CARTESIAN_POINT('',(6.07721283595898,-17.676286314285,38.989));
#181306=CARTESIAN_POINT('',(18.9913614317957,-57.4200769557629,38.988999999577));
#181307=CARTESIAN_POINT('Origin',(5.49031038273072E-15,0.,38.989));
#181308=CARTESIAN_POINT('',(24.3081989336292,-55.379134258302,38.9889999997818));
#181309=CARTESIAN_POINT('Origin',(5.49031038273072E-15,0.,38.989));
#181310=CARTESIAN_POINT('',(24.3087286055916,-55.3789017591234,38.989));
#181311=CARTESIAN_POINT('Origin',(5.49031038273072E-15,0.,38.989));
#181312=CARTESIAN_POINT('',(24.1158676331756,-54.9457289227641,38.989));
#181313=CARTESIAN_POINT('Origin',(5.49031038273072E-15,0.,38.989));
#181314=CARTESIAN_POINT('',(19.0416371860877,-57.5748148483576,39.2708017080178));
#181315=CARTESIAN_POINT('',(18.9913614315656,-57.4200769550673,38.989));
#181316=CARTESIAN_POINT('',(24.3743766271349,-55.5277679690272,39.2708017078546));
#181317=CARTESIAN_POINT('Origin',(5.52999282761009E-15,0.,39.2708017080178));
#181318=CARTESIAN_POINT('',(24.3743766270213,-55.5277679687684,39.2708017080178));
#181319=CARTESIAN_POINT('Origin',(60.71525,0.,39.3978017080178));
#181320=CARTESIAN_POINT('',(24.4643761377916,-55.7284918401499,39.3978017080178));
#181321=CARTESIAN_POINT('',(19.1090650011314,-57.7842031819383,39.3978017080178));
#181322=CARTESIAN_POINT('Origin',(5.5478765747851E-15,0.,39.3978017080178));
#181323=CARTESIAN_POINT('',(19.1557908785624,-57.9280106456676,39.3978017080178));
#181324=CARTESIAN_POINT('',(6.09975091006187,-17.7456513739111,39.3978017080178));
#181325=CARTESIAN_POINT('',(24.525878019167,-55.8666273273833,39.3978017080178));
#181326=CARTESIAN_POINT('Origin',(5.5478765747851E-15,0.,39.3978017080178));
#181327=CARTESIAN_POINT('',(24.4645917181906,-55.7289760416539,39.3978017080178));
#181328=CARTESIAN_POINT('Origin',(5.5478765747851E-15,0.,39.3978017080178));
#181329=CARTESIAN_POINT('',(24.6158705164593,-56.0673542004326,39.2708017080178));
#181330=CARTESIAN_POINT('',(19.2232259142297,-58.137396517249,39.2708017081757));
#181331=CARTESIAN_POINT('Origin',(5.52999282761008E-15,0.,39.2708017080178));
#181332=CARTESIAN_POINT('',(19.2735045526308,-58.2921333818756,38.9890000005756));
#181333=CARTESIAN_POINT('',(19.2232259141438,-58.1373965169894,39.2708017080178));
#181334=CARTESIAN_POINT('',(19.2740436149883,-58.2919551457917,38.989));
#181335=CARTESIAN_POINT('Origin',(5.49031038273072E-15,0.,38.989));
#181336=CARTESIAN_POINT('',(24.6815255140425,-56.2162173246398,38.989));
#181337=CARTESIAN_POINT('Origin',(5.49031038273072E-15,0.,38.989));
#181338=CARTESIAN_POINT('',(24.6820453786631,-56.2159890767412,38.9890000005754));
#181339=CARTESIAN_POINT('Origin',(5.49031038273072E-15,0.,38.989));
#181340=CARTESIAN_POINT('',(24.6820453788107,-56.2159890770392,38.989));
#181341=CARTESIAN_POINT('Origin',(62.2224557307631,0.,38.989));
#181342=CARTESIAN_POINT('',(19.42073522007,-58.7434254837933,38.989));
#181343=CARTESIAN_POINT('',(6.24367625034007,-18.1886080242677,38.989));
#181344=CARTESIAN_POINT('',(24.8746050278051,-56.6498810128382,38.989));
#181345=CARTESIAN_POINT('Origin',(5.49031038273072E-15,0.,38.989));
#181346=CARTESIAN_POINT('',(24.6817392198003,-56.2166973156307,38.989));
#181347=CARTESIAN_POINT('Origin',(5.57972911860581E-15,0.,39.624));
#181348=CARTESIAN_POINT('Origin',(18.8441250001654,-56.9687855447425,39.6240070731883));
#181349=CARTESIAN_POINT('Origin',(24.1156440305588,-54.9452389789697,39.6240070731883));
#181350=CARTESIAN_POINT('Origin',(5.57972911860581E-15,0.,39.624));
#181351=CARTESIAN_POINT('Origin',(19.4325497530937,-58.7796783495198,39.5552135207998));
#181352=CARTESIAN_POINT('Origin',(24.890082855091,-56.6847272350816,39.5552117598808));
#181353=CARTESIAN_POINT('Origin',(5.51210908043506E-15,0.,39.1438017080178));
#181354=CARTESIAN_POINT('Origin',(19.1606565505633,-57.9431056782032,39.1711625381345));
#181355=CARTESIAN_POINT('Origin',(24.5323241911535,-55.8810150532832,39.1712173702631));
#181356=CARTESIAN_POINT('Origin',(5.51210908043507E-15,0.,39.1438017080178));
#181357=CARTESIAN_POINT('Origin',(19.1042362097731,-57.7691948748978,39.1712175859387));
#181358=CARTESIAN_POINT('Origin',(24.457883619298,-55.7140215708725,39.1711627526749));
#181359=CARTESIAN_POINT('Origin',(60.4792282238308,0.,38.989));
#181360=CARTESIAN_POINT('',(29.7268821954849,-52.1234703131947,38.989));
#181361=CARTESIAN_POINT('',(24.6957503380306,-54.6869600343298,38.989));
#181362=CARTESIAN_POINT('Origin',(5.49031038273072E-15,0.,38.989));
#181363=CARTESIAN_POINT('',(24.8888299712411,-55.1206239907503,38.989));
#181364=CARTESIAN_POINT('',(10.295413467953,-22.3432738675264,38.989));
#181365=CARTESIAN_POINT('',(24.8893571716697,-55.1203859404113,38.988999999577));
#181366=CARTESIAN_POINT('Origin',(5.49031038273072E-15,0.,38.989));
#181367=CARTESIAN_POINT('',(29.9637318775753,-52.5348628870839,38.9889999997818));
#181368=CARTESIAN_POINT('Origin',(5.49031038273072E-15,0.,38.989));
#181369=CARTESIAN_POINT('',(29.9642343451574,-52.5345762957638,38.989));
#181370=CARTESIAN_POINT('Origin',(5.49031038273072E-15,0.,38.989));
#181371=CARTESIAN_POINT('',(29.7271509944138,-52.1239358865967,38.989));
#181372=CARTESIAN_POINT('Origin',(5.49031038273072E-15,0.,38.989));
#181373=CARTESIAN_POINT('',(24.9555320242414,-55.2690209153041,39.2708017080178));
#181374=CARTESIAN_POINT('',(24.8893571713682,-55.1203859397435,38.989));
#181375=CARTESIAN_POINT('',(30.0450834961236,-52.6757649141852,39.2708017078546));
#181376=CARTESIAN_POINT('Origin',(5.52999282761009E-15,0.,39.2708017080178));
#181377=CARTESIAN_POINT('',(30.0450834959836,-52.6757649139397,39.2708017080178));
#181378=CARTESIAN_POINT('Origin',(60.71525,0.,39.3978017080178));
#181379=CARTESIAN_POINT('',(30.1555713378337,-52.865981688396,39.3978017080178));
#181380=CARTESIAN_POINT('',(25.0444775033946,-55.4702140717967,39.3978017080178));
#181381=CARTESIAN_POINT('Origin',(5.5478765747851E-15,0.,39.3978017080178));
#181382=CARTESIAN_POINT('',(25.1059793847701,-55.6083495590302,39.3978017080178));
#181383=CARTESIAN_POINT('',(10.3344596589366,-22.4309730483565,39.3978017080178));
#181384=CARTESIAN_POINT('',(30.2311753956711,-52.9969317578288,39.3978017080178));
#181385=CARTESIAN_POINT('Origin',(5.5478765747851E-15,0.,39.3978017080178));
#181386=CARTESIAN_POINT('',(30.1558363500999,-52.8664407031057,39.3978017080178));
#181387=CARTESIAN_POINT('Origin',(5.5478765747851E-15,0.,39.3978017080178));
#181388=CARTESIAN_POINT('',(30.3416565762235,-53.1871522506176,39.2708017080178));
#181389=CARTESIAN_POINT('',(25.1949317876425,-55.80953951225,39.2708017081757));
#181390=CARTESIAN_POINT('Origin',(5.52999282761008E-15,0.,39.2708017080178));
#181391=CARTESIAN_POINT('',(25.261109401072,-55.9581731633345,38.9890000005756));
#181392=CARTESIAN_POINT('',(25.19493178753,-55.8095395120007,39.2708017080178));
#181393=CARTESIAN_POINT('',(25.2616268796456,-55.9579395562867,38.989));
#181394=CARTESIAN_POINT('Origin',(5.49031038273072E-15,0.,38.989));
#181395=CARTESIAN_POINT('',(30.422512342471,-53.3283370710513,38.989));
#181396=CARTESIAN_POINT('Origin',(5.49031038273072E-15,0.,38.989));
#181397=CARTESIAN_POINT('',(30.4230055008167,-53.3280557328687,38.9890000005754));
#181398=CARTESIAN_POINT('Origin',(5.49031038273072E-15,0.,38.989));
#181399=CARTESIAN_POINT('',(30.4230055009947,-53.3280557331496,38.989));
#181400=CARTESIAN_POINT('Origin',(62.2224557307631,0.,38.989));
#181401=CARTESIAN_POINT('',(25.4547063934082,-56.3916032444851,38.989));
#181402=CARTESIAN_POINT('',(10.5838037820516,-22.9910091182297,38.989));
#181403=CARTESIAN_POINT('',(30.6598643453574,-53.7394427993287,38.989));
#181404=CARTESIAN_POINT('Origin',(5.49031038273072E-15,0.,38.989));
#181405=CARTESIAN_POINT('',(30.422775050247,-53.3287920942668,38.989));
#181406=CARTESIAN_POINT('Origin',(5.57972911860581E-15,0.,39.624));
#181407=CARTESIAN_POINT('Origin',(24.6957545189376,-54.6869571488951,39.6240070731884));
#181408=CARTESIAN_POINT('Origin',(29.7268774036436,-52.1234719996036,39.6240070731883));
#181409=CARTESIAN_POINT('Origin',(5.57972911860581E-15,0.,39.624));
#181410=CARTESIAN_POINT('Origin',(25.470245661519,-56.4264225582401,39.5552135208038));
#181411=CARTESIAN_POINT('Origin',(30.6788998055465,-53.7724802568205,39.5552117598807));
#181412=CARTESIAN_POINT('Origin',(5.51210908043506E-15,0.,39.1438017080178));
#181413=CARTESIAN_POINT('Origin',(25.1123962626642,-55.6228532981804,39.1711625381332));
#181414=CARTESIAN_POINT('Origin',(30.2390901817301,-53.0105668578071,39.1712173702593));
#181415=CARTESIAN_POINT('Origin',(5.51210908043507E-15,0.,39.1438017080178));
#181416=CARTESIAN_POINT('Origin',(25.0381063693916,-55.4557927279735,39.1712175859357));
#181417=CARTESIAN_POINT('Origin',(30.1476018310217,-52.8522693417523,39.1711627526723));
#181418=CARTESIAN_POINT('Origin',(60.4792282238308,0.,38.989));
#181419=CARTESIAN_POINT('',(35.0124214764584,-48.7306271754177,38.989));
#181420=CARTESIAN_POINT('',(30.276808326888,-51.8059703131947,38.989));
#181421=CARTESIAN_POINT('Origin',(5.49031038273072E-15,0.,38.989));
#181422=CARTESIAN_POINT('',(30.5141604766046,-52.2170762957391,38.989));
#181423=CARTESIAN_POINT('',(15.3947701216591,-26.0295240215571,38.989));
#181424=CARTESIAN_POINT('',(30.5146599059377,-52.2167844420135,38.9889999995774));
#181425=CARTESIAN_POINT('Origin',(5.49031038273072E-15,0.,38.989));
#181426=CARTESIAN_POINT('',(35.2909759047567,-49.1150085644481,38.9889999997818));
#181427=CARTESIAN_POINT('Origin',(5.49031038273072E-15,0.,38.989));
#181428=CARTESIAN_POINT('',(35.2914456628186,-49.1146710209411,38.989));
#181429=CARTESIAN_POINT('Origin',(5.49031038273072E-15,0.,38.989));
#181430=CARTESIAN_POINT('',(35.012737468551,-48.7310621012209,38.989));
#181431=CARTESIAN_POINT('Origin',(5.49031038273072E-15,0.,38.989));
#181432=CARTESIAN_POINT('',(30.5960088312567,-52.3576880233163,39.2708017080178));
#181433=CARTESIAN_POINT('',(30.5146599055683,-52.2167844413816,38.989));
#181434=CARTESIAN_POINT('',(35.3866101429909,-49.246635155831,39.2708017078546));
#181435=CARTESIAN_POINT('Origin',(5.52999282761009E-15,0.,39.2708017080178));
#181436=CARTESIAN_POINT('',(35.3866101428259,-49.2466351556014,39.2708017080178));
#181437=CARTESIAN_POINT('Origin',(60.71525,0.,39.3978017080178));
#181438=CARTESIAN_POINT('',(35.5163757878395,-49.4242607783461,39.3978017080178));
#181439=CARTESIAN_POINT('',(30.7054974692368,-52.548481688396,39.3978017080178));
#181440=CARTESIAN_POINT('Origin',(5.5478765747851E-15,0.,39.3978017080178));
#181441=CARTESIAN_POINT('',(30.7811015270742,-52.6794317578288,39.3978017080178));
#181442=CARTESIAN_POINT('',(15.4537755657014,-26.1317244485615,39.3978017080178));
#181443=CARTESIAN_POINT('',(35.6052536882601,-49.5465907136145,39.3978017080178));
#181444=CARTESIAN_POINT('Origin',(5.5478765747851E-15,0.,39.3978017080178));
#181445=CARTESIAN_POINT('',(35.516687328443,-49.4246895772003,39.3978017080178));
#181446=CARTESIAN_POINT('Origin',(5.5478765747851E-15,0.,39.3978017080178));
#181447=CARTESIAN_POINT('',(35.7350130971388,-49.7242207306176,39.2708017080178));
#181448=CARTESIAN_POINT('',(30.8905967160115,-52.8702215134578,39.2708017081757));
#181449=CARTESIAN_POINT('Origin',(5.52999282761008E-15,0.,39.2708017080178));
#181450=CARTESIAN_POINT('',(30.971948248688,-53.0111234896154,38.9890000005756));
#181451=CARTESIAN_POINT('',(30.8905967158735,-52.8702215132217,39.2708017080178));
#181452=CARTESIAN_POINT('',(30.9724384738741,-53.0108370710513,38.989));
#181453=CARTESIAN_POINT('Origin',(5.49031038273072E-15,0.,38.989));
#181454=CARTESIAN_POINT('',(35.8301837593554,-49.8561803968404,38.989));
#181455=CARTESIAN_POINT('Origin',(5.49031038273072E-15,0.,38.989));
#181456=CARTESIAN_POINT('',(35.8306448082802,-49.8558490507737,38.9890000005754));
#181457=CARTESIAN_POINT('Origin',(5.49031038273072E-15,0.,38.989));
#181458=CARTESIAN_POINT('',(35.8306448084866,-49.8558490510345,38.989));
#181459=CARTESIAN_POINT('Origin',(62.2224557307631,0.,38.989));
#181460=CARTESIAN_POINT('',(31.2097904767605,-53.4219427993287,38.989));
#181461=CARTESIAN_POINT('',(15.8305769983922,-26.7843636743467,38.989));
#181462=CARTESIAN_POINT('',(36.1092077731528,-50.2402240048084,38.989));
#181463=CARTESIAN_POINT('Origin',(5.49031038273072E-15,0.,38.989));
#181464=CARTESIAN_POINT('',(35.8304925908681,-49.856605466951,38.989));
#181465=CARTESIAN_POINT('Origin',(5.57972911860581E-15,0.,39.624));
#181466=CARTESIAN_POINT('Origin',(30.2768121832815,-51.8059670065429,39.6240070731883));
#181467=CARTESIAN_POINT('Origin',(35.012416887145,-48.7306293534722,39.6240070731883));
#181468=CARTESIAN_POINT('Origin',(5.57972911860581E-15,0.,39.624));
#181469=CARTESIAN_POINT('Origin',(31.2288842284956,-53.4549470734246,39.5552135208005));
#181470=CARTESIAN_POINT('Origin',(36.1315923097622,-50.2710907322489,39.5552117598816));
#181471=CARTESIAN_POINT('Origin',(5.51210908043506E-15,0.,39.1438017080178));
#181472=CARTESIAN_POINT('Origin',(30.7889993062059,-52.6931852975948,39.1711625381365));
#181473=CARTESIAN_POINT('Origin',(35.6145503723398,-49.5593237986641,39.1712173702577));
#181474=CARTESIAN_POINT('Origin',(5.51210908043507E-15,0.,39.1438017080178));
#181475=CARTESIAN_POINT('Origin',(30.6976537960619,-52.5348053110497,39.171217585938));
#181476=CARTESIAN_POINT('Origin',(35.5070166083004,-49.4114565896691,39.1711627526733));
#181477=CARTESIAN_POINT('Origin',(60.4792282238308,0.,38.989));
#181478=CARTESIAN_POINT('',(39.9143573409156,-44.8038810887675,38.989));
#181479=CARTESIAN_POINT('',(35.5261472678865,-48.357383540212,38.989));
#181480=CARTESIAN_POINT('Origin',(5.49031038273072E-15,0.,38.989));
#181481=CARTESIAN_POINT('',(35.8051714542879,-48.7414273857062,38.989));
#181482=CARTESIAN_POINT('',(21.151922343707,-28.5729602337851,38.989));
#181483=CARTESIAN_POINT('',(35.8056376406738,-48.7410849262057,38.988999999577));
#181484=CARTESIAN_POINT('Origin',(5.49031038273072E-15,0.,38.989));
#181485=CARTESIAN_POINT('',(40.2315646148142,-45.1570399300039,38.9889999997818));
#181486=CARTESIAN_POINT('Origin',(5.49031038273072E-15,0.,38.989));
#181487=CARTESIAN_POINT('',(40.2319965165881,-45.1566551325072,38.989));
#181488=CARTESIAN_POINT('Origin',(5.49031038273072E-15,0.,38.989));
#181489=CARTESIAN_POINT('',(39.9147170640963,-44.8042806018338,38.989));
#181490=CARTESIAN_POINT('Origin',(5.49031038273072E-15,0.,38.989));
#181491=CARTESIAN_POINT('',(35.9012693628904,-48.8727133447944,39.2708017080178));
#181492=CARTESIAN_POINT('',(35.80563764024,-48.7410849256152,38.989));
#181493=CARTESIAN_POINT('',(40.3404336840073,-45.2779489571884,39.2708017078546));
#181494=CARTESIAN_POINT('Origin',(5.52999282761009E-15,0.,39.2708017080178));
#181495=CARTESIAN_POINT('',(40.3404336838192,-45.2779489569773,39.2708017080178));
#181496=CARTESIAN_POINT('Origin',(60.71525,0.,39.3978017080178));
#181497=CARTESIAN_POINT('',(40.4880553924343,-45.4410373245173,39.3978017080178));
#181498=CARTESIAN_POINT('',(36.0301015792676,-49.0510171431404,39.3978017080178));
#181499=CARTESIAN_POINT('Origin',(5.5478765747851E-15,0.,39.3978017080178));
#181500=CARTESIAN_POINT('',(36.1189794796882,-49.1733470784088,39.3978017080178));
#181501=CARTESIAN_POINT('',(21.2334658618522,-28.6851952578918,39.3978017080178));
#181502=CARTESIAN_POINT('',(40.5892333705622,-45.5534068532512,39.3978017080178));
#181503=CARTESIAN_POINT('Origin',(5.5478765747851E-15,0.,39.3978017080178));
#181504=CARTESIAN_POINT('',(40.488410048071,-45.4414312095059,39.3978017080178));
#181505=CARTESIAN_POINT('Origin',(5.5478765747851E-15,0.,39.3978017080178));
#181506=CARTESIAN_POINT('',(40.7368493365296,-45.7165002428308,39.2708017080178));
#181507=CARTESIAN_POINT('',(36.2478178024869,-49.351646303959,39.2708017081757));
#181508=CARTESIAN_POINT('Origin',(5.52999282761008E-15,0.,39.2708017080178));
#181509=CARTESIAN_POINT('',(36.3434519499946,-49.4832728536532,38.9890000005756));
#181510=CARTESIAN_POINT('',(36.247817802325,-49.3516463037386,39.2708017080178));
#181511=CARTESIAN_POINT('',(36.3439095507835,-49.4829367616347,38.989));
#181512=CARTESIAN_POINT('Origin',(5.49031038273072E-15,0.,38.989));
#181513=CARTESIAN_POINT('',(40.8452921850243,-45.8377889771252,38.989));
#181514=CARTESIAN_POINT('Origin',(5.49031038273072E-15,0.,38.989));
#181515=CARTESIAN_POINT('',(40.8457160731797,-45.8374112534714,38.9890000005754));
#181516=CARTESIAN_POINT('Origin',(5.49031038273072E-15,0.,38.989));
#181517=CARTESIAN_POINT('',(40.8457160734122,-45.8374112537091,38.989));
#181518=CARTESIAN_POINT('Origin',(62.2224557307631,0.,38.989));
#181519=CARTESIAN_POINT('',(36.6229335645808,-49.8669803696027,38.989));
#181520=CARTESIAN_POINT('',(21.7541926348211,-29.4019141737116,38.989));
#181521=CARTESIAN_POINT('',(41.162931164248,-46.1905628026486,38.989));
#181522=CARTESIAN_POINT('Origin',(5.49031038273072E-15,0.,38.989));
#181523=CARTESIAN_POINT('',(40.8456437566512,-45.8381794369738,38.989));
#181524=CARTESIAN_POINT('Origin',(5.57972911860581E-15,0.,39.624));
#181525=CARTESIAN_POINT('Origin',(35.5261507575148,-48.3573798485716,39.6240070731883));
#181526=CARTESIAN_POINT('Origin',(39.9143530044118,-44.8038837346041,39.6240070731883));
#181527=CARTESIAN_POINT('Origin',(5.57972911860581E-15,0.,39.624));
#181528=CARTESIAN_POINT('Origin',(36.6453726047983,-49.8978080023045,39.5552135208014));
#181529=CARTESIAN_POINT('Origin',(41.188419527604,-46.2189206177181,39.5552117598817));
#181530=CARTESIAN_POINT('Origin',(5.51210908043506E-15,0.,39.1438017080178));
#181531=CARTESIAN_POINT('Origin',(36.128271630334,-49.1861997321268,39.1711625381318));
#181532=CARTESIAN_POINT('Origin',(40.5998100962481,-45.5650984170299,39.171217370262));
#181533=CARTESIAN_POINT('Origin',(5.51210908043507E-15,0.,39.1438017080178));
#181534=CARTESIAN_POINT('Origin',(36.0208713038458,-49.0382355735244,39.1712175859395));
#181535=CARTESIAN_POINT('Origin',(40.4774090812916,-45.4292815791814,39.171162752675));
#181536=CARTESIAN_POINT('Origin',(60.4792282238308,0.,38.989));
#181537=CARTESIAN_POINT('',(44.3789831537295,-40.3862543050939,38.989));
#181538=CARTESIAN_POINT('',(40.3862543050938,-44.3789831537296,38.989));
#181539=CARTESIAN_POINT('Origin',(5.49031038273072E-15,0.,38.989));
#181540=CARTESIAN_POINT('',(40.7038934808042,-44.731757197436,38.989));
#181541=CARTESIAN_POINT('',(27.314662201079,-29.8615093742683,38.989));
#181542=CARTESIAN_POINT('',(40.7043213166065,-44.7313678842174,38.9889999995774));
#181543=CARTESIAN_POINT('Origin',(5.49031038273072E-15,0.,38.989));
#181544=CARTESIAN_POINT('',(44.7313678839555,-40.7043213163684,38.9889999997818));
#181545=CARTESIAN_POINT('Origin',(5.49031038273072E-15,0.,38.989));
#181546=CARTESIAN_POINT('',(44.7317571974354,-40.703893480804,38.989));
#181547=CARTESIAN_POINT('Origin',(5.49031038273072E-15,0.,38.989));
#181548=CARTESIAN_POINT('',(44.3793826667958,-40.3866140282746,38.989));
#181549=CARTESIAN_POINT('Origin',(5.49031038273072E-15,0.,38.989));
#181550=CARTESIAN_POINT('',(40.8131880745606,-44.8522789915942,39.2708017080178));
#181551=CARTESIAN_POINT('',(40.7043213161139,-44.7313678836761,38.989));
#181552=CARTESIAN_POINT('',(44.8522789918032,-40.813188074751,39.2708017078546));
#181553=CARTESIAN_POINT('Origin',(5.52999282761009E-15,0.,39.2708017080178));
#181554=CARTESIAN_POINT('',(44.8522789915941,-40.8131880745607,39.2708017080178));
#181555=CARTESIAN_POINT('Origin',(60.71525,0.,39.3978017080178));
#181556=CARTESIAN_POINT('',(45.0161393894793,-40.9599523566126,39.3978017080178));
#181557=CARTESIAN_POINT('',(40.9599523566124,-45.0161393894794,39.3978017080178));
#181558=CARTESIAN_POINT('Origin',(5.5478765747851E-15,0.,39.3978017080178));
#181559=CARTESIAN_POINT('',(41.0611303347403,-45.1285089182133,39.3978017080178));
#181560=CARTESIAN_POINT('',(27.4203375923833,-29.9788737863603,39.3978017080178));
#181561=CARTESIAN_POINT('',(45.1285089182132,-41.0611303347405,39.3978017080178));
#181562=CARTESIAN_POINT('Origin',(5.5478765747851E-15,0.,39.3978017080178));
#181563=CARTESIAN_POINT('',(45.0165332744679,-40.9603070122493,39.3978017080178));
#181564=CARTESIAN_POINT('Origin',(5.5478765747851E-15,0.,39.3978017080178));
#181565=CARTESIAN_POINT('',(45.2923641298556,-41.2079002115908,39.2708017080178));
#181566=CARTESIAN_POINT('',(41.2079002117747,-45.2923641300581,39.2708017081757));
#181567=CARTESIAN_POINT('Origin',(5.52999282761008E-15,0.,39.2708017080178));
#181568=CARTESIAN_POINT('',(41.3167691863808,-45.4132731252659,38.9890000005756));
#181569=CARTESIAN_POINT('',(41.2079002115907,-45.2923641298558,39.2708017080178));
#181570=CARTESIAN_POINT('',(41.3171891492024,-45.4128910420873,38.989));
#181571=CARTESIAN_POINT('Origin',(5.49031038273072E-15,0.,38.989));
#181572=CARTESIAN_POINT('',(45.4128910420872,-41.3171891492026,38.989));
#181573=CARTESIAN_POINT('Origin',(5.49031038273072E-15,0.,38.989));
#181574=CARTESIAN_POINT('',(45.4132731252658,-41.316769186381,38.9890000005754));
#181575=CARTESIAN_POINT('Origin',(5.49031038273072E-15,0.,38.989));
#181576=CARTESIAN_POINT('',(45.4132731255219,-41.3167691865932,38.989));
#181577=CARTESIAN_POINT('Origin',(62.2224557307631,0.,38.989));
#181578=CARTESIAN_POINT('',(41.6348281284261,-45.7656648676107,38.989));
#181579=CARTESIAN_POINT('',(28.0951675083324,-30.7283483363945,38.989));
#181580=CARTESIAN_POINT('',(45.7656648676106,-41.6348281284263,38.989));
#181581=CARTESIAN_POINT('Origin',(5.49031038273072E-15,0.,38.989));
#181582=CARTESIAN_POINT('',(45.4132815019358,-41.3175407208294,38.989));
#181583=CARTESIAN_POINT('Origin',(5.57972911860581E-15,0.,39.624));
#181584=CARTESIAN_POINT('Origin',(40.3862573897243,-44.3789791175468,39.6240070731883));
#181585=CARTESIAN_POINT('Origin',(44.3789791175466,-40.3862573897245,39.6240070731883));
#181586=CARTESIAN_POINT('Origin',(5.57972911860581E-15,0.,39.624));
#181587=CARTESIAN_POINT('Origin',(41.6603666103054,-45.7939781049239,39.5552135208022));
#181588=CARTESIAN_POINT('Origin',(45.793977801882,-41.6603663369584,39.5552117598818));
#181589=CARTESIAN_POINT('Origin',(5.51210908043506E-15,0.,39.1438017080178));
#181590=CARTESIAN_POINT('Origin',(41.0717150501549,-45.1403198695223,39.1711625381316));
#181591=CARTESIAN_POINT('Origin',(45.1402498046834,-41.0716522820265,39.1712173702609));
#181592=CARTESIAN_POINT('Origin',(5.51210908043507E-15,0.,39.1438017080178));
#181593=CARTESIAN_POINT('Origin',(40.9494366077774,-45.0043926651421,39.1712175859395));
#181594=CARTESIAN_POINT('Origin',(45.0043225899499,-40.9493738530219,39.171162752674));
#181595=CARTESIAN_POINT('Origin',(60.4792282238308,0.,38.989));
#181596=CARTESIAN_POINT('',(48.3573835402119,-35.5261472678866,38.989));
#181597=CARTESIAN_POINT('',(44.8038810887674,-39.9143573409157,38.989));
#181598=CARTESIAN_POINT('Origin',(5.49031038273072E-15,0.,38.989));
#181599=CARTESIAN_POINT('',(45.1566551325075,-40.2319965165887,38.989));
#181600=CARTESIAN_POINT('',(33.6129634723596,-29.8380098596982,38.989));
#181601=CARTESIAN_POINT('',(45.1570399302684,-40.2315646150501,38.9889999995771));
#181602=CARTESIAN_POINT('Origin',(5.49031038273072E-15,0.,38.989));
#181603=CARTESIAN_POINT('',(48.7410849259197,-35.805637640464,38.9889999997818));
#181604=CARTESIAN_POINT('Origin',(5.49031038273072E-15,0.,38.989));
#181605=CARTESIAN_POINT('',(48.7414273857055,-35.8051714542877,38.989));
#181606=CARTESIAN_POINT('Origin',(5.49031038273072E-15,0.,38.989));
#181607=CARTESIAN_POINT('',(48.3578184660151,-35.5264632599792,38.989));
#181608=CARTESIAN_POINT('Origin',(5.49031038273072E-15,0.,38.989));
#181609=CARTESIAN_POINT('',(45.2779489569772,-40.3404336838193,39.2708017080178));
#181610=CARTESIAN_POINT('',(45.1570399297215,-40.2315646145628,38.989));
#181611=CARTESIAN_POINT('',(48.8727133450222,-35.9012693630579,39.2708017078546));
#181612=CARTESIAN_POINT('Origin',(5.52999282761009E-15,0.,39.2708017080178));
#181613=CARTESIAN_POINT('',(48.8727133447943,-35.9012693628905,39.2708017080178));
#181614=CARTESIAN_POINT('Origin',(60.71525,0.,39.3978017080178));
#181615=CARTESIAN_POINT('',(49.0510171431403,-36.0301015792677,39.3978017080178));
#181616=CARTESIAN_POINT('',(45.4410373245171,-40.4880553924344,39.3978017080178));
#181617=CARTESIAN_POINT('Origin',(5.5478765747851E-15,0.,39.3978017080178));
#181618=CARTESIAN_POINT('',(45.5534068532511,-40.5892333705623,39.3978017080178));
#181619=CARTESIAN_POINT('',(33.7433098572246,-29.9553742717902,39.3978017080178));
#181620=CARTESIAN_POINT('',(49.1733470784087,-36.1189794796884,39.3978017080178));
#181621=CARTESIAN_POINT('Origin',(5.5478765747851E-15,0.,39.3978017080178));
#181622=CARTESIAN_POINT('',(49.0514459419945,-36.0304131198712,39.3978017080178));
#181623=CARTESIAN_POINT('Origin',(5.5478765747851E-15,0.,39.3978017080178));
#181624=CARTESIAN_POINT('',(49.3516463037384,-36.2478178023251,39.2708017080178));
#181625=CARTESIAN_POINT('',(45.7165002430348,-40.7368493367117,39.2708017081757));
#181626=CARTESIAN_POINT('Origin',(5.52999282761008E-15,0.,39.2708017080178));
#181627=CARTESIAN_POINT('',(45.8374112534712,-40.8457160731798,38.9890000005756));
#181628=CARTESIAN_POINT('',(45.7165002428306,-40.7368493365298,39.2708017080178));
#181629=CARTESIAN_POINT('',(45.8377889771251,-40.8452921850244,38.989));
#181630=CARTESIAN_POINT('Origin',(5.49031038273072E-15,0.,38.989));
#181631=CARTESIAN_POINT('',(49.4829367616345,-36.3439095507836,38.989));
#181632=CARTESIAN_POINT('Origin',(5.49031038273072E-15,0.,38.989));
#181633=CARTESIAN_POINT('',(49.4832728536532,-36.3434519499948,38.9890000005754));
#181634=CARTESIAN_POINT('Origin',(5.49031038273072E-15,0.,38.989));
#181635=CARTESIAN_POINT('',(49.48327285393,-36.3434519501791,38.989));
#181636=CARTESIAN_POINT('Origin',(62.2224557307631,0.,38.989));
#181637=CARTESIAN_POINT('',(46.1905628026484,-41.1629311642481,38.989));
#181638=CARTESIAN_POINT('',(34.5756856720385,-30.7048488218244,38.989));
#181639=CARTESIAN_POINT('',(49.8669803696025,-36.622933564581,38.989));
#181640=CARTESIAN_POINT('Origin',(5.49031038273072E-15,0.,38.989));
#181641=CARTESIAN_POINT('',(49.4833618317452,-36.3442183822964,38.989));
#181642=CARTESIAN_POINT('Origin',(5.57972911860581E-15,0.,39.624));
#181643=CARTESIAN_POINT('Origin',(44.803883734604,-39.9143530044119,39.6240070731883));
#181644=CARTESIAN_POINT('Origin',(48.3573798485713,-35.5261507575154,39.6240070731883));
#181645=CARTESIAN_POINT('Origin',(5.57972911860581E-15,0.,39.624));
#181646=CARTESIAN_POINT('Origin',(46.2189209212412,-41.1884198004176,39.5552135208008));
#181647=CARTESIAN_POINT('Origin',(49.8978076723516,-36.6453723646222,39.5552117598824));
#181648=CARTESIAN_POINT('Origin',(5.51210908043506E-15,0.,39.1438017080178));
#181649=CARTESIAN_POINT('Origin',(45.5651681650756,-40.5998732162064,39.1711625381287));
#181650=CARTESIAN_POINT('Origin',(49.1861234900558,-36.1282165298268,39.1712173702623));
#181651=CARTESIAN_POINT('Origin',(5.51210908043507E-15,0.,39.1438017080178));
#181652=CARTESIAN_POINT('Origin',(45.4293513150133,-40.4774722129475,39.1712175859372));
#181653=CARTESIAN_POINT('Origin',(49.0381593225499,-36.0208162177252,39.1711627526725));
#181654=CARTESIAN_POINT('Origin',(60.4792282238308,0.,38.989));
#181655=CARTESIAN_POINT('',(51.8059703131946,-30.2768083268882,38.989));
#181656=CARTESIAN_POINT('',(48.7306271754176,-35.0124214764585,38.989));
#181657=CARTESIAN_POINT('Origin',(5.49031038273072E-15,0.,38.989));
#181658=CARTESIAN_POINT('',(49.1146710209415,-35.2914456628191,38.989));
#181659=CARTESIAN_POINT('',(39.7707905934405,-28.502719155674,38.989));
#181660=CARTESIAN_POINT('',(49.1150085647358,-35.2909759049637,38.9889999995772));
#181661=CARTESIAN_POINT('Origin',(5.49031038273072E-15,0.,38.989));
#181662=CARTESIAN_POINT('',(52.2167844417078,-30.5146599057592,38.9889999997818));
#181663=CARTESIAN_POINT('Origin',(5.49031038273072E-15,0.,38.989));
#181664=CARTESIAN_POINT('',(52.2170762957385,-30.5141604766045,38.989));
#181665=CARTESIAN_POINT('Origin',(5.49031038273072E-15,0.,38.989));
#181666=CARTESIAN_POINT('',(51.8064358865966,-30.2770771258171,38.989));
#181667=CARTESIAN_POINT('Origin',(5.49031038273072E-15,0.,38.989));
#181668=CARTESIAN_POINT('',(49.2466351556012,-35.386610142826,39.2708017080178));
#181669=CARTESIAN_POINT('',(49.115008564141,-35.2909759045363,38.989));
#181670=CARTESIAN_POINT('',(52.3576880235603,-30.5960088313996,39.2708017078546));
#181671=CARTESIAN_POINT('Origin',(5.52999282761009E-15,0.,39.2708017080178));
#181672=CARTESIAN_POINT('',(52.3576880233162,-30.5960088312569,39.2708017080178));
#181673=CARTESIAN_POINT('Origin',(60.71525,0.,39.3978017080178));
#181674=CARTESIAN_POINT('',(52.5484816883959,-30.705497469237,39.3978017080178));
#181675=CARTESIAN_POINT('',(49.424260778346,-35.5163757878396,39.3978017080178));
#181676=CARTESIAN_POINT('Origin',(5.5478765747851E-15,0.,39.3978017080178));
#181677=CARTESIAN_POINT('',(49.5465907136144,-35.6052536882603,39.3978017080178));
#181678=CARTESIAN_POINT('',(39.9252688514646,-28.6149541797807,39.3978017080178));
#181679=CARTESIAN_POINT('',(52.6794317578287,-30.7811015270744,39.3978017080178));
#181680=CARTESIAN_POINT('Origin',(5.5478765747851E-15,0.,39.3978017080178));
#181681=CARTESIAN_POINT('',(52.5489407031056,-30.7057624815032,39.3978017080178));
#181682=CARTESIAN_POINT('Origin',(5.5478765747851E-15,0.,39.3978017080178));
#181683=CARTESIAN_POINT('',(52.8702215132216,-30.8905967158737,39.2708017080178));
#181684=CARTESIAN_POINT('',(49.7242207308395,-35.7350130972986,39.2708017081757));
#181685=CARTESIAN_POINT('Origin',(5.52999282761008E-15,0.,39.2708017080178));
#181686=CARTESIAN_POINT('',(49.8558490507736,-35.8306448082803,38.9890000005756));
#181687=CARTESIAN_POINT('',(49.7242207306174,-35.735013097139,39.2708017080178));
#181688=CARTESIAN_POINT('',(49.8561803968403,-35.8301837593555,38.989));
#181689=CARTESIAN_POINT('Origin',(5.49031038273072E-15,0.,38.989));
#181690=CARTESIAN_POINT('',(53.0108370710512,-30.9724384738743,38.989));
#181691=CARTESIAN_POINT('Origin',(5.49031038273072E-15,0.,38.989));
#181692=CARTESIAN_POINT('',(53.0111234896153,-30.9719482486883,38.9890000005754));
#181693=CARTESIAN_POINT('Origin',(5.49031038273072E-15,0.,38.989));
#181694=CARTESIAN_POINT('',(53.01112348991,-30.9719482488426,38.989));
#181695=CARTESIAN_POINT('Origin',(62.2224557307631,0.,38.989));
#181696=CARTESIAN_POINT('',(50.2402240048083,-36.1092077731529,38.989));
#181697=CARTESIAN_POINT('',(40.9117478092586,-29.3316730956005,38.989));
#181698=CARTESIAN_POINT('',(53.4219427993286,-31.2097904767607,38.989));
#181699=CARTESIAN_POINT('Origin',(5.49031038273072E-15,0.,38.989));
#181700=CARTESIAN_POINT('',(53.0112920942667,-30.9727011816503,38.989));
#181701=CARTESIAN_POINT('Origin',(5.57972911860581E-15,0.,39.624));
#181702=CARTESIAN_POINT('Origin',(48.7306293534718,-35.0124168871455,39.6240070731883));
#181703=CARTESIAN_POINT('Origin',(51.8059670065428,-30.2768121832818,39.6240070731883));
#181704=CARTESIAN_POINT('Origin',(5.57972911860581E-15,0.,39.624));
#181705=CARTESIAN_POINT('Origin',(50.2710910626291,-36.1315925493507,39.5552135208));
#181706=CARTESIAN_POINT('Origin',(53.4549467201732,-31.2288840241294,39.5552117598782));
#181707=CARTESIAN_POINT('Origin',(5.51210908043506E-15,0.,39.1438017080178));
#181708=CARTESIAN_POINT('Origin',(49.5593997624581,-35.6146058558666,39.1711625381308));
#181709=CARTESIAN_POINT('Origin',(52.6931037136124,-30.7889524770104,39.1712173702627));
#181710=CARTESIAN_POINT('Origin',(5.51210908043507E-15,0.,39.1438017080178));
#181711=CARTESIAN_POINT('Origin',(49.4115325425387,-35.507072104731,39.171217585936));
#181712=CARTESIAN_POINT('Origin',(52.5347237197204,-30.6976069821028,39.1711627526715));
#181713=CARTESIAN_POINT('Origin',(60.4792282238308,0.,38.989));
#181714=CARTESIAN_POINT('',(54.6869600343297,-24.6957503380308,38.989));
#181715=CARTESIAN_POINT('',(52.1234703131946,-29.726882195485,38.989));
#181716=CARTESIAN_POINT('Origin',(5.49031038273072E-15,0.,38.989));
#181717=CARTESIAN_POINT('',(52.5345762957643,-29.9642343451579,38.989));
#181718=CARTESIAN_POINT('',(45.518171167873,-25.9133109558556,38.989));
#181719=CARTESIAN_POINT('',(52.5348628873914,-29.9637318777509,38.9889999995773));
#181720=CARTESIAN_POINT('Origin',(5.49031038273072E-15,0.,38.989));
#181721=CARTESIAN_POINT('',(55.1203859400879,-24.8893571715239,38.9889999997818));
#181722=CARTESIAN_POINT('Origin',(5.49031038273072E-15,0.,38.989));
#181723=CARTESIAN_POINT('',(55.1206239907496,-24.888829971241,38.989));
#181724=CARTESIAN_POINT('Origin',(5.49031038273072E-15,0.,38.989));
#181725=CARTESIAN_POINT('',(54.6874511544109,-24.6959689987789,38.989));
#181726=CARTESIAN_POINT('Origin',(5.49031038273072E-15,0.,38.989));
#181727=CARTESIAN_POINT('',(52.6757649139395,-30.0450834959837,39.2708017080178));
#181728=CARTESIAN_POINT('',(52.5348628867555,-29.9637318773882,38.989));
#181729=CARTESIAN_POINT('',(55.2690209155617,-24.9555320243579,39.2708017078546));
#181730=CARTESIAN_POINT('Origin',(5.52999282761009E-15,0.,39.2708017080178));
#181731=CARTESIAN_POINT('',(55.269020915304,-24.9555320242416,39.2708017080178));
#181732=CARTESIAN_POINT('Origin',(60.71525,0.,39.3978017080178));
#181733=CARTESIAN_POINT('',(55.4702140717966,-25.0444775033948,39.3978017080178));
#181734=CARTESIAN_POINT('',(52.8659816883959,-30.1555713378339,39.3978017080178));
#181735=CARTESIAN_POINT('Origin',(5.5478765747851E-15,0.,39.3978017080178));
#181736=CARTESIAN_POINT('',(52.9969317578287,-30.2311753956713,39.3978017080178));
#181737=CARTESIAN_POINT('',(45.6951875,-26.0155113828601,39.3978017080178));
#181738=CARTESIAN_POINT('',(55.6083495590301,-25.1059793847702,39.3978017080178));
#181739=CARTESIAN_POINT('Origin',(5.5478765747851E-15,0.,39.3978017080178));
#181740=CARTESIAN_POINT('',(55.4706982733007,-25.0446930837939,39.3978017080178));
#181741=CARTESIAN_POINT('Origin',(5.5478765747851E-15,0.,39.3978017080178));
#181742=CARTESIAN_POINT('',(55.8095395120007,-25.1949317875302,39.2708017080178));
#181743=CARTESIAN_POINT('',(53.187152250855,-30.3416565763592,39.2708017081757));
#181744=CARTESIAN_POINT('Origin',(5.52999282761008E-15,0.,39.2708017080178));
#181745=CARTESIAN_POINT('',(53.3280557328685,-30.4230055008168,38.9890000005756));
#181746=CARTESIAN_POINT('',(53.1871522506175,-30.3416565762237,39.2708017080178));
#181747=CARTESIAN_POINT('',(53.3283370710512,-30.4225123424712,38.989));
#181748=CARTESIAN_POINT('Origin',(5.49031038273072E-15,0.,38.989));
#181749=CARTESIAN_POINT('',(55.9579395562866,-25.2616268796457,38.989));
#181750=CARTESIAN_POINT('Origin',(5.49031038273072E-15,0.,38.989));
#181751=CARTESIAN_POINT('',(55.9581731633345,-25.2611094010722,38.9890000005754));
#181752=CARTESIAN_POINT('Origin',(5.49031038273072E-15,0.,38.989));
#181753=CARTESIAN_POINT('',(55.9581731636437,-25.2611094011949,38.989));
#181754=CARTESIAN_POINT('Origin',(62.2224557307631,0.,38.989));
#181755=CARTESIAN_POINT('',(53.7394427993286,-30.6598643453575,38.989));
#181756=CARTESIAN_POINT('',(46.8255917980722,-26.6681506086452,38.989));
#181757=CARTESIAN_POINT('',(56.391603244485,-25.4547063934084,38.989));
#181758=CARTESIAN_POINT('Origin',(5.49031038273072E-15,0.,38.989));
#181759=CARTESIAN_POINT('',(55.9584195472775,-25.2618405854036,38.989));
#181760=CARTESIAN_POINT('Origin',(5.57972911860581E-15,0.,39.624));
#181761=CARTESIAN_POINT('Origin',(52.1234719996035,-29.7268774036438,39.6240070731883));
#181762=CARTESIAN_POINT('Origin',(54.6869571488949,-24.695754518938,39.6240070731883));
#181763=CARTESIAN_POINT('Origin',(5.57972911860581E-15,0.,39.624));
#181764=CARTESIAN_POINT('Origin',(53.7724806104346,-30.6789000092877,39.5552135208009));
#181765=CARTESIAN_POINT('Origin',(56.4264221855611,-25.4702454951992,39.5552117598807));
#181766=CARTESIAN_POINT('Origin',(5.51210908043506E-15,0.,39.1438017080178));
#181767=CARTESIAN_POINT('Origin',(53.0106482050716,-30.2391374209339,39.1711625381337));
#181768=CARTESIAN_POINT('Origin',(55.6227672661409,-25.1123582178528,39.1712173702621));
#181769=CARTESIAN_POINT('Origin',(5.51210908043507E-15,0.,39.1438017080178));
#181770=CARTESIAN_POINT('Origin',(52.852350679497,-30.1476490842092,39.1712175859328));
#181771=CARTESIAN_POINT('Origin',(55.4557066902172,-25.038068340499,39.1711627526733));
#181772=CARTESIAN_POINT('Origin',(60.4792282238308,0.,38.989));
#181773=CARTESIAN_POINT('',(56.9687879773466,-18.844120540552,38.989));
#181774=CARTESIAN_POINT('',(54.9452378026828,-24.1156489724277,38.989));
#181775=CARTESIAN_POINT('Origin',(5.49031038273072E-15,0.,38.989));
#181776=CARTESIAN_POINT('',(55.3789017591239,-24.308728605592,38.989));
#181777=CARTESIAN_POINT('',(50.6030043228557,-22.1823620689016,38.989));
#181778=CARTESIAN_POINT('',(55.3791342586264,-24.3081989337718,38.9889999995772));
#181779=CARTESIAN_POINT('Origin',(5.49031038273072E-15,0.,38.989));
#181780=CARTESIAN_POINT('',(57.4200769554261,-18.9913614316845,38.9889999997818));
#181781=CARTESIAN_POINT('Origin',(5.49031038273072E-15,0.,38.989));
#181782=CARTESIAN_POINT('',(57.420258594586,-18.9908122363901,38.989));
#181783=CARTESIAN_POINT('Origin',(5.49031038273072E-15,0.,38.989));
#181784=CARTESIAN_POINT('',(56.9692992632926,-18.8442866674262,38.989));
#181785=CARTESIAN_POINT('Origin',(5.49031038273072E-15,0.,38.989));
#181786=CARTESIAN_POINT('',(55.5277679687683,-24.3743766270215,39.2708017080178));
#181787=CARTESIAN_POINT('',(55.3791342579558,-24.3081989334774,38.989));
#181788=CARTESIAN_POINT('',(57.574814848626,-19.0416371861766,39.2708017078546));
#181789=CARTESIAN_POINT('Origin',(5.52999282761009E-15,0.,39.2708017080178));
#181790=CARTESIAN_POINT('',(57.5748148483576,-19.0416371860878,39.2708017080178));
#181791=CARTESIAN_POINT('Origin',(60.71525,0.,39.3978017080178));
#181792=CARTESIAN_POINT('',(57.7842031819382,-19.1090650011316,39.3978017080178));
#181793=CARTESIAN_POINT('',(55.7284918401498,-24.4643761377918,39.3978017080178));
#181794=CARTESIAN_POINT('Origin',(5.5478765747851E-15,0.,39.3978017080178));
#181795=CARTESIAN_POINT('',(55.8666273273833,-24.5258780191672,39.3978017080178));
#181796=CARTESIAN_POINT('',(50.7999799080414,-22.2700612497317,39.3978017080178));
#181797=CARTESIAN_POINT('',(57.9280106456676,-19.1557908785626,39.3978017080178));
#181798=CARTESIAN_POINT('Origin',(5.5478765747851E-15,0.,39.3978017080178));
#181799=CARTESIAN_POINT('',(57.7847072652236,-19.1092287877196,39.3978017080178));
#181800=CARTESIAN_POINT('Origin',(5.5478765747851E-15,0.,39.3978017080178));
#181801=CARTESIAN_POINT('',(58.1373965169893,-19.223225914144,39.2708017080178));
#181802=CARTESIAN_POINT('',(56.067354200683,-24.6158705165694,39.2708017081757));
#181803=CARTESIAN_POINT('Origin',(5.52999282761008E-15,0.,39.2708017080178));
#181804=CARTESIAN_POINT('',(56.2159890767411,-24.6820453786632,38.9890000005756));
#181805=CARTESIAN_POINT('',(56.0673542004326,-24.6158705164594,39.2708017080178));
#181806=CARTESIAN_POINT('',(56.2162173246397,-24.6815255140427,38.989));
#181807=CARTESIAN_POINT('Origin',(5.49031038273072E-15,0.,38.989));
#181808=CARTESIAN_POINT('',(58.2919551457916,-19.2740436149885,38.989));
#181809=CARTESIAN_POINT('Origin',(5.49031038273072E-15,0.,38.989));
#181810=CARTESIAN_POINT('',(58.2921333818757,-19.273504552631,38.9890000005754));
#181811=CARTESIAN_POINT('Origin',(5.49031038273072E-15,0.,38.989));
#181812=CARTESIAN_POINT('',(58.2921333821959,-19.2735045527207,38.989));
#181813=CARTESIAN_POINT('Origin',(62.2224557307631,0.,38.989));
#181814=CARTESIAN_POINT('',(56.6498810128382,-24.8746050278053,38.989));
#181815=CARTESIAN_POINT('',(52.0578415156894,-22.8300973196049,38.989));
#181816=CARTESIAN_POINT('',(58.7434254837932,-19.4207352200701,38.989));
#181817=CARTESIAN_POINT('Origin',(5.49031038273072E-15,0.,38.989));
#181818=CARTESIAN_POINT('',(58.2924548456761,-19.2742059773232,38.989));
#181819=CARTESIAN_POINT('Origin',(5.57972911860581E-15,0.,39.624));
#181820=CARTESIAN_POINT('Origin',(54.9452389789695,-24.1156440305593,39.6240070731883));
#181821=CARTESIAN_POINT('Origin',(56.9687855447424,-18.8441250001657,39.6240070731883));
#181822=CARTESIAN_POINT('Origin',(5.57972911860581E-15,0.,39.624));
#181823=CARTESIAN_POINT('Origin',(56.6847276080575,-24.8900830207517,39.5552135207979));
#181824=CARTESIAN_POINT('Origin',(58.7796779614986,-19.4325496266341,39.5552117598785));
#181825=CARTESIAN_POINT('Origin',(5.51210908043506E-15,0.,39.1438017080178));
#181826=CARTESIAN_POINT('Origin',(55.881100892759,-24.5323626684708,39.1711625381347));
#181827=CARTESIAN_POINT('Origin',(57.9430161406909,-19.1606277069622,39.1712173702642));
#181828=CARTESIAN_POINT('Origin',(5.51210908043507E-15,0.,39.1438017080178));
#181829=CARTESIAN_POINT('Origin',(55.7141074023426,-24.4579221115153,39.1712175859392));
#181830=CARTESIAN_POINT('Origin',(57.7691053333641,-19.1042073825995,39.1711627526757));
#181831=CARTESIAN_POINT('Origin',(60.4792282238308,0.,38.989));
#181832=CARTESIAN_POINT('',(58.6264539577984,-12.7860306150452,38.989));
#181833=CARTESIAN_POINT('',(57.1650137687747,-18.2401996527046,38.989));
#181834=CARTESIAN_POINT('Origin',(5.49031038273072E-15,0.,38.989));
#181835=CARTESIAN_POINT('',(57.6164843860303,-18.3868913484948,38.989));
#181836=CARTESIAN_POINT('',(54.8020887275094,-17.4724387660755,38.989));
#181837=CARTESIAN_POINT('',(57.6166602460947,-18.3863402754565,38.9889999995772));
#181838=CARTESIAN_POINT('Origin',(5.49031038273072E-15,0.,38.989));
#181839=CARTESIAN_POINT('',(59.0906615917171,-12.8852923618017,38.9889999997818));
#181840=CARTESIAN_POINT('Origin',(5.49031038273072E-15,0.,38.989));
#181841=CARTESIAN_POINT('',(59.0907848292984,-12.8847271885943,38.989));
#181842=CARTESIAN_POINT('Origin',(5.49031038273072E-15,0.,38.989));
#181843=CARTESIAN_POINT('',(58.6269798078533,-12.7861423879248,38.989));
#181844=CARTESIAN_POINT('Origin',(5.49031038273072E-15,0.,38.989));
#181845=CARTESIAN_POINT('',(57.7713971777987,-18.4366189870673,39.2708017080178));
#181846=CARTESIAN_POINT('',(57.6166602453971,-18.3863402752338,38.989));
#181847=CARTESIAN_POINT('',(59.2498070619042,-12.9191181862648,39.2708017078546));
#181848=CARTESIAN_POINT('Origin',(5.52999282761009E-15,0.,39.2708017080178));
#181849=CARTESIAN_POINT('',(59.249807061628,-12.9191181862046,39.2708017080178));
#181850=CARTESIAN_POINT('Origin',(60.71525,0.,39.3978017080178));
#181851=CARTESIAN_POINT('',(59.4650964698966,-12.9642895838871,39.3978017080178));
#181852=CARTESIAN_POINT('',(57.9804289733663,-18.5051441132842,39.3978017080178));
#181853=CARTESIAN_POINT('Origin',(5.5478765747851E-15,0.,39.3978017080178));
#181854=CARTESIAN_POINT('',(58.1242364370956,-18.5518699907151,39.3978017080178));
#181855=CARTESIAN_POINT('',(55.0155724295758,-17.5418038257016,39.3978017080178));
#181856=CARTESIAN_POINT('',(59.6130003254555,-12.9957275188824,39.3978017080178));
#181857=CARTESIAN_POINT('Origin',(5.5478765747851E-15,0.,39.3978017080178));
#181858=CARTESIAN_POINT('',(59.4656149121214,-12.9643997821838,39.3978017080178));
#181859=CARTESIAN_POINT('Origin',(5.5478765747851E-15,0.,39.3978017080178));
#181860=CARTESIAN_POINT('',(59.8282880397055,-13.0409063549239,39.2708017080178));
#181861=CARTESIAN_POINT('',(58.3332704850401,-18.620387828198,39.2708017081757));
#181862=CARTESIAN_POINT('Origin',(5.52999282761008E-15,0.,39.2708017080178));
#181863=CARTESIAN_POINT('',(58.4880082803368,-18.6706636022909,38.9890000005756));
#181864=CARTESIAN_POINT('',(58.3332704847796,-18.6203878281148,39.2708017080178));
#181865=CARTESIAN_POINT('',(58.4881809372197,-18.6701227271411,38.989));
#181866=CARTESIAN_POINT('Origin',(5.49031038273072E-15,0.,38.989));
#181867=CARTESIAN_POINT('',(59.9873118763436,-13.0752898951325,38.989));
#181868=CARTESIAN_POINT('Origin',(5.49031038273072E-15,0.,38.989));
#181869=CARTESIAN_POINT('',(59.9874327886718,-13.0747351550711,38.9890000005754));
#181870=CARTESIAN_POINT('Origin',(5.49031038273072E-15,0.,38.989));
#181871=CARTESIAN_POINT('',(59.9874327889997,-13.0747351551268,38.989));
#181872=CARTESIAN_POINT('Origin',(62.2224557307631,0.,38.989));
#181873=CARTESIAN_POINT('',(58.9396512752213,-18.8168143322227,38.989));
#181874=CARTESIAN_POINT('',(56.3788528200606,-17.9847604760582,38.989));
#181875=CARTESIAN_POINT('',(60.4516424606489,-13.1739864076107,38.989));
#181876=CARTESIAN_POINT('Origin',(5.49031038273072E-15,0.,38.989));
#181877=CARTESIAN_POINT('',(59.9878258103051,-13.0753991351683,38.989));
#181878=CARTESIAN_POINT('Origin',(5.57972911860581E-15,0.,39.624));
#181879=CARTESIAN_POINT('Origin',(57.1650144220517,-18.2401946149524,39.6240070731883));
#181880=CARTESIAN_POINT('Origin',(58.6264520046768,-12.786035304505,39.6240070731883));
#181881=CARTESIAN_POINT('Origin',(5.57972911860581E-15,0.,39.624));
#181882=CARTESIAN_POINT('Origin',(58.9759248679598,-18.828565074058,39.5552135208021));
#181883=CARTESIAN_POINT('Origin',(60.4889312852489,-13.1819466778325,39.5552117598828));
#181884=CARTESIAN_POINT('Origin',(5.51210908043506E-15,0.,39.1438017080178));
#181885=CARTESIAN_POINT('Origin',(58.1393085451921,-18.5568062168846,39.171162538134));
#181886=CARTESIAN_POINT('Origin',(59.6284292050448,-12.9989693492943,39.1712173702605));
#181887=CARTESIAN_POINT('Origin',(5.51210908043507E-15,0.,39.1438017080178));
#181888=CARTESIAN_POINT('Origin',(57.9654487055673,-18.5002290260163,39.1712175859376));
#181889=CARTESIAN_POINT('Origin',(59.4495735695174,-12.9610367308101,39.1711627526733));
#181890=CARTESIAN_POINT('Origin',(60.4792282238308,0.,38.989));
#181891=CARTESIAN_POINT('',(59.6417962403143,-6.58785426247096,38.989));
#181892=CARTESIAN_POINT('',(58.7584778814676,-12.1649068885792,38.989));
#181893=CARTESIAN_POINT('Origin',(5.49031038273072E-15,0.,38.989));
#181894=CARTESIAN_POINT('',(59.2228087529788,-12.263603462079,38.989));
#181895=CARTESIAN_POINT('',(57.9308881865554,-11.9889972685551,38.989));
#181896=CARTESIAN_POINT('',(59.2229260468457,-12.2630370254942,38.9889999995772));
#181897=CARTESIAN_POINT('Origin',(5.49031038273072E-15,0.,38.989));
#181898=CARTESIAN_POINT('',(60.1138365740932,-6.63804933238219,38.9889999997818));
#181899=CARTESIAN_POINT('Origin',(5.49031038273072E-15,0.,38.989));
#181900=CARTESIAN_POINT('',(60.1139000598794,-6.63747437341778,38.989));
#181901=CARTESIAN_POINT('Origin',(5.49031038273072E-15,0.,38.989));
#181902=CARTESIAN_POINT('',(59.6423308931549,-6.58791045674891,38.989));
#181903=CARTESIAN_POINT('Origin',(5.49031038273072E-15,0.,38.989));
#181904=CARTESIAN_POINT('',(59.3820708699071,-12.2968658913803,39.2708017080178));
#181905=CARTESIAN_POINT('',(59.2229260461285,-12.2630370253457,38.989));
#181906=CARTESIAN_POINT('',(60.2756459901929,-6.65505462400498,39.2708017078546));
#181907=CARTESIAN_POINT('Origin',(5.52999282761009E-15,0.,39.2708017080178));
#181908=CARTESIAN_POINT('',(60.2756459899119,-6.65505462397395,39.2708017080178));
#181909=CARTESIAN_POINT('Origin',(60.71525,0.,39.3978017080178));
#181910=CARTESIAN_POINT('',(60.4944777170594,-6.67747469700946,39.3978017080178));
#181911=CARTESIAN_POINT('',(59.5971203935659,-12.3431658574211,39.3978017080178));
#181912=CARTESIAN_POINT('Origin',(5.5478765747851E-15,0.,39.3978017080178));
#181913=CARTESIAN_POINT('',(59.7450242491248,-12.3746037924164,39.3978017080178));
#181914=CARTESIAN_POINT('',(58.1567073854021,-12.036996621021,39.3978017080178));
#181915=CARTESIAN_POINT('',(60.6448574988554,-6.69328024897455,39.3978017080178));
#181916=CARTESIAN_POINT('Origin',(5.5478765747851E-15,0.,39.3978017080178));
#181917=CARTESIAN_POINT('',(60.495004838062,-6.67753009965933,39.3978017080178));
#181918=CARTESIAN_POINT('Origin',(5.5478765747851E-15,0.,39.3978017080178));
#181919=CARTESIAN_POINT('',(60.8636883187845,-6.7157078966941,39.2708017080178));
#181920=CARTESIAN_POINT('',(59.9600752509415,-12.4208962742141,39.2708017081757));
#181921=CARTESIAN_POINT('Origin',(5.52999282761008E-15,0.,39.2708017080178));
#181922=CARTESIAN_POINT('',(60.1192206258106,-12.4547221284044,38.9890000005756));
#181923=CARTESIAN_POINT('',(59.9600752506737,-12.4208962741587,39.2708017080178));
#181924=CARTESIAN_POINT('',(60.1193358000128,-12.4541661686666,38.989));
#181925=CARTESIAN_POINT('Origin',(5.49031038273072E-15,0.,38.989));
#181926=CARTESIAN_POINT('',(61.0254350648262,-6.73328056300519,38.989));
#181927=CARTESIAN_POINT('Origin',(5.49031038273072E-15,0.,38.989));
#181928=CARTESIAN_POINT('',(61.025497328658,-6.73271622308798,38.9890000005754));
#181929=CARTESIAN_POINT('Origin',(5.49031038273072E-15,0.,38.989));
#181930=CARTESIAN_POINT('',(61.0254973289899,-6.73271622310909,38.989));
#181931=CARTESIAN_POINT('Origin',(62.2224557307631,0.,38.989));
#181932=CARTESIAN_POINT('',(60.5836663843182,-12.5528626811448,38.989));
#181933=CARTESIAN_POINT('',(59.5987607253194,-12.3435145206986,38.989));
#181934=CARTESIAN_POINT('',(61.4975385923862,-6.78290064323561,38.989));
#181935=CARTESIAN_POINT('Origin',(5.49031038273072E-15,0.,38.989));
#181936=CARTESIAN_POINT('',(61.0259576020968,-6.73333548388541,38.989));
#181937=CARTESIAN_POINT('Origin',(5.57972911860581E-15,0.,39.624));
#181938=CARTESIAN_POINT('Origin',(58.7584780045774,-12.1649018101385,39.6240070731883));
#181939=CARTESIAN_POINT('Origin',(59.6417947880741,-6.58785913039828,39.6240070731883));
#181940=CARTESIAN_POINT('Origin',(5.57972911860581E-15,0.,39.624));
#181941=CARTESIAN_POINT('Origin',(60.6209695535084,-12.5607574282778,39.5552135208006));
#181942=CARTESIAN_POINT('Origin',(61.5354552197178,-6.78691956273256,39.5552117598807));
#181943=CARTESIAN_POINT('Origin',(5.51210908043506E-15,0.,39.1438017080178));
#181944=CARTESIAN_POINT('Origin',(59.760529766771,-12.3779375131248,39.1711625381325));
#181945=CARTESIAN_POINT('Origin',(60.6605407209802,-6.69489156322693,39.1712173702618));
#181946=CARTESIAN_POINT('Origin',(5.51210908043507E-15,0.,39.1438017080178));
#181947=CARTESIAN_POINT('Origin',(59.5817084227223,-12.3398435598876,39.1712175859377));
#181948=CARTESIAN_POINT('Origin',(60.4786998370193,-6.67586224832376,39.1711627526732));
#181949=CARTESIAN_POINT('Origin',(57.8669800961561,0.,40.5765));
#181950=CARTESIAN_POINT('Origin',(60.4792282238308,0.,38.989));
#181951=CARTESIAN_POINT('',(60.0036905223731,-0.3175,38.989));
#181952=CARTESIAN_POINT('',(59.7081718144892,-5.95633285891211,38.989));
#181953=CARTESIAN_POINT('Origin',(5.49031038273072E-15,0.,38.989));
#181954=CARTESIAN_POINT('',(60.1802756340603,-6.00595296980872,38.989));
#181955=CARTESIAN_POINT('',(59.851607889689,-5.97140859790549,38.989));
#181956=CARTESIAN_POINT('',(60.1803330766335,-6.00537737567514,38.988999999577));
#181957=CARTESIAN_POINT('Origin',(5.49031038273072E-15,0.,38.989));
#181958=CARTESIAN_POINT('',(60.4783917833346,-0.318078445375993,38.9889999997818));
#181959=CARTESIAN_POINT('Origin',(5.49031038273072E-15,0.,38.989));
#181960=CARTESIAN_POINT('',(60.478394821762,-0.317500000025285,38.989));
#181961=CARTESIAN_POINT('Origin',(5.49031038273072E-15,0.,38.989));
#181962=CARTESIAN_POINT('',(60.004228120231,-0.3175,38.989));
#181963=CARTESIAN_POINT('Origin',(5.49031038273072E-15,0.,38.989));
#181964=CARTESIAN_POINT('',(60.3421421670675,-6.02238575970276,39.2708017080178));
#181965=CARTESIAN_POINT('',(60.1803330759045,-6.0053773756024,38.989));
#181966=CARTESIAN_POINT('',(60.6410923275233,-0.318076890624849,39.2708017078546));
#181967=CARTESIAN_POINT('Origin',(5.52999282761009E-15,0.,39.2708017080178));
#181968=CARTESIAN_POINT('',(60.6410923272405,-0.318076890623366,39.2708017080178));
#181969=CARTESIAN_POINT('Origin',(60.71525,0.,39.3978017080178));
#181970=CARTESIAN_POINT('',(60.8610688070707,-0.3175,39.3978017080178));
#181971=CARTESIAN_POINT('',(60.5608532912343,-6.04595329345061,39.3978017080178));
#181972=CARTESIAN_POINT('Origin',(5.5478765747851E-15,0.,39.3978017080178));
#181973=CARTESIAN_POINT('',(60.7112330730304,-6.0617588454157,39.3978017080178));
#181974=CARTESIAN_POINT('',(60.0850508448141,-5.99594444118207,39.3978017080178));
#181975=CARTESIAN_POINT('',(61.0122769227456,-0.3175,39.3978017080178));
#181976=CARTESIAN_POINT('Origin',(5.5478765747851E-15,0.,39.3978017080178));
#181977=CARTESIAN_POINT('',(60.8615988316031,-0.3175,39.3978017080178));
#181978=CARTESIAN_POINT('Origin',(5.5478765747851E-15,0.,39.3978017080178));
#181979=CARTESIAN_POINT('',(61.2322532920972,-0.316930737395914,39.2708017080178));
#181980=CARTESIAN_POINT('',(60.9299448849412,-6.08531878141038,39.2708017081757));
#181981=CARTESIAN_POINT('Origin',(5.52999282761008E-15,0.,39.2708017080178));
#181982=CARTESIAN_POINT('',(61.0917542093523,-6.10232411256087,38.9890000005756));
#181983=CARTESIAN_POINT('',(60.929944884669,-6.0853187813832,39.2708017080178));
#181984=CARTESIAN_POINT('',(61.0918106390012,-6.10175915944633,38.989));
#181985=CARTESIAN_POINT('Origin',(5.49031038273072E-15,0.,38.989));
#181986=CARTESIAN_POINT('',(61.3949508163454,-0.3175,38.989));
#181987=CARTESIAN_POINT('Origin',(5.49031038273072E-15,0.,38.989));
#181988=CARTESIAN_POINT('',(61.394953749505,-0.316932243253256,38.9890000005754));
#181989=CARTESIAN_POINT('Origin',(5.49031038273072E-15,0.,38.989));
#181990=CARTESIAN_POINT('',(61.3949537498373,-0.31693224323956,38.989));
#181991=CARTESIAN_POINT('Origin',(62.2224557307631,0.,38.989));
#181992=CARTESIAN_POINT('',(61.5639141665612,-6.15137923967676,38.989));
#181993=CARTESIAN_POINT('',(61.5757885448747,-6.15262728712865,38.989));
#181994=CARTESIAN_POINT('',(61.8696548221181,-0.3175,38.989));
#181995=CARTESIAN_POINT('Origin',(5.49031038273072E-15,0.,38.989));
#181996=CARTESIAN_POINT('',(61.3954762318973,-0.3175,38.989));
#181997=CARTESIAN_POINT('Origin',(63.2144358269191,0.,40.5765));
#181998=CARTESIAN_POINT('Origin',(65.,0.,38.6715));
#181999=CARTESIAN_POINT('Origin',(5.57972911860581E-15,0.,39.624));
#182000=CARTESIAN_POINT('Origin',(59.708171406083,-5.95632779542302,39.6240070731883));
#182001=CARTESIAN_POINT('Origin',(60.0036895869254,-0.317504993060752,39.6240070731883));
#182002=CARTESIAN_POINT('Origin',(5.57972911860581E-15,0.,39.624));
#182003=CARTESIAN_POINT('Origin',(61.6018382108738,-6.15533149560949,39.5552135207993));
#182004=CARTESIAN_POINT('Origin',(61.9077838296774,-0.317533536648587,39.55521175988));
#182005=CARTESIAN_POINT('Origin',(5.51210908043506E-15,0.,39.1438017080178));
#182006=CARTESIAN_POINT('Origin',(60.7270021185297,-6.06345353572125,39.1711625381299));
#182007=CARTESIAN_POINT('Origin',(61.0280426587402,-0.317463144196517,39.1712173702601));
#182008=CARTESIAN_POINT('Origin',(5.51210908043507E-15,0.,39.1438017080178));
#182009=CARTESIAN_POINT('Origin',(60.5451784741259,-6.04426018543854,39.1712175859343));
#182010=CARTESIAN_POINT('Origin',(60.8452088131256,-0.317545622030759,39.1711627526726));
#182011=CARTESIAN_POINT('Origin',(58.2637721346185,0.1905,40.10025));
#182012=CARTESIAN_POINT('',(59.0285534841296,-0.01524,40.10025));
#182013=CARTESIAN_POINT('',(62.8464427007196,-0.01524,40.10025));
#182014=CARTESIAN_POINT('',(58.2637721346185,-0.01524,40.10025));
#182015=CARTESIAN_POINT('',(62.8464427007196,0.01524,40.10025));
#182016=CARTESIAN_POINT('Origin',(-1.95097259456047E-16,0.,40.10025));
#182017=CARTESIAN_POINT('',(59.0285534841296,0.01524,40.10025));
#182018=CARTESIAN_POINT('',(58.9578504383728,0.01524,40.10025));
#182019=CARTESIAN_POINT('Origin',(4.7062627014205E-16,0.,40.10025));
#182020=CARTESIAN_POINT('Origin',(0.,0.1905,0.));
#182021=CARTESIAN_POINT('',(60.0036905223731,0.1905,39.116));
#182022=CARTESIAN_POINT('',(59.5728760150042,0.1905,39.3548010137695));
#182023=CARTESIAN_POINT('Origin',(59.9654595002501,0.1905,39.5550297832849));
#182024=CARTESIAN_POINT('',(59.2165773020941,0.190499999468626,39.92499));
#182025=CARTESIAN_POINT('',(59.5728760150042,0.1905,39.3548010137695));
#182026=CARTESIAN_POINT('',(62.6567671111299,0.190499999999999,39.92499));
#182027=CARTESIAN_POINT('',(62.9165533988763,0.1905,39.92499));
#182028=CARTESIAN_POINT('',(62.3004688883555,0.190500000605232,39.3548010137695));
#182029=CARTESIAN_POINT('',(62.6567671111299,0.1905,39.92499));
#182030=CARTESIAN_POINT('',(61.8696548221181,0.1905,39.116));
#182031=CARTESIAN_POINT('Origin',(61.907885967377,0.1905,39.5550293907185));
#182032=CARTESIAN_POINT('',(61.4682752798284,0.190500000711878,39.116));
#182033=CARTESIAN_POINT('',(5.50819412990574E-15,0.1905,39.116));
#182034=CARTESIAN_POINT('',(61.3422370451705,0.1905,39.3343017080178));
#182035=CARTESIAN_POINT('',(61.4682752798284,0.1905,39.116));
#182036=CARTESIAN_POINT('',(61.0122769227456,0.1905,39.5248017080178));
#182037=CARTESIAN_POINT('Origin',(61.0417043405058,0.190499486622398,39.1947747614266));
#182038=CARTESIAN_POINT('',(60.8610688070707,0.1905,39.5248017080178));
#182039=CARTESIAN_POINT('',(5.56576032196012E-15,0.1905,39.5248017080178));
#182040=CARTESIAN_POINT('',(60.5311086139135,0.1905,39.3343017080178));
#182041=CARTESIAN_POINT('Origin',(60.831638480741,0.190499486573503,39.19477289119));
#182042=CARTESIAN_POINT('',(60.4050703266283,0.1905,39.116));
#182043=CARTESIAN_POINT('',(60.5311086139135,0.1905,39.3343017080178));
#182044=CARTESIAN_POINT('',(5.50819412990574E-15,0.1905,39.116));
#182045=CARTESIAN_POINT('Origin',(0.,-0.1905,0.));
#182046=CARTESIAN_POINT('',(61.8696548221181,-0.1905,39.116));
#182047=CARTESIAN_POINT('',(62.3004688883555,-0.190500000000001,39.3548010137695));
#182048=CARTESIAN_POINT('Origin',(61.9078859670888,-0.1905,39.5550293912443));
#182049=CARTESIAN_POINT('',(62.6567671111299,-0.19050000045281,39.92499));
#182050=CARTESIAN_POINT('',(62.3004688883555,-0.1905,39.3548010137695));
#182051=CARTESIAN_POINT('',(59.2165773020941,-0.1905,39.92499));
#182052=CARTESIAN_POINT('',(0.,-0.1905,39.92499));
#182053=CARTESIAN_POINT('',(59.5728760150042,-0.190499999293268,39.3548010137695));
#182054=CARTESIAN_POINT('',(59.2165773020941,-0.1905,39.92499));
#182055=CARTESIAN_POINT('',(60.0036905223731,-0.1905,39.116));
#182056=CARTESIAN_POINT('Origin',(59.9654594999459,-0.1905,39.5550297827296));
#182057=CARTESIAN_POINT('',(60.4050703266283,-0.190499999258369,39.116));
#182058=CARTESIAN_POINT('',(60.4789282006569,-0.1905,39.116));
#182059=CARTESIAN_POINT('',(60.5311086139135,-0.1905,39.3343017080178));
#182060=CARTESIAN_POINT('',(60.4050703266283,-0.1905,39.116));
#182061=CARTESIAN_POINT('',(60.8610688070707,-0.1905,39.5248017080178));
#182062=CARTESIAN_POINT('Origin',(60.8316414495909,-0.190499486502558,39.1947745585603));
#182063=CARTESIAN_POINT('',(61.0122769227456,-0.1905,39.5248017080178));
#182064=CARTESIAN_POINT('',(61.0128056337175,-0.1905,39.5248017080178));
#182065=CARTESIAN_POINT('',(61.3422370451705,-0.1905,39.3343017080178));
#182066=CARTESIAN_POINT('Origin',(61.0417071743798,-0.190499486688097,39.1947728594227));
#182067=CARTESIAN_POINT('',(61.4682752798284,-0.1905,39.116));
#182068=CARTESIAN_POINT('',(61.3422370451705,-0.1905,39.3343017080178));
#182069=CARTESIAN_POINT('',(61.8701762063762,-0.1905,39.116));
#182070=CARTESIAN_POINT('Origin',(58.2637721346185,-0.01524,39.92499));
#182071=CARTESIAN_POINT('Ctrl Pts',(62.6567671111299,-0.1905,39.92499));
#182072=CARTESIAN_POINT('Ctrl Pts',(62.6673774406538,-0.1905,39.9348354642021));
#182073=CARTESIAN_POINT('Ctrl Pts',(62.6779562874465,-0.189662809673067,
39.9446440828463));
#182074=CARTESIAN_POINT('Ctrl Pts',(62.6884465439476,-0.1880036041151,39.9543641760338));
#182075=CARTESIAN_POINT('Ctrl Pts',(62.6985959295776,-0.186398312857848,
39.963768424072));
#182076=CARTESIAN_POINT('Ctrl Pts',(62.7086636500152,-0.184023290311169,
39.9730909636405));
#182077=CARTESIAN_POINT('Ctrl Pts',(62.718593962217,-0.180846261210442,
39.982280897715));
#182078=CARTESIAN_POINT('Ctrl Pts',(62.7279874260866,-0.177840987311337,
39.990974009466));
#182079=CARTESIAN_POINT('Ctrl Pts',(62.7372588214087,-0.174117798730811,
39.9995492765012));
#182080=CARTESIAN_POINT('Ctrl Pts',(62.7463424082318,-0.169611579426027,
40.0079462328706));
#182081=CARTESIAN_POINT('Ctrl Pts',(62.7547090486376,-0.165461025548246,
40.0156804369701));
#182082=CARTESIAN_POINT('Ctrl Pts',(62.7629168328863,-0.16064587058751,
40.0232638017434));
#182083=CARTESIAN_POINT('Ctrl Pts',(62.7708892610819,-0.155086395961918,
40.0306257269979));
#182084=CARTESIAN_POINT('Ctrl Pts',(62.7732017594462,-0.153473803704847,
40.032761141666));
#182085=CARTESIAN_POINT('Ctrl Pts',(62.7754942590279,-0.151798403770304,
40.0348777427275));
#182086=CARTESIAN_POINT('Ctrl Pts',(62.7777643638145,-0.150057792857652,
40.0369733168701));
#182087=CARTESIAN_POINT('Ctrl Pts',(62.780225303358,-0.148170858717032,
40.039245053974));
#182088=CARTESIAN_POINT('Ctrl Pts',(62.7826571567198,-0.14621076955376,
40.041487875195));
#182089=CARTESIAN_POINT('Ctrl Pts',(62.7850565204094,-0.144175421826142,
40.0436985701601));
#182090=CARTESIAN_POINT('Ctrl Pts',(62.791641592883,-0.138589394016614,
40.0497658398386));
#182091=CARTESIAN_POINT('Ctrl Pts',(62.7979456687653,-0.132410786669041,
40.0555581699984));
#182092=CARTESIAN_POINT('Ctrl Pts',(62.8038680995981,-0.125664597436735,
40.0609828468885));
#182093=CARTESIAN_POINT('Ctrl Pts',(62.8092868022738,-0.119492200548398,
40.0659461317304));
#182094=CARTESIAN_POINT('Ctrl Pts',(62.8143744518938,-0.112844347460372,
40.0706039980705));
#182095=CARTESIAN_POINT('Ctrl Pts',(62.8190433630432,-0.10570804383351,
40.0748843180602));
#182096=CARTESIAN_POINT('Ctrl Pts',(62.8213367169482,-0.102202714803632,
40.0769867972569));
#182097=CARTESIAN_POINT('Ctrl Pts',(62.8235285419787,-0.0985794274533726,
40.0789976708174));
#182098=CARTESIAN_POINT('Ctrl Pts',(62.8256051102647,-0.0948363533472265,
40.08090504915));
#182099=CARTESIAN_POINT('Ctrl Pts',(62.825999118871,-0.0941261414936272,
40.0812669556105));
#182100=CARTESIAN_POINT('Ctrl Pts',(62.8263888407139,-0.0934111032312788,
40.0816253922032));
#182101=CARTESIAN_POINT('Ctrl Pts',(62.826774159152,-0.0926913160160826,
40.0819801989139));
#182102=CARTESIAN_POINT('Ctrl Pts',(62.8271474363889,-0.0919940221513613,
40.0823239179149));
#182103=CARTESIAN_POINT('Ctrl Pts',(62.8275165811343,-0.0912922715310412,
40.0826642303498));
#182104=CARTESIAN_POINT('Ctrl Pts',(62.8278814873655,-0.0905861384169516,
40.0830009916099));
#182105=CARTESIAN_POINT('Ctrl Pts',(62.8318581602824,-0.0828908452418622,
40.0866709464312));
#182106=CARTESIAN_POINT('Ctrl Pts',(62.8353337180912,-0.0746698316630608,
40.0899175831877));
#182107=CARTESIAN_POINT('Ctrl Pts',(62.8381654210186,-0.0660491922297058,
40.0925642067062));
#182108=CARTESIAN_POINT('Ctrl Pts',(62.8393612667489,-0.0624086426654192,
40.0936818922527));
#182109=CARTESIAN_POINT('Ctrl Pts',(62.8404425512865,-0.0586971697057385,
40.094693009479));
#182110=CARTESIAN_POINT('Ctrl Pts',(62.8414000604479,-0.0549254519864779,
40.0955863397546));
#182111=CARTESIAN_POINT('Ctrl Pts',(62.8430124819501,-0.0485739735922166,
40.0970906856166));
#182112=CARTESIAN_POINT('Ctrl Pts',(62.8442717146911,-0.0420529246952733,
40.0982599215483));
#182113=CARTESIAN_POINT('Ctrl Pts',(62.8451307298764,-0.0354197192407095,
40.0990497370453));
#182114=CARTESIAN_POINT('Ctrl Pts',(62.8453454836727,-0.0337614178770686,
40.0992471909196));
#182115=CARTESIAN_POINT('Ctrl Pts',(62.8455349903695,-0.0320960919385888,
40.0994209989363));
#182116=CARTESIAN_POINT('Ctrl Pts',(62.8456982067485,-0.0304246312365872,
40.0995705982975));
#182117=CARTESIAN_POINT('Ctrl Pts',(62.845943031317,-0.0279174401835849,
40.0997949973393));
#182118=CARTESIAN_POINT('Ctrl Pts',(62.8461286892223,-0.0253964615339684,
40.0999649129781));
#182119=CARTESIAN_POINT('Ctrl Pts',(62.846253337618,-0.0228647168031114,
40.1000786629733));
#182120=CARTESIAN_POINT('Ctrl Pts',(62.8463779860137,-0.0203329720722545,
40.1001924129685));
#182121=CARTESIAN_POINT('Ctrl Pts',(62.8464416340693,-0.0177904683741538,
40.10025));
#182122=CARTESIAN_POINT('Ctrl Pts',(62.8464427007196,-0.01524,40.10025));
#182123=CARTESIAN_POINT('Ctrl Pts',(59.0285534841296,-0.0152400000000003,
40.10025));
#182124=CARTESIAN_POINT('Ctrl Pts',(59.0285496414744,-0.0238699985092282,
40.10025));
#182125=CARTESIAN_POINT('Ctrl Pts',(59.0292582026622,-0.0324255116353481,
40.0995786334241));
#182126=CARTESIAN_POINT('Ctrl Pts',(59.0305954788489,-0.0407807192225228,
40.0983063763366));
#182127=CARTESIAN_POINT('Ctrl Pts',(59.0314592220531,-0.0461773260301675,
40.0974846287993));
#182128=CARTESIAN_POINT('Ctrl Pts',(59.0325843328198,-0.051490526840898,
40.0964130309338));
#182129=CARTESIAN_POINT('Ctrl Pts',(59.0339399880044,-0.0566895722962414,
40.0951176960923));
#182130=CARTESIAN_POINT('Ctrl Pts',(59.0357368312949,-0.0635806092274516,
40.0934008039614));
#182131=CARTESIAN_POINT('Ctrl Pts',(59.0379438906768,-0.0702685278901257,
40.0912909372156));
#182132=CARTESIAN_POINT('Ctrl Pts',(59.0405007795597,-0.0766865040604523,
40.0888630467851));
#182133=CARTESIAN_POINT('Ctrl Pts',(59.0417792240012,-0.0798954921456156,
40.0876491015699));
#182134=CARTESIAN_POINT('Ctrl Pts',(59.0431451240706,-0.0830371938949207,
40.0863558569271));
#182135=CARTESIAN_POINT('Ctrl Pts',(59.0445909239228,-0.0861046703637865,
40.0849936342771));
#182136=CARTESIAN_POINT('Ctrl Pts',(59.0453138238489,-0.0876384085982195,
40.0843125229521));
#182137=CARTESIAN_POINT('Ctrl Pts',(59.0460566986719,-0.0891536069436217,
40.0836141747074));
#182138=CARTESIAN_POINT('Ctrl Pts',(59.0468186034776,-0.0906495011920565,
40.0828999161609));
#182139=CARTESIAN_POINT('Ctrl Pts',(59.047009079679,-0.0910234747541652,
40.0827213515243));
#182140=CARTESIAN_POINT('Ctrl Pts',(59.0472007452523,-0.0913962421596992,
40.0825417925842));
#182141=CARTESIAN_POINT('Ctrl Pts',(59.0473935854286,-0.0917677921727011,
40.082361260236));
#182142=CARTESIAN_POINT('Ctrl Pts',(59.0479721059574,-0.0928824422117066,
40.0818196631917));
#182143=CARTESIAN_POINT('Ctrl Pts',(59.0485611979309,-0.0939861339737851,
40.0812693052021));
#182144=CARTESIAN_POINT('Ctrl Pts',(59.0491604624443,-0.0950785796749054,
40.0807107531874));
#182145=CARTESIAN_POINT('Ctrl Pts',(59.0533816042977,-0.102773626133362,
40.0767763849181));
#182146=CARTESIAN_POINT('Ctrl Pts',(59.0580834293368,-0.109958823466688,
40.0724140586135));
#182147=CARTESIAN_POINT('Ctrl Pts',(59.0631465696374,-0.116642428647161,
40.0677221223765));
#182148=CARTESIAN_POINT('Ctrl Pts',(59.0656021872118,-0.119883969937114,
40.0654465383718));
#182149=CARTESIAN_POINT('Ctrl Pts',(59.068143371512,-0.123007567718246,
40.0630928000678));
#182150=CARTESIAN_POINT('Ctrl Pts',(59.0707593633743,-0.126014035556417,
40.0606689262479));
#182151=CARTESIAN_POINT('Ctrl Pts',(59.0747642641416,-0.130616727761041,
40.0569581447805));
#182152=CARTESIAN_POINT('Ctrl Pts',(59.0789414743143,-0.134943070277262,
40.0530843804605));
#182153=CARTESIAN_POINT('Ctrl Pts',(59.0832455674828,-0.138985142830725,
40.0490800251457));
#182154=CARTESIAN_POINT('Ctrl Pts',(59.0852444106167,-0.140862302235466,
40.0472203818218));
#182155=CARTESIAN_POINT('Ctrl Pts',(59.0872703932642,-0.142678271527114,
40.0453323608818));
#182156=CARTESIAN_POINT('Ctrl Pts',(59.0893195943183,-0.144431197308738,
40.0434201572162));
#182157=CARTESIAN_POINT('Ctrl Pts',(59.0894766575049,-0.144565552163021,
40.0432735943397));
#182158=CARTESIAN_POINT('Ctrl Pts',(59.0896338466134,-0.144699568925786,
40.0431268995707));
#182159=CARTESIAN_POINT('Ctrl Pts',(59.0897911602042,-0.144833247843074,
40.0429800745037));
#182160=CARTESIAN_POINT('Ctrl Pts',(59.0920009418701,-0.146711033602081,
40.0409176249753));
#182161=CARTESIAN_POINT('Ctrl Pts',(59.0942367399983,-0.148520654544882,
40.0388310783332));
#182162=CARTESIAN_POINT('Ctrl Pts',(59.0964928714566,-0.150262619641264,
40.036725739981));
#182163=CARTESIAN_POINT('Ctrl Pts',(59.1045829576263,-0.156508996678761,
40.0291763710718));
#182164=CARTESIAN_POINT('Ctrl Pts',(59.1129958342949,-0.161935290145609,
40.0213310894596));
#182165=CARTESIAN_POINT('Ctrl Pts',(59.1216309196484,-0.166622470787464,
40.0132837551322));
#182166=CARTESIAN_POINT('Ctrl Pts',(59.1311200109807,-0.171773211443903,
40.0044405431327));
#182167=CARTESIAN_POINT('Ctrl Pts',(59.1408779306737,-0.176031864362409,
39.9953528710602));
#182168=CARTESIAN_POINT('Ctrl Pts',(59.15080876581,-0.179468536017301,39.9861103629556));
#182169=CARTESIAN_POINT('Ctrl Pts',(59.1615315754581,-0.183179278917837,
39.9761307737552));
#182170=CARTESIAN_POINT('Ctrl Pts',(59.1724570142855,-0.185932239424911,
39.9659696936003));
#182171=CARTESIAN_POINT('Ctrl Pts',(59.1834936683149,-0.187766286100047,
39.9557128217493));
#182172=CARTESIAN_POINT('Ctrl Pts',(59.1944377361562,-0.189584947007891,
39.9455419945152));
#182173=CARTESIAN_POINT('Ctrl Pts',(59.205492595812,-0.1905,39.9352756289336));
#182174=CARTESIAN_POINT('Ctrl Pts',(59.2165773020941,-0.1905,39.92499));
#182175=CARTESIAN_POINT('Origin',(0.,0.01524,39.92499));
#182176=CARTESIAN_POINT('Ctrl Pts',(62.8464427007196,0.01524,40.10025));
#182177=CARTESIAN_POINT('Ctrl Pts',(62.8464391086779,0.0238289333903777,
40.10025));
#182178=CARTESIAN_POINT('Ctrl Pts',(62.8457180711405,0.0323412407623314,
40.0995859581842));
#182179=CARTESIAN_POINT('Ctrl Pts',(62.8443658068291,0.0406531130499672,
40.0983275959622));
#182180=CARTESIAN_POINT('Ctrl Pts',(62.843501774309,0.0459640037532213,
40.0975235624069));
#182181=CARTESIAN_POINT('Ctrl Pts',(62.8423809556999,0.0511932363888995,
40.0964777059491));
#182182=CARTESIAN_POINT('Ctrl Pts',(62.841033859251,0.0563116129573394,
40.0952149915961));
#182183=CARTESIAN_POINT('Ctrl Pts',(62.8391953428955,0.0632971699621427,
40.0934916398701));
#182184=CARTESIAN_POINT('Ctrl Pts',(62.8369299537504,0.0700734120983113,
40.0913643921631));
#182185=CARTESIAN_POINT('Ctrl Pts',(62.8343031482014,0.0765705776094334,
40.0889118607713));
#182186=CARTESIAN_POINT('Ctrl Pts',(62.8329897454269,0.0798191603649944,
40.0876855950754));
#182187=CARTESIAN_POINT('Ctrl Pts',(62.8315859904681,0.0829981827952882,
40.0863782327527));
#182188=CARTESIAN_POINT('Ctrl Pts',(62.8301000734874,0.0861004173278454,
40.0850006373334));
#182189=CARTESIAN_POINT('Ctrl Pts',(62.8293571149971,0.0876515345941241,
40.0843118396238));
#182190=CARTESIAN_POINT('Ctrl Pts',(62.8285936160519,0.0891834722996921,
40.0836054919165));
#182191=CARTESIAN_POINT('Ctrl Pts',(62.82781060087,0.090695436427861,40.0828829920418));
#182192=CARTESIAN_POINT('Ctrl Pts',(62.8276148470746,0.0910734274599033,
40.0827023670731));
#182193=CARTESIAN_POINT('Ctrl Pts',(62.8274178735164,0.0914501705143267,
40.0825207326933));
#182194=CARTESIAN_POINT('Ctrl Pts',(62.8272196962038,0.0918256539328356,
40.0823381109275));
#182195=CARTESIAN_POINT('Ctrl Pts',(62.8266251642659,0.0929521041883625,
40.0817902456303));
#182196=CARTESIAN_POINT('Ctrl Pts',(62.826019798519,0.0940672158686514,
40.0812334935553));
#182197=CARTESIAN_POINT('Ctrl Pts',(62.8254040313373,0.0951706907488451,
40.0806684524227));
#182198=CARTESIAN_POINT('Ctrl Pts',(62.8211486980557,0.102796386827344,
40.0767636676138));
#182199=CARTESIAN_POINT('Ctrl Pts',(62.8164204928787,0.109916699411088,
40.0724404510891));
#182200=CARTESIAN_POINT('Ctrl Pts',(62.81133770774,0.116542502759262,40.0677949937414));
#182201=CARTESIAN_POINT('Ctrl Pts',(62.8088115774778,0.119835508836132,
40.0654862141909));
#182202=CARTESIAN_POINT('Ctrl Pts',(62.8061972539434,0.123006400629168,
40.0630972003218));
#182203=CARTESIAN_POINT('Ctrl Pts',(62.8035061084565,0.126056303769965,
40.0606363359906));
#182204=CARTESIAN_POINT('Ctrl Pts',(62.7975690395531,0.132784845643283,
40.0552073017123));
#182205=CARTESIAN_POINT('Ctrl Pts',(62.7912680187377,0.138932019324687,
40.0494204304519));
#182206=CARTESIAN_POINT('Ctrl Pts',(62.7847385034067,0.14444511341317,40.0434049749851));
#182207=CARTESIAN_POINT('Ctrl Pts',(62.7823531891148,0.146459116207466,
40.0412074532442));
#182208=CARTESIAN_POINT('Ctrl Pts',(62.7799396422115,0.148396130390979,
40.0389814735788));
#182209=CARTESIAN_POINT('Ctrl Pts',(62.7775029828616,0.150257579786486,
40.0367321210016));
#182210=CARTESIAN_POINT('Ctrl Pts',(62.769318501945,0.156509991333365,40.0291767837143));
#182211=CARTESIAN_POINT('Ctrl Pts',(62.7608162581029,0.161942805717658,
40.0213235332581));
#182212=CARTESIAN_POINT('Ctrl Pts',(62.7520965944507,0.166635979460955,
40.0132649215866));
#182213=CARTESIAN_POINT('Ctrl Pts',(62.7425126511848,0.171794333347845,
40.0044075527543));
#182214=CARTESIAN_POINT('Ctrl Pts',(62.7326655363519,0.176059615357,39.9953016253733));
#182215=CARTESIAN_POINT('Ctrl Pts',(62.7226511116323,0.179500292056221,
39.9860353422374));
#182216=CARTESIAN_POINT('Ctrl Pts',(62.7118651471253,0.183206048282561,
39.9760551582714));
#182217=CARTESIAN_POINT('Ctrl Pts',(62.7008840239684,0.185955767118701,
39.9658879738179));
#182218=CARTESIAN_POINT('Ctrl Pts',(62.6897991274298,0.187785458034746,
39.9556174643281));
#182219=CARTESIAN_POINT('Ctrl Pts',(62.6788639144199,0.189590441945929,
39.9454856413922));
#182220=CARTESIAN_POINT('Ctrl Pts',(62.6678262782743,0.1905,39.9352519465122));
#182221=CARTESIAN_POINT('Ctrl Pts',(62.6567671111299,0.1905,39.92499));
#182222=CARTESIAN_POINT('Ctrl Pts',(59.2165773020941,0.1905,39.92499));
#182223=CARTESIAN_POINT('Ctrl Pts',(59.2059936184293,0.1905,39.9348107241722));
#182224=CARTESIAN_POINT('Ctrl Pts',(59.1954479901463,0.18966522548866,39.9446038383169));
#182225=CARTESIAN_POINT('Ctrl Pts',(59.1849969778462,0.188008762314096,
39.9543158069384));
#182226=CARTESIAN_POINT('Ctrl Pts',(59.17490560595,0.186409301377007,39.9636935671391));
#182227=CARTESIAN_POINT('Ctrl Pts',(59.1649012152151,0.184043455438166,
39.9729968320987));
#182228=CARTESIAN_POINT('Ctrl Pts',(59.1550396955537,0.18087742372664,39.9821731151334));
#182229=CARTESIAN_POINT('Ctrl Pts',(59.1457174710368,0.177884532219491,
39.9908475764351));
#182230=CARTESIAN_POINT('Ctrl Pts',(59.1365220583453,0.174176304386962,
39.9994093733845));
#182231=CARTESIAN_POINT('Ctrl Pts',(59.1275197082956,0.169686797572386,
40.0077966115841));
#182232=CARTESIAN_POINT('Ctrl Pts',(59.1192286949255,0.165552037113266,
40.0155211172595));
#182233=CARTESIAN_POINT('Ctrl Pts',(59.1111009786088,0.160754293903562,
40.0230979941021));
#182234=CARTESIAN_POINT('Ctrl Pts',(59.1032135992724,0.155213515013196,
40.0304554104748));
#182235=CARTESIAN_POINT('Ctrl Pts',(59.1008617419714,0.153561366595946,
40.0326492435181));
#182236=CARTESIAN_POINT('Ctrl Pts',(59.098531460358,0.151842962927709,40.0348233715061));
#182237=CARTESIAN_POINT('Ctrl Pts',(59.096225375957,0.150055686180142,40.0369753512356));
#182238=CARTESIAN_POINT('Ctrl Pts',(59.093942854056,0.148286670996707,40.0391053430352));
#182239=CARTESIAN_POINT('Ctrl Pts',(59.0916862380348,0.146452235168901,
40.041211089324));
#182240=CARTESIAN_POINT('Ctrl Pts',(59.0894604907299,0.144552116609965,
40.0432881154904));
#182241=CARTESIAN_POINT('Ctrl Pts',(59.0893057166152,0.144419986081416,
40.043432547828));
#182242=CARTESIAN_POINT('Ctrl Pts',(59.0891510807051,0.144287542502095,
40.0435768364421));
#182243=CARTESIAN_POINT('Ctrl Pts',(59.0889965840074,0.144154785043939,
40.0437209807855));
#182244=CARTESIAN_POINT('Ctrl Pts',(59.0822228828154,0.138334211749542,
40.050040796842));
#182245=CARTESIAN_POINT('Ctrl Pts',(59.0757535782846,0.131883990154185,
40.0560490279344));
#182246=CARTESIAN_POINT('Ctrl Pts',(59.0697047694308,0.124808417215433,
40.0616647108614));
#182247=CARTESIAN_POINT('Ctrl Pts',(59.0640662283033,0.118212753510261,
40.0668995033484));
#182248=CARTESIAN_POINT('Ctrl Pts',(59.0587927761314,0.111072931137642,
40.071793326748));
#182249=CARTESIAN_POINT('Ctrl Pts',(59.05400766547,0.103389544768602,40.076246030307));
#182250=CARTESIAN_POINT('Ctrl Pts',(59.0522572100838,0.100578862632908,
40.0778748868746));
#182251=CARTESIAN_POINT('Ctrl Pts',(59.0505724231958,0.0976954648439348,
40.0794443522247));
#182252=CARTESIAN_POINT('Ctrl Pts',(59.048960544286,0.094739558525343,40.0809482021492));
#182253=CARTESIAN_POINT('Ctrl Pts',(59.0485729412563,0.0940287618038469,
40.0813098278168));
#182254=CARTESIAN_POINT('Ctrl Pts',(59.0481896206934,0.0933131922167491,
40.0816679525672));
#182255=CARTESIAN_POINT('Ctrl Pts',(59.0478106940136,0.092592927197163,
40.082022419258));
#182256=CARTESIAN_POINT('Ctrl Pts',(59.0474436087926,0.0918951704594389,
40.0823658088648));
#182257=CARTESIAN_POINT('Ctrl Pts',(59.0470806471271,0.0911930071934228,
40.0827057654616));
#182258=CARTESIAN_POINT('Ctrl Pts',(59.0467219102889,0.0904865115878245,
40.0830421470151));
#182259=CARTESIAN_POINT('Ctrl Pts',(59.0427915336441,0.0827460357498801,
40.0867275956806));
#182260=CARTESIAN_POINT('Ctrl Pts',(59.039366072413,0.0744802459943286,
40.0899823432031));
#182261=CARTESIAN_POINT('Ctrl Pts',(59.036584160269,0.0658168714608708,
40.0926299529356));
#182262=CARTESIAN_POINT('Ctrl Pts',(59.0354304183829,0.0622239118143531,
40.0937279956084));
#182263=CARTESIAN_POINT('Ctrl Pts',(59.0343871039217,0.0585629032864951,
40.0947220371802));
#182264=CARTESIAN_POINT('Ctrl Pts',(59.0334626554262,0.0548440714999742,
40.0956014538692));
#182265=CARTESIAN_POINT('Ctrl Pts',(59.0318859121828,0.048501216358407,
40.097101390674));
#182266=CARTESIAN_POINT('Ctrl Pts',(59.0306571138137,0.0419914004944189,
40.0982667904316));
#182267=CARTESIAN_POINT('Ctrl Pts',(59.0298212958157,0.0353717968088257,
40.0990539325582));
#182268=CARTESIAN_POINT('Ctrl Pts',(59.0294033868167,0.032061994966029,
40.0994475036216));
#182269=CARTESIAN_POINT('Ctrl Pts',(59.0290851681639,0.0287246785546796,
40.0997467259952));
#182270=CARTESIAN_POINT('Ctrl Pts',(59.0288723192866,0.0253670368748701,
40.0999473488896));
#182271=CARTESIAN_POINT('Ctrl Pts',(59.0286594704093,0.0220093951950606,
40.100147971784));
#182272=CARTESIAN_POINT('Ctrl Pts',(59.0285519740191,0.0186314705080073,
40.10025));
#182273=CARTESIAN_POINT('Ctrl Pts',(59.0285534841296,0.01524,40.10025));
#182274=CARTESIAN_POINT('Origin',(61.4240753804089,-0.317499999706107,39.1925554495083));
#182275=CARTESIAN_POINT('Origin',(61.4683012396072,-0.317551690012947,39.116037328526));
#182276=CARTESIAN_POINT('Origin',(61.3422370451705,-0.3175,39.3343017080178));
#182277=CARTESIAN_POINT('Ctrl Pts',(61.2322532920972,-0.316930737395914,
39.2708017080178));
#182278=CARTESIAN_POINT('Ctrl Pts',(61.2327440814646,-0.190499999999994,
39.2710850691866));
#182279=CARTESIAN_POINT('Ctrl Pts',(61.3422370451705,-0.1905,39.3343017080178));
#182280=CARTESIAN_POINT('Ctrl Pts',(61.1872475084174,-0.317046579199636,
39.3487519293518));
#182281=CARTESIAN_POINT('Ctrl Pts',(61.1875064541762,-0.190500000001215,
39.3492068662928));
#182282=CARTESIAN_POINT('Ctrl Pts',(61.2747290395312,-0.1905,39.451227124874));
#182283=CARTESIAN_POINT('Ctrl Pts',(61.1019842137032,-0.31726659691349,
39.3978017080178));
#182284=CARTESIAN_POINT('Ctrl Pts',(61.1018997758106,-0.190499999999995,
39.3980347781183));
#182285=CARTESIAN_POINT('Ctrl Pts',(61.146836207171,-0.1905,39.5248015355195));
#182286=CARTESIAN_POINT('Ctrl Pts',(61.0122769227456,-0.3175,39.3978017080178));
#182287=CARTESIAN_POINT('Ctrl Pts',(61.0122769227456,-0.1905,39.3978017080178));
#182288=CARTESIAN_POINT('Ctrl Pts',(61.0122769227456,-0.1905,39.5248017080178));
#182289=CARTESIAN_POINT('Origin',(61.0122769227456,-0.3175,39.5248017080178));
#182290=CARTESIAN_POINT('Origin',(5.50819412990574E-15,-0.3175,39.116));
#182291=CARTESIAN_POINT('Origin',(61.8696548221181,-0.3175,39.116));
#182292=CARTESIAN_POINT('Origin',(5.56576032196012E-15,-0.3175,39.5248017080178));
#182293=CARTESIAN_POINT('Origin',(60.8610688070707,-0.3175,39.5248017080178));
#182294=CARTESIAN_POINT('Ctrl Pts',(62.4081695979768,-0.318048871877129,
39.2875012672119));
#182295=CARTESIAN_POINT('Ctrl Pts',(62.4086377819835,-0.190309034175017,
39.287208709576));
#182296=CARTESIAN_POINT('Ctrl Pts',(62.3003077603769,-0.190500142125054,
39.3549016990126));
#182297=CARTESIAN_POINT('Ctrl Pts',(62.2931881445371,-0.31793248988995,
39.103493917393));
#182298=CARTESIAN_POINT('Ctrl Pts',(62.2934975005738,-0.190309294367355,
39.1031692336349));
#182299=CARTESIAN_POINT('Ctrl Pts',(62.208356400327,-0.190500141995468,
39.2077507202312));
#182300=CARTESIAN_POINT('Ctrl Pts',(62.0866281564672,-0.317722686167412,
38.989));
#182301=CARTESIAN_POINT('Ctrl Pts',(62.0868143053088,-0.190309769569384,
38.9887769311152));
#182302=CARTESIAN_POINT('Ctrl Pts',(62.0431695205371,-0.190500141761867,
39.1161898712897));
#182303=CARTESIAN_POINT('Ctrl Pts',(61.8696548221181,-0.3175,38.989));
#182304=CARTESIAN_POINT('Ctrl Pts',(61.8696548221181,-0.190310267888658,
38.989));
#182305=CARTESIAN_POINT('Ctrl Pts',(61.8696548221181,-0.190500141513915,
39.116189590386));
#182306=CARTESIAN_POINT('Origin',(62.3004688883555,-0.3175,39.3548010137695));
#182307=CARTESIAN_POINT('Ctrl Pts',(60.8610688070707,-0.3175,39.3978017080178));
#182308=CARTESIAN_POINT('Ctrl Pts',(60.8610688070707,-0.1905,39.3978017080178));
#182309=CARTESIAN_POINT('Ctrl Pts',(60.8610688070707,-0.1905,39.5248017080178));
#182310=CARTESIAN_POINT('Ctrl Pts',(60.7710583184321,-0.317734773760269,
39.3978017080178));
#182311=CARTESIAN_POINT('Ctrl Pts',(60.7709717342408,-0.190499999999991,
39.3975666025021));
#182312=CARTESIAN_POINT('Ctrl Pts',(60.7260547307352,-0.1905,39.5248015517177));
#182313=CARTESIAN_POINT('Ctrl Pts',(60.6859465754578,-0.31795861791903,
39.3484894016716));
#182314=CARTESIAN_POINT('Ctrl Pts',(60.6862105562579,-0.190500000001618,
39.3480259000038));
#182315=CARTESIAN_POINT('Ctrl Pts',(60.5983892955417,-0.1905,39.4508333188945));
#182316=CARTESIAN_POINT('Ctrl Pts',(60.6410923272405,-0.318076890623366,
39.2708017080178));
#182317=CARTESIAN_POINT('Ctrl Pts',(60.6415942020421,-0.1905,39.27051194648));
#182318=CARTESIAN_POINT('Ctrl Pts',(60.5311086139135,-0.1905,39.3343017080178));
#182319=CARTESIAN_POINT('Origin',(60.5311086139135,-0.3175,39.3343017080178));
#182320=CARTESIAN_POINT('Origin',(62.4786179998489,-0.31749999997796,39.6398955068184));
#182321=CARTESIAN_POINT('Origin',(62.6567671111299,-0.3175,39.92499));
#182322=CARTESIAN_POINT('Origin',(60.4497583458782,-0.317499999994971,39.1934008539952));
#182323=CARTESIAN_POINT('Origin',(60.4050521322801,-0.317550804320654,39.1160402713849));
#182324=CARTESIAN_POINT('Ctrl Pts',(62.9541448057648,-0.0152661173108668,
40.1599502534424));
#182325=CARTESIAN_POINT('Ctrl Pts',(62.9168399481843,-0.0152570710386341,
40.10025));
#182326=CARTESIAN_POINT('Ctrl Pts',(62.8464427007196,-0.01524,40.10025));
#182327=CARTESIAN_POINT('Ctrl Pts',(62.9541233134297,-0.103381504925241,
40.1599500538463));
#182328=CARTESIAN_POINT('Ctrl Pts',(62.9168211560341,-0.0794415635236045,
40.100244835349));
#182329=CARTESIAN_POINT('Ctrl Pts',(62.8464212442881,-0.0662446030559618,
40.10025));
#182330=CARTESIAN_POINT('Ctrl Pts',(62.9290872705826,-0.184683583687744,
40.1202442001037));
#182331=CARTESIAN_POINT('Ctrl Pts',(62.8936771137448,-0.138547994784254,
40.0633873868017));
#182332=CARTESIAN_POINT('Ctrl Pts',(62.8213855864655,-0.113305567451532,
40.0772271723538));
#182333=CARTESIAN_POINT('Ctrl Pts',(62.8564203507742,-0.291340992631754,
40.0045995998164));
#182334=CARTESIAN_POINT('Ctrl Pts',(62.8329175802742,-0.201910351191398,
39.9663485808314));
#182335=CARTESIAN_POINT('Ctrl Pts',(62.7487193609389,-0.175042741957872,
40.0101727202466));
#182336=CARTESIAN_POINT('Ctrl Pts',(62.8099434033761,-0.318045276842621,
39.9304654349858));
#182337=CARTESIAN_POINT('Ctrl Pts',(62.7947175425014,-0.205831635642736,
39.905190016294));
#182338=CARTESIAN_POINT('Ctrl Pts',(62.7022409210439,-0.190500000000001,
39.9671857458183));
#182339=CARTESIAN_POINT('Ctrl Pts',(62.7644678366119,-0.318045750793045,
39.8576902534424));
#182340=CARTESIAN_POINT('Ctrl Pts',(62.7649326510148,-0.1905,39.8573998014387));
#182341=CARTESIAN_POINT('Ctrl Pts',(62.6567671111299,-0.1905,39.92499));
#182342=CARTESIAN_POINT('Origin',(62.8464427007196,-0.01524,40.22725));
#182343=CARTESIAN_POINT('Origin',(5.50819412990574E-15,-0.3175,39.116));
#182344=CARTESIAN_POINT('Origin',(60.0036905223731,-0.3175,39.116));
#182345=CARTESIAN_POINT('Origin',(-1.95097259456047E-16,0.,40.22725));
#182346=CARTESIAN_POINT('Origin',(62.8464427007196,0.01524,40.22725));
#182347=CARTESIAN_POINT('Ctrl Pts',(60.0036905223731,-0.3175,38.989));
#182348=CARTESIAN_POINT('Ctrl Pts',(60.0036905223731,-0.19030974826532,
38.989));
#182349=CARTESIAN_POINT('Ctrl Pts',(60.003690522373,-0.190500142289529,
39.116190109232));
#182350=CARTESIAN_POINT('Ctrl Pts',(59.7867137603524,-0.317270385524412,
38.989));
#182351=CARTESIAN_POINT('Ctrl Pts',(59.7869045527967,-0.190310262476384,
38.9892298989766));
#182352=CARTESIAN_POINT('Ctrl Pts',(59.8301727552493,-0.190500142032462,
39.1161900493206));
#182353=CARTESIAN_POINT('Ctrl Pts',(59.5801552670728,-0.317049440713614,
39.1034966344368));
#182354=CARTESIAN_POINT('Ctrl Pts',(59.5804765271874,-0.190310761082376,
39.1038314102564));
#182355=CARTESIAN_POINT('Ctrl Pts',(59.6649871046552,-0.190500141785105,
39.2077528789596));
#182356=CARTESIAN_POINT('Ctrl Pts',(59.4651754363832,-0.316925998273047,
39.2875012672119));
#182357=CARTESIAN_POINT('Ctrl Pts',(59.4656607446594,-0.190311035335061,
39.2878045257868));
#182358=CARTESIAN_POINT('Ctrl Pts',(59.5730368716576,-0.190500141646902,
39.3549015295898));
#182359=CARTESIAN_POINT('Origin',(59.5728760150042,-0.3175,39.3548010137695));
#182360=CARTESIAN_POINT('Ctrl Pts',(62.7644678366119,0.318045750793045,
39.8576902534424));
#182361=CARTESIAN_POINT('Ctrl Pts',(62.7649326510148,0.1905,39.8573998014387));
#182362=CARTESIAN_POINT('Ctrl Pts',(62.6567671111299,0.1905,39.92499));
#182363=CARTESIAN_POINT('Ctrl Pts',(62.8099640589334,0.318045262795179,
39.9304984902489));
#182364=CARTESIAN_POINT('Ctrl Pts',(62.7947344577637,0.205840330723205,
39.9052171569779));
#182365=CARTESIAN_POINT('Ctrl Pts',(62.7022616416345,0.1905,39.9672049726594));
#182366=CARTESIAN_POINT('Ctrl Pts',(62.8562601188215,0.29133411785554,40.0043437678664));
#182367=CARTESIAN_POINT('Ctrl Pts',(62.8328016940825,0.201836550627893,
39.9661628577643));
#182368=CARTESIAN_POINT('Ctrl Pts',(62.7485591297232,0.175038734052128,
40.0100243556235));
#182369=CARTESIAN_POINT('Ctrl Pts',(62.928611257107,0.18562218956026,40.1194874821985));
#182370=CARTESIAN_POINT('Ctrl Pts',(62.8932808767899,0.139140155999965,
40.062755148314));
#182371=CARTESIAN_POINT('Ctrl Pts',(62.8209095783125,0.113848895265745,
40.0767884282377));
#182372=CARTESIAN_POINT('Ctrl Pts',(62.9541233349674,0.103673266462929,
40.1599502015391));
#182373=CARTESIAN_POINT('Ctrl Pts',(62.9168211653022,0.0796882264537865,
40.1002449453869));
#182374=CARTESIAN_POINT('Ctrl Pts',(62.8464212664863,0.0664134143651042,
40.10025));
#182375=CARTESIAN_POINT('Ctrl Pts',(62.9541448057648,0.0152661173108668,
40.1599502534424));
#182376=CARTESIAN_POINT('Ctrl Pts',(62.9168399481843,0.0152570710386341,
40.10025));
#182377=CARTESIAN_POINT('Ctrl Pts',(62.8464427007196,0.01524,40.10025));
#182378=CARTESIAN_POINT('Origin',(62.6567671111299,0.3175,39.92499));
#182379=CARTESIAN_POINT('Origin',(59.3947266586252,-0.317499999970944,39.6398955069323));
#182380=CARTESIAN_POINT('Origin',(59.2165773020941,-0.3175,39.92499));
#182381=CARTESIAN_POINT('Origin',(62.478617999835,0.317499999978368,39.6398955068271));
#182382=CARTESIAN_POINT('Origin',(62.3004688883555,0.3175,39.3548010137695));
#182383=CARTESIAN_POINT('Ctrl Pts',(59.1088767419348,-0.316922544675689,
39.8576902534424));
#182384=CARTESIAN_POINT('Ctrl Pts',(59.1093642282367,-0.1905,39.8579948730703));
#182385=CARTESIAN_POINT('Ctrl Pts',(59.2165773020941,-0.1905,39.92499));
#182386=CARTESIAN_POINT('Ctrl Pts',(59.0634407053229,-0.316922012809157,
39.9304020711231));
#182387=CARTESIAN_POINT('Ctrl Pts',(59.0793536643045,-0.2056949737408,39.9058915297385));
#182388=CARTESIAN_POINT('Ctrl Pts',(59.1711393827295,-0.1905,39.9671523786035));
#182389=CARTESIAN_POINT('Ctrl Pts',(59.0174076205276,-0.290332993455009,
40.0043257306693));
#182390=CARTESIAN_POINT('Ctrl Pts',(59.0412846811395,-0.201480151665877,
39.9667894847835));
#182391=CARTESIAN_POINT('Ctrl Pts',(59.1251084688121,-0.175054909459681,
40.01001389752));
#182392=CARTESIAN_POINT('Ctrl Pts',(58.9458296250062,-0.184894967401558,
40.1195533054857));
#182393=CARTESIAN_POINT('Ctrl Pts',(58.9812445774292,-0.138672156931214,
40.0630813209236));
#182394=CARTESIAN_POINT('Ctrl Pts',(59.0535312451933,-0.113807322597802,
40.076826594242));
#182395=CARTESIAN_POINT('Ctrl Pts',(58.9208287018091,-0.103171606455737,
40.1599502027518));
#182396=CARTESIAN_POINT('Ctrl Pts',(58.9581363848263,-0.0793367652458399,
40.1002552791541));
#182397=CARTESIAN_POINT('Ctrl Pts',(59.0285307646513,-0.0663350652343413,
40.10025));
#182398=CARTESIAN_POINT('Ctrl Pts',(58.9208513795073,-0.0152121934559204,
40.1599502534424));
#182399=CARTESIAN_POINT('Ctrl Pts',(58.9581562369413,-0.0152218248291072,
40.10025));
#182400=CARTESIAN_POINT('Ctrl Pts',(59.0285534841296,-0.0152400000000003,
40.10025));
#182401=CARTESIAN_POINT('Origin',(59.0285534841296,-0.01524,40.22725));
#182402=CARTESIAN_POINT('Ctrl Pts',(61.8696548221181,0.3175,38.989));
#182403=CARTESIAN_POINT('Ctrl Pts',(61.8696548221181,0.190310256931022,
38.989));
#182404=CARTESIAN_POINT('Ctrl Pts',(61.8696548221181,0.190500141530249,
39.1161896013273));
#182405=CARTESIAN_POINT('Ctrl Pts',(62.0866315324121,0.31772268963223,38.989));
#182406=CARTESIAN_POINT('Ctrl Pts',(62.0868176889525,0.19030975857524,38.9887769275436));
#182407=CARTESIAN_POINT('Ctrl Pts',(62.0431722165642,0.190500141778233,
39.116189882183));
#182408=CARTESIAN_POINT('Ctrl Pts',(62.2931898887681,0.317932491655691,
39.1034967087243));
#182409=CARTESIAN_POINT('Ctrl Pts',(62.2934992458059,0.190309283351463,
39.1031720232722));
#182410=CARTESIAN_POINT('Ctrl Pts',(62.2083577878531,0.190500142011856,
39.2077529615015));
#182411=CARTESIAN_POINT('Ctrl Pts',(62.4081695979768,0.318048871877129,
39.2875012672119));
#182412=CARTESIAN_POINT('Ctrl Pts',(62.4086377820239,0.190309023146095,
39.2872087095507));
#182413=CARTESIAN_POINT('Ctrl Pts',(62.3003077510782,0.190500142141459,
39.3549017048231));
#182414=CARTESIAN_POINT('Origin',(61.8696548221181,0.3175,39.116));
#182415=CARTESIAN_POINT('Origin',(4.7062627014205E-16,0.,40.22725));
#182416=CARTESIAN_POINT('Origin',(59.0285534841296,0.01524,40.22725));
#182417=CARTESIAN_POINT('Origin',(62.2224557307631,0.3175,39.116));
#182418=CARTESIAN_POINT('Origin',(61.4683012396074,0.317551690013413,39.1160373285266));
#182419=CARTESIAN_POINT('Ctrl Pts',(58.9208513795073,0.0152121934559198,
40.1599502534424));
#182420=CARTESIAN_POINT('Ctrl Pts',(58.9581562369414,0.0152218248291069,
40.10025));
#182421=CARTESIAN_POINT('Ctrl Pts',(59.0285534841296,0.01524,40.10025));
#182422=CARTESIAN_POINT('Ctrl Pts',(58.9208288705618,0.102871702177323,
40.1599500566037));
#182423=CARTESIAN_POINT('Ctrl Pts',(58.9581365422943,0.0790852439333523,
40.1002551305372));
#182424=CARTESIAN_POINT('Ctrl Pts',(59.0285309330218,0.0661608181924836,
40.10025));
#182425=CARTESIAN_POINT('Ctrl Pts',(58.9453619764183,0.183955833237606,
40.1203070619046));
#182426=CARTESIAN_POINT('Ctrl Pts',(58.9808530699761,0.138075936736041,
40.0637098684499));
#182427=CARTESIAN_POINT('Ctrl Pts',(59.0530636028226,0.113261762368195,
40.0772636213362));
#182428=CARTESIAN_POINT('Ctrl Pts',(59.0172303255294,0.290319860890557,
40.0046102245801));
#182429=CARTESIAN_POINT('Ctrl Pts',(59.0411528690721,0.201541405841854,
39.9670001894012));
#182430=CARTESIAN_POINT('Ctrl Pts',(59.1249311745757,0.17504730955115,40.0101788811209));
#182431=CARTESIAN_POINT('Ctrl Pts',(59.0634600627912,0.316922027357347,
39.9303710930186));
#182432=CARTESIAN_POINT('Ctrl Pts',(59.0793694364691,0.20568700036727,39.9058663574113));
#182433=CARTESIAN_POINT('Ctrl Pts',(59.1711586818658,0.1905,39.9671344706364));
#182434=CARTESIAN_POINT('Ctrl Pts',(59.1088767419348,0.316922544675689,
39.8576902534424));
#182435=CARTESIAN_POINT('Ctrl Pts',(59.1093642282367,0.1905,39.8579948730703));
#182436=CARTESIAN_POINT('Ctrl Pts',(59.2165773020941,0.1905,39.92499));
#182437=CARTESIAN_POINT('Origin',(59.2165773020941,0.3175,39.92499));
#182438=CARTESIAN_POINT('Origin',(61.4240753793296,0.317499999995729,39.1925554488852));
#182439=CARTESIAN_POINT('Origin',(61.3422370451705,0.3175,39.3343017080178));
#182440=CARTESIAN_POINT('Origin',(59.3947266586076,0.317499999969843,39.6398955069213));
#182441=CARTESIAN_POINT('Origin',(59.5728760150042,0.3175,39.3548010137695));
#182442=CARTESIAN_POINT('Ctrl Pts',(61.0122769227456,0.3175,39.3978017080178));
#182443=CARTESIAN_POINT('Ctrl Pts',(61.0122769227456,0.1905,39.3978017080178));
#182444=CARTESIAN_POINT('Ctrl Pts',(61.0122769227456,0.1905,39.5248017080178));
#182445=CARTESIAN_POINT('Ctrl Pts',(61.1022873990971,0.317265808076389,
39.3978017080178));
#182446=CARTESIAN_POINT('Ctrl Pts',(61.1022028716714,0.190499999999991,
39.3980355775177));
#182447=CARTESIAN_POINT('Ctrl Pts',(61.1472909869841,0.1905,39.5248015517192));
#182448=CARTESIAN_POINT('Ctrl Pts',(61.1873990841185,0.317046189129096,
39.3484893995498));
#182449=CARTESIAN_POINT('Ctrl Pts',(61.1876587562312,0.190500000001213,
39.3489438303423));
#182450=CARTESIAN_POINT('Ctrl Pts',(61.2749563897832,0.1905,39.4508333155592));
#182451=CARTESIAN_POINT('Ctrl Pts',(61.2322532920972,0.316930737395914,
39.2708017080178));
#182452=CARTESIAN_POINT('Ctrl Pts',(61.2327440814646,0.190499999999994,
39.2710850691866));
#182453=CARTESIAN_POINT('Ctrl Pts',(61.3422370451705,0.1905,39.3343017080178));
#182454=CARTESIAN_POINT('Origin',(61.0122769227456,0.3175,39.5248017080178));
#182455=CARTESIAN_POINT('Ctrl Pts',(59.4651754363832,0.316925998273047,
39.2875012672119));
#182456=CARTESIAN_POINT('Ctrl Pts',(59.4656607446034,0.190311049925411,
39.2878045257518));
#182457=CARTESIAN_POINT('Ctrl Pts',(59.5730368592467,0.190500141625045,
39.3549015218345));
#182458=CARTESIAN_POINT('Ctrl Pts',(59.5801570044831,0.317049442579172,
39.1034938540228));
#182459=CARTESIAN_POINT('Ctrl Pts',(59.5804782634901,0.190310775688126,
39.1038286278819));
#182460=CARTESIAN_POINT('Ctrl Pts',(59.6649884842725,0.190500141763232,
39.2077506434032));
#182461=CARTESIAN_POINT('Ctrl Pts',(59.7867171285936,0.317270389088827,
38.989));
#182462=CARTESIAN_POINT('Ctrl Pts',(59.7869079131798,0.190310277118492,
38.9892298954611));
#182463=CARTESIAN_POINT('Ctrl Pts',(59.8301754438916,0.19050014201055,39.1161900347286));
#182464=CARTESIAN_POINT('Ctrl Pts',(60.0036905223731,0.3175,38.989));
#182465=CARTESIAN_POINT('Ctrl Pts',(60.0036905223731,0.190309762955091,
38.989));
#182466=CARTESIAN_POINT('Ctrl Pts',(60.0036905223731,0.190500142267573,
39.1161900945642));
#182467=CARTESIAN_POINT('Origin',(60.0036905223731,0.3175,39.116));
#182468=CARTESIAN_POINT('Origin',(60.71525,0.3175,39.5248017080178));
#182469=CARTESIAN_POINT('Origin',(60.8610688070707,0.3175,39.5248017080178));
#182470=CARTESIAN_POINT('Origin',(60.4792282238308,0.3175,39.116));
#182471=CARTESIAN_POINT('Origin',(60.4050521322803,0.317550804320378,39.1160402713846));
#182472=CARTESIAN_POINT('Ctrl Pts',(60.6410923272405,0.318076890623366,
39.2708017080178));
#182473=CARTESIAN_POINT('Ctrl Pts',(60.6415942020421,0.1905,39.27051194648));
#182474=CARTESIAN_POINT('Ctrl Pts',(60.5311086139135,0.1905,39.3343017080178));
#182475=CARTESIAN_POINT('Ctrl Pts',(60.6860981505083,0.317958218318763,
39.3487519301186));
#182476=CARTESIAN_POINT('Ctrl Pts',(60.6863613750282,0.190499999999993,
39.3482879463987));
#182477=CARTESIAN_POINT('Ctrl Pts',(60.5986166446955,0.1905,39.451227126164));
#182478=CARTESIAN_POINT('Ctrl Pts',(60.771361502534,0.317733982967541,39.3978017080178));
#182479=CARTESIAN_POINT('Ctrl Pts',(60.7712750141994,0.190499999999998,
39.3975673827397));
#182480=CARTESIAN_POINT('Ctrl Pts',(60.7265095085051,0.1905,39.524801535518));
#182481=CARTESIAN_POINT('Ctrl Pts',(60.8610688070707,0.3175,39.3978017080178));
#182482=CARTESIAN_POINT('Ctrl Pts',(60.8610688070707,0.1905,39.3978017080178));
#182483=CARTESIAN_POINT('Ctrl Pts',(60.8610688070707,0.1905,39.5248017080178));
#182484=CARTESIAN_POINT('Origin',(60.5311086139135,0.3175,39.3343017080178));
#182485=CARTESIAN_POINT('Origin',(60.449758346987,0.317500000300332,39.193400853355));
#182486=CARTESIAN_POINT('Origin',(57.9645097668785,-5.90076614434076,40.10025));
#182487=CARTESIAN_POINT('',(58.7035958781039,-6.18532049829399,40.10025));
#182488=CARTESIAN_POINT('',(62.5005702980931,-6.58439859103029,40.10025));
#182489=CARTESIAN_POINT('',(57.9430040808458,-6.10537907909383,40.10025));
#182490=CARTESIAN_POINT('',(62.5037563256535,-6.55408556365946,40.10025));
#182491=CARTESIAN_POINT('Origin',(5.50059263827931E-15,5.71025087946725E-15,
40.10025));
#182492=CARTESIAN_POINT('',(58.7067819056643,-6.15500747092316,40.10025));
#182493=CARTESIAN_POINT('',(58.63646617859,-6.14761699020186,40.10025));
#182494=CARTESIAN_POINT('Origin',(5.72291486498914E-15,5.24470718193599E-15,
40.10025));
#182495=CARTESIAN_POINT('Origin',(0.019912672252488,0.189456421067656,-2.80404091450791E-18));
#182496=CARTESIAN_POINT('',(59.6948966996543,-6.08263713962388,39.116));
#182497=CARTESIAN_POINT('',(59.2664422392336,-6.0376047612152,39.3548010137695));
#182498=CARTESIAN_POINT('Origin',(59.6568751110691,-6.07864090963206,39.555029783282));
#182499=CARTESIAN_POINT('',(58.9120953678975,-6.00036140481896,39.92499));
#182500=CARTESIAN_POINT('',(59.2664422392336,-6.0376047612152,39.3548010137695));
#182501=CARTESIAN_POINT('',(62.3334394572619,-6.35995915837802,39.92499));
#182502=CARTESIAN_POINT('',(62.5918026085422,-6.38711421981416,39.92499));
#182503=CARTESIAN_POINT('',(61.9790930734951,-6.32271585208485,39.3548010137695));
#182504=CARTESIAN_POINT('',(62.3334394572619,-6.35995915837802,39.92499));
#182505=CARTESIAN_POINT('',(61.5506390517262,-6.27768352038853,39.116));
#182506=CARTESIAN_POINT('Origin',(61.5886607627709,-6.28167976325137,39.5550293907194));
#182507=CARTESIAN_POINT('',(61.1514583086406,-6.23572793293807,39.116));
#182508=CARTESIAN_POINT('',(0.0199126722524935,0.189456421067656,39.116));
#182509=CARTESIAN_POINT('',(61.0261105245454,-6.22255335066416,39.3343017080178));
#182510=CARTESIAN_POINT('',(61.1514583085662,-6.23572793364592,39.116));
#182511=CARTESIAN_POINT('',(60.6979579581954,-6.18806312612747,39.5248017080178));
#182512=CARTESIAN_POINT('Origin',(60.7272241158256,-6.19113963944979,39.1947747614368));
#182513=CARTESIAN_POINT('',(60.5475781763993,-6.17225757416238,39.5248017080178));
#182514=CARTESIAN_POINT('',(0.0199126722524936,0.189456421067656,39.5248017080178));
#182515=CARTESIAN_POINT('',(60.2194255397045,-6.13776734223215,39.3343017080178));
#182516=CARTESIAN_POINT('Origin',(60.5183090188078,-6.16918177799145,39.1947728911918));
#182517=CARTESIAN_POINT('',(60.0940777033447,-6.12459275374935,39.116));
#182518=CARTESIAN_POINT('',(60.2194255397045,-6.13776734223215,39.3343017080178));
#182519=CARTESIAN_POINT('',(0.0199126722524935,0.189456421067656,39.116));
#182520=CARTESIAN_POINT('Origin',(-0.019912672252488,-0.189456421067656,
2.80404091450791E-18));
#182521=CARTESIAN_POINT('',(61.5108137072212,-6.65659636252384,39.116));
#182522=CARTESIAN_POINT('',(61.9392677289269,-6.70162869482172,39.3548010137695));
#182523=CARTESIAN_POINT('Origin',(61.5488354179797,-6.66059260535659,39.5550293912439));
#182524=CARTESIAN_POINT('',(62.2936141127097,-6.73887200096311,39.92499));
#182525=CARTESIAN_POINT('',(61.9392677289269,-6.70162869482172,39.3548010137695));
#182526=CARTESIAN_POINT('',(58.872270023448,-6.37927424642578,39.92499));
#182527=CARTESIAN_POINT('',(-0.019912672252488,-0.189456421067656,39.92499));
#182528=CARTESIAN_POINT('',(59.2266168948024,-6.41651760264851,39.3548010137695));
#182529=CARTESIAN_POINT('',(58.872270023448,-6.37927424642578,39.92499));
#182530=CARTESIAN_POINT('',(59.6550713551493,-6.46154998175919,39.116));
#182531=CARTESIAN_POINT('Origin',(59.6170497662622,-6.45755375173563,39.5550297827282));
#182532=CARTESIAN_POINT('',(60.0542523589173,-6.50350559514667,39.116));
#182533=CARTESIAN_POINT('',(60.1277056317065,-6.51122584595708,39.116));
#182534=CARTESIAN_POINT('',(60.1796001951995,-6.51668018436746,39.3343017080178));
#182535=CARTESIAN_POINT('',(60.0542523588397,-6.50350559588466,39.116));
#182536=CARTESIAN_POINT('',(60.5077528318944,-6.55117041629769,39.5248017080178));
#182537=CARTESIAN_POINT('Origin',(60.4784867342332,-6.54809390915787,39.1947745585596));
#182538=CARTESIAN_POINT('',(60.6581326136904,-6.56697596826278,39.5248017080178));
#182539=CARTESIAN_POINT('',(60.6586584283283,-6.56703123360819,39.5248017080178));
#182540=CARTESIAN_POINT('',(60.9862851800404,-6.60146619279947,39.3343017080178));
#182541=CARTESIAN_POINT('Origin',(60.6874016969799,-6.57005175673948,39.194772859418));
#182542=CARTESIAN_POINT('',(61.1116329640613,-6.61464077578123,39.116));
#182543=CARTESIAN_POINT('',(60.9862851800404,-6.60146619279947,39.3343017080178));
#182544=CARTESIAN_POINT('',(61.5113322352818,-6.65665086201911,39.116));
#182545=CARTESIAN_POINT('Origin',(57.030176100279,-11.9273822599894,40.10025));
#182546=CARTESIAN_POINT('',(57.7354693911204,-12.2876333308471,40.10025));
#182547=CARTESIAN_POINT('',(61.4699285681954,-13.0814171332233,40.10025));
#182548=CARTESIAN_POINT('',(56.9874003490102,-12.1286263473644,40.10025));
#182549=CARTESIAN_POINT('',(61.4762657165316,-13.0516031943529,40.10025));
#182550=CARTESIAN_POINT('Origin',(5.50299975530876E-15,5.72544881825791E-15,
40.10025));
#182551=CARTESIAN_POINT('',(57.7418065394566,-12.2578193919768,40.10025));
#182552=CARTESIAN_POINT('',(57.672648524885,-12.2431194021875,40.10025));
#182553=CARTESIAN_POINT('Origin',(5.72166156020094E-15,5.2367941269311E-15,
40.10025));
#182554=CARTESIAN_POINT('Origin',(0.0396071771007832,0.18633711793979,-5.57736016997319E-18));
#182555=CARTESIAN_POINT('',(58.7320730967338,-12.2891316338724,39.116));
#182556=CARTESIAN_POINT('',(58.3106729199896,-12.1995602612165,39.3548010137695));
#182557=CARTESIAN_POINT('Origin',(58.6946775141703,-12.281182957421,39.5550297832841));
#182558=CARTESIAN_POINT('',(57.9621601887016,-12.1254815938991,39.92499));
#182559=CARTESIAN_POINT('',(58.3106729199896,-12.1995602612165,39.3548010137695));
#182560=CARTESIAN_POINT('',(61.3271735965893,-12.8407372733098,39.92499));
#182561=CARTESIAN_POINT('',(61.581282930652,-12.8947498796465,39.92499));
#182562=CARTESIAN_POINT('',(60.9786613449626,-12.7666587067855,39.3548010137695));
#182563=CARTESIAN_POINT('',(61.3271735965893,-12.8407372733098,39.92499));
#182564=CARTESIAN_POINT('',(60.5572615995843,-12.6770874264379,39.116));
#182565=CARTESIAN_POINT('Origin',(60.5946573025927,-12.6850361284907,39.5550293907183));
#182566=CARTESIAN_POINT('',(60.164653163458,-12.5936359264446,39.116));
#182567=CARTESIAN_POINT('',(0.0396071771007887,0.18633711793979,39.116));
#182568=CARTESIAN_POINT('',(60.0413691664787,-12.5674311046654,39.3343017080178));
#182569=CARTESIAN_POINT('',(60.16465316331,-12.5936359271408,39.116));
#182570=CARTESIAN_POINT('',(59.7186194643909,-12.4988285377096,39.5248017080178));
#182571=CARTESIAN_POINT('Origin',(59.7474037157358,-12.5049473440525,39.1947747614341));
#182572=CARTESIAN_POINT('',(59.5707156088321,-12.4673906027143,39.5248017080178));
#182573=CARTESIAN_POINT('',(0.0396071771007888,0.18633711793979,39.5248017080178));
#182574=CARTESIAN_POINT('',(59.2479658375576,-12.3987880210524,39.3343017080178));
#182575=CARTESIAN_POINT('Origin',(59.5419282989939,-12.4612721960121,39.1947728911945));
#182576=CARTESIAN_POINT('',(59.124681789249,-12.3725831876352,39.116));
#182577=CARTESIAN_POINT('',(59.2479658375576,-12.3987880210524,39.3343017080178));
#182578=CARTESIAN_POINT('',(0.0396071771007887,0.18633711793979,39.116));
#182579=CARTESIAN_POINT('Origin',(-0.0396071771007832,-0.18633711793979,
5.57736016997319E-18));
#182580=CARTESIAN_POINT('',(60.4780472453827,-13.0497616623175,39.116));
#182581=CARTESIAN_POINT('',(60.8994469906352,-13.139332943257,39.3548010137695));
#182582=CARTESIAN_POINT('Origin',(60.5154429481078,-13.05771036431,39.5550293912467));
#182583=CARTESIAN_POINT('',(61.2479592422937,-13.213411509632,39.92499));
#182584=CARTESIAN_POINT('',(60.8994469906352,-13.139332943257,39.3548010137695));
#182585=CARTESIAN_POINT('',(57.8829458346105,-12.4981558292588,39.92499));
#182586=CARTESIAN_POINT('',(-0.0396071771007831,-0.186337117939789,39.92499));
#182587=CARTESIAN_POINT('',(58.2314585659349,-12.5722344964053,39.3548010137695));
#182588=CARTESIAN_POINT('',(57.8829458346105,-12.4981558292588,39.92499));
#182589=CARTESIAN_POINT('',(58.6528587425322,-12.661805869752,39.116));
#182590=CARTESIAN_POINT('Origin',(58.6154631596733,-12.6538571932378,39.5550297827333));
#182591=CARTESIAN_POINT('',(59.0454674352017,-12.7452574227892,39.116));
#182592=CARTESIAN_POINT('',(59.1177113373238,-12.7606133389842,39.116));
#182593=CARTESIAN_POINT('',(59.1687514833561,-12.771462256932,39.3343017080178));
#182594=CARTESIAN_POINT('',(59.0454674350475,-12.7452574235148,39.116));
#182595=CARTESIAN_POINT('',(59.4915012546305,-12.8400648385939,39.5248017080178));
#182596=CARTESIAN_POINT('Origin',(59.4627170622795,-12.833946044668,39.1947745585571));
#182597=CARTESIAN_POINT('',(59.6394051101893,-12.8715027735892,39.5248017080178));
#182598=CARTESIAN_POINT('',(59.639922267558,-12.8716126987813,39.5248017080178));
#182599=CARTESIAN_POINT('',(59.9621548122771,-12.940105340545,39.3343017080178));
#182600=CARTESIAN_POINT('Origin',(59.6681923469408,-12.8776211648735,39.1947728594281));
#182601=CARTESIAN_POINT('',(60.0854388091085,-12.9663101630204,39.116));
#182602=CARTESIAN_POINT('',(59.9621548122771,-12.940105340545,39.3343017080178));
#182603=CARTESIAN_POINT('',(60.4785572361439,-13.0498700642002,39.116));
#182604=CARTESIAN_POINT('Origin',(55.4710078899933,-17.8233194796324,40.10025));
#182605=CARTESIAN_POINT('',(56.1347810195642,-18.2553202812749,40.10025));
#182606=CARTESIAN_POINT('',(59.7658094374951,-19.4351129318421,40.10025));
#182607=CARTESIAN_POINT('',(55.4074307335706,-18.018989847295,40.10025));
#182608=CARTESIAN_POINT('',(59.7752282754837,-19.4061247292254,40.10025));
#182609=CARTESIAN_POINT('Origin',(5.50698230308588E-15,5.74031188890569E-15,
40.10025));
#182610=CARTESIAN_POINT('',(56.1441998575527,-18.2263320786583,40.10025));
#182611=CARTESIAN_POINT('',(56.0769572651639,-18.2044836359653,40.10025));
#182612=CARTESIAN_POINT('Origin',(5.71958798166808E-15,5.229055426493E-15,
40.10025));
#182613=CARTESIAN_POINT('Origin',(0.0588677374284276,0.181176266354227,
-8.28957270027859E-18));
#182614=CARTESIAN_POINT('',(57.1257686104891,-18.3609838302741,39.116));
#182615=CARTESIAN_POINT('',(56.7160396659414,-18.2278548260738,39.3548010137695));
#182616=CARTESIAN_POINT('Origin',(57.0894087477753,-18.349169794726,39.5550297832868));
#182617=CARTESIAN_POINT('',(56.3771794531165,-18.1177524692162,39.92499));
#182618=CARTESIAN_POINT('',(56.7160396659414,-18.2278548260738,39.3548010137695));
#182619=CARTESIAN_POINT('',(59.6489943884564,-19.1808295835782,39.92499));
#182620=CARTESIAN_POINT('',(59.8960658302617,-19.2611079613975,39.92499));
#182621=CARTESIAN_POINT('',(59.3101346421293,-19.0707273771,39.3548010137695));
#182622=CARTESIAN_POINT('',(59.6489943884564,-19.1808295835782,39.92499));
#182623=CARTESIAN_POINT('',(58.9004061169357,-18.9375985097922,39.116));
#182624=CARTESIAN_POINT('Origin',(58.9367660967592,-18.9494125833915,39.5550293907195));
#182625=CARTESIAN_POINT('',(58.5186714879536,-18.8135654093531,39.116));
#182626=CARTESIAN_POINT('',(0.0588677374284331,0.181176266354227,39.116));
#182627=CARTESIAN_POINT('',(58.3988020033598,-18.77461745358,39.3343017080178));
#182628=CARTESIAN_POINT('',(58.5186714877335,-18.8135654100303,39.116));
#182629=CARTESIAN_POINT('',(58.08499127881,-18.6726541682846,39.5248017080178));
#182630=CARTESIAN_POINT('Origin',(58.1129782575897,-18.6817482287253,39.1947747614326));
#182631=CARTESIAN_POINT('',(57.9411838150807,-18.6259282908537,39.5248017080178));
#182632=CARTESIAN_POINT('',(0.0588677374284332,0.181176266354227,39.5248017080178));
#182633=CARTESIAN_POINT('',(57.6273730232605,-18.5239649837008,39.3343017080178));
#182634=CARTESIAN_POINT('Origin',(57.9131937527906,-18.6168343081654,39.1947728911901));
#182635=CARTESIAN_POINT('',(57.5075034888353,-18.4850170109878,39.116));
#182636=CARTESIAN_POINT('',(57.6273730232605,-18.5239649837008,39.3343017080178));
#182637=CARTESIAN_POINT('',(0.0588677374284331,0.181176266354227,39.116));
#182638=CARTESIAN_POINT('Origin',(-0.0588677374284276,-0.181176266354227,
8.28957270027859E-18));
#182639=CARTESIAN_POINT('',(58.7826706420788,-19.2999510425007,39.116));
#182640=CARTESIAN_POINT('',(59.1923991670855,-19.4330799103838,39.3548010137695));
#182641=CARTESIAN_POINT('Origin',(58.8190306216277,-19.3117651160107,39.5550293912458));
#182642=CARTESIAN_POINT('',(59.5312589134599,-19.5431821167165,39.92499));
#182643=CARTESIAN_POINT('',(59.1923991670855,-19.4330799103838,39.3548010137695));
#182644=CARTESIAN_POINT('',(56.2594439784239,-18.4801050014191,39.92499));
#182645=CARTESIAN_POINT('',(-0.0588677374284273,-0.181176266354225,39.92499));
#182646=CARTESIAN_POINT('',(56.5983041913028,-18.5902073581106,39.3548010137695));
#182647=CARTESIAN_POINT('',(56.2594439784239,-18.4801050014191,39.92499));
#182648=CARTESIAN_POINT('',(57.0080331356322,-18.7233363629825,39.116));
#182649=CARTESIAN_POINT('Origin',(56.9716732726282,-18.7115223273402,39.5550297827295));
#182650=CARTESIAN_POINT('',(57.3897680142076,-18.8473695429909,39.116));
#182651=CARTESIAN_POINT('',(57.460011026353,-18.8701928819395,39.116));
#182652=CARTESIAN_POINT('',(57.5096375484037,-18.8863175164093,39.3343017080178));
#182653=CARTESIAN_POINT('',(57.3897680139784,-18.8473695436963,39.116));
#182654=CARTESIAN_POINT('',(57.8234483402239,-18.9882808235621,39.5248017080178));
#182655=CARTESIAN_POINT('Origin',(57.7954614188153,-18.9791867816364,39.194774558559));
#182656=CARTESIAN_POINT('',(57.9672558039532,-19.0350067009931,39.5248017080178));
#182657=CARTESIAN_POINT('',(57.9677586379683,-19.0351700816685,39.5248017080178));
#182658=CARTESIAN_POINT('',(58.281066528503,-19.1369699862884,39.3343017080178));
#182659=CARTESIAN_POINT('Origin',(57.995245795169,-19.0441006607084,39.1947728594241));
#182660=CARTESIAN_POINT('',(58.4009360128767,-19.1759179427387,39.116));
#182661=CARTESIAN_POINT('',(58.281066528503,-19.1369699862884,39.3343017080178));
#182662=CARTESIAN_POINT('',(58.783166507975,-19.300112159097,39.116));
#182663=CARTESIAN_POINT('Origin',(53.3040877092102,-23.5239806812872,40.10025));
#182664=CARTESIAN_POINT('',(53.9190682401995,-24.0229981225297,40.10025));
#182665=CARTESIAN_POINT('',(57.4068835917979,-25.5758735661209,40.10025));
#182666=CARTESIAN_POINT('',(53.2204057122638,-23.7119335237426,40.10025));
#182667=CARTESIAN_POINT('',(57.4192809246789,-25.5480287005719,40.10025));
#182668=CARTESIAN_POINT('Origin',(5.51249664798382E-15,5.75467724849828E-15,
40.10025));
#182669=CARTESIAN_POINT('',(53.9314655730804,-23.9951532569808,40.10025));
#182670=CARTESIAN_POINT('',(53.8668751267878,-23.9663957374944,40.10025));
#182671=CARTESIAN_POINT('Origin',(5.71671684795091E-15,5.22157586744312E-15,
40.10025));
#182672=CARTESIAN_POINT('Origin',(0.0774833305059401,0.174030409680915,
-1.09109629373751E-17));
#182673=CARTESIAN_POINT('',(54.8935822490122,-24.2316692455484,39.116));
#182674=CARTESIAN_POINT('',(54.5000136127188,-24.0564411990328,39.3548010137695));
#182675=CARTESIAN_POINT('Origin',(54.8586564724101,-24.2161192879484,39.5550297832837));
#182676=CARTESIAN_POINT('',(54.1745185417599,-23.9115214570969,39.92499));
#182677=CARTESIAN_POINT('',(54.5000136127188,-24.0564411990328,39.3548010137695));
#182678=CARTESIAN_POINT('',(57.317288315449,-25.3107727110823,39.92499));
#182679=CARTESIAN_POINT('',(57.5546148985775,-25.4164373136774,39.92499));
#182680=CARTESIAN_POINT('',(56.9917936927132,-25.1658531674647,39.3548010137695));
#182681=CARTESIAN_POINT('',(57.317288315449,-25.3107727110823,39.92499));
#182682=CARTESIAN_POINT('',(56.5982254591675,-24.9906253009259,39.116));
#182683=CARTESIAN_POINT('Origin',(56.6331513482598,-25.0061753086097,39.5550293907183));
#182684=CARTESIAN_POINT('',(56.2315470018076,-24.8273695326456,39.116));
#182685=CARTESIAN_POINT('',(0.0774833305059456,0.174030409680915,39.116));
#182686=CARTESIAN_POINT('',(56.1164053447571,-24.7761051648318,39.3343017080178));
#182687=CARTESIAN_POINT('',(56.2315470015181,-24.8273695332957,39.116));
#182688=CARTESIAN_POINT('',(55.8149717737126,-24.6418982922878,39.5248017080178));
#182689=CARTESIAN_POINT('Origin',(55.8418548487303,-24.6538679703967,39.1947747614298));
#182690=CARTESIAN_POINT('',(55.6768362864792,-24.5803964109124,39.5248017080178));
#182691=CARTESIAN_POINT('',(0.0774833305059457,0.174030409680915,39.5248017080178));
#182692=CARTESIAN_POINT('',(55.3754026508175,-24.4461895095989,39.3343017080178));
#182693=CARTESIAN_POINT('Origin',(55.6499501367123,-24.568426487814,39.1947728911939));
#182694=CARTESIAN_POINT('',(55.260260945979,-24.3949251197295,39.116));
#182695=CARTESIAN_POINT('',(55.3754026508175,-24.4461895095989,39.3343017080178));
#182696=CARTESIAN_POINT('',(0.0774833305059456,0.174030409680915,39.116));
#182697=CARTESIAN_POINT('Origin',(-0.0774833305059401,-0.174030409680915,
1.09109629373751E-17));
#182698=CARTESIAN_POINT('',(56.4432587981556,-25.3386861202878,39.116));
#182699=CARTESIAN_POINT('',(56.8368270314553,-25.513913987379,39.3548010137695));
#182700=CARTESIAN_POINT('Origin',(56.4781846869833,-25.3542361278537,39.5550293912457));
#182701=CARTESIAN_POINT('',(57.1623216542531,-25.6588335308574,39.92499));
#182702=CARTESIAN_POINT('',(56.8368270314553,-25.513913987379,39.3548010137695));
#182703=CARTESIAN_POINT('',(54.0195518809641,-24.2595822759734,39.92499));
#182704=CARTESIAN_POINT('',(-0.0774833305059396,-0.174030409680913,39.92499));
#182705=CARTESIAN_POINT('',(54.3450469519941,-24.4045020177498,39.3548010137695));
#182706=CARTESIAN_POINT('',(54.0195518809641,-24.2595822759734,39.92499));
#182707=CARTESIAN_POINT('',(54.7386155880003,-24.5797300649102,39.116));
#182708=CARTESIAN_POINT('Origin',(54.703689811123,-24.5641801071878,39.5550297827337));
#182709=CARTESIAN_POINT('',(55.1052942852688,-24.7429859384138,39.116));
#182710=CARTESIAN_POINT('',(55.1727668102971,-24.7730266428385,39.116));
#182711=CARTESIAN_POINT('',(55.2204359898056,-24.7942503289608,39.3343017080178));
#182712=CARTESIAN_POINT('',(55.1052942849672,-24.7429859390914,39.116));
#182713=CARTESIAN_POINT('',(55.5218696254673,-24.9284572302742,39.5248017080178));
#182714=CARTESIAN_POINT('Origin',(55.49498660557,-24.9164875765753,39.194774558559));
#182715=CARTESIAN_POINT('',(55.6600051127008,-24.9899591116496,39.5248017080178));
#182716=CARTESIAN_POINT('',(55.6604881142076,-24.9901741577755,39.5248017080178));
#182717=CARTESIAN_POINT('',(55.9614386837453,-25.1241659841936,39.3343017080178));
#182718=CARTESIAN_POINT('Origin',(55.6868911941832,-25.0019290044714,39.1947728594271));
#182719=CARTESIAN_POINT('',(56.0765803405063,-25.1754303526576,39.116));
#182720=CARTESIAN_POINT('',(55.9614386837453,-25.1241659841936,39.3343017080178));
#182721=CARTESIAN_POINT('',(56.4437351063763,-25.3388981863707,39.116));
#182722=CARTESIAN_POINT('Origin',(50.5531567888875,-28.9669082278884,40.10025));
#182723=CARTESIAN_POINT('',(51.1126068659047,-29.5274749692186,40.10025));
#182724=CARTESIAN_POINT('',(54.4189959163063,-31.4364195775136,40.10025));
#182725=CARTESIAN_POINT('',(50.4502867888875,-29.145084294463,40.10025));
#182726=CARTESIAN_POINT('',(54.4342359163063,-31.4100231232062,40.10025));
#182727=CARTESIAN_POINT('Origin',(5.51948237368594E-15,5.76838750714983E-15,
40.10025));
#182728=CARTESIAN_POINT('',(51.1278468659047,-29.5010785149112,40.10025));
#182729=CARTESIAN_POINT('',(51.0666162321543,-29.4657269920328,40.10025));
#182730=CARTESIAN_POINT('Origin',(5.71307961579125E-15,5.2144373973956E-15,
40.10025));
#182731=CARTESIAN_POINT('Origin',(0.0952500000000002,0.164977839420935,
-1.3412810381264E-17));
#182732=CARTESIAN_POINT('',(52.0599703131946,-29.8368674217657,39.116));
#182733=CARTESIAN_POINT('',(51.6868740054943,-29.6214601680812,39.3548010137695));
#182734=CARTESIAN_POINT('Origin',(52.0268612768236,-29.8177519107043,39.5550297832855));
#182735=CARTESIAN_POINT('',(51.3783102685129,-29.4433108120862,39.92499));
#182736=CARTESIAN_POINT('',(51.6868740054943,-29.6214601680812,39.3548010137695));
#182737=CARTESIAN_POINT('',(54.3576020372438,-31.1634057161441,39.92499));
#182738=CARTESIAN_POINT('',(54.582583561987,-31.2932988600173,39.92499));
#182739=CARTESIAN_POINT('',(54.0490387253005,-30.9852566042327,39.3548010137695));
#182740=CARTESIAN_POINT('',(54.3576020372438,-31.1634057161441,39.92499));
#182741=CARTESIAN_POINT('',(53.6759427993286,-30.7698495716382,39.116));
#182742=CARTESIAN_POINT('Origin',(53.7090519423387,-30.7889651442676,39.5550293907189));
#182743=CARTESIAN_POINT('',(53.3283379195023,-30.5691597998769,39.116));
#182744=CARTESIAN_POINT('',(0.0952500000000057,0.164977839420935,39.116));
#182745=CARTESIAN_POINT('',(53.2191856060845,-30.5061406831644,39.3343017080178));
#182746=CARTESIAN_POINT('',(53.3283379191464,-30.5691598004933,39.116));
#182747=CARTESIAN_POINT('',(52.9334317578287,-30.3411606219519,39.5248017080178));
#182748=CARTESIAN_POINT('Origin',(52.958916392489,-30.3558747754306,39.1947747614273));
#182749=CARTESIAN_POINT('',(52.8024816883959,-30.2655565641145,39.5248017080178));
#182750=CARTESIAN_POINT('',(0.0952500000000058,0.164977839420935,39.5248017080178));
#182751=CARTESIAN_POINT('',(52.5167277788841,-30.1005764675359,39.3343017080178));
#182752=CARTESIAN_POINT('Origin',(52.7769940214392,-30.2508418455899,39.1947728911908));
#182753=CARTESIAN_POINT('',(52.4075754202456,-30.0375573238933,39.116));
#182754=CARTESIAN_POINT('',(52.5167277788841,-30.1005764675359,39.3343017080178));
#182755=CARTESIAN_POINT('',(0.0952500000000057,0.164977839420935,39.116));
#182756=CARTESIAN_POINT('Origin',(-0.0952500000000002,-0.164977839420935,
1.3412810381264E-17));
#182757=CARTESIAN_POINT('',(53.4854427993286,-31.09980525048,39.116));
#182758=CARTESIAN_POINT('',(53.8585387249979,-31.3152122835987,39.3548010137695));
#182759=CARTESIAN_POINT('Origin',(53.518551942088,-31.1189208229648,39.5550293912464));
#182760=CARTESIAN_POINT('',(54.1671020370176,-31.4933613953777,39.92499));
#182761=CARTESIAN_POINT('',(53.8585387249979,-31.3152122835987,39.3548010137695));
#182762=CARTESIAN_POINT('',(51.1878102687785,-29.7732664904681,39.92499));
#182763=CARTESIAN_POINT('',(-0.0952499999999994,-0.164977839420933,39.92499));
#182764=CARTESIAN_POINT('',(51.4963740058478,-29.9514158463108,39.3548010137695));
#182765=CARTESIAN_POINT('',(51.1878102687785,-29.7732664904681,39.92499));
#182766=CARTESIAN_POINT('',(51.8694703131946,-30.1668231006075,39.116));
#182767=CARTESIAN_POINT('Origin',(51.8363612765606,-30.1477075893943,39.5550297827308));
#182768=CARTESIAN_POINT('',(52.2170754206164,-30.3675130020929,39.116));
#182769=CARTESIAN_POINT('',(52.2810382154239,-30.4044419397494,39.116));
#182770=CARTESIAN_POINT('',(52.3262277788841,-30.4305321463777,39.3343017080178));
#182771=CARTESIAN_POINT('',(52.2170754202456,-30.3675130027351,39.116));
#182772=CARTESIAN_POINT('',(52.6119816883959,-30.5955122429563,39.5248017080178));
#182773=CARTESIAN_POINT('Origin',(52.5864971060027,-30.5807981195157,39.1947745585563));
#182774=CARTESIAN_POINT('',(52.7429317578287,-30.6711163007938,39.5248017080178));
#182775=CARTESIAN_POINT('',(52.7433896349617,-30.6713806562798,39.5248017080178));
#182776=CARTESIAN_POINT('',(53.0286856060845,-30.8360963620063,39.3343017080178));
#182777=CARTESIAN_POINT('Origin',(52.7684193600401,-30.68583098207,39.1947728594247));
#182778=CARTESIAN_POINT('',(53.1378379191464,-30.8991154793352,39.116));
#182779=CARTESIAN_POINT('',(53.0286856060845,-30.8360963620063,39.3343017080178));
#182780=CARTESIAN_POINT('',(53.4858943313413,-31.1000659426091,39.116));
#182781=CARTESIAN_POINT('Origin',(47.2483549038575,-34.0924682662295,40.10025));
#182782=CARTESIAN_POINT('',(47.7461450747864,-34.7084426211232,40.10025));
#182783=CARTESIAN_POINT('',(50.8348823336486,-36.9525415975213,40.10025));
#182784=CARTESIAN_POINT('',(47.1274239660509,-34.2589154226522,40.10025));
#182785=CARTESIAN_POINT('',(50.8527980281384,-36.9278827595327,40.10025));
#182786=CARTESIAN_POINT('Origin',(5.52786294311959E-15,5.78129245239752E-15,
40.10025));
#182787=CARTESIAN_POINT('',(47.7640607692763,-34.6837837831347,40.10025));
#182788=CARTESIAN_POINT('',(47.706860803705,-34.6422255755467,40.10025));
#182789=CARTESIAN_POINT('Origin',(5.70871613546578E-15,5.20771822692212E-15,
40.10025));
#182790=CARTESIAN_POINT('Origin',(0.111973090561716,0.154117737428427,-1.57677042678047E-17));
#182791=CARTESIAN_POINT('',(48.6559784483765,-35.1151666347442,39.116));
#182792=CARTESIAN_POINT('',(48.3074421904918,-34.8619402208391,39.3548010137695));
#182793=CARTESIAN_POINT('Origin',(48.6250489017663,-35.09269500376,39.5550297832842));
#182794=CARTESIAN_POINT('',(48.019190476361,-34.6525130924099,39.92499));
#182795=CARTESIAN_POINT('',(48.3074421904918,-34.8619402208391,39.3548010137695));
#182796=CARTESIAN_POINT('',(50.8023624960591,-36.6746059268179,39.92499));
#182797=CARTESIAN_POINT('',(51.0125340177515,-36.827304475503,39.92499));
#182798=CARTESIAN_POINT('',(50.5141111791244,-36.4651790855637,39.3548010137695));
#182799=CARTESIAN_POINT('',(50.8023624960591,-36.6746059268179,39.92499));
#182800=CARTESIAN_POINT('',(50.1655752777671,-36.2119529314385,39.116));
#182801=CARTESIAN_POINT('Origin',(50.196504923995,-36.2344246347993,39.5550293907212));
#182802=CARTESIAN_POINT('',(49.8408524072787,-35.976027955333,39.116));
#182803=CARTESIAN_POINT('',(0.111973090561722,0.154117737428427,39.116));
#182804=CARTESIAN_POINT('',(49.7388853330811,-35.9019445403519,39.3343017080178));
#182805=CARTESIAN_POINT('',(49.8408524068603,-35.9760279559088,39.116));
#182806=CARTESIAN_POINT('',(49.4719419865733,-35.7079988465459,39.5248017080178));
#182807=CARTESIAN_POINT('Origin',(49.4957489658851,-35.7252962640489,39.1947747614236));
#182808=CARTESIAN_POINT('',(49.3496120513049,-35.6191209461253,39.5248017080178));
#182809=CARTESIAN_POINT('',(0.111973090561722,0.154117737428427,39.5248017080178));
#182810=CARTESIAN_POINT('',(49.0826686475734,-35.4251752107439,39.3343017080178));
#182811=CARTESIAN_POINT('Origin',(49.3258021153687,-35.6018226497085,39.1947728911923));
#182812=CARTESIAN_POINT('',(48.9807015312178,-35.3510917642534,39.116));
#182813=CARTESIAN_POINT('',(49.0826686475734,-35.4251752107439,39.3343017080178));
#182814=CARTESIAN_POINT('',(0.111973090561722,0.154117737428427,39.116));
#182815=CARTESIAN_POINT('Origin',(-0.111973090561716,-0.154117737428427,
1.57677042678047E-17));
#182816=CARTESIAN_POINT('',(49.9416290966437,-36.5201884062954,39.116));
#182817=CARTESIAN_POINT('',(50.2901649976455,-36.7734145609099,39.3548010137695));
#182818=CARTESIAN_POINT('Origin',(49.9725587426391,-36.5426601094872,39.5550293912449));
#182819=CARTESIAN_POINT('',(50.5784163146695,-36.9828414020411,39.92499));
#182820=CARTESIAN_POINT('',(50.2901649976455,-36.7734145609099,39.3548010137695));
#182821=CARTESIAN_POINT('',(47.7952442955502,-34.9607485668366,39.92499));
#182822=CARTESIAN_POINT('',(-0.111973090561715,-0.154117737428424,39.92499));
#182823=CARTESIAN_POINT('',(48.0834960097836,-35.1701756951243,39.3548010137695));
#182824=CARTESIAN_POINT('',(47.7952442955502,-34.9607485668366,39.92499));
#182825=CARTESIAN_POINT('',(48.432032267253,-35.423402109601,39.116));
#182826=CARTESIAN_POINT('Origin',(48.4011027203971,-35.4009304784382,39.5550297827298));
#182827=CARTESIAN_POINT('',(48.7567553505303,-35.6593272385103,39.116));
#182828=CARTESIAN_POINT('',(48.8165076253519,-35.7027398082299,39.116));
#182829=CARTESIAN_POINT('',(48.85872246645,-35.7334106856007,39.3343017080178));
#182830=CARTESIAN_POINT('',(48.7567553500944,-35.6593272391103,39.116));
#182831=CARTESIAN_POINT('',(49.1256658701815,-35.9273564209821,39.5248017080178));
#182832=CARTESIAN_POINT('Origin',(49.1018589397078,-35.910059038814,39.1947745585581));
#182833=CARTESIAN_POINT('',(49.2479958054498,-36.0162343214027,39.5248017080178));
#182834=CARTESIAN_POINT('',(49.2484235416113,-36.0165450899148,39.5248017080178));
#182835=CARTESIAN_POINT('',(49.5149391519577,-36.2101800152087,39.3343017080178));
#182836=CARTESIAN_POINT('Origin',(49.2718056808862,-36.0335325740054,39.1947728594183));
#182837=CARTESIAN_POINT('',(49.6169062257369,-36.2842634307656,39.116));
#182838=CARTESIAN_POINT('',(49.5149391519577,-36.2101800152087,39.3343017080178));
#182839=CARTESIAN_POINT('',(49.9420509053691,-36.5204948682731,39.116));
#182840=CARTESIAN_POINT('Origin',(43.425890155147,-38.8445040879382,40.10025));
#182841=CARTESIAN_POINT('',(43.8565665267056,-39.5091373124623,40.10025));
#182842=CARTESIAN_POINT('',(46.6938111422604,-42.0638038389701,40.10025));
#182843=CARTESIAN_POINT('',(43.2882232241948,-38.997398704332,40.10025));
#182844=CARTESIAN_POINT('',(46.7142062431422,-42.0411527846896,40.10025));
#182845=CARTESIAN_POINT('Origin',(5.5375465370123E-15,5.79325069496066E-15,
40.10025));
#182846=CARTESIAN_POINT('',(43.8769616275874,-39.4864862581817,40.10025));
#182847=CARTESIAN_POINT('',(43.8244190249878,-39.4391766863031,40.10025));
#182848=CARTESIAN_POINT('Origin',(5.70367421417806E-15,5.20149197266044E-15,
40.10025));
#182849=CARTESIAN_POINT('Origin',(0.127469380511363,0.141569089253443,-1.79498438867831E-17));
#182850=CARTESIAN_POINT('',(44.7189015017598,-40.0087367337514,39.116));
#182851=CARTESIAN_POINT('',(44.398743929868,-39.7204655612074,39.3548010137695));
#182852=CARTESIAN_POINT('Origin',(44.6904903154964,-39.9831551867365,39.5550297832852));
#182853=CARTESIAN_POINT('',(44.1339623846891,-39.482055187788,39.92499));
#182854=CARTESIAN_POINT('',(44.398743929868,-39.7204655612074,39.3548010137695));
#182855=CARTESIAN_POINT('',(46.6905216402897,-41.7839914803027,39.92499));
#182856=CARTESIAN_POINT('',(46.8835804757584,-41.9578224365462,39.92499));
#182857=CARTESIAN_POINT('',(46.425740460113,-41.5455814340034,39.3548010137695));
#182858=CARTESIAN_POINT('',(46.6905216402897,-41.7839914803027,39.92499));
#182859=CARTESIAN_POINT('',(46.1055832156409,-41.2573105570837,39.116));
#182860=CARTESIAN_POINT('Origin',(46.1339944934108,-41.2828921864915,39.5550293907218));
#182861=CARTESIAN_POINT('',(45.8073000862121,-40.9887352200425,39.116));
#182862=CARTESIAN_POINT('',(0.127469380511368,0.141569089253443,39.116));
#182863=CARTESIAN_POINT('',(45.7136354238375,-40.9043991801904,39.3343017080178));
#182864=CARTESIAN_POINT('',(45.8073000857358,-40.9887352205714,39.116));
#182865=CARTESIAN_POINT('',(45.4684272662435,-40.6836127633979,39.5248017080178));
#182866=CARTESIAN_POINT('Origin',(45.4902957559679,-40.7033039308062,39.1947747614394));
#182867=CARTESIAN_POINT('',(45.3560577375095,-40.58243478527,39.5248017080178));
#182868=CARTESIAN_POINT('',(0.127469380511368,0.141569089253443,39.5248017080178));
#182869=CARTESIAN_POINT('',(45.1108495273512,-40.3616483211485,39.3343017080178));
#182870=CARTESIAN_POINT('Origin',(45.3341863992353,-40.5627424347171,39.1947728911915));
#182871=CARTESIAN_POINT('',(45.0171848263432,-40.2773122455529,39.116));
#182872=CARTESIAN_POINT('',(45.1108495273512,-40.3616483211485,39.3343017080178));
#182873=CARTESIAN_POINT('',(0.127469380511368,0.141569089253443,39.116));
#182874=CARTESIAN_POINT('Origin',(-0.127469380511363,-0.141569089253443,
1.79498438867831E-17));
#182875=CARTESIAN_POINT('',(45.8506444546181,-41.5404487355906,39.116));
#182876=CARTESIAN_POINT('',(46.1708016986853,-41.82871961296,39.3548010137695));
#182877=CARTESIAN_POINT('Origin',(45.8790557321746,-41.5660303648061,39.5550293912458));
#182878=CARTESIAN_POINT('',(46.4355828789645,-42.0671296591456,39.92499));
#182879=CARTESIAN_POINT('',(46.1708016986853,-41.82871961296,39.3548010137695));
#182880=CARTESIAN_POINT('',(43.8790236240219,-39.7651933658999,39.92499));
#182881=CARTESIAN_POINT('',(-0.127469380511361,-0.14156908925344,39.92499));
#182882=CARTESIAN_POINT('',(44.1438051693183,-40.003603739189,39.3548010137695));
#182883=CARTESIAN_POINT('',(43.8790236240219,-39.7651933658999,39.92499));
#182884=CARTESIAN_POINT('',(44.4639627407371,-40.2918749122583,39.116));
#182885=CARTESIAN_POINT('Origin',(44.4355515542499,-40.2662933650419,39.5550297827353));
#182886=CARTESIAN_POINT('',(44.7622460658165,-40.5604504235089,39.116));
#182887=CARTESIAN_POINT('',(44.8171331622256,-40.6098709880929,39.116));
#182888=CARTESIAN_POINT('',(44.8559107663285,-40.6447864996553,39.3343017080178));
#182889=CARTESIAN_POINT('',(44.7622460653205,-40.5604504240598,39.116));
#182890=CARTESIAN_POINT('',(45.1011189764868,-40.8655729637769,39.5248017080178));
#182891=CARTESIAN_POINT('Origin',(45.0792505316454,-40.8458818366201,39.1947745585599));
#182892=CARTESIAN_POINT('',(45.2134885052208,-40.9667509419048,39.5248017080178));
#182893=CARTESIAN_POINT('',(45.2138814140438,-40.9671047185981,39.5248017080178));
#182894=CARTESIAN_POINT('',(45.4586966628148,-41.1875373586973,39.3343017080178));
#182895=CARTESIAN_POINT('Origin',(45.2353597879066,-40.9864432425598,39.1947728594184));
#182896=CARTESIAN_POINT('',(45.5523613247131,-41.2718733990783,39.116));
#182897=CARTESIAN_POINT('',(45.4586966628148,-41.1875373586973,39.3343017080178));
#182898=CARTESIAN_POINT('',(45.8510319186316,-41.5407976097554,39.116));
#182899=CARTESIAN_POINT('Origin',(39.127642266445,-43.1709513941244,40.10025));
#182900=CARTESIAN_POINT('',(39.4864862581816,-43.8769616275875,40.10025));
#182901=CARTESIAN_POINT('',(42.0411527846894,-46.7142062431423,40.10025));
#182902=CARTESIAN_POINT('',(38.9747476500513,-43.3086183250767,40.10025));
#182903=CARTESIAN_POINT('',(42.06380383897,-46.6938111422605,40.10025));
#182904=CARTESIAN_POINT('Origin',(5.54842705988296E-15,5.80413121783132E-15,
40.10025));
#182905=CARTESIAN_POINT('',(39.5091373124621,-43.8565665267057,40.10025));
#182906=CARTESIAN_POINT('',(39.4618277405835,-43.804023924106,40.10025));
#182907=CARTESIAN_POINT('Origin',(5.69800909227282E-15,5.1958268507552E-15,
40.10025));
#182908=CARTESIAN_POINT('Origin',(0.141569089253444,0.127469380511362,-1.99353212598916E-17));
#182909=CARTESIAN_POINT('',(40.2918749122581,-44.4639627407372,39.116));
#182910=CARTESIAN_POINT('',(40.0036037397142,-44.1438051688454,39.3548010137695));
#182911=CARTESIAN_POINT('Origin',(40.2662933652425,-44.4355515544729,39.5550297832825));
#182912=CARTESIAN_POINT('',(39.7651933655048,-43.8790236243778,39.92499));
#182913=CARTESIAN_POINT('',(40.0036037397142,-44.1438051688454,39.3548010137695));
#182914=CARTESIAN_POINT('',(42.0671296588095,-46.4355828792671,39.92499));
#182915=CARTESIAN_POINT('',(42.240960615053,-46.6286417147358,39.92499));
#182916=CARTESIAN_POINT('',(41.8287196134096,-46.1708016982805,39.3548010137695));
#182917=CARTESIAN_POINT('',(42.0671296588095,-46.4355828792671,39.92499));
#182918=CARTESIAN_POINT('',(41.5404487355905,-45.8506444546183,39.116));
#182919=CARTESIAN_POINT('Origin',(41.5660303649986,-45.8790557323886,39.5550293907208));
#182920=CARTESIAN_POINT('',(41.2718733996072,-45.5523613242369,39.116));
#182921=CARTESIAN_POINT('',(0.141569089253449,0.127469380511362,39.116));
#182922=CARTESIAN_POINT('',(41.1875373586971,-45.4586966628149,39.3343017080178));
#182923=CARTESIAN_POINT('',(41.2718733990782,-45.5523613247132,39.116));
#182924=CARTESIAN_POINT('',(40.9667509419047,-45.2134885052209,39.5248017080178));
#182925=CARTESIAN_POINT('Origin',(40.9864413462789,-45.2353576819716,39.1947747614227));
#182926=CARTESIAN_POINT('',(40.8655729637768,-45.101118976487,39.5248017080178));
#182927=CARTESIAN_POINT('',(0.141569089253449,0.127469380511362,39.5248017080178));
#182928=CARTESIAN_POINT('',(40.6447864996552,-44.8559107663286,39.3343017080178));
#182929=CARTESIAN_POINT('Origin',(40.8458798501228,-45.0792483253108,39.1947728911931));
#182930=CARTESIAN_POINT('',(40.5604504240596,-44.7622460653206,39.116));
#182931=CARTESIAN_POINT('',(40.6447864996552,-44.8559107663286,39.3343017080178));
#182932=CARTESIAN_POINT('',(0.141569089253449,0.127469380511362,39.116));
#182933=CARTESIAN_POINT('Origin',(-0.141569089253444,-0.127469380511362,
1.99353212598916E-17));
#182934=CARTESIAN_POINT('',(41.2573105570836,-46.105583215641,39.116));
#182935=CARTESIAN_POINT('',(41.5455814344529,-46.4257404597082,39.3548010137695));
#182936=CARTESIAN_POINT('Origin',(41.2828921862997,-46.1339944931981,39.555029391244));
#182937=CARTESIAN_POINT('',(41.7839914799665,-46.6905216405924,39.92499));
#182938=CARTESIAN_POINT('',(41.5455814344529,-46.4257404597082,39.3548010137695));
#182939=CARTESIAN_POINT('',(39.4820551873929,-44.1339623850448,39.92499));
#182940=CARTESIAN_POINT('',(-0.141569089253442,-0.127469380511358,39.92499));
#182941=CARTESIAN_POINT('',(39.7204655617324,-44.3987439293954,39.3548010137695));
#182942=CARTESIAN_POINT('',(39.4820551873929,-44.1339623850448,39.92499));
#182943=CARTESIAN_POINT('',(40.0087367337512,-44.7189015017599,39.116));
#182944=CARTESIAN_POINT('Origin',(39.9831551865335,-44.6904903152712,39.5550297827315));
#182945=CARTESIAN_POINT('',(40.2773122461036,-45.0171848258473,39.116));
#182946=CARTESIAN_POINT('',(40.3267328095859,-45.0720719232484,39.116));
#182947=CARTESIAN_POINT('',(40.3616483211483,-45.1108495273513,39.3343017080178));
#182948=CARTESIAN_POINT('',(40.2773122455527,-45.0171848263433,39.116));
#182949=CARTESIAN_POINT('',(40.5824347852699,-45.3560577375097,39.5248017080178));
#182950=CARTESIAN_POINT('Origin',(40.5627444213182,-45.3341886054734,39.1947745585617));
#182951=CARTESIAN_POINT('',(40.6836127633978,-45.4684272662437,39.5248017080178));
#182952=CARTESIAN_POINT('',(40.6839665400911,-45.4688201750666,39.5248017080178));
#182953=CARTESIAN_POINT('',(40.9043991801903,-45.7136354238376,39.3343017080178));
#182954=CARTESIAN_POINT('Origin',(40.7033058269822,-45.4902978619832,39.1947728594174));
#182955=CARTESIAN_POINT('',(40.9887352205713,-45.807300085736,39.116));
#182956=CARTESIAN_POINT('',(40.9043991801903,-45.7136354238376,39.3343017080178));
#182957=CARTESIAN_POINT('',(41.2576594312484,-46.1059706796545,39.116));
#182958=CARTESIAN_POINT('Origin',(34.4007037410862,-47.0244087227342,40.10025));
#182959=CARTESIAN_POINT('',(34.6837837831345,-47.7640607692764,40.10025));
#182960=CARTESIAN_POINT('',(36.9278827595326,-50.8527980281386,40.10025));
#182961=CARTESIAN_POINT('',(34.2342565846635,-47.1453396605409,40.10025));
#182962=CARTESIAN_POINT('',(36.9525415975211,-50.8348823336487,40.10025));
#182963=CARTESIAN_POINT('Origin',(5.5603853024461E-15,5.81381481172403E-15,
40.10025));
#182964=CARTESIAN_POINT('',(34.7084426211231,-47.7461450747865,40.10025));
#182965=CARTESIAN_POINT('',(34.6668844135351,-47.6889451092152,40.10025));
#182966=CARTESIAN_POINT('Origin',(5.69178283801114E-15,5.19078492946748E-15,
40.10025));
#182967=CARTESIAN_POINT('Origin',(0.154117737428428,0.111973090561716,-2.17023830815426E-17));
#182968=CARTESIAN_POINT('',(35.4234021096009,-48.4320322672531,39.116));
#182969=CARTESIAN_POINT('',(35.1701756956958,-48.0834960093684,39.3548010137695));
#182970=CARTESIAN_POINT('Origin',(35.4009304786184,-48.4011027206453,39.5550297832894));
#182971=CARTESIAN_POINT('',(34.9607485664066,-47.7952442958626,39.92499));
#182972=CARTESIAN_POINT('',(35.1701756956958,-48.0834960093684,39.3548010137695));
#182973=CARTESIAN_POINT('',(36.9828414016746,-50.5784163149358,39.92499));
#182974=CARTESIAN_POINT('',(37.1355399503597,-50.7885878366282,39.92499));
#182975=CARTESIAN_POINT('',(36.7734145613992,-50.29016499729,39.3548010137695));
#182976=CARTESIAN_POINT('',(36.9828414016746,-50.5784163149357,39.92499));
#182977=CARTESIAN_POINT('',(36.5201884062952,-49.9416290966438,39.116));
#182978=CARTESIAN_POINT('Origin',(36.5426601096567,-49.9725587428728,39.5550293907182));
#182979=CARTESIAN_POINT('',(36.284263431341,-49.6169062253189,39.116));
#182980=CARTESIAN_POINT('',(0.154117737428433,0.111973090561716,39.116));
#182981=CARTESIAN_POINT('',(36.2101800152086,-49.5149391519578,39.3343017080178));
#182982=CARTESIAN_POINT('',(36.2842634307655,-49.616906225737,39.116));
#182983=CARTESIAN_POINT('',(36.0162343214026,-49.24799580545,39.5248017080178));
#182984=CARTESIAN_POINT('Origin',(36.0335309082456,-49.2718033882767,39.1947747614309));
#182985=CARTESIAN_POINT('',(35.927356420982,-49.1256658701816,39.5248017080178));
#182986=CARTESIAN_POINT('',(0.154117737428433,0.111973090561716,39.5248017080178));
#182987=CARTESIAN_POINT('',(35.7334106856005,-48.8587224664501,39.3343017080178));
#182988=CARTESIAN_POINT('Origin',(35.9100572938238,-49.1018565378146,39.1947728911917));
#182989=CARTESIAN_POINT('',(35.6593272391101,-48.7567553500945,39.116));
#182990=CARTESIAN_POINT('',(35.7334106856005,-48.8587224664501,39.3343017080178));
#182991=CARTESIAN_POINT('',(0.154117737428433,0.111973090561716,39.116));
#182992=CARTESIAN_POINT('Origin',(-0.154117737428428,-0.111973090561716,
2.17023830815426E-17));
#182993=CARTESIAN_POINT('',(36.2119529314384,-50.1655752777672,39.116));
#182994=CARTESIAN_POINT('',(36.4651790860528,-50.514111178769,39.3548010137695));
#182995=CARTESIAN_POINT('Origin',(36.2344246346305,-50.196504923763,39.5550293912442));
#182996=CARTESIAN_POINT('',(36.6746059264518,-50.802362496325,39.92499));
#182997=CARTESIAN_POINT('',(36.4651790860528,-50.514111178769,39.3548010137695));
#182998=CARTESIAN_POINT('',(34.6525130919796,-48.0191904766737,39.92499));
#182999=CARTESIAN_POINT('',(-0.154117737428425,-0.111973090561711,39.92499));
#183000=CARTESIAN_POINT('',(34.8619402214101,-48.3074421900769,39.3548010137695));
#183001=CARTESIAN_POINT('',(34.6525130919796,-48.0191904766737,39.92499));
#183002=CARTESIAN_POINT('',(35.115166634744,-48.6559784483766,39.116));
#183003=CARTESIAN_POINT('Origin',(35.0926950035817,-48.6250489015213,39.5550297827311));
#183004=CARTESIAN_POINT('',(35.3510917648534,-48.9807015307819,39.116));
#183005=CARTESIAN_POINT('',(35.3945043333729,-49.0404538064755,39.116));
#183006=CARTESIAN_POINT('',(35.4251752107437,-49.0826686475735,39.3343017080178));
#183007=CARTESIAN_POINT('',(35.3510917642532,-48.9807015312179,39.116));
#183008=CARTESIAN_POINT('',(35.6191209461251,-49.349612051305,39.5248017080178));
#183009=CARTESIAN_POINT('Origin',(35.6018243948131,-49.3258045171787,39.1947745585585));
#183010=CARTESIAN_POINT('',(35.7079988465457,-49.4719419865734,39.5248017080178));
#183011=CARTESIAN_POINT('',(35.7083096150578,-49.4723697227348,39.5248017080178));
#183012=CARTESIAN_POINT('',(35.9019445403517,-49.7388853330812,39.3343017080178));
#183013=CARTESIAN_POINT('Origin',(35.7252979297061,-49.4957512585778,39.1947728594245));
#183014=CARTESIAN_POINT('',(35.9760279559086,-49.8408524068605,39.116));
#183015=CARTESIAN_POINT('',(35.9019445403517,-49.7388853330812,39.3343017080178));
#183016=CARTESIAN_POINT('',(36.2122593934161,-50.1659970864927,39.116));
#183017=CARTESIAN_POINT('Origin',(29.2968639067301,-50.3626567888876,40.10025));
#183018=CARTESIAN_POINT('',(29.501078514911,-51.1278468659048,40.10025));
#183019=CARTESIAN_POINT('',(31.410023123206,-54.4342359163064,40.10025));
#183020=CARTESIAN_POINT('',(29.1186878401555,-50.4655267888876,40.10025));
#183021=CARTESIAN_POINT('',(31.4364195775134,-54.4189959163064,40.10025));
#183022=CARTESIAN_POINT('Origin',(5.57329024769379E-15,5.82219538115768E-15,
40.10025));
#183023=CARTESIAN_POINT('',(29.5274749692184,-51.1126068659048,40.10025));
#183024=CARTESIAN_POINT('',(29.49212344634,-51.0513762321545,40.10025));
#183025=CARTESIAN_POINT('Origin',(5.68506366753766E-15,5.18642144914201E-15,
40.10025));
#183026=CARTESIAN_POINT('Origin',(0.164977839420936,0.0952499999999996,
-2.32316690526365E-17));
#183027=CARTESIAN_POINT('',(30.1668231006074,-51.8694703131947,39.116));
#183028=CARTESIAN_POINT('',(29.9514158469229,-51.4963740054944,39.3548010137695));
#183029=CARTESIAN_POINT('Origin',(30.1477075895458,-51.8363612768235,39.5550297832851));
#183030=CARTESIAN_POINT('',(29.7732664900074,-51.1878102690444,39.92499));
#183031=CARTESIAN_POINT('',(29.9514158469229,-51.4963740054944,39.3548010137695));
#183032=CARTESIAN_POINT('',(31.4933613949858,-54.1671020372439,39.92499));
#183033=CARTESIAN_POINT('',(31.623254538859,-54.3920835619871,39.92499));
#183034=CARTESIAN_POINT('',(31.3152122841232,-53.8585387246951,39.3548010137695));
#183035=CARTESIAN_POINT('',(31.4933613949858,-54.1671020372439,39.92499));
#183036=CARTESIAN_POINT('',(31.0998052504799,-53.4854427993287,39.116));
#183037=CARTESIAN_POINT('Origin',(31.1189208231087,-53.5185519423377,39.5550293907207));
#183038=CARTESIAN_POINT('',(30.8991154799516,-53.1378379187905,39.116));
#183039=CARTESIAN_POINT('',(0.164977839420941,0.0952499999999996,39.116));
#183040=CARTESIAN_POINT('',(30.8360963620061,-53.0286856060847,39.3343017080178));
#183041=CARTESIAN_POINT('',(30.899115479335,-53.1378379191465,39.116));
#183042=CARTESIAN_POINT('',(30.6711163007936,-52.7429317578288,39.5248017080178));
#183043=CARTESIAN_POINT('Origin',(30.6858295650754,-52.7684169058653,39.1947747614259));
#183044=CARTESIAN_POINT('',(30.5955122429562,-52.611981688396,39.5248017080178));
#183045=CARTESIAN_POINT('',(0.164977839420941,0.0952499999999996,39.5248017080178));
#183046=CARTESIAN_POINT('',(30.4305321463776,-52.3262277788842,39.3343017080178));
#183047=CARTESIAN_POINT('Origin',(30.5807966351526,-52.5864945348689,39.1947728911841));
#183048=CARTESIAN_POINT('',(30.367513002735,-52.2170754202457,39.116));
#183049=CARTESIAN_POINT('',(30.4305321463776,-52.3262277788842,39.3343017080178));
#183050=CARTESIAN_POINT('',(0.164977839420941,0.0952499999999996,39.116));
#183051=CARTESIAN_POINT('Origin',(-0.164977839420936,-0.0952499999999996,
2.32316690526365E-17));
#183052=CARTESIAN_POINT('',(30.769849571638,-53.6759427993287,39.116));
#183053=CARTESIAN_POINT('',(30.9852566047567,-54.0490387249979,39.3548010137695));
#183054=CARTESIAN_POINT('Origin',(30.788965144123,-53.7090519420886,39.555029391245));
#183055=CARTESIAN_POINT('',(31.163405715752,-54.3576020374702,39.92499));
#183056=CARTESIAN_POINT('',(30.9852566047567,-54.0490387249979,39.3548010137695));
#183057=CARTESIAN_POINT('',(29.443310811626,-51.3783102687785,39.92499));
#183058=CARTESIAN_POINT('',(-0.164977839420933,-0.0952499999999948,39.92499));
#183059=CARTESIAN_POINT('',(29.6214601686927,-51.6868740051412,39.3548010137695));
#183060=CARTESIAN_POINT('',(29.443310811626,-51.3783102687785,39.92499));
#183061=CARTESIAN_POINT('',(29.8368674217655,-52.0599703131947,39.116));
#183062=CARTESIAN_POINT('Origin',(29.8177519105517,-52.0268612765597,39.5550297827289));
#183063=CARTESIAN_POINT('',(30.0375573245355,-52.4075754198748,39.116));
#183064=CARTESIAN_POINT('',(30.0744862609074,-52.471538215424,39.116));
#183065=CARTESIAN_POINT('',(30.1005764675357,-52.5167277788842,39.3343017080178));
#183066=CARTESIAN_POINT('',(30.0375573238931,-52.4075754202457,39.116));
#183067=CARTESIAN_POINT('',(30.2655565641143,-52.802481688396,39.5248017080178));
#183068=CARTESIAN_POINT('Origin',(30.2508433300769,-52.7769965925048,39.1947745585576));
#183069=CARTESIAN_POINT('',(30.3411606219517,-52.9334317578288,39.5248017080178));
#183070=CARTESIAN_POINT('',(30.3414249774377,-52.9338896349618,39.5248017080178));
#183071=CARTESIAN_POINT('',(30.5061406831642,-53.2191856060846,39.3343017080178));
#183072=CARTESIAN_POINT('Origin',(30.3558761923092,-52.9589188467264,39.1947728594198));
#183073=CARTESIAN_POINT('',(30.5691598004931,-53.3283379191465,39.116));
#183074=CARTESIAN_POINT('',(30.5061406831642,-53.2191856060846,39.3343017080178));
#183075=CARTESIAN_POINT('',(30.770110263767,-53.6763943313414,39.116));
#183076=CARTESIAN_POINT('Origin',(23.8720415006489,-53.1491210481984,40.10025));
#183077=CARTESIAN_POINT('',(23.9951532569806,-53.9314655730805,40.10025));
#183078=CARTESIAN_POINT('',(25.5480287005717,-57.4192809246789,40.10025));
#183079=CARTESIAN_POINT('',(23.6840886581935,-53.2328030451448,40.10025));
#183080=CARTESIAN_POINT('',(25.5758735661207,-57.406883591798,40.10025));
#183081=CARTESIAN_POINT('Origin',(5.58700050634535E-15,5.8291811068598E-15,
40.10025));
#183082=CARTESIAN_POINT('',(24.0229981225296,-53.9190682401995,40.10025));
#183083=CARTESIAN_POINT('',(23.9942406030432,-53.8544777939069,40.10025));
#183084=CARTESIAN_POINT('Origin',(5.67792519749014E-15,5.18278421698235E-15,
40.10025));
#183085=CARTESIAN_POINT('Origin',(0.174030409680916,0.0774833305059395,
-2.45064239960505E-17));
#183086=CARTESIAN_POINT('',(24.57973006491,-54.7386155880004,39.116));
#183087=CARTESIAN_POINT('',(24.4045020183944,-54.345046951707,39.3548010137695));
#183088=CARTESIAN_POINT('Origin',(24.5641801073104,-54.7036898113989,39.5550297832849));
#183089=CARTESIAN_POINT('',(24.2595822754874,-54.0195518811805,39.92499));
#183090=CARTESIAN_POINT('',(24.4045020183944,-54.345046951707,39.3548010137695));
#183091=CARTESIAN_POINT('',(25.658833530444,-57.1623216544372,39.92499));
#183092=CARTESIAN_POINT('',(25.764498133039,-57.3996482375657,39.92499));
#183093=CARTESIAN_POINT('',(25.5139139879314,-56.8368270312094,39.3548010137695));
#183094=CARTESIAN_POINT('',(25.658833530444,-57.1623216544372,39.92499));
#183095=CARTESIAN_POINT('',(25.3386861202876,-56.4432587981557,39.116));
#183096=CARTESIAN_POINT('Origin',(25.3542361279706,-56.4781846872463,39.5550293907214));
#183097=CARTESIAN_POINT('',(25.1754303533075,-56.0765803402169,39.116));
#183098=CARTESIAN_POINT('',(0.174030409680921,0.0774833305059395,39.116));
#183099=CARTESIAN_POINT('',(25.1241659841934,-55.9614386837454,39.3343017080178));
#183100=CARTESIAN_POINT('',(25.1754303526574,-56.0765803405064,39.116));
#183101=CARTESIAN_POINT('',(24.9899591116494,-55.6600051127008,39.5248017080178));
#183102=CARTESIAN_POINT('Origin',(25.0019278517687,-55.6868886053327,39.1947747614216));
#183103=CARTESIAN_POINT('',(24.928457230274,-55.5218696254673,39.5248017080178));
#183104=CARTESIAN_POINT('',(0.174030409680921,0.0774833305059395,39.5248017080178));
#183105=CARTESIAN_POINT('',(24.7942503289606,-55.2204359898057,39.3343017080178));
#183106=CARTESIAN_POINT('Origin',(24.9164863690992,-55.4949838933603,39.1947728911913));
#183107=CARTESIAN_POINT('',(24.7429859390912,-55.1052942849672,39.116));
#183108=CARTESIAN_POINT('',(24.7942503289606,-55.2204359898057,39.3343017080178));
#183109=CARTESIAN_POINT('',(0.174030409680921,0.0774833305059395,39.116));
#183110=CARTESIAN_POINT('Origin',(-0.174030409680916,-0.0774833305059395,
2.45064239960505E-17));
#183111=CARTESIAN_POINT('',(24.9906253009257,-56.5982254591676,39.116));
#183112=CARTESIAN_POINT('',(25.165853168017,-56.9917936924673,39.3548010137695));
#183113=CARTESIAN_POINT('Origin',(25.006175308492,-56.6331513479958,39.5550293912451));
#183114=CARTESIAN_POINT('',(25.3107727106685,-57.3172883156332,39.92499));
#183115=CARTESIAN_POINT('',(25.165853168017,-56.9917936924673,39.3548010137695));
#183116=CARTESIAN_POINT('',(23.9115214566113,-54.174518541976,39.92499));
#183117=CARTESIAN_POINT('',(-0.174030409680912,-0.0774833305059344,39.92499));
#183118=CARTESIAN_POINT('',(24.0564411996773,-54.5000136124319,39.3548010137695));
#183119=CARTESIAN_POINT('',(23.9115214566113,-54.174518541976,39.92499));
#183120=CARTESIAN_POINT('',(24.2316692455482,-54.8935822490123,39.116));
#183121=CARTESIAN_POINT('Origin',(24.2161192878248,-54.8586564721328,39.5550297827294));
#183122=CARTESIAN_POINT('',(24.3949251204072,-55.2602609456773,39.116));
#183123=CARTESIAN_POINT('',(24.4249658234765,-55.3277334713091,39.116));
#183124=CARTESIAN_POINT('',(24.4461895095988,-55.3754026508175,39.3343017080178));
#183125=CARTESIAN_POINT('',(24.3949251197294,-55.2602609459791,39.116));
#183126=CARTESIAN_POINT('',(24.5803964109122,-55.6768362864792,39.5248017080178));
#183127=CARTESIAN_POINT('Origin',(24.5684276954197,-55.6499528488653,39.1947745585593));
#183128=CARTESIAN_POINT('',(24.6418982922876,-55.8149717737127,39.5248017080178));
#183129=CARTESIAN_POINT('',(24.6421133384135,-55.8154547752195,39.5248017080178));
#183130=CARTESIAN_POINT('',(24.7761051648316,-56.1164053447572,39.3343017080178));
#183131=CARTESIAN_POINT('Origin',(24.6538691229762,-55.8418574376282,39.194772859424));
#183132=CARTESIAN_POINT('',(24.8273695332956,-56.2315470015182,39.116));
#183133=CARTESIAN_POINT('',(24.7761051648316,-56.1164053447572,39.3343017080178));
#183134=CARTESIAN_POINT('',(24.9908373670086,-56.5987017673883,39.116));
#183135=CARTESIAN_POINT('Origin',(18.1856720123407,-55.3532724151365,40.10025));
#183136=CARTESIAN_POINT('',(18.2263320786581,-56.1441998575528,40.10025));
#183137=CARTESIAN_POINT('',(19.4061247292252,-59.7752282754837,40.10025));
#183138=CARTESIAN_POINT('',(17.9900016446781,-55.4168495715592,40.10025));
#183139=CARTESIAN_POINT('',(19.4351129318419,-59.7658094374952,40.10025));
#183140=CARTESIAN_POINT('Origin',(5.60136586593794E-15,5.83469545175774E-15,
40.10025));
#183141=CARTESIAN_POINT('',(18.2553202812748,-56.1347810195642,40.10025));
#183142=CARTESIAN_POINT('',(18.2334718385819,-56.0675384271753,40.10025));
#183143=CARTESIAN_POINT('Origin',(5.67044563844026E-15,5.17991308326517E-15,
40.10025));
#183144=CARTESIAN_POINT('Origin',(0.181176266354227,0.058867737428427,-2.55126814298648E-17));
#183145=CARTESIAN_POINT('',(18.7233363629823,-57.0080331356323,39.116));
#183146=CARTESIAN_POINT('',(18.5902073587821,-56.5983041910846,39.3548010137695));
#183147=CARTESIAN_POINT('Origin',(18.7115223274341,-56.9716732729178,39.5550297832854));
#183148=CARTESIAN_POINT('',(18.4801050009135,-56.2594439785882,39.92499));
#183149=CARTESIAN_POINT('',(18.5902073587821,-56.5983041910846,39.3548010137695));
#183150=CARTESIAN_POINT('',(19.5431821162865,-59.5312589135996,39.92499));
#183151=CARTESIAN_POINT('',(19.6234604941057,-59.778330355405,39.92499));
#183152=CARTESIAN_POINT('',(19.4330799109586,-59.1923991668987,39.3548010137695));
#183153=CARTESIAN_POINT('',(19.5431821162865,-59.5312589135996,39.92499));
#183154=CARTESIAN_POINT('',(19.2999510425005,-58.7826706420789,39.116));
#183155=CARTESIAN_POINT('Origin',(19.3117651160996,-58.8190306219019,39.5550293907203));
#183156=CARTESIAN_POINT('',(19.1759179434156,-58.4009360126567,39.116));
#183157=CARTESIAN_POINT('',(0.181176266354232,0.058867737428427,39.116));
#183158=CARTESIAN_POINT('',(19.1369699862882,-58.281066528503,39.3343017080178));
#183159=CARTESIAN_POINT('',(19.1759179427385,-58.4009360128767,39.116));
#183160=CARTESIAN_POINT('',(19.0350067009929,-57.9672558039532,39.5248017080178));
#183161=CARTESIAN_POINT('Origin',(19.0440997849305,-57.9952431000151,39.1947747614281));
#183162=CARTESIAN_POINT('',(18.9882808235619,-57.8234483402239,39.5248017080178));
#183163=CARTESIAN_POINT('',(0.181176266354233,0.058867737428427,39.5248017080178));
#183164=CARTESIAN_POINT('',(18.8863175164091,-57.5096375484037,39.3343017080178));
#183165=CARTESIAN_POINT('Origin',(18.9791858642777,-57.7954585952468,39.1947728911937));
#183166=CARTESIAN_POINT('',(18.8473695436961,-57.3897680139785,39.116));
#183167=CARTESIAN_POINT('',(18.8863175164091,-57.5096375484037,39.3343017080178));
#183168=CARTESIAN_POINT('',(0.181176266354232,0.058867737428427,39.116));
#183169=CARTESIAN_POINT('Origin',(-0.181176266354227,-0.058867737428427,
2.55126814298648E-17));
#183170=CARTESIAN_POINT('',(18.937598509792,-58.9004061169357,39.116));
#183171=CARTESIAN_POINT('',(19.0707273776751,-59.3101346419424,39.3548010137695));
#183172=CARTESIAN_POINT('Origin',(18.9494125833023,-58.9367660964853,39.5550293912449));
#183173=CARTESIAN_POINT('',(19.1808295831476,-59.6489943885963,39.92499));
#183174=CARTESIAN_POINT('',(19.0707273776751,-59.3101346419424,39.3548010137695));
#183175=CARTESIAN_POINT('',(18.1177524687105,-56.3771794532808,39.92499));
#183176=CARTESIAN_POINT('',(-0.181176266354223,-0.0588677374284217,39.92499));
#183177=CARTESIAN_POINT('',(18.2278548267459,-56.716039665723,39.3548010137695));
#183178=CARTESIAN_POINT('',(18.1177524687105,-56.3771794532808,39.92499));
#183179=CARTESIAN_POINT('',(18.3609838302739,-57.1257686104891,39.116));
#183180=CARTESIAN_POINT('Origin',(18.3491697946315,-57.0894087474849,39.5550297827295));
#183181=CARTESIAN_POINT('',(18.4850170116927,-57.5075034886062,39.116));
#183182=CARTESIAN_POINT('',(18.5078403492309,-57.5777465012099,39.116));
#183183=CARTESIAN_POINT('',(18.5239649837007,-57.6273730232606,39.3343017080178));
#183184=CARTESIAN_POINT('',(18.4850170109876,-57.5075034888353,39.116));
#183185=CARTESIAN_POINT('',(18.6259282908535,-57.9411838150808,39.5248017080178));
#183186=CARTESIAN_POINT('Origin',(18.6168352256581,-57.9131965763138,39.1947745585583));
#183187=CARTESIAN_POINT('',(18.6726541682844,-58.0849912788101,39.5248017080178));
#183188=CARTESIAN_POINT('',(18.6728175489599,-58.0854941128252,39.5248017080178));
#183189=CARTESIAN_POINT('',(18.7746174535798,-58.3988020033599,39.3343017080178));
#183190=CARTESIAN_POINT('Origin',(18.6817491043777,-58.1129809527839,39.1947728594284));
#183191=CARTESIAN_POINT('',(18.8135654100301,-58.5186714877336,39.116));
#183192=CARTESIAN_POINT('',(18.7746174535798,-58.3988020033599,39.3343017080178));
#183193=CARTESIAN_POINT('',(18.9377596263884,-58.9009019828319,39.116));
#183194=CARTESIAN_POINT('Origin',(12.3000564958688,-56.9509617460775,40.10025));
#183195=CARTESIAN_POINT('',(12.2578193919766,-57.7418065394566,40.10025));
#183196=CARTESIAN_POINT('',(13.0516031943527,-61.4762657165316,40.10025));
#183197=CARTESIAN_POINT('',(12.0988124084938,-56.9937374973463,40.10025));
#183198=CARTESIAN_POINT('',(13.0814171332231,-61.4699285681955,40.10025));
#183199=CARTESIAN_POINT('Origin',(5.61622893658571E-15,5.83867799953487E-15,
40.10025));
#183200=CARTESIAN_POINT('',(12.2876333308469,-57.7354693911205,40.10025));
#183201=CARTESIAN_POINT('',(12.2729333410577,-57.6663113765489,40.10025));
#183202=CARTESIAN_POINT('Origin',(5.66270693800216E-15,5.17783950473232E-15,
40.10025));
#183203=CARTESIAN_POINT('Origin',(0.18633711793979,0.0396071771007826,-2.62394165870617E-17));
#183204=CARTESIAN_POINT('',(12.6618058697518,-58.6528587425323,39.116));
#183205=CARTESIAN_POINT('',(12.5722344970959,-58.2314585657881,39.3548010137695));
#183206=CARTESIAN_POINT('Origin',(12.6538571933006,-58.6154631599697,39.5550297832864));
#183207=CARTESIAN_POINT('',(12.4981558287384,-57.8829458347211,39.92499));
#183208=CARTESIAN_POINT('',(12.5722344970959,-58.2314585657881,39.3548010137695));
#183209=CARTESIAN_POINT('',(13.2134115091892,-61.2479592423878,39.92499));
#183210=CARTESIAN_POINT('',(13.2674241155258,-61.5020685764505,39.92499));
#183211=CARTESIAN_POINT('',(13.1393329438488,-60.8994469905094,39.3548010137695));
#183212=CARTESIAN_POINT('',(13.2134115091892,-61.2479592423878,39.92499));
#183213=CARTESIAN_POINT('',(13.0497616623173,-60.4780472453828,39.116));
#183214=CARTESIAN_POINT('Origin',(13.0577103643698,-60.5154429483902,39.5550293907202));
#183215=CARTESIAN_POINT('',(12.9663101637164,-60.0854388089605,39.116));
#183216=CARTESIAN_POINT('',(0.186337117939796,0.0396071771007826,39.116));
#183217=CARTESIAN_POINT('',(12.9401053405448,-59.9621548122772,39.3343017080178));
#183218=CARTESIAN_POINT('',(12.9663101630202,-60.0854388091085,39.116));
#183219=CARTESIAN_POINT('',(12.871502773589,-59.6394051101894,39.5248017080178));
#183220=CARTESIAN_POINT('Origin',(12.8776205756134,-59.6681895750072,39.1947747614316));
#183221=CARTESIAN_POINT('',(12.8400648385937,-59.4915012546305,39.5248017080178));
#183222=CARTESIAN_POINT('',(0.186337117939796,0.0396071771007826,39.5248017080178));
#183223=CARTESIAN_POINT('',(12.7714622569318,-59.1687514833561,39.3343017080178));
#183224=CARTESIAN_POINT('Origin',(12.833945427478,-59.4627141582885,39.1947728911924));
#183225=CARTESIAN_POINT('',(12.7452574235146,-59.0454674350475,39.116));
#183226=CARTESIAN_POINT('',(12.7714622569318,-59.1687514833561,39.3343017080178));
#183227=CARTESIAN_POINT('',(0.186337117939796,0.0396071771007826,39.116));
#183228=CARTESIAN_POINT('Origin',(-0.18633711793979,-0.0396071771007826,
2.62394165870617E-17));
#183229=CARTESIAN_POINT('',(12.6770874264377,-60.5572615995844,39.116));
#183230=CARTESIAN_POINT('',(12.7666587073772,-60.9786613448368,39.3548010137695));
#183231=CARTESIAN_POINT('Origin',(12.6850361284303,-60.5946573023097,39.5550293912463));
#183232=CARTESIAN_POINT('',(12.840737272867,-61.3271735966835,39.92499));
#183233=CARTESIAN_POINT('',(12.7666587073772,-60.9786613448368,39.3548010137695));
#183234=CARTESIAN_POINT('',(12.125481593379,-57.9621601888121,39.92499));
#183235=CARTESIAN_POINT('',(-0.186337117939786,-0.0396071771007771,39.92499));
#183236=CARTESIAN_POINT('',(12.1995602619083,-58.3106729198425,39.3548010137695));
#183237=CARTESIAN_POINT('',(12.125481593379,-57.9621601888121,39.92499));
#183238=CARTESIAN_POINT('',(12.2891316338722,-58.7320730967338,39.116));
#183239=CARTESIAN_POINT('Origin',(12.281182957358,-58.6946775138747,39.5550297827326));
#183240=CARTESIAN_POINT('',(12.3725831883602,-59.1246817890949,39.116));
#183241=CARTESIAN_POINT('',(12.3879391031045,-59.1969256915254,39.116));
#183242=CARTESIAN_POINT('',(12.3987880210522,-59.2479658375577,39.3343017080178));
#183243=CARTESIAN_POINT('',(12.372583187635,-59.1246817892491,39.116));
#183244=CARTESIAN_POINT('',(12.4673906027141,-59.5707156088321,39.5248017080178));
#183245=CARTESIAN_POINT('Origin',(12.4612728133404,-59.5419312029551,39.1947745585607));
#183246=CARTESIAN_POINT('',(12.4988285377094,-59.7186194643909,39.5248017080178));
#183247=CARTESIAN_POINT('',(12.4989384629016,-59.7191366217596,39.5248017080178));
#183248=CARTESIAN_POINT('',(12.5674311046652,-60.0413691664788,39.3343017080178));
#183249=CARTESIAN_POINT('Origin',(12.5049479331829,-59.7474064876936,39.1947728594244));
#183250=CARTESIAN_POINT('',(12.5936359271406,-60.1646531633101,39.116));
#183251=CARTESIAN_POINT('',(12.5674311046652,-60.0413691664788,39.3343017080178));
#183252=CARTESIAN_POINT('',(12.6771958283204,-60.5577715903455,39.116));
#183253=CARTESIAN_POINT('Origin',(6.27967898647588,-57.9246844223735,40.10025));
#183254=CARTESIAN_POINT('',(6.15500747092297,-58.7067819056643,40.10025));
#183255=CARTESIAN_POINT('',(6.55408556365926,-62.5037563256535,40.10025));
#183256=CARTESIAN_POINT('',(6.07506605172282,-57.9461901084062,40.10025));
#183257=CARTESIAN_POINT('',(6.58439859103008,-62.5005702980931,40.10025));
#183258=CARTESIAN_POINT('Origin',(5.63142687537637E-15,5.84108511656431E-15,
40.10025));
#183259=CARTESIAN_POINT('',(6.1853204982938,-58.7035958781039,40.10025));
#183260=CARTESIAN_POINT('',(6.1779300175725,-58.6332801510296,40.10025));
#183261=CARTESIAN_POINT('Origin',(5.65479388299727E-15,5.17658619994411E-15,
40.10025));
#183262=CARTESIAN_POINT('Origin',(0.189456421067656,0.0199126722524874,
-2.66786672051798E-17));
#183263=CARTESIAN_POINT('',(6.46154998175899,-59.6550713551493,39.116));
#183264=CARTESIAN_POINT('',(6.41651760335031,-59.2266168947286,39.3548010137695));
#183265=CARTESIAN_POINT('Origin',(6.45755375176722,-59.6170497665647,39.5550297832833));
#183266=CARTESIAN_POINT('',(6.37927424589724,-58.8722700235036,39.92499));
#183267=CARTESIAN_POINT('',(6.41651760335031,-59.2266168947286,39.3548010137695));
#183268=CARTESIAN_POINT('',(6.73887200051313,-62.2936141127569,39.92499));
#183269=CARTESIAN_POINT('',(6.76602706194927,-62.5519772640372,39.92499));
#183270=CARTESIAN_POINT('',(6.70162869542395,-61.9392677288636,39.3548010137695));
#183271=CARTESIAN_POINT('',(6.73887200051313,-62.2936141127569,39.92499));
#183272=CARTESIAN_POINT('',(6.65659636252364,-61.5108137072212,39.116));
#183273=CARTESIAN_POINT('Origin',(6.66059260538629,-61.5488354182641,39.5550293907226));
#183274=CARTESIAN_POINT('',(6.61464077648889,-61.1116329639869,39.116));
#183275=CARTESIAN_POINT('',(0.189456421067662,0.0199126722524874,39.116));
#183276=CARTESIAN_POINT('',(6.60146619279927,-60.9862851800404,39.3343017080178));
#183277=CARTESIAN_POINT('',(6.61464077578103,-61.1116329640613,39.116));
#183278=CARTESIAN_POINT('',(6.56697596826259,-60.6581326136904,39.5248017080178));
#183279=CARTESIAN_POINT('Origin',(6.57005146045377,-60.68739887864,39.1947747614269));
#183280=CARTESIAN_POINT('',(6.55117041629749,-60.5077528318944,39.5248017080178));
#183281=CARTESIAN_POINT('',(0.189456421067662,0.0199126722524874,39.5248017080178));
#183282=CARTESIAN_POINT('',(6.51668018436727,-60.1796001951995,39.3343017080178));
#183283=CARTESIAN_POINT('Origin',(6.54809359889865,-60.478483781637,39.1947728911937));
#183284=CARTESIAN_POINT('',(6.50350559588446,-60.0542523588397,39.116));
#183285=CARTESIAN_POINT('',(6.51668018436727,-60.1796001951995,39.3343017080178));
#183286=CARTESIAN_POINT('',(0.189456421067662,0.0199126722524874,39.116));
#183287=CARTESIAN_POINT('Origin',(-0.189456421067656,-0.0199126722524874,
2.66786672051798E-17));
#183288=CARTESIAN_POINT('',(6.27768352038833,-61.5506390517262,39.116));
#183289=CARTESIAN_POINT('',(6.32271585268621,-61.9790930734319,39.3548010137695));
#183290=CARTESIAN_POINT('Origin',(6.2816797632211,-61.5886607624848,39.555029391244));
#183291=CARTESIAN_POINT('',(6.35995915792839,-62.3334394573092,39.92499));
#183292=CARTESIAN_POINT('',(6.32271585268621,-61.9790930734319,39.3548010137695));
#183293=CARTESIAN_POINT('',(6.00036140429027,-58.912095367953,39.92499));
#183294=CARTESIAN_POINT('',(-0.189456421067651,-0.0199126722524818,39.92499));
#183295=CARTESIAN_POINT('',(6.03760476191764,-59.2664422391598,39.3548010137695));
#183296=CARTESIAN_POINT('',(6.00036140429027,-58.912095367953,39.92499));
#183297=CARTESIAN_POINT('',(6.08263713962368,-59.6948966996543,39.116));
#183298=CARTESIAN_POINT('Origin',(6.07864090960028,-59.6568751107687,39.5550297827311));
#183299=CARTESIAN_POINT('',(6.12459275448592,-60.0940777032673,39.116));
#183300=CARTESIAN_POINT('',(6.13231300382157,-60.1675309762115,39.116));
#183301=CARTESIAN_POINT('',(6.13776734223196,-60.2194255397045,39.3343017080178));
#183302=CARTESIAN_POINT('',(6.12459275374915,-60.0940777033447,39.116));
#183303=CARTESIAN_POINT('',(6.17225757416218,-60.5475781763994,39.5248017080178));
#183304=CARTESIAN_POINT('Origin',(6.16918208839128,-60.5183119713882,39.194774558559));
#183305=CARTESIAN_POINT('',(6.18806312612727,-60.6979579581954,39.5248017080178));
#183306=CARTESIAN_POINT('',(6.18811839147268,-60.6984837728333,39.5248017080178));
#183307=CARTESIAN_POINT('',(6.22255335066396,-61.0261105245454,39.3343017080178));
#183308=CARTESIAN_POINT('Origin',(6.19113993560417,-60.7272269341768,39.1947728594245));
#183309=CARTESIAN_POINT('',(6.23572793364572,-61.1514583085662,39.116));
#183310=CARTESIAN_POINT('',(6.22255335066396,-61.0261105245454,39.3343017080178));
#183311=CARTESIAN_POINT('',(6.2777380198836,-61.5511575797868,39.116));
#183312=CARTESIAN_POINT('Origin',(0.190499999999802,-58.2637721346185,40.10025));
#183313=CARTESIAN_POINT('',(-0.0152400000002005,-59.0285534841296,40.10025));
#183314=CARTESIAN_POINT('',(-0.0152400000002138,-62.8464427007196,40.10025));
#183315=CARTESIAN_POINT('',(-0.0152400000001978,-58.2637721346185,40.10025));
#183316=CARTESIAN_POINT('',(0.0152399999997862,-62.8464427007196,40.10025));
#183317=CARTESIAN_POINT('Origin',(-4.80914138193527E-17,1.47005845636695E-16,
40.10025));
#183318=CARTESIAN_POINT('',(0.0152399999997995,-59.0285534841296,40.10025));
#183319=CARTESIAN_POINT('',(0.0152399999997998,-58.9578504383728,40.10025));
#183320=CARTESIAN_POINT('Origin',(3.94085276091011E-16,-7.6540994051039E-17,
40.10025));
#183321=CARTESIAN_POINT('Origin',(0.1905,-6.65127195049617E-16,-2.68256207625279E-17));
#183322=CARTESIAN_POINT('',(0.190499999999796,-60.0036905223731,39.116));
#183323=CARTESIAN_POINT('',(0.190499999999797,-59.5728760150042,39.3548010137695));
#183324=CARTESIAN_POINT('Origin',(0.190499999999796,-59.9654595002498,39.5550297832847));
#183325=CARTESIAN_POINT('',(0.190499999468434,-59.2165773020941,39.92499));
#183326=CARTESIAN_POINT('',(0.190499999999798,-59.5728760150042,39.3548010137695));
#183327=CARTESIAN_POINT('',(0.190499999999788,-62.6567671111299,39.92499));
#183328=CARTESIAN_POINT('',(0.190499999999786,-62.9165533988763,39.92499));
#183329=CARTESIAN_POINT('',(0.19050000060545,-62.3004688883555,39.3548010137695));
#183330=CARTESIAN_POINT('',(0.190499999999787,-62.6567671111299,39.92499));
#183331=CARTESIAN_POINT('',(0.19049999999979,-61.8696548221181,39.116));
#183332=CARTESIAN_POINT('Origin',(0.190499999999789,-61.9078859673761,39.5550293907201));
#183333=CARTESIAN_POINT('',(0.190500000711669,-61.4682752798284,39.116));
#183334=CARTESIAN_POINT('',(0.190500000000006,-6.65127195049617E-16,39.116));
#183335=CARTESIAN_POINT('',(0.190499999999791,-61.3422370451705,39.3343017080178));
#183336=CARTESIAN_POINT('',(0.190499999999791,-61.4682752798284,39.116));
#183337=CARTESIAN_POINT('',(0.190499999999793,-61.0122769227456,39.5248017080178));
#183338=CARTESIAN_POINT('Origin',(0.19049948662219,-61.0417043405089,39.1947747614312));
#183339=CARTESIAN_POINT('',(0.190499999999793,-60.8610688070707,39.5248017080178));
#183340=CARTESIAN_POINT('',(0.190500000000006,-6.65127195049617E-16,39.5248017080178));
#183341=CARTESIAN_POINT('',(0.190499999999794,-60.5311086139135,39.3343017080178));
#183342=CARTESIAN_POINT('Origin',(0.190499486573297,-60.8316384807416,39.1947728911891));
#183343=CARTESIAN_POINT('',(0.190499999999795,-60.4050703266283,39.116));
#183344=CARTESIAN_POINT('',(0.190499999999794,-60.5311086139135,39.3343017080178));
#183345=CARTESIAN_POINT('',(0.190500000000006,-6.65127195049617E-16,39.116));
#183346=CARTESIAN_POINT('Origin',(-0.1905,6.65127195049617E-16,2.68256207625279E-17));
#183347=CARTESIAN_POINT('',(-0.190500000000211,-61.8696548221181,39.116));
#183348=CARTESIAN_POINT('',(-0.190500000000213,-62.3004688883554,39.3548010137695));
#183349=CARTESIAN_POINT('Origin',(-0.190500000000211,-61.9078859670887,
39.5550293912444));
#183350=CARTESIAN_POINT('',(-0.190500000452744,-62.6567671111299,39.92499));
#183351=CARTESIAN_POINT('',(-0.190500000000212,-62.3004688883554,39.3548010137695));
#183352=CARTESIAN_POINT('',(-0.190500000000201,-59.2165773020941,39.92499));
#183353=CARTESIAN_POINT('',(-0.190499999999994,6.28724079446023E-15,39.92499));
#183354=CARTESIAN_POINT('',(-0.190499999294014,-59.5728760150042,39.3548010137695));
#183355=CARTESIAN_POINT('',(-0.190500000000201,-59.2165773020941,39.92499));
#183356=CARTESIAN_POINT('',(-0.190500000000204,-60.0036905223731,39.116));
#183357=CARTESIAN_POINT('Origin',(-0.190500000000204,-59.9654594999465,
39.5550297827309));
#183358=CARTESIAN_POINT('',(-0.190499999258436,-60.4050703266283,39.116));
#183359=CARTESIAN_POINT('',(-0.190500000000206,-60.4789282006569,39.116));
#183360=CARTESIAN_POINT('',(-0.190500000000206,-60.5311086139135,39.3343017080178));
#183361=CARTESIAN_POINT('',(-0.190500000000205,-60.4050703266283,39.116));
#183362=CARTESIAN_POINT('',(-0.190500000000207,-60.8610688070707,39.5248017080178));
#183363=CARTESIAN_POINT('Origin',(-0.190499486502767,-60.8316414495905,
39.1947745585607));
#183364=CARTESIAN_POINT('',(-0.190500000000207,-61.0122769227456,39.5248017080178));
#183365=CARTESIAN_POINT('',(-0.190500000000207,-61.0128056337175,39.5248017080178));
#183366=CARTESIAN_POINT('',(-0.190500000000209,-61.3422370451705,39.3343017080178));
#183367=CARTESIAN_POINT('Origin',(-0.190499486688308,-61.0417071743813,
39.1947728594259));
#183368=CARTESIAN_POINT('',(-0.190500000000209,-61.4682752798284,39.116));
#183369=CARTESIAN_POINT('',(-0.190500000000209,-61.3422370451705,39.3343017080178));
#183370=CARTESIAN_POINT('',(-0.190500000000211,-61.8701762063762,39.116));
#183371=CARTESIAN_POINT('Origin',(-5.90076614434095,-57.9645097668785,40.10025));
#183372=CARTESIAN_POINT('',(-6.18532049829418,-58.7035958781039,40.10025));
#183373=CARTESIAN_POINT('',(-6.58439859103049,-62.5005702980931,40.10025));
#183374=CARTESIAN_POINT('',(-6.10537907909402,-57.9430040808458,40.10025));
#183375=CARTESIAN_POINT('',(-6.55408556365967,-62.5037563256534,40.10025));
#183376=CARTESIAN_POINT('Origin',(-3.27251186835855E-17,1.46200532232821E-16,
40.10025));
#183377=CARTESIAN_POINT('',(-6.15500747092336,-58.7067819056643,40.10025));
#183378=CARTESIAN_POINT('',(-6.14761699020206,-58.6364661785899,40.10025));
#183379=CARTESIAN_POINT('Origin',(3.86084563605877E-16,-7.61216944770112E-17,
40.10025));
#183380=CARTESIAN_POINT('Origin',(0.189456421067656,-0.0199126722524887,
-2.66786672051798E-17));
#183381=CARTESIAN_POINT('',(-6.08263713962407,-59.6948966996542,39.116));
#183382=CARTESIAN_POINT('',(-6.03760476121539,-59.2664422392336,39.3548010137695));
#183383=CARTESIAN_POINT('Origin',(-6.07864090963236,-59.6568751110701,39.5550297832838));
#183384=CARTESIAN_POINT('',(-6.0003614048196,-58.9120953678974,39.92499));
#183385=CARTESIAN_POINT('',(-6.03760476121539,-59.2664422392336,39.3548010137695));
#183386=CARTESIAN_POINT('',(-6.35995915837823,-62.3334394572619,39.92499));
#183387=CARTESIAN_POINT('',(-6.38711421981437,-62.5918026085421,39.92499));
#183388=CARTESIAN_POINT('',(-6.32271585208497,-61.9790930734951,39.3548010137695));
#183389=CARTESIAN_POINT('',(-6.35995915837823,-62.3334394572619,39.92499));
#183390=CARTESIAN_POINT('',(-6.27768352038873,-61.5506390517262,39.116));
#183391=CARTESIAN_POINT('Origin',(-6.28167976325141,-61.5886607627694,39.5550293907224));
#183392=CARTESIAN_POINT('',(-6.23572793293811,-61.1514583086406,39.116));
#183393=CARTESIAN_POINT('',(0.189456421067662,-0.0199126722524887,39.116));
#183394=CARTESIAN_POINT('',(-6.22255335066436,-61.0261105245454,39.3343017080178));
#183395=CARTESIAN_POINT('',(-6.23572793364612,-61.1514583085662,39.116));
#183396=CARTESIAN_POINT('',(-6.18806312612767,-60.6979579581954,39.5248017080178));
#183397=CARTESIAN_POINT('Origin',(-6.19113963945004,-60.7272241158261,39.1947747614376));
#183398=CARTESIAN_POINT('',(-6.17225757416258,-60.5475781763993,39.5248017080178));
#183399=CARTESIAN_POINT('',(0.189456421067662,-0.0199126722524887,39.5248017080178));
#183400=CARTESIAN_POINT('',(-6.13776734223235,-60.2194255397045,39.3343017080178));
#183401=CARTESIAN_POINT('Origin',(-6.16918177799152,-60.5183090188066,39.1947728911941));
#183402=CARTESIAN_POINT('',(-6.12459275374954,-60.0940777033447,39.116));
#183403=CARTESIAN_POINT('',(-6.13776734223235,-60.2194255397045,39.3343017080178));
#183404=CARTESIAN_POINT('',(0.189456421067662,-0.0199126722524887,39.116));
#183405=CARTESIAN_POINT('Origin',(-0.189456421067656,0.0199126722524887,
2.66786672051798E-17));
#183406=CARTESIAN_POINT('',(-6.65659636252404,-61.5108137072212,39.116));
#183407=CARTESIAN_POINT('',(-6.70162869482193,-61.9392677289269,39.3548010137695));
#183408=CARTESIAN_POINT('Origin',(-6.6605926053566,-61.5488354179777,39.5550293912481));
#183409=CARTESIAN_POINT('',(-6.73887200096381,-62.2936141127096,39.92499));
#183410=CARTESIAN_POINT('',(-6.70162869482193,-61.9392677289269,39.3548010137695));
#183411=CARTESIAN_POINT('',(-6.37927424642597,-58.872270023448,39.92499));
#183412=CARTESIAN_POINT('',(-0.18945642106765,0.0199126722524943,39.92499));
#183413=CARTESIAN_POINT('',(-6.41651760264748,-59.2266168948025,39.3548010137695));
#183414=CARTESIAN_POINT('',(-6.37927424642597,-58.872270023448,39.92499));
#183415=CARTESIAN_POINT('',(-6.46154998175939,-59.6550713551492,39.116));
#183416=CARTESIAN_POINT('Origin',(-6.45755375173582,-59.6170497662621,39.5550297827283));
#183417=CARTESIAN_POINT('',(-6.5035055951475,-60.0542523589172,39.116));
#183418=CARTESIAN_POINT('',(-6.51122584595728,-60.1277056317065,39.116));
#183419=CARTESIAN_POINT('',(-6.51668018436767,-60.1796001951995,39.3343017080178));
#183420=CARTESIAN_POINT('',(-6.50350559588486,-60.0542523588397,39.116));
#183421=CARTESIAN_POINT('',(-6.55117041629789,-60.5077528318944,39.5248017080178));
#183422=CARTESIAN_POINT('Origin',(-6.54809390915818,-60.4784867342341,39.1947745585578));
#183423=CARTESIAN_POINT('',(-6.56697596826298,-60.6581326136904,39.5248017080178));
#183424=CARTESIAN_POINT('',(-6.5670312336084,-60.6586584283283,39.5248017080178));
#183425=CARTESIAN_POINT('',(-6.60146619279967,-60.9862851800404,39.3343017080178));
#183426=CARTESIAN_POINT('Origin',(-6.57005175673992,-60.687401696982,39.1947728594215));
#183427=CARTESIAN_POINT('',(-6.61464077578143,-61.1116329640612,39.116));
#183428=CARTESIAN_POINT('',(-6.60146619279967,-60.9862851800404,39.3343017080178));
#183429=CARTESIAN_POINT('',(-6.65665086201932,-61.5113322352818,39.116));
#183430=CARTESIAN_POINT('Origin',(-11.9273822599896,-57.030176100279,40.10025));
#183431=CARTESIAN_POINT('',(-12.2876333308473,-57.7354693911204,40.10025));
#183432=CARTESIAN_POINT('',(-13.0814171332235,-61.4699285681954,40.10025));
#183433=CARTESIAN_POINT('',(-12.1286263473646,-56.9874003490101,40.10025));
#183434=CARTESIAN_POINT('',(-13.0516031943531,-61.4762657165315,40.10025));
#183435=CARTESIAN_POINT('Origin',(-1.75271798929331E-17,1.43793415203377E-16,
40.10025));
#183436=CARTESIAN_POINT('',(-12.257819391977,-57.7418065394565,40.10025));
#183437=CARTESIAN_POINT('',(-12.2431194021877,-57.672648524885,40.10025));
#183438=CARTESIAN_POINT('Origin',(3.78171508600985E-16,-7.48683896888047E-17,
40.10025));
#183439=CARTESIAN_POINT('Origin',(0.18633711793979,-0.0396071771007839,
-2.62394165870617E-17));
#183440=CARTESIAN_POINT('',(-12.2891316338726,-58.7320730967337,39.116));
#183441=CARTESIAN_POINT('',(-12.1995602612167,-58.3106729199896,39.3548010137695));
#183442=CARTESIAN_POINT('Origin',(-12.281182957421,-58.6946775141692,39.5550297832827));
#183443=CARTESIAN_POINT('',(-12.1254815938996,-57.9621601887015,39.92499));
#183444=CARTESIAN_POINT('',(-12.1995602612167,-58.3106729199896,39.3548010137695));
#183445=CARTESIAN_POINT('',(-12.84073727331,-61.3271735965893,39.92499));
#183446=CARTESIAN_POINT('',(-12.8947498796467,-61.581282930652,39.92499));
#183447=CARTESIAN_POINT('',(-12.7666587067853,-60.9786613449626,39.3548010137695));
#183448=CARTESIAN_POINT('',(-12.84073727331,-61.3271735965893,39.92499));
#183449=CARTESIAN_POINT('',(-12.6770874264381,-60.5572615995843,39.116));
#183450=CARTESIAN_POINT('Origin',(-12.6850361284907,-60.5946573025919,39.5550293907204));
#183451=CARTESIAN_POINT('',(-12.5936359264447,-60.164653163458,39.116));
#183452=CARTESIAN_POINT('',(0.186337117939795,-0.0396071771007839,39.116));
#183453=CARTESIAN_POINT('',(-12.5674311046656,-60.0413691664787,39.3343017080178));
#183454=CARTESIAN_POINT('',(-12.593635927141,-60.16465316331,39.116));
#183455=CARTESIAN_POINT('',(-12.4988285377098,-59.7186194643909,39.5248017080178));
#183456=CARTESIAN_POINT('Origin',(-12.5049473440529,-59.7474037157365,39.1947747614353));
#183457=CARTESIAN_POINT('',(-12.4673906027145,-59.570715608832,39.5248017080178));
#183458=CARTESIAN_POINT('',(0.186337117939795,-0.0396071771007839,39.5248017080178));
#183459=CARTESIAN_POINT('',(-12.3987880210526,-59.2479658375576,39.3343017080178));
#183460=CARTESIAN_POINT('Origin',(-12.4612721960127,-59.5419282989955,39.1947728911913));
#183461=CARTESIAN_POINT('',(-12.3725831876354,-59.124681789249,39.116));
#183462=CARTESIAN_POINT('',(-12.3987880210526,-59.2479658375576,39.3343017080178));
#183463=CARTESIAN_POINT('',(0.186337117939795,-0.0396071771007839,39.116));
#183464=CARTESIAN_POINT('Origin',(-0.18633711793979,0.0396071771007839,
2.62394165870617E-17));
#183465=CARTESIAN_POINT('',(-13.0497616623177,-60.4780472453827,39.116));
#183466=CARTESIAN_POINT('',(-13.1393329432572,-60.8994469906352,39.3548010137695));
#183467=CARTESIAN_POINT('Origin',(-13.0577103643103,-60.5154429481083,39.5550293912458));
#183468=CARTESIAN_POINT('',(-13.2134115096323,-61.2479592422936,39.92499));
#183469=CARTESIAN_POINT('',(-13.1393329432572,-60.8994469906352,39.3548010137695));
#183470=CARTESIAN_POINT('',(-12.4981558292589,-57.8829458346105,39.92499));
#183471=CARTESIAN_POINT('',(-0.186337117939783,0.0396071771007894,39.92499));
#183472=CARTESIAN_POINT('',(-12.5722344964058,-58.2314585659347,39.3548010137695));
#183473=CARTESIAN_POINT('',(-12.4981558292589,-57.8829458346105,39.92499));
#183474=CARTESIAN_POINT('',(-12.6618058697522,-58.6528587425322,39.116));
#183475=CARTESIAN_POINT('Origin',(-12.6538571932377,-58.6154631596715,39.5550297827294));
#183476=CARTESIAN_POINT('',(-12.7452574227898,-59.0454674352015,39.116));
#183477=CARTESIAN_POINT('',(-12.7606133389844,-59.1177113373238,39.116));
#183478=CARTESIAN_POINT('',(-12.7714622569322,-59.168751483356,39.3343017080178));
#183479=CARTESIAN_POINT('',(-12.745257423515,-59.0454674350474,39.116));
#183480=CARTESIAN_POINT('',(-12.8400648385941,-59.4915012546304,39.5248017080178));
#183481=CARTESIAN_POINT('Origin',(-12.8339460446676,-59.4627170622764,39.1947745585626));
#183482=CARTESIAN_POINT('',(-12.8715027735894,-59.6394051101893,39.5248017080178));
#183483=CARTESIAN_POINT('',(-12.8716126987815,-59.639922267558,39.5248017080178));
#183484=CARTESIAN_POINT('',(-12.9401053405452,-59.9621548122771,39.3343017080178));
#183485=CARTESIAN_POINT('Origin',(-12.8776211648735,-59.6681923469399,39.1947728594259));
#183486=CARTESIAN_POINT('',(-12.9663101630206,-60.0854388091084,39.116));
#183487=CARTESIAN_POINT('',(-12.9401053405452,-59.9621548122771,39.3343017080178));
#183488=CARTESIAN_POINT('',(-13.0498700642004,-60.4785572361438,39.116));
#183489=CARTESIAN_POINT('Origin',(-17.8233194796326,-55.4710078899933,40.10025));
#183490=CARTESIAN_POINT('',(-18.2553202812751,-56.1347810195641,40.10025));
#183491=CARTESIAN_POINT('',(-19.4351129318423,-59.765809437495,40.10025));
#183492=CARTESIAN_POINT('',(-18.0189898472952,-55.4074307335706,40.10025));
#183493=CARTESIAN_POINT('',(-19.4061247292256,-59.7752282754836,40.10025));
#183494=CARTESIAN_POINT('Origin',(-2.66410924515271E-18,1.39810867426259E-16,
40.10025));
#183495=CARTESIAN_POINT('',(-18.2263320786585,-56.1441998575527,40.10025));
#183496=CARTESIAN_POINT('',(-18.2044836359655,-56.0769572651638,40.10025));
#183497=CARTESIAN_POINT('Origin',(3.70432808162889E-16,-7.27948111559479E-17,
40.10025));
#183498=CARTESIAN_POINT('Origin',(0.181176266354227,-0.0588677374284282,
-2.55126814298647E-17));
#183499=CARTESIAN_POINT('',(-18.3609838302743,-57.125768610489,39.116));
#183500=CARTESIAN_POINT('',(-18.227854826074,-56.7160396659413,39.3548010137695));
#183501=CARTESIAN_POINT('Origin',(-18.3491697947259,-57.0894087477742,39.5550297832844));
#183502=CARTESIAN_POINT('',(-18.1177524692165,-56.3771794531163,39.92499));
#183503=CARTESIAN_POINT('',(-18.227854826074,-56.7160396659413,39.3548010137695));
#183504=CARTESIAN_POINT('',(-19.1808295835784,-59.6489943884563,39.92499));
#183505=CARTESIAN_POINT('',(-19.2611079613977,-59.8960658302617,39.92499));
#183506=CARTESIAN_POINT('',(-19.0707273770997,-59.3101346421294,39.3548010137695));
#183507=CARTESIAN_POINT('',(-19.1808295835784,-59.6489943884563,39.92499));
#183508=CARTESIAN_POINT('',(-18.9375985097924,-58.9004061169356,39.116));
#183509=CARTESIAN_POINT('Origin',(-18.9494125833914,-58.936766096758,39.5550293907216));
#183510=CARTESIAN_POINT('',(-18.8135654093534,-58.5186714879534,39.116));
#183511=CARTESIAN_POINT('',(0.181176266354232,-0.0588677374284282,39.116));
#183512=CARTESIAN_POINT('',(-18.7746174535802,-58.3988020033598,39.3343017080178));
#183513=CARTESIAN_POINT('',(-18.8135654100305,-58.5186714877335,39.116));
#183514=CARTESIAN_POINT('',(-18.6726541682848,-58.08499127881,39.5248017080178));
#183515=CARTESIAN_POINT('Origin',(-18.6817482287253,-58.1129782575888,39.1947747614318));
#183516=CARTESIAN_POINT('',(-18.6259282908539,-57.9411838150807,39.5248017080178));
#183517=CARTESIAN_POINT('',(0.181176266354232,-0.0588677374284282,39.5248017080178));
#183518=CARTESIAN_POINT('',(-18.523964983701,-57.6273730232604,39.3343017080178));
#183519=CARTESIAN_POINT('Origin',(-18.6168343081655,-57.9131937527902,39.1947728911903));
#183520=CARTESIAN_POINT('',(-18.485017010988,-57.5075034888352,39.116));
#183521=CARTESIAN_POINT('',(-18.523964983701,-57.6273730232604,39.3343017080178));
#183522=CARTESIAN_POINT('',(0.181176266354232,-0.0588677374284282,39.116));
#183523=CARTESIAN_POINT('Origin',(-0.181176266354227,0.0588677374284282,
2.55126814298647E-17));
#183524=CARTESIAN_POINT('',(-19.2999510425009,-58.7826706420788,39.116));
#183525=CARTESIAN_POINT('',(-19.433079910384,-59.1923991670854,39.3548010137695));
#183526=CARTESIAN_POINT('Origin',(-19.311765116011,-58.8190306216278,39.555029391246));
#183527=CARTESIAN_POINT('',(-19.5431821167168,-59.5312589134598,39.92499));
#183528=CARTESIAN_POINT('',(-19.433079910384,-59.1923991670854,39.3548010137695));
#183529=CARTESIAN_POINT('',(-18.4801050014193,-56.2594439784238,39.92499));
#183530=CARTESIAN_POINT('',(-0.181176266354219,0.0588677374284336,39.92499));
#183531=CARTESIAN_POINT('',(-18.5902073581106,-56.5983041913028,39.3548010137695));
#183532=CARTESIAN_POINT('',(-18.4801050014193,-56.2594439784238,39.92499));
#183533=CARTESIAN_POINT('',(-18.7233363629827,-57.0080331356321,39.116));
#183534=CARTESIAN_POINT('Origin',(-18.7115223273411,-56.9716732726305,39.555029782734));
#183535=CARTESIAN_POINT('',(-18.8473695429908,-57.3897680142076,39.116));
#183536=CARTESIAN_POINT('',(-18.8701928819397,-57.4600110263529,39.116));
#183537=CARTESIAN_POINT('',(-18.8863175164095,-57.5096375484036,39.3343017080178));
#183538=CARTESIAN_POINT('',(-18.8473695436964,-57.3897680139783,39.116));
#183539=CARTESIAN_POINT('',(-18.9882808235623,-57.8234483402238,39.5248017080178));
#183540=CARTESIAN_POINT('Origin',(-18.9791867816365,-57.7954614188148,39.19477455856));
#183541=CARTESIAN_POINT('',(-19.0350067009933,-57.9672558039531,39.5248017080178));
#183542=CARTESIAN_POINT('',(-19.0351700816687,-57.9677586379682,39.5248017080178));
#183543=CARTESIAN_POINT('',(-19.1369699862886,-58.2810665285029,39.3343017080178));
#183544=CARTESIAN_POINT('Origin',(-19.0441006607084,-57.9952457951681,39.1947728594225));
#183545=CARTESIAN_POINT('',(-19.1759179427389,-58.4009360128766,39.116));
#183546=CARTESIAN_POINT('',(-19.1369699862886,-58.2810665285029,39.3343017080178));
#183547=CARTESIAN_POINT('',(-19.3001121590972,-58.7831665079749,39.116));
#183548=CARTESIAN_POINT('Origin',(-23.5239806812874,-53.3040877092101,40.10025));
#183549=CARTESIAN_POINT('',(-24.0229981225299,-53.9190682401994,40.10025));
#183550=CARTESIAN_POINT('',(-25.5758735661211,-57.4068835917978,40.10025));
#183551=CARTESIAN_POINT('',(-23.7119335237428,-53.2204057122637,40.10025));
#183552=CARTESIAN_POINT('',(-25.5480287005721,-57.4192809246788,40.10025));
#183553=CARTESIAN_POINT('Origin',(1.17012503474363E-17,1.34296522528312E-16,
40.10025));
#183554=CARTESIAN_POINT('',(-23.995153256981,-53.9314655730803,40.10025));
#183555=CARTESIAN_POINT('',(-23.9663957374946,-53.8668751267877,40.10025));
#183556=CARTESIAN_POINT('Origin',(3.62953249113008E-16,-6.99236774387749E-17,
40.10025));
#183557=CARTESIAN_POINT('Origin',(0.174030409680915,-0.0774833305059407,
-2.45064239960504E-17));
#183558=CARTESIAN_POINT('',(-24.2316692455485,-54.8935822490121,39.116));
#183559=CARTESIAN_POINT('',(-24.056441199033,-54.5000136127188,39.3548010137695));
#183560=CARTESIAN_POINT('Origin',(-24.2161192879494,-54.8586564724117,39.5550297832871));
#183561=CARTESIAN_POINT('',(-23.9115214570974,-54.1745185417596,39.92499));
#183562=CARTESIAN_POINT('',(-24.056441199033,-54.5000136127187,39.3548010137695));
#183563=CARTESIAN_POINT('',(-25.3107727110825,-57.3172883154489,39.92499));
#183564=CARTESIAN_POINT('',(-25.4164373136776,-57.5546148985774,39.92499));
#183565=CARTESIAN_POINT('',(-25.1658531674643,-56.9917936927134,39.3548010137695));
#183566=CARTESIAN_POINT('',(-25.3107727110825,-57.3172883154489,39.92499));
#183567=CARTESIAN_POINT('',(-24.9906253009261,-56.5982254591674,39.116));
#183568=CARTESIAN_POINT('Origin',(-25.0061753086093,-56.6331513482585,39.5550293907201));
#183569=CARTESIAN_POINT('',(-24.8273695326456,-56.2315470018076,39.116));
#183570=CARTESIAN_POINT('',(0.174030409680921,-0.0774833305059407,39.116));
#183571=CARTESIAN_POINT('',(-24.776105164832,-56.1164053447571,39.3343017080178));
#183572=CARTESIAN_POINT('',(-24.8273695332959,-56.2315470015181,39.116));
#183573=CARTESIAN_POINT('',(-24.641898292288,-55.8149717737125,39.5248017080178));
#183574=CARTESIAN_POINT('Origin',(-24.6538679703959,-55.841854848728,39.1947747614267));
#183575=CARTESIAN_POINT('',(-24.5803964109126,-55.6768362864791,39.5248017080178));
#183576=CARTESIAN_POINT('',(0.174030409680921,-0.0774833305059407,39.5248017080178));
#183577=CARTESIAN_POINT('',(-24.4461895095991,-55.3754026508174,39.3343017080178));
#183578=CARTESIAN_POINT('Origin',(-24.568426487815,-55.6499501367141,39.1947728911901));
#183579=CARTESIAN_POINT('',(-24.3949251197297,-55.2602609459789,39.116));
#183580=CARTESIAN_POINT('',(-24.4461895095991,-55.3754026508174,39.3343017080178));
#183581=CARTESIAN_POINT('',(0.174030409680921,-0.0774833305059407,39.116));
#183582=CARTESIAN_POINT('Origin',(-0.174030409680915,0.0774833305059407,
2.45064239960504E-17));
#183583=CARTESIAN_POINT('',(-25.338686120288,-56.4432587981556,39.116));
#183584=CARTESIAN_POINT('',(-25.5139139873792,-56.8368270314553,39.3548010137695));
#183585=CARTESIAN_POINT('Origin',(-25.3542361278543,-56.4781846869842,39.5550293912438));
#183586=CARTESIAN_POINT('',(-25.6588335308579,-57.1623216542529,39.92499));
#183587=CARTESIAN_POINT('',(-25.5139139873792,-56.8368270314553,39.3548010137695));
#183588=CARTESIAN_POINT('',(-24.2595822759735,-54.019551880964,39.92499));
#183589=CARTESIAN_POINT('',(-0.174030409680907,0.0774833305059458,39.92499));
#183590=CARTESIAN_POINT('',(-24.4045020177493,-54.3450469519942,39.3548010137695));
#183591=CARTESIAN_POINT('',(-24.2595822759735,-54.019551880964,39.92499));
#183592=CARTESIAN_POINT('',(-24.5797300649104,-54.7386155880002,39.116));
#183593=CARTESIAN_POINT('Origin',(-24.5641801071868,-54.7036898111204,39.5550297827287));
#183594=CARTESIAN_POINT('',(-24.742985938414,-55.1052942852688,39.116));
#183595=CARTESIAN_POINT('',(-24.7730266428387,-55.172766810297,39.116));
#183596=CARTESIAN_POINT('',(-24.794250328961,-55.2204359898055,39.3343017080178));
#183597=CARTESIAN_POINT('',(-24.7429859390916,-55.1052942849671,39.116));
#183598=CARTESIAN_POINT('',(-24.9284572302744,-55.5218696254672,39.5248017080178));
#183599=CARTESIAN_POINT('Origin',(-24.9164875765753,-55.4949866055695,39.1947745585593));
#183600=CARTESIAN_POINT('',(-24.9899591116498,-55.6600051127007,39.5248017080178));
#183601=CARTESIAN_POINT('',(-24.9901741577757,-55.6604881142075,39.5248017080178));
#183602=CARTESIAN_POINT('',(-25.1241659841938,-55.9614386837452,39.3343017080178));
#183603=CARTESIAN_POINT('Origin',(-25.001929004471,-55.686891194182,39.1947728594246));
#183604=CARTESIAN_POINT('',(-25.1754303526578,-56.0765803405062,39.116));
#183605=CARTESIAN_POINT('',(-25.1241659841938,-55.9614386837452,39.3343017080178));
#183606=CARTESIAN_POINT('',(-25.3388981863709,-56.4437351063763,39.116));
#183607=CARTESIAN_POINT('Origin',(-28.9669082278886,-50.5531567888874,40.10025));
#183608=CARTESIAN_POINT('',(-29.5274749692187,-51.1126068659046,40.10025));
#183609=CARTESIAN_POINT('',(-31.4364195775137,-54.4189959163062,40.10025));
#183610=CARTESIAN_POINT('',(-29.1450842944632,-50.4502867888874,40.10025));
#183611=CARTESIAN_POINT('',(-31.4100231232064,-54.4342359163062,40.10025));
#183612=CARTESIAN_POINT('Origin',(2.54115089989956E-17,1.27310796826192E-16,
40.10025));
#183613=CARTESIAN_POINT('',(-29.5010785149114,-51.1278468659046,40.10025));
#183614=CARTESIAN_POINT('',(-29.465726992033,-51.0666162321542,40.10025));
#183615=CARTESIAN_POINT('Origin',(3.55814779065492E-16,-6.62864452791125E-17,
40.10025));
#183616=CARTESIAN_POINT('Origin',(0.164977839420935,-0.0952500000000008,
-2.32316690526364E-17));
#183617=CARTESIAN_POINT('',(-29.8368674217658,-52.0599703131945,39.116));
#183618=CARTESIAN_POINT('',(-29.6214601680814,-51.6868740054942,39.3548010137695));
#183619=CARTESIAN_POINT('Origin',(-29.8177519107039,-52.0268612768225,39.5550297832829));
#183620=CARTESIAN_POINT('',(-29.4433108120869,-51.3783102685125,39.92499));
#183621=CARTESIAN_POINT('',(-29.6214601680814,-51.6868740054942,39.3548010137695));
#183622=CARTESIAN_POINT('',(-31.1634057161443,-54.3576020372437,39.92499));
#183623=CARTESIAN_POINT('',(-31.2932988600175,-54.5825835619869,39.92499));
#183624=CARTESIAN_POINT('',(-30.9852566042328,-54.0490387253004,39.3548010137695));
#183625=CARTESIAN_POINT('',(-31.1634057161443,-54.3576020372437,39.92499));
#183626=CARTESIAN_POINT('',(-30.7698495716383,-53.6759427993285,39.116));
#183627=CARTESIAN_POINT('Origin',(-30.7889651442679,-53.7090519423387,39.555029390718));
#183628=CARTESIAN_POINT('',(-30.5691597998771,-53.3283379195022,39.116));
#183629=CARTESIAN_POINT('',(0.164977839420941,-0.0952500000000008,39.116));
#183630=CARTESIAN_POINT('',(-30.5061406831646,-53.2191856060844,39.3343017080178));
#183631=CARTESIAN_POINT('',(-30.5691598004935,-53.3283379191463,39.116));
#183632=CARTESIAN_POINT('',(-30.3411606219521,-52.9334317578286,39.5248017080178));
#183633=CARTESIAN_POINT('Origin',(-30.3558747754319,-52.9589163924907,39.1947747614318));
#183634=CARTESIAN_POINT('',(-30.2655565641147,-52.8024816883958,39.5248017080178));
#183635=CARTESIAN_POINT('',(0.164977839420941,-0.0952500000000008,39.5248017080178));
#183636=CARTESIAN_POINT('',(-30.100576467536,-52.516727778884,39.3343017080178));
#183637=CARTESIAN_POINT('Origin',(-30.250841845589,-52.7769940214372,39.1947728911941));
#183638=CARTESIAN_POINT('',(-30.0375573238934,-52.4075754202455,39.116));
#183639=CARTESIAN_POINT('',(-30.100576467536,-52.516727778884,39.3343017080178));
#183640=CARTESIAN_POINT('',(0.164977839420941,-0.0952500000000008,39.116));
#183641=CARTESIAN_POINT('Origin',(-0.164977839420935,0.0952500000000008,
2.32316690526364E-17));
#183642=CARTESIAN_POINT('',(-31.0998052504802,-53.4854427993285,39.116));
#183643=CARTESIAN_POINT('',(-31.3152122835989,-53.8585387249978,39.3548010137695));
#183644=CARTESIAN_POINT('Origin',(-31.1189208229653,-53.5185519420886,39.5550293912447));
#183645=CARTESIAN_POINT('',(-31.493361395377,-54.167102037018,39.92499));
#183646=CARTESIAN_POINT('',(-31.3152122835989,-53.8585387249977,39.3548010137695));
#183647=CARTESIAN_POINT('',(-29.7732664904682,-51.1878102687783,39.92499));
#183648=CARTESIAN_POINT('',(-0.164977839420927,0.0952500000000056,39.92499));
#183649=CARTESIAN_POINT('',(-29.951415846311,-51.4963740058477,39.3548010137695));
#183650=CARTESIAN_POINT('',(-29.7732664904682,-51.1878102687783,39.92499));
#183651=CARTESIAN_POINT('',(-30.1668231006077,-51.8694703131945,39.116));
#183652=CARTESIAN_POINT('Origin',(-30.1477075893945,-51.8363612765607,39.5550297827313));
#183653=CARTESIAN_POINT('',(-30.3675130020931,-52.2170754206163,39.116));
#183654=CARTESIAN_POINT('',(-30.4044419397496,-52.2810382154238,39.116));
#183655=CARTESIAN_POINT('',(-30.4305321463779,-52.326227778884,39.3343017080178));
#183656=CARTESIAN_POINT('',(-30.3675130027353,-52.2170754202455,39.116));
#183657=CARTESIAN_POINT('',(-30.5955122429565,-52.6119816883958,39.5248017080178));
#183658=CARTESIAN_POINT('Origin',(-30.5807981195149,-52.5864971060008,39.1947745585599));
#183659=CARTESIAN_POINT('',(-30.671116300794,-52.7429317578286,39.5248017080178));
#183660=CARTESIAN_POINT('',(-30.6713806562799,-52.7433896349616,39.5248017080178));
#183661=CARTESIAN_POINT('',(-30.8360963620065,-53.0286856060844,39.3343017080178));
#183662=CARTESIAN_POINT('Origin',(-30.6858309820702,-52.7684193600399,39.1947728594235));
#183663=CARTESIAN_POINT('',(-30.8991154793354,-53.1378379191463,39.116));
#183664=CARTESIAN_POINT('',(-30.8360963620065,-53.0286856060844,39.3343017080178));
#183665=CARTESIAN_POINT('',(-31.1000659426093,-53.4858943313412,39.116));
#183666=CARTESIAN_POINT('Origin',(-34.0924682662297,-47.2483549038574,40.10025));
#183667=CARTESIAN_POINT('',(-34.7084426211234,-47.7461450747863,40.10025));
#183668=CARTESIAN_POINT('',(-36.9525415975215,-50.8348823336484,40.10025));
#183669=CARTESIAN_POINT('',(-34.2589154226524,-47.1274239660508,40.10025));
#183670=CARTESIAN_POINT('',(-36.9278827595329,-50.8527980281383,40.10025));
#183671=CARTESIAN_POINT('Origin',(3.83164542466812E-17,1.18930227392546E-16,
40.10025));
#183672=CARTESIAN_POINT('',(-34.6837837831348,-47.7640607692762,40.10025));
#183673=CARTESIAN_POINT('',(-34.6422255755468,-47.7068608037048,40.10025));
#183674=CARTESIAN_POINT('Origin',(3.49095608592005E-16,-6.19229649536416E-17,
40.10025));
#183675=CARTESIAN_POINT('Origin',(0.154117737428427,-0.111973090561717,
-2.17023830815425E-17));
#183676=CARTESIAN_POINT('',(-35.1151666347443,-48.6559784483763,39.116));
#183677=CARTESIAN_POINT('',(-34.8619402208392,-48.3074421904916,39.3548010137695));
#183678=CARTESIAN_POINT('Origin',(-35.0926950037607,-48.6250489017669,39.5550297832855));
#183679=CARTESIAN_POINT('',(-34.65251309241,-48.019190476361,39.92499));
#183680=CARTESIAN_POINT('',(-34.8619402208392,-48.3074421904916,39.3548010137695));
#183681=CARTESIAN_POINT('',(-36.674605926818,-50.8023624960589,39.92499));
#183682=CARTESIAN_POINT('',(-36.8273044755032,-51.0125340177513,39.92499));
#183683=CARTESIAN_POINT('',(-36.4651790855633,-50.5141111791247,39.3548010137695));
#183684=CARTESIAN_POINT('',(-36.674605926818,-50.8023624960589,39.92499));
#183685=CARTESIAN_POINT('',(-36.2119529314387,-50.165575277767,39.116));
#183686=CARTESIAN_POINT('Origin',(-36.2344246347989,-50.1965049239941,39.5550293907223));
#183687=CARTESIAN_POINT('',(-35.9760279553332,-49.8408524072785,39.116));
#183688=CARTESIAN_POINT('',(0.154117737428432,-0.111973090561717,39.116));
#183689=CARTESIAN_POINT('',(-35.9019445403521,-49.738885333081,39.3343017080178));
#183690=CARTESIAN_POINT('',(-35.9760279559089,-49.8408524068602,39.116));
#183691=CARTESIAN_POINT('',(-35.7079988465461,-49.4719419865731,39.5248017080178));
#183692=CARTESIAN_POINT('Origin',(-35.7252962640503,-49.4957489658867,39.1947747614277));
#183693=CARTESIAN_POINT('',(-35.6191209461254,-49.3496120513048,39.5248017080178));
#183694=CARTESIAN_POINT('',(0.154117737428432,-0.111973090561717,39.5248017080178));
#183695=CARTESIAN_POINT('',(-35.425175210744,-49.0826686475733,39.3343017080178));
#183696=CARTESIAN_POINT('Origin',(-35.6018226497073,-49.3258021153664,39.1947728911967));
#183697=CARTESIAN_POINT('',(-35.3510917642536,-48.9807015312177,39.116));
#183698=CARTESIAN_POINT('',(-35.425175210744,-49.0826686475733,39.3343017080178));
#183699=CARTESIAN_POINT('',(0.154117737428432,-0.111973090561717,39.116));
#183700=CARTESIAN_POINT('Origin',(-0.154117737428427,0.111973090561717,
2.17023830815425E-17));
#183701=CARTESIAN_POINT('',(-36.5201884062956,-49.9416290966435,39.116));
#183702=CARTESIAN_POINT('',(-36.7734145609101,-50.2901649976454,39.3548010137695));
#183703=CARTESIAN_POINT('Origin',(-36.5426601094875,-49.9725587426392,39.5550293912446));
#183704=CARTESIAN_POINT('',(-36.9828414020407,-50.5784163146697,39.92499));
#183705=CARTESIAN_POINT('',(-36.7734145609101,-50.2901649976454,39.3548010137695));
#183706=CARTESIAN_POINT('',(-34.9607485668368,-47.79524429555,39.92499));
#183707=CARTESIAN_POINT('',(-0.154117737428418,0.111973090561721,39.92499));
#183708=CARTESIAN_POINT('',(-35.1701756951245,-48.0834960097835,39.3548010137695));
#183709=CARTESIAN_POINT('',(-34.9607485668368,-47.79524429555,39.92499));
#183710=CARTESIAN_POINT('',(-35.4234021096012,-48.4320322672529,39.116));
#183711=CARTESIAN_POINT('Origin',(-35.4009304784381,-48.4011027203966,39.555029782729));
#183712=CARTESIAN_POINT('',(-35.6593272385104,-48.7567553505302,39.116));
#183713=CARTESIAN_POINT('',(-35.7027398082301,-48.8165076253518,39.116));
#183714=CARTESIAN_POINT('',(-35.7334106856009,-48.8587224664499,39.3343017080178));
#183715=CARTESIAN_POINT('',(-35.6593272391104,-48.7567553500942,39.116));
#183716=CARTESIAN_POINT('',(-35.9273564209823,-49.1256658701813,39.5248017080178));
#183717=CARTESIAN_POINT('Origin',(-35.910059038814,-49.1018589397074,39.1947745585586));
#183718=CARTESIAN_POINT('',(-36.0162343214029,-49.2479958054497,39.5248017080178));
#183719=CARTESIAN_POINT('',(-36.0165450899149,-49.2484235416111,39.5248017080178));
#183720=CARTESIAN_POINT('',(-36.2101800152089,-49.5149391519575,39.3343017080178));
#183721=CARTESIAN_POINT('Origin',(-36.0335325740062,-49.2718056808869,39.1947728594212));
#183722=CARTESIAN_POINT('',(-36.2842634307658,-49.6169062257368,39.116));
#183723=CARTESIAN_POINT('',(-36.2101800152089,-49.5149391519575,39.3343017080178));
#183724=CARTESIAN_POINT('',(-36.5204948682733,-49.942050905369,39.116));
#183725=CARTESIAN_POINT('Origin',(-38.8445040879384,-43.4258901551469,40.10025));
#183726=CARTESIAN_POINT('',(-39.5091373124624,-43.8565665267054,40.10025));
#183727=CARTESIAN_POINT('',(-42.0638038389703,-46.6938111422602,40.10025));
#183728=CARTESIAN_POINT('',(-38.9973987043321,-43.2882232241946,40.10025));
#183729=CARTESIAN_POINT('',(-42.0411527846897,-46.7142062431421,40.10025));
#183730=CARTESIAN_POINT('Origin',(5.02746968098277E-17,1.09246633499838E-16,
40.10025));
#183731=CARTESIAN_POINT('',(-39.4864862581819,-43.8769616275872,40.10025));
#183732=CARTESIAN_POINT('',(-39.4391766863032,-43.8244190249876,40.10025));
#183733=CARTESIAN_POINT('Origin',(3.42869354330331E-16,-5.68810436659251E-17,
40.10025));
#183734=CARTESIAN_POINT('Origin',(0.141569089253443,-0.127469380511363,
-1.99353212598915E-17));
#183735=CARTESIAN_POINT('',(-40.0087367337515,-44.7189015017597,39.116));
#183736=CARTESIAN_POINT('',(-39.7204655612076,-44.3987439298679,39.3548010137695));
#183737=CARTESIAN_POINT('Origin',(-39.9831551867361,-44.6904903154957,39.5550297832831));
#183738=CARTESIAN_POINT('',(-39.4820551877882,-44.1339623846889,39.92499));
#183739=CARTESIAN_POINT('',(-39.7204655612076,-44.3987439298679,39.3548010137695));
#183740=CARTESIAN_POINT('',(-41.7839914803029,-46.6905216402895,39.92499));
#183741=CARTESIAN_POINT('',(-41.9578224365464,-46.8835804757583,39.92499));
#183742=CARTESIAN_POINT('',(-41.5455814340034,-46.4257404601129,39.3548010137695));
#183743=CARTESIAN_POINT('',(-41.7839914803029,-46.6905216402895,39.92499));
#183744=CARTESIAN_POINT('',(-41.2573105570839,-46.1055832156407,39.116));
#183745=CARTESIAN_POINT('Origin',(-41.2828921864909,-46.1339944934099,39.5550293907235));
#183746=CARTESIAN_POINT('',(-40.9887352200426,-45.807300086212,39.116));
#183747=CARTESIAN_POINT('',(0.141569089253448,-0.127469380511363,39.116));
#183748=CARTESIAN_POINT('',(-40.9043991801906,-45.7136354238374,39.3343017080178));
#183749=CARTESIAN_POINT('',(-40.9887352205716,-45.8073000857357,39.116));
#183750=CARTESIAN_POINT('',(-40.6836127633981,-45.4684272662434,39.5248017080178));
#183751=CARTESIAN_POINT('Origin',(-40.7033039308042,-45.4902957559654,39.1947747614341));
#183752=CARTESIAN_POINT('',(-40.5824347852702,-45.3560577375094,39.5248017080178));
#183753=CARTESIAN_POINT('',(0.141569089253449,-0.127469380511363,39.5248017080178));
#183754=CARTESIAN_POINT('',(-40.3616483211486,-45.1108495273511,39.3343017080178));
#183755=CARTESIAN_POINT('Origin',(-40.5627424347164,-45.334186399234,39.1947728911947));
#183756=CARTESIAN_POINT('',(-40.277312245553,-45.0171848263431,39.116));
#183757=CARTESIAN_POINT('',(-40.3616483211486,-45.1108495273511,39.3343017080178));
#183758=CARTESIAN_POINT('',(0.141569089253448,-0.127469380511363,39.116));
#183759=CARTESIAN_POINT('Origin',(-0.141569089253443,0.127469380511363,
1.99353212598915E-17));
#183760=CARTESIAN_POINT('',(-41.5404487355908,-45.850644454618,39.116));
#183761=CARTESIAN_POINT('',(-41.8287196129601,-46.1708016986852,39.3548010137695));
#183762=CARTESIAN_POINT('Origin',(-41.5660303648068,-45.8790557321751,39.5550293912439));
#183763=CARTESIAN_POINT('',(-42.0671296591461,-46.435582878964,39.92499));
#183764=CARTESIAN_POINT('',(-41.8287196129601,-46.1708016986852,39.3548010137695));
#183765=CARTESIAN_POINT('',(-39.7651933659001,-43.8790236240218,39.92499));
#183766=CARTESIAN_POINT('',(-0.141569089253434,0.127469380511367,39.92499));
#183767=CARTESIAN_POINT('',(-40.0036037391898,-44.1438051693176,39.3548010137695));
#183768=CARTESIAN_POINT('',(-39.7651933659001,-43.8790236240218,39.92499));
#183769=CARTESIAN_POINT('',(-40.2918749122584,-44.4639627407369,39.116));
#183770=CARTESIAN_POINT('Origin',(-40.2662933650397,-44.4355515542471,39.555029782729));
#183771=CARTESIAN_POINT('',(-40.560450423509,-44.7622460658163,39.116));
#183772=CARTESIAN_POINT('',(-40.609870988093,-44.8171331622254,39.116));
#183773=CARTESIAN_POINT('',(-40.6447864996555,-44.8559107663283,39.3343017080178));
#183774=CARTESIAN_POINT('',(-40.5604504240599,-44.7622460653203,39.116));
#183775=CARTESIAN_POINT('',(-40.8655729637771,-45.1011189764867,39.5248017080178));
#183776=CARTESIAN_POINT('Origin',(-40.8458818366203,-45.0792505316452,39.1947745585594));
#183777=CARTESIAN_POINT('',(-40.966750941905,-45.2134885052207,39.5248017080178));
#183778=CARTESIAN_POINT('',(-40.9671047185982,-45.2138814140436,39.5248017080178));
#183779=CARTESIAN_POINT('',(-41.1875373586974,-45.4586966628146,39.3343017080178));
#183780=CARTESIAN_POINT('Origin',(-40.9864432425609,-45.2353597879075,39.1947728594213));
#183781=CARTESIAN_POINT('',(-41.2718733990785,-45.5523613247129,39.116));
#183782=CARTESIAN_POINT('',(-41.1875373586974,-45.4586966628146,39.3343017080178));
#183783=CARTESIAN_POINT('',(-41.5407976097556,-45.8510319186315,39.116));
#183784=CARTESIAN_POINT('Origin',(-43.1709513941246,-39.1276422664448,40.10025));
#183785=CARTESIAN_POINT('',(-43.8769616275876,-39.4864862581814,40.10025));
#183786=CARTESIAN_POINT('',(-46.7142062431425,-42.0411527846893,40.10025));
#183787=CARTESIAN_POINT('',(-43.3086183250768,-38.9747476500511,40.10025));
#183788=CARTESIAN_POINT('',(-46.6938111422606,-42.0638038389698,40.10025));
#183789=CARTESIAN_POINT('Origin',(6.11552196804858E-17,9.83661106291779E-17,
40.10025));
#183790=CARTESIAN_POINT('',(-43.8565665267058,-39.509137312462,40.10025));
#183791=CARTESIAN_POINT('',(-43.8040239241062,-39.4618277405834,40.10025));
#183792=CARTESIAN_POINT('Origin',(3.37204232425085E-16,-5.1215921760681E-17,
40.10025));
#183793=CARTESIAN_POINT('Origin',(0.127469380511362,-0.141569089253444,
-1.7949843886783E-17));
#183794=CARTESIAN_POINT('',(-44.4639627407373,-40.291874912258,39.116));
#183795=CARTESIAN_POINT('',(-44.1438051688456,-40.003603739714,39.3548010137695));
#183796=CARTESIAN_POINT('Origin',(-44.4355515544744,-40.2662933652435,39.5550297832866));
#183797=CARTESIAN_POINT('',(-43.8790236243775,-39.7651933655051,39.92499));
#183798=CARTESIAN_POINT('',(-44.1438051688456,-40.003603739714,39.3548010137695));
#183799=CARTESIAN_POINT('',(-46.4355828792672,-42.0671296588093,39.92499));
#183800=CARTESIAN_POINT('',(-46.6286417147359,-42.2409606150528,39.92499));
#183801=CARTESIAN_POINT('',(-46.1708016982804,-41.8287196134097,39.3548010137695));
#183802=CARTESIAN_POINT('',(-46.4355828792672,-42.0671296588093,39.92499));
#183803=CARTESIAN_POINT('',(-45.8506444546184,-41.5404487355903,39.116));
#183804=CARTESIAN_POINT('Origin',(-45.8790557323879,-41.5660303649976,39.5550293907227));
#183805=CARTESIAN_POINT('',(-45.552361324237,-41.271873399607,39.116));
#183806=CARTESIAN_POINT('',(0.127469380511367,-0.141569089253444,39.116));
#183807=CARTESIAN_POINT('',(-45.458696662815,-41.187537358697,39.3343017080178));
#183808=CARTESIAN_POINT('',(-45.5523613247134,-41.271873399078,39.116));
#183809=CARTESIAN_POINT('',(-45.2134885052211,-40.9667509419045,39.5248017080178));
#183810=CARTESIAN_POINT('Origin',(-45.2353576819754,-40.986441346282,39.1947747614315));
#183811=CARTESIAN_POINT('',(-45.1011189764871,-40.8655729637766,39.5248017080178));
#183812=CARTESIAN_POINT('',(0.127469380511367,-0.141569089253444,39.5248017080178));
#183813=CARTESIAN_POINT('',(-44.8559107663287,-40.644786499655,39.3343017080178));
#183814=CARTESIAN_POINT('Origin',(-45.0792483253096,-40.8458798501216,39.1947728911967));
#183815=CARTESIAN_POINT('',(-44.7622460653207,-40.5604504240595,39.116));
#183816=CARTESIAN_POINT('',(-44.8559107663287,-40.644786499655,39.3343017080178));
#183817=CARTESIAN_POINT('',(0.127469380511367,-0.141569089253444,39.116));
#183818=CARTESIAN_POINT('Origin',(-0.127469380511362,0.141569089253444,
1.7949843886783E-17));
#183819=CARTESIAN_POINT('',(-46.1055832156411,-41.2573105570834,39.116));
#183820=CARTESIAN_POINT('',(-46.4257404597083,-41.5455814344528,39.3548010137695));
#183821=CARTESIAN_POINT('Origin',(-46.1339944931974,-41.2828921862988,39.5550293912464));
#183822=CARTESIAN_POINT('',(-46.6905216405927,-41.7839914799662,39.92499));
#183823=CARTESIAN_POINT('',(-46.4257404597083,-41.5455814344528,39.3548010137695));
#183824=CARTESIAN_POINT('',(-44.1339623850449,-39.4820551873928,39.92499));
#183825=CARTESIAN_POINT('',(-0.127469380511352,0.141569089253448,39.92499));
#183826=CARTESIAN_POINT('',(-44.3987439293951,-39.7204655617327,39.3548010137695));
#183827=CARTESIAN_POINT('',(-44.1339623850449,-39.4820551873928,39.92499));
#183828=CARTESIAN_POINT('',(-44.7189015017601,-40.0087367337511,39.116));
#183829=CARTESIAN_POINT('Origin',(-44.6904903152715,-39.9831551865335,39.5550297827315));
#183830=CARTESIAN_POINT('',(-45.0171848258473,-40.2773122461036,39.116));
#183831=CARTESIAN_POINT('',(-45.0720719232486,-40.3267328095857,39.116));
#183832=CARTESIAN_POINT('',(-45.1108495273515,-40.3616483211481,39.3343017080178));
#183833=CARTESIAN_POINT('',(-45.0171848263434,-40.2773122455526,39.116));
#183834=CARTESIAN_POINT('',(-45.3560577375098,-40.5824347852697,39.5248017080178));
#183835=CARTESIAN_POINT('Origin',(-45.3341886054736,-40.562744421318,39.1947745585619));
#183836=CARTESIAN_POINT('',(-45.4684272662438,-40.6836127633977,39.5248017080178));
#183837=CARTESIAN_POINT('',(-45.4688201750668,-40.6839665400909,39.5248017080178));
#183838=CARTESIAN_POINT('',(-45.7136354238378,-40.9043991801901,39.3343017080178));
#183839=CARTESIAN_POINT('Origin',(-45.4902978619858,-40.7033058269843,39.1947728594229));
#183840=CARTESIAN_POINT('',(-45.8073000857361,-40.9887352205711,39.116));
#183841=CARTESIAN_POINT('',(-45.7136354238378,-40.9043991801901,39.3343017080178));
#183842=CARTESIAN_POINT('',(-46.1059706796546,-41.2576594312482,39.116));
#183843=CARTESIAN_POINT('Origin',(-47.0244087227343,-34.4007037410861,40.10025));
#183844=CARTESIAN_POINT('',(-47.7640607692765,-34.6837837831344,40.10025));
#183845=CARTESIAN_POINT('',(-50.8527980281387,-36.9278827595324,40.10025));
#183846=CARTESIAN_POINT('',(-47.145339660541,-34.2342565846634,40.10025));
#183847=CARTESIAN_POINT('',(-50.8348823336488,-36.9525415975209,40.10025));
#183848=CARTESIAN_POINT('Origin',(7.08388135731919E-17,8.64078680660324E-17,
40.10025));
#183849=CARTESIAN_POINT('',(-47.7461450747866,-34.7084426211229,40.10025));
#183850=CARTESIAN_POINT('',(-47.6889451092153,-34.6668844135349,40.10025));
#183851=CARTESIAN_POINT('Origin',(3.32162311137368E-16,-4.49896674990063E-17,
40.10025));
#183852=CARTESIAN_POINT('Origin',(0.111973090561715,-0.154117737428428,
-1.57677042678046E-17));
#183853=CARTESIAN_POINT('',(-48.4320322672532,-35.4234021096007,39.116));
#183854=CARTESIAN_POINT('',(-48.0834960093685,-35.1701756956956,39.3548010137695));
#183855=CARTESIAN_POINT('Origin',(-48.401102720643,-35.4009304786164,39.555029783284));
#183856=CARTESIAN_POINT('',(-47.7952442958628,-34.9607485664063,39.92499));
#183857=CARTESIAN_POINT('',(-48.0834960093685,-35.1701756956956,39.3548010137695));
#183858=CARTESIAN_POINT('',(-50.5784163149358,-36.9828414016744,39.92499));
#183859=CARTESIAN_POINT('',(-50.7885878366283,-37.1355399503595,39.92499));
#183860=CARTESIAN_POINT('',(-50.2901649972901,-36.773414561399,39.3548010137695));
#183861=CARTESIAN_POINT('',(-50.5784163149359,-36.9828414016744,39.92499));
#183862=CARTESIAN_POINT('',(-49.9416290966439,-36.5201884062951,39.116));
#183863=CARTESIAN_POINT('Origin',(-49.9725587428701,-36.5426601096545,39.555029390725));
#183864=CARTESIAN_POINT('',(-49.6169062253186,-36.2842634313414,39.116));
#183865=CARTESIAN_POINT('',(0.111973090561721,-0.154117737428428,39.116));
#183866=CARTESIAN_POINT('',(-49.5149391519579,-36.2101800152084,39.3343017080178));
#183867=CARTESIAN_POINT('',(-49.6169062257371,-36.2842634307653,39.116));
#183868=CARTESIAN_POINT('',(-49.2479958054501,-36.0162343214024,39.5248017080178));
#183869=CARTESIAN_POINT('Origin',(-49.2718033882782,-36.0335309082465,39.1947747614342));
#183870=CARTESIAN_POINT('',(-49.1256658701817,-35.9273564209818,39.5248017080178));
#183871=CARTESIAN_POINT('',(0.111973090561721,-0.154117737428428,39.5248017080178));
#183872=CARTESIAN_POINT('',(-48.8587224664502,-35.7334106856004,39.3343017080178));
#183873=CARTESIAN_POINT('Origin',(-49.1018565378149,-35.9100572938239,39.1947728911913));
#183874=CARTESIAN_POINT('',(-48.7567553500946,-35.6593272391099,39.116));
#183875=CARTESIAN_POINT('',(-48.8587224664502,-35.7334106856004,39.3343017080178));
#183876=CARTESIAN_POINT('',(0.111973090561721,-0.154117737428428,39.116));
#183877=CARTESIAN_POINT('Origin',(-0.111973090561715,0.154117737428428,
1.57677042678046E-17));
#183878=CARTESIAN_POINT('',(-50.1655752777673,-36.2119529314382,39.116));
#183879=CARTESIAN_POINT('',(-50.5141111787691,-36.4651790860527,39.3548010137695));
#183880=CARTESIAN_POINT('Origin',(-50.1965049237625,-36.2344246346299,39.5550293912453));
#183881=CARTESIAN_POINT('',(-50.8023624963252,-36.6746059264515,39.92499));
#183882=CARTESIAN_POINT('',(-50.5141111787691,-36.4651790860527,39.3548010137695));
#183883=CARTESIAN_POINT('',(-48.0191904766738,-34.6525130919795,39.92499));
#183884=CARTESIAN_POINT('',(-0.111973090561705,0.154117737428431,39.92499));
#183885=CARTESIAN_POINT('',(-48.3074421900765,-34.8619402214106,39.3548010137695));
#183886=CARTESIAN_POINT('',(-48.0191904766738,-34.6525130919795,39.92499));
#183887=CARTESIAN_POINT('',(-48.6559784483767,-35.1151666347439,39.116));
#183888=CARTESIAN_POINT('Origin',(-48.625048901522,-35.092695003582,39.555029782732));
#183889=CARTESIAN_POINT('',(-48.9807015307823,-35.3510917648528,39.116));
#183890=CARTESIAN_POINT('',(-49.0404538064756,-35.3945043333728,39.116));
#183891=CARTESIAN_POINT('',(-49.0826686475736,-35.4251752107435,39.3343017080178));
#183892=CARTESIAN_POINT('',(-48.980701531218,-35.3510917642531,39.116));
#183893=CARTESIAN_POINT('',(-49.3496120513051,-35.6191209461249,39.5248017080178));
#183894=CARTESIAN_POINT('Origin',(-49.325804517179,-35.6018243948132,39.1947745585582));
#183895=CARTESIAN_POINT('',(-49.4719419865735,-35.7079988465456,39.5248017080178));
#183896=CARTESIAN_POINT('',(-49.4723697227349,-35.7083096150576,39.5248017080178));
#183897=CARTESIAN_POINT('',(-49.7388853330813,-35.9019445403516,39.3343017080178));
#183898=CARTESIAN_POINT('Origin',(-49.4957512585773,-35.7252979297056,39.1947728594226));
#183899=CARTESIAN_POINT('',(-49.8408524068606,-35.9760279559084,39.116));
#183900=CARTESIAN_POINT('',(-49.7388853330813,-35.9019445403516,39.3343017080178));
#183901=CARTESIAN_POINT('',(-50.1659970864927,-36.2122593934159,39.116));
#183902=CARTESIAN_POINT('Origin',(-50.3626567888877,-29.2968639067299,40.10025));
#183903=CARTESIAN_POINT('',(-51.1278468659049,-29.5010785149108,40.10025));
#183904=CARTESIAN_POINT('',(-54.4342359163065,-31.4100231232058,40.10025));
#183905=CARTESIAN_POINT('',(-50.4655267888877,-29.1186878401553,40.10025));
#183906=CARTESIAN_POINT('',(-54.4189959163065,-31.4364195775132,40.10025));
#183907=CARTESIAN_POINT('Origin',(7.92193830068373E-17,7.35029228183466E-17,
40.10025));
#183908=CARTESIAN_POINT('',(-51.1126068659049,-29.5274749692182,40.10025));
#183909=CARTESIAN_POINT('',(-51.0513762321546,-29.4921234463398,40.10025));
#183910=CARTESIAN_POINT('Origin',(3.27798830811897E-16,-3.82704970255191E-17,
40.10025));
#183911=CARTESIAN_POINT('Origin',(0.095249999999999,-0.164977839420936,
-1.34128103812638E-17));
#183912=CARTESIAN_POINT('',(-51.8694703131948,-30.1668231006072,39.116));
#183913=CARTESIAN_POINT('',(-51.4963740054945,-29.9514158469227,39.3548010137695));
#183914=CARTESIAN_POINT('Origin',(-51.8363612768256,-30.1477075895468,39.5550297832895));
#183915=CARTESIAN_POINT('',(-51.1878102690446,-29.7732664900071,39.92499));
#183916=CARTESIAN_POINT('',(-51.4963740054945,-29.9514158469227,39.3548010137695));
#183917=CARTESIAN_POINT('',(-54.167102037244,-31.4933613949856,39.92499));
#183918=CARTESIAN_POINT('',(-54.3920835619873,-31.6232545388588,39.92499));
#183919=CARTESIAN_POINT('',(-53.8585387246954,-31.3152122841226,39.3548010137695));
#183920=CARTESIAN_POINT('',(-54.167102037244,-31.4933613949856,39.92499));
#183921=CARTESIAN_POINT('',(-53.4854427993288,-31.0998052504797,39.116));
#183922=CARTESIAN_POINT('Origin',(-53.5185519423378,-31.1189208231085,39.5550293907208));
#183923=CARTESIAN_POINT('',(-53.1378379187909,-30.8991154799509,39.116));
#183924=CARTESIAN_POINT('',(0.0952500000000046,-0.164977839420936,39.116));
#183925=CARTESIAN_POINT('',(-53.0286856060847,-30.8360963620059,39.3343017080178));
#183926=CARTESIAN_POINT('',(-53.1378379191466,-30.8991154793348,39.116));
#183927=CARTESIAN_POINT('',(-52.7429317578289,-30.6711163007934,39.5248017080178));
#183928=CARTESIAN_POINT('Origin',(-52.7684169058718,-30.685829565079,39.194774761439));
#183929=CARTESIAN_POINT('',(-52.6119816883961,-30.595512242956,39.5248017080178));
#183930=CARTESIAN_POINT('',(0.0952500000000046,-0.164977839420936,39.5248017080178));
#183931=CARTESIAN_POINT('',(-52.3262277788843,-30.4305321463774,39.3343017080178));
#183932=CARTESIAN_POINT('Origin',(-52.5864945348662,-30.5807966351507,39.1947728911897));
#183933=CARTESIAN_POINT('',(-52.2170754202458,-30.3675130027348,39.116));
#183934=CARTESIAN_POINT('',(-52.3262277788843,-30.4305321463774,39.3343017080178));
#183935=CARTESIAN_POINT('',(0.0952500000000046,-0.164977839420936,39.116));
#183936=CARTESIAN_POINT('Origin',(-0.095249999999999,0.164977839420936,
1.34128103812638E-17));
#183937=CARTESIAN_POINT('',(-53.6759427993288,-30.7698495716378,39.116));
#183938=CARTESIAN_POINT('',(-54.0490387249981,-30.9852566047565,39.3548010137695));
#183939=CARTESIAN_POINT('Origin',(-53.7090519420885,-30.7889651441227,39.555029391246));
#183940=CARTESIAN_POINT('',(-54.3576020374704,-31.1634057157515,39.92499));
#183941=CARTESIAN_POINT('',(-54.0490387249981,-30.9852566047565,39.3548010137695));
#183942=CARTESIAN_POINT('',(-51.3783102687787,-29.4433108116258,39.92499));
#183943=CARTESIAN_POINT('',(-0.0952499999999886,0.164977839420939,39.92499));
#183944=CARTESIAN_POINT('',(-51.6868740051412,-29.6214601686927,39.3548010137695));
#183945=CARTESIAN_POINT('',(-51.3783102687787,-29.4433108116258,39.92499));
#183946=CARTESIAN_POINT('',(-52.0599703131948,-29.8368674217653,39.116));
#183947=CARTESIAN_POINT('Origin',(-52.0268612765596,-29.8177519105513,39.5550297827285));
#183948=CARTESIAN_POINT('',(-52.407575419875,-30.0375573245352,39.116));
#183949=CARTESIAN_POINT('',(-52.4715382154241,-30.0744862609072,39.116));
#183950=CARTESIAN_POINT('',(-52.5167277788843,-30.1005764675355,39.3343017080178));
#183951=CARTESIAN_POINT('',(-52.4075754202458,-30.0375573238929,39.116));
#183952=CARTESIAN_POINT('',(-52.8024816883961,-30.2655565641141,39.5248017080178));
#183953=CARTESIAN_POINT('Origin',(-52.7769965925041,-30.2508433300763,39.1947745585587));
#183954=CARTESIAN_POINT('',(-52.9334317578289,-30.3411606219516,39.5248017080178));
#183955=CARTESIAN_POINT('',(-52.9338896349619,-30.3414249774375,39.5248017080178));
#183956=CARTESIAN_POINT('',(-53.2191856060847,-30.506140683164,39.3343017080178));
#183957=CARTESIAN_POINT('Origin',(-52.9589188467305,-30.3558761923113,39.1947728594283));
#183958=CARTESIAN_POINT('',(-53.3283379191466,-30.569159800493,39.116));
#183959=CARTESIAN_POINT('',(-53.2191856060847,-30.506140683164,39.3343017080178));
#183960=CARTESIAN_POINT('',(-53.6763943313415,-30.7701102637668,39.116));
#183961=CARTESIAN_POINT('Origin',(-53.1491210481985,-23.8720415006487,40.10025));
#183962=CARTESIAN_POINT('',(-53.9314655730806,-23.9951532569804,40.10025));
#183963=CARTESIAN_POINT('',(-57.419280924679,-25.5480287005715,40.10025));
#183964=CARTESIAN_POINT('',(-53.2328030451449,-23.6840886581933,40.10025));
#183965=CARTESIAN_POINT('',(-57.4068835917981,-25.5758735661205,40.10025));
#183966=CARTESIAN_POINT('Origin',(8.62051087089598E-17,5.97926641667876E-17,
40.10025));
#183967=CARTESIAN_POINT('',(-53.9190682401996,-24.0229981225294,40.10025));
#183968=CARTESIAN_POINT('',(-53.854477793907,-23.994240603043,40.10025));
#183969=CARTESIAN_POINT('Origin',(3.24161598652235E-16,-3.1132026978004E-17,
40.10025));
#183970=CARTESIAN_POINT('Origin',(0.0774833305059389,-0.174030409680916,
-1.0910962937375E-17));
#183971=CARTESIAN_POINT('',(-54.7386155880005,-24.5797300649098,39.116));
#183972=CARTESIAN_POINT('',(-54.3450469517071,-24.4045020183943,39.3548010137695));
#183973=CARTESIAN_POINT('Origin',(-54.7036898113999,-24.5641801073105,39.5550297832868));
#183974=CARTESIAN_POINT('',(-54.0195518811807,-24.2595822754869,39.92499));
#183975=CARTESIAN_POINT('',(-54.3450469517071,-24.4045020183942,39.3548010137695));
#183976=CARTESIAN_POINT('',(-57.1623216544372,-25.6588335304438,39.92499));
#183977=CARTESIAN_POINT('',(-57.3996482375658,-25.7644981330389,39.92499));
#183978=CARTESIAN_POINT('',(-56.8368270312096,-25.5139139879309,39.3548010137695));
#183979=CARTESIAN_POINT('',(-57.1623216544372,-25.6588335304438,39.92499));
#183980=CARTESIAN_POINT('',(-56.4432587981558,-25.3386861202874,39.116));
#183981=CARTESIAN_POINT('Origin',(-56.4781846872462,-25.3542361279703,39.5550293907216));
#183982=CARTESIAN_POINT('',(-56.0765803402172,-25.1754303533067,39.116));
#183983=CARTESIAN_POINT('',(0.0774833305059444,-0.174030409680916,39.116));
#183984=CARTESIAN_POINT('',(-55.9614386837454,-25.1241659841932,39.3343017080178));
#183985=CARTESIAN_POINT('',(-56.0765803405064,-25.1754303526572,39.116));
#183986=CARTESIAN_POINT('',(-55.6600051127009,-24.9899591116492,39.5248017080178));
#183987=CARTESIAN_POINT('Origin',(-55.6868886053382,-25.0019278517709,39.194774761431));
#183988=CARTESIAN_POINT('',(-55.5218696254674,-24.9284572302738,39.5248017080178));
#183989=CARTESIAN_POINT('',(0.0774833305059445,-0.174030409680916,39.5248017080178));
#183990=CARTESIAN_POINT('',(-55.2204359898058,-24.7942503289604,39.3343017080178));
#183991=CARTESIAN_POINT('Origin',(-55.4949838933598,-24.9164863690987,39.1947728911928));
#183992=CARTESIAN_POINT('',(-55.1052942849673,-24.742985939091,39.116));
#183993=CARTESIAN_POINT('',(-55.2204359898058,-24.7942503289604,39.3343017080178));
#183994=CARTESIAN_POINT('',(0.0774833305059444,-0.174030409680916,39.116));
#183995=CARTESIAN_POINT('Origin',(-0.0774833305059389,0.174030409680916,
1.0910962937375E-17));
#183996=CARTESIAN_POINT('',(-56.5982254591677,-24.9906253009256,39.116));
#183997=CARTESIAN_POINT('',(-56.9917936924674,-25.1658531680168,39.3548010137695));
#183998=CARTESIAN_POINT('Origin',(-56.633151347996,-25.0061753084918,39.5550293912444));
#183999=CARTESIAN_POINT('',(-57.3172883156331,-25.3107727106687,39.92499));
#184000=CARTESIAN_POINT('',(-56.9917936924674,-25.1658531680168,39.3548010137695));
#184001=CARTESIAN_POINT('',(-54.1745185419761,-23.9115214566112,39.92499));
#184002=CARTESIAN_POINT('',(-0.0774833305059281,0.174030409680918,39.92499));
#184003=CARTESIAN_POINT('',(-54.5000136124315,-24.0564411996782,39.3548010137695));
#184004=CARTESIAN_POINT('',(-54.1745185419761,-23.9115214566111,39.92499));
#184005=CARTESIAN_POINT('',(-54.8935822490124,-24.231669245548,39.116));
#184006=CARTESIAN_POINT('Origin',(-54.858656472134,-24.2161192878251,39.5550297827315));
#184007=CARTESIAN_POINT('',(-55.2602609456776,-24.3949251204066,39.116));
#184008=CARTESIAN_POINT('',(-55.3277334713091,-24.4249658234763,39.116));
#184009=CARTESIAN_POINT('',(-55.3754026508176,-24.4461895095986,39.3343017080178));
#184010=CARTESIAN_POINT('',(-55.2602609459792,-24.3949251197292,39.116));
#184011=CARTESIAN_POINT('',(-55.6768362864793,-24.580396410912,39.5248017080178));
#184012=CARTESIAN_POINT('Origin',(-55.6499528488661,-24.5684276954198,39.1947745585575));
#184013=CARTESIAN_POINT('',(-55.8149717737128,-24.6418982922874,39.5248017080178));
#184014=CARTESIAN_POINT('',(-55.8154547752196,-24.6421133384133,39.5248017080178));
#184015=CARTESIAN_POINT('',(-56.1164053447573,-24.7761051648314,39.3343017080178));
#184016=CARTESIAN_POINT('Origin',(-55.8418574376333,-24.6538691229782,39.1947728594331));
#184017=CARTESIAN_POINT('',(-56.2315470015183,-24.8273695332954,39.116));
#184018=CARTESIAN_POINT('',(-56.1164053447573,-24.7761051648314,39.3343017080178));
#184019=CARTESIAN_POINT('',(-56.5987017673884,-24.9908373670084,39.116));
#184020=CARTESIAN_POINT('Origin',(-55.3532724151366,-18.1856720123405,40.10025));
#184021=CARTESIAN_POINT('',(-56.1441998575528,-18.2263320786579,40.10025));
#184022=CARTESIAN_POINT('',(-59.7752282754838,-19.406124729225,40.10025));
#184023=CARTESIAN_POINT('',(-55.4168495715593,-17.9900016446779,40.10025));
#184024=CARTESIAN_POINT('',(-59.7658094374952,-19.4351129318417,40.10025));
#184025=CARTESIAN_POINT('Origin',(9.17194536069053E-17,4.54273045741979E-17,
40.10025));
#184026=CARTESIAN_POINT('',(-56.1347810195643,-18.2553202812746,40.10025));
#184027=CARTESIAN_POINT('',(-56.0675384271754,-18.2334718385816,40.10025));
#184028=CARTESIAN_POINT('Origin',(3.21290464935061E-16,-2.36524679281224E-17,
40.10025));
#184029=CARTESIAN_POINT('Origin',(0.0588677374284264,-0.181176266354227,
-8.28957270027842E-18));
#184030=CARTESIAN_POINT('',(-57.0080331356323,-18.7233363629821,39.116));
#184031=CARTESIAN_POINT('',(-56.5983041910847,-18.5902073587819,39.3548010137695));
#184032=CARTESIAN_POINT('Origin',(-56.9716732729182,-18.711522327434,39.5550297832862));
#184033=CARTESIAN_POINT('',(-56.2594439785882,-18.4801050009132,39.92499));
#184034=CARTESIAN_POINT('',(-56.5983041910847,-18.5902073587819,39.3548010137695));
#184035=CARTESIAN_POINT('',(-59.5312589135997,-19.5431821162863,39.92499));
#184036=CARTESIAN_POINT('',(-59.778330355405,-19.6234604941055,39.92499));
#184037=CARTESIAN_POINT('',(-59.1923991668986,-19.4330799109589,39.3548010137695));
#184038=CARTESIAN_POINT('',(-59.5312589135997,-19.5431821162863,39.92499));
#184039=CARTESIAN_POINT('',(-58.7826706420789,-19.2999510425003,39.116));
#184040=CARTESIAN_POINT('Origin',(-58.8190306219019,-19.3117651160994,39.5550293907208));
#184041=CARTESIAN_POINT('',(-58.4009360126569,-19.1759179434153,39.116));
#184042=CARTESIAN_POINT('',(0.0588677374284319,-0.181176266354227,39.116));
#184043=CARTESIAN_POINT('',(-58.2810665285031,-19.136969986288,39.3343017080178));
#184044=CARTESIAN_POINT('',(-58.4009360128768,-19.1759179427383,39.116));
#184045=CARTESIAN_POINT('',(-57.9672558039533,-19.0350067009927,39.5248017080178));
#184046=CARTESIAN_POINT('Origin',(-57.9952431000167,-19.0440997849308,39.1947747614299));
#184047=CARTESIAN_POINT('',(-57.823448340224,-18.9882808235617,39.5248017080178));
#184048=CARTESIAN_POINT('',(0.0588677374284319,-0.181176266354227,39.5248017080178));
#184049=CARTESIAN_POINT('',(-57.5096375484038,-18.8863175164089,39.3343017080178));
#184050=CARTESIAN_POINT('Origin',(-57.7954585952486,-18.9791858642781,39.1947728911906));
#184051=CARTESIAN_POINT('',(-57.3897680139785,-18.8473695436959,39.116));
#184052=CARTESIAN_POINT('',(-57.5096375484038,-18.8863175164089,39.3343017080178));
#184053=CARTESIAN_POINT('',(0.0588677374284319,-0.181176266354227,39.116));
#184054=CARTESIAN_POINT('Origin',(-0.0588677374284264,0.181176266354227,
8.28957270027842E-18));
#184055=CARTESIAN_POINT('',(-58.9004061169358,-18.9375985097918,39.116));
#184056=CARTESIAN_POINT('',(-59.3101346419425,-19.0707273776749,39.3548010137695));
#184057=CARTESIAN_POINT('Origin',(-58.9367660964857,-18.9494125833022,39.555029391244));
#184058=CARTESIAN_POINT('',(-59.6489943885963,-19.1808295831477,39.92499));
#184059=CARTESIAN_POINT('',(-59.3101346419425,-19.0707273776749,39.3548010137695));
#184060=CARTESIAN_POINT('',(-56.3771794532808,-18.1177524687103,39.92499));
#184061=CARTESIAN_POINT('',(-0.0588677374284154,0.181176266354229,39.92499));
#184062=CARTESIAN_POINT('',(-56.7160396657231,-18.2278548267456,39.3548010137695));
#184063=CARTESIAN_POINT('',(-56.3771794532808,-18.1177524687103,39.92499));
#184064=CARTESIAN_POINT('',(-57.1257686104892,-18.3609838302737,39.116));
#184065=CARTESIAN_POINT('Origin',(-57.0894087474847,-18.3491697946312,39.555029782729));
#184066=CARTESIAN_POINT('',(-57.5075034886062,-18.4850170116927,39.116));
#184067=CARTESIAN_POINT('',(-57.57774650121,-18.5078403492306,39.116));
#184068=CARTESIAN_POINT('',(-57.6273730232606,-18.5239649837004,39.3343017080178));
#184069=CARTESIAN_POINT('',(-57.5075034888354,-18.4850170109874,39.116));
#184070=CARTESIAN_POINT('',(-57.9411838150808,-18.6259282908533,39.5248017080178));
#184071=CARTESIAN_POINT('Origin',(-57.913196576314,-18.6168352256579,39.1947745585584));
#184072=CARTESIAN_POINT('',(-58.0849912788101,-18.6726541682842,39.5248017080178));
#184073=CARTESIAN_POINT('',(-58.0854941128252,-18.6728175489597,39.5248017080178));
#184074=CARTESIAN_POINT('',(-58.3988020033599,-18.7746174535796,39.3343017080178));
#184075=CARTESIAN_POINT('Origin',(-58.1129809527835,-18.6817491043774,39.1947728594267));
#184076=CARTESIAN_POINT('',(-58.5186714877337,-18.8135654100299,39.116));
#184077=CARTESIAN_POINT('',(-58.3988020033599,-18.7746174535796,39.3343017080178));
#184078=CARTESIAN_POINT('',(-58.900901982832,-18.9377596263882,39.116));
#184079=CARTESIAN_POINT('Origin',(-56.9509617460775,-12.3000564958686,40.10025));
#184080=CARTESIAN_POINT('',(-57.7418065394567,-12.2578193919764,40.10025));
#184081=CARTESIAN_POINT('',(-61.4762657165316,-13.0516031943525,40.10025));
#184082=CARTESIAN_POINT('',(-56.9937374973464,-12.0988124084936,40.10025));
#184083=CARTESIAN_POINT('',(-61.4699285681955,-13.0814171332228,40.10025));
#184084=CARTESIAN_POINT('Origin',(9.57020013840216E-17,3.05642339264188E-17,
40.10025));
#184085=CARTESIAN_POINT('',(-57.7354693911205,-12.2876333308468,40.10025));
#184086=CARTESIAN_POINT('',(-57.6663113765489,-12.2729333410575,40.10025));
#184087=CARTESIAN_POINT('Origin',(3.19216886402203E-16,-1.59137674900232E-17,
40.10025));
#184088=CARTESIAN_POINT('Origin',(0.039607177100782,-0.18633711793979,-5.57736016997301E-18));
#184089=CARTESIAN_POINT('',(-58.6528587425323,-12.6618058697516,39.116));
#184090=CARTESIAN_POINT('',(-58.2314585657881,-12.5722344970957,39.3548010137695));
#184091=CARTESIAN_POINT('Origin',(-58.6154631599693,-12.6538571933003,39.5550297832852));
#184092=CARTESIAN_POINT('',(-57.882945834721,-12.4981558287388,39.92499));
#184093=CARTESIAN_POINT('',(-58.2314585657881,-12.5722344970957,39.3548010137695));
#184094=CARTESIAN_POINT('',(-61.2479592423879,-13.213411509189,39.92499));
#184095=CARTESIAN_POINT('',(-61.5020685764505,-13.2674241155256,39.92499));
#184096=CARTESIAN_POINT('',(-60.8994469905094,-13.1393329438486,39.3548010137695));
#184097=CARTESIAN_POINT('',(-61.2479592423878,-13.213411509189,39.92499));
#184098=CARTESIAN_POINT('',(-60.4780472453828,-13.0497616623171,39.116));
#184099=CARTESIAN_POINT('Origin',(-60.5154429483886,-13.0577103643693,39.5550293907236));
#184100=CARTESIAN_POINT('',(-60.0854388089606,-12.966310163716,39.116));
#184101=CARTESIAN_POINT('',(0.0396071771007875,-0.18633711793979,39.116));
#184102=CARTESIAN_POINT('',(-59.9621548122772,-12.9401053405446,39.3343017080178));
#184103=CARTESIAN_POINT('',(-60.0854388091086,-12.96631016302,39.116));
#184104=CARTESIAN_POINT('',(-59.6394051101894,-12.8715027735888,39.5248017080178));
#184105=CARTESIAN_POINT('Origin',(-59.6681895750049,-12.8776205756127,39.1947747614269));
#184106=CARTESIAN_POINT('',(-59.4915012546306,-12.8400648385935,39.5248017080178));
#184107=CARTESIAN_POINT('',(0.0396071771007876,-0.18633711793979,39.5248017080178));
#184108=CARTESIAN_POINT('',(-59.1687514833561,-12.7714622569316,39.3343017080178));
#184109=CARTESIAN_POINT('Origin',(-59.4627141582876,-12.8339454274776,39.1947728911936));
#184110=CARTESIAN_POINT('',(-59.0454674350475,-12.7452574235144,39.116));
#184111=CARTESIAN_POINT('',(-59.1687514833561,-12.7714622569316,39.3343017080178));
#184112=CARTESIAN_POINT('',(0.0396071771007875,-0.18633711793979,39.116));
#184113=CARTESIAN_POINT('Origin',(-0.039607177100782,0.18633711793979,5.57736016997301E-18));
#184114=CARTESIAN_POINT('',(-60.5572615995844,-12.6770874264375,39.116));
#184115=CARTESIAN_POINT('',(-60.9786613448368,-12.766658707377,39.3548010137695));
#184116=CARTESIAN_POINT('Origin',(-60.5946573023114,-12.6850361284304,39.5550293912429));
#184117=CARTESIAN_POINT('',(-61.3271735966834,-12.8407372728674,39.92499));
#184118=CARTESIAN_POINT('',(-60.9786613448368,-12.766658707377,39.3548010137695));
#184119=CARTESIAN_POINT('',(-57.9621601888121,-12.1254815933788,39.92499));
#184120=CARTESIAN_POINT('',(-0.0396071771007709,0.186337117939791,39.92499));
#184121=CARTESIAN_POINT('',(-58.3106729198427,-12.1995602619073,39.3548010137695));
#184122=CARTESIAN_POINT('',(-57.9621601888121,-12.1254815933788,39.92499));
#184123=CARTESIAN_POINT('',(-58.7320730967339,-12.289131633872,39.116));
#184124=CARTESIAN_POINT('Origin',(-58.6946775138732,-12.2811829573575,39.5550297827297));
#184125=CARTESIAN_POINT('',(-59.1246817890949,-12.3725831883604,39.116));
#184126=CARTESIAN_POINT('',(-59.1969256915255,-12.3879391031043,39.116));
#184127=CARTESIAN_POINT('',(-59.2479658375577,-12.398788021052,39.3343017080178));
#184128=CARTESIAN_POINT('',(-59.1246817892491,-12.3725831876348,39.116));
#184129=CARTESIAN_POINT('',(-59.5707156088321,-12.4673906027139,39.5248017080178));
#184130=CARTESIAN_POINT('Origin',(-59.5419312029551,-12.4612728133403,39.19477455856));
#184131=CARTESIAN_POINT('',(-59.718619464391,-12.4988285377092,39.5248017080178));
#184132=CARTESIAN_POINT('',(-59.7191366217597,-12.4989384629014,39.5248017080178));
#184133=CARTESIAN_POINT('',(-60.0413691664788,-12.567431104665,39.3343017080178));
#184134=CARTESIAN_POINT('Origin',(-59.7474064876957,-12.5049479331832,39.1947728594283));
#184135=CARTESIAN_POINT('',(-60.1646531633101,-12.5936359271404,39.116));
#184136=CARTESIAN_POINT('',(-60.0413691664788,-12.567431104665,39.3343017080178));
#184137=CARTESIAN_POINT('',(-60.5577715903455,-12.6771958283202,39.116));
#184138=CARTESIAN_POINT('Origin',(-57.9246844223735,-6.27967898647569,40.10025));
#184139=CARTESIAN_POINT('',(-58.7067819056643,-6.15500747092277,40.10025));
#184140=CARTESIAN_POINT('',(-62.5037563256535,-6.55408556365905,40.10025));
#184141=CARTESIAN_POINT('',(-57.9461901084062,-6.07506605172262,40.10025));
#184142=CARTESIAN_POINT('',(-62.5005702980931,-6.58439859102987,40.10025));
#184143=CARTESIAN_POINT('Origin',(9.81091184134694E-17,1.53662951357646E-17,
40.10025));
#184144=CARTESIAN_POINT('',(-58.7035958781039,-6.1853204982936,40.10025));
#184145=CARTESIAN_POINT('',(-58.6332801510296,-6.1779300175723,40.10025));
#184146=CARTESIAN_POINT('Origin',(3.17963581613999E-16,-8.00071248513326E-18,
40.10025));
#184147=CARTESIAN_POINT('Origin',(0.0199126722524868,-0.189456421067656,
-2.80404091450773E-18));
#184148=CARTESIAN_POINT('',(-59.6550713551493,-6.46154998175879,39.116));
#184149=CARTESIAN_POINT('',(-59.2266168947286,-6.41651760335012,39.3548010137695));
#184150=CARTESIAN_POINT('Origin',(-59.6170497665656,-6.45755375176711,39.5550297832845));
#184151=CARTESIAN_POINT('',(-58.8722700235037,-6.3792742458964,39.92499));
#184152=CARTESIAN_POINT('',(-59.2266168947286,-6.41651760335012,39.3548010137695));
#184153=CARTESIAN_POINT('',(-62.293614112757,-6.73887200051292,39.92499));
#184154=CARTESIAN_POINT('',(-62.5519772640372,-6.76602706194906,39.92499));
#184155=CARTESIAN_POINT('',(-61.9392677288637,-6.70162869542303,39.3548010137695));
#184156=CARTESIAN_POINT('',(-62.293614112757,-6.73887200051292,39.92499));
#184157=CARTESIAN_POINT('',(-61.5108137072212,-6.65659636252343,39.116));
#184158=CARTESIAN_POINT('Origin',(-61.5488354182644,-6.66059260538611,39.5550293907221));
#184159=CARTESIAN_POINT('',(-61.1116329639869,-6.61464077648877,39.116));
#184160=CARTESIAN_POINT('',(0.0199126722524923,-0.189456421067656,39.116));
#184161=CARTESIAN_POINT('',(-60.9862851800405,-6.60146619279907,39.3343017080178));
#184162=CARTESIAN_POINT('',(-61.1116329640613,-6.61464077578082,39.116));
#184163=CARTESIAN_POINT('',(-60.6581326136904,-6.56697596826238,39.5248017080178));
#184164=CARTESIAN_POINT('Origin',(-60.6873988786444,-6.57005146045401,39.1947747614342));
#184165=CARTESIAN_POINT('',(-60.5077528318944,-6.55117041629729,39.5248017080178));
#184166=CARTESIAN_POINT('',(0.0199126722524923,-0.189456421067656,39.5248017080178));
#184167=CARTESIAN_POINT('',(-60.1796001951996,-6.51668018436707,39.3343017080178));
#184168=CARTESIAN_POINT('Origin',(-60.4784837816391,-6.54809359889867,39.1947728911901));
#184169=CARTESIAN_POINT('',(-60.0542523588397,-6.50350559588426,39.116));
#184170=CARTESIAN_POINT('',(-60.1796001951996,-6.51668018436707,39.3343017080178));
#184171=CARTESIAN_POINT('',(0.0199126722524923,-0.189456421067656,39.116));
#184172=CARTESIAN_POINT('Origin',(-0.0199126722524868,0.189456421067656,
2.80404091450773E-18));
#184173=CARTESIAN_POINT('',(-61.5506390517262,-6.27768352038812,39.116));
#184174=CARTESIAN_POINT('',(-61.9790930734319,-6.322715852686,39.3548010137695));
#184175=CARTESIAN_POINT('Origin',(-61.5886607624846,-6.28167976322088,39.555029391244));
#184176=CARTESIAN_POINT('',(-62.3334394573092,-6.35995915792788,39.92499));
#184177=CARTESIAN_POINT('',(-61.9790930734319,-6.322715852686,39.3548010137695));
#184178=CARTESIAN_POINT('',(-58.9120953679531,-6.00036140429008,39.92499));
#184179=CARTESIAN_POINT('',(-0.0199126722524756,0.189456421067657,39.92499));
#184180=CARTESIAN_POINT('',(-59.2664422391598,-6.03760476191742,39.3548010137695));
#184181=CARTESIAN_POINT('',(-58.912095367953,-6.00036140429008,39.92499));
#184182=CARTESIAN_POINT('',(-59.6948966996543,-6.08263713962348,39.116));
#184183=CARTESIAN_POINT('Origin',(-59.6568751107679,-6.07864090959999,39.5550297827291));
#184184=CARTESIAN_POINT('',(-60.0940777032672,-6.12459275448644,39.116));
#184185=CARTESIAN_POINT('',(-60.1675309762115,-6.13231300382137,39.116));
#184186=CARTESIAN_POINT('',(-60.2194255397045,-6.13776734223176,39.3343017080178));
#184187=CARTESIAN_POINT('',(-60.0940777033447,-6.12459275374895,39.116));
#184188=CARTESIAN_POINT('',(-60.5475781763994,-6.17225757416198,39.5248017080178));
#184189=CARTESIAN_POINT('Origin',(-60.5183119713893,-6.16918208839119,39.1947745585571));
#184190=CARTESIAN_POINT('',(-60.6979579581954,-6.18806312612707,39.5248017080178));
#184191=CARTESIAN_POINT('',(-60.6984837728333,-6.18811839147248,39.5248017080178));
#184192=CARTESIAN_POINT('',(-61.0261105245454,-6.22255335066375,39.3343017080178));
#184193=CARTESIAN_POINT('Origin',(-60.7272269341776,-6.19113993560405,39.1947728594259));
#184194=CARTESIAN_POINT('',(-61.1514583085663,-6.23572793364551,39.116));
#184195=CARTESIAN_POINT('',(-61.0261105245454,-6.22255335066375,39.3343017080178));
#184196=CARTESIAN_POINT('',(-61.5511575797868,-6.27773801988339,39.116));
#184197=CARTESIAN_POINT('Origin',(-58.2637721346185,-0.1905,40.10025));
#184198=CARTESIAN_POINT('',(-58.2637721346185,0.01524,40.10025));
#184199=CARTESIAN_POINT('',(-58.9578504383728,-0.01524,40.10025));
#184200=CARTESIAN_POINT('Origin',(0.,-0.1905,0.));
#184201=CARTESIAN_POINT('',(-60.0036905223731,-0.1905,39.116));
#184202=CARTESIAN_POINT('',(-59.5728760150042,-0.1905,39.3548010137695));
#184203=CARTESIAN_POINT('Origin',(-59.9654595002513,-0.1905,39.5550297832875));
#184204=CARTESIAN_POINT('',(-59.2165773020941,-0.190499999468477,39.92499));
#184205=CARTESIAN_POINT('',(-59.5728760150042,-0.1905,39.3548010137695));
#184206=CARTESIAN_POINT('',(-62.6567671111299,-0.190499999999999,39.92499));
#184207=CARTESIAN_POINT('',(-62.9165533988763,-0.1905,39.92499));
#184208=CARTESIAN_POINT('',(-62.3004688883554,-0.190500000605399,39.3548010137695));
#184209=CARTESIAN_POINT('',(-62.6567671111299,-0.1905,39.92499));
#184210=CARTESIAN_POINT('',(-61.8696548221181,-0.1905,39.116));
#184211=CARTESIAN_POINT('Origin',(-61.9078859673759,-0.1905,39.5550293907204));
#184212=CARTESIAN_POINT('',(-61.4682752798284,-0.190500000712027,39.116));
#184213=CARTESIAN_POINT('',(5.50819412990574E-15,-0.1905,39.116));
#184214=CARTESIAN_POINT('',(-61.3422370451705,-0.1905,39.3343017080178));
#184215=CARTESIAN_POINT('',(-61.4682752798284,-0.1905,39.116));
#184216=CARTESIAN_POINT('',(-61.0122769227456,-0.1905,39.5248017080178));
#184217=CARTESIAN_POINT('Origin',(-61.04170434051,-0.190499486622401,39.1947747614337));
#184218=CARTESIAN_POINT('',(-60.8610688070707,-0.1905,39.5248017080178));
#184219=CARTESIAN_POINT('',(5.56576032196012E-15,-0.1905,39.5248017080178));
#184220=CARTESIAN_POINT('',(-60.5311086139135,-0.1905,39.3343017080178));
#184221=CARTESIAN_POINT('Origin',(-60.8316384807414,-0.190499486573508,
39.1947728911889));
#184222=CARTESIAN_POINT('',(-60.4050703266282,-0.1905,39.116));
#184223=CARTESIAN_POINT('',(-60.5311086139135,-0.1905,39.3343017080178));
#184224=CARTESIAN_POINT('',(5.50819412990574E-15,-0.1905,39.116));
#184225=CARTESIAN_POINT('Origin',(0.,0.1905,0.));
#184226=CARTESIAN_POINT('',(-61.8696548221181,0.1905,39.116));
#184227=CARTESIAN_POINT('',(-62.3004688883554,0.190500000000001,39.3548010137695));
#184228=CARTESIAN_POINT('Origin',(-61.9078859670881,0.1905,39.5550293912456));
#184229=CARTESIAN_POINT('',(-62.6567671111299,0.190500000452307,39.92499));
#184230=CARTESIAN_POINT('',(-62.3004688883554,0.1905,39.3548010137695));
#184231=CARTESIAN_POINT('',(-59.2165773020941,0.1905,39.92499));
#184232=CARTESIAN_POINT('',(1.12442271988212E-14,0.1905,39.92499));
#184233=CARTESIAN_POINT('',(-59.5728760150042,0.190499999293399,39.3548010137695));
#184234=CARTESIAN_POINT('',(-59.2165773020941,0.1905,39.92499));
#184235=CARTESIAN_POINT('',(-60.003690522373,0.1905,39.116));
#184236=CARTESIAN_POINT('Origin',(-59.9654594999476,0.1905,39.5550297827329));
#184237=CARTESIAN_POINT('',(-60.4050703266283,0.190499999257743,39.116));
#184238=CARTESIAN_POINT('',(-60.4789282006568,0.1905,39.116));
#184239=CARTESIAN_POINT('',(-60.5311086139135,0.1905,39.3343017080178));
#184240=CARTESIAN_POINT('',(-60.4050703266282,0.1905,39.116));
#184241=CARTESIAN_POINT('',(-60.8610688070707,0.1905,39.5248017080178));
#184242=CARTESIAN_POINT('Origin',(-60.8316414495934,0.190499486502559,39.1947745585556));
#184243=CARTESIAN_POINT('',(-61.0122769227456,0.1905,39.5248017080178));
#184244=CARTESIAN_POINT('',(-61.0128056337175,0.1905,39.5248017080178));
#184245=CARTESIAN_POINT('',(-61.3422370451705,0.1905,39.3343017080178));
#184246=CARTESIAN_POINT('Origin',(-61.0417071743819,0.190499486688105,39.1947728594266));
#184247=CARTESIAN_POINT('',(-61.4682752798284,0.1905,39.116));
#184248=CARTESIAN_POINT('',(-61.3422370451705,0.1905,39.3343017080178));
#184249=CARTESIAN_POINT('',(-61.8701762063762,0.1905,39.116));
#184250=CARTESIAN_POINT('Origin',(-57.9645097668784,5.90076614434116,40.10025));
#184251=CARTESIAN_POINT('',(-58.7035958781038,6.18532049829439,40.10025));
#184252=CARTESIAN_POINT('',(-62.500570298093,6.58439859103072,40.10025));
#184253=CARTESIAN_POINT('',(-57.9430040808457,6.10537907909423,40.10025));
#184254=CARTESIAN_POINT('',(-62.5037563256534,6.55408556365989,40.10025));
#184255=CARTESIAN_POINT('Origin',(9.81091184134687E-17,-1.53662951357666E-17,
40.10025));
#184256=CARTESIAN_POINT('',(-58.7067819056642,6.15500747092357,40.10025));
#184257=CARTESIAN_POINT('',(-58.6364661785899,6.14761699020227,40.10025));
#184258=CARTESIAN_POINT('Origin',(3.17963581613999E-16,8.00071248513429E-18,
40.10025));
#184259=CARTESIAN_POINT('Origin',(-0.0199126722524893,-0.189456421067656,
2.8040409145081E-18));
#184260=CARTESIAN_POINT('',(-59.6948966996542,6.08263713962429,39.116));
#184261=CARTESIAN_POINT('',(-59.2664422392335,6.03760476121561,39.3548010137695));
#184262=CARTESIAN_POINT('Origin',(-59.6568751110713,6.0786409096327,39.5550297832861));
#184263=CARTESIAN_POINT('',(-58.9120953678974,6.00036140481904,39.92499));
#184264=CARTESIAN_POINT('',(-59.2664422392335,6.03760476121561,39.3548010137695));
#184265=CARTESIAN_POINT('',(-62.3334394572618,6.35995915837845,39.92499));
#184266=CARTESIAN_POINT('',(-62.5918026085421,6.38711421981459,39.92499));
#184267=CARTESIAN_POINT('',(-61.9790930734951,6.322715852085,39.3548010137695));
#184268=CARTESIAN_POINT('',(-62.3334394572618,6.35995915837845,39.92499));
#184269=CARTESIAN_POINT('',(-61.5506390517261,6.27768352038895,39.116));
#184270=CARTESIAN_POINT('Origin',(-61.5886607627699,6.2816797632517,39.5550293907212));
#184271=CARTESIAN_POINT('',(-61.1514583086406,6.23572793293842,39.116));
#184272=CARTESIAN_POINT('',(-0.0199126722524838,-0.189456421067656,39.116));
#184273=CARTESIAN_POINT('',(-61.0261105245453,6.22255335066458,39.3343017080178));
#184274=CARTESIAN_POINT('',(-61.1514583085662,6.23572793364634,39.116));
#184275=CARTESIAN_POINT('',(-60.6979579581953,6.18806312612789,39.5248017080178));
#184276=CARTESIAN_POINT('Origin',(-60.7272241158223,6.19113963944987,39.1947747614314));
#184277=CARTESIAN_POINT('',(-60.5475781763993,6.1722575741628,39.5248017080178));
#184278=CARTESIAN_POINT('',(-0.0199126722524838,-0.189456421067656,39.5248017080178));
#184279=CARTESIAN_POINT('',(-60.2194255397045,6.13776734223257,39.3343017080178));
#184280=CARTESIAN_POINT('Origin',(-60.518309018805,6.16918177799158,39.1947728911969));
#184281=CARTESIAN_POINT('',(-60.0940777033446,6.12459275374976,39.116));
#184282=CARTESIAN_POINT('',(-60.2194255397045,6.13776734223257,39.3343017080178));
#184283=CARTESIAN_POINT('',(-0.0199126722524838,-0.189456421067656,39.116));
#184284=CARTESIAN_POINT('Origin',(0.0199126722524893,0.189456421067656,
-2.8040409145081E-18));
#184285=CARTESIAN_POINT('',(-61.5108137072212,6.65659636252426,39.116));
#184286=CARTESIAN_POINT('',(-61.9392677289269,6.70162869482215,39.3548010137695));
#184287=CARTESIAN_POINT('Origin',(-61.5488354179797,6.66059260535702,39.555029391244));
#184288=CARTESIAN_POINT('',(-62.2936141127096,6.73887200096387,39.92499));
#184289=CARTESIAN_POINT('',(-61.9392677289269,6.70162869482215,39.3548010137695));
#184290=CARTESIAN_POINT('',(-58.872270023448,6.37927424642618,39.92499));
#184291=CARTESIAN_POINT('',(0.0199126722525006,0.189456421067655,39.92499));
#184292=CARTESIAN_POINT('',(-59.2266168948024,6.4165176026483,39.3548010137695));
#184293=CARTESIAN_POINT('',(-58.872270023448,6.37927424642618,39.92499));
#184294=CARTESIAN_POINT('',(-59.6550713551492,6.4615499817596,39.116));
#184295=CARTESIAN_POINT('Origin',(-59.6170497662618,6.457553751736,39.5550297827272));
#184296=CARTESIAN_POINT('',(-60.0542523589172,6.50350559514732,39.116));
#184297=CARTESIAN_POINT('',(-60.1277056317064,6.5112258459575,39.116));
#184298=CARTESIAN_POINT('',(-60.1796001951995,6.51668018436788,39.3343017080178));
#184299=CARTESIAN_POINT('',(-60.0542523588397,6.50350559588507,39.116));
#184300=CARTESIAN_POINT('',(-60.5077528318943,6.55117041629811,39.5248017080178));
#184301=CARTESIAN_POINT('Origin',(-60.4784867342325,6.54809390915823,39.1947745585609));
#184302=CARTESIAN_POINT('',(-60.6581326136904,6.5669759682632,39.5248017080178));
#184303=CARTESIAN_POINT('',(-60.6586584283283,6.56703123360861,39.5248017080178));
#184304=CARTESIAN_POINT('',(-60.9862851800404,6.60146619279989,39.3343017080178));
#184305=CARTESIAN_POINT('Origin',(-60.6874016969804,6.57005175673997,39.1947728594192));
#184306=CARTESIAN_POINT('',(-61.1116329640612,6.61464077578165,39.116));
#184307=CARTESIAN_POINT('',(-60.9862851800404,6.60146619279989,39.3343017080178));
#184308=CARTESIAN_POINT('',(-61.5113322352818,6.65665086201954,39.116));
#184309=CARTESIAN_POINT('Origin',(-57.0301761002789,11.9273822599898,40.10025));
#184310=CARTESIAN_POINT('',(-57.7354693911204,12.2876333308475,40.10025));
#184311=CARTESIAN_POINT('',(-61.4699285681953,13.0814171332237,40.10025));
#184312=CARTESIAN_POINT('',(-56.9874003490101,12.1286263473648,40.10025));
#184313=CARTESIAN_POINT('',(-61.4762657165315,13.0516031943533,40.10025));
#184314=CARTESIAN_POINT('Origin',(9.5702001384024E-17,-3.05642339264207E-17,
40.10025));
#184315=CARTESIAN_POINT('',(-57.7418065394565,12.2578193919772,40.10025));
#184316=CARTESIAN_POINT('',(-57.6726485248849,12.2431194021879,40.10025));
#184317=CARTESIAN_POINT('Origin',(3.19216886402205E-16,1.59137674900242E-17,
40.10025));
#184318=CARTESIAN_POINT('Origin',(-0.0396071771007845,-0.18633711793979,
5.57736016997337E-18));
#184319=CARTESIAN_POINT('',(-58.7320730967337,12.2891316338728,39.116));
#184320=CARTESIAN_POINT('',(-58.3106729199895,12.1995602612169,39.3548010137695));
#184321=CARTESIAN_POINT('Origin',(-58.6946775141716,12.2811829574217,39.5550297832871));
#184322=CARTESIAN_POINT('',(-57.9621601887014,12.1254815938998,39.92499));
#184323=CARTESIAN_POINT('',(-58.3106729199895,12.1995602612169,39.3548010137695));
#184324=CARTESIAN_POINT('',(-61.3271735965892,12.8407372733103,39.92499));
#184325=CARTESIAN_POINT('',(-61.5812829306519,12.8947498796469,39.92499));
#184326=CARTESIAN_POINT('',(-60.9786613449624,12.7666587067861,39.3548010137695));
#184327=CARTESIAN_POINT('',(-61.3271735965892,12.8407372733103,39.92499));
#184328=CARTESIAN_POINT('',(-60.5572615995842,12.6770874264384,39.116));
#184329=CARTESIAN_POINT('Origin',(-60.594657302592,12.6850361284909,39.5550293907194));
#184330=CARTESIAN_POINT('',(-60.164653163458,12.5936359264449,39.116));
#184331=CARTESIAN_POINT('',(-0.039607177100779,-0.18633711793979,39.116));
#184332=CARTESIAN_POINT('',(-60.0413691664786,12.5674311046659,39.3343017080178));
#184333=CARTESIAN_POINT('',(-60.1646531633099,12.5936359271413,39.116));
#184334=CARTESIAN_POINT('',(-59.7186194643908,12.49882853771,39.5248017080178));
#184335=CARTESIAN_POINT('Origin',(-59.7474037157301,12.5049473440517,39.1947747614238));
#184336=CARTESIAN_POINT('',(-59.570715608832,12.4673906027147,39.5248017080178));
#184337=CARTESIAN_POINT('',(-0.0396071771007789,-0.18633711793979,39.5248017080178));
#184338=CARTESIAN_POINT('',(-59.2479658375575,12.3987880210528,39.3343017080178));
#184339=CARTESIAN_POINT('Origin',(-59.5419282989946,12.4612721960127,39.1947728911921));
#184340=CARTESIAN_POINT('',(-59.1246817892489,12.3725831876356,39.116));
#184341=CARTESIAN_POINT('',(-59.2479658375575,12.3987880210528,39.3343017080178));
#184342=CARTESIAN_POINT('',(-0.039607177100779,-0.18633711793979,39.116));
#184343=CARTESIAN_POINT('Origin',(0.0396071771007845,0.18633711793979,-5.57736016997337E-18));
#184344=CARTESIAN_POINT('',(-60.4780472453826,13.0497616623179,39.116));
#184345=CARTESIAN_POINT('',(-60.8994469906351,13.1393329432574,39.3548010137695));
#184346=CARTESIAN_POINT('Origin',(-60.5154429481093,13.0577103643107,39.5550293912437));
#184347=CARTESIAN_POINT('',(-61.2479592422936,13.2134115096323,39.92499));
#184348=CARTESIAN_POINT('',(-60.8994469906351,13.1393329432574,39.3548010137695));
#184349=CARTESIAN_POINT('',(-57.8829458346104,12.4981558292591,39.92499));
#184350=CARTESIAN_POINT('',(0.0396071771007956,0.186337117939789,39.92499));
#184351=CARTESIAN_POINT('',(-58.2314585659347,12.5722344964058,39.3548010137695));
#184352=CARTESIAN_POINT('',(-57.8829458346104,12.4981558292591,39.92499));
#184353=CARTESIAN_POINT('',(-58.6528587425321,12.6618058697524,39.116));
#184354=CARTESIAN_POINT('Origin',(-58.6154631596727,12.6538571932381,39.555029782732));
#184355=CARTESIAN_POINT('',(-59.0454674352016,12.7452574227896,39.116));
#184356=CARTESIAN_POINT('',(-59.1177113373237,12.7606133389847,39.116));
#184357=CARTESIAN_POINT('',(-59.168751483356,12.7714622569324,39.3343017080178));
#184358=CARTESIAN_POINT('',(-59.0454674350473,12.7452574235152,39.116));
#184359=CARTESIAN_POINT('',(-59.4915012546304,12.8400648385943,39.5248017080178));
#184360=CARTESIAN_POINT('Origin',(-59.4627170622777,12.8339460446681,39.1947745585593));
#184361=CARTESIAN_POINT('',(-59.6394051101892,12.8715027735896,39.5248017080178));
#184362=CARTESIAN_POINT('',(-59.6399222675579,12.8716126987817,39.5248017080178));
#184363=CARTESIAN_POINT('',(-59.962154812277,12.9401053405454,39.3343017080178));
#184364=CARTESIAN_POINT('Origin',(-59.6681923469416,12.8776211648741,39.19477285943));
#184365=CARTESIAN_POINT('',(-60.0854388091084,12.9663101630208,39.116));
#184366=CARTESIAN_POINT('',(-59.962154812277,12.9401053405454,39.3343017080178));
#184367=CARTESIAN_POINT('',(-60.4785572361438,13.0498700642006,39.116));
#184368=CARTESIAN_POINT('Origin',(-55.4710078899932,17.8233194796328,40.10025));
#184369=CARTESIAN_POINT('',(-56.1347810195641,18.2553202812753,40.10025));
#184370=CARTESIAN_POINT('',(-59.765809437495,19.4351129318425,40.10025));
#184371=CARTESIAN_POINT('',(-55.4074307335705,18.0189898472954,40.10025));
#184372=CARTESIAN_POINT('',(-59.7752282754835,19.4061247292258,40.10025));
#184373=CARTESIAN_POINT('Origin',(9.1719453606903E-17,-4.54273045741998E-17,
40.10025));
#184374=CARTESIAN_POINT('',(-56.1441998575526,18.2263320786586,40.10025));
#184375=CARTESIAN_POINT('',(-56.0769572651637,18.2044836359657,40.10025));
#184376=CARTESIAN_POINT('Origin',(3.2129046493506E-16,2.36524679281234E-17,
40.10025));
#184377=CARTESIAN_POINT('Origin',(-0.0588677374284288,-0.181176266354226,
8.28957270027876E-18));
#184378=CARTESIAN_POINT('',(-57.1257686104889,18.3609838302744,39.116));
#184379=CARTESIAN_POINT('',(-56.7160396659413,18.2278548260742,39.3548010137695));
#184380=CARTESIAN_POINT('Origin',(-57.0894087477764,18.3491697947268,39.5550297832891));
#184381=CARTESIAN_POINT('',(-56.3771794531162,18.1177524692168,39.92499));
#184382=CARTESIAN_POINT('',(-56.7160396659413,18.2278548260742,39.3548010137695));
#184383=CARTESIAN_POINT('',(-59.6489943884562,19.1808295835786,39.92499));
#184384=CARTESIAN_POINT('',(-59.8960658302616,19.2611079613979,39.92499));
#184385=CARTESIAN_POINT('',(-59.3101346421292,19.0707273771002,39.3548010137695));
#184386=CARTESIAN_POINT('',(-59.6489943884562,19.1808295835786,39.92499));
#184387=CARTESIAN_POINT('',(-58.9004061169356,18.9375985097926,39.116));
#184388=CARTESIAN_POINT('Origin',(-58.9367660967581,18.9494125833916,39.5550293907212));
#184389=CARTESIAN_POINT('',(-58.5186714879534,18.8135654093536,39.116));
#184390=CARTESIAN_POINT('',(-0.0588677374284233,-0.181176266354226,39.116));
#184391=CARTESIAN_POINT('',(-58.3988020033597,18.7746174535804,39.3343017080178));
#184392=CARTESIAN_POINT('',(-58.5186714877334,18.8135654100307,39.116));
#184393=CARTESIAN_POINT('',(-58.0849912788099,18.672654168285,39.5248017080178));
#184394=CARTESIAN_POINT('Origin',(-58.1129782575873,18.681748228725,39.1947747614283));
#184395=CARTESIAN_POINT('',(-57.9411838150806,18.6259282908541,39.5248017080178));
#184396=CARTESIAN_POINT('',(-0.0588677374284233,-0.181176266354226,39.5248017080178));
#184397=CARTESIAN_POINT('',(-57.6273730232604,18.5239649837012,39.3343017080178));
#184398=CARTESIAN_POINT('Origin',(-57.9131937527875,18.6168343081648,39.1947728911954));
#184399=CARTESIAN_POINT('',(-57.5075034888351,18.4850170109882,39.116));
#184400=CARTESIAN_POINT('',(-57.6273730232604,18.5239649837012,39.3343017080178));
#184401=CARTESIAN_POINT('',(-0.0588677374284233,-0.181176266354226,39.116));
#184402=CARTESIAN_POINT('Origin',(0.0588677374284288,0.181176266354226,
-8.28957270027876E-18));
#184403=CARTESIAN_POINT('',(-58.7826706420787,19.2999510425011,39.116));
#184404=CARTESIAN_POINT('',(-59.1923991670854,19.4330799103842,39.3548010137695));
#184405=CARTESIAN_POINT('Origin',(-58.8190306216277,19.3117651160112,39.5550293912458));
#184406=CARTESIAN_POINT('',(-59.5312589134596,19.5431821167172,39.92499));
#184407=CARTESIAN_POINT('',(-59.1923991670854,19.4330799103842,39.3548010137695));
#184408=CARTESIAN_POINT('',(-56.2594439784237,18.4801050014195,39.92499));
#184409=CARTESIAN_POINT('',(0.0588677374284398,0.181176266354225,39.92499));
#184410=CARTESIAN_POINT('',(-56.5983041913027,18.5902073581107,39.3548010137695));
#184411=CARTESIAN_POINT('',(-56.2594439784237,18.4801050014195,39.92499));
#184412=CARTESIAN_POINT('',(-57.0080331356321,18.7233363629829,39.116));
#184413=CARTESIAN_POINT('Origin',(-56.9716732726289,18.7115223273408,39.5550297827311));
#184414=CARTESIAN_POINT('',(-57.3897680142075,18.847369542991,39.116));
#184415=CARTESIAN_POINT('',(-57.4600110263529,18.8701928819399,39.116));
#184416=CARTESIAN_POINT('',(-57.5096375484035,18.8863175164097,39.3343017080178));
#184417=CARTESIAN_POINT('',(-57.3897680139783,18.8473695436966,39.116));
#184418=CARTESIAN_POINT('',(-57.8234483402237,18.9882808235625,39.5248017080178));
#184419=CARTESIAN_POINT('Origin',(-57.7954614188134,18.9791867816362,39.1947745585618));
#184420=CARTESIAN_POINT('',(-57.967255803953,19.0350067009935,39.5248017080178));
#184421=CARTESIAN_POINT('',(-57.9677586379681,19.0351700816689,39.5248017080178));
#184422=CARTESIAN_POINT('',(-58.2810665285028,19.1369699862888,39.3343017080178));
#184423=CARTESIAN_POINT('Origin',(-57.9952457951704,19.0441006607093,39.1947728594272));
#184424=CARTESIAN_POINT('',(-58.4009360128765,19.1759179427391,39.116));
#184425=CARTESIAN_POINT('',(-58.2810665285028,19.1369699862888,39.3343017080178));
#184426=CARTESIAN_POINT('',(-58.7831665079749,19.3001121590974,39.116));
#184427=CARTESIAN_POINT('Origin',(-53.30408770921,23.5239806812876,40.10025));
#184428=CARTESIAN_POINT('',(-53.9190682401993,24.0229981225301,40.10025));
#184429=CARTESIAN_POINT('',(-57.4068835917977,25.5758735661212,40.10025));
#184430=CARTESIAN_POINT('',(-53.2204057122636,23.7119335237429,40.10025));
#184431=CARTESIAN_POINT('',(-57.4192809246787,25.5480287005723,40.10025));
#184432=CARTESIAN_POINT('Origin',(8.62051087089599E-17,-5.97926641667894E-17,
40.10025));
#184433=CARTESIAN_POINT('',(-53.9314655730802,23.9951532569811,40.10025));
#184434=CARTESIAN_POINT('',(-53.8668751267876,23.9663957374948,40.10025));
#184435=CARTESIAN_POINT('Origin',(3.24161598652236E-16,3.1132026978005E-17,
40.10025));
#184436=CARTESIAN_POINT('Origin',(-0.0774833305059413,-0.174030409680915,
1.09109629373753E-17));
#184437=CARTESIAN_POINT('',(-54.893582249012,24.2316692455487,39.116));
#184438=CARTESIAN_POINT('',(-54.5000136127187,24.0564411990331,39.3548010137695));
#184439=CARTESIAN_POINT('Origin',(-54.8586564724104,24.216119287949,39.5550297832847));
#184440=CARTESIAN_POINT('',(-54.1745185417597,23.9115214570974,39.92499));
#184441=CARTESIAN_POINT('',(-54.5000136127187,24.0564411990331,39.3548010137695));
#184442=CARTESIAN_POINT('',(-57.3172883154488,25.3107727110827,39.92499));
#184443=CARTESIAN_POINT('',(-57.5546148985774,25.4164373136778,39.92499));
#184444=CARTESIAN_POINT('',(-56.991793692713,25.1658531674651,39.3548010137695));
#184445=CARTESIAN_POINT('',(-57.3172883154488,25.3107727110827,39.92499));
#184446=CARTESIAN_POINT('',(-56.5982254591674,24.9906253009263,39.116));
#184447=CARTESIAN_POINT('Origin',(-56.6331513482564,25.0061753086086,39.5550293907245));
#184448=CARTESIAN_POINT('',(-56.2315470018074,24.8273695326461,39.116));
#184449=CARTESIAN_POINT('',(-0.0774833305059357,-0.174030409680915,39.116));
#184450=CARTESIAN_POINT('',(-56.116405344757,24.7761051648322,39.3343017080178));
#184451=CARTESIAN_POINT('',(-56.231547001518,24.8273695332961,39.116));
#184452=CARTESIAN_POINT('',(-55.8149717737125,24.6418982922882,39.5248017080178));
#184453=CARTESIAN_POINT('Origin',(-55.8418548487323,24.653867970398,39.1947747614342));
#184454=CARTESIAN_POINT('',(-55.676836286479,24.5803964109127,39.5248017080178));
#184455=CARTESIAN_POINT('',(-0.0774833305059357,-0.174030409680915,39.5248017080178));
#184456=CARTESIAN_POINT('',(-55.3754026508173,24.4461895095993,39.3343017080178));
#184457=CARTESIAN_POINT('Origin',(-55.6499501367158,24.5684264878159,39.1947728911866));
#184458=CARTESIAN_POINT('',(-55.2602609459789,24.3949251197299,39.116));
#184459=CARTESIAN_POINT('',(-55.3754026508173,24.4461895095993,39.3343017080178));
#184460=CARTESIAN_POINT('',(-0.0774833305059357,-0.174030409680915,39.116));
#184461=CARTESIAN_POINT('Origin',(0.0774833305059413,0.174030409680915,
-1.09109629373753E-17));
#184462=CARTESIAN_POINT('',(-56.4432587981555,25.3386861202881,39.116));
#184463=CARTESIAN_POINT('',(-56.8368270314552,25.5139139873794,39.3548010137695));
#184464=CARTESIAN_POINT('Origin',(-56.4781846869828,25.354236127854,39.5550293912465));
#184465=CARTESIAN_POINT('',(-57.162321654253,25.6588335308577,39.92499));
#184466=CARTESIAN_POINT('',(-56.8368270314552,25.5139139873794,39.3548010137695));
#184467=CARTESIAN_POINT('',(-54.0195518809639,24.2595822759737,39.92499));
#184468=CARTESIAN_POINT('',(0.077483330505952,0.174030409680913,39.92499));
#184469=CARTESIAN_POINT('',(-54.3450469519945,24.4045020177487,39.3548010137695));
#184470=CARTESIAN_POINT('',(-54.0195518809639,24.2595822759737,39.92499));
#184471=CARTESIAN_POINT('',(-54.7386155880002,24.5797300649105,39.116));
#184472=CARTESIAN_POINT('Origin',(-54.7036898111205,24.564180107187,39.5550297827293));
#184473=CARTESIAN_POINT('',(-55.1052942852684,24.7429859384148,39.116));
#184474=CARTESIAN_POINT('',(-55.1727668102969,24.7730266428388,39.116));
#184475=CARTESIAN_POINT('',(-55.2204359898054,24.7942503289612,39.3343017080178));
#184476=CARTESIAN_POINT('',(-55.105294284967,24.7429859390917,39.116));
#184477=CARTESIAN_POINT('',(-55.5218696254671,24.9284572302746,39.5248017080178));
#184478=CARTESIAN_POINT('Origin',(-55.4949866055697,24.9164875765756,39.1947745585588));
#184479=CARTESIAN_POINT('',(-55.6600051127006,24.98995911165,39.5248017080178));
#184480=CARTESIAN_POINT('',(-55.6604881142074,24.9901741577759,39.5248017080178));
#184481=CARTESIAN_POINT('',(-55.9614386837451,25.124165984194,39.3343017080178));
#184482=CARTESIAN_POINT('Origin',(-55.6868911941801,25.0019290044704,39.1947728594209));
#184483=CARTESIAN_POINT('',(-56.0765803405061,25.1754303526579,39.116));
#184484=CARTESIAN_POINT('',(-55.9614386837451,25.124165984194,39.3343017080178));
#184485=CARTESIAN_POINT('',(-56.4437351063762,25.338898186371,39.116));
#184486=CARTESIAN_POINT('Origin',(-50.5531567888873,28.9669082278887,40.10025));
#184487=CARTESIAN_POINT('',(-51.1126068659045,29.5274749692189,40.10025));
#184488=CARTESIAN_POINT('',(-54.4189959163061,31.4364195775139,40.10025));
#184489=CARTESIAN_POINT('',(-50.4502867888873,29.1450842944633,40.10025));
#184490=CARTESIAN_POINT('',(-54.434235916306,31.4100231232066,40.10025));
#184491=CARTESIAN_POINT('Origin',(7.92193830068374E-17,-7.35029228183484E-17,
40.10025));
#184492=CARTESIAN_POINT('',(-51.1278468659044,29.5010785149116,40.10025));
#184493=CARTESIAN_POINT('',(-51.0666162321541,29.4657269920332,40.10025));
#184494=CARTESIAN_POINT('Origin',(3.27798830811898E-16,3.82704970255201E-17,
40.10025));
#184495=CARTESIAN_POINT('Origin',(-0.0952500000000014,-0.164977839420935,
1.34128103812642E-17));
#184496=CARTESIAN_POINT('',(-52.0599703131944,29.836867421766,39.116));
#184497=CARTESIAN_POINT('',(-51.686874005494,29.6214601680816,39.3548010137695));
#184498=CARTESIAN_POINT('Origin',(-52.0268612768248,29.8177519107055,39.5550297832886));
#184499=CARTESIAN_POINT('',(-51.3783102685123,29.4433108120871,39.92499));
#184500=CARTESIAN_POINT('',(-51.686874005494,29.6214601680816,39.3548010137695));
#184501=CARTESIAN_POINT('',(-54.3576020372436,31.1634057161445,39.92499));
#184502=CARTESIAN_POINT('',(-54.5825835619868,31.2932988600177,39.92499));
#184503=CARTESIAN_POINT('',(-54.0490387253,30.9852566042336,39.3548010137695));
#184504=CARTESIAN_POINT('',(-54.3576020372436,31.1634057161445,39.92499));
#184505=CARTESIAN_POINT('',(-53.6759427993284,30.7698495716385,39.116));
#184506=CARTESIAN_POINT('Origin',(-53.7090519423364,30.7889651442668,39.5550293907229));
#184507=CARTESIAN_POINT('',(-53.328337919502,30.5691597998774,39.116));
#184508=CARTESIAN_POINT('',(-0.0952499999999959,-0.164977839420935,39.116));
#184509=CARTESIAN_POINT('',(-53.2191856060843,30.5061406831648,39.3343017080178));
#184510=CARTESIAN_POINT('',(-53.3283379191462,30.5691598004937,39.116));
#184511=CARTESIAN_POINT('',(-52.9334317578285,30.3411606219523,39.5248017080178));
#184512=CARTESIAN_POINT('Origin',(-52.958916392492,30.3558747754329,39.1947747614341));
#184513=CARTESIAN_POINT('',(-52.8024816883957,30.2655565641149,39.5248017080178));
#184514=CARTESIAN_POINT('',(-0.0952499999999958,-0.164977839420935,39.5248017080178));
#184515=CARTESIAN_POINT('',(-52.5167277788839,30.1005764675362,39.3343017080178));
#184516=CARTESIAN_POINT('Origin',(-52.7769940214391,30.2508418455903,39.1947728911909));
#184517=CARTESIAN_POINT('',(-52.4075754202454,30.0375573238936,39.116));
#184518=CARTESIAN_POINT('',(-52.5167277788839,30.1005764675362,39.3343017080178));
#184519=CARTESIAN_POINT('',(-0.0952499999999959,-0.164977839420935,39.116));
#184520=CARTESIAN_POINT('Origin',(0.0952500000000014,0.164977839420935,
-1.34128103812642E-17));
#184521=CARTESIAN_POINT('',(-53.4854427993284,31.0998052504804,39.116));
#184522=CARTESIAN_POINT('',(-53.8585387249976,31.3152122835991,39.3548010137695));
#184523=CARTESIAN_POINT('Origin',(-53.5185519420879,31.1189208229652,39.5550293912461));
#184524=CARTESIAN_POINT('',(-54.1671020370176,31.4933613953778,39.92499));
#184525=CARTESIAN_POINT('',(-53.8585387249976,31.3152122835991,39.3548010137695));
#184526=CARTESIAN_POINT('',(-51.1878102687783,29.7732664904684,39.92499));
#184527=CARTESIAN_POINT('',(0.0952500000000119,0.164977839420932,39.92499));
#184528=CARTESIAN_POINT('',(-51.4963740058469,29.9514158463123,39.3548010137695));
#184529=CARTESIAN_POINT('',(-51.1878102687783,29.7732664904684,39.92499));
#184530=CARTESIAN_POINT('',(-51.8694703131944,30.1668231006079,39.116));
#184531=CARTESIAN_POINT('Origin',(-51.8363612765597,30.1477075893942,39.5550297827294));
#184532=CARTESIAN_POINT('',(-52.2170754206163,30.3675130020931,39.116));
#184533=CARTESIAN_POINT('',(-52.2810382154237,30.4044419397498,39.116));
#184534=CARTESIAN_POINT('',(-52.3262277788839,30.4305321463781,39.3343017080178));
#184535=CARTESIAN_POINT('',(-52.2170754202454,30.3675130027355,39.116));
#184536=CARTESIAN_POINT('',(-52.6119816883956,30.5955122429567,39.5248017080178));
#184537=CARTESIAN_POINT('Origin',(-52.5864971060013,30.5807981195153,39.1947745585587));
#184538=CARTESIAN_POINT('',(-52.7429317578285,30.6711163007942,39.5248017080178));
#184539=CARTESIAN_POINT('',(-52.7433896349615,30.6713806562801,39.5248017080178));
#184540=CARTESIAN_POINT('',(-53.0286856060843,30.8360963620066,39.3343017080178));
#184541=CARTESIAN_POINT('Origin',(-52.7684193600402,30.6858309820706,39.1947728594246));
#184542=CARTESIAN_POINT('',(-53.1378379191462,30.8991154793356,39.116));
#184543=CARTESIAN_POINT('',(-53.0286856060843,30.8360963620066,39.3343017080178));
#184544=CARTESIAN_POINT('',(-53.4858943313411,31.1000659426095,39.116));
#184545=CARTESIAN_POINT('Origin',(-47.2483549038573,34.0924682662299,40.10025));
#184546=CARTESIAN_POINT('',(-47.7461450747862,34.7084426211235,40.10025));
#184547=CARTESIAN_POINT('',(-50.8348823336483,36.9525415975216,40.10025));
#184548=CARTESIAN_POINT('',(-47.1274239660506,34.2589154226526,40.10025));
#184549=CARTESIAN_POINT('',(-50.8527980281382,36.9278827595331,40.10025));
#184550=CARTESIAN_POINT('Origin',(7.08388135731921E-17,-8.6407868066034E-17,
40.10025));
#184551=CARTESIAN_POINT('',(-47.764060769276,34.683783783135,40.10025));
#184552=CARTESIAN_POINT('',(-47.7068608037047,34.642225575547,40.10025));
#184553=CARTESIAN_POINT('Origin',(3.32162311137369E-16,4.49896674990071E-17,
40.10025));
#184554=CARTESIAN_POINT('Origin',(-0.111973090561717,-0.154117737428427,
1.57677042678049E-17));
#184555=CARTESIAN_POINT('',(-48.6559784483762,35.1151666347445,39.116));
#184556=CARTESIAN_POINT('',(-48.3074421904915,34.8619402208394,39.3548010137695));
#184557=CARTESIAN_POINT('Origin',(-48.6250489017688,35.0926950037622,39.5550297832907));
#184558=CARTESIAN_POINT('',(-48.0191904763611,34.6525130924099,39.92499));
#184559=CARTESIAN_POINT('',(-48.3074421904915,34.8619402208394,39.3548010137695));
#184560=CARTESIAN_POINT('',(-50.8023624960588,36.6746059268182,39.92499));
#184561=CARTESIAN_POINT('',(-51.0125340177512,36.8273044755034,39.92499));
#184562=CARTESIAN_POINT('',(-50.5141111791242,36.465179085564,39.3548010137695));
#184563=CARTESIAN_POINT('',(-50.8023624960588,36.6746059268182,39.92499));
#184564=CARTESIAN_POINT('',(-50.1655752777668,36.2119529314389,39.116));
#184565=CARTESIAN_POINT('Origin',(-50.1965049239947,36.2344246347996,39.5550293907213));
#184566=CARTESIAN_POINT('',(-49.8408524072783,35.9760279553334,39.116));
#184567=CARTESIAN_POINT('',(-0.111973090561712,-0.154117737428427,39.116));
#184568=CARTESIAN_POINT('',(-49.7388853330808,35.9019445403522,39.3343017080178));
#184569=CARTESIAN_POINT('',(-49.8408524068601,35.9760279559091,39.116));
#184570=CARTESIAN_POINT('',(-49.471941986573,35.7079988465462,39.5248017080178));
#184571=CARTESIAN_POINT('Origin',(-49.4957489658884,35.7252962640518,39.1947747614325));
#184572=CARTESIAN_POINT('',(-49.3496120513046,35.6191209461256,39.5248017080178));
#184573=CARTESIAN_POINT('',(-0.111973090561712,-0.154117737428427,39.5248017080178));
#184574=CARTESIAN_POINT('',(-49.0826686475732,35.4251752107442,39.3343017080178));
#184575=CARTESIAN_POINT('Origin',(-49.3258021153708,35.6018226497106,39.1947728911869));
#184576=CARTESIAN_POINT('',(-48.9807015312175,35.3510917642538,39.116));
#184577=CARTESIAN_POINT('',(-49.0826686475732,35.4251752107442,39.3343017080178));
#184578=CARTESIAN_POINT('',(-0.111973090561712,-0.154117737428427,39.116));
#184579=CARTESIAN_POINT('Origin',(0.111973090561717,0.154117737428427,-1.57677042678049E-17));
#184580=CARTESIAN_POINT('',(-49.9416290966434,36.5201884062957,39.116));
#184581=CARTESIAN_POINT('',(-50.2901649976452,36.7734145609102,39.3548010137695));
#184582=CARTESIAN_POINT('Origin',(-49.9725587426391,36.5426601094878,39.5550293912443));
#184583=CARTESIAN_POINT('',(-50.5784163146694,36.9828414020412,39.92499));
#184584=CARTESIAN_POINT('',(-50.2901649976452,36.7734145609102,39.3548010137695));
#184585=CARTESIAN_POINT('',(-47.7952442955499,34.960748566837,39.92499));
#184586=CARTESIAN_POINT('',(0.111973090561728,0.154117737428423,39.92499));
#184587=CARTESIAN_POINT('',(-48.0834960097837,35.1701756951242,39.3548010137695));
#184588=CARTESIAN_POINT('',(-47.7952442955499,34.960748566837,39.92499));
#184589=CARTESIAN_POINT('',(-48.4320322672528,35.4234021096014,39.116));
#184590=CARTESIAN_POINT('Origin',(-48.4011027203979,35.4009304784394,39.5550297827317));
#184591=CARTESIAN_POINT('',(-48.7567553505297,35.659327238511,39.116));
#184592=CARTESIAN_POINT('',(-48.8165076253516,35.7027398082303,39.116));
#184593=CARTESIAN_POINT('',(-48.8587224664497,35.733410685601,39.3343017080178));
#184594=CARTESIAN_POINT('',(-48.7567553500941,35.6593272391106,39.116));
#184595=CARTESIAN_POINT('',(-49.1256658701812,35.9273564209824,39.5248017080178));
#184596=CARTESIAN_POINT('Origin',(-49.101858939706,35.9100590388132,39.1947745585612));
#184597=CARTESIAN_POINT('',(-49.2479958054496,36.0162343214031,39.5248017080178));
#184598=CARTESIAN_POINT('',(-49.248423541611,36.0165450899151,39.5248017080178));
#184599=CARTESIAN_POINT('',(-49.5149391519574,36.2101800152091,39.3343017080178));
#184600=CARTESIAN_POINT('Origin',(-49.2718056808913,36.0335325740096,39.1947728594319));
#184601=CARTESIAN_POINT('',(-49.6169062257367,36.284263430766,39.116));
#184602=CARTESIAN_POINT('',(-49.5149391519574,36.2101800152091,39.3343017080178));
#184603=CARTESIAN_POINT('',(-49.9420509053688,36.5204948682734,39.116));
#184604=CARTESIAN_POINT('Origin',(-43.4258901551468,38.8445040879385,40.10025));
#184605=CARTESIAN_POINT('',(-43.8565665267053,39.5091373124626,40.10025));
#184606=CARTESIAN_POINT('',(-46.6938111422601,42.0638038389704,40.10025));
#184607=CARTESIAN_POINT('',(-43.2882232241945,38.9973987043323,40.10025));
#184608=CARTESIAN_POINT('',(-46.7142062431419,42.0411527846899,40.10025));
#184609=CARTESIAN_POINT('Origin',(6.11552196804844E-17,-9.83661106291793E-17,
40.10025));
#184610=CARTESIAN_POINT('',(-43.8769616275871,39.486486258182,40.10025));
#184611=CARTESIAN_POINT('',(-43.8244190249875,39.4391766863034,40.10025));
#184612=CARTESIAN_POINT('Origin',(3.37204232425086E-16,5.12159217606818E-17,
40.10025));
#184613=CARTESIAN_POINT('Origin',(-0.127469380511364,-0.141569089253443,
1.79498438867833E-17));
#184614=CARTESIAN_POINT('',(-44.7189015017595,40.0087367337517,39.116));
#184615=CARTESIAN_POINT('',(-44.3987439298677,39.7204655612078,39.3548010137695));
#184616=CARTESIAN_POINT('Origin',(-44.6904903154964,39.9831551867371,39.5550297832859));
#184617=CARTESIAN_POINT('',(-44.1339623846887,39.4820551877883,39.92499));
#184618=CARTESIAN_POINT('',(-44.3987439298677,39.7204655612078,39.3548010137695));
#184619=CARTESIAN_POINT('',(-46.6905216402894,41.7839914803031,39.92499));
#184620=CARTESIAN_POINT('',(-46.8835804757581,41.9578224365465,39.92499));
#184621=CARTESIAN_POINT('',(-46.425740460113,41.5455814340033,39.3548010137695));
#184622=CARTESIAN_POINT('',(-46.6905216402894,41.7839914803031,39.92499));
#184623=CARTESIAN_POINT('',(-46.1055832156406,41.2573105570841,39.116));
#184624=CARTESIAN_POINT('Origin',(-46.1339944934112,41.2828921864924,39.5550293907205));
#184625=CARTESIAN_POINT('',(-45.8073000862117,40.9887352200428,39.116));
#184626=CARTESIAN_POINT('',(-0.127469380511358,-0.141569089253443,39.116));
#184627=CARTESIAN_POINT('',(-45.7136354238372,40.9043991801907,39.3343017080178));
#184628=CARTESIAN_POINT('',(-45.8073000857355,40.9887352205717,39.116));
#184629=CARTESIAN_POINT('',(-45.4684272662432,40.6836127633983,39.5248017080178));
#184630=CARTESIAN_POINT('Origin',(-45.4902957559641,40.7033039308033,39.1947747614306));
#184631=CARTESIAN_POINT('',(-45.3560577375092,40.5824347852704,39.5248017080178));
#184632=CARTESIAN_POINT('',(-0.127469380511358,-0.141569089253443,39.5248017080178));
#184633=CARTESIAN_POINT('',(-45.1108495273509,40.3616483211488,39.3343017080178));
#184634=CARTESIAN_POINT('Origin',(-45.3341863992356,40.562742434718,39.1947728911902));
#184635=CARTESIAN_POINT('',(-45.0171848263429,40.2773122455532,39.116));
#184636=CARTESIAN_POINT('',(-45.1108495273509,40.3616483211488,39.3343017080178));
#184637=CARTESIAN_POINT('',(-0.127469380511358,-0.141569089253443,39.116));
#184638=CARTESIAN_POINT('Origin',(0.127469380511364,0.141569089253443,-1.79498438867833E-17));
#184639=CARTESIAN_POINT('',(-45.8506444546178,41.5404487355909,39.116));
#184640=CARTESIAN_POINT('',(-46.170801698685,41.8287196129603,39.3548010137695));
#184641=CARTESIAN_POINT('Origin',(-45.8790557321747,41.5660303648068,39.5550293912447));
#184642=CARTESIAN_POINT('',(-46.4355828789641,42.067129659146,39.92499));
#184643=CARTESIAN_POINT('',(-46.170801698685,41.8287196129603,39.3548010137695));
#184644=CARTESIAN_POINT('',(-43.8790236240217,39.7651933659003,39.92499));
#184645=CARTESIAN_POINT('',(0.127469380511373,0.141569089253439,39.92499));
#184646=CARTESIAN_POINT('',(-44.1438051693171,40.0036037391903,39.3548010137695));
#184647=CARTESIAN_POINT('',(-43.8790236240217,39.7651933659002,39.92499));
#184648=CARTESIAN_POINT('',(-44.4639627407368,40.2918749122586,39.116));
#184649=CARTESIAN_POINT('Origin',(-44.4355515542491,40.2662933650416,39.555029782734));
#184650=CARTESIAN_POINT('',(-44.7622460658166,40.5604504235087,39.116));
#184651=CARTESIAN_POINT('',(-44.8171331622253,40.6098709880932,39.116));
#184652=CARTESIAN_POINT('',(-44.8559107663282,40.6447864996556,39.3343017080178));
#184653=CARTESIAN_POINT('',(-44.7622460653202,40.5604504240601,39.116));
#184654=CARTESIAN_POINT('',(-45.1011189764865,40.8655729637772,39.5248017080178));
#184655=CARTESIAN_POINT('Origin',(-45.0792505316453,40.8458818366207,39.194774558559));
#184656=CARTESIAN_POINT('',(-45.2134885052205,40.9667509419051,39.5248017080178));
#184657=CARTESIAN_POINT('',(-45.2138814140435,40.9671047185984,39.5248017080178));
#184658=CARTESIAN_POINT('',(-45.4586966628145,41.1875373586976,39.3343017080178));
#184659=CARTESIAN_POINT('Origin',(-45.2353597879103,40.9864432425637,39.1947728594292));
#184660=CARTESIAN_POINT('',(-45.5523613247128,41.2718733990786,39.116));
#184661=CARTESIAN_POINT('',(-45.4586966628145,41.1875373586976,39.3343017080178));
#184662=CARTESIAN_POINT('',(-45.8510319186313,41.5407976097557,39.116));
#184663=CARTESIAN_POINT('Origin',(-39.1276422664447,43.1709513941247,40.10025));
#184664=CARTESIAN_POINT('',(-39.4864862581813,43.8769616275878,40.10025));
#184665=CARTESIAN_POINT('',(-42.0411527846891,46.7142062431426,40.10025));
#184666=CARTESIAN_POINT('',(-38.974747650051,43.308618325077,40.10025));
#184667=CARTESIAN_POINT('',(-42.0638038389696,46.6938111422608,40.10025));
#184668=CARTESIAN_POINT('Origin',(5.02746968098233E-17,-1.09246633499839E-16,
40.10025));
#184669=CARTESIAN_POINT('',(-39.5091373124618,43.856566526706,40.10025));
#184670=CARTESIAN_POINT('',(-39.4618277405832,43.8040239241063,40.10025));
#184671=CARTESIAN_POINT('Origin',(3.4286935433033E-16,5.68810436659258E-17,
40.10025));
#184672=CARTESIAN_POINT('Origin',(-0.141569089253445,-0.127469380511361,
1.99353212598918E-17));
#184673=CARTESIAN_POINT('',(-40.2918749122578,44.4639627407375,39.116));
#184674=CARTESIAN_POINT('',(-40.0036037397139,44.1438051688457,39.3548010137695));
#184675=CARTESIAN_POINT('Origin',(-40.2662933652429,44.435551554474,39.5550297832848));
#184676=CARTESIAN_POINT('',(-39.765193365504,43.8790236243784,39.92499));
#184677=CARTESIAN_POINT('',(-40.0036037397139,44.1438051688457,39.3548010137695));
#184678=CARTESIAN_POINT('',(-42.0671296588092,46.4355828792674,39.92499));
#184679=CARTESIAN_POINT('',(-42.2409606150526,46.6286417147361,39.92499));
#184680=CARTESIAN_POINT('',(-41.8287196134094,46.1708016982806,39.3548010137695));
#184681=CARTESIAN_POINT('',(-42.0671296588092,46.4355828792674,39.92499));
#184682=CARTESIAN_POINT('',(-41.5404487355902,45.8506444546186,39.116));
#184683=CARTESIAN_POINT('Origin',(-41.5660303649983,45.8790557323889,39.5550293907209));
#184684=CARTESIAN_POINT('',(-41.2718733996071,45.552361324237,39.116));
#184685=CARTESIAN_POINT('',(-0.141569089253439,-0.127469380511361,39.116));
#184686=CARTESIAN_POINT('',(-41.1875373586968,45.4586966628152,39.3343017080178));
#184687=CARTESIAN_POINT('',(-41.2718733990778,45.5523613247135,39.116));
#184688=CARTESIAN_POINT('',(-40.9667509419044,45.2134885052212,39.5248017080178));
#184689=CARTESIAN_POINT('Origin',(-40.9864413462806,45.2353576819744,39.1947747614277));
#184690=CARTESIAN_POINT('',(-40.8655729637765,45.1011189764872,39.5248017080178));
#184691=CARTESIAN_POINT('',(-0.141569089253439,-0.127469380511361,39.5248017080178));
#184692=CARTESIAN_POINT('',(-40.6447864996549,44.8559107663289,39.3343017080178));
#184693=CARTESIAN_POINT('Origin',(-40.8458798501211,45.0792483253095,39.1947728911976));
#184694=CARTESIAN_POINT('',(-40.5604504240593,44.7622460653209,39.116));
#184695=CARTESIAN_POINT('',(-40.6447864996549,44.8559107663289,39.3343017080178));
#184696=CARTESIAN_POINT('',(-0.141569089253439,-0.127469380511361,39.116));
#184697=CARTESIAN_POINT('Origin',(0.141569089253445,0.127469380511361,-1.99353212598918E-17));
#184698=CARTESIAN_POINT('',(-41.2573105570833,46.1055832156413,39.116));
#184699=CARTESIAN_POINT('',(-41.5455814344526,46.4257404597085,39.3548010137695));
#184700=CARTESIAN_POINT('Origin',(-41.2828921862987,46.1339944931977,39.5550293912461));
#184701=CARTESIAN_POINT('',(-41.7839914799654,46.6905216405934,39.92499));
#184702=CARTESIAN_POINT('',(-41.5455814344526,46.4257404597085,39.3548010137695));
#184703=CARTESIAN_POINT('',(-39.4820551873926,44.1339623850451,39.92499));
#184704=CARTESIAN_POINT('',(0.141569089253454,0.127469380511357,39.92499));
#184705=CARTESIAN_POINT('',(-39.7204655617323,44.3987439293954,39.3548010137695));
#184706=CARTESIAN_POINT('',(-39.4820551873926,44.1339623850451,39.92499));
#184707=CARTESIAN_POINT('',(-40.0087367337509,44.7189015017602,39.116));
#184708=CARTESIAN_POINT('Origin',(-39.9831551865335,44.6904903152718,39.5550297827328));
#184709=CARTESIAN_POINT('',(-40.2773122461034,45.0171848258474,39.116));
#184710=CARTESIAN_POINT('',(-40.3267328095855,45.0720719232487,39.116));
#184711=CARTESIAN_POINT('',(-40.361648321148,45.1108495273516,39.3343017080178));
#184712=CARTESIAN_POINT('',(-40.2773122455524,45.0171848263436,39.116));
#184713=CARTESIAN_POINT('',(-40.5824347852696,45.3560577375099,39.5248017080178));
#184714=CARTESIAN_POINT('Origin',(-40.5627444213194,45.3341886054756,39.1947745585574));
#184715=CARTESIAN_POINT('',(-40.6836127633975,45.4684272662439,39.5248017080178));
#184716=CARTESIAN_POINT('',(-40.6839665400907,45.4688201750669,39.5248017080178));
#184717=CARTESIAN_POINT('',(-40.9043991801899,45.7136354238379,39.3343017080178));
#184718=CARTESIAN_POINT('Origin',(-40.7033058269857,45.4902978619877,39.1947728594267));
#184719=CARTESIAN_POINT('',(-40.988735220571,45.8073000857362,39.116));
#184720=CARTESIAN_POINT('',(-40.9043991801899,45.7136354238379,39.3343017080178));
#184721=CARTESIAN_POINT('',(-41.2576594312481,46.1059706796548,39.116));
#184722=CARTESIAN_POINT('Origin',(-34.4007037410859,47.0244087227344,40.10025));
#184723=CARTESIAN_POINT('',(-34.6837837831342,47.7640607692766,40.10025));
#184724=CARTESIAN_POINT('',(-36.9278827595322,50.8527980281388,40.10025));
#184725=CARTESIAN_POINT('',(-34.2342565846632,47.1453396605411,40.10025));
#184726=CARTESIAN_POINT('',(-36.9525415975208,50.8348823336489,40.10025));
#184727=CARTESIAN_POINT('Origin',(3.83164542466798E-17,-1.18930227392547E-16,
40.10025));
#184728=CARTESIAN_POINT('',(-34.7084426211227,47.7461450747867,40.10025));
#184729=CARTESIAN_POINT('',(-34.6668844135347,47.6889451092154,40.10025));
#184730=CARTESIAN_POINT('Origin',(3.49095608592005E-16,6.19229649536422E-17,
40.10025));
#184731=CARTESIAN_POINT('Origin',(-0.154117737428428,-0.111973090561715,
2.17023830815427E-17));
#184732=CARTESIAN_POINT('',(-35.4234021096005,48.4320322672534,39.116));
#184733=CARTESIAN_POINT('',(-35.1701756956954,48.0834960093687,39.3548010137695));
#184734=CARTESIAN_POINT('Origin',(-35.400930478617,48.4011027206441,39.5550297832863));
#184735=CARTESIAN_POINT('',(-34.9607485664064,47.7952442958627,39.92499));
#184736=CARTESIAN_POINT('',(-35.1701756956954,48.0834960093687,39.3548010137695));
#184737=CARTESIAN_POINT('',(-36.9828414016742,50.578416314936,39.92499));
#184738=CARTESIAN_POINT('',(-37.1355399503593,50.7885878366284,39.92499));
#184739=CARTESIAN_POINT('',(-36.7734145613992,50.29016499729,39.3548010137695));
#184740=CARTESIAN_POINT('',(-36.9828414016742,50.578416314936,39.92499));
#184741=CARTESIAN_POINT('',(-36.5201884062949,49.941629096644,39.116));
#184742=CARTESIAN_POINT('Origin',(-36.5426601096559,49.9725587428724,39.5550293907199));
#184743=CARTESIAN_POINT('',(-36.2842634313413,49.6169062253187,39.116));
#184744=CARTESIAN_POINT('',(-0.154117737428423,-0.111973090561715,39.116));
#184745=CARTESIAN_POINT('',(-36.2101800152082,49.514939151958,39.3343017080178));
#184746=CARTESIAN_POINT('',(-36.2842634307651,49.6169062257373,39.116));
#184747=CARTESIAN_POINT('',(-36.0162343214022,49.2479958054502,39.5248017080178));
#184748=CARTESIAN_POINT('Origin',(-36.0335309082442,49.2718033882756,39.194774761429));
#184749=CARTESIAN_POINT('',(-35.9273564209816,49.1256658701818,39.5248017080178));
#184750=CARTESIAN_POINT('',(-0.154117737428423,-0.111973090561715,39.5248017080178));
#184751=CARTESIAN_POINT('',(-35.7334106856002,48.8587224664504,39.3343017080178));
#184752=CARTESIAN_POINT('Origin',(-35.910057293824,49.1018565378156,39.1947728911897));
#184753=CARTESIAN_POINT('',(-35.6593272391098,48.7567553500947,39.116));
#184754=CARTESIAN_POINT('',(-35.7334106856002,48.8587224664504,39.3343017080178));
#184755=CARTESIAN_POINT('',(-0.154117737428423,-0.111973090561715,39.116));
#184756=CARTESIAN_POINT('Origin',(0.154117737428428,0.111973090561715,-2.17023830815427E-17));
#184757=CARTESIAN_POINT('',(-36.211952931438,50.1655752777675,39.116));
#184758=CARTESIAN_POINT('',(-36.4651790860525,50.5141111787693,39.3548010137695));
#184759=CARTESIAN_POINT('Origin',(-36.2344246346303,50.1965049237634,39.5550293912439));
#184760=CARTESIAN_POINT('',(-36.6746059264512,50.8023624963254,39.92499));
#184761=CARTESIAN_POINT('',(-36.4651790860525,50.5141111787693,39.3548010137695));
#184762=CARTESIAN_POINT('',(-34.6525130919793,48.0191904766739,39.92499));
#184763=CARTESIAN_POINT('',(0.154117737428437,0.11197309056171,39.92499));
#184764=CARTESIAN_POINT('',(-34.8619402214104,48.3074421900766,39.3548010137695));
#184765=CARTESIAN_POINT('',(-34.6525130919793,48.0191904766739,39.92499));
#184766=CARTESIAN_POINT('',(-35.1151666347437,48.6559784483768,39.116));
#184767=CARTESIAN_POINT('Origin',(-35.0926950035808,48.6250489015207,39.5550297827299));
#184768=CARTESIAN_POINT('',(-35.3510917648529,48.9807015307823,39.116));
#184769=CARTESIAN_POINT('',(-35.3945043333726,49.0404538064757,39.116));
#184770=CARTESIAN_POINT('',(-35.4251752107434,49.0826686475738,39.3343017080178));
#184771=CARTESIAN_POINT('',(-35.3510917642529,48.9807015312181,39.116));
#184772=CARTESIAN_POINT('',(-35.6191209461248,49.3496120513052,39.5248017080178));
#184773=CARTESIAN_POINT('Origin',(-35.6018243948127,49.3258045171787,39.1947745585588));
#184774=CARTESIAN_POINT('',(-35.7079988465454,49.4719419865736,39.5248017080178));
#184775=CARTESIAN_POINT('',(-35.7083096150574,49.472369722735,39.5248017080178));
#184776=CARTESIAN_POINT('',(-35.9019445403514,49.7388853330814,39.3343017080178));
#184777=CARTESIAN_POINT('Origin',(-35.7252979297055,49.4957512585776,39.1947728594227));
#184778=CARTESIAN_POINT('',(-35.9760279559083,49.8408524068607,39.116));
#184779=CARTESIAN_POINT('',(-35.9019445403514,49.7388853330814,39.3343017080178));
#184780=CARTESIAN_POINT('',(-36.2122593934157,50.1659970864929,39.116));
#184781=CARTESIAN_POINT('Origin',(-29.2968639067297,50.3626567888878,40.10025));
#184782=CARTESIAN_POINT('',(-29.5010785149107,51.127846865905,40.10025));
#184783=CARTESIAN_POINT('',(-31.4100231232056,54.4342359163066,40.10025));
#184784=CARTESIAN_POINT('',(-29.1186878401551,50.4655267888878,40.10025));
#184785=CARTESIAN_POINT('',(-31.436419577513,54.4189959163066,40.10025));
#184786=CARTESIAN_POINT('Origin',(2.54115089989943E-17,-1.27310796826193E-16,
40.10025));
#184787=CARTESIAN_POINT('',(-29.527474969218,51.112606865905,40.10025));
#184788=CARTESIAN_POINT('',(-29.4921234463396,51.0513762321547,40.10025));
#184789=CARTESIAN_POINT('Origin',(3.55814779065493E-16,6.6286445279113E-17,
40.10025));
#184790=CARTESIAN_POINT('Origin',(-0.164977839420936,-0.0952499999999985,
2.32316690526366E-17));
#184791=CARTESIAN_POINT('',(-30.166823100607,51.8694703131949,39.116));
#184792=CARTESIAN_POINT('',(-29.9514158469225,51.4963740054946,39.3548010137695));
#184793=CARTESIAN_POINT('Origin',(-30.1477075895458,51.8363612768244,39.5550297832863));
#184794=CARTESIAN_POINT('',(-29.7732664900073,51.1878102690445,39.92499));
#184795=CARTESIAN_POINT('',(-29.9514158469225,51.4963740054946,39.3548010137695));
#184796=CARTESIAN_POINT('',(-31.4933613949854,54.1671020372441,39.92499));
#184797=CARTESIAN_POINT('',(-31.6232545388586,54.3920835619874,39.92499));
#184798=CARTESIAN_POINT('',(-31.3152122841225,53.8585387246954,39.3548010137695));
#184799=CARTESIAN_POINT('',(-31.4933613949854,54.1671020372441,39.92499));
#184800=CARTESIAN_POINT('',(-31.0998052504795,53.4854427993289,39.116));
#184801=CARTESIAN_POINT('Origin',(-31.118920823109,53.5185519423391,39.5550293907184));
#184802=CARTESIAN_POINT('',(-30.8991154799509,53.1378379187909,39.116));
#184803=CARTESIAN_POINT('',(-0.164977839420931,-0.0952499999999985,39.116));
#184804=CARTESIAN_POINT('',(-30.8360963620057,53.0286856060848,39.3343017080178));
#184805=CARTESIAN_POINT('',(-30.8991154793346,53.1378379191467,39.116));
#184806=CARTESIAN_POINT('',(-30.6711163007932,52.742931757829,39.5248017080178));
#184807=CARTESIAN_POINT('Origin',(-30.6858295650774,52.7684169058696,39.1947747614331));
#184808=CARTESIAN_POINT('',(-30.5955122429558,52.6119816883962,39.5248017080178));
#184809=CARTESIAN_POINT('',(-0.164977839420931,-0.0952499999999985,39.5248017080178));
#184810=CARTESIAN_POINT('',(-30.4305321463772,52.3262277788844,39.3343017080178));
#184811=CARTESIAN_POINT('Origin',(-30.5807966351501,52.5864945348654,39.1947728911916));
#184812=CARTESIAN_POINT('',(-30.3675130027346,52.2170754202459,39.116));
#184813=CARTESIAN_POINT('',(-30.4305321463772,52.3262277788844,39.3343017080178));
#184814=CARTESIAN_POINT('',(-0.164977839420931,-0.0952499999999985,39.116));
#184815=CARTESIAN_POINT('Origin',(0.164977839420936,0.0952499999999985,
-2.32316690526366E-17));
#184816=CARTESIAN_POINT('',(-30.7698495716376,53.6759427993289,39.116));
#184817=CARTESIAN_POINT('',(-30.9852566047563,54.0490387249982,39.3548010137695));
#184818=CARTESIAN_POINT('Origin',(-30.788965144123,53.7090519420896,39.5550293912436));
#184819=CARTESIAN_POINT('',(-31.1634057157511,54.3576020374707,39.92499));
#184820=CARTESIAN_POINT('',(-30.9852566047563,54.0490387249982,39.3548010137695));
#184821=CARTESIAN_POINT('',(-29.4433108116256,51.3783102687788,39.92499));
#184822=CARTESIAN_POINT('',(0.164977839420945,0.0952499999999936,39.92499));
#184823=CARTESIAN_POINT('',(-29.6214601686921,51.6868740051415,39.3548010137695));
#184824=CARTESIAN_POINT('',(-29.4433108116256,51.3783102687788,39.92499));
#184825=CARTESIAN_POINT('',(-29.8368674217651,52.0599703131949,39.116));
#184826=CARTESIAN_POINT('Origin',(-29.8177519105508,52.026861276559,39.5550297827274));
#184827=CARTESIAN_POINT('',(-30.0375573245351,52.407575419875,39.116));
#184828=CARTESIAN_POINT('',(-30.074486260907,52.4715382154242,39.116));
#184829=CARTESIAN_POINT('',(-30.1005764675353,52.5167277788844,39.3343017080178));
#184830=CARTESIAN_POINT('',(-30.0375573238927,52.4075754202459,39.116));
#184831=CARTESIAN_POINT('',(-30.2655565641139,52.8024816883962,39.5248017080178));
#184832=CARTESIAN_POINT('Origin',(-30.2508433300758,52.7769965925036,39.1947745585601));
#184833=CARTESIAN_POINT('',(-30.3411606219514,52.933431757829,39.5248017080178));
#184834=CARTESIAN_POINT('',(-30.3414249774373,52.933889634962,39.5248017080178));
#184835=CARTESIAN_POINT('',(-30.5061406831638,53.2191856060848,39.3343017080178));
#184836=CARTESIAN_POINT('Origin',(-30.3558761923107,52.9589188467299,39.1947728594266));
#184837=CARTESIAN_POINT('',(-30.5691598004928,53.3283379191467,39.116));
#184838=CARTESIAN_POINT('',(-30.5061406831638,53.2191856060848,39.3343017080178));
#184839=CARTESIAN_POINT('',(-30.7701102637667,53.6763943313416,39.116));
#184840=CARTESIAN_POINT('Origin',(-23.8720415006485,53.1491210481985,40.10025));
#184841=CARTESIAN_POINT('',(-23.9951532569802,53.9314655730806,40.10025));
#184842=CARTESIAN_POINT('',(-25.5480287005713,57.4192809246791,40.10025));
#184843=CARTESIAN_POINT('',(-23.6840886581931,53.232803045145,40.10025));
#184844=CARTESIAN_POINT('',(-25.5758735661203,57.4068835917982,40.10025));
#184845=CARTESIAN_POINT('Origin',(1.17012503474357E-17,-1.34296522528313E-16,
40.10025));
#184846=CARTESIAN_POINT('',(-24.0229981225292,53.9190682401997,40.10025));
#184847=CARTESIAN_POINT('',(-23.9942406030429,53.8544777939071,40.10025));
#184848=CARTESIAN_POINT('Origin',(3.6295324911301E-16,6.99236774387753E-17,
40.10025));
#184849=CARTESIAN_POINT('Origin',(-0.174030409680916,-0.0774833305059384,
2.45064239960505E-17));
#184850=CARTESIAN_POINT('',(-24.5797300649096,54.7386155880006,39.116));
#184851=CARTESIAN_POINT('',(-24.4045020183941,54.3450469517072,39.3548010137695));
#184852=CARTESIAN_POINT('Origin',(-24.5641801073101,54.7036898113994,39.5550297832858));
#184853=CARTESIAN_POINT('',(-24.2595822754869,54.0195518811807,39.92499));
#184854=CARTESIAN_POINT('',(-24.4045020183941,54.3450469517072,39.3548010137695));
#184855=CARTESIAN_POINT('',(-25.6588335304436,57.1623216544373,39.92499));
#184856=CARTESIAN_POINT('',(-25.7644981330387,57.3996482375659,39.92499));
#184857=CARTESIAN_POINT('',(-25.5139139879313,56.8368270312094,39.3548010137695));
#184858=CARTESIAN_POINT('',(-25.6588335304436,57.1623216544373,39.92499));
#184859=CARTESIAN_POINT('',(-25.3386861202872,56.4432587981559,39.116));
#184860=CARTESIAN_POINT('Origin',(-25.3542361279707,56.4781846872474,39.5550293907191));
#184861=CARTESIAN_POINT('',(-25.1754303533072,56.076580340217,39.116));
#184862=CARTESIAN_POINT('',(-0.174030409680911,-0.0774833305059384,39.116));
#184863=CARTESIAN_POINT('',(-25.1241659841931,55.9614386837455,39.3343017080178));
#184864=CARTESIAN_POINT('',(-25.175430352657,56.0765803405065,39.116));
#184865=CARTESIAN_POINT('',(-24.9899591116491,55.660005112701,39.5248017080178));
#184866=CARTESIAN_POINT('Origin',(-25.00192785177,55.6868886053366,39.1947747614285));
#184867=CARTESIAN_POINT('',(-24.9284572302736,55.5218696254675,39.5248017080178));
#184868=CARTESIAN_POINT('',(-0.174030409680911,-0.0774833305059384,39.5248017080178));
#184869=CARTESIAN_POINT('',(-24.7942503289602,55.2204359898058,39.3343017080178));
#184870=CARTESIAN_POINT('Origin',(-24.9164863690984,55.4949838933597,39.1947728911931));
#184871=CARTESIAN_POINT('',(-24.7429859390908,55.1052942849674,39.116));
#184872=CARTESIAN_POINT('',(-24.7942503289602,55.2204359898058,39.3343017080178));
#184873=CARTESIAN_POINT('',(-0.174030409680911,-0.0774833305059384,39.116));
#184874=CARTESIAN_POINT('Origin',(0.174030409680916,0.0774833305059384,
-2.45064239960505E-17));
#184875=CARTESIAN_POINT('',(-24.9906253009254,56.5982254591678,39.116));
#184876=CARTESIAN_POINT('',(-25.1658531680166,56.9917936924675,39.3548010137695));
#184877=CARTESIAN_POINT('Origin',(-25.0061753084915,56.6331513479959,39.5550293912447));
#184878=CARTESIAN_POINT('',(-25.3107727106682,57.3172883156333,39.92499));
#184879=CARTESIAN_POINT('',(-25.1658531680166,56.9917936924675,39.3548010137695));
#184880=CARTESIAN_POINT('',(-23.911521456611,54.1745185419762,39.92499));
#184881=CARTESIAN_POINT('',(0.174030409680924,0.0774833305059332,39.92499));
#184882=CARTESIAN_POINT('',(-24.0564411996771,54.500013612432,39.3548010137695));
#184883=CARTESIAN_POINT('',(-23.911521456611,54.1745185419762,39.92499));
#184884=CARTESIAN_POINT('',(-24.2316692455478,54.8935822490125,39.116));
#184885=CARTESIAN_POINT('Origin',(-24.216119287825,54.8586564721344,39.5550297827321));
#184886=CARTESIAN_POINT('',(-24.3949251204065,55.2602609456776,39.116));
#184887=CARTESIAN_POINT('',(-24.4249658234761,55.3277334713092,39.116));
#184888=CARTESIAN_POINT('',(-24.4461895095984,55.3754026508177,39.3343017080178));
#184889=CARTESIAN_POINT('',(-24.394925119729,55.2602609459793,39.116));
#184890=CARTESIAN_POINT('',(-24.5803964109118,55.6768362864794,39.5248017080178));
#184891=CARTESIAN_POINT('Origin',(-24.5684276954195,55.649952848866,39.1947745585588));
#184892=CARTESIAN_POINT('',(-24.6418982922872,55.8149717737129,39.5248017080178));
#184893=CARTESIAN_POINT('',(-24.6421133384131,55.8154547752197,39.5248017080178));
#184894=CARTESIAN_POINT('',(-24.7761051648312,56.1164053447574,39.3343017080178));
#184895=CARTESIAN_POINT('Origin',(-24.653869122976,55.8418574376289,39.1947728594248));
#184896=CARTESIAN_POINT('',(-24.8273695332952,56.2315470015184,39.116));
#184897=CARTESIAN_POINT('',(-24.7761051648312,56.1164053447574,39.3343017080178));
#184898=CARTESIAN_POINT('',(-24.9908373670083,56.5987017673885,39.116));
#184899=CARTESIAN_POINT('Origin',(-18.1856720123403,55.3532724151367,40.10025));
#184900=CARTESIAN_POINT('',(-18.2263320786577,56.1441998575529,40.10025));
#184901=CARTESIAN_POINT('',(-19.4061247292248,59.7752282754838,40.10025));
#184902=CARTESIAN_POINT('',(-17.9900016446778,55.4168495715594,40.10025));
#184903=CARTESIAN_POINT('',(-19.4351129318415,59.7658094374953,40.10025));
#184904=CARTESIAN_POINT('Origin',(-2.66410924515479E-18,-1.3981086742626E-16,
40.10025));
#184905=CARTESIAN_POINT('',(-18.2553202812744,56.1347810195644,40.10025));
#184906=CARTESIAN_POINT('',(-18.2334718385814,56.0675384271755,40.10025));
#184907=CARTESIAN_POINT('Origin',(3.7043280816289E-16,7.27948111559483E-17,
40.10025));
#184908=CARTESIAN_POINT('Origin',(-0.181176266354227,-0.0588677374284257,
2.55126814298649E-17));
#184909=CARTESIAN_POINT('',(-18.7233363629819,57.0080331356324,39.116));
#184910=CARTESIAN_POINT('',(-18.5902073587817,56.5983041910847,39.3548010137695));
#184911=CARTESIAN_POINT('Origin',(-18.7115223274338,56.9716732729184,39.5550297832861));
#184912=CARTESIAN_POINT('',(-18.4801050009129,56.2594439785883,39.92499));
#184913=CARTESIAN_POINT('',(-18.5902073587817,56.5983041910847,39.3548010137695));
#184914=CARTESIAN_POINT('',(-19.5431821162861,59.5312589135997,39.92499));
#184915=CARTESIAN_POINT('',(-19.6234604941053,59.7783303554051,39.92499));
#184916=CARTESIAN_POINT('',(-19.4330799109589,59.1923991668986,39.3548010137695));
#184917=CARTESIAN_POINT('',(-19.5431821162861,59.5312589135997,39.92499));
#184918=CARTESIAN_POINT('',(-19.2999510425001,58.782670642079,39.116));
#184919=CARTESIAN_POINT('Origin',(-19.3117651160997,58.8190306219038,39.5550293907171));
#184920=CARTESIAN_POINT('',(-19.1759179434146,58.4009360126571,39.116));
#184921=CARTESIAN_POINT('',(-0.181176266354222,-0.0588677374284257,39.116));
#184922=CARTESIAN_POINT('',(-19.1369699862878,58.2810665285032,39.3343017080178));
#184923=CARTESIAN_POINT('',(-19.1759179427381,58.4009360128769,39.116));
#184924=CARTESIAN_POINT('',(-19.0350067009925,57.9672558039534,39.5248017080178));
#184925=CARTESIAN_POINT('Origin',(-19.0440997849299,57.9952431000144,39.1947747614259));
#184926=CARTESIAN_POINT('',(-18.9882808235615,57.8234483402241,39.5248017080178));
#184927=CARTESIAN_POINT('',(-0.181176266354222,-0.0588677374284257,39.5248017080178));
#184928=CARTESIAN_POINT('',(-18.8863175164087,57.5096375484038,39.3343017080178));
#184929=CARTESIAN_POINT('Origin',(-18.9791858642783,57.79545859525,39.1947728911881));
#184930=CARTESIAN_POINT('',(-18.8473695436957,57.3897680139786,39.116));
#184931=CARTESIAN_POINT('',(-18.8863175164087,57.5096375484038,39.3343017080178));
#184932=CARTESIAN_POINT('',(-0.181176266354222,-0.0588677374284257,39.116));
#184933=CARTESIAN_POINT('Origin',(0.181176266354227,0.0588677374284257,
-2.55126814298649E-17));
#184934=CARTESIAN_POINT('',(-18.9375985097916,58.9004061169359,39.116));
#184935=CARTESIAN_POINT('',(-19.0707273776747,59.3101346419425,39.3548010137695));
#184936=CARTESIAN_POINT('Origin',(-18.9494125833019,58.9367660964855,39.5550293912448));
#184937=CARTESIAN_POINT('',(-19.1808295831467,59.6489943885966,39.92499));
#184938=CARTESIAN_POINT('',(-19.0707273776747,59.3101346419425,39.3548010137695));
#184939=CARTESIAN_POINT('',(-18.1177524687101,56.3771794532809,39.92499));
#184940=CARTESIAN_POINT('',(0.181176266354235,0.0588677374284204,39.92499));
#184941=CARTESIAN_POINT('',(-18.2278548267452,56.7160396657232,39.3548010137695));
#184942=CARTESIAN_POINT('',(-18.1177524687101,56.3771794532809,39.92499));
#184943=CARTESIAN_POINT('',(-18.3609838302735,57.1257686104892,39.116));
#184944=CARTESIAN_POINT('Origin',(-18.3491697946313,57.0894087474858,39.5550297827304));
#184945=CARTESIAN_POINT('',(-18.4850170116926,57.5075034886062,39.116));
#184946=CARTESIAN_POINT('',(-18.5078403492304,57.57774650121,39.116));
#184947=CARTESIAN_POINT('',(-18.5239649837002,57.6273730232607,39.3343017080178));
#184948=CARTESIAN_POINT('',(-18.4850170109872,57.5075034888354,39.116));
#184949=CARTESIAN_POINT('',(-18.6259282908531,57.9411838150809,39.5248017080178));
#184950=CARTESIAN_POINT('Origin',(-18.6168352256568,57.9131965763112,39.1947745585637));
#184951=CARTESIAN_POINT('',(-18.672654168284,58.0849912788102,39.5248017080178));
#184952=CARTESIAN_POINT('',(-18.6728175489595,58.0854941128253,39.5248017080178));
#184953=CARTESIAN_POINT('',(-18.7746174535794,58.39880200336,39.3343017080178));
#184954=CARTESIAN_POINT('Origin',(-18.6817491043762,58.1129809527805,39.1947728594212));
#184955=CARTESIAN_POINT('',(-18.8135654100297,58.5186714877337,39.116));
#184956=CARTESIAN_POINT('',(-18.7746174535794,58.39880200336,39.3343017080178));
#184957=CARTESIAN_POINT('',(-18.937759626388,58.900901982832,39.116));
#184958=CARTESIAN_POINT('Origin',(-12.3000564958684,56.9509617460776,40.10025));
#184959=CARTESIAN_POINT('',(-12.2578193919762,57.7418065394567,40.10025));
#184960=CARTESIAN_POINT('',(-13.0516031943522,61.4762657165317,40.10025));
#184961=CARTESIAN_POINT('',(-12.0988124084934,56.9937374973464,40.10025));
#184962=CARTESIAN_POINT('',(-13.0814171332226,61.4699285681956,40.10025));
#184963=CARTESIAN_POINT('Origin',(-1.75271798929367E-17,-1.43793415203377E-16,
40.10025));
#184964=CARTESIAN_POINT('',(-12.2876333308465,57.7354693911206,40.10025));
#184965=CARTESIAN_POINT('',(-12.2729333410573,57.666311376549,40.10025));
#184966=CARTESIAN_POINT('Origin',(3.78171508600986E-16,7.48683896888049E-17,
40.10025));
#184967=CARTESIAN_POINT('Origin',(-0.18633711793979,-0.0396071771007813,
2.62394165870617E-17));
#184968=CARTESIAN_POINT('',(-12.6618058697513,58.6528587425324,39.116));
#184969=CARTESIAN_POINT('',(-12.5722344970954,58.2314585657882,39.3548010137695));
#184970=CARTESIAN_POINT('Origin',(-12.6538571933003,58.6154631599705,39.5550297832875));
#184971=CARTESIAN_POINT('',(-12.498155828738,57.8829458347212,39.92499));
#184972=CARTESIAN_POINT('',(-12.5722344970954,58.2314585657882,39.3548010137695));
#184973=CARTESIAN_POINT('',(-13.2134115091888,61.2479592423879,39.92499));
#184974=CARTESIAN_POINT('',(-13.2674241155254,61.5020685764506,39.92499));
#184975=CARTESIAN_POINT('',(-13.1393329438483,60.8994469905095,39.3548010137695));
#184976=CARTESIAN_POINT('',(-13.2134115091888,61.2479592423879,39.92499));
#184977=CARTESIAN_POINT('',(-13.0497616623169,60.4780472453829,39.116));
#184978=CARTESIAN_POINT('Origin',(-13.0577103643692,60.5154429483896,39.5550293907215));
#184979=CARTESIAN_POINT('',(-12.9663101637159,60.0854388089606,39.116));
#184980=CARTESIAN_POINT('',(-0.186337117939785,-0.0396071771007813,39.116));
#184981=CARTESIAN_POINT('',(-12.9401053405444,59.9621548122773,39.3343017080178));
#184982=CARTESIAN_POINT('',(-12.9663101630198,60.0854388091086,39.116));
#184983=CARTESIAN_POINT('',(-12.8715027735886,59.6394051101895,39.5248017080178));
#184984=CARTESIAN_POINT('Origin',(-12.8776205756126,59.6681895750056,39.1947747614283));
#184985=CARTESIAN_POINT('',(-12.8400648385932,59.4915012546306,39.5248017080178));
#184986=CARTESIAN_POINT('',(-0.186337117939785,-0.0396071771007813,39.5248017080178));
#184987=CARTESIAN_POINT('',(-12.7714622569314,59.1687514833562,39.3343017080178));
#184988=CARTESIAN_POINT('Origin',(-12.833945427478,59.4627141582908,39.1947728911885));
#184989=CARTESIAN_POINT('',(-12.7452574235141,59.0454674350476,39.116));
#184990=CARTESIAN_POINT('',(-12.7714622569314,59.1687514833562,39.3343017080178));
#184991=CARTESIAN_POINT('',(-0.186337117939785,-0.0396071771007813,39.116));
#184992=CARTESIAN_POINT('Origin',(0.18633711793979,0.0396071771007813,-2.62394165870617E-17));
#184993=CARTESIAN_POINT('',(-12.6770874264373,60.5572615995844,39.116));
#184994=CARTESIAN_POINT('',(-12.7666587073768,60.9786613448369,39.3548010137695));
#184995=CARTESIAN_POINT('Origin',(-12.6850361284299,60.5946573023103,39.5550293912455));
#184996=CARTESIAN_POINT('',(-12.8407372728669,61.3271735966835,39.92499));
#184997=CARTESIAN_POINT('',(-12.7666587073768,60.9786613448369,39.3548010137695));
#184998=CARTESIAN_POINT('',(-12.1254815933786,57.9621601888122,39.92499));
#184999=CARTESIAN_POINT('',(0.186337117939797,0.0396071771007757,39.92499));
#185000=CARTESIAN_POINT('',(-12.1995602619069,58.3106729198428,39.3548010137695));
#185001=CARTESIAN_POINT('',(-12.1254815933786,57.9621601888122,39.92499));
#185002=CARTESIAN_POINT('',(-12.2891316338718,58.7320730967339,39.116));
#185003=CARTESIAN_POINT('Origin',(-12.2811829573572,58.694677513873,39.5550297827296));
#185004=CARTESIAN_POINT('',(-12.3725831883604,59.1246817890949,39.116));
#185005=CARTESIAN_POINT('',(-12.387939103104,59.1969256915255,39.116));
#185006=CARTESIAN_POINT('',(-12.3987880210518,59.2479658375578,39.3343017080178));
#185007=CARTESIAN_POINT('',(-12.3725831876346,59.1246817892491,39.116));
#185008=CARTESIAN_POINT('',(-12.4673906027137,59.5707156088322,39.5248017080178));
#185009=CARTESIAN_POINT('Origin',(-12.4612728133405,59.5419312029573,39.1947745585561));
#185010=CARTESIAN_POINT('',(-12.498828537709,59.718619464391,39.5248017080178));
#185011=CARTESIAN_POINT('',(-12.4989384629011,59.7191366217597,39.5248017080178));
#185012=CARTESIAN_POINT('',(-12.5674311046648,60.0413691664788,39.3343017080178));
#185013=CARTESIAN_POINT('Origin',(-12.5049479331823,59.7474064876929,39.1947728594233));
#185014=CARTESIAN_POINT('',(-12.5936359271402,60.1646531633102,39.116));
#185015=CARTESIAN_POINT('',(-12.5674311046648,60.0413691664788,39.3343017080178));
#185016=CARTESIAN_POINT('',(-12.67719582832,60.5577715903456,39.116));
#185017=CARTESIAN_POINT('Origin',(-6.27967898647548,57.9246844223736,40.10025));
#185018=CARTESIAN_POINT('',(-6.15500747092256,58.7067819056644,40.10025));
#185019=CARTESIAN_POINT('',(-6.55408556365883,62.5037563256535,40.10025));
#185020=CARTESIAN_POINT('',(-6.07506605172241,57.9461901084062,40.10025));
#185021=CARTESIAN_POINT('',(-6.58439859102965,62.5005702980932,40.10025));
#185022=CARTESIAN_POINT('Origin',(-3.27251186835868E-17,-1.46200532232821E-16,
40.10025));
#185023=CARTESIAN_POINT('',(-6.18532049829339,58.7035958781039,40.10025));
#185024=CARTESIAN_POINT('',(-6.17793001757209,58.6332801510296,40.10025));
#185025=CARTESIAN_POINT('Origin',(3.86084563605879E-16,7.61216944770113E-17,
40.10025));
#185026=CARTESIAN_POINT('Origin',(-0.189456421067656,-0.0199126722524861,
2.66786672051798E-17));
#185027=CARTESIAN_POINT('',(-6.46154998175858,59.6550713551493,39.116));
#185028=CARTESIAN_POINT('',(-6.41651760334991,59.2266168947287,39.3548010137695));
#185029=CARTESIAN_POINT('Origin',(-6.45755375176684,59.617049766565,39.5550297832836));
#185030=CARTESIAN_POINT('',(-6.37927424589634,58.8722700235037,39.92499));
#185031=CARTESIAN_POINT('',(-6.4165176033499,59.2266168947287,39.3548010137695));
#185032=CARTESIAN_POINT('',(-6.7388720005127,62.293614112757,39.92499));
#185033=CARTESIAN_POINT('',(-6.76602706194884,62.5519772640373,39.92499));
#185034=CARTESIAN_POINT('',(-6.70162869542298,61.9392677288637,39.3548010137695));
#185035=CARTESIAN_POINT('',(-6.7388720005127,62.293614112757,39.92499));
#185036=CARTESIAN_POINT('',(-6.65659636252321,61.5108137072213,39.116));
#185037=CARTESIAN_POINT('Origin',(-6.66059260538601,61.5488354182655,39.55502939072));
#185038=CARTESIAN_POINT('',(-6.61464077648821,61.1116329639869,39.116));
#185039=CARTESIAN_POINT('',(-0.189456421067651,-0.0199126722524861,39.116));
#185040=CARTESIAN_POINT('',(-6.60146619279885,60.9862851800405,39.3343017080178));
#185041=CARTESIAN_POINT('',(-6.6146407757806,61.1116329640613,39.116));
#185042=CARTESIAN_POINT('',(-6.56697596826216,60.6581326136905,39.5248017080178));
#185043=CARTESIAN_POINT('Origin',(-6.57005146045362,60.6873988786426,39.1947747614312));
#185044=CARTESIAN_POINT('',(-6.55117041629707,60.5077528318944,39.5248017080178));
#185045=CARTESIAN_POINT('',(-0.189456421067651,-0.0199126722524861,39.5248017080178));
#185046=CARTESIAN_POINT('',(-6.51668018436685,60.1796001951996,39.3343017080178));
#185047=CARTESIAN_POINT('Origin',(-6.54809359889826,60.4784837816373,39.1947728911934));
#185048=CARTESIAN_POINT('',(-6.50350559588404,60.0542523588398,39.116));
#185049=CARTESIAN_POINT('',(-6.51668018436685,60.1796001951996,39.3343017080178));
#185050=CARTESIAN_POINT('',(-0.189456421067651,-0.0199126722524861,39.116));
#185051=CARTESIAN_POINT('Origin',(0.189456421067656,0.0199126722524861,
-2.66786672051798E-17));
#185052=CARTESIAN_POINT('',(-6.2776835203879,61.5506390517263,39.116));
#185053=CARTESIAN_POINT('',(-6.32271585268577,61.979093073432,39.3548010137695));
#185054=CARTESIAN_POINT('Origin',(-6.28167976322052,61.5886607624834,39.5550293912467));
#185055=CARTESIAN_POINT('',(-6.35995915792738,62.3334394573093,39.92499));
#185056=CARTESIAN_POINT('',(-6.32271585268577,61.979093073432,39.3548010137695));
#185057=CARTESIAN_POINT('',(-6.00036140428986,58.9120953679531,39.92499));
#185058=CARTESIAN_POINT('',(0.189456421067662,0.0199126722524805,39.92499));
#185059=CARTESIAN_POINT('',(-6.03760476191729,59.2664422391598,39.3548010137695));
#185060=CARTESIAN_POINT('',(-6.00036140428986,58.9120953679531,39.92499));
#185061=CARTESIAN_POINT('',(-6.08263713962327,59.6948966996543,39.116));
#185062=CARTESIAN_POINT('Origin',(-6.07864090959991,59.6568751107691,39.5550297827311));
#185063=CARTESIAN_POINT('',(-6.12459275448616,60.0940777032672,39.116));
#185064=CARTESIAN_POINT('',(-6.13231300382116,60.1675309762115,39.116));
#185065=CARTESIAN_POINT('',(-6.13776734223154,60.2194255397046,39.3343017080178));
#185066=CARTESIAN_POINT('',(-6.12459275374873,60.0940777033447,39.116));
#185067=CARTESIAN_POINT('',(-6.17225757416176,60.5475781763994,39.5248017080178));
#185068=CARTESIAN_POINT('Origin',(-6.16918208839087,60.5183119713883,39.1947745585589));
#185069=CARTESIAN_POINT('',(-6.18806312612685,60.6979579581955,39.5248017080178));
#185070=CARTESIAN_POINT('',(-6.18811839147226,60.6984837728334,39.5248017080178));
#185071=CARTESIAN_POINT('',(-6.22255335066353,61.0261105245455,39.3343017080178));
#185072=CARTESIAN_POINT('Origin',(-6.19113993560366,60.7272269341761,39.1947728594228));
#185073=CARTESIAN_POINT('',(-6.23572793364529,61.1514583085663,39.116));
#185074=CARTESIAN_POINT('',(-6.22255335066353,61.0261105245455,39.3343017080178));
#185075=CARTESIAN_POINT('',(-6.27773801988317,61.5511575797869,39.116));
#185076=CARTESIAN_POINT('Origin',(-0.190499999999384,58.2637721346185,40.10025));
#185077=CARTESIAN_POINT('',(0.0152400000006159,58.2637721346185,40.10025));
#185078=CARTESIAN_POINT('',(-0.0152399999993768,58.9578504383728,40.10025));
#185079=CARTESIAN_POINT('Origin',(-0.1905,1.99538158514885E-15,2.68256207625279E-17));
#185080=CARTESIAN_POINT('',(-0.190499999999366,60.0036905223731,39.116));
#185081=CARTESIAN_POINT('',(-0.19049999999937,59.5728760150042,39.3548010137695));
#185082=CARTESIAN_POINT('Origin',(-0.190499999999367,59.9654595002486,39.5550297832821));
#185083=CARTESIAN_POINT('',(-0.190499999467978,59.2165773020941,39.92499));
#185084=CARTESIAN_POINT('',(-0.19049999999937,59.5728760150042,39.3548010137695));
#185085=CARTESIAN_POINT('',(-0.190499999999337,62.6567671111299,39.92499));
#185086=CARTESIAN_POINT('',(-0.190499999999335,62.9165533988763,39.92499));
#185087=CARTESIAN_POINT('',(-0.190500000605309,62.3004688883555,39.3548010137695));
#185088=CARTESIAN_POINT('',(-0.190499999999338,62.6567671111299,39.92499));
#185089=CARTESIAN_POINT('',(-0.190499999999346,61.8696548221181,39.116));
#185090=CARTESIAN_POINT('Origin',(-0.190499999999346,61.9078859673755,39.5550293907214));
#185091=CARTESIAN_POINT('',(-0.190500000711194,61.4682752798284,39.116));
#185092=CARTESIAN_POINT('',(-0.190499999999995,1.99538158514885E-15,39.116));
#185093=CARTESIAN_POINT('',(-0.190499999999352,61.3422370451705,39.3343017080178));
#185094=CARTESIAN_POINT('',(-0.190499999999351,61.4682752798284,39.116));
#185095=CARTESIAN_POINT('',(-0.190499999999355,61.0122769227456,39.5248017080178));
#185096=CARTESIAN_POINT('Origin',(-0.190499486621753,61.0417043405088,39.1947747614311));
#185097=CARTESIAN_POINT('',(-0.190499999999357,60.8610688070707,39.5248017080178));
#185098=CARTESIAN_POINT('',(-0.190499999999994,1.99538158514885E-15,39.5248017080178));
#185099=CARTESIAN_POINT('',(-0.19049999999936,60.5311086139135,39.3343017080178));
#185100=CARTESIAN_POINT('Origin',(-0.190499486572862,60.831638480743,39.1947728911869));
#185101=CARTESIAN_POINT('',(-0.190499999999362,60.4050703266283,39.116));
#185102=CARTESIAN_POINT('',(-0.19049999999936,60.5311086139135,39.3343017080178));
#185103=CARTESIAN_POINT('',(-0.190499999999995,1.99538158514885E-15,39.116));
#185104=CARTESIAN_POINT('Origin',(0.1905,-1.99538158514885E-15,-2.68256207625279E-17));
#185105=CARTESIAN_POINT('',(0.190500000000654,61.8696548221181,39.116));
#185106=CARTESIAN_POINT('',(0.190500000000659,62.3004688883554,39.3548010137695));
#185107=CARTESIAN_POINT('Origin',(0.190500000000654,61.9078859670887,39.5550293912442));
#185108=CARTESIAN_POINT('',(0.190500000452942,62.6567671111299,39.92499));
#185109=CARTESIAN_POINT('',(0.190500000000658,62.3004688883554,39.3548010137695));
#185110=CARTESIAN_POINT('',(0.190500000000626,59.2165773020941,39.92499));
#185111=CARTESIAN_POINT('',(0.190500000000006,-7.61749518455946E-15,39.92499));
#185112=CARTESIAN_POINT('',(0.190499999294509,59.5728760150042,39.3548010137695));
#185113=CARTESIAN_POINT('',(0.190500000000626,59.2165773020941,39.92499));
#185114=CARTESIAN_POINT('',(0.190500000000634,60.0036905223731,39.116));
#185115=CARTESIAN_POINT('Origin',(0.190500000000634,59.9654594999465,39.5550297827309));
#185116=CARTESIAN_POINT('',(0.190499999259078,60.4050703266283,39.116));
#185117=CARTESIAN_POINT('',(0.190500000000639,60.4789282006569,39.116));
#185118=CARTESIAN_POINT('',(0.19050000000064,60.5311086139135,39.3343017080178));
#185119=CARTESIAN_POINT('',(0.190500000000638,60.4050703266283,39.116));
#185120=CARTESIAN_POINT('',(0.190500000000643,60.8610688070707,39.5248017080178));
#185121=CARTESIAN_POINT('Origin',(0.190499486503203,60.8316414495916,39.1947745585591));
#185122=CARTESIAN_POINT('',(0.190500000000645,61.0122769227456,39.5248017080178));
#185123=CARTESIAN_POINT('',(0.190500000000645,61.0128056337175,39.5248017080178));
#185124=CARTESIAN_POINT('',(0.190500000000648,61.3422370451705,39.3343017080178));
#185125=CARTESIAN_POINT('Origin',(0.190499486688745,61.0417071743813,39.1947728594256));
#185126=CARTESIAN_POINT('',(0.190500000000649,61.4682752798284,39.116));
#185127=CARTESIAN_POINT('',(0.190500000000648,61.3422370451705,39.3343017080178));
#185128=CARTESIAN_POINT('',(0.190500000000654,61.8701762063762,39.116));
#185129=CARTESIAN_POINT('Origin',(5.90076614434134,57.9645097668784,40.10025));
#185130=CARTESIAN_POINT('',(6.18532049829458,58.7035958781038,40.10025));
#185131=CARTESIAN_POINT('',(6.58439859103091,62.500570298093,40.10025));
#185132=CARTESIAN_POINT('',(6.10537907909441,57.9430040808457,40.10025));
#185133=CARTESIAN_POINT('',(6.55408556366009,62.5037563256534,40.10025));
#185134=CARTESIAN_POINT('Origin',(5.63142687537637E-15,5.54868405209867E-15,
40.10025));
#185135=CARTESIAN_POINT('',(6.15500747092375,58.7067819056642,40.10025));
#185136=CARTESIAN_POINT('',(6.14761699020245,58.6364661785899,40.10025));
#185137=CARTESIAN_POINT('Origin',(5.65479388299727E-15,5.32882958889813E-15,
40.10025));
#185138=CARTESIAN_POINT('Origin',(-0.189456421067656,0.0199126722524899,
2.66786672051798E-17));
#185139=CARTESIAN_POINT('',(6.08263713962448,59.6948966996542,39.116));
#185140=CARTESIAN_POINT('',(6.03760476121579,59.2664422392335,39.3548010137695));
#185141=CARTESIAN_POINT('Origin',(6.07864090963279,59.6568751110704,39.5550297832848));
#185142=CARTESIAN_POINT('',(6.00036140481959,58.9120953678974,39.92499));
#185143=CARTESIAN_POINT('',(6.03760476121579,59.2664422392335,39.3548010137695));
#185144=CARTESIAN_POINT('',(6.35995915837865,62.3334394572618,39.92499));
#185145=CARTESIAN_POINT('',(6.38711421981479,62.5918026085421,39.92499));
#185146=CARTESIAN_POINT('',(6.32271585208515,61.9790930734951,39.3548010137695));
#185147=CARTESIAN_POINT('',(6.35995915837864,62.3334394572618,39.92499));
#185148=CARTESIAN_POINT('',(6.27768352038914,61.5506390517261,39.116));
#185149=CARTESIAN_POINT('Origin',(6.28167976325196,61.5886607627705,39.5550293907198));
#185150=CARTESIAN_POINT('',(6.23572793293866,61.1514583086406,39.116));
#185151=CARTESIAN_POINT('',(-0.18945642106765,0.0199126722524899,39.116));
#185152=CARTESIAN_POINT('',(6.22255335066477,61.0261105245453,39.3343017080178));
#185153=CARTESIAN_POINT('',(6.23572793364653,61.1514583085662,39.116));
#185154=CARTESIAN_POINT('',(6.18806312612808,60.6979579581953,39.5248017080178));
#185155=CARTESIAN_POINT('Origin',(6.19113963945,60.7272241158218,39.1947747614305));
#185156=CARTESIAN_POINT('',(6.17225757416298,60.5475781763993,39.5248017080178));
#185157=CARTESIAN_POINT('',(-0.18945642106765,0.0199126722524899,39.5248017080178));
#185158=CARTESIAN_POINT('',(6.13776734223276,60.2194255397044,39.3343017080178));
#185159=CARTESIAN_POINT('Origin',(6.16918177799204,60.5183090188076,39.1947728911921));
#185160=CARTESIAN_POINT('',(6.12459275374995,60.0940777033446,39.116));
#185161=CARTESIAN_POINT('',(6.13776734223276,60.2194255397044,39.3343017080178));
#185162=CARTESIAN_POINT('',(-0.18945642106765,0.0199126722524899,39.116));
#185163=CARTESIAN_POINT('Origin',(0.189456421067656,-0.0199126722524899,
-2.66786672051798E-17));
#185164=CARTESIAN_POINT('',(6.65659636252446,61.5108137072211,39.116));
#185165=CARTESIAN_POINT('',(6.70162869482234,61.9392677289268,39.3548010137695));
#185166=CARTESIAN_POINT('Origin',(6.66059260535715,61.548835417979,39.5550293912451));
#185167=CARTESIAN_POINT('',(6.73887200096445,62.2936141127095,39.92499));
#185168=CARTESIAN_POINT('',(6.70162869482234,61.9392677289269,39.3548010137695));
#185169=CARTESIAN_POINT('',(6.37927424642637,58.872270023448,39.92499));
#185170=CARTESIAN_POINT('',(0.189456421067661,-0.0199126722524955,39.92499));
#185171=CARTESIAN_POINT('',(6.41651760264858,59.2266168948024,39.3548010137695));
#185172=CARTESIAN_POINT('',(6.37927424642637,58.872270023448,39.92499));
#185173=CARTESIAN_POINT('',(6.46154998175979,59.6550713551492,39.116));
#185174=CARTESIAN_POINT('Origin',(6.45755375173627,59.6170497662626,39.555029782729));
#185175=CARTESIAN_POINT('',(6.50350559514777,60.0542523589171,39.116));
#185176=CARTESIAN_POINT('',(6.51122584595768,60.1277056317064,39.116));
#185177=CARTESIAN_POINT('',(6.51668018436807,60.1796001951995,39.3343017080178));
#185178=CARTESIAN_POINT('',(6.50350559588526,60.0542523588396,39.116));
#185179=CARTESIAN_POINT('',(6.5511704162983,60.5077528318943,39.5248017080178));
#185180=CARTESIAN_POINT('Origin',(6.54809390915835,60.4784867342318,39.1947745585617));
#185181=CARTESIAN_POINT('',(6.56697596826339,60.6581326136904,39.5248017080178));
#185182=CARTESIAN_POINT('',(6.5670312336088,60.6586584283283,39.5248017080178));
#185183=CARTESIAN_POINT('',(6.60146619280008,60.9862851800404,39.3343017080178));
#185184=CARTESIAN_POINT('Origin',(6.57005175674075,60.6874016969861,39.1947728594294));
#185185=CARTESIAN_POINT('',(6.61464077578184,61.1116329640612,39.116));
#185186=CARTESIAN_POINT('',(6.60146619280008,60.9862851800404,39.3343017080178));
#185187=CARTESIAN_POINT('',(6.65665086201973,61.5113322352818,39.116));
#185188=CARTESIAN_POINT('Origin',(11.92738225999,57.0301761002789,40.10025));
#185189=CARTESIAN_POINT('',(12.2876333308477,57.7354693911203,40.10025));
#185190=CARTESIAN_POINT('',(13.0814171332239,61.4699285681953,40.10025));
#185191=CARTESIAN_POINT('',(12.128626347365,56.9874003490101,40.10025));
#185192=CARTESIAN_POINT('',(13.0516031943535,61.4762657165314,40.10025));
#185193=CARTESIAN_POINT('Origin',(5.61622893658571E-15,5.55109116912811E-15,
40.10025));
#185194=CARTESIAN_POINT('',(12.2578193919774,57.7418065394565,40.10025));
#185195=CARTESIAN_POINT('',(12.2431194021881,57.6726485248849,40.10025));
#185196=CARTESIAN_POINT('Origin',(5.66270693800216E-15,5.32757628410993E-15,
40.10025));
#185197=CARTESIAN_POINT('Origin',(-0.18633711793979,0.0396071771007852,
2.62394165870616E-17));
#185198=CARTESIAN_POINT('',(12.289131633873,58.7320730967337,39.116));
#185199=CARTESIAN_POINT('',(12.1995602612171,58.3106729199895,39.3548010137695));
#185200=CARTESIAN_POINT('Origin',(12.2811829574215,58.6946775141693,39.5550297832828));
#185201=CARTESIAN_POINT('',(12.1254815939001,57.9621601887014,39.92499));
#185202=CARTESIAN_POINT('',(12.1995602612171,58.3106729199895,39.3548010137695));
#185203=CARTESIAN_POINT('',(12.8407372733105,61.3271735965892,39.92499));
#185204=CARTESIAN_POINT('',(12.8947498796471,61.5812829306519,39.92499));
#185205=CARTESIAN_POINT('',(12.7666587067863,60.9786613449624,39.3548010137695));
#185206=CARTESIAN_POINT('',(12.8407372733105,61.3271735965892,39.92499));
#185207=CARTESIAN_POINT('',(12.6770874264386,60.5572615995842,39.116));
#185208=CARTESIAN_POINT('Origin',(12.685036128491,60.5946573025912,39.5550293907214));
#185209=CARTESIAN_POINT('',(12.5936359264456,60.1646531634578,39.116));
#185210=CARTESIAN_POINT('',(-0.186337117939784,0.0396071771007852,39.116));
#185211=CARTESIAN_POINT('',(12.5674311046661,60.0413691664786,39.3343017080178));
#185212=CARTESIAN_POINT('',(12.5936359271415,60.1646531633099,39.116));
#185213=CARTESIAN_POINT('',(12.4988285377103,59.7186194643908,39.5248017080178));
#185214=CARTESIAN_POINT('Origin',(12.5049473440533,59.7474037157363,39.1947747614349));
#185215=CARTESIAN_POINT('',(12.4673906027149,59.5707156088319,39.5248017080178));
#185216=CARTESIAN_POINT('',(-0.186337117939784,0.0396071771007852,39.5248017080178));
#185217=CARTESIAN_POINT('',(12.398788021053,59.2479658375575,39.3343017080178));
#185218=CARTESIAN_POINT('Origin',(12.4612721960133,59.5419282989966,39.1947728911891));
#185219=CARTESIAN_POINT('',(12.3725831876358,59.1246817892489,39.116));
#185220=CARTESIAN_POINT('',(12.398788021053,59.2479658375575,39.3343017080178));
#185221=CARTESIAN_POINT('',(-0.186337117939784,0.0396071771007852,39.116));
#185222=CARTESIAN_POINT('Origin',(0.18633711793979,-0.0396071771007852,
-2.62394165870616E-17));
#185223=CARTESIAN_POINT('',(13.0497616623182,60.4780472453826,39.116));
#185224=CARTESIAN_POINT('',(13.1393329432576,60.8994469906351,39.3548010137695));
#185225=CARTESIAN_POINT('Origin',(13.0577103643107,60.5154429481081,39.555029391246));
#185226=CARTESIAN_POINT('',(13.2134115096326,61.2479592422935,39.92499));
#185227=CARTESIAN_POINT('',(13.1393329432576,60.8994469906351,39.3548010137695));
#185228=CARTESIAN_POINT('',(12.4981558292594,57.8829458346104,39.92499));
#185229=CARTESIAN_POINT('',(0.186337117939794,-0.0396071771007907,39.92499));
#185230=CARTESIAN_POINT('',(12.5722344964052,58.2314585659349,39.3548010137695));
#185231=CARTESIAN_POINT('',(12.4981558292594,57.8829458346104,39.92499));
#185232=CARTESIAN_POINT('',(12.6618058697526,58.6528587425321,39.116));
#185233=CARTESIAN_POINT('Origin',(12.6538571932381,58.6154631596714,39.5550297827299));
#185234=CARTESIAN_POINT('',(12.74525742279,59.0454674352015,39.116));
#185235=CARTESIAN_POINT('',(12.7606133389849,59.1177113373237,39.116));
#185236=CARTESIAN_POINT('',(12.7714622569326,59.1687514833559,39.3343017080178));
#185237=CARTESIAN_POINT('',(12.7452574235154,59.0454674350473,39.116));
#185238=CARTESIAN_POINT('',(12.8400648385945,59.4915012546304,39.5248017080178));
#185239=CARTESIAN_POINT('Origin',(12.8339460446679,59.4627170622758,39.1947745585633));
#185240=CARTESIAN_POINT('',(12.8715027735898,59.6394051101892,39.5248017080178));
#185241=CARTESIAN_POINT('',(12.871612698782,59.6399222675579,39.5248017080178));
#185242=CARTESIAN_POINT('',(12.9401053405456,59.962154812277,39.3343017080178));
#185243=CARTESIAN_POINT('Origin',(12.8776211648729,59.668192346935,39.1947728594185));
#185244=CARTESIAN_POINT('',(12.966310163021,60.0854388091083,39.116));
#185245=CARTESIAN_POINT('',(12.9401053405456,59.962154812277,39.3343017080178));
#185246=CARTESIAN_POINT('',(13.0498700642008,60.4785572361437,39.116));
#185247=CARTESIAN_POINT('Origin',(17.823319479633,55.4710078899932,40.10025));
#185248=CARTESIAN_POINT('',(18.2553202812755,56.134781019564,40.10025));
#185249=CARTESIAN_POINT('',(19.4351129318427,59.7658094374949,40.10025));
#185250=CARTESIAN_POINT('',(18.0189898472955,55.4074307335705,40.10025));
#185251=CARTESIAN_POINT('',(19.406124729226,59.7752282754835,40.10025));
#185252=CARTESIAN_POINT('Origin',(5.60136586593793E-15,5.55507371690523E-15,
40.10025));
#185253=CARTESIAN_POINT('',(18.2263320786588,56.1441998575526,40.10025));
#185254=CARTESIAN_POINT('',(18.2044836359659,56.0769572651636,40.10025));
#185255=CARTESIAN_POINT('Origin',(5.67044563844026E-15,5.32550270557707E-15,
40.10025));
#185256=CARTESIAN_POINT('Origin',(-0.181176266354226,0.0588677374284294,
2.55126814298647E-17));
#185257=CARTESIAN_POINT('',(18.3609838302746,57.1257686104889,39.116));
#185258=CARTESIAN_POINT('',(18.2278548260744,56.7160396659412,39.3548010137695));
#185259=CARTESIAN_POINT('Origin',(18.3491697947263,57.0894087477743,39.5550297832854));
#185260=CARTESIAN_POINT('',(18.1177524692166,56.3771794531163,39.92499));
#185261=CARTESIAN_POINT('',(18.2278548260744,56.7160396659412,39.3548010137695));
#185262=CARTESIAN_POINT('',(19.1808295835788,59.6489943884562,39.92499));
#185263=CARTESIAN_POINT('',(19.261107961398,59.8960658302615,39.92499));
#185264=CARTESIAN_POINT('',(19.0707273771003,59.3101346421292,39.3548010137695));
#185265=CARTESIAN_POINT('',(19.1808295835788,59.6489943884562,39.92499));
#185266=CARTESIAN_POINT('',(18.9375985097928,58.9004061169355,39.116));
#185267=CARTESIAN_POINT('Origin',(18.9494125833917,58.9367660967579,39.555029390722));
#185268=CARTESIAN_POINT('',(18.8135654093542,58.5186714879532,39.116));
#185269=CARTESIAN_POINT('',(-0.181176266354221,0.0588677374284294,39.116));
#185270=CARTESIAN_POINT('',(18.7746174535806,58.3988020033596,39.3343017080178));
#185271=CARTESIAN_POINT('',(18.8135654100308,58.5186714877334,39.116));
#185272=CARTESIAN_POINT('',(18.6726541682852,58.0849912788098,39.5248017080178));
#185273=CARTESIAN_POINT('Origin',(18.6817482287252,58.1129782575874,39.1947747614284));
#185274=CARTESIAN_POINT('',(18.6259282908542,57.9411838150805,39.5248017080178));
#185275=CARTESIAN_POINT('',(-0.181176266354221,0.0588677374284294,39.5248017080178));
#185276=CARTESIAN_POINT('',(18.5239649837014,57.6273730232603,39.3343017080178));
#185277=CARTESIAN_POINT('Origin',(18.6168343081661,57.913193752791,39.1947728911888));
#185278=CARTESIAN_POINT('',(18.4850170109884,57.5075034888351,39.116));
#185279=CARTESIAN_POINT('',(18.5239649837014,57.6273730232603,39.3343017080178));
#185280=CARTESIAN_POINT('',(-0.181176266354221,0.0588677374284294,39.116));
#185281=CARTESIAN_POINT('Origin',(0.181176266354226,-0.0588677374284294,
-2.55126814298647E-17));
#185282=CARTESIAN_POINT('',(19.2999510425012,58.7826706420786,39.116));
#185283=CARTESIAN_POINT('',(19.4330799103844,59.1923991670853,39.3548010137695));
#185284=CARTESIAN_POINT('Origin',(19.3117651160114,58.8190306216277,39.5550293912458));
#185285=CARTESIAN_POINT('',(19.5431821167173,59.5312589134596,39.92499));
#185286=CARTESIAN_POINT('',(19.4330799103844,59.1923991670853,39.3548010137695));
#185287=CARTESIAN_POINT('',(18.4801050014197,56.2594439784237,39.92499));
#185288=CARTESIAN_POINT('',(0.18117626635423,-0.0588677374284347,39.92499));
#185289=CARTESIAN_POINT('',(18.5902073581112,56.5983041913026,39.3548010137695));
#185290=CARTESIAN_POINT('',(18.4801050014197,56.2594439784237,39.92499));
#185291=CARTESIAN_POINT('',(18.7233363629831,57.008033135632,39.116));
#185292=CARTESIAN_POINT('Origin',(18.7115223273417,56.9716732726309,39.5550297827351));
#185293=CARTESIAN_POINT('',(18.8473695429913,57.3897680142074,39.116));
#185294=CARTESIAN_POINT('',(18.8701928819401,57.4600110263528,39.116));
#185295=CARTESIAN_POINT('',(18.8863175164099,57.5096375484035,39.3343017080178));
#185296=CARTESIAN_POINT('',(18.8473695436968,57.3897680139782,39.116));
#185297=CARTESIAN_POINT('',(18.9882808235627,57.8234483402237,39.5248017080178));
#185298=CARTESIAN_POINT('Origin',(18.979186781637,57.7954614188152,39.1947745585588));
#185299=CARTESIAN_POINT('',(19.0350067009936,57.967255803953,39.5248017080178));
#185300=CARTESIAN_POINT('',(19.0351700816691,57.9677586379681,39.5248017080178));
#185301=CARTESIAN_POINT('',(19.136969986289,58.2810665285028,39.3343017080178));
#185302=CARTESIAN_POINT('Origin',(19.0441006607092,57.9952457951693,39.1947728594247));
#185303=CARTESIAN_POINT('',(19.1759179427393,58.4009360128765,39.116));
#185304=CARTESIAN_POINT('',(19.136969986289,58.2810665285028,39.3343017080178));
#185305=CARTESIAN_POINT('',(19.3001121590976,58.7831665079748,39.116));
#185306=CARTESIAN_POINT('Origin',(23.5239806812878,53.30408770921,40.10025));
#185307=CARTESIAN_POINT('',(24.0229981225303,53.9190682401992,40.10025));
#185308=CARTESIAN_POINT('',(25.5758735661215,57.4068835917977,40.10025));
#185309=CARTESIAN_POINT('',(23.7119335237431,53.2204057122635,40.10025));
#185310=CARTESIAN_POINT('',(25.5480287005725,57.4192809246786,40.10025));
#185311=CARTESIAN_POINT('Origin',(5.58700050634534E-15,5.56058806180318E-15,
40.10025));
#185312=CARTESIAN_POINT('',(23.9951532569813,53.9314655730802,40.10025));
#185313=CARTESIAN_POINT('',(23.966395737495,53.8668751267876,40.10025));
#185314=CARTESIAN_POINT('Origin',(5.67792519749014E-15,5.3226315718599E-15,
40.10025));
#185315=CARTESIAN_POINT('Origin',(-0.174030409680915,0.0774833305059419,
2.45064239960503E-17));
#185316=CARTESIAN_POINT('',(24.2316692455489,54.893582249012,39.116));
#185317=CARTESIAN_POINT('',(24.0564411990333,54.5000136127186,39.3548010137695));
#185318=CARTESIAN_POINT('Origin',(24.216119287949,54.8586564724098,39.5550297832835));
#185319=CARTESIAN_POINT('',(23.9115214570975,54.1745185417596,39.92499));
#185320=CARTESIAN_POINT('',(24.0564411990333,54.5000136127186,39.3548010137695));
#185321=CARTESIAN_POINT('',(25.3107727110829,57.3172883154487,39.92499));
#185322=CARTESIAN_POINT('',(25.416437313678,57.5546148985773,39.92499));
#185323=CARTESIAN_POINT('',(25.1658531674639,56.9917936927136,39.3548010137695));
#185324=CARTESIAN_POINT('',(25.3107727110829,57.3172883154487,39.92499));
#185325=CARTESIAN_POINT('',(24.9906253009265,56.5982254591673,39.116));
#185326=CARTESIAN_POINT('Origin',(25.0061753086094,56.6331513482574,39.5550293907218));
#185327=CARTESIAN_POINT('',(24.827369532646,56.2315470018075,39.116));
#185328=CARTESIAN_POINT('',(-0.174030409680909,0.0774833305059419,39.116));
#185329=CARTESIAN_POINT('',(24.7761051648324,56.1164053447569,39.3343017080178));
#185330=CARTESIAN_POINT('',(24.8273695332963,56.2315470015179,39.116));
#185331=CARTESIAN_POINT('',(24.6418982922884,55.8149717737124,39.5248017080178));
#185332=CARTESIAN_POINT('Origin',(24.6538679703961,55.8418548487275,39.1947747614258));
#185333=CARTESIAN_POINT('',(24.5803964109129,55.6768362864789,39.5248017080178));
#185334=CARTESIAN_POINT('',(-0.174030409680909,0.0774833305059419,39.5248017080178));
#185335=CARTESIAN_POINT('',(24.4461895095995,55.3754026508172,39.3343017080178));
#185336=CARTESIAN_POINT('Origin',(24.5684264878148,55.6499501367125,39.1947728911925));
#185337=CARTESIAN_POINT('',(24.3949251197301,55.2602609459788,39.116));
#185338=CARTESIAN_POINT('',(24.4461895095995,55.3754026508172,39.3343017080178));
#185339=CARTESIAN_POINT('',(-0.174030409680909,0.0774833305059419,39.116));
#185340=CARTESIAN_POINT('Origin',(0.174030409680915,-0.0774833305059419,
-2.45064239960503E-17));
#185341=CARTESIAN_POINT('',(25.3386861202883,56.4432587981554,39.116));
#185342=CARTESIAN_POINT('',(25.5139139873796,56.8368270314551,39.3548010137695));
#185343=CARTESIAN_POINT('Origin',(25.3542361278548,56.4781846869841,39.5550293912436));
#185344=CARTESIAN_POINT('',(25.6588335308583,57.1623216542527,39.92499));
#185345=CARTESIAN_POINT('',(25.5139139873796,56.8368270314551,39.3548010137695));
#185346=CARTESIAN_POINT('',(24.2595822759739,54.0195518809638,39.92499));
#185347=CARTESIAN_POINT('',(0.174030409680918,-0.077483330505947,39.92499));
#185348=CARTESIAN_POINT('',(24.4045020177506,54.3450469519937,39.3548010137695));
#185349=CARTESIAN_POINT('',(24.2595822759739,54.0195518809638,39.92499));
#185350=CARTESIAN_POINT('',(24.5797300649108,54.7386155880001,39.116));
#185351=CARTESIAN_POINT('Origin',(24.5641801071874,54.7036898111209,39.5550297827301));
#185352=CARTESIAN_POINT('',(24.7429859384139,55.1052942852688,39.116));
#185353=CARTESIAN_POINT('',(24.773026642839,55.1727668102968,39.116));
#185354=CARTESIAN_POINT('',(24.7942503289613,55.2204359898053,39.3343017080178));
#185355=CARTESIAN_POINT('',(24.7429859390919,55.1052942849669,39.116));
#185356=CARTESIAN_POINT('',(24.9284572302748,55.521869625467,39.5248017080178));
#185357=CARTESIAN_POINT('Origin',(24.9164875765758,55.4949866055697,39.1947745585588));
#185358=CARTESIAN_POINT('',(24.9899591116502,55.6600051127005,39.5248017080178));
#185359=CARTESIAN_POINT('',(24.9901741577761,55.6604881142073,39.5248017080178));
#185360=CARTESIAN_POINT('',(25.1241659841942,55.961438683745,39.3343017080178));
#185361=CARTESIAN_POINT('Origin',(25.0019290044727,55.6868911941847,39.1947728594294));
#185362=CARTESIAN_POINT('',(25.1754303526582,56.076580340506,39.116));
#185363=CARTESIAN_POINT('',(25.1241659841942,55.961438683745,39.3343017080178));
#185364=CARTESIAN_POINT('',(25.3388981863712,56.4437351063761,39.116));
#185365=CARTESIAN_POINT('Origin',(28.9669082278889,50.5531567888872,40.10025));
#185366=CARTESIAN_POINT('',(29.5274749692191,51.1126068659043,40.10025));
#185367=CARTESIAN_POINT('',(31.4364195775141,54.4189959163059,40.10025));
#185368=CARTESIAN_POINT('',(29.1450842944635,50.4502867888872,40.10025));
#185369=CARTESIAN_POINT('',(31.4100231232068,54.4342359163059,40.10025));
#185370=CARTESIAN_POINT('Origin',(5.57329024769379E-15,5.5675737875053E-15,
40.10025));
#185371=CARTESIAN_POINT('',(29.5010785149117,51.1278468659043,40.10025));
#185372=CARTESIAN_POINT('',(29.4657269920333,51.0666162321541,40.10025));
#185373=CARTESIAN_POINT('Origin',(5.68506366753766E-15,5.31899433970023E-15,
40.10025));
#185374=CARTESIAN_POINT('Origin',(-0.164977839420934,0.0952500000000019,
2.32316690526363E-17));
#185375=CARTESIAN_POINT('',(29.8368674217662,52.0599703131943,39.116));
#185376=CARTESIAN_POINT('',(29.6214601680818,51.6868740054939,39.3548010137695));
#185377=CARTESIAN_POINT('Origin',(29.817751910705,52.0268612768237,39.5550297832864));
#185378=CARTESIAN_POINT('',(29.4433108120868,51.3783102685125,39.92499));
#185379=CARTESIAN_POINT('',(29.6214601680818,51.6868740054939,39.3548010137695));
#185380=CARTESIAN_POINT('',(31.1634057161447,54.3576020372435,39.92499));
#185381=CARTESIAN_POINT('',(31.2932988600179,54.5825835619867,39.92499));
#185382=CARTESIAN_POINT('',(30.9852566042334,54.0490387253001,39.3548010137695));
#185383=CARTESIAN_POINT('',(31.1634057161447,54.3576020372435,39.92499));
#185384=CARTESIAN_POINT('',(30.7698495716387,53.6759427993283,39.116));
#185385=CARTESIAN_POINT('Origin',(30.788965144268,53.709051942338,39.555029390719));
#185386=CARTESIAN_POINT('',(30.5691597998772,53.3283379195021,39.116));
#185387=CARTESIAN_POINT('',(-0.164977839420929,0.0952500000000019,39.116));
#185388=CARTESIAN_POINT('',(30.506140683165,53.2191856060842,39.3343017080178));
#185389=CARTESIAN_POINT('',(30.5691598004939,53.3283379191461,39.116));
#185390=CARTESIAN_POINT('',(30.3411606219525,52.9334317578284,39.5248017080178));
#185391=CARTESIAN_POINT('Origin',(30.3558747754311,52.9589163924886,39.1947747614277));
#185392=CARTESIAN_POINT('',(30.265556564115,52.8024816883956,39.5248017080178));
#185393=CARTESIAN_POINT('',(-0.164977839420929,0.0952500000000019,39.5248017080178));
#185394=CARTESIAN_POINT('',(30.1005764675364,52.5167277788838,39.3343017080178));
#185395=CARTESIAN_POINT('Origin',(30.2508418455894,52.776994021437,39.1947728911944));
#185396=CARTESIAN_POINT('',(30.0375573238938,52.4075754202453,39.116));
#185397=CARTESIAN_POINT('',(30.1005764675364,52.5167277788838,39.3343017080178));
#185398=CARTESIAN_POINT('',(-0.164977839420929,0.0952500000000019,39.116));
#185399=CARTESIAN_POINT('Origin',(0.164977839420934,-0.0952500000000019,
-2.32316690526363E-17));
#185400=CARTESIAN_POINT('',(31.0998052504806,53.4854427993283,39.116));
#185401=CARTESIAN_POINT('',(31.3152122835993,53.8585387249975,39.3548010137695));
#185402=CARTESIAN_POINT('Origin',(31.1189208229657,53.5185519420882,39.5550293912452));
#185403=CARTESIAN_POINT('',(31.4933613953778,54.1671020370175,39.92499));
#185404=CARTESIAN_POINT('',(31.3152122835993,53.8585387249975,39.3548010137695));
#185405=CARTESIAN_POINT('',(29.7732664904686,51.1878102687781,39.92499));
#185406=CARTESIAN_POINT('',(0.164977839420937,-0.0952500000000068,39.92499));
#185407=CARTESIAN_POINT('',(29.9514158463121,51.496374005847,39.3548010137695));
#185408=CARTESIAN_POINT('',(29.7732664904686,51.1878102687781,39.92499));
#185409=CARTESIAN_POINT('',(30.1668231006081,51.8694703131943,39.116));
#185410=CARTESIAN_POINT('Origin',(30.1477075893947,51.83636127656,39.5550297827307));
#185411=CARTESIAN_POINT('',(30.3675130020937,52.2170754206159,39.116));
#185412=CARTESIAN_POINT('',(30.40444193975,52.2810382154236,39.116));
#185413=CARTESIAN_POINT('',(30.4305321463783,52.3262277788838,39.3343017080178));
#185414=CARTESIAN_POINT('',(30.3675130027357,52.2170754202453,39.116));
#185415=CARTESIAN_POINT('',(30.5955122429569,52.6119816883956,39.5248017080178));
#185416=CARTESIAN_POINT('Origin',(30.5807981195143,52.5864971059991,39.1947745585629));
#185417=CARTESIAN_POINT('',(30.6711163007943,52.7429317578284,39.5248017080178));
#185418=CARTESIAN_POINT('',(30.6713806562803,52.7433896349613,39.5248017080178));
#185419=CARTESIAN_POINT('',(30.8360963620068,53.0286856060842,39.3343017080178));
#185420=CARTESIAN_POINT('Origin',(30.6858309820708,52.7684193600401,39.1947728594248));
#185421=CARTESIAN_POINT('',(30.8991154793358,53.1378379191461,39.116));
#185422=CARTESIAN_POINT('',(30.8360963620068,53.0286856060842,39.3343017080178));
#185423=CARTESIAN_POINT('',(31.1000659426097,53.4858943313409,39.116));
#185424=CARTESIAN_POINT('Origin',(34.09246826623,47.2483549038572,40.10025));
#185425=CARTESIAN_POINT('',(34.7084426211237,47.7461450747861,40.10025));
#185426=CARTESIAN_POINT('',(36.9525415975218,50.8348823336482,40.10025));
#185427=CARTESIAN_POINT('',(34.2589154226527,47.1274239660506,40.10025));
#185428=CARTESIAN_POINT('',(36.9278827595333,50.8527980281381,40.10025));
#185429=CARTESIAN_POINT('Origin',(5.5603853024461E-15,5.57595435693894E-15,
40.10025));
#185430=CARTESIAN_POINT('',(34.6837837831351,47.7640607692759,40.10025));
#185431=CARTESIAN_POINT('',(34.6422255755471,47.7068608037046,40.10025));
#185432=CARTESIAN_POINT('Origin',(5.69178283801114E-15,5.31463085937477E-15,
40.10025));
#185433=CARTESIAN_POINT('Origin',(-0.154117737428426,0.111973090561718,
2.17023830815424E-17));
#185434=CARTESIAN_POINT('',(35.1151666347447,48.6559784483761,39.116));
#185435=CARTESIAN_POINT('',(34.8619402208396,48.3074421904914,39.3548010137695));
#185436=CARTESIAN_POINT('Origin',(35.0926950037606,48.6250489017661,39.5550297832849));
#185437=CARTESIAN_POINT('',(34.65251309241,48.019190476361,39.92499));
#185438=CARTESIAN_POINT('',(34.8619402208396,48.3074421904914,39.3548010137695));
#185439=CARTESIAN_POINT('',(36.6746059268184,50.8023624960587,39.92499));
#185440=CARTESIAN_POINT('',(36.8273044755035,51.0125340177511,39.92499));
#185441=CARTESIAN_POINT('',(36.4651790855635,50.5141111791246,39.3548010137695));
#185442=CARTESIAN_POINT('',(36.6746059268184,50.8023624960587,39.92499));
#185443=CARTESIAN_POINT('',(36.2119529314391,50.1655752777668,39.116));
#185444=CARTESIAN_POINT('Origin',(36.2344246347994,50.1965049239941,39.555029390722));
#185445=CARTESIAN_POINT('',(35.9760279553336,49.8408524072782,39.116));
#185446=CARTESIAN_POINT('',(-0.154117737428421,0.111973090561718,39.116));
#185447=CARTESIAN_POINT('',(35.9019445403524,49.7388853330807,39.3343017080178));
#185448=CARTESIAN_POINT('',(35.9760279559093,49.84085240686,39.116));
#185449=CARTESIAN_POINT('',(35.7079988465464,49.4719419865729,39.5248017080178));
#185450=CARTESIAN_POINT('Origin',(35.7252962640545,49.4957489658917,39.194774761439));
#185451=CARTESIAN_POINT('',(35.6191209461258,49.3496120513045,39.5248017080178));
#185452=CARTESIAN_POINT('',(-0.154117737428421,0.111973090561718,39.5248017080178));
#185453=CARTESIAN_POINT('',(35.4251752107443,49.0826686475731,39.3343017080178));
#185454=CARTESIAN_POINT('Origin',(35.6018226497084,49.3258021153674,39.1947728911938));
#185455=CARTESIAN_POINT('',(35.3510917642539,48.9807015312174,39.116));
#185456=CARTESIAN_POINT('',(35.4251752107443,49.0826686475731,39.3343017080178));
#185457=CARTESIAN_POINT('',(-0.154117737428421,0.111973090561718,39.116));
#185458=CARTESIAN_POINT('Origin',(0.154117737428426,-0.111973090561718,
-2.17023830815424E-17));
#185459=CARTESIAN_POINT('',(36.5201884062959,49.9416290966433,39.116));
#185460=CARTESIAN_POINT('',(36.7734145609104,50.2901649976451,39.3548010137695));
#185461=CARTESIAN_POINT('Origin',(36.5426601094884,49.9725587426398,39.5550293912424));
#185462=CARTESIAN_POINT('',(36.9828414020408,50.5784163146696,39.92499));
#185463=CARTESIAN_POINT('',(36.7734145609104,50.2901649976451,39.3548010137695));
#185464=CARTESIAN_POINT('',(34.9607485668371,47.7952442955498,39.92499));
#185465=CARTESIAN_POINT('',(0.154117737428429,-0.111973090561722,39.92499));
#185466=CARTESIAN_POINT('',(35.1701756951245,48.0834960097835,39.3548010137695));
#185467=CARTESIAN_POINT('',(34.9607485668371,47.7952442955498,39.92499));
#185468=CARTESIAN_POINT('',(35.4234021096015,48.4320322672527,39.116));
#185469=CARTESIAN_POINT('Origin',(35.4009304784386,48.4011027203966,39.5550297827295));
#185470=CARTESIAN_POINT('',(35.6593272385114,48.7567553505295,39.116));
#185471=CARTESIAN_POINT('',(35.7027398082304,48.8165076253515,39.116));
#185472=CARTESIAN_POINT('',(35.7334106856012,48.8587224664496,39.3343017080178));
#185473=CARTESIAN_POINT('',(35.6593272391108,48.756755350094,39.116));
#185474=CARTESIAN_POINT('',(35.9273564209826,49.1256658701811,39.5248017080178));
#185475=CARTESIAN_POINT('Origin',(35.9100590388139,49.1018589397066,39.1947745585602));
#185476=CARTESIAN_POINT('',(36.0162343214032,49.2479958054495,39.5248017080178));
#185477=CARTESIAN_POINT('',(36.0165450899153,49.2484235416109,39.5248017080178));
#185478=CARTESIAN_POINT('',(36.2101800152092,49.5149391519573,39.3343017080178));
#185479=CARTESIAN_POINT('Origin',(36.0335325740085,49.2718056808895,39.194772859428));
#185480=CARTESIAN_POINT('',(36.2842634307661,49.6169062257365,39.116));
#185481=CARTESIAN_POINT('',(36.2101800152092,49.5149391519573,39.3343017080178));
#185482=CARTESIAN_POINT('',(36.5204948682736,49.9420509053687,39.116));
#185483=CARTESIAN_POINT('Origin',(38.8445040879387,43.4258901551466,40.10025));
#185484=CARTESIAN_POINT('',(39.5091373124628,43.8565665267052,40.10025));
#185485=CARTESIAN_POINT('',(42.0638038389706,46.6938111422599,40.10025));
#185486=CARTESIAN_POINT('',(38.9973987043324,43.2882232241943,40.10025));
#185487=CARTESIAN_POINT('',(42.04115278469,46.7142062431418,40.10025));
#185488=CARTESIAN_POINT('Origin',(5.54842705988295E-15,5.58563795083165E-15,
40.10025));
#185489=CARTESIAN_POINT('',(39.4864862581822,43.876961627587,40.10025));
#185490=CARTESIAN_POINT('',(39.4391766863035,43.8244190249873,40.10025));
#185491=CARTESIAN_POINT('Origin',(5.69800909227282E-15,5.30958893808705E-15,
40.10025));
#185492=CARTESIAN_POINT('Origin',(-0.141569089253442,0.127469380511364,
1.99353212598914E-17));
#185493=CARTESIAN_POINT('',(40.0087367337519,44.7189015017594,39.116));
#185494=CARTESIAN_POINT('',(39.7204655612079,44.3987439298676,39.3548010137695));
#185495=CARTESIAN_POINT('Origin',(39.9831551867375,44.6904903154966,39.5550297832865));
#185496=CARTESIAN_POINT('',(39.4820551877886,44.1339623846886,39.92499));
#185497=CARTESIAN_POINT('',(39.7204655612079,44.3987439298676,39.3548010137695));
#185498=CARTESIAN_POINT('',(41.7839914803032,46.6905216402892,39.92499));
#185499=CARTESIAN_POINT('',(41.9578224365467,46.883580475758,39.92499));
#185500=CARTESIAN_POINT('',(41.5455814340041,46.4257404601123,39.3548010137695));
#185501=CARTESIAN_POINT('',(41.7839914803032,46.6905216402892,39.92499));
#185502=CARTESIAN_POINT('',(41.2573105570842,46.1055832156404,39.116));
#185503=CARTESIAN_POINT('Origin',(41.2828921864919,46.1339944934103,39.5550293907218));
#185504=CARTESIAN_POINT('',(40.988735220043,45.8073000862116,39.116));
#185505=CARTESIAN_POINT('',(-0.141569089253437,0.127469380511364,39.116));
#185506=CARTESIAN_POINT('',(40.9043991801909,45.7136354238371,39.3343017080178));
#185507=CARTESIAN_POINT('',(40.9887352205719,45.8073000857354,39.116));
#185508=CARTESIAN_POINT('',(40.6836127633984,45.4684272662431,39.5248017080178));
#185509=CARTESIAN_POINT('Origin',(40.7033039308025,45.4902957559628,39.194774761428));
#185510=CARTESIAN_POINT('',(40.5824347852705,45.3560577375091,39.5248017080178));
#185511=CARTESIAN_POINT('',(-0.141569089253437,0.127469380511364,39.5248017080178));
#185512=CARTESIAN_POINT('',(40.3616483211489,45.1108495273508,39.3343017080178));
#185513=CARTESIAN_POINT('Origin',(40.5627424347173,45.3341863992345,39.1947728911927));
#185514=CARTESIAN_POINT('',(40.2773122455534,45.0171848263428,39.116));
#185515=CARTESIAN_POINT('',(40.3616483211489,45.1108495273508,39.3343017080178));
#185516=CARTESIAN_POINT('',(-0.141569089253437,0.127469380511364,39.116));
#185517=CARTESIAN_POINT('Origin',(0.141569089253442,-0.127469380511364,
-1.99353212598914E-17));
#185518=CARTESIAN_POINT('',(41.5404487355911,45.8506444546177,39.116));
#185519=CARTESIAN_POINT('',(41.8287196129605,46.1708016986849,39.3548010137695));
#185520=CARTESIAN_POINT('Origin',(41.566030364806,45.8790557321734,39.5550293912477));
#185521=CARTESIAN_POINT('',(42.0671296591463,46.4355828789639,39.92499));
#185522=CARTESIAN_POINT('',(41.8287196129605,46.1708016986849,39.3548010137695));
#185523=CARTESIAN_POINT('',(39.7651933659004,43.8790236240215,39.92499));
#185524=CARTESIAN_POINT('',(0.141569089253444,-0.127469380511368,39.92499));
#185525=CARTESIAN_POINT('',(40.0036037391898,44.1438051693176,39.3548010137695));
#185526=CARTESIAN_POINT('',(39.7651933659004,43.8790236240215,39.92499));
#185527=CARTESIAN_POINT('',(40.2918749122587,44.4639627407367,39.116));
#185528=CARTESIAN_POINT('Origin',(40.2662933650396,44.4355515542463,39.5550297827278));
#185529=CARTESIAN_POINT('',(40.5604504235094,44.762246065816,39.116));
#185530=CARTESIAN_POINT('',(40.6098709880934,44.8171331622252,39.116));
#185531=CARTESIAN_POINT('',(40.6447864996558,44.8559107663281,39.3343017080178));
#185532=CARTESIAN_POINT('',(40.5604504240602,44.76224606532,39.116));
#185533=CARTESIAN_POINT('',(40.8655729637774,45.1011189764864,39.5248017080178));
#185534=CARTESIAN_POINT('Origin',(40.8458818366199,45.079250531644,39.1947745585614));
#185535=CARTESIAN_POINT('',(40.9667509419053,45.2134885052204,39.5248017080178));
#185536=CARTESIAN_POINT('',(40.9671047185986,45.2138814140433,39.5248017080178));
#185537=CARTESIAN_POINT('',(41.1875373586978,45.4586966628144,39.3343017080178));
#185538=CARTESIAN_POINT('Origin',(40.9864432425615,45.2353597879075,39.194772859423));
#185539=CARTESIAN_POINT('',(41.2718733990788,45.5523613247127,39.116));
#185540=CARTESIAN_POINT('',(41.1875373586978,45.4586966628144,39.3343017080178));
#185541=CARTESIAN_POINT('',(41.5407976097559,45.8510319186312,39.116));
#185542=CARTESIAN_POINT('Origin',(43.1709513941248,39.1276422664446,40.10025));
#185543=CARTESIAN_POINT('',(43.8769616275879,39.4864862581812,40.10025));
#185544=CARTESIAN_POINT('',(46.7142062431428,42.041152784689,40.10025));
#185545=CARTESIAN_POINT('',(43.3086183250771,38.9747476500508,40.10025));
#185546=CARTESIAN_POINT('',(46.6938111422609,42.0638038389695,40.10025));
#185547=CARTESIAN_POINT('Origin',(5.5375465370123E-15,5.59651847370231E-15,
40.10025));
#185548=CARTESIAN_POINT('',(43.8565665267061,39.5091373124617,40.10025));
#185549=CARTESIAN_POINT('',(43.8040239241064,39.461827740583,40.10025));
#185550=CARTESIAN_POINT('Origin',(5.70367421417806E-15,5.3039238161818E-15,
40.10025));
#185551=CARTESIAN_POINT('Origin',(-0.127469380511361,0.141569089253445,
1.79498438867829E-17));
#185552=CARTESIAN_POINT('',(44.4639627407376,40.2918749122577,39.116));
#185553=CARTESIAN_POINT('',(44.1438051688458,40.0036037397138,39.3548010137695));
#185554=CARTESIAN_POINT('Origin',(44.4355515544746,40.2662933652431,39.5550297832857));
#185555=CARTESIAN_POINT('',(43.8790236243778,39.7651933655047,39.92499));
#185556=CARTESIAN_POINT('',(44.1438051688458,40.0036037397138,39.3548010137695));
#185557=CARTESIAN_POINT('',(46.4355828792675,42.067129658809,39.92499));
#185558=CARTESIAN_POINT('',(46.6286417147362,42.2409606150525,39.92499));
#185559=CARTESIAN_POINT('',(46.1708016982805,41.8287196134095,39.3548010137695));
#185560=CARTESIAN_POINT('',(46.4355828792675,42.067129658809,39.92499));
#185561=CARTESIAN_POINT('',(45.8506444546187,41.54044873559,39.116));
#185562=CARTESIAN_POINT('Origin',(45.8790557323893,41.5660303649984,39.5550293907199));
#185563=CARTESIAN_POINT('',(45.5523613242375,41.2718733996065,39.116));
#185564=CARTESIAN_POINT('',(-0.127469380511355,0.141569089253445,39.116));
#185565=CARTESIAN_POINT('',(45.4586966628153,41.1875373586967,39.3343017080178));
#185566=CARTESIAN_POINT('',(45.5523613247136,41.2718733990777,39.116));
#185567=CARTESIAN_POINT('',(45.2134885052213,40.9667509419042,39.5248017080178));
#185568=CARTESIAN_POINT('Origin',(45.2353576819756,40.9864413462816,39.1947747614304));
#185569=CARTESIAN_POINT('',(45.1011189764874,40.8655729637763,39.5248017080178));
#185570=CARTESIAN_POINT('',(-0.127469380511355,0.141569089253445,39.5248017080178));
#185571=CARTESIAN_POINT('',(44.855910766329,40.6447864996547,39.3343017080178));
#185572=CARTESIAN_POINT('Origin',(45.0792483253111,40.8458798501223,39.1947728911937));
#185573=CARTESIAN_POINT('',(44.762246065321,40.5604504240592,39.116));
#185574=CARTESIAN_POINT('',(44.855910766329,40.6447864996547,39.3343017080178));
#185575=CARTESIAN_POINT('',(-0.127469380511355,0.141569089253445,39.116));
#185576=CARTESIAN_POINT('Origin',(0.127469380511361,-0.141569089253445,
-1.79498438867829E-17));
#185577=CARTESIAN_POINT('',(46.1055832156414,41.2573105570831,39.116));
#185578=CARTESIAN_POINT('',(46.4257404597086,41.5455814344525,39.3548010137695));
#185579=CARTESIAN_POINT('Origin',(46.1339944931977,41.2828921862985,39.5550293912464));
#185580=CARTESIAN_POINT('',(46.690521640593,41.7839914799658,39.92499));
#185581=CARTESIAN_POINT('',(46.4257404597086,41.5455814344525,39.3548010137695));
#185582=CARTESIAN_POINT('',(44.1339623850452,39.4820551873925,39.92499));
#185583=CARTESIAN_POINT('',(0.127469380511362,-0.141569089253449,39.92499));
#185584=CARTESIAN_POINT('',(44.3987439293955,39.7204655617323,39.3548010137695));
#185585=CARTESIAN_POINT('',(44.1339623850452,39.4820551873925,39.92499));
#185586=CARTESIAN_POINT('',(44.7189015017603,40.0087367337508,39.116));
#185587=CARTESIAN_POINT('Origin',(44.6904903152708,39.9831551865323,39.5550297827294));
#185588=CARTESIAN_POINT('',(45.0171848258473,40.2773122461036,39.116));
#185589=CARTESIAN_POINT('',(45.0720719232488,40.3267328095854,39.116));
#185590=CARTESIAN_POINT('',(45.1108495273517,40.3616483211478,39.3343017080178));
#185591=CARTESIAN_POINT('',(45.0171848263437,40.2773122455523,39.116));
#185592=CARTESIAN_POINT('',(45.3560577375101,40.5824347852694,39.5248017080178));
#185593=CARTESIAN_POINT('Origin',(45.3341886054765,40.5627444213201,39.1947745585557));
#185594=CARTESIAN_POINT('',(45.4684272662441,40.6836127633974,39.5248017080178));
#185595=CARTESIAN_POINT('',(45.468820175067,40.6839665400906,39.5248017080178));
#185596=CARTESIAN_POINT('',(45.7136354238381,40.9043991801898,39.3343017080178));
#185597=CARTESIAN_POINT('Origin',(45.4902978619848,40.7033058269827,39.1947728594193));
#185598=CARTESIAN_POINT('',(45.8073000857364,40.9887352205708,39.116));
#185599=CARTESIAN_POINT('',(45.7136354238381,40.9043991801898,39.3343017080178));
#185600=CARTESIAN_POINT('',(46.1059706796549,41.2576594312479,39.116));
#185601=CARTESIAN_POINT('Origin',(47.0244087227346,34.4007037410858,40.10025));
#185602=CARTESIAN_POINT('',(47.7640607692767,34.683783783134,40.10025));
#185603=CARTESIAN_POINT('',(50.8527980281389,36.9278827595321,40.10025));
#185604=CARTESIAN_POINT('',(47.1453396605412,34.2342565846631,40.10025));
#185605=CARTESIAN_POINT('',(50.8348823336491,36.9525415975206,40.10025));
#185606=CARTESIAN_POINT('Origin',(5.52786294311959E-15,5.60847671626546E-15,
40.10025));
#185607=CARTESIAN_POINT('',(47.7461450747869,34.7084426211226,40.10025));
#185608=CARTESIAN_POINT('',(47.6889451092156,34.6668844135346,40.10025));
#185609=CARTESIAN_POINT('Origin',(5.70871613546578E-15,5.29769756192013E-15,
40.10025));
#185610=CARTESIAN_POINT('Origin',(-0.111973090561714,0.154117737428429,
1.57677042678044E-17));
#185611=CARTESIAN_POINT('',(48.4320322672535,35.4234021096004,39.116));
#185612=CARTESIAN_POINT('',(48.0834960093688,35.1701756956953,39.3548010137695));
#185613=CARTESIAN_POINT('Origin',(48.4011027206445,35.400930478617,39.555029783287));
#185614=CARTESIAN_POINT('',(47.795244295863,34.960748566406,39.92499));
#185615=CARTESIAN_POINT('',(48.0834960093688,35.1701756956953,39.3548010137695));
#185616=CARTESIAN_POINT('',(50.5784163149361,36.982841401674,39.92499));
#185617=CARTESIAN_POINT('',(50.7885878366285,37.1355399503592,39.92499));
#185618=CARTESIAN_POINT('',(50.2901649972898,36.7734145613995,39.3548010137695));
#185619=CARTESIAN_POINT('',(50.5784163149361,36.982841401674,39.92499));
#185620=CARTESIAN_POINT('',(49.9416290966442,36.5201884062947,39.116));
#185621=CARTESIAN_POINT('Origin',(49.9725587428723,36.5426601096556,39.5550293907206));
#185622=CARTESIAN_POINT('',(49.6169062253194,36.2842634313403,39.116));
#185623=CARTESIAN_POINT('',(-0.111973090561709,0.154117737428429,39.116));
#185624=CARTESIAN_POINT('',(49.5149391519582,36.2101800152081,39.3343017080178));
#185625=CARTESIAN_POINT('',(49.6169062257374,36.284263430765,39.116));
#185626=CARTESIAN_POINT('',(49.2479958054503,36.0162343214021,39.5248017080178));
#185627=CARTESIAN_POINT('Origin',(49.271803388278,36.0335309082458,39.1947747614336));
#185628=CARTESIAN_POINT('',(49.1256658701819,35.9273564209815,39.5248017080178));
#185629=CARTESIAN_POINT('',(-0.111973090561709,0.154117737428429,39.5248017080178));
#185630=CARTESIAN_POINT('',(48.8587224664505,35.7334106856,39.3343017080178));
#185631=CARTESIAN_POINT('Origin',(49.1018565378157,35.9100572938239,39.1947728911905));
#185632=CARTESIAN_POINT('',(48.7567553500948,35.6593272391096,39.116));
#185633=CARTESIAN_POINT('',(48.8587224664505,35.7334106856,39.3343017080178));
#185634=CARTESIAN_POINT('',(-0.111973090561709,0.154117737428429,39.116));
#185635=CARTESIAN_POINT('Origin',(0.111973090561714,-0.154117737428429,
-1.57677042678044E-17));
#185636=CARTESIAN_POINT('',(50.1655752777676,36.2119529314379,39.116));
#185637=CARTESIAN_POINT('',(50.5141111787694,36.4651790860523,39.3548010137695));
#185638=CARTESIAN_POINT('Origin',(50.1965049237639,36.2344246346304,39.5550293912429));
#185639=CARTESIAN_POINT('',(50.8023624963257,36.6746059264508,39.92499));
#185640=CARTESIAN_POINT('',(50.5141111787694,36.4651790860523,39.3548010137695));
#185641=CARTESIAN_POINT('',(48.0191904766741,34.6525130919791,39.92499));
#185642=CARTESIAN_POINT('',(0.111973090561715,-0.154117737428432,39.92499));
#185643=CARTESIAN_POINT('',(48.3074421900769,34.8619402214101,39.3548010137695));
#185644=CARTESIAN_POINT('',(48.0191904766741,34.6525130919791,39.92499));
#185645=CARTESIAN_POINT('',(48.6559784483769,35.1151666347435,39.116));
#185646=CARTESIAN_POINT('Origin',(48.6250489015221,35.0926950035815,39.5550297827322));
#185647=CARTESIAN_POINT('',(48.9807015307826,35.3510917648525,39.116));
#185648=CARTESIAN_POINT('',(49.0404538064758,35.3945043333724,39.116));
#185649=CARTESIAN_POINT('',(49.0826686475739,35.4251752107432,39.3343017080178));
#185650=CARTESIAN_POINT('',(48.9807015312183,35.3510917642528,39.116));
#185651=CARTESIAN_POINT('',(49.3496120513054,35.6191209461246,39.5248017080178));
#185652=CARTESIAN_POINT('Origin',(49.3258045171785,35.6018243948122,39.1947745585601));
#185653=CARTESIAN_POINT('',(49.4719419865737,35.7079988465452,39.5248017080178));
#185654=CARTESIAN_POINT('',(49.4723697227352,35.7083096150572,39.5248017080178));
#185655=CARTESIAN_POINT('',(49.7388853330816,35.9019445403512,39.3343017080178));
#185656=CARTESIAN_POINT('Origin',(49.4957512585809,35.7252979297077,39.194772859431));
#185657=CARTESIAN_POINT('',(49.8408524068608,35.9760279559081,39.116));
#185658=CARTESIAN_POINT('',(49.7388853330816,35.9019445403512,39.3343017080178));
#185659=CARTESIAN_POINT('',(50.165997086493,36.2122593934156,39.116));
#185660=CARTESIAN_POINT('Origin',(50.3626567888879,29.2968639067295,40.10025));
#185661=CARTESIAN_POINT('',(51.1278468659051,29.5010785149105,40.10025));
#185662=CARTESIAN_POINT('',(54.4342359163067,31.4100231232054,40.10025));
#185663=CARTESIAN_POINT('',(50.4655267888879,29.1186878401549,40.10025));
#185664=CARTESIAN_POINT('',(54.4189959163067,31.4364195775128,40.10025));
#185665=CARTESIAN_POINT('Origin',(5.51948237368594E-15,5.62138166151314E-15,
40.10025));
#185666=CARTESIAN_POINT('',(51.1126068659051,29.5274749692178,40.10025));
#185667=CARTESIAN_POINT('',(51.0513762321548,29.4921234463394,40.10025));
#185668=CARTESIAN_POINT('Origin',(5.71307961579125E-15,5.29097839144664E-15,
40.10025));
#185669=CARTESIAN_POINT('Origin',(-0.0952499999999979,0.164977839420937,
1.34128103812637E-17));
#185670=CARTESIAN_POINT('',(51.869470313195,30.1668231006068,39.116));
#185671=CARTESIAN_POINT('',(51.4963740054947,29.9514158469224,39.3548010137695));
#185672=CARTESIAN_POINT('Origin',(51.836361276822,30.1477075895442,39.5550297832805));
#185673=CARTESIAN_POINT('',(51.1878102690448,29.7732664900068,39.92499));
#185674=CARTESIAN_POINT('',(51.4963740054947,29.9514158469224,39.3548010137695));
#185675=CARTESIAN_POINT('',(54.1671020372442,31.4933613949852,39.92499));
#185676=CARTESIAN_POINT('',(54.3920835619875,31.6232545388584,39.92499));
#185677=CARTESIAN_POINT('',(53.8585387246958,31.315212284122,39.3548010137695));
#185678=CARTESIAN_POINT('',(54.1671020372442,31.4933613949852,39.92499));
#185679=CARTESIAN_POINT('',(53.4854427993291,31.0998052504793,39.116));
#185680=CARTESIAN_POINT('Origin',(53.5185519423382,31.1189208231082,39.5550293907202));
#185681=CARTESIAN_POINT('',(53.137837918791,30.8991154799507,39.116));
#185682=CARTESIAN_POINT('',(-0.0952499999999924,0.164977839420937,39.116));
#185683=CARTESIAN_POINT('',(53.028685606085,30.8360963620055,39.3343017080178));
#185684=CARTESIAN_POINT('',(53.1378379191468,30.8991154793345,39.116));
#185685=CARTESIAN_POINT('',(52.7429317578291,30.671116300793,39.5248017080178));
#185686=CARTESIAN_POINT('Origin',(52.7684169058672,30.6858295650758,39.1947747614281));
#185687=CARTESIAN_POINT('',(52.6119816883963,30.5955122429556,39.5248017080178));
#185688=CARTESIAN_POINT('',(-0.0952499999999923,0.164977839420937,39.5248017080178));
#185689=CARTESIAN_POINT('',(52.3262277788845,30.430532146377,39.3343017080178));
#185690=CARTESIAN_POINT('Origin',(52.5864945348652,30.5807966351497,39.1947728911925));
#185691=CARTESIAN_POINT('',(52.217075420246,30.3675130027344,39.116));
#185692=CARTESIAN_POINT('',(52.3262277788845,30.430532146377,39.3343017080178));
#185693=CARTESIAN_POINT('',(-0.0952499999999924,0.164977839420937,39.116));
#185694=CARTESIAN_POINT('Origin',(0.0952499999999979,-0.164977839420937,
-1.34128103812637E-17));
#185695=CARTESIAN_POINT('',(53.675942799329,30.7698495716374,39.116));
#185696=CARTESIAN_POINT('',(54.0490387249983,30.9852566047561,39.3548010137695));
#185697=CARTESIAN_POINT('Origin',(53.7090519420883,30.7889651441222,39.5550293912471));
#185698=CARTESIAN_POINT('',(54.3576020374704,31.1634057157515,39.92499));
#185699=CARTESIAN_POINT('',(54.0490387249983,30.9852566047561,39.3548010137695));
#185700=CARTESIAN_POINT('',(51.3783102687789,29.4433108116255,39.92499));
#185701=CARTESIAN_POINT('',(0.0952499999999987,-0.16497783942094,39.92499));
#185702=CARTESIAN_POINT('',(51.6868740051415,29.6214601686922,39.3548010137695));
#185703=CARTESIAN_POINT('',(51.3783102687789,29.4433108116255,39.92499));
#185704=CARTESIAN_POINT('',(52.059970313195,29.8368674217649,39.116));
#185705=CARTESIAN_POINT('Origin',(52.0268612765588,29.8177519105504,39.5550297827267));
#185706=CARTESIAN_POINT('',(52.4075754198752,30.0375573245348,39.116));
#185707=CARTESIAN_POINT('',(52.4715382154243,30.0744862609068,39.116));
#185708=CARTESIAN_POINT('',(52.5167277788845,30.1005764675351,39.3343017080178));
#185709=CARTESIAN_POINT('',(52.407575420246,30.0375573238925,39.116));
#185710=CARTESIAN_POINT('',(52.8024816883963,30.2655565641137,39.5248017080178));
#185711=CARTESIAN_POINT('Origin',(52.7769965925056,30.2508433300767,39.1947745585566));
#185712=CARTESIAN_POINT('',(52.9334317578291,30.3411606219512,39.5248017080178));
#185713=CARTESIAN_POINT('',(52.9338896349621,30.3414249774371,39.5248017080178));
#185714=CARTESIAN_POINT('',(53.219185606085,30.5061406831637,39.3343017080178));
#185715=CARTESIAN_POINT('Origin',(52.9589188467291,30.3558761923099,39.1947728594246));
#185716=CARTESIAN_POINT('',(53.3283379191468,30.5691598004926,39.116));
#185717=CARTESIAN_POINT('',(53.219185606085,30.5061406831637,39.3343017080178));
#185718=CARTESIAN_POINT('',(53.6763943313417,30.7701102637665,39.116));
#185719=CARTESIAN_POINT('Origin',(53.1491210481986,23.8720415006483,40.10025));
#185720=CARTESIAN_POINT('',(53.9314655730807,23.9951532569801,40.10025));
#185721=CARTESIAN_POINT('',(57.4192809246792,25.5480287005711,40.10025));
#185722=CARTESIAN_POINT('',(53.2328030451451,23.6840886581929,40.10025));
#185723=CARTESIAN_POINT('',(57.4068835917983,25.5758735661201,40.10025));
#185724=CARTESIAN_POINT('Origin',(5.51249664798382E-15,5.6350919201647E-15,
40.10025));
#185725=CARTESIAN_POINT('',(53.9190682401998,24.022998122529,40.10025));
#185726=CARTESIAN_POINT('',(53.8544777939072,23.9942406030427,40.10025));
#185727=CARTESIAN_POINT('Origin',(5.71671684795091E-15,5.28383992139913E-15,
40.10025));
#185728=CARTESIAN_POINT('Origin',(-0.0774833305059378,0.174030409680916,
1.09109629373748E-17));
#185729=CARTESIAN_POINT('',(54.7386155880007,24.5797300649095,39.116));
#185730=CARTESIAN_POINT('',(54.3450469517073,24.4045020183939,39.3548010137695));
#185731=CARTESIAN_POINT('Origin',(54.7036898113993,24.5641801073098,39.5550297832851));
#185732=CARTESIAN_POINT('',(54.0195518811806,24.259582275487,39.92499));
#185733=CARTESIAN_POINT('',(54.3450469517073,24.4045020183939,39.3548010137695));
#185734=CARTESIAN_POINT('',(57.1623216544374,25.6588335304434,39.92499));
#185735=CARTESIAN_POINT('',(57.399648237566,25.7644981330385,39.92499));
#185736=CARTESIAN_POINT('',(56.8368270312096,25.5139139879309,39.3548010137695));
#185737=CARTESIAN_POINT('',(57.1623216544374,25.6588335304434,39.92499));
#185738=CARTESIAN_POINT('',(56.443258798156,25.338686120287,39.116));
#185739=CARTESIAN_POINT('Origin',(56.4781846872468,25.3542361279702,39.5550293907207));
#185740=CARTESIAN_POINT('',(56.0765803402173,25.1754303533066,39.116));
#185741=CARTESIAN_POINT('',(-0.0774833305059323,0.174030409680916,39.116));
#185742=CARTESIAN_POINT('',(55.9614386837456,25.1241659841929,39.3343017080178));
#185743=CARTESIAN_POINT('',(56.0765803405066,25.1754303526568,39.116));
#185744=CARTESIAN_POINT('',(55.6600051127011,24.9899591116489,39.5248017080178));
#185745=CARTESIAN_POINT('Origin',(55.6868886053399,25.0019278517712,39.1947747614349));
#185746=CARTESIAN_POINT('',(55.5218696254676,24.9284572302735,39.5248017080178));
#185747=CARTESIAN_POINT('',(-0.0774833305059322,0.174030409680916,39.5248017080178));
#185748=CARTESIAN_POINT('',(55.2204359898059,24.79425032896,39.3343017080178));
#185749=CARTESIAN_POINT('Origin',(55.4949838933612,24.9164863690989,39.1947728911908));
#185750=CARTESIAN_POINT('',(55.1052942849675,24.7429859390906,39.116));
#185751=CARTESIAN_POINT('',(55.2204359898059,24.79425032896,39.3343017080178));
#185752=CARTESIAN_POINT('',(-0.0774833305059323,0.174030409680916,39.116));
#185753=CARTESIAN_POINT('Origin',(0.0774833305059378,-0.174030409680916,
-1.09109629373748E-17));
#185754=CARTESIAN_POINT('',(56.5982254591679,24.9906253009252,39.116));
#185755=CARTESIAN_POINT('',(56.9917936924676,25.1658531680164,39.3548010137695));
#185756=CARTESIAN_POINT('Origin',(56.633151347996,25.0061753084914,39.5550293912448));
#185757=CARTESIAN_POINT('',(57.317288315633,25.3107727106689,39.92499));
#185758=CARTESIAN_POINT('',(56.9917936924676,25.1658531680164,39.3548010137695));
#185759=CARTESIAN_POINT('',(54.1745185419763,23.9115214566108,39.92499));
#185760=CARTESIAN_POINT('',(0.0774833305059383,-0.174030409680919,39.92499));
#185761=CARTESIAN_POINT('',(54.5000136124317,24.0564411996777,39.3548010137695));
#185762=CARTESIAN_POINT('',(54.1745185419763,23.9115214566108,39.92499));
#185763=CARTESIAN_POINT('',(54.8935822490125,24.2316692455476,39.116));
#185764=CARTESIAN_POINT('Origin',(54.858656472133,24.2161192878242,39.5550297827294));
#185765=CARTESIAN_POINT('',(55.2602609456778,24.3949251204062,39.116));
#185766=CARTESIAN_POINT('',(55.3277334713093,24.4249658234759,39.116));
#185767=CARTESIAN_POINT('',(55.3754026508178,24.4461895095982,39.3343017080178));
#185768=CARTESIAN_POINT('',(55.2602609459794,24.3949251197288,39.116));
#185769=CARTESIAN_POINT('',(55.6768362864795,24.5803964109116,39.5248017080178));
#185770=CARTESIAN_POINT('Origin',(55.6499528488663,24.5684276954194,39.1947745585578));
#185771=CARTESIAN_POINT('',(55.814971773713,24.641898292287,39.5248017080178));
#185772=CARTESIAN_POINT('',(55.8154547752198,24.6421133384129,39.5248017080178));
#185773=CARTESIAN_POINT('',(56.1164053447575,24.776105164831,39.3343017080178));
#185774=CARTESIAN_POINT('Origin',(55.8418574376285,24.6538691229756,39.1947728594241));
#185775=CARTESIAN_POINT('',(56.2315470015185,24.827369533295,39.116));
#185776=CARTESIAN_POINT('',(56.1164053447575,24.776105164831,39.3343017080178));
#185777=CARTESIAN_POINT('',(56.5987017673886,24.9908373670081,39.116));
#185778=CARTESIAN_POINT('Origin',(55.3532724151367,18.1856720123401,40.10025));
#185779=CARTESIAN_POINT('',(56.144199857553,18.2263320786575,40.10025));
#185780=CARTESIAN_POINT('',(59.7752282754839,19.4061247292246,40.10025));
#185781=CARTESIAN_POINT('',(55.4168495715594,17.9900016446776,40.10025));
#185782=CARTESIAN_POINT('',(59.7658094374954,19.4351129318413,40.10025));
#185783=CARTESIAN_POINT('Origin',(5.50698230308587E-15,5.64945727975729E-15,
40.10025));
#185784=CARTESIAN_POINT('',(56.1347810195644,18.2553202812742,40.10025));
#185785=CARTESIAN_POINT('',(56.0675384271755,18.2334718385813,40.10025));
#185786=CARTESIAN_POINT('Origin',(5.71958798166808E-15,5.27636036234925E-15,
40.10025));
#185787=CARTESIAN_POINT('Origin',(-0.0588677374284251,0.181176266354228,
8.28957270027824E-18));
#185788=CARTESIAN_POINT('',(57.0080331356325,18.7233363629817,39.116));
#185789=CARTESIAN_POINT('',(56.5983041910848,18.5902073587815,39.3548010137695));
#185790=CARTESIAN_POINT('Origin',(56.9716732729192,18.7115223274338,39.5550297832882));
#185791=CARTESIAN_POINT('',(56.2594439785883,18.4801050009129,39.92499));
#185792=CARTESIAN_POINT('',(56.5983041910848,18.5902073587815,39.3548010137695));
#185793=CARTESIAN_POINT('',(59.5312589135998,19.5431821162859,39.92499));
#185794=CARTESIAN_POINT('',(59.7783303554051,19.6234604941051,39.92499));
#185795=CARTESIAN_POINT('',(59.1923991668989,19.433079910958,39.3548010137695));
#185796=CARTESIAN_POINT('',(59.5312589135998,19.5431821162859,39.92499));
#185797=CARTESIAN_POINT('',(58.7826706420791,19.2999510424999,39.116));
#185798=CARTESIAN_POINT('Origin',(58.8190306219008,19.3117651160986,39.5550293907231));
#185799=CARTESIAN_POINT('',(58.4009360126571,19.1759179434146,39.116));
#185800=CARTESIAN_POINT('',(-0.0588677374284196,0.181176266354228,39.116));
#185801=CARTESIAN_POINT('',(58.2810665285032,19.1369699862876,39.3343017080178));
#185802=CARTESIAN_POINT('',(58.4009360128769,19.1759179427379,39.116));
#185803=CARTESIAN_POINT('',(57.9672558039534,19.0350067009923,39.5248017080178));
#185804=CARTESIAN_POINT('Origin',(57.9952431000171,19.0440997849305,39.1947747614319));
#185805=CARTESIAN_POINT('',(57.8234483402241,18.9882808235613,39.5248017080178));
#185806=CARTESIAN_POINT('',(-0.0588677374284196,0.181176266354228,39.5248017080178));
#185807=CARTESIAN_POINT('',(57.5096375484039,18.8863175164085,39.3343017080178));
#185808=CARTESIAN_POINT('Origin',(57.7954585952484,18.9791858642776,39.1947728911916));
#185809=CARTESIAN_POINT('',(57.3897680139787,18.8473695436955,39.116));
#185810=CARTESIAN_POINT('',(57.5096375484039,18.8863175164085,39.3343017080178));
#185811=CARTESIAN_POINT('',(-0.0588677374284196,0.181176266354228,39.116));
#185812=CARTESIAN_POINT('Origin',(0.0588677374284251,-0.181176266354228,
-8.28957270027824E-18));
#185813=CARTESIAN_POINT('',(58.9004061169359,18.9375985097914,39.116));
#185814=CARTESIAN_POINT('',(59.3101346419426,19.0707273776745,39.3548010137695));
#185815=CARTESIAN_POINT('Origin',(58.9367660964832,18.949412583301,39.5550293912495));
#185816=CARTESIAN_POINT('',(59.6489943885965,19.180829583147,39.92499));
#185817=CARTESIAN_POINT('',(59.3101346419426,19.0707273776745,39.3548010137695));
#185818=CARTESIAN_POINT('',(56.377179453281,18.1177524687099,39.92499));
#185819=CARTESIAN_POINT('',(0.0588677374284254,-0.181176266354229,39.92499));
#185820=CARTESIAN_POINT('',(56.7160396657233,18.2278548267449,39.3548010137695));
#185821=CARTESIAN_POINT('',(56.377179453281,18.1177524687099,39.92499));
#185822=CARTESIAN_POINT('',(57.1257686104893,18.3609838302733,39.116));
#185823=CARTESIAN_POINT('Origin',(57.0894087474837,18.3491697946304,39.5550297827266));
#185824=CARTESIAN_POINT('',(57.5075034886064,18.4850170116922,39.116));
#185825=CARTESIAN_POINT('',(57.5777465012101,18.5078403492302,39.116));
#185826=CARTESIAN_POINT('',(57.6273730232608,18.5239649837,39.3343017080178));
#185827=CARTESIAN_POINT('',(57.5075034888355,18.485017010987,39.116));
#185828=CARTESIAN_POINT('',(57.941183815081,18.6259282908529,39.5248017080178));
#185829=CARTESIAN_POINT('Origin',(57.9131965763113,18.6168352256566,39.194774558563));
#185830=CARTESIAN_POINT('',(58.0849912788103,18.6726541682838,39.5248017080178));
#185831=CARTESIAN_POINT('',(58.0854941128254,18.6728175489593,39.5248017080178));
#185832=CARTESIAN_POINT('',(58.3988020033601,18.7746174535792,39.3343017080178));
#185833=CARTESIAN_POINT('Origin',(58.1129809527781,18.6817491043752,39.1947728594169));
#185834=CARTESIAN_POINT('',(58.5186714877338,18.8135654100295,39.116));
#185835=CARTESIAN_POINT('',(58.3988020033601,18.7746174535792,39.3343017080178));
#185836=CARTESIAN_POINT('',(58.9009019828321,18.9377596263878,39.116));
#185837=CARTESIAN_POINT('Origin',(56.9509617460776,12.3000564958682,40.10025));
#185838=CARTESIAN_POINT('',(57.7418065394567,12.257819391976,40.10025));
#185839=CARTESIAN_POINT('',(61.4762657165317,13.0516031943521,40.10025));
#185840=CARTESIAN_POINT('',(56.9937374973465,12.0988124084933,40.10025));
#185841=CARTESIAN_POINT('',(61.4699285681956,13.0814171332224,40.10025));
#185842=CARTESIAN_POINT('Origin',(5.50299975530876E-15,5.66432035040507E-15,
40.10025));
#185843=CARTESIAN_POINT('',(57.7354693911206,12.2876333308464,40.10025));
#185844=CARTESIAN_POINT('',(57.666311376549,12.2729333410571,40.10025));
#185845=CARTESIAN_POINT('Origin',(5.72166156020094E-15,5.26862166191115E-15,
40.10025));
#185846=CARTESIAN_POINT('Origin',(-0.0396071771007808,0.18633711793979,
5.57736016997284E-18));
#185847=CARTESIAN_POINT('',(58.6528587425324,12.6618058697512,39.116));
#185848=CARTESIAN_POINT('',(58.2314585657882,12.5722344970953,39.3548010137695));
#185849=CARTESIAN_POINT('Origin',(58.6154631599691,12.6538571932999,39.5550297832851));
#185850=CARTESIAN_POINT('',(57.8829458347212,12.4981558287379,39.92499));
#185851=CARTESIAN_POINT('',(58.2314585657882,12.5722344970953,39.3548010137695));
#185852=CARTESIAN_POINT('',(61.2479592423879,13.2134115091886,39.92499));
#185853=CARTESIAN_POINT('',(61.5020685764506,13.2674241155252,39.92499));
#185854=CARTESIAN_POINT('',(60.8994469905094,13.1393329438488,39.3548010137695));
#185855=CARTESIAN_POINT('',(61.2479592423879,13.2134115091886,39.92499));
#185856=CARTESIAN_POINT('',(60.4780472453829,13.0497616623167,39.116));
#185857=CARTESIAN_POINT('Origin',(60.5154429483898,13.0577103643691,39.5550293907213));
#185858=CARTESIAN_POINT('',(60.0854388089607,12.9663101637158,39.116));
#185859=CARTESIAN_POINT('',(-0.0396071771007753,0.18633711793979,39.116));
#185860=CARTESIAN_POINT('',(59.9621548122773,12.9401053405442,39.3343017080178));
#185861=CARTESIAN_POINT('',(60.0854388091086,12.9663101630196,39.116));
#185862=CARTESIAN_POINT('',(59.6394051101895,12.8715027735884,39.5248017080178));
#185863=CARTESIAN_POINT('Origin',(59.6681895750054,12.8776205756125,39.1947747614281));
#185864=CARTESIAN_POINT('',(59.4915012546306,12.8400648385931,39.5248017080178));
#185865=CARTESIAN_POINT('',(-0.0396071771007752,0.18633711793979,39.5248017080178));
#185866=CARTESIAN_POINT('',(59.1687514833562,12.7714622569312,39.3343017080178));
#185867=CARTESIAN_POINT('Origin',(59.4627141582885,12.8339454274774,39.194772891192));
#185868=CARTESIAN_POINT('',(59.0454674350476,12.745257423514,39.116));
#185869=CARTESIAN_POINT('',(59.1687514833562,12.7714622569312,39.3343017080178));
#185870=CARTESIAN_POINT('',(-0.0396071771007753,0.18633711793979,39.116));
#185871=CARTESIAN_POINT('Origin',(0.0396071771007808,-0.18633711793979,
-5.57736016997284E-18));
#185872=CARTESIAN_POINT('',(60.5572615995845,12.6770874264371,39.116));
#185873=CARTESIAN_POINT('',(60.9786613448369,12.7666587073766,39.3548010137695));
#185874=CARTESIAN_POINT('Origin',(60.5946573023102,12.6850361284297,39.5550293912459));
#185875=CARTESIAN_POINT('',(61.3271735966836,12.8407372728665,39.92499));
#185876=CARTESIAN_POINT('',(60.9786613448369,12.7666587073766,39.3548010137695));
#185877=CARTESIAN_POINT('',(57.9621601888122,12.1254815933784,39.92499));
#185878=CARTESIAN_POINT('',(0.0396071771007809,-0.186337117939792,39.92499));
#185879=CARTESIAN_POINT('',(58.3106729198429,12.1995602619065,39.3548010137695));
#185880=CARTESIAN_POINT('',(57.9621601888122,12.1254815933784,39.92499));
#185881=CARTESIAN_POINT('',(58.7320730967339,12.2891316338716,39.116));
#185882=CARTESIAN_POINT('Origin',(58.6946775138724,12.2811829573569,39.5550297827283));
#185883=CARTESIAN_POINT('',(59.124681789095,12.3725831883596,39.116));
#185884=CARTESIAN_POINT('',(59.1969256915255,12.3879391031039,39.116));
#185885=CARTESIAN_POINT('',(59.2479658375578,12.3987880210516,39.3343017080178));
#185886=CARTESIAN_POINT('',(59.1246817892492,12.3725831876344,39.116));
#185887=CARTESIAN_POINT('',(59.5707156088322,12.4673906027135,39.5248017080178));
#185888=CARTESIAN_POINT('Origin',(59.5419312029547,12.4612728133398,39.1947745585609));
#185889=CARTESIAN_POINT('',(59.7186194643911,12.4988285377088,39.5248017080178));
#185890=CARTESIAN_POINT('',(59.7191366217598,12.498938462901,39.5248017080178));
#185891=CARTESIAN_POINT('',(60.0413691664789,12.5674311046646,39.3343017080178));
#185892=CARTESIAN_POINT('Origin',(59.7474064876886,12.5049479331813,39.1947728594153));
#185893=CARTESIAN_POINT('',(60.1646531633102,12.59363592714,39.116));
#185894=CARTESIAN_POINT('',(60.0413691664789,12.5674311046646,39.3343017080178));
#185895=CARTESIAN_POINT('',(60.5577715903456,12.6771958283198,39.116));
#185896=CARTESIAN_POINT('Origin',(57.9246844223736,6.27967898647528,40.10025));
#185897=CARTESIAN_POINT('',(58.7067819056644,6.15500747092236,40.10025));
#185898=CARTESIAN_POINT('',(62.5037563256536,6.55408556365861,40.10025));
#185899=CARTESIAN_POINT('',(57.9461901084063,6.07506605172221,40.10025));
#185900=CARTESIAN_POINT('',(62.5005702980932,6.58439859102944,40.10025));
#185901=CARTESIAN_POINT('Origin',(5.50059263827931E-15,5.67951828919572E-15,
40.10025));
#185902=CARTESIAN_POINT('',(58.703595878104,6.18532049829319,40.10025));
#185903=CARTESIAN_POINT('',(58.6332801510296,6.17793001757189,40.10025));
#185904=CARTESIAN_POINT('Origin',(5.72291486498914E-15,5.26070860690626E-15,
40.10025));
#185905=CARTESIAN_POINT('Origin',(-0.0199126722524855,0.189456421067656,
2.80404091450755E-18));
#185906=CARTESIAN_POINT('',(59.6550713551494,6.46154998175838,39.116));
#185907=CARTESIAN_POINT('',(59.2266168947287,6.4165176033497,39.3548010137695));
#185908=CARTESIAN_POINT('Origin',(59.6170497665651,6.45755375176664,39.5550297832836));
#185909=CARTESIAN_POINT('',(58.8722700235037,6.37927424589616,39.92499));
#185910=CARTESIAN_POINT('',(59.2266168947287,6.4165176033497,39.3548010137695));
#185911=CARTESIAN_POINT('',(62.293614112757,6.73887200051248,39.92499));
#185912=CARTESIAN_POINT('',(62.5519772640373,6.76602706194862,39.92499));
#185913=CARTESIAN_POINT('',(61.9392677288637,6.70162869542306,39.3548010137695));
#185914=CARTESIAN_POINT('',(62.293614112757,6.73887200051248,39.92499));
#185915=CARTESIAN_POINT('',(61.5108137072213,6.656596362523,39.116));
#185916=CARTESIAN_POINT('Origin',(61.5488354182638,6.66059260538561,39.5550293907231));
#185917=CARTESIAN_POINT('',(61.1116329639869,6.61464077648856,39.116));
#185918=CARTESIAN_POINT('',(-0.0199126722524799,0.189456421067656,39.116));
#185919=CARTESIAN_POINT('',(60.9862851800405,6.60146619279864,39.3343017080178));
#185920=CARTESIAN_POINT('',(61.1116329640613,6.6146407757804,39.116));
#185921=CARTESIAN_POINT('',(60.6581326136905,6.56697596826196,39.5248017080178));
#185922=CARTESIAN_POINT('Origin',(60.6873988786453,6.57005146045368,39.1947747614359));
#185923=CARTESIAN_POINT('',(60.5077528318945,6.55117041629687,39.5248017080178));
#185924=CARTESIAN_POINT('',(-0.0199126722524799,0.189456421067656,39.5248017080178));
#185925=CARTESIAN_POINT('',(60.1796001951996,6.51668018436665,39.3343017080178));
#185926=CARTESIAN_POINT('Origin',(60.4784837816392,6.54809359889824,39.1947728911902));
#185927=CARTESIAN_POINT('',(60.0542523588398,6.50350559588384,39.116));
#185928=CARTESIAN_POINT('',(60.1796001951996,6.51668018436665,39.3343017080178));
#185929=CARTESIAN_POINT('',(-0.0199126722524799,0.189456421067656,39.116));
#185930=CARTESIAN_POINT('Origin',(0.0199126722524855,-0.189456421067656,
-2.80404091450755E-18));
#185931=CARTESIAN_POINT('',(61.5506390517263,6.27768352038769,39.116));
#185932=CARTESIAN_POINT('',(61.979093073432,6.32271585268557,39.3548010137695));
#185933=CARTESIAN_POINT('Origin',(61.5886607624852,6.2816797632205,39.5550293912434));
#185934=CARTESIAN_POINT('',(62.3334394573093,6.35995915792716,39.92499));
#185935=CARTESIAN_POINT('',(61.979093073432,6.32271585268557,39.3548010137695));
#185936=CARTESIAN_POINT('',(58.9120953679531,6.00036140428966,39.92499));
#185937=CARTESIAN_POINT('',(0.0199126722524855,-0.189456421067657,39.92499));
#185938=CARTESIAN_POINT('',(59.2664422391598,6.03760476191703,39.3548010137695));
#185939=CARTESIAN_POINT('',(58.9120953679531,6.00036140428966,39.92499));
#185940=CARTESIAN_POINT('',(59.6948966996543,6.08263713962306,39.116));
#185941=CARTESIAN_POINT('Origin',(59.6568751107691,6.0786409095997,39.5550297827316));
#185942=CARTESIAN_POINT('',(60.0940777032672,6.12459275448621,39.116));
#185943=CARTESIAN_POINT('',(60.1675309762116,6.13231300382095,39.116));
#185944=CARTESIAN_POINT('',(60.2194255397046,6.13776734223133,39.3343017080178));
#185945=CARTESIAN_POINT('',(60.0940777033448,6.12459275374853,39.116));
#185946=CARTESIAN_POINT('',(60.5475781763994,6.17225757416155,39.5248017080178));
#185947=CARTESIAN_POINT('Origin',(60.5183119713874,6.16918208839056,39.1947745585607));
#185948=CARTESIAN_POINT('',(60.6979579581955,6.18806312612664,39.5248017080178));
#185949=CARTESIAN_POINT('',(60.6984837728334,6.18811839147206,39.5248017080178));
#185950=CARTESIAN_POINT('',(61.0261105245455,6.22255335066333,39.3343017080178));
#185951=CARTESIAN_POINT('Origin',(60.7272269341789,6.19113993560376,39.194772859427));
#185952=CARTESIAN_POINT('',(61.1514583085663,6.23572793364508,39.116));
#185953=CARTESIAN_POINT('',(61.0261105245455,6.22255335066333,39.3343017080178));
#185954=CARTESIAN_POINT('',(61.5511575797869,6.27773801988296,39.116));
#185955=CARTESIAN_POINT('Origin',(57.9430040808458,-6.10537907909383,39.92499));
#185956=CARTESIAN_POINT('Ctrl Pts',(62.2936141127569,-6.73887200051333,
39.92499));
#185957=CARTESIAN_POINT('Ctrl Pts',(62.3041663177862,-6.7399810819533,39.9348354642028));
#185958=CARTESIAN_POINT('Ctrl Pts',(62.3147747227683,-6.74025426844094,
39.9446440828477));
#185959=CARTESIAN_POINT('Ctrl Pts',(62.3253809467545,-6.73970068257582,
39.9543641760359));
#185960=CARTESIAN_POINT('Ctrl Pts',(62.3356425316169,-6.73916508495494,
39.9637684240747));
#185961=CARTESIAN_POINT('Ctrl Pts',(62.3459033574861,-6.737855436376,39.9730909636437));
#185962=CARTESIAN_POINT('Ctrl Pts',(62.3561113603689,-6.73573381164702,
39.9822808977187));
#185963=CARTESIAN_POINT('Ctrl Pts',(62.3657675025234,-6.73372688529553,
39.99097400947));
#185964=CARTESIAN_POINT('Ctrl Pts',(62.3753772873532,-6.73099321743661,
39.9995492765056));
#185965=CARTESIAN_POINT('Ctrl Pts',(62.3848821415168,-6.72746117704375,
40.0079462328753));
#185966=CARTESIAN_POINT('Ctrl Pts',(62.3936367996101,-6.72420791239824,
40.0156804369753));
#185967=CARTESIAN_POINT('Ctrl Pts',(62.4023029415068,-6.72027708243395,
40.0232638017489));
#185968=CARTESIAN_POINT('Ctrl Pts',(62.4108128192462,-6.71558140885914,
40.0306257270037));
#185969=CARTESIAN_POINT('Ctrl Pts',(62.4132812112908,-6.71421937245263,
40.0327611416698));
#185970=CARTESIAN_POINT('Ctrl Pts',(62.4157362792982,-6.71279278199377,
40.0348777427294));
#185971=CARTESIAN_POINT('Ctrl Pts',(62.4181758915949,-6.71129899689598,
40.0369733168701));
#185972=CARTESIAN_POINT('Ctrl Pts',(62.4208205881801,-6.70967963780669,
40.039245053974));
#185973=CARTESIAN_POINT('Ctrl Pts',(62.4234440047029,-6.70798448411175,
40.041487875195));
#185974=CARTESIAN_POINT('Ctrl Pts',(62.4260429761973,-6.70621108803123,
40.04369857016));
#185975=CARTESIAN_POINT('Ctrl Pts',(62.4331758738576,-6.70134398857268,
40.0497658398386));
#185976=CARTESIAN_POINT('Ctrl Pts',(62.4400912556838,-6.69585818364696,
40.0555581699984));
#185977=CARTESIAN_POINT('Ctrl Pts',(62.4466864116142,-6.6897680133389,40.0609828468886));
#185978=CARTESIAN_POINT('Ctrl Pts',(62.4527206212313,-6.68419583814993,
40.0659461317306));
#185979=CARTESIAN_POINT('Ctrl Pts',(62.4584752900418,-6.67811620689287,
40.0706039980709));
#185980=CARTESIAN_POINT('Ctrl Pts',(62.4638645712592,-6.67150703079124,
40.0748843180607));
#185981=CARTESIAN_POINT('Ctrl Pts',(62.466511768588,-6.66826062508022,40.0769867972572));
#185982=CARTESIAN_POINT('Ctrl Pts',(62.4690703232302,-6.66488629457962,
40.0789976708176));
#185983=CARTESIAN_POINT('Ctrl Pts',(62.4715267736418,-6.66138078591716,
40.08090504915));
#185984=CARTESIAN_POINT('Ctrl Pts',(62.4719928611813,-6.66071564979253,
40.0812669556105));
#185985=CARTESIAN_POINT('Ctrl Pts',(62.472455189938,-6.66004526560994,40.0816253922033));
#185986=CARTESIAN_POINT('Ctrl Pts',(62.4729136358129,-6.65936969820862,
40.081980198914));
#185987=CARTESIAN_POINT('Ctrl Pts',(62.4733577552542,-6.6587152422886,40.082323917915));
#185988=CARTESIAN_POINT('Ctrl Pts',(62.4737982306999,-6.65805592206456,
40.0826642303499));
#185989=CARTESIAN_POINT('Ctrl Pts',(62.4742349489459,-6.65739180030914,
40.08300099161));
#185990=CARTESIAN_POINT('Ctrl Pts',(62.4789942144022,-6.65015433826465,
40.086670946431));
#185991=CARTESIAN_POINT('Ctrl Pts',(62.4833100626573,-6.64234165497574,
40.0899175831873));
#185992=CARTESIAN_POINT('Ctrl Pts',(62.4870273554119,-6.63406423386325,
40.0925642067057));
#185993=CARTESIAN_POINT('Ctrl Pts',(62.4885971912258,-6.63056862752634,
40.0936818922524));
#185994=CARTESIAN_POINT('Ctrl Pts',(62.4900605069388,-6.62699051141436,
40.0946930094789));
#185995=CARTESIAN_POINT('Ctrl Pts',(62.4914070226221,-6.62333954252002,
40.0955863397546));
#185996=CARTESIAN_POINT('Ctrl Pts',(62.4936745213867,-6.61719140213073,
40.0970906856167));
#185997=CARTESIAN_POINT('Ctrl Pts',(62.4956084911391,-6.61083770188526,
40.0982599215483));
#185998=CARTESIAN_POINT('Ctrl Pts',(62.4971561593216,-6.6043306253614,40.0990497370454));
#185999=CARTESIAN_POINT('Ctrl Pts',(62.4975430763672,-6.60270385623043,
40.0992471909196));
#186000=CARTESIAN_POINT('Ctrl Pts',(62.4979056188877,-6.60106746196549,
40.0994209989363));
#186001=CARTESIAN_POINT('Ctrl Pts',(62.4982426563689,-6.59942221845739,
40.0995705982975));
#186002=CARTESIAN_POINT('Ctrl Pts',(62.4987482125908,-6.59695435319524,
40.0997949973393));
#186003=CARTESIAN_POINT('Ctrl Pts',(62.4991963674669,-6.59446659126598,
40.0999649129781));
#186004=CARTESIAN_POINT('Ctrl Pts',(62.4995849724118,-6.59196174500292,
40.1000786629733));
#186005=CARTESIAN_POINT('Ctrl Pts',(62.4999735773567,-6.58945689873986,
40.1001924129685));
#186006=CARTESIAN_POINT('Ctrl Pts',(62.5003026407462,-6.5869349761765,40.10025));
#186007=CARTESIAN_POINT('Ctrl Pts',(62.5005702980931,-6.58439859103029,
40.10025));
#186008=CARTESIAN_POINT('Ctrl Pts',(58.7035958781039,-6.18532049829399,
40.10025));
#186009=CARTESIAN_POINT('Ctrl Pts',(58.7026899760169,-6.19390281910185,
40.10025));
#186010=CARTESIAN_POINT('Ctrl Pts',(58.7025003609928,-6.20248552904425,
40.099578633424));
#186011=CARTESIAN_POINT('Ctrl Pts',(58.7029569544314,-6.21093474935507,
40.0983063763365));
#186012=CARTESIAN_POINT('Ctrl Pts',(58.7032518669435,-6.21639207873545,
40.0974846287991));
#186013=CARTESIAN_POINT('Ctrl Pts',(58.7038154335199,-6.22179377937535,
40.0964130309337));
#186014=CARTESIAN_POINT('Ctrl Pts',(58.7046202140516,-6.22710604846857,
40.0951176960923));
#186015=CARTESIAN_POINT('Ctrl Pts',(58.7056869045458,-6.23414715684634,
40.0934008039614));
#186016=CARTESIAN_POINT('Ctrl Pts',(58.7071827955652,-6.24102913891637,
40.0912909372156));
#186017=CARTESIAN_POINT('Ctrl Pts',(58.7090548163569,-6.24767922440741,
40.0888630467851));
#186018=CARTESIAN_POINT('Ctrl Pts',(58.7099908267528,-6.25100426715293,
40.0876491015699));
#186019=CARTESIAN_POINT('Ctrl Pts',(58.7110208470228,-6.25427153376657,
40.0863558569271));
#186020=CARTESIAN_POINT('Ctrl Pts',(58.7121380880307,-6.25747333351513,
40.0849936342771));
#186021=CARTESIAN_POINT('Ctrl Pts',(58.7126967085347,-6.25907423338942,
40.0843125229521));
#186022=CARTESIAN_POINT('Ctrl Pts',(58.7132771324571,-6.26065878288339,
40.0836141747074));
#186023=CARTESIAN_POINT('Ctrl Pts',(58.7138784999415,-6.26222612320511,
40.0828999161609));
#186024=CARTESIAN_POINT('Ctrl Pts',(58.7140288418127,-6.26261795828554,
40.0827213515243));
#186025=CARTESIAN_POINT('Ctrl Pts',(58.7141804926178,-6.26300871814006,
40.0825417925841));
#186026=CARTESIAN_POINT('Ctrl Pts',(58.7143334388436,-6.2633983900505,40.082361260236));
#186027=CARTESIAN_POINT('Ctrl Pts',(58.7147922775208,-6.26456740578181,
40.0818196631917));
#186028=CARTESIAN_POINT('Ctrl Pts',(58.715262775183,-6.26572662828366,40.0812693052021));
#186029=CARTESIAN_POINT('Ctrl Pts',(58.7157445651924,-6.26687572965161,
40.0807107531874));
#186030=CARTESIAN_POINT('Ctrl Pts',(58.7191382318078,-6.27496985131128,
40.0767763849182));
#186031=CARTESIAN_POINT('Ctrl Pts',(58.7230632421217,-6.28260716192743,
40.0724140586138));
#186032=CARTESIAN_POINT('Ctrl Pts',(58.7274000190312,-6.2897833958941,40.067722122377));
#186033=CARTESIAN_POINT('Ctrl Pts',(58.729503351146,-6.2932638616134,40.0654465383722));
#186034=CARTESIAN_POINT('Ctrl Pts',(58.731704109697,-6.29663597408912,40.063092800068));
#186035=CARTESIAN_POINT('Ctrl Pts',(58.7339915094194,-6.29989941779144,
40.0606689262479));
#186036=CARTESIAN_POINT('Ctrl Pts',(58.7374933585782,-6.30489552208934,
40.0569581447805));
#186037=CARTESIAN_POINT('Ctrl Pts',(58.7411954596217,-6.30963480180868,
40.0530843804605));
#186038=CARTESIAN_POINT('Ctrl Pts',(58.745053462885,-6.31410463171043,40.0490800251458));
#186039=CARTESIAN_POINT('Ctrl Pts',(58.7468451395591,-6.31618044384063,
40.0472203818218));
#186040=CARTESIAN_POINT('Ctrl Pts',(58.7486702031823,-6.31819823791525,
40.0453323608818));
#186041=CARTESIAN_POINT('Ctrl Pts',(58.7505249478605,-6.32015576082315,
40.0434201572162));
#186042=CARTESIAN_POINT('Ctrl Pts',(58.750667106732,-6.32030579724101,40.0432735943397));
#186043=CARTESIAN_POINT('Ctrl Pts',(58.7508094261759,-6.32045551058188,
40.0431268995707));
#186044=CARTESIAN_POINT('Ctrl Pts',(58.7509519047346,-6.32060490093997,
40.0429800745037));
#186045=CARTESIAN_POINT('Ctrl Pts',(58.7529532989256,-6.32270338507381,
40.0409176249753));
#186046=CARTESIAN_POINT('Ctrl Pts',(58.7549876922215,-6.32473679726626,
40.0388310783332));
#186047=CARTESIAN_POINT('Ctrl Pts',(58.757049379421,-6.32670504964984,40.036725739981));
#186048=CARTESIAN_POINT('Ctrl Pts',(58.7644422230598,-6.33376285265574,
40.0291763710714));
#186049=CARTESIAN_POINT('Ctrl Pts',(58.7722418109928,-6.34003880538934,
40.0213310894588));
#186050=CARTESIAN_POINT('Ctrl Pts',(58.7803396486561,-6.34560292136761,
40.013283755131));
#186051=CARTESIAN_POINT('Ctrl Pts',(58.7892383587482,-6.35171732586278,
40.004440543131));
#186052=CARTESIAN_POINT('Ctrl Pts',(58.7984976730914,-6.35697262978531,
39.9953528710581));
#186053=CARTESIAN_POINT('Ctrl Pts',(58.8080148760673,-6.36142852992911,
39.9861103629531));
#186054=CARTESIAN_POINT('Ctrl Pts',(58.8182910667897,-6.36623978380624,
39.9761307737523));
#186055=CARTESIAN_POINT('Ctrl Pts',(58.8288688921894,-6.37011968263873,
39.9659696935969));
#186056=CARTESIAN_POINT('Ctrl Pts',(58.8396533761932,-6.37309732669947,
39.9557128217455));
#186057=CARTESIAN_POINT('Ctrl Pts',(58.8503473894546,-6.37604999138532,
39.9455419945126));
#186058=CARTESIAN_POINT('Ctrl Pts',(58.861246040348,-6.37811557911247,39.9352756289323));
#186059=CARTESIAN_POINT('Ctrl Pts',(58.872270023448,-6.37927424642578,39.92499));
#186060=CARTESIAN_POINT('Origin',(0.00159301378019908,0.0151565136854131,
39.92499));
#186061=CARTESIAN_POINT('Ctrl Pts',(62.5037563256535,-6.55408556365946,
40.10025));
#186062=CARTESIAN_POINT('Ctrl Pts',(62.5046505412978,-6.54554330587368,
40.10025));
#186063=CARTESIAN_POINT('Ctrl Pts',(62.5048232320879,-6.53700226086583,
40.0995859581841));
#186064=CARTESIAN_POINT('Ctrl Pts',(62.5043472028589,-6.52859457177331,
40.0983275959619));
#186065=CARTESIAN_POINT('Ctrl Pts',(62.5040430428431,-6.52322245869402,
40.0975235624066));
#186066=CARTESIAN_POINT('Ctrl Pts',(62.5034749678471,-6.5179047148956,40.0964777059489));
#186067=CARTESIAN_POINT('Ctrl Pts',(62.5026702669707,-6.5126735674084,40.095214991596));
#186068=CARTESIAN_POINT('Ctrl Pts',(62.5015720117389,-6.50553410072647,
40.0934916398701));
#186069=CARTESIAN_POINT('Ctrl Pts',(62.5000273428098,-6.49855818190772,
40.091364392163));
#186070=CARTESIAN_POINT('Ctrl Pts',(62.4980940659029,-6.49182203260176,
40.0889118607712));
#186071=CARTESIAN_POINT('Ctrl Pts',(62.4971274274495,-6.48845395794878,
40.0876855950754));
#186072=CARTESIAN_POINT('Ctrl Pts',(62.4960636607366,-6.48514561818735,
40.0863782327526));
#186073=CARTESIAN_POINT('Ctrl Pts',(62.494910155573,-6.48190505740164,40.0850006373333));
#186074=CARTESIAN_POINT('Ctrl Pts',(62.4943334029912,-6.48028477700878,
40.0843118396237));
#186075=CARTESIAN_POINT('Ctrl Pts',(62.4937342176673,-6.47868142404681,
40.0836054919164));
#186076=CARTESIAN_POINT('Ctrl Pts',(62.4931135352114,-6.47709589524266,
40.0828829920417));
#186077=CARTESIAN_POINT('Ctrl Pts',(62.4929583645974,-6.47669951304162,
40.0827023670731));
#186078=CARTESIAN_POINT('Ctrl Pts',(62.4928018504535,-6.47630424448174,
40.0825207326932));
#186079=CARTESIAN_POINT('Ctrl Pts',(62.4926440074816,-6.47591010283074,
40.0823381109275));
#186080=CARTESIAN_POINT('Ctrl Pts',(62.4921704785661,-6.47472767787775,
40.0817902456303));
#186081=CARTESIAN_POINT('Ctrl Pts',(62.4916849899864,-6.47355539694469,
40.0812334935553));
#186082=CARTESIAN_POINT('Ctrl Pts',(62.4911879405752,-6.47239360181811,
40.0806684524227));
#186083=CARTESIAN_POINT('Ctrl Pts',(62.4877530207469,-6.46436487665163,
40.0767636676136));
#186084=CARTESIAN_POINT('Ctrl Pts',(62.4837949925046,-6.45678933786372,
40.0724404510887));
#186085=CARTESIAN_POINT('Ctrl Pts',(62.4794326364364,-6.4496685356396,40.0677949937407));
#186086=CARTESIAN_POINT('Ctrl Pts',(62.4772645574451,-6.4461295164806,40.0654862141904));
#186087=CARTESIAN_POINT('Ctrl Pts',(62.474996003895,-6.44270272394338,40.0630972003215));
#186088=CARTESIAN_POINT('Ctrl Pts',(62.4726384024734,-6.43938822718924,
40.0606363359906));
#186089=CARTESIAN_POINT('Ctrl Pts',(62.4674371815967,-6.43207595228354,
40.0552073017123));
#186090=CARTESIAN_POINT('Ctrl Pts',(62.461813233051,-6.4253038174399,40.0494204304519));
#186091=CARTESIAN_POINT('Ctrl Pts',(62.4558957623411,-6.41913840445425,
40.0434049749851));
#186092=CARTESIAN_POINT('Ctrl Pts',(62.4537340356675,-6.41688610134064,
40.0412074532442));
#186093=CARTESIAN_POINT('Ctrl Pts',(62.4515361835425,-6.41470741397467,
40.0389814735788));
#186094=CARTESIAN_POINT('Ctrl Pts',(62.4493074469123,-6.41260146153638,
40.0367321210017));
#186095=CARTESIAN_POINT('Ctrl Pts',(62.4418213564087,-6.4055277901409,40.029176783714));
#186096=CARTESIAN_POINT('Ctrl Pts',(62.4339335724863,-6.39923601079879,
40.0213235332573));
#186097=CARTESIAN_POINT('Ctrl Pts',(62.4257522463025,-6.39365709371028,
40.0132649215854));
#186098=CARTESIAN_POINT('Ctrl Pts',(62.4167599996848,-6.38752520296383,
40.0044075527527));
#186099=CARTESIAN_POINT('Ctrl Pts',(62.4074126717505,-6.38225398283454,
39.9953016253712));
#186100=CARTESIAN_POINT('Ctrl Pts',(62.3978127557447,-6.37778536209576,
39.9860353422349));
#186101=CARTESIAN_POINT('Ctrl Pts',(62.3874732348828,-6.3729724660949,39.9760551582683));
#186102=CARTESIAN_POINT('Ctrl Pts',(62.3768396913512,-6.36908997057771,
39.9658879738141));
#186103=CARTESIAN_POINT('Ctrl Pts',(62.3660067738148,-6.36611161569942,
39.9556174643237));
#186104=CARTESIAN_POINT('Ctrl Pts',(62.3553201372421,-6.36317347866826,
39.9454856413893));
#186105=CARTESIAN_POINT('Ctrl Pts',(62.3444380411296,-6.36111515612444,
39.9352519465108));
#186106=CARTESIAN_POINT('Ctrl Pts',(62.3334394572619,-6.35995915837802,
39.92499));
#186107=CARTESIAN_POINT('Ctrl Pts',(58.912095367953,-6.00036140429046,39.92499));
#186108=CARTESIAN_POINT('Ctrl Pts',(58.9015696628156,-5.99925510810136,
39.9348107241714));
#186109=CARTESIAN_POINT('Ctrl Pts',(58.8909945468917,-5.99898299131194,
39.9446038383152));
#186110=CARTESIAN_POINT('Ctrl Pts',(58.8804276387814,-5.99953795195244,
39.9543158069359));
#186111=CARTESIAN_POINT('Ctrl Pts',(58.8702243592831,-6.00007381527843,
39.963693567136));
#186112=CARTESIAN_POINT('Ctrl Pts',(58.8600274754076,-6.00138095727599,
39.9729968320952));
#186113=CARTESIAN_POINT('Ctrl Pts',(58.8498890377538,-6.00349883563849,
39.9821731151294));
#186114=CARTESIAN_POINT('Ctrl Pts',(58.8403050390087,-6.00550089396953,
39.9908475764307));
#186115=CARTESIAN_POINT('Ctrl Pts',(58.8307723843936,-6.00822762538385,
39.9994093733799));
#186116=CARTESIAN_POINT('Ctrl Pts',(58.8213500689115,-6.0117515363934,40.0077966115792));
#186117=CARTESIAN_POINT('Ctrl Pts',(58.8126722744237,-6.01499699931519,
40.0155211172544));
#186118=CARTESIAN_POINT('Ctrl Pts',(58.8040875818627,-6.01891888228866,
40.0230979940969));
#186119=CARTESIAN_POINT('Ctrl Pts',(58.7956642413131,-6.02360485257075,
40.0304554104694));
#186120=CARTESIAN_POINT('Ctrl Pts',(58.7931525711953,-6.02500211431762,
40.0326492435145));
#186121=CARTESIAN_POINT('Ctrl Pts',(58.7906554330116,-6.02646752363586,
40.0348233715043));
#186122=CARTESIAN_POINT('Ctrl Pts',(58.7881751602884,-6.02800395803705,
40.0369753512356));
#186123=CARTESIAN_POINT('Ctrl Pts',(58.7857202298425,-6.02952469386352,
40.0391053430352));
#186124=CARTESIAN_POINT('Ctrl Pts',(58.783284225042,-6.03111319985504,40.041211089324));
#186125=CARTESIAN_POINT('Ctrl Pts',(58.7808720541407,-6.0327702554203,40.0432881154904));
#186126=CARTESIAN_POINT('Ctrl Pts',(58.7807043164937,-6.03288548382362,
40.043432547828));
#186127=CARTESIAN_POINT('Ctrl Pts',(58.7805366835715,-6.0330010380091,40.0435768364421));
#186128=CARTESIAN_POINT('Ctrl Pts',(58.7803691562898,-6.03311691890562,
40.0437209807855));
#186129=CARTESIAN_POINT('Ctrl Pts',(58.7730241465597,-6.03819756191435,
40.0500407968421));
#186130=CARTESIAN_POINT('Ctrl Pts',(58.7659160498048,-6.04393622206,40.0560490279346));
#186131=CARTESIAN_POINT('Ctrl Pts',(58.7591607781928,-6.05034076157591,
40.0616647108616));
#186132=CARTESIAN_POINT('Ctrl Pts',(58.7528636909919,-6.05631090550629,
40.0668995033488));
#186133=CARTESIAN_POINT('Ctrl Pts',(58.746872812682,-6.06286038933354,40.0717933267486));
#186134=CARTESIAN_POINT('Ctrl Pts',(58.7413107827875,-6.07000150504443,
40.0762460303077));
#186135=CARTESIAN_POINT('Ctrl Pts',(58.739276120295,-6.07261381755741,40.0778748868751));
#186136=CARTESIAN_POINT('Ctrl Pts',(58.7372991657062,-6.07530531160687,
40.0794443522249));
#186137=CARTESIAN_POINT('Ctrl Pts',(58.735387140493,-6.07807653793555,40.0809482021492));
#186138=CARTESIAN_POINT('Ctrl Pts',(58.7349273623043,-6.07874292528918,
40.0813098278168));
#186139=CARTESIAN_POINT('Ctrl Pts',(58.7344713442223,-6.07941450700183,
40.0816679525672));
#186140=CARTESIAN_POINT('Ctrl Pts',(58.7340192051468,-6.08009121771075,
40.082022419258));
#186141=CARTESIAN_POINT('Ctrl Pts',(58.7335811954175,-6.08074678121001,
40.0823658088648));
#186142=CARTESIAN_POINT('Ctrl Pts',(58.7331468260468,-6.08140715812707,
40.0827057654616));
#186143=CARTESIAN_POINT('Ctrl Pts',(58.7327162055066,-6.08207228526541,
40.0830421470151));
#186144=CARTESIAN_POINT('Ctrl Pts',(58.7279982598321,-6.08935952173594,
40.0867275956805));
#186145=CARTESIAN_POINT('Ctrl Pts',(58.7237275533352,-6.09722197243172,
40.089982343203));
#186146=CARTESIAN_POINT('Ctrl Pts',(58.7200553115704,-6.1055470990915,40.0926299529354));
#186147=CARTESIAN_POINT('Ctrl Pts',(58.7185323234526,-6.10899977726292,
40.0937279956083));
#186148=CARTESIAN_POINT('Ctrl Pts',(58.7171120447816,-6.11253167434582,
40.0947220371802));
#186149=CARTESIAN_POINT('Ctrl Pts',(58.7158039367398,-6.11613350280225,
40.0956014538692));
#186150=CARTESIAN_POINT('Ctrl Pts',(58.7135728221602,-6.12227679657149,
40.097101390674));
#186151=CARTESIAN_POINT('Ctrl Pts',(58.7116702942288,-6.12862250657786,
40.0982667904316));
#186152=CARTESIAN_POINT('Ctrl Pts',(58.7101471179289,-6.13511848061099,
40.0990539325582));
#186153=CARTESIAN_POINT('Ctrl Pts',(58.7093855297789,-6.13836646762756,
40.0994475036216));
#186154=CARTESIAN_POINT('Ctrl Pts',(58.7087202098052,-6.14165223896364,
40.0997467259952));
#186155=CARTESIAN_POINT('Ctrl Pts',(58.7081575578112,-6.14496923836494,
40.0999473488896));
#186156=CARTESIAN_POINT('Ctrl Pts',(58.7075949058173,-6.14828623776625,
40.100147971784));
#186157=CARTESIAN_POINT('Ctrl Pts',(58.7071349090267,-6.15163442139592,
40.10025));
#186158=CARTESIAN_POINT('Ctrl Pts',(58.7067819056643,-6.15500747092316,
40.10025));
#186159=CARTESIAN_POINT('Origin',(56.9874003490102,-12.1286263473644,39.92499));
#186160=CARTESIAN_POINT('Ctrl Pts',(61.2479592423878,-13.2134115091894,
39.92499));
#186161=CARTESIAN_POINT('Ctrl Pts',(61.2583377107546,-13.2156175207409,
39.9348354642018));
#186162=CARTESIAN_POINT('Ctrl Pts',(61.2688594460198,-13.2169980909548,
39.9446440828459));
#186163=CARTESIAN_POINT('Ctrl Pts',(61.2794654334802,-13.2175561899854,
39.9543641760333));
#186164=CARTESIAN_POINT('Ctrl Pts',(61.2897267895027,-13.2180961541208,
39.9637684240714));
#186165=CARTESIAN_POINT('Ctrl Pts',(61.3000683010468,-13.2178662282939,
39.9730909636398));
#186166=CARTESIAN_POINT('Ctrl Pts',(61.3104421535935,-13.2168232529018,
39.9822808977143));
#186167=CARTESIAN_POINT('Ctrl Pts',(61.3202551793177,-13.2158366624037,
39.9909740094652));
#186168=CARTESIAN_POINT('Ctrl Pts',(61.3300980668405,-13.2141224659043,
39.9995492765004));
#186169=CARTESIAN_POINT('Ctrl Pts',(61.3399200511722,-13.211603302198,40.0079462328697));
#186170=CARTESIAN_POINT('Ctrl Pts',(61.3489668090858,-13.2092829702341,
40.0156804369693));
#186171=CARTESIAN_POINT('Ctrl Pts',(61.3579963605654,-13.2062795322631,
40.0232638017425));
#186172=CARTESIAN_POINT('Ctrl Pts',(61.3669504518463,-13.2024991065229,
40.030625726997));
#186173=CARTESIAN_POINT('Ctrl Pts',(61.3695476933562,-13.2014025487205,
40.0327611416654));
#186174=CARTESIAN_POINT('Ctrl Pts',(61.3721384315552,-13.2002403977584,
40.0348777427272));
#186175=CARTESIAN_POINT('Ctrl Pts',(61.374720822464,-13.1990098046947,40.0369733168701));
#186176=CARTESIAN_POINT('Ctrl Pts',(61.3775203002416,-13.1976757626938,
40.039245053974));
#186177=CARTESIAN_POINT('Ctrl Pts',(61.3803065372249,-13.1962641169258,
40.041487875195));
#186178=CARTESIAN_POINT('Ctrl Pts',(61.3830766416486,-13.194772102191,40.0436985701601));
#186179=CARTESIAN_POINT('Ctrl Pts',(61.3906792149762,-13.1906772560436,
40.0497658398386));
#186180=CARTESIAN_POINT('Ctrl Pts',(61.3981301363758,-13.1859443571664,
40.0555581699984));
#186181=CARTESIAN_POINT('Ctrl Pts',(61.4053257594953,-13.1805769309629,
40.0609828468885));
#186182=CARTESIAN_POINT('Ctrl Pts',(61.41190936399,-13.1756660273912,40.0659461317304));
#186183=CARTESIAN_POINT('Ctrl Pts',(61.418268002635,-13.1702212276779,40.0706039980705));
#186184=CARTESIAN_POINT('Ctrl Pts',(61.4243186078271,-13.1642115906185,
40.0748843180601));
#186185=CARTESIAN_POINT('Ctrl Pts',(61.4272906453324,-13.1612596765262,
40.0769867972569));
#186186=CARTESIAN_POINT('Ctrl Pts',(61.4301878975266,-13.1581712727458,
40.0789976708174));
#186187=CARTESIAN_POINT('Ctrl Pts',(61.4329973166796,-13.154941736613,40.0809050491499));
#186188=CARTESIAN_POINT('Ctrl Pts',(61.4335303765997,-13.1543289635879,
40.0812669556104));
#186189=CARTESIAN_POINT('Ctrl Pts',(61.4340602468995,-13.1537105783544,
40.0816253922032));
#186190=CARTESIAN_POINT('Ctrl Pts',(61.4345867973822,-13.1530866324248,
40.0819801989139));
#186191=CARTESIAN_POINT('Ctrl Pts',(61.4350968931623,-13.1524821848055,
40.0823239179149));
#186192=CARTESIAN_POINT('Ctrl Pts',(61.4356038733673,-13.1518725186281,
40.0826642303498));
#186193=CARTESIAN_POINT('Ctrl Pts',(61.4361076188515,-13.1512576844883,
40.0830009916099));
#186194=CARTESIAN_POINT('Ctrl Pts',(61.4415973333395,-13.1445573487221,
40.0866709464312));
#186195=CARTESIAN_POINT('Ctrl Pts',(61.4467061867047,-13.137238593115,40.0899175831877));
#186196=CARTESIAN_POINT('Ctrl Pts',(61.4512683418496,-13.1293950794801,
40.0925642067061));
#186197=CARTESIAN_POINT('Ctrl Pts',(61.453194968297,-13.1260827149661,40.0936818922527));
#186198=CARTESIAN_POINT('Ctrl Pts',(61.4550242827916,-13.1226771582918,
40.094693009479));
#186199=CARTESIAN_POINT('Ctrl Pts',(61.4567450522889,-13.1191869390028,
40.0955863397545));
#186200=CARTESIAN_POINT('Ctrl Pts',(61.4596427851248,-13.1133094969312,
40.0970906856166));
#186201=CARTESIAN_POINT('Ctrl Pts',(61.4622303029113,-13.1071927578067,
40.0982599215483));
#186202=CARTESIAN_POINT('Ctrl Pts',(61.4644496675152,-13.1008831031057,
40.0990497370453));
#186203=CARTESIAN_POINT('Ctrl Pts',(61.4650045086662,-13.0993056894304,
40.0992471909196));
#186204=CARTESIAN_POINT('Ctrl Pts',(61.4655361149186,-13.097716155517,40.0994209989363));
#186205=CARTESIAN_POINT('Ctrl Pts',(61.4660432808488,-13.096115154835,40.0995705982975));
#186206=CARTESIAN_POINT('Ctrl Pts',(61.4668040297442,-13.0937136538119,
40.0997949973393));
#186207=CARTESIAN_POINT('Ctrl Pts',(61.4675097715123,-13.0912863650433,
40.0999649129781));
#186208=CARTESIAN_POINT('Ctrl Pts',(61.4681580753693,-13.0888358608678,
40.1000786629733));
#186209=CARTESIAN_POINT('Ctrl Pts',(61.4688063792262,-13.0863853566924,
40.1001924129685));
#186210=CARTESIAN_POINT('Ctrl Pts',(61.4693972526619,-13.0839116459751,
40.10025));
#186211=CARTESIAN_POINT('Ctrl Pts',(61.4699285681954,-13.0814171332233,
40.10025));
#186212=CARTESIAN_POINT('Ctrl Pts',(57.7354693911205,-12.2876333308471,
40.10025));
#186213=CARTESIAN_POINT('Ctrl Pts',(57.7336713548546,-12.2960739442505,
40.10025));
#186214=CARTESIAN_POINT('Ctrl Pts',(57.7325856410805,-12.3045898170426,
40.0995786334241));
#186215=CARTESIAN_POINT('Ctrl Pts',(57.7321565492375,-12.3130404786508,
40.0983063763366));
#186216=CARTESIAN_POINT('Ctrl Pts',(57.7318793999343,-12.3184987389617,
40.0974846287992));
#186217=CARTESIAN_POINT('Ctrl Pts',(57.7318752477672,-12.3239297572686,
40.0964130309338));
#186218=CARTESIAN_POINT('Ctrl Pts',(57.7321203363021,-12.3292970476683,
40.0951176960924));
#186219=CARTESIAN_POINT('Ctrl Pts',(57.7324451871157,-12.3364110836358,
40.0934008039614));
#186220=CARTESIAN_POINT('Ctrl Pts',(57.7332135204776,-12.3434117286774,
40.0912909372157));
#186221=CARTESIAN_POINT('Ctrl Pts',(57.7343801629266,-12.3502210637609,
40.0888630467851));
#186222=CARTESIAN_POINT('Ctrl Pts',(57.7349634841511,-12.3536257313026,
40.0876491015699));
#186223=CARTESIAN_POINT('Ctrl Pts',(57.735646339504,-12.3569827659239,40.0863558569271));
#186224=CARTESIAN_POINT('Ctrl Pts',(57.7364227809414,-12.3602838093641,
40.0849936342771));
#186225=CARTESIAN_POINT('Ctrl Pts',(57.7368110016602,-12.3619343310841,
40.0843125229521));
#186226=CARTESIAN_POINT('Ctrl Pts',(57.737222615436,-12.3635708710708,40.0836141747074));
#186227=CARTESIAN_POINT('Ctrl Pts',(57.7376568568912,-12.3651924853573,
40.0828999161609));
#186228=CARTESIAN_POINT('Ctrl Pts',(57.737765417255,-12.3655978889289,40.0827213515243));
#186229=CARTESIAN_POINT('Ctrl Pts',(57.7378753917741,-12.3660023599857,
40.0825417925842));
#186230=CARTESIAN_POINT('Ctrl Pts',(57.7379867683384,-12.3664058844666,
40.0823612602361));
#186231=CARTESIAN_POINT('Ctrl Pts',(57.7383208980314,-12.3676164579092,
40.0818196631917));
#186232=CARTESIAN_POINT('Ctrl Pts',(57.7386676465115,-12.3688185104665,
40.0812693052021));
#186233=CARTESIAN_POINT('Ctrl Pts',(57.7390266834247,-12.3700116777062,
40.0807107531875));
#186234=CARTESIAN_POINT('Ctrl Pts',(57.7415556930806,-12.3784161936765,
40.0767763849183));
#186235=CARTESIAN_POINT('Ctrl Pts',(57.7446608854351,-12.3864219416023,
40.072414058614));
#186236=CARTESIAN_POINT('Ctrl Pts',(57.7482237843182,-12.3940121800342,
40.0677221223773));
#186237=CARTESIAN_POINT('Ctrl Pts',(57.7499517864266,-12.397693437472,40.0654465383724));
#186238=CARTESIAN_POINT('Ctrl Pts',(57.751788007257,-12.4012771190722,40.0630928000681));
#186239=CARTESIAN_POINT('Ctrl Pts',(57.7537217536093,-12.4047617836665,
40.0606689262479));
#186240=CARTESIAN_POINT('Ctrl Pts',(57.7566821841674,-12.4100965616934,
40.0569581447806));
#186241=CARTESIAN_POINT('Ctrl Pts',(57.759868615088,-12.4151968540755,40.0530843804605));
#186242=CARTESIAN_POINT('Ctrl Pts',(57.7632382593551,-12.4200454689338,
40.0490800251457));
#186243=CARTESIAN_POINT('Ctrl Pts',(57.7648031395849,-12.4222971907574,
40.0472203818218));
#186244=CARTESIAN_POINT('Ctrl Pts',(57.7664072884048,-12.4244947022408,
40.0453323608818));
#186245=CARTESIAN_POINT('Ctrl Pts',(57.7680472557362,-12.4266353752444,
40.0434201572162));
#186246=CARTESIAN_POINT('Ctrl Pts',(57.7681729527704,-12.4267994493954,
40.0432735943397));
#186247=CARTESIAN_POINT('Ctrl Pts',(57.768298843268,-12.4269632190237,40.0431268995707));
#186248=CARTESIAN_POINT('Ctrl Pts',(57.7684249257697,-12.4271266840706,
40.0429800745037));
#186249=CARTESIAN_POINT('Ctrl Pts',(57.7701960047922,-12.4294228751479,
40.0409176249753));
#186250=CARTESIAN_POINT('Ctrl Pts',(57.7720067040171,-12.4316578001005,
40.0388310783333));
#186251=CARTESIAN_POINT('Ctrl Pts',(57.7738513586814,-12.4338307751863,
40.036725739981));
#186252=CARTESIAN_POINT('Ctrl Pts',(57.7804659622464,-12.4416226773929,
40.0291763710721));
#186253=CARTESIAN_POINT('Ctrl Pts',(57.7875668075252,-12.4486795287409,
40.0213310894602));
#186254=CARTESIAN_POINT('Ctrl Pts',(57.7950386758931,-12.4550596184359,
40.0132837551331));
#186255=CARTESIAN_POINT('Ctrl Pts',(57.8032495086137,-12.462070696074,40.004440543134));
#186256=CARTESIAN_POINT('Ctrl Pts',(57.8119087706201,-12.4682650727906,
39.995352871062));
#186257=CARTESIAN_POINT('Ctrl Pts',(57.820908068967,-12.4736913816486,39.9861103629579));
#186258=CARTESIAN_POINT('Ctrl Pts',(57.830625052666,-12.4795504333977,39.9761307737582));
#186259=CARTESIAN_POINT('Ctrl Pts',(57.8407393717675,-12.484514761572,39.9659696936041));
#186260=CARTESIAN_POINT('Ctrl Pts',(57.8511535286804,-12.4886033793272,
39.9557128217538));
#186261=CARTESIAN_POINT('Ctrl Pts',(57.8614803215187,-12.4926576977809,
39.9455419945182));
#186262=CARTESIAN_POINT('Ctrl Pts',(57.8721033557542,-12.4958511892331,
39.9352756289351));
#186263=CARTESIAN_POINT('Ctrl Pts',(57.8829458346105,-12.4981558292588,
39.92499));
#186264=CARTESIAN_POINT('Origin',(0.00316857416806278,0.0149069694351844,
39.92499));
#186265=CARTESIAN_POINT('Ctrl Pts',(61.4762657165316,-13.0516031943529,
40.10025));
#186266=CARTESIAN_POINT('Ctrl Pts',(61.4780479426482,-13.0432012029365,
40.10025));
#186267=CARTESIAN_POINT('Ctrl Pts',(61.4791124697294,-13.03472499777,40.0995859581842));
#186268=CARTESIAN_POINT('Ctrl Pts',(61.4795178910588,-13.0263136082746,
40.098327595962));
#186269=CARTESIAN_POINT('Ctrl Pts',(61.4797769359881,-13.0209391308135,
40.0975235624068));
#186270=CARTESIAN_POINT('Ctrl Pts',(61.4797678285537,-13.0155911381655,
40.096477705949));
#186271=CARTESIAN_POINT('Ctrl Pts',(61.4795143397209,-13.0103045333053,
40.0952149915961));
#186272=CARTESIAN_POINT('Ctrl Pts',(61.479168378327,-13.0030893784372,40.0934916398701));
#186273=CARTESIAN_POINT('Ctrl Pts',(61.4783613533299,-12.9959902125622,
40.0913643921631));
#186274=CARTESIAN_POINT('Ctrl Pts',(61.4771427864515,-12.9890888821228,
40.0889118607713));
#186275=CARTESIAN_POINT('Ctrl Pts',(61.4765335030122,-12.9856382169031,
40.0876855950754));
#186276=CARTESIAN_POINT('Ctrl Pts',(61.4758213793959,-12.9822368066732,
40.0863782327526));
#186277=CARTESIAN_POINT('Ctrl Pts',(61.4750129240934,-12.9788934238964,
40.0850006373334));
#186278=CARTESIAN_POINT('Ctrl Pts',(61.4746086964421,-12.977221732508,40.0843118396237));
#186279=CARTESIAN_POINT('Ctrl Pts',(61.4741803895393,-12.9755645309602,
40.0836054919164));
#186280=CARTESIAN_POINT('Ctrl Pts',(61.4737288401362,-12.9739228088655,
40.0828829920418));
#186281=CARTESIAN_POINT('Ctrl Pts',(61.4736159527854,-12.9735123783418,
40.0827023670731));
#186282=CARTESIAN_POINT('Ctrl Pts',(61.4735016128575,-12.9731029149215,
40.0825207326933));
#186283=CARTESIAN_POINT('Ctrl Pts',(61.4733858335871,-12.9726944333364,
40.0823381109275));
#186284=CARTESIAN_POINT('Ctrl Pts',(61.4730384957757,-12.9714689885812,
40.0817902456303));
#186285=CARTESIAN_POINT('Ctrl Pts',(61.4726782034777,-12.9702523821505,
40.0812334935553));
#186286=CARTESIAN_POINT('Ctrl Pts',(61.4723053176144,-12.9690449956481,
40.0806684524227));
#186287=CARTESIAN_POINT('Ctrl Pts',(61.46972844494,-12.9607012057873,40.0767636676137));
#186288=CARTESIAN_POINT('Ctrl Pts',(61.4665839586187,-12.952753439984,40.0724404510889));
#186289=CARTESIAN_POINT('Ctrl Pts',(61.4629898265073,-12.9452156558837,
40.0677949937411));
#186290=CARTESIAN_POINT('Ctrl Pts',(61.4612035527136,-12.9414693978765,
40.0654862141907));
#186291=CARTESIAN_POINT('Ctrl Pts',(61.459305623895,-12.9378242492507,40.0630972003217));
#186292=CARTESIAN_POINT('Ctrl Pts',(61.4573073969127,-12.9342814732027,
40.0606363359906));
#186293=CARTESIAN_POINT('Ctrl Pts',(61.4528990097271,-12.9264655800787,
40.0552073017123));
#186294=CARTESIAN_POINT('Ctrl Pts',(61.4480137506082,-12.9191426809994,
40.0494204304519));
#186295=CARTESIAN_POINT('Ctrl Pts',(61.4427731575668,-12.9123924986714,
40.0434049749851));
#186296=CARTESIAN_POINT('Ctrl Pts',(61.4408587028414,-12.9099265719427,
40.0412074532442));
#186297=CARTESIAN_POINT('Ctrl Pts',(61.4389006256227,-12.907530081549,40.0389814735788));
#186298=CARTESIAN_POINT('Ctrl Pts',(61.436904230217,-12.9052026993235,40.0367321210016));
#186299=CARTESIAN_POINT('Ctrl Pts',(61.4301985493013,-12.8973852687041,
40.0291767837142));
#186300=CARTESIAN_POINT('Ctrl Pts',(61.4230116455107,-12.8903034584557,
40.0213235332578));
#186301=CARTESIAN_POINT('Ctrl Pts',(61.415458293118,-12.8838999218055,40.0132649215862));
#186302=CARTESIAN_POINT('Ctrl Pts',(61.407156264085,-12.876861676478,40.0044075527538));
#186303=CARTESIAN_POINT('Ctrl Pts',(61.3984111343311,-12.8706422708196,
39.9953016253726));
#186304=CARTESIAN_POINT('Ctrl Pts',(61.3893309057287,-12.8651946651852,
39.9860353422365));
#186305=CARTESIAN_POINT('Ctrl Pts',(61.3795511104669,-12.8593273605057,
39.9760551582702));
#186306=CARTESIAN_POINT('Ctrl Pts',(61.3693816498897,-12.8543546257407,
39.9658879738164));
#186307=CARTESIAN_POINT('Ctrl Pts',(61.3589193990679,-12.8502602383793,
39.9556174643262));
#186308=CARTESIAN_POINT('Ctrl Pts',(61.3485984239564,-12.8462211390713,
39.945485641391));
#186309=CARTESIAN_POINT('Ctrl Pts',(61.3379910943966,-12.8430366034496,
39.9352519465116));
#186310=CARTESIAN_POINT('Ctrl Pts',(61.3271735965893,-12.8407372733098,
39.92499));
#186311=CARTESIAN_POINT('Ctrl Pts',(57.9621601888121,-12.1254815933792,
39.92499));
#186312=CARTESIAN_POINT('Ctrl Pts',(57.9518077840279,-12.1232811218132,
39.9348107241727));
#186313=CARTESIAN_POINT('Ctrl Pts',(57.9413190436441,-12.1219050950916,
39.9446038383178));
#186314=CARTESIAN_POINT('Ctrl Pts',(57.9307520129777,-12.1213524729335,
39.9543158069397));
#186315=CARTESIAN_POINT('Ctrl Pts',(57.9205486151411,-12.120818867618,39.9636935671407));
#186316=CARTESIAN_POINT('Ctrl Pts',(57.9102709573172,-12.1210529843536,
39.9729968321007));
#186317=CARTESIAN_POINT('Ctrl Pts',(57.899966680514,-12.1220995054494,39.9821731151357));
#186318=CARTESIAN_POINT('Ctrl Pts',(57.8902259118354,-12.123088795635,39.9908475764376));
#186319=CARTESIAN_POINT('Ctrl Pts',(57.8804604570545,-12.1248041559921,
39.9994093733873));
#186320=CARTESIAN_POINT('Ctrl Pts',(57.8707214089994,-12.1273238624914,
40.007796611587));
#186321=CARTESIAN_POINT('Ctrl Pts',(57.8617519091254,-12.129644469906,40.0155211172626));
#186322=CARTESIAN_POINT('Ctrl Pts',(57.8528042960076,-12.1326475236739,
40.0230979941055));
#186323=CARTESIAN_POINT('Ctrl Pts',(57.8439372821258,-12.1364273448781,
40.0304554104783));
#186324=CARTESIAN_POINT('Ctrl Pts',(57.8412933175801,-12.13755441126,40.0326492435204));
#186325=CARTESIAN_POINT('Ctrl Pts',(57.8386566820001,-12.1387507708942,
40.0348233715072));
#186326=CARTESIAN_POINT('Ctrl Pts',(57.8360293953471,-12.140019529449,40.0369753512355));
#186327=CARTESIAN_POINT('Ctrl Pts',(57.8334289530881,-12.1412753244186,
40.0391053430352));
#186328=CARTESIAN_POINT('Ctrl Pts',(57.8308402488866,-12.1426004965698,
40.041211089324));
#186329=CARTESIAN_POINT('Ctrl Pts',(57.8282680826381,-12.1439963340938,
40.0432881154904));
#186330=CARTESIAN_POINT('Ctrl Pts',(57.8280892192276,-12.1440933979054,
40.0434325478279));
#186331=CARTESIAN_POINT('Ctrl Pts',(57.8279104259146,-12.1441907966612,
40.0435768364421));
#186332=CARTESIAN_POINT('Ctrl Pts',(57.8277317035128,-12.1442885313808,
40.0437209807855));
#186333=CARTESIAN_POINT('Ctrl Pts',(57.8198958587084,-12.1485735795158,
40.0500407968421));
#186334=CARTESIAN_POINT('Ctrl Pts',(57.8122268475249,-12.1535378042502,
40.0560490279347));
#186335=CARTESIAN_POINT('Ctrl Pts',(57.8048391253239,-12.159201140868,40.0616647108618));
#186336=CARTESIAN_POINT('Ctrl Pts',(57.797952484255,-12.1644803548773,40.0668995033491));
#186337=CARTESIAN_POINT('Ctrl Pts',(57.7913098171235,-12.1703677426436,
40.071793326749));
#186338=CARTESIAN_POINT('Ctrl Pts',(57.7850318067593,-12.1768883481381,
40.0762460303082));
#186339=CARTESIAN_POINT('Ctrl Pts',(57.7827352293485,-12.179273669986,40.0778748868754));
#186340=CARTESIAN_POINT('Ctrl Pts',(57.7804877669872,-12.1817437717241,
40.0794443522251));
#186341=CARTESIAN_POINT('Ctrl Pts',(57.7782965440188,-12.1842999559275,
40.0809482021492));
#186342=CARTESIAN_POINT('Ctrl Pts',(57.7777696280971,-12.184914632834,40.0813098278169));
#186343=CARTESIAN_POINT('Ctrl Pts',(57.7772459087255,-12.1855348686824,
40.0816679525672));
#186344=CARTESIAN_POINT('Ctrl Pts',(57.7767255109847,-12.1861606108965,
40.0820224192581));
#186345=CARTESIAN_POINT('Ctrl Pts',(57.7762213756734,-12.1867667986664,
40.0823658088648));
#186346=CARTESIAN_POINT('Ctrl Pts',(57.7757203576392,-12.1873781540068,
40.0827057654617));
#186347=CARTESIAN_POINT('Ctrl Pts',(57.7752225713658,-12.1879946254058,
40.0830421470151));
#186348=CARTESIAN_POINT('Ctrl Pts',(57.7697687474619,-12.1947487820209,
40.0867275956804));
#186349=CARTESIAN_POINT('Ctrl Pts',(57.7646995864536,-12.2021217510015,
40.0899823432026));
#186350=CARTESIAN_POINT('Ctrl Pts',(57.7601772489173,-12.2100174179573,
40.092629952935));
#186351=CARTESIAN_POINT('Ctrl Pts',(57.7583017007441,-12.2132919863894,
40.0937279956081));
#186352=CARTESIAN_POINT('Ctrl Pts',(57.7565200187335,-12.2166560758241,
40.0947220371801));
#186353=CARTESIAN_POINT('Ctrl Pts',(57.7548425830507,-12.2201014385646,
40.0956014538693));
#186354=CARTESIAN_POINT('Ctrl Pts',(57.7519815416931,-12.2259778637494,
40.097101390674));
#186355=CARTESIAN_POINT('Ctrl Pts',(57.7494261286934,-12.2320899429714,
40.0982667904316));
#186356=CARTESIAN_POINT('Ctrl Pts',(57.7472322823296,-12.2383911161012,
40.0990539325583));
#186357=CARTESIAN_POINT('Ctrl Pts',(57.7461353591478,-12.2415417026661,
40.0994475036216));
#186358=CARTESIAN_POINT('Ctrl Pts',(57.745130227238,-12.2447399293285,40.0997467259952));
#186359=CARTESIAN_POINT('Ctrl Pts',(57.7442239366604,-12.2479799447118,
40.0999473488896));
#186360=CARTESIAN_POINT('Ctrl Pts',(57.7433176460829,-12.251219960095,40.100147971784));
#186361=CARTESIAN_POINT('Ctrl Pts',(57.7425101887133,-12.2545017192668,
40.10025));
#186362=CARTESIAN_POINT('Ctrl Pts',(57.7418065394566,-12.2578193919768,
40.10025));
#186363=CARTESIAN_POINT('Origin',(55.4074307335706,-18.018989847295,39.92499));
#186364=CARTESIAN_POINT('Ctrl Pts',(59.5312589135995,-19.5431821162867,
39.92499));
#186365=CARTESIAN_POINT('Ctrl Pts',(59.5413499366334,-19.5464608884255,
39.9348354642019));
#186366=CARTESIAN_POINT('Ctrl Pts',(59.551669723849,-19.5489337165495,39.9446440828461));
#186367=CARTESIAN_POINT('Ctrl Pts',(59.5621592733664,-19.5505973858259,
39.9543641760335));
#186368=CARTESIAN_POINT('Ctrl Pts',(59.5723079749857,-19.5522069957573,
39.9637684240717));
#186369=CARTESIAN_POINT('Ctrl Pts',(59.582616868441,-19.5530593117978,39.9730909636402));
#186370=CARTESIAN_POINT('Ctrl Pts',(59.5930429125531,-19.5531064127989,
39.9822808977148));
#186371=CARTESIAN_POINT('Ctrl Pts',(59.6029053082843,-19.5531509674456,
39.9909740094658));
#186372=CARTESIAN_POINT('Ctrl Pts',(59.6128734577652,-19.5524750234008,
39.999549276501));
#186373=CARTESIAN_POINT('Ctrl Pts',(59.6229049605502,-19.5509963368653,
40.0079462328704));
#186374=CARTESIAN_POINT('Ctrl Pts',(59.6321447001119,-19.5496343596248,
40.01568043697));
#186375=CARTESIAN_POINT('Ctrl Pts',(59.6414387315194,-19.5475912199415,
40.0232638017433));
#186376=CARTESIAN_POINT('Ctrl Pts',(59.6507389334447,-19.5447674611705,
40.0306257269978));
#186377=CARTESIAN_POINT('Ctrl Pts',(59.6534365684955,-19.5439483960903,
40.032761141666));
#186378=CARTESIAN_POINT('Ctrl Pts',(59.6561345922133,-19.5430634173955,
40.0348777427275));
#186379=CARTESIAN_POINT('Ctrl Pts',(59.658831468516,-19.5421094990028,40.0369733168701));
#186380=CARTESIAN_POINT('Ctrl Pts',(59.6617550558218,-19.5410753901336,
40.039245053974));
#186381=CARTESIAN_POINT('Ctrl Pts',(59.6646735866702,-19.539962718579,40.041487875195));
#186382=CARTESIAN_POINT('Ctrl Pts',(59.6675844741795,-19.5387684320155,
40.0436985701601));
#186383=CARTESIAN_POINT('Ctrl Pts',(59.6755734277899,-19.5354907031706,
40.0497658398386));
#186384=CARTESIAN_POINT('Ctrl Pts',(59.683478254909,-19.5315625649725,40.0555581699984));
#186385=CARTESIAN_POINT('Ctrl Pts',(59.6911955084649,-19.5269766895183,
40.0609828468885));
#186386=CARTESIAN_POINT('Ctrl Pts',(59.6982563764893,-19.5227808624506,
40.0659461317306));
#186387=CARTESIAN_POINT('Ctrl Pts',(59.7051493183936,-19.5180305486456,
40.0706039980709));
#186388=CARTESIAN_POINT('Ctrl Pts',(59.7117949558642,-19.5126862934691,
40.0748843180607));
#186389=CARTESIAN_POINT('Ctrl Pts',(59.7150592712806,-19.5100612127845,
40.0769867972572));
#186390=CARTESIAN_POINT('Ctrl Pts',(59.7182634781249,-19.5072925729229,
40.0789976708176));
#186391=CARTESIAN_POINT('Ctrl Pts',(59.7213950854346,-19.5043743927939,
40.0809050491499));
#186392=CARTESIAN_POINT('Ctrl Pts',(59.7219892774193,-19.5038206965379,
40.0812669556104));
#186393=CARTESIAN_POINT('Ctrl Pts',(59.7225808838923,-19.5032610854116,
40.0816253922032));
#186394=CARTESIAN_POINT('Ctrl Pts',(59.7231697699856,-19.5026955970359,
40.0819801989139));
#186395=CARTESIAN_POINT('Ctrl Pts',(59.7237402533884,-19.5021477801719,
40.0823239179149));
#186396=CARTESIAN_POINT('Ctrl Pts',(59.7243081837714,-19.5015944476713,
40.0826642303498));
#186397=CARTESIAN_POINT('Ctrl Pts',(59.724873437353,-19.5010356373986,40.0830009916099));
#186398=CARTESIAN_POINT('Ctrl Pts',(59.7310334544115,-19.4949458381921,
40.0866709464311));
#186399=CARTESIAN_POINT('Ctrl Pts',(59.7368793392201,-19.4882011960854,
40.0899175831876));
#186400=CARTESIAN_POINT('Ctrl Pts',(59.7422363728286,-19.4808775251054,
40.092564206706));
#186401=CARTESIAN_POINT('Ctrl Pts',(59.7444986813872,-19.4777846933726,
40.0936818922526));
#186402=CARTESIAN_POINT('Ctrl Pts',(59.7466739523114,-19.474589008127,40.094693009479));
#186403=CARTESIAN_POINT('Ctrl Pts',(59.7487501225121,-19.4712977780155,
40.0955863397545));
#186404=CARTESIAN_POINT('Ctrl Pts',(59.7522463412521,-19.4657554287468,
40.0970906856166));
#186405=CARTESIAN_POINT('Ctrl Pts',(59.7554590576862,-19.4599426670171,
40.0982599215483));
#186406=CARTESIAN_POINT('Ctrl Pts',(59.758325802888,-19.4538995640362,40.0990497370453));
#186407=CARTESIAN_POINT('Ctrl Pts',(59.7590424891885,-19.4523887882909,
40.0992471909196));
#186408=CARTESIAN_POINT('Ctrl Pts',(59.7597373347835,-19.4508635299952,
40.0994209989363));
#186409=CARTESIAN_POINT('Ctrl Pts',(59.7604090725467,-19.4493243130378,
40.0995705982975));
#186410=CARTESIAN_POINT('Ctrl Pts',(59.7614166791915,-19.4470154876015,
40.0997949973393));
#186411=CARTESIAN_POINT('Ctrl Pts',(59.7623722755974,-19.4446752658773,
40.0999649129781));
#186412=CARTESIAN_POINT('Ctrl Pts',(59.7632731754137,-19.442305952026,40.1000786629733));
#186413=CARTESIAN_POINT('Ctrl Pts',(59.76417407523,-19.4399366381748,40.1001924129685));
#186414=CARTESIAN_POINT('Ctrl Pts',(59.7650202849791,-19.4375382417959,
40.10025));
#186415=CARTESIAN_POINT('Ctrl Pts',(59.7658094374951,-19.4351129318421,
40.10025));
#186416=CARTESIAN_POINT('Ctrl Pts',(56.1347810195642,-18.2553202812749,
40.10025));
#186417=CARTESIAN_POINT('Ctrl Pts',(56.1321105487811,-18.2635267101472,
40.10025));
#186418=CARTESIAN_POINT('Ctrl Pts',(56.1301406315643,-18.2718824441048,
40.0995786334241));
#186419=CARTESIAN_POINT('Ctrl Pts',(56.1288305556598,-18.2802419597937,
40.0983063763366));
#186420=CARTESIAN_POINT('Ctrl Pts',(56.1279843810471,-18.2856413491926,
40.0974846287992));
#186421=CARTESIAN_POINT('Ctrl Pts',(56.1274125556283,-18.2910421817933,
40.0964130309338));
#186422=CARTESIAN_POINT('Ctrl Pts',(56.1270952669252,-18.2964056883424,
40.0951176960924));
#186423=CARTESIAN_POINT('Ctrl Pts',(56.1266747189247,-18.3035147090328,
40.0934008039614));
#186424=CARTESIAN_POINT('Ctrl Pts',(56.1267070766081,-18.3105573165141,
40.0912909372156));
#186425=CARTESIAN_POINT('Ctrl Pts',(56.1271555587355,-18.3174512966899,
40.0888630467851));
#186426=CARTESIAN_POINT('Ctrl Pts',(56.1273797997992,-18.3208982867778,
40.0876491015699));
#186427=CARTESIAN_POINT('Ctrl Pts',(56.127708008729,-18.3243083090328,40.0863558569271));
#186428=CARTESIAN_POINT('Ctrl Pts',(56.128135143741,-18.3276724292419,40.0849936342771));
#186429=CARTESIAN_POINT('Ctrl Pts',(56.128348711247,-18.3293544893464,40.0843125229521));
#186430=CARTESIAN_POINT('Ctrl Pts',(56.1285870051495,-18.3310250895513,
40.0836141747074));
#186431=CARTESIAN_POINT('Ctrl Pts',(56.1288493629352,-18.332683211057,40.0828999161609));
#186432=CARTESIAN_POINT('Ctrl Pts',(56.1289149523817,-18.3330977414334,
40.0827213515243));
#186433=CARTESIAN_POINT('Ctrl Pts',(56.1289820457108,-18.3335114922229,
40.0825417925842));
#186434=CARTESIAN_POINT('Ctrl Pts',(56.1290506323488,-18.3339244481756,
40.082361260236));
#186435=CARTESIAN_POINT('Ctrl Pts',(56.1292563922628,-18.3351633160336,
40.0818196631917));
#186436=CARTESIAN_POINT('Ctrl Pts',(56.1294755925119,-18.336395028707,40.0812693052021));
#186437=CARTESIAN_POINT('Ctrl Pts',(56.1297079426452,-18.3376191892285,
40.0807107531874));
#186438=CARTESIAN_POINT('Ctrl Pts',(56.1313445869829,-18.3462420178743,
40.0767763849181));
#186439=CARTESIAN_POINT('Ctrl Pts',(56.1335959402409,-18.3545284904606,
40.0724140586136));
#186440=CARTESIAN_POINT('Ctrl Pts',(56.1363459252322,-18.3624495731175,
40.0677221223766));
#186441=CARTESIAN_POINT('Ctrl Pts',(56.1376796649813,-18.3662912896464,
40.0654465383719));
#186442=CARTESIAN_POINT('Ctrl Pts',(56.1391312300712,-18.3700472768051,
40.0630928000678));
#186443=CARTESIAN_POINT('Ctrl Pts',(56.1406901365234,-18.3737149835763,
40.0606689262479));
#186444=CARTESIAN_POINT('Ctrl Pts',(56.1430767133842,-18.3793299863879,
40.0569581447805));
#186445=CARTESIAN_POINT('Ctrl Pts',(56.1457125629779,-18.3847354115622,
40.0530843804605));
#186446=CARTESIAN_POINT('Ctrl Pts',(56.1485569297209,-18.3899096889379,
40.0490800251457));
#186447=CARTESIAN_POINT('Ctrl Pts',(56.1498778683512,-18.3923126501193,
40.0472203818218));
#186448=CARTESIAN_POINT('Ctrl Pts',(56.1512435269776,-18.3946658026159,
40.0453323608818));
#186449=CARTESIAN_POINT('Ctrl Pts',(56.152650749137,-18.3969661720538,40.0434201572162));
#186450=CARTESIAN_POINT('Ctrl Pts',(56.1527586071708,-18.3971424863073,
40.0432735943397));
#186451=CARTESIAN_POINT('Ctrl Pts',(56.1528666894395,-18.3973185179286,
40.0431268995707));
#186452=CARTESIAN_POINT('Ctrl Pts',(56.1529749944979,-18.397494266707,40.0429800745037));
#186453=CARTESIAN_POINT('Ctrl Pts',(56.1544963540395,-18.399963007178,40.0409176249753));
#186454=CARTESIAN_POINT('Ctrl Pts',(56.1560635207938,-18.4023749585853,
40.0388310783332));
#186455=CARTESIAN_POINT('Ctrl Pts',(56.1576709325004,-18.4047288488035,
40.036725739981));
#186456=CARTESIAN_POINT('Ctrl Pts',(56.1634348250117,-18.4131694805007,
40.0291763710717));
#186457=CARTESIAN_POINT('Ctrl Pts',(56.1697591292905,-18.4209299141239,
40.0213310894594));
#186458=CARTESIAN_POINT('Ctrl Pts',(56.1765231650107,-18.4280560759386,
40.0132837551319));
#186459=CARTESIAN_POINT('Ctrl Pts',(56.1839561607595,-18.4358870118863,
40.0044405431325));
#186460=CARTESIAN_POINT('Ctrl Pts',(56.1919204977438,-18.4429525945098,
39.9953528710602));
#186461=CARTESIAN_POINT('Ctrl Pts',(56.2003032932669,-18.4492898603069,
39.9861103629557));
#186462=CARTESIAN_POINT('Ctrl Pts',(56.209354608637,-18.456132516931,39.9761307737561));
#186463=CARTESIAN_POINT('Ctrl Pts',(56.218894606845,-18.4621268842287,39.9659696936019));
#186464=CARTESIAN_POINT('Ctrl Pts',(56.2288243369859,-18.4672816799262,
39.9557128217517));
#186465=CARTESIAN_POINT('Ctrl Pts',(56.2386707668943,-18.4723932321846,
39.9455419945168));
#186466=CARTESIAN_POINT('Ctrl Pts',(56.2489017962821,-18.4766796388,39.9352756289344));
#186467=CARTESIAN_POINT('Ctrl Pts',(56.2594439784239,-18.4801050014191,
39.92499));
#186468=CARTESIAN_POINT('Origin',(0.00470941899427448,0.0144941013083399,
39.92499));
#186469=CARTESIAN_POINT('Ctrl Pts',(59.7752282754837,-19.4061247292254,
40.10025));
#186470=CARTESIAN_POINT('Ctrl Pts',(59.7778789856303,-19.3979550581542,
40.10025));
#186471=CARTESIAN_POINT('Ctrl Pts',(59.7798236858211,-19.3896365599065,
40.0995859581841));
#186472=CARTESIAN_POINT('Ctrl Pts',(59.781106115828,-19.3813136269513,40.098327595962));
#186473=CARTESIAN_POINT('Ctrl Pts',(59.7819255275519,-19.3759956690085,
40.0975235624068));
#186474=CARTESIAN_POINT('Ctrl Pts',(59.7824754874621,-19.3706760212377,
40.096477705949));
#186475=CARTESIAN_POINT('Ctrl Pts',(59.7827759879495,-19.365391880154,40.0952149915961));
#186476=CARTESIAN_POINT('Ctrl Pts',(59.783186110819,-19.3581800878463,40.0934916398701));
#186477=CARTESIAN_POINT('Ctrl Pts',(59.7831255716887,-19.351035454862,40.0913643921631));
#186478=CARTESIAN_POINT('Ctrl Pts',(59.7826350657124,-19.3440445557096,
40.0889118607713));
#186479=CARTESIAN_POINT('Ctrl Pts',(59.7823898127243,-19.3405491061334,
40.0876855950754));
#186480=CARTESIAN_POINT('Ctrl Pts',(59.7820371343799,-19.3370918919974,
40.0863782327527));
#186481=CARTESIAN_POINT('Ctrl Pts',(59.7815825865439,-19.3336823180309,
40.0850006373334));
#186482=CARTESIAN_POINT('Ctrl Pts',(59.7813553126259,-19.3319775310477,
40.0843118396238));
#186483=CARTESIAN_POINT('Ctrl Pts',(59.7811025767643,-19.330284637561,40.0836054919165));
#186484=CARTESIAN_POINT('Ctrl Pts',(59.7808251076837,-19.3286047092264,
40.0828829920418));
#186485=CARTESIAN_POINT('Ctrl Pts',(59.7807557404135,-19.3281847271428,
40.0827023670731));
#186486=CARTESIAN_POINT('Ctrl Pts',(59.7806848274338,-19.327765555029,40.0825207326933));
#186487=CARTESIAN_POINT('Ctrl Pts',(59.7806123803667,-19.3273472089195,
40.0823381109276));
#186488=CARTESIAN_POINT('Ctrl Pts',(59.7803950391653,-19.3260921705912,
40.0817902456304));
#186489=CARTESIAN_POINT('Ctrl Pts',(59.7801638905868,-19.3248445680577,
40.0812334935553));
#186490=CARTESIAN_POINT('Ctrl Pts',(59.7799192536869,-19.3236048185586,
40.0806684524227));
#186491=CARTESIAN_POINT('Ctrl Pts',(59.7782286609226,-19.3150373803107,
40.0767636676136));
#186492=CARTESIAN_POINT('Ctrl Pts',(59.7759321681721,-19.3068044648769,
40.0724404510887));
#186493=CARTESIAN_POINT('Ctrl Pts',(59.7731456380808,-19.29893228444,40.0677949937407));
#186494=CARTESIAN_POINT('Ctrl Pts',(59.7717607402744,-19.2950198323717,
40.0654862141904));
#186495=CARTESIAN_POINT('Ctrl Pts',(59.7702542302928,-19.291196264669,40.0630972003215));
#186496=CARTESIAN_POINT('Ctrl Pts',(59.7686372707431,-19.2874640247234,
40.0606363359906));
#186497=CARTESIAN_POINT('Ctrl Pts',(59.7650700164611,-19.2792301459417,
40.0552073017123));
#186498=CARTESIAN_POINT('Ctrl Pts',(59.7609769706902,-19.2714367138414,
40.0494204304519));
#186499=CARTESIAN_POINT('Ctrl Pts',(59.7564706723513,-19.2641757185812,
40.0434049749851));
#186500=CARTESIAN_POINT('Ctrl Pts',(59.7548244647406,-19.2615231854467,
40.0412074532442));
#186501=CARTESIAN_POINT('Ctrl Pts',(59.7531276155319,-19.2589351484755,
40.0389814735788));
#186502=CARTESIAN_POINT('Ctrl Pts',(59.7513854342766,-19.2564118357496,
40.0367321210016));
#186503=CARTESIAN_POINT('Ctrl Pts',(59.7455336317916,-19.2479362953112,
40.0291767837137));
#186504=CARTESIAN_POINT('Ctrl Pts',(59.7391263493539,-19.2401420439511,
40.0213235332568));
#186505=CARTESIAN_POINT('Ctrl Pts',(59.7322837268611,-19.2329840462261,
40.0132649215847));
#186506=CARTESIAN_POINT('Ctrl Pts',(59.7247628741796,-19.2251165588058,
40.0044075527517));
#186507=CARTESIAN_POINT('Ctrl Pts',(59.7167157560769,-19.2180171087279,
39.9953016253699));
#186508=CARTESIAN_POINT('Ctrl Pts',(59.7082546997619,-19.2116502033051,
39.9860353422333));
#186509=CARTESIAN_POINT('Ctrl Pts',(59.6991417795831,-19.2047927733646,
39.9760551582665));
#186510=CARTESIAN_POINT('Ctrl Pts',(59.6895478206977,-19.1987842816745,
39.9658879738121));
#186511=CARTESIAN_POINT('Ctrl Pts',(59.6795708631988,-19.1936187207947,
39.9556174643214));
#186512=CARTESIAN_POINT('Ctrl Pts',(59.6697286283139,-19.1885229124285,
39.9454856413877));
#186513=CARTESIAN_POINT('Ctrl Pts',(59.6595122814314,-19.1842470541687,
39.93525194651));
#186514=CARTESIAN_POINT('Ctrl Pts',(59.6489943884564,-19.1808295835782,
39.92499));
#186515=CARTESIAN_POINT('Ctrl Pts',(56.3771794532807,-18.1177524687107,
39.92499));
#186516=CARTESIAN_POINT('Ctrl Pts',(56.3671137719651,-18.1144819305952,
39.934810724172));
#186517=CARTESIAN_POINT('Ctrl Pts',(56.3568263239579,-18.1120170699781,
39.9446038383165));
#186518=CARTESIAN_POINT('Ctrl Pts',(56.3463749453368,-18.1103629196652,
39.9543158069377));
#186519=CARTESIAN_POINT('Ctrl Pts',(56.3362832197254,-18.1087656919994,
39.9636935671382));
#186520=CARTESIAN_POINT('Ctrl Pts',(56.3260373921244,-18.1079242184406,
39.9729968320977));
#186521=CARTESIAN_POINT('Ctrl Pts',(56.3156801719865,-18.1078879163649,
39.9821731151321));
#186522=CARTESIAN_POINT('Ctrl Pts',(56.3058893552755,-18.1078535995342,
39.9908475764337));
#186523=CARTESIAN_POINT('Ctrl Pts',(56.2959980926961,-18.1085387949861,
39.9994093733829));
#186524=CARTESIAN_POINT('Ctrl Pts',(56.2860490151176,-18.1100266905422,
40.0077966115823));
#186525=CARTESIAN_POINT('Ctrl Pts',(56.276886081576,-18.1113970173881,40.0155211172575));
#186526=CARTESIAN_POINT('Ctrl Pts',(56.2676735798242,-18.1134483398637,
40.0230979941));
#186527=CARTESIAN_POINT('Ctrl Pts',(56.2584600414709,-18.1162805994765,
40.0304554104726));
#186528=CARTESIAN_POINT('Ctrl Pts',(56.2557127503202,-18.1171251221205,
40.0326492435166));
#186529=CARTESIAN_POINT('Ctrl Pts',(56.2529655048694,-18.1180393245068,
40.0348233715053));
#186530=CARTESIAN_POINT('Ctrl Pts',(56.2502199893831,-18.119026506434,40.0369753512355));
#186531=CARTESIAN_POINT('Ctrl Pts',(56.2475025263006,-18.1200036017942,
40.0391053430352));
#186532=CARTESIAN_POINT('Ctrl Pts',(56.244789485083,-18.1210509212416,40.041211089324));
#186533=CARTESIAN_POINT('Ctrl Pts',(56.242085504679,-18.1221702476364,40.0432881154904));
#186534=CARTESIAN_POINT('Ctrl Pts',(56.2418974751699,-18.1222480834049,
40.0434325478279));
#186535=CARTESIAN_POINT('Ctrl Pts',(56.2417094803631,-18.1223262596099,
40.0435768364421));
#186536=CARTESIAN_POINT('Ctrl Pts',(56.2415215209613,-18.1224047773504,
40.0437209807855));
#186537=CARTESIAN_POINT('Ctrl Pts',(56.2332806922381,-18.1258472827275,
40.050040796842));
#186538=CARTESIAN_POINT('Ctrl Pts',(56.2251347899176,-18.1299826829656,
40.0560490279345));
#186539=CARTESIAN_POINT('Ctrl Pts',(56.2171955585583,-18.1348427679841,
40.0616647108616));
#186540=CARTESIAN_POINT('Ctrl Pts',(56.2097948151022,-18.1393732118985,
40.0668995033488));
#186541=CARTESIAN_POINT('Ctrl Pts',(56.2025731376006,-18.1445340001513,
40.0717933267485));
#186542=CARTESIAN_POINT('Ctrl Pts',(56.1956479299622,-18.1503626543107,
40.0762460303077));
#186543=CARTESIAN_POINT('Ctrl Pts',(56.1931145994154,-18.1524948514086,
40.0778748868751));
#186544=CARTESIAN_POINT('Ctrl Pts',(56.190621252949,-18.1547164978842,40.0794443522248));
#186545=CARTESIAN_POINT('Ctrl Pts',(56.1881748397225,-18.1570296338737,
40.0809482021491));
#186546=CARTESIAN_POINT('Ctrl Pts',(56.1875865590689,-18.1575858658042,
40.0813098278168));
#186547=CARTESIAN_POINT('Ctrl Pts',(56.1870008763867,-18.1581479603547,
40.0816679525671));
#186548=CARTESIAN_POINT('Ctrl Pts',(56.1864179215672,-18.1587158783113,
40.082022419258));
#186549=CARTESIAN_POINT('Ctrl Pts',(56.1858531840858,-18.1592660488318,
40.0823658088647));
#186550=CARTESIAN_POINT('Ctrl Pts',(56.1852910066466,-18.1598216844585,
40.0827057654616));
#186551=CARTESIAN_POINT('Ctrl Pts',(56.1847315084904,-18.1603827459285,
40.083042147015));
#186552=CARTESIAN_POINT('Ctrl Pts',(56.1786015595925,-18.1665298227358,
40.0867275956805));
#186553=CARTESIAN_POINT('Ctrl Pts',(56.1727894828609,-18.1733325302111,
40.089982343203));
#186554=CARTESIAN_POINT('Ctrl Pts',(56.1674665972292,-18.1807122308848,
40.0926299529355));
#186555=CARTESIAN_POINT('Ctrl Pts',(56.1652590378994,-18.1837728127196,
40.0937279956083));
#186556=CARTESIAN_POINT('Ctrl Pts',(56.1631354730308,-18.1869322368372,
40.0947220371802));
#186557=CARTESIAN_POINT('Ctrl Pts',(56.1611070880438,-18.1901833857453,
40.0956014538692));
#186558=CARTESIAN_POINT('Ctrl Pts',(56.1576474660761,-18.1957285590017,
40.097101390674));
#186559=CARTESIAN_POINT('Ctrl Pts',(56.1544671656478,-18.2015400422203,
40.0982667904316));
#186560=CARTESIAN_POINT('Ctrl Pts',(56.1516266854597,-18.2075773774753,
40.0990539325582));
#186561=CARTESIAN_POINT('Ctrl Pts',(56.1502064453657,-18.2105960451028,
40.0994475036216));
#186562=CARTESIAN_POINT('Ctrl Pts',(56.1488725139556,-18.2136716866511,
40.0997467259952));
#186563=CARTESIAN_POINT('Ctrl Pts',(56.1476325143037,-18.2167992197297,
40.0999473488896));
#186564=CARTESIAN_POINT('Ctrl Pts',(56.1463925146518,-18.2199267528083,
40.100147971784));
#186565=CARTESIAN_POINT('Ctrl Pts',(56.1452464433752,-18.223106131882,40.10025));
#186566=CARTESIAN_POINT('Ctrl Pts',(56.1441998575527,-18.2263320786583,
40.10025));
#186567=CARTESIAN_POINT('Origin',(53.2204057122638,-23.7119335237426,39.92499));
#186568=CARTESIAN_POINT('Ctrl Pts',(57.1623216544371,-25.6588335304441,
39.92499));
#186569=CARTESIAN_POINT('Ctrl Pts',(57.172014672778,-25.6631491402567,39.9348354642022));
#186570=CARTESIAN_POINT('Ctrl Pts',(57.182019446196,-25.6666871334685,39.9446440828466));
#186571=CARTESIAN_POINT('Ctrl Pts',(57.192277632071,-25.669438145482,39.9543641760343));
#186572=CARTESIAN_POINT('Ctrl Pts',(57.2022024879886,-25.6720997659862,
39.9637684240727));
#186573=CARTESIAN_POINT('Ctrl Pts',(57.2123658169611,-25.6740249857411,
39.9730909636413));
#186574=CARTESIAN_POINT('Ctrl Pts',(57.2227298227177,-25.6751616470869,
39.982280897716));
#186575=CARTESIAN_POINT('Ctrl Pts',(57.2325335339847,-25.6762368587286,
39.9909740094672));
#186576=CARTESIAN_POINT('Ctrl Pts',(57.2425177322922,-25.6766065729228,
39.9995492765025));
#186577=CARTESIAN_POINT('Ctrl Pts',(57.2526488462867,-25.6761845643571,
40.0079462328721));
#186578=CARTESIAN_POINT('Ctrl Pts',(57.2619803349765,-25.6757958639477,
40.0156804369718));
#186579=CARTESIAN_POINT('Ctrl Pts',(57.2714370189591,-25.6747354076178,
40.0232638017452));
#186580=CARTESIAN_POINT('Ctrl Pts',(57.2809814365703,-25.6728992535079,
40.0306257269999));
#186581=CARTESIAN_POINT('Ctrl Pts',(57.2837499093073,-25.6723666549984,
40.0327611416673));
#186582=CARTESIAN_POINT('Ctrl Pts',(57.2865256584311,-25.6717685445827,
40.0348777427281));
#186583=CARTESIAN_POINT('Ctrl Pts',(57.289307472586,-25.6711017521905,40.0369733168701));
#186584=CARTESIAN_POINT('Ctrl Pts',(57.2923231379855,-25.6703789063662,
40.039245053974));
#186585=CARTESIAN_POINT('Ctrl Pts',(57.2953419866643,-25.6695773996874,
40.041487875195));
#186586=CARTESIAN_POINT('Ctrl Pts',(57.2983617649664,-25.6686939261487,
40.0436985701601));
#186587=CARTESIAN_POINT('Ctrl Pts',(57.3066495702123,-25.6662692260894,
40.0497658398386));
#186588=CARTESIAN_POINT('Ctrl Pts',(57.3149216961106,-25.6631888860745,
40.0555581699984));
#186589=CARTESIAN_POINT('Ctrl Pts',(57.323076028258,-25.6594348051807,40.0609828468885));
#186590=CARTESIAN_POINT('Ctrl Pts',(57.3305367994639,-25.6560000249767,
40.0659461317305));
#186591=CARTESIAN_POINT('Ctrl Pts',(57.3378885241132,-25.6519962425126,
40.0706039980707));
#186592=CARTESIAN_POINT('Ctrl Pts',(57.3450563828671,-25.6473759219975,
40.0748843180604));
#186593=CARTESIAN_POINT('Ctrl Pts',(57.3485772116722,-25.6451064356535,
40.076986797257));
#186594=CARTESIAN_POINT('Ctrl Pts',(57.3520532672064,-25.6426878935081,
40.0789976708175));
#186595=CARTESIAN_POINT('Ctrl Pts',(57.3554727521281,-25.6401130415747,
40.08090504915));
#186596=CARTESIAN_POINT('Ctrl Pts',(57.3561215660858,-25.6396244884997,
40.0812669556105));
#186597=CARTESIAN_POINT('Ctrl Pts',(57.3567684269677,-25.6391297826973,
40.0816253922032));
#186598=CARTESIAN_POINT('Ctrl Pts',(57.3574131967122,-25.6386289474844,
40.0819801989139));
#186599=CARTESIAN_POINT('Ctrl Pts',(57.3580378174021,-25.6381437633719,
40.0823239179149));
#186600=CARTESIAN_POINT('Ctrl Pts',(57.3586604755991,-25.6376528269749,
40.0826642303498));
#186601=CARTESIAN_POINT('Ctrl Pts',(57.3592810442415,-25.6371561630115,
40.0830009916099));
#186602=CARTESIAN_POINT('Ctrl Pts',(57.3660438734345,-25.6317436214793,
40.086670946431));
#186603=CARTESIAN_POINT('Ctrl Pts',(57.3725627409489,-25.6256469885834,
40.0899175831874));
#186604=CARTESIAN_POINT('Ctrl Pts',(57.3786559602396,-25.6189233999304,
40.0925642067058));
#186605=CARTESIAN_POINT('Ctrl Pts',(57.3812291645836,-25.6160839866903,
40.0936818922525));
#186606=CARTESIAN_POINT('Ctrl Pts',(57.3837265592141,-25.6131331854695,
40.0946930094789));
#186607=CARTESIAN_POINT('Ctrl Pts',(57.3861353831632,-25.6100770039412,
40.0955863397546));
#186608=CARTESIAN_POINT('Ctrl Pts',(57.390191782503,-25.6049304706139,40.0970906856166));
#186609=CARTESIAN_POINT('Ctrl Pts',(57.3939944983914,-25.5994853721129,
40.0982599215483));
#186610=CARTESIAN_POINT('Ctrl Pts',(57.3974772155311,-25.593775030353,40.0990497370453));
#186611=CARTESIAN_POINT('Ctrl Pts',(57.398347894816,-25.592347444913,40.0992471909196));
#186612=CARTESIAN_POINT('Ctrl Pts',(57.3991983668799,-25.5909031732841,
40.0994209989363));
#186613=CARTESIAN_POINT('Ctrl Pts',(57.4000273167765,-25.5894426040343,
40.0995705982975));
#186614=CARTESIAN_POINT('Ctrl Pts',(57.4012707416215,-25.5872517501595,
40.0997949973393));
#186615=CARTESIAN_POINT('Ctrl Pts',(57.4024657229508,-25.5850242354385,
40.0999649129781));
#186616=CARTESIAN_POINT('Ctrl Pts',(57.4036093482795,-25.5827620706098,
40.1000786629733));
#186617=CARTESIAN_POINT('Ctrl Pts',(57.4047529736082,-25.5804999057811,
40.1001924129685));
#186618=CARTESIAN_POINT('Ctrl Pts',(57.4058452484196,-25.5782031010731,
40.10025));
#186619=CARTESIAN_POINT('Ctrl Pts',(57.4068835917979,-25.5758735661209,
40.10025));
#186620=CARTESIAN_POINT('Ctrl Pts',(53.9190682401995,-24.0229981225297,
40.10025));
#186621=CARTESIAN_POINT('Ctrl Pts',(53.9155545931359,-24.0308804555185,
40.10025));
#186622=CARTESIAN_POINT('Ctrl Pts',(53.9127220553017,-24.0389845034715,
40.0995786334241));
#186623=CARTESIAN_POINT('Ctrl Pts',(53.9105453488015,-24.0471612846374,
40.0983063763367));
#186624=CARTESIAN_POINT('Ctrl Pts',(53.9091394197453,-24.0524426462847,
40.0974846287993));
#186625=CARTESIAN_POINT('Ctrl Pts',(53.9080061861138,-24.0577541205273,
40.0964130309338));
#186626=CARTESIAN_POINT('Ctrl Pts',(53.9071299964541,-24.0630550795261,
40.0951176960923));
#186627=CARTESIAN_POINT('Ctrl Pts',(53.9059686572515,-24.0700811970212,
40.0934008039614));
#186628=CARTESIAN_POINT('Ctrl Pts',(53.9052646847386,-24.0770886066606,
40.0912909372156));
#186629=CARTESIAN_POINT('Ctrl Pts',(53.9049900928805,-24.0839917000392,
40.0888630467851));
#186630=CARTESIAN_POINT('Ctrl Pts',(53.9048527969514,-24.0874432467286,
40.0876491015698));
#186631=CARTESIAN_POINT('Ctrl Pts',(53.9048227635323,-24.0908688956999,
40.0863558569271));
#186632=CARTESIAN_POINT('Ctrl Pts',(53.9048959123383,-24.0942592346729,
40.0849936342771));
#186633=CARTESIAN_POINT('Ctrl Pts',(53.9049324867413,-24.0959544041594,
40.0843125229521));
#186634=CARTESIAN_POINT('Ctrl Pts',(53.9049948499728,-24.097640761137,40.0836141747074));
#186635=CARTESIAN_POINT('Ctrl Pts',(53.9050824496422,-24.0993172231358,
40.0828999161609));
#186636=CARTESIAN_POINT('Ctrl Pts',(53.9051043495595,-24.0997363386355,
40.0827213515243));
#186637=CARTESIAN_POINT('Ctrl Pts',(53.9051278266102,-24.1001548360174,
40.0825417925841));
#186638=CARTESIAN_POINT('Ctrl Pts',(53.9051528718723,-24.10057269901,40.082361260236));
#186639=CARTESIAN_POINT('Ctrl Pts',(53.9052280076585,-24.1018262879879,
40.0818196631917));
#186640=CARTESIAN_POINT('Ctrl Pts',(53.9053172580728,-24.1030741658756,
40.0812693052021));
#186641=CARTESIAN_POINT('Ctrl Pts',(53.9054203757497,-24.10431590752,40.0807107531874));
#186642=CARTESIAN_POINT('Ctrl Pts',(53.9061467233511,-24.1130625753258,
40.0767763849181));
#186643=CARTESIAN_POINT('Ctrl Pts',(53.907519571215,-24.1215389842446,40.0724140586136));
#186644=CARTESIAN_POINT('Ctrl Pts',(53.9094265129032,-24.1297041260871,
40.0677221223766));
#186645=CARTESIAN_POINT('Ctrl Pts',(53.9103513775613,-24.1336642110573,
40.0654465383719));
#186646=CARTESIAN_POINT('Ctrl Pts',(53.91140238326,-24.1375513523935,40.0630928000678));
#186647=CARTESIAN_POINT('Ctrl Pts',(53.9125693701071,-24.1413619171791,
40.0606689262478));
#186648=CARTESIAN_POINT('Ctrl Pts',(53.914355945435,-24.1471956256295,40.0569581447805));
#186649=CARTESIAN_POINT('Ctrl Pts',(53.916412334782,-24.1528469606265,40.0530843804605));
#186650=CARTESIAN_POINT('Ctrl Pts',(53.9187002605239,-24.158290210054,40.0490800251457));
#186651=CARTESIAN_POINT('Ctrl Pts',(53.9197627850745,-24.1608180832477,
40.0472203818218));
#186652=CARTESIAN_POINT('Ctrl Pts',(53.9208749910658,-24.1633010951263,
40.0453323608818));
#186653=CARTESIAN_POINT('Ctrl Pts',(53.9220340502327,-24.1657359576695,
40.0434201572162));
#186654=CARTESIAN_POINT('Ctrl Pts',(53.9221228875509,-24.1659225802895,
40.0432735943397));
#186655=CARTESIAN_POINT('Ctrl Pts',(53.9222119774187,-24.1661089452647,
40.0431268995707));
#186656=CARTESIAN_POINT('Ctrl Pts',(53.922301318421,-24.1662950522343,40.0429800745037));
#186657=CARTESIAN_POINT('Ctrl Pts',(53.9235562901482,-24.1689092940616,
40.0409176249753));
#186658=CARTESIAN_POINT('Ctrl Pts',(53.9248627542249,-24.1714718460792,
40.0388310783332));
#186659=CARTESIAN_POINT('Ctrl Pts',(53.9262153118348,-24.173980861716,40.036725739981));
#186660=CARTESIAN_POINT('Ctrl Pts',(53.9310653428793,-24.1829777455759,
40.029176371072));
#186661=CARTESIAN_POINT('Ctrl Pts',(53.9365438157564,-24.191356736539,40.02133108946));
#186662=CARTESIAN_POINT('Ctrl Pts',(53.9425259106375,-24.1991508947526,
40.0132837551329));
#186663=CARTESIAN_POINT('Ctrl Pts',(53.9490996319571,-24.2077158916369,
40.0044405431337));
#186664=CARTESIAN_POINT('Ctrl Pts',(53.9562817849761,-24.2155752681652,
39.9953528710616));
#186665=CARTESIAN_POINT('Ctrl Pts',(53.9639562340128,-24.222754058491,39.9861103629574));
#186666=CARTESIAN_POINT('Ctrl Pts',(53.9722427129487,-24.2305053504125,
39.9761307737578));
#186667=CARTESIAN_POINT('Ctrl Pts',(53.9811038680463,-24.2374640812912,
39.9659696936037));
#186668=CARTESIAN_POINT('Ctrl Pts',(53.9904403792137,-24.2436285779109,
39.9557128217535));
#186669=CARTESIAN_POINT('Ctrl Pts',(53.9996985666468,-24.2497413607387,
39.945541994518));
#186670=CARTESIAN_POINT('Ctrl Pts',(54.0094254978893,-24.25507371975,39.935275628935));
#186671=CARTESIAN_POINT('Ctrl Pts',(54.0195518809641,-24.2595822759734,
39.92499));
#186672=CARTESIAN_POINT('Origin',(0.00619866644047569,0.0139224327744755,
39.92499));
#186673=CARTESIAN_POINT('Ctrl Pts',(57.4192809246789,-25.5480287005719,
40.10025));
#186674=CARTESIAN_POINT('Ctrl Pts',(57.4227710771202,-25.5401808584722,
40.10025));
#186675=CARTESIAN_POINT('Ctrl Pts',(57.4255746438784,-25.5321112063511,
40.0995859581842));
#186676=CARTESIAN_POINT('Ctrl Pts',(57.4277200319911,-25.5239679177318,
40.0983275959622));
#186677=CARTESIAN_POINT('Ctrl Pts',(57.4290908328636,-25.5187647439669,
40.0975235624069));
#186678=CARTESIAN_POINT('Ctrl Pts',(57.4301938346425,-25.5135317242469,
40.0964777059491));
#186679=CARTESIAN_POINT('Ctrl Pts',(57.4310450321041,-25.5083079410947,
40.0952149915961));
#186680=CARTESIAN_POINT('Ctrl Pts',(57.4322067458449,-25.5011785252532,
40.0934916398701));
#186681=CARTESIAN_POINT('Ctrl Pts',(57.4328933558607,-25.4940667032537,
40.0913643921631));
#186682=CARTESIAN_POINT('Ctrl Pts',(57.4331362848728,-25.4870628291424,
40.0889118607713));
#186683=CARTESIAN_POINT('Ctrl Pts',(57.4332577493788,-25.4835608920868,
40.0876855950755));
#186684=CARTESIAN_POINT('Ctrl Pts',(57.4332683803241,-25.4800857520062,
40.0863782327527));
#186685=CARTESIAN_POINT('Ctrl Pts',(57.4331727200758,-25.4766473428559,
40.0850006373334));
#186686=CARTESIAN_POINT('Ctrl Pts',(57.4331248899517,-25.4749281382807,
40.0843118396238));
#186687=CARTESIAN_POINT('Ctrl Pts',(57.4330504941582,-25.4732181005505,
40.0836054919165));
#186688=CARTESIAN_POINT('Ctrl Pts',(57.4329501454094,-25.4715183716225,
40.0828829920418));
#186689=CARTESIAN_POINT('Ctrl Pts',(57.4329250582223,-25.4710934393905,
40.0827023670731));
#186690=CARTESIAN_POINT('Ctrl Pts',(57.4328983491282,-25.4706691511206,
40.0825207326933));
#186691=CARTESIAN_POINT('Ctrl Pts',(57.4328700280096,-25.4702455239743,
40.0823381109276));
#186692=CARTESIAN_POINT('Ctrl Pts',(57.4327850646539,-25.4689746425355,
40.0817902456304));
#186693=CARTESIAN_POINT('Ctrl Pts',(57.4326855923071,-25.4677097128935,
40.0812334935553));
#186694=CARTESIAN_POINT('Ctrl Pts',(57.4325718846637,-25.4664511833527,
40.0806684524227));
#186695=CARTESIAN_POINT('Ctrl Pts',(57.4317860942977,-25.4577539633646,
40.0767636676138));
#186696=CARTESIAN_POINT('Ctrl Pts',(57.4303627559733,-25.4493260998452,
40.0724404510891));
#186697=CARTESIAN_POINT('Ctrl Pts',(57.4284143577092,-25.4412057723284,
40.0677949937413));
#186698=CARTESIAN_POINT('Ctrl Pts',(57.4274460091201,-25.4371699918422,
40.0654862141908));
#186699=CARTESIAN_POINT('Ctrl Pts',(57.4263474236139,-25.4332098968697,
40.0630972003217));
#186700=CARTESIAN_POINT('Ctrl Pts',(57.4251294472437,-25.4293290842279,
40.0606363359906));
#186701=CARTESIAN_POINT('Ctrl Pts',(57.4224424094497,-25.4207674318875,
40.0552073017123));
#186702=CARTESIAN_POINT('Ctrl Pts',(57.4191864212928,-25.4125888532391,
40.0494204304519));
#186703=CARTESIAN_POINT('Ctrl Pts',(57.4154637896041,-25.4048965980304,
40.0434049749851));
#186704=CARTESIAN_POINT('Ctrl Pts',(57.4141038653033,-25.4020865201982,
40.0412074532442));
#186705=CARTESIAN_POINT('Ctrl Pts',(57.4126868351396,-25.3993352917241,
40.0389814735788));
#186706=CARTESIAN_POINT('Ctrl Pts',(57.4112179557371,-25.3966436944399,
40.0367321210016));
#186707=CARTESIAN_POINT('Ctrl Pts',(57.4062841452561,-25.3876029039781,
40.029176783714));
#186708=CARTESIAN_POINT('Ctrl Pts',(57.4007266836992,-25.3791816069558,
40.0213235332574));
#186709=CARTESIAN_POINT('Ctrl Pts',(57.3946697603108,-25.3713475726777,
40.0132649215856));
#186710=CARTESIAN_POINT('Ctrl Pts',(57.3880124840173,-25.3627370410036,
40.0044075527529));
#186711=CARTESIAN_POINT('Ctrl Pts',(57.3807515434765,-25.3548353295672,
39.9953016253715));
#186712=CARTESIAN_POINT('Ctrl Pts',(57.373002360553,-25.3476188815044,39.9860353422352));
#186713=CARTESIAN_POINT('Ctrl Pts',(57.3646561585183,-25.3398464577404,
39.9760551582687));
#186714=CARTESIAN_POINT('Ctrl Pts',(57.3557428147466,-25.3328680394176,
39.9658879738145));
#186715=CARTESIAN_POINT('Ctrl Pts',(57.3463604602058,-25.3266878999853,
39.955617464324));
#186716=CARTESIAN_POINT('Ctrl Pts',(57.3371047991303,-25.3205912133023,
39.9454856413896));
#186717=CARTESIAN_POINT('Ctrl Pts',(57.3273913673573,-25.3152708796011,
39.9352519465109));
#186718=CARTESIAN_POINT('Ctrl Pts',(57.317288315449,-25.3107727110823,39.92499));
#186719=CARTESIAN_POINT('Ctrl Pts',(54.1745185419759,-23.9115214566115,
39.92499));
#186720=CARTESIAN_POINT('Ctrl Pts',(54.1648498658388,-23.9072166846463,
39.9348107241722));
#186721=CARTESIAN_POINT('Ctrl Pts',(54.1548764216404,-23.9036899956623,
39.9446038383169));
#186722=CARTESIAN_POINT('Ctrl Pts',(54.1446552025549,-23.9009524404116,
39.9543158069384));
#186723=CARTESIAN_POINT('Ctrl Pts',(54.1347857162254,-23.8983090899562,
39.9636935671391));
#186724=CARTESIAN_POINT('Ctrl Pts',(54.1246839742778,-23.8964012454636,
39.9729968320988));
#186725=CARTESIAN_POINT('Ctrl Pts',(54.1143872866754,-23.8952825179497,
39.9821731151335));
#186726=CARTESIAN_POINT('Ctrl Pts',(54.1046536921683,-23.8942249700853,
39.9908475764352));
#186727=CARTESIAN_POINT('Ctrl Pts',(54.0947449925324,-23.8938724934877,
39.9994093733846));
#186728=CARTESIAN_POINT('Ctrl Pts',(54.0846948896055,-23.8943122764062,
40.0077966115842));
#186729=CARTESIAN_POINT('Ctrl Pts',(54.075438913413,-23.8947173090963,40.0155211172595));
#186730=CARTESIAN_POINT('Ctrl Pts',(54.0660624571234,-23.8957944255619,
40.0230979941022));
#186731=CARTESIAN_POINT('Ctrl Pts',(54.0566033397521,-23.8976480927551,
40.0304554104749));
#186732=CARTESIAN_POINT('Ctrl Pts',(54.0537828218966,-23.8982008188934,
40.0326492435181));
#186733=CARTESIAN_POINT('Ctrl Pts',(54.0509550659742,-23.898822847838,40.0348233715061));
#186734=CARTESIAN_POINT('Ctrl Pts',(54.0481214021002,-23.8995176373644,
40.0369753512356));
#186735=CARTESIAN_POINT('Ctrl Pts',(54.0453166912883,-23.9002053278539,
40.0391053430352));
#186736=CARTESIAN_POINT('Ctrl Pts',(54.042509037702,-23.9009633199466,40.041211089324));
#186737=CARTESIAN_POINT('Ctrl Pts',(54.0397028685177,-23.901793871638,40.0432881154904));
#186738=CARTESIAN_POINT('Ctrl Pts',(54.0395077330006,-23.9018516265783,
40.043432547828));
#186739=CARTESIAN_POINT('Ctrl Pts',(54.0393125964105,-23.9019097237176,
40.0435768364421));
#186740=CARTESIAN_POINT('Ctrl Pts',(54.0391174593312,-23.9019681642223,
40.0437209807855));
#186741=CARTESIAN_POINT('Ctrl Pts',(54.0305619349334,-23.9045304100322,
40.0500407968419));
#186742=CARTESIAN_POINT('Ctrl Pts',(54.0220283896864,-23.9077916774635,
40.0560490279343));
#186743=CARTESIAN_POINT('Ctrl Pts',(54.0136246330491,-23.9117952627741,
40.0616647108612));
#186744=CARTESIAN_POINT('Ctrl Pts',(54.0057908713001,-23.9155273001019,
40.0668995033481));
#186745=CARTESIAN_POINT('Ctrl Pts',(53.9980693056387,-23.9199049461648,
40.0717933267476));
#186746=CARTESIAN_POINT('Ctrl Pts',(53.9905727747505,-23.9249777890342,
40.0762460303065));
#186747=CARTESIAN_POINT('Ctrl Pts',(53.9878304467668,-23.9268335005847,
40.0778748868743));
#186748=CARTESIAN_POINT('Ctrl Pts',(53.9851185338205,-23.9287823509744,
40.0794443522245));
#186749=CARTESIAN_POINT('Ctrl Pts',(53.9824437337507,-23.9308270955484,
40.0809482021492));
#186750=CARTESIAN_POINT('Ctrl Pts',(53.9818005336912,-23.9313187883095,
40.0813098278168));
#186751=CARTESIAN_POINT('Ctrl Pts',(53.9811593045604,-23.9318165831365,
40.0816679525672));
#186752=CARTESIAN_POINT('Ctrl Pts',(53.9805201796371,-23.9323204546077,
40.0820224192581));
#186753=CARTESIAN_POINT('Ctrl Pts',(53.9799010273676,-23.9328085800954,
40.0823658088648));
#186754=CARTESIAN_POINT('Ctrl Pts',(53.9792838498571,-23.9333024083482,
40.0827057654617));
#186755=CARTESIAN_POINT('Ctrl Pts',(53.9786687697971,-23.9338019127823,
40.0830421470151));
#186756=CARTESIAN_POINT('Ctrl Pts',(53.9719298569081,-23.9392745611217,
40.0867275956808));
#186757=CARTESIAN_POINT('Ctrl Pts',(53.9654385427823,-23.9454324752048,
40.0899823432033));
#186758=CARTESIAN_POINT('Ctrl Pts',(53.9593734277039,-23.9522153560512,
40.0926299529359));
#186759=CARTESIAN_POINT('Ctrl Pts',(53.9568580436995,-23.9550284189139,
40.0937279956086));
#186760=CARTESIAN_POINT('Ctrl Pts',(53.9544158621939,-23.957948562403,40.0947220371803));
#186761=CARTESIAN_POINT('Ctrl Pts',(53.9520587513132,-23.9609698772113,
40.0956014538692));
#186762=CARTESIAN_POINT('Ctrl Pts',(53.9480384530775,-23.9661230444605,
40.097101390674));
#186763=CARTESIAN_POINT('Ctrl Pts',(53.9442681092575,-23.9715702598495,
40.0982667904316));
#186764=CARTESIAN_POINT('Ctrl Pts',(53.9408121161403,-23.9772776109211,
40.0990539325582));
#186765=CARTESIAN_POINT('Ctrl Pts',(53.9390841195817,-23.9801312864569,
40.0994475036216));
#186766=CARTESIAN_POINT('Ctrl Pts',(53.9374360035029,-23.9830506455186,
40.0997467259952));
#186767=CARTESIAN_POINT('Ctrl Pts',(53.9358758804724,-23.9860314303857,
40.0999473488896));
#186768=CARTESIAN_POINT('Ctrl Pts',(53.9343157574419,-23.9890122152529,
40.100147971784));
#186769=CARTESIAN_POINT('Ctrl Pts',(53.9328436288553,-23.9920543802862,
40.10025));
#186770=CARTESIAN_POINT('Ctrl Pts',(53.9314655730804,-23.9951532569808,
40.10025));
#186771=CARTESIAN_POINT('Origin',(50.4502867888875,-29.145084294463,39.92499));
#186772=CARTESIAN_POINT('Ctrl Pts',(54.1671020372438,-31.493361394986,39.92499));
#186773=CARTESIAN_POINT('Ctrl Pts',(54.176290852154,-31.4986665597479,39.9348354642018));
#186774=CARTESIAN_POINT('Ctrl Pts',(54.1858709973826,-31.5032309550533,
39.9446440828458));
#186775=CARTESIAN_POINT('Ctrl Pts',(54.1957854287835,-31.5070391691405,
39.9543641760331));
#186776=CARTESIAN_POINT('Ctrl Pts',(54.2053777002004,-31.5107236389463,
39.9637684240711));
#186777=CARTESIAN_POINT('Ctrl Pts',(54.2152841131307,-31.513700669305,39.9730909636394));
#186778=CARTESIAN_POINT('Ctrl Pts',(54.2254725303152,-31.5159144374962,
39.9822808977138));
#186779=CARTESIAN_POINT('Ctrl Pts',(54.2351101456051,-31.518008525889,39.9909740094647));
#186780=CARTESIAN_POINT('Ctrl Pts',(54.2450010037726,-31.5194198476563,
39.9995492764997));
#186781=CARTESIAN_POINT('Ctrl Pts',(54.255120730371,-31.520059140675,40.007946232869));
#186782=CARTESIAN_POINT('Ctrl Pts',(54.2644417304454,-31.52064797578,40.0156804369684));
#186783=CARTESIAN_POINT('Ctrl Pts',(54.2739574575936,-31.5205818213852,
40.0232638017416));
#186784=CARTESIAN_POINT('Ctrl Pts',(54.2836415202534,-31.5197533892257,
40.030625726996));
#186785=CARTESIAN_POINT('Ctrl Pts',(54.2864504987124,-31.5195130925472,
40.0327611416647));
#186786=CARTESIAN_POINT('Ctrl Pts',(54.2892735615563,-31.5192084034332,
40.0348777427268));
#186787=CARTESIAN_POINT('Ctrl Pts',(54.292109835428,-31.5188360425579,40.03697331687));
#186788=CARTESIAN_POINT('Ctrl Pts',(54.2951845386601,-31.5184323794286,
40.039245053974));
#186789=CARTESIAN_POINT('Ctrl Pts',(54.2982706300314,-31.5179508191004,
40.041487875195));
#186790=CARTESIAN_POINT('Ctrl Pts',(54.3013662138033,-31.5173878381076,
40.04369857016));
#186791=CARTESIAN_POINT('Ctrl Pts',(54.3098620677559,-31.515842732355,40.0497658398386));
#186792=CARTESIAN_POINT('Ctrl Pts',(54.3184108612912,-31.5136439393732,
40.0555581699984));
#186793=CARTESIAN_POINT('Ctrl Pts',(54.3269129314607,-31.5107627835357,
40.0609828468885));
#186794=CARTESIAN_POINT('Ctrl Pts',(54.3346918640778,-31.5081266823659,
40.0659461317305));
#186795=CARTESIAN_POINT('Ctrl Pts',(54.3424218244385,-31.504913297521,40.0706039980708));
#186796=CARTESIAN_POINT('Ctrl Pts',(54.3500333719155,-31.5010675328656,
40.0748843180606));
#186797=CARTESIAN_POINT('Ctrl Pts',(54.3537721391719,-31.4991785058297,
40.0769867972571));
#186798=CARTESIAN_POINT('Ctrl Pts',(54.3574819590038,-31.4971365594545,
40.0789976708176));
#186799=CARTESIAN_POINT('Ctrl Pts',(54.3611518569451,-31.4949332463334,
40.08090504915));
#186800=CARTESIAN_POINT('Ctrl Pts',(54.3618481843341,-31.4945151891293,
40.0812669556105));
#186801=CARTESIAN_POINT('Ctrl Pts',(54.3625432124818,-31.4940908087509,
40.0816253922033));
#186802=CARTESIAN_POINT('Ctrl Pts',(54.3632368016453,-31.4936601139562,
40.081980198914));
#186803=CARTESIAN_POINT('Ctrl Pts',(54.3639087161475,-31.4932428783739,
40.0823239179149));
#186804=CARTESIAN_POINT('Ctrl Pts',(54.3645792801848,-31.4928197168823,
40.0826642303499));
#186805=CARTESIAN_POINT('Ctrl Pts',(54.365248364808,-31.4923906407827,40.08300099161));
#186806=CARTESIAN_POINT('Ctrl Pts',(54.372539911164,-31.487714657862,40.0866709464311));
#186807=CARTESIAN_POINT('Ctrl Pts',(54.379660339308,-31.4823328301624,40.0899175831876));
#186808=CARTESIAN_POINT('Ctrl Pts',(54.3864229856957,-31.4762829888801,
40.092564206706));
#186809=CARTESIAN_POINT('Ctrl Pts',(54.3892788932594,-31.4737281033387,
40.0936818922527));
#186810=CARTESIAN_POINT('Ctrl Pts',(54.3920710496176,-31.4710545157388,
40.094693009479));
#186811=CARTESIAN_POINT('Ctrl Pts',(54.3947861357355,-31.4682668669586,
40.0955863397546));
#186812=CARTESIAN_POINT('Ctrl Pts',(54.3993582729152,-31.4635725360687,
40.0970906856166));
#186813=CARTESIAN_POINT('Ctrl Pts',(54.4037093249067,-31.4585547584352,
40.0982599215483));
#186814=CARTESIAN_POINT('Ctrl Pts',(54.4077698566065,-31.4532397415955,
40.0990497370454));
#186815=CARTESIAN_POINT('Ctrl Pts',(54.4087849895314,-31.4519109873856,
40.0992471909196));
#186816=CARTESIAN_POINT('Ctrl Pts',(54.4097817701143,-31.4505635261657,
40.0994209989363));
#186817=CARTESIAN_POINT('Ctrl Pts',(54.4107588499958,-31.4491976069258,
40.0995705982975));
#186818=CARTESIAN_POINT('Ctrl Pts',(54.4122244698181,-31.4471487280661,
40.0997949973393));
#186819=CARTESIAN_POINT('Ctrl Pts',(54.4136457436054,-31.4450583254658,
40.0999649129781));
#186820=CARTESIAN_POINT('Ctrl Pts',(54.4150195646481,-31.4429280944108,
40.1000786629733));
#186821=CARTESIAN_POINT('Ctrl Pts',(54.4163933856907,-31.4407978633559,
40.1001924129685));
#186822=CARTESIAN_POINT('Ctrl Pts',(54.4177197583729,-31.4386278145919,
40.10025));
#186823=CARTESIAN_POINT('Ctrl Pts',(54.4189959163063,-31.4364195775136,
40.10025));
#186824=CARTESIAN_POINT('Ctrl Pts',(51.1126068659047,-29.5274749692186,
40.10025));
#186825=CARTESIAN_POINT('Ctrl Pts',(51.1082885388132,-29.5349468458343,
40.10025));
#186826=CARTESIAN_POINT('Ctrl Pts',(51.104624414239,-29.5427104181375,40.0995786334242));
#186827=CARTESIAN_POINT('Ctrl Pts',(51.101604925595,-29.5506148782549,40.0983063763368));
#186828=CARTESIAN_POINT('Ctrl Pts',(51.0996546457482,-29.555720348447,40.0974846287994));
#186829=CARTESIAN_POINT('Ctrl Pts',(51.0979724198488,-29.5608842707082,
40.0964130309339));
#186830=CARTESIAN_POINT('Ctrl Pts',(51.0965469289497,-29.5660646037405,
40.0951176960924));
#186831=CARTESIAN_POINT('Ctrl Pts',(51.0946575224202,-29.5729308384266,
40.0934008039615));
#186832=CARTESIAN_POINT('Ctrl Pts',(51.0932249325813,-29.5798262755779,
40.0912909372157));
#186833=CARTESIAN_POINT('Ctrl Pts',(51.0922302752234,-29.5866628504238,
40.0888630467852));
#186834=CARTESIAN_POINT('Ctrl Pts',(51.0917329465444,-29.5900811378467,
40.08764910157));
#186835=CARTESIAN_POINT('Ctrl Pts',(51.0913449998289,-29.5934848814074,
40.0863558569272));
#186836=CARTESIAN_POINT('Ctrl Pts',(51.0910633609953,-29.596864293881,40.0849936342772));
#186837=CARTESIAN_POINT('Ctrl Pts',(51.0909225415785,-29.5985540001179,
40.0843125229522));
#186838=CARTESIAN_POINT('Ctrl Pts',(51.0908082908743,-29.6002376377882,
40.0836141747075));
#186839=CARTESIAN_POINT('Ctrl Pts',(51.0907201726671,-29.6019140726116,
40.082899916161));
#186840=CARTESIAN_POINT('Ctrl Pts',(51.0906981431153,-29.6023331813174,
40.0827213515244));
#186841=CARTESIAN_POINT('Ctrl Pts',(51.090677746668,-29.602751840147,40.0825417925842));
#186842=CARTESIAN_POINT('Ctrl Pts',(51.090658976153,-29.6031700319852,40.0823612602361));
#186843=CARTESIAN_POINT('Ctrl Pts',(51.0906026646081,-29.6044246074997,
40.0818196631918));
#186844=CARTESIAN_POINT('Ctrl Pts',(51.0905609873413,-29.6056749785904,
40.0812693052022));
#186845=CARTESIAN_POINT('Ctrl Pts',(51.0905337427829,-29.6069206965765,
40.0807107531875));
#186846=CARTESIAN_POINT('Ctrl Pts',(51.0903418356317,-29.6156953732194,
40.0767763849182));
#186847=CARTESIAN_POINT('Ctrl Pts',(51.0908211368931,-29.6242688491608,
40.0724140586136));
#186848=CARTESIAN_POINT('Ctrl Pts',(51.0918641424261,-29.6325885911862,
40.0677221223766));
#186849=CARTESIAN_POINT('Ctrl Pts',(51.0923699989825,-29.6366236570779,
40.0654465383719));
#186850=CARTESIAN_POINT('Ctrl Pts',(51.0930089302516,-29.6405993642578,
40.0630928000679));
#186851=CARTESIAN_POINT('Ctrl Pts',(51.0937712117414,-29.6445110377125,
40.0606689262479));
#186852=CARTESIAN_POINT('Ctrl Pts',(51.0949382114433,-29.6504995364712,
40.0569581447805));
#186853=CARTESIAN_POINT('Ctrl Pts',(51.0963926103116,-29.656334864082,40.0530843804605));
#186854=CARTESIAN_POINT('Ctrl Pts',(51.098099028059,-29.6619874481815,40.0490800251457));
#186855=CARTESIAN_POINT('Ctrl Pts',(51.0988914972888,-29.6646125374799,
40.0472203818218));
#186856=CARTESIAN_POINT('Ctrl Pts',(51.0997380650833,-29.6671982043427,
40.0453323608818));
#186857=CARTESIAN_POINT('Ctrl Pts',(51.1006362623629,-29.6697408831276,
40.0434201572162));
#186858=CARTESIAN_POINT('Ctrl Pts',(51.1007051056453,-29.6699357694378,
40.0432735943397));
#186859=CARTESIAN_POINT('Ctrl Pts',(51.1007742270251,-29.6701304259131,
40.0431268995707));
#186860=CARTESIAN_POINT('Ctrl Pts',(51.1008436251324,-29.6703248520469,
40.0429800745037));
#186861=CARTESIAN_POINT('Ctrl Pts',(51.1018184593124,-29.67305595305,40.0409176249753));
#186862=CARTESIAN_POINT('Ctrl Pts',(51.1028499068178,-29.6757410298218,
40.0388310783332));
#186863=CARTESIAN_POINT('Ctrl Pts',(51.1039327914267,-29.6783776815769,
40.036725739981));
#186864=CARTESIAN_POINT('Ctrl Pts',(51.10781582305,-29.6878322458584,40.0291763710714));
#186865=CARTESIAN_POINT('Ctrl Pts',(51.1123884412308,-29.6967379921839,
40.0213310894586));
#186866=CARTESIAN_POINT('Ctrl Pts',(51.1175230541902,-29.705114752369,40.0132837551307));
#186867=CARTESIAN_POINT('Ctrl Pts',(51.1231654780149,-29.7143199702922,
40.0044405431309));
#186868=CARTESIAN_POINT('Ctrl Pts',(51.129486757898,-29.7228870317522,39.9953528710581));
#186869=CARTESIAN_POINT('Ctrl Pts',(51.1363687775798,-29.7308286942781,
39.9861103629531));
#186870=CARTESIAN_POINT('Ctrl Pts',(51.1437996316847,-29.7394036967207,
39.9761307737529));
#186871=CARTESIAN_POINT('Ctrl Pts',(51.1518848590033,-29.747250549869,39.9659696935981));
#186872=CARTESIAN_POINT('Ctrl Pts',(51.160525858428,-29.7543572078959,39.9557128217472));
#186873=CARTESIAN_POINT('Ctrl Pts',(51.1690943687448,-29.761404248363,39.9455419945137));
#186874=CARTESIAN_POINT('Ctrl Pts',(51.1782106315453,-29.7677241373274,
39.9352756289329));
#186875=CARTESIAN_POINT('Ctrl Pts',(51.1878102687784,-29.7732664904681,
39.92499));
#186876=CARTESIAN_POINT('Origin',(0.00762000000000077,0.0131982271536777,
39.92499));
#186877=CARTESIAN_POINT('Ctrl Pts',(54.4342359163063,-31.4100231232062,
40.10025));
#186878=CARTESIAN_POINT('Ctrl Pts',(54.4385272722023,-31.4025830926774,
40.10025));
#186879=CARTESIAN_POINT('Ctrl Pts',(54.442158989064,-31.3948506994793,40.0995859581841));
#186880=CARTESIAN_POINT('Ctrl Pts',(54.4451438299616,-31.386976274769,40.0983275959619));
#186881=CARTESIAN_POINT('Ctrl Pts',(54.4470510012009,-31.3819448922437,
40.0975235624067));
#186882=CARTESIAN_POINT('Ctrl Pts',(54.4486949601301,-31.3768558346348,
40.096477705949));
#186883=CARTESIAN_POINT('Ctrl Pts',(54.4500875286681,-31.3717496422764,
40.0952149915961));
#186884=CARTESIAN_POINT('Ctrl Pts',(54.4519881053013,-31.3647807142729,
40.0934916398701));
#186885=CARTESIAN_POINT('Ctrl Pts',(54.4534143418203,-31.3577796218683,
40.0913643921631));
#186886=CARTESIAN_POINT('Ctrl Pts',(54.4543880442396,-31.3508395087086,
40.0889118607713));
#186887=CARTESIAN_POINT('Ctrl Pts',(54.4548748954493,-31.3473694521287,
40.0876855950755));
#186888=CARTESIAN_POINT('Ctrl Pts',(54.4552487192094,-31.3439144604654,
40.0863782327527));
#186889=CARTESIAN_POINT('Ctrl Pts',(54.4555129946225,-31.3404848880614,
40.0850006373334));
#186890=CARTESIAN_POINT('Ctrl Pts',(54.4556451323291,-31.3387701018594,
40.0843118396238));
#186891=CARTESIAN_POINT('Ctrl Pts',(54.4557498916996,-31.3370616554168,
40.0836054919165));
#186892=CARTESIAN_POINT('Ctrl Pts',(54.4558277627246,-31.3353607484812,
40.0828829920418));
#186893=CARTESIAN_POINT('Ctrl Pts',(54.4558472304808,-31.3349355217473,
40.0827023670731));
#186894=CARTESIAN_POINT('Ctrl Pts',(54.4558650179028,-31.3345107659124,
40.0825207326933));
#186895=CARTESIAN_POINT('Ctrl Pts',(54.4558811330249,-31.334086499077,40.0823381109276));
#186896=CARTESIAN_POINT('Ctrl Pts',(54.4559294783911,-31.3328136985707,
40.0817902456304));
#186897=CARTESIAN_POINT('Ctrl Pts',(54.4559627721159,-31.331545300654,40.0812334935553));
#186898=CARTESIAN_POINT('Ctrl Pts',(54.4559812395338,-31.3302817797845,
40.0806684524227));
#186899=CARTESIAN_POINT('Ctrl Pts',(54.4561088608496,-31.3215500666178,
40.0767636676136));
#186900=CARTESIAN_POINT('Ctrl Pts',(54.4555742713438,-31.3130195924484,
40.0724404510887));
#186901=CARTESIAN_POINT('Ctrl Pts',(54.4544853519657,-31.3047400858587,
40.0677949937407));
#186902=CARTESIAN_POINT('Ctrl Pts',(54.4539441620239,-31.3006251938107,
40.0654862141904));
#186903=CARTESIAN_POINT('Ctrl Pts',(54.4532655373259,-31.2965719591984,
40.0630972003215));
#186904=CARTESIAN_POINT('Ctrl Pts',(54.4524598885395,-31.2925850928564,
40.0606363359906));
#186905=CARTESIAN_POINT('Ctrl Pts',(54.4506825069818,-31.283789470212,40.0552073017124));
#186906=CARTESIAN_POINT('Ctrl Pts',(54.4482992497266,-31.2753153512347,
40.0494204304519));
#186907=CARTESIAN_POINT('Ctrl Pts',(54.4454010706198,-31.2672761140351,
40.0434049749851));
#186908=CARTESIAN_POINT('Ctrl Pts',(54.4443423292441,-31.264339279306,40.0412074532442));
#186909=CARTESIAN_POINT('Ctrl Pts',(54.4432206434044,-31.2614550023639,
40.0389814735788));
#186910=CARTESIAN_POINT('Ctrl Pts',(54.4420411592048,-31.2586246102246,
40.0367321210016));
#186911=CARTESIAN_POINT('Ctrl Pts',(54.4380793965876,-31.2491176225317,
40.0291767837142));
#186912=CARTESIAN_POINT('Ctrl Pts',(54.4334326446233,-31.2401615453397,
40.021323533258));
#186913=CARTESIAN_POINT('Ctrl Pts',(54.4282277812596,-31.2317373058274,
40.0132649215865));
#186914=CARTESIAN_POINT('Ctrl Pts',(54.4225070198661,-31.2224780686866,
40.0044075527541));
#186915=CARTESIAN_POINT('Ctrl Pts',(54.4161118092713,-31.2138606686957,
39.995301625373));
#186916=CARTESIAN_POINT('Ctrl Pts',(54.4091594014093,-31.2058737429081,
39.9860353422371));
#186917=CARTESIAN_POINT('Ctrl Pts',(54.4016713602548,-31.1972714816222,
39.9760551582709));
#186918=CARTESIAN_POINT('Ctrl Pts',(54.3935362880566,-31.1893995936782,
39.9658879738171));
#186919=CARTESIAN_POINT('Ctrl Pts',(54.3848513315137,-31.1822725865945,
39.9556174643271));
#186920=CARTESIAN_POINT('Ctrl Pts',(54.3762836512073,-31.1752418181694,
39.9454856413916));
#186921=CARTESIAN_POINT('Ctrl Pts',(54.3671795569349,-31.1689352997159,
39.9352519465119));
#186922=CARTESIAN_POINT('Ctrl Pts',(54.3576020372438,-31.1634057161441,
39.92499));
#186923=CARTESIAN_POINT('Ctrl Pts',(51.3783102687785,-29.4433108116262,
39.92499));
#186924=CARTESIAN_POINT('Ctrl Pts',(51.3691445298583,-29.4380189697933,
39.9348107241731));
#186925=CARTESIAN_POINT('Ctrl Pts',(51.3595943606098,-29.4334690915847,
39.9446038383186));
#186926=CARTESIAN_POINT('Ctrl Pts',(51.3497152868745,-29.4296781246241,
39.954315806941));
#186927=CARTESIAN_POINT('Ctrl Pts',(51.3401761719842,-29.4260176124798,
39.9636935671422));
#186928=CARTESIAN_POINT('Ctrl Pts',(51.3303291924883,-29.4230642997968,
39.9729968321024));
#186929=CARTESIAN_POINT('Ctrl Pts',(51.3202058500852,-29.4208754038575,
39.9821731151375));
#186930=CARTESIAN_POINT('Ctrl Pts',(51.3106361210799,-29.4188062116752,
39.9908475764395));
#186931=CARTESIAN_POINT('Ctrl Pts',(51.300818546174,-29.4174199248356,39.9994093733891));
#186932=CARTESIAN_POINT('Ctrl Pts',(51.2907775289294,-29.4168067767629,
40.0077966115889));
#186933=CARTESIAN_POINT('Ctrl Pts',(51.281529920498,-29.4162420776743,40.0155211172644));
#186934=CARTESIAN_POINT('Ctrl Pts',(51.2720922400877,-29.4163331870167,
40.0230979941072));
#186935=CARTESIAN_POINT('Ctrl Pts',(51.2624911797676,-29.4171879526248,
40.03045541048));
#186936=CARTESIAN_POINT('Ctrl Pts',(51.2596283373925,-29.4174428264743,
40.0326492435215));
#186937=CARTESIAN_POINT('Ctrl Pts',(51.2567510524854,-29.4177658668981,
40.0348233715077));
#186938=CARTESIAN_POINT('Ctrl Pts',(51.2538602864394,-29.4181606517643,
40.0369753512356));
#186939=CARTESIAN_POINT('Ctrl Pts',(51.2509990568967,-29.4185514029023,
40.0391053430352));
#186940=CARTESIAN_POINT('Ctrl Pts',(51.2481275521818,-29.4190117629202,
40.041211089324));
#186941=CARTESIAN_POINT('Ctrl Pts',(51.2452499391939,-29.41954444021,40.0432881154904));
#186942=CARTESIAN_POINT('Ctrl Pts',(51.2450498356145,-29.4195814815469,
40.043432547828));
#186943=CARTESIAN_POINT('Ctrl Pts',(51.2448496951983,-29.4196188630961,
40.0435768364421));
#186944=CARTESIAN_POINT('Ctrl Pts',(51.2446495184043,-29.4196565860786,
40.0437209807855));
#186945=CARTESIAN_POINT('Ctrl Pts',(51.2358730344471,-29.4213104998201,
40.050040796842));
#186946=CARTESIAN_POINT('Ctrl Pts',(51.2270453415809,-29.4236619033164,
40.0560490279344));
#186947=CARTESIAN_POINT('Ctrl Pts',(51.2182691329815,-29.4267651248008,
40.0616647108614));
#186948=CARTESIAN_POINT('Ctrl Pts',(51.2100881812722,-29.4296578665605,
40.0668995033484));
#186949=CARTESIAN_POINT('Ctrl Pts',(51.2019513265394,-29.4332044080278,
40.071793326748));
#186950=CARTESIAN_POINT('Ctrl Pts',(51.1939656059621,-29.4374658604798,
40.0762460303071));
#186951=CARTESIAN_POINT('Ctrl Pts',(51.1910443260617,-29.4390247549181,
40.0778748868747));
#186952=CARTESIAN_POINT('Ctrl Pts',(51.1881435589222,-29.4406794572086,
40.0794443522247));
#186953=CARTESIAN_POINT('Ctrl Pts',(51.1852696776793,-29.4424334077168,
40.0809482021492));
#186954=CARTESIAN_POINT('Ctrl Pts',(51.1845786052483,-29.4428551742197,
40.0813098278168));
#186955=CARTESIAN_POINT('Ctrl Pts',(51.1838888551095,-29.4432832153789,
40.0816679525672));
#186956=CARTESIAN_POINT('Ctrl Pts',(51.1832005624688,-29.4437175198434,
40.082022419258));
#186957=CARTESIAN_POINT('Ctrl Pts',(51.1825337789732,-29.4441382522934,
40.0823658088648));
#186958=CARTESIAN_POINT('Ctrl Pts',(51.1818683633172,-29.4445648626866,
40.0827057654616));
#186959=CARTESIAN_POINT('Ctrl Pts',(51.1812044402993,-29.4449973374096,
40.0830421470151));
#186960=CARTESIAN_POINT('Ctrl Pts',(51.1739303963596,-29.4497355978002,
40.0867275956805));
#186961=CARTESIAN_POINT('Ctrl Pts',(51.1668309650361,-29.4551812510951,
40.089982343203));
#186962=CARTESIAN_POINT('Ctrl Pts',(51.1600900711817,-29.4612929974515,
40.0926299529354));
#186963=CARTESIAN_POINT('Ctrl Pts',(51.1572944215756,-29.4638277208372,
40.0937279956083));
#186964=CARTESIAN_POINT('Ctrl Pts',(51.1545603804839,-29.4664765899953,
40.0947220371802));
#186965=CARTESIAN_POINT('Ctrl Pts',(51.151900368709,-29.4692349685472,40.0956014538692));
#186966=CARTESIAN_POINT('Ctrl Pts',(51.1473634414341,-29.4739396706106,
40.097101390674));
#186967=CARTESIAN_POINT('Ctrl Pts',(51.1430443628984,-29.4789629373382,
40.0982667904316));
#186968=CARTESIAN_POINT('Ctrl Pts',(51.1390107214365,-29.484277773294,40.0990539325582));
#186969=CARTESIAN_POINT('Ctrl Pts',(51.1369939007055,-29.4869351912719,
40.0994475036216));
#186970=CARTESIAN_POINT('Ctrl Pts',(51.1350496570625,-29.4896662827381,
40.0997467259952));
#186971=CARTESIAN_POINT('Ctrl Pts',(51.1331865036877,-29.492467661291,40.0999473488896));
#186972=CARTESIAN_POINT('Ctrl Pts',(51.1313233503129,-29.4952690398439,
40.100147971784));
#186973=CARTESIAN_POINT('Ctrl Pts',(51.1295412933646,-29.4981406602398,
40.10025));
#186974=CARTESIAN_POINT('Ctrl Pts',(51.1278468659047,-29.5010785149112,
40.10025));
#186975=CARTESIAN_POINT('Origin',(47.1274239660509,-34.2589154226522,39.92499));
#186976=CARTESIAN_POINT('Ctrl Pts',(50.5784163149356,-36.9828414016747,
39.92499));
#186977=CARTESIAN_POINT('Ctrl Pts',(50.5870002518364,-36.9890779968908,
39.9348354642022));
#186978=CARTESIAN_POINT('Ctrl Pts',(50.5960508068002,-36.9946187858199,
39.9446440828466));
#186979=CARTESIAN_POINT('Ctrl Pts',(50.6055128591424,-36.9994424783904,
39.9543641760342));
#186980=CARTESIAN_POINT('Ctrl Pts',(50.6146674511263,-37.0041094296755,
39.9637684240726));
#186981=CARTESIAN_POINT('Ctrl Pts',(50.6242084112817,-37.0081056536706,
39.9730909636412));
#186982=CARTESIAN_POINT('Ctrl Pts',(50.6341096134641,-37.0113722741994,
39.9822808977158));
#186983=CARTESIAN_POINT('Ctrl Pts',(50.6434755410477,-37.0144622960727,
39.9909740094668));
#186984=CARTESIAN_POINT('Ctrl Pts',(50.6531646927642,-37.0168997626763,
39.9995492765021));
#186985=CARTESIAN_POINT('Ctrl Pts',(50.663162158125,-37.0185933530509,40.0079462328715));
#186986=CARTESIAN_POINT('Ctrl Pts',(50.6723705467575,-37.0201532722694,
40.0156804369711));
#186987=CARTESIAN_POINT('Ctrl Pts',(50.6818410607745,-37.021082144611,40.0232638017444));
#186988=CARTESIAN_POINT('Ctrl Pts',(50.6915586678667,-37.0212705108774,
40.0306257269989));
#186989=CARTESIAN_POINT('Ctrl Pts',(50.6943773762892,-37.021325148771,40.0327611416667));
#186990=CARTESIAN_POINT('Ctrl Pts',(50.6972168227831,-37.0213172191965,
40.0348777427279));
#186991=CARTESIAN_POINT('Ctrl Pts',(50.7000764815586,-37.0212433695024,
40.0369733168701));
#186992=CARTESIAN_POINT('Ctrl Pts',(50.7031765355313,-37.0211633116858,
40.0392450539741));
#186993=CARTESIAN_POINT('Ctrl Pts',(50.7062960577322,-37.0210069737841,
40.041487875195));
#186994=CARTESIAN_POINT('Ctrl Pts',(50.7094335311103,-37.0207706534746,
40.0436985701601));
#186995=CARTESIAN_POINT('Ctrl Pts',(50.718044351416,-37.0201220705309,40.0497658398386));
#186996=CARTESIAN_POINT('Ctrl Pts',(50.7267761502172,-37.0188289150181,
40.0555581699984));
#186997=CARTESIAN_POINT('Ctrl Pts',(50.7355328079489,-37.0168522507831,
40.0609828468885));
#186998=CARTESIAN_POINT('Ctrl Pts',(50.7435446743638,-37.0150437103237,
40.0659461317307));
#186999=CARTESIAN_POINT('Ctrl Pts',(50.7515681793728,-37.0126559296146,
40.0706039980711));
#187000=CARTESIAN_POINT('Ctrl Pts',(50.7595400218662,-37.0096268558211,
40.0748843180609));
#187001=CARTESIAN_POINT('Ctrl Pts',(50.7634557648571,-37.0081389846688,
40.0769867972574));
#187002=CARTESIAN_POINT('Ctrl Pts',(50.7673587034243,-37.0064960060557,
40.0789976708176));
#187003=CARTESIAN_POINT('Ctrl Pts',(50.771238806215,-37.0046883717067,40.0809050491499));
#187004=CARTESIAN_POINT('Ctrl Pts',(50.7719750179269,-37.0043453906956,
40.0812669556104));
#187005=CARTESIAN_POINT('Ctrl Pts',(50.7727105984664,-37.0039959853415,
40.0816253922032));
#187006=CARTESIAN_POINT('Ctrl Pts',(50.7734454079409,-37.0036401497474,
40.0819801989139));
#187007=CARTESIAN_POINT('Ctrl Pts',(50.7741572546194,-37.0032954340157,
40.0823239179149));
#187008=CARTESIAN_POINT('Ctrl Pts',(50.7748683776572,-37.0029446836753,
40.0826642303498));
#187009=CARTESIAN_POINT('Ctrl Pts',(50.7755786476302,-37.0025878964869,
40.0830009916099));
#187010=CARTESIAN_POINT('Ctrl Pts',(50.7833190234413,-36.9986997032254,
40.0866709464311));
#187011=CARTESIAN_POINT('Ctrl Pts',(50.790962999314,-36.9940916451527,40.0899175831876));
#187012=CARTESIAN_POINT('Ctrl Pts',(50.7983209798294,-36.9887818345684,
40.092564206706));
#187013=CARTESIAN_POINT('Ctrl Pts',(50.8014283006921,-36.9865394685863,
40.0936818922526));
#187014=CARTESIAN_POINT('Ctrl Pts',(50.8044846273289,-36.9841723869924,
40.094693009479));
#187015=CARTESIAN_POINT('Ctrl Pts',(50.807476228564,-36.9816838130234,40.0955863397545));
#187016=CARTESIAN_POINT('Ctrl Pts',(50.8125140102918,-36.9774931166426,
40.0970906856166));
#187017=CARTESIAN_POINT('Ctrl Pts',(50.8173657273503,-36.9729576356982,
40.0982599215483));
#187018=CARTESIAN_POINT('Ctrl Pts',(50.8219595855749,-36.9680961762154,
40.0990497370453));
#187019=CARTESIAN_POINT('Ctrl Pts',(50.8231080501311,-36.9668808113447,
40.0992471909196));
#187020=CARTESIAN_POINT('Ctrl Pts',(50.8242402182962,-36.9656449236009,
40.0994209989363));
#187021=CARTESIAN_POINT('Ctrl Pts',(50.8253547230711,-36.9643886196681,
40.0995705982975));
#187022=CARTESIAN_POINT('Ctrl Pts',(50.8270264802333,-36.9625041637689,
40.0997949973393));
#187023=CARTESIAN_POINT('Ctrl Pts',(50.8286584747055,-36.9605737761776,
40.0999649129781));
#187024=CARTESIAN_POINT('Ctrl Pts',(50.8302474395913,-36.9585988181537,
40.1000786629733));
#187025=CARTESIAN_POINT('Ctrl Pts',(50.8318364044772,-36.9566238601298,
40.1001924129685));
#187026=CARTESIAN_POINT('Ctrl Pts',(50.833382343015,-36.9546043428193,40.10025));
#187027=CARTESIAN_POINT('Ctrl Pts',(50.83488233365,-36.9525415975223,40.10025));
#187028=CARTESIAN_POINT('Ctrl Pts',(47.7461450747864,-34.7084426211232,
40.10025));
#187029=CARTESIAN_POINT('Ctrl Pts',(47.7410693801618,-34.7154221779228,
40.10025));
#187030=CARTESIAN_POINT('Ctrl Pts',(47.7366138137628,-34.7227602152543,
40.099578633424));
#187031=CARTESIAN_POINT('Ctrl Pts',(47.7327846251243,-34.7303057514049,
40.0983063763365));
#187032=CARTESIAN_POINT('Ctrl Pts',(47.7303113621615,-34.7351793935412,
40.0974846287991));
#187033=CARTESIAN_POINT('Ctrl Pts',(47.7280985748135,-34.7401391868071,
40.0964130309337));
#187034=CARTESIAN_POINT('Ctrl Pts',(47.7261394006518,-34.7451421370594,
40.0951176960923));
#187035=CARTESIAN_POINT('Ctrl Pts',(47.7235426275288,-34.7517732610324,
40.0934008039614));
#187036=CARTESIAN_POINT('Ctrl Pts',(47.721397116118,-34.7584811778432,40.0912909372156));
#187037=CARTESIAN_POINT('Ctrl Pts',(47.7196932909345,-34.7651763312116,
40.0888630467851));
#187038=CARTESIAN_POINT('Ctrl Pts',(47.7188413783428,-34.7685239078958,
40.0876491015699));
#187039=CARTESIAN_POINT('Ctrl Pts',(47.7180997687562,-34.7718684539192,
40.0863558569271));
#187040=CARTESIAN_POINT('Ctrl Pts',(47.717466427977,-34.7751999143432,40.0849936342771));
#187041=CARTESIAN_POINT('Ctrl Pts',(47.7171497575873,-34.7768656445553,
40.0843125229521));
#187042=CARTESIAN_POINT('Ctrl Pts',(47.716860144702,-34.7785281166318,40.0836141747074));
#187043=CARTESIAN_POINT('Ctrl Pts',(47.7165972740597,-34.780186156909,40.0828999161609));
#187044=CARTESIAN_POINT('Ctrl Pts',(47.7165315563991,-34.7806006669783,
40.0827213515243));
#187045=CARTESIAN_POINT('Ctrl Pts',(47.7164675099217,-34.7810149003417,
40.0825417925842));
#187046=CARTESIAN_POINT('Ctrl Pts',(47.7164051292834,-34.7814288392281,
40.0823612602361));
#187047=CARTESIAN_POINT('Ctrl Pts',(47.7162179873684,-34.7826706558875,
40.0818196631917));
#187048=CARTESIAN_POINT('Ctrl Pts',(47.7160458390454,-34.7839098208538,
40.0812693052021));
#187049=CARTESIAN_POINT('Ctrl Pts',(47.7158885307488,-34.7851458668347,
40.0807107531874));
#187050=CARTESIAN_POINT('Ctrl Pts',(47.7147804714199,-34.7938524151211,
40.0767763849181));
#187051=CARTESIAN_POINT('Ctrl Pts',(47.7143609747538,-34.8024290252884,
40.0724140586137));
#187052=CARTESIAN_POINT('Ctrl Pts',(47.7145286167446,-34.8108122146619,
40.0677221223768));
#187053=CARTESIAN_POINT('Ctrl Pts',(47.714609922929,-34.8148780524491,40.065446538372));
#187054=CARTESIAN_POINT('Ctrl Pts',(47.7148297795039,-34.8188987667928,
40.0630928000679));
#187055=CARTESIAN_POINT('Ctrl Pts',(47.7151790039209,-34.8228686918039,
40.0606689262479));
#187056=CARTESIAN_POINT('Ctrl Pts',(47.7157136421037,-34.8289463696253,
40.0569581447805));
#187057=CARTESIAN_POINT('Ctrl Pts',(47.7165501157951,-34.8349017567796,
40.0530843804605));
#187058=CARTESIAN_POINT('Ctrl Pts',(47.7176563296782,-34.8407017446568,
40.0490800251457));
#187059=CARTESIAN_POINT('Ctrl Pts',(47.7181700611282,-34.8433952890321,
40.0472203818218));
#187060=CARTESIAN_POINT('Ctrl Pts',(47.7187417155521,-34.8460552817719,
40.0453323608818));
#187061=CARTESIAN_POINT('Ctrl Pts',(47.719369210107,-34.8486779186777,40.0434201572162));
#187062=CARTESIAN_POINT('Ctrl Pts',(47.7194173050922,-34.8488789334628,
40.0432735943397));
#187063=CARTESIAN_POINT('Ctrl Pts',(47.7194657006756,-34.8490797487412,
40.0431268995707));
#187064=CARTESIAN_POINT('Ctrl Pts',(47.7195143955479,-34.8492803638658,
40.0429800745037));
#187065=CARTESIAN_POINT('Ctrl Pts',(47.7201984116934,-34.8520984015307,
40.0409176249753));
#187066=CARTESIAN_POINT('Ctrl Pts',(47.7209435418727,-34.8548765847936,
40.0388310783332));
#187067=CARTESIAN_POINT('Ctrl Pts',(47.7217448891703,-34.8576119849586,
40.036725739981));
#187068=CARTESIAN_POINT('Ctrl Pts',(47.7246183780646,-34.8674206434752,
40.0291763710721));
#187069=CARTESIAN_POINT('Ctrl Pts',(47.7282350429864,-34.8767555719411,
40.0213310894601));
#187070=CARTESIAN_POINT('Ctrl Pts',(47.732465918129,-34.8856231565589,40.013283755133));
#187071=CARTESIAN_POINT('Ctrl Pts',(47.7371152248815,-34.8953677412259,
40.004440543134));
#187072=CARTESIAN_POINT('Ctrl Pts',(47.7425063743623,-34.9045486250982,
39.995352871062));
#187073=CARTESIAN_POINT('Ctrl Pts',(47.7485205638398,-34.9131661493068,
39.9861103629579));
#187074=CARTESIAN_POINT('Ctrl Pts',(47.7550143791198,-34.9224709127486,
39.9761307737586));
#187075=CARTESIAN_POINT('Ctrl Pts',(47.7622350952152,-34.9311199164006,
39.9659696936047));
#187076=CARTESIAN_POINT('Ctrl Pts',(47.7700859102973,-34.9390908738019,
39.9557128217548));
#187077=CARTESIAN_POINT('Ctrl Pts',(47.7778708651091,-34.9469949630621,
39.9455419945188));
#187078=CARTESIAN_POINT('Ctrl Pts',(47.7862765797886,-34.9542331399568,
39.9352756289355));
#187079=CARTESIAN_POINT('Ctrl Pts',(47.7952442955502,-34.9607485668366,
39.92499));
#187080=CARTESIAN_POINT('Origin',(0.00895784724493838,0.0123294189942775,
39.92499));
#187081=CARTESIAN_POINT('Ctrl Pts',(50.8527980281385,-36.9278827595327,
40.10025));
#187082=CARTESIAN_POINT('Ctrl Pts',(50.8578435704958,-36.9209320551068,
40.10025));
#187083=CARTESIAN_POINT('Ctrl Pts',(50.8622636476109,-36.9136216385502,
40.0995859581841));
#187084=CARTESIAN_POINT('Ctrl Pts',(50.8660552387518,-36.9061023515945,
40.0983275959619));
#187085=CARTESIAN_POINT('Ctrl Pts',(50.868477884991,-36.9012978851879,40.0975235624066));
#187086=CARTESIAN_POINT('Ctrl Pts',(50.8706447895124,-36.8964085464697,
40.0964777059489));
#187087=CARTESIAN_POINT('Ctrl Pts',(50.8725634718546,-36.8914758894166,
40.095214991596));
#187088=CARTESIAN_POINT('Ctrl Pts',(50.875182088265,-36.8847438022847,40.09349163987));
#187089=CARTESIAN_POINT('Ctrl Pts',(50.8773323251414,-36.8779301449084,
40.091364392163));
#187090=CARTESIAN_POINT('Ctrl Pts',(50.8790261328804,-36.8711298300322,
40.0889118607712));
#187091=CARTESIAN_POINT('Ctrl Pts',(50.87987303675,-36.8677296725942,40.0876855950753));
#187092=CARTESIAN_POINT('Ctrl Pts',(50.8806059576336,-36.86433268296,40.0863782327526));
#187093=CARTESIAN_POINT('Ctrl Pts',(50.8812272732514,-36.8609495224152,
40.0850006373333));
#187094=CARTESIAN_POINT('Ctrl Pts',(50.8815379310603,-36.8592579421429,
40.0843118396237));
#187095=CARTESIAN_POINT('Ctrl Pts',(50.8818206978293,-36.8575698050846,
40.0836054919164));
#187096=CARTESIAN_POINT('Ctrl Pts',(50.8820759354568,-36.8558863556338,
40.0828829920417));
#187097=CARTESIAN_POINT('Ctrl Pts',(50.8821397448637,-36.8554654932711,
40.082702367073));
#187098=CARTESIAN_POINT('Ctrl Pts',(50.882201833919,-36.855044923585,40.0825207326932));
#187099=CARTESIAN_POINT('Ctrl Pts',(50.8822622087211,-36.8546246654166,
40.0823381109275));
#187100=CARTESIAN_POINT('Ctrl Pts',(50.8824433331273,-36.8533638909115,
40.0817902456303));
#187101=CARTESIAN_POINT('Ctrl Pts',(50.8826090281505,-36.8521059215532,
40.0812334935552));
#187102=CARTESIAN_POINT('Ctrl Pts',(50.8827594682968,-36.850851252754,40.0806684524226));
#187103=CARTESIAN_POINT('Ctrl Pts',(50.8837991030487,-36.842180712886,40.0767636676137));
#187104=CARTESIAN_POINT('Ctrl Pts',(50.884159119436,-36.8336410897275,40.072440451089));
#187105=CARTESIAN_POINT('Ctrl Pts',(50.8839416093727,-36.8252931160723,
40.0677949937412));
#187106=CARTESIAN_POINT('Ctrl Pts',(50.8838335074683,-36.8211441960801,
40.0654862141907));
#187107=CARTESIAN_POINT('Ctrl Pts',(50.8835822787327,-36.8170422299141,
40.0630972003217));
#187108=CARTESIAN_POINT('Ctrl Pts',(50.8831977843866,-36.8129929908131,
40.0606363359906));
#187109=CARTESIAN_POINT('Ctrl Pts',(50.8823495324296,-36.804059764547,40.0552073017123));
#187110=CARTESIAN_POINT('Ctrl Pts',(50.8808651175412,-36.7953829494616,
40.0494204304519));
#187111=CARTESIAN_POINT('Ctrl Pts',(50.8788231440731,-36.7870848098363,
40.0434049749851));
#187112=CARTESIAN_POINT('Ctrl Pts',(50.8780771854145,-36.7840533947861,
40.0412074532442));
#187113=CARTESIAN_POINT('Ctrl Pts',(50.8772631333235,-36.7810676701177,
40.0389814735788));
#187114=CARTESIAN_POINT('Ctrl Pts',(50.8763859670025,-36.7781294934919,
40.0367321210017));
#187115=CARTESIAN_POINT('Ctrl Pts',(50.8734396581493,-36.7682604691142,
40.0291767837144));
#187116=CARTESIAN_POINT('Ctrl Pts',(50.8697545265642,-36.7588677364083,
40.0213235332583));
#187117=CARTESIAN_POINT('Ctrl Pts',(50.8654587487971,-36.7499455893927,
40.0132649215869));
#187118=CARTESIAN_POINT('Ctrl Pts',(50.8607371801626,-36.7401390929248,
40.0044075527547));
#187119=CARTESIAN_POINT('Ctrl Pts',(50.8552777667792,-36.7309004184172,
39.9953016253738));
#187120=CARTESIAN_POINT('Ctrl Pts',(50.8491983060139,-36.7222305213351,
39.986035342238));
#187121=CARTESIAN_POINT('Ctrl Pts',(50.8426504662856,-36.7128926707021,
39.9760551582722));
#187122=CARTESIAN_POINT('Ctrl Pts',(50.8353827952143,-36.7042135591887,
39.9658879738187));
#187123=CARTESIAN_POINT('Ctrl Pts',(50.8274903908706,-36.6962177694347,
39.955617464329));
#187124=CARTESIAN_POINT('Ctrl Pts',(50.819704560632,-36.6883299498379,39.9454856413929));
#187125=CARTESIAN_POINT('Ctrl Pts',(50.8113095502226,-36.6811063421681,
39.9352519465126));
#187126=CARTESIAN_POINT('Ctrl Pts',(50.8023624960591,-36.6746059268179,
39.92499));
#187127=CARTESIAN_POINT('Ctrl Pts',(48.0191904766736,-34.6525130919798,
39.92499));
#187128=CARTESIAN_POINT('Ctrl Pts',(48.0106280967258,-34.6462921588067,
39.9348107241721));
#187129=CARTESIAN_POINT('Ctrl Pts',(48.0016058360818,-34.640768940792,39.9446038383167));
#187130=CARTESIAN_POINT('Ctrl Pts',(47.9921771448978,-34.6359660967493,
39.9543158069381));
#187131=CARTESIAN_POINT('Ctrl Pts',(47.9830729139868,-34.6313285282533,
39.9636935671387));
#187132=CARTESIAN_POINT('Ctrl Pts',(47.9735885825119,-34.6273621044917,
39.9729968320983));
#187133=CARTESIAN_POINT('Ctrl Pts',(47.9637494987672,-34.6241270221289,
39.9821731151329));
#187134=CARTESIAN_POINT('Ctrl Pts',(47.9544484832181,-34.6210688561309,
39.9908475764345));
#187135=CARTESIAN_POINT('Ctrl Pts',(47.9448295964483,-34.6186639474976,
39.9994093733839));
#187136=CARTESIAN_POINT('Ctrl Pts',(47.9349076763732,-34.6170045862117,
40.0077966115834));
#187137=CARTESIAN_POINT('Ctrl Pts',(47.9257697544367,-34.6154763423053,
40.0155211172588));
#187138=CARTESIAN_POINT('Ctrl Pts',(47.9163742511081,-34.6145804463108,
40.0230979941014));
#187139=CARTESIAN_POINT('Ctrl Pts',(47.906736439066,-34.614426945342,40.0304554104741));
#187140=CARTESIAN_POINT('Ctrl Pts',(47.9038626380665,-34.6143811744517,
40.0326492435176));
#187141=CARTESIAN_POINT('Ctrl Pts',(47.9009673483056,-34.6144016870564,
40.0348233715058));
#187142=CARTESIAN_POINT('Ctrl Pts',(47.8980511519205,-34.6144921419175,
40.0369753512355));
#187143=CARTESIAN_POINT('Ctrl Pts',(47.8951647518766,-34.6145816725527,
40.0391053430351));
#187144=CARTESIAN_POINT('Ctrl Pts',(47.8922608568399,-34.6147393566952,
40.041211089324));
#187145=CARTESIAN_POINT('Ctrl Pts',(47.8893433277785,-34.6149683234595,
40.0432881154904));
#187146=CARTESIAN_POINT('Ctrl Pts',(47.8891404485133,-34.6149842453605,
40.043432547828));
#187147=CARTESIAN_POINT('Ctrl Pts',(47.8889374970514,-34.6150005017596,
40.0435768364421));
#187148=CARTESIAN_POINT('Ctrl Pts',(47.8887344737214,-34.6150170939189,
40.0437209807855));
#187149=CARTESIAN_POINT('Ctrl Pts',(47.8798331871998,-34.615744554967,40.050040796842));
#187150=CARTESIAN_POINT('Ctrl Pts',(47.8708080647647,-34.6171603320593,
40.0560490279345));
#187151=CARTESIAN_POINT('Ctrl Pts',(47.8617555581812,-34.6193291901736,
40.0616647108616));
#187152=CARTESIAN_POINT('Ctrl Pts',(47.8533170487304,-34.6213509428811,
40.0668995033487));
#187153=CARTESIAN_POINT('Ctrl Pts',(47.8448540540096,-34.6240275231021,
40.0717933267483));
#187154=CARTESIAN_POINT('Ctrl Pts',(47.836466636969,-34.6274308957718,40.0762460303074));
#187155=CARTESIAN_POINT('Ctrl Pts',(47.8333984113058,-34.6286758935245,
40.0778748868749));
#187156=CARTESIAN_POINT('Ctrl Pts',(47.8303405713848,-34.6300183184511,
40.0794443522248));
#187157=CARTESIAN_POINT('Ctrl Pts',(47.827299095813,-34.6314622582449,40.0809482021492));
#187158=CARTESIAN_POINT('Ctrl Pts',(47.8265677225446,-34.6318094775275,
40.0813098278168));
#187159=CARTESIAN_POINT('Ctrl Pts',(47.8258370084447,-34.6321630753104,
40.0816679525672));
#187160=CARTESIAN_POINT('Ctrl Pts',(47.8251070891649,-34.6325230544376,
40.082022419258));
#187161=CARTESIAN_POINT('Ctrl Pts',(47.8243999798625,-34.6328717842171,
40.0823658088648));
#187162=CARTESIAN_POINT('Ctrl Pts',(47.8236936164943,-34.633226502718,40.0827057654617));
#187163=CARTESIAN_POINT('Ctrl Pts',(47.822988124598,-34.6335872094465,40.0830421470151));
#187164=CARTESIAN_POINT('Ctrl Pts',(47.8152586455547,-34.6375391685162,
40.0867275956807));
#187165=CARTESIAN_POINT('Ctrl Pts',(47.8076288798881,-34.6422128973065,
40.0899823432032));
#187166=CARTESIAN_POINT('Ctrl Pts',(47.8002860619008,-34.6475865476014,
40.0926299529357));
#187167=CARTESIAN_POINT('Ctrl Pts',(47.7972407764157,-34.6498151605499,
40.0937279956085));
#187168=CARTESIAN_POINT('Ctrl Pts',(47.794244830465,-34.6521637338115,40.0947220371803));
#187169=CARTESIAN_POINT('Ctrl Pts',(47.7913110614419,-34.6546289547338,
40.0956014538692));
#187170=CARTESIAN_POINT('Ctrl Pts',(47.7863072126526,-34.6588336459111,
40.097101390674));
#187171=CARTESIAN_POINT('Ctrl Pts',(47.7814867201294,-34.6633779280159,
40.0982667904316));
#187172=CARTESIAN_POINT('Ctrl Pts',(47.7769196237425,-34.6682420184009,
40.0990539325582));
#187173=CARTESIAN_POINT('Ctrl Pts',(47.774636075549,-34.6706740635933,40.0994475036216));
#187174=CARTESIAN_POINT('Ctrl Pts',(47.7724170058821,-34.6731869650546,
40.0997467259952));
#187175=CARTESIAN_POINT('Ctrl Pts',(47.7702712352612,-34.6757782448035,
40.0999473488896));
#187176=CARTESIAN_POINT('Ctrl Pts',(47.7681254646404,-34.6783695245524,
40.100147971784));
#187177=CARTESIAN_POINT('Ctrl Pts',(47.7660530039194,-34.681039138237,40.10025));
#187178=CARTESIAN_POINT('Ctrl Pts',(47.7640607692763,-34.6837837831347,
40.10025));
#187179=CARTESIAN_POINT('Origin',(43.2882232241948,-38.997398704332,39.92499));
#187180=CARTESIAN_POINT('Ctrl Pts',(46.435582879267,-42.0671296588096,39.92499));
#187181=CARTESIAN_POINT('Ctrl Pts',(46.4434678907493,-42.0742293550377,
39.9348354642017));
#187182=CARTESIAN_POINT('Ctrl Pts',(46.4518896956739,-42.0806858315473,
39.9446440828457));
#187183=CARTESIAN_POINT('Ctrl Pts',(46.4607957007316,-42.0864721532159,
39.9543641760331));
#187184=CARTESIAN_POINT('Ctrl Pts',(46.4694123136567,-42.0920704538855,
39.9637684240712));
#187185=CARTESIAN_POINT('Ctrl Pts',(46.4784832882808,-42.0970420880505,
39.9730909636396));
#187186=CARTESIAN_POINT('Ctrl Pts',(46.4879887958175,-42.1013257711388,
39.9822808977141));
#187187=CARTESIAN_POINT('Ctrl Pts',(46.4969804206317,-42.1053778715664,
39.9909740094651));
#187188=CARTESIAN_POINT('Ctrl Pts',(46.5063617095226,-42.1088147776121,
39.9995492765003));
#187189=CARTESIAN_POINT('Ctrl Pts',(46.5161273793226,-42.1115441100121,
40.0079462328696));
#187190=CARTESIAN_POINT('Ctrl Pts',(46.5251222674796,-42.1140580225429,
40.0156804369692));
#187191=CARTESIAN_POINT('Ctrl Pts',(46.5344438074312,-42.1159717447011,
40.0232638017425));
#187192=CARTESIAN_POINT('Ctrl Pts',(46.5440884908184,-42.1171748456134,
40.030625726997));
#187193=CARTESIAN_POINT('Ctrl Pts',(46.5468860468469,-42.1175238194548,
40.0327611416654));
#187194=CARTESIAN_POINT('Ctrl Pts',(46.5497107674229,-42.117812736298,40.0348777427272));
#187195=CARTESIAN_POINT('Ctrl Pts',(46.5525624800842,-42.1180382068975,
40.0369733168701));
#187196=CARTESIAN_POINT('Ctrl Pts',(46.5556539199574,-42.1182826315239,
40.039245053974));
#187197=CARTESIAN_POINT('Ctrl Pts',(46.5587726948499,-42.1184532289193,
40.041487875195));
#187198=CARTESIAN_POINT('Ctrl Pts',(46.5619176830194,-42.118546158468,40.0436985701601));
#187199=CARTESIAN_POINT('Ctrl Pts',(46.5705491277288,-42.1188012043435,
40.0497658398386));
#187200=CARTESIAN_POINT('Ctrl Pts',(46.5793682643811,-42.1184278543821,
40.0555581699984));
#187201=CARTESIAN_POINT('Ctrl Pts',(46.5882835699004,-42.1173773384967,
40.0609828468885));
#187202=CARTESIAN_POINT('Ctrl Pts',(46.5964405904276,-42.1164161734954,
40.0659461317306));
#187203=CARTESIAN_POINT('Ctrl Pts',(46.6046697328848,-42.1148801579475,
40.070603998071));
#187204=CARTESIAN_POINT('Ctrl Pts',(46.6129145292195,-42.1127009621825,
40.0748843180608));
#187205=CARTESIAN_POINT('Ctrl Pts',(46.6169643462458,-42.1116305483415,
40.0769867972573));
#187206=CARTESIAN_POINT('Ctrl Pts',(46.6210176421369,-42.1104045383077,
40.0789976708176));
#187207=CARTESIAN_POINT('Ctrl Pts',(46.6250654385592,-42.1090123875508,
40.08090504915));
#187208=CARTESIAN_POINT('Ctrl Pts',(46.6258334685044,-42.1087482405044,
40.0812669556105));
#187209=CARTESIAN_POINT('Ctrl Pts',(46.6266015422614,-42.1084776383328,
40.0816253922032));
#187210=CARTESIAN_POINT('Ctrl Pts',(46.6273695213206,-42.1082005605485,
40.0819801989139));
#187211=CARTESIAN_POINT('Ctrl Pts',(46.6281135010342,-42.107932141445,40.0823239179149));
#187212=CARTESIAN_POINT('Ctrl Pts',(46.6288573918596,-42.10765764515,40.0826642303498));
#187213=CARTESIAN_POINT('Ctrl Pts',(46.6296010653159,-42.107377055908,40.0830009916099));
#187214=CARTESIAN_POINT('Ctrl Pts',(46.6377054654047,-42.1043192521647,
40.086670946431));
#187215=CARTESIAN_POINT('Ctrl Pts',(46.6457892400063,-42.1005354505678,
40.0899175831874));
#187216=CARTESIAN_POINT('Ctrl Pts',(46.6536619390749,-42.0960238460778,
40.0925642067057));
#187217=CARTESIAN_POINT('Ctrl Pts',(46.6569866287793,-42.0941185674855,
40.0936818922525));
#187218=CARTESIAN_POINT('Ctrl Pts',(46.6602736399407,-42.0920839261387,
40.0946930094789));
#187219=CARTESIAN_POINT('Ctrl Pts',(46.6635089796843,-42.0899216923179,
40.0955863397546));
#187220=CARTESIAN_POINT('Ctrl Pts',(46.6689572109695,-42.0862805445926,
40.0970906856166));
#187221=CARTESIAN_POINT('Ctrl Pts',(46.6742564366675,-42.0822770520157,
40.0982599215483));
#187222=CARTESIAN_POINT('Ctrl Pts',(46.679333290145,-42.0779224130572,40.0990497370454));
#187223=CARTESIAN_POINT('Ctrl Pts',(46.6806025035144,-42.0768337533176,
40.0992471909196));
#187224=CARTESIAN_POINT('Ctrl Pts',(46.6818576549905,-42.0757229796946,
40.0994209989363));
#187225=CARTESIAN_POINT('Ctrl Pts',(46.683097373911,-42.0745900553976,40.0995705982975));
#187226=CARTESIAN_POINT('Ctrl Pts',(46.6849569522919,-42.0728906689521,
40.0997949973393));
#187227=CARTESIAN_POINT('Ctrl Pts',(46.686781786976,-42.0711414461003,40.0999649129781));
#187228=CARTESIAN_POINT('Ctrl Pts',(46.6885684866733,-42.0693433991608,
40.1000786629733));
#187229=CARTESIAN_POINT('Ctrl Pts',(46.6903551863705,-42.0675453522213,
40.1001924129685));
#187230=CARTESIAN_POINT('Ctrl Pts',(46.692103753135,-42.0656984926165,40.10025));
#187231=CARTESIAN_POINT('Ctrl Pts',(46.6938111422604,-42.0638038389701,
40.10025));
#187232=CARTESIAN_POINT('Ctrl Pts',(43.8565665267056,-39.5091373124623,
40.10025));
#187233=CARTESIAN_POINT('Ctrl Pts',(43.8507890749204,-39.5155480799606,
40.10025));
#187234=CARTESIAN_POINT('Ctrl Pts',(43.8455908828145,-39.5223801852474,
40.099578633424));
#187235=CARTESIAN_POINT('Ctrl Pts',(43.8409939475736,-39.5294841269579,
40.0983063763364));
#187236=CARTESIAN_POINT('Ctrl Pts',(43.8380247990813,-39.5340725443955,
40.097484628799));
#187237=CARTESIAN_POINT('Ctrl Pts',(43.8353056940458,-39.5387738681337,
40.0964130309337));
#187238=CARTESIAN_POINT('Ctrl Pts',(43.8328343017437,-39.5435446222363,
40.0951176960924));
#187239=CARTESIAN_POINT('Ctrl Pts',(43.8295586128169,-39.5498679835144,
40.0934008039614));
#187240=CARTESIAN_POINT('Ctrl Pts',(43.8267236865061,-39.5563148866443,
40.0912909372156));
#187241=CARTESIAN_POINT('Ctrl Pts',(43.8243293609623,-39.562795265034,40.0888630467851));
#187242=CARTESIAN_POINT('Ctrl Pts',(43.8231321981904,-39.5660354542288,
40.0876491015699));
#187243=CARTESIAN_POINT('Ctrl Pts',(43.8220450509626,-39.5692841591686,
40.0863558569271));
#187244=CARTESIAN_POINT('Ctrl Pts',(43.8210669472518,-39.5725311673655,
40.0849936342771));
#187245=CARTESIAN_POINT('Ctrl Pts',(43.8205778953964,-39.574154671464,40.0843125229521));
#187246=CARTESIAN_POINT('Ctrl Pts',(43.8201160933895,-39.5757777635547,
40.0836141747074));
#187247=CARTESIAN_POINT('Ctrl Pts',(43.8196813503779,-39.5773992434495,
40.0828999161609));
#187248=CARTESIAN_POINT('Ctrl Pts',(43.8195726646249,-39.5778046134232,
40.0827213515243));
#187249=CARTESIAN_POINT('Ctrl Pts',(43.8194656698239,-39.578209882893,40.0825417925842));
#187250=CARTESIAN_POINT('Ctrl Pts',(43.8193603625175,-39.5786150336267,
40.0823612602361));
#187251=CARTESIAN_POINT('Ctrl Pts',(43.8190444405985,-39.5798304858276,
40.0818196631917));
#187252=CARTESIAN_POINT('Ctrl Pts',(43.8187437073123,-39.581044868119,40.0812693052021));
#187253=CARTESIAN_POINT('Ctrl Pts',(43.8184580587802,-39.5822576997161,
40.0807107531875));
#187254=CARTESIAN_POINT('Ctrl Pts',(43.8164459874034,-39.5908007288813,
40.0767763849181));
#187255=CARTESIAN_POINT('Ctrl Pts',(43.8151322889031,-39.5992865061389,
40.0724140586137));
#187256=CARTESIAN_POINT('Ctrl Pts',(43.8144227306311,-39.6076412948836,
40.0677221223767));
#187257=CARTESIAN_POINT('Ctrl Pts',(43.8140785956359,-39.6116933583964,
40.065446538372));
#187258=CARTESIAN_POINT('Ctrl Pts',(43.8138769687219,-39.6157150281161,
40.0630928000679));
#187259=CARTESIAN_POINT('Ctrl Pts',(43.8138093098903,-39.6196997093542,
40.0606689262479));
#187260=CARTESIAN_POINT('Ctrl Pts',(43.8137057289464,-39.6257999779282,
40.0569581447806));
#187261=CARTESIAN_POINT('Ctrl Pts',(43.8139151128799,-39.6318101761581,
40.0530843804606));
#187262=CARTESIAN_POINT('Ctrl Pts',(43.8144090029878,-39.637694021932,40.0490800251458));
#187263=CARTESIAN_POINT('Ctrl Pts',(43.8146383681089,-39.6404265103485,
40.0472203818218));
#187264=CARTESIAN_POINT('Ctrl Pts',(43.8149288459967,-39.6431316855282,
40.0453323608818));
#187265=CARTESIAN_POINT('Ctrl Pts',(43.8152787628653,-39.6458055463961,
40.0434201572162));
#187266=CARTESIAN_POINT('Ctrl Pts',(43.8153055826145,-39.6460104872961,
40.0432735943397));
#187267=CARTESIAN_POINT('Ctrl Pts',(43.8153327221694,-39.6462152612034,
40.0431268995707));
#187268=CARTESIAN_POINT('Ctrl Pts',(43.8153601802954,-39.6464198673375,
40.0429800745037));
#187269=CARTESIAN_POINT('Ctrl Pts',(43.8157458841823,-39.6492939666537,
40.0409176249753));
#187270=CARTESIAN_POINT('Ctrl Pts',(43.8161965332334,-39.6521348180506,
40.0388310783332));
#187271=CARTESIAN_POINT('Ctrl Pts',(43.816707563491,-39.6549389970088,40.036725739981));
#187272=CARTESIAN_POINT('Ctrl Pts',(43.8185400271111,-39.664994284047,40.0291763710714));
#187273=CARTESIAN_POINT('Ctrl Pts',(43.8211611138372,-39.6746561192254,
40.0213310894587));
#187274=CARTESIAN_POINT('Ctrl Pts',(43.8244418968104,-39.6839173731645,
40.0132837551308));
#187275=CARTESIAN_POINT('Ctrl Pts',(43.8280471477141,-39.694094560868,40.004440543131));
#187276=CARTESIAN_POINT('Ctrl Pts',(43.8324491002319,-39.7037886794691,
39.9953528710582));
#187277=CARTESIAN_POINT('Ctrl Pts',(43.8375295667881,-39.7129876499629,
39.9861103629532));
#187278=CARTESIAN_POINT('Ctrl Pts',(43.8430151956457,-39.7229202294697,
39.9761307737529));
#187279=CARTESIAN_POINT('Ctrl Pts',(43.8492922888431,-39.7322766233325,
39.965969693598));
#187280=CARTESIAN_POINT('Ctrl Pts',(43.8562669044119,-39.7410245486315,
39.9557128217471));
#187281=CARTESIAN_POINT('Ctrl Pts',(43.8631830101214,-39.7496990878244,
39.9455419945137));
#187282=CARTESIAN_POINT('Ctrl Pts',(43.870786081907,-39.7577762496646,39.9352756289329));
#187283=CARTESIAN_POINT('Ctrl Pts',(43.8790236240219,-39.7651933658999,
39.92499));
#187284=CARTESIAN_POINT('Origin',(0.0101975504409105,0.0113255271402792,
39.92499));
#187285=CARTESIAN_POINT('Ctrl Pts',(46.7142062431422,-42.0411527846896,
40.10025));
#187286=CARTESIAN_POINT('Ctrl Pts',(46.7199506919422,-42.0347675597394,
40.10025));
#187287=CARTESIAN_POINT('Ctrl Pts',(46.7251107020204,-42.0279592142787,
40.0995859581842));
#187288=CARTESIAN_POINT('Ctrl Pts',(46.7296675019384,-42.0208774479599,
40.0983275959623));
#187289=CARTESIAN_POINT('Ctrl Pts',(46.7325790801588,-42.0163525364107,
40.097523562407));
#187290=CARTESIAN_POINT('Ctrl Pts',(46.7352451892137,-42.0117164852004,
40.0964777059492));
#187291=CARTESIAN_POINT('Ctrl Pts',(46.7376689638752,-42.0070114066747,
40.0952149915961));
#187292=CARTESIAN_POINT('Ctrl Pts',(46.7409769299535,-42.0005899185698,
40.0934916398701));
#187293=CARTESIAN_POINT('Ctrl Pts',(46.743827608742,-41.9940383480778,40.091364392163));
#187294=CARTESIAN_POINT('Ctrl Pts',(46.7462229640888,-41.9874523371581,
40.0889118607713));
#187295=CARTESIAN_POINT('Ctrl Pts',(46.7474206417622,-41.9841593316983,
40.0876855950754));
#187296=CARTESIAN_POINT('Ctrl Pts',(46.7485046297347,-41.9808575622224,
40.0863782327526));
#187297=CARTESIAN_POINT('Ctrl Pts',(46.7494761782933,-41.9775578801518,
40.0850006373333));
#187298=CARTESIAN_POINT('Ctrl Pts',(46.7499619525726,-41.9759080391166,
40.0843118396237));
#187299=CARTESIAN_POINT('Ctrl Pts',(46.7504196286881,-41.9742587070256,
40.0836054919164));
#187300=CARTESIAN_POINT('Ctrl Pts',(46.7508494364812,-41.972611159284,40.0828829920417));
#187301=CARTESIAN_POINT('Ctrl Pts',(46.7509568884295,-41.9721992723486,
40.0827023670731));
#187302=CARTESIAN_POINT('Ctrl Pts',(46.7510625988575,-41.9717874966607,
40.0825207326932));
#187303=CARTESIAN_POINT('Ctrl Pts',(46.7511665718606,-41.9713758515958,
40.0823381109275));
#187304=CARTESIAN_POINT('Ctrl Pts',(46.7514784908699,-41.9701409164012,
40.0817902456303));
#187305=CARTESIAN_POINT('Ctrl Pts',(46.7517747718024,-41.9689071581769,
40.0812334935553));
#187306=CARTESIAN_POINT('Ctrl Pts',(46.7520555364232,-41.9676750878619,
40.0806684524227));
#187307=CARTESIAN_POINT('Ctrl Pts',(46.7539957941553,-41.9591607175417,
40.0767636676138));
#187308=CARTESIAN_POINT('Ctrl Pts',(46.7552464720207,-41.9507055072923,
40.0724404510892));
#187309=CARTESIAN_POINT('Ctrl Pts',(46.7559027543579,-41.9423805287177,
40.0677949937415));
#187310=CARTESIAN_POINT('Ctrl Pts',(46.7562289248781,-41.9382430372173,
40.065486214191));
#187311=CARTESIAN_POINT('Ctrl Pts',(46.7564078446195,-41.9341372814972,
40.0630972003218));
#187312=CARTESIAN_POINT('Ctrl Pts',(46.7564487173143,-41.9300700339484,
40.0606363359906));
#187313=CARTESIAN_POINT('Ctrl Pts',(46.7565388885838,-41.9210970783569,
40.0552073017123));
#187314=CARTESIAN_POINT('Ctrl Pts',(46.7559695796225,-41.9123126321654,
40.0494204304519));
#187315=CARTESIAN_POINT('Ctrl Pts',(46.7548061840817,-41.9038465062684,
40.0434049749851));
#187316=CARTESIAN_POINT('Ctrl Pts',(46.7543811810194,-41.9007537237148,
40.0412074532442));
#187317=CARTESIAN_POINT('Ctrl Pts',(46.7538836816023,-41.8976992635446,
40.0389814735788));
#187318=CARTESIAN_POINT('Ctrl Pts',(46.7533184435777,-41.8946854937102,
40.0367321210017));
#187319=CARTESIAN_POINT('Ctrl Pts',(46.7514198688647,-41.8845625597432,
40.0291767837139));
#187320=CARTESIAN_POINT('Ctrl Pts',(46.7487367327314,-41.8748360802677,
40.0213235332573));
#187321=CARTESIAN_POINT('Ctrl Pts',(46.7453971060007,-41.8655137786579,
40.0132649215853));
#187322=CARTESIAN_POINT('Ctrl Pts',(46.7417264606188,-41.8552674648896,
40.0044075527525));
#187323=CARTESIAN_POINT('Ctrl Pts',(46.7372626589216,-41.8455087367158,
39.995301625371));
#187324=CARTESIAN_POINT('Ctrl Pts',(46.7321227530968,-41.8362508575454,
39.9860353422346));
#187325=CARTESIAN_POINT('Ctrl Pts',(46.726586854296,-41.8262797250103,39.9760551582681));
#187326=CARTESIAN_POINT('Ctrl Pts',(46.7202662104757,-41.8168884800889,
39.965887973814));
#187327=CARTESIAN_POINT('Ctrl Pts',(46.7132528291638,-41.80811151121,39.9556174643237));
#187328=CARTESIAN_POINT('Ctrl Pts',(46.7063341521798,-41.7994530610458,
39.9454856413893));
#187329=CARTESIAN_POINT('Ctrl Pts',(46.6987402031259,-41.7913915075188,
39.9352519465107));
#187330=CARTESIAN_POINT('Ctrl Pts',(46.6905216402897,-41.7839914803027,
39.92499));
#187331=CARTESIAN_POINT('Ctrl Pts',(44.1339623850447,-39.4820551873931,
39.92499));
#187332=CARTESIAN_POINT('Ctrl Pts',(44.1260971752941,-39.4749733207244,
39.9348107241729));
#187333=CARTESIAN_POINT('Ctrl Pts',(44.1177016730286,-39.4685372764351,
39.9446038383183));
#187334=CARTESIAN_POINT('Ctrl Pts',(44.1088266671078,-39.4627751762741,
39.9543158069405));
#187335=CARTESIAN_POINT('Ctrl Pts',(44.100257068034,-39.457211361597,39.9636935671416));
#187336=CARTESIAN_POINT('Ctrl Pts',(44.0912392968991,-39.4522752837255,
39.9729968321017));
#187337=CARTESIAN_POINT('Ctrl Pts',(44.0817922708719,-39.4480294591785,
39.9821731151368));
#187338=CARTESIAN_POINT('Ctrl Pts',(44.0728618726509,-39.4440158252717,
39.9908475764388));
#187339=CARTESIAN_POINT('Ctrl Pts',(44.0635470605524,-39.4406186435271,
39.9994093733886));
#187340=CARTESIAN_POINT('Ctrl Pts',(44.0538529442782,-39.4379312493381,
40.0077966115884));
#187341=CARTESIAN_POINT('Ctrl Pts',(44.0449248258207,-39.4354562043743,
40.015521117264));
#187342=CARTESIAN_POINT('Ctrl Pts',(44.0356744386734,-39.4335831186675,
40.0230979941068));
#187343=CARTESIAN_POINT('Ctrl Pts',(44.0261054687939,-39.4324230329113,
40.0304554104797));
#187344=CARTESIAN_POINT('Ctrl Pts',(44.0232521951402,-39.432077118757,40.0326492435213));
#187345=CARTESIAN_POINT('Ctrl Pts',(44.020370621931,-39.4317948788024,40.0348233715076));
#187346=CARTESIAN_POINT('Ctrl Pts',(44.0174609456696,-39.4315800126157,
40.0369753512355));
#187347=CARTESIAN_POINT('Ctrl Pts',(44.0145809991274,-39.4313673418318,
40.0391053430352));
#187348=CARTESIAN_POINT('Ctrl Pts',(44.0116765294504,-39.4312206224783,
40.041211089324));
#187349=CARTESIAN_POINT('Ctrl Pts',(44.0087510493745,-39.4311433701095,
40.0432881154904));
#187350=CARTESIAN_POINT('Ctrl Pts',(44.0085476172113,-39.4311379981308,
40.043432547828));
#187351=CARTESIAN_POINT('Ctrl Pts',(44.0083440782824,-39.4311329512712,
40.0435768364421));
#187352=CARTESIAN_POINT('Ctrl Pts',(44.0081404327825,-39.4311282308202,
40.0437209807855));
#187353=CARTESIAN_POINT('Ctrl Pts',(43.9992118680544,-39.4309212689594,
40.050040796842));
#187354=CARTESIAN_POINT('Ctrl Pts',(43.9900881971805,-39.4313859080977,
40.0560490279345));
#187355=CARTESIAN_POINT('Ctrl Pts',(43.9808585737696,-39.4325966403784,
40.0616647108615));
#187356=CARTESIAN_POINT('Ctrl Pts',(43.9722549606529,-39.4337252532879,
40.0668995033487));
#187357=CARTESIAN_POINT('Ctrl Pts',(43.9635585482853,-39.4355025470896,
40.0717933267483));
#187358=CARTESIAN_POINT('Ctrl Pts',(43.9548613290778,-39.4380105519136,
40.0762460303074));
#187359=CARTESIAN_POINT('Ctrl Pts',(43.9516797737739,-39.4389280125248,
40.0778748868749));
#187360=CARTESIAN_POINT('Ctrl Pts',(43.9484983634053,-39.4399434521994,
40.0794443522248));
#187361=CARTESIAN_POINT('Ctrl Pts',(43.9453226165472,-39.4410615611723,
40.0809482021492));
#187362=CARTESIAN_POINT('Ctrl Pts',(43.9445589555201,-39.4413304290276,
40.0813098278169));
#187363=CARTESIAN_POINT('Ctrl Pts',(43.9437952833156,-39.4416057093429,
40.0816679525673));
#187364=CARTESIAN_POINT('Ctrl Pts',(43.943031734545,-39.4418874191261,40.0820224192581));
#187365=CARTESIAN_POINT('Ctrl Pts',(43.9422920466734,-39.4421603254786,
40.0823658088649));
#187366=CARTESIAN_POINT('Ctrl Pts',(43.9415524746579,-39.4424392657171,
40.0827057654617));
#187367=CARTESIAN_POINT('Ctrl Pts',(43.9408131433999,-39.4427242524725,
40.0830421470151));
#187368=CARTESIAN_POINT('Ctrl Pts',(43.9327129150435,-39.4458466117306,
40.0867275956805));
#187369=CARTESIAN_POINT('Ctrl Pts',(43.9246364083438,-39.4496972096651,
40.0899823432029));
#187370=CARTESIAN_POINT('Ctrl Pts',(43.9167721156746,-39.4542738890609,
40.0926299529354));
#187371=CARTESIAN_POINT('Ctrl Pts',(43.9135105590949,-39.4561719744227,
40.0937279956083));
#187372=CARTESIAN_POINT('Ctrl Pts',(43.9102855324952,-39.4581945203283,
40.0947220371802));
#187373=CARTESIAN_POINT('Ctrl Pts',(43.9071101492109,-39.4603395741451,
40.0956014538693));
#187374=CARTESIAN_POINT('Ctrl Pts',(43.9016942021215,-39.4639981869597,
40.097101390674));
#187375=CARTESIAN_POINT('Ctrl Pts',(43.8964251099356,-39.4680136963361,
40.0982667904316));
#187376=CARTESIAN_POINT('Ctrl Pts',(43.8913745966875,-39.472373749158,40.0990539325583));
#187377=CARTESIAN_POINT('Ctrl Pts',(43.8888493400634,-39.474553775569,40.0994475036216));
#187378=CARTESIAN_POINT('Ctrl Pts',(43.8863797569642,-39.476820955151,40.0997467259952));
#187379=CARTESIAN_POINT('Ctrl Pts',(43.8839748786093,-39.4791737454928,
40.0999473488896));
#187380=CARTESIAN_POINT('Ctrl Pts',(43.8815700002543,-39.4815265358346,
40.100147971784));
#187381=CARTESIAN_POINT('Ctrl Pts',(43.879229842074,-39.4839648939618,40.10025));
#187382=CARTESIAN_POINT('Ctrl Pts',(43.8769616275874,-39.4864862581817,
40.10025));
#187383=CARTESIAN_POINT('Origin',(38.9747476500513,-43.3086183250767,39.92499));
#187384=CARTESIAN_POINT('Ctrl Pts',(41.7839914803026,-46.6905216402898,
39.92499));
#187385=CARTESIAN_POINT('Ctrl Pts',(41.7910911765308,-46.6984066517723,
39.9348354642023));
#187386=CARTESIAN_POINT('Ctrl Pts',(41.7987919603593,-46.7057080773549,
39.9446440828467));
#187387=CARTESIAN_POINT('Ctrl Pts',(41.8070443420777,-46.7123936319706,
39.9543641760345));
#187388=CARTESIAN_POINT('Ctrl Pts',(41.81502857053,-46.7188619458711,39.9637684240729));
#187389=CARTESIAN_POINT('Ctrl Pts',(41.8235301761271,-46.7247545199419,
39.9730909636415));
#187390=CARTESIAN_POINT('Ctrl Pts',(41.8325358446889,-46.7300083326616,
39.9822808977162));
#187391=CARTESIAN_POINT('Ctrl Pts',(41.8410546526111,-46.7349781159832,
39.9909740094673));
#187392=CARTESIAN_POINT('Ctrl Pts',(41.8500252953129,-46.7393768060093,
39.9995492765025));
#187393=CARTESIAN_POINT('Ctrl Pts',(41.8594521748307,-46.7431119772979,
40.007946232872));
#187394=CARTESIAN_POINT('Ctrl Pts',(41.868135012636,-46.746552340189,40.0156804369717));
#187395=CARTESIAN_POINT('Ctrl Pts',(41.8772054497804,-46.7494299450235,
40.0232638017451));
#187396=CARTESIAN_POINT('Ctrl Pts',(41.8866715402936,-46.7516345991562,
40.0306257269996));
#187397=CARTESIAN_POINT('Ctrl Pts',(41.8894172933171,-46.7522740855146,
40.0327611416671));
#187398=CARTESIAN_POINT('Ctrl Pts',(41.8921963397434,-46.7528566833418,
40.034877742728));
#187399=CARTESIAN_POINT('Ctrl Pts',(41.8950088623279,-46.7533790039317,
40.03697331687));
#187400=CARTESIAN_POINT('Ctrl Pts',(41.8980578176395,-46.7539452330336,
40.039245053974));
#187401=CARTESIAN_POINT('Ctrl Pts',(41.9011416752732,-46.7544408966254,
40.041487875195));
#187402=CARTESIAN_POINT('Ctrl Pts',(41.9042597210856,-46.7548620578767,
40.04369857016));
#187403=CARTESIAN_POINT('Ctrl Pts',(41.9128172222843,-46.7560179382354,
40.0497658398386));
#187404=CARTESIAN_POINT('Ctrl Pts',(41.921627072481,-46.7565684843259,40.0555581699984));
#187405=CARTESIAN_POINT('Ctrl Pts',(41.9306033478349,-46.7564556264619,
40.0609828468885));
#187406=CARTESIAN_POINT('Ctrl Pts',(41.9388161524506,-46.7563523676436,
40.0659461317305));
#187407=CARTESIAN_POINT('Ctrl Pts',(41.9471607721489,-46.7556849461647,
40.0706039980708));
#187408=CARTESIAN_POINT('Ctrl Pts',(41.9555881906109,-46.7543795041529,
40.0748843180606));
#187409=CARTESIAN_POINT('Ctrl Pts',(41.9597277110299,-46.7537382753012,
40.0769867972572));
#187410=CARTESIAN_POINT('Ctrl Pts',(41.9638869554869,-46.7529426662693,
40.0789976708176));
#187411=CARTESIAN_POINT('Ctrl Pts',(41.9680580970364,-46.7519812517995,
40.08090504915));
#187412=CARTESIAN_POINT('Ctrl Pts',(41.968849530518,-46.7517988327682,40.0812669556105));
#187413=CARTESIAN_POINT('Ctrl Pts',(41.9696416823158,-46.7516099985531,
40.0816253922033));
#187414=CARTESIAN_POINT('Ctrl Pts',(41.9704344168203,-46.7514147143008,
40.081980198914));
#187415=CARTESIAN_POINT('Ctrl Pts',(41.9712023783716,-46.7512255326814,
40.0823239179149));
#187416=CARTESIAN_POINT('Ctrl Pts',(41.9719708867612,-46.7510302978707,
40.0826642303499));
#187417=CARTESIAN_POINT('Ctrl Pts',(41.9727398158587,-46.7508289807694,
40.08300099161));
#187418=CARTESIAN_POINT('Ctrl Pts',(41.9811194467227,-46.7486350684818,
40.0866709464313));
#187419=CARTESIAN_POINT('Ctrl Pts',(41.9895544525281,-46.7457169794821,
40.0899175831879));
#187420=CARTESIAN_POINT('Ctrl Pts',(41.9978556152123,-46.7420530111686,
40.0925642067063));
#187421=CARTESIAN_POINT('Ctrl Pts',(42.0013612477613,-46.7405056945977,
40.0936818922528));
#187422=CARTESIAN_POINT('Ctrl Pts',(42.0048429302643,-46.7388257854547,
40.0946930094791));
#187423=CARTESIAN_POINT('Ctrl Pts',(42.0082865614562,-46.737013581669,40.0955863397546));
#187424=CARTESIAN_POINT('Ctrl Pts',(42.0140855503365,-46.7339618757756,
40.0970906856166));
#187425=CARTESIAN_POINT('Ctrl Pts',(42.0197742252486,-46.7305342346687,
40.0982599215483));
#187426=CARTESIAN_POINT('Ctrl Pts',(42.0252784509104,-46.7267341265709,
40.0990497370453));
#187427=CARTESIAN_POINT('Ctrl Pts',(42.0266545073258,-46.7257840995464,
40.0992471909196));
#187428=CARTESIAN_POINT('Ctrl Pts',(42.0280188904106,-46.7248106099125,
40.0994209989363));
#187429=CARTESIAN_POINT('Ctrl Pts',(42.029370240857,-46.7238134778069,40.0995705982975));
#187430=CARTESIAN_POINT('Ctrl Pts',(42.0313972665264,-46.7223177796486,
40.0997949973393));
#187431=CARTESIAN_POINT('Ctrl Pts',(42.0333949481518,-46.7207688863878,
40.0999649129781));
#187432=CARTESIAN_POINT('Ctrl Pts',(42.0353598072045,-46.7191674503111,
40.1000786629733));
#187433=CARTESIAN_POINT('Ctrl Pts',(42.0373246662573,-46.7175660142344,
40.1001924129685));
#187434=CARTESIAN_POINT('Ctrl Pts',(42.0392567035862,-46.7159120469163,
40.10025));
#187435=CARTESIAN_POINT('Ctrl Pts',(42.0411527846894,-46.7142062431423,
40.10025));
#187436=CARTESIAN_POINT('Ctrl Pts',(39.4864862581816,-43.8769616275875,
40.10025));
#187437=CARTESIAN_POINT('Ctrl Pts',(39.4800703482066,-43.8827333680742,
40.10025));
#187438=CARTESIAN_POINT('Ctrl Pts',(39.4741864828742,-43.8889846873409,
40.0995786334239));
#187439=CARTESIAN_POINT('Ctrl Pts',(39.4688721660153,-43.8955692023392,
40.0983063763362));
#187440=CARTESIAN_POINT('Ctrl Pts',(39.4654396626057,-43.8998221234167,
40.0974846287989));
#187441=CARTESIAN_POINT('Ctrl Pts',(39.4622440309667,-43.9042134689405,
40.0964130309336));
#187442=CARTESIAN_POINT('Ctrl Pts',(39.4592874976153,-43.9086997575132,
40.0951176960923));
#187443=CARTESIAN_POINT('Ctrl Pts',(39.4553687820182,-43.914646076027,40.0934008039614));
#187444=CARTESIAN_POINT('Ctrl Pts',(39.4518755008533,-43.9207613318563,
40.0912909372156));
#187445=CARTESIAN_POINT('Ctrl Pts',(39.4488169076809,-43.9269559348854,
40.0888630467851));
#187446=CARTESIAN_POINT('Ctrl Pts',(39.4472876110947,-43.9300532363999,
40.0876491015698));
#187447=CARTESIAN_POINT('Ctrl Pts',(39.4458668372382,-43.9331705067652,
40.0863558569271));
#187448=CARTESIAN_POINT('Ctrl Pts',(39.4445546869049,-43.9362974878336,
40.084993634277));
#187449=CARTESIAN_POINT('Ctrl Pts',(39.4438986117382,-43.9378609783679,
40.084312522952));
#187450=CARTESIAN_POINT('Ctrl Pts',(39.443269680209,-43.9394269075361,40.0836141747073));
#187451=CARTESIAN_POINT('Ctrl Pts',(39.4426678279634,-43.9409940617755,
40.0828999161609));
#187452=CARTESIAN_POINT('Ctrl Pts',(39.442517364902,-43.9413858503353,40.0827213515242));
#187453=CARTESIAN_POINT('Ctrl Pts',(39.4423685940348,-43.9417777156945,
40.0825417925841));
#187454=CARTESIAN_POINT('Ctrl Pts',(39.4422215138293,-43.9421696393591,
40.082361260236));
#187455=CARTESIAN_POINT('Ctrl Pts',(39.4417802732128,-43.943345410353,40.0818196631917));
#187456=CARTESIAN_POINT('Ctrl Pts',(39.4413542498604,-43.9445217049429,
40.0812693052021));
#187457=CARTESIAN_POINT('Ctrl Pts',(39.4409433907177,-43.9456980341195,
40.0807107531874));
#187458=CARTESIAN_POINT('Ctrl Pts',(39.4380493519682,-43.9539839449479,
40.0767763849181));
#187459=CARTESIAN_POINT('Ctrl Pts',(39.4358558447894,-43.9622859173443,
40.0724140586137));
#187460=CARTESIAN_POINT('Ctrl Pts',(39.4342768603234,-43.9705207686462,
40.0677221223768));
#187461=CARTESIAN_POINT('Ctrl Pts',(39.4335110545637,-43.974514662629,40.0654465383721));
#187462=CARTESIAN_POINT('Ctrl Pts',(39.4328901532274,-43.9784932254699,
40.0630928000679));
#187463=CARTESIAN_POINT('Ctrl Pts',(39.4324063524315,-43.9824490059336,
40.0606689262479));
#187464=CARTESIAN_POINT('Ctrl Pts',(39.4316656872153,-43.9885050294412,
40.0569581447805));
#187465=CARTESIAN_POINT('Ctrl Pts',(39.4312456873368,-43.9945041897572,
40.0530843804605));
#187466=CARTESIAN_POINT('Ctrl Pts',(39.4311218425061,-44.0004074287823,
40.0490800251457));
#187467=CARTESIAN_POINT('Ctrl Pts',(39.4310643283261,-44.0031489235249,
40.0472203818218));
#187468=CARTESIAN_POINT('Ctrl Pts',(39.4310704471411,-44.0058696426791,
40.0453323608818));
#187469=CARTESIAN_POINT('Ctrl Pts',(39.431138952561,-44.0085654321301,40.0434201572162));
#187470=CARTESIAN_POINT('Ctrl Pts',(39.4311442032315,-44.0087720537695,
40.0432735943397));
#187471=CARTESIAN_POINT('Ctrl Pts',(39.4311497894112,-44.0089785427599,
40.0431268995707));
#187472=CARTESIAN_POINT('Ctrl Pts',(39.431155709954,-44.0091848981958,40.0429800745037));
#187473=CARTESIAN_POINT('Ctrl Pts',(39.4312388757299,-44.0120835699299,
40.0409176249753));
#187474=CARTESIAN_POINT('Ctrl Pts',(39.4313901062474,-44.0149559644984,
40.0388310783332));
#187475=CARTESIAN_POINT('Ctrl Pts',(39.4316052205105,-44.0177981990784,
40.036725739981));
#187476=CARTESIAN_POINT('Ctrl Pts',(39.4323765820013,-44.027989946807,40.0291763710723));
#187477=CARTESIAN_POINT('Ctrl Pts',(39.4339733733562,-44.0378728316078,
40.0213310894606));
#187478=CARTESIAN_POINT('Ctrl Pts',(39.4362681192145,-44.0474262866303,
40.0132837551337));
#187479=CARTESIAN_POINT('Ctrl Pts',(39.4387898143851,-44.0579245739704,
40.0044405431347));
#187480=CARTESIAN_POINT('Ctrl Pts',(39.4421543412257,-44.0680257165067,
39.9953528710629));
#187481=CARTESIAN_POINT('Ctrl Pts',(39.4462454222045,-44.0777053474387,
39.9861103629589));
#187482=CARTESIAN_POINT('Ctrl Pts',(39.4506627629405,-44.0881569195897,
39.9761307737593));
#187483=CARTESIAN_POINT('Ctrl Pts',(39.4559274600916,-44.0981181930531,
39.9659696936053));
#187484=CARTESIAN_POINT('Ctrl Pts',(39.4619494607974,-44.107547242149,39.9557128217551));
#187485=CARTESIAN_POINT('Ctrl Pts',(39.4679209431059,-44.1168971912129,
39.9455419945191));
#187486=CARTESIAN_POINT('Ctrl Pts',(39.4746380711556,-44.1257248429277,
39.9352756289356));
#187487=CARTESIAN_POINT('Ctrl Pts',(39.4820551873929,-44.1339623850448,
39.92499));
#187488=CARTESIAN_POINT('Origin',(0.0113255271402773,0.0101975504409131,
39.92499));
#187489=CARTESIAN_POINT('Ctrl Pts',(42.06380383897,-46.6938111422605,40.10025));
#187490=CARTESIAN_POINT('Ctrl Pts',(42.0701842568307,-46.6880613546455,
40.10025));
#187491=CARTESIAN_POINT('Ctrl Pts',(42.0760276657227,-46.6818296739369,
40.0995859581841));
#187492=CARTESIAN_POINT('Ctrl Pts',(42.0812997491649,-46.6752630175671,
40.0983275959619));
#187493=CARTESIAN_POINT('Ctrl Pts',(42.0846683595052,-46.6710672367544,
40.0975235624067));
#187494=CARTESIAN_POINT('Ctrl Pts',(42.0878044626438,-46.6667352666009,
40.096477705949));
#187495=CARTESIAN_POINT('Ctrl Pts',(42.0907067742416,-46.662309316429,40.0952149915961));
#187496=CARTESIAN_POINT('Ctrl Pts',(42.094667847219,-46.6562687825185,40.0934916398701));
#187497=CARTESIAN_POINT('Ctrl Pts',(42.0981877352864,-46.6500510792882,
40.091364392163));
#187498=CARTESIAN_POINT('Ctrl Pts',(42.1012583942265,-46.6437515300389,
40.0889118607713));
#187499=CARTESIAN_POINT('Ctrl Pts',(42.1027937236965,-46.6406017554142,
40.0876855950754));
#187500=CARTESIAN_POINT('Ctrl Pts',(42.1042169023589,-46.6374313809739,
40.0863782327526));
#187501=CARTESIAN_POINT('Ctrl Pts',(42.1055280393689,-46.6342513293848,
40.0850006373333));
#187502=CARTESIAN_POINT('Ctrl Pts',(42.1061836078739,-46.6326613035902,
40.0843118396237));
#187503=CARTESIAN_POINT('Ctrl Pts',(42.1068111789406,-46.6310688468941,
40.0836054919164));
#187504=CARTESIAN_POINT('Ctrl Pts',(42.1074108478353,-46.6294752517395,
40.0828829920417));
#187505=CARTESIAN_POINT('Ctrl Pts',(42.107560765059,-46.6290768529508,40.0827023670731));
#187506=CARTESIAN_POINT('Ctrl Pts',(42.1077089386741,-46.6286783827619,
40.0825207326932));
#187507=CARTESIAN_POINT('Ctrl Pts',(42.1078553707282,-46.62827986087,40.0823381109275));
#187508=CARTESIAN_POINT('Ctrl Pts',(42.1082946668907,-46.6270842951943,
40.0817902456303));
#187509=CARTESIAN_POINT('Ctrl Pts',(42.1087182876164,-46.6258882654171,
40.0812334935553));
#187510=CARTESIAN_POINT('Ctrl Pts',(42.109126300596,-46.6246922924066,40.0806684524226));
#187511=CARTESIAN_POINT('Ctrl Pts',(42.1119459234384,-46.6164273768569,
40.0767636676138));
#187512=CARTESIAN_POINT('Ctrl Pts',(42.1140735600937,-46.6081492165691,
40.0724404510891));
#187513=CARTESIAN_POINT('Ctrl Pts',(42.1155964444647,-46.5999384432823,
40.0677949937414));
#187514=CARTESIAN_POINT('Ctrl Pts',(42.116353313817,-46.5958577114966,40.0654862141909));
#187515=CARTESIAN_POINT('Ctrl Pts',(42.1169604217533,-46.5917931497416,
40.0630972003217));
#187516=CARTESIAN_POINT('Ctrl Pts',(42.1174262136791,-46.5877524553605,
40.0606363359906));
#187517=CARTESIAN_POINT('Ctrl Pts',(42.11845382024,-46.5788380800229,40.0552073017123));
#187518=CARTESIAN_POINT('Ctrl Pts',(42.1188058546738,-46.5700422469559,
40.0494204304519));
#187519=CARTESIAN_POINT('Ctrl Pts',(42.1185337834653,-46.5615008914344,
40.0434049749851));
#187520=CARTESIAN_POINT('Ctrl Pts',(42.1184343924218,-46.5583806265502,
40.0412074532442));
#187521=CARTESIAN_POINT('Ctrl Pts',(42.1182588963863,-46.5552908961828,
40.0389814735788));
#187522=CARTESIAN_POINT('Ctrl Pts',(42.1180117795242,-46.5522345526328,
40.0367321210017));
#187523=CARTESIAN_POINT('Ctrl Pts',(42.1171817401335,-46.5419686180608,
40.0291767837144));
#187524=CARTESIAN_POINT('Ctrl Pts',(42.1155299964534,-46.5320149571613,
40.0213235332582));
#187525=CARTESIAN_POINT('Ctrl Pts',(42.1131831104089,-46.5223946380456,
40.0132649215868));
#187526=CARTESIAN_POINT('Ctrl Pts',(42.110603604639,-46.5118207677355,40.0044075527545));
#187527=CARTESIAN_POINT('Ctrl Pts',(42.1071843209742,-46.5016489045644,
39.9953016253735));
#187528=CARTESIAN_POINT('Ctrl Pts',(42.1030402839743,-46.4919044745678,
39.9860353422377));
#187529=CARTESIAN_POINT('Ctrl Pts',(42.0985769785676,-46.4814093059457,
39.9760551582716));
#187530=CARTESIAN_POINT('Ctrl Pts',(42.0932726122956,-46.4714088200615,
39.9658879738179));
#187531=CARTESIAN_POINT('Ctrl Pts',(42.0872150940898,-46.4619468343658,
39.955617464328));
#187532=CARTESIAN_POINT('Ctrl Pts',(42.0812393728316,-46.4526126174232,
39.9454856413922));
#187533=CARTESIAN_POINT('Ctrl Pts',(42.0745296860263,-46.4438014421041,
39.9352519465123));
#187534=CARTESIAN_POINT('Ctrl Pts',(42.0671296588095,-46.4355828792671,
39.92499));
#187535=CARTESIAN_POINT('Ctrl Pts',(39.7651933658998,-43.8790236240221,
39.92499));
#187536=CARTESIAN_POINT('Ctrl Pts',(39.7581114992314,-43.8711584142718,
39.9348107241725));
#187537=CARTESIAN_POINT('Ctrl Pts',(39.7504347382251,-43.8638800583566,
39.9446038383176));
#187538=CARTESIAN_POINT('Ctrl Pts',(39.7422106539907,-43.857221832853,39.9543158069394));
#187539=CARTESIAN_POINT('Ctrl Pts',(39.7342695770756,-43.850792730313,39.9636935671402));
#187540=CARTESIAN_POINT('Ctrl Pts',(39.7258171668693,-43.8449410790338,
39.9729968321001));
#187541=CARTESIAN_POINT('Ctrl Pts',(39.7168657021547,-43.8397310304449,
39.982173115135));
#187542=CARTESIAN_POINT('Ctrl Pts',(39.7084037645741,-43.8348059028422,
39.9908475764368));
#187543=CARTESIAN_POINT('Ctrl Pts',(39.6994950821784,-43.8304536682204,
39.9994093733864));
#187544=CARTESIAN_POINT('Ctrl Pts',(39.6901349804726,-43.826767684781,40.0077966115861));
#187545=CARTESIAN_POINT('Ctrl Pts',(39.6815144838289,-43.8233729558702,
40.0155211172616));
#187546=CARTESIAN_POINT('Ctrl Pts',(39.6725105620411,-43.8205432023696,
40.0230979941044));
#187547=CARTESIAN_POINT('Ctrl Pts',(39.6631152739614,-43.818389241968,40.0304554104772));
#187548=CARTESIAN_POINT('Ctrl Pts',(39.6603137887132,-43.8177469744569,
40.0326492435197));
#187549=CARTESIAN_POINT('Ctrl Pts',(39.6574775031712,-43.8171650742227,
40.0348233715068));
#187550=CARTESIAN_POINT('Ctrl Pts',(39.654606226052,-43.8166472411071,40.0369753512356));
#187551=CARTESIAN_POINT('Ctrl Pts',(39.6517642863086,-43.8161346989696,
40.0391053430352));
#187552=CARTESIAN_POINT('Ctrl Pts',(39.6488910639689,-43.8156851836082,
40.041211089324));
#187553=CARTESIAN_POINT('Ctrl Pts',(39.6459896850503,-43.8153025584992,
40.0432881154904));
#187554=CARTESIAN_POINT('Ctrl Pts',(39.6457879288345,-43.8152759514975,
40.043432547828));
#187555=CARTESIAN_POINT('Ctrl Pts',(39.6455860324536,-43.8152496566736,
40.0435768364421));
#187556=CARTESIAN_POINT('Ctrl Pts',(39.6453839959665,-43.8152236753306,
40.0437209807855));
#187557=CARTESIAN_POINT('Ctrl Pts',(39.6365259762555,-43.8140845580783,
40.050040796842));
#187558=CARTESIAN_POINT('Ctrl Pts',(39.6274037177903,-43.813592968579,40.0560490279344));
#187559=CARTESIAN_POINT('Ctrl Pts',(39.6180980992375,-43.8138323099899,
40.0616647108614));
#187560=CARTESIAN_POINT('Ctrl Pts',(39.6094236454408,-43.8140554177821,
40.0668995033484));
#187561=CARTESIAN_POINT('Ctrl Pts',(39.6005890951404,-43.8149139527617,
40.071793326748));
#187562=CARTESIAN_POINT('Ctrl Pts',(39.5916773623197,-43.8164991115143,
40.076246030307));
#187563=CARTESIAN_POINT('Ctrl Pts',(39.5884173351606,-43.8170789830936,
40.0778748868747));
#187564=CARTESIAN_POINT('Ctrl Pts',(39.5851472105419,-43.8177563121466,
40.0794443522247));
#187565=CARTESIAN_POINT('Ctrl Pts',(39.5818719865444,-43.8185363400628,
40.0809482021492));
#187566=CARTESIAN_POINT('Ctrl Pts',(39.5810844045886,-43.8187239107182,
40.0813098278168));
#187567=CARTESIAN_POINT('Ctrl Pts',(39.580296141232,-43.8189178575371,40.0816679525672));
#187568=CARTESIAN_POINT('Ctrl Pts',(39.5795073285707,-43.8191182115051,
40.0820224192581));
#187569=CARTESIAN_POINT('Ctrl Pts',(39.5787431663051,-43.8193123044115,
40.0823658088648));
#187570=CARTESIAN_POINT('Ctrl Pts',(39.577978488548,-43.8195124102599,40.0827057654617));
#187571=CARTESIAN_POINT('Ctrl Pts',(39.5772134181964,-43.8197185546679,
40.0830421470151));
#187572=CARTESIAN_POINT('Ctrl Pts',(39.5688311883231,-43.8219771048931,
40.0867275956807));
#187573=CARTESIAN_POINT('Ctrl Pts',(39.560396428487,-43.8249623840155,40.0899823432032));
#187574=CARTESIAN_POINT('Ctrl Pts',(39.5520968239715,-43.8286919494555,
40.0926299529357));
#187575=CARTESIAN_POINT('Ctrl Pts',(39.5486547305943,-43.8302387114098,
40.0937279956085));
#187576=CARTESIAN_POINT('Ctrl Pts',(39.5452359574128,-43.8319130705227,
40.0947220371803));
#187577=CARTESIAN_POINT('Ctrl Pts',(39.5418537500316,-43.8337144555751,
40.0956014538692));
#187578=CARTESIAN_POINT('Ctrl Pts',(39.5360850428918,-43.8367869054995,
40.097101390674));
#187579=CARTESIAN_POINT('Ctrl Pts',(39.5304250803199,-43.8402296473864,
40.0982667904316));
#187580=CARTESIAN_POINT('Ctrl Pts',(39.5249464846904,-43.8440378929941,
40.0990539325582));
#187581=CARTESIAN_POINT('Ctrl Pts',(39.5222071868757,-43.845942015798,40.0994475036216));
#187582=CARTESIAN_POINT('Ctrl Pts',(39.5195141476135,-43.8479386338067,
40.0997467259952));
#187583=CARTESIAN_POINT('Ctrl Pts',(39.516876509875,-43.8500271570781,40.0999473488896));
#187584=CARTESIAN_POINT('Ctrl Pts',(39.5142388721366,-43.8521156803494,
40.100147971784));
#187585=CARTESIAN_POINT('Ctrl Pts',(39.5116566557598,-43.8542960677574,
40.10025));
#187586=CARTESIAN_POINT('Ctrl Pts',(39.5091373124622,-43.8565665267057,
40.10025));
#187587=CARTESIAN_POINT('Origin',(34.2342565846635,-47.1453396605409,39.92499));
#187588=CARTESIAN_POINT('Ctrl Pts',(36.6746059268177,-50.8023624960592,
39.92499));
#187589=CARTESIAN_POINT('Ctrl Pts',(36.6808425220337,-50.8109464329598,
39.9348354642014));
#187590=CARTESIAN_POINT('Ctrl Pts',(36.6877379133665,-50.8190128116683,
39.944644082845));
#187591=CARTESIAN_POINT('Ctrl Pts',(36.6952462569238,-50.8265243508952,
39.9543641760321));
#187592=CARTESIAN_POINT('Ctrl Pts',(36.7025106240248,-50.8337918098256,
39.96376842407));
#187593=CARTESIAN_POINT('Ctrl Pts',(36.7103497152241,-50.8405407635272,
39.9730909636382));
#187594=CARTESIAN_POINT('Ctrl Pts',(36.7187568768207,-50.8467071440062,
39.9822808977125));
#187595=CARTESIAN_POINT('Ctrl Pts',(36.726709534008,-50.8525401602356,39.9909740094633));
#187596=CARTESIAN_POINT('Ctrl Pts',(36.735171246281,-50.8578524412735,39.9995492764984));
#187597=CARTESIAN_POINT('Ctrl Pts',(36.7441560526511,-50.8625525281322,
40.0079462328676));
#187598=CARTESIAN_POINT('Ctrl Pts',(36.7524317091156,-50.8668816480481,
40.0156804369671));
#187599=CARTESIAN_POINT('Ctrl Pts',(36.7611516658444,-50.870691607918,40.0232638017403));
#187600=CARTESIAN_POINT('Ctrl Pts',(36.7703354510142,-50.8738736606193,
40.0306257269946));
#187601=CARTESIAN_POINT('Ctrl Pts',(36.772999317991,-50.8747966531494,40.0327611416638));
#187602=CARTESIAN_POINT('Ctrl Pts',(36.7757022424567,-50.8756665488978,
40.0348777427264));
#187603=CARTESIAN_POINT('Ctrl Pts',(36.7784447603818,-50.8764799968252,
40.0369733168701));
#187604=CARTESIAN_POINT('Ctrl Pts',(36.7814178261393,-50.8773618266782,
40.039245053974));
#187605=CARTESIAN_POINT('Ctrl Pts',(36.7844329791247,-50.8781771258723,
40.041487875195));
#187606=CARTESIAN_POINT('Ctrl Pts',(36.7874899206174,-50.8789219044953,
40.0436985701601));
#187607=CARTESIAN_POINT('Ctrl Pts',(36.7958797205316,-50.8809659552704,
40.0497658398386));
#187608=CARTESIAN_POINT('Ctrl Pts',(36.8045837617103,-50.8824343655144,
40.0555581699984));
#187609=CARTESIAN_POINT('Ctrl Pts',(36.8135226609478,-50.8832604021662,
40.0609828468885));
#187610=CARTESIAN_POINT('Ctrl Pts',(36.8217012684462,-50.8840161808561,
40.0659461317306));
#187611=CARTESIAN_POINT('Ctrl Pts',(36.8300699399865,-50.8842246658555,
40.070603998071));
#187612=CARTESIAN_POINT('Ctrl Pts',(36.838587648016,-50.8838072802927,40.0748843180608));
#187613=CARTESIAN_POINT('Ctrl Pts',(36.8427715183753,-50.8836022618678,
40.0769867972572));
#187614=CARTESIAN_POINT('Ctrl Pts',(36.8469911418452,-50.8832457706969,
40.0789976708176));
#187615=CARTESIAN_POINT('Ctrl Pts',(36.8512399286217,-50.8827256259725,
40.0809050491499));
#187616=CARTESIAN_POINT('Ctrl Pts',(36.8520460945289,-50.8826269335773,
40.0812669556104));
#187617=CARTESIAN_POINT('Ctrl Pts',(36.8528536453866,-50.8825219362259,
40.0816253922032));
#187618=CARTESIAN_POINT('Ctrl Pts',(36.8536624499713,-50.8824105850807,
40.0819801989139));
#187619=CARTESIAN_POINT('Ctrl Pts',(36.8544459794128,-50.8823027136588,
40.0823239179148));
#187620=CARTESIAN_POINT('Ctrl Pts',(36.8552306854278,-50.8821888793657,
40.0826642303498));
#187621=CARTESIAN_POINT('Ctrl Pts',(36.8560164456186,-50.8820690400775,
40.0830009916099));
#187622=CARTESIAN_POINT('Ctrl Pts',(36.8645794982679,-50.8807630562079,
40.0866709464313));
#187623=CARTESIAN_POINT('Ctrl Pts',(36.8732733195879,-50.8787426509996,
40.0899175831879));
#187624=CARTESIAN_POINT('Ctrl Pts',(36.8819119966118,-50.8759664620665,
40.0925642067064));
#187625=CARTESIAN_POINT('Ctrl Pts',(36.8855601635621,-50.8747940602409,
40.0936818922528));
#187626=CARTESIAN_POINT('Ctrl Pts',(36.8891983713651,-50.8734872887376,
40.0946930094791));
#187627=CARTESIAN_POINT('Ctrl Pts',(36.8928125648617,-50.8720449698704,
40.0955863397545));
#187628=CARTESIAN_POINT('Ctrl Pts',(36.8988987764016,-50.8696161409374,
40.0970906856166));
#187629=CARTESIAN_POINT('Ctrl Pts',(36.9049145742147,-50.8668019052537,
40.0982599215483));
#187630=CARTESIAN_POINT('Ctrl Pts',(36.9107858666119,-50.8635979627951,
40.0990497370453));
#187631=CARTESIAN_POINT('Ctrl Pts',(36.9122536897111,-50.8627969771804,
40.0992471909196));
#187632=CARTESIAN_POINT('Ctrl Pts',(36.9137123559381,-50.8619714372918,
40.0994209989363));
#187633=CARTESIAN_POINT('Ctrl Pts',(36.915160532232,-50.8611210221658,40.0995705982975));
#187634=CARTESIAN_POINT('Ctrl Pts',(36.9173327966728,-50.8598453994767,
40.0997949973393));
#187635=CARTESIAN_POINT('Ctrl Pts',(36.9194814382215,-50.8585138058057,
40.0999649129781));
#187636=CARTESIAN_POINT('Ctrl Pts',(36.921602929223,-50.8571265262608,40.1000786629733));
#187637=CARTESIAN_POINT('Ctrl Pts',(36.9237244202244,-50.855739246716,40.1001924129685));
#187638=CARTESIAN_POINT('Ctrl Pts',(36.9258187603139,-50.8542962928985,
40.10025));
#187639=CARTESIAN_POINT('Ctrl Pts',(36.9278827595336,-50.85279802814,40.10025));
#187640=CARTESIAN_POINT('Ctrl Pts',(34.6837837831345,-47.7640607692764,
40.10025));
#187641=CARTESIAN_POINT('Ctrl Pts',(34.6767997090229,-47.7691302463542,
40.10025));
#187642=CARTESIAN_POINT('Ctrl Pts',(34.6702946353246,-47.7747322888382,
40.0995786334241));
#187643=CARTESIAN_POINT('Ctrl Pts',(34.6643211616157,-47.7807252357992,
40.0983063763366));
#187644=CARTESIAN_POINT('Ctrl Pts',(34.6604629105137,-47.7845960646239,
40.0974846287992));
#187645=CARTESIAN_POINT('Ctrl Pts',(34.6568257642793,-47.7886293194336,
40.0964130309338));
#187646=CARTESIAN_POINT('Ctrl Pts',(34.6534164822763,-47.7927819897609,
40.0951176960924));
#187647=CARTESIAN_POINT('Ctrl Pts',(34.6488976742769,-47.7982861164003,
40.0934008039614));
#187648=CARTESIAN_POINT('Ctrl Pts',(34.6447843113774,-47.8040027249063,
40.0912909372156));
#187649=CARTESIAN_POINT('Ctrl Pts',(34.6410949611633,-47.8098436832078,
40.0888630467851));
#187650=CARTESIAN_POINT('Ctrl Pts',(34.6392502860562,-47.8127641623586,
40.0876491015699));
#187651=CARTESIAN_POINT('Ctrl Pts',(34.6375114518666,-47.8157158446827,
40.0863558569271));
#187652=CARTESIAN_POINT('Ctrl Pts',(34.6358796311044,-47.8186885387637,
40.0849936342771));
#187653=CARTESIAN_POINT('Ctrl Pts',(34.6350637207232,-47.8201748858042,
40.0843125229521));
#187654=CARTESIAN_POINT('Ctrl Pts',(34.6342745503772,-47.8216664954025,
40.0836141747074));
#187655=CARTESIAN_POINT('Ctrl Pts',(34.6335121829169,-47.8231621539166,
40.0828999161609));
#187656=CARTESIAN_POINT('Ctrl Pts',(34.6333215910518,-47.8235360685451,
40.0827213515243));
#187657=CARTESIAN_POINT('Ctrl Pts',(34.6331326740831,-47.8239102364346,
40.0825417925842));
#187658=CARTESIAN_POINT('Ctrl Pts',(34.63294543242,-47.8242846390326,40.0823612602361));
#187659=CARTESIAN_POINT('Ctrl Pts',(34.6323837074307,-47.8254078468264,
40.0818196631917));
#187660=CARTESIAN_POINT('Ctrl Pts',(34.6318370616129,-47.8265331659851,
40.0812693052022));
#187661=CARTESIAN_POINT('Ctrl Pts',(34.6313054933184,-47.8276601046326,
40.0807107531875));
#187662=CARTESIAN_POINT('Ctrl Pts',(34.6275611948903,-47.8355981149514,
40.0767763849182));
#187663=CARTESIAN_POINT('Ctrl Pts',(34.6245119115567,-47.8436253243398,
40.0724140586137));
#187664=CARTESIAN_POINT('Ctrl Pts',(34.622080800581,-47.851650015445,40.0677221223768));
#187665=CARTESIAN_POINT('Ctrl Pts',(34.6209017143849,-47.8555419819595,
40.0654465383721));
#187666=CARTESIAN_POINT('Ctrl Pts',(34.6198683413513,-47.8594338479542,
40.0630928000679));
#187667=CARTESIAN_POINT('Ctrl Pts',(34.618973699214,-47.8633173872849,40.0606689262479));
#187668=CARTESIAN_POINT('Ctrl Pts',(34.6176040646085,-47.8692628146652,
40.0569581447805));
#187669=CARTESIAN_POINT('Ctrl Pts',(34.6165592825246,-47.8751852090113,
40.0530843804605));
#187670=CARTESIAN_POINT('Ctrl Pts',(34.6158190596252,-47.8810431641656,
40.0490800251457));
#187671=CARTESIAN_POINT('Ctrl Pts',(34.6154752962814,-47.8837636288443,
40.0472203818218));
#187672=CARTESIAN_POINT('Ctrl Pts',(34.6151969889848,-47.8864700832047,
40.0453323608818));
#187673=CARTESIAN_POINT('Ctrl Pts',(34.6149833323962,-47.8891582656052,
40.0434201572162));
#187674=CARTESIAN_POINT('Ctrl Pts',(34.6149669564605,-47.8893643041942,
40.0432735943397));
#187675=CARTESIAN_POINT('Ctrl Pts',(34.6149509280617,-47.889570245931,40.0431268995707));
#187676=CARTESIAN_POINT('Ctrl Pts',(34.6149352461545,-47.8897760897956,
40.0429800745037));
#187677=CARTESIAN_POINT('Ctrl Pts',(34.6147149626377,-47.8926675754933,
40.0409176249753));
#187678=CARTESIAN_POINT('Ctrl Pts',(34.6145651177085,-47.8955400426774,
40.0388310783332));
#187679=CARTESIAN_POINT('Ctrl Pts',(34.6144819591403,-47.8983891927623,
40.036725739981));
#187680=CARTESIAN_POINT('Ctrl Pts',(34.614183767304,-47.9086057382627,40.0291763710716));
#187681=CARTESIAN_POINT('Ctrl Pts',(34.614738768508,-47.9186013937339,40.0213310894592));
#187682=CARTESIAN_POINT('Ctrl Pts',(34.6160223355362,-47.928342380189,40.0132837551316));
#187683=CARTESIAN_POINT('Ctrl Pts',(34.6174328467544,-47.9390467457341,
40.0044405431322));
#187684=CARTESIAN_POINT('Ctrl Pts',(34.6197230854587,-47.9494442419753,
39.9953528710599));
#187685=CARTESIAN_POINT('Ctrl Pts',(34.6227799581218,-47.9594984812844,
39.9861103629555));
#187686=CARTESIAN_POINT('Ctrl Pts',(34.6260806134275,-47.9703545364682,
39.976130773756));
#187687=CARTESIAN_POINT('Ctrl Pts',(34.6302752334096,-47.9808115517359,
39.9659696936021));
#187688=CARTESIAN_POINT('Ctrl Pts',(34.6352786409534,-47.9908184179935,
39.9557128217521));
#187689=CARTESIAN_POINT('Ctrl Pts',(34.6402400750495,-48.0007413369263,
39.945541994517));
#187690=CARTESIAN_POINT('Ctrl Pts',(34.6459976651004,-48.010222760913,39.9352756289345));
#187691=CARTESIAN_POINT('Ctrl Pts',(34.6525130919796,-48.0191904766737,
39.92499));
#187692=CARTESIAN_POINT('Origin',(0.0123294189942765,0.0089578472449418,
39.92499));
#187693=CARTESIAN_POINT('Ctrl Pts',(36.9525415975211,-50.8348823336487,
40.10025));
#187694=CARTESIAN_POINT('Ctrl Pts',(36.959488079248,-50.8298309792464,40.10025));
#187695=CARTESIAN_POINT('Ctrl Pts',(36.9659508653421,-50.8242442388892,
40.0995859581843));
#187696=CARTESIAN_POINT('Ctrl Pts',(36.9718804702581,-50.8182646381311,
40.0983275959624));
#187697=CARTESIAN_POINT('Ctrl Pts',(36.9756692055198,-50.8144439579064,
40.0975235624071));
#187698=CARTESIAN_POINT('Ctrl Pts',(36.9792409429411,-50.8104635307797,
40.0964777059492));
#187699=CARTESIAN_POINT('Ctrl Pts',(36.9825899931427,-50.8063652005965,
40.0952149915962));
#187700=CARTESIAN_POINT('Ctrl Pts',(36.9871607746749,-50.800771802234,40.0934916398702));
#187701=CARTESIAN_POINT('Ctrl Pts',(36.9913113073909,-50.7949560887231,
40.0913643921631));
#187702=CARTESIAN_POINT('Ctrl Pts',(36.9950236271423,-50.7890120203239,
40.0889118607714));
#187703=CARTESIAN_POINT('Ctrl Pts',(36.996879787018,-50.7860399861243,40.0876855950755));
#187704=CARTESIAN_POINT('Ctrl Pts',(36.998626563727,-50.7830357420055,40.0863782327527));
#187705=CARTESIAN_POINT('Ctrl Pts',(37.000262924097,-50.7800101622085,40.0850006373335));
#187706=CARTESIAN_POINT('Ctrl Pts',(37.0010811042821,-50.77849737231,40.0843118396238));
#187707=CARTESIAN_POINT('Ctrl Pts',(37.0018716945001,-50.7769792382974,
40.0836054919165));
#187708=CARTESIAN_POINT('Ctrl Pts',(37.0026346543984,-50.7754570554919,
40.0828829920418));
#187709=CARTESIAN_POINT('Ctrl Pts',(37.002825394373,-50.7750765097905,40.0827023670732));
#187710=CARTESIAN_POINT('Ctrl Pts',(37.003014407754,-50.7746957108232,40.0825207326934));
#187711=CARTESIAN_POINT('Ctrl Pts',(37.0032016945189,-50.7743146783935,
40.0823381109276));
#187712=CARTESIAN_POINT('Ctrl Pts',(37.0037635548139,-50.7731715811044,
40.0817902456304));
#187713=CARTESIAN_POINT('Ctrl Pts',(37.0043098740556,-50.7720263837271,
40.0812334935554));
#187714=CARTESIAN_POINT('Ctrl Pts',(37.0048406651183,-50.7708796113516,
40.0806684524228));
#187715=CARTESIAN_POINT('Ctrl Pts',(37.0085087606932,-50.7629547027167,
40.0767636676139));
#187716=CARTESIAN_POINT('Ctrl Pts',(37.0114900453058,-50.7549442896472,
40.0724404510892));
#187717=CARTESIAN_POINT('Ctrl Pts',(37.0138628466708,-50.7469376805987,
40.0677949937416));
#187718=CARTESIAN_POINT('Ctrl Pts',(37.0150421224361,-50.7429584178789,
40.065486214191));
#187719=CARTESIAN_POINT('Ctrl Pts',(37.0160707669657,-50.7389795822781,
40.0630972003218));
#187720=CARTESIAN_POINT('Ctrl Pts',(37.0169563748089,-50.7350097117577,
40.0606363359906));
#187721=CARTESIAN_POINT('Ctrl Pts',(37.0189101579885,-50.7262515844356,
40.0552073017124));
#187722=CARTESIAN_POINT('Ctrl Pts',(37.0201796788544,-50.7175407334808,
40.049420430452));
#187723=CARTESIAN_POINT('Ctrl Pts',(37.0208019128475,-50.7090177292133,
40.0434049749851));
#187724=CARTESIAN_POINT('Ctrl Pts',(37.0210292227719,-50.7059041682736,
40.0412074532442));
#187725=CARTESIAN_POINT('Ctrl Pts',(37.0211776528892,-50.7028130194416,
40.0389814735788));
#187726=CARTESIAN_POINT('Ctrl Pts',(37.0212513646537,-50.6997475881155,
40.0367321210016));
#187727=CARTESIAN_POINT('Ctrl Pts',(37.0214989546705,-50.6894511286651,
40.0291767837141));
#187728=CARTESIAN_POINT('Ctrl Pts',(37.0208967002929,-50.6793793407328,
40.0213235332578));
#187729=CARTESIAN_POINT('Ctrl Pts',(37.019568267909,-50.6695664063399,40.0132649215862));
#187730=CARTESIAN_POINT('Ctrl Pts',(37.0181081633559,-50.6587808290235,
40.0044075527537));
#187731=CARTESIAN_POINT('Ctrl Pts',(37.0157708601105,-50.648307275916,39.9953016253725));
#187732=CARTESIAN_POINT('Ctrl Pts',(37.0126680948718,-50.638183057107,39.9860353422364));
#187733=CARTESIAN_POINT('Ctrl Pts',(37.0093262837667,-50.6272788396614,
39.9760551582701));
#187734=CARTESIAN_POINT('Ctrl Pts',(37.0050963107894,-50.6167786802299,
39.9658879738162));
#187735=CARTESIAN_POINT('Ctrl Pts',(37.0000610231261,-50.6067353452124,
39.9556174643261));
#187736=CARTESIAN_POINT('Ctrl Pts',(36.9950937288471,-50.5968276291274,
39.9454856413909));
#187737=CARTESIAN_POINT('Ctrl Pts',(36.9893418170241,-50.5873633690984,
39.9352519465116));
#187738=CARTESIAN_POINT('Ctrl Pts',(36.9828414016746,-50.5784163149358,
39.92499));
#187739=CARTESIAN_POINT('Ctrl Pts',(34.9607485668365,-47.7952442955503,
39.92499));
#187740=CARTESIAN_POINT('Ctrl Pts',(34.9545276336626,-47.7866819156013,
39.9348107241734));
#187741=CARTESIAN_POINT('Ctrl Pts',(34.9476537221147,-47.7786409912499,
39.9446038383192));
#187742=CARTESIAN_POINT('Ctrl Pts',(34.9401706643534,-47.7711595893149,
39.9543158069418));
#187743=CARTESIAN_POINT('Ctrl Pts',(34.9329451136968,-47.7639356375043,
39.9636935671432));
#187744=CARTESIAN_POINT('Ctrl Pts',(34.9251506707932,-47.757232524733,39.9729968321037));
#187745=CARTESIAN_POINT('Ctrl Pts',(34.9167928415108,-47.7511153344846,
39.982173115139));
#187746=CARTESIAN_POINT('Ctrl Pts',(34.9088920753289,-47.7453326739146,
39.9908475764412));
#187747=CARTESIAN_POINT('Ctrl Pts',(34.9004871280237,-47.7400730704088,
39.9994093733912));
#187748=CARTESIAN_POINT('Ctrl Pts',(34.8915635921182,-47.735428882125,40.0077966115912));
#187749=CARTESIAN_POINT('Ctrl Pts',(34.8833451652528,-47.7311516626277,
40.015521117267));
#187750=CARTESIAN_POINT('Ctrl Pts',(34.8746863576748,-47.7273962447052,
40.02309799411));
#187751=CARTESIAN_POINT('Ctrl Pts',(34.8655676881364,-47.7242720088992,
40.030455410483));
#187752=CARTESIAN_POINT('Ctrl Pts',(34.8628486849558,-47.7233404248499,
40.0326492435235));
#187753=CARTESIAN_POINT('Ctrl Pts',(34.8600887620223,-47.7224652397578,
40.0348233715087));
#187754=CARTESIAN_POINT('Ctrl Pts',(34.857287342362,-47.721650113202,40.0369753512355));
#187755=CARTESIAN_POINT('Ctrl Pts',(34.8545145463038,-47.7208433152299,
40.0391053430351));
#187756=CARTESIAN_POINT('Ctrl Pts',(34.8517040509267,-47.7200959288448,
40.0412110893239));
#187757=CARTESIAN_POINT('Ctrl Pts',(34.84885856128,-47.7194121231166,40.0432881154903));
#187758=CARTESIAN_POINT('Ctrl Pts',(34.8486606914949,-47.7193645726035,
40.0434325478279));
#187759=CARTESIAN_POINT('Ctrl Pts',(34.848462649681,-47.719317317907,40.0435768364421));
#187760=CARTESIAN_POINT('Ctrl Pts',(34.8482644357608,-47.719270360329,40.0437209807855));
#187761=CARTESIAN_POINT('Ctrl Pts',(34.8395740113844,-47.7172115680922,
40.050040796842));
#187762=CARTESIAN_POINT('Ctrl Pts',(34.8305531107003,-47.7157691359127,
40.0560490279346));
#187763=CARTESIAN_POINT('Ctrl Pts',(34.8212734513095,-47.7150344641792,
40.0616647108616));
#187764=CARTESIAN_POINT('Ctrl Pts',(34.8126231959634,-47.7143496224385,
40.0668995033488));
#187765=CARTESIAN_POINT('Ctrl Pts',(34.8037473009116,-47.7142799923071,
40.0717933267485));
#187766=CARTESIAN_POINT('Ctrl Pts',(34.794718693287,-47.7149249376575,40.0762460303076));
#187767=CARTESIAN_POINT('Ctrl Pts',(34.7914159118131,-47.7151608670105,
40.077874886875));
#187768=CARTESIAN_POINT('Ctrl Pts',(34.7880929011146,-47.715492664483,40.0794443522248));
#187769=CARTESIAN_POINT('Ctrl Pts',(34.7847540840179,-47.7159260651933,
40.0809482021492));
#187770=CARTESIAN_POINT('Ctrl Pts',(34.7839512100461,-47.7160302835855,
40.0813098278168));
#187771=CARTESIAN_POINT('Ctrl Pts',(34.7831469919157,-47.7161407719861,
40.0816679525672));
#187772=CARTESIAN_POINT('Ctrl Pts',(34.7823415577603,-47.7162575750188,
40.082022419258));
#187773=CARTESIAN_POINT('Ctrl Pts',(34.7815612934223,-47.7163707279567,
40.0823658088648));
#187774=CARTESIAN_POINT('Ctrl Pts',(34.7807798878931,-47.7164898070134,
40.0827057654616));
#187775=CARTESIAN_POINT('Ctrl Pts',(34.7799974607188,-47.7166148505126,
40.0830421470151));
#187776=CARTESIAN_POINT('Ctrl Pts',(34.7714250667942,-47.7179848465559,
40.0867275956804));
#187777=CARTESIAN_POINT('Ctrl Pts',(34.7627244668166,-47.720072099523,40.0899823432026));
#187778=CARTESIAN_POINT('Ctrl Pts',(34.7540804826596,-47.7229136891072,
40.092629952935));
#187779=CARTESIAN_POINT('Ctrl Pts',(34.7504955647793,-47.7240921810067,
40.0937279956081));
#187780=CARTESIAN_POINT('Ctrl Pts',(34.7469205018093,-47.7254000086985,
40.0947220371801));
#187781=CARTESIAN_POINT('Ctrl Pts',(34.7433685265021,-47.7268379886353,
40.0956014538692));
#187782=CARTESIAN_POINT('Ctrl Pts',(34.7373102624745,-47.7292906132652,
40.097101390674));
#187783=CARTESIAN_POINT('Ctrl Pts',(34.7313214412509,-47.732122868262,40.0982667904316));
#187784=CARTESIAN_POINT('Ctrl Pts',(34.7254747878805,-47.73533758272,40.0990539325582));
#187785=CARTESIAN_POINT('Ctrl Pts',(34.7225514611953,-47.736944939949,40.0994475036216));
#187786=CARTESIAN_POINT('Ctrl Pts',(34.7196644712718,-47.7386491210197,
40.0997467259952));
#187787=CARTESIAN_POINT('Ctrl Pts',(34.7168229726608,-47.7404504949226,
40.0999473488896));
#187788=CARTESIAN_POINT('Ctrl Pts',(34.7139814740497,-47.7422518688254,
40.100147971784));
#187789=CARTESIAN_POINT('Ctrl Pts',(34.7111854907792,-47.7441503967332,
40.10025));
#187790=CARTESIAN_POINT('Ctrl Pts',(34.7084426211231,-47.7461450747865,
40.10025));
#187791=CARTESIAN_POINT('Origin',(29.1186878401555,-50.4655267888876,39.92499));
#187792=CARTESIAN_POINT('Ctrl Pts',(31.1634057161439,-54.3576020372439,
39.92499));
#187793=CARTESIAN_POINT('Ctrl Pts',(31.1687108809057,-54.3667908521538,
39.934835464201));
#187794=CARTESIAN_POINT('Ctrl Pts',(31.1747253323926,-54.3755338070552,
39.9446440828443));
#187795=CARTESIAN_POINT('Ctrl Pts',(31.1814073748059,-54.3837890328978,
39.954364176031));
#187796=CARTESIAN_POINT('Ctrl Pts',(31.1878722906298,-54.3917760130574,
39.9637684240687));
#187797=CARTESIAN_POINT('Ctrl Pts',(31.194962980708,-54.3993074034408,39.9730909636366));
#187798=CARTESIAN_POINT('Ctrl Pts',(31.202679524718,-54.4063187915244,39.9822808977107));
#187799=CARTESIAN_POINT('Ctrl Pts',(31.2099789001941,-54.4129511329151,
39.9909740094612));
#187800=CARTESIAN_POINT('Ctrl Pts',(31.2178389737483,-54.4191188025021,
39.9995492764961));
#187801=CARTESIAN_POINT('Ctrl Pts',(31.226283267552,-54.4247323097957,40.0079462328652));
#187802=CARTESIAN_POINT('Ctrl Pts',(31.234061072852,-54.4299027559923,40.0156804369644));
#187803=CARTESIAN_POINT('Ctrl Pts',(31.2423350114947,-54.43460332818,40.0232638017373));
#187804=CARTESIAN_POINT('Ctrl Pts',(31.251135871849,-54.4387279162144,40.0306257269915));
#187805=CARTESIAN_POINT('Ctrl Pts',(31.2536886668942,-54.4399243024168,
40.0327611416618));
#187806=CARTESIAN_POINT('Ctrl Pts',(31.2562858555923,-54.4410719653266,
40.0348777427254));
#187807=CARTESIAN_POINT('Ctrl Pts',(31.2589283212566,-54.4421676282858,
40.03697331687));
#187808=CARTESIAN_POINT('Ctrl Pts',(31.2617929239294,-54.4433553973773,
40.039245053974));
#187809=CARTESIAN_POINT('Ctrl Pts',(31.2647063376194,-54.4444813995853,
40.041487875195));
#187810=CARTESIAN_POINT('Ctrl Pts',(31.2676686823018,-54.4455416356296,
40.04369857016));
#187811=CARTESIAN_POINT('Ctrl Pts',(31.2757988605279,-54.4484514617727,
40.0497658398386));
#187812=CARTESIAN_POINT('Ctrl Pts',(31.2843017293921,-54.4508216479603,
40.0555581699984));
#187813=CARTESIAN_POINT('Ctrl Pts',(31.2931053160624,-54.4525775288975,
40.0609828468885));
#187814=CARTESIAN_POINT('Ctrl Pts',(31.3011601199077,-54.4541840646261,
40.0659461317304));
#187815=CARTESIAN_POINT('Ctrl Pts',(31.3094611543726,-54.4552661718985,
40.0706039980705));
#187816=CARTESIAN_POINT('Ctrl Pts',(31.3179758301772,-54.4557414157485,
40.0748843180601));
#187817=CARTESIAN_POINT('Ctrl Pts',(31.3221582111182,-54.4559748539752,
40.0769867972569));
#187818=CARTESIAN_POINT('Ctrl Pts',(31.3263919825241,-54.4560613864571,
40.0789976708174));
#187819=CARTESIAN_POINT('Ctrl Pts',(31.3306718639313,-54.4559882102924,
40.08090504915));
#187820=CARTESIAN_POINT('Ctrl Pts',(31.3314839297417,-54.4559743258279,
40.0812669556105));
#187821=CARTESIAN_POINT('Ctrl Pts',(31.332298031963,-54.4559543157131,40.0816253922032));
#187822=CARTESIAN_POINT('Ctrl Pts',(31.3331140451957,-54.4559281176615,
40.0819801989139));
#187823=CARTESIAN_POINT('Ctrl Pts',(31.3339045580149,-54.4559027382989,
40.0823239179149));
#187824=CARTESIAN_POINT('Ctrl Pts',(31.334696864252,-54.4558715517159,40.0826642303498));
#187825=CARTESIAN_POINT('Ctrl Pts',(31.3354908465828,-54.4558345032251,
40.0830009916099));
#187826=CARTESIAN_POINT('Ctrl Pts',(31.3441435024208,-54.4554307564062,
40.0866709464313));
#187827=CARTESIAN_POINT('Ctrl Pts',(31.3530008879296,-54.4543301709715,
40.0899175831879));
#187828=CARTESIAN_POINT('Ctrl Pts',(31.3618824321397,-54.4524721779258,
40.0925642067064));
#187829=CARTESIAN_POINT('Ctrl Pts',(31.3656331634109,-54.4516875359251,
40.0936818922529));
#187830=CARTESIAN_POINT('Ctrl Pts',(31.369388035548,-54.4507682193235,40.0946930094791));
#187831=CARTESIAN_POINT('Ctrl Pts',(31.3731331934892,-54.4497115877221,
40.0955863397546));
#187832=CARTESIAN_POINT('Ctrl Pts',(31.3794399458813,-54.4479322465076,
40.0970906856166));
#187833=CARTESIAN_POINT('Ctrl Pts',(31.3857169562559,-54.4457622496021,
40.0982599215483));
#187834=CARTESIAN_POINT('Ctrl Pts',(31.3918909882807,-54.4431895758475,
40.0990497370454));
#187835=CARTESIAN_POINT('Ctrl Pts',(31.393434496287,-54.4425464074089,40.0992471909196));
#187836=CARTESIAN_POINT('Ctrl Pts',(31.3949714642036,-54.4418778620532,
40.0994209989363));
#187837=CARTESIAN_POINT('Ctrl Pts',(31.3965005998225,-54.4411834812328,
40.0995705982975));
#187838=CARTESIAN_POINT('Ctrl Pts',(31.3987943032508,-54.4401419100021,
40.0997949973393));
#187839=CARTESIAN_POINT('Ctrl Pts',(31.4010703637564,-54.4390422051396,
40.0999649129781));
#187840=CARTESIAN_POINT('Ctrl Pts',(31.4033252432071,-54.4378842814514,
40.1000786629733));
#187841=CARTESIAN_POINT('Ctrl Pts',(31.4055801226577,-54.4367263577632,
40.1001924129685));
#187842=CARTESIAN_POINT('Ctrl Pts',(31.4078138194781,-54.4355102267487,
40.10025));
#187843=CARTESIAN_POINT('Ctrl Pts',(31.4100231232069,-54.4342359163079,
40.10025));
#187844=CARTESIAN_POINT('Ctrl Pts',(29.501078514911,-51.1278468659048,40.10025));
#187845=CARTESIAN_POINT('Ctrl Pts',(29.4936027956392,-51.1321585373227,
40.10025));
#187846=CARTESIAN_POINT('Ctrl Pts',(29.4865477845229,-51.137049925875,40.099578633424));
#187847=CARTESIAN_POINT('Ctrl Pts',(29.4799806005914,-51.1423856448187,
40.0983063763363));
#187848=CARTESIAN_POINT('Ctrl Pts',(29.4757388736044,-51.1458319717793,
40.097484628799));
#187849=CARTESIAN_POINT('Ctrl Pts',(29.4717000621108,-51.1494629466902,
40.0964130309336));
#187850=CARTESIAN_POINT('Ctrl Pts',(29.4678753842638,-51.153236501246,40.0951176960923));
#187851=CARTESIAN_POINT('Ctrl Pts',(29.4628059928682,-51.1582381316478,
40.0934008039613));
#187852=CARTESIAN_POINT('Ctrl Pts',(29.4581176150989,-51.1634934604716,
40.0912909372156));
#187853=CARTESIAN_POINT('Ctrl Pts',(29.453837929136,-51.168916779284,40.0888630467851));
#187854=CARTESIAN_POINT('Ctrl Pts',(29.4516980861545,-51.1716284386902,
40.0876491015698));
#187855=CARTESIAN_POINT('Ctrl Pts',(29.4496602426632,-51.174382193724,40.0863558569271));
#187856=CARTESIAN_POINT('Ctrl Pts',(29.4477266300417,-51.1771680313592,
40.084993634277));
#187857=CARTESIAN_POINT('Ctrl Pts',(29.446759823731,-51.1785609501768,40.084312522952));
#187858=CARTESIAN_POINT('Ctrl Pts',(29.4458190608836,-51.179961897818,40.0836141747074));
#187859=CARTESIAN_POINT('Ctrl Pts',(29.4449045308659,-51.1813696738592,
40.0828999161609));
#187860=CARTESIAN_POINT('Ctrl Pts',(29.4446758983615,-51.1817216178695,
40.0827213515243));
#187861=CARTESIAN_POINT('Ctrl Pts',(29.4444489051053,-51.1820739888278,
40.0825417925841));
#187862=CARTESIAN_POINT('Ctrl Pts',(29.4442235534434,-51.1824267683258,
40.082361260236));
#187863=CARTESIAN_POINT('Ctrl Pts',(29.4435474984577,-51.1834851068199,
40.0818196631917));
#187864=CARTESIAN_POINT('Ctrl Pts',(29.4428862193406,-51.1845471213152,
40.0812693052021));
#187865=CARTESIAN_POINT('Ctrl Pts',(29.4422397658678,-51.185612322458,40.0807107531874));
#187866=CARTESIAN_POINT('Ctrl Pts',(29.4376862310784,-51.1931154617649,
40.0767763849182));
#187867=CARTESIAN_POINT('Ctrl Pts',(29.4338145801762,-51.2007799603592,
40.0724140586139));
#187868=CARTESIAN_POINT('Ctrl Pts',(29.4305579784515,-51.2085065710724,
40.0677221223771));
#187869=CARTESIAN_POINT('Ctrl Pts',(29.428978530134,-51.2122539689191,40.0654465383722));
#187870=CARTESIAN_POINT('Ctrl Pts',(29.4275440072543,-51.2160164979697,
40.063092800068));
#187871=CARTESIAN_POINT('Ctrl Pts',(29.4262483256618,-51.2197852472979,
40.0606689262479));
#187872=CARTESIAN_POINT('Ctrl Pts',(29.4242647276705,-51.2255549392044,
40.0569581447805));
#187873=CARTESIAN_POINT('Ctrl Pts',(29.4226066102323,-51.231335680589,40.0530843804605));
#187874=CARTESIAN_POINT('Ctrl Pts',(29.4212581193013,-51.2370841708899,
40.0490800251457));
#187875=CARTESIAN_POINT('Ctrl Pts',(29.4206318731367,-51.2397537995244,
40.0472203818218));
#187876=CARTESIAN_POINT('Ctrl Pts',(29.4200721889214,-51.2424163366105,
40.0453323608818));
#187877=CARTESIAN_POINT('Ctrl Pts',(29.4195787111907,-51.2450674596717,
40.0434201572162));
#187878=CARTESIAN_POINT('Ctrl Pts',(29.419540888067,-51.2452706578084,40.0432735943397));
#187879=CARTESIAN_POINT('Ctrl Pts',(29.4195034207002,-51.2454737959509,
40.0431268995707));
#187880=CARTESIAN_POINT('Ctrl Pts',(29.4194663081573,-51.2456768729756,
40.0429800745037));
#187881=CARTESIAN_POINT('Ctrl Pts',(29.4189449888201,-51.2485294929146,
40.0409176249753));
#187882=CARTESIAN_POINT('Ctrl Pts',(29.4184957101765,-51.2513705613628,
40.0388310783332));
#187883=CARTESIAN_POINT('Ctrl Pts',(29.4181151898796,-51.2541954110681,
40.036725739981));
#187884=CARTESIAN_POINT('Ctrl Pts',(29.4167507117685,-51.2643248197279,
40.0291763710723));
#187885=CARTESIAN_POINT('Ctrl Pts',(29.4162578421121,-51.2743237313746,
40.0213310894606));
#187886=CARTESIAN_POINT('Ctrl Pts',(29.4165161672808,-51.2841455249748,
40.0132837551338));
#187887=CARTESIAN_POINT('Ctrl Pts',(29.4168000406901,-51.2949386894547,
40.0044405431351));
#187888=CARTESIAN_POINT('Ctrl Pts',(29.4179908989229,-51.3055186222551,
39.9953528710635));
#187889=CARTESIAN_POINT('Ctrl Pts',(29.419980071533,-51.3158373135905,39.9861103629598));
#187890=CARTESIAN_POINT('Ctrl Pts',(29.4221278787377,-51.3269789105944,
39.976130773761));
#187891=CARTESIAN_POINT('Ctrl Pts',(29.4252064644159,-51.3378170984186,
39.9659696936077));
#187892=CARTESIAN_POINT('Ctrl Pts',(29.4291364604171,-51.3482921445171,
39.9557128217582));
#187893=CARTESIAN_POINT('Ctrl Pts',(29.4330334877913,-51.3586793157456,
39.9455419945212));
#187894=CARTESIAN_POINT('Ctrl Pts',(29.4377684584833,-51.3687106315419,
39.9352756289366));
#187895=CARTESIAN_POINT('Ctrl Pts',(29.443310811626,-51.3783102687785,39.92499));
#187896=CARTESIAN_POINT('Origin',(0.0131982271536777,0.00762000000000484,
39.92499));
#187897=CARTESIAN_POINT('Ctrl Pts',(31.4364195775134,-54.4189959163064,
40.10025));
#187898=CARTESIAN_POINT('Ctrl Pts',(31.4438560160002,-54.4146983388117,
40.10025));
#187899=CARTESIAN_POINT('Ctrl Pts',(31.4508673716606,-54.4098177483011,
40.0995859581842));
#187900=CARTESIAN_POINT('Ctrl Pts',(31.4573895320591,-54.4044907169108,
40.098327595962));
#187901=CARTESIAN_POINT('Ctrl Pts',(31.4615568820646,-54.4010869974472,
40.0975235624068));
#187902=CARTESIAN_POINT('Ctrl Pts',(31.4655251210647,-54.397501723741,40.096477705949));
#187903=CARTESIAN_POINT('Ctrl Pts',(31.4692842169746,-54.3937759157108,
40.095214991596));
#187904=CARTESIAN_POINT('Ctrl Pts',(31.4744146286225,-54.3886909353393,
40.09349163987));
#187905=CARTESIAN_POINT('Ctrl Pts',(31.4791503318821,-54.3833409297221,
40.091364392163));
#187906=CARTESIAN_POINT('Ctrl Pts',(31.4834636394928,-54.3778174666303,
40.0889118607712));
#187907=CARTESIAN_POINT('Ctrl Pts',(31.4856202932981,-54.3750557350844,
40.0876855950753));
#187908=CARTESIAN_POINT('Ctrl Pts',(31.4876715300026,-54.3722505364142,
40.0863782327526));
#187909=CARTESIAN_POINT('Ctrl Pts',(31.4896151854259,-54.3694125772948,
40.0850006373333));
#187910=CARTESIAN_POINT('Ctrl Pts',(31.4905870131376,-54.3679935977351,
40.0843118396237));
#187911=CARTESIAN_POINT('Ctrl Pts',(31.4915319606351,-54.3665664194,40.0836054919164));
#187912=CARTESIAN_POINT('Ctrl Pts',(31.4924498523887,-54.3651323262969,
40.0828829920417));
#187913=CARTESIAN_POINT('Ctrl Pts',(31.4926793253271,-54.3647738030211,
40.082702367073));
#187914=CARTESIAN_POINT('Ctrl Pts',(31.4929071076039,-54.3644148473886,
40.0825207326932));
#187915=CARTESIAN_POINT('Ctrl Pts',(31.4931331971267,-54.3640554790922,
40.0823381109275));
#187916=CARTESIAN_POINT('Ctrl Pts',(31.4938114656951,-54.3629773742029,
40.0817902456303));
#187917=CARTESIAN_POINT('Ctrl Pts',(31.4944744978649,-54.3618955562473,
40.0812334935552));
#187918=CARTESIAN_POINT('Ctrl Pts',(31.4951222515527,-54.360810548785,40.0806684524226));
#187919=CARTESIAN_POINT('Ctrl Pts',(31.4995986314374,-54.3533124740225,
40.0767636676138));
#187920=CARTESIAN_POINT('Ctrl Pts',(31.5034009004292,-54.3456575719331,
40.0724404510892));
#187921=CARTESIAN_POINT('Ctrl Pts',(31.5065976218799,-54.337942849207,40.0677949937415));
#187922=CARTESIAN_POINT('Ctrl Pts',(31.5081863836662,-54.3341086531882,
40.065486214191));
#187923=CARTESIAN_POINT('Ctrl Pts',(31.5096252947445,-54.330259136697,40.0630972003218));
#187924=CARTESIAN_POINT('Ctrl Pts',(31.5109210156001,-54.3264035847696,
40.0606363359906));
#187925=CARTESIAN_POINT('Ctrl Pts',(31.5137795693411,-54.3178976613386,
40.0552073017123));
#187926=CARTESIAN_POINT('Ctrl Pts',(31.515952667503,-54.309367230402,40.0494204304519));
#187927=CARTESIAN_POINT('Ctrl Pts',(31.5174623893716,-54.3009559572067,
40.0434049749851));
#187928=CARTESIAN_POINT('Ctrl Pts',(31.5180139098087,-54.2978832130367,
40.0412074532442));
#187929=CARTESIAN_POINT('Ctrl Pts',(31.5184846398474,-54.2948245130134,
40.0389814735788));
#187930=CARTESIAN_POINT('Ctrl Pts',(31.5188783726369,-54.2917835794183,
40.0367321210017));
#187931=CARTESIAN_POINT('Ctrl Pts',(31.520200879413,-54.2815694052536,40.029176783714));
#187932=CARTESIAN_POINT('Ctrl Pts',(31.5206547127627,-54.2714898389044,
40.0213235332575));
#187933=CARTESIAN_POINT('Ctrl Pts',(31.5203592886225,-54.2615918017969,
40.0132649215857));
#187934=CARTESIAN_POINT('Ctrl Pts',(31.5200345824972,-54.2507126865161,
40.004407552753));
#187935=CARTESIAN_POINT('Ctrl Pts',(31.5188048676547,-54.2400521939116,
39.9953016253716));
#187936=CARTESIAN_POINT('Ctrl Pts',(31.5167773687224,-54.2296591093501,
39.9860353422353));
#187937=CARTESIAN_POINT('Ctrl Pts',(31.5145936655009,-54.218465311969,39.9760551582688));
#187938=CARTESIAN_POINT('Ctrl Pts',(31.5114844302874,-54.2075805209344,
39.9658879738147));
#187939=CARTESIAN_POINT('Ctrl Pts',(31.5075265408321,-54.1970658734754,
39.9556174643242));
#187940=CARTESIAN_POINT('Ctrl Pts',(31.5036220962481,-54.1866932092591,
39.9454856413897));
#187941=CARTESIAN_POINT('Ctrl Pts',(31.498890978557,-54.1766795569339,39.935251946511));
#187942=CARTESIAN_POINT('Ctrl Pts',(31.4933613949858,-54.1671020372439,
39.92499));
#187943=CARTESIAN_POINT('Ctrl Pts',(29.7732664904679,-51.1878102687786,
39.92499));
#187944=CARTESIAN_POINT('Ctrl Pts',(29.7679746486359,-51.1786445298599,
39.9348107241715));
#187945=CARTESIAN_POINT('Ctrl Pts',(29.7619788985616,-51.1699291351242,
39.9446038383154));
#187946=CARTESIAN_POINT('Ctrl Pts',(29.7553188532225,-51.1617065245649,
39.9543158069362));
#187947=CARTESIAN_POINT('Ctrl Pts',(29.748887993471,-51.1537668706126,39.9636935671364));
#187948=CARTESIAN_POINT('Ctrl Pts',(29.7418369154195,-51.1462857370565,
39.9729968320956));
#187949=CARTESIAN_POINT('Ctrl Pts',(29.7341642916979,-51.1393284263657,
39.9821731151299));
#187950=CARTESIAN_POINT('Ctrl Pts',(29.7269112593639,-51.132751588868,39.9908475764313));
#187951=CARTESIAN_POINT('Ctrl Pts',(29.7191021335126,-51.1266422417952,
39.9994093733805));
#187952=CARTESIAN_POINT('Ctrl Pts',(29.7107129315363,-51.1210907313657,
40.0077966115799));
#187953=CARTESIAN_POINT('Ctrl Pts',(29.7029866172554,-51.1159778833935,
40.0155211172552));
#187954=CARTESIAN_POINT('Ctrl Pts',(29.694767791597,-51.1113379461933,40.0230979940978));
#187955=CARTESIAN_POINT('Ctrl Pts',(29.6860256466534,-51.1072776647637,
40.0304554104705));
#187956=CARTESIAN_POINT('Ctrl Pts',(29.683418915501,-51.1060669708027,40.0326492435152));
#187957=CARTESIAN_POINT('Ctrl Pts',(29.6807655934619,-51.1049080895608,
40.0348233715046));
#187958=CARTESIAN_POINT('Ctrl Pts',(29.6780647241927,-51.1038046002594,
40.0369753512356));
#187959=CARTESIAN_POINT('Ctrl Pts',(29.6753914511536,-51.1027123859001,
40.0391053430352));
#187960=CARTESIAN_POINT('Ctrl Pts',(29.6726744751146,-51.101675317013,40.041211089324));
#187961=CARTESIAN_POINT('Ctrl Pts',(29.6699160505199,-51.1006978225841,
40.0432881154904));
#187962=CARTESIAN_POINT('Ctrl Pts',(29.6697242350682,-51.1006298495331,
40.0434325478279));
#187963=CARTESIAN_POINT('Ctrl Pts',(29.6695322176089,-51.1005621526963,
40.0435768364421));
#187964=CARTESIAN_POINT('Ctrl Pts',(29.6693399979287,-51.1004947333604,
40.0437209807855));
#187965=CARTESIAN_POINT('Ctrl Pts',(29.6609123829953,-51.0975388226977,
40.0500407968418));
#187966=CARTESIAN_POINT('Ctrl Pts',(29.6520916749685,-51.095161351427,40.0560490279341));
#187967=CARTESIAN_POINT('Ctrl Pts',(29.6429396446305,-51.0934607157664,
40.061664710861));
#187968=CARTESIAN_POINT('Ctrl Pts',(29.6344083617435,-51.0918754277622,
40.0668995033479));
#187969=CARTESIAN_POINT('Ctrl Pts',(29.6255883681047,-51.0908783954021,
40.0717933267473));
#187970=CARTESIAN_POINT('Ctrl Pts',(29.6165418049916,-51.0905760611938,
40.0762460303063));
#187971=CARTESIAN_POINT('Ctrl Pts',(29.6132324551666,-51.090465463429,40.0778748868741));
#187972=CARTESIAN_POINT('Ctrl Pts',(29.6098929659876,-51.0904480940785,
40.0794443522244));
#187973=CARTESIAN_POINT('Ctrl Pts',(29.6065271365691,-51.0905301191541,
40.0809482021491));
#187974=CARTESIAN_POINT('Ctrl Pts',(29.6057177670366,-51.0905498434446,
40.0813098278168));
#187975=CARTESIAN_POINT('Ctrl Pts',(29.6049064053145,-51.0905756628929,
40.0816679525671));
#187976=CARTESIAN_POINT('Ctrl Pts',(29.6040931741702,-51.0906076352718,
40.082022419258));
#187977=CARTESIAN_POINT('Ctrl Pts',(29.6033053564991,-51.0906386085138,
40.0823658088647));
#187978=CARTESIAN_POINT('Ctrl Pts',(29.6025157844404,-51.0906753561239,
40.0827057654616));
#187979=CARTESIAN_POINT('Ctrl Pts',(29.6017245728792,-51.0907179287116,
40.083042147015));
#187980=CARTESIAN_POINT('Ctrl Pts',(29.5930559358432,-51.0911843606098,
40.0867275956808));
#187981=CARTESIAN_POINT('Ctrl Pts',(29.5841848213163,-51.0923507190418,
40.0899823432035));
#187982=CARTESIAN_POINT('Ctrl Pts',(29.5752911628152,-51.094273199721,40.0926299529361));
#187983=CARTESIAN_POINT('Ctrl Pts',(29.5716026975442,-51.0950705097614,
40.0937279956087));
#187984=CARTESIAN_POINT('Ctrl Pts',(29.5679105139256,-51.0959974771976,
40.0947220371803));
#187985=CARTESIAN_POINT('Ctrl Pts',(29.5642276868789,-51.0970562972091,
40.0956014538692));
#187986=CARTESIAN_POINT('Ctrl Pts',(29.5579462415721,-51.0988622250758,
40.097101390674));
#187987=CARTESIAN_POINT('Ctrl Pts',(29.5516941764754,-51.1010529624041,
40.0982667904316));
#187988=CARTESIAN_POINT('Ctrl Pts',(29.5455435225216,-51.1036389246275,
40.0990539325582));
#187989=CARTESIAN_POINT('Ctrl Pts',(29.5424681955447,-51.1049319057392,
40.0994475036216));
#187990=CARTESIAN_POINT('Ctrl Pts',(29.5394188854256,-51.1063249785076,
40.0997467259952));
#187991=CARTESIAN_POINT('Ctrl Pts',(29.5364046579954,-51.1078194668127,
40.0999473488896));
#187992=CARTESIAN_POINT('Ctrl Pts',(29.5333904305653,-51.1093139551177,
40.100147971784));
#187993=CARTESIAN_POINT('Ctrl Pts',(29.5304113137792,-51.1109098228567,
40.10025));
#187994=CARTESIAN_POINT('Ctrl Pts',(29.5274749692184,-51.1126068659048,
40.10025));
#187995=CARTESIAN_POINT('Origin',(23.6840886581935,-53.2328030451448,39.92499));
#187996=CARTESIAN_POINT('Ctrl Pts',(25.3107727110821,-57.317288315449,39.92499));
#187997=CARTESIAN_POINT('Ctrl Pts',(25.3150883208945,-57.3269813337896,
39.9348354642016));
#187998=CARTESIAN_POINT('Ctrl Pts',(25.3201559369468,-57.3363050752407,
39.9446440828455));
#187999=CARTESIAN_POINT('Ctrl Pts',(25.3259384683616,-57.3452135417177,
39.9543641760326));
#188000=CARTESIAN_POINT('Ctrl Pts',(25.3315331019382,-57.3538325360806,
39.9637684240707));
#188001=CARTESIAN_POINT('Ctrl Pts',(25.3377977038115,-57.3620638476571,
39.9730909636389));
#188002=CARTESIAN_POINT('Ctrl Pts',(25.3447390861647,-57.3698434251105,
39.9822808977133));
#188003=CARTESIAN_POINT('Ctrl Pts',(25.3513052064451,-57.3772024263426,
39.9909740094641));
#188004=CARTESIAN_POINT('Ctrl Pts',(25.3584775246705,-57.3841579102003,
39.9995492764992));
#188005=CARTESIAN_POINT('Ctrl Pts',(25.3662887884588,-57.3906233351686,
40.0079462328685));
#188006=CARTESIAN_POINT('Ctrl Pts',(25.3734835273328,-57.3965784591557,
40.015680436968));
#188007=CARTESIAN_POINT('Ctrl Pts',(25.3812207968871,-57.4021181432088,
40.0232638017412));
#188008=CARTESIAN_POINT('Ctrl Pts',(25.3895423083593,-57.4071400767268,
40.0306257269956));
#188009=CARTESIAN_POINT('Ctrl Pts',(25.3919560625135,-57.4085967487426,
40.0327611416645));
#188010=CARTESIAN_POINT('Ctrl Pts',(25.3944190600984,-57.4100096047774,
40.0348777427267));
#188011=CARTESIAN_POINT('Ctrl Pts',(25.3969325220924,-57.4113754784546,
40.0369733168701));
#188012=CARTESIAN_POINT('Ctrl Pts',(25.3996572764942,-57.4128561733381,
40.039245053974));
#188013=CARTESIAN_POINT('Ctrl Pts',(25.4024370309187,-57.414280541844,40.041487875195));
#188014=CARTESIAN_POINT('Ctrl Pts',(25.4052723227226,-57.4156446191417,
40.04369857016));
#188015=CARTESIAN_POINT('Ctrl Pts',(25.4130538033266,-57.4193883399888,
40.0497658398386));
#188016=CARTESIAN_POINT('Ctrl Pts',(25.4212623406656,-57.4226343338643,
40.0555581699984));
#188017=CARTESIAN_POINT('Ctrl Pts',(25.4298341608309,-57.4253008212879,
40.0609828468885));
#188018=CARTESIAN_POINT('Ctrl Pts',(25.4376769109071,-57.4277405125134,
40.0659461317303));
#188019=CARTESIAN_POINT('Ctrl Pts',(25.4458193604262,-57.4296843862652,
40.0706039980704));
#188020=CARTESIAN_POINT('Ctrl Pts',(25.4542377154365,-57.4310470526567,
40.07488431806));
#188021=CARTESIAN_POINT('Ctrl Pts',(25.4583727839181,-57.4317163899369,
40.0769867972567));
#188022=CARTESIAN_POINT('Ctrl Pts',(25.4625743171739,-57.4322449980037,
40.0789976708173));
#188023=CARTESIAN_POINT('Ctrl Pts',(25.4668384019351,-57.4326195921322,
40.0809050491499));
#188024=CARTESIAN_POINT('Ctrl Pts',(25.4676474704857,-57.4326906677195,
40.0812669556104));
#188025=CARTESIAN_POINT('Ctrl Pts',(25.4684592045965,-57.4327558640763,
40.0816253922032));
#188026=CARTESIAN_POINT('Ctrl Pts',(25.4692734860654,-57.4328151061496,
40.0819801989139));
#188027=CARTESIAN_POINT('Ctrl Pts',(25.4700623212384,-57.432872496908,40.0823239179149));
#188028=CARTESIAN_POINT('Ctrl Pts',(25.4708535470246,-57.4329242997218,
40.0826642303498));
#188029=CARTESIAN_POINT('Ctrl Pts',(25.471647052459,-57.4329704479394,40.0830009916099));
#188030=CARTESIAN_POINT('Ctrl Pts',(25.4802945111775,-57.4334733617057,
40.0866709464313));
#188031=CARTESIAN_POINT('Ctrl Pts',(25.489218417506,-57.4333046542889,40.089917583188));
#188032=CARTESIAN_POINT('Ctrl Pts',(25.4982455208455,-57.4323852136912,
40.0925642067065));
#188033=CARTESIAN_POINT('Ctrl Pts',(25.5020577226409,-57.4319969282174,
40.0936818922529));
#188034=CARTESIAN_POINT('Ctrl Pts',(25.505888119947,-57.4314751387427,40.0946930094791));
#188035=CARTESIAN_POINT('Ctrl Pts',(25.5097232095986,-57.4308157710841,
40.0955863397545));
#188036=CARTESIAN_POINT('Ctrl Pts',(25.5161814047441,-57.4297054124226,
40.0970906856166));
#188037=CARTESIAN_POINT('Ctrl Pts',(25.5226508554408,-57.4282034292356,
40.0982599215483));
#188038=CARTESIAN_POINT('Ctrl Pts',(25.5290599831064,-57.426290210937,40.0990497370453));
#188039=CARTESIAN_POINT('Ctrl Pts',(25.5306622650228,-57.4258119063624,
40.0992471909196));
#188040=CARTESIAN_POINT('Ctrl Pts',(25.532260695287,-57.4253076802625,40.0994209989363));
#188041=CARTESIAN_POINT('Ctrl Pts',(25.5338540367011,-57.4247769415292,
40.0995705982975));
#188042=CARTESIAN_POINT('Ctrl Pts',(25.5362440488221,-57.4239808334292,
40.0997949973393));
#188043=CARTESIAN_POINT('Ctrl Pts',(25.5386225912894,-57.423125065972,40.0999649129781));
#188044=CARTESIAN_POINT('Ctrl Pts',(25.5409861542582,-57.4222091845947,
40.1000786629733));
#188045=CARTESIAN_POINT('Ctrl Pts',(25.543349717227,-57.4212933032174,40.1001924129685));
#188046=CARTESIAN_POINT('Ctrl Pts',(25.5456982979279,-57.4203173191901,
40.10025));
#188047=CARTESIAN_POINT('Ctrl Pts',(25.5480287005717,-57.419280924679,40.10025));
#188048=CARTESIAN_POINT('Ctrl Pts',(23.9951532569806,-53.9314655730805,
40.10025));
#188049=CARTESIAN_POINT('Ctrl Pts',(23.9872677980943,-53.9349721992637,
40.10025));
#188050=CARTESIAN_POINT('Ctrl Pts',(23.9797401457389,-53.939099342807,40.0995786334241));
#188051=CARTESIAN_POINT('Ctrl Pts',(23.972651203027,-53.9437193744793,40.0983063763366));
#188052=CARTESIAN_POINT('Ctrl Pts',(23.9680724734026,-53.9467034408969,
40.0974846287992));
#188053=CARTESIAN_POINT('Ctrl Pts',(23.9636762467129,-53.9498923541889,
40.0964130309338));
#188054=CARTESIAN_POINT('Ctrl Pts',(23.9594780769922,-53.9532454491205,
40.0951176960924));
#188055=CARTESIAN_POINT('Ctrl Pts',(23.9539136435133,-53.9576897843753,
40.0934008039614));
#188056=CARTESIAN_POINT('Ctrl Pts',(23.948701617722,-53.9624262550345,40.0912909372156));
#188057=CARTESIAN_POINT('Ctrl Pts',(23.9438784851453,-53.967372515342,40.0888630467851));
#188058=CARTESIAN_POINT('Ctrl Pts',(23.9414669188569,-53.9698456454958,
40.0876491015699));
#188059=CARTESIAN_POINT('Ctrl Pts',(23.9391523931036,-53.9723713025228,
40.0863558569271));
#188060=CARTESIAN_POINT('Ctrl Pts',(23.9369381736874,-53.9749397614922,
40.0849936342771));
#188061=CARTESIAN_POINT('Ctrl Pts',(23.9358310639794,-53.9762239909768,
40.0843125229521));
#188062=CARTESIAN_POINT('Ctrl Pts',(23.9347490158252,-53.9775189275856,
40.0836141747074));
#188063=CARTESIAN_POINT('Ctrl Pts',(23.9336923430325,-53.978823397265,40.0828999161609));
#188064=CARTESIAN_POINT('Ctrl Pts',(23.9334281748343,-53.9791495146848,
40.0827213515243));
#188065=CARTESIAN_POINT('Ctrl Pts',(23.9331655922761,-53.9794762280618,
40.0825417925842));
#188066=CARTESIAN_POINT('Ctrl Pts',(23.9329045996154,-53.979803519334,40.082361260236));
#188067=CARTESIAN_POINT('Ctrl Pts',(23.9321216216332,-53.9807853931503,
40.0818196631917));
#188068=CARTESIAN_POINT('Ctrl Pts',(23.9313529543291,-53.9817724673292,
40.0812693052021));
#188069=CARTESIAN_POINT('Ctrl Pts',(23.9305986983576,-53.9827642604005,
40.0807107531874));
#188070=CARTESIAN_POINT('Ctrl Pts',(23.9252858166868,-53.9897503227312,
40.0767763849182));
#188071=CARTESIAN_POINT('Ctrl Pts',(23.9206342168336,-53.9969681366812,
40.0724140586139));
#188072=CARTESIAN_POINT('Ctrl Pts',(23.9165878043697,-54.0043120126387,
40.0677221223771));
#188073=CARTESIAN_POINT('Ctrl Pts',(23.9146252986972,-54.0078737845424,
40.0654465383723));
#188074=CARTESIAN_POINT('Ctrl Pts',(23.9128053429043,-54.0114657535931,
40.063092800068));
#188075=CARTESIAN_POINT('Ctrl Pts',(23.9111228176154,-54.0150784217125,
40.0606689262479));
#188076=CARTESIAN_POINT('Ctrl Pts',(23.9085469889529,-54.0206091641932,
40.0569581447806));
#188077=CARTESIAN_POINT('Ctrl Pts',(23.906293702842,-54.0261849176039,40.0530843804606));
#188078=CARTESIAN_POINT('Ctrl Pts',(23.9043517182282,-54.0317609613887,
40.0490800251458));
#188079=CARTESIAN_POINT('Ctrl Pts',(23.903449850527,-54.034350504969,40.0472203818218));
#188080=CARTESIAN_POINT('Ctrl Pts',(23.9026149214104,-54.0369399534675,
40.0453323608818));
#188081=CARTESIAN_POINT('Ctrl Pts',(23.9018470291827,-54.0395249709303,
40.0434201572162));
#188082=CARTESIAN_POINT('Ctrl Pts',(23.9017881732692,-54.0397231023333,
40.0432735943397));
#188083=CARTESIAN_POINT('Ctrl Pts',(23.9017296774346,-54.0399212112576,
40.0431268995707));
#188084=CARTESIAN_POINT('Ctrl Pts',(23.9016715408688,-54.040119296488,40.0429800745037));
#188085=CARTESIAN_POINT('Ctrl Pts',(23.9008548973949,-54.0429017967673,
40.0409176249753));
#188086=CARTESIAN_POINT('Ctrl Pts',(23.9001111074278,-54.045680339139,40.0388310783332));
#188087=CARTESIAN_POINT('Ctrl Pts',(23.8994373944623,-54.0484499388202,
40.036725739981));
#188088=CARTESIAN_POINT('Ctrl Pts',(23.8970215795839,-54.0583812307199,
40.029176371072));
#188089=CARTESIAN_POINT('Ctrl Pts',(23.8954862390503,-54.068273848375,40.02133108946));
#188090=CARTESIAN_POINT('Ctrl Pts',(23.8947164920951,-54.0780688394955,
40.0132837551328));
#188091=CARTESIAN_POINT('Ctrl Pts',(23.8938706175193,-54.0888325507427,
40.0044405431337));
#188092=CARTESIAN_POINT('Ctrl Pts',(23.8939490479891,-54.0994790041457,
39.9953528710617));
#188093=CARTESIAN_POINT('Ctrl Pts',(23.8948487267555,-54.1099490937668,
39.9861103629577));
#188094=CARTESIAN_POINT('Ctrl Pts',(23.8958201540346,-54.1212541629234,
39.9761307737585));
#188095=CARTESIAN_POINT('Ctrl Pts',(23.8977489757806,-54.132354777851,39.9659696936048));
#188096=CARTESIAN_POINT('Ctrl Pts',(23.9005625023815,-54.1431832369939,
39.955712821755));
#188097=CARTESIAN_POINT('Ctrl Pts',(23.9033524263857,-54.153920856493,39.945541994519));
#188098=CARTESIAN_POINT('Ctrl Pts',(23.9070129003878,-54.1643921589007,
39.9352756289355));
#188099=CARTESIAN_POINT('Ctrl Pts',(23.9115214566113,-54.174518541976,39.92499));
#188100=CARTESIAN_POINT('Origin',(0.0139224327744766,0.00619866644048029,
39.92499));
#188101=CARTESIAN_POINT('Ctrl Pts',(25.5758735661207,-57.406883591798,40.10025));
#188102=CARTESIAN_POINT('Ctrl Pts',(25.5837184861912,-57.4033868763695,
40.10025));
#188103=CARTESIAN_POINT('Ctrl Pts',(25.591201593538,-57.3992659084767,40.0995859581841));
#188104=CARTESIAN_POINT('Ctrl Pts',(25.5982448512649,-57.394649810525,40.0983275959618));
#188105=CARTESIAN_POINT('Ctrl Pts',(25.6027451576555,-57.391700343685,40.0975235624066));
#188106=CARTESIAN_POINT('Ctrl Pts',(25.6070664213775,-57.3885495044081,
40.0964777059489));
#188107=CARTESIAN_POINT('Ctrl Pts',(25.611194377554,-57.3852370392633,40.0952149915961));
#188108=CARTESIAN_POINT('Ctrl Pts',(25.6168282094542,-57.3807161889917,
40.0934916398701));
#188109=CARTESIAN_POINT('Ctrl Pts',(25.6220971979014,-57.3758905070493,
40.0913643921631));
#188110=CARTESIAN_POINT('Ctrl Pts',(25.6269642358707,-57.3708481654824,
40.0889118607713));
#188111=CARTESIAN_POINT('Ctrl Pts',(25.6293977548553,-57.3683269946989,
40.0876855950754));
#188112=CARTESIAN_POINT('Ctrl Pts',(25.6317309777765,-57.3657515758211,
40.0863782327527));
#188113=CARTESIAN_POINT('Ctrl Pts',(25.6339606331577,-57.3631323306532,
40.0850006373334));
#188114=CARTESIAN_POINT('Ctrl Pts',(25.6350754608483,-57.3618227080692,
40.0843118396237));
#188115=CARTESIAN_POINT('Ctrl Pts',(25.6361644125826,-57.3605021218762,
40.0836054919164));
#188116=CARTESIAN_POINT('Ctrl Pts',(25.6372271795775,-57.3591718306995,
40.0828829920417));
#188117=CARTESIAN_POINT('Ctrl Pts',(25.6374928713262,-57.3588392579054,
40.0827023670731));
#188118=CARTESIAN_POINT('Ctrl Pts',(25.6377569268685,-57.3585060784008,
40.0825207326933));
#188119=CARTESIAN_POINT('Ctrl Pts',(25.638019342065,-57.3581723115519,40.0823381109275));
#188120=CARTESIAN_POINT('Ctrl Pts',(25.6388065876546,-57.3571710110051,
40.0817902456303));
#188121=CARTESIAN_POINT('Ctrl Pts',(25.6395790684331,-57.3561644250953,
40.0812334935553));
#188122=CARTESIAN_POINT('Ctrl Pts',(25.6403366878211,-57.355153070115,40.0806684524227));
#188123=CARTESIAN_POINT('Ctrl Pts',(25.6455723078611,-57.3481639797005,
40.0767636676137));
#188124=CARTESIAN_POINT('Ctrl Pts',(25.6501539027776,-57.3409484573,40.0724404510888));
#188125=CARTESIAN_POINT('Ctrl Pts',(25.6541395203649,-57.3336101450126,
40.0677949937409));
#188126=CARTESIAN_POINT('Ctrl Pts',(25.6561203613654,-57.3299630239491,
40.0654862141906));
#188127=CARTESIAN_POINT('Ctrl Pts',(25.6579537739812,-57.3262850026762,
40.0630972003216));
#188128=CARTESIAN_POINT('Ctrl Pts',(25.6596454116602,-57.3225860115759,
40.0606363359906));
#188129=CARTESIAN_POINT('Ctrl Pts',(25.6633774170497,-57.3144254847132,
40.0552073017123));
#188130=CARTESIAN_POINT('Ctrl Pts',(25.6664302835893,-57.3061689349812,
40.0494204304519));
#188131=CARTESIAN_POINT('Ctrl Pts',(25.6688109525047,-57.2979615485274,
40.0434049749851));
#188132=CARTESIAN_POINT('Ctrl Pts',(25.6696806408813,-57.2949632867552,
40.0412074532442));
#188133=CARTESIAN_POINT('Ctrl Pts',(25.6704685134247,-57.2919705472983,
40.0389814735788));
#188134=CARTESIAN_POINT('Ctrl Pts',(25.6711779534203,-57.288987428539,40.0367321210017));
#188135=CARTESIAN_POINT('Ctrl Pts',(25.673560887295,-57.2789674482903,40.029176783714));
#188136=CARTESIAN_POINT('Ctrl Pts',(25.6750658360791,-57.268990537363,40.0213235332575));
#188137=CARTESIAN_POINT('Ctrl Pts',(25.6758066569115,-57.2591158425071,
40.0132649215858));
#188138=CARTESIAN_POINT('Ctrl Pts',(25.6766209067623,-57.248262383126,40.0044075527531));
#188139=CARTESIAN_POINT('Ctrl Pts',(25.676512253336,-57.2375317496128,39.9953016253718));
#188140=CARTESIAN_POINT('Ctrl Pts',(25.6755822344129,-57.2269836681084,
39.9860353422355));
#188141=CARTESIAN_POINT('Ctrl Pts',(25.6745805641845,-57.2156229323787,
39.9760551582691));
#188142=CARTESIAN_POINT('Ctrl Pts',(25.6726261321667,-57.2044727657896,
39.9658879738151));
#188143=CARTESIAN_POINT('Ctrl Pts',(25.6697890043847,-57.1936020065669,
39.9556174643248));
#188144=CARTESIAN_POINT('Ctrl Pts',(25.6669901874071,-57.1828780392979,
39.94548564139));
#188145=CARTESIAN_POINT('Ctrl Pts',(25.6633316989628,-57.1724247063458,
39.9352519465111));
#188146=CARTESIAN_POINT('Ctrl Pts',(25.658833530444,-57.1623216544372,39.92499));
#188147=CARTESIAN_POINT('Ctrl Pts',(24.2595822759732,-54.0195518809642,
39.92499));
#188148=CARTESIAN_POINT('Ctrl Pts',(24.2552775040085,-54.0098832048283,
39.9348107241709));
#188149=CARTESIAN_POINT('Ctrl Pts',(24.2502256060993,-54.000588827396,39.9446038383143));
#188150=CARTESIAN_POINT('Ctrl Pts',(24.2444615420317,-53.9917150968536,
39.9543158069345));
#188151=CARTESIAN_POINT('Ctrl Pts',(24.2388958310295,-53.9831467292694,
39.9636935671344));
#188152=CARTESIAN_POINT('Ctrl Pts',(24.2326653709158,-53.9749695397927,
39.9729968320933));
#188153=CARTESIAN_POINT('Ctrl Pts',(24.2257620156251,-53.9672483344113,
39.9821731151272));
#188154=CARTESIAN_POINT('Ctrl Pts',(24.2192361828782,-53.9599493771937,
39.9908475764284));
#188155=CARTESIAN_POINT('Ctrl Pts',(24.2121084368968,-53.9530572218387,
39.9994093733774));
#188156=CARTESIAN_POINT('Ctrl Pts',(24.2043454827012,-53.9466592127736,
40.0077966115766));
#188157=CARTESIAN_POINT('Ctrl Pts',(24.1971959321202,-53.9407667537592,
40.0155211172517));
#188158=CARTESIAN_POINT('Ctrl Pts',(24.1895071355543,-53.9352931334045,
40.0230979940941));
#188159=CARTESIAN_POINT('Ctrl Pts',(24.1812372959741,-53.9303412916448,
40.0304554104666));
#188160=CARTESIAN_POINT('Ctrl Pts',(24.1787713967456,-53.9288647523895,
40.0326492435127));
#188161=CARTESIAN_POINT('Ctrl Pts',(24.1762537459562,-53.9274348719442,
40.0348233715034));
#188162=CARTESIAN_POINT('Ctrl Pts',(24.1736830183708,-53.9260551099576,
40.0369753512355));
#188163=CARTESIAN_POINT('Ctrl Pts',(24.1711385572897,-53.9246894457402,
40.0391053430352));
#188164=CARTESIAN_POINT('Ctrl Pts',(24.1685448683467,-53.923374056695,40.041211089324));
#188165=CARTESIAN_POINT('Ctrl Pts',(24.1659037306811,-53.9221135831988,
40.0432881154904));
#188166=CARTESIAN_POINT('Ctrl Pts',(24.1657200711331,-53.922025932337,40.043432547828));
#188167=CARTESIAN_POINT('Ctrl Pts',(24.1655361818118,-53.9219385350606,
40.0435768364421));
#188168=CARTESIAN_POINT('Ctrl Pts',(24.1653520623708,-53.9218513926271,
40.0437209807855));
#188169=CARTESIAN_POINT('Ctrl Pts',(24.1572795915928,-53.9180307491142,
40.0500407968419));
#188170=CARTESIAN_POINT('Ctrl Pts',(24.1487557177458,-53.9147442868248,
40.0560490279343));
#188171=CARTESIAN_POINT('Ctrl Pts',(24.1398315880196,-53.9120963197573,
40.0616647108613));
#188172=CARTESIAN_POINT('Ctrl Pts',(24.1315127481117,-53.9096279542368,
40.0668995033482));
#188173=CARTESIAN_POINT('Ctrl Pts',(24.1228452895811,-53.9077144433431,
40.0717933267478));
#188174=CARTESIAN_POINT('Ctrl Pts',(24.1138798870173,-53.9064681420132,
40.0762460303068));
#188175=CARTESIAN_POINT('Ctrl Pts',(24.1106002267716,-53.906012228863,40.0778748868745));
#188176=CARTESIAN_POINT('Ctrl Pts',(24.1072808472556,-53.9056458829916,
40.0794443522246));
#188177=CARTESIAN_POINT('Ctrl Pts',(24.103924882248,-53.9053756337486,40.0809482021492));
#188178=CARTESIAN_POINT('Ctrl Pts',(24.1031178847767,-53.9053106478339,
40.0813098278168));
#188179=CARTESIAN_POINT('Ctrl Pts',(24.1023082689118,-53.9052515154466,
40.0816679525672));
#188180=CARTESIAN_POINT('Ctrl Pts',(24.1014961507091,-53.9051983068757,
40.0820224192581));
#188181=CARTESIAN_POINT('Ctrl Pts',(24.1007094112003,-53.9051467610726,
40.0823658088648));
#188182=CARTESIAN_POINT('Ctrl Pts',(24.0999203233287,-53.9051007746215,
40.0827057654617));
#188183=CARTESIAN_POINT('Ctrl Pts',(24.0991289960601,-53.9050604098635,
40.0830421470151));
#188184=CARTESIAN_POINT('Ctrl Pts',(24.0904590913157,-53.9046181672909,
40.0867275956807));
#188185=CARTESIAN_POINT('Ctrl Pts',(24.0815146560285,-53.9048508523204,
40.0899823432031));
#188186=CARTESIAN_POINT('Ctrl Pts',(24.0724687639687,-53.9058331609932,
40.0926299529357));
#188187=CARTESIAN_POINT('Ctrl Pts',(24.0687171629025,-53.9062405536792,
40.0937279956085));
#188188=CARTESIAN_POINT('Ctrl Pts',(24.0649483109699,-53.9067765048111,
40.0947220371803));
#188189=CARTESIAN_POINT('Ctrl Pts',(24.0611749820059,-53.9074445642442,
40.0956014538692));
#188190=CARTESIAN_POINT('Ctrl Pts',(24.0547391762491,-53.9085840092241,
40.097101390674));
#188191=CARTESIAN_POINT('Ctrl Pts',(24.0482923662128,-53.9101092267073,
40.0982667904316));
#188192=CARTESIAN_POINT('Ctrl Pts',(24.0419050995277,-53.9120381043533,
40.0990539325582));
#188193=CARTESIAN_POINT('Ctrl Pts',(24.0387114661851,-53.9130025431763,
40.0994475036216));
#188194=CARTESIAN_POINT('Ctrl Pts',(24.0355332447502,-53.9140692448455,
40.0997467259952));
#188195=CARTESIAN_POINT('Ctrl Pts',(24.0323793130074,-53.915240473626,40.0999473488896));
#188196=CARTESIAN_POINT('Ctrl Pts',(24.0292253812646,-53.9164117024065,
40.100147971784));
#188197=CARTESIAN_POINT('Ctrl Pts',(24.0260957707896,-53.9176874253154,
40.10025));
#188198=CARTESIAN_POINT('Ctrl Pts',(24.0229981225296,-53.9190682401995,
40.10025));
#188199=CARTESIAN_POINT('Origin',(17.9900016446781,-55.4168495715592,39.92499));
#188200=CARTESIAN_POINT('Ctrl Pts',(19.180829583578,-59.6489943884565,39.92499));
#188201=CARTESIAN_POINT('Ctrl Pts',(19.1841083557168,-59.65908541149,39.9348354642015));
#188202=CARTESIAN_POINT('Ctrl Pts',(19.1881736144723,-59.6688877866282,
39.9446440828453));
#188203=CARTESIAN_POINT('Ctrl Pts',(19.192993280264,-59.6783518907163,39.9543641760323));
#188204=CARTESIAN_POINT('Ctrl Pts',(19.1976563356167,-59.6875084677765,
39.9637684240702));
#188205=CARTESIAN_POINT('Ctrl Pts',(19.2030262129956,-59.6963495165736,
39.9730909636384));
#188206=CARTESIAN_POINT('Ctrl Pts',(19.2091163824538,-59.704812048718,39.9822808977126));
#188207=CARTESIAN_POINT('Ctrl Pts',(19.2148773077502,-59.7128170830339,
39.9909740094633));
#188208=CARTESIAN_POINT('Ctrl Pts',(19.2212832892268,-59.7204841754253,
39.9995492764982));
#188209=CARTESIAN_POINT('Ctrl Pts',(19.2283759411582,-59.727730681519,40.0079462328674));
#188210=CARTESIAN_POINT('Ctrl Pts',(19.2349087865407,-59.7344052377118,
40.0156804369667));
#188211=CARTESIAN_POINT('Ctrl Pts',(19.2420246158616,-59.7407233396923,
40.0232638017398));
#188212=CARTESIAN_POINT('Ctrl Pts',(19.2497756062298,-59.7465875973392,
40.030625726994));
#188213=CARTESIAN_POINT('Ctrl Pts',(19.2520238738993,-59.7482885955661,
40.0327611416634));
#188214=CARTESIAN_POINT('Ctrl Pts',(19.2543256952561,-59.7499511651806,
40.0348777427262));
#188215=CARTESIAN_POINT('Ctrl Pts',(19.2566826155664,-59.751572284779,40.03697331687));
#188216=CARTESIAN_POINT('Ctrl Pts',(19.2592376687177,-59.7533296826513,
40.039245053974));
#188217=CARTESIAN_POINT('Ctrl Pts',(19.2618533083056,-59.7550368117758,
40.041487875195));
#188218=CARTESIAN_POINT('Ctrl Pts',(19.2645304831806,-59.7566897852104,
40.0436985701601));
#188219=CARTESIAN_POINT('Ctrl Pts',(19.2718780106326,-59.7612263837725,
40.0497658398386));
#188220=CARTESIAN_POINT('Ctrl Pts',(19.2797022819936,-59.7653126215476,
40.0555581699984));
#188221=CARTESIAN_POINT('Ctrl Pts',(19.2879484209985,-59.7688605008634,
40.0609828468886));
#188222=CARTESIAN_POINT('Ctrl Pts',(19.2954931904948,-59.7721066178186,
40.0659461317306));
#188223=CARTESIAN_POINT('Ctrl Pts',(19.3033878446878,-59.7748909605621,
40.0706039980708));
#188224=CARTESIAN_POINT('Ctrl Pts',(19.3116176456451,-59.777126119837,40.0748843180606));
#188225=CARTESIAN_POINT('Ctrl Pts',(19.3156600969912,-59.7782240227714,
40.0769867972572));
#188226=CARTESIAN_POINT('Ctrl Pts',(19.3197833592189,-59.7791889148824,
40.0789976708176));
#188227=CARTESIAN_POINT('Ctrl Pts',(19.3239849291286,-59.7800071751723,
40.08090504915));
#188228=CARTESIAN_POINT('Ctrl Pts',(19.3247821360952,-59.7801624320923,
40.0812669556105));
#188229=CARTESIAN_POINT('Ctrl Pts',(19.3255826085666,-59.7803121206159,
40.0816253922033));
#188230=CARTESIAN_POINT('Ctrl Pts',(19.3263862368335,-59.7804561537455,
40.0819801989139));
#188231=CARTESIAN_POINT('Ctrl Pts',(19.3271647517172,-59.7805956858397,
40.0823239179149));
#188232=CARTESIAN_POINT('Ctrl Pts',(19.3279462282172,-59.7807299104878,
40.0826642303498));
#188233=CARTESIAN_POINT('Ctrl Pts',(19.3287305629435,-59.7808587498043,
40.0830009916099));
#188234=CARTESIAN_POINT('Ctrl Pts',(19.3372780811747,-59.7822628141273,
40.0866709464312));
#188235=CARTESIAN_POINT('Ctrl Pts',(19.3461707361371,-59.7830278331223,
40.0899175831877));
#188236=CARTESIAN_POINT('Ctrl Pts',(19.3552444957723,-59.7830570185563,
40.0925642067061));
#188237=CARTESIAN_POINT('Ctrl Pts',(19.3590764008117,-59.7830693437464,
40.0936818922527));
#188238=CARTESIAN_POINT('Ctrl Pts',(19.3629403566531,-59.7829507982331,
40.094693009479));
#188239=CARTESIAN_POINT('Ctrl Pts',(19.3668233599709,-59.7826959186872,
40.0955863397546));
#188240=CARTESIAN_POINT('Ctrl Pts',(19.3733622405322,-59.7822667079007,
40.0970906856167));
#188241=CARTESIAN_POINT('Ctrl Pts',(19.3799532508955,-59.7814491944743,
40.0982599215483));
#188242=CARTESIAN_POINT('Ctrl Pts',(19.3865272544576,-59.7802163932509,
40.0990497370454));
#188243=CARTESIAN_POINT('Ctrl Pts',(19.3881707553481,-59.7799081929451,
40.0992471909196));
#188244=CARTESIAN_POINT('Ctrl Pts',(19.3898131352235,-59.7795738105078,
40.0994209989363));
#188245=CARTESIAN_POINT('Ctrl Pts',(19.3914532254508,-59.7792125287463,
40.0995705982975));
#188246=CARTESIAN_POINT('Ctrl Pts',(19.3939133607917,-59.778670606104,40.0997949973393));
#188247=CARTESIAN_POINT('Ctrl Pts',(19.3963683254117,-59.7780681520195,
40.0999649129781));
#188248=CARTESIAN_POINT('Ctrl Pts',(19.3988146762082,-59.7774043475413,
40.1000786629733));
#188249=CARTESIAN_POINT('Ctrl Pts',(19.4012610270047,-59.7767405430631,
40.1001924129685));
#188250=CARTESIAN_POINT('Ctrl Pts',(19.4036987600453,-59.7760153991102,
40.10025));
#188251=CARTESIAN_POINT('Ctrl Pts',(19.4061247292252,-59.7752282754837,
40.10025));
#188252=CARTESIAN_POINT('Ctrl Pts',(18.2263320786581,-56.1441998575528,
40.10025));
#188253=CARTESIAN_POINT('Ctrl Pts',(18.2181232748944,-56.1468630191713,
40.10025));
#188254=CARTESIAN_POINT('Ctrl Pts',(18.2102054558341,-56.1501806998577,
40.0995786334241));
#188255=CARTESIAN_POINT('Ctrl Pts',(18.2026724222811,-56.1540344262252,
40.0983063763366));
#188256=CARTESIAN_POINT('Ctrl Pts',(18.1978068555398,-56.1565235380435,
40.0974846287993));
#188257=CARTESIAN_POINT('Ctrl Pts',(18.1931013796339,-56.1592354513147,
40.0964130309338));
#188258=CARTESIAN_POINT('Ctrl Pts',(18.1885757140657,-56.162131349412,40.0951176960924));
#188259=CARTESIAN_POINT('Ctrl Pts',(18.1825772036012,-56.1659696964527,
40.0934008039614));
#188260=CARTESIAN_POINT('Ctrl Pts',(18.1768986338332,-56.1701354151836,
40.0912909372157));
#188261=CARTESIAN_POINT('Ctrl Pts',(18.1715848978926,-56.1745504247233,
40.0888630467852));
#188262=CARTESIAN_POINT('Ctrl Pts',(18.1689280299222,-56.1767579294931,
40.0876491015699));
#188263=CARTESIAN_POINT('Ctrl Pts',(18.1663621803353,-56.1790278168865,
40.0863558569272));
#188264=CARTESIAN_POINT('Ctrl Pts',(18.1638916135758,-56.1813507566159,
40.0849936342771));
#188265=CARTESIAN_POINT('Ctrl Pts',(18.1626563301961,-56.1825122264807,
40.0843125229521));
#188266=CARTESIAN_POINT('Ctrl Pts',(18.1614448518812,-56.1836869644604,
40.0836141747074));
#188267=CARTESIAN_POINT('Ctrl Pts',(18.1602576134416,-56.1848738357352,
40.082899916161));
#188268=CARTESIAN_POINT('Ctrl Pts',(18.1599608038317,-56.1851705535539,
40.0827213515244));
#188269=CARTESIAN_POINT('Ctrl Pts',(18.159665508881,-56.1854680298096,40.0825417925842));
#188270=CARTESIAN_POINT('Ctrl Pts',(18.1593717347116,-56.1857662469842,
40.0823612602361));
#188271=CARTESIAN_POINT('Ctrl Pts',(18.1584904122037,-56.1866608985078,
40.0818196631918));
#188272=CARTESIAN_POINT('Ctrl Pts',(18.1576227783924,-56.1875622177789,
40.0812693052022));
#188273=CARTESIAN_POINT('Ctrl Pts',(18.1567689837085,-56.1884697364865,
40.0807107531875));
#188274=CARTESIAN_POINT('Ctrl Pts',(18.1507549641993,-56.1948621810804,
40.0767763849182));
#188275=CARTESIAN_POINT('Ctrl Pts',(18.1453743792963,-56.2015542305062,
40.0724140586136));
#188276=CARTESIAN_POINT('Ctrl Pts',(18.1405824894349,-56.2084349106665,
40.0677221223766));
#188277=CARTESIAN_POINT('Ctrl Pts',(18.1382584280304,-56.2117720331087,
40.0654465383719));
#188278=CARTESIAN_POINT('Ctrl Pts',(18.1360729791409,-56.2151540877946,
40.0630928000678));
#188279=CARTESIAN_POINT('Ctrl Pts',(18.134022044255,-56.2185710935569,40.0606689262479));
#188280=CARTESIAN_POINT('Ctrl Pts',(18.1308822062392,-56.2238022906399,
40.0569581447806));
#188281=CARTESIAN_POINT('Ctrl Pts',(18.1280584389298,-56.2291119669555,
40.0530843804606));
#188282=CARTESIAN_POINT('Ctrl Pts',(18.125544237423,-56.2344544719217,40.0490800251458));
#188283=CARTESIAN_POINT('Ctrl Pts',(18.1243766292364,-56.2369355588664,
40.0472203818218));
#188284=CARTESIAN_POINT('Ctrl Pts',(18.1232756028766,-56.2394235482376,
40.0453323608818));
#188285=CARTESIAN_POINT('Ctrl Pts',(18.12224170934,-56.2419141381097,40.0434201572162));
#188286=CARTESIAN_POINT('Ctrl Pts',(18.1221624654742,-56.24210503201,40.0432735943397));
#188287=CARTESIAN_POINT('Ctrl Pts',(18.1220835820645,-56.2422959411932,
40.0431268995707));
#188288=CARTESIAN_POINT('Ctrl Pts',(18.1220050584321,-56.2424868643661,
40.0429800745037));
#188289=CARTESIAN_POINT('Ctrl Pts',(18.1209020381385,-56.2451687593303,
40.0409176249753));
#188290=CARTESIAN_POINT('Ctrl Pts',(18.1198718859664,-56.247854333334,40.0388310783332));
#188291=CARTESIAN_POINT('Ctrl Pts',(18.1189123616725,-56.2505383386774,
40.036725739981));
#188292=CARTESIAN_POINT('Ctrl Pts',(18.1154716782,-56.2601627045047,40.0291763710716));
#188293=CARTESIAN_POINT('Ctrl Pts',(18.1129106883011,-56.2698406425792,
40.021331089459));
#188294=CARTESIAN_POINT('Ctrl Pts',(18.1111213027307,-56.2795015152478,
40.0132837551313));
#188295=CARTESIAN_POINT('Ctrl Pts',(18.1091549477485,-56.2901178437901,
40.0044405431314));
#188296=CARTESIAN_POINT('Ctrl Pts',(18.1081200911546,-56.300714173025,39.9953528710584));
#188297=CARTESIAN_POINT('Ctrl Pts',(18.1079204190084,-56.3112209484395,
39.9861103629534));
#188298=CARTESIAN_POINT('Ctrl Pts',(18.1077048232014,-56.3225656290471,
39.9761307737524));
#188299=CARTESIAN_POINT('Ctrl Pts',(18.108462748441,-56.3338070504196,39.9659696935968));
#188300=CARTESIAN_POINT('Ctrl Pts',(18.1101289800559,-56.3448702837441,
39.9557128217451));
#188301=CARTESIAN_POINT('Ctrl Pts',(18.1117812336992,-56.3558407079052,
39.9455419945123));
#188302=CARTESIAN_POINT('Ctrl Pts',(18.1143271060921,-56.3666372711414,
39.9352756289322));
#188303=CARTESIAN_POINT('Ctrl Pts',(18.1177524687105,-56.3771794532808,
39.92499));
#188304=CARTESIAN_POINT('Origin',(0.014494101308342,0.00470941899427951,
39.92499));
#188305=CARTESIAN_POINT('Ctrl Pts',(19.4351129318419,-59.7658094374952,
40.10025));
#188306=CARTESIAN_POINT('Ctrl Pts',(19.4432803829091,-59.7631518948793,
40.10025));
#188307=CARTESIAN_POINT('Ctrl Pts',(19.4511532554515,-59.7598356997914,
40.0995859581842));
#188308=CARTESIAN_POINT('Ctrl Pts',(19.4586404431003,-59.7559811102142,
40.0983275959621));
#188309=CARTESIAN_POINT('Ctrl Pts',(19.4634243995784,-59.7535182109732,
40.0975235624068));
#188310=CARTESIAN_POINT('Ctrl Pts',(19.4680513433538,-59.7508363273795,
40.096477705949));
#188311=CARTESIAN_POINT('Ctrl Pts',(19.4725029330461,-59.7479734971806,
40.0952149915961));
#188312=CARTESIAN_POINT('Ctrl Pts',(19.4785784597572,-59.7440663083907,
40.0934916398701));
#188313=CARTESIAN_POINT('Ctrl Pts',(19.4843230052521,-59.7398178213043,
40.091364392163));
#188314=CARTESIAN_POINT('Ctrl Pts',(19.4896904492933,-59.7353118462116,
40.0889118607713));
#188315=CARTESIAN_POINT('Ctrl Pts',(19.4923741713139,-59.7330588586653,
40.0876855950754));
#188316=CARTESIAN_POINT('Ctrl Pts',(19.4949638171735,-59.730741436408,40.0863782327527));
#188317=CARTESIAN_POINT('Ctrl Pts',(19.4974550439415,-59.7283696021898,
40.0850006373334));
#188318=CARTESIAN_POINT('Ctrl Pts',(19.4987006573255,-59.7271836850807,
40.0843118396238));
#188319=CARTESIAN_POINT('Ctrl Pts',(19.4999216825137,-59.7259841596484,
40.0836054919165));
#188320=CARTESIAN_POINT('Ctrl Pts',(19.5011176808521,-59.7247722453468,
40.0828829920418));
#188321=CARTESIAN_POINT('Ctrl Pts',(19.5014166804367,-59.7244692667714,
40.0827023670731));
#188322=CARTESIAN_POINT('Ctrl Pts',(19.5017141161967,-59.724165513779,40.0825207326933));
#188323=CARTESIAN_POINT('Ctrl Pts',(19.5020099819911,-59.723861005197,40.0823381109275));
#188324=CARTESIAN_POINT('Ctrl Pts',(19.5028975793744,-59.7229474794511,
40.0817902456303));
#188325=CARTESIAN_POINT('Ctrl Pts',(19.5037710453008,-59.7220271539529,
40.0812334935553));
#188326=CARTESIAN_POINT('Ctrl Pts',(19.5046302297524,-59.7211005320714,
40.0806684524227));
#188327=CARTESIAN_POINT('Ctrl Pts',(19.5105677273986,-59.7146969999425,
40.0767636676137));
#188328=CARTESIAN_POINT('Ctrl Pts',(19.515878451327,-59.7079999120046,40.0724404510888));
#188329=CARTESIAN_POINT('Ctrl Pts',(19.5206092977905,-59.7011184102413,
40.0677949937409));
#188330=CARTESIAN_POINT('Ctrl Pts',(19.5229605154969,-59.6976983227544,
40.0654862141905));
#188331=CARTESIAN_POINT('Ctrl Pts',(19.5251683423981,-59.6942320938701,
40.0630972003216));
#188332=CARTESIAN_POINT('Ctrl Pts',(19.5272373629643,-59.6907301905171,
40.0606363359906));
#188333=CARTESIAN_POINT('Ctrl Pts',(19.5318019313701,-59.6830044686627,
40.0552073017123));
#188334=CARTESIAN_POINT('Ctrl Pts',(19.5357011184427,-59.6751122606219,
40.0494204304519));
#188335=CARTESIAN_POINT('Ctrl Pts',(19.5389266512982,-59.6671986827532,
40.0434049749851));
#188336=CARTESIAN_POINT('Ctrl Pts',(19.5401049791265,-59.6643077529623,
40.0412074532442));
#188337=CARTESIAN_POINT('Ctrl Pts',(19.541201362078,-59.6614137631514,40.0389814735788));
#188338=CARTESIAN_POINT('Ctrl Pts',(19.5422187365067,-59.6585211429014,
40.0367321210016));
#188339=CARTESIAN_POINT('Ctrl Pts',(19.5456359895575,-59.6488051375696,
40.0291767837145));
#188340=CARTESIAN_POINT('Ctrl Pts',(19.5481755652419,-59.6390401911886,
40.0213235332585));
#188341=CARTESIAN_POINT('Ctrl Pts',(19.5499445144588,-59.6292970278081,
40.0132649215873));
#188342=CARTESIAN_POINT('Ctrl Pts',(19.551888799194,-59.6185881370994,40.0044075527552));
#188343=CARTESIAN_POINT('Ctrl Pts',(19.5529023976137,-59.6079049297443,
39.9953016253744));
#188344=CARTESIAN_POINT('Ctrl Pts',(19.5530800481818,-59.5973174182857,
39.9860353422388));
#188345=CARTESIAN_POINT('Ctrl Pts',(19.5532713854553,-59.5859142148059,
39.9760551582729));
#188346=CARTESIAN_POINT('Ctrl Pts',(19.5524931697996,-59.5746208362211,
39.9658879738195));
#188347=CARTESIAN_POINT('Ctrl Pts',(19.5508078878569,-59.5635130675483,
39.9556174643298));
#188348=CARTESIAN_POINT('Ctrl Pts',(19.5491453629103,-59.5525552912546,
39.9454856413934));
#188349=CARTESIAN_POINT('Ctrl Pts',(19.5465995868778,-59.5417768065773,
39.9352519465128));
#188350=CARTESIAN_POINT('Ctrl Pts',(19.5431821162865,-59.5312589135996,
39.92499));
#188351=CARTESIAN_POINT('Ctrl Pts',(18.4801050014189,-56.2594439784239,
39.92499));
#188352=CARTESIAN_POINT('Ctrl Pts',(18.4768344633035,-56.2493782971082,
39.9348107241721));
#188353=CARTESIAN_POINT('Ctrl Pts',(18.472781767209,-56.2396067681217,39.9446038383168));
#188354=CARTESIAN_POINT('Ctrl Pts',(18.4679768367038,-56.2301791400435,
39.9543158069382));
#188355=CARTESIAN_POINT('Ctrl Pts',(18.4633372535446,-56.2210759356547,
39.9636935671387));
#188356=CARTESIAN_POINT('Ctrl Pts',(18.4579956735925,-56.2122922812559,
39.9729968320983));
#188357=CARTESIAN_POINT('Ctrl Pts',(18.4519372213368,-56.203891776325,39.9821731151329));
#188358=CARTESIAN_POINT('Ctrl Pts',(18.4462100865654,-56.19595066829,39.9908475764345));
#188359=CARTESIAN_POINT('Ctrl Pts',(18.4398418135294,-56.188351216549,39.9994093733838));
#188360=CARTESIAN_POINT('Ctrl Pts',(18.4327901596639,-56.1811768067744,
40.0077966115833));
#188361=CARTESIAN_POINT('Ctrl Pts',(18.4262957047542,-56.1745692957318,
40.0155211172585));
#188362=CARTESIAN_POINT('Ctrl Pts',(18.4192211773439,-56.1683219623526,
40.0230979941011));
#188363=CARTESIAN_POINT('Ctrl Pts',(18.4115142492191,-56.1625328136775,
40.0304554104737));
#188364=CARTESIAN_POINT('Ctrl Pts',(18.4092161988262,-56.1608066064038,
40.0326492435173));
#188365=CARTESIAN_POINT('Ctrl Pts',(18.4068618031993,-56.159121392827,40.0348233715057));
#188366=CARTESIAN_POINT('Ctrl Pts',(18.4044493827314,-56.1574804751187,
40.0369753512355));
#188367=CARTESIAN_POINT('Ctrl Pts',(18.4020616112563,-56.1558563235461,
40.0391053430352));
#188368=CARTESIAN_POINT('Ctrl Pts',(18.3996196264082,-56.1542770260203,
40.041211089324));
#188369=CARTESIAN_POINT('Ctrl Pts',(18.3971247125286,-56.1527473834684,
40.0432881154904));
#188370=CARTESIAN_POINT('Ctrl Pts',(18.3969512210967,-56.1526410151168,
40.043432547828));
#188371=CARTESIAN_POINT('Ctrl Pts',(18.3967774746434,-56.1525348749437,
40.0435768364421));
#188372=CARTESIAN_POINT('Ctrl Pts',(18.3966034726925,-56.1524289641633,
40.0437209807855));
#188373=CARTESIAN_POINT('Ctrl Pts',(18.3889745897491,-56.1477854475702,
40.050040796842));
#188374=CARTESIAN_POINT('Ctrl Pts',(18.3808409394275,-56.1436260014307,
40.0560490279344));
#188375=CARTESIAN_POINT('Ctrl Pts',(18.3722424849459,-56.1400597146375,
40.0616647108614));
#188376=CARTESIAN_POINT('Ctrl Pts',(18.3642272309678,-56.1367353155297,
40.0668995033486));
#188377=CARTESIAN_POINT('Ctrl Pts',(18.3558072700349,-56.1339262909283,
40.0717933267482));
#188378=CARTESIAN_POINT('Ctrl Pts',(18.3470212548469,-56.1317496772149,
40.0762460303073));
#188379=CARTESIAN_POINT('Ctrl Pts',(18.3438072168245,-56.1309534437592,
40.0778748868748));
#188380=CARTESIAN_POINT('Ctrl Pts',(18.3405443147881,-56.1302421351291,
40.0794443522247));
#188381=CARTESIAN_POINT('Ctrl Pts',(18.3372349828464,-56.1296225724748,
40.0809482021492));
#188382=CARTESIAN_POINT('Ctrl Pts',(18.3364391990694,-56.1294735883542,
40.0813098278168));
#188383=CARTESIAN_POINT('Ctrl Pts',(18.3356401993826,-56.1293301519981,
40.0816679525672));
#188384=CARTESIAN_POINT('Ctrl Pts',(18.3348380918585,-56.1291923454416,
40.082022419258));
#188385=CARTESIAN_POINT('Ctrl Pts',(18.3340610501946,-56.1290588453399,
40.0823658088648));
#188386=CARTESIAN_POINT('Ctrl Pts',(18.333281091922,-56.1289306286648,40.0827057654616));
#188387=CARTESIAN_POINT('Ctrl Pts',(18.3324983188931,-56.1288077688058,
40.0830421470151));
#188388=CARTESIAN_POINT('Ctrl Pts',(18.3239221357307,-56.1274616970648,
40.0867275956806));
#188389=CARTESIAN_POINT('Ctrl Pts',(18.3150023767873,-56.126758159346,40.0899823432031));
#188390=CARTESIAN_POINT('Ctrl Pts',(18.3059033598548,-56.1267895336331,
40.0926299529356));
#188391=CARTESIAN_POINT('Ctrl Pts',(18.3021297263203,-56.1268025454852,
40.0937279956084));
#188392=CARTESIAN_POINT('Ctrl Pts',(18.2983254984047,-56.1269416083199,
40.0947220371802));
#188393=CARTESIAN_POINT('Ctrl Pts',(18.2945030089056,-56.1272115877755,
40.0956014538692));
#188394=CARTESIAN_POINT('Ctrl Pts',(18.2879833547333,-56.1276720658709,
40.097101390674));
#188395=CARTESIAN_POINT('Ctrl Pts',(18.2814124323572,-56.1285150529071,
40.0982667904316));
#188396=CARTESIAN_POINT('Ctrl Pts',(18.2748585331712,-56.1297657127887,
40.0990539325582));
#188397=CARTESIAN_POINT('Ctrl Pts',(18.2715815835782,-56.1303910427295,
40.0994475036216));
#188398=CARTESIAN_POINT('Ctrl Pts',(18.2683092720866,-56.1311196862928,
40.0997467259952));
#188399=CARTESIAN_POINT('Ctrl Pts',(18.2650501911673,-56.1319548233211,
40.0999473488896));
#188400=CARTESIAN_POINT('Ctrl Pts',(18.261791110248,-56.1327899603494,40.100147971784));
#188401=CARTESIAN_POINT('Ctrl Pts',(18.2585452947514,-56.1337315613409,
40.10025));
#188402=CARTESIAN_POINT('Ctrl Pts',(18.2553202812748,-56.1347810195642,
40.10025));
#188403=CARTESIAN_POINT('Origin',(12.0988124084938,-56.9937374973463,39.92499));
#188404=CARTESIAN_POINT('Ctrl Pts',(12.8407372733096,-61.3271735965894,
39.92499));
#188405=CARTESIAN_POINT('Ctrl Pts',(12.8429432848611,-61.3375520649562,
39.9348354642019));
#188406=CARTESIAN_POINT('Ctrl Pts',(12.8459616464943,-61.3477256769086,
39.944644082846));
#188407=CARTESIAN_POINT('Ctrl Pts',(12.8497656413962,-61.3576417279031,
39.9543641760335));
#188408=CARTESIAN_POINT('Ctrl Pts',(12.853446029115,-61.3672355662866,39.9637684240717));
#188409=CARTESIAN_POINT('Ctrl Pts',(12.8578623484995,-61.3765894879239,
39.9730909636401));
#188410=CARTESIAN_POINT('Ctrl Pts',(12.8630345798921,-61.3856422574865,
39.9822808977146));
#188411=CARTESIAN_POINT('Ctrl Pts',(12.8679271923017,-61.3942056200553,
39.9909740094656));
#188412=CARTESIAN_POINT('Ctrl Pts',(12.8734966517565,-61.4025003187121,
39.9995492765008));
#188413=CARTESIAN_POINT('Ctrl Pts',(12.8797929832529,-61.4104485116943,
40.0079462328702));
#188414=CARTESIAN_POINT('Ctrl Pts',(12.8855923599233,-61.4177693722588,
40.0156804369697));
#188415=CARTESIAN_POINT('Ctrl Pts',(12.8920087864963,-61.4247966697195,
40.023263801743));
#188416=CARTESIAN_POINT('Ctrl Pts',(12.8991043342887,-61.4314390014616,
40.0306257269974));
#188417=CARTESIAN_POINT('Ctrl Pts',(12.901162482981,-61.4333656894057,40.0327611416657));
#188418=CARTESIAN_POINT('Ctrl Pts',(12.9032779088716,-61.4352597571381,
40.0348777427274));
#188419=CARTESIAN_POINT('Ctrl Pts',(12.9054524645843,-61.4371183613309,
40.0369733168701));
#188420=CARTESIAN_POINT('Ctrl Pts',(12.9078098227881,-61.4391332077732,
40.039245053974));
#188421=CARTESIAN_POINT('Ctrl Pts',(12.9102326900447,-61.4411043938523,
40.041487875195));
#188422=CARTESIAN_POINT('Ctrl Pts',(12.9127224163027,-61.4430281531012,
40.0436985701601));
#188423=CARTESIAN_POINT('Ctrl Pts',(12.9195554895544,-61.448307925455,40.0497658398386));
#188424=CARTESIAN_POINT('Ctrl Pts',(12.926909770583,-61.4531896374536,40.0555581699984));
#188425=CARTESIAN_POINT('Ctrl Pts',(12.9347398820029,-61.4575800373534,
40.0609828468886));
#188426=CARTESIAN_POINT('Ctrl Pts',(12.9419040088455,-61.4615970149013,
40.0659461317305));
#188427=CARTESIAN_POINT('Ctrl Pts',(12.9494643722285,-61.4651913207947,
40.0706039980707));
#188428=CARTESIAN_POINT('Ctrl Pts',(12.9574154517107,-61.4682744840803,
40.0748843180604));
#188429=CARTESIAN_POINT('Ctrl Pts',(12.961320995979,-61.4697889238146,40.076986797257));
#188430=CARTESIAN_POINT('Ctrl Pts',(12.9653208118553,-61.47117952841,40.0789976708175));
#188431=CARTESIAN_POINT('Ctrl Pts',(12.9694138336349,-61.4724324898304,
40.08090504915));
#188432=CARTESIAN_POINT('Ctrl Pts',(12.970190444651,-61.4726702270559,40.0812669556105));
#188433=CARTESIAN_POINT('Ctrl Pts',(12.9709708853391,-61.4729027677274,
40.0816253922033));
#188434=CARTESIAN_POINT('Ctrl Pts',(12.9717550556846,-61.4731300138562,
40.0819801989139));
#188435=CARTESIAN_POINT('Ctrl Pts',(12.9725147207069,-61.4733501585435,
40.0823239179149));
#188436=CARTESIAN_POINT('Ctrl Pts',(12.9732778859006,-61.4735653344326,
40.0826642303498));
#188437=CARTESIAN_POINT('Ctrl Pts',(12.9740444565835,-61.4737754532574,
40.0830009916099));
#188438=CARTESIAN_POINT('Ctrl Pts',(12.9823983859298,-61.4760652849147,
40.0866709464313));
#188439=CARTESIAN_POINT('Ctrl Pts',(12.9911623597382,-61.4777556486132,
40.0899175831878));
#188440=CARTESIAN_POINT('Ctrl Pts',(13.0001833616604,-61.478733140317,40.0925642067063));
#188441=CARTESIAN_POINT('Ctrl Pts',(13.0039929867896,-61.4791459411335,
40.0936818922528));
#188442=CARTESIAN_POINT('Ctrl Pts',(13.0078481668567,-61.4794319383911,
40.0946930094791));
#188443=CARTESIAN_POINT('Ctrl Pts',(13.011736540843,-61.4795843394718,40.0955863397546));
#188444=CARTESIAN_POINT('Ctrl Pts',(13.0182844654763,-61.4798409790834,
40.0970906856166));
#188445=CARTESIAN_POINT('Ctrl Pts',(13.0249248230174,-61.4797168922658,
40.0982599215483));
#188446=CARTESIAN_POINT('Ctrl Pts',(13.0315916763176,-61.4791780149467,
40.0990497370454));
#188447=CARTESIAN_POINT('Ctrl Pts',(13.0332583896426,-61.4790432956169,
40.0992471909196));
#188448=CARTESIAN_POINT('Ctrl Pts',(13.0349267248715,-61.4788824204061,
40.0994209989363));
#188449=CARTESIAN_POINT('Ctrl Pts',(13.0365955947403,-61.4786945538949,
40.0995705982975));
#188450=CARTESIAN_POINT('Ctrl Pts',(13.0390988995433,-61.4784127541282,
40.0997949973393));
#188451=CARTESIAN_POINT('Ctrl Pts',(13.04160338921,-61.4780702140292,40.0999649129781));
#188452=CARTESIAN_POINT('Ctrl Pts',(13.0441057251028,-61.4776657592307,
40.1000786629733));
#188453=CARTESIAN_POINT('Ctrl Pts',(13.0466080609957,-61.4772613044321,
40.1001924129685));
#188454=CARTESIAN_POINT('Ctrl Pts',(13.0491082380627,-61.4767949453822,
40.10025));
#188455=CARTESIAN_POINT('Ctrl Pts',(13.0516031943527,-61.4762657165316,
40.10025));
#188456=CARTESIAN_POINT('Ctrl Pts',(12.2578193919766,-57.7418065394566,
40.10025));
#188457=CARTESIAN_POINT('Ctrl Pts',(12.2493771807071,-57.7435970583545,
40.10025));
#188458=CARTESIAN_POINT('Ctrl Pts',(12.2411559442239,-57.7460689269803,
40.099578633424));
#188459=CARTESIAN_POINT('Ctrl Pts',(12.2332613533216,-57.7491141258107,
40.0983063763365));
#188460=CARTESIAN_POINT('Ctrl Pts',(12.228162257631,-57.7510810117995,40.0974846287991));
#188461=CARTESIAN_POINT('Ctrl Pts',(12.223199086688,-57.7532862127606,40.0964130309337));
#188462=CARTESIAN_POINT('Ctrl Pts',(12.2183955094117,-57.7556931859579,
40.0951176960924));
#188463=CARTESIAN_POINT('Ctrl Pts',(12.2120286428976,-57.7588834910511,
40.0934008039614));
#188464=CARTESIAN_POINT('Ctrl Pts',(12.2059457447516,-57.7624328173675,
40.0912909372156));
#188465=CARTESIAN_POINT('Ctrl Pts',(12.2001996238499,-57.7662682043709,
40.0888630467851));
#188466=CARTESIAN_POINT('Ctrl Pts',(12.1973265633991,-57.7681858978726,
40.0876491015699));
#188467=CARTESIAN_POINT('Ctrl Pts',(12.1945375019637,-57.770175146271,40.0863558569271));
#188468=CARTESIAN_POINT('Ctrl Pts',(12.1918376559072,-57.7722271161468,
40.0849936342771));
#188469=CARTESIAN_POINT('Ctrl Pts',(12.190487732879,-57.7732531010847,40.0843125229521));
#188470=CARTESIAN_POINT('Ctrl Pts',(12.1891600976133,-57.7742947697603,
40.0836141747074));
#188471=CARTESIAN_POINT('Ctrl Pts',(12.1878553011596,-57.7753510390204,
40.082899916161));
#188472=CARTESIAN_POINT('Ctrl Pts',(12.1875291020462,-57.7756151063355,
40.0827213515243));
#188473=CARTESIAN_POINT('Ctrl Pts',(12.1872043300163,-57.7758800862577,
40.0825417925842));
#188474=CARTESIAN_POINT('Ctrl Pts',(12.1868809929896,-57.7761459620049,
40.0823612602361));
#188475=CARTESIAN_POINT('Ctrl Pts',(12.1859109819096,-57.7769435892465,
40.0818196631917));
#188476=CARTESIAN_POINT('Ctrl Pts',(12.1849538875689,-57.7777492785674,
40.0812693052022));
#188477=CARTESIAN_POINT('Ctrl Pts',(12.1840099085256,-57.7785625799462,
40.0807107531875));
#188478=CARTESIAN_POINT('Ctrl Pts',(12.1773606420347,-57.7842913698425,
40.0767763849181));
#188479=CARTESIAN_POINT('Ctrl Pts',(12.1713100228962,-57.7903843352499,
40.0724140586136));
#188480=CARTESIAN_POINT('Ctrl Pts',(12.1658251565855,-57.7967264334409,
40.0677221223767));
#188481=CARTESIAN_POINT('Ctrl Pts',(12.1631650023518,-57.7998023442101,
40.065446538372));
#188482=CARTESIAN_POINT('Ctrl Pts',(12.1606380046011,-57.8029374300326,
40.0630928000679));
#188483=CARTESIAN_POINT('Ctrl Pts',(12.1582411305897,-57.8061213360079,
40.0606689262479));
#188484=CARTESIAN_POINT('Ctrl Pts',(12.1545716839429,-57.8109956736032,
40.0569581447806));
#188485=CARTESIAN_POINT('Ctrl Pts',(12.1512083732206,-57.815981098899,40.0530843804605));
#188486=CARTESIAN_POINT('Ctrl Pts',(12.1481495009385,-57.8210315314441,
40.0490800251457));
#188487=CARTESIAN_POINT('Ctrl Pts',(12.1467289448262,-57.8233769784455,
40.0472203818218));
#188488=CARTESIAN_POINT('Ctrl Pts',(12.1453738842984,-57.8257362497572,
40.0453323608818));
#188489=CARTESIAN_POINT('Ctrl Pts',(12.1440853170069,-57.8281051246148,
40.0434201572162));
#188490=CARTESIAN_POINT('Ctrl Pts',(12.1439865534012,-57.8282866895388,
40.0432735943397));
#188491=CARTESIAN_POINT('Ctrl Pts',(12.1438881466795,-57.8284683073399,
40.0431268995708));
#188492=CARTESIAN_POINT('Ctrl Pts',(12.143790096302,-57.8286499766611,40.0429800745037));
#188493=CARTESIAN_POINT('Ctrl Pts',(12.1424127841096,-57.8312018829079,
40.0409176249753));
#188494=CARTESIAN_POINT('Ctrl Pts',(12.1411075562953,-57.8337650648327,
40.0388310783332));
#188495=CARTESIAN_POINT('Ctrl Pts',(12.1398727334219,-57.836334069314,40.036725739981));
#188496=CARTESIAN_POINT('Ctrl Pts',(12.1354448782036,-57.8455460625025,
40.0291763710714));
#188497=CARTESIAN_POINT('Ctrl Pts',(12.1318862976808,-57.8549032874812,
40.0213310894588));
#188498=CARTESIAN_POINT('Ctrl Pts',(12.1290968783779,-57.8643241951548,
40.0132837551309));
#188499=CARTESIAN_POINT('Ctrl Pts',(12.126031586786,-57.874676826274,40.004440543131));
#188500=CARTESIAN_POINT('Ctrl Pts',(12.1238947812336,-57.8851069357391,
39.9953528710581));
#188501=CARTESIAN_POINT('Ctrl Pts',(12.1225979458244,-57.895535282516,39.986110362953));
#188502=CARTESIAN_POINT('Ctrl Pts',(12.1211976890437,-57.9067952798775,
39.9761307737522));
#188503=CARTESIAN_POINT('Ctrl Pts',(12.1207764137885,-57.9180543443278,
39.9659696935969));
#188504=CARTESIAN_POINT('Ctrl Pts',(12.1212770948341,-57.9292311407324,
39.9557128217455));
#188505=CARTESIAN_POINT('Ctrl Pts',(12.12177357568,-57.9403141752966,39.9455419945126));
#188506=CARTESIAN_POINT('Ctrl Pts',(12.1231769533539,-57.9513177099587,
39.9352756289323));
#188507=CARTESIAN_POINT('Ctrl Pts',(12.125481593379,-57.9621601888121,39.92499));
#188508=CARTESIAN_POINT('Origin',(0.0149069694351876,0.0031685741680681,
39.92499));
#188509=CARTESIAN_POINT('Ctrl Pts',(13.0814171332231,-61.4699285681955,
40.10025));
#188510=CARTESIAN_POINT('Ctrl Pts',(13.0898176309848,-61.4681393149849,
40.10025));
#188511=CARTESIAN_POINT('Ctrl Pts',(13.0979940118843,-61.465664225629,40.0995859581841));
#188512=CARTESIAN_POINT('Ctrl Pts',(13.1058430982611,-61.4626133761158,
40.0983275959619));
#188513=CARTESIAN_POINT('Ctrl Pts',(13.1108582907976,-61.4606640285135,
40.0975235624067));
#188514=CARTESIAN_POINT('Ctrl Pts',(13.1157402208612,-61.4584804838814,
40.0964777059489));
#188515=CARTESIAN_POINT('Ctrl Pts',(13.1204666715205,-61.4560986543956,
40.0952149915961));
#188516=CARTESIAN_POINT('Ctrl Pts',(13.1269173283004,-61.4528479350654,
40.0934916398701));
#188517=CARTESIAN_POINT('Ctrl Pts',(13.1330744924004,-61.4492231901485,
40.0913643921631));
#188518=CARTESIAN_POINT('Ctrl Pts',(13.1388835356735,-61.4453029499362,
40.0889118607713));
#188519=CARTESIAN_POINT('Ctrl Pts',(13.1417880573101,-61.44334282983,40.0876855950754));
#188520=CARTESIAN_POINT('Ctrl Pts',(13.144605753406,-61.4413087943564,40.0863782327527));
#188521=CARTESIAN_POINT('Ctrl Pts',(13.147331257159,-61.4392103573999,40.0850006373334));
#188522=CARTESIAN_POINT('Ctrl Pts',(13.1486940090356,-61.4381611389217,
40.0843118396237));
#188523=CARTESIAN_POINT('Ctrl Pts',(13.1500337298701,-61.4370958165017,
40.0836054919165));
#188524=CARTESIAN_POINT('Ctrl Pts',(13.1513498559441,-61.4360155570619,
40.0828829920418));
#188525=CARTESIAN_POINT('Ctrl Pts',(13.1516788874626,-61.4357454922019,
40.0827023670731));
#188526=CARTESIAN_POINT('Ctrl Pts',(13.1520064446718,-61.4354744937031,
40.0825207326933));
#188527=CARTESIAN_POINT('Ctrl Pts',(13.1523325194966,-61.4352025796478,
40.0823381109275));
#188528=CARTESIAN_POINT('Ctrl Pts',(13.1533107439709,-61.434386837482,40.0817902456303));
#188529=CARTESIAN_POINT('Ctrl Pts',(13.1542756251696,-61.4335628556742,
40.0812334935553));
#188530=CARTESIAN_POINT('Ctrl Pts',(13.1552269612802,-61.4327311191547,
40.0806684524227));
#188531=CARTESIAN_POINT('Ctrl Pts',(13.161801284066,-61.4269833037494,40.0767636676136));
#188532=CARTESIAN_POINT('Ctrl Pts',(13.1677829516036,-61.420878024971,40.0724404510887));
#188533=CARTESIAN_POINT('Ctrl Pts',(13.1732071947995,-61.4145287289051,
40.0677949937408));
#188534=CARTESIAN_POINT('Ctrl Pts',(13.1759030287785,-61.411373146189,40.0654862141905));
#188535=CARTESIAN_POINT('Ctrl Pts',(13.1784610805514,-61.4081566864224,
40.0630972003215));
#188536=CARTESIAN_POINT('Ctrl Pts',(13.1808848153825,-61.4048902384027,
40.0606363359906));
#188537=CARTESIAN_POINT('Ctrl Pts',(13.1862319364381,-61.3976839661818,
40.0552073017124));
#188538=CARTESIAN_POINT('Ctrl Pts',(13.1909347237342,-61.3902425685152,
40.0494204304519));
#188539=CARTESIAN_POINT('Ctrl Pts',(13.1949697809168,-61.3827095020466,
40.0434049749851));
#188540=CARTESIAN_POINT('Ctrl Pts',(13.1964438381903,-61.3799575778687,
40.0412074532442));
#188541=CARTESIAN_POINT('Ctrl Pts',(13.197836719349,-61.3771940448619,40.0389814735788));
#188542=CARTESIAN_POINT('Ctrl Pts',(13.1991508816437,-61.3744236152738,
40.0367321210017));
#188543=CARTESIAN_POINT('Ctrl Pts',(13.2035650137315,-61.3651180354449,
40.0291767837139));
#188544=CARTESIAN_POINT('Ctrl Pts',(13.207111392194,-61.3556720404047,40.0213235332572));
#188545=CARTESIAN_POINT('Ctrl Pts',(13.2098890888176,-61.346167156635,40.0132649215853));
#188546=CARTESIAN_POINT('Ctrl Pts',(13.2129421064467,-61.3357201634447,
40.0044075527525));
#188547=CARTESIAN_POINT('Ctrl Pts',(13.2150668515158,-61.3252014297016,
39.9953016253709));
#188548=CARTESIAN_POINT('Ctrl Pts',(13.2163502251979,-61.3146904872786,
39.9860353422345));
#188549=CARTESIAN_POINT('Ctrl Pts',(13.2177324736417,-61.3033697519309,
39.9760551582678));
#188550=CARTESIAN_POINT('Ctrl Pts',(13.2181390006411,-61.2920568939682,
39.9658879738135));
#188551=CARTESIAN_POINT('Ctrl Pts',(13.2176240288384,-61.280833814882,39.9556174643229));
#188552=CARTESIAN_POINT('Ctrl Pts',(13.217116010894,-61.2697622852581,39.9454856413888));
#188553=CARTESIAN_POINT('Ctrl Pts',(13.2157108393287,-61.2587767401938,
39.9352519465106));
#188554=CARTESIAN_POINT('Ctrl Pts',(13.2134115091892,-61.2479592423878,
39.92499));
#188555=CARTESIAN_POINT('Ctrl Pts',(12.4981558292586,-57.8829458346106,
39.92499));
#188556=CARTESIAN_POINT('Ctrl Pts',(12.4959553576927,-57.8725934298269,
39.9348107241722));
#188557=CARTESIAN_POINT('Ctrl Pts',(12.4929462656002,-57.8624518082037,
39.944603838317));
#188558=CARTESIAN_POINT('Ctrl Pts',(12.4891531124823,-57.8525735736565,
39.9543158069385));
#188559=CARTESIAN_POINT('Ctrl Pts',(12.4854904894106,-57.8430352690759,
39.9636935671392));
#188560=CARTESIAN_POINT('Ctrl Pts',(12.4810963130884,-57.8337413853111,
39.9729968320989));
#188561=CARTESIAN_POINT('Ctrl Pts',(12.4759491415391,-57.8247536185209,
39.9821731151335));
#188562=CARTESIAN_POINT('Ctrl Pts',(12.4710834524306,-57.8162573641099,
39.9908475764353));
#188563=CARTESIAN_POINT('Ctrl Pts',(12.4655444244727,-57.8080338771665,
39.9994093733848));
#188564=CARTESIAN_POINT('Ctrl Pts',(12.4592813303333,-57.8001616710171,
40.0077966115844));
#188565=CARTESIAN_POINT('Ctrl Pts',(12.4535131257022,-57.7929115012196,
40.0155211172599));
#188566=CARTESIAN_POINT('Ctrl Pts',(12.4471303774507,-57.7859589019078,
40.0230979941026));
#188567=CARTESIAN_POINT('Ctrl Pts',(12.4400707994989,-57.7793958734413,
40.0304554104753));
#188568=CARTESIAN_POINT('Ctrl Pts',(12.4379657758606,-57.7774389108361,
40.0326492435184));
#188569=CARTESIAN_POINT('Ctrl Pts',(12.4358004306453,-57.7755168276793,
40.0348233715062));
#188570=CARTESIAN_POINT('Ctrl Pts',(12.433572748276,-57.7736327324861,40.0369753512356));
#188571=CARTESIAN_POINT('Ctrl Pts',(12.4313678273309,-57.7717678881028,
40.0391053430352));
#188572=CARTESIAN_POINT('Ctrl Pts',(12.4291043014747,-57.7699419852106,
40.041211089324));
#188573=CARTESIAN_POINT('Ctrl Pts',(12.4267829461797,-57.7681599326868,
40.0432881154904));
#188574=CARTESIAN_POINT('Ctrl Pts',(12.4266215236723,-57.7680360122395,
40.043432547828));
#188575=CARTESIAN_POINT('Ctrl Pts',(12.4264598236895,-57.7679122920635,
40.0435768364421));
#188576=CARTESIAN_POINT('Ctrl Pts',(12.4262978456307,-57.7677887733169,
40.0437209807855));
#188577=CARTESIAN_POINT('Ctrl Pts',(12.4191961341598,-57.762373258983,40.0500407968421));
#188578=CARTESIAN_POINT('Ctrl Pts',(12.4115418213385,-57.7573864007557,
40.0560490279346));
#188579=CARTESIAN_POINT('Ctrl Pts',(12.4033632485683,-57.7529408672212,
40.0616647108617));
#188580=CARTESIAN_POINT('Ctrl Pts',(12.39573939732,-57.7487968573386,40.0668995033489));
#188581=CARTESIAN_POINT('Ctrl Pts',(12.3876591848388,-57.7451230952906,
40.0717933267486));
#188582=CARTESIAN_POINT('Ctrl Pts',(12.3791488184477,-57.742040016629,40.0762460303077));
#188583=CARTESIAN_POINT('Ctrl Pts',(12.3760356163216,-57.7409121865683,
40.0778748868751));
#188584=CARTESIAN_POINT('Ctrl Pts',(12.3728649408022,-57.7398637084257,
40.0794443522249));
#188585=CARTESIAN_POINT('Ctrl Pts',(12.3696384996596,-57.7389016204182,
40.0809482021492));
#188586=CARTESIAN_POINT('Ctrl Pts',(12.3688626483506,-57.7386702703929,
40.0813098278168));
#188587=CARTESIAN_POINT('Ctrl Pts',(12.3680830188495,-57.7384441015868,
40.0816679525672));
#188588=CARTESIAN_POINT('Ctrl Pts',(12.367299710062,-57.7382232068821,40.082022419258));
#188589=CARTESIAN_POINT('Ctrl Pts',(12.3665408796741,-57.738009215137,40.0823658088648));
#188590=CARTESIAN_POINT('Ctrl Pts',(12.3657785963866,-57.7378001730065,
40.0827057654617));
#188591=CARTESIAN_POINT('Ctrl Pts',(12.3650129538224,-57.7375961641249,
40.0830421470151));
#188592=CARTESIAN_POINT('Ctrl Pts',(12.3566244546994,-57.7353610110591,
40.0867275956806));
#188593=CARTESIAN_POINT('Ctrl Pts',(12.3478270988457,-57.7337289586985,
40.0899823432029));
#188594=CARTESIAN_POINT('Ctrl Pts',(12.3387746477742,-57.7328090548568,
40.0926299529354));
#188595=CARTESIAN_POINT('Ctrl Pts',(12.3350203264899,-57.7324275433142,
40.0937279956083));
#188596=CARTESIAN_POINT('Ctrl Pts',(12.3312224025082,-57.7321681942502,
40.0947220371802));
#188597=CARTESIAN_POINT('Ctrl Pts',(12.3273926324687,-57.7320371357769,
40.0956014538693));
#188598=CARTESIAN_POINT('Ctrl Pts',(12.3208605605765,-57.7318136018935,
40.097101390674));
#188599=CARTESIAN_POINT('Ctrl Pts',(12.3142375182613,-57.7319651225402,
40.0982667904316));
#188600=CARTESIAN_POINT('Ctrl Pts',(12.3075887924653,-57.7325238621659,
40.0990539325582));
#188601=CARTESIAN_POINT('Ctrl Pts',(12.3042644295673,-57.7328032319787,
40.0994475036216));
#188602=CARTESIAN_POINT('Ctrl Pts',(12.3009338801485,-57.7331858342648,
40.0997467259952));
#188603=CARTESIAN_POINT('Ctrl Pts',(12.2976053572253,-57.7336757296049,
40.0999473488896));
#188604=CARTESIAN_POINT('Ctrl Pts',(12.294276834302,-57.734165624945,40.100147971784));
#188605=CARTESIAN_POINT('Ctrl Pts',(12.2909503756177,-57.7347627876418,
40.10025));
#188606=CARTESIAN_POINT('Ctrl Pts',(12.2876333308469,-57.7354693911205,
40.10025));
#188607=CARTESIAN_POINT('Origin',(6.07506605172281,-57.9461901084062,39.92499));
#188608=CARTESIAN_POINT('Ctrl Pts',(6.35995915837782,-62.3334394572619,
39.92499));
#188609=CARTESIAN_POINT('Ctrl Pts',(6.36106823981771,-62.3439916622904,
39.934835464202));
#188610=CARTESIAN_POINT('Ctrl Pts',(6.3630066345268,-62.3544250468352,39.9446440828461));
#188611=CARTESIAN_POINT('Ctrl Pts',(6.36575328117442,-62.3646844024062,
39.9543641760336));
#188612=CARTESIAN_POINT('Ctrl Pts',(6.36841067816121,-62.3746103900116,
39.9637684240718));
#188613=CARTESIAN_POINT('Ctrl Pts',(6.37182505343178,-62.384374700966,39.9730909636402));
#188614=CARTESIAN_POINT('Ctrl Pts',(6.37602267870886,-62.3939185239089,
39.9822808977147));
#188615=CARTESIAN_POINT('Ctrl Pts',(6.3799933737461,-62.4029463927381,39.9909740094656));
#188616=CARTESIAN_POINT('Ctrl Pts',(6.38466529101533,-62.4117778192058,
39.9995492765008));
#188617=CARTESIAN_POINT('Ctrl Pts',(6.39009631815078,-62.4203406170107,
40.0079462328701));
#188618=CARTESIAN_POINT('Ctrl Pts',(6.39509868692439,-62.4282275730663,
40.0156804369695));
#188619=CARTESIAN_POINT('Ctrl Pts',(6.4007454110367,-62.4358870734656,40.0232638017428));
#188620=CARTESIAN_POINT('Ctrl Pts',(6.40710777594629,-62.4432347045261,
40.0306257269972));
#188621=CARTESIAN_POINT('Ctrl Pts',(6.40895325615476,-62.4453659729922,
40.0327611416655));
#188622=CARTESIAN_POINT('Ctrl Pts',(6.41085910953167,-62.447470787041,40.0348777427273));
#188623=CARTESIAN_POINT('Ctrl Pts',(6.41282747576063,-62.4495465125725,
40.0369733168701));
#188624=CARTESIAN_POINT('Ctrl Pts',(6.41496131130727,-62.4517967325056,
40.039245053974));
#188625=CARTESIAN_POINT('Ctrl Pts',(6.41716486079182,-62.4540103788122,
40.041487875195));
#188626=CARTESIAN_POINT('Ctrl Pts',(6.41943986047092,-62.4561838467662,
40.04369857016));
#188627=CARTESIAN_POINT('Ctrl Pts',(6.4256836149418,-62.4621489466211,40.0497658398386));
#188628=CARTESIAN_POINT('Ctrl Pts',(6.43248733059615,-62.4677726477849,
40.0555581699984));
#188629=CARTESIAN_POINT('Ctrl Pts',(6.43981562609174,-62.4729574661286,
40.0609828468885));
#188630=CARTESIAN_POINT('Ctrl Pts',(6.4465206186082,-62.477701293423,40.0659461317308));
#188631=CARTESIAN_POINT('Ctrl Pts',(6.45366385825844,-62.482066182499,40.0706039980712));
#188632=CARTESIAN_POINT('Ctrl Pts',(6.46124910257559,-62.4859635700134,
40.0748843180612));
#188633=CARTESIAN_POINT('Ctrl Pts',(6.46497494980514,-62.4878779540286,
40.0769867972575));
#188634=CARTESIAN_POINT('Ctrl Pts',(6.46880749650979,-62.4896790353533,
40.0789976708177));
#188635=CARTESIAN_POINT('Ctrl Pts',(6.47274712615552,-62.4913529701965,
40.08090504915));
#188636=CARTESIAN_POINT('Ctrl Pts',(6.4734946325084,-62.4916705830287,40.0812669556104));
#188637=CARTESIAN_POINT('Ctrl Pts',(6.47424649074167,-62.4919834280838,
40.0816253922032));
#188638=CARTESIAN_POINT('Ctrl Pts',(6.47500261163139,-62.4922913974557,
40.0819801989139));
#188639=CARTESIAN_POINT('Ctrl Pts',(6.47573510374331,-62.4925897427847,
40.0823239179149));
#188640=CARTESIAN_POINT('Ctrl Pts',(6.47647159623326,-62.4928835124027,
40.0826642303498));
#188641=CARTESIAN_POINT('Ctrl Pts',(6.47721200416385,-62.4931726086301,
40.0830009916099));
#188642=CARTESIAN_POINT('Ctrl Pts',(6.4852808172263,-62.4963231197465,40.086670946431));
#188643=CARTESIAN_POINT('Ctrl Pts',(6.49382008994887,-62.49892030817,40.0899175831874));
#188644=CARTESIAN_POINT('Ctrl Pts',(6.5026894981724,-62.5008353965401,40.0925642067058));
#188645=CARTESIAN_POINT('Ctrl Pts',(6.50643510434215,-62.5016441502511,
40.0936818922525));
#188646=CARTESIAN_POINT('Ctrl Pts',(6.51023927047611,-62.5023315568339,
40.0946930094789));
#188647=CARTESIAN_POINT('Ctrl Pts',(6.5140904132927,-62.502889568803,40.0955863397546));
#188648=CARTESIAN_POINT('Ctrl Pts',(6.52057564156552,-62.5038292470155,
40.0970906856166));
#188649=CARTESIAN_POINT('Ctrl Pts',(6.52719259313763,-62.5043999463277,
40.0982599215483));
#188650=CARTESIAN_POINT('Ctrl Pts',(6.53387925273587,-62.5045608969643,
40.0990497370454));
#188651=CARTESIAN_POINT('Ctrl Pts',(6.53555091763542,-62.5046011346235,
40.0992471909196));
#188652=CARTESIAN_POINT('Ctrl Pts',(6.53722692958795,-62.5046155292216,
40.0994209989363));
#188653=CARTESIAN_POINT('Ctrl Pts',(6.53890629461062,-62.5046031362657,
40.0995705982975));
#188654=CARTESIAN_POINT('Ctrl Pts',(6.54142534214462,-62.5045845468319,
40.0997949973393));
#188655=CARTESIAN_POINT('Ctrl Pts',(6.54395191714495,-62.5045056736597,
40.0999649129781));
#188656=CARTESIAN_POINT('Ctrl Pts',(6.54648282201853,-62.5043649998325,
40.1000786629733));
#188657=CARTESIAN_POINT('Ctrl Pts',(6.54901372689211,-62.5042243260053,
40.1001924129685));
#188658=CARTESIAN_POINT('Ctrl Pts',(6.5515489555224,-62.5040218613861,40.10025));
#188659=CARTESIAN_POINT('Ctrl Pts',(6.55408556365926,-62.5037563256535,
40.10025));
#188660=CARTESIAN_POINT('Ctrl Pts',(6.15500747092297,-58.7067819056643,
40.10025));
#188661=CARTESIAN_POINT('Ctrl Pts',(6.14642434678156,-58.7076801645418,
40.10025));
#188662=CARTESIAN_POINT('Ctrl Pts',(6.13798976646346,-58.7092791387968,
40.0995786334241));
#188663=CARTESIAN_POINT('Ctrl Pts',(6.1298201130023,-58.7114824462541,40.0983063763366));
#188664=CARTESIAN_POINT('Ctrl Pts',(6.12454335512134,-58.7129055567991,
40.0974846287992));
#188665=CARTESIAN_POINT('Ctrl Pts',(6.11937686668017,-58.714579884807,40.0964130309338));
#188666=CARTESIAN_POINT('Ctrl Pts',(6.11434800669312,-58.7164715618025,
40.0951176960923));
#188667=CARTESIAN_POINT('Ctrl Pts',(6.10768254085112,-58.7189788712981,
40.0934008039614));
#188668=CARTESIAN_POINT('Ctrl Pts',(6.10126195983219,-58.7218729180381,
40.0912909372156));
#188669=CARTESIAN_POINT('Ctrl Pts',(6.09514640967252,-58.7250866612026,
40.0888630467851));
#188670=CARTESIAN_POINT('Ctrl Pts',(6.09208863459269,-58.7266935327848,
40.0876491015699));
#188671=CARTESIAN_POINT('Ctrl Pts',(6.08910691884952,-58.7283803475666,
40.0863558569271));
#188672=CARTESIAN_POINT('Ctrl Pts',(6.08620737357445,-58.7301388657774,
40.0849936342771));
#188673=CARTESIAN_POINT('Ctrl Pts',(6.08475760093692,-58.7310181248827,
40.0843125229521));
#188674=CARTESIAN_POINT('Ctrl Pts',(6.08332835457024,-58.7319153115143,
40.0836141747074));
#188675=CARTESIAN_POINT('Ctrl Pts',(6.08192029572551,-58.7328294060527,
40.0828999161609));
#188676=CARTESIAN_POINT('Ctrl Pts',(6.08156828101433,-58.7330579296873,
40.0827213515243));
#188677=CARTESIAN_POINT('Ctrl Pts',(6.08121759017549,-58.7332875101006,
40.0825417925841));
#188678=CARTESIAN_POINT('Ctrl Pts',(6.08086823283962,-58.7335181314301,
40.082361260236));
#188679=CARTESIAN_POINT('Ctrl Pts',(6.079820160832,-58.7342099954187,40.0818196631917));
#188680=CARTESIAN_POINT('Ctrl Pts',(6.07878409208759,-58.7349112274885,
40.0812693052021));
#188681=CARTESIAN_POINT('Ctrl Pts',(6.077760271117,-58.7356214008386,40.0807107531875));
#188682=CARTESIAN_POINT('Ctrl Pts',(6.07054860839961,-58.7406237702161,
40.0767763849182));
#188683=CARTESIAN_POINT('Ctrl Pts',(6.0638942468752,-58.746050895801,40.0724140586138));
#188684=CARTESIAN_POINT('Ctrl Pts',(6.05777649745833,-58.7517849266677,
40.067722122377));
#188685=CARTESIAN_POINT('Ctrl Pts',(6.05480939560192,-58.7545659254419,
40.0654465383722));
#188686=CARTESIAN_POINT('Ctrl Pts',(6.05196853530582,-58.7574196937447,
40.063092800068));
#188687=CARTESIAN_POINT('Ctrl Pts',(6.04925198282213,-58.7603356163931,
40.0606689262479));
#188688=CARTESIAN_POINT('Ctrl Pts',(6.04509313076973,-58.7647996902381,
40.0569581447805));
#188689=CARTESIAN_POINT('Ctrl Pts',(6.04122712577058,-58.7694062431511,
40.0530843804605));
#188690=CARTESIAN_POINT('Ctrl Pts',(6.03765709635815,-58.7741092696793,
40.0490800251457));
#188691=CARTESIAN_POINT('Ctrl Pts',(6.03599915623013,-58.7762933795292,
40.0472203818218));
#188692=CARTESIAN_POINT('Ctrl Pts',(6.03440490786102,-58.7784980841112,
40.0453323608818));
#188693=CARTESIAN_POINT('Ctrl Pts',(6.03287578462736,-58.7807192900657,
40.0434201572162));
#188694=CARTESIAN_POINT('Ctrl Pts',(6.03275858335655,-58.7808895367501,
40.0432735943397));
#188695=CARTESIAN_POINT('Ctrl Pts',(6.03264173148759,-58.7810598733265,
40.0431268995707));
#188696=CARTESIAN_POINT('Ctrl Pts',(6.03252522862529,-58.7812302983888,
40.0429800745037));
#188697=CARTESIAN_POINT('Ctrl Pts',(6.03088871465485,-58.7836242566993,
40.0409176249753));
#188698=CARTESIAN_POINT('Ctrl Pts',(6.02932271154744,-58.7860369637877,
40.0388310783332));
#188699=CARTESIAN_POINT('Ctrl Pts',(6.02782611907238,-58.7884628208563,
40.036725739981));
#188700=CARTESIAN_POINT('Ctrl Pts',(6.02245960461748,-58.7971615128793,
40.0291763710726));
#188701=CARTESIAN_POINT('Ctrl Pts',(6.01794242202427,-58.8060955050456,
40.0213310894612));
#188702=CARTESIAN_POINT('Ctrl Pts',(6.01418353045086,-58.8151732302866,
40.0132837551347));
#188703=CARTESIAN_POINT('Ctrl Pts',(6.01005288622599,-58.8251487383876,
40.0044405431366));
#188704=CARTESIAN_POINT('Ctrl Pts',(6.00683754300419,-58.8352983536189,
39.9953528710656));
#188705=CARTESIAN_POINT('Ctrl Pts',(6.00445775273193,-58.8455340166064,
39.9861103629626));
#188706=CARTESIAN_POINT('Ctrl Pts',(6.00188817648396,-58.8565859638311,
39.9761307737652));
#188707=CARTESIAN_POINT('Ctrl Pts',(6.00029231631344,-58.8677393146896,
39.9659696936133));
#188708=CARTESIAN_POINT('Ctrl Pts',(5.99962196122237,-58.8789072188508,
39.9557128217654));
#188709=CARTESIAN_POINT('Ctrl Pts',(5.99895722972124,-58.889981435779,39.945541994526));
#188710=CARTESIAN_POINT('Ctrl Pts',(5.99920273697621,-58.9010713848459,
39.935275628939));
#188711=CARTESIAN_POINT('Ctrl Pts',(6.00036140429027,-58.912095367953,39.92499));
#188712=CARTESIAN_POINT('Origin',(0.0151565136854175,0.00159301378020458,
39.92499));
#188713=CARTESIAN_POINT('Ctrl Pts',(6.58439859103009,-62.5005702980931,
40.10025));
#188714=CARTESIAN_POINT('Ctrl Pts',(6.59294009787482,-62.4996689377205,
40.10025));
#188715=CARTESIAN_POINT('Ctrl Pts',(6.60133040499131,-62.4980620716935,
40.0995859581841));
#188716=CARTESIAN_POINT('Ctrl Pts',(6.60945539386312,-62.4958483879901,
40.0983275959618));
#188717=CARTESIAN_POINT('Ctrl Pts',(6.6146468749591,-62.4944339494868,40.0975235624066));
#188718=CARTESIAN_POINT('Ctrl Pts',(6.61973030386369,-62.4927726671881,
40.0964777059489));
#188719=CARTESIAN_POINT('Ctrl Pts',(6.62467983150736,-62.4908979342377,
40.0952149915961));
#188720=CARTESIAN_POINT('Ctrl Pts',(6.63143494361066,-62.4883392999283,
40.0934916398701));
#188721=CARTESIAN_POINT('Ctrl Pts',(6.63793726713738,-62.4853780106448,
40.0913643921631));
#188722=CARTESIAN_POINT('Ctrl Pts',(6.64412426454869,-62.4820864562849,
40.0889118607713));
#188723=CARTESIAN_POINT('Ctrl Pts',(6.64721776325435,-62.480440679105,40.0876855950754));
#188724=CARTESIAN_POINT('Ctrl Pts',(6.6502326383185,-62.4787123157334,40.0863782327526));
#188725=CARTESIAN_POINT('Ctrl Pts',(6.65316255786718,-62.476910266953,40.0850006373334));
#188726=CARTESIAN_POINT('Ctrl Pts',(6.65462751764151,-62.4760092425629,
40.0843118396237));
#188727=CARTESIAN_POINT('Ctrl Pts',(6.65607125586061,-62.4750897950506,
40.0836054919164));
#188728=CARTESIAN_POINT('Ctrl Pts',(6.6574930899174,-62.474153026021,40.0828829920417));
#188729=CARTESIAN_POINT('Ctrl Pts',(6.6578485484316,-62.4739188337636,40.0827023670731));
#188730=CARTESIAN_POINT('Ctrl Pts',(6.65820263830482,-62.4736835588747,
40.0825207326932));
#188731=CARTESIAN_POINT('Ctrl Pts',(6.65855534961594,-62.4734472184934,
40.0823381109275));
#188732=CARTESIAN_POINT('Ctrl Pts',(6.65961348354927,-62.4727381973495,
40.0817902456303));
#188733=CARTESIAN_POINT('Ctrl Pts',(6.66065920857986,-62.4720195869492,
40.0812334935553));
#188734=CARTESIAN_POINT('Ctrl Pts',(6.66169227331197,-62.471291848471,40.0806684524227));
#188735=CARTESIAN_POINT('Ctrl Pts',(6.66883139158116,-62.4662627240578,
40.0767636676136));
#188736=CARTESIAN_POINT('Ctrl Pts',(6.67541846632667,-62.4608161451508,
40.0724404510887));
#188737=CARTESIAN_POINT('Ctrl Pts',(6.6814766771114,-62.4550686189988,40.0677949937407));
#188738=CARTESIAN_POINT('Ctrl Pts',(6.68448759124181,-62.452212114278,40.0654862141904));
#188739=CARTESIAN_POINT('Ctrl Pts',(6.68736784133602,-62.4492806638353,
40.0630972003215));
#188740=CARTESIAN_POINT('Ctrl Pts',(6.69011973548588,-62.4462854590369,
40.0606363359906));
#188741=CARTESIAN_POINT('Ctrl Pts',(6.69619082501401,-62.4396775898761,
40.0552073017123));
#188742=CARTESIAN_POINT('Ctrl Pts',(6.70164568781197,-62.4327685320937,
40.0494204304519));
#188743=CARTESIAN_POINT('Ctrl Pts',(6.70644606039073,-62.4256985108779,
40.0434049749851));
#188744=CARTESIAN_POINT('Ctrl Pts',(6.70819969702964,-62.42311574297,40.0412074532442));
#188745=CARTESIAN_POINT('Ctrl Pts',(6.70987381569794,-62.4205129446132,
40.0389814735788));
#188746=CARTESIAN_POINT('Ctrl Pts',(6.71147036762154,-62.4178950590935,
40.0367321210017));
#188747=CARTESIAN_POINT('Ctrl Pts',(6.71683301659107,-62.4091018586486,
40.0291767837141));
#188748=CARTESIAN_POINT('Ctrl Pts',(6.72134734296672,-62.4000783072487,
40.0213235332576));
#188749=CARTESIAN_POINT('Ctrl Pts',(6.7251033539715,-62.3909158405868,40.0132649215857));
#188750=CARTESIAN_POINT('Ctrl Pts',(6.7292316549945,-62.3808452043598,40.0044075527531));
#188751=CARTESIAN_POINT('Ctrl Pts',(6.73244426756144,-62.3706061896782,
39.9953016253718));
#188752=CARTESIAN_POINT('Ctrl Pts',(6.73481930344724,-62.3602869763768,
39.9860353422356));
#188753=CARTESIAN_POINT('Ctrl Pts',(6.7373773188584,-62.3491727415083,39.9760551582693));
#188754=CARTESIAN_POINT('Ctrl Pts',(6.73896413451842,-62.3379643502084,
39.9658879738155));
#188755=CARTESIAN_POINT('Ctrl Pts',(6.7396251149954,-62.326748923113,39.9556174643255));
#188756=CARTESIAN_POINT('Ctrl Pts',(6.74027717000425,-62.3156849421506,
39.9454856413905));
#188757=CARTESIAN_POINT('Ctrl Pts',(6.74002799825967,-62.3046126966258,
39.9352519465113));
#188758=CARTESIAN_POINT('Ctrl Pts',(6.73887200051313,-62.2936141127569,
39.92499));
#188759=CARTESIAN_POINT('Ctrl Pts',(6.37927424642559,-58.8722700234481,
39.92499));
#188760=CARTESIAN_POINT('Ctrl Pts',(6.37816795023629,-58.8617443183088,
39.9348107241731));
#188761=CARTESIAN_POINT('Ctrl Pts',(6.37623543038822,-58.8513437177768,
39.9446038383187));
#188762=CARTESIAN_POINT('Ctrl Pts',(6.37349561323655,-58.8411231047648,
39.9543158069411));
#188763=CARTESIAN_POINT('Ctrl Pts',(6.37085007871699,-58.8312542036531,
39.9636935671423));
#188764=CARTESIAN_POINT('Ctrl Pts',(6.36745144953993,-58.8215519162572,
39.9729968321024));
#188765=CARTESIAN_POINT('Ctrl Pts',(6.36327195218524,-58.8120753594613,
39.9821731151375));
#188766=CARTESIAN_POINT('Ctrl Pts',(6.35932101824761,-58.8031170454156,
39.9908475764394));
#188767=CARTESIAN_POINT('Ctrl Pts',(6.354671922117,-58.7943596215135,39.9994093733891));
#188768=CARTESIAN_POINT('Ctrl Pts',(6.34926600747357,-58.7858758685273,
40.0077966115888));
#188769=CARTESIAN_POINT('Ctrl Pts',(6.34428725077805,-58.7780624743528,
40.0155211172641));
#188770=CARTESIAN_POINT('Ctrl Pts',(6.33866621241084,-58.7704807832414,
40.0230979941068));
#188771=CARTESIAN_POINT('Ctrl Pts',(6.33233133084537,-58.7632157808971,
40.0304554104795));
#188772=CARTESIAN_POINT('Ctrl Pts',(6.33044239704174,-58.7610495038531,
40.0326492435212));
#188773=CARTESIAN_POINT('Ctrl Pts',(6.3284898262139,-58.7589116098624,40.0348233715076));
#188774=CARTESIAN_POINT('Ctrl Pts',(6.32647128889818,-58.7568049797264,
40.0369753512356));
#188775=CARTESIAN_POINT('Ctrl Pts',(6.32447337605832,-58.7547198741578,
40.0391053430352));
#188776=CARTESIAN_POINT('Ctrl Pts',(6.32241310885704,-58.7526673708734,
40.041211089324));
#188777=CARTESIAN_POINT('Ctrl Pts',(6.32029074540098,-58.7506524329181,
40.0432881154904));
#188778=CARTESIAN_POINT('Ctrl Pts',(6.32014316039693,-58.7505123180733,
40.043432547828));
#188779=CARTESIAN_POINT('Ctrl Pts',(6.31999527850335,-58.7503723733987,
40.0435768364421));
#188780=CARTESIAN_POINT('Ctrl Pts',(6.31984709900205,-58.7502325999832,
40.0437209807855));
#188781=CARTESIAN_POINT('Ctrl Pts',(6.31335036684093,-58.7441044214168,
40.050040796842));
#188782=CARTESIAN_POINT('Ctrl Pts',(6.30625925377334,-58.7383447881642,
40.0560490279344));
#188783=CARTESIAN_POINT('Ctrl Pts',(6.29859016886937,-58.7330687140843,
40.0616647108614));
#188784=CARTESIAN_POINT('Ctrl Pts',(6.29144124886088,-58.7281504960662,
40.0668995033485));
#188785=CARTESIAN_POINT('Ctrl Pts',(6.28378931333054,-58.7236522470777,
40.0717933267481));
#188786=CARTESIAN_POINT('Ctrl Pts',(6.27564783709185,-58.719696482323,40.0762460303072));
#188787=CARTESIAN_POINT('Ctrl Pts',(6.27266957975555,-58.718249412399,40.0778748868748));
#188788=CARTESIAN_POINT('Ctrl Pts',(6.26962586933712,-58.7168752520897,
40.0794443522247));
#188789=CARTESIAN_POINT('Ctrl Pts',(6.26651766855732,-58.7155811795664,
40.0809482021492));
#188790=CARTESIAN_POINT('Ctrl Pts',(6.26577025010559,-58.7152699983557,
40.0813098278168));
#188791=CARTESIAN_POINT('Ctrl Pts',(6.26501853257419,-58.7149635750523,
40.0816679525672));
#188792=CARTESIAN_POINT('Ctrl Pts',(6.26426260461821,-58.7146620123681,
40.082022419258));
#188793=CARTESIAN_POINT('Ctrl Pts',(6.26353029941086,-58.7143698735178,
40.0823658088648));
#188794=CARTESIAN_POINT('Ctrl Pts',(6.26279404284355,-58.7140822962414,
40.0827057654616));
#188795=CARTESIAN_POINT('Ctrl Pts',(6.26205391928439,-58.7137993735012,
40.0830421470151));
#188796=CARTESIAN_POINT('Ctrl Pts',(6.25394501035227,-58.7106996279152,
40.0867275956806));
#188797=CARTESIAN_POINT('Ctrl Pts',(6.24536644325941,-58.7081569420199,
40.0899823432031));
#188798=CARTESIAN_POINT('Ctrl Pts',(6.23645973859677,-58.7062958387084,
40.0926299529356));
#188799=CARTESIAN_POINT('Ctrl Pts',(6.23276586269276,-58.7055239836916,
40.0937279956084));
#188800=CARTESIAN_POINT('Ctrl Pts',(6.22901585349531,-58.7048690642115,
40.0947220371802));
#188801=CARTESIAN_POINT('Ctrl Pts',(6.22522076267779,-58.7043384037134,
40.0956014538692));
#188802=CARTESIAN_POINT('Ctrl Pts',(6.21874783981215,-58.7034333069351,
40.097101390674));
#188803=CARTESIAN_POINT('Ctrl Pts',(6.21214524099542,-58.7028917011005,
40.0982667904316));
#188804=CARTESIAN_POINT('Ctrl Pts',(6.20547453342054,-58.7027523988018,
40.0990539325582));
#188805=CARTESIAN_POINT('Ctrl Pts',(6.2021391796331,-58.7026827476525,40.0994475036216));
#188806=CARTESIAN_POINT('Ctrl Pts',(6.19878688248348,-58.7027151167906,
40.0997467259952));
#188807=CARTESIAN_POINT('Ctrl Pts',(6.19542538555006,-58.7028544030467,
40.0999473488896));
#188808=CARTESIAN_POINT('Ctrl Pts',(6.19206388861663,-58.7029936893028,
40.100147971784));
#188809=CARTESIAN_POINT('Ctrl Pts',(6.18869323212197,-58.7032398710655,
40.10025));
#188810=CARTESIAN_POINT('Ctrl Pts',(6.1853204982938,-58.7035958781039,40.10025));
#188811=CARTESIAN_POINT('Origin',(-0.0152400000001978,-58.2637721346185,
39.92499));
#188812=CARTESIAN_POINT('Ctrl Pts',(-0.190500000000213,-62.6567671111299,
39.92499));
#188813=CARTESIAN_POINT('Ctrl Pts',(-0.190500000000213,-62.6673774406538,
39.9348354642013));
#188814=CARTESIAN_POINT('Ctrl Pts',(-0.189662809673347,-62.6779562874462,
39.9446440828448));
#188815=CARTESIAN_POINT('Ctrl Pts',(-0.188003604115532,-62.6884465439468,
39.9543641760318));
#188816=CARTESIAN_POINT('Ctrl Pts',(-0.186398312858405,-62.6985959295766,
39.9637684240697));
#188817=CARTESIAN_POINT('Ctrl Pts',(-0.18402329031191,-62.7086636500137,
39.9730909636378));
#188818=CARTESIAN_POINT('Ctrl Pts',(-0.18084626121144,-62.7185939622152,
39.9822808977121));
#188819=CARTESIAN_POINT('Ctrl Pts',(-0.177840987312561,-62.7279874260843,
39.9909740094629));
#188820=CARTESIAN_POINT('Ctrl Pts',(-0.174117798732319,-62.7372588214061,
39.9995492764979));
#188821=CARTESIAN_POINT('Ctrl Pts',(-0.169611579427885,-62.7463424082288,
40.0079462328672));
#188822=CARTESIAN_POINT('Ctrl Pts',(-0.165461025550434,-62.7547090486342,
40.0156804369666));
#188823=CARTESIAN_POINT('Ctrl Pts',(-0.160645870590088,-62.7629168328826,
40.0232638017397));
#188824=CARTESIAN_POINT('Ctrl Pts',(-0.155086395964948,-62.7708892610779,
40.0306257269941));
#188825=CARTESIAN_POINT('Ctrl Pts',(-0.153473803707011,-62.7732017594436,
40.0327611416635));
#188826=CARTESIAN_POINT('Ctrl Pts',(-0.15179840377153,-62.7754942590266,
40.0348777427262));
#188827=CARTESIAN_POINT('Ctrl Pts',(-0.150057792857863,-62.7777643638146,
40.0369733168701));
#188828=CARTESIAN_POINT('Ctrl Pts',(-0.148170858717248,-62.7802253033581,
40.039245053974));
#188829=CARTESIAN_POINT('Ctrl Pts',(-0.146210769553979,-62.7826571567199,
40.041487875195));
#188830=CARTESIAN_POINT('Ctrl Pts',(-0.144175421826364,-62.7850565204095,
40.0436985701601));
#188831=CARTESIAN_POINT('Ctrl Pts',(-0.138589394016836,-62.791641592883,
40.0497658398386));
#188832=CARTESIAN_POINT('Ctrl Pts',(-0.13241078666925,-62.7979456687653,
40.0555581699984));
#188833=CARTESIAN_POINT('Ctrl Pts',(-0.125664597436941,-62.8038680995981,
40.0609828468886));
#188834=CARTESIAN_POINT('Ctrl Pts',(-0.119492200548591,-62.8092868022738,
40.0659461317304));
#188835=CARTESIAN_POINT('Ctrl Pts',(-0.11284434746055,-62.8143744518938,
40.0706039980706));
#188836=CARTESIAN_POINT('Ctrl Pts',(-0.105708043833672,-62.8190433630433,
40.0748843180602));
#188837=CARTESIAN_POINT('Ctrl Pts',(-0.102202714803807,-62.8213367169483,
40.0769867972569));
#188838=CARTESIAN_POINT('Ctrl Pts',(-0.0985794274535627,-62.8235285419788,
40.0789976708174));
#188839=CARTESIAN_POINT('Ctrl Pts',(-0.0948363533474329,-62.8256051102648,
40.08090504915));
#188840=CARTESIAN_POINT('Ctrl Pts',(-0.0941261414938337,-62.825999118871,
40.0812669556105));
#188841=CARTESIAN_POINT('Ctrl Pts',(-0.0934111032314831,-62.8263888407139,
40.0816253922032));
#188842=CARTESIAN_POINT('Ctrl Pts',(-0.0926913160162872,-62.826774159152,
40.0819801989139));
#188843=CARTESIAN_POINT('Ctrl Pts',(-0.0919940221515661,-62.8271474363889,
40.0823239179149));
#188844=CARTESIAN_POINT('Ctrl Pts',(-0.0912922715312453,-62.8275165811343,
40.0826642303498));
#188845=CARTESIAN_POINT('Ctrl Pts',(-0.0905861384171559,-62.8278814873655,
40.0830009916099));
#188846=CARTESIAN_POINT('Ctrl Pts',(-0.0828908452419125,-62.8318581602825,
40.0866709464313));
#188847=CARTESIAN_POINT('Ctrl Pts',(-0.0746698316629355,-62.8353337180914,
40.0899175831879));
#188848=CARTESIAN_POINT('Ctrl Pts',(-0.0660491922293915,-62.8381654210188,
40.0925642067063));
#188849=CARTESIAN_POINT('Ctrl Pts',(-0.0624086426652736,-62.839361266749,
40.0936818922528));
#188850=CARTESIAN_POINT('Ctrl Pts',(-0.0586971697057687,-62.8404425512865,
40.0946930094791));
#188851=CARTESIAN_POINT('Ctrl Pts',(-0.0549254519866895,-62.8414000604479,
40.0955863397546));
#188852=CARTESIAN_POINT('Ctrl Pts',(-0.0485739735924287,-62.8430124819501,
40.0970906856166));
#188853=CARTESIAN_POINT('Ctrl Pts',(-0.0420529246954846,-62.8442717146911,
40.0982599215483));
#188854=CARTESIAN_POINT('Ctrl Pts',(-0.0354197192409226,-62.8451307298764,
40.0990497370454));
#188855=CARTESIAN_POINT('Ctrl Pts',(-0.033761417877282,-62.8453454836727,
40.0992471909196));
#188856=CARTESIAN_POINT('Ctrl Pts',(-0.0320960919388051,-62.8455349903695,
40.0994209989363));
#188857=CARTESIAN_POINT('Ctrl Pts',(-0.0304246312368034,-62.8456982067485,
40.0995705982975));
#188858=CARTESIAN_POINT('Ctrl Pts',(-0.027917440183801,-62.845943031317,
40.0997949973393));
#188859=CARTESIAN_POINT('Ctrl Pts',(-0.0253964615341821,-62.8461286892223,
40.0999649129781));
#188860=CARTESIAN_POINT('Ctrl Pts',(-0.0228647168033253,-62.846253337618,
40.1000786629733));
#188861=CARTESIAN_POINT('Ctrl Pts',(-0.0203329720724685,-62.8463779860137,
40.1001924129685));
#188862=CARTESIAN_POINT('Ctrl Pts',(-0.0177904683743677,-62.8464416340693,
40.10025));
#188863=CARTESIAN_POINT('Ctrl Pts',(-0.0152400000002138,-62.8464427007196,
40.10025));
#188864=CARTESIAN_POINT('Ctrl Pts',(-0.0152400000002007,-59.0285534841296,
40.10025));
#188865=CARTESIAN_POINT('Ctrl Pts',(-0.0238699985093192,-59.0285496414744,
40.10025));
#188866=CARTESIAN_POINT('Ctrl Pts',(-0.0324255116353325,-59.0292582026621,
40.0995786334241));
#188867=CARTESIAN_POINT('Ctrl Pts',(-0.0407807192224094,-59.0305954788489,
40.0983063763367));
#188868=CARTESIAN_POINT('Ctrl Pts',(-0.046177326030172,-59.0314592220531,
40.0974846287994));
#188869=CARTESIAN_POINT('Ctrl Pts',(-0.0514905268410185,-59.0325843328198,
40.0964130309339));
#188870=CARTESIAN_POINT('Ctrl Pts',(-0.0566895722964741,-59.0339399880044,
40.0951176960924));
#188871=CARTESIAN_POINT('Ctrl Pts',(-0.063580609227685,-59.0357368312948,
40.0934008039614));
#188872=CARTESIAN_POINT('Ctrl Pts',(-0.0702685278903685,-59.0379438906768,
40.0912909372157));
#188873=CARTESIAN_POINT('Ctrl Pts',(-0.0766865040606948,-59.0405007795597,
40.0888630467852));
#188874=CARTESIAN_POINT('Ctrl Pts',(-0.079895492145858,-59.0417792240012,
40.0876491015699));
#188875=CARTESIAN_POINT('Ctrl Pts',(-0.0830371938951596,-59.0431451240706,
40.0863558569272));
#188876=CARTESIAN_POINT('Ctrl Pts',(-0.086104670364025,-59.0445909239228,
40.0849936342771));
#188877=CARTESIAN_POINT('Ctrl Pts',(-0.0876384085984576,-59.0453138238489,
40.0843125229521));
#188878=CARTESIAN_POINT('Ctrl Pts',(-0.0891536069438513,-59.0460566986719,
40.0836141747075));
#188879=CARTESIAN_POINT('Ctrl Pts',(-0.0906495011922853,-59.0468186034776,
40.082899916161));
#188880=CARTESIAN_POINT('Ctrl Pts',(-0.0910234747543938,-59.047009079679,
40.0827213515244));
#188881=CARTESIAN_POINT('Ctrl Pts',(-0.0913962421599235,-59.0472007452523,
40.0825417925842));
#188882=CARTESIAN_POINT('Ctrl Pts',(-0.0917677921729251,-59.0473935854286,
40.0823612602361));
#188883=CARTESIAN_POINT('Ctrl Pts',(-0.09288244221193,-59.0479721059574,
40.0818196631918));
#188884=CARTESIAN_POINT('Ctrl Pts',(-0.0939861339740177,-59.0485611979309,
40.0812693052022));
#188885=CARTESIAN_POINT('Ctrl Pts',(-0.0950785796751375,-59.0491604624443,
40.0807107531875));
#188886=CARTESIAN_POINT('Ctrl Pts',(-0.102773626133571,-59.0533816042977,
40.0767763849181));
#188887=CARTESIAN_POINT('Ctrl Pts',(-0.109958823466872,-59.0580834293368,
40.0724140586136));
#188888=CARTESIAN_POINT('Ctrl Pts',(-0.116642428647321,-59.0631465696374,
40.0677221223766));
#188889=CARTESIAN_POINT('Ctrl Pts',(-0.119883969937292,-59.0656021872118,
40.0654465383719));
#188890=CARTESIAN_POINT('Ctrl Pts',(-0.123007567718441,-59.068143371512,
40.0630928000678));
#188891=CARTESIAN_POINT('Ctrl Pts',(-0.126014035556628,-59.0707593633743,
40.0606689262479));
#188892=CARTESIAN_POINT('Ctrl Pts',(-0.130616727761249,-59.0747642641417,
40.0569581447806));
#188893=CARTESIAN_POINT('Ctrl Pts',(-0.13494307027746,-59.0789414743144,
40.0530843804606));
#188894=CARTESIAN_POINT('Ctrl Pts',(-0.138985142830921,-59.0832455674828,
40.0490800251458));
#188895=CARTESIAN_POINT('Ctrl Pts',(-0.140862302235661,-59.0852444106167,
40.0472203818218));
#188896=CARTESIAN_POINT('Ctrl Pts',(-0.142678271527312,-59.0872703932642,
40.0453323608818));
#188897=CARTESIAN_POINT('Ctrl Pts',(-0.144431197308936,-59.0893195943183,
40.0434201572162));
#188898=CARTESIAN_POINT('Ctrl Pts',(-0.144565552163221,-59.0894766575049,
40.0432735943397));
#188899=CARTESIAN_POINT('Ctrl Pts',(-0.144699568925986,-59.0896338466134,
40.0431268995707));
#188900=CARTESIAN_POINT('Ctrl Pts',(-0.144833247843275,-59.0897911602042,
40.0429800745037));
#188901=CARTESIAN_POINT('Ctrl Pts',(-0.146711033602282,-59.0920009418701,
40.0409176249753));
#188902=CARTESIAN_POINT('Ctrl Pts',(-0.148520654545084,-59.0942367399983,
40.0388310783332));
#188903=CARTESIAN_POINT('Ctrl Pts',(-0.150262619641468,-59.0964928714566,
40.036725739981));
#188904=CARTESIAN_POINT('Ctrl Pts',(-0.15650899667944,-59.1045829576269,
40.0291763710713));
#188905=CARTESIAN_POINT('Ctrl Pts',(-0.161935290146647,-59.1129958342961,
40.0213310894585));
#188906=CARTESIAN_POINT('Ctrl Pts',(-0.166622470788754,-59.1216309196503,
40.0132837551304));
#188907=CARTESIAN_POINT('Ctrl Pts',(-0.171773211445404,-59.1311200109833,
40.0044405431303));
#188908=CARTESIAN_POINT('Ctrl Pts',(-0.176031864364012,-59.1408779306769,
39.9953528710572));
#188909=CARTESIAN_POINT('Ctrl Pts',(-0.179468536018904,-59.1508087658139,
39.9861103629519));
#188910=CARTESIAN_POINT('Ctrl Pts',(-0.18317927891942,-59.1615315754626,
39.976130773751));
#188911=CARTESIAN_POINT('Ctrl Pts',(-0.185932239426363,-59.1724570142908,
39.9659696935954));
#188912=CARTESIAN_POINT('Ctrl Pts',(-0.187766286101261,-59.1834936683209,
39.9557128217438));
#188913=CARTESIAN_POINT('Ctrl Pts',(-0.189584947008437,-59.1944377361602,
39.9455419945115));
#188914=CARTESIAN_POINT('Ctrl Pts',(-0.190500000000201,-59.205492595814,
39.9352756289317));
#188915=CARTESIAN_POINT('Ctrl Pts',(-0.190500000000201,-59.2165773020941,
39.92499));
#188916=CARTESIAN_POINT('Origin',(0.0152400000000056,5.56890342380664E-15,
39.92499));
#188917=CARTESIAN_POINT('Ctrl Pts',(0.0152399999997863,-62.8464427007196,
40.10025));
#188918=CARTESIAN_POINT('Ctrl Pts',(0.0238289333903676,-62.8464391086779,
40.10025));
#188919=CARTESIAN_POINT('Ctrl Pts',(0.0323412407625178,-62.8457180711405,
40.0995859581842));
#188920=CARTESIAN_POINT('Ctrl Pts',(0.0406531130503384,-62.844365806829,
40.0983275959621));
#188921=CARTESIAN_POINT('Ctrl Pts',(0.0459640037534202,-62.8435017743089,
40.0975235624068));
#188922=CARTESIAN_POINT('Ctrl Pts',(0.0511932363889303,-62.8423809556998,
40.096477705949));
#188923=CARTESIAN_POINT('Ctrl Pts',(0.0563116129572096,-62.841033859251,
40.0952149915961));
#188924=CARTESIAN_POINT('Ctrl Pts',(0.0632971699619951,-62.8391953428955,
40.0934916398701));
#188925=CARTESIAN_POINT('Ctrl Pts',(0.0700734120981451,-62.8369299537504,
40.091364392163));
#188926=CARTESIAN_POINT('Ctrl Pts',(0.0765705776092501,-62.8343031482014,
40.0889118607713));
#188927=CARTESIAN_POINT('Ctrl Pts',(0.0798191603648026,-62.8329897454269,
40.0876855950754));
#188928=CARTESIAN_POINT('Ctrl Pts',(0.0829981827950912,-62.8315859904681,
40.0863782327526));
#188929=CARTESIAN_POINT('Ctrl Pts',(0.0861004173276405,-62.8301000734874,
40.0850006373334));
#188930=CARTESIAN_POINT('Ctrl Pts',(0.0876515345939151,-62.8293571149971,
40.0843118396237));
#188931=CARTESIAN_POINT('Ctrl Pts',(0.0891834722994834,-62.8285936160519,
40.0836054919164));
#188932=CARTESIAN_POINT('Ctrl Pts',(0.0906954364276482,-62.82781060087,
40.0828829920418));
#188933=CARTESIAN_POINT('Ctrl Pts',(0.0910734274596893,-62.8276148470746,
40.0827023670731));
#188934=CARTESIAN_POINT('Ctrl Pts',(0.091450170514115,-62.8274178735164,
40.0825207326933));
#188935=CARTESIAN_POINT('Ctrl Pts',(0.091825653932623,-62.8272196962038,
40.0823381109275));
#188936=CARTESIAN_POINT('Ctrl Pts',(0.092952104188147,-62.8266251642659,
40.0817902456303));
#188937=CARTESIAN_POINT('Ctrl Pts',(0.0940672158684322,-62.826019798519,
40.0812334935553));
#188938=CARTESIAN_POINT('Ctrl Pts',(0.0951706907486232,-62.8254040313373,
40.0806684524227));
#188939=CARTESIAN_POINT('Ctrl Pts',(0.102796386827374,-62.8211486980556,
40.0767636676137));
#188940=CARTESIAN_POINT('Ctrl Pts',(0.109916699411343,-62.8164204928784,
40.0724404510888));
#188941=CARTESIAN_POINT('Ctrl Pts',(0.116542502759708,-62.8113377077395,
40.0677949937409));
#188942=CARTESIAN_POINT('Ctrl Pts',(0.119835508836344,-62.8088115774775,
40.0654862141906));
#188943=CARTESIAN_POINT('Ctrl Pts',(0.123006400629162,-62.8061972539432,
40.0630972003216));
#188944=CARTESIAN_POINT('Ctrl Pts',(0.126056303769755,-62.8035061084565,
40.0606363359906));
#188945=CARTESIAN_POINT('Ctrl Pts',(0.13278484564307,-62.7975690395532,
40.0552073017123));
#188946=CARTESIAN_POINT('Ctrl Pts',(0.138932019324476,-62.7912680187378,
40.0494204304519));
#188947=CARTESIAN_POINT('Ctrl Pts',(0.144445113412955,-62.7847385034067,
40.0434049749851));
#188948=CARTESIAN_POINT('Ctrl Pts',(0.146459116207252,-62.7823531891148,
40.0412074532442));
#188949=CARTESIAN_POINT('Ctrl Pts',(0.148396130390766,-62.7799396422114,
40.0389814735788));
#188950=CARTESIAN_POINT('Ctrl Pts',(0.150257579786274,-62.7775029828616,
40.0367321210016));
#188951=CARTESIAN_POINT('Ctrl Pts',(0.156509991333158,-62.7693185019449,
40.0291767837143));
#188952=CARTESIAN_POINT('Ctrl Pts',(0.161942805717456,-62.7608162581028,
40.0213235332582));
#188953=CARTESIAN_POINT('Ctrl Pts',(0.166635979460758,-62.7520965944505,
40.0132649215867));
#188954=CARTESIAN_POINT('Ctrl Pts',(0.171794333347662,-62.7425126511844,
40.0044075527545));
#188955=CARTESIAN_POINT('Ctrl Pts',(0.176059615356826,-62.7326655363514,
39.9953016253735));
#188956=CARTESIAN_POINT('Ctrl Pts',(0.179500292056051,-62.7226511116317,
39.9860353422376));
#188957=CARTESIAN_POINT('Ctrl Pts',(0.183206048282415,-62.7118651471246,
39.9760551582716));
#188958=CARTESIAN_POINT('Ctrl Pts',(0.185955767118563,-62.7008840239675,
39.9658879738179));
#188959=CARTESIAN_POINT('Ctrl Pts',(0.1877854580346,-62.6897991274289,39.955617464328));
#188960=CARTESIAN_POINT('Ctrl Pts',(0.18959044194574,-62.6788639144192,
39.9454856413922));
#188961=CARTESIAN_POINT('Ctrl Pts',(0.190499999999787,-62.6678262782739,
39.9352519465123));
#188962=CARTESIAN_POINT('Ctrl Pts',(0.190499999999787,-62.6567671111299,
39.92499));
#188963=CARTESIAN_POINT('Ctrl Pts',(0.190499999999799,-59.2165773020941,
39.92499));
#188964=CARTESIAN_POINT('Ctrl Pts',(0.190499999999799,-59.2059936184294,
39.9348107241721));
#188965=CARTESIAN_POINT('Ctrl Pts',(0.189665225488479,-59.1954479901466,
39.9446038383166));
#188966=CARTESIAN_POINT('Ctrl Pts',(0.18800876231396,-59.1849969778467,
39.954315806938));
#188967=CARTESIAN_POINT('Ctrl Pts',(0.186409301376905,-59.1749056059505,
39.9636935671386));
#188968=CARTESIAN_POINT('Ctrl Pts',(0.184043455438109,-59.1649012152157,
39.9729968320982));
#188969=CARTESIAN_POINT('Ctrl Pts',(0.180877423726644,-59.1550396955543,
39.9821731151328));
#188970=CARTESIAN_POINT('Ctrl Pts',(0.177884532219545,-59.1457174710375,
39.9908475764344));
#188971=CARTESIAN_POINT('Ctrl Pts',(0.174176304387074,-59.136522058346,
39.9994093733838));
#188972=CARTESIAN_POINT('Ctrl Pts',(0.169686797572568,-59.1275197082963,
40.0077966115833));
#188973=CARTESIAN_POINT('Ctrl Pts',(0.16555203711349,-59.1192286949263,
40.0155211172587));
#188974=CARTESIAN_POINT('Ctrl Pts',(0.160754293903832,-59.1111009786095,
40.0230979941014));
#188975=CARTESIAN_POINT('Ctrl Pts',(0.155213515013513,-59.1032135992732,
40.0304554104741));
#188976=CARTESIAN_POINT('Ctrl Pts',(0.153561366596104,-59.1008617419719,
40.0326492435176));
#188977=CARTESIAN_POINT('Ctrl Pts',(0.151842962927694,-59.0985314603582,
40.0348233715058));
#188978=CARTESIAN_POINT('Ctrl Pts',(0.150055686179939,-59.096225375957,
40.0369753512356));
#188979=CARTESIAN_POINT('Ctrl Pts',(0.148286670996504,-59.0939428540559,
40.0391053430352));
#188980=CARTESIAN_POINT('Ctrl Pts',(0.146452235168709,-59.0916862380348,
40.041211089324));
#188981=CARTESIAN_POINT('Ctrl Pts',(0.144552116609772,-59.0894604907299,
40.0432881154904));
#188982=CARTESIAN_POINT('Ctrl Pts',(0.144419986081224,-59.0893057166152,
40.043432547828));
#188983=CARTESIAN_POINT('Ctrl Pts',(0.144287542501902,-59.0891510807051,
40.0435768364421));
#188984=CARTESIAN_POINT('Ctrl Pts',(0.144154785043746,-59.0889965840074,
40.0437209807855));
#188985=CARTESIAN_POINT('Ctrl Pts',(0.138334211749301,-59.0822228828153,
40.050040796842));
#188986=CARTESIAN_POINT('Ctrl Pts',(0.131883990153885,-59.0757535782845,
40.0560490279345));
#188987=CARTESIAN_POINT('Ctrl Pts',(0.124808417215064,-59.0697047694307,
40.0616647108615));
#188988=CARTESIAN_POINT('Ctrl Pts',(0.118212753509824,-59.0640662283031,
40.0668995033486));
#188989=CARTESIAN_POINT('Ctrl Pts',(0.111072931137127,-59.0587927761312,
40.0717933267482));
#188990=CARTESIAN_POINT('Ctrl Pts',(0.103389544768,-59.0540076654697,40.0762460303072));
#188991=CARTESIAN_POINT('Ctrl Pts',(0.100578862632434,-59.0522572100837,
40.0778748868748));
#188992=CARTESIAN_POINT('Ctrl Pts',(0.0976954648435965,-59.0505724231957,
40.0794443522248));
#188993=CARTESIAN_POINT('Ctrl Pts',(0.094739558525147,-59.048960544286,
40.0809482021492));
#188994=CARTESIAN_POINT('Ctrl Pts',(0.0940287618036509,-59.0485729412563,
40.0813098278168));
#188995=CARTESIAN_POINT('Ctrl Pts',(0.0933131922165579,-59.0481896206935,
40.0816679525672));
#188996=CARTESIAN_POINT('Ctrl Pts',(0.0925929271969717,-59.0478106940136,
40.082022419258));
#188997=CARTESIAN_POINT('Ctrl Pts',(0.0918951704592475,-59.0474436087926,
40.0823658088648));
#188998=CARTESIAN_POINT('Ctrl Pts',(0.091193007193228,-59.0470806471271,
40.0827057654616));
#188999=CARTESIAN_POINT('Ctrl Pts',(0.0904865115876297,-59.0467219102889,
40.0830421470151));
#189000=CARTESIAN_POINT('Ctrl Pts',(0.0827460357497242,-59.0427915336441,
40.0867275956806));
#189001=CARTESIAN_POINT('Ctrl Pts',(0.0744802459942153,-59.039366072413,
40.0899823432031));
#189002=CARTESIAN_POINT('Ctrl Pts',(0.0658168714608038,-59.036584160269,
40.0926299529356));
#189003=CARTESIAN_POINT('Ctrl Pts',(0.0622239118142435,-59.035430418383,
40.0937279956084));
#189004=CARTESIAN_POINT('Ctrl Pts',(0.0585629032863412,-59.0343871039217,
40.0947220371802));
#189005=CARTESIAN_POINT('Ctrl Pts',(0.0548440714997746,-59.0334626554262,
40.0956014538692));
#189006=CARTESIAN_POINT('Ctrl Pts',(0.0485012163582068,-59.0318859121827,
40.097101390674));
#189007=CARTESIAN_POINT('Ctrl Pts',(0.0419914004942192,-59.0306571138137,
40.0982667904316));
#189008=CARTESIAN_POINT('Ctrl Pts',(0.0353717968086245,-59.0298212958157,
40.0990539325582));
#189009=CARTESIAN_POINT('Ctrl Pts',(0.0320619949658271,-59.0294033868167,
40.0994475036216));
#189010=CARTESIAN_POINT('Ctrl Pts',(0.0287246785544799,-59.0290851681639,
40.0997467259952));
#189011=CARTESIAN_POINT('Ctrl Pts',(0.0253670368746702,-59.0288723192866,
40.0999473488896));
#189012=CARTESIAN_POINT('Ctrl Pts',(0.0220093951948606,-59.0286594704093,
40.100147971784));
#189013=CARTESIAN_POINT('Ctrl Pts',(0.0186314705078069,-59.0285519740191,
40.10025));
#189014=CARTESIAN_POINT('Ctrl Pts',(0.0152399999997995,-59.0285534841296,
40.10025));
#189015=CARTESIAN_POINT('Origin',(-6.10537907909402,-57.9430040808458,39.92499));
#189016=CARTESIAN_POINT('Ctrl Pts',(-6.73887200051354,-62.2936141127569,
39.92499));
#189017=CARTESIAN_POINT('Ctrl Pts',(-6.73998108195343,-62.3041663177855,
39.9348354642016));
#189018=CARTESIAN_POINT('Ctrl Pts',(-6.74025426844112,-62.3147747227668,
39.9446440828455));
#189019=CARTESIAN_POINT('Ctrl Pts',(-6.7397006825762,-62.3253809467521,
39.9543641760327));
#189020=CARTESIAN_POINT('Ctrl Pts',(-6.7391650849555,-62.3356425316138,
39.9637684240707));
#189021=CARTESIAN_POINT('Ctrl Pts',(-6.73785543637686,-62.3459033574821,
39.973090963639));
#189022=CARTESIAN_POINT('Ctrl Pts',(-6.73573381164832,-62.3561113603641,
39.9822808977133));
#189023=CARTESIAN_POINT('Ctrl Pts',(-6.73372688529723,-62.3657675025179,
39.9909740094642));
#189024=CARTESIAN_POINT('Ctrl Pts',(-6.73099321743882,-62.375377287347,
39.9995492764993));
#189025=CARTESIAN_POINT('Ctrl Pts',(-6.72746117704663,-62.3848821415098,
40.0079462328686));
#189026=CARTESIAN_POINT('Ctrl Pts',(-6.72420791240176,-62.3936367996024,
40.0156804369681));
#189027=CARTESIAN_POINT('Ctrl Pts',(-6.72027708243827,-62.4023029414984,
40.0232638017413));
#189028=CARTESIAN_POINT('Ctrl Pts',(-6.7155814088644,-62.4108128192372,
40.0306257269957));
#189029=CARTESIAN_POINT('Ctrl Pts',(-6.71421937245637,-62.4132812112848,
40.0327611416645));
#189030=CARTESIAN_POINT('Ctrl Pts',(-6.71279278199583,-62.4157362792952,
40.0348777427268));
#189031=CARTESIAN_POINT('Ctrl Pts',(-6.7112989968962,-62.418175891595,40.03697331687));
#189032=CARTESIAN_POINT('Ctrl Pts',(-6.70967963780691,-62.4208205881801,
40.039245053974));
#189033=CARTESIAN_POINT('Ctrl Pts',(-6.70798448411196,-62.4234440047029,
40.041487875195));
#189034=CARTESIAN_POINT('Ctrl Pts',(-6.70621108803145,-62.4260429761973,
40.0436985701601));
#189035=CARTESIAN_POINT('Ctrl Pts',(-6.7013439885729,-62.4331758738575,
40.0497658398386));
#189036=CARTESIAN_POINT('Ctrl Pts',(-6.69585818364715,-62.4400912556837,
40.0555581699984));
#189037=CARTESIAN_POINT('Ctrl Pts',(-6.68976801333909,-62.4466864116141,
40.0609828468885));
#189038=CARTESIAN_POINT('Ctrl Pts',(-6.68419583815052,-62.4527206212308,
40.0659461317302));
#189039=CARTESIAN_POINT('Ctrl Pts',(-6.67811620689394,-62.458475290041,
40.0706039980702));
#189040=CARTESIAN_POINT('Ctrl Pts',(-6.67150703079287,-62.463864571258,
40.0748843180598));
#189041=CARTESIAN_POINT('Ctrl Pts',(-6.6682606250814,-62.4665117685873,
40.0769867972566));
#189042=CARTESIAN_POINT('Ctrl Pts',(-6.66488629458032,-62.4690703232298,
40.0789976708173));
#189043=CARTESIAN_POINT('Ctrl Pts',(-6.66138078591733,-62.4715267736418,
40.08090504915));
#189044=CARTESIAN_POINT('Ctrl Pts',(-6.6607156497927,-62.4719928611813,
40.0812669556105));
#189045=CARTESIAN_POINT('Ctrl Pts',(-6.66004526561012,-62.472455189938,
40.0816253922033));
#189046=CARTESIAN_POINT('Ctrl Pts',(-6.65936969820881,-62.4729136358129,
40.0819801989139));
#189047=CARTESIAN_POINT('Ctrl Pts',(-6.65871524228878,-62.4733577552541,
40.0823239179149));
#189048=CARTESIAN_POINT('Ctrl Pts',(-6.65805592206474,-62.4737982306999,
40.0826642303498));
#189049=CARTESIAN_POINT('Ctrl Pts',(-6.65739180030931,-62.4742349489459,
40.0830009916099));
#189050=CARTESIAN_POINT('Ctrl Pts',(-6.65015433826397,-62.4789942144027,
40.0866709464314));
#189051=CARTESIAN_POINT('Ctrl Pts',(-6.64234165497406,-62.4833100626583,
40.0899175831881));
#189052=CARTESIAN_POINT('Ctrl Pts',(-6.63406423386048,-62.4870273554132,
40.0925642067066));
#189053=CARTESIAN_POINT('Ctrl Pts',(-6.63056862752451,-62.4885971912266,
40.093681892253));
#189054=CARTESIAN_POINT('Ctrl Pts',(-6.62699051141353,-62.4900605069391,
40.0946930094792));
#189055=CARTESIAN_POINT('Ctrl Pts',(-6.62333954252022,-62.491407022622,
40.0955863397546));
#189056=CARTESIAN_POINT('Ctrl Pts',(-6.61719140213093,-62.4936745213866,
40.0970906856166));
#189057=CARTESIAN_POINT('Ctrl Pts',(-6.61083770188548,-62.4956084911391,
40.0982599215483));
#189058=CARTESIAN_POINT('Ctrl Pts',(-6.60433062536177,-62.4971561593225,
40.0990497370453));
#189059=CARTESIAN_POINT('Ctrl Pts',(-6.60270385623084,-62.4975430763684,
40.0992471909196));
#189060=CARTESIAN_POINT('Ctrl Pts',(-6.60106746196587,-62.4979056188888,
40.0994209989363));
#189061=CARTESIAN_POINT('Ctrl Pts',(-6.59942221845775,-62.4982426563699,
40.0995705982975));
#189062=CARTESIAN_POINT('Ctrl Pts',(-6.59695435319557,-62.4987482125917,
40.0997949973393));
#189063=CARTESIAN_POINT('Ctrl Pts',(-6.59446659126629,-62.4991963674676,
40.0999649129781));
#189064=CARTESIAN_POINT('Ctrl Pts',(-6.5919617450032,-62.4995849724124,
40.1000786629733));
#189065=CARTESIAN_POINT('Ctrl Pts',(-6.58945689874012,-62.4999735773571,
40.1001924129685));
#189066=CARTESIAN_POINT('Ctrl Pts',(-6.58693497617671,-62.5003026407462,
40.10025));
#189067=CARTESIAN_POINT('Ctrl Pts',(-6.5843985910305,-62.5005702980931,
40.10025));
#189068=CARTESIAN_POINT('Ctrl Pts',(-6.18532049829418,-58.7035958781039,
40.10025));
#189069=CARTESIAN_POINT('Ctrl Pts',(-6.19390281910169,-58.702689976017,
40.10025));
#189070=CARTESIAN_POINT('Ctrl Pts',(-6.20248552904374,-58.7025003609928,
40.0995786334241));
#189071=CARTESIAN_POINT('Ctrl Pts',(-6.21093474935423,-58.7029569544313,
40.0983063763367));
#189072=CARTESIAN_POINT('Ctrl Pts',(-6.21639207873495,-58.7032518669434,
40.0974846287993));
#189073=CARTESIAN_POINT('Ctrl Pts',(-6.2217937793752,-58.7038154335198,
40.0964130309338));
#189074=CARTESIAN_POINT('Ctrl Pts',(-6.22710604846875,-58.7046202140516,
40.0951176960924));
#189075=CARTESIAN_POINT('Ctrl Pts',(-6.23414715684653,-58.7056869045457,
40.0934008039614));
#189076=CARTESIAN_POINT('Ctrl Pts',(-6.24102913891656,-58.7071827955652,
40.0912909372156));
#189077=CARTESIAN_POINT('Ctrl Pts',(-6.2476792244076,-58.7090548163569,
40.0888630467851));
#189078=CARTESIAN_POINT('Ctrl Pts',(-6.25100426715312,-58.7099908267528,
40.0876491015699));
#189079=CARTESIAN_POINT('Ctrl Pts',(-6.25427153376677,-58.7110208470228,
40.0863558569271));
#189080=CARTESIAN_POINT('Ctrl Pts',(-6.25747333351534,-58.7121380880307,
40.0849936342771));
#189081=CARTESIAN_POINT('Ctrl Pts',(-6.25907423338962,-58.7126967085347,
40.0843125229521));
#189082=CARTESIAN_POINT('Ctrl Pts',(-6.2606587828836,-58.7132771324571,
40.0836141747074));
#189083=CARTESIAN_POINT('Ctrl Pts',(-6.26222612320532,-58.7138784999415,
40.0828999161609));
#189084=CARTESIAN_POINT('Ctrl Pts',(-6.26261795828575,-58.7140288418126,
40.0827213515243));
#189085=CARTESIAN_POINT('Ctrl Pts',(-6.26300871814027,-58.7141804926178,
40.0825417925842));
#189086=CARTESIAN_POINT('Ctrl Pts',(-6.26339839005071,-58.7143334388435,
40.082361260236));
#189087=CARTESIAN_POINT('Ctrl Pts',(-6.26456740578202,-58.7147922775207,
40.0818196631917));
#189088=CARTESIAN_POINT('Ctrl Pts',(-6.26572662828387,-58.715262775183,
40.0812693052021));
#189089=CARTESIAN_POINT('Ctrl Pts',(-6.26687572965181,-58.7157445651924,
40.0807107531875));
#189090=CARTESIAN_POINT('Ctrl Pts',(-6.27496985131161,-58.7191382318078,
40.0767763849182));
#189091=CARTESIAN_POINT('Ctrl Pts',(-6.28260716192787,-58.7230632421218,
40.0724140586137));
#189092=CARTESIAN_POINT('Ctrl Pts',(-6.28978339589464,-58.7274000190313,
40.0677221223768));
#189093=CARTESIAN_POINT('Ctrl Pts',(-6.29326386161383,-58.7295033511461,
40.0654465383721));
#189094=CARTESIAN_POINT('Ctrl Pts',(-6.29663597408943,-58.731704109697,
40.0630928000679));
#189095=CARTESIAN_POINT('Ctrl Pts',(-6.29989941779165,-58.7339915094193,
40.0606689262479));
#189096=CARTESIAN_POINT('Ctrl Pts',(-6.30489552208954,-58.7374933585782,
40.0569581447805));
#189097=CARTESIAN_POINT('Ctrl Pts',(-6.30963480180889,-58.7411954596217,
40.0530843804605));
#189098=CARTESIAN_POINT('Ctrl Pts',(-6.31410463171063,-58.745053462885,
40.0490800251457));
#189099=CARTESIAN_POINT('Ctrl Pts',(-6.31618044384084,-58.7468451395592,
40.0472203818218));
#189100=CARTESIAN_POINT('Ctrl Pts',(-6.31819823791544,-58.7486702031823,
40.0453323608818));
#189101=CARTESIAN_POINT('Ctrl Pts',(-6.32015576082334,-58.7505249478605,
40.0434201572162));
#189102=CARTESIAN_POINT('Ctrl Pts',(-6.3203057972412,-58.750667106732,40.0432735943397));
#189103=CARTESIAN_POINT('Ctrl Pts',(-6.32045551058208,-58.7508094261759,
40.0431268995707));
#189104=CARTESIAN_POINT('Ctrl Pts',(-6.32060490094018,-58.7509519047346,
40.0429800745037));
#189105=CARTESIAN_POINT('Ctrl Pts',(-6.32270338507402,-58.7529532989256,
40.0409176249753));
#189106=CARTESIAN_POINT('Ctrl Pts',(-6.32473679726646,-58.7549876922215,
40.0388310783332));
#189107=CARTESIAN_POINT('Ctrl Pts',(-6.32670504965004,-58.757049379421,
40.036725739981));
#189108=CARTESIAN_POINT('Ctrl Pts',(-6.33376285265555,-58.7644422230594,
40.0291763710718));
#189109=CARTESIAN_POINT('Ctrl Pts',(-6.34003880538882,-58.772241810992,
40.0213310894596));
#189110=CARTESIAN_POINT('Ctrl Pts',(-6.34560292136685,-58.7803396486548,
40.0132837551322));
#189111=CARTESIAN_POINT('Ctrl Pts',(-6.35171732586152,-58.7892383587461,
40.0044405431331));
#189112=CARTESIAN_POINT('Ctrl Pts',(-6.35697262978372,-58.7984976730883,
39.995352871061));
#189113=CARTESIAN_POINT('Ctrl Pts',(-6.36142852992733,-58.8080148760634,
39.9861103629568));
#189114=CARTESIAN_POINT('Ctrl Pts',(-6.36623978380391,-58.818291066784,
39.9761307737578));
#189115=CARTESIAN_POINT('Ctrl Pts',(-6.37011968263616,-58.8288688921818,
39.9659696936042));
#189116=CARTESIAN_POINT('Ctrl Pts',(-6.37309732669698,-58.8396533761837,
39.9557128217545));
#189117=CARTESIAN_POINT('Ctrl Pts',(-6.37604999138425,-58.8503473894481,
39.9455419945187));
#189118=CARTESIAN_POINT('Ctrl Pts',(-6.37811557911233,-58.8612460403448,
39.9352756289354));
#189119=CARTESIAN_POINT('Ctrl Pts',(-6.37927424642597,-58.872270023448,
39.92499));
#189120=CARTESIAN_POINT('Origin',(0.0151565136854187,-0.0015930137801935,
39.92499));
#189121=CARTESIAN_POINT('Ctrl Pts',(-6.55408556365967,-62.5037563256534,
40.10025));
#189122=CARTESIAN_POINT('Ctrl Pts',(-6.54554330587437,-62.5046505412977,
40.10025));
#189123=CARTESIAN_POINT('Ctrl Pts',(-6.537002260867,-62.5048232320878,40.0995859581842));
#189124=CARTESIAN_POINT('Ctrl Pts',(-6.52859457177493,-62.5043472028589,
40.0983275959621));
#189125=CARTESIAN_POINT('Ctrl Pts',(-6.52322245869524,-62.5040430428431,
40.0975235624068));
#189126=CARTESIAN_POINT('Ctrl Pts',(-6.51790471489642,-62.5034749678471,
40.0964777059491));
#189127=CARTESIAN_POINT('Ctrl Pts',(-6.51267356740883,-62.5026702669707,
40.0952149915961));
#189128=CARTESIAN_POINT('Ctrl Pts',(-6.50553410072686,-62.5015720117389,
40.0934916398701));
#189129=CARTESIAN_POINT('Ctrl Pts',(-6.49855818190806,-62.5000273428098,
40.0913643921631));
#189130=CARTESIAN_POINT('Ctrl Pts',(-6.49182203260206,-62.4980940659029,
40.0889118607713));
#189131=CARTESIAN_POINT('Ctrl Pts',(-6.48845395794906,-62.4971274274495,
40.0876855950754));
#189132=CARTESIAN_POINT('Ctrl Pts',(-6.48514561818761,-62.4960636607365,
40.0863782327526));
#189133=CARTESIAN_POINT('Ctrl Pts',(-6.48190505740188,-62.494910155573,
40.0850006373334));
#189134=CARTESIAN_POINT('Ctrl Pts',(-6.48028477700901,-62.4943334029912,
40.0843118396237));
#189135=CARTESIAN_POINT('Ctrl Pts',(-6.47868142404705,-62.4937342176673,
40.0836054919164));
#189136=CARTESIAN_POINT('Ctrl Pts',(-6.47709589524289,-62.4931135352113,
40.0828829920417));
#189137=CARTESIAN_POINT('Ctrl Pts',(-6.47669951304185,-62.4929583645973,
40.0827023670731));
#189138=CARTESIAN_POINT('Ctrl Pts',(-6.47630424448195,-62.4928018504535,
40.0825207326933));
#189139=CARTESIAN_POINT('Ctrl Pts',(-6.47591010283095,-62.4926440074817,
40.0823381109275));
#189140=CARTESIAN_POINT('Ctrl Pts',(-6.47472767787796,-62.4921704785661,
40.0817902456303));
#189141=CARTESIAN_POINT('Ctrl Pts',(-6.47355539694489,-62.4916849899864,
40.0812334935553));
#189142=CARTESIAN_POINT('Ctrl Pts',(-6.47239360181831,-62.4911879405752,
40.0806684524227));
#189143=CARTESIAN_POINT('Ctrl Pts',(-6.46436487665219,-62.487753020747,
40.0767636676138));
#189144=CARTESIAN_POINT('Ctrl Pts',(-6.45678933786461,-62.483794992505,
40.0724404510891));
#189145=CARTESIAN_POINT('Ctrl Pts',(-6.44966853564077,-62.479432636437,
40.0677949937413));
#189146=CARTESIAN_POINT('Ctrl Pts',(-6.44612951648143,-62.4772645574455,
40.0654862141908));
#189147=CARTESIAN_POINT('Ctrl Pts',(-6.44270272394389,-62.4749960038953,
40.0630972003217));
#189148=CARTESIAN_POINT('Ctrl Pts',(-6.43938822718945,-62.4726384024734,
40.0606363359906));
#189149=CARTESIAN_POINT('Ctrl Pts',(-6.43207595228375,-62.4674371815967,
40.0552073017123));
#189150=CARTESIAN_POINT('Ctrl Pts',(-6.42530381744011,-62.461813233051,
40.0494204304519));
#189151=CARTESIAN_POINT('Ctrl Pts',(-6.41913840445446,-62.455895762341,
40.0434049749851));
#189152=CARTESIAN_POINT('Ctrl Pts',(-6.41688610134085,-62.4537340356674,
40.0412074532442));
#189153=CARTESIAN_POINT('Ctrl Pts',(-6.41470741397488,-62.4515361835425,
40.0389814735788));
#189154=CARTESIAN_POINT('Ctrl Pts',(-6.41260146153659,-62.4493074469123,
40.0367321210017));
#189155=CARTESIAN_POINT('Ctrl Pts',(-6.40552779014119,-62.4418213564088,
40.029176783714));
#189156=CARTESIAN_POINT('Ctrl Pts',(-6.39923601079914,-62.4339335724864,
40.0213235332575));
#189157=CARTESIAN_POINT('Ctrl Pts',(-6.39365709371068,-62.4257522463028,
40.0132649215856));
#189158=CARTESIAN_POINT('Ctrl Pts',(-6.3875252029643,-62.4167599996853,
40.004407552753));
#189159=CARTESIAN_POINT('Ctrl Pts',(-6.38225398283504,-62.4074126717511,
39.9953016253716));
#189160=CARTESIAN_POINT('Ctrl Pts',(-6.37778536209628,-62.3978127557455,
39.9860353422353));
#189161=CARTESIAN_POINT('Ctrl Pts',(-6.37297246609546,-62.3874732348838,
39.9760551582689));
#189162=CARTESIAN_POINT('Ctrl Pts',(-6.36908997057829,-62.3768396913524,
39.9658879738149));
#189163=CARTESIAN_POINT('Ctrl Pts',(-6.36611161569997,-62.3660067738162,
39.9556174643246));
#189164=CARTESIAN_POINT('Ctrl Pts',(-6.36317347866863,-62.355320137243,
39.9454856413899));
#189165=CARTESIAN_POINT('Ctrl Pts',(-6.3611151561247,-62.3444380411301,
39.9352519465111));
#189166=CARTESIAN_POINT('Ctrl Pts',(-6.35995915837823,-62.3334394572619,
39.92499));
#189167=CARTESIAN_POINT('Ctrl Pts',(-6.00036140429066,-58.912095367953,
39.92499));
#189168=CARTESIAN_POINT('Ctrl Pts',(-5.99925510810146,-58.9015696628146,
39.9348107241723));
#189169=CARTESIAN_POINT('Ctrl Pts',(-5.99898299131207,-58.8909945468898,
39.9446038383171));
#189170=CARTESIAN_POINT('Ctrl Pts',(-5.99953795195275,-58.8804276387785,
39.9543158069386));
#189171=CARTESIAN_POINT('Ctrl Pts',(-6.00007381527891,-58.8702243592796,
39.9636935671393));
#189172=CARTESIAN_POINT('Ctrl Pts',(-6.00138095727672,-58.8600274754035,
39.972996832099));
#189173=CARTESIAN_POINT('Ctrl Pts',(-6.00349883563959,-58.8498890377491,
39.9821731151337));
#189174=CARTESIAN_POINT('Ctrl Pts',(-6.00550089397094,-58.8403050390036,
39.9908475764353));
#189175=CARTESIAN_POINT('Ctrl Pts',(-6.00822762538565,-58.8307723843882,
39.9994093733847));
#189176=CARTESIAN_POINT('Ctrl Pts',(-6.01175153639566,-58.8213500689059,
40.0077966115843));
#189177=CARTESIAN_POINT('Ctrl Pts',(-6.01499699931784,-58.8126722744178,
40.0155211172596));
#189178=CARTESIAN_POINT('Ctrl Pts',(-6.01891888229176,-58.8040875818567,
40.0230979941022));
#189179=CARTESIAN_POINT('Ctrl Pts',(-6.02360485257435,-58.795664241307,
40.0304554104749));
#189180=CARTESIAN_POINT('Ctrl Pts',(-6.0250021143202,-58.7931525711912,
40.0326492435181));
#189181=CARTESIAN_POINT('Ctrl Pts',(-6.0264675236373,-58.7906554330095,
40.0348233715061));
#189182=CARTESIAN_POINT('Ctrl Pts',(-6.02800395803724,-58.7881751602884,
40.0369753512356));
#189183=CARTESIAN_POINT('Ctrl Pts',(-6.02952469386371,-58.7857202298425,
40.0391053430352));
#189184=CARTESIAN_POINT('Ctrl Pts',(-6.03111319985524,-58.783284225042,
40.041211089324));
#189185=CARTESIAN_POINT('Ctrl Pts',(-6.03277025542049,-58.7808720541407,
40.0432881154904));
#189186=CARTESIAN_POINT('Ctrl Pts',(-6.03288548382381,-58.7807043164937,
40.043432547828));
#189187=CARTESIAN_POINT('Ctrl Pts',(-6.0330010380093,-58.7805366835715,
40.0435768364421));
#189188=CARTESIAN_POINT('Ctrl Pts',(-6.03311691890582,-58.7803691562898,
40.0437209807855));
#189189=CARTESIAN_POINT('Ctrl Pts',(-6.03819756191453,-58.7730241465597,
40.050040796842));
#189190=CARTESIAN_POINT('Ctrl Pts',(-6.04393622206017,-58.7659160498048,
40.0560490279345));
#189191=CARTESIAN_POINT('Ctrl Pts',(-6.05034076157606,-58.7591607781928,
40.0616647108616));
#189192=CARTESIAN_POINT('Ctrl Pts',(-6.05631090550637,-58.752863690992,
40.0668995033488));
#189193=CARTESIAN_POINT('Ctrl Pts',(-6.06286038933353,-58.7468728126822,
40.0717933267484));
#189194=CARTESIAN_POINT('Ctrl Pts',(-6.07000150504434,-58.7413107827877,
40.0762460303076));
#189195=CARTESIAN_POINT('Ctrl Pts',(-6.0726138175574,-58.7392761202951,
40.077874886875));
#189196=CARTESIAN_POINT('Ctrl Pts',(-6.07530531160696,-58.7372991657063,
40.0794443522248));
#189197=CARTESIAN_POINT('Ctrl Pts',(-6.07807653793574,-58.735387140493,
40.0809482021492));
#189198=CARTESIAN_POINT('Ctrl Pts',(-6.07874292528937,-58.7349273623043,
40.0813098278168));
#189199=CARTESIAN_POINT('Ctrl Pts',(-6.07941450700203,-58.7344713442223,
40.0816679525672));
#189200=CARTESIAN_POINT('Ctrl Pts',(-6.08009121771094,-58.7340192051468,
40.082022419258));
#189201=CARTESIAN_POINT('Ctrl Pts',(-6.08074678121021,-58.7335811954175,
40.0823658088648));
#189202=CARTESIAN_POINT('Ctrl Pts',(-6.08140715812726,-58.7331468260468,
40.0827057654617));
#189203=CARTESIAN_POINT('Ctrl Pts',(-6.0820722852656,-58.7327162055066,
40.0830421470151));
#189204=CARTESIAN_POINT('Ctrl Pts',(-6.0893595217361,-58.7279982598321,
40.0867275956805));
#189205=CARTESIAN_POINT('Ctrl Pts',(-6.09722197243183,-58.7237275533352,
40.0899823432029));
#189206=CARTESIAN_POINT('Ctrl Pts',(-6.10554709909155,-58.7200553115704,
40.0926299529354));
#189207=CARTESIAN_POINT('Ctrl Pts',(-6.10899977726302,-58.7185323234526,
40.0937279956083));
#189208=CARTESIAN_POINT('Ctrl Pts',(-6.11253167434596,-58.7171120447816,
40.0947220371802));
#189209=CARTESIAN_POINT('Ctrl Pts',(-6.11613350280244,-58.7158039367398,
40.0956014538692));
#189210=CARTESIAN_POINT('Ctrl Pts',(-6.12227679657168,-58.7135728221602,
40.097101390674));
#189211=CARTESIAN_POINT('Ctrl Pts',(-6.12862250657806,-58.7116702942288,
40.0982667904316));
#189212=CARTESIAN_POINT('Ctrl Pts',(-6.13511848061117,-58.7101471179287,
40.0990539325582));
#189213=CARTESIAN_POINT('Ctrl Pts',(-6.13836646762773,-58.7093855297787,
40.0994475036216));
#189214=CARTESIAN_POINT('Ctrl Pts',(-6.14165223896381,-58.708720209805,
40.0997467259952));
#189215=CARTESIAN_POINT('Ctrl Pts',(-6.14496923836512,-58.7081575578111,
40.0999473488896));
#189216=CARTESIAN_POINT('Ctrl Pts',(-6.14828623776643,-58.7075949058171,
40.100147971784));
#189217=CARTESIAN_POINT('Ctrl Pts',(-6.15163442139611,-58.7071349090267,
40.10025));
#189218=CARTESIAN_POINT('Ctrl Pts',(-6.15500747092336,-58.7067819056643,
40.10025));
#189219=CARTESIAN_POINT('Origin',(-12.1286263473646,-56.9874003490101,39.92499));
#189220=CARTESIAN_POINT('Ctrl Pts',(-13.2134115091896,-61.2479592423877,
39.92499));
#189221=CARTESIAN_POINT('Ctrl Pts',(-13.215617520741,-61.2583377107544,
39.9348354642017));
#189222=CARTESIAN_POINT('Ctrl Pts',(-13.216998090955,-61.2688594460194,
39.9446440828456));
#189223=CARTESIAN_POINT('Ctrl Pts',(-13.2175561899856,-61.2794654334797,
39.9543641760328));
#189224=CARTESIAN_POINT('Ctrl Pts',(-13.218096154121,-61.289726789502,39.9637684240708));
#189225=CARTESIAN_POINT('Ctrl Pts',(-13.2178662282942,-61.300068301046,
39.9730909636391));
#189226=CARTESIAN_POINT('Ctrl Pts',(-13.2168232529022,-61.3104421535926,
39.9822808977134));
#189227=CARTESIAN_POINT('Ctrl Pts',(-13.2158366624041,-61.3202551793167,
39.9909740094642));
#189228=CARTESIAN_POINT('Ctrl Pts',(-13.2141224659048,-61.3300980668392,
39.9995492764992));
#189229=CARTESIAN_POINT('Ctrl Pts',(-13.2116033021987,-61.3399200511708,
40.0079462328684));
#189230=CARTESIAN_POINT('Ctrl Pts',(-13.2092829702348,-61.3489668090842,
40.0156804369678));
#189231=CARTESIAN_POINT('Ctrl Pts',(-13.2062795322641,-61.3579963605636,
40.0232638017409));
#189232=CARTESIAN_POINT('Ctrl Pts',(-13.202499106524,-61.3669504518443,
40.0306257269953));
#189233=CARTESIAN_POINT('Ctrl Pts',(-13.2014025487214,-61.3695476933549,
40.0327611416642));
#189234=CARTESIAN_POINT('Ctrl Pts',(-13.2002403977589,-61.3721384315545,
40.0348777427266));
#189235=CARTESIAN_POINT('Ctrl Pts',(-13.1990098046949,-61.374720822464,
40.03697331687));
#189236=CARTESIAN_POINT('Ctrl Pts',(-13.197675762694,-61.3775203002416,
40.039245053974));
#189237=CARTESIAN_POINT('Ctrl Pts',(-13.196264116926,-61.3803065372249,
40.041487875195));
#189238=CARTESIAN_POINT('Ctrl Pts',(-13.1947721021912,-61.3830766416486,
40.0436985701601));
#189239=CARTESIAN_POINT('Ctrl Pts',(-13.1906772560438,-61.3906792149761,
40.0497658398386));
#189240=CARTESIAN_POINT('Ctrl Pts',(-13.1859443571666,-61.3981301363758,
40.0555581699984));
#189241=CARTESIAN_POINT('Ctrl Pts',(-13.1805769309631,-61.4053257594952,
40.0609828468885));
#189242=CARTESIAN_POINT('Ctrl Pts',(-13.1756660273915,-61.4119093639898,
40.0659461317303));
#189243=CARTESIAN_POINT('Ctrl Pts',(-13.1702212276784,-61.4182680026346,
40.0706039980703));
#189244=CARTESIAN_POINT('Ctrl Pts',(-13.1642115906192,-61.4243186078266,
40.0748843180598));
#189245=CARTESIAN_POINT('Ctrl Pts',(-13.1612596765267,-61.4272906453321,
40.0769867972567));
#189246=CARTESIAN_POINT('Ctrl Pts',(-13.1581712727462,-61.4301878975264,
40.0789976708173));
#189247=CARTESIAN_POINT('Ctrl Pts',(-13.1549417366132,-61.4329973166795,
40.08090504915));
#189248=CARTESIAN_POINT('Ctrl Pts',(-13.1543289635881,-61.4335303765997,
40.0812669556105));
#189249=CARTESIAN_POINT('Ctrl Pts',(-13.1537105783546,-61.4340602468994,
40.0816253922032));
#189250=CARTESIAN_POINT('Ctrl Pts',(-13.153086632425,-61.4345867973821,
40.0819801989139));
#189251=CARTESIAN_POINT('Ctrl Pts',(-13.1524821848057,-61.4350968931622,
40.0823239179149));
#189252=CARTESIAN_POINT('Ctrl Pts',(-13.1518725186283,-61.4356038733672,
40.0826642303498));
#189253=CARTESIAN_POINT('Ctrl Pts',(-13.1512576844885,-61.4361076188515,
40.0830009916099));
#189254=CARTESIAN_POINT('Ctrl Pts',(-13.1445573487221,-61.4415973333396,
40.0866709464313));
#189255=CARTESIAN_POINT('Ctrl Pts',(-13.1372385931148,-61.446706186705,
40.0899175831879));
#189256=CARTESIAN_POINT('Ctrl Pts',(-13.1293950794796,-61.45126834185,40.0925642067064));
#189257=CARTESIAN_POINT('Ctrl Pts',(-13.1260827149658,-61.4531949682972,
40.0936818922529));
#189258=CARTESIAN_POINT('Ctrl Pts',(-13.1226771582918,-61.4550242827917,
40.0946930094791));
#189259=CARTESIAN_POINT('Ctrl Pts',(-13.119186939003,-61.4567450522888,
40.0955863397546));
#189260=CARTESIAN_POINT('Ctrl Pts',(-13.1133094969314,-61.4596427851248,
40.0970906856166));
#189261=CARTESIAN_POINT('Ctrl Pts',(-13.1071927578069,-61.4622303029112,
40.0982599215483));
#189262=CARTESIAN_POINT('Ctrl Pts',(-13.100883103106,-61.4644496675157,
40.0990497370454));
#189263=CARTESIAN_POINT('Ctrl Pts',(-13.0993056894308,-61.4650045086668,
40.0992471909196));
#189264=CARTESIAN_POINT('Ctrl Pts',(-13.0977161555174,-61.4655361149191,
40.0994209989363));
#189265=CARTESIAN_POINT('Ctrl Pts',(-13.0961151548353,-61.4660432808493,
40.0995705982975));
#189266=CARTESIAN_POINT('Ctrl Pts',(-13.0937136538122,-61.4668040297446,
40.0997949973393));
#189267=CARTESIAN_POINT('Ctrl Pts',(-13.0912863650436,-61.4675097715127,
40.0999649129781));
#189268=CARTESIAN_POINT('Ctrl Pts',(-13.0888358608681,-61.4681580753695,
40.1000786629733));
#189269=CARTESIAN_POINT('Ctrl Pts',(-13.0863853566926,-61.4688063792264,
40.1001924129685));
#189270=CARTESIAN_POINT('Ctrl Pts',(-13.0839116459753,-61.4693972526618,
40.10025));
#189271=CARTESIAN_POINT('Ctrl Pts',(-13.0814171332235,-61.4699285681954,
40.10025));
#189272=CARTESIAN_POINT('Ctrl Pts',(-12.2876333308473,-57.7354693911204,
40.10025));
#189273=CARTESIAN_POINT('Ctrl Pts',(-12.2960739442508,-57.7336713548546,
40.10025));
#189274=CARTESIAN_POINT('Ctrl Pts',(-12.3045898170431,-57.7325856410804,
40.099578633424));
#189275=CARTESIAN_POINT('Ctrl Pts',(-12.3130404786515,-57.7321565492375,
40.0983063763365));
#189276=CARTESIAN_POINT('Ctrl Pts',(-12.3184987389622,-57.7318793999343,
40.0974846287991));
#189277=CARTESIAN_POINT('Ctrl Pts',(-12.323929757269,-57.7318752477671,
40.0964130309337));
#189278=CARTESIAN_POINT('Ctrl Pts',(-12.3292970476685,-57.7321203363021,
40.0951176960924));
#189279=CARTESIAN_POINT('Ctrl Pts',(-12.336411083636,-57.7324451871157,
40.0934008039614));
#189280=CARTESIAN_POINT('Ctrl Pts',(-12.3434117286777,-57.7332135204776,
40.0912909372156));
#189281=CARTESIAN_POINT('Ctrl Pts',(-12.3502210637611,-57.7343801629266,
40.0888630467851));
#189282=CARTESIAN_POINT('Ctrl Pts',(-12.3536257313028,-57.734963484151,
40.0876491015699));
#189283=CARTESIAN_POINT('Ctrl Pts',(-12.3569827659241,-57.735646339504,
40.0863558569271));
#189284=CARTESIAN_POINT('Ctrl Pts',(-12.3602838093643,-57.7364227809414,
40.0849936342771));
#189285=CARTESIAN_POINT('Ctrl Pts',(-12.3619343310843,-57.7368110016601,
40.0843125229521));
#189286=CARTESIAN_POINT('Ctrl Pts',(-12.363570871071,-57.7372226154359,
40.0836141747074));
#189287=CARTESIAN_POINT('Ctrl Pts',(-12.3651924853575,-57.7376568568911,
40.0828999161609));
#189288=CARTESIAN_POINT('Ctrl Pts',(-12.3655978889291,-57.7377654172549,
40.0827213515243));
#189289=CARTESIAN_POINT('Ctrl Pts',(-12.3660023599859,-57.737875391774,
40.0825417925842));
#189290=CARTESIAN_POINT('Ctrl Pts',(-12.3664058844668,-57.7379867683383,
40.0823612602361));
#189291=CARTESIAN_POINT('Ctrl Pts',(-12.3676164579094,-57.7383208980313,
40.0818196631917));
#189292=CARTESIAN_POINT('Ctrl Pts',(-12.3688185104667,-57.7386676465115,
40.0812693052021));
#189293=CARTESIAN_POINT('Ctrl Pts',(-12.3700116777064,-57.7390266834246,
40.0807107531875));
#189294=CARTESIAN_POINT('Ctrl Pts',(-12.3784161936772,-57.7415556930807,
40.0767763849181));
#189295=CARTESIAN_POINT('Ctrl Pts',(-12.3864219416033,-57.7446608854354,
40.0724140586136));
#189296=CARTESIAN_POINT('Ctrl Pts',(-12.3940121800356,-57.7482237843187,
40.0677221223766));
#189297=CARTESIAN_POINT('Ctrl Pts',(-12.3976934374729,-57.749951786427,
40.0654465383719));
#189298=CARTESIAN_POINT('Ctrl Pts',(-12.4012771190728,-57.7517880072572,
40.0630928000678));
#189299=CARTESIAN_POINT('Ctrl Pts',(-12.4047617836667,-57.7537217536092,
40.0606689262479));
#189300=CARTESIAN_POINT('Ctrl Pts',(-12.4100965616936,-57.7566821841674,
40.0569581447805));
#189301=CARTESIAN_POINT('Ctrl Pts',(-12.4151968540757,-57.759868615088,
40.0530843804605));
#189302=CARTESIAN_POINT('Ctrl Pts',(-12.420045468934,-57.763238259355,40.0490800251457));
#189303=CARTESIAN_POINT('Ctrl Pts',(-12.4222971907576,-57.7648031395849,
40.0472203818218));
#189304=CARTESIAN_POINT('Ctrl Pts',(-12.424494702241,-57.7664072884047,
40.0453323608818));
#189305=CARTESIAN_POINT('Ctrl Pts',(-12.4266353752445,-57.7680472557362,
40.0434201572162));
#189306=CARTESIAN_POINT('Ctrl Pts',(-12.4267994493956,-57.7681729527703,
40.0432735943397));
#189307=CARTESIAN_POINT('Ctrl Pts',(-12.4269632190239,-57.7682988432679,
40.0431268995707));
#189308=CARTESIAN_POINT('Ctrl Pts',(-12.4271266840708,-57.7684249257696,
40.0429800745037));
#189309=CARTESIAN_POINT('Ctrl Pts',(-12.4294228751481,-57.7701960047921,
40.0409176249753));
#189310=CARTESIAN_POINT('Ctrl Pts',(-12.4316578001007,-57.772006704017,
40.0388310783332));
#189311=CARTESIAN_POINT('Ctrl Pts',(-12.4338307751865,-57.7738513586813,
40.036725739981));
#189312=CARTESIAN_POINT('Ctrl Pts',(-12.4416226773931,-57.7804659622463,
40.0291763710721));
#189313=CARTESIAN_POINT('Ctrl Pts',(-12.448679528741,-57.7875668075251,
40.0213310894602));
#189314=CARTESIAN_POINT('Ctrl Pts',(-12.455059618436,-57.7950386758929,
40.0132837551332));
#189315=CARTESIAN_POINT('Ctrl Pts',(-12.4620706960738,-57.8032495086132,
40.0044405431344));
#189316=CARTESIAN_POINT('Ctrl Pts',(-12.4682650727902,-57.8119087706193,
39.9953528710627));
#189317=CARTESIAN_POINT('Ctrl Pts',(-12.4736913816481,-57.8209080689657,
39.986110362959));
#189318=CARTESIAN_POINT('Ctrl Pts',(-12.4795504333966,-57.8306250526638,
39.9761307737604));
#189319=CARTESIAN_POINT('Ctrl Pts',(-12.4845147615706,-57.8407393717642,
39.9659696936073));
#189320=CARTESIAN_POINT('Ctrl Pts',(-12.4886033793256,-57.851153528676,
39.9557128217581));
#189321=CARTESIAN_POINT('Ctrl Pts',(-12.4926576977801,-57.8614803215156,
39.9455419945211));
#189322=CARTESIAN_POINT('Ctrl Pts',(-12.4958511892329,-57.8721033557526,
39.9352756289366));
#189323=CARTESIAN_POINT('Ctrl Pts',(-12.4981558292589,-57.8829458346105,
39.92499));
#189324=CARTESIAN_POINT('Origin',(0.0149069694351899,-0.0031685741680572,
39.92499));
#189325=CARTESIAN_POINT('Ctrl Pts',(-13.0516031943531,-61.4762657165315,
40.10025));
#189326=CARTESIAN_POINT('Ctrl Pts',(-13.0432012029365,-61.4780479426482,
40.10025));
#189327=CARTESIAN_POINT('Ctrl Pts',(-13.0347249977698,-61.4791124697294,
40.0995859581841));
#189328=CARTESIAN_POINT('Ctrl Pts',(-13.0263136082741,-61.4795178910588,
40.0983275959619));
#189329=CARTESIAN_POINT('Ctrl Pts',(-13.0209391308134,-61.479776935988,
40.0975235624067));
#189330=CARTESIAN_POINT('Ctrl Pts',(-13.0155911381655,-61.4797678285536,
40.096477705949));
#189331=CARTESIAN_POINT('Ctrl Pts',(-13.0103045333056,-61.4795143397208,
40.0952149915961));
#189332=CARTESIAN_POINT('Ctrl Pts',(-13.0030893784375,-61.4791683783269,
40.0934916398701));
#189333=CARTESIAN_POINT('Ctrl Pts',(-12.9959902125625,-61.4783613533298,
40.0913643921631));
#189334=CARTESIAN_POINT('Ctrl Pts',(-12.989088882123,-61.4771427864514,
40.0889118607713));
#189335=CARTESIAN_POINT('Ctrl Pts',(-12.9856382169033,-61.4765335030122,
40.0876855950754));
#189336=CARTESIAN_POINT('Ctrl Pts',(-12.9822368066734,-61.4758213793959,
40.0863782327526));
#189337=CARTESIAN_POINT('Ctrl Pts',(-12.9788934238966,-61.4750129240933,
40.0850006373334));
#189338=CARTESIAN_POINT('Ctrl Pts',(-12.9772217325082,-61.4746086964421,
40.0843118396237));
#189339=CARTESIAN_POINT('Ctrl Pts',(-12.9755645309605,-61.4741803895393,
40.0836054919164));
#189340=CARTESIAN_POINT('Ctrl Pts',(-12.9739228088657,-61.4737288401361,
40.0828829920418));
#189341=CARTESIAN_POINT('Ctrl Pts',(-12.973512378342,-61.4736159527853,
40.0827023670731));
#189342=CARTESIAN_POINT('Ctrl Pts',(-12.9731029149217,-61.4735016128574,
40.0825207326933));
#189343=CARTESIAN_POINT('Ctrl Pts',(-12.9726944333366,-61.473385833587,
40.0823381109275));
#189344=CARTESIAN_POINT('Ctrl Pts',(-12.9714689885814,-61.4730384957757,
40.0817902456303));
#189345=CARTESIAN_POINT('Ctrl Pts',(-12.9702523821507,-61.4726782034777,
40.0812334935553));
#189346=CARTESIAN_POINT('Ctrl Pts',(-12.9690449956483,-61.4723053176143,
40.0806684524227));
#189347=CARTESIAN_POINT('Ctrl Pts',(-12.9607012057876,-61.46972844494,40.0767636676138));
#189348=CARTESIAN_POINT('Ctrl Pts',(-12.9527534399845,-61.4665839586187,
40.0724404510891));
#189349=CARTESIAN_POINT('Ctrl Pts',(-12.9452156558843,-61.4629898265075,
40.0677949937414));
#189350=CARTESIAN_POINT('Ctrl Pts',(-12.9414693978769,-61.4612035527137,
40.0654862141909));
#189351=CARTESIAN_POINT('Ctrl Pts',(-12.937824249251,-61.459305623895,40.0630972003217));
#189352=CARTESIAN_POINT('Ctrl Pts',(-12.9342814732029,-61.4573073969127,
40.0606363359906));
#189353=CARTESIAN_POINT('Ctrl Pts',(-12.9264655800789,-61.4528990097271,
40.0552073017123));
#189354=CARTESIAN_POINT('Ctrl Pts',(-12.9191426809995,-61.4480137506082,
40.0494204304519));
#189355=CARTESIAN_POINT('Ctrl Pts',(-12.9123924986716,-61.4427731575667,
40.0434049749851));
#189356=CARTESIAN_POINT('Ctrl Pts',(-12.9099265719429,-61.4408587028413,
40.0412074532442));
#189357=CARTESIAN_POINT('Ctrl Pts',(-12.9075300815492,-61.4389006256226,
40.0389814735788));
#189358=CARTESIAN_POINT('Ctrl Pts',(-12.9052026993237,-61.4369042302169,
40.0367321210016));
#189359=CARTESIAN_POINT('Ctrl Pts',(-12.8973852687043,-61.4301985493013,
40.0291767837142));
#189360=CARTESIAN_POINT('Ctrl Pts',(-12.8903034584561,-61.4230116455107,
40.0213235332579));
#189361=CARTESIAN_POINT('Ctrl Pts',(-12.8838999218058,-61.4154582931182,
40.0132649215863));
#189362=CARTESIAN_POINT('Ctrl Pts',(-12.8768616764785,-61.4071562640854,
40.0044075527539));
#189363=CARTESIAN_POINT('Ctrl Pts',(-12.8706422708201,-61.3984111343316,
39.9953016253727));
#189364=CARTESIAN_POINT('Ctrl Pts',(-12.8651946651858,-61.3893309057294,
39.9860353422367));
#189365=CARTESIAN_POINT('Ctrl Pts',(-12.8593273605064,-61.379551110468,
39.9760551582706));
#189366=CARTESIAN_POINT('Ctrl Pts',(-12.8543546257415,-61.3693816498911,
39.9658879738169));
#189367=CARTESIAN_POINT('Ctrl Pts',(-12.85026023838,-61.3589193990694,39.955617464327));
#189368=CARTESIAN_POINT('Ctrl Pts',(-12.8462211390718,-61.3485984239575,
39.9454856413915));
#189369=CARTESIAN_POINT('Ctrl Pts',(-12.84303660345,-61.3379910943973,39.9352519465118));
#189370=CARTESIAN_POINT('Ctrl Pts',(-12.84073727331,-61.3271735965893,39.92499));
#189371=CARTESIAN_POINT('Ctrl Pts',(-12.1254815933794,-57.962160188812,
39.92499));
#189372=CARTESIAN_POINT('Ctrl Pts',(-12.1232811218133,-57.9518077840272,
39.9348107241733));
#189373=CARTESIAN_POINT('Ctrl Pts',(-12.1219050950916,-57.9413190436427,
39.944603838319));
#189374=CARTESIAN_POINT('Ctrl Pts',(-12.1213524729335,-57.9307520129756,
39.9543158069416));
#189375=CARTESIAN_POINT('Ctrl Pts',(-12.1208188676181,-57.9205486151387,
39.9636935671429));
#189376=CARTESIAN_POINT('Ctrl Pts',(-12.1210529843538,-57.9102709573144,
39.9729968321032));
#189377=CARTESIAN_POINT('Ctrl Pts',(-12.1220995054498,-57.899966680511,
39.9821731151384));
#189378=CARTESIAN_POINT('Ctrl Pts',(-12.1230887956356,-57.8902259118322,
39.9908475764405));
#189379=CARTESIAN_POINT('Ctrl Pts',(-12.1248041559929,-57.8804604570511,
39.9994093733903));
#189380=CARTESIAN_POINT('Ctrl Pts',(-12.1273238624924,-57.8707214089959,
40.0077966115901));
#189381=CARTESIAN_POINT('Ctrl Pts',(-12.1296444699072,-57.8617519091218,
40.0155211172656));
#189382=CARTESIAN_POINT('Ctrl Pts',(-12.1326475236753,-57.852804296004,
40.0230979941085));
#189383=CARTESIAN_POINT('Ctrl Pts',(-12.1364273448798,-57.8439372821223,
40.0304554104812));
#189384=CARTESIAN_POINT('Ctrl Pts',(-12.1375544112612,-57.8412933175777,
40.0326492435223));
#189385=CARTESIAN_POINT('Ctrl Pts',(-12.138750770895,-57.8386566819989,
40.0348233715081));
#189386=CARTESIAN_POINT('Ctrl Pts',(-12.1400195294492,-57.8360293953471,
40.0369753512356));
#189387=CARTESIAN_POINT('Ctrl Pts',(-12.1412753244188,-57.833428953088,
40.0391053430352));
#189388=CARTESIAN_POINT('Ctrl Pts',(-12.14260049657,-57.8308402488865,40.041211089324));
#189389=CARTESIAN_POINT('Ctrl Pts',(-12.143996334094,-57.8282680826381,
40.0432881154904));
#189390=CARTESIAN_POINT('Ctrl Pts',(-12.1440933979056,-57.8280892192275,
40.0434325478279));
#189391=CARTESIAN_POINT('Ctrl Pts',(-12.1441907966614,-57.8279104259145,
40.0435768364421));
#189392=CARTESIAN_POINT('Ctrl Pts',(-12.144288531381,-57.8277317035128,
40.0437209807855));
#189393=CARTESIAN_POINT('Ctrl Pts',(-12.1485735795159,-57.8198958587084,
40.0500407968421));
#189394=CARTESIAN_POINT('Ctrl Pts',(-12.1535378042503,-57.812226847525,
40.0560490279346));
#189395=CARTESIAN_POINT('Ctrl Pts',(-12.1592011408681,-57.804839125324,
40.0616647108617));
#189396=CARTESIAN_POINT('Ctrl Pts',(-12.1644803548773,-57.7979524842552,
40.066899503349));
#189397=CARTESIAN_POINT('Ctrl Pts',(-12.1703677426436,-57.7913098171238,
40.0717933267487));
#189398=CARTESIAN_POINT('Ctrl Pts',(-12.176888348138,-57.7850318067596,
40.0762460303079));
#189399=CARTESIAN_POINT('Ctrl Pts',(-12.179273669986,-57.7827352293487,
40.0778748868752));
#189400=CARTESIAN_POINT('Ctrl Pts',(-12.1817437717242,-57.7804877669872,
40.0794443522249));
#189401=CARTESIAN_POINT('Ctrl Pts',(-12.1842999559277,-57.7782965440188,
40.0809482021492));
#189402=CARTESIAN_POINT('Ctrl Pts',(-12.1849146328342,-57.7777696280971,
40.0813098278168));
#189403=CARTESIAN_POINT('Ctrl Pts',(-12.1855348686826,-57.7772459087254,
40.0816679525672));
#189404=CARTESIAN_POINT('Ctrl Pts',(-12.1861606108967,-57.7767255109847,
40.082022419258));
#189405=CARTESIAN_POINT('Ctrl Pts',(-12.1867667986667,-57.7762213756733,
40.0823658088648));
#189406=CARTESIAN_POINT('Ctrl Pts',(-12.1873781540071,-57.7757203576392,
40.0827057654616));
#189407=CARTESIAN_POINT('Ctrl Pts',(-12.187994625406,-57.7752225713657,
40.0830421470151));
#189408=CARTESIAN_POINT('Ctrl Pts',(-12.1947487820215,-57.7697687474616,
40.0867275956805));
#189409=CARTESIAN_POINT('Ctrl Pts',(-12.2021217510025,-57.764699586453,
40.0899823432029));
#189410=CARTESIAN_POINT('Ctrl Pts',(-12.2100174179588,-57.7601772489165,
40.0926299529354));
#189411=CARTESIAN_POINT('Ctrl Pts',(-12.2132919863905,-57.7583017007436,
40.0937279956083));
#189412=CARTESIAN_POINT('Ctrl Pts',(-12.2166560758248,-57.7565200187332,
40.0947220371802));
#189413=CARTESIAN_POINT('Ctrl Pts',(-12.2201014385647,-57.7548425830506,
40.0956014538692));
#189414=CARTESIAN_POINT('Ctrl Pts',(-12.2259778637495,-57.751981541693,
40.097101390674));
#189415=CARTESIAN_POINT('Ctrl Pts',(-12.2320899429716,-57.7494261286934,
40.0982667904316));
#189416=CARTESIAN_POINT('Ctrl Pts',(-12.2383911161013,-57.7472322823295,
40.0990539325582));
#189417=CARTESIAN_POINT('Ctrl Pts',(-12.2415417026662,-57.7461353591476,
40.0994475036216));
#189418=CARTESIAN_POINT('Ctrl Pts',(-12.2447399293287,-57.7451302272379,
40.0997467259952));
#189419=CARTESIAN_POINT('Ctrl Pts',(-12.2479799447119,-57.7442239366603,
40.0999473488896));
#189420=CARTESIAN_POINT('Ctrl Pts',(-12.2512199600952,-57.7433176460828,
40.100147971784));
#189421=CARTESIAN_POINT('Ctrl Pts',(-12.254501719267,-57.7425101887132,
40.10025));
#189422=CARTESIAN_POINT('Ctrl Pts',(-12.257819391977,-57.7418065394565,
40.10025));
#189423=CARTESIAN_POINT('Origin',(-18.0189898472952,-55.4074307335706,39.92499));
#189424=CARTESIAN_POINT('Ctrl Pts',(-19.5431821162869,-59.5312589135995,
39.92499));
#189425=CARTESIAN_POINT('Ctrl Pts',(-19.5464608884256,-59.5413499366329,
39.934835464202));
#189426=CARTESIAN_POINT('Ctrl Pts',(-19.5489337165496,-59.5516697238483,
39.9446440828461));
#189427=CARTESIAN_POINT('Ctrl Pts',(-19.550597385826,-59.5621592733656,
39.9543641760334));
#189428=CARTESIAN_POINT('Ctrl Pts',(-19.5522069957574,-59.5723079749847,
39.9637684240715));
#189429=CARTESIAN_POINT('Ctrl Pts',(-19.5530593117978,-59.5826168684398,
39.9730909636398));
#189430=CARTESIAN_POINT('Ctrl Pts',(-19.553106412799,-59.5930429125518,
39.9822808977141));
#189431=CARTESIAN_POINT('Ctrl Pts',(-19.5531509674458,-59.6029053082829,
39.9909740094649));
#189432=CARTESIAN_POINT('Ctrl Pts',(-19.5524750234012,-59.6128734577637,
39.9995492764999));
#189433=CARTESIAN_POINT('Ctrl Pts',(-19.5509963368659,-59.6229049605484,
40.0079462328691));
#189434=CARTESIAN_POINT('Ctrl Pts',(-19.5496343596255,-59.6321447001099,
40.0156804369684));
#189435=CARTESIAN_POINT('Ctrl Pts',(-19.5475912199423,-59.6414387315172,
40.0232638017415));
#189436=CARTESIAN_POINT('Ctrl Pts',(-19.5447674611716,-59.6507389334421,
40.0306257269958));
#189437=CARTESIAN_POINT('Ctrl Pts',(-19.5439483960912,-59.6534365684937,
40.0327611416646));
#189438=CARTESIAN_POINT('Ctrl Pts',(-19.5430634173961,-59.6561345922125,
40.0348777427268));
#189439=CARTESIAN_POINT('Ctrl Pts',(-19.542109499003,-59.658831468516,40.0369733168701));
#189440=CARTESIAN_POINT('Ctrl Pts',(-19.5410753901339,-59.6617550558218,
40.039245053974));
#189441=CARTESIAN_POINT('Ctrl Pts',(-19.5399627185792,-59.6646735866702,
40.041487875195));
#189442=CARTESIAN_POINT('Ctrl Pts',(-19.5387684320157,-59.6675844741794,
40.0436985701601));
#189443=CARTESIAN_POINT('Ctrl Pts',(-19.5354907031708,-59.6755734277898,
40.0497658398386));
#189444=CARTESIAN_POINT('Ctrl Pts',(-19.5315625649727,-59.6834782549089,
40.0555581699984));
#189445=CARTESIAN_POINT('Ctrl Pts',(-19.5269766895185,-59.6911955084648,
40.0609828468886));
#189446=CARTESIAN_POINT('Ctrl Pts',(-19.5227808624509,-59.698256376489,
40.0659461317305));
#189447=CARTESIAN_POINT('Ctrl Pts',(-19.518030548646,-59.7051493183932,
40.0706039980707));
#189448=CARTESIAN_POINT('Ctrl Pts',(-19.5126862934697,-59.7117949558637,
40.0748843180604));
#189449=CARTESIAN_POINT('Ctrl Pts',(-19.510061212785,-59.7150592712802,
40.076986797257));
#189450=CARTESIAN_POINT('Ctrl Pts',(-19.5072925729233,-59.7182634781247,
40.0789976708175));
#189451=CARTESIAN_POINT('Ctrl Pts',(-19.5043743927941,-59.7213950854345,
40.08090504915));
#189452=CARTESIAN_POINT('Ctrl Pts',(-19.5038206965381,-59.7219892774193,
40.0812669556105));
#189453=CARTESIAN_POINT('Ctrl Pts',(-19.5032610854118,-59.7225808838922,
40.0816253922033));
#189454=CARTESIAN_POINT('Ctrl Pts',(-19.5026955970361,-59.7231697699855,
40.0819801989139));
#189455=CARTESIAN_POINT('Ctrl Pts',(-19.5021477801721,-59.7237402533883,
40.0823239179149));
#189456=CARTESIAN_POINT('Ctrl Pts',(-19.5015944476715,-59.7243081837713,
40.0826642303498));
#189457=CARTESIAN_POINT('Ctrl Pts',(-19.5010356373988,-59.7248734373529,
40.0830009916099));
#189458=CARTESIAN_POINT('Ctrl Pts',(-19.4949458381922,-59.7310334544116,
40.0866709464312));
#189459=CARTESIAN_POINT('Ctrl Pts',(-19.4882011960853,-59.7368793392203,
40.0899175831878));
#189460=CARTESIAN_POINT('Ctrl Pts',(-19.4808775251051,-59.7422363728289,
40.0925642067062));
#189461=CARTESIAN_POINT('Ctrl Pts',(-19.4777846933724,-59.7444986813873,
40.0936818922528));
#189462=CARTESIAN_POINT('Ctrl Pts',(-19.474589008127,-59.7466739523114,
40.0946930094791));
#189463=CARTESIAN_POINT('Ctrl Pts',(-19.4712977780157,-59.748750122512,
40.0955863397546));
#189464=CARTESIAN_POINT('Ctrl Pts',(-19.465755428747,-59.752246341252,40.0970906856166));
#189465=CARTESIAN_POINT('Ctrl Pts',(-19.4599426670173,-59.7554590576861,
40.0982599215483));
#189466=CARTESIAN_POINT('Ctrl Pts',(-19.4538995640365,-59.7583258028883,
40.0990497370454));
#189467=CARTESIAN_POINT('Ctrl Pts',(-19.4523887882913,-59.7590424891888,
40.0992471909196));
#189468=CARTESIAN_POINT('Ctrl Pts',(-19.4508635299956,-59.7597373347838,
40.0994209989363));
#189469=CARTESIAN_POINT('Ctrl Pts',(-19.4493243130381,-59.760409072547,
40.0995705982975));
#189470=CARTESIAN_POINT('Ctrl Pts',(-19.4470154876019,-59.7614166791918,
40.0997949973393));
#189471=CARTESIAN_POINT('Ctrl Pts',(-19.4446752658776,-59.7623722755976,
40.0999649129781));
#189472=CARTESIAN_POINT('Ctrl Pts',(-19.4423059520263,-59.7632731754138,
40.1000786629733));
#189473=CARTESIAN_POINT('Ctrl Pts',(-19.439936638175,-59.7641740752301,
40.1001924129685));
#189474=CARTESIAN_POINT('Ctrl Pts',(-19.4375382417961,-59.765020284979,
40.10025));
#189475=CARTESIAN_POINT('Ctrl Pts',(-19.4351129318423,-59.765809437495,
40.10025));
#189476=CARTESIAN_POINT('Ctrl Pts',(-18.2553202812751,-56.1347810195641,
40.10025));
#189477=CARTESIAN_POINT('Ctrl Pts',(-18.263526710147,-56.1321105487811,
40.10025));
#189478=CARTESIAN_POINT('Ctrl Pts',(-18.2718824441042,-56.1301406315644,
40.0995786334241));
#189479=CARTESIAN_POINT('Ctrl Pts',(-18.2802419597926,-56.1288305556599,
40.0983063763368));
#189480=CARTESIAN_POINT('Ctrl Pts',(-18.285641349192,-56.1279843810471,
40.0974846287994));
#189481=CARTESIAN_POINT('Ctrl Pts',(-18.2910421817931,-56.1274125556282,
40.0964130309339));
#189482=CARTESIAN_POINT('Ctrl Pts',(-18.2964056883426,-56.1270952669252,
40.0951176960924));
#189483=CARTESIAN_POINT('Ctrl Pts',(-18.3035147090331,-56.1266747189247,
40.0934008039614));
#189484=CARTESIAN_POINT('Ctrl Pts',(-18.3105573165143,-56.126707076608,
40.0912909372157));
#189485=CARTESIAN_POINT('Ctrl Pts',(-18.3174512966901,-56.1271555587354,
40.0888630467852));
#189486=CARTESIAN_POINT('Ctrl Pts',(-18.320898286778,-56.1273797997991,
40.0876491015699));
#189487=CARTESIAN_POINT('Ctrl Pts',(-18.324308309033,-56.1277080087289,
40.0863558569272));
#189488=CARTESIAN_POINT('Ctrl Pts',(-18.3276724292421,-56.1281351437409,
40.0849936342772));
#189489=CARTESIAN_POINT('Ctrl Pts',(-18.3293544893467,-56.1283487112469,
40.0843125229521));
#189490=CARTESIAN_POINT('Ctrl Pts',(-18.3310250895515,-56.1285870051495,
40.0836141747075));
#189491=CARTESIAN_POINT('Ctrl Pts',(-18.3326832110572,-56.1288493629352,
40.082899916161));
#189492=CARTESIAN_POINT('Ctrl Pts',(-18.3330977414337,-56.1289149523816,
40.0827213515244));
#189493=CARTESIAN_POINT('Ctrl Pts',(-18.3335114922231,-56.1289820457108,
40.0825417925842));
#189494=CARTESIAN_POINT('Ctrl Pts',(-18.3339244481758,-56.1290506323488,
40.0823612602361));
#189495=CARTESIAN_POINT('Ctrl Pts',(-18.3351633160338,-56.1292563922627,
40.0818196631918));
#189496=CARTESIAN_POINT('Ctrl Pts',(-18.3363950287072,-56.1294755925118,
40.0812693052022));
#189497=CARTESIAN_POINT('Ctrl Pts',(-18.3376191892287,-56.1297079426452,
40.0807107531875));
#189498=CARTESIAN_POINT('Ctrl Pts',(-18.3462420178744,-56.1313445869828,
40.0767763849182));
#189499=CARTESIAN_POINT('Ctrl Pts',(-18.3545284904607,-56.1335959402408,
40.0724140586137));
#189500=CARTESIAN_POINT('Ctrl Pts',(-18.3624495731176,-56.136345925232,
40.0677221223768));
#189501=CARTESIAN_POINT('Ctrl Pts',(-18.3662912896465,-56.1376796649811,
40.065446538372));
#189502=CARTESIAN_POINT('Ctrl Pts',(-18.3700472768053,-56.1391312300711,
40.0630928000679));
#189503=CARTESIAN_POINT('Ctrl Pts',(-18.3737149835765,-56.1406901365233,
40.0606689262479));
#189504=CARTESIAN_POINT('Ctrl Pts',(-18.3793299863881,-56.1430767133841,
40.0569581447806));
#189505=CARTESIAN_POINT('Ctrl Pts',(-18.3847354115624,-56.1457125629778,
40.0530843804605));
#189506=CARTESIAN_POINT('Ctrl Pts',(-18.3899096889381,-56.1485569297209,
40.0490800251457));
#189507=CARTESIAN_POINT('Ctrl Pts',(-18.3923126501195,-56.1498778683512,
40.0472203818218));
#189508=CARTESIAN_POINT('Ctrl Pts',(-18.3946658026161,-56.1512435269776,
40.0453323608818));
#189509=CARTESIAN_POINT('Ctrl Pts',(-18.3969661720539,-56.1526507491369,
40.0434201572162));
#189510=CARTESIAN_POINT('Ctrl Pts',(-18.3971424863074,-56.1527586071707,
40.0432735943397));
#189511=CARTESIAN_POINT('Ctrl Pts',(-18.3973185179288,-56.1528666894394,
40.0431268995707));
#189512=CARTESIAN_POINT('Ctrl Pts',(-18.3974942667072,-56.1529749944978,
40.0429800745037));
#189513=CARTESIAN_POINT('Ctrl Pts',(-18.3999630071782,-56.1544963540395,
40.0409176249753));
#189514=CARTESIAN_POINT('Ctrl Pts',(-18.4023749585854,-56.1560635207937,
40.0388310783332));
#189515=CARTESIAN_POINT('Ctrl Pts',(-18.4047288488037,-56.1576709325003,
40.036725739981));
#189516=CARTESIAN_POINT('Ctrl Pts',(-18.413169480501,-56.1634348250117,
40.0291763710717));
#189517=CARTESIAN_POINT('Ctrl Pts',(-18.4209299141243,-56.1697591292906,
40.0213310894593));
#189518=CARTESIAN_POINT('Ctrl Pts',(-18.428056075939,-56.1765231650109,
40.0132837551317));
#189519=CARTESIAN_POINT('Ctrl Pts',(-18.4358870118869,-56.1839561607598,
40.0044405431321));
#189520=CARTESIAN_POINT('Ctrl Pts',(-18.4429525945105,-56.1919204977443,
39.9953528710596));
#189521=CARTESIAN_POINT('Ctrl Pts',(-18.4492898603077,-56.2003032932675,
39.986110362955));
#189522=CARTESIAN_POINT('Ctrl Pts',(-18.456132516932,-56.2093546086381,
39.9761307737549));
#189523=CARTESIAN_POINT('Ctrl Pts',(-18.4621268842299,-56.2188946068466,
39.9659696936003));
#189524=CARTESIAN_POINT('Ctrl Pts',(-18.4672816799275,-56.2288243369879,
39.9557128217496));
#189525=CARTESIAN_POINT('Ctrl Pts',(-18.4723932321854,-56.2386707668957,
39.9455419945154));
#189526=CARTESIAN_POINT('Ctrl Pts',(-18.4766796388004,-56.2489017962828,
39.9352756289337));
#189527=CARTESIAN_POINT('Ctrl Pts',(-18.4801050014193,-56.2594439784238,
39.92499));
#189528=CARTESIAN_POINT('Origin',(0.0144941013083455,-0.00470941899426891,
39.92499));
#189529=CARTESIAN_POINT('Ctrl Pts',(-19.4061247292256,-59.7752282754836,
40.10025));
#189530=CARTESIAN_POINT('Ctrl Pts',(-19.3979550581547,-59.7778789856301,
40.10025));
#189531=CARTESIAN_POINT('Ctrl Pts',(-19.3896365599073,-59.7798236858209,
40.0995859581842));
#189532=CARTESIAN_POINT('Ctrl Pts',(-19.3813136269524,-59.7811061158278,
40.0983275959622));
#189533=CARTESIAN_POINT('Ctrl Pts',(-19.3759956690093,-59.7819255275518,
40.0975235624069));
#189534=CARTESIAN_POINT('Ctrl Pts',(-19.3706760212382,-59.782475487462,
40.0964777059491));
#189535=CARTESIAN_POINT('Ctrl Pts',(-19.3653918801542,-59.7827759879494,
40.0952149915962));
#189536=CARTESIAN_POINT('Ctrl Pts',(-19.3581800878465,-59.7831861108189,
40.0934916398702));
#189537=CARTESIAN_POINT('Ctrl Pts',(-19.3510354548622,-59.7831255716886,
40.0913643921631));
#189538=CARTESIAN_POINT('Ctrl Pts',(-19.3440445557098,-59.7826350657123,
40.0889118607714));
#189539=CARTESIAN_POINT('Ctrl Pts',(-19.3405491061336,-59.7823898127242,
40.0876855950755));
#189540=CARTESIAN_POINT('Ctrl Pts',(-19.3370918919976,-59.7820371343798,
40.0863782327527));
#189541=CARTESIAN_POINT('Ctrl Pts',(-19.3336823180311,-59.7815825865438,
40.0850006373335));
#189542=CARTESIAN_POINT('Ctrl Pts',(-19.3319775310479,-59.7813553126258,
40.0843118396238));
#189543=CARTESIAN_POINT('Ctrl Pts',(-19.3302846375612,-59.7811025767642,
40.0836054919165));
#189544=CARTESIAN_POINT('Ctrl Pts',(-19.3286047092266,-59.7808251076836,
40.0828829920418));
#189545=CARTESIAN_POINT('Ctrl Pts',(-19.328184727143,-59.7807557404134,
40.0827023670732));
#189546=CARTESIAN_POINT('Ctrl Pts',(-19.3277655550292,-59.7806848274337,
40.0825207326934));
#189547=CARTESIAN_POINT('Ctrl Pts',(-19.3273472089197,-59.7806123803666,
40.0823381109276));
#189548=CARTESIAN_POINT('Ctrl Pts',(-19.3260921705914,-59.7803950391652,
40.0817902456304));
#189549=CARTESIAN_POINT('Ctrl Pts',(-19.3248445680579,-59.7801638905867,
40.0812334935554));
#189550=CARTESIAN_POINT('Ctrl Pts',(-19.3236048185588,-59.7799192536868,
40.0806684524228));
#189551=CARTESIAN_POINT('Ctrl Pts',(-19.3150373803109,-59.7782286609225,
40.0767636676137));
#189552=CARTESIAN_POINT('Ctrl Pts',(-19.306804464877,-59.775932168172,40.0724404510887));
#189553=CARTESIAN_POINT('Ctrl Pts',(-19.2989322844401,-59.7731456380807,
40.0677949937407));
#189554=CARTESIAN_POINT('Ctrl Pts',(-19.2950198323719,-59.7717607402743,
40.0654862141904));
#189555=CARTESIAN_POINT('Ctrl Pts',(-19.2911962646691,-59.7702542302927,
40.0630972003216));
#189556=CARTESIAN_POINT('Ctrl Pts',(-19.2874640247236,-59.768637270743,
40.0606363359906));
#189557=CARTESIAN_POINT('Ctrl Pts',(-19.2792301459419,-59.765070016461,
40.0552073017124));
#189558=CARTESIAN_POINT('Ctrl Pts',(-19.2714367138416,-59.7609769706901,
40.0494204304519));
#189559=CARTESIAN_POINT('Ctrl Pts',(-19.2641757185814,-59.7564706723512,
40.0434049749851));
#189560=CARTESIAN_POINT('Ctrl Pts',(-19.2615231854469,-59.7548244647406,
40.0412074532442));
#189561=CARTESIAN_POINT('Ctrl Pts',(-19.2589351484757,-59.7531276155318,
40.0389814735788));
#189562=CARTESIAN_POINT('Ctrl Pts',(-19.2564118357498,-59.7513854342765,
40.0367321210017));
#189563=CARTESIAN_POINT('Ctrl Pts',(-19.2479362953114,-59.7455336317915,
40.0291767837137));
#189564=CARTESIAN_POINT('Ctrl Pts',(-19.2401420439511,-59.7391263493538,
40.0213235332567));
#189565=CARTESIAN_POINT('Ctrl Pts',(-19.2329840462261,-59.7322837268608,
40.0132649215845));
#189566=CARTESIAN_POINT('Ctrl Pts',(-19.2251165588057,-59.7247628741792,
40.0044075527515));
#189567=CARTESIAN_POINT('Ctrl Pts',(-19.2180171087277,-59.7167157560764,
39.9953016253696));
#189568=CARTESIAN_POINT('Ctrl Pts',(-19.2116502033049,-59.7082546997612,
39.986035342233));
#189569=CARTESIAN_POINT('Ctrl Pts',(-19.2047927733642,-59.6991417795822,
39.976055158266));
#189570=CARTESIAN_POINT('Ctrl Pts',(-19.1987842816741,-59.6895478206965,
39.9658879738114));
#189571=CARTESIAN_POINT('Ctrl Pts',(-19.1936187207943,-59.6795708631975,
39.9556174643205));
#189572=CARTESIAN_POINT('Ctrl Pts',(-19.1885229124283,-59.6697286283129,
39.9454856413872));
#189573=CARTESIAN_POINT('Ctrl Pts',(-19.1842470541687,-59.6595122814308,
39.9352519465097));
#189574=CARTESIAN_POINT('Ctrl Pts',(-19.1808295835784,-59.6489943884563,
39.92499));
#189575=CARTESIAN_POINT('Ctrl Pts',(-18.1177524687109,-56.3771794532806,
39.92499));
#189576=CARTESIAN_POINT('Ctrl Pts',(-18.1144819305953,-56.3671137719645,
39.9348107241725));
#189577=CARTESIAN_POINT('Ctrl Pts',(-18.112017069978,-56.3568263239568,
39.9446038383174));
#189578=CARTESIAN_POINT('Ctrl Pts',(-18.1103629196651,-56.3463749453352,
39.9543158069392));
#189579=CARTESIAN_POINT('Ctrl Pts',(-18.1087656919994,-56.3362832197235,
39.9636935671399));
#189580=CARTESIAN_POINT('Ctrl Pts',(-18.1079242184407,-56.3260373921222,
39.9729968320996));
#189581=CARTESIAN_POINT('Ctrl Pts',(-18.107887916365,-56.315680171984,39.9821731151343));
#189582=CARTESIAN_POINT('Ctrl Pts',(-18.1078535995344,-56.305889355273,
39.9908475764359));
#189583=CARTESIAN_POINT('Ctrl Pts',(-18.1085387949865,-56.2959980926935,
39.9994093733852));
#189584=CARTESIAN_POINT('Ctrl Pts',(-18.1100266905428,-56.2860490151148,
40.0077966115846));
#189585=CARTESIAN_POINT('Ctrl Pts',(-18.1113970173888,-56.2768860815733,
40.0155211172598));
#189586=CARTESIAN_POINT('Ctrl Pts',(-18.1134483398646,-56.2676735798215,
40.0230979941022));
#189587=CARTESIAN_POINT('Ctrl Pts',(-18.1162805994775,-56.2584600414683,
40.0304554104747));
#189588=CARTESIAN_POINT('Ctrl Pts',(-18.1171251221212,-56.2557127503185,
40.032649243518));
#189589=CARTESIAN_POINT('Ctrl Pts',(-18.1180393245073,-56.2529655048685,
40.034823371506));
#189590=CARTESIAN_POINT('Ctrl Pts',(-18.1190265064342,-56.2502199893831,
40.0369753512356));
#189591=CARTESIAN_POINT('Ctrl Pts',(-18.1200036017944,-56.2475025263005,
40.0391053430352));
#189592=CARTESIAN_POINT('Ctrl Pts',(-18.1210509212418,-56.2447894850829,
40.041211089324));
#189593=CARTESIAN_POINT('Ctrl Pts',(-18.1221702476366,-56.242085504679,
40.0432881154904));
#189594=CARTESIAN_POINT('Ctrl Pts',(-18.1222480834051,-56.2418974751698,
40.043432547828));
#189595=CARTESIAN_POINT('Ctrl Pts',(-18.12232625961,-56.241709480363,40.0435768364421));
#189596=CARTESIAN_POINT('Ctrl Pts',(-18.1224047773506,-56.2415215209613,
40.0437209807855));
#189597=CARTESIAN_POINT('Ctrl Pts',(-18.1258472827276,-56.2332806922381,
40.050040796842));
#189598=CARTESIAN_POINT('Ctrl Pts',(-18.1299826829657,-56.2251347899177,
40.0560490279345));
#189599=CARTESIAN_POINT('Ctrl Pts',(-18.1348427679841,-56.2171955585584,
40.0616647108615));
#189600=CARTESIAN_POINT('Ctrl Pts',(-18.1393732118983,-56.2097948151026,
40.0668995033485));
#189601=CARTESIAN_POINT('Ctrl Pts',(-18.1445340001509,-56.2025731376012,
40.0717933267481));
#189602=CARTESIAN_POINT('Ctrl Pts',(-18.15036265431,-56.1956479299631,40.0762460303071));
#189603=CARTESIAN_POINT('Ctrl Pts',(-18.1524948514082,-56.193114599416,
40.0778748868747));
#189604=CARTESIAN_POINT('Ctrl Pts',(-18.1547164978841,-56.1906212529492,
40.0794443522247));
#189605=CARTESIAN_POINT('Ctrl Pts',(-18.1570296338739,-56.1881748397224,
40.0809482021492));
#189606=CARTESIAN_POINT('Ctrl Pts',(-18.1575858658044,-56.1875865590688,
40.0813098278168));
#189607=CARTESIAN_POINT('Ctrl Pts',(-18.1581479603548,-56.1870008763867,
40.0816679525672));
#189608=CARTESIAN_POINT('Ctrl Pts',(-18.1587158783115,-56.1864179215671,
40.082022419258));
#189609=CARTESIAN_POINT('Ctrl Pts',(-18.159266048832,-56.1858531840857,
40.0823658088648));
#189610=CARTESIAN_POINT('Ctrl Pts',(-18.1598216844587,-56.1852910066465,
40.0827057654616));
#189611=CARTESIAN_POINT('Ctrl Pts',(-18.1603827459286,-56.1847315084904,
40.0830421470151));
#189612=CARTESIAN_POINT('Ctrl Pts',(-18.166529822736,-56.1786015595924,
40.0867275956806));
#189613=CARTESIAN_POINT('Ctrl Pts',(-18.1733325302114,-56.1727894828607,
40.0899823432031));
#189614=CARTESIAN_POINT('Ctrl Pts',(-18.1807122308852,-56.1674665972289,
40.0926299529356));
#189615=CARTESIAN_POINT('Ctrl Pts',(-18.1837728127199,-56.1652590378992,
40.0937279956085));
#189616=CARTESIAN_POINT('Ctrl Pts',(-18.1869322368375,-56.1631354730306,
40.0947220371803));
#189617=CARTESIAN_POINT('Ctrl Pts',(-18.1901833857455,-56.1611070880438,
40.0956014538692));
#189618=CARTESIAN_POINT('Ctrl Pts',(-18.1957285590018,-56.157647466076,
40.097101390674));
#189619=CARTESIAN_POINT('Ctrl Pts',(-18.2015400422205,-56.1544671656477,
40.0982667904316));
#189620=CARTESIAN_POINT('Ctrl Pts',(-18.2075773774753,-56.1516266854593,
40.0990539325582));
#189621=CARTESIAN_POINT('Ctrl Pts',(-18.2105960451028,-56.1502064453651,
40.0994475036216));
#189622=CARTESIAN_POINT('Ctrl Pts',(-18.2136716866511,-56.1488725139551,
40.0997467259952));
#189623=CARTESIAN_POINT('Ctrl Pts',(-18.2167992197297,-56.1476325143033,
40.0999473488896));
#189624=CARTESIAN_POINT('Ctrl Pts',(-18.2199267528084,-56.1463925146515,
40.100147971784));
#189625=CARTESIAN_POINT('Ctrl Pts',(-18.2231061318822,-56.1452464433751,
40.10025));
#189626=CARTESIAN_POINT('Ctrl Pts',(-18.2263320786585,-56.1441998575527,
40.10025));
#189627=CARTESIAN_POINT('Origin',(-23.7119335237428,-53.2204057122637,39.92499));
#189628=CARTESIAN_POINT('Ctrl Pts',(-25.6588335304443,-57.162321654437,
39.92499));
#189629=CARTESIAN_POINT('Ctrl Pts',(-25.6631491402569,-57.1720146727778,
39.9348354642018));
#189630=CARTESIAN_POINT('Ctrl Pts',(-25.6666871334687,-57.1820194461957,
39.9446440828459));
#189631=CARTESIAN_POINT('Ctrl Pts',(-25.6694381454821,-57.1922776320705,
39.9543641760333));
#189632=CARTESIAN_POINT('Ctrl Pts',(-25.6720997659863,-57.2022024879878,
39.9637684240715));
#189633=CARTESIAN_POINT('Ctrl Pts',(-25.6740249857412,-57.2123658169602,
39.97309096364));
#189634=CARTESIAN_POINT('Ctrl Pts',(-25.6751616470871,-57.2227298227164,
39.9822808977145));
#189635=CARTESIAN_POINT('Ctrl Pts',(-25.6762368587287,-57.2325335339832,
39.9909740094656));
#189636=CARTESIAN_POINT('Ctrl Pts',(-25.676606572923,-57.2425177322905,
39.9995492765009));
#189637=CARTESIAN_POINT('Ctrl Pts',(-25.6761845643574,-57.2526488462847,
40.0079462328703));
#189638=CARTESIAN_POINT('Ctrl Pts',(-25.6757958639481,-57.2619803349743,
40.01568043697));
#189639=CARTESIAN_POINT('Ctrl Pts',(-25.6747354076183,-57.2714370189567,
40.0232638017433));
#189640=CARTESIAN_POINT('Ctrl Pts',(-25.6728992535086,-57.2809814365677,
40.0306257269979));
#189641=CARTESIAN_POINT('Ctrl Pts',(-25.672366654999,-57.2837499093055,
40.032761141666));
#189642=CARTESIAN_POINT('Ctrl Pts',(-25.6717685445831,-57.2865256584302,
40.0348777427275));
#189643=CARTESIAN_POINT('Ctrl Pts',(-25.6711017521907,-57.2893074725859,
40.0369733168701));
#189644=CARTESIAN_POINT('Ctrl Pts',(-25.6703789063664,-57.2923231379855,
40.039245053974));
#189645=CARTESIAN_POINT('Ctrl Pts',(-25.6695773996876,-57.2953419866642,
40.041487875195));
#189646=CARTESIAN_POINT('Ctrl Pts',(-25.6686939261489,-57.2983617649663,
40.0436985701601));
#189647=CARTESIAN_POINT('Ctrl Pts',(-25.6662692260896,-57.3066495702122,
40.0497658398386));
#189648=CARTESIAN_POINT('Ctrl Pts',(-25.6631888860747,-57.3149216961105,
40.0555581699984));
#189649=CARTESIAN_POINT('Ctrl Pts',(-25.6594348051809,-57.3230760282579,
40.0609828468886));
#189650=CARTESIAN_POINT('Ctrl Pts',(-25.656000024977,-57.3305367994636,
40.0659461317303));
#189651=CARTESIAN_POINT('Ctrl Pts',(-25.651996242513,-57.3378885241126,
40.0706039980704));
#189652=CARTESIAN_POINT('Ctrl Pts',(-25.6473759219982,-57.3450563828663,
40.07488431806));
#189653=CARTESIAN_POINT('Ctrl Pts',(-25.645106435654,-57.3485772116716,
40.0769867972568));
#189654=CARTESIAN_POINT('Ctrl Pts',(-25.6426878935085,-57.352053267206,
40.0789976708174));
#189655=CARTESIAN_POINT('Ctrl Pts',(-25.6401130415749,-57.355472752128,
40.08090504915));
#189656=CARTESIAN_POINT('Ctrl Pts',(-25.6396244884999,-57.3561215660857,
40.0812669556105));
#189657=CARTESIAN_POINT('Ctrl Pts',(-25.6391297826974,-57.3567684269676,
40.0816253922032));
#189658=CARTESIAN_POINT('Ctrl Pts',(-25.6386289474846,-57.3574131967121,
40.0819801989139));
#189659=CARTESIAN_POINT('Ctrl Pts',(-25.6381437633721,-57.3580378174021,
40.0823239179149));
#189660=CARTESIAN_POINT('Ctrl Pts',(-25.637652826975,-57.358660475599,40.0826642303498));
#189661=CARTESIAN_POINT('Ctrl Pts',(-25.6371561630117,-57.3592810442414,
40.0830009916099));
#189662=CARTESIAN_POINT('Ctrl Pts',(-25.6317436214791,-57.3660438734349,
40.0866709464313));
#189663=CARTESIAN_POINT('Ctrl Pts',(-25.6256469885827,-57.3725627409497,
40.0899175831879));
#189664=CARTESIAN_POINT('Ctrl Pts',(-25.6189233999291,-57.3786559602408,
40.0925642067064));
#189665=CARTESIAN_POINT('Ctrl Pts',(-25.6160839866894,-57.3812291645843,
40.0936818922529));
#189666=CARTESIAN_POINT('Ctrl Pts',(-25.6131331854691,-57.3837265592144,
40.0946930094791));
#189667=CARTESIAN_POINT('Ctrl Pts',(-25.6100770039414,-57.3861353831631,
40.0955863397546));
#189668=CARTESIAN_POINT('Ctrl Pts',(-25.6049304706141,-57.3901917825029,
40.0970906856166));
#189669=CARTESIAN_POINT('Ctrl Pts',(-25.5994853721131,-57.3939944983913,
40.0982599215483));
#189670=CARTESIAN_POINT('Ctrl Pts',(-25.5937750303535,-57.3974772155317,
40.0990497370454));
#189671=CARTESIAN_POINT('Ctrl Pts',(-25.5923474449136,-57.3983478948168,
40.0992471909196));
#189672=CARTESIAN_POINT('Ctrl Pts',(-25.5909031732847,-57.3991983668806,
40.0994209989363));
#189673=CARTESIAN_POINT('Ctrl Pts',(-25.5894426040348,-57.4000273167772,
40.0995705982975));
#189674=CARTESIAN_POINT('Ctrl Pts',(-25.58725175016,-57.4012707416221,40.0997949973393));
#189675=CARTESIAN_POINT('Ctrl Pts',(-25.585024235439,-57.4024657229512,
40.0999649129781));
#189676=CARTESIAN_POINT('Ctrl Pts',(-25.5827620706102,-57.4036093482798,
40.1000786629733));
#189677=CARTESIAN_POINT('Ctrl Pts',(-25.5804999057814,-57.4047529736084,
40.1001924129685));
#189678=CARTESIAN_POINT('Ctrl Pts',(-25.578203101074,-57.4058452484211,
40.10025));
#189679=CARTESIAN_POINT('Ctrl Pts',(-25.5758735661218,-57.4068835917994,
40.10025));
#189680=CARTESIAN_POINT('Ctrl Pts',(-24.0229981225299,-53.9190682401994,
40.10025));
#189681=CARTESIAN_POINT('Ctrl Pts',(-24.0308804555189,-53.9155545931357,
40.10025));
#189682=CARTESIAN_POINT('Ctrl Pts',(-24.0389845034721,-53.9127220553015,
40.0995786334241));
#189683=CARTESIAN_POINT('Ctrl Pts',(-24.0471612846382,-53.9105453488013,
40.0983063763366));
#189684=CARTESIAN_POINT('Ctrl Pts',(-24.0524426462853,-53.9091394197452,
40.0974846287992));
#189685=CARTESIAN_POINT('Ctrl Pts',(-24.0577541205276,-53.9080061861137,
40.0964130309338));
#189686=CARTESIAN_POINT('Ctrl Pts',(-24.0630550795263,-53.9071299964541,
40.0951176960924));
#189687=CARTESIAN_POINT('Ctrl Pts',(-24.0700811970213,-53.9059686572514,
40.0934008039614));
#189688=CARTESIAN_POINT('Ctrl Pts',(-24.0770886066608,-53.9052646847385,
40.0912909372156));
#189689=CARTESIAN_POINT('Ctrl Pts',(-24.0839917000394,-53.9049900928804,
40.0888630467851));
#189690=CARTESIAN_POINT('Ctrl Pts',(-24.0874432467287,-53.9048527969513,
40.0876491015699));
#189691=CARTESIAN_POINT('Ctrl Pts',(-24.0908688957001,-53.9048227635322,
40.0863558569271));
#189692=CARTESIAN_POINT('Ctrl Pts',(-24.0942592346731,-53.9048959123382,
40.0849936342771));
#189693=CARTESIAN_POINT('Ctrl Pts',(-24.0959544041596,-53.9049324867412,
40.0843125229521));
#189694=CARTESIAN_POINT('Ctrl Pts',(-24.0976407611372,-53.9049948499727,
40.0836141747074));
#189695=CARTESIAN_POINT('Ctrl Pts',(-24.099317223136,-53.9050824496421,
40.0828999161609));
#189696=CARTESIAN_POINT('Ctrl Pts',(-24.0997363386357,-53.9051043495594,
40.0827213515243));
#189697=CARTESIAN_POINT('Ctrl Pts',(-24.1001548360176,-53.9051278266101,
40.0825417925842));
#189698=CARTESIAN_POINT('Ctrl Pts',(-24.1005726990102,-53.9051528718722,
40.082361260236));
#189699=CARTESIAN_POINT('Ctrl Pts',(-24.1018262879881,-53.9052280076584,
40.0818196631917));
#189700=CARTESIAN_POINT('Ctrl Pts',(-24.1030741658758,-53.9053172580726,
40.0812693052021));
#189701=CARTESIAN_POINT('Ctrl Pts',(-24.1043159075202,-53.9054203757496,
40.0807107531875));
#189702=CARTESIAN_POINT('Ctrl Pts',(-24.1130625753257,-53.9061467233509,
40.0767763849182));
#189703=CARTESIAN_POINT('Ctrl Pts',(-24.1215389842443,-53.9075195712148,
40.0724140586139));
#189704=CARTESIAN_POINT('Ctrl Pts',(-24.1297041260866,-53.9094265129029,
40.067722122377));
#189705=CARTESIAN_POINT('Ctrl Pts',(-24.133664211057,-53.9103513775611,
40.0654465383722));
#189706=CARTESIAN_POINT('Ctrl Pts',(-24.1375513523935,-53.9114023832599,
40.063092800068));
#189707=CARTESIAN_POINT('Ctrl Pts',(-24.1413619171793,-53.912569370107,
40.0606689262479));
#189708=CARTESIAN_POINT('Ctrl Pts',(-24.1471956256297,-53.9143559454349,
40.0569581447806));
#189709=CARTESIAN_POINT('Ctrl Pts',(-24.1528469606267,-53.9164123347819,
40.0530843804605));
#189710=CARTESIAN_POINT('Ctrl Pts',(-24.1582902100542,-53.9187002605238,
40.0490800251458));
#189711=CARTESIAN_POINT('Ctrl Pts',(-24.1608180832479,-53.9197627850744,
40.0472203818218));
#189712=CARTESIAN_POINT('Ctrl Pts',(-24.1633010951265,-53.9208749910657,
40.0453323608818));
#189713=CARTESIAN_POINT('Ctrl Pts',(-24.1657359576696,-53.9220340502326,
40.0434201572162));
#189714=CARTESIAN_POINT('Ctrl Pts',(-24.1659225802897,-53.9221228875508,
40.0432735943397));
#189715=CARTESIAN_POINT('Ctrl Pts',(-24.1661089452649,-53.9222119774186,
40.0431268995707));
#189716=CARTESIAN_POINT('Ctrl Pts',(-24.1662950522344,-53.9223013184209,
40.0429800745037));
#189717=CARTESIAN_POINT('Ctrl Pts',(-24.1689092940617,-53.9235562901481,
40.0409176249753));
#189718=CARTESIAN_POINT('Ctrl Pts',(-24.1714718460793,-53.9248627542249,
40.0388310783332));
#189719=CARTESIAN_POINT('Ctrl Pts',(-24.1739808617162,-53.9262153118347,
40.036725739981));
#189720=CARTESIAN_POINT('Ctrl Pts',(-24.1829777455758,-53.9310653428791,
40.0291763710723));
#189721=CARTESIAN_POINT('Ctrl Pts',(-24.1913567365385,-53.936543815756,
40.0213310894606));
#189722=CARTESIAN_POINT('Ctrl Pts',(-24.199150894752,-53.9425259106368,
40.0132837551337));
#189723=CARTESIAN_POINT('Ctrl Pts',(-24.2077158916356,-53.9490996319559,
40.0044405431351));
#189724=CARTESIAN_POINT('Ctrl Pts',(-24.2155752681635,-53.9562817849744,
39.9953528710637));
#189725=CARTESIAN_POINT('Ctrl Pts',(-24.222754058489,-53.9639562340105,
39.9861103629602));
#189726=CARTESIAN_POINT('Ctrl Pts',(-24.2305053504095,-53.9722427129451,
39.9761307737619));
#189727=CARTESIAN_POINT('Ctrl Pts',(-24.2374640812876,-53.9811038680413,
39.9659696936093));
#189728=CARTESIAN_POINT('Ctrl Pts',(-24.2436285779068,-53.9904403792073,
39.9557128217605));
#189729=CARTESIAN_POINT('Ctrl Pts',(-24.2497413607364,-53.9996985666423,
39.9455419945227));
#189730=CARTESIAN_POINT('Ctrl Pts',(-24.2550737197492,-54.0094254978869,
39.9352756289374));
#189731=CARTESIAN_POINT('Ctrl Pts',(-24.2595822759735,-54.019551880964,
39.92499));
#189732=CARTESIAN_POINT('Origin',(0.0139224327744811,-0.00619866644047012,
39.92499));
#189733=CARTESIAN_POINT('Ctrl Pts',(-25.5480287005721,-57.4192809246788,
40.10025));
#189734=CARTESIAN_POINT('Ctrl Pts',(-25.5401808584716,-57.4227710771205,
40.10025));
#189735=CARTESIAN_POINT('Ctrl Pts',(-25.5321112063496,-57.4255746438789,
40.0995859581841));
#189736=CARTESIAN_POINT('Ctrl Pts',(-25.5239679177294,-57.4277200319917,
40.0983275959618));
#189737=CARTESIAN_POINT('Ctrl Pts',(-25.5187647439654,-57.4290908328638,
40.0975235624066));
#189738=CARTESIAN_POINT('Ctrl Pts',(-25.5135317242463,-57.4301938346426,
40.0964777059489));
#189739=CARTESIAN_POINT('Ctrl Pts',(-25.5083079410949,-57.431045032104,
40.0952149915961));
#189740=CARTESIAN_POINT('Ctrl Pts',(-25.5011785252534,-57.4322067458447,
40.0934916398701));
#189741=CARTESIAN_POINT('Ctrl Pts',(-25.4940667032539,-57.4328933558606,
40.091364392163));
#189742=CARTESIAN_POINT('Ctrl Pts',(-25.4870628291426,-57.4331362848727,
40.0889118607713));
#189743=CARTESIAN_POINT('Ctrl Pts',(-25.483560892087,-57.4332577493787,
40.0876855950754));
#189744=CARTESIAN_POINT('Ctrl Pts',(-25.4800857520064,-57.433268380324,
40.0863782327527));
#189745=CARTESIAN_POINT('Ctrl Pts',(-25.4766473428561,-57.4331727200757,
40.0850006373334));
#189746=CARTESIAN_POINT('Ctrl Pts',(-25.4749281382809,-57.4331248899516,
40.0843118396238));
#189747=CARTESIAN_POINT('Ctrl Pts',(-25.4732181005507,-57.4330504941581,
40.0836054919165));
#189748=CARTESIAN_POINT('Ctrl Pts',(-25.4715183716227,-57.4329501454093,
40.0828829920418));
#189749=CARTESIAN_POINT('Ctrl Pts',(-25.4710934393907,-57.4329250582221,
40.0827023670731));
#189750=CARTESIAN_POINT('Ctrl Pts',(-25.4706691511208,-57.4328983491281,
40.0825207326933));
#189751=CARTESIAN_POINT('Ctrl Pts',(-25.4702455239745,-57.4328700280095,
40.0823381109276));
#189752=CARTESIAN_POINT('Ctrl Pts',(-25.4689746425358,-57.4327850646537,
40.0817902456304));
#189753=CARTESIAN_POINT('Ctrl Pts',(-25.4677097128937,-57.432685592307,
40.0812334935553));
#189754=CARTESIAN_POINT('Ctrl Pts',(-25.4664511833529,-57.4325718846636,
40.0806684524227));
#189755=CARTESIAN_POINT('Ctrl Pts',(-25.4577539633643,-57.4317860942975,
40.0767636676136));
#189756=CARTESIAN_POINT('Ctrl Pts',(-25.4493260998444,-57.430362755973,
40.0724404510885));
#189757=CARTESIAN_POINT('Ctrl Pts',(-25.4412057723272,-57.4284143577087,
40.0677949937404));
#189758=CARTESIAN_POINT('Ctrl Pts',(-25.4371699918414,-57.4274460091197,
40.0654862141902));
#189759=CARTESIAN_POINT('Ctrl Pts',(-25.4332098968694,-57.4263474236137,
40.0630972003214));
#189760=CARTESIAN_POINT('Ctrl Pts',(-25.4293290842281,-57.4251294472436,
40.0606363359906));
#189761=CARTESIAN_POINT('Ctrl Pts',(-25.4207674318877,-57.4224424094496,
40.0552073017123));
#189762=CARTESIAN_POINT('Ctrl Pts',(-25.4125888532393,-57.4191864212928,
40.0494204304519));
#189763=CARTESIAN_POINT('Ctrl Pts',(-25.4048965980306,-57.415463789604,
40.0434049749851));
#189764=CARTESIAN_POINT('Ctrl Pts',(-25.4020865201984,-57.4141038653032,
40.0412074532442));
#189765=CARTESIAN_POINT('Ctrl Pts',(-25.3993352917243,-57.4126868351394,
40.0389814735788));
#189766=CARTESIAN_POINT('Ctrl Pts',(-25.3966436944401,-57.411217955737,
40.0367321210016));
#189767=CARTESIAN_POINT('Ctrl Pts',(-25.3876029039784,-57.4062841452559,
40.029176783714));
#189768=CARTESIAN_POINT('Ctrl Pts',(-25.3791816069561,-57.400726683699,
40.0213235332575));
#189769=CARTESIAN_POINT('Ctrl Pts',(-25.3713475726781,-57.3946697603108,
40.0132649215857));
#189770=CARTESIAN_POINT('Ctrl Pts',(-25.3627370410041,-57.3880124840173,
40.0044075527531));
#189771=CARTESIAN_POINT('Ctrl Pts',(-25.3548353295677,-57.3807515434767,
39.9953016253717));
#189772=CARTESIAN_POINT('Ctrl Pts',(-25.347618881505,-57.3730023605534,
39.9860353422355));
#189773=CARTESIAN_POINT('Ctrl Pts',(-25.3398464577412,-57.3646561585189,
39.9760551582691));
#189774=CARTESIAN_POINT('Ctrl Pts',(-25.3328680394184,-57.3557428147474,
39.9658879738151));
#189775=CARTESIAN_POINT('Ctrl Pts',(-25.3266878999862,-57.3463604602068,
39.9556174643249));
#189776=CARTESIAN_POINT('Ctrl Pts',(-25.3205912133029,-57.337104799131,
39.9454856413901));
#189777=CARTESIAN_POINT('Ctrl Pts',(-25.3152708796015,-57.3273913673577,
39.9352519465112));
#189778=CARTESIAN_POINT('Ctrl Pts',(-25.3107727110825,-57.3172883154489,
39.92499));
#189779=CARTESIAN_POINT('Ctrl Pts',(-23.9115214566117,-54.1745185419759,
39.92499));
#189780=CARTESIAN_POINT('Ctrl Pts',(-23.9072166846462,-54.1648498658381,
39.9348107241728));
#189781=CARTESIAN_POINT('Ctrl Pts',(-23.903689995662,-54.1548764216391,
39.9446038383182));
#189782=CARTESIAN_POINT('Ctrl Pts',(-23.9009524404112,-54.1446552025529,
39.9543158069403));
#189783=CARTESIAN_POINT('Ctrl Pts',(-23.8983090899558,-54.134785716223,
39.9636935671413));
#189784=CARTESIAN_POINT('Ctrl Pts',(-23.8964012454632,-54.124683974275,
39.9729968321014));
#189785=CARTESIAN_POINT('Ctrl Pts',(-23.8952825179495,-54.1143872866722,
39.9821731151364));
#189786=CARTESIAN_POINT('Ctrl Pts',(-23.8942249700852,-54.1046536921647,
39.9908475764383));
#189787=CARTESIAN_POINT('Ctrl Pts',(-23.8938724934878,-54.0947449925285,
39.9994093733879));
#189788=CARTESIAN_POINT('Ctrl Pts',(-23.8943122764065,-54.0846948896014,
40.0077966115876));
#189789=CARTESIAN_POINT('Ctrl Pts',(-23.8947173090968,-54.0754389134087,
40.015521117263));
#189790=CARTESIAN_POINT('Ctrl Pts',(-23.8957944255627,-54.0660624571189,
40.0230979941058));
#189791=CARTESIAN_POINT('Ctrl Pts',(-23.8976480927561,-54.0566033397473,
40.0304554104785));
#189792=CARTESIAN_POINT('Ctrl Pts',(-23.8982008188942,-54.0537828218934,
40.0326492435205));
#189793=CARTESIAN_POINT('Ctrl Pts',(-23.8988228478386,-54.0509550659726,
40.0348233715073));
#189794=CARTESIAN_POINT('Ctrl Pts',(-23.8995176373646,-54.0481214021002,
40.0369753512356));
#189795=CARTESIAN_POINT('Ctrl Pts',(-23.9002053278541,-54.0453166912882,
40.0391053430352));
#189796=CARTESIAN_POINT('Ctrl Pts',(-23.9009633199468,-54.0425090377019,
40.041211089324));
#189797=CARTESIAN_POINT('Ctrl Pts',(-23.9017938716382,-54.0397028685176,
40.0432881154904));
#189798=CARTESIAN_POINT('Ctrl Pts',(-23.9018516265785,-54.0395077330005,
40.043432547828));
#189799=CARTESIAN_POINT('Ctrl Pts',(-23.9019097237178,-54.0393125964103,
40.0435768364421));
#189800=CARTESIAN_POINT('Ctrl Pts',(-23.9019681642225,-54.0391174593311,
40.0437209807855));
#189801=CARTESIAN_POINT('Ctrl Pts',(-23.9045304100324,-54.0305619349332,
40.050040796842));
#189802=CARTESIAN_POINT('Ctrl Pts',(-23.9077916774637,-54.0220283896862,
40.0560490279344));
#189803=CARTESIAN_POINT('Ctrl Pts',(-23.9117952627744,-54.0136246330487,
40.0616647108614));
#189804=CARTESIAN_POINT('Ctrl Pts',(-23.9155273001023,-54.0057908712996,
40.0668995033484));
#189805=CARTESIAN_POINT('Ctrl Pts',(-23.9199049461654,-53.9980693056379,
40.0717933267479));
#189806=CARTESIAN_POINT('Ctrl Pts',(-23.9249777890349,-53.9905727747497,
40.076246030307));
#189807=CARTESIAN_POINT('Ctrl Pts',(-23.9268335005852,-53.9878304467662,
40.0778748868746));
#189808=CARTESIAN_POINT('Ctrl Pts',(-23.9287823509748,-53.9851185338202,
40.0794443522247));
#189809=CARTESIAN_POINT('Ctrl Pts',(-23.9308270955486,-53.9824437337506,
40.0809482021492));
#189810=CARTESIAN_POINT('Ctrl Pts',(-23.9313187883097,-53.9818005336911,
40.0813098278168));
#189811=CARTESIAN_POINT('Ctrl Pts',(-23.9318165831366,-53.9811593045603,
40.0816679525672));
#189812=CARTESIAN_POINT('Ctrl Pts',(-23.9323204546079,-53.980520179637,
40.082022419258));
#189813=CARTESIAN_POINT('Ctrl Pts',(-23.9328085800956,-53.9799010273675,
40.0823658088648));
#189814=CARTESIAN_POINT('Ctrl Pts',(-23.9333024083484,-53.979283849857,
40.0827057654616));
#189815=CARTESIAN_POINT('Ctrl Pts',(-23.9338019127824,-53.978668769797,
40.0830421470151));
#189816=CARTESIAN_POINT('Ctrl Pts',(-23.9392745611216,-53.9719298569083,
40.0867275956806));
#189817=CARTESIAN_POINT('Ctrl Pts',(-23.9454324752044,-53.9654385427828,
40.089982343203));
#189818=CARTESIAN_POINT('Ctrl Pts',(-23.9522153560504,-53.9593734277047,
40.0926299529355));
#189819=CARTESIAN_POINT('Ctrl Pts',(-23.9550284189133,-53.9568580437,40.0937279956084));
#189820=CARTESIAN_POINT('Ctrl Pts',(-23.9579485624028,-53.954415862194,
40.0947220371802));
#189821=CARTESIAN_POINT('Ctrl Pts',(-23.9609698772114,-53.9520587513131,
40.0956014538692));
#189822=CARTESIAN_POINT('Ctrl Pts',(-23.9661230444607,-53.9480384530774,
40.097101390674));
#189823=CARTESIAN_POINT('Ctrl Pts',(-23.9715702598497,-53.9442681092574,
40.0982667904316));
#189824=CARTESIAN_POINT('Ctrl Pts',(-23.9772776109213,-53.9408121161403,
40.0990539325582));
#189825=CARTESIAN_POINT('Ctrl Pts',(-23.9801312864571,-53.9390841195818,
40.0994475036216));
#189826=CARTESIAN_POINT('Ctrl Pts',(-23.9830506455188,-53.937436003503,
40.0997467259952));
#189827=CARTESIAN_POINT('Ctrl Pts',(-23.986031430386,-53.9358758804725,
40.0999473488896));
#189828=CARTESIAN_POINT('Ctrl Pts',(-23.9890122152531,-53.934315757442,
40.100147971784));
#189829=CARTESIAN_POINT('Ctrl Pts',(-23.9920543802864,-53.9328436288552,
40.10025));
#189830=CARTESIAN_POINT('Ctrl Pts',(-23.995153256981,-53.9314655730803,
40.10025));
#189831=CARTESIAN_POINT('Origin',(-29.1450842944632,-50.4502867888874,39.92499));
#189832=CARTESIAN_POINT('Ctrl Pts',(-31.4933613949861,-54.1671020372437,
39.92499));
#189833=CARTESIAN_POINT('Ctrl Pts',(-31.4986665597482,-54.1762908521541,
39.9348354642018));
#189834=CARTESIAN_POINT('Ctrl Pts',(-31.5032309550537,-54.1858709973829,
39.9446440828459));
#189835=CARTESIAN_POINT('Ctrl Pts',(-31.5070391691409,-54.195785428784,
39.9543641760333));
#189836=CARTESIAN_POINT('Ctrl Pts',(-31.5107236389468,-54.2053777002011,
39.9637684240715));
#189837=CARTESIAN_POINT('Ctrl Pts',(-31.5137006693055,-54.2152841131315,
39.97309096364));
#189838=CARTESIAN_POINT('Ctrl Pts',(-31.5159144374966,-54.2254725303162,
39.9822808977146));
#189839=CARTESIAN_POINT('Ctrl Pts',(-31.5180085258894,-54.2351101456063,
39.9909740094657));
#189840=CARTESIAN_POINT('Ctrl Pts',(-31.5194198476566,-54.245001003774,
39.999549276501));
#189841=CARTESIAN_POINT('Ctrl Pts',(-31.5200591406751,-54.2551207303727,
40.0079462328705));
#189842=CARTESIAN_POINT('Ctrl Pts',(-31.5206479757801,-54.2644417304473,
40.0156804369702));
#189843=CARTESIAN_POINT('Ctrl Pts',(-31.5205818213852,-54.2739574575959,
40.0232638017436));
#189844=CARTESIAN_POINT('Ctrl Pts',(-31.5197533892255,-54.283641520256,
40.0306257269981));
#189845=CARTESIAN_POINT('Ctrl Pts',(-31.5195130925471,-54.2864504987141,
40.0327611416661));
#189846=CARTESIAN_POINT('Ctrl Pts',(-31.5192084034331,-54.2892735615571,
40.0348777427276));
#189847=CARTESIAN_POINT('Ctrl Pts',(-31.518836042558,-54.2921098354278,
40.0369733168701));
#189848=CARTESIAN_POINT('Ctrl Pts',(-31.5184323794287,-54.29518453866,40.039245053974));
#189849=CARTESIAN_POINT('Ctrl Pts',(-31.5179508191006,-54.2982706300313,
40.041487875195));
#189850=CARTESIAN_POINT('Ctrl Pts',(-31.5173878381078,-54.3013662138032,
40.0436985701601));
#189851=CARTESIAN_POINT('Ctrl Pts',(-31.5158427323552,-54.3098620677558,
40.0497658398386));
#189852=CARTESIAN_POINT('Ctrl Pts',(-31.5136439393734,-54.3184108612911,
40.0555581699984));
#189853=CARTESIAN_POINT('Ctrl Pts',(-31.5107627835359,-54.3269129314606,
40.0609828468886));
#189854=CARTESIAN_POINT('Ctrl Pts',(-31.508126682366,-54.3346918640779,
40.0659461317307));
#189855=CARTESIAN_POINT('Ctrl Pts',(-31.504913297521,-54.3424218244388,
40.0706039980711));
#189856=CARTESIAN_POINT('Ctrl Pts',(-31.5010675328654,-54.350033371916,
40.0748843180609));
#189857=CARTESIAN_POINT('Ctrl Pts',(-31.4991785058296,-54.3537721391722,
40.0769867972573));
#189858=CARTESIAN_POINT('Ctrl Pts',(-31.4971365594545,-54.3574819590039,
40.0789976708176));
#189859=CARTESIAN_POINT('Ctrl Pts',(-31.4949332463336,-54.361151856945,
40.08090504915));
#189860=CARTESIAN_POINT('Ctrl Pts',(-31.4945151891294,-54.361848184334,
40.0812669556105));
#189861=CARTESIAN_POINT('Ctrl Pts',(-31.494090808751,-54.3625432124816,
40.0816253922033));
#189862=CARTESIAN_POINT('Ctrl Pts',(-31.4936601139564,-54.3632368016452,
40.0819801989139));
#189863=CARTESIAN_POINT('Ctrl Pts',(-31.4932428783741,-54.3639087161473,
40.0823239179149));
#189864=CARTESIAN_POINT('Ctrl Pts',(-31.4928197168825,-54.3645792801847,
40.0826642303498));
#189865=CARTESIAN_POINT('Ctrl Pts',(-31.4923906407828,-54.3652483648079,
40.0830009916099));
#189866=CARTESIAN_POINT('Ctrl Pts',(-31.4877146578622,-54.372539911164,
40.0866709464311));
#189867=CARTESIAN_POINT('Ctrl Pts',(-31.4823328301626,-54.379660339308,
40.0899175831876));
#189868=CARTESIAN_POINT('Ctrl Pts',(-31.4762829888802,-54.3864229856956,
40.092564206706));
#189869=CARTESIAN_POINT('Ctrl Pts',(-31.4737281033389,-54.3892788932593,
40.0936818922527));
#189870=CARTESIAN_POINT('Ctrl Pts',(-31.471054515739,-54.3920710496175,
40.094693009479));
#189871=CARTESIAN_POINT('Ctrl Pts',(-31.4682668669588,-54.3947861357354,
40.0955863397546));
#189872=CARTESIAN_POINT('Ctrl Pts',(-31.4635725360689,-54.3993582729151,
40.0970906856166));
#189873=CARTESIAN_POINT('Ctrl Pts',(-31.4585547584353,-54.4037093249066,
40.0982599215483));
#189874=CARTESIAN_POINT('Ctrl Pts',(-31.4532397415957,-54.4077698566064,
40.0990497370454));
#189875=CARTESIAN_POINT('Ctrl Pts',(-31.4519109873858,-54.4087849895313,
40.0992471909196));
#189876=CARTESIAN_POINT('Ctrl Pts',(-31.4505635261659,-54.4097817701142,
40.0994209989363));
#189877=CARTESIAN_POINT('Ctrl Pts',(-31.449197606926,-54.4107588499957,
40.0995705982975));
#189878=CARTESIAN_POINT('Ctrl Pts',(-31.4471487280663,-54.412224469818,
40.0997949973393));
#189879=CARTESIAN_POINT('Ctrl Pts',(-31.445058325466,-54.4136457436053,
40.0999649129781));
#189880=CARTESIAN_POINT('Ctrl Pts',(-31.442928094411,-54.4150195646479,
40.1000786629733));
#189881=CARTESIAN_POINT('Ctrl Pts',(-31.4407978633561,-54.4163933856906,
40.1001924129685));
#189882=CARTESIAN_POINT('Ctrl Pts',(-31.438627814593,-54.4177197583743,
40.10025));
#189883=CARTESIAN_POINT('Ctrl Pts',(-31.4364195775146,-54.4189959163077,
40.10025));
#189884=CARTESIAN_POINT('Ctrl Pts',(-29.5274749692187,-51.1126068659045,
40.10025));
#189885=CARTESIAN_POINT('Ctrl Pts',(-29.5349468458348,-51.1082885388128,
40.10025));
#189886=CARTESIAN_POINT('Ctrl Pts',(-29.5427104181385,-51.1046244142385,
40.0995786334241));
#189887=CARTESIAN_POINT('Ctrl Pts',(-29.5506148782564,-51.1016049255944,
40.0983063763366));
#189888=CARTESIAN_POINT('Ctrl Pts',(-29.555720348448,-51.0996546457479,
40.0974846287992));
#189889=CARTESIAN_POINT('Ctrl Pts',(-29.5608842707087,-51.0979724198486,
40.0964130309338));
#189890=CARTESIAN_POINT('Ctrl Pts',(-29.5660646037406,-51.0965469289496,
40.0951176960924));
#189891=CARTESIAN_POINT('Ctrl Pts',(-29.5729308384267,-51.0946575224201,
40.0934008039614));
#189892=CARTESIAN_POINT('Ctrl Pts',(-29.579826275578,-51.0932249325812,
40.0912909372156));
#189893=CARTESIAN_POINT('Ctrl Pts',(-29.5866628504239,-51.0922302752233,
40.0888630467851));
#189894=CARTESIAN_POINT('Ctrl Pts',(-29.5900811378468,-51.0917329465443,
40.0876491015699));
#189895=CARTESIAN_POINT('Ctrl Pts',(-29.5934848814075,-51.0913449998288,
40.0863558569271));
#189896=CARTESIAN_POINT('Ctrl Pts',(-29.5968642938812,-51.0910633609952,
40.0849936342771));
#189897=CARTESIAN_POINT('Ctrl Pts',(-29.598554000118,-51.0909225415784,
40.0843125229521));
#189898=CARTESIAN_POINT('Ctrl Pts',(-29.6002376377884,-51.0908082908742,
40.0836141747074));
#189899=CARTESIAN_POINT('Ctrl Pts',(-29.6019140726117,-51.090720172667,
40.0828999161609));
#189900=CARTESIAN_POINT('Ctrl Pts',(-29.6023331813176,-51.0906981431152,
40.0827213515243));
#189901=CARTESIAN_POINT('Ctrl Pts',(-29.6027518401471,-51.0906777466679,
40.0825417925842));
#189902=CARTESIAN_POINT('Ctrl Pts',(-29.6031700319853,-51.0906589761529,
40.0823612602361));
#189903=CARTESIAN_POINT('Ctrl Pts',(-29.6044246074998,-51.090602664608,
40.0818196631917));
#189904=CARTESIAN_POINT('Ctrl Pts',(-29.6056749785905,-51.0905609873412,
40.0812693052022));
#189905=CARTESIAN_POINT('Ctrl Pts',(-29.6069206965766,-51.0905337427829,
40.0807107531875));
#189906=CARTESIAN_POINT('Ctrl Pts',(-29.6156953732195,-51.0903418356316,
40.0767763849181));
#189907=CARTESIAN_POINT('Ctrl Pts',(-29.6242688491609,-51.090821136893,
40.0724140586136));
#189908=CARTESIAN_POINT('Ctrl Pts',(-29.6325885911862,-51.091864142426,
40.0677221223767));
#189909=CARTESIAN_POINT('Ctrl Pts',(-29.636623657078,-51.0923699989824,
40.065446538372));
#189910=CARTESIAN_POINT('Ctrl Pts',(-29.6405993642579,-51.0930089302515,
40.0630928000679));
#189911=CARTESIAN_POINT('Ctrl Pts',(-29.6445110377126,-51.0937712117413,
40.0606689262479));
#189912=CARTESIAN_POINT('Ctrl Pts',(-29.6504995364713,-51.0949382114431,
40.0569581447805));
#189913=CARTESIAN_POINT('Ctrl Pts',(-29.6563348640822,-51.0963926103115,
40.0530843804606));
#189914=CARTESIAN_POINT('Ctrl Pts',(-29.6619874481817,-51.098099028059,
40.0490800251458));
#189915=CARTESIAN_POINT('Ctrl Pts',(-29.66461253748,-51.0988914972887,40.0472203818218));
#189916=CARTESIAN_POINT('Ctrl Pts',(-29.6671982043428,-51.0997380650832,
40.0453323608819));
#189917=CARTESIAN_POINT('Ctrl Pts',(-29.6697408831278,-51.1006362623628,
40.0434201572162));
#189918=CARTESIAN_POINT('Ctrl Pts',(-29.669935769438,-51.1007051056452,
40.0432735943397));
#189919=CARTESIAN_POINT('Ctrl Pts',(-29.6701304259133,-51.1007742270249,
40.0431268995707));
#189920=CARTESIAN_POINT('Ctrl Pts',(-29.670324852047,-51.1008436251323,
40.0429800745037));
#189921=CARTESIAN_POINT('Ctrl Pts',(-29.6730559530502,-51.1018184593123,
40.0409176249753));
#189922=CARTESIAN_POINT('Ctrl Pts',(-29.675741029822,-51.1028499068177,
40.0388310783332));
#189923=CARTESIAN_POINT('Ctrl Pts',(-29.6783776815771,-51.1039327914266,
40.036725739981));
#189924=CARTESIAN_POINT('Ctrl Pts',(-29.687832245858,-51.1078158230496,
40.0291763710718));
#189925=CARTESIAN_POINT('Ctrl Pts',(-29.6967379921829,-51.1123884412301,
40.0213310894596));
#189926=CARTESIAN_POINT('Ctrl Pts',(-29.7051147523676,-51.1175230541891,
40.0132837551322));
#189927=CARTESIAN_POINT('Ctrl Pts',(-29.7143199702903,-51.1231654780134,
40.004440543133));
#189928=CARTESIAN_POINT('Ctrl Pts',(-29.7228870317498,-51.129486757896,
39.9953528710608));
#189929=CARTESIAN_POINT('Ctrl Pts',(-29.7308286942753,-51.1363687775772,
39.9861103629565));
#189930=CARTESIAN_POINT('Ctrl Pts',(-29.7394036967174,-51.1437996316814,
39.9761307737571));
#189931=CARTESIAN_POINT('Ctrl Pts',(-29.7472505498652,-51.151884858999,
39.9659696936032));
#189932=CARTESIAN_POINT('Ctrl Pts',(-29.7543572078919,-51.1605258584228,
39.9557128217532));
#189933=CARTESIAN_POINT('Ctrl Pts',(-29.7614042483606,-51.169094368741,
39.9455419945178));
#189934=CARTESIAN_POINT('Ctrl Pts',(-29.7677241373264,-51.1782106315433,
39.9352756289349));
#189935=CARTESIAN_POINT('Ctrl Pts',(-29.7732664904682,-51.1878102687783,
39.92499));
#189936=CARTESIAN_POINT('Origin',(0.0131982271536832,-0.00761999999999517,
39.92499));
#189937=CARTESIAN_POINT('Ctrl Pts',(-31.4100231232064,-54.4342359163062,
40.10025));
#189938=CARTESIAN_POINT('Ctrl Pts',(-31.402583092678,-54.438527272202,40.10025));
#189939=CARTESIAN_POINT('Ctrl Pts',(-31.3948506994802,-54.4421589890635,
40.0995859581842));
#189940=CARTESIAN_POINT('Ctrl Pts',(-31.3869762747703,-54.4451438299611,
40.0983275959621));
#189941=CARTESIAN_POINT('Ctrl Pts',(-31.3819448922446,-54.4470510012005,
40.0975235624068));
#189942=CARTESIAN_POINT('Ctrl Pts',(-31.3768558346353,-54.4486949601299,
40.096477705949));
#189943=CARTESIAN_POINT('Ctrl Pts',(-31.3717496422765,-54.450087528668,
40.0952149915961));
#189944=CARTESIAN_POINT('Ctrl Pts',(-31.364780714273,-54.4519881053012,
40.0934916398701));
#189945=CARTESIAN_POINT('Ctrl Pts',(-31.3577796218684,-54.4534143418202,
40.091364392163));
#189946=CARTESIAN_POINT('Ctrl Pts',(-31.3508395087087,-54.4543880442395,
40.0889118607713));
#189947=CARTESIAN_POINT('Ctrl Pts',(-31.3473694521288,-54.4548748954491,
40.0876855950754));
#189948=CARTESIAN_POINT('Ctrl Pts',(-31.3439144604656,-54.4552487192093,
40.0863782327526));
#189949=CARTESIAN_POINT('Ctrl Pts',(-31.3404848880616,-54.4555129946224,
40.0850006373334));
#189950=CARTESIAN_POINT('Ctrl Pts',(-31.3387701018596,-54.455645132329,
40.0843118396237));
#189951=CARTESIAN_POINT('Ctrl Pts',(-31.337061655417,-54.4557498916995,
40.0836054919164));
#189952=CARTESIAN_POINT('Ctrl Pts',(-31.3353607484814,-54.4558277627245,
40.0828829920417));
#189953=CARTESIAN_POINT('Ctrl Pts',(-31.3349355217475,-54.4558472304807,
40.0827023670731));
#189954=CARTESIAN_POINT('Ctrl Pts',(-31.3345107659126,-54.4558650179027,
40.0825207326933));
#189955=CARTESIAN_POINT('Ctrl Pts',(-31.3340864990772,-54.4558811330248,
40.0823381109275));
#189956=CARTESIAN_POINT('Ctrl Pts',(-31.3328136985709,-54.455929478391,
40.0817902456303));
#189957=CARTESIAN_POINT('Ctrl Pts',(-31.3315453006542,-54.4559627721157,
40.0812334935553));
#189958=CARTESIAN_POINT('Ctrl Pts',(-31.3302817797847,-54.4559812395336,
40.0806684524227));
#189959=CARTESIAN_POINT('Ctrl Pts',(-31.321550066618,-54.4561088608495,
40.0767636676136));
#189960=CARTESIAN_POINT('Ctrl Pts',(-31.3130195924487,-54.4555742713437,
40.0724404510887));
#189961=CARTESIAN_POINT('Ctrl Pts',(-31.304740085859,-54.4544853519656,
40.0677949937408));
#189962=CARTESIAN_POINT('Ctrl Pts',(-31.3006251938109,-54.4539441620238,
40.0654862141905));
#189963=CARTESIAN_POINT('Ctrl Pts',(-31.2965719591987,-54.4532655373258,
40.0630972003215));
#189964=CARTESIAN_POINT('Ctrl Pts',(-31.2925850928566,-54.4524598885394,
40.0606363359906));
#189965=CARTESIAN_POINT('Ctrl Pts',(-31.2837894702122,-54.4506825069817,
40.0552073017123));
#189966=CARTESIAN_POINT('Ctrl Pts',(-31.2753153512349,-54.4482992497265,
40.0494204304519));
#189967=CARTESIAN_POINT('Ctrl Pts',(-31.2672761140353,-54.4454010706196,
40.0434049749851));
#189968=CARTESIAN_POINT('Ctrl Pts',(-31.2643392793061,-54.444342329244,
40.0412074532442));
#189969=CARTESIAN_POINT('Ctrl Pts',(-31.2614550023641,-54.4432206434042,
40.0389814735788));
#189970=CARTESIAN_POINT('Ctrl Pts',(-31.2586246102248,-54.4420411592046,
40.0367321210016));
#189971=CARTESIAN_POINT('Ctrl Pts',(-31.2491176225321,-54.4380793965875,
40.0291767837144));
#189972=CARTESIAN_POINT('Ctrl Pts',(-31.2401615453402,-54.4334326446233,
40.0213235332584));
#189973=CARTESIAN_POINT('Ctrl Pts',(-31.2317373058281,-54.4282277812596,
40.0132649215871));
#189974=CARTESIAN_POINT('Ctrl Pts',(-31.2224780686874,-54.4225070198663,
40.0044075527549));
#189975=CARTESIAN_POINT('Ctrl Pts',(-31.2138606686968,-54.4161118092716,
39.995301625374));
#189976=CARTESIAN_POINT('Ctrl Pts',(-31.2058737429093,-54.4091594014098,
39.9860353422383));
#189977=CARTESIAN_POINT('Ctrl Pts',(-31.1972714816235,-54.4016713602556,
39.9760551582724));
#189978=CARTESIAN_POINT('Ctrl Pts',(-31.1893995936796,-54.3935362880577,
39.9658879738188));
#189979=CARTESIAN_POINT('Ctrl Pts',(-31.182272586596,-54.3848513315151,
39.9556174643291));
#189980=CARTESIAN_POINT('Ctrl Pts',(-31.1752418181704,-54.3762836512082,
39.9454856413929));
#189981=CARTESIAN_POINT('Ctrl Pts',(-31.1689352997164,-54.3671795569354,
39.9352519465126));
#189982=CARTESIAN_POINT('Ctrl Pts',(-31.1634057161443,-54.3576020372437,
39.92499));
#189983=CARTESIAN_POINT('Ctrl Pts',(-29.4433108116264,-51.3783102687783,
39.92499));
#189984=CARTESIAN_POINT('Ctrl Pts',(-29.4380189697943,-51.3691445298596,
39.9348107241716));
#189985=CARTESIAN_POINT('Ctrl Pts',(-29.4334690915863,-51.3595943606125,
39.9446038383157));
#189986=CARTESIAN_POINT('Ctrl Pts',(-29.429678124626,-51.3497152868788,
39.9543158069366));
#189987=CARTESIAN_POINT('Ctrl Pts',(-29.4260176124818,-51.3401761719895,
39.9636935671369));
#189988=CARTESIAN_POINT('Ctrl Pts',(-29.4230642997988,-51.3303291924946,
39.9729968320963));
#189989=CARTESIAN_POINT('Ctrl Pts',(-29.4208754038594,-51.3202058500926,
39.9821731151306));
#189990=CARTESIAN_POINT('Ctrl Pts',(-29.4188062116769,-51.3106361210879,
39.9908475764321));
#189991=CARTESIAN_POINT('Ctrl Pts',(-29.4174199248369,-51.3008185461827,
39.9994093733814));
#189992=CARTESIAN_POINT('Ctrl Pts',(-29.4168067767638,-51.2907775289389,
40.0077966115808));
#189993=CARTESIAN_POINT('Ctrl Pts',(-29.4162420776747,-51.281529920508,
40.0155211172561));
#189994=CARTESIAN_POINT('Ctrl Pts',(-29.4163331870166,-51.2720922400983,
40.0230979940988));
#189995=CARTESIAN_POINT('Ctrl Pts',(-29.4171879526239,-51.2624911797787,
40.0304554104714));
#189996=CARTESIAN_POINT('Ctrl Pts',(-29.4174428264736,-51.2596283373998,
40.0326492435158));
#189997=CARTESIAN_POINT('Ctrl Pts',(-29.4177658668977,-51.2567510524891,
40.0348233715049));
#189998=CARTESIAN_POINT('Ctrl Pts',(-29.4181606517644,-51.2538602864393,
40.0369753512355));
#189999=CARTESIAN_POINT('Ctrl Pts',(-29.4185514029024,-51.2509990568965,
40.0391053430352));
#190000=CARTESIAN_POINT('Ctrl Pts',(-29.4190117629203,-51.2481275521817,
40.041211089324));
#190001=CARTESIAN_POINT('Ctrl Pts',(-29.4195444402101,-51.2452499391938,
40.0432881154904));
#190002=CARTESIAN_POINT('Ctrl Pts',(-29.4195814815471,-51.2450498356144,
40.043432547828));
#190003=CARTESIAN_POINT('Ctrl Pts',(-29.4196188630963,-51.2448496951982,
40.0435768364421));
#190004=CARTESIAN_POINT('Ctrl Pts',(-29.4196565860788,-51.2446495184042,
40.0437209807855));
#190005=CARTESIAN_POINT('Ctrl Pts',(-29.4213104998203,-51.235873034447,
40.050040796842));
#190006=CARTESIAN_POINT('Ctrl Pts',(-29.4236619033165,-51.2270453415808,
40.0560490279344));
#190007=CARTESIAN_POINT('Ctrl Pts',(-29.426765124801,-51.2182691329814,
40.0616647108614));
#190008=CARTESIAN_POINT('Ctrl Pts',(-29.4296578665607,-51.2100881812721,
40.0668995033484));
#190009=CARTESIAN_POINT('Ctrl Pts',(-29.4332044080279,-51.2019513265394,
40.071793326748));
#190010=CARTESIAN_POINT('Ctrl Pts',(-29.4374658604799,-51.1939656059622,
40.076246030307));
#190011=CARTESIAN_POINT('Ctrl Pts',(-29.4390247549183,-51.1910443260617,
40.0778748868747));
#190012=CARTESIAN_POINT('Ctrl Pts',(-29.4406794572087,-51.1881435589222,
40.0794443522247));
#190013=CARTESIAN_POINT('Ctrl Pts',(-29.4424334077169,-51.1852696776792,
40.0809482021492));
#190014=CARTESIAN_POINT('Ctrl Pts',(-29.4428551742199,-51.1845786052482,
40.0813098278169));
#190015=CARTESIAN_POINT('Ctrl Pts',(-29.443283215379,-51.1838888551094,
40.0816679525672));
#190016=CARTESIAN_POINT('Ctrl Pts',(-29.4437175198435,-51.1832005624687,
40.0820224192581));
#190017=CARTESIAN_POINT('Ctrl Pts',(-29.4441382522935,-51.1825337789731,
40.0823658088648));
#190018=CARTESIAN_POINT('Ctrl Pts',(-29.4445648626868,-51.1818683633171,
40.0827057654617));
#190019=CARTESIAN_POINT('Ctrl Pts',(-29.4449973374098,-51.1812044402992,
40.0830421470151));
#190020=CARTESIAN_POINT('Ctrl Pts',(-29.4497355978005,-51.1739303963594,
40.0867275956807));
#190021=CARTESIAN_POINT('Ctrl Pts',(-29.4551812510955,-51.1668309650357,
40.0899823432031));
#190022=CARTESIAN_POINT('Ctrl Pts',(-29.461292997452,-51.1600900711811,
40.0926299529356));
#190023=CARTESIAN_POINT('Ctrl Pts',(-29.4638277208377,-51.1572944215752,
40.0937279956085));
#190024=CARTESIAN_POINT('Ctrl Pts',(-29.4664765899956,-51.1545603804837,
40.0947220371803));
#190025=CARTESIAN_POINT('Ctrl Pts',(-29.4692349685474,-51.1519003687089,
40.0956014538693));
#190026=CARTESIAN_POINT('Ctrl Pts',(-29.4739396706108,-51.147363441434,
40.097101390674));
#190027=CARTESIAN_POINT('Ctrl Pts',(-29.4789629373384,-51.1430443628983,
40.0982667904316));
#190028=CARTESIAN_POINT('Ctrl Pts',(-29.4842777732941,-51.1390107214363,
40.0990539325583));
#190029=CARTESIAN_POINT('Ctrl Pts',(-29.486935191272,-51.1369939007053,
40.0994475036216));
#190030=CARTESIAN_POINT('Ctrl Pts',(-29.4896662827383,-51.1350496570623,
40.0997467259952));
#190031=CARTESIAN_POINT('Ctrl Pts',(-29.4924676612911,-51.1331865036875,
40.0999473488896));
#190032=CARTESIAN_POINT('Ctrl Pts',(-29.495269039844,-51.1313233503127,
40.100147971784));
#190033=CARTESIAN_POINT('Ctrl Pts',(-29.49814066024,-51.1295412933645,40.10025));
#190034=CARTESIAN_POINT('Ctrl Pts',(-29.5010785149114,-51.1278468659046,
40.10025));
#190035=CARTESIAN_POINT('Origin',(-34.2589154226524,-47.1274239660508,39.92499));
#190036=CARTESIAN_POINT('Ctrl Pts',(-36.9828414016749,-50.5784163149355,
39.92499));
#190037=CARTESIAN_POINT('Ctrl Pts',(-36.989077996891,-50.5870002518363,
39.9348354642021));
#190038=CARTESIAN_POINT('Ctrl Pts',(-36.99461878582,-50.5960508068,39.9446440828464));
#190039=CARTESIAN_POINT('Ctrl Pts',(-36.9994424783905,-50.6055128591422,
39.9543641760339));
#190040=CARTESIAN_POINT('Ctrl Pts',(-37.0041094296757,-50.6146674511261,
39.9637684240722));
#190041=CARTESIAN_POINT('Ctrl Pts',(-37.0081056536708,-50.6242084112815,
39.9730909636407));
#190042=CARTESIAN_POINT('Ctrl Pts',(-37.0113722741996,-50.6341096134638,
39.9822808977153));
#190043=CARTESIAN_POINT('Ctrl Pts',(-37.0144622960729,-50.6434755410473,
39.9909740094663));
#190044=CARTESIAN_POINT('Ctrl Pts',(-37.0168997626766,-50.6531646927637,
39.9995492765015));
#190045=CARTESIAN_POINT('Ctrl Pts',(-37.0185933530511,-50.6631621581244,
40.0079462328709));
#190046=CARTESIAN_POINT('Ctrl Pts',(-37.0201532722697,-50.6723705467568,
40.0156804369705));
#190047=CARTESIAN_POINT('Ctrl Pts',(-37.0210821446113,-50.6818410607736,
40.0232638017438));
#190048=CARTESIAN_POINT('Ctrl Pts',(-37.0212705108777,-50.6915586678658,
40.0306257269983));
#190049=CARTESIAN_POINT('Ctrl Pts',(-37.0213251487712,-50.6943773762885,
40.0327611416662));
#190050=CARTESIAN_POINT('Ctrl Pts',(-37.0213172191968,-50.6972168227827,
40.0348777427276));
#190051=CARTESIAN_POINT('Ctrl Pts',(-37.0212433695026,-50.7000764815584,
40.0369733168701));
#190052=CARTESIAN_POINT('Ctrl Pts',(-37.021163311686,-50.7031765355312,
40.0392450539741));
#190053=CARTESIAN_POINT('Ctrl Pts',(-37.0210069737843,-50.706296057732,
40.041487875195));
#190054=CARTESIAN_POINT('Ctrl Pts',(-37.0207706534748,-50.7094335311102,
40.0436985701601));
#190055=CARTESIAN_POINT('Ctrl Pts',(-37.0201220705311,-50.7180443514158,
40.0497658398386));
#190056=CARTESIAN_POINT('Ctrl Pts',(-37.0188289150183,-50.7267761502171,
40.0555581699984));
#190057=CARTESIAN_POINT('Ctrl Pts',(-37.0168522507833,-50.7355328079488,
40.0609828468885));
#190058=CARTESIAN_POINT('Ctrl Pts',(-37.015043710324,-50.743544674363,40.0659461317303));
#190059=CARTESIAN_POINT('Ctrl Pts',(-37.0126559296152,-50.7515681793715,
40.0706039980704));
#190060=CARTESIAN_POINT('Ctrl Pts',(-37.009626855822,-50.7595400218642,
40.07488431806));
#190061=CARTESIAN_POINT('Ctrl Pts',(-37.0081389846695,-50.7634557648558,
40.0769867972568));
#190062=CARTESIAN_POINT('Ctrl Pts',(-37.0064960060562,-50.7673587034236,
40.0789976708174));
#190063=CARTESIAN_POINT('Ctrl Pts',(-37.0046883717069,-50.7712388062148,
40.08090504915));
#190064=CARTESIAN_POINT('Ctrl Pts',(-37.0043453906958,-50.7719750179268,
40.0812669556105));
#190065=CARTESIAN_POINT('Ctrl Pts',(-37.0039959853417,-50.7727105984662,
40.0816253922032));
#190066=CARTESIAN_POINT('Ctrl Pts',(-37.0036401497476,-50.7734454079408,
40.0819801989139));
#190067=CARTESIAN_POINT('Ctrl Pts',(-37.0032954340158,-50.7741572546192,
40.0823239179149));
#190068=CARTESIAN_POINT('Ctrl Pts',(-37.0029446836755,-50.774868377657,
40.0826642303498));
#190069=CARTESIAN_POINT('Ctrl Pts',(-37.0025878964871,-50.77557864763,40.0830009916099));
#190070=CARTESIAN_POINT('Ctrl Pts',(-36.9986997032254,-50.7833190234415,
40.0866709464313));
#190071=CARTESIAN_POINT('Ctrl Pts',(-36.9940916451525,-50.7909629993145,
40.0899175831879));
#190072=CARTESIAN_POINT('Ctrl Pts',(-36.988781834568,-50.7983209798302,
40.0925642067064));
#190073=CARTESIAN_POINT('Ctrl Pts',(-36.986539468586,-50.8014283006926,
40.0936818922529));
#190074=CARTESIAN_POINT('Ctrl Pts',(-36.9841723869923,-50.804484627329,
40.0946930094791));
#190075=CARTESIAN_POINT('Ctrl Pts',(-36.9816838130236,-50.8074762285638,
40.0955863397546));
#190076=CARTESIAN_POINT('Ctrl Pts',(-36.9774931166428,-50.8125140102917,
40.0970906856166));
#190077=CARTESIAN_POINT('Ctrl Pts',(-36.9729576356984,-50.8173657273501,
40.0982599215483));
#190078=CARTESIAN_POINT('Ctrl Pts',(-36.9680961762159,-50.8219595855752,
40.0990497370454));
#190079=CARTESIAN_POINT('Ctrl Pts',(-36.9668808113453,-50.8231080501314,
40.0992471909196));
#190080=CARTESIAN_POINT('Ctrl Pts',(-36.9656449236015,-50.8242402182965,
40.0994209989363));
#190081=CARTESIAN_POINT('Ctrl Pts',(-36.9643886196686,-50.8253547230713,
40.0995705982975));
#190082=CARTESIAN_POINT('Ctrl Pts',(-36.9625041637694,-50.8270264802335,
40.0997949973393));
#190083=CARTESIAN_POINT('Ctrl Pts',(-36.9605737761781,-50.8286584747056,
40.0999649129781));
#190084=CARTESIAN_POINT('Ctrl Pts',(-36.9585988181541,-50.8302474395914,
40.1000786629733));
#190085=CARTESIAN_POINT('Ctrl Pts',(-36.9566238601301,-50.8318364044772,
40.1001924129685));
#190086=CARTESIAN_POINT('Ctrl Pts',(-36.9546043428195,-50.8333823430148,
40.10025));
#190087=CARTESIAN_POINT('Ctrl Pts',(-36.9525415975225,-50.8348823336498,
40.10025));
#190088=CARTESIAN_POINT('Ctrl Pts',(-34.7084426211234,-47.7461450747863,
40.10025));
#190089=CARTESIAN_POINT('Ctrl Pts',(-34.7154221779228,-47.7410693801618,
40.10025));
#190090=CARTESIAN_POINT('Ctrl Pts',(-34.722760215254,-47.7366138137629,
40.0995786334241));
#190091=CARTESIAN_POINT('Ctrl Pts',(-34.7303057514044,-47.7327846251246,
40.0983063763366));
#190092=CARTESIAN_POINT('Ctrl Pts',(-34.7351793935409,-47.7303113621616,
40.0974846287993));
#190093=CARTESIAN_POINT('Ctrl Pts',(-34.7401391868071,-47.7280985748135,
40.0964130309338));
#190094=CARTESIAN_POINT('Ctrl Pts',(-34.7451421370596,-47.7261394006517,
40.0951176960924));
#190095=CARTESIAN_POINT('Ctrl Pts',(-34.7517732610326,-47.7235426275287,
40.0934008039614));
#190096=CARTESIAN_POINT('Ctrl Pts',(-34.7584811778434,-47.7213971161179,
40.0912909372156));
#190097=CARTESIAN_POINT('Ctrl Pts',(-34.7651763312118,-47.7196932909344,
40.0888630467851));
#190098=CARTESIAN_POINT('Ctrl Pts',(-34.768523907896,-47.7188413783427,
40.0876491015699));
#190099=CARTESIAN_POINT('Ctrl Pts',(-34.7718684539193,-47.718099768756,
40.0863558569271));
#190100=CARTESIAN_POINT('Ctrl Pts',(-34.7751999143434,-47.7174664279768,
40.0849936342771));
#190101=CARTESIAN_POINT('Ctrl Pts',(-34.7768656445554,-47.7171497575872,
40.0843125229521));
#190102=CARTESIAN_POINT('Ctrl Pts',(-34.7785281166319,-47.7168601447019,
40.0836141747074));
#190103=CARTESIAN_POINT('Ctrl Pts',(-34.7801861569092,-47.7165972740596,
40.0828999161609));
#190104=CARTESIAN_POINT('Ctrl Pts',(-34.7806006669785,-47.716531556399,
40.0827213515243));
#190105=CARTESIAN_POINT('Ctrl Pts',(-34.7810149003418,-47.7164675099216,
40.0825417925842));
#190106=CARTESIAN_POINT('Ctrl Pts',(-34.7814288392283,-47.7164051292833,
40.0823612602361));
#190107=CARTESIAN_POINT('Ctrl Pts',(-34.7826706558876,-47.7162179873683,
40.0818196631917));
#190108=CARTESIAN_POINT('Ctrl Pts',(-34.783909820854,-47.7160458390453,
40.0812693052022));
#190109=CARTESIAN_POINT('Ctrl Pts',(-34.7851458668348,-47.7158885307487,
40.0807107531875));
#190110=CARTESIAN_POINT('Ctrl Pts',(-34.7938524151213,-47.7147804714198,
40.0767763849182));
#190111=CARTESIAN_POINT('Ctrl Pts',(-34.8024290252887,-47.7143609747537,
40.0724140586137));
#190112=CARTESIAN_POINT('Ctrl Pts',(-34.8108122146622,-47.7145286167445,
40.0677221223767));
#190113=CARTESIAN_POINT('Ctrl Pts',(-34.8148780524494,-47.7146099229289,
40.065446538372));
#190114=CARTESIAN_POINT('Ctrl Pts',(-34.818898766793,-47.7148297795038,
40.0630928000679));
#190115=CARTESIAN_POINT('Ctrl Pts',(-34.8228686918041,-47.7151790039208,
40.0606689262479));
#190116=CARTESIAN_POINT('Ctrl Pts',(-34.8289463696254,-47.7157136421036,
40.0569581447806));
#190117=CARTESIAN_POINT('Ctrl Pts',(-34.8349017567798,-47.716550115795,
40.0530843804606));
#190118=CARTESIAN_POINT('Ctrl Pts',(-34.8407017446569,-47.717656329678,
40.0490800251458));
#190119=CARTESIAN_POINT('Ctrl Pts',(-34.8433952890323,-47.7181700611281,
40.0472203818218));
#190120=CARTESIAN_POINT('Ctrl Pts',(-34.8460552817721,-47.718741715552,
40.0453323608819));
#190121=CARTESIAN_POINT('Ctrl Pts',(-34.8486779186779,-47.7193692101069,
40.0434201572162));
#190122=CARTESIAN_POINT('Ctrl Pts',(-34.848878933463,-47.7194173050921,
40.0432735943397));
#190123=CARTESIAN_POINT('Ctrl Pts',(-34.8490797487414,-47.7194657006755,
40.0431268995707));
#190124=CARTESIAN_POINT('Ctrl Pts',(-34.849280363866,-47.7195143955478,
40.0429800745037));
#190125=CARTESIAN_POINT('Ctrl Pts',(-34.8520984015308,-47.7201984116933,
40.0409176249753));
#190126=CARTESIAN_POINT('Ctrl Pts',(-34.8548765847938,-47.7209435418726,
40.0388310783332));
#190127=CARTESIAN_POINT('Ctrl Pts',(-34.8576119849588,-47.7217448891702,
40.036725739981));
#190128=CARTESIAN_POINT('Ctrl Pts',(-34.8674206434757,-47.7246183780645,
40.0291763710718));
#190129=CARTESIAN_POINT('Ctrl Pts',(-34.8767555719421,-47.7282350429866,
40.0213310894595));
#190130=CARTESIAN_POINT('Ctrl Pts',(-34.8856231565602,-47.7324659181293,
40.0132837551321));
#190131=CARTESIAN_POINT('Ctrl Pts',(-34.8953677412278,-47.7371152248822,
40.0044405431325));
#190132=CARTESIAN_POINT('Ctrl Pts',(-34.9045486251006,-47.7425063743635,
39.9953528710599));
#190133=CARTESIAN_POINT('Ctrl Pts',(-34.9131661493096,-47.7485205638414,
39.9861103629552));
#190134=CARTESIAN_POINT('Ctrl Pts',(-34.9224709127524,-47.7550143791224,
39.9761307737546));
#190135=CARTESIAN_POINT('Ctrl Pts',(-34.9311199164051,-47.7622350952187,
39.9659696935995));
#190136=CARTESIAN_POINT('Ctrl Pts',(-34.939090873807,-47.7700859103021,
39.9557128217484));
#190137=CARTESIAN_POINT('Ctrl Pts',(-34.9469949630654,-47.7778708651125,
39.9455419945145));
#190138=CARTESIAN_POINT('Ctrl Pts',(-34.9542331399583,-47.7862765797904,
39.9352756289333));
#190139=CARTESIAN_POINT('Ctrl Pts',(-34.9607485668368,-47.79524429555,39.92499));
#190140=CARTESIAN_POINT('Origin',(0.0123294189942831,-0.00895784724493279,
39.92499));
#190141=CARTESIAN_POINT('Ctrl Pts',(-36.9278827595329,-50.8527980281383,
40.10025));
#190142=CARTESIAN_POINT('Ctrl Pts',(-36.920932055107,-50.8578435704956,
40.10025));
#190143=CARTESIAN_POINT('Ctrl Pts',(-36.9136216385504,-50.8622636476107,
40.0995859581841));
#190144=CARTESIAN_POINT('Ctrl Pts',(-36.9061023515947,-50.8660552387517,
40.0983275959619));
#190145=CARTESIAN_POINT('Ctrl Pts',(-36.9012978851881,-50.8684778849908,
40.0975235624067));
#190146=CARTESIAN_POINT('Ctrl Pts',(-36.8964085464699,-50.8706447895123,
40.0964777059489));
#190147=CARTESIAN_POINT('Ctrl Pts',(-36.8914758894168,-50.8725634718545,
40.0952149915961));
#190148=CARTESIAN_POINT('Ctrl Pts',(-36.8847438022849,-50.8751820882649,
40.0934916398701));
#190149=CARTESIAN_POINT('Ctrl Pts',(-36.8779301449085,-50.8773323251413,
40.091364392163));
#190150=CARTESIAN_POINT('Ctrl Pts',(-36.8711298300324,-50.8790261328804,
40.0889118607712));
#190151=CARTESIAN_POINT('Ctrl Pts',(-36.8677296725944,-50.8798730367499,
40.0876855950754));
#190152=CARTESIAN_POINT('Ctrl Pts',(-36.8643326829601,-50.8806059576335,
40.0863782327526));
#190153=CARTESIAN_POINT('Ctrl Pts',(-36.8609495224154,-50.8812272732513,
40.0850006373333));
#190154=CARTESIAN_POINT('Ctrl Pts',(-36.8592579421431,-50.8815379310602,
40.0843118396237));
#190155=CARTESIAN_POINT('Ctrl Pts',(-36.8575698050848,-50.8818206978292,
40.0836054919164));
#190156=CARTESIAN_POINT('Ctrl Pts',(-36.855886355634,-50.8820759354567,
40.0828829920417));
#190157=CARTESIAN_POINT('Ctrl Pts',(-36.8554654932713,-50.8821397448636,
40.082702367073));
#190158=CARTESIAN_POINT('Ctrl Pts',(-36.8550449235852,-50.8822018339189,
40.0825207326932));
#190159=CARTESIAN_POINT('Ctrl Pts',(-36.8546246654168,-50.8822622087209,
40.0823381109275));
#190160=CARTESIAN_POINT('Ctrl Pts',(-36.8533638909117,-50.8824433331272,
40.0817902456303));
#190161=CARTESIAN_POINT('Ctrl Pts',(-36.8521059215534,-50.8826090281504,
40.0812334935553));
#190162=CARTESIAN_POINT('Ctrl Pts',(-36.8508512527542,-50.8827594682966,
40.0806684524226));
#190163=CARTESIAN_POINT('Ctrl Pts',(-36.8421807128861,-50.8837991030486,
40.0767636676137));
#190164=CARTESIAN_POINT('Ctrl Pts',(-36.8336410897277,-50.8841591194359,
40.072440451089));
#190165=CARTESIAN_POINT('Ctrl Pts',(-36.8252931160724,-50.8839416093726,
40.0677949937412));
#190166=CARTESIAN_POINT('Ctrl Pts',(-36.8211441960803,-50.8838335074682,
40.0654862141908));
#190167=CARTESIAN_POINT('Ctrl Pts',(-36.8170422299142,-50.8835822787326,
40.0630972003217));
#190168=CARTESIAN_POINT('Ctrl Pts',(-36.8129929908133,-50.8831977843865,
40.0606363359906));
#190169=CARTESIAN_POINT('Ctrl Pts',(-36.8040597645471,-50.8823495324294,
40.0552073017123));
#190170=CARTESIAN_POINT('Ctrl Pts',(-36.7953829494618,-50.8808651175411,
40.0494204304519));
#190171=CARTESIAN_POINT('Ctrl Pts',(-36.7870848098364,-50.878823144073,
40.0434049749851));
#190172=CARTESIAN_POINT('Ctrl Pts',(-36.7840533947862,-50.8780771854144,
40.0412074532442));
#190173=CARTESIAN_POINT('Ctrl Pts',(-36.7810676701179,-50.8772631333234,
40.0389814735788));
#190174=CARTESIAN_POINT('Ctrl Pts',(-36.7781294934921,-50.8763859670025,
40.0367321210016));
#190175=CARTESIAN_POINT('Ctrl Pts',(-36.7682604691151,-50.8734396581495,
40.0291767837149));
#190176=CARTESIAN_POINT('Ctrl Pts',(-36.7588677364097,-50.8697545265647,
40.0213235332593));
#190177=CARTESIAN_POINT('Ctrl Pts',(-36.7499455893946,-50.8654587487979,
40.0132649215884));
#190178=CARTESIAN_POINT('Ctrl Pts',(-36.7401390929271,-50.8607371801638,
40.0044075527568));
#190179=CARTESIAN_POINT('Ctrl Pts',(-36.7309004184199,-50.8552777667807,
39.9953016253764));
#190180=CARTESIAN_POINT('Ctrl Pts',(-36.7222305213381,-50.8491983060158,
39.9860353422412));
#190181=CARTESIAN_POINT('Ctrl Pts',(-36.7128926707054,-50.8426504662879,
39.9760551582758));
#190182=CARTESIAN_POINT('Ctrl Pts',(-36.7042135591923,-50.835382795217,
39.9658879738229));
#190183=CARTESIAN_POINT('Ctrl Pts',(-36.6962177694384,-50.8274903908739,
39.9556174643338));
#190184=CARTESIAN_POINT('Ctrl Pts',(-36.6883299498402,-50.8197045606343,
39.9454856413961));
#190185=CARTESIAN_POINT('Ctrl Pts',(-36.6811063421692,-50.8113095502238,
39.9352519465142));
#190186=CARTESIAN_POINT('Ctrl Pts',(-36.674605926818,-50.8023624960589,
39.92499));
#190187=CARTESIAN_POINT('Ctrl Pts',(-34.6525130919799,-48.0191904766735,
39.92499));
#190188=CARTESIAN_POINT('Ctrl Pts',(-34.6462921588072,-48.0106280967261,
39.9348107241715));
#190189=CARTESIAN_POINT('Ctrl Pts',(-34.6407689407928,-48.0016058360827,
39.9446038383155));
#190190=CARTESIAN_POINT('Ctrl Pts',(-34.6359660967504,-47.9921771448993,
39.9543158069363));
#190191=CARTESIAN_POINT('Ctrl Pts',(-34.6313285282544,-47.9830729139886,
39.9636935671366));
#190192=CARTESIAN_POINT('Ctrl Pts',(-34.6273621044928,-47.9735885825141,
39.972996832096));
#190193=CARTESIAN_POINT('Ctrl Pts',(-34.62412702213,-47.9637494987697,39.9821731151303));
#190194=CARTESIAN_POINT('Ctrl Pts',(-34.6210688561319,-47.9544484832207,
39.990847576432));
#190195=CARTESIAN_POINT('Ctrl Pts',(-34.6186639474984,-47.944829596451,
39.9994093733814));
#190196=CARTESIAN_POINT('Ctrl Pts',(-34.6170045862124,-47.934907676376,
40.007796611581));
#190197=CARTESIAN_POINT('Ctrl Pts',(-34.6154763423058,-47.9257697544393,
40.0155211172565));
#190198=CARTESIAN_POINT('Ctrl Pts',(-34.6145804463111,-47.9163742511105,
40.0230979940994));
#190199=CARTESIAN_POINT('Ctrl Pts',(-34.6144269453422,-47.9067364390682,
40.0304554104723));
#190200=CARTESIAN_POINT('Ctrl Pts',(-34.6143811744519,-47.903862638068,
40.0326492435164));
#190201=CARTESIAN_POINT('Ctrl Pts',(-34.6144016870566,-47.9009673483063,
40.0348233715052));
#190202=CARTESIAN_POINT('Ctrl Pts',(-34.6144921419176,-47.8980511519204,
40.0369753512356));
#190203=CARTESIAN_POINT('Ctrl Pts',(-34.6145816725529,-47.8951647518765,
40.0391053430352));
#190204=CARTESIAN_POINT('Ctrl Pts',(-34.6147393566953,-47.8922608568397,
40.041211089324));
#190205=CARTESIAN_POINT('Ctrl Pts',(-34.6149683234597,-47.8893433277783,
40.0432881154904));
#190206=CARTESIAN_POINT('Ctrl Pts',(-34.6149842453607,-47.8891404485132,
40.043432547828));
#190207=CARTESIAN_POINT('Ctrl Pts',(-34.6150005017597,-47.8889374970513,
40.0435768364421));
#190208=CARTESIAN_POINT('Ctrl Pts',(-34.6150170939191,-47.8887344737213,
40.0437209807855));
#190209=CARTESIAN_POINT('Ctrl Pts',(-34.6157445549671,-47.8798331871998,
40.0500407968419));
#190210=CARTESIAN_POINT('Ctrl Pts',(-34.6171603320595,-47.8708080647648,
40.0560490279343));
#190211=CARTESIAN_POINT('Ctrl Pts',(-34.6193291901737,-47.8617555581815,
40.0616647108613));
#190212=CARTESIAN_POINT('Ctrl Pts',(-34.6213509428811,-47.8533170487309,
40.0668995033483));
#190213=CARTESIAN_POINT('Ctrl Pts',(-34.6240275231021,-47.8448540540103,
40.0717933267478));
#190214=CARTESIAN_POINT('Ctrl Pts',(-34.6274308957715,-47.8364666369699,
40.0762460303069));
#190215=CARTESIAN_POINT('Ctrl Pts',(-34.6286758935244,-47.8333984113063,
40.0778748868745));
#190216=CARTESIAN_POINT('Ctrl Pts',(-34.6300183184512,-47.830340571385,
40.0794443522246));
#190217=CARTESIAN_POINT('Ctrl Pts',(-34.6314622582451,-47.8272990958128,
40.0809482021492));
#190218=CARTESIAN_POINT('Ctrl Pts',(-34.6318094775277,-47.8265677225445,
40.0813098278168));
#190219=CARTESIAN_POINT('Ctrl Pts',(-34.6321630753106,-47.8258370084446,
40.0816679525672));
#190220=CARTESIAN_POINT('Ctrl Pts',(-34.6325230544378,-47.8251070891647,
40.082022419258));
#190221=CARTESIAN_POINT('Ctrl Pts',(-34.6328717842173,-47.8243999798624,
40.0823658088648));
#190222=CARTESIAN_POINT('Ctrl Pts',(-34.6332265027182,-47.8236936164942,
40.0827057654616));
#190223=CARTESIAN_POINT('Ctrl Pts',(-34.6335872094466,-47.8229881245978,
40.0830421470151));
#190224=CARTESIAN_POINT('Ctrl Pts',(-34.6375391685163,-47.8152586455546,
40.0867275956806));
#190225=CARTESIAN_POINT('Ctrl Pts',(-34.6422128973066,-47.8076288798881,
40.0899823432031));
#190226=CARTESIAN_POINT('Ctrl Pts',(-34.6475865476014,-47.8002860619008,
40.0926299529356));
#190227=CARTESIAN_POINT('Ctrl Pts',(-34.6498151605499,-47.7972407764157,
40.0937279956084));
#190228=CARTESIAN_POINT('Ctrl Pts',(-34.6521637338117,-47.7942448304649,
40.0947220371802));
#190229=CARTESIAN_POINT('Ctrl Pts',(-34.654628954734,-47.7913110614418,
40.0956014538692));
#190230=CARTESIAN_POINT('Ctrl Pts',(-34.6588336459112,-47.7863072126524,
40.097101390674));
#190231=CARTESIAN_POINT('Ctrl Pts',(-34.6633779280161,-47.7814867201292,
40.0982667904316));
#190232=CARTESIAN_POINT('Ctrl Pts',(-34.6682420184009,-47.7769196237422,
40.0990539325582));
#190233=CARTESIAN_POINT('Ctrl Pts',(-34.6706740635933,-47.7746360755486,
40.0994475036216));
#190234=CARTESIAN_POINT('Ctrl Pts',(-34.6731869650545,-47.7724170058818,
40.0997467259952));
#190235=CARTESIAN_POINT('Ctrl Pts',(-34.6757782448035,-47.7702712352609,
40.0999473488896));
#190236=CARTESIAN_POINT('Ctrl Pts',(-34.6783695245525,-47.7681254646401,
40.100147971784));
#190237=CARTESIAN_POINT('Ctrl Pts',(-34.6810391382372,-47.7660530039192,
40.10025));
#190238=CARTESIAN_POINT('Ctrl Pts',(-34.6837837831348,-47.7640607692761,
40.10025));
#190239=CARTESIAN_POINT('Origin',(-38.9973987043321,-43.2882232241946,39.92499));
#190240=CARTESIAN_POINT('Ctrl Pts',(-42.0671296588098,-46.4355828792668,
39.92499));
#190241=CARTESIAN_POINT('Ctrl Pts',(-42.0742293550381,-46.4434678907494,
39.9348354642022));
#190242=CARTESIAN_POINT('Ctrl Pts',(-42.0806858315479,-46.4518896956744,
39.9446440828466));
#190243=CARTESIAN_POINT('Ctrl Pts',(-42.0864721532166,-46.4607957007324,
39.9543641760343));
#190244=CARTESIAN_POINT('Ctrl Pts',(-42.0920704538863,-46.4694123136578,
39.9637684240728));
#190245=CARTESIAN_POINT('Ctrl Pts',(-42.0970420880514,-46.4784832882822,
39.9730909636415));
#190246=CARTESIAN_POINT('Ctrl Pts',(-42.1013257711398,-46.4879887958193,
39.9822808977163));
#190247=CARTESIAN_POINT('Ctrl Pts',(-42.1053778715674,-46.4969804206339,
39.9909740094675));
#190248=CARTESIAN_POINT('Ctrl Pts',(-42.1088147776131,-46.5063617095252,
39.999549276503));
#190249=CARTESIAN_POINT('Ctrl Pts',(-42.1115441100131,-46.5161273793256,
40.0079462328726));
#190250=CARTESIAN_POINT('Ctrl Pts',(-42.1140580225438,-46.5251222674832,
40.0156804369724));
#190251=CARTESIAN_POINT('Ctrl Pts',(-42.115971744702,-46.5344438074352,
40.023263801746));
#190252=CARTESIAN_POINT('Ctrl Pts',(-42.1171748456141,-46.544088490823,
40.0306257270007));
#190253=CARTESIAN_POINT('Ctrl Pts',(-42.1175238194552,-46.5468860468499,
40.0327611416679));
#190254=CARTESIAN_POINT('Ctrl Pts',(-42.1178127362982,-46.5497107674243,
40.0348777427284));
#190255=CARTESIAN_POINT('Ctrl Pts',(-42.1180382068977,-46.552562480084,
40.0369733168701));
#190256=CARTESIAN_POINT('Ctrl Pts',(-42.118282631524,-46.5556539199572,
40.039245053974));
#190257=CARTESIAN_POINT('Ctrl Pts',(-42.1184532289194,-46.5587726948497,
40.041487875195));
#190258=CARTESIAN_POINT('Ctrl Pts',(-42.1185461584681,-46.5619176830192,
40.0436985701601));
#190259=CARTESIAN_POINT('Ctrl Pts',(-42.1188012043436,-46.5705491277287,
40.0497658398386));
#190260=CARTESIAN_POINT('Ctrl Pts',(-42.1184278543823,-46.579368264381,
40.0555581699984));
#190261=CARTESIAN_POINT('Ctrl Pts',(-42.1173773384969,-46.5882835699002,
40.0609828468886));
#190262=CARTESIAN_POINT('Ctrl Pts',(-42.1164161734956,-46.5964405904272,
40.0659461317305));
#190263=CARTESIAN_POINT('Ctrl Pts',(-42.1148801579478,-46.604669732884,
40.0706039980707));
#190264=CARTESIAN_POINT('Ctrl Pts',(-42.1127009621828,-46.6129145292184,
40.0748843180604));
#190265=CARTESIAN_POINT('Ctrl Pts',(-42.1116305483418,-46.616964346245,
40.076986797257));
#190266=CARTESIAN_POINT('Ctrl Pts',(-42.1104045383079,-46.6210176421364,
40.0789976708175));
#190267=CARTESIAN_POINT('Ctrl Pts',(-42.109012387551,-46.6250654385591,
40.08090504915));
#190268=CARTESIAN_POINT('Ctrl Pts',(-42.1087482405046,-46.6258334685042,
40.0812669556105));
#190269=CARTESIAN_POINT('Ctrl Pts',(-42.108477638333,-46.6266015422612,
40.0816253922033));
#190270=CARTESIAN_POINT('Ctrl Pts',(-42.1082005605487,-46.6273695213204,
40.0819801989139));
#190271=CARTESIAN_POINT('Ctrl Pts',(-42.1079321414451,-46.628113501034,
40.0823239179149));
#190272=CARTESIAN_POINT('Ctrl Pts',(-42.1076576451502,-46.6288573918595,
40.0826642303498));
#190273=CARTESIAN_POINT('Ctrl Pts',(-42.1073770559081,-46.6296010653158,
40.0830009916099));
#190274=CARTESIAN_POINT('Ctrl Pts',(-42.1043192521647,-46.6377054654049,
40.0866709464312));
#190275=CARTESIAN_POINT('Ctrl Pts',(-42.1005354505675,-46.645789240007,
40.0899175831877));
#190276=CARTESIAN_POINT('Ctrl Pts',(-42.0960238460772,-46.6536619390761,
40.0925642067062));
#190277=CARTESIAN_POINT('Ctrl Pts',(-42.0941185674852,-46.65698662878,40.0936818922527));
#190278=CARTESIAN_POINT('Ctrl Pts',(-42.0920839261385,-46.660273639941,
40.094693009479));
#190279=CARTESIAN_POINT('Ctrl Pts',(-42.0899216923181,-46.6635089796842,
40.0955863397546));
#190280=CARTESIAN_POINT('Ctrl Pts',(-42.0862805445927,-46.6689572109693,
40.0970906856166));
#190281=CARTESIAN_POINT('Ctrl Pts',(-42.0822770520158,-46.6742564366674,
40.0982599215483));
#190282=CARTESIAN_POINT('Ctrl Pts',(-42.0779224130575,-46.679333290145,
40.0990497370454));
#190283=CARTESIAN_POINT('Ctrl Pts',(-42.0768337533179,-46.6806025035144,
40.0992471909196));
#190284=CARTESIAN_POINT('Ctrl Pts',(-42.0757229796949,-46.6818576549905,
40.0994209989363));
#190285=CARTESIAN_POINT('Ctrl Pts',(-42.0745900553979,-46.6830973739111,
40.0995705982975));
#190286=CARTESIAN_POINT('Ctrl Pts',(-42.0728906689524,-46.6849569522919,
40.0997949973393));
#190287=CARTESIAN_POINT('Ctrl Pts',(-42.0711414461006,-46.686781786976,
40.0999649129781));
#190288=CARTESIAN_POINT('Ctrl Pts',(-42.0693433991611,-46.6885684866732,
40.1000786629733));
#190289=CARTESIAN_POINT('Ctrl Pts',(-42.0675453522215,-46.6903551863704,
40.1001924129685));
#190290=CARTESIAN_POINT('Ctrl Pts',(-42.0656984926178,-46.6921037531361,
40.10025));
#190291=CARTESIAN_POINT('Ctrl Pts',(-42.0638038389714,-46.6938111422615,
40.10025));
#190292=CARTESIAN_POINT('Ctrl Pts',(-39.5091373124624,-43.8565665267054,
40.10025));
#190293=CARTESIAN_POINT('Ctrl Pts',(-39.5155480799606,-43.8507890749204,
40.10025));
#190294=CARTESIAN_POINT('Ctrl Pts',(-39.5223801852472,-43.8455908828145,
40.099578633424));
#190295=CARTESIAN_POINT('Ctrl Pts',(-39.5294841269576,-43.8409939475737,
40.0983063763364));
#190296=CARTESIAN_POINT('Ctrl Pts',(-39.5340725443954,-43.8380247990812,
40.0974846287991));
#190297=CARTESIAN_POINT('Ctrl Pts',(-39.5387738681337,-43.8353056940457,
40.0964130309337));
#190298=CARTESIAN_POINT('Ctrl Pts',(-39.5435446222366,-43.8328343017435,
40.0951176960924));
#190299=CARTESIAN_POINT('Ctrl Pts',(-39.5498679835146,-43.8295586128167,
40.0934008039614));
#190300=CARTESIAN_POINT('Ctrl Pts',(-39.5563148866445,-43.826723686506,
40.0912909372156));
#190301=CARTESIAN_POINT('Ctrl Pts',(-39.5627952650342,-43.8243293609622,
40.0888630467851));
#190302=CARTESIAN_POINT('Ctrl Pts',(-39.566035454229,-43.8231321981903,
40.0876491015699));
#190303=CARTESIAN_POINT('Ctrl Pts',(-39.5692841591688,-43.8220450509624,
40.0863558569271));
#190304=CARTESIAN_POINT('Ctrl Pts',(-39.5725311673657,-43.8210669472517,
40.0849936342771));
#190305=CARTESIAN_POINT('Ctrl Pts',(-39.5741546714642,-43.8205778953963,
40.0843125229521));
#190306=CARTESIAN_POINT('Ctrl Pts',(-39.5757777635549,-43.8201160933894,
40.0836141747074));
#190307=CARTESIAN_POINT('Ctrl Pts',(-39.5773992434497,-43.8196813503777,
40.082899916161));
#190308=CARTESIAN_POINT('Ctrl Pts',(-39.5778046134234,-43.8195726646248,
40.0827213515243));
#190309=CARTESIAN_POINT('Ctrl Pts',(-39.5782098828931,-43.8194656698237,
40.0825417925842));
#190310=CARTESIAN_POINT('Ctrl Pts',(-39.5786150336268,-43.8193603625174,
40.0823612602361));
#190311=CARTESIAN_POINT('Ctrl Pts',(-39.5798304858278,-43.8190444405983,
40.0818196631917));
#190312=CARTESIAN_POINT('Ctrl Pts',(-39.5810448681191,-43.8187437073122,
40.0812693052022));
#190313=CARTESIAN_POINT('Ctrl Pts',(-39.5822576997163,-43.81845805878,40.0807107531875));
#190314=CARTESIAN_POINT('Ctrl Pts',(-39.5908007288818,-43.8164459874032,
40.076776384918));
#190315=CARTESIAN_POINT('Ctrl Pts',(-39.5992865061397,-43.8151322889028,
40.0724140586133));
#190316=CARTESIAN_POINT('Ctrl Pts',(-39.6076412948847,-43.8144227306309,
40.0677221223761));
#190317=CARTESIAN_POINT('Ctrl Pts',(-39.6116933583972,-43.8140785956357,
40.0654465383716));
#190318=CARTESIAN_POINT('Ctrl Pts',(-39.6157150281166,-43.8138769687218,
40.0630928000677));
#190319=CARTESIAN_POINT('Ctrl Pts',(-39.6196997093544,-43.8138093098902,
40.0606689262479));
#190320=CARTESIAN_POINT('Ctrl Pts',(-39.6257999779283,-43.8137057289462,
40.0569581447806));
#190321=CARTESIAN_POINT('Ctrl Pts',(-39.6318101761582,-43.8139151128798,
40.0530843804606));
#190322=CARTESIAN_POINT('Ctrl Pts',(-39.6376940219322,-43.8144090029876,
40.0490800251458));
#190323=CARTESIAN_POINT('Ctrl Pts',(-39.6404265103486,-43.8146383681088,
40.0472203818218));
#190324=CARTESIAN_POINT('Ctrl Pts',(-39.6431316855283,-43.8149288459965,
40.0453323608818));
#190325=CARTESIAN_POINT('Ctrl Pts',(-39.6458055463963,-43.8152787628651,
40.0434201572162));
#190326=CARTESIAN_POINT('Ctrl Pts',(-39.6460104872963,-43.8153055826144,
40.0432735943397));
#190327=CARTESIAN_POINT('Ctrl Pts',(-39.6462152612035,-43.8153327221692,
40.0431268995707));
#190328=CARTESIAN_POINT('Ctrl Pts',(-39.6464198673376,-43.8153601802952,
40.0429800745037));
#190329=CARTESIAN_POINT('Ctrl Pts',(-39.6492939666538,-43.8157458841822,
40.0409176249753));
#190330=CARTESIAN_POINT('Ctrl Pts',(-39.6521348180507,-43.8161965332332,
40.0388310783333));
#190331=CARTESIAN_POINT('Ctrl Pts',(-39.654938997009,-43.8167075634908,
40.036725739981));
#190332=CARTESIAN_POINT('Ctrl Pts',(-39.6649942840467,-43.8185400271109,
40.0291763710718));
#190333=CARTESIAN_POINT('Ctrl Pts',(-39.6746561192247,-43.8211611138368,
40.0213310894594));
#190334=CARTESIAN_POINT('Ctrl Pts',(-39.6839173731634,-43.8244418968099,
40.0132837551319));
#190335=CARTESIAN_POINT('Ctrl Pts',(-39.6940945608669,-43.8280471477135,
40.0044405431322));
#190336=CARTESIAN_POINT('Ctrl Pts',(-39.7037886794679,-43.8324491002312,
39.9953528710595));
#190337=CARTESIAN_POINT('Ctrl Pts',(-39.7129876499617,-43.8375295667873,
39.9861103629547));
#190338=CARTESIAN_POINT('Ctrl Pts',(-39.7229202294689,-43.843015195645,
39.9761307737539));
#190339=CARTESIAN_POINT('Ctrl Pts',(-39.7322766233322,-43.8492922888427,
39.9659696935986));
#190340=CARTESIAN_POINT('Ctrl Pts',(-39.7410245486316,-43.8562669044117,
39.9557128217472));
#190341=CARTESIAN_POINT('Ctrl Pts',(-39.7496990878245,-43.8631830101212,
39.9455419945137));
#190342=CARTESIAN_POINT('Ctrl Pts',(-39.7577762496647,-43.8707860819069,
39.9352756289329));
#190343=CARTESIAN_POINT('Ctrl Pts',(-39.7651933659001,-43.8790236240218,
39.92499));
#190344=CARTESIAN_POINT('Origin',(0.0113255271402848,-0.0101975504409049,
39.92499));
#190345=CARTESIAN_POINT('Ctrl Pts',(-42.0411527846897,-46.714206243142,
40.10025));
#190346=CARTESIAN_POINT('Ctrl Pts',(-42.0347675597394,-46.7199506919421,
40.10025));
#190347=CARTESIAN_POINT('Ctrl Pts',(-42.0279592142787,-46.7251107020204,
40.0995859581842));
#190348=CARTESIAN_POINT('Ctrl Pts',(-42.0208774479597,-46.7296675019384,
40.0983275959623));
#190349=CARTESIAN_POINT('Ctrl Pts',(-42.0163525364106,-46.7325790801588,
40.097523562407));
#190350=CARTESIAN_POINT('Ctrl Pts',(-42.0117164852005,-46.7352451892135,
40.0964777059492));
#190351=CARTESIAN_POINT('Ctrl Pts',(-42.0070114066749,-46.737668963875,
40.0952149915962));
#190352=CARTESIAN_POINT('Ctrl Pts',(-42.00058991857,-46.7409769299533,40.0934916398702));
#190353=CARTESIAN_POINT('Ctrl Pts',(-41.994038348078,-46.7438276087418,
40.0913643921631));
#190354=CARTESIAN_POINT('Ctrl Pts',(-41.9874523371583,-46.7462229640886,
40.0889118607714));
#190355=CARTESIAN_POINT('Ctrl Pts',(-41.9841593316985,-46.747420641762,
40.0876855950755));
#190356=CARTESIAN_POINT('Ctrl Pts',(-41.9808575622225,-46.7485046297345,
40.0863782327527));
#190357=CARTESIAN_POINT('Ctrl Pts',(-41.977557880152,-46.7494761782931,
40.0850006373334));
#190358=CARTESIAN_POINT('Ctrl Pts',(-41.9759080391167,-46.7499619525724,
40.0843118396238));
#190359=CARTESIAN_POINT('Ctrl Pts',(-41.9742587070257,-46.7504196286879,
40.0836054919165));
#190360=CARTESIAN_POINT('Ctrl Pts',(-41.9726111592841,-46.7508494364811,
40.0828829920418));
#190361=CARTESIAN_POINT('Ctrl Pts',(-41.9721992723487,-46.7509568884294,
40.0827023670732));
#190362=CARTESIAN_POINT('Ctrl Pts',(-41.9717874966609,-46.7510625988573,
40.0825207326933));
#190363=CARTESIAN_POINT('Ctrl Pts',(-41.971375851596,-46.7511665718604,
40.0823381109276));
#190364=CARTESIAN_POINT('Ctrl Pts',(-41.9701409164013,-46.7514784908697,
40.0817902456304));
#190365=CARTESIAN_POINT('Ctrl Pts',(-41.968907158177,-46.7517747718022,
40.0812334935554));
#190366=CARTESIAN_POINT('Ctrl Pts',(-41.9676750878621,-46.7520555364231,
40.0806684524227));
#190367=CARTESIAN_POINT('Ctrl Pts',(-41.9591607175413,-46.7539957941552,
40.0767636676137));
#190368=CARTESIAN_POINT('Ctrl Pts',(-41.9507055072913,-46.7552464720207,
40.0724404510887));
#190369=CARTESIAN_POINT('Ctrl Pts',(-41.9423805287162,-46.7559027543579,
40.0677949937407));
#190370=CARTESIAN_POINT('Ctrl Pts',(-41.9382430372163,-46.756228924878,
40.0654862141904));
#190371=CARTESIAN_POINT('Ctrl Pts',(-41.9341372814968,-46.7564078446194,
40.0630972003215));
#190372=CARTESIAN_POINT('Ctrl Pts',(-41.9300700339485,-46.7564487173141,
40.0606363359906));
#190373=CARTESIAN_POINT('Ctrl Pts',(-41.9210970783571,-46.7565388885837,
40.0552073017124));
#190374=CARTESIAN_POINT('Ctrl Pts',(-41.9123126321655,-46.7559695796223,
40.0494204304519));
#190375=CARTESIAN_POINT('Ctrl Pts',(-41.9038465062686,-46.7548061840815,
40.0434049749851));
#190376=CARTESIAN_POINT('Ctrl Pts',(-41.900753723715,-46.7543811810193,
40.0412074532442));
#190377=CARTESIAN_POINT('Ctrl Pts',(-41.8976992635448,-46.7538836816022,
40.0389814735788));
#190378=CARTESIAN_POINT('Ctrl Pts',(-41.8946854937103,-46.7533184435776,
40.0367321210016));
#190379=CARTESIAN_POINT('Ctrl Pts',(-41.8845625597436,-46.7514198688647,
40.029176783714));
#190380=CARTESIAN_POINT('Ctrl Pts',(-41.8748360802682,-46.7487367327316,
40.0213235332574));
#190381=CARTESIAN_POINT('Ctrl Pts',(-41.8655137786585,-46.7453971060009,
40.0132649215856));
#190382=CARTESIAN_POINT('Ctrl Pts',(-41.8552674648902,-46.741726460619,
40.0044075527529));
#190383=CARTESIAN_POINT('Ctrl Pts',(-41.8455087367165,-46.7372626589218,
39.9953016253715));
#190384=CARTESIAN_POINT('Ctrl Pts',(-41.836250857546,-46.732122753097,39.9860353422352));
#190385=CARTESIAN_POINT('Ctrl Pts',(-41.8262797250108,-46.7265868542962,
39.9760551582687));
#190386=CARTESIAN_POINT('Ctrl Pts',(-41.8168884800893,-46.7202662104758,
39.9658879738146));
#190387=CARTESIAN_POINT('Ctrl Pts',(-41.8081115112103,-46.7132528291638,
39.9556174643242));
#190388=CARTESIAN_POINT('Ctrl Pts',(-41.799453061046,-46.7063341521797,
39.9454856413897));
#190389=CARTESIAN_POINT('Ctrl Pts',(-41.791391507519,-46.6987402031258,
39.9352519465109));
#190390=CARTESIAN_POINT('Ctrl Pts',(-41.7839914803029,-46.6905216402895,
39.92499));
#190391=CARTESIAN_POINT('Ctrl Pts',(-39.4820551873932,-44.1339623850445,
39.92499));
#190392=CARTESIAN_POINT('Ctrl Pts',(-39.4749733207259,-44.1260971752955,
39.934810724171));
#190393=CARTESIAN_POINT('Ctrl Pts',(-39.4685372764378,-44.1177016730317,
39.9446038383145));
#190394=CARTESIAN_POINT('Ctrl Pts',(-39.4627751762777,-44.1088266671127,
39.9543158069348));
#190395=CARTESIAN_POINT('Ctrl Pts',(-39.4572113616012,-44.1002570680403,
39.9636935671346));
#190396=CARTESIAN_POINT('Ctrl Pts',(-39.45227528373,-44.091239296907,39.9729968320934));
#190397=CARTESIAN_POINT('Ctrl Pts',(-39.4480294591832,-44.0817922708815,
39.9821731151272));
#190398=CARTESIAN_POINT('Ctrl Pts',(-39.4440158252765,-44.0728618726619,
39.9908475764281));
#190399=CARTESIAN_POINT('Ctrl Pts',(-39.4406186435318,-44.0635470605651,
39.9994093733768));
#190400=CARTESIAN_POINT('Ctrl Pts',(-39.4379312493424,-44.0538529442926,
40.0077966115757));
#190401=CARTESIAN_POINT('Ctrl Pts',(-39.4354562043783,-44.0449248258367,
40.0155211172504));
#190402=CARTESIAN_POINT('Ctrl Pts',(-39.4335831186709,-44.0356744386912,
40.0230979940924));
#190403=CARTESIAN_POINT('Ctrl Pts',(-39.4324230329139,-44.0261054688135,
40.0304554104645));
#190404=CARTESIAN_POINT('Ctrl Pts',(-39.4320771187584,-44.0232521951534,
40.0326492435113));
#190405=CARTESIAN_POINT('Ctrl Pts',(-39.431794878803,-44.0203706219375,
40.0348233715027));
#190406=CARTESIAN_POINT('Ctrl Pts',(-39.4315800126158,-44.0174609456694,
40.0369753512356));
#190407=CARTESIAN_POINT('Ctrl Pts',(-39.4313673418319,-44.0145809991273,
40.0391053430352));
#190408=CARTESIAN_POINT('Ctrl Pts',(-39.4312206224785,-44.0116765294503,
40.041211089324));
#190409=CARTESIAN_POINT('Ctrl Pts',(-39.4311433701096,-44.0087510493743,
40.0432881154904));
#190410=CARTESIAN_POINT('Ctrl Pts',(-39.431137998131,-44.0085476172112,
40.043432547828));
#190411=CARTESIAN_POINT('Ctrl Pts',(-39.4311329512713,-44.0083440782822,
40.0435768364421));
#190412=CARTESIAN_POINT('Ctrl Pts',(-39.4311282308204,-44.0081404327823,
40.0437209807855));
#190413=CARTESIAN_POINT('Ctrl Pts',(-39.4309212689595,-43.9992118680545,
40.0500407968419));
#190414=CARTESIAN_POINT('Ctrl Pts',(-39.4313859080978,-43.9900881971809,
40.0560490279341));
#190415=CARTESIAN_POINT('Ctrl Pts',(-39.4325966403785,-43.9808585737702,
40.061664710861));
#190416=CARTESIAN_POINT('Ctrl Pts',(-39.4337252532878,-43.9722549606539,
40.0668995033479));
#190417=CARTESIAN_POINT('Ctrl Pts',(-39.4355025470894,-43.9635585482867,
40.0717933267474));
#190418=CARTESIAN_POINT('Ctrl Pts',(-39.4380105519132,-43.9548613290796,
40.0762460303063));
#190419=CARTESIAN_POINT('Ctrl Pts',(-39.4389280125246,-43.951679773775,
40.0778748868742));
#190420=CARTESIAN_POINT('Ctrl Pts',(-39.4399434521993,-43.9484983634058,
40.0794443522244));
#190421=CARTESIAN_POINT('Ctrl Pts',(-39.4410615611725,-43.945322616547,
40.0809482021491));
#190422=CARTESIAN_POINT('Ctrl Pts',(-39.4413304290278,-43.9445589555199,
40.0813098278168));
#190423=CARTESIAN_POINT('Ctrl Pts',(-39.441605709343,-43.9437952833154,
40.0816679525671));
#190424=CARTESIAN_POINT('Ctrl Pts',(-39.4418874191263,-43.9430317345448,
40.082022419258));
#190425=CARTESIAN_POINT('Ctrl Pts',(-39.4421603254788,-43.9422920466732,
40.0823658088647));
#190426=CARTESIAN_POINT('Ctrl Pts',(-39.4424392657172,-43.9415524746577,
40.0827057654616));
#190427=CARTESIAN_POINT('Ctrl Pts',(-39.4427242524727,-43.9408131433997,
40.083042147015));
#190428=CARTESIAN_POINT('Ctrl Pts',(-39.4458466117312,-43.9327129150422,
40.086727595681));
#190429=CARTESIAN_POINT('Ctrl Pts',(-39.4496972096663,-43.9246364083414,
40.0899823432037));
#190430=CARTESIAN_POINT('Ctrl Pts',(-39.4542738890629,-43.9167721156712,
40.0926299529364));
#190431=CARTESIAN_POINT('Ctrl Pts',(-39.4561719744242,-43.9135105590926,
40.0937279956089));
#190432=CARTESIAN_POINT('Ctrl Pts',(-39.4581945203291,-43.9102855324941,
40.0947220371804));
#190433=CARTESIAN_POINT('Ctrl Pts',(-39.4603395741452,-43.9071101492107,
40.0956014538692));
#190434=CARTESIAN_POINT('Ctrl Pts',(-39.4639981869599,-43.9016942021213,
40.097101390674));
#190435=CARTESIAN_POINT('Ctrl Pts',(-39.4680136963363,-43.8964251099355,
40.0982667904316));
#190436=CARTESIAN_POINT('Ctrl Pts',(-39.472373749158,-43.8913745966872,
40.0990539325582));
#190437=CARTESIAN_POINT('Ctrl Pts',(-39.4745537755689,-43.888849340063,
40.0994475036216));
#190438=CARTESIAN_POINT('Ctrl Pts',(-39.4768209551509,-43.8863797569639,
40.0997467259952));
#190439=CARTESIAN_POINT('Ctrl Pts',(-39.4791737454928,-43.883974878609,
40.0999473488896));
#190440=CARTESIAN_POINT('Ctrl Pts',(-39.4815265358346,-43.8815700002541,
40.100147971784));
#190441=CARTESIAN_POINT('Ctrl Pts',(-39.4839648939619,-43.8792298420739,
40.10025));
#190442=CARTESIAN_POINT('Ctrl Pts',(-39.4864862581819,-43.8769616275872,
40.10025));
#190443=CARTESIAN_POINT('Origin',(-43.3086183250768,-38.9747476500511,39.92499));
#190444=CARTESIAN_POINT('Ctrl Pts',(-46.6905216402899,-41.7839914803024,
39.92499));
#190445=CARTESIAN_POINT('Ctrl Pts',(-46.6984066517724,-41.7910911765306,
39.9348354642025));
#190446=CARTESIAN_POINT('Ctrl Pts',(-46.705708077355,-41.7987919603592,
39.944644082847));
#190447=CARTESIAN_POINT('Ctrl Pts',(-46.7123936319708,-41.8070443420777,
39.9543641760349));
#190448=CARTESIAN_POINT('Ctrl Pts',(-46.7188619458713,-41.81502857053,39.9637684240734));
#190449=CARTESIAN_POINT('Ctrl Pts',(-46.7247545199422,-41.8235301761272,
39.9730909636421));
#190450=CARTESIAN_POINT('Ctrl Pts',(-46.7300083326618,-41.8325358446891,
39.9822808977169));
#190451=CARTESIAN_POINT('Ctrl Pts',(-46.7349781159835,-41.8410546526115,
39.9909740094681));
#190452=CARTESIAN_POINT('Ctrl Pts',(-46.7393768060097,-41.8500252953134,
39.9995492765035));
#190453=CARTESIAN_POINT('Ctrl Pts',(-46.7431119772982,-41.8594521748314,
40.007946232873));
#190454=CARTESIAN_POINT('Ctrl Pts',(-46.7465523401894,-41.8681350126368,
40.0156804369727));
#190455=CARTESIAN_POINT('Ctrl Pts',(-46.7494299450239,-41.8772054497814,
40.0232638017462));
#190456=CARTESIAN_POINT('Ctrl Pts',(-46.7516345991566,-41.8866715402948,
40.0306257270008));
#190457=CARTESIAN_POINT('Ctrl Pts',(-46.7522740855148,-41.8894172933178,
40.0327611416679));
#190458=CARTESIAN_POINT('Ctrl Pts',(-46.752856683342,-41.8921963397437,
40.0348777427285));
#190459=CARTESIAN_POINT('Ctrl Pts',(-46.7533790039318,-41.8950088623277,
40.0369733168701));
#190460=CARTESIAN_POINT('Ctrl Pts',(-46.7539452330337,-41.8980578176393,
40.0392450539741));
#190461=CARTESIAN_POINT('Ctrl Pts',(-46.7544408966255,-41.9011416752731,
40.0414878751951));
#190462=CARTESIAN_POINT('Ctrl Pts',(-46.7548620578768,-41.9042597210854,
40.0436985701601));
#190463=CARTESIAN_POINT('Ctrl Pts',(-46.7560179382356,-41.9128172222842,
40.0497658398386));
#190464=CARTESIAN_POINT('Ctrl Pts',(-46.756568484326,-41.9216270724808,
40.0555581699984));
#190465=CARTESIAN_POINT('Ctrl Pts',(-46.756455626462,-41.9306033478348,
40.0609828468886));
#190466=CARTESIAN_POINT('Ctrl Pts',(-46.7563523676437,-41.9388161524504,
40.0659461317305));
#190467=CARTESIAN_POINT('Ctrl Pts',(-46.7556849461648,-41.9471607721487,
40.0706039980708));
#190468=CARTESIAN_POINT('Ctrl Pts',(-46.754379504153,-41.9555881906108,
40.0748843180606));
#190469=CARTESIAN_POINT('Ctrl Pts',(-46.7537382753013,-41.9597277110297,
40.0769867972571));
#190470=CARTESIAN_POINT('Ctrl Pts',(-46.7529426662694,-41.9638869554867,
40.0789976708176));
#190471=CARTESIAN_POINT('Ctrl Pts',(-46.7519812517997,-41.9680580970362,
40.08090504915));
#190472=CARTESIAN_POINT('Ctrl Pts',(-46.7517988327683,-41.9688495305178,
40.0812669556105));
#190473=CARTESIAN_POINT('Ctrl Pts',(-46.7516099985532,-41.9696416823156,
40.0816253922033));
#190474=CARTESIAN_POINT('Ctrl Pts',(-46.7514147143009,-41.9704344168201,
40.0819801989139));
#190475=CARTESIAN_POINT('Ctrl Pts',(-46.7512255326815,-41.9712023783714,
40.0823239179149));
#190476=CARTESIAN_POINT('Ctrl Pts',(-46.7510302978708,-41.971970886761,
40.0826642303498));
#190477=CARTESIAN_POINT('Ctrl Pts',(-46.7508289807695,-41.9727398158586,
40.0830009916099));
#190478=CARTESIAN_POINT('Ctrl Pts',(-46.7486350684819,-41.9811194467225,
40.0866709464313));
#190479=CARTESIAN_POINT('Ctrl Pts',(-46.7457169794822,-41.9895544525281,
40.0899175831879));
#190480=CARTESIAN_POINT('Ctrl Pts',(-46.7420530111687,-41.9978556152123,
40.0925642067064));
#190481=CARTESIAN_POINT('Ctrl Pts',(-46.7405056945978,-42.0013612477613,
40.0936818922529));
#190482=CARTESIAN_POINT('Ctrl Pts',(-46.7388257854549,-42.0048429302643,
40.0946930094791));
#190483=CARTESIAN_POINT('Ctrl Pts',(-46.7370135816691,-42.0082865614561,
40.0955863397546));
#190484=CARTESIAN_POINT('Ctrl Pts',(-46.7339618757758,-42.0140855503364,
40.0970906856166));
#190485=CARTESIAN_POINT('Ctrl Pts',(-46.7305342346688,-42.0197742252484,
40.0982599215483));
#190486=CARTESIAN_POINT('Ctrl Pts',(-46.7267341265708,-42.02527845091,40.0990497370454));
#190487=CARTESIAN_POINT('Ctrl Pts',(-46.7257840995463,-42.0266545073254,
40.0992471909196));
#190488=CARTESIAN_POINT('Ctrl Pts',(-46.7248106099124,-42.0280188904103,
40.0994209989363));
#190489=CARTESIAN_POINT('Ctrl Pts',(-46.7238134778068,-42.0293702408566,
40.0995705982975));
#190490=CARTESIAN_POINT('Ctrl Pts',(-46.7223177796485,-42.0313972665261,
40.0997949973393));
#190491=CARTESIAN_POINT('Ctrl Pts',(-46.7207688863877,-42.0333949481515,
40.0999649129781));
#190492=CARTESIAN_POINT('Ctrl Pts',(-46.7191674503111,-42.0353598072042,
40.1000786629733));
#190493=CARTESIAN_POINT('Ctrl Pts',(-46.7175660142345,-42.037324666257,
40.1001924129685));
#190494=CARTESIAN_POINT('Ctrl Pts',(-46.7159120469165,-42.039256703586,
40.10025));
#190495=CARTESIAN_POINT('Ctrl Pts',(-46.7142062431425,-42.0411527846892,
40.10025));
#190496=CARTESIAN_POINT('Ctrl Pts',(-43.8769616275876,-39.4864862581814,
40.10025));
#190497=CARTESIAN_POINT('Ctrl Pts',(-43.8827333680735,-39.4800703482075,
40.10025));
#190498=CARTESIAN_POINT('Ctrl Pts',(-43.8889846873392,-39.4741864828759,
40.0995786334241));
#190499=CARTESIAN_POINT('Ctrl Pts',(-43.8955692023364,-39.4688721660176,
40.0983063763368));
#190500=CARTESIAN_POINT('Ctrl Pts',(-43.8998221234149,-39.465439662607,
40.0974846287994));
#190501=CARTESIAN_POINT('Ctrl Pts',(-43.9042134689397,-39.4622440309671,
40.0964130309339));
#190502=CARTESIAN_POINT('Ctrl Pts',(-43.9086997575136,-39.4592874976151,
40.0951176960923));
#190503=CARTESIAN_POINT('Ctrl Pts',(-43.9146460760273,-39.4553687820179,
40.0934008039614));
#190504=CARTESIAN_POINT('Ctrl Pts',(-43.9207613318565,-39.4518755008531,
40.0912909372156));
#190505=CARTESIAN_POINT('Ctrl Pts',(-43.9269559348856,-39.4488169076807,
40.0888630467851));
#190506=CARTESIAN_POINT('Ctrl Pts',(-43.9300532364002,-39.4472876110945,
40.0876491015699));
#190507=CARTESIAN_POINT('Ctrl Pts',(-43.9331705067654,-39.445866837238,
40.0863558569271));
#190508=CARTESIAN_POINT('Ctrl Pts',(-43.9362974878338,-39.4445546869046,
40.0849936342771));
#190509=CARTESIAN_POINT('Ctrl Pts',(-43.937860978368,-39.443898611738,40.0843125229521));
#190510=CARTESIAN_POINT('Ctrl Pts',(-43.9394269075363,-39.4432696802088,
40.0836141747074));
#190511=CARTESIAN_POINT('Ctrl Pts',(-43.9409940617757,-39.4426678279632,
40.082899916161));
#190512=CARTESIAN_POINT('Ctrl Pts',(-43.9413858503355,-39.4425173649018,
40.0827213515243));
#190513=CARTESIAN_POINT('Ctrl Pts',(-43.9417777156946,-39.4423685940346,
40.0825417925842));
#190514=CARTESIAN_POINT('Ctrl Pts',(-43.9421696393592,-39.4422215138291,
40.0823612602361));
#190515=CARTESIAN_POINT('Ctrl Pts',(-43.9433454103532,-39.4417802732126,
40.0818196631917));
#190516=CARTESIAN_POINT('Ctrl Pts',(-43.944521704943,-39.4413542498602,
40.0812693052022));
#190517=CARTESIAN_POINT('Ctrl Pts',(-43.9456980341197,-39.4409433907175,
40.0807107531875));
#190518=CARTESIAN_POINT('Ctrl Pts',(-43.9539839449482,-39.438049351968,
40.0767763849181));
#190519=CARTESIAN_POINT('Ctrl Pts',(-43.9622859173447,-39.4358558447891,
40.0724140586136));
#190520=CARTESIAN_POINT('Ctrl Pts',(-43.9705207686468,-39.4342768603232,
40.0677221223766));
#190521=CARTESIAN_POINT('Ctrl Pts',(-43.9745146626295,-39.4335110545635,
40.0654465383719));
#190522=CARTESIAN_POINT('Ctrl Pts',(-43.9784932254702,-39.4328901532272,
40.0630928000678));
#190523=CARTESIAN_POINT('Ctrl Pts',(-43.9824490059338,-39.4324063524313,
40.0606689262479));
#190524=CARTESIAN_POINT('Ctrl Pts',(-43.9885050294413,-39.4316656872151,
40.0569581447805));
#190525=CARTESIAN_POINT('Ctrl Pts',(-43.9945041897573,-39.4312456873366,
40.0530843804606));
#190526=CARTESIAN_POINT('Ctrl Pts',(-44.0004074287824,-39.431121842506,
40.0490800251458));
#190527=CARTESIAN_POINT('Ctrl Pts',(-44.003148923525,-39.4310643283259,
40.0472203818218));
#190528=CARTESIAN_POINT('Ctrl Pts',(-44.0058696426793,-39.431070447141,
40.0453323608819));
#190529=CARTESIAN_POINT('Ctrl Pts',(-44.0085654321302,-39.4311389525609,
40.0434201572162));
#190530=CARTESIAN_POINT('Ctrl Pts',(-44.0087720537697,-39.4311442032314,
40.0432735943397));
#190531=CARTESIAN_POINT('Ctrl Pts',(-44.00897854276,-39.4311497894111,40.0431268995707));
#190532=CARTESIAN_POINT('Ctrl Pts',(-44.009184898196,-39.4311557099538,
40.0429800745037));
#190533=CARTESIAN_POINT('Ctrl Pts',(-44.01208356993,-39.4312388757297,40.0409176249753));
#190534=CARTESIAN_POINT('Ctrl Pts',(-44.0149559644985,-39.4313901062472,
40.0388310783332));
#190535=CARTESIAN_POINT('Ctrl Pts',(-44.0177981990785,-39.4316052205103,
40.036725739981));
#190536=CARTESIAN_POINT('Ctrl Pts',(-44.0279899468075,-39.4323765820012,
40.029176371072));
#190537=CARTESIAN_POINT('Ctrl Pts',(-44.0378728316086,-39.4339733733562,
40.02133108946));
#190538=CARTESIAN_POINT('Ctrl Pts',(-44.0474262866314,-39.4362681192145,
40.0132837551329));
#190539=CARTESIAN_POINT('Ctrl Pts',(-44.0579245739715,-39.4387898143852,
40.0044405431339));
#190540=CARTESIAN_POINT('Ctrl Pts',(-44.0680257165077,-39.4421543412259,
39.995352871062));
#190541=CARTESIAN_POINT('Ctrl Pts',(-44.0777053474396,-39.4462454222047,
39.986110362958));
#190542=CARTESIAN_POINT('Ctrl Pts',(-44.08815691959,-39.4506627629405,39.9761307737591));
#190543=CARTESIAN_POINT('Ctrl Pts',(-44.0981181930529,-39.4559274600913,
39.9659696936056));
#190544=CARTESIAN_POINT('Ctrl Pts',(-44.1075472421482,-39.4619494607967,
39.955712821756));
#190545=CARTESIAN_POINT('Ctrl Pts',(-44.1168971912124,-39.4679209431054,
39.9455419945197));
#190546=CARTESIAN_POINT('Ctrl Pts',(-44.1257248429276,-39.4746380711552,
39.9352756289359));
#190547=CARTESIAN_POINT('Ctrl Pts',(-44.1339623850449,-39.4820551873928,
39.92499));
#190548=CARTESIAN_POINT('Origin',(0.0101975504409187,-0.0113255271402718,
39.92499));
#190549=CARTESIAN_POINT('Ctrl Pts',(-46.6938111422607,-42.0638038389698,
40.10025));
#190550=CARTESIAN_POINT('Ctrl Pts',(-46.6880613546458,-42.0701842568303,
40.10025));
#190551=CARTESIAN_POINT('Ctrl Pts',(-46.6818296739374,-42.0760276657222,
40.0995859581842));
#190552=CARTESIAN_POINT('Ctrl Pts',(-46.6752630175678,-42.0812997491642,
40.0983275959621));
#190553=CARTESIAN_POINT('Ctrl Pts',(-46.671067236755,-42.0846683595048,
40.0975235624068));
#190554=CARTESIAN_POINT('Ctrl Pts',(-46.6667352666012,-42.0878044626436,
40.096477705949));
#190555=CARTESIAN_POINT('Ctrl Pts',(-46.6623093164291,-42.0907067742415,
40.0952149915961));
#190556=CARTESIAN_POINT('Ctrl Pts',(-46.6562687825186,-42.0946678472189,
40.0934916398701));
#190557=CARTESIAN_POINT('Ctrl Pts',(-46.6500510792883,-42.0981877352863,
40.0913643921631));
#190558=CARTESIAN_POINT('Ctrl Pts',(-46.643751530039,-42.1012583942263,
40.0889118607713));
#190559=CARTESIAN_POINT('Ctrl Pts',(-46.6406017554143,-42.1027937236964,
40.0876855950754));
#190560=CARTESIAN_POINT('Ctrl Pts',(-46.637431380974,-42.1042169023588,
40.0863782327527));
#190561=CARTESIAN_POINT('Ctrl Pts',(-46.6342513293849,-42.1055280393688,
40.0850006373334));
#190562=CARTESIAN_POINT('Ctrl Pts',(-46.6326613035904,-42.1061836078738,
40.0843118396238));
#190563=CARTESIAN_POINT('Ctrl Pts',(-46.6310688468942,-42.1068111789405,
40.0836054919165));
#190564=CARTESIAN_POINT('Ctrl Pts',(-46.6294752517396,-42.1074108478352,
40.0828829920418));
#190565=CARTESIAN_POINT('Ctrl Pts',(-46.629076852951,-42.1075607650589,
40.0827023670731));
#190566=CARTESIAN_POINT('Ctrl Pts',(-46.628678382762,-42.1077089386739,
40.0825207326933));
#190567=CARTESIAN_POINT('Ctrl Pts',(-46.6282798608701,-42.1078553707281,
40.0823381109276));
#190568=CARTESIAN_POINT('Ctrl Pts',(-46.6270842951944,-42.1082946668906,
40.0817902456304));
#190569=CARTESIAN_POINT('Ctrl Pts',(-46.6258882654173,-42.1087182876163,
40.0812334935553));
#190570=CARTESIAN_POINT('Ctrl Pts',(-46.6246922924068,-42.1091263005959,
40.0806684524227));
#190571=CARTESIAN_POINT('Ctrl Pts',(-46.6164273768568,-42.1119459234384,
40.0767636676137));
#190572=CARTESIAN_POINT('Ctrl Pts',(-46.6081492165687,-42.1140735600937,
40.0724404510889));
#190573=CARTESIAN_POINT('Ctrl Pts',(-46.5999384432817,-42.1155964444647,
40.067794993741));
#190574=CARTESIAN_POINT('Ctrl Pts',(-46.5958577114962,-42.1163533138169,
40.0654862141906));
#190575=CARTESIAN_POINT('Ctrl Pts',(-46.5917931497415,-42.1169604217532,
40.0630972003216));
#190576=CARTESIAN_POINT('Ctrl Pts',(-46.5877524553607,-42.117426213679,
40.0606363359906));
#190577=CARTESIAN_POINT('Ctrl Pts',(-46.578838080023,-42.1184538202399,
40.0552073017124));
#190578=CARTESIAN_POINT('Ctrl Pts',(-46.570042246956,-42.1188058546736,
40.0494204304519));
#190579=CARTESIAN_POINT('Ctrl Pts',(-46.5615008914345,-42.1185337834651,
40.0434049749851));
#190580=CARTESIAN_POINT('Ctrl Pts',(-46.5583806265503,-42.1184343924217,
40.0412074532442));
#190581=CARTESIAN_POINT('Ctrl Pts',(-46.5552908961829,-42.1182588963861,
40.0389814735788));
#190582=CARTESIAN_POINT('Ctrl Pts',(-46.5522345526329,-42.118011779524,
40.0367321210017));
#190583=CARTESIAN_POINT('Ctrl Pts',(-46.5419686180598,-42.1171817401332,
40.0291767837136));
#190584=CARTESIAN_POINT('Ctrl Pts',(-46.5320149571592,-42.1155299964529,
40.0213235332566));
#190585=CARTESIAN_POINT('Ctrl Pts',(-46.5223946380425,-42.1131831104079,
40.0132649215844));
#190586=CARTESIAN_POINT('Ctrl Pts',(-46.5118207677315,-42.1106036046376,
40.0044075527513));
#190587=CARTESIAN_POINT('Ctrl Pts',(-46.5016489045595,-42.1071843209722,
39.9953016253694));
#190588=CARTESIAN_POINT('Ctrl Pts',(-46.4919044745621,-42.1030402839717,
39.9860353422326));
#190589=CARTESIAN_POINT('Ctrl Pts',(-46.4814093059391,-42.0985769785641,
39.9760551582655));
#190590=CARTESIAN_POINT('Ctrl Pts',(-46.471408820054,-42.0932726122912,
39.9658879738107));
#190591=CARTESIAN_POINT('Ctrl Pts',(-46.4619468343577,-42.0872150940844,
39.9556174643197));
#190592=CARTESIAN_POINT('Ctrl Pts',(-46.4526126174182,-42.0812393728275,
39.9454856413867));
#190593=CARTESIAN_POINT('Ctrl Pts',(-46.4438014421018,-42.0745296860239,
39.9352519465095));
#190594=CARTESIAN_POINT('Ctrl Pts',(-46.4355828792672,-42.0671296588093,
39.92499));
#190595=CARTESIAN_POINT('Ctrl Pts',(-43.8790236240222,-39.7651933658996,
39.92499));
#190596=CARTESIAN_POINT('Ctrl Pts',(-43.8711584142706,-39.7581114992301,
39.9348107241742));
#190597=CARTESIAN_POINT('Ctrl Pts',(-43.8638800583542,-39.7504347382225,
39.9446038383209));
#190598=CARTESIAN_POINT('Ctrl Pts',(-43.8572218328498,-39.7422106539865,
39.9543158069443));
#190599=CARTESIAN_POINT('Ctrl Pts',(-43.8507927303092,-39.7342695770704,
39.9636935671462));
#190600=CARTESIAN_POINT('Ctrl Pts',(-43.8449410790297,-39.725817166863,
39.972996832107));
#190601=CARTESIAN_POINT('Ctrl Pts',(-43.8397310304406,-39.7168657021472,
39.9821731151428));
#190602=CARTESIAN_POINT('Ctrl Pts',(-43.8348059028379,-39.7084037645658,
39.9908475764451));
#190603=CARTESIAN_POINT('Ctrl Pts',(-43.8304536682163,-39.6994950821693,
39.9994093733951));
#190604=CARTESIAN_POINT('Ctrl Pts',(-43.8267676847771,-39.6901349804625,
40.0077966115952));
#190605=CARTESIAN_POINT('Ctrl Pts',(-43.8233729558667,-39.6815144838182,
40.0155211172709));
#190606=CARTESIAN_POINT('Ctrl Pts',(-43.8205432023665,-39.6725105620296,
40.0230979941138));
#190607=CARTESIAN_POINT('Ctrl Pts',(-43.8183892419653,-39.6631152739492,
40.0304554104866));
#190608=CARTESIAN_POINT('Ctrl Pts',(-43.8177469744554,-39.660313788705,
40.0326492435259));
#190609=CARTESIAN_POINT('Ctrl Pts',(-43.8171650742221,-39.6574775031669,
40.0348233715099));
#190610=CARTESIAN_POINT('Ctrl Pts',(-43.8166472411072,-39.6546062260519,
40.0369753512356));
#190611=CARTESIAN_POINT('Ctrl Pts',(-43.8161346989697,-39.6517642863084,
40.0391053430352));
#190612=CARTESIAN_POINT('Ctrl Pts',(-43.8156851836083,-39.6488910639687,
40.041211089324));
#190613=CARTESIAN_POINT('Ctrl Pts',(-43.8153025584994,-39.6459896850502,
40.0432881154904));
#190614=CARTESIAN_POINT('Ctrl Pts',(-43.8152759514976,-39.6457879288344,
40.043432547828));
#190615=CARTESIAN_POINT('Ctrl Pts',(-43.8152496566737,-39.6455860324534,
40.0435768364421));
#190616=CARTESIAN_POINT('Ctrl Pts',(-43.8152236753307,-39.6453839959663,
40.0437209807855));
#190617=CARTESIAN_POINT('Ctrl Pts',(-43.8140845580784,-39.6365259762553,
40.050040796842));
#190618=CARTESIAN_POINT('Ctrl Pts',(-43.8135929685791,-39.62740371779,40.0560490279345));
#190619=CARTESIAN_POINT('Ctrl Pts',(-43.81383230999,-39.6180980992371,40.0616647108616));
#190620=CARTESIAN_POINT('Ctrl Pts',(-43.8140554177822,-39.6094236454403,
40.0668995033487));
#190621=CARTESIAN_POINT('Ctrl Pts',(-43.8149139527618,-39.6005890951398,
40.0717933267483));
#190622=CARTESIAN_POINT('Ctrl Pts',(-43.8164991115145,-39.591677362319,
40.0762460303074));
#190623=CARTESIAN_POINT('Ctrl Pts',(-43.8170789830938,-39.5884173351601,
40.0778748868749));
#190624=CARTESIAN_POINT('Ctrl Pts',(-43.8177563121467,-39.5851472105416,
40.0794443522248));
#190625=CARTESIAN_POINT('Ctrl Pts',(-43.8185363400629,-39.5818719865443,
40.0809482021492));
#190626=CARTESIAN_POINT('Ctrl Pts',(-43.8187239107183,-39.5810844045885,
40.0813098278169));
#190627=CARTESIAN_POINT('Ctrl Pts',(-43.8189178575372,-39.5802961412319,
40.0816679525673));
#190628=CARTESIAN_POINT('Ctrl Pts',(-43.8191182115052,-39.5795073285706,
40.0820224192581));
#190629=CARTESIAN_POINT('Ctrl Pts',(-43.8193123044117,-39.578743166305,
40.0823658088649));
#190630=CARTESIAN_POINT('Ctrl Pts',(-43.81951241026,-39.5779784885478,40.0827057654617));
#190631=CARTESIAN_POINT('Ctrl Pts',(-43.819718554668,-39.5772134181963,
40.0830421470152));
#190632=CARTESIAN_POINT('Ctrl Pts',(-43.8219771048932,-39.5688311883232,
40.0867275956806));
#190633=CARTESIAN_POINT('Ctrl Pts',(-43.8249623840155,-39.5603964284874,
40.089982343203));
#190634=CARTESIAN_POINT('Ctrl Pts',(-43.8286919494553,-39.552096823972,
40.0926299529355));
#190635=CARTESIAN_POINT('Ctrl Pts',(-43.8302387114097,-39.5486547305946,
40.0937279956084));
#190636=CARTESIAN_POINT('Ctrl Pts',(-43.8319130705227,-39.5452359574129,
40.0947220371802));
#190637=CARTESIAN_POINT('Ctrl Pts',(-43.8337144555752,-39.5418537500314,
40.0956014538693));
#190638=CARTESIAN_POINT('Ctrl Pts',(-43.8367869054997,-39.5360850428917,
40.097101390674));
#190639=CARTESIAN_POINT('Ctrl Pts',(-43.8402296473865,-39.5304250803198,
40.0982667904316));
#190640=CARTESIAN_POINT('Ctrl Pts',(-43.8440378929943,-39.5249464846903,
40.0990539325583));
#190641=CARTESIAN_POINT('Ctrl Pts',(-43.8459420157982,-39.5222071868756,
40.0994475036216));
#190642=CARTESIAN_POINT('Ctrl Pts',(-43.8479386338069,-39.5195141476134,
40.0997467259952));
#190643=CARTESIAN_POINT('Ctrl Pts',(-43.8500271570783,-39.5168765098749,
40.0999473488896));
#190644=CARTESIAN_POINT('Ctrl Pts',(-43.8521156803496,-39.5142388721364,
40.100147971784));
#190645=CARTESIAN_POINT('Ctrl Pts',(-43.8542960677575,-39.5116566557596,
40.10025));
#190646=CARTESIAN_POINT('Ctrl Pts',(-43.8565665267058,-39.509137312462,
40.10025));
#190647=CARTESIAN_POINT('Origin',(-47.145339660541,-34.2342565846634,39.92499));
#190648=CARTESIAN_POINT('Ctrl Pts',(-50.8023624960593,-36.6746059268175,
39.92499));
#190649=CARTESIAN_POINT('Ctrl Pts',(-50.8109464329598,-36.6808425220335,
39.9348354642014));
#190650=CARTESIAN_POINT('Ctrl Pts',(-50.8190128116682,-36.6877379133662,
39.944644082845));
#190651=CARTESIAN_POINT('Ctrl Pts',(-50.8265243508951,-36.6952462569234,
39.954364176032));
#190652=CARTESIAN_POINT('Ctrl Pts',(-50.8337918098254,-36.7025106240243,
39.9637684240698));
#190653=CARTESIAN_POINT('Ctrl Pts',(-50.840540763527,-36.7103497152236,
39.9730909636379));
#190654=CARTESIAN_POINT('Ctrl Pts',(-50.8467071440061,-36.7187568768201,
39.9822808977121));
#190655=CARTESIAN_POINT('Ctrl Pts',(-50.8525401602354,-36.7267095340072,
39.9909740094627));
#190656=CARTESIAN_POINT('Ctrl Pts',(-50.8578524412734,-36.7351712462802,
39.9995492764976));
#190657=CARTESIAN_POINT('Ctrl Pts',(-50.8625525281321,-36.74415605265,40.0079462328667));
#190658=CARTESIAN_POINT('Ctrl Pts',(-50.8668816480479,-36.7524317091144,
40.015680436966));
#190659=CARTESIAN_POINT('Ctrl Pts',(-50.8706916079178,-36.7611516658429,
40.023263801739));
#190660=CARTESIAN_POINT('Ctrl Pts',(-50.8738736606191,-36.7703354510124,
40.0306257269932));
#190661=CARTESIAN_POINT('Ctrl Pts',(-50.8747966531493,-36.7729993179897,
40.0327611416629));
#190662=CARTESIAN_POINT('Ctrl Pts',(-50.8756665488979,-36.775702242456,
40.034877742726));
#190663=CARTESIAN_POINT('Ctrl Pts',(-50.8764799968255,-36.7784447603817,
40.03697331687));
#190664=CARTESIAN_POINT('Ctrl Pts',(-50.8773618266784,-36.7814178261391,
40.039245053974));
#190665=CARTESIAN_POINT('Ctrl Pts',(-50.8781771258725,-36.7844329791245,
40.041487875195));
#190666=CARTESIAN_POINT('Ctrl Pts',(-50.8789219044955,-36.7874899206173,
40.0436985701601));
#190667=CARTESIAN_POINT('Ctrl Pts',(-50.8809659552704,-36.7958797205314,
40.0497658398386));
#190668=CARTESIAN_POINT('Ctrl Pts',(-50.8824343655145,-36.8045837617102,
40.0555581699984));
#190669=CARTESIAN_POINT('Ctrl Pts',(-50.8832604021663,-36.8135226609476,
40.0609828468886));
#190670=CARTESIAN_POINT('Ctrl Pts',(-50.8840161808562,-36.8217012684457,
40.0659461317305));
#190671=CARTESIAN_POINT('Ctrl Pts',(-50.8842246658556,-36.8300699399856,
40.0706039980707));
#190672=CARTESIAN_POINT('Ctrl Pts',(-50.8838072802929,-36.8385876480148,
40.0748843180603));
#190673=CARTESIAN_POINT('Ctrl Pts',(-50.883602261868,-36.8427715183744,
40.076986797257));
#190674=CARTESIAN_POINT('Ctrl Pts',(-50.8832457706971,-36.8469911418447,
40.0789976708175));
#190675=CARTESIAN_POINT('Ctrl Pts',(-50.8827256259726,-36.8512399286215,
40.08090504915));
#190676=CARTESIAN_POINT('Ctrl Pts',(-50.8826269335774,-36.8520460945287,
40.0812669556105));
#190677=CARTESIAN_POINT('Ctrl Pts',(-50.882521936226,-36.8528536453864,
40.0816253922033));
#190678=CARTESIAN_POINT('Ctrl Pts',(-50.8824105850808,-36.8536624499711,
40.0819801989139));
#190679=CARTESIAN_POINT('Ctrl Pts',(-50.8823027136589,-36.8544459794126,
40.0823239179149));
#190680=CARTESIAN_POINT('Ctrl Pts',(-50.8821888793659,-36.8552306854276,
40.0826642303498));
#190681=CARTESIAN_POINT('Ctrl Pts',(-50.8820690400776,-36.8560164456183,
40.0830009916099));
#190682=CARTESIAN_POINT('Ctrl Pts',(-50.8807630562081,-36.8645794982677,
40.0866709464313));
#190683=CARTESIAN_POINT('Ctrl Pts',(-50.8787426509998,-36.8732733195876,
40.0899175831879));
#190684=CARTESIAN_POINT('Ctrl Pts',(-50.8759664620667,-36.8819119966114,
40.0925642067064));
#190685=CARTESIAN_POINT('Ctrl Pts',(-50.874794060241,-36.8855601635618,
40.0936818922529));
#190686=CARTESIAN_POINT('Ctrl Pts',(-50.8734872887378,-36.8891983713649,
40.0946930094791));
#190687=CARTESIAN_POINT('Ctrl Pts',(-50.8720449698705,-36.8928125648615,
40.0955863397546));
#190688=CARTESIAN_POINT('Ctrl Pts',(-50.8696161409376,-36.8988987764014,
40.0970906856166));
#190689=CARTESIAN_POINT('Ctrl Pts',(-50.8668019052538,-36.9049145742146,
40.0982599215483));
#190690=CARTESIAN_POINT('Ctrl Pts',(-50.8635979627954,-36.9107858666119,
40.0990497370454));
#190691=CARTESIAN_POINT('Ctrl Pts',(-50.8627969771808,-36.9122536897112,
40.0992471909196));
#190692=CARTESIAN_POINT('Ctrl Pts',(-50.8619714372922,-36.9137123559381,
40.0994209989363));
#190693=CARTESIAN_POINT('Ctrl Pts',(-50.8611210221662,-36.915160532232,
40.0995705982975));
#190694=CARTESIAN_POINT('Ctrl Pts',(-50.8598453994771,-36.9173327966728,
40.0997949973393));
#190695=CARTESIAN_POINT('Ctrl Pts',(-50.858513805806,-36.9194814382215,
40.0999649129781));
#190696=CARTESIAN_POINT('Ctrl Pts',(-50.8571265262611,-36.9216029292229,
40.1000786629733));
#190697=CARTESIAN_POINT('Ctrl Pts',(-50.8557392467162,-36.9237244202243,
40.1001924129685));
#190698=CARTESIAN_POINT('Ctrl Pts',(-50.8542962928986,-36.9258187603138,
40.10025));
#190699=CARTESIAN_POINT('Ctrl Pts',(-50.8527980281401,-36.9278827595334,
40.10025));
#190700=CARTESIAN_POINT('Ctrl Pts',(-47.7640607692765,-34.6837837831344,
40.10025));
#190701=CARTESIAN_POINT('Ctrl Pts',(-47.7691302463542,-34.6767997090229,
40.10025));
#190702=CARTESIAN_POINT('Ctrl Pts',(-47.7747322888379,-34.6702946353247,
40.0995786334241));
#190703=CARTESIAN_POINT('Ctrl Pts',(-47.7807252357988,-34.664321161616,
40.0983063763367));
#190704=CARTESIAN_POINT('Ctrl Pts',(-47.7845960646237,-34.6604629105138,
40.0974846287993));
#190705=CARTESIAN_POINT('Ctrl Pts',(-47.7886293194335,-34.6568257642794,
40.0964130309339));
#190706=CARTESIAN_POINT('Ctrl Pts',(-47.7927819897609,-34.6534164822762,
40.0951176960924));
#190707=CARTESIAN_POINT('Ctrl Pts',(-47.7982861164003,-34.6488976742768,
40.0934008039615));
#190708=CARTESIAN_POINT('Ctrl Pts',(-47.8040027249064,-34.6447843113773,
40.0912909372157));
#190709=CARTESIAN_POINT('Ctrl Pts',(-47.8098436832079,-34.6410949611631,
40.0888630467852));
#190710=CARTESIAN_POINT('Ctrl Pts',(-47.8127641623586,-34.639250286056,
40.0876491015699));
#190711=CARTESIAN_POINT('Ctrl Pts',(-47.8157158446827,-34.6375114518665,
40.0863558569272));
#190712=CARTESIAN_POINT('Ctrl Pts',(-47.8186885387638,-34.6358796311042,
40.0849936342772));
#190713=CARTESIAN_POINT('Ctrl Pts',(-47.8201748858043,-34.6350637207231,
40.0843125229522));
#190714=CARTESIAN_POINT('Ctrl Pts',(-47.8216664954025,-34.634274550377,
40.0836141747075));
#190715=CARTESIAN_POINT('Ctrl Pts',(-47.8231621539167,-34.6335121829167,
40.082899916161));
#190716=CARTESIAN_POINT('Ctrl Pts',(-47.8235360685452,-34.6333215910516,
40.0827213515244));
#190717=CARTESIAN_POINT('Ctrl Pts',(-47.8239102364347,-34.6331326740829,
40.0825417925842));
#190718=CARTESIAN_POINT('Ctrl Pts',(-47.8242846390327,-34.6329454324198,
40.0823612602361));
#190719=CARTESIAN_POINT('Ctrl Pts',(-47.8254078468265,-34.6323837074305,
40.0818196631918));
#190720=CARTESIAN_POINT('Ctrl Pts',(-47.8265331659852,-34.6318370616127,
40.0812693052022));
#190721=CARTESIAN_POINT('Ctrl Pts',(-47.8276601046327,-34.6313054933183,
40.0807107531875));
#190722=CARTESIAN_POINT('Ctrl Pts',(-47.8355981149517,-34.6275611948901,
40.0767763849182));
#190723=CARTESIAN_POINT('Ctrl Pts',(-47.8436253243402,-34.6245119115564,
40.0724140586137));
#190724=CARTESIAN_POINT('Ctrl Pts',(-47.8516500154454,-34.6220808005807,
40.0677221223767));
#190725=CARTESIAN_POINT('Ctrl Pts',(-47.8555419819598,-34.6209017143847,
40.065446538372));
#190726=CARTESIAN_POINT('Ctrl Pts',(-47.8594338479544,-34.6198683413511,
40.0630928000679));
#190727=CARTESIAN_POINT('Ctrl Pts',(-47.863317387285,-34.6189736992138,
40.0606689262479));
#190728=CARTESIAN_POINT('Ctrl Pts',(-47.8692628146652,-34.6176040646083,
40.0569581447806));
#190729=CARTESIAN_POINT('Ctrl Pts',(-47.8751852090114,-34.6165592825244,
40.0530843804605));
#190730=CARTESIAN_POINT('Ctrl Pts',(-47.8810431641657,-34.6158190596251,
40.0490800251457));
#190731=CARTESIAN_POINT('Ctrl Pts',(-47.8837636288444,-34.6154752962812,
40.0472203818218));
#190732=CARTESIAN_POINT('Ctrl Pts',(-47.8864700832048,-34.6151969889846,
40.0453323608819));
#190733=CARTESIAN_POINT('Ctrl Pts',(-47.8891582656053,-34.614983332396,
40.0434201572162));
#190734=CARTESIAN_POINT('Ctrl Pts',(-47.8893643041943,-34.6149669564604,
40.0432735943397));
#190735=CARTESIAN_POINT('Ctrl Pts',(-47.8895702459311,-34.6149509280615,
40.0431268995707));
#190736=CARTESIAN_POINT('Ctrl Pts',(-47.8897760897957,-34.6149352461543,
40.0429800745037));
#190737=CARTESIAN_POINT('Ctrl Pts',(-47.8926675754934,-34.6147149626375,
40.0409176249753));
#190738=CARTESIAN_POINT('Ctrl Pts',(-47.8955400426775,-34.6145651177083,
40.0388310783332));
#190739=CARTESIAN_POINT('Ctrl Pts',(-47.8983891927624,-34.6144819591401,
40.036725739981));
#190740=CARTESIAN_POINT('Ctrl Pts',(-47.9086057382628,-34.6141837673038,
40.0291763710717));
#190741=CARTESIAN_POINT('Ctrl Pts',(-47.9186013937339,-34.6147387685079,
40.0213310894592));
#190742=CARTESIAN_POINT('Ctrl Pts',(-47.9283423801891,-34.616022335536,
40.0132837551316));
#190743=CARTESIAN_POINT('Ctrl Pts',(-47.9390467457342,-34.6174328467542,
40.0044405431322));
#190744=CARTESIAN_POINT('Ctrl Pts',(-47.9494442419754,-34.6197230854585,
39.9953528710599));
#190745=CARTESIAN_POINT('Ctrl Pts',(-47.9594984812846,-34.6227799581216,
39.9861103629555));
#190746=CARTESIAN_POINT('Ctrl Pts',(-47.9703545364684,-34.6260806134274,
39.9761307737559));
#190747=CARTESIAN_POINT('Ctrl Pts',(-47.9808115517362,-34.6302752334095,
39.9659696936019));
#190748=CARTESIAN_POINT('Ctrl Pts',(-47.9908184179939,-34.6352786409534,
39.9557128217518));
#190749=CARTESIAN_POINT('Ctrl Pts',(-48.0007413369265,-34.6402400750494,
39.9455419945169));
#190750=CARTESIAN_POINT('Ctrl Pts',(-48.0102227609131,-34.6459976651003,
39.9352756289345));
#190751=CARTESIAN_POINT('Ctrl Pts',(-48.0191904766738,-34.6525130919795,
39.92499));
#190752=CARTESIAN_POINT('Origin',(0.00895784724494739,-0.0123294189942709,
39.92499));
#190753=CARTESIAN_POINT('Ctrl Pts',(-50.8348823336488,-36.952541597521,
40.10025));
#190754=CARTESIAN_POINT('Ctrl Pts',(-50.8298309792457,-36.9594880792489,
40.10025));
#190755=CARTESIAN_POINT('Ctrl Pts',(-50.8242442388875,-36.965950865344,
40.0995859581841));
#190756=CARTESIAN_POINT('Ctrl Pts',(-50.8182646381283,-36.9718804702608,
40.0983275959618));
#190757=CARTESIAN_POINT('Ctrl Pts',(-50.8144439579046,-36.9756692055214,
40.0975235624066));
#190758=CARTESIAN_POINT('Ctrl Pts',(-50.8104635307789,-36.9792409429416,
40.0964777059489));
#190759=CARTESIAN_POINT('Ctrl Pts',(-50.8063652005968,-36.9825899931424,
40.0952149915962));
#190760=CARTESIAN_POINT('Ctrl Pts',(-50.8007718022343,-36.9871607746747,
40.0934916398702));
#190761=CARTESIAN_POINT('Ctrl Pts',(-50.7949560887234,-36.9913113073907,
40.0913643921631));
#190762=CARTESIAN_POINT('Ctrl Pts',(-50.7890120203241,-36.9950236271421,
40.0889118607714));
#190763=CARTESIAN_POINT('Ctrl Pts',(-50.7860399861245,-36.9968797870178,
40.0876855950755));
#190764=CARTESIAN_POINT('Ctrl Pts',(-50.7830357420057,-36.9986265637268,
40.0863782327527));
#190765=CARTESIAN_POINT('Ctrl Pts',(-50.7800101622087,-37.0002629240968,
40.0850006373334));
#190766=CARTESIAN_POINT('Ctrl Pts',(-50.7784973723102,-37.0010811042819,
40.0843118396238));
#190767=CARTESIAN_POINT('Ctrl Pts',(-50.7769792382976,-37.0018716944999,
40.0836054919165));
#190768=CARTESIAN_POINT('Ctrl Pts',(-50.775457055492,-37.0026346543982,
40.0828829920418));
#190769=CARTESIAN_POINT('Ctrl Pts',(-50.7750765097907,-37.0028253943728,
40.0827023670731));
#190770=CARTESIAN_POINT('Ctrl Pts',(-50.7746957108234,-37.0030144077538,
40.0825207326933));
#190771=CARTESIAN_POINT('Ctrl Pts',(-50.7743146783937,-37.0032016945188,
40.0823381109276));
#190772=CARTESIAN_POINT('Ctrl Pts',(-50.7731715811046,-37.0037635548137,
40.0817902456304));
#190773=CARTESIAN_POINT('Ctrl Pts',(-50.7720263837272,-37.0043098740554,
40.0812334935553));
#190774=CARTESIAN_POINT('Ctrl Pts',(-50.7708796113517,-37.0048406651181,
40.0806684524227));
#190775=CARTESIAN_POINT('Ctrl Pts',(-50.7629547027167,-37.0085087606931,
40.0767636676138));
#190776=CARTESIAN_POINT('Ctrl Pts',(-50.754944289647,-37.0114900453058,
40.072440451089));
#190777=CARTESIAN_POINT('Ctrl Pts',(-50.7469376805983,-37.0138628466708,
40.0677949937412));
#190778=CARTESIAN_POINT('Ctrl Pts',(-50.7429584178786,-37.015042122436,
40.0654862141907));
#190779=CARTESIAN_POINT('Ctrl Pts',(-50.738979582278,-37.0160707669656,
40.0630972003217));
#190780=CARTESIAN_POINT('Ctrl Pts',(-50.7350097117579,-37.0169563748087,
40.0606363359906));
#190781=CARTESIAN_POINT('Ctrl Pts',(-50.7262515844357,-37.0189101579884,
40.0552073017124));
#190782=CARTESIAN_POINT('Ctrl Pts',(-50.717540733481,-37.0201796788543,
40.0494204304519));
#190783=CARTESIAN_POINT('Ctrl Pts',(-50.7090177292134,-37.0208019128473,
40.0434049749852));
#190784=CARTESIAN_POINT('Ctrl Pts',(-50.7059041682737,-37.0210292227717,
40.0412074532442));
#190785=CARTESIAN_POINT('Ctrl Pts',(-50.7028130194416,-37.021177652889,
40.0389814735788));
#190786=CARTESIAN_POINT('Ctrl Pts',(-50.6997475881155,-37.0212513646534,
40.0367321210017));
#190787=CARTESIAN_POINT('Ctrl Pts',(-50.6894511286645,-37.0214989546702,
40.0291767837139));
#190788=CARTESIAN_POINT('Ctrl Pts',(-50.6793793407317,-37.0208967002924,
40.0213235332571));
#190789=CARTESIAN_POINT('Ctrl Pts',(-50.6695664063384,-37.0195682679084,
40.0132649215851));
#190790=CARTESIAN_POINT('Ctrl Pts',(-50.6587808290217,-37.0181081633552,
40.0044075527522));
#190791=CARTESIAN_POINT('Ctrl Pts',(-50.6483072759139,-37.0157708601097,
39.9953016253706));
#190792=CARTESIAN_POINT('Ctrl Pts',(-50.6381830571046,-37.0126680948708,
39.9860353422341));
#190793=CARTESIAN_POINT('Ctrl Pts',(-50.6272788396587,-37.0093262837655,
39.9760551582674));
#190794=CARTESIAN_POINT('Ctrl Pts',(-50.6167786802271,-37.005096310788,
39.9658879738132));
#190795=CARTESIAN_POINT('Ctrl Pts',(-50.6067353452094,-37.0000610231244,
39.9556174643228));
#190796=CARTESIAN_POINT('Ctrl Pts',(-50.5968276291256,-36.9950937288458,
39.9454856413887));
#190797=CARTESIAN_POINT('Ctrl Pts',(-50.5873633690976,-36.9893418170233,
39.9352519465104));
#190798=CARTESIAN_POINT('Ctrl Pts',(-50.5784163149359,-36.9828414016744,
39.92499));
#190799=CARTESIAN_POINT('Ctrl Pts',(-47.7952442955504,-34.9607485668363,
39.92499));
#190800=CARTESIAN_POINT('Ctrl Pts',(-47.7866819156022,-34.954527633663,
39.9348107241725));
#190801=CARTESIAN_POINT('Ctrl Pts',(-47.7786409912514,-34.9476537221158,
39.9446038383174));
#190802=CARTESIAN_POINT('Ctrl Pts',(-47.7711595893171,-34.9401706643553,
39.9543158069391));
#190803=CARTESIAN_POINT('Ctrl Pts',(-47.7639356375068,-34.9329451136992,
39.96369356714));
#190804=CARTESIAN_POINT('Ctrl Pts',(-47.7572325247358,-34.9251506707962,
39.9729968320999));
#190805=CARTESIAN_POINT('Ctrl Pts',(-47.7511153344876,-34.9167928415144,
39.9821731151347));
#190806=CARTESIAN_POINT('Ctrl Pts',(-47.7453326739177,-34.908892075333,
39.9908475764366));
#190807=CARTESIAN_POINT('Ctrl Pts',(-47.7400730704119,-34.9004871280284,
39.9994093733862));
#190808=CARTESIAN_POINT('Ctrl Pts',(-47.7354288821281,-34.8915635921236,
40.0077966115859));
#190809=CARTESIAN_POINT('Ctrl Pts',(-47.7311516626307,-34.8833451652587,
40.0155211172615));
#190810=CARTESIAN_POINT('Ctrl Pts',(-47.727396244708,-34.8746863576813,
40.0230979941043));
#190811=CARTESIAN_POINT('Ctrl Pts',(-47.7242720089018,-34.8655676881434,
40.0304554104772));
#190812=CARTESIAN_POINT('Ctrl Pts',(-47.7233404248515,-34.8628486849605,
40.0326492435196));
#190813=CARTESIAN_POINT('Ctrl Pts',(-47.7224652397586,-34.8600887620247,
40.0348233715068));
#190814=CARTESIAN_POINT('Ctrl Pts',(-47.7216501132021,-34.8572873423618,
40.0369753512356));
#190815=CARTESIAN_POINT('Ctrl Pts',(-47.72084331523,-34.8545145463036,40.0391053430352));
#190816=CARTESIAN_POINT('Ctrl Pts',(-47.720095928845,-34.8517040509265,
40.041211089324));
#190817=CARTESIAN_POINT('Ctrl Pts',(-47.7194121231167,-34.8488585612799,
40.0432881154904));
#190818=CARTESIAN_POINT('Ctrl Pts',(-47.7193645726037,-34.8486606914947,
40.043432547828));
#190819=CARTESIAN_POINT('Ctrl Pts',(-47.7193173179071,-34.8484626496808,
40.0435768364421));
#190820=CARTESIAN_POINT('Ctrl Pts',(-47.7192703603292,-34.8482644357606,
40.0437209807855));
#190821=CARTESIAN_POINT('Ctrl Pts',(-47.7172115680923,-34.8395740113842,
40.0500407968421));
#190822=CARTESIAN_POINT('Ctrl Pts',(-47.7157691359129,-34.8305531107002,
40.0560490279346));
#190823=CARTESIAN_POINT('Ctrl Pts',(-47.7150344641794,-34.8212734513095,
40.0616647108616));
#190824=CARTESIAN_POINT('Ctrl Pts',(-47.7143496224387,-34.8126231959632,
40.0668995033489));
#190825=CARTESIAN_POINT('Ctrl Pts',(-47.7142799923072,-34.8037473009113,
40.0717933267486));
#190826=CARTESIAN_POINT('Ctrl Pts',(-47.7149249376577,-34.7947186932867,
40.0762460303077));
#190827=CARTESIAN_POINT('Ctrl Pts',(-47.7151608670106,-34.7914159118128,
40.0778748868751));
#190828=CARTESIAN_POINT('Ctrl Pts',(-47.7154926644831,-34.7880929011144,
40.0794443522249));
#190829=CARTESIAN_POINT('Ctrl Pts',(-47.7159260651934,-34.7847540840178,
40.0809482021492));
#190830=CARTESIAN_POINT('Ctrl Pts',(-47.7160302835856,-34.7839512100459,
40.0813098278169));
#190831=CARTESIAN_POINT('Ctrl Pts',(-47.7161407719862,-34.7831469919156,
40.0816679525672));
#190832=CARTESIAN_POINT('Ctrl Pts',(-47.7162575750189,-34.7823415577602,
40.0820224192581));
#190833=CARTESIAN_POINT('Ctrl Pts',(-47.7163707279568,-34.7815612934222,
40.0823658088648));
#190834=CARTESIAN_POINT('Ctrl Pts',(-47.7164898070135,-34.780779887893,
40.0827057654617));
#190835=CARTESIAN_POINT('Ctrl Pts',(-47.7166148505127,-34.7799974607187,
40.0830421470151));
#190836=CARTESIAN_POINT('Ctrl Pts',(-47.717984846556,-34.7714250667938,
40.0867275956805));
#190837=CARTESIAN_POINT('Ctrl Pts',(-47.7200720995232,-34.7627244668161,
40.0899823432028));
#190838=CARTESIAN_POINT('Ctrl Pts',(-47.7229136891075,-34.7540804826588,
40.0926299529353));
#190839=CARTESIAN_POINT('Ctrl Pts',(-47.724092181007,-34.7504955647788,
40.0937279956083));
#190840=CARTESIAN_POINT('Ctrl Pts',(-47.7254000086987,-34.7469205018089,
40.0947220371802));
#190841=CARTESIAN_POINT('Ctrl Pts',(-47.7268379886354,-34.7433685265019,
40.0956014538693));
#190842=CARTESIAN_POINT('Ctrl Pts',(-47.7292906132653,-34.7373102624744,
40.097101390674));
#190843=CARTESIAN_POINT('Ctrl Pts',(-47.7321228682622,-34.7313214412508,
40.0982667904316));
#190844=CARTESIAN_POINT('Ctrl Pts',(-47.7353375827202,-34.7254747878805,
40.0990539325583));
#190845=CARTESIAN_POINT('Ctrl Pts',(-47.7369449399493,-34.7225514611953,
40.0994475036216));
#190846=CARTESIAN_POINT('Ctrl Pts',(-47.73864912102,-34.7196644712718,40.0997467259952));
#190847=CARTESIAN_POINT('Ctrl Pts',(-47.7404504949228,-34.7168229726607,
40.0999473488896));
#190848=CARTESIAN_POINT('Ctrl Pts',(-47.7422518688256,-34.7139814740496,
40.100147971784));
#190849=CARTESIAN_POINT('Ctrl Pts',(-47.7441503967333,-34.7111854907791,
40.10025));
#190850=CARTESIAN_POINT('Ctrl Pts',(-47.7461450747866,-34.7084426211229,
40.10025));
#190851=CARTESIAN_POINT('Origin',(-50.4655267888877,-29.1186878401553,39.92499));
#190852=CARTESIAN_POINT('Ctrl Pts',(-54.357602037244,-31.1634057161437,
39.92499));
#190853=CARTESIAN_POINT('Ctrl Pts',(-54.3667908521539,-31.1687108809055,
39.9348354642015));
#190854=CARTESIAN_POINT('Ctrl Pts',(-54.3755338070554,-31.1747253323925,
39.9446440828451));
#190855=CARTESIAN_POINT('Ctrl Pts',(-54.3837890328982,-31.1814073748059,
39.9543641760321));
#190856=CARTESIAN_POINT('Ctrl Pts',(-54.3917760130578,-31.18787229063,39.96376842407));
#190857=CARTESIAN_POINT('Ctrl Pts',(-54.3993074034413,-31.1949629807083,
39.9730909636381));
#190858=CARTESIAN_POINT('Ctrl Pts',(-54.406318791525,-31.2026795247186,
39.9822808977123));
#190859=CARTESIAN_POINT('Ctrl Pts',(-54.4129511329158,-31.2099789001949,
39.9909740094629));
#190860=CARTESIAN_POINT('Ctrl Pts',(-54.4191188025029,-31.2178389737493,
39.9995492764979));
#190861=CARTESIAN_POINT('Ctrl Pts',(-54.4247323097967,-31.2262832675533,
40.007946232867));
#190862=CARTESIAN_POINT('Ctrl Pts',(-54.4299027559934,-31.2340610728536,
40.0156804369663));
#190863=CARTESIAN_POINT('Ctrl Pts',(-54.4346033281811,-31.2423350114965,
40.0232638017393));
#190864=CARTESIAN_POINT('Ctrl Pts',(-54.4387279162155,-31.2511358718512,
40.0306257269936));
#190865=CARTESIAN_POINT('Ctrl Pts',(-54.4399243024176,-31.2536886668955,
40.0327611416631));
#190866=CARTESIAN_POINT('Ctrl Pts',(-54.441071965327,-31.2562858555929,
40.0348777427261));
#190867=CARTESIAN_POINT('Ctrl Pts',(-54.4421676282859,-31.2589283212564,
40.0369733168701));
#190868=CARTESIAN_POINT('Ctrl Pts',(-54.4433553973774,-31.2617929239292,
40.039245053974));
#190869=CARTESIAN_POINT('Ctrl Pts',(-54.4444813995853,-31.2647063376192,
40.041487875195));
#190870=CARTESIAN_POINT('Ctrl Pts',(-54.4455416356296,-31.2676686823016,
40.0436985701601));
#190871=CARTESIAN_POINT('Ctrl Pts',(-54.4484514617727,-31.2757988605277,
40.0497658398386));
#190872=CARTESIAN_POINT('Ctrl Pts',(-54.4508216479604,-31.2843017293919,
40.0555581699984));
#190873=CARTESIAN_POINT('Ctrl Pts',(-54.4525775288976,-31.2931053160622,
40.0609828468886));
#190874=CARTESIAN_POINT('Ctrl Pts',(-54.4541840646262,-31.3011601199077,
40.0659461317305));
#190875=CARTESIAN_POINT('Ctrl Pts',(-54.4552661718987,-31.3094611543727,
40.0706039980707));
#190876=CARTESIAN_POINT('Ctrl Pts',(-54.4557414157486,-31.3179758301776,
40.0748843180604));
#190877=CARTESIAN_POINT('Ctrl Pts',(-54.4559748539753,-31.3221582111184,
40.076986797257));
#190878=CARTESIAN_POINT('Ctrl Pts',(-54.4560613864572,-31.3263919825241,
40.0789976708175));
#190879=CARTESIAN_POINT('Ctrl Pts',(-54.4559882102925,-31.3306718639311,
40.08090504915));
#190880=CARTESIAN_POINT('Ctrl Pts',(-54.455974325828,-31.3314839297415,
40.0812669556105));
#190881=CARTESIAN_POINT('Ctrl Pts',(-54.4559543157132,-31.3322980319628,
40.0816253922032));
#190882=CARTESIAN_POINT('Ctrl Pts',(-54.4559281176616,-31.3331140451956,
40.0819801989139));
#190883=CARTESIAN_POINT('Ctrl Pts',(-54.455902738299,-31.3339045580148,
40.0823239179149));
#190884=CARTESIAN_POINT('Ctrl Pts',(-54.4558715517161,-31.3346968642518,
40.0826642303498));
#190885=CARTESIAN_POINT('Ctrl Pts',(-54.4558345032252,-31.3354908465826,
40.0830009916099));
#190886=CARTESIAN_POINT('Ctrl Pts',(-54.4554307564063,-31.3441435024201,
40.0866709464311));
#190887=CARTESIAN_POINT('Ctrl Pts',(-54.4543301709717,-31.3530008879284,
40.0899175831876));
#190888=CARTESIAN_POINT('Ctrl Pts',(-54.4524721779261,-31.361882432138,
40.092564206706));
#190889=CARTESIAN_POINT('Ctrl Pts',(-54.4516875359254,-31.3656331634098,
40.0936818922526));
#190890=CARTESIAN_POINT('Ctrl Pts',(-54.4507682193238,-31.3693880355473,
40.094693009479));
#190891=CARTESIAN_POINT('Ctrl Pts',(-54.4497115877222,-31.373133193489,
40.0955863397546));
#190892=CARTESIAN_POINT('Ctrl Pts',(-54.4479322465077,-31.3794399458811,
40.0970906856166));
#190893=CARTESIAN_POINT('Ctrl Pts',(-54.4457622496022,-31.3857169562557,
40.0982599215483));
#190894=CARTESIAN_POINT('Ctrl Pts',(-54.4431895758471,-31.3918909882803,
40.0990497370454));
#190895=CARTESIAN_POINT('Ctrl Pts',(-54.4425464074084,-31.3934344962864,
40.0992471909196));
#190896=CARTESIAN_POINT('Ctrl Pts',(-54.4418778620528,-31.3949714642032,
40.0994209989363));
#190897=CARTESIAN_POINT('Ctrl Pts',(-54.4411834812323,-31.396500599822,
40.0995705982975));
#190898=CARTESIAN_POINT('Ctrl Pts',(-54.4401419100017,-31.3987943032504,
40.0997949973393));
#190899=CARTESIAN_POINT('Ctrl Pts',(-54.4390422051394,-31.401070363756,
40.0999649129781));
#190900=CARTESIAN_POINT('Ctrl Pts',(-54.4378842814512,-31.4033252432067,
40.1000786629733));
#190901=CARTESIAN_POINT('Ctrl Pts',(-54.4367263577631,-31.4055801226574,
40.1001924129685));
#190902=CARTESIAN_POINT('Ctrl Pts',(-54.4355102267488,-31.407813819478,
40.10025));
#190903=CARTESIAN_POINT('Ctrl Pts',(-54.434235916308,-31.4100231232067,
40.10025));
#190904=CARTESIAN_POINT('Ctrl Pts',(-51.1278468659049,-29.5010785149108,
40.10025));
#190905=CARTESIAN_POINT('Ctrl Pts',(-51.1321585373226,-29.4936027956393,
40.10025));
#190906=CARTESIAN_POINT('Ctrl Pts',(-51.1370499258746,-29.4865477845233,
40.099578633424));
#190907=CARTESIAN_POINT('Ctrl Pts',(-51.142385644818,-29.4799806005921,
40.0983063763365));
#190908=CARTESIAN_POINT('Ctrl Pts',(-51.1458319717788,-29.4757388736048,
40.0974846287991));
#190909=CARTESIAN_POINT('Ctrl Pts',(-51.1494629466901,-29.4717000621109,
40.0964130309337));
#190910=CARTESIAN_POINT('Ctrl Pts',(-51.1532365012461,-29.4678753842637,
40.0951176960923));
#190911=CARTESIAN_POINT('Ctrl Pts',(-51.1582381316479,-29.462805992868,
40.0934008039614));
#190912=CARTESIAN_POINT('Ctrl Pts',(-51.1634934604717,-29.4581176150987,
40.0912909372156));
#190913=CARTESIAN_POINT('Ctrl Pts',(-51.1689167792841,-29.4538379291358,
40.0888630467851));
#190914=CARTESIAN_POINT('Ctrl Pts',(-51.1716284386903,-29.4516980861543,
40.0876491015698));
#190915=CARTESIAN_POINT('Ctrl Pts',(-51.174382193724,-29.449660242663,40.0863558569271));
#190916=CARTESIAN_POINT('Ctrl Pts',(-51.1771680313593,-29.4477266300416,
40.0849936342771));
#190917=CARTESIAN_POINT('Ctrl Pts',(-51.1785609501769,-29.4467598237308,
40.084312522952));
#190918=CARTESIAN_POINT('Ctrl Pts',(-51.1799618978181,-29.4458190608834,
40.0836141747074));
#190919=CARTESIAN_POINT('Ctrl Pts',(-51.1813696738593,-29.4449045308658,
40.0828999161609));
#190920=CARTESIAN_POINT('Ctrl Pts',(-51.1817216178696,-29.4446758983613,
40.0827213515243));
#190921=CARTESIAN_POINT('Ctrl Pts',(-51.1820739888279,-29.4444489051051,
40.0825417925841));
#190922=CARTESIAN_POINT('Ctrl Pts',(-51.182426768326,-29.4442235534432,
40.082361260236));
#190923=CARTESIAN_POINT('Ctrl Pts',(-51.1834851068201,-29.4435474984575,
40.0818196631917));
#190924=CARTESIAN_POINT('Ctrl Pts',(-51.1845471213153,-29.4428862193404,
40.0812693052021));
#190925=CARTESIAN_POINT('Ctrl Pts',(-51.1856123224581,-29.4422397658677,
40.0807107531874));
#190926=CARTESIAN_POINT('Ctrl Pts',(-51.1931154617649,-29.4376862310782,
40.0767763849183));
#190927=CARTESIAN_POINT('Ctrl Pts',(-51.2007799603592,-29.4338145801761,
40.072414058614));
#190928=CARTESIAN_POINT('Ctrl Pts',(-51.2085065710723,-29.4305579784514,
40.0677221223772));
#190929=CARTESIAN_POINT('Ctrl Pts',(-51.212253968919,-29.4289785301338,
40.0654465383723));
#190930=CARTESIAN_POINT('Ctrl Pts',(-51.2160164979697,-29.4275440072541,
40.0630928000681));
#190931=CARTESIAN_POINT('Ctrl Pts',(-51.219785247298,-29.4262483256616,
40.0606689262479));
#190932=CARTESIAN_POINT('Ctrl Pts',(-51.2255549392045,-29.4242647276703,
40.0569581447806));
#190933=CARTESIAN_POINT('Ctrl Pts',(-51.2313356805891,-29.4226066102321,
40.0530843804606));
#190934=CARTESIAN_POINT('Ctrl Pts',(-51.23708417089,-29.4212581193011,40.0490800251458));
#190935=CARTESIAN_POINT('Ctrl Pts',(-51.2397537995245,-29.4206318731365,
40.0472203818218));
#190936=CARTESIAN_POINT('Ctrl Pts',(-51.2424163366106,-29.4200721889212,
40.0453323608819));
#190937=CARTESIAN_POINT('Ctrl Pts',(-51.2450674596718,-29.4195787111905,
40.0434201572162));
#190938=CARTESIAN_POINT('Ctrl Pts',(-51.2452706578085,-29.4195408880668,
40.0432735943397));
#190939=CARTESIAN_POINT('Ctrl Pts',(-51.245473795951,-29.4195034207,40.0431268995707));
#190940=CARTESIAN_POINT('Ctrl Pts',(-51.2456768729757,-29.4194663081571,
40.0429800745037));
#190941=CARTESIAN_POINT('Ctrl Pts',(-51.2485294929147,-29.4189449888199,
40.0409176249753));
#190942=CARTESIAN_POINT('Ctrl Pts',(-51.2513705613629,-29.4184957101763,
40.0388310783332));
#190943=CARTESIAN_POINT('Ctrl Pts',(-51.2541954110682,-29.4181151898794,
40.036725739981));
#190944=CARTESIAN_POINT('Ctrl Pts',(-51.2643248197284,-29.4167507117682,
40.0291763710721));
#190945=CARTESIAN_POINT('Ctrl Pts',(-51.2743237313754,-29.4162578421119,
40.0213310894601));
#190946=CARTESIAN_POINT('Ctrl Pts',(-51.284145524976,-29.4165161672806,
40.0132837551329));
#190947=CARTESIAN_POINT('Ctrl Pts',(-51.2949386894566,-29.4168000406899,
40.0044405431337));
#190948=CARTESIAN_POINT('Ctrl Pts',(-51.3055186222576,-29.417990898923,
39.9953528710615));
#190949=CARTESIAN_POINT('Ctrl Pts',(-51.3158373135936,-29.4199800715334,
39.9861103629572));
#190950=CARTESIAN_POINT('Ctrl Pts',(-51.3269789105987,-29.4221278787384,
39.9761307737573));
#190951=CARTESIAN_POINT('Ctrl Pts',(-51.3378170984239,-29.4252064644172,
39.9659696936028));
#190952=CARTESIAN_POINT('Ctrl Pts',(-51.3482921445234,-29.4291364604192,
39.9557128217522));
#190953=CARTESIAN_POINT('Ctrl Pts',(-51.3586793157496,-29.4330334877929,
39.9455419945171));
#190954=CARTESIAN_POINT('Ctrl Pts',(-51.3687106315439,-29.4377684584842,
39.9352756289346));
#190955=CARTESIAN_POINT('Ctrl Pts',(-51.3783102687786,-29.4433108116258,
39.92499));
#190956=CARTESIAN_POINT('Origin',(0.00762000000001041,-0.0131982271536721,
39.92499));
#190957=CARTESIAN_POINT('Ctrl Pts',(-54.4189959163065,-31.4364195775132,
40.10025));
#190958=CARTESIAN_POINT('Ctrl Pts',(-54.4146983388119,-31.4438560159999,
40.10025));
#190959=CARTESIAN_POINT('Ctrl Pts',(-54.4098177483014,-31.4508673716601,
40.0995859581842));
#190960=CARTESIAN_POINT('Ctrl Pts',(-54.4044907169112,-31.4573895320586,
40.0983275959621));
#190961=CARTESIAN_POINT('Ctrl Pts',(-54.4010869974475,-31.4615568820642,
40.0975235624069));
#190962=CARTESIAN_POINT('Ctrl Pts',(-54.3975017237412,-31.4655251210644,
40.0964777059491));
#190963=CARTESIAN_POINT('Ctrl Pts',(-54.393775915711,-31.4692842169743,
40.0952149915961));
#190964=CARTESIAN_POINT('Ctrl Pts',(-54.3886909353394,-31.4744146286223,
40.0934916398701));
#190965=CARTESIAN_POINT('Ctrl Pts',(-54.3833409297223,-31.4791503318818,
40.091364392163));
#190966=CARTESIAN_POINT('Ctrl Pts',(-54.3778174666304,-31.4834636394926,
40.0889118607713));
#190967=CARTESIAN_POINT('Ctrl Pts',(-54.3750557350845,-31.4856202932979,
40.0876855950754));
#190968=CARTESIAN_POINT('Ctrl Pts',(-54.3722505364144,-31.4876715300024,
40.0863782327526));
#190969=CARTESIAN_POINT('Ctrl Pts',(-54.3694125772949,-31.4896151854257,
40.0850006373334));
#190970=CARTESIAN_POINT('Ctrl Pts',(-54.3679935977352,-31.4905870131374,
40.0843118396237));
#190971=CARTESIAN_POINT('Ctrl Pts',(-54.3665664194001,-31.4915319606349,
40.0836054919164));
#190972=CARTESIAN_POINT('Ctrl Pts',(-54.365132326297,-31.4924498523885,
40.0828829920417));
#190973=CARTESIAN_POINT('Ctrl Pts',(-54.3647738030212,-31.4926793253269,
40.0827023670731));
#190974=CARTESIAN_POINT('Ctrl Pts',(-54.3644148473887,-31.4929071076037,
40.0825207326933));
#190975=CARTESIAN_POINT('Ctrl Pts',(-54.3640554790923,-31.4931331971265,
40.0823381109275));
#190976=CARTESIAN_POINT('Ctrl Pts',(-54.362977374203,-31.493811465695,40.0817902456303));
#190977=CARTESIAN_POINT('Ctrl Pts',(-54.3618955562474,-31.4944744978647,
40.0812334935553));
#190978=CARTESIAN_POINT('Ctrl Pts',(-54.3608105487851,-31.4951222515525,
40.0806684524227));
#190979=CARTESIAN_POINT('Ctrl Pts',(-54.3533124740222,-31.4995986314374,
40.0767636676137));
#190980=CARTESIAN_POINT('Ctrl Pts',(-54.3456575719325,-31.5034009004294,
40.0724404510888));
#190981=CARTESIAN_POINT('Ctrl Pts',(-54.3379428492061,-31.5065976218801,
40.0677949937409));
#190982=CARTESIAN_POINT('Ctrl Pts',(-54.3341086531876,-31.5081863836663,
40.0654862141906));
#190983=CARTESIAN_POINT('Ctrl Pts',(-54.3302591366968,-31.5096252947444,
40.0630972003216));
#190984=CARTESIAN_POINT('Ctrl Pts',(-54.3264035847697,-31.5109210155999,
40.0606363359906));
#190985=CARTESIAN_POINT('Ctrl Pts',(-54.3178976613387,-31.5137795693409,
40.0552073017123));
#190986=CARTESIAN_POINT('Ctrl Pts',(-54.3093672304021,-31.5159526675028,
40.0494204304519));
#190987=CARTESIAN_POINT('Ctrl Pts',(-54.3009559572068,-31.5174623893714,
40.0434049749851));
#190988=CARTESIAN_POINT('Ctrl Pts',(-54.2978832130368,-31.5180139098085,
40.0412074532442));
#190989=CARTESIAN_POINT('Ctrl Pts',(-54.2948245130135,-31.5184846398473,
40.0389814735788));
#190990=CARTESIAN_POINT('Ctrl Pts',(-54.2917835794184,-31.5188783726367,
40.0367321210017));
#190991=CARTESIAN_POINT('Ctrl Pts',(-54.2815694052539,-31.5202008794129,
40.0291767837141));
#190992=CARTESIAN_POINT('Ctrl Pts',(-54.2714898389049,-31.5206547127626,
40.0213235332576));
#190993=CARTESIAN_POINT('Ctrl Pts',(-54.2615918017975,-31.5203592886225,
40.0132649215858));
#190994=CARTESIAN_POINT('Ctrl Pts',(-54.250712686517,-31.5200345824972,
40.0044075527532));
#190995=CARTESIAN_POINT('Ctrl Pts',(-54.2400521939127,-31.5188048676548,
39.9953016253719));
#190996=CARTESIAN_POINT('Ctrl Pts',(-54.2296591093513,-31.5167773687226,
39.9860353422357));
#190997=CARTESIAN_POINT('Ctrl Pts',(-54.2184653119704,-31.5145936655011,
39.9760551582693));
#190998=CARTESIAN_POINT('Ctrl Pts',(-54.207580520936,-31.5114844302878,
39.9658879738153));
#190999=CARTESIAN_POINT('Ctrl Pts',(-54.197065873477,-31.5075265408326,
39.9556174643251));
#191000=CARTESIAN_POINT('Ctrl Pts',(-54.1866932092603,-31.5036220962484,
39.9454856413903));
#191001=CARTESIAN_POINT('Ctrl Pts',(-54.1766795569346,-31.4988909785571,
39.9352519465112));
#191002=CARTESIAN_POINT('Ctrl Pts',(-54.167102037244,-31.4933613949856,
39.92499));
#191003=CARTESIAN_POINT('Ctrl Pts',(-51.1878102687787,-29.7732664904677,
39.92499));
#191004=CARTESIAN_POINT('Ctrl Pts',(-51.1786445298599,-29.7679746486356,
39.9348107241716));
#191005=CARTESIAN_POINT('Ctrl Pts',(-51.1699291351241,-29.7619788985613,
39.9446038383157));
#191006=CARTESIAN_POINT('Ctrl Pts',(-51.1617065245647,-29.7553188532221,
39.9543158069366));
#191007=CARTESIAN_POINT('Ctrl Pts',(-51.1537668706124,-29.7488879934705,
39.9636935671368));
#191008=CARTESIAN_POINT('Ctrl Pts',(-51.1462857370563,-29.741836915419,
39.9729968320961));
#191009=CARTESIAN_POINT('Ctrl Pts',(-51.1393284263655,-29.7341642916973,
39.9821731151303));
#191010=CARTESIAN_POINT('Ctrl Pts',(-51.1327515888678,-29.7269112593634,
39.9908475764318));
#191011=CARTESIAN_POINT('Ctrl Pts',(-51.126642241795,-29.719102133512,39.9994093733809));
#191012=CARTESIAN_POINT('Ctrl Pts',(-51.1210907313655,-29.7107129315358,
40.0077966115803));
#191013=CARTESIAN_POINT('Ctrl Pts',(-51.1159778833935,-29.702986617255,
40.0155211172554));
#191014=CARTESIAN_POINT('Ctrl Pts',(-51.1113379461932,-29.6947677915966,
40.023097994098));
#191015=CARTESIAN_POINT('Ctrl Pts',(-51.1072776647637,-29.6860256466531,
40.0304554104705));
#191016=CARTESIAN_POINT('Ctrl Pts',(-51.1060669708027,-29.6834189155008,
40.0326492435153));
#191017=CARTESIAN_POINT('Ctrl Pts',(-51.1049080895609,-29.6807655934617,
40.0348233715046));
#191018=CARTESIAN_POINT('Ctrl Pts',(-51.1038046002594,-29.6780647241925,
40.0369753512356));
#191019=CARTESIAN_POINT('Ctrl Pts',(-51.1027123859001,-29.6753914511534,
40.0391053430352));
#191020=CARTESIAN_POINT('Ctrl Pts',(-51.1016753170131,-29.6726744751144,
40.041211089324));
#191021=CARTESIAN_POINT('Ctrl Pts',(-51.1006978225842,-29.6699160505197,
40.0432881154904));
#191022=CARTESIAN_POINT('Ctrl Pts',(-51.1006298495333,-29.669724235068,
40.043432547828));
#191023=CARTESIAN_POINT('Ctrl Pts',(-51.1005621526964,-29.6695322176087,
40.0435768364421));
#191024=CARTESIAN_POINT('Ctrl Pts',(-51.1004947333605,-29.6693399979285,
40.0437209807855));
#191025=CARTESIAN_POINT('Ctrl Pts',(-51.0975388226978,-29.660912382995,
40.050040796842));
#191026=CARTESIAN_POINT('Ctrl Pts',(-51.095161351427,-29.652091674968,40.0560490279343));
#191027=CARTESIAN_POINT('Ctrl Pts',(-51.0934607157664,-29.6429396446298,
40.0616647108613));
#191028=CARTESIAN_POINT('Ctrl Pts',(-51.0918754277622,-29.6344083617426,
40.0668995033484));
#191029=CARTESIAN_POINT('Ctrl Pts',(-51.090878395402,-29.6255883681034,
40.071793326748));
#191030=CARTESIAN_POINT('Ctrl Pts',(-51.0905760611938,-29.61654180499,40.076246030307));
#191031=CARTESIAN_POINT('Ctrl Pts',(-51.0904654634291,-29.6132324551655,
40.0778748868746));
#191032=CARTESIAN_POINT('Ctrl Pts',(-51.0904480940785,-29.609892965987,
40.0794443522246));
#191033=CARTESIAN_POINT('Ctrl Pts',(-51.0905301191541,-29.606527136569,
40.0809482021492));
#191034=CARTESIAN_POINT('Ctrl Pts',(-51.0905498434446,-29.6057177670364,
40.0813098278168));
#191035=CARTESIAN_POINT('Ctrl Pts',(-51.090575662893,-29.6049064053144,
40.0816679525672));
#191036=CARTESIAN_POINT('Ctrl Pts',(-51.0906076352719,-29.60409317417,40.082022419258));
#191037=CARTESIAN_POINT('Ctrl Pts',(-51.0906386085139,-29.603305356499,
40.0823658088648));
#191038=CARTESIAN_POINT('Ctrl Pts',(-51.090675356124,-29.6025157844402,
40.0827057654616));
#191039=CARTESIAN_POINT('Ctrl Pts',(-51.0907179287116,-29.601724572879,
40.0830421470151));
#191040=CARTESIAN_POINT('Ctrl Pts',(-51.0911843606098,-29.5930559358435,
40.0867275956807));
#191041=CARTESIAN_POINT('Ctrl Pts',(-51.0923507190418,-29.5841848213171,
40.0899823432032));
#191042=CARTESIAN_POINT('Ctrl Pts',(-51.0942731997207,-29.5752911628165,
40.0926299529357));
#191043=CARTESIAN_POINT('Ctrl Pts',(-51.0950705097613,-29.571602697545,
40.0937279956085));
#191044=CARTESIAN_POINT('Ctrl Pts',(-51.0959974771976,-29.5679105139259,
40.0947220371803));
#191045=CARTESIAN_POINT('Ctrl Pts',(-51.0970562972092,-29.5642276868787,
40.0956014538692));
#191046=CARTESIAN_POINT('Ctrl Pts',(-51.0988622250759,-29.5579462415719,
40.097101390674));
#191047=CARTESIAN_POINT('Ctrl Pts',(-51.1010529624042,-29.5516941764752,
40.0982667904316));
#191048=CARTESIAN_POINT('Ctrl Pts',(-51.1036389246278,-29.5455435225215,
40.0990539325582));
#191049=CARTESIAN_POINT('Ctrl Pts',(-51.1049319057396,-29.5424681955446,
40.0994475036216));
#191050=CARTESIAN_POINT('Ctrl Pts',(-51.106324978508,-29.5394188854256,
40.0997467259952));
#191051=CARTESIAN_POINT('Ctrl Pts',(-51.107819466813,-29.5364046579954,
40.0999473488896));
#191052=CARTESIAN_POINT('Ctrl Pts',(-51.109313955118,-29.5333904305652,
40.100147971784));
#191053=CARTESIAN_POINT('Ctrl Pts',(-51.1109098228568,-29.530411313779,
40.10025));
#191054=CARTESIAN_POINT('Ctrl Pts',(-51.1126068659049,-29.5274749692182,
40.10025));
#191055=CARTESIAN_POINT('Origin',(-53.2328030451449,-23.6840886581933,39.92499));
#191056=CARTESIAN_POINT('Ctrl Pts',(-57.3172883154491,-25.3107727110819,
39.92499));
#191057=CARTESIAN_POINT('Ctrl Pts',(-57.3269813337899,-25.3150883208945,
39.9348354642018));
#191058=CARTESIAN_POINT('Ctrl Pts',(-57.3363050752413,-25.3201559369469,
39.9446440828457));
#191059=CARTESIAN_POINT('Ctrl Pts',(-57.3452135417184,-25.3259384683618,
39.9543641760331));
#191060=CARTESIAN_POINT('Ctrl Pts',(-57.3538325360815,-25.3315331019385,
39.9637684240712));
#191061=CARTESIAN_POINT('Ctrl Pts',(-57.3620638476581,-25.3377977038119,
39.9730909636396));
#191062=CARTESIAN_POINT('Ctrl Pts',(-57.3698434251116,-25.3447390861652,
39.9822808977141));
#191063=CARTESIAN_POINT('Ctrl Pts',(-57.3772024263438,-25.3513052064458,
39.990974009465));
#191064=CARTESIAN_POINT('Ctrl Pts',(-57.3841579102015,-25.3584775246713,
39.9995492765002));
#191065=CARTESIAN_POINT('Ctrl Pts',(-57.3906233351697,-25.3662887884596,
40.0079462328695));
#191066=CARTESIAN_POINT('Ctrl Pts',(-57.3965784591569,-25.3734835273337,
40.015680436969));
#191067=CARTESIAN_POINT('Ctrl Pts',(-57.4021181432099,-25.3812207968882,
40.0232638017423));
#191068=CARTESIAN_POINT('Ctrl Pts',(-57.4071400767278,-25.3895423083605,
40.0306257269968));
#191069=CARTESIAN_POINT('Ctrl Pts',(-57.4085967487433,-25.3919560625142,
40.0327611416652));
#191070=CARTESIAN_POINT('Ctrl Pts',(-57.4100096047778,-25.3944190600986,
40.0348777427271));
#191071=CARTESIAN_POINT('Ctrl Pts',(-57.4113754784548,-25.3969325220922,
40.0369733168701));
#191072=CARTESIAN_POINT('Ctrl Pts',(-57.4128561733382,-25.399657276494,
40.039245053974));
#191073=CARTESIAN_POINT('Ctrl Pts',(-57.4142805418441,-25.4024370309185,
40.041487875195));
#191074=CARTESIAN_POINT('Ctrl Pts',(-57.4156446191418,-25.4052723227224,
40.0436985701601));
#191075=CARTESIAN_POINT('Ctrl Pts',(-57.4193883399888,-25.4130538033264,
40.0497658398386));
#191076=CARTESIAN_POINT('Ctrl Pts',(-57.4226343338644,-25.4212623406654,
40.0555581699984));
#191077=CARTESIAN_POINT('Ctrl Pts',(-57.425300821288,-25.4298341608307,
40.0609828468886));
#191078=CARTESIAN_POINT('Ctrl Pts',(-57.4277405125136,-25.4376769109069,
40.0659461317304));
#191079=CARTESIAN_POINT('Ctrl Pts',(-57.4296843862653,-25.445819360426,
40.0706039980705));
#191080=CARTESIAN_POINT('Ctrl Pts',(-57.4310470526568,-25.4542377154364,
40.0748843180601));
#191081=CARTESIAN_POINT('Ctrl Pts',(-57.431716389937,-25.4583727839179,
40.0769867972569));
#191082=CARTESIAN_POINT('Ctrl Pts',(-57.4322449980039,-25.4625743171737,
40.0789976708174));
#191083=CARTESIAN_POINT('Ctrl Pts',(-57.4326195921323,-25.4668384019348,
40.08090504915));
#191084=CARTESIAN_POINT('Ctrl Pts',(-57.4326906677196,-25.4676474704855,
40.0812669556105));
#191085=CARTESIAN_POINT('Ctrl Pts',(-57.4327558640765,-25.4684592045962,
40.0816253922033));
#191086=CARTESIAN_POINT('Ctrl Pts',(-57.4328151061497,-25.4692734860652,
40.081980198914));
#191087=CARTESIAN_POINT('Ctrl Pts',(-57.4328724969081,-25.4700623212382,
40.082323917915));
#191088=CARTESIAN_POINT('Ctrl Pts',(-57.4329242997219,-25.4708535470243,
40.0826642303499));
#191089=CARTESIAN_POINT('Ctrl Pts',(-57.4329704479395,-25.4716470524587,
40.08300099161));
#191090=CARTESIAN_POINT('Ctrl Pts',(-57.4334733617057,-25.4802945111766,
40.0866709464311));
#191091=CARTESIAN_POINT('Ctrl Pts',(-57.433304654289,-25.4892184175044,
40.0899175831876));
#191092=CARTESIAN_POINT('Ctrl Pts',(-57.4323852136915,-25.4982455208433,
40.0925642067059));
#191093=CARTESIAN_POINT('Ctrl Pts',(-57.4319969282177,-25.5020577226393,
40.0936818922526));
#191094=CARTESIAN_POINT('Ctrl Pts',(-57.4314751387429,-25.5058881199461,
40.094693009479));
#191095=CARTESIAN_POINT('Ctrl Pts',(-57.4308157710842,-25.5097232095984,
40.0955863397546));
#191096=CARTESIAN_POINT('Ctrl Pts',(-57.4297054124227,-25.5161814047439,
40.0970906856167));
#191097=CARTESIAN_POINT('Ctrl Pts',(-57.4282034292357,-25.5226508554406,
40.0982599215483));
#191098=CARTESIAN_POINT('Ctrl Pts',(-57.426290210937,-25.5290599831061,
40.0990497370454));
#191099=CARTESIAN_POINT('Ctrl Pts',(-57.4258119063623,-25.5306622650225,
40.0992471909196));
#191100=CARTESIAN_POINT('Ctrl Pts',(-57.4253076802625,-25.5322606952868,
40.0994209989363));
#191101=CARTESIAN_POINT('Ctrl Pts',(-57.4247769415292,-25.5338540367008,
40.0995705982975));
#191102=CARTESIAN_POINT('Ctrl Pts',(-57.4239808334292,-25.5362440488219,
40.0997949973393));
#191103=CARTESIAN_POINT('Ctrl Pts',(-57.423125065972,-25.5386225912892,
40.0999649129781));
#191104=CARTESIAN_POINT('Ctrl Pts',(-57.4222091845947,-25.540986154258,
40.1000786629733));
#191105=CARTESIAN_POINT('Ctrl Pts',(-57.4212933032174,-25.5433497172268,
40.1001924129685));
#191106=CARTESIAN_POINT('Ctrl Pts',(-57.4203173191918,-25.5456982979284,
40.10025));
#191107=CARTESIAN_POINT('Ctrl Pts',(-57.4192809246806,-25.5480287005722,
40.10025));
#191108=CARTESIAN_POINT('Ctrl Pts',(-53.9314655730806,-23.9951532569804,
40.10025));
#191109=CARTESIAN_POINT('Ctrl Pts',(-53.9349721992636,-23.9872677980944,
40.10025));
#191110=CARTESIAN_POINT('Ctrl Pts',(-53.9390993428067,-23.9797401457394,
40.0995786334242));
#191111=CARTESIAN_POINT('Ctrl Pts',(-53.9437193744788,-23.9726512030277,
40.0983063763368));
#191112=CARTESIAN_POINT('Ctrl Pts',(-53.9467034408966,-23.968072473403,
40.0974846287994));
#191113=CARTESIAN_POINT('Ctrl Pts',(-53.9498923541887,-23.963676246713,
40.0964130309339));
#191114=CARTESIAN_POINT('Ctrl Pts',(-53.9532454491206,-23.9594780769919,
40.0951176960924));
#191115=CARTESIAN_POINT('Ctrl Pts',(-53.9576897843754,-23.953913643513,
40.0934008039614));
#191116=CARTESIAN_POINT('Ctrl Pts',(-53.9624262550345,-23.9487016177218,
40.0912909372157));
#191117=CARTESIAN_POINT('Ctrl Pts',(-53.9673725153421,-23.943878485145,
40.0888630467852));
#191118=CARTESIAN_POINT('Ctrl Pts',(-53.9698456454959,-23.9414669188567,
40.0876491015699));
#191119=CARTESIAN_POINT('Ctrl Pts',(-53.9723713025229,-23.9391523931033,
40.0863558569271));
#191120=CARTESIAN_POINT('Ctrl Pts',(-53.9749397614923,-23.9369381736872,
40.0849936342771));
#191121=CARTESIAN_POINT('Ctrl Pts',(-53.9762239909769,-23.9358310639792,
40.0843125229521));
#191122=CARTESIAN_POINT('Ctrl Pts',(-53.9775189275856,-23.934749015825,
40.0836141747074));
#191123=CARTESIAN_POINT('Ctrl Pts',(-53.978823397265,-23.9336923430323,
40.082899916161));
#191124=CARTESIAN_POINT('Ctrl Pts',(-53.9791495146849,-23.9334281748341,
40.0827213515243));
#191125=CARTESIAN_POINT('Ctrl Pts',(-53.9794762280619,-23.9331655922759,
40.0825417925842));
#191126=CARTESIAN_POINT('Ctrl Pts',(-53.979803519334,-23.9329045996151,
40.0823612602361));
#191127=CARTESIAN_POINT('Ctrl Pts',(-53.9807853931504,-23.932121621633,
40.0818196631917));
#191128=CARTESIAN_POINT('Ctrl Pts',(-53.9817724673293,-23.9313529543289,
40.0812693052022));
#191129=CARTESIAN_POINT('Ctrl Pts',(-53.9827642604006,-23.9305986983574,
40.0807107531875));
#191130=CARTESIAN_POINT('Ctrl Pts',(-53.9897503227313,-23.9252858166865,
40.0767763849183));
#191131=CARTESIAN_POINT('Ctrl Pts',(-53.9969681366814,-23.9206342168333,
40.0724140586139));
#191132=CARTESIAN_POINT('Ctrl Pts',(-54.0043120126389,-23.9165878043694,
40.0677221223771));
#191133=CARTESIAN_POINT('Ctrl Pts',(-54.0078737845426,-23.9146252986969,
40.0654465383722));
#191134=CARTESIAN_POINT('Ctrl Pts',(-54.0114657535932,-23.912805342904,
40.063092800068));
#191135=CARTESIAN_POINT('Ctrl Pts',(-54.0150784217125,-23.9111228176151,
40.0606689262479));
#191136=CARTESIAN_POINT('Ctrl Pts',(-54.0206091641933,-23.9085469889526,
40.0569581447805));
#191137=CARTESIAN_POINT('Ctrl Pts',(-54.026184917604,-23.9062937028418,
40.0530843804606));
#191138=CARTESIAN_POINT('Ctrl Pts',(-54.0317609613888,-23.904351718228,
40.0490800251458));
#191139=CARTESIAN_POINT('Ctrl Pts',(-54.0343505049691,-23.9034498505268,
40.0472203818218));
#191140=CARTESIAN_POINT('Ctrl Pts',(-54.0369399534675,-23.9026149214102,
40.0453323608819));
#191141=CARTESIAN_POINT('Ctrl Pts',(-54.0395249709303,-23.9018470291825,
40.0434201572162));
#191142=CARTESIAN_POINT('Ctrl Pts',(-54.0397231023334,-23.9017881732689,
40.0432735943397));
#191143=CARTESIAN_POINT('Ctrl Pts',(-54.0399212112576,-23.9017296774344,
40.0431268995707));
#191144=CARTESIAN_POINT('Ctrl Pts',(-54.040119296488,-23.9016715408685,
40.0429800745037));
#191145=CARTESIAN_POINT('Ctrl Pts',(-54.0429017967674,-23.9008548973947,
40.0409176249753));
#191146=CARTESIAN_POINT('Ctrl Pts',(-54.0456803391391,-23.9001111074276,
40.0388310783332));
#191147=CARTESIAN_POINT('Ctrl Pts',(-54.0484499388203,-23.8994373944621,
40.036725739981));
#191148=CARTESIAN_POINT('Ctrl Pts',(-54.0583812307206,-23.8970215795835,
40.0291763710715));
#191149=CARTESIAN_POINT('Ctrl Pts',(-54.0682738483764,-23.8954862390498,
40.0213310894589));
#191150=CARTESIAN_POINT('Ctrl Pts',(-54.0780688394977,-23.8947164920947,
40.0132837551311));
#191151=CARTESIAN_POINT('Ctrl Pts',(-54.0888325507459,-23.8938706175189,
40.0044405431312));
#191152=CARTESIAN_POINT('Ctrl Pts',(-54.0994790041498,-23.8939490479889,
39.9953528710584));
#191153=CARTESIAN_POINT('Ctrl Pts',(-54.1099490937719,-23.8948487267556,
39.9861103629534));
#191154=CARTESIAN_POINT('Ctrl Pts',(-54.1212541629301,-23.8958201540352,
39.9761307737527));
#191155=CARTESIAN_POINT('Ctrl Pts',(-54.1323547778592,-23.8977489757819,
39.9659696935974));
#191156=CARTESIAN_POINT('Ctrl Pts',(-54.1431832370035,-23.9005625023838,
39.955712821746));
#191157=CARTESIAN_POINT('Ctrl Pts',(-54.1539208564994,-23.9033524263876,
39.9455419945129));
#191158=CARTESIAN_POINT('Ctrl Pts',(-54.1643921589038,-23.907012900389,
39.9352756289325));
#191159=CARTESIAN_POINT('Ctrl Pts',(-54.1745185419761,-23.9115214566111,
39.92499));
#191160=CARTESIAN_POINT('Origin',(0.00619866644048587,-0.013922432774471,
39.92499));
#191161=CARTESIAN_POINT('Ctrl Pts',(-57.4068835917981,-25.5758735661205,
40.10025));
#191162=CARTESIAN_POINT('Ctrl Pts',(-57.4033868763699,-25.5837184861902,
40.10025));
#191163=CARTESIAN_POINT('Ctrl Pts',(-57.3992659084775,-25.5912015935365,
40.0995859581842));
#191164=CARTESIAN_POINT('Ctrl Pts',(-57.3946498105264,-25.5982448512628,
40.0983275959622));
#191165=CARTESIAN_POINT('Ctrl Pts',(-57.391700343686,-25.602745157654,40.0975235624069));
#191166=CARTESIAN_POINT('Ctrl Pts',(-57.3885495044088,-25.6070664213767,
40.0964777059491));
#191167=CARTESIAN_POINT('Ctrl Pts',(-57.3852370392634,-25.6111943775537,
40.0952149915962));
#191168=CARTESIAN_POINT('Ctrl Pts',(-57.3807161889919,-25.6168282094539,
40.0934916398702));
#191169=CARTESIAN_POINT('Ctrl Pts',(-57.3758905070495,-25.6220971979012,
40.0913643921631));
#191170=CARTESIAN_POINT('Ctrl Pts',(-57.3708481654825,-25.6269642358704,
40.0889118607713));
#191171=CARTESIAN_POINT('Ctrl Pts',(-57.368326994699,-25.629397754855,40.0876855950754));
#191172=CARTESIAN_POINT('Ctrl Pts',(-57.3657515758212,-25.6317309777763,
40.0863782327527));
#191173=CARTESIAN_POINT('Ctrl Pts',(-57.3631323306533,-25.6339606331575,
40.0850006373334));
#191174=CARTESIAN_POINT('Ctrl Pts',(-57.3618227080694,-25.6350754608481,
40.0843118396238));
#191175=CARTESIAN_POINT('Ctrl Pts',(-57.3605021218763,-25.6361644125824,
40.0836054919165));
#191176=CARTESIAN_POINT('Ctrl Pts',(-57.3591718306997,-25.6372271795773,
40.0828829920418));
#191177=CARTESIAN_POINT('Ctrl Pts',(-57.3588392579055,-25.637492871326,
40.0827023670731));
#191178=CARTESIAN_POINT('Ctrl Pts',(-57.3585060784009,-25.6377569268682,
40.0825207326933));
#191179=CARTESIAN_POINT('Ctrl Pts',(-57.358172311552,-25.6380193420648,
40.0823381109276));
#191180=CARTESIAN_POINT('Ctrl Pts',(-57.3571710110052,-25.6388065876544,
40.0817902456304));
#191181=CARTESIAN_POINT('Ctrl Pts',(-57.3561644250954,-25.6395790684329,
40.0812334935553));
#191182=CARTESIAN_POINT('Ctrl Pts',(-57.3551530701151,-25.6403366878209,
40.0806684524227));
#191183=CARTESIAN_POINT('Ctrl Pts',(-57.3481639797007,-25.6455723078608,
40.0767636676138));
#191184=CARTESIAN_POINT('Ctrl Pts',(-57.3409484573003,-25.6501539027773,
40.072440451089));
#191185=CARTESIAN_POINT('Ctrl Pts',(-57.3336101450131,-25.6541395203645,
40.0677949937412));
#191186=CARTESIAN_POINT('Ctrl Pts',(-57.3299630239495,-25.6561203613651,
40.0654862141907));
#191187=CARTESIAN_POINT('Ctrl Pts',(-57.3262850026764,-25.6579537739809,
40.0630972003217));
#191188=CARTESIAN_POINT('Ctrl Pts',(-57.322586011576,-25.6596454116601,
40.0606363359906));
#191189=CARTESIAN_POINT('Ctrl Pts',(-57.3144254847133,-25.6633774170495,
40.0552073017124));
#191190=CARTESIAN_POINT('Ctrl Pts',(-57.3061689349813,-25.6664302835891,
40.0494204304519));
#191191=CARTESIAN_POINT('Ctrl Pts',(-57.2979615485275,-25.6688109525045,
40.0434049749851));
#191192=CARTESIAN_POINT('Ctrl Pts',(-57.2949632867553,-25.6696806408811,
40.0412074532442));
#191193=CARTESIAN_POINT('Ctrl Pts',(-57.2919705472984,-25.6704685134245,
40.0389814735788));
#191194=CARTESIAN_POINT('Ctrl Pts',(-57.2889874285391,-25.6711779534201,
40.0367321210017));
#191195=CARTESIAN_POINT('Ctrl Pts',(-57.2789674482897,-25.6735608872949,
40.0291767837137));
#191196=CARTESIAN_POINT('Ctrl Pts',(-57.2689905373618,-25.675065836079,
40.0213235332567));
#191197=CARTESIAN_POINT('Ctrl Pts',(-57.2591158425054,-25.6758066569113,
40.0132649215845));
#191198=CARTESIAN_POINT('Ctrl Pts',(-57.2482623831237,-25.6766209067621,
40.0044075527514));
#191199=CARTESIAN_POINT('Ctrl Pts',(-57.2375317496099,-25.6765122533357,
39.9953016253696));
#191200=CARTESIAN_POINT('Ctrl Pts',(-57.226983668105,-25.6755822344123,
39.9860353422328));
#191201=CARTESIAN_POINT('Ctrl Pts',(-57.2156229323747,-25.6745805641837,
39.9760551582659));
#191202=CARTESIAN_POINT('Ctrl Pts',(-57.204472765785,-25.6726261321656,
39.9658879738112));
#191203=CARTESIAN_POINT('Ctrl Pts',(-57.1936020065619,-25.6697890043832,
39.9556174643203));
#191204=CARTESIAN_POINT('Ctrl Pts',(-57.1828780392947,-25.6669901874057,
39.9454856413871));
#191205=CARTESIAN_POINT('Ctrl Pts',(-57.1724247063442,-25.6633316989619,
39.9352519465097));
#191206=CARTESIAN_POINT('Ctrl Pts',(-57.1623216544372,-25.6588335304438,
39.92499));
#191207=CARTESIAN_POINT('Ctrl Pts',(-54.0195518809642,-24.259582275973,
39.92499));
#191208=CARTESIAN_POINT('Ctrl Pts',(-54.009883204825,-24.2552775040068,
39.9348107241744));
#191209=CARTESIAN_POINT('Ctrl Pts',(-54.0005888273895,-24.2502256060956,
39.9446038383213));
#191210=CARTESIAN_POINT('Ctrl Pts',(-53.9917150968443,-24.2444615420256,
39.9543158069449));
#191211=CARTESIAN_POINT('Ctrl Pts',(-53.9831467292584,-24.2388958310217,
39.9636935671468));
#191212=CARTESIAN_POINT('Ctrl Pts',(-53.9749695397803,-24.232665370906,
39.9729968321077));
#191213=CARTESIAN_POINT('Ctrl Pts',(-53.9672483343977,-24.2257620156131,
39.9821731151436));
#191214=CARTESIAN_POINT('Ctrl Pts',(-53.9599493771797,-24.2192361828646,
39.9908475764458));
#191215=CARTESIAN_POINT('Ctrl Pts',(-53.9530572218243,-24.2121084368813,
39.9994093733958));
#191216=CARTESIAN_POINT('Ctrl Pts',(-53.9466592127591,-24.2043454826836,
40.0077966115958));
#191217=CARTESIAN_POINT('Ctrl Pts',(-53.9407667537449,-24.197195932101,
40.0155211172713));
#191218=CARTESIAN_POINT('Ctrl Pts',(-53.9352931333904,-24.1895071355333,
40.0230979941141));
#191219=CARTESIAN_POINT('Ctrl Pts',(-53.9303412916313,-24.1812372959513,
40.0304554104869));
#191220=CARTESIAN_POINT('Ctrl Pts',(-53.9288647523808,-24.17877139673,40.0326492435261));
#191221=CARTESIAN_POINT('Ctrl Pts',(-53.9274348719401,-24.1762537459482,
40.03482337151));
#191222=CARTESIAN_POINT('Ctrl Pts',(-53.9260551099577,-24.1736830183707,
40.0369753512355));
#191223=CARTESIAN_POINT('Ctrl Pts',(-53.9246894457403,-24.1711385572896,
40.0391053430352));
#191224=CARTESIAN_POINT('Ctrl Pts',(-53.923374056695,-24.1685448683466,
40.041211089324));
#191225=CARTESIAN_POINT('Ctrl Pts',(-53.9221135831989,-24.1659037306809,
40.0432881154904));
#191226=CARTESIAN_POINT('Ctrl Pts',(-53.9220259323371,-24.1657200711329,
40.043432547828));
#191227=CARTESIAN_POINT('Ctrl Pts',(-53.9219385350607,-24.1655361818117,
40.0435768364421));
#191228=CARTESIAN_POINT('Ctrl Pts',(-53.9218513926272,-24.1653520623706,
40.0437209807855));
#191229=CARTESIAN_POINT('Ctrl Pts',(-53.9180307491142,-24.1572795915924,
40.0500407968421));
#191230=CARTESIAN_POINT('Ctrl Pts',(-53.9147442868247,-24.1487557177452,
40.0560490279346));
#191231=CARTESIAN_POINT('Ctrl Pts',(-53.9120963197572,-24.1398315880188,
40.0616647108617));
#191232=CARTESIAN_POINT('Ctrl Pts',(-53.9096279542366,-24.1315127481104,
40.0668995033489));
#191233=CARTESIAN_POINT('Ctrl Pts',(-53.9077144433429,-24.1228452895794,
40.0717933267486));
#191234=CARTESIAN_POINT('Ctrl Pts',(-53.906468142013,-24.1138798870151,
40.0762460303077));
#191235=CARTESIAN_POINT('Ctrl Pts',(-53.9060122288629,-24.1106002267701,
40.0778748868751));
#191236=CARTESIAN_POINT('Ctrl Pts',(-53.9056458829917,-24.1072808472547,
40.0794443522249));
#191237=CARTESIAN_POINT('Ctrl Pts',(-53.9053756337487,-24.1039248822478,
40.0809482021492));
#191238=CARTESIAN_POINT('Ctrl Pts',(-53.905310647834,-24.1031178847765,
40.0813098278169));
#191239=CARTESIAN_POINT('Ctrl Pts',(-53.9052515154467,-24.1023082689116,
40.0816679525672));
#191240=CARTESIAN_POINT('Ctrl Pts',(-53.9051983068758,-24.101496150709,
40.0820224192581));
#191241=CARTESIAN_POINT('Ctrl Pts',(-53.9051467610727,-24.1007094112001,
40.0823658088648));
#191242=CARTESIAN_POINT('Ctrl Pts',(-53.9051007746215,-24.0999203233285,
40.0827057654617));
#191243=CARTESIAN_POINT('Ctrl Pts',(-53.9050604098635,-24.0991289960599,
40.0830421470151));
#191244=CARTESIAN_POINT('Ctrl Pts',(-53.904618167291,-24.090459091316,40.0867275956805));
#191245=CARTESIAN_POINT('Ctrl Pts',(-53.9048508523205,-24.0815146560292,
40.0899823432028));
#191246=CARTESIAN_POINT('Ctrl Pts',(-53.9058331609931,-24.0724687639699,
40.0926299529353));
#191247=CARTESIAN_POINT('Ctrl Pts',(-53.9062405536792,-24.0687171629032,
40.0937279956083));
#191248=CARTESIAN_POINT('Ctrl Pts',(-53.9067765048111,-24.0649483109702,
40.0947220371802));
#191249=CARTESIAN_POINT('Ctrl Pts',(-53.9074445642443,-24.0611749820058,
40.0956014538693));
#191250=CARTESIAN_POINT('Ctrl Pts',(-53.9085840092242,-24.0547391762489,
40.097101390674));
#191251=CARTESIAN_POINT('Ctrl Pts',(-53.9101092267074,-24.0482923662126,
40.0982667904316));
#191252=CARTESIAN_POINT('Ctrl Pts',(-53.9120381043537,-24.0419050995276,
40.0990539325583));
#191253=CARTESIAN_POINT('Ctrl Pts',(-53.9130025431769,-24.0387114661851,
40.0994475036216));
#191254=CARTESIAN_POINT('Ctrl Pts',(-53.9140692448461,-24.0355332447502,
40.0997467259952));
#191255=CARTESIAN_POINT('Ctrl Pts',(-53.9152404736265,-24.0323793130073,
40.0999473488896));
#191256=CARTESIAN_POINT('Ctrl Pts',(-53.9164117024069,-24.0292253812645,
40.100147971784));
#191257=CARTESIAN_POINT('Ctrl Pts',(-53.9176874253155,-24.0260957707894,
40.10025));
#191258=CARTESIAN_POINT('Ctrl Pts',(-53.9190682401996,-24.0229981225294,
40.10025));
#191259=CARTESIAN_POINT('Origin',(-55.4168495715593,-17.9900016446779,39.92499));
#191260=CARTESIAN_POINT('Ctrl Pts',(-59.6489943884565,-19.1808295835778,
39.92499));
#191261=CARTESIAN_POINT('Ctrl Pts',(-59.6590854114904,-19.1841083557167,
39.934835464202));
#191262=CARTESIAN_POINT('Ctrl Pts',(-59.668887786629,-19.1881736144724,
39.9446440828463));
#191263=CARTESIAN_POINT('Ctrl Pts',(-59.6783518907174,-19.1929932802643,
39.9543641760338));
#191264=CARTESIAN_POINT('Ctrl Pts',(-59.6875084677779,-19.1976563356173,
39.9637684240721));
#191265=CARTESIAN_POINT('Ctrl Pts',(-59.6963495165753,-19.2030262129965,
39.9730909636406));
#191266=CARTESIAN_POINT('Ctrl Pts',(-59.70481204872,-19.2091163824551,39.9822808977152));
#191267=CARTESIAN_POINT('Ctrl Pts',(-59.7128170830362,-19.2148773077518,
39.9909740094662));
#191268=CARTESIAN_POINT('Ctrl Pts',(-59.7204841754278,-19.2212832892289,
39.9995492765015));
#191269=CARTESIAN_POINT('Ctrl Pts',(-59.7277306815217,-19.2283759411608,
40.0079462328709));
#191270=CARTESIAN_POINT('Ctrl Pts',(-59.7344052377148,-19.2349087865438,
40.0156804369706));
#191271=CARTESIAN_POINT('Ctrl Pts',(-59.7407233396955,-19.2420246158653,
40.0232638017439));
#191272=CARTESIAN_POINT('Ctrl Pts',(-59.7465875973425,-19.2497756062341,
40.0306257269984));
#191273=CARTESIAN_POINT('Ctrl Pts',(-59.7482885955682,-19.2520238739022,
40.0327611416664));
#191274=CARTESIAN_POINT('Ctrl Pts',(-59.7499511651817,-19.2543256952574,
40.0348777427277));
#191275=CARTESIAN_POINT('Ctrl Pts',(-59.751572284779,-19.2566826155661,
40.0369733168701));
#191276=CARTESIAN_POINT('Ctrl Pts',(-59.7533296826513,-19.2592376687175,
40.039245053974));
#191277=CARTESIAN_POINT('Ctrl Pts',(-59.7550368117758,-19.2618533083053,
40.041487875195));
#191278=CARTESIAN_POINT('Ctrl Pts',(-59.7566897852105,-19.2645304831804,
40.0436985701601));
#191279=CARTESIAN_POINT('Ctrl Pts',(-59.7612263837726,-19.2718780106324,
40.0497658398386));
#191280=CARTESIAN_POINT('Ctrl Pts',(-59.7653126215477,-19.2797022819934,
40.0555581699984));
#191281=CARTESIAN_POINT('Ctrl Pts',(-59.7688605008635,-19.2879484209983,
40.0609828468886));
#191282=CARTESIAN_POINT('Ctrl Pts',(-59.7721066178186,-19.2954931904946,
40.0659461317305));
#191283=CARTESIAN_POINT('Ctrl Pts',(-59.7748909605621,-19.3033878446875,
40.0706039980708));
#191284=CARTESIAN_POINT('Ctrl Pts',(-59.7771261198371,-19.3116176456448,
40.0748843180605));
#191285=CARTESIAN_POINT('Ctrl Pts',(-59.7782240227714,-19.3156600969909,
40.0769867972571));
#191286=CARTESIAN_POINT('Ctrl Pts',(-59.7791889148824,-19.3197833592187,
40.0789976708175));
#191287=CARTESIAN_POINT('Ctrl Pts',(-59.7800071751723,-19.3239849291284,
40.08090504915));
#191288=CARTESIAN_POINT('Ctrl Pts',(-59.7801624320924,-19.324782136095,
40.0812669556105));
#191289=CARTESIAN_POINT('Ctrl Pts',(-59.780312120616,-19.3255826085664,
40.0816253922032));
#191290=CARTESIAN_POINT('Ctrl Pts',(-59.7804561537455,-19.3263862368333,
40.0819801989139));
#191291=CARTESIAN_POINT('Ctrl Pts',(-59.7805956858398,-19.327164751717,
40.0823239179149));
#191292=CARTESIAN_POINT('Ctrl Pts',(-59.7807299104879,-19.327946228217,
40.0826642303498));
#191293=CARTESIAN_POINT('Ctrl Pts',(-59.7808587498044,-19.3287305629433,
40.0830009916099));
#191294=CARTESIAN_POINT('Ctrl Pts',(-59.7822628141274,-19.3372780811746,
40.0866709464312));
#191295=CARTESIAN_POINT('Ctrl Pts',(-59.7830278331223,-19.3461707361371,
40.0899175831877));
#191296=CARTESIAN_POINT('Ctrl Pts',(-59.7830570185564,-19.3552444957724,
40.0925642067062));
#191297=CARTESIAN_POINT('Ctrl Pts',(-59.7830693437464,-19.3590764008118,
40.0936818922527));
#191298=CARTESIAN_POINT('Ctrl Pts',(-59.7829507982331,-19.362940356653,
40.0946930094791));
#191299=CARTESIAN_POINT('Ctrl Pts',(-59.7826959186873,-19.3668233599707,
40.0955863397546));
#191300=CARTESIAN_POINT('Ctrl Pts',(-59.7822667079008,-19.373362240532,
40.0970906856166));
#191301=CARTESIAN_POINT('Ctrl Pts',(-59.7814491944743,-19.3799532508953,
40.0982599215483));
#191302=CARTESIAN_POINT('Ctrl Pts',(-59.780216393251,-19.3865272544574,
40.0990497370454));
#191303=CARTESIAN_POINT('Ctrl Pts',(-59.7799081929452,-19.3881707553479,
40.0992471909196));
#191304=CARTESIAN_POINT('Ctrl Pts',(-59.7795738105079,-19.3898131352233,
40.0994209989363));
#191305=CARTESIAN_POINT('Ctrl Pts',(-59.7792125287464,-19.3914532254506,
40.0995705982975));
#191306=CARTESIAN_POINT('Ctrl Pts',(-59.7786706061041,-19.3939133607915,
40.0997949973393));
#191307=CARTESIAN_POINT('Ctrl Pts',(-59.7780681520196,-19.3963683254115,
40.0999649129781));
#191308=CARTESIAN_POINT('Ctrl Pts',(-59.7774043475413,-19.398814676208,
40.1000786629733));
#191309=CARTESIAN_POINT('Ctrl Pts',(-59.7767405430631,-19.4012610270045,
40.1001924129685));
#191310=CARTESIAN_POINT('Ctrl Pts',(-59.7760153991102,-19.4036987600451,
40.10025));
#191311=CARTESIAN_POINT('Ctrl Pts',(-59.7752282754838,-19.406124729225,
40.10025));
#191312=CARTESIAN_POINT('Ctrl Pts',(-56.1441998575528,-18.2263320786579,
40.10025));
#191313=CARTESIAN_POINT('Ctrl Pts',(-56.1468630191714,-18.2181232748941,
40.10025));
#191314=CARTESIAN_POINT('Ctrl Pts',(-56.1501806998579,-18.2102054558337,
40.0995786334241));
#191315=CARTESIAN_POINT('Ctrl Pts',(-56.1540344262254,-18.2026724222806,
40.0983063763366));
#191316=CARTESIAN_POINT('Ctrl Pts',(-56.1565235380436,-18.1978068555394,
40.0974846287992));
#191317=CARTESIAN_POINT('Ctrl Pts',(-56.1592354513148,-18.1931013796336,
40.0964130309338));
#191318=CARTESIAN_POINT('Ctrl Pts',(-56.1621313494121,-18.1885757140655,
40.0951176960924));
#191319=CARTESIAN_POINT('Ctrl Pts',(-56.1659696964528,-18.182577203601,
40.0934008039614));
#191320=CARTESIAN_POINT('Ctrl Pts',(-56.1701354151837,-18.176898633833,
40.0912909372157));
#191321=CARTESIAN_POINT('Ctrl Pts',(-56.1745504247234,-18.1715848978924,
40.0888630467852));
#191322=CARTESIAN_POINT('Ctrl Pts',(-56.1767579294932,-18.168928029922,
40.0876491015699));
#191323=CARTESIAN_POINT('Ctrl Pts',(-56.1790278168866,-18.1663621803351,
40.0863558569271));
#191324=CARTESIAN_POINT('Ctrl Pts',(-56.181350756616,-18.1638916135756,
40.0849936342771));
#191325=CARTESIAN_POINT('Ctrl Pts',(-56.1825122264807,-18.1626563301959,
40.0843125229521));
#191326=CARTESIAN_POINT('Ctrl Pts',(-56.1836869644605,-18.161444851881,
40.0836141747074));
#191327=CARTESIAN_POINT('Ctrl Pts',(-56.1848738357353,-18.1602576134414,
40.082899916161));
#191328=CARTESIAN_POINT('Ctrl Pts',(-56.185170553554,-18.1599608038315,
40.0827213515244));
#191329=CARTESIAN_POINT('Ctrl Pts',(-56.1854680298097,-18.1596655088808,
40.0825417925842));
#191330=CARTESIAN_POINT('Ctrl Pts',(-56.1857662469842,-18.1593717347115,
40.0823612602361));
#191331=CARTESIAN_POINT('Ctrl Pts',(-56.1866608985078,-18.1584904122035,
40.0818196631918));
#191332=CARTESIAN_POINT('Ctrl Pts',(-56.187562217779,-18.1576227783922,
40.0812693052022));
#191333=CARTESIAN_POINT('Ctrl Pts',(-56.1884697364865,-18.1567689837083,
40.0807107531875));
#191334=CARTESIAN_POINT('Ctrl Pts',(-56.1948621810804,-18.1507549641992,
40.0767763849182));
#191335=CARTESIAN_POINT('Ctrl Pts',(-56.2015542305061,-18.1453743792963,
40.0724140586137));
#191336=CARTESIAN_POINT('Ctrl Pts',(-56.2084349106663,-18.1405824894349,
40.0677221223768));
#191337=CARTESIAN_POINT('Ctrl Pts',(-56.2117720331086,-18.1382584280303,
40.0654465383721));
#191338=CARTESIAN_POINT('Ctrl Pts',(-56.2151540877945,-18.1360729791408,
40.0630928000679));
#191339=CARTESIAN_POINT('Ctrl Pts',(-56.2185710935569,-18.1340220442548,
40.0606689262479));
#191340=CARTESIAN_POINT('Ctrl Pts',(-56.2238022906399,-18.130882206239,
40.0569581447806));
#191341=CARTESIAN_POINT('Ctrl Pts',(-56.2291119669556,-18.1280584389296,
40.0530843804606));
#191342=CARTESIAN_POINT('Ctrl Pts',(-56.2344544719217,-18.1255442374228,
40.0490800251458));
#191343=CARTESIAN_POINT('Ctrl Pts',(-56.2369355588664,-18.1243766292362,
40.0472203818218));
#191344=CARTESIAN_POINT('Ctrl Pts',(-56.2394235482376,-18.1232756028764,
40.0453323608819));
#191345=CARTESIAN_POINT('Ctrl Pts',(-56.2419141381098,-18.1222417093398,
40.0434201572162));
#191346=CARTESIAN_POINT('Ctrl Pts',(-56.2421050320101,-18.122162465474,
40.0432735943397));
#191347=CARTESIAN_POINT('Ctrl Pts',(-56.2422959411932,-18.1220835820643,
40.0431268995708));
#191348=CARTESIAN_POINT('Ctrl Pts',(-56.2424868643661,-18.1220050584319,
40.0429800745037));
#191349=CARTESIAN_POINT('Ctrl Pts',(-56.2451687593304,-18.1209020381383,
40.0409176249753));
#191350=CARTESIAN_POINT('Ctrl Pts',(-56.247854333334,-18.1198718859662,
40.0388310783333));
#191351=CARTESIAN_POINT('Ctrl Pts',(-56.2505383386774,-18.1189123616723,
40.036725739981));
#191352=CARTESIAN_POINT('Ctrl Pts',(-56.2601627045042,-18.1154716782,40.029176371072));
#191353=CARTESIAN_POINT('Ctrl Pts',(-56.2698406425781,-18.1129106883012,
40.0213310894599));
#191354=CARTESIAN_POINT('Ctrl Pts',(-56.2795015152461,-18.1111213027308,
40.0132837551327));
#191355=CARTESIAN_POINT('Ctrl Pts',(-56.2901178437879,-18.1091549477487,
40.0044405431333));
#191356=CARTESIAN_POINT('Ctrl Pts',(-56.3007141730221,-18.1081200911547,
39.9953528710609));
#191357=CARTESIAN_POINT('Ctrl Pts',(-56.3112209484361,-18.1079204190084,
39.9861103629564));
#191358=CARTESIAN_POINT('Ctrl Pts',(-56.3225656290429,-18.1077048232012,
39.9761307737561));
#191359=CARTESIAN_POINT('Ctrl Pts',(-56.3338070504147,-18.1084627484405,
39.9659696936013));
#191360=CARTESIAN_POINT('Ctrl Pts',(-56.3448702837385,-18.1101289800549,
39.9557128217503));
#191361=CARTESIAN_POINT('Ctrl Pts',(-56.3558407079016,-18.1117812336981,
39.9455419945158));
#191362=CARTESIAN_POINT('Ctrl Pts',(-56.3666372711396,-18.1143271060913,
39.9352756289339));
#191363=CARTESIAN_POINT('Ctrl Pts',(-56.3771794532808,-18.1177524687103,
39.92499));
#191364=CARTESIAN_POINT('Origin',(0.00470941899428508,-0.0144941013083364,
39.92499));
#191365=CARTESIAN_POINT('Ctrl Pts',(-59.7658094374952,-19.4351129318417,
40.10025));
#191366=CARTESIAN_POINT('Ctrl Pts',(-59.7631518948791,-19.4432803829096,
40.10025));
#191367=CARTESIAN_POINT('Ctrl Pts',(-59.7598356997909,-19.4511532554527,
40.0995859581841));
#191368=CARTESIAN_POINT('Ctrl Pts',(-59.7559811102133,-19.4586404431021,
40.0983275959617));
#191369=CARTESIAN_POINT('Ctrl Pts',(-59.7535182109725,-19.4634243995794,
40.0975235624065));
#191370=CARTESIAN_POINT('Ctrl Pts',(-59.7508363273792,-19.4680513433541,
40.0964777059489));
#191371=CARTESIAN_POINT('Ctrl Pts',(-59.7479734971807,-19.4725029330458,
40.0952149915961));
#191372=CARTESIAN_POINT('Ctrl Pts',(-59.7440663083908,-19.4785784597569,
40.0934916398701));
#191373=CARTESIAN_POINT('Ctrl Pts',(-59.7398178213043,-19.4843230052518,
40.0913643921631));
#191374=CARTESIAN_POINT('Ctrl Pts',(-59.7353118462117,-19.489690449293,
40.0889118607713));
#191375=CARTESIAN_POINT('Ctrl Pts',(-59.7330588586654,-19.4923741713137,
40.0876855950754));
#191376=CARTESIAN_POINT('Ctrl Pts',(-59.7307414364081,-19.4949638171732,
40.0863782327527));
#191377=CARTESIAN_POINT('Ctrl Pts',(-59.7283696021899,-19.4974550439412,
40.0850006373334));
#191378=CARTESIAN_POINT('Ctrl Pts',(-59.7271836850807,-19.4987006573253,
40.0843118396237));
#191379=CARTESIAN_POINT('Ctrl Pts',(-59.7259841596484,-19.4999216825135,
40.0836054919164));
#191380=CARTESIAN_POINT('Ctrl Pts',(-59.7247722453468,-19.5011176808519,
40.0828829920418));
#191381=CARTESIAN_POINT('Ctrl Pts',(-59.7244692667714,-19.5014166804365,
40.0827023670731));
#191382=CARTESIAN_POINT('Ctrl Pts',(-59.7241655137791,-19.5017141161965,
40.0825207326933));
#191383=CARTESIAN_POINT('Ctrl Pts',(-59.7238610051971,-19.5020099819909,
40.0823381109275));
#191384=CARTESIAN_POINT('Ctrl Pts',(-59.7229474794512,-19.5028975793742,
40.0817902456303));
#191385=CARTESIAN_POINT('Ctrl Pts',(-59.722027153953,-19.5037710453005,
40.0812334935553));
#191386=CARTESIAN_POINT('Ctrl Pts',(-59.7211005320715,-19.5046302297522,
40.0806684524227));
#191387=CARTESIAN_POINT('Ctrl Pts',(-59.7146969999426,-19.5105677273984,
40.0767636676136));
#191388=CARTESIAN_POINT('Ctrl Pts',(-59.7079999120046,-19.5158784513269,
40.0724404510887));
#191389=CARTESIAN_POINT('Ctrl Pts',(-59.7011184102413,-19.5206092977904,
40.0677949937408));
#191390=CARTESIAN_POINT('Ctrl Pts',(-59.6976983227544,-19.5229605154967,
40.0654862141905));
#191391=CARTESIAN_POINT('Ctrl Pts',(-59.6942320938702,-19.5251683423979,
40.0630972003216));
#191392=CARTESIAN_POINT('Ctrl Pts',(-59.6907301905172,-19.527237362964,
40.0606363359906));
#191393=CARTESIAN_POINT('Ctrl Pts',(-59.6830044686627,-19.5318019313699,
40.0552073017124));
#191394=CARTESIAN_POINT('Ctrl Pts',(-59.675112260622,-19.5357011184425,
40.0494204304519));
#191395=CARTESIAN_POINT('Ctrl Pts',(-59.6671986827532,-19.538926651298,
40.0434049749851));
#191396=CARTESIAN_POINT('Ctrl Pts',(-59.6643077529623,-19.5401049791262,
40.0412074532442));
#191397=CARTESIAN_POINT('Ctrl Pts',(-59.6614137631514,-19.5412013620777,
40.0389814735788));
#191398=CARTESIAN_POINT('Ctrl Pts',(-59.6585211429014,-19.5422187365065,
40.0367321210017));
#191399=CARTESIAN_POINT('Ctrl Pts',(-59.6488051375686,-19.5456359895575,
40.0291767837139));
#191400=CARTESIAN_POINT('Ctrl Pts',(-59.6390401911867,-19.5481755652421,
40.0213235332572));
#191401=CARTESIAN_POINT('Ctrl Pts',(-59.6292970278053,-19.549944514459,
40.0132649215852));
#191402=CARTESIAN_POINT('Ctrl Pts',(-59.6185881370957,-19.5518887991941,
40.0044075527524));
#191403=CARTESIAN_POINT('Ctrl Pts',(-59.6079049297397,-19.5529023976137,
39.9953016253709));
#191404=CARTESIAN_POINT('Ctrl Pts',(-59.5973174182803,-19.5530800481815,
39.9860353422344));
#191405=CARTESIAN_POINT('Ctrl Pts',(-59.5859142147997,-19.5532713854548,
39.9760551582678));
#191406=CARTESIAN_POINT('Ctrl Pts',(-59.5746208362142,-19.5524931697987,
39.9658879738135));
#191407=CARTESIAN_POINT('Ctrl Pts',(-59.5635130675406,-19.5508078878555,
39.9556174643229));
#191408=CARTESIAN_POINT('Ctrl Pts',(-59.5525552912495,-19.5491453629089,
39.9454856413888));
#191409=CARTESIAN_POINT('Ctrl Pts',(-59.5417768065749,-19.5465995868768,
39.9352519465105));
#191410=CARTESIAN_POINT('Ctrl Pts',(-59.5312589135997,-19.5431821162863,
39.92499));
#191411=CARTESIAN_POINT('Ctrl Pts',(-56.259443978424,-18.4801050014187,
39.92499));
#191412=CARTESIAN_POINT('Ctrl Pts',(-56.2493782971083,-18.4768344633033,
39.934810724172));
#191413=CARTESIAN_POINT('Ctrl Pts',(-56.2396067681219,-18.4727817672089,
39.9446038383166));
#191414=CARTESIAN_POINT('Ctrl Pts',(-56.2301791400438,-18.4679768367037,
39.9543158069379));
#191415=CARTESIAN_POINT('Ctrl Pts',(-56.221075935655,-18.4633372535445,
39.9636935671385));
#191416=CARTESIAN_POINT('Ctrl Pts',(-56.2122922812561,-18.4579956735924,
39.9729968320981));
#191417=CARTESIAN_POINT('Ctrl Pts',(-56.2038917763252,-18.4519372213367,
39.9821731151327));
#191418=CARTESIAN_POINT('Ctrl Pts',(-56.1959506682901,-18.4462100865652,
39.9908475764345));
#191419=CARTESIAN_POINT('Ctrl Pts',(-56.1883512165489,-18.4398418135292,
39.9994093733839));
#191420=CARTESIAN_POINT('Ctrl Pts',(-56.1811768067742,-18.4327901596635,
40.0077966115835));
#191421=CARTESIAN_POINT('Ctrl Pts',(-56.1745692957314,-18.4262957047536,
40.015521117259));
#191422=CARTESIAN_POINT('Ctrl Pts',(-56.1683219623521,-18.419221177343,
40.0230979941019));
#191423=CARTESIAN_POINT('Ctrl Pts',(-56.1625328136768,-18.4115142492179,
40.0304554104747));
#191424=CARTESIAN_POINT('Ctrl Pts',(-56.1608066064034,-18.4092161988253,
40.032649243518));
#191425=CARTESIAN_POINT('Ctrl Pts',(-56.1591213928268,-18.4068618031988,
40.034823371506));
#191426=CARTESIAN_POINT('Ctrl Pts',(-56.1574804751188,-18.4044493827312,
40.0369753512356));
#191427=CARTESIAN_POINT('Ctrl Pts',(-56.1558563235462,-18.4020616112561,
40.0391053430352));
#191428=CARTESIAN_POINT('Ctrl Pts',(-56.1542770260204,-18.399619626408,
40.041211089324));
#191429=CARTESIAN_POINT('Ctrl Pts',(-56.1527473834685,-18.3971247125284,
40.0432881154904));
#191430=CARTESIAN_POINT('Ctrl Pts',(-56.1526410151169,-18.3969512210965,
40.043432547828));
#191431=CARTESIAN_POINT('Ctrl Pts',(-56.1525348749437,-18.3967774746432,
40.0435768364421));
#191432=CARTESIAN_POINT('Ctrl Pts',(-56.1524289641634,-18.3966034726923,
40.0437209807855));
#191433=CARTESIAN_POINT('Ctrl Pts',(-56.1477854475702,-18.3889745897489,
40.050040796842));
#191434=CARTESIAN_POINT('Ctrl Pts',(-56.1436260014306,-18.3808409394271,
40.0560490279345));
#191435=CARTESIAN_POINT('Ctrl Pts',(-56.1400597146374,-18.3722424849456,
40.0616647108616));
#191436=CARTESIAN_POINT('Ctrl Pts',(-56.1367353155297,-18.3642272309674,
40.0668995033487));
#191437=CARTESIAN_POINT('Ctrl Pts',(-56.1339262909282,-18.3558072700344,
40.0717933267484));
#191438=CARTESIAN_POINT('Ctrl Pts',(-56.1317496772148,-18.3470212548463,
40.0762460303075));
#191439=CARTESIAN_POINT('Ctrl Pts',(-56.1309534437592,-18.343807216824,
40.077874886875));
#191440=CARTESIAN_POINT('Ctrl Pts',(-56.1302421351291,-18.3405443147878,
40.0794443522248));
#191441=CARTESIAN_POINT('Ctrl Pts',(-56.1296225724748,-18.3372349828462,
40.0809482021492));
#191442=CARTESIAN_POINT('Ctrl Pts',(-56.1294735883542,-18.3364391990693,
40.0813098278168));
#191443=CARTESIAN_POINT('Ctrl Pts',(-56.1293301519981,-18.3356401993824,
40.0816679525672));
#191444=CARTESIAN_POINT('Ctrl Pts',(-56.1291923454416,-18.3348380918583,
40.0820224192581));
#191445=CARTESIAN_POINT('Ctrl Pts',(-56.12905884534,-18.3340610501944,40.0823658088648));
#191446=CARTESIAN_POINT('Ctrl Pts',(-56.1289306286648,-18.3332810919218,
40.0827057654617));
#191447=CARTESIAN_POINT('Ctrl Pts',(-56.1288077688059,-18.3324983188929,
40.0830421470151));
#191448=CARTESIAN_POINT('Ctrl Pts',(-56.1274616970649,-18.3239221357306,
40.0867275956806));
#191449=CARTESIAN_POINT('Ctrl Pts',(-56.126758159346,-18.3150023767874,
40.089982343203));
#191450=CARTESIAN_POINT('Ctrl Pts',(-56.1267895336332,-18.3059033598551,
40.0926299529355));
#191451=CARTESIAN_POINT('Ctrl Pts',(-56.1268025454852,-18.3021297263204,
40.0937279956084));
#191452=CARTESIAN_POINT('Ctrl Pts',(-56.1269416083199,-18.2983254984046,
40.0947220371802));
#191453=CARTESIAN_POINT('Ctrl Pts',(-56.1272115877755,-18.2945030089054,
40.0956014538692));
#191454=CARTESIAN_POINT('Ctrl Pts',(-56.127672065871,-18.2879833547331,
40.097101390674));
#191455=CARTESIAN_POINT('Ctrl Pts',(-56.1285150529071,-18.2814124323571,
40.0982667904316));
#191456=CARTESIAN_POINT('Ctrl Pts',(-56.1297657127887,-18.274858533171,
40.0990539325583));
#191457=CARTESIAN_POINT('Ctrl Pts',(-56.1303910427295,-18.271581583578,
40.0994475036216));
#191458=CARTESIAN_POINT('Ctrl Pts',(-56.1311196862928,-18.2683092720864,
40.0997467259952));
#191459=CARTESIAN_POINT('Ctrl Pts',(-56.1319548233211,-18.2650501911671,
40.0999473488896));
#191460=CARTESIAN_POINT('Ctrl Pts',(-56.1327899603494,-18.2617911102478,
40.100147971784));
#191461=CARTESIAN_POINT('Ctrl Pts',(-56.1337315613409,-18.2585452947512,
40.10025));
#191462=CARTESIAN_POINT('Ctrl Pts',(-56.1347810195643,-18.2553202812746,
40.10025));
#191463=CARTESIAN_POINT('Origin',(-56.9937374973464,-12.0988124084936,39.92499));
#191464=CARTESIAN_POINT('Ctrl Pts',(-61.3271735965894,-12.8407372733094,
39.92499));
#191465=CARTESIAN_POINT('Ctrl Pts',(-61.3375520649564,-12.8429432848609,
39.9348354642022));
#191466=CARTESIAN_POINT('Ctrl Pts',(-61.347725676909,-12.8459616464942,
39.9446440828466));
#191467=CARTESIAN_POINT('Ctrl Pts',(-61.3576417279037,-12.8497656413962,
39.9543641760342));
#191468=CARTESIAN_POINT('Ctrl Pts',(-61.3672355662873,-12.8534460291151,
39.9637684240726));
#191469=CARTESIAN_POINT('Ctrl Pts',(-61.3765894879248,-12.8578623484998,
39.9730909636412));
#191470=CARTESIAN_POINT('Ctrl Pts',(-61.3856422574875,-12.8630345798924,
39.9822808977158));
#191471=CARTESIAN_POINT('Ctrl Pts',(-61.3942056200565,-12.8679271923022,
39.9909740094669));
#191472=CARTESIAN_POINT('Ctrl Pts',(-61.4025003187134,-12.8734966517571,
39.9995492765022));
#191473=CARTESIAN_POINT('Ctrl Pts',(-61.4104485116956,-12.8797929832537,
40.0079462328716));
#191474=CARTESIAN_POINT('Ctrl Pts',(-61.4177693722602,-12.8855923599243,
40.0156804369713));
#191475=CARTESIAN_POINT('Ctrl Pts',(-61.4247966697211,-12.8920087864975,
40.0232638017446));
#191476=CARTESIAN_POINT('Ctrl Pts',(-61.4314390014632,-12.8991043342901,
40.0306257269992));
#191477=CARTESIAN_POINT('Ctrl Pts',(-61.4333656894068,-12.9011624829819,
40.0327611416669));
#191478=CARTESIAN_POINT('Ctrl Pts',(-61.4352597571387,-12.9032779088719,
40.0348777427279));
#191479=CARTESIAN_POINT('Ctrl Pts',(-61.4371183613309,-12.905452464584,
40.0369733168701));
#191480=CARTESIAN_POINT('Ctrl Pts',(-61.4391332077732,-12.9078098227879,
40.039245053974));
#191481=CARTESIAN_POINT('Ctrl Pts',(-61.4411043938524,-12.9102326900445,
40.041487875195));
#191482=CARTESIAN_POINT('Ctrl Pts',(-61.4430281531012,-12.9127224163025,
40.0436985701601));
#191483=CARTESIAN_POINT('Ctrl Pts',(-61.448307925455,-12.9195554895542,
40.0497658398386));
#191484=CARTESIAN_POINT('Ctrl Pts',(-61.4531896374536,-12.9269097705828,
40.0555581699984));
#191485=CARTESIAN_POINT('Ctrl Pts',(-61.4575800373534,-12.9347398820027,
40.0609828468886));
#191486=CARTESIAN_POINT('Ctrl Pts',(-61.4615970149013,-12.9419040088453,
40.0659461317306));
#191487=CARTESIAN_POINT('Ctrl Pts',(-61.4651913207948,-12.9494643722284,
40.0706039980708));
#191488=CARTESIAN_POINT('Ctrl Pts',(-61.4682744840804,-12.9574154517107,
40.0748843180606));
#191489=CARTESIAN_POINT('Ctrl Pts',(-61.4697889238147,-12.9613209959789,
40.0769867972571));
#191490=CARTESIAN_POINT('Ctrl Pts',(-61.4711795284101,-12.9653208118552,
40.0789976708176));
#191491=CARTESIAN_POINT('Ctrl Pts',(-61.4724324898305,-12.9694138336347,
40.08090504915));
#191492=CARTESIAN_POINT('Ctrl Pts',(-61.472670227056,-12.9701904446508,
40.0812669556105));
#191493=CARTESIAN_POINT('Ctrl Pts',(-61.4729027677275,-12.9709708853389,
40.0816253922033));
#191494=CARTESIAN_POINT('Ctrl Pts',(-61.4731300138563,-12.9717550556844,
40.081980198914));
#191495=CARTESIAN_POINT('Ctrl Pts',(-61.4733501585436,-12.9725147207067,
40.0823239179149));
#191496=CARTESIAN_POINT('Ctrl Pts',(-61.4735653344326,-12.9732778859004,
40.0826642303499));
#191497=CARTESIAN_POINT('Ctrl Pts',(-61.4737754532574,-12.9740444565833,
40.08300099161));
#191498=CARTESIAN_POINT('Ctrl Pts',(-61.4760652849146,-12.9823983859292,
40.0866709464311));
#191499=CARTESIAN_POINT('Ctrl Pts',(-61.477755648613,-12.9911623597372,
40.0899175831876));
#191500=CARTESIAN_POINT('Ctrl Pts',(-61.4787331403169,-13.0001833616589,
40.0925642067059));
#191501=CARTESIAN_POINT('Ctrl Pts',(-61.4791459411335,-13.0039929867886,
40.0936818922526));
#191502=CARTESIAN_POINT('Ctrl Pts',(-61.4794319383912,-13.007848166856,
40.094693009479));
#191503=CARTESIAN_POINT('Ctrl Pts',(-61.4795843394718,-13.0117365408428,
40.0955863397546));
#191504=CARTESIAN_POINT('Ctrl Pts',(-61.4798409790835,-13.0182844654761,
40.0970906856167));
#191505=CARTESIAN_POINT('Ctrl Pts',(-61.4797168922658,-13.0249248230172,
40.0982599215483));
#191506=CARTESIAN_POINT('Ctrl Pts',(-61.4791780149462,-13.0315916763173,
40.0990497370454));
#191507=CARTESIAN_POINT('Ctrl Pts',(-61.4790432956163,-13.0332583896423,
40.0992471909196));
#191508=CARTESIAN_POINT('Ctrl Pts',(-61.4788824204055,-13.0349267248713,
40.0994209989363));
#191509=CARTESIAN_POINT('Ctrl Pts',(-61.4786945538944,-13.03659559474,40.0995705982975));
#191510=CARTESIAN_POINT('Ctrl Pts',(-61.4784127541277,-13.039098899543,
40.0997949973393));
#191511=CARTESIAN_POINT('Ctrl Pts',(-61.4780702140288,-13.0416033892097,
40.0999649129781));
#191512=CARTESIAN_POINT('Ctrl Pts',(-61.4776657592304,-13.0441057251026,
40.1000786629733));
#191513=CARTESIAN_POINT('Ctrl Pts',(-61.477261304432,-13.0466080609954,
40.1001924129685));
#191514=CARTESIAN_POINT('Ctrl Pts',(-61.4767949453822,-13.0491082380625,
40.10025));
#191515=CARTESIAN_POINT('Ctrl Pts',(-61.4762657165316,-13.0516031943525,
40.10025));
#191516=CARTESIAN_POINT('Ctrl Pts',(-57.7418065394566,-12.2578193919764,
40.10025));
#191517=CARTESIAN_POINT('Ctrl Pts',(-57.7435970583545,-12.2493771807074,
40.10025));
#191518=CARTESIAN_POINT('Ctrl Pts',(-57.7460689269801,-12.2411559442247,
40.0995786334241));
#191519=CARTESIAN_POINT('Ctrl Pts',(-57.7491141258102,-12.2332613533229,
40.0983063763367));
#191520=CARTESIAN_POINT('Ctrl Pts',(-57.7510810117991,-12.2281622576318,
40.0974846287993));
#191521=CARTESIAN_POINT('Ctrl Pts',(-57.7532862127604,-12.2231990866883,
40.0964130309338));
#191522=CARTESIAN_POINT('Ctrl Pts',(-57.7556931859579,-12.2183955094115,
40.0951176960923));
#191523=CARTESIAN_POINT('Ctrl Pts',(-57.7588834910512,-12.2120286428973,
40.0934008039614));
#191524=CARTESIAN_POINT('Ctrl Pts',(-57.7624328173676,-12.2059457447514,
40.0912909372156));
#191525=CARTESIAN_POINT('Ctrl Pts',(-57.7662682043709,-12.2001996238497,
40.0888630467851));
#191526=CARTESIAN_POINT('Ctrl Pts',(-57.7681858978726,-12.1973265633989,
40.0876491015699));
#191527=CARTESIAN_POINT('Ctrl Pts',(-57.7701751462711,-12.1945375019635,
40.0863558569271));
#191528=CARTESIAN_POINT('Ctrl Pts',(-57.7722271161468,-12.191837655907,
40.0849936342771));
#191529=CARTESIAN_POINT('Ctrl Pts',(-57.7732531010847,-12.1904877328788,
40.0843125229521));
#191530=CARTESIAN_POINT('Ctrl Pts',(-57.7742947697604,-12.1891600976131,
40.0836141747074));
#191531=CARTESIAN_POINT('Ctrl Pts',(-57.7753510390205,-12.1878553011595,
40.0828999161609));
#191532=CARTESIAN_POINT('Ctrl Pts',(-57.7756151063355,-12.187529102046,
40.0827213515243));
#191533=CARTESIAN_POINT('Ctrl Pts',(-57.7758800862578,-12.1872043300161,
40.0825417925841));
#191534=CARTESIAN_POINT('Ctrl Pts',(-57.776145962005,-12.1868809929894,
40.082361260236));
#191535=CARTESIAN_POINT('Ctrl Pts',(-57.7769435892465,-12.1859109819095,
40.0818196631917));
#191536=CARTESIAN_POINT('Ctrl Pts',(-57.7777492785674,-12.1849538875687,
40.0812693052021));
#191537=CARTESIAN_POINT('Ctrl Pts',(-57.7785625799463,-12.1840099085254,
40.0807107531875));
#191538=CARTESIAN_POINT('Ctrl Pts',(-57.7842913698424,-12.1773606420347,
40.0767763849182));
#191539=CARTESIAN_POINT('Ctrl Pts',(-57.7903843352498,-12.1713100228962,
40.0724140586138));
#191540=CARTESIAN_POINT('Ctrl Pts',(-57.7967264334407,-12.1658251565856,
40.0677221223769));
#191541=CARTESIAN_POINT('Ctrl Pts',(-57.79980234421,-12.1631650023519,40.0654465383721));
#191542=CARTESIAN_POINT('Ctrl Pts',(-57.8029374300325,-12.160638004601,
40.0630928000679));
#191543=CARTESIAN_POINT('Ctrl Pts',(-57.806121336008,-12.1582411305895,
40.0606689262479));
#191544=CARTESIAN_POINT('Ctrl Pts',(-57.8109956736033,-12.1545716839427,
40.0569581447805));
#191545=CARTESIAN_POINT('Ctrl Pts',(-57.8159810988991,-12.1512083732204,
40.0530843804606));
#191546=CARTESIAN_POINT('Ctrl Pts',(-57.8210315314441,-12.1481495009383,
40.0490800251458));
#191547=CARTESIAN_POINT('Ctrl Pts',(-57.8233769784455,-12.146728944826,
40.0472203818218));
#191548=CARTESIAN_POINT('Ctrl Pts',(-57.8257362497572,-12.1453738842982,
40.0453323608818));
#191549=CARTESIAN_POINT('Ctrl Pts',(-57.8281051246149,-12.1440853170067,
40.0434201572162));
#191550=CARTESIAN_POINT('Ctrl Pts',(-57.8282866895389,-12.143986553401,
40.0432735943397));
#191551=CARTESIAN_POINT('Ctrl Pts',(-57.82846830734,-12.1438881466793,40.0431268995708));
#191552=CARTESIAN_POINT('Ctrl Pts',(-57.8286499766611,-12.1437900963018,
40.0429800745037));
#191553=CARTESIAN_POINT('Ctrl Pts',(-57.8312018829079,-12.1424127841094,
40.0409176249753));
#191554=CARTESIAN_POINT('Ctrl Pts',(-57.8337650648327,-12.1411075562951,
40.0388310783332));
#191555=CARTESIAN_POINT('Ctrl Pts',(-57.8363340693141,-12.1398727334217,
40.036725739981));
#191556=CARTESIAN_POINT('Ctrl Pts',(-57.845546062502,-12.1354448782037,
40.0291763710719));
#191557=CARTESIAN_POINT('Ctrl Pts',(-57.8549032874802,-12.131886297681,
40.0213310894597));
#191558=CARTESIAN_POINT('Ctrl Pts',(-57.8643241951532,-12.1290968783782,
40.0132837551324));
#191559=CARTESIAN_POINT('Ctrl Pts',(-57.8746768262719,-12.1260315867863,
40.0044405431328));
#191560=CARTESIAN_POINT('Ctrl Pts',(-57.8851069357366,-12.1238947812339,
39.9953528710603));
#191561=CARTESIAN_POINT('Ctrl Pts',(-57.895535282513,-12.1225979458246,
39.9861103629557));
#191562=CARTESIAN_POINT('Ctrl Pts',(-57.9067952798742,-12.1211976890437,
39.9761307737553));
#191563=CARTESIAN_POINT('Ctrl Pts',(-57.9180543443241,-12.1207764137884,
39.9659696936003));
#191564=CARTESIAN_POINT('Ctrl Pts',(-57.9292311407285,-12.1212770948337,
39.9557128217492));
#191565=CARTESIAN_POINT('Ctrl Pts',(-57.940314175294,-12.1217735756794,
39.9455419945151));
#191566=CARTESIAN_POINT('Ctrl Pts',(-57.9513177099575,-12.1231769533535,
39.9352756289336));
#191567=CARTESIAN_POINT('Ctrl Pts',(-57.9621601888121,-12.1254815933788,
39.92499));
#191568=CARTESIAN_POINT('Origin',(0.00316857416807368,-0.0149069694351821,
39.92499));
#191569=CARTESIAN_POINT('Ctrl Pts',(-61.4699285681955,-13.0814171332229,
40.10025));
#191570=CARTESIAN_POINT('Ctrl Pts',(-61.4681393149849,-13.0898176309845,
40.10025));
#191571=CARTESIAN_POINT('Ctrl Pts',(-61.465664225629,-13.097994011884,40.0995859581841));
#191572=CARTESIAN_POINT('Ctrl Pts',(-61.4626133761159,-13.1058430982607,
40.098327595962));
#191573=CARTESIAN_POINT('Ctrl Pts',(-61.4606640285136,-13.1108582907972,
40.0975235624067));
#191574=CARTESIAN_POINT('Ctrl Pts',(-61.4584804838815,-13.1157402208609,
40.096477705949));
#191575=CARTESIAN_POINT('Ctrl Pts',(-61.4560986543957,-13.1204666715201,
40.0952149915962));
#191576=CARTESIAN_POINT('Ctrl Pts',(-61.4528479350655,-13.1269173283001,
40.0934916398702));
#191577=CARTESIAN_POINT('Ctrl Pts',(-61.4492231901485,-13.1330744924001,
40.0913643921631));
#191578=CARTESIAN_POINT('Ctrl Pts',(-61.4453029499362,-13.1388835356733,
40.0889118607714));
#191579=CARTESIAN_POINT('Ctrl Pts',(-61.44334282983,-13.1417880573098,40.0876855950755));
#191580=CARTESIAN_POINT('Ctrl Pts',(-61.4413087943565,-13.1446057534057,
40.0863782327527));
#191581=CARTESIAN_POINT('Ctrl Pts',(-61.4392103574,-13.1473312571588,40.0850006373334));
#191582=CARTESIAN_POINT('Ctrl Pts',(-61.4381611389217,-13.1486940090354,
40.0843118396238));
#191583=CARTESIAN_POINT('Ctrl Pts',(-61.4370958165018,-13.1500337298699,
40.0836054919165));
#191584=CARTESIAN_POINT('Ctrl Pts',(-61.4360155570619,-13.1513498559439,
40.0828829920418));
#191585=CARTESIAN_POINT('Ctrl Pts',(-61.4357454922019,-13.1516788874624,
40.0827023670731));
#191586=CARTESIAN_POINT('Ctrl Pts',(-61.4354744937032,-13.1520064446716,
40.0825207326933));
#191587=CARTESIAN_POINT('Ctrl Pts',(-61.4352025796479,-13.1523325194964,
40.0823381109276));
#191588=CARTESIAN_POINT('Ctrl Pts',(-61.4343868374821,-13.1533107439708,
40.0817902456304));
#191589=CARTESIAN_POINT('Ctrl Pts',(-61.4335628556743,-13.1542756251694,
40.0812334935554));
#191590=CARTESIAN_POINT('Ctrl Pts',(-61.4327311191547,-13.15522696128,40.0806684524227));
#191591=CARTESIAN_POINT('Ctrl Pts',(-61.4269833037494,-13.1618012840659,
40.0767636676136));
#191592=CARTESIAN_POINT('Ctrl Pts',(-61.4208780249709,-13.1677829516035,
40.0724404510887));
#191593=CARTESIAN_POINT('Ctrl Pts',(-61.414528728905,-13.1732071947995,
40.0677949937407));
#191594=CARTESIAN_POINT('Ctrl Pts',(-61.4113731461889,-13.1759030287784,
40.0654862141904));
#191595=CARTESIAN_POINT('Ctrl Pts',(-61.4081566864224,-13.1784610805513,
40.0630972003215));
#191596=CARTESIAN_POINT('Ctrl Pts',(-61.4048902384027,-13.1808848153823,
40.0606363359906));
#191597=CARTESIAN_POINT('Ctrl Pts',(-61.3976839661818,-13.1862319364379,
40.0552073017124));
#191598=CARTESIAN_POINT('Ctrl Pts',(-61.3902425685153,-13.190934723734,
40.0494204304519));
#191599=CARTESIAN_POINT('Ctrl Pts',(-61.3827095020467,-13.1949697809166,
40.0434049749851));
#191600=CARTESIAN_POINT('Ctrl Pts',(-61.3799575778688,-13.1964438381902,
40.0412074532442));
#191601=CARTESIAN_POINT('Ctrl Pts',(-61.377194044862,-13.1978367193488,
40.0389814735788));
#191602=CARTESIAN_POINT('Ctrl Pts',(-61.3744236152739,-13.1991508816435,
40.0367321210016));
#191603=CARTESIAN_POINT('Ctrl Pts',(-61.3651180354454,-13.2035650137312,
40.0291767837141));
#191604=CARTESIAN_POINT('Ctrl Pts',(-61.3556720404056,-13.2071113921936,
40.0213235332577));
#191605=CARTESIAN_POINT('Ctrl Pts',(-61.3461671566363,-13.2098890888172,
40.013264921586));
#191606=CARTESIAN_POINT('Ctrl Pts',(-61.3357201634464,-13.2129421064463,
40.0044075527534));
#191607=CARTESIAN_POINT('Ctrl Pts',(-61.3252014297037,-13.2150668515154,
39.9953016253721));
#191608=CARTESIAN_POINT('Ctrl Pts',(-61.314690487281,-13.2163502251975,
39.986035342236));
#191609=CARTESIAN_POINT('Ctrl Pts',(-61.3033697519337,-13.2177324736414,
39.9760551582696));
#191610=CARTESIAN_POINT('Ctrl Pts',(-61.2920568939714,-13.2181390006409,
39.9658879738157));
#191611=CARTESIAN_POINT('Ctrl Pts',(-61.2808338148855,-13.2176240288385,
39.9556174643255));
#191612=CARTESIAN_POINT('Ctrl Pts',(-61.2697622852605,-13.2171160108941,
39.9454856413905));
#191613=CARTESIAN_POINT('Ctrl Pts',(-61.2587767401951,-13.2157108393288,
39.9352519465114));
#191614=CARTESIAN_POINT('Ctrl Pts',(-61.2479592423879,-13.213411509189,
39.92499));
#191615=CARTESIAN_POINT('Ctrl Pts',(-57.8829458346106,-12.4981558292584,
39.92499));
#191616=CARTESIAN_POINT('Ctrl Pts',(-57.8725934298278,-12.4959553576927,
39.9348107241713));
#191617=CARTESIAN_POINT('Ctrl Pts',(-57.8624518082055,-12.4929462656006,
39.9446038383151));
#191618=CARTESIAN_POINT('Ctrl Pts',(-57.8525735736593,-12.4891531124831,
39.9543158069358));
#191619=CARTESIAN_POINT('Ctrl Pts',(-57.8430352690791,-12.4854904894117,
39.963693567136));
#191620=CARTESIAN_POINT('Ctrl Pts',(-57.8337413853147,-12.48109631309,39.9729968320952));
#191621=CARTESIAN_POINT('Ctrl Pts',(-57.824753618525,-12.4759491415411,
39.9821731151294));
#191622=CARTESIAN_POINT('Ctrl Pts',(-57.8162573641141,-12.471083452433,
39.990847576431));
#191623=CARTESIAN_POINT('Ctrl Pts',(-57.8080338771707,-12.4655444244754,
39.9994093733803));
#191624=CARTESIAN_POINT('Ctrl Pts',(-57.8001616710214,-12.4592813303365,
40.0077966115798));
#191625=CARTESIAN_POINT('Ctrl Pts',(-57.7929115012238,-12.4535131257056,
40.0155211172553));
#191626=CARTESIAN_POINT('Ctrl Pts',(-57.7859589019118,-12.4471303774544,
40.0230979940982));
#191627=CARTESIAN_POINT('Ctrl Pts',(-57.7793958734452,-12.4400707995028,
40.030455410471));
#191628=CARTESIAN_POINT('Ctrl Pts',(-57.7774389108387,-12.4379657758633,
40.0326492435156));
#191629=CARTESIAN_POINT('Ctrl Pts',(-57.7755168276805,-12.4358004306465,
40.0348233715048));
#191630=CARTESIAN_POINT('Ctrl Pts',(-57.7736327324861,-12.4335727482758,
40.0369753512356));
#191631=CARTESIAN_POINT('Ctrl Pts',(-57.7717678881028,-12.4313678273307,
40.0391053430352));
#191632=CARTESIAN_POINT('Ctrl Pts',(-57.7699419852106,-12.4291043014745,
40.041211089324));
#191633=CARTESIAN_POINT('Ctrl Pts',(-57.7681599326868,-12.4267829461795,
40.0432881154904));
#191634=CARTESIAN_POINT('Ctrl Pts',(-57.7680360122395,-12.4266215236722,
40.043432547828));
#191635=CARTESIAN_POINT('Ctrl Pts',(-57.7679122920635,-12.4264598236893,
40.0435768364421));
#191636=CARTESIAN_POINT('Ctrl Pts',(-57.767788773317,-12.4262978456305,
40.0437209807855));
#191637=CARTESIAN_POINT('Ctrl Pts',(-57.7623732589829,-12.4191961341595,
40.0500407968421));
#191638=CARTESIAN_POINT('Ctrl Pts',(-57.7573864007556,-12.4115418213382,
40.0560490279347));
#191639=CARTESIAN_POINT('Ctrl Pts',(-57.7529408672212,-12.4033632485679,
40.0616647108618));
#191640=CARTESIAN_POINT('Ctrl Pts',(-57.7487968573385,-12.3957393973195,
40.066899503349));
#191641=CARTESIAN_POINT('Ctrl Pts',(-57.7451230952905,-12.3876591848382,
40.0717933267488));
#191642=CARTESIAN_POINT('Ctrl Pts',(-57.7420400166289,-12.379148818447,
40.0762460303079));
#191643=CARTESIAN_POINT('Ctrl Pts',(-57.7409121865682,-12.3760356163211,
40.0778748868753));
#191644=CARTESIAN_POINT('Ctrl Pts',(-57.7398637084257,-12.3728649408019,
40.079444352225));
#191645=CARTESIAN_POINT('Ctrl Pts',(-57.7389016204182,-12.3696384996594,
40.0809482021492));
#191646=CARTESIAN_POINT('Ctrl Pts',(-57.7386702703929,-12.3688626483504,
40.0813098278168));
#191647=CARTESIAN_POINT('Ctrl Pts',(-57.7384441015868,-12.3680830188493,
40.0816679525672));
#191648=CARTESIAN_POINT('Ctrl Pts',(-57.7382232068821,-12.3672997100618,
40.0820224192581));
#191649=CARTESIAN_POINT('Ctrl Pts',(-57.738009215137,-12.3665408796739,
40.0823658088648));
#191650=CARTESIAN_POINT('Ctrl Pts',(-57.7378001730066,-12.3657785963864,
40.0827057654616));
#191651=CARTESIAN_POINT('Ctrl Pts',(-57.737596164125,-12.3650129538222,
40.0830421470151));
#191652=CARTESIAN_POINT('Ctrl Pts',(-57.7353610110592,-12.3566244546993,
40.0867275956805));
#191653=CARTESIAN_POINT('Ctrl Pts',(-57.7337289586986,-12.3478270988457,
40.0899823432029));
#191654=CARTESIAN_POINT('Ctrl Pts',(-57.7328090548569,-12.3387746477743,
40.0926299529353));
#191655=CARTESIAN_POINT('Ctrl Pts',(-57.7324275433143,-12.3350203264899,
40.0937279956083));
#191656=CARTESIAN_POINT('Ctrl Pts',(-57.7321681942503,-12.3312224025081,
40.0947220371802));
#191657=CARTESIAN_POINT('Ctrl Pts',(-57.732037135777,-12.3273926324685,
40.0956014538692));
#191658=CARTESIAN_POINT('Ctrl Pts',(-57.7318136018936,-12.3208605605763,
40.097101390674));
#191659=CARTESIAN_POINT('Ctrl Pts',(-57.7319651225403,-12.3142375182611,
40.0982667904316));
#191660=CARTESIAN_POINT('Ctrl Pts',(-57.7325238621659,-12.3075887924651,
40.0990539325582));
#191661=CARTESIAN_POINT('Ctrl Pts',(-57.7328032319787,-12.3042644295671,
40.0994475036216));
#191662=CARTESIAN_POINT('Ctrl Pts',(-57.7331858342648,-12.3009338801483,
40.0997467259952));
#191663=CARTESIAN_POINT('Ctrl Pts',(-57.7336757296049,-12.2976053572251,
40.0999473488896));
#191664=CARTESIAN_POINT('Ctrl Pts',(-57.734165624945,-12.2942768343019,
40.100147971784));
#191665=CARTESIAN_POINT('Ctrl Pts',(-57.7347627876418,-12.2909503756175,
40.10025));
#191666=CARTESIAN_POINT('Ctrl Pts',(-57.7354693911205,-12.2876333308468,
40.10025));
#191667=CARTESIAN_POINT('Origin',(-57.9461901084062,-6.07506605172262,39.92499));
#191668=CARTESIAN_POINT('Ctrl Pts',(-62.3334394572619,-6.35995915837761,
39.92499));
#191669=CARTESIAN_POINT('Ctrl Pts',(-62.3439916622905,-6.3610682398175,
39.9348354642018));
#191670=CARTESIAN_POINT('Ctrl Pts',(-62.3544250468351,-6.36300663452657,
39.9446440828458));
#191671=CARTESIAN_POINT('Ctrl Pts',(-62.364684402406,-6.36575328117415,
39.9543641760332));
#191672=CARTESIAN_POINT('Ctrl Pts',(-62.3746103900114,-6.36841067816089,
39.9637684240713));
#191673=CARTESIAN_POINT('Ctrl Pts',(-62.3843747009658,-6.37182505343141,
39.9730909636396));
#191674=CARTESIAN_POINT('Ctrl Pts',(-62.3939185239085,-6.37602267870842,
39.982280897714));
#191675=CARTESIAN_POINT('Ctrl Pts',(-62.4029463927377,-6.37999337374561,
39.9909740094649));
#191676=CARTESIAN_POINT('Ctrl Pts',(-62.4117778192053,-6.38466529101478,
39.9995492765));
#191677=CARTESIAN_POINT('Ctrl Pts',(-62.4203406170101,-6.39009631815015,
40.0079462328694));
#191678=CARTESIAN_POINT('Ctrl Pts',(-62.4282275730657,-6.39509868692369,
40.0156804369688));
#191679=CARTESIAN_POINT('Ctrl Pts',(-62.4358870734649,-6.40074541103591,
40.023263801742));
#191680=CARTESIAN_POINT('Ctrl Pts',(-62.4432347045254,-6.40710777594541,
40.0306257269964));
#191681=CARTESIAN_POINT('Ctrl Pts',(-62.4453659729917,-6.40895325615409,
40.032761141665));
#191682=CARTESIAN_POINT('Ctrl Pts',(-62.4474707870407,-6.41085910953121,
40.034877742727));
#191683=CARTESIAN_POINT('Ctrl Pts',(-62.4495465125725,-6.41282747576041,
40.0369733168701));
#191684=CARTESIAN_POINT('Ctrl Pts',(-62.4517967325056,-6.41496131130705,
40.039245053974));
#191685=CARTESIAN_POINT('Ctrl Pts',(-62.4540103788122,-6.41716486079161,
40.041487875195));
#191686=CARTESIAN_POINT('Ctrl Pts',(-62.4561838467663,-6.41943986047071,
40.0436985701601));
#191687=CARTESIAN_POINT('Ctrl Pts',(-62.4621489466211,-6.42568361494159,
40.0497658398386));
#191688=CARTESIAN_POINT('Ctrl Pts',(-62.467772647785,-6.43248733059594,
40.0555581699984));
#191689=CARTESIAN_POINT('Ctrl Pts',(-62.4729574661286,-6.43981562609152,
40.0609828468886));
#191690=CARTESIAN_POINT('Ctrl Pts',(-62.477701293423,-6.44652061860789,
40.0659461317307));
#191691=CARTESIAN_POINT('Ctrl Pts',(-62.4820661824989,-6.45366385825802,
40.0706039980711));
#191692=CARTESIAN_POINT('Ctrl Pts',(-62.4859635700132,-6.46124910257504,
40.074884318061));
#191693=CARTESIAN_POINT('Ctrl Pts',(-62.4878779540285,-6.4649749498047,
40.0769867972574));
#191694=CARTESIAN_POINT('Ctrl Pts',(-62.4896790353532,-6.46880749650946,
40.0789976708177));
#191695=CARTESIAN_POINT('Ctrl Pts',(-62.4913529701965,-6.47274712615531,
40.08090504915));
#191696=CARTESIAN_POINT('Ctrl Pts',(-62.4916705830287,-6.47349463250819,
40.0812669556105));
#191697=CARTESIAN_POINT('Ctrl Pts',(-62.4919834280839,-6.47424649074148,
40.0816253922033));
#191698=CARTESIAN_POINT('Ctrl Pts',(-62.4922913974558,-6.4750026116312,
40.0819801989139));
#191699=CARTESIAN_POINT('Ctrl Pts',(-62.4925897427848,-6.47573510374311,
40.0823239179149));
#191700=CARTESIAN_POINT('Ctrl Pts',(-62.4928835124027,-6.47647159623306,
40.0826642303498));
#191701=CARTESIAN_POINT('Ctrl Pts',(-62.4931726086301,-6.47721200416365,
40.0830009916099));
#191702=CARTESIAN_POINT('Ctrl Pts',(-62.4963231197466,-6.48528081722612,
40.086670946431));
#191703=CARTESIAN_POINT('Ctrl Pts',(-62.4989203081701,-6.4938200899487,
40.0899175831875));
#191704=CARTESIAN_POINT('Ctrl Pts',(-62.5008353965401,-6.50268949817225,
40.0925642067058));
#191705=CARTESIAN_POINT('Ctrl Pts',(-62.5016441502511,-6.50643510434198,
40.0936818922525));
#191706=CARTESIAN_POINT('Ctrl Pts',(-62.502331556834,-6.51023927047592,
40.094693009479));
#191707=CARTESIAN_POINT('Ctrl Pts',(-62.502889568803,-6.51409041329249,
40.0955863397546));
#191708=CARTESIAN_POINT('Ctrl Pts',(-62.5038292470155,-6.52057564156532,
40.0970906856166));
#191709=CARTESIAN_POINT('Ctrl Pts',(-62.5043999463277,-6.52719259313743,
40.0982599215483));
#191710=CARTESIAN_POINT('Ctrl Pts',(-62.5045608969645,-6.53387925273567,
40.0990497370454));
#191711=CARTESIAN_POINT('Ctrl Pts',(-62.5046011346237,-6.53555091763522,
40.0992471909196));
#191712=CARTESIAN_POINT('Ctrl Pts',(-62.5046155292218,-6.53722692958775,
40.0994209989363));
#191713=CARTESIAN_POINT('Ctrl Pts',(-62.5046031362659,-6.53890629461041,
40.0995705982975));
#191714=CARTESIAN_POINT('Ctrl Pts',(-62.504584546832,-6.54142534214441,
40.0997949973393));
#191715=CARTESIAN_POINT('Ctrl Pts',(-62.5045056736598,-6.54395191714475,
40.0999649129781));
#191716=CARTESIAN_POINT('Ctrl Pts',(-62.5043649998326,-6.54648282201833,
40.1000786629733));
#191717=CARTESIAN_POINT('Ctrl Pts',(-62.5042243260054,-6.54901372689191,
40.1001924129685));
#191718=CARTESIAN_POINT('Ctrl Pts',(-62.5040218613861,-6.55154895552219,
40.10025));
#191719=CARTESIAN_POINT('Ctrl Pts',(-62.5037563256535,-6.55408556365905,
40.10025));
#191720=CARTESIAN_POINT('Ctrl Pts',(-58.7067819056643,-6.15500747092277,
40.10025));
#191721=CARTESIAN_POINT('Ctrl Pts',(-58.7076801645418,-6.1464243467814,
40.10025));
#191722=CARTESIAN_POINT('Ctrl Pts',(-58.7092791387968,-6.13798976646334,
40.0995786334241));
#191723=CARTESIAN_POINT('Ctrl Pts',(-58.711482446254,-6.12982011300221,
40.0983063763366));
#191724=CARTESIAN_POINT('Ctrl Pts',(-58.712905556799,-6.12454335512122,
40.0974846287992));
#191725=CARTESIAN_POINT('Ctrl Pts',(-58.714579884807,-6.11937686668002,
40.0964130309338));
#191726=CARTESIAN_POINT('Ctrl Pts',(-58.7164715618025,-6.11434800669293,
40.0951176960924));
#191727=CARTESIAN_POINT('Ctrl Pts',(-58.7189788712981,-6.10768254085093,
40.0934008039614));
#191728=CARTESIAN_POINT('Ctrl Pts',(-58.7218729180381,-6.101261959832,40.0912909372156));
#191729=CARTESIAN_POINT('Ctrl Pts',(-58.7250866612026,-6.09514640967233,
40.0888630467851));
#191730=CARTESIAN_POINT('Ctrl Pts',(-58.7266935327848,-6.0920886345925,
40.0876491015699));
#191731=CARTESIAN_POINT('Ctrl Pts',(-58.7283803475666,-6.08910691884932,
40.0863558569271));
#191732=CARTESIAN_POINT('Ctrl Pts',(-58.7301388657774,-6.08620737357425,
40.0849936342771));
#191733=CARTESIAN_POINT('Ctrl Pts',(-58.7310181248827,-6.08475760093672,
40.0843125229521));
#191734=CARTESIAN_POINT('Ctrl Pts',(-58.7319153115143,-6.08332835457004,
40.0836141747074));
#191735=CARTESIAN_POINT('Ctrl Pts',(-58.7328294060527,-6.08192029572531,
40.0828999161609));
#191736=CARTESIAN_POINT('Ctrl Pts',(-58.7330579296874,-6.08156828101413,
40.0827213515243));
#191737=CARTESIAN_POINT('Ctrl Pts',(-58.7332875101006,-6.08121759017528,
40.0825417925842));
#191738=CARTESIAN_POINT('Ctrl Pts',(-58.7335181314301,-6.08086823283941,
40.0823612602361));
#191739=CARTESIAN_POINT('Ctrl Pts',(-58.7342099954187,-6.0798201608318,
40.0818196631917));
#191740=CARTESIAN_POINT('Ctrl Pts',(-58.7349112274885,-6.07878409208739,
40.0812693052022));
#191741=CARTESIAN_POINT('Ctrl Pts',(-58.7356214008386,-6.0777602711168,
40.0807107531875));
#191742=CARTESIAN_POINT('Ctrl Pts',(-58.7406237702161,-6.07054860839944,
40.0767763849182));
#191743=CARTESIAN_POINT('Ctrl Pts',(-58.7460508958009,-6.06389424687505,
40.0724140586139));
#191744=CARTESIAN_POINT('Ctrl Pts',(-58.7517849266676,-6.05777649745821,
40.0677221223771));
#191745=CARTESIAN_POINT('Ctrl Pts',(-58.7545659254418,-6.05480939560177,
40.0654465383722));
#191746=CARTESIAN_POINT('Ctrl Pts',(-58.7574196937447,-6.05196853530565,
40.063092800068));
#191747=CARTESIAN_POINT('Ctrl Pts',(-58.7603356163931,-6.04925198282193,
40.0606689262479));
#191748=CARTESIAN_POINT('Ctrl Pts',(-58.764799690238,-6.04509313076954,
40.0569581447806));
#191749=CARTESIAN_POINT('Ctrl Pts',(-58.7694062431511,-6.04122712577039,
40.0530843804606));
#191750=CARTESIAN_POINT('Ctrl Pts',(-58.7741092696793,-6.03765709635796,
40.0490800251458));
#191751=CARTESIAN_POINT('Ctrl Pts',(-58.7762933795292,-6.03599915622994,
40.0472203818218));
#191752=CARTESIAN_POINT('Ctrl Pts',(-58.7784980841112,-6.03440490786083,
40.0453323608819));
#191753=CARTESIAN_POINT('Ctrl Pts',(-58.7807192900657,-6.03287578462717,
40.0434201572162));
#191754=CARTESIAN_POINT('Ctrl Pts',(-58.7808895367502,-6.03275858335636,
40.0432735943397));
#191755=CARTESIAN_POINT('Ctrl Pts',(-58.7810598733265,-6.0326417314874,
40.0431268995707));
#191756=CARTESIAN_POINT('Ctrl Pts',(-58.7812302983888,-6.03252522862511,
40.0429800745037));
#191757=CARTESIAN_POINT('Ctrl Pts',(-58.7836242566993,-6.03088871465466,
40.0409176249753));
#191758=CARTESIAN_POINT('Ctrl Pts',(-58.7860369637877,-6.02932271154724,
40.0388310783332));
#191759=CARTESIAN_POINT('Ctrl Pts',(-58.7884628208563,-6.02782611907218,
40.036725739981));
#191760=CARTESIAN_POINT('Ctrl Pts',(-58.7971615128803,-6.02245960461667,
40.0291763710718));
#191761=CARTESIAN_POINT('Ctrl Pts',(-58.8060955050476,-6.01794242202301,
40.0213310894595));
#191762=CARTESIAN_POINT('Ctrl Pts',(-58.8151732302896,-6.01418353044932,
40.0132837551321));
#191763=CARTESIAN_POINT('Ctrl Pts',(-58.825148738392,-6.01005288622405,
40.0044405431328));
#191764=CARTESIAN_POINT('Ctrl Pts',(-58.8352983536247,-6.00683754300209,
39.9953528710605));
#191765=CARTESIAN_POINT('Ctrl Pts',(-58.8455340166136,-6.0044577527299,
39.9861103629562));
#191766=CARTESIAN_POINT('Ctrl Pts',(-58.8565859638406,-6.00188817648184,
39.9761307737567));
#191767=CARTESIAN_POINT('Ctrl Pts',(-58.8677393147013,-6.00029231631163,
39.9659696936026));
#191768=CARTESIAN_POINT('Ctrl Pts',(-58.8789072188648,-5.99962196122124,
39.9557128217525));
#191769=CARTESIAN_POINT('Ctrl Pts',(-58.8899814357884,-5.99895722972121,
39.9455419945173));
#191770=CARTESIAN_POINT('Ctrl Pts',(-58.9010713848505,-5.9992027369765,
39.9352756289347));
#191771=CARTESIAN_POINT('Ctrl Pts',(-58.912095367953,-6.00036140429007,
39.92499));
#191772=CARTESIAN_POINT('Origin',(0.00159301378021015,-0.0151565136854118,
39.92499));
#191773=CARTESIAN_POINT('Ctrl Pts',(-62.5005702980931,-6.58439859102987,
40.10025));
#191774=CARTESIAN_POINT('Ctrl Pts',(-62.4996689377206,-6.59294009787395,
40.10025));
#191775=CARTESIAN_POINT('Ctrl Pts',(-62.4980620716938,-6.60133040498981,
40.0995859581842));
#191776=CARTESIAN_POINT('Ctrl Pts',(-62.4958483879906,-6.60945539386104,
40.0983275959622));
#191777=CARTESIAN_POINT('Ctrl Pts',(-62.4944339494873,-6.6146468749577,
40.0975235624069));
#191778=CARTESIAN_POINT('Ctrl Pts',(-62.4927726671883,-6.61973030386296,
40.0964777059491));
#191779=CARTESIAN_POINT('Ctrl Pts',(-62.4908979342376,-6.62467983150725,
40.0952149915962));
#191780=CARTESIAN_POINT('Ctrl Pts',(-62.4883392999283,-6.63143494361054,
40.0934916398702));
#191781=CARTESIAN_POINT('Ctrl Pts',(-62.4853780106448,-6.63793726713725,
40.0913643921631));
#191782=CARTESIAN_POINT('Ctrl Pts',(-62.4820864562849,-6.64412426454855,
40.0889118607714));
#191783=CARTESIAN_POINT('Ctrl Pts',(-62.480440679105,-6.6472177632542,40.0876855950755));
#191784=CARTESIAN_POINT('Ctrl Pts',(-62.4787123157334,-6.65023263831835,
40.0863782327527));
#191785=CARTESIAN_POINT('Ctrl Pts',(-62.4769102669531,-6.65316255786702,
40.0850006373335));
#191786=CARTESIAN_POINT('Ctrl Pts',(-62.4760092425629,-6.65462751764136,
40.0843118396238));
#191787=CARTESIAN_POINT('Ctrl Pts',(-62.4750897950507,-6.65607125586043,
40.0836054919165));
#191788=CARTESIAN_POINT('Ctrl Pts',(-62.474153026021,-6.65749308991723,
40.0828829920418));
#191789=CARTESIAN_POINT('Ctrl Pts',(-62.4739188337636,-6.65784854843143,
40.0827023670732));
#191790=CARTESIAN_POINT('Ctrl Pts',(-62.4736835588747,-6.65820263830465,
40.0825207326933));
#191791=CARTESIAN_POINT('Ctrl Pts',(-62.4734472184934,-6.65855534961576,
40.0823381109276));
#191792=CARTESIAN_POINT('Ctrl Pts',(-62.4727381973496,-6.6596134835491,
40.0817902456304));
#191793=CARTESIAN_POINT('Ctrl Pts',(-62.4720195869492,-6.66065920857969,
40.0812334935554));
#191794=CARTESIAN_POINT('Ctrl Pts',(-62.471291848471,-6.66169227331179,
40.0806684524228));
#191795=CARTESIAN_POINT('Ctrl Pts',(-62.4662627240578,-6.66883139158093,
40.0767636676137));
#191796=CARTESIAN_POINT('Ctrl Pts',(-62.4608161451509,-6.67541846632637,
40.0724404510889));
#191797=CARTESIAN_POINT('Ctrl Pts',(-62.4550686189989,-6.68147667711105,
40.0677949937409));
#191798=CARTESIAN_POINT('Ctrl Pts',(-62.4522121142781,-6.68448759124153,
40.0654862141906));
#191799=CARTESIAN_POINT('Ctrl Pts',(-62.4492806638354,-6.68736784133579,
40.0630972003216));
#191800=CARTESIAN_POINT('Ctrl Pts',(-62.4462854590369,-6.69011973548569,
40.0606363359906));
#191801=CARTESIAN_POINT('Ctrl Pts',(-62.4396775898761,-6.69619082501382,
40.0552073017124));
#191802=CARTESIAN_POINT('Ctrl Pts',(-62.4327685320937,-6.70164568781174,
40.0494204304519));
#191803=CARTESIAN_POINT('Ctrl Pts',(-62.4256985108779,-6.70644606039053,
40.0434049749851));
#191804=CARTESIAN_POINT('Ctrl Pts',(-62.4231157429701,-6.70819969702944,
40.0412074532442));
#191805=CARTESIAN_POINT('Ctrl Pts',(-62.4205129446133,-6.70987381569775,
40.0389814735788));
#191806=CARTESIAN_POINT('Ctrl Pts',(-62.4178950590936,-6.71147036762136,
40.0367321210017));
#191807=CARTESIAN_POINT('Ctrl Pts',(-62.4091018586482,-6.71683301659123,
40.0291767837137));
#191808=CARTESIAN_POINT('Ctrl Pts',(-62.4000783072478,-6.72134734296709,
40.0213235332568));
#191809=CARTESIAN_POINT('Ctrl Pts',(-62.3909158405852,-6.725103353972,40.0132649215846));
#191810=CARTESIAN_POINT('Ctrl Pts',(-62.3808452043575,-6.72923165499515,
40.0044075527515));
#191811=CARTESIAN_POINT('Ctrl Pts',(-62.3706061896751,-6.73244426756212,
39.9953016253697));
#191812=CARTESIAN_POINT('Ctrl Pts',(-62.360286976373,-6.73481930344785,
39.986035342233));
#191813=CARTESIAN_POINT('Ctrl Pts',(-62.3491727415035,-6.73737731885899,
39.9760551582661));
#191814=CARTESIAN_POINT('Ctrl Pts',(-62.3379643502027,-6.73896413451883,
39.9658879738115));
#191815=CARTESIAN_POINT('Ctrl Pts',(-62.3267489231065,-6.73962511499552,
39.9556174643206));
#191816=CARTESIAN_POINT('Ctrl Pts',(-62.3156849421461,-6.74027717000391,
39.9454856413873));
#191817=CARTESIAN_POINT('Ctrl Pts',(-62.3046126966235,-6.74002799825921,
39.9352519465098));
#191818=CARTESIAN_POINT('Ctrl Pts',(-62.293614112757,-6.73887200051292,
39.92499));
#191819=CARTESIAN_POINT('Ctrl Pts',(-58.8722700234481,-6.37927424642539,
39.92499));
#191820=CARTESIAN_POINT('Ctrl Pts',(-58.8617443183087,-6.37816795023608,
39.9348107241732));
#191821=CARTESIAN_POINT('Ctrl Pts',(-58.8513437177767,-6.376235430388,39.9446038383188));
#191822=CARTESIAN_POINT('Ctrl Pts',(-58.8411231047647,-6.37349561323631,
39.9543158069412));
#191823=CARTESIAN_POINT('Ctrl Pts',(-58.8312542036529,-6.37085007871673,
39.9636935671424));
#191824=CARTESIAN_POINT('Ctrl Pts',(-58.821551916257,-6.36745144953966,
39.9729968321027));
#191825=CARTESIAN_POINT('Ctrl Pts',(-58.8120753594611,-6.36327195218493,
39.9821731151378));
#191826=CARTESIAN_POINT('Ctrl Pts',(-58.8031170454153,-6.35932101824728,
39.9908475764397));
#191827=CARTESIAN_POINT('Ctrl Pts',(-58.7943596215132,-6.35467192211664,
39.9994093733894));
#191828=CARTESIAN_POINT('Ctrl Pts',(-58.785875868527,-6.34926600747317,
40.0077966115891));
#191829=CARTESIAN_POINT('Ctrl Pts',(-58.7780624743525,-6.34428725077761,
40.0155211172645));
#191830=CARTESIAN_POINT('Ctrl Pts',(-58.770480783241,-6.33866621241035,
40.0230979941072));
#191831=CARTESIAN_POINT('Ctrl Pts',(-58.7632157808967,-6.33233133084482,
40.0304554104799));
#191832=CARTESIAN_POINT('Ctrl Pts',(-58.7610495038528,-6.33044239704131,
40.0326492435214));
#191833=CARTESIAN_POINT('Ctrl Pts',(-58.7589116098623,-6.32848982621358,
40.0348233715077));
#191834=CARTESIAN_POINT('Ctrl Pts',(-58.7568049797265,-6.32647128889798,
40.0369753512356));
#191835=CARTESIAN_POINT('Ctrl Pts',(-58.7547198741578,-6.32447337605812,
40.0391053430352));
#191836=CARTESIAN_POINT('Ctrl Pts',(-58.7526673708734,-6.32241310885685,
40.041211089324));
#191837=CARTESIAN_POINT('Ctrl Pts',(-58.7506524329181,-6.32029074540079,
40.0432881154904));
#191838=CARTESIAN_POINT('Ctrl Pts',(-58.7505123180733,-6.32014316039674,
40.043432547828));
#191839=CARTESIAN_POINT('Ctrl Pts',(-58.7503723733987,-6.31999527850315,
40.0435768364421));
#191840=CARTESIAN_POINT('Ctrl Pts',(-58.7502325999832,-6.31984709900185,
40.0437209807855));
#191841=CARTESIAN_POINT('Ctrl Pts',(-58.7441044214167,-6.31335036684059,
40.0500407968421));
#191842=CARTESIAN_POINT('Ctrl Pts',(-58.738344788164,-6.30625925377284,
40.0560490279347));
#191843=CARTESIAN_POINT('Ctrl Pts',(-58.7330687140839,-6.29859016886869,
40.0616647108618));
#191844=CARTESIAN_POINT('Ctrl Pts',(-58.7281504960658,-6.2914412488599,
40.066899503349));
#191845=CARTESIAN_POINT('Ctrl Pts',(-58.7236522470771,-6.28378931332922,
40.0717933267488));
#191846=CARTESIAN_POINT('Ctrl Pts',(-58.7196964823223,-6.27564783709016,
40.076246030308));
#191847=CARTESIAN_POINT('Ctrl Pts',(-58.7182494123986,-6.27266957975434,
40.0778748868753));
#191848=CARTESIAN_POINT('Ctrl Pts',(-58.7168752520896,-6.26962586933641,
40.079444352225));
#191849=CARTESIAN_POINT('Ctrl Pts',(-58.7155811795664,-6.26651766855713,
40.0809482021492));
#191850=CARTESIAN_POINT('Ctrl Pts',(-58.7152699983557,-6.26577025010539,
40.0813098278169));
#191851=CARTESIAN_POINT('Ctrl Pts',(-58.7149635750523,-6.26501853257399,
40.0816679525672));
#191852=CARTESIAN_POINT('Ctrl Pts',(-58.7146620123681,-6.26426260461801,
40.082022419258));
#191853=CARTESIAN_POINT('Ctrl Pts',(-58.7143698735178,-6.26353029941065,
40.0823658088648));
#191854=CARTESIAN_POINT('Ctrl Pts',(-58.7140822962414,-6.26279404284336,
40.0827057654617));
#191855=CARTESIAN_POINT('Ctrl Pts',(-58.7137993735012,-6.2620539192842,
40.0830421470151));
#191856=CARTESIAN_POINT('Ctrl Pts',(-58.7106996279153,-6.25394501035234,
40.0867275956805));
#191857=CARTESIAN_POINT('Ctrl Pts',(-58.7081569420201,-6.24536644325977,
40.0899823432029));
#191858=CARTESIAN_POINT('Ctrl Pts',(-58.7062958387086,-6.23645973859744,
40.0926299529353));
#191859=CARTESIAN_POINT('Ctrl Pts',(-58.7055239836917,-6.23276586269315,
40.0937279956083));
#191860=CARTESIAN_POINT('Ctrl Pts',(-58.7048690642116,-6.22901585349541,
40.0947220371802));
#191861=CARTESIAN_POINT('Ctrl Pts',(-58.7043384037134,-6.2252207626776,
40.0956014538692));
#191862=CARTESIAN_POINT('Ctrl Pts',(-58.7034333069351,-6.21874783981196,
40.097101390674));
#191863=CARTESIAN_POINT('Ctrl Pts',(-58.7028917011005,-6.21214524099522,
40.0982667904316));
#191864=CARTESIAN_POINT('Ctrl Pts',(-58.7027523988021,-6.20547453342035,
40.0990539325583));
#191865=CARTESIAN_POINT('Ctrl Pts',(-58.7026827476529,-6.20213917963292,
40.0994475036216));
#191866=CARTESIAN_POINT('Ctrl Pts',(-58.7027151167909,-6.19878688248331,
40.0997467259952));
#191867=CARTESIAN_POINT('Ctrl Pts',(-58.7028544030469,-6.19542538554988,
40.0999473488896));
#191868=CARTESIAN_POINT('Ctrl Pts',(-58.7029936893029,-6.19206388861645,
40.100147971784));
#191869=CARTESIAN_POINT('Ctrl Pts',(-58.7032398710655,-6.18869323212177,
40.10025));
#191870=CARTESIAN_POINT('Ctrl Pts',(-58.7035958781039,-6.1853204982936,
40.10025));
#191871=CARTESIAN_POINT('Origin',(-58.2637721346185,0.01524,39.92499));
#191872=CARTESIAN_POINT('Ctrl Pts',(-62.6567671111299,0.1905,39.92499));
#191873=CARTESIAN_POINT('Ctrl Pts',(-62.6673774406538,0.1905,39.9348354642018));
#191874=CARTESIAN_POINT('Ctrl Pts',(-62.6779562874464,0.189662809673088,
39.9446440828458));
#191875=CARTESIAN_POINT('Ctrl Pts',(-62.6884465439472,0.188003604115171,
39.9543641760331));
#191876=CARTESIAN_POINT('Ctrl Pts',(-62.6985959295772,0.186398312857959,
39.9637684240713));
#191877=CARTESIAN_POINT('Ctrl Pts',(-62.7086636500146,0.184023290311342,
39.9730909636396));
#191878=CARTESIAN_POINT('Ctrl Pts',(-62.7185939622163,0.180846261210701,
39.9822808977141));
#191879=CARTESIAN_POINT('Ctrl Pts',(-62.7279874260857,0.177840987311675,
39.990974009465));
#191880=CARTESIAN_POINT('Ctrl Pts',(-62.7372588214078,0.17411779873125,
39.9995492765001));
#191881=CARTESIAN_POINT('Ctrl Pts',(-62.7463424082307,0.169611579426592,
40.0079462328694));
#191882=CARTESIAN_POINT('Ctrl Pts',(-62.7547090486364,0.165461025548926,
40.0156804369689));
#191883=CARTESIAN_POINT('Ctrl Pts',(-62.762916832885,0.160645870588327,
40.0232638017421));
#191884=CARTESIAN_POINT('Ctrl Pts',(-62.7708892610805,0.155086395962896,
40.0306257269966));
#191885=CARTESIAN_POINT('Ctrl Pts',(-62.7732017594453,0.153473803705521,
40.0327611416651));
#191886=CARTESIAN_POINT('Ctrl Pts',(-62.7754942590274,0.151798403770651,
40.0348777427271));
#191887=CARTESIAN_POINT('Ctrl Pts',(-62.7777643638145,0.150057792857645,
40.0369733168701));
#191888=CARTESIAN_POINT('Ctrl Pts',(-62.780225303358,0.148170858717027,
40.039245053974));
#191889=CARTESIAN_POINT('Ctrl Pts',(-62.7826571567198,0.146210769553757,
40.041487875195));
#191890=CARTESIAN_POINT('Ctrl Pts',(-62.7850565204094,0.144175421826141,
40.0436985701601));
#191891=CARTESIAN_POINT('Ctrl Pts',(-62.791641592883,0.138589394016616,
40.0497658398386));
#191892=CARTESIAN_POINT('Ctrl Pts',(-62.7979456687653,0.132410786669038,
40.0555581699984));
#191893=CARTESIAN_POINT('Ctrl Pts',(-62.8038680995981,0.12566459743673,
40.0609828468886));
#191894=CARTESIAN_POINT('Ctrl Pts',(-62.8092868022738,0.119492200548389,
40.0659461317304));
#191895=CARTESIAN_POINT('Ctrl Pts',(-62.8143744518938,0.112844347460359,
40.0706039980705));
#191896=CARTESIAN_POINT('Ctrl Pts',(-62.8190433630432,0.105708043833492,
40.0748843180602));
#191897=CARTESIAN_POINT('Ctrl Pts',(-62.8213367169482,0.102202714803617,
40.0769867972569));
#191898=CARTESIAN_POINT('Ctrl Pts',(-62.8235285419787,0.0985794274533612,
40.0789976708174));
#191899=CARTESIAN_POINT('Ctrl Pts',(-62.8256051102647,0.0948363533472193,
40.08090504915));
#191900=CARTESIAN_POINT('Ctrl Pts',(-62.8259991188709,0.09412614149362,
40.0812669556104));
#191901=CARTESIAN_POINT('Ctrl Pts',(-62.8263888407139,0.093411103231266,
40.0816253922033));
#191902=CARTESIAN_POINT('Ctrl Pts',(-62.826774159152,0.09269131601607,40.0819801989139));
#191903=CARTESIAN_POINT('Ctrl Pts',(-62.8271474363889,0.0919940221513489,
40.0823239179149));
#191904=CARTESIAN_POINT('Ctrl Pts',(-62.8275165811343,0.0912922715310365,
40.0826642303498));
#191905=CARTESIAN_POINT('Ctrl Pts',(-62.8278814873655,0.0905861384169469,
40.0830009916099));
#191906=CARTESIAN_POINT('Ctrl Pts',(-62.8318581602824,0.0828908452418441,
40.0866709464312));
#191907=CARTESIAN_POINT('Ctrl Pts',(-62.8353337180912,0.0746698316630267,
40.0899175831877));
#191908=CARTESIAN_POINT('Ctrl Pts',(-62.8381654210186,0.0660491922296554,
40.0925642067062));
#191909=CARTESIAN_POINT('Ctrl Pts',(-62.8393612667489,0.0624086426653834,
40.0936818922528));
#191910=CARTESIAN_POINT('Ctrl Pts',(-62.8404425512865,0.0586971697057181,
40.0946930094791));
#191911=CARTESIAN_POINT('Ctrl Pts',(-62.8414000604479,0.0549254519864736,
40.0955863397546));
#191912=CARTESIAN_POINT('Ctrl Pts',(-62.8430124819501,0.048573973592213,
40.0970906856166));
#191913=CARTESIAN_POINT('Ctrl Pts',(-62.8442717146912,0.0420529246952702,
40.0982599215483));
#191914=CARTESIAN_POINT('Ctrl Pts',(-62.8451307298764,0.0354197192407063,
40.0990497370454));
#191915=CARTESIAN_POINT('Ctrl Pts',(-62.8453454836727,0.0337614178770653,
40.0992471909196));
#191916=CARTESIAN_POINT('Ctrl Pts',(-62.8455349903695,0.032096091938589,
40.0994209989363));
#191917=CARTESIAN_POINT('Ctrl Pts',(-62.8456982067485,0.0304246312365876,
40.0995705982975));
#191918=CARTESIAN_POINT('Ctrl Pts',(-62.845943031317,0.0279174401835856,
40.0997949973393));
#191919=CARTESIAN_POINT('Ctrl Pts',(-62.8461286892223,0.0253964615339666,
40.0999649129781));
#191920=CARTESIAN_POINT('Ctrl Pts',(-62.846253337618,0.0228647168031101,
40.1000786629733));
#191921=CARTESIAN_POINT('Ctrl Pts',(-62.8463779860137,0.0203329720722537,
40.1001924129685));
#191922=CARTESIAN_POINT('Ctrl Pts',(-62.8464416340693,0.017790468374154,
40.10025));
#191923=CARTESIAN_POINT('Ctrl Pts',(-62.8464427007196,0.01524,40.10025));
#191924=CARTESIAN_POINT('Ctrl Pts',(-59.0285534841296,0.0152400000000004,
40.10025));
#191925=CARTESIAN_POINT('Ctrl Pts',(-59.0285496414744,0.0238699985096171,
40.10025));
#191926=CARTESIAN_POINT('Ctrl Pts',(-59.0292582026622,0.032425511636119,
40.099578633424));
#191927=CARTESIAN_POINT('Ctrl Pts',(-59.0305954788491,0.0407807192236517,
40.0983063763365));
#191928=CARTESIAN_POINT('Ctrl Pts',(-59.0314592220533,0.0461773260308832,
40.0974846287991));
#191929=CARTESIAN_POINT('Ctrl Pts',(-59.0325843328199,0.0514905268412107,
40.0964130309337));
#191930=CARTESIAN_POINT('Ctrl Pts',(-59.0339399880044,0.0566895722961695,
40.0951176960924));
#191931=CARTESIAN_POINT('Ctrl Pts',(-59.0357368312948,0.0635806092273947,
40.0934008039614));
#191932=CARTESIAN_POINT('Ctrl Pts',(-59.0379438906768,0.0702685278900844,
40.0912909372157));
#191933=CARTESIAN_POINT('Ctrl Pts',(-59.0405007795597,0.0766865040604244,
40.0888630467851));
#191934=CARTESIAN_POINT('Ctrl Pts',(-59.0417792240012,0.0798954921455943,
40.0876491015699));
#191935=CARTESIAN_POINT('Ctrl Pts',(-59.0431451240705,0.0830371938949132,
40.0863558569271));
#191936=CARTESIAN_POINT('Ctrl Pts',(-59.0445909239228,0.0861046703637849,
40.0849936342771));
#191937=CARTESIAN_POINT('Ctrl Pts',(-59.0453138238489,0.0876384085982208,
40.0843125229521));
#191938=CARTESIAN_POINT('Ctrl Pts',(-59.0460566986719,0.0891536069436204,
40.0836141747074));
#191939=CARTESIAN_POINT('Ctrl Pts',(-59.0468186034775,0.0906495011920575,
40.0828999161609));
#191940=CARTESIAN_POINT('Ctrl Pts',(-59.047009079679,0.0910234747541668,
40.0827213515243));
#191941=CARTESIAN_POINT('Ctrl Pts',(-59.0472007452523,0.0913962421596926,
40.0825417925842));
#191942=CARTESIAN_POINT('Ctrl Pts',(-59.0473935854286,0.091767792172695,
40.0823612602361));
#191943=CARTESIAN_POINT('Ctrl Pts',(-59.0479721059574,0.0928824422117024,
40.0818196631917));
#191944=CARTESIAN_POINT('Ctrl Pts',(-59.0485611979309,0.0939861339737884,
40.0812693052021));
#191945=CARTESIAN_POINT('Ctrl Pts',(-59.0491604624443,0.0950785796749106,
40.0807107531875));
#191946=CARTESIAN_POINT('Ctrl Pts',(-59.0533816042976,0.102773626133156,
40.0767763849182));
#191947=CARTESIAN_POINT('Ctrl Pts',(-59.0580834293366,0.109958823466292,
40.0724140586138));
#191948=CARTESIAN_POINT('Ctrl Pts',(-59.063146569637,0.116642428646605,
40.0677221223769));
#191949=CARTESIAN_POINT('Ctrl Pts',(-59.0656021872115,0.119883969936752,
40.0654465383721));
#191950=CARTESIAN_POINT('Ctrl Pts',(-59.0681433715119,0.123007567718065,
40.063092800068));
#191951=CARTESIAN_POINT('Ctrl Pts',(-59.0707593633743,0.126014035556406,
40.0606689262479));
#191952=CARTESIAN_POINT('Ctrl Pts',(-59.0747642641417,0.130616727761033,
40.0569581447806));
#191953=CARTESIAN_POINT('Ctrl Pts',(-59.0789414743143,0.134943070277265,
40.0530843804606));
#191954=CARTESIAN_POINT('Ctrl Pts',(-59.0832455674828,0.138985142830727,
40.0490800251458));
#191955=CARTESIAN_POINT('Ctrl Pts',(-59.0852444106166,0.140862302235468,
40.0472203818218));
#191956=CARTESIAN_POINT('Ctrl Pts',(-59.0872703932641,0.142678271527114,
40.0453323608819));
#191957=CARTESIAN_POINT('Ctrl Pts',(-59.0893195943183,0.144431197308737,
40.0434201572162));
#191958=CARTESIAN_POINT('Ctrl Pts',(-59.0894766575049,0.144565552163021,
40.0432735943397));
#191959=CARTESIAN_POINT('Ctrl Pts',(-59.0896338466133,0.144699568925786,
40.0431268995707));
#191960=CARTESIAN_POINT('Ctrl Pts',(-59.0897911602042,0.144833247843074,
40.0429800745037));
#191961=CARTESIAN_POINT('Ctrl Pts',(-59.0920009418701,0.14671103360208,
40.0409176249753));
#191962=CARTESIAN_POINT('Ctrl Pts',(-59.0942367399983,0.148520654544882,
40.0388310783332));
#191963=CARTESIAN_POINT('Ctrl Pts',(-59.0964928714566,0.150262619641264,
40.036725739981));
#191964=CARTESIAN_POINT('Ctrl Pts',(-59.1045829576263,0.156508996678799,
40.0291763710718));
#191965=CARTESIAN_POINT('Ctrl Pts',(-59.112995834295,0.161935290145674,
40.0213310894595));
#191966=CARTESIAN_POINT('Ctrl Pts',(-59.1216309196485,0.166622470787548,
40.0132837551321));
#191967=CARTESIAN_POINT('Ctrl Pts',(-59.1311200109809,0.171773211443978,
40.0044405431325));
#191968=CARTESIAN_POINT('Ctrl Pts',(-59.1408779306738,0.176031864362474,
39.99535287106));
#191969=CARTESIAN_POINT('Ctrl Pts',(-59.1508087658101,0.179468536017358,
39.9861103629554));
#191970=CARTESIAN_POINT('Ctrl Pts',(-59.1615315754582,0.183179278917879,
39.9761307737551));
#191971=CARTESIAN_POINT('Ctrl Pts',(-59.1724570142857,0.185932239424941,
39.9659696936002));
#191972=CARTESIAN_POINT('Ctrl Pts',(-59.1834936683151,0.187766286100067,
39.9557128217492));
#191973=CARTESIAN_POINT('Ctrl Pts',(-59.1944377361563,0.189584947007898,
39.9455419945151));
#191974=CARTESIAN_POINT('Ctrl Pts',(-59.205492595812,0.1905,39.9352756289336));
#191975=CARTESIAN_POINT('Ctrl Pts',(-59.2165773020941,0.1905,39.92499));
#191976=CARTESIAN_POINT('Origin',(1.12442271988212E-14,-0.01524,39.92499));
#191977=CARTESIAN_POINT('Ctrl Pts',(-62.8464427007196,-0.01524,40.10025));
#191978=CARTESIAN_POINT('Ctrl Pts',(-62.8464391086779,-0.0238289333904583,
40.10025));
#191979=CARTESIAN_POINT('Ctrl Pts',(-62.8457180711405,-0.0323412407624883,
40.0995859581842));
#191980=CARTESIAN_POINT('Ctrl Pts',(-62.8443658068291,-0.0406531130501973,
40.0983275959621));
#191981=CARTESIAN_POINT('Ctrl Pts',(-62.843501774309,-0.0459640037533824,
40.0975235624069));
#191982=CARTESIAN_POINT('Ctrl Pts',(-62.8423809556999,-0.0511932363889938,
40.0964777059491));
#191983=CARTESIAN_POINT('Ctrl Pts',(-62.841033859251,-0.0563116129573706,
40.0952149915961));
#191984=CARTESIAN_POINT('Ctrl Pts',(-62.8391953428955,-0.0632971699621705,
40.0934916398701));
#191985=CARTESIAN_POINT('Ctrl Pts',(-62.8369299537504,-0.070073412098335,
40.0913643921631));
#191986=CARTESIAN_POINT('Ctrl Pts',(-62.8343031482014,-0.0765705776094529,
40.0889118607713));
#191987=CARTESIAN_POINT('Ctrl Pts',(-62.8329897454269,-0.0798191603650119,
40.0876855950755));
#191988=CARTESIAN_POINT('Ctrl Pts',(-62.8315859904681,-0.08299818279531,
40.0863782327527));
#191989=CARTESIAN_POINT('Ctrl Pts',(-62.8301000734874,-0.0861004173278655,
40.0850006373334));
#191990=CARTESIAN_POINT('Ctrl Pts',(-62.8293571149971,-0.0876515345941433,
40.0843118396238));
#191991=CARTESIAN_POINT('Ctrl Pts',(-62.8285936160519,-0.0891834722997116,
40.0836054919165));
#191992=CARTESIAN_POINT('Ctrl Pts',(-62.82781060087,-0.0906954364278793,
40.0828829920418));
#191993=CARTESIAN_POINT('Ctrl Pts',(-62.8276148470746,-0.0910734274599212,
40.0827023670731));
#191994=CARTESIAN_POINT('Ctrl Pts',(-62.8274178735164,-0.0914501705143456,
40.0825207326933));
#191995=CARTESIAN_POINT('Ctrl Pts',(-62.8272196962038,-0.0918256539328543,
40.0823381109276));
#191996=CARTESIAN_POINT('Ctrl Pts',(-62.8266251642659,-0.0929521041883804,
40.0817902456304));
#191997=CARTESIAN_POINT('Ctrl Pts',(-62.826019798519,-0.0940672158686678,
40.0812334935554));
#191998=CARTESIAN_POINT('Ctrl Pts',(-62.8254040313373,-0.0951706907488606,
40.0806684524227));
#191999=CARTESIAN_POINT('Ctrl Pts',(-62.8211486980557,-0.102796386827432,
40.0767636676138));
#192000=CARTESIAN_POINT('Ctrl Pts',(-62.8164204928786,-0.109916699411237,
40.0724404510891));
#192001=CARTESIAN_POINT('Ctrl Pts',(-62.8113377077399,-0.116542502759463,
40.0677949937413));
#192002=CARTESIAN_POINT('Ctrl Pts',(-62.8088115774777,-0.119835508836266,
40.0654862141908));
#192003=CARTESIAN_POINT('Ctrl Pts',(-62.8061972539434,-0.123006400629238,
40.0630972003217));
#192004=CARTESIAN_POINT('Ctrl Pts',(-62.8035061084565,-0.126056303769975,
40.0606363359906));
#192005=CARTESIAN_POINT('Ctrl Pts',(-62.7975690395532,-0.132784845643289,
40.0552073017124));
#192006=CARTESIAN_POINT('Ctrl Pts',(-62.7912680187378,-0.138932019324687,
40.0494204304519));
#192007=CARTESIAN_POINT('Ctrl Pts',(-62.7847385034067,-0.144445113413174,
40.0434049749851));
#192008=CARTESIAN_POINT('Ctrl Pts',(-62.7823531891148,-0.146459116207472,
40.0412074532442));
#192009=CARTESIAN_POINT('Ctrl Pts',(-62.7799396422115,-0.148396130390986,
40.0389814735788));
#192010=CARTESIAN_POINT('Ctrl Pts',(-62.7775029828616,-0.150257579786495,
40.0367321210016));
#192011=CARTESIAN_POINT('Ctrl Pts',(-62.7693185019448,-0.156509991333542,
40.0291767837141));
#192012=CARTESIAN_POINT('Ctrl Pts',(-62.7608162581025,-0.161942805717962,
40.0213235332578));
#192013=CARTESIAN_POINT('Ctrl Pts',(-62.7520965944499,-0.166635979461348,
40.0132649215861));
#192014=CARTESIAN_POINT('Ctrl Pts',(-62.7425126511837,-0.17179433334833,
40.0044075527536));
#192015=CARTESIAN_POINT('Ctrl Pts',(-62.7326655363505,-0.176059615357533,
39.9953016253724));
#192016=CARTESIAN_POINT('Ctrl Pts',(-62.7226511116306,-0.179500292056757,
39.9860353422363));
#192017=CARTESIAN_POINT('Ctrl Pts',(-62.7118651471232,-0.183206048283122,
39.97605515827));
#192018=CARTESIAN_POINT('Ctrl Pts',(-62.7008840239659,-0.185955767119226,
39.9658879738161));
#192019=CARTESIAN_POINT('Ctrl Pts',(-62.689799127427,-0.187785458035178,
39.955617464326));
#192020=CARTESIAN_POINT('Ctrl Pts',(-62.6788639144179,-0.189590441946077,
39.9454856413909));
#192021=CARTESIAN_POINT('Ctrl Pts',(-62.6678262782733,-0.1905,39.9352519465115));
#192022=CARTESIAN_POINT('Ctrl Pts',(-62.6567671111299,-0.1905,39.92499));
#192023=CARTESIAN_POINT('Ctrl Pts',(-59.2165773020941,-0.1905,39.92499));
#192024=CARTESIAN_POINT('Ctrl Pts',(-59.2059936184286,-0.1905,39.9348107241729));
#192025=CARTESIAN_POINT('Ctrl Pts',(-59.1954479901449,-0.18966522548857,
39.9446038383182));
#192026=CARTESIAN_POINT('Ctrl Pts',(-59.1849969778442,-0.188008762313808,
39.9543158069403));
#192027=CARTESIAN_POINT('Ctrl Pts',(-59.1749056059476,-0.186409301376566,
39.9636935671413));
#192028=CARTESIAN_POINT('Ctrl Pts',(-59.1649012152123,-0.184043455437504,
39.9729968321014));
#192029=CARTESIAN_POINT('Ctrl Pts',(-59.1550396955505,-0.180877423725678,
39.9821731151364));
#192030=CARTESIAN_POINT('Ctrl Pts',(-59.1457174710335,-0.177884532218296,
39.9908475764383));
#192031=CARTESIAN_POINT('Ctrl Pts',(-59.1365220583417,-0.174176304385485,
39.9994093733879));
#192032=CARTESIAN_POINT('Ctrl Pts',(-59.1275197082918,-0.169686797570574,
40.0077966115876));
#192033=CARTESIAN_POINT('Ctrl Pts',(-59.1192286949217,-0.165552037111176,
40.015521117263));
#192034=CARTESIAN_POINT('Ctrl Pts',(-59.1111009786049,-0.16075429390116,
40.0230979941058));
#192035=CARTESIAN_POINT('Ctrl Pts',(-59.1032135992685,-0.155213515010445,
40.0304554104785));
#192036=CARTESIAN_POINT('Ctrl Pts',(-59.1008617419687,-0.15356136659404,
40.0326492435205));
#192037=CARTESIAN_POINT('Ctrl Pts',(-59.0985314603567,-0.151842962926721,
40.0348233715073));
#192038=CARTESIAN_POINT('Ctrl Pts',(-59.096225375957,-0.150055686180148,
40.0369753512356));
#192039=CARTESIAN_POINT('Ctrl Pts',(-59.0939428540559,-0.148286670996711,
40.0391053430352));
#192040=CARTESIAN_POINT('Ctrl Pts',(-59.0916862380348,-0.146452235168912,
40.041211089324));
#192041=CARTESIAN_POINT('Ctrl Pts',(-59.0894604907299,-0.144552116609974,
40.0432881154904));
#192042=CARTESIAN_POINT('Ctrl Pts',(-59.0893057166152,-0.144419986081426,
40.043432547828));
#192043=CARTESIAN_POINT('Ctrl Pts',(-59.089151080705,-0.144287542502105,
40.0435768364421));
#192044=CARTESIAN_POINT('Ctrl Pts',(-59.0889965840074,-0.144154785043949,
40.0437209807855));
#192045=CARTESIAN_POINT('Ctrl Pts',(-59.0822228828153,-0.138334211749519,
40.050040796842));
#192046=CARTESIAN_POINT('Ctrl Pts',(-59.0757535782845,-0.131883990154123,
40.0560490279344));
#192047=CARTESIAN_POINT('Ctrl Pts',(-59.0697047694307,-0.124808417215326,
40.0616647108615));
#192048=CARTESIAN_POINT('Ctrl Pts',(-59.0640662283031,-0.118212753510071,
40.0668995033485));
#192049=CARTESIAN_POINT('Ctrl Pts',(-59.0587927761312,-0.111072931137358,
40.0717933267482));
#192050=CARTESIAN_POINT('Ctrl Pts',(-59.0540076654697,-0.103389544768211,
40.0762460303072));
#192051=CARTESIAN_POINT('Ctrl Pts',(-59.0522572100836,-0.100578862632643,
40.0778748868748));
#192052=CARTESIAN_POINT('Ctrl Pts',(-59.0505724231957,-0.0976954648438018,
40.0794443522247));
#192053=CARTESIAN_POINT('Ctrl Pts',(-59.048960544286,-0.0947395585253491,
40.0809482021492));
#192054=CARTESIAN_POINT('Ctrl Pts',(-59.0485729412563,-0.0940287618038531,
40.0813098278168));
#192055=CARTESIAN_POINT('Ctrl Pts',(-59.0481896206935,-0.0933131922167578,
40.0816679525672));
#192056=CARTESIAN_POINT('Ctrl Pts',(-59.0478106940136,-0.0925929271971714,
40.082022419258));
#192057=CARTESIAN_POINT('Ctrl Pts',(-59.0474436087926,-0.0918951704594471,
40.0823658088648));
#192058=CARTESIAN_POINT('Ctrl Pts',(-59.047080647127,-0.0911930071934237,
40.0827057654616));
#192059=CARTESIAN_POINT('Ctrl Pts',(-59.0467219102889,-0.0904865115878252,
40.0830421470151));
#192060=CARTESIAN_POINT('Ctrl Pts',(-59.042791533644,-0.0827460357497621,
40.0867275956807));
#192061=CARTESIAN_POINT('Ctrl Pts',(-59.0393660724129,-0.0744802459940775,
40.0899823432032));
#192062=CARTESIAN_POINT('Ctrl Pts',(-59.0365841602688,-0.0658168714604773,
40.0926299529357));
#192063=CARTESIAN_POINT('Ctrl Pts',(-59.0354304183829,-0.0622239118140861,
40.0937279956085));
#192064=CARTESIAN_POINT('Ctrl Pts',(-59.0343871039216,-0.05856290328636,
40.0947220371803));
#192065=CARTESIAN_POINT('Ctrl Pts',(-59.0334626554261,-0.0548440714999749,
40.0956014538692));
#192066=CARTESIAN_POINT('Ctrl Pts',(-59.0318859121827,-0.048501216358408,
40.097101390674));
#192067=CARTESIAN_POINT('Ctrl Pts',(-59.0306571138137,-0.041991400494417,
40.0982667904316));
#192068=CARTESIAN_POINT('Ctrl Pts',(-59.0298212958158,-0.0353717968088207,
40.0990539325583));
#192069=CARTESIAN_POINT('Ctrl Pts',(-59.0294033868168,-0.0320619949660225,
40.0994475036216));
#192070=CARTESIAN_POINT('Ctrl Pts',(-59.029085168164,-0.0287246785546771,
40.0997467259952));
#192071=CARTESIAN_POINT('Ctrl Pts',(-59.0288723192866,-0.0253670368748687,
40.0999473488896));
#192072=CARTESIAN_POINT('Ctrl Pts',(-59.0286594704093,-0.0220093951950603,
40.100147971784));
#192073=CARTESIAN_POINT('Ctrl Pts',(-59.0285519740191,-0.0186314705080073,
40.10025));
#192074=CARTESIAN_POINT('Ctrl Pts',(-59.0285534841296,-0.01524,40.10025));
#192075=CARTESIAN_POINT('Origin',(-57.9430040808457,6.10537907909423,39.92499));
#192076=CARTESIAN_POINT('Ctrl Pts',(-62.2936141127569,6.73887200051376,
39.92499));
#192077=CARTESIAN_POINT('Ctrl Pts',(-62.3041663177853,6.73998108195364,
39.9348354642015));
#192078=CARTESIAN_POINT('Ctrl Pts',(-62.3147747227664,6.74025426844133,
39.9446440828452));
#192079=CARTESIAN_POINT('Ctrl Pts',(-62.3253809467515,6.73970068257644,
39.9543641760322));
#192080=CARTESIAN_POINT('Ctrl Pts',(-62.3356425316131,6.73916508495577,
39.9637684240701));
#192081=CARTESIAN_POINT('Ctrl Pts',(-62.3459033574813,6.73785543637718,
39.9730909636382));
#192082=CARTESIAN_POINT('Ctrl Pts',(-62.3561113603631,6.73573381164871,
39.9822808977125));
#192083=CARTESIAN_POINT('Ctrl Pts',(-62.3657675025168,6.73372688529769,
39.9909740094633));
#192084=CARTESIAN_POINT('Ctrl Pts',(-62.3753772873457,6.73099321743938,
39.9995492764983));
#192085=CARTESIAN_POINT('Ctrl Pts',(-62.3848821415084,6.72746117704732,
40.0079462328675));
#192086=CARTESIAN_POINT('Ctrl Pts',(-62.3936367996008,6.72420791240257,
40.0156804369668));
#192087=CARTESIAN_POINT('Ctrl Pts',(-62.4023029414968,6.72027708243923,
40.02326380174));
#192088=CARTESIAN_POINT('Ctrl Pts',(-62.4108128192354,6.71558140886554,
40.0306257269943));
#192089=CARTESIAN_POINT('Ctrl Pts',(-62.4132812112836,6.71421937245723,
40.0327611416636));
#192090=CARTESIAN_POINT('Ctrl Pts',(-62.4157362792946,6.71279278199639,
40.0348777427263));
#192091=CARTESIAN_POINT('Ctrl Pts',(-62.4181758915949,6.71129899689642,
40.03697331687));
#192092=CARTESIAN_POINT('Ctrl Pts',(-62.4208205881801,6.70967963780713,
40.039245053974));
#192093=CARTESIAN_POINT('Ctrl Pts',(-62.4234440047028,6.70798448411218,
40.041487875195));
#192094=CARTESIAN_POINT('Ctrl Pts',(-62.4260429761973,6.70621108803167,
40.0436985701601));
#192095=CARTESIAN_POINT('Ctrl Pts',(-62.4331758738575,6.70134398857313,
40.0497658398386));
#192096=CARTESIAN_POINT('Ctrl Pts',(-62.4400912556837,6.69585818364737,
40.0555581699984));
#192097=CARTESIAN_POINT('Ctrl Pts',(-62.4466864116141,6.6897680133393,40.0609828468885));
#192098=CARTESIAN_POINT('Ctrl Pts',(-62.4527206212309,6.68419583815059,
40.0659461317303));
#192099=CARTESIAN_POINT('Ctrl Pts',(-62.4584752900412,6.67811620689384,
40.0706039980705));
#192100=CARTESIAN_POINT('Ctrl Pts',(-62.4638645712584,6.67150703079258,
40.0748843180601));
#192101=CARTESIAN_POINT('Ctrl Pts',(-62.4665117685875,6.66826062508126,
40.0769867972568));
#192102=CARTESIAN_POINT('Ctrl Pts',(-62.4690703232299,6.66488629458035,
40.0789976708174));
#192103=CARTESIAN_POINT('Ctrl Pts',(-62.4715267736418,6.66138078591754,
40.08090504915));
#192104=CARTESIAN_POINT('Ctrl Pts',(-62.4719928611813,6.66071564979291,
40.0812669556104));
#192105=CARTESIAN_POINT('Ctrl Pts',(-62.472455189938,6.66004526561032,40.0816253922032));
#192106=CARTESIAN_POINT('Ctrl Pts',(-62.4729136358128,6.659369698209,40.0819801989139));
#192107=CARTESIAN_POINT('Ctrl Pts',(-62.4733577552541,6.65871524228898,
40.0823239179149));
#192108=CARTESIAN_POINT('Ctrl Pts',(-62.4737982306999,6.65805592206494,
40.0826642303498));
#192109=CARTESIAN_POINT('Ctrl Pts',(-62.4742349489459,6.65739180030952,
40.0830009916099));
#192110=CARTESIAN_POINT('Ctrl Pts',(-62.4789942144025,6.65015433826453,
40.0866709464312));
#192111=CARTESIAN_POINT('Ctrl Pts',(-62.4833100626578,6.64234165497502,
40.0899175831877));
#192112=CARTESIAN_POINT('Ctrl Pts',(-62.4870273554127,6.63406423386189,
40.0925642067062));
#192113=CARTESIAN_POINT('Ctrl Pts',(-62.4885971912263,6.63056862752554,
40.0936818922527));
#192114=CARTESIAN_POINT('Ctrl Pts',(-62.4900605069389,6.62699051141415,
40.0946930094791));
#192115=CARTESIAN_POINT('Ctrl Pts',(-62.491407022622,6.62333954252043,40.0955863397546));
#192116=CARTESIAN_POINT('Ctrl Pts',(-62.4936745213866,6.61719140213115,
40.0970906856166));
#192117=CARTESIAN_POINT('Ctrl Pts',(-62.495608491139,6.61083770188569,40.0982599215483));
#192118=CARTESIAN_POINT('Ctrl Pts',(-62.4971561593219,6.60433062536189,
40.0990497370453));
#192119=CARTESIAN_POINT('Ctrl Pts',(-62.4975430763677,6.60270385623094,
40.0992471909196));
#192120=CARTESIAN_POINT('Ctrl Pts',(-62.4979056188881,6.60106746196599,
40.0994209989363));
#192121=CARTESIAN_POINT('Ctrl Pts',(-62.4982426563693,6.59942221845788,
40.0995705982975));
#192122=CARTESIAN_POINT('Ctrl Pts',(-62.4987482125911,6.59695435319572,
40.0997949973393));
#192123=CARTESIAN_POINT('Ctrl Pts',(-62.4991963674672,6.59446659126645,
40.0999649129781));
#192124=CARTESIAN_POINT('Ctrl Pts',(-62.499584972412,6.59196174500338,40.1000786629733));
#192125=CARTESIAN_POINT('Ctrl Pts',(-62.4999735773569,6.58945689874031,
40.1001924129685));
#192126=CARTESIAN_POINT('Ctrl Pts',(-62.5003026407461,6.58693497617694,
40.10025));
#192127=CARTESIAN_POINT('Ctrl Pts',(-62.500570298093,6.58439859103072,40.10025));
#192128=CARTESIAN_POINT('Ctrl Pts',(-58.7035958781038,6.18532049829439,
40.10025));
#192129=CARTESIAN_POINT('Ctrl Pts',(-58.7026899760169,6.19390281910191,
40.10025));
#192130=CARTESIAN_POINT('Ctrl Pts',(-58.7025003609928,6.20248552904397,
40.0995786334241));
#192131=CARTESIAN_POINT('Ctrl Pts',(-58.7029569544313,6.21093474935446,
40.0983063763367));
#192132=CARTESIAN_POINT('Ctrl Pts',(-58.7032518669434,6.21639207873522,
40.0974846287993));
#192133=CARTESIAN_POINT('Ctrl Pts',(-58.7038154335198,6.22179377937549,
40.0964130309338));
#192134=CARTESIAN_POINT('Ctrl Pts',(-58.7046202140516,6.22710604846907,
40.0951176960924));
#192135=CARTESIAN_POINT('Ctrl Pts',(-58.7056869045457,6.23414715684684,
40.0934008039614));
#192136=CARTESIAN_POINT('Ctrl Pts',(-58.7071827955652,6.24102913891686,
40.0912909372157));
#192137=CARTESIAN_POINT('Ctrl Pts',(-58.7090548163569,6.24767922440788,
40.0888630467852));
#192138=CARTESIAN_POINT('Ctrl Pts',(-58.7099908267527,6.25100426715339,
40.0876491015699));
#192139=CARTESIAN_POINT('Ctrl Pts',(-58.7110208470227,6.25427153376702,
40.0863558569271));
#192140=CARTESIAN_POINT('Ctrl Pts',(-58.7121380880307,6.25747333351558,
40.0849936342771));
#192141=CARTESIAN_POINT('Ctrl Pts',(-58.7126967085346,6.25907423338986,
40.0843125229521));
#192142=CARTESIAN_POINT('Ctrl Pts',(-58.713277132457,6.26065878288383,40.0836141747074));
#192143=CARTESIAN_POINT('Ctrl Pts',(-58.7138784999414,6.26222612320555,
40.082899916161));
#192144=CARTESIAN_POINT('Ctrl Pts',(-58.7140288418126,6.26261795828598,
40.0827213515243));
#192145=CARTESIAN_POINT('Ctrl Pts',(-58.7141804926178,6.26300871814051,
40.0825417925842));
#192146=CARTESIAN_POINT('Ctrl Pts',(-58.7143334388435,6.26339839005094,
40.0823612602361));
#192147=CARTESIAN_POINT('Ctrl Pts',(-58.7147922775207,6.26456740578226,
40.0818196631917));
#192148=CARTESIAN_POINT('Ctrl Pts',(-58.7152627751829,6.2657266282841,40.0812693052022));
#192149=CARTESIAN_POINT('Ctrl Pts',(-58.7157445651923,6.26687572965204,
40.0807107531875));
#192150=CARTESIAN_POINT('Ctrl Pts',(-58.7191382318077,6.27496985131173,
40.0767763849182));
#192151=CARTESIAN_POINT('Ctrl Pts',(-58.7230632421216,6.2826071619279,40.0724140586139));
#192152=CARTESIAN_POINT('Ctrl Pts',(-58.7274000190312,6.28978339589459,
40.067722122377));
#192153=CARTESIAN_POINT('Ctrl Pts',(-58.729503351146,6.29326386161387,40.0654465383722));
#192154=CARTESIAN_POINT('Ctrl Pts',(-58.731704109697,6.29663597408956,40.063092800068));
#192155=CARTESIAN_POINT('Ctrl Pts',(-58.7339915094193,6.29989941779187,
40.0606689262479));
#192156=CARTESIAN_POINT('Ctrl Pts',(-58.7374933585782,6.30489552208976,
40.0569581447806));
#192157=CARTESIAN_POINT('Ctrl Pts',(-58.7411954596216,6.3096348018091,40.0530843804606));
#192158=CARTESIAN_POINT('Ctrl Pts',(-58.7450534628849,6.31410463171084,
40.0490800251458));
#192159=CARTESIAN_POINT('Ctrl Pts',(-58.7468451395591,6.31618044384105,
40.0472203818218));
#192160=CARTESIAN_POINT('Ctrl Pts',(-58.7486702031823,6.31819823791566,
40.0453323608819));
#192161=CARTESIAN_POINT('Ctrl Pts',(-58.7505249478605,6.32015576082356,
40.0434201572162));
#192162=CARTESIAN_POINT('Ctrl Pts',(-58.750667106732,6.32030579724142,40.0432735943397));
#192163=CARTESIAN_POINT('Ctrl Pts',(-58.7508094261758,6.32045551058229,
40.0431268995707));
#192164=CARTESIAN_POINT('Ctrl Pts',(-58.7509519047345,6.32060490094039,
40.0429800745037));
#192165=CARTESIAN_POINT('Ctrl Pts',(-58.7529532989256,6.32270338507423,
40.0409176249753));
#192166=CARTESIAN_POINT('Ctrl Pts',(-58.7549876922214,6.32473679726668,
40.0388310783332));
#192167=CARTESIAN_POINT('Ctrl Pts',(-58.7570493794209,6.32670504965026,
40.036725739981));
#192168=CARTESIAN_POINT('Ctrl Pts',(-58.7644422230594,6.33376285265585,
40.0291763710718));
#192169=CARTESIAN_POINT('Ctrl Pts',(-58.7722418109921,6.34003880538919,
40.0213310894595));
#192170=CARTESIAN_POINT('Ctrl Pts',(-58.780339648655,6.34560292136727,40.013283755132));
#192171=CARTESIAN_POINT('Ctrl Pts',(-58.7892383587467,6.35171732586219,
40.0044405431325));
#192172=CARTESIAN_POINT('Ctrl Pts',(-58.7984976730893,6.35697262978456,
39.9953528710601));
#192173=CARTESIAN_POINT('Ctrl Pts',(-58.8080148760648,6.36142852992827,
39.9861103629555));
#192174=CARTESIAN_POINT('Ctrl Pts',(-58.8182910667864,6.36623978380521,
39.9761307737555));
#192175=CARTESIAN_POINT('Ctrl Pts',(-58.8288688921852,6.37011968263765,
39.9659696936009));
#192176=CARTESIAN_POINT('Ctrl Pts',(-58.8396533761882,6.37309732669848,
39.9557128217502));
#192177=CARTESIAN_POINT('Ctrl Pts',(-58.8503473894511,6.37604999138507,
39.9455419945158));
#192178=CARTESIAN_POINT('Ctrl Pts',(-58.8612460403463,6.3781155791127,39.9352756289339));
#192179=CARTESIAN_POINT('Ctrl Pts',(-58.872270023448,6.37927424642618,39.92499));
#192180=CARTESIAN_POINT('Origin',(-0.00159301378018793,-0.015156513685413,
39.92499));
#192181=CARTESIAN_POINT('Ctrl Pts',(-62.5037563256534,6.5540855636599,40.10025));
#192182=CARTESIAN_POINT('Ctrl Pts',(-62.5046505412977,6.54554330587477,
40.10025));
#192183=CARTESIAN_POINT('Ctrl Pts',(-62.5048232320878,6.53700226086759,
40.0995859581842));
#192184=CARTESIAN_POINT('Ctrl Pts',(-62.5043472028589,6.5285945717757,40.0983275959622));
#192185=CARTESIAN_POINT('Ctrl Pts',(-62.5040430428431,6.52322245869582,
40.0975235624069));
#192186=CARTESIAN_POINT('Ctrl Pts',(-62.5034749678471,6.51790471489682,
40.0964777059491));
#192187=CARTESIAN_POINT('Ctrl Pts',(-62.5026702669707,6.51267356740905,
40.0952149915962));
#192188=CARTESIAN_POINT('Ctrl Pts',(-62.5015720117389,6.50553410072708,
40.0934916398702));
#192189=CARTESIAN_POINT('Ctrl Pts',(-62.5000273428098,6.49855818190828,
40.0913643921631));
#192190=CARTESIAN_POINT('Ctrl Pts',(-62.4980940659029,6.49182203260229,
40.0889118607714));
#192191=CARTESIAN_POINT('Ctrl Pts',(-62.4971274274494,6.48845395794929,
40.0876855950755));
#192192=CARTESIAN_POINT('Ctrl Pts',(-62.4960636607365,6.48514561818783,
40.0863782327527));
#192193=CARTESIAN_POINT('Ctrl Pts',(-62.4949101555729,6.4819050574021,40.0850006373334));
#192194=CARTESIAN_POINT('Ctrl Pts',(-62.4943334029912,6.48028477700923,
40.0843118396238));
#192195=CARTESIAN_POINT('Ctrl Pts',(-62.4937342176673,6.47868142404725,
40.0836054919165));
#192196=CARTESIAN_POINT('Ctrl Pts',(-62.4931135352113,6.4770958952431,40.0828829920418));
#192197=CARTESIAN_POINT('Ctrl Pts',(-62.4929583645973,6.47669951304206,
40.0827023670731));
#192198=CARTESIAN_POINT('Ctrl Pts',(-62.4928018504535,6.47630424448216,
40.0825207326933));
#192199=CARTESIAN_POINT('Ctrl Pts',(-62.4926440074816,6.47591010283116,
40.0823381109276));
#192200=CARTESIAN_POINT('Ctrl Pts',(-62.4921704785661,6.47472767787817,
40.0817902456304));
#192201=CARTESIAN_POINT('Ctrl Pts',(-62.4916849899864,6.4735553969451,40.0812334935553));
#192202=CARTESIAN_POINT('Ctrl Pts',(-62.4911879405752,6.47239360181852,
40.0806684524227));
#192203=CARTESIAN_POINT('Ctrl Pts',(-62.4877530207469,6.46436487665211,
40.0767636676137));
#192204=CARTESIAN_POINT('Ctrl Pts',(-62.4837949925047,6.45678933786425,
40.0724404510888));
#192205=CARTESIAN_POINT('Ctrl Pts',(-62.4794326364365,6.44966853564018,
40.0677949937409));
#192206=CARTESIAN_POINT('Ctrl Pts',(-62.4772645574451,6.44612951648112,
40.0654862141905));
#192207=CARTESIAN_POINT('Ctrl Pts',(-62.4749960038951,6.44270272394384,
40.0630972003216));
#192208=CARTESIAN_POINT('Ctrl Pts',(-62.4726384024734,6.43938822718966,
40.0606363359906));
#192209=CARTESIAN_POINT('Ctrl Pts',(-62.4674371815967,6.43207595228396,
40.0552073017124));
#192210=CARTESIAN_POINT('Ctrl Pts',(-62.461813233051,6.42530381744033,40.049420430452));
#192211=CARTESIAN_POINT('Ctrl Pts',(-62.455895762341,6.41913840445467,40.0434049749852));
#192212=CARTESIAN_POINT('Ctrl Pts',(-62.4537340356674,6.41688610134107,
40.0412074532442));
#192213=CARTESIAN_POINT('Ctrl Pts',(-62.4515361835425,6.4147074139751,40.0389814735788));
#192214=CARTESIAN_POINT('Ctrl Pts',(-62.4493074469123,6.4126014615368,40.0367321210017));
#192215=CARTESIAN_POINT('Ctrl Pts',(-62.4418213564085,6.40552779014114,
40.0291767837138));
#192216=CARTESIAN_POINT('Ctrl Pts',(-62.4339335724859,6.39923601079889,
40.0213235332569));
#192217=CARTESIAN_POINT('Ctrl Pts',(-62.4257522463019,6.39365709371027,
40.0132649215848));
#192218=CARTESIAN_POINT('Ctrl Pts',(-62.416759999684,6.38752520296373,40.0044075527519));
#192219=CARTESIAN_POINT('Ctrl Pts',(-62.4074126717495,6.38225398283438,
39.9953016253702));
#192220=CARTESIAN_POINT('Ctrl Pts',(-62.3978127557435,6.37778536209557,
39.9860353422336));
#192221=CARTESIAN_POINT('Ctrl Pts',(-62.3874732348813,6.37297246609468,
39.9760551582668));
#192222=CARTESIAN_POINT('Ctrl Pts',(-62.3768396913494,6.36908997057751,
39.9658879738124));
#192223=CARTESIAN_POINT('Ctrl Pts',(-62.3660067738128,6.36611161569927,
39.9556174643217));
#192224=CARTESIAN_POINT('Ctrl Pts',(-62.3553201372407,6.36317347866842,
39.945485641388));
#192225=CARTESIAN_POINT('Ctrl Pts',(-62.3444380411289,6.3611151561248,39.9352519465101));
#192226=CARTESIAN_POINT('Ctrl Pts',(-62.3334394572618,6.35995915837845,
39.92499));
#192227=CARTESIAN_POINT('Ctrl Pts',(-58.9120953679529,6.00036140429087,
39.92499));
#192228=CARTESIAN_POINT('Ctrl Pts',(-58.9015696628139,5.9992551081016,39.9348107241729));
#192229=CARTESIAN_POINT('Ctrl Pts',(-58.8909945468885,5.99898299131223,
39.9446038383182));
#192230=CARTESIAN_POINT('Ctrl Pts',(-58.8804276387766,5.99953795195303,
39.9543158069403));
#192231=CARTESIAN_POINT('Ctrl Pts',(-58.8702243592773,6.00007381527929,
39.9636935671413));
#192232=CARTESIAN_POINT('Ctrl Pts',(-58.8600274754009,6.00138095727726,
39.9729968321014));
#192233=CARTESIAN_POINT('Ctrl Pts',(-58.8498890377462,6.00349883564037,
39.9821731151364));
#192234=CARTESIAN_POINT('Ctrl Pts',(-58.8403050390005,6.00550089397191,
39.9908475764382));
#192235=CARTESIAN_POINT('Ctrl Pts',(-58.8307723843848,6.00822762538685,
39.9994093733878));
#192236=CARTESIAN_POINT('Ctrl Pts',(-58.8213500689023,6.01175153639715,
40.0077966115874));
#192237=CARTESIAN_POINT('Ctrl Pts',(-58.8126722744142,6.01499699931957,
40.0155211172628));
#192238=CARTESIAN_POINT('Ctrl Pts',(-58.804087581853,6.01891888229376,40.0230979941055));
#192239=CARTESIAN_POINT('Ctrl Pts',(-58.7956642413032,6.02360485257665,
40.0304554104781));
#192240=CARTESIAN_POINT('Ctrl Pts',(-58.7931525711886,6.02500211432187,
40.0326492435203));
#192241=CARTESIAN_POINT('Ctrl Pts',(-58.7906554330083,6.02646752363828,
40.0348233715071));
#192242=CARTESIAN_POINT('Ctrl Pts',(-58.7881751602883,6.02800395803745,
40.0369753512356));
#192243=CARTESIAN_POINT('Ctrl Pts',(-58.7857202298424,6.02952469386392,
40.0391053430352));
#192244=CARTESIAN_POINT('Ctrl Pts',(-58.7832842250419,6.03111319985544,
40.041211089324));
#192245=CARTESIAN_POINT('Ctrl Pts',(-58.7808720541407,6.0327702554207,40.0432881154904));
#192246=CARTESIAN_POINT('Ctrl Pts',(-58.7807043164937,6.03288548382402,
40.043432547828));
#192247=CARTESIAN_POINT('Ctrl Pts',(-58.7805366835714,6.03300103800951,
40.0435768364421));
#192248=CARTESIAN_POINT('Ctrl Pts',(-58.7803691562897,6.03311691890603,
40.0437209807855));
#192249=CARTESIAN_POINT('Ctrl Pts',(-58.7730241465597,6.03819756191476,
40.0500407968421));
#192250=CARTESIAN_POINT('Ctrl Pts',(-58.7659160498048,6.04393622206041,
40.0560490279346));
#192251=CARTESIAN_POINT('Ctrl Pts',(-58.7591607781927,6.05034076157632,
40.0616647108616));
#192252=CARTESIAN_POINT('Ctrl Pts',(-58.7528636909919,6.05631090550667,
40.0668995033488));
#192253=CARTESIAN_POINT('Ctrl Pts',(-58.746872812682,6.06286038933388,40.0717933267485));
#192254=CARTESIAN_POINT('Ctrl Pts',(-58.7413107827875,6.07000150504474,
40.0762460303077));
#192255=CARTESIAN_POINT('Ctrl Pts',(-58.739276120295,6.07261381755775,40.0778748868751));
#192256=CARTESIAN_POINT('Ctrl Pts',(-58.7372991657062,6.07530531160724,
40.0794443522249));
#192257=CARTESIAN_POINT('Ctrl Pts',(-58.735387140493,6.07807653793596,40.0809482021492));
#192258=CARTESIAN_POINT('Ctrl Pts',(-58.7349273623042,6.07874292528959,
40.0813098278168));
#192259=CARTESIAN_POINT('Ctrl Pts',(-58.7344713442223,6.07941450700224,
40.0816679525672));
#192260=CARTESIAN_POINT('Ctrl Pts',(-58.7340192051468,6.08009121771116,
40.0820224192581));
#192261=CARTESIAN_POINT('Ctrl Pts',(-58.7335811954175,6.08074678121042,
40.0823658088648));
#192262=CARTESIAN_POINT('Ctrl Pts',(-58.7331468260467,6.08140715812747,
40.0827057654617));
#192263=CARTESIAN_POINT('Ctrl Pts',(-58.7327162055066,6.08207228526581,
40.0830421470151));
#192264=CARTESIAN_POINT('Ctrl Pts',(-58.7279982598322,6.08935952173621,
40.0867275956805));
#192265=CARTESIAN_POINT('Ctrl Pts',(-58.7237275533353,6.09722197243184,
40.0899823432029));
#192266=CARTESIAN_POINT('Ctrl Pts',(-58.7200553115705,6.10554709909145,
40.0926299529353));
#192267=CARTESIAN_POINT('Ctrl Pts',(-58.7185323234527,6.10899977726302,
40.0937279956083));
#192268=CARTESIAN_POINT('Ctrl Pts',(-58.7171120447816,6.11253167434606,
40.0947220371802));
#192269=CARTESIAN_POINT('Ctrl Pts',(-58.7158039367398,6.11613350280266,
40.0956014538693));
#192270=CARTESIAN_POINT('Ctrl Pts',(-58.7135728221601,6.12227679657189,
40.097101390674));
#192271=CARTESIAN_POINT('Ctrl Pts',(-58.7116702942287,6.12862250657827,
40.0982667904316));
#192272=CARTESIAN_POINT('Ctrl Pts',(-58.7101471179288,6.13511848061139,
40.0990539325583));
#192273=CARTESIAN_POINT('Ctrl Pts',(-58.7093855297788,6.13836646762795,
40.0994475036216));
#192274=CARTESIAN_POINT('Ctrl Pts',(-58.7087202098051,6.14165223896403,
40.0997467259952));
#192275=CARTESIAN_POINT('Ctrl Pts',(-58.7081575578111,6.14496923836534,
40.0999473488896));
#192276=CARTESIAN_POINT('Ctrl Pts',(-58.7075949058172,6.14828623776664,
40.100147971784));
#192277=CARTESIAN_POINT('Ctrl Pts',(-58.7071349090267,6.15163442139633,
40.10025));
#192278=CARTESIAN_POINT('Ctrl Pts',(-58.7067819056642,6.15500747092357,
40.10025));
#192279=CARTESIAN_POINT('Origin',(-56.9874003490101,12.1286263473648,39.92499));
#192280=CARTESIAN_POINT('Ctrl Pts',(-61.2479592423877,13.2134115091898,
39.92499));
#192281=CARTESIAN_POINT('Ctrl Pts',(-61.2583377107548,13.2156175207413,
39.934835464202));
#192282=CARTESIAN_POINT('Ctrl Pts',(-61.2688594460202,13.2169980909553,
39.9446440828463));
#192283=CARTESIAN_POINT('Ctrl Pts',(-61.2794654334808,13.2175561899859,
39.9543641760338));
#192284=CARTESIAN_POINT('Ctrl Pts',(-61.2897267895035,13.2180961541212,
39.9637684240722));
#192285=CARTESIAN_POINT('Ctrl Pts',(-61.3000683010478,13.2178662282943,
39.9730909636408));
#192286=CARTESIAN_POINT('Ctrl Pts',(-61.3104421535948,13.2168232529021,
39.9822808977154));
#192287=CARTESIAN_POINT('Ctrl Pts',(-61.3202551793192,13.2158366624039,
39.9909740094666));
#192288=CARTESIAN_POINT('Ctrl Pts',(-61.3300980668421,13.2141224659043,
39.9995492765019));
#192289=CARTESIAN_POINT('Ctrl Pts',(-61.3399200511741,13.2116033021979,
40.0079462328714));
#192290=CARTESIAN_POINT('Ctrl Pts',(-61.3489668090879,13.2092829702338,
40.0156804369712));
#192291=CARTESIAN_POINT('Ctrl Pts',(-61.3579963605677,13.2062795322627,
40.0232638017446));
#192292=CARTESIAN_POINT('Ctrl Pts',(-61.3669504518488,13.2024991065222,
40.0306257269992));
#192293=CARTESIAN_POINT('Ctrl Pts',(-61.3695476933578,13.2014025487201,
40.0327611416669));
#192294=CARTESIAN_POINT('Ctrl Pts',(-61.372138431556,13.2002403977583,40.0348777427279));
#192295=CARTESIAN_POINT('Ctrl Pts',(-61.3747208224639,13.1990098046951,
40.0369733168701));
#192296=CARTESIAN_POINT('Ctrl Pts',(-61.3775203002415,13.1976757626942,
40.0392450539741));
#192297=CARTESIAN_POINT('Ctrl Pts',(-61.3803065372248,13.1962641169262,
40.0414878751951));
#192298=CARTESIAN_POINT('Ctrl Pts',(-61.3830766416485,13.1947721021914,
40.0436985701601));
#192299=CARTESIAN_POINT('Ctrl Pts',(-61.3906792149761,13.190677256044,40.0497658398386));
#192300=CARTESIAN_POINT('Ctrl Pts',(-61.3981301363757,13.1859443571668,
40.0555581699984));
#192301=CARTESIAN_POINT('Ctrl Pts',(-61.4053257594952,13.1805769309634,
40.0609828468886));
#192302=CARTESIAN_POINT('Ctrl Pts',(-61.4119093639902,13.1756660273914,
40.0659461317306));
#192303=CARTESIAN_POINT('Ctrl Pts',(-61.4182680026354,13.170221227678,40.0706039980708));
#192304=CARTESIAN_POINT('Ctrl Pts',(-61.4243186078276,13.1642115906184,
40.0748843180606));
#192305=CARTESIAN_POINT('Ctrl Pts',(-61.4272906453327,13.1612596765262,
40.0769867972571));
#192306=CARTESIAN_POINT('Ctrl Pts',(-61.4301878975267,13.158171272746,40.0789976708175));
#192307=CARTESIAN_POINT('Ctrl Pts',(-61.4329973166795,13.1549417366134,
40.08090504915));
#192308=CARTESIAN_POINT('Ctrl Pts',(-61.4335303765996,13.1543289635883,
40.0812669556104));
#192309=CARTESIAN_POINT('Ctrl Pts',(-61.4340602468994,13.1537105783548,
40.0816253922033));
#192310=CARTESIAN_POINT('Ctrl Pts',(-61.4345867973821,13.1530866324252,
40.0819801989139));
#192311=CARTESIAN_POINT('Ctrl Pts',(-61.4350968931622,13.1524821848059,
40.0823239179149));
#192312=CARTESIAN_POINT('Ctrl Pts',(-61.4356038733672,13.1518725186285,
40.0826642303498));
#192313=CARTESIAN_POINT('Ctrl Pts',(-61.4361076188514,13.1512576844887,
40.0830009916099));
#192314=CARTESIAN_POINT('Ctrl Pts',(-61.4415973333393,13.1445573487227,
40.0866709464311));
#192315=CARTESIAN_POINT('Ctrl Pts',(-61.4467061867045,13.1372385931157,
40.0899175831876));
#192316=CARTESIAN_POINT('Ctrl Pts',(-61.4512683418493,13.1293950794809,
40.092564206706));
#192317=CARTESIAN_POINT('Ctrl Pts',(-61.4531949682968,13.1260827149668,
40.0936818922526));
#192318=CARTESIAN_POINT('Ctrl Pts',(-61.4550242827915,13.1226771582924,
40.094693009479));
#192319=CARTESIAN_POINT('Ctrl Pts',(-61.4567450522888,13.1191869390032,
40.0955863397546));
#192320=CARTESIAN_POINT('Ctrl Pts',(-61.4596427851247,13.1133094969316,
40.0970906856166));
#192321=CARTESIAN_POINT('Ctrl Pts',(-61.4622303029112,13.1071927578071,
40.0982599215483));
#192322=CARTESIAN_POINT('Ctrl Pts',(-61.4644496675148,13.100883103106,40.0990497370454));
#192323=CARTESIAN_POINT('Ctrl Pts',(-61.4650045086657,13.0993056894308,
40.0992471909196));
#192324=CARTESIAN_POINT('Ctrl Pts',(-61.4655361149182,13.0977161555174,
40.0994209989363));
#192325=CARTESIAN_POINT('Ctrl Pts',(-61.4660432808484,13.0961151548353,
40.0995705982975));
#192326=CARTESIAN_POINT('Ctrl Pts',(-61.4668040297438,13.0937136538123,
40.0997949973393));
#192327=CARTESIAN_POINT('Ctrl Pts',(-61.467509771512,13.0912863650436,40.0999649129781));
#192328=CARTESIAN_POINT('Ctrl Pts',(-61.468158075369,13.0888358608682,40.1000786629733));
#192329=CARTESIAN_POINT('Ctrl Pts',(-61.468806379226,13.0863853566928,40.1001924129685));
#192330=CARTESIAN_POINT('Ctrl Pts',(-61.4693972526618,13.0839116459755,
40.10025));
#192331=CARTESIAN_POINT('Ctrl Pts',(-61.4699285681953,13.0814171332237,
40.10025));
#192332=CARTESIAN_POINT('Ctrl Pts',(-57.7354693911204,12.2876333308475,
40.10025));
#192333=CARTESIAN_POINT('Ctrl Pts',(-57.7336713548545,12.2960739442511,
40.10025));
#192334=CARTESIAN_POINT('Ctrl Pts',(-57.7325856410804,12.3045898170434,
40.099578633424));
#192335=CARTESIAN_POINT('Ctrl Pts',(-57.7321565492374,12.3130404786519,
40.0983063763365));
#192336=CARTESIAN_POINT('Ctrl Pts',(-57.7318793999343,12.3184987389625,
40.0974846287992));
#192337=CARTESIAN_POINT('Ctrl Pts',(-57.7318752477671,12.3239297572693,
40.0964130309338));
#192338=CARTESIAN_POINT('Ctrl Pts',(-57.7321203363021,12.3292970476687,
40.0951176960924));
#192339=CARTESIAN_POINT('Ctrl Pts',(-57.7324451871156,12.3364110836362,
40.0934008039614));
#192340=CARTESIAN_POINT('Ctrl Pts',(-57.7332135204775,12.3434117286779,
40.0912909372157));
#192341=CARTESIAN_POINT('Ctrl Pts',(-57.7343801629265,12.3502210637613,
40.0888630467852));
#192342=CARTESIAN_POINT('Ctrl Pts',(-57.734963484151,12.3536257313031,40.0876491015699));
#192343=CARTESIAN_POINT('Ctrl Pts',(-57.735646339504,12.3569827659243,40.0863558569272));
#192344=CARTESIAN_POINT('Ctrl Pts',(-57.7364227809414,12.3602838093645,
40.0849936342771));
#192345=CARTESIAN_POINT('Ctrl Pts',(-57.7368110016601,12.3619343310846,
40.0843125229521));
#192346=CARTESIAN_POINT('Ctrl Pts',(-57.7372226154359,12.3635708710713,
40.0836141747074));
#192347=CARTESIAN_POINT('Ctrl Pts',(-57.7376568568911,12.3651924853577,
40.082899916161));
#192348=CARTESIAN_POINT('Ctrl Pts',(-57.7377654172549,12.3655978889293,
40.0827213515244));
#192349=CARTESIAN_POINT('Ctrl Pts',(-57.737875391774,12.3660023599861,40.0825417925842));
#192350=CARTESIAN_POINT('Ctrl Pts',(-57.7379867683383,12.366405884467,40.0823612602361));
#192351=CARTESIAN_POINT('Ctrl Pts',(-57.7383208980313,12.3676164579096,
40.0818196631918));
#192352=CARTESIAN_POINT('Ctrl Pts',(-57.7386676465114,12.3688185104669,
40.0812693052022));
#192353=CARTESIAN_POINT('Ctrl Pts',(-57.7390266834246,12.3700116777066,
40.0807107531875));
#192354=CARTESIAN_POINT('Ctrl Pts',(-57.7415556930807,12.3784161936775,
40.0767763849181));
#192355=CARTESIAN_POINT('Ctrl Pts',(-57.7446608854354,12.3864219416038,
40.0724140586135));
#192356=CARTESIAN_POINT('Ctrl Pts',(-57.7482237843189,12.3940121800362,
40.0677221223764));
#192357=CARTESIAN_POINT('Ctrl Pts',(-57.7499517864271,12.3976934374734,
40.0654465383717));
#192358=CARTESIAN_POINT('Ctrl Pts',(-57.7517880072572,12.4012771190731,
40.0630928000678));
#192359=CARTESIAN_POINT('Ctrl Pts',(-57.7537217536092,12.4047617836669,
40.0606689262479));
#192360=CARTESIAN_POINT('Ctrl Pts',(-57.7566821841673,12.4100965616938,
40.0569581447806));
#192361=CARTESIAN_POINT('Ctrl Pts',(-57.7598686150879,12.4151968540759,
40.0530843804606));
#192362=CARTESIAN_POINT('Ctrl Pts',(-57.763238259355,12.4200454689342,40.0490800251458));
#192363=CARTESIAN_POINT('Ctrl Pts',(-57.7648031395849,12.4222971907578,
40.0472203818218));
#192364=CARTESIAN_POINT('Ctrl Pts',(-57.7664072884047,12.4244947022412,
40.0453323608819));
#192365=CARTESIAN_POINT('Ctrl Pts',(-57.7680472557361,12.4266353752448,
40.0434201572162));
#192366=CARTESIAN_POINT('Ctrl Pts',(-57.7681729527703,12.4267994493958,
40.0432735943397));
#192367=CARTESIAN_POINT('Ctrl Pts',(-57.7682988432679,12.4269632190241,
40.0431268995708));
#192368=CARTESIAN_POINT('Ctrl Pts',(-57.7684249257696,12.427126684071,40.0429800745037));
#192369=CARTESIAN_POINT('Ctrl Pts',(-57.7701960047921,12.4294228751483,
40.0409176249753));
#192370=CARTESIAN_POINT('Ctrl Pts',(-57.772006704017,12.4316578001009,40.0388310783332));
#192371=CARTESIAN_POINT('Ctrl Pts',(-57.7738513586813,12.4338307751867,
40.036725739981));
#192372=CARTESIAN_POINT('Ctrl Pts',(-57.780465962247,12.4416226773942,40.0291763710713));
#192373=CARTESIAN_POINT('Ctrl Pts',(-57.7875668075266,12.4486795287429,
40.0213310894585));
#192374=CARTESIAN_POINT('Ctrl Pts',(-57.7950386758954,12.4550596184385,
40.0132837551305));
#192375=CARTESIAN_POINT('Ctrl Pts',(-57.803249508617,12.4620706960771,40.0044405431304));
#192376=CARTESIAN_POINT('Ctrl Pts',(-57.8119087706244,12.4682650727941,
39.9953528710574));
#192377=CARTESIAN_POINT('Ctrl Pts',(-57.8209080689723,12.4736913816524,
39.9861103629522));
#192378=CARTESIAN_POINT('Ctrl Pts',(-57.8306250526725,12.4795504334018,
39.9761307737515));
#192379=CARTESIAN_POINT('Ctrl Pts',(-57.8407393717752,12.4845147615762,
39.9659696935962));
#192380=CARTESIAN_POINT('Ctrl Pts',(-57.8511535286894,12.4886033793312,
39.9557128217448));
#192381=CARTESIAN_POINT('Ctrl Pts',(-57.8614803215248,12.4926576977832,
39.9455419945121));
#192382=CARTESIAN_POINT('Ctrl Pts',(-57.8721033557573,12.4958511892341,
39.9352756289321));
#192383=CARTESIAN_POINT('Ctrl Pts',(-57.8829458346104,12.4981558292591,
39.92499));
#192384=CARTESIAN_POINT('Origin',(-0.00316857416805164,-0.0149069694351843,
39.92499));
#192385=CARTESIAN_POINT('Ctrl Pts',(-61.4762657165315,13.0516031943533,
40.10025));
#192386=CARTESIAN_POINT('Ctrl Pts',(-61.4780479426481,13.0432012029369,
40.10025));
#192387=CARTESIAN_POINT('Ctrl Pts',(-61.4791124697293,13.0347249977705,
40.0995859581842));
#192388=CARTESIAN_POINT('Ctrl Pts',(-61.4795178910587,13.026313608275,40.0983275959621));
#192389=CARTESIAN_POINT('Ctrl Pts',(-61.479776935988,13.020939130814,40.0975235624068));
#192390=CARTESIAN_POINT('Ctrl Pts',(-61.4797678285536,13.0155911381659,
40.096477705949));
#192391=CARTESIAN_POINT('Ctrl Pts',(-61.4795143397207,13.0103045333057,
40.0952149915961));
#192392=CARTESIAN_POINT('Ctrl Pts',(-61.4791683783269,13.0030893784376,
40.0934916398701));
#192393=CARTESIAN_POINT('Ctrl Pts',(-61.4783613533298,12.9959902125626,
40.0913643921631));
#192394=CARTESIAN_POINT('Ctrl Pts',(-61.4771427864514,12.9890888821232,
40.0889118607713));
#192395=CARTESIAN_POINT('Ctrl Pts',(-61.4765335030122,12.9856382169035,
40.0876855950755));
#192396=CARTESIAN_POINT('Ctrl Pts',(-61.4758213793958,12.9822368066736,
40.0863782327527));
#192397=CARTESIAN_POINT('Ctrl Pts',(-61.4750129240933,12.9788934238968,
40.0850006373334));
#192398=CARTESIAN_POINT('Ctrl Pts',(-61.474608696442,12.9772217325084,40.0843118396238));
#192399=CARTESIAN_POINT('Ctrl Pts',(-61.4741803895392,12.9755645309606,
40.0836054919165));
#192400=CARTESIAN_POINT('Ctrl Pts',(-61.4737288401361,12.9739228088659,
40.0828829920418));
#192401=CARTESIAN_POINT('Ctrl Pts',(-61.4736159527853,12.9735123783422,
40.0827023670731));
#192402=CARTESIAN_POINT('Ctrl Pts',(-61.4735016128574,12.9731029149219,
40.0825207326933));
#192403=CARTESIAN_POINT('Ctrl Pts',(-61.473385833587,12.9726944333368,40.0823381109276));
#192404=CARTESIAN_POINT('Ctrl Pts',(-61.4730384957757,12.9714689885816,
40.0817902456304));
#192405=CARTESIAN_POINT('Ctrl Pts',(-61.4726782034776,12.9702523821509,
40.0812334935553));
#192406=CARTESIAN_POINT('Ctrl Pts',(-61.4723053176143,12.9690449956485,
40.0806684524227));
#192407=CARTESIAN_POINT('Ctrl Pts',(-61.46972844494,12.9607012057877,40.0767636676138));
#192408=CARTESIAN_POINT('Ctrl Pts',(-61.4665839586186,12.9527534399845,
40.072440451089));
#192409=CARTESIAN_POINT('Ctrl Pts',(-61.4629898265073,12.9452156558842,
40.0677949937413));
#192410=CARTESIAN_POINT('Ctrl Pts',(-61.4612035527136,12.941469397877,40.0654862141908));
#192411=CARTESIAN_POINT('Ctrl Pts',(-61.4593056238949,12.9378242492511,
40.0630972003217));
#192412=CARTESIAN_POINT('Ctrl Pts',(-61.4573073969126,12.9342814732032,
40.0606363359906));
#192413=CARTESIAN_POINT('Ctrl Pts',(-61.452899009727,12.9264655800791,40.0552073017124));
#192414=CARTESIAN_POINT('Ctrl Pts',(-61.4480137506081,12.9191426809998,
40.049420430452));
#192415=CARTESIAN_POINT('Ctrl Pts',(-61.4427731575667,12.9123924986718,
40.0434049749852));
#192416=CARTESIAN_POINT('Ctrl Pts',(-61.4408587028413,12.9099265719431,
40.0412074532442));
#192417=CARTESIAN_POINT('Ctrl Pts',(-61.4389006256225,12.9075300815494,
40.0389814735788));
#192418=CARTESIAN_POINT('Ctrl Pts',(-61.4369042302168,12.9052026993239,
40.0367321210017));
#192419=CARTESIAN_POINT('Ctrl Pts',(-61.4301985493006,12.8973852687039,
40.0291767837136));
#192420=CARTESIAN_POINT('Ctrl Pts',(-61.4230116455093,12.890303458455,40.0213235332567));
#192421=CARTESIAN_POINT('Ctrl Pts',(-61.415458293116,12.8838999218043,40.0132649215844));
#192422=CARTESIAN_POINT('Ctrl Pts',(-61.4071562640824,12.8768616764765,
40.0044075527513));
#192423=CARTESIAN_POINT('Ctrl Pts',(-61.3984111343277,12.8706422708178,
39.9953016253694));
#192424=CARTESIAN_POINT('Ctrl Pts',(-61.3893309057246,12.8651946651833,
39.9860353422326));
#192425=CARTESIAN_POINT('Ctrl Pts',(-61.3795511104622,12.8593273605036,
39.9760551582656));
#192426=CARTESIAN_POINT('Ctrl Pts',(-61.3693816498842,12.8543546257386,
39.965887973811));
#192427=CARTESIAN_POINT('Ctrl Pts',(-61.3589193990615,12.8502602383772,
39.95561746432));
#192428=CARTESIAN_POINT('Ctrl Pts',(-61.348598423952,12.8462211390704,39.9454856413869));
#192429=CARTESIAN_POINT('Ctrl Pts',(-61.3379910943943,12.8430366034496,
39.9352519465096));
#192430=CARTESIAN_POINT('Ctrl Pts',(-61.3271735965892,12.8407372733102,
39.92499));
#192431=CARTESIAN_POINT('Ctrl Pts',(-57.962160188812,12.1254815933796,39.92499));
#192432=CARTESIAN_POINT('Ctrl Pts',(-57.9518077840282,12.1232811218137,
39.9348107241723));
#192433=CARTESIAN_POINT('Ctrl Pts',(-57.9413190436447,12.1219050950921,
39.9446038383171));
#192434=CARTESIAN_POINT('Ctrl Pts',(-57.9307520129787,12.1213524729339,
39.9543158069387));
#192435=CARTESIAN_POINT('Ctrl Pts',(-57.9205486151424,12.1208188676184,
39.9636935671395));
#192436=CARTESIAN_POINT('Ctrl Pts',(-57.9102709573187,12.1210529843539,
39.9729968320992));
#192437=CARTESIAN_POINT('Ctrl Pts',(-57.8999666805159,12.1220995054496,
39.9821731151339));
#192438=CARTESIAN_POINT('Ctrl Pts',(-57.8902259118375,12.1230887956351,
39.9908475764357));
#192439=CARTESIAN_POINT('Ctrl Pts',(-57.8804604570568,12.1248041559921,
39.9994093733852));
#192440=CARTESIAN_POINT('Ctrl Pts',(-57.870721409002,12.1273238624911,40.0077966115848));
#192441=CARTESIAN_POINT('Ctrl Pts',(-57.8617519091282,12.1296444699055,
40.0155211172602));
#192442=CARTESIAN_POINT('Ctrl Pts',(-57.8528042960106,12.1326475236732,
40.0230979941029));
#192443=CARTESIAN_POINT('Ctrl Pts',(-57.8439372821291,12.1364273448771,
40.0304554104756));
#192444=CARTESIAN_POINT('Ctrl Pts',(-57.8412933175822,12.1375544112594,
40.0326492435186));
#192445=CARTESIAN_POINT('Ctrl Pts',(-57.8386566820011,12.1387507708941,
40.0348233715063));
#192446=CARTESIAN_POINT('Ctrl Pts',(-57.836029395347,12.1400195294494,40.0369753512356));
#192447=CARTESIAN_POINT('Ctrl Pts',(-57.833428953088,12.141275324419,40.0391053430352));
#192448=CARTESIAN_POINT('Ctrl Pts',(-57.8308402488865,12.1426004965702,
40.041211089324));
#192449=CARTESIAN_POINT('Ctrl Pts',(-57.828268082638,12.1439963340942,40.0432881154904));
#192450=CARTESIAN_POINT('Ctrl Pts',(-57.8280892192275,12.1440933979058,
40.043432547828));
#192451=CARTESIAN_POINT('Ctrl Pts',(-57.8279104259145,12.1441907966616,
40.0435768364421));
#192452=CARTESIAN_POINT('Ctrl Pts',(-57.8277317035127,12.1442885313812,
40.0437209807855));
#192453=CARTESIAN_POINT('Ctrl Pts',(-57.8198958587085,12.1485735795161,
40.050040796842));
#192454=CARTESIAN_POINT('Ctrl Pts',(-57.8122268475251,12.1535378042504,
40.0560490279344));
#192455=CARTESIAN_POINT('Ctrl Pts',(-57.8048391253243,12.1592011408681,
40.0616647108615));
#192456=CARTESIAN_POINT('Ctrl Pts',(-57.7979524842556,12.1644803548771,
40.0668995033486));
#192457=CARTESIAN_POINT('Ctrl Pts',(-57.7913098171243,12.1703677426432,
40.0717933267483));
#192458=CARTESIAN_POINT('Ctrl Pts',(-57.7850318067603,12.1768883481374,
40.0762460303074));
#192459=CARTESIAN_POINT('Ctrl Pts',(-57.7827352293492,12.1792736699856,
40.0778748868749));
#192460=CARTESIAN_POINT('Ctrl Pts',(-57.7804877669874,12.1817437717241,
40.0794443522248));
#192461=CARTESIAN_POINT('Ctrl Pts',(-57.7782965440187,12.1842999559279,
40.0809482021492));
#192462=CARTESIAN_POINT('Ctrl Pts',(-57.777769628097,12.1849146328344,40.0813098278168));
#192463=CARTESIAN_POINT('Ctrl Pts',(-57.7772459087254,12.1855348686828,
40.0816679525672));
#192464=CARTESIAN_POINT('Ctrl Pts',(-57.7767255109846,12.1861606108969,
40.082022419258));
#192465=CARTESIAN_POINT('Ctrl Pts',(-57.7762213756733,12.1867667986668,
40.0823658088648));
#192466=CARTESIAN_POINT('Ctrl Pts',(-57.7757203576391,12.1873781540072,
40.0827057654616));
#192467=CARTESIAN_POINT('Ctrl Pts',(-57.7752225713656,12.1879946254062,
40.0830421470151));
#192468=CARTESIAN_POINT('Ctrl Pts',(-57.7697687474614,12.1947487820219,
40.0867275956806));
#192469=CARTESIAN_POINT('Ctrl Pts',(-57.7646995864527,12.202121751003,40.0899823432031));
#192470=CARTESIAN_POINT('Ctrl Pts',(-57.7601772489162,12.2100174179596,
40.0926299529356));
#192471=CARTESIAN_POINT('Ctrl Pts',(-57.7583017007433,12.2132919863911,
40.0937279956084));
#192472=CARTESIAN_POINT('Ctrl Pts',(-57.7565200187331,12.2166560758252,
40.0947220371802));
#192473=CARTESIAN_POINT('Ctrl Pts',(-57.7548425830506,12.220101438565,40.0956014538692));
#192474=CARTESIAN_POINT('Ctrl Pts',(-57.751981541693,12.2259778637498,40.097101390674));
#192475=CARTESIAN_POINT('Ctrl Pts',(-57.7494261286933,12.2320899429718,
40.0982667904316));
#192476=CARTESIAN_POINT('Ctrl Pts',(-57.7472322823293,12.2383911161015,
40.0990539325583));
#192477=CARTESIAN_POINT('Ctrl Pts',(-57.7461353591473,12.2415417026664,
40.0994475036216));
#192478=CARTESIAN_POINT('Ctrl Pts',(-57.7451302272376,12.2447399293288,
40.0997467259952));
#192479=CARTESIAN_POINT('Ctrl Pts',(-57.7442239366601,12.2479799447121,
40.0999473488896));
#192480=CARTESIAN_POINT('Ctrl Pts',(-57.7433176460826,12.2512199600953,
40.100147971784));
#192481=CARTESIAN_POINT('Ctrl Pts',(-57.7425101887131,12.2545017192672,
40.10025));
#192482=CARTESIAN_POINT('Ctrl Pts',(-57.7418065394565,12.2578193919772,
40.10025));
#192483=CARTESIAN_POINT('Origin',(-55.4074307335705,18.0189898472954,39.92499));
#192484=CARTESIAN_POINT('Ctrl Pts',(-59.5312589135994,19.5431821162871,
39.92499));
#192485=CARTESIAN_POINT('Ctrl Pts',(-59.5413499366325,19.5464608884257,
39.9348354642013));
#192486=CARTESIAN_POINT('Ctrl Pts',(-59.5516697238474,19.5489337165496,
39.9446440828448));
#192487=CARTESIAN_POINT('Ctrl Pts',(-59.5621592733641,19.550597385826,39.9543641760316));
#192488=CARTESIAN_POINT('Ctrl Pts',(-59.5723079749828,19.5522069957574,
39.9637684240692));
#192489=CARTESIAN_POINT('Ctrl Pts',(-59.5826168684374,19.5530593117979,
39.9730909636371));
#192490=CARTESIAN_POINT('Ctrl Pts',(-59.5930429125488,19.5531064127993,
39.982280897711));
#192491=CARTESIAN_POINT('Ctrl Pts',(-59.6029053082795,19.5531509674463,
39.9909740094615));
#192492=CARTESIAN_POINT('Ctrl Pts',(-59.6128734577597,19.5524750234018,
39.9995492764962));
#192493=CARTESIAN_POINT('Ctrl Pts',(-59.622904960544,19.5509963368668,40.0079462328651));
#192494=CARTESIAN_POINT('Ctrl Pts',(-59.6321447001049,19.5496343596267,
40.0156804369641));
#192495=CARTESIAN_POINT('Ctrl Pts',(-59.6414387315116,19.5475912199439,
40.0232638017369));
#192496=CARTESIAN_POINT('Ctrl Pts',(-59.650738933436,19.5447674611737,40.0306257269909));
#192497=CARTESIAN_POINT('Ctrl Pts',(-59.6534365684897,19.5439483960927,
40.0327611416613));
#192498=CARTESIAN_POINT('Ctrl Pts',(-59.6561345922104,19.543063417397,40.0348777427252));
#192499=CARTESIAN_POINT('Ctrl Pts',(-59.658831468516,19.5421094990033,40.03697331687));
#192500=CARTESIAN_POINT('Ctrl Pts',(-59.6617550558217,19.5410753901341,
40.039245053974));
#192501=CARTESIAN_POINT('Ctrl Pts',(-59.6646735866701,19.5399627185794,
40.041487875195));
#192502=CARTESIAN_POINT('Ctrl Pts',(-59.6675844741793,19.5387684320159,
40.0436985701601));
#192503=CARTESIAN_POINT('Ctrl Pts',(-59.6755734277898,19.535490703171,40.0497658398386));
#192504=CARTESIAN_POINT('Ctrl Pts',(-59.6834782549088,19.5315625649729,
40.0555581699984));
#192505=CARTESIAN_POINT('Ctrl Pts',(-59.6911955084647,19.5269766895187,
40.0609828468885));
#192506=CARTESIAN_POINT('Ctrl Pts',(-59.698256376489,19.522780862451,40.0659461317305));
#192507=CARTESIAN_POINT('Ctrl Pts',(-59.7051493183932,19.5180305486462,
40.0706039980708));
#192508=CARTESIAN_POINT('Ctrl Pts',(-59.7117949558637,19.5126862934698,
40.0748843180605));
#192509=CARTESIAN_POINT('Ctrl Pts',(-59.7150592712802,19.5100612127851,
40.0769867972571));
#192510=CARTESIAN_POINT('Ctrl Pts',(-59.7182634781246,19.5072925729234,
40.0789976708175));
#192511=CARTESIAN_POINT('Ctrl Pts',(-59.7213950854344,19.5043743927943,
40.08090504915));
#192512=CARTESIAN_POINT('Ctrl Pts',(-59.7219892774191,19.5038206965383,
40.0812669556104));
#192513=CARTESIAN_POINT('Ctrl Pts',(-59.7225808838921,19.503261085412,40.0816253922032));
#192514=CARTESIAN_POINT('Ctrl Pts',(-59.7231697699854,19.5026955970363,
40.0819801989139));
#192515=CARTESIAN_POINT('Ctrl Pts',(-59.7237402533882,19.5021477801723,
40.0823239179149));
#192516=CARTESIAN_POINT('Ctrl Pts',(-59.7243081837712,19.5015944476717,
40.0826642303498));
#192517=CARTESIAN_POINT('Ctrl Pts',(-59.7248734373528,19.501035637399,40.0830009916099));
#192518=CARTESIAN_POINT('Ctrl Pts',(-59.7310334544114,19.4949458381924,
40.0866709464312));
#192519=CARTESIAN_POINT('Ctrl Pts',(-59.7368793392201,19.4882011960855,
40.0899175831877));
#192520=CARTESIAN_POINT('Ctrl Pts',(-59.7422363728287,19.4808775251053,
40.0925642067062));
#192521=CARTESIAN_POINT('Ctrl Pts',(-59.7444986813872,19.4777846933727,
40.0936818922527));
#192522=CARTESIAN_POINT('Ctrl Pts',(-59.7466739523113,19.4745890081272,
40.094693009479));
#192523=CARTESIAN_POINT('Ctrl Pts',(-59.7487501225119,19.4712977780159,
40.0955863397546));
#192524=CARTESIAN_POINT('Ctrl Pts',(-59.7522463412518,19.4657554287472,
40.0970906856166));
#192525=CARTESIAN_POINT('Ctrl Pts',(-59.755459057686,19.4599426670175,40.0982599215483));
#192526=CARTESIAN_POINT('Ctrl Pts',(-59.7583258028879,19.4538995640366,
40.0990497370454));
#192527=CARTESIAN_POINT('Ctrl Pts',(-59.7590424891884,19.4523887882914,
40.0992471909196));
#192528=CARTESIAN_POINT('Ctrl Pts',(-59.7597373347834,19.4508635299957,
40.0994209989363));
#192529=CARTESIAN_POINT('Ctrl Pts',(-59.7604090725466,19.4493243130382,
40.0995705982975));
#192530=CARTESIAN_POINT('Ctrl Pts',(-59.7614166791914,19.447015487602,40.0997949973393));
#192531=CARTESIAN_POINT('Ctrl Pts',(-59.7623722755973,19.4446752658777,
40.0999649129781));
#192532=CARTESIAN_POINT('Ctrl Pts',(-59.7632731754136,19.4423059520264,
40.1000786629733));
#192533=CARTESIAN_POINT('Ctrl Pts',(-59.7641740752299,19.4399366381752,
40.1001924129685));
#192534=CARTESIAN_POINT('Ctrl Pts',(-59.765020284979,19.4375382417963,40.10025));
#192535=CARTESIAN_POINT('Ctrl Pts',(-59.765809437495,19.4351129318425,40.10025));
#192536=CARTESIAN_POINT('Ctrl Pts',(-56.134781019564,18.2553202812753,40.10025));
#192537=CARTESIAN_POINT('Ctrl Pts',(-56.1321105487809,18.2635267101475,
40.10025));
#192538=CARTESIAN_POINT('Ctrl Pts',(-56.1301406315642,18.2718824441051,
40.0995786334241));
#192539=CARTESIAN_POINT('Ctrl Pts',(-56.1288305556597,18.2802419597939,
40.0983063763366));
#192540=CARTESIAN_POINT('Ctrl Pts',(-56.1279843810469,18.2856413491929,
40.0974846287992));
#192541=CARTESIAN_POINT('Ctrl Pts',(-56.1274125556282,18.2910421817937,
40.0964130309338));
#192542=CARTESIAN_POINT('Ctrl Pts',(-56.1270952669251,18.2964056883429,
40.0951176960923));
#192543=CARTESIAN_POINT('Ctrl Pts',(-56.1266747189246,18.3035147090333,
40.0934008039614));
#192544=CARTESIAN_POINT('Ctrl Pts',(-56.126707076608,18.3105573165145,40.0912909372156));
#192545=CARTESIAN_POINT('Ctrl Pts',(-56.1271555587354,18.3174512966903,
40.0888630467851));
#192546=CARTESIAN_POINT('Ctrl Pts',(-56.1273797997991,18.3208982867782,
40.0876491015699));
#192547=CARTESIAN_POINT('Ctrl Pts',(-56.1277080087289,18.3243083090332,
40.0863558569271));
#192548=CARTESIAN_POINT('Ctrl Pts',(-56.1281351437408,18.3276724292423,
40.0849936342771));
#192549=CARTESIAN_POINT('Ctrl Pts',(-56.1283487112468,18.3293544893468,
40.0843125229521));
#192550=CARTESIAN_POINT('Ctrl Pts',(-56.1285870051494,18.3310250895517,
40.0836141747074));
#192551=CARTESIAN_POINT('Ctrl Pts',(-56.1288493629351,18.3326832110574,
40.0828999161609));
#192552=CARTESIAN_POINT('Ctrl Pts',(-56.1289149523815,18.3330977414338,
40.0827213515243));
#192553=CARTESIAN_POINT('Ctrl Pts',(-56.1289820457107,18.3335114922233,
40.0825417925842));
#192554=CARTESIAN_POINT('Ctrl Pts',(-56.1290506323487,18.333924448176,40.082361260236));
#192555=CARTESIAN_POINT('Ctrl Pts',(-56.1292563922627,18.335163316034,40.0818196631917));
#192556=CARTESIAN_POINT('Ctrl Pts',(-56.1294755925117,18.3363950287073,
40.0812693052021));
#192557=CARTESIAN_POINT('Ctrl Pts',(-56.1297079426451,18.3376191892289,
40.0807107531875));
#192558=CARTESIAN_POINT('Ctrl Pts',(-56.1313445869827,18.3462420178745,
40.0767763849182));
#192559=CARTESIAN_POINT('Ctrl Pts',(-56.1335959402407,18.3545284904607,
40.0724140586137));
#192560=CARTESIAN_POINT('Ctrl Pts',(-56.1363459252319,18.3624495731175,
40.0677221223769));
#192561=CARTESIAN_POINT('Ctrl Pts',(-56.1376796649811,18.3662912896465,
40.0654465383721));
#192562=CARTESIAN_POINT('Ctrl Pts',(-56.139131230071,18.3700472768054,40.0630928000679));
#192563=CARTESIAN_POINT('Ctrl Pts',(-56.1406901365233,18.3737149835767,
40.0606689262479));
#192564=CARTESIAN_POINT('Ctrl Pts',(-56.143076713384,18.3793299863883,40.0569581447805));
#192565=CARTESIAN_POINT('Ctrl Pts',(-56.1457125629777,18.3847354115625,
40.0530843804606));
#192566=CARTESIAN_POINT('Ctrl Pts',(-56.1485569297208,18.3899096889383,
40.0490800251458));
#192567=CARTESIAN_POINT('Ctrl Pts',(-56.1498778683511,18.3923126501197,
40.0472203818218));
#192568=CARTESIAN_POINT('Ctrl Pts',(-56.1512435269775,18.3946658026163,
40.0453323608818));
#192569=CARTESIAN_POINT('Ctrl Pts',(-56.1526507491369,18.3969661720541,
40.0434201572162));
#192570=CARTESIAN_POINT('Ctrl Pts',(-56.1527586071707,18.3971424863076,
40.0432735943397));
#192571=CARTESIAN_POINT('Ctrl Pts',(-56.1528666894394,18.397318517929,40.0431268995707));
#192572=CARTESIAN_POINT('Ctrl Pts',(-56.1529749944978,18.3974942667074,
40.0429800745037));
#192573=CARTESIAN_POINT('Ctrl Pts',(-56.1544963540394,18.3999630071783,
40.0409176249753));
#192574=CARTESIAN_POINT('Ctrl Pts',(-56.1560635207937,18.4023749585856,
40.0388310783332));
#192575=CARTESIAN_POINT('Ctrl Pts',(-56.1576709325003,18.4047288488038,
40.036725739981));
#192576=CARTESIAN_POINT('Ctrl Pts',(-56.1634348250113,18.4131694805007,
40.0291763710721));
#192577=CARTESIAN_POINT('Ctrl Pts',(-56.1697591292898,18.4209299141236,
40.0213310894601));
#192578=CARTESIAN_POINT('Ctrl Pts',(-56.1765231650097,18.4280560759379,
40.013283755133));
#192579=CARTESIAN_POINT('Ctrl Pts',(-56.1839561607582,18.4358870118855,
40.004440543134));
#192580=CARTESIAN_POINT('Ctrl Pts',(-56.1919204977421,18.4429525945088,
39.995352871062));
#192581=CARTESIAN_POINT('Ctrl Pts',(-56.2003032932647,18.4492898603057,
39.986110362958));
#192582=CARTESIAN_POINT('Ctrl Pts',(-56.2093546086345,18.4561325169297,
39.9761307737587));
#192583=CARTESIAN_POINT('Ctrl Pts',(-56.2188946068421,18.4621268842274,
39.9659696936049));
#192584=CARTESIAN_POINT('Ctrl Pts',(-56.2288243369826,18.4672816799249,
39.955712821755));
#192585=CARTESIAN_POINT('Ctrl Pts',(-56.238670766892,18.4723932321841,39.945541994519));
#192586=CARTESIAN_POINT('Ctrl Pts',(-56.2489017962809,18.4766796388,39.9352756289355));
#192587=CARTESIAN_POINT('Ctrl Pts',(-56.2594439784237,18.4801050014195,
39.92499));
#192588=CARTESIAN_POINT('Origin',(-0.00470941899426334,-0.0144941013083398,
39.92499));
#192589=CARTESIAN_POINT('Ctrl Pts',(-59.7752282754835,19.4061247292258,
40.10025));
#192590=CARTESIAN_POINT('Ctrl Pts',(-59.7778789856303,19.3979550581542,
40.10025));
#192591=CARTESIAN_POINT('Ctrl Pts',(-59.7798236858212,19.3896365599059,
40.0995859581841));
#192592=CARTESIAN_POINT('Ctrl Pts',(-59.7811061158281,19.3813136269502,
40.0983275959618));
#192593=CARTESIAN_POINT('Ctrl Pts',(-59.7819255275519,19.3759956690079,
40.0975235624066));
#192594=CARTESIAN_POINT('Ctrl Pts',(-59.782475487462,19.3706760212375,40.0964777059489));
#192595=CARTESIAN_POINT('Ctrl Pts',(-59.7827759879494,19.3653918801542,
40.0952149915961));
#192596=CARTESIAN_POINT('Ctrl Pts',(-59.7831861108188,19.3581800878466,
40.0934916398701));
#192597=CARTESIAN_POINT('Ctrl Pts',(-59.7831255716886,19.3510354548623,
40.091364392163));
#192598=CARTESIAN_POINT('Ctrl Pts',(-59.7826350657123,19.3440445557099,
40.0889118607713));
#192599=CARTESIAN_POINT('Ctrl Pts',(-59.7823898127242,19.3405491061338,
40.0876855950754));
#192600=CARTESIAN_POINT('Ctrl Pts',(-59.7820371343798,19.3370918919978,
40.0863782327527));
#192601=CARTESIAN_POINT('Ctrl Pts',(-59.7815825865438,19.3336823180313,
40.0850006373334));
#192602=CARTESIAN_POINT('Ctrl Pts',(-59.7813553126258,19.331977531048,40.0843118396237));
#192603=CARTESIAN_POINT('Ctrl Pts',(-59.7811025767641,19.3302846375614,
40.0836054919165));
#192604=CARTESIAN_POINT('Ctrl Pts',(-59.7808251076835,19.3286047092268,
40.0828829920418));
#192605=CARTESIAN_POINT('Ctrl Pts',(-59.7807557404133,19.3281847271432,
40.0827023670731));
#192606=CARTESIAN_POINT('Ctrl Pts',(-59.7806848274336,19.3277655550294,
40.0825207326933));
#192607=CARTESIAN_POINT('Ctrl Pts',(-59.7806123803665,19.3273472089199,
40.0823381109276));
#192608=CARTESIAN_POINT('Ctrl Pts',(-59.7803950391652,19.3260921705916,
40.0817902456304));
#192609=CARTESIAN_POINT('Ctrl Pts',(-59.7801638905866,19.3248445680581,
40.0812334935553));
#192610=CARTESIAN_POINT('Ctrl Pts',(-59.7799192536868,19.323604818559,40.0806684524227));
#192611=CARTESIAN_POINT('Ctrl Pts',(-59.7782286609225,19.3150373803111,
40.0767636676136));
#192612=CARTESIAN_POINT('Ctrl Pts',(-59.7759321681719,19.3068044648773,
40.0724404510887));
#192613=CARTESIAN_POINT('Ctrl Pts',(-59.7731456380807,19.2989322844405,
40.0677949937408));
#192614=CARTESIAN_POINT('Ctrl Pts',(-59.7717607402743,19.2950198323722,
40.0654862141905));
#192615=CARTESIAN_POINT('Ctrl Pts',(-59.7702542302926,19.2911962646694,
40.0630972003215));
#192616=CARTESIAN_POINT('Ctrl Pts',(-59.7686372707429,19.2874640247238,
40.0606363359906));
#192617=CARTESIAN_POINT('Ctrl Pts',(-59.7650700164609,19.2792301459421,
40.0552073017124));
#192618=CARTESIAN_POINT('Ctrl Pts',(-59.7609769706901,19.2714367138418,
40.0494204304519));
#192619=CARTESIAN_POINT('Ctrl Pts',(-59.7564706723511,19.2641757185816,
40.0434049749851));
#192620=CARTESIAN_POINT('Ctrl Pts',(-59.7548244647405,19.2615231854471,
40.0412074532442));
#192621=CARTESIAN_POINT('Ctrl Pts',(-59.7531276155318,19.2589351484759,
40.0389814735788));
#192622=CARTESIAN_POINT('Ctrl Pts',(-59.7513854342765,19.25641183575,40.0367321210017));
#192623=CARTESIAN_POINT('Ctrl Pts',(-59.7455336317917,19.247936295312,40.029176783714));
#192624=CARTESIAN_POINT('Ctrl Pts',(-59.7391263493543,19.2401420439521,
40.0213235332574));
#192625=CARTESIAN_POINT('Ctrl Pts',(-59.7322837268617,19.2329840462273,
40.0132649215856));
#192626=CARTESIAN_POINT('Ctrl Pts',(-59.7247628741805,19.2251165588073,
40.0044075527529));
#192627=CARTESIAN_POINT('Ctrl Pts',(-59.7167157560782,19.2180171087295,
39.9953016253715));
#192628=CARTESIAN_POINT('Ctrl Pts',(-59.7082546997634,19.2116502033068,
39.9860353422352));
#192629=CARTESIAN_POINT('Ctrl Pts',(-59.699141779585,19.2047927733664,39.9760551582687));
#192630=CARTESIAN_POINT('Ctrl Pts',(-59.6895478207,19.1987842816764,39.9658879738147));
#192631=CARTESIAN_POINT('Ctrl Pts',(-59.6795708632015,19.1936187207966,
39.9556174643244));
#192632=CARTESIAN_POINT('Ctrl Pts',(-59.6697286283157,19.1885229124297,
39.9454856413898));
#192633=CARTESIAN_POINT('Ctrl Pts',(-59.6595122814323,19.1842470541694,
39.935251946511));
#192634=CARTESIAN_POINT('Ctrl Pts',(-59.6489943884562,19.1808295835786,
39.92499));
#192635=CARTESIAN_POINT('Ctrl Pts',(-56.3771794532806,18.117752468711,39.92499));
#192636=CARTESIAN_POINT('Ctrl Pts',(-56.3671137719635,18.1144819305951,
39.9348107241734));
#192637=CARTESIAN_POINT('Ctrl Pts',(-56.3568263239548,18.1120170699777,
39.9446038383193));
#192638=CARTESIAN_POINT('Ctrl Pts',(-56.3463749453322,18.1103629196648,
39.9543158069419));
#192639=CARTESIAN_POINT('Ctrl Pts',(-56.3362832197197,18.1087656919991,
39.9636935671433));
#192640=CARTESIAN_POINT('Ctrl Pts',(-56.3260373921176,18.1079242184405,
39.9729968321037));
#192641=CARTESIAN_POINT('Ctrl Pts',(-56.3156801719786,18.1078879163651,
39.9821731151391));
#192642=CARTESIAN_POINT('Ctrl Pts',(-56.3058893552668,18.1078535995347,
39.9908475764413));
#192643=CARTESIAN_POINT('Ctrl Pts',(-56.2959980926866,18.1085387949872,
39.9994093733911));
#192644=CARTESIAN_POINT('Ctrl Pts',(-56.2860490151071,18.1100266905441,
40.0077966115911));
#192645=CARTESIAN_POINT('Ctrl Pts',(-56.2768860815648,18.1113970173906,
40.0155211172668));
#192646=CARTESIAN_POINT('Ctrl Pts',(-56.2676735798122,18.113448339867,40.0230979941098));
#192647=CARTESIAN_POINT('Ctrl Pts',(-56.2584600414581,18.1162805994807,
40.0304554104827));
#192648=CARTESIAN_POINT('Ctrl Pts',(-56.2557127503117,18.1171251221236,
40.0326492435233));
#192649=CARTESIAN_POINT('Ctrl Pts',(-56.252965504865,18.1180393245087,40.0348233715086));
#192650=CARTESIAN_POINT('Ctrl Pts',(-56.250219989383,18.1190265064344,40.0369753512356));
#192651=CARTESIAN_POINT('Ctrl Pts',(-56.2475025263004,18.1200036017945,
40.0391053430352));
#192652=CARTESIAN_POINT('Ctrl Pts',(-56.2447894850829,18.121050921242,40.041211089324));
#192653=CARTESIAN_POINT('Ctrl Pts',(-56.2420855046789,18.1221702476368,
40.0432881154904));
#192654=CARTESIAN_POINT('Ctrl Pts',(-56.2418974751697,18.1222480834052,
40.043432547828));
#192655=CARTESIAN_POINT('Ctrl Pts',(-56.241709480363,18.1223262596102,40.0435768364421));
#192656=CARTESIAN_POINT('Ctrl Pts',(-56.2415215209612,18.1224047773507,
40.0437209807855));
#192657=CARTESIAN_POINT('Ctrl Pts',(-56.233280692238,18.1258472827278,40.050040796842));
#192658=CARTESIAN_POINT('Ctrl Pts',(-56.2251347899175,18.1299826829659,
40.0560490279345));
#192659=CARTESIAN_POINT('Ctrl Pts',(-56.2171955585582,18.1348427679844,
40.0616647108616));
#192660=CARTESIAN_POINT('Ctrl Pts',(-56.2097948151022,18.1393732118987,
40.0668995033488));
#192661=CARTESIAN_POINT('Ctrl Pts',(-56.2025731376007,18.1445340001514,
40.0717933267484));
#192662=CARTESIAN_POINT('Ctrl Pts',(-56.1956479299625,18.1503626543107,
40.0762460303075));
#192663=CARTESIAN_POINT('Ctrl Pts',(-56.1931145994155,18.1524948514087,
40.077874886875));
#192664=CARTESIAN_POINT('Ctrl Pts',(-56.190621252949,18.1547164978844,40.0794443522248));
#192665=CARTESIAN_POINT('Ctrl Pts',(-56.1881748397224,18.1570296338741,
40.0809482021492));
#192666=CARTESIAN_POINT('Ctrl Pts',(-56.1875865590688,18.1575858658046,
40.0813098278169));
#192667=CARTESIAN_POINT('Ctrl Pts',(-56.1870008763866,18.158147960355,40.0816679525672));
#192668=CARTESIAN_POINT('Ctrl Pts',(-56.186417921567,18.1587158783117,40.0820224192581));
#192669=CARTESIAN_POINT('Ctrl Pts',(-56.1858531840856,18.1592660488322,
40.0823658088648));
#192670=CARTESIAN_POINT('Ctrl Pts',(-56.1852910066464,18.1598216844589,
40.0827057654617));
#192671=CARTESIAN_POINT('Ctrl Pts',(-56.1847315084903,18.1603827459288,
40.0830421470151));
#192672=CARTESIAN_POINT('Ctrl Pts',(-56.1786015595925,18.166529822736,40.0867275956805));
#192673=CARTESIAN_POINT('Ctrl Pts',(-56.172789482861,18.1733325302111,40.0899823432029));
#192674=CARTESIAN_POINT('Ctrl Pts',(-56.1674665972294,18.1807122308847,
40.0926299529354));
#192675=CARTESIAN_POINT('Ctrl Pts',(-56.1652590378995,18.1837728127196,
40.0937279956083));
#192676=CARTESIAN_POINT('Ctrl Pts',(-56.1631354730307,18.1869322368374,
40.0947220371802));
#192677=CARTESIAN_POINT('Ctrl Pts',(-56.1611070880437,18.1901833857457,
40.0956014538693));
#192678=CARTESIAN_POINT('Ctrl Pts',(-56.1576474660759,18.195728559002,40.097101390674));
#192679=CARTESIAN_POINT('Ctrl Pts',(-56.1544671656476,18.2015400422207,
40.0982667904316));
#192680=CARTESIAN_POINT('Ctrl Pts',(-56.1516266854594,18.2075773774756,
40.0990539325583));
#192681=CARTESIAN_POINT('Ctrl Pts',(-56.1502064453653,18.210596045103,40.0994475036216));
#192682=CARTESIAN_POINT('Ctrl Pts',(-56.1488725139552,18.2136716866513,
40.0997467259952));
#192683=CARTESIAN_POINT('Ctrl Pts',(-56.1476325143034,18.21679921973,40.0999473488896));
#192684=CARTESIAN_POINT('Ctrl Pts',(-56.1463925146515,18.2199267528086,
40.100147971784));
#192685=CARTESIAN_POINT('Ctrl Pts',(-56.145246443375,18.2231061318824,40.10025));
#192686=CARTESIAN_POINT('Ctrl Pts',(-56.1441998575526,18.2263320786586,
40.10025));
#192687=CARTESIAN_POINT('Origin',(-53.2204057122636,23.7119335237429,39.92499));
#192688=CARTESIAN_POINT('Ctrl Pts',(-57.1623216544369,25.6588335304445,
39.92499));
#192689=CARTESIAN_POINT('Ctrl Pts',(-57.1720146727776,25.663149140257,39.9348354642022));
#192690=CARTESIAN_POINT('Ctrl Pts',(-57.1820194461954,25.6666871334687,
39.9446440828466));
#192691=CARTESIAN_POINT('Ctrl Pts',(-57.1922776320703,25.6694381454822,
39.9543641760342));
#192692=CARTESIAN_POINT('Ctrl Pts',(-57.2022024879877,25.6720997659864,
39.9637684240726));
#192693=CARTESIAN_POINT('Ctrl Pts',(-57.2123658169602,25.6740249857413,
39.9730909636411));
#192694=CARTESIAN_POINT('Ctrl Pts',(-57.2227298227166,25.6751616470872,
39.9822808977157));
#192695=CARTESIAN_POINT('Ctrl Pts',(-57.2325335339835,25.6762368587288,
39.9909740094667));
#192696=CARTESIAN_POINT('Ctrl Pts',(-57.242517732291,25.6766065729231,39.9995492765019));
#192697=CARTESIAN_POINT('Ctrl Pts',(-57.2526488462854,25.6761845643575,
40.0079462328713));
#192698=CARTESIAN_POINT('Ctrl Pts',(-57.261980334975,25.6757958639482,40.0156804369709));
#192699=CARTESIAN_POINT('Ctrl Pts',(-57.2714370189575,25.6747354076183,
40.0232638017442));
#192700=CARTESIAN_POINT('Ctrl Pts',(-57.2809814365685,25.6728992535086,
40.0306257269986));
#192701=CARTESIAN_POINT('Ctrl Pts',(-57.283749909306,25.672366654999,40.0327611416665));
#192702=CARTESIAN_POINT('Ctrl Pts',(-57.2865256584303,25.6717685445833,
40.0348777427277));
#192703=CARTESIAN_POINT('Ctrl Pts',(-57.2893074725858,25.6711017521909,
40.0369733168701));
#192704=CARTESIAN_POINT('Ctrl Pts',(-57.2923231379853,25.6703789063666,
40.039245053974));
#192705=CARTESIAN_POINT('Ctrl Pts',(-57.2953419866641,25.6695773996878,
40.041487875195));
#192706=CARTESIAN_POINT('Ctrl Pts',(-57.2983617649662,25.6686939261491,
40.0436985701601));
#192707=CARTESIAN_POINT('Ctrl Pts',(-57.3066495702121,25.6662692260898,
40.0497658398386));
#192708=CARTESIAN_POINT('Ctrl Pts',(-57.3149216961104,25.6631888860749,
40.0555581699984));
#192709=CARTESIAN_POINT('Ctrl Pts',(-57.3230760282578,25.6594348051811,
40.0609828468886));
#192710=CARTESIAN_POINT('Ctrl Pts',(-57.3305367994637,25.6560000249771,
40.0659461317305));
#192711=CARTESIAN_POINT('Ctrl Pts',(-57.3378885241129,25.651996242513,40.0706039980707));
#192712=CARTESIAN_POINT('Ctrl Pts',(-57.3450563828669,25.647375921998,40.0748843180603));
#192713=CARTESIAN_POINT('Ctrl Pts',(-57.3485772116719,25.6451064356539,
40.076986797257));
#192714=CARTESIAN_POINT('Ctrl Pts',(-57.3520532672061,25.6426878935086,
40.0789976708175));
#192715=CARTESIAN_POINT('Ctrl Pts',(-57.3554727521279,25.6401130415751,
40.08090504915));
#192716=CARTESIAN_POINT('Ctrl Pts',(-57.3561215660856,25.6396244885001,
40.0812669556104));
#192717=CARTESIAN_POINT('Ctrl Pts',(-57.3567684269675,25.6391297826976,
40.0816253922032));
#192718=CARTESIAN_POINT('Ctrl Pts',(-57.357413196712,25.6386289474847,40.0819801989139));
#192719=CARTESIAN_POINT('Ctrl Pts',(-57.358037817402,25.6381437633723,40.0823239179149));
#192720=CARTESIAN_POINT('Ctrl Pts',(-57.3586604755989,25.6376528269752,
40.0826642303498));
#192721=CARTESIAN_POINT('Ctrl Pts',(-57.3592810442413,25.6371561630119,
40.0830009916099));
#192722=CARTESIAN_POINT('Ctrl Pts',(-57.3660438734347,25.6317436214794,
40.0866709464312));
#192723=CARTESIAN_POINT('Ctrl Pts',(-57.3725627409494,25.6256469885832,
40.0899175831878));
#192724=CARTESIAN_POINT('Ctrl Pts',(-57.3786559602404,25.6189233999297,
40.0925642067062));
#192725=CARTESIAN_POINT('Ctrl Pts',(-57.381229164584,25.6160839866899,40.0936818922528));
#192726=CARTESIAN_POINT('Ctrl Pts',(-57.3837265592142,25.6131331854695,
40.094693009479));
#192727=CARTESIAN_POINT('Ctrl Pts',(-57.386135383163,25.6100770039416,40.0955863397546));
#192728=CARTESIAN_POINT('Ctrl Pts',(-57.3901917825029,25.6049304706143,
40.0970906856166));
#192729=CARTESIAN_POINT('Ctrl Pts',(-57.3939944983912,25.5994853721133,
40.0982599215483));
#192730=CARTESIAN_POINT('Ctrl Pts',(-57.3974772155309,25.5937750303534,
40.0990497370454));
#192731=CARTESIAN_POINT('Ctrl Pts',(-57.3983478948158,25.5923474449134,
40.0992471909196));
#192732=CARTESIAN_POINT('Ctrl Pts',(-57.3991983668797,25.5909031732845,
40.0994209989363));
#192733=CARTESIAN_POINT('Ctrl Pts',(-57.4000273167764,25.5894426040346,
40.0995705982975));
#192734=CARTESIAN_POINT('Ctrl Pts',(-57.4012707416213,25.5872517501599,
40.0997949973393));
#192735=CARTESIAN_POINT('Ctrl Pts',(-57.4024657229506,25.5850242354389,
40.0999649129781));
#192736=CARTESIAN_POINT('Ctrl Pts',(-57.4036093482793,25.5827620706102,
40.1000786629733));
#192737=CARTESIAN_POINT('Ctrl Pts',(-57.404752973608,25.5804999057814,40.1001924129685));
#192738=CARTESIAN_POINT('Ctrl Pts',(-57.4058452484194,25.5782031010735,
40.10025));
#192739=CARTESIAN_POINT('Ctrl Pts',(-57.4068835917977,25.5758735661212,
40.10025));
#192740=CARTESIAN_POINT('Ctrl Pts',(-53.9190682401993,24.0229981225301,
40.10025));
#192741=CARTESIAN_POINT('Ctrl Pts',(-53.9155545931357,24.030880455519,40.10025));
#192742=CARTESIAN_POINT('Ctrl Pts',(-53.9127220553015,24.038984503472,40.0995786334241));
#192743=CARTESIAN_POINT('Ctrl Pts',(-53.9105453488013,24.047161284638,40.0983063763367));
#192744=CARTESIAN_POINT('Ctrl Pts',(-53.9091394197451,24.0524426462852,
40.0974846287993));
#192745=CARTESIAN_POINT('Ctrl Pts',(-53.9080061861137,24.0577541205278,
40.0964130309338));
#192746=CARTESIAN_POINT('Ctrl Pts',(-53.907129996454,24.0630550795266,40.0951176960924));
#192747=CARTESIAN_POINT('Ctrl Pts',(-53.9059686572513,24.0700811970216,
40.0934008039614));
#192748=CARTESIAN_POINT('Ctrl Pts',(-53.9052646847384,24.077088606661,40.0912909372157));
#192749=CARTESIAN_POINT('Ctrl Pts',(-53.9049900928803,24.0839917000397,
40.0888630467852));
#192750=CARTESIAN_POINT('Ctrl Pts',(-53.9048527969512,24.087443246729,40.0876491015699));
#192751=CARTESIAN_POINT('Ctrl Pts',(-53.9048227635321,24.0908688957003,
40.0863558569271));
#192752=CARTESIAN_POINT('Ctrl Pts',(-53.9048959123381,24.0942592346733,
40.0849936342771));
#192753=CARTESIAN_POINT('Ctrl Pts',(-53.9049324867411,24.0959544041598,
40.0843125229521));
#192754=CARTESIAN_POINT('Ctrl Pts',(-53.9049948499726,24.0976407611374,
40.0836141747074));
#192755=CARTESIAN_POINT('Ctrl Pts',(-53.905082449642,24.0993172231362,40.082899916161));
#192756=CARTESIAN_POINT('Ctrl Pts',(-53.9051043495593,24.0997363386359,
40.0827213515244));
#192757=CARTESIAN_POINT('Ctrl Pts',(-53.90512782661,24.1001548360178,40.0825417925842));
#192758=CARTESIAN_POINT('Ctrl Pts',(-53.9051528718721,24.1005726990104,
40.0823612602361));
#192759=CARTESIAN_POINT('Ctrl Pts',(-53.9052280076583,24.1018262879883,
40.0818196631918));
#192760=CARTESIAN_POINT('Ctrl Pts',(-53.9053172580726,24.103074165876,40.0812693052022));
#192761=CARTESIAN_POINT('Ctrl Pts',(-53.9054203757495,24.1043159075204,
40.0807107531875));
#192762=CARTESIAN_POINT('Ctrl Pts',(-53.9061467233509,24.1130625753261,
40.0767763849182));
#192763=CARTESIAN_POINT('Ctrl Pts',(-53.9075195712147,24.1215389842448,
40.0724140586138));
#192764=CARTESIAN_POINT('Ctrl Pts',(-53.909426512903,24.1297041260872,40.0677221223768));
#192765=CARTESIAN_POINT('Ctrl Pts',(-53.9103513775611,24.1336642110574,
40.0654465383721));
#192766=CARTESIAN_POINT('Ctrl Pts',(-53.9114023832598,24.1375513523938,
40.0630928000679));
#192767=CARTESIAN_POINT('Ctrl Pts',(-53.9125693701069,24.1413619171795,
40.0606689262479));
#192768=CARTESIAN_POINT('Ctrl Pts',(-53.9143559454348,24.1471956256299,
40.0569581447806));
#192769=CARTESIAN_POINT('Ctrl Pts',(-53.9164123347818,24.1528469606268,
40.0530843804606));
#192770=CARTESIAN_POINT('Ctrl Pts',(-53.9187002605237,24.1582902100543,
40.0490800251458));
#192771=CARTESIAN_POINT('Ctrl Pts',(-53.9197627850744,24.1608180832481,
40.0472203818218));
#192772=CARTESIAN_POINT('Ctrl Pts',(-53.9208749910656,24.1633010951267,
40.0453323608819));
#192773=CARTESIAN_POINT('Ctrl Pts',(-53.9220340502325,24.1657359576698,
40.0434201572162));
#192774=CARTESIAN_POINT('Ctrl Pts',(-53.9221228875507,24.1659225802899,
40.0432735943397));
#192775=CARTESIAN_POINT('Ctrl Pts',(-53.9222119774186,24.1661089452651,
40.0431268995707));
#192776=CARTESIAN_POINT('Ctrl Pts',(-53.9223013184208,24.1662950522346,
40.0429800745037));
#192777=CARTESIAN_POINT('Ctrl Pts',(-53.9235562901481,24.1689092940619,
40.0409176249753));
#192778=CARTESIAN_POINT('Ctrl Pts',(-53.9248627542248,24.1714718460795,
40.0388310783333));
#192779=CARTESIAN_POINT('Ctrl Pts',(-53.9262153118346,24.1739808617164,
40.036725739981));
#192780=CARTESIAN_POINT('Ctrl Pts',(-53.9310653428793,24.1829777455765,
40.0291763710719));
#192781=CARTESIAN_POINT('Ctrl Pts',(-53.9365438157565,24.1913567365397,
40.0213310894597));
#192782=CARTESIAN_POINT('Ctrl Pts',(-53.9425259106377,24.1991508947535,
40.0132837551323));
#192783=CARTESIAN_POINT('Ctrl Pts',(-53.9490996319574,24.2077158916377,
40.0044405431331));
#192784=CARTESIAN_POINT('Ctrl Pts',(-53.9562817849765,24.2155752681661,
39.995352871061));
#192785=CARTESIAN_POINT('Ctrl Pts',(-53.9639562340132,24.222754058492,39.9861103629567));
#192786=CARTESIAN_POINT('Ctrl Pts',(-53.972242712949,24.2305053504132,39.9761307737573));
#192787=CARTESIAN_POINT('Ctrl Pts',(-53.9811038680465,24.2374640812918,
39.9659696936033));
#192788=CARTESIAN_POINT('Ctrl Pts',(-53.9904403792137,24.2436285779114,
39.9557128217533));
#192789=CARTESIAN_POINT('Ctrl Pts',(-53.9996985666468,24.2497413607391,
39.9455419945179));
#192790=CARTESIAN_POINT('Ctrl Pts',(-54.0094254978892,24.2550737197504,
39.935275628935));
#192791=CARTESIAN_POINT('Ctrl Pts',(-54.0195518809639,24.2595822759737,
39.92499));
#192792=CARTESIAN_POINT('Origin',(-0.00619866644046454,-0.0139224327744755,
39.92499));
#192793=CARTESIAN_POINT('Ctrl Pts',(-57.4192809246787,25.5480287005723,
40.10025));
#192794=CARTESIAN_POINT('Ctrl Pts',(-57.4227710771204,25.5401808584719,
40.10025));
#192795=CARTESIAN_POINT('Ctrl Pts',(-57.4255746438788,25.53211120635,40.0995859581841));
#192796=CARTESIAN_POINT('Ctrl Pts',(-57.4277200319916,25.5239679177298,
40.0983275959618));
#192797=CARTESIAN_POINT('Ctrl Pts',(-57.4290908328637,25.5187647439658,
40.0975235624066));
#192798=CARTESIAN_POINT('Ctrl Pts',(-57.4301938346425,25.5135317242467,
40.0964777059489));
#192799=CARTESIAN_POINT('Ctrl Pts',(-57.4310450321039,25.5083079410952,
40.0952149915961));
#192800=CARTESIAN_POINT('Ctrl Pts',(-57.4322067458447,25.5011785252537,
40.0934916398701));
#192801=CARTESIAN_POINT('Ctrl Pts',(-57.4328933558605,25.4940667032542,
40.0913643921631));
#192802=CARTESIAN_POINT('Ctrl Pts',(-57.4331362848726,25.4870628291429,
40.0889118607713));
#192803=CARTESIAN_POINT('Ctrl Pts',(-57.4332577493786,25.4835608920873,
40.0876855950754));
#192804=CARTESIAN_POINT('Ctrl Pts',(-57.4332683803239,25.4800857520067,
40.0863782327526));
#192805=CARTESIAN_POINT('Ctrl Pts',(-57.4331727200756,25.4766473428563,
40.0850006373334));
#192806=CARTESIAN_POINT('Ctrl Pts',(-57.4331248899515,25.4749281382812,
40.0843118396237));
#192807=CARTESIAN_POINT('Ctrl Pts',(-57.433050494158,25.4732181005509,40.0836054919164));
#192808=CARTESIAN_POINT('Ctrl Pts',(-57.4329501454092,25.4715183716229,
40.0828829920417));
#192809=CARTESIAN_POINT('Ctrl Pts',(-57.4329250582221,25.4710934393909,
40.0827023670731));
#192810=CARTESIAN_POINT('Ctrl Pts',(-57.432898349128,25.470669151121,40.0825207326933));
#192811=CARTESIAN_POINT('Ctrl Pts',(-57.4328700280094,25.4702455239748,
40.0823381109275));
#192812=CARTESIAN_POINT('Ctrl Pts',(-57.4327850646537,25.468974642536,40.0817902456303));
#192813=CARTESIAN_POINT('Ctrl Pts',(-57.4326855923069,25.467709712894,40.0812334935553));
#192814=CARTESIAN_POINT('Ctrl Pts',(-57.4325718846635,25.4664511833531,
40.0806684524227));
#192815=CARTESIAN_POINT('Ctrl Pts',(-57.4317860942974,25.4577539633646,
40.0767636676136));
#192816=CARTESIAN_POINT('Ctrl Pts',(-57.430362755973,25.4493260998447,40.0724404510886));
#192817=CARTESIAN_POINT('Ctrl Pts',(-57.4284143577087,25.4412057723275,
40.0677949937405));
#192818=CARTESIAN_POINT('Ctrl Pts',(-57.4274460091197,25.4371699918417,
40.0654862141903));
#192819=CARTESIAN_POINT('Ctrl Pts',(-57.4263474236136,25.4332098968697,
40.0630972003214));
#192820=CARTESIAN_POINT('Ctrl Pts',(-57.4251294472435,25.4293290842283,
40.0606363359906));
#192821=CARTESIAN_POINT('Ctrl Pts',(-57.4224424094495,25.4207674318879,
40.0552073017123));
#192822=CARTESIAN_POINT('Ctrl Pts',(-57.4191864212927,25.4125888532395,
40.0494204304519));
#192823=CARTESIAN_POINT('Ctrl Pts',(-57.4154637896039,25.4048965980308,
40.0434049749851));
#192824=CARTESIAN_POINT('Ctrl Pts',(-57.4141038653031,25.4020865201986,
40.0412074532442));
#192825=CARTESIAN_POINT('Ctrl Pts',(-57.4126868351393,25.3993352917245,
40.0389814735788));
#192826=CARTESIAN_POINT('Ctrl Pts',(-57.4112179557368,25.3966436944403,
40.0367321210017));
#192827=CARTESIAN_POINT('Ctrl Pts',(-57.4062841452556,25.3876029039784,
40.0291767837139));
#192828=CARTESIAN_POINT('Ctrl Pts',(-57.4007266836985,25.3791816069559,
40.0213235332573));
#192829=CARTESIAN_POINT('Ctrl Pts',(-57.39466976031,25.3713475726776,40.0132649215853));
#192830=CARTESIAN_POINT('Ctrl Pts',(-57.3880124840164,25.3627370410035,
40.0044075527525));
#192831=CARTESIAN_POINT('Ctrl Pts',(-57.3807515434754,25.3548353295669,
39.995301625371));
#192832=CARTESIAN_POINT('Ctrl Pts',(-57.3730023605519,25.3476188815041,
39.9860353422346));
#192833=CARTESIAN_POINT('Ctrl Pts',(-57.3646561585171,25.3398464577401,
39.9760551582679));
#192834=CARTESIAN_POINT('Ctrl Pts',(-57.3557428147453,25.3328680394173,
39.9658879738137));
#192835=CARTESIAN_POINT('Ctrl Pts',(-57.3463604602045,25.326687899985,39.9556174643232));
#192836=CARTESIAN_POINT('Ctrl Pts',(-57.3371047991293,25.3205912133023,
39.945485641389));
#192837=CARTESIAN_POINT('Ctrl Pts',(-57.3273913673568,25.3152708796013,
39.9352519465106));
#192838=CARTESIAN_POINT('Ctrl Pts',(-57.3172883154488,25.3107727110827,
39.92499));
#192839=CARTESIAN_POINT('Ctrl Pts',(-54.1745185419758,23.9115214566119,
39.92499));
#192840=CARTESIAN_POINT('Ctrl Pts',(-54.164849865839,23.9072166846468,39.9348107241718));
#192841=CARTESIAN_POINT('Ctrl Pts',(-54.154876421641,23.903689995663,39.9446038383162));
#192842=CARTESIAN_POINT('Ctrl Pts',(-54.144655202556,23.9009524404123,39.9543158069373));
#192843=CARTESIAN_POINT('Ctrl Pts',(-54.1347857162268,23.8983090899569,
39.9636935671377));
#192844=CARTESIAN_POINT('Ctrl Pts',(-54.1246839742795,23.8964012454643,
39.9729968320972));
#192845=CARTESIAN_POINT('Ctrl Pts',(-54.1143872866774,23.8952825179503,
39.9821731151316));
#192846=CARTESIAN_POINT('Ctrl Pts',(-54.1046536921704,23.8942249700858,
39.9908475764331));
#192847=CARTESIAN_POINT('Ctrl Pts',(-54.0947449925347,23.8938724934881,
39.9994093733825));
#192848=CARTESIAN_POINT('Ctrl Pts',(-54.084694889608,23.8943122764065,40.0077966115819));
#192849=CARTESIAN_POINT('Ctrl Pts',(-54.0754389134156,23.8947173090964,
40.0155211172572));
#192850=CARTESIAN_POINT('Ctrl Pts',(-54.0660624571261,23.8957944255618,
40.0230979940999));
#192851=CARTESIAN_POINT('Ctrl Pts',(-54.0566033397549,23.8976480927548,
40.0304554104726));
#192852=CARTESIAN_POINT('Ctrl Pts',(-54.0537828218984,23.8982008188933,
40.0326492435166));
#192853=CARTESIAN_POINT('Ctrl Pts',(-54.050955065975,23.8988228478381,40.0348233715053));
#192854=CARTESIAN_POINT('Ctrl Pts',(-54.0481214021001,23.8995176373648,
40.0369753512355));
#192855=CARTESIAN_POINT('Ctrl Pts',(-54.0453166912881,23.9002053278543,
40.0391053430352));
#192856=CARTESIAN_POINT('Ctrl Pts',(-54.0425090377018,23.900963319947,40.041211089324));
#192857=CARTESIAN_POINT('Ctrl Pts',(-54.0397028685175,23.9017938716384,
40.0432881154904));
#192858=CARTESIAN_POINT('Ctrl Pts',(-54.0395077330004,23.9018516265787,
40.043432547828));
#192859=CARTESIAN_POINT('Ctrl Pts',(-54.0393125964103,23.901909723718,40.0435768364421));
#192860=CARTESIAN_POINT('Ctrl Pts',(-54.039117459331,23.9019681642227,40.0437209807855));
#192861=CARTESIAN_POINT('Ctrl Pts',(-54.0305619349331,23.9045304100326,
40.0500407968419));
#192862=CARTESIAN_POINT('Ctrl Pts',(-54.0220283896861,23.9077916774639,
40.0560490279344));
#192863=CARTESIAN_POINT('Ctrl Pts',(-54.0136246330487,23.9117952627745,
40.0616647108613));
#192864=CARTESIAN_POINT('Ctrl Pts',(-54.0057908712997,23.9155273001024,
40.0668995033483));
#192865=CARTESIAN_POINT('Ctrl Pts',(-53.9980693056381,23.9199049461654,
40.0717933267479));
#192866=CARTESIAN_POINT('Ctrl Pts',(-53.9905727747499,23.9249777890349,
40.0762460303068));
#192867=CARTESIAN_POINT('Ctrl Pts',(-53.9878304467663,23.9268335005853,
40.0778748868746));
#192868=CARTESIAN_POINT('Ctrl Pts',(-53.9851185338202,23.9287823509749,
40.0794443522246));
#192869=CARTESIAN_POINT('Ctrl Pts',(-53.9824437337505,23.9308270955488,
40.0809482021492));
#192870=CARTESIAN_POINT('Ctrl Pts',(-53.981800533691,23.9313187883098,40.0813098278169));
#192871=CARTESIAN_POINT('Ctrl Pts',(-53.9811593045603,23.9318165831368,
40.0816679525672));
#192872=CARTESIAN_POINT('Ctrl Pts',(-53.9805201796369,23.932320454608,40.0820224192581));
#192873=CARTESIAN_POINT('Ctrl Pts',(-53.9799010273675,23.9328085800958,
40.0823658088648));
#192874=CARTESIAN_POINT('Ctrl Pts',(-53.9792838498569,23.9333024083486,
40.0827057654617));
#192875=CARTESIAN_POINT('Ctrl Pts',(-53.9786687697969,23.9338019127826,
40.0830421470151));
#192876=CARTESIAN_POINT('Ctrl Pts',(-53.9719298569082,23.9392745611218,
40.0867275956807));
#192877=CARTESIAN_POINT('Ctrl Pts',(-53.9654385427826,23.9454324752047,
40.0899823432031));
#192878=CARTESIAN_POINT('Ctrl Pts',(-53.9593734277044,23.9522153560508,
40.0926299529356));
#192879=CARTESIAN_POINT('Ctrl Pts',(-53.9568580436998,23.9550284189137,
40.0937279956085));
#192880=CARTESIAN_POINT('Ctrl Pts',(-53.9544158621939,23.9579485624031,
40.0947220371803));
#192881=CARTESIAN_POINT('Ctrl Pts',(-53.952058751313,23.9609698772116,40.0956014538693));
#192882=CARTESIAN_POINT('Ctrl Pts',(-53.9480384530773,23.9661230444609,
40.097101390674));
#192883=CARTESIAN_POINT('Ctrl Pts',(-53.9442681092574,23.9715702598499,
40.0982667904316));
#192884=CARTESIAN_POINT('Ctrl Pts',(-53.9408121161402,23.9772776109215,
40.0990539325583));
#192885=CARTESIAN_POINT('Ctrl Pts',(-53.9390841195816,23.9801312864573,
40.0994475036216));
#192886=CARTESIAN_POINT('Ctrl Pts',(-53.9374360035028,23.983050645519,40.0997467259952));
#192887=CARTESIAN_POINT('Ctrl Pts',(-53.9358758804723,23.9860314303861,
40.0999473488896));
#192888=CARTESIAN_POINT('Ctrl Pts',(-53.9343157574418,23.9890122152533,
40.100147971784));
#192889=CARTESIAN_POINT('Ctrl Pts',(-53.9328436288551,23.9920543802865,
40.10025));
#192890=CARTESIAN_POINT('Ctrl Pts',(-53.9314655730802,23.9951532569811,
40.10025));
#192891=CARTESIAN_POINT('Origin',(-50.4502867888873,29.1450842944633,39.92499));
#192892=CARTESIAN_POINT('Ctrl Pts',(-54.1671020372436,31.4933613949863,
39.92499));
#192893=CARTESIAN_POINT('Ctrl Pts',(-54.1762908521541,31.4986665597485,
39.9348354642022));
#192894=CARTESIAN_POINT('Ctrl Pts',(-54.185870997383,31.503230955054,39.9446440828465));
#192895=CARTESIAN_POINT('Ctrl Pts',(-54.1957854287843,31.5070391691412,
39.9543641760342));
#192896=CARTESIAN_POINT('Ctrl Pts',(-54.2053777002016,31.5107236389471,
39.9637684240726));
#192897=CARTESIAN_POINT('Ctrl Pts',(-54.2152841131322,31.5137006693058,
39.9730909636412));
#192898=CARTESIAN_POINT('Ctrl Pts',(-54.225472530317,31.5159144374969,39.982280897716));
#192899=CARTESIAN_POINT('Ctrl Pts',(-54.2351101456073,31.5180085258897,
39.9909740094671));
#192900=CARTESIAN_POINT('Ctrl Pts',(-54.2450010037753,31.5194198476569,
39.9995492765025));
#192901=CARTESIAN_POINT('Ctrl Pts',(-54.2551207303742,31.5200591406754,
40.0079462328721));
#192902=CARTESIAN_POINT('Ctrl Pts',(-54.264441730449,31.5206479757802,40.0156804369718));
#192903=CARTESIAN_POINT('Ctrl Pts',(-54.2739574575979,31.5205818213853,
40.0232638017453));
#192904=CARTESIAN_POINT('Ctrl Pts',(-54.2836415202582,31.5197533892255,
40.0306257269999));
#192905=CARTESIAN_POINT('Ctrl Pts',(-54.2864504987155,31.5195130925471,
40.0327611416674));
#192906=CARTESIAN_POINT('Ctrl Pts',(-54.2892735615578,31.5192084034332,
40.0348777427282));
#192907=CARTESIAN_POINT('Ctrl Pts',(-54.2921098354277,31.5188360425582,
40.0369733168701));
#192908=CARTESIAN_POINT('Ctrl Pts',(-54.2951845386599,31.5184323794289,
40.039245053974));
#192909=CARTESIAN_POINT('Ctrl Pts',(-54.2982706300311,31.5179508191008,
40.041487875195));
#192910=CARTESIAN_POINT('Ctrl Pts',(-54.301366213803,31.5173878381079,40.0436985701601));
#192911=CARTESIAN_POINT('Ctrl Pts',(-54.3098620677557,31.5158427323554,
40.0497658398386));
#192912=CARTESIAN_POINT('Ctrl Pts',(-54.3184108612909,31.5136439393736,
40.0555581699984));
#192913=CARTESIAN_POINT('Ctrl Pts',(-54.3269129314605,31.5107627835361,
40.0609828468885));
#192914=CARTESIAN_POINT('Ctrl Pts',(-54.3346918640774,31.5081266823664,
40.0659461317304));
#192915=CARTESIAN_POINT('Ctrl Pts',(-54.3424218244378,31.5049132975215,
40.0706039980706));
#192916=CARTESIAN_POINT('Ctrl Pts',(-54.3500333719147,31.5010675328662,
40.0748843180602));
#192917=CARTESIAN_POINT('Ctrl Pts',(-54.3537721391712,31.4991785058302,
40.0769867972569));
#192918=CARTESIAN_POINT('Ctrl Pts',(-54.3574819590034,31.497136559455,40.0789976708174));
#192919=CARTESIAN_POINT('Ctrl Pts',(-54.3611518569448,31.4949332463338,
40.08090504915));
#192920=CARTESIAN_POINT('Ctrl Pts',(-54.3618481843339,31.4945151891296,
40.0812669556105));
#192921=CARTESIAN_POINT('Ctrl Pts',(-54.3625432124815,31.4940908087512,
40.0816253922032));
#192922=CARTESIAN_POINT('Ctrl Pts',(-54.3632368016451,31.4936601139566,
40.0819801989139));
#192923=CARTESIAN_POINT('Ctrl Pts',(-54.3639087161472,31.4932428783743,
40.0823239179149));
#192924=CARTESIAN_POINT('Ctrl Pts',(-54.3645792801846,31.4928197168827,
40.0826642303498));
#192925=CARTESIAN_POINT('Ctrl Pts',(-54.3652483648078,31.492390640783,40.0830009916099));
#192926=CARTESIAN_POINT('Ctrl Pts',(-54.3725399111639,31.4877146578623,
40.0866709464311));
#192927=CARTESIAN_POINT('Ctrl Pts',(-54.3796603393079,31.4823328301627,
40.0899175831876));
#192928=CARTESIAN_POINT('Ctrl Pts',(-54.3864229856956,31.4762829888804,
40.0925642067061));
#192929=CARTESIAN_POINT('Ctrl Pts',(-54.3892788932592,31.473728103339,40.0936818922527));
#192930=CARTESIAN_POINT('Ctrl Pts',(-54.3920710496174,31.4710545157392,
40.094693009479));
#192931=CARTESIAN_POINT('Ctrl Pts',(-54.3947861357353,31.468266866959,40.0955863397546));
#192932=CARTESIAN_POINT('Ctrl Pts',(-54.399358272915,31.4635725360691,40.0970906856166));
#192933=CARTESIAN_POINT('Ctrl Pts',(-54.4037093249065,31.4585547584355,
40.0982599215483));
#192934=CARTESIAN_POINT('Ctrl Pts',(-54.4077698566062,31.4532397415958,
40.0990497370454));
#192935=CARTESIAN_POINT('Ctrl Pts',(-54.4087849895311,31.4519109873859,
40.0992471909196));
#192936=CARTESIAN_POINT('Ctrl Pts',(-54.4097817701139,31.450563526166,40.0994209989363));
#192937=CARTESIAN_POINT('Ctrl Pts',(-54.4107588499955,31.4491976069261,
40.0995705982975));
#192938=CARTESIAN_POINT('Ctrl Pts',(-54.4122244698178,31.4471487280664,
40.0997949973393));
#192939=CARTESIAN_POINT('Ctrl Pts',(-54.4136457436051,31.4450583254661,
40.0999649129781));
#192940=CARTESIAN_POINT('Ctrl Pts',(-54.4150195646478,31.4429280944112,
40.1000786629733));
#192941=CARTESIAN_POINT('Ctrl Pts',(-54.4163933856905,31.4407978633562,
40.1001924129685));
#192942=CARTESIAN_POINT('Ctrl Pts',(-54.4177197583742,31.4386278145932,
40.10025));
#192943=CARTESIAN_POINT('Ctrl Pts',(-54.4189959163076,31.4364195775148,
40.10025));
#192944=CARTESIAN_POINT('Ctrl Pts',(-51.1126068659044,29.5274749692189,
40.10025));
#192945=CARTESIAN_POINT('Ctrl Pts',(-51.1082885388128,29.534946845835,40.10025));
#192946=CARTESIAN_POINT('Ctrl Pts',(-51.1046244142384,29.5427104181386,
40.0995786334241));
#192947=CARTESIAN_POINT('Ctrl Pts',(-51.1016049255944,29.5506148782564,
40.0983063763366));
#192948=CARTESIAN_POINT('Ctrl Pts',(-51.0996546457477,29.5557203484481,
40.0974846287992));
#192949=CARTESIAN_POINT('Ctrl Pts',(-51.0979724198485,29.5608842707089,
40.0964130309338));
#192950=CARTESIAN_POINT('Ctrl Pts',(-51.0965469289494,29.5660646037408,
40.0951176960923));
#192951=CARTESIAN_POINT('Ctrl Pts',(-51.09465752242,29.5729308384269,40.0934008039614));
#192952=CARTESIAN_POINT('Ctrl Pts',(-51.0932249325811,29.5798262755782,
40.0912909372156));
#192953=CARTESIAN_POINT('Ctrl Pts',(-51.0922302752232,29.586662850424,40.0888630467851));
#192954=CARTESIAN_POINT('Ctrl Pts',(-51.0917329465443,29.590081137847,40.0876491015698));
#192955=CARTESIAN_POINT('Ctrl Pts',(-51.0913449998287,29.5934848814077,
40.0863558569271));
#192956=CARTESIAN_POINT('Ctrl Pts',(-51.0910633609951,29.5968642938813,
40.0849936342771));
#192957=CARTESIAN_POINT('Ctrl Pts',(-51.0909225415783,29.5985540001181,
40.084312522952));
#192958=CARTESIAN_POINT('Ctrl Pts',(-51.0908082908741,29.6002376377885,
40.0836141747074));
#192959=CARTESIAN_POINT('Ctrl Pts',(-51.0907201726668,29.6019140726119,
40.0828999161609));
#192960=CARTESIAN_POINT('Ctrl Pts',(-51.090698143115,29.6023331813177,40.0827213515243));
#192961=CARTESIAN_POINT('Ctrl Pts',(-51.0906777466678,29.6027518401473,
40.0825417925841));
#192962=CARTESIAN_POINT('Ctrl Pts',(-51.0906589761528,29.6031700319854,
40.082361260236));
#192963=CARTESIAN_POINT('Ctrl Pts',(-51.0906026646079,29.6044246075,40.0818196631917));
#192964=CARTESIAN_POINT('Ctrl Pts',(-51.0905609873411,29.6056749785907,
40.0812693052021));
#192965=CARTESIAN_POINT('Ctrl Pts',(-51.0905337427828,29.6069206965768,
40.0807107531874));
#192966=CARTESIAN_POINT('Ctrl Pts',(-51.0903418356315,29.6156953732196,
40.0767763849181));
#192967=CARTESIAN_POINT('Ctrl Pts',(-51.0908211368928,29.6242688491608,
40.0724140586137));
#192968=CARTESIAN_POINT('Ctrl Pts',(-51.0918641424258,29.6325885911861,
40.0677221223768));
#192969=CARTESIAN_POINT('Ctrl Pts',(-51.0923699989822,29.636623657078,40.065446538372));
#192970=CARTESIAN_POINT('Ctrl Pts',(-51.0930089302514,29.640599364258,40.0630928000679));
#192971=CARTESIAN_POINT('Ctrl Pts',(-51.0937712117412,29.6445110377128,
40.0606689262479));
#192972=CARTESIAN_POINT('Ctrl Pts',(-51.094938211443,29.6504995364715,40.0569581447805));
#192973=CARTESIAN_POINT('Ctrl Pts',(-51.0963926103114,29.6563348640824,
40.0530843804605));
#192974=CARTESIAN_POINT('Ctrl Pts',(-51.0980990280588,29.6619874481818,
40.0490800251458));
#192975=CARTESIAN_POINT('Ctrl Pts',(-51.0988914972885,29.6646125374802,
40.0472203818218));
#192976=CARTESIAN_POINT('Ctrl Pts',(-51.0997380650831,29.667198204343,40.0453323608818));
#192977=CARTESIAN_POINT('Ctrl Pts',(-51.1006362623626,29.6697408831279,
40.0434201572162));
#192978=CARTESIAN_POINT('Ctrl Pts',(-51.100705105645,29.6699357694381,40.0432735943397));
#192979=CARTESIAN_POINT('Ctrl Pts',(-51.1007742270248,29.6701304259135,
40.0431268995707));
#192980=CARTESIAN_POINT('Ctrl Pts',(-51.1008436251322,29.6703248520472,
40.0429800745037));
#192981=CARTESIAN_POINT('Ctrl Pts',(-51.1018184593122,29.6730559530504,
40.0409176249753));
#192982=CARTESIAN_POINT('Ctrl Pts',(-51.1028499068175,29.6757410298221,
40.0388310783332));
#192983=CARTESIAN_POINT('Ctrl Pts',(-51.1039327914265,29.6783776815772,
40.036725739981));
#192984=CARTESIAN_POINT('Ctrl Pts',(-51.1078158230491,29.6878322458572,
40.0291763710725));
#192985=CARTESIAN_POINT('Ctrl Pts',(-51.1123884412291,29.6967379921813,
40.0213310894611));
#192986=CARTESIAN_POINT('Ctrl Pts',(-51.1175230541875,29.7051147523653,
40.0132837551345));
#192987=CARTESIAN_POINT('Ctrl Pts',(-51.1231654780111,29.7143199702871,
40.0044405431362));
#192988=CARTESIAN_POINT('Ctrl Pts',(-51.129486757893,29.7228870317459,39.995352871065));
#192989=CARTESIAN_POINT('Ctrl Pts',(-51.1363687775732,29.7308286942709,
39.9861103629617));
#192990=CARTESIAN_POINT('Ctrl Pts',(-51.1437996316763,29.7394036967122,
39.9761307737635));
#192991=CARTESIAN_POINT('Ctrl Pts',(-51.1518848589927,29.7472505498595,
39.9659696936109));
#192992=CARTESIAN_POINT('Ctrl Pts',(-51.1605258584151,29.7543572078857,
39.9557128217622));
#192993=CARTESIAN_POINT('Ctrl Pts',(-51.1690943687355,29.7614042483571,
39.9455419945238));
#192994=CARTESIAN_POINT('Ctrl Pts',(-51.1782106315403,29.767724137325,39.935275628938));
#192995=CARTESIAN_POINT('Ctrl Pts',(-51.1878102687782,29.7732664904684,
39.92499));
#192996=CARTESIAN_POINT('Origin',(-0.00761999999998962,-0.0131982271536776,
39.92499));
#192997=CARTESIAN_POINT('Ctrl Pts',(-54.4342359163061,31.4100231232066,
40.10025));
#192998=CARTESIAN_POINT('Ctrl Pts',(-54.4385272722018,31.4025830926783,
40.10025));
#192999=CARTESIAN_POINT('Ctrl Pts',(-54.4421589890633,31.3948506994807,
40.0995859581842));
#193000=CARTESIAN_POINT('Ctrl Pts',(-54.4451438299608,31.386976274771,40.0983275959622));
#193001=CARTESIAN_POINT('Ctrl Pts',(-54.4470510012003,31.3819448922451,
40.0975235624069));
#193002=CARTESIAN_POINT('Ctrl Pts',(-54.4486949601297,31.3768558346356,
40.0964777059491));
#193003=CARTESIAN_POINT('Ctrl Pts',(-54.4500875286679,31.3717496422767,
40.0952149915961));
#193004=CARTESIAN_POINT('Ctrl Pts',(-54.4519881053011,31.3647807142732,
40.0934916398701));
#193005=CARTESIAN_POINT('Ctrl Pts',(-54.4534143418201,31.3577796218686,
40.091364392163));
#193006=CARTESIAN_POINT('Ctrl Pts',(-54.4543880442394,31.3508395087089,
40.0889118607713));
#193007=CARTESIAN_POINT('Ctrl Pts',(-54.454874895449,31.347369452129,40.0876855950754));
#193008=CARTESIAN_POINT('Ctrl Pts',(-54.4552487192092,31.3439144604658,
40.0863782327526));
#193009=CARTESIAN_POINT('Ctrl Pts',(-54.4555129946223,31.3404848880618,
40.0850006373334));
#193010=CARTESIAN_POINT('Ctrl Pts',(-54.4556451323288,31.3387701018598,
40.0843118396237));
#193011=CARTESIAN_POINT('Ctrl Pts',(-54.4557498916994,31.3370616554172,
40.0836054919164));
#193012=CARTESIAN_POINT('Ctrl Pts',(-54.4558277627244,31.3353607484816,
40.0828829920417));
#193013=CARTESIAN_POINT('Ctrl Pts',(-54.4558472304806,31.3349355217477,
40.0827023670731));
#193014=CARTESIAN_POINT('Ctrl Pts',(-54.4558650179026,31.3345107659128,
40.0825207326933));
#193015=CARTESIAN_POINT('Ctrl Pts',(-54.4558811330247,31.3340864990774,
40.0823381109275));
#193016=CARTESIAN_POINT('Ctrl Pts',(-54.4559294783909,31.3328136985711,
40.0817902456303));
#193017=CARTESIAN_POINT('Ctrl Pts',(-54.4559627721156,31.3315453006544,
40.0812334935553));
#193018=CARTESIAN_POINT('Ctrl Pts',(-54.4559812395335,31.3302817797849,
40.0806684524227));
#193019=CARTESIAN_POINT('Ctrl Pts',(-54.4561088608494,31.3215500666185,
40.0767636676138));
#193020=CARTESIAN_POINT('Ctrl Pts',(-54.4555742713436,31.3130195924495,
40.072440451089));
#193021=CARTESIAN_POINT('Ctrl Pts',(-54.4544853519656,31.30474008586,40.0677949937412));
#193022=CARTESIAN_POINT('Ctrl Pts',(-54.4539441620237,31.3006251938117,
40.0654862141908));
#193023=CARTESIAN_POINT('Ctrl Pts',(-54.4532655373257,31.2965719591991,
40.0630972003217));
#193024=CARTESIAN_POINT('Ctrl Pts',(-54.4524598885392,31.2925850928568,
40.0606363359906));
#193025=CARTESIAN_POINT('Ctrl Pts',(-54.4506825069816,31.2837894702124,
40.0552073017124));
#193026=CARTESIAN_POINT('Ctrl Pts',(-54.4482992497264,31.2753153512351,
40.0494204304519));
#193027=CARTESIAN_POINT('Ctrl Pts',(-54.4454010706195,31.2672761140355,
40.0434049749852));
#193028=CARTESIAN_POINT('Ctrl Pts',(-54.4443423292438,31.2643392793063,
40.0412074532442));
#193029=CARTESIAN_POINT('Ctrl Pts',(-54.443220643404,31.2614550023643,40.0389814735788));
#193030=CARTESIAN_POINT('Ctrl Pts',(-54.4420411592044,31.258624610225,40.0367321210017));
#193031=CARTESIAN_POINT('Ctrl Pts',(-54.438079396587,31.2491176225317,40.029176783714));
#193032=CARTESIAN_POINT('Ctrl Pts',(-54.4334326446225,31.2401615453394,
40.0213235332575));
#193033=CARTESIAN_POINT('Ctrl Pts',(-54.4282277812585,31.2317373058269,
40.0132649215856));
#193034=CARTESIAN_POINT('Ctrl Pts',(-54.422507019865,31.2224780686858,40.004407552753));
#193035=CARTESIAN_POINT('Ctrl Pts',(-54.4161118092699,31.2138606686949,
39.9953016253715));
#193036=CARTESIAN_POINT('Ctrl Pts',(-54.4091594014078,31.2058737429071,
39.9860353422353));
#193037=CARTESIAN_POINT('Ctrl Pts',(-54.4016713602533,31.1972714816212,
39.9760551582689));
#193038=CARTESIAN_POINT('Ctrl Pts',(-54.393536288055,31.1893995936773,39.965887973815));
#193039=CARTESIAN_POINT('Ctrl Pts',(-54.3848513315119,31.1822725865936,
39.9556174643248));
#193040=CARTESIAN_POINT('Ctrl Pts',(-54.376283651206,31.1752418181691,39.94548564139));
#193041=CARTESIAN_POINT('Ctrl Pts',(-54.3671795569342,31.168935299716,39.9352519465111));
#193042=CARTESIAN_POINT('Ctrl Pts',(-54.3576020372436,31.1634057161445,
39.92499));
#193043=CARTESIAN_POINT('Ctrl Pts',(-51.3783102687782,29.4433108116265,
39.92499));
#193044=CARTESIAN_POINT('Ctrl Pts',(-51.3691445298596,29.4380189697945,
39.9348107241715));
#193045=CARTESIAN_POINT('Ctrl Pts',(-51.3595943606127,29.4334690915866,
39.9446038383154));
#193046=CARTESIAN_POINT('Ctrl Pts',(-51.3497152868792,29.4296781246264,
39.9543158069362));
#193047=CARTESIAN_POINT('Ctrl Pts',(-51.3401761719901,29.4260176124823,
39.9636935671362));
#193048=CARTESIAN_POINT('Ctrl Pts',(-51.3303291924955,29.4230642997994,
39.9729968320954));
#193049=CARTESIAN_POINT('Ctrl Pts',(-51.3202058500938,29.4208754038599,
39.9821731151294));
#193050=CARTESIAN_POINT('Ctrl Pts',(-51.3106361210895,29.4188062116774,
39.9908475764306));
#193051=CARTESIAN_POINT('Ctrl Pts',(-51.3008185461848,29.4174199248374,
39.9994093733795));
#193052=CARTESIAN_POINT('Ctrl Pts',(-51.2907775289415,29.4168067767642,
40.0077966115786));
#193053=CARTESIAN_POINT('Ctrl Pts',(-51.2815299205112,29.416242077675,40.0155211172534));
#193054=CARTESIAN_POINT('Ctrl Pts',(-51.2720922401022,29.4163331870167,
40.0230979940956));
#193055=CARTESIAN_POINT('Ctrl Pts',(-51.2624911797833,29.4171879526237,
40.0304554104678));
#193056=CARTESIAN_POINT('Ctrl Pts',(-51.2596283374029,29.4174428264735,
40.0326492435135));
#193057=CARTESIAN_POINT('Ctrl Pts',(-51.2567510524905,29.4177658668977,
40.0348233715038));
#193058=CARTESIAN_POINT('Ctrl Pts',(-51.2538602864392,29.4181606517646,
40.0369753512356));
#193059=CARTESIAN_POINT('Ctrl Pts',(-51.2509990568965,29.4185514029026,
40.0391053430352));
#193060=CARTESIAN_POINT('Ctrl Pts',(-51.2481275521816,29.4190117629205,
40.041211089324));
#193061=CARTESIAN_POINT('Ctrl Pts',(-51.2452499391937,29.4195444402103,
40.0432881154904));
#193062=CARTESIAN_POINT('Ctrl Pts',(-51.2450498356143,29.4195814815473,
40.043432547828));
#193063=CARTESIAN_POINT('Ctrl Pts',(-51.2448496951981,29.4196188630965,
40.0435768364421));
#193064=CARTESIAN_POINT('Ctrl Pts',(-51.244649518404,29.419656586079,40.0437209807855));
#193065=CARTESIAN_POINT('Ctrl Pts',(-51.2358730344468,29.4213104998205,
40.050040796842));
#193066=CARTESIAN_POINT('Ctrl Pts',(-51.2270453415805,29.4236619033168,
40.0560490279345));
#193067=CARTESIAN_POINT('Ctrl Pts',(-51.2182691329811,29.4267651248012,
40.0616647108615));
#193068=CARTESIAN_POINT('Ctrl Pts',(-51.2100881812716,29.429657866561,40.0668995033487));
#193069=CARTESIAN_POINT('Ctrl Pts',(-51.2019513265387,29.4332044080284,
40.0717933267483));
#193070=CARTESIAN_POINT('Ctrl Pts',(-51.1939656059613,29.4374658604804,
40.0762460303074));
#193071=CARTESIAN_POINT('Ctrl Pts',(-51.1910443260611,29.4390247549187,
40.0778748868749));
#193072=CARTESIAN_POINT('Ctrl Pts',(-51.1881435589218,29.440679457209,40.0794443522248));
#193073=CARTESIAN_POINT('Ctrl Pts',(-51.1852696776791,29.4424334077171,
40.0809482021492));
#193074=CARTESIAN_POINT('Ctrl Pts',(-51.184578605248,29.44285517422,40.0813098278168));
#193075=CARTESIAN_POINT('Ctrl Pts',(-51.1838888551093,29.4432832153792,
40.0816679525672));
#193076=CARTESIAN_POINT('Ctrl Pts',(-51.1832005624686,29.4437175198438,
40.0820224192581));
#193077=CARTESIAN_POINT('Ctrl Pts',(-51.1825337789729,29.4441382522937,
40.0823658088648));
#193078=CARTESIAN_POINT('Ctrl Pts',(-51.181868363317,29.4445648626869,40.0827057654616));
#193079=CARTESIAN_POINT('Ctrl Pts',(-51.1812044402991,29.44499733741,40.0830421470151));
#193080=CARTESIAN_POINT('Ctrl Pts',(-51.1739303963593,29.4497355978007,
40.0867275956806));
#193081=CARTESIAN_POINT('Ctrl Pts',(-51.1668309650356,29.4551812510958,
40.0899823432031));
#193082=CARTESIAN_POINT('Ctrl Pts',(-51.160090071181,29.4612929974523,40.0926299529356));
#193083=CARTESIAN_POINT('Ctrl Pts',(-51.1572944215751,29.4638277208379,
40.0937279956085));
#193084=CARTESIAN_POINT('Ctrl Pts',(-51.1545603804836,29.4664765899958,
40.0947220371803));
#193085=CARTESIAN_POINT('Ctrl Pts',(-51.1519003687088,29.4692349685476,
40.0956014538692));
#193086=CARTESIAN_POINT('Ctrl Pts',(-51.1473634414339,29.473939670611,40.097101390674));
#193087=CARTESIAN_POINT('Ctrl Pts',(-51.1430443628982,29.4789629373386,
40.0982667904316));
#193088=CARTESIAN_POINT('Ctrl Pts',(-51.1390107214363,29.4842777732944,
40.0990539325582));
#193089=CARTESIAN_POINT('Ctrl Pts',(-51.1369939007054,29.4869351912723,
40.0994475036216));
#193090=CARTESIAN_POINT('Ctrl Pts',(-51.1350496570624,29.4896662827386,
40.0997467259952));
#193091=CARTESIAN_POINT('Ctrl Pts',(-51.1331865036876,29.4924676612914,
40.0999473488896));
#193092=CARTESIAN_POINT('Ctrl Pts',(-51.1313233503127,29.4952690398443,
40.100147971784));
#193093=CARTESIAN_POINT('Ctrl Pts',(-51.1295412933643,29.4981406602402,
40.10025));
#193094=CARTESIAN_POINT('Ctrl Pts',(-51.1278468659044,29.5010785149115,
40.10025));
#193095=CARTESIAN_POINT('Origin',(-47.1274239660506,34.2589154226526,39.92499));
#193096=CARTESIAN_POINT('Ctrl Pts',(-50.5784163149354,36.9828414016751,
39.92499));
#193097=CARTESIAN_POINT('Ctrl Pts',(-50.5870002518362,36.9890779968912,
39.9348354642021));
#193098=CARTESIAN_POINT('Ctrl Pts',(-50.5960508068,36.9946187858203,39.9446440828463));
#193099=CARTESIAN_POINT('Ctrl Pts',(-50.6055128591422,36.9994424783908,
39.9543641760339));
#193100=CARTESIAN_POINT('Ctrl Pts',(-50.6146674511261,37.004109429676,39.9637684240722));
#193101=CARTESIAN_POINT('Ctrl Pts',(-50.6242084112814,37.008105653671,39.9730909636407));
#193102=CARTESIAN_POINT('Ctrl Pts',(-50.6341096134637,37.0113722741998,
39.9822808977152));
#193103=CARTESIAN_POINT('Ctrl Pts',(-50.6434755410472,37.0144622960732,
39.9909740094662));
#193104=CARTESIAN_POINT('Ctrl Pts',(-50.6531646927636,37.0168997626768,
39.9995492765014));
#193105=CARTESIAN_POINT('Ctrl Pts',(-50.6631621581243,37.0185933530514,
40.0079462328707));
#193106=CARTESIAN_POINT('Ctrl Pts',(-50.6723705467566,37.0201532722699,
40.0156804369703));
#193107=CARTESIAN_POINT('Ctrl Pts',(-50.6818410607734,37.0210821446115,
40.0232638017436));
#193108=CARTESIAN_POINT('Ctrl Pts',(-50.6915586678655,37.0212705108779,
40.030625726998));
#193109=CARTESIAN_POINT('Ctrl Pts',(-50.6943773762883,37.0213251487714,
40.0327611416661));
#193110=CARTESIAN_POINT('Ctrl Pts',(-50.6972168227826,37.021317219197,40.0348777427276));
#193111=CARTESIAN_POINT('Ctrl Pts',(-50.7000764815584,37.0212433695028,
40.0369733168701));
#193112=CARTESIAN_POINT('Ctrl Pts',(-50.7031765355311,37.0211633116862,
40.039245053974));
#193113=CARTESIAN_POINT('Ctrl Pts',(-50.7062960577319,37.0210069737845,
40.041487875195));
#193114=CARTESIAN_POINT('Ctrl Pts',(-50.7094335311101,37.020770653475,40.0436985701601));
#193115=CARTESIAN_POINT('Ctrl Pts',(-50.7180443514157,37.0201220705313,
40.0497658398386));
#193116=CARTESIAN_POINT('Ctrl Pts',(-50.726776150217,37.0188289150185,40.0555581699984));
#193117=CARTESIAN_POINT('Ctrl Pts',(-50.7355328079486,37.0168522507835,
40.0609828468886));
#193118=CARTESIAN_POINT('Ctrl Pts',(-50.7435446743629,37.0150437103242,
40.0659461317304));
#193119=CARTESIAN_POINT('Ctrl Pts',(-50.7515681793714,37.0126559296153,
40.0706039980705));
#193120=CARTESIAN_POINT('Ctrl Pts',(-50.7595400218642,37.0096268558221,
40.0748843180601));
#193121=CARTESIAN_POINT('Ctrl Pts',(-50.7634557648557,37.0081389846697,
40.0769867972568));
#193122=CARTESIAN_POINT('Ctrl Pts',(-50.7673587034235,37.0064960060563,
40.0789976708174));
#193123=CARTESIAN_POINT('Ctrl Pts',(-50.7712388062147,37.0046883717071,
40.08090504915));
#193124=CARTESIAN_POINT('Ctrl Pts',(-50.7719750179266,37.004345390696,40.0812669556105));
#193125=CARTESIAN_POINT('Ctrl Pts',(-50.7727105984661,37.0039959853419,
40.0816253922033));
#193126=CARTESIAN_POINT('Ctrl Pts',(-50.7734454079406,37.0036401497478,
40.081980198914));
#193127=CARTESIAN_POINT('Ctrl Pts',(-50.7741572546191,37.003295434016,40.0823239179149));
#193128=CARTESIAN_POINT('Ctrl Pts',(-50.7748683776569,37.0029446836757,
40.0826642303498));
#193129=CARTESIAN_POINT('Ctrl Pts',(-50.7755786476299,37.0025878964873,
40.0830009916099));
#193130=CARTESIAN_POINT('Ctrl Pts',(-50.7833190234412,36.9986997032257,
40.0866709464312));
#193131=CARTESIAN_POINT('Ctrl Pts',(-50.790962999314,36.9940916451529,40.0899175831878));
#193132=CARTESIAN_POINT('Ctrl Pts',(-50.7983209798296,36.9887818345685,
40.0925642067062));
#193133=CARTESIAN_POINT('Ctrl Pts',(-50.8014283006921,36.9865394685864,
40.0936818922528));
#193134=CARTESIAN_POINT('Ctrl Pts',(-50.8044846273287,36.9841723869926,
40.0946930094791));
#193135=CARTESIAN_POINT('Ctrl Pts',(-50.8074762285637,36.9816838130238,
40.0955863397546));
#193136=CARTESIAN_POINT('Ctrl Pts',(-50.8125140102916,36.9774931166429,
40.0970906856166));
#193137=CARTESIAN_POINT('Ctrl Pts',(-50.81736572735,36.9729576356985,40.0982599215483));
#193138=CARTESIAN_POINT('Ctrl Pts',(-50.8219595855748,36.9680961762159,
40.0990497370454));
#193139=CARTESIAN_POINT('Ctrl Pts',(-50.823108050131,36.9668808113452,40.0992471909196));
#193140=CARTESIAN_POINT('Ctrl Pts',(-50.8242402182961,36.9656449236014,
40.0994209989363));
#193141=CARTESIAN_POINT('Ctrl Pts',(-50.8253547230709,36.9643886196686,
40.0995705982975));
#193142=CARTESIAN_POINT('Ctrl Pts',(-50.8270264802332,36.9625041637694,
40.0997949973393));
#193143=CARTESIAN_POINT('Ctrl Pts',(-50.8286584747053,36.9605737761781,
40.0999649129781));
#193144=CARTESIAN_POINT('Ctrl Pts',(-50.8302474395911,36.9585988181541,
40.1000786629733));
#193145=CARTESIAN_POINT('Ctrl Pts',(-50.831836404477,36.9566238601302,40.1001924129685));
#193146=CARTESIAN_POINT('Ctrl Pts',(-50.8333823430133,36.9546043428186,
40.10025));
#193147=CARTESIAN_POINT('Ctrl Pts',(-50.8348823336483,36.9525415975216,
40.10025));
#193148=CARTESIAN_POINT('Ctrl Pts',(-47.7461450747862,34.7084426211235,
40.10025));
#193149=CARTESIAN_POINT('Ctrl Pts',(-47.7410693801614,34.7154221779233,
40.10025));
#193150=CARTESIAN_POINT('Ctrl Pts',(-47.7366138137623,34.722760215255,40.099578633424));
#193151=CARTESIAN_POINT('Ctrl Pts',(-47.7327846251238,34.7303057514058,
40.0983063763364));
#193152=CARTESIAN_POINT('Ctrl Pts',(-47.7303113621611,34.7351793935419,
40.097484628799));
#193153=CARTESIAN_POINT('Ctrl Pts',(-47.7280985748132,34.7401391868077,
40.0964130309337));
#193154=CARTESIAN_POINT('Ctrl Pts',(-47.7261394006516,34.7451421370598,
40.0951176960923));
#193155=CARTESIAN_POINT('Ctrl Pts',(-47.7235426275286,34.7517732610328,
40.0934008039614));
#193156=CARTESIAN_POINT('Ctrl Pts',(-47.7213971161177,34.7584811778435,
40.0912909372156));
#193157=CARTESIAN_POINT('Ctrl Pts',(-47.7196932909343,34.7651763312119,
40.0888630467851));
#193158=CARTESIAN_POINT('Ctrl Pts',(-47.7188413783425,34.7685239078962,
40.0876491015698));
#193159=CARTESIAN_POINT('Ctrl Pts',(-47.7180997687559,34.7718684539195,
40.0863558569271));
#193160=CARTESIAN_POINT('Ctrl Pts',(-47.7174664279767,34.7751999143435,
40.0849936342771));
#193161=CARTESIAN_POINT('Ctrl Pts',(-47.7171497575871,34.7768656445556,
40.0843125229521));
#193162=CARTESIAN_POINT('Ctrl Pts',(-47.7168601447018,34.7785281166321,
40.0836141747074));
#193163=CARTESIAN_POINT('Ctrl Pts',(-47.7165972740595,34.7801861569093,
40.0828999161609));
#193164=CARTESIAN_POINT('Ctrl Pts',(-47.7165315563989,34.7806006669786,
40.0827213515243));
#193165=CARTESIAN_POINT('Ctrl Pts',(-47.7164675099214,34.781014900342,40.0825417925841));
#193166=CARTESIAN_POINT('Ctrl Pts',(-47.7164051292831,34.7814288392284,
40.082361260236));
#193167=CARTESIAN_POINT('Ctrl Pts',(-47.7162179873681,34.7826706558878,
40.0818196631917));
#193168=CARTESIAN_POINT('Ctrl Pts',(-47.7160458390452,34.7839098208541,
40.0812693052021));
#193169=CARTESIAN_POINT('Ctrl Pts',(-47.7158885307486,34.785145866835,40.0807107531874));
#193170=CARTESIAN_POINT('Ctrl Pts',(-47.7147804714196,34.7938524151218,
40.076776384918));
#193171=CARTESIAN_POINT('Ctrl Pts',(-47.7143609747535,34.8024290252895,
40.0724140586133));
#193172=CARTESIAN_POINT('Ctrl Pts',(-47.7145286167444,34.8108122146634,
40.0677221223761));
#193173=CARTESIAN_POINT('Ctrl Pts',(-47.7146099229288,34.8148780524502,
40.0654465383716));
#193174=CARTESIAN_POINT('Ctrl Pts',(-47.7148297795037,34.8188987667935,
40.0630928000677));
#193175=CARTESIAN_POINT('Ctrl Pts',(-47.7151790039206,34.8228686918042,
40.0606689262479));
#193176=CARTESIAN_POINT('Ctrl Pts',(-47.7157136421035,34.8289463696256,
40.0569581447805));
#193177=CARTESIAN_POINT('Ctrl Pts',(-47.7165501157949,34.8349017567799,
40.0530843804605));
#193178=CARTESIAN_POINT('Ctrl Pts',(-47.7176563296779,34.8407017446571,
40.0490800251457));
#193179=CARTESIAN_POINT('Ctrl Pts',(-47.718170061128,34.8433952890324,40.0472203818218));
#193180=CARTESIAN_POINT('Ctrl Pts',(-47.7187417155519,34.8460552817722,
40.0453323608818));
#193181=CARTESIAN_POINT('Ctrl Pts',(-47.7193692101068,34.848677918678,40.0434201572162));
#193182=CARTESIAN_POINT('Ctrl Pts',(-47.719417305092,34.8488789334632,40.0432735943397));
#193183=CARTESIAN_POINT('Ctrl Pts',(-47.7194657006753,34.8490797487416,
40.0431268995707));
#193184=CARTESIAN_POINT('Ctrl Pts',(-47.7195143955476,34.8492803638661,
40.0429800745037));
#193185=CARTESIAN_POINT('Ctrl Pts',(-47.7201984116931,34.852098401531,40.0409176249753));
#193186=CARTESIAN_POINT('Ctrl Pts',(-47.7209435418724,34.8548765847939,
40.0388310783333));
#193187=CARTESIAN_POINT('Ctrl Pts',(-47.72174488917,34.8576119849589,40.036725739981));
#193188=CARTESIAN_POINT('Ctrl Pts',(-47.7246183780643,34.8674206434755,
40.0291763710721));
#193189=CARTESIAN_POINT('Ctrl Pts',(-47.7282350429862,34.8767555719415,
40.0213310894601));
#193190=CARTESIAN_POINT('Ctrl Pts',(-47.7324659181288,34.8856231565592,
40.013283755133));
#193191=CARTESIAN_POINT('Ctrl Pts',(-47.7371152248812,34.895367741226,40.0044405431341));
#193192=CARTESIAN_POINT('Ctrl Pts',(-47.7425063743619,34.9045486250982,
39.9953528710623));
#193193=CARTESIAN_POINT('Ctrl Pts',(-47.7485205638392,34.9131661493066,
39.9861103629584));
#193194=CARTESIAN_POINT('Ctrl Pts',(-47.7550143791189,34.922470912748,39.9761307737596));
#193195=CARTESIAN_POINT('Ctrl Pts',(-47.7622350952138,34.9311199163996,
39.9659696936062));
#193196=CARTESIAN_POINT('Ctrl Pts',(-47.7700859102955,34.9390908738006,
39.9557128217568));
#193197=CARTESIAN_POINT('Ctrl Pts',(-47.7778708651077,34.9469949630615,
39.9455419945202));
#193198=CARTESIAN_POINT('Ctrl Pts',(-47.7862765797878,34.9542331399567,
39.9352756289362));
#193199=CARTESIAN_POINT('Ctrl Pts',(-47.7952442955499,34.960748566837,39.92499));
#193200=CARTESIAN_POINT('Origin',(-0.00895784724492722,-0.0123294189942774,
39.92499));
#193201=CARTESIAN_POINT('Ctrl Pts',(-50.8527980281382,36.9278827595331,
40.10025));
#193202=CARTESIAN_POINT('Ctrl Pts',(-50.8578435704955,36.9209320551071,
40.10025));
#193203=CARTESIAN_POINT('Ctrl Pts',(-50.8622636476106,36.9136216385506,
40.0995859581841));
#193204=CARTESIAN_POINT('Ctrl Pts',(-50.8660552387516,36.9061023515948,
40.0983275959619));
#193205=CARTESIAN_POINT('Ctrl Pts',(-50.8684778849907,36.9012978851883,
40.0975235624067));
#193206=CARTESIAN_POINT('Ctrl Pts',(-50.8706447895121,36.8964085464701,
40.096477705949));
#193207=CARTESIAN_POINT('Ctrl Pts',(-50.8725634718543,36.8914758894172,
40.0952149915962));
#193208=CARTESIAN_POINT('Ctrl Pts',(-50.8751820882648,36.8847438022852,
40.0934916398702));
#193209=CARTESIAN_POINT('Ctrl Pts',(-50.8773323251411,36.8779301449088,
40.0913643921631));
#193210=CARTESIAN_POINT('Ctrl Pts',(-50.8790261328802,36.8711298300327,
40.0889118607713));
#193211=CARTESIAN_POINT('Ctrl Pts',(-50.8798730367497,36.8677296725946,
40.0876855950755));
#193212=CARTESIAN_POINT('Ctrl Pts',(-50.8806059576334,36.8643326829604,
40.0863782327527));
#193213=CARTESIAN_POINT('Ctrl Pts',(-50.8812272732512,36.8609495224156,
40.0850006373334));
#193214=CARTESIAN_POINT('Ctrl Pts',(-50.8815379310601,36.8592579421432,
40.0843118396238));
#193215=CARTESIAN_POINT('Ctrl Pts',(-50.881820697829,36.857569805085,40.0836054919165));
#193216=CARTESIAN_POINT('Ctrl Pts',(-50.8820759354566,36.8558863556342,
40.0828829920418));
#193217=CARTESIAN_POINT('Ctrl Pts',(-50.8821397448634,36.8554654932715,
40.0827023670731));
#193218=CARTESIAN_POINT('Ctrl Pts',(-50.8822018339187,36.8550449235853,
40.0825207326933));
#193219=CARTESIAN_POINT('Ctrl Pts',(-50.8822622087208,36.854624665417,40.0823381109276));
#193220=CARTESIAN_POINT('Ctrl Pts',(-50.882443333127,36.8533638909118,40.0817902456304));
#193221=CARTESIAN_POINT('Ctrl Pts',(-50.8826090281503,36.8521059215536,
40.0812334935553));
#193222=CARTESIAN_POINT('Ctrl Pts',(-50.8827594682965,36.8508512527543,
40.0806684524227));
#193223=CARTESIAN_POINT('Ctrl Pts',(-50.8837991030485,36.8421807128858,
40.0767636676135));
#193224=CARTESIAN_POINT('Ctrl Pts',(-50.8841591194358,36.8336410897268,
40.0724404510885));
#193225=CARTESIAN_POINT('Ctrl Pts',(-50.8839416093724,36.8252931160711,
40.0677949937404));
#193226=CARTESIAN_POINT('Ctrl Pts',(-50.883833507468,36.8211441960794,40.0654862141902));
#193227=CARTESIAN_POINT('Ctrl Pts',(-50.8835822787324,36.8170422299139,
40.0630972003214));
#193228=CARTESIAN_POINT('Ctrl Pts',(-50.8831977843863,36.8129929908134,
40.0606363359906));
#193229=CARTESIAN_POINT('Ctrl Pts',(-50.8823495324293,36.8040597645473,
40.0552073017123));
#193230=CARTESIAN_POINT('Ctrl Pts',(-50.880865117541,36.795382949462,40.0494204304519));
#193231=CARTESIAN_POINT('Ctrl Pts',(-50.8788231440728,36.7870848098366,
40.0434049749852));
#193232=CARTESIAN_POINT('Ctrl Pts',(-50.8780771854142,36.7840533947864,
40.0412074532442));
#193233=CARTESIAN_POINT('Ctrl Pts',(-50.8772631333232,36.7810676701181,
40.0389814735788));
#193234=CARTESIAN_POINT('Ctrl Pts',(-50.8763859670022,36.7781294934923,
40.0367321210017));
#193235=CARTESIAN_POINT('Ctrl Pts',(-50.8734396581486,36.7682604691132,
40.0291767837134));
#193236=CARTESIAN_POINT('Ctrl Pts',(-50.8697545265629,36.758867736406,40.0213235332562));
#193237=CARTESIAN_POINT('Ctrl Pts',(-50.865458748795,36.7499455893893,40.0132649215836));
#193238=CARTESIAN_POINT('Ctrl Pts',(-50.8607371801598,36.7401390929203,
40.0044075527503));
#193239=CARTESIAN_POINT('Ctrl Pts',(-50.8552777667754,36.7309004184117,
39.9953016253681));
#193240=CARTESIAN_POINT('Ctrl Pts',(-50.8491983060091,36.7222305213288,
39.9860353422311));
#193241=CARTESIAN_POINT('Ctrl Pts',(-50.8426504662796,36.712892670695,39.9760551582639));
#193242=CARTESIAN_POINT('Ctrl Pts',(-50.835382795207,36.7042135591809,39.965887973809));
#193243=CARTESIAN_POINT('Ctrl Pts',(-50.8274903908619,36.6962177694265,
39.955617464318));
#193244=CARTESIAN_POINT('Ctrl Pts',(-50.8197045606257,36.688329949833,39.9454856413854));
#193245=CARTESIAN_POINT('Ctrl Pts',(-50.8113095502191,36.6811063421661,
39.9352519465088));
#193246=CARTESIAN_POINT('Ctrl Pts',(-50.8023624960588,36.6746059268182,
39.92499));
#193247=CARTESIAN_POINT('Ctrl Pts',(-48.0191904766733,34.6525130919801,
39.92499));
#193248=CARTESIAN_POINT('Ctrl Pts',(-48.010628096725,34.6462921588067,39.9348107241726));
#193249=CARTESIAN_POINT('Ctrl Pts',(-48.0016058360806,34.6407689407917,
39.9446038383178));
#193250=CARTESIAN_POINT('Ctrl Pts',(-47.9921771448961,34.6359660967489,
39.9543158069396));
#193251=CARTESIAN_POINT('Ctrl Pts',(-47.9830729139848,34.6313285282528,
39.9636935671405));
#193252=CARTESIAN_POINT('Ctrl Pts',(-47.9735885825097,34.6273621044913,
39.9729968321003));
#193253=CARTESIAN_POINT('Ctrl Pts',(-47.9637494987646,34.6241270221285,
39.9821731151351));
#193254=CARTESIAN_POINT('Ctrl Pts',(-47.9544484832155,34.6210688561306,
39.9908475764368));
#193255=CARTESIAN_POINT('Ctrl Pts',(-47.9448295964456,34.6186639474974,
39.9994093733862));
#193256=CARTESIAN_POINT('Ctrl Pts',(-47.9349076763704,34.6170045862116,
40.0077966115857));
#193257=CARTESIAN_POINT('Ctrl Pts',(-47.925769754434,34.6154763423054,40.0155211172608));
#193258=CARTESIAN_POINT('Ctrl Pts',(-47.9163742511055,34.614580446311,40.0230979941034));
#193259=CARTESIAN_POINT('Ctrl Pts',(-47.9067364390635,34.6144269453423,
40.0304554104759));
#193260=CARTESIAN_POINT('Ctrl Pts',(-47.9038626380648,34.614381174452,40.0326492435188));
#193261=CARTESIAN_POINT('Ctrl Pts',(-47.9009673483046,34.6144016870568,
40.0348233715064));
#193262=CARTESIAN_POINT('Ctrl Pts',(-47.8980511519203,34.6144921419178,
40.0369753512356));
#193263=CARTESIAN_POINT('Ctrl Pts',(-47.8951647518764,34.614581672553,40.0391053430352));
#193264=CARTESIAN_POINT('Ctrl Pts',(-47.8922608568396,34.6147393566955,
40.041211089324));
#193265=CARTESIAN_POINT('Ctrl Pts',(-47.8893433277782,34.6149683234599,
40.0432881154904));
#193266=CARTESIAN_POINT('Ctrl Pts',(-47.8891404485131,34.6149842453609,
40.043432547828));
#193267=CARTESIAN_POINT('Ctrl Pts',(-47.8889374970512,34.6150005017599,
40.0435768364421));
#193268=CARTESIAN_POINT('Ctrl Pts',(-47.8887344737211,34.6150170939192,
40.0437209807855));
#193269=CARTESIAN_POINT('Ctrl Pts',(-47.8798331871996,34.6157445549673,
40.050040796842));
#193270=CARTESIAN_POINT('Ctrl Pts',(-47.8708080647645,34.6171603320597,
40.0560490279345));
#193271=CARTESIAN_POINT('Ctrl Pts',(-47.8617555581811,34.6193291901739,
40.0616647108615));
#193272=CARTESIAN_POINT('Ctrl Pts',(-47.8533170487303,34.6213509428814,
40.0668995033486));
#193273=CARTESIAN_POINT('Ctrl Pts',(-47.8448540540095,34.6240275231024,
40.0717933267482));
#193274=CARTESIAN_POINT('Ctrl Pts',(-47.836466636969,34.627430895772,40.0762460303073));
#193275=CARTESIAN_POINT('Ctrl Pts',(-47.8333984113056,34.6286758935248,
40.0778748868749));
#193276=CARTESIAN_POINT('Ctrl Pts',(-47.8303405713846,34.6300183184515,
40.0794443522248));
#193277=CARTESIAN_POINT('Ctrl Pts',(-47.8272990958127,34.6314622582452,
40.0809482021492));
#193278=CARTESIAN_POINT('Ctrl Pts',(-47.8265677225444,34.6318094775279,
40.0813098278168));
#193279=CARTESIAN_POINT('Ctrl Pts',(-47.8258370084445,34.6321630753108,
40.0816679525672));
#193280=CARTESIAN_POINT('Ctrl Pts',(-47.8251070891646,34.632523054438,40.082022419258));
#193281=CARTESIAN_POINT('Ctrl Pts',(-47.8243999798623,34.6328717842175,
40.0823658088648));
#193282=CARTESIAN_POINT('Ctrl Pts',(-47.8236936164941,34.6332265027183,
40.0827057654616));
#193283=CARTESIAN_POINT('Ctrl Pts',(-47.8229881245977,34.6335872094468,
40.0830421470151));
#193284=CARTESIAN_POINT('Ctrl Pts',(-47.8152586455543,34.6375391685166,
40.0867275956807));
#193285=CARTESIAN_POINT('Ctrl Pts',(-47.8076288798876,34.642212897307,40.0899823432033));
#193286=CARTESIAN_POINT('Ctrl Pts',(-47.8002860619002,34.647586547602,40.0926299529359));
#193287=CARTESIAN_POINT('Ctrl Pts',(-47.7972407764152,34.6498151605504,
40.0937279956086));
#193288=CARTESIAN_POINT('Ctrl Pts',(-47.7942448304646,34.652163733812,40.0947220371803));
#193289=CARTESIAN_POINT('Ctrl Pts',(-47.7913110614416,34.6546289547342,
40.0956014538692));
#193290=CARTESIAN_POINT('Ctrl Pts',(-47.7863072126523,34.6588336459114,
40.097101390674));
#193291=CARTESIAN_POINT('Ctrl Pts',(-47.7814867201291,34.6633779280163,
40.0982667904316));
#193292=CARTESIAN_POINT('Ctrl Pts',(-47.7769196237422,34.6682420184012,
40.0990539325583));
#193293=CARTESIAN_POINT('Ctrl Pts',(-47.7746360755488,34.6706740635937,
40.0994475036216));
#193294=CARTESIAN_POINT('Ctrl Pts',(-47.7724170058819,34.6731869650549,
40.0997467259952));
#193295=CARTESIAN_POINT('Ctrl Pts',(-47.770271235261,34.6757782448038,40.0999473488896));
#193296=CARTESIAN_POINT('Ctrl Pts',(-47.7681254646401,34.6783695245527,
40.100147971784));
#193297=CARTESIAN_POINT('Ctrl Pts',(-47.7660530039191,34.6810391382374,
40.10025));
#193298=CARTESIAN_POINT('Ctrl Pts',(-47.764060769276,34.683783783135,40.10025));
#193299=CARTESIAN_POINT('Origin',(-43.2882232241945,38.9973987043323,39.92499));
#193300=CARTESIAN_POINT('Ctrl Pts',(-46.4355828792667,42.06712965881,39.92499));
#193301=CARTESIAN_POINT('Ctrl Pts',(-46.443467890749,42.074229355038,39.934835464202));
#193302=CARTESIAN_POINT('Ctrl Pts',(-46.4518896956737,42.0806858315476,
39.9446440828461));
#193303=CARTESIAN_POINT('Ctrl Pts',(-46.4607957007314,42.0864721532162,
39.9543641760336));
#193304=CARTESIAN_POINT('Ctrl Pts',(-46.4694123136565,42.0920704538858,
39.9637684240718));
#193305=CARTESIAN_POINT('Ctrl Pts',(-46.4784832882807,42.0970420880509,
39.9730909636402));
#193306=CARTESIAN_POINT('Ctrl Pts',(-46.4879887958175,42.1013257711392,
39.9822808977148));
#193307=CARTESIAN_POINT('Ctrl Pts',(-46.4969804206318,42.1053778715668,
39.9909740094658));
#193308=CARTESIAN_POINT('Ctrl Pts',(-46.5063617095229,42.1088147776126,
39.999549276501));
#193309=CARTESIAN_POINT('Ctrl Pts',(-46.516127379323,42.1115441100126,40.0079462328704));
#193310=CARTESIAN_POINT('Ctrl Pts',(-46.5251222674801,42.1140580225433,
40.01568043697));
#193311=CARTESIAN_POINT('Ctrl Pts',(-46.5344438074317,42.1159717447016,
40.0232638017433));
#193312=CARTESIAN_POINT('Ctrl Pts',(-46.544088490819,42.1171748456138,40.0306257269978));
#193313=CARTESIAN_POINT('Ctrl Pts',(-46.5468860468472,42.1175238194551,
40.0327611416659));
#193314=CARTESIAN_POINT('Ctrl Pts',(-46.5497107674229,42.1178127362983,
40.0348777427275));
#193315=CARTESIAN_POINT('Ctrl Pts',(-46.5525624800839,42.1180382068978,
40.0369733168701));
#193316=CARTESIAN_POINT('Ctrl Pts',(-46.5556539199571,42.1182826315242,
40.039245053974));
#193317=CARTESIAN_POINT('Ctrl Pts',(-46.5587726948496,42.1184532289196,
40.041487875195));
#193318=CARTESIAN_POINT('Ctrl Pts',(-46.5619176830191,42.1185461584682,
40.0436985701601));
#193319=CARTESIAN_POINT('Ctrl Pts',(-46.5705491277285,42.1188012043438,
40.0497658398386));
#193320=CARTESIAN_POINT('Ctrl Pts',(-46.5793682643808,42.1184278543824,
40.0555581699984));
#193321=CARTESIAN_POINT('Ctrl Pts',(-46.5882835699001,42.117377338497,40.0609828468885));
#193322=CARTESIAN_POINT('Ctrl Pts',(-46.596440590427,42.1164161734957,40.0659461317304));
#193323=CARTESIAN_POINT('Ctrl Pts',(-46.6046697328837,42.114880157948,40.0706039980706));
#193324=CARTESIAN_POINT('Ctrl Pts',(-46.6129145292181,42.1127009621831,
40.0748843180603));
#193325=CARTESIAN_POINT('Ctrl Pts',(-46.6169643462448,42.111630548342,40.076986797257));
#193326=CARTESIAN_POINT('Ctrl Pts',(-46.6210176421362,42.1104045383081,
40.0789976708175));
#193327=CARTESIAN_POINT('Ctrl Pts',(-46.6250654385589,42.1090123875511,
40.08090504915));
#193328=CARTESIAN_POINT('Ctrl Pts',(-46.6258334685041,42.1087482405047,
40.0812669556105));
#193329=CARTESIAN_POINT('Ctrl Pts',(-46.6266015422611,42.1084776383331,
40.0816253922033));
#193330=CARTESIAN_POINT('Ctrl Pts',(-46.6273695213203,42.1082005605488,
40.0819801989139));
#193331=CARTESIAN_POINT('Ctrl Pts',(-46.6281135010338,42.1079321414453,
40.0823239179149));
#193332=CARTESIAN_POINT('Ctrl Pts',(-46.6288573918593,42.1076576451504,
40.0826642303498));
#193333=CARTESIAN_POINT('Ctrl Pts',(-46.6296010653156,42.1073770559083,
40.0830009916099));
#193334=CARTESIAN_POINT('Ctrl Pts',(-46.6377054654047,42.1043192521649,
40.0866709464311));
#193335=CARTESIAN_POINT('Ctrl Pts',(-46.6457892400066,42.1005354505678,
40.0899175831876));
#193336=CARTESIAN_POINT('Ctrl Pts',(-46.6536619390755,42.0960238460775,
40.092564206706));
#193337=CARTESIAN_POINT('Ctrl Pts',(-46.6569866287796,42.0941185674854,
40.0936818922527));
#193338=CARTESIAN_POINT('Ctrl Pts',(-46.6602736399407,42.0920839261387,
40.094693009479));
#193339=CARTESIAN_POINT('Ctrl Pts',(-46.663508979684,42.0899216923182,40.0955863397546));
#193340=CARTESIAN_POINT('Ctrl Pts',(-46.6689572109691,42.0862805445929,
40.0970906856166));
#193341=CARTESIAN_POINT('Ctrl Pts',(-46.6742564366672,42.082277052016,40.0982599215483));
#193342=CARTESIAN_POINT('Ctrl Pts',(-46.6793332901452,42.0779224130581,
40.0990497370454));
#193343=CARTESIAN_POINT('Ctrl Pts',(-46.6806025035147,42.0768337533186,
40.0992471909196));
#193344=CARTESIAN_POINT('Ctrl Pts',(-46.6818576549908,42.0757229796955,
40.0994209989363));
#193345=CARTESIAN_POINT('Ctrl Pts',(-46.6830973739113,42.0745900553985,
40.0995705982975));
#193346=CARTESIAN_POINT('Ctrl Pts',(-46.6849569522921,42.0728906689529,
40.0997949973393));
#193347=CARTESIAN_POINT('Ctrl Pts',(-46.6867817869761,42.0711414461011,
40.0999649129781));
#193348=CARTESIAN_POINT('Ctrl Pts',(-46.6885684866733,42.0693433991615,
40.1000786629733));
#193349=CARTESIAN_POINT('Ctrl Pts',(-46.6903551863704,42.0675453522219,
40.1001924129685));
#193350=CARTESIAN_POINT('Ctrl Pts',(-46.692103753136,42.065698492618,40.10025));
#193351=CARTESIAN_POINT('Ctrl Pts',(-46.6938111422614,42.0638038389716,
40.10025));
#193352=CARTESIAN_POINT('Ctrl Pts',(-43.8565665267053,39.5091373124626,
40.10025));
#193353=CARTESIAN_POINT('Ctrl Pts',(-43.8507890749205,39.5155480799605,
40.10025));
#193354=CARTESIAN_POINT('Ctrl Pts',(-43.8455908828149,39.5223801852468,
40.0995786334241));
#193355=CARTESIAN_POINT('Ctrl Pts',(-43.8409939475741,39.5294841269568,
40.0983063763366));
#193356=CARTESIAN_POINT('Ctrl Pts',(-43.8380247990815,39.5340725443949,
40.0974846287992));
#193357=CARTESIAN_POINT('Ctrl Pts',(-43.8353056940458,39.5387738681335,
40.0964130309338));
#193358=CARTESIAN_POINT('Ctrl Pts',(-43.8328343017434,39.5435446222366,
40.0951176960924));
#193359=CARTESIAN_POINT('Ctrl Pts',(-43.8295586128166,39.5498679835147,
40.0934008039614));
#193360=CARTESIAN_POINT('Ctrl Pts',(-43.8267236865058,39.5563148866446,
40.0912909372157));
#193361=CARTESIAN_POINT('Ctrl Pts',(-43.824329360962,39.5627952650343,40.0888630467851));
#193362=CARTESIAN_POINT('Ctrl Pts',(-43.8231321981901,39.5660354542291,
40.0876491015699));
#193363=CARTESIAN_POINT('Ctrl Pts',(-43.8220450509623,39.5692841591689,
40.0863558569271));
#193364=CARTESIAN_POINT('Ctrl Pts',(-43.8210669472515,39.5725311673658,
40.0849936342771));
#193365=CARTESIAN_POINT('Ctrl Pts',(-43.8205778953961,39.5741546714643,
40.0843125229521));
#193366=CARTESIAN_POINT('Ctrl Pts',(-43.8201160933892,39.575777763555,40.0836141747074));
#193367=CARTESIAN_POINT('Ctrl Pts',(-43.8196813503776,39.5773992434498,
40.0828999161609));
#193368=CARTESIAN_POINT('Ctrl Pts',(-43.8195726646246,39.5778046134235,
40.0827213515243));
#193369=CARTESIAN_POINT('Ctrl Pts',(-43.8194656698236,39.5782098828933,
40.0825417925842));
#193370=CARTESIAN_POINT('Ctrl Pts',(-43.8193603625172,39.578615033627,40.0823612602361));
#193371=CARTESIAN_POINT('Ctrl Pts',(-43.8190444405982,39.5798304858279,
40.0818196631917));
#193372=CARTESIAN_POINT('Ctrl Pts',(-43.8187437073121,39.5810448681193,
40.0812693052022));
#193373=CARTESIAN_POINT('Ctrl Pts',(-43.8184580587799,39.5822576997164,
40.0807107531875));
#193374=CARTESIAN_POINT('Ctrl Pts',(-43.8164459874032,39.5908007288814,
40.0767763849182));
#193375=CARTESIAN_POINT('Ctrl Pts',(-43.8151322889029,39.5992865061389,
40.0724140586138));
#193376=CARTESIAN_POINT('Ctrl Pts',(-43.8144227306309,39.6076412948835,
40.067722122377));
#193377=CARTESIAN_POINT('Ctrl Pts',(-43.8140785956357,39.6116933583964,
40.0654465383722));
#193378=CARTESIAN_POINT('Ctrl Pts',(-43.8138769687216,39.6157150281163,
40.063092800068));
#193379=CARTESIAN_POINT('Ctrl Pts',(-43.81380930989,39.6196997093545,40.0606689262479));
#193380=CARTESIAN_POINT('Ctrl Pts',(-43.8137057289461,39.6257999779285,
40.0569581447806));
#193381=CARTESIAN_POINT('Ctrl Pts',(-43.8139151128796,39.6318101761584,
40.0530843804606));
#193382=CARTESIAN_POINT('Ctrl Pts',(-43.8144090029875,39.6376940219324,
40.0490800251458));
#193383=CARTESIAN_POINT('Ctrl Pts',(-43.8146383681086,39.6404265103488,
40.0472203818218));
#193384=CARTESIAN_POINT('Ctrl Pts',(-43.8149288459964,39.6431316855285,
40.0453323608818));
#193385=CARTESIAN_POINT('Ctrl Pts',(-43.815278762865,39.6458055463964,40.0434201572162));
#193386=CARTESIAN_POINT('Ctrl Pts',(-43.8153055826142,39.6460104872964,
40.0432735943397));
#193387=CARTESIAN_POINT('Ctrl Pts',(-43.8153327221691,39.6462152612037,
40.0431268995707));
#193388=CARTESIAN_POINT('Ctrl Pts',(-43.8153601802951,39.6464198673378,
40.0429800745037));
#193389=CARTESIAN_POINT('Ctrl Pts',(-43.815745884182,39.649293966654,40.0409176249753));
#193390=CARTESIAN_POINT('Ctrl Pts',(-43.8161965332331,39.6521348180509,
40.0388310783332));
#193391=CARTESIAN_POINT('Ctrl Pts',(-43.8167075634907,39.6549389970091,
40.036725739981));
#193392=CARTESIAN_POINT('Ctrl Pts',(-43.8185400271108,39.664994284047,40.0291763710717));
#193393=CARTESIAN_POINT('Ctrl Pts',(-43.8211611138367,39.6746561192251,
40.0213310894592));
#193394=CARTESIAN_POINT('Ctrl Pts',(-43.8244418968098,39.6839173731639,
40.0132837551316));
#193395=CARTESIAN_POINT('Ctrl Pts',(-43.8280471477135,39.6940945608674,
40.0044405431319));
#193396=CARTESIAN_POINT('Ctrl Pts',(-43.8324491002312,39.7037886794685,
39.9953528710591));
#193397=CARTESIAN_POINT('Ctrl Pts',(-43.8375295667874,39.7129876499623,
39.9861103629542));
#193398=CARTESIAN_POINT('Ctrl Pts',(-43.8430151956451,39.7229202294695,
39.9761307737535));
#193399=CARTESIAN_POINT('Ctrl Pts',(-43.8492922888428,39.7322766233327,
39.9659696935982));
#193400=CARTESIAN_POINT('Ctrl Pts',(-43.8562669044119,39.7410245486321,
39.9557128217468));
#193401=CARTESIAN_POINT('Ctrl Pts',(-43.8631830101213,39.7496990878249,
39.9455419945135));
#193402=CARTESIAN_POINT('Ctrl Pts',(-43.8707860819068,39.757776249665,39.9352756289328));
#193403=CARTESIAN_POINT('Ctrl Pts',(-43.8790236240217,39.7651933659002,
39.92499));
#193404=CARTESIAN_POINT('Origin',(-0.0101975504408993,-0.0113255271402792,
39.92499));
#193405=CARTESIAN_POINT('Ctrl Pts',(-46.7142062431419,42.0411527846899,
40.10025));
#193406=CARTESIAN_POINT('Ctrl Pts',(-46.7199506919431,42.0347675597384,
40.10025));
#193407=CARTESIAN_POINT('Ctrl Pts',(-46.7251107020222,42.0279592142763,
40.099585958184));
#193408=CARTESIAN_POINT('Ctrl Pts',(-46.7296675019408,42.0208774479559,
40.0983275959616));
#193409=CARTESIAN_POINT('Ctrl Pts',(-46.7325790801602,42.0163525364081,
40.0975235624064));
#193410=CARTESIAN_POINT('Ctrl Pts',(-46.7352451892141,42.0117164851992,
40.0964777059487));
#193411=CARTESIAN_POINT('Ctrl Pts',(-46.737668963875,42.007011406675,40.0952149915961));
#193412=CARTESIAN_POINT('Ctrl Pts',(-46.7409769299532,42.00058991857,40.09349163987));
#193413=CARTESIAN_POINT('Ctrl Pts',(-46.7438276087417,41.9940383480781,
40.091364392163));
#193414=CARTESIAN_POINT('Ctrl Pts',(-46.7462229640885,41.9874523371584,
40.0889118607712));
#193415=CARTESIAN_POINT('Ctrl Pts',(-46.7474206417619,41.9841593316986,
40.0876855950754));
#193416=CARTESIAN_POINT('Ctrl Pts',(-46.7485046297344,41.9808575622227,
40.0863782327526));
#193417=CARTESIAN_POINT('Ctrl Pts',(-46.749476178293,41.9775578801521,40.0850006373333));
#193418=CARTESIAN_POINT('Ctrl Pts',(-46.7499619525723,41.9759080391169,
40.0843118396237));
#193419=CARTESIAN_POINT('Ctrl Pts',(-46.7504196286878,41.9742587070259,
40.0836054919164));
#193420=CARTESIAN_POINT('Ctrl Pts',(-46.7508494364809,41.9726111592843,
40.0828829920417));
#193421=CARTESIAN_POINT('Ctrl Pts',(-46.7509568884292,41.9721992723489,
40.082702367073));
#193422=CARTESIAN_POINT('Ctrl Pts',(-46.7510625988572,41.9717874966611,
40.0825207326932));
#193423=CARTESIAN_POINT('Ctrl Pts',(-46.7511665718603,41.9713758515962,
40.0823381109275));
#193424=CARTESIAN_POINT('Ctrl Pts',(-46.7514784908696,41.9701409164016,
40.0817902456303));
#193425=CARTESIAN_POINT('Ctrl Pts',(-46.751774771802,41.9689071581772,40.0812334935553));
#193426=CARTESIAN_POINT('Ctrl Pts',(-46.7520555364229,41.9676750878623,
40.0806684524226));
#193427=CARTESIAN_POINT('Ctrl Pts',(-46.753995794155,41.9591607175415,40.0767636676136));
#193428=CARTESIAN_POINT('Ctrl Pts',(-46.7552464720206,41.9507055072916,
40.0724404510887));
#193429=CARTESIAN_POINT('Ctrl Pts',(-46.7559027543577,41.9423805287165,
40.0677949937407));
#193430=CARTESIAN_POINT('Ctrl Pts',(-46.7562289248778,41.9382430372166,
40.0654862141904));
#193431=CARTESIAN_POINT('Ctrl Pts',(-46.7564078446192,41.934137281497,40.0630972003215));
#193432=CARTESIAN_POINT('Ctrl Pts',(-46.756448717314,41.9300700339487,40.0606363359906));
#193433=CARTESIAN_POINT('Ctrl Pts',(-46.7565388885835,41.9210970783572,
40.0552073017123));
#193434=CARTESIAN_POINT('Ctrl Pts',(-46.7559695796222,41.9123126321657,
40.0494204304519));
#193435=CARTESIAN_POINT('Ctrl Pts',(-46.7548061840814,41.9038465062688,
40.0434049749851));
#193436=CARTESIAN_POINT('Ctrl Pts',(-46.7543811810191,41.9007537237152,
40.0412074532442));
#193437=CARTESIAN_POINT('Ctrl Pts',(-46.753883681602,41.8976992635449,40.0389814735788));
#193438=CARTESIAN_POINT('Ctrl Pts',(-46.7533184435774,41.8946854937105,
40.0367321210017));
#193439=CARTESIAN_POINT('Ctrl Pts',(-46.7514198688646,41.8845625597445,
40.0291767837145));
#193440=CARTESIAN_POINT('Ctrl Pts',(-46.7487367327317,41.8748360802697,
40.0213235332586));
#193441=CARTESIAN_POINT('Ctrl Pts',(-46.7453971060013,41.8655137786607,
40.0132649215873));
#193442=CARTESIAN_POINT('Ctrl Pts',(-46.7417264606198,41.855267464893,40.0044075527552));
#193443=CARTESIAN_POINT('Ctrl Pts',(-46.737262658923,41.8455087367198,39.9953016253744));
#193444=CARTESIAN_POINT('Ctrl Pts',(-46.7321227530987,41.8362508575498,
39.9860353422388));
#193445=CARTESIAN_POINT('Ctrl Pts',(-46.7265868542985,41.8262797250152,
39.9760551582731));
#193446=CARTESIAN_POINT('Ctrl Pts',(-46.7202662104789,41.8168884800942,
39.9658879738197));
#193447=CARTESIAN_POINT('Ctrl Pts',(-46.7132528291677,41.8081115112156,
39.9556174643302));
#193448=CARTESIAN_POINT('Ctrl Pts',(-46.7063341521825,41.7994530610494,
39.9454856413937));
#193449=CARTESIAN_POINT('Ctrl Pts',(-46.6987402031273,41.7913915075206,
39.9352519465129));
#193450=CARTESIAN_POINT('Ctrl Pts',(-46.6905216402894,41.7839914803031,
39.92499));
#193451=CARTESIAN_POINT('Ctrl Pts',(-44.1339623850444,39.4820551873934,
39.92499));
#193452=CARTESIAN_POINT('Ctrl Pts',(-44.1260971752947,39.4749733207255,
39.9348107241718));
#193453=CARTESIAN_POINT('Ctrl Pts',(-44.1177016730302,39.4685372764368,
39.9446038383161));
#193454=CARTESIAN_POINT('Ctrl Pts',(-44.1088266671104,39.4627751762764,
39.9543158069372));
#193455=CARTESIAN_POINT('Ctrl Pts',(-44.1002570680373,39.4572113615995,
39.9636935671376));
#193456=CARTESIAN_POINT('Ctrl Pts',(-44.0912392969033,39.4522752837282,
39.9729968320971));
#193457=CARTESIAN_POINT('Ctrl Pts',(-44.0817922708769,39.4480294591813,
39.9821731151315));
#193458=CARTESIAN_POINT('Ctrl Pts',(-44.0728618726566,39.4440158252744,
39.9908475764331));
#193459=CARTESIAN_POINT('Ctrl Pts',(-44.0635470605588,39.4406186435298,
39.9994093733824));
#193460=CARTESIAN_POINT('Ctrl Pts',(-44.0538529442853,39.4379312493405,
40.0077966115819));
#193461=CARTESIAN_POINT('Ctrl Pts',(-44.0449248258284,39.4354562043765,
40.0155211172573));
#193462=CARTESIAN_POINT('Ctrl Pts',(-44.0356744386817,39.4335831186693,
40.0230979941));
#193463=CARTESIAN_POINT('Ctrl Pts',(-44.0261054688028,39.4324230329128,
40.0304554104726));
#193464=CARTESIAN_POINT('Ctrl Pts',(-44.0232521951461,39.4320771187579,
40.0326492435167));
#193465=CARTESIAN_POINT('Ctrl Pts',(-44.0203706219338,39.4317948788029,
40.0348233715053));
#193466=CARTESIAN_POINT('Ctrl Pts',(-44.0174609456693,39.431580012616,40.0369753512356));
#193467=CARTESIAN_POINT('Ctrl Pts',(-44.0145809991271,39.4313673418321,
40.0391053430352));
#193468=CARTESIAN_POINT('Ctrl Pts',(-44.0116765294501,39.4312206224786,
40.041211089324));
#193469=CARTESIAN_POINT('Ctrl Pts',(-44.0087510493742,39.4311433701098,
40.0432881154904));
#193470=CARTESIAN_POINT('Ctrl Pts',(-44.0085476172111,39.4311379981311,
40.043432547828));
#193471=CARTESIAN_POINT('Ctrl Pts',(-44.0083440782821,39.4311329512714,
40.0435768364421));
#193472=CARTESIAN_POINT('Ctrl Pts',(-44.0081404327822,39.4311282308205,
40.0437209807855));
#193473=CARTESIAN_POINT('Ctrl Pts',(-43.999211868054,39.4309212689597,40.0500407968421));
#193474=CARTESIAN_POINT('Ctrl Pts',(-43.9900881971801,39.431385908098,40.0560490279346));
#193475=CARTESIAN_POINT('Ctrl Pts',(-43.9808585737691,39.4325966403787,
40.0616647108616));
#193476=CARTESIAN_POINT('Ctrl Pts',(-43.9722549606523,39.4337252532882,
40.0668995033489));
#193477=CARTESIAN_POINT('Ctrl Pts',(-43.9635585482845,39.43550254709,40.0717933267486));
#193478=CARTESIAN_POINT('Ctrl Pts',(-43.9548613290768,39.4380105519141,
40.0762460303077));
#193479=CARTESIAN_POINT('Ctrl Pts',(-43.9516797737731,39.4389280125252,
40.0778748868751));
#193480=CARTESIAN_POINT('Ctrl Pts',(-43.9484983634048,39.4399434521998,
40.0794443522249));
#193481=CARTESIAN_POINT('Ctrl Pts',(-43.9453226165469,39.4410615611726,
40.0809482021492));
#193482=CARTESIAN_POINT('Ctrl Pts',(-43.9445589555198,39.4413304290279,
40.0813098278168));
#193483=CARTESIAN_POINT('Ctrl Pts',(-43.9437952833153,39.4416057093431,
40.0816679525672));
#193484=CARTESIAN_POINT('Ctrl Pts',(-43.9430317345447,39.4418874191264,
40.082022419258));
#193485=CARTESIAN_POINT('Ctrl Pts',(-43.9422920466731,39.4421603254789,
40.0823658088648));
#193486=CARTESIAN_POINT('Ctrl Pts',(-43.9415524746576,39.4424392657174,
40.0827057654617));
#193487=CARTESIAN_POINT('Ctrl Pts',(-43.9408131433996,39.4427242524729,
40.0830421470151));
#193488=CARTESIAN_POINT('Ctrl Pts',(-43.9327129150431,39.445846611731,40.0867275956806));
#193489=CARTESIAN_POINT('Ctrl Pts',(-43.9246364083432,39.4496972096656,
40.089982343203));
#193490=CARTESIAN_POINT('Ctrl Pts',(-43.9167721156739,39.4542738890614,
40.0926299529355));
#193491=CARTESIAN_POINT('Ctrl Pts',(-43.9135105590943,39.4561719744232,
40.0937279956084));
#193492=CARTESIAN_POINT('Ctrl Pts',(-43.9102855324948,39.4581945203286,
40.0947220371802));
#193493=CARTESIAN_POINT('Ctrl Pts',(-43.9071101492106,39.4603395741454,
40.0956014538692));
#193494=CARTESIAN_POINT('Ctrl Pts',(-43.9016942021212,39.46399818696,40.097101390674));
#193495=CARTESIAN_POINT('Ctrl Pts',(-43.8964251099353,39.4680136963364,
40.0982667904316));
#193496=CARTESIAN_POINT('Ctrl Pts',(-43.8913745966873,39.4723737491584,
40.0990539325583));
#193497=CARTESIAN_POINT('Ctrl Pts',(-43.8888493400632,39.4745537755694,
40.0994475036216));
#193498=CARTESIAN_POINT('Ctrl Pts',(-43.8863797569641,39.4768209551514,
40.0997467259952));
#193499=CARTESIAN_POINT('Ctrl Pts',(-43.8839748786091,39.4791737454931,
40.0999473488896));
#193500=CARTESIAN_POINT('Ctrl Pts',(-43.8815700002541,39.4815265358349,
40.100147971784));
#193501=CARTESIAN_POINT('Ctrl Pts',(-43.8792298420738,39.4839648939621,
40.10025));
#193502=CARTESIAN_POINT('Ctrl Pts',(-43.8769616275871,39.486486258182,40.10025));
#193503=CARTESIAN_POINT('Origin',(-38.974747650051,43.308618325077,39.92499));
#193504=CARTESIAN_POINT('Ctrl Pts',(-41.7839914803023,46.6905216402901,
39.92499));
#193505=CARTESIAN_POINT('Ctrl Pts',(-41.7910911765302,46.6984066517723,
39.9348354642018));
#193506=CARTESIAN_POINT('Ctrl Pts',(-41.7987919603585,46.7057080773547,
39.9446440828458));
#193507=CARTESIAN_POINT('Ctrl Pts',(-41.8070443420765,46.7123936319702,
39.9543641760331));
#193508=CARTESIAN_POINT('Ctrl Pts',(-41.8150285705285,46.7188619458705,
39.9637684240712));
#193509=CARTESIAN_POINT('Ctrl Pts',(-41.8235301761253,46.7247545199412,
39.9730909636396));
#193510=CARTESIAN_POINT('Ctrl Pts',(-41.8325358446866,46.7300083326607,
39.982280897714));
#193511=CARTESIAN_POINT('Ctrl Pts',(-41.8410546526086,46.7349781159823,
39.9909740094649));
#193512=CARTESIAN_POINT('Ctrl Pts',(-41.85002529531,46.7393768060084,39.9995492765));
#193513=CARTESIAN_POINT('Ctrl Pts',(-41.8594521748275,46.7431119772969,
40.0079462328693));
#193514=CARTESIAN_POINT('Ctrl Pts',(-41.8681350126323,46.7465523401881,
40.0156804369688));
#193515=CARTESIAN_POINT('Ctrl Pts',(-41.8772054497763,46.7494299450226,
40.023263801742));
#193516=CARTESIAN_POINT('Ctrl Pts',(-41.8866715402891,46.7516345991555,
40.0306257269964));
#193517=CARTESIAN_POINT('Ctrl Pts',(-41.8894172933139,46.7522740855142,
40.032761141665));
#193518=CARTESIAN_POINT('Ctrl Pts',(-41.8921963397416,46.7528566833418,
40.034877742727));
#193519=CARTESIAN_POINT('Ctrl Pts',(-41.8950088623276,46.753379003932,40.0369733168701));
#193520=CARTESIAN_POINT('Ctrl Pts',(-41.8980578176392,46.7539452330339,
40.039245053974));
#193521=CARTESIAN_POINT('Ctrl Pts',(-41.9011416752729,46.7544408966257,
40.041487875195));
#193522=CARTESIAN_POINT('Ctrl Pts',(-41.9042597210852,46.7548620578769,
40.0436985701601));
#193523=CARTESIAN_POINT('Ctrl Pts',(-41.912817222284,46.7560179382357,40.0497658398386));
#193524=CARTESIAN_POINT('Ctrl Pts',(-41.9216270724807,46.7565684843261,
40.0555581699984));
#193525=CARTESIAN_POINT('Ctrl Pts',(-41.9306033478346,46.7564556264622,
40.0609828468885));
#193526=CARTESIAN_POINT('Ctrl Pts',(-41.93881615245,46.7563523676438,40.0659461317303));
#193527=CARTESIAN_POINT('Ctrl Pts',(-41.947160772148,46.755684946165,40.0706039980704));
#193528=CARTESIAN_POINT('Ctrl Pts',(-41.9555881906097,46.7543795041533,
40.0748843180601));
#193529=CARTESIAN_POINT('Ctrl Pts',(-41.959727711029,46.7537382753016,40.0769867972568));
#193530=CARTESIAN_POINT('Ctrl Pts',(-41.9638869554863,46.7529426662696,
40.0789976708174));
#193531=CARTESIAN_POINT('Ctrl Pts',(-41.9680580970361,46.7519812517998,
40.08090504915));
#193532=CARTESIAN_POINT('Ctrl Pts',(-41.9688495305177,46.7517988327685,
40.0812669556104));
#193533=CARTESIAN_POINT('Ctrl Pts',(-41.9696416823154,46.7516099985534,
40.0816253922032));
#193534=CARTESIAN_POINT('Ctrl Pts',(-41.97043441682,46.7514147143011,40.0819801989139));
#193535=CARTESIAN_POINT('Ctrl Pts',(-41.9712023783712,46.7512255326816,
40.0823239179149));
#193536=CARTESIAN_POINT('Ctrl Pts',(-41.9719708867608,46.7510302978709,
40.0826642303498));
#193537=CARTESIAN_POINT('Ctrl Pts',(-41.9727398158584,46.7508289807696,
40.0830009916099));
#193538=CARTESIAN_POINT('Ctrl Pts',(-41.9811194467224,46.7486350684821,
40.0866709464312));
#193539=CARTESIAN_POINT('Ctrl Pts',(-41.9895544525278,46.7457169794824,
40.0899175831878));
#193540=CARTESIAN_POINT('Ctrl Pts',(-41.9978556152119,46.7420530111689,
40.0925642067063));
#193541=CARTESIAN_POINT('Ctrl Pts',(-42.001361247761,46.740505694598,40.0936818922528));
#193542=CARTESIAN_POINT('Ctrl Pts',(-42.004842930264,46.738825785455,40.0946930094791));
#193543=CARTESIAN_POINT('Ctrl Pts',(-42.0082865614559,46.7370135816692,
40.0955863397546));
#193544=CARTESIAN_POINT('Ctrl Pts',(-42.0140855503362,46.7339618757759,
40.0970906856166));
#193545=CARTESIAN_POINT('Ctrl Pts',(-42.0197742252482,46.730534234669,40.0982599215483));
#193546=CARTESIAN_POINT('Ctrl Pts',(-42.0252784509101,46.7267341265712,
40.0990497370454));
#193547=CARTESIAN_POINT('Ctrl Pts',(-42.0266545073256,46.7257840995468,
40.0992471909196));
#193548=CARTESIAN_POINT('Ctrl Pts',(-42.0280188904104,46.7248106099129,
40.0994209989363));
#193549=CARTESIAN_POINT('Ctrl Pts',(-42.0293702408567,46.7238134778073,
40.0995705982975));
#193550=CARTESIAN_POINT('Ctrl Pts',(-42.0313972665262,46.722317779649,40.0997949973393));
#193551=CARTESIAN_POINT('Ctrl Pts',(-42.0333949481515,46.7207688863881,
40.0999649129781));
#193552=CARTESIAN_POINT('Ctrl Pts',(-42.0353598072042,46.7191674503114,
40.1000786629733));
#193553=CARTESIAN_POINT('Ctrl Pts',(-42.037324666257,46.7175660142347,40.1001924129685));
#193554=CARTESIAN_POINT('Ctrl Pts',(-42.0392567035859,46.7159120469166,
40.10025));
#193555=CARTESIAN_POINT('Ctrl Pts',(-42.0411527846891,46.7142062431426,
40.10025));
#193556=CARTESIAN_POINT('Ctrl Pts',(-39.4864862581813,43.8769616275878,
40.10025));
#193557=CARTESIAN_POINT('Ctrl Pts',(-39.4800703482072,43.8827333680737,
40.10025));
#193558=CARTESIAN_POINT('Ctrl Pts',(-39.4741864828755,43.8889846873396,
40.0995786334241));
#193559=CARTESIAN_POINT('Ctrl Pts',(-39.4688721660171,43.8955692023369,
40.0983063763367));
#193560=CARTESIAN_POINT('Ctrl Pts',(-39.4654396626067,43.8998221234152,
40.0974846287993));
#193561=CARTESIAN_POINT('Ctrl Pts',(-39.4622440309669,43.9042134689399,
40.0964130309338));
#193562=CARTESIAN_POINT('Ctrl Pts',(-39.459287497615,43.9086997575136,40.0951176960923));
#193563=CARTESIAN_POINT('Ctrl Pts',(-39.4553687820178,43.9146460760273,
40.0934008039614));
#193564=CARTESIAN_POINT('Ctrl Pts',(-39.451875500853,43.9207613318566,40.0912909372156));
#193565=CARTESIAN_POINT('Ctrl Pts',(-39.4488169076806,43.9269559348857,
40.0888630467851));
#193566=CARTESIAN_POINT('Ctrl Pts',(-39.4472876110944,43.9300532364003,
40.0876491015699));
#193567=CARTESIAN_POINT('Ctrl Pts',(-39.4458668372378,43.9331705067655,
40.0863558569271));
#193568=CARTESIAN_POINT('Ctrl Pts',(-39.4445546869045,43.9362974878339,
40.0849936342771));
#193569=CARTESIAN_POINT('Ctrl Pts',(-39.4438986117379,43.9378609783681,
40.0843125229521));
#193570=CARTESIAN_POINT('Ctrl Pts',(-39.4432696802086,43.9394269075364,
40.0836141747074));
#193571=CARTESIAN_POINT('Ctrl Pts',(-39.4426678279631,43.9409940617758,
40.0828999161609));
#193572=CARTESIAN_POINT('Ctrl Pts',(-39.4425173649017,43.9413858503356,
40.0827213515243));
#193573=CARTESIAN_POINT('Ctrl Pts',(-39.4423685940344,43.9417777156947,
40.0825417925842));
#193574=CARTESIAN_POINT('Ctrl Pts',(-39.4422215138289,43.9421696393594,
40.082361260236));
#193575=CARTESIAN_POINT('Ctrl Pts',(-39.4417802732125,43.9433454103533,
40.0818196631917));
#193576=CARTESIAN_POINT('Ctrl Pts',(-39.44135424986,43.9445217049432,40.0812693052021));
#193577=CARTESIAN_POINT('Ctrl Pts',(-39.4409433907174,43.9456980341198,
40.0807107531874));
#193578=CARTESIAN_POINT('Ctrl Pts',(-39.4380493519679,43.953983944948,40.0767763849182));
#193579=CARTESIAN_POINT('Ctrl Pts',(-39.4358558447891,43.9622859173442,
40.0724140586139));
#193580=CARTESIAN_POINT('Ctrl Pts',(-39.4342768603232,43.970520768646,40.0677221223771));
#193581=CARTESIAN_POINT('Ctrl Pts',(-39.4335110545634,43.974514662629,40.0654465383723));
#193582=CARTESIAN_POINT('Ctrl Pts',(-39.4328901532271,43.97849322547,40.063092800068));
#193583=CARTESIAN_POINT('Ctrl Pts',(-39.4324063524312,43.9824490059339,
40.0606689262479));
#193584=CARTESIAN_POINT('Ctrl Pts',(-39.4316656872149,43.9885050294414,
40.0569581447805));
#193585=CARTESIAN_POINT('Ctrl Pts',(-39.4312456873365,43.9945041897574,
40.0530843804606));
#193586=CARTESIAN_POINT('Ctrl Pts',(-39.4311218425058,44.0004074287826,
40.0490800251458));
#193587=CARTESIAN_POINT('Ctrl Pts',(-39.4310643283257,44.0031489235252,
40.0472203818218));
#193588=CARTESIAN_POINT('Ctrl Pts',(-39.4310704471408,44.0058696426794,
40.0453323608819));
#193589=CARTESIAN_POINT('Ctrl Pts',(-39.4311389525607,44.0085654321303,
40.0434201572162));
#193590=CARTESIAN_POINT('Ctrl Pts',(-39.4311442032312,44.0087720537698,
40.0432735943397));
#193591=CARTESIAN_POINT('Ctrl Pts',(-39.4311497894109,44.0089785427601,
40.0431268995708));
#193592=CARTESIAN_POINT('Ctrl Pts',(-39.4311557099537,44.0091848981961,
40.0429800745037));
#193593=CARTESIAN_POINT('Ctrl Pts',(-39.4312388757296,44.0120835699301,
40.0409176249753));
#193594=CARTESIAN_POINT('Ctrl Pts',(-39.4313901062471,44.0149559644986,
40.0388310783332));
#193595=CARTESIAN_POINT('Ctrl Pts',(-39.4316052205102,44.0177981990786,
40.036725739981));
#193596=CARTESIAN_POINT('Ctrl Pts',(-39.432376582001,44.0279899468076,40.0291763710721));
#193597=CARTESIAN_POINT('Ctrl Pts',(-39.433973373356,44.0378728316087,40.0213310894601));
#193598=CARTESIAN_POINT('Ctrl Pts',(-39.4362681192144,44.0474262866314,
40.0132837551329));
#193599=CARTESIAN_POINT('Ctrl Pts',(-39.438789814385,44.0579245739714,40.0044405431341));
#193600=CARTESIAN_POINT('Ctrl Pts',(-39.4421543412256,44.0680257165074,
39.9953528710623));
#193601=CARTESIAN_POINT('Ctrl Pts',(-39.4462454222044,44.0777053474392,
39.9861103629585));
#193602=CARTESIAN_POINT('Ctrl Pts',(-39.4506627629399,44.0881569195892,
39.9761307737599));
#193603=CARTESIAN_POINT('Ctrl Pts',(-39.4559274600905,44.0981181930518,
39.9659696936068));
#193604=CARTESIAN_POINT('Ctrl Pts',(-39.4619494607956,44.1075472421469,
39.9557128217576));
#193605=CARTESIAN_POINT('Ctrl Pts',(-39.4679209431045,44.1168971912117,
39.9455419945208));
#193606=CARTESIAN_POINT('Ctrl Pts',(-39.4746380711547,44.1257248429273,
39.9352756289364));
#193607=CARTESIAN_POINT('Ctrl Pts',(-39.4820551873926,44.1339623850451,
39.92499));
#193608=CARTESIAN_POINT('Origin',(-0.0113255271402662,-0.0101975504409131,
39.92499));
#193609=CARTESIAN_POINT('Ctrl Pts',(-42.0638038389696,46.6938111422608,
40.10025));
#193610=CARTESIAN_POINT('Ctrl Pts',(-42.07018425683,46.6880613546461,40.10025));
#193611=CARTESIAN_POINT('Ctrl Pts',(-42.0760276657216,46.681829673938,40.0995859581842));
#193612=CARTESIAN_POINT('Ctrl Pts',(-42.0812997491636,46.6752630175686,
40.0983275959622));
#193613=CARTESIAN_POINT('Ctrl Pts',(-42.0846683595043,46.6710672367555,
40.0975235624069));
#193614=CARTESIAN_POINT('Ctrl Pts',(-42.0878044626433,46.6667352666015,
40.0964777059491));
#193615=CARTESIAN_POINT('Ctrl Pts',(-42.0907067742414,46.6623093164292,
40.0952149915961));
#193616=CARTESIAN_POINT('Ctrl Pts',(-42.0946678472188,46.6562687825187,
40.0934916398701));
#193617=CARTESIAN_POINT('Ctrl Pts',(-42.0981877352862,46.6500510792884,
40.0913643921631));
#193618=CARTESIAN_POINT('Ctrl Pts',(-42.1012583942262,46.6437515300391,
40.0889118607713));
#193619=CARTESIAN_POINT('Ctrl Pts',(-42.1027937236962,46.6406017554144,
40.0876855950755));
#193620=CARTESIAN_POINT('Ctrl Pts',(-42.1042169023586,46.6374313809741,
40.0863782327527));
#193621=CARTESIAN_POINT('Ctrl Pts',(-42.1055280393686,46.634251329385,40.0850006373334));
#193622=CARTESIAN_POINT('Ctrl Pts',(-42.1061836078736,46.6326613035905,
40.0843118396238));
#193623=CARTESIAN_POINT('Ctrl Pts',(-42.1068111789404,46.6310688468943,
40.0836054919165));
#193624=CARTESIAN_POINT('Ctrl Pts',(-42.1074108478351,46.6294752517397,
40.0828829920418));
#193625=CARTESIAN_POINT('Ctrl Pts',(-42.1075607650587,46.6290768529511,
40.0827023670731));
#193626=CARTESIAN_POINT('Ctrl Pts',(-42.1077089386738,46.6286783827621,
40.0825207326933));
#193627=CARTESIAN_POINT('Ctrl Pts',(-42.1078553707279,46.6282798608702,
40.0823381109276));
#193628=CARTESIAN_POINT('Ctrl Pts',(-42.1082946668904,46.6270842951945,
40.0817902456304));
#193629=CARTESIAN_POINT('Ctrl Pts',(-42.1087182876161,46.6258882654174,
40.0812334935554));
#193630=CARTESIAN_POINT('Ctrl Pts',(-42.1091263005957,46.6246922924069,
40.0806684524227));
#193631=CARTESIAN_POINT('Ctrl Pts',(-42.1119459234382,46.6164273768569,
40.0767636676138));
#193632=CARTESIAN_POINT('Ctrl Pts',(-42.1140735600935,46.608149216569,40.072440451089));
#193633=CARTESIAN_POINT('Ctrl Pts',(-42.1155964444645,46.599938443282,40.0677949937411));
#193634=CARTESIAN_POINT('Ctrl Pts',(-42.1163533138167,46.5958577114964,
40.0654862141907));
#193635=CARTESIAN_POINT('Ctrl Pts',(-42.116960421753,46.5917931497417,40.0630972003216));
#193636=CARTESIAN_POINT('Ctrl Pts',(-42.1174262136788,46.5877524553608,
40.0606363359906));
#193637=CARTESIAN_POINT('Ctrl Pts',(-42.1184538202397,46.5788380800231,
40.0552073017124));
#193638=CARTESIAN_POINT('Ctrl Pts',(-42.1188058546734,46.5700422469561,
40.0494204304519));
#193639=CARTESIAN_POINT('Ctrl Pts',(-42.118533783465,46.5615008914347,40.0434049749851));
#193640=CARTESIAN_POINT('Ctrl Pts',(-42.1184343924215,46.5583806265505,
40.0412074532442));
#193641=CARTESIAN_POINT('Ctrl Pts',(-42.118258896386,46.5552908961831,40.0389814735788));
#193642=CARTESIAN_POINT('Ctrl Pts',(-42.1180117795239,46.5522345526331,
40.0367321210016));
#193643=CARTESIAN_POINT('Ctrl Pts',(-42.1171817401332,46.5419686180606,
40.029176783714));
#193644=CARTESIAN_POINT('Ctrl Pts',(-42.1155299964531,46.5320149571607,
40.0213235332574));
#193645=CARTESIAN_POINT('Ctrl Pts',(-42.1131831104084,46.5223946380446,
40.0132649215855));
#193646=CARTESIAN_POINT('Ctrl Pts',(-42.1106036046384,46.5118207677343,
40.0044075527528));
#193647=CARTESIAN_POINT('Ctrl Pts',(-42.1071843209734,46.5016489045629,
39.9953016253713));
#193648=CARTESIAN_POINT('Ctrl Pts',(-42.1030402839734,46.491904474566,39.986035342235));
#193649=CARTESIAN_POINT('Ctrl Pts',(-42.0985769785664,46.4814093059437,
39.9760551582686));
#193650=CARTESIAN_POINT('Ctrl Pts',(-42.0932726122941,46.4714088200593,
39.9658879738145));
#193651=CARTESIAN_POINT('Ctrl Pts',(-42.0872150940878,46.4619468343633,
39.9556174643243));
#193652=CARTESIAN_POINT('Ctrl Pts',(-42.0812393728301,46.4526126174219,
39.9454856413897));
#193653=CARTESIAN_POINT('Ctrl Pts',(-42.0745296860254,46.4438014421037,
39.9352519465109));
#193654=CARTESIAN_POINT('Ctrl Pts',(-42.0671296588092,46.4355828792674,
39.92499));
#193655=CARTESIAN_POINT('Ctrl Pts',(-39.7651933658995,43.8790236240223,
39.92499));
#193656=CARTESIAN_POINT('Ctrl Pts',(-39.7581114992309,43.8711584142718,
39.9348107241729));
#193657=CARTESIAN_POINT('Ctrl Pts',(-39.7504347382243,43.8638800583564,
39.9446038383182));
#193658=CARTESIAN_POINT('Ctrl Pts',(-39.7422106539896,43.8572218328526,
39.9543158069403));
#193659=CARTESIAN_POINT('Ctrl Pts',(-39.7342695770743,43.8507927303124,
39.9636935671414));
#193660=CARTESIAN_POINT('Ctrl Pts',(-39.7258171668678,43.8449410790332,
39.9729968321016));
#193661=CARTESIAN_POINT('Ctrl Pts',(-39.7168657021529,43.8397310304442,
39.9821731151366));
#193662=CARTESIAN_POINT('Ctrl Pts',(-39.7084037645721,43.8348059028415,
39.9908475764386));
#193663=CARTESIAN_POINT('Ctrl Pts',(-39.6994950821762,43.8304536682197,
39.9994093733883));
#193664=CARTESIAN_POINT('Ctrl Pts',(-39.6901349804701,43.8267676847803,
40.0077966115881));
#193665=CARTESIAN_POINT('Ctrl Pts',(-39.6815144838262,43.8233729558697,
40.0155211172637));
#193666=CARTESIAN_POINT('Ctrl Pts',(-39.6725105620382,43.8205432023691,
40.0230979941066));
#193667=CARTESIAN_POINT('Ctrl Pts',(-39.6631152739582,43.8183892419676,
40.0304554104794));
#193668=CARTESIAN_POINT('Ctrl Pts',(-39.660313788711,43.8177469744568,40.0326492435211));
#193669=CARTESIAN_POINT('Ctrl Pts',(-39.6574775031699,43.8171650742228,
40.0348233715075));
#193670=CARTESIAN_POINT('Ctrl Pts',(-39.6546062260517,43.8166472411073,
40.0369753512356));
#193671=CARTESIAN_POINT('Ctrl Pts',(-39.6517642863083,43.8161346989699,
40.0391053430352));
#193672=CARTESIAN_POINT('Ctrl Pts',(-39.6488910639686,43.8156851836085,
40.041211089324));
#193673=CARTESIAN_POINT('Ctrl Pts',(-39.64598968505,43.8153025584995,40.0432881154904));
#193674=CARTESIAN_POINT('Ctrl Pts',(-39.6457879288342,43.8152759514977,
40.043432547828));
#193675=CARTESIAN_POINT('Ctrl Pts',(-39.6455860324533,43.8152496566738,
40.0435768364421));
#193676=CARTESIAN_POINT('Ctrl Pts',(-39.6453839959662,43.8152236753309,
40.0437209807855));
#193677=CARTESIAN_POINT('Ctrl Pts',(-39.6365259762552,43.8140845580785,
40.050040796842));
#193678=CARTESIAN_POINT('Ctrl Pts',(-39.6274037177901,43.8135929685793,
40.0560490279344));
#193679=CARTESIAN_POINT('Ctrl Pts',(-39.6180980992373,43.8138323099901,
40.0616647108614));
#193680=CARTESIAN_POINT('Ctrl Pts',(-39.6094236454406,43.8140554177823,
40.0668995033484));
#193681=CARTESIAN_POINT('Ctrl Pts',(-39.6005890951403,43.8149139527619,
40.0717933267479));
#193682=CARTESIAN_POINT('Ctrl Pts',(-39.5916773623197,43.8164991115145,
40.0762460303069));
#193683=CARTESIAN_POINT('Ctrl Pts',(-39.5884173351605,43.8170789830938,
40.0778748868746));
#193684=CARTESIAN_POINT('Ctrl Pts',(-39.5851472105417,43.8177563121468,
40.0794443522247));
#193685=CARTESIAN_POINT('Ctrl Pts',(-39.5818719865441,43.818536340063,40.0809482021492));
#193686=CARTESIAN_POINT('Ctrl Pts',(-39.5810844045883,43.8187239107184,
40.0813098278169));
#193687=CARTESIAN_POINT('Ctrl Pts',(-39.5802961412317,43.8189178575374,
40.0816679525672));
#193688=CARTESIAN_POINT('Ctrl Pts',(-39.5795073285704,43.8191182115053,
40.0820224192581));
#193689=CARTESIAN_POINT('Ctrl Pts',(-39.5787431663048,43.8193123044118,
40.0823658088648));
#193690=CARTESIAN_POINT('Ctrl Pts',(-39.5779784885477,43.8195124102602,
40.0827057654617));
#193691=CARTESIAN_POINT('Ctrl Pts',(-39.5772134181961,43.8197185546681,
40.0830421470151));
#193692=CARTESIAN_POINT('Ctrl Pts',(-39.568831188323,43.8219771048933,40.0867275956806));
#193693=CARTESIAN_POINT('Ctrl Pts',(-39.5603964284872,43.8249623840156,
40.089982343203));
#193694=CARTESIAN_POINT('Ctrl Pts',(-39.5520968239719,43.8286919494554,
40.0926299529355));
#193695=CARTESIAN_POINT('Ctrl Pts',(-39.5486547305945,43.8302387114099,
40.0937279956084));
#193696=CARTESIAN_POINT('Ctrl Pts',(-39.5452359574127,43.8319130705228,
40.0947220371802));
#193697=CARTESIAN_POINT('Ctrl Pts',(-39.5418537500313,43.8337144555753,
40.0956014538693));
#193698=CARTESIAN_POINT('Ctrl Pts',(-39.5360850428915,43.8367869054998,
40.097101390674));
#193699=CARTESIAN_POINT('Ctrl Pts',(-39.5304250803196,43.8402296473866,
40.0982667904316));
#193700=CARTESIAN_POINT('Ctrl Pts',(-39.5249464846901,43.8440378929943,
40.0990539325583));
#193701=CARTESIAN_POINT('Ctrl Pts',(-39.5222071868753,43.8459420157981,
40.0994475036216));
#193702=CARTESIAN_POINT('Ctrl Pts',(-39.5195141476131,43.8479386338069,
40.0997467259952));
#193703=CARTESIAN_POINT('Ctrl Pts',(-39.5168765098747,43.8500271570783,
40.0999473488896));
#193704=CARTESIAN_POINT('Ctrl Pts',(-39.5142388721362,43.8521156803497,
40.100147971784));
#193705=CARTESIAN_POINT('Ctrl Pts',(-39.5116566557594,43.8542960677577,
40.10025));
#193706=CARTESIAN_POINT('Ctrl Pts',(-39.5091373124618,43.856566526706,40.10025));
#193707=CARTESIAN_POINT('Origin',(-34.2342565846632,47.1453396605411,39.92499));
#193708=CARTESIAN_POINT('Ctrl Pts',(-36.6746059268174,50.8023624960594,
39.92499));
#193709=CARTESIAN_POINT('Ctrl Pts',(-36.6808425220335,50.8109464329603,
39.9348354642022));
#193710=CARTESIAN_POINT('Ctrl Pts',(-36.6877379133667,50.819012811669,39.9446440828465));
#193711=CARTESIAN_POINT('Ctrl Pts',(-36.6952462569244,50.8265243508963,
39.9543641760341));
#193712=CARTESIAN_POINT('Ctrl Pts',(-36.7025106240257,50.8337918098269,
39.9637684240725));
#193713=CARTESIAN_POINT('Ctrl Pts',(-36.7103497152254,50.8405407635287,
39.973090963641));
#193714=CARTESIAN_POINT('Ctrl Pts',(-36.7187568768225,50.8467071440079,
39.9822808977156));
#193715=CARTESIAN_POINT('Ctrl Pts',(-36.7267095340102,50.8525401602375,
39.9909740094666));
#193716=CARTESIAN_POINT('Ctrl Pts',(-36.7351712462837,50.8578524412756,
39.9995492765018));
#193717=CARTESIAN_POINT('Ctrl Pts',(-36.7441560526543,50.8625525281344,
40.0079462328713));
#193718=CARTESIAN_POINT('Ctrl Pts',(-36.7524317091193,50.8668816480503,
40.0156804369708));
#193719=CARTESIAN_POINT('Ctrl Pts',(-36.7611516658486,50.8706916079202,
40.0232638017442));
#193720=CARTESIAN_POINT('Ctrl Pts',(-36.7703354510189,50.8738736606214,
40.0306257269987));
#193721=CARTESIAN_POINT('Ctrl Pts',(-36.772999317994,50.8747966531508,40.0327611416665));
#193722=CARTESIAN_POINT('Ctrl Pts',(-36.7757022424581,50.8756665488987,
40.0348777427278));
#193723=CARTESIAN_POINT('Ctrl Pts',(-36.7784447603815,50.8764799968256,
40.0369733168701));
#193724=CARTESIAN_POINT('Ctrl Pts',(-36.7814178261389,50.8773618266785,
40.039245053974));
#193725=CARTESIAN_POINT('Ctrl Pts',(-36.7844329791243,50.8781771258726,
40.041487875195));
#193726=CARTESIAN_POINT('Ctrl Pts',(-36.7874899206171,50.8789219044956,
40.0436985701601));
#193727=CARTESIAN_POINT('Ctrl Pts',(-36.7958797205313,50.8809659552706,
40.0497658398386));
#193728=CARTESIAN_POINT('Ctrl Pts',(-36.80458376171,50.8824343655146,40.0555581699984));
#193729=CARTESIAN_POINT('Ctrl Pts',(-36.8135226609474,50.8832604021664,
40.0609828468886));
#193730=CARTESIAN_POINT('Ctrl Pts',(-36.8217012684457,50.8840161808563,
40.0659461317305));
#193731=CARTESIAN_POINT('Ctrl Pts',(-36.8300699399857,50.8842246658557,
40.0706039980708));
#193732=CARTESIAN_POINT('Ctrl Pts',(-36.8385876480149,50.8838072802931,
40.0748843180605));
#193733=CARTESIAN_POINT('Ctrl Pts',(-36.8427715183744,50.8836022618681,
40.0769867972571));
#193734=CARTESIAN_POINT('Ctrl Pts',(-36.8469911418446,50.8832457706972,
40.0789976708176));
#193735=CARTESIAN_POINT('Ctrl Pts',(-36.8512399286213,50.8827256259728,
40.08090504915));
#193736=CARTESIAN_POINT('Ctrl Pts',(-36.8520460945285,50.8826269335776,
40.0812669556105));
#193737=CARTESIAN_POINT('Ctrl Pts',(-36.8528536453862,50.8825219362262,
40.0816253922033));
#193738=CARTESIAN_POINT('Ctrl Pts',(-36.8536624499709,50.8824105850809,
40.0819801989139));
#193739=CARTESIAN_POINT('Ctrl Pts',(-36.8544459794124,50.882302713659,40.0823239179149));
#193740=CARTESIAN_POINT('Ctrl Pts',(-36.8552306854274,50.882188879366,40.0826642303499));
#193741=CARTESIAN_POINT('Ctrl Pts',(-36.8560164456182,50.8820690400778,
40.08300099161));
#193742=CARTESIAN_POINT('Ctrl Pts',(-36.8645794982669,50.8807630562083,
40.0866709464311));
#193743=CARTESIAN_POINT('Ctrl Pts',(-36.8732733195863,50.8787426510002,
40.0899175831875));
#193744=CARTESIAN_POINT('Ctrl Pts',(-36.8819119966095,50.8759664620674,
40.0925642067059));
#193745=CARTESIAN_POINT('Ctrl Pts',(-36.8855601635605,50.8747940602416,
40.0936818922526));
#193746=CARTESIAN_POINT('Ctrl Pts',(-36.8891983713641,50.8734872887381,
40.094693009479));
#193747=CARTESIAN_POINT('Ctrl Pts',(-36.8928125648613,50.8720449698707,
40.0955863397546));
#193748=CARTESIAN_POINT('Ctrl Pts',(-36.8988987764012,50.8696161409377,
40.0970906856166));
#193749=CARTESIAN_POINT('Ctrl Pts',(-36.9049145742144,50.8668019052539,
40.0982599215483));
#193750=CARTESIAN_POINT('Ctrl Pts',(-36.9107858666115,50.8635979627953,
40.0990497370454));
#193751=CARTESIAN_POINT('Ctrl Pts',(-36.9122536897107,50.8627969771806,
40.0992471909196));
#193752=CARTESIAN_POINT('Ctrl Pts',(-36.9137123559377,50.861971437292,40.0994209989363));
#193753=CARTESIAN_POINT('Ctrl Pts',(-36.9151605322316,50.861121022166,40.0995705982975));
#193754=CARTESIAN_POINT('Ctrl Pts',(-36.9173327966724,50.8598453994769,
40.0997949973393));
#193755=CARTESIAN_POINT('Ctrl Pts',(-36.9194814382212,50.8585138058059,
40.0999649129781));
#193756=CARTESIAN_POINT('Ctrl Pts',(-36.9216029292226,50.8571265262611,
40.1000786629733));
#193757=CARTESIAN_POINT('Ctrl Pts',(-36.923724420224,50.8557392467162,40.1001924129685));
#193758=CARTESIAN_POINT('Ctrl Pts',(-36.9258187603126,50.8542962928973,
40.10025));
#193759=CARTESIAN_POINT('Ctrl Pts',(-36.9278827595322,50.8527980281388,
40.10025));
#193760=CARTESIAN_POINT('Ctrl Pts',(-34.6837837831342,47.7640607692766,
40.10025));
#193761=CARTESIAN_POINT('Ctrl Pts',(-34.6767997090225,47.7691302463545,
40.10025));
#193762=CARTESIAN_POINT('Ctrl Pts',(-34.6702946353241,47.7747322888385,
40.0995786334241));
#193763=CARTESIAN_POINT('Ctrl Pts',(-34.6643211616152,47.7807252357995,
40.0983063763365));
#193764=CARTESIAN_POINT('Ctrl Pts',(-34.6604629105133,47.7845960646243,
40.0974846287992));
#193765=CARTESIAN_POINT('Ctrl Pts',(-34.6568257642789,47.7886293194339,
40.0964130309337));
#193766=CARTESIAN_POINT('Ctrl Pts',(-34.6534164822759,47.7927819897612,
40.0951176960923));
#193767=CARTESIAN_POINT('Ctrl Pts',(-34.6488976742765,47.7982861164005,
40.0934008039614));
#193768=CARTESIAN_POINT('Ctrl Pts',(-34.6447843113771,47.8040027249066,
40.0912909372156));
#193769=CARTESIAN_POINT('Ctrl Pts',(-34.6410949611629,47.8098436832081,
40.0888630467851));
#193770=CARTESIAN_POINT('Ctrl Pts',(-34.6392502860559,47.8127641623588,
40.0876491015699));
#193771=CARTESIAN_POINT('Ctrl Pts',(-34.6375114518663,47.8157158446829,
40.0863558569271));
#193772=CARTESIAN_POINT('Ctrl Pts',(-34.635879631104,47.818688538764,40.0849936342771));
#193773=CARTESIAN_POINT('Ctrl Pts',(-34.6350637207229,47.8201748858045,
40.0843125229521));
#193774=CARTESIAN_POINT('Ctrl Pts',(-34.6342745503769,47.8216664954027,
40.0836141747074));
#193775=CARTESIAN_POINT('Ctrl Pts',(-34.6335121829165,47.8231621539168,
40.0828999161609));
#193776=CARTESIAN_POINT('Ctrl Pts',(-34.6333215910514,47.8235360685453,
40.0827213515243));
#193777=CARTESIAN_POINT('Ctrl Pts',(-34.6331326740828,47.8239102364349,
40.0825417925842));
#193778=CARTESIAN_POINT('Ctrl Pts',(-34.6329454324196,47.8242846390328,
40.0823612602361));
#193779=CARTESIAN_POINT('Ctrl Pts',(-34.6323837074303,47.8254078468266,
40.0818196631917));
#193780=CARTESIAN_POINT('Ctrl Pts',(-34.6318370616126,47.8265331659853,
40.0812693052022));
#193781=CARTESIAN_POINT('Ctrl Pts',(-34.6313054933181,47.8276601046328,
40.0807107531875));
#193782=CARTESIAN_POINT('Ctrl Pts',(-34.6275611948899,47.8355981149519,
40.0767763849181));
#193783=CARTESIAN_POINT('Ctrl Pts',(-34.6245119115562,47.8436253243405,
40.0724140586135));
#193784=CARTESIAN_POINT('Ctrl Pts',(-34.6220808005805,47.8516500154458,
40.0677221223765));
#193785=CARTESIAN_POINT('Ctrl Pts',(-34.6209017143844,47.8555419819601,
40.0654465383718));
#193786=CARTESIAN_POINT('Ctrl Pts',(-34.6198683413509,47.8594338479546,
40.0630928000678));
#193787=CARTESIAN_POINT('Ctrl Pts',(-34.6189736992136,47.8633173872851,
40.0606689262479));
#193788=CARTESIAN_POINT('Ctrl Pts',(-34.6176040646081,47.8692628146654,
40.0569581447806));
#193789=CARTESIAN_POINT('Ctrl Pts',(-34.6165592825243,47.8751852090116,
40.0530843804606));
#193790=CARTESIAN_POINT('Ctrl Pts',(-34.6158190596249,47.8810431641658,
40.0490800251458));
#193791=CARTESIAN_POINT('Ctrl Pts',(-34.6154752962811,47.8837636288445,
40.0472203818218));
#193792=CARTESIAN_POINT('Ctrl Pts',(-34.6151969889845,47.8864700832049,
40.0453323608819));
#193793=CARTESIAN_POINT('Ctrl Pts',(-34.6149833323959,47.8891582656054,
40.0434201572162));
#193794=CARTESIAN_POINT('Ctrl Pts',(-34.6149669564602,47.8893643041944,
40.0432735943397));
#193795=CARTESIAN_POINT('Ctrl Pts',(-34.6149509280614,47.8895702459313,
40.0431268995707));
#193796=CARTESIAN_POINT('Ctrl Pts',(-34.6149352461542,47.8897760897958,
40.0429800745037));
#193797=CARTESIAN_POINT('Ctrl Pts',(-34.6147149626374,47.8926675754935,
40.0409176249753));
#193798=CARTESIAN_POINT('Ctrl Pts',(-34.6145651177081,47.8955400426777,
40.0388310783332));
#193799=CARTESIAN_POINT('Ctrl Pts',(-34.6144819591399,47.8983891927626,
40.036725739981));
#193800=CARTESIAN_POINT('Ctrl Pts',(-34.6141837673037,47.908605738263,40.0291763710716));
#193801=CARTESIAN_POINT('Ctrl Pts',(-34.6147387685077,47.9186013937342,
40.0213310894592));
#193802=CARTESIAN_POINT('Ctrl Pts',(-34.6160223355359,47.9283423801894,
40.0132837551316));
#193803=CARTESIAN_POINT('Ctrl Pts',(-34.6174328467541,47.9390467457347,
40.0044405431319));
#193804=CARTESIAN_POINT('Ctrl Pts',(-34.6197230854584,47.9494442419762,
39.9953528710594));
#193805=CARTESIAN_POINT('Ctrl Pts',(-34.6227799581217,47.9594984812856,
39.9861103629547));
#193806=CARTESIAN_POINT('Ctrl Pts',(-34.6260806134277,47.97035453647,39.9761307737546));
#193807=CARTESIAN_POINT('Ctrl Pts',(-34.6302752334102,47.9808115517384,
39.9659696935999));
#193808=CARTESIAN_POINT('Ctrl Pts',(-34.6352786409545,47.9908184179967,
39.9557128217491));
#193809=CARTESIAN_POINT('Ctrl Pts',(-34.6402400750502,48.0007413369283,
39.9455419945151));
#193810=CARTESIAN_POINT('Ctrl Pts',(-34.6459976651007,48.010222760914,39.9352756289336));
#193811=CARTESIAN_POINT('Ctrl Pts',(-34.6525130919793,48.0191904766739,
39.92499));
#193812=CARTESIAN_POINT('Origin',(-0.0123294189942654,-0.00895784724494174,
39.92499));
#193813=CARTESIAN_POINT('Ctrl Pts',(-36.9525415975208,50.8348823336489,
40.10025));
#193814=CARTESIAN_POINT('Ctrl Pts',(-36.9594880792485,50.829830979246,40.10025));
#193815=CARTESIAN_POINT('Ctrl Pts',(-36.9659508653433,50.824244238888,40.0995859581841));
#193816=CARTESIAN_POINT('Ctrl Pts',(-36.97188047026,50.8182646381292,40.0983275959619));
#193817=CARTESIAN_POINT('Ctrl Pts',(-36.9756692055208,50.8144439579052,
40.0975235624067));
#193818=CARTESIAN_POINT('Ctrl Pts',(-36.9792409429413,50.8104635307792,
40.0964777059489));
#193819=CARTESIAN_POINT('Ctrl Pts',(-36.9825899931423,50.8063652005969,
40.0952149915961));
#193820=CARTESIAN_POINT('Ctrl Pts',(-36.9871607746745,50.8007718022344,
40.0934916398701));
#193821=CARTESIAN_POINT('Ctrl Pts',(-36.9913113073905,50.7949560887235,
40.0913643921631));
#193822=CARTESIAN_POINT('Ctrl Pts',(-36.9950236271419,50.7890120203242,
40.0889118607713));
#193823=CARTESIAN_POINT('Ctrl Pts',(-36.9968797870176,50.7860399861246,
40.0876855950754));
#193824=CARTESIAN_POINT('Ctrl Pts',(-36.9986265637266,50.7830357420058,
40.0863782327526));
#193825=CARTESIAN_POINT('Ctrl Pts',(-37.0002629240967,50.7800101622088,
40.0850006373334));
#193826=CARTESIAN_POINT('Ctrl Pts',(-37.0010811042817,50.7784973723103,
40.0843118396237));
#193827=CARTESIAN_POINT('Ctrl Pts',(-37.0018716944997,50.7769792382977,
40.0836054919164));
#193828=CARTESIAN_POINT('Ctrl Pts',(-37.002634654398,50.7754570554922,40.0828829920417));
#193829=CARTESIAN_POINT('Ctrl Pts',(-37.0028253943726,50.7750765097908,
40.0827023670731));
#193830=CARTESIAN_POINT('Ctrl Pts',(-37.0030144077536,50.7746957108235,
40.0825207326932));
#193831=CARTESIAN_POINT('Ctrl Pts',(-37.0032016945186,50.7743146783938,
40.0823381109275));
#193832=CARTESIAN_POINT('Ctrl Pts',(-37.0037635548135,50.7731715811047,
40.0817902456303));
#193833=CARTESIAN_POINT('Ctrl Pts',(-37.0043098740552,50.7720263837273,
40.0812334935553));
#193834=CARTESIAN_POINT('Ctrl Pts',(-37.0048406651179,50.7708796113519,
40.0806684524227));
#193835=CARTESIAN_POINT('Ctrl Pts',(-37.0085087606929,50.7629547027167,
40.0767636676137));
#193836=CARTESIAN_POINT('Ctrl Pts',(-37.0114900453056,50.7549442896469,
40.0724404510888));
#193837=CARTESIAN_POINT('Ctrl Pts',(-37.0138628466707,50.7469376805981,
40.067794993741));
#193838=CARTESIAN_POINT('Ctrl Pts',(-37.0150421224359,50.7429584178785,
40.0654862141906));
#193839=CARTESIAN_POINT('Ctrl Pts',(-37.0160707669654,50.738979582278,40.0630972003216));
#193840=CARTESIAN_POINT('Ctrl Pts',(-37.0169563748085,50.735009711758,40.0606363359906));
#193841=CARTESIAN_POINT('Ctrl Pts',(-37.0189101579882,50.7262515844358,
40.0552073017123));
#193842=CARTESIAN_POINT('Ctrl Pts',(-37.0201796788542,50.7175407334811,
40.0494204304519));
#193843=CARTESIAN_POINT('Ctrl Pts',(-37.0208019128471,50.7090177292135,
40.0434049749852));
#193844=CARTESIAN_POINT('Ctrl Pts',(-37.0210292227715,50.7059041682738,
40.0412074532443));
#193845=CARTESIAN_POINT('Ctrl Pts',(-37.0211776528887,50.7028130194417,
40.0389814735788));
#193846=CARTESIAN_POINT('Ctrl Pts',(-37.0212513646531,50.6997475881155,
40.0367321210017));
#193847=CARTESIAN_POINT('Ctrl Pts',(-37.0214989546698,50.6894511286642,
40.0291767837136));
#193848=CARTESIAN_POINT('Ctrl Pts',(-37.0208967002921,50.6793793407311,
40.0213235332566));
#193849=CARTESIAN_POINT('Ctrl Pts',(-37.0195682679079,50.6695664063375,
40.0132649215843));
#193850=CARTESIAN_POINT('Ctrl Pts',(-37.0181081633546,50.6587808290205,
40.0044075527512));
#193851=CARTESIAN_POINT('Ctrl Pts',(-37.015770860109,50.6483072759125,39.9953016253693));
#193852=CARTESIAN_POINT('Ctrl Pts',(-37.01266809487,50.638183057103,39.9860353422325));
#193853=CARTESIAN_POINT('Ctrl Pts',(-37.0093262837647,50.6272788396571,
39.9760551582657));
#193854=CARTESIAN_POINT('Ctrl Pts',(-37.005096310787,50.6167786802254,39.9658879738112));
#193855=CARTESIAN_POINT('Ctrl Pts',(-37.0000610231232,50.6067353452076,
39.9556174643206));
#193856=CARTESIAN_POINT('Ctrl Pts',(-36.9950937288449,50.5968276291246,
39.9454856413871));
#193857=CARTESIAN_POINT('Ctrl Pts',(-36.9893418170227,50.5873633690972,
39.9352519465096));
#193858=CARTESIAN_POINT('Ctrl Pts',(-36.9828414016742,50.578416314936,39.92499));
#193859=CARTESIAN_POINT('Ctrl Pts',(-34.9607485668361,47.7952442955505,
39.92499));
#193860=CARTESIAN_POINT('Ctrl Pts',(-34.9545276336625,47.7866819156019,
39.934810724173));
#193861=CARTESIAN_POINT('Ctrl Pts',(-34.9476537221149,47.7786409912507,
39.9446038383184));
#193862=CARTESIAN_POINT('Ctrl Pts',(-34.940170664354,47.7711595893161,39.9543158069406));
#193863=CARTESIAN_POINT('Ctrl Pts',(-34.9329451136977,47.7639356375057,
39.9636935671417));
#193864=CARTESIAN_POINT('Ctrl Pts',(-34.9251506707945,47.7572325247346,
39.9729968321018));
#193865=CARTESIAN_POINT('Ctrl Pts',(-34.9167928415125,47.7511153344864,
39.9821731151368));
#193866=CARTESIAN_POINT('Ctrl Pts',(-34.908892075331,47.7453326739166,39.9908475764386));
#193867=CARTESIAN_POINT('Ctrl Pts',(-34.9004871280263,47.7400730704109,
39.9994093733882));
#193868=CARTESIAN_POINT('Ctrl Pts',(-34.8915635921215,47.7354288821272,
40.0077966115878));
#193869=CARTESIAN_POINT('Ctrl Pts',(-34.8833451652567,47.73115166263,40.0155211172631));
#193870=CARTESIAN_POINT('Ctrl Pts',(-34.8746863576795,47.7273962447075,
40.0230979941058));
#193871=CARTESIAN_POINT('Ctrl Pts',(-34.8655676881418,47.7242720089015,
40.0304554104784));
#193872=CARTESIAN_POINT('Ctrl Pts',(-34.8628486849594,47.7233404248514,
40.0326492435204));
#193873=CARTESIAN_POINT('Ctrl Pts',(-34.860088762024,47.7224652397586,40.0348233715072));
#193874=CARTESIAN_POINT('Ctrl Pts',(-34.8572873423617,47.7216501132022,
40.0369753512356));
#193875=CARTESIAN_POINT('Ctrl Pts',(-34.8545145463035,47.7208433152301,
40.0391053430352));
#193876=CARTESIAN_POINT('Ctrl Pts',(-34.8517040509264,47.7200959288451,
40.041211089324));
#193877=CARTESIAN_POINT('Ctrl Pts',(-34.8488585612797,47.7194121231168,
40.0432881154904));
#193878=CARTESIAN_POINT('Ctrl Pts',(-34.8486606914946,47.7193645726038,
40.043432547828));
#193879=CARTESIAN_POINT('Ctrl Pts',(-34.8484626496807,47.7193173179073,
40.0435768364421));
#193880=CARTESIAN_POINT('Ctrl Pts',(-34.8482644357605,47.7192703603293,
40.0437209807855));
#193881=CARTESIAN_POINT('Ctrl Pts',(-34.8395740113842,47.7172115680925,
40.050040796842));
#193882=CARTESIAN_POINT('Ctrl Pts',(-34.8305531107003,47.715769135913,40.0560490279343));
#193883=CARTESIAN_POINT('Ctrl Pts',(-34.8212734513098,47.7150344641795,
40.0616647108613));
#193884=CARTESIAN_POINT('Ctrl Pts',(-34.8126231959637,47.7143496224388,
40.0668995033484));
#193885=CARTESIAN_POINT('Ctrl Pts',(-34.8037473009119,47.7142799923074,
40.0717933267481));
#193886=CARTESIAN_POINT('Ctrl Pts',(-34.7947186932874,47.7149249376578,
40.0762460303072));
#193887=CARTESIAN_POINT('Ctrl Pts',(-34.7914159118133,47.7151608670107,
40.0778748868748));
#193888=CARTESIAN_POINT('Ctrl Pts',(-34.7880929011146,47.7154926644832,
40.0794443522247));
#193889=CARTESIAN_POINT('Ctrl Pts',(-34.7847540840176,47.7159260651935,
40.0809482021491));
#193890=CARTESIAN_POINT('Ctrl Pts',(-34.7839512100458,47.7160302835857,
40.0813098278168));
#193891=CARTESIAN_POINT('Ctrl Pts',(-34.7831469919154,47.7161407719864,
40.0816679525672));
#193892=CARTESIAN_POINT('Ctrl Pts',(-34.78234155776,47.716257575019,40.082022419258));
#193893=CARTESIAN_POINT('Ctrl Pts',(-34.781561293422,47.7163707279569,40.0823658088648));
#193894=CARTESIAN_POINT('Ctrl Pts',(-34.7807798878928,47.7164898070137,
40.0827057654616));
#193895=CARTESIAN_POINT('Ctrl Pts',(-34.7799974607185,47.7166148505129,
40.083042147015));
#193896=CARTESIAN_POINT('Ctrl Pts',(-34.7714250667933,47.7179848465562,
40.0867275956806));
#193897=CARTESIAN_POINT('Ctrl Pts',(-34.7627244668151,47.7200720995235,
40.0899823432031));
#193898=CARTESIAN_POINT('Ctrl Pts',(-34.7540804826574,47.722913689108,40.0926299529356));
#193899=CARTESIAN_POINT('Ctrl Pts',(-34.7504955647778,47.7240921810074,
40.0937279956084));
#193900=CARTESIAN_POINT('Ctrl Pts',(-34.7469205018084,47.7254000086989,
40.0947220371802));
#193901=CARTESIAN_POINT('Ctrl Pts',(-34.7433685265017,47.7268379886355,
40.0956014538692));
#193902=CARTESIAN_POINT('Ctrl Pts',(-34.7373102624742,47.7292906132654,
40.097101390674));
#193903=CARTESIAN_POINT('Ctrl Pts',(-34.7313214412506,47.7321228682622,
40.0982667904316));
#193904=CARTESIAN_POINT('Ctrl Pts',(-34.7254747878803,47.7353375827203,
40.0990539325582));
#193905=CARTESIAN_POINT('Ctrl Pts',(-34.7225514611951,47.7369449399494,
40.0994475036216));
#193906=CARTESIAN_POINT('Ctrl Pts',(-34.7196644712716,47.7386491210201,
40.0997467259952));
#193907=CARTESIAN_POINT('Ctrl Pts',(-34.7168229726605,47.7404504949229,
40.0999473488896));
#193908=CARTESIAN_POINT('Ctrl Pts',(-34.7139814740494,47.7422518688257,
40.100147971784));
#193909=CARTESIAN_POINT('Ctrl Pts',(-34.7111854907789,47.7441503967335,
40.10025));
#193910=CARTESIAN_POINT('Ctrl Pts',(-34.7084426211227,47.7461450747867,
40.10025));
#193911=CARTESIAN_POINT('Origin',(-29.1186878401551,50.4655267888878,39.92499));
#193912=CARTESIAN_POINT('Ctrl Pts',(-31.1634057161435,54.3576020372441,
39.92499));
#193913=CARTESIAN_POINT('Ctrl Pts',(-31.1687108809055,54.3667908521544,
39.9348354642014));
#193914=CARTESIAN_POINT('Ctrl Pts',(-31.1747253323927,54.3755338070562,
39.9446440828452));
#193915=CARTESIAN_POINT('Ctrl Pts',(-31.1814073748063,54.3837890328991,
39.9543641760323));
#193916=CARTESIAN_POINT('Ctrl Pts',(-31.1878722906305,54.3917760130589,
39.9637684240703));
#193917=CARTESIAN_POINT('Ctrl Pts',(-31.194962980709,54.3993074034425,39.9730909636386));
#193918=CARTESIAN_POINT('Ctrl Pts',(-31.2026795247194,54.4063187915262,
39.982280897713));
#193919=CARTESIAN_POINT('Ctrl Pts',(-31.2099789001959,54.4129511329171,
39.9909740094639));
#193920=CARTESIAN_POINT('Ctrl Pts',(-31.2178389737506,54.4191188025042,
39.999549276499));
#193921=CARTESIAN_POINT('Ctrl Pts',(-31.2262832675547,54.4247323097979,
40.0079462328684));
#193922=CARTESIAN_POINT('Ctrl Pts',(-31.2340610728553,54.4299027559947,
40.0156804369679));
#193923=CARTESIAN_POINT('Ctrl Pts',(-31.2423350114985,54.4346033281824,
40.0232638017412));
#193924=CARTESIAN_POINT('Ctrl Pts',(-31.2511358718535,54.4387279162168,
40.0306257269957));
#193925=CARTESIAN_POINT('Ctrl Pts',(-31.2536886668971,54.4399243024184,
40.0327611416645));
#193926=CARTESIAN_POINT('Ctrl Pts',(-31.2562858555935,54.4410719653274,
40.0348777427268));
#193927=CARTESIAN_POINT('Ctrl Pts',(-31.2589283212562,54.442167628286,40.03697331687));
#193928=CARTESIAN_POINT('Ctrl Pts',(-31.261792923929,54.4433553973775,40.039245053974));
#193929=CARTESIAN_POINT('Ctrl Pts',(-31.264706337619,54.4444813995855,40.041487875195));
#193930=CARTESIAN_POINT('Ctrl Pts',(-31.2676686823014,54.4455416356298,
40.0436985701601));
#193931=CARTESIAN_POINT('Ctrl Pts',(-31.2757988605275,54.4484514617729,
40.0497658398386));
#193932=CARTESIAN_POINT('Ctrl Pts',(-31.2843017293917,54.4508216479606,
40.0555581699984));
#193933=CARTESIAN_POINT('Ctrl Pts',(-31.293105316062,54.4525775288978,40.0609828468885));
#193934=CARTESIAN_POINT('Ctrl Pts',(-31.3011601199074,54.4541840646263,
40.0659461317304));
#193935=CARTESIAN_POINT('Ctrl Pts',(-31.3094611543724,54.4552661718987,
40.0706039980706));
#193936=CARTESIAN_POINT('Ctrl Pts',(-31.3179758301772,54.4557414157487,
40.0748843180603));
#193937=CARTESIAN_POINT('Ctrl Pts',(-31.3221582111181,54.4559748539754,
40.076986797257));
#193938=CARTESIAN_POINT('Ctrl Pts',(-31.3263919825238,54.4560613864573,
40.0789976708175));
#193939=CARTESIAN_POINT('Ctrl Pts',(-31.3306718639309,54.4559882102926,
40.08090504915));
#193940=CARTESIAN_POINT('Ctrl Pts',(-31.3314839297413,54.4559743258281,
40.0812669556105));
#193941=CARTESIAN_POINT('Ctrl Pts',(-31.3322980319626,54.4559543157133,
40.0816253922033));
#193942=CARTESIAN_POINT('Ctrl Pts',(-31.3331140451953,54.4559281176617,
40.0819801989139));
#193943=CARTESIAN_POINT('Ctrl Pts',(-31.3339045580145,54.4559027382991,
40.0823239179149));
#193944=CARTESIAN_POINT('Ctrl Pts',(-31.3346968642515,54.4558715517162,
40.0826642303498));
#193945=CARTESIAN_POINT('Ctrl Pts',(-31.3354908465824,54.4558345032253,
40.0830009916099));
#193946=CARTESIAN_POINT('Ctrl Pts',(-31.3441435024199,54.4554307564064,
40.0866709464312));
#193947=CARTESIAN_POINT('Ctrl Pts',(-31.3530008879283,54.4543301709717,
40.0899175831877));
#193948=CARTESIAN_POINT('Ctrl Pts',(-31.3618824321381,54.4524721779262,
40.0925642067061));
#193949=CARTESIAN_POINT('Ctrl Pts',(-31.3656331634097,54.4516875359255,
40.0936818922527));
#193950=CARTESIAN_POINT('Ctrl Pts',(-31.3693880355472,54.4507682193238,
40.094693009479));
#193951=CARTESIAN_POINT('Ctrl Pts',(-31.3731331934888,54.4497115877223,
40.0955863397546));
#193952=CARTESIAN_POINT('Ctrl Pts',(-31.3794399458809,54.4479322465077,
40.0970906856167));
#193953=CARTESIAN_POINT('Ctrl Pts',(-31.3857169562555,54.4457622496023,
40.0982599215483));
#193954=CARTESIAN_POINT('Ctrl Pts',(-31.3918909882804,54.4431895758479,
40.0990497370454));
#193955=CARTESIAN_POINT('Ctrl Pts',(-31.3934344962867,54.4425464074094,
40.0992471909196));
#193956=CARTESIAN_POINT('Ctrl Pts',(-31.3949714642034,54.4418778620537,
40.0994209989363));
#193957=CARTESIAN_POINT('Ctrl Pts',(-31.3965005998222,54.4411834812332,
40.0995705982975));
#193958=CARTESIAN_POINT('Ctrl Pts',(-31.3987943032505,54.4401419100025,
40.0997949973393));
#193959=CARTESIAN_POINT('Ctrl Pts',(-31.4010703637561,54.43904220514,40.0999649129781));
#193960=CARTESIAN_POINT('Ctrl Pts',(-31.4033252432067,54.4378842814518,
40.1000786629733));
#193961=CARTESIAN_POINT('Ctrl Pts',(-31.4055801226574,54.4367263577635,
40.1001924129685));
#193962=CARTESIAN_POINT('Ctrl Pts',(-31.4078138194769,54.4355102267474,
40.10025));
#193963=CARTESIAN_POINT('Ctrl Pts',(-31.4100231232056,54.4342359163066,
40.10025));
#193964=CARTESIAN_POINT('Ctrl Pts',(-29.5010785149107,51.127846865905,40.10025));
#193965=CARTESIAN_POINT('Ctrl Pts',(-29.4936027956391,51.1321585373228,
40.10025));
#193966=CARTESIAN_POINT('Ctrl Pts',(-29.486547784523,51.1370499258748,40.099578633424));
#193967=CARTESIAN_POINT('Ctrl Pts',(-29.4799806005917,51.1423856448183,
40.0983063763365));
#193968=CARTESIAN_POINT('Ctrl Pts',(-29.4757388736045,51.145831971779,40.0974846287991));
#193969=CARTESIAN_POINT('Ctrl Pts',(-29.4717000621107,51.1494629466902,
40.0964130309337));
#193970=CARTESIAN_POINT('Ctrl Pts',(-29.4678753842635,51.1532365012462,
40.0951176960923));
#193971=CARTESIAN_POINT('Ctrl Pts',(-29.4628059928679,51.158238131648,40.0934008039614));
#193972=CARTESIAN_POINT('Ctrl Pts',(-29.4581176150985,51.1634934604718,
40.0912909372156));
#193973=CARTESIAN_POINT('Ctrl Pts',(-29.4538379291356,51.1689167792842,
40.0888630467851));
#193974=CARTESIAN_POINT('Ctrl Pts',(-29.4516980861541,51.1716284386904,
40.0876491015699));
#193975=CARTESIAN_POINT('Ctrl Pts',(-29.4496602426628,51.1743821937242,
40.0863558569271));
#193976=CARTESIAN_POINT('Ctrl Pts',(-29.4477266300414,51.1771680313594,
40.0849936342771));
#193977=CARTESIAN_POINT('Ctrl Pts',(-29.4467598237307,51.178560950177,40.0843125229521));
#193978=CARTESIAN_POINT('Ctrl Pts',(-29.4458190608832,51.1799618978182,
40.0836141747074));
#193979=CARTESIAN_POINT('Ctrl Pts',(-29.4449045308656,51.1813696738594,
40.0828999161609));
#193980=CARTESIAN_POINT('Ctrl Pts',(-29.4446758983612,51.1817216178698,
40.0827213515243));
#193981=CARTESIAN_POINT('Ctrl Pts',(-29.4444489051049,51.182073988828,40.0825417925842));
#193982=CARTESIAN_POINT('Ctrl Pts',(-29.444223553443,51.1824267683261,40.082361260236));
#193983=CARTESIAN_POINT('Ctrl Pts',(-29.4435474984573,51.1834851068201,
40.0818196631917));
#193984=CARTESIAN_POINT('Ctrl Pts',(-29.4428862193402,51.1845471213154,
40.0812693052022));
#193985=CARTESIAN_POINT('Ctrl Pts',(-29.4422397658675,51.1856123224582,
40.0807107531875));
#193986=CARTESIAN_POINT('Ctrl Pts',(-29.4376862310779,51.1931154617653,
40.0767763849181));
#193987=CARTESIAN_POINT('Ctrl Pts',(-29.4338145801756,51.20077996036,40.0724140586136));
#193988=CARTESIAN_POINT('Ctrl Pts',(-29.4305579784508,51.2085065710734,
40.0677221223766));
#193989=CARTESIAN_POINT('Ctrl Pts',(-29.4289785301334,51.2122539689198,
40.0654465383719));
#193990=CARTESIAN_POINT('Ctrl Pts',(-29.4275440072538,51.2160164979701,
40.0630928000679));
#193991=CARTESIAN_POINT('Ctrl Pts',(-29.4262483256614,51.2197852472981,
40.0606689262479));
#193992=CARTESIAN_POINT('Ctrl Pts',(-29.4242647276701,51.2255549392046,
40.0569581447806));
#193993=CARTESIAN_POINT('Ctrl Pts',(-29.4226066102319,51.2313356805892,
40.0530843804606));
#193994=CARTESIAN_POINT('Ctrl Pts',(-29.4212581193009,51.2370841708901,
40.0490800251458));
#193995=CARTESIAN_POINT('Ctrl Pts',(-29.4206318731364,51.2397537995246,
40.0472203818218));
#193996=CARTESIAN_POINT('Ctrl Pts',(-29.4200721889211,51.2424163366107,
40.0453323608818));
#193997=CARTESIAN_POINT('Ctrl Pts',(-29.4195787111903,51.2450674596719,
40.0434201572162));
#193998=CARTESIAN_POINT('Ctrl Pts',(-29.4195408880667,51.2452706578086,
40.0432735943397));
#193999=CARTESIAN_POINT('Ctrl Pts',(-29.4195034206998,51.2454737959511,
40.0431268995707));
#194000=CARTESIAN_POINT('Ctrl Pts',(-29.4194663081569,51.2456768729758,
40.0429800745037));
#194001=CARTESIAN_POINT('Ctrl Pts',(-29.4189449888197,51.2485294929148,
40.0409176249753));
#194002=CARTESIAN_POINT('Ctrl Pts',(-29.4184957101761,51.251370561363,40.0388310783332));
#194003=CARTESIAN_POINT('Ctrl Pts',(-29.4181151898793,51.2541954110683,
40.036725739981));
#194004=CARTESIAN_POINT('Ctrl Pts',(-29.416750711768,51.2643248197292,40.0291763710715));
#194005=CARTESIAN_POINT('Ctrl Pts',(-29.4162578421116,51.2743237313769,
40.0213310894589));
#194006=CARTESIAN_POINT('Ctrl Pts',(-29.4165161672804,51.2841455249782,
40.0132837551312));
#194007=CARTESIAN_POINT('Ctrl Pts',(-29.4168000406899,51.2949386894592,
40.0044405431316));
#194008=CARTESIAN_POINT('Ctrl Pts',(-29.4179908989231,51.3055186222606,
39.995352871059));
#194009=CARTESIAN_POINT('Ctrl Pts',(-29.4199800715338,51.315837313597,39.9861103629543));
#194010=CARTESIAN_POINT('Ctrl Pts',(-29.422127878739,51.3269789106019,39.9761307737543));
#194011=CARTESIAN_POINT('Ctrl Pts',(-29.4252064644179,51.3378170984271,
39.9659696935998));
#194012=CARTESIAN_POINT('Ctrl Pts',(-29.4291364604201,51.3482921445265,
39.9557128217493));
#194013=CARTESIAN_POINT('Ctrl Pts',(-29.4330334877936,51.3586793157517,
39.9455419945152));
#194014=CARTESIAN_POINT('Ctrl Pts',(-29.4377684584846,51.3687106315449,
39.9352756289336));
#194015=CARTESIAN_POINT('Ctrl Pts',(-29.4433108116256,51.3783102687788,
39.92499));
#194016=CARTESIAN_POINT('Origin',(-0.0131982271536665,-0.00762000000000475,
39.92499));
#194017=CARTESIAN_POINT('Ctrl Pts',(-31.436419577513,54.4189959163066,40.10025));
#194018=CARTESIAN_POINT('Ctrl Pts',(-31.4438560159996,54.414698338812,40.10025));
#194019=CARTESIAN_POINT('Ctrl Pts',(-31.4508673716598,54.4098177483016,
40.0995859581842));
#194020=CARTESIAN_POINT('Ctrl Pts',(-31.4573895320582,54.4044907169115,
40.0983275959622));
#194021=CARTESIAN_POINT('Ctrl Pts',(-31.4615568820638,54.4010869974478,
40.0975235624069));
#194022=CARTESIAN_POINT('Ctrl Pts',(-31.4655251210641,54.3975017237414,
40.0964777059491));
#194023=CARTESIAN_POINT('Ctrl Pts',(-31.469284216974,54.3937759157112,40.0952149915962));
#194024=CARTESIAN_POINT('Ctrl Pts',(-31.474414628622,54.3886909353396,40.0934916398702));
#194025=CARTESIAN_POINT('Ctrl Pts',(-31.4791503318816,54.3833409297224,
40.0913643921631));
#194026=CARTESIAN_POINT('Ctrl Pts',(-31.4834636394924,54.3778174666306,
40.0889118607713));
#194027=CARTESIAN_POINT('Ctrl Pts',(-31.4856202932977,54.3750557350847,
40.0876855950755));
#194028=CARTESIAN_POINT('Ctrl Pts',(-31.4876715300021,54.3722505364145,
40.0863782327527));
#194029=CARTESIAN_POINT('Ctrl Pts',(-31.4896151854255,54.369412577295,40.0850006373334));
#194030=CARTESIAN_POINT('Ctrl Pts',(-31.4905870131372,54.3679935977353,
40.0843118396238));
#194031=CARTESIAN_POINT('Ctrl Pts',(-31.4915319606347,54.3665664194002,
40.0836054919165));
#194032=CARTESIAN_POINT('Ctrl Pts',(-31.4924498523883,54.3651323262971,
40.0828829920418));
#194033=CARTESIAN_POINT('Ctrl Pts',(-31.4926793253267,54.3647738030213,
40.0827023670731));
#194034=CARTESIAN_POINT('Ctrl Pts',(-31.4929071076035,54.3644148473888,
40.0825207326933));
#194035=CARTESIAN_POINT('Ctrl Pts',(-31.4931331971263,54.3640554790924,
40.0823381109276));
#194036=CARTESIAN_POINT('Ctrl Pts',(-31.4938114656948,54.3629773742031,
40.0817902456304));
#194037=CARTESIAN_POINT('Ctrl Pts',(-31.4944744978645,54.3618955562475,
40.0812334935553));
#194038=CARTESIAN_POINT('Ctrl Pts',(-31.4951222515523,54.3608105487852,
40.0806684524227));
#194039=CARTESIAN_POINT('Ctrl Pts',(-31.499598631437,54.3533124740227,40.0767636676139));
#194040=CARTESIAN_POINT('Ctrl Pts',(-31.5034009004289,54.3456575719332,
40.0724404510892));
#194041=CARTESIAN_POINT('Ctrl Pts',(-31.5065976218795,54.3379428492072,
40.0677949937415));
#194042=CARTESIAN_POINT('Ctrl Pts',(-31.5081863836659,54.3341086531883,
40.065486214191));
#194043=CARTESIAN_POINT('Ctrl Pts',(-31.5096252947441,54.3302591366972,
40.0630972003218));
#194044=CARTESIAN_POINT('Ctrl Pts',(-31.5109210155997,54.3264035847699,
40.0606363359906));
#194045=CARTESIAN_POINT('Ctrl Pts',(-31.5137795693407,54.3178976613389,
40.0552073017124));
#194046=CARTESIAN_POINT('Ctrl Pts',(-31.5159526675026,54.3093672304022,
40.0494204304519));
#194047=CARTESIAN_POINT('Ctrl Pts',(-31.5174623893712,54.3009559572069,
40.0434049749851));
#194048=CARTESIAN_POINT('Ctrl Pts',(-31.5180139098083,54.2978832130369,
40.0412074532442));
#194049=CARTESIAN_POINT('Ctrl Pts',(-31.5184846398471,54.2948245130136,
40.0389814735788));
#194050=CARTESIAN_POINT('Ctrl Pts',(-31.5188783726365,54.2917835794185,
40.0367321210017));
#194051=CARTESIAN_POINT('Ctrl Pts',(-31.5202008794128,54.2815694052538,
40.0291767837139));
#194052=CARTESIAN_POINT('Ctrl Pts',(-31.5206547127625,54.2714898389046,
40.0213235332572));
#194053=CARTESIAN_POINT('Ctrl Pts',(-31.5203592886224,54.261591801797,40.0132649215852));
#194054=CARTESIAN_POINT('Ctrl Pts',(-31.520034582497,54.2507126865162,40.0044075527524));
#194055=CARTESIAN_POINT('Ctrl Pts',(-31.5188048676546,54.2400521939118,
39.9953016253709));
#194056=CARTESIAN_POINT('Ctrl Pts',(-31.5167773687222,54.2296591093502,
39.9860353422345));
#194057=CARTESIAN_POINT('Ctrl Pts',(-31.5145936655006,54.2184653119691,
39.9760551582679));
#194058=CARTESIAN_POINT('Ctrl Pts',(-31.5114844302871,54.2075805209345,
39.9658879738137));
#194059=CARTESIAN_POINT('Ctrl Pts',(-31.5075265408317,54.1970658734753,
39.9556174643232));
#194060=CARTESIAN_POINT('Ctrl Pts',(-31.5036220962477,54.1866932092592,
39.945485641389));
#194061=CARTESIAN_POINT('Ctrl Pts',(-31.4988909785566,54.1766795569341,
39.9352519465106));
#194062=CARTESIAN_POINT('Ctrl Pts',(-31.4933613949854,54.1671020372441,
39.92499));
#194063=CARTESIAN_POINT('Ctrl Pts',(-29.7732664904675,51.1878102687788,
39.92499));
#194064=CARTESIAN_POINT('Ctrl Pts',(-29.767974648635,51.1786445298592,39.9348107241724));
#194065=CARTESIAN_POINT('Ctrl Pts',(-29.7619788985601,51.1699291351227,
39.9446038383174));
#194066=CARTESIAN_POINT('Ctrl Pts',(-29.7553188532203,51.1617065245628,
39.9543158069391));
#194067=CARTESIAN_POINT('Ctrl Pts',(-29.7488879934682,51.1537668706101,
39.9636935671398));
#194068=CARTESIAN_POINT('Ctrl Pts',(-29.7418369154162,51.1462857370536,
39.9729968320996));
#194069=CARTESIAN_POINT('Ctrl Pts',(-29.734164291694,51.1393284263626,39.9821731151343));
#194070=CARTESIAN_POINT('Ctrl Pts',(-29.7269112593595,51.1327515888649,
39.990847576436));
#194071=CARTESIAN_POINT('Ctrl Pts',(-29.7191021335077,51.126642241792,39.9994093733854));
#194072=CARTESIAN_POINT('Ctrl Pts',(-29.7107129315309,51.1210907313625,
40.007796611585));
#194073=CARTESIAN_POINT('Ctrl Pts',(-29.7029866172497,51.1159778833906,
40.0155211172603));
#194074=CARTESIAN_POINT('Ctrl Pts',(-29.694767791591,51.1113379461905,40.0230979941029));
#194075=CARTESIAN_POINT('Ctrl Pts',(-29.686025646647,51.1072776647611,40.0304554104755));
#194076=CARTESIAN_POINT('Ctrl Pts',(-29.6834189154966,51.1060669708011,
40.0326492435186));
#194077=CARTESIAN_POINT('Ctrl Pts',(-29.6807655934595,51.1049080895602,
40.0348233715063));
#194078=CARTESIAN_POINT('Ctrl Pts',(-29.6780647241923,51.1038046002596,
40.0369753512356));
#194079=CARTESIAN_POINT('Ctrl Pts',(-29.6753914511533,51.1027123859003,
40.0391053430352));
#194080=CARTESIAN_POINT('Ctrl Pts',(-29.6726744751142,51.1016753170132,
40.041211089324));
#194081=CARTESIAN_POINT('Ctrl Pts',(-29.6699160505195,51.1006978225843,
40.0432881154904));
#194082=CARTESIAN_POINT('Ctrl Pts',(-29.6697242350678,51.1006298495334,
40.043432547828));
#194083=CARTESIAN_POINT('Ctrl Pts',(-29.6695322176085,51.1005621526965,
40.0435768364421));
#194084=CARTESIAN_POINT('Ctrl Pts',(-29.6693399979284,51.1004947333606,
40.0437209807855));
#194085=CARTESIAN_POINT('Ctrl Pts',(-29.6609123829948,51.0975388226979,
40.050040796842));
#194086=CARTESIAN_POINT('Ctrl Pts',(-29.6520916749677,51.0951613514271,
40.0560490279344));
#194087=CARTESIAN_POINT('Ctrl Pts',(-29.6429396446295,51.0934607157664,
40.0616647108614));
#194088=CARTESIAN_POINT('Ctrl Pts',(-29.6344083617421,51.0918754277623,
40.0668995033485));
#194089=CARTESIAN_POINT('Ctrl Pts',(-29.6255883681029,51.0908783954021,
40.0717933267481));
#194090=CARTESIAN_POINT('Ctrl Pts',(-29.6165418049893,51.0905760611939,
40.0762460303072));
#194091=CARTESIAN_POINT('Ctrl Pts',(-29.6132324551649,51.0904654634292,
40.0778748868748));
#194092=CARTESIAN_POINT('Ctrl Pts',(-29.6098929659866,51.0904480940786,
40.0794443522247));
#194093=CARTESIAN_POINT('Ctrl Pts',(-29.6065271365688,51.0905301191542,
40.0809482021492));
#194094=CARTESIAN_POINT('Ctrl Pts',(-29.6057177670362,51.0905498434447,
40.0813098278168));
#194095=CARTESIAN_POINT('Ctrl Pts',(-29.6049064053142,51.0905756628931,
40.0816679525672));
#194096=CARTESIAN_POINT('Ctrl Pts',(-29.6040931741699,51.090607635272,40.082022419258));
#194097=CARTESIAN_POINT('Ctrl Pts',(-29.6033053564988,51.090638608514,40.0823658088648));
#194098=CARTESIAN_POINT('Ctrl Pts',(-29.60251578444,51.0906753561241,40.0827057654616));
#194099=CARTESIAN_POINT('Ctrl Pts',(-29.6017245728788,51.0907179287118,
40.0830421470151));
#194100=CARTESIAN_POINT('Ctrl Pts',(-29.5930559358432,51.0911843606099,
40.0867275956807));
#194101=CARTESIAN_POINT('Ctrl Pts',(-29.5841848213168,51.0923507190419,
40.0899823432032));
#194102=CARTESIAN_POINT('Ctrl Pts',(-29.5752911628161,51.0942731997209,
40.0926299529358));
#194103=CARTESIAN_POINT('Ctrl Pts',(-29.5716026975446,51.0950705097614,
40.0937279956086));
#194104=CARTESIAN_POINT('Ctrl Pts',(-29.5679105139256,51.0959974771977,
40.0947220371803));
#194105=CARTESIAN_POINT('Ctrl Pts',(-29.5642276868785,51.0970562972093,
40.0956014538692));
#194106=CARTESIAN_POINT('Ctrl Pts',(-29.5579462415717,51.098862225076,40.097101390674));
#194107=CARTESIAN_POINT('Ctrl Pts',(-29.551694176475,51.1010529624043,40.0982667904316));
#194108=CARTESIAN_POINT('Ctrl Pts',(-29.5455435225214,51.103638924628,40.0990539325582));
#194109=CARTESIAN_POINT('Ctrl Pts',(-29.5424681955445,51.1049319057399,
40.0994475036216));
#194110=CARTESIAN_POINT('Ctrl Pts',(-29.5394188854254,51.1063249785082,
40.0997467259952));
#194111=CARTESIAN_POINT('Ctrl Pts',(-29.5364046579953,51.1078194668132,
40.0999473488896));
#194112=CARTESIAN_POINT('Ctrl Pts',(-29.5333904305651,51.1093139551182,
40.100147971784));
#194113=CARTESIAN_POINT('Ctrl Pts',(-29.5304113137788,51.1109098228569,
40.10025));
#194114=CARTESIAN_POINT('Ctrl Pts',(-29.527474969218,51.112606865905,40.10025));
#194115=CARTESIAN_POINT('Origin',(-23.6840886581931,53.232803045145,39.92499));
#194116=CARTESIAN_POINT('Ctrl Pts',(-25.3107727110817,57.3172883154492,
39.92499));
#194117=CARTESIAN_POINT('Ctrl Pts',(-25.3150883208942,57.3269813337898,
39.9348354642014));
#194118=CARTESIAN_POINT('Ctrl Pts',(-25.3201559369465,57.336305075241,39.9446440828451));
#194119=CARTESIAN_POINT('Ctrl Pts',(-25.3259384683613,57.345213541718,39.9543641760322));
#194120=CARTESIAN_POINT('Ctrl Pts',(-25.3315331019378,57.3538325360809,
39.9637684240701));
#194121=CARTESIAN_POINT('Ctrl Pts',(-25.337797703811,57.3620638476573,39.9730909636383));
#194122=CARTESIAN_POINT('Ctrl Pts',(-25.3447390861641,57.3698434251107,
39.9822808977126));
#194123=CARTESIAN_POINT('Ctrl Pts',(-25.3513052064445,57.3772024263428,
39.9909740094634));
#194124=CARTESIAN_POINT('Ctrl Pts',(-25.3584775246698,57.3841579102004,
39.9995492764985));
#194125=CARTESIAN_POINT('Ctrl Pts',(-25.3662887884579,57.3906233351685,
40.0079462328677));
#194126=CARTESIAN_POINT('Ctrl Pts',(-25.3734835273317,57.3965784591556,
40.0156804369671));
#194127=CARTESIAN_POINT('Ctrl Pts',(-25.3812207968859,57.4021181432086,
40.0232638017402));
#194128=CARTESIAN_POINT('Ctrl Pts',(-25.3895423083579,57.4071400767265,
40.0306257269946));
#194129=CARTESIAN_POINT('Ctrl Pts',(-25.3919560625124,57.4085967487425,
40.0327611416638));
#194130=CARTESIAN_POINT('Ctrl Pts',(-25.3944190600976,57.4100096047775,
40.0348777427264));
#194131=CARTESIAN_POINT('Ctrl Pts',(-25.396932522092,57.4113754784549,40.0369733168701));
#194132=CARTESIAN_POINT('Ctrl Pts',(-25.3996572764938,57.4128561733383,
40.039245053974));
#194133=CARTESIAN_POINT('Ctrl Pts',(-25.4024370309183,57.4142805418442,
40.041487875195));
#194134=CARTESIAN_POINT('Ctrl Pts',(-25.4052723227222,57.4156446191419,
40.0436985701601));
#194135=CARTESIAN_POINT('Ctrl Pts',(-25.4130538033262,57.419388339989,40.0497658398386));
#194136=CARTESIAN_POINT('Ctrl Pts',(-25.4212623406652,57.4226343338644,
40.0555581699984));
#194137=CARTESIAN_POINT('Ctrl Pts',(-25.4298341608305,57.425300821288,40.0609828468886));
#194138=CARTESIAN_POINT('Ctrl Pts',(-25.4376769109072,57.4277405125137,
40.0659461317306));
#194139=CARTESIAN_POINT('Ctrl Pts',(-25.4458193604268,57.4296843862656,
40.070603998071));
#194140=CARTESIAN_POINT('Ctrl Pts',(-25.4542377154376,57.4310470526571,
40.0748843180608));
#194141=CARTESIAN_POINT('Ctrl Pts',(-25.4583727839187,57.4317163899372,
40.0769867972573));
#194142=CARTESIAN_POINT('Ctrl Pts',(-25.462574317174,57.432244998004,40.0789976708176));
#194143=CARTESIAN_POINT('Ctrl Pts',(-25.4668384019346,57.4326195921324,
40.08090504915));
#194144=CARTESIAN_POINT('Ctrl Pts',(-25.4676474704853,57.4326906677196,
40.0812669556105));
#194145=CARTESIAN_POINT('Ctrl Pts',(-25.4684592045961,57.4327558640765,
40.0816253922033));
#194146=CARTESIAN_POINT('Ctrl Pts',(-25.469273486065,57.4328151061498,40.0819801989139));
#194147=CARTESIAN_POINT('Ctrl Pts',(-25.470062321238,57.4328724969082,40.0823239179149));
#194148=CARTESIAN_POINT('Ctrl Pts',(-25.4708535470242,57.432924299722,40.0826642303498));
#194149=CARTESIAN_POINT('Ctrl Pts',(-25.4716470524585,57.4329704479396,
40.0830009916099));
#194150=CARTESIAN_POINT('Ctrl Pts',(-25.4802945111763,57.4334733617058,
40.086670946431));
#194151=CARTESIAN_POINT('Ctrl Pts',(-25.4892184175041,57.4333046542891,
40.0899175831875));
#194152=CARTESIAN_POINT('Ctrl Pts',(-25.4982455208428,57.4323852136917,
40.0925642067058));
#194153=CARTESIAN_POINT('Ctrl Pts',(-25.502057722639,57.4319969282178,40.0936818922525));
#194154=CARTESIAN_POINT('Ctrl Pts',(-25.5058881199459,57.431475138743,40.094693009479));
#194155=CARTESIAN_POINT('Ctrl Pts',(-25.5097232095982,57.4308157710843,
40.0955863397546));
#194156=CARTESIAN_POINT('Ctrl Pts',(-25.5161814047437,57.4297054124228,
40.0970906856166));
#194157=CARTESIAN_POINT('Ctrl Pts',(-25.5226508554405,57.4282034292358,
40.0982599215483));
#194158=CARTESIAN_POINT('Ctrl Pts',(-25.5290599831058,57.4262902109365,
40.0990497370454));
#194159=CARTESIAN_POINT('Ctrl Pts',(-25.5306622650221,57.4258119063617,
40.0992471909196));
#194160=CARTESIAN_POINT('Ctrl Pts',(-25.5322606952864,57.4253076802619,
40.0994209989363));
#194161=CARTESIAN_POINT('Ctrl Pts',(-25.5338540367004,57.4247769415286,
40.0995705982975));
#194162=CARTESIAN_POINT('Ctrl Pts',(-25.5362440488215,57.4239808334287,
40.0997949973393));
#194163=CARTESIAN_POINT('Ctrl Pts',(-25.5386225912888,57.4231250659716,
40.0999649129781));
#194164=CARTESIAN_POINT('Ctrl Pts',(-25.5409861542577,57.4222091845945,
40.1000786629733));
#194165=CARTESIAN_POINT('Ctrl Pts',(-25.5433497172265,57.4212933032173,
40.1001924129685));
#194166=CARTESIAN_POINT('Ctrl Pts',(-25.5456982979275,57.4203173191903,
40.10025));
#194167=CARTESIAN_POINT('Ctrl Pts',(-25.5480287005713,57.4192809246791,
40.10025));
#194168=CARTESIAN_POINT('Ctrl Pts',(-23.9951532569802,53.9314655730806,
40.10025));
#194169=CARTESIAN_POINT('Ctrl Pts',(-23.9872677980933,53.9349721992642,
40.10025));
#194170=CARTESIAN_POINT('Ctrl Pts',(-23.9797401457373,53.9390993428078,
40.099578633424));
#194171=CARTESIAN_POINT('Ctrl Pts',(-23.9726512030249,53.9437193744806,
40.0983063763363));
#194172=CARTESIAN_POINT('Ctrl Pts',(-23.9680724734011,53.9467034408979,
40.097484628799));
#194173=CARTESIAN_POINT('Ctrl Pts',(-23.9636762467119,53.9498923541895,
40.0964130309336));
#194174=CARTESIAN_POINT('Ctrl Pts',(-23.9594780769917,53.9532454491207,
40.0951176960923));
#194175=CARTESIAN_POINT('Ctrl Pts',(-23.9539136435128,53.9576897843755,
40.0934008039614));
#194176=CARTESIAN_POINT('Ctrl Pts',(-23.9487016177215,53.9624262550347,
40.0912909372156));
#194177=CARTESIAN_POINT('Ctrl Pts',(-23.9438784851449,53.9673725153422,
40.0888630467851));
#194178=CARTESIAN_POINT('Ctrl Pts',(-23.9414669188565,53.969845645496,40.0876491015699));
#194179=CARTESIAN_POINT('Ctrl Pts',(-23.9391523931032,53.972371302523,40.0863558569271));
#194180=CARTESIAN_POINT('Ctrl Pts',(-23.9369381736871,53.9749397614923,
40.0849936342771));
#194181=CARTESIAN_POINT('Ctrl Pts',(-23.935831063979,53.976223990977,40.0843125229521));
#194182=CARTESIAN_POINT('Ctrl Pts',(-23.9347490158249,53.9775189275857,
40.0836141747074));
#194183=CARTESIAN_POINT('Ctrl Pts',(-23.9336923430321,53.9788233972651,
40.0828999161609));
#194184=CARTESIAN_POINT('Ctrl Pts',(-23.9334281748339,53.9791495146849,
40.0827213515243));
#194185=CARTESIAN_POINT('Ctrl Pts',(-23.9331655922757,53.979476228062,40.0825417925842));
#194186=CARTESIAN_POINT('Ctrl Pts',(-23.932904599615,53.9798035193341,40.0823612602361));
#194187=CARTESIAN_POINT('Ctrl Pts',(-23.9321216216328,53.9807853931505,
40.0818196631917));
#194188=CARTESIAN_POINT('Ctrl Pts',(-23.9313529543287,53.9817724673293,
40.0812693052022));
#194189=CARTESIAN_POINT('Ctrl Pts',(-23.9305986983573,53.9827642604007,
40.0807107531875));
#194190=CARTESIAN_POINT('Ctrl Pts',(-23.925285816686,53.9897503227319,40.076776384918));
#194191=CARTESIAN_POINT('Ctrl Pts',(-23.9206342168325,53.9969681366825,
40.0724140586132));
#194192=CARTESIAN_POINT('Ctrl Pts',(-23.9165878043684,54.0043120126406,
40.067722122376));
#194193=CARTESIAN_POINT('Ctrl Pts',(-23.9146252986962,54.0078737845438,
40.0654465383715));
#194194=CARTESIAN_POINT('Ctrl Pts',(-23.9128053429036,54.0114657535938,
40.0630928000676));
#194195=CARTESIAN_POINT('Ctrl Pts',(-23.911122817615,54.0150784217126,40.0606689262479));
#194196=CARTESIAN_POINT('Ctrl Pts',(-23.9085469889525,54.0206091641934,
40.0569581447805));
#194197=CARTESIAN_POINT('Ctrl Pts',(-23.9062937028417,54.0261849176041,
40.0530843804606));
#194198=CARTESIAN_POINT('Ctrl Pts',(-23.9043517182278,54.0317609613889,
40.0490800251458));
#194199=CARTESIAN_POINT('Ctrl Pts',(-23.9034498505266,54.0343505049692,
40.0472203818218));
#194200=CARTESIAN_POINT('Ctrl Pts',(-23.90261492141,54.0369399534676,40.0453323608819));
#194201=CARTESIAN_POINT('Ctrl Pts',(-23.9018470291824,54.0395249709304,
40.0434201572162));
#194202=CARTESIAN_POINT('Ctrl Pts',(-23.9017881732688,54.0397231023335,
40.0432735943397));
#194203=CARTESIAN_POINT('Ctrl Pts',(-23.9017296774342,54.0399212112578,
40.0431268995707));
#194204=CARTESIAN_POINT('Ctrl Pts',(-23.9016715408684,54.0401192964882,
40.0429800745037));
#194205=CARTESIAN_POINT('Ctrl Pts',(-23.9008548973946,54.0429017967675,
40.0409176249753));
#194206=CARTESIAN_POINT('Ctrl Pts',(-23.9001111074275,54.0456803391392,
40.0388310783332));
#194207=CARTESIAN_POINT('Ctrl Pts',(-23.899437394462,54.0484499388204,40.036725739981));
#194208=CARTESIAN_POINT('Ctrl Pts',(-23.8970215795833,54.0583812307209,
40.0291763710714));
#194209=CARTESIAN_POINT('Ctrl Pts',(-23.8954862390496,54.0682738483768,
40.0213310894587));
#194210=CARTESIAN_POINT('Ctrl Pts',(-23.8947164920945,54.0780688394982,
40.0132837551308));
#194211=CARTESIAN_POINT('Ctrl Pts',(-23.8938706175187,54.0888325507465,
40.0044405431308));
#194212=CARTESIAN_POINT('Ctrl Pts',(-23.8939490479888,54.0994790041506,
39.9953528710578));
#194213=CARTESIAN_POINT('Ctrl Pts',(-23.8948487267555,54.1099490937727,
39.9861103629527));
#194214=CARTESIAN_POINT('Ctrl Pts',(-23.8958201540351,54.1212541629309,
39.976130773752));
#194215=CARTESIAN_POINT('Ctrl Pts',(-23.8977489757819,54.13235477786,39.9659696935967));
#194216=CARTESIAN_POINT('Ctrl Pts',(-23.9005625023837,54.1431832370043,
39.9557128217453));
#194217=CARTESIAN_POINT('Ctrl Pts',(-23.9033524263876,54.1539208564999,
39.9455419945125));
#194218=CARTESIAN_POINT('Ctrl Pts',(-23.9070129003889,54.1643921589041,
39.9352756289323));
#194219=CARTESIAN_POINT('Ctrl Pts',(-23.911521456611,54.1745185419761,39.92499));
#194220=CARTESIAN_POINT('Origin',(-0.0139224327744654,-0.0061986664404802,
39.92499));
#194221=CARTESIAN_POINT('Ctrl Pts',(-25.5758735661203,57.4068835917982,
40.10025));
#194222=CARTESIAN_POINT('Ctrl Pts',(-25.5837184861901,57.4033868763699,
40.10025));
#194223=CARTESIAN_POINT('Ctrl Pts',(-25.5912015935364,57.3992659084775,
40.0995859581842));
#194224=CARTESIAN_POINT('Ctrl Pts',(-25.5982448512627,57.3946498105263,
40.0983275959621));
#194225=CARTESIAN_POINT('Ctrl Pts',(-25.6027451576539,57.3917003436859,
40.0975235624068));
#194226=CARTESIAN_POINT('Ctrl Pts',(-25.6070664213767,57.3885495044087,
40.0964777059491));
#194227=CARTESIAN_POINT('Ctrl Pts',(-25.6111943775537,57.3852370392634,
40.0952149915961));
#194228=CARTESIAN_POINT('Ctrl Pts',(-25.6168282094538,57.3807161889918,
40.0934916398701));
#194229=CARTESIAN_POINT('Ctrl Pts',(-25.6220971979011,57.3758905070494,
40.091364392163));
#194230=CARTESIAN_POINT('Ctrl Pts',(-25.6269642358703,57.3708481654825,
40.0889118607713));
#194231=CARTESIAN_POINT('Ctrl Pts',(-25.6293977548549,57.3683269946991,
40.0876855950754));
#194232=CARTESIAN_POINT('Ctrl Pts',(-25.6317309777762,57.3657515758212,
40.0863782327526));
#194233=CARTESIAN_POINT('Ctrl Pts',(-25.6339606331573,57.3631323306533,
40.0850006373334));
#194234=CARTESIAN_POINT('Ctrl Pts',(-25.6350754608479,57.3618227080694,
40.0843118396237));
#194235=CARTESIAN_POINT('Ctrl Pts',(-25.6361644125823,57.3605021218764,
40.0836054919164));
#194236=CARTESIAN_POINT('Ctrl Pts',(-25.6372271795771,57.3591718306997,
40.0828829920418));
#194237=CARTESIAN_POINT('Ctrl Pts',(-25.6374928713258,57.3588392579056,
40.0827023670731));
#194238=CARTESIAN_POINT('Ctrl Pts',(-25.6377569268681,57.358506078401,40.0825207326933));
#194239=CARTESIAN_POINT('Ctrl Pts',(-25.6380193420646,57.358172311552,40.0823381109275));
#194240=CARTESIAN_POINT('Ctrl Pts',(-25.6388065876542,57.3571710110053,
40.0817902456303));
#194241=CARTESIAN_POINT('Ctrl Pts',(-25.6395790684327,57.3561644250955,
40.0812334935553));
#194242=CARTESIAN_POINT('Ctrl Pts',(-25.6403366878207,57.3551530701152,
40.0806684524227));
#194243=CARTESIAN_POINT('Ctrl Pts',(-25.6455723078606,57.3481639797008,
40.0767636676137));
#194244=CARTESIAN_POINT('Ctrl Pts',(-25.6501539027771,57.3409484573004,
40.0724404510889));
#194245=CARTESIAN_POINT('Ctrl Pts',(-25.6541395203643,57.3336101450131,
40.0677949937411));
#194246=CARTESIAN_POINT('Ctrl Pts',(-25.656120361365,57.3299630239495,40.0654862141907));
#194247=CARTESIAN_POINT('Ctrl Pts',(-25.6579537739808,57.3262850026765,
40.0630972003217));
#194248=CARTESIAN_POINT('Ctrl Pts',(-25.6596454116599,57.3225860115761,
40.0606363359906));
#194249=CARTESIAN_POINT('Ctrl Pts',(-25.6633774170493,57.3144254847134,
40.0552073017124));
#194250=CARTESIAN_POINT('Ctrl Pts',(-25.6664302835889,57.3061689349814,
40.0494204304519));
#194251=CARTESIAN_POINT('Ctrl Pts',(-25.6688109525044,57.2979615485276,
40.0434049749851));
#194252=CARTESIAN_POINT('Ctrl Pts',(-25.669680640881,57.2949632867554,40.0412074532442));
#194253=CARTESIAN_POINT('Ctrl Pts',(-25.6704685134244,57.2919705472985,
40.0389814735788));
#194254=CARTESIAN_POINT('Ctrl Pts',(-25.67117795342,57.2889874285393,40.0367321210017));
#194255=CARTESIAN_POINT('Ctrl Pts',(-25.6735608872945,57.2789674482913,
40.0291767837146));
#194256=CARTESIAN_POINT('Ctrl Pts',(-25.6750658360785,57.2689905373647,
40.0213235332587));
#194257=CARTESIAN_POINT('Ctrl Pts',(-25.675806656911,57.2591158425095,40.0132649215875));
#194258=CARTESIAN_POINT('Ctrl Pts',(-25.6766209067618,57.248262383129,40.0044075527555));
#194259=CARTESIAN_POINT('Ctrl Pts',(-25.6765122533358,57.2375317496164,
39.9953016253747));
#194260=CARTESIAN_POINT('Ctrl Pts',(-25.6755822344128,57.2269836681125,
39.9860353422391));
#194261=CARTESIAN_POINT('Ctrl Pts',(-25.6745805641847,57.2156229323833,
39.9760551582733));
#194262=CARTESIAN_POINT('Ctrl Pts',(-25.6726261321672,57.2044727657947,
39.9658879738199));
#194263=CARTESIAN_POINT('Ctrl Pts',(-25.6697890043857,57.1936020065725,
39.9556174643302));
#194264=CARTESIAN_POINT('Ctrl Pts',(-25.6669901874079,57.1828780393016,
39.9454856413937));
#194265=CARTESIAN_POINT('Ctrl Pts',(-25.6633316989632,57.1724247063476,
39.935251946513));
#194266=CARTESIAN_POINT('Ctrl Pts',(-25.6588335304436,57.1623216544373,
39.92499));
#194267=CARTESIAN_POINT('Ctrl Pts',(-24.2595822759728,54.0195518809643,
39.92499));
#194268=CARTESIAN_POINT('Ctrl Pts',(-24.2552775040072,54.0098832048262,
39.9348107241732));
#194269=CARTESIAN_POINT('Ctrl Pts',(-24.2502256060967,54.0005888273918,
39.9446038383189));
#194270=CARTESIAN_POINT('Ctrl Pts',(-24.2444615420275,53.9917150968476,
39.9543158069413));
#194271=CARTESIAN_POINT('Ctrl Pts',(-24.2388958310241,53.9831467292621,
39.9636935671426));
#194272=CARTESIAN_POINT('Ctrl Pts',(-24.232665370909,53.9749695397845,39.972996832103));
#194273=CARTESIAN_POINT('Ctrl Pts',(-24.2257620156167,53.9672483344021,
39.9821731151383));
#194274=CARTESIAN_POINT('Ctrl Pts',(-24.2192361828685,53.959949377184,39.9908475764405));
#194275=CARTESIAN_POINT('Ctrl Pts',(-24.2121084368856,53.9530572218286,
39.9994093733904));
#194276=CARTESIAN_POINT('Ctrl Pts',(-24.2043454826882,53.9466592127632,
40.0077966115905));
#194277=CARTESIAN_POINT('Ctrl Pts',(-24.1971959321057,53.9407667537486,
40.0155211172663));
#194278=CARTESIAN_POINT('Ctrl Pts',(-24.1895071355381,53.9352931333939,
40.0230979941094));
#194279=CARTESIAN_POINT('Ctrl Pts',(-24.181237295956,53.9303412916343,40.0304554104825));
#194280=CARTESIAN_POINT('Ctrl Pts',(-24.1787713967332,53.9288647523828,
40.0326492435231));
#194281=CARTESIAN_POINT('Ctrl Pts',(-24.1762537459497,53.9274348719411,
40.0348233715086));
#194282=CARTESIAN_POINT('Ctrl Pts',(-24.1736830183705,53.9260551099578,
40.0369753512356));
#194283=CARTESIAN_POINT('Ctrl Pts',(-24.1711385572894,53.9246894457404,
40.0391053430352));
#194284=CARTESIAN_POINT('Ctrl Pts',(-24.1685448683464,53.9233740566951,
40.041211089324));
#194285=CARTESIAN_POINT('Ctrl Pts',(-24.1659037306808,53.922113583199,40.0432881154904));
#194286=CARTESIAN_POINT('Ctrl Pts',(-24.1657200711328,53.9220259323371,
40.0434325478279));
#194287=CARTESIAN_POINT('Ctrl Pts',(-24.1655361818115,53.9219385350607,
40.0435768364421));
#194288=CARTESIAN_POINT('Ctrl Pts',(-24.1653520623704,53.9218513926272,
40.0437209807855));
#194289=CARTESIAN_POINT('Ctrl Pts',(-24.1572795915922,53.9180307491142,
40.0500407968422));
#194290=CARTESIAN_POINT('Ctrl Pts',(-24.1487557177448,53.9147442868247,
40.0560490279348));
#194291=CARTESIAN_POINT('Ctrl Pts',(-24.1398315880183,53.9120963197571,
40.0616647108619));
#194292=CARTESIAN_POINT('Ctrl Pts',(-24.1315127481097,53.9096279542365,
40.0668995033492));
#194293=CARTESIAN_POINT('Ctrl Pts',(-24.1228452895785,53.9077144433428,
40.071793326749));
#194294=CARTESIAN_POINT('Ctrl Pts',(-24.113879887014,53.906468142013,40.0762460303083));
#194295=CARTESIAN_POINT('Ctrl Pts',(-24.1106002267692,53.9060122288629,
40.0778748868755));
#194296=CARTESIAN_POINT('Ctrl Pts',(-24.1072808472542,53.9056458829917,
40.0794443522251));
#194297=CARTESIAN_POINT('Ctrl Pts',(-24.1039248822477,53.9053756337488,
40.0809482021492));
#194298=CARTESIAN_POINT('Ctrl Pts',(-24.1031178847763,53.9053106478341,
40.0813098278169));
#194299=CARTESIAN_POINT('Ctrl Pts',(-24.1023082689114,53.9052515154468,
40.0816679525672));
#194300=CARTESIAN_POINT('Ctrl Pts',(-24.1014961507088,53.9051983068758,
40.0820224192581));
#194301=CARTESIAN_POINT('Ctrl Pts',(-24.1007094112,53.9051467610727,40.0823658088648));
#194302=CARTESIAN_POINT('Ctrl Pts',(-24.0999203233284,53.9051007746216,
40.0827057654617));
#194303=CARTESIAN_POINT('Ctrl Pts',(-24.0991289960597,53.9050604098636,
40.0830421470151));
#194304=CARTESIAN_POINT('Ctrl Pts',(-24.0904590913156,53.9046181672911,
40.0867275956806));
#194305=CARTESIAN_POINT('Ctrl Pts',(-24.0815146560285,53.9048508523206,
40.089982343203));
#194306=CARTESIAN_POINT('Ctrl Pts',(-24.072468763969,53.9058331609933,40.0926299529355));
#194307=CARTESIAN_POINT('Ctrl Pts',(-24.0687171629026,53.9062405536793,
40.0937279956084));
#194308=CARTESIAN_POINT('Ctrl Pts',(-24.0649483109698,53.9067765048112,
40.0947220371802));
#194309=CARTESIAN_POINT('Ctrl Pts',(-24.0611749820056,53.9074445642444,
40.0956014538693));
#194310=CARTESIAN_POINT('Ctrl Pts',(-24.0547391762487,53.9085840092243,
40.097101390674));
#194311=CARTESIAN_POINT('Ctrl Pts',(-24.0482923662124,53.9101092267075,
40.0982667904316));
#194312=CARTESIAN_POINT('Ctrl Pts',(-24.0419050995275,53.9120381043539,
40.0990539325583));
#194313=CARTESIAN_POINT('Ctrl Pts',(-24.038711466185,53.9130025431771,40.0994475036216));
#194314=CARTESIAN_POINT('Ctrl Pts',(-24.03553324475,53.9140692448462,40.0997467259952));
#194315=CARTESIAN_POINT('Ctrl Pts',(-24.0323793130072,53.9152404736266,
40.0999473488896));
#194316=CARTESIAN_POINT('Ctrl Pts',(-24.0292253812643,53.916411702407,40.100147971784));
#194317=CARTESIAN_POINT('Ctrl Pts',(-24.0260957707892,53.9176874253155,
40.10025));
#194318=CARTESIAN_POINT('Ctrl Pts',(-24.0229981225292,53.9190682401997,
40.10025));
#194319=CARTESIAN_POINT('Origin',(-17.9900016446778,55.4168495715594,39.92499));
#194320=CARTESIAN_POINT('Ctrl Pts',(-19.1808295835776,59.6489943884566,
39.92499));
#194321=CARTESIAN_POINT('Ctrl Pts',(-19.1841083557164,59.6590854114903,
39.9348354642017));
#194322=CARTESIAN_POINT('Ctrl Pts',(-19.188173614472,59.6688877866287,39.9446440828455));
#194323=CARTESIAN_POINT('Ctrl Pts',(-19.1929932802638,59.6783518907168,
39.9543641760327));
#194324=CARTESIAN_POINT('Ctrl Pts',(-19.1976563356165,59.6875084677772,
39.9637684240707));
#194325=CARTESIAN_POINT('Ctrl Pts',(-19.2030262129955,59.6963495165744,
39.973090963639));
#194326=CARTESIAN_POINT('Ctrl Pts',(-19.2091163824538,59.7048120487189,
39.9822808977133));
#194327=CARTESIAN_POINT('Ctrl Pts',(-19.2148773077503,59.7128170830349,
39.9909740094641));
#194328=CARTESIAN_POINT('Ctrl Pts',(-19.2212832892271,59.7204841754264,
39.9995492764992));
#194329=CARTESIAN_POINT('Ctrl Pts',(-19.2283759411587,59.72773068152,40.0079462328684));
#194330=CARTESIAN_POINT('Ctrl Pts',(-19.2349087865413,59.7344052377129,
40.0156804369678));
#194331=CARTESIAN_POINT('Ctrl Pts',(-19.2420246158623,59.7407233396934,
40.0232638017409));
#194332=CARTESIAN_POINT('Ctrl Pts',(-19.2497756062306,59.7465875973403,
40.0306257269953));
#194333=CARTESIAN_POINT('Ctrl Pts',(-19.2520238738997,59.7482885955669,
40.0327611416643));
#194334=CARTESIAN_POINT('Ctrl Pts',(-19.2543256952561,59.7499511651811,
40.0348777427266));
#194335=CARTESIAN_POINT('Ctrl Pts',(-19.2566826155659,59.7515722847792,
40.03697331687));
#194336=CARTESIAN_POINT('Ctrl Pts',(-19.2592376687173,59.7533296826515,
40.039245053974));
#194337=CARTESIAN_POINT('Ctrl Pts',(-19.2618533083051,59.7550368117759,
40.041487875195));
#194338=CARTESIAN_POINT('Ctrl Pts',(-19.2645304831802,59.7566897852106,
40.0436985701601));
#194339=CARTESIAN_POINT('Ctrl Pts',(-19.2718780106322,59.7612263837726,
40.0497658398386));
#194340=CARTESIAN_POINT('Ctrl Pts',(-19.2797022819932,59.7653126215478,
40.0555581699984));
#194341=CARTESIAN_POINT('Ctrl Pts',(-19.2879484209981,59.7688605008636,
40.0609828468886));
#194342=CARTESIAN_POINT('Ctrl Pts',(-19.2954931904943,59.7721066178187,
40.0659461317305));
#194343=CARTESIAN_POINT('Ctrl Pts',(-19.3033878446872,59.7748909605621,
40.0706039980708));
#194344=CARTESIAN_POINT('Ctrl Pts',(-19.3116176456444,59.7771261198371,
40.0748843180605));
#194345=CARTESIAN_POINT('Ctrl Pts',(-19.3156600969906,59.7782240227715,
40.0769867972571));
#194346=CARTESIAN_POINT('Ctrl Pts',(-19.3197833592184,59.7791889148825,
40.0789976708176));
#194347=CARTESIAN_POINT('Ctrl Pts',(-19.3239849291282,59.7800071751724,
40.08090504915));
#194348=CARTESIAN_POINT('Ctrl Pts',(-19.3247821360948,59.7801624320925,
40.0812669556105));
#194349=CARTESIAN_POINT('Ctrl Pts',(-19.3255826085661,59.7803121206161,
40.0816253922033));
#194350=CARTESIAN_POINT('Ctrl Pts',(-19.3263862368331,59.7804561537456,
40.081980198914));
#194351=CARTESIAN_POINT('Ctrl Pts',(-19.3271647517167,59.7805956858399,
40.0823239179149));
#194352=CARTESIAN_POINT('Ctrl Pts',(-19.3279462282167,59.780729910488,40.0826642303499));
#194353=CARTESIAN_POINT('Ctrl Pts',(-19.328730562943,59.7808587498045,40.08300099161));
#194354=CARTESIAN_POINT('Ctrl Pts',(-19.3372780811743,59.7822628141275,
40.0866709464312));
#194355=CARTESIAN_POINT('Ctrl Pts',(-19.3461707361367,59.7830278331224,
40.0899175831877));
#194356=CARTESIAN_POINT('Ctrl Pts',(-19.3552444957718,59.7830570185564,
40.0925642067061));
#194357=CARTESIAN_POINT('Ctrl Pts',(-19.3590764008113,59.7830693437465,
40.0936818922527));
#194358=CARTESIAN_POINT('Ctrl Pts',(-19.3629403566526,59.7829507982332,
40.094693009479));
#194359=CARTESIAN_POINT('Ctrl Pts',(-19.3668233599705,59.7826959186873,
40.0955863397546));
#194360=CARTESIAN_POINT('Ctrl Pts',(-19.3733622405317,59.7822667079008,
40.0970906856167));
#194361=CARTESIAN_POINT('Ctrl Pts',(-19.3799532508951,59.7814491944744,
40.0982599215483));
#194362=CARTESIAN_POINT('Ctrl Pts',(-19.3865272544572,59.780216393251,40.0990497370454));
#194363=CARTESIAN_POINT('Ctrl Pts',(-19.3881707553477,59.7799081929452,
40.0992471909196));
#194364=CARTESIAN_POINT('Ctrl Pts',(-19.3898131352231,59.7795738105079,
40.0994209989363));
#194365=CARTESIAN_POINT('Ctrl Pts',(-19.3914532254504,59.7792125287464,
40.0995705982975));
#194366=CARTESIAN_POINT('Ctrl Pts',(-19.3939133607912,59.7786706061041,
40.0997949973393));
#194367=CARTESIAN_POINT('Ctrl Pts',(-19.3963683254113,59.7780681520196,
40.0999649129781));
#194368=CARTESIAN_POINT('Ctrl Pts',(-19.3988146762078,59.7774043475414,
40.1000786629733));
#194369=CARTESIAN_POINT('Ctrl Pts',(-19.4012610270042,59.7767405430632,
40.1001924129685));
#194370=CARTESIAN_POINT('Ctrl Pts',(-19.4036987600454,59.7760153991119,
40.10025));
#194371=CARTESIAN_POINT('Ctrl Pts',(-19.4061247292253,59.7752282754855,
40.10025));
#194372=CARTESIAN_POINT('Ctrl Pts',(-18.2263320786577,56.1441998575529,
40.10025));
#194373=CARTESIAN_POINT('Ctrl Pts',(-18.2181232748938,56.1468630191715,
40.10025));
#194374=CARTESIAN_POINT('Ctrl Pts',(-18.2102054558333,56.150180699858,40.0995786334241));
#194375=CARTESIAN_POINT('Ctrl Pts',(-18.2026724222802,56.1540344262256,
40.0983063763366));
#194376=CARTESIAN_POINT('Ctrl Pts',(-18.1978068555391,56.1565235380438,
40.0974846287992));
#194377=CARTESIAN_POINT('Ctrl Pts',(-18.1931013796334,56.1592354513149,
40.0964130309338));
#194378=CARTESIAN_POINT('Ctrl Pts',(-18.1885757140654,56.1621313494121,
40.0951176960924));
#194379=CARTESIAN_POINT('Ctrl Pts',(-18.1825772036009,56.1659696964529,
40.0934008039615));
#194380=CARTESIAN_POINT('Ctrl Pts',(-18.1768986338329,56.1701354151837,
40.0912909372157));
#194381=CARTESIAN_POINT('Ctrl Pts',(-18.1715848978922,56.1745504247234,
40.0888630467852));
#194382=CARTESIAN_POINT('Ctrl Pts',(-18.1689280299218,56.1767579294932,
40.0876491015699));
#194383=CARTESIAN_POINT('Ctrl Pts',(-18.1663621803349,56.1790278168866,
40.0863558569272));
#194384=CARTESIAN_POINT('Ctrl Pts',(-18.1638916135754,56.1813507566161,
40.0849936342771));
#194385=CARTESIAN_POINT('Ctrl Pts',(-18.1626563301957,56.1825122264808,
40.0843125229521));
#194386=CARTESIAN_POINT('Ctrl Pts',(-18.1614448518808,56.1836869644605,
40.0836141747075));
#194387=CARTESIAN_POINT('Ctrl Pts',(-18.1602576134412,56.1848738357354,
40.082899916161));
#194388=CARTESIAN_POINT('Ctrl Pts',(-18.1599608038313,56.1851705535541,
40.0827213515244));
#194389=CARTESIAN_POINT('Ctrl Pts',(-18.1596655088806,56.1854680298098,
40.0825417925842));
#194390=CARTESIAN_POINT('Ctrl Pts',(-18.1593717347113,56.1857662469843,
40.0823612602361));
#194391=CARTESIAN_POINT('Ctrl Pts',(-18.1584904122033,56.1866608985079,
40.0818196631918));
#194392=CARTESIAN_POINT('Ctrl Pts',(-18.157622778392,56.1875622177791,40.0812693052022));
#194393=CARTESIAN_POINT('Ctrl Pts',(-18.156768983708,56.1884697364866,40.0807107531875));
#194394=CARTESIAN_POINT('Ctrl Pts',(-18.1507549641989,56.1948621810806,
40.0767763849181));
#194395=CARTESIAN_POINT('Ctrl Pts',(-18.1453743792958,56.2015542305065,
40.0724140586135));
#194396=CARTESIAN_POINT('Ctrl Pts',(-18.1405824894343,56.2084349106669,
40.0677221223765));
#194397=CARTESIAN_POINT('Ctrl Pts',(-18.1382584280299,56.211772033109,40.0654465383718));
#194398=CARTESIAN_POINT('Ctrl Pts',(-18.1360729791405,56.2151540877948,
40.0630928000678));
#194399=CARTESIAN_POINT('Ctrl Pts',(-18.1340220442546,56.218571093557,40.0606689262479));
#194400=CARTESIAN_POINT('Ctrl Pts',(-18.1308822062388,56.22380229064,40.0569581447806));
#194401=CARTESIAN_POINT('Ctrl Pts',(-18.1280584389294,56.2291119669557,
40.0530843804606));
#194402=CARTESIAN_POINT('Ctrl Pts',(-18.1255442374226,56.2344544719218,
40.0490800251458));
#194403=CARTESIAN_POINT('Ctrl Pts',(-18.124376629236,56.2369355588665,40.0472203818218));
#194404=CARTESIAN_POINT('Ctrl Pts',(-18.1232756028762,56.2394235482377,
40.0453323608819));
#194405=CARTESIAN_POINT('Ctrl Pts',(-18.1222417093396,56.2419141381098,
40.0434201572162));
#194406=CARTESIAN_POINT('Ctrl Pts',(-18.1221624654738,56.2421050320101,
40.0432735943397));
#194407=CARTESIAN_POINT('Ctrl Pts',(-18.1220835820641,56.2422959411933,
40.0431268995708));
#194408=CARTESIAN_POINT('Ctrl Pts',(-18.1220050584317,56.2424868643661,
40.0429800745037));
#194409=CARTESIAN_POINT('Ctrl Pts',(-18.1209020381381,56.2451687593305,
40.0409176249753));
#194410=CARTESIAN_POINT('Ctrl Pts',(-18.119871885966,56.2478543333341,40.0388310783333));
#194411=CARTESIAN_POINT('Ctrl Pts',(-18.1189123616721,56.2505383386775,
40.036725739981));
#194412=CARTESIAN_POINT('Ctrl Pts',(-18.1154716782,56.2601627045038,40.0291763710724));
#194413=CARTESIAN_POINT('Ctrl Pts',(-18.1129106883013,56.2698406425772,
40.0213310894607));
#194414=CARTESIAN_POINT('Ctrl Pts',(-18.111121302731,56.2795015152448,40.0132837551339));
#194415=CARTESIAN_POINT('Ctrl Pts',(-18.1091549477489,56.2901178437856,
40.0044405431352));
#194416=CARTESIAN_POINT('Ctrl Pts',(-18.1081200911549,56.300714173019,39.9953528710635));
#194417=CARTESIAN_POINT('Ctrl Pts',(-18.1079204190083,56.3112209484322,
39.9861103629598));
#194418=CARTESIAN_POINT('Ctrl Pts',(-18.1077048232009,56.3225656290374,
39.976130773761));
#194419=CARTESIAN_POINT('Ctrl Pts',(-18.1084627484397,56.3338070504076,
39.9659696936077));
#194420=CARTESIAN_POINT('Ctrl Pts',(-18.1101289800535,56.3448702837299,
39.9557128217582));
#194421=CARTESIAN_POINT('Ctrl Pts',(-18.1117812336966,56.355840707896,39.9455419945212));
#194422=CARTESIAN_POINT('Ctrl Pts',(-18.1143271060902,56.3666372711369,
39.9352756289366));
#194423=CARTESIAN_POINT('Ctrl Pts',(-18.1177524687101,56.3771794532809,
39.92499));
#194424=CARTESIAN_POINT('Origin',(-0.0144941013083308,-0.0047094189942794,
39.92499));
#194425=CARTESIAN_POINT('Ctrl Pts',(-19.4351129318415,59.7658094374953,
40.10025));
#194426=CARTESIAN_POINT('Ctrl Pts',(-19.4432803829089,59.7631518948793,
40.10025));
#194427=CARTESIAN_POINT('Ctrl Pts',(-19.4511532554514,59.7598356997914,
40.0995859581841));
#194428=CARTESIAN_POINT('Ctrl Pts',(-19.4586404431004,59.7559811102141,
40.098327595962));
#194429=CARTESIAN_POINT('Ctrl Pts',(-19.4634243995782,59.7535182109732,
40.0975235624067));
#194430=CARTESIAN_POINT('Ctrl Pts',(-19.4680513433534,59.7508363273796,
40.096477705949));
#194431=CARTESIAN_POINT('Ctrl Pts',(-19.4725029330456,59.7479734971808,
40.0952149915961));
#194432=CARTESIAN_POINT('Ctrl Pts',(-19.4785784597567,59.7440663083909,
40.0934916398701));
#194433=CARTESIAN_POINT('Ctrl Pts',(-19.4843230052516,59.7398178213044,
40.091364392163));
#194434=CARTESIAN_POINT('Ctrl Pts',(-19.4896904492928,59.7353118462118,
40.0889118607713));
#194435=CARTESIAN_POINT('Ctrl Pts',(-19.4923741713134,59.7330588586655,
40.0876855950754));
#194436=CARTESIAN_POINT('Ctrl Pts',(-19.494963817173,59.7307414364082,40.0863782327526));
#194437=CARTESIAN_POINT('Ctrl Pts',(-19.497455043941,59.72836960219,40.0850006373333));
#194438=CARTESIAN_POINT('Ctrl Pts',(-19.498700657325,59.7271836850808,40.0843118396237));
#194439=CARTESIAN_POINT('Ctrl Pts',(-19.4999216825132,59.7259841596485,
40.0836054919164));
#194440=CARTESIAN_POINT('Ctrl Pts',(-19.5011176808517,59.7247722453469,
40.0828829920417));
#194441=CARTESIAN_POINT('Ctrl Pts',(-19.5014166804363,59.7244692667715,
40.082702367073));
#194442=CARTESIAN_POINT('Ctrl Pts',(-19.5017141161962,59.7241655137792,
40.0825207326932));
#194443=CARTESIAN_POINT('Ctrl Pts',(-19.5020099819907,59.7238610051972,
40.0823381109275));
#194444=CARTESIAN_POINT('Ctrl Pts',(-19.502897579374,59.7229474794513,40.0817902456303));
#194445=CARTESIAN_POINT('Ctrl Pts',(-19.5037710453003,59.7220271539531,
40.0812334935553));
#194446=CARTESIAN_POINT('Ctrl Pts',(-19.5046302297519,59.7211005320715,
40.0806684524226));
#194447=CARTESIAN_POINT('Ctrl Pts',(-19.5105677273981,59.7146969999428,
40.0767636676137));
#194448=CARTESIAN_POINT('Ctrl Pts',(-19.5158784513264,59.707999912005,40.0724404510889));
#194449=CARTESIAN_POINT('Ctrl Pts',(-19.5206092977898,59.7011184102419,
40.0677949937411));
#194450=CARTESIAN_POINT('Ctrl Pts',(-19.5229605154963,59.6976983227548,
40.0654862141907));
#194451=CARTESIAN_POINT('Ctrl Pts',(-19.5251683423975,59.6942320938704,
40.0630972003217));
#194452=CARTESIAN_POINT('Ctrl Pts',(-19.5272373629638,59.6907301905173,
40.0606363359906));
#194453=CARTESIAN_POINT('Ctrl Pts',(-19.5318019313697,59.6830044686628,
40.0552073017123));
#194454=CARTESIAN_POINT('Ctrl Pts',(-19.5357011184423,59.6751122606221,
40.0494204304519));
#194455=CARTESIAN_POINT('Ctrl Pts',(-19.5389266512978,59.6671986827533,
40.0434049749851));
#194456=CARTESIAN_POINT('Ctrl Pts',(-19.540104979126,59.6643077529624,40.0412074532442));
#194457=CARTESIAN_POINT('Ctrl Pts',(-19.5412013620775,59.6614137631515,
40.0389814735788));
#194458=CARTESIAN_POINT('Ctrl Pts',(-19.5422187365062,59.6585211429014,
40.0367321210017));
#194459=CARTESIAN_POINT('Ctrl Pts',(-19.5456359895572,59.6488051375689,
40.0291767837141));
#194460=CARTESIAN_POINT('Ctrl Pts',(-19.5481755652417,59.6390401911873,
40.0213235332577));
#194461=CARTESIAN_POINT('Ctrl Pts',(-19.5499445144585,59.6292970278063,
40.013264921586));
#194462=CARTESIAN_POINT('Ctrl Pts',(-19.5518887991937,59.6185881370969,
40.0044075527534));
#194463=CARTESIAN_POINT('Ctrl Pts',(-19.5529023976133,59.6079049297412,
39.9953016253721));
#194464=CARTESIAN_POINT('Ctrl Pts',(-19.5530800481813,59.5973174182821,
39.9860353422359));
#194465=CARTESIAN_POINT('Ctrl Pts',(-19.5532713854546,59.5859142148018,
39.9760551582696));
#194466=CARTESIAN_POINT('Ctrl Pts',(-19.5524931697987,59.5746208362166,
39.9658879738156));
#194467=CARTESIAN_POINT('Ctrl Pts',(-19.5508078878557,59.5635130675434,
39.9556174643253));
#194468=CARTESIAN_POINT('Ctrl Pts',(-19.5491453629091,59.5525552912514,
39.9454856413904));
#194469=CARTESIAN_POINT('Ctrl Pts',(-19.5465995868769,59.5417768065758,
39.9352519465114));
#194470=CARTESIAN_POINT('Ctrl Pts',(-19.5431821162861,59.5312589135997,
39.92499));
#194471=CARTESIAN_POINT('Ctrl Pts',(-18.4801050014185,56.259443978424,39.92499));
#194472=CARTESIAN_POINT('Ctrl Pts',(-18.4768344633031,56.2493782971084,
39.934810724172));
#194473=CARTESIAN_POINT('Ctrl Pts',(-18.4727817672087,56.239606768122,39.9446038383166));
#194474=CARTESIAN_POINT('Ctrl Pts',(-18.4679768367035,56.2301791400439,
39.9543158069379));
#194475=CARTESIAN_POINT('Ctrl Pts',(-18.4633372535444,56.2210759356552,
39.9636935671383));
#194476=CARTESIAN_POINT('Ctrl Pts',(-18.4579956735924,56.2122922812566,
39.9729968320978));
#194477=CARTESIAN_POINT('Ctrl Pts',(-18.4519372213368,56.2038917763258,
39.9821731151322));
#194478=CARTESIAN_POINT('Ctrl Pts',(-18.4462100865656,56.195950668291,39.9908475764336));
#194479=CARTESIAN_POINT('Ctrl Pts',(-18.4398418135299,56.1883512165501,
39.9994093733827));
#194480=CARTESIAN_POINT('Ctrl Pts',(-18.4327901596646,56.1811768067756,
40.007796611582));
#194481=CARTESIAN_POINT('Ctrl Pts',(-18.4262957047551,56.1745692957332,
40.015521117257));
#194482=CARTESIAN_POINT('Ctrl Pts',(-18.4192211773452,56.1683219623542,
40.0230979940993));
#194483=CARTESIAN_POINT('Ctrl Pts',(-18.4115142492208,56.1625328136792,
40.0304554104717));
#194484=CARTESIAN_POINT('Ctrl Pts',(-18.4092161988273,56.160806606405,40.032649243516));
#194485=CARTESIAN_POINT('Ctrl Pts',(-18.4068618031996,56.1591213928276,
40.034823371505));
#194486=CARTESIAN_POINT('Ctrl Pts',(-18.4044493827309,56.1574804751188,
40.0369753512355));
#194487=CARTESIAN_POINT('Ctrl Pts',(-18.4020616112559,56.1558563235462,
40.0391053430352));
#194488=CARTESIAN_POINT('Ctrl Pts',(-18.3996196264078,56.1542770260204,
40.041211089324));
#194489=CARTESIAN_POINT('Ctrl Pts',(-18.3971247125282,56.1527473834685,
40.0432881154904));
#194490=CARTESIAN_POINT('Ctrl Pts',(-18.3969512210963,56.152641015117,40.043432547828));
#194491=CARTESIAN_POINT('Ctrl Pts',(-18.3967774746429,56.1525348749438,
40.0435768364421));
#194492=CARTESIAN_POINT('Ctrl Pts',(-18.3966034726921,56.1524289641634,
40.0437209807855));
#194493=CARTESIAN_POINT('Ctrl Pts',(-18.3889745897489,56.1477854475704,
40.0500407968419));
#194494=CARTESIAN_POINT('Ctrl Pts',(-18.3808409394273,56.143626001431,40.0560490279342));
#194495=CARTESIAN_POINT('Ctrl Pts',(-18.372242484946,56.1400597146378,40.0616647108612));
#194496=CARTESIAN_POINT('Ctrl Pts',(-18.3642272309682,56.1367353155302,
40.066899503348));
#194497=CARTESIAN_POINT('Ctrl Pts',(-18.3558072700357,56.1339262909288,
40.0717933267475));
#194498=CARTESIAN_POINT('Ctrl Pts',(-18.3470212548482,56.1317496772155,
40.0762460303064));
#194499=CARTESIAN_POINT('Ctrl Pts',(-18.3438072168252,56.1309534437596,
40.0778748868742));
#194500=CARTESIAN_POINT('Ctrl Pts',(-18.3405443147883,56.1302421351294,
40.0794443522245));
#194501=CARTESIAN_POINT('Ctrl Pts',(-18.337234982846,56.1296225724749,40.0809482021492));
#194502=CARTESIAN_POINT('Ctrl Pts',(-18.336439199069,56.1294735883543,40.0813098278168));
#194503=CARTESIAN_POINT('Ctrl Pts',(-18.3356401993822,56.1293301519982,
40.0816679525672));
#194504=CARTESIAN_POINT('Ctrl Pts',(-18.3348380918581,56.1291923454417,
40.082022419258));
#194505=CARTESIAN_POINT('Ctrl Pts',(-18.3340610501942,56.1290588453401,
40.0823658088648));
#194506=CARTESIAN_POINT('Ctrl Pts',(-18.3332810919216,56.1289306286649,
40.0827057654616));
#194507=CARTESIAN_POINT('Ctrl Pts',(-18.3324983188927,56.1288077688059,
40.0830421470151));
#194508=CARTESIAN_POINT('Ctrl Pts',(-18.3239221357297,56.1274616970648,
40.0867275956808));
#194509=CARTESIAN_POINT('Ctrl Pts',(-18.3150023767858,56.126758159346,40.0899823432035));
#194510=CARTESIAN_POINT('Ctrl Pts',(-18.3059033598527,56.1267895336332,
40.0926299529361));
#194511=CARTESIAN_POINT('Ctrl Pts',(-18.3021297263188,56.1268025454853,
40.0937279956087));
#194512=CARTESIAN_POINT('Ctrl Pts',(-18.2983254984037,56.12694160832,40.0947220371804));
#194513=CARTESIAN_POINT('Ctrl Pts',(-18.2945030089052,56.1272115877756,
40.0956014538692));
#194514=CARTESIAN_POINT('Ctrl Pts',(-18.2879833547329,56.127672065871,40.097101390674));
#194515=CARTESIAN_POINT('Ctrl Pts',(-18.2814124323569,56.1285150529072,
40.0982667904316));
#194516=CARTESIAN_POINT('Ctrl Pts',(-18.2748585331707,56.1297657127884,
40.0990539325582));
#194517=CARTESIAN_POINT('Ctrl Pts',(-18.2715815835777,56.130391042729,40.0994475036216));
#194518=CARTESIAN_POINT('Ctrl Pts',(-18.2683092720861,56.1311196862925,
40.0997467259952));
#194519=CARTESIAN_POINT('Ctrl Pts',(-18.2650501911668,56.1319548233208,
40.0999473488896));
#194520=CARTESIAN_POINT('Ctrl Pts',(-18.2617911102475,56.1327899603492,
40.100147971784));
#194521=CARTESIAN_POINT('Ctrl Pts',(-18.258545294751,56.133731561341,40.10025));
#194522=CARTESIAN_POINT('Ctrl Pts',(-18.2553202812744,56.1347810195644,
40.10025));
#194523=CARTESIAN_POINT('Origin',(-12.0988124084934,56.9937374973464,39.92499));
#194524=CARTESIAN_POINT('Ctrl Pts',(-12.8407372733092,61.3271735965895,
39.92499));
#194525=CARTESIAN_POINT('Ctrl Pts',(-12.8429432848607,61.3375520649564,
39.9348354642016));
#194526=CARTESIAN_POINT('Ctrl Pts',(-12.8459616464938,61.3477256769088,
39.9446440828454));
#194527=CARTESIAN_POINT('Ctrl Pts',(-12.8497656413956,61.3576417279032,
39.9543641760326));
#194528=CARTESIAN_POINT('Ctrl Pts',(-12.8534460291144,61.3672355662866,
39.9637684240707));
#194529=CARTESIAN_POINT('Ctrl Pts',(-12.8578623484989,61.3765894879238,
39.973090963639));
#194530=CARTESIAN_POINT('Ctrl Pts',(-12.8630345798913,61.3856422574863,
39.9822808977135));
#194531=CARTESIAN_POINT('Ctrl Pts',(-12.8679271923008,61.394205620055,39.9909740094644));
#194532=CARTESIAN_POINT('Ctrl Pts',(-12.8734966517555,61.4025003187116,
39.9995492764996));
#194533=CARTESIAN_POINT('Ctrl Pts',(-12.8797929832517,61.4104485116936,
40.0079462328689));
#194534=CARTESIAN_POINT('Ctrl Pts',(-12.885592359922,61.417769372258,40.0156804369685));
#194535=CARTESIAN_POINT('Ctrl Pts',(-12.8920087864949,61.4247966697187,
40.0232638017417));
#194536=CARTESIAN_POINT('Ctrl Pts',(-12.8991043342871,61.4314390014606,
40.0306257269962));
#194537=CARTESIAN_POINT('Ctrl Pts',(-12.9011624829797,61.4333656894051,
40.0327611416649));
#194538=CARTESIAN_POINT('Ctrl Pts',(-12.9032779088707,61.4352597571379,
40.0348777427269));
#194539=CARTESIAN_POINT('Ctrl Pts',(-12.9054524645838,61.437118361331,40.0369733168701));
#194540=CARTESIAN_POINT('Ctrl Pts',(-12.9078098227877,61.4391332077733,
40.039245053974));
#194541=CARTESIAN_POINT('Ctrl Pts',(-12.9102326900442,61.4411043938524,
40.041487875195));
#194542=CARTESIAN_POINT('Ctrl Pts',(-12.9127224163023,61.4430281531013,
40.0436985701601));
#194543=CARTESIAN_POINT('Ctrl Pts',(-12.9195554895539,61.4483079254551,
40.0497658398386));
#194544=CARTESIAN_POINT('Ctrl Pts',(-12.9269097705825,61.4531896374537,
40.0555581699984));
#194545=CARTESIAN_POINT('Ctrl Pts',(-12.9347398820024,61.4575800373534,
40.0609828468885));
#194546=CARTESIAN_POINT('Ctrl Pts',(-12.941904008845,61.4615970149014,40.0659461317305));
#194547=CARTESIAN_POINT('Ctrl Pts',(-12.9494643722281,61.4651913207948,
40.0706039980708));
#194548=CARTESIAN_POINT('Ctrl Pts',(-12.9574154517104,61.4682744840804,
40.0748843180605));
#194549=CARTESIAN_POINT('Ctrl Pts',(-12.9613209959786,61.4697889238147,
40.0769867972571));
#194550=CARTESIAN_POINT('Ctrl Pts',(-12.9653208118549,61.4711795284101,
40.0789976708175));
#194551=CARTESIAN_POINT('Ctrl Pts',(-12.9694138336344,61.4724324898305,
40.08090504915));
#194552=CARTESIAN_POINT('Ctrl Pts',(-12.9701904446506,61.472670227056,40.0812669556105));
#194553=CARTESIAN_POINT('Ctrl Pts',(-12.9709708853386,61.4729027677275,
40.0816253922033));
#194554=CARTESIAN_POINT('Ctrl Pts',(-12.9717550556842,61.4731300138563,
40.0819801989139));
#194555=CARTESIAN_POINT('Ctrl Pts',(-12.9725147207064,61.4733501585436,
40.0823239179149));
#194556=CARTESIAN_POINT('Ctrl Pts',(-12.9732778859002,61.4735653344326,
40.0826642303498));
#194557=CARTESIAN_POINT('Ctrl Pts',(-12.974044456583,61.4737754532575,40.0830009916099));
#194558=CARTESIAN_POINT('Ctrl Pts',(-12.9823983859291,61.4760652849147,
40.0866709464312));
#194559=CARTESIAN_POINT('Ctrl Pts',(-12.9911623597373,61.4777556486131,
40.0899175831877));
#194560=CARTESIAN_POINT('Ctrl Pts',(-13.0001833616592,61.4787331403171,
40.0925642067061));
#194561=CARTESIAN_POINT('Ctrl Pts',(-13.0039929867887,61.4791459411336,
40.0936818922527));
#194562=CARTESIAN_POINT('Ctrl Pts',(-13.007848166856,61.4794319383913,40.094693009479));
#194563=CARTESIAN_POINT('Ctrl Pts',(-13.0117365408425,61.4795843394719,
40.0955863397546));
#194564=CARTESIAN_POINT('Ctrl Pts',(-13.0182844654758,61.4798409790836,
40.0970906856166));
#194565=CARTESIAN_POINT('Ctrl Pts',(-13.024924823017,61.4797168922659,40.0982599215483));
#194566=CARTESIAN_POINT('Ctrl Pts',(-13.0315916763171,61.4791780149468,
40.0990497370453));
#194567=CARTESIAN_POINT('Ctrl Pts',(-13.0332583896422,61.479043295617,40.0992471909196));
#194568=CARTESIAN_POINT('Ctrl Pts',(-13.0349267248711,61.4788824204062,
40.0994209989363));
#194569=CARTESIAN_POINT('Ctrl Pts',(-13.0365955947398,61.478694553895,40.0995705982975));
#194570=CARTESIAN_POINT('Ctrl Pts',(-13.0390988995429,61.4784127541283,
40.0997949973393));
#194571=CARTESIAN_POINT('Ctrl Pts',(-13.0416033892095,61.4780702140293,
40.0999649129781));
#194572=CARTESIAN_POINT('Ctrl Pts',(-13.0441057251024,61.4776657592308,
40.1000786629733));
#194573=CARTESIAN_POINT('Ctrl Pts',(-13.0466080609952,61.4772613044322,
40.1001924129685));
#194574=CARTESIAN_POINT('Ctrl Pts',(-13.0491082380622,61.4767949453823,
40.10025));
#194575=CARTESIAN_POINT('Ctrl Pts',(-13.0516031943522,61.4762657165317,
40.10025));
#194576=CARTESIAN_POINT('Ctrl Pts',(-12.2578193919762,57.7418065394567,
40.10025));
#194577=CARTESIAN_POINT('Ctrl Pts',(-12.2493771807071,57.7435970583545,
40.10025));
#194578=CARTESIAN_POINT('Ctrl Pts',(-12.2411559442244,57.7460689269802,
40.0995786334241));
#194579=CARTESIAN_POINT('Ctrl Pts',(-12.2332613533225,57.7491141258103,
40.0983063763367));
#194580=CARTESIAN_POINT('Ctrl Pts',(-12.2281622576314,57.7510810117992,
40.0974846287993));
#194581=CARTESIAN_POINT('Ctrl Pts',(-12.223199086688,57.7532862127605,40.0964130309338));
#194582=CARTESIAN_POINT('Ctrl Pts',(-12.2183955094113,57.755693185958,40.0951176960924));
#194583=CARTESIAN_POINT('Ctrl Pts',(-12.2120286428972,57.7588834910513,
40.0934008039614));
#194584=CARTESIAN_POINT('Ctrl Pts',(-12.2059457447512,57.7624328173676,
40.0912909372156));
#194585=CARTESIAN_POINT('Ctrl Pts',(-12.2001996238495,57.766268204371,40.0888630467851));
#194586=CARTESIAN_POINT('Ctrl Pts',(-12.1973265633987,57.7681858978727,
40.0876491015699));
#194587=CARTESIAN_POINT('Ctrl Pts',(-12.1945375019633,57.7701751462711,
40.0863558569271));
#194588=CARTESIAN_POINT('Ctrl Pts',(-12.1918376559068,57.7722271161469,
40.0849936342771));
#194589=CARTESIAN_POINT('Ctrl Pts',(-12.1904877328785,57.7732531010848,
40.0843125229521));
#194590=CARTESIAN_POINT('Ctrl Pts',(-12.1891600976129,57.7742947697604,
40.0836141747074));
#194591=CARTESIAN_POINT('Ctrl Pts',(-12.1878553011592,57.7753510390206,
40.082899916161));
#194592=CARTESIAN_POINT('Ctrl Pts',(-12.1875291020458,57.7756151063356,
40.0827213515243));
#194593=CARTESIAN_POINT('Ctrl Pts',(-12.1872043300158,57.7758800862578,
40.0825417925842));
#194594=CARTESIAN_POINT('Ctrl Pts',(-12.1868809929892,57.776145962005,40.0823612602361));
#194595=CARTESIAN_POINT('Ctrl Pts',(-12.1859109819092,57.7769435892466,
40.0818196631917));
#194596=CARTESIAN_POINT('Ctrl Pts',(-12.1849538875684,57.7777492785675,
40.0812693052022));
#194597=CARTESIAN_POINT('Ctrl Pts',(-12.1840099085252,57.7785625799463,
40.0807107531875));
#194598=CARTESIAN_POINT('Ctrl Pts',(-12.1773606420345,57.7842913698424,
40.0767763849183));
#194599=CARTESIAN_POINT('Ctrl Pts',(-12.1713100228961,57.7903843352497,
40.0724140586139));
#194600=CARTESIAN_POINT('Ctrl Pts',(-12.1658251565855,57.7967264334405,
40.0677221223771));
#194601=CARTESIAN_POINT('Ctrl Pts',(-12.1631650023517,57.7998023442099,
40.0654465383722));
#194602=CARTESIAN_POINT('Ctrl Pts',(-12.1606380046008,57.8029374300325,
40.063092800068));
#194603=CARTESIAN_POINT('Ctrl Pts',(-12.1582411305893,57.806121336008,40.0606689262479));
#194604=CARTESIAN_POINT('Ctrl Pts',(-12.1545716839425,57.8109956736034,
40.0569581447805));
#194605=CARTESIAN_POINT('Ctrl Pts',(-12.1512083732202,57.8159810988991,
40.0530843804605));
#194606=CARTESIAN_POINT('Ctrl Pts',(-12.1481495009381,57.8210315314442,
40.0490800251457));
#194607=CARTESIAN_POINT('Ctrl Pts',(-12.1467289448258,57.8233769784456,
40.0472203818217));
#194608=CARTESIAN_POINT('Ctrl Pts',(-12.145373884298,57.8257362497573,40.0453323608818));
#194609=CARTESIAN_POINT('Ctrl Pts',(-12.1440853170064,57.8281051246149,
40.0434201572162));
#194610=CARTESIAN_POINT('Ctrl Pts',(-12.1439865534007,57.8282866895389,
40.0432735943397));
#194611=CARTESIAN_POINT('Ctrl Pts',(-12.1438881466791,57.82846830734,40.0431268995707));
#194612=CARTESIAN_POINT('Ctrl Pts',(-12.1437900963016,57.8286499766612,
40.0429800745037));
#194613=CARTESIAN_POINT('Ctrl Pts',(-12.1424127841092,57.831201882908,40.0409176249753));
#194614=CARTESIAN_POINT('Ctrl Pts',(-12.1411075562949,57.8337650648328,
40.0388310783332));
#194615=CARTESIAN_POINT('Ctrl Pts',(-12.1398727334215,57.8363340693142,
40.036725739981));
#194616=CARTESIAN_POINT('Ctrl Pts',(-12.1354448782034,57.8455460625021,
40.0291763710718));
#194617=CARTESIAN_POINT('Ctrl Pts',(-12.1318862976808,57.8549032874803,
40.0213310894597));
#194618=CARTESIAN_POINT('Ctrl Pts',(-12.129096878378,57.8643241951533,40.0132837551323));
#194619=CARTESIAN_POINT('Ctrl Pts',(-12.1260315867862,57.8746768262719,
40.0044405431329));
#194620=CARTESIAN_POINT('Ctrl Pts',(-12.1238947812338,57.8851069357363,
39.9953528710605));
#194621=CARTESIAN_POINT('Ctrl Pts',(-12.1225979458245,57.8955352825126,
39.9861103629561));
#194622=CARTESIAN_POINT('Ctrl Pts',(-12.1211976890436,57.9067952798732,
39.9761307737561));
#194623=CARTESIAN_POINT('Ctrl Pts',(-12.1207764137882,57.9180543443226,
39.9659696936017));
#194624=CARTESIAN_POINT('Ctrl Pts',(-12.1212770948334,57.9292311407264,
39.9557128217511));
#194625=CARTESIAN_POINT('Ctrl Pts',(-12.121773575679,57.9403141752926,39.9455419945164));
#194626=CARTESIAN_POINT('Ctrl Pts',(-12.1231769533531,57.9513177099568,
39.9352756289342));
#194627=CARTESIAN_POINT('Ctrl Pts',(-12.1254815933786,57.9621601888122,
39.92499));
#194628=CARTESIAN_POINT('Origin',(-0.0149069694351764,-0.00316857416806799,
39.92499));
#194629=CARTESIAN_POINT('Ctrl Pts',(-13.0814171332226,61.4699285681956,
40.10025));
#194630=CARTESIAN_POINT('Ctrl Pts',(-13.089817630984,61.468139314985,40.10025));
#194631=CARTESIAN_POINT('Ctrl Pts',(-13.0979940118833,61.4656642256292,
40.0995859581842));
#194632=CARTESIAN_POINT('Ctrl Pts',(-13.1058430982598,61.4626133761162,
40.098327595962));
#194633=CARTESIAN_POINT('Ctrl Pts',(-13.1108582907966,61.4606640285138,
40.0975235624068));
#194634=CARTESIAN_POINT('Ctrl Pts',(-13.1157402208606,61.4584804838816,
40.096477705949));
#194635=CARTESIAN_POINT('Ctrl Pts',(-13.1204666715201,61.4560986543957,
40.0952149915961));
#194636=CARTESIAN_POINT('Ctrl Pts',(-13.1269173283,61.4528479350654,40.0934916398701));
#194637=CARTESIAN_POINT('Ctrl Pts',(-13.1330744924,61.4492231901485,40.091364392163));
#194638=CARTESIAN_POINT('Ctrl Pts',(-13.1388835356731,61.4453029499362,
40.0889118607713));
#194639=CARTESIAN_POINT('Ctrl Pts',(-13.1417880573096,61.4433428298301,
40.0876855950754));
#194640=CARTESIAN_POINT('Ctrl Pts',(-13.1446057534055,61.4413087943565,
40.0863782327526));
#194641=CARTESIAN_POINT('Ctrl Pts',(-13.1473312571586,61.4392103574,40.0850006373334));
#194642=CARTESIAN_POINT('Ctrl Pts',(-13.1486940090351,61.4381611389218,
40.0843118396237));
#194643=CARTESIAN_POINT('Ctrl Pts',(-13.1500337298697,61.4370958165018,
40.0836054919164));
#194644=CARTESIAN_POINT('Ctrl Pts',(-13.1513498559436,61.4360155570619,
40.0828829920417));
#194645=CARTESIAN_POINT('Ctrl Pts',(-13.1516788874621,61.435745492202,40.0827023670731));
#194646=CARTESIAN_POINT('Ctrl Pts',(-13.1520064446714,61.4354744937032,
40.0825207326933));
#194647=CARTESIAN_POINT('Ctrl Pts',(-13.1523325194961,61.4352025796479,
40.0823381109275));
#194648=CARTESIAN_POINT('Ctrl Pts',(-13.1533107439705,61.4343868374821,
40.0817902456303));
#194649=CARTESIAN_POINT('Ctrl Pts',(-13.1542756251691,61.4335628556743,
40.0812334935553));
#194650=CARTESIAN_POINT('Ctrl Pts',(-13.1552269612797,61.4327311191548,
40.0806684524227));
#194651=CARTESIAN_POINT('Ctrl Pts',(-13.1618012840655,61.4269833037496,
40.0767636676137));
#194652=CARTESIAN_POINT('Ctrl Pts',(-13.167782951603,61.4208780249712,40.0724404510888));
#194653=CARTESIAN_POINT('Ctrl Pts',(-13.1732071947989,61.4145287289054,
40.0677949937409));
#194654=CARTESIAN_POINT('Ctrl Pts',(-13.1759030287779,61.4113731461892,
40.0654862141906));
#194655=CARTESIAN_POINT('Ctrl Pts',(-13.1784610805509,61.4081566864226,
40.0630972003216));
#194656=CARTESIAN_POINT('Ctrl Pts',(-13.180884815382,61.4048902384027,40.0606363359906));
#194657=CARTESIAN_POINT('Ctrl Pts',(-13.1862319364376,61.3976839661819,
40.0552073017123));
#194658=CARTESIAN_POINT('Ctrl Pts',(-13.1909347237338,61.3902425685153,
40.0494204304519));
#194659=CARTESIAN_POINT('Ctrl Pts',(-13.1949697809163,61.3827095020467,
40.0434049749851));
#194660=CARTESIAN_POINT('Ctrl Pts',(-13.1964438381899,61.3799575778687,
40.0412074532442));
#194661=CARTESIAN_POINT('Ctrl Pts',(-13.1978367193485,61.377194044862,40.0389814735788));
#194662=CARTESIAN_POINT('Ctrl Pts',(-13.1991508816432,61.3744236152739,
40.0367321210017));
#194663=CARTESIAN_POINT('Ctrl Pts',(-13.203565013731,61.365118035445,40.029176783714));
#194664=CARTESIAN_POINT('Ctrl Pts',(-13.2071113921934,61.355672040405,40.0213235332573));
#194665=CARTESIAN_POINT('Ctrl Pts',(-13.209889088817,61.3461671566355,40.0132649215854));
#194666=CARTESIAN_POINT('Ctrl Pts',(-13.2129421064461,61.3357201634454,
40.0044075527526));
#194667=CARTESIAN_POINT('Ctrl Pts',(-13.2150668515152,61.3252014297026,
39.9953016253711));
#194668=CARTESIAN_POINT('Ctrl Pts',(-13.2163502251974,61.3146904872798,
39.9860353422348));
#194669=CARTESIAN_POINT('Ctrl Pts',(-13.2177324736412,61.3033697519324,
39.9760551582683));
#194670=CARTESIAN_POINT('Ctrl Pts',(-13.2181390006407,61.2920568939702,
39.9658879738142));
#194671=CARTESIAN_POINT('Ctrl Pts',(-13.2176240288381,61.2808338148841,
39.955617464324));
#194672=CARTESIAN_POINT('Ctrl Pts',(-13.2171160108937,61.2697622852597,
39.9454856413894));
#194673=CARTESIAN_POINT('Ctrl Pts',(-13.2157108393285,61.2587767401948,
39.9352519465108));
#194674=CARTESIAN_POINT('Ctrl Pts',(-13.2134115091888,61.2479592423879,
39.92499));
#194675=CARTESIAN_POINT('Ctrl Pts',(-12.4981558292581,57.8829458346106,
39.92499));
#194676=CARTESIAN_POINT('Ctrl Pts',(-12.4959553576922,57.8725934298266,
39.9348107241725));
#194677=CARTESIAN_POINT('Ctrl Pts',(-12.4929462655996,57.8624518082032,
39.9446038383175));
#194678=CARTESIAN_POINT('Ctrl Pts',(-12.4891531124815,57.8525735736558,
39.9543158069393));
#194679=CARTESIAN_POINT('Ctrl Pts',(-12.4854904894097,57.8430352690751,
39.9636935671401));
#194680=CARTESIAN_POINT('Ctrl Pts',(-12.4810963130876,57.8337413853103,
39.9729968320998));
#194681=CARTESIAN_POINT('Ctrl Pts',(-12.4759491415381,57.8247536185201,
39.9821731151346));
#194682=CARTESIAN_POINT('Ctrl Pts',(-12.4710834524297,57.8162573641093,
39.9908475764361));
#194683=CARTESIAN_POINT('Ctrl Pts',(-12.4655444244719,57.808033877166,39.9994093733854));
#194684=CARTESIAN_POINT('Ctrl Pts',(-12.4592813303326,57.8001616710168,
40.0077966115849));
#194685=CARTESIAN_POINT('Ctrl Pts',(-12.4535131257017,57.7929115012196,
40.01552111726));
#194686=CARTESIAN_POINT('Ctrl Pts',(-12.4471303774504,57.785958901908,40.0230979941024));
#194687=CARTESIAN_POINT('Ctrl Pts',(-12.4400707994989,57.7793958734419,
40.0304554104748));
#194688=CARTESIAN_POINT('Ctrl Pts',(-12.4379657758605,57.7774389108365,
40.0326492435181));
#194689=CARTESIAN_POINT('Ctrl Pts',(-12.435800430645,57.7755168276795,40.034823371506));
#194690=CARTESIAN_POINT('Ctrl Pts',(-12.4335727482756,57.7736327324861,
40.0369753512355));
#194691=CARTESIAN_POINT('Ctrl Pts',(-12.4313678273305,57.7717678881029,
40.0391053430352));
#194692=CARTESIAN_POINT('Ctrl Pts',(-12.4291043014743,57.7699419852107,
40.0412110893239));
#194693=CARTESIAN_POINT('Ctrl Pts',(-12.4267829461793,57.7681599326869,
40.0432881154903));
#194694=CARTESIAN_POINT('Ctrl Pts',(-12.4266215236719,57.7680360122395,
40.0434325478279));
#194695=CARTESIAN_POINT('Ctrl Pts',(-12.426459823689,57.7679122920636,40.0435768364421));
#194696=CARTESIAN_POINT('Ctrl Pts',(-12.4262978456302,57.767788773317,40.0437209807855));
#194697=CARTESIAN_POINT('Ctrl Pts',(-12.4191961341593,57.762373258983,40.0500407968421));
#194698=CARTESIAN_POINT('Ctrl Pts',(-12.4115418213381,57.7573864007557,
40.0560490279346));
#194699=CARTESIAN_POINT('Ctrl Pts',(-12.4033632485678,57.7529408672213,
40.0616647108617));
#194700=CARTESIAN_POINT('Ctrl Pts',(-12.3957393973196,57.7487968573387,
40.0668995033488));
#194701=CARTESIAN_POINT('Ctrl Pts',(-12.3876591848384,57.7451230952908,
40.0717933267485));
#194702=CARTESIAN_POINT('Ctrl Pts',(-12.3791488184475,57.7420400166292,
40.0762460303076));
#194703=CARTESIAN_POINT('Ctrl Pts',(-12.3760356163213,57.7409121865684,
40.077874886875));
#194704=CARTESIAN_POINT('Ctrl Pts',(-12.3728649408019,57.7398637084259,
40.0794443522249));
#194705=CARTESIAN_POINT('Ctrl Pts',(-12.3696384996592,57.7389016204183,
40.0809482021492));
#194706=CARTESIAN_POINT('Ctrl Pts',(-12.3688626483502,57.738670270393,40.0813098278168));
#194707=CARTESIAN_POINT('Ctrl Pts',(-12.3680830188491,57.7384441015869,
40.0816679525672));
#194708=CARTESIAN_POINT('Ctrl Pts',(-12.3672997100616,57.7382232068822,
40.082022419258));
#194709=CARTESIAN_POINT('Ctrl Pts',(-12.3665408796737,57.7380092151371,
40.0823658088648));
#194710=CARTESIAN_POINT('Ctrl Pts',(-12.3657785963861,57.7378001730066,
40.0827057654617));
#194711=CARTESIAN_POINT('Ctrl Pts',(-12.365012953822,57.737596164125,40.0830421470151));
#194712=CARTESIAN_POINT('Ctrl Pts',(-12.3566244546988,57.7353610110591,
40.0867275956806));
#194713=CARTESIAN_POINT('Ctrl Pts',(-12.3478270988448,57.7337289586985,
40.0899823432031));
#194714=CARTESIAN_POINT('Ctrl Pts',(-12.338774647773,57.7328090548568,40.0926299529356));
#194715=CARTESIAN_POINT('Ctrl Pts',(-12.335020326489,57.7324275433143,40.0937279956085));
#194716=CARTESIAN_POINT('Ctrl Pts',(-12.3312224025075,57.7321681942503,
40.0947220371803));
#194717=CARTESIAN_POINT('Ctrl Pts',(-12.3273926324683,57.7320371357771,
40.0956014538692));
#194718=CARTESIAN_POINT('Ctrl Pts',(-12.320860560576,57.7318136018936,40.097101390674));
#194719=CARTESIAN_POINT('Ctrl Pts',(-12.3142375182609,57.7319651225404,
40.0982667904316));
#194720=CARTESIAN_POINT('Ctrl Pts',(-12.3075887924648,57.7325238621659,
40.0990539325582));
#194721=CARTESIAN_POINT('Ctrl Pts',(-12.3042644295668,57.7328032319787,
40.0994475036216));
#194722=CARTESIAN_POINT('Ctrl Pts',(-12.300933880148,57.7331858342648,40.0997467259952));
#194723=CARTESIAN_POINT('Ctrl Pts',(-12.2976053572248,57.7336757296049,
40.0999473488896));
#194724=CARTESIAN_POINT('Ctrl Pts',(-12.2942768343016,57.734165624945,40.100147971784));
#194725=CARTESIAN_POINT('Ctrl Pts',(-12.2909503756172,57.7347627876419,
40.10025));
#194726=CARTESIAN_POINT('Ctrl Pts',(-12.2876333308465,57.7354693911206,
40.10025));
#194727=CARTESIAN_POINT('Origin',(-6.07506605172241,57.9461901084062,39.92499));
#194728=CARTESIAN_POINT('Ctrl Pts',(-6.35995915837738,62.333439457262,39.92499));
#194729=CARTESIAN_POINT('Ctrl Pts',(-6.36106823981726,62.3439916622903,
39.9348354642018));
#194730=CARTESIAN_POINT('Ctrl Pts',(-6.3630066345263,62.3544250468349,39.9446440828457));
#194731=CARTESIAN_POINT('Ctrl Pts',(-6.36575328117383,62.3646844024057,
39.9543641760329));
#194732=CARTESIAN_POINT('Ctrl Pts',(-6.36841067816053,62.3746103900109,
39.9637684240709));
#194733=CARTESIAN_POINT('Ctrl Pts',(-6.37182505343099,62.3843747009652,
39.9730909636391));
#194734=CARTESIAN_POINT('Ctrl Pts',(-6.37602267870792,62.393918523908,39.9822808977135));
#194735=CARTESIAN_POINT('Ctrl Pts',(-6.37999337374501,62.402946392737,39.9909740094642));
#194736=CARTESIAN_POINT('Ctrl Pts',(-6.38466529101406,62.4117778192045,
39.9995492764992));
#194737=CARTESIAN_POINT('Ctrl Pts',(-6.39009631814929,62.4203406170093,
40.0079462328684));
#194738=CARTESIAN_POINT('Ctrl Pts',(-6.39509868692269,62.4282275730647,
40.0156804369677));
#194739=CARTESIAN_POINT('Ctrl Pts',(-6.40074541103475,62.4358870734638,
40.0232638017408));
#194740=CARTESIAN_POINT('Ctrl Pts',(-6.40710777594406,62.4432347045242,
40.0306257269951));
#194741=CARTESIAN_POINT('Ctrl Pts',(-6.40895325615309,62.4453659729909,
40.0327611416641));
#194742=CARTESIAN_POINT('Ctrl Pts',(-6.41085910953059,62.4474707870404,
40.0348777427266));
#194743=CARTESIAN_POINT('Ctrl Pts',(-6.41282747576019,62.4495465125725,
40.0369733168701));
#194744=CARTESIAN_POINT('Ctrl Pts',(-6.41496131130683,62.4517967325057,
40.039245053974));
#194745=CARTESIAN_POINT('Ctrl Pts',(-6.41716486079138,62.4540103788122,
40.041487875195));
#194746=CARTESIAN_POINT('Ctrl Pts',(-6.41943986047048,62.4561838467663,
40.0436985701601));
#194747=CARTESIAN_POINT('Ctrl Pts',(-6.42568361494137,62.4621489466211,
40.0497658398386));
#194748=CARTESIAN_POINT('Ctrl Pts',(-6.43248733059572,62.467772647785,40.0555581699984));
#194749=CARTESIAN_POINT('Ctrl Pts',(-6.4398156260913,62.4729574661286,40.0609828468886));
#194750=CARTESIAN_POINT('Ctrl Pts',(-6.44652061860732,62.4777012934227,
40.0659461317305));
#194751=CARTESIAN_POINT('Ctrl Pts',(-6.45366385825704,62.4820661824985,
40.0706039980706));
#194752=CARTESIAN_POINT('Ctrl Pts',(-6.46124910257362,62.4859635700126,
40.0748843180603));
#194753=CARTESIAN_POINT('Ctrl Pts',(-6.46497494980365,62.4878779540282,
40.076986797257));
#194754=CARTESIAN_POINT('Ctrl Pts',(-6.46880749650881,62.4896790353531,
40.0789976708175));
#194755=CARTESIAN_POINT('Ctrl Pts',(-6.47274712615508,62.4913529701965,
40.08090504915));
#194756=CARTESIAN_POINT('Ctrl Pts',(-6.47349463250796,62.4916705830287,
40.0812669556105));
#194757=CARTESIAN_POINT('Ctrl Pts',(-6.47424649074124,62.4919834280839,
40.0816253922033));
#194758=CARTESIAN_POINT('Ctrl Pts',(-6.47500261163096,62.4922913974558,
40.0819801989139));
#194759=CARTESIAN_POINT('Ctrl Pts',(-6.47573510374288,62.4925897427848,
40.0823239179149));
#194760=CARTESIAN_POINT('Ctrl Pts',(-6.47647159623284,62.4928835124027,
40.0826642303499));
#194761=CARTESIAN_POINT('Ctrl Pts',(-6.47721200416343,62.4931726086301,
40.08300099161));
#194762=CARTESIAN_POINT('Ctrl Pts',(-6.4852808172262,62.4963231197467,40.0866709464312));
#194763=CARTESIAN_POINT('Ctrl Pts',(-6.49382008994911,62.4989203081703,
40.0899175831877));
#194764=CARTESIAN_POINT('Ctrl Pts',(-6.50268949817301,62.5008353965404,
40.0925642067061));
#194765=CARTESIAN_POINT('Ctrl Pts',(-6.50643510434242,62.5016441502512,
40.0936818922527));
#194766=CARTESIAN_POINT('Ctrl Pts',(-6.51023927047603,62.502331556834,40.094693009479));
#194767=CARTESIAN_POINT('Ctrl Pts',(-6.51409041329226,62.502889568803,40.0955863397546));
#194768=CARTESIAN_POINT('Ctrl Pts',(-6.52057564156509,62.5038292470156,
40.0970906856166));
#194769=CARTESIAN_POINT('Ctrl Pts',(-6.52719259313719,62.5043999463278,
40.0982599215483));
#194770=CARTESIAN_POINT('Ctrl Pts',(-6.53387925273545,62.5045608969649,
40.0990497370454));
#194771=CARTESIAN_POINT('Ctrl Pts',(-6.53555091763502,62.5046011346242,
40.0992471909196));
#194772=CARTESIAN_POINT('Ctrl Pts',(-6.53722692958755,62.5046155292223,
40.0994209989363));
#194773=CARTESIAN_POINT('Ctrl Pts',(-6.53890629461021,62.5046031362664,
40.0995705982975));
#194774=CARTESIAN_POINT('Ctrl Pts',(-6.54142534214421,62.5045845468324,
40.0997949973393));
#194775=CARTESIAN_POINT('Ctrl Pts',(-6.54395191714455,62.5045056736602,
40.0999649129781));
#194776=CARTESIAN_POINT('Ctrl Pts',(-6.54648282201812,62.5043649998329,
40.1000786629733));
#194777=CARTESIAN_POINT('Ctrl Pts',(-6.5490137268917,62.5042243260056,40.1001924129685));
#194778=CARTESIAN_POINT('Ctrl Pts',(-6.55154895552196,62.5040218613862,
40.10025));
#194779=CARTESIAN_POINT('Ctrl Pts',(-6.55408556365883,62.5037563256535,
40.10025));
#194780=CARTESIAN_POINT('Ctrl Pts',(-6.15500747092256,58.7067819056643,
40.10025));
#194781=CARTESIAN_POINT('Ctrl Pts',(-6.14642434678091,58.7076801645418,
40.10025));
#194782=CARTESIAN_POINT('Ctrl Pts',(-6.13798976646259,58.7092791387969,
40.099578633424));
#194783=CARTESIAN_POINT('Ctrl Pts',(-6.12982011300122,58.7114824462543,
40.0983063763365));
#194784=CARTESIAN_POINT('Ctrl Pts',(-6.12454335512051,58.7129055567992,
40.0974846287991));
#194785=CARTESIAN_POINT('Ctrl Pts',(-6.11937686667958,58.7145798848071,
40.0964130309337));
#194786=CARTESIAN_POINT('Ctrl Pts',(-6.11434800669275,58.7164715618025,
40.0951176960924));
#194787=CARTESIAN_POINT('Ctrl Pts',(-6.10768254085074,58.7189788712981,
40.0934008039614));
#194788=CARTESIAN_POINT('Ctrl Pts',(-6.10126195983181,58.7218729180382,
40.0912909372156));
#194789=CARTESIAN_POINT('Ctrl Pts',(-6.09514640967214,58.7250866612027,
40.0888630467851));
#194790=CARTESIAN_POINT('Ctrl Pts',(-6.0920886345923,58.7266935327849,40.0876491015699));
#194791=CARTESIAN_POINT('Ctrl Pts',(-6.08910691884912,58.7283803475666,
40.0863558569271));
#194792=CARTESIAN_POINT('Ctrl Pts',(-6.08620737357405,58.7301388657774,
40.0849936342771));
#194793=CARTESIAN_POINT('Ctrl Pts',(-6.08475760093651,58.7310181248828,
40.0843125229521));
#194794=CARTESIAN_POINT('Ctrl Pts',(-6.08332835456984,58.7319153115143,
40.0836141747074));
#194795=CARTESIAN_POINT('Ctrl Pts',(-6.08192029572511,58.7328294060528,
40.0828999161609));
#194796=CARTESIAN_POINT('Ctrl Pts',(-6.08156828101392,58.7330579296874,
40.0827213515243));
#194797=CARTESIAN_POINT('Ctrl Pts',(-6.08121759017508,58.7332875101007,
40.0825417925842));
#194798=CARTESIAN_POINT('Ctrl Pts',(-6.08086823283921,58.7335181314302,
40.0823612602361));
#194799=CARTESIAN_POINT('Ctrl Pts',(-6.07982016083159,58.7342099954187,
40.0818196631917));
#194800=CARTESIAN_POINT('Ctrl Pts',(-6.07878409208717,58.7349112274886,
40.0812693052021));
#194801=CARTESIAN_POINT('Ctrl Pts',(-6.07776027111658,58.7356214008386,
40.0807107531875));
#194802=CARTESIAN_POINT('Ctrl Pts',(-6.07054860839909,58.7406237702162,
40.0767763849182));
#194803=CARTESIAN_POINT('Ctrl Pts',(-6.06389424687459,58.7460508958012,
40.0724140586137));
#194804=CARTESIAN_POINT('Ctrl Pts',(-6.05777649745766,58.751784926668,40.0677221223768));
#194805=CARTESIAN_POINT('Ctrl Pts',(-6.05480939560134,58.7545659254421,
40.0654465383721));
#194806=CARTESIAN_POINT('Ctrl Pts',(-6.05196853530533,58.7574196937449,
40.0630928000679));
#194807=CARTESIAN_POINT('Ctrl Pts',(-6.04925198282172,58.7603356163932,
40.0606689262479));
#194808=CARTESIAN_POINT('Ctrl Pts',(-6.04509313076933,58.7647996902381,
40.0569581447806));
#194809=CARTESIAN_POINT('Ctrl Pts',(-6.04122712577018,58.7694062431512,
40.0530843804606));
#194810=CARTESIAN_POINT('Ctrl Pts',(-6.03765709635775,58.7741092696794,
40.0490800251458));
#194811=CARTESIAN_POINT('Ctrl Pts',(-6.03599915622974,58.7762933795293,
40.0472203818218));
#194812=CARTESIAN_POINT('Ctrl Pts',(-6.03440490786063,58.7784980841112,
40.0453323608819));
#194813=CARTESIAN_POINT('Ctrl Pts',(-6.03287578462697,58.7807192900658,
40.0434201572162));
#194814=CARTESIAN_POINT('Ctrl Pts',(-6.03275858335616,58.7808895367502,
40.0432735943397));
#194815=CARTESIAN_POINT('Ctrl Pts',(-6.03264173148719,58.7810598733266,
40.0431268995708));
#194816=CARTESIAN_POINT('Ctrl Pts',(-6.03252522862489,58.7812302983889,
40.0429800745037));
#194817=CARTESIAN_POINT('Ctrl Pts',(-6.03088871465445,58.7836242566994,
40.0409176249753));
#194818=CARTESIAN_POINT('Ctrl Pts',(-6.02932271154703,58.7860369637878,
40.0388310783332));
#194819=CARTESIAN_POINT('Ctrl Pts',(-6.02782611907197,58.7884628208564,
40.036725739981));
#194820=CARTESIAN_POINT('Ctrl Pts',(-6.02245960461632,58.7971615128805,
40.0291763710716));
#194821=CARTESIAN_POINT('Ctrl Pts',(-6.01794242202257,58.8060955050481,
40.0213310894592));
#194822=CARTESIAN_POINT('Ctrl Pts',(-6.01418353044881,58.8151732302903,
40.0132837551315));
#194823=CARTESIAN_POINT('Ctrl Pts',(-6.01005288622337,58.8251487383932,
40.0044405431318));
#194824=CARTESIAN_POINT('Ctrl Pts',(-6.00683754300133,58.8352983536264,
39.9953528710591));
#194825=CARTESIAN_POINT('Ctrl Pts',(-6.00445775272914,58.8455340166158,
39.9861103629543));
#194826=CARTESIAN_POINT('Ctrl Pts',(-6.00188817648097,58.8565859638438,
39.9761307737539));
#194827=CARTESIAN_POINT('Ctrl Pts',(-6.00029231631084,58.8677393147055,
39.9659696935989));
#194828=CARTESIAN_POINT('Ctrl Pts',(-5.99962196122069,58.8789072188699,
39.9557128217479));
#194829=CARTESIAN_POINT('Ctrl Pts',(-5.99895722972105,58.8899814357918,
39.9455419945142));
#194830=CARTESIAN_POINT('Ctrl Pts',(-5.99920273697647,58.9010713848523,
39.9352756289331));
#194831=CARTESIAN_POINT('Ctrl Pts',(-6.00036140428986,58.9120953679531,
39.92499));
#194832=CARTESIAN_POINT('Origin',(-0.0151565136854063,-0.00159301378020448,
39.92499));
#194833=CARTESIAN_POINT('Ctrl Pts',(-6.58439859102965,62.5005702980932,
40.10025));
#194834=CARTESIAN_POINT('Ctrl Pts',(-6.59294009787387,62.4996689377206,
40.10025));
#194835=CARTESIAN_POINT('Ctrl Pts',(-6.60133040498987,62.4980620716937,
40.0995859581842));
#194836=CARTESIAN_POINT('Ctrl Pts',(-6.60945539386123,62.4958483879905,
40.0983275959621));
#194837=CARTESIAN_POINT('Ctrl Pts',(-6.61464687495778,62.4944339494872,
40.0975235624068));
#194838=CARTESIAN_POINT('Ctrl Pts',(-6.61973030386294,62.4927726671883,
40.096477705949));
#194839=CARTESIAN_POINT('Ctrl Pts',(-6.62467983150713,62.4908979342377,
40.0952149915961));
#194840=CARTESIAN_POINT('Ctrl Pts',(-6.6314349436104,62.4883392999283,40.0934916398701));
#194841=CARTESIAN_POINT('Ctrl Pts',(-6.63793726713709,62.4853780106448,
40.0913643921631));
#194842=CARTESIAN_POINT('Ctrl Pts',(-6.64412426454837,62.4820864562849,
40.0889118607713));
#194843=CARTESIAN_POINT('Ctrl Pts',(-6.64721776325402,62.480440679105,40.0876855950754));
#194844=CARTESIAN_POINT('Ctrl Pts',(-6.65023263831815,62.4787123157334,
40.0863782327527));
#194845=CARTESIAN_POINT('Ctrl Pts',(-6.65316255786681,62.4769102669531,
40.0850006373334));
#194846=CARTESIAN_POINT('Ctrl Pts',(-6.65462751764114,62.4760092425629,
40.0843118396238));
#194847=CARTESIAN_POINT('Ctrl Pts',(-6.65607125586022,62.4750897950507,
40.0836054919165));
#194848=CARTESIAN_POINT('Ctrl Pts',(-6.65749308991701,62.474153026021,40.0828829920418));
#194849=CARTESIAN_POINT('Ctrl Pts',(-6.65784854843121,62.4739188337636,
40.0827023670731));
#194850=CARTESIAN_POINT('Ctrl Pts',(-6.65820263830443,62.4736835588747,
40.0825207326933));
#194851=CARTESIAN_POINT('Ctrl Pts',(-6.65855534961554,62.4734472184934,
40.0823381109276));
#194852=CARTESIAN_POINT('Ctrl Pts',(-6.65961348354888,62.4727381973496,
40.0817902456304));
#194853=CARTESIAN_POINT('Ctrl Pts',(-6.66065920857946,62.4720195869493,
40.0812334935554));
#194854=CARTESIAN_POINT('Ctrl Pts',(-6.66169227331156,62.4712918484711,
40.0806684524227));
#194855=CARTESIAN_POINT('Ctrl Pts',(-6.66883139158091,62.4662627240577,
40.0767636676136));
#194856=CARTESIAN_POINT('Ctrl Pts',(-6.67541846632655,62.4608161451506,
40.0724404510886));
#194857=CARTESIAN_POINT('Ctrl Pts',(-6.68147667711138,62.4550686189984,
40.0677949937405));
#194858=CARTESIAN_POINT('Ctrl Pts',(-6.68448759124166,62.4522121142777,
40.0654862141903));
#194859=CARTESIAN_POINT('Ctrl Pts',(-6.68736784133573,62.4492806638352,
40.0630972003214));
#194860=CARTESIAN_POINT('Ctrl Pts',(-6.69011973548547,62.4462854590369,
40.0606363359906));
#194861=CARTESIAN_POINT('Ctrl Pts',(-6.6961908250136,62.4396775898761,40.0552073017123));
#194862=CARTESIAN_POINT('Ctrl Pts',(-6.70164568781152,62.4327685320937,
40.0494204304519));
#194863=CARTESIAN_POINT('Ctrl Pts',(-6.70644606039031,62.425698510878,40.0434049749851));
#194864=CARTESIAN_POINT('Ctrl Pts',(-6.70819969702922,62.4231157429702,
40.0412074532442));
#194865=CARTESIAN_POINT('Ctrl Pts',(-6.70987381569753,62.4205129446134,
40.0389814735788));
#194866=CARTESIAN_POINT('Ctrl Pts',(-6.71147036762114,62.4178950590937,
40.0367321210016));
#194867=CARTESIAN_POINT('Ctrl Pts',(-6.71683301659055,62.4091018586491,
40.0291767837142));
#194868=CARTESIAN_POINT('Ctrl Pts',(-6.72134734296609,62.4000783072496,
40.0213235332579));
#194869=CARTESIAN_POINT('Ctrl Pts',(-6.72510335397081,62.390915840588,40.0132649215864));
#194870=CARTESIAN_POINT('Ctrl Pts',(-6.72923165499376,62.3808452043613,
40.004407552754));
#194871=CARTESIAN_POINT('Ctrl Pts',(-6.73244426756069,62.37060618968,39.9953016253729));
#194872=CARTESIAN_POINT('Ctrl Pts',(-6.7348193034465,62.3602869763789,39.986035342237));
#194873=CARTESIAN_POINT('Ctrl Pts',(-6.7373773188577,62.3491727415105,39.976055158271));
#194874=CARTESIAN_POINT('Ctrl Pts',(-6.73896413451778,62.3379643502108,
39.9658879738174));
#194875=CARTESIAN_POINT('Ctrl Pts',(-6.73962511499487,62.3267489231156,
39.9556174643277));
#194876=CARTESIAN_POINT('Ctrl Pts',(-6.74027717000387,62.3156849421523,
39.9454856413919));
#194877=CARTESIAN_POINT('Ctrl Pts',(-6.74002799825933,62.3046126966267,
39.935251946512));
#194878=CARTESIAN_POINT('Ctrl Pts',(-6.7388720005127,62.293614112757,39.92499));
#194879=CARTESIAN_POINT('Ctrl Pts',(-6.37927424642518,58.8722700234481,
39.92499));
#194880=CARTESIAN_POINT('Ctrl Pts',(-6.37816795023605,58.8617443183104,
39.9348107241716));
#194881=CARTESIAN_POINT('Ctrl Pts',(-6.37623543038835,58.85134371778,39.9446038383158));
#194882=CARTESIAN_POINT('Ctrl Pts',(-6.37349561323731,58.8411231047695,
39.9543158069367));
#194883=CARTESIAN_POINT('Ctrl Pts',(-6.37085007871821,58.8312542036586,
39.9636935671369));
#194884=CARTESIAN_POINT('Ctrl Pts',(-6.36745144954177,58.8215519162636,
39.9729968320962));
#194885=CARTESIAN_POINT('Ctrl Pts',(-6.36327195218786,58.8120753594685,
39.9821731151305));
#194886=CARTESIAN_POINT('Ctrl Pts',(-6.35932101825085,58.8031170454232,
39.990847576432));
#194887=CARTESIAN_POINT('Ctrl Pts',(-6.35467192212096,58.7943596215215,
39.9994093733811));
#194888=CARTESIAN_POINT('Ctrl Pts',(-6.34926600747837,58.7858758685357,
40.0077966115805));
#194889=CARTESIAN_POINT('Ctrl Pts',(-6.34428725078353,58.7780624743613,
40.0155211172557));
#194890=CARTESIAN_POINT('Ctrl Pts',(-6.33866621241707,58.77048078325,40.0230979940982));
#194891=CARTESIAN_POINT('Ctrl Pts',(-6.33233133085242,58.7632157809057,
40.0304554104708));
#194892=CARTESIAN_POINT('Ctrl Pts',(-6.33044239704648,58.7610495038588,
40.0326492435154));
#194893=CARTESIAN_POINT('Ctrl Pts',(-6.32848982621615,58.7589116098653,
40.0348233715047));
#194894=CARTESIAN_POINT('Ctrl Pts',(-6.32647128889777,58.7568049797265,
40.0369753512356));
#194895=CARTESIAN_POINT('Ctrl Pts',(-6.32447337605791,58.7547198741579,
40.0391053430352));
#194896=CARTESIAN_POINT('Ctrl Pts',(-6.32241310885664,58.7526673708734,
40.041211089324));
#194897=CARTESIAN_POINT('Ctrl Pts',(-6.32029074540058,58.7506524329181,
40.0432881154904));
#194898=CARTESIAN_POINT('Ctrl Pts',(-6.32014316039653,58.7505123180733,
40.043432547828));
#194899=CARTESIAN_POINT('Ctrl Pts',(-6.31999527850295,58.7503723733987,
40.0435768364421));
#194900=CARTESIAN_POINT('Ctrl Pts',(-6.31984709900165,58.7502325999832,
40.0437209807855));
#194901=CARTESIAN_POINT('Ctrl Pts',(-6.31335036684046,58.7441044214168,
40.050040796842));
#194902=CARTESIAN_POINT('Ctrl Pts',(-6.3062592537728,58.7383447881641,40.0560490279345));
#194903=CARTESIAN_POINT('Ctrl Pts',(-6.29859016886874,58.7330687140842,
40.0616647108615));
#194904=CARTESIAN_POINT('Ctrl Pts',(-6.29144124886015,58.7281504960661,
40.0668995033487));
#194905=CARTESIAN_POINT('Ctrl Pts',(-6.28378931332969,58.7236522470775,
40.0717933267484));
#194906=CARTESIAN_POINT('Ctrl Pts',(-6.27564783709088,58.7196964823228,
40.0762460303075));
#194907=CARTESIAN_POINT('Ctrl Pts',(-6.27266957975476,58.7182494123989,
40.077874886875));
#194908=CARTESIAN_POINT('Ctrl Pts',(-6.26962586933651,58.7168752520897,
40.0794443522248));
#194909=CARTESIAN_POINT('Ctrl Pts',(-6.26651766855691,58.7155811795665,
40.0809482021492));
#194910=CARTESIAN_POINT('Ctrl Pts',(-6.26577025010518,58.7152699983557,
40.0813098278168));
#194911=CARTESIAN_POINT('Ctrl Pts',(-6.26501853257377,58.7149635750523,
40.0816679525672));
#194912=CARTESIAN_POINT('Ctrl Pts',(-6.2642626046178,58.7146620123682,40.082022419258));
#194913=CARTESIAN_POINT('Ctrl Pts',(-6.26353029941044,58.7143698735179,
40.0823658088648));
#194914=CARTESIAN_POINT('Ctrl Pts',(-6.26279404284314,58.7140822962415,
40.0827057654616));
#194915=CARTESIAN_POINT('Ctrl Pts',(-6.26205391928398,58.7137993735012,
40.0830421470151));
#194916=CARTESIAN_POINT('Ctrl Pts',(-6.25394501035177,58.7106996279152,
40.0867275956807));
#194917=CARTESIAN_POINT('Ctrl Pts',(-6.24536644325881,58.7081569420199,
40.0899823432031));
#194918=CARTESIAN_POINT('Ctrl Pts',(-6.23645973859607,58.7062958387084,
40.0926299529357));
#194919=CARTESIAN_POINT('Ctrl Pts',(-6.23276586269216,58.7055239836916,
40.0937279956085));
#194920=CARTESIAN_POINT('Ctrl Pts',(-6.22901585349481,58.7048690642116,
40.0947220371803));
#194921=CARTESIAN_POINT('Ctrl Pts',(-6.22522076267739,58.7043384037134,
40.0956014538692));
#194922=CARTESIAN_POINT('Ctrl Pts',(-6.21874783981175,58.7034333069352,
40.097101390674));
#194923=CARTESIAN_POINT('Ctrl Pts',(-6.21214524099501,58.7028917011006,
40.0982667904316));
#194924=CARTESIAN_POINT('Ctrl Pts',(-6.20547453342014,58.702752398802,40.0990539325582));
#194925=CARTESIAN_POINT('Ctrl Pts',(-6.2021391796327,58.7026827476527,40.0994475036216));
#194926=CARTESIAN_POINT('Ctrl Pts',(-6.19878688248309,58.7027151167908,
40.0997467259952));
#194927=CARTESIAN_POINT('Ctrl Pts',(-6.19542538554966,58.7028544030468,
40.0999473488896));
#194928=CARTESIAN_POINT('Ctrl Pts',(-6.19206388861623,58.7029936893029,
40.100147971784));
#194929=CARTESIAN_POINT('Ctrl Pts',(-6.18869323212156,58.7032398710655,
40.10025));
#194930=CARTESIAN_POINT('Ctrl Pts',(-6.18532049829339,58.7035958781039,
40.10025));
#194931=CARTESIAN_POINT('Origin',(0.0152400000006159,58.2637721346185,39.92499));
#194932=CARTESIAN_POINT('Ctrl Pts',(0.190500000000662,62.6567671111299,
39.92499));
#194933=CARTESIAN_POINT('Ctrl Pts',(0.190500000000662,62.6673774406537,
39.9348354642018));
#194934=CARTESIAN_POINT('Ctrl Pts',(0.189662809673755,62.6779562874463,
39.9446440828457));
#194935=CARTESIAN_POINT('Ctrl Pts',(0.188003604115847,62.6884465439472,
39.954364176033));
#194936=CARTESIAN_POINT('Ctrl Pts',(0.186398312858645,62.6985959295771,
39.9637684240711));
#194937=CARTESIAN_POINT('Ctrl Pts',(0.18402329031204,62.7086636500145,39.9730909636395));
#194938=CARTESIAN_POINT('Ctrl Pts',(0.180846261211417,62.7185939622162,
39.9822808977139));
#194939=CARTESIAN_POINT('Ctrl Pts',(0.177840987312408,62.7279874260856,
39.9909740094648));
#194940=CARTESIAN_POINT('Ctrl Pts',(0.174117798732004,62.7372588214076,
39.9995492764999));
#194941=CARTESIAN_POINT('Ctrl Pts',(0.169611579427374,62.7463424082305,
40.0079462328692));
#194942=CARTESIAN_POINT('Ctrl Pts',(0.165461025549738,62.7547090486361,
40.0156804369687));
#194943=CARTESIAN_POINT('Ctrl Pts',(0.160645870589174,62.7629168328847,
40.0232638017419));
#194944=CARTESIAN_POINT('Ctrl Pts',(0.155086395963785,62.7708892610802,
40.0306257269963));
#194945=CARTESIAN_POINT('Ctrl Pts',(0.153473803706341,62.7732017594451,
40.0327611416649));
#194946=CARTESIAN_POINT('Ctrl Pts',(0.151798403771396,62.7754942590273,
40.034877742727));
#194947=CARTESIAN_POINT('Ctrl Pts',(0.150057792858308,62.7777643638146,
40.0369733168701));
#194948=CARTESIAN_POINT('Ctrl Pts',(0.148170858717694,62.7802253033581,
40.039245053974));
#194949=CARTESIAN_POINT('Ctrl Pts',(0.146210769554428,62.7826571567199,
40.041487875195));
#194950=CARTESIAN_POINT('Ctrl Pts',(0.144175421826815,62.7850565204095,
40.0436985701601));
#194951=CARTESIAN_POINT('Ctrl Pts',(0.138589394017285,62.791641592883,40.0497658398386));
#194952=CARTESIAN_POINT('Ctrl Pts',(0.132410786669698,62.7979456687654,
40.0555581699984));
#194953=CARTESIAN_POINT('Ctrl Pts',(0.125664597437386,62.8038680995982,
40.0609828468886));
#194954=CARTESIAN_POINT('Ctrl Pts',(0.119492200549089,62.8092868022738,
40.0659461317304));
#194955=CARTESIAN_POINT('Ctrl Pts',(0.112844347461111,62.8143744518937,
40.0706039980705));
#194956=CARTESIAN_POINT('Ctrl Pts',(0.105708043834302,62.8190433630431,
40.0748843180601));
#194957=CARTESIAN_POINT('Ctrl Pts',(0.102202714804381,62.8213367169482,
40.0769867972568));
#194958=CARTESIAN_POINT('Ctrl Pts',(0.098579427454075,62.8235285419787,
40.0789976708174));
#194959=CARTESIAN_POINT('Ctrl Pts',(0.0948363533478791,62.8256051102647,
40.08090504915));
#194960=CARTESIAN_POINT('Ctrl Pts',(0.0941261414942798,62.8259991188709,
40.0812669556104));
#194961=CARTESIAN_POINT('Ctrl Pts',(0.0934111032319379,62.8263888407139,
40.0816253922032));
#194962=CARTESIAN_POINT('Ctrl Pts',(0.0926913160167418,62.826774159152,
40.0819801989139));
#194963=CARTESIAN_POINT('Ctrl Pts',(0.0919940221520205,62.8271474363889,
40.0823239179149));
#194964=CARTESIAN_POINT('Ctrl Pts',(0.091292271531703,62.8275165811343,
40.0826642303498));
#194965=CARTESIAN_POINT('Ctrl Pts',(0.0905861384176134,62.8278814873655,
40.0830009916099));
#194966=CARTESIAN_POINT('Ctrl Pts',(0.0828908452426149,62.8318581602824,
40.0866709464311));
#194967=CARTESIAN_POINT('Ctrl Pts',(0.0746698316639147,62.8353337180911,
40.0899175831877));
#194968=CARTESIAN_POINT('Ctrl Pts',(0.0660491922306701,62.8381654210185,
40.0925642067061));
#194969=CARTESIAN_POINT('Ctrl Pts',(0.0624086426662855,62.8393612667488,
40.0936818922527));
#194970=CARTESIAN_POINT('Ctrl Pts',(0.0586971697065028,62.8404425512864,
40.094693009479));
#194971=CARTESIAN_POINT('Ctrl Pts',(0.0549254519871374,62.8414000604479,
40.0955863397546));
#194972=CARTESIAN_POINT('Ctrl Pts',(0.0485739735928769,62.8430124819501,
40.0970906856166));
#194973=CARTESIAN_POINT('Ctrl Pts',(0.0420529246959365,62.8442717146911,
40.0982599215483));
#194974=CARTESIAN_POINT('Ctrl Pts',(0.0354197192413731,62.8451307298764,
40.0990497370454));
#194975=CARTESIAN_POINT('Ctrl Pts',(0.0337614178777322,62.8453454836727,
40.0992471909196));
#194976=CARTESIAN_POINT('Ctrl Pts',(0.0320960919392539,62.8455349903695,
40.0994209989363));
#194977=CARTESIAN_POINT('Ctrl Pts',(0.0304246312372522,62.8456982067485,
40.0995705982975));
#194978=CARTESIAN_POINT('Ctrl Pts',(0.0279174401842497,62.845943031317,
40.0997949973393));
#194979=CARTESIAN_POINT('Ctrl Pts',(0.0253964615346316,62.8461286892223,
40.0999649129781));
#194980=CARTESIAN_POINT('Ctrl Pts',(0.0228647168037747,62.846253337618,
40.1000786629733));
#194981=CARTESIAN_POINT('Ctrl Pts',(0.0203329720729179,62.8463779860137,
40.1001924129685));
#194982=CARTESIAN_POINT('Ctrl Pts',(0.0177904683748178,62.8464416340693,
40.10025));
#194983=CARTESIAN_POINT('Ctrl Pts',(0.0152400000006639,62.8464427007196,
40.10025));
#194984=CARTESIAN_POINT('Ctrl Pts',(0.0152400000006241,59.0285534841296,
40.10025));
#194985=CARTESIAN_POINT('Ctrl Pts',(0.0238699985097099,59.0285496414744,
40.10025));
#194986=CARTESIAN_POINT('Ctrl Pts',(0.0324255116356922,59.0292582026621,
40.0995786334241));
#194987=CARTESIAN_POINT('Ctrl Pts',(0.0407807192227396,59.0305954788488,
40.0983063763367));
#194988=CARTESIAN_POINT('Ctrl Pts',(0.0461773260305022,59.031459222053,
40.0974846287994));
#194989=CARTESIAN_POINT('Ctrl Pts',(0.0514905268413487,59.0325843328198,
40.0964130309339));
#194990=CARTESIAN_POINT('Ctrl Pts',(0.0566895722968041,59.0339399880044,
40.0951176960924));
#194991=CARTESIAN_POINT('Ctrl Pts',(0.0635806092280323,59.0357368312948,
40.0934008039614));
#194992=CARTESIAN_POINT('Ctrl Pts',(0.0702685278907234,59.0379438906768,
40.0912909372157));
#194993=CARTESIAN_POINT('Ctrl Pts',(0.0766865040610644,59.0405007795597,
40.0888630467852));
#194994=CARTESIAN_POINT('Ctrl Pts',(0.079895492146235,59.0417792240012,
40.0876491015699));
#194995=CARTESIAN_POINT('Ctrl Pts',(0.0830371938955519,59.0431451240706,
40.0863558569272));
#194996=CARTESIAN_POINT('Ctrl Pts',(0.0861046703644237,59.0445909239228,
40.0849936342772));
#194997=CARTESIAN_POINT('Ctrl Pts',(0.0876384085988596,59.0453138238489,
40.0843125229521));
#194998=CARTESIAN_POINT('Ctrl Pts',(0.0891536069442622,59.0460566986719,
40.0836141747074));
#194999=CARTESIAN_POINT('Ctrl Pts',(0.0906495011926997,59.0468186034776,
40.082899916161));
#195000=CARTESIAN_POINT('Ctrl Pts',(0.0910234747548091,59.047009079679,
40.0827213515244));
#195001=CARTESIAN_POINT('Ctrl Pts',(0.0913962421603369,59.0472007452523,
40.0825417925842));
#195002=CARTESIAN_POINT('Ctrl Pts',(0.0917677921733394,59.0473935854286,
40.0823612602361));
#195003=CARTESIAN_POINT('Ctrl Pts',(0.0928824422123469,59.0479721059574,
40.0818196631918));
#195004=CARTESIAN_POINT('Ctrl Pts',(0.0939861339744371,59.048561197931,
40.0812693052022));
#195005=CARTESIAN_POINT('Ctrl Pts',(0.0950785796755595,59.0491604624444,
40.0807107531875));
#195006=CARTESIAN_POINT('Ctrl Pts',(0.102773626133803,59.0533816042976,
40.0767763849182));
#195007=CARTESIAN_POINT('Ctrl Pts',(0.109958823466934,59.0580834293366,
40.0724140586138));
#195008=CARTESIAN_POINT('Ctrl Pts',(0.11664242864724,59.063146569637,40.0677221223769));
#195009=CARTESIAN_POINT('Ctrl Pts',(0.119883969937389,59.0656021872115,
40.0654465383721));
#195010=CARTESIAN_POINT('Ctrl Pts',(0.123007567718702,59.0681433715119,
40.063092800068));
#195011=CARTESIAN_POINT('Ctrl Pts',(0.126014035557044,59.0707593633743,
40.0606689262479));
#195012=CARTESIAN_POINT('Ctrl Pts',(0.130616727761667,59.0747642641417,
40.0569581447806));
#195013=CARTESIAN_POINT('Ctrl Pts',(0.134943070277899,59.0789414743143,
40.0530843804606));
#195014=CARTESIAN_POINT('Ctrl Pts',(0.138985142831358,59.0832455674828,
40.0490800251458));
#195015=CARTESIAN_POINT('Ctrl Pts',(0.140862302236097,59.0852444106167,
40.0472203818218));
#195016=CARTESIAN_POINT('Ctrl Pts',(0.142678271527742,59.0872703932641,
40.0453323608818));
#195017=CARTESIAN_POINT('Ctrl Pts',(0.144431197309365,59.0893195943183,
40.0434201572162));
#195018=CARTESIAN_POINT('Ctrl Pts',(0.144565552163648,59.0894766575049,
40.0432735943397));
#195019=CARTESIAN_POINT('Ctrl Pts',(0.144699568926413,59.0896338466133,
40.0431268995707));
#195020=CARTESIAN_POINT('Ctrl Pts',(0.144833247843701,59.0897911602042,
40.0429800745037));
#195021=CARTESIAN_POINT('Ctrl Pts',(0.146711033602707,59.0920009418701,
40.0409176249753));
#195022=CARTESIAN_POINT('Ctrl Pts',(0.14852065454551,59.0942367399983,40.0388310783332));
#195023=CARTESIAN_POINT('Ctrl Pts',(0.150262619641892,59.0964928714566,
40.036725739981));
#195024=CARTESIAN_POINT('Ctrl Pts',(0.156508996679636,59.1045829576266,
40.0291763710715));
#195025=CARTESIAN_POINT('Ctrl Pts',(0.161935290146665,59.1129958342955,
40.021331089459));
#195026=CARTESIAN_POINT('Ctrl Pts',(0.166622470788645,59.1216309196494,
40.0132837551312));
#195027=CARTESIAN_POINT('Ctrl Pts',(0.171773211445055,59.1311200109818,
40.0044405431316));
#195028=CARTESIAN_POINT('Ctrl Pts',(0.17603186436352,59.1408779306748,39.995352871059));
#195029=CARTESIAN_POINT('Ctrl Pts',(0.179468536018366,59.1508087658112,
39.9861103629543));
#195030=CARTESIAN_POINT('Ctrl Pts',(0.18317927891867,59.1615315754589,39.9761307737543));
#195031=CARTESIAN_POINT('Ctrl Pts',(0.185932239425596,59.172457014286,39.9659696935999));
#195032=CARTESIAN_POINT('Ctrl Pts',(0.187766286100662,59.1834936683149,
39.9557128217493));
#195033=CARTESIAN_POINT('Ctrl Pts',(0.189584947008509,59.1944377361562,
39.9455419945152));
#195034=CARTESIAN_POINT('Ctrl Pts',(0.190500000000626,59.205492595812,39.9352756289336));
#195035=CARTESIAN_POINT('Ctrl Pts',(0.190500000000626,59.2165773020941,
39.92499));
#195036=CARTESIAN_POINT('Origin',(-0.0152399999999944,-5.4624830725987E-15,
39.92499));
#195037=CARTESIAN_POINT('Ctrl Pts',(-0.0152399999993361,62.8464427007196,
40.10025));
#195038=CARTESIAN_POINT('Ctrl Pts',(-0.0238289333898259,62.8464391086779,
40.10025));
#195039=CARTESIAN_POINT('Ctrl Pts',(-0.0323412407618862,62.8457180711405,
40.0995859581842));
#195040=CARTESIAN_POINT('Ctrl Pts',(-0.0406531130496237,62.8443658068291,
40.0983275959621));
#195041=CARTESIAN_POINT('Ctrl Pts',(-0.0459640037527979,62.8435017743089,
40.0975235624069));
#195042=CARTESIAN_POINT('Ctrl Pts',(-0.0511932363883983,62.8423809556999,
40.0964777059491));
#195043=CARTESIAN_POINT('Ctrl Pts',(-0.0563116129567646,62.841033859251,
40.0952149915961));
#195044=CARTESIAN_POINT('Ctrl Pts',(-0.0632971699615518,62.8391953428955,
40.0934916398701));
#195045=CARTESIAN_POINT('Ctrl Pts',(-0.0700734120977075,62.8369299537504,
40.0913643921631));
#195046=CARTESIAN_POINT('Ctrl Pts',(-0.0765705776088136,62.8343031482014,
40.0889118607713));
#195047=CARTESIAN_POINT('Ctrl Pts',(-0.0798191603643667,62.8329897454269,
40.0876855950754));
#195048=CARTESIAN_POINT('Ctrl Pts',(-0.082998182794656,62.8315859904681,
40.0863782327527));
#195049=CARTESIAN_POINT('Ctrl Pts',(-0.0861004173272054,62.8301000734874,
40.0850006373334));
#195050=CARTESIAN_POINT('Ctrl Pts',(-0.0876515345934802,62.8293571149971,
40.0843118396238));
#195051=CARTESIAN_POINT('Ctrl Pts',(-0.0891834722990432,62.8285936160519,
40.0836054919165));
#195052=CARTESIAN_POINT('Ctrl Pts',(-0.0906954364272085,62.82781060087,
40.0828829920418));
#195053=CARTESIAN_POINT('Ctrl Pts',(-0.0910734274592499,62.8276148470746,
40.0827023670731));
#195054=CARTESIAN_POINT('Ctrl Pts',(-0.0914501705136822,62.8274178735164,
40.0825207326933));
#195055=CARTESIAN_POINT('Ctrl Pts',(-0.0918256539321903,62.8272196962038,
40.0823381109276));
#195056=CARTESIAN_POINT('Ctrl Pts',(-0.0929521041877145,62.826625164266,
40.0817902456304));
#195057=CARTESIAN_POINT('Ctrl Pts',(-0.0940672158679963,62.826019798519,
40.0812334935553));
#195058=CARTESIAN_POINT('Ctrl Pts',(-0.0951706907481875,62.8254040313373,
40.0806684524227));
#195059=CARTESIAN_POINT('Ctrl Pts',(-0.102796386827119,62.8211486980555,
40.0767636676136));
#195060=CARTESIAN_POINT('Ctrl Pts',(-0.109916699411247,62.8164204928781,
40.0724404510886));
#195061=CARTESIAN_POINT('Ctrl Pts',(-0.116542502759745,62.8113377077391,
40.0677949937406));
#195062=CARTESIAN_POINT('Ctrl Pts',(-0.119835508836212,62.8088115774772,
40.0654862141904));
#195063=CARTESIAN_POINT('Ctrl Pts',(-0.123006400628873,62.8061972539431,
40.0630972003215));
#195064=CARTESIAN_POINT('Ctrl Pts',(-0.126056303769318,62.8035061084565,
40.0606363359906));
#195065=CARTESIAN_POINT('Ctrl Pts',(-0.13278484564263,62.7975690395531,
40.0552073017123));
#195066=CARTESIAN_POINT('Ctrl Pts',(-0.138932019324023,62.7912680187378,
40.0494204304519));
#195067=CARTESIAN_POINT('Ctrl Pts',(-0.144445113412509,62.7847385034067,
40.0434049749851));
#195068=CARTESIAN_POINT('Ctrl Pts',(-0.146459116206807,62.7823531891148,
40.0412074532442));
#195069=CARTESIAN_POINT('Ctrl Pts',(-0.148396130390321,62.7799396422115,
40.0389814735788));
#195070=CARTESIAN_POINT('Ctrl Pts',(-0.150257579785831,62.7775029828616,
40.0367321210016));
#195071=CARTESIAN_POINT('Ctrl Pts',(-0.156509991333007,62.7693185019446,
40.029176783714));
#195072=CARTESIAN_POINT('Ctrl Pts',(-0.161942805717527,62.760816258102,
40.0213235332575));
#195073=CARTESIAN_POINT('Ctrl Pts',(-0.166635979460982,62.7520965944493,
40.0132649215857));
#195074=CARTESIAN_POINT('Ctrl Pts',(-0.171794333348042,62.7425126511828,
40.0044075527531));
#195075=CARTESIAN_POINT('Ctrl Pts',(-0.176059615357286,62.7326655363493,
39.9953016253717));
#195076=CARTESIAN_POINT('Ctrl Pts',(-0.179500292056516,62.7226511116291,
39.9860353422354));
#195077=CARTESIAN_POINT('Ctrl Pts',(-0.18320604828291,62.7118651471214,
39.9760551582689));
#195078=CARTESIAN_POINT('Ctrl Pts',(-0.185955767118991,62.7008840239637,
39.9658879738147));
#195079=CARTESIAN_POINT('Ctrl Pts',(-0.187785458034871,62.6897991274246,
39.9556174643243));
#195080=CARTESIAN_POINT('Ctrl Pts',(-0.189590441945537,62.6788639144162,
39.9454856413897));
#195081=CARTESIAN_POINT('Ctrl Pts',(-0.190499999999338,62.6678262782724,
39.935251946511));
#195082=CARTESIAN_POINT('Ctrl Pts',(-0.190499999999338,62.6567671111299,
39.92499));
#195083=CARTESIAN_POINT('Ctrl Pts',(-0.190499999999374,59.2165773020941,
39.92499));
#195084=CARTESIAN_POINT('Ctrl Pts',(-0.190499999999374,59.2059936184292,
39.9348107241723));
#195085=CARTESIAN_POINT('Ctrl Pts',(-0.189665225488023,59.1954479901461,
39.9446038383171));
#195086=CARTESIAN_POINT('Ctrl Pts',(-0.188008762313435,59.184996977846,
39.9543158069386));
#195087=CARTESIAN_POINT('Ctrl Pts',(-0.186409301376326,59.1749056059497,
39.9636935671394));
#195088=CARTESIAN_POINT('Ctrl Pts',(-0.184043455437455,59.1649012152147,
39.9729968320991));
#195089=CARTESIAN_POINT('Ctrl Pts',(-0.180877423725887,59.1550396955532,
39.9821731151338));
#195090=CARTESIAN_POINT('Ctrl Pts',(-0.177884532218707,59.1457174710364,
39.9908475764355));
#195091=CARTESIAN_POINT('Ctrl Pts',(-0.174176304386139,59.1365220583447,
39.999409373385));
#195092=CARTESIAN_POINT('Ctrl Pts',(-0.169686797571517,59.127519708295,
40.0077966115846));
#195093=CARTESIAN_POINT('Ctrl Pts',(-0.165552037112346,59.1192286949249,
40.01552111726));
#195094=CARTESIAN_POINT('Ctrl Pts',(-0.160754293902584,59.1111009786082,
40.0230979941027));
#195095=CARTESIAN_POINT('Ctrl Pts',(-0.15521351501215,59.1032135992718,
40.0304554104754));
#195096=CARTESIAN_POINT('Ctrl Pts',(-0.153561366595031,59.100861741971,
40.0326492435185));
#195097=CARTESIAN_POINT('Ctrl Pts',(-0.151842962926936,59.0985314603578,
40.0348233715062));
#195098=CARTESIAN_POINT('Ctrl Pts',(-0.150055686179523,59.096225375957,
40.0369753512356));
#195099=CARTESIAN_POINT('Ctrl Pts',(-0.148286670996087,59.0939428540559,
40.0391053430352));
#195100=CARTESIAN_POINT('Ctrl Pts',(-0.146452235168277,59.0916862380348,
40.041211089324));
#195101=CARTESIAN_POINT('Ctrl Pts',(-0.14455211660934,59.0894604907299,
40.0432881154904));
#195102=CARTESIAN_POINT('Ctrl Pts',(-0.144419986080793,59.0893057166152,
40.043432547828));
#195103=CARTESIAN_POINT('Ctrl Pts',(-0.144287542501473,59.0891510807051,
40.0435768364421));
#195104=CARTESIAN_POINT('Ctrl Pts',(-0.144154785043317,59.0889965840074,
40.0437209807855));
#195105=CARTESIAN_POINT('Ctrl Pts',(-0.138334211748934,59.0822228828154,
40.0500407968419));
#195106=CARTESIAN_POINT('Ctrl Pts',(-0.131883990153598,59.0757535782847,
40.0560490279343));
#195107=CARTESIAN_POINT('Ctrl Pts',(-0.12480841721487,59.0697047694309,
40.0616647108613));
#195108=CARTESIAN_POINT('Ctrl Pts',(-0.118212753509711,59.0640662283034,
40.0668995033484));
#195109=CARTESIAN_POINT('Ctrl Pts',(-0.111072931137106,59.0587927761315,
40.0717933267479));
#195110=CARTESIAN_POINT('Ctrl Pts',(-0.10338954476808,59.05400766547,40.076246030307));
#195111=CARTESIAN_POINT('Ctrl Pts',(-0.100578862632356,59.0522572100839,
40.0778748868746));
#195112=CARTESIAN_POINT('Ctrl Pts',(-0.0976954648433502,59.0505724231958,
40.0794443522247));
#195113=CARTESIAN_POINT('Ctrl Pts',(-0.0947395585247239,59.048960544286,
40.0809482021492));
#195114=CARTESIAN_POINT('Ctrl Pts',(-0.0940287618032278,59.0485729412563,
40.0813098278168));
#195115=CARTESIAN_POINT('Ctrl Pts',(-0.0933131922161319,59.0481896206935,
40.0816679525672));
#195116=CARTESIAN_POINT('Ctrl Pts',(-0.0925929271965458,59.0478106940136,
40.082022419258));
#195117=CARTESIAN_POINT('Ctrl Pts',(-0.0918951704588219,59.0474436087926,
40.0823658088648));
#195118=CARTESIAN_POINT('Ctrl Pts',(-0.0911930071928013,59.047080647127,
40.0827057654616));
#195119=CARTESIAN_POINT('Ctrl Pts',(-0.090486511587203,59.0467219102889,
40.0830421470151));
#195120=CARTESIAN_POINT('Ctrl Pts',(-0.0827460357491811,59.0427915336441,
40.0867275956807));
#195121=CARTESIAN_POINT('Ctrl Pts',(-0.0744802459935432,59.0393660724129,
40.0899823432031));
#195122=CARTESIAN_POINT('Ctrl Pts',(-0.0658168714599912,59.0365841602689,
40.0926299529357));
#195123=CARTESIAN_POINT('Ctrl Pts',(-0.0622239118135568,59.0354304183829,
40.0937279956085));
#195124=CARTESIAN_POINT('Ctrl Pts',(-0.0585629032857854,59.0343871039216,
40.0947220371803));
#195125=CARTESIAN_POINT('Ctrl Pts',(-0.0548440714993534,59.0334626554262,
40.0956014538693));
#195126=CARTESIAN_POINT('Ctrl Pts',(-0.0485012163577852,59.0318859121827,
40.097101390674));
#195127=CARTESIAN_POINT('Ctrl Pts',(-0.0419914004937971,59.0306571138137,
40.0982667904316));
#195128=CARTESIAN_POINT('Ctrl Pts',(-0.0353717968082022,59.0298212958157,
40.0990539325583));
#195129=CARTESIAN_POINT('Ctrl Pts',(-0.0320619949654048,59.0294033868167,
40.0994475036216));
#195130=CARTESIAN_POINT('Ctrl Pts',(-0.0287246785540554,59.0290851681639,
40.0997467259952));
#195131=CARTESIAN_POINT('Ctrl Pts',(-0.0253670368742458,59.0288723192866,
40.0999473488896));
#195132=CARTESIAN_POINT('Ctrl Pts',(-0.0220093951944362,59.0286594704093,
40.100147971784));
#195133=CARTESIAN_POINT('Ctrl Pts',(-0.0186314705073834,59.0285519740191,
40.10025));
#195134=CARTESIAN_POINT('Ctrl Pts',(-0.0152399999993761,59.0285534841296,
40.10025));
#195135=CARTESIAN_POINT('Origin',(6.10537907909441,57.9430040808457,39.92499));
#195136=CARTESIAN_POINT('Ctrl Pts',(6.73887200051396,62.2936141127569,39.92499));
#195137=CARTESIAN_POINT('Ctrl Pts',(6.73998108195387,62.3041663177856,39.934835464202));
#195138=CARTESIAN_POINT('Ctrl Pts',(6.74025426844153,62.3147747227671,39.9446440828461));
#195139=CARTESIAN_POINT('Ctrl Pts',(6.73970068257655,62.3253809467526,39.9543641760336));
#195140=CARTESIAN_POINT('Ctrl Pts',(6.73916508495579,62.3356425316146,39.9637684240719));
#195141=CARTESIAN_POINT('Ctrl Pts',(6.73785543637705,62.3459033574831,39.9730909636404));
#195142=CARTESIAN_POINT('Ctrl Pts',(6.73573381164837,62.3561113603653,39.982280897715));
#195143=CARTESIAN_POINT('Ctrl Pts',(6.73372688529716,62.3657675025193,39.990974009466));
#195144=CARTESIAN_POINT('Ctrl Pts',(6.73099321743859,62.3753772873486,39.9995492765013));
#195145=CARTESIAN_POINT('Ctrl Pts',(6.72746117704619,62.3848821415117,40.0079462328707));
#195146=CARTESIAN_POINT('Ctrl Pts',(6.72420791240112,62.3936367996045,40.0156804369703));
#195147=CARTESIAN_POINT('Ctrl Pts',(6.72027708243738,62.4023029415008,40.0232638017437));
#195148=CARTESIAN_POINT('Ctrl Pts',(6.71558140886323,62.4108128192398,40.0306257269982));
#195149=CARTESIAN_POINT('Ctrl Pts',(6.71421937245567,62.4132812112865,40.0327611416662));
#195150=CARTESIAN_POINT('Ctrl Pts',(6.71279278199565,62.415736279296,40.0348777427276));
#195151=CARTESIAN_POINT('Ctrl Pts',(6.71129899689659,62.4181758915948,40.0369733168701));
#195152=CARTESIAN_POINT('Ctrl Pts',(6.70967963780731,62.42082058818,40.039245053974));
#195153=CARTESIAN_POINT('Ctrl Pts',(6.70798448411237,62.4234440047028,40.041487875195));
#195154=CARTESIAN_POINT('Ctrl Pts',(6.70621108803186,62.4260429761972,40.0436985701601));
#195155=CARTESIAN_POINT('Ctrl Pts',(6.70134398857332,62.4331758738575,40.0497658398386));
#195156=CARTESIAN_POINT('Ctrl Pts',(6.69585818364757,62.4400912556837,40.0555581699984));
#195157=CARTESIAN_POINT('Ctrl Pts',(6.68976801333951,62.4466864116141,40.0609828468885));
#195158=CARTESIAN_POINT('Ctrl Pts',(6.68419583815079,62.4527206212309,40.0659461317303));
#195159=CARTESIAN_POINT('Ctrl Pts',(6.67811620689403,62.4584752900412,40.0706039980705));
#195160=CARTESIAN_POINT('Ctrl Pts',(6.67150703079275,62.4638645712583,40.0748843180601));
#195161=CARTESIAN_POINT('Ctrl Pts',(6.66826062508144,62.4665117685875,40.0769867972568));
#195162=CARTESIAN_POINT('Ctrl Pts',(6.66488629458054,62.4690703232299,40.0789976708174));
#195163=CARTESIAN_POINT('Ctrl Pts',(6.66138078591774,62.4715267736418,40.08090504915));
#195164=CARTESIAN_POINT('Ctrl Pts',(6.66071564979311,62.4719928611813,40.0812669556104));
#195165=CARTESIAN_POINT('Ctrl Pts',(6.66004526561052,62.4724551899379,40.0816253922032));
#195166=CARTESIAN_POINT('Ctrl Pts',(6.65936969820921,62.4729136358128,40.0819801989139));
#195167=CARTESIAN_POINT('Ctrl Pts',(6.65871524228918,62.4733577552541,40.0823239179149));
#195168=CARTESIAN_POINT('Ctrl Pts',(6.65805592206515,62.4737982306999,40.0826642303498));
#195169=CARTESIAN_POINT('Ctrl Pts',(6.65739180030973,62.4742349489458,40.0830009916099));
#195170=CARTESIAN_POINT('Ctrl Pts',(6.65015433826458,62.4789942144025,40.0866709464313));
#195171=CARTESIAN_POINT('Ctrl Pts',(6.6423416549749,62.483310062658,40.0899175831879));
#195172=CARTESIAN_POINT('Ctrl Pts',(6.63406423386157,62.4870273554129,40.0925642067064));
#195173=CARTESIAN_POINT('Ctrl Pts',(6.63056862752539,62.4885971912264,40.0936818922529));
#195174=CARTESIAN_POINT('Ctrl Pts',(6.62699051141418,62.490060506939,40.0946930094791));
#195175=CARTESIAN_POINT('Ctrl Pts',(6.62333954252063,62.491407022622,40.0955863397546));
#195176=CARTESIAN_POINT('Ctrl Pts',(6.61719140213135,62.4936745213866,40.0970906856166));
#195177=CARTESIAN_POINT('Ctrl Pts',(6.61083770188589,62.495608491139,40.0982599215483));
#195178=CARTESIAN_POINT('Ctrl Pts',(6.60433062536211,62.4971561593221,40.0990497370454));
#195179=CARTESIAN_POINT('Ctrl Pts',(6.60270385623117,62.4975430763678,40.0992471909196));
#195180=CARTESIAN_POINT('Ctrl Pts',(6.60106746196622,62.4979056188883,40.0994209989363));
#195181=CARTESIAN_POINT('Ctrl Pts',(6.5994222184581,62.4982426563695,40.0995705982975));
#195182=CARTESIAN_POINT('Ctrl Pts',(6.59695435319593,62.4987482125912,40.0997949973393));
#195183=CARTESIAN_POINT('Ctrl Pts',(6.59446659126666,62.4991963674672,40.0999649129781));
#195184=CARTESIAN_POINT('Ctrl Pts',(6.59196174500359,62.4995849724121,40.1000786629733));
#195185=CARTESIAN_POINT('Ctrl Pts',(6.58945689874052,62.4999735773569,40.1001924129685));
#195186=CARTESIAN_POINT('Ctrl Pts',(6.58693497617713,62.5003026407461,40.10025));
#195187=CARTESIAN_POINT('Ctrl Pts',(6.58439859103091,62.500570298093,40.10025));
#195188=CARTESIAN_POINT('Ctrl Pts',(6.18532049829458,58.7035958781038,40.10025));
#195189=CARTESIAN_POINT('Ctrl Pts',(6.19390281910209,58.7026899760169,40.10025));
#195190=CARTESIAN_POINT('Ctrl Pts',(6.20248552904414,58.7025003609928,40.0995786334241));
#195191=CARTESIAN_POINT('Ctrl Pts',(6.21093474935464,58.7029569544313,40.0983063763367));
#195192=CARTESIAN_POINT('Ctrl Pts',(6.21639207873535,58.7032518669434,40.0974846287993));
#195193=CARTESIAN_POINT('Ctrl Pts',(6.22179377937559,58.7038154335198,40.0964130309338));
#195194=CARTESIAN_POINT('Ctrl Pts',(6.22710604846914,58.7046202140515,40.0951176960924));
#195195=CARTESIAN_POINT('Ctrl Pts',(6.23414715684692,58.7056869045457,40.0934008039614));
#195196=CARTESIAN_POINT('Ctrl Pts',(6.24102913891695,58.7071827955651,40.0912909372156));
#195197=CARTESIAN_POINT('Ctrl Pts',(6.247679224408,58.7090548163569,40.0888630467851));
#195198=CARTESIAN_POINT('Ctrl Pts',(6.25100426715352,58.7099908267527,40.0876491015699));
#195199=CARTESIAN_POINT('Ctrl Pts',(6.25427153376716,58.7110208470227,40.0863558569271));
#195200=CARTESIAN_POINT('Ctrl Pts',(6.25747333351573,58.7121380880307,40.0849936342771));
#195201=CARTESIAN_POINT('Ctrl Pts',(6.25907423339001,58.7126967085346,40.0843125229521));
#195202=CARTESIAN_POINT('Ctrl Pts',(6.26065878288398,58.713277132457,40.0836141747074));
#195203=CARTESIAN_POINT('Ctrl Pts',(6.2622261232057,58.7138784999415,40.0828999161609));
#195204=CARTESIAN_POINT('Ctrl Pts',(6.26261795828614,58.7140288418126,40.0827213515243));
#195205=CARTESIAN_POINT('Ctrl Pts',(6.26300871814066,58.7141804926177,40.0825417925842));
#195206=CARTESIAN_POINT('Ctrl Pts',(6.2633983900511,58.7143334388435,40.082361260236));
#195207=CARTESIAN_POINT('Ctrl Pts',(6.26456740578241,58.7147922775207,40.0818196631917));
#195208=CARTESIAN_POINT('Ctrl Pts',(6.26572662828426,58.715262775183,40.0812693052021));
#195209=CARTESIAN_POINT('Ctrl Pts',(6.2668757296522,58.7157445651923,40.0807107531875));
#195210=CARTESIAN_POINT('Ctrl Pts',(6.27496985131196,58.7191382318077,40.0767763849182));
#195211=CARTESIAN_POINT('Ctrl Pts',(6.2826071619282,58.7230632421217,40.0724140586138));
#195212=CARTESIAN_POINT('Ctrl Pts',(6.28978339589494,58.7274000190313,40.0677221223769));
#195213=CARTESIAN_POINT('Ctrl Pts',(6.29326386161416,58.7295033511461,40.0654465383721));
#195214=CARTESIAN_POINT('Ctrl Pts',(6.2966359740898,58.731704109697,40.0630928000679));
#195215=CARTESIAN_POINT('Ctrl Pts',(6.29989941779205,58.7339915094193,40.0606689262479));
#195216=CARTESIAN_POINT('Ctrl Pts',(6.30489552208994,58.7374933585781,40.0569581447805));
#195217=CARTESIAN_POINT('Ctrl Pts',(6.30963480180928,58.7411954596216,40.0530843804605));
#195218=CARTESIAN_POINT('Ctrl Pts',(6.31410463171103,58.7450534628849,40.0490800251457));
#195219=CARTESIAN_POINT('Ctrl Pts',(6.31618044384123,58.7468451395591,40.0472203818218));
#195220=CARTESIAN_POINT('Ctrl Pts',(6.31819823791584,58.7486702031823,40.0453323608818));
#195221=CARTESIAN_POINT('Ctrl Pts',(6.32015576082374,58.7505249478604,40.0434201572162));
#195222=CARTESIAN_POINT('Ctrl Pts',(6.3203057972416,58.750667106732,40.0432735943397));
#195223=CARTESIAN_POINT('Ctrl Pts',(6.32045551058247,58.7508094261758,40.0431268995707));
#195224=CARTESIAN_POINT('Ctrl Pts',(6.32060490094056,58.7509519047345,40.0429800745037));
#195225=CARTESIAN_POINT('Ctrl Pts',(6.3227033850744,58.7529532989256,40.0409176249753));
#195226=CARTESIAN_POINT('Ctrl Pts',(6.32473679726686,58.7549876922214,40.0388310783332));
#195227=CARTESIAN_POINT('Ctrl Pts',(6.32670504965044,58.7570493794209,40.036725739981));
#195228=CARTESIAN_POINT('Ctrl Pts',(6.3337628526564,58.7644422230598,40.0291763710714));
#195229=CARTESIAN_POINT('Ctrl Pts',(6.34003880539004,58.7722418109929,40.0213310894587));
#195230=CARTESIAN_POINT('Ctrl Pts',(6.34560292136835,58.7803396486563,40.0132837551308));
#195231=CARTESIAN_POINT('Ctrl Pts',(6.35171732586353,58.7892383587484,40.0044405431308));
#195232=CARTESIAN_POINT('Ctrl Pts',(6.35697262978608,58.7984976730916,39.9953528710578));
#195233=CARTESIAN_POINT('Ctrl Pts',(6.36142852992988,58.8080148760677,39.9861103629527));
#195234=CARTESIAN_POINT('Ctrl Pts',(6.36623978380702,58.8182910667901,39.9761307737519));
#195235=CARTESIAN_POINT('Ctrl Pts',(6.3701196826395,58.8288688921899,39.9659696935964));
#195236=CARTESIAN_POINT('Ctrl Pts',(6.37309732670023,58.8396533761938,39.9557128217449));
#195237=CARTESIAN_POINT('Ctrl Pts',(6.37604999138599,58.8503473894549,39.9455419945122));
#195238=CARTESIAN_POINT('Ctrl Pts',(6.37811557911308,58.8612460403482,39.9352756289321));
#195239=CARTESIAN_POINT('Ctrl Pts',(6.37927424642637,58.872270023448,39.92499));
#195240=CARTESIAN_POINT('Origin',(-0.0151565136854075,0.0015930137801936,
39.92499));
#195241=CARTESIAN_POINT('Ctrl Pts',(6.55408556366009,62.5037563256534,40.10025));
#195242=CARTESIAN_POINT('Ctrl Pts',(6.54554330587477,62.5046505412977,40.10025));
#195243=CARTESIAN_POINT('Ctrl Pts',(6.53700226086738,62.5048232320878,40.0995859581842));
#195244=CARTESIAN_POINT('Ctrl Pts',(6.5285945717753,62.5043472028589,40.0983275959621));
#195245=CARTESIAN_POINT('Ctrl Pts',(6.52322245869558,62.5040430428431,40.0975235624068));
#195246=CARTESIAN_POINT('Ctrl Pts',(6.51790471489673,62.5034749678471,40.096477705949));
#195247=CARTESIAN_POINT('Ctrl Pts',(6.51267356740911,62.5026702669706,40.0952149915961));
#195248=CARTESIAN_POINT('Ctrl Pts',(6.50553410072716,62.5015720117389,40.0934916398701));
#195249=CARTESIAN_POINT('Ctrl Pts',(6.49855818190839,62.5000273428097,40.091364392163));
#195250=CARTESIAN_POINT('Ctrl Pts',(6.49182203260242,62.4980940659028,40.0889118607713));
#195251=CARTESIAN_POINT('Ctrl Pts',(6.48845395794943,62.4971274274494,40.0876855950754));
#195252=CARTESIAN_POINT('Ctrl Pts',(6.48514561818799,62.4960636607365,40.0863782327526));
#195253=CARTESIAN_POINT('Ctrl Pts',(6.48190505740227,62.4949101555729,40.0850006373334));
#195254=CARTESIAN_POINT('Ctrl Pts',(6.48028477700941,62.4943334029911,40.0843118396237));
#195255=CARTESIAN_POINT('Ctrl Pts',(6.47868142404744,62.4937342176672,40.0836054919164));
#195256=CARTESIAN_POINT('Ctrl Pts',(6.47709589524329,62.4931135352113,40.0828829920417));
#195257=CARTESIAN_POINT('Ctrl Pts',(6.47669951304225,62.4929583645973,40.0827023670731));
#195258=CARTESIAN_POINT('Ctrl Pts',(6.47630424448236,62.4928018504534,40.0825207326933));
#195259=CARTESIAN_POINT('Ctrl Pts',(6.47591010283136,62.4926440074816,40.0823381109275));
#195260=CARTESIAN_POINT('Ctrl Pts',(6.47472767787837,62.492170478566,40.0817902456303));
#195261=CARTESIAN_POINT('Ctrl Pts',(6.47355539694531,62.4916849899863,40.0812334935553));
#195262=CARTESIAN_POINT('Ctrl Pts',(6.47239360181873,62.4911879405751,40.0806684524227));
#195263=CARTESIAN_POINT('Ctrl Pts',(6.46436487665231,62.4877530207468,40.0767636676136));
#195264=CARTESIAN_POINT('Ctrl Pts',(6.45678933786444,62.4837949925046,40.0724404510887));
#195265=CARTESIAN_POINT('Ctrl Pts',(6.44966853564036,62.4794326364364,40.0677949937408));
#195266=CARTESIAN_POINT('Ctrl Pts',(6.44612951648131,62.4772645574451,40.0654862141905));
#195267=CARTESIAN_POINT('Ctrl Pts',(6.44270272394404,62.474996003895,40.0630972003215));
#195268=CARTESIAN_POINT('Ctrl Pts',(6.43938822718986,62.4726384024733,40.0606363359906));
#195269=CARTESIAN_POINT('Ctrl Pts',(6.43207595228416,62.4674371815966,40.0552073017123));
#195270=CARTESIAN_POINT('Ctrl Pts',(6.42530381744052,62.4618132330509,40.0494204304519));
#195271=CARTESIAN_POINT('Ctrl Pts',(6.41913840445487,62.455895762341,40.0434049749851));
#195272=CARTESIAN_POINT('Ctrl Pts',(6.41688610134127,62.4537340356674,40.0412074532442));
#195273=CARTESIAN_POINT('Ctrl Pts',(6.4147074139753,62.4515361835425,40.0389814735788));
#195274=CARTESIAN_POINT('Ctrl Pts',(6.41260146153701,62.4493074469122,40.0367321210017));
#195275=CARTESIAN_POINT('Ctrl Pts',(6.40552779014142,62.4418213564085,40.0291767837138));
#195276=CARTESIAN_POINT('Ctrl Pts',(6.39923601079921,62.4339335724859,40.0213235332571));
#195277=CARTESIAN_POINT('Ctrl Pts',(6.39365709371064,62.4257522463021,40.0132649215851));
#195278=CARTESIAN_POINT('Ctrl Pts',(6.38752520296412,62.4167599996842,40.0044075527522));
#195279=CARTESIAN_POINT('Ctrl Pts',(6.38225398283479,62.4074126717497,39.9953016253706));
#195280=CARTESIAN_POINT('Ctrl Pts',(6.37778536209598,62.3978127557438,39.9860353422341));
#195281=CARTESIAN_POINT('Ctrl Pts',(6.3729724660951,62.3874732348817,39.9760551582674));
#195282=CARTESIAN_POINT('Ctrl Pts',(6.36908997057791,62.3768396913499,39.9658879738131));
#195283=CARTESIAN_POINT('Ctrl Pts',(6.36611161569965,62.3660067738133,39.9556174643225));
#195284=CARTESIAN_POINT('Ctrl Pts',(6.36317347866869,62.355320137241,39.9454856413885));
#195285=CARTESIAN_POINT('Ctrl Pts',(6.36111515612501,62.344438041129,39.9352519465104));
#195286=CARTESIAN_POINT('Ctrl Pts',(6.35995915837865,62.3334394572618,39.92499));
#195287=CARTESIAN_POINT('Ctrl Pts',(6.00036140429106,58.9120953679529,39.92499));
#195288=CARTESIAN_POINT('Ctrl Pts',(5.99925510810176,58.9015696628136,39.9348107241731));
#195289=CARTESIAN_POINT('Ctrl Pts',(5.99898299131239,58.8909945468879,39.9446038383187));
#195290=CARTESIAN_POINT('Ctrl Pts',(5.99953795195324,58.8804276387757,39.9543158069411));
#195291=CARTESIAN_POINT('Ctrl Pts',(6.00007381527955,58.8702243592762,39.9636935671423));
#195292=CARTESIAN_POINT('Ctrl Pts',(6.0013809572776,58.8600274753995,39.9729968321026));
#195293=CARTESIAN_POINT('Ctrl Pts',(6.00349883564084,58.8498890377446,39.9821731151378));
#195294=CARTESIAN_POINT('Ctrl Pts',(6.00550089397251,58.8403050389987,39.9908475764398));
#195295=CARTESIAN_POINT('Ctrl Pts',(6.00822762538762,58.8307723843828,39.9994093733896));
#195296=CARTESIAN_POINT('Ctrl Pts',(6.01175153639814,58.8213500689001,40.0077966115894));
#195297=CARTESIAN_POINT('Ctrl Pts',(6.01499699932078,58.8126722744117,40.015521117265));
#195298=CARTESIAN_POINT('Ctrl Pts',(6.01891888229525,58.8040875818502,40.0230979941079));
#195299=CARTESIAN_POINT('Ctrl Pts',(6.02360485257848,58.7956642413002,40.0304554104807));
#195300=CARTESIAN_POINT('Ctrl Pts',(6.0250021143232,58.7931525711866,40.032649243522));
#195301=CARTESIAN_POINT('Ctrl Pts',(6.02646752363906,58.7906554330073,40.034823371508));
#195302=CARTESIAN_POINT('Ctrl Pts',(6.02800395803763,58.7881751602883,40.0369753512355));
#195303=CARTESIAN_POINT('Ctrl Pts',(6.0295246938641,58.7857202298424,40.0391053430351));
#195304=CARTESIAN_POINT('Ctrl Pts',(6.03111319985562,58.7832842250419,40.041211089324));
#195305=CARTESIAN_POINT('Ctrl Pts',(6.03277025542088,58.7808720541406,40.0432881154904));
#195306=CARTESIAN_POINT('Ctrl Pts',(6.0328854838242,58.7807043164936,40.0434325478279));
#195307=CARTESIAN_POINT('Ctrl Pts',(6.03300103800968,58.7805366835714,40.0435768364421));
#195308=CARTESIAN_POINT('Ctrl Pts',(6.0331169189062,58.7803691562897,40.0437209807855));
#195309=CARTESIAN_POINT('Ctrl Pts',(6.03819756191488,58.7730241465597,40.050040796842));
#195310=CARTESIAN_POINT('Ctrl Pts',(6.04393622206048,58.7659160498049,40.0560490279345));
#195311=CARTESIAN_POINT('Ctrl Pts',(6.05034076157633,58.7591607781928,40.0616647108615));
#195312=CARTESIAN_POINT('Ctrl Pts',(6.05631090550653,58.7528636909922,40.0668995033486));
#195313=CARTESIAN_POINT('Ctrl Pts',(6.06286038933357,58.7468728126824,40.0717933267482));
#195314=CARTESIAN_POINT('Ctrl Pts',(6.07000150504423,58.741310782788,40.0762460303072));
#195315=CARTESIAN_POINT('Ctrl Pts',(6.07261381755745,58.7392761202953,40.0778748868748));
#195316=CARTESIAN_POINT('Ctrl Pts',(6.07530531160718,58.7372991657064,40.0794443522247));
#195317=CARTESIAN_POINT('Ctrl Pts',(6.07807653793614,58.735387140493,40.0809482021492));
#195318=CARTESIAN_POINT('Ctrl Pts',(6.07874292528977,58.7349273623042,40.0813098278168));
#195319=CARTESIAN_POINT('Ctrl Pts',(6.07941450700242,58.7344713442222,40.0816679525672));
#195320=CARTESIAN_POINT('Ctrl Pts',(6.08009121771133,58.7340192051468,40.082022419258));
#195321=CARTESIAN_POINT('Ctrl Pts',(6.0807467812106,58.7335811954174,40.0823658088648));
#195322=CARTESIAN_POINT('Ctrl Pts',(6.08140715812765,58.7331468260467,40.0827057654616));
#195323=CARTESIAN_POINT('Ctrl Pts',(6.08207228526599,58.7327162055065,40.0830421470151));
#195324=CARTESIAN_POINT('Ctrl Pts',(6.08935952173653,58.727998259832,40.0867275956806));
#195325=CARTESIAN_POINT('Ctrl Pts',(6.09722197243233,58.7237275533351,40.089982343203));
#195326=CARTESIAN_POINT('Ctrl Pts',(6.10554709909211,58.7200553115703,40.0926299529355));
#195327=CARTESIAN_POINT('Ctrl Pts',(6.10899977726353,58.7185323234525,40.0937279956084));
#195328=CARTESIAN_POINT('Ctrl Pts',(6.11253167434641,58.7171120447815,40.0947220371802));
#195329=CARTESIAN_POINT('Ctrl Pts',(6.11613350280284,58.7158039367398,40.0956014538692));
#195330=CARTESIAN_POINT('Ctrl Pts',(6.12227679657208,58.7135728221601,40.097101390674));
#195331=CARTESIAN_POINT('Ctrl Pts',(6.12862250657844,58.7116702942287,40.0982667904316));
#195332=CARTESIAN_POINT('Ctrl Pts',(6.13511848061154,58.7101471179285,40.0990539325582));
#195333=CARTESIAN_POINT('Ctrl Pts',(6.13836646762808,58.7093855297784,40.0994475036216));
#195334=CARTESIAN_POINT('Ctrl Pts',(6.14165223896418,58.7087202098048,40.0997467259952));
#195335=CARTESIAN_POINT('Ctrl Pts',(6.14496923836549,58.7081575578109,40.0999473488896));
#195336=CARTESIAN_POINT('Ctrl Pts',(6.14828623776681,58.707594905817,40.100147971784));
#195337=CARTESIAN_POINT('Ctrl Pts',(6.15163442139651,58.7071349090266,40.10025));
#195338=CARTESIAN_POINT('Ctrl Pts',(6.15500747092375,58.7067819056642,40.10025));
#195339=CARTESIAN_POINT('Origin',(12.128626347365,56.9874003490101,39.92499));
#195340=CARTESIAN_POINT('Ctrl Pts',(13.21341150919,61.2479592423876,39.92499));
#195341=CARTESIAN_POINT('Ctrl Pts',(13.2156175207415,61.2583377107545,39.9348354642021));
#195342=CARTESIAN_POINT('Ctrl Pts',(13.2169980909554,61.2688594460197,39.9446440828464));
#195343=CARTESIAN_POINT('Ctrl Pts',(13.217556189986,61.2794654334803,39.954364176034));
#195344=CARTESIAN_POINT('Ctrl Pts',(13.2180961541214,61.2897267895029,39.9637684240723));
#195345=CARTESIAN_POINT('Ctrl Pts',(13.2178662282945,61.3000683010471,39.9730909636408));
#195346=CARTESIAN_POINT('Ctrl Pts',(13.2168232529023,61.310442153594,39.9822808977153));
#195347=CARTESIAN_POINT('Ctrl Pts',(13.2158366624041,61.3202551793184,39.9909740094663));
#195348=CARTESIAN_POINT('Ctrl Pts',(13.2141224659046,61.3300980668413,39.9995492765015));
#195349=CARTESIAN_POINT('Ctrl Pts',(13.2116033021983,61.3399200511732,40.0079462328709));
#195350=CARTESIAN_POINT('Ctrl Pts',(13.2092829702343,61.3489668090869,40.0156804369705));
#195351=CARTESIAN_POINT('Ctrl Pts',(13.2062795322632,61.3579963605666,40.0232638017438));
#195352=CARTESIAN_POINT('Ctrl Pts',(13.2024991065229,61.3669504518477,40.0306257269983));
#195353=CARTESIAN_POINT('Ctrl Pts',(13.2014025487207,61.3695476933571,40.0327611416663));
#195354=CARTESIAN_POINT('Ctrl Pts',(13.2002403977587,61.3721384315556,40.0348777427276));
#195355=CARTESIAN_POINT('Ctrl Pts',(13.1990098046953,61.3747208224638,40.0369733168701));
#195356=CARTESIAN_POINT('Ctrl Pts',(13.1976757626944,61.3775203002415,40.039245053974));
#195357=CARTESIAN_POINT('Ctrl Pts',(13.1962641169264,61.3803065372248,40.041487875195));
#195358=CARTESIAN_POINT('Ctrl Pts',(13.1947721021916,61.3830766416485,40.0436985701601));
#195359=CARTESIAN_POINT('Ctrl Pts',(13.1906772560442,61.390679214976,40.0497658398386));
#195360=CARTESIAN_POINT('Ctrl Pts',(13.185944357167,61.3981301363757,40.0555581699984));
#195361=CARTESIAN_POINT('Ctrl Pts',(13.1805769309636,61.4053257594952,40.0609828468885));
#195362=CARTESIAN_POINT('Ctrl Pts',(13.1756660273918,61.41190936399,40.0659461317304));
#195363=CARTESIAN_POINT('Ctrl Pts',(13.1702212276784,61.418268002635,40.0706039980706));
#195364=CARTESIAN_POINT('Ctrl Pts',(13.164211590619,61.4243186078272,40.0748843180603));
#195365=CARTESIAN_POINT('Ctrl Pts',(13.1612596765267,61.4272906453324,40.0769867972569));
#195366=CARTESIAN_POINT('Ctrl Pts',(13.1581712727464,61.4301878975265,40.0789976708174));
#195367=CARTESIAN_POINT('Ctrl Pts',(13.1549417366136,61.4329973166794,40.0809050491499));
#195368=CARTESIAN_POINT('Ctrl Pts',(13.1543289635885,61.4335303765996,40.0812669556104));
#195369=CARTESIAN_POINT('Ctrl Pts',(13.1537105783551,61.4340602468993,40.0816253922032));
#195370=CARTESIAN_POINT('Ctrl Pts',(13.1530866324254,61.434586797382,40.0819801989139));
#195371=CARTESIAN_POINT('Ctrl Pts',(13.1524821848061,61.4350968931621,40.0823239179149));
#195372=CARTESIAN_POINT('Ctrl Pts',(13.1518725186287,61.4356038733671,40.0826642303498));
#195373=CARTESIAN_POINT('Ctrl Pts',(13.1512576844889,61.4361076188514,40.0830009916099));
#195374=CARTESIAN_POINT('Ctrl Pts',(13.1445573487227,61.4415973333394,40.0866709464312));
#195375=CARTESIAN_POINT('Ctrl Pts',(13.1372385931155,61.4467061867047,40.0899175831878));
#195376=CARTESIAN_POINT('Ctrl Pts',(13.1293950794805,61.4512683418497,40.0925642067062));
#195377=CARTESIAN_POINT('Ctrl Pts',(13.1260827149666,61.453194968297,40.0936818922528));
#195378=CARTESIAN_POINT('Ctrl Pts',(13.1226771582924,61.4550242827915,40.094693009479));
#195379=CARTESIAN_POINT('Ctrl Pts',(13.1191869390034,61.4567450522887,40.0955863397545));
#195380=CARTESIAN_POINT('Ctrl Pts',(13.1133094969318,61.4596427851247,40.0970906856166));
#195381=CARTESIAN_POINT('Ctrl Pts',(13.1071927578073,61.4622303029111,40.0982599215483));
#195382=CARTESIAN_POINT('Ctrl Pts',(13.1008831031063,61.464449667515,40.0990497370454));
#195383=CARTESIAN_POINT('Ctrl Pts',(13.0993056894311,61.465004508666,40.0992471909196));
#195384=CARTESIAN_POINT('Ctrl Pts',(13.0977161555177,61.4655361149184,40.0994209989363));
#195385=CARTESIAN_POINT('Ctrl Pts',(13.0961151548356,61.4660432808487,40.0995705982975));
#195386=CARTESIAN_POINT('Ctrl Pts',(13.0937136538125,61.466804029744,40.0997949973393));
#195387=CARTESIAN_POINT('Ctrl Pts',(13.0912863650439,61.4675097715122,40.0999649129781));
#195388=CARTESIAN_POINT('Ctrl Pts',(13.0888358608685,61.4681580753691,40.1000786629733));
#195389=CARTESIAN_POINT('Ctrl Pts',(13.086385356693,61.4688063792261,40.1001924129685));
#195390=CARTESIAN_POINT('Ctrl Pts',(13.0839116459757,61.4693972526618,40.10025));
#195391=CARTESIAN_POINT('Ctrl Pts',(13.0814171332239,61.4699285681953,40.10025));
#195392=CARTESIAN_POINT('Ctrl Pts',(12.2876333308477,57.7354693911203,40.10025));
#195393=CARTESIAN_POINT('Ctrl Pts',(12.2960739442514,57.7336713548545,40.10025));
#195394=CARTESIAN_POINT('Ctrl Pts',(12.3045898170438,57.7325856410803,40.099578633424));
#195395=CARTESIAN_POINT('Ctrl Pts',(12.3130404786523,57.7321565492374,40.0983063763364));
#195396=CARTESIAN_POINT('Ctrl Pts',(12.3184987389629,57.7318793999342,40.0974846287991));
#195397=CARTESIAN_POINT('Ctrl Pts',(12.3239297572695,57.731875247767,40.0964130309337));
#195398=CARTESIAN_POINT('Ctrl Pts',(12.3292970476689,57.732120336302,40.0951176960923));
#195399=CARTESIAN_POINT('Ctrl Pts',(12.3364110836364,57.7324451871156,40.0934008039614));
#195400=CARTESIAN_POINT('Ctrl Pts',(12.3434117286781,57.7332135204775,40.0912909372156));
#195401=CARTESIAN_POINT('Ctrl Pts',(12.3502210637615,57.7343801629265,40.0888630467851));
#195402=CARTESIAN_POINT('Ctrl Pts',(12.3536257313032,57.734963484151,40.0876491015699));
#195403=CARTESIAN_POINT('Ctrl Pts',(12.3569827659245,57.735646339504,40.0863558569271));
#195404=CARTESIAN_POINT('Ctrl Pts',(12.3602838093647,57.7364227809414,40.0849936342771));
#195405=CARTESIAN_POINT('Ctrl Pts',(12.3619343310847,57.7368110016601,40.0843125229521));
#195406=CARTESIAN_POINT('Ctrl Pts',(12.3635708710714,57.7372226154359,40.0836141747074));
#195407=CARTESIAN_POINT('Ctrl Pts',(12.3651924853579,57.7376568568911,40.0828999161609));
#195408=CARTESIAN_POINT('Ctrl Pts',(12.3655978889295,57.7377654172549,40.0827213515243));
#195409=CARTESIAN_POINT('Ctrl Pts',(12.3660023599863,57.737875391774,40.0825417925841));
#195410=CARTESIAN_POINT('Ctrl Pts',(12.3664058844671,57.7379867683383,40.082361260236));
#195411=CARTESIAN_POINT('Ctrl Pts',(12.3676164579098,57.7383208980313,40.0818196631917));
#195412=CARTESIAN_POINT('Ctrl Pts',(12.3688185104671,57.7386676465114,40.0812693052021));
#195413=CARTESIAN_POINT('Ctrl Pts',(12.3700116777068,57.7390266834245,40.0807107531874));
#195414=CARTESIAN_POINT('Ctrl Pts',(12.3784161936773,57.7415556930806,40.0767763849182));
#195415=CARTESIAN_POINT('Ctrl Pts',(12.3864219416033,57.7446608854351,40.0724140586138));
#195416=CARTESIAN_POINT('Ctrl Pts',(12.3940121800354,57.7482237843184,40.0677221223769));
#195417=CARTESIAN_POINT('Ctrl Pts',(12.397693437473,57.7499517864267,40.0654465383721));
#195418=CARTESIAN_POINT('Ctrl Pts',(12.401277119073,57.751788007257,40.0630928000679));
#195419=CARTESIAN_POINT('Ctrl Pts',(12.4047617836671,57.7537217536092,40.0606689262479));
#195420=CARTESIAN_POINT('Ctrl Pts',(12.410096561694,57.7566821841673,40.0569581447805));
#195421=CARTESIAN_POINT('Ctrl Pts',(12.4151968540761,57.7598686150879,40.0530843804606));
#195422=CARTESIAN_POINT('Ctrl Pts',(12.4200454689344,57.763238259355,40.0490800251458));
#195423=CARTESIAN_POINT('Ctrl Pts',(12.422297190758,57.7648031395848,40.0472203818218));
#195424=CARTESIAN_POINT('Ctrl Pts',(12.4244947022414,57.7664072884047,40.0453323608818));
#195425=CARTESIAN_POINT('Ctrl Pts',(12.426635375245,57.7680472557361,40.0434201572162));
#195426=CARTESIAN_POINT('Ctrl Pts',(12.426799449396,57.7681729527702,40.0432735943397));
#195427=CARTESIAN_POINT('Ctrl Pts',(12.4269632190243,57.7682988432678,40.0431268995707));
#195428=CARTESIAN_POINT('Ctrl Pts',(12.4271266840712,57.7684249257695,40.0429800745037));
#195429=CARTESIAN_POINT('Ctrl Pts',(12.4294228751485,57.7701960047921,40.0409176249753));
#195430=CARTESIAN_POINT('Ctrl Pts',(12.4316578001011,57.7720067040169,40.0388310783332));
#195431=CARTESIAN_POINT('Ctrl Pts',(12.4338307751869,57.7738513586812,40.036725739981));
#195432=CARTESIAN_POINT('Ctrl Pts',(12.4416226773936,57.7804659622463,40.029176371072));
#195433=CARTESIAN_POINT('Ctrl Pts',(12.4486795287417,57.7875668075252,40.02133108946));
#195434=CARTESIAN_POINT('Ctrl Pts',(12.4550596184368,57.7950386758933,40.0132837551328));
#195435=CARTESIAN_POINT('Ctrl Pts',(12.4620706960749,57.8032495086139,40.0044405431337));
#195436=CARTESIAN_POINT('Ctrl Pts',(12.4682650727914,57.8119087706204,39.9953528710616));
#195437=CARTESIAN_POINT('Ctrl Pts',(12.4736913816495,57.8209080689672,39.9861103629574));
#195438=CARTESIAN_POINT('Ctrl Pts',(12.4795504333984,57.8306250526661,39.9761307737579));
#195439=CARTESIAN_POINT('Ctrl Pts',(12.4845147615727,57.8407393717674,39.965969693604));
#195440=CARTESIAN_POINT('Ctrl Pts',(12.4886033793277,57.8511535286802,39.9557128217539));
#195441=CARTESIAN_POINT('Ctrl Pts',(12.4926576977815,57.8614803215184,39.9455419945183));
#195442=CARTESIAN_POINT('Ctrl Pts',(12.4958511892337,57.872103355754,39.9352756289352));
#195443=CARTESIAN_POINT('Ctrl Pts',(12.4981558292594,57.8829458346104,39.92499));
#195444=CARTESIAN_POINT('Origin',(-0.0149069694351787,0.0031685741680573,
39.92499));
#195445=CARTESIAN_POINT('Ctrl Pts',(13.0516031943535,61.4762657165314,40.10025));
#195446=CARTESIAN_POINT('Ctrl Pts',(13.0432012029373,61.478047942648,40.10025));
#195447=CARTESIAN_POINT('Ctrl Pts',(13.0347249977711,61.4791124697292,40.0995859581842));
#195448=CARTESIAN_POINT('Ctrl Pts',(13.0263136082758,61.4795178910586,40.0983275959621));
#195449=CARTESIAN_POINT('Ctrl Pts',(13.0209391308145,61.4797769359879,40.0975235624068));
#195450=CARTESIAN_POINT('Ctrl Pts',(13.0155911381662,61.4797678285535,40.096477705949));
#195451=CARTESIAN_POINT('Ctrl Pts',(13.0103045333058,61.4795143397207,40.0952149915961));
#195452=CARTESIAN_POINT('Ctrl Pts',(13.0030893784377,61.4791683783268,40.0934916398701));
#195453=CARTESIAN_POINT('Ctrl Pts',(12.9959902125627,61.4783613533297,40.091364392163));
#195454=CARTESIAN_POINT('Ctrl Pts',(12.9890888821233,61.4771427864513,40.0889118607713));
#195455=CARTESIAN_POINT('Ctrl Pts',(12.9856382169037,61.4765335030121,40.0876855950754));
#195456=CARTESIAN_POINT('Ctrl Pts',(12.9822368066738,61.4758213793958,40.0863782327526));
#195457=CARTESIAN_POINT('Ctrl Pts',(12.978893423897,61.4750129240932,40.0850006373334));
#195458=CARTESIAN_POINT('Ctrl Pts',(12.9772217325086,61.474608696442,40.0843118396237));
#195459=CARTESIAN_POINT('Ctrl Pts',(12.9755645309608,61.4741803895392,40.0836054919164));
#195460=CARTESIAN_POINT('Ctrl Pts',(12.9739228088661,61.473728840136,40.0828829920417));
#195461=CARTESIAN_POINT('Ctrl Pts',(12.9735123783424,61.4736159527852,40.0827023670731));
#195462=CARTESIAN_POINT('Ctrl Pts',(12.9731029149221,61.4735016128573,40.0825207326933));
#195463=CARTESIAN_POINT('Ctrl Pts',(12.972694433337,61.4733858335869,40.0823381109275));
#195464=CARTESIAN_POINT('Ctrl Pts',(12.9714689885818,61.4730384957756,40.0817902456303));
#195465=CARTESIAN_POINT('Ctrl Pts',(12.9702523821512,61.4726782034776,40.0812334935553));
#195466=CARTESIAN_POINT('Ctrl Pts',(12.9690449956487,61.4723053176142,40.0806684524227));
#195467=CARTESIAN_POINT('Ctrl Pts',(12.9607012057877,61.4697284449398,40.0767636676136));
#195468=CARTESIAN_POINT('Ctrl Pts',(12.9527534399842,61.4665839586184,40.0724404510887));
#195469=CARTESIAN_POINT('Ctrl Pts',(12.9452156558837,61.4629898265069,40.0677949937407));
#195470=CARTESIAN_POINT('Ctrl Pts',(12.9414693978767,61.4612035527132,40.0654862141904));
#195471=CARTESIAN_POINT('Ctrl Pts',(12.9378242492511,61.4593056238947,40.0630972003215));
#195472=CARTESIAN_POINT('Ctrl Pts',(12.9342814732034,61.4573073969126,40.0606363359906));
#195473=CARTESIAN_POINT('Ctrl Pts',(12.9264655800794,61.4528990097269,40.0552073017123));
#195474=CARTESIAN_POINT('Ctrl Pts',(12.919142681,61.4480137506081,40.0494204304519));
#195475=CARTESIAN_POINT('Ctrl Pts',(12.912392498672,61.4427731575666,40.0434049749851));
#195476=CARTESIAN_POINT('Ctrl Pts',(12.9099265719433,61.4408587028412,40.0412074532442));
#195477=CARTESIAN_POINT('Ctrl Pts',(12.9075300815496,61.4389006256225,40.0389814735788));
#195478=CARTESIAN_POINT('Ctrl Pts',(12.9052026993241,61.4369042302168,40.0367321210016));
#195479=CARTESIAN_POINT('Ctrl Pts',(12.8973852687046,61.430198549301,40.029176783714));
#195480=CARTESIAN_POINT('Ctrl Pts',(12.8903034584561,61.4230116455102,40.0213235332574));
#195481=CARTESIAN_POINT('Ctrl Pts',(12.8838999218057,61.4154582931175,40.0132649215856));
#195482=CARTESIAN_POINT('Ctrl Pts',(12.8768616764782,61.4071562640844,40.004407552753));
#195483=CARTESIAN_POINT('Ctrl Pts',(12.8706422708197,61.3984111343304,39.9953016253716));
#195484=CARTESIAN_POINT('Ctrl Pts',(12.8651946651854,61.3893309057279,39.9860353422353));
#195485=CARTESIAN_POINT('Ctrl Pts',(12.8593273605059,61.3795511104661,39.9760551582689));
#195486=CARTESIAN_POINT('Ctrl Pts',(12.8543546257409,61.3693816498889,39.9658879738149));
#195487=CARTESIAN_POINT('Ctrl Pts',(12.8502602383795,61.3589193990669,39.9556174643247));
#195488=CARTESIAN_POINT('Ctrl Pts',(12.8462211390717,61.3485984239558,39.94548564139));
#195489=CARTESIAN_POINT('Ctrl Pts',(12.8430366034502,61.3379910943963,39.9352519465111));
#195490=CARTESIAN_POINT('Ctrl Pts',(12.8407372733105,61.3271735965892,39.92499));
#195491=CARTESIAN_POINT('Ctrl Pts',(12.1254815933798,57.9621601888119,39.92499));
#195492=CARTESIAN_POINT('Ctrl Pts',(12.1232811218139,57.9518077840282,39.9348107241723));
#195493=CARTESIAN_POINT('Ctrl Pts',(12.1219050950923,57.9413190436447,39.944603838317));
#195494=CARTESIAN_POINT('Ctrl Pts',(12.1213524729341,57.9307520129788,39.9543158069386));
#195495=CARTESIAN_POINT('Ctrl Pts',(12.1208188676186,57.9205486151425,39.9636935671393));
#195496=CARTESIAN_POINT('Ctrl Pts',(12.1210529843541,57.9102709573189,39.972996832099));
#195497=CARTESIAN_POINT('Ctrl Pts',(12.1220995054498,57.8999666805161,39.9821731151337));
#195498=CARTESIAN_POINT('Ctrl Pts',(12.1230887956353,57.8902259118377,39.9908475764355));
#195499=CARTESIAN_POINT('Ctrl Pts',(12.1248041559922,57.880460457057,39.9994093733849));
#195500=CARTESIAN_POINT('Ctrl Pts',(12.1273238624912,57.8707214090022,40.0077966115845));
#195501=CARTESIAN_POINT('Ctrl Pts',(12.1296444699056,57.8617519091283,40.01552111726));
#195502=CARTESIAN_POINT('Ctrl Pts',(12.1326475236733,57.8528042960108,40.0230979941027));
#195503=CARTESIAN_POINT('Ctrl Pts',(12.1364273448772,57.8439372821293,40.0304554104754));
#195504=CARTESIAN_POINT('Ctrl Pts',(12.1375544112595,57.8412933175823,40.0326492435185));
#195505=CARTESIAN_POINT('Ctrl Pts',(12.1387507708943,57.8386566820012,40.0348233715062));
#195506=CARTESIAN_POINT('Ctrl Pts',(12.1400195294497,57.836029395347,40.0369753512356));
#195507=CARTESIAN_POINT('Ctrl Pts',(12.1412753244192,57.833428953088,40.0391053430352));
#195508=CARTESIAN_POINT('Ctrl Pts',(12.1426004965704,57.8308402488864,40.041211089324));
#195509=CARTESIAN_POINT('Ctrl Pts',(12.1439963340944,57.828268082638,40.0432881154904));
#195510=CARTESIAN_POINT('Ctrl Pts',(12.144093397906,57.8280892192274,40.043432547828));
#195511=CARTESIAN_POINT('Ctrl Pts',(12.1441907966618,57.8279104259145,40.0435768364421));
#195512=CARTESIAN_POINT('Ctrl Pts',(12.1442885313814,57.8277317035127,40.0437209807855));
#195513=CARTESIAN_POINT('Ctrl Pts',(12.1485735795163,57.8198958587083,40.050040796842));
#195514=CARTESIAN_POINT('Ctrl Pts',(12.1535378042507,57.812226847525,40.0560490279346));
#195515=CARTESIAN_POINT('Ctrl Pts',(12.1592011408685,57.804839125324,40.0616647108616));
#195516=CARTESIAN_POINT('Ctrl Pts',(12.1644803548775,57.7979524842553,40.0668995033488));
#195517=CARTESIAN_POINT('Ctrl Pts',(12.1703677426437,57.791309817124,40.0717933267485));
#195518=CARTESIAN_POINT('Ctrl Pts',(12.176888348138,57.7850318067599,40.0762460303076));
#195519=CARTESIAN_POINT('Ctrl Pts',(12.1792736699861,57.7827352293489,40.0778748868751));
#195520=CARTESIAN_POINT('Ctrl Pts',(12.1817437717245,57.7804877669873,40.0794443522249));
#195521=CARTESIAN_POINT('Ctrl Pts',(12.1842999559281,57.7782965440187,40.0809482021492));
#195522=CARTESIAN_POINT('Ctrl Pts',(12.1849146328346,57.777769628097,40.0813098278168));
#195523=CARTESIAN_POINT('Ctrl Pts',(12.185534868683,57.7772459087254,40.0816679525672));
#195524=CARTESIAN_POINT('Ctrl Pts',(12.1861606108972,57.7767255109846,40.082022419258));
#195525=CARTESIAN_POINT('Ctrl Pts',(12.1867667986671,57.7762213756732,40.0823658088648));
#195526=CARTESIAN_POINT('Ctrl Pts',(12.1873781540075,57.7757203576391,40.0827057654616));
#195527=CARTESIAN_POINT('Ctrl Pts',(12.1879946254064,57.7752225713656,40.0830421470151));
#195528=CARTESIAN_POINT('Ctrl Pts',(12.194748782022,57.7697687474614,40.0867275956806));
#195529=CARTESIAN_POINT('Ctrl Pts',(12.202121751003,57.7646995864528,40.089982343203));
#195530=CARTESIAN_POINT('Ctrl Pts',(12.2100174179595,57.7601772489163,40.0926299529355));
#195531=CARTESIAN_POINT('Ctrl Pts',(12.2132919863911,57.7583017007434,40.0937279956084));
#195532=CARTESIAN_POINT('Ctrl Pts',(12.2166560758253,57.7565200187331,40.0947220371802));
#195533=CARTESIAN_POINT('Ctrl Pts',(12.2201014385652,57.7548425830506,40.0956014538692));
#195534=CARTESIAN_POINT('Ctrl Pts',(12.22597786375,57.7519815416929,40.097101390674));
#195535=CARTESIAN_POINT('Ctrl Pts',(12.232089942972,57.7494261286933,40.0982667904316));
#195536=CARTESIAN_POINT('Ctrl Pts',(12.2383911161017,57.7472322823293,40.0990539325582));
#195537=CARTESIAN_POINT('Ctrl Pts',(12.2415417026666,57.7461353591472,40.0994475036216));
#195538=CARTESIAN_POINT('Ctrl Pts',(12.2447399293291,57.7451302272376,40.0997467259952));
#195539=CARTESIAN_POINT('Ctrl Pts',(12.2479799447123,57.7442239366601,40.0999473488896));
#195540=CARTESIAN_POINT('Ctrl Pts',(12.2512199600955,57.7433176460826,40.100147971784));
#195541=CARTESIAN_POINT('Ctrl Pts',(12.2545017192674,57.7425101887131,40.10025));
#195542=CARTESIAN_POINT('Ctrl Pts',(12.2578193919774,57.7418065394564,40.10025));
#195543=CARTESIAN_POINT('Origin',(18.0189898472955,55.4074307335705,39.92499));
#195544=CARTESIAN_POINT('Ctrl Pts',(19.5431821162873,59.5312589135993,39.92499));
#195545=CARTESIAN_POINT('Ctrl Pts',(19.5464608884259,59.5413499366324,39.9348354642013));
#195546=CARTESIAN_POINT('Ctrl Pts',(19.5489337165498,59.5516697238473,39.9446440828447));
#195547=CARTESIAN_POINT('Ctrl Pts',(19.5505973858261,59.562159273364,39.9543641760315));
#195548=CARTESIAN_POINT('Ctrl Pts',(19.5522069957576,59.5723079749826,39.9637684240691));
#195549=CARTESIAN_POINT('Ctrl Pts',(19.5530593117981,59.5826168684372,39.973090963637));
#195550=CARTESIAN_POINT('Ctrl Pts',(19.5531064127995,59.5930429125487,39.982280897711));
#195551=CARTESIAN_POINT('Ctrl Pts',(19.5531509674464,59.6029053082793,39.9909740094614));
#195552=CARTESIAN_POINT('Ctrl Pts',(19.552475023402,59.6128734577595,39.999549276496));
#195553=CARTESIAN_POINT('Ctrl Pts',(19.550996336867,59.6229049605437,40.0079462328649));
#195554=CARTESIAN_POINT('Ctrl Pts',(19.549634359627,59.6321447001047,40.0156804369639));
#195555=CARTESIAN_POINT('Ctrl Pts',(19.5475912199442,59.6414387315114,40.0232638017367));
#195556=CARTESIAN_POINT('Ctrl Pts',(19.5447674611739,59.6507389334358,40.0306257269907));
#195557=CARTESIAN_POINT('Ctrl Pts',(19.543948396093,59.6534365684895,40.0327611416612));
#195558=CARTESIAN_POINT('Ctrl Pts',(19.5430634173972,59.6561345922103,40.0348777427251));
#195559=CARTESIAN_POINT('Ctrl Pts',(19.5421094990035,59.6588314685159,40.03697331687));
#195560=CARTESIAN_POINT('Ctrl Pts',(19.5410753901343,59.6617550558217,40.039245053974));
#195561=CARTESIAN_POINT('Ctrl Pts',(19.5399627185796,59.66467358667,40.041487875195));
#195562=CARTESIAN_POINT('Ctrl Pts',(19.5387684320161,59.6675844741793,40.04369857016));
#195563=CARTESIAN_POINT('Ctrl Pts',(19.5354907031712,59.6755734277897,40.0497658398386));
#195564=CARTESIAN_POINT('Ctrl Pts',(19.5315625649731,59.6834782549088,40.0555581699984));
#195565=CARTESIAN_POINT('Ctrl Pts',(19.5269766895189,59.6911955084647,40.0609828468885));
#195566=CARTESIAN_POINT('Ctrl Pts',(19.5227808624515,59.6982563764886,40.0659461317302));
#195567=CARTESIAN_POINT('Ctrl Pts',(19.5180305486469,59.7051493183924,40.0706039980703));
#195568=CARTESIAN_POINT('Ctrl Pts',(19.5126862934709,59.7117949558626,40.0748843180598));
#195569=CARTESIAN_POINT('Ctrl Pts',(19.5100612127859,59.7150592712795,40.0769867972566));
#195570=CARTESIAN_POINT('Ctrl Pts',(19.507292572924,59.7182634781242,40.0789976708173));
#195571=CARTESIAN_POINT('Ctrl Pts',(19.5043743927945,59.7213950854343,40.0809050491499));
#195572=CARTESIAN_POINT('Ctrl Pts',(19.5038206965385,59.7219892774191,40.0812669556104));
#195573=CARTESIAN_POINT('Ctrl Pts',(19.5032610854122,59.7225808838921,40.0816253922032));
#195574=CARTESIAN_POINT('Ctrl Pts',(19.5026955970365,59.7231697699853,40.0819801989139));
#195575=CARTESIAN_POINT('Ctrl Pts',(19.5021477801725,59.7237402533881,40.0823239179149));
#195576=CARTESIAN_POINT('Ctrl Pts',(19.5015944476719,59.7243081837712,40.0826642303498));
#195577=CARTESIAN_POINT('Ctrl Pts',(19.5010356373992,59.7248734373528,40.0830009916099));
#195578=CARTESIAN_POINT('Ctrl Pts',(19.4949458381923,59.7310334544117,40.0866709464313));
#195579=CARTESIAN_POINT('Ctrl Pts',(19.4882011960852,59.7368793392206,40.089917583188));
#195580=CARTESIAN_POINT('Ctrl Pts',(19.4808775251046,59.7422363728294,40.0925642067065));
#195581=CARTESIAN_POINT('Ctrl Pts',(19.4777846933723,59.7444986813876,40.093681892253));
#195582=CARTESIAN_POINT('Ctrl Pts',(19.4745890081271,59.7466739523115,40.0946930094791));
#195583=CARTESIAN_POINT('Ctrl Pts',(19.4712977780161,59.7487501225118,40.0955863397546));
#195584=CARTESIAN_POINT('Ctrl Pts',(19.4657554287474,59.7522463412518,40.0970906856166));
#195585=CARTESIAN_POINT('Ctrl Pts',(19.4599426670177,59.755459057686,40.0982599215483));
#195586=CARTESIAN_POINT('Ctrl Pts',(19.453899564037,59.7583258028885,40.0990497370453));
#195587=CARTESIAN_POINT('Ctrl Pts',(19.4523887882919,59.7590424891891,40.0992471909196));
#195588=CARTESIAN_POINT('Ctrl Pts',(19.4508635299961,59.7597373347841,40.0994209989363));
#195589=CARTESIAN_POINT('Ctrl Pts',(19.4493243130386,59.7604090725472,40.0995705982975));
#195590=CARTESIAN_POINT('Ctrl Pts',(19.4470154876024,59.761416679192,40.0997949973393));
#195591=CARTESIAN_POINT('Ctrl Pts',(19.4446752658781,59.7623722755977,40.0999649129781));
#195592=CARTESIAN_POINT('Ctrl Pts',(19.4423059520268,59.7632731754139,40.1000786629733));
#195593=CARTESIAN_POINT('Ctrl Pts',(19.4399366381755,59.7641740752301,40.1001924129685));
#195594=CARTESIAN_POINT('Ctrl Pts',(19.4375382417965,59.7650202849789,40.10025));
#195595=CARTESIAN_POINT('Ctrl Pts',(19.4351129318427,59.7658094374949,40.10025));
#195596=CARTESIAN_POINT('Ctrl Pts',(18.2553202812755,56.134781019564,40.10025));
#195597=CARTESIAN_POINT('Ctrl Pts',(18.2635267101477,56.1321105487809,40.10025));
#195598=CARTESIAN_POINT('Ctrl Pts',(18.2718824441053,56.1301406315641,40.0995786334241));
#195599=CARTESIAN_POINT('Ctrl Pts',(18.2802419597942,56.1288305556596,40.0983063763366));
#195600=CARTESIAN_POINT('Ctrl Pts',(18.2856413491931,56.1279843810469,40.0974846287992));
#195601=CARTESIAN_POINT('Ctrl Pts',(18.2910421817938,56.1274125556281,40.0964130309338));
#195602=CARTESIAN_POINT('Ctrl Pts',(18.296405688343,56.127095266925,40.0951176960924));
#195603=CARTESIAN_POINT('Ctrl Pts',(18.3035147090335,56.1266747189246,40.0934008039614));
#195604=CARTESIAN_POINT('Ctrl Pts',(18.3105573165147,56.1267070766079,40.0912909372156));
#195605=CARTESIAN_POINT('Ctrl Pts',(18.3174512966905,56.1271555587353,40.0888630467851));
#195606=CARTESIAN_POINT('Ctrl Pts',(18.3208982867784,56.127379799799,40.0876491015699));
#195607=CARTESIAN_POINT('Ctrl Pts',(18.3243083090334,56.1277080087288,40.0863558569271));
#195608=CARTESIAN_POINT('Ctrl Pts',(18.3276724292425,56.1281351437408,40.0849936342771));
#195609=CARTESIAN_POINT('Ctrl Pts',(18.329354489347,56.1283487112468,40.0843125229521));
#195610=CARTESIAN_POINT('Ctrl Pts',(18.3310250895519,56.1285870051494,40.0836141747074));
#195611=CARTESIAN_POINT('Ctrl Pts',(18.3326832110576,56.1288493629351,40.0828999161609));
#195612=CARTESIAN_POINT('Ctrl Pts',(18.333097741434,56.1289149523815,40.0827213515243));
#195613=CARTESIAN_POINT('Ctrl Pts',(18.3335114922235,56.1289820457107,40.0825417925842));
#195614=CARTESIAN_POINT('Ctrl Pts',(18.3339244481761,56.1290506323486,40.0823612602361));
#195615=CARTESIAN_POINT('Ctrl Pts',(18.3351633160341,56.1292563922626,40.0818196631917));
#195616=CARTESIAN_POINT('Ctrl Pts',(18.3363950287075,56.1294755925117,40.0812693052022));
#195617=CARTESIAN_POINT('Ctrl Pts',(18.337619189229,56.129707942645,40.0807107531875));
#195618=CARTESIAN_POINT('Ctrl Pts',(18.3462420178748,56.1313445869827,40.0767763849182));
#195619=CARTESIAN_POINT('Ctrl Pts',(18.354528490461,56.1335959402407,40.0724140586137));
#195620=CARTESIAN_POINT('Ctrl Pts',(18.3624495731179,56.136345925232,40.0677221223768));
#195621=CARTESIAN_POINT('Ctrl Pts',(18.3662912896469,56.1376796649811,40.065446538372));
#195622=CARTESIAN_POINT('Ctrl Pts',(18.3700472768056,56.139131230071,40.0630928000679));
#195623=CARTESIAN_POINT('Ctrl Pts',(18.3737149835769,56.1406901365232,40.0606689262479));
#195624=CARTESIAN_POINT('Ctrl Pts',(18.3793299863885,56.143076713384,40.0569581447805));
#195625=CARTESIAN_POINT('Ctrl Pts',(18.3847354115627,56.1457125629777,40.0530843804605));
#195626=CARTESIAN_POINT('Ctrl Pts',(18.3899096889384,56.1485569297208,40.0490800251457));
#195627=CARTESIAN_POINT('Ctrl Pts',(18.3923126501199,56.1498778683511,40.0472203818218));
#195628=CARTESIAN_POINT('Ctrl Pts',(18.3946658026165,56.1512435269775,40.0453323608818));
#195629=CARTESIAN_POINT('Ctrl Pts',(18.3969661720543,56.1526507491368,40.0434201572162));
#195630=CARTESIAN_POINT('Ctrl Pts',(18.3971424863078,56.1527586071706,40.0432735943397));
#195631=CARTESIAN_POINT('Ctrl Pts',(18.3973185179292,56.1528666894393,40.0431268995707));
#195632=CARTESIAN_POINT('Ctrl Pts',(18.3974942667076,56.1529749944977,40.0429800745037));
#195633=CARTESIAN_POINT('Ctrl Pts',(18.3999630071785,56.1544963540394,40.0409176249753));
#195634=CARTESIAN_POINT('Ctrl Pts',(18.4023749585858,56.1560635207936,40.0388310783332));
#195635=CARTESIAN_POINT('Ctrl Pts',(18.404728848804,56.1576709325002,40.036725739981));
#195636=CARTESIAN_POINT('Ctrl Pts',(18.4131694805014,56.1634348250116,40.0291763710716));
#195637=CARTESIAN_POINT('Ctrl Pts',(18.4209299141247,56.1697591292905,40.0213310894592));
#195638=CARTESIAN_POINT('Ctrl Pts',(18.4280560759394,56.1765231650108,40.0132837551316));
#195639=CARTESIAN_POINT('Ctrl Pts',(18.4358870118872,56.1839561607597,40.0044405431321));
#195640=CARTESIAN_POINT('Ctrl Pts',(18.4429525945108,56.1919204977441,39.9953528710597));
#195641=CARTESIAN_POINT('Ctrl Pts',(18.4492898603079,56.2003032932673,39.9861103629551));
#195642=CARTESIAN_POINT('Ctrl Pts',(18.4561325169321,56.2093546086376,39.9761307737553));
#195643=CARTESIAN_POINT('Ctrl Pts',(18.4621268842298,56.2188946068458,39.965969693601));
#195644=CARTESIAN_POINT('Ctrl Pts',(18.4672816799273,56.2288243369868,39.9557128217506));
#195645=CARTESIAN_POINT('Ctrl Pts',(18.4723932321855,56.2386707668949,39.945541994516));
#195646=CARTESIAN_POINT('Ctrl Pts',(18.4766796388007,56.2489017962824,39.9352756289341));
#195647=CARTESIAN_POINT('Ctrl Pts',(18.4801050014197,56.2594439784237,39.92499));
#195648=CARTESIAN_POINT('Origin',(-0.0144941013083342,0.004709418994269,
39.92499));
#195649=CARTESIAN_POINT('Ctrl Pts',(19.406124729226,59.7752282754835,40.10025));
#195650=CARTESIAN_POINT('Ctrl Pts',(19.3979550581551,59.77787898563,40.10025));
#195651=CARTESIAN_POINT('Ctrl Pts',(19.3896365599076,59.7798236858208,40.0995859581842));
#195652=CARTESIAN_POINT('Ctrl Pts',(19.3813136269527,59.7811061158277,40.0983275959621));
#195653=CARTESIAN_POINT('Ctrl Pts',(19.3759956690096,59.7819255275517,40.0975235624069));
#195654=CARTESIAN_POINT('Ctrl Pts',(19.3706760212385,59.7824754874619,40.0964777059491));
#195655=CARTESIAN_POINT('Ctrl Pts',(19.3653918801545,59.7827759879493,40.0952149915961));
#195656=CARTESIAN_POINT('Ctrl Pts',(19.3581800878468,59.7831861108188,40.0934916398701));
#195657=CARTESIAN_POINT('Ctrl Pts',(19.3510354548625,59.7831255716885,40.0913643921631));
#195658=CARTESIAN_POINT('Ctrl Pts',(19.3440445557102,59.7826350657122,40.0889118607713));
#195659=CARTESIAN_POINT('Ctrl Pts',(19.340549106134,59.7823898127241,40.0876855950754));
#195660=CARTESIAN_POINT('Ctrl Pts',(19.337091891998,59.7820371343797,40.0863782327527));
#195661=CARTESIAN_POINT('Ctrl Pts',(19.3336823180315,59.7815825865437,40.0850006373334));
#195662=CARTESIAN_POINT('Ctrl Pts',(19.3319775310482,59.7813553126257,40.0843118396238));
#195663=CARTESIAN_POINT('Ctrl Pts',(19.3302846375616,59.781102576764,40.0836054919165));
#195664=CARTESIAN_POINT('Ctrl Pts',(19.328604709227,59.7808251076834,40.0828829920418));
#195665=CARTESIAN_POINT('Ctrl Pts',(19.3281847271434,59.7807557404133,40.0827023670731));
#195666=CARTESIAN_POINT('Ctrl Pts',(19.3277655550296,59.7806848274336,40.0825207326933));
#195667=CARTESIAN_POINT('Ctrl Pts',(19.3273472089201,59.7806123803664,40.0823381109276));
#195668=CARTESIAN_POINT('Ctrl Pts',(19.3260921705918,59.7803950391651,40.0817902456304));
#195669=CARTESIAN_POINT('Ctrl Pts',(19.3248445680583,59.7801638905866,40.0812334935553));
#195670=CARTESIAN_POINT('Ctrl Pts',(19.3236048185592,59.7799192536867,40.0806684524227));
#195671=CARTESIAN_POINT('Ctrl Pts',(19.3150373803115,59.7782286609224,40.0767636676137));
#195672=CARTESIAN_POINT('Ctrl Pts',(19.3068044648779,59.775932168172,40.0724404510889));
#195673=CARTESIAN_POINT('Ctrl Pts',(19.2989322844411,59.7731456380808,40.067794993741));
#195674=CARTESIAN_POINT('Ctrl Pts',(19.2950198323727,59.7717607402743,40.0654862141906));
#195675=CARTESIAN_POINT('Ctrl Pts',(19.2911962646697,59.7702542302926,40.0630972003216));
#195676=CARTESIAN_POINT('Ctrl Pts',(19.287464024724,59.7686372707428,40.0606363359906));
#195677=CARTESIAN_POINT('Ctrl Pts',(19.2792301459423,59.7650700164608,40.0552073017123));
#195678=CARTESIAN_POINT('Ctrl Pts',(19.271436713842,59.76097697069,40.0494204304519));
#195679=CARTESIAN_POINT('Ctrl Pts',(19.2641757185818,59.7564706723511,40.0434049749851));
#195680=CARTESIAN_POINT('Ctrl Pts',(19.2615231854473,59.7548244647405,40.0412074532442));
#195681=CARTESIAN_POINT('Ctrl Pts',(19.2589351484761,59.7531276155317,40.0389814735788));
#195682=CARTESIAN_POINT('Ctrl Pts',(19.2564118357502,59.7513854342764,40.0367321210016));
#195683=CARTESIAN_POINT('Ctrl Pts',(19.247936295312,59.7455336317916,40.0291767837139));
#195684=CARTESIAN_POINT('Ctrl Pts',(19.240142043952,59.739126349354,40.0213235332572));
#195685=CARTESIAN_POINT('Ctrl Pts',(19.2329840462272,59.7322837268613,40.0132649215853));
#195686=CARTESIAN_POINT('Ctrl Pts',(19.225116558807,59.7247628741799,40.0044075527525));
#195687=CARTESIAN_POINT('Ctrl Pts',(19.2180171087291,59.7167157560773,39.995301625371));
#195688=CARTESIAN_POINT('Ctrl Pts',(19.2116502033063,59.7082546997624,39.9860353422346));
#195689=CARTESIAN_POINT('Ctrl Pts',(19.2047927733658,59.6991417795837,39.9760551582679));
#195690=CARTESIAN_POINT('Ctrl Pts',(19.1987842816757,59.6895478206984,39.9658879738136));
#195691=CARTESIAN_POINT('Ctrl Pts',(19.1936187207959,59.6795708631997,39.9556174643231));
#195692=CARTESIAN_POINT('Ctrl Pts',(19.1885229124294,59.6697286283143,39.9454856413889));
#195693=CARTESIAN_POINT('Ctrl Pts',(19.1842470541694,59.6595122814315,39.9352519465106));
#195694=CARTESIAN_POINT('Ctrl Pts',(19.1808295835788,59.6489943884562,39.92499));
#195695=CARTESIAN_POINT('Ctrl Pts',(18.1177524687112,56.3771794532805,39.92499));
#195696=CARTESIAN_POINT('Ctrl Pts',(18.1144819305957,56.3671137719648,39.9348107241721));
#195697=CARTESIAN_POINT('Ctrl Pts',(18.1120170699786,56.3568263239574,39.9446038383167));
#195698=CARTESIAN_POINT('Ctrl Pts',(18.1103629196656,56.3463749453362,39.9543158069381));
#195699=CARTESIAN_POINT('Ctrl Pts',(18.1087656919999,56.3362832197247,39.9636935671387));
#195700=CARTESIAN_POINT('Ctrl Pts',(18.1079242184411,56.3260373921235,39.9729968320983));
#195701=CARTESIAN_POINT('Ctrl Pts',(18.1078879163654,56.3156801719855,39.9821731151329));
#195702=CARTESIAN_POINT('Ctrl Pts',(18.1078535995347,56.3058893552744,39.9908475764345));
#195703=CARTESIAN_POINT('Ctrl Pts',(18.1085387949867,56.2959980926949,39.9994093733839));
#195704=CARTESIAN_POINT('Ctrl Pts',(18.110026690543,56.2860490151161,40.0077966115834));
#195705=CARTESIAN_POINT('Ctrl Pts',(18.1113970173889,56.2768860815744,40.0155211172587));
#195706=CARTESIAN_POINT('Ctrl Pts',(18.1134483398646,56.2676735798224,40.0230979941013));
#195707=CARTESIAN_POINT('Ctrl Pts',(18.1162805994776,56.258460041469,40.030455410474));
#195708=CARTESIAN_POINT('Ctrl Pts',(18.1171251221214,56.2557127503189,40.0326492435175));
#195709=CARTESIAN_POINT('Ctrl Pts',(18.1180393245076,56.2529655048686,40.0348233715058));
#195710=CARTESIAN_POINT('Ctrl Pts',(18.1190265064346,56.250219989383,40.0369753512355));
#195711=CARTESIAN_POINT('Ctrl Pts',(18.1200036017947,56.2475025263004,40.0391053430352));
#195712=CARTESIAN_POINT('Ctrl Pts',(18.1210509212422,56.2447894850828,40.041211089324));
#195713=CARTESIAN_POINT('Ctrl Pts',(18.122170247637,56.2420855046789,40.0432881154904));
#195714=CARTESIAN_POINT('Ctrl Pts',(18.1222480834054,56.2418974751697,40.0434325478279));
#195715=CARTESIAN_POINT('Ctrl Pts',(18.1223262596104,56.2417094803629,40.0435768364421));
#195716=CARTESIAN_POINT('Ctrl Pts',(18.1224047773509,56.2415215209612,40.0437209807855));
#195717=CARTESIAN_POINT('Ctrl Pts',(18.125847282728,56.233280692238,40.050040796842));
#195718=CARTESIAN_POINT('Ctrl Pts',(18.129982682966,56.2251347899176,40.0560490279344));
#195719=CARTESIAN_POINT('Ctrl Pts',(18.1348427679844,56.2171955585584,40.0616647108614));
#195720=CARTESIAN_POINT('Ctrl Pts',(18.1393732118986,56.2097948151026,40.0668995033484));
#195721=CARTESIAN_POINT('Ctrl Pts',(18.1445340001512,56.2025731376012,40.071793326748));
#195722=CARTESIAN_POINT('Ctrl Pts',(18.1503626543103,56.1956479299631,40.076246030307));
#195723=CARTESIAN_POINT('Ctrl Pts',(18.1524948514085,56.1931145994159,40.0778748868747));
#195724=CARTESIAN_POINT('Ctrl Pts',(18.1547164978844,56.1906212529491,40.0794443522247));
#195725=CARTESIAN_POINT('Ctrl Pts',(18.1570296338743,56.1881748397223,40.0809482021492));
#195726=CARTESIAN_POINT('Ctrl Pts',(18.1575858658048,56.1875865590687,40.0813098278168));
#195727=CARTESIAN_POINT('Ctrl Pts',(18.1581479603552,56.1870008763865,40.0816679525672));
#195728=CARTESIAN_POINT('Ctrl Pts',(18.1587158783119,56.186417921567,40.082022419258));
#195729=CARTESIAN_POINT('Ctrl Pts',(18.1592660488324,56.1858531840856,40.0823658088648));
#195730=CARTESIAN_POINT('Ctrl Pts',(18.1598216844591,56.1852910066464,40.0827057654616));
#195731=CARTESIAN_POINT('Ctrl Pts',(18.160382745929,56.1847315084902,40.0830421470151));
#195732=CARTESIAN_POINT('Ctrl Pts',(18.1665298227365,56.1786015595921,40.0867275956807));
#195733=CARTESIAN_POINT('Ctrl Pts',(18.1733325302119,56.1727894828604,40.0899823432032));
#195734=CARTESIAN_POINT('Ctrl Pts',(18.1807122308859,56.1674665972286,40.0926299529357));
#195735=CARTESIAN_POINT('Ctrl Pts',(18.1837728127205,56.165259037899,40.0937279956085));
#195736=CARTESIAN_POINT('Ctrl Pts',(18.186932236838,56.1631354730305,40.0947220371803));
#195737=CARTESIAN_POINT('Ctrl Pts',(18.1901833857459,56.1611070880436,40.0956014538692));
#195738=CARTESIAN_POINT('Ctrl Pts',(18.1957285590022,56.1576474660758,40.097101390674));
#195739=CARTESIAN_POINT('Ctrl Pts',(18.2015400422208,56.1544671656476,40.0982667904316));
#195740=CARTESIAN_POINT('Ctrl Pts',(18.2075773774757,56.1516266854592,40.0990539325582));
#195741=CARTESIAN_POINT('Ctrl Pts',(18.2105960451031,56.150206445365,40.0994475036216));
#195742=CARTESIAN_POINT('Ctrl Pts',(18.2136716866515,56.148872513955,40.0997467259952));
#195743=CARTESIAN_POINT('Ctrl Pts',(18.2167992197301,56.1476325143032,40.0999473488896));
#195744=CARTESIAN_POINT('Ctrl Pts',(18.2199267528088,56.1463925146513,40.100147971784));
#195745=CARTESIAN_POINT('Ctrl Pts',(18.2231061318825,56.145246443375,40.10025));
#195746=CARTESIAN_POINT('Ctrl Pts',(18.2263320786588,56.1441998575526,40.10025));
#195747=CARTESIAN_POINT('Origin',(23.7119335237431,53.2204057122635,39.92499));
#195748=CARTESIAN_POINT('Ctrl Pts',(25.6588335304447,57.1623216544368,39.92499));
#195749=CARTESIAN_POINT('Ctrl Pts',(25.6631491402573,57.1720146727777,39.9348354642023));
#195750=CARTESIAN_POINT('Ctrl Pts',(25.6666871334692,57.1820194461958,39.9446440828468));
#195751=CARTESIAN_POINT('Ctrl Pts',(25.6694381454826,57.1922776320709,39.9543641760345));
#195752=CARTESIAN_POINT('Ctrl Pts',(25.6720997659869,57.2022024879885,39.963768424073));
#195753=CARTESIAN_POINT('Ctrl Pts',(25.6740249857417,57.2123658169611,39.9730909636417));
#195754=CARTESIAN_POINT('Ctrl Pts',(25.6751616470875,57.2227298227177,39.9822808977164));
#195755=CARTESIAN_POINT('Ctrl Pts',(25.6762368587291,57.2325335339847,39.9909740094676));
#195756=CARTESIAN_POINT('Ctrl Pts',(25.6766065729233,57.2425177322924,39.999549276503));
#195757=CARTESIAN_POINT('Ctrl Pts',(25.6761845643577,57.2526488462869,40.0079462328725));
#195758=CARTESIAN_POINT('Ctrl Pts',(25.6757958639483,57.2619803349768,40.0156804369723));
#195759=CARTESIAN_POINT('Ctrl Pts',(25.6747354076183,57.2714370189594,40.0232638017457));
#195760=CARTESIAN_POINT('Ctrl Pts',(25.6728992535084,57.2809814365707,40.0306257270004));
#195761=CARTESIAN_POINT('Ctrl Pts',(25.6723666549989,57.2837499093074,40.0327611416676));
#195762=CARTESIAN_POINT('Ctrl Pts',(25.6717685445833,57.286525658431,40.0348777427283));
#195763=CARTESIAN_POINT('Ctrl Pts',(25.6711017521911,57.2893074725857,40.0369733168701));
#195764=CARTESIAN_POINT('Ctrl Pts',(25.6703789063668,57.2923231379853,40.039245053974));
#195765=CARTESIAN_POINT('Ctrl Pts',(25.669577399688,57.295341986664,40.041487875195));
#195766=CARTESIAN_POINT('Ctrl Pts',(25.6686939261493,57.2983617649661,40.0436985701601));
#195767=CARTESIAN_POINT('Ctrl Pts',(25.66626922609,57.306649570212,40.0497658398386));
#195768=CARTESIAN_POINT('Ctrl Pts',(25.6631888860751,57.3149216961103,40.0555581699984));
#195769=CARTESIAN_POINT('Ctrl Pts',(25.6594348051813,57.3230760282577,40.0609828468885));
#195770=CARTESIAN_POINT('Ctrl Pts',(25.6560000249773,57.3305367994636,40.0659461317305));
#195771=CARTESIAN_POINT('Ctrl Pts',(25.6519962425132,57.3378885241129,40.0706039980707));
#195772=CARTESIAN_POINT('Ctrl Pts',(25.6473759219981,57.3450563828668,40.0748843180604));
#195773=CARTESIAN_POINT('Ctrl Pts',(25.6451064356541,57.3485772116719,40.076986797257));
#195774=CARTESIAN_POINT('Ctrl Pts',(25.6426878935087,57.3520532672061,40.0789976708175));
#195775=CARTESIAN_POINT('Ctrl Pts',(25.6401130415753,57.3554727521278,40.08090504915));
#195776=CARTESIAN_POINT('Ctrl Pts',(25.6396244885003,57.3561215660855,40.0812669556105));
#195777=CARTESIAN_POINT('Ctrl Pts',(25.6391297826978,57.3567684269674,40.0816253922033));
#195778=CARTESIAN_POINT('Ctrl Pts',(25.638628947485,57.3574131967119,40.0819801989139));
#195779=CARTESIAN_POINT('Ctrl Pts',(25.6381437633725,57.3580378174019,40.0823239179149));
#195780=CARTESIAN_POINT('Ctrl Pts',(25.6376528269754,57.3586604755988,40.0826642303498));
#195781=CARTESIAN_POINT('Ctrl Pts',(25.6371561630121,57.3592810442412,40.0830009916099));
#195782=CARTESIAN_POINT('Ctrl Pts',(25.6317436214796,57.3660438734344,40.0866709464312));
#195783=CARTESIAN_POINT('Ctrl Pts',(25.6256469885835,57.3725627409491,40.0899175831877));
#195784=CARTESIAN_POINT('Ctrl Pts',(25.6189233999302,57.3786559602401,40.0925642067061));
#195785=CARTESIAN_POINT('Ctrl Pts',(25.6160839866903,57.3812291645838,40.0936818922527));
#195786=CARTESIAN_POINT('Ctrl Pts',(25.6131331854698,57.383726559214,40.094693009479));
#195787=CARTESIAN_POINT('Ctrl Pts',(25.6100770039418,57.3861353831629,40.0955863397546));
#195788=CARTESIAN_POINT('Ctrl Pts',(25.6049304706145,57.3901917825028,40.0970906856166));
#195789=CARTESIAN_POINT('Ctrl Pts',(25.5994853721135,57.3939944983911,40.0982599215483));
#195790=CARTESIAN_POINT('Ctrl Pts',(25.5937750303537,57.397477215531,40.0990497370454));
#195791=CARTESIAN_POINT('Ctrl Pts',(25.5923474449137,57.398347894816,40.0992471909196));
#195792=CARTESIAN_POINT('Ctrl Pts',(25.5909031732848,57.3991983668799,40.0994209989363));
#195793=CARTESIAN_POINT('Ctrl Pts',(25.589442604035,57.4000273167765,40.0995705982975));
#195794=CARTESIAN_POINT('Ctrl Pts',(25.5872517501602,57.4012707416214,40.0997949973393));
#195795=CARTESIAN_POINT('Ctrl Pts',(25.5850242354392,57.4024657229507,40.0999649129781));
#195796=CARTESIAN_POINT('Ctrl Pts',(25.5827620706104,57.4036093482794,40.1000786629733));
#195797=CARTESIAN_POINT('Ctrl Pts',(25.5804999057817,57.404752973608,40.1001924129685));
#195798=CARTESIAN_POINT('Ctrl Pts',(25.5782031010737,57.4058452484193,40.10025));
#195799=CARTESIAN_POINT('Ctrl Pts',(25.5758735661215,57.4068835917977,40.10025));
#195800=CARTESIAN_POINT('Ctrl Pts',(24.0229981225303,53.9190682401992,40.10025));
#195801=CARTESIAN_POINT('Ctrl Pts',(24.0308804555195,53.9155545931355,40.10025));
#195802=CARTESIAN_POINT('Ctrl Pts',(24.0389845034729,53.9127220553012,40.099578633424));
#195803=CARTESIAN_POINT('Ctrl Pts',(24.0471612846392,53.910545348801,40.0983063763365));
#195804=CARTESIAN_POINT('Ctrl Pts',(24.052442646286,53.9091394197449,40.0974846287991));
#195805=CARTESIAN_POINT('Ctrl Pts',(24.0577541205282,53.9080061861136,40.0964130309337));
#195806=CARTESIAN_POINT('Ctrl Pts',(24.0630550795266,53.9071299964539,40.0951176960924));
#195807=CARTESIAN_POINT('Ctrl Pts',(24.0700811970216,53.9059686572513,40.0934008039614));
#195808=CARTESIAN_POINT('Ctrl Pts',(24.0770886066611,53.9052646847383,40.0912909372156));
#195809=CARTESIAN_POINT('Ctrl Pts',(24.0839917000397,53.9049900928802,40.0888630467851));
#195810=CARTESIAN_POINT('Ctrl Pts',(24.0874432467291,53.9048527969511,40.0876491015699));
#195811=CARTESIAN_POINT('Ctrl Pts',(24.0908688957004,53.904822763532,40.0863558569271));
#195812=CARTESIAN_POINT('Ctrl Pts',(24.0942592346735,53.904895912338,40.0849936342771));
#195813=CARTESIAN_POINT('Ctrl Pts',(24.09595440416,53.904932486741,40.0843125229521));
#195814=CARTESIAN_POINT('Ctrl Pts',(24.0976407611376,53.9049948499725,40.0836141747074));
#195815=CARTESIAN_POINT('Ctrl Pts',(24.0993172231363,53.9050824496419,40.0828999161609));
#195816=CARTESIAN_POINT('Ctrl Pts',(24.099736338636,53.9051043495593,40.0827213515243));
#195817=CARTESIAN_POINT('Ctrl Pts',(24.100154836018,53.90512782661,40.0825417925842));
#195818=CARTESIAN_POINT('Ctrl Pts',(24.1005726990106,53.9051528718721,40.082361260236));
#195819=CARTESIAN_POINT('Ctrl Pts',(24.1018262879885,53.9052280076583,40.0818196631917));
#195820=CARTESIAN_POINT('Ctrl Pts',(24.1030741658761,53.9053172580725,40.0812693052021));
#195821=CARTESIAN_POINT('Ctrl Pts',(24.1043159075206,53.9054203757494,40.0807107531874));
#195822=CARTESIAN_POINT('Ctrl Pts',(24.1130625753263,53.9061467233508,40.0767763849181));
#195823=CARTESIAN_POINT('Ctrl Pts',(24.121538984245,53.9075195712147,40.0724140586137));
#195824=CARTESIAN_POINT('Ctrl Pts',(24.1297041260875,53.9094265129029,40.0677221223767));
#195825=CARTESIAN_POINT('Ctrl Pts',(24.1336642110577,53.910351377561,40.065446538372));
#195826=CARTESIAN_POINT('Ctrl Pts',(24.137551352394,53.9114023832598,40.0630928000679));
#195827=CARTESIAN_POINT('Ctrl Pts',(24.1413619171797,53.9125693701068,40.0606689262479));
#195828=CARTESIAN_POINT('Ctrl Pts',(24.1471956256301,53.9143559454347,40.0569581447805));
#195829=CARTESIAN_POINT('Ctrl Pts',(24.152846960627,53.9164123347818,40.0530843804605));
#195830=CARTESIAN_POINT('Ctrl Pts',(24.1582902100545,53.9187002605236,40.0490800251457));
#195831=CARTESIAN_POINT('Ctrl Pts',(24.1608180832483,53.9197627850743,40.0472203818218));
#195832=CARTESIAN_POINT('Ctrl Pts',(24.1633010951269,53.9208749910655,40.0453323608818));
#195833=CARTESIAN_POINT('Ctrl Pts',(24.16573595767,53.9220340502324,40.0434201572162));
#195834=CARTESIAN_POINT('Ctrl Pts',(24.1659225802901,53.9221228875506,40.0432735943397));
#195835=CARTESIAN_POINT('Ctrl Pts',(24.1661089452653,53.9222119774185,40.0431268995707));
#195836=CARTESIAN_POINT('Ctrl Pts',(24.1662950522348,53.9223013184207,40.0429800745037));
#195837=CARTESIAN_POINT('Ctrl Pts',(24.1689092940621,53.923556290148,40.0409176249753));
#195838=CARTESIAN_POINT('Ctrl Pts',(24.1714718460797,53.9248627542247,40.0388310783332));
#195839=CARTESIAN_POINT('Ctrl Pts',(24.1739808617166,53.9262153118346,40.036725739981));
#195840=CARTESIAN_POINT('Ctrl Pts',(24.182977745577,53.9310653428794,40.0291763710716));
#195841=CARTESIAN_POINT('Ctrl Pts',(24.1913567365406,53.9365438157568,40.0213310894591));
#195842=CARTESIAN_POINT('Ctrl Pts',(24.1991508947546,53.9425259106383,40.0132837551314));
#195843=CARTESIAN_POINT('Ctrl Pts',(24.2077158916391,53.9490996319582,40.0044405431318));
#195844=CARTESIAN_POINT('Ctrl Pts',(24.2155752681678,53.9562817849777,39.9953528710593));
#195845=CARTESIAN_POINT('Ctrl Pts',(24.2227540584938,53.9639562340148,39.9861103629547));
#195846=CARTESIAN_POINT('Ctrl Pts',(24.2305053504153,53.972242712951,39.9761307737548));
#195847=CARTESIAN_POINT('Ctrl Pts',(24.2374640812941,53.9811038680491,39.9659696936003));
#195848=CARTESIAN_POINT('Ctrl Pts',(24.2436285779137,53.9904403792169,39.9557128217498));
#195849=CARTESIAN_POINT('Ctrl Pts',(24.2497413607405,53.999698566649,39.9455419945155));
#195850=CARTESIAN_POINT('Ctrl Pts',(24.2550737197511,54.0094254978903,39.9352756289338));
#195851=CARTESIAN_POINT('Ctrl Pts',(24.2595822759739,54.0195518809638,39.92499));
#195852=CARTESIAN_POINT('Origin',(-0.0139224327744698,0.0061986664404702,
39.92499));
#195853=CARTESIAN_POINT('Ctrl Pts',(25.5480287005725,57.4192809246786,40.10025));
#195854=CARTESIAN_POINT('Ctrl Pts',(25.5401808584723,57.4227710771202,40.10025));
#195855=CARTESIAN_POINT('Ctrl Pts',(25.5321112063506,57.4255746438785,40.0995859581841));
#195856=CARTESIAN_POINT('Ctrl Pts',(25.5239679177306,57.4277200319913,40.0983275959619));
#195857=CARTESIAN_POINT('Ctrl Pts',(25.5187647439664,57.4290908328635,40.0975235624067));
#195858=CARTESIAN_POINT('Ctrl Pts',(25.5135317242471,57.4301938346423,40.0964777059489));
#195859=CARTESIAN_POINT('Ctrl Pts',(25.5083079410954,57.4310450321038,40.0952149915961));
#195860=CARTESIAN_POINT('Ctrl Pts',(25.5011785252539,57.4322067458446,40.0934916398701));
#195861=CARTESIAN_POINT('Ctrl Pts',(25.4940667032544,57.4328933558604,40.091364392163));
#195862=CARTESIAN_POINT('Ctrl Pts',(25.4870628291431,57.4331362848725,40.0889118607713));
#195863=CARTESIAN_POINT('Ctrl Pts',(25.4835608920875,57.4332577493785,40.0876855950754));
#195864=CARTESIAN_POINT('Ctrl Pts',(25.4800857520069,57.4332683803238,40.0863782327526));
#195865=CARTESIAN_POINT('Ctrl Pts',(25.4766473428565,57.4331727200755,40.0850006373333));
#195866=CARTESIAN_POINT('Ctrl Pts',(25.4749281382814,57.4331248899514,40.0843118396237));
#195867=CARTESIAN_POINT('Ctrl Pts',(25.4732181005511,57.4330504941579,40.0836054919164));
#195868=CARTESIAN_POINT('Ctrl Pts',(25.4715183716231,57.4329501454091,40.0828829920417));
#195869=CARTESIAN_POINT('Ctrl Pts',(25.4710934393911,57.4329250582219,40.082702367073));
#195870=CARTESIAN_POINT('Ctrl Pts',(25.4706691511212,57.4328983491279,40.0825207326932));
#195871=CARTESIAN_POINT('Ctrl Pts',(25.470245523975,57.4328700280093,40.0823381109275));
#195872=CARTESIAN_POINT('Ctrl Pts',(25.4689746425362,57.4327850646536,40.0817902456303));
#195873=CARTESIAN_POINT('Ctrl Pts',(25.4677097128942,57.4326855923068,40.0812334935553));
#195874=CARTESIAN_POINT('Ctrl Pts',(25.4664511833533,57.4325718846634,40.0806684524226));
#195875=CARTESIAN_POINT('Ctrl Pts',(25.457753963365,57.4317860942974,40.0767636676136));
#195876=CARTESIAN_POINT('Ctrl Pts',(25.4493260998454,57.4303627559729,40.0724404510888));
#195877=CARTESIAN_POINT('Ctrl Pts',(25.4412057723283,57.4284143577088,40.0677949937408));
#195878=CARTESIAN_POINT('Ctrl Pts',(25.4371699918423,57.4274460091197,40.0654862141905));
#195879=CARTESIAN_POINT('Ctrl Pts',(25.4332098968701,57.4263474236136,40.0630972003215));
#195880=CARTESIAN_POINT('Ctrl Pts',(25.4293290842285,57.4251294472435,40.0606363359906));
#195881=CARTESIAN_POINT('Ctrl Pts',(25.4207674318881,57.4224424094494,40.0552073017123));
#195882=CARTESIAN_POINT('Ctrl Pts',(25.4125888532397,57.4191864212926,40.0494204304519));
#195883=CARTESIAN_POINT('Ctrl Pts',(25.404896598031,57.4154637896038,40.0434049749851));
#195884=CARTESIAN_POINT('Ctrl Pts',(25.4020865201988,57.414103865303,40.0412074532442));
#195885=CARTESIAN_POINT('Ctrl Pts',(25.3993352917247,57.4126868351392,40.0389814735788));
#195886=CARTESIAN_POINT('Ctrl Pts',(25.3966436944405,57.4112179557367,40.0367321210016));
#195887=CARTESIAN_POINT('Ctrl Pts',(25.387602903979,57.4062841452558,40.0291767837142));
#195888=CARTESIAN_POINT('Ctrl Pts',(25.379181606957,57.4007266836991,40.0213235332579));
#195889=CARTESIAN_POINT('Ctrl Pts',(25.3713475726791,57.394669760311,40.0132649215864));
#195890=CARTESIAN_POINT('Ctrl Pts',(25.3627370410054,57.3880124840178,40.004407552754));
#195891=CARTESIAN_POINT('Ctrl Pts',(25.3548353295691,57.3807515434774,39.9953016253728));
#195892=CARTESIAN_POINT('Ctrl Pts',(25.3476188815065,57.3730023605543,39.9860353422369));
#195893=CARTESIAN_POINT('Ctrl Pts',(25.3398464577429,57.3646561585202,39.9760551582708));
#195894=CARTESIAN_POINT('Ctrl Pts',(25.3328680394203,57.3557428147491,39.9658879738171));
#195895=CARTESIAN_POINT('Ctrl Pts',(25.3266878999881,57.3463604602089,39.9556174643273));
#195896=CARTESIAN_POINT('Ctrl Pts',(25.3205912133042,57.3371047991325,39.9454856413917));
#195897=CARTESIAN_POINT('Ctrl Pts',(25.3152708796023,57.3273913673584,39.9352519465119));
#195898=CARTESIAN_POINT('Ctrl Pts',(25.3107727110829,57.3172883154487,39.92499));
#195899=CARTESIAN_POINT('Ctrl Pts',(23.9115214566121,54.1745185419757,39.92499));
#195900=CARTESIAN_POINT('Ctrl Pts',(23.9072166846468,54.1648498658383,39.9348107241724));
#195901=CARTESIAN_POINT('Ctrl Pts',(23.9036899956627,54.1548764216397,39.9446038383174));
#195902=CARTESIAN_POINT('Ctrl Pts',(23.9009524404119,54.144655202554,39.9543158069391));
#195903=CARTESIAN_POINT('Ctrl Pts',(23.8983090899566,54.1347857162244,39.9636935671399));
#195904=CARTESIAN_POINT('Ctrl Pts',(23.8964012454639,54.1246839742766,39.9729968320997));
#195905=CARTESIAN_POINT('Ctrl Pts',(23.8952825179501,54.1143872866741,39.9821731151345));
#195906=CARTESIAN_POINT('Ctrl Pts',(23.8942249700857,54.1046536921668,39.9908475764363));
#195907=CARTESIAN_POINT('Ctrl Pts',(23.8938724934883,54.0947449925308,39.9994093733858));
#195908=CARTESIAN_POINT('Ctrl Pts',(23.8943122764069,54.0846948896039,40.0077966115854));
#195909=CARTESIAN_POINT('Ctrl Pts',(23.894717309097,54.0754389134112,40.0155211172608));
#195910=CARTESIAN_POINT('Ctrl Pts',(23.8957944255627,54.0660624571215,40.0230979941035));
#195911=CARTESIAN_POINT('Ctrl Pts',(23.8976480927559,54.0566033397501,40.0304554104762));
#195912=CARTESIAN_POINT('Ctrl Pts',(23.8982008188942,54.0537828218952,40.032649243519));
#195913=CARTESIAN_POINT('Ctrl Pts',(23.8988228478387,54.0509550659734,40.0348233715065));
#195914=CARTESIAN_POINT('Ctrl Pts',(23.899517637365,54.0481214021,40.0369753512355));
#195915=CARTESIAN_POINT('Ctrl Pts',(23.9002053278545,54.0453166912881,40.0391053430352));
#195916=CARTESIAN_POINT('Ctrl Pts',(23.9009633199472,54.0425090377017,40.041211089324));
#195917=CARTESIAN_POINT('Ctrl Pts',(23.9017938716385,54.0397028685174,40.0432881154904));
#195918=CARTESIAN_POINT('Ctrl Pts',(23.9018516265789,54.0395077330003,40.0434325478279));
#195919=CARTESIAN_POINT('Ctrl Pts',(23.9019097237182,54.0393125964102,40.0435768364421));
#195920=CARTESIAN_POINT('Ctrl Pts',(23.9019681642229,54.0391174593309,40.0437209807855));
#195921=CARTESIAN_POINT('Ctrl Pts',(23.9045304100328,54.030561934933,40.050040796842));
#195922=CARTESIAN_POINT('Ctrl Pts',(23.9077916774641,54.022028389686,40.0560490279344));
#195923=CARTESIAN_POINT('Ctrl Pts',(23.9117952627748,54.0136246330485,40.0616647108614));
#195924=CARTESIAN_POINT('Ctrl Pts',(23.9155273001027,54.0057908712994,40.0668995033484));
#195925=CARTESIAN_POINT('Ctrl Pts',(23.9199049461658,53.9980693056376,40.071793326748));
#195926=CARTESIAN_POINT('Ctrl Pts',(23.9249777890354,53.9905727747493,40.0762460303071));
#195927=CARTESIAN_POINT('Ctrl Pts',(23.9268335005857,53.9878304467659,40.0778748868747));
#195928=CARTESIAN_POINT('Ctrl Pts',(23.9287823509752,53.9851185338199,40.0794443522247));
#195929=CARTESIAN_POINT('Ctrl Pts',(23.930827095549,53.9824437337504,40.0809482021492));
#195930=CARTESIAN_POINT('Ctrl Pts',(23.9313187883101,53.9818005336909,40.0813098278168));
#195931=CARTESIAN_POINT('Ctrl Pts',(23.931816583137,53.9811593045602,40.0816679525672));
#195932=CARTESIAN_POINT('Ctrl Pts',(23.9323204546083,53.9805201796369,40.082022419258));
#195933=CARTESIAN_POINT('Ctrl Pts',(23.932808580096,53.9799010273674,40.0823658088648));
#195934=CARTESIAN_POINT('Ctrl Pts',(23.9333024083488,53.9792838498568,40.0827057654616));
#195935=CARTESIAN_POINT('Ctrl Pts',(23.9338019127828,53.9786687697969,40.0830421470151));
#195936=CARTESIAN_POINT('Ctrl Pts',(23.939274561122,53.9719298569081,40.0867275956806));
#195937=CARTESIAN_POINT('Ctrl Pts',(23.9454324752048,53.9654385427825,40.089982343203));
#195938=CARTESIAN_POINT('Ctrl Pts',(23.9522153560509,53.9593734277044,40.0926299529355));
#195939=CARTESIAN_POINT('Ctrl Pts',(23.9550284189138,53.9568580436998,40.0937279956084));
#195940=CARTESIAN_POINT('Ctrl Pts',(23.9579485624032,53.9544158621938,40.0947220371802));
#195941=CARTESIAN_POINT('Ctrl Pts',(23.9609698772118,53.9520587513129,40.0956014538692));
#195942=CARTESIAN_POINT('Ctrl Pts',(23.966123044461,53.9480384530772,40.097101390674));
#195943=CARTESIAN_POINT('Ctrl Pts',(23.9715702598501,53.9442681092573,40.0982667904315));
#195944=CARTESIAN_POINT('Ctrl Pts',(23.9772776109217,53.9408121161403,40.0990539325582));
#195945=CARTESIAN_POINT('Ctrl Pts',(23.9801312864576,53.9390841195818,40.0994475036216));
#195946=CARTESIAN_POINT('Ctrl Pts',(23.9830506455193,53.937436003503,40.0997467259952));
#195947=CARTESIAN_POINT('Ctrl Pts',(23.9860314303864,53.9358758804724,40.0999473488896));
#195948=CARTESIAN_POINT('Ctrl Pts',(23.9890122152535,53.9343157574419,40.100147971784));
#195949=CARTESIAN_POINT('Ctrl Pts',(23.9920543802867,53.932843628855,40.10025));
#195950=CARTESIAN_POINT('Ctrl Pts',(23.9951532569813,53.9314655730802,40.10025));
#195951=CARTESIAN_POINT('Origin',(29.1450842944635,50.4502867888872,39.92499));
#195952=CARTESIAN_POINT('Ctrl Pts',(31.4933613949865,54.1671020372435,39.92499));
#195953=CARTESIAN_POINT('Ctrl Pts',(31.498666559748,54.1762908521529,39.9348354642007));
#195954=CARTESIAN_POINT('Ctrl Pts',(31.503230955053,54.1858709973805,39.9446440828436));
#195955=CARTESIAN_POINT('Ctrl Pts',(31.50703916914,54.1957854287804,39.9543641760299));
#195956=CARTESIAN_POINT('Ctrl Pts',(31.5107236389456,54.2053777001966,39.9637684240672));
#195957=CARTESIAN_POINT('Ctrl Pts',(31.5137006693043,54.2152841131259,39.9730909636348));
#195958=CARTESIAN_POINT('Ctrl Pts',(31.5159144374956,54.2254725303094,39.9822808977085));
#195959=CARTESIAN_POINT('Ctrl Pts',(31.5180085258885,54.2351101455984,39.9909740094586));
#195960=CARTESIAN_POINT('Ctrl Pts',(31.519419847656,54.245001003765,39.9995492764931));
#195961=CARTESIAN_POINT('Ctrl Pts',(31.520059140675,54.2551207303624,40.0079462328618));
#195962=CARTESIAN_POINT('Ctrl Pts',(31.5206479757804,54.2644417304357,40.0156804369606));
#195963=CARTESIAN_POINT('Ctrl Pts',(31.5205818213861,54.2739574575829,40.0232638017333));
#195964=CARTESIAN_POINT('Ctrl Pts',(31.5197533892273,54.2836415202415,40.0306257269871));
#195965=CARTESIAN_POINT('Ctrl Pts',(31.5195130925487,54.2864504987044,40.0327611416589));
#195966=CARTESIAN_POINT('Ctrl Pts',(31.5192084034343,54.2892735615522,40.0348777427239));
#195967=CARTESIAN_POINT('Ctrl Pts',(31.5188360425585,54.2921098354277,40.03697331687));
#195968=CARTESIAN_POINT('Ctrl Pts',(31.5184323794292,54.2951845386598,40.039245053974));
#195969=CARTESIAN_POINT('Ctrl Pts',(31.517950819101,54.2982706300311,40.041487875195));
#195970=CARTESIAN_POINT('Ctrl Pts',(31.5173878381082,54.301366213803,40.0436985701601));
#195971=CARTESIAN_POINT('Ctrl Pts',(31.5158427323556,54.3098620677556,40.0497658398386));
#195972=CARTESIAN_POINT('Ctrl Pts',(31.5136439393738,54.3184108612909,40.0555581699984));
#195973=CARTESIAN_POINT('Ctrl Pts',(31.5107627835363,54.3269129314604,40.0609828468885));
#195974=CARTESIAN_POINT('Ctrl Pts',(31.5081266823666,54.3346918640771,40.0659461317303));
#195975=CARTESIAN_POINT('Ctrl Pts',(31.5049132975218,54.3424218244375,40.0706039980704));
#195976=CARTESIAN_POINT('Ctrl Pts',(31.5010675328665,54.3500333719143,40.07488431806));
#195977=CARTESIAN_POINT('Ctrl Pts',(31.4991785058305,54.3537721391709,40.0769867972568));
#195978=CARTESIAN_POINT('Ctrl Pts',(31.4971365594552,54.3574819590032,40.0789976708174));
#195979=CARTESIAN_POINT('Ctrl Pts',(31.494933246334,54.3611518569447,40.0809050491499));
#195980=CARTESIAN_POINT('Ctrl Pts',(31.4945151891298,54.3618481843338,40.0812669556104));
#195981=CARTESIAN_POINT('Ctrl Pts',(31.4940908087514,54.3625432124814,40.0816253922032));
#195982=CARTESIAN_POINT('Ctrl Pts',(31.4936601139568,54.363236801645,40.0819801989139));
#195983=CARTESIAN_POINT('Ctrl Pts',(31.4932428783745,54.3639087161471,40.0823239179149));
#195984=CARTESIAN_POINT('Ctrl Pts',(31.4928197168828,54.3645792801845,40.0826642303498));
#195985=CARTESIAN_POINT('Ctrl Pts',(31.4923906407832,54.3652483648077,40.0830009916099));
#195986=CARTESIAN_POINT('Ctrl Pts',(31.4877146578623,54.3725399111641,40.0866709464313));
#195987=CARTESIAN_POINT('Ctrl Pts',(31.4823328301623,54.3796603393085,40.089917583188));
#195988=CARTESIAN_POINT('Ctrl Pts',(31.4762829888796,54.3864229856965,40.0925642067064));
#195989=CARTESIAN_POINT('Ctrl Pts',(31.4737281033385,54.3892788932598,40.0936818922529));
#195990=CARTESIAN_POINT('Ctrl Pts',(31.471054515739,54.3920710496177,40.0946930094791));
#195991=CARTESIAN_POINT('Ctrl Pts',(31.4682668669592,54.3947861357352,40.0955863397545));
#195992=CARTESIAN_POINT('Ctrl Pts',(31.4635725360693,54.3993582729149,40.0970906856166));
#195993=CARTESIAN_POINT('Ctrl Pts',(31.4585547584357,54.4037093249064,40.0982599215483));
#195994=CARTESIAN_POINT('Ctrl Pts',(31.4532397415962,54.4077698566063,40.0990497370453));
#195995=CARTESIAN_POINT('Ctrl Pts',(31.4519109873863,54.4087849895313,40.0992471909196));
#195996=CARTESIAN_POINT('Ctrl Pts',(31.4505635261664,54.4097817701141,40.0994209989363));
#195997=CARTESIAN_POINT('Ctrl Pts',(31.4491976069265,54.4107588499956,40.0995705982975));
#195998=CARTESIAN_POINT('Ctrl Pts',(31.4471487280667,54.412224469818,40.0997949973393));
#195999=CARTESIAN_POINT('Ctrl Pts',(31.4450583254664,54.4136457436052,40.0999649129781));
#196000=CARTESIAN_POINT('Ctrl Pts',(31.4429280944115,54.4150195646478,40.1000786629733));
#196001=CARTESIAN_POINT('Ctrl Pts',(31.4407978633565,54.4163933856905,40.1001924129685));
#196002=CARTESIAN_POINT('Ctrl Pts',(31.4386278145925,54.4177197583726,40.10025));
#196003=CARTESIAN_POINT('Ctrl Pts',(31.4364195775141,54.418995916306,40.10025));
#196004=CARTESIAN_POINT('Ctrl Pts',(29.5274749692191,51.1126068659043,40.10025));
#196005=CARTESIAN_POINT('Ctrl Pts',(29.534946845835,51.1082885388128,40.10025));
#196006=CARTESIAN_POINT('Ctrl Pts',(29.5427104181384,51.1046244142385,40.0995786334241));
#196007=CARTESIAN_POINT('Ctrl Pts',(29.550614878256,51.1016049255945,40.0983063763367));
#196008=CARTESIAN_POINT('Ctrl Pts',(29.5557203484479,51.0996546457478,40.0974846287993));
#196009=CARTESIAN_POINT('Ctrl Pts',(29.5608842707089,51.0979724198484,40.0964130309339));
#196010=CARTESIAN_POINT('Ctrl Pts',(29.5660646037411,51.0965469289494,40.0951176960924));
#196011=CARTESIAN_POINT('Ctrl Pts',(29.5729308384271,51.0946575224199,40.0934008039614));
#196012=CARTESIAN_POINT('Ctrl Pts',(29.5798262755784,51.093224932581,40.0912909372156));
#196013=CARTESIAN_POINT('Ctrl Pts',(29.5866628504243,51.0922302752231,40.0888630467851));
#196014=CARTESIAN_POINT('Ctrl Pts',(29.5900811378472,51.0917329465441,40.0876491015699));
#196015=CARTESIAN_POINT('Ctrl Pts',(29.5934848814079,51.0913449998286,40.0863558569271));
#196016=CARTESIAN_POINT('Ctrl Pts',(29.5968642938815,51.091063360995,40.0849936342771));
#196017=CARTESIAN_POINT('Ctrl Pts',(29.5985540001184,51.0909225415782,40.0843125229521));
#196018=CARTESIAN_POINT('Ctrl Pts',(29.6002376377887,51.090808290874,40.0836141747074));
#196019=CARTESIAN_POINT('Ctrl Pts',(29.6019140726121,51.0907201726668,40.0828999161609));
#196020=CARTESIAN_POINT('Ctrl Pts',(29.6023331813179,51.090698143115,40.0827213515243));
#196021=CARTESIAN_POINT('Ctrl Pts',(29.6027518401475,51.0906777466677,40.0825417925842));
#196022=CARTESIAN_POINT('Ctrl Pts',(29.6031700319857,51.0906589761527,40.0823612602361));
#196023=CARTESIAN_POINT('Ctrl Pts',(29.6044246075002,51.0906026646078,40.0818196631917));
#196024=CARTESIAN_POINT('Ctrl Pts',(29.6056749785909,51.090560987341,40.0812693052022));
#196025=CARTESIAN_POINT('Ctrl Pts',(29.606920696577,51.0905337427827,40.0807107531875));
#196026=CARTESIAN_POINT('Ctrl Pts',(29.6156953732198,51.0903418356314,40.0767763849182));
#196027=CARTESIAN_POINT('Ctrl Pts',(29.6242688491611,51.0908211368928,40.0724140586137));
#196028=CARTESIAN_POINT('Ctrl Pts',(29.6325885911864,51.0918641424257,40.0677221223768));
#196029=CARTESIAN_POINT('Ctrl Pts',(29.6366236570783,51.0923699989822,40.065446538372));
#196030=CARTESIAN_POINT('Ctrl Pts',(29.6405993642582,51.0930089302513,40.0630928000679));
#196031=CARTESIAN_POINT('Ctrl Pts',(29.644511037713,51.0937712117411,40.0606689262479));
#196032=CARTESIAN_POINT('Ctrl Pts',(29.6504995364717,51.0949382114429,40.0569581447805));
#196033=CARTESIAN_POINT('Ctrl Pts',(29.6563348640826,51.0963926103113,40.0530843804605));
#196034=CARTESIAN_POINT('Ctrl Pts',(29.661987448182,51.0980990280587,40.0490800251457));
#196035=CARTESIAN_POINT('Ctrl Pts',(29.6646125374804,51.0988914972884,40.0472203818218));
#196036=CARTESIAN_POINT('Ctrl Pts',(29.6671982043432,51.099738065083,40.0453323608818));
#196037=CARTESIAN_POINT('Ctrl Pts',(29.6697408831281,51.1006362623625,40.0434201572162));
#196038=CARTESIAN_POINT('Ctrl Pts',(29.6699357694383,51.1007051056449,40.0432735943397));
#196039=CARTESIAN_POINT('Ctrl Pts',(29.6701304259137,51.1007742270247,40.0431268995707));
#196040=CARTESIAN_POINT('Ctrl Pts',(29.6703248520474,51.1008436251321,40.0429800745037));
#196041=CARTESIAN_POINT('Ctrl Pts',(29.6730559530505,51.1018184593121,40.0409176249753));
#196042=CARTESIAN_POINT('Ctrl Pts',(29.6757410298223,51.1028499068175,40.0388310783332));
#196043=CARTESIAN_POINT('Ctrl Pts',(29.6783776815774,51.1039327914264,40.036725739981));
#196044=CARTESIAN_POINT('Ctrl Pts',(29.6878322458589,51.1078158230496,40.0291763710714));
#196045=CARTESIAN_POINT('Ctrl Pts',(29.6967379921843,51.1123884412304,40.0213310894587));
#196046=CARTESIAN_POINT('Ctrl Pts',(29.7051147523695,51.1175230541898,40.0132837551309));
#196047=CARTESIAN_POINT('Ctrl Pts',(29.7143199702928,51.1231654780145,40.0044405431309));
#196048=CARTESIAN_POINT('Ctrl Pts',(29.7228870317529,51.1294867578978,39.995352871058));
#196049=CARTESIAN_POINT('Ctrl Pts',(29.7308286942788,51.1363687775796,39.9861103629529));
#196050=CARTESIAN_POINT('Ctrl Pts',(29.7394036967218,51.1437996316849,39.9761307737523));
#196051=CARTESIAN_POINT('Ctrl Pts',(29.7472505498704,51.1518848590038,39.965969693597));
#196052=CARTESIAN_POINT('Ctrl Pts',(29.7543572078975,51.1605258584289,39.9557128217457));
#196053=CARTESIAN_POINT('Ctrl Pts',(29.7614042483641,51.1690943687453,39.9455419945127));
#196054=CARTESIAN_POINT('Ctrl Pts',(29.7677241373282,51.1782106315454,39.9352756289324));
#196055=CARTESIAN_POINT('Ctrl Pts',(29.7732664904686,51.1878102687781,39.92499));
#196056=CARTESIAN_POINT('Origin',(-0.0131982271536719,0.00761999999999528,
39.92499));
#196057=CARTESIAN_POINT('Ctrl Pts',(31.4100231232068,54.434235916306,40.10025));
#196058=CARTESIAN_POINT('Ctrl Pts',(31.4025830926779,54.4385272722021,40.10025));
#196059=CARTESIAN_POINT('Ctrl Pts',(31.3948506994797,54.4421589890638,40.0995859581841));
#196060=CARTESIAN_POINT('Ctrl Pts',(31.3869762747693,54.4451438299614,40.0983275959619));
#196061=CARTESIAN_POINT('Ctrl Pts',(31.3819448922441,54.4470510012006,40.0975235624067));
#196062=CARTESIAN_POINT('Ctrl Pts',(31.3768558346353,54.4486949601298,40.096477705949));
#196063=CARTESIAN_POINT('Ctrl Pts',(31.3717496422771,54.4500875286677,40.0952149915962));
#196064=CARTESIAN_POINT('Ctrl Pts',(31.3647807142736,54.451988105301,40.0934916398702));
#196065=CARTESIAN_POINT('Ctrl Pts',(31.3577796218689,54.45341434182,40.0913643921631));
#196066=CARTESIAN_POINT('Ctrl Pts',(31.3508395087091,54.4543880442393,40.0889118607714));
#196067=CARTESIAN_POINT('Ctrl Pts',(31.3473694521293,54.454874895449,40.0876855950755));
#196068=CARTESIAN_POINT('Ctrl Pts',(31.343914460466,54.4552487192091,40.0863782327527));
#196069=CARTESIAN_POINT('Ctrl Pts',(31.340484888062,54.4555129946222,40.0850006373334));
#196070=CARTESIAN_POINT('Ctrl Pts',(31.33877010186,54.4556451323288,40.0843118396238));
#196071=CARTESIAN_POINT('Ctrl Pts',(31.3370616554174,54.4557498916993,40.0836054919165));
#196072=CARTESIAN_POINT('Ctrl Pts',(31.3353607484818,54.4558277627243,40.0828829920418));
#196073=CARTESIAN_POINT('Ctrl Pts',(31.3349355217479,54.4558472304805,40.0827023670731));
#196074=CARTESIAN_POINT('Ctrl Pts',(31.334510765913,54.4558650179025,40.0825207326933));
#196075=CARTESIAN_POINT('Ctrl Pts',(31.3340864990776,54.4558811330246,40.0823381109276));
#196076=CARTESIAN_POINT('Ctrl Pts',(31.3328136985713,54.4559294783908,40.0817902456304));
#196077=CARTESIAN_POINT('Ctrl Pts',(31.3315453006546,54.4559627721155,40.0812334935553));
#196078=CARTESIAN_POINT('Ctrl Pts',(31.3302817797851,54.4559812395334,40.0806684524227));
#196079=CARTESIAN_POINT('Ctrl Pts',(31.3215500666183,54.4561088608493,40.0767636676136));
#196080=CARTESIAN_POINT('Ctrl Pts',(31.313019592449,54.4555742713435,40.0724404510887));
#196081=CARTESIAN_POINT('Ctrl Pts',(31.3047400858592,54.4544853519654,40.0677949937407));
#196082=CARTESIAN_POINT('Ctrl Pts',(31.3006251938112,54.4539441620235,40.0654862141904));
#196083=CARTESIAN_POINT('Ctrl Pts',(31.296571959199,54.4532655373256,40.0630972003215));
#196084=CARTESIAN_POINT('Ctrl Pts',(31.2925850928569,54.4524598885392,40.0606363359906));
#196085=CARTESIAN_POINT('Ctrl Pts',(31.2837894702125,54.4506825069815,40.0552073017124));
#196086=CARTESIAN_POINT('Ctrl Pts',(31.2753153512353,54.4482992497263,40.0494204304519));
#196087=CARTESIAN_POINT('Ctrl Pts',(31.2672761140357,54.4454010706195,40.0434049749851));
#196088=CARTESIAN_POINT('Ctrl Pts',(31.2643392793066,54.4443423292438,40.0412074532442));
#196089=CARTESIAN_POINT('Ctrl Pts',(31.2614550023645,54.443220643404,40.0389814735788));
#196090=CARTESIAN_POINT('Ctrl Pts',(31.2586246102252,54.4420411592045,40.0367321210016));
#196091=CARTESIAN_POINT('Ctrl Pts',(31.2491176225323,54.4380793965873,40.0291767837142));
#196092=CARTESIAN_POINT('Ctrl Pts',(31.2401615453403,54.433432644623,40.021323533258));
#196093=CARTESIAN_POINT('Ctrl Pts',(31.2317373058279,54.4282277812592,40.0132649215865));
#196094=CARTESIAN_POINT('Ctrl Pts',(31.222478068687,54.4225070198657,40.0044075527542));
#196095=CARTESIAN_POINT('Ctrl Pts',(31.2138606686962,54.4161118092708,39.9953016253731));
#196096=CARTESIAN_POINT('Ctrl Pts',(31.2058737429085,54.4091594014087,39.9860353422371));
#196097=CARTESIAN_POINT('Ctrl Pts',(31.1972714816225,54.4016713602542,39.9760551582709));
#196098=CARTESIAN_POINT('Ctrl Pts',(31.1893995936785,54.3935362880559,39.9658879738171));
#196099=CARTESIAN_POINT('Ctrl Pts',(31.1822725865947,54.3848513315129,39.9556174643269));
#196100=CARTESIAN_POINT('Ctrl Pts',(31.1752418181697,54.3762836512066,39.9454856413915));
#196101=CARTESIAN_POINT('Ctrl Pts',(31.1689352997164,54.3671795569343,39.9352519465119));
#196102=CARTESIAN_POINT('Ctrl Pts',(31.1634057161447,54.3576020372435,39.92499));
#196103=CARTESIAN_POINT('Ctrl Pts',(29.4433108116267,51.3783102687781,39.92499));
#196104=CARTESIAN_POINT('Ctrl Pts',(29.4380189697937,51.3691445298578,39.9348107241733));
#196105=CARTESIAN_POINT('Ctrl Pts',(29.433469091585,51.3595943606091,39.9446038383191));
#196106=CARTESIAN_POINT('Ctrl Pts',(29.4296781246243,51.3497152868736,39.9543158069416));
#196107=CARTESIAN_POINT('Ctrl Pts',(29.42601761248,51.3401761719831,39.963693567143));
#196108=CARTESIAN_POINT('Ctrl Pts',(29.423064299797,51.330329192487,39.9729968321034));
#196109=CARTESIAN_POINT('Ctrl Pts',(29.4208754038577,51.3202058500836,39.9821731151387));
#196110=CARTESIAN_POINT('Ctrl Pts',(29.4188062116754,51.310636121078,39.9908475764409));
#196111=CARTESIAN_POINT('Ctrl Pts',(29.4174199248359,51.3008185461718,39.9994093733908));
#196112=CARTESIAN_POINT('Ctrl Pts',(29.4168067767633,51.290777528927,40.0077966115908));
#196113=CARTESIAN_POINT('Ctrl Pts',(29.4162420776748,51.2815299204951,40.0155211172665));
#196114=CARTESIAN_POINT('Ctrl Pts',(29.4163331870173,51.2720922400845,40.0230979941095));
#196115=CARTESIAN_POINT('Ctrl Pts',(29.4171879526256,51.262491179764,40.0304554104825));
#196116=CARTESIAN_POINT('Ctrl Pts',(29.4174428264751,51.2596283373899,40.0326492435232));
#196117=CARTESIAN_POINT('Ctrl Pts',(29.4177658668987,51.256751052484,40.0348233715086));
#196118=CARTESIAN_POINT('Ctrl Pts',(29.4181606517648,51.2538602864391,40.0369753512356));
#196119=CARTESIAN_POINT('Ctrl Pts',(29.4185514029028,51.2509990568964,40.0391053430352));
#196120=CARTESIAN_POINT('Ctrl Pts',(29.4190117629207,51.2481275521815,40.041211089324));
#196121=CARTESIAN_POINT('Ctrl Pts',(29.4195444402105,51.2452499391936,40.0432881154904));
#196122=CARTESIAN_POINT('Ctrl Pts',(29.4195814815475,51.2450498356142,40.043432547828));
#196123=CARTESIAN_POINT('Ctrl Pts',(29.4196188630967,51.244849695198,40.0435768364421));
#196124=CARTESIAN_POINT('Ctrl Pts',(29.4196565860791,51.2446495184039,40.0437209807855));
#196125=CARTESIAN_POINT('Ctrl Pts',(29.4213104998207,51.2358730344468,40.0500407968419));
#196126=CARTESIAN_POINT('Ctrl Pts',(29.4236619033169,51.2270453415806,40.0560490279344));
#196127=CARTESIAN_POINT('Ctrl Pts',(29.4267651248013,51.2182691329813,40.0616647108614));
#196128=CARTESIAN_POINT('Ctrl Pts',(29.429657866561,51.210088181272,40.0668995033484));
#196129=CARTESIAN_POINT('Ctrl Pts',(29.4332044080282,51.2019513265394,40.0717933267479));
#196130=CARTESIAN_POINT('Ctrl Pts',(29.4374658604801,51.1939656059622,40.0762460303069));
#196131=CARTESIAN_POINT('Ctrl Pts',(29.4390247549186,51.1910443260617,40.0778748868746));
#196132=CARTESIAN_POINT('Ctrl Pts',(29.440679457209,51.1881435589221,40.0794443522246));
#196133=CARTESIAN_POINT('Ctrl Pts',(29.4424334077173,51.185269677679,40.0809482021492));
#196134=CARTESIAN_POINT('Ctrl Pts',(29.4428551742202,51.184578605248,40.0813098278168));
#196135=CARTESIAN_POINT('Ctrl Pts',(29.4432832153794,51.1838888551092,40.0816679525672));
#196136=CARTESIAN_POINT('Ctrl Pts',(29.4437175198439,51.1832005624685,40.0820224192581));
#196137=CARTESIAN_POINT('Ctrl Pts',(29.4441382522939,51.1825337789729,40.0823658088648));
#196138=CARTESIAN_POINT('Ctrl Pts',(29.4445648626871,51.1818683633169,40.0827057654617));
#196139=CARTESIAN_POINT('Ctrl Pts',(29.4449973374102,51.181204440299,40.0830421470151));
#196140=CARTESIAN_POINT('Ctrl Pts',(29.4497355978007,51.1739303963593,40.0867275956806));
#196141=CARTESIAN_POINT('Ctrl Pts',(29.4551812510957,51.1668309650357,40.089982343203));
#196142=CARTESIAN_POINT('Ctrl Pts',(29.4612929974521,51.1600900711813,40.0926299529355));
#196143=CARTESIAN_POINT('Ctrl Pts',(29.4638277208378,51.1572944215752,40.0937279956084));
#196144=CARTESIAN_POINT('Ctrl Pts',(29.4664765899958,51.1545603804836,40.0947220371802));
#196145=CARTESIAN_POINT('Ctrl Pts',(29.4692349685477,51.1519003687086,40.0956014538692));
#196146=CARTESIAN_POINT('Ctrl Pts',(29.4739396706111,51.1473634414338,40.097101390674));
#196147=CARTESIAN_POINT('Ctrl Pts',(29.4789629373388,51.1430443628981,40.0982667904316));
#196148=CARTESIAN_POINT('Ctrl Pts',(29.4842777732944,51.139010721436,40.0990539325583));
#196149=CARTESIAN_POINT('Ctrl Pts',(29.4869351912722,51.1369939007049,40.0994475036216));
#196150=CARTESIAN_POINT('Ctrl Pts',(29.4896662827385,51.135049657062,40.0997467259952));
#196151=CARTESIAN_POINT('Ctrl Pts',(29.4924676612914,51.1331865036872,40.0999473488896));
#196152=CARTESIAN_POINT('Ctrl Pts',(29.4952690398443,51.1313233503124,40.100147971784));
#196153=CARTESIAN_POINT('Ctrl Pts',(29.4981406602403,51.1295412933643,40.10025));
#196154=CARTESIAN_POINT('Ctrl Pts',(29.5010785149117,51.1278468659044,40.10025));
#196155=CARTESIAN_POINT('Origin',(34.2589154226527,47.1274239660506,39.92499));
#196156=CARTESIAN_POINT('Ctrl Pts',(36.9828414016752,50.5784163149353,39.92499));
#196157=CARTESIAN_POINT('Ctrl Pts',(36.9890779968915,50.5870002518363,39.9348354642018));
#196158=CARTESIAN_POINT('Ctrl Pts',(36.9946187858206,50.5960508068001,39.9446440828459));
#196159=CARTESIAN_POINT('Ctrl Pts',(36.9994424783912,50.6055128591423,39.9543641760333));
#196160=CARTESIAN_POINT('Ctrl Pts',(37.0041094296764,50.6146674511263,39.9637684240716));
#196161=CARTESIAN_POINT('Ctrl Pts',(37.0081056536714,50.6242084112816,39.9730909636401));
#196162=CARTESIAN_POINT('Ctrl Pts',(37.0113722742002,50.6341096134638,39.9822808977147));
#196163=CARTESIAN_POINT('Ctrl Pts',(37.0144622960735,50.6434755410474,39.9909740094658));
#196164=CARTESIAN_POINT('Ctrl Pts',(37.0168997626771,50.6531646927637,39.9995492765011));
#196165=CARTESIAN_POINT('Ctrl Pts',(37.0185933530516,50.6631621581244,40.0079462328707));
#196166=CARTESIAN_POINT('Ctrl Pts',(37.0201532722701,50.6723705467567,40.0156804369703));
#196167=CARTESIAN_POINT('Ctrl Pts',(37.0210821446117,50.6818410607736,40.0232638017438));
#196168=CARTESIAN_POINT('Ctrl Pts',(37.021270510878,50.6915586678658,40.0306257269984));
#196169=CARTESIAN_POINT('Ctrl Pts',(37.0213251487716,50.6943773762884,40.0327611416663));
#196170=CARTESIAN_POINT('Ctrl Pts',(37.0213172191971,50.6972168227826,40.0348777427277));
#196171=CARTESIAN_POINT('Ctrl Pts',(37.0212433695029,50.7000764815582,40.0369733168701));
#196172=CARTESIAN_POINT('Ctrl Pts',(37.0211633116864,50.7031765355309,40.039245053974));
#196173=CARTESIAN_POINT('Ctrl Pts',(37.0210069737846,50.7062960577318,40.041487875195));
#196174=CARTESIAN_POINT('Ctrl Pts',(37.0207706534752,50.70943353111,40.0436985701601));
#196175=CARTESIAN_POINT('Ctrl Pts',(37.0201220705314,50.7180443514156,40.0497658398386));
#196176=CARTESIAN_POINT('Ctrl Pts',(37.0188289150186,50.7267761502169,40.0555581699984));
#196177=CARTESIAN_POINT('Ctrl Pts',(37.0168522507837,50.7355328079485,40.0609828468886));
#196178=CARTESIAN_POINT('Ctrl Pts',(37.0150437103243,50.743544674363,40.0659461317305));
#196179=CARTESIAN_POINT('Ctrl Pts',(37.0126559296154,50.7515681793716,40.0706039980706));
#196180=CARTESIAN_POINT('Ctrl Pts',(37.0096268558221,50.7595400218645,40.0748843180603));
#196181=CARTESIAN_POINT('Ctrl Pts',(37.0081389846697,50.7634557648559,40.076986797257));
#196182=CARTESIAN_POINT('Ctrl Pts',(37.0064960060565,50.7673587034235,40.0789976708175));
#196183=CARTESIAN_POINT('Ctrl Pts',(37.0046883717073,50.7712388062146,40.08090504915));
#196184=CARTESIAN_POINT('Ctrl Pts',(37.0043453906961,50.7719750179265,40.0812669556105));
#196185=CARTESIAN_POINT('Ctrl Pts',(37.003995985342,50.772710598466,40.0816253922033));
#196186=CARTESIAN_POINT('Ctrl Pts',(37.003640149748,50.7734454079405,40.0819801989139));
#196187=CARTESIAN_POINT('Ctrl Pts',(37.0032954340162,50.774157254619,40.0823239179149));
#196188=CARTESIAN_POINT('Ctrl Pts',(37.0029446836758,50.7748683776568,40.0826642303498));
#196189=CARTESIAN_POINT('Ctrl Pts',(37.0025878964874,50.7755786476298,40.0830009916099));
#196190=CARTESIAN_POINT('Ctrl Pts',(36.9986997032258,50.7833190234411,40.0866709464312));
#196191=CARTESIAN_POINT('Ctrl Pts',(36.9940916451531,50.7909629993138,40.0899175831877));
#196192=CARTESIAN_POINT('Ctrl Pts',(36.9887818345687,50.7983209798294,40.0925642067062));
#196193=CARTESIAN_POINT('Ctrl Pts',(36.9865394685866,50.8014283006919,40.0936818922527));
#196194=CARTESIAN_POINT('Ctrl Pts',(36.9841723869928,50.8044846273286,40.0946930094791));
#196195=CARTESIAN_POINT('Ctrl Pts',(36.9816838130239,50.8074762285636,40.0955863397546));
#196196=CARTESIAN_POINT('Ctrl Pts',(36.9774931166431,50.8125140102914,40.0970906856166));
#196197=CARTESIAN_POINT('Ctrl Pts',(36.9729576356987,50.8173657273499,40.0982599215483));
#196198=CARTESIAN_POINT('Ctrl Pts',(36.9680961762161,50.8219595855747,40.0990497370453));
#196199=CARTESIAN_POINT('Ctrl Pts',(36.9668808113454,50.8231080501309,40.0992471909196));
#196200=CARTESIAN_POINT('Ctrl Pts',(36.9656449236016,50.8242402182961,40.0994209989363));
#196201=CARTESIAN_POINT('Ctrl Pts',(36.9643886196688,50.8253547230709,40.0995705982975));
#196202=CARTESIAN_POINT('Ctrl Pts',(36.9625041637695,50.8270264802331,40.0997949973393));
#196203=CARTESIAN_POINT('Ctrl Pts',(36.9605737761782,50.8286584747052,40.0999649129781));
#196204=CARTESIAN_POINT('Ctrl Pts',(36.9585988181543,50.830247439591,40.1000786629733));
#196205=CARTESIAN_POINT('Ctrl Pts',(36.9566238601303,50.8318364044769,40.1001924129685));
#196206=CARTESIAN_POINT('Ctrl Pts',(36.9546043428198,50.8333823430146,40.10025));
#196207=CARTESIAN_POINT('Ctrl Pts',(36.9525415975228,50.8348823336496,40.10025));
#196208=CARTESIAN_POINT('Ctrl Pts',(34.7084426211237,47.746145074786,40.10025));
#196209=CARTESIAN_POINT('Ctrl Pts',(34.7154221779238,47.7410693801611,40.10025));
#196210=CARTESIAN_POINT('Ctrl Pts',(34.7227602152557,47.7366138137618,40.0995786334239));
#196211=CARTESIAN_POINT('Ctrl Pts',(34.7303057514069,47.7327846251232,40.0983063763362));
#196212=CARTESIAN_POINT('Ctrl Pts',(34.7351793935427,47.7303113621607,40.0974846287989));
#196213=CARTESIAN_POINT('Ctrl Pts',(34.7401391868082,47.7280985748129,40.0964130309336));
#196214=CARTESIAN_POINT('Ctrl Pts',(34.74514213706,47.7261394006514,40.0951176960923));
#196215=CARTESIAN_POINT('Ctrl Pts',(34.751773261033,47.7235426275284,40.0934008039614));
#196216=CARTESIAN_POINT('Ctrl Pts',(34.7584811778437,47.7213971161176,40.0912909372156));
#196217=CARTESIAN_POINT('Ctrl Pts',(34.7651763312121,47.7196932909341,40.0888630467851));
#196218=CARTESIAN_POINT('Ctrl Pts',(34.7685239078963,47.7188413783424,40.0876491015699));
#196219=CARTESIAN_POINT('Ctrl Pts',(34.7718684539197,47.7180997687558,40.0863558569271));
#196220=CARTESIAN_POINT('Ctrl Pts',(34.7751999143437,47.7174664279766,40.0849936342771));
#196221=CARTESIAN_POINT('Ctrl Pts',(34.7768656445557,47.7171497575869,40.0843125229521));
#196222=CARTESIAN_POINT('Ctrl Pts',(34.7785281166323,47.7168601447017,40.0836141747074));
#196223=CARTESIAN_POINT('Ctrl Pts',(34.7801861569095,47.7165972740594,40.0828999161609));
#196224=CARTESIAN_POINT('Ctrl Pts',(34.7806006669788,47.7165315563988,40.0827213515243));
#196225=CARTESIAN_POINT('Ctrl Pts',(34.7810149003422,47.7164675099213,40.0825417925842));
#196226=CARTESIAN_POINT('Ctrl Pts',(34.7814288392286,47.716405129283,40.082361260236));
#196227=CARTESIAN_POINT('Ctrl Pts',(34.7826706558879,47.716217987368,40.0818196631917));
#196228=CARTESIAN_POINT('Ctrl Pts',(34.7839098208543,47.7160458390451,40.0812693052021));
#196229=CARTESIAN_POINT('Ctrl Pts',(34.7851458668351,47.7158885307485,40.0807107531875));
#196230=CARTESIAN_POINT('Ctrl Pts',(34.793852415122,47.7147804714195,40.076776384918));
#196231=CARTESIAN_POINT('Ctrl Pts',(34.8024290252897,47.7143609747534,40.0724140586133));
#196232=CARTESIAN_POINT('Ctrl Pts',(34.8108122146636,47.7145286167443,40.0677221223761));
#196233=CARTESIAN_POINT('Ctrl Pts',(34.8148780524504,47.7146099229287,40.0654465383716));
#196234=CARTESIAN_POINT('Ctrl Pts',(34.8188987667937,47.7148297795036,40.0630928000677));
#196235=CARTESIAN_POINT('Ctrl Pts',(34.8228686918044,47.7151790039206,40.0606689262479));
#196236=CARTESIAN_POINT('Ctrl Pts',(34.8289463696258,47.7157136421034,40.0569581447805));
#196237=CARTESIAN_POINT('Ctrl Pts',(34.8349017567801,47.7165501157948,40.0530843804605));
#196238=CARTESIAN_POINT('Ctrl Pts',(34.8407017446573,47.7176563296778,40.0490800251458));
#196239=CARTESIAN_POINT('Ctrl Pts',(34.8433952890326,47.7181700611279,40.0472203818218));
#196240=CARTESIAN_POINT('Ctrl Pts',(34.8460552817724,47.7187417155518,40.0453323608818));
#196241=CARTESIAN_POINT('Ctrl Pts',(34.8486779186782,47.7193692101067,40.0434201572162));
#196242=CARTESIAN_POINT('Ctrl Pts',(34.8488789334633,47.7194173050919,40.0432735943397));
#196243=CARTESIAN_POINT('Ctrl Pts',(34.8490797487417,47.7194657006753,40.0431268995707));
#196244=CARTESIAN_POINT('Ctrl Pts',(34.8492803638663,47.7195143955475,40.0429800745037));
#196245=CARTESIAN_POINT('Ctrl Pts',(34.8520984015311,47.720198411693,40.0409176249753));
#196246=CARTESIAN_POINT('Ctrl Pts',(34.8548765847941,47.7209435418723,40.0388310783332));
#196247=CARTESIAN_POINT('Ctrl Pts',(34.8576119849591,47.7217448891699,40.036725739981));
#196248=CARTESIAN_POINT('Ctrl Pts',(34.8674206434763,47.7246183780644,40.0291763710716));
#196249=CARTESIAN_POINT('Ctrl Pts',(34.8767555719428,47.7282350429865,40.0213310894592));
#196250=CARTESIAN_POINT('Ctrl Pts',(34.885623156561,47.7324659181294,40.0132837551315));
#196251=CARTESIAN_POINT('Ctrl Pts',(34.8953677412285,47.7371152248823,40.004440543132));
#196252=CARTESIAN_POINT('Ctrl Pts',(34.9045486251012,47.7425063743635,39.9953528710595));
#196253=CARTESIAN_POINT('Ctrl Pts',(34.9131661493101,47.7485205638414,39.9861103629549));
#196254=CARTESIAN_POINT('Ctrl Pts',(34.9224709127522,47.7550143791219,39.976130773755));
#196255=CARTESIAN_POINT('Ctrl Pts',(34.9311199164044,47.7622350952177,39.9659696936006));
#196256=CARTESIAN_POINT('Ctrl Pts',(34.9390908738059,47.7700859103005,39.9557128217502));
#196257=CARTESIAN_POINT('Ctrl Pts',(34.9469949630648,47.7778708651112,39.9455419945158));
#196258=CARTESIAN_POINT('Ctrl Pts',(34.9542331399582,47.7862765797896,39.9352756289339));
#196259=CARTESIAN_POINT('Ctrl Pts',(34.9607485668371,47.7952442955498,39.92499));
#196260=CARTESIAN_POINT('Origin',(-0.0123294189942718,0.00895784724493288,
39.92499));
#196261=CARTESIAN_POINT('Ctrl Pts',(36.9278827595333,50.8527980281381,40.10025));
#196262=CARTESIAN_POINT('Ctrl Pts',(36.9209320551076,50.8578435704952,40.10025));
#196263=CARTESIAN_POINT('Ctrl Pts',(36.9136216385513,50.8622636476101,40.0995859581842));
#196264=CARTESIAN_POINT('Ctrl Pts',(36.9061023515959,50.866055238751,40.0983275959621));
#196265=CARTESIAN_POINT('Ctrl Pts',(36.9012978851891,50.8684778849903,40.0975235624068));
#196266=CARTESIAN_POINT('Ctrl Pts',(36.8964085464706,50.8706447895119,40.0964777059491));
#196267=CARTESIAN_POINT('Ctrl Pts',(36.8914758894172,50.8725634718542,40.0952149915962));
#196268=CARTESIAN_POINT('Ctrl Pts',(36.8847438022853,50.8751820882647,40.0934916398702));
#196269=CARTESIAN_POINT('Ctrl Pts',(36.8779301449089,50.8773323251411,40.0913643921631));
#196270=CARTESIAN_POINT('Ctrl Pts',(36.8711298300328,50.8790261328801,40.0889118607714));
#196271=CARTESIAN_POINT('Ctrl Pts',(36.8677296725947,50.8798730367497,40.0876855950755));
#196272=CARTESIAN_POINT('Ctrl Pts',(36.8643326829605,50.8806059576333,40.0863782327527));
#196273=CARTESIAN_POINT('Ctrl Pts',(36.8609495224157,50.8812272732511,40.0850006373334));
#196274=CARTESIAN_POINT('Ctrl Pts',(36.8592579421434,50.88153793106,40.0843118396238));
#196275=CARTESIAN_POINT('Ctrl Pts',(36.8575698050851,50.881820697829,40.0836054919165));
#196276=CARTESIAN_POINT('Ctrl Pts',(36.8558863556343,50.8820759354565,40.0828829920418));
#196277=CARTESIAN_POINT('Ctrl Pts',(36.8554654932716,50.8821397448634,40.0827023670731));
#196278=CARTESIAN_POINT('Ctrl Pts',(36.8550449235855,50.8822018339186,40.0825207326933));
#196279=CARTESIAN_POINT('Ctrl Pts',(36.8546246654171,50.8822622087207,40.0823381109276));
#196280=CARTESIAN_POINT('Ctrl Pts',(36.853363890912,50.8824433331269,40.0817902456304));
#196281=CARTESIAN_POINT('Ctrl Pts',(36.8521059215537,50.8826090281502,40.0812334935553));
#196282=CARTESIAN_POINT('Ctrl Pts',(36.8508512527545,50.8827594682965,40.0806684524227));
#196283=CARTESIAN_POINT('Ctrl Pts',(36.8421807128862,50.8837991030484,40.0767636676137));
#196284=CARTESIAN_POINT('Ctrl Pts',(36.8336410897275,50.8841591194357,40.0724404510888));
#196285=CARTESIAN_POINT('Ctrl Pts',(36.825293116072,50.8839416093724,40.0677949937408));
#196286=CARTESIAN_POINT('Ctrl Pts',(36.8211441960801,50.8838335074679,40.0654862141905));
#196287=CARTESIAN_POINT('Ctrl Pts',(36.8170422299143,50.8835822787324,40.0630972003216));
#196288=CARTESIAN_POINT('Ctrl Pts',(36.8129929908136,50.8831977843863,40.0606363359906));
#196289=CARTESIAN_POINT('Ctrl Pts',(36.8040597645475,50.8823495324292,40.0552073017124));
#196290=CARTESIAN_POINT('Ctrl Pts',(36.7953829494622,50.8808651175409,40.0494204304519));
#196291=CARTESIAN_POINT('Ctrl Pts',(36.7870848098368,50.8788231440727,40.0434049749851));
#196292=CARTESIAN_POINT('Ctrl Pts',(36.7840533947866,50.8780771854142,40.0412074532442));
#196293=CARTESIAN_POINT('Ctrl Pts',(36.7810676701183,50.8772631333232,40.0389814735788));
#196294=CARTESIAN_POINT('Ctrl Pts',(36.7781294934924,50.8763859670022,40.0367321210017));
#196295=CARTESIAN_POINT('Ctrl Pts',(36.7682604691136,50.8734396581487,40.0291767837136));
#196296=CARTESIAN_POINT('Ctrl Pts',(36.7588677364067,50.8697545265632,40.0213235332565));
#196297=CARTESIAN_POINT('Ctrl Pts',(36.7499455893902,50.8654587487954,40.0132649215842));
#196298=CARTESIAN_POINT('Ctrl Pts',(36.7401390929214,50.8607371801604,40.004407552751));
#196299=CARTESIAN_POINT('Ctrl Pts',(36.730900418413,50.8552777667761,39.995301625369));
#196300=CARTESIAN_POINT('Ctrl Pts',(36.7222305213302,50.84919830601,39.9860353422322));
#196301=CARTESIAN_POINT('Ctrl Pts',(36.7128926706965,50.8426504662806,39.9760551582652));
#196302=CARTESIAN_POINT('Ctrl Pts',(36.7042135591825,50.8353827952082,39.9658879738106));
#196303=CARTESIAN_POINT('Ctrl Pts',(36.696217769428,50.8274903908632,39.9556174643197));
#196304=CARTESIAN_POINT('Ctrl Pts',(36.688329949834,50.8197045606266,39.9454856413866));
#196305=CARTESIAN_POINT('Ctrl Pts',(36.6811063421666,50.8113095502195,39.9352519465094));
#196306=CARTESIAN_POINT('Ctrl Pts',(36.6746059268184,50.8023624960587,39.92499));
#196307=CARTESIAN_POINT('Ctrl Pts',(34.6525130919802,48.0191904766733,39.92499));
#196308=CARTESIAN_POINT('Ctrl Pts',(34.6462921588066,48.0106280967246,39.934810724173));
#196309=CARTESIAN_POINT('Ctrl Pts',(34.6407689407914,48.0016058360797,39.9446038383186));
#196310=CARTESIAN_POINT('Ctrl Pts',(34.6359660967484,47.9921771448948,39.9543158069409));
#196311=CARTESIAN_POINT('Ctrl Pts',(34.6313285282523,47.9830729139833,39.9636935671419));
#196312=CARTESIAN_POINT('Ctrl Pts',(34.6273621044907,47.9735885825078,39.972996832102));
#196313=CARTESIAN_POINT('Ctrl Pts',(34.6241270221279,47.9637494987625,39.9821731151371));
#196314=CARTESIAN_POINT('Ctrl Pts',(34.6210688561301,47.9544484832132,39.9908475764388));
#196315=CARTESIAN_POINT('Ctrl Pts',(34.6186639474969,47.9448295964431,39.9994093733883));
#196316=CARTESIAN_POINT('Ctrl Pts',(34.6170045862113,47.9349076763676,40.007796611588));
#196317=CARTESIAN_POINT('Ctrl Pts',(34.6154763423052,47.925769754431,40.0155211172632));
#196318=CARTESIAN_POINT('Ctrl Pts',(34.6145804463109,47.9163742511024,40.0230979941057));
#196319=CARTESIAN_POINT('Ctrl Pts',(34.6144269453424,47.9067364390602,40.0304554104783));
#196320=CARTESIAN_POINT('Ctrl Pts',(34.6143811744522,47.9038626380626,40.0326492435204));
#196321=CARTESIAN_POINT('Ctrl Pts',(34.614401687057,47.9009673483035,40.0348233715072));
#196322=CARTESIAN_POINT('Ctrl Pts',(34.614492141918,47.8980511519202,40.0369753512356));
#196323=CARTESIAN_POINT('Ctrl Pts',(34.6145816725532,47.8951647518763,40.0391053430352));
#196324=CARTESIAN_POINT('Ctrl Pts',(34.6147393566957,47.8922608568395,40.041211089324));
#196325=CARTESIAN_POINT('Ctrl Pts',(34.61496832346,47.8893433277781,40.0432881154904));
#196326=CARTESIAN_POINT('Ctrl Pts',(34.614984245361,47.889140448513,40.043432547828));
#196327=CARTESIAN_POINT('Ctrl Pts',(34.6150005017601,47.8889374970511,40.0435768364421));
#196328=CARTESIAN_POINT('Ctrl Pts',(34.6150170939194,47.888734473721,40.0437209807855));
#196329=CARTESIAN_POINT('Ctrl Pts',(34.6157445549675,47.8798331871997,40.0500407968419));
#196330=CARTESIAN_POINT('Ctrl Pts',(34.6171603320598,47.8708080647648,40.0560490279342));
#196331=CARTESIAN_POINT('Ctrl Pts',(34.6193291901739,47.8617555581816,40.0616647108611));
#196332=CARTESIAN_POINT('Ctrl Pts',(34.6213509428813,47.8533170487311,40.0668995033481));
#196333=CARTESIAN_POINT('Ctrl Pts',(34.6240275231022,47.8448540540106,40.0717933267476));
#196334=CARTESIAN_POINT('Ctrl Pts',(34.6274308957716,47.8364666369703,40.0762460303065));
#196335=CARTESIAN_POINT('Ctrl Pts',(34.6286758935245,47.8333984113065,40.0778748868743));
#196336=CARTESIAN_POINT('Ctrl Pts',(34.6300183184514,47.830340571385,40.0794443522245));
#196337=CARTESIAN_POINT('Ctrl Pts',(34.6314622582454,47.8272990958126,40.0809482021492));
#196338=CARTESIAN_POINT('Ctrl Pts',(34.631809477528,47.8265677225443,40.0813098278168));
#196339=CARTESIAN_POINT('Ctrl Pts',(34.6321630753109,47.8258370084444,40.0816679525672));
#196340=CARTESIAN_POINT('Ctrl Pts',(34.6325230544381,47.8251070891645,40.082022419258));
#196341=CARTESIAN_POINT('Ctrl Pts',(34.6328717842176,47.8243999798622,40.0823658088648));
#196342=CARTESIAN_POINT('Ctrl Pts',(34.6332265027185,47.823693616494,40.0827057654616));
#196343=CARTESIAN_POINT('Ctrl Pts',(34.6335872094469,47.8229881245976,40.0830421470151));
#196344=CARTESIAN_POINT('Ctrl Pts',(34.6375391685168,47.815258645554,40.0867275956808));
#196345=CARTESIAN_POINT('Ctrl Pts',(34.6422128973073,47.8076288798872,40.0899823432034));
#196346=CARTESIAN_POINT('Ctrl Pts',(34.6475865476024,47.8002860618997,40.092629952936));
#196347=CARTESIAN_POINT('Ctrl Pts',(34.6498151605508,47.7972407764148,40.0937279956087));
#196348=CARTESIAN_POINT('Ctrl Pts',(34.6521637338122,47.7942448304644,40.0947220371803));
#196349=CARTESIAN_POINT('Ctrl Pts',(34.6546289547343,47.7913110614415,40.0956014538692));
#196350=CARTESIAN_POINT('Ctrl Pts',(34.6588336459116,47.7863072126522,40.097101390674));
#196351=CARTESIAN_POINT('Ctrl Pts',(34.6633779280164,47.781486720129,40.0982667904316));
#196352=CARTESIAN_POINT('Ctrl Pts',(34.6682420184012,47.776919623742,40.0990539325582));
#196353=CARTESIAN_POINT('Ctrl Pts',(34.6706740635936,47.7746360755484,40.0994475036216));
#196354=CARTESIAN_POINT('Ctrl Pts',(34.6731869650549,47.7724170058816,40.0997467259952));
#196355=CARTESIAN_POINT('Ctrl Pts',(34.6757782448039,47.7702712352608,40.0999473488896));
#196356=CARTESIAN_POINT('Ctrl Pts',(34.6783695245528,47.7681254646399,40.100147971784));
#196357=CARTESIAN_POINT('Ctrl Pts',(34.6810391382375,47.766053003919,40.10025));
#196358=CARTESIAN_POINT('Ctrl Pts',(34.6837837831351,47.7640607692759,40.10025));
#196359=CARTESIAN_POINT('Origin',(38.9973987043324,43.2882232241944,39.92499));
#196360=CARTESIAN_POINT('Ctrl Pts',(42.0671296588101,46.4355828792665,39.92499));
#196361=CARTESIAN_POINT('Ctrl Pts',(42.0742293550387,46.4434678907495,39.9348354642026));
#196362=CARTESIAN_POINT('Ctrl Pts',(42.0806858315487,46.4518896956747,39.9446440828474));
#196363=CARTESIAN_POINT('Ctrl Pts',(42.0864721532177,46.4607957007331,39.9543641760356));
#196364=CARTESIAN_POINT('Ctrl Pts',(42.0920704538875,46.4694123136588,39.9637684240743));
#196365=CARTESIAN_POINT('Ctrl Pts',(42.0970420880528,46.4784832882836,39.9730909636433));
#196366=CARTESIAN_POINT('Ctrl Pts',(42.1013257711412,46.487988795821,39.9822808977183));
#196367=CARTESIAN_POINT('Ctrl Pts',(42.1053778715688,46.496980420636,39.9909740094698));
#196368=CARTESIAN_POINT('Ctrl Pts',(42.1088147776146,46.5063617095277,39.9995492765054));
#196369=CARTESIAN_POINT('Ctrl Pts',(42.1115441100144,46.5161273793285,40.0079462328752));
#196370=CARTESIAN_POINT('Ctrl Pts',(42.1140580225451,46.5251222674863,40.0156804369753));
#196371=CARTESIAN_POINT('Ctrl Pts',(42.1159717447031,46.5344438074388,40.023263801749));
#196372=CARTESIAN_POINT('Ctrl Pts',(42.1171748456151,46.5440884908269,40.0306257270039));
#196373=CARTESIAN_POINT('Ctrl Pts',(42.1175238194559,46.5468860468525,40.0327611416699));
#196374=CARTESIAN_POINT('Ctrl Pts',(42.1178127362988,46.5497107674255,40.0348777427294));
#196375=CARTESIAN_POINT('Ctrl Pts',(42.118038206898,46.5525624800837,40.03697331687));
#196376=CARTESIAN_POINT('Ctrl Pts',(42.1182826315244,46.5556539199569,40.039245053974));
#196377=CARTESIAN_POINT('Ctrl Pts',(42.1184532289198,46.5587726948494,40.041487875195));
#196378=CARTESIAN_POINT('Ctrl Pts',(42.1185461584685,46.5619176830189,40.0436985701601));
#196379=CARTESIAN_POINT('Ctrl Pts',(42.118801204344,46.5705491277284,40.0497658398386));
#196380=CARTESIAN_POINT('Ctrl Pts',(42.1184278543826,46.5793682643807,40.0555581699984));
#196381=CARTESIAN_POINT('Ctrl Pts',(42.1173773384972,46.5882835698999,40.0609828468886));
#196382=CARTESIAN_POINT('Ctrl Pts',(42.1164161734959,46.5964405904273,40.0659461317308));
#196383=CARTESIAN_POINT('Ctrl Pts',(42.114880157948,46.6046697328847,40.0706039980713));
#196384=CARTESIAN_POINT('Ctrl Pts',(42.1127009621828,46.6129145292196,40.0748843180612));
#196385=CARTESIAN_POINT('Ctrl Pts',(42.1116305483418,46.6169643462457,40.0769867972576));
#196386=CARTESIAN_POINT('Ctrl Pts',(42.1104045383081,46.6210176421366,40.0789976708178));
#196387=CARTESIAN_POINT('Ctrl Pts',(42.1090123875513,46.6250654385587,40.08090504915));
#196388=CARTESIAN_POINT('Ctrl Pts',(42.1087482405049,46.6258334685039,40.0812669556105));
#196389=CARTESIAN_POINT('Ctrl Pts',(42.1084776383333,46.6266015422609,40.0816253922033));
#196390=CARTESIAN_POINT('Ctrl Pts',(42.1082005605491,46.6273695213201,40.081980198914));
#196391=CARTESIAN_POINT('Ctrl Pts',(42.1079321414455,46.6281135010337,40.082323917915));
#196392=CARTESIAN_POINT('Ctrl Pts',(42.1076576451506,46.6288573918592,40.0826642303499));
#196393=CARTESIAN_POINT('Ctrl Pts',(42.1073770559085,46.6296010653155,40.08300099161));
#196394=CARTESIAN_POINT('Ctrl Pts',(42.1043192521653,46.6377054654042,40.0866709464311));
#196395=CARTESIAN_POINT('Ctrl Pts',(42.1005354505683,46.6457892400059,40.0899175831875));
#196396=CARTESIAN_POINT('Ctrl Pts',(42.0960238460782,46.6536619390745,40.0925642067058));
#196397=CARTESIAN_POINT('Ctrl Pts',(42.094118567486,46.6569866287789,40.0936818922525));
#196398=CARTESIAN_POINT('Ctrl Pts',(42.0920839261391,46.6602736399403,40.094693009479));
#196399=CARTESIAN_POINT('Ctrl Pts',(42.0899216923184,46.6635089796838,40.0955863397546));
#196400=CARTESIAN_POINT('Ctrl Pts',(42.0862805445931,46.668957210969,40.0970906856167));
#196401=CARTESIAN_POINT('Ctrl Pts',(42.0822770520161,46.674256436667,40.0982599215483));
#196402=CARTESIAN_POINT('Ctrl Pts',(42.0779224130577,46.6793332901445,40.0990497370454));
#196403=CARTESIAN_POINT('Ctrl Pts',(42.0768337533181,46.6806025035139,40.0992471909196));
#196404=CARTESIAN_POINT('Ctrl Pts',(42.0757229796951,46.68185765499,40.0994209989363));
#196405=CARTESIAN_POINT('Ctrl Pts',(42.0745900553981,46.6830973739106,40.0995705982975));
#196406=CARTESIAN_POINT('Ctrl Pts',(42.0728906689526,46.6849569522914,40.0997949973393));
#196407=CARTESIAN_POINT('Ctrl Pts',(42.0711414461008,46.6867817869756,40.0999649129781));
#196408=CARTESIAN_POINT('Ctrl Pts',(42.0693433991613,46.6885684866728,40.1000786629733));
#196409=CARTESIAN_POINT('Ctrl Pts',(42.0675453522218,46.69035518637,40.1001924129685));
#196410=CARTESIAN_POINT('Ctrl Pts',(42.0656984926182,46.6921037531358,40.10025));
#196411=CARTESIAN_POINT('Ctrl Pts',(42.0638038389718,46.6938111422612,40.10025));
#196412=CARTESIAN_POINT('Ctrl Pts',(39.5091373124628,43.8565665267052,40.10025));
#196413=CARTESIAN_POINT('Ctrl Pts',(39.5155480799608,43.8507890749202,40.10025));
#196414=CARTESIAN_POINT('Ctrl Pts',(39.5223801852473,43.8455908828145,40.099578633424));
#196415=CARTESIAN_POINT('Ctrl Pts',(39.5294841269575,43.8409939475737,40.0983063763365));
#196416=CARTESIAN_POINT('Ctrl Pts',(39.5340725443954,43.8380247990812,40.0974846287991));
#196417=CARTESIAN_POINT('Ctrl Pts',(39.5387738681339,43.8353056940455,40.0964130309337));
#196418=CARTESIAN_POINT('Ctrl Pts',(39.5435446222369,43.8328343017432,40.0951176960924));
#196419=CARTESIAN_POINT('Ctrl Pts',(39.5498679835149,43.8295586128165,40.0934008039614));
#196420=CARTESIAN_POINT('Ctrl Pts',(39.5563148866448,43.8267236865057,40.0912909372156));
#196421=CARTESIAN_POINT('Ctrl Pts',(39.5627952650345,43.8243293609619,40.0888630467851));
#196422=CARTESIAN_POINT('Ctrl Pts',(39.5660354542293,43.82313219819,40.0876491015699));
#196423=CARTESIAN_POINT('Ctrl Pts',(39.5692841591691,43.8220450509621,40.0863558569271));
#196424=CARTESIAN_POINT('Ctrl Pts',(39.572531167366,43.8210669472514,40.0849936342771));
#196425=CARTESIAN_POINT('Ctrl Pts',(39.5741546714645,43.820577895396,40.0843125229521));
#196426=CARTESIAN_POINT('Ctrl Pts',(39.5757777635552,43.8201160933891,40.0836141747074));
#196427=CARTESIAN_POINT('Ctrl Pts',(39.57739924345,43.8196813503774,40.0828999161609));
#196428=CARTESIAN_POINT('Ctrl Pts',(39.5778046134237,43.8195726646245,40.0827213515243));
#196429=CARTESIAN_POINT('Ctrl Pts',(39.5782098828935,43.8194656698234,40.0825417925842));
#196430=CARTESIAN_POINT('Ctrl Pts',(39.5786150336271,43.8193603625171,40.0823612602361));
#196431=CARTESIAN_POINT('Ctrl Pts',(39.5798304858281,43.819044440598,40.0818196631917));
#196432=CARTESIAN_POINT('Ctrl Pts',(39.5810448681195,43.8187437073119,40.0812693052022));
#196433=CARTESIAN_POINT('Ctrl Pts',(39.5822576997166,43.8184580587797,40.0807107531875));
#196434=CARTESIAN_POINT('Ctrl Pts',(39.5908007288817,43.816445987403,40.0767763849182));
#196435=CARTESIAN_POINT('Ctrl Pts',(39.5992865061392,43.8151322889027,40.0724140586137));
#196436=CARTESIAN_POINT('Ctrl Pts',(39.6076412948839,43.8144227306307,40.0677221223768));
#196437=CARTESIAN_POINT('Ctrl Pts',(39.6116933583968,43.8140785956355,40.065446538372));
#196438=CARTESIAN_POINT('Ctrl Pts',(39.6157150281166,43.8138769687215,40.0630928000679));
#196439=CARTESIAN_POINT('Ctrl Pts',(39.6196997093547,43.8138093098899,40.0606689262479));
#196440=CARTESIAN_POINT('Ctrl Pts',(39.6257999779287,43.8137057289459,40.0569581447805));
#196441=CARTESIAN_POINT('Ctrl Pts',(39.6318101761586,43.8139151128795,40.0530843804605));
#196442=CARTESIAN_POINT('Ctrl Pts',(39.6376940219325,43.8144090029874,40.0490800251457));
#196443=CARTESIAN_POINT('Ctrl Pts',(39.6404265103489,43.8146383681085,40.0472203818218));
#196444=CARTESIAN_POINT('Ctrl Pts',(39.6431316855286,43.8149288459962,40.0453323608818));
#196445=CARTESIAN_POINT('Ctrl Pts',(39.6458055463966,43.8152787628648,40.0434201572162));
#196446=CARTESIAN_POINT('Ctrl Pts',(39.6460104872966,43.8153055826141,40.0432735943397));
#196447=CARTESIAN_POINT('Ctrl Pts',(39.6462152612038,43.8153327221689,40.0431268995707));
#196448=CARTESIAN_POINT('Ctrl Pts',(39.6464198673379,43.815360180295,40.0429800745037));
#196449=CARTESIAN_POINT('Ctrl Pts',(39.6492939666541,43.8157458841819,40.0409176249753));
#196450=CARTESIAN_POINT('Ctrl Pts',(39.6521348180511,43.816196533233,40.0388310783332));
#196451=CARTESIAN_POINT('Ctrl Pts',(39.6549389970093,43.8167075634905,40.036725739981));
#196452=CARTESIAN_POINT('Ctrl Pts',(39.6649942840468,43.8185400271106,40.029176371072));
#196453=CARTESIAN_POINT('Ctrl Pts',(39.6746561192245,43.8211611138364,40.0213310894599));
#196454=CARTESIAN_POINT('Ctrl Pts',(39.6839173731629,43.8244418968093,40.0132837551326));
#196455=CARTESIAN_POINT('Ctrl Pts',(39.6940945608659,43.8280471477127,40.0044405431333));
#196456=CARTESIAN_POINT('Ctrl Pts',(39.7037886794665,43.8324491002301,39.995352871061));
#196457=CARTESIAN_POINT('Ctrl Pts',(39.7129876499599,43.8375295667859,39.9861103629567));
#196458=CARTESIAN_POINT('Ctrl Pts',(39.7229202294665,43.8430151956431,39.9761307737567));
#196459=CARTESIAN_POINT('Ctrl Pts',(39.7322766233292,43.8492922888401,39.9659696936022));
#196460=CARTESIAN_POINT('Ctrl Pts',(39.7410245486281,43.8562669044084,39.9557128217517));
#196461=CARTESIAN_POINT('Ctrl Pts',(39.7496990878225,43.8631830101187,39.9455419945167));
#196462=CARTESIAN_POINT('Ctrl Pts',(39.7577762496639,43.8707860819054,39.9352756289344));
#196463=CARTESIAN_POINT('Ctrl Pts',(39.7651933659004,43.8790236240215,39.92499));
#196464=CARTESIAN_POINT('Origin',(-0.0113255271402735,0.010197550440905,
39.92499));
#196465=CARTESIAN_POINT('Ctrl Pts',(42.0411527846901,46.7142062431418,40.10025));
#196466=CARTESIAN_POINT('Ctrl Pts',(42.0347675597388,46.7199506919427,40.10025));
#196467=CARTESIAN_POINT('Ctrl Pts',(42.027959214277,46.7251107020217,40.099585958184));
#196468=CARTESIAN_POINT('Ctrl Pts',(42.0208774479568,46.7296675019402,40.0983275959617));
#196469=CARTESIAN_POINT('Ctrl Pts',(42.0163525364088,46.7325790801597,40.0975235624065));
#196470=CARTESIAN_POINT('Ctrl Pts',(42.0117164851997,46.7352451892138,40.0964777059488));
#196471=CARTESIAN_POINT('Ctrl Pts',(42.0070114066753,46.7376689638747,40.0952149915961));
#196472=CARTESIAN_POINT('Ctrl Pts',(42.0005899185703,46.740976929953,40.0934916398701));
#196473=CARTESIAN_POINT('Ctrl Pts',(41.9940383480783,46.7438276087415,40.0913643921631));
#196474=CARTESIAN_POINT('Ctrl Pts',(41.9874523371586,46.7462229640883,40.0889118607713));
#196475=CARTESIAN_POINT('Ctrl Pts',(41.9841593316988,46.7474206417617,40.0876855950754));
#196476=CARTESIAN_POINT('Ctrl Pts',(41.9808575622229,46.7485046297342,40.0863782327526));
#196477=CARTESIAN_POINT('Ctrl Pts',(41.9775578801523,46.7494761782928,40.0850006373334));
#196478=CARTESIAN_POINT('Ctrl Pts',(41.9759080391171,46.7499619525721,40.0843118396237));
#196479=CARTESIAN_POINT('Ctrl Pts',(41.9742587070261,46.7504196286876,40.0836054919164));
#196480=CARTESIAN_POINT('Ctrl Pts',(41.9726111592845,46.7508494364808,40.0828829920417));
#196481=CARTESIAN_POINT('Ctrl Pts',(41.9721992723491,46.7509568884291,40.0827023670731));
#196482=CARTESIAN_POINT('Ctrl Pts',(41.9717874966612,46.751062598857,40.0825207326932));
#196483=CARTESIAN_POINT('Ctrl Pts',(41.9713758515963,46.7511665718601,40.0823381109275));
#196484=CARTESIAN_POINT('Ctrl Pts',(41.9701409164017,46.7514784908694,40.0817902456303));
#196485=CARTESIAN_POINT('Ctrl Pts',(41.9689071581774,46.7517747718019,40.0812334935553));
#196486=CARTESIAN_POINT('Ctrl Pts',(41.9676750878624,46.7520555364228,40.0806684524227));
#196487=CARTESIAN_POINT('Ctrl Pts',(41.9591607175417,46.7539957941549,40.0767636676136));
#196488=CARTESIAN_POINT('Ctrl Pts',(41.9507055072917,46.7552464720204,40.0724404510887));
#196489=CARTESIAN_POINT('Ctrl Pts',(41.9423805287167,46.7559027543576,40.0677949937407));
#196490=CARTESIAN_POINT('Ctrl Pts',(41.9382430372167,46.7562289248776,40.0654862141904));
#196491=CARTESIAN_POINT('Ctrl Pts',(41.9341372814972,46.756407844619,40.0630972003215));
#196492=CARTESIAN_POINT('Ctrl Pts',(41.9300700339489,46.7564487173138,40.0606363359906));
#196493=CARTESIAN_POINT('Ctrl Pts',(41.9210970783574,46.7565388885834,40.0552073017123));
#196494=CARTESIAN_POINT('Ctrl Pts',(41.9123126321659,46.7559695796221,40.0494204304519));
#196495=CARTESIAN_POINT('Ctrl Pts',(41.903846506269,46.7548061840812,40.0434049749851));
#196496=CARTESIAN_POINT('Ctrl Pts',(41.9007537237153,46.754381181019,40.0412074532442));
#196497=CARTESIAN_POINT('Ctrl Pts',(41.8976992635451,46.7538836816018,40.0389814735788));
#196498=CARTESIAN_POINT('Ctrl Pts',(41.8946854937106,46.7533184435772,40.0367321210017));
#196499=CARTESIAN_POINT('Ctrl Pts',(41.8845625597433,46.7514198688641,40.0291767837137));
#196500=CARTESIAN_POINT('Ctrl Pts',(41.8748360802674,46.7487367327307,40.0213235332568));
#196501=CARTESIAN_POINT('Ctrl Pts',(41.8655137786572,46.7453971059997,40.0132649215846));
#196502=CARTESIAN_POINT('Ctrl Pts',(41.8552674648883,46.7417264606175,40.0044075527515));
#196503=CARTESIAN_POINT('Ctrl Pts',(41.8455087367141,46.7372626589199,39.9953016253697));
#196504=CARTESIAN_POINT('Ctrl Pts',(41.8362508575433,46.7321227530947,39.986035342233));
#196505=CARTESIAN_POINT('Ctrl Pts',(41.8262797250076,46.7265868542934,39.976055158266));
#196506=CARTESIAN_POINT('Ctrl Pts',(41.8168884800858,46.7202662104726,39.9658879738113));
#196507=CARTESIAN_POINT('Ctrl Pts',(41.8081115112066,46.7132528291601,39.9556174643203));
#196508=CARTESIAN_POINT('Ctrl Pts',(41.7994530610437,46.7063341521769,39.9454856413871));
#196509=CARTESIAN_POINT('Ctrl Pts',(41.791391507518,46.6987402031241,39.9352519465097));
#196510=CARTESIAN_POINT('Ctrl Pts',(41.7839914803032,46.6905216402892,39.92499));
#196511=CARTESIAN_POINT('Ctrl Pts',(39.4820551873935,44.1339623850442,39.92499));
#196512=CARTESIAN_POINT('Ctrl Pts',(39.4749733207254,44.1260971752943,39.9348107241722));
#196513=CARTESIAN_POINT('Ctrl Pts',(39.4685372764365,44.1177016730294,39.9446038383168));
#196514=CARTESIAN_POINT('Ctrl Pts',(39.4627751762759,44.1088266671093,39.9543158069383));
#196515=CARTESIAN_POINT('Ctrl Pts',(39.457211361599,44.100257068036,39.9636935671389));
#196516=CARTESIAN_POINT('Ctrl Pts',(39.4522752837276,44.0912392969017,39.9729968320986));
#196517=CARTESIAN_POINT('Ctrl Pts',(39.4480294591806,44.0817922708751,39.9821731151332));
#196518=CARTESIAN_POINT('Ctrl Pts',(39.4440158252738,44.0728618726545,39.9908475764349));
#196519=CARTESIAN_POINT('Ctrl Pts',(39.4406186435292,44.0635470605566,39.9994093733843));
#196520=CARTESIAN_POINT('Ctrl Pts',(39.43793124934,44.0538529442829,40.0077966115839));
#196521=CARTESIAN_POINT('Ctrl Pts',(39.4354562043761,44.0449248258259,40.0155211172592));
#196522=CARTESIAN_POINT('Ctrl Pts',(39.4335831186691,44.0356744386791,40.0230979941019));
#196523=CARTESIAN_POINT('Ctrl Pts',(39.4324230329126,44.0261054688002,40.0304554104745));
#196524=CARTESIAN_POINT('Ctrl Pts',(39.4320771187579,44.0232521951443,40.0326492435179));
#196525=CARTESIAN_POINT('Ctrl Pts',(39.431794878803,44.0203706219328,40.0348233715059));
#196526=CARTESIAN_POINT('Ctrl Pts',(39.4315800126161,44.0174609456692,40.0369753512355));
#196527=CARTESIAN_POINT('Ctrl Pts',(39.4313673418322,44.014580999127,40.0391053430352));
#196528=CARTESIAN_POINT('Ctrl Pts',(39.4312206224788,44.01167652945,40.041211089324));
#196529=CARTESIAN_POINT('Ctrl Pts',(39.4311433701099,44.0087510493741,40.0432881154904));
#196530=CARTESIAN_POINT('Ctrl Pts',(39.4311379981313,44.0085476172109,40.043432547828));
#196531=CARTESIAN_POINT('Ctrl Pts',(39.4311329512716,44.0083440782819,40.0435768364421));
#196532=CARTESIAN_POINT('Ctrl Pts',(39.4311282308207,44.008140432782,40.0437209807855));
#196533=CARTESIAN_POINT('Ctrl Pts',(39.4309212689598,43.9992118680539,40.0500407968421));
#196534=CARTESIAN_POINT('Ctrl Pts',(39.4313859080982,43.99008819718,40.0560490279346));
#196535=CARTESIAN_POINT('Ctrl Pts',(39.4325966403789,43.980858573769,40.0616647108617));
#196536=CARTESIAN_POINT('Ctrl Pts',(39.4337252532884,43.9722549606522,40.0668995033488));
#196537=CARTESIAN_POINT('Ctrl Pts',(39.4355025470901,43.9635585482846,40.0717933267485));
#196538=CARTESIAN_POINT('Ctrl Pts',(39.4380105519142,43.954861329077,40.0762460303076));
#196539=CARTESIAN_POINT('Ctrl Pts',(39.4389280125254,43.9516797737732,40.077874886875));
#196540=CARTESIAN_POINT('Ctrl Pts',(39.4399434521999,43.9484983634047,40.0794443522249));
#196541=CARTESIAN_POINT('Ctrl Pts',(39.4410615611728,43.9453226165467,40.0809482021492));
#196542=CARTESIAN_POINT('Ctrl Pts',(39.441330429028,43.9445589555196,40.0813098278169));
#196543=CARTESIAN_POINT('Ctrl Pts',(39.4416057093433,43.9437952833152,40.0816679525672));
#196544=CARTESIAN_POINT('Ctrl Pts',(39.4418874191266,43.9430317345445,40.0820224192581));
#196545=CARTESIAN_POINT('Ctrl Pts',(39.4421603254791,43.942292046673,40.0823658088648));
#196546=CARTESIAN_POINT('Ctrl Pts',(39.4424392657175,43.9415524746574,40.0827057654617));
#196547=CARTESIAN_POINT('Ctrl Pts',(39.442724252473,43.9408131433995,40.0830421470151));
#196548=CARTESIAN_POINT('Ctrl Pts',(39.445846611731,43.9327129150432,40.0867275956805));
#196549=CARTESIAN_POINT('Ctrl Pts',(39.4496972096654,43.9246364083437,40.0899823432028));
#196550=CARTESIAN_POINT('Ctrl Pts',(39.4542738890611,43.9167721156746,40.0926299529352));
#196551=CARTESIAN_POINT('Ctrl Pts',(39.456171974423,43.9135105590948,40.0937279956082));
#196552=CARTESIAN_POINT('Ctrl Pts',(39.4581945203286,43.910285532495,40.0947220371802));
#196553=CARTESIAN_POINT('Ctrl Pts',(39.4603395741455,43.9071101492104,40.0956014538693));
#196554=CARTESIAN_POINT('Ctrl Pts',(39.4639981869602,43.9016942021211,40.097101390674));
#196555=CARTESIAN_POINT('Ctrl Pts',(39.4680136963365,43.8964251099352,40.0982667904316));
#196556=CARTESIAN_POINT('Ctrl Pts',(39.4723737491585,43.8913745966871,40.0990539325582));
#196557=CARTESIAN_POINT('Ctrl Pts',(39.4745537755695,43.888849340063,40.0994475036216));
#196558=CARTESIAN_POINT('Ctrl Pts',(39.4768209551515,43.8863797569638,40.0997467259952));
#196559=CARTESIAN_POINT('Ctrl Pts',(39.4791737454933,43.8839748786089,40.0999473488896));
#196560=CARTESIAN_POINT('Ctrl Pts',(39.481526535835,43.8815700002539,40.100147971784));
#196561=CARTESIAN_POINT('Ctrl Pts',(39.4839648939622,43.8792298420736,40.10025));
#196562=CARTESIAN_POINT('Ctrl Pts',(39.4864862581822,43.876961627587,40.10025));
#196563=CARTESIAN_POINT('Origin',(43.3086183250771,38.9747476500508,39.92499));
#196564=CARTESIAN_POINT('Ctrl Pts',(46.6905216402902,41.7839914803021,39.92499));
#196565=CARTESIAN_POINT('Ctrl Pts',(46.6984066517725,41.7910911765301,39.9348354642018));
#196566=CARTESIAN_POINT('Ctrl Pts',(46.7057080773548,41.7987919603583,39.9446440828458));
#196567=CARTESIAN_POINT('Ctrl Pts',(46.7123936319703,41.8070443420764,39.9543641760331));
#196568=CARTESIAN_POINT('Ctrl Pts',(46.7188619458706,41.8150285705283,39.9637684240712));
#196569=CARTESIAN_POINT('Ctrl Pts',(46.7247545199412,41.8235301761251,39.9730909636396));
#196570=CARTESIAN_POINT('Ctrl Pts',(46.7300083326608,41.8325358446865,39.982280897714));
#196571=CARTESIAN_POINT('Ctrl Pts',(46.7349781159823,41.8410546526084,39.9909740094649));
#196572=CARTESIAN_POINT('Ctrl Pts',(46.7393768060084,41.8500252953099,39.9995492765001));
#196573=CARTESIAN_POINT('Ctrl Pts',(46.743111977297,41.8594521748273,40.0079462328694));
#196574=CARTESIAN_POINT('Ctrl Pts',(46.7465523401882,41.8681350126322,40.0156804369689));
#196575=CARTESIAN_POINT('Ctrl Pts',(46.7494299450227,41.8772054497762,40.0232638017421));
#196576=CARTESIAN_POINT('Ctrl Pts',(46.7516345991556,41.8866715402891,40.0306257269965));
#196577=CARTESIAN_POINT('Ctrl Pts',(46.7522740855143,41.8894172933139,40.0327611416651));
#196578=CARTESIAN_POINT('Ctrl Pts',(46.7528566833419,41.8921963397415,40.0348777427271));
#196579=CARTESIAN_POINT('Ctrl Pts',(46.7533790039321,41.8950088623274,40.0369733168701));
#196580=CARTESIAN_POINT('Ctrl Pts',(46.753945233034,41.898057817639,40.039245053974));
#196581=CARTESIAN_POINT('Ctrl Pts',(46.7544408966258,41.9011416752728,40.041487875195));
#196582=CARTESIAN_POINT('Ctrl Pts',(46.7548620578771,41.9042597210851,40.0436985701601));
#196583=CARTESIAN_POINT('Ctrl Pts',(46.7560179382359,41.9128172222839,40.0497658398386));
#196584=CARTESIAN_POINT('Ctrl Pts',(46.7565684843263,41.9216270724806,40.0555581699984));
#196585=CARTESIAN_POINT('Ctrl Pts',(46.7564556264623,41.9306033478345,40.0609828468885));
#196586=CARTESIAN_POINT('Ctrl Pts',(46.7563523676439,41.9388161524503,40.0659461317306));
#196587=CARTESIAN_POINT('Ctrl Pts',(46.7556849461651,41.9471607721488,40.070603998071));
#196588=CARTESIAN_POINT('Ctrl Pts',(46.7543795041532,41.955588190611,40.0748843180608));
#196589=CARTESIAN_POINT('Ctrl Pts',(46.7537382753015,41.9597277110298,40.0769867972572));
#196590=CARTESIAN_POINT('Ctrl Pts',(46.7529426662697,41.9638869554867,40.0789976708176));
#196591=CARTESIAN_POINT('Ctrl Pts',(46.7519812518,41.968058097036,40.0809050491499));
#196592=CARTESIAN_POINT('Ctrl Pts',(46.7517988327686,41.9688495305176,40.0812669556104));
#196593=CARTESIAN_POINT('Ctrl Pts',(46.7516099985535,41.9696416823153,40.0816253922032));
#196594=CARTESIAN_POINT('Ctrl Pts',(46.7514147143012,41.9704344168199,40.0819801989139));
#196595=CARTESIAN_POINT('Ctrl Pts',(46.7512255326818,41.9712023783711,40.0823239179149));
#196596=CARTESIAN_POINT('Ctrl Pts',(46.751030297871,41.9719708867607,40.0826642303498));
#196597=CARTESIAN_POINT('Ctrl Pts',(46.7508289807697,41.9727398158583,40.0830009916099));
#196598=CARTESIAN_POINT('Ctrl Pts',(46.7486350684821,41.9811194467227,40.0866709464314));
#196599=CARTESIAN_POINT('Ctrl Pts',(46.7457169794822,41.9895544525285,40.0899175831881));
#196600=CARTESIAN_POINT('Ctrl Pts',(46.7420530111684,41.9978556152131,40.0925642067066));
#196601=CARTESIAN_POINT('Ctrl Pts',(46.7405056945977,42.0013612477617,40.093681892253));
#196602=CARTESIAN_POINT('Ctrl Pts',(46.7388257854549,42.0048429302643,40.0946930094791));
#196603=CARTESIAN_POINT('Ctrl Pts',(46.7370135816694,42.0082865614558,40.0955863397545));
#196604=CARTESIAN_POINT('Ctrl Pts',(46.733961875776,42.0140855503361,40.0970906856166));
#196605=CARTESIAN_POINT('Ctrl Pts',(46.7305342346691,42.0197742252481,40.0982599215483));
#196606=CARTESIAN_POINT('Ctrl Pts',(46.7267341265709,42.0252784509096,40.0990497370453));
#196607=CARTESIAN_POINT('Ctrl Pts',(46.7257840995464,42.026654507325,40.0992471909196));
#196608=CARTESIAN_POINT('Ctrl Pts',(46.7248106099125,42.0280188904098,40.0994209989363));
#196609=CARTESIAN_POINT('Ctrl Pts',(46.723813477807,42.0293702408562,40.0995705982975));
#196610=CARTESIAN_POINT('Ctrl Pts',(46.7223177796487,42.0313972665257,40.0997949973393));
#196611=CARTESIAN_POINT('Ctrl Pts',(46.7207688863879,42.0333949481511,40.0999649129781));
#196612=CARTESIAN_POINT('Ctrl Pts',(46.7191674503113,42.0353598072039,40.1000786629733));
#196613=CARTESIAN_POINT('Ctrl Pts',(46.7175660142347,42.0373246662567,40.1001924129685));
#196614=CARTESIAN_POINT('Ctrl Pts',(46.7159120469168,42.0392567035858,40.10025));
#196615=CARTESIAN_POINT('Ctrl Pts',(46.7142062431428,42.041152784689,40.10025));
#196616=CARTESIAN_POINT('Ctrl Pts',(43.8769616275879,39.4864862581812,40.10025));
#196617=CARTESIAN_POINT('Ctrl Pts',(43.8827333680738,39.4800703482071,40.10025));
#196618=CARTESIAN_POINT('Ctrl Pts',(43.8889846873397,39.4741864828754,40.0995786334241));
#196619=CARTESIAN_POINT('Ctrl Pts',(43.895569202337,39.468872166017,40.0983063763367));
#196620=CARTESIAN_POINT('Ctrl Pts',(43.8998221234153,39.4654396626066,40.0974846287993));
#196621=CARTESIAN_POINT('Ctrl Pts',(43.90421346894,39.4622440309668,40.0964130309338));
#196622=CARTESIAN_POINT('Ctrl Pts',(43.9086997575138,39.4592874976149,40.0951176960923));
#196623=CARTESIAN_POINT('Ctrl Pts',(43.9146460760275,39.4553687820177,40.0934008039613));
#196624=CARTESIAN_POINT('Ctrl Pts',(43.9207613318567,39.4518755008528,40.0912909372156));
#196625=CARTESIAN_POINT('Ctrl Pts',(43.9269559348858,39.4488169076804,40.0888630467851));
#196626=CARTESIAN_POINT('Ctrl Pts',(43.9300532364004,39.4472876110942,40.0876491015698));
#196627=CARTESIAN_POINT('Ctrl Pts',(43.9331705067656,39.4458668372377,40.0863558569271));
#196628=CARTESIAN_POINT('Ctrl Pts',(43.936297487834,39.4445546869044,40.084993634277));
#196629=CARTESIAN_POINT('Ctrl Pts',(43.9378609783682,39.4438986117377,40.084312522952));
#196630=CARTESIAN_POINT('Ctrl Pts',(43.9394269075365,39.4432696802085,40.0836141747073));
#196631=CARTESIAN_POINT('Ctrl Pts',(43.9409940617759,39.4426678279629,40.0828999161609));
#196632=CARTESIAN_POINT('Ctrl Pts',(43.9413858503357,39.4425173649016,40.0827213515243));
#196633=CARTESIAN_POINT('Ctrl Pts',(43.9417777156948,39.4423685940343,40.0825417925841));
#196634=CARTESIAN_POINT('Ctrl Pts',(43.9421696393595,39.4422215138288,40.082361260236));
#196635=CARTESIAN_POINT('Ctrl Pts',(43.9433454103534,39.4417802732124,40.0818196631917));
#196636=CARTESIAN_POINT('Ctrl Pts',(43.9445217049433,39.4413542498599,40.0812693052021));
#196637=CARTESIAN_POINT('Ctrl Pts',(43.9456980341199,39.4409433907172,40.0807107531874));
#196638=CARTESIAN_POINT('Ctrl Pts',(43.953983944948,39.4380493519679,40.0767763849183));
#196639=CARTESIAN_POINT('Ctrl Pts',(43.962285917344,39.4358558447891,40.0724140586141));
#196640=CARTESIAN_POINT('Ctrl Pts',(43.9705207686456,39.4342768603232,40.0677221223774));
#196641=CARTESIAN_POINT('Ctrl Pts',(43.9745146626288,39.4335110545633,40.0654465383724));
#196642=CARTESIAN_POINT('Ctrl Pts',(43.97849322547,39.432890153227,40.0630928000681));
#196643=CARTESIAN_POINT('Ctrl Pts',(43.982449005934,39.4324063524311,40.0606689262479));
#196644=CARTESIAN_POINT('Ctrl Pts',(43.9885050294416,39.4316656872148,40.0569581447805));
#196645=CARTESIAN_POINT('Ctrl Pts',(43.9945041897575,39.4312456873364,40.0530843804605));
#196646=CARTESIAN_POINT('Ctrl Pts',(44.0004074287827,39.4311218425057,40.0490800251457));
#196647=CARTESIAN_POINT('Ctrl Pts',(44.0031489235253,39.4310643283256,40.0472203818218));
#196648=CARTESIAN_POINT('Ctrl Pts',(44.0058696426795,39.4310704471407,40.0453323608818));
#196649=CARTESIAN_POINT('Ctrl Pts',(44.0085654321305,39.4311389525606,40.0434201572162));
#196650=CARTESIAN_POINT('Ctrl Pts',(44.0087720537699,39.4311442032311,40.0432735943397));
#196651=CARTESIAN_POINT('Ctrl Pts',(44.0089785427603,39.4311497894108,40.0431268995707));
#196652=CARTESIAN_POINT('Ctrl Pts',(44.0091848981962,39.4311557099535,40.0429800745037));
#196653=CARTESIAN_POINT('Ctrl Pts',(44.0120835699302,39.4312388757294,40.0409176249753));
#196654=CARTESIAN_POINT('Ctrl Pts',(44.0149559644988,39.4313901062469,40.0388310783332));
#196655=CARTESIAN_POINT('Ctrl Pts',(44.0177981990788,39.4316052205101,40.036725739981));
#196656=CARTESIAN_POINT('Ctrl Pts',(44.0279899468071,39.4323765820008,40.0291763710725));
#196657=CARTESIAN_POINT('Ctrl Pts',(44.0378728316076,39.4339733733557,40.021331089461));
#196658=CARTESIAN_POINT('Ctrl Pts',(44.0474262866297,39.4362681192138,40.0132837551344));
#196659=CARTESIAN_POINT('Ctrl Pts',(44.057924573969,39.4387898143842,40.0044405431362));
#196660=CARTESIAN_POINT('Ctrl Pts',(44.0680257165045,39.4421543412245,39.9953528710651));
#196661=CARTESIAN_POINT('Ctrl Pts',(44.0777053474358,39.4462454222028,39.9861103629619));
#196662=CARTESIAN_POINT('Ctrl Pts',(44.088156919585,39.4506627629378,39.9761307737641));
#196663=CARTESIAN_POINT('Ctrl Pts',(44.0981181930469,39.4559274600877,39.9659696936119));
#196664=CARTESIAN_POINT('Ctrl Pts',(44.1075472421415,39.461949460792,39.9557128217636));
#196665=CARTESIAN_POINT('Ctrl Pts',(44.1168971912083,39.4679209431018,39.9455419945248));
#196666=CARTESIAN_POINT('Ctrl Pts',(44.1257248429258,39.4746380711531,39.9352756289384));
#196667=CARTESIAN_POINT('Ctrl Pts',(44.1339623850452,39.4820551873925,39.92499));
#196668=CARTESIAN_POINT('Origin',(-0.0101975504409074,0.0113255271402718,
39.92499));
#196669=CARTESIAN_POINT('Ctrl Pts',(46.6938111422609,42.0638038389695,40.10025));
#196670=CARTESIAN_POINT('Ctrl Pts',(46.6880613546461,42.07018425683,40.10025));
#196671=CARTESIAN_POINT('Ctrl Pts',(46.6818296739378,42.0760276657218,40.0995859581842));
#196672=CARTESIAN_POINT('Ctrl Pts',(46.6752630175681,42.0812997491639,40.0983275959621));
#196673=CARTESIAN_POINT('Ctrl Pts',(46.6710672367553,42.0846683595044,40.0975235624068));
#196674=CARTESIAN_POINT('Ctrl Pts',(46.6667352666015,42.0878044626432,40.096477705949));
#196675=CARTESIAN_POINT('Ctrl Pts',(46.6623093164294,42.0907067742411,40.0952149915961));
#196676=CARTESIAN_POINT('Ctrl Pts',(46.6562687825189,42.0946678472186,40.0934916398701));
#196677=CARTESIAN_POINT('Ctrl Pts',(46.6500510792886,42.098187735286,40.0913643921631));
#196678=CARTESIAN_POINT('Ctrl Pts',(46.6437515300393,42.101258394226,40.0889118607713));
#196679=CARTESIAN_POINT('Ctrl Pts',(46.6406017554146,42.1027937236961,40.0876855950755));
#196680=CARTESIAN_POINT('Ctrl Pts',(46.6374313809743,42.1042169023584,40.0863782327527));
#196681=CARTESIAN_POINT('Ctrl Pts',(46.6342513293852,42.1055280393685,40.0850006373334));
#196682=CARTESIAN_POINT('Ctrl Pts',(46.6326613035906,42.1061836078735,40.0843118396238));
#196683=CARTESIAN_POINT('Ctrl Pts',(46.6310688468945,42.1068111789402,40.0836054919165));
#196684=CARTESIAN_POINT('Ctrl Pts',(46.6294752517399,42.1074108478349,40.0828829920418));
#196685=CARTESIAN_POINT('Ctrl Pts',(46.6290768529512,42.1075607650586,40.0827023670731));
#196686=CARTESIAN_POINT('Ctrl Pts',(46.6286783827623,42.1077089386736,40.0825207326933));
#196687=CARTESIAN_POINT('Ctrl Pts',(46.6282798608704,42.1078553707278,40.0823381109276));
#196688=CARTESIAN_POINT('Ctrl Pts',(46.6270842951947,42.1082946668902,40.0817902456304));
#196689=CARTESIAN_POINT('Ctrl Pts',(46.6258882654176,42.108718287616,40.0812334935553));
#196690=CARTESIAN_POINT('Ctrl Pts',(46.6246922924071,42.1091263005955,40.0806684524227));
#196691=CARTESIAN_POINT('Ctrl Pts',(46.616427376857,42.1119459234381,40.0767636676137));
#196692=CARTESIAN_POINT('Ctrl Pts',(46.608149216569,42.1140735600934,40.0724404510889));
#196693=CARTESIAN_POINT('Ctrl Pts',(46.599938443282,42.1155964444644,40.067794993741));
#196694=CARTESIAN_POINT('Ctrl Pts',(46.5958577114965,42.1163533138166,40.0654862141906));
#196695=CARTESIAN_POINT('Ctrl Pts',(46.5917931497418,42.1169604217528,40.0630972003216));
#196696=CARTESIAN_POINT('Ctrl Pts',(46.5877524553609,42.1174262136787,40.0606363359906));
#196697=CARTESIAN_POINT('Ctrl Pts',(46.5788380800233,42.1184538202395,40.0552073017124));
#196698=CARTESIAN_POINT('Ctrl Pts',(46.5700422469563,42.1188058546733,40.0494204304519));
#196699=CARTESIAN_POINT('Ctrl Pts',(46.5615008914348,42.1185337834648,40.0434049749851));
#196700=CARTESIAN_POINT('Ctrl Pts',(46.5583806265506,42.1184343924214,40.0412074532442));
#196701=CARTESIAN_POINT('Ctrl Pts',(46.5552908961832,42.1182588963858,40.0389814735788));
#196702=CARTESIAN_POINT('Ctrl Pts',(46.5522345526332,42.1180117795237,40.0367321210016));
#196703=CARTESIAN_POINT('Ctrl Pts',(46.5419686180606,42.117181740133,40.0291767837139));
#196704=CARTESIAN_POINT('Ctrl Pts',(46.5320149571606,42.1155299964529,40.0213235332572));
#196705=CARTESIAN_POINT('Ctrl Pts',(46.5223946380443,42.1131831104082,40.0132649215852));
#196706=CARTESIAN_POINT('Ctrl Pts',(46.5118207677339,42.1106036046381,40.0044075527524));
#196707=CARTESIAN_POINT('Ctrl Pts',(46.5016489045623,42.107184320973,39.9953016253708));
#196708=CARTESIAN_POINT('Ctrl Pts',(46.4919044745653,42.1030402839728,39.9860353422344));
#196709=CARTESIAN_POINT('Ctrl Pts',(46.4814093059429,42.0985769785657,39.9760551582678));
#196710=CARTESIAN_POINT('Ctrl Pts',(46.4714088200582,42.0932726122933,39.9658879738136));
#196711=CARTESIAN_POINT('Ctrl Pts',(46.4619468343622,42.0872150940869,39.9556174643231));
#196712=CARTESIAN_POINT('Ctrl Pts',(46.4526126174212,42.0812393728293,39.9454856413889));
#196713=CARTESIAN_POINT('Ctrl Pts',(46.4438014421035,42.0745296860248,39.9352519465105));
#196714=CARTESIAN_POINT('Ctrl Pts',(46.4355828792675,42.067129658809,39.92499));
#196715=CARTESIAN_POINT('Ctrl Pts',(43.8790236240225,39.7651933658994,39.92499));
#196716=CARTESIAN_POINT('Ctrl Pts',(43.8711584142728,39.7581114992315,39.9348107241718));
#196717=CARTESIAN_POINT('Ctrl Pts',(43.8638800583581,39.7504347382259,39.9446038383161));
#196718=CARTESIAN_POINT('Ctrl Pts',(43.857221832855,39.7422106539921,39.9543158069372));
#196719=CARTESIAN_POINT('Ctrl Pts',(43.8507927303151,39.7342695770775,39.9636935671376));
#196720=CARTESIAN_POINT('Ctrl Pts',(43.8449410790361,39.7258171668717,39.972996832097));
#196721=CARTESIAN_POINT('Ctrl Pts',(43.8397310304473,39.7168657021576,39.9821731151314));
#196722=CARTESIAN_POINT('Ctrl Pts',(43.8348059028446,39.7084037645775,39.990847576433));
#196723=CARTESIAN_POINT('Ctrl Pts',(43.8304536682228,39.6994950821822,39.9994093733823));
#196724=CARTESIAN_POINT('Ctrl Pts',(43.8267676847832,39.6901349804769,40.0077966115818));
#196725=CARTESIAN_POINT('Ctrl Pts',(43.8233729558724,39.6815144838336,40.0155211172571));
#196726=CARTESIAN_POINT('Ctrl Pts',(43.8205432023716,39.6725105620462,40.0230979940998));
#196727=CARTESIAN_POINT('Ctrl Pts',(43.8183892419697,39.6631152739669,40.0304554104725));
#196728=CARTESIAN_POINT('Ctrl Pts',(43.8177469744581,39.6603137887169,40.0326492435165));
#196729=CARTESIAN_POINT('Ctrl Pts',(43.8171650742235,39.6574775031728,40.0348233715053));
#196730=CARTESIAN_POINT('Ctrl Pts',(43.8166472411075,39.6546062260516,40.0369753512355));
#196731=CARTESIAN_POINT('Ctrl Pts',(43.81613469897,39.6517642863081,40.0391053430352));
#196732=CARTESIAN_POINT('Ctrl Pts',(43.8156851836086,39.6488910639685,40.041211089324));
#196733=CARTESIAN_POINT('Ctrl Pts',(43.8153025584996,39.6459896850499,40.0432881154904));
#196734=CARTESIAN_POINT('Ctrl Pts',(43.8152759514979,39.6457879288341,40.043432547828));
#196735=CARTESIAN_POINT('Ctrl Pts',(43.815249656674,39.6455860324532,40.0435768364421));
#196736=CARTESIAN_POINT('Ctrl Pts',(43.815223675331,39.6453839959661,40.0437209807855));
#196737=CARTESIAN_POINT('Ctrl Pts',(43.8140845580787,39.6365259762551,40.050040796842));
#196738=CARTESIAN_POINT('Ctrl Pts',(43.8135929685794,39.6274037177898,40.0560490279344));
#196739=CARTESIAN_POINT('Ctrl Pts',(43.8138323099903,39.618098099237,40.0616647108614));
#196740=CARTESIAN_POINT('Ctrl Pts',(43.8140554177825,39.6094236454401,40.0668995033485));
#196741=CARTESIAN_POINT('Ctrl Pts',(43.8149139527621,39.6005890951397,40.0717933267481));
#196742=CARTESIAN_POINT('Ctrl Pts',(43.8164991115148,39.5916773623189,40.0762460303072));
#196743=CARTESIAN_POINT('Ctrl Pts',(43.817078983094,39.5884173351599,40.0778748868748));
#196744=CARTESIAN_POINT('Ctrl Pts',(43.817756312147,39.5851472105413,40.0794443522247));
#196745=CARTESIAN_POINT('Ctrl Pts',(43.8185363400632,39.581871986544,40.0809482021491));
#196746=CARTESIAN_POINT('Ctrl Pts',(43.8187239107186,39.5810844045881,40.0813098278168));
#196747=CARTESIAN_POINT('Ctrl Pts',(43.8189178575375,39.5802961412316,40.0816679525672));
#196748=CARTESIAN_POINT('Ctrl Pts',(43.8191182115055,39.5795073285703,40.082022419258));
#196749=CARTESIAN_POINT('Ctrl Pts',(43.819312304412,39.5787431663046,40.0823658088648));
#196750=CARTESIAN_POINT('Ctrl Pts',(43.8195124102603,39.5779784885475,40.0827057654616));
#196751=CARTESIAN_POINT('Ctrl Pts',(43.8197185546683,39.577213418196,40.0830421470151));
#196752=CARTESIAN_POINT('Ctrl Pts',(43.8219771048936,39.5688311883225,40.0867275956807));
#196753=CARTESIAN_POINT('Ctrl Pts',(43.824962384016,39.5603964284863,40.0899823432032));
#196754=CARTESIAN_POINT('Ctrl Pts',(43.8286919494561,39.5520968239707,40.0926299529357));
#196755=CARTESIAN_POINT('Ctrl Pts',(43.8302387114104,39.5486547305936,40.0937279956085));
#196756=CARTESIAN_POINT('Ctrl Pts',(43.8319130705232,39.5452359574122,40.0947220371803));
#196757=CARTESIAN_POINT('Ctrl Pts',(43.8337144555755,39.5418537500311,40.0956014538692));
#196758=CARTESIAN_POINT('Ctrl Pts',(43.8367869054999,39.5360850428914,40.097101390674));
#196759=CARTESIAN_POINT('Ctrl Pts',(43.8402296473868,39.5304250803195,40.0982667904316));
#196760=CARTESIAN_POINT('Ctrl Pts',(43.8440378929946,39.52494648469,40.0990539325582));
#196761=CARTESIAN_POINT('Ctrl Pts',(43.8459420157984,39.5222071868753,40.0994475036216));
#196762=CARTESIAN_POINT('Ctrl Pts',(43.8479386338072,39.5195141476131,40.0997467259952));
#196763=CARTESIAN_POINT('Ctrl Pts',(43.8500271570785,39.5168765098746,40.0999473488896));
#196764=CARTESIAN_POINT('Ctrl Pts',(43.8521156803499,39.5142388721361,40.100147971784));
#196765=CARTESIAN_POINT('Ctrl Pts',(43.8542960677578,39.5116566557593,40.10025));
#196766=CARTESIAN_POINT('Ctrl Pts',(43.8565665267061,39.5091373124617,40.10025));
#196767=CARTESIAN_POINT('Origin',(47.1453396605412,34.2342565846631,39.92499));
#196768=CARTESIAN_POINT('Ctrl Pts',(50.8023624960595,36.6746059268172,39.92499));
#196769=CARTESIAN_POINT('Ctrl Pts',(50.8109464329608,36.6808425220337,39.9348354642024));
#196770=CARTESIAN_POINT('Ctrl Pts',(50.8190128116699,36.6877379133671,39.944644082847));
#196771=CARTESIAN_POINT('Ctrl Pts',(50.8265243508974,36.6952462569251,39.9543641760349));
#196772=CARTESIAN_POINT('Ctrl Pts',(50.8337918098282,36.7025106240267,39.9637684240734));
#196773=CARTESIAN_POINT('Ctrl Pts',(50.8405407635302,36.7103497152267,39.9730909636422));
#196774=CARTESIAN_POINT('Ctrl Pts',(50.8467071440096,36.7187568768241,39.9822808977171));
#196775=CARTESIAN_POINT('Ctrl Pts',(50.8525401602392,36.726709534012,39.9909740094683));
#196776=CARTESIAN_POINT('Ctrl Pts',(50.8578524412773,36.7351712462859,39.9995492765038));
#196777=CARTESIAN_POINT('Ctrl Pts',(50.8625525281361,36.7441560526567,40.0079462328735));
#196778=CARTESIAN_POINT('Ctrl Pts',(50.866881648052,36.7524317091221,40.0156804369733));
#196779=CARTESIAN_POINT('Ctrl Pts',(50.8706916079218,36.7611516658517,40.0232638017468));
#196780=CARTESIAN_POINT('Ctrl Pts',(50.8738736606229,36.7703354510224,40.0306257270015));
#196781=CARTESIAN_POINT('Ctrl Pts',(50.8747966531518,36.7729993179964,40.0327611416684));
#196782=CARTESIAN_POINT('Ctrl Pts',(50.8756665488992,36.7757022424592,40.0348777427287));
#196783=CARTESIAN_POINT('Ctrl Pts',(50.8764799968257,36.7784447603813,40.03697331687));
#196784=CARTESIAN_POINT('Ctrl Pts',(50.8773618266786,36.7814178261388,40.039245053974));
#196785=CARTESIAN_POINT('Ctrl Pts',(50.8781771258728,36.7844329791242,40.041487875195));
#196786=CARTESIAN_POINT('Ctrl Pts',(50.8789219044958,36.7874899206169,40.0436985701601));
#196787=CARTESIAN_POINT('Ctrl Pts',(50.8809659552707,36.7958797205311,40.0497658398386));
#196788=CARTESIAN_POINT('Ctrl Pts',(50.8824343655147,36.8045837617098,40.0555581699984));
#196789=CARTESIAN_POINT('Ctrl Pts',(50.8832604021666,36.8135226609472,40.0609828468886));
#196790=CARTESIAN_POINT('Ctrl Pts',(50.8840161808564,36.8217012684452,40.0659461317304));
#196791=CARTESIAN_POINT('Ctrl Pts',(50.8842246658559,36.8300699399849,40.0706039980705));
#196792=CARTESIAN_POINT('Ctrl Pts',(50.8838072802932,36.8385876480138,40.0748843180601));
#196793=CARTESIAN_POINT('Ctrl Pts',(50.8836022618683,36.8427715183736,40.0769867972569));
#196794=CARTESIAN_POINT('Ctrl Pts',(50.8832457706974,36.8469911418441,40.0789976708175));
#196795=CARTESIAN_POINT('Ctrl Pts',(50.8827256259729,36.8512399286211,40.0809050491501));
#196796=CARTESIAN_POINT('Ctrl Pts',(50.8826269335777,36.8520460945283,40.0812669556106));
#196797=CARTESIAN_POINT('Ctrl Pts',(50.8825219362263,36.8528536453859,40.0816253922033));
#196798=CARTESIAN_POINT('Ctrl Pts',(50.8824105850811,36.8536624499707,40.081980198914));
#196799=CARTESIAN_POINT('Ctrl Pts',(50.8823027136591,36.8544459794122,40.082323917915));
#196800=CARTESIAN_POINT('Ctrl Pts',(50.8821888793662,36.8552306854272,40.0826642303499));
#196801=CARTESIAN_POINT('Ctrl Pts',(50.8820690400779,36.856016445618,40.08300099161));
#196802=CARTESIAN_POINT('Ctrl Pts',(50.8807630562085,36.8645794982668,40.0866709464312));
#196803=CARTESIAN_POINT('Ctrl Pts',(50.8787426510003,36.8732733195862,40.0899175831876));
#196804=CARTESIAN_POINT('Ctrl Pts',(50.8759664620674,36.8819119966094,40.092564206706));
#196805=CARTESIAN_POINT('Ctrl Pts',(50.8747940602417,36.8855601635604,40.0936818922527));
#196806=CARTESIAN_POINT('Ctrl Pts',(50.8734872887382,36.889198371364,40.094693009479));
#196807=CARTESIAN_POINT('Ctrl Pts',(50.8720449698708,36.8928125648611,40.0955863397546));
#196808=CARTESIAN_POINT('Ctrl Pts',(50.8696161409378,36.898898776401,40.0970906856167));
#196809=CARTESIAN_POINT('Ctrl Pts',(50.8668019052541,36.9049145742142,40.0982599215483));
#196810=CARTESIAN_POINT('Ctrl Pts',(50.863597962796,36.9107858666116,40.0990497370454));
#196811=CARTESIAN_POINT('Ctrl Pts',(50.8627969771814,36.912253689711,40.0992471909196));
#196812=CARTESIAN_POINT('Ctrl Pts',(50.8619714372928,36.913712355938,40.0994209989363));
#196813=CARTESIAN_POINT('Ctrl Pts',(50.8611210221667,36.9151605322318,40.0995705982975));
#196814=CARTESIAN_POINT('Ctrl Pts',(50.8598453994776,36.9173327966726,40.0997949973393));
#196815=CARTESIAN_POINT('Ctrl Pts',(50.8585138058065,36.9194814382213,40.0999649129781));
#196816=CARTESIAN_POINT('Ctrl Pts',(50.8571265262615,36.9216029292227,40.1000786629733));
#196817=CARTESIAN_POINT('Ctrl Pts',(50.8557392467166,36.923724420224,40.1001924129685));
#196818=CARTESIAN_POINT('Ctrl Pts',(50.8542962928989,36.9258187603134,40.10025));
#196819=CARTESIAN_POINT('Ctrl Pts',(50.8527980281403,36.9278827595331,40.10025));
#196820=CARTESIAN_POINT('Ctrl Pts',(47.7640607692767,34.683783783134,40.10025));
#196821=CARTESIAN_POINT('Ctrl Pts',(47.7691302463545,34.6767997090224,40.10025));
#196822=CARTESIAN_POINT('Ctrl Pts',(47.7747322888384,34.6702946353241,40.0995786334241));
#196823=CARTESIAN_POINT('Ctrl Pts',(47.7807252357994,34.6643211616153,40.0983063763366));
#196824=CARTESIAN_POINT('Ctrl Pts',(47.7845960646242,34.6604629105133,40.0974846287992));
#196825=CARTESIAN_POINT('Ctrl Pts',(47.7886293194339,34.6568257642789,40.0964130309338));
#196826=CARTESIAN_POINT('Ctrl Pts',(47.7927819897612,34.6534164822759,40.0951176960924));
#196827=CARTESIAN_POINT('Ctrl Pts',(47.7982861164005,34.6488976742765,40.0934008039614));
#196828=CARTESIAN_POINT('Ctrl Pts',(47.8040027249066,34.644784311377,40.0912909372157));
#196829=CARTESIAN_POINT('Ctrl Pts',(47.8098436832081,34.6410949611628,40.0888630467852));
#196830=CARTESIAN_POINT('Ctrl Pts',(47.8127641623589,34.6392502860557,40.0876491015699));
#196831=CARTESIAN_POINT('Ctrl Pts',(47.815715844683,34.6375114518661,40.0863558569271));
#196832=CARTESIAN_POINT('Ctrl Pts',(47.8186885387641,34.6358796311039,40.0849936342771));
#196833=CARTESIAN_POINT('Ctrl Pts',(47.8201748858046,34.6350637207227,40.0843125229521));
#196834=CARTESIAN_POINT('Ctrl Pts',(47.8216664954028,34.6342745503767,40.0836141747074));
#196835=CARTESIAN_POINT('Ctrl Pts',(47.8231621539169,34.6335121829164,40.082899916161));
#196836=CARTESIAN_POINT('Ctrl Pts',(47.8235360685455,34.6333215910513,40.0827213515243));
#196837=CARTESIAN_POINT('Ctrl Pts',(47.823910236435,34.6331326740826,40.0825417925842));
#196838=CARTESIAN_POINT('Ctrl Pts',(47.824284639033,34.6329454324195,40.0823612602361));
#196839=CARTESIAN_POINT('Ctrl Pts',(47.8254078468268,34.6323837074302,40.0818196631917));
#196840=CARTESIAN_POINT('Ctrl Pts',(47.8265331659854,34.6318370616124,40.0812693052022));
#196841=CARTESIAN_POINT('Ctrl Pts',(47.827660104633,34.631305493318,40.0807107531875));
#196842=CARTESIAN_POINT('Ctrl Pts',(47.8355981149521,34.6275611948897,40.076776384918));
#196843=CARTESIAN_POINT('Ctrl Pts',(47.8436253243409,34.6245119115559,40.0724140586133));
#196844=CARTESIAN_POINT('Ctrl Pts',(47.8516500154464,34.6220808005802,40.0677221223762));
#196845=CARTESIAN_POINT('Ctrl Pts',(47.8555419819605,34.6209017143842,40.0654465383716));
#196846=CARTESIAN_POINT('Ctrl Pts',(47.8594338479549,34.6198683413508,40.0630928000677));
#196847=CARTESIAN_POINT('Ctrl Pts',(47.8633173872852,34.6189736992135,40.0606689262479));
#196848=CARTESIAN_POINT('Ctrl Pts',(47.8692628146655,34.617604064608,40.0569581447805));
#196849=CARTESIAN_POINT('Ctrl Pts',(47.8751852090117,34.6165592825241,40.0530843804606));
#196850=CARTESIAN_POINT('Ctrl Pts',(47.881043164166,34.6158190596248,40.0490800251458));
#196851=CARTESIAN_POINT('Ctrl Pts',(47.8837636288446,34.6154752962809,40.0472203818218));
#196852=CARTESIAN_POINT('Ctrl Pts',(47.886470083205,34.6151969889843,40.0453323608818));
#196853=CARTESIAN_POINT('Ctrl Pts',(47.8891582656055,34.6149833323957,40.0434201572162));
#196854=CARTESIAN_POINT('Ctrl Pts',(47.8893643041946,34.61496695646,40.0432735943397));
#196855=CARTESIAN_POINT('Ctrl Pts',(47.8895702459314,34.6149509280612,40.0431268995707));
#196856=CARTESIAN_POINT('Ctrl Pts',(47.8897760897959,34.614935246154,40.0429800745037));
#196857=CARTESIAN_POINT('Ctrl Pts',(47.8926675754936,34.6147149626372,40.0409176249753));
#196858=CARTESIAN_POINT('Ctrl Pts',(47.8955400426778,34.614565117708,40.0388310783332));
#196859=CARTESIAN_POINT('Ctrl Pts',(47.8983891927627,34.6144819591398,40.036725739981));
#196860=CARTESIAN_POINT('Ctrl Pts',(47.9086057382628,34.6141837673035,40.0291763710718));
#196861=CARTESIAN_POINT('Ctrl Pts',(47.9186013937337,34.6147387685075,40.0213310894596));
#196862=CARTESIAN_POINT('Ctrl Pts',(47.9283423801886,34.6160223355356,40.0132837551323));
#196863=CARTESIAN_POINT('Ctrl Pts',(47.9390467457337,34.6174328467537,40.0044405431329));
#196864=CARTESIAN_POINT('Ctrl Pts',(47.9494442419749,34.619723085458,39.9953528710606));
#196865=CARTESIAN_POINT('Ctrl Pts',(47.959498481284,34.6227799581211,39.9861103629562));
#196866=CARTESIAN_POINT('Ctrl Pts',(47.9703545364683,34.6260806134269,39.9761307737563));
#196867=CARTESIAN_POINT('Ctrl Pts',(47.9808115517364,34.6302752334091,39.965969693602));
#196868=CARTESIAN_POINT('Ctrl Pts',(47.9908184179945,34.6352786409532,39.9557128217515));
#196869=CARTESIAN_POINT('Ctrl Pts',(48.000741336927,34.6402400750492,39.9455419945166));
#196870=CARTESIAN_POINT('Ctrl Pts',(48.0102227609135,34.6459976651,39.9352756289343));
#196871=CARTESIAN_POINT('Ctrl Pts',(48.019190476674,34.6525130919791,39.92499));
#196872=CARTESIAN_POINT('Origin',(-0.00895784724493606,0.012329418994271,
39.92499));
#196873=CARTESIAN_POINT('Ctrl Pts',(50.8348823336491,36.9525415975206,40.10025));
#196874=CARTESIAN_POINT('Ctrl Pts',(50.829830979246,36.9594880792485,40.10025));
#196875=CARTESIAN_POINT('Ctrl Pts',(50.8242442388878,36.9659508653435,40.0995859581841));
#196876=CARTESIAN_POINT('Ctrl Pts',(50.8182646381287,36.9718804702604,40.0983275959618));
#196877=CARTESIAN_POINT('Ctrl Pts',(50.8144439579048,36.9756692055211,40.0975235624065));
#196878=CARTESIAN_POINT('Ctrl Pts',(50.810463530779,36.9792409429414,40.0964777059488));
#196879=CARTESIAN_POINT('Ctrl Pts',(50.8063652005968,36.9825899931423,40.095214991596));
#196880=CARTESIAN_POINT('Ctrl Pts',(50.8007718022343,36.9871607746745,40.09349163987));
#196881=CARTESIAN_POINT('Ctrl Pts',(50.7949560887235,36.9913113073904,40.091364392163));
#196882=CARTESIAN_POINT('Ctrl Pts',(50.7890120203243,36.9950236271418,40.0889118607712));
#196883=CARTESIAN_POINT('Ctrl Pts',(50.7860399861247,36.9968797870175,40.0876855950754));
#196884=CARTESIAN_POINT('Ctrl Pts',(50.7830357420058,36.9986265637265,40.0863782327526));
#196885=CARTESIAN_POINT('Ctrl Pts',(50.7800101622089,37.0002629240965,40.0850006373333));
#196886=CARTESIAN_POINT('Ctrl Pts',(50.7784973723104,37.0010811042815,40.0843118396237));
#196887=CARTESIAN_POINT('Ctrl Pts',(50.7769792382978,37.0018716944995,40.0836054919164));
#196888=CARTESIAN_POINT('Ctrl Pts',(50.7754570554923,37.0026346543979,40.0828829920417));
#196889=CARTESIAN_POINT('Ctrl Pts',(50.7750765097909,37.0028253943725,40.082702367073));
#196890=CARTESIAN_POINT('Ctrl Pts',(50.7746957108236,37.0030144077534,40.0825207326932));
#196891=CARTESIAN_POINT('Ctrl Pts',(50.7743146783939,37.0032016945184,40.0823381109275));
#196892=CARTESIAN_POINT('Ctrl Pts',(50.7731715811049,37.0037635548134,40.0817902456303));
#196893=CARTESIAN_POINT('Ctrl Pts',(50.7720263837275,37.004309874055,40.0812334935552));
#196894=CARTESIAN_POINT('Ctrl Pts',(50.770879611352,37.0048406651177,40.0806684524226));
#196895=CARTESIAN_POINT('Ctrl Pts',(50.7629547027171,37.0085087606927,40.0767636676138));
#196896=CARTESIAN_POINT('Ctrl Pts',(50.7549442896476,37.0114900453053,40.0724404510891));
#196897=CARTESIAN_POINT('Ctrl Pts',(50.746937680599,37.0138628466703,40.0677949937414));
#196898=CARTESIAN_POINT('Ctrl Pts',(50.7429584178792,37.0150421224356,40.0654862141909));
#196899=CARTESIAN_POINT('Ctrl Pts',(50.7389795822785,37.0160707669652,40.0630972003217));
#196900=CARTESIAN_POINT('Ctrl Pts',(50.7350097117581,37.0169563748084,40.0606363359906));
#196901=CARTESIAN_POINT('Ctrl Pts',(50.726251584436,37.018910157988,40.0552073017123));
#196902=CARTESIAN_POINT('Ctrl Pts',(50.7175407334812,37.020179678854,40.0494204304519));
#196903=CARTESIAN_POINT('Ctrl Pts',(50.7090177292136,37.0208019128469,40.0434049749851));
#196904=CARTESIAN_POINT('Ctrl Pts',(50.7059041682739,37.0210292227713,40.0412074532442));
#196905=CARTESIAN_POINT('Ctrl Pts',(50.7028130194418,37.0211776528886,40.0389814735788));
#196906=CARTESIAN_POINT('Ctrl Pts',(50.6997475881157,37.021251364653,40.0367321210017));
#196907=CARTESIAN_POINT('Ctrl Pts',(50.6894511286649,37.0214989546697,40.029176783714));
#196908=CARTESIAN_POINT('Ctrl Pts',(50.6793793407323,37.020896700292,40.0213235332574));
#196909=CARTESIAN_POINT('Ctrl Pts',(50.6695664063391,37.019568267908,40.0132649215856));
#196910=CARTESIAN_POINT('Ctrl Pts',(50.6587808290224,37.0181081633547,40.0044075527529));
#196911=CARTESIAN_POINT('Ctrl Pts',(50.6483072759147,37.0157708601093,39.9953016253715));
#196912=CARTESIAN_POINT('Ctrl Pts',(50.6381830571056,37.0126680948705,39.9860353422352));
#196913=CARTESIAN_POINT('Ctrl Pts',(50.6272788396598,37.0093262837653,39.9760551582688));
#196914=CARTESIAN_POINT('Ctrl Pts',(50.6167786802283,37.0050963107879,39.9658879738147));
#196915=CARTESIAN_POINT('Ctrl Pts',(50.6067353452107,37.0000610231245,39.9556174643244));
#196916=CARTESIAN_POINT('Ctrl Pts',(50.5968276291265,36.9950937288458,39.9454856413898));
#196917=CARTESIAN_POINT('Ctrl Pts',(50.5873633690981,36.9893418170231,39.935251946511));
#196918=CARTESIAN_POINT('Ctrl Pts',(50.5784163149361,36.982841401674,39.92499));
#196919=CARTESIAN_POINT('Ctrl Pts',(47.7952442955506,34.960748566836,39.92499));
#196920=CARTESIAN_POINT('Ctrl Pts',(47.786681915603,34.9545276336631,39.9348107241719));
#196921=CARTESIAN_POINT('Ctrl Pts',(47.7786409912526,34.9476537221162,39.9446038383163));
#196922=CARTESIAN_POINT('Ctrl Pts',(47.7711595893187,34.9401706643562,39.9543158069375));
#196923=CARTESIAN_POINT('Ctrl Pts',(47.7639356375086,34.9329451137005,39.963693567138));
#196924=CARTESIAN_POINT('Ctrl Pts',(47.7572325247378,34.9251506707979,39.9729968320975));
#196925=CARTESIAN_POINT('Ctrl Pts',(47.7511153344897,34.9167928415166,39.9821731151319));
#196926=CARTESIAN_POINT('Ctrl Pts',(47.7453326739199,34.9088920753355,39.9908475764335));
#196927=CARTESIAN_POINT('Ctrl Pts',(47.7400730704142,34.9004871280313,39.9994093733829));
#196928=CARTESIAN_POINT('Ctrl Pts',(47.7354288821303,34.8915635921269,40.0077966115824));
#196929=CARTESIAN_POINT('Ctrl Pts',(47.7311516626329,34.8833451652624,40.0155211172578));
#196930=CARTESIAN_POINT('Ctrl Pts',(47.7273962447101,34.8746863576854,40.0230979941005));
#196931=CARTESIAN_POINT('Ctrl Pts',(47.7242720089038,34.865567688148,40.0304554104732));
#196932=CARTESIAN_POINT('Ctrl Pts',(47.7233404248529,34.8628486849635,40.032649243517));
#196933=CARTESIAN_POINT('Ctrl Pts',(47.7224652397594,34.860088762026,40.0348233715055));
#196934=CARTESIAN_POINT('Ctrl Pts',(47.7216501132023,34.8572873423615,40.0369753512355));
#196935=CARTESIAN_POINT('Ctrl Pts',(47.7208433152302,34.8545145463033,40.0391053430352));
#196936=CARTESIAN_POINT('Ctrl Pts',(47.7200959288452,34.8517040509262,40.041211089324));
#196937=CARTESIAN_POINT('Ctrl Pts',(47.7194121231169,34.8488585612795,40.0432881154904));
#196938=CARTESIAN_POINT('Ctrl Pts',(47.7193645726039,34.8486606914944,40.0434325478279));
#196939=CARTESIAN_POINT('Ctrl Pts',(47.7193173179074,34.8484626496805,40.0435768364421));
#196940=CARTESIAN_POINT('Ctrl Pts',(47.7192703603294,34.8482644357603,40.0437209807855));
#196941=CARTESIAN_POINT('Ctrl Pts',(47.7172115680926,34.8395740113841,40.0500407968419));
#196942=CARTESIAN_POINT('Ctrl Pts',(47.7157691359132,34.8305531107003,40.0560490279342));
#196943=CARTESIAN_POINT('Ctrl Pts',(47.7150344641797,34.8212734513099,40.0616647108611));
#196944=CARTESIAN_POINT('Ctrl Pts',(47.714349622439,34.8126231959642,40.0668995033481));
#196945=CARTESIAN_POINT('Ctrl Pts',(47.7142799923075,34.8037473009128,40.0717933267476));
#196946=CARTESIAN_POINT('Ctrl Pts',(47.7149249376578,34.7947186932888,40.0762460303065));
#196947=CARTESIAN_POINT('Ctrl Pts',(47.7151608670107,34.7914159118141,40.0778748868743));
#196948=CARTESIAN_POINT('Ctrl Pts',(47.7154926644833,34.7880929011149,40.0794443522245));
#196949=CARTESIAN_POINT('Ctrl Pts',(47.7159260651937,34.7847540840174,40.0809482021492));
#196950=CARTESIAN_POINT('Ctrl Pts',(47.7160302835859,34.7839512100456,40.0813098278168));
#196951=CARTESIAN_POINT('Ctrl Pts',(47.7161407719865,34.7831469919153,40.0816679525672));
#196952=CARTESIAN_POINT('Ctrl Pts',(47.7162575750192,34.7823415577599,40.082022419258));
#196953=CARTESIAN_POINT('Ctrl Pts',(47.716370727957,34.7815612934218,40.0823658088648));
#196954=CARTESIAN_POINT('Ctrl Pts',(47.7164898070138,34.7807798878926,40.0827057654616));
#196955=CARTESIAN_POINT('Ctrl Pts',(47.716614850513,34.7799974607183,40.0830421470151));
#196956=CARTESIAN_POINT('Ctrl Pts',(47.7179848465564,34.7714250667928,40.0867275956807));
#196957=CARTESIAN_POINT('Ctrl Pts',(47.7200720995238,34.7627244668144,40.0899823432033));
#196958=CARTESIAN_POINT('Ctrl Pts',(47.7229136891084,34.7540804826564,40.0926299529359));
#196959=CARTESIAN_POINT('Ctrl Pts',(47.7240921810077,34.7504955647771,40.0937279956086));
#196960=CARTESIAN_POINT('Ctrl Pts',(47.7254000086992,34.7469205018079,40.0947220371803));
#196961=CARTESIAN_POINT('Ctrl Pts',(47.7268379886356,34.7433685265016,40.0956014538692));
#196962=CARTESIAN_POINT('Ctrl Pts',(47.7292906132656,34.737310262474,40.097101390674));
#196963=CARTESIAN_POINT('Ctrl Pts',(47.7321228682624,34.7313214412505,40.0982667904316));
#196964=CARTESIAN_POINT('Ctrl Pts',(47.7353375827201,34.7254747878799,40.0990539325582));
#196965=CARTESIAN_POINT('Ctrl Pts',(47.7369449399489,34.7225514611946,40.0994475036216));
#196966=CARTESIAN_POINT('Ctrl Pts',(47.7386491210198,34.7196644712711,40.0997467259952));
#196967=CARTESIAN_POINT('Ctrl Pts',(47.7404504949227,34.7168229726601,40.0999473488896));
#196968=CARTESIAN_POINT('Ctrl Pts',(47.7422518688256,34.7139814740491,40.100147971784));
#196969=CARTESIAN_POINT('Ctrl Pts',(47.7441503967336,34.7111854907788,40.10025));
#196970=CARTESIAN_POINT('Ctrl Pts',(47.7461450747869,34.7084426211226,40.10025));
#196971=CARTESIAN_POINT('Origin',(50.4655267888879,29.1186878401549,39.92499));
#196972=CARTESIAN_POINT('Ctrl Pts',(54.3576020372442,31.1634057161433,39.92499));
#196973=CARTESIAN_POINT('Ctrl Pts',(54.3667908521541,31.1687108809051,39.9348354642012));
#196974=CARTESIAN_POINT('Ctrl Pts',(54.3755338070554,31.174725332392,39.9446440828447));
#196975=CARTESIAN_POINT('Ctrl Pts',(54.3837890328981,31.1814073748053,39.9543641760315));
#196976=CARTESIAN_POINT('Ctrl Pts',(54.3917760130576,31.1878722906292,39.9637684240692));
#196977=CARTESIAN_POINT('Ctrl Pts',(54.3993074034411,31.1949629807075,39.9730909636371));
#196978=CARTESIAN_POINT('Ctrl Pts',(54.4063187915247,31.2026795247176,39.9822808977112));
#196979=CARTESIAN_POINT('Ctrl Pts',(54.4129511329155,31.2099789001937,39.9909740094617));
#196980=CARTESIAN_POINT('Ctrl Pts',(54.4191188025025,31.2178389737479,39.9995492764965));
#196981=CARTESIAN_POINT('Ctrl Pts',(54.4247323097961,31.2262832675516,40.0079462328655));
#196982=CARTESIAN_POINT('Ctrl Pts',(54.4299027559928,31.2340610728517,40.0156804369646));
#196983=CARTESIAN_POINT('Ctrl Pts',(54.4346033281805,31.2423350114943,40.0232638017375));
#196984=CARTESIAN_POINT('Ctrl Pts',(54.4387279162148,31.2511358718486,40.0306257269917));
#196985=CARTESIAN_POINT('Ctrl Pts',(54.4399243024172,31.2536886668937,40.0327611416619));
#196986=CARTESIAN_POINT('Ctrl Pts',(54.4410719653269,31.2562858555917,40.0348777427254));
#196987=CARTESIAN_POINT('Ctrl Pts',(54.4421676282861,31.258928321256,40.03697331687));
#196988=CARTESIAN_POINT('Ctrl Pts',(54.4433553973776,31.2617929239288,40.039245053974));
#196989=CARTESIAN_POINT('Ctrl Pts',(54.4444813995856,31.2647063376188,40.041487875195));
#196990=CARTESIAN_POINT('Ctrl Pts',(54.4455416356299,31.2676686823013,40.04369857016));
#196991=CARTESIAN_POINT('Ctrl Pts',(54.448451461773,31.2757988605273,40.0497658398386));
#196992=CARTESIAN_POINT('Ctrl Pts',(54.4508216479607,31.2843017293915,40.0555581699984));
#196993=CARTESIAN_POINT('Ctrl Pts',(54.4525775288979,31.2931053160618,40.0609828468885));
#196994=CARTESIAN_POINT('Ctrl Pts',(54.4541840646265,31.3011601199075,40.0659461317306));
#196995=CARTESIAN_POINT('Ctrl Pts',(54.4552661718989,31.3094611543726,40.0706039980708));
#196996=CARTESIAN_POINT('Ctrl Pts',(54.4557414157489,31.3179758301775,40.0748843180606));
#196997=CARTESIAN_POINT('Ctrl Pts',(54.4559748539755,31.3221582111183,40.0769867972571));
#196998=CARTESIAN_POINT('Ctrl Pts',(54.4560613864574,31.3263919825238,40.0789976708176));
#196999=CARTESIAN_POINT('Ctrl Pts',(54.4559882102927,31.3306718639307,40.08090504915));
#197000=CARTESIAN_POINT('Ctrl Pts',(54.4559743258282,31.3314839297411,40.0812669556105));
#197001=CARTESIAN_POINT('Ctrl Pts',(54.4559543157134,31.3322980319624,40.0816253922032));
#197002=CARTESIAN_POINT('Ctrl Pts',(54.4559281176618,31.3331140451952,40.0819801989139));
#197003=CARTESIAN_POINT('Ctrl Pts',(54.4559027382992,31.3339045580144,40.0823239179149));
#197004=CARTESIAN_POINT('Ctrl Pts',(54.4558715517163,31.3346968642514,40.0826642303498));
#197005=CARTESIAN_POINT('Ctrl Pts',(54.4558345032254,31.3354908465822,40.0830009916099));
#197006=CARTESIAN_POINT('Ctrl Pts',(54.4554307564065,31.34414350242,40.0866709464312));
#197007=CARTESIAN_POINT('Ctrl Pts',(54.4543301709718,31.3530008879285,40.0899175831878));
#197008=CARTESIAN_POINT('Ctrl Pts',(54.4524721779262,31.3618824321384,40.0925642067062));
#197009=CARTESIAN_POINT('Ctrl Pts',(54.4516875359255,31.3656331634099,40.0936818922528));
#197010=CARTESIAN_POINT('Ctrl Pts',(54.4507682193239,31.3693880355472,40.0946930094791));
#197011=CARTESIAN_POINT('Ctrl Pts',(54.4497115877225,31.3731331934886,40.0955863397546));
#197012=CARTESIAN_POINT('Ctrl Pts',(54.4479322465079,31.3794399458808,40.0970906856166));
#197013=CARTESIAN_POINT('Ctrl Pts',(54.4457622496024,31.3857169562553,40.0982599215483));
#197014=CARTESIAN_POINT('Ctrl Pts',(54.4431895758475,31.39189098828,40.0990497370453));
#197015=CARTESIAN_POINT('Ctrl Pts',(54.4425464074088,31.3934344962862,40.0992471909196));
#197016=CARTESIAN_POINT('Ctrl Pts',(54.4418778620531,31.3949714642028,40.0994209989363));
#197017=CARTESIAN_POINT('Ctrl Pts',(54.4411834812327,31.3965005998217,40.0995705982975));
#197018=CARTESIAN_POINT('Ctrl Pts',(54.4401419100021,31.39879430325,40.0997949973393));
#197019=CARTESIAN_POINT('Ctrl Pts',(54.4390422051397,31.4010703637557,40.0999649129781));
#197020=CARTESIAN_POINT('Ctrl Pts',(54.4378842814515,31.4033252432064,40.1000786629733));
#197021=CARTESIAN_POINT('Ctrl Pts',(54.4367263577634,31.4055801226571,40.1001924129685));
#197022=CARTESIAN_POINT('Ctrl Pts',(54.435510226749,31.4078138194776,40.10025));
#197023=CARTESIAN_POINT('Ctrl Pts',(54.4342359163082,31.4100231232063,40.10025));
#197024=CARTESIAN_POINT('Ctrl Pts',(51.1278468659051,29.5010785149105,40.10025));
#197025=CARTESIAN_POINT('Ctrl Pts',(51.1321585373228,29.493602795639,40.10025));
#197026=CARTESIAN_POINT('Ctrl Pts',(51.1370499258748,29.486547784523,40.099578633424));
#197027=CARTESIAN_POINT('Ctrl Pts',(51.1423856448182,29.4799806005918,40.0983063763365));
#197028=CARTESIAN_POINT('Ctrl Pts',(51.145831971779,29.4757388736045,40.0974846287991));
#197029=CARTESIAN_POINT('Ctrl Pts',(51.1494629466902,29.4717000621106,40.0964130309337));
#197030=CARTESIAN_POINT('Ctrl Pts',(51.1532365012463,29.4678753842634,40.0951176960923));
#197031=CARTESIAN_POINT('Ctrl Pts',(51.158238131648,29.4628059928677,40.0934008039614));
#197032=CARTESIAN_POINT('Ctrl Pts',(51.1634934604718,29.4581176150984,40.0912909372156));
#197033=CARTESIAN_POINT('Ctrl Pts',(51.1689167792842,29.4538379291355,40.0888630467851));
#197034=CARTESIAN_POINT('Ctrl Pts',(51.1716284386905,29.451698086154,40.0876491015699));
#197035=CARTESIAN_POINT('Ctrl Pts',(51.1743821937243,29.4496602426627,40.0863558569271));
#197036=CARTESIAN_POINT('Ctrl Pts',(51.1771680313595,29.4477266300412,40.0849936342771));
#197037=CARTESIAN_POINT('Ctrl Pts',(51.1785609501771,29.4467598237305,40.0843125229521));
#197038=CARTESIAN_POINT('Ctrl Pts',(51.1799618978183,29.4458190608831,40.0836141747074));
#197039=CARTESIAN_POINT('Ctrl Pts',(51.1813696738596,29.4449045308654,40.0828999161609));
#197040=CARTESIAN_POINT('Ctrl Pts',(51.1817216178699,29.444675898361,40.0827213515243));
#197041=CARTESIAN_POINT('Ctrl Pts',(51.1820739888281,29.4444489051048,40.0825417925841));
#197042=CARTESIAN_POINT('Ctrl Pts',(51.1824267683262,29.4442235534429,40.082361260236));
#197043=CARTESIAN_POINT('Ctrl Pts',(51.1834851068203,29.4435474984572,40.0818196631917));
#197044=CARTESIAN_POINT('Ctrl Pts',(51.1845471213155,29.44288621934,40.0812693052021));
#197045=CARTESIAN_POINT('Ctrl Pts',(51.1856123224583,29.4422397658673,40.0807107531874));
#197046=CARTESIAN_POINT('Ctrl Pts',(51.1931154617654,29.4376862310777,40.0767763849181));
#197047=CARTESIAN_POINT('Ctrl Pts',(51.20077996036,29.4338145801754,40.0724140586136));
#197048=CARTESIAN_POINT('Ctrl Pts',(51.2085065710735,29.4305579784506,40.0677221223766));
#197049=CARTESIAN_POINT('Ctrl Pts',(51.2122539689199,29.4289785301332,40.0654465383719));
#197050=CARTESIAN_POINT('Ctrl Pts',(51.2160164979702,29.4275440072536,40.0630928000678));
#197051=CARTESIAN_POINT('Ctrl Pts',(51.2197852472982,29.4262483256613,40.0606689262479));
#197052=CARTESIAN_POINT('Ctrl Pts',(51.2255549392047,29.4242647276699,40.0569581447805));
#197053=CARTESIAN_POINT('Ctrl Pts',(51.2313356805893,29.4226066102317,40.0530843804605));
#197054=CARTESIAN_POINT('Ctrl Pts',(51.2370841708902,29.4212581193007,40.0490800251457));
#197055=CARTESIAN_POINT('Ctrl Pts',(51.2397537995247,29.4206318731362,40.0472203818218));
#197056=CARTESIAN_POINT('Ctrl Pts',(51.2424163366108,29.4200721889209,40.0453323608818));
#197057=CARTESIAN_POINT('Ctrl Pts',(51.245067459672,29.4195787111901,40.0434201572162));
#197058=CARTESIAN_POINT('Ctrl Pts',(51.2452706578087,29.4195408880665,40.0432735943397));
#197059=CARTESIAN_POINT('Ctrl Pts',(51.2454737959512,29.4195034206996,40.0431268995707));
#197060=CARTESIAN_POINT('Ctrl Pts',(51.2456768729759,29.4194663081567,40.0429800745037));
#197061=CARTESIAN_POINT('Ctrl Pts',(51.2485294929149,29.4189449888195,40.0409176249753));
#197062=CARTESIAN_POINT('Ctrl Pts',(51.2513705613631,29.4184957101759,40.0388310783332));
#197063=CARTESIAN_POINT('Ctrl Pts',(51.2541954110684,29.4181151898791,40.036725739981));
#197064=CARTESIAN_POINT('Ctrl Pts',(51.2643248197289,29.4167507117679,40.0291763710718));
#197065=CARTESIAN_POINT('Ctrl Pts',(51.2743237313762,29.4162578421115,40.0213310894596));
#197066=CARTESIAN_POINT('Ctrl Pts',(51.2841455249771,29.4165161672802,40.0132837551322));
#197067=CARTESIAN_POINT('Ctrl Pts',(51.2949386894578,29.4168000406897,40.0044405431328));
#197068=CARTESIAN_POINT('Ctrl Pts',(51.305518622259,29.4179908989228,39.9953528710605));
#197069=CARTESIAN_POINT('Ctrl Pts',(51.3158373135951,29.4199800715332,39.986110362956));
#197070=CARTESIAN_POINT('Ctrl Pts',(51.3269789106,29.4221278787384,39.9761307737562));
#197071=CARTESIAN_POINT('Ctrl Pts',(51.3378170984252,29.4252064644171,39.9659696936018));
#197072=CARTESIAN_POINT('Ctrl Pts',(51.3482921445245,29.4291364604191,39.9557128217513));
#197073=CARTESIAN_POINT('Ctrl Pts',(51.3586793157504,29.4330334877928,39.9455419945165));
#197074=CARTESIAN_POINT('Ctrl Pts',(51.3687106315444,29.437768458484,39.9352756289343));
#197075=CARTESIAN_POINT('Ctrl Pts',(51.3783102687789,29.4433108116255,39.92499));
#197076=CARTESIAN_POINT('Origin',(-0.00761999999999908,0.0131982271536721,
39.92499));
#197077=CARTESIAN_POINT('Ctrl Pts',(54.4189959163067,31.4364195775128,40.10025));
#197078=CARTESIAN_POINT('Ctrl Pts',(54.4146983388121,31.4438560159995,40.10025));
#197079=CARTESIAN_POINT('Ctrl Pts',(54.4098177483016,31.4508673716598,40.0995859581842));
#197080=CARTESIAN_POINT('Ctrl Pts',(54.4044907169114,31.4573895320582,40.0983275959621));
#197081=CARTESIAN_POINT('Ctrl Pts',(54.4010869974477,31.4615568820638,40.0975235624069));
#197082=CARTESIAN_POINT('Ctrl Pts',(54.3975017237414,31.4655251210641,40.0964777059491));
#197083=CARTESIAN_POINT('Ctrl Pts',(54.3937759157112,31.469284216974,40.0952149915961));
#197084=CARTESIAN_POINT('Ctrl Pts',(54.3886909353396,31.474414628622,40.0934916398701));
#197085=CARTESIAN_POINT('Ctrl Pts',(54.3833409297224,31.4791503318816,40.0913643921631));
#197086=CARTESIAN_POINT('Ctrl Pts',(54.3778174666306,31.4834636394923,40.0889118607713));
#197087=CARTESIAN_POINT('Ctrl Pts',(54.3750557350847,31.4856202932976,40.0876855950754));
#197088=CARTESIAN_POINT('Ctrl Pts',(54.3722505364145,31.487671530002,40.0863782327527));
#197089=CARTESIAN_POINT('Ctrl Pts',(54.3694125772951,31.4896151854254,40.0850006373334));
#197090=CARTESIAN_POINT('Ctrl Pts',(54.3679935977354,31.4905870131371,40.0843118396238));
#197091=CARTESIAN_POINT('Ctrl Pts',(54.3665664194003,31.4915319606345,40.0836054919165));
#197092=CARTESIAN_POINT('Ctrl Pts',(54.3651323262972,31.4924498523882,40.0828829920418));
#197093=CARTESIAN_POINT('Ctrl Pts',(54.3647738030214,31.4926793253266,40.0827023670731));
#197094=CARTESIAN_POINT('Ctrl Pts',(54.3644148473889,31.4929071076033,40.0825207326933));
#197095=CARTESIAN_POINT('Ctrl Pts',(54.3640554790925,31.4931331971262,40.0823381109276));
#197096=CARTESIAN_POINT('Ctrl Pts',(54.3629773742032,31.4938114656946,40.0817902456304));
#197097=CARTESIAN_POINT('Ctrl Pts',(54.3618955562477,31.4944744978644,40.0812334935553));
#197098=CARTESIAN_POINT('Ctrl Pts',(54.3608105487854,31.4951222515522,40.0806684524227));
#197099=CARTESIAN_POINT('Ctrl Pts',(54.3533124740225,31.499598631437,40.0767636676137));
#197100=CARTESIAN_POINT('Ctrl Pts',(54.3456575719328,31.503400900429,40.0724404510889));
#197101=CARTESIAN_POINT('Ctrl Pts',(54.3379428492064,31.5065976218797,40.067794993741));
#197102=CARTESIAN_POINT('Ctrl Pts',(54.3341086531879,31.5081863836659,40.0654862141906));
#197103=CARTESIAN_POINT('Ctrl Pts',(54.330259136697,31.509625294744,40.0630972003216));
#197104=CARTESIAN_POINT('Ctrl Pts',(54.3264035847699,31.5109210155995,40.0606363359906));
#197105=CARTESIAN_POINT('Ctrl Pts',(54.3178976613389,31.5137795693406,40.0552073017123));
#197106=CARTESIAN_POINT('Ctrl Pts',(54.3093672304024,31.5159526675024,40.0494204304519));
#197107=CARTESIAN_POINT('Ctrl Pts',(54.300955957207,31.517462389371,40.0434049749851));
#197108=CARTESIAN_POINT('Ctrl Pts',(54.297883213037,31.5180139098082,40.0412074532442));
#197109=CARTESIAN_POINT('Ctrl Pts',(54.2948245130138,31.5184846398469,40.0389814735788));
#197110=CARTESIAN_POINT('Ctrl Pts',(54.2917835794187,31.5188783726364,40.0367321210016));
#197111=CARTESIAN_POINT('Ctrl Pts',(54.2815694052538,31.5202008794127,40.0291767837137));
#197112=CARTESIAN_POINT('Ctrl Pts',(54.2714898389044,31.5206547127624,40.0213235332569));
#197113=CARTESIAN_POINT('Ctrl Pts',(54.2615918017967,31.5203592886222,40.0132649215848));
#197114=CARTESIAN_POINT('Ctrl Pts',(54.2507126865157,31.5200345824968,40.0044075527519));
#197115=CARTESIAN_POINT('Ctrl Pts',(54.240052193911,31.5188048676543,39.9953016253702));
#197116=CARTESIAN_POINT('Ctrl Pts',(54.2296591093493,31.5167773687219,39.9860353422336));
#197117=CARTESIAN_POINT('Ctrl Pts',(54.2184653119679,31.5145936655002,39.9760551582668));
#197118=CARTESIAN_POINT('Ctrl Pts',(54.2075805209331,31.5114844302865,39.9658879738124));
#197119=CARTESIAN_POINT('Ctrl Pts',(54.1970658734737,31.5075265408309,39.9556174643217));
#197120=CARTESIAN_POINT('Ctrl Pts',(54.1866932092582,31.503622096247,39.945485641388));
#197121=CARTESIAN_POINT('Ctrl Pts',(54.1766795569337,31.4988909785561,39.9352519465101));
#197122=CARTESIAN_POINT('Ctrl Pts',(54.1671020372442,31.4933613949852,39.92499));
#197123=CARTESIAN_POINT('Ctrl Pts',(51.1878102687789,29.7732664904673,39.92499));
#197124=CARTESIAN_POINT('Ctrl Pts',(51.1786445298598,29.7679746486351,39.9348107241719));
#197125=CARTESIAN_POINT('Ctrl Pts',(51.1699291351238,29.7619788985606,39.9446038383162));
#197126=CARTESIAN_POINT('Ctrl Pts',(51.1617065245643,29.7553188532212,39.9543158069374));
#197127=CARTESIAN_POINT('Ctrl Pts',(51.1537668706118,29.7488879934694,39.9636935671378));
#197128=CARTESIAN_POINT('Ctrl Pts',(51.1462857370555,29.7418369154177,39.9729968320973));
#197129=CARTESIAN_POINT('Ctrl Pts',(51.1393284263646,29.7341642916958,39.9821731151318));
#197130=CARTESIAN_POINT('Ctrl Pts',(51.1327515888668,29.7269112593616,39.9908475764334));
#197131=CARTESIAN_POINT('Ctrl Pts',(51.1266422417939,29.71910213351,39.9994093733828));
#197132=CARTESIAN_POINT('Ctrl Pts',(51.1210907313644,29.7107129315334,40.0077966115823));
#197133=CARTESIAN_POINT('Ctrl Pts',(51.1159778833923,29.7029866172523,40.0155211172576));
#197134=CARTESIAN_POINT('Ctrl Pts',(51.1113379461921,29.6947677915936,40.0230979941003));
#197135=CARTESIAN_POINT('Ctrl Pts',(51.1072776647626,29.6860256466498,40.030455410473));
#197136=CARTESIAN_POINT('Ctrl Pts',(51.1060669708021,29.6834189154984,40.0326492435169));
#197137=CARTESIAN_POINT('Ctrl Pts',(51.1049080895607,29.6807655934603,40.0348233715054));
#197138=CARTESIAN_POINT('Ctrl Pts',(51.1038046002597,29.6780647241921,40.0369753512355));
#197139=CARTESIAN_POINT('Ctrl Pts',(51.1027123859004,29.6753914511531,40.0391053430352));
#197140=CARTESIAN_POINT('Ctrl Pts',(51.1016753170134,29.672674475114,40.041211089324));
#197141=CARTESIAN_POINT('Ctrl Pts',(51.1006978225844,29.6699160505193,40.0432881154904));
#197142=CARTESIAN_POINT('Ctrl Pts',(51.1006298495335,29.6697242350676,40.043432547828));
#197143=CARTESIAN_POINT('Ctrl Pts',(51.1005621526966,29.6695322176083,40.0435768364421));
#197144=CARTESIAN_POINT('Ctrl Pts',(51.1004947333607,29.6693399979282,40.0437209807855));
#197145=CARTESIAN_POINT('Ctrl Pts',(51.097538822698,29.6609123829947,40.0500407968419));
#197146=CARTESIAN_POINT('Ctrl Pts',(51.0951613514272,29.6520916749677,40.0560490279343));
#197147=CARTESIAN_POINT('Ctrl Pts',(51.0934607157666,29.6429396446296,40.0616647108612));
#197148=CARTESIAN_POINT('Ctrl Pts',(51.0918754277624,29.6344083617422,40.0668995033483));
#197149=CARTESIAN_POINT('Ctrl Pts',(51.0908783954022,29.6255883681029,40.071793326748));
#197150=CARTESIAN_POINT('Ctrl Pts',(51.090576061194,29.6165418049894,40.0762460303071));
#197151=CARTESIAN_POINT('Ctrl Pts',(51.0904654634293,29.613232455165,40.0778748868747));
#197152=CARTESIAN_POINT('Ctrl Pts',(51.0904480940787,29.6098929659865,40.0794443522246));
#197153=CARTESIAN_POINT('Ctrl Pts',(51.0905301191544,29.6065271365686,40.0809482021491));
#197154=CARTESIAN_POINT('Ctrl Pts',(51.0905498434448,29.605717767036,40.0813098278168));
#197155=CARTESIAN_POINT('Ctrl Pts',(51.0905756628932,29.604906405314,40.0816679525672));
#197156=CARTESIAN_POINT('Ctrl Pts',(51.0906076352721,29.6040931741697,40.082022419258));
#197157=CARTESIAN_POINT('Ctrl Pts',(51.0906386085141,29.6033053564986,40.0823658088648));
#197158=CARTESIAN_POINT('Ctrl Pts',(51.0906753561242,29.6025157844399,40.0827057654616));
#197159=CARTESIAN_POINT('Ctrl Pts',(51.0907179287118,29.6017245728787,40.083042147015));
#197160=CARTESIAN_POINT('Ctrl Pts',(51.09118436061,29.5930559358433,40.0867275956805));
#197161=CARTESIAN_POINT('Ctrl Pts',(51.0923507190419,29.5841848213171,40.089982343203));
#197162=CARTESIAN_POINT('Ctrl Pts',(51.0942731997208,29.5752911628167,40.0926299529355));
#197163=CARTESIAN_POINT('Ctrl Pts',(51.0950705097614,29.571602697545,40.0937279956084));
#197164=CARTESIAN_POINT('Ctrl Pts',(51.0959974771977,29.5679105139257,40.0947220371802));
#197165=CARTESIAN_POINT('Ctrl Pts',(51.0970562972094,29.5642276868784,40.0956014538692));
#197166=CARTESIAN_POINT('Ctrl Pts',(51.0988622250761,29.5579462415715,40.097101390674));
#197167=CARTESIAN_POINT('Ctrl Pts',(51.1010529624044,29.5516941764749,40.0982667904315));
#197168=CARTESIAN_POINT('Ctrl Pts',(51.1036389246282,29.5455435225212,40.0990539325582));
#197169=CARTESIAN_POINT('Ctrl Pts',(51.1049319057401,29.5424681955444,40.0994475036216));
#197170=CARTESIAN_POINT('Ctrl Pts',(51.1063249785084,29.5394188854253,40.0997467259952));
#197171=CARTESIAN_POINT('Ctrl Pts',(51.1078194668134,29.5364046579951,40.0999473488896));
#197172=CARTESIAN_POINT('Ctrl Pts',(51.1093139551183,29.5333904305649,40.100147971784));
#197173=CARTESIAN_POINT('Ctrl Pts',(51.110909822857,29.5304113137787,40.10025));
#197174=CARTESIAN_POINT('Ctrl Pts',(51.1126068659051,29.5274749692178,40.10025));
#197175=CARTESIAN_POINT('Origin',(53.2328030451451,23.6840886581929,39.92499));
#197176=CARTESIAN_POINT('Ctrl Pts',(57.3172883154493,25.3107727110816,39.92499));
#197177=CARTESIAN_POINT('Ctrl Pts',(57.3269813337904,25.3150883208943,39.9348354642023));
#197178=CARTESIAN_POINT('Ctrl Pts',(57.3363050752422,25.3201559369469,39.9446440828468));
#197179=CARTESIAN_POINT('Ctrl Pts',(57.3452135417197,25.3259384683622,39.9543641760346));
#197180=CARTESIAN_POINT('Ctrl Pts',(57.3538325360831,25.3315331019391,39.9637684240732));
#197181=CARTESIAN_POINT('Ctrl Pts',(57.3620638476599,25.3377977038129,39.9730909636419));
#197182=CARTESIAN_POINT('Ctrl Pts',(57.3698434251136,25.3447390861666,39.9822808977167));
#197183=CARTESIAN_POINT('Ctrl Pts',(57.3772024263461,25.3513052064475,39.9909740094679));
#197184=CARTESIAN_POINT('Ctrl Pts',(57.3841579102039,25.3584775246735,39.9995492765034));
#197185=CARTESIAN_POINT('Ctrl Pts',(57.3906233351723,25.3662887884623,40.007946232873));
#197186=CARTESIAN_POINT('Ctrl Pts',(57.3965784591597,25.3734835273369,40.0156804369728));
#197187=CARTESIAN_POINT('Ctrl Pts',(57.4021181432129,25.381220796892,40.0232638017464));
#197188=CARTESIAN_POINT('Ctrl Pts',(57.4071400767309,25.389542308365,40.0306257270011));
#197189=CARTESIAN_POINT('Ctrl Pts',(57.4085967487453,25.3919560625171,40.0327611416681));
#197190=CARTESIAN_POINT('Ctrl Pts',(57.4100096047789,25.3944190601,40.0348777427285));
#197191=CARTESIAN_POINT('Ctrl Pts',(57.4113754784549,25.3969325220918,40.0369733168701));
#197192=CARTESIAN_POINT('Ctrl Pts',(57.4128561733383,25.3996572764936,40.039245053974));
#197193=CARTESIAN_POINT('Ctrl Pts',(57.4142805418443,25.4024370309181,40.041487875195));
#197194=CARTESIAN_POINT('Ctrl Pts',(57.4156446191419,25.405272322722,40.04369857016));
#197195=CARTESIAN_POINT('Ctrl Pts',(57.419388339989,25.413053803326,40.0497658398386));
#197196=CARTESIAN_POINT('Ctrl Pts',(57.4226343338645,25.421262340665,40.0555581699984));
#197197=CARTESIAN_POINT('Ctrl Pts',(57.4253008212881,25.4298341608304,40.0609828468885));
#197198=CARTESIAN_POINT('Ctrl Pts',(57.4277405125138,25.4376769109067,40.0659461317304));
#197199=CARTESIAN_POINT('Ctrl Pts',(57.4296843862655,25.445819360426,40.0706039980707));
#197200=CARTESIAN_POINT('Ctrl Pts',(57.431047052657,25.4542377154365,40.0748843180603));
#197201=CARTESIAN_POINT('Ctrl Pts',(57.4317163899372,25.4583727839179,40.076986797257));
#197202=CARTESIAN_POINT('Ctrl Pts',(57.432244998004,25.4625743171735,40.0789976708175));
#197203=CARTESIAN_POINT('Ctrl Pts',(57.4326195921325,25.4668384019344,40.08090504915));
#197204=CARTESIAN_POINT('Ctrl Pts',(57.4326906677197,25.4676474704851,40.0812669556105));
#197205=CARTESIAN_POINT('Ctrl Pts',(57.4327558640766,25.4684592045959,40.0816253922033));
#197206=CARTESIAN_POINT('Ctrl Pts',(57.4328151061499,25.4692734860648,40.081980198914));
#197207=CARTESIAN_POINT('Ctrl Pts',(57.4328724969083,25.4700623212378,40.0823239179149));
#197208=CARTESIAN_POINT('Ctrl Pts',(57.4329242997221,25.470853547024,40.0826642303499));
#197209=CARTESIAN_POINT('Ctrl Pts',(57.4329704479396,25.4716470524583,40.08300099161));
#197210=CARTESIAN_POINT('Ctrl Pts',(57.4334733617059,25.4802945111765,40.0866709464312));
#197211=CARTESIAN_POINT('Ctrl Pts',(57.4333046542892,25.4892184175045,40.0899175831877));
#197212=CARTESIAN_POINT('Ctrl Pts',(57.4323852136916,25.4982455208437,40.0925642067062));
#197213=CARTESIAN_POINT('Ctrl Pts',(57.4319969282178,25.5020577226394,40.0936818922527));
#197214=CARTESIAN_POINT('Ctrl Pts',(57.431475138743,25.505888119946,40.0946930094791));
#197215=CARTESIAN_POINT('Ctrl Pts',(57.4308157710843,25.509723209598,40.0955863397546));
#197216=CARTESIAN_POINT('Ctrl Pts',(57.4297054124229,25.5161814047435,40.0970906856166));
#197217=CARTESIAN_POINT('Ctrl Pts',(57.4282034292359,25.5226508554403,40.0982599215483));
#197218=CARTESIAN_POINT('Ctrl Pts',(57.4262902109372,25.5290599831058,40.0990497370454));
#197219=CARTESIAN_POINT('Ctrl Pts',(57.4258119063625,25.5306622650222,40.0992471909196));
#197220=CARTESIAN_POINT('Ctrl Pts',(57.4253076802627,25.5322606952864,40.0994209989363));
#197221=CARTESIAN_POINT('Ctrl Pts',(57.4247769415294,25.5338540367005,40.0995705982975));
#197222=CARTESIAN_POINT('Ctrl Pts',(57.4239808334294,25.5362440488215,40.0997949973393));
#197223=CARTESIAN_POINT('Ctrl Pts',(57.4231250659722,25.5386225912888,40.0999649129781));
#197224=CARTESIAN_POINT('Ctrl Pts',(57.4222091845949,25.5409861542576,40.1000786629733));
#197225=CARTESIAN_POINT('Ctrl Pts',(57.4212933032176,25.5433497172264,40.1001924129685));
#197226=CARTESIAN_POINT('Ctrl Pts',(57.4203173191904,25.5456982979273,40.10025));
#197227=CARTESIAN_POINT('Ctrl Pts',(57.4192809246792,25.5480287005711,40.10025));
#197228=CARTESIAN_POINT('Ctrl Pts',(53.9314655730807,23.9951532569801,40.10025));
#197229=CARTESIAN_POINT('Ctrl Pts',(53.934972199264,23.9872677980937,40.10025));
#197230=CARTESIAN_POINT('Ctrl Pts',(53.9390993428073,23.9797401457383,40.0995786334241));
#197231=CARTESIAN_POINT('Ctrl Pts',(53.9437193744796,23.9726512030264,40.0983063763366));
#197232=CARTESIAN_POINT('Ctrl Pts',(53.9467034408972,23.968072473402,40.0974846287992));
#197233=CARTESIAN_POINT('Ctrl Pts',(53.9498923541892,23.9636762467123,40.0964130309338));
#197234=CARTESIAN_POINT('Ctrl Pts',(53.9532454491208,23.9594780769915,40.0951176960923));
#197235=CARTESIAN_POINT('Ctrl Pts',(53.9576897843756,23.9539136435126,40.0934008039614));
#197236=CARTESIAN_POINT('Ctrl Pts',(53.9624262550348,23.9487016177214,40.0912909372156));
#197237=CARTESIAN_POINT('Ctrl Pts',(53.9673725153423,23.9438784851447,40.0888630467851));
#197238=CARTESIAN_POINT('Ctrl Pts',(53.9698456454961,23.9414669188563,40.0876491015699));
#197239=CARTESIAN_POINT('Ctrl Pts',(53.9723713025231,23.9391523931029,40.0863558569271));
#197240=CARTESIAN_POINT('Ctrl Pts',(53.9749397614924,23.9369381736868,40.0849936342771));
#197241=CARTESIAN_POINT('Ctrl Pts',(53.9762239909771,23.9358310639788,40.0843125229521));
#197242=CARTESIAN_POINT('Ctrl Pts',(53.9775189275858,23.9347490158246,40.0836141747074));
#197243=CARTESIAN_POINT('Ctrl Pts',(53.9788233972652,23.9336923430319,40.0828999161609));
#197244=CARTESIAN_POINT('Ctrl Pts',(53.9791495146851,23.9334281748337,40.0827213515243));
#197245=CARTESIAN_POINT('Ctrl Pts',(53.9794762280621,23.9331655922755,40.0825417925842));
#197246=CARTESIAN_POINT('Ctrl Pts',(53.9798035193342,23.9329045996148,40.0823612602361));
#197247=CARTESIAN_POINT('Ctrl Pts',(53.9807853931506,23.9321216216326,40.0818196631917));
#197248=CARTESIAN_POINT('Ctrl Pts',(53.9817724673294,23.9313529543285,40.0812693052022));
#197249=CARTESIAN_POINT('Ctrl Pts',(53.9827642604008,23.930598698357,40.0807107531875));
#197250=CARTESIAN_POINT('Ctrl Pts',(53.9897503227319,23.9252858166859,40.076776384918));
#197251=CARTESIAN_POINT('Ctrl Pts',(53.9969681366824,23.9206342168324,40.0724140586134));
#197252=CARTESIAN_POINT('Ctrl Pts',(54.0043120126403,23.9165878043684,40.0677221223762));
#197253=CARTESIAN_POINT('Ctrl Pts',(54.0078737845436,23.9146252986961,40.0654465383717));
#197254=CARTESIAN_POINT('Ctrl Pts',(54.0114657535938,23.9128053429035,40.0630928000677));
#197255=CARTESIAN_POINT('Ctrl Pts',(54.0150784217127,23.9111228176148,40.0606689262479));
#197256=CARTESIAN_POINT('Ctrl Pts',(54.0206091641934,23.9085469889523,40.0569581447805));
#197257=CARTESIAN_POINT('Ctrl Pts',(54.0261849176042,23.9062937028415,40.0530843804605));
#197258=CARTESIAN_POINT('Ctrl Pts',(54.0317609613889,23.9043517182276,40.0490800251457));
#197259=CARTESIAN_POINT('Ctrl Pts',(54.0343505049692,23.9034498505265,40.0472203818218));
#197260=CARTESIAN_POINT('Ctrl Pts',(54.0369399534677,23.9026149214098,40.0453323608818));
#197261=CARTESIAN_POINT('Ctrl Pts',(54.0395249709305,23.9018470291822,40.0434201572162));
#197262=CARTESIAN_POINT('Ctrl Pts',(54.0397231023336,23.9017881732686,40.0432735943397));
#197263=CARTESIAN_POINT('Ctrl Pts',(54.0399212112578,23.901729677434,40.0431268995707));
#197264=CARTESIAN_POINT('Ctrl Pts',(54.0401192964882,23.9016715408682,40.0429800745037));
#197265=CARTESIAN_POINT('Ctrl Pts',(54.0429017967675,23.9008548973944,40.0409176249753));
#197266=CARTESIAN_POINT('Ctrl Pts',(54.0456803391393,23.9001111074273,40.0388310783332));
#197267=CARTESIAN_POINT('Ctrl Pts',(54.0484499388205,23.8994373944618,40.036725739981));
#197268=CARTESIAN_POINT('Ctrl Pts',(54.0583812307207,23.8970215795832,40.0291763710716));
#197269=CARTESIAN_POINT('Ctrl Pts',(54.0682738483763,23.8954862390495,40.0213310894591));
#197270=CARTESIAN_POINT('Ctrl Pts',(54.0780688394974,23.8947164920944,40.0132837551314));
#197271=CARTESIAN_POINT('Ctrl Pts',(54.0888325507452,23.8938706175186,40.0044405431318));
#197272=CARTESIAN_POINT('Ctrl Pts',(54.0994790041488,23.8939490479886,39.9953528710593));
#197273=CARTESIAN_POINT('Ctrl Pts',(54.1099490937704,23.8948487267552,39.9861103629547));
#197274=CARTESIAN_POINT('Ctrl Pts',(54.1212541629277,23.8958201540345,39.9761307737549));
#197275=CARTESIAN_POINT('Ctrl Pts',(54.1323547778559,23.897748975781,39.9659696936005));
#197276=CARTESIAN_POINT('Ctrl Pts',(54.1431832369993,23.9005625023823,39.9557128217501));
#197277=CARTESIAN_POINT('Ctrl Pts',(54.1539208564967,23.9033524263863,39.9455419945157));
#197278=CARTESIAN_POINT('Ctrl Pts',(54.1643921589026,23.907012900388,39.9352756289339));
#197279=CARTESIAN_POINT('Ctrl Pts',(54.1745185419763,23.9115214566108,39.92499));
#197280=CARTESIAN_POINT('Origin',(-0.00619866644047451,0.013922432774471,
39.92499));
#197281=CARTESIAN_POINT('Ctrl Pts',(57.4068835917983,25.5758735661201,40.10025));
#197282=CARTESIAN_POINT('Ctrl Pts',(57.40338687637,25.5837184861902,40.10025));
#197283=CARTESIAN_POINT('Ctrl Pts',(57.3992659084774,25.5912015935366,40.0995859581842));
#197284=CARTESIAN_POINT('Ctrl Pts',(57.394649810526,25.5982448512631,40.098327595962));
#197285=CARTESIAN_POINT('Ctrl Pts',(57.3917003436858,25.6027451576541,40.0975235624068));
#197286=CARTESIAN_POINT('Ctrl Pts',(57.3885495044087,25.6070664213766,40.096477705949));
#197287=CARTESIAN_POINT('Ctrl Pts',(57.3852370392635,25.6111943775534,40.0952149915961));
#197288=CARTESIAN_POINT('Ctrl Pts',(57.380716188992,25.6168282094536,40.0934916398701));
#197289=CARTESIAN_POINT('Ctrl Pts',(57.3758905070496,25.6220971979008,40.0913643921631));
#197290=CARTESIAN_POINT('Ctrl Pts',(57.3708481654827,25.6269642358701,40.0889118607713));
#197291=CARTESIAN_POINT('Ctrl Pts',(57.3683269946992,25.6293977548547,40.0876855950754));
#197292=CARTESIAN_POINT('Ctrl Pts',(57.3657515758214,25.631730977776,40.0863782327527));
#197293=CARTESIAN_POINT('Ctrl Pts',(57.3631323306535,25.6339606331571,40.0850006373334));
#197294=CARTESIAN_POINT('Ctrl Pts',(57.3618227080695,25.6350754608477,40.0843118396237));
#197295=CARTESIAN_POINT('Ctrl Pts',(57.3605021218765,25.6361644125821,40.0836054919164));
#197296=CARTESIAN_POINT('Ctrl Pts',(57.3591718306999,25.6372271795769,40.0828829920418));
#197297=CARTESIAN_POINT('Ctrl Pts',(57.3588392579057,25.6374928713256,40.0827023670731));
#197298=CARTESIAN_POINT('Ctrl Pts',(57.3585060784011,25.6377569268679,40.0825207326933));
#197299=CARTESIAN_POINT('Ctrl Pts',(57.3581723115522,25.6380193420644,40.0823381109275));
#197300=CARTESIAN_POINT('Ctrl Pts',(57.3571710110054,25.638806587654,40.0817902456303));
#197301=CARTESIAN_POINT('Ctrl Pts',(57.3561644250956,25.6395790684325,40.0812334935553));
#197302=CARTESIAN_POINT('Ctrl Pts',(57.3551530701153,25.6403366878206,40.0806684524227));
#197303=CARTESIAN_POINT('Ctrl Pts',(57.3481639797008,25.6455723078605,40.0767636676136));
#197304=CARTESIAN_POINT('Ctrl Pts',(57.3409484573002,25.6501539027771,40.0724404510887));
#197305=CARTESIAN_POINT('Ctrl Pts',(57.3336101450127,25.6541395203644,40.0677949937408));
#197306=CARTESIAN_POINT('Ctrl Pts',(57.3299630239493,25.6561203613649,40.0654862141905));
#197307=CARTESIAN_POINT('Ctrl Pts',(57.3262850026764,25.6579537739806,40.0630972003215));
#197308=CARTESIAN_POINT('Ctrl Pts',(57.3225860115762,25.6596454116597,40.0606363359906));
#197309=CARTESIAN_POINT('Ctrl Pts',(57.3144254847134,25.6633774170491,40.0552073017123));
#197310=CARTESIAN_POINT('Ctrl Pts',(57.3061689349815,25.6664302835887,40.0494204304519));
#197311=CARTESIAN_POINT('Ctrl Pts',(57.2979615485277,25.6688109525042,40.0434049749851));
#197312=CARTESIAN_POINT('Ctrl Pts',(57.2949632867555,25.6696806408808,40.0412074532442));
#197313=CARTESIAN_POINT('Ctrl Pts',(57.2919705472986,25.6704685134241,40.0389814735788));
#197314=CARTESIAN_POINT('Ctrl Pts',(57.2889874285393,25.6711779534198,40.0367321210016));
#197315=CARTESIAN_POINT('Ctrl Pts',(57.278967448291,25.6735608872944,40.0291767837143));
#197316=CARTESIAN_POINT('Ctrl Pts',(57.2689905373642,25.6750658360784,40.0213235332581));
#197317=CARTESIAN_POINT('Ctrl Pts',(57.2591158425087,25.6758066569109,40.0132649215867));
#197318=CARTESIAN_POINT('Ctrl Pts',(57.2482623831279,25.6766209067617,40.0044075527544));
#197319=CARTESIAN_POINT('Ctrl Pts',(57.2375317496152,25.6765122533356,39.9953016253734));
#197320=CARTESIAN_POINT('Ctrl Pts',(57.2269836681111,25.6755822344125,39.9860353422375));
#197321=CARTESIAN_POINT('Ctrl Pts',(57.2156229323817,25.6745805641843,39.9760551582714));
#197322=CARTESIAN_POINT('Ctrl Pts',(57.2044727657929,25.6726261321667,39.9658879738178));
#197323=CARTESIAN_POINT('Ctrl Pts',(57.1936020065706,25.669789004385,39.9556174643279));
#197324=CARTESIAN_POINT('Ctrl Pts',(57.1828780393004,25.6669901874073,39.9454856413921));
#197325=CARTESIAN_POINT('Ctrl Pts',(57.1724247063471,25.6633316989627,39.9352519465122));
#197326=CARTESIAN_POINT('Ctrl Pts',(57.1623216544374,25.6588335304434,39.92499));
#197327=CARTESIAN_POINT('Ctrl Pts',(54.0195518809644,24.2595822759726,39.92499));
#197328=CARTESIAN_POINT('Ctrl Pts',(54.0098832048288,24.2552775040081,39.9348107241706));
#197329=CARTESIAN_POINT('Ctrl Pts',(54.0005888273967,24.250225606099,39.9446038383138));
#197330=CARTESIAN_POINT('Ctrl Pts',(53.9917150968546,24.2444615420316,39.9543158069337));
#197331=CARTESIAN_POINT('Ctrl Pts',(53.9831467292703,24.2388958310295,39.9636935671335));
#197332=CARTESIAN_POINT('Ctrl Pts',(53.9749695397937,24.2326653709158,39.9729968320924));
#197333=CARTESIAN_POINT('Ctrl Pts',(53.9672483344123,24.2257620156253,39.9821731151263));
#197334=CARTESIAN_POINT('Ctrl Pts',(53.9599493771946,24.2192361828783,39.9908475764277));
#197335=CARTESIAN_POINT('Ctrl Pts',(53.9530572218394,24.2121084368968,39.9994093733768));
#197336=CARTESIAN_POINT('Ctrl Pts',(53.9466592127742,24.204345482701,40.0077966115762));
#197337=CARTESIAN_POINT('Ctrl Pts',(53.9407667537595,24.1971959321197,40.0155211172516));
#197338=CARTESIAN_POINT('Ctrl Pts',(53.9352931334045,24.1895071355534,40.0230979940944));
#197339=CARTESIAN_POINT('Ctrl Pts',(53.9303412916447,24.1812372959729,40.0304554104673));
#197340=CARTESIAN_POINT('Ctrl Pts',(53.9288647523896,24.1787713967446,40.0326492435131));
#197341=CARTESIAN_POINT('Ctrl Pts',(53.9274348719444,24.1762537459554,40.0348233715036));
#197342=CARTESIAN_POINT('Ctrl Pts',(53.9260551099579,24.1736830183703,40.0369753512356));
#197343=CARTESIAN_POINT('Ctrl Pts',(53.9246894457405,24.1711385572892,40.0391053430352));
#197344=CARTESIAN_POINT('Ctrl Pts',(53.9233740566953,24.1685448683462,40.041211089324));
#197345=CARTESIAN_POINT('Ctrl Pts',(53.9221135831991,24.1659037306806,40.0432881154904));
#197346=CARTESIAN_POINT('Ctrl Pts',(53.9220259323373,24.1657200711326,40.043432547828));
#197347=CARTESIAN_POINT('Ctrl Pts',(53.9219385350609,24.1655361818113,40.0435768364421));
#197348=CARTESIAN_POINT('Ctrl Pts',(53.9218513926274,24.1653520623703,40.0437209807855));
#197349=CARTESIAN_POINT('Ctrl Pts',(53.9180307491145,24.1572795915923,40.0500407968419));
#197350=CARTESIAN_POINT('Ctrl Pts',(53.9147442868251,24.1487557177452,40.0560490279343));
#197351=CARTESIAN_POINT('Ctrl Pts',(53.9120963197575,24.139831588019,40.0616647108613));
#197352=CARTESIAN_POINT('Ctrl Pts',(53.909627954237,24.131512748111,40.0668995033483));
#197353=CARTESIAN_POINT('Ctrl Pts',(53.9077144433433,24.1228452895804,40.0717933267478));
#197354=CARTESIAN_POINT('Ctrl Pts',(53.9064681420134,24.1138798870166,40.0762460303068));
#197355=CARTESIAN_POINT('Ctrl Pts',(53.9060122288632,24.1106002267709,40.0778748868745));
#197356=CARTESIAN_POINT('Ctrl Pts',(53.9056458829919,24.107280847255,40.0794443522246));
#197357=CARTESIAN_POINT('Ctrl Pts',(53.9053756337488,24.1039248822475,40.0809482021492));
#197358=CARTESIAN_POINT('Ctrl Pts',(53.9053106478341,24.1031178847761,40.0813098278168));
#197359=CARTESIAN_POINT('Ctrl Pts',(53.9052515154469,24.1023082689112,40.0816679525672));
#197360=CARTESIAN_POINT('Ctrl Pts',(53.9051983068759,24.1014961507086,40.082022419258));
#197361=CARTESIAN_POINT('Ctrl Pts',(53.9051467610728,24.1007094111998,40.0823658088648));
#197362=CARTESIAN_POINT('Ctrl Pts',(53.9051007746217,24.0999203233282,40.0827057654617));
#197363=CARTESIAN_POINT('Ctrl Pts',(53.9050604098637,24.0991289960595,40.0830421470151));
#197364=CARTESIAN_POINT('Ctrl Pts',(53.9046181672912,24.0904590913151,40.0867275956807));
#197365=CARTESIAN_POINT('Ctrl Pts',(53.9048508523207,24.0815146560278,40.0899823432032));
#197366=CARTESIAN_POINT('Ctrl Pts',(53.9058331609935,24.072468763968,40.0926299529357));
#197367=CARTESIAN_POINT('Ctrl Pts',(53.9062405536795,24.0687171629018,40.0937279956085));
#197368=CARTESIAN_POINT('Ctrl Pts',(53.9067765048114,24.0649483109693,40.0947220371803));
#197369=CARTESIAN_POINT('Ctrl Pts',(53.9074445642445,24.0611749820054,40.0956014538692));
#197370=CARTESIAN_POINT('Ctrl Pts',(53.9085840092244,24.0547391762485,40.097101390674));
#197371=CARTESIAN_POINT('Ctrl Pts',(53.9101092267075,24.0482923662123,40.0982667904316));
#197372=CARTESIAN_POINT('Ctrl Pts',(53.9120381043535,24.0419050995271,40.0990539325582));
#197373=CARTESIAN_POINT('Ctrl Pts',(53.9130025431765,24.0387114661845,40.0994475036216));
#197374=CARTESIAN_POINT('Ctrl Pts',(53.9140692448457,24.0355332447496,40.0997467259952));
#197375=CARTESIAN_POINT('Ctrl Pts',(53.9152404736262,24.0323793130068,40.0999473488896));
#197376=CARTESIAN_POINT('Ctrl Pts',(53.9164117024067,24.029225381264,40.100147971784));
#197377=CARTESIAN_POINT('Ctrl Pts',(53.9176874253156,24.026095770789,40.10025));
#197378=CARTESIAN_POINT('Ctrl Pts',(53.9190682401998,24.022998122529,40.10025));
#197379=CARTESIAN_POINT('Origin',(55.4168495715594,17.9900016446776,39.92499));
#197380=CARTESIAN_POINT('Ctrl Pts',(59.6489943884567,19.1808295835774,39.92499));
#197381=CARTESIAN_POINT('Ctrl Pts',(59.6590854114904,19.1841083557162,39.9348354642021));
#197382=CARTESIAN_POINT('Ctrl Pts',(59.668887786629,19.1881736144719,39.9446440828463));
#197383=CARTESIAN_POINT('Ctrl Pts',(59.6783518907173,19.1929932802638,39.9543641760339));
#197384=CARTESIAN_POINT('Ctrl Pts',(59.6875084677778,19.1976563356168,39.9637684240722));
#197385=CARTESIAN_POINT('Ctrl Pts',(59.6963495165752,19.203026212996,39.9730909636406));
#197386=CARTESIAN_POINT('Ctrl Pts',(59.7048120487199,19.2091163824545,39.9822808977152));
#197387=CARTESIAN_POINT('Ctrl Pts',(59.712817083036,19.2148773077512,39.9909740094661));
#197388=CARTESIAN_POINT('Ctrl Pts',(59.7204841754277,19.2212832892283,39.9995492765013));
#197389=CARTESIAN_POINT('Ctrl Pts',(59.7277306815216,19.2283759411601,40.0079462328707));
#197390=CARTESIAN_POINT('Ctrl Pts',(59.7344052377146,19.234908786543,40.0156804369702));
#197391=CARTESIAN_POINT('Ctrl Pts',(59.7407233396953,19.2420246158644,40.0232638017434));
#197392=CARTESIAN_POINT('Ctrl Pts',(59.7465875973423,19.2497756062331,40.0306257269979));
#197393=CARTESIAN_POINT('Ctrl Pts',(59.7482885955682,19.2520238739014,40.032761141666));
#197394=CARTESIAN_POINT('Ctrl Pts',(59.7499511651817,19.2543256952568,40.0348777427275));
#197395=CARTESIAN_POINT('Ctrl Pts',(59.7515722847792,19.2566826155657,40.0369733168701));
#197396=CARTESIAN_POINT('Ctrl Pts',(59.7533296826515,19.2592376687171,40.039245053974));
#197397=CARTESIAN_POINT('Ctrl Pts',(59.755036811776,19.2618533083049,40.041487875195));
#197398=CARTESIAN_POINT('Ctrl Pts',(59.7566897852106,19.26453048318,40.04369857016));
#197399=CARTESIAN_POINT('Ctrl Pts',(59.7612263837727,19.271878010632,40.0497658398386));
#197400=CARTESIAN_POINT('Ctrl Pts',(59.7653126215478,19.279702281993,40.0555581699984));
#197401=CARTESIAN_POINT('Ctrl Pts',(59.7688605008636,19.2879484209979,40.0609828468885));
#197402=CARTESIAN_POINT('Ctrl Pts',(59.7721066178187,19.2954931904941,40.0659461317305));
#197403=CARTESIAN_POINT('Ctrl Pts',(59.7748909605622,19.303387844687,40.0706039980707));
#197404=CARTESIAN_POINT('Ctrl Pts',(59.7771261198371,19.3116176456442,40.0748843180604));
#197405=CARTESIAN_POINT('Ctrl Pts',(59.7782240227715,19.3156600969904,40.076986797257));
#197406=CARTESIAN_POINT('Ctrl Pts',(59.7791889148826,19.3197833592182,40.0789976708175));
#197407=CARTESIAN_POINT('Ctrl Pts',(59.7800071751725,19.323984929128,40.08090504915));
#197408=CARTESIAN_POINT('Ctrl Pts',(59.7801624320925,19.3247821360946,40.0812669556104));
#197409=CARTESIAN_POINT('Ctrl Pts',(59.7803121206161,19.3255826085659,40.0816253922032));
#197410=CARTESIAN_POINT('Ctrl Pts',(59.7804561537457,19.3263862368329,40.0819801989139));
#197411=CARTESIAN_POINT('Ctrl Pts',(59.7805956858399,19.3271647517165,40.0823239179149));
#197412=CARTESIAN_POINT('Ctrl Pts',(59.780729910488,19.3279462282165,40.0826642303498));
#197413=CARTESIAN_POINT('Ctrl Pts',(59.7808587498045,19.3287305629428,40.0830009916099));
#197414=CARTESIAN_POINT('Ctrl Pts',(59.7822628141275,19.3372780811743,40.0866709464312));
#197415=CARTESIAN_POINT('Ctrl Pts',(59.7830278331225,19.3461707361368,40.0899175831878));
#197416=CARTESIAN_POINT('Ctrl Pts',(59.7830570185565,19.3552444957722,40.0925642067062));
#197417=CARTESIAN_POINT('Ctrl Pts',(59.7830693437465,19.3590764008114,40.0936818922528));
#197418=CARTESIAN_POINT('Ctrl Pts',(59.7829507982332,19.3629403566526,40.094693009479));
#197419=CARTESIAN_POINT('Ctrl Pts',(59.7826959186874,19.3668233599702,40.0955863397546));
#197420=CARTESIAN_POINT('Ctrl Pts',(59.7822667079009,19.3733622405315,40.0970906856166));
#197421=CARTESIAN_POINT('Ctrl Pts',(59.7814491944745,19.3799532508949,40.0982599215483));
#197422=CARTESIAN_POINT('Ctrl Pts',(59.7802163932513,19.386527254457,40.0990497370454));
#197423=CARTESIAN_POINT('Ctrl Pts',(59.7799081929455,19.3881707553476,40.0992471909196));
#197424=CARTESIAN_POINT('Ctrl Pts',(59.7795738105081,19.3898131352229,40.0994209989363));
#197425=CARTESIAN_POINT('Ctrl Pts',(59.7792125287466,19.3914532254502,40.0995705982975));
#197426=CARTESIAN_POINT('Ctrl Pts',(59.7786706061044,19.3939133607911,40.0997949973393));
#197427=CARTESIAN_POINT('Ctrl Pts',(59.7780681520198,19.3963683254111,40.0999649129781));
#197428=CARTESIAN_POINT('Ctrl Pts',(59.7774043475416,19.3988146762076,40.1000786629733));
#197429=CARTESIAN_POINT('Ctrl Pts',(59.7767405430633,19.4012610270041,40.1001924129685));
#197430=CARTESIAN_POINT('Ctrl Pts',(59.7760153991104,19.4036987600447,40.10025));
#197431=CARTESIAN_POINT('Ctrl Pts',(59.7752282754839,19.4061247292246,40.10025));
#197432=CARTESIAN_POINT('Ctrl Pts',(56.144199857553,18.2263320786575,40.10025));
#197433=CARTESIAN_POINT('Ctrl Pts',(56.1468630191714,18.2181232748942,40.10025));
#197434=CARTESIAN_POINT('Ctrl Pts',(56.1501806998576,18.2102054558342,40.0995786334241));
#197435=CARTESIAN_POINT('Ctrl Pts',(56.1540344262249,18.2026724222816,40.0983063763368));
#197436=CARTESIAN_POINT('Ctrl Pts',(56.1565235380433,18.1978068555399,40.0974846287994));
#197437=CARTESIAN_POINT('Ctrl Pts',(56.1592354513147,18.1931013796336,40.0964130309339));
#197438=CARTESIAN_POINT('Ctrl Pts',(56.1621313494122,18.1885757140651,40.0951176960924));
#197439=CARTESIAN_POINT('Ctrl Pts',(56.165969696453,18.1825772036006,40.0934008039614));
#197440=CARTESIAN_POINT('Ctrl Pts',(56.1701354151838,18.1768986338326,40.0912909372156));
#197441=CARTESIAN_POINT('Ctrl Pts',(56.1745504247235,18.171584897892,40.0888630467851));
#197442=CARTESIAN_POINT('Ctrl Pts',(56.1767579294933,18.1689280299216,40.0876491015699));
#197443=CARTESIAN_POINT('Ctrl Pts',(56.1790278168867,18.1663621803347,40.0863558569271));
#197444=CARTESIAN_POINT('Ctrl Pts',(56.1813507566161,18.1638916135752,40.0849936342771));
#197445=CARTESIAN_POINT('Ctrl Pts',(56.1825122264809,18.1626563301955,40.0843125229521));
#197446=CARTESIAN_POINT('Ctrl Pts',(56.1836869644606,18.1614448518806,40.0836141747074));
#197447=CARTESIAN_POINT('Ctrl Pts',(56.1848738357354,18.160257613441,40.0828999161609));
#197448=CARTESIAN_POINT('Ctrl Pts',(56.1851705535541,18.1599608038311,40.0827213515243));
#197449=CARTESIAN_POINT('Ctrl Pts',(56.1854680298098,18.1596655088804,40.0825417925842));
#197450=CARTESIAN_POINT('Ctrl Pts',(56.1857662469844,18.1593717347111,40.082361260236));
#197451=CARTESIAN_POINT('Ctrl Pts',(56.186660898508,18.1584904122031,40.0818196631917));
#197452=CARTESIAN_POINT('Ctrl Pts',(56.1875622177791,18.1576227783918,40.0812693052021));
#197453=CARTESIAN_POINT('Ctrl Pts',(56.1884697364866,18.1567689837079,40.0807107531874));
#197454=CARTESIAN_POINT('Ctrl Pts',(56.1948621810804,18.150754964199,40.0767763849182));
#197455=CARTESIAN_POINT('Ctrl Pts',(56.2015542305059,18.1453743792962,40.0724140586139));
#197456=CARTESIAN_POINT('Ctrl Pts',(56.2084349106659,18.1405824894349,40.0677221223771));
#197457=CARTESIAN_POINT('Ctrl Pts',(56.2117720331084,18.1382584280302,40.0654465383723));
#197458=CARTESIAN_POINT('Ctrl Pts',(56.2151540877945,18.1360729791405,40.063092800068));
#197459=CARTESIAN_POINT('Ctrl Pts',(56.2185710935571,18.1340220442544,40.0606689262479));
#197460=CARTESIAN_POINT('Ctrl Pts',(56.22380229064,18.1308822062386,40.0569581447805));
#197461=CARTESIAN_POINT('Ctrl Pts',(56.2291119669557,18.1280584389292,40.0530843804605));
#197462=CARTESIAN_POINT('Ctrl Pts',(56.2344544719219,18.1255442374224,40.0490800251457));
#197463=CARTESIAN_POINT('Ctrl Pts',(56.2369355588666,18.1243766292358,40.0472203818218));
#197464=CARTESIAN_POINT('Ctrl Pts',(56.2394235482377,18.123275602876,40.0453323608818));
#197465=CARTESIAN_POINT('Ctrl Pts',(56.2419141381099,18.1222417093394,40.0434201572162));
#197466=CARTESIAN_POINT('Ctrl Pts',(56.2421050320102,18.1221624654736,40.0432735943397));
#197467=CARTESIAN_POINT('Ctrl Pts',(56.2422959411933,18.1220835820639,40.0431268995707));
#197468=CARTESIAN_POINT('Ctrl Pts',(56.2424868643662,18.1220050584315,40.0429800745037));
#197469=CARTESIAN_POINT('Ctrl Pts',(56.2451687593305,18.1209020381379,40.0409176249753));
#197470=CARTESIAN_POINT('Ctrl Pts',(56.2478543333342,18.1198718859658,40.0388310783332));
#197471=CARTESIAN_POINT('Ctrl Pts',(56.2505383386776,18.1189123616719,40.036725739981));
#197472=CARTESIAN_POINT('Ctrl Pts',(56.2601627045041,18.1154716781997,40.0291763710722));
#197473=CARTESIAN_POINT('Ctrl Pts',(56.2698406425778,18.112910688301,40.0213310894603));
#197474=CARTESIAN_POINT('Ctrl Pts',(56.2795015152455,18.1111213027306,40.0132837551333));
#197475=CARTESIAN_POINT('Ctrl Pts',(56.2901178437866,18.1091549477485,40.0044405431344));
#197476=CARTESIAN_POINT('Ctrl Pts',(56.3007141730202,18.1081200911546,39.9953528710626));
#197477=CARTESIAN_POINT('Ctrl Pts',(56.3112209484336,18.1079204190081,39.9861103629587));
#197478=CARTESIAN_POINT('Ctrl Pts',(56.3225656290391,18.1077048232008,39.9761307737596));
#197479=CARTESIAN_POINT('Ctrl Pts',(56.3338070504095,18.1084627484397,39.965969693606));
#197480=CARTESIAN_POINT('Ctrl Pts',(56.3448702837321,18.1101289800536,39.9557128217563));
#197481=CARTESIAN_POINT('Ctrl Pts',(56.3558407078974,18.1117812336967,39.9455419945199));
#197482=CARTESIAN_POINT('Ctrl Pts',(56.3666372711377,18.1143271060903,39.935275628936));
#197483=CARTESIAN_POINT('Ctrl Pts',(56.377179453281,18.1177524687099,39.92499));
#197484=CARTESIAN_POINT('Origin',(-0.00470941899427373,0.0144941013083365,
39.92499));
#197485=CARTESIAN_POINT('Ctrl Pts',(59.7658094374954,19.4351129318413,40.10025));
#197486=CARTESIAN_POINT('Ctrl Pts',(59.7631518948792,19.4432803829093,40.10025));
#197487=CARTESIAN_POINT('Ctrl Pts',(59.759835699791,19.4511532554524,40.099585958184));
#197488=CARTESIAN_POINT('Ctrl Pts',(59.7559811102134,19.4586404431018,40.0983275959617));
#197489=CARTESIAN_POINT('Ctrl Pts',(59.7535182109726,19.4634243995791,40.0975235624065));
#197490=CARTESIAN_POINT('Ctrl Pts',(59.7508363273794,19.4680513433538,40.0964777059488));
#197491=CARTESIAN_POINT('Ctrl Pts',(59.7479734971809,19.4725029330454,40.0952149915961));
#197492=CARTESIAN_POINT('Ctrl Pts',(59.744066308391,19.4785784597565,40.0934916398701));
#197493=CARTESIAN_POINT('Ctrl Pts',(59.7398178213045,19.4843230052514,40.0913643921631));
#197494=CARTESIAN_POINT('Ctrl Pts',(59.7353118462119,19.4896904492926,40.0889118607713));
#197495=CARTESIAN_POINT('Ctrl Pts',(59.7330588586655,19.4923741713132,40.0876855950754));
#197496=CARTESIAN_POINT('Ctrl Pts',(59.7307414364082,19.4949638171728,40.0863782327526));
#197497=CARTESIAN_POINT('Ctrl Pts',(59.72836960219,19.4974550439408,40.0850006373334));
#197498=CARTESIAN_POINT('Ctrl Pts',(59.7271836850809,19.4987006573248,40.0843118396237));
#197499=CARTESIAN_POINT('Ctrl Pts',(59.7259841596486,19.499921682513,40.0836054919164));
#197500=CARTESIAN_POINT('Ctrl Pts',(59.724772245347,19.5011176808515,40.0828829920418));
#197501=CARTESIAN_POINT('Ctrl Pts',(59.7244692667716,19.5014166804361,40.0827023670731));
#197502=CARTESIAN_POINT('Ctrl Pts',(59.7241655137792,19.5017141161961,40.0825207326933));
#197503=CARTESIAN_POINT('Ctrl Pts',(59.7238610051972,19.5020099819905,40.0823381109275));
#197504=CARTESIAN_POINT('Ctrl Pts',(59.7229474794513,19.5028975793738,40.0817902456303));
#197505=CARTESIAN_POINT('Ctrl Pts',(59.7220271539531,19.5037710453001,40.0812334935553));
#197506=CARTESIAN_POINT('Ctrl Pts',(59.7211005320716,19.5046302297518,40.0806684524227));
#197507=CARTESIAN_POINT('Ctrl Pts',(59.7146969999425,19.5105677273982,40.0767636676135));
#197508=CARTESIAN_POINT('Ctrl Pts',(59.7079999120043,19.5158784513267,40.0724404510885));
#197509=CARTESIAN_POINT('Ctrl Pts',(59.7011184102408,19.5206092977904,40.0677949937404));
#197510=CARTESIAN_POINT('Ctrl Pts',(59.6976983227541,19.5229605154966,40.0654862141902));
#197511=CARTESIAN_POINT('Ctrl Pts',(59.6942320938701,19.5251683423976,40.0630972003214));
#197512=CARTESIAN_POINT('Ctrl Pts',(59.6907301905173,19.5272373629636,40.0606363359906));
#197513=CARTESIAN_POINT('Ctrl Pts',(59.6830044686629,19.5318019313695,40.0552073017123));
#197514=CARTESIAN_POINT('Ctrl Pts',(59.6751122606222,19.5357011184421,40.0494204304519));
#197515=CARTESIAN_POINT('Ctrl Pts',(59.6671986827534,19.5389266512976,40.0434049749851));
#197516=CARTESIAN_POINT('Ctrl Pts',(59.6643077529625,19.5401049791258,40.0412074532442));
#197517=CARTESIAN_POINT('Ctrl Pts',(59.6614137631516,19.5412013620773,40.0389814735788));
#197518=CARTESIAN_POINT('Ctrl Pts',(59.6585211429015,19.5422187365061,40.0367321210016));
#197519=CARTESIAN_POINT('Ctrl Pts',(59.6488051375691,19.545635989557,40.0291767837141));
#197520=CARTESIAN_POINT('Ctrl Pts',(59.6390401911876,19.5481755652415,40.0213235332577));
#197521=CARTESIAN_POINT('Ctrl Pts',(59.6292970278066,19.5499445144584,40.0132649215861));
#197522=CARTESIAN_POINT('Ctrl Pts',(59.6185881370972,19.5518887991936,40.0044075527536));
#197523=CARTESIAN_POINT('Ctrl Pts',(59.6079049297416,19.5529023976132,39.9953016253723));
#197524=CARTESIAN_POINT('Ctrl Pts',(59.5973174182825,19.5530800481811,39.9860353422362));
#197525=CARTESIAN_POINT('Ctrl Pts',(59.5859142148021,19.5532713854545,39.9760551582698));
#197526=CARTESIAN_POINT('Ctrl Pts',(59.5746208362169,19.5524931697985,39.9658879738159));
#197527=CARTESIAN_POINT('Ctrl Pts',(59.5635130675436,19.5508078878555,39.9556174643256));
#197528=CARTESIAN_POINT('Ctrl Pts',(59.5525552912515,19.5491453629089,39.9454856413906));
#197529=CARTESIAN_POINT('Ctrl Pts',(59.5417768065759,19.5465995868767,39.9352519465114));
#197530=CARTESIAN_POINT('Ctrl Pts',(59.5312589135998,19.5431821162859,39.92499));
#197531=CARTESIAN_POINT('Ctrl Pts',(56.2594439784241,18.4801050014183,39.92499));
#197532=CARTESIAN_POINT('Ctrl Pts',(56.249378297109,18.4768344633031,39.9348107241714));
#197533=CARTESIAN_POINT('Ctrl Pts',(56.2396067681233,18.472781767209,39.9446038383154));
#197534=CARTESIAN_POINT('Ctrl Pts',(56.2301791400456,18.4679768367041,39.9543158069361));
#197535=CARTESIAN_POINT('Ctrl Pts',(56.2210759356573,18.4633372535452,39.9636935671363));
#197536=CARTESIAN_POINT('Ctrl Pts',(56.2122922812589,18.4579956735935,39.9729968320954));
#197537=CARTESIAN_POINT('Ctrl Pts',(56.2038917763283,18.4519372213383,39.9821731151296));
#197538=CARTESIAN_POINT('Ctrl Pts',(56.1959506682935,18.4462100865672,39.9908475764309));
#197539=CARTESIAN_POINT('Ctrl Pts',(56.1883512165526,18.4398418135318,39.9994093733799));
#197540=CARTESIAN_POINT('Ctrl Pts',(56.1811768067782,18.4327901596668,40.0077966115791));
#197541=CARTESIAN_POINT('Ctrl Pts',(56.1745692957356,18.4262957047575,40.0155211172542));
#197542=CARTESIAN_POINT('Ctrl Pts',(56.1683219623566,18.4192211773477,40.0230979940965));
#197543=CARTESIAN_POINT('Ctrl Pts',(56.1625328136815,18.4115142492234,40.0304554104689));
#197544=CARTESIAN_POINT('Ctrl Pts',(56.1608066064065,18.409216198829,40.0326492435142));
#197545=CARTESIAN_POINT('Ctrl Pts',(56.1591213928284,18.4068618032005,40.0348233715041));
#197546=CARTESIAN_POINT('Ctrl Pts',(56.1574804751189,18.4044493827308,40.0369753512356));
#197547=CARTESIAN_POINT('Ctrl Pts',(56.1558563235463,18.4020616112557,40.0391053430352));
#197548=CARTESIAN_POINT('Ctrl Pts',(56.1542770260205,18.3996196264076,40.041211089324));
#197549=CARTESIAN_POINT('Ctrl Pts',(56.1527473834686,18.397124712528,40.0432881154904));
#197550=CARTESIAN_POINT('Ctrl Pts',(56.152641015117,18.3969512210961,40.043432547828));
#197551=CARTESIAN_POINT('Ctrl Pts',(56.1525348749439,18.3967774746428,40.0435768364421));
#197552=CARTESIAN_POINT('Ctrl Pts',(56.1524289641635,18.3966034726919,40.0437209807855));
#197553=CARTESIAN_POINT('Ctrl Pts',(56.1477854475703,18.3889745897485,40.050040796842));
#197554=CARTESIAN_POINT('Ctrl Pts',(56.1436260014308,18.3808409394268,40.0560490279345));
#197555=CARTESIAN_POINT('Ctrl Pts',(56.1400597146376,18.3722424849452,40.0616647108616));
#197556=CARTESIAN_POINT('Ctrl Pts',(56.1367353155299,18.364227230967,40.0668995033487));
#197557=CARTESIAN_POINT('Ctrl Pts',(56.1339262909284,18.3558072700341,40.0717933267483));
#197558=CARTESIAN_POINT('Ctrl Pts',(56.131749677215,18.347021254846,40.0762460303074));
#197559=CARTESIAN_POINT('Ctrl Pts',(56.1309534437593,18.3438072168237,40.0778748868749));
#197560=CARTESIAN_POINT('Ctrl Pts',(56.1302421351293,18.3405443147874,40.0794443522248));
#197561=CARTESIAN_POINT('Ctrl Pts',(56.1296225724749,18.3372349828458,40.0809482021492));
#197562=CARTESIAN_POINT('Ctrl Pts',(56.1294735883543,18.3364391990689,40.0813098278168));
#197563=CARTESIAN_POINT('Ctrl Pts',(56.1293301519983,18.335640199382,40.0816679525672));
#197564=CARTESIAN_POINT('Ctrl Pts',(56.1291923454417,18.334838091858,40.082022419258));
#197565=CARTESIAN_POINT('Ctrl Pts',(56.1290588453401,18.3340610501941,40.0823658088648));
#197566=CARTESIAN_POINT('Ctrl Pts',(56.1289306286649,18.3332810919215,40.0827057654616));
#197567=CARTESIAN_POINT('Ctrl Pts',(56.128807768806,18.3324983188925,40.0830421470151));
#197568=CARTESIAN_POINT('Ctrl Pts',(56.127461697065,18.3239221357303,40.0867275956805));
#197569=CARTESIAN_POINT('Ctrl Pts',(56.1267581593462,18.3150023767871,40.089982343203));
#197570=CARTESIAN_POINT('Ctrl Pts',(56.1267895336333,18.3059033598548,40.0926299529354));
#197571=CARTESIAN_POINT('Ctrl Pts',(56.1268025454853,18.3021297263201,40.0937279956083));
#197572=CARTESIAN_POINT('Ctrl Pts',(56.12694160832,18.2983254984043,40.0947220371802));
#197573=CARTESIAN_POINT('Ctrl Pts',(56.1272115877757,18.294503008905,40.0956014538692));
#197574=CARTESIAN_POINT('Ctrl Pts',(56.1276720658711,18.2879833547327,40.097101390674));
#197575=CARTESIAN_POINT('Ctrl Pts',(56.1285150529072,18.2814124323567,40.0982667904316));
#197576=CARTESIAN_POINT('Ctrl Pts',(56.1297657127889,18.2748585331707,40.0990539325582));
#197577=CARTESIAN_POINT('Ctrl Pts',(56.1303910427298,18.2715815835777,40.0994475036216));
#197578=CARTESIAN_POINT('Ctrl Pts',(56.1311196862931,18.2683092720861,40.0997467259952));
#197579=CARTESIAN_POINT('Ctrl Pts',(56.1319548233213,18.2650501911668,40.0999473488896));
#197580=CARTESIAN_POINT('Ctrl Pts',(56.1327899603496,18.2617911102474,40.100147971784));
#197581=CARTESIAN_POINT('Ctrl Pts',(56.1337315613411,18.2585452947508,40.10025));
#197582=CARTESIAN_POINT('Ctrl Pts',(56.1347810195644,18.2553202812742,40.10025));
#197583=CARTESIAN_POINT('Origin',(56.9937374973465,12.0988124084933,39.92499));
#197584=CARTESIAN_POINT('Ctrl Pts',(61.3271735965895,12.840737273309,39.92499));
#197585=CARTESIAN_POINT('Ctrl Pts',(61.3375520649562,12.8429432848604,39.9348354642016));
#197586=CARTESIAN_POINT('Ctrl Pts',(61.3477256769083,12.8459616464936,39.9446440828453));
#197587=CARTESIAN_POINT('Ctrl Pts',(61.3576417279026,12.8497656413953,39.9543641760325));
#197588=CARTESIAN_POINT('Ctrl Pts',(61.3672355662859,12.853446029114,39.9637684240705));
#197589=CARTESIAN_POINT('Ctrl Pts',(61.376589487923,12.8578623484984,39.9730909636387));
#197590=CARTESIAN_POINT('Ctrl Pts',(61.3856422574854,12.8630345798907,39.982280897713));
#197591=CARTESIAN_POINT('Ctrl Pts',(61.394205620054,12.8679271923002,39.9909740094639));
#197592=CARTESIAN_POINT('Ctrl Pts',(61.4025003187107,12.8734966517548,39.9995492764989));
#197593=CARTESIAN_POINT('Ctrl Pts',(61.4104485116927,12.8797929832509,40.0079462328682));
#197594=CARTESIAN_POINT('Ctrl Pts',(61.417769372257,12.8855923599211,40.0156804369676));
#197595=CARTESIAN_POINT('Ctrl Pts',(61.4247966697177,12.8920087864938,40.0232638017408));
#197596=CARTESIAN_POINT('Ctrl Pts',(61.4314390014596,12.8991043342859,40.0306257269952));
#197597=CARTESIAN_POINT('Ctrl Pts',(61.4333656894045,12.9011624829789,40.0327611416642));
#197598=CARTESIAN_POINT('Ctrl Pts',(61.4352597571376,12.9032779088702,40.0348777427266));
#197599=CARTESIAN_POINT('Ctrl Pts',(61.4371183613309,12.9054524645837,40.0369733168701));
#197600=CARTESIAN_POINT('Ctrl Pts',(61.4391332077733,12.9078098227875,40.039245053974));
#197601=CARTESIAN_POINT('Ctrl Pts',(61.4411043938524,12.9102326900441,40.041487875195));
#197602=CARTESIAN_POINT('Ctrl Pts',(61.4430281531013,12.9127224163021,40.0436985701601));
#197603=CARTESIAN_POINT('Ctrl Pts',(61.4483079254551,12.9195554895538,40.0497658398386));
#197604=CARTESIAN_POINT('Ctrl Pts',(61.4531896374537,12.9269097705824,40.0555581699984));
#197605=CARTESIAN_POINT('Ctrl Pts',(61.4575800373535,12.9347398820023,40.0609828468885));
#197606=CARTESIAN_POINT('Ctrl Pts',(61.4615970149013,12.9419040088446,40.0659461317303));
#197607=CARTESIAN_POINT('Ctrl Pts',(61.4651913207946,12.9494643722274,40.0706039980704));
#197608=CARTESIAN_POINT('Ctrl Pts',(61.4682744840801,12.9574154517093,40.07488431806));
#197609=CARTESIAN_POINT('Ctrl Pts',(61.4697889238145,12.9613209959778,40.0769867972567));
#197610=CARTESIAN_POINT('Ctrl Pts',(61.4711795284101,12.9653208118544,40.0789976708173));
#197611=CARTESIAN_POINT('Ctrl Pts',(61.4724324898305,12.9694138336343,40.0809050491499));
#197612=CARTESIAN_POINT('Ctrl Pts',(61.4726702270561,12.9701904446504,40.0812669556104));
#197613=CARTESIAN_POINT('Ctrl Pts',(61.4729027677276,12.9709708853385,40.0816253922032));
#197614=CARTESIAN_POINT('Ctrl Pts',(61.4731300138564,12.9717550556841,40.0819801989139));
#197615=CARTESIAN_POINT('Ctrl Pts',(61.4733501585437,12.9725147207063,40.0823239179149));
#197616=CARTESIAN_POINT('Ctrl Pts',(61.4735653344327,12.9732778859001,40.0826642303498));
#197617=CARTESIAN_POINT('Ctrl Pts',(61.4737754532575,12.9740444565829,40.0830009916099));
#197618=CARTESIAN_POINT('Ctrl Pts',(61.4760652849148,12.9823983859293,40.0866709464313));
#197619=CARTESIAN_POINT('Ctrl Pts',(61.4777556486134,12.9911623597379,40.0899175831879));
#197620=CARTESIAN_POINT('Ctrl Pts',(61.4787331403172,13.0001833616603,40.0925642067064));
#197621=CARTESIAN_POINT('Ctrl Pts',(61.4791459411337,13.0039929867894,40.0936818922529));
#197622=CARTESIAN_POINT('Ctrl Pts',(61.4794319383913,13.0078481668562,40.0946930094791));
#197623=CARTESIAN_POINT('Ctrl Pts',(61.4795843394719,13.0117365408424,40.0955863397545));
#197624=CARTESIAN_POINT('Ctrl Pts',(61.4798409790836,13.0182844654757,40.0970906856166));
#197625=CARTESIAN_POINT('Ctrl Pts',(61.4797168922659,13.0249248230168,40.0982599215483));
#197626=CARTESIAN_POINT('Ctrl Pts',(61.4791780149468,13.031591676317,40.0990497370453));
#197627=CARTESIAN_POINT('Ctrl Pts',(61.4790432956171,13.033258389642,40.0992471909196));
#197628=CARTESIAN_POINT('Ctrl Pts',(61.4788824204062,13.0349267248709,40.0994209989363));
#197629=CARTESIAN_POINT('Ctrl Pts',(61.478694553895,13.0365955947397,40.0995705982975));
#197630=CARTESIAN_POINT('Ctrl Pts',(61.4784127541283,13.0390988995427,40.0997949973393));
#197631=CARTESIAN_POINT('Ctrl Pts',(61.4780702140293,13.0416033892093,40.0999649129781));
#197632=CARTESIAN_POINT('Ctrl Pts',(61.4776657592308,13.0441057251022,40.1000786629733));
#197633=CARTESIAN_POINT('Ctrl Pts',(61.4772613044323,13.0466080609951,40.1001924129685));
#197634=CARTESIAN_POINT('Ctrl Pts',(61.4767949453823,13.0491082380621,40.10025));
#197635=CARTESIAN_POINT('Ctrl Pts',(61.4762657165317,13.0516031943521,40.10025));
#197636=CARTESIAN_POINT('Ctrl Pts',(57.7418065394567,12.257819391976,40.10025));
#197637=CARTESIAN_POINT('Ctrl Pts',(57.7435970583547,12.2493771807065,40.10025));
#197638=CARTESIAN_POINT('Ctrl Pts',(57.7460689269805,12.2411559442234,40.099578633424));
#197639=CARTESIAN_POINT('Ctrl Pts',(57.7491141258108,12.2332613533211,40.0983063763364));
#197640=CARTESIAN_POINT('Ctrl Pts',(57.7510810117996,12.2281622576305,40.0974846287991));
#197641=CARTESIAN_POINT('Ctrl Pts',(57.7532862127607,12.2231990866875,40.0964130309337));
#197642=CARTESIAN_POINT('Ctrl Pts',(57.755693185958,12.2183955094112,40.0951176960923));
#197643=CARTESIAN_POINT('Ctrl Pts',(57.7588834910513,12.212028642897,40.0934008039613));
#197644=CARTESIAN_POINT('Ctrl Pts',(57.7624328173676,12.2059457447511,40.0912909372156));
#197645=CARTESIAN_POINT('Ctrl Pts',(57.766268204371,12.2001996238494,40.0888630467851));
#197646=CARTESIAN_POINT('Ctrl Pts',(57.7681858978727,12.1973265633985,40.0876491015698));
#197647=CARTESIAN_POINT('Ctrl Pts',(57.7701751462712,12.1945375019631,40.086355856927));
#197648=CARTESIAN_POINT('Ctrl Pts',(57.7722271161469,12.1918376559067,40.084993634277));
#197649=CARTESIAN_POINT('Ctrl Pts',(57.7732531010848,12.1904877328784,40.084312522952));
#197650=CARTESIAN_POINT('Ctrl Pts',(57.7742947697605,12.1891600976128,40.0836141747073));
#197651=CARTESIAN_POINT('Ctrl Pts',(57.7753510390206,12.1878553011591,40.0828999161609));
#197652=CARTESIAN_POINT('Ctrl Pts',(57.7756151063356,12.1875291020457,40.0827213515243));
#197653=CARTESIAN_POINT('Ctrl Pts',(57.7758800862579,12.1872043300158,40.0825417925841));
#197654=CARTESIAN_POINT('Ctrl Pts',(57.7761459620051,12.1868809929891,40.082361260236));
#197655=CARTESIAN_POINT('Ctrl Pts',(57.7769435892466,12.1859109819091,40.0818196631917));
#197656=CARTESIAN_POINT('Ctrl Pts',(57.7777492785675,12.1849538875683,40.0812693052021));
#197657=CARTESIAN_POINT('Ctrl Pts',(57.7785625799463,12.1840099085251,40.0807107531874));
#197658=CARTESIAN_POINT('Ctrl Pts',(57.7842913698425,12.1773606420343,40.0767763849182));
#197659=CARTESIAN_POINT('Ctrl Pts',(57.7903843352498,12.171310022896,40.0724140586138));
#197660=CARTESIAN_POINT('Ctrl Pts',(57.7967264334406,12.1658251565853,40.067722122377));
#197661=CARTESIAN_POINT('Ctrl Pts',(57.7998023442099,12.1631650023516,40.0654465383722));
#197662=CARTESIAN_POINT('Ctrl Pts',(57.8029374300325,12.1606380046006,40.063092800068));
#197663=CARTESIAN_POINT('Ctrl Pts',(57.8061213360081,12.1582411305891,40.0606689262479));
#197664=CARTESIAN_POINT('Ctrl Pts',(57.8109956736034,12.1545716839424,40.0569581447805));
#197665=CARTESIAN_POINT('Ctrl Pts',(57.8159810988991,12.15120837322,40.0530843804605));
#197666=CARTESIAN_POINT('Ctrl Pts',(57.8210315314442,12.148149500938,40.0490800251457));
#197667=CARTESIAN_POINT('Ctrl Pts',(57.8233769784456,12.1467289448257,40.0472203818218));
#197668=CARTESIAN_POINT('Ctrl Pts',(57.8257362497573,12.1453738842979,40.0453323608818));
#197669=CARTESIAN_POINT('Ctrl Pts',(57.828105124615,12.1440853170063,40.0434201572162));
#197670=CARTESIAN_POINT('Ctrl Pts',(57.828286689539,12.1439865534006,40.0432735943397));
#197671=CARTESIAN_POINT('Ctrl Pts',(57.8284683073401,12.143888146679,40.0431268995707));
#197672=CARTESIAN_POINT('Ctrl Pts',(57.8286499766612,12.1437900963014,40.0429800745037));
#197673=CARTESIAN_POINT('Ctrl Pts',(57.831201882908,12.1424127841091,40.0409176249753));
#197674=CARTESIAN_POINT('Ctrl Pts',(57.8337650648328,12.1411075562948,40.0388310783332));
#197675=CARTESIAN_POINT('Ctrl Pts',(57.8363340693142,12.1398727334214,40.036725739981));
#197676=CARTESIAN_POINT('Ctrl Pts',(57.8455460625016,12.1354448782036,40.0291763710723));
#197677=CARTESIAN_POINT('Ctrl Pts',(57.8549032874792,12.1318862976811,40.0213310894606));
#197678=CARTESIAN_POINT('Ctrl Pts',(57.8643241951516,12.1290968783783,40.0132837551337));
#197679=CARTESIAN_POINT('Ctrl Pts',(57.8746768262695,12.1260315867866,40.0044405431349));
#197680=CARTESIAN_POINT('Ctrl Pts',(57.8851069357333,12.1238947812343,39.9953528710631));
#197681=CARTESIAN_POINT('Ctrl Pts',(57.8955352825089,12.1225979458248,39.9861103629593));
#197682=CARTESIAN_POINT('Ctrl Pts',(57.9067952798687,12.1211976890439,39.9761307737602));
#197683=CARTESIAN_POINT('Ctrl Pts',(57.9180543443172,12.1207764137882,39.9659696936065));
#197684=CARTESIAN_POINT('Ctrl Pts',(57.9292311407202,12.121277094833,39.9557128217568));
#197685=CARTESIAN_POINT('Ctrl Pts',(57.9403141752885,12.1217735756784,39.9455419945202));
#197686=CARTESIAN_POINT('Ctrl Pts',(57.9513177099548,12.1231769533525,39.9352756289361));
#197687=CARTESIAN_POINT('Ctrl Pts',(57.9621601888122,12.1254815933784,39.92499));
#197688=CARTESIAN_POINT('Origin',(-0.00316857416806234,0.0149069694351821,
39.92499));
#197689=CARTESIAN_POINT('Ctrl Pts',(61.4699285681956,13.0814171332224,40.10025));
#197690=CARTESIAN_POINT('Ctrl Pts',(61.468139314985,13.0898176309843,40.10025));
#197691=CARTESIAN_POINT('Ctrl Pts',(61.465664225629,13.097994011884,40.0995859581841));
#197692=CARTESIAN_POINT('Ctrl Pts',(61.4626133761157,13.1058430982609,40.0983275959618));
#197693=CARTESIAN_POINT('Ctrl Pts',(61.4606640285135,13.1108582907973,40.0975235624066));
#197694=CARTESIAN_POINT('Ctrl Pts',(61.4584804838814,13.1157402208608,40.0964777059489));
#197695=CARTESIAN_POINT('Ctrl Pts',(61.4560986543957,13.12046667152,40.095214991596));
#197696=CARTESIAN_POINT('Ctrl Pts',(61.4528479350655,13.1269173282999,40.09349163987));
#197697=CARTESIAN_POINT('Ctrl Pts',(61.4492231901485,13.1330744923999,40.091364392163));
#197698=CARTESIAN_POINT('Ctrl Pts',(61.4453029499362,13.1388835356729,40.0889118607712));
#197699=CARTESIAN_POINT('Ctrl Pts',(61.4433428298301,13.1417880573095,40.0876855950754));
#197700=CARTESIAN_POINT('Ctrl Pts',(61.4413087943565,13.1446057534054,40.0863782327526));
#197701=CARTESIAN_POINT('Ctrl Pts',(61.4392103574,13.1473312571584,40.0850006373333));
#197702=CARTESIAN_POINT('Ctrl Pts',(61.4381611389218,13.148694009035,40.0843118396237));
#197703=CARTESIAN_POINT('Ctrl Pts',(61.4370958165018,13.1500337298695,40.0836054919164));
#197704=CARTESIAN_POINT('Ctrl Pts',(61.436015557062,13.1513498559435,40.0828829920417));
#197705=CARTESIAN_POINT('Ctrl Pts',(61.435745492202,13.151678887462,40.0827023670731));
#197706=CARTESIAN_POINT('Ctrl Pts',(61.4354744937032,13.1520064446712,40.0825207326932));
#197707=CARTESIAN_POINT('Ctrl Pts',(61.435202579648,13.152332519496,40.0823381109275));
#197708=CARTESIAN_POINT('Ctrl Pts',(61.4343868374822,13.1533107439703,40.0817902456303));
#197709=CARTESIAN_POINT('Ctrl Pts',(61.4335628556744,13.1542756251689,40.0812334935553));
#197710=CARTESIAN_POINT('Ctrl Pts',(61.4327311191548,13.1552269612796,40.0806684524227));
#197711=CARTESIAN_POINT('Ctrl Pts',(61.4269833037496,13.1618012840653,40.0767636676137));
#197712=CARTESIAN_POINT('Ctrl Pts',(61.4208780249712,13.1677829516029,40.0724404510888));
#197713=CARTESIAN_POINT('Ctrl Pts',(61.4145287289054,13.1732071947987,40.0677949937409));
#197714=CARTESIAN_POINT('Ctrl Pts',(61.4113731461892,13.1759030287778,40.0654862141905));
#197715=CARTESIAN_POINT('Ctrl Pts',(61.4081566864226,13.1784610805508,40.0630972003216));
#197716=CARTESIAN_POINT('Ctrl Pts',(61.4048902384028,13.1808848153819,40.0606363359906));
#197717=CARTESIAN_POINT('Ctrl Pts',(61.3976839661819,13.1862319364375,40.0552073017123));
#197718=CARTESIAN_POINT('Ctrl Pts',(61.3902425685154,13.1909347237336,40.0494204304519));
#197719=CARTESIAN_POINT('Ctrl Pts',(61.3827095020468,13.1949697809162,40.0434049749851));
#197720=CARTESIAN_POINT('Ctrl Pts',(61.3799575778688,13.1964438381897,40.0412074532442));
#197721=CARTESIAN_POINT('Ctrl Pts',(61.377194044862,13.1978367193484,40.0389814735788));
#197722=CARTESIAN_POINT('Ctrl Pts',(61.374423615274,13.1991508816431,40.0367321210016));
#197723=CARTESIAN_POINT('Ctrl Pts',(61.3651180354457,13.2035650137306,40.0291767837143));
#197724=CARTESIAN_POINT('Ctrl Pts',(61.3556720404061,13.2071113921929,40.0213235332581));
#197725=CARTESIAN_POINT('Ctrl Pts',(61.3461671566372,13.2098890888164,40.0132649215866));
#197726=CARTESIAN_POINT('Ctrl Pts',(61.3357201634477,13.2129421064455,40.0044075527543));
#197727=CARTESIAN_POINT('Ctrl Pts',(61.3252014297054,13.2150668515146,39.9953016253732));
#197728=CARTESIAN_POINT('Ctrl Pts',(61.3146904872832,13.2163502251969,39.9860353422374));
#197729=CARTESIAN_POINT('Ctrl Pts',(61.3033697519365,13.2177324736408,39.9760551582714));
#197730=CARTESIAN_POINT('Ctrl Pts',(61.2920568939748,13.2181390006405,39.9658879738179));
#197731=CARTESIAN_POINT('Ctrl Pts',(61.2808338148893,13.2176240288382,39.9556174643282));
#197732=CARTESIAN_POINT('Ctrl Pts',(61.2697622852632,13.217116010894,39.9454856413923));
#197733=CARTESIAN_POINT('Ctrl Pts',(61.2587767401965,13.2157108393287,39.9352519465122));
#197734=CARTESIAN_POINT('Ctrl Pts',(61.2479592423879,13.2134115091886,39.92499));
#197735=CARTESIAN_POINT('Ctrl Pts',(57.8829458346107,12.498155829258,39.92499));
#197736=CARTESIAN_POINT('Ctrl Pts',(57.8725934298277,12.4959553576923,39.9348107241715));
#197737=CARTESIAN_POINT('Ctrl Pts',(57.8624518082053,12.4929462656001,39.9446038383155));
#197738=CARTESIAN_POINT('Ctrl Pts',(57.8525735736588,12.4891531124825,39.9543158069363));
#197739=CARTESIAN_POINT('Ctrl Pts',(57.8430352690785,12.485490489411,39.9636935671367));
#197740=CARTESIAN_POINT('Ctrl Pts',(57.833741385314,12.4810963130892,39.972996832096));
#197741=CARTESIAN_POINT('Ctrl Pts',(57.8247536185241,12.4759491415402,39.9821731151303));
#197742=CARTESIAN_POINT('Ctrl Pts',(57.8162573641132,12.471083452432,39.990847576432));
#197743=CARTESIAN_POINT('Ctrl Pts',(57.8080338771698,12.4655444244744,39.9994093733814));
#197744=CARTESIAN_POINT('Ctrl Pts',(57.8001616710205,12.4592813303353,40.0077966115809));
#197745=CARTESIAN_POINT('Ctrl Pts',(57.7929115012229,12.4535131257044,40.0155211172564));
#197746=CARTESIAN_POINT('Ctrl Pts',(57.7859589019109,12.447130377453,40.0230979940993));
#197747=CARTESIAN_POINT('Ctrl Pts',(57.7793958734443,12.4400707995013,40.0304554104721));
#197748=CARTESIAN_POINT('Ctrl Pts',(57.7774389108381,12.4379657758621,40.0326492435163));
#197749=CARTESIAN_POINT('Ctrl Pts',(57.7755168276803,12.4358004306458,40.0348233715052));
#197750=CARTESIAN_POINT('Ctrl Pts',(57.7736327324862,12.4335727482754,40.0369753512355));
#197751=CARTESIAN_POINT('Ctrl Pts',(57.7717678881029,12.4313678273303,40.0391053430352));
#197752=CARTESIAN_POINT('Ctrl Pts',(57.7699419852107,12.4291043014742,40.041211089324));
#197753=CARTESIAN_POINT('Ctrl Pts',(57.7681599326869,12.4267829461791,40.0432881154904));
#197754=CARTESIAN_POINT('Ctrl Pts',(57.7680360122396,12.4266215236718,40.043432547828));
#197755=CARTESIAN_POINT('Ctrl Pts',(57.7679122920636,12.4264598236889,40.0435768364421));
#197756=CARTESIAN_POINT('Ctrl Pts',(57.7677887733171,12.4262978456301,40.0437209807855));
#197757=CARTESIAN_POINT('Ctrl Pts',(57.7623732589831,12.4191961341592,40.0500407968421));
#197758=CARTESIAN_POINT('Ctrl Pts',(57.7573864007558,12.4115418213379,40.0560490279346));
#197759=CARTESIAN_POINT('Ctrl Pts',(57.7529408672214,12.4033632485677,40.0616647108616));
#197760=CARTESIAN_POINT('Ctrl Pts',(57.7487968573387,12.3957393973195,40.0668995033488));
#197761=CARTESIAN_POINT('Ctrl Pts',(57.7451230952908,12.3876591848383,40.0717933267485));
#197762=CARTESIAN_POINT('Ctrl Pts',(57.7420400166293,12.3791488184473,40.0762460303076));
#197763=CARTESIAN_POINT('Ctrl Pts',(57.7409121865685,12.3760356163212,40.077874886875));
#197764=CARTESIAN_POINT('Ctrl Pts',(57.7398637084259,12.3728649408017,40.0794443522248));
#197765=CARTESIAN_POINT('Ctrl Pts',(57.7389016204183,12.3696384996591,40.0809482021492));
#197766=CARTESIAN_POINT('Ctrl Pts',(57.738670270393,12.3688626483501,40.0813098278168));
#197767=CARTESIAN_POINT('Ctrl Pts',(57.7384441015869,12.3680830188489,40.0816679525672));
#197768=CARTESIAN_POINT('Ctrl Pts',(57.7382232068823,12.3672997100614,40.082022419258));
#197769=CARTESIAN_POINT('Ctrl Pts',(57.7380092151371,12.3665408796735,40.0823658088648));
#197770=CARTESIAN_POINT('Ctrl Pts',(57.7378001730067,12.365778596386,40.0827057654616));
#197771=CARTESIAN_POINT('Ctrl Pts',(57.7375961641251,12.3650129538219,40.0830421470151));
#197772=CARTESIAN_POINT('Ctrl Pts',(57.7353610110592,12.3566244546988,40.0867275956806));
#197773=CARTESIAN_POINT('Ctrl Pts',(57.7337289586986,12.3478270988449,40.089982343203));
#197774=CARTESIAN_POINT('Ctrl Pts',(57.7328090548569,12.3387746477733,40.0926299529355));
#197775=CARTESIAN_POINT('Ctrl Pts',(57.7324275433144,12.3350203264891,40.0937279956084));
#197776=CARTESIAN_POINT('Ctrl Pts',(57.7321681942504,12.3312224025075,40.0947220371802));
#197777=CARTESIAN_POINT('Ctrl Pts',(57.7320371357771,12.3273926324681,40.0956014538692));
#197778=CARTESIAN_POINT('Ctrl Pts',(57.7318136018936,12.3208605605759,40.097101390674));
#197779=CARTESIAN_POINT('Ctrl Pts',(57.7319651225404,12.3142375182607,40.0982667904316));
#197780=CARTESIAN_POINT('Ctrl Pts',(57.7325238621659,12.3075887924647,40.0990539325582));
#197781=CARTESIAN_POINT('Ctrl Pts',(57.7328032319787,12.3042644295667,40.0994475036216));
#197782=CARTESIAN_POINT('Ctrl Pts',(57.7331858342648,12.3009338801479,40.0997467259952));
#197783=CARTESIAN_POINT('Ctrl Pts',(57.7336757296049,12.2976053572247,40.0999473488896));
#197784=CARTESIAN_POINT('Ctrl Pts',(57.734165624945,12.2942768343015,40.100147971784));
#197785=CARTESIAN_POINT('Ctrl Pts',(57.7347627876419,12.2909503756171,40.10025));
#197786=CARTESIAN_POINT('Ctrl Pts',(57.7354693911206,12.2876333308464,40.10025));
#197787=CARTESIAN_POINT('Origin',(57.9461901084063,6.07506605172221,39.92499));
#197788=CARTESIAN_POINT('Ctrl Pts',(62.333439457262,6.35995915837717,39.92499));
#197789=CARTESIAN_POINT('Ctrl Pts',(62.3439916622903,6.36106823981704,39.9348354642019));
#197790=CARTESIAN_POINT('Ctrl Pts',(62.3544250468349,6.3630066345261,39.944644082846));
#197791=CARTESIAN_POINT('Ctrl Pts',(62.3646844024058,6.36575328117367,39.9543641760333));
#197792=CARTESIAN_POINT('Ctrl Pts',(62.374610390011,6.36841067816039,39.9637684240714));
#197793=CARTESIAN_POINT('Ctrl Pts',(62.3843747009654,6.37182505343089,39.9730909636397));
#197794=CARTESIAN_POINT('Ctrl Pts',(62.3939185239082,6.37602267870788,39.9822808977141));
#197795=CARTESIAN_POINT('Ctrl Pts',(62.4029463927373,6.37999337374501,39.9909740094648));
#197796=CARTESIAN_POINT('Ctrl Pts',(62.4117778192049,6.38466529101412,39.9995492764998));
#197797=CARTESIAN_POINT('Ctrl Pts',(62.4203406170097,6.3900963181494,40.007946232869));
#197798=CARTESIAN_POINT('Ctrl Pts',(62.4282275730652,6.39509868692286,40.0156804369683));
#197799=CARTESIAN_POINT('Ctrl Pts',(62.4358870734644,6.40074541103499,40.0232638017414));
#197800=CARTESIAN_POINT('Ctrl Pts',(62.4432347045248,6.40710777594438,40.0306257269957));
#197801=CARTESIAN_POINT('Ctrl Pts',(62.4453659729914,6.40895325615324,40.0327611416646));
#197802=CARTESIAN_POINT('Ctrl Pts',(62.4474707870406,6.41085910953056,40.0348777427268));
#197803=CARTESIAN_POINT('Ctrl Pts',(62.4495465125726,6.41282747575996,40.03697331687));
#197804=CARTESIAN_POINT('Ctrl Pts',(62.4517967325057,6.41496131130661,40.039245053974));
#197805=CARTESIAN_POINT('Ctrl Pts',(62.4540103788123,6.41716486079117,40.041487875195));
#197806=CARTESIAN_POINT('Ctrl Pts',(62.4561838467663,6.41943986047027,40.04369857016));
#197807=CARTESIAN_POINT('Ctrl Pts',(62.4621489466212,6.42568361494116,40.0497658398386));
#197808=CARTESIAN_POINT('Ctrl Pts',(62.467772647785,6.4324873305955,40.0555581699984));
#197809=CARTESIAN_POINT('Ctrl Pts',(62.4729574661287,6.43981562609108,40.0609828468885));
#197810=CARTESIAN_POINT('Ctrl Pts',(62.4777012934231,6.44652061860752,40.0659461317308));
#197811=CARTESIAN_POINT('Ctrl Pts',(62.4820661824991,6.45366385825773,40.0706039980712));
#197812=CARTESIAN_POINT('Ctrl Pts',(62.4859635700134,6.46124910257484,40.0748843180611));
#197813=CARTESIAN_POINT('Ctrl Pts',(62.4878779540287,6.46497494980442,40.0769867972575));
#197814=CARTESIAN_POINT('Ctrl Pts',(62.4896790353534,6.4688074965091,40.0789976708177));
#197815=CARTESIAN_POINT('Ctrl Pts',(62.4913529701966,6.47274712615487,40.08090504915));
#197816=CARTESIAN_POINT('Ctrl Pts',(62.4916705830287,6.47349463250775,40.0812669556104));
#197817=CARTESIAN_POINT('Ctrl Pts',(62.4919834280839,6.47424649074103,40.0816253922032));
#197818=CARTESIAN_POINT('Ctrl Pts',(62.4922913974558,6.47500261163075,40.0819801989139));
#197819=CARTESIAN_POINT('Ctrl Pts',(62.4925897427848,6.47573510374267,40.0823239179149));
#197820=CARTESIAN_POINT('Ctrl Pts',(62.4928835124027,6.47647159623262,40.0826642303498));
#197821=CARTESIAN_POINT('Ctrl Pts',(62.4931726086302,6.47721200416321,40.0830009916099));
#197822=CARTESIAN_POINT('Ctrl Pts',(62.4963231197467,6.48528081722581,40.0866709464311));
#197823=CARTESIAN_POINT('Ctrl Pts',(62.4989203081702,6.49382008994854,40.0899175831876));
#197824=CARTESIAN_POINT('Ctrl Pts',(62.5008353965403,6.50268949817224,40.0925642067059));
#197825=CARTESIAN_POINT('Ctrl Pts',(62.5016441502512,6.50643510434183,40.0936818922526));
#197826=CARTESIAN_POINT('Ctrl Pts',(62.5023315568341,6.51023927047563,40.094693009479));
#197827=CARTESIAN_POINT('Ctrl Pts',(62.5028895688031,6.51409041329205,40.0955863397546));
#197828=CARTESIAN_POINT('Ctrl Pts',(62.5038292470156,6.52057564156488,40.0970906856166));
#197829=CARTESIAN_POINT('Ctrl Pts',(62.5043999463278,6.52719259313698,40.0982599215483));
#197830=CARTESIAN_POINT('Ctrl Pts',(62.5045608969644,6.53387925273521,40.0990497370454));
#197831=CARTESIAN_POINT('Ctrl Pts',(62.5046011346236,6.53555091763477,40.0992471909196));
#197832=CARTESIAN_POINT('Ctrl Pts',(62.5046155292217,6.5372269295873,40.0994209989363));
#197833=CARTESIAN_POINT('Ctrl Pts',(62.5046031362658,6.53890629460996,40.0995705982975));
#197834=CARTESIAN_POINT('Ctrl Pts',(62.5045845468319,6.54142534214396,40.0997949973393));
#197835=CARTESIAN_POINT('Ctrl Pts',(62.5045056736598,6.5439519171443,40.0999649129781));
#197836=CARTESIAN_POINT('Ctrl Pts',(62.5043649998326,6.54648282201788,40.1000786629733));
#197837=CARTESIAN_POINT('Ctrl Pts',(62.5042243260054,6.54901372689146,40.1001924129685));
#197838=CARTESIAN_POINT('Ctrl Pts',(62.5040218613862,6.55154895552175,40.10025));
#197839=CARTESIAN_POINT('Ctrl Pts',(62.5037563256536,6.55408556365861,40.10025));
#197840=CARTESIAN_POINT('Ctrl Pts',(58.7067819056644,6.15500747092236,40.10025));
#197841=CARTESIAN_POINT('Ctrl Pts',(58.7076801645418,6.14642434678071,40.10025));
#197842=CARTESIAN_POINT('Ctrl Pts',(58.7092791387969,6.13798976646238,40.099578633424));
#197843=CARTESIAN_POINT('Ctrl Pts',(58.7114824462543,6.12982011300101,40.0983063763365));
#197844=CARTESIAN_POINT('Ctrl Pts',(58.7129055567993,6.1245433551203,40.0974846287991));
#197845=CARTESIAN_POINT('Ctrl Pts',(58.7145798848071,6.11937686667937,40.0964130309337));
#197846=CARTESIAN_POINT('Ctrl Pts',(58.7164715618026,6.11434800669255,40.0951176960923));
#197847=CARTESIAN_POINT('Ctrl Pts',(58.7189788712982,6.10768254085054,40.0934008039614));
#197848=CARTESIAN_POINT('Ctrl Pts',(58.7218729180382,6.10126195983161,40.0912909372156));
#197849=CARTESIAN_POINT('Ctrl Pts',(58.7250866612027,6.09514640967194,40.0888630467851));
#197850=CARTESIAN_POINT('Ctrl Pts',(58.7266935327849,6.0920886345921,40.0876491015698));
#197851=CARTESIAN_POINT('Ctrl Pts',(58.7283803475667,6.08910691884893,40.0863558569271));
#197852=CARTESIAN_POINT('Ctrl Pts',(58.7301388657774,6.08620737357386,40.0849936342771));
#197853=CARTESIAN_POINT('Ctrl Pts',(58.7310181248828,6.08475760093632,40.0843125229521));
#197854=CARTESIAN_POINT('Ctrl Pts',(58.7319153115143,6.08332835456963,40.0836141747074));
#197855=CARTESIAN_POINT('Ctrl Pts',(58.7328294060528,6.0819202957249,40.0828999161609));
#197856=CARTESIAN_POINT('Ctrl Pts',(58.7330579296874,6.08156828101372,40.0827213515243));
#197857=CARTESIAN_POINT('Ctrl Pts',(58.7332875101007,6.08121759017488,40.0825417925841));
#197858=CARTESIAN_POINT('Ctrl Pts',(58.7335181314302,6.08086823283901,40.082361260236));
#197859=CARTESIAN_POINT('Ctrl Pts',(58.7342099954187,6.0798201608314,40.0818196631917));
#197860=CARTESIAN_POINT('Ctrl Pts',(58.7349112274886,6.07878409208698,40.0812693052021));
#197861=CARTESIAN_POINT('Ctrl Pts',(58.7356214008386,6.07776027111639,40.0807107531874));
#197862=CARTESIAN_POINT('Ctrl Pts',(58.7406237702163,6.07054860839872,40.076776384918));
#197863=CARTESIAN_POINT('Ctrl Pts',(58.7460508958015,6.06389424687405,40.0724140586135));
#197864=CARTESIAN_POINT('Ctrl Pts',(58.7517849266684,6.05777649745699,40.0677221223764));
#197865=CARTESIAN_POINT('Ctrl Pts',(58.7545659254424,6.05480939560084,40.0654465383718));
#197866=CARTESIAN_POINT('Ctrl Pts',(58.757419693745,6.05196853530499,40.0630928000678));
#197867=CARTESIAN_POINT('Ctrl Pts',(58.7603356163932,6.04925198282152,40.0606689262479));
#197868=CARTESIAN_POINT('Ctrl Pts',(58.7647996902381,6.04509313076913,40.0569581447805));
#197869=CARTESIAN_POINT('Ctrl Pts',(58.7694062431512,6.04122712576998,40.0530843804605));
#197870=CARTESIAN_POINT('Ctrl Pts',(58.7741092696794,6.03765709635755,40.0490800251457));
#197871=CARTESIAN_POINT('Ctrl Pts',(58.7762933795293,6.03599915622953,40.0472203818218));
#197872=CARTESIAN_POINT('Ctrl Pts',(58.7784980841112,6.03440490786043,40.0453323608818));
#197873=CARTESIAN_POINT('Ctrl Pts',(58.7807192900658,6.03287578462677,40.0434201572162));
#197874=CARTESIAN_POINT('Ctrl Pts',(58.7808895367502,6.03275858335596,40.0432735943397));
#197875=CARTESIAN_POINT('Ctrl Pts',(58.7810598733266,6.03264173148699,40.0431268995707));
#197876=CARTESIAN_POINT('Ctrl Pts',(58.7812302983889,6.0325252286247,40.0429800745037));
#197877=CARTESIAN_POINT('Ctrl Pts',(58.7836242566994,6.03088871465425,40.0409176249753));
#197878=CARTESIAN_POINT('Ctrl Pts',(58.7860369637877,6.02932271154683,40.0388310783332));
#197879=CARTESIAN_POINT('Ctrl Pts',(58.7884628208564,6.02782611907177,40.036725739981));
#197880=CARTESIAN_POINT('Ctrl Pts',(58.7971615128802,6.02245960461633,40.0291763710719));
#197881=CARTESIAN_POINT('Ctrl Pts',(58.8060955050474,6.01794242202273,40.0213310894597));
#197882=CARTESIAN_POINT('Ctrl Pts',(58.8151732302893,6.01418353044908,40.0132837551324));
#197883=CARTESIAN_POINT('Ctrl Pts',(58.8251487383915,6.01005288622384,40.0044405431332));
#197884=CARTESIAN_POINT('Ctrl Pts',(58.8352983536241,6.0068375430019,39.9953528710611));
#197885=CARTESIAN_POINT('Ctrl Pts',(58.8455340166129,6.0044577527297,39.9861103629569));
#197886=CARTESIAN_POINT('Ctrl Pts',(58.8565859638396,6.00188817648163,39.9761307737576));
#197887=CARTESIAN_POINT('Ctrl Pts',(58.8677393147001,6.00029231631139,39.9659696936038));
#197888=CARTESIAN_POINT('Ctrl Pts',(58.8789072188634,5.99962196122093,39.9557128217539));
#197889=CARTESIAN_POINT('Ctrl Pts',(58.8899814357874,5.99895722972078,39.9455419945182));
#197890=CARTESIAN_POINT('Ctrl Pts',(58.9010713848501,5.99920273697604,39.9352756289351));
#197891=CARTESIAN_POINT('Ctrl Pts',(58.9120953679531,6.00036140428966,39.92499));
#197892=CARTESIAN_POINT('Origin',(-0.00159301378019881,0.0151565136854119,
39.92499));
#197893=CARTESIAN_POINT('Ctrl Pts',(62.5005702980932,6.58439859102944,40.10025));
#197894=CARTESIAN_POINT('Ctrl Pts',(62.4996689377206,6.59294009787364,40.10025));
#197895=CARTESIAN_POINT('Ctrl Pts',(62.4980620716938,6.60133040498961,40.0995859581842));
#197896=CARTESIAN_POINT('Ctrl Pts',(62.4958483879906,6.60945539386096,40.0983275959621));
#197897=CARTESIAN_POINT('Ctrl Pts',(62.4944339494872,6.61464687495747,40.0975235624068));
#197898=CARTESIAN_POINT('Ctrl Pts',(62.4927726671884,6.61973030386259,40.096477705949));
#197899=CARTESIAN_POINT('Ctrl Pts',(62.4908979342377,6.62467983150676,40.0952149915961));
#197900=CARTESIAN_POINT('Ctrl Pts',(62.4883392999284,6.63143494361006,40.0934916398701));
#197901=CARTESIAN_POINT('Ctrl Pts',(62.4853780106449,6.63793726713676,40.0913643921631));
#197902=CARTESIAN_POINT('Ctrl Pts',(62.482086456285,6.64412426454807,40.0889118607713));
#197903=CARTESIAN_POINT('Ctrl Pts',(62.4804406791051,6.64721776325373,40.0876855950754));
#197904=CARTESIAN_POINT('Ctrl Pts',(62.4787123157335,6.65023263831788,40.0863782327527));
#197905=CARTESIAN_POINT('Ctrl Pts',(62.4769102669531,6.65316255786655,40.0850006373334));
#197906=CARTESIAN_POINT('Ctrl Pts',(62.476009242563,6.65462751764088,40.0843118396237));
#197907=CARTESIAN_POINT('Ctrl Pts',(62.4750897950507,6.65607125585996,40.0836054919164));
#197908=CARTESIAN_POINT('Ctrl Pts',(62.4741530260211,6.65749308991676,40.0828829920418));
#197909=CARTESIAN_POINT('Ctrl Pts',(62.4739188337637,6.65784854843096,40.0827023670731));
#197910=CARTESIAN_POINT('Ctrl Pts',(62.4736835588747,6.65820263830418,40.0825207326933));
#197911=CARTESIAN_POINT('Ctrl Pts',(62.4734472184935,6.65855534961529,40.0823381109275));
#197912=CARTESIAN_POINT('Ctrl Pts',(62.4727381973496,6.65961348354863,40.0817902456303));
#197913=CARTESIAN_POINT('Ctrl Pts',(62.4720195869493,6.66065920857923,40.0812334935553));
#197914=CARTESIAN_POINT('Ctrl Pts',(62.4712918484711,6.66169227331133,40.0806684524227));
#197915=CARTESIAN_POINT('Ctrl Pts',(62.4662627240579,6.66883139158041,40.0767636676137));
#197916=CARTESIAN_POINT('Ctrl Pts',(62.460816145151,6.67541846632582,40.0724404510889));
#197917=CARTESIAN_POINT('Ctrl Pts',(62.4550686189991,6.68147667711046,40.067794993741));
#197918=CARTESIAN_POINT('Ctrl Pts',(62.4522121142782,6.68448759124099,40.0654862141906));
#197919=CARTESIAN_POINT('Ctrl Pts',(62.4492806638355,6.6873678413353,40.0630972003216));
#197920=CARTESIAN_POINT('Ctrl Pts',(62.4462854590369,6.69011973548525,40.0606363359906));
#197921=CARTESIAN_POINT('Ctrl Pts',(62.4396775898762,6.69619082501338,40.0552073017123));
#197922=CARTESIAN_POINT('Ctrl Pts',(62.4327685320937,6.70164568781131,40.0494204304519));
#197923=CARTESIAN_POINT('Ctrl Pts',(62.425698510878,6.7064460603901,40.0434049749851));
#197924=CARTESIAN_POINT('Ctrl Pts',(62.4231157429702,6.70819969702901,40.0412074532442));
#197925=CARTESIAN_POINT('Ctrl Pts',(62.4205129446134,6.70987381569732,40.0389814735788));
#197926=CARTESIAN_POINT('Ctrl Pts',(62.4178950590936,6.71147036762092,40.0367321210016));
#197927=CARTESIAN_POINT('Ctrl Pts',(62.409101858649,6.71683301659034,40.0291767837143));
#197928=CARTESIAN_POINT('Ctrl Pts',(62.4000783072493,6.72134734296589,40.021323533258));
#197929=CARTESIAN_POINT('Ctrl Pts',(62.3909158405875,6.7251033539706,40.0132649215865));
#197930=CARTESIAN_POINT('Ctrl Pts',(62.3808452043606,6.72923165499357,40.0044075527542));
#197931=CARTESIAN_POINT('Ctrl Pts',(62.370606189679,6.73244426756049,39.9953016253731));
#197932=CARTESIAN_POINT('Ctrl Pts',(62.3602869763777,6.73481930344629,39.9860353422371));
#197933=CARTESIAN_POINT('Ctrl Pts',(62.349172741509,6.73737731885751,39.976055158271));
#197934=CARTESIAN_POINT('Ctrl Pts',(62.3379643502091,6.73896413451758,39.9658879738172));
#197935=CARTESIAN_POINT('Ctrl Pts',(62.3267489231138,6.73962511499463,39.9556174643272));
#197936=CARTESIAN_POINT('Ctrl Pts',(62.315684942151,6.74027717000357,39.9454856413917));
#197937=CARTESIAN_POINT('Ctrl Pts',(62.304612696626,6.74002799825903,39.935251946512));
#197938=CARTESIAN_POINT('Ctrl Pts',(62.293614112757,6.73887200051249,39.92499));
#197939=CARTESIAN_POINT('Ctrl Pts',(58.8722700234481,6.37927424642498,39.92499));
#197940=CARTESIAN_POINT('Ctrl Pts',(58.8617443183096,6.37816795023576,39.9348107241724));
#197941=CARTESIAN_POINT('Ctrl Pts',(58.8513437177784,6.37623543038788,39.9446038383172));
#197942=CARTESIAN_POINT('Ctrl Pts',(58.8411231047672,6.37349561323652,39.9543158069389));
#197943=CARTESIAN_POINT('Ctrl Pts',(58.8312542036559,6.37085007871718,39.9636935671396));
#197944=CARTESIAN_POINT('Ctrl Pts',(58.8215519162604,6.36745144954042,39.9729968320994));
#197945=CARTESIAN_POINT('Ctrl Pts',(58.8120753594649,6.36327195218611,39.9821731151341));
#197946=CARTESIAN_POINT('Ctrl Pts',(58.8031170454193,6.35932101824877,39.9908475764358));
#197947=CARTESIAN_POINT('Ctrl Pts',(58.7943596215174,6.35467192211852,39.9994093733852));
#197948=CARTESIAN_POINT('Ctrl Pts',(58.7858758685314,6.34926600747549,40.0077966115847));
#197949=CARTESIAN_POINT('Ctrl Pts',(58.778062474357,6.34428725078029,40.01552111726));
#197950=CARTESIAN_POINT('Ctrl Pts',(58.7704807832456,6.33866621241343,40.0230979941026));
#197951=CARTESIAN_POINT('Ctrl Pts',(58.7632157809012,6.33233133084835,40.0304554104753));
#197952=CARTESIAN_POINT('Ctrl Pts',(58.7610495038559,6.33044239704361,40.0326492435184));
#197953=CARTESIAN_POINT('Ctrl Pts',(58.7589116098638,6.32848982621457,40.0348233715062));
#197954=CARTESIAN_POINT('Ctrl Pts',(58.7568049797265,6.32647128889757,40.0369753512356));
#197955=CARTESIAN_POINT('Ctrl Pts',(58.7547198741579,6.32447337605771,40.0391053430352));
#197956=CARTESIAN_POINT('Ctrl Pts',(58.7526673708734,6.32241310885643,40.041211089324));
#197957=CARTESIAN_POINT('Ctrl Pts',(58.7506524329182,6.32029074540037,40.0432881154904));
#197958=CARTESIAN_POINT('Ctrl Pts',(58.7505123180733,6.32014316039632,40.043432547828));
#197959=CARTESIAN_POINT('Ctrl Pts',(58.7503723733987,6.31999527850274,40.0435768364421));
#197960=CARTESIAN_POINT('Ctrl Pts',(58.7502325999832,6.31984709900144,40.0437209807855));
#197961=CARTESIAN_POINT('Ctrl Pts',(58.7441044214169,6.31335036684033,40.050040796842));
#197962=CARTESIAN_POINT('Ctrl Pts',(58.7383447881643,6.30625925377274,40.0560490279344));
#197963=CARTESIAN_POINT('Ctrl Pts',(58.7330687140843,6.29859016886878,40.0616647108614));
#197964=CARTESIAN_POINT('Ctrl Pts',(58.7281504960664,6.29144124886035,40.0668995033484));
#197965=CARTESIAN_POINT('Ctrl Pts',(58.7236522470779,6.28378931333009,40.071793326748));
#197966=CARTESIAN_POINT('Ctrl Pts',(58.7196964823232,6.27564783709148,40.076246030307));
#197967=CARTESIAN_POINT('Ctrl Pts',(58.7182494123992,6.2726695797551,40.0778748868747));
#197968=CARTESIAN_POINT('Ctrl Pts',(58.7168752520898,6.26962586933659,40.0794443522247));
#197969=CARTESIAN_POINT('Ctrl Pts',(58.7155811795664,6.26651766855671,40.0809482021492));
#197970=CARTESIAN_POINT('Ctrl Pts',(58.7152699983557,6.26577025010498,40.0813098278168));
#197971=CARTESIAN_POINT('Ctrl Pts',(58.7149635750523,6.26501853257358,40.0816679525672));
#197972=CARTESIAN_POINT('Ctrl Pts',(58.7146620123681,6.2642626046176,40.082022419258));
#197973=CARTESIAN_POINT('Ctrl Pts',(58.7143698735178,6.26353029941025,40.0823658088648));
#197974=CARTESIAN_POINT('Ctrl Pts',(58.7140822962415,6.26279404284295,40.0827057654616));
#197975=CARTESIAN_POINT('Ctrl Pts',(58.7137993735012,6.26205391928379,40.0830421470151));
#197976=CARTESIAN_POINT('Ctrl Pts',(58.7106996279153,6.2539450103517,40.0867275956806));
#197977=CARTESIAN_POINT('Ctrl Pts',(58.70815694202,6.24536644325887,40.089982343203));
#197978=CARTESIAN_POINT('Ctrl Pts',(58.7062958387085,6.23645973859628,40.0926299529355));
#197979=CARTESIAN_POINT('Ctrl Pts',(58.7055239836916,6.23276586269223,40.0937279956084));
#197980=CARTESIAN_POINT('Ctrl Pts',(58.7048690642116,6.22901585349474,40.0947220371802));
#197981=CARTESIAN_POINT('Ctrl Pts',(58.7043384037134,6.22522076267719,40.0956014538692));
#197982=CARTESIAN_POINT('Ctrl Pts',(58.7034333069352,6.21874783981155,40.097101390674));
#197983=CARTESIAN_POINT('Ctrl Pts',(58.7028917011006,6.21214524099482,40.0982667904316));
#197984=CARTESIAN_POINT('Ctrl Pts',(58.7027523988018,6.20547453341993,40.0990539325582));
#197985=CARTESIAN_POINT('Ctrl Pts',(58.7026827476524,6.20213917963249,40.0994475036216));
#197986=CARTESIAN_POINT('Ctrl Pts',(58.7027151167905,6.19878688248287,40.0997467259952));
#197987=CARTESIAN_POINT('Ctrl Pts',(58.7028544030466,6.19542538554944,40.0999473488896));
#197988=CARTESIAN_POINT('Ctrl Pts',(58.7029936893027,6.19206388861602,40.100147971784));
#197989=CARTESIAN_POINT('Ctrl Pts',(58.7032398710655,6.18869323212136,40.10025));
#197990=CARTESIAN_POINT('Ctrl Pts',(58.703595878104,6.18532049829319,40.10025));
#197991=CARTESIAN_POINT('Origin',(61.0544000815101,-6.73632490863785,39.1925554495077));
#197992=CARTESIAN_POINT('Origin',(61.0983782637162,-6.74099917687776,39.1160373285247));
#197993=CARTESIAN_POINT('Origin',(60.9730100652054,-6.72777047351124,39.3343017080178));
#197994=CARTESIAN_POINT('Ctrl Pts',(60.8636883187845,-6.7157078966941,39.2708017080178));
#197995=CARTESIAN_POINT('Ctrl Pts',(60.8773920302461,-6.59002106156467,
39.2710850691866));
#197996=CARTESIAN_POINT('Ctrl Pts',(60.9862851800404,-6.60146619279947,
39.3343017080178));
#197997=CARTESIAN_POINT('Ctrl Pts',(60.818916972731,-6.71111871849805,39.3487519293518));
#197998=CARTESIAN_POINT('Ctrl Pts',(60.8324022194113,-6.58529244190234,
39.3492068662923));
#197999=CARTESIAN_POINT('Ctrl Pts',(60.9191469903169,-6.59440968471146,
39.4512271248733));
#198000=CARTESIAN_POINT('Ctrl Pts',(60.7340977611529,-6.7024250897622,39.3978017080178));
#198001=CARTESIAN_POINT('Ctrl Pts',(60.7472645033904,-6.57634410736721,
39.3980347781183));
#198002=CARTESIAN_POINT('Ctrl Pts',(60.7919547682785,-6.58104124348236,
39.5248015355195));
#198003=CARTESIAN_POINT('Ctrl Pts',(60.6448574988554,-6.69328024897455,
39.3978017080178));
#198004=CARTESIAN_POINT('Ctrl Pts',(60.6581326136904,-6.56697596826278,
39.3978017080178));
#198005=CARTESIAN_POINT('Ctrl Pts',(60.6581326136904,-6.56697596826278,
39.5248017080178));
#198006=CARTESIAN_POINT('Origin',(60.6448574988554,-6.69328024897455,39.5248017080178));
#198007=CARTESIAN_POINT('Origin',(-0.0331877870874745,-0.315760701779427,
39.116));
#198008=CARTESIAN_POINT('Origin',(61.4975385923862,-6.78290064323561,39.116));
#198009=CARTESIAN_POINT('Origin',(-0.0331877870874745,-0.315760701779427,
39.5248017080178));
#198010=CARTESIAN_POINT('Origin',(60.4944777170594,-6.67747469700946,39.5248017080178));
#198011=CARTESIAN_POINT('Ctrl Pts',(62.0330459552232,-6.8397366303026,39.2875012672119));
#198012=CARTESIAN_POINT('Ctrl Pts',(62.046864023402,-6.71274550335202,39.287208709576));
#198013=CARTESIAN_POINT('Ctrl Pts',(61.9391074687683,-6.70161199370823,
39.3549016990124));
#198014=CARTESIAN_POINT('Ctrl Pts',(61.9187065474465,-6.82760205123564,
39.103493917393));
#198015=CARTESIAN_POINT('Ctrl Pts',(61.9323544653035,-6.70071032544322,
39.1031692336349));
#198016=CARTESIAN_POINT('Ctrl Pts',(61.8476598279018,-6.6920004592178,39.2077507202315));
#198017=CARTESIAN_POINT('Ctrl Pts',(61.7133000470647,-6.80580199871467,
38.989));
#198018=CARTESIAN_POINT('Ctrl Pts',(61.7268034525359,-6.67910652125777,
38.9887769311152));
#198019=CARTESIAN_POINT('Ctrl Pts',(61.6833778591502,-6.67473372828934,
39.1161898712895));
#198020=CARTESIAN_POINT('Ctrl Pts',(61.4975385923862,-6.78290064323561,
38.989));
#198021=CARTESIAN_POINT('Ctrl Pts',(61.5108335396272,-6.65640766978507,
38.989));
#198022=CARTESIAN_POINT('Ctrl Pts',(61.510813692429,-6.65659650326253,39.1161895903858));
#198023=CARTESIAN_POINT('Origin',(61.9259926140919,-6.82793297553349,39.3548010137695));
#198024=CARTESIAN_POINT('Ctrl Pts',(60.4944777170594,-6.67747469700946,
39.3978017080178));
#198025=CARTESIAN_POINT('Ctrl Pts',(60.5077528318944,-6.55117041629769,
39.3978017080178));
#198026=CARTESIAN_POINT('Ctrl Pts',(60.5077528318944,-6.55117041629769,
39.5248017080178));
#198027=CARTESIAN_POINT('Ctrl Pts',(60.404935774755,-6.66829952659935,39.3978017080178));
#198028=CARTESIAN_POINT('Ctrl Pts',(60.4181493202566,-6.5417527077301,39.3975666025021));
#198029=CARTESIAN_POINT('Ctrl Pts',(60.3734783767965,-6.53705760237891,
39.5248015517177));
#198030=CARTESIAN_POINT('Ctrl Pts',(60.3202668847283,-6.65962554481688,
39.3484894016716));
#198031=CARTESIAN_POINT('Ctrl Pts',(60.333852472875,-6.53289275204992,39.3480259000039));
#198032=CARTESIAN_POINT('Ctrl Pts',(60.2465123062132,-6.52371293062557,
39.4508333188947));
#198033=CARTESIAN_POINT('Ctrl Pts',(60.2756459899119,-6.65505462397395,
39.2708017080178));
#198034=CARTESIAN_POINT('Ctrl Pts',(60.2894805317162,-6.52822907310778,
39.27051194648));
#198035=CARTESIAN_POINT('Ctrl Pts',(60.1796001951995,-6.51668018436747,
39.3343017080178));
#198036=CARTESIAN_POINT('Origin',(60.1663250803646,-6.64298446507924,39.3343017080178));
#198037=CARTESIAN_POINT('Origin',(62.1031658061135,-6.84655462836804,39.6398955068193));
#198038=CARTESIAN_POINT('Origin',(62.2803389979219,-6.8651762812251,39.92499));
#198039=CARTESIAN_POINT('Origin',(60.0854204576119,-6.634481046568,39.1934008539943));
#198040=CARTESIAN_POINT('Origin',(60.0409538388296,-6.62985850077847,39.1160402713849));
#198041=CARTESIAN_POINT('Ctrl Pts',(62.6076796697354,-6.59568250079886,
40.1599502534424));
#198042=CARTESIAN_POINT('Ctrl Pts',(62.5705801176609,-6.59177408464774,
40.10025));
#198043=CARTESIAN_POINT('Ctrl Pts',(62.5005702980931,-6.58439859103029,
40.10025));
#198044=CARTESIAN_POINT('Ctrl Pts',(62.598447729079,-6.68331293653951,40.1599500538448));
#198045=CARTESIAN_POINT('Ctrl Pts',(62.5638523220891,-6.65560500345244,
40.1002448353502));
#198046=CARTESIAN_POINT('Ctrl Pts',(62.4952175264232,-6.63512154272615,
40.10025));
#198047=CARTESIAN_POINT('Ctrl Pts',(62.565050454942,-6.76155265492241,40.1202442001041));
#198048=CARTESIAN_POINT('Ctrl Pts',(62.5346567608587,-6.71196843232399,
40.063387386802));
#198049=CARTESIAN_POINT('Ctrl Pts',(62.4653998062676,-6.67930776339544,
40.077227172354));
#198050=CARTESIAN_POINT('Ctrl Pts',(62.4816328770699,-6.86003002196291,
40.004599599816));
#198051=CARTESIAN_POINT('Ctrl Pts',(62.4676069047243,-6.7686325824506,39.9663485808311));
#198052=CARTESIAN_POINT('Ctrl Pts',(62.3866783619496,-6.7331110463148,40.0101727202463));
#198053=CARTESIAN_POINT('Ctrl Pts',(62.4326191774619,-6.88172985342165,
39.9304654349861));
#198054=CARTESIAN_POINT('Ctrl Pts',(62.429206244915,-6.76853939445059,39.9051900162963));
#198055=CARTESIAN_POINT('Ctrl Pts',(62.338838812382,-6.74362530798255,39.9671857458188));
#198056=CARTESIAN_POINT('Ctrl Pts',(62.3873926810691,-6.87697683366565,
39.8576902534424));
#198057=CARTESIAN_POINT('Ctrl Pts',(62.4011871104969,-6.75017837817602,
39.8573998014387));
#198058=CARTESIAN_POINT('Ctrl Pts',(62.2936141127569,-6.73887200051333,
39.92499));
#198059=CARTESIAN_POINT('Origin',(62.5005702980931,-6.58439859103029,40.22725));
#198060=CARTESIAN_POINT('Origin',(-0.0331877870874745,-0.315760701779427,
39.116));
#198061=CARTESIAN_POINT('Origin',(59.6417962403143,-6.58785426247096,39.116));
#198062=CARTESIAN_POINT('Origin',(5.50069060731754E-15,5.71212024007692E-15,
40.22725));
#198063=CARTESIAN_POINT('Origin',(62.5037563256535,-6.55408556365946,40.22725));
#198064=CARTESIAN_POINT('Ctrl Pts',(59.6417962403143,-6.58785426247096,
38.989));
#198065=CARTESIAN_POINT('Ctrl Pts',(59.6550912418708,-6.46136077224313,
38.989));
#198066=CARTESIAN_POINT('Ctrl Pts',(59.655071340276,-6.46155012326924,39.1161901092323));
#198067=CARTESIAN_POINT('Ctrl Pts',(59.4260321009469,-6.56494565834876,
38.989));
#198068=CARTESIAN_POINT('Ctrl Pts',(59.4394927947735,-6.43870097938002,
38.989229898976));
#198069=CARTESIAN_POINT('Ctrl Pts',(59.4825041216649,-6.44341257746672,
39.1161900493203));
#198070=CARTESIAN_POINT('Ctrl Pts',(59.2206282517276,-6.54313468201959,
39.1034966344368));
#198071=CARTESIAN_POINT('Ctrl Pts',(59.234195551358,-6.41712387095933,39.1038314102551));
#198072=CARTESIAN_POINT('Ctrl Pts',(59.3182233753697,-6.42614597500977,
39.2077528789596));
#198073=CARTESIAN_POINT('Ctrl Pts',(59.1062911958296,-6.53099325080055,
39.2875012672119));
#198074=CARTESIAN_POINT('Ctrl Pts',(59.1200087130389,-6.40512262640552,
39.2878045257868));
#198075=CARTESIAN_POINT('Ctrl Pts',(59.2267768553865,-6.41653455832026,
39.35490152959));
#198076=CARTESIAN_POINT('Origin',(59.2133417798936,-6.54282188406228,39.3548010137695));
#198077=CARTESIAN_POINT('Ctrl Pts',(62.4538823482275,-6.2443699078806,39.8576902534424));
#198078=CARTESIAN_POINT('Ctrl Pts',(62.4410124550018,-6.37126553604071,
39.8573998014387));
#198079=CARTESIAN_POINT('Ctrl Pts',(62.3334394572619,-6.35995915837802,
39.92499));
#198080=CARTESIAN_POINT('Ctrl Pts',(62.4991292864732,-6.24912604340899,
39.930498490249));
#198081=CARTESIAN_POINT('Ctrl Pts',(62.4722545055303,-6.3591243783161,39.9052171569792));
#198082=CARTESIAN_POINT('Ctrl Pts',(62.3786847639676,-6.36471463173867,
39.9672049726604));
#198083=CARTESIAN_POINT('Ctrl Pts',(62.5423796567684,-6.28053011789743,
40.0043437678662));
#198084=CARTESIAN_POINT('Ctrl Pts',(62.509694696565,-6.367085334999,39.9661628577642));
#198085=CARTESIAN_POINT('Ctrl Pts',(62.4231124872028,-6.38493060453713,
40.0100243556236));
#198086=CARTESIAN_POINT('Ctrl Pts',(62.6032845425345,-6.39322569848883,
40.1194874821987));
#198087=CARTESIAN_POINT('Ctrl Pts',(62.5632890102007,-6.43576006824441,
40.062755148314));
#198088=CARTESIAN_POINT('Ctrl Pts',(62.4886705126496,-6.45334792019192,
40.0767884282376));
#198089=CARTESIAN_POINT('Ctrl Pts',(62.6200908675645,-6.4773924351049,40.1599502015381));
#198090=CARTESIAN_POINT('Ctrl Pts',(62.5804859237118,-6.49734694408353,
40.1002449453872));
#198091=CARTESIAN_POINT('Ctrl Pts',(62.5090840872014,-6.50319024212508,
40.10025));
#198092=CARTESIAN_POINT('Ctrl Pts',(62.6108711573006,-6.56531752495302,
40.1599502534424));
#198093=CARTESIAN_POINT('Ctrl Pts',(62.5737697140402,-6.56142710223352,
40.10025));
#198094=CARTESIAN_POINT('Ctrl Pts',(62.5037563256535,-6.55408556365946,
40.10025));
#198095=CARTESIAN_POINT('Origin',(62.3467145720969,-6.23365487766625,39.92499));
#198096=CARTESIAN_POINT('Origin',(59.0361683443304,-6.52420020557798,39.6398955069312));
#198097=CARTESIAN_POINT('Origin',(58.858994908613,-6.50557852713755,39.92499));
#198098=CARTESIAN_POINT('Origin',(62.169541380269,-6.21503322484993,39.6398955068287));
#198099=CARTESIAN_POINT('Origin',(61.9923681882669,-6.19641157197464,39.3548010137695));
#198100=CARTESIAN_POINT('Ctrl Pts',(58.7519447039088,-6.49374646112741,
39.8576902534424));
#198101=CARTESIAN_POINT('Ctrl Pts',(58.7656442740271,-6.36806742857326,
39.8579948730703));
#198102=CARTESIAN_POINT('Ctrl Pts',(58.872270023448,-6.37927424642578,39.92499));
#198103=CARTESIAN_POINT('Ctrl Pts',(58.7067576262547,-6.48899657309051,
39.930402071123));
#198104=CARTESIAN_POINT('Ctrl Pts',(58.7342098038494,-6.38004220452783,
39.9058915297388));
#198105=CARTESIAN_POINT('Ctrl Pts',(58.8270810177601,-6.37452469054053,
39.9671523786039));
#198106=CARTESIAN_POINT('Ctrl Pts',(58.6637560248473,-6.45774144355308,
40.0043257306694));
#198107=CARTESIAN_POINT('Ctrl Pts',(58.6967899354326,-6.37187117938123,
39.9667894847835));
#198108=CARTESIAN_POINT('Ctrl Pts',(58.7829167175848,-6.3543526691276,40.0100138975201));
#198109=CARTESIAN_POINT('Ctrl Pts',(58.6035914159081,-6.34539908016329,
40.1195533054856));
#198110=CARTESIAN_POINT('Ctrl Pts',(58.6436439608621,-6.30313135363851,
40.0630813209236));
#198111=CARTESIAN_POINT('Ctrl Pts',(58.7181337176191,-6.28595874576521,
40.0768265942419));
#198112=CARTESIAN_POINT('Ctrl Pts',(58.5872698677174,-6.26151010025721,
40.1599502027509));
#198113=CARTESIAN_POINT('Ctrl Pts',(58.6268645946692,-6.24170554357537,
40.1002552791541));
#198114=CARTESIAN_POINT('Ctrl Pts',(58.6982323944365,-6.23613328458267,
40.10025));
#198115=CARTESIAN_POINT('Ctrl Pts',(58.5964866834551,-6.1740349085902,40.1599502534424));
#198116=CARTESIAN_POINT('Ctrl Pts',(58.6335861742242,-6.17794390662172,
40.10025));
#198117=CARTESIAN_POINT('Ctrl Pts',(58.7035958781039,-6.18532049829399,
40.10025));
#198118=CARTESIAN_POINT('Origin',(58.7035958781039,-6.18532049829399,40.22725));
#198119=CARTESIAN_POINT('Ctrl Pts',(61.5639141665612,-6.15137923967676,
38.989));
#198120=CARTESIAN_POINT('Ctrl Pts',(61.5506192181748,-6.2778722240245,38.989));
#198121=CARTESIAN_POINT('Ctrl Pts',(61.5506390665201,-6.2776833796336,39.1161896013267));
#198122=CARTESIAN_POINT('Ctrl Pts',(61.7797255331386,-6.17383801205359,
38.989));
#198123=CARTESIAN_POINT('Ctrl Pts',(61.7665923920133,-6.30057242039953,
38.988776927546));
#198124=CARTESIAN_POINT('Ctrl Pts',(61.7232059145528,-6.29582088597892,
39.1161898821824));
#198125=CARTESIAN_POINT('Ctrl Pts',(61.9851742714891,-6.19522058691241,
39.1034967087243));
#198126=CARTESIAN_POINT('Ctrl Pts',(61.9721416759911,-6.32217699854488,
39.1031720232716));
#198127=CARTESIAN_POINT('Ctrl Pts',(61.887486582017,-6.31308747966678,39.2077529615019));
#198128=CARTESIAN_POINT('Ctrl Pts',(62.0995362748659,-6.20712349654464,
39.2875012672119));
#198129=CARTESIAN_POINT('Ctrl Pts',(62.086649444066,-6.33421251157703,39.2872087095507));
#198130=CARTESIAN_POINT('Ctrl Pts',(61.9789328337398,-6.3226988678917,39.3549017048228));
#198131=CARTESIAN_POINT('Origin',(61.5639141665612,-6.15137923967676,39.116));
#198132=CARTESIAN_POINT('Origin',(5.72301283402738E-15,5.24657654254566E-15,
40.22725));
#198133=CARTESIAN_POINT('Origin',(58.7067819056643,-6.15500747092316,40.22725));
#198134=CARTESIAN_POINT('Origin',(61.5757885448747,-6.15262728712865,39.116));
#198135=CARTESIAN_POINT('Origin',(61.1647646440473,-6.1093749596204,39.1160373285264));
#198136=CARTESIAN_POINT('Ctrl Pts',(58.5996668978648,-6.14377718965322,
40.1599502534424));
#198137=CARTESIAN_POINT('Ctrl Pts',(58.6367684021392,-6.14766703046171,
40.10025));
#198138=CARTESIAN_POINT('Ctrl Pts',(58.7067819056643,-6.15500747092316,
40.10025));
#198139=CARTESIAN_POINT('Ctrl Pts',(58.6088074259634,-6.05659553606703,
40.1599500566034));
#198140=CARTESIAN_POINT('Ctrl Pts',(58.6434243604386,-6.08415140319802,
40.1002551305369));
#198141=CARTESIAN_POINT('Ctrl Pts',(58.7120821529696,-6.10436324506821,
40.10025));
#198142=CARTESIAN_POINT('Ctrl Pts',(58.641681736514,-5.97852000021518,40.1203070619046));
#198143=CARTESIAN_POINT('Ctrl Pts',(58.6721826510718,-6.02785839131264,
40.0637098684499));
#198144=CARTESIAN_POINT('Ctrl Pts',(58.7414038195498,-6.06008468706693,
40.0772636213363));
#198145=CARTESIAN_POINT('Ctrl Pts',(58.7242744516463,-5.88025093392472,
40.0046102245802));
#198146=CARTESIAN_POINT('Ctrl Pts',(58.7387860695147,-5.97104363802146,
39.9670001894012));
#198147=CARTESIAN_POINT('Ctrl Pts',(58.8193360415241,-6.00614981441022,
40.0101788811209));
#198148=CARTESIAN_POINT('Ctrl Pts',(58.7730316211507,-5.85862682030274,
39.9303710930186));
#198149=CARTESIAN_POINT('Ctrl Pts',(58.7772266151804,-5.97091547255841,
39.9058663574101));
#198150=CARTESIAN_POINT('Ctrl Pts',(58.8669255556781,-5.99561386571421,
39.9671344706357));
#198151=CARTESIAN_POINT('Ctrl Pts',(58.8181995570485,-5.8633736414958,39.8576902534424));
#198152=CARTESIAN_POINT('Ctrl Pts',(58.805469618532,-5.98915458643795,39.8579948730703));
#198153=CARTESIAN_POINT('Ctrl Pts',(58.912095367953,-6.00036140429046,39.92499));
#198154=CARTESIAN_POINT('Origin',(58.925370482788,-5.87405712357869,39.92499));
#198155=CARTESIAN_POINT('Origin',(61.1207756545813,-6.10480350526346,39.192555448885));
#198156=CARTESIAN_POINT('Origin',(61.0393856393804,-6.09624906995239,39.3343017080178));
#198157=CARTESIAN_POINT('Origin',(59.1025439184835,-5.89267880207615,39.6398955069214));
#198158=CARTESIAN_POINT('Origin',(59.2797173540686,-5.91130048050343,39.3548010137695));
#198159=CARTESIAN_POINT('Ctrl Pts',(60.7112330730304,-6.0617588454157,39.3978017080178));
#198160=CARTESIAN_POINT('Ctrl Pts',(60.6979579581954,-6.18806312612747,
39.3978017080178));
#198161=CARTESIAN_POINT('Ctrl Pts',(60.6979579581954,-6.18806312612747,
39.5248017080178));
#198162=CARTESIAN_POINT('Ctrl Pts',(60.8007259828526,-6.07140041118235,
39.3978017080178));
#198163=CARTESIAN_POINT('Ctrl Pts',(60.7873912833632,-6.19746294737652,
39.3980355775177));
#198164=CARTESIAN_POINT('Ctrl Pts',(60.832232401263,-6.20217593878182,39.5248015517192));
#198165=CARTESIAN_POINT('Ctrl Pts',(60.885348460727,-6.08051542067561,39.3484893995498));
#198166=CARTESIAN_POINT('Ctrl Pts',(60.8723790316477,-6.20639551966723,
39.3489438303425));
#198167=CARTESIAN_POINT('Ctrl Pts',(60.9591984396283,-6.21552060714891,
39.4508333155593));
#198168=CARTESIAN_POINT('Ctrl Pts',(60.929944884669,-6.0853187813832,39.2708017080178));
#198169=CARTESIAN_POINT('Ctrl Pts',(60.917217374751,-6.21110821942935,39.2710850691866));
#198170=CARTESIAN_POINT('Ctrl Pts',(61.0261105245454,-6.22255335066416,
39.3343017080178));
#198171=CARTESIAN_POINT('Origin',(60.7112330730304,-6.0617588454157,39.5248017080178));
#198172=CARTESIAN_POINT('Ctrl Pts',(59.1725467709677,-5.90061356181257,
39.2875012672119));
#198173=CARTESIAN_POINT('Ctrl Pts',(59.1597945546413,-6.02658562874793,
39.2878045257519));
#198174=CARTESIAN_POINT('Ctrl Pts',(59.2666022171586,-6.03762143316751,
39.3549015218347));
#198175=CARTESIAN_POINT('Ctrl Pts',(59.2869113614505,-5.91250964036448,
39.1034938540228));
#198176=CARTESIAN_POINT('Ctrl Pts',(59.2739830624786,-6.03858760028837,
39.1038286278814));
#198177=CARTESIAN_POINT('Ctrl Pts',(59.3580501215753,-6.04723299508892,
39.2077506434033));
#198178=CARTESIAN_POINT('Ctrl Pts',(59.4923630227875,-5.93388131656882,
38.989));
#198179=CARTESIAN_POINT('Ctrl Pts',(59.4792818168365,-6.06016587018146,
38.9892298954611));
#198180=CARTESIAN_POINT('Ctrl Pts',(59.5223321697726,-6.06449973388389,
39.1161900347288));
#198181=CARTESIAN_POINT('Ctrl Pts',(59.7081718144892,-5.9563328589121,38.989));
#198182=CARTESIAN_POINT('Ctrl Pts',(59.6948768144683,-6.08282633453058,
38.989));
#198183=CARTESIAN_POINT('Ctrl Pts',(59.6948967145253,-6.08263699813566,
39.1161900945645));
#198184=CARTESIAN_POINT('Origin',(59.7081718144892,-5.95633285891211,39.116));
#198185=CARTESIAN_POINT('Origin',(60.0850508448141,-5.99594444118207,39.5248017080178));
#198186=CARTESIAN_POINT('Origin',(60.5608532912343,-6.04595329345061,39.5248017080178));
#198187=CARTESIAN_POINT('Origin',(59.851607889689,-5.97140859790549,39.116));
#198188=CARTESIAN_POINT('Origin',(60.1073400339997,-5.99823604520099,39.1160402713849));
#198189=CARTESIAN_POINT('Ctrl Pts',(60.3421421670675,-6.02238575970276,
39.2708017080178));
#198190=CARTESIAN_POINT('Ctrl Pts',(60.3293058762211,-6.14931623097247,
39.27051194648));
#198191=CARTESIAN_POINT('Ctrl Pts',(60.2194255397045,-6.13776734223215,
39.3343017080178));
#198192=CARTESIAN_POINT('Ctrl Pts',(60.3868890390928,-6.02720817145206,
39.3487519301185));
#198193=CARTESIAN_POINT('Ctrl Pts',(60.3738278099516,-6.15399567476902,
39.3482879463981));
#198194=CARTESIAN_POINT('Ctrl Pts',(60.2865637544299,-6.14482385294797,
39.4512271261641));
#198195=CARTESIAN_POINT('Ctrl Pts',(60.4716618705782,-6.03634362557897,
39.3978017080178));
#198196=CARTESIAN_POINT('Ctrl Pts',(60.4582762833192,-6.16287156698251,
39.3975673827397));
#198197=CARTESIAN_POINT('Ctrl Pts',(60.4137560077509,-6.15819229746499,
39.524801535518));
#198198=CARTESIAN_POINT('Ctrl Pts',(60.5608532912343,-6.04595329345061,
39.3978017080178));
#198199=CARTESIAN_POINT('Ctrl Pts',(60.5475781763993,-6.17225757416238,
39.3978017080178));
#198200=CARTESIAN_POINT('Ctrl Pts',(60.5475781763993,-6.17225757416238,
39.5248017080178));
#198201=CARTESIAN_POINT('Origin',(60.2327006545395,-6.01146306152038,39.3343017080178));
#198202=CARTESIAN_POINT('Origin',(60.1517960329188,-6.00295964283163,39.193400853355));
#198203=CARTESIAN_POINT('Origin',(60.0157999988656,-13.0813452322044,39.1925554495083));
#198204=CARTESIAN_POINT('Origin',(60.0590486699125,-13.0905908661188,39.1160373285276));
#198205=CARTESIAN_POINT('Origin',(59.9357500275433,-13.0643300858382,39.3343017080178));
#198206=CARTESIAN_POINT('Ctrl Pts',(59.8282880397055,-13.0409063549239,
39.2708017080178));
#198207=CARTESIAN_POINT('Ctrl Pts',(59.8550545325309,-12.9173404733283,
39.2710850691866));
#198208=CARTESIAN_POINT('Ctrl Pts',(59.9621548122771,-12.940105340545,39.3343017080178));
#198209=CARTESIAN_POINT('Ctrl Pts',(59.7842416555146,-13.0316624367248,
39.3487519293518));
#198210=CARTESIAN_POINT('Ctrl Pts',(59.8108054559361,-12.9079350417513,
39.349206866293));
#198211=CARTESIAN_POINT('Ctrl Pts',(59.8961220185298,-12.9260696369486,
39.4512271248737));
#198212=CARTESIAN_POINT('Ctrl Pts',(59.7007958241044,-13.014150410755,39.3978017080178));
#198213=CARTESIAN_POINT('Ctrl Pts',(59.7270694888854,-12.8901364125059,
39.3980347781183));
#198214=CARTESIAN_POINT('Ctrl Pts',(59.7710239514072,-12.8994792219295,
39.5248015355195));
#198215=CARTESIAN_POINT('Ctrl Pts',(59.6130003254555,-12.9957275188824,
39.3978017080178));
#198216=CARTESIAN_POINT('Ctrl Pts',(59.6394051101893,-12.8715027735892,
39.3978017080178));
#198217=CARTESIAN_POINT('Ctrl Pts',(59.6394051101893,-12.8715027735892,
39.5248017080178));
#198218=CARTESIAN_POINT('Origin',(59.6130003254555,-12.9957275188824,39.5248017080178));
#198219=CARTESIAN_POINT('Origin',(-0.0660119618346332,-0.310561863232983,
39.116));
#198220=CARTESIAN_POINT('Origin',(60.4516424606489,-13.1739864076107,39.116));
#198221=CARTESIAN_POINT('Origin',(-0.0660119618346331,-0.310561863232983,
39.5248017080178));
#198222=CARTESIAN_POINT('Origin',(59.4650964698966,-12.9642895838871,39.5248017080178));
#198223=CARTESIAN_POINT('Ctrl Pts',(60.9782752797348,-13.2864868028996,
39.2875012672119));
#198224=CARTESIAN_POINT('Ctrl Pts',(61.0052918384389,-13.1616357280625,
39.287208709576));
#198225=CARTESIAN_POINT('Ctrl Pts',(60.8992893541409,-13.139299581886,39.354901699012));
#198226=CARTESIAN_POINT('Ctrl Pts',(60.8658306440996,-13.2624669757406,
39.103493917393));
#198227=CARTESIAN_POINT('Ctrl Pts',(60.8926675943295,-13.13769697198,39.1031692336354));
#198228=CARTESIAN_POINT('Ctrl Pts',(60.8093473519447,-13.120181819017,39.207750720232));
#198229=CARTESIAN_POINT('Ctrl Pts',(60.663828108008,-13.2193155203585,38.989));
#198230=CARTESIAN_POINT('Ctrl Pts',(60.690500823975,-13.0947255842078,38.9887769311158));
#198231=CARTESIAN_POINT('Ctrl Pts',(60.6477702018642,-13.0858375353126,
39.1161898712887));
#198232=CARTESIAN_POINT('Ctrl Pts',(60.4516424606489,-13.1739864076107,
38.989));
#198233=CARTESIAN_POINT('Ctrl Pts',(60.4780866929066,-13.049576076309,38.989));
#198234=CARTESIAN_POINT('Ctrl Pts',(60.4780472159604,-13.049761800739,39.116189590385));
#198235=CARTESIAN_POINT('Origin',(60.8730422059013,-13.2635576885502,39.3548010137695));
#198236=CARTESIAN_POINT('Ctrl Pts',(59.4650964698966,-12.9642895838871,
39.3978017080178));
#198237=CARTESIAN_POINT('Ctrl Pts',(59.4915012546305,-12.8400648385939,
39.3978017080178));
#198238=CARTESIAN_POINT('Ctrl Pts',(59.4915012546305,-12.8400648385939,
39.5248017080178));
#198239=CARTESIAN_POINT('Ctrl Pts',(59.3770041141843,-12.9458049943939,
39.3978017080178));
#198240=CARTESIAN_POINT('Ctrl Pts',(59.4033730190112,-12.8213326038453,
39.3975666025021));
#198241=CARTESIAN_POINT('Ctrl Pts',(59.3594375597982,-12.8119938336989,
39.5248015517177));
#198242=CARTESIAN_POINT('Ctrl Pts',(59.2937057271824,-12.9283282206295,
39.3484894016716));
#198243=CARTESIAN_POINT('Ctrl Pts',(59.3204640761264,-12.803709764012,39.3480259000047));
#198244=CARTESIAN_POINT('Ctrl Pts',(59.2345619206657,-12.7854506972085,
39.4508333188947));
#198245=CARTESIAN_POINT('Ctrl Pts',(59.2498070616279,-12.9191181862046,
39.2708017080178));
#198246=CARTESIAN_POINT('Ctrl Pts',(59.2768226962998,-12.7944335023708,
39.27051194648));
#198247=CARTESIAN_POINT('Ctrl Pts',(59.1687514833561,-12.771462256932,39.3343017080178));
#198248=CARTESIAN_POINT('Origin',(59.1423466986222,-12.8956870022252,39.3343017080178));
#198249=CARTESIAN_POINT('Origin',(61.047298331886,-13.3005969715158,39.6398955068186));
#198250=CARTESIAN_POINT('Origin',(61.2215544576539,-13.3376362544826,39.92499));
#198251=CARTESIAN_POINT('Origin',(59.062774129127,-12.8787733304434,39.1934008539945));
#198252=CARTESIAN_POINT('Origin',(59.0190342907435,-12.8695280801147,39.1160402713849));
#198253=CARTESIAN_POINT('Ctrl Pts',(61.5752716937451,-13.1038352065728,
40.1599502534424));
#198254=CARTESIAN_POINT('Ctrl Pts',(61.5387839176328,-13.096070241968,40.10025));
#198255=CARTESIAN_POINT('Ctrl Pts',(61.4699285681954,-13.0814171332233,
40.10025));
#198256=CARTESIAN_POINT('Ctrl Pts',(61.5569304518434,-13.1900205930478,
40.1599500538467));
#198257=CARTESIAN_POINT('Ctrl Pts',(61.5254208297825,-13.1588482421895,
40.1002448353503));
#198258=CARTESIAN_POINT('Ctrl Pts',(61.4593031273768,-13.1313027022857,
40.10025));
#198259=CARTESIAN_POINT('Ctrl Pts',(61.515537853938,-13.2643407403244,40.120244200104));
#198260=CARTESIAN_POINT('Ctrl Pts',(61.4904936222818,-13.2118511391498,
40.0633873868018));
#198261=CARTESIAN_POINT('Ctrl Pts',(61.4250300340666,-13.172130065749,40.0772271723537));
#198262=CARTESIAN_POINT('Ctrl Pts',(61.4222835584426,-13.3535591268193,
40.0045995998161));
#198263=CARTESIAN_POINT('Ctrl Pts',(61.4178880557397,-13.2611962587088,
39.9663485808315));
#198264=CARTESIAN_POINT('Ctrl Pts',(61.3411158595754,-13.2174099770538,
40.0101727202466));
#198265=CARTESIAN_POINT('Ctrl Pts',(61.3712701109737,-13.370016757632,39.930465434986));
#198266=CARTESIAN_POINT('Ctrl Pts',(61.3797074995639,-13.2570896192432,
39.9051900162951));
#198267=CARTESIAN_POINT('Ctrl Pts',(61.2924393404518,-13.2228660458967,
39.9671857458178));
#198268=CARTESIAN_POINT('Ctrl Pts',(61.3267881959113,-13.3605623192487,
39.8576902534424));
#198269=CARTESIAN_POINT('Ctrl Pts',(61.3537611057083,-13.2359003894751,
39.8573998014387));
#198270=CARTESIAN_POINT('Ctrl Pts',(61.2479592423878,-13.2134115091894,
39.92499));
#198271=CARTESIAN_POINT('Origin',(61.4699285681954,-13.0814171332233,40.22725));
#198272=CARTESIAN_POINT('Origin',(-0.0660119618346332,-0.310561863232983,
39.116));
#198273=CARTESIAN_POINT('Origin',(58.6264539577984,-12.7860306150452,39.116));
#198274=CARTESIAN_POINT('Origin',(5.5033905580924E-15,5.72916705837122E-15,
40.22725));
#198275=CARTESIAN_POINT('Origin',(61.4762657165316,-13.0516031943529,40.22725));
#198276=CARTESIAN_POINT('Ctrl Pts',(58.6264539577984,-12.7860306150452,
38.989));
#198277=CARTESIAN_POINT('Ctrl Pts',(58.6528982980922,-12.6616197754736,
38.989));
#198278=CARTESIAN_POINT('Ctrl Pts',(58.6528587129486,-12.6618060089321,
39.1161901092325));
#198279=CARTESIAN_POINT('Ctrl Pts',(58.4142663981466,-12.7406940127373,
38.989));
#198280=CARTESIAN_POINT('Ctrl Pts',(58.4408495151711,-12.616547940969,38.989229898976));
#198281=CARTESIAN_POINT('Ctrl Pts',(58.4831327254079,-12.6257296363316,
39.1161900493205));
#198282=CARTESIAN_POINT('Ctrl Pts',(58.2122676405433,-12.6975319705099,
39.1034966344368));
#198283=CARTESIAN_POINT('Ctrl Pts',(58.2389323335232,-12.5736296288409,
39.1038314102556));
#198284=CARTESIAN_POINT('Ctrl Pts',(58.3215567776494,-12.5913856081746,
39.2077528789596));
#198285=CARTESIAN_POINT('Ctrl Pts',(58.099826060148,-12.6735055745741,39.2875012672119));
#198286=CARTESIAN_POINT('Ctrl Pts',(58.1266254943013,-12.5497583536231,
39.2878045257868));
#198287=CARTESIAN_POINT('Ctrl Pts',(58.231615877888,-12.5722680796265,39.3549015295901));
#198288=CARTESIAN_POINT('Origin',(58.2050537810542,-12.6964592423893,39.3548010137695));
#198289=CARTESIAN_POINT('Ctrl Pts',(61.4590390555209,-12.7383709431251,
39.8576902534424));
#198290=CARTESIAN_POINT('Ctrl Pts',(61.4329754599099,-12.8632261535955,
39.8573998014387));
#198291=CARTESIAN_POINT('Ctrl Pts',(61.3271735965893,-12.8407372733098,
39.92499));
#198292=CARTESIAN_POINT('Ctrl Pts',(61.5035409747667,-12.7478306169679,
39.9304984902491));
#198293=CARTESIAN_POINT('Ctrl Pts',(61.4653154597762,-12.8544171899347,
39.9052171569788));
#198294=CARTESIAN_POINT('Ctrl Pts',(61.3716739624479,-12.8501961180698,
39.9672049726605));
#198295=CARTESIAN_POINT('Ctrl Pts',(61.5432717953614,-12.783583551393,40.0043437678662));
#198296=CARTESIAN_POINT('Ctrl Pts',(61.501718402959,-12.8662481012965,39.9661628577646));
#198297=CARTESIAN_POINT('Ctrl Pts',(61.4137451613974,-12.8749453072904,
40.0100243556235));
#198298=CARTESIAN_POINT('Ctrl Pts',(61.5920631419345,-12.9020280679171,
40.1194874821987));
#198299=CARTESIAN_POINT('Ctrl Pts',(61.5478406570046,-12.9401487584127,
40.0627551483138));
#198300=CARTESIAN_POINT('Ctrl Pts',(61.4717924962542,-12.9498405053861,
40.0767884282377));
#198301=CARTESIAN_POINT('Ctrl Pts',(61.5999795805211,-12.987490469672,40.1599502015386));
#198302=CARTESIAN_POINT('Ctrl Pts',(61.5585057825379,-13.003195821844,40.1002449453872));
#198303=CARTESIAN_POINT('Ctrl Pts',(61.4868843017925,-13.0015435854425,
40.10025));
#198304=CARTESIAN_POINT('Ctrl Pts',(61.5816197022698,-13.0739701745325,
40.1599502534424));
#198305=CARTESIAN_POINT('Ctrl Pts',(61.5451281645059,-13.0662229071067,
40.10025));
#198306=CARTESIAN_POINT('Ctrl Pts',(61.4762657165316,-13.0516031943529,
40.10025));
#198307=CARTESIAN_POINT('Origin',(61.3535783813232,-12.7165125280166,39.92499));
#198308=CARTESIAN_POINT('Origin',(58.0307974155447,-12.6594199084569,39.6398955069314));
#198309=CARTESIAN_POINT('Origin',(57.8565410498767,-12.6223805745519,39.92499));
#198310=CARTESIAN_POINT('Origin',(61.1793222555322,-12.6794732450928,39.6398955068271));
#198311=CARTESIAN_POINT('Origin',(61.0050661295706,-12.6424339620842,39.3548010137695));
#198312=CARTESIAN_POINT('Ctrl Pts',(57.751314065072,-12.5994235324472,39.8576902534424));
#198313=CARTESIAN_POINT('Ctrl Pts',(57.7780756236495,-12.4758649777953,
39.8579948730703));
#198314=CARTESIAN_POINT('Ctrl Pts',(57.8829458346105,-12.4981558292588,
39.92499));
#198315=CARTESIAN_POINT('Ctrl Pts',(57.7068710254545,-12.5899763290071,
39.930402071123));
#198316=CARTESIAN_POINT('Ctrl Pts',(57.7455616498603,-12.4844883578131,
39.9058915297386));
#198317=CARTESIAN_POINT('Ctrl Pts',(57.8385008428013,-12.4887087546163,
39.967152378603));
#198318=CARTESIAN_POINT('Ctrl Pts',(57.6673720419786,-12.5543975270268,
40.0043257306693));
#198319=CARTESIAN_POINT('Ctrl Pts',(57.709200876099,-12.4724506530559,39.9667894847835));
#198320=CARTESIAN_POINT('Ctrl Pts',(57.7966870296826,-12.4640308112188,
40.01001389752));
#198321=CARTESIAN_POINT('Ctrl Pts',(57.6192799956674,-12.4363816727421,
40.1195533054857));
#198322=CARTESIAN_POINT('Ctrl Pts',(57.6635313090893,-12.39853212422,40.0630813209236));
#198323=CARTESIAN_POINT('Ctrl Pts',(57.7394080294762,-12.3892398894926,
40.076826594242));
#198324=CARTESIAN_POINT('Ctrl Pts',(57.6118166447792,-12.3512461790953,
40.1599502027523));
#198325=CARTESIAN_POINT('Ctrl Pts',(57.6532646075463,-12.3356888898082,
40.1002552791529));
#198326=CARTESIAN_POINT('Ctrl Pts',(57.7248239067121,-12.3376071226704,
40.10025));
#198327=CARTESIAN_POINT('Ctrl Pts',(57.6301266171957,-12.2652136052661,
40.1599502534424));
#198328=CARTESIAN_POINT('Ctrl Pts',(57.6666142715155,-12.2729791421555,
40.10025));
#198329=CARTESIAN_POINT('Ctrl Pts',(57.7354693911205,-12.2876333308471,
40.10025));
#198330=CARTESIAN_POINT('Origin',(57.7354693911204,-12.2876333308471,40.22725));
#198331=CARTESIAN_POINT('Ctrl Pts',(60.5836663843182,-12.5528626811448,
38.989));
#198332=CARTESIAN_POINT('Ctrl Pts',(60.5572221497821,-12.6772730231653,
38.989));
#198333=CARTESIAN_POINT('Ctrl Pts',(60.5572616290101,-12.6770872880005,
39.1161896013269));
#198334=CARTESIAN_POINT('Ctrl Pts',(60.7959479326852,-12.597756852521,38.989));
#198335=CARTESIAN_POINT('Ctrl Pts',(60.7696393833305,-12.7224242094576,
38.9887769275436));
#198336=CARTESIAN_POINT('Ctrl Pts',(60.7269872521261,-12.7131635826238,
39.1161898821827));
#198337=CARTESIAN_POINT('Ctrl Pts',(60.9980361136598,-12.6404975322982,
39.1034967087243));
#198338=CARTESIAN_POINT('Ctrl Pts',(60.9718043534777,-12.7653961862451,
39.1031720232722));
#198339=CARTESIAN_POINT('Ctrl Pts',(60.8885631224039,-12.74750759382,39.2077529615016));
#198340=CARTESIAN_POINT('Ctrl Pts',(61.1105274371641,-12.6642893210142,
39.2875012672119));
#198341=CARTESIAN_POINT('Ctrl Pts',(61.0844267823321,-12.789335088505,39.2872087095507));
#198342=CARTESIAN_POINT('Ctrl Pts',(60.9785037583488,-12.7666250660184,
39.3549017048229));
#198343=CARTESIAN_POINT('Origin',(60.5836663843182,-12.5528626811448,39.116));
#198344=CARTESIAN_POINT('Origin',(5.72205236298458E-15,5.24051236704441E-15,
40.22725));
#198345=CARTESIAN_POINT('Origin',(57.7418065394566,-12.2578193919768,40.22725));
#198346=CARTESIAN_POINT('Origin',(59.5987607253194,-12.3435145206986,39.116));
#198347=CARTESIAN_POINT('Origin',(60.1910940874965,-12.4693660187271,39.1160373285252));
#198348=CARTESIAN_POINT('Ctrl Pts',(57.6364522029207,-12.2354540642045,
40.1599502534424));
#198349=CARTESIAN_POINT('Ctrl Pts',(57.6729438621906,-12.2432007592847,
40.10025));
#198350=CARTESIAN_POINT('Ctrl Pts',(57.7418065394566,-12.2578193919768,
40.10025));
#198351=CARTESIAN_POINT('Ctrl Pts',(57.654655622525,-12.1497054461942,40.1599500566025));
#198352=CARTESIAN_POINT('Ctrl Pts',(57.6862025493675,-12.1807288143661,
40.1002551305369));
#198353=CARTESIAN_POINT('Ctrl Pts',(57.7523715145553,-12.2080066271958,
40.10025));
#198354=CARTESIAN_POINT('Ctrl Pts',(57.6955109599433,-12.0754939174599,
40.1203070619049));
#198355=CARTESIAN_POINT('Ctrl Pts',(57.7206875210982,-12.1277502414153,
40.0637098684502));
#198356=CARTESIAN_POINT('Ctrl Pts',(57.7861609236007,-12.1670355805164,
40.0772636213365));
#198357=CARTESIAN_POINT('Ctrl Pts',(57.7879231380269,-11.9863964689862,
40.0046102245799));
#198358=CARTESIAN_POINT('Ctrl Pts',(57.7928648378991,-12.0782086782658,
39.9670001894009));
#198359=CARTESIAN_POINT('Ctrl Pts',(57.8693039540645,-12.1215423041371,
40.0101788811207));
#198360=CARTESIAN_POINT('Ctrl Pts',(57.8386735460213,-11.9699873265228,
39.9303710930188));
#198361=CARTESIAN_POINT('Ctrl Pts',(57.8311081991733,-12.0820993460726,
39.9058663574113));
#198362=CARTESIAN_POINT('Ctrl Pts',(57.917734074407,-12.1160385312529,39.9671344706364));
#198363=CARTESIAN_POINT('Ctrl Pts',(57.8830978693156,-11.9794294790612,
39.8576902534424));
#198364=CARTESIAN_POINT('Ctrl Pts',(57.8572899778511,-12.1031907419157,
39.8579948730703));
#198365=CARTESIAN_POINT('Ctrl Pts',(57.9621601888121,-12.1254815933792,
39.92499));
#198366=CARTESIAN_POINT('Origin',(57.9885649735459,-12.001256848086,39.92499));
#198367=CARTESIAN_POINT('Origin',(60.1478239214166,-12.4602215058058,39.1925554488848));
#198368=CARTESIAN_POINT('Origin',(60.0677739512126,-12.4432063593722,39.3343017080178));
#198369=CARTESIAN_POINT('Origin',(58.1628213391873,-12.038296182045,39.6398955069221));
#198370=CARTESIAN_POINT('Origin',(58.3370777047235,-12.0753355159233,39.3548010137695));
#198371=CARTESIAN_POINT('Ctrl Pts',(59.7450242491248,-12.3746037924164,
39.3978017080178));
#198372=CARTESIAN_POINT('Ctrl Pts',(59.7186194643909,-12.4988285377096,
39.3978017080178));
#198373=CARTESIAN_POINT('Ctrl Pts',(59.7186194643909,-12.4988285377096,
39.5248017080178));
#198374=CARTESIAN_POINT('Ctrl Pts',(59.8330190893701,-12.393547097014,39.3978017080178));
#198375=CARTESIAN_POINT('Ctrl Pts',(59.8065803155759,-12.5175251937991,
39.3980355775177));
#198376=CARTESIAN_POINT('Ctrl Pts',(59.8506831473905,-12.5268995400895,
39.5248015517192));
#198377=CARTESIAN_POINT('Ctrl Pts',(59.9162252185215,-12.4114576311016,
39.3484893995498));
#198378=CARTESIAN_POINT('Ctrl Pts',(59.8901687840278,-12.5352924712485,
39.3489438303424));
#198379=CARTESIAN_POINT('Ctrl Pts',(59.9755587548367,-12.5534426698447,
39.4508333155594));
#198380=CARTESIAN_POINT('Ctrl Pts',(59.9600752506737,-12.4208962741587,
39.2708017080178));
#198381=CARTESIAN_POINT('Ctrl Pts',(59.9342688867325,-12.5446662374487,
39.2710850691866));
#198382=CARTESIAN_POINT('Ctrl Pts',(60.0413691664787,-12.5674311046654,
39.3343017080178));
#198383=CARTESIAN_POINT('Origin',(59.7450242491248,-12.3746037924164,39.5248017080178));
#198384=CARTESIAN_POINT('Ctrl Pts',(58.2316113004781,-12.0535047649322,
39.2875012672119));
#198385=CARTESIAN_POINT('Ctrl Pts',(58.2057612755556,-12.1774537741283,
39.2878045257518));
#198386=CARTESIAN_POINT('Ctrl Pts',(58.3108302788452,-12.1995935640848,
39.3549015218346));
#198387=CARTESIAN_POINT('Ctrl Pts',(58.344105910958,-12.0772900304171,39.1034938540228));
#198388=CARTESIAN_POINT('Ctrl Pts',(58.3180696991572,-12.2013259468575,
39.1038286278792));
#198389=CARTESIAN_POINT('Ctrl Pts',(58.400772540276,-12.2187113817821,39.2077506434033));
#198390=CARTESIAN_POINT('Ctrl Pts',(58.5461981381265,-12.1200201767772,
38.989));
#198391=CARTESIAN_POINT('Ctrl Pts',(58.5199882620678,-12.2442455720362,
38.9892298954635));
#198392=CARTESIAN_POINT('Ctrl Pts',(58.562349768552,-12.2530556816157,39.1161900347287));
#198393=CARTESIAN_POINT('Ctrl Pts',(58.7584778814676,-12.1649068885792,
38.989));
#198394=CARTESIAN_POINT('Ctrl Pts',(58.7320335442281,-12.2893177137816,
38.989));
#198395=CARTESIAN_POINT('Ctrl Pts',(58.7320731263129,-12.2891314947137,
39.1161900945644));
#198396=CARTESIAN_POINT('Origin',(58.7584778814676,-12.1649068885792,39.116));
#198397=CARTESIAN_POINT('Origin',(58.1567073854021,-12.036996621021,39.5248017080178));
#198398=CARTESIAN_POINT('Origin',(59.5971203935659,-12.3431658574211,39.5248017080178));
#198399=CARTESIAN_POINT('Origin',(57.9308881865554,-11.9889972685551,39.116));
#198400=CARTESIAN_POINT('Origin',(59.1510793400372,-12.2483049654002,39.1160402713847));
#198401=CARTESIAN_POINT('Ctrl Pts',(59.3820708699071,-12.2968658913803,
39.2708017080178));
#198402=CARTESIAN_POINT('Ctrl Pts',(59.3560370505014,-12.4217592664913,
39.27051194648));
#198403=CARTESIAN_POINT('Ctrl Pts',(59.2479658375576,-12.3987880210524,
39.3343017080178));
#198404=CARTESIAN_POINT('Ctrl Pts',(59.4260685345961,-12.3063392072221,
39.3487519301185));
#198405=CARTESIAN_POINT('Ctrl Pts',(59.3998259533489,-12.4310668851215,
39.3482879464001));
#198406=CARTESIAN_POINT('Ctrl Pts',(59.3139986558974,-12.4128237298761,
39.4512271261639));
#198407=CARTESIAN_POINT('Ctrl Pts',(59.5094220566594,-12.324285790178,39.3978017080178));
#198408=CARTESIAN_POINT('Ctrl Pts',(59.4828840257742,-12.448721423414,39.3975673827378));
#198409=CARTESIAN_POINT('Ctrl Pts',(59.4390967537837,-12.4394141514343,
39.524801535518));
#198410=CARTESIAN_POINT('Ctrl Pts',(59.5971203935659,-12.3431658574211,
39.3978017080178));
#198411=CARTESIAN_POINT('Ctrl Pts',(59.570715608832,-12.4673906027143,39.3978017080178));
#198412=CARTESIAN_POINT('Ctrl Pts',(59.5707156088321,-12.4673906027143,
39.5248017080178));
#198413=CARTESIAN_POINT('Origin',(59.2743706222915,-12.2745632757592,39.3343017080178));
#198414=CARTESIAN_POINT('Origin',(59.1947980539408,-12.257649603918,39.1934008533553));
#198415=CARTESIAN_POINT('Origin',(58.3196542523186,-19.283043599959,39.192555449508));
#198416=CARTESIAN_POINT('Origin',(58.3616995707151,-19.2967593024457,39.1160373285266));
#198417=CARTESIAN_POINT('Origin',(58.2418213702174,-19.2577541638579,39.3343017080178));
#198418=CARTESIAN_POINT('Ctrl Pts',(58.1373965169893,-19.223225914144,39.2708017080178));
#198419=CARTESIAN_POINT('Ctrl Pts',(58.1769325318819,-19.1031347997388,
39.2710850691866));
#198420=CARTESIAN_POINT('Ctrl Pts',(58.281066528503,-19.1369699862884,39.3343017080178));
#198421=CARTESIAN_POINT('Ctrl Pts',(58.094557676063,-19.209428534246,39.3487519293517));
#198422=CARTESIAN_POINT('Ctrl Pts',(58.1339089916609,-19.0891556041226,
39.3492068662912));
#198423=CARTESIAN_POINT('Ctrl Pts',(58.2168625998349,-19.1161088652886,
39.4512271248732));
#198424=CARTESIAN_POINT('Ctrl Pts',(58.0133994748126,-19.1832899764602,
39.3978017080178));
#198425=CARTESIAN_POINT('Ctrl Pts',(58.0524922023745,-19.0627016856742,
39.3980347781183));
#198426=CARTESIAN_POINT('Ctrl Pts',(58.095229288236,-19.0765878066321,39.5248015355195));
#198427=CARTESIAN_POINT('Ctrl Pts',(57.9280106456676,-19.1557908785626,
39.3978017080178));
#198428=CARTESIAN_POINT('Ctrl Pts',(57.9672558039532,-19.0350067009931,
39.3978017080178));
#198429=CARTESIAN_POINT('Ctrl Pts',(57.9672558039532,-19.0350067009931,
39.5248017080178));
#198430=CARTESIAN_POINT('Origin',(57.9280106456676,-19.1557908785626,39.5248017080178));
#198431=CARTESIAN_POINT('Origin',(-0.0981128957140405,-0.301960443923711,
39.116));
#198432=CARTESIAN_POINT('Origin',(58.7434254837932,-19.4207352200701,39.116));
#198433=CARTESIAN_POINT('Origin',(-0.0981128957140404,-0.301960443923711,
39.5248017080178));
#198434=CARTESIAN_POINT('Origin',(57.7842031819383,-19.1090650011316,39.5248017080178));
#198435=CARTESIAN_POINT('Ctrl Pts',(59.2554138597571,-19.5876674457079,
39.2875012672119));
#198436=CARTESIAN_POINT('Ctrl Pts',(59.2953329099159,-19.4663243174861,
39.287208709576));
#198437=CARTESIAN_POINT('Ctrl Pts',(59.1922458813531,-19.4330302542693,
39.3549016990121));
#198438=CARTESIAN_POINT('Ctrl Pts',(59.1460959632223,-19.5520255367093,
39.1034939173931));
#198439=CARTESIAN_POINT('Ctrl Pts',(59.185827914589,-19.4307442612481,39.1031692336334));
#198440=CARTESIAN_POINT('Ctrl Pts',(59.1047949412315,-19.4046157212334,
39.2077507202299));
#198441=CARTESIAN_POINT('Ctrl Pts',(58.9497105734782,-19.4879954548404,
38.989));
#198442=CARTESIAN_POINT('Ctrl Pts',(58.9892603680794,-19.3668760934057,
38.9887769311176));
#198443=CARTESIAN_POINT('Ctrl Pts',(58.9476928828796,-19.3535701679106,
39.1161898712914));
#198444=CARTESIAN_POINT('Ctrl Pts',(58.7434254837932,-19.4207352200701,
38.989));
#198445=CARTESIAN_POINT('Ctrl Pts',(58.7827292725254,-19.2997705965405,
38.989));
#198446=CARTESIAN_POINT('Ctrl Pts',(58.7826705983486,-19.2999511770884,
39.1161895903853));
#198447=CARTESIAN_POINT('Origin',(59.1531540087999,-19.5538640879533,39.3548010137695));
#198448=CARTESIAN_POINT('Ctrl Pts',(57.7842031819382,-19.1090650011316,
39.3978017080178));
#198449=CARTESIAN_POINT('Ctrl Pts',(57.8234483402239,-18.9882808235621,
39.3978017080178));
#198450=CARTESIAN_POINT('Ctrl Pts',(57.8234483402239,-18.9882808235621,
39.5248017080178));
#198451=CARTESIAN_POINT('Ctrl Pts',(57.698525571102,-19.0814735135845,39.3978017080178));
#198452=CARTESIAN_POINT('Ctrl Pts',(57.737760932012,-18.9604392969146,39.3975666025026));
#198453=CARTESIAN_POINT('Ctrl Pts',(57.695042323134,-18.9465591794948,39.5248015517177));
#198454=CARTESIAN_POINT('Ctrl Pts',(57.6175103216835,-19.0553854270314,
39.3484894016716));
#198455=CARTESIAN_POINT('Ctrl Pts',(57.6571482613574,-18.934246652454,39.3480259000042));
#198456=CARTESIAN_POINT('Ctrl Pts',(57.5736252790861,-18.9071083904253,
39.4508333188947));
#198457=CARTESIAN_POINT('Ctrl Pts',(57.5748148483576,-19.0416371860878,
39.2708017080178));
#198458=CARTESIAN_POINT('Ctrl Pts',(57.6147155869502,-18.9204594407746,
39.27051194648));
#198459=CARTESIAN_POINT('Ctrl Pts',(57.5096375484037,-18.8863175164093,
39.3343017080178));
#198460=CARTESIAN_POINT('Origin',(57.4703923901181,-19.0071016939788,39.3343017080178));
#198461=CARTESIAN_POINT('Origin',(59.3225838821613,-19.608915190917,39.6398955068204));
#198462=CARTESIAN_POINT('Origin',(59.4920137553139,-19.6639662938562,39.92499));
#198463=CARTESIAN_POINT('Origin',(57.3930236876035,-18.9819630786538,39.1934008539947));
#198464=CARTESIAN_POINT('Origin',(57.3504898524414,-18.9681964166828,39.1160402713844));
#198465=CARTESIAN_POINT('Ctrl Pts',(59.8682321556242,-19.4684195516697,
40.1599502534424));
#198466=CARTESIAN_POINT('Ctrl Pts',(59.8327559231846,-19.4568831131884,
40.10025));
#198467=CARTESIAN_POINT('Ctrl Pts',(59.7658094374951,-19.4351129318421,
40.10025));
#198468=CARTESIAN_POINT('Ctrl Pts',(59.8409825629599,-19.5522156237493,
40.159950053846));
#198469=CARTESIAN_POINT('Ctrl Pts',(59.812903951836,-19.5179203859178,40.1002448353493));
#198470=CARTESIAN_POINT('Ctrl Pts',(59.7500277420787,-19.4836145615369,
40.10025));
#198471=CARTESIAN_POINT('Ctrl Pts',(59.7920481472525,-19.6218019328334,
40.1202442001039));
#198472=CARTESIAN_POINT('Ctrl Pts',(59.7726277678658,-19.5669820401377,
40.0633873868017));
#198473=CARTESIAN_POINT('Ctrl Pts',(59.7116747787989,-19.5206357546568,
40.0772271723536));
#198474=CARTESIAN_POINT('Ctrl Pts',(59.6899788477098,-19.7007838434707,
40.0045995998162));
#198475=CARTESIAN_POINT('Ctrl Pts',(59.6952619726974,-19.6084674936726,
39.9663485808314));
#198476=CARTESIAN_POINT('Ctrl Pts',(59.6234872553896,-19.5568961981634,
40.0101727202467));
#198477=CARTESIAN_POINT('Ctrl Pts',(59.6375245663856,-19.7118189603903,
39.9304654349859));
#198478=CARTESIAN_POINT('Ctrl Pts',(59.6577198343148,-19.600392395946,39.9051900162946));
#198479=CARTESIAN_POINT('Ctrl Pts',(59.5745070768395,-19.5572342963492,
39.9671857458179));
#198480=CARTESIAN_POINT('Ctrl Pts',(59.5942745858236,-19.6977666881846,
39.8576902534424));
#198481=CARTESIAN_POINT('Ctrl Pts',(59.6341304551457,-19.5766071063169,
39.8573998014387));
#198482=CARTESIAN_POINT('Ctrl Pts',(59.5312589135995,-19.5431821162867,
39.92499));
#198483=CARTESIAN_POINT('Origin',(59.7658094374951,-19.4351129318421,40.22725));
#198484=CARTESIAN_POINT('Origin',(-0.0981128957140405,-0.301960443923711,
39.116));
#198485=CARTESIAN_POINT('Origin',(56.9687879773466,-18.844120540552,39.116));
#198486=CARTESIAN_POINT('Origin',(5.50785759597432E-15,5.74583827070587E-15,
40.22725));
#198487=CARTESIAN_POINT('Origin',(59.7752282754837,-19.4061247292254,40.22725));
#198488=CARTESIAN_POINT('Ctrl Pts',(56.9687879773466,-18.844120540552,38.989));
#198489=CARTESIAN_POINT('Ctrl Pts',(57.0080919266514,-18.7231554228306,
38.989));
#198490=CARTESIAN_POINT('Ctrl Pts',(57.0080330916623,-18.7233364983079,
39.1161901092319));
#198491=CARTESIAN_POINT('Ctrl Pts',(56.7625017687173,-18.7768526573602,
38.989));
#198492=CARTESIAN_POINT('Ctrl Pts',(56.8019160587434,-18.6561653631331,
38.989229898976));
#198493=CARTESIAN_POINT('Ctrl Pts',(56.8430078886248,-18.6697165591959,
39.1161900493199));
#198494=CARTESIAN_POINT('Ctrl Pts',(56.5661212433894,-18.7128124416009,
39.1034966344368));
#198495=CARTESIAN_POINT('Ctrl Pts',(56.6055911857666,-18.5923760693073,
39.1038314102573));
#198496=CARTESIAN_POINT('Ctrl Pts',(56.6859069993073,-18.6186713857008,
39.2077528789603));
#198497=CARTESIAN_POINT('Ctrl Pts',(56.4568070719811,-18.677164319171,39.2875012672119));
#198498=CARTESIAN_POINT('Ctrl Pts',(56.4963948028695,-18.5568963021133,
39.2878045257868));
#198499=CARTESIAN_POINT('Ctrl Pts',(56.5984571310816,-18.590257200936,39.3549015295897));
#198500=CARTESIAN_POINT('Origin',(56.5590590327989,-18.7109915363517,39.3548010137695));
#198501=CARTESIAN_POINT('Ctrl Pts',(59.7908376697911,-19.0928077206412,
39.8576902534424));
#198502=CARTESIAN_POINT('Ctrl Pts',(59.7518659300026,-19.2142545736084,
39.8573998014387));
#198503=CARTESIAN_POINT('Ctrl Pts',(59.6489943884564,-19.1808295835782,
39.92499));
#198504=CARTESIAN_POINT('Ctrl Pts',(59.8341069976972,-19.1068672906321,
39.9304984902491));
#198505=CARTESIAN_POINT('Ctrl Pts',(59.7849495554016,-19.2088743168612,
39.9052171569785));
#198506=CARTESIAN_POINT('Ctrl Pts',(59.6922622581486,-19.1948881666553,
39.9672049726599));
#198507=CARTESIAN_POINT('Ctrl Pts',(59.8698829694067,-19.1465773683628,
40.0043437678661));
#198508=CARTESIAN_POINT('Ctrl Pts',(59.8199164124673,-19.2244455609615,
39.966162857764));
#198509=CARTESIAN_POINT('Ctrl Pts',(59.7315159919505,-19.2238994150012,
40.0100243556235));
#198510=CARTESIAN_POINT('Ctrl Pts',(59.9060262085836,-19.2694731179102,
40.1194874821988));
#198511=CARTESIAN_POINT('Ctrl Pts',(59.8580612818573,-19.3027624708828,
40.0627551483143));
#198512=CARTESIAN_POINT('Ctrl Pts',(59.7814166574712,-19.3044519280752,
40.0767884282378));
#198513=CARTESIAN_POINT('Ctrl Pts',(59.9049660265691,-19.3552948408465,
40.1599502015395));
#198514=CARTESIAN_POINT('Ctrl Pts',(59.8620777700652,-19.3665789650879,
40.1002449453869));
#198515=CARTESIAN_POINT('Ctrl Pts',(59.7910213450144,-19.3574492964897,
40.10025));
#198516=CARTESIAN_POINT('Ctrl Pts',(59.8776671349985,-19.4393816709757,
40.1599502534424));
#198517=CARTESIAN_POINT('Ctrl Pts',(59.8421853116552,-19.4278624395267,
40.10025));
#198518=CARTESIAN_POINT('Ctrl Pts',(59.7752282754837,-19.4061247292254,
40.10025));
#198519=CARTESIAN_POINT('Origin',(59.688239546742,-19.0600454060087,39.92499));
#198520=CARTESIAN_POINT('Origin',(56.3896289265489,-18.6559403576676,39.639895506932));
#198521=CARTESIAN_POINT('Origin',(56.2201988201383,-18.6008891789886,39.92499));
#198522=CARTESIAN_POINT('Origin',(59.5188096735645,-19.0049943031082,39.6398955068277));
#198523=CARTESIAN_POINT('Origin',(59.349379800228,-18.9499432001058,39.3548010137695));
#198524=CARTESIAN_POINT('Ctrl Pts',(56.1179479440988,-18.5670586829466,
39.8576902534424));
#198525=CARTESIAN_POINT('Ctrl Pts',(56.1574782858997,-18.446974339578,39.8579948730703));
#198526=CARTESIAN_POINT('Ctrl Pts',(56.2594439784239,-18.4801050014191,
39.92499));
#198527=CARTESIAN_POINT('Ctrl Pts',(56.0747358697604,-18.5530176696407,
39.9304020711232));
#198528=CARTESIAN_POINT('Ctrl Pts',(56.1242410383992,-18.4521518441035,
39.9058915297388));
#198529=CARTESIAN_POINT('Ctrl Pts',(56.2162299491247,-18.4660639121462,
39.9671523786032));
#198530=CARTESIAN_POINT('Ctrl Pts',(56.0391722633447,-18.5135050040175,
40.0043257306691));
#198531=CARTESIAN_POINT('Ctrl Pts',(56.0893377355418,-18.436379347347,39.9667894847835));
#198532=CARTESIAN_POINT('Ctrl Pts',(56.17722474395,-18.4371504234763,40.0100138975201));
#198533=CARTESIAN_POINT('Ctrl Pts',(56.0036796861845,-18.3911086652346,
40.1195533054859));
#198534=CARTESIAN_POINT('Ctrl Pts',(56.051644941423,-18.3580919822894,40.0630813209236));
#198535=CARTESIAN_POINT('Ctrl Pts',(56.1280773042132,-18.3567819283754,
40.076826594242));
#198536=CARTESIAN_POINT('Ctrl Pts',(56.0051563026344,-18.3056594201306,
40.1599502027516));
#198537=CARTESIAN_POINT('Ctrl Pts',(56.0480033886682,-18.2945198471559,
40.1002552791553));
#198538=CARTESIAN_POINT('Ctrl Pts',(56.1189701685708,-18.3039075553119,
40.10025));
#198539=CARTESIAN_POINT('Ctrl Pts',(56.0323588238391,-18.2220120550217,
40.1599502534424));
#198540=CARTESIAN_POINT('Ctrl Pts',(56.0678348753332,-18.2335490499218,
40.10025));
#198541=CARTESIAN_POINT('Ctrl Pts',(56.1347810195642,-18.2553202812749,
40.10025));
#198542=CARTESIAN_POINT('Origin',(56.1347810195642,-18.2553202812749,40.22725));
#198543=CARTESIAN_POINT('Ctrl Pts',(58.9396512752213,-18.8168143322227,
38.989));
#198544=CARTESIAN_POINT('Ctrl Pts',(58.9003474831029,-18.9377789661741,
38.989));
#198545=CARTESIAN_POINT('Ctrl Pts',(58.9004061606709,-18.9375983751889,
39.116189601327));
#198546=CARTESIAN_POINT('Ctrl Pts',(59.1460772043118,-18.8836520326604,
38.989));
#198547=CARTESIAN_POINT('Ctrl Pts',(59.1068814887033,-19.0048864565372,
38.9887769275436));
#198548=CARTESIAN_POINT('Ctrl Pts',(59.0654310094272,-18.991218198657,39.1161898821827));
#198549=CARTESIAN_POINT('Ctrl Pts',(59.3425907075097,-18.9472825415245,
39.1034967087243));
#198550=CARTESIAN_POINT('Ctrl Pts',(59.3034471832928,-19.0687550219954,
39.1031720232724));
#198551=CARTESIAN_POINT('Ctrl Pts',(59.2225318234694,-19.0422633471879,
39.2077529615016));
#198552=CARTESIAN_POINT('Ctrl Pts',(59.4519788726607,-18.9827025415097,
39.2875012672119));
#198553=CARTESIAN_POINT('Ctrl Pts',(59.4129503580329,-19.1043350338627,
39.2872087095507));
#198554=CARTESIAN_POINT('Ctrl Pts',(59.3099814352092,-19.0706774483338,
39.3549017048229));
#198555=CARTESIAN_POINT('Origin',(58.9396512752213,-18.8168143322227,39.116));
#198556=CARTESIAN_POINT('Origin',(5.72046327455653E-15,5.23458180829319E-15,
40.22725));
#198557=CARTESIAN_POINT('Origin',(56.1441998575527,-18.2263320786583,40.22725));
#198558=CARTESIAN_POINT('Origin',(56.3788528200606,-17.9847604760582,39.116));
#198559=CARTESIAN_POINT('Origin',(58.5579573083287,-18.6927400943497,39.1160373285264));
#198560=CARTESIAN_POINT('Ctrl Pts',(56.0417604764383,-18.193076743595,40.1599502534424));
#198561=CARTESIAN_POINT('Ctrl Pts',(56.0772424804484,-18.2045954185346,
40.10025));
#198562=CARTESIAN_POINT('Ctrl Pts',(56.1441998575527,-18.2263320786583,
40.10025));
#198563=CARTESIAN_POINT('Ctrl Pts',(56.0688273470726,-18.1097006409636,
40.1599500566036));
#198564=CARTESIAN_POINT('Ctrl Pts',(56.0969586315475,-18.1438516116618,
40.1002551305369));
#198565=CARTESIAN_POINT('Ctrl Pts',(56.1599138083653,-18.1778965340263,
40.10025));
#198566=CARTESIAN_POINT('Ctrl Pts',(56.1172160917342,-18.040166196385,40.1203070619044));
#198567=CARTESIAN_POINT('Ctrl Pts',(56.1367924598137,-18.0947679219781,
40.0637098684496));
#198568=CARTESIAN_POINT('Ctrl Pts',(56.1978007560413,-18.1406818860294,
40.0772636213361));
#198569=CARTESIAN_POINT('Ctrl Pts',(56.2184352456062,-17.9612165360192,
40.0046102245804));
#198570=CARTESIAN_POINT('Ctrl Pts',(56.2137528851844,-18.0530423367033,
39.9670001894015));
#198571=CARTESIAN_POINT('Ctrl Pts',(56.2852436625535,-18.1041286397846,
40.0101788811211));
#198572=CARTESIAN_POINT('Ctrl Pts',(56.2706228600015,-17.9502021467126,
39.9303710930184));
#198573=CARTESIAN_POINT('Ctrl Pts',(56.2513800597972,-18.0609092108094,
39.9058663574111));
#198574=CARTESIAN_POINT('Ctrl Pts',(56.3339837785517,-18.1037173431991,
39.9671344706364));
#198575=CARTESIAN_POINT('Ctrl Pts',(56.3138168485095,-17.9642361803973,
39.8576902534424));
#198576=CARTESIAN_POINT('Ctrl Pts',(56.2752137607566,-18.0846218068695,
39.8579948730703));
#198577=CARTESIAN_POINT('Ctrl Pts',(56.3771794532807,-18.1177524687107,
39.92499));
#198578=CARTESIAN_POINT('Origin',(56.4164246115663,-17.9969682911412,39.92499));
#198579=CARTESIAN_POINT('Origin',(58.5158800426272,-18.6791227120619,39.1925554488844));
#198580=CARTESIAN_POINT('Origin',(58.4380471616454,-18.6538332760105,39.3343017080178));
#198581=CARTESIAN_POINT('Origin',(56.5858547179429,-18.0520194698694,39.6398955069213));
#198582=CARTESIAN_POINT('Origin',(56.755284824227,-18.1070706485043,39.3548010137695));
#198583=CARTESIAN_POINT('Ctrl Pts',(58.1242364370956,-18.5518699907151,
39.3978017080178));
#198584=CARTESIAN_POINT('Ctrl Pts',(58.08499127881,-18.6726541682846,39.3978017080178));
#198585=CARTESIAN_POINT('Ctrl Pts',(58.08499127881,-18.6726541682846,39.5248017080178));
#198586=CARTESIAN_POINT('Ctrl Pts',(58.2097691178803,-18.5799074873343,
39.3978017080178));
#198587=CARTESIAN_POINT('Ctrl Pts',(58.1705159385207,-18.7004428147369,
39.3980355775177));
#198588=CARTESIAN_POINT('Ctrl Pts',(58.2133972843949,-18.7143758086137,
39.5248015517192));
#198589=CARTESIAN_POINT('Ctrl Pts',(58.2906472745453,-18.6064173144581,
39.3484893995498));
#198590=CARTESIAN_POINT('Ctrl Pts',(58.2517893143854,-18.7268501353373,
39.3489438303421));
#198591=CARTESIAN_POINT('Ctrl Pts',(58.3348142976339,-18.7538265876729,
39.4508333155594));
#198592=CARTESIAN_POINT('Ctrl Pts',(58.3332704847796,-18.6203878281148,
39.2708017080178));
#198593=CARTESIAN_POINT('Ctrl Pts',(58.2946680067388,-18.7407822670303,
39.2710850691866));
#198594=CARTESIAN_POINT('Ctrl Pts',(58.3988020033598,-18.77461745358,39.3343017080178));
#198595=CARTESIAN_POINT('Origin',(58.1242364370957,-18.5518699907151,39.5248017080178));
#198596=CARTESIAN_POINT('Ctrl Pts',(56.6526781108323,-18.0743352474892,
39.2875012672119));
#198597=CARTESIAN_POINT('Ctrl Pts',(56.6140134955962,-18.1949031876634,
39.2878045257519));
#198598=CARTESIAN_POINT('Ctrl Pts',(56.7161926816711,-18.2279043949848,
39.3549015218347));
#198599=CARTESIAN_POINT('Ctrl Pts',(56.7620702268162,-18.1097491035597,
39.1034938540228));
#198600=CARTESIAN_POINT('Ctrl Pts',(56.7232113603685,-18.2303840130645,
39.1038286278802));
#198601=CARTESIAN_POINT('Ctrl Pts',(56.803643873878,-18.2563190096466,39.2077506434033));
#198602=CARTESIAN_POINT('Ctrl Pts',(56.9585888550845,-18.1733695596523,
38.989));
#198603=CARTESIAN_POINT('Ctrl Pts',(56.9195374698062,-18.294174757132,38.9892298954611));
#198604=CARTESIAN_POINT('Ctrl Pts',(56.9607460083078,-18.307364587183,39.1161900347288));
#198605=CARTESIAN_POINT('Ctrl Pts',(57.1650137687747,-18.2401996527046,
38.989));
#198606=CARTESIAN_POINT('Ctrl Pts',(57.1257098240092,-18.3611647564555,
38.989));
#198607=CARTESIAN_POINT('Ctrl Pts',(57.1257686544522,-18.3609836949695,
39.1161900945645));
#198608=CARTESIAN_POINT('Origin',(57.1650137687747,-18.2401996527046,39.116));
#198609=CARTESIAN_POINT('Origin',(55.0155724295758,-17.5418038257016,39.5248017080178));
#198610=CARTESIAN_POINT('Origin',(57.9804289733664,-18.5051441132842,39.5248017080178));
#198611=CARTESIAN_POINT('Origin',(54.8020887275094,-17.4724387660755,39.116));
#198612=CARTESIAN_POINT('Origin',(57.5467470426661,-18.3641788932756,39.1160402713847));
#198613=CARTESIAN_POINT('Ctrl Pts',(57.7713971777987,-18.4366189870673,
39.2708017080178));
#198614=CARTESIAN_POINT('Ctrl Pts',(57.732451061807,-18.5581069080661,39.27051194648));
#198615=CARTESIAN_POINT('Ctrl Pts',(57.6273730232605,-18.5239649837008,
39.3343017080178));
#198616=CARTESIAN_POINT('Ctrl Pts',(57.8141635875301,-18.4506394153709,
39.3487519301186));
#198617=CARTESIAN_POINT('Ctrl Pts',(57.7750271733926,-18.5719407253083,
39.3482879463999));
#198618=CARTESIAN_POINT('Ctrl Pts',(57.6915769758382,-18.5448261124693,
39.451227126164));
#198619=CARTESIAN_POINT('Ctrl Pts',(57.8951845615408,-18.4772005006368,
39.3978017080178));
#198620=CARTESIAN_POINT('Ctrl Pts',(57.8557848432467,-18.5981804828678,
39.3975673827378));
#198621=CARTESIAN_POINT('Ctrl Pts',(57.8132103173517,-18.5843471808457,
39.524801535518));
#198622=CARTESIAN_POINT('Ctrl Pts',(57.9804289733664,-18.5051441132842,
39.3978017080178));
#198623=CARTESIAN_POINT('Ctrl Pts',(57.9411838150807,-18.6259282908537,
39.3978017080178));
#198624=CARTESIAN_POINT('Ctrl Pts',(57.9411838150807,-18.6259282908537,
39.5248017080178));
#198625=CARTESIAN_POINT('Origin',(57.6666181815461,-18.4031808061313,39.3343017080178));
#198626=CARTESIAN_POINT('Origin',(57.5892494801768,-18.3780421908668,39.1934008533551));
#198627=CARTESIAN_POINT('Origin',(55.9845461696115,-25.273472906795,39.1925554495078));
#198628=CARTESIAN_POINT('Origin',(56.0249274780511,-25.2915084057492,39.1160373285264));
#198629=CARTESIAN_POINT('Origin',(55.9097831300746,-25.2401862573142,39.3343017080178));
#198630=CARTESIAN_POINT('Ctrl Pts',(55.8095395120007,-25.1949317875302,
39.2708017080178));
#198631=CARTESIAN_POINT('Ctrl Pts',(55.8614118841079,-25.0796311836954,
39.2710850691866));
#198632=CARTESIAN_POINT('Ctrl Pts',(55.9614386837453,-25.1241659841936,
39.3343017080178));
#198633=CARTESIAN_POINT('Ctrl Pts',(55.7683775656457,-25.1767321129114,
39.3487519293518));
#198634=CARTESIAN_POINT('Ctrl Pts',(55.8200852551805,-25.0612313830316,
39.3492068662923));
#198635=CARTESIAN_POINT('Ctrl Pts',(55.8997670518367,-25.0967080045981,
39.4512271248733));
#198636=CARTESIAN_POINT('Ctrl Pts',(55.6903961807902,-25.1422534028232,
39.3978017080178));
#198637=CARTESIAN_POINT('Ctrl Pts',(55.7418796630219,-25.026412010048,39.3980347781178));
#198638=CARTESIAN_POINT('Ctrl Pts',(55.7829311357729,-25.0446893032922,
39.5248015355195));
#198639=CARTESIAN_POINT('Ctrl Pts',(55.6083495590301,-25.1059793847702,
39.3978017080178));
#198640=CARTESIAN_POINT('Ctrl Pts',(55.6600051127008,-24.9899591116496,
39.3978017080178));
#198641=CARTESIAN_POINT('Ctrl Pts',(55.6600051127007,-24.9899591116496,
39.5248017080178));
#198642=CARTESIAN_POINT('Origin',(55.6083495590301,-25.1059793847702,39.5248017080178));
#198643=CARTESIAN_POINT('Origin',(-0.129138884176561,-0.290050682801526,
39.116));
#198644=CARTESIAN_POINT('Origin',(56.391603244485,-25.4547063934084,39.116));
#198645=CARTESIAN_POINT('Origin',(-0.129138884176561,-0.290050682801526,
39.5248017080178));
#198646=CARTESIAN_POINT('Origin',(55.4702140717966,-25.0444775033948,39.5248017080178));
#198647=CARTESIAN_POINT('Ctrl Pts',(56.8833377255394,-25.6742415049981,
39.2875012672119));
#198648=CARTESIAN_POINT('Ctrl Pts',(56.9357219056859,-25.5577357840968,
39.287208709576));
#198649=CARTESIAN_POINT('Ctrl Pts',(56.8366797759152,-25.5138485805637,
39.3549016990124));
#198650=CARTESIAN_POINT('Ctrl Pts',(56.7783442778552,-25.6273680143744,
39.103493917393));
#198651=CARTESIAN_POINT('Ctrl Pts',(56.8305359187841,-25.510904250251,39.1031692336322));
#198652=CARTESIAN_POINT('Ctrl Pts',(56.7526780286692,-25.4764485929319,
39.2077507202294));
#198653=CARTESIAN_POINT('Ctrl Pts',(56.589727673885,-25.5431608329955,38.989));
#198654=CARTESIAN_POINT('Ctrl Pts',(56.6417212312941,-25.4268390553472,
38.9887769311182));
#198655=CARTESIAN_POINT('Ctrl Pts',(56.6017723050717,-25.4092610357534,
39.1161898712918));
#198656=CARTESIAN_POINT('Ctrl Pts',(56.391603244485,-25.4547063934084,38.989));
#198657=CARTESIAN_POINT('Ctrl Pts',(56.4433359691576,-25.3385127913796,
38.989));
#198658=CARTESIAN_POINT('Ctrl Pts',(56.4432587405967,-25.3386862495672,
39.1161895903857));
#198659=CARTESIAN_POINT('Origin',(56.7851714777847,-25.6299342604996,39.3548010137695));
#198660=CARTESIAN_POINT('Ctrl Pts',(55.4702140717966,-25.0444775033948,
39.3978017080178));
#198661=CARTESIAN_POINT('Ctrl Pts',(55.5218696254673,-24.9284572302742,
39.3978017080178));
#198662=CARTESIAN_POINT('Ctrl Pts',(55.5218696254673,-24.9284572302742,
39.5248017080178));
#198663=CARTESIAN_POINT('Ctrl Pts',(55.3878899076696,-25.0080814159061,
39.3978017080178));
#198664=CARTESIAN_POINT('Ctrl Pts',(55.4395618538391,-24.8918114493207,
39.3975666025007));
#198665=CARTESIAN_POINT('Ctrl Pts',(55.3985281293138,-24.8735420580978,
39.5248015517177));
#198666=CARTESIAN_POINT('Ctrl Pts',(55.310045415862,-24.9736678430965,39.3484894016716));
#198667=CARTESIAN_POINT('Ctrl Pts',(55.3621286647035,-24.8573359723221,
39.3480259000056));
#198668=CARTESIAN_POINT('Ctrl Pts',(55.2818999508933,-24.8216158475497,
39.4508333188947));
#198669=CARTESIAN_POINT('Ctrl Pts',(55.269020915304,-24.9555320242416,39.2708017080178));
#198670=CARTESIAN_POINT('Ctrl Pts',(55.3213695969755,-24.8391888661845,
39.27051194648));
#198671=CARTESIAN_POINT('Ctrl Pts',(55.2204359898056,-24.7942503289608,
39.3343017080178));
#198672=CARTESIAN_POINT('Origin',(55.168780436135,-24.9102706020814,39.3343017080178));
#198673=CARTESIAN_POINT('Origin',(56.9479187893821,-25.7023940320519,39.639895506819));
#198674=CARTESIAN_POINT('Origin',(57.1106661007665,-25.7748538035648,39.92499));
#198675=CARTESIAN_POINT('Origin',(55.0944632682975,-24.8771824671421,39.1934008539943));
#198676=CARTESIAN_POINT('Origin',(55.0536014459542,-24.8590452239599,39.1160402713843));
#198677=CARTESIAN_POINT('Ctrl Pts',(57.5052637377732,-25.6197038181298,
40.1599502534424));
#198678=CARTESIAN_POINT('Ctrl Pts',(57.4711877340329,-25.6045223014062,
40.10025));
#198679=CARTESIAN_POINT('Ctrl Pts',(57.4068835917979,-25.5758735661209,
40.10025));
#198680=CARTESIAN_POINT('Ctrl Pts',(57.4694043465863,-25.7001924885131,
40.1599500538461));
#198681=CARTESIAN_POINT('Ctrl Pts',(57.4450643815388,-25.6631501095107,
40.1002448353478));
#198682=CARTESIAN_POINT('Ctrl Pts',(57.3861185493426,-25.622459862444,40.10025));
#198683=CARTESIAN_POINT('Ctrl Pts',(57.4134642487753,-25.76428255724,40.1202442001039));
#198684=CARTESIAN_POINT('Ctrl Pts',(57.3998804953989,-25.7077329912391,
40.0633873868017));
#198685=CARTESIAN_POINT('Ctrl Pts',(57.3441059191831,-25.6552692732805,
40.0772271723538));
#198686=CARTESIAN_POINT('Ctrl Pts',(57.3036982377902,-25.8321626496791,
40.0045995998162));
#198687=CARTESIAN_POINT('Ctrl Pts',(57.3186021074451,-25.7409042554406,
39.9663485808314));
#198688=CARTESIAN_POINT('Ctrl Pts',(57.2526112478171,-25.6821129719826,
40.0101727202466));
#198689=CARTESIAN_POINT('Ctrl Pts',(57.2503778226941,-25.8376543496545,
39.9304654349859));
#198690=CARTESIAN_POINT('Ctrl Pts',(57.28210970638,-25.7289491719111,39.905190016295));
#198691=CARTESIAN_POINT('Ctrl Pts',(57.203864046926,-25.6773293952366,39.9671857458181));
#198692=CARTESIAN_POINT('Ctrl Pts',(57.2088336324698,-25.8191582032621,
39.8576902534424));
#198693=CARTESIAN_POINT('Ctrl Pts',(57.2611357920724,-25.7028284190334,
39.8573998014387));
#198694=CARTESIAN_POINT('Ctrl Pts',(57.1623216544371,-25.6588335304441,
39.92499));
#198695=CARTESIAN_POINT('Origin',(57.4068835917979,-25.5758735661209,40.22725));
#198696=CARTESIAN_POINT('Origin',(-0.129138884176561,-0.290050682801526,
39.116));
#198697=CARTESIAN_POINT('Origin',(54.6869600343297,-24.6957503380308,39.116));
#198698=CARTESIAN_POINT('Origin',(5.51404277916147E-15,5.76195122378986E-15,
40.22725));
#198699=CARTESIAN_POINT('Origin',(57.4192809246789,-25.5480287005719,40.22725));
#198700=CARTESIAN_POINT('Ctrl Pts',(54.6869600343297,-24.6957503380308,
38.989));
#198701=CARTESIAN_POINT('Ctrl Pts',(54.7386929703524,-24.5795562613018,
38.989));
#198702=CARTESIAN_POINT('Ctrl Pts',(54.738615530126,-24.5797301948982,39.1161901092324));
#198703=CARTESIAN_POINT('Ctrl Pts',(54.4888352915926,-24.6072881749603,
38.989));
#198704=CARTESIAN_POINT('Ctrl Pts',(54.5406489234191,-24.4913819335269,
38.9892298989766));
#198705=CARTESIAN_POINT('Ctrl Pts',(54.5800991622563,-24.5091541605502,
39.1161900493204));
#198706=CARTESIAN_POINT('Ctrl Pts',(54.3002245846702,-24.5230714236766,
39.1034966344368));
#198707=CARTESIAN_POINT('Ctrl Pts',(54.3520673354864,-24.4074205468509,
39.1038314102554));
#198708=CARTESIAN_POINT('Ctrl Pts',(54.4291945615848,-24.4419671033155,
39.2077528789597));
#198709=CARTESIAN_POINT('Ctrl Pts',(54.1952354911872,-24.4761921430393,
39.2875012672119));
#198710=CARTESIAN_POINT('Ctrl Pts',(54.2471777873472,-24.3607210114364,
39.2878045257868));
#198711=CARTESIAN_POINT('Ctrl Pts',(54.3451938439593,-24.4045675740909,
39.35490152959));
#198712=CARTESIAN_POINT('Origin',(54.2933913980363,-24.5205222915152,39.3548010137695));
#198713=CARTESIAN_POINT('Ctrl Pts',(57.467555354514,-25.2380597013431,39.8576902534424));
#198714=CARTESIAN_POINT('Ctrl Pts',(57.4161024530843,-25.3547675996716,
39.8573998014387));
#198715=CARTESIAN_POINT('Ctrl Pts',(57.317288315449,-25.3107727110823,39.92499));
#198716=CARTESIAN_POINT('Ctrl Pts',(57.5091180232691,-25.256565127891,39.9304984902491));
#198717=CARTESIAN_POINT('Ctrl Pts',(57.4495672328902,-25.3528749970549,
39.9052171569785));
#198718=CARTESIAN_POINT('Ctrl Pts',(57.3588496371383,-25.3292770036978,
39.9672049726604));
#198719=CARTESIAN_POINT('Ctrl Pts',(57.540547177061,-25.2997972770056,40.0043437678662));
#198720=CARTESIAN_POINT('Ctrl Pts',(57.4827148996401,-25.372015972086,39.9661628577643));
#198721=CARTESIAN_POINT('Ctrl Pts',(57.3948558336735,-25.3622324578621,
40.0100243556233));
#198722=CARTESIAN_POINT('Ctrl Pts',(57.5636463159493,-25.4257977880273,
40.1194874821987));
#198723=CARTESIAN_POINT('Ctrl Pts',(57.5124644611998,-25.4538910783597,
40.062755148314));
#198724=CARTESIAN_POINT('Ctrl Pts',(57.4360631077221,-25.4475597357237,
40.0767884282379));
#198725=CARTESIAN_POINT('Ctrl Pts',(57.5536211289093,-25.5110385513885,
40.159950201539));
#198726=CARTESIAN_POINT('Ctrl Pts',(57.5097883065949,-25.5177778164711,
40.1002449453884));
#198727=CARTESIAN_POINT('Ctrl Pts',(57.4400754463057,-25.5012707422382,
40.10025));
#198728=CARTESIAN_POINT('Ctrl Pts',(57.5176823163888,-25.5918112338795,
40.1599502534424));
#198729=CARTESIAN_POINT('Ctrl Pts',(57.4835989537477,-25.5766462455177,
40.10025));
#198730=CARTESIAN_POINT('Ctrl Pts',(57.4192809246789,-25.5480287005719,
40.10025));
#198731=CARTESIAN_POINT('Origin',(57.3689438691196,-25.1947524379617,39.92499));
#198732=CARTESIAN_POINT('Origin',(54.1306438627446,-24.4480624203072,39.6398955069309));
#198733=CARTESIAN_POINT('Origin',(53.9678963272934,-24.375602549094,39.92499));
#198734=CARTESIAN_POINT('Origin',(57.2061965577021,-25.1222926664875,39.639895506828));
#198735=CARTESIAN_POINT('Origin',(57.0434492461379,-25.0498328948966,39.3548010137695));
#198736=CARTESIAN_POINT('Ctrl Pts',(53.8697418420145,-24.3312692531089,
39.8576902534424));
#198737=CARTESIAN_POINT('Ctrl Pts',(53.9216078643417,-24.2159747902187,
39.8579948730703));
#198738=CARTESIAN_POINT('Ctrl Pts',(54.0195518809641,-24.2595822759734,
39.92499));
#198739=CARTESIAN_POINT('Ctrl Pts',(53.8282341734846,-24.3127882662175,
39.9304020711228));
#198740=CARTESIAN_POINT('Ctrl Pts',(53.88801149737,-24.2176496934284,39.905891529739));
#198741=CARTESIAN_POINT('Ctrl Pts',(53.9780422761236,-24.2411010091825,
39.9671523786032));
#198742=CARTESIAN_POINT('Ctrl Pts',(53.7969955864427,-24.2697746459838,
40.0043257306697));
#198743=CARTESIAN_POINT('Ctrl Pts',(53.8549480733038,-24.1983152114488,
39.9667894847838));
#198744=CARTESIAN_POINT('Ctrl Pts',(53.9422730280819,-24.2082687574721,
40.0100138975202));
#198745=CARTESIAN_POINT('Ctrl Pts',(53.7744913425366,-24.1443388226042,
40.1195533054853));
#198746=CARTESIAN_POINT('Ctrl Pts',(53.8256450222193,-24.1165167429224,
40.0630813209234));
#198747=CARTESIAN_POINT('Ctrl Pts',(53.9017956184508,-24.1232032230476,
40.0768265942419));
#198748=CARTESIAN_POINT('Ctrl Pts',(53.7848917482049,-24.0595120258532,
40.1599502027519));
#198749=CARTESIAN_POINT('Ctrl Pts',(53.828668515863,-24.052912216684,40.1002552791553));
#198750=CARTESIAN_POINT('Ctrl Pts',(53.8982652496115,-24.0696665464379,
40.10025));
#198751=CARTESIAN_POINT('Ctrl Pts',(53.8206887816836,-23.9791663275014,
40.1599502534424));
#198752=CARTESIAN_POINT('Ctrl Pts',(53.8547645473081,-23.9943483786818,
40.10025));
#198753=CARTESIAN_POINT('Ctrl Pts',(53.9190682401995,-24.0229981225297,
40.10025));
#198754=CARTESIAN_POINT('Origin',(53.9190682401995,-24.0229981225297,40.22725));
#198755=CARTESIAN_POINT('Ctrl Pts',(56.6498810128382,-24.8746050278053,
38.989));
#198756=CARTESIAN_POINT('Ctrl Pts',(56.5981482837089,-24.9907986398441,
38.989));
#198757=CARTESIAN_POINT('Ctrl Pts',(56.5982255167331,-24.9906251716316,
39.1161896013266));
#198758=CARTESIAN_POINT('Ctrl Pts',(56.8481896769747,-24.9626539694743,
38.989));
#198759=CARTESIAN_POINT('Ctrl Pts',(56.7965362315769,-25.0791271905737,
38.9887769275436));
#198760=CARTESIAN_POINT('Ctrl Pts',(56.756741544355,-25.0612010539386,39.1161898821824));
#198761=CARTESIAN_POINT('Ctrl Pts',(57.0369754593327,-25.0464771582524,
39.1034967087243));
#198762=CARTESIAN_POINT('Ctrl Pts',(56.9853490357212,-25.1631925873307,
39.1031720232733));
#198763=CARTESIAN_POINT('Ctrl Pts',(56.9076460727631,-25.1283880784731,
39.207752961502));
#198764=CARTESIAN_POINT('Ctrl Pts',(57.1420619865021,-25.0931373005746,
39.2875012672119));
#198765=CARTESIAN_POINT('Ctrl Pts',(57.0905332166521,-25.2100238867499,
39.2872087095507));
#198766=CARTESIAN_POINT('Ctrl Pts',(56.9916465440542,-25.1657874977295,
39.3549017048227));
#198767=CARTESIAN_POINT('Origin',(56.6498810128382,-24.8746050278053,39.116));
#198768=CARTESIAN_POINT('Origin',(5.71826297912856E-15,5.2288498427347E-15,
40.22725));
#198769=CARTESIAN_POINT('Origin',(53.9314655730804,-23.9951532569808,40.22725));
#198770=CARTESIAN_POINT('Origin',(52.0578415156894,-22.8300973196049,39.116));
#198771=CARTESIAN_POINT('Origin',(56.2832472948507,-24.7113125977907,39.1160373285278));
#198772=CARTESIAN_POINT('Ctrl Pts',(53.8330634946837,-23.9513722670365,
40.1599502534424));
#198773=CARTESIAN_POINT('Ctrl Pts',(53.867147095173,-23.9665367208225,40.10025));
#198774=CARTESIAN_POINT('Ctrl Pts',(53.9314655730804,-23.9951532569808,
40.10025));
#198775=CARTESIAN_POINT('Ctrl Pts',(53.8686972660496,-23.8712821658118,
40.1599500566043));
#198776=CARTESIAN_POINT('Ctrl Pts',(53.8931046959182,-23.9081865738548,
40.1002551305372));
#198777=CARTESIAN_POINT('Ctrl Pts',(53.9521563342717,-23.9486256024593,
40.10025));
#198778=CARTESIAN_POINT('Ctrl Pts',(53.9240892607411,-23.8071866393154,
40.1203070619045));
#198779=CARTESIAN_POINT('Ctrl Pts',(53.93785095296,-23.8635355386145,40.0637098684499));
#198780=CARTESIAN_POINT('Ctrl Pts',(53.9937257232527,-23.9155750846179,
40.0772636213363));
#198781=CARTESIAN_POINT('Ctrl Pts',(54.0330064121713,-23.739249756057,40.0046102245803));
#198782=CARTESIAN_POINT('Ctrl Pts',(54.018751292376,-23.8300830854575,39.9670001894012));
#198783=CARTESIAN_POINT('Ctrl Pts',(54.0845104630313,-23.8883623535216,
40.0101788811209));
#198784=CARTESIAN_POINT('Ctrl Pts',(54.0860594545423,-23.7337507958619,
39.9303710930185));
#198785=CARTESIAN_POINT('Ctrl Pts',(54.055350029128,-23.8418399747435,39.9058663574109));
#198786=CARTESIAN_POINT('Ctrl Pts',(54.1330265677739,-23.8930480394867,
39.9671344706363));
#198787=CARTESIAN_POINT('Ctrl Pts',(54.1275498658873,-23.7522229508828,
39.8576902534424));
#198788=CARTESIAN_POINT('Ctrl Pts',(54.0765745253536,-23.8679139708569,
39.8579948730703));
#198789=CARTESIAN_POINT('Ctrl Pts',(54.1745185419759,-23.9115214566115,
39.92499));
#198790=CARTESIAN_POINT('Origin',(54.2261740956466,-23.7955011834909,39.92499));
#198791=CARTESIAN_POINT('Origin',(56.2428239368584,-24.6933715410261,39.1925554488854));
#198792=CARTESIAN_POINT('Origin',(56.1680608984278,-24.6600848917112,39.3343017080178));
#198793=CARTESIAN_POINT('Origin',(54.3889216310581,-23.8679610547541,39.639895506921));
#198794=CARTESIAN_POINT('Origin',(54.5516691663895,-23.9404209259122,39.3548010137695));
#198795=CARTESIAN_POINT('Ctrl Pts',(55.8666273273833,-24.5258780191672,
39.3978017080178));
#198796=CARTESIAN_POINT('Ctrl Pts',(55.8149717737126,-24.6418982922878,
39.3978017080178));
#198797=CARTESIAN_POINT('Ctrl Pts',(55.8149717737126,-24.6418982922878,
39.5248017080178));
#198798=CARTESIAN_POINT('Ctrl Pts',(55.9487607347573,-24.5627025231285,
39.3978017080178));
#198799=CARTESIAN_POINT('Ctrl Pts',(55.8971232158787,-24.6784744708791,
39.3980355775201));
#198800=CARTESIAN_POINT('Ctrl Pts',(55.9383132588166,-24.6968134595446,
39.5248015517192));
#198801=CARTESIAN_POINT('Ctrl Pts',(56.0264248009279,-24.5975211960716,
39.3484893995498));
#198802=CARTESIAN_POINT('Ctrl Pts',(55.9751910510459,-24.7132325104956,
39.3489438303403));
#198803=CARTESIAN_POINT('Ctrl Pts',(56.0549414076394,-24.748739656915,39.4508333155588));
#198804=CARTESIAN_POINT('Ctrl Pts',(56.0673542004326,-24.6158705164594,
39.2708017080178));
#198805=CARTESIAN_POINT('Ctrl Pts',(56.0163785451197,-24.7315703643336,
39.2710850691866));
#198806=CARTESIAN_POINT('Ctrl Pts',(56.1164053447572,-24.7761051648318,
39.3343017080178));
#198807=CARTESIAN_POINT('Origin',(55.8666273273833,-24.5258780191672,39.5248017080178));
#198808=CARTESIAN_POINT('Ctrl Pts',(54.4530463244692,-23.8971395307769,
39.2875012672119));
#198809=CARTESIAN_POINT('Ctrl Pts',(54.4019907365351,-24.0130054343463,
39.2878045257519));
#198810=CARTESIAN_POINT('Ctrl Pts',(54.5001606088505,-24.0565064908993,
39.3549015218348));
#198811=CARTESIAN_POINT('Ctrl Pts',(54.5581374230424,-23.9437939758158,
39.1034938540228));
#198812=CARTESIAN_POINT('Ctrl Pts',(54.5068816478264,-24.0597061770704,
39.1038286278777));
#198813=CARTESIAN_POINT('Ctrl Pts',(54.5841625982698,-24.0939065860605,
39.207750643403));
#198814=CARTESIAN_POINT('Ctrl Pts',(54.7469293531951,-24.02760770261,38.989));
#198815=CARTESIAN_POINT('Ctrl Pts',(54.6954643138426,-24.1436691352852,
38.9892298954653));
#198816=CARTESIAN_POINT('Ctrl Pts',(54.7350683949955,-24.1610941752714,
39.116190034729));
#198817=CARTESIAN_POINT('Ctrl Pts',(54.9452378026828,-24.1156489724277,
38.989));
#198818=CARTESIAN_POINT('Ctrl Pts',(54.893504872635,-24.231843035737,38.989));
#198819=CARTESIAN_POINT('Ctrl Pts',(54.8935823068776,-24.2316691155805,
39.1161900945647));
#198820=CARTESIAN_POINT('Origin',(54.9452378026828,-24.1156489724277,39.116));
#198821=CARTESIAN_POINT('Origin',(50.7999799080414,-22.2700612497317,39.5248017080178));
#198822=CARTESIAN_POINT('Origin',(55.7284918401498,-24.4643761377918,39.5248017080178));
#198823=CARTESIAN_POINT('Origin',(50.6030043228557,-22.1823620689016,39.116));
#198824=CARTESIAN_POINT('Origin',(55.3119205422644,-24.2788510342443,39.116040271385));
#198825=CARTESIAN_POINT('Ctrl Pts',(55.5277679687683,-24.3743766270215,
39.2708017080178));
#198826=CARTESIAN_POINT('Ctrl Pts',(55.4763362579874,-24.4911280468227,
39.27051194648));
#198827=CARTESIAN_POINT('Ctrl Pts',(55.3754026508175,-24.4461895095989,
39.3343017080178));
#198828=CARTESIAN_POINT('Ctrl Pts',(55.5688345658079,-24.3927905570397,
39.3487519301186));
#198829=CARTESIAN_POINT('Ctrl Pts',(55.5172331055236,-24.5093364964848,
39.3482879463991));
#198830=CARTESIAN_POINT('Ctrl Pts',(55.4370743056947,-24.4736474994207,
39.4512271261635));
#198831=CARTESIAN_POINT('Ctrl Pts',(55.6466353090197,-24.4276751358079,
39.3978017080178));
#198832=CARTESIAN_POINT('Ctrl Pts',(55.5948055748743,-24.5438739850305,
39.3975673827378));
#198833=CARTESIAN_POINT('Ctrl Pts',(55.5539102504896,-24.5256662135185,
39.524801535518));
#198834=CARTESIAN_POINT('Ctrl Pts',(55.7284918401498,-24.4643761377918,
39.3978017080178));
#198835=CARTESIAN_POINT('Ctrl Pts',(55.6768362864792,-24.5803964109124,
39.3978017080178));
#198836=CARTESIAN_POINT('Ctrl Pts',(55.6768362864792,-24.5803964109124,
39.5248017080178));
#198837=CARTESIAN_POINT('Origin',(55.4270582044881,-24.3301692364783,39.3343017080178));
#198838=CARTESIAN_POINT('Origin',(55.3527410377822,-24.2970811017181,39.1934008533554));
#198839=CARTESIAN_POINT('Origin',(53.0360596835511,-30.9870007556522,39.1925554495084));
#198840=CARTESIAN_POINT('Origin',(53.0743345559682,-31.0091584503702,39.1160373285271));
#198841=CARTESIAN_POINT('Origin',(52.9651856060845,-30.9460815882869,39.3343017080178));
#198842=CARTESIAN_POINT('Ctrl Pts',(52.8702215132216,-30.8905967158737,
39.2708017080178));
#198843=CARTESIAN_POINT('Ctrl Pts',(52.9338619179795,-30.7813498801533,
39.2710850691866));
#198844=CARTESIAN_POINT('Ctrl Pts',(53.0286856060846,-30.8360963620063,
39.3343017080178));
#198845=CARTESIAN_POINT('Ctrl Pts',(52.8311874403366,-30.8681941459771,
39.3487519293518));
#198846=CARTESIAN_POINT('Ctrl Pts',(52.8946849835388,-30.7587310665065,
39.3492068662923));
#198847=CARTESIAN_POINT('Ctrl Pts',(52.9702219582398,-30.8023423591853,
39.4512271248733));
#198848=CARTESIAN_POINT('Ctrl Pts',(52.7572372522455,-30.8257530395517,
39.3978017080178));
#198849=CARTESIAN_POINT('Ctrl Pts',(52.8205474253444,-30.7159277273278,
39.3980347781178));
#198850=CARTESIAN_POINT('Ctrl Pts',(52.8594635164578,-30.7383959430075,
39.5248015355195));
#198851=CARTESIAN_POINT('Ctrl Pts',(52.6794317578287,-30.7811015270744,
39.3978017080178));
#198852=CARTESIAN_POINT('Ctrl Pts',(52.7429317578287,-30.6711163007938,
39.3978017080178));
#198853=CARTESIAN_POINT('Ctrl Pts',(52.7429317578287,-30.6711163007938,
39.5248017080178));
#198854=CARTESIAN_POINT('Origin',(52.6794317578287,-30.7811015270744,39.5248017080178));
#198855=CARTESIAN_POINT('Origin',(-0.158749999999995,-0.274963065701559,
39.116));
#198856=CARTESIAN_POINT('Origin',(53.4219427993286,-31.2097904767607,39.116));
#198857=CARTESIAN_POINT('Origin',(-0.158749999999995,-0.274963065701559,
39.5248017080178));
#198858=CARTESIAN_POINT('Origin',(52.5484816883959,-30.705497469237,39.5248017080178));
#198859=CARTESIAN_POINT('Ctrl Pts',(53.888035839597,-31.479523201679,39.2875012672119));
#198860=CARTESIAN_POINT('Ctrl Pts',(53.9523112176912,-31.3691313491576,
39.287208709576));
#198861=CARTESIAN_POINT('Ctrl Pts',(53.8583991130131,-31.3151318426936,
39.3549016990122));
#198862=CARTESIAN_POINT('Ctrl Pts',(53.7885171709483,-31.4219316852008,
39.1034939173931));
#198863=CARTESIAN_POINT('Ctrl Pts',(53.8525966788904,-31.3115614337832,
39.1031692336328));
#198864=CARTESIAN_POINT('Ctrl Pts',(53.7787668993595,-31.2691561625549,
39.2077507202297));
#198865=CARTESIAN_POINT('Ctrl Pts',(53.6097358757348,-31.3184699958138,
38.989));
#198866=CARTESIAN_POINT('Ctrl Pts',(53.673603543663,-31.2082202476927,38.98877693112));
#198867=CARTESIAN_POINT('Ctrl Pts',(53.6357108652107,-31.1865627224601,
39.1161898712915));
#198868=CARTESIAN_POINT('Ctrl Pts',(53.4219427993286,-31.2097904767607,
38.989));
#198869=CARTESIAN_POINT('Ctrl Pts',(53.485537665384,-31.0996409376522,38.989));
#198870=CARTESIAN_POINT('Ctrl Pts',(53.4854427285717,-31.0998053730347,
39.1161895903854));
#198871=CARTESIAN_POINT('Origin',(53.7950387249979,-31.4251975098794,39.3548010137695));
#198872=CARTESIAN_POINT('Ctrl Pts',(52.5484816883959,-30.705497469237,39.3978017080178));
#198873=CARTESIAN_POINT('Ctrl Pts',(52.6119816883959,-30.5955122429563,
39.3978017080178));
#198874=CARTESIAN_POINT('Ctrl Pts',(52.6119816883959,-30.5955122429563,
39.5248017080178));
#198875=CARTESIAN_POINT('Ctrl Pts',(52.4704129317475,-30.6606955449584,
39.3978017080178));
#198876=CARTESIAN_POINT('Ctrl Pts',(52.5339553345207,-30.5504637065424,
39.3975666025026));
#198877=CARTESIAN_POINT('Ctrl Pts',(52.495056068421,-30.5280052047887,39.5248015517177));
#198878=CARTESIAN_POINT('Ctrl Pts',(52.3965920780923,-30.6183335281988,
39.3484894016716));
#198879=CARTESIAN_POINT('Ctrl Pts',(52.4605500011273,-30.5080831175497,
39.3480259000042));
#198880=CARTESIAN_POINT('Ctrl Pts',(52.3844945583579,-30.4641724871917,
39.4508333188945));
#198881=CARTESIAN_POINT('Ctrl Pts',(52.3576880233162,-30.5960088312569,
39.2708017080178));
#198882=CARTESIAN_POINT('Ctrl Pts',(52.4219111049556,-30.4857749404421,
39.27051194648));
#198883=CARTESIAN_POINT('Ctrl Pts',(52.3262277788841,-30.4305321463777,
39.3343017080178));
#198884=CARTESIAN_POINT('Origin',(52.2627277788841,-30.5405173726584,39.3343017080178));
#198885=CARTESIAN_POINT('Origin',(53.9493203812237,-31.5142720656047,39.6398955068192));
#198886=CARTESIAN_POINT('Origin',(54.1036020372438,-31.6033466212666,39.92499));
#198887=CARTESIAN_POINT('Origin',(52.1922763801647,-30.4998422386361,39.1934008539946));
#198888=CARTESIAN_POINT('Origin',(52.1535342613175,-30.4775331296741,39.1160402713851));
#198889=CARTESIAN_POINT('Ctrl Pts',(54.5122556166611,-31.4902932482909,
40.1599502534424));
#198890=CARTESIAN_POINT('Ctrl Pts',(54.4799531854479,-31.471632985199,40.10025));
#198891=CARTESIAN_POINT('Ctrl Pts',(54.4189959163063,-31.4364195775136,
40.10025));
#198892=CARTESIAN_POINT('Ctrl Pts',(54.4681793099457,-31.5665926662617,
40.1599500538463));
#198893=CARTESIAN_POINT('Ctrl Pts',(54.4478446647267,-31.5272089901453,
40.1002448353502));
#198894=CARTESIAN_POINT('Ctrl Pts',(54.3934750329626,-31.4805801312538,
40.10025));
#198895=CARTESIAN_POINT('Ctrl Pts',(54.4058464214488,-31.624484310427,40.120244200104));
#198896=CARTESIAN_POINT('Ctrl Pts',(54.3982481205269,-31.5668246399991,
40.0633873868021));
#198897=CARTESIAN_POINT('Ctrl Pts',(54.3482630350907,-31.5088182930358,
40.0772271723539));
#198898=CARTESIAN_POINT('Ctrl Pts',(54.2895863184075,-31.68051887617,40.0045995998161));
#198899=CARTESIAN_POINT('Ctrl Pts',(54.3139476428155,-31.5913182835559,
39.9663485808311));
#198900=CARTESIAN_POINT('Ctrl Pts',(54.2544636505348,-31.5259511417534,
40.0101727202464));
#198901=CARTESIAN_POINT('Ctrl Pts',(54.2359839591653,-31.6804069909876,
39.930465434986));
#198902=CARTESIAN_POINT('Ctrl Pts',(54.2789047974524,-31.5756141966193,
39.9051900162949));
#198903=CARTESIAN_POINT('Ctrl Pts',(54.2064835118365,-31.5160982999431,
39.9671857458177));
#198904=CARTESIAN_POINT('Ctrl Pts',(54.1966007261207,-31.6576696180585,
39.8576902534424));
#198905=CARTESIAN_POINT('Ctrl Pts',(54.2607761425982,-31.5474441649284,
39.8573998014387));
#198906=CARTESIAN_POINT('Ctrl Pts',(54.1671020372438,-31.493361394986,39.92499));
#198907=CARTESIAN_POINT('Origin',(54.4189959163063,-31.4364195775136,40.22725));
#198908=CARTESIAN_POINT('Origin',(-0.158749999999995,-0.274963065701559,
39.116));
#198909=CARTESIAN_POINT('Origin',(51.8059703131946,-30.2768083268881,39.116));
#198910=CARTESIAN_POINT('Origin',(5.52187834149254E-15,5.77732938073734E-15,
40.22725));
#198911=CARTESIAN_POINT('Origin',(54.4342359163063,-31.4100231232062,40.22725));
#198912=CARTESIAN_POINT('Ctrl Pts',(51.8059703131946,-30.2768083268881,
38.989));
#198913=CARTESIAN_POINT('Ctrl Pts',(51.8695654390622,-30.1666583377718,
38.989));
#198914=CARTESIAN_POINT('Ctrl Pts',(51.8694702420498,-30.1668232238339,
39.1161901092325));
#198915=CARTESIAN_POINT('Ctrl Pts',(51.6181777324916,-30.1681210939088,
38.989));
#198916=CARTESIAN_POINT('Ctrl Pts',(51.6818230251202,-30.0582657983057,
38.989229898976));
#198917=CARTESIAN_POINT('Ctrl Pts',(51.7191994478434,-30.0800643400506,
39.1161900493205));
#198918=CARTESIAN_POINT('Ctrl Pts',(51.4394033023489,-30.0646505034511,
39.1034966344368));
#198919=CARTESIAN_POINT('Ctrl Pts',(51.5030508615836,-29.9550522173033,
39.1038314102562));
#198920=CARTESIAN_POINT('Ctrl Pts',(51.5761444782074,-29.9974715145367,
39.2077528789596));
#198921=CARTESIAN_POINT('Ctrl Pts',(51.3398895692697,-30.0070536838159,
39.2875012672119));
#198922=CARTESIAN_POINT('Ctrl Pts',(51.4036173400347,-29.89764456355,39.2878045257868));
#198923=CARTESIAN_POINT('Ctrl Pts',(51.4965132406194,-29.9514963979198,
39.3549015295901));
#198924=CARTESIAN_POINT('Origin',(51.4328740054943,-30.0614010732037,39.3548010137695));
#198925=CARTESIAN_POINT('Ctrl Pts',(54.5146464769138,-31.1067982185536,
39.8576902534424));
#198926=CARTESIAN_POINT('Ctrl Pts',(54.4512761425982,-31.2174884860866,
39.8573998014387));
#198927=CARTESIAN_POINT('Ctrl Pts',(54.3576020372438,-31.1634057161441,
39.92499));
#198928=CARTESIAN_POINT('Ctrl Pts',(54.5540471172213,-31.1295467523332,
39.930498490249));
#198929=CARTESIAN_POINT('Ctrl Pts',(54.4847554296804,-31.2191042733502,
39.9052171569796));
#198930=CARTESIAN_POINT('Ctrl Pts',(54.3970014563933,-31.186152981396,39.9672049726602));
#198931=CARTESIAN_POINT('Ctrl Pts',(54.5807851087098,-31.1758273123588,
40.0043437678663));
#198932=CARTESIAN_POINT('Ctrl Pts',(54.5157207333391,-31.2416052667848,
39.9661628577649));
#198933=CARTESIAN_POINT('Ctrl Pts',(54.4293656242365,-31.2226915745263,
40.0100243556234));
#198934=CARTESIAN_POINT('Ctrl Pts',(54.5905870683102,-31.3035520968883,
40.1194874821986));
#198935=CARTESIAN_POINT('Ctrl Pts',(54.5367490446502,-31.3261415286131,
40.0627551483135));
#198936=CARTESIAN_POINT('Ctrl Pts',(54.4614280312964,-31.3118587536634,
40.0767884282378));
#198937=CARTESIAN_POINT('Ctrl Pts',(54.5717067142913,-31.3872779850332,
40.1599502015378));
#198938=CARTESIAN_POINT('Ctrl Pts',(54.5274095677394,-31.3893985541585,
40.1002449453863));
#198939=CARTESIAN_POINT('Ctrl Pts',(54.4598040608964,-31.3656949292499,
40.10025));
#198940=CARTESIAN_POINT('Ctrl Pts',(54.5275217339719,-31.4638515574741,
40.1599502534424));
#198941=CARTESIAN_POINT('Ctrl Pts',(54.4952102564865,-31.4452069629854,
40.10025));
#198942=CARTESIAN_POINT('Ctrl Pts',(54.4342359163063,-31.4100231232062,
40.10025));
#198943=CARTESIAN_POINT('Origin',(54.4211020372438,-31.0534204898635,39.92499));
#198944=CARTESIAN_POINT('Origin',(51.2785921372171,-29.9723263949888,39.6398955069324));
#198945=CARTESIAN_POINT('Origin',(51.1243102687785,-29.8832517167487,39.92499));
#198946=CARTESIAN_POINT('Origin',(54.2668203811903,-30.9643459342374,39.6398955068261));
#198947=CARTESIAN_POINT('Origin',(54.1125387249979,-30.8752713784762,39.3548010137695));
#198948=CARTESIAN_POINT('Ctrl Pts',(51.0313275753408,-29.8289013456886,
39.8576902534424));
#198949=CARTESIAN_POINT('Ctrl Pts',(51.0949610232001,-29.7196599535393,
39.8579948730703));
#198950=CARTESIAN_POINT('Ctrl Pts',(51.1878102687784,-29.7732664904681,
39.92499));
#198951=CARTESIAN_POINT('Ctrl Pts',(50.9919790793208,-29.8061828667725,
39.9304020711234));
#198952=CARTESIAN_POINT('Ctrl Pts',(51.0613736255819,-29.7178139048433,
39.9058915297385));
#198953=CARTESIAN_POINT('Ctrl Pts',(51.1484598763128,-29.7505475307853,
39.9671523786031));
#198954=CARTESIAN_POINT('Ctrl Pts',(50.9654077681509,-29.7601395581528,
40.0043257306689));
#198955=CARTESIAN_POINT('Ctrl Pts',(51.0305123301031,-29.695129270271,39.9667894847832));
#198956=CARTESIAN_POINT('Ctrl Pts',(51.1163184807719,-29.7141562330558,
40.0100138975197));
#198957=CARTESIAN_POINT('Ctrl Pts',(50.9561384187037,-29.6330385513047,
40.1195533054861));
#198958=CARTESIAN_POINT('Ctrl Pts',(51.009920072411,-29.6107158994144,40.0630813209239));
#198959=CARTESIAN_POINT('Ctrl Pts',(51.0849545802166,-29.6253256551027,
40.0768265942423));
#198960=CARTESIAN_POINT('Ctrl Pts',(50.9753486645701,-29.5497635830446,
40.1599502027516));
#198961=CARTESIAN_POINT('Ctrl Pts',(51.0195754864255,-29.5477758465709,
40.1002552791557));
#198962=CARTESIAN_POINT('Ctrl Pts',(51.087039657642,-29.5717132339806,40.10025));
#198963=CARTESIAN_POINT('Ctrl Pts',(51.0193480105327,-29.4735998357338,
40.1599502534424));
#198964=CARTESIAN_POINT('Ctrl Pts',(51.0516501490686,-29.4922606054647,
40.10025));
#198965=CARTESIAN_POINT('Ctrl Pts',(51.1126068659047,-29.5274749692186,
40.10025));
#198966=CARTESIAN_POINT('Origin',(51.1126068659047,-29.5274749692186,40.22725));
#198967=CARTESIAN_POINT('Ctrl Pts',(53.7394427993286,-30.6598643453575,
38.989));
#198968=CARTESIAN_POINT('Ctrl Pts',(53.6758479277944,-30.7700138939557,
38.989));
#198969=CARTESIAN_POINT('Ctrl Pts',(53.6759428700937,-30.7698494490694,
39.1161896013268));
#198970=CARTESIAN_POINT('Ctrl Pts',(53.9274614872889,-30.7681598456259,
38.989));
#198971=CARTESIAN_POINT('Ctrl Pts',(53.8639162380529,-30.8785957589612,
38.9887769275478));
#198972=CARTESIAN_POINT('Ctrl Pts',(53.8262133418071,-30.856608146078,39.116189882185));
#198973=CARTESIAN_POINT('Ctrl Pts',(54.1064511722697,-30.8712573299205,
39.1034967087243));
#198974=CARTESIAN_POINT('Ctrl Pts',(54.0429074791709,-30.9819369489461,
39.1031720232688));
#198975=CARTESIAN_POINT('Ctrl Pts',(53.9692682429978,-30.9392009315196,
39.2077529614995));
#198976=CARTESIAN_POINT('Ctrl Pts',(54.2060847114741,-30.9286463962979,
39.2875012672119));
#198977=CARTESIAN_POINT('Ctrl Pts',(54.1426202463873,-31.0395064423977,
39.2872087095507));
#198978=CARTESIAN_POINT('Ctrl Pts',(54.0488992470933,-30.9851759130203,
39.3549017048228));
#198979=CARTESIAN_POINT('Origin',(53.7394427993286,-30.6598643453575,39.116));
#198980=CARTESIAN_POINT('Origin',(5.71547558359784E-15,5.22337927098311E-15,
40.22725));
#198981=CARTESIAN_POINT('Origin',(51.1278468659047,-29.5010785149112,40.22725));
#198982=CARTESIAN_POINT('Origin',(46.8255917980722,-26.6681506086452,39.116));
#198983=CARTESIAN_POINT('Origin',(53.3918862459806,-30.4591427892376,39.1160373285258));
#198984=CARTESIAN_POINT('Ctrl Pts',(51.0345602039887,-29.4472515437736,
40.1599502534424));
#198985=CARTESIAN_POINT('Ctrl Pts',(51.0668719738977,-29.4658956314768,
40.10025));
#198986=CARTESIAN_POINT('Ctrl Pts',(51.1278468659047,-29.5010785149112,
40.10025));
#198987=CARTESIAN_POINT('Ctrl Pts',(51.0783704650306,-29.3713249278649,
40.159950056604));
#198988=CARTESIAN_POINT('Ctrl Pts',(51.0987866273847,-29.4105784408364,
40.1002551305372));
#198989=CARTESIAN_POINT('Ctrl Pts',(51.1532877451689,-29.4569685172212,
40.10025));
#198990=CARTESIAN_POINT('Ctrl Pts',(51.1401588234665,-29.313370563451,40.1203070619045));
#198991=CARTESIAN_POINT('Ctrl Pts',(51.1479550638452,-29.3708492661234,
40.0637098684496));
#198992=CARTESIAN_POINT('Ctrl Pts',(51.1980841325266,-29.4284442379231,
40.0772636213363));
#198993=CARTESIAN_POINT('Ctrl Pts',(51.2555806533509,-29.2571907880104,
40.0046102245803));
#198994=CARTESIAN_POINT('Ctrl Pts',(51.2319089562572,-29.3460364571626,
39.9670001894015));
#198995=CARTESIAN_POINT('Ctrl Pts',(51.2912160489646,-29.4108701703525,
40.0101788811209));
#198996=CARTESIAN_POINT('Ctrl Pts',(51.3089178634638,-29.2572675046848,
39.9303710930185));
#198997=CARTESIAN_POINT('Ctrl Pts',(51.2670782717319,-29.3615545506881,
39.9058663574108));
#198998=CARTESIAN_POINT('Ctrl Pts',(51.3389765898564,-29.4206015015123,
39.967134470637));
#198999=CARTESIAN_POINT('Ctrl Pts',(51.3482501200165,-29.2799753962463,
39.8576902534424));
#199000=CARTESIAN_POINT('Ctrl Pts',(51.2854610232001,-29.3897042746975,
39.8579948730703));
#199001=CARTESIAN_POINT('Ctrl Pts',(51.3783102687785,-29.4433108116262,
39.92499));
#199002=CARTESIAN_POINT('Origin',(51.4418102687785,-29.3333255853456,39.92499));
#199003=CARTESIAN_POINT('Origin',(53.3535596824668,-30.4370746239674,39.1925554488849));
#199004=CARTESIAN_POINT('Origin',(53.2826856060845,-30.3961554568838,39.3343017080178));
#199005=CARTESIAN_POINT('Origin',(51.5960921371721,-29.4224002636276,39.6398955069211));
#199006=CARTESIAN_POINT('Origin',(51.7503740054943,-29.5114749418006,39.3548010137695));
#199007=CARTESIAN_POINT('Ctrl Pts',(52.9969317578287,-30.2311753956713,
39.3978017080178));
#199008=CARTESIAN_POINT('Ctrl Pts',(52.9334317578287,-30.3411606219519,
39.3978017080178));
#199009=CARTESIAN_POINT('Ctrl Pts',(52.9334317578287,-30.3411606219519,
39.5248017080178));
#199010=CARTESIAN_POINT('Ctrl Pts',(53.0747660209943,-30.2763834500017,
39.3978017080178));
#199011=CARTESIAN_POINT('Ctrl Pts',(53.01130991406,-30.3861235964155,39.3980355775177));
#199012=CARTESIAN_POINT('Ctrl Pts',(53.0503573673287,-30.4086676540719,
39.5248015517192));
#199013=CARTESIAN_POINT('Ctrl Pts',(53.1483650929077,-30.3191294881007,
39.3484893995498));
#199014=CARTESIAN_POINT('Ctrl Pts',(53.0853168809867,-30.4288515386937,
39.3489438303415));
#199015=CARTESIAN_POINT('Ctrl Pts',(53.1609188493341,-30.4725003554697,
39.4508333155587));
#199016=CARTESIAN_POINT('Ctrl Pts',(53.1871522506175,-30.3416565762237,
39.2708017080178));
#199017=CARTESIAN_POINT('Ctrl Pts',(53.1243619179795,-30.4513942013114,
39.2710850691866));
#199018=CARTESIAN_POINT('Ctrl Pts',(53.2191856060846,-30.5061406831644,
39.3343017080178));
#199019=CARTESIAN_POINT('Origin',(52.9969317578287,-30.2311753956713,39.5248017080178));
#199020=CARTESIAN_POINT('Ctrl Pts',(51.6568155675427,-29.4581217525674,
39.2875012672119));
#199021=CARTESIAN_POINT('Ctrl Pts',(51.5939283826162,-29.5680161684457,
39.2878045257519));
#199022=CARTESIAN_POINT('Ctrl Pts',(51.6870133715071,-29.6215404675517,
39.3549015218347));
#199023=CARTESIAN_POINT('Ctrl Pts',(51.7564542486366,-29.5155056307135,
39.1034938540228));
#199024=CARTESIAN_POINT('Ctrl Pts',(51.6933631336526,-29.6254251653838,
39.1038286278802));
#199025=CARTESIAN_POINT('Ctrl Pts',(51.7666458147672,-29.6675162799446,
39.2077506434033));
#199026=CARTESIAN_POINT('Ctrl Pts',(51.9354510367802,-29.6185943474781,
38.989));
#199027=CARTESIAN_POINT('Ctrl Pts',(51.8721362050942,-29.7286404220051,
38.9892298954629));
#199028=CARTESIAN_POINT('Ctrl Pts',(51.9097019182957,-29.7501097595404,
39.1161900347288));
#199029=CARTESIAN_POINT('Ctrl Pts',(52.1234703131946,-29.726882195485,38.989));
#199030=CARTESIAN_POINT('Ctrl Pts',(52.059875194672,-29.8370321718795,38.989));
#199031=CARTESIAN_POINT('Ctrl Pts',(52.0599703843284,-29.8368672985583,
39.1161900945645));
#199032=CARTESIAN_POINT('Origin',(52.1234703131946,-29.726882195485,39.116));
#199033=CARTESIAN_POINT('Origin',(45.6951875,-26.0155113828601,39.5248017080178));
#199034=CARTESIAN_POINT('Origin',(52.8659816883959,-30.1555713378339,39.5248017080178));
#199035=CARTESIAN_POINT('Origin',(45.518171167873,-25.9133109558556,39.116));
#199036=CARTESIAN_POINT('Origin',(52.4710850656383,-29.9275190026069,39.1160402713844));
#199037=CARTESIAN_POINT('Ctrl Pts',(52.6757649139395,-30.0450834959837,
39.2708017080178));
#199038=CARTESIAN_POINT('Ctrl Pts',(52.6124111049556,-30.1558192616002,
39.27051194648));
#199039=CARTESIAN_POINT('Ctrl Pts',(52.5167277788841,-30.1005764675359,
39.3343017080178));
#199040=CARTESIAN_POINT('Ctrl Pts',(52.7146817640556,-30.0676891808479,
39.3487519301186));
#199041=CARTESIAN_POINT('Ctrl Pts',(52.6511806140165,-30.1782028480937,
39.3482879463998));
#199042=CARTESIAN_POINT('Ctrl Pts',(52.5751914485008,-30.1343304829269,
39.451227126164));
#199043=CARTESIAN_POINT('Ctrl Pts',(52.7884098752456,-30.1105150503719,
39.3978017080178));
#199044=CARTESIAN_POINT('Ctrl Pts',(52.7247179826675,-30.2206596676788,
39.3975673827383));
#199045=CARTESIAN_POINT('Ctrl Pts',(52.6859499175227,-30.1982769148317,
39.524801535518));
#199046=CARTESIAN_POINT('Ctrl Pts',(52.8659816883959,-30.1555713378339,
39.3978017080178));
#199047=CARTESIAN_POINT('Ctrl Pts',(52.8024816883959,-30.2655565641145,
39.3978017080178));
#199048=CARTESIAN_POINT('Ctrl Pts',(52.8024816883959,-30.2655565641145,
39.5248017080178));
#199049=CARTESIAN_POINT('Origin',(52.5802277788841,-29.9905912412552,39.3343017080178));
#199050=CARTESIAN_POINT('Origin',(52.5097763812718,-29.9499161075303,39.1934008533552));
#199051=CARTESIAN_POINT('Origin',(49.5064990290885,-36.3610285397819,39.1925554495083));
#199052=CARTESIAN_POINT('Origin',(49.5422481179708,-36.3870656659259,39.1160373285269));
#199053=CARTESIAN_POINT('Origin',(49.4402904249165,-36.3129251734944,39.3343017080178));
#199054=CARTESIAN_POINT('Ctrl Pts',(49.3516463037385,-36.2478178023251,
39.2708017080178));
#199055=CARTESIAN_POINT('Ctrl Pts',(49.4263574835551,-36.1458216659126,
39.2710850691866));
#199056=CARTESIAN_POINT('Ctrl Pts',(49.5149391519577,-36.2101800152087,
39.3343017080178));
#199057=CARTESIAN_POINT('Ctrl Pts',(49.3151677697926,-36.221457784398,39.3487519293518));
#199058=CARTESIAN_POINT('Ctrl Pts',(49.3897594742889,-36.1192316557404,
39.3492068662938));
#199059=CARTESIAN_POINT('Ctrl Pts',(49.4603240281391,-36.1704998050822,
39.4512271248739));
#199060=CARTESIAN_POINT('Ctrl Pts',(49.2460589922044,-36.1715192752735,
39.3978017080178));
#199061=CARTESIAN_POINT('Ctrl Pts',(49.3205022166686,-36.0689133127034,
39.398034778115));
#199062=CARTESIAN_POINT('Ctrl Pts',(49.3568565533009,-36.0953262843471,
39.5248015355195));
#199063=CARTESIAN_POINT('Ctrl Pts',(49.1733470784087,-36.1189794796884,
39.3978017080178));
#199064=CARTESIAN_POINT('Ctrl Pts',(49.2479958054498,-36.0162343214027,
39.3978017080178));
#199065=CARTESIAN_POINT('Ctrl Pts',(49.2479958054498,-36.0162343214027,
39.5248017080178));
#199066=CARTESIAN_POINT('Origin',(49.1733470784087,-36.1189794796884,39.5248017080178));
#199067=CARTESIAN_POINT('Origin',(-0.186621817602855,-0.256862895714046,
39.116));
#199068=CARTESIAN_POINT('Origin',(49.8669803696025,-36.622933564581,39.116));
#199069=CARTESIAN_POINT('Origin',(-0.186621817602855,-0.256862895714046,
39.5248017080178));
#199070=CARTESIAN_POINT('Origin',(49.0510171431403,-36.0301015792677,39.5248017080178));
#199071=CARTESIAN_POINT('Ctrl Pts',(50.3023253561995,-36.9399086546487,
39.2875012672119));
#199072=CARTESIAN_POINT('Ctrl Pts',(50.3777877177488,-36.8368401467437,
39.287208709576));
#199073=CARTESIAN_POINT('Ctrl Pts',(50.2900345588337,-36.7733199672421,
39.3549016990124));
#199074=CARTESIAN_POINT('Ctrl Pts',(50.2093718139448,-36.8722300970239,
39.1034939173931));
#199075=CARTESIAN_POINT('Ctrl Pts',(50.2846371204137,-36.7691625978866,
39.1031692336317));
#199076=CARTESIAN_POINT('Ctrl Pts',(50.2156443459739,-36.7192723137719,
39.207750720229));
#199077=CARTESIAN_POINT('Ctrl Pts',(50.0423845927703,-36.7506474475485,
38.989));
#199078=CARTESIAN_POINT('Ctrl Pts',(50.1174266236752,-36.6476776482607,
38.9887769311194));
#199079=CARTESIAN_POINT('Ctrl Pts',(50.0820053531129,-36.6221779017697,
39.1161898712918));
#199080=CARTESIAN_POINT('Ctrl Pts',(49.8669803696025,-36.622933564581,38.989));
#199081=CARTESIAN_POINT('Ctrl Pts',(49.9417406183804,-36.5200349097932,
38.989));
#199082=CARTESIAN_POINT('Ctrl Pts',(49.9416290134639,-36.5201885207826,
39.1161895903857));
#199083=CARTESIAN_POINT('Origin',(50.2155162706044,-36.8761597191955,39.3548010137695));
#199084=CARTESIAN_POINT('Ctrl Pts',(49.0510171431403,-36.0301015792677,
39.3978017080178));
#199085=CARTESIAN_POINT('Ctrl Pts',(49.1256658701815,-35.9273564209821,
39.3978017080178));
#199086=CARTESIAN_POINT('Ctrl Pts',(49.1256658701815,-35.9273564209821,
39.5248017080178));
#199087=CARTESIAN_POINT('Ctrl Pts',(48.9780591316059,-35.977384677456,39.3978017080178));
#199088=CARTESIAN_POINT('Ctrl Pts',(49.0527758071209,-35.8743986902987,
39.3975666025003));
#199089=CARTESIAN_POINT('Ctrl Pts',(49.0164371879474,-35.8479971380611,
39.5248015517177));
#199090=CARTESIAN_POINT('Ctrl Pts',(48.9090707128239,-35.9275383438668,
39.3484894016716));
#199091=CARTESIAN_POINT('Ctrl Pts',(48.9842025736662,-35.8245773199091,
39.348025900006));
#199092=CARTESIAN_POINT('Ctrl Pts',(48.9131536812787,-35.7729572780248,
39.450833318895));
#199093=CARTESIAN_POINT('Ctrl Pts',(48.8727133447943,-35.9012693628905,
39.2708017080178));
#199094=CARTESIAN_POINT('Ctrl Pts',(48.9481071848796,-35.7983524848936,
39.27051194648));
#199095=CARTESIAN_POINT('Ctrl Pts',(48.85872246645,-35.7334106856007,39.3343017080178));
#199096=CARTESIAN_POINT('Origin',(48.7840737394089,-35.8361558438863,39.3343017080178));
#199097=CARTESIAN_POINT('Origin',(50.3596419293498,-36.9808731396198,39.6398955068187));
#199098=CARTESIAN_POINT('Origin',(50.5037675878945,-37.0855865599603,39.92499));
#199099=CARTESIAN_POINT('Origin',(48.7182599900762,-35.788339356061,39.1934008539944));
#199100=CARTESIAN_POINT('Origin',(48.6820620414866,-35.7621028045849,39.1160402713842));
#199101=CARTESIAN_POINT('Ctrl Pts',(50.9219998155899,-37.015868435856,40.1599502534424));
#199102=CARTESIAN_POINT('Ctrl Pts',(50.8918248691,-36.9939338721434,40.10025));
#199103=CARTESIAN_POINT('Ctrl Pts',(50.8348823336486,-36.9525415975213,
40.10025));
#199104=CARTESIAN_POINT('Ctrl Pts',(50.8701895025857,-37.0871426490242,
40.1599500538461));
#199105=CARTESIAN_POINT('Ctrl Pts',(50.8540829678232,-37.0458491715906,
40.1002448353499));
#199106=CARTESIAN_POINT('Ctrl Pts',(50.8048852215543,-36.9937925764098,
40.10025));
#199107=CARTESIAN_POINT('Ctrl Pts',(50.8021467555734,-37.1382015956601,
40.120244200104));
#199108=CARTESIAN_POINT('Ctrl Pts',(50.8006171556815,-37.0800635522214,
40.0633873868017));
#199109=CARTESIAN_POINT('Ctrl Pts',(50.7569692080814,-37.0171501059293,
40.0772271723536));
#199110=CARTESIAN_POINT('Ctrl Pts',(50.6806663304943,-37.1817767082786,
40.0045995998161));
#199111=CARTESIAN_POINT('Ctrl Pts',(50.7142182018865,-37.0956112176473,
39.9663485808314));
#199112=CARTESIAN_POINT('Ctrl Pts',(50.66189279602,-37.0243843935847,40.0101727202468));
#199113=CARTESIAN_POINT('Ctrl Pts',(50.627369305771,-37.1760624637753,39.930465434986));
#199114=CARTESIAN_POINT('Ctrl Pts',(50.6810088489711,-37.0763301845677,
39.9051900162952));
#199115=CARTESIAN_POINT('Ctrl Pts',(50.6152053999547,-37.0095702365075,
39.9671857458188));
#199116=CARTESIAN_POINT('Ctrl Pts',(50.5905785208484,-37.1493329797261,
39.8576902534424));
#199117=CARTESIAN_POINT('Ctrl Pts',(50.6659240749083,-37.0464195108254,
39.8573998014387));
#199118=CARTESIAN_POINT('Ctrl Pts',(50.5784163149356,-36.9828414016747,
39.92499));
#199119=CARTESIAN_POINT('Origin',(50.8348823336486,-36.9525415975213,40.22725));
#199120=CARTESIAN_POINT('Origin',(-0.186621817602855,-0.256862895714046,
39.116));
#199121=CARTESIAN_POINT('Origin',(48.3573835402119,-35.5261472678866,39.116));
#199122=CARTESIAN_POINT('Origin',(5.53127843490691E-15,5.79180425524272E-15,
40.22725));
#199123=CARTESIAN_POINT('Origin',(50.8527980281384,-36.9278827595327,40.22725));
#199124=CARTESIAN_POINT('Ctrl Pts',(48.3573835402119,-35.5261472678866,
38.989));
#199125=CARTESIAN_POINT('Ctrl Pts',(48.4321440944169,-35.4232481927144,
38.989));
#199126=CARTESIAN_POINT('Ctrl Pts',(48.4320321836173,-35.4234022247157,
39.116190109232));
#199127=CARTESIAN_POINT('Ctrl Pts',(48.1819806163554,-35.3984257650676,
38.989));
#199128=CARTESIAN_POINT('Ctrl Pts',(48.2567602586447,-35.2958250128969,
38.9892298989754));
#199129=CARTESIAN_POINT('Ctrl Pts',(48.2916533613393,-35.3214110399816,
39.11619004932));
#199130=CARTESIAN_POINT('Ctrl Pts',(48.015001153061,-35.2768349808754,39.1034966344368));
#199131=CARTESIAN_POINT('Ctrl Pts',(48.0897561847329,-35.174490067168,39.103831410257));
#199132=CARTESIAN_POINT('Ctrl Pts',(48.1580153629272,-35.224317350472,39.2077528789602));
#199133=CARTESIAN_POINT('Ctrl Pts',(47.9220530736687,-35.2091516650529,
39.2875012672119));
#199134=CARTESIAN_POINT('Ctrl Pts',(47.9968681042461,-35.1070032653414,
39.2878045257868));
#199135=CARTESIAN_POINT('Ctrl Pts',(48.0836260618767,-35.1702703594593,
39.3549015295898));
#199136=CARTESIAN_POINT('Origin',(48.0088472823272,-35.2729208539816,39.3548010137695));
#199137=CARTESIAN_POINT('Ctrl Pts',(50.9644637245892,-36.6347241449655,
39.8576902534424));
#199138=CARTESIAN_POINT('Ctrl Pts',(50.8898702560317,-36.7381840359685,
39.8573998014387));
#199139=CARTESIAN_POINT('Ctrl Pts',(50.8023624960591,-36.6746059268179,
39.92499));
#199140=CARTESIAN_POINT('Ctrl Pts',(51.0012706547892,-36.6614665482797,
39.930498490249));
#199141=CARTESIAN_POINT('Ctrl Pts',(50.9229972443175,-36.7432905102106,
39.9052171569798));
#199142=CARTESIAN_POINT('Ctrl Pts',(50.8391683443881,-36.7013469409082,
39.9672049726599));
#199143=CARTESIAN_POINT('Ctrl Pts',(51.0230245369438,-36.7102884597167,
40.0043437678662));
#199144=CARTESIAN_POINT('Ctrl Pts',(50.9514409225347,-36.7689049964551,
39.9661628577646));
#199145=CARTESIAN_POINT('Ctrl Pts',(50.8675358949426,-36.7410683485315,
40.0100243556238));
#199146=CARTESIAN_POINT('Ctrl Pts',(51.0194219249361,-36.8383381382862,
40.1194874821987));
#199147=CARTESIAN_POINT('Ctrl Pts',(50.9635175930198,-36.8551762168616,
40.0627551483138));
#199148=CARTESIAN_POINT('Ctrl Pts',(50.8901021525742,-36.8330984946703,
40.0767884282374));
#199149=CARTESIAN_POINT('Ctrl Pts',(50.9918932610486,-36.9196318328644,
40.1599502015385));
#199150=CARTESIAN_POINT('Ctrl Pts',(50.9476171190673,-36.9171104726339,
40.1002449453869));
#199151=CARTESIAN_POINT('Ctrl Pts',(50.8828596657514,-36.8864699989243,
40.10025));
#199152=CARTESIAN_POINT('Ctrl Pts',(50.9399462128201,-36.9911673391708,
40.1599502534424));
#199153=CARTESIAN_POINT('Ctrl Pts',(50.9097606317993,-36.9692474126341,
40.10025));
#199154=CARTESIAN_POINT('Ctrl Pts',(50.8527980281385,-36.9278827595327,
40.10025));
#199155=CARTESIAN_POINT('Origin',(50.8770112231002,-36.5718607685322,39.92499));
#199156=CARTESIAN_POINT('Origin',(47.8647214254963,-35.1682072895739,39.6398955069324));
#199157=CARTESIAN_POINT('Origin',(47.720595568509,-35.0634937251222,39.92499));
#199158=CARTESIAN_POINT('Origin',(50.7328855645148,-36.4671473482219,39.6398955068281));
#199159=CARTESIAN_POINT('Origin',(50.5887599058101,-36.3624339277674,39.3548010137695));
#199160=CARTESIAN_POINT('Ctrl Pts',(47.6338034047599,-34.9997217530261,
39.8576902534424));
#199161=CARTESIAN_POINT('Ctrl Pts',(47.7085070967803,-34.8977303031703,
39.8579948730703));
#199162=CARTESIAN_POINT('Ctrl Pts',(47.7952442955502,-34.9607485668366,
39.92499));
#199163=CARTESIAN_POINT('Ctrl Pts',(47.5970451916076,-34.9730146904934,
39.9304020711229));
#199164=CARTESIAN_POINT('Ctrl Pts',(47.6752966590745,-34.8923835282623,
39.905891529738));
#199165=CARTESIAN_POINT('Ctrl Pts',(47.7584842465947,-34.9340408279389,
39.9671523786029));
#199166=CARTESIAN_POINT('Ctrl Pts',(47.5754322771535,-34.9244461536122,
40.0043257306695));
#199167=CARTESIAN_POINT('Ctrl Pts',(47.646975614992,-34.866597278702,39.9667894847838));
#199168=CARTESIAN_POINT('Ctrl Pts',(47.7303228514092,-34.8944891948622,
40.0100138975201));
#199169=CARTESIAN_POINT('Ctrl Pts',(47.5794993790985,-34.7970725085259,
40.1195533054855));
#199170=CARTESIAN_POINT('Ctrl Pts',(47.6353197637778,-34.7804938560726,
40.0630813209234));
#199171=CARTESIAN_POINT('Ctrl Pts',(47.7084160893875,-34.8028668197834,
40.076826594242));
#199172=CARTESIAN_POINT('Ctrl Pts',(47.607308993689,-34.7162617467342,40.1599502027513));
#199173=CARTESIAN_POINT('Ctrl Pts',(47.6515013114247,-34.7189078610121,
40.1002552791553));
#199174=CARTESIAN_POINT('Ctrl Pts',(47.7160937685333,-34.7497660430526,
40.10025));
#199175=CARTESIAN_POINT('Ctrl Pts',(47.6590285860935,-34.6451144164186,
40.1599502534424));
#199176=CARTESIAN_POINT('Ctrl Pts',(47.6892031885513,-34.6670494534018,
40.10025));
#199177=CARTESIAN_POINT('Ctrl Pts',(47.7461450747864,-34.7084426211232,
40.10025));
#199178=CARTESIAN_POINT('Origin',(47.7461450747864,-34.7084426211232,40.22725));
#199179=CARTESIAN_POINT('Ctrl Pts',(50.2402240048083,-36.1092077731529,
38.989));
#199180=CARTESIAN_POINT('Ctrl Pts',(50.1654637495898,-36.2121064368054,
38.989));
#199181=CARTESIAN_POINT('Ctrl Pts',(50.1655753609565,-36.2119528169382,
39.1161896013266));
#199182=CARTESIAN_POINT('Ctrl Pts',(50.4158927445019,-36.2365633238569,
38.989));
#199183=CARTESIAN_POINT('Ctrl Pts',(50.3411519064808,-36.3397519704545,
38.988776927546));
#199184=CARTESIAN_POINT('Ctrl Pts',(50.305953882031,-36.3139437822107,39.1161898821848));
#199185=CARTESIAN_POINT('Ctrl Pts',(50.5831252836581,-36.3578055460602,
39.1034967087243));
#199186=CARTESIAN_POINT('Ctrl Pts',(50.5083605190648,-36.4612367259614,
39.1031720232708));
#199187=CARTESIAN_POINT('Ctrl Pts',(50.4395918165621,-36.4110374247136,
39.2077529615001));
#199188=CARTESIAN_POINT('Ctrl Pts',(50.6762142289948,-36.4252947698679,
39.2875012672119));
#199189=CARTESIAN_POINT('Ctrl Pts',(50.6015093986316,-36.5289136700279,
39.2872087095507));
#199190=CARTESIAN_POINT('Ctrl Pts',(50.5139808995223,-36.4650842569433,
39.3549017048227));
#199191=CARTESIAN_POINT('Origin',(50.2402240048083,-36.1092077731529,39.116));
#199192=CARTESIAN_POINT('Origin',(5.7121316272531E-15,5.21823002976732E-15,
40.22725));
#199193=CARTESIAN_POINT('Origin',(47.7640607692763,-34.6837837831347,40.22725));
#199194=CARTESIAN_POINT('Origin',(40.9117478092586,-29.3316730956005,39.116));
#199195=CARTESIAN_POINT('Origin',(49.915552518432,-35.8732562382992,39.1160373285272));
#199196=CARTESIAN_POINT('Ctrl Pts',(47.6769115920304,-34.6205005703635,
40.1599502534424));
#199197=CARTESIAN_POINT('Ctrl Pts',(47.7070975168464,-34.6424200234575,
40.10025));
#199198=CARTESIAN_POINT('Ctrl Pts',(47.7640607692763,-34.6837837831347,
40.10025));
#199199=CARTESIAN_POINT('Ctrl Pts',(47.7284183483606,-34.5495693076631,
40.1599500566037));
#199200=CARTESIAN_POINT('Ctrl Pts',(47.7446195594518,-34.5907418558593,
40.1002551305372));
#199201=CARTESIAN_POINT('Ctrl Pts',(47.7939730310155,-34.6425747206412,
40.10025));
#199202=CARTESIAN_POINT('Ctrl Pts',(47.7959261043554,-34.4983910654767,
40.1203070619046));
#199203=CARTESIAN_POINT('Ctrl Pts',(47.797671475652,-34.5563698228277,40.0637098684499));
#199204=CARTESIAN_POINT('Ctrl Pts',(47.8415056181568,-34.61888919786,40.0772636213363));
#199205=CARTESIAN_POINT('Ctrl Pts',(47.9165880269728,-34.4545839152292,
40.0046102245802));
#199206=CARTESIAN_POINT('Ctrl Pts',(47.8837591046489,-34.5404685123897,
39.9670001894012));
#199207=CARTESIAN_POINT('Ctrl Pts',(47.9359643384884,-34.6111463389765,
40.0101788811208));
#199208=CARTESIAN_POINT('Ctrl Pts',(47.9696250311906,-34.4602354682513,
39.9303710930186));
#199209=CARTESIAN_POINT('Ctrl Pts',(47.9171136764635,-34.5595777906764,
39.9058663574114));
#199210=CARTESIAN_POINT('Ctrl Pts',(47.9824460410477,-34.62581669683,39.9671344706362));
#199211=CARTESIAN_POINT('Ctrl Pts',(48.0063682005187,-34.4869303039397,
39.8576902534424));
#199212=CARTESIAN_POINT('Ctrl Pts',(47.9324532779037,-34.5894948283134,
39.8579948730703));
#199213=CARTESIAN_POINT('Ctrl Pts',(48.0191904766736,-34.6525130919798,
39.92499));
#199214=CARTESIAN_POINT('Origin',(48.0938392037147,-34.5497679336941,39.92499));
#199215=CARTESIAN_POINT('Origin',(49.8797426632453,-35.8473027479611,39.1925554488851));
#199216=CARTESIAN_POINT('Origin',(49.8135340601223,-35.7991993820663,39.3343017080178));
#199217=CARTESIAN_POINT('Origin',(48.237965060651,-34.6544814981838,39.6398955069206));
#199218=CARTESIAN_POINT('Origin',(48.3820909175329,-34.7591950625535,39.3548010137695));
#199219=CARTESIAN_POINT('Ctrl Pts',(49.5465907136144,-35.6052536882603,
39.3978017080178));
#199220=CARTESIAN_POINT('Ctrl Pts',(49.4719419865733,-35.7079988465459,
39.3978017080178));
#199221=CARTESIAN_POINT('Ctrl Pts',(49.4719419865733,-35.7079988465459,
39.5248017080178));
#199222=CARTESIAN_POINT('Ctrl Pts',(49.6192730640956,-35.6583499840576,
39.3978017080178));
#199223=CARTESIAN_POINT('Ctrl Pts',(49.544693607491,-35.7608559931226,39.3980355775163));
#199224=CARTESIAN_POINT('Ctrl Pts',(49.5811706590223,-35.7873581223577,
39.5248015517192));
#199225=CARTESIAN_POINT('Ctrl Pts',(49.6880007749198,-35.7085550527712,
39.3484893995498));
#199226=CARTESIAN_POINT('Ctrl Pts',(49.6138288703675,-35.8110857017868,
39.348943830343));
#199227=CARTESIAN_POINT('Ctrl Pts',(49.6844541394794,-35.8623979633502,
39.450833315559));
#199228=CARTESIAN_POINT('Ctrl Pts',(49.7242207306175,-35.735013097139,39.2708017080178));
#199229=CARTESIAN_POINT('Ctrl Pts',(49.6503036646785,-35.8375861910557,
39.2710850691866));
#199230=CARTESIAN_POINT('Ctrl Pts',(49.7388853330811,-35.9019445403519,
39.3343017080178));
#199231=CARTESIAN_POINT('Origin',(49.5465907136144,-35.6052536882603,39.5248017080178));
#199232=CARTESIAN_POINT('Ctrl Pts',(48.2946219293746,-34.6963546279286,
39.2875012672119));
#199233=CARTESIAN_POINT('Ctrl Pts',(48.2205921526136,-34.7990735298986,
39.2878045257519));
#199234=CARTESIAN_POINT('Ctrl Pts',(48.3075723994627,-34.8620346481358,
39.3549015218347));
#199235=CARTESIAN_POINT('Ctrl Pts',(48.3877165307504,-34.7638392294009,
39.1034938540228));
#199236=CARTESIAN_POINT('Ctrl Pts',(48.3134813154502,-34.8665617960632,
39.1038286278789));
#199237=CARTESIAN_POINT('Ctrl Pts',(48.3819628268489,-34.9160824571376,
39.207750643403));
#199238=CARTESIAN_POINT('Ctrl Pts',(48.5549570506147,-34.8850734745854,
38.989));
#199239=CARTESIAN_POINT('Ctrl Pts',(48.4804861171459,-34.9878985031429,
38.9892298954635));
#199240=CARTESIAN_POINT('Ctrl Pts',(48.5156018845772,-35.0131769156741,
39.1161900347288));
#199241=CARTESIAN_POINT('Ctrl Pts',(48.7306271754176,-35.0124214764585,
38.989));
#199242=CARTESIAN_POINT('Ctrl Pts',(48.6558666298469,-35.1153205397466,
38.989));
#199243=CARTESIAN_POINT('Ctrl Pts',(48.6559785319992,-35.1151665196473,
39.1161900945645));
#199244=CARTESIAN_POINT('Origin',(48.7306271754176,-35.0124214764585,39.116));
#199245=CARTESIAN_POINT('Origin',(39.9252688514646,-28.6149541797807,39.5248017080178));
#199246=CARTESIAN_POINT('Origin',(49.424260778346,-35.5163757878396,39.5248017080178));
#199247=CARTESIAN_POINT('Origin',(39.7707905934405,-28.502719155674,39.116));
#199248=CARTESIAN_POINT('Origin',(49.0553654007526,-35.2482948100397,39.1160402713847));
#199249=CARTESIAN_POINT('Ctrl Pts',(49.2466351556012,-35.386610142826,39.2708017080178));
#199250=CARTESIAN_POINT('Ctrl Pts',(49.1720533660031,-35.4901170100368,
39.27051194648));
#199251=CARTESIAN_POINT('Ctrl Pts',(49.0826686475734,-35.4251752107438,
39.3343017080178));
#199252=CARTESIAN_POINT('Ctrl Pts',(49.282975877639,-35.4131599099231,39.3487519301185));
#199253=CARTESIAN_POINT('Ctrl Pts',(49.2082707697374,-35.5164304941056,
39.3482879463985));
#199254=CARTESIAN_POINT('Ctrl Pts',(49.1372837917337,-35.4648554356494,
39.4512271261637));
#199255=CARTESIAN_POINT('Ctrl Pts',(49.3518235761932,-35.4634578610138,
39.3978017080178));
#199256=CARTESIAN_POINT('Ctrl Pts',(49.2769673468822,-35.5663414789297,
39.3975673827401));
#199257=CARTESIAN_POINT('Ctrl Pts',(49.2407512920135,-35.5400289748691,
39.524801535518));
#199258=CARTESIAN_POINT('Ctrl Pts',(49.424260778346,-35.5163757878396,39.3978017080178));
#199259=CARTESIAN_POINT('Ctrl Pts',(49.3496120513049,-35.6191209461252,
39.3978017080178));
#199260=CARTESIAN_POINT('Ctrl Pts',(49.3496120513049,-35.6191209461252,
39.5248017080178));
#199261=CARTESIAN_POINT('Origin',(49.1573173746146,-35.3224300524582,39.3343017080178));
#199262=CARTESIAN_POINT('Origin',(49.0915036263516,-35.2746135650469,39.1934008533543));
#199263=CARTESIAN_POINT('Origin',(45.4345348113611,-41.3366772861974,39.1925554495085));
#199264=CARTESIAN_POINT('Origin',(45.4673664422103,-41.3663085755639,39.116037328527));
#199265=CARTESIAN_POINT('Origin',(45.3737170758072,-41.2819167515329,39.3343017080178));
#199266=CARTESIAN_POINT('Ctrl Pts',(45.2923641298557,-41.2079002115908,
39.2708017080178));
#199267=CARTESIAN_POINT('Ctrl Pts',(45.3773275334105,-41.1142722655007,
39.2710850691866));
#199268=CARTESIAN_POINT('Ctrl Pts',(45.4586966628148,-41.1875373586973,
39.3343017080178));
#199269=CARTESIAN_POINT('Ctrl Pts',(45.2588408013013,-41.1778715515042,
39.3487519293518));
#199270=CARTESIAN_POINT('Ctrl Pts',(45.3437094247724,-41.084002384522,39.3492068662926));
#199271=CARTESIAN_POINT('Ctrl Pts',(45.4085284377449,-41.1423656859491,
39.451227124874));
#199272=CARTESIAN_POINT('Ctrl Pts',(45.1953306044459,-41.1209827764365,
39.3978017080178));
#199273=CARTESIAN_POINT('Ctrl Pts',(45.280091264722,-41.0267203359205,39.3980347781178));
#199274=CARTESIAN_POINT('Ctrl Pts',(45.313485541162,-41.0567886774841,39.524801535519));
#199275=CARTESIAN_POINT('Ctrl Pts',(45.1285089182132,-41.0611303347405,
39.3978017080178));
#199276=CARTESIAN_POINT('Ctrl Pts',(45.2134885052208,-40.9667509419048,
39.3978017080178));
#199277=CARTESIAN_POINT('Ctrl Pts',(45.2134885052208,-40.9667509419048,
39.5248017080178));
#199278=CARTESIAN_POINT('Origin',(45.1285089182132,-41.0611303347405,39.5248017080178));
#199279=CARTESIAN_POINT('Origin',(-0.212448967518932,-0.235948482089072,
39.116));
#199280=CARTESIAN_POINT('Origin',(45.7656648676106,-41.6348281284263,39.116));
#199281=CARTESIAN_POINT('Origin',(-0.212448967518932,-0.235948482089072,
39.5248017080178));
#199282=CARTESIAN_POINT('Origin',(45.0161393894793,-40.9599523566126,39.5248017080178));
#199283=CARTESIAN_POINT('Ctrl Pts',(46.1654920697611,-41.9955727382251,
39.2875012672119));
#199284=CARTESIAN_POINT('Ctrl Pts',(46.2513146333407,-41.900956815078,39.287208709576));
#199285=CARTESIAN_POINT('Ctrl Pts',(46.1706818621617,-41.8286119029176,
39.3549016990124));
#199286=CARTESIAN_POINT('Ctrl Pts',(46.0801220723611,-41.9185486398936,
39.103493917393));
#199287=CARTESIAN_POINT('Ctrl Pts',(46.1657485549058,-41.823913122125,39.1031692336314));
#199288=CARTESIAN_POINT('Ctrl Pts',(46.1023486848322,-41.767084433516,39.207750720229));
#199289=CARTESIAN_POINT('Ctrl Pts',(45.9267584721677,-41.780177115277,38.989));
#199290=CARTESIAN_POINT('Ctrl Pts',(46.0121526898533,-41.6856154234966,
38.9887769311188));
#199291=CARTESIAN_POINT('Ctrl Pts',(45.979590910035,-41.6565528363053,39.1161898712919));
#199292=CARTESIAN_POINT('Ctrl Pts',(45.7656648676106,-41.6348281284263,
38.989));
#199293=CARTESIAN_POINT('Ctrl Pts',(45.8507714101807,-41.540307737154,38.989));
#199294=CARTESIAN_POINT('Ctrl Pts',(45.8506443599268,-41.5404488407559,
39.1161895903858));
#199295=CARTESIAN_POINT('Origin',(46.0858221116777,-41.9230990057956,39.3548010137695));
#199296=CARTESIAN_POINT('Ctrl Pts',(45.0161393894793,-40.9599523566126,
39.3978017080178));
#199297=CARTESIAN_POINT('Ctrl Pts',(45.1011189764868,-40.8655729637769,
39.3978017080178));
#199298=CARTESIAN_POINT('Ctrl Pts',(45.1011189764868,-40.8655729637769,
39.5248017080178));
#199299=CARTESIAN_POINT('Ctrl Pts',(44.9490914662989,-40.8998980546777,
39.3978017080178));
#199300=CARTESIAN_POINT('Ctrl Pts',(45.0341638030263,-40.8052862548056,
39.3975666025017));
#199301=CARTESIAN_POINT('Ctrl Pts',(45.0007839642924,-40.7752309130124,
39.5248015517177));
#199302=CARTESIAN_POINT('Ctrl Pts',(44.8856913339435,-40.8431135311203,
39.3484894016716));
#199303=CARTESIAN_POINT('Ctrl Pts',(44.9711739721975,-40.7485699563814,
39.3480259000057));
#199304=CARTESIAN_POINT('Ctrl Pts',(44.9059100567339,-40.6898060629484,
39.4508333188949));
#199305=CARTESIAN_POINT('Ctrl Pts',(44.8522789915941,-40.8131880745607,
39.2708017080178));
#199306=CARTESIAN_POINT('Ctrl Pts',(44.9380175594362,-40.7187157882338,
39.27051194648));
#199307=CARTESIAN_POINT('Ctrl Pts',(44.8559107663285,-40.6447864996553,
39.3343017080178));
#199308=CARTESIAN_POINT('Origin',(44.7709311793209,-40.739165892491,39.3343017080178));
#199309=CARTESIAN_POINT('Origin',(46.2182127020628,-42.0423040287724,39.6398955068193));
#199310=CARTESIAN_POINT('Origin',(46.3506032922594,-42.1615090516453,39.92499));
#199311=CARTESIAN_POINT('Origin',(44.7104761485842,-40.6847319383096,39.1934008539945));
#199312=CARTESIAN_POINT('Origin',(44.6772189625507,-40.6548553974685,39.1160402713855));
#199313=CARTESIAN_POINT('Ctrl Pts',(46.7738319284257,-42.1358900227696,
40.1599502534424));
#199314=CARTESIAN_POINT('Ctrl Pts',(46.7461150696872,-42.1109214781062,
40.10025));
#199315=CARTESIAN_POINT('Ctrl Pts',(46.6938111422604,-42.0638038389701,
40.10025));
#199316=CARTESIAN_POINT('Ctrl Pts',(46.7148552537636,-42.2013581359407,
40.1599500538455));
#199317=CARTESIAN_POINT('Ctrl Pts',(46.703153296022,-42.1586072771686,40.100244835349));
#199318=CARTESIAN_POINT('Ctrl Pts',(46.6596664560525,-42.1016932886499,
40.10025));
#199319=CARTESIAN_POINT('Ctrl Pts',(46.6418481388116,-42.2450249725426,
40.120244200104));
#199320=CARTESIAN_POINT('Ctrl Pts',(46.646403998566,-42.1870455286631,40.0633873868017));
#199321=CARTESIAN_POINT('Ctrl Pts',(46.6095714048493,-42.1199142759248,
40.0772271723538));
#199322=CARTESIAN_POINT('Ctrl Pts',(46.5164783566526,-42.2756632139847,
40.0045995998161));
#199323=CARTESIAN_POINT('Ctrl Pts',(46.5588531737051,-42.1934768724827,
39.9663485808314));
#199324=CARTESIAN_POINT('Ctrl Pts',(46.5142596423498,-42.1171707421502,
40.0101727202466));
#199325=CARTESIAN_POINT('Ctrl Pts',(46.4640705998044,-42.2644092166192,
39.930465434986));
#199326=CARTESIAN_POINT('Ctrl Pts',(46.5278411618568,-42.1708301402936,
39.9051900162956));
#199327=CARTESIAN_POINT('Ctrl Pts',(46.4693765058,-42.0975575768115,39.9671857458174));
#199328=CARTESIAN_POINT('Ctrl Pts',(46.4302753505424,-42.2339804752702,
39.8576902534424));
#199329=CARTESIAN_POINT('Ctrl Pts',(46.5159655405274,-42.1395065321,39.8573998014387));
#199330=CARTESIAN_POINT('Ctrl Pts',(46.435582879267,-42.0671296588096,39.92499));
#199331=CARTESIAN_POINT('Origin',(46.6938111422604,-42.0638038389701,40.22725));
#199332=CARTESIAN_POINT('Origin',(-0.212448967518932,-0.235948482089072,
39.116));
#199333=CARTESIAN_POINT('Origin',(44.3789831537295,-40.3862543050939,39.116));
#199334=CARTESIAN_POINT('Origin',(5.54214007001405E-15,5.80521725755185E-15,
40.22725));
#199335=CARTESIAN_POINT('Origin',(46.7142062431422,-42.0411527846896,40.22725));
#199336=CARTESIAN_POINT('Ctrl Pts',(44.3789831537295,-40.3862543050939,
38.989));
#199337=CARTESIAN_POINT('Ctrl Pts',(44.4640900439955,-40.2917335276662,
38.989));
#199338=CARTESIAN_POINT('Ctrl Pts',(44.4639626455268,-40.291875018,39.1161901092318));
#199339=CARTESIAN_POINT('Ctrl Pts',(44.2178916378581,-40.2408978759481,
38.989));
#199340=CARTESIAN_POINT('Ctrl Pts',(44.3029863283941,-40.1466757825273,
38.989229898976));
#199341=CARTESIAN_POINT('Ctrl Pts',(44.335013814932,-40.1757689690791,39.1161900493198));
#199342=CARTESIAN_POINT('Ctrl Pts',(44.0645366033547,-40.102519072098,39.1034966344368));
#199343=CARTESIAN_POINT('Ctrl Pts',(44.1495800756973,-40.0085488431172,
39.1038314102568));
#199344=CARTESIAN_POINT('Ctrl Pts',(44.2122569536161,-40.0652381943521,
39.2077528789601));
#199345=CARTESIAN_POINT('Ctrl Pts',(43.9791725362582,-40.0254908126589,
39.2875012672119));
#199346=CARTESIAN_POINT('Ctrl Pts',(44.0642551375171,-39.9317222927448,
39.2878045257868));
#199347=CARTESIAN_POINT('Ctrl Pts',(44.1439246138545,-40.0037114790884,
39.3549015295897));
#199348=CARTESIAN_POINT('Origin',(44.0588255818377,-40.09798313255,39.3548010137695));
#199349=CARTESIAN_POINT('Ctrl Pts',(46.8559036426985,-41.7612723673363,
39.8576902534424));
#199350=CARTESIAN_POINT('Ctrl Pts',(46.7709043015502,-41.8563683535931,
39.8573998014387));
#199351=CARTESIAN_POINT('Ctrl Pts',(46.6905216402897,-41.7839914803027,
39.92499));
#199352=CARTESIAN_POINT('Ctrl Pts',(46.8897135983611,-41.7917156448187,
39.9304984902491));
#199353=CARTESIAN_POINT('Ctrl Pts',(46.8033160448235,-41.8649095672142,
39.9052171569788));
#199354=CARTESIAN_POINT('Ctrl Pts',(46.7243306652218,-41.8144332630854,
39.9672049726596));
#199355=CARTESIAN_POINT('Ctrl Pts',(46.9062450310968,-41.8425440045878,
40.0043437678661));
#199356=CARTESIAN_POINT('Ctrl Pts',(46.8289264627109,-41.8933569085955,
39.9661628577642));
#199357=CARTESIAN_POINT('Ctrl Pts',(46.748390797668,-41.8569022891471,40.0100243556237));
#199358=CARTESIAN_POINT('Ctrl Pts',(46.8892773184517,-41.9695156381235,
40.1194874821988));
#199359=CARTESIAN_POINT('Ctrl Pts',(46.8319191778365,-41.9804178820374,
40.062755148314));
#199360=CARTESIAN_POINT('Ctrl Pts',(46.7612136652292,-41.9507871007487,
40.0767884282376));
#199361=CARTESIAN_POINT('Ctrl Pts',(46.8534019544983,-42.047486468405,40.1599502015393));
#199362=CARTESIAN_POINT('Ctrl Pts',(46.8096319157679,-42.0403508033703,
40.1002449453869));
#199363=CARTESIAN_POINT('Ctrl Pts',(46.7484320121873,-42.0031091843017,
40.10025));
#199364=CARTESIAN_POINT('Ctrl Pts',(46.7942619810916,-42.1132001506002,
40.1599502534424));
#199365=CARTESIAN_POINT('Ctrl Pts',(46.7665330160779,-42.0882450513176,
40.10025));
#199366=CARTESIAN_POINT('Ctrl Pts',(46.7142062431422,-42.0411527846896,
40.10025));
#199367=CARTESIAN_POINT('Origin',(46.7755012272973,-41.6896120874671,39.92499));
#199368=CARTESIAN_POINT('Origin',(43.9264348095014,-39.9787779456746,39.639895506933));
#199369=CARTESIAN_POINT('Origin',(43.7940440370144,-39.8595727587356,39.92499));
#199370=CARTESIAN_POINT('Origin',(46.6431106370589,-41.5704070646205,39.6398955068277));
#199371=CARTESIAN_POINT('Origin',(46.5107200467156,-41.4512020416175,39.3548010137695));
#199372=CARTESIAN_POINT('Ctrl Pts',(43.7143933160623,-39.7870778846748,
39.8576902534424));
#199373=CARTESIAN_POINT('Ctrl Pts',(43.7993487829612,-39.6934538167801,
39.8579948730703));
#199374=CARTESIAN_POINT('Ctrl Pts',(43.8790236240219,-39.7651933658999,
39.92499));
#199375=CARTESIAN_POINT('Ctrl Pts',(43.6806281164521,-39.7566748466922,
39.9304020711231));
#199376=CARTESIAN_POINT('Ctrl Pts',(43.7668791656721,-39.684664896048,39.9058915297382));
#199377=CARTESIAN_POINT('Ctrl Pts',(43.8452566693654,-39.7347894633636,
39.9671523786035));
#199378=CARTESIAN_POINT('Ctrl Pts',(43.6642103943287,-39.7061132086029,
40.0043257306693));
#199379=CARTESIAN_POINT('Ctrl Pts',(43.7414086642734,-39.656059551044,39.9667894847838));
#199380=CARTESIAN_POINT('Ctrl Pts',(43.8213838166748,-39.6925108309093,
40.01001389752));
#199381=CARTESIAN_POINT('Ctrl Pts',(43.6815693876452,-39.5798624575878,
40.1195533054857));
#199382=CARTESIAN_POINT('Ctrl Pts',(43.7388169234803,-39.5692094437564,
40.0630813209233));
#199383=CARTESIAN_POINT('Ctrl Pts',(43.8091742082547,-39.5991004926177,
40.076826594242));
#199384=CARTESIAN_POINT('Ctrl Pts',(43.7176736830029,-39.5024012818818,
40.1599502027513));
#199385=CARTESIAN_POINT('Ctrl Pts',(43.76134731634,-39.5096522555309,40.1002552791529));
#199386=CARTESIAN_POINT('Ctrl Pts',(43.822360370862,-39.5470931435016,40.10025));
#199387=CARTESIAN_POINT('Ctrl Pts',(43.7765468711722,-39.4370498736009,
40.1599502534424));
#199388=CARTESIAN_POINT('Ctrl Pts',(43.8042633382929,-39.462018852981,40.10025));
#199389=CARTESIAN_POINT('Ctrl Pts',(43.8565665267056,-39.5091373124623,
40.10025));
#199390=CARTESIAN_POINT('Origin',(43.8565665267056,-39.5091373124623,40.22725));
#199391=CARTESIAN_POINT('Ctrl Pts',(46.1905628026484,-41.1629311642481,
38.989));
#199392=CARTESIAN_POINT('Ctrl Pts',(46.1054562527464,-41.2574515636633,
38.989));
#199393=CARTESIAN_POINT('Ctrl Pts',(46.1055833103431,-41.2573104519063,
39.1161896013268));
#199394=CARTESIAN_POINT('Ctrl Pts',(46.3519569306012,-41.307951431325,38.989));
#199395=CARTESIAN_POINT('Ctrl Pts',(46.2668393800559,-41.4027622547783,
38.988776927546));
#199396=CARTESIAN_POINT('Ctrl Pts',(46.2345318643234,-41.3734162510828,
39.1161898821849));
#199397=CARTESIAN_POINT('Ctrl Pts',(46.5056000892405,-41.446010036275,39.1034967087243));
#199398=CARTESIAN_POINT('Ctrl Pts',(46.4204333915643,-41.541059563397,39.103172023271));
#199399=CARTESIAN_POINT('Ctrl Pts',(46.3572886670237,-41.4839469723849,
39.2077529614999));
#199400=CARTESIAN_POINT('Ctrl Pts',(46.5911245387429,-41.5228599914563,
39.2875012672119));
#199401=CARTESIAN_POINT('Ctrl Pts',(46.5059978248576,-41.618102475323,39.2872087095507));
#199402=CARTESIAN_POINT('Ctrl Pts',(46.4256208064858,-41.5454735069376,
39.3549017048228));
#199403=CARTESIAN_POINT('Origin',(46.1905628026484,-41.1629311642481,39.116));
#199404=CARTESIAN_POINT('Origin',(5.70826774717982E-15,5.21345853525163E-15,
40.22725));
#199405=CARTESIAN_POINT('Origin',(43.8769616275874,-39.4864862581817,40.22725));
#199406=CARTESIAN_POINT('Origin',(34.5756856720385,-30.7048488218244,39.116));
#199407=CARTESIAN_POINT('Origin',(45.8923335519876,-40.8943347850527,39.1160373285247));
#199408=CARTESIAN_POINT('Ctrl Pts',(43.7969047596346,-39.414440147899,40.1599502534424));
#199409=CARTESIAN_POINT('Ctrl Pts',(43.8246341160485,-39.4393948122689,
40.10025));
#199410=CARTESIAN_POINT('Ctrl Pts',(43.8769616275874,-39.4864862581817,
40.10025));
#199411=CARTESIAN_POINT('Ctrl Pts',(43.8555436924521,-39.3492813761645,
40.1599500566037));
#199412=CARTESIAN_POINT('Ctrl Pts',(43.8673524484227,-39.3919218645331,
40.100255130536));
#199413=CARTESIAN_POINT('Ctrl Pts',(43.9110175468023,-39.4486296259968,
40.10025));
#199414=CARTESIAN_POINT('Ctrl Pts',(43.9280312169046,-39.3054399757363,
40.1203070619049));
#199415=CARTESIAN_POINT('Ctrl Pts',(43.9237065964669,-39.3632835603675,
40.0637098684502));
#199416=CARTESIAN_POINT('Ctrl Pts',(43.9607655567556,-39.4300423632768,
40.0772636213365));
#199417=CARTESIAN_POINT('Ctrl Pts',(44.0526112349805,-39.2744854109878,
40.0046102245799));
#199418=CARTESIAN_POINT('Ctrl Pts',(44.0109847679681,-39.3564679665376,
39.9670001894009));
#199419=CARTESIAN_POINT('Ctrl Pts',(44.0555161714745,-39.4322155454628,
40.0101788811207));
#199420=CARTESIAN_POINT('Ctrl Pts',(44.1047669487881,-39.2856498807571,
39.9303710930188));
#199421=CARTESIAN_POINT('Ctrl Pts',(44.0421591564547,-39.3789590643325,
39.9058663574113));
#199422=CARTESIAN_POINT('Ctrl Pts',(44.1002097724418,-39.4516641984998,
39.9671344706366));
#199423=CARTESIAN_POINT('Ctrl Pts',(44.1385184650375,-39.316039186369,39.8576902534424));
#199424=CARTESIAN_POINT('Ctrl Pts',(44.054287543984,-39.4103156382732,39.8579948730703));
#199425=CARTESIAN_POINT('Ctrl Pts',(44.1339623850447,-39.4820551873931,
39.92499));
#199426=CARTESIAN_POINT('Origin',(44.2189419720523,-39.3876757945574,39.92499));
#199427=CARTESIAN_POINT('Origin',(45.8594327453956,-40.8647803215175,39.1925554488842));
#199428=CARTESIAN_POINT('Origin',(45.7986150108451,-40.8100197873548,39.3343017080178));
#199429=CARTESIAN_POINT('Origin',(44.3513327444874,-39.5068809815262,39.6398955069214));
#199430=CARTESIAN_POINT('Origin',(44.4837235168756,-39.6260861683718,39.3548010137695));
#199431=CARTESIAN_POINT('Ctrl Pts',(45.5534068532511,-40.5892333705623,
39.3978017080178));
#199432=CARTESIAN_POINT('Ctrl Pts',(45.4684272662435,-40.6836127633979,
39.3978017080178));
#199433=CARTESIAN_POINT('Ctrl Pts',(45.4684272662435,-40.683612763398,39.5248017080178));
#199434=CARTESIAN_POINT('Ctrl Pts',(45.6201409680063,-40.6496361736986,
39.3978017080178));
#199435=CARTESIAN_POINT('Ctrl Pts',(45.5352552698599,-40.7437849681286,
39.3980355775196));
#199436=CARTESIAN_POINT('Ctrl Pts',(45.5687622694472,-40.7739548060672,
39.5248015517192));
#199437=CARTESIAN_POINT('Ctrl Pts',(45.6832443225597,-40.7067502157879,
39.3484893995498));
#199438=CARTESIAN_POINT('Ctrl Pts',(45.5987613682844,-40.8009661159867,
39.3489438303423));
#199439=CARTESIAN_POINT('Ctrl Pts',(45.6636361529341,-40.8593796344571,
39.4508333155601));
#199440=CARTESIAN_POINT('Ctrl Pts',(45.7165002428306,-40.7368493365298,
39.2708017080178));
#199441=CARTESIAN_POINT('Ctrl Pts',(45.6322662944332,-40.8311340869938,
39.2710850691866));
#199442=CARTESIAN_POINT('Ctrl Pts',(45.7136354238375,-40.9043991801904,
39.3343017080178));
#199443=CARTESIAN_POINT('Origin',(45.5534068532511,-40.5892333705623,39.5248017080178));
#199444=CARTESIAN_POINT('Ctrl Pts',(44.4033023070489,-39.5544469813071,
39.2875012672119));
#199445=CARTESIAN_POINT('Ctrl Pts',(44.3189410241795,-39.6488649595835,
39.2878045257519));
#199446=CARTESIAN_POINT('Ctrl Pts',(44.3988635552003,-39.7205730817651,
39.3549015218346));
#199447=CARTESIAN_POINT('Ctrl Pts',(44.4888328647691,-39.6312929306947,
39.1034938540228));
#199448=CARTESIAN_POINT('Ctrl Pts',(44.4042668857107,-39.7256930794144,
39.1038286278794));
#199449=CARTESIAN_POINT('Ctrl Pts',(44.4671969296255,-39.7821007282721,
39.2077506434035));
#199450=CARTESIAN_POINT('Ctrl Pts',(44.6424847942248,-39.7693444365338,
38.989));
#199451=CARTESIAN_POINT('Ctrl Pts',(44.5576736780985,-39.8638218465935,
38.9892298954635));
#199452=CARTESIAN_POINT('Ctrl Pts',(44.5899547640672,-39.8926323785399,
39.1161900347286));
#199453=CARTESIAN_POINT('Ctrl Pts',(44.8038810887674,-39.9143573409157,
38.989));
#199454=CARTESIAN_POINT('Ctrl Pts',(44.7187742083306,-40.008878107427,38.989));
#199455=CARTESIAN_POINT('Ctrl Pts',(44.7189015969554,-40.008736628026,39.1161900945643));
#199456=CARTESIAN_POINT('Origin',(44.8038810887674,-39.9143573409157,39.116));
#199457=CARTESIAN_POINT('Origin',(33.7433098572246,-29.9553742717902,39.5248017080178));
#199458=CARTESIAN_POINT('Origin',(45.4410373245171,-40.4880553924344,39.5248017080178));
#199459=CARTESIAN_POINT('Origin',(33.6129634723596,-29.8380098596982,39.116));
#199460=CARTESIAN_POINT('Origin',(45.1021848870409,-40.1828829233545,39.1160402713845));
#199461=CARTESIAN_POINT('Ctrl Pts',(45.2779489569772,-40.3404336838193,
39.2708017080178));
#199462=CARTESIAN_POINT('Ctrl Pts',(45.1929563204589,-40.4355776097269,
39.27051194648));
#199463=CARTESIAN_POINT('Ctrl Pts',(45.1108495273512,-40.3616483211485,
39.3343017080178));
#199464=CARTESIAN_POINT('Ctrl Pts',(45.3113153943832,-40.370636648342,39.3487519301186));
#199465=CARTESIAN_POINT('Ctrl Pts',(45.2262248134205,-40.465532695337,39.3482879463991));
#199466=CARTESIAN_POINT('Ctrl Pts',(45.1610177711089,-40.4068200107232,
39.4512271261626));
#199467=CARTESIAN_POINT('Ctrl Pts',(45.3745283705085,-40.4278556061229,
39.3978017080178));
#199468=CARTESIAN_POINT('Ctrl Pts',(45.2893279449735,-40.5223510101945,
39.3975673827364));
#199469=CARTESIAN_POINT('Ctrl Pts',(45.2560606910578,-40.492397040227,39.524801535518));
#199470=CARTESIAN_POINT('Ctrl Pts',(45.4410373245171,-40.4880553924344,
39.3978017080178));
#199471=CARTESIAN_POINT('Ctrl Pts',(45.3560577375095,-40.58243478527,39.3978017080178));
#199472=CARTESIAN_POINT('Ctrl Pts',(45.3560577375095,-40.58243478527,39.5248017080178));
#199473=CARTESIAN_POINT('Origin',(45.1958291143588,-40.2672689283128,39.3343017080178));
#199474=CARTESIAN_POINT('Origin',(45.1353740846438,-40.2128349746504,39.1934008533557));
#199475=CARTESIAN_POINT('Origin',(40.8647803224533,-45.8594327460076,39.1925554495083));
#199476=CARTESIAN_POINT('Origin',(40.8943347850522,-45.8923335519897,39.1160373285272));
#199477=CARTESIAN_POINT('Origin',(40.8100197873546,-45.7986150108452,39.3343017080178));
#199478=CARTESIAN_POINT('Ctrl Pts',(40.7368493365296,-45.7165002428308,
39.2708017080178));
#199479=CARTESIAN_POINT('Ctrl Pts',(40.8311340869937,-45.6322662944333,
39.2710850691866));
#199480=CARTESIAN_POINT('Ctrl Pts',(40.9043991801903,-45.7136354238377,
39.3343017080178));
#199481=CARTESIAN_POINT('Ctrl Pts',(40.7066485019706,-45.6831319408677,
39.3487519293518));
#199482=CARTESIAN_POINT('Ctrl Pts',(40.8008642060144,-45.5986481857943,
39.3492068662913));
#199483=CARTESIAN_POINT('Ctrl Pts',(40.8592275074406,-45.6634671987661,
39.4512271248735));
#199484=CARTESIAN_POINT('Ctrl Pts',(40.6494327168505,-45.6199161851861,
39.3978017080178));
#199485=CARTESIAN_POINT('Ctrl Pts',(40.7435821574126,-45.5350300257468,
39.3980347781192));
#199486=CARTESIAN_POINT('Ctrl Pts',(40.7736504989782,-45.5684243021861,
39.524801535519));
#199487=CARTESIAN_POINT('Ctrl Pts',(40.5892333705622,-45.5534068532512,
39.3978017080178));
#199488=CARTESIAN_POINT('Ctrl Pts',(40.6836127633978,-45.4684272662437,
39.3978017080178));
#199489=CARTESIAN_POINT('Ctrl Pts',(40.6836127633978,-45.4684272662437,
39.5248017080178));
#199490=CARTESIAN_POINT('Origin',(40.5892333705622,-45.5534068532512,39.5248017080178));
#199491=CARTESIAN_POINT('Origin',(-0.235948482089068,-0.212448967518937,
39.116));
#199492=CARTESIAN_POINT('Origin',(41.162931164248,-46.1905628026486,39.116));
#199493=CARTESIAN_POINT('Origin',(-0.235948482089068,-0.212448967518937,
39.5248017080178));
#199494=CARTESIAN_POINT('Origin',(40.4880553924343,-45.4410373245173,39.5248017080178));
#199495=CARTESIAN_POINT('Ctrl Pts',(41.5228599914562,-46.5911245387431,
39.2875012672119));
#199496=CARTESIAN_POINT('Ctrl Pts',(41.6181024670999,-46.5059978322074,
39.287208709576));
#199497=CARTESIAN_POINT('Ctrl Pts',(41.5454735131716,-46.4256208133851,
39.3549016990124));
#199498=CARTESIAN_POINT('Ctrl Pts',(41.4460088704669,-46.5055987918445,
39.1034939173931));
#199499=CARTESIAN_POINT('Ctrl Pts',(41.5410583874238,-46.4204321019783,
39.103169233633));
#199500=CARTESIAN_POINT('Ctrl Pts',(41.4839460439617,-46.3572876358811,
39.2077507202293));
#199501=CARTESIAN_POINT('Ctrl Pts',(41.3079491749537,-46.3519544194652,
38.989));
#199502=CARTESIAN_POINT('Ctrl Pts',(41.4027599825089,-46.2668368728713,
38.988776931117));
#199503=CARTESIAN_POINT('Ctrl Pts',(41.3734144470997,-46.234529860773,39.1161898712918));
#199504=CARTESIAN_POINT('Ctrl Pts',(41.162931164248,-46.1905628026486,38.989));
#199505=CARTESIAN_POINT('Ctrl Pts',(41.2574515555201,-46.1054562600785,
38.989));
#199506=CARTESIAN_POINT('Ctrl Pts',(41.2573104519183,-46.1055833103323,
39.1161895903857));
#199507=CARTESIAN_POINT('Origin',(41.4512020416173,-46.5107200467158,39.3548010137695));
#199508=CARTESIAN_POINT('Ctrl Pts',(40.4880553924343,-45.4410373245172,
39.3978017080178));
#199509=CARTESIAN_POINT('Ctrl Pts',(40.5824347852699,-45.3560577375097,
39.3978017080178));
#199510=CARTESIAN_POINT('Ctrl Pts',(40.5824347852699,-45.3560577375097,
39.5248017080178));
#199511=CARTESIAN_POINT('Ctrl Pts',(40.4276521486881,-45.3743035899551,
39.3978017080178));
#199512=CARTESIAN_POINT('Ctrl Pts',(40.5221480763004,-45.2891025640488,
39.3975666025036));
#199513=CARTESIAN_POINT('Ctrl Pts',(40.4920927345059,-45.2557227253158,
39.5248015517196));
#199514=CARTESIAN_POINT('Ctrl Pts',(40.370534927875,-45.3112030195541,39.3484894016716));
#199515=CARTESIAN_POINT('Ctrl Pts',(40.4654317778746,-45.2261127332183,
39.3480259000047));
#199516=CARTESIAN_POINT('Ctrl Pts',(40.4066678844406,-45.1608488177559,
39.4508333188937));
#199517=CARTESIAN_POINT('Ctrl Pts',(40.3404336838192,-45.2779489569773,
39.2708017080178));
#199518=CARTESIAN_POINT('Ctrl Pts',(40.4355776097268,-45.192956320459,39.27051194648));
#199519=CARTESIAN_POINT('Ctrl Pts',(40.3616483211483,-45.1108495273513,
39.3343017080178));
#199520=CARTESIAN_POINT('Origin',(40.2672689283127,-45.1958291143589,39.3343017080178));
#199521=CARTESIAN_POINT('Origin',(41.5704070646291,-46.64311063707,39.639895506819));
#199522=CARTESIAN_POINT('Origin',(41.689612087467,-46.7755012272974,39.92499));
#199523=CARTESIAN_POINT('Origin',(40.2128349741407,-45.1353740836146,39.1934008539941));
#199524=CARTESIAN_POINT('Origin',(40.182882923354,-45.1021848870412,39.1160402713849));
#199525=CARTESIAN_POINT('Ctrl Pts',(42.1132001506,-46.7942619810918,40.1599502534424));
#199526=CARTESIAN_POINT('Ctrl Pts',(42.0882450513174,-46.766533016078,40.10025));
#199527=CARTESIAN_POINT('Ctrl Pts',(42.0411527846894,-46.7142062431423,
40.10025));
#199528=CARTESIAN_POINT('Ctrl Pts',(42.0477032750703,-46.8532067119187,
40.1599500538472));
#199529=CARTESIAN_POINT('Ctrl Pts',(42.0405341034511,-46.8094668591672,
40.1002448353499));
#199530=CARTESIAN_POINT('Ctrl Pts',(42.0032346206983,-46.7483190388769,
40.10025));
#199531=CARTESIAN_POINT('Ctrl Pts',(41.9705316734067,-46.8890030154862,
40.120244200104));
#199532=CARTESIAN_POINT('Ctrl Pts',(41.9811230778542,-46.8318174060854,
40.0633873868017));
#199533=CARTESIAN_POINT('Ctrl Pts',(41.9515093836259,-46.7612038509546,
40.0772271723539));
#199534=CARTESIAN_POINT('Ctrl Pts',(41.8426461117365,-46.906368706767,40.0045995998161));
#199535=CARTESIAN_POINT('Ctrl Pts',(41.8933796070866,-46.8290619651512,
39.9663485808314));
#199536=CARTESIAN_POINT('Ctrl Pts',(41.8570065263034,-46.7485125544801,
40.0101727202464));
#199537=CARTESIAN_POINT('Ctrl Pts',(41.7917018131133,-46.8896982576907,
39.930465434986));
#199538=CARTESIAN_POINT('Ctrl Pts',(41.8649047103979,-46.8032976561885,
39.9051900162954));
#199539=CARTESIAN_POINT('Ctrl Pts',(41.8144193983038,-46.7243152668222,
39.9671857458183));
#199540=CARTESIAN_POINT('Ctrl Pts',(41.7612723673362,-46.8559036426986,
39.8576902534424));
#199541=CARTESIAN_POINT('Ctrl Pts',(41.8563683535929,-46.7709043015503,
39.8573998014387));
#199542=CARTESIAN_POINT('Ctrl Pts',(41.7839914803026,-46.6905216402898,
39.92499));
#199543=CARTESIAN_POINT('Origin',(42.0411527846894,-46.7142062431423,40.22725));
#199544=CARTESIAN_POINT('Origin',(-0.235948482089068,-0.212448967518937,
39.116));
#199545=CARTESIAN_POINT('Origin',(39.9143573409156,-44.8038810887675,39.116));
#199546=CARTESIAN_POINT('Origin',(5.55434424446679E-15,5.81742143200459E-15,
40.22725));
#199547=CARTESIAN_POINT('Origin',(42.06380383897,-46.6938111422605,40.22725));
#199548=CARTESIAN_POINT('Ctrl Pts',(39.9143573409156,-44.8038810887675,
38.989));
#199549=CARTESIAN_POINT('Ctrl Pts',(40.0088781183437,-44.7187741985011,
38.989));
#199550=CARTESIAN_POINT('Ctrl Pts',(40.0087366280095,-44.7189015969702,
39.1161901092324));
#199551=CARTESIAN_POINT('Ctrl Pts',(39.7693421853883,-44.6424822887497,
38.989));
#199552=CARTESIAN_POINT('Ctrl Pts',(39.8638196089385,-44.5576711710515,
38.9892298989766));
#199553=CARTESIAN_POINT('Ctrl Pts',(39.8926305794723,-44.5899527660332,
39.1161900493204));
#199554=CARTESIAN_POINT('Ctrl Pts',(39.6312917695235,-44.4888315723763,
39.1034966344367));
#199555=CARTESIAN_POINT('Ctrl Pts',(39.7256919284523,-44.4042655856149,
39.1038314102555));
#199556=CARTESIAN_POINT('Ctrl Pts',(39.7820998051095,-44.4671959043825,
39.2077528789597));
#199557=CARTESIAN_POINT('Ctrl Pts',(39.554446981307,-44.403302307049,39.2875012672119));
#199558=CARTESIAN_POINT('Ctrl Pts',(39.6488649704638,-44.3189410144581,
39.2878045257868));
#199559=CARTESIAN_POINT('Ctrl Pts',(39.7205730900534,-44.3988635644383,
39.35490152959));
#199560=CARTESIAN_POINT('Origin',(39.6260861683717,-44.4837235168757,39.3548010137695));
#199561=CARTESIAN_POINT('Ctrl Pts',(42.2339804752701,-46.4302753505426,
39.8576902534424));
#199562=CARTESIAN_POINT('Ctrl Pts',(42.1395065320998,-46.5159655405276,
39.8573998014387));
#199563=CARTESIAN_POINT('Ctrl Pts',(42.0671296588095,-46.4355828792671,
39.92499));
#199564=CARTESIAN_POINT('Ctrl Pts',(42.2644230274452,-46.4640859592745,
39.9304984902489));
#199565=CARTESIAN_POINT('Ctrl Pts',(42.1708479205168,-46.5278479142009,
39.9052171569801));
#199566=CARTESIAN_POINT('Ctrl Pts',(42.0975714415913,-46.4693919041982,
39.9672049726605));
#199567=CARTESIAN_POINT('Ctrl Pts',(42.2755508889261,-46.51636388123,40.0043437678664));
#199568=CARTESIAN_POINT('Ctrl Pts',(42.1933444849779,-46.5588164356977,
39.9661628577643));
#199569=CARTESIAN_POINT('Ctrl Pts',(42.1170605480851,-46.5141432491637,
40.0100243556237));
#199570=CARTESIAN_POINT('Ctrl Pts',(42.2454039774546,-46.6408663419432,
40.1194874821985));
#199571=CARTESIAN_POINT('Ctrl Pts',(42.1872204559323,-46.6457133039297,
40.062755148314));
#199572=CARTESIAN_POINT('Ctrl Pts',(42.1199995355544,-46.6088541045838,
40.0767884282375));
#199573=CARTESIAN_POINT('Ctrl Pts',(42.2015749714288,-46.7146600431953,
40.1599502015385));
#199574=CARTESIAN_POINT('Ctrl Pts',(42.1587905896505,-46.7029882531943,
40.1002449453872));
#199575=CARTESIAN_POINT('Ctrl Pts',(42.1018187547553,-46.6595535157369,
40.10025));
#199576=CARTESIAN_POINT('Ctrl Pts',(42.1358900227694,-46.7738319284258,
40.1599502534424));
#199577=CARTESIAN_POINT('Ctrl Pts',(42.110921478106,-46.7461150696873,40.10025));
#199578=CARTESIAN_POINT('Ctrl Pts',(42.06380383897,-46.6938111422605,40.10025));
#199579=CARTESIAN_POINT('Origin',(42.1615090516451,-46.3506032922595,39.92499));
#199580=CARTESIAN_POINT('Origin',(39.5068809815359,-44.3513327445003,39.6398955069314));
#199581=CARTESIAN_POINT('Origin',(39.3876757945573,-44.2189419720524,39.92499));
#199582=CARTESIAN_POINT('Origin',(42.0423040287636,-46.2182127020529,39.6398955068275));
#199583=CARTESIAN_POINT('Origin',(41.9230990057955,-46.0858221116779,39.3548010137695));
#199584=CARTESIAN_POINT('Ctrl Pts',(39.3160391863689,-44.1385184650377,
39.8576902534424));
#199585=CARTESIAN_POINT('Ctrl Pts',(39.4103156382731,-44.0542875439841,
39.8579948730703));
#199586=CARTESIAN_POINT('Ctrl Pts',(39.4820551873929,-44.1339623850448,
39.92499));
#199587=CARTESIAN_POINT('Ctrl Pts',(39.285636938894,-44.1047525536513,39.9304020711229));
#199588=CARTESIAN_POINT('Ctrl Pts',(39.3789425853238,-44.0421527706792,
39.905891529738));
#199589=CARTESIAN_POINT('Ctrl Pts',(39.4516512848569,-44.1001954303886,
39.9671523786034));
#199590=CARTESIAN_POINT('Ctrl Pts',(39.2745942850999,-44.0527517782417,
40.0043257306695));
#199591=CARTESIAN_POINT('Ctrl Pts',(39.3566016867496,-44.0110417363798,
39.9667894847838));
#199592=CARTESIAN_POINT('Ctrl Pts',(39.4323285306301,-44.0556530121001,
40.0100138975203));
#199593=CARTESIAN_POINT('Ctrl Pts',(39.3050549810251,-43.9290071509457,
40.1195533054855));
#199594=CARTESIAN_POINT('Ctrl Pts',(39.3631024520342,-43.9243964923859,
40.0630813209234));
#199595=CARTESIAN_POINT('Ctrl Pts',(39.4299498468379,-43.9614781338113,
40.0768265942418));
#199596=CARTESIAN_POINT('Ctrl Pts',(39.3490583909343,-43.8557442421764,
40.1599502027513));
#199597=CARTESIAN_POINT('Ctrl Pts',(39.3917348424054,-43.8675206320107,
40.1002552791541));
#199598=CARTESIAN_POINT('Ctrl Pts',(39.4485000225483,-43.9111340157082,
40.10025));
#199599=CARTESIAN_POINT('Ctrl Pts',(39.4144401478989,-43.7969047596347,
40.1599502534424));
#199600=CARTESIAN_POINT('Ctrl Pts',(39.4393948122687,-43.8246341160486,
40.10025));
#199601=CARTESIAN_POINT('Ctrl Pts',(39.4864862581816,-43.8769616275875,
40.10025));
#199602=CARTESIAN_POINT('Origin',(39.4864862581816,-43.8769616275875,40.22725));
#199603=CARTESIAN_POINT('Ctrl Pts',(41.6348281284261,-45.7656648676107,
38.989));
#199604=CARTESIAN_POINT('Ctrl Pts',(41.5403077290112,-45.8507714175125,
38.989));
#199605=CARTESIAN_POINT('Ctrl Pts',(41.540448840768,-45.8506443599161,39.1161896013264));
#199606=CARTESIAN_POINT('Ctrl Pts',(41.7801793767999,-45.926760978665,38.989));
#199607=CARTESIAN_POINT('Ctrl Pts',(41.6856176794255,-46.0121552117511,
38.9887769275454));
#199608=CARTESIAN_POINT('Ctrl Pts',(41.6565546403139,-45.9795929135655,
39.1161898821845));
#199609=CARTESIAN_POINT('Ctrl Pts',(41.9185498083238,-46.0801233673961,
39.1034967087243));
#199610=CARTESIAN_POINT('Ctrl Pts',(41.8239142817211,-46.1657498592376,
39.1031720232711));
#199611=CARTESIAN_POINT('Ctrl Pts',(41.7670853619614,-46.1023497159511,
39.2077529615));
#199612=CARTESIAN_POINT('Ctrl Pts',(41.995572738225,-46.1654920697613,39.2875012672119));
#199613=CARTESIAN_POINT('Ctrl Pts',(41.9009568069092,-46.2513146407502,
39.2872087095507));
#199614=CARTESIAN_POINT('Ctrl Pts',(41.828611896708,-46.170681855241,39.3549017048226));
#199615=CARTESIAN_POINT('Origin',(41.6348281284261,-45.7656648676107,39.116));
#199616=CARTESIAN_POINT('Origin',(5.70392627685665E-15,5.20911706492846E-15,
40.22725));
#199617=CARTESIAN_POINT('Origin',(39.5091373124621,-43.8565665267057,40.22725));
#199618=CARTESIAN_POINT('Origin',(28.0951675083324,-30.7283483363945,39.116));
#199619=CARTESIAN_POINT('Origin',(41.3663085755633,-45.4673664422111,39.1160373285272));
#199620=CARTESIAN_POINT('Ctrl Pts',(39.4370498736007,-43.7765468711723,
40.1599502534424));
#199621=CARTESIAN_POINT('Ctrl Pts',(39.4620188529809,-43.804263338293,40.10025));
#199622=CARTESIAN_POINT('Ctrl Pts',(39.5091373124622,-43.8565665267057,
40.10025));
#199623=CARTESIAN_POINT('Ctrl Pts',(39.5021785224865,-43.717874483542,40.159950056604));
#199624=CARTESIAN_POINT('Ctrl Pts',(39.509465444133,-43.7615157339673,40.1002551305381));
#199625=CARTESIAN_POINT('Ctrl Pts',(39.5469637653745,-43.8224770900131,
40.10025));
#199626=CARTESIAN_POINT('Ctrl Pts',(39.57885162691,-43.6818502604296,40.1203070619049));
#199627=CARTESIAN_POINT('Ctrl Pts',(39.5685043961841,-43.7389249259232,
40.0637098684502));
#199628=CARTESIAN_POINT('Ctrl Pts',(39.5983821485331,-43.8091917332944,
40.0772636213363));
#199629=CARTESIAN_POINT('Ctrl Pts',(39.7059848156959,-43.6640874258692,
40.0046102245799));
#199630=CARTESIAN_POINT('Ctrl Pts',(39.656016872279,-43.7412697217739,39.9670001894009));
#199631=CARTESIAN_POINT('Ctrl Pts',(39.6923865500763,-43.8212571467117,
40.0101788811209));
#199632=CARTESIAN_POINT('Ctrl Pts',(39.7566878101774,-43.6806424921204,
39.9303710930188));
#199633=CARTESIAN_POINT('Ctrl Pts',(39.6846695243114,-43.7668962219027,
39.9058663574106));
#199634=CARTESIAN_POINT('Ctrl Pts',(39.7348023770065,-43.8452710114192,
39.9671344706366));
#199635=CARTESIAN_POINT('Ctrl Pts',(39.7870778846746,-43.7143933160624,
39.8576902534424));
#199636=CARTESIAN_POINT('Ctrl Pts',(39.69345381678,-43.7993487829614,39.8579948730703));
#199637=CARTESIAN_POINT('Ctrl Pts',(39.7651933658998,-43.8790236240221,
39.92499));
#199638=CARTESIAN_POINT('Origin',(39.8595727587354,-43.7940440370145,39.92499));
#199639=CARTESIAN_POINT('Origin',(41.3366772856869,-45.4345348103663,39.1925554488845));
#199640=CARTESIAN_POINT('Origin',(41.2819167515328,-45.3737170758073,39.3343017080178));
#199641=CARTESIAN_POINT('Origin',(39.9787779456623,-43.9264348094891,39.6398955069222));
#199642=CARTESIAN_POINT('Origin',(40.0979831325498,-44.0588255818379,39.3548010137695));
#199643=CARTESIAN_POINT('Ctrl Pts',(41.0611303347403,-45.1285089182134,
39.3978017080178));
#199644=CARTESIAN_POINT('Ctrl Pts',(40.9667509419047,-45.2134885052209,
39.3978017080178));
#199645=CARTESIAN_POINT('Ctrl Pts',(40.9667509419047,-45.2134885052209,
39.5248017080178));
#199646=CARTESIAN_POINT('Ctrl Pts',(41.1211850608443,-45.1955564429362,
39.3978017080178));
#199647=CARTESIAN_POINT('Ctrl Pts',(41.0269231466362,-45.2803165088384,
39.3980355775172));
#199648=CARTESIAN_POINT('Ctrl Pts',(41.057092984575,-45.3138235084259,39.5248015517192));
#199649=CARTESIAN_POINT('Ctrl Pts',(41.177972685568,-45.2589537050056,39.3484893995498));
#199650=CARTESIAN_POINT('Ctrl Pts',(41.0841042944919,-45.3438226072607,
39.3489438303435));
#199651=CARTESIAN_POINT('Ctrl Pts',(41.1425178129623,-45.4086973919099,
39.4508333155595));
#199652=CARTESIAN_POINT('Ctrl Pts',(41.2079002115907,-45.2923641298558,
39.2708017080178));
#199653=CARTESIAN_POINT('Ctrl Pts',(41.1142722655005,-45.3773275334106,
39.2710850691866));
#199654=CARTESIAN_POINT('Ctrl Pts',(41.1875373586971,-45.4586966628149,
39.3343017080178));
#199655=CARTESIAN_POINT('Origin',(41.0611303347403,-45.1285089182134,39.5248017080178));
#199656=CARTESIAN_POINT('Ctrl Pts',(40.0254908126588,-43.9791725362583,
39.2875012672119));
#199657=CARTESIAN_POINT('Ctrl Pts',(39.9317223035496,-44.0642551277131,
39.2878045257518));
#199658=CARTESIAN_POINT('Ctrl Pts',(40.0037114707678,-44.1439246046465,
39.3549015218347));
#199659=CARTESIAN_POINT('Ctrl Pts',(40.1025202360375,-44.0645378932548,
39.1034938540228));
#199660=CARTESIAN_POINT('Ctrl Pts',(40.0085500157865,-44.149581356248,39.1038286278812));
#199661=CARTESIAN_POINT('Ctrl Pts',(40.0652391174793,-44.2122579788857,
39.2077506434032));
#199662=CARTESIAN_POINT('Ctrl Pts',(40.2409001323908,-44.2178941385635,
38.989));
#199663=CARTESIAN_POINT('Ctrl Pts',(40.1466780419433,-44.3029888158473,
38.9892298954623));
#199664=CARTESIAN_POINT('Ctrl Pts',(40.1757707681161,-44.3350158129981,
39.1161900347288));
#199665=CARTESIAN_POINT('Ctrl Pts',(40.3862543050938,-44.3789831537296,
38.989));
#199666=CARTESIAN_POINT('Ctrl Pts',(40.2917335385824,-44.4640900341666,
38.989));
#199667=CARTESIAN_POINT('Ctrl Pts',(40.2918750179835,-44.4639626455416,
39.1161900945645));
#199668=CARTESIAN_POINT('Origin',(40.3862543050938,-44.3789831537296,39.116));
#199669=CARTESIAN_POINT('Origin',(27.4203375923833,-29.9788737863603,39.5248017080178));
#199670=CARTESIAN_POINT('Origin',(40.9599523566124,-45.0161393894794,39.5248017080178));
#199671=CARTESIAN_POINT('Origin',(27.314662201079,-29.8615093742683,39.116));
#199672=CARTESIAN_POINT('Origin',(40.654855397468,-44.6772189625516,39.1160402713848));
#199673=CARTESIAN_POINT('Ctrl Pts',(40.8131880745606,-44.8522789915942,
39.2708017080178));
#199674=CARTESIAN_POINT('Ctrl Pts',(40.7187157882337,-44.9380175594363,
39.27051194648));
#199675=CARTESIAN_POINT('Ctrl Pts',(40.6447864996552,-44.8559107663286,
39.3343017080178));
#199676=CARTESIAN_POINT('Ctrl Pts',(40.8432146576643,-44.8858042435433,
39.3487519301185));
#199677=CARTESIAN_POINT('Ctrl Pts',(40.7486708738394,-44.9712860523915,
39.3482879463973));
#199678=CARTESIAN_POINT('Ctrl Pts',(40.6899581892273,-44.9060790100834,
39.4512271261623));
#199679=CARTESIAN_POINT('Ctrl Pts',(40.9001003367647,-44.9493173051403,
39.3978017080178));
#199680=CARTESIAN_POINT('Ctrl Pts',(40.8054891887053,-45.034389183955,39.3975673827415));
#199681=CARTESIAN_POINT('Ctrl Pts',(40.7755352187358,-45.0011219300374,
39.5248015355199));
#199682=CARTESIAN_POINT('Ctrl Pts',(40.9599523566124,-45.0161393894794,
39.3978017080178));
#199683=CARTESIAN_POINT('Ctrl Pts',(40.8655729637768,-45.1011189764869,
39.3978017080178));
#199684=CARTESIAN_POINT('Ctrl Pts',(40.8655729637768,-45.101118976487,39.5248017080178));
#199685=CARTESIAN_POINT('Origin',(40.7391658924908,-44.7709311793211,39.3343017080178));
#199686=CARTESIAN_POINT('Origin',(40.684731939279,-44.710476149201,39.1934008533553));
#199687=CARTESIAN_POINT('Origin',(35.8473027488288,-49.8797426639489,39.1925554495083));
#199688=CARTESIAN_POINT('Origin',(35.8732562382987,-49.9155525184317,39.1160373285263));
#199689=CARTESIAN_POINT('Origin',(35.7991993820661,-49.8135340601224,39.3343017080178));
#199690=CARTESIAN_POINT('Ctrl Pts',(35.7350130971388,-49.7242207306176,
39.2708017080178));
#199691=CARTESIAN_POINT('Ctrl Pts',(35.8375861910555,-49.6503036646786,
39.2710850691866));
#199692=CARTESIAN_POINT('Ctrl Pts',(35.9019445403517,-49.7388853330812,
39.3343017080178));
#199693=CARTESIAN_POINT('Ctrl Pts',(35.7084656432366,-49.6878783768789,
39.3487519293518));
#199694=CARTESIAN_POINT('Ctrl Pts',(35.8109961808879,-49.6137056554146,
39.3492068662942));
#199695=CARTESIAN_POINT('Ctrl Pts',(35.8622643302253,-49.6842702092628,
39.4512271248743));
#199696=CARTESIAN_POINT('Ctrl Pts',(35.6581711379713,-49.6190282456268,
39.3978017080178));
#199697=CARTESIAN_POINT('Ctrl Pts',(35.7606778378466,-49.5444483977879,
39.3980347781159));
#199698=CARTESIAN_POINT('Ctrl Pts',(35.78709080949,-49.5808027344244,39.524801535519));
#199699=CARTESIAN_POINT('Ctrl Pts',(35.6052536882601,-49.5465907136145,
39.3978017080178));
#199700=CARTESIAN_POINT('Ctrl Pts',(35.7079988465457,-49.4719419865734,
39.3978017080178));
#199701=CARTESIAN_POINT('Ctrl Pts',(35.7079988465457,-49.4719419865734,
39.5248017080178));
#199702=CARTESIAN_POINT('Origin',(35.6052536882601,-49.5465907136145,39.5248017080178));
#199703=CARTESIAN_POINT('Origin',(-0.256862895714041,-0.18662181760286,
39.116));
#199704=CARTESIAN_POINT('Origin',(36.1092077731528,-50.2402240048084,39.116));
#199705=CARTESIAN_POINT('Origin',(-0.256862895714041,-0.18662181760286,
39.5248017080178));
#199706=CARTESIAN_POINT('Origin',(35.5163757878395,-49.4242607783462,39.5248017080178));
#199707=CARTESIAN_POINT('Ctrl Pts',(36.4252947698678,-50.6762142289949,
39.2875012672119));
#199708=CARTESIAN_POINT('Ctrl Pts',(36.5289136610815,-50.6015094050816,
39.287208709576));
#199709=CARTESIAN_POINT('Ctrl Pts',(36.465084262422,-50.5139809070355,39.3549016990122));
#199710=CARTESIAN_POINT('Ctrl Pts',(36.3578045222547,-50.5831238715082,
39.1034939173931));
#199711=CARTESIAN_POINT('Ctrl Pts',(36.4612356912236,-50.5083591136214,
39.1031692336309));
#199712=CARTESIAN_POINT('Ctrl Pts',(36.4110366091595,-50.4395906940207,
39.2077507202297));
#199713=CARTESIAN_POINT('Ctrl Pts',(36.2365613423298,-50.4158900112683,
38.989));
#199714=CARTESIAN_POINT('Ctrl Pts',(36.3397499727042,-50.3411491755169,
38.9887769311206));
#199715=CARTESIAN_POINT('Ctrl Pts',(36.3139421975387,-50.3059517008895,
39.1161898712915));
#199716=CARTESIAN_POINT('Ctrl Pts',(36.1092077731528,-50.2402240048084,
38.989));
#199717=CARTESIAN_POINT('Ctrl Pts',(36.2121064279403,-50.1654637560306,
38.989));
#199718=CARTESIAN_POINT('Ctrl Pts',(36.2119528169512,-50.165575360947,39.1161895903854));
#199719=CARTESIAN_POINT('Origin',(36.3624339277672,-50.5887599058102,39.3548010137695));
#199720=CARTESIAN_POINT('Ctrl Pts',(35.5163757878395,-49.4242607783461,
39.3978017080178));
#199721=CARTESIAN_POINT('Ctrl Pts',(35.6191209461251,-49.349612051305,39.3978017080178));
#199722=CARTESIAN_POINT('Ctrl Pts',(35.6191209461251,-49.349612051305,39.5248017080178));
#199723=CARTESIAN_POINT('Ctrl Pts',(35.463279014105,-49.3515787599188,39.3978017080178));
#199724=CARTESIAN_POINT('Ctrl Pts',(35.5661632154433,-49.2767219882452,
39.3975666025064));
#199725=CARTESIAN_POINT('Ctrl Pts',(35.5397616632044,-49.2403833690714,
39.5248015517196));
#199726=CARTESIAN_POINT('Ctrl Pts',(35.4130704930576,-49.2828534857283,
39.3484894016717));
#199727=CARTESIAN_POINT('Ctrl Pts',(35.5163418450515,-49.2081487547874,
39.348025900002));
#199728=CARTESIAN_POINT('Ctrl Pts',(35.4647218031673,-49.1370998624016,
39.4508333188939));
#199729=CARTESIAN_POINT('Ctrl Pts',(35.3866101428259,-49.2466351556013,
39.2708017080178));
#199730=CARTESIAN_POINT('Ctrl Pts',(35.4901170100366,-49.1720533660032,
39.27051194648));
#199731=CARTESIAN_POINT('Ctrl Pts',(35.4251752107437,-49.0826686475735,
39.3343017080178));
#199732=CARTESIAN_POINT('Origin',(35.3224300524581,-49.1573173746147,39.3343017080178));
#199733=CARTESIAN_POINT('Origin',(36.4671473482325,-50.7328855645261,39.6398955068185));
#199734=CARTESIAN_POINT('Origin',(36.5718607685321,-50.8770112231003,39.92499));
#199735=CARTESIAN_POINT('Origin',(35.2746135646418,-49.0915036252741,39.193400853995));
#199736=CARTESIAN_POINT('Origin',(35.248294810039,-49.0553654007527,39.1160402713851));
#199737=CARTESIAN_POINT('Ctrl Pts',(36.9911673391707,-50.9399462128202,
40.1599502534424));
#199738=CARTESIAN_POINT('Ctrl Pts',(36.9692474126339,-50.9097606317995,
40.10025));
#199739=CARTESIAN_POINT('Ctrl Pts',(36.9278827595326,-50.8527980281386,
40.10025));
#199740=CARTESIAN_POINT('Ctrl Pts',(36.9198678602471,-50.9917217504954,
40.159950053846));
#199741=CARTESIAN_POINT('Ctrl Pts',(36.9173100216891,-50.9474721267378,
40.100244835349));
#199742=CARTESIAN_POINT('Ctrl Pts',(36.8866065570941,-50.8827604229948,
40.10025));
#199743=CARTESIAN_POINT('Ctrl Pts',(36.8393772800888,-51.019255329238,40.1202442001039));
#199744=CARTESIAN_POINT('Ctrl Pts',(36.8558881875866,-50.96349009182,40.0633873868017));
#199745=CARTESIAN_POINT('Ctrl Pts',(36.8338178466776,-50.890167891183,40.0772271723535));
#199746=CARTESIAN_POINT('Ctrl Pts',(36.7103770798844,-51.0231582082087,
40.0045995998162));
#199747=CARTESIAN_POINT('Ctrl Pts',(36.7689134067395,-50.951578055317,39.9663485808314));
#199748=CARTESIAN_POINT('Ctrl Pts',(36.7411592876131,-50.8676678805073,
40.0101727202468));
#199749=CARTESIAN_POINT('Ctrl Pts',(36.6614543958834,-51.0012539523492,
39.9304654349859));
#199750=CARTESIAN_POINT('Ctrl Pts',(36.7432876021378,-50.9229784487434,
39.9051900162952));
#199751=CARTESIAN_POINT('Ctrl Pts',(36.7013347616514,-50.8391515810796,
39.9671857458171));
#199752=CARTESIAN_POINT('Ctrl Pts',(36.6347241449653,-50.9644637245894,
39.8576902534424));
#199753=CARTESIAN_POINT('Ctrl Pts',(36.7381840359683,-50.8898702560319,
39.8573998014387));
#199754=CARTESIAN_POINT('Ctrl Pts',(36.6746059268177,-50.8023624960592,
39.92499));
#199755=CARTESIAN_POINT('Origin',(36.9278827595326,-50.8527980281386,40.22725));
#199756=CARTESIAN_POINT('Origin',(-0.256862895714041,-0.18662181760286,
39.116));
#199757=CARTESIAN_POINT('Origin',(35.0124214764584,-48.7306271754177,39.116));
#199758=CARTESIAN_POINT('Origin',(5.56775724677592E-15,5.82828306711173E-15,
40.22725));
#199759=CARTESIAN_POINT('Origin',(36.9525415975211,-50.8348823336487,40.22725));
#199760=CARTESIAN_POINT('Ctrl Pts',(35.0124214764584,-48.7306271754177,
38.989));
#199761=CARTESIAN_POINT('Ctrl Pts',(35.115320551631,-48.6558666212124,38.989));
#199762=CARTESIAN_POINT('Ctrl Pts',(35.1151665196293,-48.6559785320122,
39.1161901092325));
#199763=CARTESIAN_POINT('Ctrl Pts',(34.8850714976643,-48.5549543235569,
38.989));
#199764=CARTESIAN_POINT('Ctrl Pts',(34.9878965398057,-48.4804833899301,
38.9892298989718));
#199765=CARTESIAN_POINT('Ctrl Pts',(35.0131753353122,-48.5155997094333,
39.1161900493187));
#199766=CARTESIAN_POINT('Ctrl Pts',(34.7638382096871,-48.3877151240587,
39.1034966344368));
#199767=CARTESIAN_POINT('Ctrl Pts',(34.8665607873104,-48.3134799021662,
39.1038314102594));
#199768=CARTESIAN_POINT('Ctrl Pts',(34.9160816462009,-48.3819617107278,
39.2077528789613));
#199769=CARTESIAN_POINT('Ctrl Pts',(34.6963546279284,-48.2946219293747,
39.2875012672119));
#199770=CARTESIAN_POINT('Ctrl Pts',(34.7990735417353,-48.2205921440829,
39.2878045257868));
#199771=CARTESIAN_POINT('Ctrl Pts',(34.862034655413,-48.3075724095164,39.35490152959));
#199772=CARTESIAN_POINT('Origin',(34.7591950625533,-48.382090917533,39.3548010137695));
#199773=CARTESIAN_POINT('Ctrl Pts',(37.149332979726,-50.5905785208485,39.8576902534424));
#199774=CARTESIAN_POINT('Ctrl Pts',(37.0464195108252,-50.6659240749084,
39.8573998014387));
#199775=CARTESIAN_POINT('Ctrl Pts',(36.9828414016746,-50.5784163149358,
39.92499));
#199776=CARTESIAN_POINT('Ctrl Pts',(37.1760745934432,-50.6273860247244,
39.9304984902492));
#199777=CARTESIAN_POINT('Ctrl Pts',(37.0763471615772,-50.6810174228634,
39.9052171569798));
#199778=CARTESIAN_POINT('Ctrl Pts',(37.0095824157648,-50.6152221632646,
39.96720497266));
#199779=CARTESIAN_POINT('Ctrl Pts',(37.1816769644889,-50.6805407410137,
40.004343767866));
#199780=CARTESIAN_POINT('Ctrl Pts',(37.0954833955433,-50.7141678268707,
39.9661628577643));
#199781=CARTESIAN_POINT('Ctrl Pts',(37.0242869695758,-50.6617655220317,
40.0100243556233));
#199782=CARTESIAN_POINT('Ctrl Pts',(37.138681150061,-50.8012099538926,40.1194874821989));
#199783=CARTESIAN_POINT('Ctrl Pts',(37.0803097184689,-50.799948529622,40.0627551483141));
#199784=CARTESIAN_POINT('Ctrl Pts',(37.0173098767915,-50.7562647493197,
40.0767884282379));
#199785=CARTESIAN_POINT('Ctrl Pts',(37.0873787017263,-50.8700180268817,
40.1599502015399));
#199786=CARTESIAN_POINT('Ctrl Pts',(37.0460487315422,-50.8539379904903,
40.1002449453869));
#199787=CARTESIAN_POINT('Ctrl Pts',(36.9939291606774,-50.8047860147175,
40.10025));
#199788=CARTESIAN_POINT('Ctrl Pts',(37.0158684358559,-50.9219998155901,
40.1599502534424));
#199789=CARTESIAN_POINT('Ctrl Pts',(36.9939338721432,-50.8918248691001,
40.10025));
#199790=CARTESIAN_POINT('Ctrl Pts',(36.9525415975211,-50.8348823336487,
40.10025));
#199791=CARTESIAN_POINT('Origin',(37.0855865599602,-50.5037675878946,39.92499));
#199792=CARTESIAN_POINT('Origin',(34.6544814981912,-48.2379650606676,39.6398955069316));
#199793=CARTESIAN_POINT('Origin',(34.549767933694,-48.0938392037149,39.92499));
#199794=CARTESIAN_POINT('Origin',(36.980873139611,-50.35964192934,39.6398955068268));
#199795=CARTESIAN_POINT('Origin',(36.8761597191953,-50.2155162706045,39.3548010137695));
#199796=CARTESIAN_POINT('Ctrl Pts',(34.4869303039396,-48.0063682005188,
39.8576902534424));
#199797=CARTESIAN_POINT('Ctrl Pts',(34.5894948283132,-47.9324532779038,
39.8579948730703));
#199798=CARTESIAN_POINT('Ctrl Pts',(34.6525130919796,-48.0191904766737,
39.92499));
#199799=CARTESIAN_POINT('Ctrl Pts',(34.4602241019854,-47.9696093621194,
39.9304020711232));
#199800=CARTESIAN_POINT('Ctrl Pts',(34.5595620694348,-47.9171056031439,
39.9058915297378));
#199801=CARTESIAN_POINT('Ctrl Pts',(34.6258053530817,-47.982430427718,39.9671523786029));
#199802=CARTESIAN_POINT('Ctrl Pts',(34.4546775021467,-47.9167391807672,
40.0043257306691));
#199803=CARTESIAN_POINT('Ctrl Pts',(34.5405955452487,-47.8838297385501,
39.9667894847831));
#199804=CARTESIAN_POINT('Ctrl Pts',(34.611244401459,-47.9361122396534,40.01001389752));
#199805=CARTESIAN_POINT('Ctrl Pts',(34.4979061669209,-47.796856449222,40.1195533054859));
#199806=CARTESIAN_POINT('Ctrl Pts',(34.5561175928638,-47.7983386612733,
40.0630813209239));
#199807=CARTESIAN_POINT('Ctrl Pts',(34.6187227036512,-47.8422046210389,
40.0768265942421));
#199808=CARTESIAN_POINT('Ctrl Pts',(34.5493265808148,-47.7285944911488,
40.1599502027517));
#199809=CARTESIAN_POINT('Ctrl Pts',(34.5905382782863,-47.7447672725759,
40.1002552791544));
#199810=CARTESIAN_POINT('Ctrl Pts',(34.6424336528575,-47.7940753146429,
40.10025));
#199811=CARTESIAN_POINT('Ctrl Pts',(34.6205005703634,-47.6769115920305,
40.1599502534424));
#199812=CARTESIAN_POINT('Ctrl Pts',(34.6424200234574,-47.7070975168465,
40.10025));
#199813=CARTESIAN_POINT('Ctrl Pts',(34.6837837831345,-47.7640607692764,
40.10025));
#199814=CARTESIAN_POINT('Origin',(34.6837837831345,-47.7640607692764,40.22725));
#199815=CARTESIAN_POINT('Ctrl Pts',(36.6229335645808,-49.8669803696027,
38.989));
#199816=CARTESIAN_POINT('Ctrl Pts',(36.5200349009287,-49.9417406248209,
38.989));
#199817=CARTESIAN_POINT('Ctrl Pts',(36.5201885207956,-49.9416290134544,
39.1161896013263));
#199818=CARTESIAN_POINT('Ctrl Pts',(36.7506494346807,-50.0423873219315,
38.989));
#199819=CARTESIAN_POINT('Ctrl Pts',(36.647679628225,-50.1174293675636,38.988776927546));
#199820=CARTESIAN_POINT('Ctrl Pts',(36.6221794864701,-50.0820075342383,
39.1161898821844));
#199821=CARTESIAN_POINT('Ctrl Pts',(36.872231123687,-50.2093732240185,39.1034967087243));
#199822=CARTESIAN_POINT('Ctrl Pts',(36.7691636147949,-50.2846385388079,
39.1031720232715));
#199823=CARTESIAN_POINT('Ctrl Pts',(36.7192731293496,-50.2156454684929,
39.2077529615002));
#199824=CARTESIAN_POINT('Ctrl Pts',(36.9399086546485,-50.3023253561996,
39.2875012672119));
#199825=CARTESIAN_POINT('Ctrl Pts',(36.8368401378453,-50.3777877242638,
39.2872087095508));
#199826=CARTESIAN_POINT('Ctrl Pts',(36.7733199617899,-50.2900345513019,
39.3549017048226));
#199827=CARTESIAN_POINT('Origin',(36.6229335645808,-49.8669803696026,39.116));
#199828=CARTESIAN_POINT('Origin',(5.69915478234096E-15,5.20525318485518E-15,
40.22725));
#199829=CARTESIAN_POINT('Origin',(34.7084426211231,-47.7461450747865,40.22725));
#199830=CARTESIAN_POINT('Origin',(21.7541926348211,-29.4019141737116,39.116));
#199831=CARTESIAN_POINT('Origin',(36.3870656659257,-49.5422481179703,39.1160373285258));
#199832=CARTESIAN_POINT('Ctrl Pts',(34.6451144164185,-47.6590285860936,
40.1599502534424));
#199833=CARTESIAN_POINT('Ctrl Pts',(34.6670494534017,-47.6892031885514,
40.10025));
#199834=CARTESIAN_POINT('Ctrl Pts',(34.7084426211231,-47.7461450747865,
40.10025));
#199835=CARTESIAN_POINT('Ctrl Pts',(34.7160192182665,-47.6074854095245,
40.1599500566037));
#199836=CARTESIAN_POINT('Ctrl Pts',(34.718704468552,-47.6516492793353,40.1002551305372));
#199837=CARTESIAN_POINT('Ctrl Pts',(34.7496251732003,-47.7161963245896,
40.10025));
#199838=CARTESIAN_POINT('Ctrl Pts',(34.7960378560836,-47.5796730526551,
40.1203070619048));
#199839=CARTESIAN_POINT('Ctrl Pts',(34.7797813814945,-47.6353534770325,
40.0637098684496));
#199840=CARTESIAN_POINT('Ctrl Pts',(34.8021505789969,-47.7083584310193,
40.0772636213363));
#199841=CARTESIAN_POINT('Ctrl Pts',(34.9243313177593,-47.5752965616148,
40.00461022458));
#199842=CARTESIAN_POINT('Ctrl Pts',(34.8665693571826,-47.6468329724886,
39.9670001894015));
#199843=CARTESIAN_POINT('Ctrl Pts',(34.8943788354697,-47.7301838844735,
40.0101788811209));
#199844=CARTESIAN_POINT('Ctrl Pts',(34.973026080298,-47.5970608435766,39.9303710930188));
#199845=CARTESIAN_POINT('Ctrl Pts',(34.8923863483134,-47.6753141056561,
39.9058663574116));
#199846=CARTESIAN_POINT('Ctrl Pts',(34.9340521716871,-47.7584998599249,
39.9671344706372));
#199847=CARTESIAN_POINT('Ctrl Pts',(34.9997217530259,-47.63380340476,39.8576902534424));
#199848=CARTESIAN_POINT('Ctrl Pts',(34.8977303031701,-47.7085070967804,
39.8579948730703));
#199849=CARTESIAN_POINT('Ctrl Pts',(34.9607485668365,-47.7952442955503,
39.92499));
#199850=CARTESIAN_POINT('Origin',(35.0634937251221,-47.7205955685091,39.92499));
#199851=CARTESIAN_POINT('Origin',(36.3610285393807,-49.5064990280457,39.1925554488851));
#199852=CARTESIAN_POINT('Origin',(36.3129251734942,-49.4402904249166,39.3343017080178));
#199853=CARTESIAN_POINT('Origin',(35.1682072895601,-47.8647214254832,39.6398955069207));
#199854=CARTESIAN_POINT('Origin',(35.2729208539814,-48.0088472823273,39.3548010137695));
#199855=CARTESIAN_POINT('Ctrl Pts',(36.1189794796882,-49.1733470784088,
39.3978017080178));
#199856=CARTESIAN_POINT('Ctrl Pts',(36.0162343214026,-49.24799580545,39.3978017080178));
#199857=CARTESIAN_POINT('Ctrl Pts',(36.0162343214026,-49.24799580545,39.5248017080178));
#199858=CARTESIAN_POINT('Ctrl Pts',(36.1716968449935,-49.2463047380076,
39.3978017080178));
#199859=CARTESIAN_POINT('Ctrl Pts',(36.0690914679803,-49.3207474263657,
39.3980355775177));
#199860=CARTESIAN_POINT('Ctrl Pts',(36.0955935972132,-49.3572244778974,
39.5248015517192));
#199861=CARTESIAN_POINT('Ctrl Pts',(36.221546562787,-49.3152906263877,39.3484893995498));
#199862=CARTESIAN_POINT('Ctrl Pts',(36.1193211766474,-49.389882689243,39.3489438303423));
#199863=CARTESIAN_POINT('Ctrl Pts',(36.1706334382084,-49.4605079583582,
39.4508333155597));
#199864=CARTESIAN_POINT('Ctrl Pts',(36.247817802325,-49.3516463037386,39.2708017080178));
#199865=CARTESIAN_POINT('Ctrl Pts',(36.1458216659124,-49.4263574835552,
39.2710850691866));
#199866=CARTESIAN_POINT('Ctrl Pts',(36.2101800152086,-49.5149391519578,
39.3343017080178));
#199867=CARTESIAN_POINT('Origin',(36.1189794796882,-49.1733470784088,39.5248017080178));
#199868=CARTESIAN_POINT('Ctrl Pts',(35.2091516650527,-47.9220530736688,
39.2875012672119));
#199869=CARTESIAN_POINT('Ctrl Pts',(35.1070032771119,-47.9968680956252,
39.2878045257518));
#199870=CARTESIAN_POINT('Ctrl Pts',(35.1702703521467,-48.0836260518493,
39.3549015218348));
#199871=CARTESIAN_POINT('Ctrl Pts',(35.2768360036064,-48.0150025575606,
39.1034938540228));
#199872=CARTESIAN_POINT('Ctrl Pts',(35.1744910995523,-48.0897575808465,
39.1038286278812));
#199873=CARTESIAN_POINT('Ctrl Pts',(35.2243181613714,-48.158016479072,39.2077506434027));
#199874=CARTESIAN_POINT('Ctrl Pts',(35.3984277477543,-48.1819833392241,
38.989));
#199875=CARTESIAN_POINT('Ctrl Pts',(35.2958269999289,-48.2567629686459,
38.9892298954605));
#199876=CARTESIAN_POINT('Ctrl Pts',(35.3214126203093,-48.2916555365114,
39.1161900347289));
#199877=CARTESIAN_POINT('Ctrl Pts',(35.5261472678865,-48.357383540212,38.989));
#199878=CARTESIAN_POINT('Ctrl Pts',(35.4232482045983,-48.4321440857828,
38.989));
#199879=CARTESIAN_POINT('Ctrl Pts',(35.4234022246977,-48.4320321836304,
39.1161900945646));
#199880=CARTESIAN_POINT('Origin',(35.5261472678865,-48.357383540212,39.116));
#199881=CARTESIAN_POINT('Origin',(21.2334658618522,-28.6851952578918,39.5248017080178));
#199882=CARTESIAN_POINT('Origin',(36.0301015792676,-49.0510171431404,39.5248017080178));
#199883=CARTESIAN_POINT('Origin',(21.151922343707,-28.5729602337851,39.116));
#199884=CARTESIAN_POINT('Origin',(35.762102804585,-48.6820620414862,39.1160402713848));
#199885=CARTESIAN_POINT('Ctrl Pts',(35.9012693628904,-48.8727133447944,
39.2708017080178));
#199886=CARTESIAN_POINT('Ctrl Pts',(35.7983524848935,-48.9481071848797,
39.27051194648));
#199887=CARTESIAN_POINT('Ctrl Pts',(35.7334106856005,-48.8587224664501,
39.3343017080178));
#199888=CARTESIAN_POINT('Ctrl Pts',(35.9276271141644,-48.9091935744936,
39.3487519301186));
#199889=CARTESIAN_POINT('Ctrl Pts',(35.8246659689634,-48.9843245886171,
39.3482879463969));
#199890=CARTESIAN_POINT('Ctrl Pts',(35.773090910506,-48.9133376106102,39.4512271261627));
#199891=CARTESIAN_POINT('Ctrl Pts',(35.9775622448344,-48.9783048775136,
39.3978017080178));
#199892=CARTESIAN_POINT('Ctrl Pts',(35.8745769537838,-49.0530211657578,
39.3975673827411));
#199893=CARTESIAN_POINT('Ctrl Pts',(35.8482644497259,-49.0168051108904,
39.5248015355194));
#199894=CARTESIAN_POINT('Ctrl Pts',(36.0301015792676,-49.0510171431404,
39.3978017080178));
#199895=CARTESIAN_POINT('Ctrl Pts',(35.927356420982,-49.1256658701816,39.3978017080178));
#199896=CARTESIAN_POINT('Ctrl Pts',(35.927356420982,-49.1256658701816,39.5248017080178));
#199897=CARTESIAN_POINT('Origin',(35.8361558438862,-48.784073739409,39.3343017080178));
#199898=CARTESIAN_POINT('Origin',(35.7883393569609,-48.7182599907918,39.1934008533547));
#199899=CARTESIAN_POINT('Origin',(30.4370746247567,-53.3535596832589,39.1925554495088));
#199900=CARTESIAN_POINT('Origin',(30.4591427892365,-53.3918862459835,39.1160373285291));
#199901=CARTESIAN_POINT('Origin',(30.3961554568836,-53.2826856060846,39.3343017080178));
#199902=CARTESIAN_POINT('Ctrl Pts',(30.3416565762235,-53.1871522506176,
39.2708017080178));
#199903=CARTESIAN_POINT('Ctrl Pts',(30.4513942013112,-53.1243619179796,
39.2710850691866));
#199904=CARTESIAN_POINT('Ctrl Pts',(30.5061406831642,-53.2191856060846,
39.3343017080178));
#199905=CARTESIAN_POINT('Ctrl Pts',(30.3190533624391,-53.1482340195353,
39.3487519293518));
#199906=CARTESIAN_POINT('Ctrl Pts',(30.4287753876654,-53.0851849835372,
39.3492068662939));
#199907=CARTESIAN_POINT('Ctrl Pts',(30.4723866803437,-53.1607219582407,
39.4512271248739));
#199908=CARTESIAN_POINT('Ctrl Pts',(30.2762311741517,-53.0745038491598,
39.3978017080178));
#199909=CARTESIAN_POINT('Ctrl Pts',(30.3859720484856,-53.0110474253454,
39.3980347781155));
#199910=CARTESIAN_POINT('Ctrl Pts',(30.4084402641651,-53.0499635164573,
39.524801535519));
#199911=CARTESIAN_POINT('Ctrl Pts',(30.2311753956711,-52.9969317578288,
39.3978017080178));
#199912=CARTESIAN_POINT('Ctrl Pts',(30.3411606219517,-52.9334317578288,
39.3978017080178));
#199913=CARTESIAN_POINT('Ctrl Pts',(30.3411606219517,-52.9334317578288,
39.5248017080178));
#199914=CARTESIAN_POINT('Origin',(30.2311753956711,-52.9969317578288,39.5248017080178));
#199915=CARTESIAN_POINT('Origin',(-0.274963065701554,-0.158749999999999,
39.116));
#199916=CARTESIAN_POINT('Origin',(30.6598643453574,-53.7394427993287,39.116));
#199917=CARTESIAN_POINT('Origin',(-0.274963065701554,-0.158749999999999,
39.5248017080178));
#199918=CARTESIAN_POINT('Origin',(30.1555713378337,-52.865981688396,39.5248017080178));
#199919=CARTESIAN_POINT('Ctrl Pts',(30.9286463962977,-54.2060847114742,
39.2875012672119));
#199920=CARTESIAN_POINT('Ctrl Pts',(31.0395064328261,-54.1426202518668,
39.287208709576));
#199921=CARTESIAN_POINT('Ctrl Pts',(30.9851759176836,-54.048899255138,39.3549016990124));
#199922=CARTESIAN_POINT('Ctrl Pts',(30.8712564593359,-54.1064496608375,
39.1034939173931));
#199923=CARTESIAN_POINT('Ctrl Pts',(30.9819360667855,-54.0429059732659,
39.1031692336342));
#199924=CARTESIAN_POINT('Ctrl Pts',(30.9392002377702,-53.9692670413563,
39.2077507202308));
#199925=CARTESIAN_POINT('Ctrl Pts',(30.7681581606542,-53.9274585619024,
38.989));
#199926=CARTESIAN_POINT('Ctrl Pts',(30.8785940576193,-53.8639133132281,
38.9887769311158));
#199927=CARTESIAN_POINT('Ctrl Pts',(30.8566067980787,-53.8262110069715,
39.11618987129));
#199928=CARTESIAN_POINT('Ctrl Pts',(30.6598643453574,-53.7394427993287,
38.989));
#199929=CARTESIAN_POINT('Ctrl Pts',(30.770013884466,-53.6758479332732,38.989));
#199930=CARTESIAN_POINT('Ctrl Pts',(30.7698494490833,-53.6759428700857,
39.1161895903856));
#199931=CARTESIAN_POINT('Origin',(30.8752713784761,-54.112538724998,39.3548010137695));
#199932=CARTESIAN_POINT('Ctrl Pts',(30.1555713378337,-52.865981688396,39.3978017080178));
#199933=CARTESIAN_POINT('Ctrl Pts',(30.2655565641143,-52.802481688396,39.3978017080178));
#199934=CARTESIAN_POINT('Ctrl Pts',(30.2655565641143,-52.802481688396,39.5248017080178));
#199935=CARTESIAN_POINT('Ctrl Pts',(30.1103627734745,-52.7881477055076,
39.3978017080178));
#199936=CARTESIAN_POINT('Ctrl Pts',(30.2205080277021,-52.7244553345209,
39.397566602504));
#199937=CARTESIAN_POINT('Ctrl Pts',(30.1980495259466,-52.6855560684211,
39.5248015517196));
#199938=CARTESIAN_POINT('Ctrl Pts',(30.0676130472596,-52.7145506960108,
39.3484894016716));
#199939=CARTESIAN_POINT('Ctrl Pts',(30.1781274387069,-52.6510500011263,
39.3480259000035));
#199940=CARTESIAN_POINT('Ctrl Pts',(30.1342168083496,-52.5749945583579,
39.4508333188932));
#199941=CARTESIAN_POINT('Ctrl Pts',(30.0450834959835,-52.6757649139396,
39.2708017080178));
#199942=CARTESIAN_POINT('Ctrl Pts',(30.1558192616,-52.6124111049557,39.27051194648));
#199943=CARTESIAN_POINT('Ctrl Pts',(30.1005764675357,-52.5167277788842,
39.3343017080178));
#199944=CARTESIAN_POINT('Origin',(29.9905912412551,-52.5802277788842,39.3343017080178));
#199945=CARTESIAN_POINT('Origin',(30.9643459342435,-54.2668203812016,39.6398955068181));
#199946=CARTESIAN_POINT('Origin',(31.0534204898633,-54.4211020372439,39.92499));
#199947=CARTESIAN_POINT('Origin',(29.9499161072417,-52.5097763801582,39.1934008539954));
#199948=CARTESIAN_POINT('Origin',(29.9275190026059,-52.4710850656384,39.116040271385));
#199949=CARTESIAN_POINT('Ctrl Pts',(31.4638515574739,-54.527521733972,40.1599502534424));
#199950=CARTESIAN_POINT('Ctrl Pts',(31.4452069629852,-54.4952102564866,
40.10025));
#199951=CARTESIAN_POINT('Ctrl Pts',(31.410023123206,-54.4342359163064,40.10025));
#199952=CARTESIAN_POINT('Ctrl Pts',(31.3875306471682,-54.5715608148713,
40.1599500538469));
#199953=CARTESIAN_POINT('Ctrl Pts',(31.3896121658908,-54.5272862282519,
40.100244835349));
#199954=CARTESIAN_POINT('Ctrl Pts',(31.365841113034,-54.4597196360198,40.10025));
#199955=CARTESIAN_POINT('Ctrl Pts',(31.3046029601556,-54.5905300051366,
40.1202442001039));
#199956=CARTESIAN_POINT('Ctrl Pts',(31.3268524737457,-54.5367961153117,
40.0633873868018));
#199957=CARTESIAN_POINT('Ctrl Pts',(31.3125672934292,-54.4615686025423,
40.0772271723537));
#199958=CARTESIAN_POINT('Ctrl Pts',(31.1759014746041,-54.5809273110395,
40.0045995998162));
#199959=CARTESIAN_POINT('Ctrl Pts',(31.2415992967183,-54.5158579940066,
39.9663485808315));
#199960=CARTESIAN_POINT('Ctrl Pts',(31.2227682191859,-54.4295063924928,
40.0101727202466));
#199961=CARTESIAN_POINT('Ctrl Pts',(31.1295364123887,-54.554029236008,39.9304654349859));
#199962=CARTESIAN_POINT('Ctrl Pts',(31.2191033458799,-54.4847364330952,
39.905190016295));
#199963=CARTESIAN_POINT('Ctrl Pts',(31.1861426211016,-54.3969835118376,
39.9671857458165));
#199964=CARTESIAN_POINT('Ctrl Pts',(31.1067982185534,-54.5146464769138,
39.8576902534424));
#199965=CARTESIAN_POINT('Ctrl Pts',(31.2174884860864,-54.4512761425983,
39.8573998014387));
#199966=CARTESIAN_POINT('Ctrl Pts',(31.1634057161439,-54.3576020372439,
39.92499));
#199967=CARTESIAN_POINT('Origin',(31.410023123206,-54.4342359163064,40.22725));
#199968=CARTESIAN_POINT('Origin',(-0.274963065701554,-0.158749999999999,
39.116));
#199969=CARTESIAN_POINT('Origin',(29.7268821954849,-52.1234703131947,39.116));
#199970=CARTESIAN_POINT('Origin',(5.5822321212813E-15,5.8376831605261E-15,
40.22725));
#199971=CARTESIAN_POINT('Origin',(31.4364195775134,-54.4189959163064,40.22725));
#199972=CARTESIAN_POINT('Ctrl Pts',(29.7268821954848,-52.1234703131947,
38.989));
#199973=CARTESIAN_POINT('Ctrl Pts',(29.8370321846012,-52.0598751873271,
38.989));
#199974=CARTESIAN_POINT('Ctrl Pts',(29.8368672985391,-52.0599703843395,
39.1161901092324));
#199975=CARTESIAN_POINT('Ctrl Pts',(29.6185926664433,-51.9354481180161,
38.989));
#199976=CARTESIAN_POINT('Ctrl Pts',(29.7286387544941,-51.8721332875975,
38.9892298989718));
#199977=CARTESIAN_POINT('Ctrl Pts',(29.7501084152006,-51.909699589875,39.1161900493186));
#199978=CARTESIAN_POINT('Ctrl Pts',(29.5155047636238,-51.7564527430626,
39.1034966344367));
#199979=CARTESIAN_POINT('Ctrl Pts',(29.6254243098799,-51.6933616226663,
39.1038314102593));
#199980=CARTESIAN_POINT('Ctrl Pts',(29.6675155901163,-51.7666446199937,
39.2077528789613));
#199981=CARTESIAN_POINT('Ctrl Pts',(29.4581217525673,-51.6568155675428,
39.2875012672119));
#199982=CARTESIAN_POINT('Ctrl Pts',(29.5680161811093,-51.5939283753694,
39.2878045257868));
#199983=CARTESIAN_POINT('Ctrl Pts',(29.6215404737381,-51.6870133822663,
39.35490152959));
#199984=CARTESIAN_POINT('Origin',(29.5114749418004,-51.7503740054944,39.3548010137695));
#199985=CARTESIAN_POINT('Ctrl Pts',(31.6576696180583,-54.1966007261208,
39.8576902534424));
#199986=CARTESIAN_POINT('Ctrl Pts',(31.5474441649283,-54.2607761425983,
39.8573998014387));
#199987=CARTESIAN_POINT('Ctrl Pts',(31.4933613949858,-54.1671020372439,
39.92499));
#199988=CARTESIAN_POINT('Ctrl Pts',(31.6804173065997,-54.236001854427,39.9304984902492));
#199989=CARTESIAN_POINT('Ctrl Pts',(31.5756301844092,-54.2789150989588,
39.9052171569805));
#199990=CARTESIAN_POINT('Ctrl Pts',(31.5161086602375,-54.2065014563931,
39.9672049726609));
#199991=CARTESIAN_POINT('Ctrl Pts',(31.6804328064621,-54.2894509908545,
40.004343767866));
#199992=CARTESIAN_POINT('Ctrl Pts',(31.5911964272957,-54.3138841827105,
39.9661628577643));
#199993=CARTESIAN_POINT('Ctrl Pts',(31.5258675551963,-54.2543268901839,
40.0100243556238));
#199994=CARTESIAN_POINT('Ctrl Pts',(31.6250591602192,-54.4049648787499,
40.1194874821989));
#199995=CARTESIAN_POINT('Ctrl Pts',(31.5671393481785,-54.397608888651,40.062755148314));
#199996=CARTESIAN_POINT('Ctrl Pts',(31.5090508246496,-54.3475791360314,
40.0767884282374));
#199997=CARTESIAN_POINT('Ctrl Pts',(31.5668453499337,-54.4680334478297,
40.1599502015398));
#199998=CARTESIAN_POINT('Ctrl Pts',(31.5274226111431,-54.4477213412894,
40.1002449453872));
#199999=CARTESIAN_POINT('Ctrl Pts',(31.4807263372353,-54.3933906465337,
40.10025));
#200000=CARTESIAN_POINT('Ctrl Pts',(31.4902932482907,-54.5122556166611,
40.1599502534424));
#200001=CARTESIAN_POINT('Ctrl Pts',(31.4716329851988,-54.479953185448,40.10025));
#200002=CARTESIAN_POINT('Ctrl Pts',(31.4364195775134,-54.4189959163064,
40.10025));
#200003=CARTESIAN_POINT('Origin',(31.6033466212664,-54.1036020372439,39.92499));
#200004=CARTESIAN_POINT('Origin',(29.4224002636353,-51.5960921371865,39.6398955069314));
#200005=CARTESIAN_POINT('Origin',(29.3333255853454,-51.4418102687786,39.92499));
#200006=CARTESIAN_POINT('Origin',(31.5142720655984,-53.9493203812121,39.6398955068274));
#200007=CARTESIAN_POINT('Origin',(31.4251975098792,-53.795038724998,39.3548010137695));
#200008=CARTESIAN_POINT('Ctrl Pts',(29.2799753962461,-51.3482501200166,
39.8576902534424));
#200009=CARTESIAN_POINT('Ctrl Pts',(29.3897042746973,-51.2854610232002,
39.8579948730703));
#200010=CARTESIAN_POINT('Ctrl Pts',(29.443310811626,-51.3783102687785,39.92499));
#200011=CARTESIAN_POINT('Ctrl Pts',(29.2572578385502,-51.3089010921302,
39.9304020711229));
#200012=CARTESIAN_POINT('Ctrl Pts',(29.3615397594609,-51.2670685993237,
39.9058915297382));
#200013=CARTESIAN_POINT('Ctrl Pts',(29.4205918519434,-51.3389598763132,
39.9671523786028));
#200014=CARTESIAN_POINT('Ctrl Pts',(29.2572680623749,-51.2557407616056,
40.0043257306695));
#200015=CARTESIAN_POINT('Ctrl Pts',(29.3461554108688,-51.2319924817688,
39.9667894847835));
#200016=CARTESIAN_POINT('Ctrl Pts',(29.4109522357567,-51.2913733902315,
40.0100138975202));
#200017=CARTESIAN_POINT('Ctrl Pts',(29.3127910737013,-51.1410333861057,
40.1195533054855));
#200018=CARTESIAN_POINT('Ctrl Pts',(29.3705286780144,-51.1485922293424,
40.0630813209237));
#200019=CARTESIAN_POINT('Ctrl Pts',(29.4282055900901,-51.1987619028146,
40.0768265942419));
#200020=CARTESIAN_POINT('Ctrl Pts',(29.3710651187649,-51.0785202710263,
40.1599502027508));
#200021=CARTESIAN_POINT('Ctrl Pts',(29.410360538257,-51.0989122516717,40.1002552791554));
#200022=CARTESIAN_POINT('Ctrl Pts',(29.4568175306717,-51.1533747228777,
40.10025));
#200023=CARTESIAN_POINT('Ctrl Pts',(29.4472515437734,-51.0345602039887,
40.1599502534424));
#200024=CARTESIAN_POINT('Ctrl Pts',(29.4658956314766,-51.0668719738978,
40.10025));
#200025=CARTESIAN_POINT('Ctrl Pts',(29.501078514911,-51.1278468659048,40.10025));
#200026=CARTESIAN_POINT('Origin',(29.501078514911,-51.1278468659048,40.22725));
#200027=CARTESIAN_POINT('Ctrl Pts',(31.2097904767605,-53.4219427993287,
38.989));
#200028=CARTESIAN_POINT('Ctrl Pts',(31.0996409281621,-53.4855376708631,
38.989));
#200029=CARTESIAN_POINT('Ctrl Pts',(31.0998053730487,-53.4854427285636,
39.1161896013271));
#200030=CARTESIAN_POINT('Ctrl Pts',(31.3184716867874,-53.609738797656,38.989));
#200031=CARTESIAN_POINT('Ctrl Pts',(31.2082219299917,-53.6736064794771,
38.988776927543));
#200032=CARTESIAN_POINT('Ctrl Pts',(31.1865640704867,-53.6357132000289,
39.1161898821828));
#200033=CARTESIAN_POINT('Ctrl Pts',(31.4219325588463,-53.7885186806134,
39.1034967087243));
#200034=CARTESIAN_POINT('Ctrl Pts',(31.3115622968597,-53.8525981958206,
39.1031720232726));
#200035=CARTESIAN_POINT('Ctrl Pts',(31.269156856333,-53.7787681009861,39.2077529615015));
#200036=CARTESIAN_POINT('Ctrl Pts',(31.4795232016789,-53.8880358395971,
39.2875012672119));
#200037=CARTESIAN_POINT('Ctrl Pts',(31.369131339626,-53.9523112232409,39.2872087095507));
#200038=CARTESIAN_POINT('Ctrl Pts',(31.3151318380581,-53.8583991049518,
39.354901704823));
#200039=CARTESIAN_POINT('Origin',(31.2097904767605,-53.4219427993287,39.116));
#200040=CARTESIAN_POINT('Origin',(5.69400554112516E-15,5.20190922851043E-15,
40.22725));
#200041=CARTESIAN_POINT('Origin',(29.5274749692184,-51.1126068659048,40.22725));
#200042=CARTESIAN_POINT('Origin',(15.8305769983922,-26.7843636743467,39.116));
#200043=CARTESIAN_POINT('Origin',(31.0091584503693,-53.0743345559677,39.1160373285256));
#200044=CARTESIAN_POINT('Ctrl Pts',(29.4735998357337,-51.0193480105328,
40.1599502534424));
#200045=CARTESIAN_POINT('Ctrl Pts',(29.4922606054645,-51.0516501490687,
40.10025));
#200046=CARTESIAN_POINT('Ctrl Pts',(29.5274749692184,-51.1126068659048,
40.10025));
#200047=CARTESIAN_POINT('Ctrl Pts',(29.5495039426969,-50.9754987628534,
40.1599500566039));
#200048=CARTESIAN_POINT('Ctrl Pts',(29.5475581014577,-51.019701383452,40.1002551305372));
#200049=CARTESIAN_POINT('Ctrl Pts',(29.5715624157998,-51.0871269269751,
40.10025));
#200050=CARTESIAN_POINT('Ctrl Pts',(29.6319914129672,-50.956202990229,40.1203070619044));
#200051=CARTESIAN_POINT('Ctrl Pts',(29.6100038038528,-51.0098791271087,
40.0637098684496));
#200052=CARTESIAN_POINT('Ctrl Pts',(29.6246193648995,-51.0848223701583,
40.077263621336));
#200053=CARTESIAN_POINT('Ctrl Pts',(29.7600395375189,-50.9652607924604,
40.0046102245804));
#200054=CARTESIAN_POINT('Ctrl Pts',(29.6951164119093,-51.0303675504162,
39.9670001894015));
#200055=CARTESIAN_POINT('Ctrl Pts',(29.7140610042231,-51.1161687394138,
40.0101788811211));
#200056=CARTESIAN_POINT('Ctrl Pts',(29.8061925581062,-50.9919958361061,
39.9303710930185));
#200057=CARTESIAN_POINT('Ctrl Pts',(29.7178148857788,-51.0613912713643,
39.9058663574108));
#200058=CARTESIAN_POINT('Ctrl Pts',(29.7505571803536,-51.1484765898558,
39.9671344706362));
#200059=CARTESIAN_POINT('Ctrl Pts',(29.8289013456884,-51.0313275753409,
39.8576902534424));
#200060=CARTESIAN_POINT('Ctrl Pts',(29.7196599535391,-51.0949610232002,
39.8579948730703));
#200061=CARTESIAN_POINT('Ctrl Pts',(29.7732664904679,-51.1878102687786,
39.92499));
#200062=CARTESIAN_POINT('Origin',(29.8832517167485,-51.1243102687785,39.92499));
#200063=CARTESIAN_POINT('Origin',(30.9870007553618,-53.0360596824716,39.1925554488848));
#200064=CARTESIAN_POINT('Origin',(30.9460815882867,-52.9651856060847,39.3343017080178));
#200065=CARTESIAN_POINT('Origin',(29.9723263949823,-51.2785921372022,39.6398955069223));
#200066=CARTESIAN_POINT('Origin',(30.0614010732035,-51.4328740054944,39.3548010137695));
#200067=CARTESIAN_POINT('Ctrl Pts',(30.7811015270742,-52.6794317578288,
39.3978017080178));
#200068=CARTESIAN_POINT('Ctrl Pts',(30.6711163007936,-52.7429317578288,
39.3978017080178));
#200069=CARTESIAN_POINT('Ctrl Pts',(30.6711163007936,-52.7429317578288,
39.5248017080178));
#200070=CARTESIAN_POINT('Ctrl Pts',(30.8259039490945,-52.7575002129179,
39.3978017080178));
#200071=CARTESIAN_POINT('Ctrl Pts',(30.7160792752579,-52.820809914058,39.3980355775196));
#200072=CARTESIAN_POINT('Ctrl Pts',(30.7386233329129,-52.8598573673276,
39.5248015517192));
#200073=CARTESIAN_POINT('Ctrl Pts',(30.8682695960185,-52.8313189037786,
39.3484893995498));
#200074=CARTESIAN_POINT('Ctrl Pts',(30.7588072175367,-52.8948168809884,
39.3489438303406));
#200075=CARTESIAN_POINT('Ctrl Pts',(30.8024560343124,-52.9704188493359,
39.4508333155592));
#200076=CARTESIAN_POINT('Ctrl Pts',(30.8905967158735,-52.8702215132217,
39.2708017080178));
#200077=CARTESIAN_POINT('Ctrl Pts',(30.7813498801531,-52.9338619179796,
39.2710850691866));
#200078=CARTESIAN_POINT('Ctrl Pts',(30.8360963620061,-53.0286856060847,
39.3343017080178));
#200079=CARTESIAN_POINT('Origin',(30.7811015270742,-52.6794317578288,39.5248017080178));
#200080=CARTESIAN_POINT('Ctrl Pts',(30.0070536838157,-51.3398895692698,
39.2875012672119));
#200081=CARTESIAN_POINT('Ctrl Pts',(29.8976445761572,-51.4036173326914,
39.2878045257519));
#200082=CARTESIAN_POINT('Ctrl Pts',(29.9514963916954,-51.4965132298826,
39.354901521835));
#200083=CARTESIAN_POINT('Ctrl Pts',(30.0646513737714,-51.4394048060578,
39.1034938540228));
#200084=CARTESIAN_POINT('Ctrl Pts',(29.9550530981044,-51.5030523579581,
39.1038286278815));
#200085=CARTESIAN_POINT('Ctrl Pts',(29.9974722043256,-51.576145673001,39.2077506434039));
#200086=CARTESIAN_POINT('Ctrl Pts',(30.1681227811155,-51.6181806476923,
38.989));
#200087=CARTESIAN_POINT('Ctrl Pts',(30.0582674911768,-51.6818259279801,
38.9892298954593));
#200088=CARTESIAN_POINT('Ctrl Pts',(30.0800656843532,-51.7192017762879,
39.1161900347276));
#200089=CARTESIAN_POINT('Ctrl Pts',(30.276808326888,-51.8059703131947,38.989));
#200090=CARTESIAN_POINT('Ctrl Pts',(30.166658350493,-51.8695654317175,38.989));
#200091=CARTESIAN_POINT('Ctrl Pts',(30.1668232238147,-51.8694702420609,
39.116190094565));
#200092=CARTESIAN_POINT('Origin',(30.276808326888,-51.8059703131947,39.116));
#200093=CARTESIAN_POINT('Origin',(15.4537755657014,-26.1317244485615,39.5248017080178));
#200094=CARTESIAN_POINT('Origin',(30.7054974692368,-52.548481688396,39.5248017080178));
#200095=CARTESIAN_POINT('Origin',(15.3947701216591,-26.0295240215571,39.116));
#200096=CARTESIAN_POINT('Origin',(30.4775331296737,-52.1535342613181,39.1160402713845));
#200097=CARTESIAN_POINT('Ctrl Pts',(30.5960088312567,-52.3576880233163,
39.2708017080178));
#200098=CARTESIAN_POINT('Ctrl Pts',(30.4857749404419,-52.4219111049557,
39.27051194648));
#200099=CARTESIAN_POINT('Ctrl Pts',(30.4305321463775,-52.3262277788842,
39.3343017080178));
#200100=CARTESIAN_POINT('Ctrl Pts',(30.6184089696605,-52.3967235457366,
39.3487519301185));
#200101=CARTESIAN_POINT('Ctrl Pts',(30.5081585269353,-52.4606806140183,
39.348287946398));
#200102=CARTESIAN_POINT('Ctrl Pts',(30.4642861617686,-52.3846914485009,
39.4512271261629));
#200103=CARTESIAN_POINT('Ctrl Pts',(30.6608464521624,-52.4706758922784,
39.3978017080178));
#200104=CARTESIAN_POINT('Ctrl Pts',(30.5506153465204,-52.5342179826664,
39.3975673827401));
#200105=CARTESIAN_POINT('Ctrl Pts',(30.5282325936734,-52.4954499175227,
39.5248015355194));
#200106=CARTESIAN_POINT('Ctrl Pts',(30.7054974692368,-52.548481688396,39.3978017080178));
#200107=CARTESIAN_POINT('Ctrl Pts',(30.5955122429562,-52.611981688396,39.3978017080178));
#200108=CARTESIAN_POINT('Ctrl Pts',(30.5955122429562,-52.611981688396,39.5248017080178));
#200109=CARTESIAN_POINT('Origin',(30.5405173726582,-52.2627277788842,39.3343017080178));
#200110=CARTESIAN_POINT('Origin',(30.4998422394562,-52.1922763809696,39.1934008533555));
#200111=CARTESIAN_POINT('Origin',(24.6933715417282,-56.2428239377257,39.1925554495077));
#200112=CARTESIAN_POINT('Origin',(24.7113125977915,-56.2832472948485,39.1160373285247));
#200113=CARTESIAN_POINT('Origin',(24.660084891711,-56.1680608984279,39.3343017080178));
#200114=CARTESIAN_POINT('Ctrl Pts',(24.6158705164593,-56.0673542004326,
39.2708017080178));
#200115=CARTESIAN_POINT('Ctrl Pts',(24.7315703643334,-56.0163785451198,
39.2710850691866));
#200116=CARTESIAN_POINT('Ctrl Pts',(24.7761051648316,-56.1164053447572,
39.3343017080178));
#200117=CARTESIAN_POINT('Ctrl Pts',(24.5974591883334,-56.0262864882904,
39.3487519293518));
#200118=CARTESIAN_POINT('Ctrl Pts',(24.7131705636691,-55.9750519161932,
39.3492068662935));
#200119=CARTESIAN_POINT('Ctrl Pts',(24.748647185237,-56.0547337128505,39.4512271248753));
#200120=CARTESIAN_POINT('Ctrl Pts',(24.5625784858799,-55.9484840819673,
39.3978017080178));
#200121=CARTESIAN_POINT('Ctrl Pts',(24.6783511906875,-55.8968463240328,
39.3980347781164));
#200122=CARTESIAN_POINT('Ctrl Pts',(24.6966284839296,-55.9378977967835,
39.5248015355176));
#200123=CARTESIAN_POINT('Ctrl Pts',(24.525878019167,-55.8666273273833,39.3978017080178));
#200124=CARTESIAN_POINT('Ctrl Pts',(24.6418982922876,-55.8149717737127,
39.3978017080178));
#200125=CARTESIAN_POINT('Ctrl Pts',(24.6418982922876,-55.8149717737127,
39.5248017080178));
#200126=CARTESIAN_POINT('Origin',(24.525878019167,-55.8666273273833,39.5248017080178));
#200127=CARTESIAN_POINT('Origin',(-0.290050682801521,-0.129138884176566,
39.116));
#200128=CARTESIAN_POINT('Origin',(24.8746050278051,-56.6498810128382,39.116));
#200129=CARTESIAN_POINT('Origin',(-0.29005068280152,-0.129138884176566,
39.5248017080178));
#200130=CARTESIAN_POINT('Origin',(24.4643761377916,-55.7284918401499,39.5248017080178));
#200131=CARTESIAN_POINT('Ctrl Pts',(25.0931373005745,-57.1420619865022,
39.2875012672119));
#200132=CARTESIAN_POINT('Ctrl Pts',(25.210023876658,-57.090533221101,39.287208709576));
#200133=CARTESIAN_POINT('Ctrl Pts',(25.1657875015263,-56.9916465525422,
39.3549016990123));
#200134=CARTESIAN_POINT('Ctrl Pts',(25.0464764504219,-57.0369738651805,
39.103493917393));
#200135=CARTESIAN_POINT('Ctrl Pts',(25.1631918674162,-56.9853474458573,
39.1031692336327));
#200136=CARTESIAN_POINT('Ctrl Pts',(25.1283875141308,-56.9076448051896,
39.207750720231));
#200137=CARTESIAN_POINT('Ctrl Pts',(24.9626525995183,-56.8481865914868,
38.989));
#200138=CARTESIAN_POINT('Ctrl Pts',(25.0791258042758,-56.7965331449343,
38.9887769311182));
#200139=CARTESIAN_POINT('Ctrl Pts',(25.0611999573799,-56.7567390814041,
39.1161898712898));
#200140=CARTESIAN_POINT('Ctrl Pts',(24.8746050278051,-56.6498810128382,
38.989));
#200141=CARTESIAN_POINT('Ctrl Pts',(24.9907986298338,-56.5981482881658,
38.989));
#200142=CARTESIAN_POINT('Ctrl Pts',(24.9906251716464,-56.5982255167265,
39.1161895903855));
#200143=CARTESIAN_POINT('Origin',(25.0498328948964,-57.0434492461379,39.3548010137695));
#200144=CARTESIAN_POINT('Ctrl Pts',(24.4643761377916,-55.7284918401499,
39.3978017080178));
#200145=CARTESIAN_POINT('Ctrl Pts',(24.5803964109122,-55.6768362864792,
39.3978017080178));
#200146=CARTESIAN_POINT('Ctrl Pts',(24.5803964109122,-55.6768362864792,
39.5248017080178));
#200147=CARTESIAN_POINT('Ctrl Pts',(24.4275510972985,-55.6463586582051,
39.3978017080178));
#200148=CARTESIAN_POINT('Ctrl Pts',(24.5437506299576,-55.594528514849,39.3975666025031));
#200149=CARTESIAN_POINT('Ctrl Pts',(24.5254812387363,-55.5534947903269,
39.5248015517182));
#200150=CARTESIAN_POINT('Ctrl Pts',(24.3927285408595,-55.568696257641,39.3484894016716));
#200151=CARTESIAN_POINT('Ctrl Pts',(24.509275152962,-55.5170953257179,39.3480259000031));
#200152=CARTESIAN_POINT('Ctrl Pts',(24.473555028187,-55.4368666119038,39.4508333188948));
#200153=CARTESIAN_POINT('Ctrl Pts',(24.3743766270213,-55.5277679687683,
39.2708017080178));
#200154=CARTESIAN_POINT('Ctrl Pts',(24.4911280468225,-55.4763362579875,
39.27051194648));
#200155=CARTESIAN_POINT('Ctrl Pts',(24.4461895095988,-55.3754026508175,
39.3343017080178));
#200156=CARTESIAN_POINT('Origin',(24.3301692364782,-55.4270582044882,39.3343017080178));
#200157=CARTESIAN_POINT('Origin',(25.1222926664938,-57.2061965577167,39.6398955068181));
#200158=CARTESIAN_POINT('Origin',(25.1947524379615,-57.3689438691197,39.92499));
#200159=CARTESIAN_POINT('Origin',(24.2970811015499,-55.3527410366444,39.1934008539951));
#200160=CARTESIAN_POINT('Origin',(24.2788510342446,-55.3119205422646,39.1160402713846));
#200161=CARTESIAN_POINT('Ctrl Pts',(25.5918112338793,-57.5176823163889,
40.1599502534424));
#200162=CARTESIAN_POINT('Ctrl Pts',(25.5766462455175,-57.4835989537478,
40.10025));
#200163=CARTESIAN_POINT('Ctrl Pts',(25.5480287005717,-57.419280924679,40.10025));
#200164=CARTESIAN_POINT('Ctrl Pts',(25.5113050800558,-57.5535024391256,
40.1599500538468));
#200165=CARTESIAN_POINT('Ctrl Pts',(25.518003150502,-57.5096879712785,40.1002448353481));
#200166=CARTESIAN_POINT('Ctrl Pts',(25.5014249500148,-57.4400067642829,
40.10025));
#200167=CARTESIAN_POINT('Ctrl Pts',(25.4268488592815,-57.5636994104961,
40.1202442001038));
#200168=CARTESIAN_POINT('Ctrl Pts',(25.4545932086373,-57.5125855880057,
40.0633873868015));
#200169=CARTESIAN_POINT('Ctrl Pts',(25.4482497003382,-57.4362769714772,
40.0772271723536));
#200170=CARTESIAN_POINT('Ctrl Pts',(25.2998561687915,-57.5406963524571,
40.0045995998163));
#200171=CARTESIAN_POINT('Ctrl Pts',(25.371995687077,-57.4828507843371,39.9663485808318));
#200172=CARTESIAN_POINT('Ctrl Pts',(25.3622939683648,-57.3950038423346,
40.0101727202467));
#200173=CARTESIAN_POINT('Ctrl Pts',(25.2565567136857,-57.5090991591923,
39.9304654349858));
#200174=CARTESIAN_POINT('Ctrl Pts',(25.3528760603499,-57.4495482434202,
39.9051900162955));
#200175=CARTESIAN_POINT('Ctrl Pts',(25.3292685758747,-57.3588307079383,
39.9671857458176));
#200176=CARTESIAN_POINT('Ctrl Pts',(25.2380597013429,-57.4675553545141,
39.8576902534424));
#200177=CARTESIAN_POINT('Ctrl Pts',(25.3547675996714,-57.4161024530844,
39.8573998014387));
#200178=CARTESIAN_POINT('Ctrl Pts',(25.3107727110821,-57.317288315449,39.92499));
#200179=CARTESIAN_POINT('Origin',(25.5480287005717,-57.419280924679,40.22725));
#200180=CARTESIAN_POINT('Origin',(-0.290050682801521,-0.129138884176566,
39.116));
#200181=CARTESIAN_POINT('Origin',(24.1156489724276,-54.9452378026829,39.116));
#200182=CARTESIAN_POINT('Origin',(5.59761027822878E-15,5.84551872285717E-15,
40.22725));
#200183=CARTESIAN_POINT('Origin',(25.5758735661207,-57.406883591798,40.22725));
#200184=CARTESIAN_POINT('Ctrl Pts',(24.1156489724276,-54.9452378026829,
38.989));
#200185=CARTESIAN_POINT('Ctrl Pts',(24.2318430491565,-54.8935048666603,
38.989));
#200186=CARTESIAN_POINT('Ctrl Pts',(24.2316691155602,-54.8935823068866,
39.1161901092323));
#200187=CARTESIAN_POINT('Ctrl Pts',(24.0276063358807,-54.7469262747032,
38.989));
#200188=CARTESIAN_POINT('Ctrl Pts',(24.1436677818728,-54.6954612380236,
38.9892298989724));
#200189=CARTESIAN_POINT('Ctrl Pts',(24.1610930816817,-54.7350659388072,
39.1161900493185));
#200190=CARTESIAN_POINT('Ctrl Pts',(23.9437932708506,-54.5581358350809,
39.1034966344368));
#200191=CARTESIAN_POINT('Ctrl Pts',(24.0597054841937,-54.5068800556947,
39.1038314102585));
#200192=CARTESIAN_POINT('Ctrl Pts',(24.0939060248995,-54.5841613379358,
39.2077528789612));
#200193=CARTESIAN_POINT('Ctrl Pts',(23.8971395307767,-54.4530463244693,
39.2875012672119));
#200194=CARTESIAN_POINT('Ctrl Pts',(24.0130054476977,-54.4019907306519,
39.2878045257868));
#200195=CARTESIAN_POINT('Ctrl Pts',(24.056506495927,-54.5001606201971,39.35490152959));
#200196=CARTESIAN_POINT('Origin',(23.940420925912,-54.5516691663895,39.3548010137695));
#200197=CARTESIAN_POINT('Ctrl Pts',(25.8191582032619,-57.2088336324699,
39.8576902534424));
#200198=CARTESIAN_POINT('Ctrl Pts',(25.7028284190332,-57.2611357920725,
39.8573998014387));
#200199=CARTESIAN_POINT('Ctrl Pts',(25.658833530444,-57.1623216544372,39.92499));
#200200=CARTESIAN_POINT('Ctrl Pts',(25.8376627381929,-57.2503966981986,
39.9304984902491));
#200201=CARTESIAN_POINT('Ctrl Pts',(25.7289639953175,-57.2821216226331,
39.9052171569798));
#200202=CARTESIAN_POINT('Ctrl Pts',(25.6773378230594,-57.2038829761266,
39.9672049726603));
#200203=CARTESIAN_POINT('Ctrl Pts',(25.8320911970517,-57.3035546548412,
40.0043437678662));
#200204=CARTESIAN_POINT('Ctrl Pts',(25.7407897001106,-57.3185262575349,
39.9661628577643));
#200205=CARTESIAN_POINT('Ctrl Pts',(25.6820441386715,-57.25246649948,40.0100243556235));
#200206=CARTESIAN_POINT('Ctrl Pts',(25.7649464042482,-57.4126476234251,
40.1194874821987));
#200207=CARTESIAN_POINT('Ctrl Pts',(25.7081127933384,-57.3992776612634,
40.062755148314));
#200208=CARTESIAN_POINT('Ctrl Pts',(25.6555720179789,-57.343450072766,40.0767884282377));
#200209=CARTESIAN_POINT('Ctrl Pts',(25.7004590347003,-57.4692856961534,
40.1599502015384));
#200210=CARTESIAN_POINT('Ctrl Pts',(25.663375451079,-57.4449640631517,40.1002449453881));
#200211=CARTESIAN_POINT('Ctrl Pts',(25.622614088277,-57.3860499078761,40.10025));
#200212=CARTESIAN_POINT('Ctrl Pts',(25.6197038181297,-57.5052637377733,
40.1599502534424));
#200213=CARTESIAN_POINT('Ctrl Pts',(25.604522301406,-57.471187734033,40.10025));
#200214=CARTESIAN_POINT('Ctrl Pts',(25.5758735661207,-57.406883591798,40.10025));
#200215=CARTESIAN_POINT('Origin',(25.7748538035646,-57.1106661007665,39.92499));
#200216=CARTESIAN_POINT('Origin',(23.8679610547593,-54.3889216310736,39.6398955069312));
#200217=CARTESIAN_POINT('Origin',(23.7955011834907,-54.2261740956467,39.92499));
#200218=CARTESIAN_POINT('Origin',(25.7023940320485,-56.9479187893674,39.6398955068282));
#200219=CARTESIAN_POINT('Origin',(25.6299342604994,-56.7851714777848,39.3548010137695));
#200220=CARTESIAN_POINT('Ctrl Pts',(23.7522229508827,-54.1275498658874,
39.8576902534424));
#200221=CARTESIAN_POINT('Ctrl Pts',(23.8679139708567,-54.0765745253536,
39.8579948730703));
#200222=CARTESIAN_POINT('Ctrl Pts',(23.9115214566113,-54.174518541976,39.92499));
#200223=CARTESIAN_POINT('Ctrl Pts',(23.7337429357606,-54.0860417646979,
39.9304020711229));
#200224=CARTESIAN_POINT('Ctrl Pts',(23.8418262755855,-54.0553388636016,
39.9058915297373));
#200225=CARTESIAN_POINT('Ctrl Pts',(23.8930401898204,-54.1330089371351,
39.9671523786029));
#200226=CARTESIAN_POINT('Ctrl Pts',(23.7393098712348,-54.0331737207068,
40.0043257306695));
#200227=CARTESIAN_POINT('Ctrl Pts',(23.8301926567299,-54.0188467943736,
39.9667894847838));
#200228=CARTESIAN_POINT('Ctrl Pts',(23.8884275227222,-54.0846755205371,
40.0100138975201));
#200229=CARTESIAN_POINT('Ctrl Pts',(23.8065189073823,-53.9248984592618,
40.1195533054855));
#200230=CARTESIAN_POINT('Ctrl Pts',(23.86315010479,-53.9384511174162,40.0630813209233));
#200231=CARTESIAN_POINT('Ctrl Pts',(23.9152668978359,-53.9943748351526,
40.076826594242));
#200232=CARTESIAN_POINT('Ctrl Pts',(23.8710081209825,-53.8688190939457,
40.1599502027523));
#200233=CARTESIAN_POINT('Ctrl Pts',(23.9079567336543,-53.8932068549978,
40.1002552791544));
#200234=CARTESIAN_POINT('Ctrl Pts',(23.9484663513833,-53.952227053115,40.10025));
#200235=CARTESIAN_POINT('Ctrl Pts',(23.9513722670364,-53.8330634946838,
40.1599502534424));
#200236=CARTESIAN_POINT('Ctrl Pts',(23.9665367208223,-53.8671470951731,
40.10025));
#200237=CARTESIAN_POINT('Ctrl Pts',(23.9951532569806,-53.9314655730805,
40.10025));
#200238=CARTESIAN_POINT('Origin',(23.9951532569806,-53.9314655730805,40.22725));
#200239=CARTESIAN_POINT('Ctrl Pts',(25.4547063934082,-56.3916032444851,
38.989));
#200240=CARTESIAN_POINT('Ctrl Pts',(25.3385127813692,-56.4433359736145,
38.989));
#200241=CARTESIAN_POINT('Ctrl Pts',(25.3386862495819,-56.4432587405902,
39.1161896013269));
#200242=CARTESIAN_POINT('Ctrl Pts',(25.5431622092827,-56.5897307565541,
38.989));
#200243=CARTESIAN_POINT('Ctrl Pts',(25.4268404215568,-56.6417243268789,
38.9887769275436));
#200244=CARTESIAN_POINT('Ctrl Pts',(25.4092621323414,-56.601774768009,39.1161898821826));
#200245=CARTESIAN_POINT('Ctrl Pts',(25.6273687254298,-56.7783458705714,
39.1034967087243));
#200246=CARTESIAN_POINT('Ctrl Pts',(25.5109049500366,-56.830537517612,39.1031720232724));
#200247=CARTESIAN_POINT('Ctrl Pts',(25.4764491573041,-56.7526792962301,
39.2077529615017));
#200248=CARTESIAN_POINT('Ctrl Pts',(25.6742415049979,-56.8833377255395,
39.2875012672119));
#200249=CARTESIAN_POINT('Ctrl Pts',(25.5577357740377,-56.9357219102088,
39.2872087095508));
#200250=CARTESIAN_POINT('Ctrl Pts',(25.5138485767964,-56.8366797674139,
39.3549017048229));
#200251=CARTESIAN_POINT('Origin',(25.4547063934082,-56.3916032444851,39.116));
#200252=CARTESIAN_POINT('Origin',(5.68853496937358E-15,5.19912183297972E-15,
40.22725));
#200253=CARTESIAN_POINT('Origin',(24.0229981225296,-53.9190682401995,40.22725));
#200254=CARTESIAN_POINT('Origin',(10.5838037820516,-22.9910091182297,39.116));
#200255=CARTESIAN_POINT('Origin',(25.2915084057492,-56.0249274780511,39.1160373285268));
#200256=CARTESIAN_POINT('Ctrl Pts',(23.9791663275012,-53.8206887816837,
40.1599502534424));
#200257=CARTESIAN_POINT('Ctrl Pts',(23.9943483786816,-53.8547645473081,
40.10025));
#200258=CARTESIAN_POINT('Ctrl Pts',(24.0229981225296,-53.9190682401995,
40.10025));
#200259=CARTESIAN_POINT('Ctrl Pts',(24.0592381183001,-53.7850138844278,
40.1599500566035));
#200260=CARTESIAN_POINT('Ctrl Pts',(24.0526825045793,-53.8287709626516,
40.1002551305357));
#200261=CARTESIAN_POINT('Ctrl Pts',(24.0695074323267,-53.8983362760826,
40.10025));
#200262=CARTESIAN_POINT('Ctrl Pts',(24.1432906710371,-53.7744461045708,
40.1203070619045));
#200263=CARTESIAN_POINT('Ctrl Pts',(24.1158128282441,-53.8255298669645,
40.0637098684499));
#200264=CARTESIAN_POINT('Ctrl Pts',(24.1225146216897,-53.901590305224,40.0772636213363));
#200265=CARTESIAN_POINT('Ctrl Pts',(24.2696905364172,-53.7968389608975,
40.0046102245803));
#200266=CARTESIAN_POINT('Ctrl Pts',(24.198317557125,-53.8548027426708,39.9670001894012));
#200267=CARTESIAN_POINT('Ctrl Pts',(24.2081897025475,-53.9421141528985,
40.0101788811208));
#200268=CARTESIAN_POINT('Ctrl Pts',(24.3127961529013,-53.8282518514936,
39.9303710930185));
#200269=CARTESIAN_POINT('Ctrl Pts',(24.2176488245051,-53.8880291490197,
39.9058663574099));
#200270=CARTESIAN_POINT('Ctrl Pts',(24.241108858848,-53.9780599067614,39.9671344706353));
#200271=CARTESIAN_POINT('Ctrl Pts',(24.3312692531087,-53.8697418420146,
39.8576902534424));
#200272=CARTESIAN_POINT('Ctrl Pts',(24.2159747902185,-53.9216078643418,
39.8579948730703));
#200273=CARTESIAN_POINT('Ctrl Pts',(24.2595822759732,-54.0195518809642,
39.92499));
#200274=CARTESIAN_POINT('Origin',(24.3756025490938,-53.9678963272935,39.92499));
#200275=CARTESIAN_POINT('Origin',(25.2734729066189,-55.9845461685081,39.1925554488845));
#200276=CARTESIAN_POINT('Origin',(25.2401862573141,-55.9097831300747,39.3343017080178));
#200277=CARTESIAN_POINT('Origin',(24.4480624203036,-54.1306438627315,39.6398955069225));
#200278=CARTESIAN_POINT('Origin',(24.5205222915151,-54.2933913980364,39.3548010137695));
#200279=CARTESIAN_POINT('Ctrl Pts',(25.10597938477,-55.6083495590302,39.3978017080178));
#200280=CARTESIAN_POINT('Ctrl Pts',(24.9899591116494,-55.6600051127008,
39.3978017080178));
#200281=CARTESIAN_POINT('Ctrl Pts',(24.9899591116494,-55.6600051127008,
39.5248017080178));
#200282=CARTESIAN_POINT('Ctrl Pts',(25.1423759987949,-55.6906734752781,
39.3978017080178));
#200283=CARTESIAN_POINT('Ctrl Pts',(25.0265352902399,-55.742156554866,39.3980355775168));
#200284=CARTESIAN_POINT('Ctrl Pts',(25.0448742789057,-55.7833465978035,
39.5248015517178));
#200285=CARTESIAN_POINT('Ctrl Pts',(25.1767934079551,-55.7685161955953,
39.3484893995498));
#200286=CARTESIAN_POINT('Ctrl Pts',(25.0612933298571,-55.8202243900358,
39.3489438303432));
#200287=CARTESIAN_POINT('Ctrl Pts',(25.0968004762774,-55.8999747466294,
39.4508333155604));
#200288=CARTESIAN_POINT('Ctrl Pts',(25.19493178753,-55.8095395120008,39.2708017080178));
#200289=CARTESIAN_POINT('Ctrl Pts',(25.0796311836953,-55.8614118841079,
39.2710850691866));
#200290=CARTESIAN_POINT('Ctrl Pts',(25.1241659841935,-55.9614386837454,
39.3343017080178));
#200291=CARTESIAN_POINT('Origin',(25.10597938477,-55.6083495590302,39.5248017080178));
#200292=CARTESIAN_POINT('Ctrl Pts',(24.4761921430391,-54.1952354911873,
39.2875012672119));
#200293=CARTESIAN_POINT('Ctrl Pts',(24.3607210247425,-54.2471777813617,
39.2878045257519));
#200294=CARTESIAN_POINT('Ctrl Pts',(24.4045675690228,-54.3451938326304,
39.3549015218347));
#200295=CARTESIAN_POINT('Ctrl Pts',(24.5230721320475,-54.3002261711154,
39.1034938540228));
#200296=CARTESIAN_POINT('Ctrl Pts',(24.4074212664131,-54.352068915742,39.1038286278836));
#200297=CARTESIAN_POINT('Ctrl Pts',(24.4419676644372,-54.4291958219391,
39.2077506434048));
#200298=CARTESIAN_POINT('Ctrl Pts',(24.6072895482034,-54.4888383671843,
38.989));
#200299=CARTESIAN_POINT('Ctrl Pts',(24.4913833136921,-54.5406519873231,
38.9892298954593));
#200300=CARTESIAN_POINT('Ctrl Pts',(24.5091552540986,-54.5801016184604,
39.1161900347271));
#200301=CARTESIAN_POINT('Ctrl Pts',(24.6957503380306,-54.6869600343298,
38.989));
#200302=CARTESIAN_POINT('Ctrl Pts',(24.5795562747214,-54.7386929643776,
38.989));
#200303=CARTESIAN_POINT('Ctrl Pts',(24.5797301948779,-54.738615530135,39.1161900945646));
#200304=CARTESIAN_POINT('Origin',(24.6957503380306,-54.6869600343298,39.116));
#200305=CARTESIAN_POINT('Origin',(10.3344596589366,-22.4309730483565,39.5248017080178));
#200306=CARTESIAN_POINT('Origin',(25.0444775033946,-55.4702140717967,39.5248017080178));
#200307=CARTESIAN_POINT('Origin',(10.295413467953,-22.3432738675264,39.116));
#200308=CARTESIAN_POINT('Origin',(24.8590452239601,-55.0536014459537,39.1160402713849));
#200309=CARTESIAN_POINT('Ctrl Pts',(24.9555320242414,-55.2690209153041,
39.2708017080178));
#200310=CARTESIAN_POINT('Ctrl Pts',(24.8391888661843,-55.3213695969756,
39.27051194648));
#200311=CARTESIAN_POINT('Ctrl Pts',(24.7942503289606,-55.2204359898057,
39.3343017080178));
#200312=CARTESIAN_POINT('Ctrl Pts',(24.9737291291708,-55.3101840490929,
39.3487519301186));
#200313=CARTESIAN_POINT('Ctrl Pts',(24.8573973158434,-55.3622664445116,
39.3482879463981));
#200314=CARTESIAN_POINT('Ctrl Pts',(24.8217083187823,-55.2821076446826,
39.4512271261636));
#200315=CARTESIAN_POINT('Ctrl Pts',(25.0082040095654,-55.3881672017729,
39.3978017080178));
#200316=CARTESIAN_POINT('Ctrl Pts',(24.8919348043925,-55.4398389138634,
39.3975673827397));
#200317=CARTESIAN_POINT('Ctrl Pts',(24.8737270328803,-55.398943589478,39.5248015355181));
#200318=CARTESIAN_POINT('Ctrl Pts',(25.0444775033946,-55.4702140717967,
39.3978017080178));
#200319=CARTESIAN_POINT('Ctrl Pts',(24.928457230274,-55.5218696254674,39.3978017080178));
#200320=CARTESIAN_POINT('Ctrl Pts',(24.928457230274,-55.5218696254674,39.5248017080178));
#200321=CARTESIAN_POINT('Origin',(24.9102706020812,-55.168780436135,39.3343017080178));
#200322=CARTESIAN_POINT('Origin',(24.8771824678742,-55.0944632691847,39.1934008533544));
#200323=CARTESIAN_POINT('Origin',(18.6791227126689,-58.5158800435653,39.1925554495079));
#200324=CARTESIAN_POINT('Origin',(18.6927400943506,-58.557957308327,39.1160373285241));
#200325=CARTESIAN_POINT('Origin',(18.6538332760103,-58.4380471616455,39.3343017080178));
#200326=CARTESIAN_POINT('Ctrl Pts',(18.6203878281146,-58.3332704847796,
39.2708017080178));
#200327=CARTESIAN_POINT('Ctrl Pts',(18.7407822670301,-58.2946680067388,
39.2710850691866));
#200328=CARTESIAN_POINT('Ctrl Pts',(18.7746174535798,-58.3988020033599,
39.3343017080178));
#200329=CARTESIAN_POINT('Ctrl Pts',(18.6063701040112,-58.2905032380256,
39.3487519293518));
#200330=CARTESIAN_POINT('Ctrl Pts',(18.7268030714131,-58.2516444665215,
39.3492068662938));
#200331=CARTESIAN_POINT('Ctrl Pts',(18.7537563325802,-58.3345980746926,
39.4512271248748));
#200332=CARTESIAN_POINT('Ctrl Pts',(18.579813047667,-58.2094810151997,39.3978017080178));
#200333=CARTESIAN_POINT('Ctrl Pts',(18.700349152967,-58.1702276772284,39.398034778116));
#200334=CARTESIAN_POINT('Ctrl Pts',(18.7142352739233,-58.2129647630923,
39.5248015355176));
#200335=CARTESIAN_POINT('Ctrl Pts',(18.5518699907149,-58.1242364370957,
39.3978017080178));
#200336=CARTESIAN_POINT('Ctrl Pts',(18.6726541682844,-58.0849912788101,
39.3978017080178));
#200337=CARTESIAN_POINT('Ctrl Pts',(18.6726541682844,-58.0849912788101,
39.5248017080178));
#200338=CARTESIAN_POINT('Origin',(18.5518699907149,-58.1242364370957,39.5248017080178));
#200339=CARTESIAN_POINT('Origin',(-0.301960443923706,-0.098112895714045,
39.116));
#200340=CARTESIAN_POINT('Origin',(18.8168143322225,-58.9396512752214,39.116));
#200341=CARTESIAN_POINT('Origin',(-0.301960443923706,-0.098112895714045,
39.5248017080178));
#200342=CARTESIAN_POINT('Origin',(18.505144113284,-57.9804289733664,39.5248017080178));
#200343=CARTESIAN_POINT('Ctrl Pts',(18.9827025415095,-59.4519788726608,
39.2875012672119));
#200344=CARTESIAN_POINT('Ctrl Pts',(19.1043350233607,-59.4129503614027,
39.287208709576));
#200345=CARTESIAN_POINT('Ctrl Pts',(19.0706774512227,-59.3099814440479,
39.3549016990123));
#200346=CARTESIAN_POINT('Ctrl Pts',(18.9472820042064,-59.3425890481019,
39.1034939173931));
#200347=CARTESIAN_POINT('Ctrl Pts',(19.0687544722092,-59.3034455268815,
39.1031692336348));
#200348=CARTESIAN_POINT('Ctrl Pts',(19.0422629184334,-59.2225305038466,
39.2077507202313));
#200349=CARTESIAN_POINT('Ctrl Pts',(18.8836509927318,-59.1460739925267,
38.989));
#200350=CARTESIAN_POINT('Ctrl Pts',(19.0048854004789,-59.1068782740656,
38.9887769311164));
#200351=CARTESIAN_POINT('Ctrl Pts',(18.9912173655547,-59.0654284453498,
39.1161898712898));
#200352=CARTESIAN_POINT('Ctrl Pts',(18.8168143322225,-58.9396512752214,
38.989));
#200353=CARTESIAN_POINT('Ctrl Pts',(18.9377789557524,-58.9003474864891,
38.989));
#200354=CARTESIAN_POINT('Ctrl Pts',(18.9375983752043,-58.900406160666,39.1161895903855));
#200355=CARTESIAN_POINT('Origin',(18.9499432001057,-59.349379800228,39.3548010137695));
#200356=CARTESIAN_POINT('Ctrl Pts',(18.505144113284,-57.9804289733664,39.3978017080178));
#200357=CARTESIAN_POINT('Ctrl Pts',(18.6259282908535,-57.9411838150808,
39.3978017080178));
#200358=CARTESIAN_POINT('Ctrl Pts',(18.6259282908535,-57.9411838150808,
39.5248017080178));
#200359=CARTESIAN_POINT('Ctrl Pts',(18.4771060595094,-57.894896460693,39.3978017080178));
#200360=CARTESIAN_POINT('Ctrl Pts',(18.5980867642078,-57.8554964068678,
39.3975666025021));
#200361=CARTESIAN_POINT('Ctrl Pts',(18.5842066467862,-57.8127777979909,
39.5248015517178));
#200362=CARTESIAN_POINT('Ctrl Pts',(18.4505921960617,-57.8140195545739,
39.3484894016716));
#200363=CARTESIAN_POINT('Ctrl Pts',(18.5718941197436,-57.7748837362156,
39.3480259000044));
#200364=CARTESIAN_POINT('Ctrl Pts',(18.5447558577167,-57.6913607539431,
39.4508333188947));
#200365=CARTESIAN_POINT('Ctrl Pts',(18.4366189870672,-57.7713971777987,
39.2708017080178));
#200366=CARTESIAN_POINT('Ctrl Pts',(18.5581069080659,-57.7324510618071,
39.27051194648));
#200367=CARTESIAN_POINT('Ctrl Pts',(18.5239649837007,-57.6273730232606,
39.3343017080178));
#200368=CARTESIAN_POINT('Origin',(18.4031808061312,-57.6666181815462,39.3343017080178));
#200369=CARTESIAN_POINT('Origin',(19.0049943031108,-59.5188096735779,39.6398955068193));
#200370=CARTESIAN_POINT('Origin',(19.0600454060086,-59.6882395467421,39.92499));
#200371=CARTESIAN_POINT('Origin',(18.378042190817,-57.5892494790284,39.1934008539945));
#200372=CARTESIAN_POINT('Origin',(18.3641788932754,-57.5467470426662,39.1160402713846));
#200373=CARTESIAN_POINT('Ctrl Pts',(19.4393816709755,-59.8776671349986,
40.1599502534424));
#200374=CARTESIAN_POINT('Ctrl Pts',(19.4278624395265,-59.8421853116553,
40.10025));
#200375=CARTESIAN_POINT('Ctrl Pts',(19.4061247292252,-59.7752282754837,
40.10025));
#200376=CARTESIAN_POINT('Ctrl Pts',(19.355572315902,-59.9048758468122,40.1599500538465));
#200377=CARTESIAN_POINT('Ctrl Pts',(19.3668135526099,-59.8620015382123,
40.1002448353478));
#200378=CARTESIAN_POINT('Ctrl Pts',(19.3576098387254,-59.7909691583392,
40.10025));
#200379=CARTESIAN_POINT('Ctrl Pts',(19.2705128813954,-59.9061888791355,
40.1202442001037));
#200380=CARTESIAN_POINT('Ctrl Pts',(19.3034480936187,-59.8582551377152,
40.0633873868015));
#200381=CARTESIAN_POINT('Ctrl Pts',(19.3051157581417,-59.7817014705979,
40.0772271723538));
#200382=CARTESIAN_POINT('Ctrl Pts',(19.1466203444578,-59.8700374834726,
40.0045995998164));
#200383=CARTESIAN_POINT('Ctrl Pts',(19.2244111832567,-59.8200494324147,
39.9663485808318));
#200384=CARTESIAN_POINT('Ctrl Pts',(19.2239451174251,-59.7316696194042,
40.0101727202465));
#200385=CARTESIAN_POINT('Ctrl Pts',(19.1068608943534,-59.8340873574359,
39.9304654349858));
#200386=CARTESIAN_POINT('Ctrl Pts',(19.208877359269,-59.7849307811027,39.9051900162941));
#200387=CARTESIAN_POINT('Ctrl Pts',(19.1948817636406,-59.6922425516964,
39.9671857458175));
#200388=CARTESIAN_POINT('Ctrl Pts',(19.092807720641,-59.7908376697912,39.8576902534424));
#200389=CARTESIAN_POINT('Ctrl Pts',(19.2142545736082,-59.7518659300026,
39.8573998014387));
#200390=CARTESIAN_POINT('Ctrl Pts',(19.180829583578,-59.6489943884565,39.92499));
#200391=CARTESIAN_POINT('Origin',(19.4061247292252,-59.7752282754837,40.22725));
#200392=CARTESIAN_POINT('Origin',(-0.301960443923706,-0.098112895714045,
39.116));
#200393=CARTESIAN_POINT('Origin',(18.2401996527044,-57.1650137687747,39.116));
#200394=CARTESIAN_POINT('Origin',(5.61372323131277E-15,5.85170390604432E-15,
40.22725));
#200395=CARTESIAN_POINT('Origin',(19.4351129318419,-59.7658094374952,40.22725));
#200396=CARTESIAN_POINT('Ctrl Pts',(18.2401996527044,-57.1650137687747,
38.989));
#200397=CARTESIAN_POINT('Ctrl Pts',(18.3611647704264,-57.1257098194697,
38.989));
#200398=CARTESIAN_POINT('Ctrl Pts',(18.3609836949485,-57.125768654459,39.1161901092325));
#200399=CARTESIAN_POINT('Ctrl Pts',(18.1733685221991,-56.9585856505952,
38.989));
#200400=CARTESIAN_POINT('Ctrl Pts',(18.2941737326426,-56.9195342693655,
38.9892298989742));
#200401=CARTESIAN_POINT('Ctrl Pts',(18.3073637563263,-56.9607434512653,
39.1161900493187));
#200402=CARTESIAN_POINT('Ctrl Pts',(18.1097485684451,-56.7620685738642,
39.1034966344368));
#200403=CARTESIAN_POINT('Ctrl Pts',(18.2303834904095,-56.7232097045349,
39.1038314102571));
#200404=CARTESIAN_POINT('Ctrl Pts',(18.2563185832999,-56.8036425617893,
39.2077528789613));
#200405=CARTESIAN_POINT('Ctrl Pts',(18.074335247489,-56.6526781108324,39.2875012672119));
#200406=CARTESIAN_POINT('Ctrl Pts',(18.194903201557,-56.6140134911407,39.2878045257868));
#200407=CARTESIAN_POINT('Ctrl Pts',(18.2279043987991,-56.7161926934816,
39.3549015295901));
#200408=CARTESIAN_POINT('Origin',(18.1070706485041,-56.7552848242271,39.3548010137695));
#200409=CARTESIAN_POINT('Ctrl Pts',(19.6977666881844,-59.5942745858236,
39.8576902534424));
#200410=CARTESIAN_POINT('Ctrl Pts',(19.5766071063167,-59.6341304551457,
39.8573998014387));
#200411=CARTESIAN_POINT('Ctrl Pts',(19.5431821162865,-59.5312589135996,
39.92499));
#200412=CARTESIAN_POINT('Ctrl Pts',(19.7118253299484,-59.6375442153288,
39.930498490249));
#200413=CARTESIAN_POINT('Ctrl Pts',(19.6004058925601,-59.6577332347592,
39.9052171569784));
#200414=CARTESIAN_POINT('Ctrl Pts',(19.5572406993632,-59.5745267832908,
39.9672049726602));
#200415=CARTESIAN_POINT('Ctrl Pts',(19.7007277907734,-59.6898285824899,
40.0043437678663));
#200416=CARTESIAN_POINT('Ctrl Pts',(19.6083614943636,-59.695174564008,39.9661628577646));
#200417=CARTESIAN_POINT('Ctrl Pts',(19.55684287225,-59.6233361049593,40.0100243556235));
#200418=CARTESIAN_POINT('Ctrl Pts',(19.6225475038109,-59.791305386369,40.1194874821986));
#200419=CARTESIAN_POINT('Ctrl Pts',(19.5674227749668,-59.7720679362488,
40.0627551483138));
#200420=CARTESIAN_POINT('Ctrl Pts',(19.5210053955058,-59.7110541706146,
40.0767884282377));
#200421=CARTESIAN_POINT('Ctrl Pts',(19.5524931121163,-59.8408924241702,
40.159950201539));
#200422=CARTESIAN_POINT('Ctrl Pts',(19.5181549791688,-59.8128277376124,
40.1002449453872));
#200423=CARTESIAN_POINT('Ctrl Pts',(19.4837751174925,-59.7499755976286,
40.10025));
#200424=CARTESIAN_POINT('Ctrl Pts',(19.4684195516695,-59.8682321556242,
40.1599502534424));
#200425=CARTESIAN_POINT('Ctrl Pts',(19.4568831131883,-59.8327559231846,
40.10025));
#200426=CARTESIAN_POINT('Ctrl Pts',(19.4351129318419,-59.7658094374952,
40.10025));
#200427=CARTESIAN_POINT('Origin',(19.663966293856,-59.492013755314,39.92499));
#200428=CARTESIAN_POINT('Origin',(18.0520194698745,-56.5858547179583,39.6398955069314));
#200429=CARTESIAN_POINT('Origin',(17.996968291141,-56.4164246115664,39.92499));
#200430=CARTESIAN_POINT('Origin',(19.6089151909103,-59.3225838821502,39.6398955068283));
#200431=CARTESIAN_POINT('Origin',(19.5538640879531,-59.1531540087999,39.3548010137695));
#200432=CARTESIAN_POINT('Ctrl Pts',(17.9642361803971,-56.3138168485095,
39.8576902534424));
#200433=CARTESIAN_POINT('Ctrl Pts',(18.0846218068694,-56.2752137607566,
39.8579948730703));
#200434=CARTESIAN_POINT('Ctrl Pts',(18.1177524687105,-56.3771794532808,
39.92499));
#200435=CARTESIAN_POINT('Ctrl Pts',(17.9501961787629,-56.2706044454591,
39.9304020711231));
#200436=CARTESIAN_POINT('Ctrl Pts',(18.0608967538138,-56.2513675234836,
39.9058915297377));
#200437=CARTESIAN_POINT('Ctrl Pts',(18.1037113794378,-56.3339654239822,
39.9671523786037));
#200438=CARTESIAN_POINT('Ctrl Pts',(17.9612588333756,-56.2186079213554,
40.0043257306693));
#200439=CARTESIAN_POINT('Ctrl Pts',(18.0531413250551,-56.2138593173289,
39.9667894847839));
#200440=CARTESIAN_POINT('Ctrl Pts',(18.1041761987737,-56.2854146278934,
40.0100138975199));
#200441=CARTESIAN_POINT('Ctrl Pts',(18.0394175380795,-56.1179510603876,
40.1195533054857));
#200442=CARTESIAN_POINT('Ctrl Pts',(18.0943218653327,-56.1373490477006,
40.0630813209234));
#200443=CARTESIAN_POINT('Ctrl Pts',(18.140307536858,-56.1984140977477,40.0768265942422));
#200444=CARTESIAN_POINT('Ctrl Pts',(18.1094153628979,-56.0689198620982,
40.1599502027512));
#200445=CARTESIAN_POINT('Ctrl Pts',(18.1436123520191,-56.0970362061497,
40.1002552791541));
#200446=CARTESIAN_POINT('Ctrl Pts',(18.1777307632117,-56.1599674935319,
40.10025));
#200447=CARTESIAN_POINT('Ctrl Pts',(18.1930767435948,-56.0417604764384,
40.1599502534424));
#200448=CARTESIAN_POINT('Ctrl Pts',(18.2045954185344,-56.0772424804485,
40.10025));
#200449=CARTESIAN_POINT('Ctrl Pts',(18.2263320786581,-56.1441998575528,
40.10025));
#200450=CARTESIAN_POINT('Origin',(18.2263320786581,-56.1441998575528,40.22725));
#200451=CARTESIAN_POINT('Ctrl Pts',(19.42073522007,-58.7434254837933,38.989));
#200452=CARTESIAN_POINT('Ctrl Pts',(19.2997705861194,-58.7827292759114,
38.989));
#200453=CARTESIAN_POINT('Ctrl Pts',(19.2999511771037,-58.7826705983436,
39.1161896013261));
#200454=CARTESIAN_POINT('Ctrl Pts',(19.4879965013588,-58.9497137831223,
38.989));
#200455=CARTESIAN_POINT('Ctrl Pts',(19.3668771285546,-58.9892635895195,
38.9887769275436));
#200456=CARTESIAN_POINT('Ctrl Pts',(19.3535710010449,-58.947695446951,39.1161898821819));
#200457=CARTESIAN_POINT('Ctrl Pts',(19.5520260773869,-59.1460976215385,
39.1034967087243));
#200458=CARTESIAN_POINT('Ctrl Pts',(19.4307447900779,-59.1858295777984,
39.103172023275));
#200459=CARTESIAN_POINT('Ctrl Pts',(19.4046161500171,-59.1047962608395,
39.2077529615026));
#200460=CARTESIAN_POINT('Ctrl Pts',(19.5876674457077,-59.2554138597572,
39.2875012672119));
#200461=CARTESIAN_POINT('Ctrl Pts',(19.4663243070096,-59.2953329133624,
39.2872087095508));
#200462=CARTESIAN_POINT('Ctrl Pts',(19.4330302514114,-59.1922458725048,
39.3549017048225));
#200463=CARTESIAN_POINT('Origin',(19.42073522007,-58.7434254837933,39.116));
#200464=CARTESIAN_POINT('Origin',(5.68280300381509E-15,5.19692153755175E-15,
40.22725));
#200465=CARTESIAN_POINT('Origin',(18.2553202812748,-56.1347810195642,40.22725));
#200466=CARTESIAN_POINT('Origin',(6.24367625034007,-18.1886080242677,39.116));
#200467=CARTESIAN_POINT('Origin',(19.2967593024463,-58.3616995707159,39.1160373285276));
#200468=CARTESIAN_POINT('Ctrl Pts',(18.2220120550216,-56.0323588238392,
40.1599502534424));
#200469=CARTESIAN_POINT('Ctrl Pts',(18.2335490499217,-56.0678348753333,
40.10025));
#200470=CARTESIAN_POINT('Ctrl Pts',(18.2553202812748,-56.1347810195643,
40.10025));
#200471=CARTESIAN_POINT('Ctrl Pts',(18.3053742463598,-56.0052491386465,
40.1599500566035));
#200472=CARTESIAN_POINT('Ctrl Pts',(18.2942806848329,-56.0480812627881,
40.1002551305372));
#200473=CARTESIAN_POINT('Ctrl Pts',(18.3037418885565,-56.1190241739981,
40.10025));
#200474=CARTESIAN_POINT('Ctrl Pts',(18.3900709842069,-56.0035251343647,
40.1203070619044));
#200475=CARTESIAN_POINT('Ctrl Pts',(18.3574039607305,-56.0514568378823,
40.0637098684496));
#200476=CARTESIAN_POINT('Ctrl Pts',(18.3561185603241,-56.1278011372721,
40.0772636213362));
#200477=CARTESIAN_POINT('Ctrl Pts',(18.513437727039,-56.0390077039667,40.0046102245804));
#200478=CARTESIAN_POINT('Ctrl Pts',(18.4363968713616,-56.0891934462338,
39.9670001894015));
#200479=CARTESIAN_POINT('Ctrl Pts',(18.4370884086013,-56.1770584756118,
40.010178881121));
#200480=CARTESIAN_POINT('Ctrl Pts',(18.5530236652638,-56.0747542753111,
39.9303710930184));
#200481=CARTESIAN_POINT('Ctrl Pts',(18.4521491348396,-56.1242585025267,
39.9058663574108));
#200482=CARTESIAN_POINT('Ctrl Pts',(18.4660698759074,-56.2162483036948,
39.9671344706364));
#200483=CARTESIAN_POINT('Ctrl Pts',(18.5670586829464,-56.1179479440989,
39.8576902534424));
#200484=CARTESIAN_POINT('Ctrl Pts',(18.4469743395778,-56.1574782858998,
39.8579948730703));
#200485=CARTESIAN_POINT('Ctrl Pts',(18.4801050014189,-56.2594439784239,
39.92499));
#200486=CARTESIAN_POINT('Origin',(18.6008891789884,-56.2201988201383,39.92499));
#200487=CARTESIAN_POINT('Origin',(19.2830435998985,-58.3196542512026,39.1925554488844));
#200488=CARTESIAN_POINT('Origin',(19.2577541638577,-58.2418213702174,39.3343017080178));
#200489=CARTESIAN_POINT('Origin',(18.6559403576616,-56.389628926533,39.6398955069214));
#200490=CARTESIAN_POINT('Origin',(18.7109915363516,-56.559059032799,39.3548010137695));
#200491=CARTESIAN_POINT('Ctrl Pts',(19.1557908785624,-57.9280106456676,
39.3978017080178));
#200492=CARTESIAN_POINT('Ctrl Pts',(19.0350067009929,-57.9672558039532,
39.3978017080178));
#200493=CARTESIAN_POINT('Ctrl Pts',(19.0350067009929,-57.9672558039532,
39.5248017080178));
#200494=CARTESIAN_POINT('Ctrl Pts',(19.1833829156713,-58.013688065021,39.3978017080178));
#200495=CARTESIAN_POINT('Ctrl Pts',(19.0627953474457,-58.052780463663,39.3980355775177));
#200496=CARTESIAN_POINT('Ctrl Pts',(19.0767283413222,-58.0956618095388,
39.5248015517178));
#200497=CARTESIAN_POINT('Ctrl Pts',(19.2094750027322,-58.0947019536604,
39.3484893995498));
#200498=CARTESIAN_POINT('Ctrl Pts',(19.0892026680444,-58.13405383953,39.3489438303424));
#200499=CARTESIAN_POINT('Ctrl Pts',(19.1161791203808,-58.2170788227761,
39.4508333155602));
#200500=CARTESIAN_POINT('Ctrl Pts',(19.2232259141438,-58.1373965169894,
39.2708017080178));
#200501=CARTESIAN_POINT('Ctrl Pts',(19.1031347997386,-58.176932531882,39.2710850691866));
#200502=CARTESIAN_POINT('Ctrl Pts',(19.1369699862882,-58.281066528503,39.3343017080178));
#200503=CARTESIAN_POINT('Origin',(19.1557908785624,-57.9280106456676,39.5248017080178));
#200504=CARTESIAN_POINT('Ctrl Pts',(18.6771643191709,-56.4568070719812,
39.2875012672119));
#200505=CARTESIAN_POINT('Ctrl Pts',(18.5568963159717,-56.4963947983079,
39.2878045257518));
#200506=CARTESIAN_POINT('Ctrl Pts',(18.59025719708,-56.5984571192853,39.3549015218347));
#200507=CARTESIAN_POINT('Ctrl Pts',(18.7128129802643,-56.5661228951883,
39.1034938540228));
#200508=CARTESIAN_POINT('Ctrl Pts',(18.5923766197439,-56.605592832571,39.1038286278807));
#200509=CARTESIAN_POINT('Ctrl Pts',(18.6186718120043,-56.6859083114058,
39.2077506434026));
#200510=CARTESIAN_POINT('Ctrl Pts',(18.7768537015931,-56.7625049710038,
38.989));
#200511=CARTESIAN_POINT('Ctrl Pts',(18.6561664154745,-56.8019192501362,
38.9892298954617));
#200512=CARTESIAN_POINT('Ctrl Pts',(18.6697173900117,-56.8430104456845,
39.1161900347295));
#200513=CARTESIAN_POINT('Ctrl Pts',(18.8441205405518,-56.9687879773467,
38.989));
#200514=CARTESIAN_POINT('Ctrl Pts',(18.7231554368008,-57.0080919221122,
38.989));
#200515=CARTESIAN_POINT('Ctrl Pts',(18.7233364982868,-57.0080330916692,
39.1161900945646));
#200516=CARTESIAN_POINT('Origin',(18.8441205405518,-56.9687879773467,39.116));
#200517=CARTESIAN_POINT('Origin',(6.09975091006187,-17.7456513739111,39.5248017080178));
#200518=CARTESIAN_POINT('Origin',(19.1090650011314,-57.7842031819383,39.5248017080178));
#200519=CARTESIAN_POINT('Origin',(6.07721283595898,-17.676286314285,39.116));
#200520=CARTESIAN_POINT('Origin',(18.9681964166832,-57.3504898524408,39.1160402713852));
#200521=CARTESIAN_POINT('Ctrl Pts',(19.0416371860877,-57.5748148483576,
39.2708017080178));
#200522=CARTESIAN_POINT('Ctrl Pts',(18.9204594407744,-57.6147155869502,
39.27051194648));
#200523=CARTESIAN_POINT('Ctrl Pts',(18.8863175164091,-57.5096375484037,
39.3343017080178));
#200524=CARTESIAN_POINT('Ctrl Pts',(19.0554318862548,-57.6176546016065,
39.3487519301185));
#200525=CARTESIAN_POINT('Ctrl Pts',(18.9342932580175,-57.657291698537,39.3482879463977));
#200526=CARTESIAN_POINT('Ctrl Pts',(18.9071786451782,-57.5738415009833,
39.4512271261633));
#200527=CARTESIAN_POINT('Ctrl Pts',(19.0815664505371,-57.6988141606857,
39.3978017080178));
#200528=CARTESIAN_POINT('Ctrl Pts',(18.960533015575,-57.7380493683891,39.3975673827401));
#200529=CARTESIAN_POINT('Ctrl Pts',(18.9466997135535,-57.6954748424935,
39.5248015355181));
#200530=CARTESIAN_POINT('Ctrl Pts',(19.1090650011314,-57.7842031819383,
39.3978017080178));
#200531=CARTESIAN_POINT('Ctrl Pts',(18.9882808235619,-57.8234483402239,
39.3978017080178));
#200532=CARTESIAN_POINT('Ctrl Pts',(18.9882808235619,-57.8234483402239,
39.5248017080178));
#200533=CARTESIAN_POINT('Origin',(19.0071016939786,-57.4703923901181,39.3343017080178));
#200534=CARTESIAN_POINT('Origin',(18.9819630792892,-57.3930236885616,39.1934008533552));
#200535=CARTESIAN_POINT('Origin',(12.4602215063119,-60.1478239224126,39.192555449508));
#200536=CARTESIAN_POINT('Origin',(12.4693660187275,-60.1910940874965,39.116037328525));
#200537=CARTESIAN_POINT('Origin',(12.443206359372,-60.0677739512126,39.3343017080178));
#200538=CARTESIAN_POINT('Ctrl Pts',(12.4208962741585,-59.9600752506737,
39.2708017080178));
#200539=CARTESIAN_POINT('Ctrl Pts',(12.5446662374485,-59.9342688867325,
39.2710850691866));
#200540=CARTESIAN_POINT('Ctrl Pts',(12.5674311046652,-60.0413691664788,
39.3343017080178));
#200541=CARTESIAN_POINT('Ctrl Pts',(12.4114257351943,-59.9160770362135,
39.3487519293518));
#200542=CARTESIAN_POINT('Ctrl Pts',(12.5352608058713,-59.8900198101361,
39.3492068662929));
#200543=CARTESIAN_POINT('Ctrl Pts',(12.553395401069,-59.975336372732,39.4512271248739));
#200544=CARTESIAN_POINT('Ctrl Pts',(12.3934832896272,-59.8327226933129,
39.3978017080178));
#200545=CARTESIAN_POINT('Ctrl Pts',(12.5174621766264,-59.8062838430882,
39.3980347781178));
#200546=CARTESIAN_POINT('Ctrl Pts',(12.5268049860496,-59.8502383056083,
39.5248015355195));
#200547=CARTESIAN_POINT('Ctrl Pts',(12.3746037924162,-59.7450242491248,
39.3978017080178));
#200548=CARTESIAN_POINT('Ctrl Pts',(12.4988285377094,-59.7186194643909,
39.3978017080178));
#200549=CARTESIAN_POINT('Ctrl Pts',(12.4988285377094,-59.7186194643909,
39.5248017080178));
#200550=CARTESIAN_POINT('Origin',(12.3746037924162,-59.7450242491248,39.5248017080178));
#200551=CARTESIAN_POINT('Origin',(-0.310561863232978,-0.0660119618346377,
39.116));
#200552=CARTESIAN_POINT('Origin',(12.5528626811445,-60.5836663843182,39.116));
#200553=CARTESIAN_POINT('Origin',(-0.310561863232978,-0.0660119618346377,
39.5248017080178));
#200554=CARTESIAN_POINT('Origin',(12.3431658574209,-59.5971203935659,39.5248017080178));
#200555=CARTESIAN_POINT('Ctrl Pts',(12.664289321014,-61.1105274371641,39.2875012672119));
#200556=CARTESIAN_POINT('Ctrl Pts',(12.7893350777082,-61.0844267845857,
39.287208709576));
#200557=CARTESIAN_POINT('Ctrl Pts',(12.7666250679676,-60.9785037674412,
39.3549016990122));
#200558=CARTESIAN_POINT('Ctrl Pts',(12.6404971713781,-60.9980344071775,
39.1034939173931));
#200559=CARTESIAN_POINT('Ctrl Pts',(12.7653958126118,-60.9718026486705,
39.1031692336359));
#200560=CARTESIAN_POINT('Ctrl Pts',(12.7475073053525,-60.8885617651932,
39.2077507202317));
#200561=CARTESIAN_POINT('Ctrl Pts',(12.5977561540111,-60.7959446297926,
38.989));
#200562=CARTESIAN_POINT('Ctrl Pts',(12.7224234952041,-60.7696360759163,
38.9887769311152));
#200563=CARTESIAN_POINT('Ctrl Pts',(12.7131630221044,-60.7269846150121,
39.1161898712891));
#200564=CARTESIAN_POINT('Ctrl Pts',(12.5528626811445,-60.5836663843182,
38.989));
#200565=CARTESIAN_POINT('Ctrl Pts',(12.6772730124466,-60.5572221520604,
38.989));
#200566=CARTESIAN_POINT('Ctrl Pts',(12.6770872880162,-60.5572616290068,
39.1161895903854));
#200567=CARTESIAN_POINT('Origin',(12.642433962084,-61.0050661295707,39.3548010137695));
#200568=CARTESIAN_POINT('Ctrl Pts',(12.3431658574209,-59.5971203935659,
39.3978017080178));
#200569=CARTESIAN_POINT('Ctrl Pts',(12.4673906027141,-59.5707156088321,
39.3978017080178));
#200570=CARTESIAN_POINT('Ctrl Pts',(12.4673906027141,-59.5707156088321,
39.5248017080178));
#200571=CARTESIAN_POINT('Ctrl Pts',(12.3242219811461,-59.5091256622727,
39.3978017080178));
#200572=CARTESIAN_POINT('Ctrl Pts',(12.4486583679645,-59.4825873732142,
39.3975666025021));
#200573=CARTESIAN_POINT('Ctrl Pts',(12.4393195978195,-59.4386519140016,
39.5248015517178));
#200574=CARTESIAN_POINT('Ctrl Pts',(12.3063073021301,-59.4259203549055,
39.3484894016716));
#200575=CARTESIAN_POINT('Ctrl Pts',(12.4310355281337,-59.3996784303259,
39.3480259000051));
#200576=CARTESIAN_POINT('Ctrl Pts',(12.4127764613282,-59.3137762748649,
39.4508333188953));
#200577=CARTESIAN_POINT('Ctrl Pts',(12.2968658913801,-59.3820708699071,
39.2708017080178));
#200578=CARTESIAN_POINT('Ctrl Pts',(12.4217592664911,-59.3560370505014,
39.27051194648));
#200579=CARTESIAN_POINT('Ctrl Pts',(12.3987880210522,-59.2479658375577,
39.3343017080178));
#200580=CARTESIAN_POINT('Origin',(12.274563275759,-59.2743706222915,39.3343017080178));
#200581=CARTESIAN_POINT('Origin',(12.6794732450922,-61.1793222555443,39.6398955068198));
#200582=CARTESIAN_POINT('Origin',(12.7165125280164,-61.3535783813232,39.92499));
#200583=CARTESIAN_POINT('Origin',(12.2576496039896,-59.1947980527942,39.1934008539943));
#200584=CARTESIAN_POINT('Origin',(12.2483049653993,-59.151079340037,39.1160402713853));
#200585=CARTESIAN_POINT('Ctrl Pts',(13.0739701745323,-61.5816197022698,
40.1599502534424));
#200586=CARTESIAN_POINT('Ctrl Pts',(13.0662229071065,-61.5451281645059,
40.10025));
#200587=CARTESIAN_POINT('Ctrl Pts',(13.0516031943527,-61.4762657165316,
40.10025));
#200588=CARTESIAN_POINT('Ctrl Pts',(12.9877758510419,-61.5999188988202,
40.1599500538472));
#200589=CARTESIAN_POINT('Ctrl Pts',(13.0034370926714,-61.5584544893711,
40.100244835349));
#200590=CARTESIAN_POINT('Ctrl Pts',(13.0017087032042,-61.4868491822357,
40.10025));
#200591=CARTESIAN_POINT('Ctrl Pts',(12.9030451317659,-61.5923336062396,
40.1202442001039));
#200592=CARTESIAN_POINT('Ctrl Pts',(12.9408103617801,-61.5481051179917,
40.0633873868018));
#200593=CARTESIAN_POINT('Ctrl Pts',(12.9504709278438,-61.4721451382825,
40.0772271723538));
#200594=CARTESIAN_POINT('Ctrl Pts',(12.7836101409429,-61.5434299552079,
40.0045995998162));
#200595=CARTESIAN_POINT('Ctrl Pts',(12.8662000075463,-61.5018471007595,
39.9663485808315));
#200596=CARTESIAN_POINT('Ctrl Pts',(12.8749747009097,-61.4139027244671,
40.0101727202466));
#200597=CARTESIAN_POINT('Ctrl Pts',(12.7478263086951,-61.5035207735036,
39.9304654349859));
#200598=CARTESIAN_POINT('Ctrl Pts',(12.8544221781243,-61.465297106343,39.9051900162953));
#200599=CARTESIAN_POINT('Ctrl Pts',(12.8501918100168,-61.3716536946533,
39.9671857458179));
#200600=CARTESIAN_POINT('Ctrl Pts',(12.7383709431249,-61.4590390555209,
39.8576902534424));
#200601=CARTESIAN_POINT('Ctrl Pts',(12.8632261535953,-61.4329754599099,
39.8573998014387));
#200602=CARTESIAN_POINT('Ctrl Pts',(12.8407372733096,-61.3271735965894,
39.92499));
#200603=CARTESIAN_POINT('Origin',(13.0516031943527,-61.4762657165316,40.22725));
#200604=CARTESIAN_POINT('Origin',(-0.310561863232978,-0.0660119618346377,
39.116));
#200605=CARTESIAN_POINT('Origin',(12.164906888579,-58.7584778814677,39.116));
#200606=CARTESIAN_POINT('Origin',(5.63039444364742E-15,5.85617094392624E-15,
40.22725));
#200607=CARTESIAN_POINT('Origin',(13.0814171332231,-61.4699285681955,40.22725));
#200608=CARTESIAN_POINT('Ctrl Pts',(12.164906888579,-58.7584778814677,38.989));
#200609=CARTESIAN_POINT('Ctrl Pts',(12.2893177281499,-58.732033541174,38.989));
#200610=CARTESIAN_POINT('Ctrl Pts',(12.289131494692,-58.7320731263175,39.1161901092319));
#200611=CARTESIAN_POINT('Ctrl Pts',(12.1200194799681,-58.5461948427482,
38.989));
#200612=CARTESIAN_POINT('Ctrl Pts',(12.2442448876954,-58.5199849720709,
38.9892298989766));
#200613=CARTESIAN_POINT('Ctrl Pts',(12.2530551225939,-58.5623471386674,
39.1161900493205));
#200614=CARTESIAN_POINT('Ctrl Pts',(12.0772896710129,-58.3441042111267,
39.1034966344368));
#200615=CARTESIAN_POINT('Ctrl Pts',(12.201325600148,-58.3180679977624,39.1038314102563));
#200616=CARTESIAN_POINT('Ctrl Pts',(12.2187110949219,-58.4007711908112,
39.2077528789595));
#200617=CARTESIAN_POINT('Ctrl Pts',(12.053504764932,-58.2316113004781,39.2875012672119));
#200618=CARTESIAN_POINT('Ctrl Pts',(12.1774537884109,-58.2057612725768,
39.2878045257868));
#200619=CARTESIAN_POINT('Ctrl Pts',(12.1995935666435,-58.3108302909891,
39.3549015295897));
#200620=CARTESIAN_POINT('Origin',(12.0753355159231,-58.3370777047235,39.3548010137695));
#200621=CARTESIAN_POINT('Ctrl Pts',(13.3605623192485,-61.3267881959113,
39.8576902534424));
#200622=CARTESIAN_POINT('Ctrl Pts',(13.2359003894749,-61.3537611057083,
39.8573998014387));
#200623=CARTESIAN_POINT('Ctrl Pts',(13.2134115091892,-61.2479592423878,
39.92499));
#200624=CARTESIAN_POINT('Ctrl Pts',(13.3700210384233,-61.371290318078,39.9304984902491));
#200625=CARTESIAN_POINT('Ctrl Pts',(13.2571016411968,-61.3797222373779,
39.9052171569789));
#200626=CARTESIAN_POINT('Ctrl Pts',(13.2228703539491,-61.2924596082463,
39.9672049726608));
#200627=CARTESIAN_POINT('Ctrl Pts',(13.3535190881771,-61.422128257289,40.0043437678663));
#200628=CARTESIAN_POINT('Ctrl Pts',(13.2610999767702,-61.4177900459393,
39.9661628577643));
#200629=CARTESIAN_POINT('Ctrl Pts',(13.2173727427872,-61.3409599630865,
40.0100243556235));
#200630=CARTESIAN_POINT('Ctrl Pts',(13.2651598666398,-61.5148770953648,
40.1194874821986));
#200631=CARTESIAN_POINT('Ctrl Pts',(13.2123479779268,-61.4899829268154,
40.062755148314));
#200632=CARTESIAN_POINT('Ctrl Pts',(13.1725625528868,-61.4244514636296,
40.0767884282377));
#200633=CARTESIAN_POINT('Ctrl Pts',(13.1903059833735,-61.5568698122755,
40.1599502015388));
#200634=CARTESIAN_POINT('Ctrl Pts',(13.1590895168688,-61.5253695547383,
40.100244945386));
#200635=CARTESIAN_POINT('Ctrl Pts',(13.1314678292776,-61.4592680512443,
40.10025));
#200636=CARTESIAN_POINT('Ctrl Pts',(13.1038352065726,-61.5752716937452,
40.1599502534424));
#200637=CARTESIAN_POINT('Ctrl Pts',(13.0960702419678,-61.5387839176328,
40.10025));
#200638=CARTESIAN_POINT('Ctrl Pts',(13.0814171332231,-61.4699285681955,
40.10025));
#200639=CARTESIAN_POINT('Origin',(13.3376362544824,-61.2215544576539,39.92499));
#200640=CARTESIAN_POINT('Origin',(12.0382961820475,-58.1628213392055,39.6398955069336));
#200641=CARTESIAN_POINT('Origin',(12.0012568480858,-57.988564973546,39.92499));
#200642=CARTESIAN_POINT('Origin',(13.3005969715137,-61.0472983318708,39.6398955068282));
#200643=CARTESIAN_POINT('Origin',(13.26355768855,-60.8730422059014,39.3548010137695));
#200644=CARTESIAN_POINT('Ctrl Pts',(11.9794294790611,-57.8830978693156,
39.8576902534424));
#200645=CARTESIAN_POINT('Ctrl Pts',(12.1031907419155,-57.8572899778511,
39.8579948730703));
#200646=CARTESIAN_POINT('Ctrl Pts',(12.125481593379,-57.9621601888121,39.92499));
#200647=CARTESIAN_POINT('Ctrl Pts',(11.9699833161086,-57.8386546085355,
39.9304020711231));
#200648=CARTESIAN_POINT('Ctrl Pts',(12.0820882677174,-57.8310944294283,
39.9058915297392));
#200649=CARTESIAN_POINT('Ctrl Pts',(12.1160345187366,-57.9177151970032,
39.9671523786037));
#200650=CARTESIAN_POINT('Ctrl Pts',(11.986420485103,-57.7880992891175,40.0043257306692));
#200651=CARTESIAN_POINT('Ctrl Pts',(12.0782959991611,-57.7929810340975,
39.9667894847835));
#200652=CARTESIAN_POINT('Ctrl Pts',(12.1215717318493,-57.8694789541066,
40.01001389752));
#200653=CARTESIAN_POINT('Ctrl Pts',(12.0746725352387,-57.6961636462597,
40.1195533054858));
#200654=CARTESIAN_POINT('Ctrl Pts',(12.1272484490378,-57.7211944343229,
40.0630813209236));
#200655=CARTESIAN_POINT('Ctrl Pts',(12.1665991704024,-57.7867317752132,
40.0768265942421));
#200656=CARTESIAN_POINT('Ctrl Pts',(12.1494120604582,-57.654717811065,40.1599502027512));
#200657=CARTESIAN_POINT('Ctrl Pts',(12.1804827566585,-57.6862546895626,
40.1002552791541));
#200658=CARTESIAN_POINT('Ctrl Pts',(12.2078361528634,-57.7524075778604,
40.10025));
#200659=CARTESIAN_POINT('Ctrl Pts',(12.2354540642043,-57.6364522029207,
40.1599502534424));
#200660=CARTESIAN_POINT('Ctrl Pts',(12.2432007592846,-57.6729438621906,
40.10025));
#200661=CARTESIAN_POINT('Ctrl Pts',(12.2578193919766,-57.7418065394566,
40.10025));
#200662=CARTESIAN_POINT('Origin',(12.2578193919766,-57.7418065394566,40.22725));
#200663=CARTESIAN_POINT('Ctrl Pts',(13.1739864076105,-60.4516424606489,
38.989));
#200664=CARTESIAN_POINT('Ctrl Pts',(13.0495760655905,-60.4780866951849,
38.989));
#200665=CARTESIAN_POINT('Ctrl Pts',(13.0497618007548,-60.478047215957,39.1161896013264));
#200666=CARTESIAN_POINT('Ctrl Pts',(13.2193162256451,-60.6638314094601,
38.989));
#200667=CARTESIAN_POINT('Ctrl Pts',(13.0947262769526,-60.6905041359647,
38.988776927546));
#200668=CARTESIAN_POINT('Ctrl Pts',(13.0858380958638,-60.6477728389725,
39.1161898821822));
#200669=CARTESIAN_POINT('Ctrl Pts',(13.2624673401144,-60.8658323498478,
39.1034967087243));
#200670=CARTESIAN_POINT('Ctrl Pts',(13.1376973240545,-60.8926693037143,
39.1031720232717));
#200671=CARTESIAN_POINT('Ctrl Pts',(13.1201821075159,-60.8093487091476,
39.2077529615022));
#200672=CARTESIAN_POINT('Ctrl Pts',(13.2864868028994,-60.9782752797348,
39.2875012672119));
#200673=CARTESIAN_POINT('Ctrl Pts',(13.1616357172827,-61.0052918407715,
39.2872087095507));
#200674=CARTESIAN_POINT('Ctrl Pts',(13.1392995799685,-60.8992893450419,
39.3549017048226));
#200675=CARTESIAN_POINT('Origin',(13.1739864076105,-60.4516424606489,39.116));
#200676=CARTESIAN_POINT('Origin',(5.67687244506386E-15,5.19533244912369E-15,
40.22725));
#200677=CARTESIAN_POINT('Origin',(12.2876333308469,-57.7354693911205,40.22725));
#200678=CARTESIAN_POINT('Origin',(3.00026883051124,-12.5880644220968,39.116));
#200679=CARTESIAN_POINT('Origin',(13.0905908661165,-60.0590486699117,39.1160373285255));
#200680=CARTESIAN_POINT('Ctrl Pts',(12.2652136052659,-57.6301266171958,
40.1599502534424));
#200681=CARTESIAN_POINT('Ctrl Pts',(12.2729791421553,-57.6666142715155,
40.10025));
#200682=CARTESIAN_POINT('Ctrl Pts',(12.2876333308469,-57.7354693911205,
40.10025));
#200683=CARTESIAN_POINT('Ctrl Pts',(12.3509528635304,-57.61187916345,40.159950056604));
#200684=CARTESIAN_POINT('Ctrl Pts',(12.3354428975794,-57.6533170557954,
40.100255130536));
#200685=CARTESIAN_POINT('Ctrl Pts',(12.3374367183506,-57.7248602994014,
40.10025));
#200686=CARTESIAN_POINT('Ctrl Pts',(12.4353658313041,-57.6190178232951,
40.1203070619047));
#200687=CARTESIAN_POINT('Ctrl Pts',(12.3978675338896,-57.6632723181624,
40.0637098684499));
#200688=CARTESIAN_POINT('Ctrl Pts',(12.3886090227466,-57.7390640345628,
40.0772636213363));
#200689=CARTESIAN_POINT('Ctrl Pts',(12.5543478197374,-57.6672013517152,
40.0046102245801));
#200690=CARTESIAN_POINT('Ctrl Pts',(12.4724831634114,-57.7090592089822,
39.9670001894012));
#200691=CARTESIAN_POINT('Ctrl Pts',(12.463986515842,-57.7965151898608,40.0101788811209));
#200692=CARTESIAN_POINT('Ctrl Pts',(12.5899803678813,-57.7068899568909,
39.9303710930187));
#200693=CARTESIAN_POINT('Ctrl Pts',(12.4844838378943,-57.7455787351216,
39.9058663574104));
#200694=CARTESIAN_POINT('Ctrl Pts',(12.4887127671323,-57.8385197202055,
39.9671344706363));
#200695=CARTESIAN_POINT('Ctrl Pts',(12.599423532447,-57.751314065072,39.8576902534424));
#200696=CARTESIAN_POINT('Ctrl Pts',(12.4758649777951,-57.7780756236496,
39.8579948730703));
#200697=CARTESIAN_POINT('Ctrl Pts',(12.4981558292586,-57.8829458346106,
39.92499));
#200698=CARTESIAN_POINT('Origin',(12.6223805745518,-57.8565410498767,39.92499));
#200699=CARTESIAN_POINT('Origin',(13.081345232263,-60.0157999977505,39.1925554488856));
#200700=CARTESIAN_POINT('Origin',(13.064330085838,-59.9357500275433,39.3343017080178));
#200701=CARTESIAN_POINT('Origin',(12.6594199084528,-58.0307974155296,39.6398955069217));
#200702=CARTESIAN_POINT('Origin',(12.6964592423891,-58.2050537810542,39.3548010137695));
#200703=CARTESIAN_POINT('Ctrl Pts',(12.9957275188822,-59.6130003254555,
39.3978017080178));
#200704=CARTESIAN_POINT('Ctrl Pts',(12.871502773589,-59.6394051101894,39.3978017080178));
#200705=CARTESIAN_POINT('Ctrl Pts',(12.871502773589,-59.6394051101894,39.5248017080178));
#200706=CARTESIAN_POINT('Ctrl Pts',(13.0142126749438,-59.7010925481784,
39.3978017080178));
#200707=CARTESIAN_POINT('Ctrl Pts',(12.8901994296791,-59.7273659613754,
39.3980355775177));
#200708=CARTESIAN_POINT('Ctrl Pts',(12.899573775969,-59.7714687931893,39.5248015517192));
#200709=CARTESIAN_POINT('Ctrl Pts',(13.0316935695382,-59.7843900000233,
39.3484893995498));
#200710=CARTESIAN_POINT('Ctrl Pts',(12.9079667071292,-59.8109544298246,
39.3489438303421));
#200711=CARTESIAN_POINT('Ctrl Pts',(12.926116905724,-59.8963444006346,39.4508333155593));
#200712=CARTESIAN_POINT('Ctrl Pts',(13.0409063549237,-59.8282880397055,
39.2708017080178));
#200713=CARTESIAN_POINT('Ctrl Pts',(12.9173404733281,-59.855054532531,39.2710850691866));
#200714=CARTESIAN_POINT('Ctrl Pts',(12.9401053405448,-59.9621548122772,
39.3343017080178));
#200715=CARTESIAN_POINT('Origin',(12.9957275188822,-59.6130003254555,39.5248017080178));
#200716=CARTESIAN_POINT('Ctrl Pts',(12.6735055745739,-58.099826060148,39.2875012672119));
#200717=CARTESIAN_POINT('Ctrl Pts',(12.549758367883,-58.1266254912131,39.2878045257518));
#200718=CARTESIAN_POINT('Ctrl Pts',(12.5722680770246,-58.2316158657527,
39.3549015218347));
#200719=CARTESIAN_POINT('Ctrl Pts',(12.697532333562,-58.2122693395992,39.1034938540228));
#200720=CARTESIAN_POINT('Ctrl Pts',(12.5736300041254,-58.2389340288469,
39.1038286278789));
#200721=CARTESIAN_POINT('Ctrl Pts',(12.5913858949919,-58.3215581271248,
39.2077506434029));
#200722=CARTESIAN_POINT('Ctrl Pts',(12.7406947165197,-58.4142696920427,
38.989));
#200723=CARTESIAN_POINT('Ctrl Pts',(12.6165486539537,-58.4408527990775,
38.9892298954635));
#200724=CARTESIAN_POINT('Ctrl Pts',(12.6257301953099,-58.4831353553001,
39.1161900347288));
#200725=CARTESIAN_POINT('Ctrl Pts',(12.786030615045,-58.6264539577984,38.989));
#200726=CARTESIAN_POINT('Ctrl Pts',(12.6616197898425,-58.652898295038,38.989));
#200727=CARTESIAN_POINT('Ctrl Pts',(12.6618060089105,-58.6528587129532,
39.1161900945645));
#200728=CARTESIAN_POINT('Origin',(12.786030615045,-58.6264539577984,39.116));
#200729=CARTESIAN_POINT('Origin',(2.93511643966546,-12.2815465224192,39.5248017080178));
#200730=CARTESIAN_POINT('Origin',(12.9642895838869,-59.4650964698967,39.5248017080178));
#200731=CARTESIAN_POINT('Origin',(2.92491386234291,-12.2335471699533,39.116));
#200732=CARTESIAN_POINT('Origin',(12.8695280801142,-59.0190342907437,39.1160402713847));
#200733=CARTESIAN_POINT('Ctrl Pts',(12.9191181862044,-59.249807061628,39.2708017080178));
#200734=CARTESIAN_POINT('Ctrl Pts',(12.7944335023706,-59.2768226962998,
39.27051194648));
#200735=CARTESIAN_POINT('Ctrl Pts',(12.7714622569318,-59.1687514833561,
39.3343017080178));
#200736=CARTESIAN_POINT('Ctrl Pts',(12.9283593439858,-59.2938540730361,
39.3487519301186));
#200737=CARTESIAN_POINT('Ctrl Pts',(12.8037411209993,-59.3206115991491,
39.3482879463997));
#200738=CARTESIAN_POINT('Ctrl Pts',(12.7854979657559,-59.2347843016977,
39.4512271261635));
#200739=CARTESIAN_POINT('Ctrl Pts',(12.9458672564005,-59.3773008374013,
39.3978017080178));
#200740=CARTESIAN_POINT('Ctrl Pts',(12.8213956592929,-59.4036696715717,
39.3975673827378));
#200741=CARTESIAN_POINT('Ctrl Pts',(12.8120883873134,-59.3598823995808,
39.5248015355181));
#200742=CARTESIAN_POINT('Ctrl Pts',(12.9642895838869,-59.4650964698967,
39.3978017080178));
#200743=CARTESIAN_POINT('Ctrl Pts',(12.8400648385937,-59.4915012546305,
39.3978017080178));
#200744=CARTESIAN_POINT('Ctrl Pts',(12.8400648385937,-59.4915012546305,
39.5248017080178));
#200745=CARTESIAN_POINT('Origin',(12.895687002225,-59.1423466986222,39.3343017080178));
#200746=CARTESIAN_POINT('Origin',(12.8787733309747,-59.0627741301463,39.1934008533551));
#200747=CARTESIAN_POINT('Origin',(6.10480350566306,-61.1207756556249,39.1925554495084));
#200748=CARTESIAN_POINT('Origin',(6.10937495962084,-61.1647646440469,39.1160373285258));
#200749=CARTESIAN_POINT('Origin',(6.09624906995219,-61.0393856393804,39.3343017080178));
#200750=CARTESIAN_POINT('Ctrl Pts',(6.08531878138301,-60.929944884669,39.2708017080178));
#200751=CARTESIAN_POINT('Ctrl Pts',(6.21110821942915,-60.9172173747511,
39.2710850691866));
#200752=CARTESIAN_POINT('Ctrl Pts',(6.22255335066396,-61.0261105245454,
39.3343017080178));
#200753=CARTESIAN_POINT('Ctrl Pts',(6.08049918876647,-60.885197756147,39.3487519293518));
#200754=CARTESIAN_POINT('Ctrl Pts',(6.20637959976528,-60.8722275639167,
39.3492068662927));
#200755=CARTESIAN_POINT('Ctrl Pts',(6.21549684257599,-60.9589723348223,
39.4512271248734));
#200756=CARTESIAN_POINT('Ctrl Pts',(6.07136793516305,-60.800424540796,39.3978017080178));
#200757=CARTESIAN_POINT('Ctrl Pts',(6.19743126523188,-60.7870898478952,
39.3980347781178));
#200758=CARTESIAN_POINT('Ctrl Pts',(6.20212840134683,-60.8317801127832,
39.5248015355195));
#200759=CARTESIAN_POINT('Ctrl Pts',(6.0617588454155,-60.7112330730304,39.3978017080178));
#200760=CARTESIAN_POINT('Ctrl Pts',(6.18806312612727,-60.6979579581954,
39.3978017080178));
#200761=CARTESIAN_POINT('Ctrl Pts',(6.18806312612727,-60.6979579581954,
39.5248017080178));
#200762=CARTESIAN_POINT('Origin',(6.0617588454155,-60.7112330730304,39.5248017080178));
#200763=CARTESIAN_POINT('Origin',(-0.315760701779421,-0.033187787087479,
39.116));
#200764=CARTESIAN_POINT('Origin',(6.15137923967656,-61.5639141665612,39.116));
#200765=CARTESIAN_POINT('Origin',(-0.315760701779421,-0.033187787087479,
39.5248017080178));
#200766=CARTESIAN_POINT('Origin',(6.04595329345041,-60.5608532912344,39.5248017080178));
#200767=CARTESIAN_POINT('Ctrl Pts',(6.20712349654444,-62.0995362748659,
39.2875012672119));
#200768=CARTESIAN_POINT('Ctrl Pts',(6.33421250060443,-62.0866494451786,
39.287208709576));
#200769=CARTESIAN_POINT('Ctrl Pts',(6.32269886887976,-61.9789328429856,
39.3549016990124));
#200770=CARTESIAN_POINT('Ctrl Pts',(6.19522040634661,-61.9851725366286,
39.1034939173931));
#200771=CARTESIAN_POINT('Ctrl Pts',(6.32217680516354,-61.9721399414744,
39.1031692336332));
#200772=CARTESIAN_POINT('Ctrl Pts',(6.31308733464728,-61.8874852020939,
39.2077507202291));
#200773=CARTESIAN_POINT('Ctrl Pts',(6.17383766261684,-61.7797221753254,
38.989));
#200774=CARTESIAN_POINT('Ctrl Pts',(6.30057205577867,-61.7665890280522,
38.9887769311176));
#200775=CARTESIAN_POINT('Ctrl Pts',(6.29582060418312,-61.7232032332902,
39.1161898712918));
#200776=CARTESIAN_POINT('Ctrl Pts',(6.15137923967656,-61.5639141665612,
38.989));
#200777=CARTESIAN_POINT('Ctrl Pts',(6.27787221312702,-61.5506192193202,
38.989));
#200778=CARTESIAN_POINT('Ctrl Pts',(6.27768337964964,-61.5506390665185,
39.1161895903857));
#200779=CARTESIAN_POINT('Origin',(6.19641157197444,-61.9923681882669,39.3548010137695));
#200780=CARTESIAN_POINT('Ctrl Pts',(6.04595329345041,-60.5608532912344,
39.3978017080178));
#200781=CARTESIAN_POINT('Ctrl Pts',(6.17225757416218,-60.5475781763994,
39.3978017080178));
#200782=CARTESIAN_POINT('Ctrl Pts',(6.17225757416218,-60.5475781763994,
39.5248017080178));
#200783=CARTESIAN_POINT('Ctrl Pts',(6.03631114775037,-60.4713604300107,
39.3978017080178));
#200784=CARTESIAN_POINT('Ctrl Pts',(6.16283986559496,-60.4579746647645,
39.3975666025021));
#200785=CARTESIAN_POINT('Ctrl Pts',(6.1581447602436,-60.4133037213034,39.5248015517178));
#200786=CARTESIAN_POINT('Ctrl Pts',(6.02719193013407,-60.3867383361558,
39.3484894016716));
#200787=CARTESIAN_POINT('Ctrl Pts',(6.1539799099135,-60.3736778173762,39.3480259000049));
#200788=CARTESIAN_POINT('Ctrl Pts',(6.14480008848979,-60.2863376507156,
39.4508333188954));
#200789=CARTESIAN_POINT('Ctrl Pts',(6.02238575970256,-60.3421421670675,
39.2708017080178));
#200790=CARTESIAN_POINT('Ctrl Pts',(6.14931623097228,-60.3293058762212,
39.27051194648));
#200791=CARTESIAN_POINT('Ctrl Pts',(6.13776734223196,-60.2194255397045,
39.3343017080178));
#200792=CARTESIAN_POINT('Origin',(6.01146306152019,-60.2327006545395,39.3343017080178));
#200793=CARTESIAN_POINT('Origin',(6.21503322485551,-62.1695413802827,39.6398955068198));
#200794=CARTESIAN_POINT('Origin',(6.23365487766605,-62.3467145720969,39.92499));
#200795=CARTESIAN_POINT('Origin',(6.00295964302158,-60.1517960317859,39.193400853994));
#200796=CARTESIAN_POINT('Origin',(5.99823604520051,-60.1073400339996,39.1160402713852));
#200797=CARTESIAN_POINT('Ctrl Pts',(6.56531752495282,-62.6108711573006,
40.1599502534424));
#200798=CARTESIAN_POINT('Ctrl Pts',(6.56142710223332,-62.5737697140402,
40.10025));
#200799=CARTESIAN_POINT('Ctrl Pts',(6.55408556365926,-62.5037563256535,
40.10025));
#200800=CARTESIAN_POINT('Ctrl Pts',(6.47768259609056,-62.6200603487595,
40.159950053845));
#200801=CARTESIAN_POINT('Ctrl Pts',(6.49759225479931,-62.5804601311999,
40.1002448353481));
#200802=CARTESIAN_POINT('Ctrl Pts',(6.50335812634734,-62.5090664195357,
40.10025));
#200803=CARTESIAN_POINT('Ctrl Pts',(6.39420891953743,-62.603659837329,40.1202442001038));
#200804=CARTESIAN_POINT('Ctrl Pts',(6.43639040357922,-62.5636211788254,
40.0633873868017));
#200805=CARTESIAN_POINT('Ctrl Pts',(6.45393802800009,-62.489087119958,40.0772271723538));
#200806=CARTESIAN_POINT('Ctrl Pts',(6.28054002958119,-62.5425397295636,
40.0045995998163));
#200807=CARTESIAN_POINT('Ctrl Pts',(6.36702405212767,-62.5098176621807,
39.9663485808314));
#200808=CARTESIAN_POINT('Ctrl Pts',(6.3849433673096,-62.423272259596,40.0101727202465));
#200809=CARTESIAN_POINT('Ctrl Pts',(6.24912387034454,-62.4991087455376,
39.9304654349858));
#200810=CARTESIAN_POINT('Ctrl Pts',(6.35913125763746,-62.4722367740488,
39.9051900162944));
#200811=CARTESIAN_POINT('Ctrl Pts',(6.36471246584704,-62.3786641568871,
39.9671857458182));
#200812=CARTESIAN_POINT('Ctrl Pts',(6.24436990788039,-62.4538823482276,
39.8576902534424));
#200813=CARTESIAN_POINT('Ctrl Pts',(6.37126553604051,-62.4410124550018,
39.8573998014387));
#200814=CARTESIAN_POINT('Ctrl Pts',(6.35995915837782,-62.3334394572619,
39.92499));
#200815=CARTESIAN_POINT('Origin',(6.55408556365926,-62.5037563256535,40.22725));
#200816=CARTESIAN_POINT('Origin',(-0.315760701779421,-0.033187787087479,
39.116));
#200817=CARTESIAN_POINT('Origin',(5.95633285891191,-59.7081718144893,39.116));
#200818=CARTESIAN_POINT('Origin',(5.64744126194172E-15,5.8588708947011E-15,
40.22725));
#200819=CARTESIAN_POINT('Origin',(6.58439859103008,-62.5005702980931,40.22725));
#200820=CARTESIAN_POINT('Ctrl Pts',(5.95633285891191,-59.7081718144893,
38.989));
#200821=CARTESIAN_POINT('Ctrl Pts',(6.08282634913978,-59.6948768129328,
38.989));
#200822=CARTESIAN_POINT('Ctrl Pts',(6.08263699811363,-59.6948967145276,
39.1161901092323));
#200823=CARTESIAN_POINT('Ctrl Pts',(5.93388096803615,-59.4923596726254,
38.989));
#200824=CARTESIAN_POINT('Ctrl Pts',(6.06016553348747,-59.479278473332,38.9892298989736));
#200825=CARTESIAN_POINT('Ctrl Pts',(6.06449945282236,-59.5223294958622,
39.1161900493203));
#200826=CARTESIAN_POINT('Ctrl Pts',(5.91250946061109,-59.286909633363,39.1034966344368));
#200827=CARTESIAN_POINT('Ctrl Pts',(6.03858743331853,-59.2739813341604,
39.103831410258));
#200828=CARTESIAN_POINT('Ctrl Pts',(6.04723285085757,-59.3580487495167,
39.2077528789598));
#200829=CARTESIAN_POINT('Ctrl Pts',(5.90061356181238,-59.1725467709678,
39.2875012672119));
#200830=CARTESIAN_POINT('Ctrl Pts',(6.0265856432641,-59.1597945531718,39.2878045257868));
#200831=CARTESIAN_POINT('Ctrl Pts',(6.03762143444287,-59.2666022295038,
39.35490152959));
#200832=CARTESIAN_POINT('Origin',(5.91130048050323,-59.2797173540686,39.3548010137695));
#200833=CARTESIAN_POINT('Ctrl Pts',(6.87697683366544,-62.3873926810691,
39.8576902534424));
#200834=CARTESIAN_POINT('Ctrl Pts',(6.75017837817581,-62.4011871104969,
39.8573998014387));
#200835=CARTESIAN_POINT('Ctrl Pts',(6.73887200051313,-62.2936141127569,
39.92499));
#200836=CARTESIAN_POINT('Ctrl Pts',(6.88173199854475,-62.4326397213341,
39.9304984902491));
#200837=CARTESIAN_POINT('Ctrl Pts',(6.76854981002449,-62.4292221586344,
39.9052171569777));
#200838=CARTESIAN_POINT('Ctrl Pts',(6.74362747387393,-62.338859419464,39.967204972659));
#200839=CARTESIAN_POINT('Ctrl Pts',(6.8600064360469,-62.4814742414947,40.0043437678662));
#200840=CARTESIAN_POINT('Ctrl Pts',(6.7685470727683,-62.4674993676294,39.966162857764));
#200841=CARTESIAN_POINT('Ctrl Pts',(6.73309031164146,-62.3865194274371,
40.0100243556237));
#200842=CARTESIAN_POINT('Ctrl Pts',(6.76243636205699,-62.5644789380883,
40.1194874821987));
#200843=CARTESIAN_POINT('Ctrl Pts',(6.71251593157865,-62.5342007968287,
40.0627551483143));
#200844=CARTESIAN_POINT('Ctrl Pts',(6.6797983584025,-62.4648696125161,40.0767884282376));
#200845=CARTESIAN_POINT('Ctrl Pts',(6.6836031020277,-62.5984172531142,40.1599502015384));
#200846=CARTESIAN_POINT('Ctrl Pts',(6.65585031610595,-62.5638265480122,
40.1002449453885));
#200847=CARTESIAN_POINT('Ctrl Pts',(6.63528943158912,-62.4951999029129,
40.10025));
#200848=CARTESIAN_POINT('Ctrl Pts',(6.59568250079866,-62.6076796697354,
40.1599502534424));
#200849=CARTESIAN_POINT('Ctrl Pts',(6.59177408464754,-62.5705801176609,
40.10025));
#200850=CARTESIAN_POINT('Ctrl Pts',(6.58439859103009,-62.5005702980931,
40.10025));
#200851=CARTESIAN_POINT('Origin',(6.8651762812249,-62.2803389979219,39.92499));
#200852=CARTESIAN_POINT('Origin',(5.8926788020772,-59.1025439185011,39.6398955069324));
#200853=CARTESIAN_POINT('Origin',(5.8740571235785,-58.925370482788,39.92499));
#200854=CARTESIAN_POINT('Origin',(6.84655462836501,-62.1031658061012,39.6398955068271));
#200855=CARTESIAN_POINT('Origin',(6.82793297553329,-61.925992614092,39.3548010137695));
#200856=CARTESIAN_POINT('Ctrl Pts',(5.86337364149561,-58.8181995570485,
39.8576902534424));
#200857=CARTESIAN_POINT('Ctrl Pts',(5.98915458643775,-58.8054696185321,
39.8579948730703));
#200858=CARTESIAN_POINT('Ctrl Pts',(6.00036140429027,-58.912095367953,39.92499));
#200859=CARTESIAN_POINT('Ctrl Pts',(5.85862481136451,-58.7730123682041,
39.930402071123));
#200860=CARTESIAN_POINT('Ctrl Pts',(5.97090589422215,-58.777211762863,39.9058915297377));
#200861=CARTESIAN_POINT('Ctrl Pts',(5.99561184840486,-58.8669063622634,
39.9671523786019));
#200862=CARTESIAN_POINT('Ctrl Pts',(5.88025640567557,-58.7244521481307,
40.0043257306694));
#200863=CARTESIAN_POINT('Ctrl Pts',(5.97111833475366,-58.7389107566976,
39.9667894847838));
#200864=CARTESIAN_POINT('Ctrl Pts',(6.00616078842874,-58.819513158931,40.0100138975201));
#200865=CARTESIAN_POINT('Ctrl Pts',(5.97763489331428,-58.642244989525,40.1195533054856));
#200866=CARTESIAN_POINT('Ctrl Pts',(6.02730636094602,-58.6726343357862,
40.0630813209234));
#200867=CARTESIAN_POINT('Ctrl Pts',(6.05959099741146,-58.7419259266991,
40.076826594242));
#200868=CARTESIAN_POINT('Ctrl Pts',(6.05629725705608,-58.608838606668,40.1599502027522));
#200869=CARTESIAN_POINT('Ctrl Pts',(6.08390124328572,-58.6434504949695,
40.1002552791541));
#200870=CARTESIAN_POINT('Ctrl Pts',(6.10418993496999,-58.712100199295,40.10025));
#200871=CARTESIAN_POINT('Ctrl Pts',(6.14377718965303,-58.5996668978649,
40.1599502534424));
#200872=CARTESIAN_POINT('Ctrl Pts',(6.14766703046152,-58.6367684021393,
40.10025));
#200873=CARTESIAN_POINT('Ctrl Pts',(6.15500747092297,-58.7067819056643,
40.10025));
#200874=CARTESIAN_POINT('Origin',(6.15500747092297,-58.7067819056643,40.22725));
#200875=CARTESIAN_POINT('Ctrl Pts',(6.78290064323541,-61.4975385923862,
38.989));
#200876=CARTESIAN_POINT('Ctrl Pts',(6.65640765888775,-61.5108335407726,
38.989));
#200877=CARTESIAN_POINT('Ctrl Pts',(6.65659650327857,-61.5108136924273,
39.1161896013266));
#200878=CARTESIAN_POINT('Ctrl Pts',(6.80580235504215,-61.7133034041536,
38.989));
#200879=CARTESIAN_POINT('Ctrl Pts',(6.67910686401115,-61.7268068187933,
38.988776927546));
#200880=CARTESIAN_POINT('Ctrl Pts',(6.67473401011708,-61.6833805404075,
39.1161898821847));
#200881=CARTESIAN_POINT('Ctrl Pts',(6.82760223531318,-61.9187082819379,
39.1034967087243));
#200882=CARTESIAN_POINT('Ctrl Pts',(6.70071049691542,-61.9323562021257,
39.1031720232707));
#200883=CARTESIAN_POINT('Ctrl Pts',(6.69200060426978,-61.8476612078244,
39.2077529614998));
#200884=CARTESIAN_POINT('Ctrl Pts',(6.8397366303024,-62.0330459552232,39.2875012672119));
#200885=CARTESIAN_POINT('Ctrl Pts',(6.71274549238803,-62.046864024595,39.2872087095507));
#200886=CARTESIAN_POINT('Ctrl Pts',(6.7016119927524,-61.9391074595193,39.3549017048227));
#200887=CARTESIAN_POINT('Origin',(6.78290064323541,-61.4975385923862,39.116));
#200888=CARTESIAN_POINT('Origin',(5.67080826956262E-15,5.1943719780809E-15,
40.22725));
#200889=CARTESIAN_POINT('Origin',(6.1853204982938,-58.7035958781039,40.22725));
#200890=CARTESIAN_POINT('Origin',(0.995615674755264,-6.4352002018204,39.116));
#200891=CARTESIAN_POINT('Origin',(6.74099917688066,-61.0983782637179,39.1160373285285));
#200892=CARTESIAN_POINT('Ctrl Pts',(6.17403490859001,-58.5964866834551,
40.1599502534424));
#200893=CARTESIAN_POINT('Ctrl Pts',(6.17794390662153,-58.6335861742242,
40.10025));
#200894=CARTESIAN_POINT('Ctrl Pts',(6.1853204982938,-58.7035958781039,40.10025));
#200895=CARTESIAN_POINT('Ctrl Pts',(6.26121185652522,-58.5873013840786,
40.1599500566036));
#200896=CARTESIAN_POINT('Ctrl Pts',(6.2414554165825,-58.6268910424075,40.1002551305369));
#200897=CARTESIAN_POINT('Ctrl Pts',(6.23596000968374,-58.6982507756602,
40.10025));
#200898=CARTESIAN_POINT('Ctrl Pts',(6.34441620808589,-58.603224495399,40.1203070619047));
#200899=CARTESIAN_POINT('Ctrl Pts',(6.30249747592711,-58.6433169201088,
40.06370986845));
#200900=CARTESIAN_POINT('Ctrl Pts',(6.28536729223303,-58.7177256636152,
40.0772636213363));
#200901=CARTESIAN_POINT('Ctrl Pts',(6.45770985055653,-58.6635810738165,
40.0046102245801));
#200902=CARTESIAN_POINT('Ctrl Pts',(6.37191831988761,-58.6966524426403,
39.9670001894012));
#200903=CARTESIAN_POINT('Ctrl Pts',(6.35432657855794,-58.7827411889911,
40.0101788811209));
#200904=CARTESIAN_POINT('Ctrl Pts',(6.48899861096521,-58.7067768761601,
39.9303710930186));
#200905=CARTESIAN_POINT('Ctrl Pts',(6.38003592347219,-58.7342263230566,
39.9058663574114));
#200906=CARTESIAN_POINT('Ctrl Pts',(6.37452670784946,-58.8271002111743,
39.967134470637));
#200907=CARTESIAN_POINT('Ctrl Pts',(6.49374646112722,-58.7519447039089,
39.8576902534424));
#200908=CARTESIAN_POINT('Ctrl Pts',(6.36806742857306,-58.7656442740271,
39.8579948730703));
#200909=CARTESIAN_POINT('Ctrl Pts',(6.37927424642559,-58.8722700234481,
39.92499));
#200910=CARTESIAN_POINT('Origin',(6.50557852713736,-58.8589949086131,39.92499));
#200911=CARTESIAN_POINT('Origin',(6.73632490881042,-61.0544000804059,39.1925554488841));
#200912=CARTESIAN_POINT('Origin',(6.72777047351104,-60.9730100652055,39.3343017080178));
#200913=CARTESIAN_POINT('Origin',(6.5242002055762,-59.036168344314,39.639895506921));
#200914=CARTESIAN_POINT('Origin',(6.54282188406209,-59.2133417798936,39.3548010137695));
#200915=CARTESIAN_POINT('Ctrl Pts',(6.69328024897436,-60.6448574988554,
39.3978017080178));
#200916=CARTESIAN_POINT('Ctrl Pts',(6.56697596826259,-60.6581326136904,
39.3978017080178));
#200917=CARTESIAN_POINT('Ctrl Pts',(6.56697596826259,-60.6581326136904,
39.5248017080178));
#200918=CARTESIAN_POINT('Ctrl Pts',(6.70245599674994,-60.7343993681214,
39.3978017080178));
#200919=CARTESIAN_POINT('Ctrl Pts',(6.57637578951157,-60.7475659388567,
39.3980355775177));
#200920=CARTESIAN_POINT('Ctrl Pts',(6.58108878091675,-60.7924070567563,
39.5248015517192));
#200921=CARTESIAN_POINT('Ctrl Pts',(6.71113417453894,-60.819067758858,39.3484893995498));
#200922=CARTESIAN_POINT('Ctrl Pts',(6.58530836180071,-60.8325536871448,
39.348943830343));
#200923=CARTESIAN_POINT('Ctrl Pts',(6.59443344928427,-60.9193730951256,
39.4508333155599));
#200924=CARTESIAN_POINT('Ctrl Pts',(6.7157078966939,-60.8636883187845,39.2708017080178));
#200925=CARTESIAN_POINT('Ctrl Pts',(6.59002106156447,-60.8773920302461,
39.2710850691866));
#200926=CARTESIAN_POINT('Ctrl Pts',(6.60146619279927,-60.9862851800404,
39.3343017080178));
#200927=CARTESIAN_POINT('Origin',(6.69328024897435,-60.6448574988554,39.5248017080178));
#200928=CARTESIAN_POINT('Ctrl Pts',(6.53099325080036,-59.1062911958297,
39.2875012672119));
#200929=CARTESIAN_POINT('Ctrl Pts',(6.40512264090967,-59.1200087114582,
39.2878045257519));
#200930=CARTESIAN_POINT('Ctrl Pts',(6.41653455700107,-59.2267768430462,
39.3549015218348));
#200931=CARTESIAN_POINT('Ctrl Pts',(6.54313486548324,-59.2206299794251,
39.1034938540228));
#200932=CARTESIAN_POINT('Ctrl Pts',(6.41712406698121,-59.2341972766239,
39.1038286278807));
#200933=CARTESIAN_POINT('Ctrl Pts',(6.42614611919711,-59.3182247474317,
39.2077506434029));
#200934=CARTESIAN_POINT('Ctrl Pts',(6.56494601397037,-59.426035450364,38.989));
#200935=CARTESIAN_POINT('Ctrl Pts',(6.43870134519723,-59.4394961352161,
38.9892298954611));
#200936=CARTESIAN_POINT('Ctrl Pts',(6.4434128584844,-59.482506795581,39.1161900347291));
#200937=CARTESIAN_POINT('Ctrl Pts',(6.58785426247077,-59.6417962403143,
38.989));
#200938=CARTESIAN_POINT('Ctrl Pts',(6.461360786852,-59.6550912403353,38.989));
#200939=CARTESIAN_POINT('Ctrl Pts',(6.46155012324721,-59.6550713402783,
39.1161900945647));
#200940=CARTESIAN_POINT('Origin',(6.58785426247077,-59.6417962403143,39.116));
#200941=CARTESIAN_POINT('Origin',(0.979147644052797,-6.27851735587382,39.5248017080178));
#200942=CARTESIAN_POINT('Origin',(6.67747469700926,-60.4944777170594,39.5248017080178));
#200943=CARTESIAN_POINT('Origin',(0.976568823008617,-6.25398151259724,39.116));
#200944=CARTESIAN_POINT('Origin',(6.62985850077836,-60.0409538388296,39.116040271385));
#200945=CARTESIAN_POINT('Ctrl Pts',(6.65505462397376,-60.2756459899119,
39.2708017080178));
#200946=CARTESIAN_POINT('Ctrl Pts',(6.52822907310758,-60.2894805317162,
39.27051194648));
#200947=CARTESIAN_POINT('Ctrl Pts',(6.51668018436727,-60.1796001951995,
39.3343017080178));
#200948=CARTESIAN_POINT('Ctrl Pts',(6.65964099131233,-60.3204176712045,
39.3487519301186));
#200949=CARTESIAN_POINT('Ctrl Pts',(6.53290851690466,-60.3340024654484,
39.3482879463988));
#200950=CARTESIAN_POINT('Ctrl Pts',(6.52373669508343,-60.2467384099282,
39.4512271261633));
#200951=CARTESIAN_POINT('Ctrl Pts',(6.6683304315064,-60.4052373806432,39.3978017080178));
#200952=CARTESIAN_POINT('Ctrl Pts',(6.54178440911728,-60.4184509388129,
39.3975673827383));
#200953=CARTESIAN_POINT('Ctrl Pts',(6.53710513959985,-60.3739306632435,
39.5248015355181));
#200954=CARTESIAN_POINT('Ctrl Pts',(6.67747469700926,-60.4944777170594,
39.3978017080178));
#200955=CARTESIAN_POINT('Ctrl Pts',(6.5511704162975,-60.5077528318944,39.3978017080178));
#200956=CARTESIAN_POINT('Ctrl Pts',(6.55117041629749,-60.5077528318944,
39.5248017080178));
#200957=CARTESIAN_POINT('Origin',(6.64298446507904,-60.1663250803646,39.3343017080178));
#200958=CARTESIAN_POINT('Origin',(6.6344810469906,-60.085420458681,39.1934008533549));
#200959=CARTESIAN_POINT('Origin',(-0.317499999708329,-61.4240753804096,
39.1925554495087));
#200960=CARTESIAN_POINT('Origin',(-0.31755169001553,-61.4683012396086,39.1160373285286));
#200961=CARTESIAN_POINT('Origin',(-0.317500000000209,-61.3422370451705,
39.3343017080178));
#200962=CARTESIAN_POINT('Ctrl Pts',(-0.316930737396123,-61.2322532920972,
39.2708017080178));
#200963=CARTESIAN_POINT('Ctrl Pts',(-0.190500000000209,-61.2327440814645,
39.2710850691866));
#200964=CARTESIAN_POINT('Ctrl Pts',(-0.190500000000209,-61.3422370451705,
39.3343017080178));
#200965=CARTESIAN_POINT('Ctrl Pts',(-0.317046579199844,-61.1872475084174,
39.3487519293518));
#200966=CARTESIAN_POINT('Ctrl Pts',(-0.190500000000221,-61.187506454175,
39.3492068662925));
#200967=CARTESIAN_POINT('Ctrl Pts',(-0.190500000000208,-61.2747290395312,
39.451227124874));
#200968=CARTESIAN_POINT('Ctrl Pts',(-0.317266596913697,-61.1019842137032,
39.3978017080178));
#200969=CARTESIAN_POINT('Ctrl Pts',(-0.190500000000202,-61.1018997758114,
39.3980347781183));
#200970=CARTESIAN_POINT('Ctrl Pts',(-0.190500000000208,-61.146836207171,
39.5248015355195));
#200971=CARTESIAN_POINT('Ctrl Pts',(-0.317500000000208,-61.0122769227456,
39.3978017080178));
#200972=CARTESIAN_POINT('Ctrl Pts',(-0.190500000000207,-61.0122769227456,
39.3978017080178));
#200973=CARTESIAN_POINT('Ctrl Pts',(-0.190500000000207,-61.0122769227456,
39.5248017080178));
#200974=CARTESIAN_POINT('Origin',(-0.317500000000208,-61.0122769227456,
39.5248017080178));
#200975=CARTESIAN_POINT('Origin',(-0.317499999999994,1.10854532508269E-15,
39.116));
#200976=CARTESIAN_POINT('Origin',(-0.317500000000211,-61.8696548221181,
39.116));
#200977=CARTESIAN_POINT('Origin',(-0.317499999999994,1.10854532508269E-15,
39.5248017080178));
#200978=CARTESIAN_POINT('Origin',(-0.317500000000207,-60.8610688070707,
39.5248017080178));
#200979=CARTESIAN_POINT('Ctrl Pts',(-0.318048871877342,-62.4081695979768,
39.2875012672119));
#200980=CARTESIAN_POINT('Ctrl Pts',(-0.190309034175712,-62.4086377819835,
39.287208709576));
#200981=CARTESIAN_POINT('Ctrl Pts',(-0.190500142125266,-62.3003077603773,
39.3549016990123));
#200982=CARTESIAN_POINT('Ctrl Pts',(-0.317932489890162,-62.2931881445371,
39.1034939173931));
#200983=CARTESIAN_POINT('Ctrl Pts',(-0.190309294368566,-62.2934975005725,
39.1031692336334));
#200984=CARTESIAN_POINT('Ctrl Pts',(-0.190500141995678,-62.2083564003264,
39.2077507202293));
#200985=CARTESIAN_POINT('Ctrl Pts',(-0.317722686167617,-62.0866281564673,
38.989));
#200986=CARTESIAN_POINT('Ctrl Pts',(-0.190309769570069,-62.0868143053097,
38.9887769311176));
#200987=CARTESIAN_POINT('Ctrl Pts',(-0.190500141762077,-62.043169520538,
39.1161898712916));
#200988=CARTESIAN_POINT('Ctrl Pts',(-0.31750000000021,-61.8696548221181,
38.989));
#200989=CARTESIAN_POINT('Ctrl Pts',(-0.190310267889348,-61.8696548221181,
38.989));
#200990=CARTESIAN_POINT('Ctrl Pts',(-0.190500141514125,-61.8696548221181,
39.1161895903855));
#200991=CARTESIAN_POINT('Origin',(-0.317500000000212,-62.3004688883554,
39.3548010137695));
#200992=CARTESIAN_POINT('Ctrl Pts',(-0.317500000000207,-60.8610688070707,
39.3978017080178));
#200993=CARTESIAN_POINT('Ctrl Pts',(-0.190500000000207,-60.8610688070707,
39.3978017080178));
#200994=CARTESIAN_POINT('Ctrl Pts',(-0.190500000000207,-60.8610688070707,
39.5248017080178));
#200995=CARTESIAN_POINT('Ctrl Pts',(-0.317734773760476,-60.7710583184321,
39.3978017080178));
#200996=CARTESIAN_POINT('Ctrl Pts',(-0.190500000000205,-60.770971734242,
39.3975666025021));
#200997=CARTESIAN_POINT('Ctrl Pts',(-0.190500000000206,-60.7260547307358,
39.5248015517178));
#200998=CARTESIAN_POINT('Ctrl Pts',(-0.317958617919243,-60.6859465754578,
39.3484894016716));
#200999=CARTESIAN_POINT('Ctrl Pts',(-0.190500000000603,-60.6862105562563,
39.3480259000043));
#201000=CARTESIAN_POINT('Ctrl Pts',(-0.190500000000206,-60.5983892955408,
39.4508333188947));
#201001=CARTESIAN_POINT('Ctrl Pts',(-0.318076890623573,-60.6410923272405,
39.2708017080178));
#201002=CARTESIAN_POINT('Ctrl Pts',(-0.190500000000206,-60.6415942020422,
39.27051194648));
#201003=CARTESIAN_POINT('Ctrl Pts',(-0.190500000000206,-60.5311086139135,
39.3343017080178));
#201004=CARTESIAN_POINT('Origin',(-0.317500000000206,-60.5311086139135,
39.3343017080178));
#201005=CARTESIAN_POINT('Origin',(-0.317499999976942,-62.4786179998487,
39.6398955068185));
#201006=CARTESIAN_POINT('Origin',(-0.317500000000213,-62.6567671111299,
39.92499));
#201007=CARTESIAN_POINT('Origin',(-0.31749999999388,-60.4497583458792,39.1934008539947));
#201008=CARTESIAN_POINT('Origin',(-0.317550804320733,-60.4050521322802,
39.1160402713848));
#201009=CARTESIAN_POINT('Ctrl Pts',(-0.015266117311081,-62.9541448057648,
40.1599502534424));
#201010=CARTESIAN_POINT('Ctrl Pts',(-0.0152570710388482,-62.9168399481843,
40.10025));
#201011=CARTESIAN_POINT('Ctrl Pts',(-0.0152400000002138,-62.8464427007196,
40.10025));
#201012=CARTESIAN_POINT('Ctrl Pts',(-0.103381504925368,-62.9541233134297,
40.1599500538463));
#201013=CARTESIAN_POINT('Ctrl Pts',(-0.0794415635237479,-62.9168211560341,
40.100244835349));
#201014=CARTESIAN_POINT('Ctrl Pts',(-0.0662446030561434,-62.8464212442881,
40.10025));
#201015=CARTESIAN_POINT('Ctrl Pts',(-0.184683583688078,-62.9290872705826,
40.1202442001037));
#201016=CARTESIAN_POINT('Ctrl Pts',(-0.138547994784559,-62.8936771137448,
40.0633873868015));
#201017=CARTESIAN_POINT('Ctrl Pts',(-0.11330556745179,-62.8213855864655,
40.0772271723537));
#201018=CARTESIAN_POINT('Ctrl Pts',(-0.29134099263186,-62.8564203507742,
40.0045995998164));
#201019=CARTESIAN_POINT('Ctrl Pts',(-0.20191035119152,-62.8329175802742,
39.9663485808317));
#201020=CARTESIAN_POINT('Ctrl Pts',(-0.175042741958046,-62.7487193609389,
40.0101727202466));
#201021=CARTESIAN_POINT('Ctrl Pts',(-0.318045276842851,-62.8099434033761,
39.9304654349858));
#201022=CARTESIAN_POINT('Ctrl Pts',(-0.205831635643045,-62.7947175425015,
39.9051900162937));
#201023=CARTESIAN_POINT('Ctrl Pts',(-0.190500000000215,-62.7022409210455,
39.9671857458166));
#201024=CARTESIAN_POINT('Ctrl Pts',(-0.318045750793259,-62.7644678366119,
39.8576902534424));
#201025=CARTESIAN_POINT('Ctrl Pts',(-0.190500000000209,-62.7649326510149,
39.8573998014387));
#201026=CARTESIAN_POINT('Ctrl Pts',(-0.190500000000213,-62.6567671111299,
39.92499));
#201027=CARTESIAN_POINT('Origin',(-0.0152400000002138,-62.8464427007196,
40.22725));
#201028=CARTESIAN_POINT('Origin',(-0.317499999999994,1.10854532508269E-15,
39.116));
#201029=CARTESIAN_POINT('Origin',(-0.317500000000204,-60.0036905223731,
39.116));
#201030=CARTESIAN_POINT('Origin',(-3.02076666443335E-17,1.64889592811714E-16,
40.22725));
#201031=CARTESIAN_POINT('Origin',(0.0152399999997862,-62.8464427007196,
40.22725));
#201032=CARTESIAN_POINT('Ctrl Pts',(-0.317500000000204,-60.0036905223731,
38.989));
#201033=CARTESIAN_POINT('Ctrl Pts',(-0.19030974826544,-60.003690522373,
38.989));
#201034=CARTESIAN_POINT('Ctrl Pts',(-0.190500142289733,-60.0036905223731,
39.1161901092321));
#201035=CARTESIAN_POINT('Ctrl Pts',(-0.317270385524616,-59.7867137603524,
38.989));
#201036=CARTESIAN_POINT('Ctrl Pts',(-0.190310262476514,-59.786904552798,
38.989229898976));
#201037=CARTESIAN_POINT('Ctrl Pts',(-0.190500142032665,-59.8301727552495,
39.1161900493201));
#201038=CARTESIAN_POINT('Ctrl Pts',(-0.317049440713822,-59.5801552670728,
39.1034966344368));
#201039=CARTESIAN_POINT('Ctrl Pts',(-0.190310761081983,-59.5804765271857,
39.1038314102564));
#201040=CARTESIAN_POINT('Ctrl Pts',(-0.190500141785309,-59.664987104655,
39.2077528789601));
#201041=CARTESIAN_POINT('Ctrl Pts',(-0.316925998273249,-59.4651754363832,
39.2875012672119));
#201042=CARTESIAN_POINT('Ctrl Pts',(-0.19031103533518,-59.4656607446593,
39.2878045257868));
#201043=CARTESIAN_POINT('Ctrl Pts',(-0.190500141647105,-59.5730368716576,
39.3549015295899));
#201044=CARTESIAN_POINT('Origin',(-0.317500000000203,-59.5728760150042,
39.3548010137695));
#201045=CARTESIAN_POINT('Ctrl Pts',(0.318045750792832,-62.7644678366119,
39.8576902534424));
#201046=CARTESIAN_POINT('Ctrl Pts',(0.190499999999787,-62.7649326510149,
39.8573998014387));
#201047=CARTESIAN_POINT('Ctrl Pts',(0.190499999999787,-62.6567671111299,
39.92499));
#201048=CARTESIAN_POINT('Ctrl Pts',(0.318045262794968,-62.8099640589334,
39.930498490249));
#201049=CARTESIAN_POINT('Ctrl Pts',(0.205840330722736,-62.794734457763,
39.9052171569785));
#201050=CARTESIAN_POINT('Ctrl Pts',(0.190499999999787,-62.7022616416336,
39.9672049726603));
#201051=CARTESIAN_POINT('Ctrl Pts',(0.291334117855151,-62.8562601188215,
40.0043437678664));
#201052=CARTESIAN_POINT('Ctrl Pts',(0.201836550627533,-62.8328016940825,
39.9661628577643));
#201053=CARTESIAN_POINT('Ctrl Pts',(0.175038734051849,-62.7485591297232,
40.0100243556236));
#201054=CARTESIAN_POINT('Ctrl Pts',(0.18562218956022,-62.928611257107,40.1194874821985));
#201055=CARTESIAN_POINT('Ctrl Pts',(0.139140155999885,-62.8932808767899,
40.062755148314));
#201056=CARTESIAN_POINT('Ctrl Pts',(0.113848895265595,-62.8209095783125,
40.0767884282376));
#201057=CARTESIAN_POINT('Ctrl Pts',(0.10367326646258,-62.9541233349674,
40.1599502015391));
#201058=CARTESIAN_POINT('Ctrl Pts',(0.0796882264534641,-62.9168211653022,
40.1002449453869));
#201059=CARTESIAN_POINT('Ctrl Pts',(0.0664134143648399,-62.8464212664863,
40.10025));
#201060=CARTESIAN_POINT('Ctrl Pts',(0.0152661173106522,-62.9541448057648,
40.1599502534424));
#201061=CARTESIAN_POINT('Ctrl Pts',(0.0152570710384197,-62.9168399481843,
40.10025));
#201062=CARTESIAN_POINT('Ctrl Pts',(0.0152399999997859,-62.8464427007196,
40.10025));
#201063=CARTESIAN_POINT('Origin',(0.317499999999787,-62.6567671111299,39.92499));
#201064=CARTESIAN_POINT('Origin',(-0.31749999997078,-59.3947266586231,39.639895506931));
#201065=CARTESIAN_POINT('Origin',(-0.317500000000201,-59.2165773020941,
39.92499));
#201066=CARTESIAN_POINT('Origin',(0.317499999978187,-62.4786179998349,39.6398955068271));
#201067=CARTESIAN_POINT('Origin',(0.317499999999788,-62.3004688883555,39.3548010137695));
#201068=CARTESIAN_POINT('Ctrl Pts',(-0.316922544675889,-59.1088767419348,
39.8576902534424));
#201069=CARTESIAN_POINT('Ctrl Pts',(-0.190500000000201,-59.1093642282367,
39.8579948730703));
#201070=CARTESIAN_POINT('Ctrl Pts',(-0.190500000000201,-59.2165773020941,
39.92499));
#201071=CARTESIAN_POINT('Ctrl Pts',(-0.316922012809372,-59.0634407053228,
39.9304020711232));
#201072=CARTESIAN_POINT('Ctrl Pts',(-0.205694973740961,-59.0793536643045,
39.9058915297389));
#201073=CARTESIAN_POINT('Ctrl Pts',(-0.190500000000201,-59.1711393827293,
39.9671523786037));
#201074=CARTESIAN_POINT('Ctrl Pts',(-0.290332993455254,-59.0174076205277,
40.0043257306692));
#201075=CARTESIAN_POINT('Ctrl Pts',(-0.201480151666078,-59.0412846811398,
39.9667894847832));
#201076=CARTESIAN_POINT('Ctrl Pts',(-0.175054909460048,-59.1251084688124,
40.0100138975199));
#201077=CARTESIAN_POINT('Ctrl Pts',(-0.184894967401715,-58.9458296250061,
40.1195533054858));
#201078=CARTESIAN_POINT('Ctrl Pts',(-0.138672156931401,-58.9812445774289,
40.0630813209239));
#201079=CARTESIAN_POINT('Ctrl Pts',(-0.113807322597838,-59.053531245193,
40.0768265942422));
#201080=CARTESIAN_POINT('Ctrl Pts',(-0.103171606455975,-58.9208287018091,
40.1599502027518));
#201081=CARTESIAN_POINT('Ctrl Pts',(-0.0793367652460264,-58.9581363848269,
40.1002552791538));
#201082=CARTESIAN_POINT('Ctrl Pts',(-0.0663350652346691,-59.0285307646513,
40.10025));
#201083=CARTESIAN_POINT('Ctrl Pts',(-0.0152121934561203,-58.9208513795073,
40.1599502534424));
#201084=CARTESIAN_POINT('Ctrl Pts',(-0.0152218248293074,-58.9581562369413,
40.10025));
#201085=CARTESIAN_POINT('Ctrl Pts',(-0.0152400000002007,-59.0285534841296,
40.10025));
#201086=CARTESIAN_POINT('Origin',(-0.0152400000002004,-59.0285534841296,
40.22725));
#201087=CARTESIAN_POINT('Ctrl Pts',(0.31749999999979,-61.8696548221181,
38.989));
#201088=CARTESIAN_POINT('Ctrl Pts',(0.190310256931471,-61.8696548221181,
38.989));
#201089=CARTESIAN_POINT('Ctrl Pts',(0.190500141530038,-61.8696548221181,
39.1161896013266));
#201090=CARTESIAN_POINT('Ctrl Pts',(0.317722689632019,-62.0866315324121,
38.989));
#201091=CARTESIAN_POINT('Ctrl Pts',(0.190309758575691,-62.0868176889529,
38.988776927546));
#201092=CARTESIAN_POINT('Ctrl Pts',(0.190500141778021,-62.043172216566,
39.1161898821848));
#201093=CARTESIAN_POINT('Ctrl Pts',(0.31793249165548,-62.2931898887681,
39.1034967087243));
#201094=CARTESIAN_POINT('Ctrl Pts',(0.190309283350388,-62.2934992458053,
39.1031720232706));
#201095=CARTESIAN_POINT('Ctrl Pts',(0.190500142011646,-62.2083577878513,
39.2077529614998));
#201096=CARTESIAN_POINT('Ctrl Pts',(0.318048871876917,-62.4081695979768,
39.2875012672119));
#201097=CARTESIAN_POINT('Ctrl Pts',(0.190309023146547,-62.4086377820239,
39.2872087095508));
#201098=CARTESIAN_POINT('Ctrl Pts',(0.190500142141246,-62.3003077510787,
39.3549017048227));
#201099=CARTESIAN_POINT('Origin',(0.31749999999979,-61.8696548221181,39.116));
#201100=CARTESIAN_POINT('Origin',(4.1196902326603E-16,-5.86572468760199E-17,
40.22725));
#201101=CARTESIAN_POINT('Origin',(0.0152399999997996,-59.0285534841296,
40.22725));
#201102=CARTESIAN_POINT('Origin',(0.317500000000005,2.1613999771587E-13,
39.116));
#201103=CARTESIAN_POINT('Origin',(0.317551690012274,-61.4683012396062,39.1160373285252));
#201104=CARTESIAN_POINT('Ctrl Pts',(0.0152121934557198,-58.9208513795073,
40.1599502534424));
#201105=CARTESIAN_POINT('Ctrl Pts',(0.0152218248289066,-58.9581562369413,
40.10025));
#201106=CARTESIAN_POINT('Ctrl Pts',(0.0152399999997995,-59.0285534841296,
40.10025));
#201107=CARTESIAN_POINT('Ctrl Pts',(0.102871702177192,-58.9208288705618,
40.1599500566038));
#201108=CARTESIAN_POINT('Ctrl Pts',(0.0790852439331834,-58.9581365422964,
40.100255130536));
#201109=CARTESIAN_POINT('Ctrl Pts',(0.0661608181923067,-59.0285309330218,
40.10025));
#201110=CARTESIAN_POINT('Ctrl Pts',(0.183955833237311,-58.9453619764183,
40.1203070619046));
#201111=CARTESIAN_POINT('Ctrl Pts',(0.138075936735767,-58.9808530699761,
40.0637098684499));
#201112=CARTESIAN_POINT('Ctrl Pts',(0.113261762367961,-59.0530636028226,
40.0772636213363));
#201113=CARTESIAN_POINT('Ctrl Pts',(0.290319860890461,-59.0172303255294,
40.0046102245801));
#201114=CARTESIAN_POINT('Ctrl Pts',(0.201541405841739,-59.0411528690721,
39.9670001894012));
#201115=CARTESIAN_POINT('Ctrl Pts',(0.175047309550988,-59.1249311745757,
40.0101788811209));
#201116=CARTESIAN_POINT('Ctrl Pts',(0.316922027357148,-59.0634600627911,
39.9303710930187));
#201117=CARTESIAN_POINT('Ctrl Pts',(0.20568700036638,-59.0793694364682,
39.905866357411));
#201118=CARTESIAN_POINT('Ctrl Pts',(0.190499999999799,-59.1711586818657,
39.9671344706363));
#201119=CARTESIAN_POINT('Ctrl Pts',(0.316922544675488,-59.1088767419348,
39.8576902534424));
#201120=CARTESIAN_POINT('Ctrl Pts',(0.190499999999799,-59.1093642282366,
39.8579948730703));
#201121=CARTESIAN_POINT('Ctrl Pts',(0.190499999999799,-59.2165773020941,
39.92499));
#201122=CARTESIAN_POINT('Origin',(0.317499999999799,-59.2165773020941,39.92499));
#201123=CARTESIAN_POINT('Origin',(0.317499999994104,-61.4240753793282,39.1925554488844));
#201124=CARTESIAN_POINT('Origin',(0.317499999999791,-61.3422370451705,39.3343017080178));
#201125=CARTESIAN_POINT('Origin',(0.317499999970067,-59.3947266586071,39.639895506921));
#201126=CARTESIAN_POINT('Origin',(0.317499999999798,-59.5728760150042,39.3548010137695));
#201127=CARTESIAN_POINT('Ctrl Pts',(0.317499999999793,-61.0122769227456,
39.3978017080178));
#201128=CARTESIAN_POINT('Ctrl Pts',(0.190499999999793,-61.0122769227456,
39.3978017080178));
#201129=CARTESIAN_POINT('Ctrl Pts',(0.190499999999793,-61.0122769227456,
39.5248017080178));
#201130=CARTESIAN_POINT('Ctrl Pts',(0.317265808076182,-61.1022873990971,
39.3978017080178));
#201131=CARTESIAN_POINT('Ctrl Pts',(0.190499999999776,-61.1022028716704,
39.3980355775177));
#201132=CARTESIAN_POINT('Ctrl Pts',(0.190499999999792,-61.1472909869838,
39.5248015517192));
#201133=CARTESIAN_POINT('Ctrl Pts',(0.31704618912888,-61.1873990841185,
39.3484893995498));
#201134=CARTESIAN_POINT('Ctrl Pts',(0.190500000001004,-61.1876587562325,
39.3489438303426));
#201135=CARTESIAN_POINT('Ctrl Pts',(0.190499999999792,-61.2749563897836,
39.4508333155593));
#201136=CARTESIAN_POINT('Ctrl Pts',(0.316930737395706,-61.2322532920972,
39.2708017080178));
#201137=CARTESIAN_POINT('Ctrl Pts',(0.190499999999785,-61.2327440814646,
39.2710850691866));
#201138=CARTESIAN_POINT('Ctrl Pts',(0.190499999999791,-61.3422370451705,
39.3343017080178));
#201139=CARTESIAN_POINT('Origin',(0.317499999999793,-61.0122769227456,39.5248017080178));
#201140=CARTESIAN_POINT('Ctrl Pts',(0.316925998272845,-59.4651754363832,
39.2875012672119));
#201141=CARTESIAN_POINT('Ctrl Pts',(0.190311049925075,-59.4656607446034,
39.2878045257519));
#201142=CARTESIAN_POINT('Ctrl Pts',(0.190500141624843,-59.5730368592469,
39.3549015218346));
#201143=CARTESIAN_POINT('Ctrl Pts',(0.317049442578974,-59.5801570044831,
39.1034938540228));
#201144=CARTESIAN_POINT('Ctrl Pts',(0.19031077568779,-59.5804782634875,
39.1038286278812));
#201145=CARTESIAN_POINT('Ctrl Pts',(0.190500141763029,-59.6649884842717,
39.2077506434031));
#201146=CARTESIAN_POINT('Ctrl Pts',(0.317270389088641,-59.7867171285936,
38.989));
#201147=CARTESIAN_POINT('Ctrl Pts',(0.190310277118154,-59.7869079131817,
38.9892298954611));
#201148=CARTESIAN_POINT('Ctrl Pts',(0.190500142010347,-59.8301754438924,
39.1161900347287));
#201149=CARTESIAN_POINT('Ctrl Pts',(0.317499999999796,-60.0036905223731,
38.989));
#201150=CARTESIAN_POINT('Ctrl Pts',(0.190309762954753,-60.0036905223731,
38.989));
#201151=CARTESIAN_POINT('Ctrl Pts',(0.190500142267369,-60.0036905223731,
39.1161900945644));
#201152=CARTESIAN_POINT('Origin',(0.317499999999796,-60.0036905223731,39.116));
#201153=CARTESIAN_POINT('Origin',(0.317500000000005,2.10877617033113E-13,
39.5248017080178));
#201154=CARTESIAN_POINT('Origin',(0.317499999999793,-60.8610688070707,39.5248017080178));
#201155=CARTESIAN_POINT('Origin',(0.317500000000005,2.10053551406057E-13,
39.116));
#201156=CARTESIAN_POINT('Origin',(0.317550804320415,-60.4050521322802,39.1160402713848));
#201157=CARTESIAN_POINT('Ctrl Pts',(0.31807689062316,-60.6410923272405,
39.2708017080178));
#201158=CARTESIAN_POINT('Ctrl Pts',(0.1904999999998,-60.6415942020422,39.27051194648));
#201159=CARTESIAN_POINT('Ctrl Pts',(0.190499999999794,-60.5311086139135,
39.3343017080178));
#201160=CARTESIAN_POINT('Ctrl Pts',(0.317958218318564,-60.6860981505083,
39.3487519301186));
#201161=CARTESIAN_POINT('Ctrl Pts',(0.190499999998582,-60.6863613750267,
39.348287946399));
#201162=CARTESIAN_POINT('Ctrl Pts',(0.190499999999794,-60.598616644694,
39.4512271261644));
#201163=CARTESIAN_POINT('Ctrl Pts',(0.317733982967334,-60.771361502534,
39.3978017080178));
#201164=CARTESIAN_POINT('Ctrl Pts',(0.190499999999793,-60.7712750142006,
39.3975673827397));
#201165=CARTESIAN_POINT('Ctrl Pts',(0.190499999999794,-60.7265095085063,
39.5248015355181));
#201166=CARTESIAN_POINT('Ctrl Pts',(0.317499999999793,-60.8610688070707,
39.3978017080178));
#201167=CARTESIAN_POINT('Ctrl Pts',(0.190499999999793,-60.8610688070707,
39.3978017080178));
#201168=CARTESIAN_POINT('Ctrl Pts',(0.190499999999793,-60.8610688070707,
39.5248017080178));
#201169=CARTESIAN_POINT('Origin',(0.317499999999794,-60.5311086139135,39.3343017080178));
#201170=CARTESIAN_POINT('Origin',(0.317500000300197,-60.4497583469878,39.1934008533546));
#201171=CARTESIAN_POINT('Origin',(-6.73632490863922,-61.0544000815109,39.1925554495083));
#201172=CARTESIAN_POINT('Origin',(-6.74099917688029,-61.0983782637176,39.1160373285273));
#201173=CARTESIAN_POINT('Origin',(-6.72777047351144,-60.9730100652054,39.3343017080178));
#201174=CARTESIAN_POINT('Ctrl Pts',(-6.7157078966943,-60.8636883187844,
39.2708017080178));
#201175=CARTESIAN_POINT('Ctrl Pts',(-6.59002106156486,-60.877392030246,
39.2710850691866));
#201176=CARTESIAN_POINT('Ctrl Pts',(-6.60146619279967,-60.9862851800404,
39.3343017080178));
#201177=CARTESIAN_POINT('Ctrl Pts',(-6.71111871849837,-60.8189169727309,
39.3487519293517));
#201178=CARTESIAN_POINT('Ctrl Pts',(-6.58529244190256,-60.832402219412,
39.3492068662929));
#201179=CARTESIAN_POINT('Ctrl Pts',(-6.59440968471164,-60.9191469903167,
39.4512271248736));
#201180=CARTESIAN_POINT('Ctrl Pts',(-6.70242508976246,-60.7340977611528,
39.3978017080178));
#201181=CARTESIAN_POINT('Ctrl Pts',(-6.57634410736735,-60.7472645033898,
39.3980347781178));
#201182=CARTESIAN_POINT('Ctrl Pts',(-6.58104124348259,-60.7919547682786,
39.524801535519));
#201183=CARTESIAN_POINT('Ctrl Pts',(-6.69328024897476,-60.6448574988554,
39.3978017080178));
#201184=CARTESIAN_POINT('Ctrl Pts',(-6.56697596826299,-60.6581326136904,
39.3978017080178));
#201185=CARTESIAN_POINT('Ctrl Pts',(-6.56697596826298,-60.6581326136904,
39.5248017080178));
#201186=CARTESIAN_POINT('Origin',(-6.69328024897475,-60.6448574988554,39.5248017080178));
#201187=CARTESIAN_POINT('Origin',(-0.315760701779421,0.0331877870874811,
39.116));
#201188=CARTESIAN_POINT('Origin',(-6.78290064323581,-61.4975385923862,39.116));
#201189=CARTESIAN_POINT('Origin',(-0.315760701779421,0.0331877870874811,
39.5248017080178));
#201190=CARTESIAN_POINT('Origin',(-6.67747469700966,-60.4944777170594,39.5248017080178));
#201191=CARTESIAN_POINT('Ctrl Pts',(-6.83973663030281,-62.0330459552232,
39.2875012672119));
#201192=CARTESIAN_POINT('Ctrl Pts',(-6.71274550335251,-62.0468640234019,
39.287208709576));
#201193=CARTESIAN_POINT('Ctrl Pts',(-6.70161199370846,-61.9391074687685,
39.3549016990123));
#201194=CARTESIAN_POINT('Ctrl Pts',(-6.82760205123578,-61.9187065474465,
39.1034939173931));
#201195=CARTESIAN_POINT('Ctrl Pts',(-6.70071032544293,-61.9323544653044,
39.1031692336329));
#201196=CARTESIAN_POINT('Ctrl Pts',(-6.69200045921796,-61.8476598279013,
39.2077507202296));
#201197=CARTESIAN_POINT('Ctrl Pts',(-6.80580199871494,-61.7133000470646,
38.989));
#201198=CARTESIAN_POINT('Ctrl Pts',(-6.67910652125822,-61.7268034525352,
38.9887769311176));
#201199=CARTESIAN_POINT('Ctrl Pts',(-6.67473372828961,-61.6833778591508,
39.1161898712916));
#201200=CARTESIAN_POINT('Ctrl Pts',(-6.78290064323581,-61.4975385923862,
38.989));
#201201=CARTESIAN_POINT('Ctrl Pts',(-6.65640766978554,-61.5108335396272,
38.989));
#201202=CARTESIAN_POINT('Ctrl Pts',(-6.65659650326273,-61.510813692429,
39.1161895903855));
#201203=CARTESIAN_POINT('Origin',(-6.8279329755337,-61.9259926140919,39.3548010137695));
#201204=CARTESIAN_POINT('Ctrl Pts',(-6.67747469700966,-60.4944777170594,
39.3978017080178));
#201205=CARTESIAN_POINT('Ctrl Pts',(-6.55117041629789,-60.5077528318944,
39.3978017080178));
#201206=CARTESIAN_POINT('Ctrl Pts',(-6.55117041629789,-60.5077528318944,
39.5248017080178));
#201207=CARTESIAN_POINT('Ctrl Pts',(-6.66829952659983,-60.404935774755,
39.3978017080178));
#201208=CARTESIAN_POINT('Ctrl Pts',(-6.54175270773085,-60.4181493202587,
39.397566602504));
#201209=CARTESIAN_POINT('Ctrl Pts',(-6.53705760237928,-60.373478376798,
39.5248015517196));
#201210=CARTESIAN_POINT('Ctrl Pts',(-6.65962554481717,-60.3202668847283,
39.3484894016716));
#201211=CARTESIAN_POINT('Ctrl Pts',(-6.53289275205199,-60.3338524728719,
39.3480259000033));
#201212=CARTESIAN_POINT('Ctrl Pts',(-6.52371293062554,-60.246512306211,
39.4508333188939));
#201213=CARTESIAN_POINT('Ctrl Pts',(-6.65505462397415,-60.2756459899119,
39.2708017080178));
#201214=CARTESIAN_POINT('Ctrl Pts',(-6.52822907310799,-60.2894805317161,
39.27051194648));
#201215=CARTESIAN_POINT('Ctrl Pts',(-6.51668018436767,-60.1796001951995,
39.3343017080178));
#201216=CARTESIAN_POINT('Origin',(-6.64298446507943,-60.1663250803645,39.3343017080178));
#201217=CARTESIAN_POINT('Origin',(-6.84655462836824,-62.1031658061144,39.6398955068187));
#201218=CARTESIAN_POINT('Origin',(-6.86517628122531,-62.2803389979219,39.92499));
#201219=CARTESIAN_POINT('Origin',(-6.63448104656953,-60.0854204576115,39.1934008539944));
#201220=CARTESIAN_POINT('Origin',(-6.62985850077867,-60.0409538388295,39.1160402713849));
#201221=CARTESIAN_POINT('Ctrl Pts',(-6.59568250079906,-62.6076796697354,
40.1599502534424));
#201222=CARTESIAN_POINT('Ctrl Pts',(-6.59177408464795,-62.5705801176609,
40.10025));
#201223=CARTESIAN_POINT('Ctrl Pts',(-6.58439859103049,-62.5005702980931,
40.10025));
#201224=CARTESIAN_POINT('Ctrl Pts',(-6.68331293653979,-62.5984477290802,
40.1599500538468));
#201225=CARTESIAN_POINT('Ctrl Pts',(-6.65560500345307,-62.5638523220933,
40.1002448353502));
#201226=CARTESIAN_POINT('Ctrl Pts',(-6.6351215427267,-62.4952175264275,
40.10025));
#201227=CARTESIAN_POINT('Ctrl Pts',(-6.76155265492271,-62.5650504549418,
40.1202442001039));
#201228=CARTESIAN_POINT('Ctrl Pts',(-6.71196843232426,-62.5346567608587,
40.0633873868018));
#201229=CARTESIAN_POINT('Ctrl Pts',(-6.6793077633958,-62.4653998062673,
40.0772271723538));
#201230=CARTESIAN_POINT('Ctrl Pts',(-6.86003002196301,-62.48163287707,40.0045995998162));
#201231=CARTESIAN_POINT('Ctrl Pts',(-6.76863258245072,-62.4676069047243,
39.9663485808315));
#201232=CARTESIAN_POINT('Ctrl Pts',(-6.73311104631486,-62.3866783619499,
40.0101727202465));
#201233=CARTESIAN_POINT('Ctrl Pts',(-6.88172985342185,-62.4326191774618,
39.930465434986));
#201234=CARTESIAN_POINT('Ctrl Pts',(-6.76853939445034,-62.4292062449171,
39.9051900162951));
#201235=CARTESIAN_POINT('Ctrl Pts',(-6.74362530798287,-62.3388388123831,
39.9671857458173));
#201236=CARTESIAN_POINT('Ctrl Pts',(-6.87697683366585,-62.3873926810691,
39.8576902534424));
#201237=CARTESIAN_POINT('Ctrl Pts',(-6.75017837817623,-62.4011871104968,
39.8573998014387));
#201238=CARTESIAN_POINT('Ctrl Pts',(-6.73887200051354,-62.2936141127569,
39.92499));
#201239=CARTESIAN_POINT('Origin',(-6.58439859103049,-62.5005702980931,40.22725));
#201240=CARTESIAN_POINT('Origin',(-0.315760701779421,0.0331877870874811,
39.116));
#201241=CARTESIAN_POINT('Origin',(-6.58785426247116,-59.6417962403142,39.116));
#201242=CARTESIAN_POINT('Origin',(-1.29720108988942E-17,1.63986310369608E-16,
40.22725));
#201243=CARTESIAN_POINT('Origin',(-6.55408556365967,-62.5037563256534,40.22725));
#201244=CARTESIAN_POINT('Ctrl Pts',(-6.58785426247116,-59.6417962403142,
38.989));
#201245=CARTESIAN_POINT('Ctrl Pts',(-6.46136077224317,-59.6550912418708,
38.989));
#201246=CARTESIAN_POINT('Ctrl Pts',(-6.46155012326944,-59.6550713402759,
39.1161901092324));
#201247=CARTESIAN_POINT('Ctrl Pts',(-6.56494565834866,-59.4260321009469,
38.989));
#201248=CARTESIAN_POINT('Ctrl Pts',(-6.43870097937981,-59.4394927947734,
38.989229898976));
#201249=CARTESIAN_POINT('Ctrl Pts',(-6.44341257746702,-59.4825041216658,
39.1161900493204));
#201250=CARTESIAN_POINT('Ctrl Pts',(-6.543134682019,-59.2206282517276,39.1034966344368));
#201251=CARTESIAN_POINT('Ctrl Pts',(-6.41712387096028,-59.234195551358,
39.1038314102552));
#201252=CARTESIAN_POINT('Ctrl Pts',(-6.42614597500986,-59.3182233753686,
39.2077528789594));
#201253=CARTESIAN_POINT('Ctrl Pts',(-6.53099325080075,-59.1062911958296,
39.2875012672119));
#201254=CARTESIAN_POINT('Ctrl Pts',(-6.40512262640556,-59.1200087130389,
39.2878045257868));
#201255=CARTESIAN_POINT('Ctrl Pts',(-6.41653455832048,-59.2267768553867,
39.3549015295901));
#201256=CARTESIAN_POINT('Origin',(-6.54282188406247,-59.2133417798936,39.3548010137695));
#201257=CARTESIAN_POINT('Ctrl Pts',(-6.2443699078808,-62.4538823482275,
39.8576902534424));
#201258=CARTESIAN_POINT('Ctrl Pts',(-6.37126553604092,-62.4410124550018,
39.8573998014387));
#201259=CARTESIAN_POINT('Ctrl Pts',(-6.35995915837823,-62.3334394572619,
39.92499));
#201260=CARTESIAN_POINT('Ctrl Pts',(-6.24912604340947,-62.4991292864732,
39.9304984902492));
#201261=CARTESIAN_POINT('Ctrl Pts',(-6.3591243783171,-62.4722545055304,
39.9052171569797));
#201262=CARTESIAN_POINT('Ctrl Pts',(-6.36471463173893,-62.378684763968,
39.9672049726599));
#201263=CARTESIAN_POINT('Ctrl Pts',(-6.28053011789757,-62.5423796567682,
40.004343767866));
#201264=CARTESIAN_POINT('Ctrl Pts',(-6.36708533499896,-62.5096946965644,
39.9661628577643));
#201265=CARTESIAN_POINT('Ctrl Pts',(-6.38493060453732,-62.4231124872028,
40.0100243556236));
#201266=CARTESIAN_POINT('Ctrl Pts',(-6.39322569848911,-62.6032845425346,
40.1194874821989));
#201267=CARTESIAN_POINT('Ctrl Pts',(-6.43576006824497,-62.5632890102013,
40.062755148314));
#201268=CARTESIAN_POINT('Ctrl Pts',(-6.45334792019214,-62.4886705126496,
40.0767884282376));
#201269=CARTESIAN_POINT('Ctrl Pts',(-6.47739243510511,-62.620090867565,
40.1599502015389));
#201270=CARTESIAN_POINT('Ctrl Pts',(-6.49734694408379,-62.5804859237136,
40.1002449453872));
#201271=CARTESIAN_POINT('Ctrl Pts',(-6.50319024212544,-62.5090840872032,
40.10025));
#201272=CARTESIAN_POINT('Ctrl Pts',(-6.56531752495323,-62.6108711573005,
40.1599502534424));
#201273=CARTESIAN_POINT('Ctrl Pts',(-6.56142710223373,-62.5737697140402,
40.10025));
#201274=CARTESIAN_POINT('Ctrl Pts',(-6.55408556365967,-62.5037563256534,
40.10025));
#201275=CARTESIAN_POINT('Origin',(-6.23365487766645,-62.3467145720969,39.92499));
#201276=CARTESIAN_POINT('Origin',(-6.52420020558083,-59.0361683443333,39.6398955069332));
#201277=CARTESIAN_POINT('Origin',(-6.50557852713774,-58.858994908613,39.92499));
#201278=CARTESIAN_POINT('Origin',(-6.21503322485401,-62.1695413802712,39.6398955068271));
#201279=CARTESIAN_POINT('Origin',(-6.19641157197484,-61.9923681882669,39.3548010137695));
#201280=CARTESIAN_POINT('Ctrl Pts',(-6.4937464611276,-58.7519447039088,
39.8576902534424));
#201281=CARTESIAN_POINT('Ctrl Pts',(-6.36806742857345,-58.765644274027,
39.8579948730703));
#201282=CARTESIAN_POINT('Ctrl Pts',(-6.37927424642597,-58.872270023448,
39.92499));
#201283=CARTESIAN_POINT('Ctrl Pts',(-6.48899657309077,-58.7067576262546,
39.9304020711232));
#201284=CARTESIAN_POINT('Ctrl Pts',(-6.3800422045293,-58.7342098038493,
39.905891529738));
#201285=CARTESIAN_POINT('Ctrl Pts',(-6.37452469054062,-58.827081017759,
39.9671523786028));
#201286=CARTESIAN_POINT('Ctrl Pts',(-6.45774144355347,-58.6637560248474,
40.0043257306692));
#201287=CARTESIAN_POINT('Ctrl Pts',(-6.37187117938172,-58.6967899354323,
39.9667894847838));
#201288=CARTESIAN_POINT('Ctrl Pts',(-6.35435266912786,-58.7829167175848,
40.01001389752));
#201289=CARTESIAN_POINT('Ctrl Pts',(-6.34539908016329,-58.603591415908,
40.1195533054858));
#201290=CARTESIAN_POINT('Ctrl Pts',(-6.30313135363842,-58.6436439608623,
40.0630813209233));
#201291=CARTESIAN_POINT('Ctrl Pts',(-6.28595874576534,-58.7181337176191,
40.076826594242));
#201292=CARTESIAN_POINT('Ctrl Pts',(-6.26151010025752,-58.587269867717,
40.1599502027514));
#201293=CARTESIAN_POINT('Ctrl Pts',(-6.24170554357568,-58.626864594668,
40.1002552791541));
#201294=CARTESIAN_POINT('Ctrl Pts',(-6.23613328458281,-58.6982323944353,
40.10025));
#201295=CARTESIAN_POINT('Ctrl Pts',(-6.1740349085904,-58.5964866834551,
40.1599502534424));
#201296=CARTESIAN_POINT('Ctrl Pts',(-6.17794390662191,-58.6335861742242,
40.10025));
#201297=CARTESIAN_POINT('Ctrl Pts',(-6.18532049829418,-58.7035958781039,
40.10025));
#201298=CARTESIAN_POINT('Origin',(-6.18532049829418,-58.7035958781039,40.22725));
#201299=CARTESIAN_POINT('Ctrl Pts',(-6.15137923967696,-61.5639141665612,
38.989));
#201300=CARTESIAN_POINT('Ctrl Pts',(-6.27787222402478,-61.5506192181748,
38.989));
#201301=CARTESIAN_POINT('Ctrl Pts',(-6.2776833796338,-61.5506390665201,
39.1161896013267));
#201302=CARTESIAN_POINT('Ctrl Pts',(-6.17383801205357,-61.7797255331386,
38.989));
#201303=CARTESIAN_POINT('Ctrl Pts',(-6.30057242039932,-61.7665923920114,
38.988776927546));
#201304=CARTESIAN_POINT('Ctrl Pts',(-6.29582088597906,-61.723205914552,
39.1161898821849));
#201305=CARTESIAN_POINT('Ctrl Pts',(-6.19522058691281,-61.985174271489,
39.1034967087243));
#201306=CARTESIAN_POINT('Ctrl Pts',(-6.32217699854699,-61.9721416759935,
39.1031720232709));
#201307=CARTESIAN_POINT('Ctrl Pts',(-6.31308747966708,-61.8874865820179,
39.2077529615));
#201308=CARTESIAN_POINT('Ctrl Pts',(-6.20712349654484,-62.0995362748658,
39.2875012672119));
#201309=CARTESIAN_POINT('Ctrl Pts',(-6.33421251157731,-62.0866494440659,
39.2872087095507));
#201310=CARTESIAN_POINT('Ctrl Pts',(-6.3226988678919,-61.9789328337398,
39.3549017048228));
#201311=CARTESIAN_POINT('Origin',(-6.15137923967696,-61.5639141665612,39.116));
#201312=CARTESIAN_POINT('Origin',(4.05837671390568E-16,-5.83359163402241E-17,
40.22725));
#201313=CARTESIAN_POINT('Origin',(-6.15500747092336,-58.7067819056643,40.22725));
#201314=CARTESIAN_POINT('Origin',(0.995615674755347,6.43520020182081,39.116));
#201315=CARTESIAN_POINT('Origin',(-6.1093749596203,-61.1647646440474,39.1160373285266));
#201316=CARTESIAN_POINT('Ctrl Pts',(-6.14377718965342,-58.5996668978648,
40.1599502534424));
#201317=CARTESIAN_POINT('Ctrl Pts',(-6.1476670304619,-58.6367684021392,
40.10025));
#201318=CARTESIAN_POINT('Ctrl Pts',(-6.15500747092336,-58.7067819056643,
40.10025));
#201319=CARTESIAN_POINT('Ctrl Pts',(-6.0565955360672,-58.6088074259633,
40.1599500566035));
#201320=CARTESIAN_POINT('Ctrl Pts',(-6.08415140319836,-58.6434243604401,
40.1002551305372));
#201321=CARTESIAN_POINT('Ctrl Pts',(-6.10436324506832,-58.712082152969,
40.10025));
#201322=CARTESIAN_POINT('Ctrl Pts',(-5.97852000021541,-58.641681736514,
40.1203070619045));
#201323=CARTESIAN_POINT('Ctrl Pts',(-6.02785839131288,-58.6721826510718,
40.0637098684497));
#201324=CARTESIAN_POINT('Ctrl Pts',(-6.06008468706716,-58.7414038195498,
40.0772636213363));
#201325=CARTESIAN_POINT('Ctrl Pts',(-5.88025093392488,-58.7242744516463,
40.0046102245802));
#201326=CARTESIAN_POINT('Ctrl Pts',(-5.97104363802162,-58.7387860695147,
39.9670001894015));
#201327=CARTESIAN_POINT('Ctrl Pts',(-6.00614981441038,-58.8193360415241,
40.0101788811209));
#201328=CARTESIAN_POINT('Ctrl Pts',(-5.85862682030279,-58.7730316211507,
39.9303710930186));
#201329=CARTESIAN_POINT('Ctrl Pts',(-5.97091547255937,-58.7772266151797,
39.9058663574098));
#201330=CARTESIAN_POINT('Ctrl Pts',(-5.99561386571446,-58.8669255556785,
39.9671344706363));
#201331=CARTESIAN_POINT('Ctrl Pts',(-5.863373641496,-58.8181995570485,39.8576902534424));
#201332=CARTESIAN_POINT('Ctrl Pts',(-5.98915458643814,-58.805469618532,
39.8579948730703));
#201333=CARTESIAN_POINT('Ctrl Pts',(-6.00036140429066,-58.912095367953,
39.92499));
#201334=CARTESIAN_POINT('Origin',(-5.87405712357889,-58.925370482788,39.92499));
#201335=CARTESIAN_POINT('Origin',(-6.10480350526348,-61.1207756545809,39.1925554488848));
#201336=CARTESIAN_POINT('Origin',(-6.09624906995259,-61.0393856393804,39.3343017080178));
#201337=CARTESIAN_POINT('Origin',(-5.89267880207433,-59.1025439184843,39.6398955069217));
#201338=CARTESIAN_POINT('Origin',(-5.91130048050362,-59.2797173540686,39.3548010137695));
#201339=CARTESIAN_POINT('Ctrl Pts',(-6.0617588454159,-60.7112330730304,
39.3978017080178));
#201340=CARTESIAN_POINT('Ctrl Pts',(-6.18806312612767,-60.6979579581954,
39.3978017080178));
#201341=CARTESIAN_POINT('Ctrl Pts',(-6.18806312612767,-60.6979579581954,
39.5248017080178));
#201342=CARTESIAN_POINT('Ctrl Pts',(-6.07140041118272,-60.8007259828525,
39.3978017080178));
#201343=CARTESIAN_POINT('Ctrl Pts',(-6.19746294737672,-60.787391283361,
39.3980355775196));
#201344=CARTESIAN_POINT('Ctrl Pts',(-6.20217593878193,-60.8322324012621,
39.5248015517192));
#201345=CARTESIAN_POINT('Ctrl Pts',(-6.08051542067571,-60.885348460727,
39.3484893995498));
#201346=CARTESIAN_POINT('Ctrl Pts',(-6.20639551966706,-60.8723790316504,
39.3489438303418));
#201347=CARTESIAN_POINT('Ctrl Pts',(-6.21552060714923,-60.9591984396293,
39.4508333155596));
#201348=CARTESIAN_POINT('Ctrl Pts',(-6.08531878138341,-60.929944884669,
39.2708017080178));
#201349=CARTESIAN_POINT('Ctrl Pts',(-6.21110821942955,-60.917217374751,
39.2710850691866));
#201350=CARTESIAN_POINT('Ctrl Pts',(-6.22255335066436,-61.0261105245454,
39.3343017080178));
#201351=CARTESIAN_POINT('Origin',(-6.0617588454159,-60.7112330730304,39.5248017080178));
#201352=CARTESIAN_POINT('Ctrl Pts',(-5.90061356181277,-59.1725467709677,
39.2875012672119));
#201353=CARTESIAN_POINT('Ctrl Pts',(-6.02658562874827,-59.1597945546412,
39.2878045257519));
#201354=CARTESIAN_POINT('Ctrl Pts',(-6.03762143316772,-59.2666022171587,
39.3549015218348));
#201355=CARTESIAN_POINT('Ctrl Pts',(-5.91250964036485,-59.2869113614505,
39.1034938540228));
#201356=CARTESIAN_POINT('Ctrl Pts',(-6.03858760028461,-59.2739830624742,
39.1038286278801));
#201357=CARTESIAN_POINT('Ctrl Pts',(-6.0472329950889,-59.3580501215732,
39.2077506434028));
#201358=CARTESIAN_POINT('Ctrl Pts',(-5.93388131656949,-59.4923630227874,
38.989));
#201359=CARTESIAN_POINT('Ctrl Pts',(-6.06016587018276,-59.47928181684,38.9892298954611));
#201360=CARTESIAN_POINT('Ctrl Pts',(-6.06449973388426,-59.5223321697742,
39.1161900347289));
#201361=CARTESIAN_POINT('Ctrl Pts',(-5.9563328589123,-59.7081718144892,
38.989));
#201362=CARTESIAN_POINT('Ctrl Pts',(-6.08282633453093,-59.6948768144682,
38.989));
#201363=CARTESIAN_POINT('Ctrl Pts',(-6.08263699813586,-59.6948967145252,
39.1161900945646));
#201364=CARTESIAN_POINT('Origin',(-5.9563328589123,-59.7081718144892,39.116));
#201365=CARTESIAN_POINT('Origin',(0.97914764405288,6.27851735587422,39.5248017080178));
#201366=CARTESIAN_POINT('Origin',(-6.04595329345081,-60.5608532912343,39.5248017080178));
#201367=CARTESIAN_POINT('Origin',(0.9765688230087,6.25398151259764,39.116));
#201368=CARTESIAN_POINT('Origin',(-5.99823604520128,-60.1073400339997,39.1160402713849));
#201369=CARTESIAN_POINT('Ctrl Pts',(-6.02238575970296,-60.3421421670675,
39.2708017080178));
#201370=CARTESIAN_POINT('Ctrl Pts',(-6.14931623097267,-60.3293058762211,
39.27051194648));
#201371=CARTESIAN_POINT('Ctrl Pts',(-6.13776734223235,-60.2194255397045,
39.3343017080178));
#201372=CARTESIAN_POINT('Ctrl Pts',(-6.02720817145255,-60.3868890390928,
39.3487519301185));
#201373=CARTESIAN_POINT('Ctrl Pts',(-6.1539956747704,-60.3738278099523,
39.3482879463979));
#201374=CARTESIAN_POINT('Ctrl Pts',(-6.14482385294844,-60.2865637544324,
39.4512271261634));
#201375=CARTESIAN_POINT('Ctrl Pts',(-6.03634362557914,-60.4716618705782,
39.3978017080178));
#201376=CARTESIAN_POINT('Ctrl Pts',(-6.16287156698238,-60.4582762833186,
39.3975673827397));
#201377=CARTESIAN_POINT('Ctrl Pts',(-6.15819229746499,-60.413756007749,
39.5248015355181));
#201378=CARTESIAN_POINT('Ctrl Pts',(-6.04595329345081,-60.5608532912343,
39.3978017080178));
#201379=CARTESIAN_POINT('Ctrl Pts',(-6.17225757416258,-60.5475781763993,
39.3978017080178));
#201380=CARTESIAN_POINT('Ctrl Pts',(-6.17225757416258,-60.5475781763993,
39.5248017080178));
#201381=CARTESIAN_POINT('Origin',(-6.01146306152058,-60.2327006545395,39.3343017080178));
#201382=CARTESIAN_POINT('Origin',(-6.00295964283318,-60.151796032919,39.1934008533548));
#201383=CARTESIAN_POINT('Origin',(-13.0813452322046,-60.0157999988656,39.1925554495083));
#201384=CARTESIAN_POINT('Origin',(-13.0905908661199,-60.0590486699125,39.116037328528));
#201385=CARTESIAN_POINT('Origin',(-13.0643300858384,-59.9357500275432,39.3343017080178));
#201386=CARTESIAN_POINT('Ctrl Pts',(-13.0409063549241,-59.8282880397054,
39.2708017080178));
#201387=CARTESIAN_POINT('Ctrl Pts',(-12.9173404733285,-59.8550545325309,
39.2710850691866));
#201388=CARTESIAN_POINT('Ctrl Pts',(-12.9401053405452,-59.9621548122771,
39.3343017080178));
#201389=CARTESIAN_POINT('Ctrl Pts',(-13.0316624367249,-59.7842416555146,
39.3487519293518));
#201390=CARTESIAN_POINT('Ctrl Pts',(-12.9079350417483,-59.8108054559364,
39.3492068662935));
#201391=CARTESIAN_POINT('Ctrl Pts',(-12.9260696369488,-59.8961220185296,
39.451227124874));
#201392=CARTESIAN_POINT('Ctrl Pts',(-13.0141504107554,-59.7007958241043,
39.3978017080178));
#201393=CARTESIAN_POINT('Ctrl Pts',(-12.8901364125064,-59.7270694888856,
39.3980347781174));
#201394=CARTESIAN_POINT('Ctrl Pts',(-12.8994792219297,-59.7710239514073,
39.524801535519));
#201395=CARTESIAN_POINT('Ctrl Pts',(-12.9957275188826,-59.6130003254554,
39.3978017080178));
#201396=CARTESIAN_POINT('Ctrl Pts',(-12.8715027735894,-59.6394051101893,
39.3978017080178));
#201397=CARTESIAN_POINT('Ctrl Pts',(-12.8715027735894,-59.6394051101893,
39.5248017080178));
#201398=CARTESIAN_POINT('Origin',(-12.9957275188826,-59.6130003254554,39.5248017080178));
#201399=CARTESIAN_POINT('Origin',(-0.310561863232978,0.0660119618346398,
39.116));
#201400=CARTESIAN_POINT('Origin',(-13.1739864076109,-60.4516424606488,39.116));
#201401=CARTESIAN_POINT('Origin',(-0.310561863232978,0.0660119618346398,
39.5248017080178));
#201402=CARTESIAN_POINT('Origin',(-12.9642895838873,-59.4650964698966,39.5248017080178));
#201403=CARTESIAN_POINT('Ctrl Pts',(-13.2864868028998,-60.9782752797347,
39.2875012672119));
#201404=CARTESIAN_POINT('Ctrl Pts',(-13.1616357280625,-61.0052918384389,
39.287208709576));
#201405=CARTESIAN_POINT('Ctrl Pts',(-13.1392995818862,-60.8992893541407,
39.3549016990122));
#201406=CARTESIAN_POINT('Ctrl Pts',(-13.2624669757412,-60.8658306440995,
39.1034939173931));
#201407=CARTESIAN_POINT('Ctrl Pts',(-13.1376969719812,-60.8926675943312,
39.1031692336336));
#201408=CARTESIAN_POINT('Ctrl Pts',(-13.1201818190176,-60.8093473519465,
39.2077507202299));
#201409=CARTESIAN_POINT('Ctrl Pts',(-13.2193155203585,-60.663828108008,
38.989));
#201410=CARTESIAN_POINT('Ctrl Pts',(-13.0947255842069,-60.6905008239737,
38.9887769311176));
#201411=CARTESIAN_POINT('Ctrl Pts',(-13.0858375353125,-60.6477702018626,
39.1161898712914));
#201412=CARTESIAN_POINT('Ctrl Pts',(-13.1739864076109,-60.4516424606489,
38.989));
#201413=CARTESIAN_POINT('Ctrl Pts',(-13.049576076309,-60.4780866929066,
38.989));
#201414=CARTESIAN_POINT('Ctrl Pts',(-13.0497618007392,-60.4780472159603,
39.1161895903853));
#201415=CARTESIAN_POINT('Origin',(-13.2635576885504,-60.8730422059013,39.3548010137695));
#201416=CARTESIAN_POINT('Ctrl Pts',(-12.9642895838873,-59.4650964698966,
39.3978017080178));
#201417=CARTESIAN_POINT('Ctrl Pts',(-12.8400648385941,-59.4915012546304,
39.3978017080178));
#201418=CARTESIAN_POINT('Ctrl Pts',(-12.8400648385941,-59.4915012546304,
39.5248017080178));
#201419=CARTESIAN_POINT('Ctrl Pts',(-12.9458049943937,-59.3770041141843,
39.3978017080178));
#201420=CARTESIAN_POINT('Ctrl Pts',(-12.8213326038448,-59.4033730190105,
39.3975666025045));
#201421=CARTESIAN_POINT('Ctrl Pts',(-12.8119938336989,-59.3594375597974,
39.5248015517196));
#201422=CARTESIAN_POINT('Ctrl Pts',(-12.9283282206293,-59.2937057271824,
39.3484894016716));
#201423=CARTESIAN_POINT('Ctrl Pts',(-12.8037097640135,-59.320464076127,
39.3480259000027));
#201424=CARTESIAN_POINT('Ctrl Pts',(-12.7854506972089,-59.2345619206666,
39.450833318893));
#201425=CARTESIAN_POINT('Ctrl Pts',(-12.9191181862048,-59.2498070616279,
39.2708017080178));
#201426=CARTESIAN_POINT('Ctrl Pts',(-12.794433502371,-59.2768226962998,
39.2705119464801));
#201427=CARTESIAN_POINT('Ctrl Pts',(-12.7714622569322,-59.168751483356,
39.3343017080178));
#201428=CARTESIAN_POINT('Origin',(-12.8956870022254,-59.1423466986221,39.3343017080178));
#201429=CARTESIAN_POINT('Origin',(-13.3005969715153,-61.0472983318868,39.6398955068182));
#201430=CARTESIAN_POINT('Origin',(-13.3376362544828,-61.2215544576539,39.92499));
#201431=CARTESIAN_POINT('Origin',(-12.8787733304449,-59.0627741291261,39.1934008539949));
#201432=CARTESIAN_POINT('Origin',(-12.8695280801149,-59.0190342907433,39.116040271385));
#201433=CARTESIAN_POINT('Ctrl Pts',(-13.103835206573,-61.5752716937451,
40.1599502534424));
#201434=CARTESIAN_POINT('Ctrl Pts',(-13.0960702419682,-61.5387839176327,
40.10025));
#201435=CARTESIAN_POINT('Ctrl Pts',(-13.0814171332235,-61.4699285681954,
40.10025));
#201436=CARTESIAN_POINT('Ctrl Pts',(-13.1900205930483,-61.556930451844,
40.1599500538479));
#201437=CARTESIAN_POINT('Ctrl Pts',(-13.15884824219,-61.5254208297837,40.100244835349));
#201438=CARTESIAN_POINT('Ctrl Pts',(-13.1313027022865,-61.4593031273792,
40.10025));
#201439=CARTESIAN_POINT('Ctrl Pts',(-13.2643407403244,-61.5155378539379,
40.1202442001038));
#201440=CARTESIAN_POINT('Ctrl Pts',(-13.2118511391498,-61.4904936222814,
40.0633873868017));
#201441=CARTESIAN_POINT('Ctrl Pts',(-13.1721300657491,-61.4250300340662,
40.0772271723538));
#201442=CARTESIAN_POINT('Ctrl Pts',(-13.3535591268198,-61.4222835584426,
40.0045995998163));
#201443=CARTESIAN_POINT('Ctrl Pts',(-13.2611962587091,-61.41788805574,39.9663485808314));
#201444=CARTESIAN_POINT('Ctrl Pts',(-13.2174099770541,-61.3411158595757,
40.0101727202465));
#201445=CARTESIAN_POINT('Ctrl Pts',(-13.3700167576322,-61.3712701109736,
39.9304654349859));
#201446=CARTESIAN_POINT('Ctrl Pts',(-13.2570896192442,-61.379707499563,
39.9051900162951));
#201447=CARTESIAN_POINT('Ctrl Pts',(-13.2228660458969,-61.2924393404518,
39.9671857458177));
#201448=CARTESIAN_POINT('Ctrl Pts',(-13.3605623192489,-61.3267881959112,
39.8576902534424));
#201449=CARTESIAN_POINT('Ctrl Pts',(-13.2359003894753,-61.3537611057082,
39.8573998014387));
#201450=CARTESIAN_POINT('Ctrl Pts',(-13.2134115091896,-61.2479592423877,
39.92499));
#201451=CARTESIAN_POINT('Origin',(-13.0814171332235,-61.4699285681954,40.22725));
#201452=CARTESIAN_POINT('Origin',(-0.310561863232978,0.0660119618346398,
39.116));
#201453=CARTESIAN_POINT('Origin',(-12.7860306150453,-58.6264539577983,39.116));
#201454=CARTESIAN_POINT('Origin',(4.07480739540194E-18,1.61286359594752E-16,
40.22725));
#201455=CARTESIAN_POINT('Origin',(-13.0516031943531,-61.4762657165315,40.22725));
#201456=CARTESIAN_POINT('Ctrl Pts',(-12.7860306150453,-58.6264539577983,
38.989));
#201457=CARTESIAN_POINT('Ctrl Pts',(-12.6616197754742,-58.652898298092,
38.989));
#201458=CARTESIAN_POINT('Ctrl Pts',(-12.6618060089323,-58.6528587129485,
39.1161901092321));
#201459=CARTESIAN_POINT('Ctrl Pts',(-12.740694012737,-58.4142663981467,
38.989));
#201460=CARTESIAN_POINT('Ctrl Pts',(-12.6165479409688,-58.4408495151692,
38.989229898976));
#201461=CARTESIAN_POINT('Ctrl Pts',(-12.6257296363315,-58.4831327254063,
39.1161900493201));
#201462=CARTESIAN_POINT('Ctrl Pts',(-12.6975319705099,-58.2122676405433,
39.1034966344368));
#201463=CARTESIAN_POINT('Ctrl Pts',(-12.5736296288407,-58.2389323335259,
39.1038314102563));
#201464=CARTESIAN_POINT('Ctrl Pts',(-12.5913856081751,-58.3215567776509,
39.2077528789598));
#201465=CARTESIAN_POINT('Ctrl Pts',(-12.6735055745743,-58.0998260601479,
39.2875012672119));
#201466=CARTESIAN_POINT('Ctrl Pts',(-12.5497583536237,-58.1266254943012,
39.2878045257868));
#201467=CARTESIAN_POINT('Ctrl Pts',(-12.5722680796266,-58.2316158778876,
39.3549015295899));
#201468=CARTESIAN_POINT('Origin',(-12.6964592423895,-58.2050537810541,39.3548010137695));
#201469=CARTESIAN_POINT('Ctrl Pts',(-12.7383709431253,-61.4590390555208,
39.8576902534424));
#201470=CARTESIAN_POINT('Ctrl Pts',(-12.8632261535957,-61.4329754599098,
39.8573998014387));
#201471=CARTESIAN_POINT('Ctrl Pts',(-12.84073727331,-61.3271735965893,39.92499));
#201472=CARTESIAN_POINT('Ctrl Pts',(-12.7478306169676,-61.5035409747668,
39.9304984902492));
#201473=CARTESIAN_POINT('Ctrl Pts',(-12.8544171899343,-61.4653154597763,
39.9052171569791));
#201474=CARTESIAN_POINT('Ctrl Pts',(-12.8501961180702,-61.3716739624489,
39.9672049726596));
#201475=CARTESIAN_POINT('Ctrl Pts',(-12.7835835513933,-61.5432717953612,
40.004343767866));
#201476=CARTESIAN_POINT('Ctrl Pts',(-12.8662481012968,-61.5017184029583,
39.9661628577643));
#201477=CARTESIAN_POINT('Ctrl Pts',(-12.8749453072906,-61.4137451613971,
40.0100243556236));
#201478=CARTESIAN_POINT('Ctrl Pts',(-12.9020280679172,-61.5920631419345,
40.1194874821989));
#201479=CARTESIAN_POINT('Ctrl Pts',(-12.9401487584128,-61.5478406570052,
40.0627551483141));
#201480=CARTESIAN_POINT('Ctrl Pts',(-12.9498405053863,-61.4717924962545,
40.0767884282376));
#201481=CARTESIAN_POINT('Ctrl Pts',(-12.9874904696724,-61.5999795805213,
40.1599502015392));
#201482=CARTESIAN_POINT('Ctrl Pts',(-13.0031958218444,-61.5585057825378,
40.1002449453869));
#201483=CARTESIAN_POINT('Ctrl Pts',(-13.0015435854427,-61.4868843017924,
40.10025));
#201484=CARTESIAN_POINT('Ctrl Pts',(-13.0739701745327,-61.5816197022697,
40.1599502534424));
#201485=CARTESIAN_POINT('Ctrl Pts',(-13.0662229071069,-61.5451281645058,
40.10025));
#201486=CARTESIAN_POINT('Ctrl Pts',(-13.0516031943531,-61.4762657165315,
40.10025));
#201487=CARTESIAN_POINT('Origin',(-12.7165125280168,-61.3535783813231,39.92499));
#201488=CARTESIAN_POINT('Origin',(-12.6594199084569,-58.0307974155441,39.6398955069311));
#201489=CARTESIAN_POINT('Origin',(-12.6223805745521,-57.8565410498766,39.92499));
#201490=CARTESIAN_POINT('Origin',(-12.6794732450936,-61.1793222555334,39.6398955068263));
#201491=CARTESIAN_POINT('Origin',(-12.6424339620844,-61.0050661295706,39.3548010137695));
#201492=CARTESIAN_POINT('Ctrl Pts',(-12.5994235324474,-57.751314065072,
39.8576902534424));
#201493=CARTESIAN_POINT('Ctrl Pts',(-12.4758649777955,-57.7780756236495,
39.8579948730703));
#201494=CARTESIAN_POINT('Ctrl Pts',(-12.4981558292589,-57.8829458346105,
39.92499));
#201495=CARTESIAN_POINT('Ctrl Pts',(-12.5899763290075,-57.7068710254543,
39.9304020711231));
#201496=CARTESIAN_POINT('Ctrl Pts',(-12.4844883578144,-57.7455616498582,
39.9058915297372));
#201497=CARTESIAN_POINT('Ctrl Pts',(-12.4887087546164,-57.8385008428006,
39.9671523786025));
#201498=CARTESIAN_POINT('Ctrl Pts',(-12.5543975270269,-57.6673720419787,
40.0043257306692));
#201499=CARTESIAN_POINT('Ctrl Pts',(-12.4724506530561,-57.7092008760993,
39.9667894847835));
#201500=CARTESIAN_POINT('Ctrl Pts',(-12.4640308112191,-57.7966870296829,
40.01001389752));
#201501=CARTESIAN_POINT('Ctrl Pts',(-12.4363816727424,-57.6192799956673,
40.1195533054858));
#201502=CARTESIAN_POINT('Ctrl Pts',(-12.3985321242201,-57.663531309089,
40.0630813209236));
#201503=CARTESIAN_POINT('Ctrl Pts',(-12.3892398894927,-57.7394080294759,
40.076826594242));
#201504=CARTESIAN_POINT('Ctrl Pts',(-12.3512461790954,-57.6118166447794,
40.1599502027519));
#201505=CARTESIAN_POINT('Ctrl Pts',(-12.3356888898088,-57.6532646075484,
40.1002552791541));
#201506=CARTESIAN_POINT('Ctrl Pts',(-12.3376071226707,-57.7248239067129,
40.10025));
#201507=CARTESIAN_POINT('Ctrl Pts',(-12.2652136052663,-57.6301266171957,
40.1599502534424));
#201508=CARTESIAN_POINT('Ctrl Pts',(-12.2729791421557,-57.6666142715155,
40.10025));
#201509=CARTESIAN_POINT('Ctrl Pts',(-12.2876333308473,-57.7354693911204,
40.10025));
#201510=CARTESIAN_POINT('Origin',(-12.2876333308473,-57.7354693911204,40.22725));
#201511=CARTESIAN_POINT('Ctrl Pts',(-12.5528626811449,-60.5836663843181,
38.989));
#201512=CARTESIAN_POINT('Ctrl Pts',(-12.6772730231648,-60.5572221497822,
38.989));
#201513=CARTESIAN_POINT('Ctrl Pts',(-12.6770872880007,-60.55726162901,39.1161896013262));
#201514=CARTESIAN_POINT('Ctrl Pts',(-12.5977568525207,-60.7959479326852,
38.989));
#201515=CARTESIAN_POINT('Ctrl Pts',(-12.722424209458,-60.7696393833347,
38.988776927546));
#201516=CARTESIAN_POINT('Ctrl Pts',(-12.7131635826247,-60.7269872521295,
39.1161898821844));
#201517=CARTESIAN_POINT('Ctrl Pts',(-12.6404975322974,-60.9980361136599,
39.1034967087243));
#201518=CARTESIAN_POINT('Ctrl Pts',(-12.765396186243,-60.9718043534724,
39.1031720232721));
#201519=CARTESIAN_POINT('Ctrl Pts',(-12.7475075938194,-60.8885631224,39.2077529615005));
#201520=CARTESIAN_POINT('Ctrl Pts',(-12.6642893210144,-61.1105274371641,
39.2875012672119));
#201521=CARTESIAN_POINT('Ctrl Pts',(-12.7893350885046,-61.0844267823322,
39.2872087095508));
#201522=CARTESIAN_POINT('Ctrl Pts',(-12.7666250660187,-60.9785037583493,
39.3549017048226));
#201523=CARTESIAN_POINT('Origin',(-12.5528626811449,-60.5836663843181,39.116));
#201524=CARTESIAN_POINT('Origin',(3.9977349588932E-16,-5.73754452974295E-17,
40.22725));
#201525=CARTESIAN_POINT('Origin',(-12.257819391977,-57.7418065394565,40.22725));
#201526=CARTESIAN_POINT('Origin',(3.00026883051142,12.5880644220972,39.116));
#201527=CARTESIAN_POINT('Origin',(-12.469366018727,-60.1910940874972,39.1160373285259));
#201528=CARTESIAN_POINT('Ctrl Pts',(-12.2354540642047,-57.6364522029206,
40.1599502534424));
#201529=CARTESIAN_POINT('Ctrl Pts',(-12.2432007592849,-57.6729438621906,
40.10025));
#201530=CARTESIAN_POINT('Ctrl Pts',(-12.257819391977,-57.7418065394565,
40.10025));
#201531=CARTESIAN_POINT('Ctrl Pts',(-12.1497054461945,-57.6546556225247,
40.1599500566029));
#201532=CARTESIAN_POINT('Ctrl Pts',(-12.1807288143664,-57.6862025493679,
40.1002551305372));
#201533=CARTESIAN_POINT('Ctrl Pts',(-12.2080066271961,-57.7523715145548,
40.10025));
#201534=CARTESIAN_POINT('Ctrl Pts',(-12.0754939174599,-57.6955109599434,
40.1203070619046));
#201535=CARTESIAN_POINT('Ctrl Pts',(-12.1277502414153,-57.720687521098,
40.0637098684499));
#201536=CARTESIAN_POINT('Ctrl Pts',(-12.1670355805164,-57.7861609236007,
40.0772636213363));
#201537=CARTESIAN_POINT('Ctrl Pts',(-11.9863964689866,-57.7879231380266,
40.0046102245801));
#201538=CARTESIAN_POINT('Ctrl Pts',(-12.0782086782661,-57.7928648378994,
39.9670001894012));
#201539=CARTESIAN_POINT('Ctrl Pts',(-12.1215423041375,-57.8693039540645,
40.0101788811209));
#201540=CARTESIAN_POINT('Ctrl Pts',(-11.9699873265229,-57.8386735460214,
39.9303710930186));
#201541=CARTESIAN_POINT('Ctrl Pts',(-12.0820993460742,-57.8311081991722,
39.9058663574113));
#201542=CARTESIAN_POINT('Ctrl Pts',(-12.1160385312532,-57.9177340744077,
39.9671344706371));
#201543=CARTESIAN_POINT('Ctrl Pts',(-11.9794294790614,-57.8830978693155,
39.8576902534424));
#201544=CARTESIAN_POINT('Ctrl Pts',(-12.1031907419159,-57.8572899778511,
39.8579948730703));
#201545=CARTESIAN_POINT('Ctrl Pts',(-12.1254815933794,-57.962160188812,
39.92499));
#201546=CARTESIAN_POINT('Origin',(-12.0012568480862,-57.9885649735459,39.92499));
#201547=CARTESIAN_POINT('Origin',(-12.4602215058057,-60.1478239214168,39.1925554488849));
#201548=CARTESIAN_POINT('Origin',(-12.4432063593724,-60.0677739512125,39.3343017080178));
#201549=CARTESIAN_POINT('Origin',(-12.038296182044,-58.1628213391889,39.639895506923));
#201550=CARTESIAN_POINT('Origin',(-12.0753355159235,-58.3370777047234,39.3548010137695));
#201551=CARTESIAN_POINT('Ctrl Pts',(-12.3746037924166,-59.7450242491247,
39.3978017080178));
#201552=CARTESIAN_POINT('Ctrl Pts',(-12.4988285377098,-59.7186194643909,
39.3978017080178));
#201553=CARTESIAN_POINT('Ctrl Pts',(-12.4988285377098,-59.7186194643909,
39.5248017080178));
#201554=CARTESIAN_POINT('Ctrl Pts',(-12.3935470970146,-59.8330190893699,
39.3978017080178));
#201555=CARTESIAN_POINT('Ctrl Pts',(-12.5175251938,-59.8065803155777,39.3980355775177));
#201556=CARTESIAN_POINT('Ctrl Pts',(-12.5268995400901,-59.8506831473923,
39.5248015517192));
#201557=CARTESIAN_POINT('Ctrl Pts',(-12.411457631102,-59.9162252185215,
39.3484893995498));
#201558=CARTESIAN_POINT('Ctrl Pts',(-12.5352924712471,-59.8901687840256,
39.3489438303418));
#201559=CARTESIAN_POINT('Ctrl Pts',(-12.5534426698444,-59.9755587548341,
39.4508333155588));
#201560=CARTESIAN_POINT('Ctrl Pts',(-12.4208962741589,-59.9600752506737,
39.2708017080178));
#201561=CARTESIAN_POINT('Ctrl Pts',(-12.5446662374489,-59.9342688867324,
39.2710850691866));
#201562=CARTESIAN_POINT('Ctrl Pts',(-12.5674311046656,-60.0413691664787,
39.3343017080178));
#201563=CARTESIAN_POINT('Origin',(-12.3746037924166,-59.7450242491247,39.5248017080178));
#201564=CARTESIAN_POINT('Ctrl Pts',(-12.0535047649324,-58.2316113004781,
39.2875012672119));
#201565=CARTESIAN_POINT('Ctrl Pts',(-12.1774537741287,-58.2057612755555,
39.2878045257518));
#201566=CARTESIAN_POINT('Ctrl Pts',(-12.199593564085,-58.3108302788453,
39.3549015218347));
#201567=CARTESIAN_POINT('Ctrl Pts',(-12.0772900304169,-58.344105910958,
39.1034938540228));
#201568=CARTESIAN_POINT('Ctrl Pts',(-12.2013259468593,-58.3180696991549,
39.1038286278806));
#201569=CARTESIAN_POINT('Ctrl Pts',(-12.2187113817821,-58.4007725402752,
39.2077506434031));
#201570=CARTESIAN_POINT('Ctrl Pts',(-12.1200201767776,-58.5461981381264,
38.989));
#201571=CARTESIAN_POINT('Ctrl Pts',(-12.2442455720364,-58.5199882620691,
38.9892298954611));
#201572=CARTESIAN_POINT('Ctrl Pts',(-12.2530556816161,-58.5623497685526,
39.1161900347289));
#201573=CARTESIAN_POINT('Ctrl Pts',(-12.1649068885794,-58.7584778814676,
38.989));
#201574=CARTESIAN_POINT('Ctrl Pts',(-12.289317713782,-58.732033544228,38.989));
#201575=CARTESIAN_POINT('Ctrl Pts',(-12.2891314947139,-58.7320731263128,
39.1161900945646));
#201576=CARTESIAN_POINT('Origin',(-12.1649068885794,-58.7584778814676,39.116));
#201577=CARTESIAN_POINT('Origin',(2.93511643966563,12.2815465224196,39.5248017080178));
#201578=CARTESIAN_POINT('Origin',(-12.3431658574213,-59.5971203935659,39.5248017080178));
#201579=CARTESIAN_POINT('Origin',(2.92491386234308,12.2335471699536,39.116));
#201580=CARTESIAN_POINT('Origin',(-12.2483049654005,-59.1510793400372,39.1160402713846));
#201581=CARTESIAN_POINT('Ctrl Pts',(-12.2968658913805,-59.382070869907,
39.2708017080178));
#201582=CARTESIAN_POINT('Ctrl Pts',(-12.4217592664914,-59.3560370505013,
39.27051194648));
#201583=CARTESIAN_POINT('Ctrl Pts',(-12.3987880210526,-59.2479658375576,
39.3343017080178));
#201584=CARTESIAN_POINT('Ctrl Pts',(-12.3063392072228,-59.426068534596,
39.3487519301186));
#201585=CARTESIAN_POINT('Ctrl Pts',(-12.4310668851217,-59.3998259533469,
39.3482879463995));
#201586=CARTESIAN_POINT('Ctrl Pts',(-12.4128237298761,-59.3139986558962,
39.4512271261633));
#201587=CARTESIAN_POINT('Ctrl Pts',(-12.3242857901775,-59.5094220566595,
39.3978017080178));
#201588=CARTESIAN_POINT('Ctrl Pts',(-12.4487214234138,-59.4828840257757,
39.3975673827392));
#201589=CARTESIAN_POINT('Ctrl Pts',(-12.4394141514347,-59.4390967537845,
39.5248015355194));
#201590=CARTESIAN_POINT('Ctrl Pts',(-12.3431658574213,-59.5971203935659,
39.3978017080178));
#201591=CARTESIAN_POINT('Ctrl Pts',(-12.4673906027145,-59.570715608832,
39.3978017080178));
#201592=CARTESIAN_POINT('Ctrl Pts',(-12.4673906027145,-59.570715608832,
39.5248017080178));
#201593=CARTESIAN_POINT('Origin',(-12.2745632757594,-59.2743706222914,39.3343017080178));
#201594=CARTESIAN_POINT('Origin',(-12.2576496039189,-59.1947980539411,39.193400853355));
#201595=CARTESIAN_POINT('Origin',(-19.2830435999589,-58.3196542523186,39.192555449508));
#201596=CARTESIAN_POINT('Origin',(-19.296759302446,-58.3616995707147,39.1160373285266));
#201597=CARTESIAN_POINT('Origin',(-19.2577541638581,-58.2418213702173,39.3343017080178));
#201598=CARTESIAN_POINT('Ctrl Pts',(-19.2232259141442,-58.1373965169892,
39.2708017080178));
#201599=CARTESIAN_POINT('Ctrl Pts',(-19.103134799739,-58.1769325318819,
39.2710850691866));
#201600=CARTESIAN_POINT('Ctrl Pts',(-19.1369699862886,-58.2810665285029,
39.3343017080178));
#201601=CARTESIAN_POINT('Ctrl Pts',(-19.2094285342437,-58.0945576760637,
39.3487519293518));
#201602=CARTESIAN_POINT('Ctrl Pts',(-19.0891556041211,-58.1339089916654,
39.3492068662929));
#201603=CARTESIAN_POINT('Ctrl Pts',(-19.1161088652898,-58.2168625998377,
39.4512271248744));
#201604=CARTESIAN_POINT('Ctrl Pts',(-19.1832899764611,-58.0133994748124,
39.3978017080178));
#201605=CARTESIAN_POINT('Ctrl Pts',(-19.0627016856737,-58.0524922023716,
39.3980347781174));
#201606=CARTESIAN_POINT('Ctrl Pts',(-19.0765878066316,-58.0952292882338,
39.524801535519));
#201607=CARTESIAN_POINT('Ctrl Pts',(-19.1557908785627,-57.9280106456675,
39.3978017080178));
#201608=CARTESIAN_POINT('Ctrl Pts',(-19.0350067009933,-57.9672558039531,
39.3978017080178));
#201609=CARTESIAN_POINT('Ctrl Pts',(-19.0350067009933,-57.9672558039531,
39.5248017080178));
#201610=CARTESIAN_POINT('Origin',(-19.1557908785627,-57.9280106456675,39.5248017080178));
#201611=CARTESIAN_POINT('Origin',(-0.301960443923705,0.0981128957140471,
39.116));
#201612=CARTESIAN_POINT('Origin',(-19.4207352200703,-58.7434254837931,39.116));
#201613=CARTESIAN_POINT('Origin',(-0.301960443923705,0.0981128957140471,
39.5248017080178));
#201614=CARTESIAN_POINT('Origin',(-19.1090650011318,-57.7842031819382,39.5248017080178));
#201615=CARTESIAN_POINT('Ctrl Pts',(-19.5876674457081,-59.255413859757,
39.2875012672119));
#201616=CARTESIAN_POINT('Ctrl Pts',(-19.4663243174858,-59.295332909916,
39.287208709576));
#201617=CARTESIAN_POINT('Ctrl Pts',(-19.4330302542694,-59.1922458813525,
39.3549016990124));
#201618=CARTESIAN_POINT('Ctrl Pts',(-19.5520255367085,-59.1460959632225,
39.1034939173931));
#201619=CARTESIAN_POINT('Ctrl Pts',(-19.4307442612488,-59.1858279145903,
39.1031692336344));
#201620=CARTESIAN_POINT('Ctrl Pts',(-19.4046157212345,-59.104794941234,
39.2077507202309));
#201621=CARTESIAN_POINT('Ctrl Pts',(-19.4879954548414,-58.9497105734779,
38.989));
#201622=CARTESIAN_POINT('Ctrl Pts',(-19.3668760934073,-58.9892603680778,
38.9887769311158));
#201623=CARTESIAN_POINT('Ctrl Pts',(-19.35357016791,-58.9476928828771,39.1161898712901));
#201624=CARTESIAN_POINT('Ctrl Pts',(-19.4207352200704,-58.7434254837931,
38.989));
#201625=CARTESIAN_POINT('Ctrl Pts',(-19.2997705965402,-58.7827292725255,
38.989));
#201626=CARTESIAN_POINT('Ctrl Pts',(-19.2999511770886,-58.7826705983486,
39.1161895903858));
#201627=CARTESIAN_POINT('Origin',(-19.5538640879535,-59.1531540087998,39.3548010137695));
#201628=CARTESIAN_POINT('Ctrl Pts',(-19.1090650011318,-57.7842031819382,
39.3978017080178));
#201629=CARTESIAN_POINT('Ctrl Pts',(-18.9882808235623,-57.8234483402238,
39.3978017080178));
#201630=CARTESIAN_POINT('Ctrl Pts',(-18.9882808235623,-57.8234483402238,
39.5248017080178));
#201631=CARTESIAN_POINT('Ctrl Pts',(-19.081473513585,-57.6985255711017,
39.3978017080178));
#201632=CARTESIAN_POINT('Ctrl Pts',(-18.9604392969164,-57.7377609320145,
39.397566602504));
#201633=CARTESIAN_POINT('Ctrl Pts',(-18.9465591794958,-57.6950423231364,
39.5248015517196));
#201634=CARTESIAN_POINT('Ctrl Pts',(-19.0553854270307,-57.6175103216838,
39.3484894016716));
#201635=CARTESIAN_POINT('Ctrl Pts',(-18.934246652452,-57.657148261354,39.3480259000042));
#201636=CARTESIAN_POINT('Ctrl Pts',(-18.9071083904244,-57.5736252790828,
39.4508333188942));
#201637=CARTESIAN_POINT('Ctrl Pts',(-19.041637186088,-57.5748148483575,
39.2708017080178));
#201638=CARTESIAN_POINT('Ctrl Pts',(-18.9204594407748,-57.6147155869501,
39.27051194648));
#201639=CARTESIAN_POINT('Ctrl Pts',(-18.8863175164095,-57.5096375484036,
39.3343017080178));
#201640=CARTESIAN_POINT('Origin',(-19.007101693979,-57.470392390118,39.3343017080178));
#201641=CARTESIAN_POINT('Origin',(-19.6089151909176,-59.3225838821614,39.6398955068202));
#201642=CARTESIAN_POINT('Origin',(-19.6639662938564,-59.4920137553138,39.92499));
#201643=CARTESIAN_POINT('Origin',(-18.9819630786536,-57.3930236876028,39.1934008539951));
#201644=CARTESIAN_POINT('Origin',(-18.9681964166836,-57.3504898524408,39.1160402713851));
#201645=CARTESIAN_POINT('Ctrl Pts',(-19.4684195516699,-59.8682321556241,
40.1599502534424));
#201646=CARTESIAN_POINT('Ctrl Pts',(-19.4568831131887,-59.8327559231845,
40.10025));
#201647=CARTESIAN_POINT('Ctrl Pts',(-19.4351129318423,-59.765809437495,
40.10025));
#201648=CARTESIAN_POINT('Ctrl Pts',(-19.5522156237499,-59.8409825629603,
40.1599500538469));
#201649=CARTESIAN_POINT('Ctrl Pts',(-19.5179203859188,-59.8129039518375,
40.100244835349));
#201650=CARTESIAN_POINT('Ctrl Pts',(-19.4836145615377,-59.7500277420804,
40.10025));
#201651=CARTESIAN_POINT('Ctrl Pts',(-19.6218019328333,-59.7920481472525,
40.1202442001039));
#201652=CARTESIAN_POINT('Ctrl Pts',(-19.5669820401374,-59.7726277678654,
40.0633873868017));
#201653=CARTESIAN_POINT('Ctrl Pts',(-19.5206357546566,-59.7116747787981,
40.0772271723538));
#201654=CARTESIAN_POINT('Ctrl Pts',(-19.7007838434712,-59.6899788477096,
40.0045995998162));
#201655=CARTESIAN_POINT('Ctrl Pts',(-19.6084674936732,-59.6952619726976,
39.9663485808314));
#201656=CARTESIAN_POINT('Ctrl Pts',(-19.556896198164,-59.6234872553901,
40.0101727202466));
#201657=CARTESIAN_POINT('Ctrl Pts',(-19.7118189603903,-59.6375245663857,
39.930465434986));
#201658=CARTESIAN_POINT('Ctrl Pts',(-19.6003923959451,-59.6577198343135,
39.9051900162954));
#201659=CARTESIAN_POINT('Ctrl Pts',(-19.5572342963491,-59.5745070768384,
39.9671857458186));
#201660=CARTESIAN_POINT('Ctrl Pts',(-19.6977666881848,-59.5942745858235,
39.8576902534424));
#201661=CARTESIAN_POINT('Ctrl Pts',(-19.5766071063171,-59.6341304551456,
39.8573998014387));
#201662=CARTESIAN_POINT('Ctrl Pts',(-19.5431821162869,-59.5312589135995,
39.92499));
#201663=CARTESIAN_POINT('Origin',(-19.4351129318423,-59.765809437495,40.22725));
#201664=CARTESIAN_POINT('Origin',(-0.301960443923705,0.0981128957140471,
39.116));
#201665=CARTESIAN_POINT('Origin',(-18.8441205405522,-56.9687879773465,39.116));
#201666=CARTESIAN_POINT('Origin',(2.07460197300515E-17,1.56819321712835E-16,
40.22725));
#201667=CARTESIAN_POINT('Origin',(-19.4061247292256,-59.7752282754836,40.22725));
#201668=CARTESIAN_POINT('Ctrl Pts',(-18.8441205405522,-56.9687879773465,
38.989));
#201669=CARTESIAN_POINT('Ctrl Pts',(-18.7231554228301,-57.0080919266516,
38.989));
#201670=CARTESIAN_POINT('Ctrl Pts',(-18.7233364983081,-57.0080330916622,
39.1161901092326));
#201671=CARTESIAN_POINT('Ctrl Pts',(-18.7768526573593,-56.7625017687175,
38.989));
#201672=CARTESIAN_POINT('Ctrl Pts',(-18.6561653631324,-56.8019160587458,
38.9892298989742));
#201673=CARTESIAN_POINT('Ctrl Pts',(-18.6697165591974,-56.8430078886289,
39.1161900493188));
#201674=CARTESIAN_POINT('Ctrl Pts',(-18.7128124416024,-56.5661212433889,
39.1034966344368));
#201675=CARTESIAN_POINT('Ctrl Pts',(-18.5923760693053,-56.6055911857644,
39.1038314102579));
#201676=CARTESIAN_POINT('Ctrl Pts',(-18.6186713856995,-56.6859069993025,
39.2077528789608));
#201677=CARTESIAN_POINT('Ctrl Pts',(-18.6771643191712,-56.456807071981,
39.2875012672119));
#201678=CARTESIAN_POINT('Ctrl Pts',(-18.5568963021129,-56.4963948028697,
39.2878045257868));
#201679=CARTESIAN_POINT('Ctrl Pts',(-18.5902572009364,-56.5984571310821,
39.3549015295901));
#201680=CARTESIAN_POINT('Origin',(-18.7109915363519,-56.5590590327989,39.3548010137695));
#201681=CARTESIAN_POINT('Ctrl Pts',(-19.0928077206414,-59.7908376697911,
39.8576902534424));
#201682=CARTESIAN_POINT('Ctrl Pts',(-19.2142545736086,-59.7518659300025,
39.8573998014387));
#201683=CARTESIAN_POINT('Ctrl Pts',(-19.1808295835784,-59.6489943884563,
39.92499));
#201684=CARTESIAN_POINT('Ctrl Pts',(-19.1068672906322,-59.8341069976972,
39.9304984902492));
#201685=CARTESIAN_POINT('Ctrl Pts',(-19.2088743168615,-59.7849495553993,
39.9052171569797));
#201686=CARTESIAN_POINT('Ctrl Pts',(-19.1948881666553,-59.6922622581479,
39.9672049726605));
#201687=CARTESIAN_POINT('Ctrl Pts',(-19.1465773683627,-59.8698829694067,
40.004343767866));
#201688=CARTESIAN_POINT('Ctrl Pts',(-19.2244455609613,-59.8199164124675,
39.9661628577643));
#201689=CARTESIAN_POINT('Ctrl Pts',(-19.2238994150014,-59.7315159919507,
40.0100243556234));
#201690=CARTESIAN_POINT('Ctrl Pts',(-19.2694731179107,-59.9060262085835,
40.1194874821989));
#201691=CARTESIAN_POINT('Ctrl Pts',(-19.3027624708833,-59.8580612818569,
40.062755148314));
#201692=CARTESIAN_POINT('Ctrl Pts',(-19.3044519280755,-59.7814166574708,
40.0767884282379));
#201693=CARTESIAN_POINT('Ctrl Pts',(-19.3552948408465,-59.9049660265689,
40.1599502015391));
#201694=CARTESIAN_POINT('Ctrl Pts',(-19.3665789650869,-59.8620777700625,
40.1002449453872));
#201695=CARTESIAN_POINT('Ctrl Pts',(-19.3574492964901,-59.7910213450151,
40.10025));
#201696=CARTESIAN_POINT('Ctrl Pts',(-19.4393816709759,-59.8776671349984,
40.1599502534424));
#201697=CARTESIAN_POINT('Ctrl Pts',(-19.4278624395269,-59.8421853116552,
40.10025));
#201698=CARTESIAN_POINT('Ctrl Pts',(-19.4061247292256,-59.7752282754836,
40.10025));
#201699=CARTESIAN_POINT('Origin',(-19.0600454060089,-59.6882395467419,39.92499));
#201700=CARTESIAN_POINT('Origin',(-18.6559403576665,-56.3896289265494,39.6398955069321));
#201701=CARTESIAN_POINT('Origin',(-18.6008891789888,-56.2201988201382,39.92499));
#201702=CARTESIAN_POINT('Origin',(-19.0049943031084,-59.518809673565,39.6398955068274));
#201703=CARTESIAN_POINT('Origin',(-18.949943200106,-59.3493798002279,39.3548010137695));
#201704=CARTESIAN_POINT('Ctrl Pts',(-18.5670586829468,-56.1179479440987,
39.8576902534424));
#201705=CARTESIAN_POINT('Ctrl Pts',(-18.4469743395782,-56.1574782858996,
39.8579948730703));
#201706=CARTESIAN_POINT('Ctrl Pts',(-18.4801050014193,-56.2594439784238,
39.92499));
#201707=CARTESIAN_POINT('Ctrl Pts',(-18.5530176696414,-56.0747358697601,
39.9304020711232));
#201708=CARTESIAN_POINT('Ctrl Pts',(-18.4521518441042,-56.1242410383992,
39.9058915297385));
#201709=CARTESIAN_POINT('Ctrl Pts',(-18.4660639121464,-56.2162299491246,
39.9671523786031));
#201710=CARTESIAN_POINT('Ctrl Pts',(-18.5135050040175,-56.0391722633447,
40.0043257306692));
#201711=CARTESIAN_POINT('Ctrl Pts',(-18.4363793473476,-56.0893377355411,
39.9667894847836));
#201712=CARTESIAN_POINT('Ctrl Pts',(-18.4371504234766,-56.1772247439496,
40.0100138975199));
#201713=CARTESIAN_POINT('Ctrl Pts',(-18.3911086652349,-56.0036796861844,
40.1195533054859));
#201714=CARTESIAN_POINT('Ctrl Pts',(-18.3580919822891,-56.0516449414235,
40.0630813209237));
#201715=CARTESIAN_POINT('Ctrl Pts',(-18.3567819283755,-56.1280773042135,
40.0768265942422));
#201716=CARTESIAN_POINT('Ctrl Pts',(-18.3056594201306,-56.005156302634,
40.1599502027521));
#201717=CARTESIAN_POINT('Ctrl Pts',(-18.2945198471561,-56.0480033886671,
40.1002552791554));
#201718=CARTESIAN_POINT('Ctrl Pts',(-18.3039075553119,-56.1189701685697,
40.10025));
#201719=CARTESIAN_POINT('Ctrl Pts',(-18.2220120550219,-56.032358823839,
40.1599502534424));
#201720=CARTESIAN_POINT('Ctrl Pts',(-18.233549049922,-56.0678348753331,
40.10025));
#201721=CARTESIAN_POINT('Ctrl Pts',(-18.2553202812751,-56.1347810195641,
40.10025));
#201722=CARTESIAN_POINT('Origin',(-18.2553202812751,-56.1347810195641,40.22725));
#201723=CARTESIAN_POINT('Ctrl Pts',(-18.8168143322229,-58.9396512752212,
38.989));
#201724=CARTESIAN_POINT('Ctrl Pts',(-18.9377789661743,-58.9003474831028,
38.989));
#201725=CARTESIAN_POINT('Ctrl Pts',(-18.9375983751891,-58.9004061606709,
39.116189601327));
#201726=CARTESIAN_POINT('Ctrl Pts',(-18.8836520326609,-59.1460772043116,
38.989));
#201727=CARTESIAN_POINT('Ctrl Pts',(-19.0048864565382,-59.1068814887035,
38.988776927543));
#201728=CARTESIAN_POINT('Ctrl Pts',(-18.9912181986571,-59.0654310094269,
39.1161898821828));
#201729=CARTESIAN_POINT('Ctrl Pts',(-18.947282541524,-59.3425907075099,
39.1034967087243));
#201730=CARTESIAN_POINT('Ctrl Pts',(-19.0687550219947,-59.3034471832924,
39.1031720232731));
#201731=CARTESIAN_POINT('Ctrl Pts',(-19.0422633471882,-59.2225318234696,
39.2077529615015));
#201732=CARTESIAN_POINT('Ctrl Pts',(-18.9827025415099,-59.4519788726607,
39.2875012672119));
#201733=CARTESIAN_POINT('Ctrl Pts',(-19.1043350338629,-59.4129503580328,
39.2872087095508));
#201734=CARTESIAN_POINT('Ctrl Pts',(-19.070677448334,-59.3099814352091,
39.354901704823));
#201735=CARTESIAN_POINT('Origin',(-18.8168143322229,-58.9396512752212,39.116));
#201736=CARTESIAN_POINT('Origin',(3.93842937138093E-16,-5.57863568693716E-17,
40.22725));
#201737=CARTESIAN_POINT('Origin',(-18.2263320786585,-56.1441998575527,40.22725));
#201738=CARTESIAN_POINT('Origin',(6.24367625034032,18.1886080242681,39.116));
#201739=CARTESIAN_POINT('Origin',(-18.6927400943499,-58.5579573083284,39.116037328526));
#201740=CARTESIAN_POINT('Ctrl Pts',(-18.1930767435952,-56.0417604764382,
40.1599502534424));
#201741=CARTESIAN_POINT('Ctrl Pts',(-18.2045954185348,-56.0772424804484,
40.10025));
#201742=CARTESIAN_POINT('Ctrl Pts',(-18.2263320786585,-56.1441998575527,
40.10025));
#201743=CARTESIAN_POINT('Ctrl Pts',(-18.1097006409636,-56.0688273470723,
40.159950056604));
#201744=CARTESIAN_POINT('Ctrl Pts',(-18.1438516116611,-56.0969586315449,
40.1002551305372));
#201745=CARTESIAN_POINT('Ctrl Pts',(-18.1778965340257,-56.1599138083632,
40.10025));
#201746=CARTESIAN_POINT('Ctrl Pts',(-18.0401661963854,-56.117216091734,
40.1203070619045));
#201747=CARTESIAN_POINT('Ctrl Pts',(-18.0947679219784,-56.1367924598139,
40.0637098684499));
#201748=CARTESIAN_POINT('Ctrl Pts',(-18.1406818860299,-56.1978007560415,
40.0772636213363));
#201749=CARTESIAN_POINT('Ctrl Pts',(-17.9612165360192,-56.2184352456063,
40.0046102245803));
#201750=CARTESIAN_POINT('Ctrl Pts',(-18.0530423367033,-56.2137528851841,
39.9670001894012));
#201751=CARTESIAN_POINT('Ctrl Pts',(-18.1041286397845,-56.2852436625531,
40.0101788811209));
#201752=CARTESIAN_POINT('Ctrl Pts',(-17.9502021467135,-56.2706228600011,
39.9303710930185));
#201753=CARTESIAN_POINT('Ctrl Pts',(-18.0609092108089,-56.2513800597974,
39.9058663574109));
#201754=CARTESIAN_POINT('Ctrl Pts',(-18.1037173431994,-56.3339837785518,
39.9671344706364));
#201755=CARTESIAN_POINT('Ctrl Pts',(-17.9642361803975,-56.3138168485094,
39.8576902534424));
#201756=CARTESIAN_POINT('Ctrl Pts',(-18.0846218068697,-56.2752137607565,
39.8579948730704));
#201757=CARTESIAN_POINT('Ctrl Pts',(-18.1177524687109,-56.3771794532806,
39.92499));
#201758=CARTESIAN_POINT('Origin',(-17.9969682911414,-56.4164246115663,39.92499));
#201759=CARTESIAN_POINT('Origin',(-18.6791227120623,-58.5158800426268,39.1925554488843));
#201760=CARTESIAN_POINT('Origin',(-18.6538332760107,-58.4380471616454,39.3343017080178));
#201761=CARTESIAN_POINT('Origin',(-18.0520194698702,-56.585854717942,39.6398955069209));
#201762=CARTESIAN_POINT('Origin',(-18.1070706485045,-56.755284824227,39.3548010137695));
#201763=CARTESIAN_POINT('Ctrl Pts',(-18.5518699907153,-58.1242364370956,
39.3978017080178));
#201764=CARTESIAN_POINT('Ctrl Pts',(-18.6726541682848,-58.08499127881,39.3978017080178));
#201765=CARTESIAN_POINT('Ctrl Pts',(-18.6726541682848,-58.08499127881,39.5248017080178));
#201766=CARTESIAN_POINT('Ctrl Pts',(-18.5799074873334,-58.2097691178805,
39.3978017080178));
#201767=CARTESIAN_POINT('Ctrl Pts',(-18.7004428147371,-58.1705159385216,
39.3980355775177));
#201768=CARTESIAN_POINT('Ctrl Pts',(-18.7143758086142,-58.2133972843956,
39.5248015517192));
#201769=CARTESIAN_POINT('Ctrl Pts',(-18.6064173144578,-58.2906472745454,
39.3484893995498));
#201770=CARTESIAN_POINT('Ctrl Pts',(-18.7268501353366,-58.2517893143844,
39.3489438303419));
#201771=CARTESIAN_POINT('Ctrl Pts',(-18.7538265876727,-58.3348142976328,
39.4508333155592));
#201772=CARTESIAN_POINT('Ctrl Pts',(-18.620387828115,-58.3332704847795,
39.2708017080178));
#201773=CARTESIAN_POINT('Ctrl Pts',(-18.7407822670305,-58.2946680067387,
39.2710850691866));
#201774=CARTESIAN_POINT('Ctrl Pts',(-18.7746174535802,-58.3988020033598,
39.3343017080178));
#201775=CARTESIAN_POINT('Origin',(-18.5518699907153,-58.1242364370956,39.5248017080178));
#201776=CARTESIAN_POINT('Ctrl Pts',(-18.0743352474894,-56.6526781108323,
39.2875012672119));
#201777=CARTESIAN_POINT('Ctrl Pts',(-18.1949031876641,-56.614013495596,
39.2878045257519));
#201778=CARTESIAN_POINT('Ctrl Pts',(-18.2279043949852,-56.7161926816715,
39.354901521835));
#201779=CARTESIAN_POINT('Ctrl Pts',(-18.109749103561,-56.7620702268158,
39.1034938540228));
#201780=CARTESIAN_POINT('Ctrl Pts',(-18.2303840130662,-56.7232113603657,
39.103828627881));
#201781=CARTESIAN_POINT('Ctrl Pts',(-18.256319009646,-56.8036438738754,
39.2077506434042));
#201782=CARTESIAN_POINT('Ctrl Pts',(-18.1733695596538,-56.9585888550841,
38.989));
#201783=CARTESIAN_POINT('Ctrl Pts',(-18.2941747571346,-56.9195374698071,
38.9892298954593));
#201784=CARTESIAN_POINT('Ctrl Pts',(-18.307364587184,-56.9607460083102,
39.1161900347276));
#201785=CARTESIAN_POINT('Ctrl Pts',(-18.2401996527048,-57.1650137687746,
38.989));
#201786=CARTESIAN_POINT('Ctrl Pts',(-18.3611647564562,-57.1257098240089,
38.989));
#201787=CARTESIAN_POINT('Ctrl Pts',(-18.3609836949697,-57.1257686544521,
39.116190094565));
#201788=CARTESIAN_POINT('Origin',(-18.2401996527048,-57.1650137687746,39.116));
#201789=CARTESIAN_POINT('Origin',(6.09975091006211,17.7456513739114,39.5248017080178));
#201790=CARTESIAN_POINT('Origin',(-18.5051441132844,-57.9804289733663,39.5248017080178));
#201791=CARTESIAN_POINT('Origin',(6.07721283595922,17.6762863142854,39.116));
#201792=CARTESIAN_POINT('Origin',(-18.3641788932757,-57.5467470426659,39.1160402713847));
#201793=CARTESIAN_POINT('Ctrl Pts',(-18.4366189870675,-57.7713971777986,
39.2708017080178));
#201794=CARTESIAN_POINT('Ctrl Pts',(-18.5581069080663,-57.732451061807,
39.2705119464801));
#201795=CARTESIAN_POINT('Ctrl Pts',(-18.523964983701,-57.6273730232604,
39.3343017080178));
#201796=CARTESIAN_POINT('Ctrl Pts',(-18.4506394153724,-57.8141635875296,
39.3487519301186));
#201797=CARTESIAN_POINT('Ctrl Pts',(-18.5719407253097,-57.7750271733953,
39.348287946398));
#201798=CARTESIAN_POINT('Ctrl Pts',(-18.5448261124702,-57.6915769758401,
39.4512271261624));
#201799=CARTESIAN_POINT('Ctrl Pts',(-18.4772005006362,-57.895184561541,
39.3978017080178));
#201800=CARTESIAN_POINT('Ctrl Pts',(-18.5981804828667,-57.8557848432447,
39.3975673827392));
#201801=CARTESIAN_POINT('Ctrl Pts',(-18.5843471808454,-57.8132103173501,
39.5248015355194));
#201802=CARTESIAN_POINT('Ctrl Pts',(-18.5051441132844,-57.9804289733663,
39.3978017080178));
#201803=CARTESIAN_POINT('Ctrl Pts',(-18.6259282908539,-57.9411838150807,
39.3978017080178));
#201804=CARTESIAN_POINT('Ctrl Pts',(-18.6259282908539,-57.9411838150807,
39.5248017080178));
#201805=CARTESIAN_POINT('Origin',(-18.4031808061315,-57.6666181815461,39.3343017080178));
#201806=CARTESIAN_POINT('Origin',(-18.3780421908663,-57.5892494801765,39.1934008533553));
#201807=CARTESIAN_POINT('Origin',(-25.2734729067959,-55.9845461696115,39.1925554495081));
#201808=CARTESIAN_POINT('Origin',(-25.2915084057485,-56.0249274780511,39.1160373285261));
#201809=CARTESIAN_POINT('Origin',(-25.2401862573144,-55.9097831300745,39.3343017080178));
#201810=CARTESIAN_POINT('Ctrl Pts',(-25.1949317875303,-55.8095395120006,
39.2708017080178));
#201811=CARTESIAN_POINT('Ctrl Pts',(-25.0796311836956,-55.8614118841077,
39.2710850691867));
#201812=CARTESIAN_POINT('Ctrl Pts',(-25.1241659841938,-55.9614386837452,
39.3343017080178));
#201813=CARTESIAN_POINT('Ctrl Pts',(-25.1767321129116,-55.7683775656456,
39.3487519293518));
#201814=CARTESIAN_POINT('Ctrl Pts',(-25.0612313830313,-55.820085255182,
39.3492068662941));
#201815=CARTESIAN_POINT('Ctrl Pts',(-25.0967080045988,-55.8997670518376,
39.451227124875));
#201816=CARTESIAN_POINT('Ctrl Pts',(-25.1422534028251,-55.6903961807894,
39.3978017080178));
#201817=CARTESIAN_POINT('Ctrl Pts',(-25.0264120100489,-55.7418796630205,
39.398034778116));
#201818=CARTESIAN_POINT('Ctrl Pts',(-25.0446893032921,-55.782931135772,
39.5248015355176));
#201819=CARTESIAN_POINT('Ctrl Pts',(-25.1059793847704,-55.60834955903,39.3978017080178));
#201820=CARTESIAN_POINT('Ctrl Pts',(-24.9899591116498,-55.6600051127007,
39.3978017080178));
#201821=CARTESIAN_POINT('Ctrl Pts',(-24.9899591116498,-55.6600051127007,
39.5248017080178));
#201822=CARTESIAN_POINT('Origin',(-25.1059793847704,-55.60834955903,39.5248017080178));
#201823=CARTESIAN_POINT('Origin',(-0.29005068280152,0.129138884176568,39.116));
#201824=CARTESIAN_POINT('Origin',(-25.4547063934086,-56.3916032444849,39.116));
#201825=CARTESIAN_POINT('Origin',(-0.29005068280152,0.129138884176568,39.5248017080178));
#201826=CARTESIAN_POINT('Origin',(-25.044477503395,-55.4702140717966,39.5248017080178));
#201827=CARTESIAN_POINT('Ctrl Pts',(-25.6742415049982,-56.8833377255393,
39.2875012672119));
#201828=CARTESIAN_POINT('Ctrl Pts',(-25.5577357840971,-56.9357219056858,
39.287208709576));
#201829=CARTESIAN_POINT('Ctrl Pts',(-25.5138485805639,-56.8366797759152,
39.3549016990123));
#201830=CARTESIAN_POINT('Ctrl Pts',(-25.6273680143765,-56.7783442778542,
39.1034939173931));
#201831=CARTESIAN_POINT('Ctrl Pts',(-25.5109042502547,-56.8305359187812,
39.1031692336344));
#201832=CARTESIAN_POINT('Ctrl Pts',(-25.4764485929318,-56.7526780286685,
39.2077507202309));
#201833=CARTESIAN_POINT('Ctrl Pts',(-25.543160832995,-56.5897276738852,
38.989));
#201834=CARTESIAN_POINT('Ctrl Pts',(-25.4268390553472,-56.6417212312951,
38.9887769311158));
#201835=CARTESIAN_POINT('Ctrl Pts',(-25.4092610357538,-56.6017723050722,
39.1161898712899));
#201836=CARTESIAN_POINT('Ctrl Pts',(-25.4547063934086,-56.3916032444849,
38.989));
#201837=CARTESIAN_POINT('Ctrl Pts',(-25.3385127913799,-56.4433359691574,
38.989));
#201838=CARTESIAN_POINT('Ctrl Pts',(-25.3386862495673,-56.4432587405967,
39.1161895903856));
#201839=CARTESIAN_POINT('Origin',(-25.6299342604998,-56.7851714777846,39.3548010137695));
#201840=CARTESIAN_POINT('Ctrl Pts',(-25.044477503395,-55.4702140717966,
39.3978017080178));
#201841=CARTESIAN_POINT('Ctrl Pts',(-24.9284572302744,-55.5218696254672,
39.3978017080178));
#201842=CARTESIAN_POINT('Ctrl Pts',(-24.9284572302744,-55.5218696254672,
39.5248017080178));
#201843=CARTESIAN_POINT('Ctrl Pts',(-25.0080814159056,-55.3878899076699,
39.3978017080178));
#201844=CARTESIAN_POINT('Ctrl Pts',(-24.8918114493205,-55.4395618538397,
39.3975666025031));
#201845=CARTESIAN_POINT('Ctrl Pts',(-24.8735420580984,-55.3985281293147,
39.5248015517182));
#201846=CARTESIAN_POINT('Ctrl Pts',(-24.9736678430976,-55.3100454158615,
39.3484894016716));
#201847=CARTESIAN_POINT('Ctrl Pts',(-24.8573359723236,-55.362128664702,
39.3480259000042));
#201848=CARTESIAN_POINT('Ctrl Pts',(-24.8216158475493,-55.2818999508919,
39.4508333188947));
#201849=CARTESIAN_POINT('Ctrl Pts',(-24.9555320242418,-55.2690209153039,
39.2708017080178));
#201850=CARTESIAN_POINT('Ctrl Pts',(-24.8391888661847,-55.3213695969755,
39.27051194648));
#201851=CARTESIAN_POINT('Ctrl Pts',(-24.794250328961,-55.2204359898055,
39.3343017080178));
#201852=CARTESIAN_POINT('Origin',(-24.9102706020816,-55.1687804361349,39.3343017080178));
#201853=CARTESIAN_POINT('Origin',(-25.7023940320537,-56.9479187893842,39.6398955068173));
#201854=CARTESIAN_POINT('Origin',(-25.774853803565,-57.1106661007664,39.92499));
#201855=CARTESIAN_POINT('Origin',(-24.8771824671422,-55.0944632682979,39.1934008539941));
#201856=CARTESIAN_POINT('Origin',(-24.8590452239607,-55.0536014459531,39.1160402713853));
#201857=CARTESIAN_POINT('Ctrl Pts',(-25.61970381813,-57.5052637377731,40.1599502534424));
#201858=CARTESIAN_POINT('Ctrl Pts',(-25.6045223014064,-57.4711877340328,
40.10025));
#201859=CARTESIAN_POINT('Ctrl Pts',(-25.5758735661211,-57.4068835917978,
40.10025));
#201860=CARTESIAN_POINT('Ctrl Pts',(-25.7001924885134,-57.469404346587,
40.1599500538473));
#201861=CARTESIAN_POINT('Ctrl Pts',(-25.663150109512,-57.4450643815409,
40.1002448353499));
#201862=CARTESIAN_POINT('Ctrl Pts',(-25.6224598624455,-57.3861185493457,
40.10025));
#201863=CARTESIAN_POINT('Ctrl Pts',(-25.7642825572405,-57.4134642487751,
40.1202442001039));
#201864=CARTESIAN_POINT('Ctrl Pts',(-25.7077329912392,-57.3998804953991,
40.0633873868018));
#201865=CARTESIAN_POINT('Ctrl Pts',(-25.6552692732808,-57.344105919183,
40.0772271723537));
#201866=CARTESIAN_POINT('Ctrl Pts',(-25.8321626496791,-57.3036982377902,
40.0045995998162));
#201867=CARTESIAN_POINT('Ctrl Pts',(-25.7409042554408,-57.3186021074447,
39.9663485808315));
#201868=CARTESIAN_POINT('Ctrl Pts',(-25.6821129719827,-57.2526112478169,
40.0101727202466));
#201869=CARTESIAN_POINT('Ctrl Pts',(-25.8376543496551,-57.2503778226939,
39.930465434986));
#201870=CARTESIAN_POINT('Ctrl Pts',(-25.7289491719104,-57.2821097063817,
39.9051900162949));
#201871=CARTESIAN_POINT('Ctrl Pts',(-25.677329395237,-57.2038640469266,
39.9671857458174));
#201872=CARTESIAN_POINT('Ctrl Pts',(-25.8191582032623,-57.2088336324698,
39.8576902534424));
#201873=CARTESIAN_POINT('Ctrl Pts',(-25.7028284190336,-57.2611357920724,
39.8573998014387));
#201874=CARTESIAN_POINT('Ctrl Pts',(-25.6588335304443,-57.162321654437,
39.92499));
#201875=CARTESIAN_POINT('Origin',(-25.5758735661211,-57.4068835917978,40.22725));
#201876=CARTESIAN_POINT('Origin',(-0.29005068280152,0.129138884176568,39.116));
#201877=CARTESIAN_POINT('Origin',(-24.695750338031,-54.6869600343296,39.116));
#201878=CARTESIAN_POINT('Origin',(3.68589728140384E-17,1.50634138525679E-16,
40.22725));
#201879=CARTESIAN_POINT('Origin',(-25.5480287005721,-57.4192809246788,40.22725));
#201880=CARTESIAN_POINT('Ctrl Pts',(-24.695750338031,-54.6869600343296,
38.989));
#201881=CARTESIAN_POINT('Ctrl Pts',(-24.5795562613021,-54.7386929703522,
38.989));
#201882=CARTESIAN_POINT('Ctrl Pts',(-24.5797301948983,-54.7386155301259,
39.1161901092322));
#201883=CARTESIAN_POINT('Ctrl Pts',(-24.6072881749585,-54.4888352915933,
38.989));
#201884=CARTESIAN_POINT('Ctrl Pts',(-24.491381933525,-54.540648923419,38.9892298989742));
#201885=CARTESIAN_POINT('Ctrl Pts',(-24.5091541605496,-54.5800991622545,
39.1161900493184));
#201886=CARTESIAN_POINT('Ctrl Pts',(-24.5230714236759,-54.3002245846705,
39.1034966344368));
#201887=CARTESIAN_POINT('Ctrl Pts',(-24.4074205468501,-54.352067335488,
39.1038314102576));
#201888=CARTESIAN_POINT('Ctrl Pts',(-24.4419671033166,-54.4291945615868,
39.2077528789616));
#201889=CARTESIAN_POINT('Ctrl Pts',(-24.4761921430394,-54.1952354911871,
39.2875012672119));
#201890=CARTESIAN_POINT('Ctrl Pts',(-24.3607210114368,-54.247177787347,
39.2878045257868));
#201891=CARTESIAN_POINT('Ctrl Pts',(-24.404567574091,-54.3451938439591,
39.3549015295899));
#201892=CARTESIAN_POINT('Origin',(-24.5205222915154,-54.2933913980362,39.3548010137695));
#201893=CARTESIAN_POINT('Ctrl Pts',(-25.2380597013433,-57.4675553545139,
39.8576902534424));
#201894=CARTESIAN_POINT('Ctrl Pts',(-25.3547675996718,-57.4161024530842,
39.8573998014387));
#201895=CARTESIAN_POINT('Ctrl Pts',(-25.3107727110825,-57.3172883154489,
39.92499));
#201896=CARTESIAN_POINT('Ctrl Pts',(-25.2565651278915,-57.509118023269,
39.9304984902491));
#201897=CARTESIAN_POINT('Ctrl Pts',(-25.352874997054,-57.44956723289,39.9052171569792));
#201898=CARTESIAN_POINT('Ctrl Pts',(-25.3292770036982,-57.3588496371387,
39.9672049726599));
#201899=CARTESIAN_POINT('Ctrl Pts',(-25.2997972770059,-57.5405471770609,
40.0043437678661));
#201900=CARTESIAN_POINT('Ctrl Pts',(-25.3720159720861,-57.4827148996387,
39.9661628577643));
#201901=CARTESIAN_POINT('Ctrl Pts',(-25.3622324578623,-57.3948558336731,
40.0100243556235));
#201902=CARTESIAN_POINT('Ctrl Pts',(-25.4257977880274,-57.5636463159493,
40.1194874821988));
#201903=CARTESIAN_POINT('Ctrl Pts',(-25.4538910783601,-57.5124644612009,
40.0627551483141));
#201904=CARTESIAN_POINT('Ctrl Pts',(-25.4475597357239,-57.4360631077223,
40.0767884282377));
#201905=CARTESIAN_POINT('Ctrl Pts',(-25.5110385513887,-57.553621128909,
40.1599502015387));
#201906=CARTESIAN_POINT('Ctrl Pts',(-25.5177778164707,-57.5097883065925,
40.1002449453854));
#201907=CARTESIAN_POINT('Ctrl Pts',(-25.5012707422378,-57.4400754463039,
40.10025));
#201908=CARTESIAN_POINT('Ctrl Pts',(-25.5918112338797,-57.5176823163887,
40.1599502534424));
#201909=CARTESIAN_POINT('Ctrl Pts',(-25.5766462455179,-57.4835989537476,
40.10025));
#201910=CARTESIAN_POINT('Ctrl Pts',(-25.5480287005721,-57.4192809246788,
40.10025));
#201911=CARTESIAN_POINT('Origin',(-25.1947524379619,-57.3689438691195,39.92499));
#201912=CARTESIAN_POINT('Origin',(-24.4480624203116,-54.1306438627471,39.6398955069335));
#201913=CARTESIAN_POINT('Origin',(-24.3756025490941,-53.9678963272934,39.92499));
#201914=CARTESIAN_POINT('Origin',(-25.1222926664881,-57.2061965577042,39.6398955068267));
#201915=CARTESIAN_POINT('Origin',(-25.0498328948967,-57.0434492461378,39.3548010137695));
#201916=CARTESIAN_POINT('Ctrl Pts',(-24.331269253109,-53.8697418420144,
39.8576902534424));
#201917=CARTESIAN_POINT('Ctrl Pts',(-24.2159747902189,-53.9216078643416,
39.8579948730703));
#201918=CARTESIAN_POINT('Ctrl Pts',(-24.2595822759735,-54.019551880964,
39.92499));
#201919=CARTESIAN_POINT('Ctrl Pts',(-24.3127882662189,-53.8282341734838,
39.930402071123));
#201920=CARTESIAN_POINT('Ctrl Pts',(-24.2176496934291,-53.8880114973683,
39.905891529738));
#201921=CARTESIAN_POINT('Ctrl Pts',(-24.2411010091823,-53.9780422761226,
39.9671523786023));
#201922=CARTESIAN_POINT('Ctrl Pts',(-24.2697746459841,-53.7969955864427,
40.0043257306694));
#201923=CARTESIAN_POINT('Ctrl Pts',(-24.198315211449,-53.854948073304,39.9667894847838));
#201924=CARTESIAN_POINT('Ctrl Pts',(-24.2082687574724,-53.9422730280818,
40.0100138975201));
#201925=CARTESIAN_POINT('Ctrl Pts',(-24.1443388226042,-53.7744913425364,
40.1195533054856));
#201926=CARTESIAN_POINT('Ctrl Pts',(-24.1165167429226,-53.8256450222189,
40.0630813209233));
#201927=CARTESIAN_POINT('Ctrl Pts',(-24.1232032230477,-53.9017956184507,
40.076826594242));
#201928=CARTESIAN_POINT('Ctrl Pts',(-24.0595120258535,-53.7848917482049,
40.1599502027517));
#201929=CARTESIAN_POINT('Ctrl Pts',(-24.0529122166833,-53.828668515861,
40.1002552791541));
#201930=CARTESIAN_POINT('Ctrl Pts',(-24.0696665464382,-53.8982652496117,
40.10025));
#201931=CARTESIAN_POINT('Ctrl Pts',(-23.9791663275016,-53.8206887816835,
40.1599502534424));
#201932=CARTESIAN_POINT('Ctrl Pts',(-23.994348378682,-53.854764547308,40.10025));
#201933=CARTESIAN_POINT('Ctrl Pts',(-24.0229981225299,-53.9190682401994,
40.10025));
#201934=CARTESIAN_POINT('Origin',(-24.0229981225299,-53.9190682401994,40.22725));
#201935=CARTESIAN_POINT('Ctrl Pts',(-24.8746050278055,-56.6498810128381,
38.989));
#201936=CARTESIAN_POINT('Ctrl Pts',(-24.9907986398447,-56.5981482837086,
38.989));
#201937=CARTESIAN_POINT('Ctrl Pts',(-24.9906251716318,-56.598225516733,
39.1161896013271));
#201938=CARTESIAN_POINT('Ctrl Pts',(-24.9626539694736,-56.848189676975,
38.989));
#201939=CARTESIAN_POINT('Ctrl Pts',(-25.0791271905724,-56.7965362315742,
38.9887769275436));
#201940=CARTESIAN_POINT('Ctrl Pts',(-25.0612010539377,-56.7567415443524,
39.1161898821829));
#201941=CARTESIAN_POINT('Ctrl Pts',(-25.0464771582516,-57.036975459333,
39.1034967087243));
#201942=CARTESIAN_POINT('Ctrl Pts',(-25.1631925873323,-56.9853490357247,
39.1031720232723));
#201943=CARTESIAN_POINT('Ctrl Pts',(-25.1283880784746,-56.907646072766,
39.2077529615014));
#201944=CARTESIAN_POINT('Ctrl Pts',(-25.0931373005748,-57.142061986502,
39.2875012672119));
#201945=CARTESIAN_POINT('Ctrl Pts',(-25.2100238867505,-57.0905332166518,
39.2872087095507));
#201946=CARTESIAN_POINT('Ctrl Pts',(-25.1657874977295,-56.9916465440537,
39.354901704823));
#201947=CARTESIAN_POINT('Origin',(-24.8746050278055,-56.6498810128381,39.116));
#201948=CARTESIAN_POINT('Origin',(3.8811097157961E-16,-5.3586061441408E-17,
40.22725));
#201949=CARTESIAN_POINT('Origin',(-23.995153256981,-53.9314655730803,40.22725));
#201950=CARTESIAN_POINT('Origin',(10.5838037820519,22.99100911823,39.116));
#201951=CARTESIAN_POINT('Origin',(-24.7113125977908,-56.2832472948502,39.1160373285277));
#201952=CARTESIAN_POINT('Ctrl Pts',(-23.9513722670367,-53.8330634946837,
40.1599502534424));
#201953=CARTESIAN_POINT('Ctrl Pts',(-23.9665367208226,-53.8671470951729,
40.10025));
#201954=CARTESIAN_POINT('Ctrl Pts',(-23.995153256981,-53.9314655730803,
40.10025));
#201955=CARTESIAN_POINT('Ctrl Pts',(-23.8712821658119,-53.8686972660497,
40.1599500566041));
#201956=CARTESIAN_POINT('Ctrl Pts',(-23.9081865738556,-53.8931046959193,
40.100255130536));
#201957=CARTESIAN_POINT('Ctrl Pts',(-23.9486256024598,-53.9521563342723,
40.10025));
#201958=CARTESIAN_POINT('Ctrl Pts',(-23.8071866393157,-53.9240892607409,
40.1203070619047));
#201959=CARTESIAN_POINT('Ctrl Pts',(-23.8635355386145,-53.9378509529596,
40.0637098684497));
#201960=CARTESIAN_POINT('Ctrl Pts',(-23.915575084618,-53.9937257232526,
40.0772636213363));
#201961=CARTESIAN_POINT('Ctrl Pts',(-23.7392497560571,-54.0330064121714,
40.0046102245801));
#201962=CARTESIAN_POINT('Ctrl Pts',(-23.8300830854579,-54.0187512923762,
39.9670001894015));
#201963=CARTESIAN_POINT('Ctrl Pts',(-23.8883623535218,-54.0845104630312,
40.0101788811209));
#201964=CARTESIAN_POINT('Ctrl Pts',(-23.7337507958619,-54.0860594545422,
39.9303710930186));
#201965=CARTESIAN_POINT('Ctrl Pts',(-23.8418399747443,-54.0553500291285,
39.9058663574115));
#201966=CARTESIAN_POINT('Ctrl Pts',(-23.8930480394871,-54.1330265677743,
39.9671344706369));
#201967=CARTESIAN_POINT('Ctrl Pts',(-23.752222950883,-54.1275498658872,
39.8576902534424));
#201968=CARTESIAN_POINT('Ctrl Pts',(-23.8679139708571,-54.0765745253535,
39.8579948730703));
#201969=CARTESIAN_POINT('Ctrl Pts',(-23.9115214566117,-54.1745185419759,
39.92499));
#201970=CARTESIAN_POINT('Origin',(-23.7955011834911,-54.2261740956465,39.92499));
#201971=CARTESIAN_POINT('Origin',(-24.6933715410276,-56.2428239368544,39.1925554488836));
#201972=CARTESIAN_POINT('Origin',(-24.6600848917114,-56.1680608984277,39.3343017080178));
#201973=CARTESIAN_POINT('Origin',(-23.8679610547539,-54.3889216310586,39.6398955069213));
#201974=CARTESIAN_POINT('Origin',(-23.9404209259123,-54.5516691663894,39.3548010137695));
#201975=CARTESIAN_POINT('Ctrl Pts',(-24.5258780191674,-55.8666273273832,
39.3978017080178));
#201976=CARTESIAN_POINT('Ctrl Pts',(-24.641898292288,-55.8149717737125,
39.3978017080178));
#201977=CARTESIAN_POINT('Ctrl Pts',(-24.641898292288,-55.8149717737125,
39.5248017080178));
#201978=CARTESIAN_POINT('Ctrl Pts',(-24.5627025231283,-55.9487607347574,
39.3978017080178));
#201979=CARTESIAN_POINT('Ctrl Pts',(-24.6784744708792,-55.8971232158788,
39.3980355775163));
#201980=CARTESIAN_POINT('Ctrl Pts',(-24.6968134595441,-55.938313258815,
39.5248015517178));
#201981=CARTESIAN_POINT('Ctrl Pts',(-24.5975211960713,-56.0264248009281,
39.3484893995498));
#201982=CARTESIAN_POINT('Ctrl Pts',(-24.713232510496,-55.9751910510455,
39.3489438303431));
#201983=CARTESIAN_POINT('Ctrl Pts',(-24.7487396569161,-56.0549414076414,
39.4508333155604));
#201984=CARTESIAN_POINT('Ctrl Pts',(-24.6158705164596,-56.0673542004325,
39.2708017080178));
#201985=CARTESIAN_POINT('Ctrl Pts',(-24.7315703643338,-56.0163785451196,
39.2710850691866));
#201986=CARTESIAN_POINT('Ctrl Pts',(-24.776105164832,-56.1164053447571,
39.3343017080178));
#201987=CARTESIAN_POINT('Origin',(-24.5258780191674,-55.8666273273832,39.5248017080178));
#201988=CARTESIAN_POINT('Ctrl Pts',(-23.8971395307771,-54.4530463244691,
39.2875012672119));
#201989=CARTESIAN_POINT('Ctrl Pts',(-24.0130054343468,-54.4019907365348,
39.2878045257519));
#201990=CARTESIAN_POINT('Ctrl Pts',(-24.0565064908996,-54.5001606088507,
39.354901521835));
#201991=CARTESIAN_POINT('Ctrl Pts',(-23.9437939758168,-54.5581374230419,
39.1034938540228));
#201992=CARTESIAN_POINT('Ctrl Pts',(-24.0597061770695,-54.5068816478228,
39.1038286278817));
#201993=CARTESIAN_POINT('Ctrl Pts',(-24.0939065860602,-54.5841625982685,
39.2077506434042));
#201994=CARTESIAN_POINT('Ctrl Pts',(-24.0276077026095,-54.7469293531954,
38.989));
#201995=CARTESIAN_POINT('Ctrl Pts',(-24.1436691352872,-54.6954643138447,
38.9892298954587));
#201996=CARTESIAN_POINT('Ctrl Pts',(-24.1610941752721,-54.7350683949965,
39.1161900347276));
#201997=CARTESIAN_POINT('Ctrl Pts',(-24.1156489724279,-54.9452378026827,
38.989));
#201998=CARTESIAN_POINT('Ctrl Pts',(-24.2318430357375,-54.8935048726347,
38.989));
#201999=CARTESIAN_POINT('Ctrl Pts',(-24.2316691155806,-54.8935823068775,
39.116190094565));
#202000=CARTESIAN_POINT('Origin',(-24.1156489724279,-54.9452378026828,39.116));
#202001=CARTESIAN_POINT('Origin',(10.3344596589369,22.4309730483568,39.5248017080178));
#202002=CARTESIAN_POINT('Origin',(-24.4643761377919,-55.7284918401497,39.5248017080178));
#202003=CARTESIAN_POINT('Origin',(10.2954134679533,22.3432738675267,39.116));
#202004=CARTESIAN_POINT('Origin',(-24.2788510342447,-55.3119205422644,39.1160402713849));
#202005=CARTESIAN_POINT('Ctrl Pts',(-24.3743766270216,-55.5277679687682,
39.2708017080178));
#202006=CARTESIAN_POINT('Ctrl Pts',(-24.4911280468229,-55.4763362579873,
39.27051194648));
#202007=CARTESIAN_POINT('Ctrl Pts',(-24.4461895095991,-55.3754026508174,
39.3343017080178));
#202008=CARTESIAN_POINT('Ctrl Pts',(-24.3927905570426,-55.5688345658066,
39.3487519301186));
#202009=CARTESIAN_POINT('Ctrl Pts',(-24.5093364964831,-55.5172331055199,
39.3482879463987));
#202010=CARTESIAN_POINT('Ctrl Pts',(-24.4736474994194,-55.4370743056912,
39.4512271261644));
#202011=CARTESIAN_POINT('Ctrl Pts',(-24.4276751358079,-55.6466353090196,
39.3978017080178));
#202012=CARTESIAN_POINT('Ctrl Pts',(-24.543873985031,-55.5948055748773,
39.3975673827397));
#202013=CARTESIAN_POINT('Ctrl Pts',(-24.5256662135199,-55.553910250492,
39.5248015355181));
#202014=CARTESIAN_POINT('Ctrl Pts',(-24.4643761377919,-55.7284918401497,
39.3978017080178));
#202015=CARTESIAN_POINT('Ctrl Pts',(-24.5803964109126,-55.6768362864791,
39.3978017080178));
#202016=CARTESIAN_POINT('Ctrl Pts',(-24.5803964109126,-55.6768362864791,
39.5248017080178));
#202017=CARTESIAN_POINT('Origin',(-24.3301692364785,-55.427058204488,39.3343017080178));
#202018=CARTESIAN_POINT('Origin',(-24.2970811017213,-55.3527410377814,39.1934008533551));
#202019=CARTESIAN_POINT('Origin',(-30.9870007556527,-53.0360596835509,39.1925554495085));
#202020=CARTESIAN_POINT('Origin',(-31.0091584503705,-53.0743345559677,39.1160373285265));
#202021=CARTESIAN_POINT('Origin',(-30.9460815882871,-52.9651856060844,39.3343017080178));
#202022=CARTESIAN_POINT('Ctrl Pts',(-30.8905967158739,-52.8702215132214,
39.2708017080178));
#202023=CARTESIAN_POINT('Ctrl Pts',(-30.7813498801535,-52.9338619179794,
39.2710850691866));
#202024=CARTESIAN_POINT('Ctrl Pts',(-30.8360963620065,-53.0286856060844,
39.3343017080178));
#202025=CARTESIAN_POINT('Ctrl Pts',(-30.868194145979,-52.8311874403355,
39.3487519293518));
#202026=CARTESIAN_POINT('Ctrl Pts',(-30.7587310665072,-52.894684983538,
39.3492068662937));
#202027=CARTESIAN_POINT('Ctrl Pts',(-30.8023423591855,-52.9702219582397,
39.4512271248747));
#202028=CARTESIAN_POINT('Ctrl Pts',(-30.8257530395505,-52.7572372522462,
39.3978017080178));
#202029=CARTESIAN_POINT('Ctrl Pts',(-30.7159277273266,-52.8205474253453,
39.398034778116));
#202030=CARTESIAN_POINT('Ctrl Pts',(-30.7383959430076,-52.8594635164577,
39.5248015355176));
#202031=CARTESIAN_POINT('Ctrl Pts',(-30.7811015270746,-52.6794317578286,
39.3978017080178));
#202032=CARTESIAN_POINT('Ctrl Pts',(-30.671116300794,-52.7429317578286,
39.3978017080178));
#202033=CARTESIAN_POINT('Ctrl Pts',(-30.671116300794,-52.7429317578286,
39.5248017080178));
#202034=CARTESIAN_POINT('Origin',(-30.7811015270746,-52.6794317578286,39.5248017080178));
#202035=CARTESIAN_POINT('Origin',(-0.274963065701553,0.158750000000001,
39.116));
#202036=CARTESIAN_POINT('Origin',(-31.2097904767608,-53.4219427993285,39.116));
#202037=CARTESIAN_POINT('Origin',(-0.274963065701553,0.158750000000001,
39.5248017080178));
#202038=CARTESIAN_POINT('Origin',(-30.7054974692372,-52.5484816883958,39.5248017080178));
#202039=CARTESIAN_POINT('Ctrl Pts',(-31.4795232016792,-53.8880358395969,
39.2875012672119));
#202040=CARTESIAN_POINT('Ctrl Pts',(-31.3691313491575,-53.9523112176912,
39.287208709576));
#202041=CARTESIAN_POINT('Ctrl Pts',(-31.3151318426937,-53.8583991130128,
39.3549016990124));
#202042=CARTESIAN_POINT('Ctrl Pts',(-31.4219316852012,-53.7885171709481,
39.1034939173931));
#202043=CARTESIAN_POINT('Ctrl Pts',(-31.3115614337855,-53.8525966788964,
39.1031692336333));
#202044=CARTESIAN_POINT('Ctrl Pts',(-31.2691561625558,-53.7787668993605,
39.2077507202313));
#202045=CARTESIAN_POINT('Ctrl Pts',(-31.3184699958134,-53.6097358757351,
38.989));
#202046=CARTESIAN_POINT('Ctrl Pts',(-31.2082202476906,-53.6736035436587,
38.988776931117));
#202047=CARTESIAN_POINT('Ctrl Pts',(-31.1865627224597,-53.6357108652095,
39.1161898712894));
#202048=CARTESIAN_POINT('Ctrl Pts',(-31.2097904767608,-53.4219427993285,
38.989));
#202049=CARTESIAN_POINT('Ctrl Pts',(-31.0996409376522,-53.485537665384,
38.989));
#202050=CARTESIAN_POINT('Ctrl Pts',(-31.0998053730349,-53.4854427285716,
39.1161895903857));
#202051=CARTESIAN_POINT('Origin',(-31.4251975098795,-53.7950387249977,39.3548010137695));
#202052=CARTESIAN_POINT('Ctrl Pts',(-30.7054974692372,-52.5484816883958,
39.3978017080178));
#202053=CARTESIAN_POINT('Ctrl Pts',(-30.5955122429565,-52.6119816883958,
39.3978017080178));
#202054=CARTESIAN_POINT('Ctrl Pts',(-30.5955122429565,-52.6119816883958,
39.5248017080178));
#202055=CARTESIAN_POINT('Ctrl Pts',(-30.6606955449582,-52.4704129317476,
39.3978017080178));
#202056=CARTESIAN_POINT('Ctrl Pts',(-30.5504637065407,-52.5339553345193,
39.3975666025021));
#202057=CARTESIAN_POINT('Ctrl Pts',(-30.5280052047889,-52.4950560684209,
39.5248015517178));
#202058=CARTESIAN_POINT('Ctrl Pts',(-30.6183335281985,-52.3965920780925,
39.3484894016717));
#202059=CARTESIAN_POINT('Ctrl Pts',(-30.5080831175518,-52.4605500011291,
39.3480259000039));
#202060=CARTESIAN_POINT('Ctrl Pts',(-30.4641724871919,-52.3844945583577,
39.4508333188946));
#202061=CARTESIAN_POINT('Ctrl Pts',(-30.5960088312571,-52.3576880233161,
39.2708017080178));
#202062=CARTESIAN_POINT('Ctrl Pts',(-30.4857749404423,-52.4219111049555,
39.27051194648));
#202063=CARTESIAN_POINT('Ctrl Pts',(-30.4305321463779,-52.326227778884,
39.3343017080178));
#202064=CARTESIAN_POINT('Origin',(-30.5405173726585,-52.262727778884,39.3343017080178));
#202065=CARTESIAN_POINT('Origin',(-31.5142720656056,-53.9493203812217,39.63989550682));
#202066=CARTESIAN_POINT('Origin',(-31.6033466212668,-54.1036020372437,39.92499));
#202067=CARTESIAN_POINT('Origin',(-30.4998422386362,-52.1922763801648,39.1934008539946));
#202068=CARTESIAN_POINT('Origin',(-30.4775331296743,-52.1535342613172,39.1160402713852));
#202069=CARTESIAN_POINT('Ctrl Pts',(-31.490293248291,-54.5122556166609,
40.1599502534424));
#202070=CARTESIAN_POINT('Ctrl Pts',(-31.4716329851992,-54.4799531854478,
40.10025));
#202071=CARTESIAN_POINT('Ctrl Pts',(-31.4364195775137,-54.4189959163062,
40.10025));
#202072=CARTESIAN_POINT('Ctrl Pts',(-31.5665926662616,-54.4681793099457,
40.1599500538464));
#202073=CARTESIAN_POINT('Ctrl Pts',(-31.5272089901454,-54.4478446647266,
40.1002448353503));
#202074=CARTESIAN_POINT('Ctrl Pts',(-31.4805801312539,-54.3934750329625,
40.10025));
#202075=CARTESIAN_POINT('Ctrl Pts',(-31.6244843104275,-54.4058464214485,
40.120244200104));
#202076=CARTESIAN_POINT('Ctrl Pts',(-31.5668246399996,-54.3982481205271,
40.0633873868015));
#202077=CARTESIAN_POINT('Ctrl Pts',(-31.5088182930364,-54.3482630350911,
40.0772271723538));
#202078=CARTESIAN_POINT('Ctrl Pts',(-31.6805188761698,-54.2895863184076,
40.0045995998161));
#202079=CARTESIAN_POINT('Ctrl Pts',(-31.5913182835557,-54.3139476428151,
39.9663485808318));
#202080=CARTESIAN_POINT('Ctrl Pts',(-31.5259511417531,-54.2544636505341,
40.0101727202466));
#202081=CARTESIAN_POINT('Ctrl Pts',(-31.6804069909878,-54.2359839591652,
39.930465434986));
#202082=CARTESIAN_POINT('Ctrl Pts',(-31.5756141966199,-54.2789047974526,
39.9051900162944));
#202083=CARTESIAN_POINT('Ctrl Pts',(-31.5160982999437,-54.2064835118371,
39.9671857458173));
#202084=CARTESIAN_POINT('Ctrl Pts',(-31.6576696180587,-54.1966007261206,
39.8576902534424));
#202085=CARTESIAN_POINT('Ctrl Pts',(-31.5474441649286,-54.2607761425981,
39.8573998014387));
#202086=CARTESIAN_POINT('Ctrl Pts',(-31.4933613949861,-54.1671020372437,
39.92499));
#202087=CARTESIAN_POINT('Origin',(-31.4364195775137,-54.4189959163062,40.22725));
#202088=CARTESIAN_POINT('Origin',(-0.274963065701553,0.158750000000001,
39.116));
#202089=CARTESIAN_POINT('Origin',(-30.2768083268883,-51.8059703131945,39.116));
#202090=CARTESIAN_POINT('Origin',(5.22371297615238E-17,1.42798576194616E-16,
40.22725));
#202091=CARTESIAN_POINT('Origin',(-31.4100231232064,-54.4342359163062,40.22725));
#202092=CARTESIAN_POINT('Ctrl Pts',(-30.2768083268883,-51.8059703131945,
38.989));
#202093=CARTESIAN_POINT('Ctrl Pts',(-30.1666583377715,-51.8695654390623,
38.989));
#202094=CARTESIAN_POINT('Ctrl Pts',(-30.166823223834,-51.8694702420497,
39.1161901092329));
#202095=CARTESIAN_POINT('Ctrl Pts',(-30.1681210939101,-51.6181777324909,
38.989));
#202096=CARTESIAN_POINT('Ctrl Pts',(-30.0582657983061,-51.6818230251232,
38.9892298989718));
#202097=CARTESIAN_POINT('Ctrl Pts',(-30.0800643400517,-51.7191994478448,
39.1161900493191));
#202098=CARTESIAN_POINT('Ctrl Pts',(-30.0646505034512,-51.4394033023488,
39.1034966344368));
#202099=CARTESIAN_POINT('Ctrl Pts',(-29.9550522173005,-51.5030508615808,
39.1038314102583));
#202100=CARTESIAN_POINT('Ctrl Pts',(-29.9974715145359,-51.5761444782056,
39.2077528789608));
#202101=CARTESIAN_POINT('Ctrl Pts',(-30.007053683816,-51.3398895692696,
39.2875012672119));
#202102=CARTESIAN_POINT('Ctrl Pts',(-29.8976445635498,-51.4036173400348,
39.2878045257868));
#202103=CARTESIAN_POINT('Ctrl Pts',(-29.9514963979202,-51.4965132406196,
39.3549015295903));
#202104=CARTESIAN_POINT('Origin',(-30.0614010732039,-51.4328740054941,39.3548010137695));
#202105=CARTESIAN_POINT('Ctrl Pts',(-31.1067982185537,-54.5146464769136,
39.8576902534424));
#202106=CARTESIAN_POINT('Ctrl Pts',(-31.2174884860867,-54.4512761425981,
39.8573998014387));
#202107=CARTESIAN_POINT('Ctrl Pts',(-31.1634057161443,-54.3576020372437,
39.92499));
#202108=CARTESIAN_POINT('Ctrl Pts',(-31.1295467523325,-54.5540471172216,
39.930498490249));
#202109=CARTESIAN_POINT('Ctrl Pts',(-31.2191042733518,-54.4847554296818,
39.9052171569786));
#202110=CARTESIAN_POINT('Ctrl Pts',(-31.1861529813961,-54.3970014563931,
39.9672049726603));
#202111=CARTESIAN_POINT('Ctrl Pts',(-31.1758273123592,-54.5807851087096,
40.0043437678664));
#202112=CARTESIAN_POINT('Ctrl Pts',(-31.2416052667856,-54.515720733339,
39.9661628577646));
#202113=CARTESIAN_POINT('Ctrl Pts',(-31.2226915745266,-54.4293656242362,
40.0100243556236));
#202114=CARTESIAN_POINT('Ctrl Pts',(-31.3035520968882,-54.5905870683101,
40.1194874821985));
#202115=CARTESIAN_POINT('Ctrl Pts',(-31.3261415286127,-54.53674904465,40.0627551483138));
#202116=CARTESIAN_POINT('Ctrl Pts',(-31.3118587536634,-54.4614280312965,
40.0767884282376));
#202117=CARTESIAN_POINT('Ctrl Pts',(-31.3872779850339,-54.5717067142918,
40.1599502015391));
#202118=CARTESIAN_POINT('Ctrl Pts',(-31.3893985541603,-54.5274095677415,
40.1002449453869));
#202119=CARTESIAN_POINT('Ctrl Pts',(-31.3656949292512,-54.459804060898,
40.10025));
#202120=CARTESIAN_POINT('Ctrl Pts',(-31.4638515574743,-54.5275217339718,
40.1599502534424));
#202121=CARTESIAN_POINT('Ctrl Pts',(-31.4452069629856,-54.4952102564864,
40.10025));
#202122=CARTESIAN_POINT('Ctrl Pts',(-31.4100231232064,-54.4342359163062,
40.10025));
#202123=CARTESIAN_POINT('Origin',(-31.0534204898636,-54.4211020372437,39.92499));
#202124=CARTESIAN_POINT('Origin',(-29.9723263949891,-51.278592137217,39.6398955069325));
#202125=CARTESIAN_POINT('Origin',(-29.8832517167489,-51.1243102687783,39.92499));
#202126=CARTESIAN_POINT('Origin',(-30.9643459342343,-54.2668203811893,39.6398955068276));
#202127=CARTESIAN_POINT('Origin',(-30.8752713784764,-54.1125387249977,39.3548010137695));
#202128=CARTESIAN_POINT('Ctrl Pts',(-29.8289013456888,-51.0313275753407,
39.8576902534424));
#202129=CARTESIAN_POINT('Ctrl Pts',(-29.7196599535395,-51.0949610232,39.8579948730704));
#202130=CARTESIAN_POINT('Ctrl Pts',(-29.7732664904682,-51.1878102687783,
39.92499));
#202131=CARTESIAN_POINT('Ctrl Pts',(-29.8061828667729,-50.9919790793207,
39.9304020711232));
#202132=CARTESIAN_POINT('Ctrl Pts',(-29.7178139048428,-51.0613736255828,
39.9058915297387));
#202133=CARTESIAN_POINT('Ctrl Pts',(-29.7505475307855,-51.1484598763128,
39.967152378603));
#202134=CARTESIAN_POINT('Ctrl Pts',(-29.7601395581529,-50.9654077681506,
40.0043257306691));
#202135=CARTESIAN_POINT('Ctrl Pts',(-29.695129270271,-51.030512330103,39.9667894847838));
#202136=CARTESIAN_POINT('Ctrl Pts',(-29.7141562330557,-51.1163184807719,
40.01001389752));
#202137=CARTESIAN_POINT('Ctrl Pts',(-29.6330385513049,-50.9561384187037,
40.1195533054859));
#202138=CARTESIAN_POINT('Ctrl Pts',(-29.6107158994147,-51.0099200724109,
40.0630813209234));
#202139=CARTESIAN_POINT('Ctrl Pts',(-29.6253256551032,-51.0849545802163,
40.076826594242));
#202140=CARTESIAN_POINT('Ctrl Pts',(-29.5497635830448,-50.9753486645701,
40.1599502027514));
#202141=CARTESIAN_POINT('Ctrl Pts',(-29.5477758465707,-51.0195754864248,
40.1002552791554));
#202142=CARTESIAN_POINT('Ctrl Pts',(-29.5717132339809,-51.0870396576426,
40.10025));
#202143=CARTESIAN_POINT('Ctrl Pts',(-29.473599835734,-51.0193480105326,
40.1599502534424));
#202144=CARTESIAN_POINT('Ctrl Pts',(-29.4922606054649,-51.0516501490685,
40.10025));
#202145=CARTESIAN_POINT('Ctrl Pts',(-29.5274749692187,-51.1126068659045,
40.10025));
#202146=CARTESIAN_POINT('Origin',(-29.5274749692187,-51.1126068659046,40.22725));
#202147=CARTESIAN_POINT('Ctrl Pts',(-30.6598643453577,-53.7394427993285,
38.989));
#202148=CARTESIAN_POINT('Ctrl Pts',(-30.7700138939555,-53.6758479277944,
38.989));
#202149=CARTESIAN_POINT('Ctrl Pts',(-30.7698494490696,-53.6759428700936,
39.1161896013264));
#202150=CARTESIAN_POINT('Ctrl Pts',(-30.7681598456261,-53.9274614872887,
38.989));
#202151=CARTESIAN_POINT('Ctrl Pts',(-30.8785957589626,-53.8639162380558,
38.9887769275436));
#202152=CARTESIAN_POINT('Ctrl Pts',(-30.85660814608,-53.8262133418101,39.1161898821822));
#202153=CARTESIAN_POINT('Ctrl Pts',(-30.8712573299222,-54.1064511722687,
39.1034967087243));
#202154=CARTESIAN_POINT('Ctrl Pts',(-30.9819369489432,-54.0429074791677,
39.1031720232731));
#202155=CARTESIAN_POINT('Ctrl Pts',(-30.9392009315176,-53.9692682429941,
39.2077529615022));
#202156=CARTESIAN_POINT('Ctrl Pts',(-30.9286463962981,-54.206084711474,
39.2875012672119));
#202157=CARTESIAN_POINT('Ctrl Pts',(-31.0395064423976,-54.1426202463874,
39.2872087095507));
#202158=CARTESIAN_POINT('Ctrl Pts',(-30.9851759130207,-54.0488992470935,
39.3549017048226));
#202159=CARTESIAN_POINT('Origin',(-30.6598643453577,-53.7394427993285,39.116));
#202160=CARTESIAN_POINT('Origin',(3.8264039982802E-16,-5.07986659106881E-17,
40.22725));
#202161=CARTESIAN_POINT('Origin',(-29.5010785149114,-51.1278468659046,40.22725));
#202162=CARTESIAN_POINT('Origin',(15.8305769983926,26.7843636743469,39.116));
#202163=CARTESIAN_POINT('Origin',(-30.4591427892373,-53.3918862459816,39.1160373285268));
#202164=CARTESIAN_POINT('Ctrl Pts',(-29.4472515437738,-51.0345602039885,
40.1599502534424));
#202165=CARTESIAN_POINT('Ctrl Pts',(-29.4658956314769,-51.0668719738976,
40.10025));
#202166=CARTESIAN_POINT('Ctrl Pts',(-29.5010785149114,-51.1278468659046,
40.10025));
#202167=CARTESIAN_POINT('Ctrl Pts',(-29.3713249278648,-51.0783704650304,
40.1599500566043));
#202168=CARTESIAN_POINT('Ctrl Pts',(-29.4105784408359,-51.098786627384,
40.1002551305372));
#202169=CARTESIAN_POINT('Ctrl Pts',(-29.4569685172211,-51.1532877451684,
40.10025));
#202170=CARTESIAN_POINT('Ctrl Pts',(-29.3133705634514,-51.1401588234662,
40.1203070619046));
#202171=CARTESIAN_POINT('Ctrl Pts',(-29.3708492661238,-51.1479550638448,
40.0637098684497));
#202172=CARTESIAN_POINT('Ctrl Pts',(-29.4284442379234,-51.1980841325266,
40.0772636213363));
#202173=CARTESIAN_POINT('Ctrl Pts',(-29.2571907880104,-51.255580653351,
40.0046102245802));
#202174=CARTESIAN_POINT('Ctrl Pts',(-29.3460364571625,-51.2319089562574,
39.9670001894015));
#202175=CARTESIAN_POINT('Ctrl Pts',(-29.4108701703525,-51.2912160489645,
40.0101788811209));
#202176=CARTESIAN_POINT('Ctrl Pts',(-29.2572675046853,-51.3089178634634,
39.9303710930186));
#202177=CARTESIAN_POINT('Ctrl Pts',(-29.3615545506885,-51.2670782717308,
39.9058663574106));
#202178=CARTESIAN_POINT('Ctrl Pts',(-29.4206015015119,-51.3389765898554,
39.9671344706358));
#202179=CARTESIAN_POINT('Ctrl Pts',(-29.2799753962465,-51.3482501200164,
39.8576902534424));
#202180=CARTESIAN_POINT('Ctrl Pts',(-29.3897042746976,-51.2854610232,39.8579948730703));
#202181=CARTESIAN_POINT('Ctrl Pts',(-29.4433108116264,-51.3783102687783,
39.92499));
#202182=CARTESIAN_POINT('Origin',(-29.3333255853457,-51.4418102687783,39.92499));
#202183=CARTESIAN_POINT('Origin',(-30.4370746239675,-53.3535596824668,39.192555448885));
#202184=CARTESIAN_POINT('Origin',(-30.396155456884,-53.2826856060844,39.3343017080178));
#202185=CARTESIAN_POINT('Origin',(-29.4224002636276,-51.5960921371731,39.6398955069217));
#202186=CARTESIAN_POINT('Origin',(-29.5114749418008,-51.7503740054942,39.3548010137695));
#202187=CARTESIAN_POINT('Ctrl Pts',(-30.2311753956715,-52.9969317578286,
39.3978017080178));
#202188=CARTESIAN_POINT('Ctrl Pts',(-30.3411606219521,-52.9334317578286,
39.3978017080178));
#202189=CARTESIAN_POINT('Ctrl Pts',(-30.3411606219521,-52.9334317578286,
39.5248017080178));
#202190=CARTESIAN_POINT('Ctrl Pts',(-30.2763834500022,-53.074766020994,
39.3978017080178));
#202191=CARTESIAN_POINT('Ctrl Pts',(-30.386123596414,-53.0113099140565,
39.3980355775163));
#202192=CARTESIAN_POINT('Ctrl Pts',(-30.4086676540711,-53.0503573673268,
39.5248015517178));
#202193=CARTESIAN_POINT('Ctrl Pts',(-30.3191294881007,-53.1483650929077,
39.3484893995498));
#202194=CARTESIAN_POINT('Ctrl Pts',(-30.4288515386962,-53.0853168809912,
39.3489438303439));
#202195=CARTESIAN_POINT('Ctrl Pts',(-30.4725003554712,-53.1609188493363,
39.4508333155605));
#202196=CARTESIAN_POINT('Ctrl Pts',(-30.3416565762239,-53.1871522506173,
39.2708017080178));
#202197=CARTESIAN_POINT('Ctrl Pts',(-30.4513942013116,-53.1243619179794,
39.2710850691866));
#202198=CARTESIAN_POINT('Ctrl Pts',(-30.5061406831646,-53.2191856060844,
39.3343017080178));
#202199=CARTESIAN_POINT('Origin',(-30.2311753956715,-52.9969317578286,39.5248017080178));
#202200=CARTESIAN_POINT('Ctrl Pts',(-29.4581217525676,-51.6568155675426,
39.2875012672119));
#202201=CARTESIAN_POINT('Ctrl Pts',(-29.5680161684459,-51.5939283826161,
39.2878045257519));
#202202=CARTESIAN_POINT('Ctrl Pts',(-29.6215404675519,-51.6870133715069,
39.3549015218347));
#202203=CARTESIAN_POINT('Ctrl Pts',(-29.515505630711,-51.756454248638,39.1034938540228));
#202204=CARTESIAN_POINT('Ctrl Pts',(-29.6254251653826,-51.6933631336547,
39.1038286278833));
#202205=CARTESIAN_POINT('Ctrl Pts',(-29.6675162799448,-51.7666458147672,
39.2077506434047));
#202206=CARTESIAN_POINT('Ctrl Pts',(-29.6185943474775,-51.9354510367806,
38.989));
#202207=CARTESIAN_POINT('Ctrl Pts',(-29.7286404220049,-51.8721362050931,
38.9892298954593));
#202208=CARTESIAN_POINT('Ctrl Pts',(-29.7501097595406,-51.9097019182955,
39.116190034727));
#202209=CARTESIAN_POINT('Ctrl Pts',(-29.7268821954852,-52.1234703131945,
38.989));
#202210=CARTESIAN_POINT('Ctrl Pts',(-29.8370321718797,-52.0598751946719,
38.989));
#202211=CARTESIAN_POINT('Ctrl Pts',(-29.8368672985585,-52.0599703843283,
39.1161900945645));
#202212=CARTESIAN_POINT('Origin',(-29.7268821954852,-52.1234703131945,39.116));
#202213=CARTESIAN_POINT('Origin',(15.4537755657018,26.1317244485617,39.5248017080178));
#202214=CARTESIAN_POINT('Origin',(-30.155571337834,-52.8659816883958,39.5248017080178));
#202215=CARTESIAN_POINT('Origin',(15.3947701216595,26.0295240215573,39.116));
#202216=CARTESIAN_POINT('Origin',(-29.9275190026066,-52.4710850656382,39.1160402713848));
#202217=CARTESIAN_POINT('Ctrl Pts',(-30.0450834959839,-52.6757649139394,
39.2708017080178));
#202218=CARTESIAN_POINT('Ctrl Pts',(-30.1558192616004,-52.6124111049555,
39.27051194648));
#202219=CARTESIAN_POINT('Ctrl Pts',(-30.100576467536,-52.516727778884,39.3343017080178));
#202220=CARTESIAN_POINT('Ctrl Pts',(-30.0676891808491,-52.7146817640549,
39.3487519301185));
#202221=CARTESIAN_POINT('Ctrl Pts',(-30.1782028480944,-52.6511806140169,
39.3482879463976));
#202222=CARTESIAN_POINT('Ctrl Pts',(-30.1343304829276,-52.5751914485016,
39.4512271261638));
#202223=CARTESIAN_POINT('Ctrl Pts',(-30.1105150503711,-52.7884098752461,
39.3978017080178));
#202224=CARTESIAN_POINT('Ctrl Pts',(-30.220659667678,-52.7247179826673,
39.3975673827411));
#202225=CARTESIAN_POINT('Ctrl Pts',(-30.1982769148315,-52.6859499175219,
39.5248015355181));
#202226=CARTESIAN_POINT('Ctrl Pts',(-30.155571337834,-52.8659816883958,
39.3978017080178));
#202227=CARTESIAN_POINT('Ctrl Pts',(-30.2655565641147,-52.8024816883958,
39.3978017080178));
#202228=CARTESIAN_POINT('Ctrl Pts',(-30.2655565641147,-52.8024816883958,
39.5248017080178));
#202229=CARTESIAN_POINT('Origin',(-29.9905912412554,-52.580227778884,39.3343017080178));
#202230=CARTESIAN_POINT('Origin',(-29.9499161075309,-52.5097763812719,39.1934008533551));
#202231=CARTESIAN_POINT('Origin',(-36.3610285397812,-49.5064990290886,39.1925554495082));
#202232=CARTESIAN_POINT('Origin',(-36.3870656659254,-49.5422481179707,39.1160373285265));
#202233=CARTESIAN_POINT('Origin',(-36.3129251734945,-49.4402904249164,39.3343017080178));
#202234=CARTESIAN_POINT('Ctrl Pts',(-36.2478178023253,-49.3516463037383,
39.2708017080178));
#202235=CARTESIAN_POINT('Ctrl Pts',(-36.1458216659127,-49.4263574835549,
39.2710850691866));
#202236=CARTESIAN_POINT('Ctrl Pts',(-36.2101800152089,-49.5149391519575,
39.3343017080178));
#202237=CARTESIAN_POINT('Ctrl Pts',(-36.2214577843979,-49.3151677697927,
39.3487519293518));
#202238=CARTESIAN_POINT('Ctrl Pts',(-36.1192316557451,-49.3897594742963,
39.349206866295));
#202239=CARTESIAN_POINT('Ctrl Pts',(-36.1704998050836,-49.4603240281405,
39.4512271248759));
#202240=CARTESIAN_POINT('Ctrl Pts',(-36.1715192752727,-49.2460589922049,
39.3978017080178));
#202241=CARTESIAN_POINT('Ctrl Pts',(-36.0689133127003,-49.3205022166628,
39.3980347781164));
#202242=CARTESIAN_POINT('Ctrl Pts',(-36.0953262843463,-49.3568565532996,
39.5248015355176));
#202243=CARTESIAN_POINT('Ctrl Pts',(-36.1189794796885,-49.1733470784086,
39.3978017080178));
#202244=CARTESIAN_POINT('Ctrl Pts',(-36.0162343214029,-49.2479958054497,
39.3978017080178));
#202245=CARTESIAN_POINT('Ctrl Pts',(-36.0162343214029,-49.2479958054497,
39.5248017080178));
#202246=CARTESIAN_POINT('Origin',(-36.1189794796885,-49.1733470784086,39.5248017080178));
#202247=CARTESIAN_POINT('Origin',(-0.256862895714039,0.186621817602861,
39.116));
#202248=CARTESIAN_POINT('Origin',(-36.6229335645812,-49.8669803696024,39.116));
#202249=CARTESIAN_POINT('Origin',(-0.256862895714039,0.186621817602861,
39.5248017080178));
#202250=CARTESIAN_POINT('Origin',(-36.0301015792679,-49.0510171431402,39.5248017080178));
#202251=CARTESIAN_POINT('Ctrl Pts',(-36.9399086546489,-50.3023253561993,
39.2875012672119));
#202252=CARTESIAN_POINT('Ctrl Pts',(-36.8368401467438,-50.3777877177486,
39.287208709576));
#202253=CARTESIAN_POINT('Ctrl Pts',(-36.7733199672422,-50.2900345588336,
39.3549016990124));
#202254=CARTESIAN_POINT('Ctrl Pts',(-36.8722300970233,-50.2093718139452,
39.1034939173931));
#202255=CARTESIAN_POINT('Ctrl Pts',(-36.7691625978848,-50.2846371204143,
39.103169233635));
#202256=CARTESIAN_POINT('Ctrl Pts',(-36.7192723137706,-50.2156443459718,
39.2077507202315));
#202257=CARTESIAN_POINT('Ctrl Pts',(-36.7506474475454,-50.0423845927726,
38.989));
#202258=CARTESIAN_POINT('Ctrl Pts',(-36.6476776482595,-50.1174266236766,
38.9887769311152));
#202259=CARTESIAN_POINT('Ctrl Pts',(-36.622177901771,-50.0820053531142,
39.1161898712895));
#202260=CARTESIAN_POINT('Ctrl Pts',(-36.6229335645812,-49.8669803696024,
38.989));
#202261=CARTESIAN_POINT('Ctrl Pts',(-36.5200349097933,-49.9417406183803,
38.989));
#202262=CARTESIAN_POINT('Ctrl Pts',(-36.5201885207827,-49.9416290134637,
39.1161895903858));
#202263=CARTESIAN_POINT('Origin',(-36.8761597191957,-50.2155162706042,39.3548010137695));
#202264=CARTESIAN_POINT('Ctrl Pts',(-36.0301015792679,-49.0510171431402,
39.3978017080178));
#202265=CARTESIAN_POINT('Ctrl Pts',(-35.9273564209823,-49.1256658701813,
39.3978017080178));
#202266=CARTESIAN_POINT('Ctrl Pts',(-35.9273564209823,-49.1256658701813,
39.5248017080178));
#202267=CARTESIAN_POINT('Ctrl Pts',(-35.9773846774553,-48.9780591316064,
39.3978017080178));
#202268=CARTESIAN_POINT('Ctrl Pts',(-35.8743986902985,-49.0527758071202,
39.3975666025021));
#202269=CARTESIAN_POINT('Ctrl Pts',(-35.8479971380609,-49.0164371879468,
39.5248015517178));
#202270=CARTESIAN_POINT('Ctrl Pts',(-35.9275383438679,-48.9090707128231,
39.3484894016716));
#202271=CARTESIAN_POINT('Ctrl Pts',(-35.8245773199107,-48.984202573666,
39.3480259000044));
#202272=CARTESIAN_POINT('Ctrl Pts',(-35.7729572780254,-48.9131536812792,
39.4508333188948));
#202273=CARTESIAN_POINT('Ctrl Pts',(-35.9012693628907,-48.8727133447942,
39.2708017080178));
#202274=CARTESIAN_POINT('Ctrl Pts',(-35.7983524848938,-48.9481071848795,
39.27051194648));
#202275=CARTESIAN_POINT('Ctrl Pts',(-35.7334106856009,-48.8587224664499,
39.3343017080178));
#202276=CARTESIAN_POINT('Origin',(-35.8361558438865,-48.7840737394087,39.3343017080178));
#202277=CARTESIAN_POINT('Origin',(-36.980873139623,-50.3596419293452,39.6398955068198));
#202278=CARTESIAN_POINT('Origin',(-37.0855865599605,-50.5037675878943,39.92499));
#202279=CARTESIAN_POINT('Origin',(-35.7883393560614,-48.7182599900754,39.1934008539946));
#202280=CARTESIAN_POINT('Origin',(-35.7621028045852,-48.6820620414863,39.1160402713845));
#202281=CARTESIAN_POINT('Ctrl Pts',(-37.0158684358562,-50.9219998155898,
40.1599502534424));
#202282=CARTESIAN_POINT('Ctrl Pts',(-36.9939338721435,-50.8918248690998,
40.10025));
#202283=CARTESIAN_POINT('Ctrl Pts',(-36.9525415975215,-50.8348823336484,
40.10025));
#202284=CARTESIAN_POINT('Ctrl Pts',(-37.0871426490248,-50.870189502586,
40.1599500538471));
#202285=CARTESIAN_POINT('Ctrl Pts',(-37.0458491715921,-50.8540829678249,
40.100244835349));
#202286=CARTESIAN_POINT('Ctrl Pts',(-36.9937925764114,-50.8048852215559,
40.10025));
#202287=CARTESIAN_POINT('Ctrl Pts',(-37.1382015956602,-50.8021467555732,
40.1202442001038));
#202288=CARTESIAN_POINT('Ctrl Pts',(-37.0800635522215,-50.8006171556814,
40.0633873868017));
#202289=CARTESIAN_POINT('Ctrl Pts',(-37.0171501059293,-50.7569692080812,
40.0772271723537));
#202290=CARTESIAN_POINT('Ctrl Pts',(-37.1817767082789,-50.6806663304942,
40.0045995998163));
#202291=CARTESIAN_POINT('Ctrl Pts',(-37.0956112176475,-50.7142182018864,
39.9663485808314));
#202292=CARTESIAN_POINT('Ctrl Pts',(-37.0243843935851,-50.6618927960199,
40.0101727202466));
#202293=CARTESIAN_POINT('Ctrl Pts',(-37.1760624637761,-50.6273693057704,
39.9304654349858));
#202294=CARTESIAN_POINT('Ctrl Pts',(-37.0763301845679,-50.6810088489693,
39.9051900162958));
#202295=CARTESIAN_POINT('Ctrl Pts',(-37.0095702365079,-50.6152053999548,
39.9671857458184));
#202296=CARTESIAN_POINT('Ctrl Pts',(-37.1493329797263,-50.5905785208482,
39.8576902534424));
#202297=CARTESIAN_POINT('Ctrl Pts',(-37.0464195108255,-50.6659240749081,
39.8573998014387));
#202298=CARTESIAN_POINT('Ctrl Pts',(-36.9828414016749,-50.5784163149355,
39.92499));
#202299=CARTESIAN_POINT('Origin',(-36.9525415975215,-50.8348823336484,40.22725));
#202300=CARTESIAN_POINT('Origin',(-0.256862895714039,0.186621817602861,
39.116));
#202301=CARTESIAN_POINT('Origin',(-35.5261472678868,-48.3573835402117,39.116));
#202302=CARTESIAN_POINT('Origin',(6.67120042669033E-17,1.33398482780241E-16,
40.22725));
#202303=CARTESIAN_POINT('Origin',(-36.9278827595329,-50.8527980281383,40.22725));
#202304=CARTESIAN_POINT('Ctrl Pts',(-35.5261472678868,-48.3573835402117,
38.989));
#202305=CARTESIAN_POINT('Ctrl Pts',(-35.4232481927144,-48.432144094417,
38.989));
#202306=CARTESIAN_POINT('Ctrl Pts',(-35.4234022247158,-48.4320321836172,
39.1161901092323));
#202307=CARTESIAN_POINT('Ctrl Pts',(-35.3984257650695,-48.1819806163539,
38.989));
#202308=CARTESIAN_POINT('Ctrl Pts',(-35.2958250128989,-48.2567602586425,
38.9892298989718));
#202309=CARTESIAN_POINT('Ctrl Pts',(-35.3214110399822,-48.2916533613397,
39.1161900493185));
#202310=CARTESIAN_POINT('Ctrl Pts',(-35.276834980876,-48.0150011530606,
39.1034966344368));
#202311=CARTESIAN_POINT('Ctrl Pts',(-35.1744900671661,-48.0897561847353,
39.1038314102599));
#202312=CARTESIAN_POINT('Ctrl Pts',(-35.2243173504718,-48.1580153629267,
39.2077528789615));
#202313=CARTESIAN_POINT('Ctrl Pts',(-35.209151665053,-47.9220530736685,
39.2875012672119));
#202314=CARTESIAN_POINT('Ctrl Pts',(-35.1070032653413,-47.9968681042462,
39.2878045257868));
#202315=CARTESIAN_POINT('Ctrl Pts',(-35.1702703594596,-48.0836260618767,
39.35490152959));
#202316=CARTESIAN_POINT('Origin',(-35.2729208539817,-48.008847282327,39.3548010137695));
#202317=CARTESIAN_POINT('Ctrl Pts',(-36.6347241449657,-50.9644637245891,
39.8576902534424));
#202318=CARTESIAN_POINT('Ctrl Pts',(-36.7381840359687,-50.8898702560316,
39.8573998014387));
#202319=CARTESIAN_POINT('Ctrl Pts',(-36.674605926818,-50.8023624960589,
39.92499));
#202320=CARTESIAN_POINT('Ctrl Pts',(-36.6614665482806,-51.0012706547885,
39.9304984902489));
#202321=CARTESIAN_POINT('Ctrl Pts',(-36.7432905102115,-50.9229972443173,
39.9052171569796));
#202322=CARTESIAN_POINT('Ctrl Pts',(-36.701346940908,-50.8391683443875,
39.96720497266));
#202323=CARTESIAN_POINT('Ctrl Pts',(-36.710288459717,-51.0230245369437,
40.0043437678665));
#202324=CARTESIAN_POINT('Ctrl Pts',(-36.768904996455,-50.9514409225352,
39.9661628577646));
#202325=CARTESIAN_POINT('Ctrl Pts',(-36.7410683485321,-50.867535894943,
40.0100243556238));
#202326=CARTESIAN_POINT('Ctrl Pts',(-36.8383381382862,-51.0194219249359,
40.1194874821985));
#202327=CARTESIAN_POINT('Ctrl Pts',(-36.8551762168621,-50.9635175930191,
40.0627551483138));
#202328=CARTESIAN_POINT('Ctrl Pts',(-36.8330984946702,-50.8901021525735,
40.0767884282375));
#202329=CARTESIAN_POINT('Ctrl Pts',(-36.9196318328647,-50.9918932610485,
40.1599502015387));
#202330=CARTESIAN_POINT('Ctrl Pts',(-36.9171104726346,-50.9476171190686,
40.1002449453872));
#202331=CARTESIAN_POINT('Ctrl Pts',(-36.8864699989248,-50.8828596657519,
40.10025));
#202332=CARTESIAN_POINT('Ctrl Pts',(-36.991167339171,-50.93994621282,40.1599502534424));
#202333=CARTESIAN_POINT('Ctrl Pts',(-36.9692474126343,-50.9097606317992,
40.10025));
#202334=CARTESIAN_POINT('Ctrl Pts',(-36.9278827595329,-50.8527980281383,
40.10025));
#202335=CARTESIAN_POINT('Origin',(-36.5718607685324,-50.8770112231001,39.92499));
#202336=CARTESIAN_POINT('Origin',(-35.1682072895736,-47.864721425495,39.6398955069317));
#202337=CARTESIAN_POINT('Origin',(-35.0634937251224,-47.7205955685089,39.92499));
#202338=CARTESIAN_POINT('Origin',(-36.467147348224,-50.7328855645163,39.6398955068266));
#202339=CARTESIAN_POINT('Origin',(-36.3624339277676,-50.5887599058099,39.3548010137695));
#202340=CARTESIAN_POINT('Ctrl Pts',(-34.9997217530263,-47.6338034047598,
39.8576902534424));
#202341=CARTESIAN_POINT('Ctrl Pts',(-34.8977303031704,-47.7085070967802,
39.8579948730703));
#202342=CARTESIAN_POINT('Ctrl Pts',(-34.9607485668368,-47.79524429555,39.92499));
#202343=CARTESIAN_POINT('Ctrl Pts',(-34.9730146904946,-47.5970451916066,
39.9304020711231));
#202344=CARTESIAN_POINT('Ctrl Pts',(-34.8923835282626,-47.6752966590742,
39.9058915297382));
#202345=CARTESIAN_POINT('Ctrl Pts',(-34.9340408279395,-47.7584842465951,
39.9671523786036));
#202346=CARTESIAN_POINT('Ctrl Pts',(-34.9244461536127,-47.5754322771534,
40.0043257306692));
#202347=CARTESIAN_POINT('Ctrl Pts',(-34.8665972787028,-47.6469756149919,
39.9667894847835));
#202348=CARTESIAN_POINT('Ctrl Pts',(-34.8944891948624,-47.7303228514091,
40.0100138975201));
#202349=CARTESIAN_POINT('Ctrl Pts',(-34.7970725085258,-47.5794993790984,
40.1195533054858));
#202350=CARTESIAN_POINT('Ctrl Pts',(-34.7804938560721,-47.6353197637777,
40.0630813209237));
#202351=CARTESIAN_POINT('Ctrl Pts',(-34.8028668197836,-47.7084160893873,
40.076826594242));
#202352=CARTESIAN_POINT('Ctrl Pts',(-34.7162617467342,-47.6073089936882,
40.1599502027523));
#202353=CARTESIAN_POINT('Ctrl Pts',(-34.7189078610131,-47.6515013114252,
40.100255279155));
#202354=CARTESIAN_POINT('Ctrl Pts',(-34.7497660430524,-47.7160937685325,
40.10025));
#202355=CARTESIAN_POINT('Ctrl Pts',(-34.6451144164188,-47.6590285860934,
40.1599502534424));
#202356=CARTESIAN_POINT('Ctrl Pts',(-34.667049453402,-47.6892031885512,
40.10025));
#202357=CARTESIAN_POINT('Ctrl Pts',(-34.7084426211234,-47.7461450747863,
40.10025));
#202358=CARTESIAN_POINT('Origin',(-34.7084426211234,-47.7461450747863,40.22725));
#202359=CARTESIAN_POINT('Ctrl Pts',(-36.1092077731531,-50.2402240048081,
38.989));
#202360=CARTESIAN_POINT('Ctrl Pts',(-36.2121064368057,-50.1654637495896,
38.989));
#202361=CARTESIAN_POINT('Ctrl Pts',(-36.2119528169383,-50.1655753609564,
39.1161896013268));
#202362=CARTESIAN_POINT('Ctrl Pts',(-36.2365633238574,-50.4158927445015,
38.989));
#202363=CARTESIAN_POINT('Ctrl Pts',(-36.3397519704563,-50.3411519064829,
38.9887769275436));
#202364=CARTESIAN_POINT('Ctrl Pts',(-36.313943782211,-50.3059538820309,
39.1161898821826));
#202365=CARTESIAN_POINT('Ctrl Pts',(-36.3578055460618,-50.583125283657,
39.1034967087243));
#202366=CARTESIAN_POINT('Ctrl Pts',(-36.4612367259587,-50.5083605190624,
39.1031720232736));
#202367=CARTESIAN_POINT('Ctrl Pts',(-36.4110374247136,-50.4395918165618,
39.2077529615021));
#202368=CARTESIAN_POINT('Ctrl Pts',(-36.4252947698681,-50.6762142289946,
39.2875012672119));
#202369=CARTESIAN_POINT('Ctrl Pts',(-36.5289136700283,-50.6015093986314,
39.2872087095507));
#202370=CARTESIAN_POINT('Ctrl Pts',(-36.4650842569434,-50.513980899522,
39.3549017048229));
#202371=CARTESIAN_POINT('Origin',(-36.1092077731531,-50.2402240048081,39.116));
#202372=CARTESIAN_POINT('Origin',(3.77491158612227E-16,-4.74547095659465E-17,
40.22725));
#202373=CARTESIAN_POINT('Origin',(-34.6837837831348,-47.7640607692761,40.22725));
#202374=CARTESIAN_POINT('Origin',(21.7541926348216,29.4019141737117,39.116));
#202375=CARTESIAN_POINT('Origin',(-35.8732562382988,-49.9155525184322,39.1160373285271));
#202376=CARTESIAN_POINT('Ctrl Pts',(-34.6205005703637,-47.6769115920302,
40.1599502534424));
#202377=CARTESIAN_POINT('Ctrl Pts',(-34.6424200234577,-47.7070975168462,
40.10025));
#202378=CARTESIAN_POINT('Ctrl Pts',(-34.6837837831348,-47.7640607692761,
40.10025));
#202379=CARTESIAN_POINT('Ctrl Pts',(-34.5495693076632,-47.72841834836,40.1599500566044));
#202380=CARTESIAN_POINT('Ctrl Pts',(-34.5907418558587,-47.7446195594503,
40.1002551305372));
#202381=CARTESIAN_POINT('Ctrl Pts',(-34.6425747206407,-47.7939730310144,
40.10025));
#202382=CARTESIAN_POINT('Ctrl Pts',(-34.4983910654766,-47.7959261043554,
40.1203070619047));
#202383=CARTESIAN_POINT('Ctrl Pts',(-34.5563698228278,-47.7976714756522,
40.0637098684499));
#202384=CARTESIAN_POINT('Ctrl Pts',(-34.6188891978597,-47.8415056181563,
40.0772636213362));
#202385=CARTESIAN_POINT('Ctrl Pts',(-34.4545839152296,-47.9165880269726,
40.0046102245801));
#202386=CARTESIAN_POINT('Ctrl Pts',(-34.5404685123898,-47.8837591046485,
39.9670001894012));
#202387=CARTESIAN_POINT('Ctrl Pts',(-34.6111463389772,-47.9359643384887,
40.010178881121));
#202388=CARTESIAN_POINT('Ctrl Pts',(-34.460235468251,-47.9696250311907,
39.9303710930187));
#202389=CARTESIAN_POINT('Ctrl Pts',(-34.559577790676,-47.9171136764605,
39.9058663574101));
#202390=CARTESIAN_POINT('Ctrl Pts',(-34.6258166968299,-47.9824460410472,
39.9671344706361));
#202391=CARTESIAN_POINT('Ctrl Pts',(-34.4869303039399,-48.0063682005185,
39.8576902534424));
#202392=CARTESIAN_POINT('Ctrl Pts',(-34.5894948283136,-47.9324532779036,
39.8579948730704));
#202393=CARTESIAN_POINT('Ctrl Pts',(-34.6525130919799,-48.0191904766735,
39.92499));
#202394=CARTESIAN_POINT('Origin',(-34.5497679336943,-48.0938392037146,39.92499));
#202395=CARTESIAN_POINT('Origin',(-35.8473027479613,-49.8797426632443,39.1925554488848));
#202396=CARTESIAN_POINT('Origin',(-35.7991993820664,-49.8135340601221,39.3343017080178));
#202397=CARTESIAN_POINT('Origin',(-34.6544814981818,-48.237965060654,39.6398955069213));
#202398=CARTESIAN_POINT('Origin',(-34.7591950625536,-48.3820909175328,39.3548010137695));
#202399=CARTESIAN_POINT('Ctrl Pts',(-35.6052536882604,-49.5465907136143,
39.3978017080178));
#202400=CARTESIAN_POINT('Ctrl Pts',(-35.707998846546,-49.4719419865731,
39.3978017080178));
#202401=CARTESIAN_POINT('Ctrl Pts',(-35.707998846546,-49.4719419865731,
39.5248017080178));
#202402=CARTESIAN_POINT('Ctrl Pts',(-35.6583499840584,-49.6192730640951,
39.3978017080178));
#202403=CARTESIAN_POINT('Ctrl Pts',(-35.760855993121,-49.5446936074878,
39.3980355775182));
#202404=CARTESIAN_POINT('Ctrl Pts',(-35.7873581223566,-49.5811706590204,
39.5248015517173));
#202405=CARTESIAN_POINT('Ctrl Pts',(-35.7085550527717,-49.6880007749195,
39.3484893995498));
#202406=CARTESIAN_POINT('Ctrl Pts',(-35.8110857017893,-49.6138288703715,
39.3489438303428));
#202407=CARTESIAN_POINT('Ctrl Pts',(-35.862397963352,-49.6844541394816,
39.4508333155612));
#202408=CARTESIAN_POINT('Ctrl Pts',(-35.7350130971391,-49.7242207306173,
39.2708017080178));
#202409=CARTESIAN_POINT('Ctrl Pts',(-35.8375861910559,-49.6503036646783,
39.2710850691866));
#202410=CARTESIAN_POINT('Ctrl Pts',(-35.9019445403521,-49.738885333081,
39.3343017080178));
#202411=CARTESIAN_POINT('Origin',(-35.6052536882604,-49.5465907136143,39.5248017080178));
#202412=CARTESIAN_POINT('Ctrl Pts',(-34.6963546279287,-48.2946219293745,
39.2875012672119));
#202413=CARTESIAN_POINT('Ctrl Pts',(-34.7990735298985,-48.2205921526137,
39.2878045257519));
#202414=CARTESIAN_POINT('Ctrl Pts',(-34.8620346481358,-48.3075723994624,
39.3549015218345));
#202415=CARTESIAN_POINT('Ctrl Pts',(-34.7638392294011,-48.3877165307503,
39.1034938540228));
#202416=CARTESIAN_POINT('Ctrl Pts',(-34.866561796066,-48.3134813154549,
39.1038286278822));
#202417=CARTESIAN_POINT('Ctrl Pts',(-34.9160824571397,-48.3819628268515,
39.2077506434037));
#202418=CARTESIAN_POINT('Ctrl Pts',(-34.8850734745837,-48.5549570506159,
38.989));
#202419=CARTESIAN_POINT('Ctrl Pts',(-34.9878985031412,-48.4804861171421,
38.9892298954611));
#202420=CARTESIAN_POINT('Ctrl Pts',(-35.0131769156726,-48.5156018845749,
39.1161900347285));
#202421=CARTESIAN_POINT('Ctrl Pts',(-35.0124214764587,-48.7306271754175,
38.989));
#202422=CARTESIAN_POINT('Ctrl Pts',(-35.1153205397465,-48.6558666298469,
38.989));
#202423=CARTESIAN_POINT('Ctrl Pts',(-35.1151665196475,-48.6559785319991,
39.1161900945641));
#202424=CARTESIAN_POINT('Origin',(-35.0124214764587,-48.7306271754175,39.116));
#202425=CARTESIAN_POINT('Origin',(21.2334658618526,28.6851952578919,39.5248017080178));
#202426=CARTESIAN_POINT('Origin',(-35.5163757878398,-49.4242607783459,39.5248017080178));
#202427=CARTESIAN_POINT('Origin',(21.1519223437074,28.5729602337852,39.116));
#202428=CARTESIAN_POINT('Origin',(-35.2482948100398,-49.0553654007524,39.1160402713849));
#202429=CARTESIAN_POINT('Ctrl Pts',(-35.3866101428262,-49.2466351556011,
39.2708017080178));
#202430=CARTESIAN_POINT('Ctrl Pts',(-35.4901170100369,-49.1720533660029,
39.27051194648));
#202431=CARTESIAN_POINT('Ctrl Pts',(-35.425175210744,-49.0826686475733,
39.3343017080178));
#202432=CARTESIAN_POINT('Ctrl Pts',(-35.4131599099205,-49.2829758776409,
39.3487519301186));
#202433=CARTESIAN_POINT('Ctrl Pts',(-35.5164304941039,-49.2082707697416,
39.3482879463972));
#202434=CARTESIAN_POINT('Ctrl Pts',(-35.4648554356498,-49.1372837917339,
39.4512271261637));
#202435=CARTESIAN_POINT('Ctrl Pts',(-35.4634578610141,-49.351823576193,
39.3978017080178));
#202436=CARTESIAN_POINT('Ctrl Pts',(-35.5663414789288,-49.2769673468807,
39.3975673827411));
#202437=CARTESIAN_POINT('Ctrl Pts',(-35.5400289748692,-49.2407512920132,
39.5248015355181));
#202438=CARTESIAN_POINT('Ctrl Pts',(-35.5163757878398,-49.4242607783459,
39.3978017080178));
#202439=CARTESIAN_POINT('Ctrl Pts',(-35.6191209461254,-49.3496120513047,
39.3978017080178));
#202440=CARTESIAN_POINT('Ctrl Pts',(-35.6191209461254,-49.3496120513047,
39.5248017080178));
#202441=CARTESIAN_POINT('Origin',(-35.3224300524584,-49.1573173746145,39.3343017080178));
#202442=CARTESIAN_POINT('Origin',(-35.2746135650462,-49.091503626351,39.1934008533548));
#202443=CARTESIAN_POINT('Origin',(-41.3366772861974,-45.4345348113607,39.1925554495084));
#202444=CARTESIAN_POINT('Origin',(-41.3663085755628,-45.4673664422104,39.1160373285261));
#202445=CARTESIAN_POINT('Origin',(-41.2819167515331,-45.3737170758071,39.3343017080178));
#202446=CARTESIAN_POINT('Ctrl Pts',(-41.2079002115909,-45.2923641298555,
39.2708017080178));
#202447=CARTESIAN_POINT('Ctrl Pts',(-41.1142722655008,-45.3773275334104,
39.2710850691866));
#202448=CARTESIAN_POINT('Ctrl Pts',(-41.1875373586974,-45.4586966628146,
39.3343017080178));
#202449=CARTESIAN_POINT('Ctrl Pts',(-41.1778715515046,-45.2588408013009,
39.3487519293518));
#202450=CARTESIAN_POINT('Ctrl Pts',(-41.0840023845238,-45.3437094247749,
39.3492068662931));
#202451=CARTESIAN_POINT('Ctrl Pts',(-41.1423656859494,-45.4085284377449,
39.4512271248737));
#202452=CARTESIAN_POINT('Ctrl Pts',(-41.1209827764384,-45.1953306044442,
39.3978017080178));
#202453=CARTESIAN_POINT('Ctrl Pts',(-41.0267203359206,-45.2800912647189,
39.3980347781183));
#202454=CARTESIAN_POINT('Ctrl Pts',(-41.0567886774842,-45.3134855411618,
39.5248015355195));
#202455=CARTESIAN_POINT('Ctrl Pts',(-41.0611303347406,-45.1285089182131,
39.3978017080178));
#202456=CARTESIAN_POINT('Ctrl Pts',(-40.966750941905,-45.2134885052206,
39.3978017080178));
#202457=CARTESIAN_POINT('Ctrl Pts',(-40.966750941905,-45.2134885052206,
39.5248017080178));
#202458=CARTESIAN_POINT('Origin',(-41.0611303347406,-45.1285089182131,39.5248017080178));
#202459=CARTESIAN_POINT('Origin',(-0.235948482089066,0.212448967518939,
39.116));
#202460=CARTESIAN_POINT('Origin',(-41.6348281284264,-45.7656648676104,39.116));
#202461=CARTESIAN_POINT('Origin',(-0.235948482089066,0.212448967518939,
39.5248017080178));
#202462=CARTESIAN_POINT('Origin',(-40.9599523566127,-45.0161393894791,39.5248017080178));
#202463=CARTESIAN_POINT('Ctrl Pts',(-41.9955727382253,-46.165492069761,
39.2875012672119));
#202464=CARTESIAN_POINT('Ctrl Pts',(-41.900956815078,-46.2513146333406,
39.287208709576));
#202465=CARTESIAN_POINT('Ctrl Pts',(-41.8286119029177,-46.1706818621615,
39.3549016990125));
#202466=CARTESIAN_POINT('Ctrl Pts',(-41.9185486398931,-46.0801220723616,
39.1034939173931));
#202467=CARTESIAN_POINT('Ctrl Pts',(-41.8239131221214,-46.1657485549032,
39.1031692336336));
#202468=CARTESIAN_POINT('Ctrl Pts',(-41.7670844335159,-46.1023486848317,
39.2077507202291));
#202469=CARTESIAN_POINT('Ctrl Pts',(-41.7801771152787,-45.926758472166,
38.989));
#202470=CARTESIAN_POINT('Ctrl Pts',(-41.6856154234971,-46.0121526898573,
38.9887769311176));
#202471=CARTESIAN_POINT('Ctrl Pts',(-41.6565528363056,-45.9795909100351,
39.116189871292));
#202472=CARTESIAN_POINT('Ctrl Pts',(-41.6348281284264,-45.7656648676104,
38.989));
#202473=CARTESIAN_POINT('Ctrl Pts',(-41.5403077371541,-45.8507714101806,
38.989));
#202474=CARTESIAN_POINT('Ctrl Pts',(-41.5404488407561,-45.8506443599267,
39.1161895903859));
#202475=CARTESIAN_POINT('Origin',(-41.9230990057958,-46.0858221116776,39.3548010137695));
#202476=CARTESIAN_POINT('Ctrl Pts',(-40.9599523566127,-45.0161393894791,
39.3978017080178));
#202477=CARTESIAN_POINT('Ctrl Pts',(-40.8655729637771,-45.1011189764867,
39.3978017080178));
#202478=CARTESIAN_POINT('Ctrl Pts',(-40.8655729637771,-45.1011189764867,
39.5248017080178));
#202479=CARTESIAN_POINT('Ctrl Pts',(-40.8998980546769,-44.9490914662996,
39.3978017080178));
#202480=CARTESIAN_POINT('Ctrl Pts',(-40.8052862548041,-45.0341638030234,
39.3975666025026));
#202481=CARTESIAN_POINT('Ctrl Pts',(-40.7752309130114,-45.000783964291,
39.5248015517178));
#202482=CARTESIAN_POINT('Ctrl Pts',(-40.8431135311195,-44.8856913339442,
39.3484894016717));
#202483=CARTESIAN_POINT('Ctrl Pts',(-40.7485699563835,-44.9711739722012,
39.3480259000039));
#202484=CARTESIAN_POINT('Ctrl Pts',(-40.68980606295,-44.9059100567353,39.4508333188944));
#202485=CARTESIAN_POINT('Ctrl Pts',(-40.8131880745608,-44.8522789915939,
39.2708017080178));
#202486=CARTESIAN_POINT('Ctrl Pts',(-40.7187157882339,-44.938017559436,
39.27051194648));
#202487=CARTESIAN_POINT('Ctrl Pts',(-40.6447864996555,-44.8559107663283,
39.3343017080178));
#202488=CARTESIAN_POINT('Origin',(-40.7391658924911,-44.7709311793208,39.3343017080178));
#202489=CARTESIAN_POINT('Origin',(-42.0423040287729,-46.2182127020652,39.639895506818));
#202490=CARTESIAN_POINT('Origin',(-42.1615090516454,-46.3506032922592,39.92499));
#202491=CARTESIAN_POINT('Origin',(-40.6847319383099,-44.7104761485843,39.1934008539943));
#202492=CARTESIAN_POINT('Origin',(-40.6548553974683,-44.6772189625516,39.1160402713845));
#202493=CARTESIAN_POINT('Ctrl Pts',(-42.1358900227697,-46.7738319284255,
40.1599502534424));
#202494=CARTESIAN_POINT('Ctrl Pts',(-42.1109214781063,-46.746115069687,
40.10025));
#202495=CARTESIAN_POINT('Ctrl Pts',(-42.0638038389703,-46.6938111422602,
40.10025));
#202496=CARTESIAN_POINT('Ctrl Pts',(-42.2013581359409,-46.7148552537637,
40.1599500538459));
#202497=CARTESIAN_POINT('Ctrl Pts',(-42.1586072771693,-46.7031532960222,
40.1002448353478));
#202498=CARTESIAN_POINT('Ctrl Pts',(-42.1016932886507,-46.659666456053,
40.10025));
#202499=CARTESIAN_POINT('Ctrl Pts',(-42.2450249725429,-46.6418481388113,
40.1202442001041));
#202500=CARTESIAN_POINT('Ctrl Pts',(-42.1870455286633,-46.6464039985661,
40.0633873868017));
#202501=CARTESIAN_POINT('Ctrl Pts',(-42.1199142759252,-46.6095714048494,
40.0772271723538));
#202502=CARTESIAN_POINT('Ctrl Pts',(-42.2756632139847,-46.5164783566525,
40.004599599816));
#202503=CARTESIAN_POINT('Ctrl Pts',(-42.1934768724829,-46.5588531737045,
39.9663485808314));
#202504=CARTESIAN_POINT('Ctrl Pts',(-42.1171707421501,-46.5142596423493,
40.0101727202466));
#202505=CARTESIAN_POINT('Ctrl Pts',(-42.2644092166189,-46.4640705998047,
39.9304654349861));
#202506=CARTESIAN_POINT('Ctrl Pts',(-42.1708301402941,-46.527841161857,
39.9051900162953));
#202507=CARTESIAN_POINT('Ctrl Pts',(-42.0975575768116,-46.4693765057998,
39.9671857458178));
#202508=CARTESIAN_POINT('Ctrl Pts',(-42.2339804752703,-46.4302753505423,
39.8576902534424));
#202509=CARTESIAN_POINT('Ctrl Pts',(-42.1395065321001,-46.5159655405273,
39.8573998014387));
#202510=CARTESIAN_POINT('Ctrl Pts',(-42.0671296588098,-46.4355828792668,
39.92499));
#202511=CARTESIAN_POINT('Origin',(-42.0638038389703,-46.6938111422602,40.22725));
#202512=CARTESIAN_POINT('Origin',(-0.235948482089066,0.212448967518939,
39.116));
#202513=CARTESIAN_POINT('Origin',(-40.386254305094,-44.3789831537294,39.116));
#202514=CARTESIAN_POINT('Origin',(8.01250065760356E-17,1.22536847673099E-16,
40.22725));
#202515=CARTESIAN_POINT('Origin',(-42.0411527846897,-46.714206243142,40.22725));
#202516=CARTESIAN_POINT('Ctrl Pts',(-40.386254305094,-44.3789831537294,
38.989));
#202517=CARTESIAN_POINT('Ctrl Pts',(-40.2917335276658,-44.4640900439959,
38.989));
#202518=CARTESIAN_POINT('Ctrl Pts',(-40.2918750180001,-44.4639626455266,
39.1161901092326));
#202519=CARTESIAN_POINT('Ctrl Pts',(-40.2408978759466,-44.2178916378594,
38.989));
#202520=CARTESIAN_POINT('Ctrl Pts',(-40.1466757825259,-44.3029863283988,
38.9892298989778));
#202521=CARTESIAN_POINT('Ctrl Pts',(-40.1757689690818,-44.3350138149348,
39.1161900493206));
#202522=CARTESIAN_POINT('Ctrl Pts',(-40.1025190720984,-44.0645366033543,
39.1034966344368));
#202523=CARTESIAN_POINT('Ctrl Pts',(-40.008548843116,-44.1495800756938,
39.1038314102545));
#202524=CARTESIAN_POINT('Ctrl Pts',(-40.0652381943494,-44.2122569536128,
39.2077528789595));
#202525=CARTESIAN_POINT('Ctrl Pts',(-40.025490812659,-43.9791725362581,
39.2875012672119));
#202526=CARTESIAN_POINT('Ctrl Pts',(-39.9317222927443,-44.0642551375175,
39.2878045257868));
#202527=CARTESIAN_POINT('Ctrl Pts',(-40.003711479089,-44.1439246138549,
39.3549015295901));
#202528=CARTESIAN_POINT('Origin',(-40.0979831325501,-44.0588255818376,39.3548010137695));
#202529=CARTESIAN_POINT('Ctrl Pts',(-41.7612723673365,-46.8559036426983,
39.8576902534424));
#202530=CARTESIAN_POINT('Ctrl Pts',(-41.8563683535933,-46.77090430155,39.8573998014387));
#202531=CARTESIAN_POINT('Ctrl Pts',(-41.7839914803029,-46.6905216402895,
39.92499));
#202532=CARTESIAN_POINT('Ctrl Pts',(-41.7917156448185,-46.8897135983612,
39.9304984902492));
#202533=CARTESIAN_POINT('Ctrl Pts',(-41.8649095672158,-46.8033160448228,
39.9052171569793));
#202534=CARTESIAN_POINT('Ctrl Pts',(-41.8144332630852,-46.7243306652213,
39.96720497266));
#202535=CARTESIAN_POINT('Ctrl Pts',(-41.8425440045879,-46.9062450310967,
40.0043437678661));
#202536=CARTESIAN_POINT('Ctrl Pts',(-41.8933569085957,-46.8289264627104,
39.9661628577639));
#202537=CARTESIAN_POINT('Ctrl Pts',(-41.8569022891475,-46.7483907976685,
40.0100243556234));
#202538=CARTESIAN_POINT('Ctrl Pts',(-41.9695156381237,-46.8892773184516,
40.1194874821988));
#202539=CARTESIAN_POINT('Ctrl Pts',(-41.9804178820376,-46.8319191778366,
40.0627551483143));
#202540=CARTESIAN_POINT('Ctrl Pts',(-41.9507871007486,-46.7612136652284,
40.0767884282378));
#202541=CARTESIAN_POINT('Ctrl Pts',(-42.0474864684053,-46.8534019544983,
40.1599502015396));
#202542=CARTESIAN_POINT('Ctrl Pts',(-42.0403508033715,-46.8096319157686,
40.1002449453872));
#202543=CARTESIAN_POINT('Ctrl Pts',(-42.003109184301,-46.7484320121865,
40.10025));
#202544=CARTESIAN_POINT('Ctrl Pts',(-42.1132001506003,-46.7942619810915,
40.1599502534424));
#202545=CARTESIAN_POINT('Ctrl Pts',(-42.0882450513177,-46.7665330160777,
40.10025));
#202546=CARTESIAN_POINT('Ctrl Pts',(-42.0411527846897,-46.7142062431421,
40.10025));
#202547=CARTESIAN_POINT('Origin',(-41.6896120874673,-46.7755012272971,39.92499));
#202548=CARTESIAN_POINT('Origin',(-39.9787779456718,-43.9264348095002,39.6398955069313));
#202549=CARTESIAN_POINT('Origin',(-39.8595727587357,-43.7940440370142,39.92499));
#202550=CARTESIAN_POINT('Origin',(-41.5704070646213,-46.6431106370585,39.6398955068276));
#202551=CARTESIAN_POINT('Origin',(-41.4512020416176,-46.5107200467155,39.3548010137695));
#202552=CARTESIAN_POINT('Ctrl Pts',(-39.7870778846749,-43.7143933160621,
39.8576902534424));
#202553=CARTESIAN_POINT('Ctrl Pts',(-39.6934538167802,-43.7993487829611,
39.8579948730704));
#202554=CARTESIAN_POINT('Ctrl Pts',(-39.7651933659001,-43.8790236240218,
39.92499));
#202555=CARTESIAN_POINT('Ctrl Pts',(-39.7566748466928,-43.6806281164515,
39.9304020711232));
#202556=CARTESIAN_POINT('Ctrl Pts',(-39.6846648960483,-43.7668791656733,
39.9058915297392));
#202557=CARTESIAN_POINT('Ctrl Pts',(-39.734789463364,-43.8452566693656,
39.9671523786036));
#202558=CARTESIAN_POINT('Ctrl Pts',(-39.7061132086033,-43.6642103943285,
40.0043257306692));
#202559=CARTESIAN_POINT('Ctrl Pts',(-39.6560595510438,-43.7414086642729,
39.9667894847835));
#202560=CARTESIAN_POINT('Ctrl Pts',(-39.692510830909,-43.8213838166742,
40.01001389752));
#202561=CARTESIAN_POINT('Ctrl Pts',(-39.5798624575878,-43.6815693876451,
40.1195533054859));
#202562=CARTESIAN_POINT('Ctrl Pts',(-39.5692094437568,-43.7388169234804,
40.0630813209237));
#202563=CARTESIAN_POINT('Ctrl Pts',(-39.5991004926183,-43.8091742082551,
40.0768265942421));
#202564=CARTESIAN_POINT('Ctrl Pts',(-39.5024012818821,-43.7176736830026,
40.1599502027513));
#202565=CARTESIAN_POINT('Ctrl Pts',(-39.5096522555305,-43.7613473163394,
40.1002552791529));
#202566=CARTESIAN_POINT('Ctrl Pts',(-39.5470931435017,-43.8223603708618,
40.10025));
#202567=CARTESIAN_POINT('Ctrl Pts',(-39.437049873601,-43.776546871172,40.1599502534424));
#202568=CARTESIAN_POINT('Ctrl Pts',(-39.4620188529811,-43.8042633382927,
40.10025));
#202569=CARTESIAN_POINT('Ctrl Pts',(-39.5091373124624,-43.8565665267054,
40.10025));
#202570=CARTESIAN_POINT('Origin',(-39.5091373124624,-43.8565665267054,40.22725));
#202571=CARTESIAN_POINT('Ctrl Pts',(-41.1629311642483,-46.1905628026483,
38.989));
#202572=CARTESIAN_POINT('Ctrl Pts',(-41.2574515636636,-46.1054562527462,
38.989));
#202573=CARTESIAN_POINT('Ctrl Pts',(-41.2573104519064,-46.1055833103429,
39.116189601327));
#202574=CARTESIAN_POINT('Ctrl Pts',(-41.3079514313262,-46.3519569306001,
38.989));
#202575=CARTESIAN_POINT('Ctrl Pts',(-41.4027622547797,-46.2668393800548,
38.9887769275436));
#202576=CARTESIAN_POINT('Ctrl Pts',(-41.373416251083,-46.2345318643232,
39.1161898821827));
#202577=CARTESIAN_POINT('Ctrl Pts',(-41.4460100362725,-46.5056000892427,
39.1034967087243));
#202578=CARTESIAN_POINT('Ctrl Pts',(-41.5410595633946,-46.4204333915663,
39.1031720232727));
#202579=CARTESIAN_POINT('Ctrl Pts',(-41.4839469723849,-46.3572886670234,
39.2077529615019));
#202580=CARTESIAN_POINT('Ctrl Pts',(-41.5228599914565,-46.5911245387428,
39.2875012672119));
#202581=CARTESIAN_POINT('Ctrl Pts',(-41.6181024753233,-46.5059978248574,
39.2872087095508));
#202582=CARTESIAN_POINT('Ctrl Pts',(-41.5454735069377,-46.4256208064855,
39.3549017048229));
#202583=CARTESIAN_POINT('Origin',(-41.1629311642483,-46.1905628026483,39.116));
#202584=CARTESIAN_POINT('Origin',(3.72719664096539E-16,-4.35908294926639E-17,
40.22725));
#202585=CARTESIAN_POINT('Origin',(-39.4864862581819,-43.8769616275872,40.22725));
#202586=CARTESIAN_POINT('Origin',(28.0951675083328,30.7283483363946,39.116));
#202587=CARTESIAN_POINT('Origin',(-40.8943347850526,-45.8923335519886,39.1160373285264));
#202588=CARTESIAN_POINT('Ctrl Pts',(-39.4144401478992,-43.7969047596345,
40.1599502534424));
#202589=CARTESIAN_POINT('Ctrl Pts',(-39.439394812269,-43.8246341160483,
40.10025));
#202590=CARTESIAN_POINT('Ctrl Pts',(-39.4864862581819,-43.8769616275872,
40.10025));
#202591=CARTESIAN_POINT('Ctrl Pts',(-39.3492813761645,-43.8555436924519,
40.159950056604));
#202592=CARTESIAN_POINT('Ctrl Pts',(-39.3919218645327,-43.8673524484222,
40.1002551305372));
#202593=CARTESIAN_POINT('Ctrl Pts',(-39.4486296259963,-43.911017546801,
40.10025));
#202594=CARTESIAN_POINT('Ctrl Pts',(-39.3054399757367,-43.9280312169047,
40.1203070619043));
#202595=CARTESIAN_POINT('Ctrl Pts',(-39.3632835603682,-43.923706596467,
40.0637098684494));
#202596=CARTESIAN_POINT('Ctrl Pts',(-39.4300423632771,-43.9607655567562,
40.0772636213361));
#202597=CARTESIAN_POINT('Ctrl Pts',(-39.2744854109877,-44.0526112349801,
40.0046102245805));
#202598=CARTESIAN_POINT('Ctrl Pts',(-39.3564679665371,-44.0109847679676,
39.9670001894019));
#202599=CARTESIAN_POINT('Ctrl Pts',(-39.4322155454628,-44.0555161714737,
40.0101788811211));
#202600=CARTESIAN_POINT('Ctrl Pts',(-39.285649880758,-44.1047669487876,
39.9303710930184));
#202601=CARTESIAN_POINT('Ctrl Pts',(-39.3789590643341,-44.0421591564532,
39.9058663574109));
#202602=CARTESIAN_POINT('Ctrl Pts',(-39.4516641984998,-44.1002097724415,
39.9671344706356));
#202603=CARTESIAN_POINT('Ctrl Pts',(-39.3160391863692,-44.1385184650374,
39.8576902534424));
#202604=CARTESIAN_POINT('Ctrl Pts',(-39.4103156382734,-44.0542875439838,
39.8579948730703));
#202605=CARTESIAN_POINT('Ctrl Pts',(-39.4820551873932,-44.1339623850445,
39.92499));
#202606=CARTESIAN_POINT('Origin',(-39.3876757945576,-44.2189419720521,39.92499));
#202607=CARTESIAN_POINT('Origin',(-40.8647803215177,-45.8594327453957,39.1925554488843));
#202608=CARTESIAN_POINT('Origin',(-40.8100197873549,-45.7986150108449,39.3343017080178));
#202609=CARTESIAN_POINT('Origin',(-39.5068809815269,-44.351332744487,39.6398955069215));
#202610=CARTESIAN_POINT('Origin',(-39.626086168372,-44.4837235168755,39.3548010137695));
#202611=CARTESIAN_POINT('Ctrl Pts',(-40.5892333705625,-45.553406853251,
39.3978017080178));
#202612=CARTESIAN_POINT('Ctrl Pts',(-40.6836127633981,-45.4684272662434,
39.3978017080178));
#202613=CARTESIAN_POINT('Ctrl Pts',(-40.6836127633981,-45.4684272662434,
39.5248017080178));
#202614=CARTESIAN_POINT('Ctrl Pts',(-40.6496361736976,-45.6201409680071,
39.3978017080178));
#202615=CARTESIAN_POINT('Ctrl Pts',(-40.7437849681275,-45.5352552698635,
39.3980355775177));
#202616=CARTESIAN_POINT('Ctrl Pts',(-40.773954806069,-45.5687622694489,
39.5248015517192));
#202617=CARTESIAN_POINT('Ctrl Pts',(-40.7067502157901,-45.6832443225576,
39.3484893995498));
#202618=CARTESIAN_POINT('Ctrl Pts',(-40.8009661159847,-45.5987613682826,
39.3489438303429));
#202619=CARTESIAN_POINT('Ctrl Pts',(-40.859379634455,-45.6636361529315,
39.4508333155592));
#202620=CARTESIAN_POINT('Ctrl Pts',(-40.7368493365299,-45.7165002428305,
39.2708017080178));
#202621=CARTESIAN_POINT('Ctrl Pts',(-40.8311340869939,-45.6322662944331,
39.2710850691866));
#202622=CARTESIAN_POINT('Ctrl Pts',(-40.9043991801906,-45.7136354238374,
39.3343017080178));
#202623=CARTESIAN_POINT('Origin',(-40.5892333705625,-45.5534068532509,39.5248017080178));
#202624=CARTESIAN_POINT('Ctrl Pts',(-39.5544469813073,-44.4033023070487,
39.2875012672119));
#202625=CARTESIAN_POINT('Ctrl Pts',(-39.6488649595838,-44.3189410241793,
39.2878045257519));
#202626=CARTESIAN_POINT('Ctrl Pts',(-39.7205730817653,-44.3988635552002,
39.3549015218347));
#202627=CARTESIAN_POINT('Ctrl Pts',(-39.6312929306913,-44.4888328647721,
39.1034938540228));
#202628=CARTESIAN_POINT('Ctrl Pts',(-39.7256930794109,-44.404266885711,
39.1038286278806));
#202629=CARTESIAN_POINT('Ctrl Pts',(-39.7821007282717,-44.4671969296246,
39.2077506434033));
#202630=CARTESIAN_POINT('Ctrl Pts',(-39.7693444365328,-44.6424847942257,
38.989));
#202631=CARTESIAN_POINT('Ctrl Pts',(-39.8638218465937,-44.5576736781004,
38.9892298954611));
#202632=CARTESIAN_POINT('Ctrl Pts',(-39.8926323785405,-44.5899547640676,
39.1161900347287));
#202633=CARTESIAN_POINT('Ctrl Pts',(-39.9143573409159,-44.8038810887672,
38.989));
#202634=CARTESIAN_POINT('Ctrl Pts',(-40.0088781074272,-44.7187742083303,
38.989));
#202635=CARTESIAN_POINT('Ctrl Pts',(-40.0087366280261,-44.7189015969553,
39.1161900945644));
#202636=CARTESIAN_POINT('Origin',(-39.9143573409159,-44.8038810887672,39.116));
#202637=CARTESIAN_POINT('Origin',(27.4203375923837,29.9788737863604,39.5248017080178));
#202638=CARTESIAN_POINT('Origin',(-40.4880553924346,-45.441037324517,39.5248017080178));
#202639=CARTESIAN_POINT('Origin',(27.3146622010794,29.8615093742684,39.116));
#202640=CARTESIAN_POINT('Origin',(-40.1828829233543,-45.1021848870409,39.1160402713849));
#202641=CARTESIAN_POINT('Ctrl Pts',(-40.3404336838195,-45.2779489569771,
39.2708017080178));
#202642=CARTESIAN_POINT('Ctrl Pts',(-40.4355776097271,-45.1929563204587,
39.27051194648));
#202643=CARTESIAN_POINT('Ctrl Pts',(-40.3616483211486,-45.1108495273511,
39.3343017080178));
#202644=CARTESIAN_POINT('Ctrl Pts',(-40.3706366483425,-45.3113153943828,
39.3487519301186));
#202645=CARTESIAN_POINT('Ctrl Pts',(-40.4655326953338,-45.226224813414,
39.3482879463985));
#202646=CARTESIAN_POINT('Ctrl Pts',(-40.4068200107203,-45.1610177711054,
39.4512271261638));
#202647=CARTESIAN_POINT('Ctrl Pts',(-40.427855606124,-45.3745283705075,
39.3978017080178));
#202648=CARTESIAN_POINT('Ctrl Pts',(-40.5223510101992,-45.2893279449762,
39.3975673827397));
#202649=CARTESIAN_POINT('Ctrl Pts',(-40.4923970402295,-45.2560606910602,
39.5248015355181));
#202650=CARTESIAN_POINT('Ctrl Pts',(-40.4880553924346,-45.441037324517,
39.3978017080178));
#202651=CARTESIAN_POINT('Ctrl Pts',(-40.5824347852702,-45.3560577375094,
39.3978017080178));
#202652=CARTESIAN_POINT('Ctrl Pts',(-40.5824347852702,-45.3560577375094,
39.5248017080178));
#202653=CARTESIAN_POINT('Origin',(-40.267268928313,-45.1958291143586,39.3343017080178));
#202654=CARTESIAN_POINT('Origin',(-40.2128349746545,-45.1353740846424,39.1934008533546));
#202655=CARTESIAN_POINT('Origin',(-45.8594327460075,-40.864780322453,39.1925554495082));
#202656=CARTESIAN_POINT('Origin',(-45.8923335519897,-40.8943347850517,39.116037328527));
#202657=CARTESIAN_POINT('Origin',(-45.7986150108453,-40.8100197873545,39.3343017080178));
#202658=CARTESIAN_POINT('Ctrl Pts',(-45.7165002428309,-40.7368493365295,
39.2708017080178));
#202659=CARTESIAN_POINT('Ctrl Pts',(-45.6322662944335,-40.8311340869935,
39.2710850691866));
#202660=CARTESIAN_POINT('Ctrl Pts',(-45.7136354238378,-40.9043991801901,
39.3343017080178));
#202661=CARTESIAN_POINT('Ctrl Pts',(-45.6831319408677,-40.7066485019706,
39.3487519293518));
#202662=CARTESIAN_POINT('Ctrl Pts',(-45.5986481857991,-40.8008642060175,
39.3492068662924));
#202663=CARTESIAN_POINT('Ctrl Pts',(-45.663467198768,-40.859227507442,39.4512271248737));
#202664=CARTESIAN_POINT('Ctrl Pts',(-45.6199161851841,-40.6494327168526,
39.3978017080178));
#202665=CARTESIAN_POINT('Ctrl Pts',(-45.5350300257406,-40.7435821574131,
39.3980347781197));
#202666=CARTESIAN_POINT('Ctrl Pts',(-45.5684243021849,-40.7736504989768,
39.5248015355195));
#202667=CARTESIAN_POINT('Ctrl Pts',(-45.5534068532514,-40.589233370562,
39.3978017080178));
#202668=CARTESIAN_POINT('Ctrl Pts',(-45.4684272662438,-40.6836127633977,
39.3978017080178));
#202669=CARTESIAN_POINT('Ctrl Pts',(-45.4684272662438,-40.6836127633977,
39.5248017080178));
#202670=CARTESIAN_POINT('Origin',(-45.5534068532514,-40.589233370562,39.5248017080178));
#202671=CARTESIAN_POINT('Origin',(-0.212448967518931,0.235948482089074,
39.116));
#202672=CARTESIAN_POINT('Origin',(-46.1905628026487,-41.1629311642478,39.116));
#202673=CARTESIAN_POINT('Origin',(-0.212448967518931,0.235948482089074,
39.5248017080178));
#202674=CARTESIAN_POINT('Origin',(-45.4410373245174,-40.4880553924341,39.5248017080178));
#202675=CARTESIAN_POINT('Ctrl Pts',(-46.5911245387432,-41.522859991456,
39.2875012672119));
#202676=CARTESIAN_POINT('Ctrl Pts',(-46.5059978322079,-41.6181024670993,
39.287208709576));
#202677=CARTESIAN_POINT('Ctrl Pts',(-46.4256208133856,-41.5454735131718,
39.3549016990121));
#202678=CARTESIAN_POINT('Ctrl Pts',(-46.5055987918453,-41.4460088704659,
39.103493917393));
#202679=CARTESIAN_POINT('Ctrl Pts',(-46.4204321019767,-41.5410583874205,
39.1031692336335));
#202680=CARTESIAN_POINT('Ctrl Pts',(-46.3572876358789,-41.4839460439595,
39.2077507202298));
#202681=CARTESIAN_POINT('Ctrl Pts',(-46.3519544194668,-41.307949174952,
38.989));
#202682=CARTESIAN_POINT('Ctrl Pts',(-46.2668368728755,-41.4027599825081,
38.9887769311176));
#202683=CARTESIAN_POINT('Ctrl Pts',(-46.2345298607753,-41.3734144471015,
39.1161898712912));
#202684=CARTESIAN_POINT('Ctrl Pts',(-46.1905628026487,-41.1629311642478,
38.989));
#202685=CARTESIAN_POINT('Ctrl Pts',(-46.105456260079,-41.2574515555195,
38.989));
#202686=CARTESIAN_POINT('Ctrl Pts',(-46.1055833103324,-41.2573104519181,
39.1161895903851));
#202687=CARTESIAN_POINT('Origin',(-46.5107200467159,-41.4512020416172,39.3548010137695));
#202688=CARTESIAN_POINT('Ctrl Pts',(-45.4410373245174,-40.4880553924341,
39.3978017080178));
#202689=CARTESIAN_POINT('Ctrl Pts',(-45.3560577375098,-40.5824347852697,
39.3978017080178));
#202690=CARTESIAN_POINT('Ctrl Pts',(-45.3560577375098,-40.5824347852697,
39.5248017080178));
#202691=CARTESIAN_POINT('Ctrl Pts',(-45.3743035899552,-40.4276521486879,
39.3978017080178));
#202692=CARTESIAN_POINT('Ctrl Pts',(-45.2891025640473,-40.5221480762974,
39.3975666025007));
#202693=CARTESIAN_POINT('Ctrl Pts',(-45.2557227253151,-40.492092734505,
39.5248015517178));
#202694=CARTESIAN_POINT('Ctrl Pts',(-45.3112030195551,-40.3705349278739,
39.3484894016716));
#202695=CARTESIAN_POINT('Ctrl Pts',(-45.226112733224,-40.4654317778745,
39.3480259000057));
#202696=CARTESIAN_POINT('Ctrl Pts',(-45.1608488177571,-40.4066678844414,
39.4508333188948));
#202697=CARTESIAN_POINT('Ctrl Pts',(-45.2779489569775,-40.340433683819,
39.2708017080178));
#202698=CARTESIAN_POINT('Ctrl Pts',(-45.1929563204591,-40.4355776097266,
39.27051194648));
#202699=CARTESIAN_POINT('Ctrl Pts',(-45.1108495273515,-40.3616483211481,
39.3343017080178));
#202700=CARTESIAN_POINT('Origin',(-45.1958291143591,-40.2672689283125,39.3343017080178));
#202701=CARTESIAN_POINT('Origin',(-46.6431106370695,-41.5704070646303,39.6398955068187));
#202702=CARTESIAN_POINT('Origin',(-46.7755012272975,-41.6896120874668,39.92499));
#202703=CARTESIAN_POINT('Origin',(-45.1353740836144,-40.2128349741382,39.1934008539952));
#202704=CARTESIAN_POINT('Origin',(-45.1021848870414,-40.1828829233533,39.1160402713854));
#202705=CARTESIAN_POINT('Ctrl Pts',(-46.7942619810919,-42.1132001505999,
40.1599502534424));
#202706=CARTESIAN_POINT('Ctrl Pts',(-46.7665330160781,-42.0882450513173,
40.10025));
#202707=CARTESIAN_POINT('Ctrl Pts',(-46.7142062431425,-42.0411527846893,
40.10025));
#202708=CARTESIAN_POINT('Ctrl Pts',(-46.8532067119186,-42.0477032750701,
40.1599500538469));
#202709=CARTESIAN_POINT('Ctrl Pts',(-46.8094668591651,-42.0405341034489,
40.100244835349));
#202710=CARTESIAN_POINT('Ctrl Pts',(-46.7483190388761,-42.0032346206974,
40.10025));
#202711=CARTESIAN_POINT('Ctrl Pts',(-46.8890030154865,-41.9705316734063,
40.1202442001039));
#202712=CARTESIAN_POINT('Ctrl Pts',(-46.8318174060858,-41.9811230778543,
40.0633873868017));
#202713=CARTESIAN_POINT('Ctrl Pts',(-46.761203850955,-41.9515093836258,
40.0772271723538));
#202714=CARTESIAN_POINT('Ctrl Pts',(-46.906368706767,-41.8426461117366,
40.0045995998162));
#202715=CARTESIAN_POINT('Ctrl Pts',(-46.829061965151,-41.8933796070861,
39.9663485808314));
#202716=CARTESIAN_POINT('Ctrl Pts',(-46.74851255448,-41.8570065263031,40.0101727202465));
#202717=CARTESIAN_POINT('Ctrl Pts',(-46.8896982576908,-41.7917018131131,
39.9304654349859));
#202718=CARTESIAN_POINT('Ctrl Pts',(-46.8032976561895,-41.8649047103977,
39.9051900162951));
#202719=CARTESIAN_POINT('Ctrl Pts',(-46.724315266822,-41.8144193983034,
39.9671857458188));
#202720=CARTESIAN_POINT('Ctrl Pts',(-46.8559036426987,-41.761272367336,
39.8576902534424));
#202721=CARTESIAN_POINT('Ctrl Pts',(-46.7709043015504,-41.8563683535928,
39.8573998014387));
#202722=CARTESIAN_POINT('Ctrl Pts',(-46.6905216402899,-41.7839914803024,
39.92499));
#202723=CARTESIAN_POINT('Origin',(-46.7142062431425,-42.0411527846893,40.22725));
#202724=CARTESIAN_POINT('Origin',(-0.212448967518931,0.235948482089074,
39.116));
#202725=CARTESIAN_POINT('Origin',(-44.8038810887676,-39.9143573409155,39.116));
#202726=CARTESIAN_POINT('Origin',(9.23291810287662E-17,1.10332673220367E-16,
40.22725));
#202727=CARTESIAN_POINT('Origin',(-46.6938111422607,-42.0638038389698,40.22725));
#202728=CARTESIAN_POINT('Ctrl Pts',(-44.8038810887676,-39.9143573409155,
38.989));
#202729=CARTESIAN_POINT('Ctrl Pts',(-44.7187741985013,-40.0088781183435,
38.989));
#202730=CARTESIAN_POINT('Ctrl Pts',(-44.7189015969703,-40.0087366280094,
39.1161901092323));
#202731=CARTESIAN_POINT('Ctrl Pts',(-44.6424822887487,-39.7693421853894,
38.989));
#202732=CARTESIAN_POINT('Ctrl Pts',(-44.5576711710495,-39.8638196089396,
38.9892298989784));
#202733=CARTESIAN_POINT('Ctrl Pts',(-44.589952766033,-39.8926305794718,
39.1161900493203));
#202734=CARTESIAN_POINT('Ctrl Pts',(-44.4888315723759,-39.6312917695239,
39.1034966344368));
#202735=CARTESIAN_POINT('Ctrl Pts',(-44.4042655856137,-39.7256919284549,
39.1038314102544));
#202736=CARTESIAN_POINT('Ctrl Pts',(-44.467195904383,-39.7820998051097,
39.2077528789598));
#202737=CARTESIAN_POINT('Ctrl Pts',(-44.4033023070491,-39.5544469813068,
39.2875012672119));
#202738=CARTESIAN_POINT('Ctrl Pts',(-44.3189410144583,-39.6488649704636,
39.2878045257868));
#202739=CARTESIAN_POINT('Ctrl Pts',(-44.3988635644384,-39.7205730900532,
39.35490152959));
#202740=CARTESIAN_POINT('Origin',(-44.4837235168759,-39.6260861683715,39.3548010137695));
#202741=CARTESIAN_POINT('Ctrl Pts',(-46.4302753505427,-42.2339804752699,
39.8576902534424));
#202742=CARTESIAN_POINT('Ctrl Pts',(-46.5159655405277,-42.1395065320997,
39.8573998014387));
#202743=CARTESIAN_POINT('Ctrl Pts',(-46.4355828792672,-42.0671296588093,
39.92499));
#202744=CARTESIAN_POINT('Ctrl Pts',(-46.4640859592741,-42.264423027446,
39.9304984902493));
#202745=CARTESIAN_POINT('Ctrl Pts',(-46.5278479142027,-42.1708479205167,
39.9052171569797));
#202746=CARTESIAN_POINT('Ctrl Pts',(-46.4693919041982,-42.0975714415909,
39.9672049726614));
#202747=CARTESIAN_POINT('Ctrl Pts',(-46.5163638812298,-42.2755508889259,
40.0043437678659));
#202748=CARTESIAN_POINT('Ctrl Pts',(-46.5588164356976,-42.1933444849778,
39.9661628577643));
#202749=CARTESIAN_POINT('Ctrl Pts',(-46.5141432491634,-42.1170605480847,
40.0100243556235));
#202750=CARTESIAN_POINT('Ctrl Pts',(-46.6408663419437,-42.2454039774545,
40.119487482199));
#202751=CARTESIAN_POINT('Ctrl Pts',(-46.6457133039302,-42.1872204559322,
40.0627551483141));
#202752=CARTESIAN_POINT('Ctrl Pts',(-46.6088541045843,-42.1199995355544,
40.0767884282377));
#202753=CARTESIAN_POINT('Ctrl Pts',(-46.7146600431957,-42.2015749714291,
40.1599502015393));
#202754=CARTESIAN_POINT('Ctrl Pts',(-46.7029882531949,-42.1587905896511,
40.1002449453875));
#202755=CARTESIAN_POINT('Ctrl Pts',(-46.6595535157373,-42.1018187547555,
40.10025));
#202756=CARTESIAN_POINT('Ctrl Pts',(-46.773831928426,-42.1358900227693,
40.1599502534424));
#202757=CARTESIAN_POINT('Ctrl Pts',(-46.7461150696875,-42.1109214781059,
40.10025));
#202758=CARTESIAN_POINT('Ctrl Pts',(-46.6938111422607,-42.0638038389698,
40.10025));
#202759=CARTESIAN_POINT('Origin',(-46.3506032922596,-42.161509051645,39.92499));
#202760=CARTESIAN_POINT('Origin',(-44.3513327445024,-39.5068809815374,39.6398955069331));
#202761=CARTESIAN_POINT('Origin',(-44.2189419720525,-39.3876757945571,39.92499));
#202762=CARTESIAN_POINT('Origin',(-46.2182127020509,-42.0423040287663,39.6398955068274));
#202763=CARTESIAN_POINT('Origin',(-46.085822111678,-41.9230990057953,39.3548010137695));
#202764=CARTESIAN_POINT('Ctrl Pts',(-44.1385184650378,-39.3160391863687,
39.8576902534424));
#202765=CARTESIAN_POINT('Ctrl Pts',(-44.0542875439842,-39.4103156382729,
39.8579948730703));
#202766=CARTESIAN_POINT('Ctrl Pts',(-44.1339623850449,-39.4820551873928,
39.92499));
#202767=CARTESIAN_POINT('Ctrl Pts',(-44.1047525536513,-39.285636938894,
39.9304020711229));
#202768=CARTESIAN_POINT('Ctrl Pts',(-44.0421527706808,-39.3789425853227,
39.9058915297381));
#202769=CARTESIAN_POINT('Ctrl Pts',(-44.100195430388,-39.451651284856,39.9671523786027));
#202770=CARTESIAN_POINT('Ctrl Pts',(-44.0527517782418,-39.2745942850998,
40.0043257306695));
#202771=CARTESIAN_POINT('Ctrl Pts',(-44.0110417363802,-39.3566016867495,
39.9667894847835));
#202772=CARTESIAN_POINT('Ctrl Pts',(-44.0556530121005,-39.4323285306299,
40.01001389752));
#202773=CARTESIAN_POINT('Ctrl Pts',(-43.9290071509458,-39.3050549810249,
40.1195533054855));
#202774=CARTESIAN_POINT('Ctrl Pts',(-43.9243964923857,-39.3631024520341,
40.0630813209236));
#202775=CARTESIAN_POINT('Ctrl Pts',(-43.9614781338111,-39.4299498468377,
40.0768265942421));
#202776=CARTESIAN_POINT('Ctrl Pts',(-43.8557442421763,-39.3490583909339,
40.1599502027517));
#202777=CARTESIAN_POINT('Ctrl Pts',(-43.8675206320097,-39.3917348424039,
40.1002552791553));
#202778=CARTESIAN_POINT('Ctrl Pts',(-43.9111340157071,-39.4485000225468,
40.10025));
#202779=CARTESIAN_POINT('Ctrl Pts',(-43.7969047596348,-39.4144401478987,
40.1599502534424));
#202780=CARTESIAN_POINT('Ctrl Pts',(-43.8246341160487,-39.4393948122686,
40.10025));
#202781=CARTESIAN_POINT('Ctrl Pts',(-43.8769616275876,-39.4864862581814,
40.10025));
#202782=CARTESIAN_POINT('Origin',(-43.8769616275876,-39.4864862581814,40.22725));
#202783=CARTESIAN_POINT('Ctrl Pts',(-45.7656648676108,-41.634828128426,
38.989));
#202784=CARTESIAN_POINT('Ctrl Pts',(-45.8507714175129,-41.5403077290107,
38.989));
#202785=CARTESIAN_POINT('Ctrl Pts',(-45.8506443599162,-41.5404488407678,
39.1161896013269));
#202786=CARTESIAN_POINT('Ctrl Pts',(-45.9267609786668,-41.7801793767981,
38.989));
#202787=CARTESIAN_POINT('Ctrl Pts',(-46.0121552117527,-41.6856176794253,
38.9887769275485));
#202788=CARTESIAN_POINT('Ctrl Pts',(-45.9795929135641,-41.6565546403125,
39.1161898821851));
#202789=CARTESIAN_POINT('Ctrl Pts',(-46.0801233673977,-41.9185498083221,
39.1034967087243));
#202790=CARTESIAN_POINT('Ctrl Pts',(-46.165749859237,-41.8239142817197,
39.1031720232693));
#202791=CARTESIAN_POINT('Ctrl Pts',(-46.1023497159528,-41.7670853619627,
39.2077529614997));
#202792=CARTESIAN_POINT('Ctrl Pts',(-46.1654920697614,-41.9955727382249,
39.2875012672119));
#202793=CARTESIAN_POINT('Ctrl Pts',(-46.2513146407507,-41.9009568069087,
39.2872087095508));
#202794=CARTESIAN_POINT('Ctrl Pts',(-46.1706818552408,-41.8286118967075,
39.3549017048229));
#202795=CARTESIAN_POINT('Origin',(-45.7656648676108,-41.634828128426,39.116));
#202796=CARTESIAN_POINT('Origin',(3.68378193773366E-16,-3.92493591694921E-17,
40.22725));
#202797=CARTESIAN_POINT('Origin',(-43.8565665267058,-39.509137312462,40.22725));
#202798=CARTESIAN_POINT('Origin',(34.5756856720389,30.7048488218244,39.116));
#202799=CARTESIAN_POINT('Origin',(-45.4673664422114,-41.3663085755624,39.116037328527));
#202800=CARTESIAN_POINT('Ctrl Pts',(-43.7765468711724,-39.4370498736006,
40.1599502534424));
#202801=CARTESIAN_POINT('Ctrl Pts',(-43.8042633382931,-39.4620188529807,
40.10025));
#202802=CARTESIAN_POINT('Ctrl Pts',(-43.8565665267058,-39.509137312462,
40.10025));
#202803=CARTESIAN_POINT('Ctrl Pts',(-43.7178744835419,-39.5021785224865,
40.159950056604));
#202804=CARTESIAN_POINT('Ctrl Pts',(-43.7615157339672,-39.5094654441334,
40.1002551305381));
#202805=CARTESIAN_POINT('Ctrl Pts',(-43.8224770900135,-39.5469637653747,
40.10025));
#202806=CARTESIAN_POINT('Ctrl Pts',(-43.6818502604301,-39.5788516269096,
40.1203070619047));
#202807=CARTESIAN_POINT('Ctrl Pts',(-43.7389249259241,-39.5685043961836,
40.0637098684497));
#202808=CARTESIAN_POINT('Ctrl Pts',(-43.8091917332948,-39.598382148533,
40.0772636213364));
#202809=CARTESIAN_POINT('Ctrl Pts',(-43.664087425869,-39.705984815696,40.0046102245801));
#202810=CARTESIAN_POINT('Ctrl Pts',(-43.7412697217731,-39.6560168722791,
39.9670001894016));
#202811=CARTESIAN_POINT('Ctrl Pts',(-43.8212571467115,-39.6923865500761,
40.0101788811207));
#202812=CARTESIAN_POINT('Ctrl Pts',(-43.68064249212,-39.7566878101779,39.9303710930186));
#202813=CARTESIAN_POINT('Ctrl Pts',(-43.7668962219046,-39.6846695243128,
39.9058663574113));
#202814=CARTESIAN_POINT('Ctrl Pts',(-43.84527101142,-39.734802377007,39.9671344706375));
#202815=CARTESIAN_POINT('Ctrl Pts',(-43.7143933160625,-39.7870778846745,
39.8576902534424));
#202816=CARTESIAN_POINT('Ctrl Pts',(-43.7993487829615,-39.6934538167798,
39.8579948730704));
#202817=CARTESIAN_POINT('Ctrl Pts',(-43.8790236240222,-39.7651933658996,
39.92499));
#202818=CARTESIAN_POINT('Origin',(-43.7940440370146,-39.8595727587353,39.92499));
#202819=CARTESIAN_POINT('Origin',(-45.4345348103664,-41.3366772856882,39.192555448885));
#202820=CARTESIAN_POINT('Origin',(-45.3737170758075,-41.2819167515326,39.3343017080178));
#202821=CARTESIAN_POINT('Origin',(-43.9264348094887,-39.9787779456578,39.6398955069202));
#202822=CARTESIAN_POINT('Origin',(-44.058825581838,-40.0979831325497,39.3548010137695));
#202823=CARTESIAN_POINT('Ctrl Pts',(-45.1285089182135,-41.0611303347402,
39.3978017080178));
#202824=CARTESIAN_POINT('Ctrl Pts',(-45.2134885052211,-40.9667509419046,
39.3978017080178));
#202825=CARTESIAN_POINT('Ctrl Pts',(-45.2134885052211,-40.9667509419045,
39.5248017080178));
#202826=CARTESIAN_POINT('Ctrl Pts',(-45.1955564429372,-41.1211850608431,
39.3978017080178));
#202827=CARTESIAN_POINT('Ctrl Pts',(-45.2803165088391,-41.026923146635,
39.3980355775229));
#202828=CARTESIAN_POINT('Ctrl Pts',(-45.3138235084264,-41.0570929845753,
39.5248015517192));
#202829=CARTESIAN_POINT('Ctrl Pts',(-45.2589537050076,-41.1779726855658,
39.3484893995498));
#202830=CARTESIAN_POINT('Ctrl Pts',(-45.3438226072617,-41.0841042944915,
39.3489438303395));
#202831=CARTESIAN_POINT('Ctrl Pts',(-45.4086973919094,-41.1425178129616,
39.4508333155593));
#202832=CARTESIAN_POINT('Ctrl Pts',(-45.2923641298559,-41.2079002115905,
39.2708017080178));
#202833=CARTESIAN_POINT('Ctrl Pts',(-45.3773275334108,-41.1142722655004,
39.2710850691866));
#202834=CARTESIAN_POINT('Ctrl Pts',(-45.4586966628151,-41.187537358697,
39.3343017080178));
#202835=CARTESIAN_POINT('Origin',(-45.1285089182135,-41.0611303347402,39.5248017080178));
#202836=CARTESIAN_POINT('Ctrl Pts',(-43.9791725362585,-40.0254908126586,
39.2875012672119));
#202837=CARTESIAN_POINT('Ctrl Pts',(-44.0642551277132,-39.9317223035495,
39.2878045257519));
#202838=CARTESIAN_POINT('Ctrl Pts',(-44.1439246046466,-40.0037114707676,
39.3549015218347));
#202839=CARTESIAN_POINT('Ctrl Pts',(-44.0645378932555,-40.1025202360368,
39.1034938540228));
#202840=CARTESIAN_POINT('Ctrl Pts',(-44.1495813562482,-40.0085500157871,
39.103828627881));
#202841=CARTESIAN_POINT('Ctrl Pts',(-44.2122579788861,-40.0652391174794,
39.2077506434033));
#202842=CARTESIAN_POINT('Ctrl Pts',(-44.2178941385633,-40.240900132391,
38.989));
#202843=CARTESIAN_POINT('Ctrl Pts',(-44.3029888158476,-40.1466780419424,
38.989229895463));
#202844=CARTESIAN_POINT('Ctrl Pts',(-44.335015812998,-40.1757707681158,
39.1161900347288));
#202845=CARTESIAN_POINT('Ctrl Pts',(-44.3789831537298,-40.3862543050936,
38.989));
#202846=CARTESIAN_POINT('Ctrl Pts',(-44.4640900341667,-40.2917335385823,
38.989));
#202847=CARTESIAN_POINT('Ctrl Pts',(-44.4639626455417,-40.2918750179834,
39.1161900945645));
#202848=CARTESIAN_POINT('Origin',(-44.3789831537298,-40.3862543050936,39.116));
#202849=CARTESIAN_POINT('Origin',(33.743309857225,29.9553742717902,39.5248017080178));
#202850=CARTESIAN_POINT('Origin',(-45.0161393894795,-40.9599523566123,39.5248017080178));
#202851=CARTESIAN_POINT('Origin',(33.61296347236,29.8380098596982,39.116));
#202852=CARTESIAN_POINT('Origin',(-44.6772189625516,-40.654855397468,39.1160402713849));
#202853=CARTESIAN_POINT('Ctrl Pts',(-44.8522789915944,-40.8131880745604,
39.2708017080178));
#202854=CARTESIAN_POINT('Ctrl Pts',(-44.9380175594364,-40.7187157882335,
39.27051194648));
#202855=CARTESIAN_POINT('Ctrl Pts',(-44.8559107663287,-40.644786499655,
39.3343017080178));
#202856=CARTESIAN_POINT('Ctrl Pts',(-44.8858042435438,-40.8432146576637,
39.3487519301186));
#202857=CARTESIAN_POINT('Ctrl Pts',(-44.97128605239,-40.7486708738366,39.3482879464018));
#202858=CARTESIAN_POINT('Ctrl Pts',(-44.906079010081,-40.6899581892249,
39.4512271261645));
#202859=CARTESIAN_POINT('Ctrl Pts',(-44.9493173051404,-40.9001003367645,
39.3978017080178));
#202860=CARTESIAN_POINT('Ctrl Pts',(-45.0343891839553,-40.8054891887082,
39.3975673827364));
#202861=CARTESIAN_POINT('Ctrl Pts',(-45.0011219300394,-40.7755352187373,
39.5248015355181));
#202862=CARTESIAN_POINT('Ctrl Pts',(-45.0161393894795,-40.9599523566123,
39.3978017080178));
#202863=CARTESIAN_POINT('Ctrl Pts',(-45.1011189764871,-40.8655729637766,
39.3978017080178));
#202864=CARTESIAN_POINT('Ctrl Pts',(-45.1011189764871,-40.8655729637766,
39.5248017080178));
#202865=CARTESIAN_POINT('Origin',(-44.7709311793212,-40.7391658924907,39.3343017080178));
#202866=CARTESIAN_POINT('Origin',(-44.7104761492019,-40.6847319392791,39.1934008533549));
#202867=CARTESIAN_POINT('Origin',(-49.8797426639499,-35.8473027488279,39.1925554495084));
#202868=CARTESIAN_POINT('Origin',(-49.9155525184331,-35.8732562382984,39.116037328528));
#202869=CARTESIAN_POINT('Origin',(-49.8135340601225,-35.799199382066,39.3343017080178));
#202870=CARTESIAN_POINT('Ctrl Pts',(-49.7242207306177,-35.7350130971387,
39.2708017080178));
#202871=CARTESIAN_POINT('Ctrl Pts',(-49.6503036646787,-35.8375861910554,
39.2710850691866));
#202872=CARTESIAN_POINT('Ctrl Pts',(-49.7388853330813,-35.9019445403516,
39.3343017080178));
#202873=CARTESIAN_POINT('Ctrl Pts',(-49.6878783768805,-35.7084656432344,
39.3487519293518));
#202874=CARTESIAN_POINT('Ctrl Pts',(-49.6137056554148,-35.8109961808816,
39.3492068662919));
#202875=CARTESIAN_POINT('Ctrl Pts',(-49.6842702092604,-35.8622643302234,
39.4512271248732));
#202876=CARTESIAN_POINT('Ctrl Pts',(-49.6190282456266,-35.6581711379714,
39.3978017080178));
#202877=CARTESIAN_POINT('Ctrl Pts',(-49.5444483977901,-35.7606778378481,
39.3980347781178));
#202878=CARTESIAN_POINT('Ctrl Pts',(-49.5808027344264,-35.7870908094911,
39.5248015355195));
#202879=CARTESIAN_POINT('Ctrl Pts',(-49.5465907136146,-35.6052536882599,
39.3978017080178));
#202880=CARTESIAN_POINT('Ctrl Pts',(-49.4719419865735,-35.7079988465456,
39.3978017080178));
#202881=CARTESIAN_POINT('Ctrl Pts',(-49.4719419865735,-35.7079988465456,
39.5248017080178));
#202882=CARTESIAN_POINT('Origin',(-49.5465907136146,-35.6052536882599,39.5248017080178));
#202883=CARTESIAN_POINT('Origin',(-0.186621817602853,0.256862895714047,
39.116));
#202884=CARTESIAN_POINT('Origin',(-50.2402240048085,-36.1092077731526,39.116));
#202885=CARTESIAN_POINT('Origin',(-0.186621817602853,0.256862895714047,
39.5248017080178));
#202886=CARTESIAN_POINT('Origin',(-49.4242607783462,-35.5163757878393,39.5248017080178));
#202887=CARTESIAN_POINT('Ctrl Pts',(-50.676214228995,-36.4252947698676,
39.2875012672119));
#202888=CARTESIAN_POINT('Ctrl Pts',(-50.6015094050817,-36.5289136610813,
39.287208709576));
#202889=CARTESIAN_POINT('Ctrl Pts',(-50.5139809070357,-36.4650842624219,
39.3549016990122));
#202890=CARTESIAN_POINT('Ctrl Pts',(-50.5831238715085,-36.3578045222543,
39.1034939173931));
#202891=CARTESIAN_POINT('Ctrl Pts',(-50.5083591136198,-36.4612356912225,
39.1031692336333));
#202892=CARTESIAN_POINT('Ctrl Pts',(-50.4395906940211,-36.4110366091596,
39.2077507202295));
#202893=CARTESIAN_POINT('Ctrl Pts',(-50.415890011269,-36.2365613423289,
38.989));
#202894=CARTESIAN_POINT('Ctrl Pts',(-50.3411491755196,-36.339749972703,
38.9887769311182));
#202895=CARTESIAN_POINT('Ctrl Pts',(-50.3059517008894,-36.3139421975384,
39.1161898712915));
#202896=CARTESIAN_POINT('Ctrl Pts',(-50.2402240048085,-36.1092077731526,
38.989));
#202897=CARTESIAN_POINT('Ctrl Pts',(-50.1654637560308,-36.2121064279401,
38.989));
#202898=CARTESIAN_POINT('Ctrl Pts',(-50.1655753609471,-36.2119528169511,
39.1161895903853));
#202899=CARTESIAN_POINT('Origin',(-50.5887599058103,-36.3624339277671,39.3548010137695));
#202900=CARTESIAN_POINT('Ctrl Pts',(-49.4242607783463,-35.5163757878393,
39.3978017080178));
#202901=CARTESIAN_POINT('Ctrl Pts',(-49.3496120513051,-35.619120946125,
39.3978017080178));
#202902=CARTESIAN_POINT('Ctrl Pts',(-49.3496120513051,-35.6191209461249,
39.5248017080178));
#202903=CARTESIAN_POINT('Ctrl Pts',(-49.3515787599185,-35.4632790141053,
39.3978017080178));
#202904=CARTESIAN_POINT('Ctrl Pts',(-49.2767219882448,-35.5661632154432,
39.3975666025054));
#202905=CARTESIAN_POINT('Ctrl Pts',(-49.2403833690709,-35.5397616632038,
39.5248015517178));
#202906=CARTESIAN_POINT('Ctrl Pts',(-49.2828534857277,-35.4130704930583,
39.3484894016716));
#202907=CARTESIAN_POINT('Ctrl Pts',(-49.208148754787,-35.5163418450528,
39.3480259000026));
#202908=CARTESIAN_POINT('Ctrl Pts',(-49.1370998624026,-35.4647218031678,
39.4508333188949));
#202909=CARTESIAN_POINT('Ctrl Pts',(-49.2466351556014,-35.3866101428257,
39.2708017080178));
#202910=CARTESIAN_POINT('Ctrl Pts',(-49.1720533660033,-35.4901170100364,
39.2705119464801));
#202911=CARTESIAN_POINT('Ctrl Pts',(-49.0826686475736,-35.4251752107435,
39.3343017080178));
#202912=CARTESIAN_POINT('Origin',(-49.1573173746148,-35.3224300524579,39.3343017080178));
#202913=CARTESIAN_POINT('Origin',(-50.732885564526,-36.4671473482319,39.6398955068188));
#202914=CARTESIAN_POINT('Origin',(-50.8770112231004,-36.5718607685319,39.92499));
#202915=CARTESIAN_POINT('Origin',(-49.0915036252757,-35.2746135646437,39.1934008539937));
#202916=CARTESIAN_POINT('Origin',(-49.0553654007528,-35.2482948100394,39.1160402713847));
#202917=CARTESIAN_POINT('Ctrl Pts',(-50.9399462128204,-36.9911673391705,
40.1599502534424));
#202918=CARTESIAN_POINT('Ctrl Pts',(-50.9097606317996,-36.9692474126338,
40.10025));
#202919=CARTESIAN_POINT('Ctrl Pts',(-50.8527980281387,-36.9278827595324,
40.10025));
#202920=CARTESIAN_POINT('Ctrl Pts',(-50.9917217504962,-36.9198678602471,
40.1599500538471));
#202921=CARTESIAN_POINT('Ctrl Pts',(-50.9474721267406,-36.9173100216903,
40.100244835349));
#202922=CARTESIAN_POINT('Ctrl Pts',(-50.8827604229961,-36.8866065570947,
40.10025));
#202923=CARTESIAN_POINT('Ctrl Pts',(-51.0192553292378,-36.8393772800889,
40.1202442001037));
#202924=CARTESIAN_POINT('Ctrl Pts',(-50.9634900918192,-36.8558881875865,
40.0633873868015));
#202925=CARTESIAN_POINT('Ctrl Pts',(-50.8901678911824,-36.8338178466772,
40.0772271723538));
#202926=CARTESIAN_POINT('Ctrl Pts',(-51.0231582082091,-36.710377079884,
40.0045995998164));
#202927=CARTESIAN_POINT('Ctrl Pts',(-50.951578055318,-36.7689134067394,
39.9663485808318));
#202928=CARTESIAN_POINT('Ctrl Pts',(-50.8676678805081,-36.7411592876131,
40.0101727202465));
#202929=CARTESIAN_POINT('Ctrl Pts',(-51.0012539523496,-36.6614543958826,
39.9304654349858));
#202930=CARTESIAN_POINT('Ctrl Pts',(-50.922978448743,-36.7432876021378,
39.9051900162949));
#202931=CARTESIAN_POINT('Ctrl Pts',(-50.8391515810792,-36.7013347616509,
39.9671857458173));
#202932=CARTESIAN_POINT('Ctrl Pts',(-50.9644637245895,-36.6347241449652,
39.8576902534424));
#202933=CARTESIAN_POINT('Ctrl Pts',(-50.8898702560319,-36.7381840359682,
39.8573998014387));
#202934=CARTESIAN_POINT('Ctrl Pts',(-50.8023624960593,-36.6746059268175,
39.92499));
#202935=CARTESIAN_POINT('Origin',(-50.8527980281387,-36.9278827595324,40.22725));
#202936=CARTESIAN_POINT('Origin',(-0.186621817602853,0.256862895714047,
39.116));
#202937=CARTESIAN_POINT('Origin',(-48.7306271754178,-35.0124214764582,39.116));
#202938=CARTESIAN_POINT('Origin',(1.03190816135906E-16,9.69196709112357E-17,
40.22725));
#202939=CARTESIAN_POINT('Origin',(-50.8348823336488,-36.9525415975209,40.22725));
#202940=CARTESIAN_POINT('Ctrl Pts',(-48.7306271754178,-35.0124214764582,
38.989));
#202941=CARTESIAN_POINT('Ctrl Pts',(-48.6558666212126,-35.1153205516308,
38.989));
#202942=CARTESIAN_POINT('Ctrl Pts',(-48.6559785320123,-35.1151665196292,
39.1161901092324));
#202943=CARTESIAN_POINT('Ctrl Pts',(-48.5549543235573,-34.8850714976637,
38.989));
#202944=CARTESIAN_POINT('Ctrl Pts',(-48.4804833899316,-34.9878965398047,
38.9892298989778));
#202945=CARTESIAN_POINT('Ctrl Pts',(-48.5155997094345,-35.0131753353128,
39.1161900493204));
#202946=CARTESIAN_POINT('Ctrl Pts',(-48.3877151240598,-34.7638382096857,
39.1034966344368));
#202947=CARTESIAN_POINT('Ctrl Pts',(-48.3134799021657,-34.8665607873099,
39.1038314102547));
#202948=CARTESIAN_POINT('Ctrl Pts',(-48.3819617107265,-34.9160816461997,
39.2077528789594));
#202949=CARTESIAN_POINT('Ctrl Pts',(-48.2946219293748,-34.6963546279283,
39.2875012672119));
#202950=CARTESIAN_POINT('Ctrl Pts',(-48.220592144083,-34.7990735417351,
39.2878045257868));
#202951=CARTESIAN_POINT('Ctrl Pts',(-48.3075724095165,-34.8620346554128,
39.35490152959));
#202952=CARTESIAN_POINT('Origin',(-48.3820909175331,-34.7591950625531,39.3548010137695));
#202953=CARTESIAN_POINT('Ctrl Pts',(-50.5905785208486,-37.1493329797258,
39.8576902534424));
#202954=CARTESIAN_POINT('Ctrl Pts',(-50.6659240749085,-37.046419510825,
39.8573998014387));
#202955=CARTESIAN_POINT('Ctrl Pts',(-50.5784163149359,-36.9828414016744,
39.92499));
#202956=CARTESIAN_POINT('Ctrl Pts',(-50.6273860247248,-37.1760745934426,
39.9304984902492));
#202957=CARTESIAN_POINT('Ctrl Pts',(-50.681017422865,-37.0763471615773,
39.9052171569793));
#202958=CARTESIAN_POINT('Ctrl Pts',(-50.6152221632652,-37.009582415765,
39.9672049726598));
#202959=CARTESIAN_POINT('Ctrl Pts',(-50.6805407410139,-37.1816769644887,
40.0043437678661));
#202960=CARTESIAN_POINT('Ctrl Pts',(-50.7141678268705,-37.0954833955425,
39.9661628577643));
#202961=CARTESIAN_POINT('Ctrl Pts',(-50.6617655220313,-37.024286969575,
40.0100243556235));
#202962=CARTESIAN_POINT('Ctrl Pts',(-50.8012099538927,-37.1386811500609,
40.1194874821989));
#202963=CARTESIAN_POINT('Ctrl Pts',(-50.7999485296224,-37.0803097184694,
40.062755148314));
#202964=CARTESIAN_POINT('Ctrl Pts',(-50.7562647493204,-37.0173098767919,
40.0767884282377));
#202965=CARTESIAN_POINT('Ctrl Pts',(-50.8700180268809,-37.0873787017254,
40.159950201538));
#202966=CARTESIAN_POINT('Ctrl Pts',(-50.8539379904865,-37.0460487315389,
40.100244945386));
#202967=CARTESIAN_POINT('Ctrl Pts',(-50.8047860147144,-36.9939291606747,
40.10025));
#202968=CARTESIAN_POINT('Ctrl Pts',(-50.9219998155902,-37.0158684358557,
40.1599502534424));
#202969=CARTESIAN_POINT('Ctrl Pts',(-50.8918248691002,-36.993933872143,
40.10025));
#202970=CARTESIAN_POINT('Ctrl Pts',(-50.8348823336488,-36.952541597521,
40.10025));
#202971=CARTESIAN_POINT('Origin',(-50.5037675878947,-37.08558655996,39.92499));
#202972=CARTESIAN_POINT('Origin',(-48.2379650606702,-34.6544814981901,39.6398955069326));
#202973=CARTESIAN_POINT('Origin',(-48.093839203715,-34.5497679336938,39.92499));
#202974=CARTESIAN_POINT('Origin',(-50.3596419293373,-36.9808731396128,39.6398955068275));
#202975=CARTESIAN_POINT('Origin',(-50.2155162706046,-36.8761597191952,39.3548010137695));
#202976=CARTESIAN_POINT('Ctrl Pts',(-48.0063682005189,-34.4869303039394,
39.8576902534424));
#202977=CARTESIAN_POINT('Ctrl Pts',(-47.9324532779039,-34.5894948283131,
39.8579948730703));
#202978=CARTESIAN_POINT('Ctrl Pts',(-48.0191904766738,-34.6525130919795,
39.92499));
#202979=CARTESIAN_POINT('Ctrl Pts',(-47.9696093621197,-34.460224101985,
39.9304020711231));
#202980=CARTESIAN_POINT('Ctrl Pts',(-47.9171056031471,-34.559562069433,
39.9058915297378));
#202981=CARTESIAN_POINT('Ctrl Pts',(-47.9824304277179,-34.6258053530815,
39.9671523786028));
#202982=CARTESIAN_POINT('Ctrl Pts',(-47.9167391807674,-34.4546775021463,
40.0043257306692));
#202983=CARTESIAN_POINT('Ctrl Pts',(-47.8838297385504,-34.5405955452482,
39.9667894847832));
#202984=CARTESIAN_POINT('Ctrl Pts',(-47.9361122396534,-34.6112444014587,
40.0100138975199));
#202985=CARTESIAN_POINT('Ctrl Pts',(-47.796856449222,-34.497906166921,40.1195533054858));
#202986=CARTESIAN_POINT('Ctrl Pts',(-47.798338661273,-34.5561175928639,
40.0630813209239));
#202987=CARTESIAN_POINT('Ctrl Pts',(-47.8422046210391,-34.6187227036512,
40.0768265942422));
#202988=CARTESIAN_POINT('Ctrl Pts',(-47.7285944911485,-34.5493265808141,
40.1599502027527));
#202989=CARTESIAN_POINT('Ctrl Pts',(-47.7447672725766,-34.5905382782862,
40.100255279155));
#202990=CARTESIAN_POINT('Ctrl Pts',(-47.7940753146424,-34.6424336528568,
40.10025));
#202991=CARTESIAN_POINT('Ctrl Pts',(-47.6769115920305,-34.6205005703632,
40.1599502534424));
#202992=CARTESIAN_POINT('Ctrl Pts',(-47.7070975168466,-34.6424200234572,
40.10025));
#202993=CARTESIAN_POINT('Ctrl Pts',(-47.7640607692765,-34.6837837831344,
40.10025));
#202994=CARTESIAN_POINT('Origin',(-47.7640607692765,-34.6837837831344,40.22725));
#202995=CARTESIAN_POINT('Ctrl Pts',(-49.8669803696028,-36.6229335645807,
38.989));
#202996=CARTESIAN_POINT('Ctrl Pts',(-49.941740624821,-36.5200349009285,
38.989));
#202997=CARTESIAN_POINT('Ctrl Pts',(-49.9416290134545,-36.5201885207954,
39.1161896013263));
#202998=CARTESIAN_POINT('Ctrl Pts',(-50.0423873219314,-36.7506494346809,
38.989));
#202999=CARTESIAN_POINT('Ctrl Pts',(-50.1174293675647,-36.6476796282247,
38.9887769275478));
#203000=CARTESIAN_POINT('Ctrl Pts',(-50.0820075342382,-36.6221794864698,
39.1161898821845));
#203001=CARTESIAN_POINT('Ctrl Pts',(-50.2093732240197,-36.8722311236853,
39.1034967087243));
#203002=CARTESIAN_POINT('Ctrl Pts',(-50.2846385388084,-36.7691636147926,
39.1031720232704));
#203003=CARTESIAN_POINT('Ctrl Pts',(-50.2156454684932,-36.7192731293496,
39.2077529615001));
#203004=CARTESIAN_POINT('Ctrl Pts',(-50.3023253561997,-36.9399086546484,
39.2875012672119));
#203005=CARTESIAN_POINT('Ctrl Pts',(-50.377787724264,-36.8368401378451,
39.2872087095508));
#203006=CARTESIAN_POINT('Ctrl Pts',(-50.290034551302,-36.7733199617897,
39.3549017048226));
#203007=CARTESIAN_POINT('Origin',(-49.8669803696028,-36.6229335645807,39.116));
#203008=CARTESIAN_POINT('Origin',(3.64514313700082E-16,-3.44778646538029E-17,
40.22725));
#203009=CARTESIAN_POINT('Origin',(-47.7461450747866,-34.7084426211229,40.22725));
#203010=CARTESIAN_POINT('Origin',(40.911747809259,29.3316730956003,39.116));
#203011=CARTESIAN_POINT('Origin',(-49.5422481179709,-36.3870656659258,39.1160373285268));
#203012=CARTESIAN_POINT('Ctrl Pts',(-47.6590285860937,-34.6451144164183,
40.1599502534424));
#203013=CARTESIAN_POINT('Ctrl Pts',(-47.6892031885515,-34.6670494534015,
40.10025));
#203014=CARTESIAN_POINT('Ctrl Pts',(-47.7461450747866,-34.7084426211229,
40.10025));
#203015=CARTESIAN_POINT('Ctrl Pts',(-47.6074854095246,-34.7160192182665,
40.1599500566037));
#203016=CARTESIAN_POINT('Ctrl Pts',(-47.6516492793365,-34.7187044685528,
40.100255130536));
#203017=CARTESIAN_POINT('Ctrl Pts',(-47.7161963245903,-34.7496251732006,
40.10025));
#203018=CARTESIAN_POINT('Ctrl Pts',(-47.5796730526553,-34.7960378560833,
40.1203070619047));
#203019=CARTESIAN_POINT('Ctrl Pts',(-47.6353534770329,-34.7797813814943,
40.0637098684497));
#203020=CARTESIAN_POINT('Ctrl Pts',(-47.7083584310196,-34.8021505789969,
40.0772636213364));
#203021=CARTESIAN_POINT('Ctrl Pts',(-47.5752965616147,-34.9243313177593,
40.0046102245801));
#203022=CARTESIAN_POINT('Ctrl Pts',(-47.6468329724884,-34.8665693571824,
39.9670001894015));
#203023=CARTESIAN_POINT('Ctrl Pts',(-47.7301838844734,-34.8943788354695,
40.0101788811208));
#203024=CARTESIAN_POINT('Ctrl Pts',(-47.5970608435773,-34.9730260802972,
39.9303710930187));
#203025=CARTESIAN_POINT('Ctrl Pts',(-47.675314105656,-34.8923863483126,
39.9058663574112));
#203026=CARTESIAN_POINT('Ctrl Pts',(-47.7584998599245,-34.9340521716866,
39.9671344706364));
#203027=CARTESIAN_POINT('Ctrl Pts',(-47.6338034047601,-34.9997217530258,
39.8576902534424));
#203028=CARTESIAN_POINT('Ctrl Pts',(-47.7085070967805,-34.89773030317,39.8579948730703));
#203029=CARTESIAN_POINT('Ctrl Pts',(-47.7952442955504,-34.9607485668363,
39.92499));
#203030=CARTESIAN_POINT('Origin',(-47.7205955685092,-35.0634937251219,39.92499));
#203031=CARTESIAN_POINT('Origin',(-49.5064990280448,-36.3610285393809,39.1925554488848));
#203032=CARTESIAN_POINT('Origin',(-49.4402904249167,-36.312925173494,39.3343017080178));
#203033=CARTESIAN_POINT('Origin',(-47.8647214254841,-35.1682072895607,39.6398955069214));
#203034=CARTESIAN_POINT('Origin',(-48.0088472823274,-35.2729208539812,39.3548010137695));
#203035=CARTESIAN_POINT('Ctrl Pts',(-49.1733470784089,-36.118979479688,
39.3978017080178));
#203036=CARTESIAN_POINT('Ctrl Pts',(-49.2479958054501,-36.0162343214024,
39.3978017080178));
#203037=CARTESIAN_POINT('Ctrl Pts',(-49.2479958054501,-36.0162343214024,
39.5248017080178));
#203038=CARTESIAN_POINT('Ctrl Pts',(-49.2463047380079,-36.1716968449931,
39.3978017080178));
#203039=CARTESIAN_POINT('Ctrl Pts',(-49.3207474263653,-36.0690914679774,
39.3980355775177));
#203040=CARTESIAN_POINT('Ctrl Pts',(-49.357224477898,-36.0955935972134,
39.5248015517192));
#203041=CARTESIAN_POINT('Ctrl Pts',(-49.3152906263885,-36.2215465627859,
39.3484893995498));
#203042=CARTESIAN_POINT('Ctrl Pts',(-49.3898826892454,-36.1193211766487,
39.348943830343));
#203043=CARTESIAN_POINT('Ctrl Pts',(-49.4605079583576,-36.1706334382077,
39.4508333155595));
#203044=CARTESIAN_POINT('Ctrl Pts',(-49.3516463037387,-36.2478178023248,
39.2708017080178));
#203045=CARTESIAN_POINT('Ctrl Pts',(-49.4263574835553,-36.1458216659123,
39.2710850691867));
#203046=CARTESIAN_POINT('Ctrl Pts',(-49.5149391519579,-36.2101800152084,
39.3343017080178));
#203047=CARTESIAN_POINT('Origin',(-49.1733470784089,-36.118979479688,39.5248017080178));
#203048=CARTESIAN_POINT('Ctrl Pts',(-47.9220530736689,-35.2091516650526,
39.2875012672119));
#203049=CARTESIAN_POINT('Ctrl Pts',(-47.9968680956251,-35.1070032771121,
39.2878045257519));
#203050=CARTESIAN_POINT('Ctrl Pts',(-48.0836260518491,-35.1702703521464,
39.3549015218345));
#203051=CARTESIAN_POINT('Ctrl Pts',(-48.015002557559,-35.2768360036086,
39.1034938540228));
#203052=CARTESIAN_POINT('Ctrl Pts',(-48.0897575808459,-35.1744910995526,
39.1038286278798));
#203053=CARTESIAN_POINT('Ctrl Pts',(-48.1580164790744,-35.2243181613729,
39.2077506434033));
#203054=CARTESIAN_POINT('Ctrl Pts',(-48.181983339224,-35.3984277477545,
38.989));
#203055=CARTESIAN_POINT('Ctrl Pts',(-48.2567629686467,-35.2958269999282,
38.9892298954623));
#203056=CARTESIAN_POINT('Ctrl Pts',(-48.2916555365094,-35.3214126203077,
39.1161900347285));
#203057=CARTESIAN_POINT('Ctrl Pts',(-48.3573835402121,-35.5261472678863,
38.989));
#203058=CARTESIAN_POINT('Ctrl Pts',(-48.4321440857827,-35.4232482045984,
38.989));
#203059=CARTESIAN_POINT('Ctrl Pts',(-48.4320321836305,-35.4234022246976,
39.1161900945642));
#203060=CARTESIAN_POINT('Origin',(-48.3573835402121,-35.5261472678863,39.116));
#203061=CARTESIAN_POINT('Origin',(39.9252688514649,28.6149541797805,39.5248017080178));
#203062=CARTESIAN_POINT('Origin',(-49.0510171431405,-36.0301015792674,39.5248017080178));
#203063=CARTESIAN_POINT('Origin',(39.7707905934409,28.5027191556739,39.116));
#203064=CARTESIAN_POINT('Origin',(-48.6820620414869,-35.7621028045845,39.1160402713842));
#203065=CARTESIAN_POINT('Ctrl Pts',(-48.8727133447945,-35.9012693628902,
39.2708017080178));
#203066=CARTESIAN_POINT('Ctrl Pts',(-48.9481071848799,-35.7983524848933,
39.27051194648));
#203067=CARTESIAN_POINT('Ctrl Pts',(-48.8587224664502,-35.7334106856004,
39.3343017080178));
#203068=CARTESIAN_POINT('Ctrl Pts',(-48.9091935744932,-35.9276271141649,
39.3487519301186));
#203069=CARTESIAN_POINT('Ctrl Pts',(-48.9843245886175,-35.824665968965,
39.3482879464002));
#203070=CARTESIAN_POINT('Ctrl Pts',(-48.9133376106101,-35.7730909105057,
39.4512271261638));
#203071=CARTESIAN_POINT('Ctrl Pts',(-48.978304877513,-35.9775622448352,
39.3978017080178));
#203072=CARTESIAN_POINT('Ctrl Pts',(-49.0530211657568,-35.8745769537837,
39.3975673827364));
#203073=CARTESIAN_POINT('Ctrl Pts',(-49.0168051108907,-35.8482644497259,
39.5248015355181));
#203074=CARTESIAN_POINT('Ctrl Pts',(-49.0510171431405,-36.0301015792674,
39.3978017080178));
#203075=CARTESIAN_POINT('Ctrl Pts',(-49.1256658701817,-35.9273564209818,
39.3978017080178));
#203076=CARTESIAN_POINT('Ctrl Pts',(-49.1256658701817,-35.9273564209818,
39.5248017080178));
#203077=CARTESIAN_POINT('Origin',(-48.7840737394091,-35.836155843886,39.3343017080178));
#203078=CARTESIAN_POINT('Origin',(-48.7182599907933,-35.7883393569604,39.1934008533543));
#203079=CARTESIAN_POINT('Origin',(-53.3535596832587,-30.4370746247561,39.1925554495086));
#203080=CARTESIAN_POINT('Origin',(-53.3918862459828,-30.4591427892365,39.1160373285277));
#203081=CARTESIAN_POINT('Origin',(-53.2826856060847,-30.3961554568834,39.3343017080178));
#203082=CARTESIAN_POINT('Ctrl Pts',(-53.1871522506177,-30.3416565762233,
39.2708017080178));
#203083=CARTESIAN_POINT('Ctrl Pts',(-53.1243619179797,-30.451394201311,
39.2710850691866));
#203084=CARTESIAN_POINT('Ctrl Pts',(-53.2191856060847,-30.506140683164,
39.3343017080178));
#203085=CARTESIAN_POINT('Ctrl Pts',(-53.1482340195362,-30.3190533624374,
39.3487519293518));
#203086=CARTESIAN_POINT('Ctrl Pts',(-53.0851849835388,-30.4287753876648,
39.3492068662924));
#203087=CARTESIAN_POINT('Ctrl Pts',(-53.1607219582406,-30.4723866803434,
39.4512271248735));
#203088=CARTESIAN_POINT('Ctrl Pts',(-53.0745038491603,-30.2762311741509,
39.3978017080178));
#203089=CARTESIAN_POINT('Ctrl Pts',(-53.0110474253452,-30.3859720484844,
39.3980347781178));
#203090=CARTESIAN_POINT('Ctrl Pts',(-53.0499635164576,-30.408440264165,
39.5248015355195));
#203091=CARTESIAN_POINT('Ctrl Pts',(-52.9969317578289,-30.2311753956709,
39.3978017080178));
#203092=CARTESIAN_POINT('Ctrl Pts',(-52.9334317578289,-30.3411606219515,
39.3978017080178));
#203093=CARTESIAN_POINT('Ctrl Pts',(-52.9334317578289,-30.3411606219515,
39.5248017080178));
#203094=CARTESIAN_POINT('Origin',(-52.9969317578289,-30.2311753956709,39.5248017080178));
#203095=CARTESIAN_POINT('Origin',(-0.158749999999993,0.27496306570156,39.116));
#203096=CARTESIAN_POINT('Origin',(-53.7394427993288,-30.6598643453572,39.116));
#203097=CARTESIAN_POINT('Origin',(-0.158749999999993,0.27496306570156,39.5248017080178));
#203098=CARTESIAN_POINT('Origin',(-52.8659816883961,-30.1555713378335,39.5248017080178));
#203099=CARTESIAN_POINT('Ctrl Pts',(-54.2060847114743,-30.9286463962975,
39.2875012672119));
#203100=CARTESIAN_POINT('Ctrl Pts',(-54.1426202518671,-31.0395064328255,
39.287208709576));
#203101=CARTESIAN_POINT('Ctrl Pts',(-54.0488992551384,-30.9851759176836,
39.3549016990122));
#203102=CARTESIAN_POINT('Ctrl Pts',(-54.1064496608377,-30.8712564593355,
39.1034939173931));
#203103=CARTESIAN_POINT('Ctrl Pts',(-54.0429059732646,-30.981936066785,
39.1031692336346));
#203104=CARTESIAN_POINT('Ctrl Pts',(-53.9692670413541,-30.9392002377687,
39.2077507202299));
#203105=CARTESIAN_POINT('Ctrl Pts',(-53.9274585619034,-30.7681581606525,
38.989));
#203106=CARTESIAN_POINT('Ctrl Pts',(-53.8639133132304,-30.8785940576174,
38.9887769311158));
#203107=CARTESIAN_POINT('Ctrl Pts',(-53.8262110069737,-30.8566067980797,
39.1161898712914));
#203108=CARTESIAN_POINT('Ctrl Pts',(-53.7394427993288,-30.6598643453572,
38.989));
#203109=CARTESIAN_POINT('Ctrl Pts',(-53.6758479332735,-30.7700138844655,
38.989));
#203110=CARTESIAN_POINT('Ctrl Pts',(-53.6759428700858,-30.7698494490832,
39.1161895903853));
#203111=CARTESIAN_POINT('Origin',(-54.1125387249981,-30.8752713784759,39.3548010137695));
#203112=CARTESIAN_POINT('Ctrl Pts',(-52.8659816883961,-30.1555713378335,
39.3978017080178));
#203113=CARTESIAN_POINT('Ctrl Pts',(-52.8024816883961,-30.2655565641141,
39.3978017080178));
#203114=CARTESIAN_POINT('Ctrl Pts',(-52.8024816883961,-30.2655565641141,
39.5248017080178));
#203115=CARTESIAN_POINT('Ctrl Pts',(-52.7881477055078,-30.1103627734741,
39.3978017080178));
#203116=CARTESIAN_POINT('Ctrl Pts',(-52.7244553345201,-30.2205080277005,
39.3975666025026));
#203117=CARTESIAN_POINT('Ctrl Pts',(-52.6855560684216,-30.1980495259467,
39.5248015517178));
#203118=CARTESIAN_POINT('Ctrl Pts',(-52.7145506960112,-30.0676130472589,
39.3484894016717));
#203119=CARTESIAN_POINT('Ctrl Pts',(-52.651050001129,-30.1781274387059,
39.3480259000041));
#203120=CARTESIAN_POINT('Ctrl Pts',(-52.5749945583575,-30.1342168083492,
39.4508333188947));
#203121=CARTESIAN_POINT('Ctrl Pts',(-52.6757649139397,-30.0450834959833,
39.2708017080178));
#203122=CARTESIAN_POINT('Ctrl Pts',(-52.6124111049558,-30.1558192615998,
39.27051194648));
#203123=CARTESIAN_POINT('Ctrl Pts',(-52.5167277788843,-30.1005764675355,
39.3343017080178));
#203124=CARTESIAN_POINT('Origin',(-52.5802277788843,-29.9905912412549,39.3343017080178));
#203125=CARTESIAN_POINT('Origin',(-54.2668203812025,-30.9643459342458,39.6398955068168));
#203126=CARTESIAN_POINT('Origin',(-54.421102037244,-31.0534204898631,39.92499));
#203127=CARTESIAN_POINT('Origin',(-52.5097763801588,-29.949916107243,39.1934008539947));
#203128=CARTESIAN_POINT('Origin',(-52.4710850656385,-29.927519002606,39.1160402713848));
#203129=CARTESIAN_POINT('Ctrl Pts',(-54.5275217339721,-31.4638515574737,
40.1599502534424));
#203130=CARTESIAN_POINT('Ctrl Pts',(-54.4952102564867,-31.445206962985,
40.10025));
#203131=CARTESIAN_POINT('Ctrl Pts',(-54.4342359163065,-31.4100231232058,
40.10025));
#203132=CARTESIAN_POINT('Ctrl Pts',(-54.5715608148707,-31.3875306471678,
40.1599500538458));
#203133=CARTESIAN_POINT('Ctrl Pts',(-54.5272862282506,-31.3896121658898,
40.100244835349));
#203134=CARTESIAN_POINT('Ctrl Pts',(-54.4597196360178,-31.3658411130326,
40.10025));
#203135=CARTESIAN_POINT('Ctrl Pts',(-54.5905300051367,-31.3046029601553,
40.1202442001039));
#203136=CARTESIAN_POINT('Ctrl Pts',(-54.5367961153118,-31.3268524737455,
40.0633873868018));
#203137=CARTESIAN_POINT('Ctrl Pts',(-54.4615686025424,-31.312567293429,
40.0772271723537));
#203138=CARTESIAN_POINT('Ctrl Pts',(-54.5809273110395,-31.1759014746041,
40.0045995998163));
#203139=CARTESIAN_POINT('Ctrl Pts',(-54.5158579940067,-31.2415992967182,
39.9663485808315));
#203140=CARTESIAN_POINT('Ctrl Pts',(-54.4295063924929,-31.2227682191857,
40.0101727202466));
#203141=CARTESIAN_POINT('Ctrl Pts',(-54.5540292360078,-31.1295364123889,
39.9304654349859));
#203142=CARTESIAN_POINT('Ctrl Pts',(-54.4847364330945,-31.2191033458793,
39.9051900162955));
#203143=CARTESIAN_POINT('Ctrl Pts',(-54.3969835118368,-31.1861426211009,
39.9671857458175));
#203144=CARTESIAN_POINT('Ctrl Pts',(-54.514646476914,-31.1067982185532,
39.8576902534424));
#203145=CARTESIAN_POINT('Ctrl Pts',(-54.4512761425984,-31.2174884860862,
39.8573998014387));
#203146=CARTESIAN_POINT('Ctrl Pts',(-54.357602037244,-31.1634057161437,
39.92499));
#203147=CARTESIAN_POINT('Origin',(-54.4342359163065,-31.4100231232058,40.22725));
#203148=CARTESIAN_POINT('Origin',(-0.158749999999993,0.27496306570156,39.116));
#203149=CARTESIAN_POINT('Origin',(-52.1234703131948,-29.7268821954847,39.116));
#203150=CARTESIAN_POINT('Origin',(1.12590909550281E-16,8.2444796405856E-17,
40.22725));
#203151=CARTESIAN_POINT('Origin',(-54.4189959163065,-31.4364195775132,40.22725));
#203152=CARTESIAN_POINT('Ctrl Pts',(-52.1234703131948,-29.7268821954847,
38.989));
#203153=CARTESIAN_POINT('Ctrl Pts',(-52.0598751873274,-29.8370321846007,
38.989));
#203154=CARTESIAN_POINT('Ctrl Pts',(-52.0599703843396,-29.8368672985389,
39.1161901092321));
#203155=CARTESIAN_POINT('Ctrl Pts',(-51.9354481180167,-29.6185926664424,
38.989));
#203156=CARTESIAN_POINT('Ctrl Pts',(-51.872133287597,-29.72863875449,38.9892298989754));
#203157=CARTESIAN_POINT('Ctrl Pts',(-51.909699589874,-29.7501084151998,
39.1161900493201));
#203158=CARTESIAN_POINT('Ctrl Pts',(-51.7564527430629,-29.5155047636231,
39.1034966344368));
#203159=CARTESIAN_POINT('Ctrl Pts',(-51.6933616226679,-29.6254243098839,
39.1038314102575));
#203160=CARTESIAN_POINT('Ctrl Pts',(-51.7666446199949,-29.6675155901168,
39.2077528789601));
#203161=CARTESIAN_POINT('Ctrl Pts',(-51.6568155675429,-29.4581217525671,
39.2875012672119));
#203162=CARTESIAN_POINT('Ctrl Pts',(-51.5939283753697,-29.5680161811087,
39.2878045257868));
#203163=CARTESIAN_POINT('Ctrl Pts',(-51.6870133822662,-29.6215404737378,
39.3549015295899));
#203164=CARTESIAN_POINT('Origin',(-51.7503740054945,-29.5114749418002,39.3548010137695));
#203165=CARTESIAN_POINT('Ctrl Pts',(-54.1966007261209,-31.6576696180581,
39.8576902534424));
#203166=CARTESIAN_POINT('Ctrl Pts',(-54.2607761425984,-31.5474441649281,
39.8573998014387));
#203167=CARTESIAN_POINT('Ctrl Pts',(-54.167102037244,-31.4933613949856,
39.92499));
#203168=CARTESIAN_POINT('Ctrl Pts',(-54.2360018544267,-31.6804173066003,
39.9304984902492));
#203169=CARTESIAN_POINT('Ctrl Pts',(-54.2789150989584,-31.5756301844103,
39.9052171569797));
#203170=CARTESIAN_POINT('Ctrl Pts',(-54.2065014563939,-31.5161086602377,
39.9672049726601));
#203171=CARTESIAN_POINT('Ctrl Pts',(-54.2894509908545,-31.6804328064622,
40.0043437678661));
#203172=CARTESIAN_POINT('Ctrl Pts',(-54.3138841827106,-31.5911964272959,
39.9661628577643));
#203173=CARTESIAN_POINT('Ctrl Pts',(-54.2543268901841,-31.5258675551963,
40.0100243556237));
#203174=CARTESIAN_POINT('Ctrl Pts',(-54.4049648787501,-31.6250591602187,
40.1194874821989));
#203175=CARTESIAN_POINT('Ctrl Pts',(-54.3976088886511,-31.5671393481781,
40.062755148314));
#203176=CARTESIAN_POINT('Ctrl Pts',(-54.3475791360314,-31.5090508246492,
40.0767884282375));
#203177=CARTESIAN_POINT('Ctrl Pts',(-54.4680334478296,-31.5668453499336,
40.1599502015396));
#203178=CARTESIAN_POINT('Ctrl Pts',(-54.4477213412895,-31.5274226111431,
40.1002449453875));
#203179=CARTESIAN_POINT('Ctrl Pts',(-54.393390646534,-31.4807263372353,
40.10025));
#203180=CARTESIAN_POINT('Ctrl Pts',(-54.5122556166612,-31.4902932482905,
40.1599502534424));
#203181=CARTESIAN_POINT('Ctrl Pts',(-54.4799531854481,-31.4716329851986,
40.10025));
#203182=CARTESIAN_POINT('Ctrl Pts',(-54.4189959163065,-31.4364195775132,
40.10025));
#203183=CARTESIAN_POINT('Origin',(-54.103602037244,-31.6033466212662,39.92499));
#203184=CARTESIAN_POINT('Origin',(-51.5960921371862,-29.4224002636365,39.6398955069316));
#203185=CARTESIAN_POINT('Origin',(-51.4418102687787,-29.3333255853452,39.92499));
#203186=CARTESIAN_POINT('Origin',(-53.9493203812131,-31.5142720655985,39.6398955068269));
#203187=CARTESIAN_POINT('Origin',(-53.7950387249981,-31.425197509879,39.3548010137695));
#203188=CARTESIAN_POINT('Ctrl Pts',(-51.3482501200167,-29.2799753962459,
39.8576902534424));
#203189=CARTESIAN_POINT('Ctrl Pts',(-51.2854610232003,-29.3897042746971,
39.8579948730703));
#203190=CARTESIAN_POINT('Ctrl Pts',(-51.3783102687786,-29.4433108116258,
39.92499));
#203191=CARTESIAN_POINT('Ctrl Pts',(-51.3089010921303,-29.25725783855,39.9304020711229));
#203192=CARTESIAN_POINT('Ctrl Pts',(-51.2670685993226,-29.3615397594614,
39.9058915297381));
#203193=CARTESIAN_POINT('Ctrl Pts',(-51.3389598763138,-29.4205918519435,
39.9671523786034));
#203194=CARTESIAN_POINT('Ctrl Pts',(-51.2557407616057,-29.2572680623747,
40.0043257306695));
#203195=CARTESIAN_POINT('Ctrl Pts',(-51.231992481769,-29.3461554108685,
39.9667894847835));
#203196=CARTESIAN_POINT('Ctrl Pts',(-51.2913733902316,-29.4109522357565,
40.0100138975202));
#203197=CARTESIAN_POINT('Ctrl Pts',(-51.1410333861058,-29.3127910737011,
40.1195533054855));
#203198=CARTESIAN_POINT('Ctrl Pts',(-51.1485922293426,-29.3705286780142,
40.0630813209236));
#203199=CARTESIAN_POINT('Ctrl Pts',(-51.1987619028147,-29.4282055900899,
40.0768265942419));
#203200=CARTESIAN_POINT('Ctrl Pts',(-51.0785202710257,-29.3710651187643,
40.1599502027521));
#203201=CARTESIAN_POINT('Ctrl Pts',(-51.0989122516715,-29.4103605382566,
40.1002552791547));
#203202=CARTESIAN_POINT('Ctrl Pts',(-51.1533747228767,-29.4568175306708,
40.10025));
#203203=CARTESIAN_POINT('Ctrl Pts',(-51.0345602039888,-29.4472515437732,
40.1599502534424));
#203204=CARTESIAN_POINT('Ctrl Pts',(-51.0668719738979,-29.4658956314764,
40.10025));
#203205=CARTESIAN_POINT('Ctrl Pts',(-51.1278468659049,-29.5010785149108,
40.10025));
#203206=CARTESIAN_POINT('Origin',(-51.1278468659049,-29.5010785149108,40.22725));
#203207=CARTESIAN_POINT('Ctrl Pts',(-53.4219427993288,-31.2097904767603,
38.989));
#203208=CARTESIAN_POINT('Ctrl Pts',(-53.4855376708629,-31.0996409281624,
38.989));
#203209=CARTESIAN_POINT('Ctrl Pts',(-53.4854427285637,-31.0998053730485,
39.1161896013265));
#203210=CARTESIAN_POINT('Ctrl Pts',(-53.6097387976566,-31.3184716867864,
38.989));
#203211=CARTESIAN_POINT('Ctrl Pts',(-53.673606479479,-31.2082219299921,
38.9887769275485));
#203212=CARTESIAN_POINT('Ctrl Pts',(-53.6357132000306,-31.1865640704875,
39.1161898821847));
#203213=CARTESIAN_POINT('Ctrl Pts',(-53.7885186806131,-31.4219325588467,
39.1034967087243));
#203214=CARTESIAN_POINT('Ctrl Pts',(-53.8525981958179,-31.3115622968592,
39.1031720232692));
#203215=CARTESIAN_POINT('Ctrl Pts',(-53.7787681009845,-31.2691568563318,
39.2077529614999));
#203216=CARTESIAN_POINT('Ctrl Pts',(-53.8880358395972,-31.4795232016787,
39.2875012672119));
#203217=CARTESIAN_POINT('Ctrl Pts',(-53.9523112232408,-31.3691313396262,
39.2872087095508));
#203218=CARTESIAN_POINT('Ctrl Pts',(-53.8583991049523,-31.3151318380581,
39.3549017048227));
#203219=CARTESIAN_POINT('Origin',(-53.4219427993288,-31.2097904767603,39.116));
#203220=CARTESIAN_POINT('Origin',(3.61170357355341E-16,-2.93286234380096E-17,
40.22725));
#203221=CARTESIAN_POINT('Origin',(-51.1126068659049,-29.5274749692182,40.22725));
#203222=CARTESIAN_POINT('Origin',(46.8255917980726,26.668150608645,39.116));
#203223=CARTESIAN_POINT('Origin',(-53.0743345559669,-31.0091584503666,39.1160373285225));
#203224=CARTESIAN_POINT('Ctrl Pts',(-51.0193480105329,-29.4735998357335,
40.1599502534424));
#203225=CARTESIAN_POINT('Ctrl Pts',(-51.0516501490688,-29.4922606054643,
40.10025));
#203226=CARTESIAN_POINT('Ctrl Pts',(-51.1126068659049,-29.5274749692182,
40.10025));
#203227=CARTESIAN_POINT('Ctrl Pts',(-50.9754987628538,-29.5495039426968,
40.1599500566034));
#203228=CARTESIAN_POINT('Ctrl Pts',(-51.0197013834521,-29.5475581014576,
40.1002551305372));
#203229=CARTESIAN_POINT('Ctrl Pts',(-51.0871269269763,-29.5715624158004,
40.10025));
#203230=CARTESIAN_POINT('Ctrl Pts',(-50.9562029902289,-29.6319914129669,
40.1203070619047));
#203231=CARTESIAN_POINT('Ctrl Pts',(-51.0098791271085,-29.6100038038525,
40.0637098684499));
#203232=CARTESIAN_POINT('Ctrl Pts',(-51.0848223701588,-29.6246193648993,
40.0772636213362));
#203233=CARTESIAN_POINT('Ctrl Pts',(-50.9652607924606,-29.7600395375188,
40.0046102245802));
#203234=CARTESIAN_POINT('Ctrl Pts',(-51.0303675504166,-29.6951164119093,
39.9670001894012));
#203235=CARTESIAN_POINT('Ctrl Pts',(-51.1161687394136,-29.7140610042229,
40.010178881121));
#203236=CARTESIAN_POINT('Ctrl Pts',(-50.9919958361064,-29.8061925581054,
39.9303710930186));
#203237=CARTESIAN_POINT('Ctrl Pts',(-51.061391271364,-29.71781488578,39.905866357411));
#203238=CARTESIAN_POINT('Ctrl Pts',(-51.1484765898559,-29.7505571803534,
39.967134470636));
#203239=CARTESIAN_POINT('Ctrl Pts',(-51.031327575341,-29.8289013456883,
39.8576902534424));
#203240=CARTESIAN_POINT('Ctrl Pts',(-51.0949610232003,-29.719659953539,
39.8579948730703));
#203241=CARTESIAN_POINT('Ctrl Pts',(-51.1878102687787,-29.7732664904677,
39.92499));
#203242=CARTESIAN_POINT('Origin',(-51.1243102687787,-29.8832517167483,39.92499));
#203243=CARTESIAN_POINT('Origin',(-53.0360596824723,-30.9870007553603,39.1925554488847));
#203244=CARTESIAN_POINT('Origin',(-52.9651856060848,-30.9460815882865,39.3343017080178));
#203245=CARTESIAN_POINT('Origin',(-51.2785921372023,-29.9723263949832,39.6398955069226));
#203246=CARTESIAN_POINT('Origin',(-51.4328740054945,-30.0614010732033,39.3548010137695));
#203247=CARTESIAN_POINT('Ctrl Pts',(-52.6794317578289,-30.781101527074,
39.3978017080178));
#203248=CARTESIAN_POINT('Ctrl Pts',(-52.7429317578289,-30.6711163007934,
39.3978017080178));
#203249=CARTESIAN_POINT('Ctrl Pts',(-52.7429317578289,-30.6711163007934,
39.5248017080178));
#203250=CARTESIAN_POINT('Ctrl Pts',(-52.7575002129172,-30.8259039490956,
39.3978017080178));
#203251=CARTESIAN_POINT('Ctrl Pts',(-52.820809914056,-30.7160792752574,
39.3980355775177));
#203252=CARTESIAN_POINT('Ctrl Pts',(-52.8598573673265,-30.738623332912,
39.5248015517192));
#203253=CARTESIAN_POINT('Ctrl Pts',(-52.8313189037791,-30.8682695960175,
39.3484893995498));
#203254=CARTESIAN_POINT('Ctrl Pts',(-52.8948168809914,-30.7588072175368,
39.3489438303428));
#203255=CARTESIAN_POINT('Ctrl Pts',(-52.9704188493375,-30.8024560343131,
39.4508333155596));
#203256=CARTESIAN_POINT('Ctrl Pts',(-52.8702215132218,-30.8905967158733,
39.2708017080178));
#203257=CARTESIAN_POINT('Ctrl Pts',(-52.9338619179797,-30.7813498801529,
39.2710850691866));
#203258=CARTESIAN_POINT('Ctrl Pts',(-53.0286856060847,-30.8360963620059,
39.3343017080178));
#203259=CARTESIAN_POINT('Origin',(-52.6794317578289,-30.781101527074,39.5248017080178));
#203260=CARTESIAN_POINT('Ctrl Pts',(-51.3398895692699,-30.0070536838155,
39.2875012672119));
#203261=CARTESIAN_POINT('Ctrl Pts',(-51.4036173326911,-29.8976445761577,
39.2878045257519));
#203262=CARTESIAN_POINT('Ctrl Pts',(-51.496513229882,-29.9514963916949,
39.3549015218345));
#203263=CARTESIAN_POINT('Ctrl Pts',(-51.4394048060578,-30.0646513737712,
39.1034938540228));
#203264=CARTESIAN_POINT('Ctrl Pts',(-51.5030523579637,-29.9550530981071,
39.1038286278806));
#203265=CARTESIAN_POINT('Ctrl Pts',(-51.576145673005,-29.9974722043277,
39.2077506434033));
#203266=CARTESIAN_POINT('Ctrl Pts',(-51.6181806476914,-30.168122781117,
38.989));
#203267=CARTESIAN_POINT('Ctrl Pts',(-51.6818259279747,-30.0582674911768,
38.989229895463));
#203268=CARTESIAN_POINT('Ctrl Pts',(-51.7192017762845,-30.0800656843509,
39.1161900347285));
#203269=CARTESIAN_POINT('Ctrl Pts',(-51.8059703131948,-30.2768083268878,
38.989));
#203270=CARTESIAN_POINT('Ctrl Pts',(-51.8695654317172,-30.1666583504936,
38.989));
#203271=CARTESIAN_POINT('Ctrl Pts',(-51.869470242061,-30.1668232238145,
39.1161900945642));
#203272=CARTESIAN_POINT('Origin',(-51.8059703131948,-30.2768083268878,39.116));
#203273=CARTESIAN_POINT('Origin',(45.6951875000003,26.0155113828598,39.5248017080178));
#203274=CARTESIAN_POINT('Origin',(-52.5484816883961,-30.7054974692366,39.5248017080178));
#203275=CARTESIAN_POINT('Origin',(45.5181711678734,25.9133109558554,39.116));
#203276=CARTESIAN_POINT('Origin',(-52.1535342613174,-30.4775331296738,39.1160402713853));
#203277=CARTESIAN_POINT('Ctrl Pts',(-52.3576880233164,-30.5960088312565,
39.2708017080178));
#203278=CARTESIAN_POINT('Ctrl Pts',(-52.4219111049558,-30.4857749404417,
39.2705119464801));
#203279=CARTESIAN_POINT('Ctrl Pts',(-52.3262277788843,-30.4305321463774,
39.3343017080178));
#203280=CARTESIAN_POINT('Ctrl Pts',(-52.3967235457367,-30.6184089696602,
39.3487519301186));
#203281=CARTESIAN_POINT('Ctrl Pts',(-52.4606806140216,-30.5081585269385,
39.3482879463983));
#203282=CARTESIAN_POINT('Ctrl Pts',(-52.3846914485048,-30.4642861617706,
39.4512271261628));
#203283=CARTESIAN_POINT('Ctrl Pts',(-52.4706758922785,-30.6608464521622,
39.3978017080178));
#203284=CARTESIAN_POINT('Ctrl Pts',(-52.5342179826636,-30.5506153465186,
39.3975673827383));
#203285=CARTESIAN_POINT('Ctrl Pts',(-52.49544991752,-30.5282325936716,39.5248015355181));
#203286=CARTESIAN_POINT('Ctrl Pts',(-52.5484816883961,-30.7054974692366,
39.3978017080178));
#203287=CARTESIAN_POINT('Ctrl Pts',(-52.6119816883961,-30.595512242956,
39.3978017080178));
#203288=CARTESIAN_POINT('Ctrl Pts',(-52.6119816883961,-30.595512242956,
39.5248017080178));
#203289=CARTESIAN_POINT('Origin',(-52.2627277788843,-30.540517372658,39.3343017080178));
#203290=CARTESIAN_POINT('Origin',(-52.1922763809707,-30.499842239456,39.193400853355));
#203291=CARTESIAN_POINT('Origin',(-56.242823937725,-24.6933715417292,39.1925554495076));
#203292=CARTESIAN_POINT('Origin',(-56.2832472948486,-24.7113125977911,39.1160373285244));
#203293=CARTESIAN_POINT('Origin',(-56.1680608984279,-24.6600848917108,39.3343017080178));
#203294=CARTESIAN_POINT('Ctrl Pts',(-56.0673542004327,-24.6158705164591,
39.2708017080178));
#203295=CARTESIAN_POINT('Ctrl Pts',(-56.0163785451199,-24.7315703643332,
39.2710850691866));
#203296=CARTESIAN_POINT('Ctrl Pts',(-56.1164053447573,-24.7761051648314,
39.3343017080178));
#203297=CARTESIAN_POINT('Ctrl Pts',(-56.0262864882905,-24.5974591883331,
39.3487519293518));
#203298=CARTESIAN_POINT('Ctrl Pts',(-55.9750519161917,-24.7131705636681,
39.349206866292));
#203299=CARTESIAN_POINT('Ctrl Pts',(-56.0547337128487,-24.7486471852359,
39.4512271248737));
#203300=CARTESIAN_POINT('Ctrl Pts',(-55.9484840819671,-24.5625784858803,
39.3978017080178));
#203301=CARTESIAN_POINT('Ctrl Pts',(-55.8968463240338,-24.6783511906885,
39.3980347781178));
#203302=CARTESIAN_POINT('Ctrl Pts',(-55.937897796785,-24.6966284839301,
39.524801535519));
#203303=CARTESIAN_POINT('Ctrl Pts',(-55.8666273273834,-24.5258780191668,
39.3978017080178));
#203304=CARTESIAN_POINT('Ctrl Pts',(-55.8149717737128,-24.6418982922874,
39.3978017080178));
#203305=CARTESIAN_POINT('Ctrl Pts',(-55.8149717737128,-24.6418982922874,
39.5248017080178));
#203306=CARTESIAN_POINT('Origin',(-55.8666273273834,-24.5258780191668,39.5248017080178));
#203307=CARTESIAN_POINT('Origin',(-0.129138884176559,0.290050682801527,
39.116));
#203308=CARTESIAN_POINT('Origin',(-56.6498810128383,-24.8746050278049,39.116));
#203309=CARTESIAN_POINT('Origin',(-0.129138884176559,0.290050682801527,
39.5248017080178));
#203310=CARTESIAN_POINT('Origin',(-55.7284918401499,-24.4643761377914,39.5248017080178));
#203311=CARTESIAN_POINT('Ctrl Pts',(-57.1420619865023,-25.0931373005742,
39.2875012672119));
#203312=CARTESIAN_POINT('Ctrl Pts',(-57.0905332211012,-25.2100238766575,
39.287208709576));
#203313=CARTESIAN_POINT('Ctrl Pts',(-56.9916465525425,-25.1657875015262,
39.3549016990122));
#203314=CARTESIAN_POINT('Ctrl Pts',(-57.0369738651806,-25.0464764504217,
39.1034939173931));
#203315=CARTESIAN_POINT('Ctrl Pts',(-56.9853474458546,-25.1631918674178,
39.1031692336355));
#203316=CARTESIAN_POINT('Ctrl Pts',(-56.9076448051892,-25.1283875141303,
39.2077507202296));
#203317=CARTESIAN_POINT('Ctrl Pts',(-56.8481865914866,-24.9626525995185,
38.989));
#203318=CARTESIAN_POINT('Ctrl Pts',(-56.7965331449355,-25.0791258042767,
38.9887769311152));
#203319=CARTESIAN_POINT('Ctrl Pts',(-56.7567390814047,-25.06119995738,39.1161898712914));
#203320=CARTESIAN_POINT('Ctrl Pts',(-56.6498810128383,-24.8746050278049,
38.989));
#203321=CARTESIAN_POINT('Ctrl Pts',(-56.5981482881659,-24.9907986298333,
38.989));
#203322=CARTESIAN_POINT('Ctrl Pts',(-56.5982255167266,-24.9906251716462,
39.1161895903852));
#203323=CARTESIAN_POINT('Origin',(-57.043449246138,-25.0498328948962,39.3548010137695));
#203324=CARTESIAN_POINT('Ctrl Pts',(-55.7284918401499,-24.4643761377914,
39.3978017080178));
#203325=CARTESIAN_POINT('Ctrl Pts',(-55.6768362864793,-24.580396410912,
39.3978017080178));
#203326=CARTESIAN_POINT('Ctrl Pts',(-55.6768362864793,-24.580396410912,
39.5248017080178));
#203327=CARTESIAN_POINT('Ctrl Pts',(-55.6463586582056,-24.4275510972974,
39.3978017080178));
#203328=CARTESIAN_POINT('Ctrl Pts',(-55.5945285148507,-24.5437506299579,
39.397566602504));
#203329=CARTESIAN_POINT('Ctrl Pts',(-55.5534947903273,-24.5254812387363,
39.5248015517196));
#203330=CARTESIAN_POINT('Ctrl Pts',(-55.5686962576408,-24.39272854086,39.3484894016716));
#203331=CARTESIAN_POINT('Ctrl Pts',(-55.517095325717,-24.5092751529583,
39.3480259000031));
#203332=CARTESIAN_POINT('Ctrl Pts',(-55.4368666119034,-24.4735550281866,
39.4508333188939));
#203333=CARTESIAN_POINT('Ctrl Pts',(-55.5277679687684,-24.3743766270211,
39.2708017080178));
#203334=CARTESIAN_POINT('Ctrl Pts',(-55.4763362579876,-24.4911280468223,
39.27051194648));
#203335=CARTESIAN_POINT('Ctrl Pts',(-55.3754026508176,-24.4461895095986,
39.3343017080178));
#203336=CARTESIAN_POINT('Origin',(-55.4270582044882,-24.330169236478,39.3343017080178));
#203337=CARTESIAN_POINT('Origin',(-57.206196557715,-25.1222926664907,39.6398955068199));
#203338=CARTESIAN_POINT('Origin',(-57.3689438691197,-25.1947524379613,39.92499));
#203339=CARTESIAN_POINT('Origin',(-55.3527410366459,-24.2970811015516,39.1934008539938));
#203340=CARTESIAN_POINT('Origin',(-55.3119205422647,-24.2788510342449,39.1160402713843));
#203341=CARTESIAN_POINT('Ctrl Pts',(-57.517682316389,-25.5918112338791,
40.1599502534424));
#203342=CARTESIAN_POINT('Ctrl Pts',(-57.4835989537479,-25.5766462455173,
40.10025));
#203343=CARTESIAN_POINT('Ctrl Pts',(-57.419280924679,-25.5480287005715,
40.10025));
#203344=CARTESIAN_POINT('Ctrl Pts',(-57.553502439126,-25.5113050800555,
40.1599500538472));
#203345=CARTESIAN_POINT('Ctrl Pts',(-57.5096879712806,-25.5180031505023,
40.1002448353506));
#203346=CARTESIAN_POINT('Ctrl Pts',(-57.4400067642827,-25.5014249500142,
40.10025));
#203347=CARTESIAN_POINT('Ctrl Pts',(-57.5636994104963,-25.4268488592816,
40.1202442001041));
#203348=CARTESIAN_POINT('Ctrl Pts',(-57.5125855880052,-25.4545932086374,
40.0633873868015));
#203349=CARTESIAN_POINT('Ctrl Pts',(-57.4362769714769,-25.4482497003382,
40.0772271723539));
#203350=CARTESIAN_POINT('Ctrl Pts',(-57.5406963524571,-25.2998561687909,
40.004599599816));
#203351=CARTESIAN_POINT('Ctrl Pts',(-57.4828507843379,-25.3719956870764,
39.9663485808318));
#203352=CARTESIAN_POINT('Ctrl Pts',(-57.395003842335,-25.3622939683644,
40.0101727202465));
#203353=CARTESIAN_POINT('Ctrl Pts',(-57.5090991591924,-25.2565567136861,
39.9304654349861));
#203354=CARTESIAN_POINT('Ctrl Pts',(-57.4495482434214,-25.3528760603493,
39.9051900162944));
#203355=CARTESIAN_POINT('Ctrl Pts',(-57.3588307079386,-25.3292685758746,
39.9671857458173));
#203356=CARTESIAN_POINT('Ctrl Pts',(-57.4675553545142,-25.2380597013427,
39.8576902534424));
#203357=CARTESIAN_POINT('Ctrl Pts',(-57.4161024530845,-25.3547675996712,
39.8573998014387));
#203358=CARTESIAN_POINT('Ctrl Pts',(-57.3172883154491,-25.3107727110819,
39.92499));
#203359=CARTESIAN_POINT('Origin',(-57.419280924679,-25.5480287005715,40.22725));
#203360=CARTESIAN_POINT('Origin',(-0.129138884176559,0.290050682801527,
39.116));
#203361=CARTESIAN_POINT('Origin',(-54.945237802683,-24.1156489724274,39.116));
#203362=CARTESIAN_POINT('Origin',(1.20426471881346E-16,6.70666394583711E-17,
40.22725));
#203363=CARTESIAN_POINT('Origin',(-57.4068835917981,-25.5758735661205,40.22725));
#203364=CARTESIAN_POINT('Ctrl Pts',(-54.945237802683,-24.1156489724274,
38.989));
#203365=CARTESIAN_POINT('Ctrl Pts',(-54.8935048666604,-24.2318430491562,
38.989));
#203366=CARTESIAN_POINT('Ctrl Pts',(-54.8935823068867,-24.23166911556,39.1161901092322));
#203367=CARTESIAN_POINT('Ctrl Pts',(-54.746926274704,-24.027606335879,38.989));
#203368=CARTESIAN_POINT('Ctrl Pts',(-54.6954612380238,-24.1436677818706,
38.9892298989736));
#203369=CARTESIAN_POINT('Ctrl Pts',(-54.7350659388068,-24.1610930816813,
39.1161900493202));
#203370=CARTESIAN_POINT('Ctrl Pts',(-54.5581358350805,-23.9437932708512,
39.1034966344368));
#203371=CARTESIAN_POINT('Ctrl Pts',(-54.5068800556949,-24.0597054841957,
39.1038314102579));
#203372=CARTESIAN_POINT('Ctrl Pts',(-54.5841613379365,-24.0939060248996,
39.20775287896));
#203373=CARTESIAN_POINT('Ctrl Pts',(-54.4530463244694,-23.8971395307765,
39.2875012672119));
#203374=CARTESIAN_POINT('Ctrl Pts',(-54.401990730652,-24.0130054476974,
39.2878045257868));
#203375=CARTESIAN_POINT('Ctrl Pts',(-54.5001606201971,-24.0565064959268,
39.3549015295899));
#203376=CARTESIAN_POINT('Origin',(-54.5516691663896,-23.9404209259118,39.3548010137695));
#203377=CARTESIAN_POINT('Ctrl Pts',(-57.20883363247,-25.8191582032617,39.8576902534424));
#203378=CARTESIAN_POINT('Ctrl Pts',(-57.2611357920726,-25.702828419033,
39.8573998014387));
#203379=CARTESIAN_POINT('Ctrl Pts',(-57.1623216544372,-25.6588335304438,
39.92499));
#203380=CARTESIAN_POINT('Ctrl Pts',(-57.2503966981984,-25.8376627381934,
39.9304984902492));
#203381=CARTESIAN_POINT('Ctrl Pts',(-57.2821216226325,-25.7289639953181,
39.9052171569799));
#203382=CARTESIAN_POINT('Ctrl Pts',(-57.2038829761264,-25.6773378230591,
39.9672049726609));
#203383=CARTESIAN_POINT('Ctrl Pts',(-57.3035546548412,-25.8320911970516,
40.0043437678661));
#203384=CARTESIAN_POINT('Ctrl Pts',(-57.3185262575343,-25.74078970011,39.9661628577643));
#203385=CARTESIAN_POINT('Ctrl Pts',(-57.2524664994798,-25.6820441386712,
40.0100243556236));
#203386=CARTESIAN_POINT('Ctrl Pts',(-57.4126476234253,-25.7649464042479,
40.1194874821989));
#203387=CARTESIAN_POINT('Ctrl Pts',(-57.3992776612641,-25.7081127933386,
40.062755148314));
#203388=CARTESIAN_POINT('Ctrl Pts',(-57.3434500727664,-25.6555720179788,
40.0767884282377));
#203389=CARTESIAN_POINT('Ctrl Pts',(-57.4692856961541,-25.7004590347005,
40.1599502015396));
#203390=CARTESIAN_POINT('Ctrl Pts',(-57.4449640631542,-25.6633754510798,
40.1002449453872));
#203391=CARTESIAN_POINT('Ctrl Pts',(-57.3860499078785,-25.6226140882779,
40.10025));
#203392=CARTESIAN_POINT('Ctrl Pts',(-57.5052637377733,-25.6197038181295,
40.1599502534424));
#203393=CARTESIAN_POINT('Ctrl Pts',(-57.471187734033,-25.6045223014058,
40.10025));
#203394=CARTESIAN_POINT('Ctrl Pts',(-57.4068835917981,-25.5758735661205,
40.10025));
#203395=CARTESIAN_POINT('Origin',(-57.1106661007666,-25.7748538035644,39.92499));
#203396=CARTESIAN_POINT('Origin',(-54.3889216310786,-23.8679610547564,39.6398955069333));
#203397=CARTESIAN_POINT('Origin',(-54.2261740956467,-23.7955011834905,39.92499));
#203398=CARTESIAN_POINT('Origin',(-56.9479187893687,-25.7023940320469,39.6398955068279));
#203399=CARTESIAN_POINT('Origin',(-56.7851714777849,-25.6299342604992,39.3548010137695));
#203400=CARTESIAN_POINT('Ctrl Pts',(-54.1275498658875,-23.7522229508825,
39.8576902534424));
#203401=CARTESIAN_POINT('Ctrl Pts',(-54.0765745253537,-23.8679139708565,
39.8579948730704));
#203402=CARTESIAN_POINT('Ctrl Pts',(-54.1745185419761,-23.9115214566111,
39.92499));
#203403=CARTESIAN_POINT('Ctrl Pts',(-54.0860417646976,-23.7337429357609,
39.9304020711231));
#203404=CARTESIAN_POINT('Ctrl Pts',(-54.0553388636007,-23.8418262755865,
39.9058915297382));
#203405=CARTESIAN_POINT('Ctrl Pts',(-54.1330089371358,-23.8930401898204,
39.9671523786037));
#203406=CARTESIAN_POINT('Ctrl Pts',(-54.0331737207069,-23.7393098712348,
40.0043257306692));
#203407=CARTESIAN_POINT('Ctrl Pts',(-54.018846794374,-23.83019265673,39.9667894847832));
#203408=CARTESIAN_POINT('Ctrl Pts',(-54.0846755205373,-23.888427522722,
40.01001389752));
#203409=CARTESIAN_POINT('Ctrl Pts',(-53.9248984592618,-23.8065189073819,
40.1195533054858));
#203410=CARTESIAN_POINT('Ctrl Pts',(-53.938451117416,-23.8631501047895,
40.0630813209239));
#203411=CARTESIAN_POINT('Ctrl Pts',(-53.9943748351526,-23.9152668978358,
40.0768265942421));
#203412=CARTESIAN_POINT('Ctrl Pts',(-53.8688190939453,-23.8710081209822,
40.1599502027532));
#203413=CARTESIAN_POINT('Ctrl Pts',(-53.8932068549987,-23.9079567336545,
40.1002552791566));
#203414=CARTESIAN_POINT('Ctrl Pts',(-53.9522270531151,-23.9484663513831,
40.10025));
#203415=CARTESIAN_POINT('Ctrl Pts',(-53.8330634946839,-23.9513722670362,
40.1599502534424));
#203416=CARTESIAN_POINT('Ctrl Pts',(-53.8671470951732,-23.9665367208221,
40.10025));
#203417=CARTESIAN_POINT('Ctrl Pts',(-53.9314655730806,-23.9951532569804,
40.10025));
#203418=CARTESIAN_POINT('Origin',(-53.9314655730806,-23.9951532569804,40.22725));
#203419=CARTESIAN_POINT('Ctrl Pts',(-56.3916032444852,-25.454706393408,
38.989));
#203420=CARTESIAN_POINT('Ctrl Pts',(-56.4433359736143,-25.3385127813695,
38.989));
#203421=CARTESIAN_POINT('Ctrl Pts',(-56.4432587405903,-25.3386862495817,
39.1161896013263));
#203422=CARTESIAN_POINT('Ctrl Pts',(-56.5897307565552,-25.5431622092801,
38.989));
#203423=CARTESIAN_POINT('Ctrl Pts',(-56.6417243268827,-25.4268404215574,
38.9887769275485));
#203424=CARTESIAN_POINT('Ctrl Pts',(-56.6017747680112,-25.4092621323421,
39.1161898821845));
#203425=CARTESIAN_POINT('Ctrl Pts',(-56.7783458705719,-25.6273687254288,
39.1034967087244));
#203426=CARTESIAN_POINT('Ctrl Pts',(-56.8305375176085,-25.5109049500324,
39.1031720232701));
#203427=CARTESIAN_POINT('Ctrl Pts',(-56.7526792962279,-25.4764491573029,
39.2077529615002));
#203428=CARTESIAN_POINT('Ctrl Pts',(-56.8833377255396,-25.6742415049977,
39.2875012672119));
#203429=CARTESIAN_POINT('Ctrl Pts',(-56.9357219102086,-25.5577357740381,
39.2872087095508));
#203430=CARTESIAN_POINT('Ctrl Pts',(-56.8366797674145,-25.5138485767964,
39.3549017048226));
#203431=CARTESIAN_POINT('Origin',(-56.3916032444852,-25.454706393408,39.116));
#203432=CARTESIAN_POINT('Origin',(3.58382961824622E-16,-2.38580516864205E-17,
40.22725));
#203433=CARTESIAN_POINT('Origin',(-53.9190682401996,-24.0229981225294,40.22725));
#203434=CARTESIAN_POINT('Origin',(52.0578415156897,22.8300973196046,39.116));
#203435=CARTESIAN_POINT('Origin',(-56.0249274780499,-25.2915084057458,39.1160373285229));
#203436=CARTESIAN_POINT('Ctrl Pts',(-53.8206887816837,-23.9791663275011,
40.1599502534424));
#203437=CARTESIAN_POINT('Ctrl Pts',(-53.8547645473082,-23.9943483786814,
40.10025));
#203438=CARTESIAN_POINT('Ctrl Pts',(-53.9190682401996,-24.0229981225294,
40.10025));
#203439=CARTESIAN_POINT('Ctrl Pts',(-53.7850138844279,-24.0592381182999,
40.1599500566036));
#203440=CARTESIAN_POINT('Ctrl Pts',(-53.8287709626504,-24.052682504579,
40.1002551305357));
#203441=CARTESIAN_POINT('Ctrl Pts',(-53.8983362760846,-24.0695074323273,
40.10025));
#203442=CARTESIAN_POINT('Ctrl Pts',(-53.7744461045708,-24.143290671037,
40.1203070619046));
#203443=CARTESIAN_POINT('Ctrl Pts',(-53.8255298669651,-24.1158128282434,
40.0637098684497));
#203444=CARTESIAN_POINT('Ctrl Pts',(-53.9015903052241,-24.1225146216896,
40.0772636213363));
#203445=CARTESIAN_POINT('Ctrl Pts',(-53.7968389608977,-24.2696905364169,
40.0046102245802));
#203446=CARTESIAN_POINT('Ctrl Pts',(-53.8548027426702,-24.1983175571252,
39.9670001894016));
#203447=CARTESIAN_POINT('Ctrl Pts',(-53.9421141528986,-24.2081897025473,
40.0101788811209));
#203448=CARTESIAN_POINT('Ctrl Pts',(-53.8282518514941,-24.3127961529,39.9303710930186));
#203449=CARTESIAN_POINT('Ctrl Pts',(-53.8880291490215,-24.217648824503,
39.9058663574108));
#203450=CARTESIAN_POINT('Ctrl Pts',(-53.9780599067636,-24.2411088588488,
39.9671344706378));
#203451=CARTESIAN_POINT('Ctrl Pts',(-53.8697418420146,-24.3312692531085,
39.8576902534424));
#203452=CARTESIAN_POINT('Ctrl Pts',(-53.9216078643418,-24.2159747902184,
39.8579948730703));
#203453=CARTESIAN_POINT('Ctrl Pts',(-54.0195518809642,-24.259582275973,
39.92499));
#203454=CARTESIAN_POINT('Origin',(-53.9678963272936,-24.3756025490936,39.92499));
#203455=CARTESIAN_POINT('Origin',(-55.984546168509,-25.2734729066183,39.1925554488849));
#203456=CARTESIAN_POINT('Origin',(-55.9097831300748,-25.2401862573139,39.3343017080178));
#203457=CARTESIAN_POINT('Origin',(-54.1306438627326,-24.4480624203039,39.6398955069233));
#203458=CARTESIAN_POINT('Origin',(-54.2933913980365,-24.5205222915149,39.3548010137695));
#203459=CARTESIAN_POINT('Ctrl Pts',(-55.6083495590303,-25.1059793847698,
39.3978017080178));
#203460=CARTESIAN_POINT('Ctrl Pts',(-55.6600051127009,-24.9899591116492,
39.3978017080178));
#203461=CARTESIAN_POINT('Ctrl Pts',(-55.6600051127009,-24.9899591116492,
39.5248017080178));
#203462=CARTESIAN_POINT('Ctrl Pts',(-55.6906734752781,-25.1423759987951,
39.3978017080178));
#203463=CARTESIAN_POINT('Ctrl Pts',(-55.7421565548654,-25.02653529024,39.3980355775177));
#203464=CARTESIAN_POINT('Ctrl Pts',(-55.7833465978032,-25.0448742789053,
39.5248015517192));
#203465=CARTESIAN_POINT('Ctrl Pts',(-55.7685161955951,-25.1767934079555,
39.3484893995498));
#203466=CARTESIAN_POINT('Ctrl Pts',(-55.8202243900357,-25.0612933298591,
39.3489438303427));
#203467=CARTESIAN_POINT('Ctrl Pts',(-55.89997474663,-25.0968004762774,39.4508333155595));
#203468=CARTESIAN_POINT('Ctrl Pts',(-55.8095395120008,-25.1949317875298,
39.2708017080178));
#203469=CARTESIAN_POINT('Ctrl Pts',(-55.861411884108,-25.079631183695,39.2710850691866));
#203470=CARTESIAN_POINT('Ctrl Pts',(-55.9614386837454,-25.1241659841932,
39.3343017080178));
#203471=CARTESIAN_POINT('Origin',(-55.6083495590303,-25.1059793847698,39.5248017080178));
#203472=CARTESIAN_POINT('Ctrl Pts',(-54.1952354911873,-24.4761921430389,
39.2875012672119));
#203473=CARTESIAN_POINT('Ctrl Pts',(-54.2471777813617,-24.3607210247424,
39.2878045257519));
#203474=CARTESIAN_POINT('Ctrl Pts',(-54.3451938326303,-24.4045675690225,
39.3549015218347));
#203475=CARTESIAN_POINT('Ctrl Pts',(-54.3002261711149,-24.5230721320486,
39.1034938540228));
#203476=CARTESIAN_POINT('Ctrl Pts',(-54.3520689157368,-24.4074212664111,
39.1038286278808));
#203477=CARTESIAN_POINT('Ctrl Pts',(-54.4291958219391,-24.441967664437,
39.2077506434033));
#203478=CARTESIAN_POINT('Ctrl Pts',(-54.4888383671852,-24.6072895482014,
38.989));
#203479=CARTESIAN_POINT('Ctrl Pts',(-54.5406519873274,-24.4913833136928,
38.9892298954611));
#203480=CARTESIAN_POINT('Ctrl Pts',(-54.5801016184605,-24.5091552540984,
39.1161900347287));
#203481=CARTESIAN_POINT('Ctrl Pts',(-54.6869600343299,-24.6957503380304,
38.989));
#203482=CARTESIAN_POINT('Ctrl Pts',(-54.7386929643776,-24.5795562747214,
38.989));
#203483=CARTESIAN_POINT('Ctrl Pts',(-54.7386155301351,-24.5797301948777,
39.1161900945644));
#203484=CARTESIAN_POINT('Origin',(-54.6869600343299,-24.6957503380304,39.116));
#203485=CARTESIAN_POINT('Origin',(50.7999799080417,22.2700612497314,39.5248017080178));
#203486=CARTESIAN_POINT('Origin',(-55.4702140717968,-25.0444775033944,39.5248017080178));
#203487=CARTESIAN_POINT('Origin',(50.603004322856,22.1823620689013,39.116));
#203488=CARTESIAN_POINT('Origin',(-55.0536014459539,-24.8590452239598,39.1160402713848));
#203489=CARTESIAN_POINT('Ctrl Pts',(-55.2690209153042,-24.9555320242412,
39.2708017080178));
#203490=CARTESIAN_POINT('Ctrl Pts',(-55.3213695969757,-24.8391888661841,
39.2705119464801));
#203491=CARTESIAN_POINT('Ctrl Pts',(-55.2204359898058,-24.7942503289604,
39.3343017080178));
#203492=CARTESIAN_POINT('Ctrl Pts',(-55.3101840490925,-24.9737291291718,
39.3487519301186));
#203493=CARTESIAN_POINT('Ctrl Pts',(-55.3622664445122,-24.8573973158467,
39.3482879463976));
#203494=CARTESIAN_POINT('Ctrl Pts',(-55.2821076446841,-24.8217083187827,
39.4512271261631));
#203495=CARTESIAN_POINT('Ctrl Pts',(-55.3881672017734,-25.0082040095644,
39.3978017080178));
#203496=CARTESIAN_POINT('Ctrl Pts',(-55.4398389138625,-24.891934804391,
39.3975673827397));
#203497=CARTESIAN_POINT('Ctrl Pts',(-55.398943589477,-24.8737270328796,
39.5248015355181));
#203498=CARTESIAN_POINT('Ctrl Pts',(-55.4702140717968,-25.0444775033944,
39.3978017080178));
#203499=CARTESIAN_POINT('Ctrl Pts',(-55.5218696254675,-24.9284572302738,
39.3978017080178));
#203500=CARTESIAN_POINT('Ctrl Pts',(-55.5218696254674,-24.9284572302738,
39.5248017080178));
#203501=CARTESIAN_POINT('Origin',(-55.1687804361351,-24.910270602081,39.3343017080178));
#203502=CARTESIAN_POINT('Origin',(-55.094463269184,-24.877182467873,39.1934008533551));
#203503=CARTESIAN_POINT('Origin',(-58.5158800435658,-18.6791227126686,39.1925554495081));
#203504=CARTESIAN_POINT('Origin',(-58.5579573083275,-18.6927400943506,39.116037328525));
#203505=CARTESIAN_POINT('Origin',(-58.4380471616456,-18.6538332760101,39.3343017080178));
#203506=CARTESIAN_POINT('Ctrl Pts',(-58.3332704847797,-18.6203878281144,
39.2708017080178));
#203507=CARTESIAN_POINT('Ctrl Pts',(-58.2946680067389,-18.7407822670299,
39.2710850691866));
#203508=CARTESIAN_POINT('Ctrl Pts',(-58.3988020033599,-18.7746174535796,
39.3343017080178));
#203509=CARTESIAN_POINT('Ctrl Pts',(-58.290503238026,-18.6063701040101,
39.3487519293518));
#203510=CARTESIAN_POINT('Ctrl Pts',(-58.2516444665226,-18.7268030714108,
39.3492068662929));
#203511=CARTESIAN_POINT('Ctrl Pts',(-58.3345980746913,-18.7537563325796,
39.4512271248734));
#203512=CARTESIAN_POINT('Ctrl Pts',(-58.2094810152002,-18.5798130476653,
39.3978017080178));
#203513=CARTESIAN_POINT('Ctrl Pts',(-58.1702276772286,-18.7003491529652,
39.3980347781174));
#203514=CARTESIAN_POINT('Ctrl Pts',(-58.2129647630934,-18.7142352739234,
39.524801535519));
#203515=CARTESIAN_POINT('Ctrl Pts',(-58.1242364370958,-18.5518699907147,
39.3978017080178));
#203516=CARTESIAN_POINT('Ctrl Pts',(-58.0849912788101,-18.6726541682842,
39.3978017080178));
#203517=CARTESIAN_POINT('Ctrl Pts',(-58.0849912788101,-18.6726541682842,
39.5248017080178));
#203518=CARTESIAN_POINT('Origin',(-58.1242364370958,-18.5518699907147,39.5248017080178));
#203519=CARTESIAN_POINT('Origin',(-0.0981128957140385,0.301960443923712,
39.116));
#203520=CARTESIAN_POINT('Origin',(-58.9396512752214,-18.8168143322223,39.116));
#203521=CARTESIAN_POINT('Origin',(-0.0981128957140384,0.301960443923712,
39.5248017080178));
#203522=CARTESIAN_POINT('Origin',(-57.9804289733665,-18.5051441132838,39.5248017080178));
#203523=CARTESIAN_POINT('Ctrl Pts',(-59.4519788726609,-18.9827025415093,
39.2875012672119));
#203524=CARTESIAN_POINT('Ctrl Pts',(-59.4129503614028,-19.1043350233604,
39.287208709576));
#203525=CARTESIAN_POINT('Ctrl Pts',(-59.3099814440481,-19.0706774512225,
39.3549016990122));
#203526=CARTESIAN_POINT('Ctrl Pts',(-59.3425890481023,-18.947282004205,
39.103493917393));
#203527=CARTESIAN_POINT('Ctrl Pts',(-59.3034455268852,-19.0687544722082,
39.103169233633));
#203528=CARTESIAN_POINT('Ctrl Pts',(-59.222530503847,-19.0422629184333,
39.2077507202298));
#203529=CARTESIAN_POINT('Ctrl Pts',(-59.1460739925266,-18.8836509927321,
38.989));
#203530=CARTESIAN_POINT('Ctrl Pts',(-59.1068782740634,-19.0048854004771,
38.9887769311176));
#203531=CARTESIAN_POINT('Ctrl Pts',(-59.0654284453497,-18.9912173655545,
39.1161898712915));
#203532=CARTESIAN_POINT('Ctrl Pts',(-58.9396512752214,-18.8168143322223,
38.989));
#203533=CARTESIAN_POINT('Ctrl Pts',(-58.9003474864892,-18.937778955752,
38.989));
#203534=CARTESIAN_POINT('Ctrl Pts',(-58.900406160666,-18.9375983752041,
39.1161895903854));
#203535=CARTESIAN_POINT('Origin',(-59.3493798002281,-18.9499432001054,39.3548010137695));
#203536=CARTESIAN_POINT('Ctrl Pts',(-57.9804289733665,-18.5051441132838,
39.3978017080178));
#203537=CARTESIAN_POINT('Ctrl Pts',(-57.9411838150808,-18.6259282908533,
39.3978017080178));
#203538=CARTESIAN_POINT('Ctrl Pts',(-57.9411838150808,-18.6259282908533,
39.5248017080178));
#203539=CARTESIAN_POINT('Ctrl Pts',(-57.8948964606935,-18.4771060595081,
39.3978017080178));
#203540=CARTESIAN_POINT('Ctrl Pts',(-57.8554964068714,-18.5980867642071,
39.3975666025045));
#203541=CARTESIAN_POINT('Ctrl Pts',(-57.8127777979941,-18.584206646787,
39.5248015517196));
#203542=CARTESIAN_POINT('Ctrl Pts',(-57.8140195545737,-18.4505921960625,
39.3484894016716));
#203543=CARTESIAN_POINT('Ctrl Pts',(-57.7748837362118,-18.5718941197414,
39.3480259000037));
#203544=CARTESIAN_POINT('Ctrl Pts',(-57.691360753939,-18.5447558577151,
39.4508333188944));
#203545=CARTESIAN_POINT('Ctrl Pts',(-57.7713971777988,-18.4366189870669,
39.2708017080178));
#203546=CARTESIAN_POINT('Ctrl Pts',(-57.7324510618071,-18.5581069080657,
39.27051194648));
#203547=CARTESIAN_POINT('Ctrl Pts',(-57.6273730232606,-18.5239649837004,
39.3343017080178));
#203548=CARTESIAN_POINT('Origin',(-57.6666181815462,-18.403180806131,39.3343017080178));
#203549=CARTESIAN_POINT('Origin',(-59.5188096735778,-19.0049943031116,39.6398955068191));
#203550=CARTESIAN_POINT('Origin',(-59.6882395467421,-19.0600454060083,39.92499));
#203551=CARTESIAN_POINT('Origin',(-57.5892494790283,-18.3780421908171,39.1934008539945));
#203552=CARTESIAN_POINT('Origin',(-57.5467470426661,-18.3641788932745,39.1160402713852));
#203553=CARTESIAN_POINT('Ctrl Pts',(-59.8776671349986,-19.4393816709753,
40.1599502534424));
#203554=CARTESIAN_POINT('Ctrl Pts',(-59.8421853116554,-19.4278624395263,
40.10025));
#203555=CARTESIAN_POINT('Ctrl Pts',(-59.7752282754838,-19.406124729225,
40.10025));
#203556=CARTESIAN_POINT('Ctrl Pts',(-59.9048758468122,-19.3555723159019,
40.1599500538466));
#203557=CARTESIAN_POINT('Ctrl Pts',(-59.8620015382124,-19.3668135526099,
40.1002448353481));
#203558=CARTESIAN_POINT('Ctrl Pts',(-59.7909691583393,-19.3576098387253,
40.10025));
#203559=CARTESIAN_POINT('Ctrl Pts',(-59.9061888791358,-19.270512881395,
40.120244200104));
#203560=CARTESIAN_POINT('Ctrl Pts',(-59.8582551377155,-19.3034480936182,
40.0633873868017));
#203561=CARTESIAN_POINT('Ctrl Pts',(-59.7817014705985,-19.3051157581416,
40.0772271723537));
#203562=CARTESIAN_POINT('Ctrl Pts',(-59.8700374834723,-19.1466203444577,
40.0045995998161));
#203563=CARTESIAN_POINT('Ctrl Pts',(-59.8200494324144,-19.2244111832568,
39.9663485808314));
#203564=CARTESIAN_POINT('Ctrl Pts',(-59.7316696194037,-19.2239451174248,
40.0101727202466));
#203565=CARTESIAN_POINT('Ctrl Pts',(-59.834087357436,-19.1068608943535,
39.930465434986));
#203566=CARTESIAN_POINT('Ctrl Pts',(-59.7849307811025,-19.2088773592673,
39.9051900162943));
#203567=CARTESIAN_POINT('Ctrl Pts',(-59.6922425516964,-19.1948817636404,
39.967185745818));
#203568=CARTESIAN_POINT('Ctrl Pts',(-59.7908376697913,-19.0928077206408,
39.8576902534424));
#203569=CARTESIAN_POINT('Ctrl Pts',(-59.7518659300027,-19.214254573608,
39.8573998014387));
#203570=CARTESIAN_POINT('Ctrl Pts',(-59.6489943884565,-19.1808295835778,
39.92499));
#203571=CARTESIAN_POINT('Origin',(-59.7752282754838,-19.406124729225,40.22725));
#203572=CARTESIAN_POINT('Origin',(-0.0981128957140385,0.301960443923712,
39.116));
#203573=CARTESIAN_POINT('Origin',(-57.1650137687748,-18.2401996527042,39.116));
#203574=CARTESIAN_POINT('Origin',(1.26611655068502E-16,5.09536863743838E-17,
40.22725));
#203575=CARTESIAN_POINT('Origin',(-59.7658094374952,-19.4351129318417,40.22725));
#203576=CARTESIAN_POINT('Ctrl Pts',(-57.1650137687748,-18.2401996527042,
38.989));
#203577=CARTESIAN_POINT('Ctrl Pts',(-57.12570981947,-18.3611647704257,38.989));
#203578=CARTESIAN_POINT('Ctrl Pts',(-57.1257686544591,-18.3609836949483,
39.1161901092321));
#203579=CARTESIAN_POINT('Ctrl Pts',(-56.958585650595,-18.1733685221997,
38.989));
#203580=CARTESIAN_POINT('Ctrl Pts',(-56.9195342693626,-18.2941737326415,
38.989229898976));
#203581=CARTESIAN_POINT('Ctrl Pts',(-56.9607434512643,-18.3073637563258,
39.11619004932));
#203582=CARTESIAN_POINT('Ctrl Pts',(-56.7620685738646,-18.109748568444,
39.1034966344368));
#203583=CARTESIAN_POINT('Ctrl Pts',(-56.72320970454,-18.230383490407,39.103831410257));
#203584=CARTESIAN_POINT('Ctrl Pts',(-56.8036425617902,-18.2563185833,39.2077528789599));
#203585=CARTESIAN_POINT('Ctrl Pts',(-56.6526781108325,-18.0743352474888,
39.2875012672119));
#203586=CARTESIAN_POINT('Ctrl Pts',(-56.6140134911409,-18.1949032015563,
39.2878045257868));
#203587=CARTESIAN_POINT('Ctrl Pts',(-56.7161926934812,-18.2279043987988,
39.3549015295898));
#203588=CARTESIAN_POINT('Origin',(-56.7552848242271,-18.1070706485039,39.3548010137695));
#203589=CARTESIAN_POINT('Ctrl Pts',(-59.5942745858237,-19.6977666881842,
39.8576902534424));
#203590=CARTESIAN_POINT('Ctrl Pts',(-59.6341304551458,-19.5766071063165,
39.8573998014387));
#203591=CARTESIAN_POINT('Ctrl Pts',(-59.5312589135996,-19.5431821162863,
39.92499));
#203592=CARTESIAN_POINT('Ctrl Pts',(-59.6375442153292,-19.7118253299473,
39.9304984902491));
#203593=CARTESIAN_POINT('Ctrl Pts',(-59.6577332347575,-19.6004058925596,
39.9052171569799));
#203594=CARTESIAN_POINT('Ctrl Pts',(-59.5745267832909,-19.557240699363,
39.9672049726607));
#203595=CARTESIAN_POINT('Ctrl Pts',(-59.6898285824899,-19.7007277907731,
40.0043437678662));
#203596=CARTESIAN_POINT('Ctrl Pts',(-59.6951745640074,-19.6083614943628,
39.9661628577642));
#203597=CARTESIAN_POINT('Ctrl Pts',(-59.6233361049588,-19.5568428722495,
40.0100243556236));
#203598=CARTESIAN_POINT('Ctrl Pts',(-59.7913053863691,-19.6225475038108,
40.1194874821987));
#203599=CARTESIAN_POINT('Ctrl Pts',(-59.7720679362494,-19.5674227749672,
40.062755148314));
#203600=CARTESIAN_POINT('Ctrl Pts',(-59.7110541706153,-19.5210053955058,
40.0767884282377));
#203601=CARTESIAN_POINT('Ctrl Pts',(-59.8408924241699,-19.5524931121159,
40.1599502015383));
#203602=CARTESIAN_POINT('Ctrl Pts',(-59.8128277376112,-19.518154979168,
40.1002449453878));
#203603=CARTESIAN_POINT('Ctrl Pts',(-59.7499755976267,-19.4837751174916,
40.10025));
#203604=CARTESIAN_POINT('Ctrl Pts',(-59.8682321556243,-19.4684195516693,
40.1599502534424));
#203605=CARTESIAN_POINT('Ctrl Pts',(-59.8327559231847,-19.456883113188,
40.10025));
#203606=CARTESIAN_POINT('Ctrl Pts',(-59.7658094374952,-19.4351129318417,
40.10025));
#203607=CARTESIAN_POINT('Origin',(-59.492013755314,-19.6639662938558,39.92499));
#203608=CARTESIAN_POINT('Origin',(-56.5858547179577,-18.0520194698753,39.6398955069312));
#203609=CARTESIAN_POINT('Origin',(-56.4164246115664,-17.9969682911408,39.92499));
#203610=CARTESIAN_POINT('Origin',(-59.322583882151,-19.6089151909104,39.6398955068277));
#203611=CARTESIAN_POINT('Origin',(-59.1531540088,-19.5538640879529,39.3548010137695));
#203612=CARTESIAN_POINT('Ctrl Pts',(-56.3138168485096,-17.9642361803969,
39.8576902534424));
#203613=CARTESIAN_POINT('Ctrl Pts',(-56.2752137607567,-18.0846218068692,
39.8579948730704));
#203614=CARTESIAN_POINT('Ctrl Pts',(-56.3771794532808,-18.1177524687103,
39.92499));
#203615=CARTESIAN_POINT('Ctrl Pts',(-56.2706044454594,-17.9501961787622,
39.930402071123));
#203616=CARTESIAN_POINT('Ctrl Pts',(-56.2513675234837,-18.0608967538131,
39.9058915297375));
#203617=CARTESIAN_POINT('Ctrl Pts',(-56.3339654239822,-18.1037113794376,
39.9671523786033));
#203618=CARTESIAN_POINT('Ctrl Pts',(-56.2186079213553,-17.9612588333755,
40.0043257306694));
#203619=CARTESIAN_POINT('Ctrl Pts',(-56.2138593173284,-18.0531413250549,
39.9667894847836));
#203620=CARTESIAN_POINT('Ctrl Pts',(-56.2854146278931,-18.1041761987734,
40.0100138975199));
#203621=CARTESIAN_POINT('Ctrl Pts',(-56.1179510603878,-18.0394175380792,
40.1195533054856));
#203622=CARTESIAN_POINT('Ctrl Pts',(-56.1373490477012,-18.0943218653325,
40.0630813209237));
#203623=CARTESIAN_POINT('Ctrl Pts',(-56.198414097748,-18.1403075368578,
40.0768265942421));
#203624=CARTESIAN_POINT('Ctrl Pts',(-56.0689198620976,-18.1094153628975,
40.1599502027523));
#203625=CARTESIAN_POINT('Ctrl Pts',(-56.0970362061497,-18.1436123520189,
40.1002552791554));
#203626=CARTESIAN_POINT('Ctrl Pts',(-56.1599674935319,-18.1777307632115,
40.10025));
#203627=CARTESIAN_POINT('Ctrl Pts',(-56.0417604764384,-18.1930767435946,
40.1599502534424));
#203628=CARTESIAN_POINT('Ctrl Pts',(-56.0772424804485,-18.2045954185342,
40.10025));
#203629=CARTESIAN_POINT('Ctrl Pts',(-56.1441998575528,-18.2263320786579,
40.10025));
#203630=CARTESIAN_POINT('Origin',(-56.1441998575528,-18.2263320786579,40.22725));
#203631=CARTESIAN_POINT('Ctrl Pts',(-58.7434254837933,-19.4207352200698,
38.989));
#203632=CARTESIAN_POINT('Ctrl Pts',(-58.7827292759115,-19.299770586119,
38.989));
#203633=CARTESIAN_POINT('Ctrl Pts',(-58.7826705983437,-19.2999511771035,
39.1161896013263));
#203634=CARTESIAN_POINT('Ctrl Pts',(-58.9497137831222,-19.4879965013589,
38.989));
#203635=CARTESIAN_POINT('Ctrl Pts',(-58.9892635895143,-19.3668771285525,
38.9887769275485));
#203636=CARTESIAN_POINT('Ctrl Pts',(-58.9476954469492,-19.3535710010441,
39.1161898821845));
#203637=CARTESIAN_POINT('Ctrl Pts',(-59.1460976215389,-19.5520260773857,
39.1034967087243));
#203638=CARTESIAN_POINT('Ctrl Pts',(-59.1858295778064,-19.4307447900771,
39.1031720232694));
#203639=CARTESIAN_POINT('Ctrl Pts',(-59.1047962608419,-19.4046161500177,
39.2077529615002));
#203640=CARTESIAN_POINT('Ctrl Pts',(-59.2554138597572,-19.5876674457075,
39.2875012672119));
#203641=CARTESIAN_POINT('Ctrl Pts',(-59.2953329133625,-19.4663243070093,
39.2872087095508));
#203642=CARTESIAN_POINT('Ctrl Pts',(-59.1922458725047,-19.4330302514111,
39.3549017048226));
#203643=CARTESIAN_POINT('Origin',(-58.7434254837933,-19.4207352200698,39.116));
#203644=CARTESIAN_POINT('Origin',(3.56182666396657E-16,-1.81260861279366E-17,
40.22725));
#203645=CARTESIAN_POINT('Origin',(-56.1347810195643,-18.2553202812746,40.22725));
#203646=CARTESIAN_POINT('Origin',(56.3788528200609,17.9847604760579,39.116));
#203647=CARTESIAN_POINT('Origin',(-58.3616995707157,-19.2967593024458,39.1160373285271));
#203648=CARTESIAN_POINT('Ctrl Pts',(-56.0323588238392,-18.2220120550214,
40.1599502534424));
#203649=CARTESIAN_POINT('Ctrl Pts',(-56.0678348753333,-18.2335490499215,
40.10025));
#203650=CARTESIAN_POINT('Ctrl Pts',(-56.1347810195643,-18.2553202812746,
40.10025));
#203651=CARTESIAN_POINT('Ctrl Pts',(-56.0052491386463,-18.3053742463596,
40.1599500566039));
#203652=CARTESIAN_POINT('Ctrl Pts',(-56.0480812627871,-18.2942806848323,
40.1002551305381));
#203653=CARTESIAN_POINT('Ctrl Pts',(-56.119024173998,-18.3037418885563,
40.10025));
#203654=CARTESIAN_POINT('Ctrl Pts',(-56.0035251343645,-18.3900709842066,
40.1203070619048));
#203655=CARTESIAN_POINT('Ctrl Pts',(-56.0514568378818,-18.3574039607304,
40.0637098684502));
#203656=CARTESIAN_POINT('Ctrl Pts',(-56.1278011372719,-18.3561185603238,
40.0772636213363));
#203657=CARTESIAN_POINT('Ctrl Pts',(-56.039007703967,-18.5134377270389,
40.0046102245801));
#203658=CARTESIAN_POINT('Ctrl Pts',(-56.0891934462345,-18.4363968713614,
39.9670001894009));
#203659=CARTESIAN_POINT('Ctrl Pts',(-56.177058475612,-18.4370884086013,
40.0101788811209));
#203660=CARTESIAN_POINT('Ctrl Pts',(-56.0747542753109,-18.5530236652639,
39.9303710930187));
#203661=CARTESIAN_POINT('Ctrl Pts',(-56.1242585025264,-18.4521491348386,
39.9058663574113));
#203662=CARTESIAN_POINT('Ctrl Pts',(-56.2162483036945,-18.4660698759071,
39.9671344706363));
#203663=CARTESIAN_POINT('Ctrl Pts',(-56.1179479440989,-18.5670586829462,
39.8576902534424));
#203664=CARTESIAN_POINT('Ctrl Pts',(-56.1574782858998,-18.4469743395776,
39.8579948730703));
#203665=CARTESIAN_POINT('Ctrl Pts',(-56.259443978424,-18.4801050014187,
39.92499));
#203666=CARTESIAN_POINT('Origin',(-56.2201988201384,-18.6008891789882,39.92499));
#203667=CARTESIAN_POINT('Origin',(-58.319654251203,-19.2830435998987,39.1925554488847));
#203668=CARTESIAN_POINT('Origin',(-58.2418213702175,-19.2577541638575,39.3343017080178));
#203669=CARTESIAN_POINT('Origin',(-56.3896289265332,-18.6559403576609,39.6398955069214));
#203670=CARTESIAN_POINT('Origin',(-56.559059032799,-18.7109915363514,39.3548010137695));
#203671=CARTESIAN_POINT('Ctrl Pts',(-57.9280106456677,-19.1557908785622,
39.3978017080178));
#203672=CARTESIAN_POINT('Ctrl Pts',(-57.9672558039533,-19.0350067009927,
39.3978017080178));
#203673=CARTESIAN_POINT('Ctrl Pts',(-57.9672558039533,-19.0350067009927,
39.5248017080178));
#203674=CARTESIAN_POINT('Ctrl Pts',(-58.0136880650209,-19.1833829156714,
39.3978017080178));
#203675=CARTESIAN_POINT('Ctrl Pts',(-58.0527804636624,-19.0627953474463,
39.3980355775177));
#203676=CARTESIAN_POINT('Ctrl Pts',(-58.0956618095384,-19.0767283413219,
39.5248015517192));
#203677=CARTESIAN_POINT('Ctrl Pts',(-58.0947019536606,-19.2094750027316,
39.3484893995498));
#203678=CARTESIAN_POINT('Ctrl Pts',(-58.1340538395301,-19.0892026680456,
39.3489438303425));
#203679=CARTESIAN_POINT('Ctrl Pts',(-58.2170788227769,-19.1161791203808,
39.4508333155594));
#203680=CARTESIAN_POINT('Ctrl Pts',(-58.1373965169895,-19.2232259141436,
39.2708017080178));
#203681=CARTESIAN_POINT('Ctrl Pts',(-58.1769325318821,-19.1031347997384,
39.2710850691866));
#203682=CARTESIAN_POINT('Ctrl Pts',(-58.2810665285031,-19.136969986288,
39.3343017080178));
#203683=CARTESIAN_POINT('Origin',(-57.9280106456677,-19.1557908785622,39.5248017080178));
#203684=CARTESIAN_POINT('Ctrl Pts',(-56.4568070719812,-18.6771643191707,
39.2875012672119));
#203685=CARTESIAN_POINT('Ctrl Pts',(-56.4963947983079,-18.5568963159714,
39.2878045257519));
#203686=CARTESIAN_POINT('Ctrl Pts',(-56.5984571192854,-18.5902571970798,
39.3549015218348));
#203687=CARTESIAN_POINT('Ctrl Pts',(-56.566122895188,-18.7128129802652,
39.1034938540228));
#203688=CARTESIAN_POINT('Ctrl Pts',(-56.6055928325706,-18.5923766197444,
39.1038286278815));
#203689=CARTESIAN_POINT('Ctrl Pts',(-56.6859083114046,-18.6186718120036,
39.2077506434028));
#203690=CARTESIAN_POINT('Ctrl Pts',(-56.7625049710037,-18.7768537015935,
38.989));
#203691=CARTESIAN_POINT('Ctrl Pts',(-56.8019192501367,-18.6561664154735,
38.9892298954606));
#203692=CARTESIAN_POINT('Ctrl Pts',(-56.8430104456856,-18.6697173900118,
39.116190034729));
#203693=CARTESIAN_POINT('Ctrl Pts',(-56.9687879773467,-18.8441205405516,
38.989));
#203694=CARTESIAN_POINT('Ctrl Pts',(-57.0080919221123,-18.7231554368005,
38.989));
#203695=CARTESIAN_POINT('Ctrl Pts',(-57.0080330916692,-18.7233364982866,
39.1161900945646));
#203696=CARTESIAN_POINT('Origin',(-56.9687879773467,-18.8441205405516,39.116));
#203697=CARTESIAN_POINT('Origin',(55.0155724295761,17.5418038257013,39.5248017080178));
#203698=CARTESIAN_POINT('Origin',(-57.7842031819384,-19.1090650011312,39.5248017080178));
#203699=CARTESIAN_POINT('Origin',(54.8020887275097,17.4724387660752,39.116));
#203700=CARTESIAN_POINT('Origin',(-57.3504898524412,-18.9681964166827,39.1160402713849));
#203701=CARTESIAN_POINT('Ctrl Pts',(-57.5748148483577,-19.0416371860875,
39.2708017080178));
#203702=CARTESIAN_POINT('Ctrl Pts',(-57.6147155869503,-18.9204594407742,
39.2705119464801));
#203703=CARTESIAN_POINT('Ctrl Pts',(-57.5096375484038,-18.8863175164089,
39.3343017080178));
#203704=CARTESIAN_POINT('Ctrl Pts',(-57.6176546016066,-19.0554318862547,
39.3487519301186));
#203705=CARTESIAN_POINT('Ctrl Pts',(-57.6572916985351,-18.9342932580167,
39.3482879463972));
#203706=CARTESIAN_POINT('Ctrl Pts',(-57.5738415009812,-18.9071786451773,
39.4512271261625));
#203707=CARTESIAN_POINT('Ctrl Pts',(-57.6988141606861,-19.0815664505358,
39.3978017080178));
#203708=CARTESIAN_POINT('Ctrl Pts',(-57.7380493683907,-18.960533015575,
39.3975673827415));
#203709=CARTESIAN_POINT('Ctrl Pts',(-57.6954748424951,-18.9466997135538,
39.5248015355199));
#203710=CARTESIAN_POINT('Ctrl Pts',(-57.7842031819384,-19.1090650011312,
39.3978017080178));
#203711=CARTESIAN_POINT('Ctrl Pts',(-57.823448340224,-18.9882808235617,
39.3978017080178));
#203712=CARTESIAN_POINT('Ctrl Pts',(-57.823448340224,-18.9882808235617,
39.5248017080178));
#203713=CARTESIAN_POINT('Origin',(-57.4703923901182,-19.0071016939784,39.3343017080178));
#203714=CARTESIAN_POINT('Origin',(-57.3930236885614,-18.9819630792891,39.1934008533553));
#203715=CARTESIAN_POINT('Origin',(-60.1478239224126,-12.4602215063121,39.1925554495081));
#203716=CARTESIAN_POINT('Origin',(-60.1910940874976,-12.4693660187259,39.1160373285263));
#203717=CARTESIAN_POINT('Origin',(-60.0677739512127,-12.4432063593718,39.3343017080178));
#203718=CARTESIAN_POINT('Ctrl Pts',(-59.9600752506738,-12.4208962741583,
39.2708017080178));
#203719=CARTESIAN_POINT('Ctrl Pts',(-59.9342688867326,-12.5446662374483,
39.2710850691866));
#203720=CARTESIAN_POINT('Ctrl Pts',(-60.0413691664788,-12.567431104665,
39.3343017080178));
#203721=CARTESIAN_POINT('Ctrl Pts',(-59.9160770362135,-12.4114257351942,
39.3487519293518));
#203722=CARTESIAN_POINT('Ctrl Pts',(-59.890019810135,-12.535260805871,39.3492068662926));
#203723=CARTESIAN_POINT('Ctrl Pts',(-59.9753363727317,-12.5533954010687,
39.4512271248741));
#203724=CARTESIAN_POINT('Ctrl Pts',(-59.8327226933131,-12.3934832896267,
39.3978017080178));
#203725=CARTESIAN_POINT('Ctrl Pts',(-59.8062838430892,-12.517462176626,
39.3980347781178));
#203726=CARTESIAN_POINT('Ctrl Pts',(-59.8502383056086,-12.5268049860494,
39.524801535519));
#203727=CARTESIAN_POINT('Ctrl Pts',(-59.7450242491248,-12.374603792416,
39.3978017080178));
#203728=CARTESIAN_POINT('Ctrl Pts',(-59.718619464391,-12.4988285377092,
39.3978017080178));
#203729=CARTESIAN_POINT('Ctrl Pts',(-59.718619464391,-12.4988285377092,
39.5248017080178));
#203730=CARTESIAN_POINT('Origin',(-59.7450242491248,-12.374603792416,39.5248017080178));
#203731=CARTESIAN_POINT('Origin',(-0.0660119618346311,0.310561863232984,
39.116));
#203732=CARTESIAN_POINT('Origin',(-60.5836663843182,-12.5528626811443,39.116));
#203733=CARTESIAN_POINT('Origin',(-0.0660119618346311,0.310561863232984,
39.5248017080178));
#203734=CARTESIAN_POINT('Origin',(-59.597120393566,-12.3431658574207,39.5248017080178));
#203735=CARTESIAN_POINT('Ctrl Pts',(-61.1105274371642,-12.6642893210138,
39.2875012672119));
#203736=CARTESIAN_POINT('Ctrl Pts',(-61.0844267845857,-12.7893350777081,
39.287208709576));
#203737=CARTESIAN_POINT('Ctrl Pts',(-60.9785037674411,-12.7666250679674,
39.3549016990123));
#203738=CARTESIAN_POINT('Ctrl Pts',(-60.9980344071775,-12.6404971713783,
39.1034939173931));
#203739=CARTESIAN_POINT('Ctrl Pts',(-60.9718026486717,-12.765395812612,
39.1031692336333));
#203740=CARTESIAN_POINT('Ctrl Pts',(-60.8885617651955,-12.7475073053528,
39.2077507202293));
#203741=CARTESIAN_POINT('Ctrl Pts',(-60.7959446297925,-12.5977561540114,
38.989));
#203742=CARTESIAN_POINT('Ctrl Pts',(-60.7696360759153,-12.7224234952044,
38.9887769311182));
#203743=CARTESIAN_POINT('Ctrl Pts',(-60.7269846150103,-12.7131630221038,
39.1161898712916));
#203744=CARTESIAN_POINT('Ctrl Pts',(-60.5836663843182,-12.5528626811443,
38.989));
#203745=CARTESIAN_POINT('Ctrl Pts',(-60.5572221520604,-12.6772730124465,
38.989));
#203746=CARTESIAN_POINT('Ctrl Pts',(-60.5572616290068,-12.677087288016,
39.1161895903855));
#203747=CARTESIAN_POINT('Origin',(-61.0050661295707,-12.6424339620838,39.3548010137695));
#203748=CARTESIAN_POINT('Ctrl Pts',(-59.597120393566,-12.3431658574207,
39.3978017080178));
#203749=CARTESIAN_POINT('Ctrl Pts',(-59.5707156088321,-12.4673906027139,
39.3978017080178));
#203750=CARTESIAN_POINT('Ctrl Pts',(-59.5707156088321,-12.4673906027139,
39.5248017080178));
#203751=CARTESIAN_POINT('Ctrl Pts',(-59.5091256622727,-12.3242219811464,
39.3978017080178));
#203752=CARTESIAN_POINT('Ctrl Pts',(-59.4825873732107,-12.4486583679641,
39.397566602504));
#203753=CARTESIAN_POINT('Ctrl Pts',(-59.4386519140003,-12.439319597819,
39.5248015517196));
#203754=CARTESIAN_POINT('Ctrl Pts',(-59.4259203549057,-12.306307302129,
39.3484894016716));
#203755=CARTESIAN_POINT('Ctrl Pts',(-59.3996784303305,-12.4310355281343,
39.3480259000026));
#203756=CARTESIAN_POINT('Ctrl Pts',(-59.3137762748666,-12.4127764613284,
39.4508333188935));
#203757=CARTESIAN_POINT('Ctrl Pts',(-59.3820708699071,-12.2968658913799,
39.2708017080178));
#203758=CARTESIAN_POINT('Ctrl Pts',(-59.3560370505014,-12.4217592664909,
39.27051194648));
#203759=CARTESIAN_POINT('Ctrl Pts',(-59.2479658375577,-12.398788021052,
39.3343017080178));
#203760=CARTESIAN_POINT('Origin',(-59.2743706222916,-12.2745632757588,39.3343017080178));
#203761=CARTESIAN_POINT('Origin',(-61.1793222555435,-12.6794732450911,39.6398955068204));
#203762=CARTESIAN_POINT('Origin',(-61.3535783813233,-12.7165125280162,39.92499));
#203763=CARTESIAN_POINT('Origin',(-59.1947980527939,-12.25764960399,39.1934008539944));
#203764=CARTESIAN_POINT('Origin',(-59.1510793400371,-12.2483049653992,39.1160402713851));
#203765=CARTESIAN_POINT('Ctrl Pts',(-61.5816197022698,-13.0739701745321,
40.1599502534424));
#203766=CARTESIAN_POINT('Ctrl Pts',(-61.545128164506,-13.0662229071063,
40.10025));
#203767=CARTESIAN_POINT('Ctrl Pts',(-61.4762657165316,-13.0516031943525,
40.10025));
#203768=CARTESIAN_POINT('Ctrl Pts',(-61.5999188988197,-12.9877758510415,
40.1599500538462));
#203769=CARTESIAN_POINT('Ctrl Pts',(-61.558454489368,-13.0034370926705,
40.100244835349));
#203770=CARTESIAN_POINT('Ctrl Pts',(-61.4868491822336,-13.0017087032035,
40.10025));
#203771=CARTESIAN_POINT('Ctrl Pts',(-61.5923336062396,-12.9030451317659,
40.1202442001039));
#203772=CARTESIAN_POINT('Ctrl Pts',(-61.5481051179917,-12.9408103617798,
40.0633873868018));
#203773=CARTESIAN_POINT('Ctrl Pts',(-61.4721451382825,-12.9504709278437,
40.0772271723538));
#203774=CARTESIAN_POINT('Ctrl Pts',(-61.5434299552079,-12.7836101409426,
40.0045995998162));
#203775=CARTESIAN_POINT('Ctrl Pts',(-61.5018471007596,-12.8662000075461,
39.9663485808315));
#203776=CARTESIAN_POINT('Ctrl Pts',(-61.4139027244671,-12.8749747009095,
40.0101727202465));
#203777=CARTESIAN_POINT('Ctrl Pts',(-61.5035207735036,-12.7478263086951,
39.9304654349859));
#203778=CARTESIAN_POINT('Ctrl Pts',(-61.465297106342,-12.8544221781231,
39.9051900162958));
#203779=CARTESIAN_POINT('Ctrl Pts',(-61.3716536946531,-12.8501918100166,
39.9671857458182));
#203780=CARTESIAN_POINT('Ctrl Pts',(-61.4590390555209,-12.7383709431247,
39.8576902534424));
#203781=CARTESIAN_POINT('Ctrl Pts',(-61.43297545991,-12.8632261535951,39.8573998014387));
#203782=CARTESIAN_POINT('Ctrl Pts',(-61.3271735965894,-12.8407372733094,
39.92499));
#203783=CARTESIAN_POINT('Origin',(-61.4762657165316,-13.0516031943525,40.22725));
#203784=CARTESIAN_POINT('Origin',(-0.0660119618346311,0.310561863232984,
39.116));
#203785=CARTESIAN_POINT('Origin',(-58.7584778814677,-12.1649068885788,39.116));
#203786=CARTESIAN_POINT('Origin',(1.31078692950416E-16,3.42824740397342E-17,
40.22725));
#203787=CARTESIAN_POINT('Origin',(-61.4699285681955,-13.0814171332228,40.22725));
#203788=CARTESIAN_POINT('Ctrl Pts',(-58.7584778814677,-12.1649068885788,
38.989));
#203789=CARTESIAN_POINT('Ctrl Pts',(-58.732033541174,-12.28931772815,38.989));
#203790=CARTESIAN_POINT('Ctrl Pts',(-58.7320731263175,-12.2891314946918,
39.1161901092323));
#203791=CARTESIAN_POINT('Ctrl Pts',(-58.5461948427484,-12.1200194799672,
38.989));
#203792=CARTESIAN_POINT('Ctrl Pts',(-58.5199849720729,-12.2442448876955,
38.989229898976));
#203793=CARTESIAN_POINT('Ctrl Pts',(-58.5623471386685,-12.2530551225939,
39.1161900493202));
#203794=CARTESIAN_POINT('Ctrl Pts',(-58.3441042111266,-12.0772896710131,
39.1034966344368));
#203795=CARTESIAN_POINT('Ctrl Pts',(-58.3180679977598,-12.201325600148,
39.1038314102561));
#203796=CARTESIAN_POINT('Ctrl Pts',(-58.4007711908102,-12.2187110949215,
39.2077528789599));
#203797=CARTESIAN_POINT('Ctrl Pts',(-58.2316113004782,-12.0535047649318,
39.2875012672119));
#203798=CARTESIAN_POINT('Ctrl Pts',(-58.2057612725768,-12.1774537884111,
39.2878045257868));
#203799=CARTESIAN_POINT('Ctrl Pts',(-58.3108302909895,-12.1995935666434,
39.3549015295899));
#203800=CARTESIAN_POINT('Origin',(-58.3370777047235,-12.0753355159229,39.3548010137695));
#203801=CARTESIAN_POINT('Ctrl Pts',(-61.3267881959114,-13.3605623192483,
39.8576902534424));
#203802=CARTESIAN_POINT('Ctrl Pts',(-61.3537611057084,-13.2359003894747,
39.8573998014387));
#203803=CARTESIAN_POINT('Ctrl Pts',(-61.2479592423879,-13.213411509189,
39.92499));
#203804=CARTESIAN_POINT('Ctrl Pts',(-61.3712903180782,-13.370021038423,
39.9304984902492));
#203805=CARTESIAN_POINT('Ctrl Pts',(-61.3797222373792,-13.2571016411956,
39.9052171569788));
#203806=CARTESIAN_POINT('Ctrl Pts',(-61.2924596082469,-13.2228703539491,
39.96720497266));
#203807=CARTESIAN_POINT('Ctrl Pts',(-61.4221282572889,-13.3535190881769,
40.0043437678661));
#203808=CARTESIAN_POINT('Ctrl Pts',(-61.4177900459394,-13.26109997677,39.966162857764));
#203809=CARTESIAN_POINT('Ctrl Pts',(-61.3409599630868,-13.2173727427872,
40.0100243556234));
#203810=CARTESIAN_POINT('Ctrl Pts',(-61.514877095365,-13.2651598666396,
40.1194874821989));
#203811=CARTESIAN_POINT('Ctrl Pts',(-61.4899829268154,-13.2123479779266,
40.0627551483143));
#203812=CARTESIAN_POINT('Ctrl Pts',(-61.4244514636294,-13.1725625528864,
40.0767884282378));
#203813=CARTESIAN_POINT('Ctrl Pts',(-61.5568698122754,-13.1903059833733,
40.1599502015386));
#203814=CARTESIAN_POINT('Ctrl Pts',(-61.5253695547376,-13.1590895168684,
40.100244945386));
#203815=CARTESIAN_POINT('Ctrl Pts',(-61.4592680512438,-13.1314678292773,
40.10025));
#203816=CARTESIAN_POINT('Ctrl Pts',(-61.5752716937452,-13.1038352065724,
40.1599502534424));
#203817=CARTESIAN_POINT('Ctrl Pts',(-61.5387839176329,-13.0960702419676,
40.10025));
#203818=CARTESIAN_POINT('Ctrl Pts',(-61.4699285681955,-13.0814171332229,
40.10025));
#203819=CARTESIAN_POINT('Origin',(-61.221554457654,-13.3376362544822,39.92499));
#203820=CARTESIAN_POINT('Origin',(-58.1628213392047,-12.038296182048,39.6398955069332));
#203821=CARTESIAN_POINT('Origin',(-57.988564973546,-12.0012568480856,39.92499));
#203822=CARTESIAN_POINT('Origin',(-61.0472983318727,-13.3005969715127,39.6398955068272));
#203823=CARTESIAN_POINT('Origin',(-60.8730422059014,-13.2635576885498,39.3548010137695));
#203824=CARTESIAN_POINT('Ctrl Pts',(-57.8830978693156,-11.9794294790609,
39.8576902534424));
#203825=CARTESIAN_POINT('Ctrl Pts',(-57.8572899778512,-12.1031907419153,
39.8579948730704));
#203826=CARTESIAN_POINT('Ctrl Pts',(-57.9621601888121,-12.1254815933788,
39.92499));
#203827=CARTESIAN_POINT('Ctrl Pts',(-57.8386546085357,-11.9699833161083,
39.930402071123));
#203828=CARTESIAN_POINT('Ctrl Pts',(-57.8310944294263,-12.0820882677187,
39.9058915297384));
#203829=CARTESIAN_POINT('Ctrl Pts',(-57.9177151970035,-12.1160345187365,
39.9671523786037));
#203830=CARTESIAN_POINT('Ctrl Pts',(-57.7880992891175,-11.9864204851027,
40.0043257306694));
#203831=CARTESIAN_POINT('Ctrl Pts',(-57.7929810340972,-12.0782959991608,
39.9667894847838));
#203832=CARTESIAN_POINT('Ctrl Pts',(-57.8694789541063,-12.1215717318492,
40.0100138975201));
#203833=CARTESIAN_POINT('Ctrl Pts',(-57.6961636462598,-12.0746725352386,
40.1195533054856));
#203834=CARTESIAN_POINT('Ctrl Pts',(-57.7211944343232,-12.1272484490377,
40.0630813209234));
#203835=CARTESIAN_POINT('Ctrl Pts',(-57.7867317752136,-12.1665991704021,
40.0768265942419));
#203836=CARTESIAN_POINT('Ctrl Pts',(-57.6547178110643,-12.1494120604578,
40.1599502027525));
#203837=CARTESIAN_POINT('Ctrl Pts',(-57.6862546895618,-12.1804827566582,
40.1002552791553));
#203838=CARTESIAN_POINT('Ctrl Pts',(-57.7524075778586,-12.2078361528629,
40.10025));
#203839=CARTESIAN_POINT('Ctrl Pts',(-57.6364522029208,-12.2354540642041,
40.1599502534424));
#203840=CARTESIAN_POINT('Ctrl Pts',(-57.6729438621907,-12.2432007592844,
40.10025));
#203841=CARTESIAN_POINT('Ctrl Pts',(-57.7418065394566,-12.2578193919764,
40.10025));
#203842=CARTESIAN_POINT('Origin',(-57.7418065394566,-12.2578193919764,40.22725));
#203843=CARTESIAN_POINT('Ctrl Pts',(-60.451642460649,-13.1739864076103,
38.989));
#203844=CARTESIAN_POINT('Ctrl Pts',(-60.478086695185,-13.0495760655901,
38.989));
#203845=CARTESIAN_POINT('Ctrl Pts',(-60.478047215957,-13.0497618007546,
39.1161896013266));
#203846=CARTESIAN_POINT('Ctrl Pts',(-60.6638314094602,-13.2193162256447,
38.989));
#203847=CARTESIAN_POINT('Ctrl Pts',(-60.6905041359633,-13.0947262769507,
38.988776927546));
#203848=CARTESIAN_POINT('Ctrl Pts',(-60.6477728389708,-13.0858380958632,
39.1161898821847));
#203849=CARTESIAN_POINT('Ctrl Pts',(-60.8658323498479,-13.2624673401139,
39.1034967087243));
#203850=CARTESIAN_POINT('Ctrl Pts',(-60.8926693037164,-13.1376973240559,
39.1031720232711));
#203851=CARTESIAN_POINT('Ctrl Pts',(-60.8093487091498,-13.1201821075162,
39.2077529614998));
#203852=CARTESIAN_POINT('Ctrl Pts',(-60.9782752797349,-13.2864868028992,
39.2875012672119));
#203853=CARTESIAN_POINT('Ctrl Pts',(-61.0052918407716,-13.1616357172824,
39.2872087095508));
#203854=CARTESIAN_POINT('Ctrl Pts',(-60.8992893450419,-13.1392995799683,
39.3549017048227));
#203855=CARTESIAN_POINT('Origin',(-60.451642460649,-13.1739864076103,39.116));
#203856=CARTESIAN_POINT('Origin',(3.54593577968597E-16,-1.21955273767077E-17,
40.22725));
#203857=CARTESIAN_POINT('Origin',(-57.7354693911205,-12.2876333308468,40.22725));
#203858=CARTESIAN_POINT('Origin',(59.5987607253196,12.3435145206982,39.116));
#203859=CARTESIAN_POINT('Origin',(-60.0590486699117,-13.0905908661169,39.1160373285254));
#203860=CARTESIAN_POINT('Ctrl Pts',(-57.6301266171958,-12.2652136052657,
40.1599502534424));
#203861=CARTESIAN_POINT('Ctrl Pts',(-57.6666142715156,-12.2729791421551,
40.10025));
#203862=CARTESIAN_POINT('Ctrl Pts',(-57.7354693911205,-12.2876333308468,
40.10025));
#203863=CARTESIAN_POINT('Ctrl Pts',(-57.6118791634503,-12.3509528635302,
40.1599500566036));
#203864=CARTESIAN_POINT('Ctrl Pts',(-57.6533170557966,-12.3354428975793,
40.100255130536));
#203865=CARTESIAN_POINT('Ctrl Pts',(-57.7248602994014,-12.3374367183504,
40.10025));
#203866=CARTESIAN_POINT('Ctrl Pts',(-57.619017823295,-12.4353658313039,
40.1203070619049));
#203867=CARTESIAN_POINT('Ctrl Pts',(-57.6632723181618,-12.3978675338895,
40.06370986845));
#203868=CARTESIAN_POINT('Ctrl Pts',(-57.7390640345625,-12.3886090227464,
40.0772636213363));
#203869=CARTESIAN_POINT('Ctrl Pts',(-57.6672013517154,-12.5543478197371,
40.00461022458));
#203870=CARTESIAN_POINT('Ctrl Pts',(-57.7090592089829,-12.4724831634111,
39.9670001894012));
#203871=CARTESIAN_POINT('Ctrl Pts',(-57.7965151898611,-12.4639865158418,
40.0101788811209));
#203872=CARTESIAN_POINT('Ctrl Pts',(-57.7068899568908,-12.5899803678811,
39.9303710930188));
#203873=CARTESIAN_POINT('Ctrl Pts',(-57.745578735121,-12.4844838378934,
39.9058663574104));
#203874=CARTESIAN_POINT('Ctrl Pts',(-57.8385197202049,-12.4887127671319,
39.9671344706358));
#203875=CARTESIAN_POINT('Ctrl Pts',(-57.7513140650721,-12.5994235324468,
39.8576902534424));
#203876=CARTESIAN_POINT('Ctrl Pts',(-57.7780756236496,-12.4758649777949,
39.8579948730704));
#203877=CARTESIAN_POINT('Ctrl Pts',(-57.8829458346106,-12.4981558292584,
39.92499));
#203878=CARTESIAN_POINT('Origin',(-57.8565410498767,-12.6223805745516,39.92499));
#203879=CARTESIAN_POINT('Origin',(-60.01579999775,-13.0813452322614,39.1925554488851));
#203880=CARTESIAN_POINT('Origin',(-59.9357500275434,-13.0643300858378,39.3343017080178));
#203881=CARTESIAN_POINT('Origin',(-58.030797415528,-12.6594199084519,39.6398955069206));
#203882=CARTESIAN_POINT('Origin',(-58.2050537810542,-12.6964592423889,39.3548010137695));
#203883=CARTESIAN_POINT('Ctrl Pts',(-59.6130003254556,-12.995727518882,
39.3978017080178));
#203884=CARTESIAN_POINT('Ctrl Pts',(-59.6394051101894,-12.8715027735888,
39.3978017080178));
#203885=CARTESIAN_POINT('Ctrl Pts',(-59.6394051101894,-12.8715027735888,
39.5248017080178));
#203886=CARTESIAN_POINT('Ctrl Pts',(-59.7010925481785,-13.0142126749435,
39.3978017080178));
#203887=CARTESIAN_POINT('Ctrl Pts',(-59.7273659613755,-12.8901994296787,
39.3980355775178));
#203888=CARTESIAN_POINT('Ctrl Pts',(-59.7714687931904,-12.899573775969,
39.5248015517192));
#203889=CARTESIAN_POINT('Ctrl Pts',(-59.7843900000232,-13.0316935695386,
39.3484893995498));
#203890=CARTESIAN_POINT('Ctrl Pts',(-59.810954429825,-12.9079667071265,
39.3489438303421));
#203891=CARTESIAN_POINT('Ctrl Pts',(-59.8963444006333,-12.9261169057235,
39.450833315559));
#203892=CARTESIAN_POINT('Ctrl Pts',(-59.8282880397056,-13.0409063549235,
39.2708017080178));
#203893=CARTESIAN_POINT('Ctrl Pts',(-59.855054532531,-12.9173404733279,
39.2710850691866));
#203894=CARTESIAN_POINT('Ctrl Pts',(-59.9621548122772,-12.9401053405446,
39.3343017080178));
#203895=CARTESIAN_POINT('Origin',(-59.6130003254556,-12.995727518882,39.5248017080178));
#203896=CARTESIAN_POINT('Ctrl Pts',(-58.0998260601481,-12.6735055745737,
39.2875012672119));
#203897=CARTESIAN_POINT('Ctrl Pts',(-58.1266254912132,-12.5497583678825,
39.2878045257519));
#203898=CARTESIAN_POINT('Ctrl Pts',(-58.231615865753,-12.5722680770244,
39.3549015218348));
#203899=CARTESIAN_POINT('Ctrl Pts',(-58.2122693395992,-12.6975323335621,
39.1034938540228));
#203900=CARTESIAN_POINT('Ctrl Pts',(-58.2389340288436,-12.5736300041245,
39.1038286278802));
#203901=CARTESIAN_POINT('Ctrl Pts',(-58.321558127123,-12.5913858949913,
39.2077506434026));
#203902=CARTESIAN_POINT('Ctrl Pts',(-58.4142696920427,-12.7406947165201,
38.989));
#203903=CARTESIAN_POINT('Ctrl Pts',(-58.4408527990799,-12.6165486539543,
38.9892298954605));
#203904=CARTESIAN_POINT('Ctrl Pts',(-58.4831353553018,-12.62573019531,39.1161900347291));
#203905=CARTESIAN_POINT('Ctrl Pts',(-58.6264539577984,-12.7860306150448,
38.989));
#203906=CARTESIAN_POINT('Ctrl Pts',(-58.652898295038,-12.661619789842,38.989));
#203907=CARTESIAN_POINT('Ctrl Pts',(-58.6528587129532,-12.6618060089103,
39.1161900945648));
#203908=CARTESIAN_POINT('Origin',(-58.6264539577984,-12.7860306150448,39.116));
#203909=CARTESIAN_POINT('Origin',(58.1567073854023,12.0369966210207,39.5248017080178));
#203910=CARTESIAN_POINT('Origin',(-59.4650964698967,-12.9642895838867,39.5248017080178));
#203911=CARTESIAN_POINT('Origin',(57.9308881865556,11.9889972685547,39.116));
#203912=CARTESIAN_POINT('Origin',(-59.0190342907425,-12.8695280801153,39.116040271386));
#203913=CARTESIAN_POINT('Ctrl Pts',(-59.249807061628,-12.9191181862042,
39.2708017080178));
#203914=CARTESIAN_POINT('Ctrl Pts',(-59.2768226962999,-12.7944335023704,
39.27051194648));
#203915=CARTESIAN_POINT('Ctrl Pts',(-59.1687514833561,-12.7714622569316,
39.3343017080178));
#203916=CARTESIAN_POINT('Ctrl Pts',(-59.2938540730361,-12.9283593439862,
39.3487519301186));
#203917=CARTESIAN_POINT('Ctrl Pts',(-59.320611599148,-12.8037411209984,
39.3482879463986));
#203918=CARTESIAN_POINT('Ctrl Pts',(-59.2347843016965,-12.7854979657554,
39.4512271261625));
#203919=CARTESIAN_POINT('Ctrl Pts',(-59.3773008374014,-12.9458672564001,
39.3978017080178));
#203920=CARTESIAN_POINT('Ctrl Pts',(-59.4036696715727,-12.8213956592927,
39.3975673827397));
#203921=CARTESIAN_POINT('Ctrl Pts',(-59.3598823995817,-12.8120883873134,
39.5248015355199));
#203922=CARTESIAN_POINT('Ctrl Pts',(-59.4650964698967,-12.9642895838867,
39.3978017080178));
#203923=CARTESIAN_POINT('Ctrl Pts',(-59.4915012546306,-12.8400648385935,
39.3978017080178));
#203924=CARTESIAN_POINT('Ctrl Pts',(-59.4915012546306,-12.8400648385935,
39.5248017080178));
#203925=CARTESIAN_POINT('Origin',(-59.1423466986223,-12.8956870022248,39.3343017080178));
#203926=CARTESIAN_POINT('Origin',(-59.0627741301462,-12.8787733309739,39.1934008533553));
#203927=CARTESIAN_POINT('Origin',(-61.1207756556245,-6.10480350566274,39.1925554495082));
#203928=CARTESIAN_POINT('Origin',(-61.1647646440472,-6.10937495961999,39.1160373285259));
#203929=CARTESIAN_POINT('Origin',(-61.0393856393804,-6.09624906995198,39.3343017080178));
#203930=CARTESIAN_POINT('Ctrl Pts',(-60.9299448846691,-6.0853187813828,
39.2708017080178));
#203931=CARTESIAN_POINT('Ctrl Pts',(-60.9172173747511,-6.21110821942895,
39.2710850691866));
#203932=CARTESIAN_POINT('Ctrl Pts',(-61.0261105245455,-6.22255335066376,
39.3343017080178));
#203933=CARTESIAN_POINT('Ctrl Pts',(-60.885197756147,-6.08049918876655,
39.3487519293518));
#203934=CARTESIAN_POINT('Ctrl Pts',(-60.8722275639182,-6.20637959976686,
39.3492068662932));
#203935=CARTESIAN_POINT('Ctrl Pts',(-60.958972334824,-6.21549684257596,
39.4512271248742));
#203936=CARTESIAN_POINT('Ctrl Pts',(-60.800424540796,-6.07136793516307,
39.3978017080178));
#203937=CARTESIAN_POINT('Ctrl Pts',(-60.7870898478939,-6.19743126523177,
39.3980347781178));
#203938=CARTESIAN_POINT('Ctrl Pts',(-60.8317801127819,-6.20212840134649,
39.524801535519));
#203939=CARTESIAN_POINT('Ctrl Pts',(-60.7112330730304,-6.0617588454153,
39.3978017080178));
#203940=CARTESIAN_POINT('Ctrl Pts',(-60.6979579581954,-6.18806312612707,
39.3978017080178));
#203941=CARTESIAN_POINT('Ctrl Pts',(-60.6979579581954,-6.18806312612707,
39.5248017080178));
#203942=CARTESIAN_POINT('Origin',(-60.7112330730304,-6.0617588454153,39.5248017080178));
#203943=CARTESIAN_POINT('Origin',(-0.0331877870874725,0.315760701779427,
39.116));
#203944=CARTESIAN_POINT('Origin',(-61.5639141665612,-6.15137923967635,39.116));
#203945=CARTESIAN_POINT('Origin',(-0.0331877870874724,0.315760701779427,
39.5248017080178));
#203946=CARTESIAN_POINT('Origin',(-60.5608532912344,-6.04595329345021,39.5248017080178));
#203947=CARTESIAN_POINT('Ctrl Pts',(-62.0995362748659,-6.20712349654423,
39.2875012672119));
#203948=CARTESIAN_POINT('Ctrl Pts',(-62.0866494451786,-6.33421250060381,
39.287208709576));
#203949=CARTESIAN_POINT('Ctrl Pts',(-61.978932842986,-6.32269886887959,
39.3549016990122));
#203950=CARTESIAN_POINT('Ctrl Pts',(-61.9851725366286,-6.19522040634658,
39.1034939173931));
#203951=CARTESIAN_POINT('Ctrl Pts',(-61.9721399414719,-6.32217680516044,
39.1031692336341));
#203952=CARTESIAN_POINT('Ctrl Pts',(-61.8874852020914,-6.31308733464682,
39.2077507202295));
#203953=CARTESIAN_POINT('Ctrl Pts',(-61.7797221753254,-6.17383766261664,
38.989));
#203954=CARTESIAN_POINT('Ctrl Pts',(-61.7665890280543,-6.30057205577826,
38.9887769311176));
#203955=CARTESIAN_POINT('Ctrl Pts',(-61.7232032332924,-6.29582060418315,
39.1161898712914));
#203956=CARTESIAN_POINT('Ctrl Pts',(-61.5639141665612,-6.15137923967635,
38.989));
#203957=CARTESIAN_POINT('Ctrl Pts',(-61.5506192193203,-6.27787221312641,
38.989));
#203958=CARTESIAN_POINT('Ctrl Pts',(-61.5506390665185,-6.27768337964943,
39.1161895903853));
#203959=CARTESIAN_POINT('Origin',(-61.9923681882669,-6.19641157197423,39.3548010137695));
#203960=CARTESIAN_POINT('Ctrl Pts',(-60.5608532912344,-6.04595329345021,
39.3978017080178));
#203961=CARTESIAN_POINT('Ctrl Pts',(-60.5475781763994,-6.17225757416198,
39.3978017080178));
#203962=CARTESIAN_POINT('Ctrl Pts',(-60.5475781763994,-6.17225757416198,
39.5248017080178));
#203963=CARTESIAN_POINT('Ctrl Pts',(-60.4713604300108,-6.03631114775,39.3978017080178));
#203964=CARTESIAN_POINT('Ctrl Pts',(-60.4579746647643,-6.16283986559456,
39.397566602504));
#203965=CARTESIAN_POINT('Ctrl Pts',(-60.4133037213016,-6.15814476024322,
39.5248015517196));
#203966=CARTESIAN_POINT('Ctrl Pts',(-60.3867383361559,-6.02719193013317,
39.3484894016717));
#203967=CARTESIAN_POINT('Ctrl Pts',(-60.3736778173763,-6.15397990991425,
39.3480259000034));
#203968=CARTESIAN_POINT('Ctrl Pts',(-60.2863376507179,-6.14480008848983,
39.4508333188934));
#203969=CARTESIAN_POINT('Ctrl Pts',(-60.3421421670675,-6.02238575970236,
39.2708017080178));
#203970=CARTESIAN_POINT('Ctrl Pts',(-60.3293058762212,-6.14931623097207,
39.2705119464801));
#203971=CARTESIAN_POINT('Ctrl Pts',(-60.2194255397045,-6.13776734223176,
39.3343017080178));
#203972=CARTESIAN_POINT('Origin',(-60.2327006545395,-6.01146306151998,39.3343017080178));
#203973=CARTESIAN_POINT('Origin',(-62.1695413802841,-6.21503322485303,39.6398955068191));
#203974=CARTESIAN_POINT('Origin',(-62.3467145720969,-6.23365487766584,39.92499));
#203975=CARTESIAN_POINT('Origin',(-60.1517960317849,-6.00295964302187,39.1934008539946));
#203976=CARTESIAN_POINT('Origin',(-60.1073400339997,-5.9982360452005,39.116040271385));
#203977=CARTESIAN_POINT('Ctrl Pts',(-62.6108711573006,-6.56531752495261,
40.1599502534424));
#203978=CARTESIAN_POINT('Ctrl Pts',(-62.5737697140402,-6.56142710223311,
40.10025));
#203979=CARTESIAN_POINT('Ctrl Pts',(-62.5037563256535,-6.55408556365905,
40.10025));
#203980=CARTESIAN_POINT('Ctrl Pts',(-62.6200603487601,-6.47768259609045,
40.159950053846));
#203981=CARTESIAN_POINT('Ctrl Pts',(-62.5804601312005,-6.49759225479912,
40.100244835349));
#203982=CARTESIAN_POINT('Ctrl Pts',(-62.5090664195363,-6.50335812634718,
40.10025));
#203983=CARTESIAN_POINT('Ctrl Pts',(-62.603659837329,-6.39420891953715,
40.1202442001038));
#203984=CARTESIAN_POINT('Ctrl Pts',(-62.5636211788254,-6.43639040357905,
40.0633873868018));
#203985=CARTESIAN_POINT('Ctrl Pts',(-62.4890871199581,-6.45393802799988,
40.0772271723538));
#203986=CARTESIAN_POINT('Ctrl Pts',(-62.5425397295636,-6.28054002958106,
40.0045995998164));
#203987=CARTESIAN_POINT('Ctrl Pts',(-62.5098176621807,-6.36702405212743,
39.9663485808315));
#203988=CARTESIAN_POINT('Ctrl Pts',(-62.423272259596,-6.38494336730939,
40.0101727202466));
#203989=CARTESIAN_POINT('Ctrl Pts',(-62.4991087455376,-6.24912387034439,
39.9304654349858));
#203990=CARTESIAN_POINT('Ctrl Pts',(-62.4722367740483,-6.35913125763767,
39.9051900162948));
#203991=CARTESIAN_POINT('Ctrl Pts',(-62.3786641568876,-6.36471246584688,
39.9671857458179));
#203992=CARTESIAN_POINT('Ctrl Pts',(-62.4538823482276,-6.24436990788019,
39.8576902534424));
#203993=CARTESIAN_POINT('Ctrl Pts',(-62.4410124550019,-6.37126553604029,
39.8573998014388));
#203994=CARTESIAN_POINT('Ctrl Pts',(-62.3334394572619,-6.35995915837761,
39.92499));
#203995=CARTESIAN_POINT('Origin',(-62.5037563256535,-6.55408556365905,40.22725));
#203996=CARTESIAN_POINT('Origin',(-0.0331877870874725,0.315760701779427,
39.116));
#203997=CARTESIAN_POINT('Origin',(-59.7081718144893,-5.95633285891171,39.116));
#203998=CARTESIAN_POINT('Origin',(1.33778643725276E-16,1.72356557454365E-17,
40.22725));
#203999=CARTESIAN_POINT('Origin',(-62.5005702980931,-6.58439859102987,40.22725));
#204000=CARTESIAN_POINT('Ctrl Pts',(-59.7081718144893,-5.95633285891171,
38.989));
#204001=CARTESIAN_POINT('Ctrl Pts',(-59.6948768129328,-6.08282634913946,
38.989));
#204002=CARTESIAN_POINT('Ctrl Pts',(-59.6948967145276,-6.08263699811343,
39.1161901092322));
#204003=CARTESIAN_POINT('Ctrl Pts',(-59.4923596726254,-5.93388096803599,
38.989));
#204004=CARTESIAN_POINT('Ctrl Pts',(-59.4792784733316,-6.06016553348717,
38.989229898976));
#204005=CARTESIAN_POINT('Ctrl Pts',(-59.5223294958616,-6.0644994528221,
39.1161900493202));
#204006=CARTESIAN_POINT('Ctrl Pts',(-59.286909633363,-5.91250946061102,
39.1034966344368));
#204007=CARTESIAN_POINT('Ctrl Pts',(-59.2739813341608,-6.03858743332049,
39.1038314102564));
#204008=CARTESIAN_POINT('Ctrl Pts',(-59.3580487495174,-6.04723285085744,
39.20775287896));
#204009=CARTESIAN_POINT('Ctrl Pts',(-59.1725467709678,-5.90061356181218,
39.2875012672119));
#204010=CARTESIAN_POINT('Ctrl Pts',(-59.1597945531718,-6.02658564326377,
39.2878045257868));
#204011=CARTESIAN_POINT('Ctrl Pts',(-59.2666022295037,-6.03762143444266,
39.3549015295899));
#204012=CARTESIAN_POINT('Origin',(-59.2797173540686,-5.91130048050303,39.3548010137695));
#204013=CARTESIAN_POINT('Ctrl Pts',(-62.3873926810692,-6.87697683366523,
39.8576902534424));
#204014=CARTESIAN_POINT('Ctrl Pts',(-62.4011871104969,-6.7501783781756,
39.8573998014387));
#204015=CARTESIAN_POINT('Ctrl Pts',(-62.293614112757,-6.73887200051292,
39.92499));
#204016=CARTESIAN_POINT('Ctrl Pts',(-62.4326397213343,-6.88173199854445,
39.9304984902493));
#204017=CARTESIAN_POINT('Ctrl Pts',(-62.4292221586313,-6.76854981002466,
39.9052171569797));
#204018=CARTESIAN_POINT('Ctrl Pts',(-62.3388594194626,-6.74362747387357,
39.9672049726606));
#204019=CARTESIAN_POINT('Ctrl Pts',(-62.4814742414945,-6.86000643604701,
40.004343767866));
#204020=CARTESIAN_POINT('Ctrl Pts',(-62.4674993676288,-6.768547072768,39.9661628577639));
#204021=CARTESIAN_POINT('Ctrl Pts',(-62.3865194274374,-6.73309031164153,
40.0100243556234));
#204022=CARTESIAN_POINT('Ctrl Pts',(-62.5644789380885,-6.76243636205646,
40.1194874821989));
#204023=CARTESIAN_POINT('Ctrl Pts',(-62.5342007968293,-6.71251593157857,
40.0627551483143));
#204024=CARTESIAN_POINT('Ctrl Pts',(-62.4648696125158,-6.679798358402,40.0767884282379));
#204025=CARTESIAN_POINT('Ctrl Pts',(-62.5984172531147,-6.68360310202781,
40.1599502015393));
#204026=CARTESIAN_POINT('Ctrl Pts',(-62.563826548014,-6.65585031610596,
40.1002449453885));
#204027=CARTESIAN_POINT('Ctrl Pts',(-62.4951999029147,-6.63528943158931,
40.10025));
#204028=CARTESIAN_POINT('Ctrl Pts',(-62.6076796697355,-6.59568250079845,
40.1599502534424));
#204029=CARTESIAN_POINT('Ctrl Pts',(-62.570580117661,-6.59177408464733,
40.10025));
#204030=CARTESIAN_POINT('Ctrl Pts',(-62.5005702980931,-6.58439859102987,
40.10025));
#204031=CARTESIAN_POINT('Origin',(-62.280338997922,-6.86517628122469,39.92499));
#204032=CARTESIAN_POINT('Origin',(-59.1025439185015,-5.89267880207714,39.6398955069327));
#204033=CARTESIAN_POINT('Origin',(-58.925370482788,-5.8740571235783,39.92499));
#204034=CARTESIAN_POINT('Origin',(-62.1031658061012,-6.84655462836385,39.6398955068272));
#204035=CARTESIAN_POINT('Origin',(-61.925992614092,-6.82793297553308,39.3548010137695));
#204036=CARTESIAN_POINT('Ctrl Pts',(-58.8181995570485,-5.86337364149541,
39.8576902534424));
#204037=CARTESIAN_POINT('Ctrl Pts',(-58.8054696185321,-5.98915458643755,
39.8579948730704));
#204038=CARTESIAN_POINT('Ctrl Pts',(-58.912095367953,-6.00036140429007,
39.92499));
#204039=CARTESIAN_POINT('Ctrl Pts',(-58.773012368204,-5.8586248113641,39.9304020711231));
#204040=CARTESIAN_POINT('Ctrl Pts',(-58.7772117628631,-5.97090589422308,
39.9058915297379));
#204041=CARTESIAN_POINT('Ctrl Pts',(-58.8669063622643,-5.99561184840474,
39.967152378603));
#204042=CARTESIAN_POINT('Ctrl Pts',(-58.7244521481309,-5.88025640567524,
40.0043257306693));
#204043=CARTESIAN_POINT('Ctrl Pts',(-58.7389107566976,-5.9711183347532,
39.9667894847842));
#204044=CARTESIAN_POINT('Ctrl Pts',(-58.8195131589313,-6.00616078842852,
40.01001389752));
#204045=CARTESIAN_POINT('Ctrl Pts',(-58.6422449895249,-5.97763489331421,
40.1195533054857));
#204046=CARTESIAN_POINT('Ctrl Pts',(-58.6726343357863,-6.02730636094608,
40.0630813209231));
#204047=CARTESIAN_POINT('Ctrl Pts',(-58.7419259266988,-6.05959099741128,
40.076826594242));
#204048=CARTESIAN_POINT('Ctrl Pts',(-58.6088386066675,-6.05629725705572,
40.1599502027529));
#204049=CARTESIAN_POINT('Ctrl Pts',(-58.6434504949707,-6.08390124328546,
40.1002552791553));
#204050=CARTESIAN_POINT('Ctrl Pts',(-58.7121001992953,-6.10418993496979,
40.10025));
#204051=CARTESIAN_POINT('Ctrl Pts',(-58.5996668978649,-6.14377718965283,
40.1599502534424));
#204052=CARTESIAN_POINT('Ctrl Pts',(-58.6367684021393,-6.14766703046132,
40.10025));
#204053=CARTESIAN_POINT('Ctrl Pts',(-58.7067819056643,-6.15500747092277,
40.10025));
#204054=CARTESIAN_POINT('Origin',(-58.7067819056643,-6.15500747092277,40.22725));
#204055=CARTESIAN_POINT('Ctrl Pts',(-61.4975385923863,-6.7829006432352,
38.989));
#204056=CARTESIAN_POINT('Ctrl Pts',(-61.5108335407726,-6.6564076588874,
38.989));
#204057=CARTESIAN_POINT('Ctrl Pts',(-61.5108136924273,-6.65659650327836,
39.1161896013267));
#204058=CARTESIAN_POINT('Ctrl Pts',(-61.7133034041536,-6.80580235504166,
38.989));
#204059=CARTESIAN_POINT('Ctrl Pts',(-61.7268068187953,-6.67910686401061,
38.988776927546));
#204060=CARTESIAN_POINT('Ctrl Pts',(-61.6833805404074,-6.67473401011687,
39.1161898821849));
#204061=CARTESIAN_POINT('Ctrl Pts',(-61.9187082819379,-6.82760223531334,
39.1034967087243));
#204062=CARTESIAN_POINT('Ctrl Pts',(-61.9323562021234,-6.70071049691222,
39.1031720232715));
#204063=CARTESIAN_POINT('Ctrl Pts',(-61.8476612078244,-6.69200060426958,
39.2077529615));
#204064=CARTESIAN_POINT('Ctrl Pts',(-62.0330459552233,-6.83973663030219,
39.2875012672119));
#204065=CARTESIAN_POINT('Ctrl Pts',(-62.046864024595,-6.71274549238769,
39.2872087095508));
#204066=CARTESIAN_POINT('Ctrl Pts',(-61.9391074595192,-6.70161199275219,
39.3549017048228));
#204067=CARTESIAN_POINT('Origin',(-61.4975385923863,-6.7829006432352,39.116));
#204068=CARTESIAN_POINT('Origin',(3.53633106925806E-16,-6.13135187546137E-18,
40.22725));
#204069=CARTESIAN_POINT('Origin',(-58.7035958781039,-6.1853204982936,40.22725));
#204070=CARTESIAN_POINT('Origin',(61.5757885448748,6.15262728712825,39.116));
#204071=CARTESIAN_POINT('Origin',(-61.0983782637168,-6.74099917687867,39.1160373285262));
#204072=CARTESIAN_POINT('Ctrl Pts',(-58.5964866834551,-6.17403490858981,
40.1599502534424));
#204073=CARTESIAN_POINT('Ctrl Pts',(-58.6335861742242,-6.17794390662133,
40.10025));
#204074=CARTESIAN_POINT('Ctrl Pts',(-58.7035958781039,-6.1853204982936,
40.10025));
#204075=CARTESIAN_POINT('Ctrl Pts',(-58.5873013840787,-6.26121185652503,
40.1599500566034));
#204076=CARTESIAN_POINT('Ctrl Pts',(-58.6268910424087,-6.24145541658243,
40.1002551305363));
#204077=CARTESIAN_POINT('Ctrl Pts',(-58.6982507756617,-6.23596000968369,
40.10025));
#204078=CARTESIAN_POINT('Ctrl Pts',(-58.603224495399,-6.34441620808569,
40.1203070619047));
#204079=CARTESIAN_POINT('Ctrl Pts',(-58.6433169201088,-6.30249747592687,
40.06370986845));
#204080=CARTESIAN_POINT('Ctrl Pts',(-58.7177256636152,-6.28536729223281,
40.0772636213363));
#204081=CARTESIAN_POINT('Ctrl Pts',(-58.6635810738165,-6.45770985055632,
40.0046102245801));
#204082=CARTESIAN_POINT('Ctrl Pts',(-58.6966524426403,-6.37191831988744,
39.9670001894012));
#204083=CARTESIAN_POINT('Ctrl Pts',(-58.7827411889911,-6.35432657855775,
40.0101788811209));
#204084=CARTESIAN_POINT('Ctrl Pts',(-58.7067768761601,-6.4889986109649,
39.9303710930187));
#204085=CARTESIAN_POINT('Ctrl Pts',(-58.7342263230564,-6.38003592347196,
39.9058663574113));
#204086=CARTESIAN_POINT('Ctrl Pts',(-58.8271002111743,-6.37452670784926,
39.967134470637));
#204087=CARTESIAN_POINT('Ctrl Pts',(-58.7519447039089,-6.49374646112702,
39.8576902534424));
#204088=CARTESIAN_POINT('Ctrl Pts',(-58.7656442740271,-6.36806742857287,
39.8579948730703));
#204089=CARTESIAN_POINT('Ctrl Pts',(-58.8722700234481,-6.37927424642539,
39.92499));
#204090=CARTESIAN_POINT('Origin',(-58.8589949086131,-6.50557852713716,39.92499));
#204091=CARTESIAN_POINT('Origin',(-61.054400080406,-6.73632490881056,39.1925554488841));
#204092=CARTESIAN_POINT('Origin',(-60.9730100652055,-6.72777047351084,39.3343017080178));
#204093=CARTESIAN_POINT('Origin',(-59.0361683443172,-6.52420020557848,39.6398955069231));
#204094=CARTESIAN_POINT('Origin',(-59.2133417798937,-6.54282188406189,39.3548010137695));
#204095=CARTESIAN_POINT('Ctrl Pts',(-60.6448574988555,-6.69328024897415,
39.3978017080178));
#204096=CARTESIAN_POINT('Ctrl Pts',(-60.6581326136904,-6.56697596826238,
39.3978017080178));
#204097=CARTESIAN_POINT('Ctrl Pts',(-60.6581326136904,-6.56697596826238,
39.5248017080178));
#204098=CARTESIAN_POINT('Ctrl Pts',(-60.7343993681214,-6.70245599674926,
39.3978017080178));
#204099=CARTESIAN_POINT('Ctrl Pts',(-60.7475659388568,-6.57637578951094,
39.3980355775196));
#204100=CARTESIAN_POINT('Ctrl Pts',(-60.7924070567575,-6.58108878091667,
39.5248015517192));
#204101=CARTESIAN_POINT('Ctrl Pts',(-60.819067758858,-6.71113417453915,
39.3484893995498));
#204102=CARTESIAN_POINT('Ctrl Pts',(-60.8325536871445,-6.58530836180368,
39.3489438303417));
#204103=CARTESIAN_POINT('Ctrl Pts',(-60.919373095124,-6.59443344928389,
39.4508333155595));
#204104=CARTESIAN_POINT('Ctrl Pts',(-60.8636883187845,-6.7157078966937,
39.2708017080178));
#204105=CARTESIAN_POINT('Ctrl Pts',(-60.8773920302461,-6.59002106156426,
39.2710850691866));
#204106=CARTESIAN_POINT('Ctrl Pts',(-60.9862851800405,-6.60146619279907,
39.3343017080178));
#204107=CARTESIAN_POINT('Origin',(-60.6448574988555,-6.69328024897415,39.5248017080178));
#204108=CARTESIAN_POINT('Ctrl Pts',(-59.1062911958297,-6.53099325080016,
39.2875012672119));
#204109=CARTESIAN_POINT('Ctrl Pts',(-59.1200087114582,-6.40512264090962,
39.2878045257519));
#204110=CARTESIAN_POINT('Ctrl Pts',(-59.2267768430461,-6.41653455700086,
39.3549015218348));
#204111=CARTESIAN_POINT('Ctrl Pts',(-59.2206299794252,-6.54313486548303,
39.1034938540228));
#204112=CARTESIAN_POINT('Ctrl Pts',(-59.2341972766252,-6.41712406698078,
39.103828627881));
#204113=CARTESIAN_POINT('Ctrl Pts',(-59.318224747433,-6.42614611919703,
39.2077506434031));
#204114=CARTESIAN_POINT('Ctrl Pts',(-59.426035450364,-6.56494601397012,
38.989));
#204115=CARTESIAN_POINT('Ctrl Pts',(-59.4394961352152,-6.43870134519683,
38.9892298954611));
#204116=CARTESIAN_POINT('Ctrl Pts',(-59.4825067955799,-6.44341285848409,
39.1161900347289));
#204117=CARTESIAN_POINT('Ctrl Pts',(-59.6417962403143,-6.58785426247057,
38.989));
#204118=CARTESIAN_POINT('Ctrl Pts',(-59.6550912403353,-6.46136078685196,
38.989));
#204119=CARTESIAN_POINT('Ctrl Pts',(-59.6550713402783,-6.46155012324701,
39.1161900945646));
#204120=CARTESIAN_POINT('Origin',(-59.6417962403143,-6.58785426247057,39.116));
#204121=CARTESIAN_POINT('Origin',(60.0850508448142,5.99594444118168,39.5248017080178));
#204122=CARTESIAN_POINT('Origin',(-60.4944777170594,-6.67747469700906,39.5248017080178));
#204123=CARTESIAN_POINT('Origin',(59.8516078896891,5.9714085979051,39.116));
#204124=CARTESIAN_POINT('Origin',(-60.0409538388299,-6.62985850077773,39.1160402713847));
#204125=CARTESIAN_POINT('Ctrl Pts',(-60.2756459899119,-6.65505462397356,
39.2708017080178));
#204126=CARTESIAN_POINT('Ctrl Pts',(-60.2894805317162,-6.52822907310738,
39.2705119464801));
#204127=CARTESIAN_POINT('Ctrl Pts',(-60.1796001951996,-6.51668018436707,
39.3343017080178));
#204128=CARTESIAN_POINT('Ctrl Pts',(-60.3204176712045,-6.65964099131245,
39.3487519301186));
#204129=CARTESIAN_POINT('Ctrl Pts',(-60.3340024654448,-6.53290851690434,
39.3482879463971));
#204130=CARTESIAN_POINT('Ctrl Pts',(-60.2467384099268,-6.52373669508308,
39.4512271261623));
#204131=CARTESIAN_POINT('Ctrl Pts',(-60.4052373806432,-6.66833043150608,
39.3978017080178));
#204132=CARTESIAN_POINT('Ctrl Pts',(-60.4184509388156,-6.54178440911727,
39.3975673827415));
#204133=CARTESIAN_POINT('Ctrl Pts',(-60.3739306632446,-6.53710513959975,
39.5248015355199));
#204134=CARTESIAN_POINT('Ctrl Pts',(-60.4944777170594,-6.67747469700906,
39.3978017080178));
#204135=CARTESIAN_POINT('Ctrl Pts',(-60.5077528318944,-6.55117041629729,
39.3978017080178));
#204136=CARTESIAN_POINT('Ctrl Pts',(-60.5077528318944,-6.55117041629729,
39.5248017080178));
#204137=CARTESIAN_POINT('Origin',(-60.1663250803646,-6.64298446507884,39.3343017080178));
#204138=CARTESIAN_POINT('Origin',(-60.0854204586811,-6.63448104699053,39.1934008533548));
#204139=CARTESIAN_POINT('Origin',(-61.4240753804085,0.317499999705897,39.1925554495081));
#204140=CARTESIAN_POINT('Origin',(-61.4683012396063,0.317551690012599,39.1160373285251));
#204141=CARTESIAN_POINT('Origin',(-61.3422370451705,0.3175,39.3343017080178));
#204142=CARTESIAN_POINT('Ctrl Pts',(-61.2322532920972,0.316930737395914,
39.2708017080178));
#204143=CARTESIAN_POINT('Ctrl Pts',(-61.2327440814645,0.1905,39.2710850691866));
#204144=CARTESIAN_POINT('Ctrl Pts',(-61.3422370451705,0.1905,39.3343017080178));
#204145=CARTESIAN_POINT('Ctrl Pts',(-61.1872475084174,0.317046579199636,
39.3487519293518));
#204146=CARTESIAN_POINT('Ctrl Pts',(-61.1875064541755,0.190499999998394,
39.349206866293));
#204147=CARTESIAN_POINT('Ctrl Pts',(-61.274729039531,0.1905,39.4512271248743));
#204148=CARTESIAN_POINT('Ctrl Pts',(-61.1019842137032,0.317266596913493,
39.3978017080178));
#204149=CARTESIAN_POINT('Ctrl Pts',(-61.1018997758111,0.190499999999993,
39.3980347781178));
#204150=CARTESIAN_POINT('Ctrl Pts',(-61.1468362071712,0.1905,39.524801535519));
#204151=CARTESIAN_POINT('Ctrl Pts',(-61.0122769227456,0.3175,39.3978017080178));
#204152=CARTESIAN_POINT('Ctrl Pts',(-61.0122769227456,0.1905,39.3978017080178));
#204153=CARTESIAN_POINT('Ctrl Pts',(-61.0122769227456,0.1905,39.5248017080178));
#204154=CARTESIAN_POINT('Origin',(-61.0122769227456,0.3175,39.5248017080178));
#204155=CARTESIAN_POINT('Origin',(5.50819412990574E-15,0.3175,39.116));
#204156=CARTESIAN_POINT('Origin',(-61.8696548221181,0.3175,39.116));
#204157=CARTESIAN_POINT('Origin',(5.56576032196012E-15,0.3175,39.5248017080178));
#204158=CARTESIAN_POINT('Origin',(-60.8610688070707,0.3175,39.5248017080178));
#204159=CARTESIAN_POINT('Ctrl Pts',(-62.4081695979768,0.318048871877129,
39.2875012672119));
#204160=CARTESIAN_POINT('Ctrl Pts',(-62.4086377819835,0.190309034175427,
39.287208709576));
#204161=CARTESIAN_POINT('Ctrl Pts',(-62.3003077603772,0.190500142125054,
39.3549016990124));
#204162=CARTESIAN_POINT('Ctrl Pts',(-62.2931881445371,0.317932489889954,
39.1034939173931));
#204163=CARTESIAN_POINT('Ctrl Pts',(-62.2934975005749,0.190309294367765,
39.1031692336328));
#204164=CARTESIAN_POINT('Ctrl Pts',(-62.2083564003268,0.190500141995467,
39.2077507202292));
#204165=CARTESIAN_POINT('Ctrl Pts',(-62.0866281564672,0.317722686167411,
38.989));
#204166=CARTESIAN_POINT('Ctrl Pts',(-62.0868143053079,0.190309769569793,
38.9887769311176));
#204167=CARTESIAN_POINT('Ctrl Pts',(-62.0431695205376,0.190500141761866,
39.1161898712917));
#204168=CARTESIAN_POINT('Ctrl Pts',(-61.8696548221181,0.3175,38.989));
#204169=CARTESIAN_POINT('Ctrl Pts',(-61.8696548221181,0.190310267889066,
38.989));
#204170=CARTESIAN_POINT('Ctrl Pts',(-61.8696548221181,0.190500141513915,
39.1161895903856));
#204171=CARTESIAN_POINT('Origin',(-62.3004688883554,0.3175,39.3548010137695));
#204172=CARTESIAN_POINT('Ctrl Pts',(-60.8610688070707,0.3175,39.3978017080178));
#204173=CARTESIAN_POINT('Ctrl Pts',(-60.8610688070707,0.1905,39.3978017080178));
#204174=CARTESIAN_POINT('Ctrl Pts',(-60.8610688070707,0.1905,39.5248017080178));
#204175=CARTESIAN_POINT('Ctrl Pts',(-60.7710583184321,0.317734773760269,
39.3978017080178));
#204176=CARTESIAN_POINT('Ctrl Pts',(-60.7709717342448,0.1905,39.397566602504));
#204177=CARTESIAN_POINT('Ctrl Pts',(-60.7260547307367,0.1905,39.5248015517196));
#204178=CARTESIAN_POINT('Ctrl Pts',(-60.6859465754578,0.317958617919043,
39.3484894016717));
#204179=CARTESIAN_POINT('Ctrl Pts',(-60.6862105562525,0.190499999999993,
39.3480259000038));
#204180=CARTESIAN_POINT('Ctrl Pts',(-60.5983892955396,0.1905,39.4508333188936));
#204181=CARTESIAN_POINT('Ctrl Pts',(-60.6410923272405,0.318076890623366,
39.2708017080178));
#204182=CARTESIAN_POINT('Ctrl Pts',(-60.6415942020421,0.1905,39.2705119464801));
#204183=CARTESIAN_POINT('Ctrl Pts',(-60.5311086139135,0.1905,39.3343017080178));
#204184=CARTESIAN_POINT('Origin',(-60.5311086139134,0.3175,39.3343017080178));
#204185=CARTESIAN_POINT('Origin',(-62.4786179998484,0.317499999976884,39.6398955068187));
#204186=CARTESIAN_POINT('Origin',(-62.6567671111299,0.3175,39.92499));
#204187=CARTESIAN_POINT('Origin',(-60.4497583458796,0.317499999992453,39.1934008539944));
#204188=CARTESIAN_POINT('Origin',(-60.4050521322801,0.317550804320716,39.116040271385));
#204189=CARTESIAN_POINT('Ctrl Pts',(-62.9541448057648,0.0152661173108668,
40.1599502534424));
#204190=CARTESIAN_POINT('Ctrl Pts',(-62.9168399481843,0.0152570710386341,
40.10025));
#204191=CARTESIAN_POINT('Ctrl Pts',(-62.8464427007196,0.01524,40.10025));
#204192=CARTESIAN_POINT('Ctrl Pts',(-62.9541233134297,0.103381504925153,
40.1599500538463));
#204193=CARTESIAN_POINT('Ctrl Pts',(-62.9168211560341,0.0794415635235332,
40.100244835349));
#204194=CARTESIAN_POINT('Ctrl Pts',(-62.8464212442881,0.0662446030559308,
40.10025));
#204195=CARTESIAN_POINT('Ctrl Pts',(-62.9290872705826,0.184683583687856,
40.1202442001037));
#204196=CARTESIAN_POINT('Ctrl Pts',(-62.8936771137448,0.138547994784339,
40.0633873868018));
#204197=CARTESIAN_POINT('Ctrl Pts',(-62.8213855864655,0.113305567451571,
40.0772271723537));
#204198=CARTESIAN_POINT('Ctrl Pts',(-62.8564203507742,0.291340992631635,
40.0045995998164));
#204199=CARTESIAN_POINT('Ctrl Pts',(-62.8329175802742,0.201910351191299,
39.9663485808314));
#204200=CARTESIAN_POINT('Ctrl Pts',(-62.7487193609389,0.175042741957826,
40.0101727202466));
#204201=CARTESIAN_POINT('Ctrl Pts',(-62.8099434033761,0.318045276842632,
39.9304654349858));
#204202=CARTESIAN_POINT('Ctrl Pts',(-62.7947175425018,0.205831635642382,
39.9051900162939));
#204203=CARTESIAN_POINT('Ctrl Pts',(-62.7022409210443,0.190499999999998,
39.9671857458178));
#204204=CARTESIAN_POINT('Ctrl Pts',(-62.7644678366119,0.318045750793045,
39.8576902534424));
#204205=CARTESIAN_POINT('Ctrl Pts',(-62.7649326510149,0.190500000000004,
39.8573998014387));
#204206=CARTESIAN_POINT('Ctrl Pts',(-62.6567671111299,0.1905,39.92499));
#204207=CARTESIAN_POINT('Origin',(5.50819412990574E-15,0.3175,39.116));
#204208=CARTESIAN_POINT('Origin',(-60.003690522373,0.3175,39.116));
#204209=CARTESIAN_POINT('Ctrl Pts',(-60.003690522373,0.3175,38.989));
#204210=CARTESIAN_POINT('Ctrl Pts',(-60.003690522373,0.190309748265386,
38.989));
#204211=CARTESIAN_POINT('Ctrl Pts',(-60.003690522373,0.190500142289529,
39.1161901092319));
#204212=CARTESIAN_POINT('Ctrl Pts',(-59.7867137603524,0.317270385524416,
38.989));
#204213=CARTESIAN_POINT('Ctrl Pts',(-59.7869045527969,0.190310262476459,
38.989229898976));
#204214=CARTESIAN_POINT('Ctrl Pts',(-59.8301727552494,0.190500142032462,
39.1161900493199));
#204215=CARTESIAN_POINT('Ctrl Pts',(-59.5801552670728,0.317049440713614,
39.1034966344368));
#204216=CARTESIAN_POINT('Ctrl Pts',(-59.5804765271871,0.190310761081929,
39.1038314102569));
#204217=CARTESIAN_POINT('Ctrl Pts',(-59.6649871046549,0.190500141785106,
39.20775287896));
#204218=CARTESIAN_POINT('Ctrl Pts',(-59.4651754363832,0.316925998273047,
39.2875012672119));
#204219=CARTESIAN_POINT('Ctrl Pts',(-59.4656607446594,0.190311035335126,
39.2878045257868));
#204220=CARTESIAN_POINT('Ctrl Pts',(-59.5730368716575,0.190500141646902,
39.3549015295898));
#204221=CARTESIAN_POINT('Origin',(-59.5728760150042,0.3175,39.3548010137695));
#204222=CARTESIAN_POINT('Ctrl Pts',(-62.7644678366119,-0.318045750793045,
39.8576902534424));
#204223=CARTESIAN_POINT('Ctrl Pts',(-62.7649326510148,-0.1905,39.8573998014387));
#204224=CARTESIAN_POINT('Ctrl Pts',(-62.6567671111299,-0.1905,39.92499));
#204225=CARTESIAN_POINT('Ctrl Pts',(-62.8099640589335,-0.318045262795181,
39.9304984902491));
#204226=CARTESIAN_POINT('Ctrl Pts',(-62.7947344577634,-0.205840330723031,
39.9052171569785));
#204227=CARTESIAN_POINT('Ctrl Pts',(-62.7022616416339,-0.1905,39.9672049726601));
#204228=CARTESIAN_POINT('Ctrl Pts',(-62.8562601188214,-0.291334117855409,
40.0043437678662));
#204229=CARTESIAN_POINT('Ctrl Pts',(-62.8328016940825,-0.201836550627716,
39.966162857764));
#204230=CARTESIAN_POINT('Ctrl Pts',(-62.7485591297232,-0.1750387340522,
40.0100243556234));
#204231=CARTESIAN_POINT('Ctrl Pts',(-62.9286112571071,-0.185622189560398,
40.1194874821988));
#204232=CARTESIAN_POINT('Ctrl Pts',(-62.8932808767899,-0.139140156000136,
40.0627551483143));
#204233=CARTESIAN_POINT('Ctrl Pts',(-62.8209095783125,-0.113848895265678,
40.0767884282378));
#204234=CARTESIAN_POINT('Ctrl Pts',(-62.9541233349674,-0.103673266462822,
40.1599502015391));
#204235=CARTESIAN_POINT('Ctrl Pts',(-62.9168211653022,-0.0796882264536551,
40.1002449453869));
#204236=CARTESIAN_POINT('Ctrl Pts',(-62.8464212664863,-0.0664134143651546,
40.10025));
#204237=CARTESIAN_POINT('Ctrl Pts',(-62.9541448057648,-0.0152661173108661,
40.1599502534424));
#204238=CARTESIAN_POINT('Ctrl Pts',(-62.9168399481843,-0.0152570710386336,
40.10025));
#204239=CARTESIAN_POINT('Ctrl Pts',(-62.8464427007196,-0.0152399999999996,
40.10025));
#204240=CARTESIAN_POINT('Origin',(-62.6567671111299,-0.3175,39.92499));
#204241=CARTESIAN_POINT('Origin',(-59.3947266586251,0.317499999970926,39.6398955069322));
#204242=CARTESIAN_POINT('Origin',(-59.2165773020941,0.3175,39.92499));
#204243=CARTESIAN_POINT('Origin',(-62.4786179998343,-0.317499999976807,
39.6398955068275));
#204244=CARTESIAN_POINT('Origin',(-62.3004688883554,-0.3175,39.3548010137695));
#204245=CARTESIAN_POINT('Ctrl Pts',(-59.1088767419348,0.316922544675689,
39.8576902534424));
#204246=CARTESIAN_POINT('Ctrl Pts',(-59.1093642282367,0.190499999999994,
39.8579948730703));
#204247=CARTESIAN_POINT('Ctrl Pts',(-59.2165773020941,0.1905,39.92499));
#204248=CARTESIAN_POINT('Ctrl Pts',(-59.063440705323,0.316922012809165,
39.9304020711229));
#204249=CARTESIAN_POINT('Ctrl Pts',(-59.0793536643041,0.205694973741121,
39.9058915297382));
#204250=CARTESIAN_POINT('Ctrl Pts',(-59.1711393827295,0.1905,39.9671523786035));
#204251=CARTESIAN_POINT('Ctrl Pts',(-59.0174076205275,0.290332993454962,
40.0043257306695));
#204252=CARTESIAN_POINT('Ctrl Pts',(-59.0412846811395,0.201480151665867,
39.9667894847835));
#204253=CARTESIAN_POINT('Ctrl Pts',(-59.1251084688121,0.175054909459692,
40.01001389752));
#204254=CARTESIAN_POINT('Ctrl Pts',(-58.9458296250063,0.184894967401607,
40.1195533054855));
#204255=CARTESIAN_POINT('Ctrl Pts',(-58.9812445774292,0.138672156931206,
40.0630813209236));
#204256=CARTESIAN_POINT('Ctrl Pts',(-59.0535312451933,0.113807322597792,
40.076826594242));
#204257=CARTESIAN_POINT('Ctrl Pts',(-58.9208287018089,0.10317160645571,
40.1599502027521));
#204258=CARTESIAN_POINT('Ctrl Pts',(-58.9581363848278,0.0793367652458316,
40.1002552791554));
#204259=CARTESIAN_POINT('Ctrl Pts',(-59.0285307646525,0.0663350652343385,
40.10025));
#204260=CARTESIAN_POINT('Ctrl Pts',(-58.9208513795073,0.0152121934559205,
40.1599502534424));
#204261=CARTESIAN_POINT('Ctrl Pts',(-58.9581562369413,0.0152218248291074,
40.10025));
#204262=CARTESIAN_POINT('Ctrl Pts',(-59.0285534841296,0.0152400000000004,
40.10025));
#204263=CARTESIAN_POINT('Ctrl Pts',(-61.8696548221181,-0.3175,38.989));
#204264=CARTESIAN_POINT('Ctrl Pts',(-61.8696548221181,-0.190310256931795,
38.989));
#204265=CARTESIAN_POINT('Ctrl Pts',(-61.8696548221181,-0.190500141530248,
39.1161896013265));
#204266=CARTESIAN_POINT('Ctrl Pts',(-62.0866315324121,-0.31772268963223,
38.989));
#204267=CARTESIAN_POINT('Ctrl Pts',(-62.0868176889526,-0.190309758576012,
38.988776927546));
#204268=CARTESIAN_POINT('Ctrl Pts',(-62.0431722165666,-0.190500141778232,
39.1161898821847));
#204269=CARTESIAN_POINT('Ctrl Pts',(-62.2931898887681,-0.317932491655698,
39.1034967087244));
#204270=CARTESIAN_POINT('Ctrl Pts',(-62.2934992458057,-0.190309283350195,
39.1031720232705));
#204271=CARTESIAN_POINT('Ctrl Pts',(-62.2083577878507,-0.190500142011858,
39.2077529614999));
#204272=CARTESIAN_POINT('Ctrl Pts',(-62.4081695979768,-0.318048871877129,
39.2875012672119));
#204273=CARTESIAN_POINT('Ctrl Pts',(-62.4086377820239,-0.190309023146872,
39.2872087095507));
#204274=CARTESIAN_POINT('Ctrl Pts',(-62.3003077510788,-0.190500142141458,
39.3549017048227));
#204275=CARTESIAN_POINT('Origin',(-61.8696548221181,-0.3175,39.116));
#204276=CARTESIAN_POINT('Origin',(62.2224557307631,-0.3175,39.116));
#204277=CARTESIAN_POINT('Origin',(-61.4683012396084,-0.317551690014637,
39.1160373285281));
#204278=CARTESIAN_POINT('Ctrl Pts',(-58.9208513795073,-0.0152121934559198,
40.1599502534424));
#204279=CARTESIAN_POINT('Ctrl Pts',(-58.9581562369413,-0.0152218248291069,
40.10025));
#204280=CARTESIAN_POINT('Ctrl Pts',(-59.0285534841296,-0.01524,40.10025));
#204281=CARTESIAN_POINT('Ctrl Pts',(-58.9208288705619,-0.102871702177371,
40.1599500566036));
#204282=CARTESIAN_POINT('Ctrl Pts',(-58.9581365422967,-0.0790852439332833,
40.100255130536));
#204283=CARTESIAN_POINT('Ctrl Pts',(-59.0285309330221,-0.0661608181924982,
40.10025));
#204284=CARTESIAN_POINT('Ctrl Pts',(-58.9453619764183,-0.183955833237535,
40.1203070619047));
#204285=CARTESIAN_POINT('Ctrl Pts',(-58.9808530699758,-0.138075936736132,
40.0637098684499));
#204286=CARTESIAN_POINT('Ctrl Pts',(-59.0530636028226,-0.113261762368167,
40.0772636213363));
#204287=CARTESIAN_POINT('Ctrl Pts',(-59.0172303255293,-0.290319860890624,
40.0046102245802));
#204288=CARTESIAN_POINT('Ctrl Pts',(-59.0411528690725,-0.201541405841779,
39.9670001894012));
#204289=CARTESIAN_POINT('Ctrl Pts',(-59.1249311745757,-0.175047309551177,
40.0101788811209));
#204290=CARTESIAN_POINT('Ctrl Pts',(-59.0634600627912,-0.316922027357334,
39.9303710930186));
#204291=CARTESIAN_POINT('Ctrl Pts',(-59.079369436468,-0.205687000366196,
39.9058663574111));
#204292=CARTESIAN_POINT('Ctrl Pts',(-59.1711586818662,-0.190499999999998,
39.9671344706369));
#204293=CARTESIAN_POINT('Ctrl Pts',(-59.1088767419348,-0.316922544675689,
39.8576902534424));
#204294=CARTESIAN_POINT('Ctrl Pts',(-59.1093642282366,-0.190500000000004,
39.8579948730704));
#204295=CARTESIAN_POINT('Ctrl Pts',(-59.2165773020941,-0.1905,39.92499));
#204296=CARTESIAN_POINT('Origin',(-59.2165773020941,-0.3175,39.92499));
#204297=CARTESIAN_POINT('Origin',(-61.4240753793289,-0.317499999995429,
39.1925554488848));
#204298=CARTESIAN_POINT('Origin',(-61.3422370451705,-0.3175,39.3343017080178));
#204299=CARTESIAN_POINT('Origin',(-59.3947266586079,-0.317499999970831,
39.6398955069215));
#204300=CARTESIAN_POINT('Origin',(-59.5728760150042,-0.3175,39.3548010137695));
#204301=CARTESIAN_POINT('Ctrl Pts',(-61.0122769227456,-0.3175,39.3978017080178));
#204302=CARTESIAN_POINT('Ctrl Pts',(-61.0122769227456,-0.1905,39.3978017080178));
#204303=CARTESIAN_POINT('Ctrl Pts',(-61.0122769227456,-0.1905,39.5248017080178));
#204304=CARTESIAN_POINT('Ctrl Pts',(-61.102287399097,-0.317265808076389,
39.3978017080178));
#204305=CARTESIAN_POINT('Ctrl Pts',(-61.1022028716714,-0.190499999999991,
39.3980355775177));
#204306=CARTESIAN_POINT('Ctrl Pts',(-61.1472909869838,-0.1905,39.5248015517192));
#204307=CARTESIAN_POINT('Ctrl Pts',(-61.1873990841185,-0.317046189129109,
39.3484893995498));
#204308=CARTESIAN_POINT('Ctrl Pts',(-61.1876587562312,-0.190500000000015,
39.3489438303423));
#204309=CARTESIAN_POINT('Ctrl Pts',(-61.2749563897835,-0.1905,39.4508333155593));
#204310=CARTESIAN_POINT('Ctrl Pts',(-61.2322532920972,-0.316930737395914,
39.2708017080178));
#204311=CARTESIAN_POINT('Ctrl Pts',(-61.2327440814645,-0.1905,39.2710850691866));
#204312=CARTESIAN_POINT('Ctrl Pts',(-61.3422370451705,-0.1905,39.3343017080178));
#204313=CARTESIAN_POINT('Origin',(-61.0122769227456,-0.3175,39.5248017080178));
#204314=CARTESIAN_POINT('Ctrl Pts',(-59.4651754363832,-0.316925998273047,
39.2875012672119));
#204315=CARTESIAN_POINT('Ctrl Pts',(-59.4656607446034,-0.190311049925011,
39.2878045257519));
#204316=CARTESIAN_POINT('Ctrl Pts',(-59.5730368592471,-0.190500141625046,
39.3549015218348));
#204317=CARTESIAN_POINT('Ctrl Pts',(-59.5801570044831,-0.317049442579187,
39.1034938540228));
#204318=CARTESIAN_POINT('Ctrl Pts',(-59.5804782634865,-0.190310775687219,
39.1038286278809));
#204319=CARTESIAN_POINT('Ctrl Pts',(-59.6649884842712,-0.190500141763233,
39.2077506434031));
#204320=CARTESIAN_POINT('Ctrl Pts',(-59.7867171285936,-0.317270389088839,
38.989));
#204321=CARTESIAN_POINT('Ctrl Pts',(-59.7869079131825,-0.190310277118105,
38.9892298954611));
#204322=CARTESIAN_POINT('Ctrl Pts',(-59.8301754438929,-0.19050014201055,
39.116190034729));
#204323=CARTESIAN_POINT('Ctrl Pts',(-60.003690522373,-0.3175,38.989));
#204324=CARTESIAN_POINT('Ctrl Pts',(-60.003690522373,-0.190309762954695,
38.989));
#204325=CARTESIAN_POINT('Ctrl Pts',(-60.003690522373,-0.190500142267574,
39.1161900945646));
#204326=CARTESIAN_POINT('Origin',(-60.0036905223731,-0.3175,39.116));
#204327=CARTESIAN_POINT('Origin',(60.71525,-0.3175,39.5248017080178));
#204328=CARTESIAN_POINT('Origin',(-60.8610688070707,-0.3175,39.5248017080178));
#204329=CARTESIAN_POINT('Origin',(60.4792282238308,-0.3175,39.116));
#204330=CARTESIAN_POINT('Origin',(-60.40505213228,-0.317550804320886,39.1160402713852));
#204331=CARTESIAN_POINT('Ctrl Pts',(-60.6410923272405,-0.318076890623366,
39.2708017080178));
#204332=CARTESIAN_POINT('Ctrl Pts',(-60.6415942020421,-0.1905,39.2705119464801));
#204333=CARTESIAN_POINT('Ctrl Pts',(-60.5311086139134,-0.1905,39.3343017080178));
#204334=CARTESIAN_POINT('Ctrl Pts',(-60.6860981505083,-0.317958218318758,
39.3487519301186));
#204335=CARTESIAN_POINT('Ctrl Pts',(-60.68636137503,-0.190499999997976,
39.3482879463971));
#204336=CARTESIAN_POINT('Ctrl Pts',(-60.5986166446964,-0.1905,39.4512271261627));
#204337=CARTESIAN_POINT('Ctrl Pts',(-60.771361502534,-0.317733982967541,
39.3978017080178));
#204338=CARTESIAN_POINT('Ctrl Pts',(-60.771275014198,-0.1905,39.3975673827411));
#204339=CARTESIAN_POINT('Ctrl Pts',(-60.7265095085044,-0.1905,39.5248015355195));
#204340=CARTESIAN_POINT('Ctrl Pts',(-60.8610688070707,-0.3175,39.3978017080178));
#204341=CARTESIAN_POINT('Ctrl Pts',(-60.8610688070707,-0.1905,39.3978017080178));
#204342=CARTESIAN_POINT('Ctrl Pts',(-60.8610688070707,-0.1905,39.5248017080178));
#204343=CARTESIAN_POINT('Origin',(-60.5311086139135,-0.3175,39.3343017080178));
#204344=CARTESIAN_POINT('Origin',(-60.4497583469873,-0.31750000030155,39.1934008533549));
#204345=CARTESIAN_POINT('Origin',(-61.0544000815112,6.73632490863974,39.1925554495085));
#204346=CARTESIAN_POINT('Origin',(-61.0983782637182,6.74099917688121,39.1160373285283));
#204347=CARTESIAN_POINT('Origin',(-60.9730100652054,6.72777047351166,39.3343017080178));
#204348=CARTESIAN_POINT('Ctrl Pts',(-60.8636883187844,6.71570789669452,
39.2708017080178));
#204349=CARTESIAN_POINT('Ctrl Pts',(-60.877392030246,6.59002106156508,39.2710850691866));
#204350=CARTESIAN_POINT('Ctrl Pts',(-60.9862851800404,6.60146619279989,
39.3343017080178));
#204351=CARTESIAN_POINT('Ctrl Pts',(-60.8189169727309,6.71111871849841,
39.3487519293518));
#204352=CARTESIAN_POINT('Ctrl Pts',(-60.8324022194118,6.58529244190258,
39.3492068662932));
#204353=CARTESIAN_POINT('Ctrl Pts',(-60.9191469903167,6.59440968471186,
39.4512271248736));
#204354=CARTESIAN_POINT('Ctrl Pts',(-60.7340977611528,6.70242508976258,
39.3978017080178));
#204355=CARTESIAN_POINT('Ctrl Pts',(-60.7472645033899,6.5763441073677,39.3980347781174));
#204356=CARTESIAN_POINT('Ctrl Pts',(-60.7919547682785,6.5810412434828,39.524801535519));
#204357=CARTESIAN_POINT('Ctrl Pts',(-60.6448574988554,6.69328024897497,
39.3978017080178));
#204358=CARTESIAN_POINT('Ctrl Pts',(-60.6581326136904,6.5669759682632,39.3978017080178));
#204359=CARTESIAN_POINT('Ctrl Pts',(-60.6581326136904,6.5669759682632,39.5248017080178));
#204360=CARTESIAN_POINT('Origin',(-60.6448574988554,6.69328024897497,39.5248017080178));
#204361=CARTESIAN_POINT('Origin',(0.0331877870874877,0.315760701779427,
39.116));
#204362=CARTESIAN_POINT('Origin',(-61.4975385923862,6.78290064323603,39.116));
#204363=CARTESIAN_POINT('Origin',(0.0331877870874878,0.315760701779427,
39.5248017080178));
#204364=CARTESIAN_POINT('Origin',(-60.4944777170593,6.67747469700988,39.5248017080178));
#204365=CARTESIAN_POINT('Ctrl Pts',(-62.0330459552232,6.83973663030303,
39.2875012672119));
#204366=CARTESIAN_POINT('Ctrl Pts',(-62.0468640234019,6.71274550335285,
39.287208709576));
#204367=CARTESIAN_POINT('Ctrl Pts',(-61.9391074687686,6.70161199370869,
39.3549016990123));
#204368=CARTESIAN_POINT('Ctrl Pts',(-61.9187065474464,6.82760205123632,
39.103493917393));
#204369=CARTESIAN_POINT('Ctrl Pts',(-61.9323544653015,6.70071032544359,
39.1031692336337));
#204370=CARTESIAN_POINT('Ctrl Pts',(-61.8476598279006,6.6920004592181,39.2077507202297));
#204371=CARTESIAN_POINT('Ctrl Pts',(-61.7133000470647,6.80580199871487,
38.989));
#204372=CARTESIAN_POINT('Ctrl Pts',(-61.7268034525372,6.67910652125848,
38.9887769311176));
#204373=CARTESIAN_POINT('Ctrl Pts',(-61.6833778591514,6.67473372828989,
39.1161898712915));
#204374=CARTESIAN_POINT('Ctrl Pts',(-61.4975385923862,6.78290064323603,
38.989));
#204375=CARTESIAN_POINT('Ctrl Pts',(-61.5108335396271,6.65640766978589,
38.989));
#204376=CARTESIAN_POINT('Ctrl Pts',(-61.5108136924289,6.65659650326295,
39.1161895903854));
#204377=CARTESIAN_POINT('Origin',(-61.9259926140919,6.82793297553392,39.3548010137695));
#204378=CARTESIAN_POINT('Ctrl Pts',(-60.4944777170593,6.67747469700988,
39.3978017080178));
#204379=CARTESIAN_POINT('Ctrl Pts',(-60.5077528318943,6.55117041629811,
39.3978017080178));
#204380=CARTESIAN_POINT('Ctrl Pts',(-60.5077528318943,6.55117041629811,
39.5248017080178));
#204381=CARTESIAN_POINT('Ctrl Pts',(-60.4049357747551,6.66829952659918,
39.3978017080178));
#204382=CARTESIAN_POINT('Ctrl Pts',(-60.4181493202576,6.54175270773008,
39.397566602504));
#204383=CARTESIAN_POINT('Ctrl Pts',(-60.3734783767973,6.53705760237942,
39.5248015517196));
#204384=CARTESIAN_POINT('Ctrl Pts',(-60.3202668847282,6.65962554481747,
39.3484894016716));
#204385=CARTESIAN_POINT('Ctrl Pts',(-60.3338524728735,6.53289275205061,
39.3480259000029));
#204386=CARTESIAN_POINT('Ctrl Pts',(-60.2465123062119,6.52371293062585,
39.4508333188936));
#204387=CARTESIAN_POINT('Ctrl Pts',(-60.2756459899118,6.65505462397437,
39.2708017080178));
#204388=CARTESIAN_POINT('Ctrl Pts',(-60.2894805317161,6.5282290731082,39.2705119464801));
#204389=CARTESIAN_POINT('Ctrl Pts',(-60.1796001951995,6.51668018436788,
39.3343017080178));
#204390=CARTESIAN_POINT('Origin',(-60.1663250803645,6.64298446507965,39.3343017080178));
#204391=CARTESIAN_POINT('Origin',(-62.1031658061144,6.8465546283679,39.6398955068187));
#204392=CARTESIAN_POINT('Origin',(-62.2803389979219,6.86517628122553,39.92499));
#204393=CARTESIAN_POINT('Origin',(-60.0854204576109,6.63448104656938,39.1934008539947));
#204394=CARTESIAN_POINT('Origin',(-60.0409538388295,6.62985850077888,39.1160402713849));
#204395=CARTESIAN_POINT('Ctrl Pts',(-62.6076796697354,6.59568250079929,
40.1599502534424));
#204396=CARTESIAN_POINT('Ctrl Pts',(-62.5705801176609,6.59177408464818,
40.10025));
#204397=CARTESIAN_POINT('Ctrl Pts',(-62.500570298093,6.58439859103072,40.10025));
#204398=CARTESIAN_POINT('Ctrl Pts',(-62.5984477290795,6.68331293653975,
40.1599500538457));
#204399=CARTESIAN_POINT('Ctrl Pts',(-62.5638523220909,6.65560500345286,
40.1002448353503));
#204400=CARTESIAN_POINT('Ctrl Pts',(-62.495217526425,6.63512154272658,40.10025));
#204401=CARTESIAN_POINT('Ctrl Pts',(-62.5650504549418,6.76155265492316,
40.1202442001039));
#204402=CARTESIAN_POINT('Ctrl Pts',(-62.5346567608586,6.71196843232467,
40.0633873868018));
#204403=CARTESIAN_POINT('Ctrl Pts',(-62.4653998062672,6.67930776339611,
40.0772271723537));
#204404=CARTESIAN_POINT('Ctrl Pts',(-62.48163287707,6.86003002196301,40.0045995998162));
#204405=CARTESIAN_POINT('Ctrl Pts',(-62.4676069047243,6.76863258245075,
39.9663485808315));
#204406=CARTESIAN_POINT('Ctrl Pts',(-62.3866783619498,6.73311104631499,
40.0101727202466));
#204407=CARTESIAN_POINT('Ctrl Pts',(-62.4326191774618,6.88172985342207,
39.930465434986));
#204408=CARTESIAN_POINT('Ctrl Pts',(-62.4292062449178,6.76853939445011,
39.9051900162948));
#204409=CARTESIAN_POINT('Ctrl Pts',(-62.338838812383,6.74362530798309,39.9671857458173));
#204410=CARTESIAN_POINT('Ctrl Pts',(-62.3873926810691,6.87697683366608,
39.8576902534424));
#204411=CARTESIAN_POINT('Ctrl Pts',(-62.4011871104968,6.75017837817646,
39.8573998014387));
#204412=CARTESIAN_POINT('Ctrl Pts',(-62.2936141127569,6.73887200051376,
39.92499));
#204413=CARTESIAN_POINT('Origin',(-62.500570298093,6.58439859103072,40.22725));
#204414=CARTESIAN_POINT('Origin',(0.0331877870874877,0.315760701779427,
39.116));
#204415=CARTESIAN_POINT('Origin',(-59.6417962403142,6.58785426247137,39.116));
#204416=CARTESIAN_POINT('Origin',(1.33778643725275E-16,-1.72356557454387E-17,
40.22725));
#204417=CARTESIAN_POINT('Origin',(-62.5037563256534,6.55408556365989,40.22725));
#204418=CARTESIAN_POINT('Ctrl Pts',(-59.6417962403142,6.58785426247137,
38.989));
#204419=CARTESIAN_POINT('Ctrl Pts',(-59.6550912418707,6.46136077224392,
38.989));
#204420=CARTESIAN_POINT('Ctrl Pts',(-59.6550713402759,6.46155012326965,
39.1161901092319));
#204421=CARTESIAN_POINT('Ctrl Pts',(-59.4260321009469,6.56494565834894,
38.989));
#204422=CARTESIAN_POINT('Ctrl Pts',(-59.43949279477,6.43870097938019,38.989229898976));
#204423=CARTESIAN_POINT('Ctrl Pts',(-59.4825041216627,6.4434125774669,39.1161900493199));
#204424=CARTESIAN_POINT('Ctrl Pts',(-59.2206282517276,6.54313468201949,
39.1034966344368));
#204425=CARTESIAN_POINT('Ctrl Pts',(-59.2341955513627,6.41712387095977,
39.1038314102564));
#204426=CARTESIAN_POINT('Ctrl Pts',(-59.3182233753722,6.42614597501045,
39.2077528789601));
#204427=CARTESIAN_POINT('Ctrl Pts',(-59.1062911958296,6.53099325080096,
39.2875012672119));
#204428=CARTESIAN_POINT('Ctrl Pts',(-59.1200087130388,6.4051226264063,39.2878045257868));
#204429=CARTESIAN_POINT('Ctrl Pts',(-59.2267768553862,6.41653455832064,
39.3549015295898));
#204430=CARTESIAN_POINT('Origin',(-59.2133417798936,6.54282188406269,39.3548010137695));
#204431=CARTESIAN_POINT('Ctrl Pts',(-62.4538823482275,6.24436990788103,
39.8576902534424));
#204432=CARTESIAN_POINT('Ctrl Pts',(-62.4410124550018,6.37126553604114,
39.8573998014387));
#204433=CARTESIAN_POINT('Ctrl Pts',(-62.3334394572618,6.35995915837845,
39.92499));
#204434=CARTESIAN_POINT('Ctrl Pts',(-62.4991292864733,6.24912604340955,
39.9304984902494));
#204435=CARTESIAN_POINT('Ctrl Pts',(-62.4722545055303,6.35912437831612,
39.9052171569796));
#204436=CARTESIAN_POINT('Ctrl Pts',(-62.3786847639677,6.36471463173913,
39.9672049726603));
#204437=CARTESIAN_POINT('Ctrl Pts',(-62.542379656768,6.28053011789782,40.0043437678658));
#204438=CARTESIAN_POINT('Ctrl Pts',(-62.5096946965644,6.36708533499936,
39.966162857764));
#204439=CARTESIAN_POINT('Ctrl Pts',(-62.4231124872028,6.38493060453743,
40.0100243556235));
#204440=CARTESIAN_POINT('Ctrl Pts',(-62.6032845425347,6.39322569848931,
40.1194874821992));
#204441=CARTESIAN_POINT('Ctrl Pts',(-62.5632890102013,6.43576006824499,
40.0627551483143));
#204442=CARTESIAN_POINT('Ctrl Pts',(-62.4886705126495,6.45334792019248,
40.0767884282378));
#204443=CARTESIAN_POINT('Ctrl Pts',(-62.620090867565,6.47739243510536,40.1599502015389));
#204444=CARTESIAN_POINT('Ctrl Pts',(-62.5804859237135,6.49734694408414,
40.1002449453872));
#204445=CARTESIAN_POINT('Ctrl Pts',(-62.5090840872032,6.50319024212558,
40.10025));
#204446=CARTESIAN_POINT('Ctrl Pts',(-62.6108711573005,6.56531752495346,
40.1599502534424));
#204447=CARTESIAN_POINT('Ctrl Pts',(-62.5737697140401,6.56142710223395,
40.10025));
#204448=CARTESIAN_POINT('Ctrl Pts',(-62.5037563256534,6.5540855636599,40.10025));
#204449=CARTESIAN_POINT('Origin',(-62.3467145720969,6.23365487766668,39.92499));
#204450=CARTESIAN_POINT('Origin',(-59.0361683443313,6.52420020558017,39.639895506932));
#204451=CARTESIAN_POINT('Origin',(-58.858994908613,6.50557852713795,39.92499));
#204452=CARTESIAN_POINT('Origin',(-62.1695413802715,6.21503322485432,39.6398955068269));
#204453=CARTESIAN_POINT('Origin',(-61.9923681882668,6.19641157197507,39.3548010137695));
#204454=CARTESIAN_POINT('Ctrl Pts',(-58.7519447039088,6.49374646112781,
39.8576902534424));
#204455=CARTESIAN_POINT('Ctrl Pts',(-58.765644274027,6.36806742857366,39.8579948730703));
#204456=CARTESIAN_POINT('Ctrl Pts',(-58.872270023448,6.37927424642618,39.92499));
#204457=CARTESIAN_POINT('Ctrl Pts',(-58.7067576262547,6.48899657309089,
39.9304020711231));
#204458=CARTESIAN_POINT('Ctrl Pts',(-58.7342098038487,6.38004220452875,
39.9058915297381));
#204459=CARTESIAN_POINT('Ctrl Pts',(-58.8270810177595,6.37452469054088,
39.9671523786032));
#204460=CARTESIAN_POINT('Ctrl Pts',(-58.6637560248473,6.4577414435536,40.0043257306693));
#204461=CARTESIAN_POINT('Ctrl Pts',(-58.6967899354322,6.37187117938164,
39.9667894847835));
#204462=CARTESIAN_POINT('Ctrl Pts',(-58.7829167175845,6.35435266912814,
40.01001389752));
#204463=CARTESIAN_POINT('Ctrl Pts',(-58.603591415908,6.34539908016358,40.1195533054857));
#204464=CARTESIAN_POINT('Ctrl Pts',(-58.6436439608623,6.30313135363892,
40.0630813209236));
#204465=CARTESIAN_POINT('Ctrl Pts',(-58.7181337176194,6.28595874576549,
40.0768265942421));
#204466=CARTESIAN_POINT('Ctrl Pts',(-58.5872698677166,6.26151010025763,
40.1599502027522));
#204467=CARTESIAN_POINT('Ctrl Pts',(-58.6268645946683,6.24170554357573,
40.1002552791554));
#204468=CARTESIAN_POINT('Ctrl Pts',(-58.6982323944355,6.23613328458312,
40.10025));
#204469=CARTESIAN_POINT('Ctrl Pts',(-58.596486683455,6.17403490859061,40.1599502534424));
#204470=CARTESIAN_POINT('Ctrl Pts',(-58.6335861742241,6.17794390662212,
40.10025));
#204471=CARTESIAN_POINT('Ctrl Pts',(-58.7035958781038,6.18532049829439,
40.10025));
#204472=CARTESIAN_POINT('Origin',(-58.7035958781038,6.18532049829439,40.22725));
#204473=CARTESIAN_POINT('Ctrl Pts',(-61.5639141665611,6.15137923967718,
38.989));
#204474=CARTESIAN_POINT('Ctrl Pts',(-61.5506192181748,6.27787222402454,
38.989));
#204475=CARTESIAN_POINT('Ctrl Pts',(-61.5506390665201,6.27768337963402,
39.1161896013263));
#204476=CARTESIAN_POINT('Ctrl Pts',(-61.7797255331385,6.17383801205393,
38.989));
#204477=CARTESIAN_POINT('Ctrl Pts',(-61.766592392013,6.30057242039937,38.988776927546));
#204478=CARTESIAN_POINT('Ctrl Pts',(-61.7232059145547,6.29582088597956,
39.1161898821845));
#204479=CARTESIAN_POINT('Ctrl Pts',(-61.985174271489,6.19522058691287,39.1034967087243));
#204480=CARTESIAN_POINT('Ctrl Pts',(-61.9721416759917,6.32217699854306,
39.1031720232715));
#204481=CARTESIAN_POINT('Ctrl Pts',(-61.8874865820147,6.31308747966697,
39.2077529615005));
#204482=CARTESIAN_POINT('Ctrl Pts',(-62.0995362748658,6.20712349654507,
39.2875012672119));
#204483=CARTESIAN_POINT('Ctrl Pts',(-62.0866494440659,6.33421251157707,
39.2872087095507));
#204484=CARTESIAN_POINT('Ctrl Pts',(-61.9789328337401,6.32269886789217,
39.3549017048226));
#204485=CARTESIAN_POINT('Origin',(-61.5639141665611,6.15137923967718,39.116));
#204486=CARTESIAN_POINT('Origin',(3.53633106925806E-16,6.13135187546216E-18,
40.22725));
#204487=CARTESIAN_POINT('Origin',(-58.7067819056642,6.15500747092357,40.22725));
#204488=CARTESIAN_POINT('Origin',(61.5094129706996,-6.78414869068793,39.116));
#204489=CARTESIAN_POINT('Origin',(-61.1647646440474,6.10937495962054,39.1160373285262));
#204490=CARTESIAN_POINT('Ctrl Pts',(-58.5996668978648,6.14377718965363,
40.1599502534424));
#204491=CARTESIAN_POINT('Ctrl Pts',(-58.6367684021392,6.14766703046211,
40.10025));
#204492=CARTESIAN_POINT('Ctrl Pts',(-58.7067819056642,6.15500747092357,
40.10025));
#204493=CARTESIAN_POINT('Ctrl Pts',(-58.6088074259633,6.05659553606742,
40.1599500566034));
#204494=CARTESIAN_POINT('Ctrl Pts',(-58.6434243604373,6.08415140319827,
40.1002551305372));
#204495=CARTESIAN_POINT('Ctrl Pts',(-58.7120821529693,6.10436324506856,
40.10025));
#204496=CARTESIAN_POINT('Ctrl Pts',(-58.6416817365139,5.97852000021562,
40.1203070619046));
#204497=CARTESIAN_POINT('Ctrl Pts',(-58.6721826510718,6.02785839131309,
40.06370986845));
#204498=CARTESIAN_POINT('Ctrl Pts',(-58.7414038195498,6.06008468706738,
40.0772636213363));
#204499=CARTESIAN_POINT('Ctrl Pts',(-58.7242744516463,5.88025093392509,
40.0046102245803));
#204500=CARTESIAN_POINT('Ctrl Pts',(-58.7387860695146,5.97104363802183,
39.9670001894012));
#204501=CARTESIAN_POINT('Ctrl Pts',(-58.819336041524,6.00614981441059,40.0101788811209));
#204502=CARTESIAN_POINT('Ctrl Pts',(-58.7730316211507,5.85862682030306,
39.9303710930186));
#204503=CARTESIAN_POINT('Ctrl Pts',(-58.77722661518,5.97091547255942,39.9058663574101));
#204504=CARTESIAN_POINT('Ctrl Pts',(-58.866925555679,5.99561386571472,39.9671344706368));
#204505=CARTESIAN_POINT('Ctrl Pts',(-58.8181995570484,5.8633736414962,39.8576902534424));
#204506=CARTESIAN_POINT('Ctrl Pts',(-58.805469618532,5.98915458643835,39.8579948730704));
#204507=CARTESIAN_POINT('Ctrl Pts',(-58.9120953679529,6.00036140429087,
39.92499));
#204508=CARTESIAN_POINT('Origin',(-58.925370482788,5.8740571235791,39.92499));
#204509=CARTESIAN_POINT('Origin',(-61.1207756545813,6.10480350526353,39.1925554488851));
#204510=CARTESIAN_POINT('Origin',(-61.0393856393803,6.09624906995281,39.3343017080178));
#204511=CARTESIAN_POINT('Origin',(-59.1025439184822,5.89267880207721,39.6398955069206));
#204512=CARTESIAN_POINT('Origin',(-59.2797173540685,5.91130048050383,39.3548010137695));
#204513=CARTESIAN_POINT('Ctrl Pts',(-60.7112330730303,6.06175884541612,
39.3978017080178));
#204514=CARTESIAN_POINT('Ctrl Pts',(-60.6979579581953,6.18806312612789,
39.3978017080178));
#204515=CARTESIAN_POINT('Ctrl Pts',(-60.6979579581953,6.18806312612789,
39.5248017080178));
#204516=CARTESIAN_POINT('Ctrl Pts',(-60.8007259828525,6.07140041118273,
39.3978017080178));
#204517=CARTESIAN_POINT('Ctrl Pts',(-60.787391283362,6.19746294737678,39.3980355775177));
#204518=CARTESIAN_POINT('Ctrl Pts',(-60.832232401261,6.20217593878204,39.5248015517192));
#204519=CARTESIAN_POINT('Ctrl Pts',(-60.885348460727,6.08051542067576,39.3484893995498));
#204520=CARTESIAN_POINT('Ctrl Pts',(-60.8723790316489,6.20639551966831,
39.3489438303429));
#204521=CARTESIAN_POINT('Ctrl Pts',(-60.9591984396307,6.2155206071496,39.45083331556));
#204522=CARTESIAN_POINT('Ctrl Pts',(-60.929944884669,6.08531878138363,39.2708017080178));
#204523=CARTESIAN_POINT('Ctrl Pts',(-60.917217374751,6.21110821942976,39.2710850691866));
#204524=CARTESIAN_POINT('Ctrl Pts',(-61.0261105245453,6.22255335066458,
39.3343017080178));
#204525=CARTESIAN_POINT('Origin',(-60.7112330730303,6.06175884541612,39.5248017080178));
#204526=CARTESIAN_POINT('Ctrl Pts',(-59.1725467709677,5.90061356181298,
39.2875012672119));
#204527=CARTESIAN_POINT('Ctrl Pts',(-59.1597945546412,6.02658562874862,
39.2878045257519));
#204528=CARTESIAN_POINT('Ctrl Pts',(-59.2666022171588,6.03762143316794,
39.3549015218348));
#204529=CARTESIAN_POINT('Ctrl Pts',(-59.2869113614504,5.91250964036551,
39.1034938540228));
#204530=CARTESIAN_POINT('Ctrl Pts',(-59.2739830624754,6.03858760028937,
39.1038286278806));
#204531=CARTESIAN_POINT('Ctrl Pts',(-59.3580501215732,6.04723299508913,
39.2077506434029));
#204532=CARTESIAN_POINT('Ctrl Pts',(-59.4923630227875,5.93388131656941,
38.989));
#204533=CARTESIAN_POINT('Ctrl Pts',(-59.4792818168387,6.06016587018228,
38.9892298954611));
#204534=CARTESIAN_POINT('Ctrl Pts',(-59.5223321697741,6.06449973388448,
39.1161900347291));
#204535=CARTESIAN_POINT('Ctrl Pts',(-59.7081718144892,5.95633285891252,
38.989));
#204536=CARTESIAN_POINT('Ctrl Pts',(-59.6948768144682,6.08282633453128,
38.989));
#204537=CARTESIAN_POINT('Ctrl Pts',(-59.6948967145252,6.08263699813607,
39.1161900945648));
#204538=CARTESIAN_POINT('Origin',(-59.7081718144892,5.95633285891252,39.116));
#204539=CARTESIAN_POINT('Origin',(60.0186752706391,-6.62746584474133,39.5248017080178));
#204540=CARTESIAN_POINT('Origin',(-60.5608532912343,6.04595329345103,39.5248017080178));
#204541=CARTESIAN_POINT('Origin',(59.785232315514,-6.60293000146475,39.116));
#204542=CARTESIAN_POINT('Origin',(-60.1073400340001,5.99823604520212,39.1160402713844));
#204543=CARTESIAN_POINT('Ctrl Pts',(-60.3421421670674,6.02238575970317,
39.2708017080178));
#204544=CARTESIAN_POINT('Ctrl Pts',(-60.3293058762211,6.14931623097289,
39.27051194648));
#204545=CARTESIAN_POINT('Ctrl Pts',(-60.2194255397044,6.13776734223257,
39.3343017080178));
#204546=CARTESIAN_POINT('Ctrl Pts',(-60.3868890390927,6.02720817145296,
39.3487519301186));
#204547=CARTESIAN_POINT('Ctrl Pts',(-60.3738278099533,6.15399567477046,
39.3482879463963));
#204548=CARTESIAN_POINT('Ctrl Pts',(-60.2865637544332,6.14482385294874,
39.4512271261618));
#204549=CARTESIAN_POINT('Ctrl Pts',(-60.4716618705782,6.03634362557922,
39.3978017080178));
#204550=CARTESIAN_POINT('Ctrl Pts',(-60.4582762833178,6.1628715669826,39.3975673827415));
#204551=CARTESIAN_POINT('Ctrl Pts',(-60.4137560077483,6.15819229746514,
39.5248015355199));
#204552=CARTESIAN_POINT('Ctrl Pts',(-60.5608532912343,6.04595329345103,
39.3978017080178));
#204553=CARTESIAN_POINT('Ctrl Pts',(-60.5475781763993,6.1722575741628,39.3978017080178));
#204554=CARTESIAN_POINT('Ctrl Pts',(-60.5475781763993,6.1722575741628,39.5248017080178));
#204555=CARTESIAN_POINT('Origin',(-60.2327006545395,6.0114630615208,39.3343017080178));
#204556=CARTESIAN_POINT('Origin',(-60.1517960329186,6.00295964283188,39.1934008533551));
#204557=CARTESIAN_POINT('Origin',(-60.0157999988656,13.0813452322065,39.1925554495085));
#204558=CARTESIAN_POINT('Origin',(-60.0590486699127,13.0905908661204,39.1160373285284));
#204559=CARTESIAN_POINT('Origin',(-59.9357500275432,13.0643300858386,39.3343017080178));
#204560=CARTESIAN_POINT('Ctrl Pts',(-59.8282880397054,13.0409063549243,
39.2708017080178));
#204561=CARTESIAN_POINT('Ctrl Pts',(-59.8550545325308,12.9173404733287,
39.2710850691866));
#204562=CARTESIAN_POINT('Ctrl Pts',(-59.9621548122771,12.9401053405454,
39.3343017080178));
#204563=CARTESIAN_POINT('Ctrl Pts',(-59.7842416555146,13.0316624367251,
39.3487519293518));
#204564=CARTESIAN_POINT('Ctrl Pts',(-59.8108054559344,12.9079350417481,
39.349206866293));
#204565=CARTESIAN_POINT('Ctrl Pts',(-59.8961220185276,12.9260696369486,
39.4512271248735));
#204566=CARTESIAN_POINT('Ctrl Pts',(-59.7007958241042,13.0141504107556,
39.3978017080178));
#204567=CARTESIAN_POINT('Ctrl Pts',(-59.727069488887,12.8901364125065,39.3980347781174));
#204568=CARTESIAN_POINT('Ctrl Pts',(-59.7710239514086,12.8994792219302,
39.524801535519));
#204569=CARTESIAN_POINT('Ctrl Pts',(-59.6130003254554,12.9957275188828,
39.3978017080178));
#204570=CARTESIAN_POINT('Ctrl Pts',(-59.6394051101892,12.8715027735896,
39.3978017080178));
#204571=CARTESIAN_POINT('Ctrl Pts',(-59.6394051101892,12.8715027735896,
39.5248017080178));
#204572=CARTESIAN_POINT('Origin',(-59.6130003254554,12.9957275188828,39.5248017080178));
#204573=CARTESIAN_POINT('Origin',(0.0660119618346463,0.310561863232983,
39.116));
#204574=CARTESIAN_POINT('Origin',(-60.4516424606488,13.1739864076111,39.116));
#204575=CARTESIAN_POINT('Origin',(0.0660119618346464,0.310561863232983,
39.5248017080178));
#204576=CARTESIAN_POINT('Origin',(-59.4650964698965,12.9642895838875,39.5248017080178));
#204577=CARTESIAN_POINT('Ctrl Pts',(-60.9782752797347,13.2864868029,39.2875012672119));
#204578=CARTESIAN_POINT('Ctrl Pts',(-61.0052918384388,13.1616357280628,
39.287208709576));
#204579=CARTESIAN_POINT('Ctrl Pts',(-60.8992893541407,13.1392995818864,
39.3549016990121));
#204580=CARTESIAN_POINT('Ctrl Pts',(-60.8658306440996,13.2624669757409,
39.1034939173931));
#204581=CARTESIAN_POINT('Ctrl Pts',(-60.8926675943332,13.1376969719829,
39.1031692336329));
#204582=CARTESIAN_POINT('Ctrl Pts',(-60.809347351947,13.1201818190179,39.2077507202297));
#204583=CARTESIAN_POINT('Ctrl Pts',(-60.663828108008,13.2193155203584,38.989));
#204584=CARTESIAN_POINT('Ctrl Pts',(-60.6905008239721,13.0947255842063,
38.9887769311176));
#204585=CARTESIAN_POINT('Ctrl Pts',(-60.6477702018622,13.0858375353126,
39.1161898712913));
#204586=CARTESIAN_POINT('Ctrl Pts',(-60.4516424606488,13.1739864076111,
38.989));
#204587=CARTESIAN_POINT('Ctrl Pts',(-60.4780866929065,13.0495760763092,
38.989));
#204588=CARTESIAN_POINT('Ctrl Pts',(-60.4780472159603,13.0497618007394,
39.1161895903852));
#204589=CARTESIAN_POINT('Origin',(-60.8730422059013,13.2635576885506,39.3548010137695));
#204590=CARTESIAN_POINT('Ctrl Pts',(-59.4650964698965,12.9642895838875,
39.3978017080178));
#204591=CARTESIAN_POINT('Ctrl Pts',(-59.4915012546304,12.8400648385943,
39.3978017080178));
#204592=CARTESIAN_POINT('Ctrl Pts',(-59.4915012546304,12.8400648385943,
39.5248017080178));
#204593=CARTESIAN_POINT('Ctrl Pts',(-59.3770041141843,12.9458049943934,
39.3978017080178));
#204594=CARTESIAN_POINT('Ctrl Pts',(-59.4033730190104,12.8213326038441,
39.397566602504));
#204595=CARTESIAN_POINT('Ctrl Pts',(-59.3594375597973,12.8119938336991,
39.5248015517196));
#204596=CARTESIAN_POINT('Ctrl Pts',(-59.2937057271822,12.9283282206303,
39.3484894016716));
#204597=CARTESIAN_POINT('Ctrl Pts',(-59.3204640761271,12.8037097640145,
39.348025900003));
#204598=CARTESIAN_POINT('Ctrl Pts',(-59.2345619206666,12.7854506972091,
39.450833318893));
#204599=CARTESIAN_POINT('Ctrl Pts',(-59.2498070616278,12.919118186205,39.2708017080178));
#204600=CARTESIAN_POINT('Ctrl Pts',(-59.2768226962997,12.7944335023712,
39.2705119464801));
#204601=CARTESIAN_POINT('Ctrl Pts',(-59.168751483356,12.7714622569324,39.3343017080178));
#204602=CARTESIAN_POINT('Origin',(-59.1423466986221,12.8956870022256,39.3343017080178));
#204603=CARTESIAN_POINT('Origin',(-61.0472983318862,13.3005969715151,39.6398955068186));
#204604=CARTESIAN_POINT('Origin',(-61.2215544576538,13.337636254483,39.92499));
#204605=CARTESIAN_POINT('Origin',(-59.0627741291273,12.8787733304436,39.1934008539943));
#204606=CARTESIAN_POINT('Origin',(-59.0190342907434,12.8695280801151,39.1160402713849));
#204607=CARTESIAN_POINT('Ctrl Pts',(-61.575271693745,13.1038352065732,40.1599502534424));
#204608=CARTESIAN_POINT('Ctrl Pts',(-61.5387839176327,13.0960702419685,
40.10025));
#204609=CARTESIAN_POINT('Ctrl Pts',(-61.4699285681953,13.0814171332237,
40.10025));
#204610=CARTESIAN_POINT('Ctrl Pts',(-61.5569304518429,13.1900205930481,
40.1599500538462));
#204611=CARTESIAN_POINT('Ctrl Pts',(-61.5254208297815,13.1588482421897,
40.1002448353506));
#204612=CARTESIAN_POINT('Ctrl Pts',(-61.4593031273755,13.1313027022859,
40.10025));
#204613=CARTESIAN_POINT('Ctrl Pts',(-61.5155378539379,13.2643407403248,
40.120244200104));
#204614=CARTESIAN_POINT('Ctrl Pts',(-61.4904936222817,13.2118511391503,
40.0633873868018));
#204615=CARTESIAN_POINT('Ctrl Pts',(-61.4250300340668,13.1721300657495,
40.0772271723538));
#204616=CARTESIAN_POINT('Ctrl Pts',(-61.4222835584425,13.3535591268197,
40.0045995998161));
#204617=CARTESIAN_POINT('Ctrl Pts',(-61.4178880557396,13.2611962587091,
39.9663485808315));
#204618=CARTESIAN_POINT('Ctrl Pts',(-61.341115859575,13.2174099770542,40.0101727202466));
#204619=CARTESIAN_POINT('Ctrl Pts',(-61.3712701109735,13.3700167576329,
39.930465434986));
#204620=CARTESIAN_POINT('Ctrl Pts',(-61.3797074995629,13.2570896192454,
39.9051900162948));
#204621=CARTESIAN_POINT('Ctrl Pts',(-61.2924393404521,13.2228660458971,
39.9671857458177));
#204622=CARTESIAN_POINT('Ctrl Pts',(-61.3267881959112,13.3605623192491,
39.8576902534424));
#204623=CARTESIAN_POINT('Ctrl Pts',(-61.3537611057082,13.2359003894755,
39.8573998014387));
#204624=CARTESIAN_POINT('Ctrl Pts',(-61.2479592423877,13.2134115091898,
39.92499));
#204625=CARTESIAN_POINT('Origin',(-61.4699285681953,13.0814171332237,40.22725));
#204626=CARTESIAN_POINT('Origin',(0.0660119618346463,0.310561863232983,
39.116));
#204627=CARTESIAN_POINT('Origin',(-58.6264539577983,12.7860306150456,39.116));
#204628=CARTESIAN_POINT('Origin',(1.31078692950418E-16,-3.42824740397364E-17,
40.22725));
#204629=CARTESIAN_POINT('Origin',(-61.4762657165315,13.0516031943533,40.22725));
#204630=CARTESIAN_POINT('Ctrl Pts',(-58.6264539577983,12.7860306150456,
38.989));
#204631=CARTESIAN_POINT('Ctrl Pts',(-58.6528982980921,12.6616197754741,
38.989));
#204632=CARTESIAN_POINT('Ctrl Pts',(-58.6528587129484,12.6618060089325,
39.1161901092325));
#204633=CARTESIAN_POINT('Ctrl Pts',(-58.4142663981466,12.7406940127372,
38.989));
#204634=CARTESIAN_POINT('Ctrl Pts',(-58.4408495151712,12.6165479409689,
38.989229898976));
#204635=CARTESIAN_POINT('Ctrl Pts',(-58.4831327254077,12.625729636332,39.1161900493205));
#204636=CARTESIAN_POINT('Ctrl Pts',(-58.2122676405432,12.6975319705102,
39.1034966344368));
#204637=CARTESIAN_POINT('Ctrl Pts',(-58.2389323335231,12.5736296288405,
39.1038314102556));
#204638=CARTESIAN_POINT('Ctrl Pts',(-58.3215567776493,12.591385608175,39.2077528789596));
#204639=CARTESIAN_POINT('Ctrl Pts',(-58.0998260601479,12.6735055745745,
39.2875012672119));
#204640=CARTESIAN_POINT('Ctrl Pts',(-58.1266254943012,12.5497583536235,
39.2878045257868));
#204641=CARTESIAN_POINT('Ctrl Pts',(-58.2316158778879,12.5722680796269,
39.3549015295901));
#204642=CARTESIAN_POINT('Origin',(-58.2050537810541,12.6964592423897,39.3548010137695));
#204643=CARTESIAN_POINT('Ctrl Pts',(-61.4590390555208,12.7383709431255,
39.8576902534424));
#204644=CARTESIAN_POINT('Ctrl Pts',(-61.4329754599098,12.8632261535959,
39.8573998014387));
#204645=CARTESIAN_POINT('Ctrl Pts',(-61.3271735965892,12.8407372733102,
39.92499));
#204646=CARTESIAN_POINT('Ctrl Pts',(-61.5035409747668,12.7478306169679,
39.9304984902493));
#204647=CARTESIAN_POINT('Ctrl Pts',(-61.4653154597751,12.8544171899343,
39.9052171569796));
#204648=CARTESIAN_POINT('Ctrl Pts',(-61.3716739624481,12.8501961180703,
39.9672049726606));
#204649=CARTESIAN_POINT('Ctrl Pts',(-61.5432717953611,12.7835835513933,
40.004343767866));
#204650=CARTESIAN_POINT('Ctrl Pts',(-61.5017184029588,12.8662481012971,
39.9661628577639));
#204651=CARTESIAN_POINT('Ctrl Pts',(-61.4137451613968,12.8749453072906,
40.0100243556235));
#204652=CARTESIAN_POINT('Ctrl Pts',(-61.5920631419345,12.9020280679176,
40.119487482199));
#204653=CARTESIAN_POINT('Ctrl Pts',(-61.5478406570045,12.9401487584129,
40.0627551483143));
#204654=CARTESIAN_POINT('Ctrl Pts',(-61.4717924962547,12.9498405053867,
40.0767884282377));
#204655=CARTESIAN_POINT('Ctrl Pts',(-61.5999795805214,12.9874904696725,
40.1599502015393));
#204656=CARTESIAN_POINT('Ctrl Pts',(-61.5585057825381,13.0031958218446,
40.1002449453872));
#204657=CARTESIAN_POINT('Ctrl Pts',(-61.4868843017924,13.0015435854429,
40.10025));
#204658=CARTESIAN_POINT('Ctrl Pts',(-61.5816197022697,13.0739701745329,
40.1599502534424));
#204659=CARTESIAN_POINT('Ctrl Pts',(-61.5451281645058,13.0662229071071,
40.10025));
#204660=CARTESIAN_POINT('Ctrl Pts',(-61.4762657165315,13.0516031943533,
40.10025));
#204661=CARTESIAN_POINT('Origin',(-61.3535783813231,12.7165125280171,39.92499));
#204662=CARTESIAN_POINT('Origin',(-58.0307974155445,12.6594199084583,39.6398955069315));
#204663=CARTESIAN_POINT('Origin',(-57.8565410498766,12.6223805745523,39.92499));
#204664=CARTESIAN_POINT('Origin',(-61.1793222555316,12.6794732450921,39.6398955068276));
#204665=CARTESIAN_POINT('Origin',(-61.0050661295705,12.6424339620847,39.3548010137695));
#204666=CARTESIAN_POINT('Ctrl Pts',(-57.7513140650719,12.5994235324476,
39.8576902534424));
#204667=CARTESIAN_POINT('Ctrl Pts',(-57.7780756236494,12.4758649777957,
39.8579948730703));
#204668=CARTESIAN_POINT('Ctrl Pts',(-57.8829458346104,12.4981558292591,
39.92499));
#204669=CARTESIAN_POINT('Ctrl Pts',(-57.7068710254542,12.589976329008,39.9304020711232));
#204670=CARTESIAN_POINT('Ctrl Pts',(-57.7455616498597,12.4844883578133,
39.9058915297387));
#204671=CARTESIAN_POINT('Ctrl Pts',(-57.8385008428012,12.4887087546167,
39.9671523786036));
#204672=CARTESIAN_POINT('Ctrl Pts',(-57.6673720419787,12.5543975270271,
40.0043257306691));
#204673=CARTESIAN_POINT('Ctrl Pts',(-57.7092008760999,12.4724506530563,
39.9667894847835));
#204674=CARTESIAN_POINT('Ctrl Pts',(-57.7966870296831,12.4640308112195,
40.0100138975199));
#204675=CARTESIAN_POINT('Ctrl Pts',(-57.6192799956671,12.4363816727426,
40.119553305486));
#204676=CARTESIAN_POINT('Ctrl Pts',(-57.6635313090883,12.3985321242203,
40.0630813209237));
#204677=CARTESIAN_POINT('Ctrl Pts',(-57.7394080294755,12.3892398894927,
40.0768265942422));
#204678=CARTESIAN_POINT('Ctrl Pts',(-57.611816644779,12.3512461790955,40.1599502027525));
#204679=CARTESIAN_POINT('Ctrl Pts',(-57.6532646075487,12.3356888898089,
40.1002552791541));
#204680=CARTESIAN_POINT('Ctrl Pts',(-57.7248239067135,12.3376071226711,
40.10025));
#204681=CARTESIAN_POINT('Ctrl Pts',(-57.6301266171956,12.2652136052665,
40.1599502534424));
#204682=CARTESIAN_POINT('Ctrl Pts',(-57.6666142715154,12.2729791421559,
40.10025));
#204683=CARTESIAN_POINT('Ctrl Pts',(-57.7354693911204,12.2876333308475,
40.10025));
#204684=CARTESIAN_POINT('Origin',(-57.7354693911203,12.2876333308475,40.22725));
#204685=CARTESIAN_POINT('Ctrl Pts',(-60.5836663843181,12.5528626811452,
38.989));
#204686=CARTESIAN_POINT('Ctrl Pts',(-60.5572221497821,12.677273023165,38.989));
#204687=CARTESIAN_POINT('Ctrl Pts',(-60.55726162901,12.6770872880009,39.1161896013262));
#204688=CARTESIAN_POINT('Ctrl Pts',(-60.7959479326852,12.5977568525207,
38.989));
#204689=CARTESIAN_POINT('Ctrl Pts',(-60.7696393833354,12.7224242094577,
38.9887769275485));
#204690=CARTESIAN_POINT('Ctrl Pts',(-60.7269872521295,12.713163582625,39.1161898821844));
#204691=CARTESIAN_POINT('Ctrl Pts',(-60.99803611366,12.6404975322971,39.1034967087243));
#204692=CARTESIAN_POINT('Ctrl Pts',(-60.9718043534717,12.7653961862424,
39.1031720232704));
#204693=CARTESIAN_POINT('Ctrl Pts',(-60.8885631223998,12.7475075938196,
39.2077529615006));
#204694=CARTESIAN_POINT('Ctrl Pts',(-61.110527437164,12.6642893210146,39.2875012672119));
#204695=CARTESIAN_POINT('Ctrl Pts',(-61.0844267823321,12.7893350885048,
39.2872087095508));
#204696=CARTESIAN_POINT('Ctrl Pts',(-60.9785037583493,12.7666250660189,
39.3549017048226));
#204697=CARTESIAN_POINT('Origin',(-60.5836663843181,12.5528626811452,39.116));
#204698=CARTESIAN_POINT('Origin',(3.545935779686E-16,1.21955273767085E-17,
40.22725));
#204699=CARTESIAN_POINT('Origin',(-57.7418065394565,12.2578193919772,40.22725));
#204700=CARTESIAN_POINT('Origin',(59.4667368016499,-12.964638247165,39.116));
#204701=CARTESIAN_POINT('Origin',(-60.191094087497,12.4693660187274,39.1160373285259));
#204702=CARTESIAN_POINT('Ctrl Pts',(-57.6364522029206,12.2354540642049,
40.1599502534424));
#204703=CARTESIAN_POINT('Ctrl Pts',(-57.6729438621905,12.2432007592851,
40.10025));
#204704=CARTESIAN_POINT('Ctrl Pts',(-57.7418065394565,12.2578193919772,
40.10025));
#204705=CARTESIAN_POINT('Ctrl Pts',(-57.6546556225243,12.1497054461947,
40.1599500566034));
#204706=CARTESIAN_POINT('Ctrl Pts',(-57.6862025493677,12.1807288143667,
40.1002551305381));
#204707=CARTESIAN_POINT('Ctrl Pts',(-57.7523715145536,12.208006627196,40.10025));
#204708=CARTESIAN_POINT('Ctrl Pts',(-57.6955109599434,12.0754939174601,
40.1203070619047));
#204709=CARTESIAN_POINT('Ctrl Pts',(-57.7206875210979,12.1277502414154,
40.0637098684499));
#204710=CARTESIAN_POINT('Ctrl Pts',(-57.7861609236006,12.1670355805166,
40.0772636213362));
#204711=CARTESIAN_POINT('Ctrl Pts',(-57.7879231380266,11.9863964689869,
40.0046102245801));
#204712=CARTESIAN_POINT('Ctrl Pts',(-57.7928648378994,12.0782086782664,
39.9670001894012));
#204713=CARTESIAN_POINT('Ctrl Pts',(-57.8693039540644,12.1215423041377,
40.0101788811209));
#204714=CARTESIAN_POINT('Ctrl Pts',(-57.8386735460213,11.9699873265229,
39.9303710930187));
#204715=CARTESIAN_POINT('Ctrl Pts',(-57.8311081991708,12.0820993460745,
39.9058663574107));
#204716=CARTESIAN_POINT('Ctrl Pts',(-57.9177340744071,12.1160385312533,
39.9671344706365));
#204717=CARTESIAN_POINT('Ctrl Pts',(-57.8830978693155,11.9794294790616,
39.8576902534424));
#204718=CARTESIAN_POINT('Ctrl Pts',(-57.857289977851,12.1031907419161,39.8579948730704));
#204719=CARTESIAN_POINT('Ctrl Pts',(-57.962160188812,12.1254815933796,39.92499));
#204720=CARTESIAN_POINT('Origin',(-57.9885649735458,12.0012568480864,39.92499));
#204721=CARTESIAN_POINT('Origin',(-60.1478239214169,12.460221505806,39.192555448885));
#204722=CARTESIAN_POINT('Origin',(-60.0677739512125,12.4432063593727,39.3343017080178));
#204723=CARTESIAN_POINT('Origin',(-58.1628213391877,12.0382961820444,39.6398955069223));
#204724=CARTESIAN_POINT('Origin',(-58.3370777047234,12.0753355159237,39.3548010137695));
#204725=CARTESIAN_POINT('Ctrl Pts',(-59.7450242491247,12.3746037924168,
39.3978017080178));
#204726=CARTESIAN_POINT('Ctrl Pts',(-59.7186194643908,12.49882853771,39.3978017080178));
#204727=CARTESIAN_POINT('Ctrl Pts',(-59.7186194643908,12.49882853771,39.5248017080178));
#204728=CARTESIAN_POINT('Ctrl Pts',(-59.83301908937,12.3935470970144,39.3978017080178));
#204729=CARTESIAN_POINT('Ctrl Pts',(-59.8065803155741,12.5175251937995,
39.3980355775177));
#204730=CARTESIAN_POINT('Ctrl Pts',(-59.8506831473907,12.52689954009,39.5248015517192));
#204731=CARTESIAN_POINT('Ctrl Pts',(-59.9162252185216,12.411457631101,39.3484893995498));
#204732=CARTESIAN_POINT('Ctrl Pts',(-59.8901687840302,12.5352924712482,
39.3489438303431));
#204733=CARTESIAN_POINT('Ctrl Pts',(-59.9755587548362,12.553442669845,39.4508333155594));
#204734=CARTESIAN_POINT('Ctrl Pts',(-59.9600752506736,12.4208962741591,
39.2708017080178));
#204735=CARTESIAN_POINT('Ctrl Pts',(-59.9342688867324,12.5446662374491,
39.2710850691866));
#204736=CARTESIAN_POINT('Ctrl Pts',(-60.0413691664786,12.5674311046659,
39.3343017080178));
#204737=CARTESIAN_POINT('Origin',(-59.7450242491247,12.3746037924168,39.5248017080178));
#204738=CARTESIAN_POINT('Ctrl Pts',(-58.231611300478,12.0535047649326,39.2875012672119));
#204739=CARTESIAN_POINT('Ctrl Pts',(-58.2057612755554,12.1774537741288,
39.2878045257519));
#204740=CARTESIAN_POINT('Ctrl Pts',(-58.3108302788452,12.1995935640852,
39.3549015218347));
#204741=CARTESIAN_POINT('Ctrl Pts',(-58.3441059109579,12.0772900304171,
39.1034938540228));
#204742=CARTESIAN_POINT('Ctrl Pts',(-58.3180696991556,12.2013259468607,
39.1038286278809));
#204743=CARTESIAN_POINT('Ctrl Pts',(-58.4007725402744,12.2187113817821,
39.2077506434029));
#204744=CARTESIAN_POINT('Ctrl Pts',(-58.5461981381262,12.120020176779,38.989));
#204745=CARTESIAN_POINT('Ctrl Pts',(-58.5199882620682,12.2442455720376,
38.9892298954611));
#204746=CARTESIAN_POINT('Ctrl Pts',(-58.5623497685531,12.2530556816164,
39.1161900347289));
#204747=CARTESIAN_POINT('Ctrl Pts',(-58.7584778814675,12.1649068885796,
38.989));
#204748=CARTESIAN_POINT('Ctrl Pts',(-58.732033544228,12.2893177137821,38.989));
#204749=CARTESIAN_POINT('Ctrl Pts',(-58.7320731263128,12.2891314947141,
39.1161900945645));
#204750=CARTESIAN_POINT('Origin',(-58.7584778814675,12.1649068885796,39.116));
#204751=CARTESIAN_POINT('Origin',(58.0246834617327,-12.6581203474874,39.5248017080178));
#204752=CARTESIAN_POINT('Origin',(-59.5971203935658,12.3431658574215,39.5248017080178));
#204753=CARTESIAN_POINT('Origin',(57.798864262886,-12.6101209950214,39.116));
#204754=CARTESIAN_POINT('Origin',(-59.1510793400376,12.2483049654019,39.1160402713836));
#204755=CARTESIAN_POINT('Ctrl Pts',(-59.382070869907,12.2968658913807,39.2708017080178));
#204756=CARTESIAN_POINT('Ctrl Pts',(-59.3560370505013,12.4217592664917,
39.27051194648));
#204757=CARTESIAN_POINT('Ctrl Pts',(-59.2479658375575,12.3987880210528,
39.3343017080178));
#204758=CARTESIAN_POINT('Ctrl Pts',(-59.4260685345959,12.3063392072229,
39.3487519301185));
#204759=CARTESIAN_POINT('Ctrl Pts',(-59.3998259533518,12.4310668851203,
39.3482879463966));
#204760=CARTESIAN_POINT('Ctrl Pts',(-59.3139986558985,12.4128237298768,
39.4512271261623));
#204761=CARTESIAN_POINT('Ctrl Pts',(-59.5094220566594,12.3242857901781,
39.3978017080178));
#204762=CARTESIAN_POINT('Ctrl Pts',(-59.4828840257723,12.4487214234132,
39.3975673827415));
#204763=CARTESIAN_POINT('Ctrl Pts',(-59.4390967537827,12.4394141514345,
39.5248015355199));
#204764=CARTESIAN_POINT('Ctrl Pts',(-59.5971203935658,12.3431658574215,
39.3978017080178));
#204765=CARTESIAN_POINT('Ctrl Pts',(-59.570715608832,12.4673906027147,39.3978017080178));
#204766=CARTESIAN_POINT('Ctrl Pts',(-59.570715608832,12.4673906027147,39.5248017080178));
#204767=CARTESIAN_POINT('Origin',(-59.2743706222914,12.2745632757596,39.3343017080178));
#204768=CARTESIAN_POINT('Origin',(-59.1947980539414,12.2576496039199,39.1934008533547));
#204769=CARTESIAN_POINT('Origin',(-58.3196542523184,19.2830435999574,39.1925554495077));
#204770=CARTESIAN_POINT('Origin',(-58.3616995707146,19.2967593024446,39.1160373285253));
#204771=CARTESIAN_POINT('Origin',(-58.2418213702172,19.2577541638583,39.3343017080178));
#204772=CARTESIAN_POINT('Ctrl Pts',(-58.1373965169892,19.2232259141444,
39.2708017080178));
#204773=CARTESIAN_POINT('Ctrl Pts',(-58.1769325318818,19.1031347997392,
39.2710850691866));
#204774=CARTESIAN_POINT('Ctrl Pts',(-58.2810665285028,19.1369699862888,
39.3343017080178));
#204775=CARTESIAN_POINT('Ctrl Pts',(-58.0945576760634,19.2094285342449,
39.3487519293518));
#204776=CARTESIAN_POINT('Ctrl Pts',(-58.1339089916615,19.0891556041209,
39.349206866292));
#204777=CARTESIAN_POINT('Ctrl Pts',(-58.2168625998337,19.1161088652887,
39.4512271248733));
#204778=CARTESIAN_POINT('Ctrl Pts',(-58.0133994748122,19.1832899764614,
39.3978017080178));
#204779=CARTESIAN_POINT('Ctrl Pts',(-58.0524922023739,19.0627016856755,
39.3980347781174));
#204780=CARTESIAN_POINT('Ctrl Pts',(-58.0952292882366,19.0765878066328,
39.524801535519));
#204781=CARTESIAN_POINT('Ctrl Pts',(-57.9280106456674,19.155790878563,39.3978017080178));
#204782=CARTESIAN_POINT('Ctrl Pts',(-57.967255803953,19.0350067009935,39.3978017080178));
#204783=CARTESIAN_POINT('Ctrl Pts',(-57.967255803953,19.0350067009935,39.5248017080178));
#204784=CARTESIAN_POINT('Origin',(-57.9280106456674,19.1557908785629,39.5248017080178));
#204785=CARTESIAN_POINT('Origin',(0.0981128957140535,0.301960443923711,
39.116));
#204786=CARTESIAN_POINT('Origin',(-58.7434254837931,19.4207352200705,39.116));
#204787=CARTESIAN_POINT('Origin',(0.0981128957140536,0.301960443923711,
39.5248017080178));
#204788=CARTESIAN_POINT('Origin',(-57.7842031819381,19.109065001132,39.5248017080178));
#204789=CARTESIAN_POINT('Ctrl Pts',(-59.255413859757,19.5876674457083,39.2875012672119));
#204790=CARTESIAN_POINT('Ctrl Pts',(-59.2953329099158,19.4663243174863,
39.287208709576));
#204791=CARTESIAN_POINT('Ctrl Pts',(-59.1922458813527,19.4330302542696,
39.3549016990123));
#204792=CARTESIAN_POINT('Ctrl Pts',(-59.1460959632216,19.5520255367114,
39.1034939173931));
#204793=CARTESIAN_POINT('Ctrl Pts',(-59.1858279145868,19.4307442612513,
39.1031692336319));
#204794=CARTESIAN_POINT('Ctrl Pts',(-59.1047949412326,19.4046157212343,
39.2077507202296));
#204795=CARTESIAN_POINT('Ctrl Pts',(-58.949710573478,19.4879954548411,38.989));
#204796=CARTESIAN_POINT('Ctrl Pts',(-58.9892603680799,19.3668760934068,
38.98877693112));
#204797=CARTESIAN_POINT('Ctrl Pts',(-58.9476928828783,19.3535701679106,
39.1161898712916));
#204798=CARTESIAN_POINT('Ctrl Pts',(-58.7434254837931,19.4207352200705,
38.989));
#204799=CARTESIAN_POINT('Ctrl Pts',(-58.7827292725253,19.2997705965407,
38.989));
#204800=CARTESIAN_POINT('Ctrl Pts',(-58.7826705983485,19.2999511770888,
39.1161895903855));
#204801=CARTESIAN_POINT('Origin',(-59.1531540087997,19.5538640879537,39.3548010137695));
#204802=CARTESIAN_POINT('Ctrl Pts',(-57.7842031819381,19.109065001132,39.3978017080178));
#204803=CARTESIAN_POINT('Ctrl Pts',(-57.8234483402237,18.9882808235625,
39.3978017080178));
#204804=CARTESIAN_POINT('Ctrl Pts',(-57.8234483402237,18.9882808235625,
39.5248017080178));
#204805=CARTESIAN_POINT('Ctrl Pts',(-57.6985255711015,19.0814735135857,
39.3978017080178));
#204806=CARTESIAN_POINT('Ctrl Pts',(-57.7377609320107,18.9604392969153,
39.3975666025021));
#204807=CARTESIAN_POINT('Ctrl Pts',(-57.6950423231344,18.9465591794954,
39.5248015517196));
#204808=CARTESIAN_POINT('Ctrl Pts',(-57.6175103216837,19.0553854270309,
39.3484894016717));
#204809=CARTESIAN_POINT('Ctrl Pts',(-57.6571482613595,18.9342466524521,
39.3480259000043));
#204810=CARTESIAN_POINT('Ctrl Pts',(-57.5736252790853,18.9071083904254,
39.4508333188935));
#204811=CARTESIAN_POINT('Ctrl Pts',(-57.5748148483574,19.0416371860882,
39.2708017080178));
#204812=CARTESIAN_POINT('Ctrl Pts',(-57.61471558695,18.920459440775,39.27051194648));
#204813=CARTESIAN_POINT('Ctrl Pts',(-57.5096375484035,18.8863175164097,
39.3343017080178));
#204814=CARTESIAN_POINT('Origin',(-57.4703923901179,19.0071016939792,39.3343017080178));
#204815=CARTESIAN_POINT('Origin',(-59.322583882164,19.6089151909166,39.6398955068188));
#204816=CARTESIAN_POINT('Origin',(-59.4920137553138,19.6639662938566,39.92499));
#204817=CARTESIAN_POINT('Origin',(-57.393023687604,18.9819630786532,39.1934008539945));
#204818=CARTESIAN_POINT('Origin',(-57.3504898524412,18.9681964166833,39.1160402713845));
#204819=CARTESIAN_POINT('Ctrl Pts',(-59.868232155624,19.4684195516701,40.1599502534424));
#204820=CARTESIAN_POINT('Ctrl Pts',(-59.8327559231845,19.4568831131889,
40.10025));
#204821=CARTESIAN_POINT('Ctrl Pts',(-59.765809437495,19.4351129318425,40.10025));
#204822=CARTESIAN_POINT('Ctrl Pts',(-59.8409825629598,19.5522156237499,
40.1599500538463));
#204823=CARTESIAN_POINT('Ctrl Pts',(-59.8129039518352,19.5179203859182,
40.100244835349));
#204824=CARTESIAN_POINT('Ctrl Pts',(-59.750027742079,19.4836145615375,40.10025));
#204825=CARTESIAN_POINT('Ctrl Pts',(-59.7920481472522,19.6218019328335,
40.1202442001036));
#204826=CARTESIAN_POINT('Ctrl Pts',(-59.7726277678653,19.5669820401376,
40.0633873868015));
#204827=CARTESIAN_POINT('Ctrl Pts',(-59.7116747787978,19.5206357546568,
40.0772271723537));
#204828=CARTESIAN_POINT('Ctrl Pts',(-59.6899788477097,19.7007838434714,
40.0045995998165));
#204829=CARTESIAN_POINT('Ctrl Pts',(-59.6952619726975,19.6084674936735,
39.9663485808317));
#204830=CARTESIAN_POINT('Ctrl Pts',(-59.6234872553903,19.5568961981642,
40.0101727202466));
#204831=CARTESIAN_POINT('Ctrl Pts',(-59.6375245663854,19.7118189603904,
39.9304654349857));
#204832=CARTESIAN_POINT('Ctrl Pts',(-59.6577198343148,19.6003923959452,
39.9051900162946));
#204833=CARTESIAN_POINT('Ctrl Pts',(-59.5745070768387,19.5572342963495,
39.9671857458178));
#204834=CARTESIAN_POINT('Ctrl Pts',(-59.5942745858234,19.697766688185,39.8576902534424));
#204835=CARTESIAN_POINT('Ctrl Pts',(-59.6341304551456,19.5766071063173,
39.8573998014387));
#204836=CARTESIAN_POINT('Ctrl Pts',(-59.5312589135994,19.5431821162871,
39.92499));
#204837=CARTESIAN_POINT('Origin',(-59.765809437495,19.4351129318425,40.22725));
#204838=CARTESIAN_POINT('Origin',(0.0981128957140535,0.301960443923711,
39.116));
#204839=CARTESIAN_POINT('Origin',(-56.9687879773464,18.8441205405524,39.116));
#204840=CARTESIAN_POINT('Origin',(1.26611655068499E-16,-5.09536863743859E-17,
40.22725));
#204841=CARTESIAN_POINT('Origin',(-59.7752282754835,19.4061247292258,40.22725));
#204842=CARTESIAN_POINT('Ctrl Pts',(-56.9687879773464,18.8441205405524,
38.989));
#204843=CARTESIAN_POINT('Ctrl Pts',(-57.0080919266514,18.7231554228306,
38.989));
#204844=CARTESIAN_POINT('Ctrl Pts',(-57.0080330916622,18.7233364983083,
39.1161901092323));
#204845=CARTESIAN_POINT('Ctrl Pts',(-56.762501768717,18.776852657361,38.989));
#204846=CARTESIAN_POINT('Ctrl Pts',(-56.801916058748,18.6561653631345,38.989229898976));
#204847=CARTESIAN_POINT('Ctrl Pts',(-56.8430078886277,18.6697165591972,
39.1161900493203));
#204848=CARTESIAN_POINT('Ctrl Pts',(-56.5661212433882,18.7128124416044,
39.1034966344368));
#204849=CARTESIAN_POINT('Ctrl Pts',(-56.60559118576,18.5923760693073,39.1038314102556));
#204850=CARTESIAN_POINT('Ctrl Pts',(-56.6859069993035,18.6186713857,39.2077528789596));
#204851=CARTESIAN_POINT('Ctrl Pts',(-56.456807071981,18.6771643191714,39.2875012672119));
#204852=CARTESIAN_POINT('Ctrl Pts',(-56.4963948028695,18.5568963021134,
39.2878045257868));
#204853=CARTESIAN_POINT('Ctrl Pts',(-56.5984571310817,18.5902572009365,
39.35490152959));
#204854=CARTESIAN_POINT('Origin',(-56.5590590327988,18.7109915363521,39.3548010137695));
#204855=CARTESIAN_POINT('Ctrl Pts',(-59.790837669791,19.0928077206416,39.8576902534424));
#204856=CARTESIAN_POINT('Ctrl Pts',(-59.7518659300024,19.2142545736088,
39.8573998014387));
#204857=CARTESIAN_POINT('Ctrl Pts',(-59.6489943884562,19.1808295835786,
39.92499));
#204858=CARTESIAN_POINT('Ctrl Pts',(-59.834106997697,19.1068672906329,39.9304984902492));
#204859=CARTESIAN_POINT('Ctrl Pts',(-59.7849495554007,19.2088743168613,
39.9052171569785));
#204860=CARTESIAN_POINT('Ctrl Pts',(-59.6922622581482,19.1948881666556,
39.9672049726599));
#204861=CARTESIAN_POINT('Ctrl Pts',(-59.8698829694066,19.146577368363,40.0043437678661));
#204862=CARTESIAN_POINT('Ctrl Pts',(-59.8199164124675,19.2244455609614,
39.9661628577646));
#204863=CARTESIAN_POINT('Ctrl Pts',(-59.7315159919505,19.2238994150017,
40.0100243556235));
#204864=CARTESIAN_POINT('Ctrl Pts',(-59.9060262085834,19.2694731179107,
40.1194874821988));
#204865=CARTESIAN_POINT('Ctrl Pts',(-59.8580612818569,19.3027624708837,
40.0627551483138));
#204866=CARTESIAN_POINT('Ctrl Pts',(-59.7814166574708,19.3044519280755,
40.0767884282377));
#204867=CARTESIAN_POINT('Ctrl Pts',(-59.9049660265685,19.3552948408467,
40.1599502015386));
#204868=CARTESIAN_POINT('Ctrl Pts',(-59.8620777700628,19.3665789650872,
40.1002449453863));
#204869=CARTESIAN_POINT('Ctrl Pts',(-59.791021345013,19.3574492964898,40.10025));
#204870=CARTESIAN_POINT('Ctrl Pts',(-59.8776671349984,19.4393816709761,
40.1599502534424));
#204871=CARTESIAN_POINT('Ctrl Pts',(-59.8421853116551,19.4278624395271,
40.10025));
#204872=CARTESIAN_POINT('Ctrl Pts',(-59.7752282754835,19.4061247292258,
40.10025));
#204873=CARTESIAN_POINT('Origin',(-59.6882395467419,19.0600454060092,39.92499));
#204874=CARTESIAN_POINT('Origin',(-56.3896289265485,18.655940357667,39.6398955069316));
#204875=CARTESIAN_POINT('Origin',(-56.2201988201381,18.600889178989,39.92499));
#204876=CARTESIAN_POINT('Origin',(-59.5188096735653,19.004994303108,39.6398955068273));
#204877=CARTESIAN_POINT('Origin',(-59.3493798002278,18.9499432001062,39.3548010137695));
#204878=CARTESIAN_POINT('Ctrl Pts',(-56.1179479440987,18.567058682947,39.8576902534424));
#204879=CARTESIAN_POINT('Ctrl Pts',(-56.1574782858996,18.4469743395784,
39.8579948730703));
#204880=CARTESIAN_POINT('Ctrl Pts',(-56.2594439784237,18.4801050014195,
39.92499));
#204881=CARTESIAN_POINT('Ctrl Pts',(-56.0747358697602,18.5530176696414,
39.930402071123));
#204882=CARTESIAN_POINT('Ctrl Pts',(-56.1242410384002,18.4521518441034,
39.9058915297388));
#204883=CARTESIAN_POINT('Ctrl Pts',(-56.2162299491246,18.4660639121466,
39.967152378603));
#204884=CARTESIAN_POINT('Ctrl Pts',(-56.0391722633446,18.5135050040176,
40.0043257306694));
#204885=CARTESIAN_POINT('Ctrl Pts',(-56.0893377355407,18.4363793473478,
39.9667894847842));
#204886=CARTESIAN_POINT('Ctrl Pts',(-56.1772247439496,18.4371504234765,
40.0100138975201));
#204887=CARTESIAN_POINT('Ctrl Pts',(-56.0036796861844,18.3911086652353,
40.1195533054856));
#204888=CARTESIAN_POINT('Ctrl Pts',(-56.0516449414237,18.3580919822893,
40.0630813209231));
#204889=CARTESIAN_POINT('Ctrl Pts',(-56.1280773042134,18.3567819283759,
40.076826594242));
#204890=CARTESIAN_POINT('Ctrl Pts',(-56.0051563026338,18.3056594201307,
40.1599502027523));
#204891=CARTESIAN_POINT('Ctrl Pts',(-56.0480033886678,18.2945198471566,
40.1002552791563));
#204892=CARTESIAN_POINT('Ctrl Pts',(-56.1189701685705,18.3039075553122,
40.10025));
#204893=CARTESIAN_POINT('Ctrl Pts',(-56.032358823839,18.2220120550221,40.1599502534424));
#204894=CARTESIAN_POINT('Ctrl Pts',(-56.0678348753331,18.2335490499222,
40.10025));
#204895=CARTESIAN_POINT('Ctrl Pts',(-56.134781019564,18.2553202812753,40.10025));
#204896=CARTESIAN_POINT('Origin',(-56.1347810195641,18.2553202812753,40.22725));
#204897=CARTESIAN_POINT('Ctrl Pts',(-58.9396512752212,18.8168143322231,
38.989));
#204898=CARTESIAN_POINT('Ctrl Pts',(-58.9003474831028,18.9377789661744,
38.989));
#204899=CARTESIAN_POINT('Ctrl Pts',(-58.9004061606708,18.9375983751893,
39.1161896013269));
#204900=CARTESIAN_POINT('Ctrl Pts',(-59.1460772043116,18.8836520326607,
38.989));
#204901=CARTESIAN_POINT('Ctrl Pts',(-59.1068814887041,19.0048864565377,
38.988776927546));
#204902=CARTESIAN_POINT('Ctrl Pts',(-59.0654310094273,18.9912181986575,
39.116189882185));
#204903=CARTESIAN_POINT('Ctrl Pts',(-59.3425907075095,18.947282541525,39.1034967087243));
#204904=CARTESIAN_POINT('Ctrl Pts',(-59.3034471832914,19.0687550219954,
39.103172023271));
#204905=CARTESIAN_POINT('Ctrl Pts',(-59.222531823469,19.0422633471882,39.2077529614998));
#204906=CARTESIAN_POINT('Ctrl Pts',(-59.4519788726606,18.9827025415101,
39.2875012672119));
#204907=CARTESIAN_POINT('Ctrl Pts',(-59.4129503580328,19.104335033863,39.2872087095507));
#204908=CARTESIAN_POINT('Ctrl Pts',(-59.3099814352091,19.0706774483342,
39.3549017048229));
#204909=CARTESIAN_POINT('Origin',(-58.9396512752212,18.8168143322231,39.116));
#204910=CARTESIAN_POINT('Origin',(3.56182666396656E-16,1.81260861279374E-17,
40.22725));
#204911=CARTESIAN_POINT('Origin',(-56.1441998575526,18.2263320786586,40.22725));
#204912=CARTESIAN_POINT('Origin',(56.1826270286323,-18.588681363906,39.116));
#204913=CARTESIAN_POINT('Origin',(-58.5579573083284,18.6927400943502,39.116037328526));
#204914=CARTESIAN_POINT('Ctrl Pts',(-56.0417604764382,18.1930767435953,
40.1599502534424));
#204915=CARTESIAN_POINT('Ctrl Pts',(-56.0772424804483,18.204595418535,40.10025));
#204916=CARTESIAN_POINT('Ctrl Pts',(-56.1441998575526,18.2263320786586,
40.10025));
#204917=CARTESIAN_POINT('Ctrl Pts',(-56.0688273470725,18.1097006409638,
40.1599500566036));
#204918=CARTESIAN_POINT('Ctrl Pts',(-56.0969586315472,18.1438516116619,
40.1002551305369));
#204919=CARTESIAN_POINT('Ctrl Pts',(-56.1599138083641,18.1778965340261,
40.10025));
#204920=CARTESIAN_POINT('Ctrl Pts',(-56.1172160917338,18.0401661963856,
40.1203070619047));
#204921=CARTESIAN_POINT('Ctrl Pts',(-56.136792459813,18.0947679219786,40.0637098684496));
#204922=CARTESIAN_POINT('Ctrl Pts',(-56.1978007560409,18.14068188603,40.0772636213364));
#204923=CARTESIAN_POINT('Ctrl Pts',(-56.2184352456064,17.9612165360194,
40.0046102245801));
#204924=CARTESIAN_POINT('Ctrl Pts',(-56.2137528851849,18.0530423367035,
39.9670001894015));
#204925=CARTESIAN_POINT('Ctrl Pts',(-56.2852436625537,18.1041286397848,
40.0101788811208));
#204926=CARTESIAN_POINT('Ctrl Pts',(-56.2706228600015,17.9502021467121,
39.9303710930187));
#204927=CARTESIAN_POINT('Ctrl Pts',(-56.2513800597996,18.0609092108084,
39.9058663574117));
#204928=CARTESIAN_POINT('Ctrl Pts',(-56.3339837785519,18.1037173431996,
39.9671344706371));
#204929=CARTESIAN_POINT('Ctrl Pts',(-56.3138168485093,17.9642361803977,
39.8576902534424));
#204930=CARTESIAN_POINT('Ctrl Pts',(-56.2752137607564,18.0846218068699,
39.8579948730703));
#204931=CARTESIAN_POINT('Ctrl Pts',(-56.3771794532806,18.117752468711,39.92499));
#204932=CARTESIAN_POINT('Origin',(-56.4164246115662,17.9969682911416,39.92499));
#204933=CARTESIAN_POINT('Origin',(-58.5158800426271,18.6791227120623,39.1925554488845));
#204934=CARTESIAN_POINT('Origin',(-58.4380471616453,18.6538332760109,39.3343017080178));
#204935=CARTESIAN_POINT('Origin',(-56.5858547179449,18.0520194698678,39.6398955069221));
#204936=CARTESIAN_POINT('Origin',(-56.7552848242269,18.1070706485047,39.3548010137695));
#204937=CARTESIAN_POINT('Ctrl Pts',(-58.1242364370955,18.5518699907155,
39.3978017080178));
#204938=CARTESIAN_POINT('Ctrl Pts',(-58.0849912788099,18.672654168285,39.3978017080178));
#204939=CARTESIAN_POINT('Ctrl Pts',(-58.0849912788099,18.672654168285,39.5248017080178));
#204940=CARTESIAN_POINT('Ctrl Pts',(-58.2097691178803,18.5799074873342,
39.3978017080178));
#204941=CARTESIAN_POINT('Ctrl Pts',(-58.1705159385189,18.7004428147377,
39.3980355775196));
#204942=CARTESIAN_POINT('Ctrl Pts',(-58.213397284395,18.7143758086142,39.5248015517192));
#204943=CARTESIAN_POINT('Ctrl Pts',(-58.2906472745457,18.6064173144569,
39.3484893995498));
#204944=CARTESIAN_POINT('Ctrl Pts',(-58.2517893143875,18.7268501353373,
39.3489438303413));
#204945=CARTESIAN_POINT('Ctrl Pts',(-58.3348142976334,18.7538265876731,
39.4508333155594));
#204946=CARTESIAN_POINT('Ctrl Pts',(-58.3332704847794,18.6203878281152,
39.2708017080178));
#204947=CARTESIAN_POINT('Ctrl Pts',(-58.2946680067386,18.7407822670307,
39.2710850691867));
#204948=CARTESIAN_POINT('Ctrl Pts',(-58.3988020033597,18.7746174535804,
39.3343017080178));
#204949=CARTESIAN_POINT('Origin',(-58.1242364370955,18.5518699907155,39.5248017080178));
#204950=CARTESIAN_POINT('Ctrl Pts',(-56.6526781108322,18.0743352474896,
39.2875012672119));
#204951=CARTESIAN_POINT('Ctrl Pts',(-56.6140134955961,18.1949031876638,
39.2878045257519));
#204952=CARTESIAN_POINT('Ctrl Pts',(-56.716192681671,18.2279043949852,39.3549015218347));
#204953=CARTESIAN_POINT('Ctrl Pts',(-56.7620702268159,18.1097491035606,
39.1034938540228));
#204954=CARTESIAN_POINT('Ctrl Pts',(-56.7232113603681,18.2303840130666,
39.1038286278784));
#204955=CARTESIAN_POINT('Ctrl Pts',(-56.8036438738767,18.2563190096466,
39.207750643403));
#204956=CARTESIAN_POINT('Ctrl Pts',(-56.958588855084,18.1733695596541,38.989));
#204957=CARTESIAN_POINT('Ctrl Pts',(-56.9195374698056,18.2941747571335,
38.9892298954636));
#204958=CARTESIAN_POINT('Ctrl Pts',(-56.9607460083086,18.3073645871837,
39.1161900347288));
#204959=CARTESIAN_POINT('Ctrl Pts',(-57.1650137687746,18.240199652705,38.989));
#204960=CARTESIAN_POINT('Ctrl Pts',(-57.125709824009,18.3611647564559,38.989));
#204961=CARTESIAN_POINT('Ctrl Pts',(-57.125768654452,18.3609836949699,39.1161900945645));
#204962=CARTESIAN_POINT('Origin',(-57.1650137687745,18.240199652705,39.116));
#204963=CARTESIAN_POINT('Origin',(54.8193466381475,-18.1457247135494,39.5248017080178));
#204964=CARTESIAN_POINT('Origin',(-57.9804289733662,18.5051441132846,39.5248017080178));
#204965=CARTESIAN_POINT('Origin',(54.6058629360811,-18.0763596539233,39.116));
#204966=CARTESIAN_POINT('Origin',(-57.5467470426658,18.3641788932756,39.116040271385));
#204967=CARTESIAN_POINT('Ctrl Pts',(-57.7713971777985,18.4366189870677,
39.2708017080178));
#204968=CARTESIAN_POINT('Ctrl Pts',(-57.7324510618069,18.5581069080665,
39.27051194648));
#204969=CARTESIAN_POINT('Ctrl Pts',(-57.6273730232604,18.5239649837012,
39.3343017080178));
#204970=CARTESIAN_POINT('Ctrl Pts',(-57.8141635875298,18.450639415372,39.3487519301186));
#204971=CARTESIAN_POINT('Ctrl Pts',(-57.7750271733919,18.5719407253113,
39.3482879463966));
#204972=CARTESIAN_POINT('Ctrl Pts',(-57.6915769758397,18.5448261124702,
39.4512271261621));
#204973=CARTESIAN_POINT('Ctrl Pts',(-57.8951845615401,18.477200500639,39.3978017080178));
#204974=CARTESIAN_POINT('Ctrl Pts',(-57.8557848432464,18.5981804828681,
39.397567382742));
#204975=CARTESIAN_POINT('Ctrl Pts',(-57.8132103173504,18.5843471808457,
39.5248015355199));
#204976=CARTESIAN_POINT('Ctrl Pts',(-57.9804289733662,18.5051441132846,
39.3978017080178));
#204977=CARTESIAN_POINT('Ctrl Pts',(-57.9411838150806,18.6259282908541,
39.3978017080178));
#204978=CARTESIAN_POINT('Ctrl Pts',(-57.9411838150806,18.6259282908541,
39.5248017080178));
#204979=CARTESIAN_POINT('Origin',(-57.666618181546,18.4031808061317,39.3343017080178));
#204980=CARTESIAN_POINT('Origin',(-57.5892494801772,18.3780421908681,39.1934008533546));
#204981=CARTESIAN_POINT('Origin',(-55.9845461696107,25.273472906794,39.1925554495072));
#204982=CARTESIAN_POINT('Origin',(-56.0249274780501,25.2915084057467,39.1160373285231));
#204983=CARTESIAN_POINT('Origin',(-55.9097831300745,25.2401862573146,39.3343017080178));
#204984=CARTESIAN_POINT('Ctrl Pts',(-55.8095395120005,25.1949317875305,
39.2708017080178));
#204985=CARTESIAN_POINT('Ctrl Pts',(-55.8614118841076,25.0796311836958,
39.2710850691866));
#204986=CARTESIAN_POINT('Ctrl Pts',(-55.9614386837451,25.124165984194,39.3343017080178));
#204987=CARTESIAN_POINT('Ctrl Pts',(-55.7683775656457,25.1767321129114,
39.3487519293518));
#204988=CARTESIAN_POINT('Ctrl Pts',(-55.8200852551826,25.0612313830313,
39.3492068662946));
#204989=CARTESIAN_POINT('Ctrl Pts',(-55.8997670518381,25.0967080045992,
39.4512271248741));
#204990=CARTESIAN_POINT('Ctrl Pts',(-55.6903961807893,25.1422534028253,
39.3978017080178));
#204991=CARTESIAN_POINT('Ctrl Pts',(-55.7418796630199,25.0264120100489,
39.3980347781155));
#204992=CARTESIAN_POINT('Ctrl Pts',(-55.7829311357716,25.0446893032921,
39.524801535519));
#204993=CARTESIAN_POINT('Ctrl Pts',(-55.6083495590299,25.1059793847706,
39.3978017080178));
#204994=CARTESIAN_POINT('Ctrl Pts',(-55.6600051127006,24.98995911165,39.3978017080178));
#204995=CARTESIAN_POINT('Ctrl Pts',(-55.6600051127006,24.98995911165,39.5248017080178));
#204996=CARTESIAN_POINT('Origin',(-55.6083495590299,25.1059793847706,39.5248017080178));
#204997=CARTESIAN_POINT('Origin',(0.129138884176574,0.290050682801525,39.116));
#204998=CARTESIAN_POINT('Origin',(-56.3916032444848,25.4547063934087,39.116));
#204999=CARTESIAN_POINT('Origin',(0.129138884176574,0.290050682801525,39.5248017080178));
#205000=CARTESIAN_POINT('Origin',(-55.4702140717965,25.0444775033952,39.5248017080178));
#205001=CARTESIAN_POINT('Ctrl Pts',(-56.8833377255392,25.6742415049984,
39.2875012672119));
#205002=CARTESIAN_POINT('Ctrl Pts',(-56.9357219056856,25.5577357840976,
39.287208709576));
#205003=CARTESIAN_POINT('Ctrl Pts',(-56.8366797759153,25.5138485805642,
39.3549016990122));
#205004=CARTESIAN_POINT('Ctrl Pts',(-56.7783442778555,25.6273680143737,
39.1034939173931));
#205005=CARTESIAN_POINT('Ctrl Pts',(-56.8305359187831,25.5109042502482,
39.1031692336329));
#205006=CARTESIAN_POINT('Ctrl Pts',(-56.7526780286664,25.4764485929311,
39.2077507202299));
#205007=CARTESIAN_POINT('Ctrl Pts',(-56.5897276738849,25.5431608329955,
38.989));
#205008=CARTESIAN_POINT('Ctrl Pts',(-56.6417212312953,25.4268390553483,
38.9887769311182));
#205009=CARTESIAN_POINT('Ctrl Pts',(-56.6017723050738,25.4092610357547,
39.1161898712914));
#205010=CARTESIAN_POINT('Ctrl Pts',(-56.3916032444848,25.4547063934087,
38.989));
#205011=CARTESIAN_POINT('Ctrl Pts',(-56.4433359691572,25.3385127913803,
38.989));
#205012=CARTESIAN_POINT('Ctrl Pts',(-56.4432587405966,25.3386862495675,
39.1161895903853));
#205013=CARTESIAN_POINT('Origin',(-56.7851714777845,25.6299342605,39.3548010137695));
#205014=CARTESIAN_POINT('Ctrl Pts',(-55.4702140717965,25.0444775033952,
39.3978017080178));
#205015=CARTESIAN_POINT('Ctrl Pts',(-55.5218696254671,24.9284572302746,
39.3978017080178));
#205016=CARTESIAN_POINT('Ctrl Pts',(-55.5218696254671,24.9284572302746,
39.5248017080178));
#205017=CARTESIAN_POINT('Ctrl Pts',(-55.3878899076691,25.0080814159073,
39.3978017080178));
#205018=CARTESIAN_POINT('Ctrl Pts',(-55.4395618538405,24.8918114493237,
39.3975666025045));
#205019=CARTESIAN_POINT('Ctrl Pts',(-55.3985281293149,24.8735420580987,
39.5248015517196));
#205020=CARTESIAN_POINT('Ctrl Pts',(-55.3100454158619,24.9736678430968,
39.3484894016716));
#205021=CARTESIAN_POINT('Ctrl Pts',(-55.3621286647,24.8573359723215,39.3480259000037));
#205022=CARTESIAN_POINT('Ctrl Pts',(-55.2818999508914,24.8216158475493,
39.4508333188938));
#205023=CARTESIAN_POINT('Ctrl Pts',(-55.2690209153038,24.9555320242419,
39.2708017080178));
#205024=CARTESIAN_POINT('Ctrl Pts',(-55.3213695969754,24.8391888661849,
39.27051194648));
#205025=CARTESIAN_POINT('Ctrl Pts',(-55.2204359898054,24.7942503289611,
39.3343017080178));
#205026=CARTESIAN_POINT('Origin',(-55.1687804361348,24.9102706020818,39.3343017080178));
#205027=CARTESIAN_POINT('Origin',(-56.9479187893799,25.7023940320541,39.6398955068197));
#205028=CARTESIAN_POINT('Origin',(-57.1106661007663,25.7748538035651,39.92499));
#205029=CARTESIAN_POINT('Origin',(-55.0944632682976,24.8771824671432,39.1934008539939));
#205030=CARTESIAN_POINT('Origin',(-55.0536014459533,24.8590452239608,39.1160402713851));
#205031=CARTESIAN_POINT('Ctrl Pts',(-57.505263737773,25.6197038181302,40.1599502534424));
#205032=CARTESIAN_POINT('Ctrl Pts',(-57.4711877340327,25.6045223014066,
40.10025));
#205033=CARTESIAN_POINT('Ctrl Pts',(-57.4068835917977,25.5758735661212,
40.10025));
#205034=CARTESIAN_POINT('Ctrl Pts',(-57.4694043465862,25.7001924885134,
40.1599500538462));
#205035=CARTESIAN_POINT('Ctrl Pts',(-57.4450643815399,25.6631501095118,
40.1002448353478));
#205036=CARTESIAN_POINT('Ctrl Pts',(-57.3861185493425,25.6224598624443,
40.10025));
#205037=CARTESIAN_POINT('Ctrl Pts',(-57.413464248775,25.7642825572405,40.1202442001038));
#205038=CARTESIAN_POINT('Ctrl Pts',(-57.3998804953985,25.7077329912391,
40.0633873868015));
#205039=CARTESIAN_POINT('Ctrl Pts',(-57.3441059191826,25.6552692732808,
40.0772271723537));
#205040=CARTESIAN_POINT('Ctrl Pts',(-57.3036982377901,25.8321626496794,
40.0045995998164));
#205041=CARTESIAN_POINT('Ctrl Pts',(-57.3186021074453,25.7409042554413,
39.9663485808318));
#205042=CARTESIAN_POINT('Ctrl Pts',(-57.2526112478171,25.6821129719831,
40.0101727202466));
#205043=CARTESIAN_POINT('Ctrl Pts',(-57.2503778226939,25.8376543496548,
39.9304654349858));
#205044=CARTESIAN_POINT('Ctrl Pts',(-57.2821097063785,25.728949171911,39.9051900162956));
#205045=CARTESIAN_POINT('Ctrl Pts',(-57.2038640469252,25.6773293952367,
39.9671857458187));
#205046=CARTESIAN_POINT('Ctrl Pts',(-57.2088336324697,25.8191582032625,
39.8576902534424));
#205047=CARTESIAN_POINT('Ctrl Pts',(-57.2611357920723,25.7028284190338,
39.8573998014387));
#205048=CARTESIAN_POINT('Ctrl Pts',(-57.1623216544369,25.6588335304445,
39.92499));
#205049=CARTESIAN_POINT('Origin',(-57.4068835917977,25.5758735661212,40.22725));
#205050=CARTESIAN_POINT('Origin',(0.129138884176574,0.290050682801525,39.116));
#205051=CARTESIAN_POINT('Origin',(-54.6869600343295,24.6957503380312,39.116));
#205052=CARTESIAN_POINT('Origin',(1.20426471881346E-16,-6.70666394583731E-17,
40.22725));
#205053=CARTESIAN_POINT('Origin',(-57.4192809246787,25.5480287005723,40.22725));
#205054=CARTESIAN_POINT('Ctrl Pts',(-54.6869600343295,24.6957503380312,
38.989));
#205055=CARTESIAN_POINT('Ctrl Pts',(-54.7386929703522,24.5795562613022,
38.989));
#205056=CARTESIAN_POINT('Ctrl Pts',(-54.7386155301258,24.5797301948985,
39.1161901092324));
#205057=CARTESIAN_POINT('Ctrl Pts',(-54.4888352915933,24.6072881749587,
38.989));
#205058=CARTESIAN_POINT('Ctrl Pts',(-54.5406489234191,24.4913819335262,
38.989229898976));
#205059=CARTESIAN_POINT('Ctrl Pts',(-54.5800991622559,24.5091541605505,
39.1161900493204));
#205060=CARTESIAN_POINT('Ctrl Pts',(-54.3002245846697,24.5230714236777,
39.1034966344368));
#205061=CARTESIAN_POINT('Ctrl Pts',(-54.3520673354865,24.4074205468518,
39.103831410256));
#205062=CARTESIAN_POINT('Ctrl Pts',(-54.4291945615849,24.441967103316,39.2077528789598));
#205063=CARTESIAN_POINT('Ctrl Pts',(-54.195235491187,24.4761921430396,39.2875012672119));
#205064=CARTESIAN_POINT('Ctrl Pts',(-54.247177787347,24.3607210114368,39.2878045257868));
#205065=CARTESIAN_POINT('Ctrl Pts',(-54.3451938439591,24.4045675740912,
39.35490152959));
#205066=CARTESIAN_POINT('Origin',(-54.2933913980362,24.5205222915156,39.3548010137695));
#205067=CARTESIAN_POINT('Ctrl Pts',(-57.4675553545138,25.2380597013435,
39.8576902534424));
#205068=CARTESIAN_POINT('Ctrl Pts',(-57.4161024530841,25.354767599672,39.8573998014387));
#205069=CARTESIAN_POINT('Ctrl Pts',(-57.3172883154488,25.3107727110827,
39.92499));
#205070=CARTESIAN_POINT('Ctrl Pts',(-57.5091180232691,25.2565651278913,
39.9304984902492));
#205071=CARTESIAN_POINT('Ctrl Pts',(-57.4495672328895,25.3528749970536,
39.9052171569797));
#205072=CARTESIAN_POINT('Ctrl Pts',(-57.358849637138,25.3292770036981,39.9672049726607));
#205073=CARTESIAN_POINT('Ctrl Pts',(-57.5405471770606,25.2997972770063,
40.004343767866));
#205074=CARTESIAN_POINT('Ctrl Pts',(-57.482714899638,25.3720159720864,39.9661628577643));
#205075=CARTESIAN_POINT('Ctrl Pts',(-57.3948558336728,25.3622324578625,
40.0100243556236));
#205076=CARTESIAN_POINT('Ctrl Pts',(-57.5636463159494,25.4257977880274,
40.1194874821989));
#205077=CARTESIAN_POINT('Ctrl Pts',(-57.5124644612013,25.4538910783601,
40.062755148314));
#205078=CARTESIAN_POINT('Ctrl Pts',(-57.4360631077225,25.4475597357241,
40.0767884282376));
#205079=CARTESIAN_POINT('Ctrl Pts',(-57.5536211289088,25.511038551389,40.1599502015387));
#205080=CARTESIAN_POINT('Ctrl Pts',(-57.509788306592,25.517777816471,40.1002449453875));
#205081=CARTESIAN_POINT('Ctrl Pts',(-57.4400754463037,25.5012707422381,
40.10025));
#205082=CARTESIAN_POINT('Ctrl Pts',(-57.5176823163886,25.5918112338799,
40.1599502534424));
#205083=CARTESIAN_POINT('Ctrl Pts',(-57.4835989537475,25.5766462455181,
40.10025));
#205084=CARTESIAN_POINT('Ctrl Pts',(-57.4192809246787,25.5480287005723,
40.10025));
#205085=CARTESIAN_POINT('Origin',(-57.3689438691194,25.1947524379621,39.92499));
#205086=CARTESIAN_POINT('Origin',(-54.1306438627472,24.4480624203115,39.6398955069335));
#205087=CARTESIAN_POINT('Origin',(-53.9678963272933,24.3756025490943,39.92499));
#205088=CARTESIAN_POINT('Origin',(-57.2061965577014,25.1222926664875,39.6398955068285));
#205089=CARTESIAN_POINT('Origin',(-57.0434492461377,25.0498328948969,39.3548010137695));
#205090=CARTESIAN_POINT('Ctrl Pts',(-53.8697418420143,24.3312692531092,
39.8576902534424));
#205091=CARTESIAN_POINT('Ctrl Pts',(-53.9216078643415,24.2159747902191,
39.8579948730703));
#205092=CARTESIAN_POINT('Ctrl Pts',(-54.0195518809639,24.2595822759737,
39.92499));
#205093=CARTESIAN_POINT('Ctrl Pts',(-53.8282341734838,24.3127882662188,
39.9304020711231));
#205094=CARTESIAN_POINT('Ctrl Pts',(-53.8880114973681,24.2176496934286,
39.9058915297379));
#205095=CARTESIAN_POINT('Ctrl Pts',(-53.9780422761229,24.2411010091827,
39.9671523786028));
#205096=CARTESIAN_POINT('Ctrl Pts',(-53.7969955864425,24.2697746459846,
40.0043257306693));
#205097=CARTESIAN_POINT('Ctrl Pts',(-53.8549480733036,24.1983152114492,
39.9667894847835));
#205098=CARTESIAN_POINT('Ctrl Pts',(-53.9422730280817,24.2082687574727,
40.0100138975199));
#205099=CARTESIAN_POINT('Ctrl Pts',(-53.7744913425364,24.1443388226041,
40.1195533054857));
#205100=CARTESIAN_POINT('Ctrl Pts',(-53.8256450222191,24.1165167429228,
40.0630813209236));
#205101=CARTESIAN_POINT('Ctrl Pts',(-53.9017956184507,24.1232032230478,
40.0768265942421));
#205102=CARTESIAN_POINT('Ctrl Pts',(-53.7848917482045,24.0595120258538,
40.1599502027521));
#205103=CARTESIAN_POINT('Ctrl Pts',(-53.8286685158632,24.0529122166846,
40.1002552791554));
#205104=CARTESIAN_POINT('Ctrl Pts',(-53.8982652496121,24.0696665464387,
40.10025));
#205105=CARTESIAN_POINT('Ctrl Pts',(-53.8206887816834,23.9791663275018,
40.1599502534424));
#205106=CARTESIAN_POINT('Ctrl Pts',(-53.8547645473079,23.9943483786821,
40.10025));
#205107=CARTESIAN_POINT('Ctrl Pts',(-53.9190682401993,24.0229981225301,
40.10025));
#205108=CARTESIAN_POINT('Origin',(-53.9190682401993,24.0229981225301,40.22725));
#205109=CARTESIAN_POINT('Ctrl Pts',(-56.649881012838,24.8746050278057,38.989));
#205110=CARTESIAN_POINT('Ctrl Pts',(-56.5981482837086,24.9907986398447,
38.989));
#205111=CARTESIAN_POINT('Ctrl Pts',(-56.5982255167329,24.990625171632,39.1161896013268));
#205112=CARTESIAN_POINT('Ctrl Pts',(-56.8481896769747,24.9626539694743,
38.989));
#205113=CARTESIAN_POINT('Ctrl Pts',(-56.7965362315768,25.0791271905752,
38.9887769275485));
#205114=CARTESIAN_POINT('Ctrl Pts',(-56.7567415443537,25.0612010539385,
39.116189882185));
#205115=CARTESIAN_POINT('Ctrl Pts',(-57.036975459333,25.0464771582517,39.1034967087243));
#205116=CARTESIAN_POINT('Ctrl Pts',(-56.9853490357206,25.1631925873301,
39.10317202327));
#205117=CARTESIAN_POINT('Ctrl Pts',(-56.9076460727643,25.1283880784741,
39.2077529614999));
#205118=CARTESIAN_POINT('Ctrl Pts',(-57.1420619865019,25.093137300575,39.2875012672119));
#205119=CARTESIAN_POINT('Ctrl Pts',(-57.0905332166518,25.2100238867504,
39.2872087095507));
#205120=CARTESIAN_POINT('Ctrl Pts',(-56.9916465440539,25.1657874977298,
39.3549017048228));
#205121=CARTESIAN_POINT('Origin',(-56.649881012838,24.8746050278057,39.116));
#205122=CARTESIAN_POINT('Origin',(3.58382961824623E-16,2.38580516864212E-17,
40.22725));
#205123=CARTESIAN_POINT('Origin',(-53.9314655730802,23.9951532569811,40.22725));
#205124=CARTESIAN_POINT('Origin',(51.799563747336,-23.4101986852082,39.116));
#205125=CARTESIAN_POINT('Origin',(-56.2832472948488,24.7113125977917,39.1160373285251));
#205126=CARTESIAN_POINT('Ctrl Pts',(-53.8330634946836,23.9513722670369,
40.1599502534424));
#205127=CARTESIAN_POINT('Ctrl Pts',(-53.8671470951728,23.9665367208228,
40.10025));
#205128=CARTESIAN_POINT('Ctrl Pts',(-53.9314655730802,23.9951532569811,
40.10025));
#205129=CARTESIAN_POINT('Ctrl Pts',(-53.8686972660497,23.871282165812,40.159950056604));
#205130=CARTESIAN_POINT('Ctrl Pts',(-53.8931046959165,23.9081865738544,
40.1002551305369));
#205131=CARTESIAN_POINT('Ctrl Pts',(-53.9521563342718,23.9486256024597,
40.10025));
#205132=CARTESIAN_POINT('Ctrl Pts',(-53.9240892607408,23.807186639316,40.1203070619047));
#205133=CARTESIAN_POINT('Ctrl Pts',(-53.9378509529599,23.863535538615,40.0637098684499));
#205134=CARTESIAN_POINT('Ctrl Pts',(-53.9937257232526,23.9155750846183,
40.0772636213364));
#205135=CARTESIAN_POINT('Ctrl Pts',(-54.0330064121714,23.7392497560572,
40.0046102245801));
#205136=CARTESIAN_POINT('Ctrl Pts',(-54.0187512923758,23.8300830854577,
39.9670001894012));
#205137=CARTESIAN_POINT('Ctrl Pts',(-54.0845104630311,23.8883623535219,
40.0101788811208));
#205138=CARTESIAN_POINT('Ctrl Pts',(-54.0860594545419,23.7337507958625,
39.9303710930187));
#205139=CARTESIAN_POINT('Ctrl Pts',(-54.0553500291278,23.8418399747429,
39.9058663574104));
#205140=CARTESIAN_POINT('Ctrl Pts',(-54.1330265677735,23.8930480394869,
39.9671344706359));
#205141=CARTESIAN_POINT('Ctrl Pts',(-54.1275498658872,23.7522229508832,
39.8576902534424));
#205142=CARTESIAN_POINT('Ctrl Pts',(-54.0765745253534,23.8679139708573,
39.8579948730703));
#205143=CARTESIAN_POINT('Ctrl Pts',(-54.1745185419758,23.9115214566119,
39.92499));
#205144=CARTESIAN_POINT('Origin',(-54.2261740956464,23.7955011834913,39.92499));
#205145=CARTESIAN_POINT('Origin',(-56.2428239368561,24.6933715410274,39.1925554488845));
#205146=CARTESIAN_POINT('Origin',(-56.1680608984276,24.6600848917116,39.3343017080178));
#205147=CARTESIAN_POINT('Origin',(-54.3889216310588,23.8679610547526,39.639895506921));
#205148=CARTESIAN_POINT('Origin',(-54.5516691663893,23.9404209259125,39.3548010137695));
#205149=CARTESIAN_POINT('Ctrl Pts',(-55.8666273273831,24.5258780191675,
39.3978017080178));
#205150=CARTESIAN_POINT('Ctrl Pts',(-55.8149717737125,24.6418982922882,
39.3978017080178));
#205151=CARTESIAN_POINT('Ctrl Pts',(-55.8149717737125,24.6418982922882,
39.5248017080178));
#205152=CARTESIAN_POINT('Ctrl Pts',(-55.9487607347574,24.5627025231283,
39.3978017080178));
#205153=CARTESIAN_POINT('Ctrl Pts',(-55.8971232158786,24.6784744708797,
39.3980355775182));
#205154=CARTESIAN_POINT('Ctrl Pts',(-55.9383132588147,24.6968134595443,
39.5248015517192));
#205155=CARTESIAN_POINT('Ctrl Pts',(-56.0264248009273,24.597521196073,39.3484893995498));
#205156=CARTESIAN_POINT('Ctrl Pts',(-55.9751910510454,24.7132325104962,
39.3489438303417));
#205157=CARTESIAN_POINT('Ctrl Pts',(-56.0549414076415,24.7487396569164,
39.4508333155595));
#205158=CARTESIAN_POINT('Ctrl Pts',(-56.0673542004324,24.6158705164598,
39.2708017080178));
#205159=CARTESIAN_POINT('Ctrl Pts',(-56.0163785451196,24.731570364334,39.2710850691866));
#205160=CARTESIAN_POINT('Ctrl Pts',(-56.116405344757,24.7761051648322,39.3343017080178));
#205161=CARTESIAN_POINT('Origin',(-55.8666273273831,24.5258780191675,39.5248017080178));
#205162=CARTESIAN_POINT('Ctrl Pts',(-54.4530463244691,23.8971395307773,
39.2875012672119));
#205163=CARTESIAN_POINT('Ctrl Pts',(-54.401990736535,24.0130054343465,39.2878045257519));
#205164=CARTESIAN_POINT('Ctrl Pts',(-54.5001606088501,24.0565064908996,
39.3549015218347));
#205165=CARTESIAN_POINT('Ctrl Pts',(-54.5581374230423,23.9437939758161,
39.1034938540228));
#205166=CARTESIAN_POINT('Ctrl Pts',(-54.506881647828,24.0597061770709,39.1038286278813));
#205167=CARTESIAN_POINT('Ctrl Pts',(-54.5841625982711,24.0939065860615,
39.2077506434033));
#205168=CARTESIAN_POINT('Ctrl Pts',(-54.7469293531953,24.0276077026093,
38.989));
#205169=CARTESIAN_POINT('Ctrl Pts',(-54.6954643138415,24.1436691352846,
38.9892298954611));
#205170=CARTESIAN_POINT('Ctrl Pts',(-54.735068394994,24.1610941752712,39.1161900347288));
#205171=CARTESIAN_POINT('Ctrl Pts',(-54.9452378026827,24.1156489724281,
38.989));
#205172=CARTESIAN_POINT('Ctrl Pts',(-54.8935048726349,24.2318430357372,
38.989));
#205173=CARTESIAN_POINT('Ctrl Pts',(-54.8935823068775,24.2316691155808,
39.1161900945645));
#205174=CARTESIAN_POINT('Origin',(-54.9452378026827,24.1156489724281,39.116));
#205175=CARTESIAN_POINT('Origin',(50.541702139688,-22.850162615335,39.5248017080178));
#205176=CARTESIAN_POINT('Origin',(-55.7284918401496,24.4643761377921,39.5248017080178));
#205177=CARTESIAN_POINT('Origin',(50.3447265545023,-22.7624634345049,39.116));
#205178=CARTESIAN_POINT('Origin',(-55.3119205422643,24.2788510342452,39.1160402713846));
#205179=CARTESIAN_POINT('Ctrl Pts',(-55.5277679687681,24.3743766270218,
39.2708017080178));
#205180=CARTESIAN_POINT('Ctrl Pts',(-55.4763362579872,24.491128046823,39.2705119464801));
#205181=CARTESIAN_POINT('Ctrl Pts',(-55.3754026508173,24.4461895095993,
39.3343017080178));
#205182=CARTESIAN_POINT('Ctrl Pts',(-55.5688345658067,24.3927905570423,
39.3487519301186));
#205183=CARTESIAN_POINT('Ctrl Pts',(-55.5172331055191,24.5093364964835,
39.3482879463986));
#205184=CARTESIAN_POINT('Ctrl Pts',(-55.4370743056935,24.4736474994206,
39.4512271261638));
#205185=CARTESIAN_POINT('Ctrl Pts',(-55.6466353090197,24.4276751358079,
39.3978017080178));
#205186=CARTESIAN_POINT('Ctrl Pts',(-55.5948055748778,24.543873985031,39.3975673827401));
#205187=CARTESIAN_POINT('Ctrl Pts',(-55.5539102504902,24.5256662135193,
39.5248015355181));
#205188=CARTESIAN_POINT('Ctrl Pts',(-55.7284918401496,24.4643761377921,
39.3978017080178));
#205189=CARTESIAN_POINT('Ctrl Pts',(-55.676836286479,24.5803964109127,39.3978017080178));
#205190=CARTESIAN_POINT('Ctrl Pts',(-55.676836286479,24.5803964109127,39.5248017080178));
#205191=CARTESIAN_POINT('Origin',(-55.4270582044879,24.3301692364787,39.3343017080178));
#205192=CARTESIAN_POINT('Origin',(-55.3527410377818,24.2970811017172,39.1934008533559));
#205193=CARTESIAN_POINT('Origin',(-53.0360596835504,30.9870007556532,39.1925554495084));
#205194=CARTESIAN_POINT('Origin',(-53.0743345559671,31.0091584503694,39.1160373285251));
#205195=CARTESIAN_POINT('Origin',(-52.9651856060843,30.9460815882873,39.3343017080178));
#205196=CARTESIAN_POINT('Ctrl Pts',(-52.8702215132213,30.8905967158741,
39.2708017080178));
#205197=CARTESIAN_POINT('Ctrl Pts',(-52.9338619179793,30.7813498801536,
39.2710850691866));
#205198=CARTESIAN_POINT('Ctrl Pts',(-53.0286856060843,30.8360963620066,
39.3343017080178));
#205199=CARTESIAN_POINT('Ctrl Pts',(-52.8311874403355,30.868194145979,39.3487519293518));
#205200=CARTESIAN_POINT('Ctrl Pts',(-52.8946849835385,30.7587310665085,
39.3492068662926));
#205201=CARTESIAN_POINT('Ctrl Pts',(-52.9702219582401,30.802342359186,39.4512271248735));
#205202=CARTESIAN_POINT('Ctrl Pts',(-52.7572372522463,30.8257530395504,
39.3978017080178));
#205203=CARTESIAN_POINT('Ctrl Pts',(-52.8205474253443,30.7159277273269,
39.3980347781178));
#205204=CARTESIAN_POINT('Ctrl Pts',(-52.8594635164572,30.7383959430076,
39.5248015355195));
#205205=CARTESIAN_POINT('Ctrl Pts',(-52.6794317578285,30.7811015270748,
39.3978017080178));
#205206=CARTESIAN_POINT('Ctrl Pts',(-52.7429317578285,30.6711163007942,
39.3978017080178));
#205207=CARTESIAN_POINT('Ctrl Pts',(-52.7429317578285,30.6711163007942,
39.5248017080178));
#205208=CARTESIAN_POINT('Origin',(-52.6794317578285,30.7811015270748,39.5248017080178));
#205209=CARTESIAN_POINT('Origin',(0.158750000000008,0.274963065701558,39.116));
#205210=CARTESIAN_POINT('Origin',(-53.4219427993284,31.209790476761,39.116));
#205211=CARTESIAN_POINT('Origin',(0.158750000000008,0.274963065701558,39.5248017080178));
#205212=CARTESIAN_POINT('Origin',(-52.5484816883957,30.7054974692373,39.5248017080178));
#205213=CARTESIAN_POINT('Ctrl Pts',(-53.8880358395968,31.4795232016794,
39.2875012672119));
#205214=CARTESIAN_POINT('Ctrl Pts',(-53.9523112176908,31.3691313491582,
39.287208709576));
#205215=CARTESIAN_POINT('Ctrl Pts',(-53.8583991130131,31.3151318426941,
39.3549016990121));
#205216=CARTESIAN_POINT('Ctrl Pts',(-53.7885171709481,31.4219316852012,
39.1034939173931));
#205217=CARTESIAN_POINT('Ctrl Pts',(-53.8525966788897,31.3115614337837,
39.1031692336348));
#205218=CARTESIAN_POINT('Ctrl Pts',(-53.7787668993583,31.2691561625547,
39.2077507202298));
#205219=CARTESIAN_POINT('Ctrl Pts',(-53.6097358757354,31.3184699958127,
38.989));
#205220=CARTESIAN_POINT('Ctrl Pts',(-53.6736035436633,31.2082202476928,
38.9887769311176));
#205221=CARTESIAN_POINT('Ctrl Pts',(-53.6357108652113,31.186562722461,39.1161898712912));
#205222=CARTESIAN_POINT('Ctrl Pts',(-53.4219427993284,31.209790476761,38.989));
#205223=CARTESIAN_POINT('Ctrl Pts',(-53.4855376653836,31.0996409376529,
38.989));
#205224=CARTESIAN_POINT('Ctrl Pts',(-53.4854427285714,31.0998053730351,
39.1161895903851));
#205225=CARTESIAN_POINT('Origin',(-53.7950387249976,31.4251975098797,39.3548010137695));
#205226=CARTESIAN_POINT('Ctrl Pts',(-52.5484816883957,30.7054974692373,
39.3978017080178));
#205227=CARTESIAN_POINT('Ctrl Pts',(-52.6119816883957,30.5955122429567,
39.3978017080178));
#205228=CARTESIAN_POINT('Ctrl Pts',(-52.6119816883957,30.5955122429567,
39.5248017080178));
#205229=CARTESIAN_POINT('Ctrl Pts',(-52.4704129317472,30.6606955449589,
39.3978017080178));
#205230=CARTESIAN_POINT('Ctrl Pts',(-52.5339553345217,30.5504637065431,
39.3975666025022));
#205231=CARTESIAN_POINT('Ctrl Pts',(-52.4950560684217,30.5280052047896,
39.5248015517178));
#205232=CARTESIAN_POINT('Ctrl Pts',(-52.3965920780924,30.6183335281986,
39.3484894016716));
#205233=CARTESIAN_POINT('Ctrl Pts',(-52.4605500011258,30.5080831175487,
39.348025900005));
#205234=CARTESIAN_POINT('Ctrl Pts',(-52.3844945583563,30.4641724871913,
39.450833318895));
#205235=CARTESIAN_POINT('Ctrl Pts',(-52.357688023316,30.5960088312573,39.2708017080178));
#205236=CARTESIAN_POINT('Ctrl Pts',(-52.4219111049554,30.4857749404424,
39.2705119464801));
#205237=CARTESIAN_POINT('Ctrl Pts',(-52.3262277788839,30.4305321463781,
39.3343017080178));
#205238=CARTESIAN_POINT('Origin',(-52.2627277788839,30.5405173726587,39.3343017080178));
#205239=CARTESIAN_POINT('Origin',(-53.9493203812208,31.5142720656068,39.6398955068201));
#205240=CARTESIAN_POINT('Origin',(-54.1036020372436,31.603346621267,39.92499));
#205241=CARTESIAN_POINT('Origin',(-52.1922763801643,30.4998422386362,39.1934008539949));
#205242=CARTESIAN_POINT('Origin',(-52.1535342613176,30.4775331296743,39.1160402713847));
#205243=CARTESIAN_POINT('Ctrl Pts',(-54.5122556166608,31.4902932482912,
40.1599502534424));
#205244=CARTESIAN_POINT('Ctrl Pts',(-54.4799531854476,31.4716329851994,
40.10025));
#205245=CARTESIAN_POINT('Ctrl Pts',(-54.4189959163061,31.4364195775139,
40.10025));
#205246=CARTESIAN_POINT('Ctrl Pts',(-54.4681793099456,31.5665926662618,
40.1599500538464));
#205247=CARTESIAN_POINT('Ctrl Pts',(-54.4478446647269,31.5272089901459,
40.100244835349));
#205248=CARTESIAN_POINT('Ctrl Pts',(-54.3934750329619,31.4805801312537,
40.10025));
#205249=CARTESIAN_POINT('Ctrl Pts',(-54.4058464214484,31.6244843104277,
40.120244200104));
#205250=CARTESIAN_POINT('Ctrl Pts',(-54.398248120527,31.5668246399998,40.0633873868015));
#205251=CARTESIAN_POINT('Ctrl Pts',(-54.3482630350909,31.5088182930366,
40.0772271723538));
#205252=CARTESIAN_POINT('Ctrl Pts',(-54.2895863184075,31.68051887617,40.0045995998161));
#205253=CARTESIAN_POINT('Ctrl Pts',(-54.313947642815,31.5913182835559,39.9663485808318));
#205254=CARTESIAN_POINT('Ctrl Pts',(-54.254463650534,31.5259511417533,40.0101727202466));
#205255=CARTESIAN_POINT('Ctrl Pts',(-54.2359839591645,31.680406990989,39.930465434986));
#205256=CARTESIAN_POINT('Ctrl Pts',(-54.278904797451,31.5756141966208,39.9051900162946));
#205257=CARTESIAN_POINT('Ctrl Pts',(-54.2064835118365,31.5160982999436,
39.9671857458179));
#205258=CARTESIAN_POINT('Ctrl Pts',(-54.1966007261205,31.6576696180589,
39.8576902534424));
#205259=CARTESIAN_POINT('Ctrl Pts',(-54.260776142598,31.5474441649288,39.8573998014387));
#205260=CARTESIAN_POINT('Ctrl Pts',(-54.1671020372436,31.4933613949863,
39.92499));
#205261=CARTESIAN_POINT('Origin',(-54.4189959163061,31.4364195775139,40.22725));
#205262=CARTESIAN_POINT('Origin',(0.158750000000008,0.274963065701558,39.116));
#205263=CARTESIAN_POINT('Origin',(-51.8059703131944,30.2768083268885,39.116));
#205264=CARTESIAN_POINT('Origin',(1.12590909550281E-16,-8.24447964058581E-17,
40.22725));
#205265=CARTESIAN_POINT('Origin',(-54.4342359163061,31.4100231232066,40.22725));
#205266=CARTESIAN_POINT('Ctrl Pts',(-51.8059703131944,30.2768083268885,
38.989));
#205267=CARTESIAN_POINT('Ctrl Pts',(-51.8695654390618,30.1666583377723,
38.989));
#205268=CARTESIAN_POINT('Ctrl Pts',(-51.8694702420496,30.1668232238342,
39.1161901092323));
#205269=CARTESIAN_POINT('Ctrl Pts',(-51.6181777324919,30.1681210939084,
38.989));
#205270=CARTESIAN_POINT('Ctrl Pts',(-51.6818230251198,30.0582657983037,
38.989229898976));
#205271=CARTESIAN_POINT('Ctrl Pts',(-51.7191994478421,30.0800643400504,
39.1161900493203));
#205272=CARTESIAN_POINT('Ctrl Pts',(-51.43940330235,30.0646505034491,39.1034966344368));
#205273=CARTESIAN_POINT('Ctrl Pts',(-51.5030508615843,29.9550522173057,
39.1038314102567));
#205274=CARTESIAN_POINT('Ctrl Pts',(-51.5761444782083,29.9974715145378,
39.2077528789599));
#205275=CARTESIAN_POINT('Ctrl Pts',(-51.3398895692694,30.0070536838162,
39.2875012672119));
#205276=CARTESIAN_POINT('Ctrl Pts',(-51.4036173400344,29.8976445635505,
39.2878045257868));
#205277=CARTESIAN_POINT('Ctrl Pts',(-51.496513240619,29.9514963979201,39.35490152959));
#205278=CARTESIAN_POINT('Origin',(-51.432874005494,30.0614010732041,39.3548010137695));
#205279=CARTESIAN_POINT('Ctrl Pts',(-54.5146464769135,31.1067982185539,
39.8576902534424));
#205280=CARTESIAN_POINT('Ctrl Pts',(-54.451276142598,31.2174884860869,39.8573998014387));
#205281=CARTESIAN_POINT('Ctrl Pts',(-54.3576020372436,31.1634057161445,
39.92499));
#205282=CARTESIAN_POINT('Ctrl Pts',(-54.5540471172209,31.1295467523339,
39.9304984902491));
#205283=CARTESIAN_POINT('Ctrl Pts',(-54.4847554296815,31.2191042733502,
39.9052171569793));
#205284=CARTESIAN_POINT('Ctrl Pts',(-54.3970014563939,31.1861529813968,
39.9672049726597));
#205285=CARTESIAN_POINT('Ctrl Pts',(-54.5807851087093,31.1758273123595,
40.0043437678661));
#205286=CARTESIAN_POINT('Ctrl Pts',(-54.515720733338,31.2416052667855,39.9661628577646));
#205287=CARTESIAN_POINT('Ctrl Pts',(-54.4293656242355,31.2226915745265,
40.0100243556237));
#205288=CARTESIAN_POINT('Ctrl Pts',(-54.5905870683102,31.3035520968883,
40.1194874821988));
#205289=CARTESIAN_POINT('Ctrl Pts',(-54.5367490446508,31.3261415286131,
40.0627551483138));
#205290=CARTESIAN_POINT('Ctrl Pts',(-54.461428031297,31.311858753664,40.0767884282376));
#205291=CARTESIAN_POINT('Ctrl Pts',(-54.5717067142918,31.3872779850343,
40.1599502015394));
#205292=CARTESIAN_POINT('Ctrl Pts',(-54.5274095677426,31.3893985541613,
40.1002449453872));
#205293=CARTESIAN_POINT('Ctrl Pts',(-54.4598040608988,31.3656949292519,
40.10025));
#205294=CARTESIAN_POINT('Ctrl Pts',(-54.5275217339717,31.4638515574745,
40.1599502534424));
#205295=CARTESIAN_POINT('Ctrl Pts',(-54.4952102564863,31.4452069629858,
40.10025));
#205296=CARTESIAN_POINT('Ctrl Pts',(-54.4342359163061,31.4100231232066,
40.10025));
#205297=CARTESIAN_POINT('Origin',(-54.4211020372436,31.0534204898638,39.92499));
#205298=CARTESIAN_POINT('Origin',(-51.2785921372153,29.9723263949871,39.6398955069309));
#205299=CARTESIAN_POINT('Origin',(-51.1243102687782,29.883251716749,39.92499));
#205300=CARTESIAN_POINT('Origin',(-54.2668203811871,30.9643459342335,39.639895506829));
#205301=CARTESIAN_POINT('Origin',(-54.1125387249976,30.8752713784766,39.3548010137695));
#205302=CARTESIAN_POINT('Ctrl Pts',(-51.0313275753406,29.828901345689,39.8576902534424));
#205303=CARTESIAN_POINT('Ctrl Pts',(-51.0949610231999,29.7196599535397,
39.8579948730704));
#205304=CARTESIAN_POINT('Ctrl Pts',(-51.1878102687782,29.7732664904684,
39.92499));
#205305=CARTESIAN_POINT('Ctrl Pts',(-50.9919790793206,29.8061828667735,
39.9304020711229));
#205306=CARTESIAN_POINT('Ctrl Pts',(-51.0613736255811,29.7178139048431,
39.9058915297375));
#205307=CARTESIAN_POINT('Ctrl Pts',(-51.1484598763126,29.7505475307857,
39.9671523786024));
#205308=CARTESIAN_POINT('Ctrl Pts',(-50.9654077681504,29.7601395581529,
40.0043257306695));
#205309=CARTESIAN_POINT('Ctrl Pts',(-51.0305123301025,29.6951292702712,
39.9667894847838));
#205310=CARTESIAN_POINT('Ctrl Pts',(-51.1163184807716,29.7141562330556,
40.0100138975202));
#205311=CARTESIAN_POINT('Ctrl Pts',(-50.9561384187038,29.6330385513053,
40.1195533054855));
#205312=CARTESIAN_POINT('Ctrl Pts',(-51.0099200724111,29.6107158994149,
40.0630813209233));
#205313=CARTESIAN_POINT('Ctrl Pts',(-51.0849545802164,29.6253256551036,
40.0768265942419));
#205314=CARTESIAN_POINT('Ctrl Pts',(-50.9753486645695,29.5497635830446,
40.1599502027523));
#205315=CARTESIAN_POINT('Ctrl Pts',(-51.0195754864236,29.5477758465704,
40.100255279156));
#205316=CARTESIAN_POINT('Ctrl Pts',(-51.087039657642,29.5717132339807,40.10025));
#205317=CARTESIAN_POINT('Ctrl Pts',(-51.0193480105325,29.4735998357342,
40.1599502534424));
#205318=CARTESIAN_POINT('Ctrl Pts',(-51.0516501490684,29.492260605465,40.10025));
#205319=CARTESIAN_POINT('Ctrl Pts',(-51.1126068659044,29.5274749692189,
40.10025));
#205320=CARTESIAN_POINT('Origin',(-51.1126068659044,29.5274749692189,40.22725));
#205321=CARTESIAN_POINT('Ctrl Pts',(-53.7394427993284,30.6598643453579,
38.989));
#205322=CARTESIAN_POINT('Ctrl Pts',(-53.6758479277944,30.7700138939557,
38.989));
#205323=CARTESIAN_POINT('Ctrl Pts',(-53.6759428700935,30.7698494490698,
39.1161896013264));
#205324=CARTESIAN_POINT('Ctrl Pts',(-53.9274614872882,30.7681598456269,
38.989));
#205325=CARTESIAN_POINT('Ctrl Pts',(-53.8639162380569,30.8785957589629,
38.9887769275479));
#205326=CARTESIAN_POINT('Ctrl Pts',(-53.8262133418093,30.8566081460798,
39.1161898821845));
#205327=CARTESIAN_POINT('Ctrl Pts',(-54.1064511722685,30.8712573299225,
39.1034967087244));
#205328=CARTESIAN_POINT('Ctrl Pts',(-54.0429074791663,30.9819369489427,
39.1031720232703));
#205329=CARTESIAN_POINT('Ctrl Pts',(-53.9692682429949,30.9392009315184,
39.2077529615001));
#205330=CARTESIAN_POINT('Ctrl Pts',(-54.2060847114739,30.9286463962983,
39.2875012672119));
#205331=CARTESIAN_POINT('Ctrl Pts',(-54.1426202463873,31.0395064423977,
39.2872087095508));
#205332=CARTESIAN_POINT('Ctrl Pts',(-54.0488992470934,30.9851759130209,
39.3549017048226));
#205333=CARTESIAN_POINT('Origin',(-53.7394427993284,30.6598643453579,39.116));
#205334=CARTESIAN_POINT('Origin',(3.61170357355341E-16,2.93286234380104E-17,
40.22725));
#205335=CARTESIAN_POINT('Origin',(-51.1278468659044,29.5010785149116,40.22725));
#205336=CARTESIAN_POINT('Origin',(46.5080917980719,-27.2180767400485,39.116));
#205337=CARTESIAN_POINT('Origin',(-53.3918862459816,30.4591427892373,39.1160373285273));
#205338=CARTESIAN_POINT('Ctrl Pts',(-51.0345602039884,29.447251543774,40.1599502534424));
#205339=CARTESIAN_POINT('Ctrl Pts',(-51.0668719738975,29.4658956314771,
40.10025));
#205340=CARTESIAN_POINT('Ctrl Pts',(-51.1278468659044,29.5010785149116,
40.10025));
#205341=CARTESIAN_POINT('Ctrl Pts',(-51.0783704650304,29.3713249278651,
40.159950056604));
#205342=CARTESIAN_POINT('Ctrl Pts',(-51.0987866273836,29.4105784408359,
40.100255130536));
#205343=CARTESIAN_POINT('Ctrl Pts',(-51.1532877451691,29.4569685172218,
40.10025));
#205344=CARTESIAN_POINT('Ctrl Pts',(-51.1401588234662,29.3133705634516,
40.1203070619044));
#205345=CARTESIAN_POINT('Ctrl Pts',(-51.1479550638447,29.3708492661242,
40.0637098684497));
#205346=CARTESIAN_POINT('Ctrl Pts',(-51.198084132527,29.4284442379238,40.0772636213363));
#205347=CARTESIAN_POINT('Ctrl Pts',(-51.2555806533507,29.2571907880105,
40.0046102245804));
#205348=CARTESIAN_POINT('Ctrl Pts',(-51.2319089562573,29.3460364571625,
39.9670001894016));
#205349=CARTESIAN_POINT('Ctrl Pts',(-51.2912160489638,29.4108701703525,
40.0101788811209));
#205350=CARTESIAN_POINT('Ctrl Pts',(-51.3089178634635,29.2572675046854,
39.9303710930185));
#205351=CARTESIAN_POINT('Ctrl Pts',(-51.2670782717317,29.3615545506876,
39.9058663574103));
#205352=CARTESIAN_POINT('Ctrl Pts',(-51.3389765898556,29.4206015015123,
39.9671344706357));
#205353=CARTESIAN_POINT('Ctrl Pts',(-51.3482501200163,29.2799753962467,
39.8576902534424));
#205354=CARTESIAN_POINT('Ctrl Pts',(-51.2854610231999,29.3897042746978,
39.8579948730704));
#205355=CARTESIAN_POINT('Ctrl Pts',(-51.3783102687782,29.4433108116265,
39.92499));
#205356=CARTESIAN_POINT('Origin',(-51.4418102687782,29.3333255853459,39.92499));
#205357=CARTESIAN_POINT('Origin',(-53.3535596824659,30.437074623968,39.1925554488847));
#205358=CARTESIAN_POINT('Origin',(-53.2826856060843,30.3961554568841,39.3343017080178));
#205359=CARTESIAN_POINT('Origin',(-51.5960921371744,29.4224002636274,39.6398955069223));
#205360=CARTESIAN_POINT('Origin',(-51.750374005494,29.5114749418009,39.3548010137695));
#205361=CARTESIAN_POINT('Ctrl Pts',(-52.9969317578285,30.2311753956717,
39.3978017080178));
#205362=CARTESIAN_POINT('Ctrl Pts',(-52.9334317578285,30.3411606219523,
39.3978017080178));
#205363=CARTESIAN_POINT('Ctrl Pts',(-52.9334317578285,30.3411606219523,
39.5248017080178));
#205364=CARTESIAN_POINT('Ctrl Pts',(-53.0747660209932,30.2763834500036,
39.3978017080178));
#205365=CARTESIAN_POINT('Ctrl Pts',(-53.0113099140572,30.3861235964154,
39.3980355775173));
#205366=CARTESIAN_POINT('Ctrl Pts',(-53.0503573673261,30.4086676540709,
39.5248015517192));
#205367=CARTESIAN_POINT('Ctrl Pts',(-53.1483650929077,30.3191294881006,
39.3484893995498));
#205368=CARTESIAN_POINT('Ctrl Pts',(-53.0853168809894,30.4288515386957,
39.3489438303427));
#205369=CARTESIAN_POINT('Ctrl Pts',(-53.1609188493371,30.472500355472,39.4508333155597));
#205370=CARTESIAN_POINT('Ctrl Pts',(-53.1871522506172,30.3416565762241,
39.2708017080178));
#205371=CARTESIAN_POINT('Ctrl Pts',(-53.1243619179793,30.4513942013118,
39.2710850691866));
#205372=CARTESIAN_POINT('Ctrl Pts',(-53.2191856060843,30.5061406831648,
39.3343017080178));
#205373=CARTESIAN_POINT('Origin',(-52.9969317578285,30.2311753956717,39.5248017080178));
#205374=CARTESIAN_POINT('Ctrl Pts',(-51.6568155675425,29.4581217525678,
39.2875012672119));
#205375=CARTESIAN_POINT('Ctrl Pts',(-51.5939283826159,29.5680161684461,
39.2878045257519));
#205376=CARTESIAN_POINT('Ctrl Pts',(-51.6870133715069,29.6215404675521,
39.3549015218347));
#205377=CARTESIAN_POINT('Ctrl Pts',(-51.7564542486366,29.5155056307134,
39.1034938540228));
#205378=CARTESIAN_POINT('Ctrl Pts',(-51.6933631336501,29.6254251653837,
39.1038286278814));
#205379=CARTESIAN_POINT('Ctrl Pts',(-51.7666458147666,29.6675162799448,
39.2077506434032));
#205380=CARTESIAN_POINT('Ctrl Pts',(-51.9354510367808,29.6185943474771,
38.989));
#205381=CARTESIAN_POINT('Ctrl Pts',(-51.8721362050962,29.7286404220048,
38.9892298954605));
#205382=CARTESIAN_POINT('Ctrl Pts',(-51.9097019182958,29.750109759541,39.1161900347289));
#205383=CARTESIAN_POINT('Ctrl Pts',(-52.1234703131944,29.7268821954854,
38.989));
#205384=CARTESIAN_POINT('Ctrl Pts',(-52.0598751946718,29.8370321718799,
38.989));
#205385=CARTESIAN_POINT('Ctrl Pts',(-52.0599703843282,29.8368672985587,
39.1161900945646));
#205386=CARTESIAN_POINT('Origin',(-52.1234703131944,29.7268821954854,39.116));
#205387=CARTESIAN_POINT('Origin',(45.3776874999996,-26.5654375142634,39.5248017080178));
#205388=CARTESIAN_POINT('Origin',(-52.8659816883957,30.1555713378342,39.5248017080178));
#205389=CARTESIAN_POINT('Origin',(45.2006711678726,-26.4632370872589,39.116));
#205390=CARTESIAN_POINT('Origin',(-52.4710850656381,29.9275190026063,39.1160402713852));
#205391=CARTESIAN_POINT('Ctrl Pts',(-52.6757649139393,30.0450834959841,
39.2708017080178));
#205392=CARTESIAN_POINT('Ctrl Pts',(-52.6124111049554,30.1558192616006,
39.27051194648));
#205393=CARTESIAN_POINT('Ctrl Pts',(-52.5167277788839,30.1005764675362,
39.3343017080178));
#205394=CARTESIAN_POINT('Ctrl Pts',(-52.7146817640547,30.0676891808493,
39.3487519301185));
#205395=CARTESIAN_POINT('Ctrl Pts',(-52.6511806140165,30.1782028480957,
39.3482879463988));
#205396=CARTESIAN_POINT('Ctrl Pts',(-52.5751914484999,30.1343304829268,
39.4512271261642));
#205397=CARTESIAN_POINT('Ctrl Pts',(-52.788409875246,30.1105150503713,39.3978017080178));
#205398=CARTESIAN_POINT('Ctrl Pts',(-52.7247179826667,30.2206596676787,
39.3975673827392));
#205399=CARTESIAN_POINT('Ctrl Pts',(-52.685949917523,30.1982769148324,39.5248015355181));
#205400=CARTESIAN_POINT('Ctrl Pts',(-52.8659816883957,30.1555713378342,
39.3978017080178));
#205401=CARTESIAN_POINT('Ctrl Pts',(-52.8024816883957,30.2655565641149,
39.3978017080178));
#205402=CARTESIAN_POINT('Ctrl Pts',(-52.8024816883957,30.2655565641149,
39.5248017080178));
#205403=CARTESIAN_POINT('Origin',(-52.5802277788839,29.9905912412556,39.3343017080178));
#205404=CARTESIAN_POINT('Origin',(-52.509776381272,29.9499161075316,39.1934008533548));
#205405=CARTESIAN_POINT('Origin',(-49.5064990290873,36.3610285397835,39.1925554495084));
#205406=CARTESIAN_POINT('Origin',(-49.5422481179704,36.3870656659293,39.1160373285299));
#205407=CARTESIAN_POINT('Origin',(-49.4402904249163,36.3129251734947,39.3343017080178));
#205408=CARTESIAN_POINT('Ctrl Pts',(-49.3516463037382,36.2478178023255,
39.2708017080178));
#205409=CARTESIAN_POINT('Ctrl Pts',(-49.4263574835548,36.1458216659129,
39.2710850691866));
#205410=CARTESIAN_POINT('Ctrl Pts',(-49.5149391519574,36.2101800152091,
39.3343017080178));
#205411=CARTESIAN_POINT('Ctrl Pts',(-49.3151677697924,36.2214577843983,
39.3487519293518));
#205412=CARTESIAN_POINT('Ctrl Pts',(-49.3897594742873,36.1192316557419,
39.3492068662902));
#205413=CARTESIAN_POINT('Ctrl Pts',(-49.4603240281357,36.1704998050804,
39.451227124873));
#205414=CARTESIAN_POINT('Ctrl Pts',(-49.2460589922052,36.1715192752722,
39.3978017080178));
#205415=CARTESIAN_POINT('Ctrl Pts',(-49.3205022166676,36.0689133127054,
39.3980347781197));
#205416=CARTESIAN_POINT('Ctrl Pts',(-49.356856553303,36.0953262843491,39.5248015355195));
#205417=CARTESIAN_POINT('Ctrl Pts',(-49.1733470784084,36.1189794796887,
39.3978017080178));
#205418=CARTESIAN_POINT('Ctrl Pts',(-49.2479958054496,36.0162343214031,
39.3978017080178));
#205419=CARTESIAN_POINT('Ctrl Pts',(-49.2479958054496,36.0162343214031,
39.5248017080178));
#205420=CARTESIAN_POINT('Origin',(-49.1733470784084,36.1189794796887,39.5248017080178));
#205421=CARTESIAN_POINT('Origin',(0.186621817602868,0.256862895714044,39.116));
#205422=CARTESIAN_POINT('Origin',(-49.8669803696023,36.6229335645814,39.116));
#205423=CARTESIAN_POINT('Origin',(0.186621817602868,0.256862895714044,39.5248017080178));
#205424=CARTESIAN_POINT('Origin',(-49.05101714314,36.0301015792681,39.5248017080178));
#205425=CARTESIAN_POINT('Ctrl Pts',(-50.3023253561992,36.939908654649,39.2875012672119));
#205426=CARTESIAN_POINT('Ctrl Pts',(-50.377787717748,36.8368401467448,39.287208709576));
#205427=CARTESIAN_POINT('Ctrl Pts',(-50.2900345588341,36.7733199672428,
39.354901699012));
#205428=CARTESIAN_POINT('Ctrl Pts',(-50.2093718139431,36.8722300970262,
39.1034939173931));
#205429=CARTESIAN_POINT('Ctrl Pts',(-50.2846371204121,36.7691625978866,
39.1031692336331));
#205430=CARTESIAN_POINT('Ctrl Pts',(-50.2156443459689,36.7192723137688,
39.2077507202301));
#205431=CARTESIAN_POINT('Ctrl Pts',(-50.0423845927714,36.750647447547,38.989));
#205432=CARTESIAN_POINT('Ctrl Pts',(-50.1174266236757,36.6476776482617,
38.9887769311182));
#205433=CARTESIAN_POINT('Ctrl Pts',(-50.0820053531167,36.6221779017731,
39.116189871291));
#205434=CARTESIAN_POINT('Ctrl Pts',(-49.8669803696023,36.6229335645814,
38.989));
#205435=CARTESIAN_POINT('Ctrl Pts',(-49.9417406183797,36.5200349097942,
38.989));
#205436=CARTESIAN_POINT('Ctrl Pts',(-49.9416290134636,36.5201885207829,
39.1161895903849));
#205437=CARTESIAN_POINT('Origin',(-50.2155162706041,36.8761597191958,39.3548010137695));
#205438=CARTESIAN_POINT('Ctrl Pts',(-49.05101714314,36.0301015792681,39.3978017080178));
#205439=CARTESIAN_POINT('Ctrl Pts',(-49.1256658701812,35.9273564209825,
39.3978017080178));
#205440=CARTESIAN_POINT('Ctrl Pts',(-49.1256658701812,35.9273564209825,
39.5248017080178));
#205441=CARTESIAN_POINT('Ctrl Pts',(-48.9780591316057,35.9773846774561,
39.3978017080178));
#205442=CARTESIAN_POINT('Ctrl Pts',(-49.0527758071224,35.874398690299,39.3975666025017));
#205443=CARTESIAN_POINT('Ctrl Pts',(-49.016437187947,35.8479971380613,39.5248015517178));
#205444=CARTESIAN_POINT('Ctrl Pts',(-48.9090707128232,35.9275383438678,
39.3484894016716));
#205445=CARTESIAN_POINT('Ctrl Pts',(-48.9842025736629,35.8245773199103,
39.3480259000054));
#205446=CARTESIAN_POINT('Ctrl Pts',(-48.9131536812787,35.7729572780253,
39.4508333188949));
#205447=CARTESIAN_POINT('Ctrl Pts',(-48.872713344794,35.9012693628909,39.2708017080178));
#205448=CARTESIAN_POINT('Ctrl Pts',(-48.9481071848794,35.7983524848939,
39.27051194648));
#205449=CARTESIAN_POINT('Ctrl Pts',(-48.8587224664497,35.733410685601,39.3343017080178));
#205450=CARTESIAN_POINT('Origin',(-48.7840737394086,35.8361558438867,39.3343017080178));
#205451=CARTESIAN_POINT('Origin',(-50.3596419293478,36.9808731396215,39.6398955068191));
#205452=CARTESIAN_POINT('Origin',(-50.5037675878942,37.0855865599607,39.92499));
#205453=CARTESIAN_POINT('Origin',(-48.7182599900743,35.7883393560622,39.1934008539949));
#205454=CARTESIAN_POINT('Origin',(-48.6820620414858,35.7621028045855,39.1160402713848));
#205455=CARTESIAN_POINT('Ctrl Pts',(-50.9219998155897,37.0158684358564,
40.1599502534424));
#205456=CARTESIAN_POINT('Ctrl Pts',(-50.8918248690997,36.9939338721437,
40.10025));
#205457=CARTESIAN_POINT('Ctrl Pts',(-50.8348823336483,36.9525415975216,
40.10025));
#205458=CARTESIAN_POINT('Ctrl Pts',(-50.8701895025857,37.0871426490249,
40.1599500538467));
#205459=CARTESIAN_POINT('Ctrl Pts',(-50.8540829678241,37.0458491715919,
40.100244835349));
#205460=CARTESIAN_POINT('Ctrl Pts',(-50.8048852215546,36.9937925764108,
40.10025));
#205461=CARTESIAN_POINT('Ctrl Pts',(-50.8021467555731,37.1382015956604,
40.1202442001038));
#205462=CARTESIAN_POINT('Ctrl Pts',(-50.8006171556815,37.0800635522217,
40.0633873868018));
#205463=CARTESIAN_POINT('Ctrl Pts',(-50.756969208081,37.0171501059292,40.0772271723538));
#205464=CARTESIAN_POINT('Ctrl Pts',(-50.6806663304941,37.1817767082791,
40.0045995998163));
#205465=CARTESIAN_POINT('Ctrl Pts',(-50.7142182018859,37.0956112176477,
39.9663485808315));
#205466=CARTESIAN_POINT('Ctrl Pts',(-50.6618927960199,37.0243843935855,
40.0101727202465));
#205467=CARTESIAN_POINT('Ctrl Pts',(-50.6273693057704,37.1760624637761,
39.9304654349858));
#205468=CARTESIAN_POINT('Ctrl Pts',(-50.6810088489711,37.0763301845675,
39.9051900162956));
#205469=CARTESIAN_POINT('Ctrl Pts',(-50.6152053999548,37.0095702365081,
39.9671857458182));
#205470=CARTESIAN_POINT('Ctrl Pts',(-50.5905785208481,37.1493329797265,
39.8576902534424));
#205471=CARTESIAN_POINT('Ctrl Pts',(-50.665924074908,37.0464195108257,39.8573998014387));
#205472=CARTESIAN_POINT('Ctrl Pts',(-50.5784163149354,36.9828414016751,
39.92499));
#205473=CARTESIAN_POINT('Origin',(-50.8348823336483,36.9525415975216,40.22725));
#205474=CARTESIAN_POINT('Origin',(0.186621817602868,0.256862895714044,39.116));
#205475=CARTESIAN_POINT('Origin',(-48.3573835402116,35.526147267887,39.116));
#205476=CARTESIAN_POINT('Origin',(1.03190816135906E-16,-9.69196709112375E-17,
40.22725));
#205477=CARTESIAN_POINT('Origin',(-50.8527980281382,36.9278827595331,40.22725));
#205478=CARTESIAN_POINT('Ctrl Pts',(-48.3573835402116,35.526147267887,38.989));
#205479=CARTESIAN_POINT('Ctrl Pts',(-48.4321440944166,35.4232481927149,
38.989));
#205480=CARTESIAN_POINT('Ctrl Pts',(-48.4320321836171,35.423402224716,39.1161901092319));
#205481=CARTESIAN_POINT('Ctrl Pts',(-48.1819806163548,35.3984257650683,
38.989));
#205482=CARTESIAN_POINT('Ctrl Pts',(-48.2567602586406,35.2958250128989,
38.989229898976));
#205483=CARTESIAN_POINT('Ctrl Pts',(-48.2916533613388,35.3214110399818,
39.1161900493199));
#205484=CARTESIAN_POINT('Ctrl Pts',(-48.0150011530602,35.2768349808766,
39.1034966344368));
#205485=CARTESIAN_POINT('Ctrl Pts',(-48.0897561847363,35.1744900671682,
39.1038314102573));
#205486=CARTESIAN_POINT('Ctrl Pts',(-48.1580153629271,35.2243173504724,
39.2077528789601));
#205487=CARTESIAN_POINT('Ctrl Pts',(-47.9220530736684,35.2091516650532,
39.2875012672119));
#205488=CARTESIAN_POINT('Ctrl Pts',(-47.9968681042458,35.1070032653419,
39.2878045257868));
#205489=CARTESIAN_POINT('Ctrl Pts',(-48.0836260618763,35.1702703594596,
39.3549015295897));
#205490=CARTESIAN_POINT('Origin',(-48.0088472823269,35.2729208539819,39.3548010137695));
#205491=CARTESIAN_POINT('Ctrl Pts',(-50.964463724589,36.6347241449659,39.8576902534424));
#205492=CARTESIAN_POINT('Ctrl Pts',(-50.8898702560315,36.7381840359688,
39.8573998014387));
#205493=CARTESIAN_POINT('Ctrl Pts',(-50.8023624960588,36.6746059268182,
39.92499));
#205494=CARTESIAN_POINT('Ctrl Pts',(-51.0012706547886,36.6614665482809,
39.9304984902493));
#205495=CARTESIAN_POINT('Ctrl Pts',(-50.9229972443165,36.7432905102103,
39.9052171569806));
#205496=CARTESIAN_POINT('Ctrl Pts',(-50.8391683443882,36.7013469409088,
39.9672049726601));
#205497=CARTESIAN_POINT('Ctrl Pts',(-51.0230245369435,36.7102884597167,
40.004343767866));
#205498=CARTESIAN_POINT('Ctrl Pts',(-50.9514409225344,36.7689049964548,
39.9661628577642));
#205499=CARTESIAN_POINT('Ctrl Pts',(-50.867535894942,36.7410683485313,40.0100243556235));
#205500=CARTESIAN_POINT('Ctrl Pts',(-51.0194219249358,36.8383381382868,
40.119487482199));
#205501=CARTESIAN_POINT('Ctrl Pts',(-50.9635175930195,36.8551762168625,
40.062755148314));
#205502=CARTESIAN_POINT('Ctrl Pts',(-50.8901021525742,36.8330984946713,
40.0767884282377));
#205503=CARTESIAN_POINT('Ctrl Pts',(-50.9918932610483,36.9196318328646,
40.1599502015384));
#205504=CARTESIAN_POINT('Ctrl Pts',(-50.9476171190676,36.9171104726342,
40.1002449453869));
#205505=CARTESIAN_POINT('Ctrl Pts',(-50.882859665751,36.8864699989243,40.10025));
#205506=CARTESIAN_POINT('Ctrl Pts',(-50.9399462128199,36.9911673391712,
40.1599502534424));
#205507=CARTESIAN_POINT('Ctrl Pts',(-50.9097606317991,36.9692474126344,
40.10025));
#205508=CARTESIAN_POINT('Ctrl Pts',(-50.8527980281382,36.9278827595331,
40.10025));
#205509=CARTESIAN_POINT('Origin',(-50.8770112230999,36.5718607685326,39.92499));
#205510=CARTESIAN_POINT('Origin',(-47.864721425496,35.1682072895758,39.6398955069329));
#205511=CARTESIAN_POINT('Origin',(-47.7205955685088,35.0634937251226,39.92499));
#205512=CARTESIAN_POINT('Origin',(-50.7328855645153,36.4671473482232,39.6398955068274));
#205513=CARTESIAN_POINT('Origin',(-50.5887599058098,36.3624339277678,39.3548010137695));
#205514=CARTESIAN_POINT('Ctrl Pts',(-47.6338034047597,34.9997217530264,
39.8576902534424));
#205515=CARTESIAN_POINT('Ctrl Pts',(-47.7085070967801,34.8977303031706,
39.8579948730704));
#205516=CARTESIAN_POINT('Ctrl Pts',(-47.7952442955499,34.960748566837,39.92499));
#205517=CARTESIAN_POINT('Ctrl Pts',(-47.597045191607,34.9730146904941,39.9304020711231));
#205518=CARTESIAN_POINT('Ctrl Pts',(-47.675296659073,34.8923835282623,39.9058915297375));
#205519=CARTESIAN_POINT('Ctrl Pts',(-47.7584842465943,34.9340408279391,
39.9671523786028));
#205520=CARTESIAN_POINT('Ctrl Pts',(-47.5754322771533,34.9244461536127,
40.0043257306693));
#205521=CARTESIAN_POINT('Ctrl Pts',(-47.6469756149924,34.8665972787026,
39.9667894847838));
#205522=CARTESIAN_POINT('Ctrl Pts',(-47.7303228514092,34.8944891948627,
40.0100138975202));
#205523=CARTESIAN_POINT('Ctrl Pts',(-47.5794993790982,34.7970725085261,
40.1195533054857));
#205524=CARTESIAN_POINT('Ctrl Pts',(-47.635319763777,34.7804938560726,40.0630813209234));
#205525=CARTESIAN_POINT('Ctrl Pts',(-47.708416089387,34.8028668197837,40.0768265942419));
#205526=CARTESIAN_POINT('Ctrl Pts',(-47.6073089936885,34.7162617467345,
40.1599502027516));
#205527=CARTESIAN_POINT('Ctrl Pts',(-47.651501311427,34.7189078610141,40.1002552791553));
#205528=CARTESIAN_POINT('Ctrl Pts',(-47.7160937685338,34.7497660430534,
40.10025));
#205529=CARTESIAN_POINT('Ctrl Pts',(-47.6590285860933,34.645114416419,40.1599502534424));
#205530=CARTESIAN_POINT('Ctrl Pts',(-47.689203188551,34.6670494534022,40.10025));
#205531=CARTESIAN_POINT('Ctrl Pts',(-47.7461450747862,34.7084426211235,
40.10025));
#205532=CARTESIAN_POINT('Origin',(-47.7461450747862,34.7084426211235,40.22725));
#205533=CARTESIAN_POINT('Ctrl Pts',(-50.240224004808,36.1092077731533,38.989));
#205534=CARTESIAN_POINT('Ctrl Pts',(-50.1654637495897,36.2121064368056,
38.989));
#205535=CARTESIAN_POINT('Ctrl Pts',(-50.1655753609562,36.2119528169385,
39.1161896013264));
#205536=CARTESIAN_POINT('Ctrl Pts',(-50.4158927445024,36.2365633238561,
38.989));
#205537=CARTESIAN_POINT('Ctrl Pts',(-50.3411519064795,36.339751970454,38.988776927543));
#205538=CARTESIAN_POINT('Ctrl Pts',(-50.3059538820317,36.3139437822118,
39.1161898821846));
#205539=CARTESIAN_POINT('Ctrl Pts',(-50.5831252836573,36.3578055460614,
39.1034967087244));
#205540=CARTESIAN_POINT('Ctrl Pts',(-50.5083605190661,36.4612367259627,
39.1031720232725));
#205541=CARTESIAN_POINT('Ctrl Pts',(-50.4395918165607,36.4110374247131,
39.2077529615003));
#205542=CARTESIAN_POINT('Ctrl Pts',(-50.6762142289945,36.4252947698683,
39.2875012672119));
#205543=CARTESIAN_POINT('Ctrl Pts',(-50.6015093986314,36.5289136700281,
39.2872087095508));
#205544=CARTESIAN_POINT('Ctrl Pts',(-50.5139808995221,36.4650842569438,
39.3549017048227));
#205545=CARTESIAN_POINT('Origin',(-50.240224004808,36.1092077731533,39.116));
#205546=CARTESIAN_POINT('Origin',(3.64514313700083E-16,3.44778646538036E-17,
40.22725));
#205547=CARTESIAN_POINT('Origin',(-47.764060769276,34.683783783135,40.22725));
#205548=CARTESIAN_POINT('Origin',(40.5385041740525,-29.8453988870287,39.116));
#205549=CARTESIAN_POINT('Origin',(-49.9155525184323,35.8732562382991,39.1160373285273));
#205550=CARTESIAN_POINT('Ctrl Pts',(-47.6769115920301,34.6205005703638,
40.1599502534424));
#205551=CARTESIAN_POINT('Ctrl Pts',(-47.7070975168461,34.6424200234579,
40.10025));
#205552=CARTESIAN_POINT('Ctrl Pts',(-47.764060769276,34.683783783135,40.10025));
#205553=CARTESIAN_POINT('Ctrl Pts',(-47.7284183483602,34.5495693076633,
40.1599500566042));
#205554=CARTESIAN_POINT('Ctrl Pts',(-47.7446195594519,34.5907418558602,
40.100255130536));
#205555=CARTESIAN_POINT('Ctrl Pts',(-47.7939730310155,34.6425747206417,
40.10025));
#205556=CARTESIAN_POINT('Ctrl Pts',(-47.7959261043552,34.498391065477,40.1203070619046));
#205557=CARTESIAN_POINT('Ctrl Pts',(-47.7976714756521,34.556369822828,40.0637098684497));
#205558=CARTESIAN_POINT('Ctrl Pts',(-47.8415056181568,34.6188891978604,
40.0772636213363));
#205559=CARTESIAN_POINT('Ctrl Pts',(-47.9165880269726,34.4545839152295,
40.0046102245802));
#205560=CARTESIAN_POINT('Ctrl Pts',(-47.8837591046483,34.54046851239,39.9670001894016));
#205561=CARTESIAN_POINT('Ctrl Pts',(-47.9359643384879,34.6111463389768,
40.0101788811209));
#205562=CARTESIAN_POINT('Ctrl Pts',(-47.9696250311905,34.4602354682514,
39.9303710930186));
#205563=CARTESIAN_POINT('Ctrl Pts',(-47.9171136764619,34.5595777906768,
39.9058663574108));
#205564=CARTESIAN_POINT('Ctrl Pts',(-47.982446041048,34.6258166968307,39.9671344706366));
#205565=CARTESIAN_POINT('Ctrl Pts',(-48.0063682005184,34.4869303039401,
39.8576902534424));
#205566=CARTESIAN_POINT('Ctrl Pts',(-47.9324532779035,34.5894948283137,
39.8579948730703));
#205567=CARTESIAN_POINT('Ctrl Pts',(-48.0191904766733,34.6525130919801,
39.92499));
#205568=CARTESIAN_POINT('Origin',(-48.0938392037145,34.5497679336945,39.92499));
#205569=CARTESIAN_POINT('Origin',(-49.8797426632439,35.8473027479618,39.1925554488847));
#205570=CARTESIAN_POINT('Origin',(-49.813534060122,35.7991993820666,39.3343017080178));
#205571=CARTESIAN_POINT('Origin',(-48.2379650606559,34.6544814981802,39.6398955069217));
#205572=CARTESIAN_POINT('Origin',(-48.3820909175326,34.7591950625538,39.3548010137695));
#205573=CARTESIAN_POINT('Ctrl Pts',(-49.5465907136142,35.6052536882606,
39.3978017080178));
#205574=CARTESIAN_POINT('Ctrl Pts',(-49.471941986573,35.7079988465462,39.3978017080178));
#205575=CARTESIAN_POINT('Ctrl Pts',(-49.471941986573,35.7079988465462,39.5248017080178));
#205576=CARTESIAN_POINT('Ctrl Pts',(-49.6192730640965,35.6583499840564,
39.3978017080178));
#205577=CARTESIAN_POINT('Ctrl Pts',(-49.5446936074929,35.7608559931221,
39.3980355775182));
#205578=CARTESIAN_POINT('Ctrl Pts',(-49.5811706590224,35.7873581223583,
39.5248015517192));
#205579=CARTESIAN_POINT('Ctrl Pts',(-49.6880007749199,35.7085550527711,
39.3484893995498));
#205580=CARTESIAN_POINT('Ctrl Pts',(-49.6138288703648,35.8110857017878,
39.3489438303412));
#205581=CARTESIAN_POINT('Ctrl Pts',(-49.6844541394787,35.8623979633502,
39.4508333155589));
#205582=CARTESIAN_POINT('Ctrl Pts',(-49.7242207306172,35.7350130971393,
39.2708017080178));
#205583=CARTESIAN_POINT('Ctrl Pts',(-49.6503036646782,35.8375861910561,
39.2710850691866));
#205584=CARTESIAN_POINT('Ctrl Pts',(-49.7388853330808,35.9019445403522,
39.3343017080178));
#205585=CARTESIAN_POINT('Origin',(-49.5465907136142,35.6052536882606,39.5248017080178));
#205586=CARTESIAN_POINT('Ctrl Pts',(-48.2946219293743,34.6963546279289,
39.2875012672119));
#205587=CARTESIAN_POINT('Ctrl Pts',(-48.2205921526132,34.7990735298992,
39.2878045257519));
#205588=CARTESIAN_POINT('Ctrl Pts',(-48.3075723994626,34.8620346481363,
39.3549015218348));
#205589=CARTESIAN_POINT('Ctrl Pts',(-48.3877165307502,34.7638392294012,
39.1034938540228));
#205590=CARTESIAN_POINT('Ctrl Pts',(-48.3134813154478,34.8665617960639,
39.1038286278799));
#205591=CARTESIAN_POINT('Ctrl Pts',(-48.3819628268478,34.9160824571373,
39.2077506434029));
#205592=CARTESIAN_POINT('Ctrl Pts',(-48.5549570506144,34.8850734745857,
38.989));
#205593=CARTESIAN_POINT('Ctrl Pts',(-48.480486117147,34.9878985031432,38.9892298954618));
#205594=CARTESIAN_POINT('Ctrl Pts',(-48.5156018845779,35.0131769156751,
39.1161900347291));
#205595=CARTESIAN_POINT('Ctrl Pts',(-48.7306271754173,35.0124214764589,
38.989));
#205596=CARTESIAN_POINT('Ctrl Pts',(-48.6558666298464,35.1153205397472,
38.989));
#205597=CARTESIAN_POINT('Ctrl Pts',(-48.655978531999,35.1151665196476,39.1161900945647));
#205598=CARTESIAN_POINT('Origin',(-48.7306271754173,35.0124214764589,39.116));
#205599=CARTESIAN_POINT('Origin',(39.5520252162584,-29.1286799712089,39.5248017080178));
#205600=CARTESIAN_POINT('Origin',(-49.4242607783458,35.51637578784,39.5248017080178));
#205601=CARTESIAN_POINT('Origin',(39.3975469582344,-29.0164449471022,39.116));
#205602=CARTESIAN_POINT('Origin',(-49.0553654007523,35.2482948100397,39.1160402713849));
#205603=CARTESIAN_POINT('Ctrl Pts',(-49.246635155601,35.3866101428264,39.2708017080178));
#205604=CARTESIAN_POINT('Ctrl Pts',(-49.1720533660028,35.4901170100371,
39.27051194648));
#205605=CARTESIAN_POINT('Ctrl Pts',(-49.0826686475732,35.4251752107442,
39.3343017080178));
#205606=CARTESIAN_POINT('Ctrl Pts',(-49.2829758776396,35.4131599099222,
39.3487519301186));
#205607=CARTESIAN_POINT('Ctrl Pts',(-49.2082707697373,35.5164304941041,
39.3482879463997));
#205608=CARTESIAN_POINT('Ctrl Pts',(-49.1372837917323,35.4648554356489,
39.4512271261641));
#205609=CARTESIAN_POINT('Ctrl Pts',(-49.3518235761942,35.4634578610125,
39.3978017080178));
#205610=CARTESIAN_POINT('Ctrl Pts',(-49.276967346883,35.5663414789297,39.3975673827387));
#205611=CARTESIAN_POINT('Ctrl Pts',(-49.2407512920142,35.5400289748701,
39.5248015355181));
#205612=CARTESIAN_POINT('Ctrl Pts',(-49.4242607783458,35.51637578784,39.3978017080178));
#205613=CARTESIAN_POINT('Ctrl Pts',(-49.3496120513046,35.6191209461256,
39.3978017080178));
#205614=CARTESIAN_POINT('Ctrl Pts',(-49.3496120513046,35.6191209461256,
39.5248017080178));
#205615=CARTESIAN_POINT('Origin',(-49.1573173746143,35.3224300524586,39.3343017080178));
#205616=CARTESIAN_POINT('Origin',(-49.0915036263502,35.2746135650466,39.1934008533551));
#205617=CARTESIAN_POINT('Origin',(-45.4345348113613,41.3366772861953,39.1925554495078));
#205618=CARTESIAN_POINT('Origin',(-45.4673664422111,41.3663085755596,39.1160373285232));
#205619=CARTESIAN_POINT('Origin',(-45.3737170758069,41.2819167515332,39.3343017080178));
#205620=CARTESIAN_POINT('Ctrl Pts',(-45.2923641298554,41.2079002115911,
39.2708017080178));
#205621=CARTESIAN_POINT('Ctrl Pts',(-45.3773275334102,41.114272265501,39.2710850691866));
#205622=CARTESIAN_POINT('Ctrl Pts',(-45.4586966628145,41.1875373586976,
39.3343017080178));
#205623=CARTESIAN_POINT('Ctrl Pts',(-45.2588408013008,41.1778715515047,
39.3487519293518));
#205624=CARTESIAN_POINT('Ctrl Pts',(-45.3437094247727,41.0840023845234,
39.3492068662929));
#205625=CARTESIAN_POINT('Ctrl Pts',(-45.4085284377449,41.1423656859497,
39.4512271248738));
#205626=CARTESIAN_POINT('Ctrl Pts',(-45.1953306044444,41.1209827764383,
39.3978017080178));
#205627=CARTESIAN_POINT('Ctrl Pts',(-45.280091264719,41.0267203359225,39.3980347781178));
#205628=CARTESIAN_POINT('Ctrl Pts',(-45.3134855411615,41.0567886774842,
39.5248015355195));
#205629=CARTESIAN_POINT('Ctrl Pts',(-45.1285089182129,41.0611303347408,
39.3978017080178));
#205630=CARTESIAN_POINT('Ctrl Pts',(-45.2134885052205,40.9667509419051,
39.3978017080178));
#205631=CARTESIAN_POINT('Ctrl Pts',(-45.2134885052205,40.9667509419051,
39.5248017080178));
#205632=CARTESIAN_POINT('Origin',(-45.1285089182129,41.0611303347408,39.5248017080178));
#205633=CARTESIAN_POINT('Origin',(0.212448967518945,0.235948482089071,39.116));
#205634=CARTESIAN_POINT('Origin',(-45.7656648676103,41.6348281284266,39.116));
#205635=CARTESIAN_POINT('Origin',(0.212448967518945,0.235948482089071,39.5248017080178));
#205636=CARTESIAN_POINT('Origin',(-45.016139389479,40.9599523566129,39.5248017080178));
#205637=CARTESIAN_POINT('Ctrl Pts',(-46.1654920697608,41.9955727382255,
39.2875012672119));
#205638=CARTESIAN_POINT('Ctrl Pts',(-46.2513146333399,41.9009568150788,
39.287208709576));
#205639=CARTESIAN_POINT('Ctrl Pts',(-46.1706818621619,41.8286119029183,
39.354901699012));
#205640=CARTESIAN_POINT('Ctrl Pts',(-46.0801220723621,41.9185486398925,
39.1034939173931));
#205641=CARTESIAN_POINT('Ctrl Pts',(-46.1657485549033,41.8239131221199,
39.1031692336338));
#205642=CARTESIAN_POINT('Ctrl Pts',(-46.1023486848284,41.7670844335132,
39.2077507202299));
#205643=CARTESIAN_POINT('Ctrl Pts',(-45.9267584721682,41.7801771152764,
38.989));
#205644=CARTESIAN_POINT('Ctrl Pts',(-46.0121526898595,41.6856154234958,
38.9887769311176));
#205645=CARTESIAN_POINT('Ctrl Pts',(-45.9795909100378,41.6565528363084,
39.1161898712912));
#205646=CARTESIAN_POINT('Ctrl Pts',(-45.7656648676103,41.6348281284266,
38.989));
#205647=CARTESIAN_POINT('Ctrl Pts',(-45.8507714101799,41.5403077371549,
38.989));
#205648=CARTESIAN_POINT('Ctrl Pts',(-45.8506443599266,41.5404488407563,
39.1161895903851));
#205649=CARTESIAN_POINT('Origin',(-46.0858221116775,41.9230990057959,39.3548010137695));
#205650=CARTESIAN_POINT('Ctrl Pts',(-45.016139389479,40.9599523566129,39.3978017080178));
#205651=CARTESIAN_POINT('Ctrl Pts',(-45.1011189764865,40.8655729637772,
39.3978017080178));
#205652=CARTESIAN_POINT('Ctrl Pts',(-45.1011189764865,40.8655729637772,
39.5248017080178));
#205653=CARTESIAN_POINT('Ctrl Pts',(-44.9490914662995,40.8998980546771,
39.3978017080178));
#205654=CARTESIAN_POINT('Ctrl Pts',(-45.0341638030233,40.8052862548047,
39.3975666025003));
#205655=CARTESIAN_POINT('Ctrl Pts',(-45.0007839642914,40.7752309130121,
39.5248015517178));
#205656=CARTESIAN_POINT('Ctrl Pts',(-44.885691333944,40.8431135311197,39.3484894016716));
#205657=CARTESIAN_POINT('Ctrl Pts',(-44.9711739722005,40.7485699563835,
39.3480259000058));
#205658=CARTESIAN_POINT('Ctrl Pts',(-44.9059100567345,40.6898060629495,
39.4508333188946));
#205659=CARTESIAN_POINT('Ctrl Pts',(-44.8522789915938,40.813188074561,39.2708017080178));
#205660=CARTESIAN_POINT('Ctrl Pts',(-44.9380175594359,40.7187157882341,
39.27051194648));
#205661=CARTESIAN_POINT('Ctrl Pts',(-44.8559107663282,40.6447864996556,
39.3343017080178));
#205662=CARTESIAN_POINT('Origin',(-44.7709311793206,40.7391658924913,39.3343017080178));
#205663=CARTESIAN_POINT('Origin',(-46.2182127020652,42.0423040287734,39.6398955068177));
#205664=CARTESIAN_POINT('Origin',(-46.3506032922591,42.1615090516456,39.92499));
#205665=CARTESIAN_POINT('Origin',(-44.7104761485858,40.684731938309,39.193400853994));
#205666=CARTESIAN_POINT('Origin',(-44.6772189625514,40.6548553974684,39.1160402713846));
#205667=CARTESIAN_POINT('Ctrl Pts',(-46.7738319284254,42.1358900227699,
40.1599502534424));
#205668=CARTESIAN_POINT('Ctrl Pts',(-46.7461150696869,42.1109214781065,
40.10025));
#205669=CARTESIAN_POINT('Ctrl Pts',(-46.6938111422601,42.0638038389704,
40.10025));
#205670=CARTESIAN_POINT('Ctrl Pts',(-46.714855253764,42.2013581359417,40.1599500538471));
#205671=CARTESIAN_POINT('Ctrl Pts',(-46.7031532960251,42.1586072771723,
40.1002448353478));
#205672=CARTESIAN_POINT('Ctrl Pts',(-46.6596664560547,42.1016932886526,
40.10025));
#205673=CARTESIAN_POINT('Ctrl Pts',(-46.6418481388114,42.245024972543,40.1202442001042));
#205674=CARTESIAN_POINT('Ctrl Pts',(-46.6464039985657,42.1870455286632,
40.0633873868017));
#205675=CARTESIAN_POINT('Ctrl Pts',(-46.609571404849,42.1199142759251,40.0772271723538));
#205676=CARTESIAN_POINT('Ctrl Pts',(-46.5164783566522,42.275663213985,40.0045995998159));
#205677=CARTESIAN_POINT('Ctrl Pts',(-46.5588531737047,42.1934768724834,
39.9663485808314));
#205678=CARTESIAN_POINT('Ctrl Pts',(-46.5142596423495,42.1171707421506,
40.0101727202466));
#205679=CARTESIAN_POINT('Ctrl Pts',(-46.4640705998041,42.2644092166196,
39.9304654349861));
#205680=CARTESIAN_POINT('Ctrl Pts',(-46.5278411618548,42.1708301402928,
39.9051900162966));
#205681=CARTESIAN_POINT('Ctrl Pts',(-46.4693765057993,42.0975575768115,
39.9671857458179));
#205682=CARTESIAN_POINT('Ctrl Pts',(-46.4302753505421,42.2339804752705,
39.8576902534424));
#205683=CARTESIAN_POINT('Ctrl Pts',(-46.5159655405271,42.1395065321003,
39.8573998014387));
#205684=CARTESIAN_POINT('Ctrl Pts',(-46.4355828792667,42.06712965881,39.92499));
#205685=CARTESIAN_POINT('Origin',(-46.6938111422601,42.0638038389704,40.22725));
#205686=CARTESIAN_POINT('Origin',(0.212448967518945,0.235948482089071,39.116));
#205687=CARTESIAN_POINT('Origin',(-44.3789831537292,40.3862543050942,39.116));
#205688=CARTESIAN_POINT('Origin',(9.23291810287646E-17,-1.10332673220368E-16,
40.22725));
#205689=CARTESIAN_POINT('Origin',(-46.7142062431419,42.0411527846899,40.22725));
#205690=CARTESIAN_POINT('Ctrl Pts',(-44.3789831537292,40.3862543050942,
38.989));
#205691=CARTESIAN_POINT('Ctrl Pts',(-44.4640900439955,40.2917335276662,
38.989));
#205692=CARTESIAN_POINT('Ctrl Pts',(-44.4639626455265,40.2918750180003,
39.1161901092322));
#205693=CARTESIAN_POINT('Ctrl Pts',(-44.2178916378592,40.2408978759468,
38.989));
#205694=CARTESIAN_POINT('Ctrl Pts',(-44.3029863283978,40.1466757825274,
38.9892298989754));
#205695=CARTESIAN_POINT('Ctrl Pts',(-44.3350138149328,40.1757689690803,
39.1161900493202));
#205696=CARTESIAN_POINT('Ctrl Pts',(-44.0645366033547,40.1025190720979,
39.1034966344368));
#205697=CARTESIAN_POINT('Ctrl Pts',(-44.1495800756942,40.0085488431148,
39.1038314102563));
#205698=CARTESIAN_POINT('Ctrl Pts',(-44.2122569536148,40.0652381943514,
39.20775287896));
#205699=CARTESIAN_POINT('Ctrl Pts',(-43.9791725362579,40.0254908126592,
39.2875012672119));
#205700=CARTESIAN_POINT('Ctrl Pts',(-44.0642551375171,39.9317222927448,
39.2878045257868));
#205701=CARTESIAN_POINT('Ctrl Pts',(-44.1439246138545,40.0037114790889,
39.3549015295899));
#205702=CARTESIAN_POINT('Origin',(-44.0588255818374,40.0979831325503,39.3548010137695));
#205703=CARTESIAN_POINT('Ctrl Pts',(-46.8559036426982,41.7612723673367,
39.8576902534424));
#205704=CARTESIAN_POINT('Ctrl Pts',(-46.7709043015499,41.8563683535934,
39.8573998014387));
#205705=CARTESIAN_POINT('Ctrl Pts',(-46.6905216402894,41.7839914803031,
39.92499));
#205706=CARTESIAN_POINT('Ctrl Pts',(-46.8897135983598,41.7917156448197,
39.9304984902488));
#205707=CARTESIAN_POINT('Ctrl Pts',(-46.8033160448216,41.8649095672156,
39.9052171569791));
#205708=CARTESIAN_POINT('Ctrl Pts',(-46.7243306652211,41.8144332630853,
39.9672049726598));
#205709=CARTESIAN_POINT('Ctrl Pts',(-46.9062450310964,41.8425440045886,
40.0043437678665));
#205710=CARTESIAN_POINT('Ctrl Pts',(-46.8289264627112,41.8933569085961,
39.9661628577649));
#205711=CARTESIAN_POINT('Ctrl Pts',(-46.7483907976682,41.8569022891479,
40.0100243556237));
#205712=CARTESIAN_POINT('Ctrl Pts',(-46.8892773184515,41.9695156381233,
40.1194874821984));
#205713=CARTESIAN_POINT('Ctrl Pts',(-46.8319191778356,41.9804178820375,
40.0627551483134));
#205714=CARTESIAN_POINT('Ctrl Pts',(-46.7612136652285,41.9507871007485,
40.0767884282375));
#205715=CARTESIAN_POINT('Ctrl Pts',(-46.8534019544973,42.0474864684051,
40.1599502015382));
#205716=CARTESIAN_POINT('Ctrl Pts',(-46.8096319157665,42.0403508033695,
40.1002449453869));
#205717=CARTESIAN_POINT('Ctrl Pts',(-46.7484320121836,42.003109184299,40.10025));
#205718=CARTESIAN_POINT('Ctrl Pts',(-46.7942619810913,42.1132001506005,
40.1599502534424));
#205719=CARTESIAN_POINT('Ctrl Pts',(-46.7665330160776,42.0882450513179,
40.10025));
#205720=CARTESIAN_POINT('Ctrl Pts',(-46.7142062431419,42.0411527846899,
40.10025));
#205721=CARTESIAN_POINT('Origin',(-46.7755012272969,41.6896120874674,39.92499));
#205722=CARTESIAN_POINT('Origin',(-43.9264348094991,39.9787779456715,39.6398955069307));
#205723=CARTESIAN_POINT('Origin',(-43.7940440370141,39.8595727587359,39.92499));
#205724=CARTESIAN_POINT('Origin',(-46.6431106370596,41.5704070646253,39.6398955068254));
#205725=CARTESIAN_POINT('Origin',(-46.5107200467153,41.4512020416178,39.3548010137695));
#205726=CARTESIAN_POINT('Ctrl Pts',(-43.714393316062,39.7870778846751,39.8576902534424));
#205727=CARTESIAN_POINT('Ctrl Pts',(-43.799348782961,39.6934538167804,39.8579948730704));
#205728=CARTESIAN_POINT('Ctrl Pts',(-43.8790236240217,39.7651933659002,
39.92499));
#205729=CARTESIAN_POINT('Ctrl Pts',(-43.6806281164518,39.7566748466926,
39.9304020711229));
#205730=CARTESIAN_POINT('Ctrl Pts',(-43.7668791656724,39.6846648960486,
39.9058915297384));
#205731=CARTESIAN_POINT('Ctrl Pts',(-43.8452566693655,39.7347894633642,
39.9671523786037));
#205732=CARTESIAN_POINT('Ctrl Pts',(-43.6642103943284,39.7061132086031,
40.0043257306695));
#205733=CARTESIAN_POINT('Ctrl Pts',(-43.7414086642728,39.656059551044,39.9667894847838));
#205734=CARTESIAN_POINT('Ctrl Pts',(-43.8213838166742,39.6925108309093,
40.01001389752));
#205735=CARTESIAN_POINT('Ctrl Pts',(-43.681569387645,39.5798624575882,40.1195533054856));
#205736=CARTESIAN_POINT('Ctrl Pts',(-43.7388169234803,39.569209443757,40.0630813209234));
#205737=CARTESIAN_POINT('Ctrl Pts',(-43.8091742082548,39.5991004926183,
40.076826594242));
#205738=CARTESIAN_POINT('Ctrl Pts',(-43.7176736830024,39.502401281882,40.1599502027517));
#205739=CARTESIAN_POINT('Ctrl Pts',(-43.7613473163384,39.50965225553,40.1002552791541));
#205740=CARTESIAN_POINT('Ctrl Pts',(-43.8223603708606,39.5470931435009,
40.10025));
#205741=CARTESIAN_POINT('Ctrl Pts',(-43.7765468711719,39.4370498736012,
40.1599502534424));
#205742=CARTESIAN_POINT('Ctrl Pts',(-43.8042633382926,39.4620188529813,
40.10025));
#205743=CARTESIAN_POINT('Ctrl Pts',(-43.8565665267053,39.5091373124626,
40.10025));
#205744=CARTESIAN_POINT('Origin',(-43.8565665267053,39.5091373124626,40.22725));
#205745=CARTESIAN_POINT('Ctrl Pts',(-46.1905628026481,41.1629311642484,
38.989));
#205746=CARTESIAN_POINT('Ctrl Pts',(-46.1054562527463,41.2574515636633,
38.989));
#205747=CARTESIAN_POINT('Ctrl Pts',(-46.1055833103428,41.2573104519066,
39.1161896013265));
#205748=CARTESIAN_POINT('Ctrl Pts',(-46.3519569306006,41.3079514313256,
38.989));
#205749=CARTESIAN_POINT('Ctrl Pts',(-46.2668393800556,41.4027622547787,
38.988776927546));
#205750=CARTESIAN_POINT('Ctrl Pts',(-46.2345318643238,41.3734162510838,
39.1161898821846));
#205751=CARTESIAN_POINT('Ctrl Pts',(-46.5056000892403,41.4460100362752,
39.1034967087244));
#205752=CARTESIAN_POINT('Ctrl Pts',(-46.420433391565,41.541059563396,39.103172023271));
#205753=CARTESIAN_POINT('Ctrl Pts',(-46.3572886670226,41.4839469723845,
39.2077529615));
#205754=CARTESIAN_POINT('Ctrl Pts',(-46.5911245387426,41.5228599914567,
39.2875012672119));
#205755=CARTESIAN_POINT('Ctrl Pts',(-46.5059978248576,41.6181024753231,
39.2872087095508));
#205756=CARTESIAN_POINT('Ctrl Pts',(-46.4256208064857,41.5454735069382,
39.3549017048227));
#205757=CARTESIAN_POINT('Origin',(-46.1905628026481,41.1629311642484,39.116));
#205758=CARTESIAN_POINT('Origin',(3.68378193773366E-16,3.92493591694927E-17,
40.22725));
#205759=CARTESIAN_POINT('Origin',(-43.8769616275871,39.486486258182,40.22725));
#205760=CARTESIAN_POINT('Origin',(34.1507877370002,-31.1767457860026,39.116));
#205761=CARTESIAN_POINT('Origin',(-45.892333551989,40.8943347850521,39.1160373285266));
#205762=CARTESIAN_POINT('Ctrl Pts',(-43.7969047596343,39.4144401478993,
40.1599502534424));
#205763=CARTESIAN_POINT('Ctrl Pts',(-43.8246341160482,39.4393948122691,
40.10025));
#205764=CARTESIAN_POINT('Ctrl Pts',(-43.8769616275871,39.486486258182,40.10025));
#205765=CARTESIAN_POINT('Ctrl Pts',(-43.8555436924522,39.3492813761649,
40.1599500566032));
#205766=CARTESIAN_POINT('Ctrl Pts',(-43.8673524484236,39.3919218645342,
40.1002551305372));
#205767=CARTESIAN_POINT('Ctrl Pts',(-43.9110175468025,39.4486296259977,
40.10025));
#205768=CARTESIAN_POINT('Ctrl Pts',(-43.9280312169043,39.3054399757369,
40.1203070619046));
#205769=CARTESIAN_POINT('Ctrl Pts',(-43.9237065964667,39.3632835603681,
40.0637098684499));
#205770=CARTESIAN_POINT('Ctrl Pts',(-43.9607655567554,39.430042363277,40.0772636213363));
#205771=CARTESIAN_POINT('Ctrl Pts',(-44.0526112349802,39.2744854109879,
40.0046102245802));
#205772=CARTESIAN_POINT('Ctrl Pts',(-44.0109847679678,39.3564679665376,
39.9670001894012));
#205773=CARTESIAN_POINT('Ctrl Pts',(-44.0555161714742,39.4322155454632,
40.0101788811209));
#205774=CARTESIAN_POINT('Ctrl Pts',(-44.1047669487885,39.2856498807568,
39.9303710930186));
#205775=CARTESIAN_POINT('Ctrl Pts',(-44.0421591564523,39.3789590643314,
39.9058663574094));
#205776=CARTESIAN_POINT('Ctrl Pts',(-44.1002097724411,39.4516641984998,
39.967134470636));
#205777=CARTESIAN_POINT('Ctrl Pts',(-44.1385184650372,39.3160391863694,
39.8576902534424));
#205778=CARTESIAN_POINT('Ctrl Pts',(-44.0542875439837,39.4103156382735,
39.8579948730703));
#205779=CARTESIAN_POINT('Ctrl Pts',(-44.1339623850444,39.4820551873934,
39.92499));
#205780=CARTESIAN_POINT('Origin',(-44.218941972052,39.3876757945577,39.92499));
#205781=CARTESIAN_POINT('Origin',(-45.8594327453955,40.8647803215178,39.1925554488843));
#205782=CARTESIAN_POINT('Origin',(-45.7986150108448,40.8100197873551,39.3343017080178));
#205783=CARTESIAN_POINT('Origin',(-44.3513327444881,39.5068809815262,39.6398955069218));
#205784=CARTESIAN_POINT('Origin',(-44.4837235168753,39.6260861683721,39.3548010137695));
#205785=CARTESIAN_POINT('Ctrl Pts',(-45.5534068532508,40.5892333705626,
39.3978017080178));
#205786=CARTESIAN_POINT('Ctrl Pts',(-45.4684272662432,40.6836127633983,
39.3978017080178));
#205787=CARTESIAN_POINT('Ctrl Pts',(-45.4684272662432,40.6836127633983,
39.5248017080178));
#205788=CARTESIAN_POINT('Ctrl Pts',(-45.6201409680064,40.6496361736984,
39.3978017080178));
#205789=CARTESIAN_POINT('Ctrl Pts',(-45.5352552698605,40.7437849681284,
39.3980355775196));
#205790=CARTESIAN_POINT('Ctrl Pts',(-45.5687622694472,40.7739548060677,
39.5248015517192));
#205791=CARTESIAN_POINT('Ctrl Pts',(-45.6832443225586,40.7067502157891,
39.3484893995498));
#205792=CARTESIAN_POINT('Ctrl Pts',(-45.5987613682854,40.800966115985,39.3489438303422));
#205793=CARTESIAN_POINT('Ctrl Pts',(-45.6636361529334,40.859379634457,39.45083331556));
#205794=CARTESIAN_POINT('Ctrl Pts',(-45.7165002428303,40.7368493365301,
39.2708017080178));
#205795=CARTESIAN_POINT('Ctrl Pts',(-45.6322662944329,40.8311340869941,
39.2710850691866));
#205796=CARTESIAN_POINT('Ctrl Pts',(-45.7136354238372,40.9043991801907,
39.3343017080178));
#205797=CARTESIAN_POINT('Origin',(-45.5534068532508,40.5892333705626,39.5248017080178));
#205798=CARTESIAN_POINT('Ctrl Pts',(-44.4033023070486,39.5544469813075,
39.2875012672119));
#205799=CARTESIAN_POINT('Ctrl Pts',(-44.3189410241787,39.6488649595845,
39.2878045257519));
#205800=CARTESIAN_POINT('Ctrl Pts',(-44.3988635552005,39.7205730817659,
39.3549015218351));
#205801=CARTESIAN_POINT('Ctrl Pts',(-44.4888328647704,39.6312929306932,
39.1034938540228));
#205802=CARTESIAN_POINT('Ctrl Pts',(-44.4042668857084,39.7256930794085,
39.1038286278778));
#205803=CARTESIAN_POINT('Ctrl Pts',(-44.4671969296207,39.7821007282684,
39.2077506434024));
#205804=CARTESIAN_POINT('Ctrl Pts',(-44.6424847942264,39.769344436532,38.989));
#205805=CARTESIAN_POINT('Ctrl Pts',(-44.5576736781015,39.8638218465963,
38.9892298954636));
#205806=CARTESIAN_POINT('Ctrl Pts',(-44.5899547640708,39.8926323785438,
39.1161900347295));
#205807=CARTESIAN_POINT('Ctrl Pts',(-44.8038810887671,39.9143573409161,
38.989));
#205808=CARTESIAN_POINT('Ctrl Pts',(-44.7187742083296,40.0088781074279,
38.989));
#205809=CARTESIAN_POINT('Ctrl Pts',(-44.7189015969551,40.0087366280263,
39.1161900945652));
#205810=CARTESIAN_POINT('Origin',(-44.8038810887671,39.9143573409161,39.116));
#205811=CARTESIAN_POINT('Origin',(33.3184119221863,-30.4272712359684,39.5248017080178));
#205812=CARTESIAN_POINT('Origin',(-45.4410373245168,40.4880553924347,39.5248017080178));
#205813=CARTESIAN_POINT('Origin',(33.1880655373213,-30.3099068238764,39.116));
#205814=CARTESIAN_POINT('Origin',(-45.1021848870407,40.1828829233541,39.1160402713851));
#205815=CARTESIAN_POINT('Ctrl Pts',(-45.2779489569769,40.3404336838196,
39.2708017080178));
#205816=CARTESIAN_POINT('Ctrl Pts',(-45.1929563204586,40.4355776097272,
39.2705119464801));
#205817=CARTESIAN_POINT('Ctrl Pts',(-45.1108495273509,40.3616483211487,
39.3343017080178));
#205818=CARTESIAN_POINT('Ctrl Pts',(-45.3113153943826,40.3706366483427,
39.3487519301185));
#205819=CARTESIAN_POINT('Ctrl Pts',(-45.2262248134191,40.4655326953387,
39.3482879463977));
#205820=CARTESIAN_POINT('Ctrl Pts',(-45.1610177711094,40.4068200107242,
39.4512271261624));
#205821=CARTESIAN_POINT('Ctrl Pts',(-45.3745283705082,40.4278556061232,
39.3978017080178));
#205822=CARTESIAN_POINT('Ctrl Pts',(-45.2893279449732,40.5223510101947,
39.3975673827383));
#205823=CARTESIAN_POINT('Ctrl Pts',(-45.2560606910569,40.4923970402268,
39.5248015355181));
#205824=CARTESIAN_POINT('Ctrl Pts',(-45.4410373245168,40.4880553924347,
39.3978017080178));
#205825=CARTESIAN_POINT('Ctrl Pts',(-45.3560577375092,40.5824347852704,
39.3978017080178));
#205826=CARTESIAN_POINT('Ctrl Pts',(-45.3560577375093,40.5824347852704,
39.5248017080178));
#205827=CARTESIAN_POINT('Origin',(-45.1958291143585,40.2672689283131,39.3343017080178));
#205828=CARTESIAN_POINT('Origin',(-45.1353740846424,40.2128349746537,39.193400853355));
#205829=CARTESIAN_POINT('Origin',(-40.8647803224532,45.8594327460079,39.1925554495084));
#205830=CARTESIAN_POINT('Origin',(-40.8943347850518,45.8923335519894,39.1160373285266));
#205831=CARTESIAN_POINT('Origin',(-40.8100197873543,45.7986150108455,39.3343017080178));
#205832=CARTESIAN_POINT('Ctrl Pts',(-40.7368493365293,45.716500242831,39.2708017080178));
#205833=CARTESIAN_POINT('Ctrl Pts',(-40.8311340869933,45.6322662944336,
39.2710850691866));
#205834=CARTESIAN_POINT('Ctrl Pts',(-40.9043991801899,45.7136354238379,
39.3343017080178));
#205835=CARTESIAN_POINT('Ctrl Pts',(-40.7066485019697,45.6831319408686,
39.3487519293518));
#205836=CARTESIAN_POINT('Ctrl Pts',(-40.8008642060156,45.5986481857975,
39.3492068662932));
#205837=CARTESIAN_POINT('Ctrl Pts',(-40.8592275074407,45.6634671987668,
39.4512271248733));
#205838=CARTESIAN_POINT('Ctrl Pts',(-40.649432716852,45.6199161851846,39.3978017080178));
#205839=CARTESIAN_POINT('Ctrl Pts',(-40.7435821574136,45.5350300257427,
39.3980347781178));
#205840=CARTESIAN_POINT('Ctrl Pts',(-40.7736504989776,45.5684243021861,
39.5248015355195));
#205841=CARTESIAN_POINT('Ctrl Pts',(-40.5892333705618,45.5534068532515,
39.3978017080178));
#205842=CARTESIAN_POINT('Ctrl Pts',(-40.6836127633975,45.4684272662439,
39.3978017080178));
#205843=CARTESIAN_POINT('Ctrl Pts',(-40.6836127633975,45.4684272662439,
39.5248017080178));
#205844=CARTESIAN_POINT('Origin',(-40.5892333705618,45.5534068532515,39.5248017080178));
#205845=CARTESIAN_POINT('Origin',(0.23594848208908,0.212448967518935,39.116));
#205846=CARTESIAN_POINT('Origin',(-41.1629311642476,46.1905628026488,39.116));
#205847=CARTESIAN_POINT('Origin',(0.23594848208908,0.212448967518935,39.5248017080178));
#205848=CARTESIAN_POINT('Origin',(-40.4880553924339,45.4410373245175,39.5248017080178));
#205849=CARTESIAN_POINT('Ctrl Pts',(-41.5228599914559,46.5911245387433,
39.2875012672119));
#205850=CARTESIAN_POINT('Ctrl Pts',(-41.6181024670991,46.5059978322081,
39.287208709576));
#205851=CARTESIAN_POINT('Ctrl Pts',(-41.5454735131716,46.4256208133857,
39.3549016990121));
#205852=CARTESIAN_POINT('Ctrl Pts',(-41.4460088704665,46.5055987918449,
39.1034939173931));
#205853=CARTESIAN_POINT('Ctrl Pts',(-41.5410583874207,46.4204321019766,
39.1031692336335));
#205854=CARTESIAN_POINT('Ctrl Pts',(-41.4839460439595,46.3572876358793,
39.2077507202297));
#205855=CARTESIAN_POINT('Ctrl Pts',(-41.3079491749511,46.3519544194674,
38.989));
#205856=CARTESIAN_POINT('Ctrl Pts',(-41.4027599825073,46.2668368728761,
38.9887769311176));
#205857=CARTESIAN_POINT('Ctrl Pts',(-41.3734144471011,46.2345298607752,
39.1161898712913));
#205858=CARTESIAN_POINT('Ctrl Pts',(-41.1629311642476,46.1905628026488,
38.989));
#205859=CARTESIAN_POINT('Ctrl Pts',(-41.2574515555194,46.1054562600791,
38.989));
#205860=CARTESIAN_POINT('Ctrl Pts',(-41.2573104519179,46.1055833103326,
39.1161895903852));
#205861=CARTESIAN_POINT('Origin',(-41.451202041617,46.510720046716,39.3548010137695));
#205862=CARTESIAN_POINT('Ctrl Pts',(-40.4880553924339,45.4410373245175,
39.3978017080178));
#205863=CARTESIAN_POINT('Ctrl Pts',(-40.5824347852696,45.3560577375099,
39.3978017080178));
#205864=CARTESIAN_POINT('Ctrl Pts',(-40.5824347852696,45.3560577375099,
39.5248017080178));
#205865=CARTESIAN_POINT('Ctrl Pts',(-40.427652148688,45.3743035899551,39.3978017080178));
#205866=CARTESIAN_POINT('Ctrl Pts',(-40.5221480762998,45.2891025640498,
39.3975666025003));
#205867=CARTESIAN_POINT('Ctrl Pts',(-40.4920927345059,45.2557227253165,
39.5248015517178));
#205868=CARTESIAN_POINT('Ctrl Pts',(-40.3705349278749,45.3112030195542,
39.3484894016716));
#205869=CARTESIAN_POINT('Ctrl Pts',(-40.4654317778737,45.2261127332184,
39.3480259000072));
#205870=CARTESIAN_POINT('Ctrl Pts',(-40.4066678844398,45.1608488177557,
39.4508333188954));
#205871=CARTESIAN_POINT('Ctrl Pts',(-40.3404336838189,45.2779489569776,
39.2708017080178));
#205872=CARTESIAN_POINT('Ctrl Pts',(-40.4355776097265,45.1929563204593,
39.27051194648));
#205873=CARTESIAN_POINT('Ctrl Pts',(-40.361648321148,45.1108495273516,39.3343017080178));
#205874=CARTESIAN_POINT('Origin',(-40.2672689283123,45.1958291143592,39.3343017080178));
#205875=CARTESIAN_POINT('Origin',(-41.5704070646319,46.6431106370705,39.6398955068176));
#205876=CARTESIAN_POINT('Origin',(-41.6896120874666,46.7755012272977,39.92499));
#205877=CARTESIAN_POINT('Origin',(-40.2128349741375,45.1353740836144,39.1934008539954));
#205878=CARTESIAN_POINT('Origin',(-40.1828829233547,45.1021848870412,39.116040271384));
#205879=CARTESIAN_POINT('Ctrl Pts',(-42.1132001505997,46.794261981092,40.1599502534424));
#205880=CARTESIAN_POINT('Ctrl Pts',(-42.0882450513171,46.7665330160783,
40.10025));
#205881=CARTESIAN_POINT('Ctrl Pts',(-42.0411527846891,46.7142062431426,
40.10025));
#205882=CARTESIAN_POINT('Ctrl Pts',(-42.0477032750704,46.8532067119191,
40.1599500538478));
#205883=CARTESIAN_POINT('Ctrl Pts',(-42.0405341034509,46.8094668591674,
40.100244835349));
#205884=CARTESIAN_POINT('Ctrl Pts',(-42.0032346206984,46.7483190388774,
40.10025));
#205885=CARTESIAN_POINT('Ctrl Pts',(-41.9705316734061,46.8890030154868,
40.120244200104));
#205886=CARTESIAN_POINT('Ctrl Pts',(-41.9811230778539,46.831817406086,40.0633873868017));
#205887=CARTESIAN_POINT('Ctrl Pts',(-41.9515093836254,46.761203850955,40.0772271723537));
#205888=CARTESIAN_POINT('Ctrl Pts',(-41.8426461117365,46.906368706767,40.0045995998161));
#205889=CARTESIAN_POINT('Ctrl Pts',(-41.8933796070862,46.8290619651512,
39.9663485808314));
#205890=CARTESIAN_POINT('Ctrl Pts',(-41.8570065263032,46.7485125544803,
40.0101727202466));
#205891=CARTESIAN_POINT('Ctrl Pts',(-41.7917018131136,46.8896982576904,
39.930465434986));
#205892=CARTESIAN_POINT('Ctrl Pts',(-41.8649047103985,46.8032976561882,
39.9051900162957));
#205893=CARTESIAN_POINT('Ctrl Pts',(-41.8144193983037,46.7243152668227,
39.9671857458179));
#205894=CARTESIAN_POINT('Ctrl Pts',(-41.7612723673359,46.8559036426989,
39.8576902534424));
#205895=CARTESIAN_POINT('Ctrl Pts',(-41.8563683535926,46.7709043015506,
39.8573998014387));
#205896=CARTESIAN_POINT('Ctrl Pts',(-41.7839914803023,46.6905216402901,
39.92499));
#205897=CARTESIAN_POINT('Origin',(-42.0411527846891,46.7142062431426,40.22725));
#205898=CARTESIAN_POINT('Origin',(0.23594848208908,0.212448967518935,39.116));
#205899=CARTESIAN_POINT('Origin',(-39.9143573409153,44.8038810887678,39.116));
#205900=CARTESIAN_POINT('Origin',(8.0125006576031E-17,-1.22536847673101E-16,
40.22725));
#205901=CARTESIAN_POINT('Origin',(-42.0638038389696,46.6938111422608,40.22725));
#205902=CARTESIAN_POINT('Ctrl Pts',(-39.9143573409153,44.8038810887678,
38.989));
#205903=CARTESIAN_POINT('Ctrl Pts',(-40.0088781183431,44.7187741985016,
38.989));
#205904=CARTESIAN_POINT('Ctrl Pts',(-40.0087366280092,44.7189015969705,
39.116190109232));
#205905=CARTESIAN_POINT('Ctrl Pts',(-39.7693421853879,44.6424822887502,
38.989));
#205906=CARTESIAN_POINT('Ctrl Pts',(-39.863819608937,44.5576711710514,38.9892298989736));
#205907=CARTESIAN_POINT('Ctrl Pts',(-39.8926305794711,44.5899527660325,
39.11619004932));
#205908=CARTESIAN_POINT('Ctrl Pts',(-39.6312917695235,44.4888315723763,
39.1034966344368));
#205909=CARTESIAN_POINT('Ctrl Pts',(-39.7256919284545,44.4042655856146,
39.1038314102582));
#205910=CARTESIAN_POINT('Ctrl Pts',(-39.7820998051101,44.4671959043838,
39.2077528789599));
#205911=CARTESIAN_POINT('Ctrl Pts',(-39.5544469813067,44.4033023070493,
39.2875012672119));
#205912=CARTESIAN_POINT('Ctrl Pts',(-39.6488649704632,44.3189410144587,
39.2878045257868));
#205913=CARTESIAN_POINT('Ctrl Pts',(-39.7205730900529,44.3988635644383,
39.3549015295898));
#205914=CARTESIAN_POINT('Origin',(-39.6260861683714,44.483723516876,39.3548010137695));
#205915=CARTESIAN_POINT('Ctrl Pts',(-42.2339804752697,46.4302753505428,
39.8576902534424));
#205916=CARTESIAN_POINT('Ctrl Pts',(-42.1395065320995,46.5159655405278,
39.8573998014387));
#205917=CARTESIAN_POINT('Ctrl Pts',(-42.0671296588092,46.4355828792674,
39.92499));
#205918=CARTESIAN_POINT('Ctrl Pts',(-42.2644230274451,46.4640859592749,
39.9304984902493));
#205919=CARTESIAN_POINT('Ctrl Pts',(-42.1708479205184,46.5278479142039,
39.9052171569784));
#205920=CARTESIAN_POINT('Ctrl Pts',(-42.0975714415917,46.4693919041994,
39.9672049726596));
#205921=CARTESIAN_POINT('Ctrl Pts',(-42.2755508889257,46.5163638812299,
40.0043437678659));
#205922=CARTESIAN_POINT('Ctrl Pts',(-42.1933444849776,46.5588164356977,
39.966162857764));
#205923=CARTESIAN_POINT('Ctrl Pts',(-42.1170605480848,46.5141432491636,
40.0100243556234));
#205924=CARTESIAN_POINT('Ctrl Pts',(-42.2454039774543,46.6408663419438,
40.119487482199));
#205925=CARTESIAN_POINT('Ctrl Pts',(-42.187220455932,46.6457133039303,40.0627551483144));
#205926=CARTESIAN_POINT('Ctrl Pts',(-42.1199995355541,46.6088541045844,
40.0767884282378));
#205927=CARTESIAN_POINT('Ctrl Pts',(-42.2015749714289,46.7146600431958,
40.1599502015393));
#205928=CARTESIAN_POINT('Ctrl Pts',(-42.1587905896512,46.7029882531954,
40.1002449453881));
#205929=CARTESIAN_POINT('Ctrl Pts',(-42.1018187547561,46.6595535157382,
40.10025));
#205930=CARTESIAN_POINT('Ctrl Pts',(-42.1358900227691,46.7738319284261,
40.1599502534424));
#205931=CARTESIAN_POINT('Ctrl Pts',(-42.1109214781057,46.7461150696876,
40.10025));
#205932=CARTESIAN_POINT('Ctrl Pts',(-42.0638038389696,46.6938111422608,
40.10025));
#205933=CARTESIAN_POINT('Origin',(-42.1615090516448,46.3506032922598,39.92499));
#205934=CARTESIAN_POINT('Origin',(-39.5068809815375,44.3513327445023,39.6398955069331));
#205935=CARTESIAN_POINT('Origin',(-39.387675794557,44.2189419720526,39.92499));
#205936=CARTESIAN_POINT('Origin',(-42.0423040287649,46.2182127020538,39.6398955068266));
#205937=CARTESIAN_POINT('Origin',(-41.9230990057951,46.0858221116782,39.3548010137695));
#205938=CARTESIAN_POINT('Ctrl Pts',(-39.3160391863686,44.1385184650379,
39.8576902534424));
#205939=CARTESIAN_POINT('Ctrl Pts',(-39.4103156382728,44.0542875439844,
39.8579948730703));
#205940=CARTESIAN_POINT('Ctrl Pts',(-39.4820551873926,44.1339623850451,
39.92499));
#205941=CARTESIAN_POINT('Ctrl Pts',(-39.2856369388936,44.1047525536515,
39.9304020711232));
#205942=CARTESIAN_POINT('Ctrl Pts',(-39.3789425853219,44.0421527706803,
39.9058915297377));
#205943=CARTESIAN_POINT('Ctrl Pts',(-39.4516512848558,44.100195430388,39.9671523786027));
#205944=CARTESIAN_POINT('Ctrl Pts',(-39.2745942850996,44.0527517782423,
40.0043257306692));
#205945=CARTESIAN_POINT('Ctrl Pts',(-39.3566016867499,44.0110417363804,
39.9667894847835));
#205946=CARTESIAN_POINT('Ctrl Pts',(-39.43232853063,44.0556530121007,40.0100138975201));
#205947=CARTESIAN_POINT('Ctrl Pts',(-39.3050549810248,43.9290071509457,
40.1195533054858));
#205948=CARTESIAN_POINT('Ctrl Pts',(-39.3631024520333,43.9243964923859,
40.0630813209236));
#205949=CARTESIAN_POINT('Ctrl Pts',(-39.4299498468374,43.9614781338112,
40.0768265942419));
#205950=CARTESIAN_POINT('Ctrl Pts',(-39.3490583909335,43.8557442421763,
40.1599502027522));
#205951=CARTESIAN_POINT('Ctrl Pts',(-39.3917348424042,43.8675206320098,
40.1002552791541));
#205952=CARTESIAN_POINT('Ctrl Pts',(-39.4485000225464,43.9111340157069,
40.10025));
#205953=CARTESIAN_POINT('Ctrl Pts',(-39.4144401478986,43.796904759635,40.1599502534424));
#205954=CARTESIAN_POINT('Ctrl Pts',(-39.4393948122684,43.8246341160488,
40.10025));
#205955=CARTESIAN_POINT('Ctrl Pts',(-39.4864862581813,43.8769616275878,
40.10025));
#205956=CARTESIAN_POINT('Origin',(-39.4864862581813,43.8769616275878,40.22725));
#205957=CARTESIAN_POINT('Ctrl Pts',(-41.6348281284258,45.765664867611,38.989));
#205958=CARTESIAN_POINT('Ctrl Pts',(-41.5403077290107,45.8507714175129,
38.989));
#205959=CARTESIAN_POINT('Ctrl Pts',(-41.5404488407676,45.8506443599163,
39.1161896013267));
#205960=CARTESIAN_POINT('Ctrl Pts',(-41.7801793767997,45.9267609786653,
38.989));
#205961=CARTESIAN_POINT('Ctrl Pts',(-41.6856176794227,46.012155211749,38.988776927543));
#205962=CARTESIAN_POINT('Ctrl Pts',(-41.6565546403132,45.9795929135653,
39.1161898821824));
#205963=CARTESIAN_POINT('Ctrl Pts',(-41.9185498083232,46.0801233673967,
39.1034967087243));
#205964=CARTESIAN_POINT('Ctrl Pts',(-41.8239142817226,46.1657498592425,
39.1031720232716));
#205965=CARTESIAN_POINT('Ctrl Pts',(-41.7670853619614,46.1023497159518,
39.2077529615019));
#205966=CARTESIAN_POINT('Ctrl Pts',(-41.9955727382247,46.1654920697616,
39.2875012672119));
#205967=CARTESIAN_POINT('Ctrl Pts',(-41.9009568069087,46.2513146407507,
39.2872087095508));
#205968=CARTESIAN_POINT('Ctrl Pts',(-41.8286118967075,46.1706818552411,
39.3549017048228));
#205969=CARTESIAN_POINT('Origin',(-41.6348281284258,45.765664867611,39.116));
#205970=CARTESIAN_POINT('Origin',(3.72719664096538E-16,4.35908294926644E-17,
40.22725));
#205971=CARTESIAN_POINT('Origin',(-39.5091373124618,43.856566526706,40.22725));
#205972=CARTESIAN_POINT('Origin',(27.6232705441538,-31.1532462714324,39.116));
#205973=CARTESIAN_POINT('Origin',(-41.3663085755636,45.4673664422112,39.1160373285278));
#205974=CARTESIAN_POINT('Ctrl Pts',(-39.4370498736004,43.7765468711726,
40.1599502534424));
#205975=CARTESIAN_POINT('Ctrl Pts',(-39.4620188529806,43.8042633382933,
40.10025));
#205976=CARTESIAN_POINT('Ctrl Pts',(-39.5091373124618,43.856566526706,40.10025));
#205977=CARTESIAN_POINT('Ctrl Pts',(-39.5021785224862,43.7178744835423,
40.159950056604));
#205978=CARTESIAN_POINT('Ctrl Pts',(-39.5094654441321,43.761515733967,40.1002551305381));
#205979=CARTESIAN_POINT('Ctrl Pts',(-39.5469637653738,43.8224770900129,
40.10025));
#205980=CARTESIAN_POINT('Ctrl Pts',(-39.5788516269098,43.6818502604299,
40.1203070619047));
#205981=CARTESIAN_POINT('Ctrl Pts',(-39.5685043961838,43.7389249259234,
40.06370986845));
#205982=CARTESIAN_POINT('Ctrl Pts',(-39.5983821485328,43.8091917332947,
40.0772636213363));
#205983=CARTESIAN_POINT('Ctrl Pts',(-39.7059848156956,43.6640874258694,
40.0046102245801));
#205984=CARTESIAN_POINT('Ctrl Pts',(-39.6560168722787,43.7412697217741,
39.9670001894012));
#205985=CARTESIAN_POINT('Ctrl Pts',(-39.692386550076,43.8212571467119,40.0101788811208));
#205986=CARTESIAN_POINT('Ctrl Pts',(-39.7566878101776,43.6806424921203,
39.9303710930186));
#205987=CARTESIAN_POINT('Ctrl Pts',(-39.6846695243124,43.7668962219029,
39.9058663574106));
#205988=CARTESIAN_POINT('Ctrl Pts',(-39.7348023770063,43.8452710114195,
39.9671344706368));
#205989=CARTESIAN_POINT('Ctrl Pts',(-39.7870778846743,43.7143933160627,
39.8576902534424));
#205990=CARTESIAN_POINT('Ctrl Pts',(-39.6934538167797,43.7993487829616,
39.8579948730704));
#205991=CARTESIAN_POINT('Ctrl Pts',(-39.7651933658995,43.8790236240223,
39.92499));
#205992=CARTESIAN_POINT('Origin',(-39.8595727587351,43.7940440370148,39.92499));
#205993=CARTESIAN_POINT('Origin',(-41.3366772856866,45.434534810366,39.1925554488842));
#205994=CARTESIAN_POINT('Origin',(-41.2819167515325,45.3737170758076,39.3343017080178));
#205995=CARTESIAN_POINT('Origin',(-39.9787779456617,43.9264348094905,39.6398955069226));
#205996=CARTESIAN_POINT('Origin',(-40.0979831325495,44.0588255818381,39.3548010137695));
#205997=CARTESIAN_POINT('Ctrl Pts',(-41.06113033474,45.1285089182136,39.3978017080178));
#205998=CARTESIAN_POINT('Ctrl Pts',(-40.9667509419044,45.2134885052212,
39.3978017080178));
#205999=CARTESIAN_POINT('Ctrl Pts',(-40.9667509419044,45.2134885052212,
39.5248017080178));
#206000=CARTESIAN_POINT('Ctrl Pts',(-41.1211850608437,45.1955564429366,
39.3978017080178));
#206001=CARTESIAN_POINT('Ctrl Pts',(-41.0269231466371,45.28031650884,39.3980355775177));
#206002=CARTESIAN_POINT('Ctrl Pts',(-41.0570929845756,45.3138235084271,
39.5248015517192));
#206003=CARTESIAN_POINT('Ctrl Pts',(-41.1779726855659,45.2589537050075,
39.3484893995498));
#206004=CARTESIAN_POINT('Ctrl Pts',(-41.0841042944899,45.3438226072592,
39.3489438303425));
#206005=CARTESIAN_POINT('Ctrl Pts',(-41.1425178129608,45.4086973919089,
39.4508333155591));
#206006=CARTESIAN_POINT('Ctrl Pts',(-41.2079002115903,45.2923641298561,
39.2708017080178));
#206007=CARTESIAN_POINT('Ctrl Pts',(-41.1142722655002,45.3773275334109,
39.2710850691866));
#206008=CARTESIAN_POINT('Ctrl Pts',(-41.1875373586968,45.4586966628152,
39.3343017080178));
#206009=CARTESIAN_POINT('Origin',(-41.06113033474,45.1285089182136,39.5248017080178));
#206010=CARTESIAN_POINT('Ctrl Pts',(-40.0254908126584,43.9791725362586,
39.2875012672119));
#206011=CARTESIAN_POINT('Ctrl Pts',(-39.9317223035497,44.064255127713,39.2878045257519));
#206012=CARTESIAN_POINT('Ctrl Pts',(-40.0037114707672,44.1439246046464,
39.3549015218344));
#206013=CARTESIAN_POINT('Ctrl Pts',(-40.1025202360379,44.0645378932545,
39.1034938540228));
#206014=CARTESIAN_POINT('Ctrl Pts',(-40.0085500157897,44.1495813562492,
39.1038286278834));
#206015=CARTESIAN_POINT('Ctrl Pts',(-40.0652391174805,44.2122579788877,
39.2077506434036));
#206016=CARTESIAN_POINT('Ctrl Pts',(-40.2409001323909,44.2178941385634,
38.989));
#206017=CARTESIAN_POINT('Ctrl Pts',(-40.1466780419426,44.3029888158449,
38.9892298954605));
#206018=CARTESIAN_POINT('Ctrl Pts',(-40.1757707681144,44.3350158129969,
39.1161900347283));
#206019=CARTESIAN_POINT('Ctrl Pts',(-40.3862543050934,44.3789831537299,
38.989));
#206020=CARTESIAN_POINT('Ctrl Pts',(-40.2917335385825,44.4640900341665,
38.989));
#206021=CARTESIAN_POINT('Ctrl Pts',(-40.2918750179832,44.4639626455419,
39.116190094564));
#206022=CARTESIAN_POINT('Origin',(-40.3862543050934,44.3789831537299,39.116));
#206023=CARTESIAN_POINT('Origin',(26.9484406282047,-30.4037717213982,39.5248017080178));
#206024=CARTESIAN_POINT('Origin',(-40.9599523566121,45.0161393894797,39.5248017080178));
#206025=CARTESIAN_POINT('Origin',(26.8427652369004,-30.2864073093061,39.116));
#206026=CARTESIAN_POINT('Origin',(-40.6548553974679,44.6772189625514,39.1160402713853));
#206027=CARTESIAN_POINT('Ctrl Pts',(-40.8131880745603,44.8522789915945,
39.2708017080178));
#206028=CARTESIAN_POINT('Ctrl Pts',(-40.7187157882333,44.9380175594366,
39.27051194648));
#206029=CARTESIAN_POINT('Ctrl Pts',(-40.6447864996549,44.8559107663289,
39.3343017080178));
#206030=CARTESIAN_POINT('Ctrl Pts',(-40.8432146576646,44.8858042435429,
39.3487519301185));
#206031=CARTESIAN_POINT('Ctrl Pts',(-40.748670873839,44.9712860523926,39.3482879463985));
#206032=CARTESIAN_POINT('Ctrl Pts',(-40.6899581892264,44.906079010083,39.4512271261639));
#206033=CARTESIAN_POINT('Ctrl Pts',(-40.9001003367641,44.9493173051408,
39.3978017080178));
#206034=CARTESIAN_POINT('Ctrl Pts',(-40.8054891887044,45.0343891839552,
39.3975673827397));
#206035=CARTESIAN_POINT('Ctrl Pts',(-40.7755352187359,45.0011219300382,
39.5248015355181));
#206036=CARTESIAN_POINT('Ctrl Pts',(-40.9599523566121,45.0161393894797,
39.3978017080178));
#206037=CARTESIAN_POINT('Ctrl Pts',(-40.8655729637765,45.1011189764872,
39.3978017080178));
#206038=CARTESIAN_POINT('Ctrl Pts',(-40.8655729637765,45.1011189764872,
39.5248017080178));
#206039=CARTESIAN_POINT('Origin',(-40.7391658924905,44.7709311793213,39.3343017080178));
#206040=CARTESIAN_POINT('Origin',(-40.6847319392783,44.7104761492014,39.1934008533554));
#206041=CARTESIAN_POINT('Origin',(-35.8473027488275,49.8797426639498,39.1925554495083));
#206042=CARTESIAN_POINT('Origin',(-35.8732562382978,49.9155525184337,39.1160373285282));
#206043=CARTESIAN_POINT('Origin',(-35.7991993820658,49.8135340601226,39.3343017080178));
#206044=CARTESIAN_POINT('Ctrl Pts',(-35.7350130971385,49.7242207306178,
39.2708017080178));
#206045=CARTESIAN_POINT('Ctrl Pts',(-35.8375861910552,49.6503036646788,
39.2710850691866));
#206046=CARTESIAN_POINT('Ctrl Pts',(-35.9019445403514,49.7388853330815,
39.3343017080178));
#206047=CARTESIAN_POINT('Ctrl Pts',(-35.7084656432366,49.6878783768789,
39.3487519293518));
#206048=CARTESIAN_POINT('Ctrl Pts',(-35.8109961808828,49.6137056554138,
39.3492068662929));
#206049=CARTESIAN_POINT('Ctrl Pts',(-35.8622643302213,49.6842702092578,
39.4512271248737));
#206050=CARTESIAN_POINT('Ctrl Pts',(-35.6581711379707,49.6190282456271,
39.3978017080178));
#206051=CARTESIAN_POINT('Ctrl Pts',(-35.7606778378473,49.5444483977908,
39.3980347781164));
#206052=CARTESIAN_POINT('Ctrl Pts',(-35.7870908094924,49.5808027344285,
39.5248015355176));
#206053=CARTESIAN_POINT('Ctrl Pts',(-35.6052536882598,49.5465907136148,
39.3978017080178));
#206054=CARTESIAN_POINT('Ctrl Pts',(-35.7079988465454,49.4719419865736,
39.3978017080178));
#206055=CARTESIAN_POINT('Ctrl Pts',(-35.7079988465454,49.4719419865736,
39.5248017080178));
#206056=CARTESIAN_POINT('Origin',(-35.6052536882598,49.5465907136148,39.5248017080178));
#206057=CARTESIAN_POINT('Origin',(0.256862895714053,0.186621817602858,39.116));
#206058=CARTESIAN_POINT('Origin',(-36.1092077731524,50.2402240048086,39.116));
#206059=CARTESIAN_POINT('Origin',(0.256862895714053,0.186621817602858,39.5248017080178));
#206060=CARTESIAN_POINT('Origin',(-35.5163757878391,49.4242607783464,39.5248017080178));
#206061=CARTESIAN_POINT('Ctrl Pts',(-36.4252947698674,50.6762142289951,
39.2875012672119));
#206062=CARTESIAN_POINT('Ctrl Pts',(-36.5289136610809,50.601509405082,39.287208709576));
#206063=CARTESIAN_POINT('Ctrl Pts',(-36.4650842624219,50.513980907036,39.3549016990121));
#206064=CARTESIAN_POINT('Ctrl Pts',(-36.3578045222537,50.5831238715089,
39.103493917393));
#206065=CARTESIAN_POINT('Ctrl Pts',(-36.4612356912194,50.5083591136189,
39.1031692336376));
#206066=CARTESIAN_POINT('Ctrl Pts',(-36.4110366091576,50.4395906940187,
39.2077507202321));
#206067=CARTESIAN_POINT('Ctrl Pts',(-36.2365613423287,50.4158900112692,
38.989));
#206068=CARTESIAN_POINT('Ctrl Pts',(-36.3397499727032,50.3411491755218,
38.9887769311134));
#206069=CARTESIAN_POINT('Ctrl Pts',(-36.3139421975398,50.3059517008917,
39.1161898712888));
#206070=CARTESIAN_POINT('Ctrl Pts',(-36.1092077731524,50.2402240048086,
38.989));
#206071=CARTESIAN_POINT('Ctrl Pts',(-36.2121064279397,50.1654637560311,
38.989));
#206072=CARTESIAN_POINT('Ctrl Pts',(-36.2119528169509,50.1655753609473,
39.1161895903851));
#206073=CARTESIAN_POINT('Origin',(-36.3624339277669,50.5887599058104,39.3548010137695));
#206074=CARTESIAN_POINT('Ctrl Pts',(-35.5163757878391,49.4242607783464,
39.3978017080178));
#206075=CARTESIAN_POINT('Ctrl Pts',(-35.6191209461248,49.3496120513052,
39.3978017080178));
#206076=CARTESIAN_POINT('Ctrl Pts',(-35.6191209461248,49.3496120513052,
39.5248017080178));
#206077=CARTESIAN_POINT('Ctrl Pts',(-35.4632790141033,49.3515787599201,
39.3978017080178));
#206078=CARTESIAN_POINT('Ctrl Pts',(-35.5661632154413,49.276721988248,39.3975666025022));
#206079=CARTESIAN_POINT('Ctrl Pts',(-35.5397616632048,49.2403833690727,
39.5248015517178));
#206080=CARTESIAN_POINT('Ctrl Pts',(-35.4130704930569,49.2828534857288,
39.3484894016717));
#206081=CARTESIAN_POINT('Ctrl Pts',(-35.5163418450511,49.2081487547859,
39.3480259000055));
#206082=CARTESIAN_POINT('Ctrl Pts',(-35.464721803166,49.1370998624006,39.4508333188956));
#206083=CARTESIAN_POINT('Ctrl Pts',(-35.3866101428255,49.2466351556016,
39.2708017080178));
#206084=CARTESIAN_POINT('Ctrl Pts',(-35.4901170100363,49.1720533660034,
39.2705119464801));
#206085=CARTESIAN_POINT('Ctrl Pts',(-35.4251752107434,49.0826686475738,
39.3343017080178));
#206086=CARTESIAN_POINT('Origin',(-35.3224300524577,49.1573173746149,39.3343017080178));
#206087=CARTESIAN_POINT('Origin',(-36.4671473482338,50.7328855645276,39.6398955068173));
#206088=CARTESIAN_POINT('Origin',(-36.5718607685317,50.8770112231006,39.92499));
#206089=CARTESIAN_POINT('Origin',(-35.2746135646439,49.0915036252753,39.1934008539938));
#206090=CARTESIAN_POINT('Origin',(-35.2482948100384,49.055365400753,39.1160402713854));
#206091=CARTESIAN_POINT('Ctrl Pts',(-36.9911673391703,50.9399462128205,
40.1599502534424));
#206092=CARTESIAN_POINT('Ctrl Pts',(-36.9692474126336,50.9097606317997,
40.10025));
#206093=CARTESIAN_POINT('Ctrl Pts',(-36.9278827595322,50.8527980281388,
40.10025));
#206094=CARTESIAN_POINT('Ctrl Pts',(-36.9198678602466,50.991721750496,40.1599500538463));
#206095=CARTESIAN_POINT('Ctrl Pts',(-36.9173100216895,50.9474721267403,
40.100244835349));
#206096=CARTESIAN_POINT('Ctrl Pts',(-36.8866065570935,50.8827604229949,
40.10025));
#206097=CARTESIAN_POINT('Ctrl Pts',(-36.8393772800889,51.0192553292381,
40.1202442001041));
#206098=CARTESIAN_POINT('Ctrl Pts',(-36.8558881875866,50.9634900918193,
40.0633873868015));
#206099=CARTESIAN_POINT('Ctrl Pts',(-36.8338178466773,50.8901678911828,
40.0772271723539));
#206100=CARTESIAN_POINT('Ctrl Pts',(-36.7103770798836,51.0231582082091,
40.004599599816));
#206101=CARTESIAN_POINT('Ctrl Pts',(-36.7689134067389,50.9515780553181,
39.9663485808318));
#206102=CARTESIAN_POINT('Ctrl Pts',(-36.7411592876127,50.8676678805079,
40.0101727202465));
#206103=CARTESIAN_POINT('Ctrl Pts',(-36.6614543958819,51.0012539523503,
39.9304654349861));
#206104=CARTESIAN_POINT('Ctrl Pts',(-36.7432876021362,50.9229784487436,
39.9051900162947));
#206105=CARTESIAN_POINT('Ctrl Pts',(-36.7013347616503,50.8391515810788,
39.9671857458184));
#206106=CARTESIAN_POINT('Ctrl Pts',(-36.634724144965,50.9644637245896,39.8576902534424));
#206107=CARTESIAN_POINT('Ctrl Pts',(-36.738184035968,50.8898702560321,39.8573998014387));
#206108=CARTESIAN_POINT('Ctrl Pts',(-36.6746059268174,50.8023624960594,
39.92499));
#206109=CARTESIAN_POINT('Origin',(-36.9278827595322,50.8527980281388,40.22725));
#206110=CARTESIAN_POINT('Origin',(0.256862895714053,0.186621817602858,39.116));
#206111=CARTESIAN_POINT('Origin',(-35.0124214764581,48.7306271754179,39.116));
#206112=CARTESIAN_POINT('Origin',(6.67120042669018E-17,-1.33398482780243E-16,
40.22725));
#206113=CARTESIAN_POINT('Origin',(-36.9525415975208,50.8348823336489,40.22725));
#206114=CARTESIAN_POINT('Ctrl Pts',(-35.0124214764581,48.7306271754179,
38.989));
#206115=CARTESIAN_POINT('Ctrl Pts',(-35.1153205516305,48.6558666212127,
38.989));
#206116=CARTESIAN_POINT('Ctrl Pts',(-35.115166519629,48.6559785320125,39.1161901092323));
#206117=CARTESIAN_POINT('Ctrl Pts',(-34.8850714976646,48.5549543235566,
38.989));
#206118=CARTESIAN_POINT('Ctrl Pts',(-34.9878965398059,48.4804833899298,
38.9892298989718));
#206119=CARTESIAN_POINT('Ctrl Pts',(-35.0131753353115,48.515599709433,39.1161900493185));
#206120=CARTESIAN_POINT('Ctrl Pts',(-34.7638382096882,48.3877151240579,
39.1034966344368));
#206121=CARTESIAN_POINT('Ctrl Pts',(-34.8665607873115,48.3134799021656,
39.1038314102594));
#206122=CARTESIAN_POINT('Ctrl Pts',(-34.916081646201,48.3819617107287,39.2077528789615));
#206123=CARTESIAN_POINT('Ctrl Pts',(-34.6963546279281,48.2946219293749,
39.2875012672119));
#206124=CARTESIAN_POINT('Ctrl Pts',(-34.7990735417349,48.2205921440832,
39.2878045257868));
#206125=CARTESIAN_POINT('Ctrl Pts',(-34.8620346554126,48.3075724095165,
39.35490152959));
#206126=CARTESIAN_POINT('Origin',(-34.759195062553,48.3820909175332,39.3548010137695));
#206127=CARTESIAN_POINT('Ctrl Pts',(-37.1493329797256,50.5905785208487,
39.8576902534424));
#206128=CARTESIAN_POINT('Ctrl Pts',(-37.0464195108248,50.6659240749087,
39.8573998014387));
#206129=CARTESIAN_POINT('Ctrl Pts',(-36.9828414016742,50.578416314936,39.92499));
#206130=CARTESIAN_POINT('Ctrl Pts',(-37.1760745934428,50.6273860247245,
39.930498490249));
#206131=CARTESIAN_POINT('Ctrl Pts',(-37.0763471615787,50.6810174228644,
39.905217156979));
#206132=CARTESIAN_POINT('Ctrl Pts',(-37.0095824157651,50.6152221632658,
39.9672049726596));
#206133=CARTESIAN_POINT('Ctrl Pts',(-37.1816769644883,50.6805407410144,
40.0043437678663));
#206134=CARTESIAN_POINT('Ctrl Pts',(-37.0954833955414,50.7141678268705,
39.9661628577642));
#206135=CARTESIAN_POINT('Ctrl Pts',(-37.0242869695743,50.661765522031,40.0100243556237));
#206136=CARTESIAN_POINT('Ctrl Pts',(-37.1386811500609,50.8012099538924,
40.1194874821986));
#206137=CARTESIAN_POINT('Ctrl Pts',(-37.08030971847,50.7999485296225,40.062755148314));
#206138=CARTESIAN_POINT('Ctrl Pts',(-37.0173098767922,50.7562647493209,
40.0767884282375));
#206139=CARTESIAN_POINT('Ctrl Pts',(-37.0873787017255,50.8700180268819,
40.1599502015394));
#206140=CARTESIAN_POINT('Ctrl Pts',(-37.0460487315402,50.8539379904895,
40.1002449453872));
#206141=CARTESIAN_POINT('Ctrl Pts',(-36.9939291606758,50.8047860147164,
40.10025));
#206142=CARTESIAN_POINT('Ctrl Pts',(-37.0158684358555,50.9219998155903,
40.1599502534424));
#206143=CARTESIAN_POINT('Ctrl Pts',(-36.9939338721428,50.8918248691003,
40.10025));
#206144=CARTESIAN_POINT('Ctrl Pts',(-36.9525415975208,50.8348823336489,
40.10025));
#206145=CARTESIAN_POINT('Origin',(-37.0855865599598,50.5037675878948,39.92499));
#206146=CARTESIAN_POINT('Origin',(-34.6544814981902,48.2379650606699,39.6398955069325));
#206147=CARTESIAN_POINT('Origin',(-34.5497679336937,48.0938392037151,39.92499));
#206148=CARTESIAN_POINT('Origin',(-36.980873139614,50.3596419293373,39.6398955068271));
#206149=CARTESIAN_POINT('Origin',(-36.876159719195,50.2155162706047,39.3548010137695));
#206150=CARTESIAN_POINT('Ctrl Pts',(-34.4869303039392,48.006368200519,39.8576902534424));
#206151=CARTESIAN_POINT('Ctrl Pts',(-34.5894948283129,47.9324532779041,
39.8579948730703));
#206152=CARTESIAN_POINT('Ctrl Pts',(-34.6525130919793,48.0191904766739,
39.92499));
#206153=CARTESIAN_POINT('Ctrl Pts',(-34.4602241019849,47.9696093621198,
39.930402071123));
#206154=CARTESIAN_POINT('Ctrl Pts',(-34.559562069435,47.9171056031468,39.9058915297386));
#206155=CARTESIAN_POINT('Ctrl Pts',(-34.6258053530817,47.9824304277186,
39.9671523786034));
#206156=CARTESIAN_POINT('Ctrl Pts',(-34.4546775021463,47.9167391807674,
40.0043257306694));
#206157=CARTESIAN_POINT('Ctrl Pts',(-34.5405955452481,47.8838297385506,
39.9667894847838));
#206158=CARTESIAN_POINT('Ctrl Pts',(-34.6112444014586,47.9361122396534,
40.01001389752));
#206159=CARTESIAN_POINT('Ctrl Pts',(-34.4979061669207,47.7968564492224,
40.1195533054857));
#206160=CARTESIAN_POINT('Ctrl Pts',(-34.5561175928638,47.7983386612732,
40.0630813209234));
#206161=CARTESIAN_POINT('Ctrl Pts',(-34.6187227036509,47.8422046210393,
40.076826594242));
#206162=CARTESIAN_POINT('Ctrl Pts',(-34.5493265808147,47.7285944911493,
40.1599502027511));
#206163=CARTESIAN_POINT('Ctrl Pts',(-34.5905382782876,47.7447672725789,
40.1002552791554));
#206164=CARTESIAN_POINT('Ctrl Pts',(-34.6424336528575,47.7940753146434,
40.10025));
#206165=CARTESIAN_POINT('Ctrl Pts',(-34.620500570363,47.6769115920307,40.1599502534424));
#206166=CARTESIAN_POINT('Ctrl Pts',(-34.642420023457,47.7070975168467,40.10025));
#206167=CARTESIAN_POINT('Ctrl Pts',(-34.6837837831342,47.7640607692766,
40.10025));
#206168=CARTESIAN_POINT('Origin',(-34.6837837831342,47.7640607692766,40.22725));
#206169=CARTESIAN_POINT('Ctrl Pts',(-36.6229335645805,49.8669803696029,
38.989));
#206170=CARTESIAN_POINT('Ctrl Pts',(-36.5200349009277,49.9417406248216,
38.989));
#206171=CARTESIAN_POINT('Ctrl Pts',(-36.5201885207953,49.9416290134547,
39.1161896013271));
#206172=CARTESIAN_POINT('Ctrl Pts',(-36.7506494346786,50.042387321933,38.989));
#206173=CARTESIAN_POINT('Ctrl Pts',(-36.6476796282208,50.1174293675617,
38.9887769275442));
#206174=CARTESIAN_POINT('Ctrl Pts',(-36.6221794864683,50.0820075342366,
39.1161898821828));
#206175=CARTESIAN_POINT('Ctrl Pts',(-36.8722311236856,50.2093732240195,
39.1034967087243));
#206176=CARTESIAN_POINT('Ctrl Pts',(-36.7691636147928,50.284638538816,39.1031720232712));
#206177=CARTESIAN_POINT('Ctrl Pts',(-36.7192731293507,50.2156454684951,
39.2077529615018));
#206178=CARTESIAN_POINT('Ctrl Pts',(-36.9399086546482,50.3023253561999,
39.2875012672119));
#206179=CARTESIAN_POINT('Ctrl Pts',(-36.8368401378443,50.3777877242645,
39.2872087095508));
#206180=CARTESIAN_POINT('Ctrl Pts',(-36.7733199617892,50.2900345513016,
39.354901704823));
#206181=CARTESIAN_POINT('Origin',(-36.6229335645805,49.8669803696029,39.116));
#206182=CARTESIAN_POINT('Origin',(3.77491158612227E-16,4.74547095659469E-17,
40.22725));
#206183=CARTESIAN_POINT('Origin',(-34.7084426211227,47.7461450747867,40.22725));
#206184=CARTESIAN_POINT('Origin',(21.2404668433927,-29.7751578089172,39.116));
#206185=CARTESIAN_POINT('Origin',(-36.3870656659264,49.5422481179711,39.116037328528));
#206186=CARTESIAN_POINT('Ctrl Pts',(-34.6451144164181,47.6590285860939,
40.1599502534424));
#206187=CARTESIAN_POINT('Ctrl Pts',(-34.6670494534013,47.6892031885516,
40.10025));
#206188=CARTESIAN_POINT('Ctrl Pts',(-34.7084426211227,47.7461450747867,
40.10025));
#206189=CARTESIAN_POINT('Ctrl Pts',(-34.7160192182661,47.6074854095251,
40.1599500566034));
#206190=CARTESIAN_POINT('Ctrl Pts',(-34.7187044685518,47.6516492793364,
40.1002551305369));
#206191=CARTESIAN_POINT('Ctrl Pts',(-34.7496251732003,47.7161963245905,
40.10025));
#206192=CARTESIAN_POINT('Ctrl Pts',(-34.7960378560837,47.5796730526554,
40.1203070619043));
#206193=CARTESIAN_POINT('Ctrl Pts',(-34.7797813814947,47.6353534770327,
40.0637098684494));
#206194=CARTESIAN_POINT('Ctrl Pts',(-34.802150578997,47.7083584310198,40.0772636213361));
#206195=CARTESIAN_POINT('Ctrl Pts',(-34.9243313177586,47.5752965616149,
40.0046102245805));
#206196=CARTESIAN_POINT('Ctrl Pts',(-34.8665693571816,47.6468329724888,
39.9670001894019));
#206197=CARTESIAN_POINT('Ctrl Pts',(-34.894378835469,47.7301838844735,40.0101788811211));
#206198=CARTESIAN_POINT('Ctrl Pts',(-34.9730260802977,47.5970608435772,
39.9303710930184));
#206199=CARTESIAN_POINT('Ctrl Pts',(-34.8923863483135,47.6753141056551,
39.9058663574106));
#206200=CARTESIAN_POINT('Ctrl Pts',(-34.934052171687,47.7584998599255,39.9671344706371));
#206201=CARTESIAN_POINT('Ctrl Pts',(-34.9997217530256,47.6338034047603,
39.8576902534424));
#206202=CARTESIAN_POINT('Ctrl Pts',(-34.8977303031698,47.7085070967806,
39.8579948730703));
#206203=CARTESIAN_POINT('Ctrl Pts',(-34.9607485668361,47.7952442955505,
39.92499));
#206204=CARTESIAN_POINT('Origin',(-35.0634937251217,47.7205955685094,39.92499));
#206205=CARTESIAN_POINT('Origin',(-36.3610285393802,49.5064990280449,39.1925554488846));
#206206=CARTESIAN_POINT('Origin',(-36.3129251734939,49.4402904249169,39.3343017080178));
#206207=CARTESIAN_POINT('Origin',(-35.1682072895617,47.8647214254821,39.6398955069207));
#206208=CARTESIAN_POINT('Origin',(-35.2729208539811,48.0088472823275,39.3548010137695));
#206209=CARTESIAN_POINT('Ctrl Pts',(-36.1189794796879,49.1733470784091,
39.3978017080178));
#206210=CARTESIAN_POINT('Ctrl Pts',(-36.0162343214022,49.2479958054502,
39.3978017080178));
#206211=CARTESIAN_POINT('Ctrl Pts',(-36.0162343214022,49.2479958054502,
39.5248017080178));
#206212=CARTESIAN_POINT('Ctrl Pts',(-36.1716968449934,49.2463047380077,
39.3978017080178));
#206213=CARTESIAN_POINT('Ctrl Pts',(-36.0690914679777,49.3207474263656,
39.3980355775191));
#206214=CARTESIAN_POINT('Ctrl Pts',(-36.0955935972134,49.3572244778984,
39.5248015517192));
#206215=CARTESIAN_POINT('Ctrl Pts',(-36.2215465627857,49.3152906263886,
39.3484893995498));
#206216=CARTESIAN_POINT('Ctrl Pts',(-36.1193211766481,49.3898826892451,
39.3489438303418));
#206217=CARTESIAN_POINT('Ctrl Pts',(-36.1706334382073,49.4605079583574,
39.4508333155594));
#206218=CARTESIAN_POINT('Ctrl Pts',(-36.2478178023246,49.3516463037388,
39.2708017080178));
#206219=CARTESIAN_POINT('Ctrl Pts',(-36.1458216659121,49.4263574835554,
39.2710850691866));
#206220=CARTESIAN_POINT('Ctrl Pts',(-36.2101800152082,49.514939151958,39.3343017080178));
#206221=CARTESIAN_POINT('Origin',(-36.1189794796879,49.1733470784091,39.5248017080178));
#206222=CARTESIAN_POINT('Ctrl Pts',(-35.2091516650524,47.922053073669,39.2875012672119));
#206223=CARTESIAN_POINT('Ctrl Pts',(-35.1070032771116,47.9968680956254,
39.2878045257519));
#206224=CARTESIAN_POINT('Ctrl Pts',(-35.1702703521464,48.0836260518495,
39.3549015218347));
#206225=CARTESIAN_POINT('Ctrl Pts',(-35.2768360036062,48.0150025575607,
39.1034938540228));
#206226=CARTESIAN_POINT('Ctrl Pts',(-35.1744910995566,48.0897575808481,
39.1038286278809));
#206227=CARTESIAN_POINT('Ctrl Pts',(-35.2243181613712,48.1580164790724,
39.2077506434028));
#206228=CARTESIAN_POINT('Ctrl Pts',(-35.398427747753,48.181983339225,38.989));
#206229=CARTESIAN_POINT('Ctrl Pts',(-35.2958269999255,48.2567629686449,
38.9892298954624));
#206230=CARTESIAN_POINT('Ctrl Pts',(-35.3214126203088,48.2916555365114,
39.1161900347289));
#206231=CARTESIAN_POINT('Ctrl Pts',(-35.5261472678861,48.3573835402122,
38.989));
#206232=CARTESIAN_POINT('Ctrl Pts',(-35.4232482045979,48.432144085783,38.989));
#206233=CARTESIAN_POINT('Ctrl Pts',(-35.4234022246974,48.4320321836306,
39.1161900945646));
#206234=CARTESIAN_POINT('Origin',(-35.5261472678861,48.3573835402122,39.116));
#206235=CARTESIAN_POINT('Origin',(20.7197400704237,-29.0584388930974,39.5248017080178));
#206236=CARTESIAN_POINT('Origin',(-36.0301015792672,49.0510171431407,39.5248017080178));
#206237=CARTESIAN_POINT('Origin',(20.6381965522785,-28.9462038689907,39.116));
#206238=CARTESIAN_POINT('Origin',(-35.7621028045848,48.6820620414861,39.1160402713851));
#206239=CARTESIAN_POINT('Ctrl Pts',(-35.90126936289,48.8727133447947,39.2708017080178));
#206240=CARTESIAN_POINT('Ctrl Pts',(-35.7983524848931,48.94810718488,39.27051194648));
#206241=CARTESIAN_POINT('Ctrl Pts',(-35.7334106856002,48.8587224664504,
39.3343017080178));
#206242=CARTESIAN_POINT('Ctrl Pts',(-35.9276271141638,48.909193574494,39.3487519301185));
#206243=CARTESIAN_POINT('Ctrl Pts',(-35.8246659689621,48.9843245886183,
39.3482879463976));
#206244=CARTESIAN_POINT('Ctrl Pts',(-35.7730909105055,48.9133376106103,
39.4512271261638));
#206245=CARTESIAN_POINT('Ctrl Pts',(-35.9775622448353,48.978304877513,39.3978017080178));
#206246=CARTESIAN_POINT('Ctrl Pts',(-35.8745769537837,49.0530211657577,
39.3975673827401));
#206247=CARTESIAN_POINT('Ctrl Pts',(-35.8482644497257,49.0168051108908,
39.5248015355181));
#206248=CARTESIAN_POINT('Ctrl Pts',(-36.0301015792672,49.0510171431407,
39.3978017080178));
#206249=CARTESIAN_POINT('Ctrl Pts',(-35.9273564209816,49.1256658701818,
39.3978017080178));
#206250=CARTESIAN_POINT('Ctrl Pts',(-35.9273564209816,49.1256658701818,
39.5248017080178));
#206251=CARTESIAN_POINT('Origin',(-35.8361558438858,48.7840737394092,39.3343017080178));
#206252=CARTESIAN_POINT('Origin',(-35.7883393569606,48.7182599907915,39.193400853355));
#206253=CARTESIAN_POINT('Origin',(-30.437074624756,53.3535596832575,39.192555449508));
#206254=CARTESIAN_POINT('Origin',(-30.4591427892374,53.3918862459807,39.1160373285255));
#206255=CARTESIAN_POINT('Origin',(-30.3961554568832,53.2826856060848,39.3343017080178));
#206256=CARTESIAN_POINT('Ctrl Pts',(-30.3416565762231,53.1871522506178,
39.2708017080178));
#206257=CARTESIAN_POINT('Ctrl Pts',(-30.4513942013108,53.1243619179798,
39.2710850691867));
#206258=CARTESIAN_POINT('Ctrl Pts',(-30.5061406831638,53.2191856060848,
39.3343017080178));
#206259=CARTESIAN_POINT('Ctrl Pts',(-30.3190533624385,53.1482340195356,
39.3487519293518));
#206260=CARTESIAN_POINT('Ctrl Pts',(-30.4287753876661,53.0851849835386,
39.3492068662939));
#206261=CARTESIAN_POINT('Ctrl Pts',(-30.4723866803431,53.1607219582405,
39.4512271248748));
#206262=CARTESIAN_POINT('Ctrl Pts',(-30.2762311741509,53.0745038491602,
39.3978017080178));
#206263=CARTESIAN_POINT('Ctrl Pts',(-30.3859720484835,53.0110474253453,
39.398034778116));
#206264=CARTESIAN_POINT('Ctrl Pts',(-30.4084402641648,53.0499635164578,
39.5248015355176));
#206265=CARTESIAN_POINT('Ctrl Pts',(-30.2311753956707,52.996931757829,39.3978017080178));
#206266=CARTESIAN_POINT('Ctrl Pts',(-30.3411606219514,52.933431757829,39.3978017080178));
#206267=CARTESIAN_POINT('Ctrl Pts',(-30.3411606219514,52.933431757829,39.5248017080178));
#206268=CARTESIAN_POINT('Origin',(-30.2311753956707,52.996931757829,39.5248017080178));
#206269=CARTESIAN_POINT('Origin',(0.274963065701566,0.158749999999997,39.116));
#206270=CARTESIAN_POINT('Origin',(-30.659864345357,53.7394427993289,39.116));
#206271=CARTESIAN_POINT('Origin',(0.274963065701566,0.158749999999997,39.5248017080178));
#206272=CARTESIAN_POINT('Origin',(-30.1555713378333,52.8659816883962,39.5248017080178));
#206273=CARTESIAN_POINT('Ctrl Pts',(-30.9286463962973,54.2060847114744,
39.2875012672119));
#206274=CARTESIAN_POINT('Ctrl Pts',(-31.039506432826,54.1426202518668,39.287208709576));
#206275=CARTESIAN_POINT('Ctrl Pts',(-30.9851759176831,54.048899255138,39.3549016990126));
#206276=CARTESIAN_POINT('Ctrl Pts',(-30.8712564593345,54.1064496608383,
39.1034939173931));
#206277=CARTESIAN_POINT('Ctrl Pts',(-30.9819360667873,54.0429059732653,
39.1031692336345));
#206278=CARTESIAN_POINT('Ctrl Pts',(-30.9392002377703,53.9692670413573,
39.2077507202313));
#206279=CARTESIAN_POINT('Ctrl Pts',(-30.7681581606534,53.9274585619029,
38.989));
#206280=CARTESIAN_POINT('Ctrl Pts',(-30.8785940576184,53.8639133132283,
38.9887769311152));
#206281=CARTESIAN_POINT('Ctrl Pts',(-30.8566067980778,53.8262110069709,
39.1161898712897));
#206282=CARTESIAN_POINT('Ctrl Pts',(-30.659864345357,53.7394427993289,38.989));
#206283=CARTESIAN_POINT('Ctrl Pts',(-30.7700138844659,53.6758479332733,
38.989));
#206284=CARTESIAN_POINT('Ctrl Pts',(-30.769849449083,53.6759428700859,39.116189590386));
#206285=CARTESIAN_POINT('Origin',(-30.8752713784757,54.1125387249982,39.3548010137695));
#206286=CARTESIAN_POINT('Ctrl Pts',(-30.1555713378333,52.8659816883962,
39.3978017080178));
#206287=CARTESIAN_POINT('Ctrl Pts',(-30.2655565641139,52.8024816883962,
39.3978017080178));
#206288=CARTESIAN_POINT('Ctrl Pts',(-30.2655565641139,52.8024816883962,
39.5248017080178));
#206289=CARTESIAN_POINT('Ctrl Pts',(-30.1103627734739,52.7881477055079,
39.3978017080178));
#206290=CARTESIAN_POINT('Ctrl Pts',(-30.2205080276998,52.7244553345187,
39.3975666025021));
#206291=CARTESIAN_POINT('Ctrl Pts',(-30.1980495259467,52.685556068422,39.5248015517178));
#206292=CARTESIAN_POINT('Ctrl Pts',(-30.0676130472578,52.7145506960118,
39.3484894016716));
#206293=CARTESIAN_POINT('Ctrl Pts',(-30.1781274387052,52.6510500011318,
39.3480259000039));
#206294=CARTESIAN_POINT('Ctrl Pts',(-30.1342168083487,52.5749945583572,
39.4508333188949));
#206295=CARTESIAN_POINT('Ctrl Pts',(-30.0450834959832,52.6757649139399,
39.2708017080178));
#206296=CARTESIAN_POINT('Ctrl Pts',(-30.1558192615997,52.6124111049559,
39.27051194648));
#206297=CARTESIAN_POINT('Ctrl Pts',(-30.1005764675353,52.5167277788844,
39.3343017080178));
#206298=CARTESIAN_POINT('Origin',(-29.9905912412547,52.5802277788844,39.3343017080178));
#206299=CARTESIAN_POINT('Origin',(-30.9643459342459,54.2668203812029,39.6398955068166));
#206300=CARTESIAN_POINT('Origin',(-31.0534204898629,54.4211020372441,39.92499));
#206301=CARTESIAN_POINT('Origin',(-29.9499161072434,52.5097763801591,39.1934008539945));
#206302=CARTESIAN_POINT('Origin',(-29.9275190026058,52.4710850656386,39.1160402713848));
#206303=CARTESIAN_POINT('Ctrl Pts',(-31.4638515574735,54.5275217339722,
40.1599502534424));
#206304=CARTESIAN_POINT('Ctrl Pts',(-31.4452069629848,54.4952102564868,
40.10025));
#206305=CARTESIAN_POINT('Ctrl Pts',(-31.4100231232056,54.4342359163066,
40.10025));
#206306=CARTESIAN_POINT('Ctrl Pts',(-31.3875306471679,54.5715608148717,
40.1599500538472));
#206307=CARTESIAN_POINT('Ctrl Pts',(-31.3896121658909,54.5272862282532,
40.100244835349));
#206308=CARTESIAN_POINT('Ctrl Pts',(-31.365841113034,54.4597196360208,40.10025));
#206309=CARTESIAN_POINT('Ctrl Pts',(-31.3046029601553,54.5905300051369,
40.1202442001041));
#206310=CARTESIAN_POINT('Ctrl Pts',(-31.3268524737456,54.5367961153122,
40.0633873868015));
#206311=CARTESIAN_POINT('Ctrl Pts',(-31.3125672934291,54.4615686025428,
40.0772271723538));
#206312=CARTESIAN_POINT('Ctrl Pts',(-31.1759014746037,54.5809273110396,
40.0045995998161));
#206313=CARTESIAN_POINT('Ctrl Pts',(-31.2415992967176,54.5158579940065,
39.9663485808318));
#206314=CARTESIAN_POINT('Ctrl Pts',(-31.2227682191853,54.4295063924926,
40.0101727202466));
#206315=CARTESIAN_POINT('Ctrl Pts',(-31.1295364123884,54.5540292360083,
39.9304654349861));
#206316=CARTESIAN_POINT('Ctrl Pts',(-31.2191033458797,54.4847364330961,
39.9051900162944));
#206317=CARTESIAN_POINT('Ctrl Pts',(-31.1861426211014,54.3969835118379,
39.9671857458167));
#206318=CARTESIAN_POINT('Ctrl Pts',(-31.106798218553,54.5146464769141,39.8576902534424));
#206319=CARTESIAN_POINT('Ctrl Pts',(-31.217488486086,54.4512761425985,39.8573998014387));
#206320=CARTESIAN_POINT('Ctrl Pts',(-31.1634057161435,54.3576020372441,
39.92499));
#206321=CARTESIAN_POINT('Origin',(-31.4100231232056,54.4342359163066,40.22725));
#206322=CARTESIAN_POINT('Origin',(0.274963065701566,0.158749999999997,39.116));
#206323=CARTESIAN_POINT('Origin',(-29.7268821954845,52.1234703131949,39.116));
#206324=CARTESIAN_POINT('Origin',(5.22371297615222E-17,-1.42798576194617E-16,
40.22725));
#206325=CARTESIAN_POINT('Origin',(-31.436419577513,54.4189959163066,40.22725));
#206326=CARTESIAN_POINT('Ctrl Pts',(-29.7268821954845,52.1234703131949,
38.989));
#206327=CARTESIAN_POINT('Ctrl Pts',(-29.8370321846011,52.0598751873272,
38.989));
#206328=CARTESIAN_POINT('Ctrl Pts',(-29.8368672985388,52.0599703843397,
39.1161901092328));
#206329=CARTESIAN_POINT('Ctrl Pts',(-29.6185926664413,51.9354481180173,
38.989));
#206330=CARTESIAN_POINT('Ctrl Pts',(-29.7286387544932,51.8721332876001,
38.9892298989718));
#206331=CARTESIAN_POINT('Ctrl Pts',(-29.7501084152017,51.9096995898778,
39.116190049319));
#206332=CARTESIAN_POINT('Ctrl Pts',(-29.5155047636231,51.7564527430629,
39.1034966344368));
#206333=CARTESIAN_POINT('Ctrl Pts',(-29.6254243098796,51.6933616226636,
39.1038314102586));
#206334=CARTESIAN_POINT('Ctrl Pts',(-29.6675155901142,51.7666446199909,
39.2077528789606));
#206335=CARTESIAN_POINT('Ctrl Pts',(-29.4581217525669,51.656815567543,39.2875012672119));
#206336=CARTESIAN_POINT('Ctrl Pts',(-29.5680161811092,51.5939283753695,
39.2878045257868));
#206337=CARTESIAN_POINT('Ctrl Pts',(-29.6215404737379,51.6870133822668,
39.3549015295902));
#206338=CARTESIAN_POINT('Origin',(-29.5114749418,51.7503740054946,39.3548010137695));
#206339=CARTESIAN_POINT('Ctrl Pts',(-31.6576696180579,54.196600726121,39.8576902534424));
#206340=CARTESIAN_POINT('Ctrl Pts',(-31.5474441649279,54.2607761425985,
39.8573998014387));
#206341=CARTESIAN_POINT('Ctrl Pts',(-31.4933613949854,54.1671020372441,
39.92499));
#206342=CARTESIAN_POINT('Ctrl Pts',(-31.6804173066001,54.2360018544268,
39.9304984902494));
#206343=CARTESIAN_POINT('Ctrl Pts',(-31.5756301844101,54.2789150989593,
39.9052171569796));
#206344=CARTESIAN_POINT('Ctrl Pts',(-31.5161086602375,54.2065014563941,
39.96720497266));
#206345=CARTESIAN_POINT('Ctrl Pts',(-31.6804328064619,54.2894509908545,
40.0043437678659));
#206346=CARTESIAN_POINT('Ctrl Pts',(-31.5911964272957,54.313884182711,39.966162857764));
#206347=CARTESIAN_POINT('Ctrl Pts',(-31.5258675551963,54.2543268901841,
40.0100243556235));
#206348=CARTESIAN_POINT('Ctrl Pts',(-31.6250591602186,54.4049648787503,
40.1194874821991));
#206349=CARTESIAN_POINT('Ctrl Pts',(-31.5671393481779,54.397608888651,40.0627551483143));
#206350=CARTESIAN_POINT('Ctrl Pts',(-31.5090508246489,54.3475791360316,
40.0767884282377));
#206351=CARTESIAN_POINT('Ctrl Pts',(-31.5668453499335,54.4680334478298,
40.1599502015398));
#206352=CARTESIAN_POINT('Ctrl Pts',(-31.5274226111428,54.4477213412897,
40.100244945386));
#206353=CARTESIAN_POINT('Ctrl Pts',(-31.4807263372351,54.3933906465338,
40.10025));
#206354=CARTESIAN_POINT('Ctrl Pts',(-31.4902932482903,54.5122556166614,
40.1599502534424));
#206355=CARTESIAN_POINT('Ctrl Pts',(-31.4716329851984,54.4799531854482,
40.10025));
#206356=CARTESIAN_POINT('Ctrl Pts',(-31.436419577513,54.4189959163066,40.10025));
#206357=CARTESIAN_POINT('Origin',(-31.603346621266,54.1036020372441,39.92499));
#206358=CARTESIAN_POINT('Origin',(-29.4224002636351,51.596092137187,39.6398955069316));
#206359=CARTESIAN_POINT('Origin',(-29.333325585345,51.4418102687788,39.92499));
#206360=CARTESIAN_POINT('Origin',(-31.5142720655972,53.9493203812116,39.6398955068281));
#206361=CARTESIAN_POINT('Origin',(-31.4251975098788,53.7950387249982,39.3548010137695));
#206362=CARTESIAN_POINT('Ctrl Pts',(-29.2799753962458,51.3482501200168,
39.8576902534424));
#206363=CARTESIAN_POINT('Ctrl Pts',(-29.3897042746969,51.2854610232004,
39.8579948730703));
#206364=CARTESIAN_POINT('Ctrl Pts',(-29.4433108116256,51.3783102687788,
39.92499));
#206365=CARTESIAN_POINT('Ctrl Pts',(-29.2572578385493,51.3089010921306,
39.9304020711231));
#206366=CARTESIAN_POINT('Ctrl Pts',(-29.3615397594605,51.2670685993242,
39.9058915297385));
#206367=CARTESIAN_POINT('Ctrl Pts',(-29.4205918519431,51.3389598763134,
39.9671523786034));
#206368=CARTESIAN_POINT('Ctrl Pts',(-29.2572680623744,51.255740761606,40.0043257306693));
#206369=CARTESIAN_POINT('Ctrl Pts',(-29.3461554108688,51.2319924817694,
39.9667894847835));
#206370=CARTESIAN_POINT('Ctrl Pts',(-29.4109522357566,51.2913733902323,
40.0100138975201));
#206371=CARTESIAN_POINT('Ctrl Pts',(-29.312791073701,51.1410333861057,40.1195533054858));
#206372=CARTESIAN_POINT('Ctrl Pts',(-29.3705286780136,51.1485922293424,
40.0630813209236));
#206373=CARTESIAN_POINT('Ctrl Pts',(-29.4282055900895,51.1987619028143,
40.076826594242));
#206374=CARTESIAN_POINT('Ctrl Pts',(-29.3710651187643,51.0785202710265,
40.159950202751));
#206375=CARTESIAN_POINT('Ctrl Pts',(-29.4103605382572,51.0989122516725,
40.1002552791547));
#206376=CARTESIAN_POINT('Ctrl Pts',(-29.4568175306711,51.1533747228777,
40.10025));
#206377=CARTESIAN_POINT('Ctrl Pts',(-29.4472515437731,51.0345602039889,
40.1599502534424));
#206378=CARTESIAN_POINT('Ctrl Pts',(-29.4658956314762,51.066871973898,40.10025));
#206379=CARTESIAN_POINT('Ctrl Pts',(-29.5010785149107,51.127846865905,40.10025));
#206380=CARTESIAN_POINT('Origin',(-29.5010785149107,51.127846865905,40.22725));
#206381=CARTESIAN_POINT('Ctrl Pts',(-31.2097904767601,53.4219427993289,
38.989));
#206382=CARTESIAN_POINT('Ctrl Pts',(-31.0996409281616,53.4855376708634,
38.989));
#206383=CARTESIAN_POINT('Ctrl Pts',(-31.0998053730483,53.4854427285638,
39.1161896013272));
#206384=CARTESIAN_POINT('Ctrl Pts',(-31.3184716867872,53.6097387976561,
38.989));
#206385=CARTESIAN_POINT('Ctrl Pts',(-31.2082219299917,53.6736064794776,
38.9887769275436));
#206386=CARTESIAN_POINT('Ctrl Pts',(-31.1865640704865,53.6357132000293,
39.1161898821829));
#206387=CARTESIAN_POINT('Ctrl Pts',(-31.4219325588441,53.7885186806146,
39.1034967087243));
#206388=CARTESIAN_POINT('Ctrl Pts',(-31.3115622968571,53.8525981958214,
39.1031720232723));
#206389=CARTESIAN_POINT('Ctrl Pts',(-31.2691568563324,53.7787681009859,
39.2077529615016));
#206390=CARTESIAN_POINT('Ctrl Pts',(-31.4795232016785,53.8880358395973,
39.2875012672119));
#206391=CARTESIAN_POINT('Ctrl Pts',(-31.3691313396255,53.9523112232412,
39.2872087095508));
#206392=CARTESIAN_POINT('Ctrl Pts',(-31.3151318380577,53.8583991049519,
39.354901704823));
#206393=CARTESIAN_POINT('Origin',(-31.2097904767601,53.4219427993289,39.116));
#206394=CARTESIAN_POINT('Origin',(3.82640399828021E-16,5.07986659106885E-17,
40.22725));
#206395=CARTESIAN_POINT('Origin',(-29.527474969218,51.112606865905,40.22725));
#206396=CARTESIAN_POINT('Origin',(15.2806508669887,-27.1018636743464,39.116));
#206397=CARTESIAN_POINT('Origin',(-31.0091584503668,53.0743345559679,39.1160373285238));
#206398=CARTESIAN_POINT('Ctrl Pts',(-29.4735998357333,51.019348010533,40.1599502534424));
#206399=CARTESIAN_POINT('Ctrl Pts',(-29.4922606054642,51.0516501490689,
40.10025));
#206400=CARTESIAN_POINT('Ctrl Pts',(-29.527474969218,51.112606865905,40.10025));
#206401=CARTESIAN_POINT('Ctrl Pts',(-29.5495039426964,50.9754987628535,
40.1599500566041));
#206402=CARTESIAN_POINT('Ctrl Pts',(-29.5475581014565,51.0197013834509,
40.100255130536));
#206403=CARTESIAN_POINT('Ctrl Pts',(-29.5715624158006,51.0871269269771,
40.10025));
#206404=CARTESIAN_POINT('Ctrl Pts',(-29.6319914129668,50.9562029902291,
40.1203070619046));
#206405=CARTESIAN_POINT('Ctrl Pts',(-29.6100038038524,51.0098791271086,
40.0637098684499));
#206406=CARTESIAN_POINT('Ctrl Pts',(-29.6246193648992,51.0848223701589,
40.0772636213362));
#206407=CARTESIAN_POINT('Ctrl Pts',(-29.7600395375186,50.9652607924608,
40.0046102245801));
#206408=CARTESIAN_POINT('Ctrl Pts',(-29.695116411909,51.0303675504167,39.9670001894012));
#206409=CARTESIAN_POINT('Ctrl Pts',(-29.7140610042227,51.1161687394137,
40.010178881121));
#206410=CARTESIAN_POINT('Ctrl Pts',(-29.8061925581062,50.9919958361059,
39.9303710930186));
#206411=CARTESIAN_POINT('Ctrl Pts',(-29.7178148857793,51.0613912713645,
39.9058663574112));
#206412=CARTESIAN_POINT('Ctrl Pts',(-29.7505571803535,51.1484765898565,
39.9671344706366));
#206413=CARTESIAN_POINT('Ctrl Pts',(-29.8289013456881,51.0313275753412,
39.8576902534424));
#206414=CARTESIAN_POINT('Ctrl Pts',(-29.7196599535388,51.0949610232004,
39.8579948730704));
#206415=CARTESIAN_POINT('Ctrl Pts',(-29.7732664904675,51.1878102687788,
39.92499));
#206416=CARTESIAN_POINT('Origin',(-29.8832517167481,51.1243102687788,39.92499));
#206417=CARTESIAN_POINT('Origin',(-30.9870007553615,53.0360596824725,39.1925554488852));
#206418=CARTESIAN_POINT('Origin',(-30.9460815882863,52.9651856060848,39.3343017080178));
#206419=CARTESIAN_POINT('Origin',(-29.9723263949791,51.2785921372021,39.6398955069213));
#206420=CARTESIAN_POINT('Origin',(-30.0614010732032,51.4328740054946,39.3548010137695));
#206421=CARTESIAN_POINT('Ctrl Pts',(-30.7811015270739,52.679431757829,39.3978017080178));
#206422=CARTESIAN_POINT('Ctrl Pts',(-30.6711163007932,52.742931757829,39.3978017080178));
#206423=CARTESIAN_POINT('Ctrl Pts',(-30.6711163007932,52.742931757829,39.5248017080178));
#206424=CARTESIAN_POINT('Ctrl Pts',(-30.8259039490945,52.7575002129179,
39.3978017080178));
#206425=CARTESIAN_POINT('Ctrl Pts',(-30.7160792752572,52.8208099140567,
39.3980355775187));
#206426=CARTESIAN_POINT('Ctrl Pts',(-30.7386233329133,52.8598573673291,
39.5248015517178));
#206427=CARTESIAN_POINT('Ctrl Pts',(-30.868269596017,52.8313189037794,39.3484893995498));
#206428=CARTESIAN_POINT('Ctrl Pts',(-30.7588072175368,52.8948168809906,
39.3489438303419));
#206429=CARTESIAN_POINT('Ctrl Pts',(-30.802456034311,52.9704188493343,39.4508333155597));
#206430=CARTESIAN_POINT('Ctrl Pts',(-30.8905967158731,52.8702215132219,
39.2708017080178));
#206431=CARTESIAN_POINT('Ctrl Pts',(-30.7813498801527,52.9338619179798,
39.2710850691866));
#206432=CARTESIAN_POINT('Ctrl Pts',(-30.8360963620057,53.0286856060849,
39.3343017080178));
#206433=CARTESIAN_POINT('Origin',(-30.7811015270739,52.679431757829,39.5248017080178));
#206434=CARTESIAN_POINT('Ctrl Pts',(-30.0070536838153,51.33988956927,39.2875012672119));
#206435=CARTESIAN_POINT('Ctrl Pts',(-29.897644576157,51.4036173326915,39.2878045257519));
#206436=CARTESIAN_POINT('Ctrl Pts',(-29.9514963916949,51.4965132298826,
39.3549015218349));
#206437=CARTESIAN_POINT('Ctrl Pts',(-30.0646513737685,51.4394048060594,
39.1034938540228));
#206438=CARTESIAN_POINT('Ctrl Pts',(-29.9550530981037,51.5030523579604,
39.103828627882));
#206439=CARTESIAN_POINT('Ctrl Pts',(-29.9974722043259,51.5761456730022,
39.2077506434042));
#206440=CARTESIAN_POINT('Ctrl Pts',(-30.1681227811168,51.6181806476915,
38.989));
#206441=CARTESIAN_POINT('Ctrl Pts',(-30.058267491178,51.6818259279779,38.9892298954593));
#206442=CARTESIAN_POINT('Ctrl Pts',(-30.0800656843523,51.7192017762872,
39.1161900347273));
#206443=CARTESIAN_POINT('Ctrl Pts',(-30.2768083268876,51.8059703131949,
38.989));
#206444=CARTESIAN_POINT('Ctrl Pts',(-30.1666583504929,51.8695654317176,
38.989));
#206445=CARTESIAN_POINT('Ctrl Pts',(-30.1668232238143,51.8694702420611,
39.1161900945648));
#206446=CARTESIAN_POINT('Origin',(-30.2768083268876,51.8059703131949,39.116));
#206447=CARTESIAN_POINT('Origin',(14.903849434298,-26.4492244485613,39.5248017080178));
#206448=CARTESIAN_POINT('Origin',(-30.7054974692364,52.5484816883962,39.5248017080178));
#206449=CARTESIAN_POINT('Origin',(14.8448439902557,-26.3470240215568,39.116));
#206450=CARTESIAN_POINT('Origin',(-30.4775331296737,52.1535342613176,39.1160402713853));
#206451=CARTESIAN_POINT('Ctrl Pts',(-30.5960088312564,52.3576880233165,
39.2708017080178));
#206452=CARTESIAN_POINT('Ctrl Pts',(-30.4857749404415,52.4219111049559,
39.2705119464801));
#206453=CARTESIAN_POINT('Ctrl Pts',(-30.4305321463772,52.3262277788844,
39.3343017080178));
#206454=CARTESIAN_POINT('Ctrl Pts',(-30.6184089696597,52.396723545737,39.3487519301186));
#206455=CARTESIAN_POINT('Ctrl Pts',(-30.5081585269339,52.4606806140172,
39.3482879463988));
#206456=CARTESIAN_POINT('Ctrl Pts',(-30.4642861617682,52.384691448501,39.451227126164));
#206457=CARTESIAN_POINT('Ctrl Pts',(-30.660846452162,52.4706758922786,39.3978017080178));
#206458=CARTESIAN_POINT('Ctrl Pts',(-30.5506153465205,52.5342179826678,
39.3975673827397));
#206459=CARTESIAN_POINT('Ctrl Pts',(-30.528232593673,52.4954499175231,39.5248015355181));
#206460=CARTESIAN_POINT('Ctrl Pts',(-30.7054974692364,52.5484816883962,
39.3978017080178));
#206461=CARTESIAN_POINT('Ctrl Pts',(-30.5955122429558,52.6119816883962,
39.3978017080178));
#206462=CARTESIAN_POINT('Ctrl Pts',(-30.5955122429558,52.6119816883962,
39.5248017080178));
#206463=CARTESIAN_POINT('Origin',(-30.5405173726578,52.2627277788844,39.3343017080178));
#206464=CARTESIAN_POINT('Origin',(-30.4998422394556,52.1922763809708,39.193400853355));
#206465=CARTESIAN_POINT('Origin',(-24.6933715417274,56.2428239377275,39.1925554495085));
#206466=CARTESIAN_POINT('Origin',(-24.7113125977903,56.2832472948513,39.1160373285287));
#206467=CARTESIAN_POINT('Origin',(-24.6600848917106,56.168060898428,39.3343017080178));
#206468=CARTESIAN_POINT('Ctrl Pts',(-24.6158705164589,56.0673542004328,
39.2708017080178));
#206469=CARTESIAN_POINT('Ctrl Pts',(-24.731570364333,56.01637854512,39.2710850691866));
#206470=CARTESIAN_POINT('Ctrl Pts',(-24.7761051648312,56.1164053447574,
39.3343017080178));
#206471=CARTESIAN_POINT('Ctrl Pts',(-24.5974591883321,56.0262864882909,
39.3487519293518));
#206472=CARTESIAN_POINT('Ctrl Pts',(-24.7131705636667,55.9750519161912,
39.3492068662931));
#206473=CARTESIAN_POINT('Ctrl Pts',(-24.7486471852354,56.0547337128479,
39.4512271248745));
#206474=CARTESIAN_POINT('Ctrl Pts',(-24.5625784858788,55.9484840819677,
39.3978017080178));
#206475=CARTESIAN_POINT('Ctrl Pts',(-24.6783511906864,55.8968463240355,
39.398034778116));
#206476=CARTESIAN_POINT('Ctrl Pts',(-24.6966284839301,55.9378977967857,
39.5248015355176));
#206477=CARTESIAN_POINT('Ctrl Pts',(-24.5258780191666,55.8666273273835,
39.3978017080178));
#206478=CARTESIAN_POINT('Ctrl Pts',(-24.6418982922872,55.8149717737129,
39.3978017080178));
#206479=CARTESIAN_POINT('Ctrl Pts',(-24.6418982922872,55.8149717737129,
39.5248017080178));
#206480=CARTESIAN_POINT('Origin',(-24.5258780191666,55.8666273273835,39.5248017080178));
#206481=CARTESIAN_POINT('Origin',(0.290050682801532,0.129138884176564,39.116));
#206482=CARTESIAN_POINT('Origin',(-24.8746050278048,56.6498810128384,39.116));
#206483=CARTESIAN_POINT('Origin',(0.290050682801533,0.129138884176564,39.5248017080178));
#206484=CARTESIAN_POINT('Origin',(-24.4643761377912,55.72849184015,39.5248017080178));
#206485=CARTESIAN_POINT('Ctrl Pts',(-25.0931373005741,57.1420619865023,
39.2875012672119));
#206486=CARTESIAN_POINT('Ctrl Pts',(-25.2100238766574,57.0905332211013,
39.287208709576));
#206487=CARTESIAN_POINT('Ctrl Pts',(-25.165787501526,56.9916465525425,39.3549016990122));
#206488=CARTESIAN_POINT('Ctrl Pts',(-25.0464764504208,57.0369738651811,
39.1034939173931));
#206489=CARTESIAN_POINT('Ctrl Pts',(-25.1631918674125,56.9853474458547,
39.103169233632));
#206490=CARTESIAN_POINT('Ctrl Pts',(-25.1283875141299,56.9076448051888,
39.2077507202312));
#206491=CARTESIAN_POINT('Ctrl Pts',(-24.9626525995179,56.8481865914869,
38.989));
#206492=CARTESIAN_POINT('Ctrl Pts',(-25.0791258042768,56.7965331449371,
38.9887769311206));
#206493=CARTESIAN_POINT('Ctrl Pts',(-25.0611999573799,56.7567390814052,
39.1161898712896));
#206494=CARTESIAN_POINT('Ctrl Pts',(-24.8746050278048,56.6498810128384,
38.989));
#206495=CARTESIAN_POINT('Ctrl Pts',(-24.9907986298332,56.598148288166,38.989));
#206496=CARTESIAN_POINT('Ctrl Pts',(-24.990625171646,56.5982255167267,39.1161895903853));
#206497=CARTESIAN_POINT('Origin',(-25.049832894896,57.0434492461381,39.3548010137695));
#206498=CARTESIAN_POINT('Ctrl Pts',(-24.4643761377912,55.72849184015,39.3978017080178));
#206499=CARTESIAN_POINT('Ctrl Pts',(-24.5803964109118,55.6768362864794,
39.3978017080178));
#206500=CARTESIAN_POINT('Ctrl Pts',(-24.5803964109118,55.6768362864794,
39.5248017080178));
#206501=CARTESIAN_POINT('Ctrl Pts',(-24.4275510972981,55.6463586582053,
39.3978017080178));
#206502=CARTESIAN_POINT('Ctrl Pts',(-24.5437506299587,55.5945285148505,
39.3975666025031));
#206503=CARTESIAN_POINT('Ctrl Pts',(-24.5254812387358,55.5534947903269,
39.5248015517182));
#206504=CARTESIAN_POINT('Ctrl Pts',(-24.3927285408598,55.5686962576409,
39.3484894016716));
#206505=CARTESIAN_POINT('Ctrl Pts',(-24.5092751529634,55.5170953257147,
39.3480259000038));
#206506=CARTESIAN_POINT('Ctrl Pts',(-24.4735550281868,55.4368666119041,
39.4508333188947));
#206507=CARTESIAN_POINT('Ctrl Pts',(-24.3743766270209,55.5277679687685,
39.2708017080178));
#206508=CARTESIAN_POINT('Ctrl Pts',(-24.4911280468221,55.4763362579877,
39.27051194648));
#206509=CARTESIAN_POINT('Ctrl Pts',(-24.4461895095984,55.3754026508177,
39.3343017080178));
#206510=CARTESIAN_POINT('Origin',(-24.3301692364778,55.4270582044883,39.3343017080178));
#206511=CARTESIAN_POINT('Origin',(-25.1222926664929,57.2061965577165,39.6398955068185));
#206512=CARTESIAN_POINT('Origin',(-25.1947524379611,57.3689438691198,39.92499));
#206513=CARTESIAN_POINT('Origin',(-24.2970811015489,55.3527410366449,39.193400853995));
#206514=CARTESIAN_POINT('Origin',(-24.2788510342437,55.3119205422647,39.1160402713851));
#206515=CARTESIAN_POINT('Ctrl Pts',(-25.5918112338789,57.5176823163891,
40.1599502534424));
#206516=CARTESIAN_POINT('Ctrl Pts',(-25.5766462455171,57.483598953748,40.10025));
#206517=CARTESIAN_POINT('Ctrl Pts',(-25.5480287005713,57.4192809246791,
40.10025));
#206518=CARTESIAN_POINT('Ctrl Pts',(-25.5113050800551,57.5535024391257,
40.1599500538466));
#206519=CARTESIAN_POINT('Ctrl Pts',(-25.5180031505006,57.509687971276,40.1002448353478));
#206520=CARTESIAN_POINT('Ctrl Pts',(-25.501424950013,57.4400067642803,40.10025));
#206521=CARTESIAN_POINT('Ctrl Pts',(-25.4268488592814,57.5636994104962,
40.1202442001039));
#206522=CARTESIAN_POINT('Ctrl Pts',(-25.4545932086369,57.5125855880061,
40.0633873868018));
#206523=CARTESIAN_POINT('Ctrl Pts',(-25.4482497003379,57.436276971477,40.0772271723538));
#206524=CARTESIAN_POINT('Ctrl Pts',(-25.2998561687908,57.5406963524573,
40.0045995998162));
#206525=CARTESIAN_POINT('Ctrl Pts',(-25.3719956870765,57.482850784337,39.9663485808315));
#206526=CARTESIAN_POINT('Ctrl Pts',(-25.3622939683643,57.3950038423351,
40.0101727202465));
#206527=CARTESIAN_POINT('Ctrl Pts',(-25.2565567136854,57.5090991591925,
39.9304654349859));
#206528=CARTESIAN_POINT('Ctrl Pts',(-25.3528760603481,57.4495482434222,
39.9051900162946));
#206529=CARTESIAN_POINT('Ctrl Pts',(-25.3292685758745,57.3588307079389,
39.9671857458169));
#206530=CARTESIAN_POINT('Ctrl Pts',(-25.2380597013425,57.4675553545143,
39.8576902534424));
#206531=CARTESIAN_POINT('Ctrl Pts',(-25.354767599671,57.4161024530845,39.8573998014387));
#206532=CARTESIAN_POINT('Ctrl Pts',(-25.3107727110817,57.3172883154492,
39.92499));
#206533=CARTESIAN_POINT('Origin',(-25.5480287005713,57.4192809246791,40.22725));
#206534=CARTESIAN_POINT('Origin',(0.290050682801532,0.129138884176564,39.116));
#206535=CARTESIAN_POINT('Origin',(-24.1156489724272,54.9452378026831,39.116));
#206536=CARTESIAN_POINT('Origin',(3.68589728140376E-17,-1.5063413852568E-16,
40.22725));
#206537=CARTESIAN_POINT('Origin',(-25.5758735661203,57.4068835917982,40.22725));
#206538=CARTESIAN_POINT('Ctrl Pts',(-24.1156489724272,54.9452378026831,
38.989));
#206539=CARTESIAN_POINT('Ctrl Pts',(-24.2318430491562,54.8935048666604,
38.989));
#206540=CARTESIAN_POINT('Ctrl Pts',(-24.2316691155599,54.8935823068868,
39.1161901092324));
#206541=CARTESIAN_POINT('Ctrl Pts',(-24.0276063358803,54.7469262747034,
38.989));
#206542=CARTESIAN_POINT('Ctrl Pts',(-24.1436677818718,54.695461238022,38.9892298989742));
#206543=CARTESIAN_POINT('Ctrl Pts',(-24.1610930816816,54.7350659388079,
39.1161900493186));
#206544=CARTESIAN_POINT('Ctrl Pts',(-23.9437932708526,54.55813583508,39.1034966344368));
#206545=CARTESIAN_POINT('Ctrl Pts',(-24.0597054841957,54.5068800556966,
39.1038314102578));
#206546=CARTESIAN_POINT('Ctrl Pts',(-24.0939060248989,54.5841613379354,
39.2077528789611));
#206547=CARTESIAN_POINT('Ctrl Pts',(-23.8971395307763,54.4530463244695,
39.2875012672119));
#206548=CARTESIAN_POINT('Ctrl Pts',(-24.0130054476974,54.401990730652,39.2878045257868));
#206549=CARTESIAN_POINT('Ctrl Pts',(-24.0565064959267,54.5001606201974,
39.35490152959));
#206550=CARTESIAN_POINT('Origin',(-23.9404209259116,54.5516691663897,39.3548010137695));
#206551=CARTESIAN_POINT('Ctrl Pts',(-25.8191582032616,57.2088336324701,
39.8576902534424));
#206552=CARTESIAN_POINT('Ctrl Pts',(-25.7028284190329,57.2611357920727,
39.8573998014387));
#206553=CARTESIAN_POINT('Ctrl Pts',(-25.6588335304436,57.1623216544373,
39.92499));
#206554=CARTESIAN_POINT('Ctrl Pts',(-25.837662738193,57.2503966981984,39.930498490249));
#206555=CARTESIAN_POINT('Ctrl Pts',(-25.7289639953175,57.2821216226318,
39.9052171569806));
#206556=CARTESIAN_POINT('Ctrl Pts',(-25.6773378230588,57.2038829761261,
39.9672049726605));
#206557=CARTESIAN_POINT('Ctrl Pts',(-25.8320911970515,57.3035546548414,
40.0043437678664));
#206558=CARTESIAN_POINT('Ctrl Pts',(-25.7407897001101,57.3185262575347,
39.966162857764));
#206559=CARTESIAN_POINT('Ctrl Pts',(-25.6820441386713,57.2524664994808,
40.0100243556236));
#206560=CARTESIAN_POINT('Ctrl Pts',(-25.7649464042476,57.4126476234252,
40.1194874821986));
#206561=CARTESIAN_POINT('Ctrl Pts',(-25.7081127933381,57.3992776612639,
40.0627551483143));
#206562=CARTESIAN_POINT('Ctrl Pts',(-25.6555720179783,57.3434500727656,
40.0767884282376));
#206563=CARTESIAN_POINT('Ctrl Pts',(-25.7004590347003,57.4692856961542,
40.1599502015394));
#206564=CARTESIAN_POINT('Ctrl Pts',(-25.6633754510794,57.4449640631536,
40.1002449453872));
#206565=CARTESIAN_POINT('Ctrl Pts',(-25.6226140882776,57.3860499078786,
40.10025));
#206566=CARTESIAN_POINT('Ctrl Pts',(-25.6197038181293,57.5052637377734,
40.1599502534424));
#206567=CARTESIAN_POINT('Ctrl Pts',(-25.6045223014057,57.4711877340331,
40.10025));
#206568=CARTESIAN_POINT('Ctrl Pts',(-25.5758735661203,57.4068835917982,
40.10025));
#206569=CARTESIAN_POINT('Origin',(-25.7748538035642,57.1106661007667,39.92499));
#206570=CARTESIAN_POINT('Origin',(-23.8679610547577,54.3889216310751,39.6398955069317));
#206571=CARTESIAN_POINT('Origin',(-23.7955011834904,54.2261740956468,39.92499));
#206572=CARTESIAN_POINT('Origin',(-25.7023940320476,56.9479187893687,39.6398955068277));
#206573=CARTESIAN_POINT('Origin',(-25.629934260499,56.785171477785,39.3548010137695));
#206574=CARTESIAN_POINT('Ctrl Pts',(-23.7522229508823,54.1275498658876,
39.8576902534424));
#206575=CARTESIAN_POINT('Ctrl Pts',(-23.8679139708563,54.0765745253538,
39.8579948730703));
#206576=CARTESIAN_POINT('Ctrl Pts',(-23.911521456611,54.1745185419762,39.92499));
#206577=CARTESIAN_POINT('Ctrl Pts',(-23.7337429357603,54.0860417646979,
39.930402071123));
#206578=CARTESIAN_POINT('Ctrl Pts',(-23.841826275586,54.0553388636023,39.9058915297381));
#206579=CARTESIAN_POINT('Ctrl Pts',(-23.8930401898202,54.1330089371358,
39.9671523786038));
#206580=CARTESIAN_POINT('Ctrl Pts',(-23.7393098712344,54.033173720707,40.0043257306694));
#206581=CARTESIAN_POINT('Ctrl Pts',(-23.8301926567295,54.018846794374,39.9667894847838));
#206582=CARTESIAN_POINT('Ctrl Pts',(-23.8884275227219,54.0846755205375,
40.01001389752));
#206583=CARTESIAN_POINT('Ctrl Pts',(-23.806518907382,53.9248984592618,40.1195533054857));
#206584=CARTESIAN_POINT('Ctrl Pts',(-23.8631501047896,53.938451117416,40.0630813209234));
#206585=CARTESIAN_POINT('Ctrl Pts',(-23.9152668978355,53.9943748351525,
40.076826594242));
#206586=CARTESIAN_POINT('Ctrl Pts',(-23.8710081209824,53.8688190939466,
40.1599502027512));
#206587=CARTESIAN_POINT('Ctrl Pts',(-23.9079567336554,53.8932068550015,
40.1002552791541));
#206588=CARTESIAN_POINT('Ctrl Pts',(-23.948466351384,53.9522270531176,40.10025));
#206589=CARTESIAN_POINT('Ctrl Pts',(-23.951372267036,53.833063494684,40.1599502534424));
#206590=CARTESIAN_POINT('Ctrl Pts',(-23.9665367208219,53.8671470951733,
40.10025));
#206591=CARTESIAN_POINT('Ctrl Pts',(-23.9951532569802,53.9314655730806,
40.10025));
#206592=CARTESIAN_POINT('Origin',(-23.9951532569802,53.9314655730806,40.22725));
#206593=CARTESIAN_POINT('Ctrl Pts',(-25.4547063934078,56.3916032444853,
38.989));
#206594=CARTESIAN_POINT('Ctrl Pts',(-25.3385127813683,56.4433359736149,
38.989));
#206595=CARTESIAN_POINT('Ctrl Pts',(-25.3386862495815,56.4432587405904,
39.1161896013274));
#206596=CARTESIAN_POINT('Ctrl Pts',(-25.5431622092821,56.5897307565543,
38.989));
#206597=CARTESIAN_POINT('Ctrl Pts',(-25.426840421553,56.6417243268743,38.988776927543));
#206598=CARTESIAN_POINT('Ctrl Pts',(-25.4092621323401,56.6017747680072,
39.1161898821832));
#206599=CARTESIAN_POINT('Ctrl Pts',(-25.627368725429,56.7783458705718,39.1034967087243));
#206600=CARTESIAN_POINT('Ctrl Pts',(-25.5109049500366,56.8305375176205,
39.1031720232707));
#206601=CARTESIAN_POINT('Ctrl Pts',(-25.4764491573047,56.7526792962324,
39.2077529615013));
#206602=CARTESIAN_POINT('Ctrl Pts',(-25.6742415049975,56.8833377255396,
39.2875012672119));
#206603=CARTESIAN_POINT('Ctrl Pts',(-25.5577357740368,56.9357219102092,
39.2872087095508));
#206604=CARTESIAN_POINT('Ctrl Pts',(-25.5138485767958,56.8366797674136,
39.3549017048232));
#206605=CARTESIAN_POINT('Origin',(-25.4547063934078,56.3916032444853,39.116));
#206606=CARTESIAN_POINT('Origin',(3.88110971579612E-16,5.35860614414083E-17,
40.22725));
#206607=CARTESIAN_POINT('Origin',(-24.0229981225292,53.9190682401997,40.22725));
#206608=CARTESIAN_POINT('Origin',(10.0037024164483,-23.2492868865826,39.116));
#206609=CARTESIAN_POINT('Origin',(-25.2915084057502,56.0249274780519,39.1160373285286));
#206610=CARTESIAN_POINT('Ctrl Pts',(-23.9791663275009,53.8206887816838,
40.1599502534424));
#206611=CARTESIAN_POINT('Ctrl Pts',(-23.9943483786813,53.8547645473083,
40.10025));
#206612=CARTESIAN_POINT('Ctrl Pts',(-24.0229981225292,53.9190682401997,
40.10025));
#206613=CARTESIAN_POINT('Ctrl Pts',(-24.0592381182997,53.785013884428,40.1599500566034));
#206614=CARTESIAN_POINT('Ctrl Pts',(-24.0526825045793,53.8287709626519,
40.100255130536));
#206615=CARTESIAN_POINT('Ctrl Pts',(-24.0695074323274,53.8983362760852,
40.10025));
#206616=CARTESIAN_POINT('Ctrl Pts',(-24.1432906710367,53.7744461045707,
40.1203070619049));
#206617=CARTESIAN_POINT('Ctrl Pts',(-24.115812828243,53.8255298669644,40.06370986845));
#206618=CARTESIAN_POINT('Ctrl Pts',(-24.1225146216891,53.9015903052236,
40.0772636213363));
#206619=CARTESIAN_POINT('Ctrl Pts',(-24.2696905364168,53.796838960898,40.0046102245799));
#206620=CARTESIAN_POINT('Ctrl Pts',(-24.1983175571254,53.8548027426712,
39.9670001894012));
#206621=CARTESIAN_POINT('Ctrl Pts',(-24.2081897025474,53.9421141528993,
40.0101788811208));
#206622=CARTESIAN_POINT('Ctrl Pts',(-24.3127961528998,53.8282518514941,
39.9303710930188));
#206623=CARTESIAN_POINT('Ctrl Pts',(-24.2176488245027,53.8880291490223,
39.9058663574119));
#206624=CARTESIAN_POINT('Ctrl Pts',(-24.2411088588481,53.9780599067625,
39.967134470637));
#206625=CARTESIAN_POINT('Ctrl Pts',(-24.3312692531083,53.8697418420147,
39.8576902534424));
#206626=CARTESIAN_POINT('Ctrl Pts',(-24.2159747902182,53.9216078643419,
39.8579948730703));
#206627=CARTESIAN_POINT('Ctrl Pts',(-24.2595822759728,54.0195518809643,
39.92499));
#206628=CARTESIAN_POINT('Origin',(-24.3756025490934,53.9678963272937,39.92499));
#206629=CARTESIAN_POINT('Origin',(-25.273472906618,55.984546168508,39.1925554488842));
#206630=CARTESIAN_POINT('Origin',(-25.2401862573137,55.9097831300749,39.3343017080178));
#206631=CARTESIAN_POINT('Origin',(-24.4480624203039,54.1306438627321,39.639895506923));
#206632=CARTESIAN_POINT('Origin',(-24.5205222915147,54.2933913980366,39.3548010137695));
#206633=CARTESIAN_POINT('Ctrl Pts',(-25.1059793847697,55.6083495590304,
39.3978017080178));
#206634=CARTESIAN_POINT('Ctrl Pts',(-24.9899591116491,55.660005112701,39.3978017080178));
#206635=CARTESIAN_POINT('Ctrl Pts',(-24.9899591116491,55.660005112701,39.5248017080178));
#206636=CARTESIAN_POINT('Ctrl Pts',(-25.1423759987949,55.6906734752782,
39.3978017080178));
#206637=CARTESIAN_POINT('Ctrl Pts',(-25.0265352902402,55.7421565548672,
39.3980355775163));
#206638=CARTESIAN_POINT('Ctrl Pts',(-25.0448742789051,55.7833465978032,
39.5248015517178));
#206639=CARTESIAN_POINT('Ctrl Pts',(-25.1767934079549,55.7685161955953,
39.3484893995498));
#206640=CARTESIAN_POINT('Ctrl Pts',(-25.0612933298573,55.820224390034,39.3489438303431));
#206641=CARTESIAN_POINT('Ctrl Pts',(-25.0968004762773,55.8999747466301,
39.4508333155605));
#206642=CARTESIAN_POINT('Ctrl Pts',(-25.1949317875296,55.8095395120009,
39.2708017080178));
#206643=CARTESIAN_POINT('Ctrl Pts',(-25.0796311836949,55.8614118841081,
39.2710850691866));
#206644=CARTESIAN_POINT('Ctrl Pts',(-25.1241659841931,55.9614386837455,
39.3343017080178));
#206645=CARTESIAN_POINT('Origin',(-25.1059793847697,55.6083495590304,39.5248017080178));
#206646=CARTESIAN_POINT('Ctrl Pts',(-24.4761921430387,54.1952354911874,
39.2875012672119));
#206647=CARTESIAN_POINT('Ctrl Pts',(-24.3607210247419,54.247177781362,39.2878045257519));
#206648=CARTESIAN_POINT('Ctrl Pts',(-24.4045675690225,54.3451938326307,
39.3549015218349));
#206649=CARTESIAN_POINT('Ctrl Pts',(-24.523072132049,54.3002261711148,39.1034938540228));
#206650=CARTESIAN_POINT('Ctrl Pts',(-24.4074212664148,54.3520689157386,
39.1038286278812));
#206651=CARTESIAN_POINT('Ctrl Pts',(-24.4419676644362,54.4291958219377,
39.2077506434045));
#206652=CARTESIAN_POINT('Ctrl Pts',(-24.6072895482032,54.4888383671844,
38.989));
#206653=CARTESIAN_POINT('Ctrl Pts',(-24.4913833136934,54.5406519873246,
38.9892298954618));
#206654=CARTESIAN_POINT('Ctrl Pts',(-24.5091552540989,54.580101618462,39.1161900347274));
#206655=CARTESIAN_POINT('Ctrl Pts',(-24.6957503380303,54.6869600343299,
38.989));
#206656=CARTESIAN_POINT('Ctrl Pts',(-24.5795562747208,54.7386929643778,
38.989));
#206657=CARTESIAN_POINT('Ctrl Pts',(-24.5797301948775,54.7386155301351,
39.1161900945648));
#206658=CARTESIAN_POINT('Origin',(-24.6957503380303,54.6869600343299,39.116));
#206659=CARTESIAN_POINT('Origin',(9.75435829333325,-22.6892508167094,39.5248017080178));
#206660=CARTESIAN_POINT('Origin',(-25.0444775033943,55.4702140717969,39.5248017080178));
#206661=CARTESIAN_POINT('Origin',(9.71531210234964,-22.6015516358793,39.116));
#206662=CARTESIAN_POINT('Origin',(-24.8590452239599,55.0536014459538,39.1160402713851));
#206663=CARTESIAN_POINT('Ctrl Pts',(-24.955532024241,55.2690209153042,39.2708017080178));
#206664=CARTESIAN_POINT('Ctrl Pts',(-24.839188866184,55.3213695969758,39.27051194648));
#206665=CARTESIAN_POINT('Ctrl Pts',(-24.7942503289602,55.2204359898058,
39.3343017080178));
#206666=CARTESIAN_POINT('Ctrl Pts',(-24.9737291291715,55.3101840490926,
39.3487519301186));
#206667=CARTESIAN_POINT('Ctrl Pts',(-24.8573973158448,55.362266444506,39.3482879463992));
#206668=CARTESIAN_POINT('Ctrl Pts',(-24.8217083187807,55.2821076446801,
39.4512271261643));
#206669=CARTESIAN_POINT('Ctrl Pts',(-25.0082040095649,55.3881672017732,
39.3978017080178));
#206670=CARTESIAN_POINT('Ctrl Pts',(-24.8919348043934,55.4398389138667,
39.3975673827397));
#206671=CARTESIAN_POINT('Ctrl Pts',(-24.8737270328808,55.3989435894802,
39.5248015355181));
#206672=CARTESIAN_POINT('Ctrl Pts',(-25.0444775033943,55.4702140717969,
39.3978017080178));
#206673=CARTESIAN_POINT('Ctrl Pts',(-24.9284572302737,55.5218696254675,
39.3978017080178));
#206674=CARTESIAN_POINT('Ctrl Pts',(-24.9284572302736,55.5218696254675,
39.5248017080178));
#206675=CARTESIAN_POINT('Origin',(-24.9102706020808,55.1687804361352,39.3343017080178));
#206676=CARTESIAN_POINT('Origin',(-24.8771824678736,55.0944632691849,39.1934008533545));
#206677=CARTESIAN_POINT('Origin',(-18.6791227126682,58.5158800435661,39.1925554495081));
#206678=CARTESIAN_POINT('Origin',(-18.6927400943481,58.5579573083294,39.1160373285272));
#206679=CARTESIAN_POINT('Origin',(-18.6538332760099,58.4380471616456,39.3343017080178));
#206680=CARTESIAN_POINT('Ctrl Pts',(-18.6203878281142,58.3332704847798,
39.2708017080178));
#206681=CARTESIAN_POINT('Ctrl Pts',(-18.7407822670297,58.294668006739,39.2710850691866));
#206682=CARTESIAN_POINT('Ctrl Pts',(-18.7746174535794,58.39880200336,39.3343017080178));
#206683=CARTESIAN_POINT('Ctrl Pts',(-18.6063701040097,58.2905032380261,
39.3487519293518));
#206684=CARTESIAN_POINT('Ctrl Pts',(-18.7268030714138,58.2516444665218,
39.3492068662926));
#206685=CARTESIAN_POINT('Ctrl Pts',(-18.7537563325798,58.3345980746928,
39.4512271248738));
#206686=CARTESIAN_POINT('Ctrl Pts',(-18.5798130476652,58.2094810152003,
39.3978017080178));
#206687=CARTESIAN_POINT('Ctrl Pts',(-18.7003491529649,58.1702276772286,
39.3980347781178));
#206688=CARTESIAN_POINT('Ctrl Pts',(-18.7142352739229,58.2129647630925,
39.524801535519));
#206689=CARTESIAN_POINT('Ctrl Pts',(-18.5518699907145,58.1242364370958,
39.3978017080178));
#206690=CARTESIAN_POINT('Ctrl Pts',(-18.672654168284,58.0849912788102,39.3978017080178));
#206691=CARTESIAN_POINT('Ctrl Pts',(-18.672654168284,58.0849912788102,39.5248017080178));
#206692=CARTESIAN_POINT('Origin',(-18.5518699907145,58.1242364370958,39.5248017080178));
#206693=CARTESIAN_POINT('Origin',(0.301960443923718,0.0981128957140429,
39.116));
#206694=CARTESIAN_POINT('Origin',(-18.8168143322221,58.9396512752215,39.116));
#206695=CARTESIAN_POINT('Origin',(0.301960443923718,0.0981128957140429,
39.5248017080178));
#206696=CARTESIAN_POINT('Origin',(-18.5051441132836,57.9804289733665,39.5248017080178));
#206697=CARTESIAN_POINT('Ctrl Pts',(-18.9827025415091,59.4519788726609,
39.2875012672119));
#206698=CARTESIAN_POINT('Ctrl Pts',(-19.1043350233607,59.4129503614027,
39.287208709576));
#206699=CARTESIAN_POINT('Ctrl Pts',(-19.0706774512221,59.3099814440477,
39.3549016990125));
#206700=CARTESIAN_POINT('Ctrl Pts',(-18.9472820042043,59.3425890481026,
39.1034939173931));
#206701=CARTESIAN_POINT('Ctrl Pts',(-19.0687544722108,59.3034455268866,
39.1031692336336));
#206702=CARTESIAN_POINT('Ctrl Pts',(-19.042262918434,59.2225305038497,39.2077507202307));
#206703=CARTESIAN_POINT('Ctrl Pts',(-18.8836509927328,59.1460739925263,
38.989));
#206704=CARTESIAN_POINT('Ctrl Pts',(-19.0048854004771,59.1068782740618,
38.9887769311158));
#206705=CARTESIAN_POINT('Ctrl Pts',(-18.9912173655535,59.0654284453474,
39.1161898712903));
#206706=CARTESIAN_POINT('Ctrl Pts',(-18.8168143322221,58.9396512752215,
38.989));
#206707=CARTESIAN_POINT('Ctrl Pts',(-18.9377789557524,58.9003474864891,
38.989));
#206708=CARTESIAN_POINT('Ctrl Pts',(-18.9375983752039,58.9004061606661,
39.116189590386));
#206709=CARTESIAN_POINT('Origin',(-18.9499432001052,59.3493798002282,39.3548010137695));
#206710=CARTESIAN_POINT('Ctrl Pts',(-18.5051441132836,57.9804289733665,
39.3978017080178));
#206711=CARTESIAN_POINT('Ctrl Pts',(-18.6259282908531,57.9411838150809,
39.3978017080178));
#206712=CARTESIAN_POINT('Ctrl Pts',(-18.6259282908531,57.9411838150809,
39.5248017080178));
#206713=CARTESIAN_POINT('Ctrl Pts',(-18.477106059507,57.8948964606938,39.3978017080178));
#206714=CARTESIAN_POINT('Ctrl Pts',(-18.5980867642062,57.8554964068695,
39.3975666025045));
#206715=CARTESIAN_POINT('Ctrl Pts',(-18.5842066467862,57.8127777979925,
39.5248015517196));
#206716=CARTESIAN_POINT('Ctrl Pts',(-18.4505921960625,57.8140195545737,
39.3484894016716));
#206717=CARTESIAN_POINT('Ctrl Pts',(-18.5718941197448,57.7748837362136,
39.348025900003));
#206718=CARTESIAN_POINT('Ctrl Pts',(-18.5447558577156,57.6913607539413,
39.4508333188939));
#206719=CARTESIAN_POINT('Ctrl Pts',(-18.4366189870667,57.7713971777989,
39.2708017080178));
#206720=CARTESIAN_POINT('Ctrl Pts',(-18.5581069080655,57.7324510618072,
39.27051194648));
#206721=CARTESIAN_POINT('Ctrl Pts',(-18.5239649837002,57.6273730232607,
39.3343017080178));
#206722=CARTESIAN_POINT('Origin',(-18.4031808061308,57.6666181815463,39.3343017080178));
#206723=CARTESIAN_POINT('Origin',(-19.0049943031126,59.5188096735815,39.6398955068167));
#206724=CARTESIAN_POINT('Origin',(-19.0600454060081,59.6882395467422,39.92499));
#206725=CARTESIAN_POINT('Origin',(-18.3780421908181,57.5892494790287,39.1934008539941));
#206726=CARTESIAN_POINT('Origin',(-18.3641788932749,57.5467470426663,39.1160402713848));
#206727=CARTESIAN_POINT('Ctrl Pts',(-19.4393816709751,59.8776671349987,
40.1599502534424));
#206728=CARTESIAN_POINT('Ctrl Pts',(-19.4278624395261,59.8421853116554,
40.10025));
#206729=CARTESIAN_POINT('Ctrl Pts',(-19.4061247292248,59.7752282754839,
40.10025));
#206730=CARTESIAN_POINT('Ctrl Pts',(-19.3555723159017,59.9048758468123,
40.1599500538465));
#206731=CARTESIAN_POINT('Ctrl Pts',(-19.3668135526094,59.8620015382124,
40.100244835349));
#206732=CARTESIAN_POINT('Ctrl Pts',(-19.357609838725,59.7909691583393,40.10025));
#206733=CARTESIAN_POINT('Ctrl Pts',(-19.2705128813948,59.9061888791357,
40.1202442001037));
#206734=CARTESIAN_POINT('Ctrl Pts',(-19.3034480936183,59.8582551377153,
40.0633873868015));
#206735=CARTESIAN_POINT('Ctrl Pts',(-19.3051157581413,59.7817014705981,
40.0772271723539));
#206736=CARTESIAN_POINT('Ctrl Pts',(-19.1466203444575,59.8700374834727,
40.0045995998165));
#206737=CARTESIAN_POINT('Ctrl Pts',(-19.2244111832563,59.8200494324148,
39.9663485808318));
#206738=CARTESIAN_POINT('Ctrl Pts',(-19.2239451174246,59.7316696194043,
40.0101727202464));
#206739=CARTESIAN_POINT('Ctrl Pts',(-19.1068608943535,59.8340873574358,
39.9304654349858));
#206740=CARTESIAN_POINT('Ctrl Pts',(-19.2088773592686,59.7849307811033,
39.9051900162937));
#206741=CARTESIAN_POINT('Ctrl Pts',(-19.1948817636402,59.6922425516967,
39.9671857458174));
#206742=CARTESIAN_POINT('Ctrl Pts',(-19.0928077206406,59.7908376697913,
39.8576902534424));
#206743=CARTESIAN_POINT('Ctrl Pts',(-19.2142545736078,59.7518659300027,
39.8573998014387));
#206744=CARTESIAN_POINT('Ctrl Pts',(-19.1808295835776,59.6489943884566,
39.92499));
#206745=CARTESIAN_POINT('Origin',(-19.4061247292248,59.7752282754839,40.22725));
#206746=CARTESIAN_POINT('Origin',(0.301960443923718,0.0981128957140429,
39.116));
#206747=CARTESIAN_POINT('Origin',(-18.240199652704,57.1650137687749,39.116));
#206748=CARTESIAN_POINT('Origin',(2.07460197300492E-17,-1.56819321712836E-16,
40.22725));
#206749=CARTESIAN_POINT('Origin',(-19.4351129318415,59.7658094374953,40.22725));
#206750=CARTESIAN_POINT('Ctrl Pts',(-18.240199652704,57.1650137687749,38.989));
#206751=CARTESIAN_POINT('Ctrl Pts',(-18.3611647704257,57.12570981947,38.989));
#206752=CARTESIAN_POINT('Ctrl Pts',(-18.3609836949481,57.1257686544591,
39.1161901092322));
#206753=CARTESIAN_POINT('Ctrl Pts',(-18.1733685221997,56.958585650595,38.989));
#206754=CARTESIAN_POINT('Ctrl Pts',(-18.2941737326416,56.9195342693631,
38.9892298989724));
#206755=CARTESIAN_POINT('Ctrl Pts',(-18.3073637563256,56.9607434512644,
39.1161900493184));
#206756=CARTESIAN_POINT('Ctrl Pts',(-18.1097485684441,56.7620685738645,
39.1034966344368));
#206757=CARTESIAN_POINT('Ctrl Pts',(-18.2303834904091,56.7232097045386,
39.1038314102595));
#206758=CARTESIAN_POINT('Ctrl Pts',(-18.2563185832998,56.8036425617904,
39.2077528789613));
#206759=CARTESIAN_POINT('Ctrl Pts',(-18.0743352474886,56.6526781108325,
39.2875012672119));
#206760=CARTESIAN_POINT('Ctrl Pts',(-18.1949032015563,56.6140134911409,
39.2878045257868));
#206761=CARTESIAN_POINT('Ctrl Pts',(-18.2279043987986,56.7161926934814,
39.3549015295899));
#206762=CARTESIAN_POINT('Origin',(-18.1070706485037,56.7552848242272,39.3548010137695));
#206763=CARTESIAN_POINT('Ctrl Pts',(-19.697766688184,59.5942745858238,39.8576902534424));
#206764=CARTESIAN_POINT('Ctrl Pts',(-19.5766071063163,59.6341304551459,
39.8573998014387));
#206765=CARTESIAN_POINT('Ctrl Pts',(-19.5431821162861,59.5312589135997,
39.92499));
#206766=CARTESIAN_POINT('Ctrl Pts',(-19.7118253299475,59.6375442153291,
39.9304984902489));
#206767=CARTESIAN_POINT('Ctrl Pts',(-19.6004058925609,59.6577332347567,
39.9052171569792));
#206768=CARTESIAN_POINT('Ctrl Pts',(-19.5572406993628,59.574526783291,39.9672049726606));
#206769=CARTESIAN_POINT('Ctrl Pts',(-19.700727790773,59.6898285824901,40.0043437678664));
#206770=CARTESIAN_POINT('Ctrl Pts',(-19.6083614943627,59.6951745640082,
39.9661628577646));
#206771=CARTESIAN_POINT('Ctrl Pts',(-19.5568428722492,59.6233361049589,
40.0100243556237));
#206772=CARTESIAN_POINT('Ctrl Pts',(-19.6225475038105,59.791305386369,40.1194874821985));
#206773=CARTESIAN_POINT('Ctrl Pts',(-19.5674227749668,59.7720679362489,
40.0627551483138));
#206774=CARTESIAN_POINT('Ctrl Pts',(-19.5210053955057,59.7110541706153,
40.0767884282375));
#206775=CARTESIAN_POINT('Ctrl Pts',(-19.5524931121158,59.8408924241704,
40.1599502015391));
#206776=CARTESIAN_POINT('Ctrl Pts',(-19.5181549791682,59.8128277376128,
40.1002449453872));
#206777=CARTESIAN_POINT('Ctrl Pts',(-19.4837751174919,59.7499755976288,
40.10025));
#206778=CARTESIAN_POINT('Ctrl Pts',(-19.4684195516691,59.8682321556243,
40.1599502534424));
#206779=CARTESIAN_POINT('Ctrl Pts',(-19.4568831131878,59.8327559231848,
40.10025));
#206780=CARTESIAN_POINT('Ctrl Pts',(-19.4351129318415,59.7658094374953,
40.10025));
#206781=CARTESIAN_POINT('Origin',(-19.6639662938556,59.4920137553141,39.92499));
#206782=CARTESIAN_POINT('Origin',(-18.0520194698729,56.5858547179589,39.6398955069315));
#206783=CARTESIAN_POINT('Origin',(-17.9969682911406,56.4164246115665,39.92499));
#206784=CARTESIAN_POINT('Origin',(-19.6089151909109,59.3225838821518,39.6398955068272));
#206785=CARTESIAN_POINT('Origin',(-19.5538640879527,59.1531540088001,39.3548010137695));
#206786=CARTESIAN_POINT('Ctrl Pts',(-17.9642361803967,56.3138168485097,
39.8576902534424));
#206787=CARTESIAN_POINT('Ctrl Pts',(-18.084621806869,56.2752137607567,39.8579948730703));
#206788=CARTESIAN_POINT('Ctrl Pts',(-18.1177524687101,56.3771794532809,
39.92499));
#206789=CARTESIAN_POINT('Ctrl Pts',(-17.9501961787623,56.2706044454594,
39.930402071123));
#206790=CARTESIAN_POINT('Ctrl Pts',(-18.060896753812,56.2513675234857,39.9058915297379));
#206791=CARTESIAN_POINT('Ctrl Pts',(-18.1037113794371,56.3339654239813,
39.9671523786023));
#206792=CARTESIAN_POINT('Ctrl Pts',(-17.9612588333752,56.2186079213554,
40.0043257306694));
#206793=CARTESIAN_POINT('Ctrl Pts',(-18.0531413250546,56.2138593173285,
39.9667894847835));
#206794=CARTESIAN_POINT('Ctrl Pts',(-18.1041761987731,56.2854146278932,
40.0100138975199));
#206795=CARTESIAN_POINT('Ctrl Pts',(-18.0394175380792,56.1179510603878,
40.1195533054856));
#206796=CARTESIAN_POINT('Ctrl Pts',(-18.0943218653324,56.1373490477013,
40.0630813209237));
#206797=CARTESIAN_POINT('Ctrl Pts',(-18.1403075368577,56.1984140977481,
40.0768265942422));
#206798=CARTESIAN_POINT('Ctrl Pts',(-18.1094153628975,56.0689198620986,
40.1599502027507));
#206799=CARTESIAN_POINT('Ctrl Pts',(-18.1436123520187,56.0970362061498,
40.1002552791544));
#206800=CARTESIAN_POINT('Ctrl Pts',(-18.1777307632117,56.1599674935332,
40.10025));
#206801=CARTESIAN_POINT('Ctrl Pts',(-18.1930767435944,56.0417604764385,
40.1599502534424));
#206802=CARTESIAN_POINT('Ctrl Pts',(-18.204595418534,56.0772424804486,40.10025));
#206803=CARTESIAN_POINT('Ctrl Pts',(-18.2263320786577,56.1441998575529,
40.10025));
#206804=CARTESIAN_POINT('Origin',(-18.2263320786577,56.1441998575529,40.22725));
#206805=CARTESIAN_POINT('Ctrl Pts',(-19.4207352200695,58.7434254837934,
38.989));
#206806=CARTESIAN_POINT('Ctrl Pts',(-19.2997705861184,58.7827292759117,
38.989));
#206807=CARTESIAN_POINT('Ctrl Pts',(-19.2999511771033,58.7826705983438,
39.1161896013267));
#206808=CARTESIAN_POINT('Ctrl Pts',(-19.4879965013594,58.9497137831221,
38.989));
#206809=CARTESIAN_POINT('Ctrl Pts',(-19.3668771285512,58.9892635895131,
38.9887769275436));
#206810=CARTESIAN_POINT('Ctrl Pts',(-19.3535710010434,58.947695446948,39.1161898821825));
#206811=CARTESIAN_POINT('Ctrl Pts',(-19.5520260773864,59.1460976215386,
39.1034967087243));
#206812=CARTESIAN_POINT('Ctrl Pts',(-19.4307447900772,59.1858295778086,
39.1031720232724));
#206813=CARTESIAN_POINT('Ctrl Pts',(-19.4046161500179,59.1047962608432,
39.2077529615019));
#206814=CARTESIAN_POINT('Ctrl Pts',(-19.5876674457073,59.2554138597573,
39.2875012672119));
#206815=CARTESIAN_POINT('Ctrl Pts',(-19.4663243070086,59.2953329133627,
39.2872087095508));
#206816=CARTESIAN_POINT('Ctrl Pts',(-19.4330302514108,59.1922458725044,
39.3549017048228));
#206817=CARTESIAN_POINT('Origin',(-19.4207352200695,58.7434254837934,39.116));
#206818=CARTESIAN_POINT('Origin',(3.93842937138094E-16,5.57863568693718E-17,
40.22725));
#206819=CARTESIAN_POINT('Origin',(-18.2553202812744,56.1347810195644,40.22725));
#206820=CARTESIAN_POINT('Origin',(5.6397553624924,-18.3848338156955,39.116));
#206821=CARTESIAN_POINT('Origin',(-19.2967593024422,58.3616995707148,39.1160373285237));
#206822=CARTESIAN_POINT('Ctrl Pts',(-18.2220120550212,56.0323588238393,
40.1599502534424));
#206823=CARTESIAN_POINT('Ctrl Pts',(-18.2335490499213,56.0678348753334,
40.10025));
#206824=CARTESIAN_POINT('Ctrl Pts',(-18.2553202812744,56.1347810195644,
40.10025));
#206825=CARTESIAN_POINT('Ctrl Pts',(-18.3053742463592,56.0052491386463,
40.1599500566041));
#206826=CARTESIAN_POINT('Ctrl Pts',(-18.2942806848318,56.0480812627856,
40.1002551305372));
#206827=CARTESIAN_POINT('Ctrl Pts',(-18.3037418885554,56.1190241739962,
40.10025));
#206828=CARTESIAN_POINT('Ctrl Pts',(-18.3900709842067,56.0035251343648,
40.1203070619042));
#206829=CARTESIAN_POINT('Ctrl Pts',(-18.3574039607301,56.051456837883,40.0637098684494));
#206830=CARTESIAN_POINT('Ctrl Pts',(-18.3561185603239,56.1278011372725,
40.0772636213361));
#206831=CARTESIAN_POINT('Ctrl Pts',(-18.5134377270384,56.0390077039668,
40.0046102245806));
#206832=CARTESIAN_POINT('Ctrl Pts',(-18.4363968713612,56.0891934462333,
39.9670001894019));
#206833=CARTESIAN_POINT('Ctrl Pts',(-18.4370884086008,56.1770584756116,
40.010178881121));
#206834=CARTESIAN_POINT('Ctrl Pts',(-18.5530236652643,56.0747542753111,
39.9303710930183));
#206835=CARTESIAN_POINT('Ctrl Pts',(-18.452149134841,56.1242585025261,39.9058663574096));
#206836=CARTESIAN_POINT('Ctrl Pts',(-18.466069875907,56.2162483036951,39.9671344706363));
#206837=CARTESIAN_POINT('Ctrl Pts',(-18.567058682946,56.117947944099,39.8576902534424));
#206838=CARTESIAN_POINT('Ctrl Pts',(-18.4469743395774,56.1574782858999,
39.8579948730704));
#206839=CARTESIAN_POINT('Ctrl Pts',(-18.4801050014185,56.259443978424,39.92499));
#206840=CARTESIAN_POINT('Origin',(-18.600889178988,56.2201988201384,39.92499));
#206841=CARTESIAN_POINT('Origin',(-19.2830435998994,58.3196542512046,39.1925554488857));
#206842=CARTESIAN_POINT('Origin',(-19.2577541638573,58.2418213702175,39.3343017080178));
#206843=CARTESIAN_POINT('Origin',(-18.6559403576601,56.3896289265348,39.6398955069222));
#206844=CARTESIAN_POINT('Origin',(-18.7109915363512,56.5590590327991,39.3548010137695));
#206845=CARTESIAN_POINT('Ctrl Pts',(-19.155790878562,57.9280106456677,39.3978017080178));
#206846=CARTESIAN_POINT('Ctrl Pts',(-19.0350067009925,57.9672558039534,
39.3978017080178));
#206847=CARTESIAN_POINT('Ctrl Pts',(-19.0350067009925,57.9672558039534,
39.5248017080178));
#206848=CARTESIAN_POINT('Ctrl Pts',(-19.1833829156718,58.0136880650208,
39.3978017080178));
#206849=CARTESIAN_POINT('Ctrl Pts',(-19.0627953474461,58.0527804636625,
39.3980355775177));
#206850=CARTESIAN_POINT('Ctrl Pts',(-19.0767283413218,58.0956618095388,
39.5248015517192));
#206851=CARTESIAN_POINT('Ctrl Pts',(-19.2094750027316,58.0947019536606,
39.3484893995498));
#206852=CARTESIAN_POINT('Ctrl Pts',(-19.089202668042,58.1340538395312,39.3489438303425));
#206853=CARTESIAN_POINT('Ctrl Pts',(-19.1161791203805,58.2170788227765,
39.4508333155592));
#206854=CARTESIAN_POINT('Ctrl Pts',(-19.2232259141434,58.1373965169895,
39.2708017080178));
#206855=CARTESIAN_POINT('Ctrl Pts',(-19.1031347997382,58.1769325318821,
39.2710850691866));
#206856=CARTESIAN_POINT('Ctrl Pts',(-19.1369699862878,58.2810665285032,
39.3343017080178));
#206857=CARTESIAN_POINT('Origin',(-19.155790878562,57.9280106456677,39.5248017080178));
#206858=CARTESIAN_POINT('Ctrl Pts',(-18.6771643191705,56.4568070719813,
39.2875012672119));
#206859=CARTESIAN_POINT('Ctrl Pts',(-18.5568963159711,56.4963947983081,
39.2878045257519));
#206860=CARTESIAN_POINT('Ctrl Pts',(-18.5902571970796,56.5984571192857,
39.3549015218349));
#206861=CARTESIAN_POINT('Ctrl Pts',(-18.7128129802632,56.5661228951886,
39.1034938540228));
#206862=CARTESIAN_POINT('Ctrl Pts',(-18.5923766197454,56.6055928325716,
39.1038286278827));
#206863=CARTESIAN_POINT('Ctrl Pts',(-18.6186718120038,56.6859083114056,
39.2077506434045));
#206864=CARTESIAN_POINT('Ctrl Pts',(-18.7768537015926,56.7625049710039,
38.989));
#206865=CARTESIAN_POINT('Ctrl Pts',(-18.6561664154737,56.8019192501357,
38.9892298954593));
#206866=CARTESIAN_POINT('Ctrl Pts',(-18.6697173900114,56.843010445685,39.1161900347273));
#206867=CARTESIAN_POINT('Ctrl Pts',(-18.8441205405514,56.9687879773468,
38.989));
#206868=CARTESIAN_POINT('Ctrl Pts',(-18.7231554368002,57.0080919221124,
38.989));
#206869=CARTESIAN_POINT('Ctrl Pts',(-18.7233364982864,57.0080330916693,
39.1161900945648));
#206870=CARTESIAN_POINT('Origin',(-18.8441205405514,56.9687879773468,39.116));
#206871=CARTESIAN_POINT('Origin',(5.49583002221419,-17.9418771653389,39.5248017080178));
#206872=CARTESIAN_POINT('Origin',(-19.109065001131,57.7842031819385,39.5248017080178));
#206873=CARTESIAN_POINT('Origin',(5.4732919481113,-17.8725121057128,39.116));
#206874=CARTESIAN_POINT('Origin',(-18.9681964166823,57.3504898524415,39.1160402713845));
#206875=CARTESIAN_POINT('Ctrl Pts',(-19.0416371860872,57.5748148483578,
39.2708017080178));
#206876=CARTESIAN_POINT('Ctrl Pts',(-18.920459440774,57.6147155869504,39.27051194648));
#206877=CARTESIAN_POINT('Ctrl Pts',(-18.8863175164087,57.5096375484038,
39.3343017080178));
#206878=CARTESIAN_POINT('Ctrl Pts',(-19.0554318862554,57.6176546016064,
39.3487519301186));
#206879=CARTESIAN_POINT('Ctrl Pts',(-18.9342932580167,57.6572916985375,
39.3482879463984));
#206880=CARTESIAN_POINT('Ctrl Pts',(-18.907178645177,57.5738415009809,39.4512271261631));
#206881=CARTESIAN_POINT('Ctrl Pts',(-19.0815664505357,57.6988141606861,
39.3978017080178));
#206882=CARTESIAN_POINT('Ctrl Pts',(-18.9605330155739,57.7380493683893,
39.3975673827392));
#206883=CARTESIAN_POINT('Ctrl Pts',(-18.9466997135537,57.6954748424955,
39.5248015355194));
#206884=CARTESIAN_POINT('Ctrl Pts',(-19.109065001131,57.7842031819385,39.3978017080178));
#206885=CARTESIAN_POINT('Ctrl Pts',(-18.9882808235615,57.8234483402241,
39.3978017080178));
#206886=CARTESIAN_POINT('Ctrl Pts',(-18.9882808235615,57.8234483402241,
39.5248017080178));
#206887=CARTESIAN_POINT('Origin',(-19.0071016939782,57.4703923901182,39.3343017080178));
#206888=CARTESIAN_POINT('Origin',(-18.9819630792879,57.393023688563,39.1934008533546));
#206889=CARTESIAN_POINT('Origin',(-12.4602215063111,60.1478239224134,39.1925554495084));
#206890=CARTESIAN_POINT('Origin',(-12.4693660187272,60.1910940874968,39.1160373285258));
#206891=CARTESIAN_POINT('Origin',(-12.4432063593716,60.0677739512127,39.3343017080178));
#206892=CARTESIAN_POINT('Ctrl Pts',(-12.420896274158,59.9600752506738,39.2708017080178));
#206893=CARTESIAN_POINT('Ctrl Pts',(-12.544666237448,59.9342688867326,39.2710850691866));
#206894=CARTESIAN_POINT('Ctrl Pts',(-12.5674311046648,60.0413691664789,
39.3343017080178));
#206895=CARTESIAN_POINT('Ctrl Pts',(-12.4114257351939,59.9160770362136,
39.3487519293518));
#206896=CARTESIAN_POINT('Ctrl Pts',(-12.5352608058714,59.8900198101348,
39.3492068662926));
#206897=CARTESIAN_POINT('Ctrl Pts',(-12.5533954010684,59.9753363727317,
39.4512271248741));
#206898=CARTESIAN_POINT('Ctrl Pts',(-12.3934832896268,59.832722693313,39.3978017080178));
#206899=CARTESIAN_POINT('Ctrl Pts',(-12.5174621766263,59.8062838430892,
39.3980347781178));
#206900=CARTESIAN_POINT('Ctrl Pts',(-12.5268049860492,59.8502383056087,
39.524801535519));
#206901=CARTESIAN_POINT('Ctrl Pts',(-12.3746037924158,59.7450242491249,
39.3978017080178));
#206902=CARTESIAN_POINT('Ctrl Pts',(-12.498828537709,59.718619464391,39.3978017080178));
#206903=CARTESIAN_POINT('Ctrl Pts',(-12.498828537709,59.718619464391,39.5248017080178));
#206904=CARTESIAN_POINT('Origin',(-12.3746037924158,59.7450242491249,39.5248017080178));
#206905=CARTESIAN_POINT('Origin',(0.31056186323299,0.0660119618346354,39.116));
#206906=CARTESIAN_POINT('Origin',(-12.5528626811441,60.5836663843183,39.116));
#206907=CARTESIAN_POINT('Origin',(0.31056186323299,0.0660119618346354,39.5248017080178));
#206908=CARTESIAN_POINT('Origin',(-12.3431658574205,59.597120393566,39.5248017080178));
#206909=CARTESIAN_POINT('Ctrl Pts',(-12.6642893210135,61.1105274371642,
39.2875012672119));
#206910=CARTESIAN_POINT('Ctrl Pts',(-12.7893350777075,61.0844267845858,
39.287208709576));
#206911=CARTESIAN_POINT('Ctrl Pts',(-12.7666250679672,60.9785037674415,
39.3549016990121));
#206912=CARTESIAN_POINT('Ctrl Pts',(-12.6404971713777,60.9980344071776,
39.1034939173931));
#206913=CARTESIAN_POINT('Ctrl Pts',(-12.7653958126085,60.9718026486694,
39.1031692336342));
#206914=CARTESIAN_POINT('Ctrl Pts',(-12.747507305352,60.888561765193,39.2077507202298));
#206915=CARTESIAN_POINT('Ctrl Pts',(-12.5977561540109,60.7959446297927,
38.989));
#206916=CARTESIAN_POINT('Ctrl Pts',(-12.7224234952038,60.7696360759178,
38.9887769311182));
#206917=CARTESIAN_POINT('Ctrl Pts',(-12.7131630221041,60.7269846150126,
39.1161898712912));
#206918=CARTESIAN_POINT('Ctrl Pts',(-12.5528626811441,60.5836663843183,
38.989));
#206919=CARTESIAN_POINT('Ctrl Pts',(-12.6772730124459,60.5572221520606,
38.989));
#206920=CARTESIAN_POINT('Ctrl Pts',(-12.6770872880158,60.5572616290068,
39.1161895903851));
#206921=CARTESIAN_POINT('Origin',(-12.6424339620836,61.0050661295708,39.3548010137695));
#206922=CARTESIAN_POINT('Ctrl Pts',(-12.3431658574205,59.597120393566,39.3978017080178));
#206923=CARTESIAN_POINT('Ctrl Pts',(-12.4673906027137,59.5707156088322,
39.3978017080178));
#206924=CARTESIAN_POINT('Ctrl Pts',(-12.4673906027137,59.5707156088322,
39.5248017080178));
#206925=CARTESIAN_POINT('Ctrl Pts',(-12.3242219811461,59.5091256622727,
39.3978017080178));
#206926=CARTESIAN_POINT('Ctrl Pts',(-12.448658367964,59.4825873732114,39.397566602504));
#206927=CARTESIAN_POINT('Ctrl Pts',(-12.4393195978188,59.4386519140005,
39.5248015517196));
#206928=CARTESIAN_POINT('Ctrl Pts',(-12.3063073021287,59.4259203549058,
39.3484894016716));
#206929=CARTESIAN_POINT('Ctrl Pts',(-12.4310355281329,59.3996784303299,
39.3480259000028));
#206930=CARTESIAN_POINT('Ctrl Pts',(-12.4127764613281,59.3137762748665,
39.4508333188936));
#206931=CARTESIAN_POINT('Ctrl Pts',(-12.2968658913797,59.3820708699072,
39.2708017080178));
#206932=CARTESIAN_POINT('Ctrl Pts',(-12.4217592664906,59.3560370505015,
39.27051194648));
#206933=CARTESIAN_POINT('Ctrl Pts',(-12.3987880210518,59.2479658375578,
39.3343017080178));
#206934=CARTESIAN_POINT('Origin',(-12.2745632757586,59.2743706222916,39.3343017080178));
#206935=CARTESIAN_POINT('Origin',(-12.6794732450919,61.1793222555445,39.6398955068197));
#206936=CARTESIAN_POINT('Origin',(-12.716512528016,61.3535783813233,39.92499));
#206937=CARTESIAN_POINT('Origin',(-12.25764960399,59.1947980527935,39.1934008539946));
#206938=CARTESIAN_POINT('Origin',(-12.2483049653994,59.1510793400374,39.1160402713848));
#206939=CARTESIAN_POINT('Ctrl Pts',(-13.0739701745318,61.5816197022699,
40.1599502534424));
#206940=CARTESIAN_POINT('Ctrl Pts',(-13.066222907106,61.545128164506,40.10025));
#206941=CARTESIAN_POINT('Ctrl Pts',(-13.0516031943522,61.4762657165317,
40.10025));
#206942=CARTESIAN_POINT('Ctrl Pts',(-12.9877758510414,61.5999188988203,
40.1599500538471));
#206943=CARTESIAN_POINT('Ctrl Pts',(-13.0034370926704,61.5584544893691,
40.100244835349));
#206944=CARTESIAN_POINT('Ctrl Pts',(-13.0017087032037,61.4868491822358,
40.10025));
#206945=CARTESIAN_POINT('Ctrl Pts',(-12.9030451317656,61.5923336062397,
40.1202442001039));
#206946=CARTESIAN_POINT('Ctrl Pts',(-12.9408103617797,61.5481051179917,
40.0633873868017));
#206947=CARTESIAN_POINT('Ctrl Pts',(-12.9504709278434,61.4721451382826,
40.0772271723538));
#206948=CARTESIAN_POINT('Ctrl Pts',(-12.7836101409423,61.543429955208,40.0045995998162));
#206949=CARTESIAN_POINT('Ctrl Pts',(-12.8662000075457,61.5018471007596,
39.9663485808314));
#206950=CARTESIAN_POINT('Ctrl Pts',(-12.8749747009092,61.4139027244671,
40.0101727202465));
#206951=CARTESIAN_POINT('Ctrl Pts',(-12.7478263086949,61.5035207735037,
39.9304654349859));
#206952=CARTESIAN_POINT('Ctrl Pts',(-12.8544221781243,61.4652971063446,
39.9051900162944));
#206953=CARTESIAN_POINT('Ctrl Pts',(-12.8501918100166,61.3716536946544,
39.9671857458169));
#206954=CARTESIAN_POINT('Ctrl Pts',(-12.7383709431244,61.459039055521,39.8576902534424));
#206955=CARTESIAN_POINT('Ctrl Pts',(-12.8632261535949,61.43297545991,39.8573998014387));
#206956=CARTESIAN_POINT('Ctrl Pts',(-12.8407372733092,61.3271735965895,
39.92499));
#206957=CARTESIAN_POINT('Origin',(-13.0516031943522,61.4762657165317,40.22725));
#206958=CARTESIAN_POINT('Origin',(0.31056186323299,0.0660119618346354,39.116));
#206959=CARTESIAN_POINT('Origin',(-12.1649068885786,58.7584778814678,39.116));
#206960=CARTESIAN_POINT('Origin',(4.07480739539809E-18,-1.61286359594752E-16,
40.22725));
#206961=CARTESIAN_POINT('Origin',(-13.0814171332226,61.4699285681956,40.22725));
#206962=CARTESIAN_POINT('Ctrl Pts',(-12.1649068885786,58.7584778814678,
38.989));
#206963=CARTESIAN_POINT('Ctrl Pts',(-12.28931772815,58.732033541174,38.989));
#206964=CARTESIAN_POINT('Ctrl Pts',(-12.2891314946916,58.7320731263176,
39.1161901092324));
#206965=CARTESIAN_POINT('Ctrl Pts',(-12.1200194799675,58.5461948427483,
38.989));
#206966=CARTESIAN_POINT('Ctrl Pts',(-12.2442448876963,58.5199849720741,
38.9892298989736));
#206967=CARTESIAN_POINT('Ctrl Pts',(-12.2530551225939,58.5623471386696,
39.1161900493204));
#206968=CARTESIAN_POINT('Ctrl Pts',(-12.0772896710125,58.3441042111268,
39.1034966344368));
#206969=CARTESIAN_POINT('Ctrl Pts',(-12.2013256001473,58.3180679977581,
39.1038314102574));
#206970=CARTESIAN_POINT('Ctrl Pts',(-12.218711094921,58.4007711908091,39.2077528789597));
#206971=CARTESIAN_POINT('Ctrl Pts',(-12.0535047649316,58.2316113004782,
39.2875012672119));
#206972=CARTESIAN_POINT('Ctrl Pts',(-12.1774537884111,58.2057612725768,
39.2878045257868));
#206973=CARTESIAN_POINT('Ctrl Pts',(-12.1995935666432,58.3108302909897,
39.3549015295901));
#206974=CARTESIAN_POINT('Origin',(-12.0753355159227,58.3370777047236,39.3548010137695));
#206975=CARTESIAN_POINT('Ctrl Pts',(-13.360562319248,61.3267881959114,39.8576902534424));
#206976=CARTESIAN_POINT('Ctrl Pts',(-13.2359003894744,61.3537611057084,
39.8573998014387));
#206977=CARTESIAN_POINT('Ctrl Pts',(-13.2134115091888,61.2479592423879,
39.92499));
#206978=CARTESIAN_POINT('Ctrl Pts',(-13.3700210384232,61.3712903180781,
39.9304984902491));
#206979=CARTESIAN_POINT('Ctrl Pts',(-13.2571016411962,61.3797222373784,
39.9052171569785));
#206980=CARTESIAN_POINT('Ctrl Pts',(-13.2228703539489,61.2924596082476,
39.9672049726597));
#206981=CARTESIAN_POINT('Ctrl Pts',(-13.3535190881765,61.4221282572892,
40.0043437678663));
#206982=CARTESIAN_POINT('Ctrl Pts',(-13.2610999767698,61.4177900459397,
39.9661628577642));
#206983=CARTESIAN_POINT('Ctrl Pts',(-13.2173727427866,61.3409599630863,
40.0100243556236));
#206984=CARTESIAN_POINT('Ctrl Pts',(-13.2651598666396,61.5148770953649,
40.1194874821987));
#206985=CARTESIAN_POINT('Ctrl Pts',(-13.2123479779264,61.4899829268152,
40.062755148314));
#206986=CARTESIAN_POINT('Ctrl Pts',(-13.1725625528865,61.42445146363,40.0767884282376));
#206987=CARTESIAN_POINT('Ctrl Pts',(-13.1903059833729,61.5568698122756,
40.1599502015388));
#206988=CARTESIAN_POINT('Ctrl Pts',(-13.1590895168684,61.5253695547385,
40.1002449453881));
#206989=CARTESIAN_POINT('Ctrl Pts',(-13.1314678292774,61.4592680512459,
40.10025));
#206990=CARTESIAN_POINT('Ctrl Pts',(-13.1038352065721,61.5752716937453,
40.1599502534424));
#206991=CARTESIAN_POINT('Ctrl Pts',(-13.0960702419674,61.5387839176329,
40.10025));
#206992=CARTESIAN_POINT('Ctrl Pts',(-13.0814171332226,61.4699285681956,
40.10025));
#206993=CARTESIAN_POINT('Origin',(-13.3376362544819,61.221554457654,39.92499));
#206994=CARTESIAN_POINT('Origin',(-12.0382961820468,58.1628213392039,39.6398955069326));
#206995=CARTESIAN_POINT('Origin',(-12.0012568480854,57.9885649735461,39.92499));
#206996=CARTESIAN_POINT('Origin',(-13.300596971511,61.0472983318734,39.6398955068269));
#206997=CARTESIAN_POINT('Origin',(-13.2635576885496,60.8730422059015,39.3548010137695));
#206998=CARTESIAN_POINT('Ctrl Pts',(-11.9794294790606,57.8830978693157,
39.8576902534424));
#206999=CARTESIAN_POINT('Ctrl Pts',(-12.1031907419151,57.8572899778512,
39.8579948730703));
#207000=CARTESIAN_POINT('Ctrl Pts',(-12.1254815933786,57.9621601888122,
39.92499));
#207001=CARTESIAN_POINT('Ctrl Pts',(-11.9699833161084,57.8386546085356,
39.9304020711231));
#207002=CARTESIAN_POINT('Ctrl Pts',(-12.0820882677171,57.8310944294267,
39.9058915297383));
#207003=CARTESIAN_POINT('Ctrl Pts',(-12.1160345187361,57.9177151970029,
39.9671523786031));
#207004=CARTESIAN_POINT('Ctrl Pts',(-11.9864204851024,57.7880992891177,
40.0043257306692));
#207005=CARTESIAN_POINT('Ctrl Pts',(-12.0782959991605,57.7929810340973,
39.9667894847835));
#207006=CARTESIAN_POINT('Ctrl Pts',(-12.1215717318488,57.8694789541064,
40.0100138975199));
#207007=CARTESIAN_POINT('Ctrl Pts',(-12.0746725352384,57.6961636462597,
40.1195533054858));
#207008=CARTESIAN_POINT('Ctrl Pts',(-12.1272484490375,57.7211944343233,
40.0630813209236));
#207009=CARTESIAN_POINT('Ctrl Pts',(-12.1665991704021,57.7867317752136,
40.0768265942421));
#207010=CARTESIAN_POINT('Ctrl Pts',(-12.1494120604577,57.6547178110651,
40.1599502027512));
#207011=CARTESIAN_POINT('Ctrl Pts',(-12.180482756658,57.6862546895627,40.100255279155));
#207012=CARTESIAN_POINT('Ctrl Pts',(-12.2078361528627,57.7524075778595,
40.10025));
#207013=CARTESIAN_POINT('Ctrl Pts',(-12.2354540642039,57.6364522029208,
40.1599502534424));
#207014=CARTESIAN_POINT('Ctrl Pts',(-12.2432007592841,57.6729438621907,
40.10025));
#207015=CARTESIAN_POINT('Ctrl Pts',(-12.2578193919762,57.7418065394567,
40.10025));
#207016=CARTESIAN_POINT('Origin',(-12.2578193919762,57.7418065394567,40.22725));
#207017=CARTESIAN_POINT('Ctrl Pts',(-13.1739864076101,60.451642460649,38.989));
#207018=CARTESIAN_POINT('Ctrl Pts',(-13.0495760655898,60.478086695185,38.989));
#207019=CARTESIAN_POINT('Ctrl Pts',(-13.0497618007543,60.4780472159571,
39.1161896013266));
#207020=CARTESIAN_POINT('Ctrl Pts',(-13.2193162256439,60.6638314094604,
38.989));
#207021=CARTESIAN_POINT('Ctrl Pts',(-13.0947262769505,60.6905041359636,
38.988776927546));
#207022=CARTESIAN_POINT('Ctrl Pts',(-13.085838095863,60.647772838971,39.1161898821848));
#207023=CARTESIAN_POINT('Ctrl Pts',(-13.2624673401135,60.8658323498479,
39.1034967087243));
#207024=CARTESIAN_POINT('Ctrl Pts',(-13.1376973240554,60.8926693037162,
39.1031720232711));
#207025=CARTESIAN_POINT('Ctrl Pts',(-13.1201821075158,60.8093487091495,
39.2077529615));
#207026=CARTESIAN_POINT('Ctrl Pts',(-13.2864868028989,60.9782752797349,
39.2875012672119));
#207027=CARTESIAN_POINT('Ctrl Pts',(-13.161635717282,61.0052918407716,39.2872087095508));
#207028=CARTESIAN_POINT('Ctrl Pts',(-13.139299579968,60.8992893450419,39.3549017048228));
#207029=CARTESIAN_POINT('Origin',(-13.1739864076101,60.451642460649,39.116));
#207030=CARTESIAN_POINT('Origin',(3.9977349588932E-16,5.73754452974297E-17,
40.22725));
#207031=CARTESIAN_POINT('Origin',(-12.2876333308465,57.7354693911206,40.22725));
#207032=CARTESIAN_POINT('Origin',(2.37914510404509,-12.7200883457656,39.116));
#207033=CARTESIAN_POINT('Origin',(-13.0905908661173,60.0590486699123,39.1160373285265));
#207034=CARTESIAN_POINT('Ctrl Pts',(-12.2652136052655,57.6301266171959,
40.1599502534424));
#207035=CARTESIAN_POINT('Ctrl Pts',(-12.2729791421549,57.6666142715156,
40.10025));
#207036=CARTESIAN_POINT('Ctrl Pts',(-12.2876333308465,57.7354693911206,
40.10025));
#207037=CARTESIAN_POINT('Ctrl Pts',(-12.3509528635302,57.6118791634504,
40.1599500566036));
#207038=CARTESIAN_POINT('Ctrl Pts',(-12.3354428975791,57.6533170557961,
40.1002551305363));
#207039=CARTESIAN_POINT('Ctrl Pts',(-12.3374367183502,57.7248602994012,
40.10025));
#207040=CARTESIAN_POINT('Ctrl Pts',(-12.4353658313035,57.6190178232954,
40.1203070619044));
#207041=CARTESIAN_POINT('Ctrl Pts',(-12.3978675338892,57.6632723181628,
40.0637098684499));
#207042=CARTESIAN_POINT('Ctrl Pts',(-12.3886090227463,57.7390640345635,
40.0772636213363));
#207043=CARTESIAN_POINT('Ctrl Pts',(-12.5543478197371,57.6672013517152,
40.0046102245803));
#207044=CARTESIAN_POINT('Ctrl Pts',(-12.4724831634109,57.709059208982,39.9670001894012));
#207045=CARTESIAN_POINT('Ctrl Pts',(-12.4639865158414,57.7965151898603,
40.0101788811208));
#207046=CARTESIAN_POINT('Ctrl Pts',(-12.5899803678808,57.7068899568911,
39.9303710930185));
#207047=CARTESIAN_POINT('Ctrl Pts',(-12.4844838378932,57.7455787351226,
39.905866357411));
#207048=CARTESIAN_POINT('Ctrl Pts',(-12.4887127671319,57.838519720206,39.9671344706364));
#207049=CARTESIAN_POINT('Ctrl Pts',(-12.5994235324466,57.7513140650721,
39.8576902534424));
#207050=CARTESIAN_POINT('Ctrl Pts',(-12.4758649777947,57.7780756236497,
39.8579948730703));
#207051=CARTESIAN_POINT('Ctrl Pts',(-12.4981558292581,57.8829458346106,
39.92499));
#207052=CARTESIAN_POINT('Origin',(-12.6223805745513,57.8565410498768,39.92499));
#207053=CARTESIAN_POINT('Origin',(-13.0813452322613,60.01579999775,39.192555448885));
#207054=CARTESIAN_POINT('Origin',(-13.0643300858376,59.9357500275434,39.3343017080178));
#207055=CARTESIAN_POINT('Origin',(-12.6594199084536,58.03079741553,39.639895506922));
#207056=CARTESIAN_POINT('Origin',(-12.6964592423886,58.2050537810543,39.3548010137695));
#207057=CARTESIAN_POINT('Ctrl Pts',(-12.9957275188818,59.6130003254556,
39.3978017080178));
#207058=CARTESIAN_POINT('Ctrl Pts',(-12.8715027735886,59.6394051101895,
39.3978017080178));
#207059=CARTESIAN_POINT('Ctrl Pts',(-12.8715027735886,59.6394051101895,
39.5248017080178));
#207060=CARTESIAN_POINT('Ctrl Pts',(-13.0142126749433,59.7010925481785,
39.3978017080178));
#207061=CARTESIAN_POINT('Ctrl Pts',(-12.8901994296779,59.727365961373,39.3980355775177));
#207062=CARTESIAN_POINT('Ctrl Pts',(-12.8995737759685,59.7714687931892,
39.5248015517192));
#207063=CARTESIAN_POINT('Ctrl Pts',(-13.0316935695382,59.7843900000233,
39.3484893995498));
#207064=CARTESIAN_POINT('Ctrl Pts',(-12.9079667071272,59.8109544298284,
39.348943830343));
#207065=CARTESIAN_POINT('Ctrl Pts',(-12.9261169057236,59.896344400635,39.4508333155594));
#207066=CARTESIAN_POINT('Ctrl Pts',(-13.0409063549232,59.8282880397056,
39.2708017080178));
#207067=CARTESIAN_POINT('Ctrl Pts',(-12.9173404733276,59.855054532531,39.2710850691866));
#207068=CARTESIAN_POINT('Ctrl Pts',(-12.9401053405444,59.9621548122773,
39.3343017080178));
#207069=CARTESIAN_POINT('Origin',(-12.9957275188818,59.6130003254556,39.5248017080178));
#207070=CARTESIAN_POINT('Ctrl Pts',(-12.6735055745735,58.0998260601481,
39.2875012672119));
#207071=CARTESIAN_POINT('Ctrl Pts',(-12.5497583678825,58.1266254912132,
39.2878045257519));
#207072=CARTESIAN_POINT('Ctrl Pts',(-12.5722680770241,58.2316158657529,
39.3549015218347));
#207073=CARTESIAN_POINT('Ctrl Pts',(-12.697532333562,58.2122693395992,39.1034938540228));
#207074=CARTESIAN_POINT('Ctrl Pts',(-12.5736300041235,58.2389340288477,
39.1038286278794));
#207075=CARTESIAN_POINT('Ctrl Pts',(-12.5913858949916,58.3215581271253,
39.2077506434031));
#207076=CARTESIAN_POINT('Ctrl Pts',(-12.7406947165199,58.4142696920427,
38.989));
#207077=CARTESIAN_POINT('Ctrl Pts',(-12.6165486539538,58.4408527990771,
38.9892298954629));
#207078=CARTESIAN_POINT('Ctrl Pts',(-12.6257301953094,58.4831353553,39.1161900347289));
#207079=CARTESIAN_POINT('Ctrl Pts',(-12.7860306150445,58.6264539577985,
38.989));
#207080=CARTESIAN_POINT('Ctrl Pts',(-12.6616197898419,58.6528982950381,
38.989));
#207081=CARTESIAN_POINT('Ctrl Pts',(-12.66180600891,58.6528587129533,39.1161900945646));
#207082=CARTESIAN_POINT('Origin',(-12.7860306150445,58.6264539577985,39.116));
#207083=CARTESIAN_POINT('Origin',(2.31399271319931,-12.4135704460881,39.5248017080178));
#207084=CARTESIAN_POINT('Origin',(-12.9642895838864,59.4650964698968,39.5248017080178));
#207085=CARTESIAN_POINT('Origin',(2.30379013587677,-12.3655710936221,39.116));
#207086=CARTESIAN_POINT('Origin',(-12.8695280801141,59.0190342907435,39.1160402713851));
#207087=CARTESIAN_POINT('Ctrl Pts',(-12.9191181862039,59.2498070616281,
39.2708017080178));
#207088=CARTESIAN_POINT('Ctrl Pts',(-12.7944335023702,59.2768226962999,
39.27051194648));
#207089=CARTESIAN_POINT('Ctrl Pts',(-12.7714622569314,59.1687514833562,
39.3343017080178));
#207090=CARTESIAN_POINT('Ctrl Pts',(-12.9283593439867,59.293854073036,39.3487519301186));
#207091=CARTESIAN_POINT('Ctrl Pts',(-12.8037411210015,59.3206115991496,
39.3482879463984));
#207092=CARTESIAN_POINT('Ctrl Pts',(-12.7854979657552,59.2347843016968,
39.4512271261627));
#207093=CARTESIAN_POINT('Ctrl Pts',(-12.9458672563998,59.3773008374015,
39.3978017080178));
#207094=CARTESIAN_POINT('Ctrl Pts',(-12.821395659292,59.4036696715712,39.3975673827392));
#207095=CARTESIAN_POINT('Ctrl Pts',(-12.8120883873131,59.3598823995816,
39.5248015355194));
#207096=CARTESIAN_POINT('Ctrl Pts',(-12.9642895838864,59.4650964698968,
39.3978017080178));
#207097=CARTESIAN_POINT('Ctrl Pts',(-12.8400648385932,59.4915012546306,
39.3978017080178));
#207098=CARTESIAN_POINT('Ctrl Pts',(-12.8400648385932,59.4915012546306,
39.5248017080178));
#207099=CARTESIAN_POINT('Origin',(-12.8956870022246,59.1423466986223,39.3343017080178));
#207100=CARTESIAN_POINT('Origin',(-12.8787733309733,59.0627741301469,39.193400853355));
#207101=CARTESIAN_POINT('Origin',(-6.10480350566275,61.1207756556245,39.1925554495081));
#207102=CARTESIAN_POINT('Origin',(-6.10937495962055,61.1647646440466,39.116037328525));
#207103=CARTESIAN_POINT('Origin',(-6.09624906995176,61.0393856393804,39.3343017080178));
#207104=CARTESIAN_POINT('Ctrl Pts',(-6.08531878138258,60.9299448846691,
39.2708017080178));
#207105=CARTESIAN_POINT('Ctrl Pts',(-6.21110821942872,60.9172173747511,
39.2710850691866));
#207106=CARTESIAN_POINT('Ctrl Pts',(-6.22255335066354,61.0261105245455,
39.3343017080178));
#207107=CARTESIAN_POINT('Ctrl Pts',(-6.08049918876613,60.885197756147,39.3487519293518));
#207108=CARTESIAN_POINT('Ctrl Pts',(-6.20637959976764,60.8722275639175,
39.349206866293));
#207109=CARTESIAN_POINT('Ctrl Pts',(-6.2154968425757,60.9589723348237,39.4512271248741));
#207110=CARTESIAN_POINT('Ctrl Pts',(-6.0713679351625,60.800424540796,39.3978017080178));
#207111=CARTESIAN_POINT('Ctrl Pts',(-6.19743126523124,60.7870898478945,
39.3980347781178));
#207112=CARTESIAN_POINT('Ctrl Pts',(-6.2021284013463,60.8317801127822,39.524801535519));
#207113=CARTESIAN_POINT('Ctrl Pts',(-6.06175884541508,60.7112330730304,
39.3978017080178));
#207114=CARTESIAN_POINT('Ctrl Pts',(-6.18806312612685,60.6979579581955,
39.3978017080178));
#207115=CARTESIAN_POINT('Ctrl Pts',(-6.18806312612685,60.6979579581955,
39.5248017080178));
#207116=CARTESIAN_POINT('Origin',(-6.06175884541508,60.7112330730304,39.5248017080178));
#207117=CARTESIAN_POINT('Origin',(0.315760701779433,0.0331877870874769,
39.116));
#207118=CARTESIAN_POINT('Origin',(-6.15137923967613,61.5639141665612,39.116));
#207119=CARTESIAN_POINT('Origin',(0.315760701779433,0.0331877870874769,
39.5248017080178));
#207120=CARTESIAN_POINT('Origin',(-6.04595329344999,60.5608532912344,39.5248017080178));
#207121=CARTESIAN_POINT('Ctrl Pts',(-6.207123496544,62.0995362748659,39.2875012672119));
#207122=CARTESIAN_POINT('Ctrl Pts',(-6.33421250060359,62.0866494451786,
39.287208709576));
#207123=CARTESIAN_POINT('Ctrl Pts',(-6.32269886887937,61.978932842986,39.3549016990122));
#207124=CARTESIAN_POINT('Ctrl Pts',(-6.19522040634688,61.9851725366286,
39.1034939173931));
#207125=CARTESIAN_POINT('Ctrl Pts',(-6.32217680516144,61.9721399414732,
39.1031692336336));
#207126=CARTESIAN_POINT('Ctrl Pts',(-6.31308733464659,61.8874852020914,
39.2077507202295));
#207127=CARTESIAN_POINT('Ctrl Pts',(-6.17383766261612,61.7797221753254,
38.989));
#207128=CARTESIAN_POINT('Ctrl Pts',(-6.30057205577764,61.7665890280533,
38.9887769311176));
#207129=CARTESIAN_POINT('Ctrl Pts',(-6.29582060418292,61.7232032332924,
39.1161898712914));
#207130=CARTESIAN_POINT('Ctrl Pts',(-6.15137923967613,61.5639141665612,
38.989));
#207131=CARTESIAN_POINT('Ctrl Pts',(-6.2778722131262,61.5506192193203,38.989));
#207132=CARTESIAN_POINT('Ctrl Pts',(-6.27768337964921,61.5506390665185,
39.1161895903853));
#207133=CARTESIAN_POINT('Origin',(-6.19641157197401,61.9923681882669,39.3548010137695));
#207134=CARTESIAN_POINT('Ctrl Pts',(-6.04595329344999,60.5608532912344,
39.3978017080178));
#207135=CARTESIAN_POINT('Ctrl Pts',(-6.17225757416176,60.5475781763994,
39.3978017080178));
#207136=CARTESIAN_POINT('Ctrl Pts',(-6.17225757416176,60.5475781763994,
39.5248017080178));
#207137=CARTESIAN_POINT('Ctrl Pts',(-6.03631114774952,60.4713604300109,
39.3978017080178));
#207138=CARTESIAN_POINT('Ctrl Pts',(-6.16283986559437,60.4579746647649,
39.397566602504));
#207139=CARTESIAN_POINT('Ctrl Pts',(-6.158144760243,60.4133037213017,39.5248015517196));
#207140=CARTESIAN_POINT('Ctrl Pts',(-6.0271919301333,60.3867383361559,39.3484894016716));
#207141=CARTESIAN_POINT('Ctrl Pts',(-6.15397990991402,60.3736778173757,
39.3480259000036));
#207142=CARTESIAN_POINT('Ctrl Pts',(-6.14480008848961,60.286337650718,39.4508333188934));
#207143=CARTESIAN_POINT('Ctrl Pts',(-6.02238575970214,60.3421421670676,
39.2708017080178));
#207144=CARTESIAN_POINT('Ctrl Pts',(-6.14931623097185,60.3293058762212,
39.27051194648));
#207145=CARTESIAN_POINT('Ctrl Pts',(-6.13776734223154,60.2194255397046,
39.3343017080178));
#207146=CARTESIAN_POINT('Origin',(-6.01146306151977,60.2327006545396,39.3343017080178));
#207147=CARTESIAN_POINT('Origin',(-6.21503322485447,62.169541380285,39.6398955068184));
#207148=CARTESIAN_POINT('Origin',(-6.23365487766561,62.346714572097,39.92499));
#207149=CARTESIAN_POINT('Origin',(-6.00295964302103,60.1517960317845,39.1934008539949));
#207150=CARTESIAN_POINT('Origin',(-5.99823604520081,60.107340034,39.1160402713845));
#207151=CARTESIAN_POINT('Ctrl Pts',(-6.56531752495238,62.6108711573006,
40.1599502534424));
#207152=CARTESIAN_POINT('Ctrl Pts',(-6.56142710223288,62.5737697140403,
40.10025));
#207153=CARTESIAN_POINT('Ctrl Pts',(-6.55408556365883,62.5037563256535,
40.10025));
#207154=CARTESIAN_POINT('Ctrl Pts',(-6.47768259609018,62.6200603487606,
40.1599500538468));
#207155=CARTESIAN_POINT('Ctrl Pts',(-6.49759225479899,62.5804601312023,
40.100244835349));
#207156=CARTESIAN_POINT('Ctrl Pts',(-6.50335812634711,62.5090664195381,
40.10025));
#207157=CARTESIAN_POINT('Ctrl Pts',(-6.39420891953703,62.603659837329,40.1202442001038));
#207158=CARTESIAN_POINT('Ctrl Pts',(-6.43639040357899,62.5636211788254,
40.0633873868015));
#207159=CARTESIAN_POINT('Ctrl Pts',(-6.45393802799966,62.4890871199578,
40.0772271723538));
#207160=CARTESIAN_POINT('Ctrl Pts',(-6.28054002958072,62.5425397295636,
40.0045995998163));
#207161=CARTESIAN_POINT('Ctrl Pts',(-6.36702405212707,62.5098176621808,
39.9663485808318));
#207162=CARTESIAN_POINT('Ctrl Pts',(-6.38494336730917,62.4232722595963,
40.0101727202465));
#207163=CARTESIAN_POINT('Ctrl Pts',(-6.24912387034407,62.4991087455376,
39.9304654349858));
#207164=CARTESIAN_POINT('Ctrl Pts',(-6.35913125763593,62.4722367740482,
39.9051900162944));
#207165=CARTESIAN_POINT('Ctrl Pts',(-6.36471246584663,62.3786641568873,
39.967185745818));
#207166=CARTESIAN_POINT('Ctrl Pts',(-6.24436990787996,62.4538823482276,
39.8576902534424));
#207167=CARTESIAN_POINT('Ctrl Pts',(-6.37126553604008,62.4410124550019,
39.8573998014387));
#207168=CARTESIAN_POINT('Ctrl Pts',(-6.35995915837738,62.333439457262,39.92499));
#207169=CARTESIAN_POINT('Origin',(-6.55408556365882,62.5037563256535,40.22725));
#207170=CARTESIAN_POINT('Origin',(0.315760701779433,0.0331877870874769,
39.116));
#207171=CARTESIAN_POINT('Origin',(-5.9563328589115,59.7081718144893,39.116));
#207172=CARTESIAN_POINT('Origin',(-1.29720108988958E-17,-1.63986310369608E-16,
40.22725));
#207173=CARTESIAN_POINT('Origin',(-6.58439859102965,62.5005702980931,40.22725));
#207174=CARTESIAN_POINT('Ctrl Pts',(-5.9563328589115,59.7081718144893,38.989));
#207175=CARTESIAN_POINT('Ctrl Pts',(-6.08282634913902,59.6948768129328,
38.989));
#207176=CARTESIAN_POINT('Ctrl Pts',(-6.08263699811321,59.6948967145276,
39.116190109232));
#207177=CARTESIAN_POINT('Ctrl Pts',(-5.93388096803544,59.4923596726254,
38.989));
#207178=CARTESIAN_POINT('Ctrl Pts',(-6.06016553348636,59.4792784733305,
38.9892298989736));
#207179=CARTESIAN_POINT('Ctrl Pts',(-6.06449945282174,59.5223294958602,
39.11619004932));
#207180=CARTESIAN_POINT('Ctrl Pts',(-5.91250946061117,59.286909633363,39.1034966344368));
#207181=CARTESIAN_POINT('Ctrl Pts',(-6.03858743331817,59.2739813341626,
39.1038314102587));
#207182=CARTESIAN_POINT('Ctrl Pts',(-6.0472328508574,59.358048749519,39.2077528789603));
#207183=CARTESIAN_POINT('Ctrl Pts',(-5.90061356181196,59.1725467709678,
39.2875012672119));
#207184=CARTESIAN_POINT('Ctrl Pts',(-6.02658564326333,59.1597945531718,
39.2878045257868));
#207185=CARTESIAN_POINT('Ctrl Pts',(-6.03762143444243,59.2666022295036,
39.3549015295898));
#207186=CARTESIAN_POINT('Origin',(-5.91130048050282,59.2797173540686,39.3548010137695));
#207187=CARTESIAN_POINT('Ctrl Pts',(-6.87697683366501,62.3873926810692,
39.8576902534424));
#207188=CARTESIAN_POINT('Ctrl Pts',(-6.75017837817539,62.4011871104969,
39.8573998014387));
#207189=CARTESIAN_POINT('Ctrl Pts',(-6.7388720005127,62.293614112757,39.92499));
#207190=CARTESIAN_POINT('Ctrl Pts',(-6.88173199854425,62.4326397213343,
39.9304984902493));
#207191=CARTESIAN_POINT('Ctrl Pts',(-6.76854981002517,62.4292221586323,
39.9052171569784));
#207192=CARTESIAN_POINT('Ctrl Pts',(-6.7436274738735,62.338859419464,39.9672049726588));
#207193=CARTESIAN_POINT('Ctrl Pts',(-6.86000643604672,62.4814742414946,
40.004343767866));
#207194=CARTESIAN_POINT('Ctrl Pts',(-6.76854707276804,62.4674993676295,
39.966162857764));
#207195=CARTESIAN_POINT('Ctrl Pts',(-6.73309031164129,62.3865194274377,
40.0100243556234));
#207196=CARTESIAN_POINT('Ctrl Pts',(-6.76243636205631,62.5644789380885,
40.1194874821989));
#207197=CARTESIAN_POINT('Ctrl Pts',(-6.71251593157802,62.5342007968288,
40.0627551483144));
#207198=CARTESIAN_POINT('Ctrl Pts',(-6.6797983584018,62.4648696125156,40.0767884282378));
#207199=CARTESIAN_POINT('Ctrl Pts',(-6.68360310202759,62.5984172531152,
40.1599502015401));
#207200=CARTESIAN_POINT('Ctrl Pts',(-6.65585031610573,62.5638265480135,
40.1002449453869));
#207201=CARTESIAN_POINT('Ctrl Pts',(-6.63528943158898,62.4951999029141,
40.10025));
#207202=CARTESIAN_POINT('Ctrl Pts',(-6.59568250079822,62.6076796697355,
40.1599502534424));
#207203=CARTESIAN_POINT('Ctrl Pts',(-6.5917740846471,62.570580117661,40.10025));
#207204=CARTESIAN_POINT('Ctrl Pts',(-6.58439859102965,62.5005702980932,
40.10025));
#207205=CARTESIAN_POINT('Origin',(-6.86517628122447,62.280338997922,39.92499));
#207206=CARTESIAN_POINT('Origin',(-5.89267880207669,59.102543918501,39.6398955069323));
#207207=CARTESIAN_POINT('Origin',(-5.87405712357809,58.9253704827881,39.92499));
#207208=CARTESIAN_POINT('Origin',(-6.84655462836599,62.1031658061002,39.6398955068277));
#207209=CARTESIAN_POINT('Origin',(-6.82793297553286,61.925992614092,39.3548010137695));
#207210=CARTESIAN_POINT('Ctrl Pts',(-5.8633736414952,58.8181995570485,39.8576902534424));
#207211=CARTESIAN_POINT('Ctrl Pts',(-5.98915458643735,58.8054696185321,
39.8579948730703));
#207212=CARTESIAN_POINT('Ctrl Pts',(-6.00036140428986,58.9120953679531,
39.92499));
#207213=CARTESIAN_POINT('Ctrl Pts',(-5.85862481136388,58.773012368204,39.9304020711231));
#207214=CARTESIAN_POINT('Ctrl Pts',(-5.97090589422178,58.7772117628642,
39.9058915297384));
#207215=CARTESIAN_POINT('Ctrl Pts',(-5.99561184840459,58.8669063622649,
39.9671523786036));
#207216=CARTESIAN_POINT('Ctrl Pts',(-5.8802564056751,58.7244521481309,40.0043257306693));
#207217=CARTESIAN_POINT('Ctrl Pts',(-5.97111833475339,58.7389107566976,
39.9667894847838));
#207218=CARTESIAN_POINT('Ctrl Pts',(-6.00616078842833,58.8195131589313,
40.0100138975201));
#207219=CARTESIAN_POINT('Ctrl Pts',(-5.97763489331393,58.642244989525,40.1195533054857));
#207220=CARTESIAN_POINT('Ctrl Pts',(-6.02730636094545,58.6726343357863,
40.0630813209234));
#207221=CARTESIAN_POINT('Ctrl Pts',(-6.05959099741105,58.7419259266988,
40.076826594242));
#207222=CARTESIAN_POINT('Ctrl Pts',(-6.05629725705567,58.6088386066683,
40.1599502027516));
#207223=CARTESIAN_POINT('Ctrl Pts',(-6.08390124328572,58.6434504949722,
40.1002552791541));
#207224=CARTESIAN_POINT('Ctrl Pts',(-6.1041899349697,58.7121001992962,40.10025));
#207225=CARTESIAN_POINT('Ctrl Pts',(-6.14377718965262,58.5996668978649,
40.1599502534424));
#207226=CARTESIAN_POINT('Ctrl Pts',(-6.14766703046111,58.6367684021393,
40.10025));
#207227=CARTESIAN_POINT('Ctrl Pts',(-6.15500747092256,58.7067819056643,
40.10025));
#207228=CARTESIAN_POINT('Origin',(-6.15500747092256,58.7067819056643,40.22725));
#207229=CARTESIAN_POINT('Ctrl Pts',(-6.78290064323498,61.4975385923863,
38.989));
#207230=CARTESIAN_POINT('Ctrl Pts',(-6.65640765888762,61.5108335407726,
38.989));
#207231=CARTESIAN_POINT('Ctrl Pts',(-6.65659650327814,61.5108136924273,
39.1161896013263));
#207232=CARTESIAN_POINT('Ctrl Pts',(-6.80580235504196,61.7133034041536,
38.989));
#207233=CARTESIAN_POINT('Ctrl Pts',(-6.67910686401144,61.7268068187953,
38.988776927546));
#207234=CARTESIAN_POINT('Ctrl Pts',(-6.67473401011693,61.6833805404101,
39.1161898821844));
#207235=CARTESIAN_POINT('Ctrl Pts',(-6.82760223531305,61.9187082819379,
39.1034967087243));
#207236=CARTESIAN_POINT('Ctrl Pts',(-6.70071049691168,61.9323562021233,
39.1031720232714));
#207237=CARTESIAN_POINT('Ctrl Pts',(-6.69200060426903,61.8476612078213,
39.2077529615005));
#207238=CARTESIAN_POINT('Ctrl Pts',(-6.83973663030197,62.0330459552233,
39.2875012672119));
#207239=CARTESIAN_POINT('Ctrl Pts',(-6.71274549238791,62.046864024595,39.2872087095508));
#207240=CARTESIAN_POINT('Ctrl Pts',(-6.701611992752,61.9391074595196,39.3549017048226));
#207241=CARTESIAN_POINT('Origin',(-6.78290064323498,61.4975385923863,39.116));
#207242=CARTESIAN_POINT('Origin',(4.0583767139057E-16,5.83359163402242E-17,
40.22725));
#207243=CARTESIAN_POINT('Origin',(-6.18532049829339,58.7035958781039,40.22725));
#207244=CARTESIAN_POINT('Origin',(0.364094271196318,-6.50157577599494,39.116));
#207245=CARTESIAN_POINT('Origin',(-6.74099917687859,61.0983782637168,39.1160373285255));
#207246=CARTESIAN_POINT('Ctrl Pts',(-6.17403490858961,58.5964866834551,
40.1599502534424));
#207247=CARTESIAN_POINT('Ctrl Pts',(-6.17794390662112,58.6335861742242,
40.10025));
#207248=CARTESIAN_POINT('Ctrl Pts',(-6.18532049829339,58.7035958781039,
40.10025));
#207249=CARTESIAN_POINT('Ctrl Pts',(-6.2612118565248,58.5873013840788,40.1599500566034));
#207250=CARTESIAN_POINT('Ctrl Pts',(-6.24145541658216,58.6268910424085,
40.1002551305381));
#207251=CARTESIAN_POINT('Ctrl Pts',(-6.23596000968337,58.6982507756608,
40.10025));
#207252=CARTESIAN_POINT('Ctrl Pts',(-6.34441620808552,58.6032244953991,
40.1203070619047));
#207253=CARTESIAN_POINT('Ctrl Pts',(-6.30249747592673,58.6433169201089,
40.0637098684497));
#207254=CARTESIAN_POINT('Ctrl Pts',(-6.28536729223264,58.7177256636153,
40.0772636213362));
#207255=CARTESIAN_POINT('Ctrl Pts',(-6.45770985055608,58.6635810738165,
40.0046102245801));
#207256=CARTESIAN_POINT('Ctrl Pts',(-6.37191831988716,58.6966524426404,
39.9670001894015));
#207257=CARTESIAN_POINT('Ctrl Pts',(-6.35432657855751,58.7827411889911,
40.0101788811209));
#207258=CARTESIAN_POINT('Ctrl Pts',(-6.48899861096501,58.7067768761601,
39.9303710930187));
#207259=CARTESIAN_POINT('Ctrl Pts',(-6.38003592347278,58.7342263230558,
39.9058663574104));
#207260=CARTESIAN_POINT('Ctrl Pts',(-6.37452670784895,58.8271002111734,
39.967134470636));
#207261=CARTESIAN_POINT('Ctrl Pts',(-6.49374646112681,58.7519447039089,
39.8576902534424));
#207262=CARTESIAN_POINT('Ctrl Pts',(-6.36806742857265,58.7656442740271,
39.8579948730703));
#207263=CARTESIAN_POINT('Ctrl Pts',(-6.37927424642518,58.8722700234481,
39.92499));
#207264=CARTESIAN_POINT('Origin',(-6.50557852713695,58.8589949086131,39.92499));
#207265=CARTESIAN_POINT('Origin',(-6.73632490881093,61.0544000804071,39.1925554488848));
#207266=CARTESIAN_POINT('Origin',(-6.72777047351062,60.9730100652055,39.3343017080178));
#207267=CARTESIAN_POINT('Origin',(-6.52420020557747,59.0361683443156,39.639895506922));
#207268=CARTESIAN_POINT('Origin',(-6.54282188406168,59.2133417798937,39.3548010137695));
#207269=CARTESIAN_POINT('Ctrl Pts',(-6.69328024897394,60.6448574988555,
39.3978017080178));
#207270=CARTESIAN_POINT('Ctrl Pts',(-6.56697596826217,60.6581326136905,
39.3978017080178));
#207271=CARTESIAN_POINT('Ctrl Pts',(-6.56697596826216,60.6581326136905,
39.5248017080178));
#207272=CARTESIAN_POINT('Ctrl Pts',(-6.70245599674905,60.7343993681215,
39.3978017080178));
#207273=CARTESIAN_POINT('Ctrl Pts',(-6.5763757895108,60.7475659388583,39.3980355775177));
#207274=CARTESIAN_POINT('Ctrl Pts',(-6.58108878091646,60.7924070567576,
39.5248015517192));
#207275=CARTESIAN_POINT('Ctrl Pts',(-6.7111341745387,60.819067758858,39.3484893995498));
#207276=CARTESIAN_POINT('Ctrl Pts',(-6.58530836180002,60.8325536871429,
39.3489438303426));
#207277=CARTESIAN_POINT('Ctrl Pts',(-6.59443344928367,60.919373095124,39.4508333155595));
#207278=CARTESIAN_POINT('Ctrl Pts',(-6.71570789669348,60.8636883187845,
39.2708017080178));
#207279=CARTESIAN_POINT('Ctrl Pts',(-6.59002106156404,60.8773920302461,
39.2710850691866));
#207280=CARTESIAN_POINT('Ctrl Pts',(-6.60146619279885,60.9862851800405,
39.3343017080178));
#207281=CARTESIAN_POINT('Origin',(-6.69328024897394,60.6448574988555,39.5248017080178));
#207282=CARTESIAN_POINT('Ctrl Pts',(-6.53099325079995,59.1062911958297,
39.2875012672119));
#207283=CARTESIAN_POINT('Ctrl Pts',(-6.40512264090925,59.1200087114583,
39.2878045257519));
#207284=CARTESIAN_POINT('Ctrl Pts',(-6.41653455700066,59.2267768430462,
39.3549015218348));
#207285=CARTESIAN_POINT('Ctrl Pts',(-6.54313486548275,59.2206299794252,
39.1034938540228));
#207286=CARTESIAN_POINT('Ctrl Pts',(-6.41712406698103,59.2341972766234,
39.1038286278805));
#207287=CARTESIAN_POINT('Ctrl Pts',(-6.4261461191967,59.3182247474318,39.2077506434029));
#207288=CARTESIAN_POINT('Ctrl Pts',(-6.56494601396936,59.426035450364,38.989));
#207289=CARTESIAN_POINT('Ctrl Pts',(-6.43870134519624,59.4394961352166,
38.9892298954611));
#207290=CARTESIAN_POINT('Ctrl Pts',(-6.44341285848398,59.482506795581,39.1161900347291));
#207291=CARTESIAN_POINT('Ctrl Pts',(-6.58785426247035,59.6417962403143,
38.989));
#207292=CARTESIAN_POINT('Ctrl Pts',(-6.46136078685158,59.6550912403354,
38.989));
#207293=CARTESIAN_POINT('Ctrl Pts',(-6.4615501232468,59.6550713402783,39.1161900945648));
#207294=CARTESIAN_POINT('Origin',(-6.58785426247035,59.6417962403143,39.116));
#207295=CARTESIAN_POINT('Origin',(0.347626240493858,-6.34489293004837,39.5248017080178));
#207296=CARTESIAN_POINT('Origin',(-6.67747469700884,60.4944777170594,39.5248017080178));
#207297=CARTESIAN_POINT('Origin',(0.345047419449677,-6.32035708677179,39.116));
#207298=CARTESIAN_POINT('Origin',(-6.62985850077849,60.0409538388293,39.1160402713855));
#207299=CARTESIAN_POINT('Ctrl Pts',(-6.65505462397334,60.2756459899119,
39.2708017080178));
#207300=CARTESIAN_POINT('Ctrl Pts',(-6.52822907310717,60.2894805317162,
39.27051194648));
#207301=CARTESIAN_POINT('Ctrl Pts',(-6.51668018436685,60.1796001951996,
39.3343017080178));
#207302=CARTESIAN_POINT('Ctrl Pts',(-6.65964099131221,60.3204176712045,
39.3487519301185));
#207303=CARTESIAN_POINT('Ctrl Pts',(-6.53290851690289,60.334002465445,39.3482879464));
#207304=CARTESIAN_POINT('Ctrl Pts',(-6.52373669508281,60.2467384099263,
39.4512271261638));
#207305=CARTESIAN_POINT('Ctrl Pts',(-6.6683304315061,60.4052373806432,39.3978017080178));
#207306=CARTESIAN_POINT('Ctrl Pts',(-6.54178440911703,60.4184509388156,
39.3975673827378));
#207307=CARTESIAN_POINT('Ctrl Pts',(-6.53710513959958,60.373930663245,39.5248015355181));
#207308=CARTESIAN_POINT('Ctrl Pts',(-6.67747469700884,60.4944777170594,
39.3978017080178));
#207309=CARTESIAN_POINT('Ctrl Pts',(-6.55117041629707,60.5077528318944,
39.3978017080178));
#207310=CARTESIAN_POINT('Ctrl Pts',(-6.55117041629707,60.5077528318944,
39.5248017080178));
#207311=CARTESIAN_POINT('Origin',(-6.64298446507862,60.1663250803646,39.3343017080178));
#207312=CARTESIAN_POINT('Origin',(-6.63448104698998,60.0854204586817,39.1934008533545));
#207313=CARTESIAN_POINT('Origin',(0.317499999708719,61.4240753804094,39.1925554495086));
#207314=CARTESIAN_POINT('Origin',(0.317551690014633,61.4683012396074,39.1160373285273));
#207315=CARTESIAN_POINT('Origin',(0.317500000000648,61.3422370451705,39.3343017080178));
#207316=CARTESIAN_POINT('Ctrl Pts',(0.316930737396561,61.2322532920972,
39.2708017080178));
#207317=CARTESIAN_POINT('Ctrl Pts',(0.190500000000648,61.2327440814646,
39.2710850691866));
#207318=CARTESIAN_POINT('Ctrl Pts',(0.190500000000648,61.3422370451705,
39.3343017080178));
#207319=CARTESIAN_POINT('Ctrl Pts',(0.317046579200286,61.1872475084174,
39.3487519293518));
#207320=CARTESIAN_POINT('Ctrl Pts',(0.190500000000646,61.1875064541748,
39.3492068662925));
#207321=CARTESIAN_POINT('Ctrl Pts',(0.190500000000647,61.2747290395312,
39.451227124874));
#207322=CARTESIAN_POINT('Ctrl Pts',(0.317266596914152,61.1019842137032,
39.3978017080178));
#207323=CARTESIAN_POINT('Ctrl Pts',(0.19050000000065,61.1018997758116,39.3980347781183));
#207324=CARTESIAN_POINT('Ctrl Pts',(0.190500000000646,61.146836207171,39.5248015355195));
#207325=CARTESIAN_POINT('Ctrl Pts',(0.317500000000645,61.0122769227456,
39.3978017080178));
#207326=CARTESIAN_POINT('Ctrl Pts',(0.190500000000645,61.0122769227456,
39.3978017080178));
#207327=CARTESIAN_POINT('Ctrl Pts',(0.190500000000645,61.0122769227456,
39.5248017080178));
#207328=CARTESIAN_POINT('Origin',(0.317500000000645,61.0122769227456,39.5248017080178));
#207329=CARTESIAN_POINT('Origin',(0.317500000000006,-3.32563597524808E-15,
39.116));
#207330=CARTESIAN_POINT('Origin',(0.317500000000654,61.8696548221181,39.116));
#207331=CARTESIAN_POINT('Origin',(0.317500000000006,-3.32563597524808E-15,
39.5248017080178));
#207332=CARTESIAN_POINT('Origin',(0.317500000000643,60.8610688070707,39.5248017080178));
#207333=CARTESIAN_POINT('Ctrl Pts',(0.318048871877788,62.4081695979768,
39.2875012672119));
#207334=CARTESIAN_POINT('Ctrl Pts',(0.19030903417629,62.4086377819835,39.287208709576));
#207335=CARTESIAN_POINT('Ctrl Pts',(0.190500142125712,62.3003077603774,
39.3549016990122));
#207336=CARTESIAN_POINT('Ctrl Pts',(0.317932489890632,62.2931881445371,
39.1034939173931));
#207337=CARTESIAN_POINT('Ctrl Pts',(0.190309294369134,62.2934975005705,
39.103169233634));
#207338=CARTESIAN_POINT('Ctrl Pts',(0.190500141996123,62.2083564003244,
39.2077507202297));
#207339=CARTESIAN_POINT('Ctrl Pts',(0.317722686168063,62.0866281564673,
38.989));
#207340=CARTESIAN_POINT('Ctrl Pts',(0.190309769570643,62.0868143053113,
38.9887769311176));
#207341=CARTESIAN_POINT('Ctrl Pts',(0.190500141762521,62.0431695205396,
39.1161898712915));
#207342=CARTESIAN_POINT('Ctrl Pts',(0.317500000000654,61.8696548221181,
38.989));
#207343=CARTESIAN_POINT('Ctrl Pts',(0.190310267889922,61.8696548221181,
38.989));
#207344=CARTESIAN_POINT('Ctrl Pts',(0.190500141514568,61.8696548221181,
39.1161895903854));
#207345=CARTESIAN_POINT('Origin',(0.317500000000658,62.3004688883554,39.3548010137695));
#207346=CARTESIAN_POINT('Ctrl Pts',(0.317500000000643,60.8610688070707,
39.3978017080178));
#207347=CARTESIAN_POINT('Ctrl Pts',(0.190500000000643,60.8610688070707,
39.3978017080178));
#207348=CARTESIAN_POINT('Ctrl Pts',(0.190500000000643,60.8610688070707,
39.5248017080178));
#207349=CARTESIAN_POINT('Ctrl Pts',(0.317734773760909,60.7710583184321,
39.3978017080178));
#207350=CARTESIAN_POINT('Ctrl Pts',(0.190500000000643,60.7709717342408,
39.3975666025021));
#207351=CARTESIAN_POINT('Ctrl Pts',(0.190500000000642,60.7260547307358,
39.5248015517178));
#207352=CARTESIAN_POINT('Ctrl Pts',(0.317958617919677,60.6859465754578,
39.3484894016716));
#207353=CARTESIAN_POINT('Ctrl Pts',(0.190500000001051,60.6862105562579,
39.3480259000038));
#207354=CARTESIAN_POINT('Ctrl Pts',(0.19050000000064,60.5983892955408,39.4508333188947));
#207355=CARTESIAN_POINT('Ctrl Pts',(0.318076890624007,60.6410923272405,
39.2708017080178));
#207356=CARTESIAN_POINT('Ctrl Pts',(0.19050000000064,60.6415942020421,39.27051194648));
#207357=CARTESIAN_POINT('Ctrl Pts',(0.19050000000064,60.5311086139135,39.3343017080178));
#207358=CARTESIAN_POINT('Origin',(0.317500000000639,60.5311086139135,39.3343017080178));
#207359=CARTESIAN_POINT('Origin',(0.317499999979629,62.4786179998468,39.6398955068197));
#207360=CARTESIAN_POINT('Origin',(0.317500000000662,62.6567671111299,39.92499));
#207361=CARTESIAN_POINT('Origin',(0.317499999994473,60.4497583458796,39.1934008539944));
#207362=CARTESIAN_POINT('Origin',(0.317550804321697,60.4050521322799,39.1160402713852));
#207363=CARTESIAN_POINT('Ctrl Pts',(0.0152661173115319,62.9541448057648,
40.1599502534424));
#207364=CARTESIAN_POINT('Ctrl Pts',(0.0152570710392988,62.9168399481843,
40.10025));
#207365=CARTESIAN_POINT('Ctrl Pts',(0.0152400000006639,62.8464427007196,
40.10025));
#207366=CARTESIAN_POINT('Ctrl Pts',(0.103381504925819,62.9541233134297,
40.1599500538463));
#207367=CARTESIAN_POINT('Ctrl Pts',(0.0794415635241996,62.9168211560341,
40.100244835349));
#207368=CARTESIAN_POINT('Ctrl Pts',(0.0662446030565934,62.8464212442881,
40.10025));
#207369=CARTESIAN_POINT('Ctrl Pts',(0.184683583688528,62.9290872705826,
40.1202442001037));
#207370=CARTESIAN_POINT('Ctrl Pts',(0.138547994785008,62.8936771137448,
40.0633873868015));
#207371=CARTESIAN_POINT('Ctrl Pts',(0.11330556745224,62.8213855864655,40.0772271723537));
#207372=CARTESIAN_POINT('Ctrl Pts',(0.29134099263231,62.8564203507742,40.0045995998164));
#207373=CARTESIAN_POINT('Ctrl Pts',(0.201910351191971,62.8329175802742,
39.9663485808318));
#207374=CARTESIAN_POINT('Ctrl Pts',(0.175042741958496,62.7487193609389,
40.0101727202466));
#207375=CARTESIAN_POINT('Ctrl Pts',(0.318045276843284,62.8099434033761,
39.9304654349858));
#207376=CARTESIAN_POINT('Ctrl Pts',(0.205831635643775,62.7947175424999,
39.9051900162947));
#207377=CARTESIAN_POINT('Ctrl Pts',(0.190500000000664,62.7022409210443,
39.9671857458178));
#207378=CARTESIAN_POINT('Ctrl Pts',(0.318045750793708,62.7644678366119,
39.8576902534424));
#207379=CARTESIAN_POINT('Ctrl Pts',(0.190500000000658,62.7649326510149,
39.8573998014387));
#207380=CARTESIAN_POINT('Ctrl Pts',(0.190500000000662,62.6567671111299,
39.92499));
#207381=CARTESIAN_POINT('Origin',(0.317500000000006,-3.32563597524808E-15,
39.116));
#207382=CARTESIAN_POINT('Origin',(0.317500000000634,60.0036905223731,39.116));
#207383=CARTESIAN_POINT('Ctrl Pts',(0.317500000000634,60.0036905223731,
38.989));
#207384=CARTESIAN_POINT('Ctrl Pts',(0.190309748265858,60.003690522373,38.989));
#207385=CARTESIAN_POINT('Ctrl Pts',(0.190500142290163,60.0036905223731,
39.1161901092321));
#207386=CARTESIAN_POINT('Ctrl Pts',(0.31727038552505,59.7867137603524,38.989));
#207387=CARTESIAN_POINT('Ctrl Pts',(0.190310262476932,59.7869045527987,
38.989229898976));
#207388=CARTESIAN_POINT('Ctrl Pts',(0.190500142033094,59.8301727552495,
39.1161900493201));
#207389=CARTESIAN_POINT('Ctrl Pts',(0.317049440714262,59.5801552670728,
39.1034966344368));
#207390=CARTESIAN_POINT('Ctrl Pts',(0.190310761082396,59.5804765271847,
39.1038314102561));
#207391=CARTESIAN_POINT('Ctrl Pts',(0.190500141785737,59.664987104655,39.2077528789601));
#207392=CARTESIAN_POINT('Ctrl Pts',(0.316925998273675,59.4651754363832,
39.2875012672119));
#207393=CARTESIAN_POINT('Ctrl Pts',(0.190311035335595,59.4656607446593,
39.2878045257868));
#207394=CARTESIAN_POINT('Ctrl Pts',(0.190500141647532,59.5730368716576,
39.3549015295899));
#207395=CARTESIAN_POINT('Origin',(0.31750000000063,59.5728760150042,39.3548010137695));
#207396=CARTESIAN_POINT('Ctrl Pts',(-0.318045750792382,62.7644678366119,
39.8576902534424));
#207397=CARTESIAN_POINT('Ctrl Pts',(-0.190499999999334,62.7649326510149,
39.8573998014387));
#207398=CARTESIAN_POINT('Ctrl Pts',(-0.190499999999338,62.6567671111299,
39.92499));
#207399=CARTESIAN_POINT('Ctrl Pts',(-0.318045262794513,62.8099640589335,
39.9304984902491));
#207400=CARTESIAN_POINT('Ctrl Pts',(-0.20584033072329,62.7947344577613,
39.9052171569794));
#207401=CARTESIAN_POINT('Ctrl Pts',(-0.190499999999339,62.7022616416333,
39.9672049726608));
#207402=CARTESIAN_POINT('Ctrl Pts',(-0.291334117854747,62.8562601188214,
40.0043437678662));
#207403=CARTESIAN_POINT('Ctrl Pts',(-0.201836550627054,62.8328016940825,
39.9661628577639));
#207404=CARTESIAN_POINT('Ctrl Pts',(-0.175038734051537,62.7485591297232,
40.0100243556234));
#207405=CARTESIAN_POINT('Ctrl Pts',(-0.185622189559732,62.9286112571071,
40.1194874821987));
#207406=CARTESIAN_POINT('Ctrl Pts',(-0.139140155999468,62.8932808767899,
40.0627551483143));
#207407=CARTESIAN_POINT('Ctrl Pts',(-0.113848895265012,62.8209095783125,
40.0767884282378));
#207408=CARTESIAN_POINT('Ctrl Pts',(-0.103673266462164,62.9541233349674,
40.1599502015391));
#207409=CARTESIAN_POINT('Ctrl Pts',(-0.0796882264529957,62.9168211653022,
40.1002449453869));
#207410=CARTESIAN_POINT('Ctrl Pts',(-0.0664134143644937,62.8464212664863,
40.10025));
#207411=CARTESIAN_POINT('Ctrl Pts',(-0.0152661173102017,62.9541448057648,
40.1599502534424));
#207412=CARTESIAN_POINT('Ctrl Pts',(-0.0152570710379694,62.9168399481843,
40.10025));
#207413=CARTESIAN_POINT('Ctrl Pts',(-0.015239999999336,62.8464427007196,
40.10025));
#207414=CARTESIAN_POINT('Origin',(-0.317499999999338,62.6567671111299,39.92499));
#207415=CARTESIAN_POINT('Origin',(0.317499999970736,59.3947266586226,39.6398955069306));
#207416=CARTESIAN_POINT('Origin',(0.317500000000626,59.2165773020941,39.92499));
#207417=CARTESIAN_POINT('Origin',(-0.317499999976485,62.4786179998354,39.6398955068269));
#207418=CARTESIAN_POINT('Origin',(-0.317499999999342,62.3004688883555,39.3548010137695));
#207419=CARTESIAN_POINT('Ctrl Pts',(0.316922544676314,59.1088767419348,
39.8576902534424));
#207420=CARTESIAN_POINT('Ctrl Pts',(0.190500000000626,59.1093642282366,
39.8579948730703));
#207421=CARTESIAN_POINT('Ctrl Pts',(0.190500000000626,59.2165773020941,
39.92499));
#207422=CARTESIAN_POINT('Ctrl Pts',(0.316922012809789,59.0634407053228,
39.9304020711232));
#207423=CARTESIAN_POINT('Ctrl Pts',(0.205694973741221,59.0793536643037,
39.9058915297385));
#207424=CARTESIAN_POINT('Ctrl Pts',(0.190500000000625,59.1711393827287,
39.9671523786031));
#207425=CARTESIAN_POINT('Ctrl Pts',(0.290332993455678,59.0174076205277,
40.0043257306692));
#207426=CARTESIAN_POINT('Ctrl Pts',(0.201480151666502,59.0412846811398,
39.9667894847832));
#207427=CARTESIAN_POINT('Ctrl Pts',(0.175054909460471,59.1251084688124,
40.0100138975199));
#207428=CARTESIAN_POINT('Ctrl Pts',(0.184894967402138,58.9458296250061,
40.1195533054858));
#207429=CARTESIAN_POINT('Ctrl Pts',(0.138672156931825,58.9812445774289,
40.0630813209239));
#207430=CARTESIAN_POINT('Ctrl Pts',(0.113807322598262,59.053531245193,40.0768265942422));
#207431=CARTESIAN_POINT('Ctrl Pts',(0.103171606456398,58.9208287018091,
40.1599502027518));
#207432=CARTESIAN_POINT('Ctrl Pts',(0.0793367652464492,58.9581363848269,
40.1002552791538));
#207433=CARTESIAN_POINT('Ctrl Pts',(0.0663350652350921,59.0285307646513,
40.10025));
#207434=CARTESIAN_POINT('Ctrl Pts',(0.015212193456543,58.9208513795073,
40.1599502534424));
#207435=CARTESIAN_POINT('Ctrl Pts',(0.0152218248297303,58.9581562369413,
40.10025));
#207436=CARTESIAN_POINT('Ctrl Pts',(0.0152400000006241,59.0285534841296,
40.10025));
#207437=CARTESIAN_POINT('Ctrl Pts',(-0.317499999999346,61.8696548221181,
38.989));
#207438=CARTESIAN_POINT('Ctrl Pts',(-0.190310256931028,61.8696548221181,
38.989));
#207439=CARTESIAN_POINT('Ctrl Pts',(-0.190500141529595,61.8696548221181,
39.1161896013266));
#207440=CARTESIAN_POINT('Ctrl Pts',(-0.317722689631595,62.0866315324121,
38.989));
#207441=CARTESIAN_POINT('Ctrl Pts',(-0.190309758575247,62.0868176889541,
38.988776927546));
#207442=CARTESIAN_POINT('Ctrl Pts',(-0.190500141777577,62.0431722165661,
39.1161898821848));
#207443=CARTESIAN_POINT('Ctrl Pts',(-0.317932491655033,62.2931898887681,
39.1034967087243));
#207444=CARTESIAN_POINT('Ctrl Pts',(-0.190309283349939,62.2934992458037,
39.103172023271));
#207445=CARTESIAN_POINT('Ctrl Pts',(-0.1905001420112,62.2083577878513,39.2077529614998));
#207446=CARTESIAN_POINT('Ctrl Pts',(-0.31804887187647,62.4081695979768,
39.2875012672119));
#207447=CARTESIAN_POINT('Ctrl Pts',(-0.1903090231461,62.4086377820239,39.2872087095508));
#207448=CARTESIAN_POINT('Ctrl Pts',(-0.1905001421408,62.3003077510787,39.3549017048228));
#207449=CARTESIAN_POINT('Origin',(-0.317499999999346,61.8696548221181,39.116));
#207450=CARTESIAN_POINT('Origin',(-0.317499999999998,6.55071265098105E-13,
39.116));
#207451=CARTESIAN_POINT('Origin',(-0.317551690012418,61.4683012396066,39.1160373285255));
#207452=CARTESIAN_POINT('Ctrl Pts',(-0.015212193455297,58.9208513795073,
40.1599502534424));
#207453=CARTESIAN_POINT('Ctrl Pts',(-0.0152218248284836,58.9581562369413,
40.10025));
#207454=CARTESIAN_POINT('Ctrl Pts',(-0.0152399999993761,59.0285534841296,
40.10025));
#207455=CARTESIAN_POINT('Ctrl Pts',(-0.102871702176771,58.9208288705618,
40.1599500566038));
#207456=CARTESIAN_POINT('Ctrl Pts',(-0.0790852439327617,58.9581365422965,
40.100255130536));
#207457=CARTESIAN_POINT('Ctrl Pts',(-0.0661608181918845,59.0285309330218,
40.10025));
#207458=CARTESIAN_POINT('Ctrl Pts',(-0.183955833236888,58.9453619764183,
40.1203070619046));
#207459=CARTESIAN_POINT('Ctrl Pts',(-0.138075936735343,58.9808530699761,
40.0637098684499));
#207460=CARTESIAN_POINT('Ctrl Pts',(-0.113261762367537,59.0530636028226,
40.0772636213363));
#207461=CARTESIAN_POINT('Ctrl Pts',(-0.290319860890038,59.0172303255294,
40.0046102245801));
#207462=CARTESIAN_POINT('Ctrl Pts',(-0.201541405841316,59.0411528690721,
39.9670001894012));
#207463=CARTESIAN_POINT('Ctrl Pts',(-0.175047309550564,59.1249311745757,
40.0101788811209));
#207464=CARTESIAN_POINT('Ctrl Pts',(-0.316922027356722,59.0634600627912,
39.9303710930187));
#207465=CARTESIAN_POINT('Ctrl Pts',(-0.20568700036667,59.0793694364685,
39.9058663574109));
#207466=CARTESIAN_POINT('Ctrl Pts',(-0.190499999999374,59.1711586818658,
39.9671344706364));
#207467=CARTESIAN_POINT('Ctrl Pts',(-0.316922544675064,59.1088767419348,
39.8576902534424));
#207468=CARTESIAN_POINT('Ctrl Pts',(-0.190499999999374,59.1093642282366,
39.8579948730703));
#207469=CARTESIAN_POINT('Ctrl Pts',(-0.190499999999374,59.2165773020941,
39.92499));
#207470=CARTESIAN_POINT('Origin',(-0.317499999999374,59.2165773020941,39.92499));
#207471=CARTESIAN_POINT('Origin',(-0.317499999993373,61.4240753793279,39.1925554488842));
#207472=CARTESIAN_POINT('Origin',(-0.317499999999352,61.3422370451705,39.3343017080178));
#207473=CARTESIAN_POINT('Origin',(-0.317499999969898,59.3947266586074,39.6398955069212));
#207474=CARTESIAN_POINT('Origin',(-0.31749999999937,59.5728760150042,39.3548010137695));
#207475=CARTESIAN_POINT('Ctrl Pts',(-0.317499999999355,61.0122769227456,
39.3978017080178));
#207476=CARTESIAN_POINT('Ctrl Pts',(-0.190499999999355,61.0122769227456,
39.3978017080178));
#207477=CARTESIAN_POINT('Ctrl Pts',(-0.190499999999355,61.0122769227456,
39.5248017080178));
#207478=CARTESIAN_POINT('Ctrl Pts',(-0.317265808075748,61.1022873990971,
39.3978017080178));
#207479=CARTESIAN_POINT('Ctrl Pts',(-0.190499999999328,61.1022028716704,
39.3980355775177));
#207480=CARTESIAN_POINT('Ctrl Pts',(-0.190499999999354,61.1472909869838,
39.5248015517192));
#207481=CARTESIAN_POINT('Ctrl Pts',(-0.317046189128453,61.1873990841185,
39.3484893995498));
#207482=CARTESIAN_POINT('Ctrl Pts',(-0.190500000000547,61.1876587562325,
39.3489438303426));
#207483=CARTESIAN_POINT('Ctrl Pts',(-0.190499999999353,61.2749563897836,
39.4508333155593));
#207484=CARTESIAN_POINT('Ctrl Pts',(-0.316930737395267,61.2322532920972,
39.2708017080178));
#207485=CARTESIAN_POINT('Ctrl Pts',(-0.190499999999346,61.2327440814646,
39.2710850691866));
#207486=CARTESIAN_POINT('Ctrl Pts',(-0.190499999999352,61.3422370451705,
39.3343017080178));
#207487=CARTESIAN_POINT('Origin',(-0.317499999999355,61.0122769227456,39.5248017080178));
#207488=CARTESIAN_POINT('Ctrl Pts',(-0.316925998272419,59.4651754363832,
39.2875012672119));
#207489=CARTESIAN_POINT('Ctrl Pts',(-0.190311049924531,59.4656607446034,
39.2878045257519));
#207490=CARTESIAN_POINT('Ctrl Pts',(-0.190500141624416,59.5730368592469,
39.3549015218347));
#207491=CARTESIAN_POINT('Ctrl Pts',(-0.31704944257856,59.5801570044831,
39.1034938540228));
#207492=CARTESIAN_POINT('Ctrl Pts',(-0.190310775688781,59.5804782634853,
39.1038286278806));
#207493=CARTESIAN_POINT('Ctrl Pts',(-0.190500141762599,59.664988484272,
39.2077506434032));
#207494=CARTESIAN_POINT('Ctrl Pts',(-0.317270389088207,59.7867171285936,
38.989));
#207495=CARTESIAN_POINT('Ctrl Pts',(-0.190310277117612,59.7869079131834,
38.9892298954611));
#207496=CARTESIAN_POINT('Ctrl Pts',(-0.190500142009918,59.8301754438923,
39.1161900347288));
#207497=CARTESIAN_POINT('Ctrl Pts',(-0.317499999999366,60.0036905223731,
38.989));
#207498=CARTESIAN_POINT('Ctrl Pts',(-0.190309762954212,60.0036905223731,
38.989));
#207499=CARTESIAN_POINT('Ctrl Pts',(-0.19050014226694,60.0036905223731,
39.1161900945645));
#207500=CARTESIAN_POINT('Origin',(-0.317499999999366,60.0036905223731,39.116));
#207501=CARTESIAN_POINT('Origin',(-0.317499999999991,6.39284123049835E-13,
39.5248017080178));
#207502=CARTESIAN_POINT('Origin',(-0.317499999999357,60.8610688070707,39.5248017080178));
#207503=CARTESIAN_POINT('Origin',(-0.317499999999991,6.36811926168668E-13,
39.116));
#207504=CARTESIAN_POINT('Origin',(-0.317550804320187,60.4050521322801,39.116040271385));
#207505=CARTESIAN_POINT('Ctrl Pts',(-0.318076890622726,60.6410923272405,
39.2708017080178));
#207506=CARTESIAN_POINT('Ctrl Pts',(-0.190499999999366,60.6415942020422,
39.27051194648));
#207507=CARTESIAN_POINT('Ctrl Pts',(-0.19049999999936,60.5311086139135,
39.3343017080178));
#207508=CARTESIAN_POINT('Ctrl Pts',(-0.317958218318119,60.6860981505084,
39.3487519301186));
#207509=CARTESIAN_POINT('Ctrl Pts',(-0.190499999998138,60.6863613750267,
39.348287946399));
#207510=CARTESIAN_POINT('Ctrl Pts',(-0.19049999999936,60.598616644694,39.4512271261644));
#207511=CARTESIAN_POINT('Ctrl Pts',(-0.317733982966902,60.771361502534,
39.3978017080178));
#207512=CARTESIAN_POINT('Ctrl Pts',(-0.190499999999357,60.7712750142006,
39.3975673827397));
#207513=CARTESIAN_POINT('Ctrl Pts',(-0.190499999999358,60.7265095085063,
39.5248015355181));
#207514=CARTESIAN_POINT('Ctrl Pts',(-0.317499999999357,60.8610688070707,
39.3978017080178));
#207515=CARTESIAN_POINT('Ctrl Pts',(-0.190499999999357,60.8610688070707,
39.3978017080178));
#207516=CARTESIAN_POINT('Ctrl Pts',(-0.190499999999357,60.8610688070707,
39.5248017080178));
#207517=CARTESIAN_POINT('Origin',(-0.31749999999936,60.5311086139135,39.3343017080178));
#207518=CARTESIAN_POINT('Origin',(-0.317500000299763,60.4497583469878,39.1934008533546));
#207519=CARTESIAN_POINT('Origin',(6.73632490863968,61.054400081511,39.1925554495083));
#207520=CARTESIAN_POINT('Origin',(6.74099917688,61.0983782637173,39.1160373285268));
#207521=CARTESIAN_POINT('Origin',(6.72777047351185,60.9730100652054,39.3343017080178));
#207522=CARTESIAN_POINT('Ctrl Pts',(6.71570789669471,60.8636883187844,39.2708017080178));
#207523=CARTESIAN_POINT('Ctrl Pts',(6.59002106156527,60.877392030246,39.2710850691866));
#207524=CARTESIAN_POINT('Ctrl Pts',(6.60146619280008,60.9862851800404,39.3343017080178));
#207525=CARTESIAN_POINT('Ctrl Pts',(6.71111871849892,60.8189169727308,39.3487519293518));
#207526=CARTESIAN_POINT('Ctrl Pts',(6.58529244190356,60.8324022194127,39.3492068662927));
#207527=CARTESIAN_POINT('Ctrl Pts',(6.59440968471234,60.9191469903194,39.451227124874));
#207528=CARTESIAN_POINT('Ctrl Pts',(6.70242508976313,60.7340977611528,39.3978017080178));
#207529=CARTESIAN_POINT('Ctrl Pts',(6.57634410736793,60.7472645033892,39.3980347781183));
#207530=CARTESIAN_POINT('Ctrl Pts',(6.58104124348278,60.7919547682765,39.5248015355195));
#207531=CARTESIAN_POINT('Ctrl Pts',(6.69328024897516,60.6448574988554,39.3978017080178));
#207532=CARTESIAN_POINT('Ctrl Pts',(6.56697596826339,60.6581326136904,39.3978017080178));
#207533=CARTESIAN_POINT('Ctrl Pts',(6.56697596826339,60.6581326136904,39.5248017080178));
#207534=CARTESIAN_POINT('Origin',(6.69328024897516,60.6448574988554,39.5248017080178));
#207535=CARTESIAN_POINT('Origin',(0.315760701779432,-0.0331877870874832,
39.116));
#207536=CARTESIAN_POINT('Origin',(6.78290064323623,61.4975385923861,39.116));
#207537=CARTESIAN_POINT('Origin',(0.315760701779432,-0.0331877870874832,
39.5248017080178));
#207538=CARTESIAN_POINT('Origin',(6.67747469701007,60.4944777170593,39.5248017080178));
#207539=CARTESIAN_POINT('Ctrl Pts',(6.83973663030323,62.0330459552232,39.2875012672119));
#207540=CARTESIAN_POINT('Ctrl Pts',(6.71274550335304,62.0468640234019,39.287208709576));
#207541=CARTESIAN_POINT('Ctrl Pts',(6.70161199370888,61.9391074687686,39.3549016990123));
#207542=CARTESIAN_POINT('Ctrl Pts',(6.82760205123604,61.9187065474465,39.1034939173931));
#207543=CARTESIAN_POINT('Ctrl Pts',(6.70071032544346,61.932354465302,39.1031692336335));
#207544=CARTESIAN_POINT('Ctrl Pts',(6.69200045921829,61.8476598279005,39.2077507202298));
#207545=CARTESIAN_POINT('Ctrl Pts',(6.80580199871536,61.7133000470645,38.989));
#207546=CARTESIAN_POINT('Ctrl Pts',(6.67910652125894,61.7268034525369,38.9887769311176));
#207547=CARTESIAN_POINT('Ctrl Pts',(6.67473372829009,61.6833778591514,39.1161898712915));
#207548=CARTESIAN_POINT('Ctrl Pts',(6.78290064323623,61.4975385923861,38.989));
#207549=CARTESIAN_POINT('Ctrl Pts',(6.65640766978607,61.5108335396271,38.989));
#207550=CARTESIAN_POINT('Ctrl Pts',(6.65659650326314,61.5108136924289,39.1161895903854));
#207551=CARTESIAN_POINT('Origin',(6.82793297553411,61.9259926140919,39.3548010137695));
#207552=CARTESIAN_POINT('Ctrl Pts',(6.67747469701007,60.4944777170593,39.3978017080178));
#207553=CARTESIAN_POINT('Ctrl Pts',(6.5511704162983,60.5077528318943,39.3978017080178));
#207554=CARTESIAN_POINT('Ctrl Pts',(6.5511704162983,60.5077528318943,39.5248017080178));
#207555=CARTESIAN_POINT('Ctrl Pts',(6.66829952659994,60.404935774755,39.3978017080178));
#207556=CARTESIAN_POINT('Ctrl Pts',(6.54175270773074,60.4181493202563,39.3975666025021));
#207557=CARTESIAN_POINT('Ctrl Pts',(6.53705760237946,60.3734783767959,39.5248015517178));
#207558=CARTESIAN_POINT('Ctrl Pts',(6.65962554481765,60.3202668847282,39.3484894016717));
#207559=CARTESIAN_POINT('Ctrl Pts',(6.53289275204912,60.3338524728754,39.3480259000038));
#207560=CARTESIAN_POINT('Ctrl Pts',(6.52371293062624,60.2465123062138,39.4508333188945));
#207561=CARTESIAN_POINT('Ctrl Pts',(6.65505462397456,60.2756459899118,39.2708017080178));
#207562=CARTESIAN_POINT('Ctrl Pts',(6.52822907310839,60.2894805317161,39.27051194648));
#207563=CARTESIAN_POINT('Ctrl Pts',(6.51668018436807,60.1796001951995,39.3343017080178));
#207564=CARTESIAN_POINT('Origin',(6.64298446507984,60.1663250803645,39.3343017080178));
#207565=CARTESIAN_POINT('Origin',(6.84655462836781,62.1031658061145,39.6398955068186));
#207566=CARTESIAN_POINT('Origin',(6.86517628122572,62.2803389979219,39.92499));
#207567=CARTESIAN_POINT('Origin',(6.63448104656917,60.0854204576121,39.193400853994));
#207568=CARTESIAN_POINT('Origin',(6.62985850077975,60.040953838829,39.1160402713856));
#207569=CARTESIAN_POINT('Ctrl Pts',(6.59568250079948,62.6076796697354,40.1599502534424));
#207570=CARTESIAN_POINT('Ctrl Pts',(6.59177408464837,62.5705801176609,40.10025));
#207571=CARTESIAN_POINT('Ctrl Pts',(6.58439859103091,62.500570298093,40.10025));
#207572=CARTESIAN_POINT('Ctrl Pts',(6.68331293653994,62.5984477290793,40.1599500538453));
#207573=CARTESIAN_POINT('Ctrl Pts',(6.6556050034532,62.5638523220915,40.1002448353493));
#207574=CARTESIAN_POINT('Ctrl Pts',(6.63512154272685,62.4952175264256,40.10025));
#207575=CARTESIAN_POINT('Ctrl Pts',(6.76155265492332,62.5650504549417,40.1202442001039));
#207576=CARTESIAN_POINT('Ctrl Pts',(6.71196843232468,62.534656760858,40.0633873868015));
#207577=CARTESIAN_POINT('Ctrl Pts',(6.67930776339633,62.4653998062675,40.0772271723537));
#207578=CARTESIAN_POINT('Ctrl Pts',(6.86003002196325,62.48163287707,40.0045995998162));
#207579=CARTESIAN_POINT('Ctrl Pts',(6.76863258245113,62.4676069047249,39.9663485808318));
#207580=CARTESIAN_POINT('Ctrl Pts',(6.73311104631518,62.3866783619495,40.0101727202466));
#207581=CARTESIAN_POINT('Ctrl Pts',(6.88172985342223,62.4326191774618,39.9304654349859));
#207582=CARTESIAN_POINT('Ctrl Pts',(6.76853939445079,62.4292062449162,39.905190016295));
#207583=CARTESIAN_POINT('Ctrl Pts',(6.74362530798325,62.3388388123827,39.9671857458179));
#207584=CARTESIAN_POINT('Ctrl Pts',(6.87697683366627,62.387392681069,39.8576902534424));
#207585=CARTESIAN_POINT('Ctrl Pts',(6.75017837817664,62.4011871104968,39.8573998014387));
#207586=CARTESIAN_POINT('Ctrl Pts',(6.73887200051396,62.2936141127569,39.92499));
#207587=CARTESIAN_POINT('Origin',(6.58439859103091,62.500570298093,40.22725));
#207588=CARTESIAN_POINT('Origin',(0.315760701779432,-0.0331877870874832,
39.116));
#207589=CARTESIAN_POINT('Origin',(6.58785426247156,59.6417962403142,39.116));
#207590=CARTESIAN_POINT('Origin',(5.64744126194171E-15,5.53089827396188E-15,
40.22725));
#207591=CARTESIAN_POINT('Origin',(6.55408556366009,62.5037563256534,40.22725));
#207592=CARTESIAN_POINT('Ctrl Pts',(6.58785426247156,59.6417962403142,38.989));
#207593=CARTESIAN_POINT('Ctrl Pts',(6.4613607722442,59.6550912418706,38.989));
#207594=CARTESIAN_POINT('Ctrl Pts',(6.46155012326984,59.6550713402759,39.1161901092318));
#207595=CARTESIAN_POINT('Ctrl Pts',(6.56494565834935,59.4260321009468,38.989));
#207596=CARTESIAN_POINT('Ctrl Pts',(6.43870097938069,59.4394927947694,38.989229898976));
#207597=CARTESIAN_POINT('Ctrl Pts',(6.44341257746704,59.4825041216622,39.1161900493198));
#207598=CARTESIAN_POINT('Ctrl Pts',(6.54313468201973,59.2206282517276,39.1034966344368));
#207599=CARTESIAN_POINT('Ctrl Pts',(6.41712387096456,59.2341955513628,39.1038314102566));
#207600=CARTESIAN_POINT('Ctrl Pts',(6.42614597501067,59.3182233753726,39.2077528789601));
#207601=CARTESIAN_POINT('Ctrl Pts',(6.53099325080115,59.1062911958296,39.2875012672119));
#207602=CARTESIAN_POINT('Ctrl Pts',(6.40512262640657,59.1200087130388,39.2878045257868));
#207603=CARTESIAN_POINT('Ctrl Pts',(6.41653455832081,59.2267768553861,39.3549015295897));
#207604=CARTESIAN_POINT('Origin',(6.54282188406287,59.2133417798936,39.3548010137695));
#207605=CARTESIAN_POINT('Ctrl Pts',(6.24436990788122,62.4538823482275,39.8576902534424));
#207606=CARTESIAN_POINT('Ctrl Pts',(6.37126553604133,62.4410124550017,39.8573998014387));
#207607=CARTESIAN_POINT('Ctrl Pts',(6.35995915837864,62.3334394572618,39.92499));
#207608=CARTESIAN_POINT('Ctrl Pts',(6.24912604340989,62.4991292864732,39.9304984902492));
#207609=CARTESIAN_POINT('Ctrl Pts',(6.35912437831703,62.4722545055303,39.9052171569795));
#207610=CARTESIAN_POINT('Ctrl Pts',(6.36471463173929,62.3786847639674,39.9672049726605));
#207611=CARTESIAN_POINT('Ctrl Pts',(6.28053011789799,62.5423796567681,40.004343767866));
#207612=CARTESIAN_POINT('Ctrl Pts',(6.3670853349994,62.5096946965644,39.9661628577643));
#207613=CARTESIAN_POINT('Ctrl Pts',(6.38493060453772,62.4231124872027,40.0100243556236));
#207614=CARTESIAN_POINT('Ctrl Pts',(6.39322569848953,62.6032845425346,40.1194874821989));
#207615=CARTESIAN_POINT('Ctrl Pts',(6.43576006824533,62.5632890102012,40.062755148314));
#207616=CARTESIAN_POINT('Ctrl Pts',(6.45334792019258,62.4886705126495,40.0767884282376));
#207617=CARTESIAN_POINT('Ctrl Pts',(6.47739243510552,62.620090867565,40.1599502015389));
#207618=CARTESIAN_POINT('Ctrl Pts',(6.49734694408422,62.5804859237135,40.1002449453872));
#207619=CARTESIAN_POINT('Ctrl Pts',(6.50319024212585,62.5090840872032,40.10025));
#207620=CARTESIAN_POINT('Ctrl Pts',(6.56531752495365,62.6108711573005,40.1599502534424));
#207621=CARTESIAN_POINT('Ctrl Pts',(6.56142710223415,62.5737697140401,40.10025));
#207622=CARTESIAN_POINT('Ctrl Pts',(6.55408556366009,62.5037563256534,40.10025));
#207623=CARTESIAN_POINT('Origin',(6.23365487766687,62.3467145720968,39.92499));
#207624=CARTESIAN_POINT('Origin',(6.52420020557921,59.0361683443322,39.6398955069324));
#207625=CARTESIAN_POINT('Origin',(6.50557852713814,58.858994908613,39.92499));
#207626=CARTESIAN_POINT('Origin',(6.2150332248537,62.1695413802714,39.639895506827));
#207627=CARTESIAN_POINT('Origin',(6.19641157197526,61.9923681882668,39.3548010137695));
#207628=CARTESIAN_POINT('Ctrl Pts',(6.493746461128,58.7519447039088,39.8576902534424));
#207629=CARTESIAN_POINT('Ctrl Pts',(6.36806742857384,58.765644274027,39.8579948730703));
#207630=CARTESIAN_POINT('Ctrl Pts',(6.37927424642637,58.872270023448,39.92499));
#207631=CARTESIAN_POINT('Ctrl Pts',(6.48899657309109,58.7067576262548,39.9304020711229));
#207632=CARTESIAN_POINT('Ctrl Pts',(6.38004220453006,58.7342098038497,39.9058915297385));
#207633=CARTESIAN_POINT('Ctrl Pts',(6.37452469054112,58.82708101776,39.9671523786039));
#207634=CARTESIAN_POINT('Ctrl Pts',(6.45774144355365,58.6637560248471,40.0043257306696));
#207635=CARTESIAN_POINT('Ctrl Pts',(6.37187117938174,58.6967899354329,39.9667894847838));
#207636=CARTESIAN_POINT('Ctrl Pts',(6.35435266912822,58.7829167175848,40.0100138975201));
#207637=CARTESIAN_POINT('Ctrl Pts',(6.34539908016389,58.6035914159082,40.1195533054854));
#207638=CARTESIAN_POINT('Ctrl Pts',(6.30313135363918,58.6436439608617,40.0630813209233));
#207639=CARTESIAN_POINT('Ctrl Pts',(6.28595874576577,58.7181337176191,40.076826594242));
#207640=CARTESIAN_POINT('Ctrl Pts',(6.26151010025777,58.587269867717,40.1599502027514));
#207641=CARTESIAN_POINT('Ctrl Pts',(6.24170554357575,58.6268645946676,40.1002552791553));
#207642=CARTESIAN_POINT('Ctrl Pts',(6.23613328458318,58.6982323944352,40.10025));
#207643=CARTESIAN_POINT('Ctrl Pts',(6.17403490859079,58.596486683455,40.1599502534424));
#207644=CARTESIAN_POINT('Ctrl Pts',(6.17794390662231,58.6335861742241,40.10025));
#207645=CARTESIAN_POINT('Ctrl Pts',(6.18532049829458,58.7035958781038,40.10025));
#207646=CARTESIAN_POINT('Origin',(6.18532049829458,58.7035958781038,40.22725));
#207647=CARTESIAN_POINT('Ctrl Pts',(6.15137923967737,61.5639141665611,38.989));
#207648=CARTESIAN_POINT('Ctrl Pts',(6.27787222402492,61.5506192181748,38.989));
#207649=CARTESIAN_POINT('Ctrl Pts',(6.27768337963421,61.5506390665201,39.1161896013264));
#207650=CARTESIAN_POINT('Ctrl Pts',(6.17383801205405,61.7797255331385,38.989));
#207651=CARTESIAN_POINT('Ctrl Pts',(6.3005724203996,61.7665923920118,38.988776927546));
#207652=CARTESIAN_POINT('Ctrl Pts',(6.29582088597955,61.7232059145528,39.1161898821846));
#207653=CARTESIAN_POINT('Ctrl Pts',(6.19522058691312,61.985174271489,39.1034967087243));
#207654=CARTESIAN_POINT('Ctrl Pts',(6.3221769985456,61.972141675993,39.103172023271));
#207655=CARTESIAN_POINT('Ctrl Pts',(6.31308747966742,61.8874865820171,39.2077529615));
#207656=CARTESIAN_POINT('Ctrl Pts',(6.20712349654526,62.0995362748658,39.2875012672119));
#207657=CARTESIAN_POINT('Ctrl Pts',(6.33421251157745,62.0866494440659,39.2872087095508));
#207658=CARTESIAN_POINT('Ctrl Pts',(6.32269886789234,61.9789328337399,39.3549017048227));
#207659=CARTESIAN_POINT('Origin',(6.15137923967737,61.5639141665611,39.116));
#207660=CARTESIAN_POINT('Origin',(5.67080826956262E-15,5.31104381076135E-15,
40.22725));
#207661=CARTESIAN_POINT('Origin',(6.15500747092375,58.7067819056642,40.22725));
#207662=CARTESIAN_POINT('Origin',(0.364094271196581,6.50157577599617,39.116));
#207663=CARTESIAN_POINT('Origin',(6.10937495962157,61.1647646440465,39.116037328525));
#207664=CARTESIAN_POINT('Ctrl Pts',(6.14377718965381,58.5996668978648,40.1599502534424));
#207665=CARTESIAN_POINT('Ctrl Pts',(6.1476670304623,58.6367684021392,40.10025));
#207666=CARTESIAN_POINT('Ctrl Pts',(6.15500747092375,58.7067819056642,40.10025));
#207667=CARTESIAN_POINT('Ctrl Pts',(6.05659553606757,58.6088074259629,40.1599500566041));
#207668=CARTESIAN_POINT('Ctrl Pts',(6.08415140319854,58.6434243604373,40.1002551305372));
#207669=CARTESIAN_POINT('Ctrl Pts',(6.10436324506862,58.712082152968,40.10025));
#207670=CARTESIAN_POINT('Ctrl Pts',(5.97852000021575,58.6416817365139,40.1203070619047));
#207671=CARTESIAN_POINT('Ctrl Pts',(6.02785839131313,58.6721826510715,40.06370986845));
#207672=CARTESIAN_POINT('Ctrl Pts',(6.06008468706751,58.7414038195495,40.0772636213363));
#207673=CARTESIAN_POINT('Ctrl Pts',(5.88025093392533,58.7242744516464,40.0046102245801));
#207674=CARTESIAN_POINT('Ctrl Pts',(5.97104363802217,58.7387860695149,39.9670001894012));
#207675=CARTESIAN_POINT('Ctrl Pts',(6.00614981441082,58.8193360415243,40.0101788811209));
#207676=CARTESIAN_POINT('Ctrl Pts',(5.85862682030321,58.7730316211506,39.9303710930187));
#207677=CARTESIAN_POINT('Ctrl Pts',(5.97091547255935,58.777226615181,39.9058663574108));
#207678=CARTESIAN_POINT('Ctrl Pts',(5.99561386571491,58.866925555679,39.967134470637));
#207679=CARTESIAN_POINT('Ctrl Pts',(5.86337364149639,58.8181995570484,39.8576902534424));
#207680=CARTESIAN_POINT('Ctrl Pts',(5.98915458643854,58.805469618532,39.8579948730703));
#207681=CARTESIAN_POINT('Ctrl Pts',(6.00036140429106,58.9120953679529,39.92499));
#207682=CARTESIAN_POINT('Origin',(5.87405712357929,58.9253704827879,39.92499));
#207683=CARTESIAN_POINT('Origin',(6.10480350526343,61.1207756545817,39.1925554488853));
#207684=CARTESIAN_POINT('Origin',(6.096249069953,61.0393856393803,39.3343017080178));
#207685=CARTESIAN_POINT('Origin',(5.89267880207684,59.1025439184842,39.6398955069219));
#207686=CARTESIAN_POINT('Origin',(5.91130048050402,59.2797173540685,39.3548010137695));
#207687=CARTESIAN_POINT('Ctrl Pts',(6.06175884541631,60.7112330730303,39.3978017080178));
#207688=CARTESIAN_POINT('Ctrl Pts',(6.18806312612808,60.6979579581953,39.3978017080178));
#207689=CARTESIAN_POINT('Ctrl Pts',(6.18806312612808,60.6979579581953,39.5248017080178));
#207690=CARTESIAN_POINT('Ctrl Pts',(6.07140041118295,60.8007259828525,39.3978017080178));
#207691=CARTESIAN_POINT('Ctrl Pts',(6.19746294737696,60.7873912833615,39.3980355775177));
#207692=CARTESIAN_POINT('Ctrl Pts',(6.20217593878221,60.8322324012609,39.5248015517192));
#207693=CARTESIAN_POINT('Ctrl Pts',(6.08051542067653,60.8853484607269,39.3484893995498));
#207694=CARTESIAN_POINT('Ctrl Pts',(6.206395519668,60.8723790316496,39.3489438303431));
#207695=CARTESIAN_POINT('Ctrl Pts',(6.21552060714981,60.9591984396309,39.45083331556));
#207696=CARTESIAN_POINT('Ctrl Pts',(6.08531878138382,60.929944884669,39.2708017080178));
#207697=CARTESIAN_POINT('Ctrl Pts',(6.21110821942996,60.917217374751,39.2710850691866));
#207698=CARTESIAN_POINT('Ctrl Pts',(6.22255335066477,61.0261105245453,39.3343017080178));
#207699=CARTESIAN_POINT('Origin',(6.06175884541631,60.7112330730303,39.5248017080178));
#207700=CARTESIAN_POINT('Ctrl Pts',(5.90061356181316,59.1725467709677,39.2875012672119));
#207701=CARTESIAN_POINT('Ctrl Pts',(6.02658562874881,59.1597945546411,39.2878045257519));
#207702=CARTESIAN_POINT('Ctrl Pts',(6.03762143316813,59.2666022171588,39.3549015218348));
#207703=CARTESIAN_POINT('Ctrl Pts',(5.91250964036517,59.2869113614504,39.1034938540228));
#207704=CARTESIAN_POINT('Ctrl Pts',(6.03858760028819,59.2739830624739,39.1038286278801));
#207705=CARTESIAN_POINT('Ctrl Pts',(6.04723299508931,59.3580501215732,39.2077506434029));
#207706=CARTESIAN_POINT('Ctrl Pts',(5.93388131656935,59.4923630227874,38.989));
#207707=CARTESIAN_POINT('Ctrl Pts',(6.06016587018271,59.4792818168399,38.9892298954611));
#207708=CARTESIAN_POINT('Ctrl Pts',(6.06449973388467,59.5223321697741,39.1161900347291));
#207709=CARTESIAN_POINT('Ctrl Pts',(5.95633285891271,59.7081718144892,38.989));
#207710=CARTESIAN_POINT('Ctrl Pts',(6.08282633453148,59.6948768144682,38.989));
#207711=CARTESIAN_POINT('Ctrl Pts',(6.08263699813626,59.6948967145252,39.1161900945648));
#207712=CARTESIAN_POINT('Origin',(5.95633285891271,59.7081718144892,39.116));
#207713=CARTESIAN_POINT('Origin',(0.347626240494121,6.34489293004957,39.5248017080178));
#207714=CARTESIAN_POINT('Origin',(6.04595329345122,60.5608532912343,39.5248017080178));
#207715=CARTESIAN_POINT('Origin',(0.345047419449927,6.32035708677299,39.116));
#207716=CARTESIAN_POINT('Origin',(5.99823604520107,60.1073400339994,39.1160402713854));
#207717=CARTESIAN_POINT('Ctrl Pts',(6.02238575970336,60.3421421670674,39.2708017080178));
#207718=CARTESIAN_POINT('Ctrl Pts',(6.14931623097308,60.3293058762211,39.27051194648));
#207719=CARTESIAN_POINT('Ctrl Pts',(6.13776734223276,60.2194255397044,39.3343017080178));
#207720=CARTESIAN_POINT('Ctrl Pts',(6.02720817145297,60.3868890390927,39.3487519301186));
#207721=CARTESIAN_POINT('Ctrl Pts',(6.15399567476866,60.3738278099515,39.3482879463982));
#207722=CARTESIAN_POINT('Ctrl Pts',(6.14482385294874,60.2865637544314,39.4512271261636));
#207723=CARTESIAN_POINT('Ctrl Pts',(6.03634362557985,60.4716618705781,39.3978017080178));
#207724=CARTESIAN_POINT('Ctrl Pts',(6.16287156698308,60.4582762833192,39.3975673827397));
#207725=CARTESIAN_POINT('Ctrl Pts',(6.15819229746547,60.4137560077496,39.5248015355181));
#207726=CARTESIAN_POINT('Ctrl Pts',(6.04595329345122,60.5608532912343,39.3978017080178));
#207727=CARTESIAN_POINT('Ctrl Pts',(6.17225757416299,60.5475781763993,39.3978017080178));
#207728=CARTESIAN_POINT('Ctrl Pts',(6.17225757416299,60.5475781763993,39.5248017080178));
#207729=CARTESIAN_POINT('Origin',(6.01146306152099,60.2327006545394,39.3343017080178));
#207730=CARTESIAN_POINT('Origin',(6.00295964283411,60.1517960329196,39.1934008533544));
#207731=CARTESIAN_POINT('Origin',(13.0813452322048,60.0157999988651,39.192555449508));
#207732=CARTESIAN_POINT('Origin',(13.0905908661203,60.0590486699119,39.1160373285273));
#207733=CARTESIAN_POINT('Origin',(13.0643300858388,59.9357500275432,39.3343017080178));
#207734=CARTESIAN_POINT('Ctrl Pts',(13.0409063549245,59.8282880397053,39.2708017080178));
#207735=CARTESIAN_POINT('Ctrl Pts',(12.9173404733289,59.8550545325308,39.2710850691866));
#207736=CARTESIAN_POINT('Ctrl Pts',(12.9401053405456,59.962154812277,39.3343017080178));
#207737=CARTESIAN_POINT('Ctrl Pts',(13.0316624367254,59.7842416555145,39.3487519293518));
#207738=CARTESIAN_POINT('Ctrl Pts',(12.9079350417484,59.8108054559338,39.3492068662936));
#207739=CARTESIAN_POINT('Ctrl Pts',(12.926069636949,59.8961220185284,39.4512271248748));
#207740=CARTESIAN_POINT('Ctrl Pts',(13.0141504107554,59.7007958241043,39.3978017080178));
#207741=CARTESIAN_POINT('Ctrl Pts',(12.8901364125069,59.7270694888874,39.3980347781164));
#207742=CARTESIAN_POINT('Ctrl Pts',(12.8994792219303,59.771023951408,39.5248015355176));
#207743=CARTESIAN_POINT('Ctrl Pts',(12.995727518883,59.6130003254553,39.3978017080178));
#207744=CARTESIAN_POINT('Ctrl Pts',(12.8715027735898,59.6394051101892,39.3978017080178));
#207745=CARTESIAN_POINT('Ctrl Pts',(12.8715027735898,59.6394051101892,39.5248017080178));
#207746=CARTESIAN_POINT('Origin',(12.995727518883,59.6130003254553,39.5248017080178));
#207747=CARTESIAN_POINT('Origin',(0.310561863232988,-0.0660119618346419,
39.116));
#207748=CARTESIAN_POINT('Origin',(13.1739864076113,60.4516424606487,39.116));
#207749=CARTESIAN_POINT('Origin',(0.310561863232988,-0.0660119618346419,
39.5248017080178));
#207750=CARTESIAN_POINT('Origin',(12.9642895838877,59.4650964698965,39.5248017080178));
#207751=CARTESIAN_POINT('Ctrl Pts',(13.2864868029002,60.9782752797347,39.2875012672119));
#207752=CARTESIAN_POINT('Ctrl Pts',(13.1616357280628,61.0052918384388,39.287208709576));
#207753=CARTESIAN_POINT('Ctrl Pts',(13.1392995818866,60.8992893541404,39.3549016990123));
#207754=CARTESIAN_POINT('Ctrl Pts',(13.2624669757413,60.8658306440995,39.103493917393));
#207755=CARTESIAN_POINT('Ctrl Pts',(13.1376969719802,60.8926675943325,39.1031692336351));
#207756=CARTESIAN_POINT('Ctrl Pts',(13.1201818190182,60.8093473519472,39.2077507202316));
#207757=CARTESIAN_POINT('Ctrl Pts',(13.2193155203587,60.663828108008,38.989));
#207758=CARTESIAN_POINT('Ctrl Pts',(13.0947255842066,60.690500823973,38.9887769311152));
#207759=CARTESIAN_POINT('Ctrl Pts',(13.0858375353127,60.6477702018618,39.1161898712892));
#207760=CARTESIAN_POINT('Ctrl Pts',(13.1739864076113,60.4516424606487,38.989));
#207761=CARTESIAN_POINT('Ctrl Pts',(13.0495760763092,60.4780866929065,38.989));
#207762=CARTESIAN_POINT('Ctrl Pts',(13.0497618007396,60.4780472159602,39.1161895903854));
#207763=CARTESIAN_POINT('Origin',(13.2635576885508,60.8730422059012,39.3548010137695));
#207764=CARTESIAN_POINT('Ctrl Pts',(12.9642895838877,59.4650964698965,39.3978017080178));
#207765=CARTESIAN_POINT('Ctrl Pts',(12.8400648385945,59.4915012546304,39.3978017080178));
#207766=CARTESIAN_POINT('Ctrl Pts',(12.8400648385945,59.4915012546304,39.5248017080178));
#207767=CARTESIAN_POINT('Ctrl Pts',(12.9458049943937,59.3770041141843,39.3978017080178));
#207768=CARTESIAN_POINT('Ctrl Pts',(12.8213326038448,59.4033730190106,39.3975666025021));
#207769=CARTESIAN_POINT('Ctrl Pts',(12.8119938336996,59.3594375597987,39.5248015517178));
#207770=CARTESIAN_POINT('Ctrl Pts',(12.92832822063,59.2937057271823,39.3484894016716));
#207771=CARTESIAN_POINT('Ctrl Pts',(12.803709764015,59.3204640761266,39.3480259000045));
#207772=CARTESIAN_POINT('Ctrl Pts',(12.785450697209,59.2345619206646,39.4508333188949));
#207773=CARTESIAN_POINT('Ctrl Pts',(12.9191181862052,59.2498070616278,39.2708017080178));
#207774=CARTESIAN_POINT('Ctrl Pts',(12.7944335023714,59.2768226962997,39.27051194648));
#207775=CARTESIAN_POINT('Ctrl Pts',(12.7714622569326,59.1687514833559,39.3343017080178));
#207776=CARTESIAN_POINT('Origin',(12.8956870022258,59.1423466986221,39.3343017080178));
#207777=CARTESIAN_POINT('Origin',(13.300596971516,61.0472983318851,39.6398955068192));
#207778=CARTESIAN_POINT('Origin',(13.3376362544832,61.2215544576538,39.92499));
#207779=CARTESIAN_POINT('Origin',(12.8787733304445,59.0627741291271,39.1934008539943));
#207780=CARTESIAN_POINT('Origin',(12.869528080115,59.0190342907435,39.1160402713846));
#207781=CARTESIAN_POINT('Ctrl Pts',(13.1038352065734,61.575271693745,40.1599502534424));
#207782=CARTESIAN_POINT('Ctrl Pts',(13.0960702419687,61.5387839176326,40.10025));
#207783=CARTESIAN_POINT('Ctrl Pts',(13.0814171332239,61.4699285681953,40.10025));
#207784=CARTESIAN_POINT('Ctrl Pts',(13.1900205930483,61.5569304518429,40.1599500538461));
#207785=CARTESIAN_POINT('Ctrl Pts',(13.1588482421898,61.5254208297812,40.1002448353481));
#207786=CARTESIAN_POINT('Ctrl Pts',(13.1313027022863,61.4593031273767,40.10025));
#207787=CARTESIAN_POINT('Ctrl Pts',(13.2643407403251,61.5155378539378,40.1202442001038));
#207788=CARTESIAN_POINT('Ctrl Pts',(13.2118511391503,61.4904936222811,40.0633873868015));
#207789=CARTESIAN_POINT('Ctrl Pts',(13.1721300657497,61.4250300340665,40.0772271723537));
#207790=CARTESIAN_POINT('Ctrl Pts',(13.3535591268199,61.4222835584426,40.0045995998163));
#207791=CARTESIAN_POINT('Ctrl Pts',(13.2611962587095,61.4178880557402,39.9663485808318));
#207792=CARTESIAN_POINT('Ctrl Pts',(13.2174099770544,61.3411158595752,40.0101727202466));
#207793=CARTESIAN_POINT('Ctrl Pts',(13.3700167576327,61.3712701109735,39.9304654349859));
#207794=CARTESIAN_POINT('Ctrl Pts',(13.2570896192449,61.3797074995622,39.905190016295));
#207795=CARTESIAN_POINT('Ctrl Pts',(13.2228660458972,61.2924393404512,39.9671857458184));
#207796=CARTESIAN_POINT('Ctrl Pts',(13.3605623192493,61.3267881959111,39.8576902534424));
#207797=CARTESIAN_POINT('Ctrl Pts',(13.2359003894757,61.3537611057082,39.8573998014387));
#207798=CARTESIAN_POINT('Ctrl Pts',(13.21341150919,61.2479592423876,39.92499));
#207799=CARTESIAN_POINT('Origin',(13.0814171332239,61.4699285681953,40.22725));
#207800=CARTESIAN_POINT('Origin',(0.310561863232988,-0.0660119618346419,
39.116));
#207801=CARTESIAN_POINT('Origin',(12.7860306150458,58.6264539577982,39.116));
#207802=CARTESIAN_POINT('Origin',(5.63039444364742E-15,5.53359822473674E-15,
40.22725));
#207803=CARTESIAN_POINT('Origin',(13.0516031943535,61.4762657165314,40.22725));
#207804=CARTESIAN_POINT('Ctrl Pts',(12.7860306150458,58.6264539577982,38.989));
#207805=CARTESIAN_POINT('Ctrl Pts',(12.6616197754744,58.652898298092,38.989));
#207806=CARTESIAN_POINT('Ctrl Pts',(12.6618060089327,58.6528587129484,39.1161901092324));
#207807=CARTESIAN_POINT('Ctrl Pts',(12.7406940127379,58.4142663981465,38.989));
#207808=CARTESIAN_POINT('Ctrl Pts',(12.6165479409694,58.4408495151684,38.9892298989742));
#207809=CARTESIAN_POINT('Ctrl Pts',(12.6257296363319,58.4831327254061,39.1161900493186));
#207810=CARTESIAN_POINT('Ctrl Pts',(12.6975319705105,58.2122676405432,39.1034966344368));
#207811=CARTESIAN_POINT('Ctrl Pts',(12.5736296288419,58.2389323335264,39.1038314102579));
#207812=CARTESIAN_POINT('Ctrl Pts',(12.5913856081756,58.3215567776513,39.2077528789614));
#207813=CARTESIAN_POINT('Ctrl Pts',(12.6735055745747,58.0998260601478,39.2875012672119));
#207814=CARTESIAN_POINT('Ctrl Pts',(12.5497583536238,58.1266254943011,39.2878045257868));
#207815=CARTESIAN_POINT('Ctrl Pts',(12.5722680796271,58.2316158778877,39.35490152959));
#207816=CARTESIAN_POINT('Origin',(12.6964592423899,58.205053781054,39.3548010137695));
#207817=CARTESIAN_POINT('Ctrl Pts',(12.7383709431257,61.4590390555207,39.8576902534424));
#207818=CARTESIAN_POINT('Ctrl Pts',(12.8632261535962,61.4329754599097,39.8573998014387));
#207819=CARTESIAN_POINT('Ctrl Pts',(12.8407372733105,61.3271735965892,39.92499));
#207820=CARTESIAN_POINT('Ctrl Pts',(12.7478306169683,61.5035409747666,39.9304984902492));
#207821=CARTESIAN_POINT('Ctrl Pts',(12.8544171899353,61.4653154597758,39.905217156979));
#207822=CARTESIAN_POINT('Ctrl Pts',(12.8501961180706,61.3716739624487,39.9672049726598));
#207823=CARTESIAN_POINT('Ctrl Pts',(12.7835835513936,61.5432717953611,40.004343767866));
#207824=CARTESIAN_POINT('Ctrl Pts',(12.866248101297,61.5017184029585,39.9661628577646));
#207825=CARTESIAN_POINT('Ctrl Pts',(12.874945307291,61.413745161397,40.0100243556235));
#207826=CARTESIAN_POINT('Ctrl Pts',(12.9020280679178,61.5920631419344,40.1194874821989));
#207827=CARTESIAN_POINT('Ctrl Pts',(12.9401487584136,61.5478406570048,40.0627551483138));
#207828=CARTESIAN_POINT('Ctrl Pts',(12.9498405053869,61.4717924962544,40.0767884282377));
#207829=CARTESIAN_POINT('Ctrl Pts',(12.9874904696727,61.5999795805214,40.1599502015394));
#207830=CARTESIAN_POINT('Ctrl Pts',(13.0031958218447,61.5585057825384,40.1002449453869));
#207831=CARTESIAN_POINT('Ctrl Pts',(13.0015435854432,61.4868843017929,40.10025));
#207832=CARTESIAN_POINT('Ctrl Pts',(13.0739701745332,61.5816197022696,40.1599502534424));
#207833=CARTESIAN_POINT('Ctrl Pts',(13.0662229071073,61.5451281645058,40.10025));
#207834=CARTESIAN_POINT('Ctrl Pts',(13.0516031943535,61.4762657165314,40.10025));
#207835=CARTESIAN_POINT('Origin',(12.7165125280173,61.353578381323,39.92499));
#207836=CARTESIAN_POINT('Origin',(12.659419908459,58.0307974155464,39.6398955069327));
#207837=CARTESIAN_POINT('Origin',(12.6223805745526,57.8565410498765,39.92499));
#207838=CARTESIAN_POINT('Origin',(12.6794732450915,61.1793222555321,39.6398955068273));
#207839=CARTESIAN_POINT('Origin',(12.6424339620849,61.0050661295705,39.3548010137695));
#207840=CARTESIAN_POINT('Ctrl Pts',(12.5994235324478,57.7513140650719,39.8576902534424));
#207841=CARTESIAN_POINT('Ctrl Pts',(12.4758649777959,57.7780756236494,39.8579948730703));
#207842=CARTESIAN_POINT('Ctrl Pts',(12.4981558292594,57.8829458346104,39.92499));
#207843=CARTESIAN_POINT('Ctrl Pts',(12.5899763290081,57.7068710254543,39.930402071123));
#207844=CARTESIAN_POINT('Ctrl Pts',(12.4844883578143,57.7455616498591,39.9058915297379));
#207845=CARTESIAN_POINT('Ctrl Pts',(12.4887087546169,57.8385008428011,39.967152378603));
#207846=CARTESIAN_POINT('Ctrl Pts',(12.5543975270271,57.6673720419785,40.0043257306694));
#207847=CARTESIAN_POINT('Ctrl Pts',(12.4724506530562,57.7092008760995,39.9667894847838));
#207848=CARTESIAN_POINT('Ctrl Pts',(12.4640308112194,57.7966870296828,40.0100138975201));
#207849=CARTESIAN_POINT('Ctrl Pts',(12.436381672743,57.6192799956673,40.1195533054856));
#207850=CARTESIAN_POINT('Ctrl Pts',(12.3985321242208,57.6635313090886,40.0630813209233));
#207851=CARTESIAN_POINT('Ctrl Pts',(12.3892398894932,57.7394080294758,40.076826594242));
#207852=CARTESIAN_POINT('Ctrl Pts',(12.3512461790957,57.6118166447793,40.1599502027519));
#207853=CARTESIAN_POINT('Ctrl Pts',(12.3356888898087,57.6532646075471,40.1002552791541));
#207854=CARTESIAN_POINT('Ctrl Pts',(12.3376071226711,57.7248239067128,40.10025));
#207855=CARTESIAN_POINT('Ctrl Pts',(12.2652136052667,57.6301266171956,40.1599502534424));
#207856=CARTESIAN_POINT('Ctrl Pts',(12.2729791421561,57.6666142715154,40.10025));
#207857=CARTESIAN_POINT('Ctrl Pts',(12.2876333308477,57.7354693911203,40.10025));
#207858=CARTESIAN_POINT('Origin',(12.2876333308477,57.7354693911203,40.22725));
#207859=CARTESIAN_POINT('Ctrl Pts',(12.5528626811454,60.583666384318,38.989));
#207860=CARTESIAN_POINT('Ctrl Pts',(12.6772730231654,60.5572221497821,38.989));
#207861=CARTESIAN_POINT('Ctrl Pts',(12.6770872880011,60.55726162901,39.1161896013264));
#207862=CARTESIAN_POINT('Ctrl Pts',(12.5977568525216,60.795947932685,38.989));
#207863=CARTESIAN_POINT('Ctrl Pts',(12.7224242094588,60.7696393833351,38.9887769275436));
#207864=CARTESIAN_POINT('Ctrl Pts',(12.713163582625,60.7269872521286,39.1161898821822));
#207865=CARTESIAN_POINT('Ctrl Pts',(12.6404975322983,60.9980361136597,39.1034967087243));
#207866=CARTESIAN_POINT('Ctrl Pts',(12.7653961862444,60.9718043534714,39.103172023274));
#207867=CARTESIAN_POINT('Ctrl Pts',(12.74750759382,60.8885631224008,39.2077529615022));
#207868=CARTESIAN_POINT('Ctrl Pts',(12.6642893210148,61.110527437164,39.2875012672119));
#207869=CARTESIAN_POINT('Ctrl Pts',(12.7893350885052,61.084426782332,39.2872087095507));
#207870=CARTESIAN_POINT('Ctrl Pts',(12.7666250660191,60.9785037583491,39.3549017048226));
#207871=CARTESIAN_POINT('Origin',(12.5528626811454,60.583666384318,39.116));
#207872=CARTESIAN_POINT('Origin',(5.67687244506386E-15,5.31008333971855E-15,
40.22725));
#207873=CARTESIAN_POINT('Origin',(12.2578193919774,57.7418065394565,40.22725));
#207874=CARTESIAN_POINT('Origin',(2.3791451040456,12.7200883457668,39.116));
#207875=CARTESIAN_POINT('Origin',(12.4693660187268,60.1910940874971,39.1160373285255));
#207876=CARTESIAN_POINT('Ctrl Pts',(12.2354540642051,57.6364522029206,40.1599502534424));
#207877=CARTESIAN_POINT('Ctrl Pts',(12.2432007592853,57.6729438621905,40.10025));
#207878=CARTESIAN_POINT('Ctrl Pts',(12.2578193919774,57.7418065394565,40.10025));
#207879=CARTESIAN_POINT('Ctrl Pts',(12.1497054461948,57.6546556225243,40.1599500566034));
#207880=CARTESIAN_POINT('Ctrl Pts',(12.1807288143669,57.6862025493687,40.1002551305369));
#207881=CARTESIAN_POINT('Ctrl Pts',(12.2080066271962,57.7523715145536,40.10025));
#207882=CARTESIAN_POINT('Ctrl Pts',(12.0754939174604,57.6955109599433,40.1203070619046));
#207883=CARTESIAN_POINT('Ctrl Pts',(12.127750241416,57.7206875210984,40.0637098684496));
#207884=CARTESIAN_POINT('Ctrl Pts',(12.1670355805169,57.7861609236006,40.0772636213363));
#207885=CARTESIAN_POINT('Ctrl Pts',(11.9863964689869,57.7879231380266,40.0046102245801));
#207886=CARTESIAN_POINT('Ctrl Pts',(12.0782086782662,57.7928648378987,39.9670001894015));
#207887=CARTESIAN_POINT('Ctrl Pts',(12.1215423041379,57.8693039540644,40.0101788811209));
#207888=CARTESIAN_POINT('Ctrl Pts',(11.9699873265234,57.8386735460213,39.9303710930186));
#207889=CARTESIAN_POINT('Ctrl Pts',(12.0820993460723,57.8311081991742,39.9058663574109));
#207890=CARTESIAN_POINT('Ctrl Pts',(12.1160385312535,57.917734074407,39.9671344706364));
#207891=CARTESIAN_POINT('Ctrl Pts',(11.9794294790618,57.8830978693154,39.8576902534424));
#207892=CARTESIAN_POINT('Ctrl Pts',(12.1031907419163,57.857289977851,39.8579948730703));
#207893=CARTESIAN_POINT('Ctrl Pts',(12.1254815933798,57.9621601888119,39.92499));
#207894=CARTESIAN_POINT('Origin',(12.0012568480866,57.9885649735458,39.92499));
#207895=CARTESIAN_POINT('Origin',(12.4602215058074,60.1478239214161,39.1925554488847));
#207896=CARTESIAN_POINT('Origin',(12.4432063593729,60.0677739512124,39.3343017080178));
#207897=CARTESIAN_POINT('Origin',(12.0382961820458,58.1628213391881,39.6398955069227));
#207898=CARTESIAN_POINT('Origin',(12.0753355159239,58.3370777047233,39.3548010137695));
#207899=CARTESIAN_POINT('Ctrl Pts',(12.3746037924171,59.7450242491246,39.3978017080178));
#207900=CARTESIAN_POINT('Ctrl Pts',(12.4988285377102,59.7186194643908,39.3978017080178));
#207901=CARTESIAN_POINT('Ctrl Pts',(12.4988285377102,59.7186194643908,39.5248017080178));
#207902=CARTESIAN_POINT('Ctrl Pts',(12.3935470970145,59.8330190893699,39.3978017080178));
#207903=CARTESIAN_POINT('Ctrl Pts',(12.5175251937997,59.8065803155747,39.3980355775177));
#207904=CARTESIAN_POINT('Ctrl Pts',(12.5268995400901,59.8506831473904,39.5248015517192));
#207905=CARTESIAN_POINT('Ctrl Pts',(12.4114576311024,59.9162252185214,39.3484893995498));
#207906=CARTESIAN_POINT('Ctrl Pts',(12.5352924712502,59.8901687840289,39.3489438303428));
#207907=CARTESIAN_POINT('Ctrl Pts',(12.5534426698453,59.9755587548363,39.4508333155594));
#207908=CARTESIAN_POINT('Ctrl Pts',(12.4208962741593,59.9600752506736,39.2708017080178));
#207909=CARTESIAN_POINT('Ctrl Pts',(12.5446662374493,59.9342688867323,39.2710850691866));
#207910=CARTESIAN_POINT('Ctrl Pts',(12.5674311046661,60.0413691664786,39.3343017080178));
#207911=CARTESIAN_POINT('Origin',(12.3746037924171,59.7450242491246,39.5248017080178));
#207912=CARTESIAN_POINT('Ctrl Pts',(12.0535047649328,58.231611300478,39.2875012672119));
#207913=CARTESIAN_POINT('Ctrl Pts',(12.177453774129,58.2057612755554,39.2878045257519));
#207914=CARTESIAN_POINT('Ctrl Pts',(12.1995935640854,58.3108302788451,39.3549015218347));
#207915=CARTESIAN_POINT('Ctrl Pts',(12.077290030418,58.3441059109578,39.1034938540228));
#207916=CARTESIAN_POINT('Ctrl Pts',(12.2013259468594,58.318069699157,39.1038286278812));
#207917=CARTESIAN_POINT('Ctrl Pts',(12.2187113817826,58.4007725402757,39.2077506434032));
#207918=CARTESIAN_POINT('Ctrl Pts',(12.1200201767774,58.5461981381265,38.989));
#207919=CARTESIAN_POINT('Ctrl Pts',(12.2442455720365,58.5199882620676,38.9892298954612));
#207920=CARTESIAN_POINT('Ctrl Pts',(12.2530556816164,58.5623497685521,39.1161900347288));
#207921=CARTESIAN_POINT('Ctrl Pts',(12.1649068885798,58.7584778814675,38.989));
#207922=CARTESIAN_POINT('Ctrl Pts',(12.2893177137823,58.7320335442279,38.989));
#207923=CARTESIAN_POINT('Ctrl Pts',(12.2891314947143,58.7320731263127,39.1161900945645));
#207924=CARTESIAN_POINT('Origin',(12.1649068885798,58.7584778814675,39.116));
#207925=CARTESIAN_POINT('Origin',(2.31399271319982,12.4135704460892,39.5248017080178));
#207926=CARTESIAN_POINT('Origin',(12.3431658574217,59.5971203935658,39.5248017080178));
#207927=CARTESIAN_POINT('Origin',(2.30379013587727,12.3655710936233,39.116));
#207928=CARTESIAN_POINT('Origin',(12.2483049654007,59.1510793400371,39.1160402713848));
#207929=CARTESIAN_POINT('Ctrl Pts',(12.296865891381,59.3820708699069,39.2708017080178));
#207930=CARTESIAN_POINT('Ctrl Pts',(12.4217592664919,59.3560370505013,39.27051194648));
#207931=CARTESIAN_POINT('Ctrl Pts',(12.398788021053,59.2479658375575,39.3343017080178));
#207932=CARTESIAN_POINT('Ctrl Pts',(12.3063392072231,59.4260685345959,39.3487519301186));
#207933=CARTESIAN_POINT('Ctrl Pts',(12.4310668851193,59.3998259533523,39.3482879463979));
#207934=CARTESIAN_POINT('Ctrl Pts',(12.4128237298768,59.3139986558978,39.4512271261639));
#207935=CARTESIAN_POINT('Ctrl Pts',(12.3242857901782,59.5094220566594,39.3978017080178));
#207936=CARTESIAN_POINT('Ctrl Pts',(12.4487214234133,59.4828840257721,39.3975673827397));
#207937=CARTESIAN_POINT('Ctrl Pts',(12.4394141514348,59.4390967537832,39.5248015355181));
#207938=CARTESIAN_POINT('Ctrl Pts',(12.3431658574217,59.5971203935658,39.3978017080178));
#207939=CARTESIAN_POINT('Ctrl Pts',(12.4673906027149,59.5707156088319,39.3978017080178));
#207940=CARTESIAN_POINT('Ctrl Pts',(12.4673906027149,59.5707156088319,39.5248017080178));
#207941=CARTESIAN_POINT('Origin',(12.2745632757598,59.2743706222914,39.3343017080178));
#207942=CARTESIAN_POINT('Origin',(12.2576496039196,59.194798053941,39.193400853355));
#207943=CARTESIAN_POINT('Origin',(19.2830435999582,58.3196542523187,39.1925554495079));
#207944=CARTESIAN_POINT('Origin',(19.2967593024445,58.3616995707149,39.1160373285249));
#207945=CARTESIAN_POINT('Origin',(19.2577541638585,58.2418213702172,39.3343017080178));
#207946=CARTESIAN_POINT('Ctrl Pts',(19.2232259141446,58.1373965169891,39.2708017080178));
#207947=CARTESIAN_POINT('Ctrl Pts',(19.1031347997394,58.1769325318817,39.2710850691866));
#207948=CARTESIAN_POINT('Ctrl Pts',(19.136969986289,58.2810665285028,39.3343017080178));
#207949=CARTESIAN_POINT('Ctrl Pts',(19.2094285342446,58.0945576760635,39.3487519293518));
#207950=CARTESIAN_POINT('Ctrl Pts',(19.0891556041211,58.1339089916632,39.3492068662935));
#207951=CARTESIAN_POINT('Ctrl Pts',(19.1161088652894,58.2168625998353,39.4512271248748));
#207952=CARTESIAN_POINT('Ctrl Pts',(19.1832899764616,58.0133994748122,39.3978017080178));
#207953=CARTESIAN_POINT('Ctrl Pts',(19.0627016856753,58.0524922023727,39.398034778116));
#207954=CARTESIAN_POINT('Ctrl Pts',(19.0765878066325,58.0952292882353,39.5248015355176));
#207955=CARTESIAN_POINT('Ctrl Pts',(19.1557908785631,57.9280106456674,39.3978017080178));
#207956=CARTESIAN_POINT('Ctrl Pts',(19.0350067009936,57.967255803953,39.3978017080178));
#207957=CARTESIAN_POINT('Ctrl Pts',(19.0350067009936,57.967255803953,39.5248017080178));
#207958=CARTESIAN_POINT('Origin',(19.1557908785631,57.9280106456674,39.5248017080178));
#207959=CARTESIAN_POINT('Origin',(0.301960443923716,-0.098112895714049,
39.116));
#207960=CARTESIAN_POINT('Origin',(19.4207352200707,58.743425483793,39.116));
#207961=CARTESIAN_POINT('Origin',(0.301960443923716,-0.098112895714049,
39.5248017080178));
#207962=CARTESIAN_POINT('Origin',(19.1090650011322,57.7842031819381,39.5248017080178));
#207963=CARTESIAN_POINT('Ctrl Pts',(19.5876674457085,59.2554138597569,39.2875012672119));
#207964=CARTESIAN_POINT('Ctrl Pts',(19.4663243174862,59.2953329099158,39.287208709576));
#207965=CARTESIAN_POINT('Ctrl Pts',(19.4330302542698,59.1922458813525,39.3549016990124));
#207966=CARTESIAN_POINT('Ctrl Pts',(19.5520255367116,59.1460959632215,39.1034939173931));
#207967=CARTESIAN_POINT('Ctrl Pts',(19.4307442612541,59.1858279145874,39.1031692336328));
#207968=CARTESIAN_POINT('Ctrl Pts',(19.4046157212346,59.1047949412331,39.207750720231));
#207969=CARTESIAN_POINT('Ctrl Pts',(19.4879954548418,58.9497105734778,38.989));
#207970=CARTESIAN_POINT('Ctrl Pts',(19.366876093407,58.9892603680788,38.9887769311182));
#207971=CARTESIAN_POINT('Ctrl Pts',(19.3535701679106,58.9476928828777,39.11618987129));
#207972=CARTESIAN_POINT('Ctrl Pts',(19.4207352200707,58.743425483793,38.989));
#207973=CARTESIAN_POINT('Ctrl Pts',(19.2997705965407,58.7827292725253,38.989));
#207974=CARTESIAN_POINT('Ctrl Pts',(19.299951177089,58.7826705983484,39.1161895903857));
#207975=CARTESIAN_POINT('Origin',(19.5538640879539,59.1531540087997,39.3548010137695));
#207976=CARTESIAN_POINT('Ctrl Pts',(19.1090650011322,57.7842031819381,39.3978017080178));
#207977=CARTESIAN_POINT('Ctrl Pts',(18.9882808235627,57.8234483402237,39.3978017080178));
#207978=CARTESIAN_POINT('Ctrl Pts',(18.9882808235627,57.8234483402237,39.5248017080178));
#207979=CARTESIAN_POINT('Ctrl Pts',(19.0814735135856,57.6985255711016,39.3978017080178));
#207980=CARTESIAN_POINT('Ctrl Pts',(18.9604392969159,57.7377609320109,39.3975666025035));
#207981=CARTESIAN_POINT('Ctrl Pts',(18.9465591794953,57.6950423231336,39.5248015517178));
#207982=CARTESIAN_POINT('Ctrl Pts',(19.0553854270312,57.6175103216836,39.3484894016716));
#207983=CARTESIAN_POINT('Ctrl Pts',(18.9342466524546,57.6571482613582,39.3480259000032));
#207984=CARTESIAN_POINT('Ctrl Pts',(18.9071083904259,57.5736252790862,39.4508333188947));
#207985=CARTESIAN_POINT('Ctrl Pts',(19.0416371860884,57.5748148483574,39.2708017080178));
#207986=CARTESIAN_POINT('Ctrl Pts',(18.9204594407751,57.61471558695,39.2705119464801));
#207987=CARTESIAN_POINT('Ctrl Pts',(18.8863175164099,57.5096375484035,39.3343017080178));
#207988=CARTESIAN_POINT('Origin',(19.0071016939793,57.4703923901179,39.3343017080178));
#207989=CARTESIAN_POINT('Origin',(19.6089151909165,59.3225838821656,39.6398955068179));
#207990=CARTESIAN_POINT('Origin',(19.6639662938568,59.4920137553137,39.92499));
#207991=CARTESIAN_POINT('Origin',(18.9819630786535,57.3930236876039,39.1934008539944));
#207992=CARTESIAN_POINT('Origin',(18.9681964166836,57.350489852441,39.1160402713847));
#207993=CARTESIAN_POINT('Ctrl Pts',(19.4684195516703,59.868232155624,40.1599502534424));
#207994=CARTESIAN_POINT('Ctrl Pts',(19.456883113189,59.8327559231844,40.10025));
#207995=CARTESIAN_POINT('Ctrl Pts',(19.4351129318427,59.7658094374949,40.10025));
#207996=CARTESIAN_POINT('Ctrl Pts',(19.55221562375,59.8409825629602,40.159950053847));
#207997=CARTESIAN_POINT('Ctrl Pts',(19.5179203859198,59.8129039518391,40.1002448353493));
#207998=CARTESIAN_POINT('Ctrl Pts',(19.4836145615386,59.7500277420817,40.10025));
#207999=CARTESIAN_POINT('Ctrl Pts',(19.621801932834,59.7920481472521,40.1202442001036));
#208000=CARTESIAN_POINT('Ctrl Pts',(19.5669820401376,59.7726277678653,40.0633873868015));
#208001=CARTESIAN_POINT('Ctrl Pts',(19.520635754657,59.7116747787977,40.0772271723537));
#208002=CARTESIAN_POINT('Ctrl Pts',(19.7007838434713,59.6899788477097,40.0045995998165));
#208003=CARTESIAN_POINT('Ctrl Pts',(19.6084674936738,59.6952619726975,39.9663485808318));
#208004=CARTESIAN_POINT('Ctrl Pts',(19.5568961981644,59.6234872553903,40.0101727202466));
#208005=CARTESIAN_POINT('Ctrl Pts',(19.7118189603907,59.6375245663853,39.9304654349857));
#208006=CARTESIAN_POINT('Ctrl Pts',(19.6003923959459,59.6577198343137,39.9051900162949));
#208007=CARTESIAN_POINT('Ctrl Pts',(19.5572342963496,59.5745070768387,39.9671857458178));
#208008=CARTESIAN_POINT('Ctrl Pts',(19.6977666881852,59.5942745858234,39.8576902534424));
#208009=CARTESIAN_POINT('Ctrl Pts',(19.5766071063175,59.6341304551455,39.8573998014387));
#208010=CARTESIAN_POINT('Ctrl Pts',(19.5431821162873,59.5312589135993,39.92499));
#208011=CARTESIAN_POINT('Origin',(19.4351129318427,59.7658094374949,40.22725));
#208012=CARTESIAN_POINT('Origin',(0.301960443923716,-0.098112895714049,
39.116));
#208013=CARTESIAN_POINT('Origin',(18.8441205405526,56.9687879773464,39.116));
#208014=CARTESIAN_POINT('Origin',(5.61372323131277E-15,5.53806526261865E-15,
40.22725));
#208015=CARTESIAN_POINT('Origin',(19.406124729226,59.7752282754835,40.22725));
#208016=CARTESIAN_POINT('Ctrl Pts',(18.8441205405526,56.9687879773464,38.989));
#208017=CARTESIAN_POINT('Ctrl Pts',(18.7231554228307,57.0080919266514,38.989));
#208018=CARTESIAN_POINT('Ctrl Pts',(18.7233364983085,57.0080330916621,39.1161901092324));
#208019=CARTESIAN_POINT('Ctrl Pts',(18.7768526573605,56.7625017687172,38.989));
#208020=CARTESIAN_POINT('Ctrl Pts',(18.656165363134,56.8019160587468,38.9892298989742));
#208021=CARTESIAN_POINT('Ctrl Pts',(18.6697165591974,56.8430078886276,39.1161900493186));
#208022=CARTESIAN_POINT('Ctrl Pts',(18.712812441602,56.566121243389,39.1034966344368));
#208023=CARTESIAN_POINT('Ctrl Pts',(18.5923760693066,56.605591185762,39.1038314102574));
#208024=CARTESIAN_POINT('Ctrl Pts',(18.6186713857003,56.6859069993037,39.2077528789611));
#208025=CARTESIAN_POINT('Ctrl Pts',(18.6771643191716,56.4568070719809,39.2875012672119));
#208026=CARTESIAN_POINT('Ctrl Pts',(18.5568963021134,56.4963948028695,39.2878045257868));
#208027=CARTESIAN_POINT('Ctrl Pts',(18.5902572009367,56.5984571310818,39.35490152959));
#208028=CARTESIAN_POINT('Origin',(18.7109915363523,56.5590590327987,39.3548010137695));
#208029=CARTESIAN_POINT('Ctrl Pts',(19.0928077206418,59.7908376697909,39.8576902534424));
#208030=CARTESIAN_POINT('Ctrl Pts',(19.214254573609,59.7518659300023,39.8573998014387));
#208031=CARTESIAN_POINT('Ctrl Pts',(19.1808295835788,59.6489943884562,39.92499));
#208032=CARTESIAN_POINT('Ctrl Pts',(19.1068672906319,59.8341069976972,39.9304984902491));
#208033=CARTESIAN_POINT('Ctrl Pts',(19.2088743168593,59.7849495554005,39.9052171569788));
#208034=CARTESIAN_POINT('Ctrl Pts',(19.1948881666556,59.6922622581476,39.9672049726605));
#208035=CARTESIAN_POINT('Ctrl Pts',(19.1465773683635,59.8698829694065,40.0043437678661));
#208036=CARTESIAN_POINT('Ctrl Pts',(19.224445560962,59.8199164124671,39.9661628577643));
#208037=CARTESIAN_POINT('Ctrl Pts',(19.2238994150019,59.7315159919506,40.0100243556235));
#208038=CARTESIAN_POINT('Ctrl Pts',(19.2694731179107,59.9060262085834,40.1194874821988));
#208039=CARTESIAN_POINT('Ctrl Pts',(19.3027624708836,59.8580612818571,40.0627551483141));
#208040=CARTESIAN_POINT('Ctrl Pts',(19.3044519280757,59.7814166574707,40.0767884282377));
#208041=CARTESIAN_POINT('Ctrl Pts',(19.3552948408472,59.9049660265687,40.1599502015391));
#208042=CARTESIAN_POINT('Ctrl Pts',(19.3665789650881,59.862077770064,40.1002449453885));
#208043=CARTESIAN_POINT('Ctrl Pts',(19.3574492964906,59.7910213450152,40.10025));
#208044=CARTESIAN_POINT('Ctrl Pts',(19.4393816709763,59.8776671349983,40.1599502534424));
#208045=CARTESIAN_POINT('Ctrl Pts',(19.4278624395273,59.842185311655,40.10025));
#208046=CARTESIAN_POINT('Ctrl Pts',(19.406124729226,59.7752282754835,40.10025));
#208047=CARTESIAN_POINT('Origin',(19.0600454060093,59.6882395467418,39.92499));
#208048=CARTESIAN_POINT('Origin',(18.6559403576659,56.3896289265475,39.6398955069309));
#208049=CARTESIAN_POINT('Origin',(18.6008891789892,56.2201988201381,39.92499));
#208050=CARTESIAN_POINT('Origin',(19.0049943031095,59.5188096735647,39.6398955068273));
#208051=CARTESIAN_POINT('Origin',(18.9499432001064,59.3493798002278,39.3548010137695));
#208052=CARTESIAN_POINT('Ctrl Pts',(18.5670586829472,56.1179479440986,39.8576902534424));
#208053=CARTESIAN_POINT('Ctrl Pts',(18.4469743395785,56.1574782858995,39.8579948730703));
#208054=CARTESIAN_POINT('Ctrl Pts',(18.4801050014197,56.2594439784237,39.92499));
#208055=CARTESIAN_POINT('Ctrl Pts',(18.5530176696416,56.0747358697601,39.9304020711231));
#208056=CARTESIAN_POINT('Ctrl Pts',(18.4521518441046,56.1242410383984,39.9058915297382));
#208057=CARTESIAN_POINT('Ctrl Pts',(18.4660639121468,56.2162299491245,39.9671523786031));
#208058=CARTESIAN_POINT('Ctrl Pts',(18.5135050040178,56.0391722633446,40.0043257306692));
#208059=CARTESIAN_POINT('Ctrl Pts',(18.4363793473476,56.0893377355413,39.9667894847835));
#208060=CARTESIAN_POINT('Ctrl Pts',(18.4371504234769,56.1772247439498,40.01001389752));
#208061=CARTESIAN_POINT('Ctrl Pts',(18.3911086652354,56.0036796861842,40.1195533054858));
#208062=CARTESIAN_POINT('Ctrl Pts',(18.3580919822899,56.0516449414231,40.0630813209236));
#208063=CARTESIAN_POINT('Ctrl Pts',(18.3567819283759,56.1280773042131,40.0768265942421));
#208064=CARTESIAN_POINT('Ctrl Pts',(18.305659420131,56.0051563026342,40.1599502027515));
#208065=CARTESIAN_POINT('Ctrl Pts',(18.2945198471564,56.0480033886679,40.1002552791541));
#208066=CARTESIAN_POINT('Ctrl Pts',(18.3039075553125,56.1189701685706,40.10025));
#208067=CARTESIAN_POINT('Ctrl Pts',(18.2220120550223,56.0323588238389,40.1599502534424));
#208068=CARTESIAN_POINT('Ctrl Pts',(18.2335490499224,56.067834875333,40.10025));
#208069=CARTESIAN_POINT('Ctrl Pts',(18.2553202812755,56.134781019564,40.10025));
#208070=CARTESIAN_POINT('Origin',(18.2553202812755,56.134781019564,40.22725));
#208071=CARTESIAN_POINT('Ctrl Pts',(18.8168143322233,58.9396512752211,38.989));
#208072=CARTESIAN_POINT('Ctrl Pts',(18.9377789661745,58.9003474831028,38.989));
#208073=CARTESIAN_POINT('Ctrl Pts',(18.9375983751895,58.9004061606707,39.1161896013268));
#208074=CARTESIAN_POINT('Ctrl Pts',(18.8836520326613,59.1460772043115,38.989));
#208075=CARTESIAN_POINT('Ctrl Pts',(19.004886456538,59.1068814887034,38.9887769275436));
#208076=CARTESIAN_POINT('Ctrl Pts',(18.9912181986579,59.0654310094279,39.1161898821825));
#208077=CARTESIAN_POINT('Ctrl Pts',(18.9472825415237,59.3425907075099,39.1034967087243));
#208078=CARTESIAN_POINT('Ctrl Pts',(19.0687550219952,59.3034471832925,39.1031720232725));
#208079=CARTESIAN_POINT('Ctrl Pts',(19.0422633471881,59.2225318234682,39.2077529615018));
#208080=CARTESIAN_POINT('Ctrl Pts',(18.9827025415103,59.4519788726605,39.2875012672119));
#208081=CARTESIAN_POINT('Ctrl Pts',(19.1043350338631,59.4129503580328,39.2872087095507));
#208082=CARTESIAN_POINT('Ctrl Pts',(19.0706774483344,59.3099814352091,39.3549017048228));
#208083=CARTESIAN_POINT('Origin',(18.8168143322233,58.9396512752211,39.116));
#208084=CARTESIAN_POINT('Origin',(5.68280300381509E-15,5.3084942512905E-15,
40.22725));
#208085=CARTESIAN_POINT('Origin',(18.2263320786588,56.1441998575526,40.22725));
#208086=CARTESIAN_POINT('Origin',(5.63975536249314,18.3848338156965,39.116));
#208087=CARTESIAN_POINT('Origin',(18.6927400943511,58.557957308326,39.1160373285235));
#208088=CARTESIAN_POINT('Ctrl Pts',(18.1930767435955,56.0417604764381,40.1599502534424));
#208089=CARTESIAN_POINT('Ctrl Pts',(18.2045954185351,56.0772424804482,40.10025));
#208090=CARTESIAN_POINT('Ctrl Pts',(18.2263320786588,56.1441998575526,40.10025));
#208091=CARTESIAN_POINT('Ctrl Pts',(18.109700640964,56.0688273470721,40.1599500566042));
#208092=CARTESIAN_POINT('Ctrl Pts',(18.1438516116619,56.0969586315456,40.1002551305369));
#208093=CARTESIAN_POINT('Ctrl Pts',(18.1778965340261,56.1599138083631,40.10025));
#208094=CARTESIAN_POINT('Ctrl Pts',(18.0401661963857,56.1172160917338,40.1203070619046));
#208095=CARTESIAN_POINT('Ctrl Pts',(18.0947679219785,56.1367924598132,40.0637098684499));
#208096=CARTESIAN_POINT('Ctrl Pts',(18.1406818860301,56.1978007560411,40.0772636213362));
#208097=CARTESIAN_POINT('Ctrl Pts',(17.9612165360197,56.2184352456062,40.0046102245802));
#208098=CARTESIAN_POINT('Ctrl Pts',(18.053042336704,56.2137528851846,39.9670001894012));
#208099=CARTESIAN_POINT('Ctrl Pts',(18.104128639785,56.2852436625533,40.0101788811209));
#208100=CARTESIAN_POINT('Ctrl Pts',(17.9502021467132,56.2706228600011,39.9303710930186));
#208101=CARTESIAN_POINT('Ctrl Pts',(18.0609092108094,56.2513800597966,39.9058663574109));
#208102=CARTESIAN_POINT('Ctrl Pts',(18.1037173431996,56.3339837785513,39.9671344706363));
#208103=CARTESIAN_POINT('Ctrl Pts',(17.9642361803979,56.3138168485093,39.8576902534424));
#208104=CARTESIAN_POINT('Ctrl Pts',(18.0846218068701,56.2752137607564,39.8579948730703));
#208105=CARTESIAN_POINT('Ctrl Pts',(18.1177524687112,56.3771794532805,39.92499));
#208106=CARTESIAN_POINT('Origin',(17.9969682911417,56.4164246115661,39.92499));
#208107=CARTESIAN_POINT('Origin',(18.6791227120638,58.5158800426259,39.1925554488841));
#208108=CARTESIAN_POINT('Origin',(18.6538332760111,58.4380471616453,39.3343017080178));
#208109=CARTESIAN_POINT('Origin',(18.0520194698704,56.5858547179429,39.6398955069215));
#208110=CARTESIAN_POINT('Origin',(18.1070706485049,56.7552848242268,39.3548010137695));
#208111=CARTESIAN_POINT('Ctrl Pts',(18.5518699907157,58.1242364370955,39.3978017080178));
#208112=CARTESIAN_POINT('Ctrl Pts',(18.6726541682852,58.0849912788098,39.3978017080178));
#208113=CARTESIAN_POINT('Ctrl Pts',(18.6726541682852,58.0849912788098,39.5248017080178));
#208114=CARTESIAN_POINT('Ctrl Pts',(18.5799074873344,58.2097691178802,39.3978017080178));
#208115=CARTESIAN_POINT('Ctrl Pts',(18.7004428147375,58.1705159385202,39.3980355775163));
#208116=CARTESIAN_POINT('Ctrl Pts',(18.7143758086146,58.2133972843955,39.5248015517178));
#208117=CARTESIAN_POINT('Ctrl Pts',(18.6064173144583,58.2906472745453,39.3484893995498));
#208118=CARTESIAN_POINT('Ctrl Pts',(18.7268501353397,58.2517893143851,39.3489438303433));
#208119=CARTESIAN_POINT('Ctrl Pts',(18.7538265876731,58.3348142976327,39.4508333155602));
#208120=CARTESIAN_POINT('Ctrl Pts',(18.6203878281154,58.3332704847794,39.2708017080178));
#208121=CARTESIAN_POINT('Ctrl Pts',(18.7407822670309,58.2946680067386,39.2710850691866));
#208122=CARTESIAN_POINT('Ctrl Pts',(18.7746174535806,58.3988020033596,39.3343017080178));
#208123=CARTESIAN_POINT('Origin',(18.5518699907157,58.1242364370955,39.5248017080178));
#208124=CARTESIAN_POINT('Ctrl Pts',(18.0743352474898,56.6526781108321,39.2875012672119));
#208125=CARTESIAN_POINT('Ctrl Pts',(18.1949031876639,56.614013495596,39.2878045257519));
#208126=CARTESIAN_POINT('Ctrl Pts',(18.2279043949854,56.7161926816709,39.3549015218347));
#208127=CARTESIAN_POINT('Ctrl Pts',(18.1097491035613,56.7620702268156,39.1034938540228));
#208128=CARTESIAN_POINT('Ctrl Pts',(18.2303840130663,56.7232113603676,39.1038286278797));
#208129=CARTESIAN_POINT('Ctrl Pts',(18.2563190096467,56.8036438738764,39.2077506434024));
#208130=CARTESIAN_POINT('Ctrl Pts',(18.1733695596542,56.9585888550839,38.989));
#208131=CARTESIAN_POINT('Ctrl Pts',(18.2941747571336,56.919537469806,38.9892298954617));
#208132=CARTESIAN_POINT('Ctrl Pts',(18.307364587184,56.9607460083087,39.1161900347294));
#208133=CARTESIAN_POINT('Ctrl Pts',(18.2401996527051,57.1650137687745,38.989));
#208134=CARTESIAN_POINT('Ctrl Pts',(18.361164756456,57.125709824009,38.989));
#208135=CARTESIAN_POINT('Ctrl Pts',(18.3609836949701,57.125768654452,39.1161900945644));
#208136=CARTESIAN_POINT('Origin',(18.2401996527051,57.1650137687745,39.116));
#208137=CARTESIAN_POINT('Origin',(5.49583002221492,17.9418771653399,39.5248017080178));
#208138=CARTESIAN_POINT('Origin',(18.5051441132848,57.9804289733662,39.5248017080178));
#208139=CARTESIAN_POINT('Origin',(5.47329194811203,17.8725121057138,39.116));
#208140=CARTESIAN_POINT('Origin',(18.3641788932758,57.5467470426658,39.116040271385));
#208141=CARTESIAN_POINT('Ctrl Pts',(18.4366189870679,57.7713971777985,39.2708017080178));
#208142=CARTESIAN_POINT('Ctrl Pts',(18.5581069080667,57.7324510618068,39.27051194648));
#208143=CARTESIAN_POINT('Ctrl Pts',(18.5239649837014,57.6273730232603,39.3343017080178));
#208144=CARTESIAN_POINT('Ctrl Pts',(18.4506394153725,57.8141635875296,39.3487519301186));
#208145=CARTESIAN_POINT('Ctrl Pts',(18.5719407253098,57.7750271733906,39.3482879463984));
#208146=CARTESIAN_POINT('Ctrl Pts',(18.5448261124699,57.6915769758379,39.451227126164));
#208147=CARTESIAN_POINT('Ctrl Pts',(18.4772005006382,57.8951845615404,39.3978017080178));
#208148=CARTESIAN_POINT('Ctrl Pts',(18.5981804828681,57.8557848432477,39.3975673827401));
#208149=CARTESIAN_POINT('Ctrl Pts',(18.5843471808463,57.8132103173516,39.5248015355181));
#208150=CARTESIAN_POINT('Ctrl Pts',(18.5051441132848,57.9804289733662,39.3978017080178));
#208151=CARTESIAN_POINT('Ctrl Pts',(18.6259282908542,57.9411838150805,39.3978017080178));
#208152=CARTESIAN_POINT('Ctrl Pts',(18.6259282908542,57.9411838150805,39.5248017080178));
#208153=CARTESIAN_POINT('Origin',(18.4031808061319,57.666618181546,39.3343017080178));
#208154=CARTESIAN_POINT('Origin',(18.3780421908675,57.5892494801764,39.1934008533551));
#208155=CARTESIAN_POINT('Origin',(25.273472906796,55.9845461696116,39.1925554495081));
#208156=CARTESIAN_POINT('Origin',(25.2915084057467,56.0249274780509,39.1160373285247));
#208157=CARTESIAN_POINT('Origin',(25.2401862573148,55.9097831300744,39.3343017080178));
#208158=CARTESIAN_POINT('Ctrl Pts',(25.1949317875307,55.8095395120004,39.2708017080178));
#208159=CARTESIAN_POINT('Ctrl Pts',(25.079631183696,55.8614118841076,39.2710850691866));
#208160=CARTESIAN_POINT('Ctrl Pts',(25.1241659841942,55.961438683745,39.3343017080178));
#208161=CARTESIAN_POINT('Ctrl Pts',(25.1767321129116,55.7683775656456,39.3487519293517));
#208162=CARTESIAN_POINT('Ctrl Pts',(25.0612313830309,55.8200852551827,39.3492068662942));
#208163=CARTESIAN_POINT('Ctrl Pts',(25.0967080045995,55.8997670518382,39.4512271248752));
#208164=CARTESIAN_POINT('Ctrl Pts',(25.1422534028249,55.6903961807895,39.3978017080178));
#208165=CARTESIAN_POINT('Ctrl Pts',(25.0264120100491,55.74187966302,39.398034778116));
#208166=CARTESIAN_POINT('Ctrl Pts',(25.0446893032922,55.7829311357713,39.5248015355176));
#208167=CARTESIAN_POINT('Ctrl Pts',(25.1059793847708,55.6083495590299,39.3978017080178));
#208168=CARTESIAN_POINT('Ctrl Pts',(24.9899591116502,55.6600051127005,39.3978017080178));
#208169=CARTESIAN_POINT('Ctrl Pts',(24.9899591116502,55.6600051127005,39.5248017080178));
#208170=CARTESIAN_POINT('Origin',(25.1059793847708,55.6083495590299,39.5248017080178));
#208171=CARTESIAN_POINT('Origin',(0.29005068280153,-0.12913888417657,39.116));
#208172=CARTESIAN_POINT('Origin',(25.454706393409,56.3916032444848,39.116));
#208173=CARTESIAN_POINT('Origin',(0.29005068280153,-0.12913888417657,39.5248017080178));
#208174=CARTESIAN_POINT('Origin',(25.0444775033954,55.4702140717964,39.5248017080178));
#208175=CARTESIAN_POINT('Ctrl Pts',(25.6742415049986,56.8833377255391,39.2875012672119));
#208176=CARTESIAN_POINT('Ctrl Pts',(25.5577357840972,56.9357219056858,39.287208709576));
#208177=CARTESIAN_POINT('Ctrl Pts',(25.5138485805642,56.8366797759148,39.3549016990125));
#208178=CARTESIAN_POINT('Ctrl Pts',(25.627368014374,56.7783442778554,39.1034939173931));
#208179=CARTESIAN_POINT('Ctrl Pts',(25.510904250253,56.8305359187817,39.1031692336344));
#208180=CARTESIAN_POINT('Ctrl Pts',(25.4764485929327,56.7526780286695,39.2077507202307));
#208181=CARTESIAN_POINT('Ctrl Pts',(25.5431608329957,56.5897276738848,38.989));
#208182=CARTESIAN_POINT('Ctrl Pts',(25.4268390553479,56.6417212312948,38.9887769311158));
#208183=CARTESIAN_POINT('Ctrl Pts',(25.4092610357536,56.6017723050709,39.1161898712902));
#208184=CARTESIAN_POINT('Ctrl Pts',(25.454706393409,56.3916032444848,38.989));
#208185=CARTESIAN_POINT('Ctrl Pts',(25.33851279138,56.4433359691574,38.989));
#208186=CARTESIAN_POINT('Ctrl Pts',(25.3386862495677,56.4432587405965,39.1161895903859));
#208187=CARTESIAN_POINT('Origin',(25.6299342605002,56.7851714777844,39.3548010137695));
#208188=CARTESIAN_POINT('Ctrl Pts',(25.0444775033954,55.4702140717964,39.3978017080178));
#208189=CARTESIAN_POINT('Ctrl Pts',(24.9284572302748,55.521869625467,39.3978017080178));
#208190=CARTESIAN_POINT('Ctrl Pts',(24.9284572302748,55.521869625467,39.5248017080178));
#208191=CARTESIAN_POINT('Ctrl Pts',(25.0080814159069,55.3878899076694,39.3978017080178));
#208192=CARTESIAN_POINT('Ctrl Pts',(24.891811449322,55.4395618538376,39.3975666025031));
#208193=CARTESIAN_POINT('Ctrl Pts',(24.8735420580987,55.3985281293144,39.5248015517182));
#208194=CARTESIAN_POINT('Ctrl Pts',(24.9736678430993,55.3100454158607,39.3484894016716));
#208195=CARTESIAN_POINT('Ctrl Pts',(24.857335972326,55.362128664703,39.3480259000036));
#208196=CARTESIAN_POINT('Ctrl Pts',(24.8216158475498,55.281899950892,39.4508333188946));
#208197=CARTESIAN_POINT('Ctrl Pts',(24.9555320242421,55.2690209153037,39.2708017080178));
#208198=CARTESIAN_POINT('Ctrl Pts',(24.8391888661851,55.3213695969753,39.27051194648));
#208199=CARTESIAN_POINT('Ctrl Pts',(24.7942503289613,55.2204359898053,39.3343017080178));
#208200=CARTESIAN_POINT('Origin',(24.910270602082,55.1687804361347,39.3343017080178));
#208201=CARTESIAN_POINT('Origin',(25.7023940320534,56.9479187893822,39.6398955068185));
#208202=CARTESIAN_POINT('Origin',(25.7748538035653,57.1106661007662,39.92499));
#208203=CARTESIAN_POINT('Origin',(24.877182467142,55.0944632682965,39.1934008539949));
#208204=CARTESIAN_POINT('Origin',(24.8590452239608,55.0536014459534,39.1160402713848));
#208205=CARTESIAN_POINT('Ctrl Pts',(25.6197038181304,57.5052637377729,40.1599502534424));
#208206=CARTESIAN_POINT('Ctrl Pts',(25.6045223014068,57.4711877340326,40.10025));
#208207=CARTESIAN_POINT('Ctrl Pts',(25.5758735661215,57.4068835917977,40.10025));
#208208=CARTESIAN_POINT('Ctrl Pts',(25.7001924885135,57.4694043465857,40.1599500538455));
#208209=CARTESIAN_POINT('Ctrl Pts',(25.6631501095111,57.4450643815376,40.1002448353481));
#208210=CARTESIAN_POINT('Ctrl Pts',(25.622459862445,57.3861185493433,40.10025));
#208211=CARTESIAN_POINT('Ctrl Pts',(25.7642825572406,57.413464248775,40.1202442001039));
#208212=CARTESIAN_POINT('Ctrl Pts',(25.7077329912395,57.399880495399,40.0633873868017));
#208213=CARTESIAN_POINT('Ctrl Pts',(25.6552692732811,57.3441059191828,40.0772271723538));
#208214=CARTESIAN_POINT('Ctrl Pts',(25.8321626496797,57.3036982377899,40.0045995998162));
#208215=CARTESIAN_POINT('Ctrl Pts',(25.7409042554413,57.3186021074446,39.9663485808314));
#208216=CARTESIAN_POINT('Ctrl Pts',(25.6821129719832,57.2526112478168,40.0101727202466));
#208217=CARTESIAN_POINT('Ctrl Pts',(25.8376543496551,57.2503778226938,39.9304654349859));
#208218=CARTESIAN_POINT('Ctrl Pts',(25.7289491719115,57.28210970638,39.9051900162952));
#208219=CARTESIAN_POINT('Ctrl Pts',(25.6773293952371,57.2038640469256,39.9671857458183));
#208220=CARTESIAN_POINT('Ctrl Pts',(25.8191582032627,57.2088336324696,39.8576902534424));
#208221=CARTESIAN_POINT('Ctrl Pts',(25.702828419034,57.2611357920722,39.8573998014387));
#208222=CARTESIAN_POINT('Ctrl Pts',(25.6588335304447,57.1623216544368,39.92499));
#208223=CARTESIAN_POINT('Origin',(25.5758735661215,57.4068835917977,40.22725));
#208224=CARTESIAN_POINT('Origin',(0.29005068280153,-0.12913888417657,39.116));
#208225=CARTESIAN_POINT('Origin',(24.6957503380314,54.6869600343295,39.116));
#208226=CARTESIAN_POINT('Origin',(5.59761027822878E-15,5.54425044580581E-15,
40.22725));
#208227=CARTESIAN_POINT('Origin',(25.5480287005725,57.4192809246786,40.22725));
#208228=CARTESIAN_POINT('Ctrl Pts',(24.6957503380314,54.6869600343295,38.989));
#208229=CARTESIAN_POINT('Ctrl Pts',(24.5795562613026,54.738692970352,38.989));
#208230=CARTESIAN_POINT('Ctrl Pts',(24.5797301948987,54.7386155301257,39.1161901092321));
#208231=CARTESIAN_POINT('Ctrl Pts',(24.6072881749609,54.4888352915923,38.989));
#208232=CARTESIAN_POINT('Ctrl Pts',(24.4913819335275,54.540648923418,38.989229898976));
#208233=CARTESIAN_POINT('Ctrl Pts',(24.5091541605501,54.5800991622545,39.1161900493183));
#208234=CARTESIAN_POINT('Ctrl Pts',(24.5230714236775,54.3002245846698,39.1034966344368));
#208235=CARTESIAN_POINT('Ctrl Pts',(24.4074205468513,54.3520673354873,39.1038314102562));
#208236=CARTESIAN_POINT('Ctrl Pts',(24.4419671033168,54.4291945615862,39.2077528789614));
#208237=CARTESIAN_POINT('Ctrl Pts',(24.4761921430398,54.1952354911869,39.2875012672119));
#208238=CARTESIAN_POINT('Ctrl Pts',(24.3607210114372,54.2471777873468,39.2878045257868));
#208239=CARTESIAN_POINT('Ctrl Pts',(24.4045675740913,54.3451938439588,39.3549015295899));
#208240=CARTESIAN_POINT('Origin',(24.5205222915158,54.2933913980361,39.3548010137695));
#208241=CARTESIAN_POINT('Ctrl Pts',(25.2380597013437,57.4675553545137,39.8576902534424));
#208242=CARTESIAN_POINT('Ctrl Pts',(25.3547675996722,57.416102453084,39.8573998014387));
#208243=CARTESIAN_POINT('Ctrl Pts',(25.3107727110829,57.3172883154487,39.92499));
#208244=CARTESIAN_POINT('Ctrl Pts',(25.2565651278917,57.5091180232689,39.9304984902492));
#208245=CARTESIAN_POINT('Ctrl Pts',(25.3528749970543,57.44956723289,39.905217156979));
#208246=CARTESIAN_POINT('Ctrl Pts',(25.3292770036986,57.3588496371387,39.9672049726596));
#208247=CARTESIAN_POINT('Ctrl Pts',(25.2997972770066,57.5405471770605,40.0043437678661));
#208248=CARTESIAN_POINT('Ctrl Pts',(25.3720159720868,57.4827148996386,39.9661628577646));
#208249=CARTESIAN_POINT('Ctrl Pts',(25.3622324578628,57.3948558336727,40.0100243556237));
#208250=CARTESIAN_POINT('Ctrl Pts',(25.4257977880274,57.5636463159493,40.1194874821989));
#208251=CARTESIAN_POINT('Ctrl Pts',(25.4538910783602,57.5124644612007,40.0627551483138));
#208252=CARTESIAN_POINT('Ctrl Pts',(25.4475597357242,57.4360631077224,40.0767884282375));
#208253=CARTESIAN_POINT('Ctrl Pts',(25.5110385513892,57.5536211289084,40.1599502015382));
#208254=CARTESIAN_POINT('Ctrl Pts',(25.517777816472,57.509788306594,40.1002449453885));
#208255=CARTESIAN_POINT('Ctrl Pts',(25.5012707422386,57.4400754463044,40.10025));
#208256=CARTESIAN_POINT('Ctrl Pts',(25.5918112338801,57.5176823163886,40.1599502534424));
#208257=CARTESIAN_POINT('Ctrl Pts',(25.5766462455183,57.4835989537475,40.10025));
#208258=CARTESIAN_POINT('Ctrl Pts',(25.5480287005725,57.4192809246786,40.10025));
#208259=CARTESIAN_POINT('Origin',(25.1947524379623,57.3689438691193,39.92499));
#208260=CARTESIAN_POINT('Origin',(24.4480624203082,54.1306438627435,39.6398955069306));
#208261=CARTESIAN_POINT('Origin',(24.3756025490945,53.9678963272932,39.92499));
#208262=CARTESIAN_POINT('Origin',(25.1222926664914,57.2061965577052,39.6398955068253));
#208263=CARTESIAN_POINT('Origin',(25.0498328948971,57.0434492461376,39.3548010137695));
#208264=CARTESIAN_POINT('Ctrl Pts',(24.3312692531094,53.8697418420142,39.8576902534424));
#208265=CARTESIAN_POINT('Ctrl Pts',(24.2159747902193,53.9216078643414,39.8579948730703));
#208266=CARTESIAN_POINT('Ctrl Pts',(24.2595822759739,54.0195518809638,39.92499));
#208267=CARTESIAN_POINT('Ctrl Pts',(24.3127882662185,53.828234173484,39.930402071123));
#208268=CARTESIAN_POINT('Ctrl Pts',(24.2176496934292,53.8880114973686,39.9058915297383));
#208269=CARTESIAN_POINT('Ctrl Pts',(24.241101009183,53.9780422761231,39.9671523786034));
#208270=CARTESIAN_POINT('Ctrl Pts',(24.2697746459846,53.7969955864425,40.0043257306694));
#208271=CARTESIAN_POINT('Ctrl Pts',(24.1983152114497,53.8549480733036,39.9667894847835));
#208272=CARTESIAN_POINT('Ctrl Pts',(24.2082687574729,53.9422730280819,40.0100138975201));
#208273=CARTESIAN_POINT('Ctrl Pts',(24.1443388226044,53.7744913425363,40.1195533054856));
#208274=CARTESIAN_POINT('Ctrl Pts',(24.1165167429227,53.825645022219,40.0630813209236));
#208275=CARTESIAN_POINT('Ctrl Pts',(24.123203223048,53.9017956184502,40.076826594242));
#208276=CARTESIAN_POINT('Ctrl Pts',(24.0595120258541,53.7848917482049,40.1599502027513));
#208277=CARTESIAN_POINT('Ctrl Pts',(24.0529122166853,53.8286685158639,40.100255279155));
#208278=CARTESIAN_POINT('Ctrl Pts',(24.069666546439,53.8982652496125,40.10025));
#208279=CARTESIAN_POINT('Ctrl Pts',(23.979166327502,53.8206887816833,40.1599502534424));
#208280=CARTESIAN_POINT('Ctrl Pts',(23.9943483786823,53.8547645473078,40.10025));
#208281=CARTESIAN_POINT('Ctrl Pts',(24.0229981225303,53.9190682401992,40.10025));
#208282=CARTESIAN_POINT('Origin',(24.0229981225303,53.9190682401992,40.22725));
#208283=CARTESIAN_POINT('Ctrl Pts',(24.8746050278059,56.6498810128379,38.989));
#208284=CARTESIAN_POINT('Ctrl Pts',(24.9907986398451,56.5981482837085,38.989));
#208285=CARTESIAN_POINT('Ctrl Pts',(24.9906251716322,56.5982255167328,39.1161896013271));
#208286=CARTESIAN_POINT('Ctrl Pts',(24.9626539694757,56.8481896769742,38.989));
#208287=CARTESIAN_POINT('Ctrl Pts',(25.079127190575,56.7965362315748,38.9887769275466));
#208288=CARTESIAN_POINT('Ctrl Pts',(25.0612010539382,56.7567415443525,39.1161898821828));
#208289=CARTESIAN_POINT('Ctrl Pts',(25.046477158254,57.0369754593319,39.1034967087243));
#208290=CARTESIAN_POINT('Ctrl Pts',(25.1631925873332,56.985349035722,39.1031720232705));
#208291=CARTESIAN_POINT('Ctrl Pts',(25.1283880784749,56.9076460727655,39.2077529615015));
#208292=CARTESIAN_POINT('Ctrl Pts',(25.0931373005752,57.1420619865018,39.2875012672119));
#208293=CARTESIAN_POINT('Ctrl Pts',(25.2100238867509,57.0905332166516,39.2872087095507));
#208294=CARTESIAN_POINT('Ctrl Pts',(25.1657874977299,56.9916465440536,39.354901704823));
#208295=CARTESIAN_POINT('Origin',(24.8746050278059,56.6498810128379,39.116));
#208296=CARTESIAN_POINT('Origin',(5.68853496937358E-15,5.30629395586253E-15,
40.22725));
#208297=CARTESIAN_POINT('Origin',(23.9951532569813,53.9314655730802,40.22725));
#208298=CARTESIAN_POINT('Origin',(10.0037024164492,23.2492868865834,39.116));
#208299=CARTESIAN_POINT('Origin',(24.7113125977913,56.2832472948504,39.1160373285276));
#208300=CARTESIAN_POINT('Ctrl Pts',(23.9513722670371,53.8330634946835,40.1599502534424));
#208301=CARTESIAN_POINT('Ctrl Pts',(23.966536720823,53.8671470951728,40.10025));
#208302=CARTESIAN_POINT('Ctrl Pts',(23.9951532569813,53.9314655730802,40.10025));
#208303=CARTESIAN_POINT('Ctrl Pts',(23.8712821658127,53.8686972660498,40.1599500566034));
#208304=CARTESIAN_POINT('Ctrl Pts',(23.9081865738562,53.8931046959194,40.1002551305381));
#208305=CARTESIAN_POINT('Ctrl Pts',(23.9486256024605,53.9521563342729,40.10025));
#208306=CARTESIAN_POINT('Ctrl Pts',(23.8071866393158,53.9240892607409,40.1203070619045));
#208307=CARTESIAN_POINT('Ctrl Pts',(23.8635355386149,53.9378509529598,40.0637098684499));
#208308=CARTESIAN_POINT('Ctrl Pts',(23.9155750846183,53.9937257232524,40.0772636213362));
#208309=CARTESIAN_POINT('Ctrl Pts',(23.7392497560577,54.033006412171,40.0046102245802));
#208310=CARTESIAN_POINT('Ctrl Pts',(23.8300830854582,54.0187512923757,39.9670001894012));
#208311=CARTESIAN_POINT('Ctrl Pts',(23.8883623535222,54.0845104630311,40.0101788811209));
#208312=CARTESIAN_POINT('Ctrl Pts',(23.7337507958623,54.0860594545421,39.9303710930186));
#208313=CARTESIAN_POINT('Ctrl Pts',(23.8418399747433,54.0553500291283,39.9058663574109));
#208314=CARTESIAN_POINT('Ctrl Pts',(23.8930480394874,54.1330265677739,39.9671344706365));
#208315=CARTESIAN_POINT('Ctrl Pts',(23.7522229508834,54.1275498658871,39.8576902534424));
#208316=CARTESIAN_POINT('Ctrl Pts',(23.8679139708575,54.0765745253533,39.8579948730703));
#208317=CARTESIAN_POINT('Ctrl Pts',(23.9115214566121,54.1745185419757,39.92499));
#208318=CARTESIAN_POINT('Origin',(23.7955011834915,54.2261740956463,39.92499));
#208319=CARTESIAN_POINT('Origin',(24.6933715410276,56.2428239368548,39.1925554488838));
#208320=CARTESIAN_POINT('Origin',(24.6600848917118,56.1680608984275,39.3343017080178));
#208321=CARTESIAN_POINT('Origin',(23.8679610547522,54.388921631059,39.6398955069211));
#208322=CARTESIAN_POINT('Origin',(23.9404209259127,54.5516691663892,39.3548010137695));
#208323=CARTESIAN_POINT('Ctrl Pts',(24.5258780191677,55.866627327383,39.3978017080178));
#208324=CARTESIAN_POINT('Ctrl Pts',(24.6418982922884,55.8149717737124,39.3978017080178));
#208325=CARTESIAN_POINT('Ctrl Pts',(24.6418982922884,55.8149717737124,39.5248017080178));
#208326=CARTESIAN_POINT('Ctrl Pts',(24.5627025231295,55.9487607347569,39.3978017080178));
#208327=CARTESIAN_POINT('Ctrl Pts',(24.6784744708811,55.8971232158781,39.3980355775159));
#208328=CARTESIAN_POINT('Ctrl Pts',(24.6968134595448,55.9383132588155,39.5248015517178));
#208329=CARTESIAN_POINT('Ctrl Pts',(24.5975211960713,56.026424800928,39.3484893995498));
#208330=CARTESIAN_POINT('Ctrl Pts',(24.7132325104948,55.9751910510458,39.3489438303434));
#208331=CARTESIAN_POINT('Ctrl Pts',(24.7487396569161,56.0549414076403,39.4508333155602));
#208332=CARTESIAN_POINT('Ctrl Pts',(24.61587051646,56.0673542004323,39.2708017080178));
#208333=CARTESIAN_POINT('Ctrl Pts',(24.7315703643342,56.0163785451195,39.2710850691866));
#208334=CARTESIAN_POINT('Ctrl Pts',(24.7761051648324,56.1164053447569,39.3343017080178));
#208335=CARTESIAN_POINT('Origin',(24.5258780191677,55.866627327383,39.5248017080178));
#208336=CARTESIAN_POINT('Ctrl Pts',(23.8971395307774,54.453046324469,39.2875012672119));
#208337=CARTESIAN_POINT('Ctrl Pts',(24.0130054343475,54.4019907365345,39.2878045257519));
#208338=CARTESIAN_POINT('Ctrl Pts',(24.0565064909001,54.5001606088507,39.3549015218351));
#208339=CARTESIAN_POINT('Ctrl Pts',(23.9437939758161,54.5581374230423,39.1034938540228));
#208340=CARTESIAN_POINT('Ctrl Pts',(24.059706177069,54.5068816478247,39.1038286278798));
#208341=CARTESIAN_POINT('Ctrl Pts',(24.0939065860597,54.5841625982665,39.2077506434038));
#208342=CARTESIAN_POINT('Ctrl Pts',(24.0276077026109,54.7469293531947,38.989));
#208343=CARTESIAN_POINT('Ctrl Pts',(24.1436691352865,54.6954643138438,38.9892298954617));
#208344=CARTESIAN_POINT('Ctrl Pts',(24.1610941752732,54.735068394998,39.1161900347279));
#208345=CARTESIAN_POINT('Ctrl Pts',(24.1156489724283,54.9452378026826,38.989));
#208346=CARTESIAN_POINT('Ctrl Pts',(24.2318430357382,54.8935048726345,38.989));
#208347=CARTESIAN_POINT('Ctrl Pts',(24.231669115581,54.8935823068774,39.1161900945654));
#208348=CARTESIAN_POINT('Origin',(24.1156489724283,54.9452378026826,39.116));
#208349=CARTESIAN_POINT('Origin',(9.75435829333415,22.6892508167102,39.5248017080178));
#208350=CARTESIAN_POINT('Origin',(24.4643761377923,55.7284918401495,39.5248017080178));
#208351=CARTESIAN_POINT('Origin',(9.71531210235053,22.6015516358801,39.116));
#208352=CARTESIAN_POINT('Origin',(24.278851034245,55.3119205422642,39.1160402713849));
#208353=CARTESIAN_POINT('Ctrl Pts',(24.374376627022,55.527767968768,39.2708017080178));
#208354=CARTESIAN_POINT('Ctrl Pts',(24.4911280468232,55.4763362579872,39.27051194648));
#208355=CARTESIAN_POINT('Ctrl Pts',(24.4461895095995,55.3754026508172,39.3343017080178));
#208356=CARTESIAN_POINT('Ctrl Pts',(24.3927905570414,55.5688345658071,39.3487519301186));
#208357=CARTESIAN_POINT('Ctrl Pts',(24.5093364964834,55.5172331055225,39.3482879463981));
#208358=CARTESIAN_POINT('Ctrl Pts',(24.4736474994209,55.4370743056936,39.4512271261637));
#208359=CARTESIAN_POINT('Ctrl Pts',(24.4276751358087,55.6466353090193,39.3978017080178));
#208360=CARTESIAN_POINT('Ctrl Pts',(24.543873985031,55.5948055748752,39.3975673827397));
#208361=CARTESIAN_POINT('Ctrl Pts',(24.5256662135194,55.5539102504899,39.5248015355181));
#208362=CARTESIAN_POINT('Ctrl Pts',(24.4643761377923,55.7284918401495,39.3978017080178));
#208363=CARTESIAN_POINT('Ctrl Pts',(24.5803964109129,55.6768362864789,39.3978017080178));
#208364=CARTESIAN_POINT('Ctrl Pts',(24.5803964109129,55.6768362864789,39.5248017080178));
#208365=CARTESIAN_POINT('Origin',(24.3301692364789,55.4270582044878,39.3343017080178));
#208366=CARTESIAN_POINT('Origin',(24.2970811017216,55.3527410377811,39.1934008533552));
#208367=CARTESIAN_POINT('Origin',(30.9870007556516,53.0360596835508,39.1925554495081));
#208368=CARTESIAN_POINT('Origin',(31.0091584503715,53.0743345559674,39.1160373285272));
#208369=CARTESIAN_POINT('Origin',(30.9460815882875,52.9651856060842,39.3343017080178));
#208370=CARTESIAN_POINT('Ctrl Pts',(30.8905967158742,52.8702215132212,39.2708017080178));
#208371=CARTESIAN_POINT('Ctrl Pts',(30.7813498801538,52.9338619179792,39.2710850691866));
#208372=CARTESIAN_POINT('Ctrl Pts',(30.8360963620068,53.0286856060842,39.3343017080178));
#208373=CARTESIAN_POINT('Ctrl Pts',(30.8681941459793,52.8311874403353,39.3487519293517));
#208374=CARTESIAN_POINT('Ctrl Pts',(30.7587310665105,52.8946849835399,39.3492068662932));
#208375=CARTESIAN_POINT('Ctrl Pts',(30.8023423591876,52.9702219582425,39.4512271248746));
#208376=CARTESIAN_POINT('Ctrl Pts',(30.8257530395504,52.7572372522463,39.3978017080178));
#208377=CARTESIAN_POINT('Ctrl Pts',(30.715927727326,52.8205474253429,39.3980347781178));
#208378=CARTESIAN_POINT('Ctrl Pts',(30.7383959430067,52.8594635164552,39.524801535519));
#208379=CARTESIAN_POINT('Ctrl Pts',(30.781101527075,52.6794317578284,39.3978017080178));
#208380=CARTESIAN_POINT('Ctrl Pts',(30.6711163007943,52.7429317578284,39.3978017080178));
#208381=CARTESIAN_POINT('Ctrl Pts',(30.6711163007943,52.7429317578284,39.5248017080178));
#208382=CARTESIAN_POINT('Origin',(30.781101527075,52.6794317578284,39.5248017080178));
#208383=CARTESIAN_POINT('Origin',(0.274963065701563,-0.158750000000003,
39.116));
#208384=CARTESIAN_POINT('Origin',(31.2097904767612,53.4219427993283,39.116));
#208385=CARTESIAN_POINT('Origin',(0.274963065701563,-0.158750000000003,
39.5248017080178));
#208386=CARTESIAN_POINT('Origin',(30.7054974692375,52.5484816883956,39.5248017080178));
#208387=CARTESIAN_POINT('Ctrl Pts',(31.4795232016796,53.8880358395966,39.2875012672119));
#208388=CARTESIAN_POINT('Ctrl Pts',(31.369131349158,53.9523112176909,39.287208709576));
#208389=CARTESIAN_POINT('Ctrl Pts',(31.3151318426941,53.8583991130126,39.3549016990123));
#208390=CARTESIAN_POINT('Ctrl Pts',(31.4219316852027,53.7885171709472,39.1034939173931));
#208391=CARTESIAN_POINT('Ctrl Pts',(31.3115614337849,53.8525966788984,39.1031692336334));
#208392=CARTESIAN_POINT('Ctrl Pts',(31.269156162556,53.7787668993601,39.2077507202308));
#208393=CARTESIAN_POINT('Ctrl Pts',(31.3184699958138,53.6097358757348,38.989));
#208394=CARTESIAN_POINT('Ctrl Pts',(31.2082202476905,53.6736035436575,38.9887769311164));
#208395=CARTESIAN_POINT('Ctrl Pts',(31.1865627224602,53.6357108652095,39.1161898712899));
#208396=CARTESIAN_POINT('Ctrl Pts',(31.2097904767612,53.4219427993283,38.989));
#208397=CARTESIAN_POINT('Ctrl Pts',(31.0996409376526,53.4855376653837,38.989));
#208398=CARTESIAN_POINT('Ctrl Pts',(31.0998053730352,53.4854427285713,39.1161895903856));
#208399=CARTESIAN_POINT('Origin',(31.4251975098799,53.7950387249975,39.3548010137695));
#208400=CARTESIAN_POINT('Ctrl Pts',(30.7054974692375,52.5484816883955,39.3978017080178));
#208401=CARTESIAN_POINT('Ctrl Pts',(30.5955122429569,52.6119816883956,39.3978017080178));
#208402=CARTESIAN_POINT('Ctrl Pts',(30.5955122429569,52.6119816883956,39.5248017080178));
#208403=CARTESIAN_POINT('Ctrl Pts',(30.6606955449583,52.4704129317475,39.3978017080178));
#208404=CARTESIAN_POINT('Ctrl Pts',(30.5504637065433,52.5339553345216,39.397566602504));
#208405=CARTESIAN_POINT('Ctrl Pts',(30.5280052047894,52.4950560684209,39.5248015517196));
#208406=CARTESIAN_POINT('Ctrl Pts',(30.618333528198,52.3965920780928,39.3484894016716));
#208407=CARTESIAN_POINT('Ctrl Pts',(30.5080831175492,52.4605500011255,39.3480259000037));
#208408=CARTESIAN_POINT('Ctrl Pts',(30.4641724871921,52.3844945583571,39.4508333188932));
#208409=CARTESIAN_POINT('Ctrl Pts',(30.5960088312575,52.3576880233159,39.2708017080178));
#208410=CARTESIAN_POINT('Ctrl Pts',(30.4857749404426,52.4219111049553,39.27051194648));
#208411=CARTESIAN_POINT('Ctrl Pts',(30.4305321463783,52.3262277788838,39.3343017080178));
#208412=CARTESIAN_POINT('Origin',(30.5405173726589,52.2627277788838,39.3343017080178));
#208413=CARTESIAN_POINT('Origin',(31.5142720656045,53.9493203812239,39.6398955068191));
#208414=CARTESIAN_POINT('Origin',(31.6033466212672,54.1036020372434,39.92499));
#208415=CARTESIAN_POINT('Origin',(30.499842238637,52.1922763801646,39.1934008539944));
#208416=CARTESIAN_POINT('Origin',(30.4775331296744,52.1535342613176,39.1160402713846));
#208417=CARTESIAN_POINT('Ctrl Pts',(31.4902932482914,54.5122556166607,40.1599502534424));
#208418=CARTESIAN_POINT('Ctrl Pts',(31.4716329851996,54.4799531854475,40.10025));
#208419=CARTESIAN_POINT('Ctrl Pts',(31.4364195775141,54.4189959163059,40.10025));
#208420=CARTESIAN_POINT('Ctrl Pts',(31.5665926662623,54.4681793099456,40.1599500538468));
#208421=CARTESIAN_POINT('Ctrl Pts',(31.5272089901464,54.4478446647271,40.100244835349));
#208422=CARTESIAN_POINT('Ctrl Pts',(31.4805801312546,54.3934750329631,40.10025));
#208423=CARTESIAN_POINT('Ctrl Pts',(31.6244843104276,54.4058464214482,40.1202442001037));
#208424=CARTESIAN_POINT('Ctrl Pts',(31.5668246399994,54.3982481205263,40.0633873868012));
#208425=CARTESIAN_POINT('Ctrl Pts',(31.5088182930364,54.3482630350898,40.0772271723536));
#208426=CARTESIAN_POINT('Ctrl Pts',(31.6805188761705,54.2895863184075,40.0045995998164));
#208427=CARTESIAN_POINT('Ctrl Pts',(31.5913182835567,54.3139476428155,39.9663485808321));
#208428=CARTESIAN_POINT('Ctrl Pts',(31.5259511417539,54.2544636505349,40.0101727202467));
#208429=CARTESIAN_POINT('Ctrl Pts',(31.6804069909882,54.2359839591648,39.9304654349857));
#208430=CARTESIAN_POINT('Ctrl Pts',(31.5756141966203,54.2789047974524,39.9051900162937));
#208431=CARTESIAN_POINT('Ctrl Pts',(31.5160982999439,54.2064835118364,39.9671857458168));
#208432=CARTESIAN_POINT('Ctrl Pts',(31.6576696180591,54.1966007261204,39.8576902534424));
#208433=CARTESIAN_POINT('Ctrl Pts',(31.547444164929,54.2607761425979,39.8573998014387));
#208434=CARTESIAN_POINT('Ctrl Pts',(31.4933613949865,54.1671020372435,39.92499));
#208435=CARTESIAN_POINT('Origin',(31.4364195775141,54.4189959163059,40.22725));
#208436=CARTESIAN_POINT('Origin',(0.274963065701563,-0.158750000000003,
39.116));
#208437=CARTESIAN_POINT('Origin',(30.2768083268887,51.8059703131943,39.116));
#208438=CARTESIAN_POINT('Origin',(5.58223212128129E-15,5.55208600813687E-15,
40.22725));
#208439=CARTESIAN_POINT('Origin',(31.4100231232068,54.4342359163059,40.22725));
#208440=CARTESIAN_POINT('Ctrl Pts',(30.2768083268887,51.8059703131943,38.989));
#208441=CARTESIAN_POINT('Ctrl Pts',(30.1666583377722,51.8695654390619,38.989));
#208442=CARTESIAN_POINT('Ctrl Pts',(30.1668232238344,51.8694702420495,39.1161901092326));
#208443=CARTESIAN_POINT('Ctrl Pts',(30.1681210939104,51.6181777324908,38.989));
#208444=CARTESIAN_POINT('Ctrl Pts',(30.0582657983062,51.6818230251226,38.9892298989718));
#208445=CARTESIAN_POINT('Ctrl Pts',(30.0800643400511,51.7191994478429,39.1161900493188));
#208446=CARTESIAN_POINT('Ctrl Pts',(30.0646505034505,51.4394033023492,39.1034966344368));
#208447=CARTESIAN_POINT('Ctrl Pts',(29.9550522173037,51.5030508615797,39.1038314102585));
#208448=CARTESIAN_POINT('Ctrl Pts',(29.9974715145374,51.5761444782073,39.2077528789611));
#208449=CARTESIAN_POINT('Ctrl Pts',(30.0070536838164,51.3398895692694,39.2875012672119));
#208450=CARTESIAN_POINT('Ctrl Pts',(29.8976445635504,51.4036173400345,39.2878045257868));
#208451=CARTESIAN_POINT('Ctrl Pts',(29.9514963979204,51.4965132406191,39.3549015295901));
#208452=CARTESIAN_POINT('Origin',(30.0614010732043,51.4328740054939,39.3548010137695));
#208453=CARTESIAN_POINT('Ctrl Pts',(31.1067982185541,54.5146464769134,39.8576902534424));
#208454=CARTESIAN_POINT('Ctrl Pts',(31.2174884860871,54.4512761425979,39.8573998014387));
#208455=CARTESIAN_POINT('Ctrl Pts',(31.1634057161447,54.3576020372435,39.92499));
#208456=CARTESIAN_POINT('Ctrl Pts',(31.1295467523335,54.5540471172212,39.9304984902491));
#208457=CARTESIAN_POINT('Ctrl Pts',(31.2191042733517,54.4847554296812,39.9052171569791));
#208458=CARTESIAN_POINT('Ctrl Pts',(31.1861529813963,54.3970014563925,39.9672049726606));
#208459=CARTESIAN_POINT('Ctrl Pts',(31.1758273123594,54.5807851087095,40.0043437678663));
#208460=CARTESIAN_POINT('Ctrl Pts',(31.241605266786,54.5157207333391,39.966162857764));
#208461=CARTESIAN_POINT('Ctrl Pts',(31.2226915745269,54.4293656242364,40.0100243556234));
#208462=CARTESIAN_POINT('Ctrl Pts',(31.3035520968889,54.5905870683099,40.1194874821986));
#208463=CARTESIAN_POINT('Ctrl Pts',(31.326141528613,54.5367490446495,40.0627551483143));
#208464=CARTESIAN_POINT('Ctrl Pts',(31.3118587536639,54.461428031296,40.0767884282378));
#208465=CARTESIAN_POINT('Ctrl Pts',(31.3872779850339,54.5717067142911,40.1599502015381));
#208466=CARTESIAN_POINT('Ctrl Pts',(31.3893985541595,54.5274095677394,40.100244945386));
#208467=CARTESIAN_POINT('Ctrl Pts',(31.3656949292504,54.459804060896,40.10025));
#208468=CARTESIAN_POINT('Ctrl Pts',(31.4638515574747,54.5275217339716,40.1599502534424));
#208469=CARTESIAN_POINT('Ctrl Pts',(31.445206962986,54.4952102564862,40.10025));
#208470=CARTESIAN_POINT('Ctrl Pts',(31.4100231232068,54.434235916306,40.10025));
#208471=CARTESIAN_POINT('Origin',(31.053420489864,54.4211020372435,39.92499));
#208472=CARTESIAN_POINT('Origin',(29.9723263949888,51.278592137215,39.6398955069312));
#208473=CARTESIAN_POINT('Origin',(29.8832517167492,51.1243102687781,39.92499));
#208474=CARTESIAN_POINT('Origin',(30.9643459342367,54.2668203811885,39.6398955068273));
#208475=CARTESIAN_POINT('Origin',(30.8752713784768,54.1125387249975,39.3548010137695));
#208476=CARTESIAN_POINT('Ctrl Pts',(29.8289013456892,51.0313275753405,39.8576902534424));
#208477=CARTESIAN_POINT('Ctrl Pts',(29.7196599535399,51.0949610231998,39.8579948730703));
#208478=CARTESIAN_POINT('Ctrl Pts',(29.7732664904686,51.1878102687781,39.92499));
#208479=CARTESIAN_POINT('Ctrl Pts',(29.8061828667731,50.9919790793207,39.930402071123));
#208480=CARTESIAN_POINT('Ctrl Pts',(29.7178139048433,51.0613736255825,39.9058915297388));
#208481=CARTESIAN_POINT('Ctrl Pts',(29.7505475307862,51.1484598763131,39.9671523786037));
#208482=CARTESIAN_POINT('Ctrl Pts',(29.7601395581531,50.9654077681504,40.0043257306694));
#208483=CARTESIAN_POINT('Ctrl Pts',(29.6951292702712,51.0305123301031,39.9667894847838));
#208484=CARTESIAN_POINT('Ctrl Pts',(29.7141562330561,51.1163184807718,40.01001389752));
#208485=CARTESIAN_POINT('Ctrl Pts',(29.6330385513055,50.9561384187036,40.1195533054856));
#208486=CARTESIAN_POINT('Ctrl Pts',(29.6107158994153,51.0099200724104,40.0630813209234));
#208487=CARTESIAN_POINT('Ctrl Pts',(29.6253256551034,51.0849545802161,40.0768265942421));
#208488=CARTESIAN_POINT('Ctrl Pts',(29.5497635830449,50.9753486645696,40.1599502027521));
#208489=CARTESIAN_POINT('Ctrl Pts',(29.5477758465702,51.0195754864235,40.1002552791541));
#208490=CARTESIAN_POINT('Ctrl Pts',(29.5717132339806,51.0870396576411,40.10025));
#208491=CARTESIAN_POINT('Ctrl Pts',(29.4735998357344,51.0193480105324,40.1599502534424));
#208492=CARTESIAN_POINT('Ctrl Pts',(29.4922606054652,51.0516501490683,40.10025));
#208493=CARTESIAN_POINT('Ctrl Pts',(29.5274749692191,51.1126068659043,40.10025));
#208494=CARTESIAN_POINT('Origin',(29.5274749692191,51.1126068659043,40.22725));
#208495=CARTESIAN_POINT('Ctrl Pts',(30.6598643453581,53.7394427993283,38.989));
#208496=CARTESIAN_POINT('Ctrl Pts',(30.7700138939565,53.6758479277939,38.989));
#208497=CARTESIAN_POINT('Ctrl Pts',(30.7698494490699,53.6759428700934,39.1161896013271));
#208498=CARTESIAN_POINT('Ctrl Pts',(30.7681598456269,53.9274614872883,38.989));
#208499=CARTESIAN_POINT('Ctrl Pts',(30.8785957589617,53.8639162380512,38.9887769275436));
#208500=CARTESIAN_POINT('Ctrl Pts',(30.8566081460784,53.8262133418065,39.1161898821829));
#208501=CARTESIAN_POINT('Ctrl Pts',(30.8712573299201,54.1064511722699,39.1034967087243));
#208502=CARTESIAN_POINT('Ctrl Pts',(30.9819369489468,54.0429074791724,39.1031720232714));
#208503=CARTESIAN_POINT('Ctrl Pts',(30.9392009315203,53.9692682429977,39.2077529615014));
#208504=CARTESIAN_POINT('Ctrl Pts',(30.9286463962985,54.2060847114738,39.2875012672119));
#208505=CARTESIAN_POINT('Ctrl Pts',(31.0395064423985,54.1426202463868,39.2872087095507));
#208506=CARTESIAN_POINT('Ctrl Pts',(30.9851759130208,54.0488992470928,39.354901704823));
#208507=CARTESIAN_POINT('Origin',(30.6598643453581,53.7394427993283,39.116));
#208508=CARTESIAN_POINT('Origin',(5.69400554112517E-15,5.30350656033181E-15,
40.22725));
#208509=CARTESIAN_POINT('Origin',(29.5010785149117,51.1278468659043,40.22725));
#208510=CARTESIAN_POINT('Origin',(15.2806508669898,27.1018636743471,39.116));
#208511=CARTESIAN_POINT('Origin',(30.4591427892375,53.3918862459818,39.1160373285273));
#208512=CARTESIAN_POINT('Ctrl Pts',(29.4472515437741,51.0345602039883,40.1599502534424));
#208513=CARTESIAN_POINT('Ctrl Pts',(29.4658956314773,51.0668719738974,40.10025));
#208514=CARTESIAN_POINT('Ctrl Pts',(29.5010785149117,51.1278468659044,40.10025));
#208515=CARTESIAN_POINT('Ctrl Pts',(29.3713249278651,51.0783704650302,40.1599500566043));
#208516=CARTESIAN_POINT('Ctrl Pts',(29.410578440836,51.0987866273836,40.100255130536));
#208517=CARTESIAN_POINT('Ctrl Pts',(29.4569685172211,51.1532877451675,40.10025));
#208518=CARTESIAN_POINT('Ctrl Pts',(29.3133705634517,51.1401588234659,40.1203070619047));
#208519=CARTESIAN_POINT('Ctrl Pts',(29.3708492661241,51.1479550638441,40.0637098684496));
#208520=CARTESIAN_POINT('Ctrl Pts',(29.4284442379235,51.198084132526,40.0772636213363));
#208521=CARTESIAN_POINT('Ctrl Pts',(29.2571907880108,51.2555806533508,40.0046102245801));
#208522=CARTESIAN_POINT('Ctrl Pts',(29.346036457163,51.2319089562579,39.9670001894015));
#208523=CARTESIAN_POINT('Ctrl Pts',(29.4108701703532,51.2912160489646,40.0101788811209));
#208524=CARTESIAN_POINT('Ctrl Pts',(29.2572675046855,51.3089178634633,39.9303710930187));
#208525=CARTESIAN_POINT('Ctrl Pts',(29.3615545506891,51.2670782717306,39.9058663574108));
#208526=CARTESIAN_POINT('Ctrl Pts',(29.4206015015128,51.338976589856,39.9671344706372));
#208527=CARTESIAN_POINT('Ctrl Pts',(29.2799753962468,51.3482501200162,39.8576902534424));
#208528=CARTESIAN_POINT('Ctrl Pts',(29.389704274698,51.2854610231998,39.8579948730703));
#208529=CARTESIAN_POINT('Ctrl Pts',(29.4433108116267,51.3783102687781,39.92499));
#208530=CARTESIAN_POINT('Origin',(29.3333255853461,51.4418102687781,39.92499));
#208531=CARTESIAN_POINT('Origin',(30.4370746239673,53.3535596824664,39.1925554488847));
#208532=CARTESIAN_POINT('Origin',(30.3961554568843,53.2826856060842,39.3343017080178));
#208533=CARTESIAN_POINT('Origin',(29.4224002636289,51.5960921371705,39.6398955069207));
#208534=CARTESIAN_POINT('Origin',(29.5114749418011,51.750374005494,39.3548010137695));
#208535=CARTESIAN_POINT('Ctrl Pts',(30.2311753956719,52.9969317578284,39.3978017080178));
#208536=CARTESIAN_POINT('Ctrl Pts',(30.3411606219525,52.9334317578284,39.3978017080178));
#208537=CARTESIAN_POINT('Ctrl Pts',(30.3411606219525,52.9334317578284,39.5248017080178));
#208538=CARTESIAN_POINT('Ctrl Pts',(30.2763834500039,53.0747660209931,39.3978017080178));
#208539=CARTESIAN_POINT('Ctrl Pts',(30.3861235964158,53.0113099140559,39.3980355775196));
#208540=CARTESIAN_POINT('Ctrl Pts',(30.4086676540716,53.0503573673268,39.5248015517192));
#208541=CARTESIAN_POINT('Ctrl Pts',(30.319129488101,53.1483650929075,39.3484893995498));
#208542=CARTESIAN_POINT('Ctrl Pts',(30.4288515386952,53.0853168809912,39.3489438303413));
#208543=CARTESIAN_POINT('Ctrl Pts',(30.4725003554715,53.1609188493359,39.4508333155594));
#208544=CARTESIAN_POINT('Ctrl Pts',(30.3416565762243,53.1871522506172,39.2708017080178));
#208545=CARTESIAN_POINT('Ctrl Pts',(30.451394201312,53.1243619179792,39.2710850691866));
#208546=CARTESIAN_POINT('Ctrl Pts',(30.506140683165,53.2191856060842,39.3343017080178));
#208547=CARTESIAN_POINT('Origin',(30.2311753956718,52.9969317578284,39.5248017080178));
#208548=CARTESIAN_POINT('Ctrl Pts',(29.458121752568,51.6568155675424,39.2875012672119));
#208549=CARTESIAN_POINT('Ctrl Pts',(29.5680161684464,51.5939283826158,39.2878045257519));
#208550=CARTESIAN_POINT('Ctrl Pts',(29.6215404675523,51.6870133715069,39.3549015218348));
#208551=CARTESIAN_POINT('Ctrl Pts',(29.5155056307115,51.7564542486377,39.1034938540228));
#208552=CARTESIAN_POINT('Ctrl Pts',(29.625425165382,51.6933631336519,39.1038286278807));
#208553=CARTESIAN_POINT('Ctrl Pts',(29.6675162799446,51.7666458147659,39.2077506434044));
#208554=CARTESIAN_POINT('Ctrl Pts',(29.6185943474785,51.93545103678,38.989));
#208555=CARTESIAN_POINT('Ctrl Pts',(29.7286404220058,51.872136205095,38.9892298954617));
#208556=CARTESIAN_POINT('Ctrl Pts',(29.7501097595415,51.9097019182962,39.1161900347272));
#208557=CARTESIAN_POINT('Ctrl Pts',(29.7268821954856,52.1234703131943,38.989));
#208558=CARTESIAN_POINT('Ctrl Pts',(29.8370321718802,52.0598751946716,38.989));
#208559=CARTESIAN_POINT('Ctrl Pts',(29.8368672985589,52.0599703843281,39.1161900945647));
#208560=CARTESIAN_POINT('Origin',(29.7268821954856,52.1234703131943,39.116));
#208561=CARTESIAN_POINT('Origin',(14.9038494342991,26.4492244485619,39.5248017080178));
#208562=CARTESIAN_POINT('Origin',(30.1555713378344,52.8659816883956,39.5248017080178));
#208563=CARTESIAN_POINT('Origin',(14.8448439902567,26.3470240215575,39.116));
#208564=CARTESIAN_POINT('Origin',(29.9275190026064,52.471085065638,39.1160402713852));
#208565=CARTESIAN_POINT('Ctrl Pts',(30.0450834959843,52.6757649139392,39.2708017080178));
#208566=CARTESIAN_POINT('Ctrl Pts',(30.1558192616008,52.6124111049553,39.27051194648));
#208567=CARTESIAN_POINT('Ctrl Pts',(30.1005764675364,52.5167277788838,39.3343017080178));
#208568=CARTESIAN_POINT('Ctrl Pts',(30.0676891808479,52.7146817640556,39.3487519301186));
#208569=CARTESIAN_POINT('Ctrl Pts',(30.1782028480943,52.6511806140172,39.3482879463985));
#208570=CARTESIAN_POINT('Ctrl Pts',(30.1343304829269,52.5751914484995,39.4512271261632));
#208571=CARTESIAN_POINT('Ctrl Pts',(30.1105150503725,52.7884098752453,39.3978017080178));
#208572=CARTESIAN_POINT('Ctrl Pts',(30.2206596676791,52.7247179826666,39.3975673827397));
#208573=CARTESIAN_POINT('Ctrl Pts',(30.1982769148327,52.6859499175231,39.5248015355194));
#208574=CARTESIAN_POINT('Ctrl Pts',(30.1555713378344,52.8659816883956,39.3978017080178));
#208575=CARTESIAN_POINT('Ctrl Pts',(30.265556564115,52.8024816883956,39.3978017080178));
#208576=CARTESIAN_POINT('Ctrl Pts',(30.265556564115,52.8024816883956,39.5248017080178));
#208577=CARTESIAN_POINT('Origin',(29.9905912412558,52.5802277788838,39.3343017080178));
#208578=CARTESIAN_POINT('Origin',(29.9499161075313,52.5097763812713,39.1934008533552));
#208579=CARTESIAN_POINT('Origin',(36.361028539783,49.5064990290875,39.1925554495082));
#208580=CARTESIAN_POINT('Origin',(36.3870656659288,49.5422481179703,39.1160373285292));
#208581=CARTESIAN_POINT('Origin',(36.3129251734949,49.4402904249162,39.3343017080178));
#208582=CARTESIAN_POINT('Ctrl Pts',(36.2478178023256,49.3516463037381,39.2708017080178));
#208583=CARTESIAN_POINT('Ctrl Pts',(36.1458216659131,49.4263574835547,39.2710850691866));
#208584=CARTESIAN_POINT('Ctrl Pts',(36.2101800152093,49.5149391519573,39.3343017080178));
#208585=CARTESIAN_POINT('Ctrl Pts',(36.2214577843992,49.3151677697917,39.3487519293518));
#208586=CARTESIAN_POINT('Ctrl Pts',(36.1192316557432,49.389759474291,39.3492068662919));
#208587=CARTESIAN_POINT('Ctrl Pts',(36.1704998050828,49.4603240281388,39.4512271248743));
#208588=CARTESIAN_POINT('Ctrl Pts',(36.1715192752727,49.246058992205,39.3978017080178));
#208589=CARTESIAN_POINT('Ctrl Pts',(36.068913312703,49.3205022166658,39.3980347781187));
#208590=CARTESIAN_POINT('Ctrl Pts',(36.0953262843475,49.3568565533005,39.524801535519));
#208591=CARTESIAN_POINT('Ctrl Pts',(36.1189794796889,49.1733470784083,39.3978017080178));
#208592=CARTESIAN_POINT('Ctrl Pts',(36.0162343214032,49.2479958054495,39.3978017080178));
#208593=CARTESIAN_POINT('Ctrl Pts',(36.0162343214032,49.2479958054495,39.5248017080178));
#208594=CARTESIAN_POINT('Origin',(36.1189794796889,49.1733470784083,39.5248017080178));
#208595=CARTESIAN_POINT('Origin',(0.256862895714049,-0.186621817602863,
39.116));
#208596=CARTESIAN_POINT('Origin',(36.6229335645815,49.8669803696022,39.116));
#208597=CARTESIAN_POINT('Origin',(0.256862895714049,-0.186621817602863,
39.5248017080178));
#208598=CARTESIAN_POINT('Origin',(36.0301015792682,49.0510171431399,39.5248017080178));
#208599=CARTESIAN_POINT('Ctrl Pts',(36.9399086546492,50.3023253561991,39.2875012672119));
#208600=CARTESIAN_POINT('Ctrl Pts',(36.8368401467444,50.3777877177482,39.287208709576));
#208601=CARTESIAN_POINT('Ctrl Pts',(36.7733199672427,50.2900345588335,39.3549016990123));
#208602=CARTESIAN_POINT('Ctrl Pts',(36.8722300970248,50.2093718139441,39.1034939173931));
#208603=CARTESIAN_POINT('Ctrl Pts',(36.7691625978877,50.2846371204152,39.1031692336321));
#208604=CARTESIAN_POINT('Ctrl Pts',(36.7192723137716,50.2156443459724,39.2077507202293));
#208605=CARTESIAN_POINT('Ctrl Pts',(36.7506474475478,50.0423845927708,38.989));
#208606=CARTESIAN_POINT('Ctrl Pts',(36.6476776482611,50.1174266236732,38.9887769311182));
#208607=CARTESIAN_POINT('Ctrl Pts',(36.622177901771,50.0820053531135,39.1161898712916));
#208608=CARTESIAN_POINT('Ctrl Pts',(36.6229335645815,49.8669803696022,38.989));
#208609=CARTESIAN_POINT('Ctrl Pts',(36.5200349097939,49.9417406183799,38.989));
#208610=CARTESIAN_POINT('Ctrl Pts',(36.5201885207831,49.9416290134635,39.1161895903855));
#208611=CARTESIAN_POINT('Origin',(36.876159719196,50.215516270604,39.3548010137695));
#208612=CARTESIAN_POINT('Ctrl Pts',(36.0301015792682,49.0510171431399,39.3978017080178));
#208613=CARTESIAN_POINT('Ctrl Pts',(35.9273564209826,49.1256658701811,39.3978017080178));
#208614=CARTESIAN_POINT('Ctrl Pts',(35.9273564209826,49.1256658701811,39.5248017080178));
#208615=CARTESIAN_POINT('Ctrl Pts',(35.9773846774565,48.9780591316055,39.3978017080178));
#208616=CARTESIAN_POINT('Ctrl Pts',(35.8743986903,49.0527758071216,39.3975666025035));
#208617=CARTESIAN_POINT('Ctrl Pts',(35.8479971380625,49.0164371879483,39.5248015517196));
#208618=CARTESIAN_POINT('Ctrl Pts',(35.9275383438686,48.9090707128226,39.3484894016716));
#208619=CARTESIAN_POINT('Ctrl Pts',(35.8245773199098,48.9842025736633,39.348025900004));
#208620=CARTESIAN_POINT('Ctrl Pts',(35.772957278024,48.9131536812767,39.4508333188941));
#208621=CARTESIAN_POINT('Ctrl Pts',(35.901269362891,48.8727133447939,39.2708017080178));
#208622=CARTESIAN_POINT('Ctrl Pts',(35.7983524848941,48.9481071848793,39.27051194648));
#208623=CARTESIAN_POINT('Ctrl Pts',(35.7334106856012,48.8587224664496,39.3343017080178));
#208624=CARTESIAN_POINT('Origin',(35.8361558438868,48.7840737394085,39.3343017080178));
#208625=CARTESIAN_POINT('Origin',(36.9808731396208,50.3596419293477,39.6398955068193));
#208626=CARTESIAN_POINT('Origin',(37.0855865599608,50.5037675878941,39.92499));
#208627=CARTESIAN_POINT('Origin',(35.7883393560629,48.7182599900743,39.1934008539946));
#208628=CARTESIAN_POINT('Origin',(35.7621028045855,48.682062041486,39.1160402713846));
#208629=CARTESIAN_POINT('Ctrl Pts',(37.0158684358566,50.9219998155896,40.1599502534424));
#208630=CARTESIAN_POINT('Ctrl Pts',(36.9939338721439,50.8918248690996,40.10025));
#208631=CARTESIAN_POINT('Ctrl Pts',(36.9525415975218,50.8348823336482,40.10025));
#208632=CARTESIAN_POINT('Ctrl Pts',(37.087142649025,50.8701895025857,40.1599500538468));
#208633=CARTESIAN_POINT('Ctrl Pts',(37.0458491715926,50.8540829678248,40.100244835349));
#208634=CARTESIAN_POINT('Ctrl Pts',(36.993792576411,50.8048852215546,40.10025));
#208635=CARTESIAN_POINT('Ctrl Pts',(37.1382015956606,50.802146755573,40.120244200104));
#208636=CARTESIAN_POINT('Ctrl Pts',(37.0800635522221,50.8006171556817,40.0633873868018));
#208637=CARTESIAN_POINT('Ctrl Pts',(37.0171501059297,50.7569692080812,40.0772271723538));
#208638=CARTESIAN_POINT('Ctrl Pts',(37.1817767082791,50.6806663304939,40.0045995998161));
#208639=CARTESIAN_POINT('Ctrl Pts',(37.0956112176475,50.7142182018855,39.9663485808314));
#208640=CARTESIAN_POINT('Ctrl Pts',(37.0243843935853,50.6618927960195,40.0101727202465));
#208641=CARTESIAN_POINT('Ctrl Pts',(37.1760624637757,50.6273693057707,39.9304654349859));
#208642=CARTESIAN_POINT('Ctrl Pts',(37.0763301845697,50.6810088489719,39.9051900162942));
#208643=CARTESIAN_POINT('Ctrl Pts',(37.009570236509,50.6152053999557,39.9671857458172));
#208644=CARTESIAN_POINT('Ctrl Pts',(37.1493329797266,50.590578520848,39.8576902534424));
#208645=CARTESIAN_POINT('Ctrl Pts',(37.0464195108259,50.6659240749079,39.8573998014387));
#208646=CARTESIAN_POINT('Ctrl Pts',(36.9828414016752,50.5784163149353,39.92499));
#208647=CARTESIAN_POINT('Origin',(36.9525415975218,50.8348823336482,40.22725));
#208648=CARTESIAN_POINT('Origin',(0.256862895714049,-0.186621817602863,
39.116));
#208649=CARTESIAN_POINT('Origin',(35.5261472678871,48.3573835402115,39.116));
#208650=CARTESIAN_POINT('Origin',(5.56775724677591E-15,5.56148610155125E-15,
40.22725));
#208651=CARTESIAN_POINT('Origin',(36.9278827595332,50.8527980281381,40.22725));
#208652=CARTESIAN_POINT('Ctrl Pts',(35.5261472678871,48.3573835402115,38.989));
#208653=CARTESIAN_POINT('Ctrl Pts',(35.4232481927143,48.432144094417,38.989));
#208654=CARTESIAN_POINT('Ctrl Pts',(35.4234022247162,48.432032183617,39.1161901092328));
#208655=CARTESIAN_POINT('Ctrl Pts',(35.3984257650696,48.1819806163539,38.989));
#208656=CARTESIAN_POINT('Ctrl Pts',(35.2958250128997,48.2567602586438,38.9892298989718));
#208657=CARTESIAN_POINT('Ctrl Pts',(35.3214110399842,48.2916533613418,39.116190049319));
#208658=CARTESIAN_POINT('Ctrl Pts',(35.2768349808764,48.0150011530603,39.1034966344368));
#208659=CARTESIAN_POINT('Ctrl Pts',(35.1744900671637,48.0897561847345,39.1038314102594));
#208660=CARTESIAN_POINT('Ctrl Pts',(35.2243173504702,48.1580153629237,39.2077528789609));
#208661=CARTESIAN_POINT('Ctrl Pts',(35.2091516650533,47.9220530736683,39.2875012672119));
#208662=CARTESIAN_POINT('Ctrl Pts',(35.1070032653412,47.9968681042462,39.2878045257868));
#208663=CARTESIAN_POINT('Ctrl Pts',(35.1702703594602,48.0836260618768,39.3549015295903));
#208664=CARTESIAN_POINT('Origin',(35.272920853982,48.0088472823268,39.3548010137695));
#208665=CARTESIAN_POINT('Ctrl Pts',(36.634724144966,50.9644637245889,39.8576902534424));
#208666=CARTESIAN_POINT('Ctrl Pts',(36.738184035969,50.8898702560314,39.8573998014387));
#208667=CARTESIAN_POINT('Ctrl Pts',(36.6746059268184,50.8023624960587,39.92499));
#208668=CARTESIAN_POINT('Ctrl Pts',(36.6614665482798,51.0012706547895,39.9304984902494));
#208669=CARTESIAN_POINT('Ctrl Pts',(36.7432905102111,50.9229972443178,39.9052171569795));
#208670=CARTESIAN_POINT('Ctrl Pts',(36.7013469409089,50.839168344388,39.96720497266));
#208671=CARTESIAN_POINT('Ctrl Pts',(36.710288459717,51.0230245369432,40.0043437678658));
#208672=CARTESIAN_POINT('Ctrl Pts',(36.7689049964553,50.951440922535,39.966162857764));
#208673=CARTESIAN_POINT('Ctrl Pts',(36.7410683485316,50.8675358949423,40.0100243556234));
#208674=CARTESIAN_POINT('Ctrl Pts',(36.8383381382869,51.0194219249359,40.1194874821991));
#208675=CARTESIAN_POINT('Ctrl Pts',(36.8551762168624,50.9635175930189,40.0627551483143));
#208676=CARTESIAN_POINT('Ctrl Pts',(36.8330984946713,50.8901021525737,40.0767884282378));
#208677=CARTESIAN_POINT('Ctrl Pts',(36.9196318328649,50.9918932610482,40.1599502015385));
#208678=CARTESIAN_POINT('Ctrl Pts',(36.9171104726343,50.9476171190675,40.1002449453875));
#208679=CARTESIAN_POINT('Ctrl Pts',(36.8864699989244,50.8828596657509,40.10025));
#208680=CARTESIAN_POINT('Ctrl Pts',(36.9911673391713,50.9399462128198,40.1599502534424));
#208681=CARTESIAN_POINT('Ctrl Pts',(36.9692474126346,50.909760631799,40.10025));
#208682=CARTESIAN_POINT('Ctrl Pts',(36.9278827595333,50.8527980281381,40.10025));
#208683=CARTESIAN_POINT('Origin',(36.5718607685328,50.8770112230998,39.92499));
#208684=CARTESIAN_POINT('Origin',(35.1682072895768,47.8647214254969,39.6398955069337));
#208685=CARTESIAN_POINT('Origin',(35.0634937251227,47.7205955685087,39.92499));
#208686=CARTESIAN_POINT('Origin',(36.4671473482256,50.7328855645163,39.6398955068261));
#208687=CARTESIAN_POINT('Origin',(36.3624339277679,50.5887599058097,39.3548010137695));
#208688=CARTESIAN_POINT('Ctrl Pts',(34.9997217530266,47.6338034047596,39.8576902534424));
#208689=CARTESIAN_POINT('Ctrl Pts',(34.8977303031707,47.70850709678,39.8579948730703));
#208690=CARTESIAN_POINT('Ctrl Pts',(34.9607485668371,47.7952442955498,39.92499));
#208691=CARTESIAN_POINT('Ctrl Pts',(34.9730146904946,47.5970451916066,39.930402071123));
#208692=CARTESIAN_POINT('Ctrl Pts',(34.8923835282618,47.6752966590737,39.9058915297377));
#208693=CARTESIAN_POINT('Ctrl Pts',(34.9340408279394,47.7584842465943,39.9671523786032));
#208694=CARTESIAN_POINT('Ctrl Pts',(34.9244461536129,47.5754322771532,40.0043257306693));
#208695=CARTESIAN_POINT('Ctrl Pts',(34.8665972787031,47.6469756149917,39.9667894847838));
#208696=CARTESIAN_POINT('Ctrl Pts',(34.894489194863,47.7303228514092,40.01001389752));
#208697=CARTESIAN_POINT('Ctrl Pts',(34.7970725085263,47.5794993790981,40.1195533054857));
#208698=CARTESIAN_POINT('Ctrl Pts',(34.7804938560725,47.6353197637775,40.0630813209234));
#208699=CARTESIAN_POINT('Ctrl Pts',(34.8028668197837,47.7084160893868,40.076826594242));
#208700=CARTESIAN_POINT('Ctrl Pts',(34.716261746735,47.607308993689,40.1599502027505));
#208701=CARTESIAN_POINT('Ctrl Pts',(34.7189078610147,47.6515013114269,40.1002552791544));
#208702=CARTESIAN_POINT('Ctrl Pts',(34.7497660430541,47.7160937685343,40.10025));
#208703=CARTESIAN_POINT('Ctrl Pts',(34.6451144164191,47.6590285860932,40.1599502534424));
#208704=CARTESIAN_POINT('Ctrl Pts',(34.6670494534023,47.6892031885509,40.10025));
#208705=CARTESIAN_POINT('Ctrl Pts',(34.7084426211237,47.746145074786,40.10025));
#208706=CARTESIAN_POINT('Origin',(34.7084426211237,47.7461450747861,40.22725));
#208707=CARTESIAN_POINT('Ctrl Pts',(36.1092077731534,50.2402240048079,38.989));
#208708=CARTESIAN_POINT('Ctrl Pts',(36.2121064368061,50.1654637495893,38.989));
#208709=CARTESIAN_POINT('Ctrl Pts',(36.2119528169387,50.1655753609561,39.1161896013269));
#208710=CARTESIAN_POINT('Ctrl Pts',(36.2365633238594,50.4158927445001,38.989));
#208711=CARTESIAN_POINT('Ctrl Pts',(36.3397519704551,50.3411519064778,38.9887769275466));
#208712=CARTESIAN_POINT('Ctrl Pts',(36.3139437822104,50.3059538820295,39.116189882185));
#208713=CARTESIAN_POINT('Ctrl Pts',(36.3578055460604,50.5831252836579,39.1034967087243));
#208714=CARTESIAN_POINT('Ctrl Pts',(36.4612367259619,50.5083605190678,39.1031720232695));
#208715=CARTESIAN_POINT('Ctrl Pts',(36.411037424715,50.439591816563,39.2077529614998));
#208716=CARTESIAN_POINT('Ctrl Pts',(36.4252947698684,50.6762142289944,39.2875012672119));
#208717=CARTESIAN_POINT('Ctrl Pts',(36.5289136700287,50.6015093986311,39.2872087095508));
#208718=CARTESIAN_POINT('Ctrl Pts',(36.4650842569437,50.5139808995218,39.3549017048229));
#208719=CARTESIAN_POINT('Origin',(36.1092077731534,50.2402240048079,39.116));
#208720=CARTESIAN_POINT('Origin',(5.69915478234096E-15,5.30016260398707E-15,
40.22725));
#208721=CARTESIAN_POINT('Origin',(34.6837837831351,47.7640607692759,40.22725));
#208722=CARTESIAN_POINT('Origin',(21.2404668433939,29.7751578089175,39.116));
#208723=CARTESIAN_POINT('Origin',(35.873256238299,49.9155525184323,39.1160373285273));
#208724=CARTESIAN_POINT('Ctrl Pts',(34.620500570364,47.67691159203,40.1599502534424));
#208725=CARTESIAN_POINT('Ctrl Pts',(34.642420023458,47.707097516846,40.10025));
#208726=CARTESIAN_POINT('Ctrl Pts',(34.6837837831352,47.7640607692759,40.10025));
#208727=CARTESIAN_POINT('Ctrl Pts',(34.5495693076632,47.7284183483598,40.1599500566048));
#208728=CARTESIAN_POINT('Ctrl Pts',(34.5907418558588,47.7446195594498,40.1002551305351));
#208729=CARTESIAN_POINT('Ctrl Pts',(34.6425747206411,47.7939730310143,40.10025));
#208730=CARTESIAN_POINT('Ctrl Pts',(34.4983910654774,47.7959261043552,40.1203070619042));
#208731=CARTESIAN_POINT('Ctrl Pts',(34.5563698228282,47.797671475652,40.0637098684499));
#208732=CARTESIAN_POINT('Ctrl Pts',(34.6188891978606,47.8415056181567,40.0772636213362));
#208733=CARTESIAN_POINT('Ctrl Pts',(34.4545839152295,47.9165880269723,40.0046102245806));
#208734=CARTESIAN_POINT('Ctrl Pts',(34.5404685123901,47.8837591046483,39.9670001894012));
#208735=CARTESIAN_POINT('Ctrl Pts',(34.6111463389769,47.9359643384878,40.0101788811209));
#208736=CARTESIAN_POINT('Ctrl Pts',(34.4602354682508,47.9696250311912,39.9303710930183));
#208737=CARTESIAN_POINT('Ctrl Pts',(34.5595777906775,47.9171136764607,39.905866357411));
#208738=CARTESIAN_POINT('Ctrl Pts',(34.625816696831,47.9824460410481,39.9671344706369));
#208739=CARTESIAN_POINT('Ctrl Pts',(34.4869303039402,48.0063682005183,39.8576902534424));
#208740=CARTESIAN_POINT('Ctrl Pts',(34.5894948283139,47.9324532779034,39.8579948730703));
#208741=CARTESIAN_POINT('Ctrl Pts',(34.6525130919802,48.0191904766733,39.92499));
#208742=CARTESIAN_POINT('Origin',(34.5497679336946,48.0938392037144,39.92499));
#208743=CARTESIAN_POINT('Origin',(35.8473027479618,49.8797426632445,39.192555448885));
#208744=CARTESIAN_POINT('Origin',(35.7991993820668,49.8135340601219,39.3343017080178));
#208745=CARTESIAN_POINT('Origin',(34.6544814981813,48.2379650606536,39.6398955069209));
#208746=CARTESIAN_POINT('Origin',(34.759195062554,48.3820909175325,39.3548010137695));
#208747=CARTESIAN_POINT('Ctrl Pts',(35.6052536882608,49.5465907136141,39.3978017080178));
#208748=CARTESIAN_POINT('Ctrl Pts',(35.7079988465464,49.4719419865729,39.3978017080178));
#208749=CARTESIAN_POINT('Ctrl Pts',(35.7079988465464,49.4719419865729,39.5248017080178));
#208750=CARTESIAN_POINT('Ctrl Pts',(35.6583499840587,49.6192730640949,39.3978017080178));
#208751=CARTESIAN_POINT('Ctrl Pts',(35.7608559931214,49.5446936074884,39.3980355775201));
#208752=CARTESIAN_POINT('Ctrl Pts',(35.7873581223574,49.5811706590209,39.5248015517192));
#208753=CARTESIAN_POINT('Ctrl Pts',(35.7085550527699,49.6880007749208,39.3484893995498));
#208754=CARTESIAN_POINT('Ctrl Pts',(35.8110857017869,49.6138288703721,39.3489438303412));
#208755=CARTESIAN_POINT('Ctrl Pts',(35.8623979633517,49.6844541394804,39.4508333155595));
#208756=CARTESIAN_POINT('Ctrl Pts',(35.7350130971395,49.7242207306171,39.2708017080178));
#208757=CARTESIAN_POINT('Ctrl Pts',(35.8375861910562,49.6503036646781,39.2710850691866));
#208758=CARTESIAN_POINT('Ctrl Pts',(35.9019445403524,49.7388853330807,39.3343017080178));
#208759=CARTESIAN_POINT('Origin',(35.6052536882608,49.5465907136141,39.5248017080178));
#208760=CARTESIAN_POINT('Ctrl Pts',(34.6963546279291,48.2946219293742,39.2875012672119));
#208761=CARTESIAN_POINT('Ctrl Pts',(34.7990735298991,48.2205921526132,39.2878045257519));
#208762=CARTESIAN_POINT('Ctrl Pts',(34.8620346481364,48.3075723994624,39.3549015218347));
#208763=CARTESIAN_POINT('Ctrl Pts',(34.7638392294029,48.387716530749,39.1034938540228));
#208764=CARTESIAN_POINT('Ctrl Pts',(34.8665617960674,48.3134813154523,39.1038286278818));
#208765=CARTESIAN_POINT('Ctrl Pts',(34.916082457139,48.3819628268498,39.2077506434048));
#208766=CARTESIAN_POINT('Ctrl Pts',(34.885073474582,48.5549570506171,38.989));
#208767=CARTESIAN_POINT('Ctrl Pts',(34.9878985031391,48.4804861171447,38.9892298954611));
#208768=CARTESIAN_POINT('Ctrl Pts',(35.013176915674,48.515601884576,39.1161900347271));
#208769=CARTESIAN_POINT('Ctrl Pts',(35.012421476459,48.7306271754172,38.989));
#208770=CARTESIAN_POINT('Ctrl Pts',(35.1153205397472,48.6558666298465,38.989));
#208771=CARTESIAN_POINT('Ctrl Pts',(35.1151665196478,48.6559785319989,39.1161900945645));
#208772=CARTESIAN_POINT('Origin',(35.012421476459,48.7306271754172,39.116));
#208773=CARTESIAN_POINT('Origin',(20.7197400704249,29.0584388930977,39.5248017080178));
#208774=CARTESIAN_POINT('Origin',(35.5163757878401,49.4242607783457,39.5248017080178));
#208775=CARTESIAN_POINT('Origin',(20.6381965522797,28.9462038689911,39.116));
#208776=CARTESIAN_POINT('Origin',(35.2482948100405,49.0553654007522,39.1160402713845));
#208777=CARTESIAN_POINT('Ctrl Pts',(35.3866101428265,49.2466351556009,39.2708017080178));
#208778=CARTESIAN_POINT('Ctrl Pts',(35.4901170100373,49.1720533660027,39.27051194648));
#208779=CARTESIAN_POINT('Ctrl Pts',(35.4251752107443,49.0826686475731,39.3343017080178));
#208780=CARTESIAN_POINT('Ctrl Pts',(35.4131599099226,49.2829758776393,39.3487519301185));
#208781=CARTESIAN_POINT('Ctrl Pts',(35.5164304941056,49.2082707697385,39.3482879463972));
#208782=CARTESIAN_POINT('Ctrl Pts',(35.4648554356505,49.1372837917341,39.4512271261624));
#208783=CARTESIAN_POINT('Ctrl Pts',(35.4634578610134,49.3518235761936,39.3978017080178));
#208784=CARTESIAN_POINT('Ctrl Pts',(35.5663414789288,49.2769673468819,39.3975673827415));
#208785=CARTESIAN_POINT('Ctrl Pts',(35.5400289748693,49.2407512920126,39.5248015355194));
#208786=CARTESIAN_POINT('Ctrl Pts',(35.5163757878401,49.4242607783457,39.3978017080178));
#208787=CARTESIAN_POINT('Ctrl Pts',(35.6191209461258,49.3496120513045,39.3978017080178));
#208788=CARTESIAN_POINT('Ctrl Pts',(35.6191209461258,49.3496120513045,39.5248017080178));
#208789=CARTESIAN_POINT('Origin',(35.3224300524587,49.1573173746142,39.3343017080178));
#208790=CARTESIAN_POINT('Origin',(35.274613565047,49.0915036263512,39.1934008533544));
#208791=CARTESIAN_POINT('Origin',(41.3366772861977,45.4345348113602,39.1925554495083));
#208792=CARTESIAN_POINT('Origin',(41.366308575564,45.4673664422105,39.1160373285273));
#208793=CARTESIAN_POINT('Origin',(41.2819167515334,45.3737170758068,39.3343017080178));
#208794=CARTESIAN_POINT('Ctrl Pts',(41.2079002115913,45.2923641298552,39.2708017080178));
#208795=CARTESIAN_POINT('Ctrl Pts',(41.1142722655012,45.3773275334101,39.2710850691866));
#208796=CARTESIAN_POINT('Ctrl Pts',(41.1875373586978,45.4586966628144,39.3343017080178));
#208797=CARTESIAN_POINT('Ctrl Pts',(41.1778715515039,45.2588408013016,39.3487519293518));
#208798=CARTESIAN_POINT('Ctrl Pts',(41.0840023845219,45.343709424771,39.349206866291));
#208799=CARTESIAN_POINT('Ctrl Pts',(41.1423656859486,45.4085284377433,39.4512271248737));
#208800=CARTESIAN_POINT('Ctrl Pts',(41.1209827764384,45.1953306044442,39.3978017080178));
#208801=CARTESIAN_POINT('Ctrl Pts',(41.026720335924,45.2800912647201,39.3980347781197));
#208802=CARTESIAN_POINT('Ctrl Pts',(41.0567886774853,45.3134855411624,39.524801535519));
#208803=CARTESIAN_POINT('Ctrl Pts',(41.0611303347409,45.1285089182128,39.3978017080178));
#208804=CARTESIAN_POINT('Ctrl Pts',(40.9667509419053,45.2134885052204,39.3978017080178));
#208805=CARTESIAN_POINT('Ctrl Pts',(40.9667509419053,45.2134885052204,39.5248017080178));
#208806=CARTESIAN_POINT('Origin',(41.0611303347409,45.1285089182128,39.5248017080178));
#208807=CARTESIAN_POINT('Origin',(0.235948482089076,-0.21244896751894,39.116));
#208808=CARTESIAN_POINT('Origin',(41.6348281284267,45.7656648676101,39.116));
#208809=CARTESIAN_POINT('Origin',(0.235948482089076,-0.21244896751894,39.5248017080178));
#208810=CARTESIAN_POINT('Origin',(40.959952356613,45.0161393894788,39.5248017080178));
#208811=CARTESIAN_POINT('Ctrl Pts',(41.9955727382256,46.1654920697607,39.2875012672119));
#208812=CARTESIAN_POINT('Ctrl Pts',(41.9009568150788,46.2513146333399,39.287208709576));
#208813=CARTESIAN_POINT('Ctrl Pts',(41.8286119029184,46.1706818621616,39.3549016990121));
#208814=CARTESIAN_POINT('Ctrl Pts',(41.9185486398962,46.0801220723588,39.1034939173931));
#208815=CARTESIAN_POINT('Ctrl Pts',(41.8239131221214,46.165748554905,39.1031692336345));
#208816=CARTESIAN_POINT('Ctrl Pts',(41.7670844335144,46.1023486848294,39.2077507202296));
#208817=CARTESIAN_POINT('Ctrl Pts',(41.7801771152788,45.926758472166,38.989));
#208818=CARTESIAN_POINT('Ctrl Pts',(41.6856154234981,46.0121526898551,38.9887769311158));
#208819=CARTESIAN_POINT('Ctrl Pts',(41.6565528363077,45.9795909100367,39.1161898712914));
#208820=CARTESIAN_POINT('Ctrl Pts',(41.6348281284267,45.7656648676101,38.989));
#208821=CARTESIAN_POINT('Ctrl Pts',(41.5403077371549,45.8507714101799,38.989));
#208822=CARTESIAN_POINT('Ctrl Pts',(41.5404488407565,45.8506443599264,39.1161895903853));
#208823=CARTESIAN_POINT('Origin',(41.9230990057961,46.0858221116773,39.3548010137695));
#208824=CARTESIAN_POINT('Ctrl Pts',(40.959952356613,45.0161393894788,39.3978017080178));
#208825=CARTESIAN_POINT('Ctrl Pts',(40.8655729637774,45.1011189764864,39.3978017080178));
#208826=CARTESIAN_POINT('Ctrl Pts',(40.8655729637774,45.1011189764864,39.5248017080178));
#208827=CARTESIAN_POINT('Ctrl Pts',(40.899898054678,44.9490914662986,39.3978017080178));
#208828=CARTESIAN_POINT('Ctrl Pts',(40.8052862548051,45.0341638030236,39.3975666025031));
#208829=CARTESIAN_POINT('Ctrl Pts',(40.7752309130129,45.000783964292,39.5248015517196));
#208830=CARTESIAN_POINT('Ctrl Pts',(40.8431135311188,44.8856913339448,39.3484894016716));
#208831=CARTESIAN_POINT('Ctrl Pts',(40.7485699563816,44.9711739722015,39.3480259000038));
#208832=CARTESIAN_POINT('Ctrl Pts',(40.6898060629487,44.9059100567333,39.4508333188935));
#208833=CARTESIAN_POINT('Ctrl Pts',(40.8131880745612,44.8522789915937,39.2708017080178));
#208834=CARTESIAN_POINT('Ctrl Pts',(40.7187157882343,44.9380175594357,39.27051194648));
#208835=CARTESIAN_POINT('Ctrl Pts',(40.6447864996558,44.8559107663281,39.3343017080178));
#208836=CARTESIAN_POINT('Origin',(40.7391658924914,44.7709311793205,39.3343017080178));
#208837=CARTESIAN_POINT('Origin',(42.0423040287729,46.218212702065,39.639895506818));
#208838=CARTESIAN_POINT('Origin',(42.1615090516458,46.3506032922589,39.92499));
#208839=CARTESIAN_POINT('Origin',(40.6847319383107,44.7104761485831,39.1934008539946));
#208840=CARTESIAN_POINT('Origin',(40.6548553974685,44.6772189625516,39.1160402713843));
#208841=CARTESIAN_POINT('Ctrl Pts',(42.1358900227701,46.7738319284252,40.1599502534424));
#208842=CARTESIAN_POINT('Ctrl Pts',(42.1109214781067,46.7461150696867,40.10025));
#208843=CARTESIAN_POINT('Ctrl Pts',(42.0638038389706,46.6938111422599,40.10025));
#208844=CARTESIAN_POINT('Ctrl Pts',(42.2013581359415,46.7148552537629,40.1599500538455));
#208845=CARTESIAN_POINT('Ctrl Pts',(42.1586072771699,46.7031532960216,40.100244835349));
#208846=CARTESIAN_POINT('Ctrl Pts',(42.1016932886506,46.6596664560519,40.10025));
#208847=CARTESIAN_POINT('Ctrl Pts',(42.2450249725429,46.6418481388115,40.1202442001042));
#208848=CARTESIAN_POINT('Ctrl Pts',(42.187045528663,46.6464039985659,40.0633873868017));
#208849=CARTESIAN_POINT('Ctrl Pts',(42.1199142759252,46.6095714048492,40.0772271723541));
#208850=CARTESIAN_POINT('Ctrl Pts',(42.2756632139854,46.5164783566517,40.0045995998159));
#208851=CARTESIAN_POINT('Ctrl Pts',(42.1934768724838,46.5588531737043,39.9663485808314));
#208852=CARTESIAN_POINT('Ctrl Pts',(42.1171707421508,46.514259642349,40.0101727202462));
#208853=CARTESIAN_POINT('Ctrl Pts',(42.2644092166203,46.4640705998035,39.9304654349861));
#208854=CARTESIAN_POINT('Ctrl Pts',(42.1708301402944,46.5278411618565,39.9051900162951));
#208855=CARTESIAN_POINT('Ctrl Pts',(42.0975575768118,46.4693765057994,39.967185745818));
#208856=CARTESIAN_POINT('Ctrl Pts',(42.2339804752707,46.430275350542,39.8576902534424));
#208857=CARTESIAN_POINT('Ctrl Pts',(42.1395065321005,46.515965540527,39.8573998014387));
#208858=CARTESIAN_POINT('Ctrl Pts',(42.0671296588101,46.4355828792665,39.92499));
#208859=CARTESIAN_POINT('Origin',(42.0638038389706,46.6938111422599,40.22725));
#208860=CARTESIAN_POINT('Origin',(0.235948482089076,-0.21244896751894,39.116));
#208861=CARTESIAN_POINT('Origin',(40.3862543050944,44.3789831537291,39.116));
#208862=CARTESIAN_POINT('Origin',(5.55434424446678E-15,5.57234773665839E-15,
40.22725));
#208863=CARTESIAN_POINT('Origin',(42.0411527846901,46.7142062431418,40.22725));
#208864=CARTESIAN_POINT('Ctrl Pts',(40.3862543050944,44.3789831537291,38.989));
#208865=CARTESIAN_POINT('Ctrl Pts',(40.2917335276659,44.4640900439958,38.989));
#208866=CARTESIAN_POINT('Ctrl Pts',(40.2918750180005,44.4639626455264,39.1161901092328));
#208867=CARTESIAN_POINT('Ctrl Pts',(40.240897875948,44.2178916378582,38.989));
#208868=CARTESIAN_POINT('Ctrl Pts',(40.1466757825285,44.3029863283993,38.9892298989778));
#208869=CARTESIAN_POINT('Ctrl Pts',(40.1757689690828,44.3350138149353,39.1161900493208));
#208870=CARTESIAN_POINT('Ctrl Pts',(40.1025190720977,44.0645366033549,39.1034966344368));
#208871=CARTESIAN_POINT('Ctrl Pts',(40.0085488431135,44.1495800756922,39.1038314102538));
#208872=CARTESIAN_POINT('Ctrl Pts',(40.0652381943489,44.2122569536116,39.2077528789592));
#208873=CARTESIAN_POINT('Ctrl Pts',(40.0254908126594,43.9791725362578,39.2875012672119));
#208874=CARTESIAN_POINT('Ctrl Pts',(39.9317222927445,44.0642551375174,39.2878045257868));
#208875=CARTESIAN_POINT('Ctrl Pts',(40.0037114790895,44.1439246138547,39.3549015295903));
#208876=CARTESIAN_POINT('Origin',(40.0979831325504,44.0588255818373,39.3548010137695));
#208877=CARTESIAN_POINT('Ctrl Pts',(41.7612723673368,46.855903642698,39.8576902534424));
#208878=CARTESIAN_POINT('Ctrl Pts',(41.8563683535936,46.7709043015497,39.8573998014387));
#208879=CARTESIAN_POINT('Ctrl Pts',(41.7839914803032,46.6905216402892,39.92499));
#208880=CARTESIAN_POINT('Ctrl Pts',(41.7917156448194,46.8897135983604,39.9304984902491));
#208881=CARTESIAN_POINT('Ctrl Pts',(41.8649095672154,46.8033160448216,39.90521715698));
#208882=CARTESIAN_POINT('Ctrl Pts',(41.8144332630849,46.7243306652203,39.9672049726612));
#208883=CARTESIAN_POINT('Ctrl Pts',(41.8425440045886,46.9062450310961,40.0043437678661));
#208884=CARTESIAN_POINT('Ctrl Pts',(41.8933569085963,46.8289264627101,39.9661628577639));
#208885=CARTESIAN_POINT('Ctrl Pts',(41.8569022891477,46.7483907976678,40.0100243556236));
#208886=CARTESIAN_POINT('Ctrl Pts',(41.9695156381237,46.8892773184516,40.1194874821988));
#208887=CARTESIAN_POINT('Ctrl Pts',(41.9804178820376,46.8319191778363,40.0627551483143));
#208888=CARTESIAN_POINT('Ctrl Pts',(41.9507871007491,46.7612136652286,40.0767884282376));
#208889=CARTESIAN_POINT('Ctrl Pts',(42.0474864684053,46.8534019544971,40.1599502015382));
#208890=CARTESIAN_POINT('Ctrl Pts',(42.0403508033701,46.8096319157661,40.1002449453869));
#208891=CARTESIAN_POINT('Ctrl Pts',(42.0031091842997,46.7484320121841,40.10025));
#208892=CARTESIAN_POINT('Ctrl Pts',(42.1132001506006,46.7942619810912,40.1599502534424));
#208893=CARTESIAN_POINT('Ctrl Pts',(42.0882450513181,46.7665330160774,40.10025));
#208894=CARTESIAN_POINT('Ctrl Pts',(42.0411527846901,46.7142062431418,40.10025));
#208895=CARTESIAN_POINT('Origin',(41.6896120874676,46.7755012272968,39.92499));
#208896=CARTESIAN_POINT('Origin',(39.9787779456735,43.9264348094991,39.6398955069315));
#208897=CARTESIAN_POINT('Origin',(39.859572758736,43.794044037014,39.92499));
#208898=CARTESIAN_POINT('Origin',(41.5704070646205,46.6431106370574,39.6398955068284));
#208899=CARTESIAN_POINT('Origin',(41.451202041618,46.5107200467152,39.3548010137695));
#208900=CARTESIAN_POINT('Ctrl Pts',(39.7870778846752,43.7143933160618,39.8576902534424));
#208901=CARTESIAN_POINT('Ctrl Pts',(39.6934538167806,43.7993487829608,39.8579948730703));
#208902=CARTESIAN_POINT('Ctrl Pts',(39.7651933659004,43.8790236240215,39.92499));
#208903=CARTESIAN_POINT('Ctrl Pts',(39.7566748466922,43.6806281164521,39.9304020711231));
#208904=CARTESIAN_POINT('Ctrl Pts',(39.6846648960476,43.7668791656722,39.9058915297384));
#208905=CARTESIAN_POINT('Ctrl Pts',(39.7347894633641,43.845256669365,39.9671523786032));
#208906=CARTESIAN_POINT('Ctrl Pts',(39.7061132086034,43.6642103943284,40.0043257306692));
#208907=CARTESIAN_POINT('Ctrl Pts',(39.6560595510438,43.7414086642726,39.9667894847835));
#208908=CARTESIAN_POINT('Ctrl Pts',(39.6925108309094,43.8213838166739,40.01001389752));
#208909=CARTESIAN_POINT('Ctrl Pts',(39.5798624575883,43.6815693876447,40.1195533054858));
#208910=CARTESIAN_POINT('Ctrl Pts',(39.5692094437574,43.7388169234802,40.0630813209236));
#208911=CARTESIAN_POINT('Ctrl Pts',(39.5991004926186,43.8091742082548,40.0768265942421));
#208912=CARTESIAN_POINT('Ctrl Pts',(39.5024012818823,43.7176736830024,40.1599502027513));
#208913=CARTESIAN_POINT('Ctrl Pts',(39.5096522555304,43.7613473163387,40.1002552791553));
#208914=CARTESIAN_POINT('Ctrl Pts',(39.5470931435016,43.8223603708611,40.10025));
#208915=CARTESIAN_POINT('Ctrl Pts',(39.4370498736014,43.7765468711718,40.1599502534424));
#208916=CARTESIAN_POINT('Ctrl Pts',(39.4620188529815,43.8042633382925,40.10025));
#208917=CARTESIAN_POINT('Ctrl Pts',(39.5091373124628,43.8565665267052,40.10025));
#208918=CARTESIAN_POINT('Origin',(39.5091373124628,43.8565665267052,40.22725));
#208919=CARTESIAN_POINT('Ctrl Pts',(41.1629311642486,46.190562802648,38.989));
#208920=CARTESIAN_POINT('Ctrl Pts',(41.2574515636637,46.1054562527461,38.989));
#208921=CARTESIAN_POINT('Ctrl Pts',(41.2573104519068,46.1055833103427,39.1161896013266));
#208922=CARTESIAN_POINT('Ctrl Pts',(41.3079514313265,46.3519569305998,38.989));
#208923=CARTESIAN_POINT('Ctrl Pts',(41.4027622547802,46.2668393800551,38.9887769275466));
#208924=CARTESIAN_POINT('Ctrl Pts',(41.3734162510838,46.2345318643235,39.1161898821848));
#208925=CARTESIAN_POINT('Ctrl Pts',(41.4460100362754,46.5056000892402,39.1034967087243));
#208926=CARTESIAN_POINT('Ctrl Pts',(41.5410595633975,46.4204333915625,39.1031720232707));
#208927=CARTESIAN_POINT('Ctrl Pts',(41.4839469723848,46.3572886670227,39.2077529615));
#208928=CARTESIAN_POINT('Ctrl Pts',(41.5228599914568,46.5911245387425,39.2875012672119));
#208929=CARTESIAN_POINT('Ctrl Pts',(41.6181024753234,46.5059978248573,39.2872087095507));
#208930=CARTESIAN_POINT('Ctrl Pts',(41.5454735069382,46.4256208064854,39.3549017048228));
#208931=CARTESIAN_POINT('Origin',(41.1629311642486,46.190562802648,39.116));
#208932=CARTESIAN_POINT('Origin',(5.70392627685665E-15,5.29629872391379E-15,
40.22725));
#208933=CARTESIAN_POINT('Origin',(39.4864862581822,43.876961627587,40.22725));
#208934=CARTESIAN_POINT('Origin',(27.6232705441551,31.1532462714325,39.116));
#208935=CARTESIAN_POINT('Origin',(40.8943347850524,45.8923335519894,39.1160373285266));
#208936=CARTESIAN_POINT('Ctrl Pts',(39.4144401478995,43.7969047596342,40.1599502534424));
#208937=CARTESIAN_POINT('Ctrl Pts',(39.4393948122693,43.824634116048,40.10025));
#208938=CARTESIAN_POINT('Ctrl Pts',(39.4864862581822,43.876961627587,40.10025));
#208939=CARTESIAN_POINT('Ctrl Pts',(39.3492813761647,43.855543692452,40.1599500566037));
#208940=CARTESIAN_POINT('Ctrl Pts',(39.3919218645339,43.8673524484232,40.1002551305372));
#208941=CARTESIAN_POINT('Ctrl Pts',(39.4486296259974,43.9110175468021,40.10025));
#208942=CARTESIAN_POINT('Ctrl Pts',(39.3054399757372,43.928031216904,40.1203070619045));
#208943=CARTESIAN_POINT('Ctrl Pts',(39.3632835603686,43.9237065964665,40.0637098684499));
#208944=CARTESIAN_POINT('Ctrl Pts',(39.4300423632773,43.9607655567554,40.0772636213364));
#208945=CARTESIAN_POINT('Ctrl Pts',(39.2744854109878,44.0526112349802,40.0046102245803));
#208946=CARTESIAN_POINT('Ctrl Pts',(39.3564679665374,44.0109847679677,39.9670001894012));
#208947=CARTESIAN_POINT('Ctrl Pts',(39.4322155454632,44.0555161714739,40.0101788811208));
#208948=CARTESIAN_POINT('Ctrl Pts',(39.2856498807583,44.1047669487872,39.9303710930185));
#208949=CARTESIAN_POINT('Ctrl Pts',(39.3789590643339,44.0421591564552,39.9058663574116));
#208950=CARTESIAN_POINT('Ctrl Pts',(39.4516641985,44.1002097724411,39.9671344706361));
#208951=CARTESIAN_POINT('Ctrl Pts',(39.3160391863695,44.1385184650371,39.8576902534424));
#208952=CARTESIAN_POINT('Ctrl Pts',(39.4103156382737,44.0542875439835,39.8579948730703));
#208953=CARTESIAN_POINT('Ctrl Pts',(39.4820551873935,44.1339623850442,39.92499));
#208954=CARTESIAN_POINT('Origin',(39.3876757945579,44.2189419720518,39.92499));
#208955=CARTESIAN_POINT('Origin',(40.8647803215182,45.8594327453949,39.1925554488842));
#208956=CARTESIAN_POINT('Origin',(40.8100197873553,45.7986150108446,39.3343017080178));
#208957=CARTESIAN_POINT('Origin',(39.5068809815259,44.351332744489,39.639895506922));
#208958=CARTESIAN_POINT('Origin',(39.6260861683723,44.4837235168752,39.3548010137695));
#208959=CARTESIAN_POINT('Ctrl Pts',(40.5892333705628,45.5534068532507,39.3978017080178));
#208960=CARTESIAN_POINT('Ctrl Pts',(40.6836127633984,45.4684272662431,39.3978017080178));
#208961=CARTESIAN_POINT('Ctrl Pts',(40.6836127633984,45.4684272662431,39.5248017080178));
#208962=CARTESIAN_POINT('Ctrl Pts',(40.649636173698,45.6201409680068,39.3978017080178));
#208963=CARTESIAN_POINT('Ctrl Pts',(40.7437849681284,45.5352552698624,39.3980355775182));
#208964=CARTESIAN_POINT('Ctrl Pts',(40.7739548060691,45.5687622694484,39.5248015517192));
#208965=CARTESIAN_POINT('Ctrl Pts',(40.7067502157887,45.6832443225589,39.3484893995498));
#208966=CARTESIAN_POINT('Ctrl Pts',(40.8009661159848,45.598761368283,39.3489438303427));
#208967=CARTESIAN_POINT('Ctrl Pts',(40.8593796344556,45.6636361529315,39.4508333155593));
#208968=CARTESIAN_POINT('Ctrl Pts',(40.7368493365303,45.7165002428302,39.2708017080178));
#208969=CARTESIAN_POINT('Ctrl Pts',(40.8311340869943,45.6322662944328,39.2710850691866));
#208970=CARTESIAN_POINT('Ctrl Pts',(40.9043991801909,45.7136354238371,39.3343017080178));
#208971=CARTESIAN_POINT('Origin',(40.5892333705628,45.5534068532507,39.5248017080178));
#208972=CARTESIAN_POINT('Ctrl Pts',(39.5544469813076,44.4033023070485,39.2875012672119));
#208973=CARTESIAN_POINT('Ctrl Pts',(39.648864959584,44.3189410241791,39.2878045257518));
#208974=CARTESIAN_POINT('Ctrl Pts',(39.7205730817656,44.3988635551999,39.3549015218346));
#208975=CARTESIAN_POINT('Ctrl Pts',(39.6312929306926,44.4888328647709,39.1034938540228));
#208976=CARTESIAN_POINT('Ctrl Pts',(39.7256930794107,44.4042668857132,39.1038286278792));
#208977=CARTESIAN_POINT('Ctrl Pts',(39.7821007282715,44.4671969296239,39.2077506434031));
#208978=CARTESIAN_POINT('Ctrl Pts',(39.7693444365344,44.6424847942243,38.989));
#208979=CARTESIAN_POINT('Ctrl Pts',(39.8638218465944,44.5576736780982,38.9892298954635));
#208980=CARTESIAN_POINT('Ctrl Pts',(39.8926323785412,44.5899547640677,39.1161900347287));
#208981=CARTESIAN_POINT('Ctrl Pts',(39.9143573409162,44.803881088767,38.989));
#208982=CARTESIAN_POINT('Ctrl Pts',(40.0088781074275,44.7187742083301,38.989));
#208983=CARTESIAN_POINT('Ctrl Pts',(40.0087366280265,44.718901596955,39.1161900945644));
#208984=CARTESIAN_POINT('Origin',(39.9143573409162,44.803881088767,39.116));
#208985=CARTESIAN_POINT('Origin',(26.948440628206,30.4037717213983,39.5248017080178));
#208986=CARTESIAN_POINT('Origin',(40.4880553924349,45.4410373245167,39.5248017080178));
#208987=CARTESIAN_POINT('Origin',(26.8427652369017,30.2864073093063,39.116));
#208988=CARTESIAN_POINT('Origin',(40.1828829233537,45.1021848870408,39.1160402713856));
#208989=CARTESIAN_POINT('Ctrl Pts',(40.3404336838198,45.2779489569768,39.2708017080178));
#208990=CARTESIAN_POINT('Ctrl Pts',(40.4355776097274,45.1929563204585,39.27051194648));
#208991=CARTESIAN_POINT('Ctrl Pts',(40.3616483211489,45.1108495273508,39.3343017080178));
#208992=CARTESIAN_POINT('Ctrl Pts',(40.3706366483424,45.3113153943829,39.3487519301185));
#208993=CARTESIAN_POINT('Ctrl Pts',(40.4655326953331,45.2262248134121,39.3482879463962));
#208994=CARTESIAN_POINT('Ctrl Pts',(40.4068200107198,45.1610177711042,39.4512271261628));
#208995=CARTESIAN_POINT('Ctrl Pts',(40.4278556061236,45.3745283705079,39.3978017080178));
#208996=CARTESIAN_POINT('Ctrl Pts',(40.5223510102012,45.2893279449763,39.3975673827434));
#208997=CARTESIAN_POINT('Ctrl Pts',(40.4923970402304,45.2560606910606,39.5248015355199));
#208998=CARTESIAN_POINT('Ctrl Pts',(40.4880553924349,45.4410373245167,39.3978017080178));
#208999=CARTESIAN_POINT('Ctrl Pts',(40.5824347852705,45.3560577375091,39.3978017080178));
#209000=CARTESIAN_POINT('Ctrl Pts',(40.5824347852705,45.3560577375091,39.5248017080178));
#209001=CARTESIAN_POINT('Origin',(40.2672689283133,45.1958291143584,39.3343017080178));
#209002=CARTESIAN_POINT('Origin',(40.2128349746544,45.1353740846425,39.1934008533546));
#209003=CARTESIAN_POINT('Origin',(45.8594327460071,40.8647803224529,39.1925554495079));
#209004=CARTESIAN_POINT('Origin',(45.8923335519876,40.894334785052,39.1160373285244));
#209005=CARTESIAN_POINT('Origin',(45.7986150108456,40.8100197873542,39.3343017080178));
#209006=CARTESIAN_POINT('Ctrl Pts',(45.7165002428312,40.7368493365292,39.2708017080178));
#209007=CARTESIAN_POINT('Ctrl Pts',(45.6322662944338,40.8311340869932,39.2710850691866));
#209008=CARTESIAN_POINT('Ctrl Pts',(45.7136354238381,40.9043991801898,39.3343017080178));
#209009=CARTESIAN_POINT('Ctrl Pts',(45.6831319408695,40.7066485019686,39.3487519293518));
#209010=CARTESIAN_POINT('Ctrl Pts',(45.5986481858001,40.800864206016,39.3492068662937));
#209011=CARTESIAN_POINT('Ctrl Pts',(45.6634671987692,40.8592275074425,39.4512271248741));
#209012=CARTESIAN_POINT('Ctrl Pts',(45.6199161851854,40.6494327168512,39.3978017080178));
#209013=CARTESIAN_POINT('Ctrl Pts',(45.5350300257422,40.7435821574116,39.3980347781178));
#209014=CARTESIAN_POINT('Ctrl Pts',(45.5684243021845,40.773650498976,39.5248015355195));
#209015=CARTESIAN_POINT('Ctrl Pts',(45.5534068532516,40.5892333705617,39.3978017080178));
#209016=CARTESIAN_POINT('Ctrl Pts',(45.468427266244,40.6836127633974,39.3978017080178));
#209017=CARTESIAN_POINT('Ctrl Pts',(45.4684272662441,40.6836127633974,39.5248017080178));
#209018=CARTESIAN_POINT('Origin',(45.5534068532516,40.5892333705617,39.5248017080178));
#209019=CARTESIAN_POINT('Origin',(0.21244896751894,-0.235948482089075,39.116));
#209020=CARTESIAN_POINT('Origin',(46.190562802649,41.1629311642475,39.116));
#209021=CARTESIAN_POINT('Origin',(0.21244896751894,-0.235948482089075,39.5248017080178));
#209022=CARTESIAN_POINT('Origin',(45.4410373245177,40.4880553924338,39.5248017080178));
#209023=CARTESIAN_POINT('Ctrl Pts',(46.5911245387435,41.5228599914557,39.2875012672119));
#209024=CARTESIAN_POINT('Ctrl Pts',(46.5059978322081,41.6181024670992,39.287208709576));
#209025=CARTESIAN_POINT('Ctrl Pts',(46.4256208133857,41.5454735131714,39.3549016990122));
#209026=CARTESIAN_POINT('Ctrl Pts',(46.5055987918431,41.4460088704685,39.1034939173931));
#209027=CARTESIAN_POINT('Ctrl Pts',(46.4204321019733,41.5410583874199,39.1031692336321));
#209028=CARTESIAN_POINT('Ctrl Pts',(46.3572876358796,41.4839460439595,39.2077507202298));
#209029=CARTESIAN_POINT('Ctrl Pts',(46.3519544194676,41.307949174951,38.989));
#209030=CARTESIAN_POINT('Ctrl Pts',(46.2668368728777,41.402759982509,38.9887769311206));
#209031=CARTESIAN_POINT('Ctrl Pts',(46.2345298607752,41.3734144471008,39.1161898712915));
#209032=CARTESIAN_POINT('Ctrl Pts',(46.190562802649,41.1629311642475,38.989));
#209033=CARTESIAN_POINT('Ctrl Pts',(46.1054562600791,41.2574515555194,38.989));
#209034=CARTESIAN_POINT('Ctrl Pts',(46.1055833103327,41.2573104519178,39.1161895903854));
#209035=CARTESIAN_POINT('Origin',(46.5107200467162,41.4512020416168,39.3548010137695));
#209036=CARTESIAN_POINT('Ctrl Pts',(45.4410373245177,40.4880553924338,39.3978017080178));
#209037=CARTESIAN_POINT('Ctrl Pts',(45.3560577375101,40.5824347852694,39.3978017080178));
#209038=CARTESIAN_POINT('Ctrl Pts',(45.3560577375101,40.5824347852694,39.5248017080178));
#209039=CARTESIAN_POINT('Ctrl Pts',(45.374303589957,40.427652148686,39.3978017080178));
#209040=CARTESIAN_POINT('Ctrl Pts',(45.2891025640496,40.522148076296,39.3975666025003));
#209041=CARTESIAN_POINT('Ctrl Pts',(45.2557227253159,40.4920927345052,39.5248015517177));
#209042=CARTESIAN_POINT('Ctrl Pts',(45.3112030195537,40.3705349278756,39.3484894016716));
#209043=CARTESIAN_POINT('Ctrl Pts',(45.2261127332216,40.4654317778756,39.3480259000063));
#209044=CARTESIAN_POINT('Ctrl Pts',(45.1608488177568,40.4066678844405,39.4508333188951));
#209045=CARTESIAN_POINT('Ctrl Pts',(45.2779489569777,40.3404336838187,39.2708017080178));
#209046=CARTESIAN_POINT('Ctrl Pts',(45.1929563204594,40.4355776097263,39.27051194648));
#209047=CARTESIAN_POINT('Ctrl Pts',(45.1108495273517,40.3616483211478,39.3343017080178));
#209048=CARTESIAN_POINT('Origin',(45.1958291143593,40.2672689283122,39.3343017080178));
#209049=CARTESIAN_POINT('Origin',(46.6431106370703,41.5704070646306,39.6398955068182));
#209050=CARTESIAN_POINT('Origin',(46.7755012272978,41.6896120874665,39.92499));
#209051=CARTESIAN_POINT('Origin',(45.135374083614,40.2128349741385,39.1934008539952));
#209052=CARTESIAN_POINT('Origin',(45.1021848870414,40.1828829233542,39.1160402713843));
#209053=CARTESIAN_POINT('Ctrl Pts',(46.7942619810922,42.1132001505995,40.1599502534424));
#209054=CARTESIAN_POINT('Ctrl Pts',(46.7665330160784,42.088245051317,40.10025));
#209055=CARTESIAN_POINT('Ctrl Pts',(46.7142062431428,42.041152784689,40.10025));
#209056=CARTESIAN_POINT('Ctrl Pts',(46.8532067119185,42.0477032750699,40.1599500538466));
#209057=CARTESIAN_POINT('Ctrl Pts',(46.8094668591648,42.0405341034486,40.1002448353493));
#209058=CARTESIAN_POINT('Ctrl Pts',(46.7483190388756,42.0032346206966,40.10025));
#209059=CARTESIAN_POINT('Ctrl Pts',(46.889003015487,41.9705316734057,40.1202442001039));
#209060=CARTESIAN_POINT('Ctrl Pts',(46.8318174060864,41.9811230778537,40.0633873868017));
#209061=CARTESIAN_POINT('Ctrl Pts',(46.7612038509554,41.9515093836254,40.0772271723536));
#209062=CARTESIAN_POINT('Ctrl Pts',(46.906368706767,41.8426461117366,40.0045995998162));
#209063=CARTESIAN_POINT('Ctrl Pts',(46.829061965151,41.8933796070861,39.9663485808314));
#209064=CARTESIAN_POINT('Ctrl Pts',(46.7485125544802,41.8570065263029,40.0101727202467));
#209065=CARTESIAN_POINT('Ctrl Pts',(46.8896982576911,41.7917018131128,39.9304654349859));
#209066=CARTESIAN_POINT('Ctrl Pts',(46.8032976561906,41.8649047103976,39.9051900162946));
#209067=CARTESIAN_POINT('Ctrl Pts',(46.7243152668228,41.8144193983036,39.9671857458179));
#209068=CARTESIAN_POINT('Ctrl Pts',(46.855903642699,41.7612723673357,39.8576902534424));
#209069=CARTESIAN_POINT('Ctrl Pts',(46.7709043015507,41.8563683535925,39.8573998014387));
#209070=CARTESIAN_POINT('Ctrl Pts',(46.6905216402902,41.7839914803021,39.92499));
#209071=CARTESIAN_POINT('Origin',(46.7142062431428,42.041152784689,40.22725));
#209072=CARTESIAN_POINT('Origin',(0.21244896751894,-0.235948482089075,39.116));
#209073=CARTESIAN_POINT('Origin',(44.8038810887679,39.9143573409152,39.116));
#209074=CARTESIAN_POINT('Origin',(5.54214007001405E-15,5.58455191111112E-15,
40.22725));
#209075=CARTESIAN_POINT('Origin',(46.6938111422609,42.0638038389695,40.22725));
#209076=CARTESIAN_POINT('Ctrl Pts',(44.8038810887679,39.9143573409152,38.989));
#209077=CARTESIAN_POINT('Ctrl Pts',(44.7187741985015,40.0088781183433,38.989));
#209078=CARTESIAN_POINT('Ctrl Pts',(44.7189015969706,40.0087366280091,39.1161901092324));
#209079=CARTESIAN_POINT('Ctrl Pts',(44.642482288749,39.7693421853891,38.989));
#209080=CARTESIAN_POINT('Ctrl Pts',(44.5576711710494,39.8638196089392,38.9892298989784));
#209081=CARTESIAN_POINT('Ctrl Pts',(44.5899527660337,39.8926305794719,39.1161900493204));
#209082=CARTESIAN_POINT('Ctrl Pts',(44.4888315723744,39.6312917695255,39.1034966344368));
#209083=CARTESIAN_POINT('Ctrl Pts',(44.4042655856142,39.7256919284549,39.1038314102545));
#209084=CARTESIAN_POINT('Ctrl Pts',(44.4671959043828,39.782099805109,39.2077528789597));
#209085=CARTESIAN_POINT('Ctrl Pts',(44.4033023070494,39.5544469813066,39.2875012672119));
#209086=CARTESIAN_POINT('Ctrl Pts',(44.3189410144585,39.6488649704634,39.2878045257868));
#209087=CARTESIAN_POINT('Ctrl Pts',(44.3988635644387,39.720573090053,39.35490152959));
#209088=CARTESIAN_POINT('Origin',(44.4837235168761,39.6260861683712,39.3548010137695));
#209089=CARTESIAN_POINT('Ctrl Pts',(46.430275350543,42.2339804752696,39.8576902534424));
#209090=CARTESIAN_POINT('Ctrl Pts',(46.515965540528,42.1395065320994,39.8573998014387));
#209091=CARTESIAN_POINT('Ctrl Pts',(46.4355828792675,42.067129658809,39.92499));
#209092=CARTESIAN_POINT('Ctrl Pts',(46.4640859592749,42.2644230274448,39.930498490249));
#209093=CARTESIAN_POINT('Ctrl Pts',(46.5278479142031,42.1708479205164,39.9052171569796));
#209094=CARTESIAN_POINT('Ctrl Pts',(46.4693919041993,42.0975714415914,39.9672049726599));
#209095=CARTESIAN_POINT('Ctrl Pts',(46.5163638812303,42.2755508889258,40.0043437678663));
#209096=CARTESIAN_POINT('Ctrl Pts',(46.5588164356978,42.1933444849778,39.9661628577643));
#209097=CARTESIAN_POINT('Ctrl Pts',(46.5141432491637,42.1170605480846,40.0100243556234));
#209098=CARTESIAN_POINT('Ctrl Pts',(46.6408663419438,42.245403977454,40.1194874821986));
#209099=CARTESIAN_POINT('Ctrl Pts',(46.6457133039304,42.1872204559316,40.062755148314));
#209100=CARTESIAN_POINT('Ctrl Pts',(46.6088541045845,42.1199995355539,40.0767884282378));
#209101=CARTESIAN_POINT('Ctrl Pts',(46.7146600431958,42.2015749714286,40.1599502015389));
#209102=CARTESIAN_POINT('Ctrl Pts',(46.7029882531942,42.15879058965,40.1002449453872));
#209103=CARTESIAN_POINT('Ctrl Pts',(46.6595535157374,42.1018187547551,40.10025));
#209104=CARTESIAN_POINT('Ctrl Pts',(46.7738319284262,42.1358900227689,40.1599502534424));
#209105=CARTESIAN_POINT('Ctrl Pts',(46.7461150696877,42.1109214781056,40.10025));
#209106=CARTESIAN_POINT('Ctrl Pts',(46.6938111422609,42.0638038389695,40.10025));
#209107=CARTESIAN_POINT('Origin',(46.3506032922599,42.1615090516447,39.92499));
#209108=CARTESIAN_POINT('Origin',(44.3513327445049,39.5068809815356,39.6398955069335));
#209109=CARTESIAN_POINT('Origin',(44.2189419720528,39.3876757945569,39.92499));
#209110=CARTESIAN_POINT('Origin',(46.2182127020518,42.0423040287654,39.6398955068273));
#209111=CARTESIAN_POINT('Origin',(46.0858221116783,41.923099005795,39.3548010137695));
#209112=CARTESIAN_POINT('Ctrl Pts',(44.1385184650381,39.3160391863685,39.8576902534424));
#209113=CARTESIAN_POINT('Ctrl Pts',(44.0542875439845,39.4103156382726,39.8579948730703));
#209114=CARTESIAN_POINT('Ctrl Pts',(44.1339623850452,39.4820551873925,39.92499));
#209115=CARTESIAN_POINT('Ctrl Pts',(44.1047525536511,39.2856369388941,39.9304020711231));
#209116=CARTESIAN_POINT('Ctrl Pts',(44.0421527706783,39.3789425853227,39.9058915297377));
#209117=CARTESIAN_POINT('Ctrl Pts',(44.1001954303881,39.4516512848556,39.9671523786023));
#209118=CARTESIAN_POINT('Ctrl Pts',(44.0527517782422,39.2745942850996,40.0043257306693));
#209119=CARTESIAN_POINT('Ctrl Pts',(44.0110417363802,39.3566016867498,39.9667894847835));
#209120=CARTESIAN_POINT('Ctrl Pts',(44.0556530121006,39.4323285306298,40.0100138975202));
#209121=CARTESIAN_POINT('Ctrl Pts',(43.929007150946,39.3050549810245,40.1195533054857));
#209122=CARTESIAN_POINT('Ctrl Pts',(43.9243964923863,39.3631024520332,40.0630813209236));
#209123=CARTESIAN_POINT('Ctrl Pts',(43.9614781338115,39.4299498468373,40.0768265942418));
#209124=CARTESIAN_POINT('Ctrl Pts',(43.8557442421764,39.3490583909335,40.1599502027521));
#209125=CARTESIAN_POINT('Ctrl Pts',(43.867520632009,39.3917348424035,40.1002552791553));
#209126=CARTESIAN_POINT('Ctrl Pts',(43.9111340157067,39.4485000225461,40.10025));
#209127=CARTESIAN_POINT('Ctrl Pts',(43.7969047596351,39.4144401478985,40.1599502534424));
#209128=CARTESIAN_POINT('Ctrl Pts',(43.824634116049,39.4393948122683,40.10025));
#209129=CARTESIAN_POINT('Ctrl Pts',(43.8769616275879,39.4864862581812,40.10025));
#209130=CARTESIAN_POINT('Origin',(43.8769616275879,39.4864862581812,40.22725));
#209131=CARTESIAN_POINT('Ctrl Pts',(45.7656648676111,41.6348281284257,38.989));
#209132=CARTESIAN_POINT('Ctrl Pts',(45.8507714175132,41.5403077290104,38.989));
#209133=CARTESIAN_POINT('Ctrl Pts',(45.8506443599165,41.5404488407675,39.1161896013269));
#209134=CARTESIAN_POINT('Ctrl Pts',(45.9267609786665,41.7801793767983,38.989));
#209135=CARTESIAN_POINT('Ctrl Pts',(46.0121552117524,41.6856176794247,38.9887769275484));
#209136=CARTESIAN_POINT('Ctrl Pts',(45.9795929135641,41.6565546403119,39.1161898821851));
#209137=CARTESIAN_POINT('Ctrl Pts',(46.0801233673968,41.9185498083232,39.1034967087243));
#209138=CARTESIAN_POINT('Ctrl Pts',(46.1657498592349,41.8239142817232,39.103172023269));
#209139=CARTESIAN_POINT('Ctrl Pts',(46.1023497159534,41.7670853619627,39.2077529614997));
#209140=CARTESIAN_POINT('Ctrl Pts',(46.1654920697617,41.9955727382246,39.2875012672119));
#209141=CARTESIAN_POINT('Ctrl Pts',(46.251314640751,41.9009568069084,39.2872087095507));
#209142=CARTESIAN_POINT('Ctrl Pts',(46.1706818552411,41.8286118967072,39.3549017048229));
#209143=CARTESIAN_POINT('Origin',(45.7656648676111,41.6348281284257,39.116));
#209144=CARTESIAN_POINT('Origin',(5.70826774717982E-15,5.29195725359062E-15,
40.22725));
#209145=CARTESIAN_POINT('Origin',(43.8565665267061,39.5091373124617,40.22725));
#209146=CARTESIAN_POINT('Origin',(34.1507877370015,31.1767457860025,39.116));
#209147=CARTESIAN_POINT('Origin',(45.4673664422111,41.3663085755622,39.1160373285261));
#209148=CARTESIAN_POINT('Ctrl Pts',(43.7765468711727,39.4370498736003,40.1599502534424));
#209149=CARTESIAN_POINT('Ctrl Pts',(43.8042633382934,39.4620188529804,40.10025));
#209150=CARTESIAN_POINT('Ctrl Pts',(43.8565665267061,39.5091373124617,40.10025));
#209151=CARTESIAN_POINT('Ctrl Pts',(43.7178744835426,39.502178522486,40.1599500566038));
#209152=CARTESIAN_POINT('Ctrl Pts',(43.7615157339678,39.5094654441326,40.1002551305372));
#209153=CARTESIAN_POINT('Ctrl Pts',(43.8224770900139,39.5469637653742,40.10025));
#209154=CARTESIAN_POINT('Ctrl Pts',(43.68185026043,39.5788516269098,40.1203070619046));
#209155=CARTESIAN_POINT('Ctrl Pts',(43.7389249259235,39.5685043961837,40.0637098684499));
#209156=CARTESIAN_POINT('Ctrl Pts',(43.8091917332947,39.5983821485328,40.0772636213361));
#209157=CARTESIAN_POINT('Ctrl Pts',(43.6640874258696,39.7059848156952,40.0046102245802));
#209158=CARTESIAN_POINT('Ctrl Pts',(43.7412697217743,39.6560168722786,39.9670001894012));
#209159=CARTESIAN_POINT('Ctrl Pts',(43.8212571467122,39.6923865500758,40.010178881121));
#209160=CARTESIAN_POINT('Ctrl Pts',(43.6806424921205,39.7566878101775,39.9303710930186));
#209161=CARTESIAN_POINT('Ctrl Pts',(43.766896221903,39.6846695243133,39.9058663574107));
#209162=CARTESIAN_POINT('Ctrl Pts',(43.8452710114194,39.734802377006,39.9671344706363));
#209163=CARTESIAN_POINT('Ctrl Pts',(43.7143933160628,39.7870778846742,39.8576902534424));
#209164=CARTESIAN_POINT('Ctrl Pts',(43.7993487829618,39.6934538167795,39.8579948730703));
#209165=CARTESIAN_POINT('Ctrl Pts',(43.8790236240225,39.7651933658994,39.92499));
#209166=CARTESIAN_POINT('Origin',(43.7940440370149,39.859572758735,39.92499));
#209167=CARTESIAN_POINT('Origin',(45.4345348103669,41.3366772856866,39.1925554488846));
#209168=CARTESIAN_POINT('Origin',(45.3737170758078,41.2819167515323,39.3343017080178));
#209169=CARTESIAN_POINT('Origin',(43.9264348094888,39.9787779456578,39.6398955069202));
#209170=CARTESIAN_POINT('Origin',(44.0588255818383,40.0979831325494,39.3548010137695));
#209171=CARTESIAN_POINT('Ctrl Pts',(45.1285089182138,41.0611303347399,39.3978017080178));
#209172=CARTESIAN_POINT('Ctrl Pts',(45.2134885052213,40.9667509419042,39.3978017080178));
#209173=CARTESIAN_POINT('Ctrl Pts',(45.2134885052213,40.9667509419042,39.5248017080178));
#209174=CARTESIAN_POINT('Ctrl Pts',(45.1955564429368,41.1211850608436,39.3978017080178));
#209175=CARTESIAN_POINT('Ctrl Pts',(45.2803165088404,41.0269231466362,39.398035577521));
#209176=CARTESIAN_POINT('Ctrl Pts',(45.3138235084273,41.0570929845756,39.5248015517192));
#209177=CARTESIAN_POINT('Ctrl Pts',(45.2589537050069,41.1779726855665,39.3484893995498));
#209178=CARTESIAN_POINT('Ctrl Pts',(45.3438226072591,41.0841042944907,39.3489438303402));
#209179=CARTESIAN_POINT('Ctrl Pts',(45.4086973919088,41.1425178129605,39.450833315559));
#209180=CARTESIAN_POINT('Ctrl Pts',(45.2923641298562,41.2079002115902,39.2708017080178));
#209181=CARTESIAN_POINT('Ctrl Pts',(45.377327533411,41.1142722655001,39.2710850691866));
#209182=CARTESIAN_POINT('Ctrl Pts',(45.4586966628153,41.1875373586967,39.3343017080178));
#209183=CARTESIAN_POINT('Origin',(45.1285089182138,41.0611303347399,39.5248017080178));
#209184=CARTESIAN_POINT('Ctrl Pts',(43.9791725362587,40.0254908126583,39.2875012672119));
#209185=CARTESIAN_POINT('Ctrl Pts',(44.0642551277135,39.9317223035491,39.2878045257519));
#209186=CARTESIAN_POINT('Ctrl Pts',(44.1439246046469,40.0037114707674,39.3549015218347));
#209187=CARTESIAN_POINT('Ctrl Pts',(44.0645378932547,40.1025202360377,39.1034938540227));
#209188=CARTESIAN_POINT('Ctrl Pts',(44.1495813562438,40.0085500157857,39.1038286278816));
#209189=CARTESIAN_POINT('Ctrl Pts',(44.212257978885,40.0652391174778,39.2077506434029));
#209190=CARTESIAN_POINT('Ctrl Pts',(44.2178941385635,40.2409001323907,38.989));
#209191=CARTESIAN_POINT('Ctrl Pts',(44.3029888158492,40.1466780419453,38.9892298954605));
#209192=CARTESIAN_POINT('Ctrl Pts',(44.3350158129994,40.1757707681164,39.1161900347289));
#209193=CARTESIAN_POINT('Ctrl Pts',(44.37898315373,40.3862543050933,38.989));
#209194=CARTESIAN_POINT('Ctrl Pts',(44.464090034167,40.2917335385819,38.989));
#209195=CARTESIAN_POINT('Ctrl Pts',(44.463962645542,40.2918750179831,39.1161900945645));
#209196=CARTESIAN_POINT('Origin',(44.37898315373,40.3862543050933,39.116));
#209197=CARTESIAN_POINT('Origin',(33.3184119221875,30.4272712359683,39.5248017080178));
#209198=CARTESIAN_POINT('Origin',(45.0161393894798,40.959952356612,39.5248017080178));
#209199=CARTESIAN_POINT('Origin',(33.1880655373225,30.3099068238763,39.116));
#209200=CARTESIAN_POINT('Origin',(44.6772189625519,40.6548553974676,39.1160402713849));
#209201=CARTESIAN_POINT('Ctrl Pts',(44.8522789915946,40.8131880745601,39.2708017080178));
#209202=CARTESIAN_POINT('Ctrl Pts',(44.9380175594367,40.7187157882332,39.27051194648));
#209203=CARTESIAN_POINT('Ctrl Pts',(44.855910766329,40.6447864996547,39.3343017080178));
#209204=CARTESIAN_POINT('Ctrl Pts',(44.885804243544,40.8432146576635,39.3487519301186));
#209205=CARTESIAN_POINT('Ctrl Pts',(44.9712860523918,40.7486708738366,39.3482879463991));
#209206=CARTESIAN_POINT('Ctrl Pts',(44.9060790100825,40.6899581892257,39.4512271261641));
#209207=CARTESIAN_POINT('Ctrl Pts',(44.9493173051407,40.9001003367642,39.3978017080178));
#209208=CARTESIAN_POINT('Ctrl Pts',(45.0343891839563,40.8054891887056,39.3975673827397));
#209209=CARTESIAN_POINT('Ctrl Pts',(45.0011219300388,40.7755352187362,39.524801535518));
#209210=CARTESIAN_POINT('Ctrl Pts',(45.0161393894798,40.959952356612,39.3978017080178));
#209211=CARTESIAN_POINT('Ctrl Pts',(45.1011189764874,40.8655729637763,39.3978017080178));
#209212=CARTESIAN_POINT('Ctrl Pts',(45.1011189764874,40.8655729637763,39.5248017080178));
#209213=CARTESIAN_POINT('Origin',(44.7709311793215,40.7391658924904,39.3343017080178));
#209214=CARTESIAN_POINT('Origin',(44.7104761492018,40.6847319392788,39.1934008533551));
#209215=CARTESIAN_POINT('Origin',(49.8797426639511,35.8473027488275,39.1925554495088));
#209216=CARTESIAN_POINT('Origin',(49.9155525184341,35.8732562382978,39.116037328529));
#209217=CARTESIAN_POINT('Origin',(49.8135340601227,35.7991993820656,39.3343017080178));
#209218=CARTESIAN_POINT('Ctrl Pts',(49.7242207306179,35.7350130971383,39.2708017080178));
#209219=CARTESIAN_POINT('Ctrl Pts',(49.650303664679,35.8375861910551,39.2710850691866));
#209220=CARTESIAN_POINT('Ctrl Pts',(49.7388853330816,35.9019445403512,39.3343017080178));
#209221=CARTESIAN_POINT('Ctrl Pts',(49.6878783768803,35.7084656432346,39.3487519293517));
#209222=CARTESIAN_POINT('Ctrl Pts',(49.6137056554176,35.8109961808839,39.3492068662914));
#209223=CARTESIAN_POINT('Ctrl Pts',(49.6842702092628,35.8622643302246,39.4512271248739));
#209224=CARTESIAN_POINT('Ctrl Pts',(49.6190282456266,35.6581711379715,39.3978017080178));
#209225=CARTESIAN_POINT('Ctrl Pts',(49.5444483977887,35.7606778378455,39.3980347781197));
#209226=CARTESIAN_POINT('Ctrl Pts',(49.580802734425,35.7870908094896,39.5248015355195));
#209227=CARTESIAN_POINT('Ctrl Pts',(49.5465907136149,35.6052536882596,39.3978017080178));
#209228=CARTESIAN_POINT('Ctrl Pts',(49.4719419865738,35.7079988465452,39.3978017080178));
#209229=CARTESIAN_POINT('Ctrl Pts',(49.4719419865738,35.7079988465452,39.5248017080178));
#209230=CARTESIAN_POINT('Origin',(49.5465907136149,35.6052536882596,39.5248017080178));
#209231=CARTESIAN_POINT('Origin',(0.186621817602863,-0.256862895714048,
39.116));
#209232=CARTESIAN_POINT('Origin',(50.2402240048087,36.1092077731522,39.116));
#209233=CARTESIAN_POINT('Origin',(0.186621817602863,-0.256862895714048,
39.5248017080178));
#209234=CARTESIAN_POINT('Origin',(49.4242607783465,35.516375787839,39.5248017080178));
#209235=CARTESIAN_POINT('Ctrl Pts',(50.6762142289952,36.4252947698673,39.2875012672119));
#209236=CARTESIAN_POINT('Ctrl Pts',(50.6015094050819,36.528913661081,39.287208709576));
#209237=CARTESIAN_POINT('Ctrl Pts',(50.5139809070359,36.4650842624215,39.3549016990122));
#209238=CARTESIAN_POINT('Ctrl Pts',(50.5831238715085,36.3578045222543,39.1034939173931));
#209239=CARTESIAN_POINT('Ctrl Pts',(50.508359113622,36.461235691223,39.1031692336331));
#209240=CARTESIAN_POINT('Ctrl Pts',(50.4395906940219,36.4110366091596,39.2077507202294));
#209241=CARTESIAN_POINT('Ctrl Pts',(50.4158900112696,36.2365613423281,38.989));
#209242=CARTESIAN_POINT('Ctrl Pts',(50.3411491755186,36.3397499727017,38.9887769311176));
#209243=CARTESIAN_POINT('Ctrl Pts',(50.3059517008893,36.3139421975377,39.1161898712915));
#209244=CARTESIAN_POINT('Ctrl Pts',(50.2402240048087,36.1092077731522,38.989));
#209245=CARTESIAN_POINT('Ctrl Pts',(50.165463756031,36.2121064279398,38.989));
#209246=CARTESIAN_POINT('Ctrl Pts',(50.1655753609474,36.2119528169507,39.1161895903854));
#209247=CARTESIAN_POINT('Origin',(50.5887599058106,36.3624339277667,39.3548010137695));
#209248=CARTESIAN_POINT('Ctrl Pts',(49.4242607783465,35.516375787839,39.3978017080178));
#209249=CARTESIAN_POINT('Ctrl Pts',(49.3496120513054,35.6191209461246,39.3978017080178));
#209250=CARTESIAN_POINT('Ctrl Pts',(49.3496120513054,35.6191209461246,39.5248017080178));
#209251=CARTESIAN_POINT('Ctrl Pts',(49.3515787599206,35.4632790141025,39.3978017080178));
#209252=CARTESIAN_POINT('Ctrl Pts',(49.2767219882426,35.5661632154381,39.3975666025007));
#209253=CARTESIAN_POINT('Ctrl Pts',(49.2403833690702,35.5397616632027,39.5248015517177));
#209254=CARTESIAN_POINT('Ctrl Pts',(49.2828534857273,35.413070493059,39.3484894016716));
#209255=CARTESIAN_POINT('Ctrl Pts',(49.208148754793,35.5163418450557,39.3480259000045));
#209256=CARTESIAN_POINT('Ctrl Pts',(49.1370998624041,35.4647218031684,39.4508333188946));
#209257=CARTESIAN_POINT('Ctrl Pts',(49.2466351556017,35.3866101428254,39.2708017080178));
#209258=CARTESIAN_POINT('Ctrl Pts',(49.1720533660035,35.4901170100361,39.27051194648));
#209259=CARTESIAN_POINT('Ctrl Pts',(49.0826686475739,35.4251752107432,39.3343017080178));
#209260=CARTESIAN_POINT('Origin',(49.1573173746151,35.3224300524576,39.3343017080178));
#209261=CARTESIAN_POINT('Origin',(50.7328855645276,36.4671473482311,39.6398955068182));
#209262=CARTESIAN_POINT('Origin',(50.8770112231007,36.5718607685316,39.92499));
#209263=CARTESIAN_POINT('Origin',(49.0915036252755,35.274613564642,39.1934008539943));
#209264=CARTESIAN_POINT('Origin',(49.0553654007531,35.2482948100385,39.1160402713852));
#209265=CARTESIAN_POINT('Ctrl Pts',(50.9399462128206,36.9911673391701,40.1599502534424));
#209266=CARTESIAN_POINT('Ctrl Pts',(50.9097606317998,36.9692474126334,40.10025));
#209267=CARTESIAN_POINT('Ctrl Pts',(50.8527980281389,36.9278827595321,40.10025));
#209268=CARTESIAN_POINT('Ctrl Pts',(50.9917217504968,36.9198678602467,40.1599500538475));
#209269=CARTESIAN_POINT('Ctrl Pts',(50.9474721267427,36.9173100216912,40.100244835349));
#209270=CARTESIAN_POINT('Ctrl Pts',(50.8827604229976,36.8866065570948,40.10025));
#209271=CARTESIAN_POINT('Ctrl Pts',(51.0192553292382,36.8393772800889,40.1202442001042));
#209272=CARTESIAN_POINT('Ctrl Pts',(50.9634900918198,36.8558881875864,40.0633873868023));
#209273=CARTESIAN_POINT('Ctrl Pts',(50.8901678911828,36.8338178466774,40.0772271723542));
#209274=CARTESIAN_POINT('Ctrl Pts',(51.0231582082093,36.7103770798833,40.0045995998159));
#209275=CARTESIAN_POINT('Ctrl Pts',(50.951578055318,36.7689134067387,39.9663485808308));
#209276=CARTESIAN_POINT('Ctrl Pts',(50.8676678805082,36.7411592876123,40.0101727202462));
#209277=CARTESIAN_POINT('Ctrl Pts',(51.0012539523509,36.6614543958812,39.9304654349861));
#209278=CARTESIAN_POINT('Ctrl Pts',(50.922978448746,36.7432876021354,39.905190016294));
#209279=CARTESIAN_POINT('Ctrl Pts',(50.8391515810794,36.7013347616505,39.9671857458178));
#209280=CARTESIAN_POINT('Ctrl Pts',(50.9644637245897,36.6347241449648,39.8576902534424));
#209281=CARTESIAN_POINT('Ctrl Pts',(50.8898702560322,36.7381840359678,39.8573998014387));
#209282=CARTESIAN_POINT('Ctrl Pts',(50.8023624960595,36.6746059268172,39.92499));
#209283=CARTESIAN_POINT('Origin',(50.8527980281389,36.9278827595321,40.22725));
#209284=CARTESIAN_POINT('Origin',(0.186621817602863,-0.256862895714048,
39.116));
#209285=CARTESIAN_POINT('Origin',(48.7306271754181,35.0124214764579,39.116));
#209286=CARTESIAN_POINT('Origin',(5.53127843490691E-15,5.59796491342025E-15,
40.22725));
#209287=CARTESIAN_POINT('Origin',(50.8348823336491,36.9525415975206,40.22725));
#209288=CARTESIAN_POINT('Ctrl Pts',(48.7306271754181,35.0124214764579,38.989));
#209289=CARTESIAN_POINT('Ctrl Pts',(48.6558666212131,35.11532055163,38.989));
#209290=CARTESIAN_POINT('Ctrl Pts',(48.6559785320126,35.1151665196289,39.1161901092319));
#209291=CARTESIAN_POINT('Ctrl Pts',(48.5549543235576,34.8850714976633,38.989));
#209292=CARTESIAN_POINT('Ctrl Pts',(48.4804833899293,34.9878965398005,38.989229898976));
#209293=CARTESIAN_POINT('Ctrl Pts',(48.5155997094323,35.0131753353107,39.1161900493199));
#209294=CARTESIAN_POINT('Ctrl Pts',(48.3877151240586,34.7638382096872,39.1034966344368));
#209295=CARTESIAN_POINT('Ctrl Pts',(48.3134799021736,34.8665607873086,39.1038314102576));
#209296=CARTESIAN_POINT('Ctrl Pts',(48.3819617107294,34.9160816462013,39.20775287896));
#209297=CARTESIAN_POINT('Ctrl Pts',(48.2946219293751,34.6963546279279,39.2875012672119));
#209298=CARTESIAN_POINT('Ctrl Pts',(48.2205921440835,34.7990735417344,39.2878045257868));
#209299=CARTESIAN_POINT('Ctrl Pts',(48.3075724095164,34.8620346554122,39.3549015295898));
#209300=CARTESIAN_POINT('Origin',(48.3820909175334,34.7591950625528,39.3548010137695));
#209301=CARTESIAN_POINT('Ctrl Pts',(50.5905785208489,37.1493329797255,39.8576902534424));
#209302=CARTESIAN_POINT('Ctrl Pts',(50.6659240749088,37.0464195108247,39.8573998014387));
#209303=CARTESIAN_POINT('Ctrl Pts',(50.5784163149361,36.982841401674,39.92499));
#209304=CARTESIAN_POINT('Ctrl Pts',(50.6273860247246,37.1760745934428,39.9304984902491));
#209305=CARTESIAN_POINT('Ctrl Pts',(50.6810174228649,37.0763471615767,39.9052171569796));
#209306=CARTESIAN_POINT('Ctrl Pts',(50.6152221632648,37.0095824157642,39.9672049726605));
#209307=CARTESIAN_POINT('Ctrl Pts',(50.6805407410142,37.1816769644885,40.0043437678663));
#209308=CARTESIAN_POINT('Ctrl Pts',(50.7141678268707,37.0954833955422,39.9661628577642));
#209309=CARTESIAN_POINT('Ctrl Pts',(50.6617655220317,37.0242869695745,40.0100243556237));
#209310=CARTESIAN_POINT('Ctrl Pts',(50.8012099538928,37.1386811500604,40.1194874821986));
#209311=CARTESIAN_POINT('Ctrl Pts',(50.7999485296226,37.080309718469,40.062755148314));
#209312=CARTESIAN_POINT('Ctrl Pts',(50.7562647493206,37.0173098767917,40.0767884282375));
#209313=CARTESIAN_POINT('Ctrl Pts',(50.8700180268812,37.0873787017251,40.159950201538));
#209314=CARTESIAN_POINT('Ctrl Pts',(50.8539379904875,37.0460487315392,40.1002449453885));
#209315=CARTESIAN_POINT('Ctrl Pts',(50.804786014715,36.9939291606744,40.10025));
#209316=CARTESIAN_POINT('Ctrl Pts',(50.9219998155904,37.0158684358554,40.1599502534424));
#209317=CARTESIAN_POINT('Ctrl Pts',(50.8918248691005,36.9939338721427,40.10025));
#209318=CARTESIAN_POINT('Ctrl Pts',(50.8348823336491,36.9525415975206,40.10025));
#209319=CARTESIAN_POINT('Origin',(50.503767587895,37.0855865599597,39.92499));
#209320=CARTESIAN_POINT('Origin',(48.2379650606683,34.6544814981897,39.6398955069315));
#209321=CARTESIAN_POINT('Origin',(48.0938392037152,34.5497679336935,39.92499));
#209322=CARTESIAN_POINT('Origin',(50.3596419293387,36.9808731396133,39.6398955068266));
#209323=CARTESIAN_POINT('Origin',(50.2155162706049,36.8761597191948,39.3548010137695));
#209324=CARTESIAN_POINT('Ctrl Pts',(48.0063682005191,34.4869303039391,39.8576902534424));
#209325=CARTESIAN_POINT('Ctrl Pts',(47.9324532779042,34.5894948283128,39.8579948730703));
#209326=CARTESIAN_POINT('Ctrl Pts',(48.019190476674,34.6525130919791,39.92499));
#209327=CARTESIAN_POINT('Ctrl Pts',(47.9696093621204,34.4602241019841,39.9304020711231));
#209328=CARTESIAN_POINT('Ctrl Pts',(47.9171056031474,34.5595620694331,39.9058915297376));
#209329=CARTESIAN_POINT('Ctrl Pts',(47.9824304277187,34.6258053530815,39.9671523786031));
#209330=CARTESIAN_POINT('Ctrl Pts',(47.9167391807674,34.4546775021463,40.0043257306692));
#209331=CARTESIAN_POINT('Ctrl Pts',(47.88382973855,34.5405955452479,39.9667894847839));
#209332=CARTESIAN_POINT('Ctrl Pts',(47.9361122396534,34.6112444014583,40.01001389752));
#209333=CARTESIAN_POINT('Ctrl Pts',(47.7968564492225,34.4979061669203,40.1195533054858));
#209334=CARTESIAN_POINT('Ctrl Pts',(47.7983386612738,34.5561175928636,40.0630813209234));
#209335=CARTESIAN_POINT('Ctrl Pts',(47.8422046210396,34.618722703651,40.0768265942421));
#209336=CARTESIAN_POINT('Ctrl Pts',(47.7285944911492,34.5493265808145,40.1599502027515));
#209337=CARTESIAN_POINT('Ctrl Pts',(47.7447672725774,34.5905382782867,40.1002552791541));
#209338=CARTESIAN_POINT('Ctrl Pts',(47.794075314643,34.6424336528569,40.10025));
#209339=CARTESIAN_POINT('Ctrl Pts',(47.6769115920308,34.6205005703629,40.1599502534424));
#209340=CARTESIAN_POINT('Ctrl Pts',(47.7070975168468,34.6424200234569,40.10025));
#209341=CARTESIAN_POINT('Ctrl Pts',(47.7640607692767,34.683783783134,40.10025));
#209342=CARTESIAN_POINT('Origin',(47.7640607692768,34.683783783134,40.22725));
#209343=CARTESIAN_POINT('Ctrl Pts',(49.866980369603,36.6229335645803,38.989));
#209344=CARTESIAN_POINT('Ctrl Pts',(49.9417406248217,36.5200349009276,38.989));
#209345=CARTESIAN_POINT('Ctrl Pts',(49.9416290134548,36.5201885207951,39.116189601327));
#209346=CARTESIAN_POINT('Ctrl Pts',(50.0423873219322,36.7506494346797,38.989));
#209347=CARTESIAN_POINT('Ctrl Pts',(50.1174293675626,36.6476796282206,38.9887769275478));
#209348=CARTESIAN_POINT('Ctrl Pts',(50.0820075342354,36.6221794864672,39.1161898821852));
#209349=CARTESIAN_POINT('Ctrl Pts',(50.2093732240192,36.872231123686,39.1034967087243));
#209350=CARTESIAN_POINT('Ctrl Pts',(50.2846385388134,36.7691636147952,39.1031720232688));
#209351=CARTESIAN_POINT('Ctrl Pts',(50.215645468497,36.7192731293518,39.2077529614993));
#209352=CARTESIAN_POINT('Ctrl Pts',(50.3023253562,36.939908654648,39.2875012672119));
#209353=CARTESIAN_POINT('Ctrl Pts',(50.3777877242646,36.8368401378442,39.2872087095507));
#209354=CARTESIAN_POINT('Ctrl Pts',(50.2900345513018,36.773319961789,39.354901704823));
#209355=CARTESIAN_POINT('Origin',(49.866980369603,36.6229335645803,39.116));
#209356=CARTESIAN_POINT('Origin',(5.7121316272531E-15,5.28718575907493E-15,
40.22725));
#209357=CARTESIAN_POINT('Origin',(47.7461450747869,34.7084426211226,40.22725));
#209358=CARTESIAN_POINT('Origin',(40.5385041740537,29.8453988870283,39.116));
#209359=CARTESIAN_POINT('Origin',(49.5422481179707,36.3870656659227,39.1160373285231));
#209360=CARTESIAN_POINT('Ctrl Pts',(47.659028586094,34.645114416418,40.1599502534424));
#209361=CARTESIAN_POINT('Ctrl Pts',(47.6892031885518,34.6670494534012,40.10025));
#209362=CARTESIAN_POINT('Ctrl Pts',(47.7461450747869,34.7084426211226,40.10025));
#209363=CARTESIAN_POINT('Ctrl Pts',(47.6074854095246,34.7160192182659,40.1599500566043));
#209364=CARTESIAN_POINT('Ctrl Pts',(47.6516492793354,34.7187044685513,40.1002551305372));
#209365=CARTESIAN_POINT('Ctrl Pts',(47.7161963245886,34.7496251731987,40.10025));
#209366=CARTESIAN_POINT('Ctrl Pts',(47.5796730526558,34.7960378560832,40.1203070619043));
#209367=CARTESIAN_POINT('Ctrl Pts',(47.6353534770331,34.7797813814943,40.0637098684496));
#209368=CARTESIAN_POINT('Ctrl Pts',(47.7083584310198,34.8021505789967,40.0772636213362));
#209369=CARTESIAN_POINT('Ctrl Pts',(47.5752965616148,34.9243313177588,40.0046102245805));
#209370=CARTESIAN_POINT('Ctrl Pts',(47.6468329724886,34.8665693571818,39.9670001894015));
#209371=CARTESIAN_POINT('Ctrl Pts',(47.7301838844737,34.894378835469,40.010178881121));
#209372=CARTESIAN_POINT('Ctrl Pts',(47.5970608435776,34.9730260802971,39.9303710930184));
#209373=CARTESIAN_POINT('Ctrl Pts',(47.6753141056553,34.8923863483124,39.9058663574105));
#209374=CARTESIAN_POINT('Ctrl Pts',(47.7584998599247,34.9340521716862,39.9671344706362));
#209375=CARTESIAN_POINT('Ctrl Pts',(47.6338034047604,34.9997217530255,39.8576902534424));
#209376=CARTESIAN_POINT('Ctrl Pts',(47.7085070967808,34.8977303031696,39.8579948730703));
#209377=CARTESIAN_POINT('Ctrl Pts',(47.7952442955506,34.960748566836,39.92499));
#209378=CARTESIAN_POINT('Origin',(47.7205955685095,35.0634937251216,39.92499));
#209379=CARTESIAN_POINT('Origin',(49.5064990280466,36.3610285393793,39.1925554488851));
#209380=CARTESIAN_POINT('Origin',(49.440290424917,36.3129251734937,39.3343017080178));
#209381=CARTESIAN_POINT('Origin',(47.8647214254837,35.168207289561,39.6398955069212));
#209382=CARTESIAN_POINT('Origin',(48.0088472823277,35.2729208539809,39.3548010137695));
#209383=CARTESIAN_POINT('Ctrl Pts',(49.1733470784092,36.1189794796877,39.3978017080178));
#209384=CARTESIAN_POINT('Ctrl Pts',(49.2479958054503,36.0162343214021,39.3978017080178));
#209385=CARTESIAN_POINT('Ctrl Pts',(49.2479958054503,36.0162343214021,39.5248017080178));
#209386=CARTESIAN_POINT('Ctrl Pts',(49.246304738008,36.1716968449931,39.3978017080178));
#209387=CARTESIAN_POINT('Ctrl Pts',(49.3207474263632,36.0690914679777,39.3980355775182));
#209388=CARTESIAN_POINT('Ctrl Pts',(49.3572244778978,36.0955935972127,39.5248015517192));
#209389=CARTESIAN_POINT('Ctrl Pts',(49.3152906263885,36.2215465627858,39.3484893995498));
#209390=CARTESIAN_POINT('Ctrl Pts',(49.3898826892472,36.1193211766498,39.3489438303432));
#209391=CARTESIAN_POINT('Ctrl Pts',(49.4605079583586,36.1706334382079,39.4508333155597));
#209392=CARTESIAN_POINT('Ctrl Pts',(49.3516463037389,36.2478178023245,39.2708017080178));
#209393=CARTESIAN_POINT('Ctrl Pts',(49.4263574835555,36.1458216659119,39.2710850691866));
#209394=CARTESIAN_POINT('Ctrl Pts',(49.5149391519582,36.2101800152081,39.3343017080178));
#209395=CARTESIAN_POINT('Origin',(49.1733470784092,36.1189794796877,39.5248017080178));
#209396=CARTESIAN_POINT('Ctrl Pts',(47.9220530736691,35.2091516650522,39.2875012672119));
#209397=CARTESIAN_POINT('Ctrl Pts',(47.9968680956257,35.1070032771113,39.2878045257518));
#209398=CARTESIAN_POINT('Ctrl Pts',(48.0836260518497,35.1702703521463,39.3549015218348));
#209399=CARTESIAN_POINT('Ctrl Pts',(48.015002557561,35.2768360036059,39.1034938540228));
#209400=CARTESIAN_POINT('Ctrl Pts',(48.0897575808479,35.1744910995541,39.1038286278818));
#209401=CARTESIAN_POINT('Ctrl Pts',(48.1580164790724,35.2243181613709,39.2077506434029));
#209402=CARTESIAN_POINT('Ctrl Pts',(48.1819833392242,35.3984277477542,38.989));
#209403=CARTESIAN_POINT('Ctrl Pts',(48.2567629686452,35.2958269999271,38.9892298954605));
#209404=CARTESIAN_POINT('Ctrl Pts',(48.2916555365118,35.3214126203089,39.1161900347291));
#209405=CARTESIAN_POINT('Ctrl Pts',(48.3573835402124,35.526147267886,38.989));
#209406=CARTESIAN_POINT('Ctrl Pts',(48.4321440857833,35.4232482045976,38.989));
#209407=CARTESIAN_POINT('Ctrl Pts',(48.4320321836307,35.4234022246972,39.1161900945648));
#209408=CARTESIAN_POINT('Origin',(48.3573835402124,35.526147267886,39.116));
#209409=CARTESIAN_POINT('Origin',(39.5520252162596,29.1286799712085,39.5248017080178));
#209410=CARTESIAN_POINT('Origin',(49.0510171431408,36.0301015792671,39.5248017080178));
#209411=CARTESIAN_POINT('Origin',(39.3975469582356,29.0164449471018,39.116));
#209412=CARTESIAN_POINT('Origin',(48.6820620414863,35.7621028045846,39.116040271385));
#209413=CARTESIAN_POINT('Ctrl Pts',(48.8727133447948,35.9012693628899,39.2708017080178));
#209414=CARTESIAN_POINT('Ctrl Pts',(48.9481071848801,35.798352484893,39.27051194648));
#209415=CARTESIAN_POINT('Ctrl Pts',(48.8587224664505,35.7334106856,39.3343017080178));
#209416=CARTESIAN_POINT('Ctrl Pts',(48.9091935744939,35.927627114164,39.3487519301185));
#209417=CARTESIAN_POINT('Ctrl Pts',(48.9843245886202,35.8246659689635,39.3482879463985));
#209418=CARTESIAN_POINT('Ctrl Pts',(48.9133376106112,35.7730909105059,39.4512271261636));
#209419=CARTESIAN_POINT('Ctrl Pts',(48.978304877513,35.9775622448351,39.3978017080178));
#209420=CARTESIAN_POINT('Ctrl Pts',(49.0530211657558,35.8745769537834,39.3975673827383));
#209421=CARTESIAN_POINT('Ctrl Pts',(49.0168051108903,35.8482644497251,39.524801535518));
#209422=CARTESIAN_POINT('Ctrl Pts',(49.0510171431408,36.0301015792671,39.3978017080178));
#209423=CARTESIAN_POINT('Ctrl Pts',(49.1256658701819,35.9273564209814,39.3978017080178));
#209424=CARTESIAN_POINT('Ctrl Pts',(49.1256658701819,35.9273564209814,39.5248017080178));
#209425=CARTESIAN_POINT('Origin',(48.7840737394093,35.8361558438857,39.3343017080178));
#209426=CARTESIAN_POINT('Origin',(48.7182599907926,35.7883393569599,39.1934008533547));
#209427=CARTESIAN_POINT('Origin',(53.3535596832587,30.4370746247553,39.1925554495084));
#209428=CARTESIAN_POINT('Origin',(53.3918862459839,30.4591427892357,39.1160373285289));
#209429=CARTESIAN_POINT('Origin',(53.282685606085,30.396155456883,39.3343017080178));
#209430=CARTESIAN_POINT('Ctrl Pts',(53.1871522506179,30.3416565762229,39.2708017080178));
#209431=CARTESIAN_POINT('Ctrl Pts',(53.1243619179799,30.4513942013107,39.2710850691866));
#209432=CARTESIAN_POINT('Ctrl Pts',(53.219185606085,30.5061406831637,39.3343017080178));
#209433=CARTESIAN_POINT('Ctrl Pts',(53.1482340195352,30.3190533624392,39.3487519293517));
#209434=CARTESIAN_POINT('Ctrl Pts',(53.0851849835376,30.4287753876668,39.3492068662928));
#209435=CARTESIAN_POINT('Ctrl Pts',(53.1607219582396,30.4723866803423,39.4512271248731));
#209436=CARTESIAN_POINT('Ctrl Pts',(53.0745038491601,30.2762311741512,39.3978017080178));
#209437=CARTESIAN_POINT('Ctrl Pts',(53.0110474253454,30.3859720484841,39.3980347781174));
#209438=CARTESIAN_POINT('Ctrl Pts',(53.0499635164587,30.4084402641651,39.5248015355195));
#209439=CARTESIAN_POINT('Ctrl Pts',(52.9969317578291,30.2311753956706,39.3978017080178));
#209440=CARTESIAN_POINT('Ctrl Pts',(52.9334317578291,30.3411606219512,39.3978017080178));
#209441=CARTESIAN_POINT('Ctrl Pts',(52.9334317578291,30.3411606219512,39.5248017080178));
#209442=CARTESIAN_POINT('Origin',(52.9969317578291,30.2311753956706,39.5248017080178));
#209443=CARTESIAN_POINT('Origin',(0.158750000000002,-0.274963065701561,
39.116));
#209444=CARTESIAN_POINT('Origin',(53.739442799329,30.6598643453568,39.116));
#209445=CARTESIAN_POINT('Origin',(0.158750000000002,-0.274963065701561,
39.5248017080178));
#209446=CARTESIAN_POINT('Origin',(52.8659816883963,30.1555713378331,39.5248017080178));
#209447=CARTESIAN_POINT('Ctrl Pts',(54.2060847114746,30.9286463962971,39.2875012672119));
#209448=CARTESIAN_POINT('Ctrl Pts',(54.1426202518673,31.0395064328251,39.287208709576));
#209449=CARTESIAN_POINT('Ctrl Pts',(54.0488992551387,30.9851759176832,39.3549016990121));
#209450=CARTESIAN_POINT('Ctrl Pts',(54.1064496608385,30.8712564593342,39.1034939173931));
#209451=CARTESIAN_POINT('Ctrl Pts',(54.0429059732607,30.981936066786,39.1031692336358));
#209452=CARTESIAN_POINT('Ctrl Pts',(53.9692670413543,30.9392002377683,39.2077507202299));
#209453=CARTESIAN_POINT('Ctrl Pts',(53.927458561903,30.768158160653,38.989));
#209454=CARTESIAN_POINT('Ctrl Pts',(53.8639133132318,30.8785940576193,38.9887769311152));
#209455=CARTESIAN_POINT('Ctrl Pts',(53.8262110069739,30.8566067980793,39.1161898712914));
#209456=CARTESIAN_POINT('Ctrl Pts',(53.7394427993291,30.6598643453568,38.989));
#209457=CARTESIAN_POINT('Ctrl Pts',(53.6758479332738,30.7700138844651,38.989));
#209458=CARTESIAN_POINT('Ctrl Pts',(53.675942870086,30.7698494490828,39.1161895903852));
#209459=CARTESIAN_POINT('Origin',(54.1125387249983,30.8752713784755,39.3548010137695));
#209460=CARTESIAN_POINT('Ctrl Pts',(52.8659816883963,30.1555713378331,39.3978017080178));
#209461=CARTESIAN_POINT('Ctrl Pts',(52.8024816883963,30.2655565641137,39.3978017080178));
#209462=CARTESIAN_POINT('Ctrl Pts',(52.8024816883963,30.2655565641137,39.5248017080178));
#209463=CARTESIAN_POINT('Ctrl Pts',(52.788147705508,30.1103627734738,39.3978017080178));
#209464=CARTESIAN_POINT('Ctrl Pts',(52.7244553345199,30.2205080277001,39.3975666025026));
#209465=CARTESIAN_POINT('Ctrl Pts',(52.6855560684224,30.1980495259467,39.5248015517177));
#209466=CARTESIAN_POINT('Ctrl Pts',(52.7145506960115,30.0676130472584,39.3484894016716));
#209467=CARTESIAN_POINT('Ctrl Pts',(52.6510500011311,30.1781274387036,39.348025900004));
#209468=CARTESIAN_POINT('Ctrl Pts',(52.5749945583569,30.1342168083483,39.450833318895));
#209469=CARTESIAN_POINT('Ctrl Pts',(52.67576491394,30.045083495983,39.2708017080178));
#209470=CARTESIAN_POINT('Ctrl Pts',(52.612411104956,30.1558192615995,39.27051194648));
#209471=CARTESIAN_POINT('Ctrl Pts',(52.5167277788845,30.1005764675351,39.3343017080178));
#209472=CARTESIAN_POINT('Origin',(52.5802277788845,29.9905912412545,39.3343017080178));
#209473=CARTESIAN_POINT('Origin',(54.2668203812004,30.9643459342443,39.6398955068184));
#209474=CARTESIAN_POINT('Origin',(54.4211020372442,31.0534204898627,39.92499));
#209475=CARTESIAN_POINT('Origin',(52.5097763801592,29.949916107243,39.1934008539945));
#209476=CARTESIAN_POINT('Origin',(52.4710850656387,29.9275190026056,39.1160402713849));
#209477=CARTESIAN_POINT('Ctrl Pts',(54.5275217339724,31.4638515574734,40.1599502534424));
#209478=CARTESIAN_POINT('Ctrl Pts',(54.4952102564869,31.4452069629847,40.10025));
#209479=CARTESIAN_POINT('Ctrl Pts',(54.4342359163067,31.4100231232054,40.10025));
#209480=CARTESIAN_POINT('Ctrl Pts',(54.5715608148713,31.3875306471674,40.1599500538462));
#209481=CARTESIAN_POINT('Ctrl Pts',(54.5272862282505,31.389612165889,40.100244835349));
#209482=CARTESIAN_POINT('Ctrl Pts',(54.4597196360186,31.3658411130325,40.10025));
#209483=CARTESIAN_POINT('Ctrl Pts',(54.5905300051369,31.3046029601552,40.120244200104));
#209484=CARTESIAN_POINT('Ctrl Pts',(54.5367961153114,31.3268524737451,40.0633873868015));
#209485=CARTESIAN_POINT('Ctrl Pts',(54.4615686025423,31.3125672934286,40.0772271723538));
#209486=CARTESIAN_POINT('Ctrl Pts',(54.5809273110398,31.1759014746034,40.0045995998161));
#209487=CARTESIAN_POINT('Ctrl Pts',(54.5158579940075,31.2415992967178,39.9663485808318));
#209488=CARTESIAN_POINT('Ctrl Pts',(54.4295063924934,31.2227682191854,40.0101727202465));
#209489=CARTESIAN_POINT('Ctrl Pts',(54.5540292360084,31.1295364123882,39.930465434986));
#209490=CARTESIAN_POINT('Ctrl Pts',(54.4847364330958,31.2191033458804,39.9051900162941));
#209491=CARTESIAN_POINT('Ctrl Pts',(54.3969835118372,31.1861426211007,39.9671857458171));
#209492=CARTESIAN_POINT('Ctrl Pts',(54.5146464769142,31.1067982185528,39.8576902534424));
#209493=CARTESIAN_POINT('Ctrl Pts',(54.4512761425986,31.2174884860858,39.8573998014387));
#209494=CARTESIAN_POINT('Ctrl Pts',(54.3576020372442,31.1634057161433,39.92499));
#209495=CARTESIAN_POINT('Origin',(54.4342359163067,31.4100231232054,40.22725));
#209496=CARTESIAN_POINT('Origin',(0.158750000000002,-0.274963065701561,
39.116));
#209497=CARTESIAN_POINT('Origin',(52.123470313195,29.7268821954843,39.116));
#209498=CARTESIAN_POINT('Origin',(5.52187834149254E-15,5.61243978792563E-15,
40.22725));
#209499=CARTESIAN_POINT('Origin',(54.4189959163067,31.4364195775128,40.22725));
#209500=CARTESIAN_POINT('Ctrl Pts',(52.123470313195,29.7268821954843,38.989));
#209501=CARTESIAN_POINT('Ctrl Pts',(52.0598751873274,29.8370321846007,38.989));
#209502=CARTESIAN_POINT('Ctrl Pts',(52.0599703843398,29.8368672985386,39.1161901092325));
#209503=CARTESIAN_POINT('Ctrl Pts',(51.9354481180158,29.618592666444,38.989));
#209504=CARTESIAN_POINT('Ctrl Pts',(51.8721332875999,29.7286387544943,38.9892298989754));
#209505=CARTESIAN_POINT('Ctrl Pts',(51.9096995898764,29.7501084152007,39.1161900493205));
#209506=CARTESIAN_POINT('Ctrl Pts',(51.7564527430627,29.5155047636236,39.1034966344368));
#209507=CARTESIAN_POINT('Ctrl Pts',(51.693361622663,29.6254243098798,39.1038314102557));
#209508=CARTESIAN_POINT('Ctrl Pts',(51.7666446199927,29.667515590115,39.2077528789596));
#209509=CARTESIAN_POINT('Ctrl Pts',(51.6568155675431,29.4581217525667,39.2875012672119));
#209510=CARTESIAN_POINT('Ctrl Pts',(51.5939283753697,29.5680161811088,39.2878045257868));
#209511=CARTESIAN_POINT('Ctrl Pts',(51.6870133822667,29.6215404737376,39.3549015295901));
#209512=CARTESIAN_POINT('Origin',(51.7503740054947,29.5114749417999,39.3548010137695));
#209513=CARTESIAN_POINT('Ctrl Pts',(54.1966007261211,31.6576696180577,39.8576902534424));
#209514=CARTESIAN_POINT('Ctrl Pts',(54.2607761425987,31.5474441649277,39.8573998014387));
#209515=CARTESIAN_POINT('Ctrl Pts',(54.1671020372442,31.4933613949852,39.92499));
#209516=CARTESIAN_POINT('Ctrl Pts',(54.236001854427,31.6804173066,39.9304984902494));
#209517=CARTESIAN_POINT('Ctrl Pts',(54.2789150989591,31.5756301844099,39.9052171569793));
#209518=CARTESIAN_POINT('Ctrl Pts',(54.2065014563941,31.5161086602373,39.9672049726602));
#209519=CARTESIAN_POINT('Ctrl Pts',(54.2894509908546,31.6804328064617,40.0043437678658));
#209520=CARTESIAN_POINT('Ctrl Pts',(54.3138841827112,31.5911964272961,39.9661628577643));
#209521=CARTESIAN_POINT('Ctrl Pts',(54.2543268901843,31.5258675551963,40.0100243556234));
#209522=CARTESIAN_POINT('Ctrl Pts',(54.4049648787505,31.6250591602184,40.1194874821991));
#209523=CARTESIAN_POINT('Ctrl Pts',(54.3976088886511,31.5671393481771,40.0627551483141));
#209524=CARTESIAN_POINT('Ctrl Pts',(54.3475791360317,31.5090508246486,40.0767884282378));
#209525=CARTESIAN_POINT('Ctrl Pts',(54.4680334478299,31.5668453499333,40.1599502015398));
#209526=CARTESIAN_POINT('Ctrl Pts',(54.4477213412897,31.527422611143,40.1002449453872));
#209527=CARTESIAN_POINT('Ctrl Pts',(54.3933906465338,31.4807263372349,40.10025));
#209528=CARTESIAN_POINT('Ctrl Pts',(54.5122556166615,31.4902932482901,40.1599502534424));
#209529=CARTESIAN_POINT('Ctrl Pts',(54.4799531854483,31.4716329851982,40.10025));
#209530=CARTESIAN_POINT('Ctrl Pts',(54.4189959163067,31.4364195775128,40.10025));
#209531=CARTESIAN_POINT('Origin',(54.1036020372442,31.6033466212658,39.92499));
#209532=CARTESIAN_POINT('Origin',(51.5960921371897,29.422400263634,39.6398955069326));
#209533=CARTESIAN_POINT('Origin',(51.4418102687789,29.3333255853448,39.92499));
#209534=CARTESIAN_POINT('Origin',(53.9493203812093,31.5142720655996,39.6398955068286));
#209535=CARTESIAN_POINT('Origin',(53.7950387249983,31.4251975098786,39.3548010137695));
#209536=CARTESIAN_POINT('Ctrl Pts',(51.3482501200169,29.2799753962456,39.8576902534424));
#209537=CARTESIAN_POINT('Ctrl Pts',(51.2854610232005,29.3897042746967,39.8579948730703));
#209538=CARTESIAN_POINT('Ctrl Pts',(51.3783102687789,29.4433108116255,39.92499));
#209539=CARTESIAN_POINT('Ctrl Pts',(51.3089010921305,29.2572578385496,39.930402071123));
#209540=CARTESIAN_POINT('Ctrl Pts',(51.2670685993228,29.3615397594612,39.9058915297379));
#209541=CARTESIAN_POINT('Ctrl Pts',(51.3389598763137,29.420591851943,39.9671523786033));
#209542=CARTESIAN_POINT('Ctrl Pts',(51.255740761606,29.2572680623744,40.0043257306694));
#209543=CARTESIAN_POINT('Ctrl Pts',(51.2319924817695,29.3461554108682,39.9667894847842));
#209544=CARTESIAN_POINT('Ctrl Pts',(51.2913733902321,29.4109522357562,40.0100138975201));
#209545=CARTESIAN_POINT('Ctrl Pts',(51.141033386106,29.3127910737008,40.1195533054856));
#209546=CARTESIAN_POINT('Ctrl Pts',(51.1485922293425,29.3705286780139,40.0630813209231));
#209547=CARTESIAN_POINT('Ctrl Pts',(51.1987619028147,29.4282055900895,40.076826594242));
#209548=CARTESIAN_POINT('Ctrl Pts',(51.0785202710266,29.3710651187643,40.159950202751));
#209549=CARTESIAN_POINT('Ctrl Pts',(51.0989122516729,29.4103605382569,40.1002552791538));
#209550=CARTESIAN_POINT('Ctrl Pts',(51.1533747228781,29.4568175306711,40.10025));
#209551=CARTESIAN_POINT('Ctrl Pts',(51.0345602039891,29.4472515437729,40.1599502534424));
#209552=CARTESIAN_POINT('Ctrl Pts',(51.0668719738981,29.4658956314761,40.10025));
#209553=CARTESIAN_POINT('Ctrl Pts',(51.1278468659051,29.5010785149105,40.10025));
#209554=CARTESIAN_POINT('Origin',(51.1278468659051,29.5010785149105,40.22725));
#209555=CARTESIAN_POINT('Ctrl Pts',(53.421942799329,31.2097904767599,38.989));
#209556=CARTESIAN_POINT('Ctrl Pts',(53.4855376708633,31.0996409281618,38.989));
#209557=CARTESIAN_POINT('Ctrl Pts',(53.4854427285639,31.0998053730481,39.1161896013268));
#209558=CARTESIAN_POINT('Ctrl Pts',(53.6097387976563,31.3184716867868,38.989));
#209559=CARTESIAN_POINT('Ctrl Pts',(53.6736064794797,31.2082219299913,38.9887769275484));
#209560=CARTESIAN_POINT('Ctrl Pts',(53.6357132000302,31.1865640704867,39.116189882185));
#209561=CARTESIAN_POINT('Ctrl Pts',(53.788518680614,31.4219325588453,39.1034967087244));
#209562=CARTESIAN_POINT('Ctrl Pts',(53.8525981958187,31.3115622968575,39.1031720232692));
#209563=CARTESIAN_POINT('Ctrl Pts',(53.7787681009852,31.2691568563318,39.2077529614999));
#209564=CARTESIAN_POINT('Ctrl Pts',(53.8880358395974,31.4795232016783,39.2875012672119));
#209565=CARTESIAN_POINT('Ctrl Pts',(53.9523112232411,31.3691313396256,39.2872087095507));
#209566=CARTESIAN_POINT('Ctrl Pts',(53.8583991049523,31.3151318380577,39.3549017048228));
#209567=CARTESIAN_POINT('Origin',(53.421942799329,31.2097904767599,39.116));
#209568=CARTESIAN_POINT('Origin',(5.71547558359784E-15,5.28203651785913E-15,
40.22725));
#209569=CARTESIAN_POINT('Origin',(51.1126068659051,29.5274749692178,40.22725));
#209570=CARTESIAN_POINT('Origin',(46.508091798073,27.2180767400479,39.116));
#209571=CARTESIAN_POINT('Origin',(53.0743345559669,31.0091584503662,39.1160373285227));
#209572=CARTESIAN_POINT('Ctrl Pts',(51.0193480105331,29.4735998357331,40.1599502534424));
#209573=CARTESIAN_POINT('Ctrl Pts',(51.051650149069,29.492260605464,40.10025));
#209574=CARTESIAN_POINT('Ctrl Pts',(51.1126068659051,29.5274749692178,40.10025));
#209575=CARTESIAN_POINT('Ctrl Pts',(50.9754987628539,29.5495039426964,40.1599500566036));
#209576=CARTESIAN_POINT('Ctrl Pts',(51.0197013834521,29.547558101457,40.1002551305369));
#209577=CARTESIAN_POINT('Ctrl Pts',(51.0871269269775,29.5715624158005,40.10025));
#209578=CARTESIAN_POINT('Ctrl Pts',(50.9562029902292,29.6319914129666,40.1203070619046));
#209579=CARTESIAN_POINT('Ctrl Pts',(51.0098791271087,29.6100038038523,40.0637098684499));
#209580=CARTESIAN_POINT('Ctrl Pts',(51.0848223701587,29.6246193648989,40.0772636213361));
#209581=CARTESIAN_POINT('Ctrl Pts',(50.9652607924609,29.7600395375184,40.0046102245801));
#209582=CARTESIAN_POINT('Ctrl Pts',(51.0303675504168,29.6951164119088,39.9670001894011));
#209583=CARTESIAN_POINT('Ctrl Pts',(51.1161687394141,29.7140610042226,40.010178881121));
#209584=CARTESIAN_POINT('Ctrl Pts',(50.9919958361062,29.8061925581057,39.9303710930186));
#209585=CARTESIAN_POINT('Ctrl Pts',(51.061391271364,29.7178148857794,39.9058663574107));
#209586=CARTESIAN_POINT('Ctrl Pts',(51.1484765898563,29.7505571803532,39.9671344706363));
#209587=CARTESIAN_POINT('Ctrl Pts',(51.0313275753413,29.8289013456879,39.8576902534424));
#209588=CARTESIAN_POINT('Ctrl Pts',(51.0949610232005,29.7196599535386,39.8579948730703));
#209589=CARTESIAN_POINT('Ctrl Pts',(51.1878102687789,29.7732664904673,39.92499));
#209590=CARTESIAN_POINT('Origin',(51.1243102687789,29.883251716748,39.92499));
#209591=CARTESIAN_POINT('Origin',(53.036059682472,30.9870007553596,39.1925554488844));
#209592=CARTESIAN_POINT('Origin',(52.965185606085,30.9460815882862,39.3343017080178));
#209593=CARTESIAN_POINT('Origin',(51.2785921372027,29.9723263949817,39.6398955069224));
#209594=CARTESIAN_POINT('Origin',(51.4328740054947,30.061401073203,39.3548010137695));
#209595=CARTESIAN_POINT('Ctrl Pts',(52.6794317578291,30.7811015270737,39.3978017080178));
#209596=CARTESIAN_POINT('Ctrl Pts',(52.7429317578291,30.6711163007931,39.3978017080178));
#209597=CARTESIAN_POINT('Ctrl Pts',(52.7429317578291,30.671116300793,39.5248017080178));
#209598=CARTESIAN_POINT('Ctrl Pts',(52.7575002129179,30.8259039490945,39.3978017080178));
#209599=CARTESIAN_POINT('Ctrl Pts',(52.8208099140593,30.7160792752579,39.3980355775163));
#209600=CARTESIAN_POINT('Ctrl Pts',(52.8598573673292,30.7386233329131,39.5248015517192));
#209601=CARTESIAN_POINT('Ctrl Pts',(52.8313189037793,30.8682695960172,39.3484893995498));
#209602=CARTESIAN_POINT('Ctrl Pts',(52.8948168809868,30.7588072175363,39.3489438303427));
#209603=CARTESIAN_POINT('Ctrl Pts',(52.9704188493344,30.8024560343108,39.4508333155587));
#209604=CARTESIAN_POINT('Ctrl Pts',(52.870221513222,30.8905967158729,39.2708017080178));
#209605=CARTESIAN_POINT('Ctrl Pts',(52.9338619179799,30.7813498801525,39.2710850691866));
#209606=CARTESIAN_POINT('Ctrl Pts',(53.028685606085,30.8360963620055,39.3343017080178));
#209607=CARTESIAN_POINT('Origin',(52.6794317578291,30.7811015270737,39.5248017080178));
#209608=CARTESIAN_POINT('Ctrl Pts',(51.3398895692701,30.0070536838151,39.2875012672119));
#209609=CARTESIAN_POINT('Ctrl Pts',(51.4036173326916,29.8976445761568,39.2878045257519));
#209610=CARTESIAN_POINT('Ctrl Pts',(51.4965132298827,29.9514963916948,39.3549015218349));
#209611=CARTESIAN_POINT('Ctrl Pts',(51.439404806058,30.0646513737711,39.1034938540228));
#209612=CARTESIAN_POINT('Ctrl Pts',(51.5030523579595,29.9550530981016,39.1038286278801));
#209613=CARTESIAN_POINT('Ctrl Pts',(51.5761456730019,29.9974722043254,39.2077506434027));
#209614=CARTESIAN_POINT('Ctrl Pts',(51.6181806476922,30.1681227811157,38.989));
#209615=CARTESIAN_POINT('Ctrl Pts',(51.68182592798,30.0582674911773,38.9892298954611));
#209616=CARTESIAN_POINT('Ctrl Pts',(51.7192017762877,30.0800656843523,39.1161900347292));
#209617=CARTESIAN_POINT('Ctrl Pts',(51.805970313195,30.2768083268874,38.989));
#209618=CARTESIAN_POINT('Ctrl Pts',(51.8695654317178,30.1666583504926,38.989));
#209619=CARTESIAN_POINT('Ctrl Pts',(51.8694702420612,30.1668232238141,39.1161900945648));
#209620=CARTESIAN_POINT('Origin',(51.805970313195,30.2768083268874,39.116));
#209621=CARTESIAN_POINT('Origin',(45.3776875000007,26.5654375142628,39.5248017080178));
#209622=CARTESIAN_POINT('Origin',(52.5484816883963,30.7054974692362,39.5248017080178));
#209623=CARTESIAN_POINT('Origin',(45.2006711678738,26.4632370872583,39.116));
#209624=CARTESIAN_POINT('Origin',(52.1535342613181,30.4775331296733,39.1160402713849));
#209625=CARTESIAN_POINT('Ctrl Pts',(52.3576880233166,30.5960088312562,39.2708017080178));
#209626=CARTESIAN_POINT('Ctrl Pts',(52.421911104956,30.4857749404413,39.27051194648));
#209627=CARTESIAN_POINT('Ctrl Pts',(52.3262277788845,30.430532146377,39.3343017080178));
#209628=CARTESIAN_POINT('Ctrl Pts',(52.3967235457366,30.6184089696604,39.3487519301186));
#209629=CARTESIAN_POINT('Ctrl Pts',(52.4606806140229,30.5081585269356,39.3482879463987));
#209630=CARTESIAN_POINT('Ctrl Pts',(52.3846914485017,30.4642861617683,39.4512271261638));
#209631=CARTESIAN_POINT('Ctrl Pts',(52.4706758922783,30.6608464521626,39.3978017080178));
#209632=CARTESIAN_POINT('Ctrl Pts',(52.5342179826637,30.5506153465189,39.3975673827378));
#209633=CARTESIAN_POINT('Ctrl Pts',(52.4954499175228,30.5282325936726,39.524801535518));
#209634=CARTESIAN_POINT('Ctrl Pts',(52.5484816883963,30.7054974692362,39.3978017080178));
#209635=CARTESIAN_POINT('Ctrl Pts',(52.6119816883963,30.5955122429556,39.3978017080178));
#209636=CARTESIAN_POINT('Ctrl Pts',(52.6119816883963,30.5955122429556,39.5248017080178));
#209637=CARTESIAN_POINT('Origin',(52.2627277788845,30.5405173726576,39.3343017080178));
#209638=CARTESIAN_POINT('Origin',(52.1922763809709,30.4998422394554,39.1934008533551));
#209639=CARTESIAN_POINT('Origin',(56.2428239377263,24.693371541728,39.192555449508));
#209640=CARTESIAN_POINT('Origin',(56.2832472948506,24.7113125977902,39.1160373285274));
#209641=CARTESIAN_POINT('Origin',(56.1680608984281,24.6600848917104,39.3343017080178));
#209642=CARTESIAN_POINT('Ctrl Pts',(56.0673542004329,24.6158705164587,39.2708017080178));
#209643=CARTESIAN_POINT('Ctrl Pts',(56.0163785451201,24.7315703643328,39.2710850691866));
#209644=CARTESIAN_POINT('Ctrl Pts',(56.1164053447575,24.776105164831,39.3343017080178));
#209645=CARTESIAN_POINT('Ctrl Pts',(56.0262864882908,24.5974591883324,39.3487519293518));
#209646=CARTESIAN_POINT('Ctrl Pts',(55.9750519161942,24.7131705636675,39.3492068662925));
#209647=CARTESIAN_POINT('Ctrl Pts',(56.0547337128493,24.7486471852357,39.4512271248734));
#209648=CARTESIAN_POINT('Ctrl Pts',(55.9484840819673,24.5625784858799,39.3978017080178));
#209649=CARTESIAN_POINT('Ctrl Pts',(55.8968463240326,24.6783511906874,39.3980347781178));
#209650=CARTESIAN_POINT('Ctrl Pts',(55.9378977967849,24.6966284839295,39.5248015355195));
#209651=CARTESIAN_POINT('Ctrl Pts',(55.8666273273836,24.5258780191664,39.3978017080178));
#209652=CARTESIAN_POINT('Ctrl Pts',(55.814971773713,24.641898292287,39.3978017080178));
#209653=CARTESIAN_POINT('Ctrl Pts',(55.814971773713,24.641898292287,39.5248017080178));
#209654=CARTESIAN_POINT('Origin',(55.8666273273836,24.5258780191664,39.5248017080178));
#209655=CARTESIAN_POINT('Origin',(0.129138884176568,-0.290050682801527,
39.116));
#209656=CARTESIAN_POINT('Origin',(56.6498810128385,24.8746050278046,39.116));
#209657=CARTESIAN_POINT('Origin',(0.129138884176569,-0.290050682801527,
39.5248017080178));
#209658=CARTESIAN_POINT('Origin',(55.7284918401501,24.464376137791,39.5248017080178));
#209659=CARTESIAN_POINT('Ctrl Pts',(57.1420619865024,25.0931373005739,39.2875012672119));
#209660=CARTESIAN_POINT('Ctrl Pts',(57.0905332211014,25.2100238766572,39.287208709576));
#209661=CARTESIAN_POINT('Ctrl Pts',(56.9916465525426,25.1657875015258,39.3549016990122));
#209662=CARTESIAN_POINT('Ctrl Pts',(57.0369738651805,25.0464764504221,39.103493917393));
#209663=CARTESIAN_POINT('Ctrl Pts',(56.9853474458591,25.163191867418,39.1031692336325));
#209664=CARTESIAN_POINT('Ctrl Pts',(56.907644805189,25.1283875141298,39.2077507202298));
#209665=CARTESIAN_POINT('Ctrl Pts',(56.8481865914868,24.9626525995183,38.989));
#209666=CARTESIAN_POINT('Ctrl Pts',(56.7965331449327,25.0791258042751,38.9887769311176));
#209667=CARTESIAN_POINT('Ctrl Pts',(56.7567390814052,25.0611999573797,39.1161898712914));
#209668=CARTESIAN_POINT('Ctrl Pts',(56.6498810128385,24.8746050278046,38.989));
#209669=CARTESIAN_POINT('Ctrl Pts',(56.5981482881661,24.9907986298331,38.989));
#209670=CARTESIAN_POINT('Ctrl Pts',(56.5982255167267,24.9906251716458,39.1161895903853));
#209671=CARTESIAN_POINT('Origin',(57.0434492461382,25.0498328948958,39.3548010137695));
#209672=CARTESIAN_POINT('Ctrl Pts',(55.7284918401501,24.464376137791,39.3978017080178));
#209673=CARTESIAN_POINT('Ctrl Pts',(55.6768362864795,24.5803964109116,39.3978017080178));
#209674=CARTESIAN_POINT('Ctrl Pts',(55.6768362864795,24.5803964109116,39.5248017080178));
#209675=CARTESIAN_POINT('Ctrl Pts',(55.6463586582052,24.4275510972984,39.3978017080178));
#209676=CARTESIAN_POINT('Ctrl Pts',(55.5945285148525,24.5437506299592,39.3975666025021));
#209677=CARTESIAN_POINT('Ctrl Pts',(55.5534947903273,24.5254812387358,39.5248015517177));
#209678=CARTESIAN_POINT('Ctrl Pts',(55.5686962576402,24.3927285408614,39.3484894016716));
#209679=CARTESIAN_POINT('Ctrl Pts',(55.5170953257129,24.5092751529609,39.3480259000051));
#209680=CARTESIAN_POINT('Ctrl Pts',(55.4368666119038,24.4735550281864,39.4508333188952));
#209681=CARTESIAN_POINT('Ctrl Pts',(55.5277679687686,24.3743766270207,39.2708017080178));
#209682=CARTESIAN_POINT('Ctrl Pts',(55.4763362579877,24.4911280468219,39.27051194648));
#209683=CARTESIAN_POINT('Ctrl Pts',(55.3754026508178,24.4461895095982,39.3343017080178));
#209684=CARTESIAN_POINT('Origin',(55.4270582044884,24.3301692364776,39.3343017080178));
#209685=CARTESIAN_POINT('Origin',(57.2061965577142,25.1222926664913,39.6398955068201));
#209686=CARTESIAN_POINT('Origin',(57.3689438691199,25.1947524379609,39.92499));
#209687=CARTESIAN_POINT('Origin',(55.3527410366463,24.2970811015511,39.1934008539938));
#209688=CARTESIAN_POINT('Origin',(55.3119205422648,24.2788510342435,39.1160402713851));
#209689=CARTESIAN_POINT('Ctrl Pts',(57.5176823163891,25.5918112338787,40.1599502534424));
#209690=CARTESIAN_POINT('Ctrl Pts',(57.4835989537481,25.5766462455169,40.10025));
#209691=CARTESIAN_POINT('Ctrl Pts',(57.4192809246792,25.5480287005711,40.10025));
#209692=CARTESIAN_POINT('Ctrl Pts',(57.5535024391262,25.511305080055,40.1599500538472));
#209693=CARTESIAN_POINT('Ctrl Pts',(57.5096879712787,25.5180031505012,40.1002448353493));
#209694=CARTESIAN_POINT('Ctrl Pts',(57.4400067642829,25.5014249500138,40.10025));
#209695=CARTESIAN_POINT('Ctrl Pts',(57.5636994104965,25.4268488592814,40.1202442001043));
#209696=CARTESIAN_POINT('Ctrl Pts',(57.5125855880059,25.454593208637,40.0633873868017));
#209697=CARTESIAN_POINT('Ctrl Pts',(57.4362769714774,25.448249700338,40.0772271723539));
#209698=CARTESIAN_POINT('Ctrl Pts',(57.5406963524572,25.2998561687904,40.0045995998158));
#209699=CARTESIAN_POINT('Ctrl Pts',(57.4828507843374,25.371995687076,39.9663485808314));
#209700=CARTESIAN_POINT('Ctrl Pts',(57.3950038423349,25.3622939683639,40.0101727202464));
#209701=CARTESIAN_POINT('Ctrl Pts',(57.5090991591926,25.2565567136858,39.9304654349862));
#209702=CARTESIAN_POINT('Ctrl Pts',(57.4495482434219,25.3528760603468,39.9051900162946));
#209703=CARTESIAN_POINT('Ctrl Pts',(57.3588307079385,25.3292685758741,39.9671857458179));
#209704=CARTESIAN_POINT('Ctrl Pts',(57.4675553545144,25.2380597013423,39.8576902534424));
#209705=CARTESIAN_POINT('Ctrl Pts',(57.4161024530847,25.3547675996708,39.8573998014387));
#209706=CARTESIAN_POINT('Ctrl Pts',(57.3172883154493,25.3107727110816,39.92499));
#209707=CARTESIAN_POINT('Origin',(57.4192809246792,25.5480287005711,40.22725));
#209708=CARTESIAN_POINT('Origin',(0.129138884176568,-0.290050682801527,
39.116));
#209709=CARTESIAN_POINT('Origin',(54.9452378026832,24.115648972427,39.116));
#209710=CARTESIAN_POINT('Origin',(5.51404277916147E-15,5.62781794487312E-15,
40.22725));
#209711=CARTESIAN_POINT('Origin',(57.4068835917983,25.5758735661201,40.22725));
#209712=CARTESIAN_POINT('Ctrl Pts',(54.9452378026832,24.115648972427,38.989));
#209713=CARTESIAN_POINT('Ctrl Pts',(54.8935048666606,24.2318430491557,38.989));
#209714=CARTESIAN_POINT('Ctrl Pts',(54.8935823068869,24.2316691155597,39.1161901092321));
#209715=CARTESIAN_POINT('Ctrl Pts',(54.7469262747045,24.0276063358778,38.989));
#209716=CARTESIAN_POINT('Ctrl Pts',(54.6954612380262,24.14366778187,38.989229898976));
#209717=CARTESIAN_POINT('Ctrl Pts',(54.7350659388069,24.1610930816809,39.1161900493201));
#209718=CARTESIAN_POINT('Ctrl Pts',(54.5581358350802,23.9437932708521,39.1034966344368));
#209719=CARTESIAN_POINT('Ctrl Pts',(54.5068800556915,24.0597054841971,39.1038314102553));
#209720=CARTESIAN_POINT('Ctrl Pts',(54.5841613379366,24.0939060248992,39.2077528789598));
#209721=CARTESIAN_POINT('Ctrl Pts',(54.4530463244696,23.8971395307762,39.2875012672119));
#209722=CARTESIAN_POINT('Ctrl Pts',(54.4019907306522,24.0130054476969,39.2878045257868));
#209723=CARTESIAN_POINT('Ctrl Pts',(54.5001606201972,24.0565064959264,39.3549015295898));
#209724=CARTESIAN_POINT('Origin',(54.5516691663898,23.9404209259114,39.3548010137695));
#209725=CARTESIAN_POINT('Ctrl Pts',(57.2088336324702,25.8191582032614,39.8576902534424));
#209726=CARTESIAN_POINT('Ctrl Pts',(57.2611357920728,25.7028284190327,39.8573998014387));
#209727=CARTESIAN_POINT('Ctrl Pts',(57.1623216544374,25.6588335304434,39.92499));
#209728=CARTESIAN_POINT('Ctrl Pts',(57.2503966981987,25.8376627381923,39.9304984902489));
#209729=CARTESIAN_POINT('Ctrl Pts',(57.2821216226336,25.7289639953167,39.9052171569796));
#209730=CARTESIAN_POINT('Ctrl Pts',(57.2038829761268,25.6773378230588,39.9672049726602));
#209731=CARTESIAN_POINT('Ctrl Pts',(57.3035546548415,25.8320911970513,40.0043437678664));
#209732=CARTESIAN_POINT('Ctrl Pts',(57.3185262575354,25.7407897001102,39.9661628577643));
#209733=CARTESIAN_POINT('Ctrl Pts',(57.2524664994806,25.6820441386711,40.0100243556235));
#209734=CARTESIAN_POINT('Ctrl Pts',(57.4126476234253,25.7649464042474,40.1194874821986));
#209735=CARTESIAN_POINT('Ctrl Pts',(57.3992776612634,25.7081127933376,40.062755148314));
#209736=CARTESIAN_POINT('Ctrl Pts',(57.3434500727659,25.6555720179782,40.0767884282377));
#209737=CARTESIAN_POINT('Ctrl Pts',(57.4692856961537,25.7004590346998,40.1599502015384));
#209738=CARTESIAN_POINT('Ctrl Pts',(57.4449640631527,25.6633754510788,40.1002449453869));
#209739=CARTESIAN_POINT('Ctrl Pts',(57.3860499078766,25.6226140882765,40.10025));
#209740=CARTESIAN_POINT('Ctrl Pts',(57.5052637377735,25.6197038181291,40.1599502534424));
#209741=CARTESIAN_POINT('Ctrl Pts',(57.4711877340332,25.6045223014054,40.10025));
#209742=CARTESIAN_POINT('Ctrl Pts',(57.4068835917983,25.5758735661201,40.10025));
#209743=CARTESIAN_POINT('Origin',(57.1106661007668,25.774853803564,39.92499));
#209744=CARTESIAN_POINT('Origin',(54.3889216310757,23.8679610547579,39.639895506932));
#209745=CARTESIAN_POINT('Origin',(54.2261740956469,23.7955011834902,39.92499));
#209746=CARTESIAN_POINT('Origin',(56.9479187893705,25.7023940320462,39.6398955068271));
#209747=CARTESIAN_POINT('Origin',(56.7851714777851,25.6299342604988,39.3548010137695));
#209748=CARTESIAN_POINT('Ctrl Pts',(54.1275498658877,23.7522229508821,39.8576902534424));
#209749=CARTESIAN_POINT('Ctrl Pts',(54.0765745253539,23.8679139708562,39.8579948730703));
#209750=CARTESIAN_POINT('Ctrl Pts',(54.1745185419763,23.9115214566108,39.92499));
#209751=CARTESIAN_POINT('Ctrl Pts',(54.0860417646979,23.7337429357601,39.9304020711232));
#209752=CARTESIAN_POINT('Ctrl Pts',(54.0553388636001,23.8418262755854,39.905891529737));
#209753=CARTESIAN_POINT('Ctrl Pts',(54.1330089371354,23.8930401898198,39.9671523786031));
#209754=CARTESIAN_POINT('Ctrl Pts',(54.0331737207073,23.7393098712341,40.0043257306692));
#209755=CARTESIAN_POINT('Ctrl Pts',(54.0188467943745,23.8301926567289,39.9667894847835));
#209756=CARTESIAN_POINT('Ctrl Pts',(54.0846755205376,23.8884275227217,40.01001389752));
#209757=CARTESIAN_POINT('Ctrl Pts',(53.9248984592617,23.8065189073819,40.1195533054859));
#209758=CARTESIAN_POINT('Ctrl Pts',(53.9384511174158,23.8631501047899,40.0630813209236));
#209759=CARTESIAN_POINT('Ctrl Pts',(53.9943748351526,23.9152668978354,40.0768265942421));
#209760=CARTESIAN_POINT('Ctrl Pts',(53.8688190939463,23.8710081209819,40.1599502027519));
#209761=CARTESIAN_POINT('Ctrl Pts',(53.8932068549991,23.9079567336536,40.1002552791553));
#209762=CARTESIAN_POINT('Ctrl Pts',(53.952227053116,23.948466351383,40.10025));
#209763=CARTESIAN_POINT('Ctrl Pts',(53.8330634946841,23.9513722670358,40.1599502534424));
#209764=CARTESIAN_POINT('Ctrl Pts',(53.8671470951733,23.9665367208217,40.10025));
#209765=CARTESIAN_POINT('Ctrl Pts',(53.9314655730807,23.9951532569801,40.10025));
#209766=CARTESIAN_POINT('Origin',(53.9314655730807,23.9951532569801,40.22725));
#209767=CARTESIAN_POINT('Ctrl Pts',(56.3916032444854,25.4547063934076,38.989));
#209768=CARTESIAN_POINT('Ctrl Pts',(56.4433359736148,25.3385127813685,38.989));
#209769=CARTESIAN_POINT('Ctrl Pts',(56.4432587405905,25.3386862495813,39.116189601327));
#209770=CARTESIAN_POINT('Ctrl Pts',(56.589730756555,25.5431622092807,38.989));
#209771=CARTESIAN_POINT('Ctrl Pts',(56.6417243268786,25.426840421554,38.9887769275436));
#209772=CARTESIAN_POINT('Ctrl Pts',(56.6017747680085,25.4092621323405,39.1161898821828));
#209773=CARTESIAN_POINT('Ctrl Pts',(56.7783458705717,25.6273687254292,39.1034967087243));
#209774=CARTESIAN_POINT('Ctrl Pts',(56.8305375176146,25.5109049500354,39.1031720232718));
#209775=CARTESIAN_POINT('Ctrl Pts',(56.7526792962312,25.4764491573039,39.2077529615015));
#209776=CARTESIAN_POINT('Ctrl Pts',(56.8833377255397,25.6742415049973,39.2875012672119));
#209777=CARTESIAN_POINT('Ctrl Pts',(56.9357219102091,25.557735774037,39.2872087095508));
#209778=CARTESIAN_POINT('Ctrl Pts',(56.836679767414,25.5138485767958,39.354901704823));
#209779=CARTESIAN_POINT('Origin',(56.3916032444854,25.4547063934076,39.116));
#209780=CARTESIAN_POINT('Origin',(5.71826297912856E-15,5.27656594610754E-15,
40.22725));
#209781=CARTESIAN_POINT('Origin',(53.9190682401998,24.022998122529,40.22725));
#209782=CARTESIAN_POINT('Origin',(51.7995637473369,23.4101986852074,39.116));
#209783=CARTESIAN_POINT('Origin',(56.0249274780513,25.2915084057482,39.1160373285258));
#209784=CARTESIAN_POINT('Ctrl Pts',(53.8206887816839,23.9791663275007,40.1599502534424));
#209785=CARTESIAN_POINT('Ctrl Pts',(53.8547645473084,23.9943483786811,40.10025));
#209786=CARTESIAN_POINT('Ctrl Pts',(53.9190682401998,24.022998122529,40.10025));
#209787=CARTESIAN_POINT('Ctrl Pts',(53.7850138844278,24.0592381182994,40.159950056604));
#209788=CARTESIAN_POINT('Ctrl Pts',(53.8287709626494,24.0526825045778,40.1002551305369));
#209789=CARTESIAN_POINT('Ctrl Pts',(53.8983362760826,24.069507432326,40.10025));
#209790=CARTESIAN_POINT('Ctrl Pts',(53.7744461045709,24.1432906710366,40.1203070619048));
#209791=CARTESIAN_POINT('Ctrl Pts',(53.8255298669647,24.1158128282433,40.0637098684499));
#209792=CARTESIAN_POINT('Ctrl Pts',(53.9015903052237,24.122514621689,40.0772636213363));
#209793=CARTESIAN_POINT('Ctrl Pts',(53.796838960898,24.2696905364166,40.00461022458));
#209794=CARTESIAN_POINT('Ctrl Pts',(53.854802742671,24.1983175571248,39.9670001894012));
#209795=CARTESIAN_POINT('Ctrl Pts',(53.9421141528994,24.2081897025472,40.0101788811209));
#209796=CARTESIAN_POINT('Ctrl Pts',(53.8282518514941,24.3127961529,39.9303710930187));
#209797=CARTESIAN_POINT('Ctrl Pts',(53.8880291490201,24.2176488245059,39.90586635741));
#209798=CARTESIAN_POINT('Ctrl Pts',(53.9780599067612,24.2411088588473,39.9671344706352));
#209799=CARTESIAN_POINT('Ctrl Pts',(53.8697418420148,24.3312692531081,39.8576902534424));
#209800=CARTESIAN_POINT('Ctrl Pts',(53.921607864342,24.215974790218,39.8579948730703));
#209801=CARTESIAN_POINT('Ctrl Pts',(54.0195518809644,24.2595822759726,39.92499));
#209802=CARTESIAN_POINT('Origin',(53.9678963272938,24.3756025490932,39.92499));
#209803=CARTESIAN_POINT('Origin',(55.9845461685092,25.2734729066187,39.192555448885));
#209804=CARTESIAN_POINT('Origin',(55.909783130075,25.2401862573135,39.3343017080178));
#209805=CARTESIAN_POINT('Origin',(54.1306438627302,24.448062420301,39.6398955069211));
#209806=CARTESIAN_POINT('Origin',(54.2933913980367,24.5205222915145,39.3548010137695));
#209807=CARTESIAN_POINT('Ctrl Pts',(55.6083495590305,25.1059793847695,39.3978017080178));
#209808=CARTESIAN_POINT('Ctrl Pts',(55.6600051127011,24.9899591116489,39.3978017080178));
#209809=CARTESIAN_POINT('Ctrl Pts',(55.6600051127011,24.9899591116489,39.5248017080178));
#209810=CARTESIAN_POINT('Ctrl Pts',(55.6906734752783,25.1423759987946,39.3978017080178));
#209811=CARTESIAN_POINT('Ctrl Pts',(55.7421565548657,25.0265352902402,39.3980355775196));
#209812=CARTESIAN_POINT('Ctrl Pts',(55.7833465978042,25.0448742789053,39.5248015517192));
#209813=CARTESIAN_POINT('Ctrl Pts',(55.768516195596,25.1767934079536,39.3484893995498));
#209814=CARTESIAN_POINT('Ctrl Pts',(55.8202243900357,25.0612933298582,39.3489438303412));
#209815=CARTESIAN_POINT('Ctrl Pts',(55.899974746629,25.0968004762766,39.4508333155591));
#209816=CARTESIAN_POINT('Ctrl Pts',(55.809539512001,25.1949317875294,39.2708017080178));
#209817=CARTESIAN_POINT('Ctrl Pts',(55.8614118841082,25.0796311836947,39.2710850691866));
#209818=CARTESIAN_POINT('Ctrl Pts',(55.9614386837456,25.1241659841929,39.3343017080178));
#209819=CARTESIAN_POINT('Origin',(55.6083495590305,25.1059793847695,39.5248017080178));
#209820=CARTESIAN_POINT('Ctrl Pts',(54.1952354911875,24.4761921430385,39.2875012672119));
#209821=CARTESIAN_POINT('Ctrl Pts',(54.2471777813619,24.360721024742,39.2878045257519));
#209822=CARTESIAN_POINT('Ctrl Pts',(54.3451938326306,24.4045675690222,39.3549015218347));
#209823=CARTESIAN_POINT('Ctrl Pts',(54.3002261711149,24.5230721320487,39.1034938540228));
#209824=CARTESIAN_POINT('Ctrl Pts',(54.3520689157361,24.407421266411,39.1038286278805));
#209825=CARTESIAN_POINT('Ctrl Pts',(54.4291958219375,24.4419676644359,39.2077506434029));
#209826=CARTESIAN_POINT('Ctrl Pts',(54.4888383671844,24.6072895482032,38.989));
#209827=CARTESIAN_POINT('Ctrl Pts',(54.5406519873275,24.4913833136937,38.9892298954611));
#209828=CARTESIAN_POINT('Ctrl Pts',(54.5801016184621,24.5091552540987,39.1161900347288));
#209829=CARTESIAN_POINT('Ctrl Pts',(54.68696003433,24.6957503380301,38.989));
#209830=CARTESIAN_POINT('Ctrl Pts',(54.7386929643778,24.5795562747209,38.989));
#209831=CARTESIAN_POINT('Ctrl Pts',(54.7386155301352,24.5797301948774,39.1161900945645));
#209832=CARTESIAN_POINT('Origin',(54.68696003433,24.6957503380301,39.116));
#209833=CARTESIAN_POINT('Origin',(50.5417021396889,22.8501626153342,39.5248017080178));
#209834=CARTESIAN_POINT('Origin',(55.470214071797,25.0444775033941,39.5248017080178));
#209835=CARTESIAN_POINT('Origin',(50.3447265545032,22.7624634345041,39.116));
#209836=CARTESIAN_POINT('Origin',(55.0536014459541,24.8590452239595,39.1160402713848));
#209837=CARTESIAN_POINT('Ctrl Pts',(55.2690209153043,24.9555320242408,39.2708017080178));
#209838=CARTESIAN_POINT('Ctrl Pts',(55.3213695969759,24.8391888661838,39.27051194648));
#209839=CARTESIAN_POINT('Ctrl Pts',(55.2204359898059,24.79425032896,39.3343017080178));
#209840=CARTESIAN_POINT('Ctrl Pts',(55.3101840490931,24.9737291291706,39.3487519301186));
#209841=CARTESIAN_POINT('Ctrl Pts',(55.3622664445099,24.8573973158458,39.3482879463992));
#209842=CARTESIAN_POINT('Ctrl Pts',(55.2821076446824,24.8217083187815,39.4512271261636));
#209843=CARTESIAN_POINT('Ctrl Pts',(55.3881672017734,25.0082040095645,39.3978017080178));
#209844=CARTESIAN_POINT('Ctrl Pts',(55.4398389138645,24.8919348043911,39.3975673827383));
#209845=CARTESIAN_POINT('Ctrl Pts',(55.3989435894786,24.8737270328799,39.524801535518));
#209846=CARTESIAN_POINT('Ctrl Pts',(55.470214071797,25.0444775033941,39.3978017080178));
#209847=CARTESIAN_POINT('Ctrl Pts',(55.5218696254676,24.9284572302735,39.3978017080178));
#209848=CARTESIAN_POINT('Ctrl Pts',(55.5218696254676,24.9284572302735,39.5248017080178));
#209849=CARTESIAN_POINT('Origin',(55.1687804361353,24.9102706020807,39.3343017080178));
#209850=CARTESIAN_POINT('Origin',(55.0944632691829,24.8771824678734,39.1934008533556));
#209851=CARTESIAN_POINT('Origin',(58.5158800435652,18.6791227126689,39.1925554495078));
#209852=CARTESIAN_POINT('Origin',(58.5579573083286,18.6927400943489,39.1160373285261));
#209853=CARTESIAN_POINT('Origin',(58.4380471616457,18.6538332760097,39.3343017080178));
#209854=CARTESIAN_POINT('Ctrl Pts',(58.3332704847798,18.620387828114,39.2708017080178));
#209855=CARTESIAN_POINT('Ctrl Pts',(58.2946680067391,18.7407822670295,39.2710850691866));
#209856=CARTESIAN_POINT('Ctrl Pts',(58.3988020033601,18.7746174535792,39.3343017080178));
#209857=CARTESIAN_POINT('Ctrl Pts',(58.2905032380261,18.6063701040097,39.3487519293518));
#209858=CARTESIAN_POINT('Ctrl Pts',(58.2516444665234,18.7268030714124,39.3492068662928));
#209859=CARTESIAN_POINT('Ctrl Pts',(58.3345980746935,18.7537563325799,39.4512271248736));
#209860=CARTESIAN_POINT('Ctrl Pts',(58.2094810152003,18.5798130476652,39.3978017080178));
#209861=CARTESIAN_POINT('Ctrl Pts',(58.1702276772277,18.7003491529652,39.3980347781178));
#209862=CARTESIAN_POINT('Ctrl Pts',(58.2129647630919,18.7142352739225,39.5248015355195));
#209863=CARTESIAN_POINT('Ctrl Pts',(58.1242364370959,18.5518699907143,39.3978017080178));
#209864=CARTESIAN_POINT('Ctrl Pts',(58.0849912788103,18.6726541682838,39.3978017080178));
#209865=CARTESIAN_POINT('Ctrl Pts',(58.0849912788103,18.6726541682838,39.5248017080178));
#209866=CARTESIAN_POINT('Origin',(58.1242364370959,18.5518699907143,39.5248017080178));
#209867=CARTESIAN_POINT('Origin',(0.0981128957140474,-0.301960443923713,
39.116));
#209868=CARTESIAN_POINT('Origin',(58.9396512752216,18.8168143322219,39.116));
#209869=CARTESIAN_POINT('Origin',(0.0981128957140474,-0.301960443923713,
39.5248017080178));
#209870=CARTESIAN_POINT('Origin',(57.9804289733666,18.5051441132834,39.5248017080178));
#209871=CARTESIAN_POINT('Ctrl Pts',(59.451978872661,18.9827025415089,39.2875012672119));
#209872=CARTESIAN_POINT('Ctrl Pts',(59.4129503614028,19.1043350233602,39.287208709576));
#209873=CARTESIAN_POINT('Ctrl Pts',(59.309981444048,19.070677451222,39.3549016990123));
#209874=CARTESIAN_POINT('Ctrl Pts',(59.3425890481026,18.9472820042042,39.1034939173931));
#209875=CARTESIAN_POINT('Ctrl Pts',(59.3034455268856,19.0687544722107,39.1031692336326));
#209876=CARTESIAN_POINT('Ctrl Pts',(59.2225305038488,19.0422629184335,39.2077507202294));
#209877=CARTESIAN_POINT('Ctrl Pts',(59.1460739925267,18.8836509927317,38.989));
#209878=CARTESIAN_POINT('Ctrl Pts',(59.1068782740625,19.0048854004773,38.9887769311176));
#209879=CARTESIAN_POINT('Ctrl Pts',(59.0654284453484,18.9912173655536,39.1161898712917));
#209880=CARTESIAN_POINT('Ctrl Pts',(58.9396512752216,18.8168143322219,38.989));
#209881=CARTESIAN_POINT('Ctrl Pts',(58.9003474864893,18.9377789557519,38.989));
#209882=CARTESIAN_POINT('Ctrl Pts',(58.9004061606662,18.9375983752037,39.1161895903856));
#209883=CARTESIAN_POINT('Origin',(59.3493798002282,18.949943200105,39.3548010137695));
#209884=CARTESIAN_POINT('Ctrl Pts',(57.9804289733666,18.5051441132834,39.3978017080178));
#209885=CARTESIAN_POINT('Ctrl Pts',(57.941183815081,18.6259282908529,39.3978017080178));
#209886=CARTESIAN_POINT('Ctrl Pts',(57.941183815081,18.6259282908529,39.5248017080178));
#209887=CARTESIAN_POINT('Ctrl Pts',(57.8948964606935,18.4771060595082,39.3978017080178));
#209888=CARTESIAN_POINT('Ctrl Pts',(57.8554964068674,18.5980867642064,39.3975666025026));
#209889=CARTESIAN_POINT('Ctrl Pts',(57.8127777979911,18.5842066467856,39.5248015517177));
#209890=CARTESIAN_POINT('Ctrl Pts',(57.8140195545736,18.4505921960626,39.3484894016716));
#209891=CARTESIAN_POINT('Ctrl Pts',(57.7748837362164,18.5718941197449,39.3480259000037));
#209892=CARTESIAN_POINT('Ctrl Pts',(57.6913607539432,18.544755857716,39.4508333188947));
#209893=CARTESIAN_POINT('Ctrl Pts',(57.7713971777989,18.4366189870665,39.2708017080178));
#209894=CARTESIAN_POINT('Ctrl Pts',(57.7324510618073,18.5581069080653,39.27051194648));
#209895=CARTESIAN_POINT('Ctrl Pts',(57.6273730232608,18.5239649837,39.3343017080178));
#209896=CARTESIAN_POINT('Origin',(57.6666181815464,18.4031808061306,39.3343017080178));
#209897=CARTESIAN_POINT('Origin',(59.5188096735781,19.0049943031103,39.6398955068192));
#209898=CARTESIAN_POINT('Origin',(59.6882395467423,19.0600454060079,39.92499));
#209899=CARTESIAN_POINT('Origin',(57.5892494790285,18.3780421908169,39.1934008539945));
#209900=CARTESIAN_POINT('Origin',(57.5467470426663,18.3641788932747,39.1160402713848));
#209901=CARTESIAN_POINT('Ctrl Pts',(59.8776671349988,19.4393816709748,40.1599502534424));
#209902=CARTESIAN_POINT('Ctrl Pts',(59.8421853116555,19.4278624395259,40.10025));
#209903=CARTESIAN_POINT('Ctrl Pts',(59.7752282754839,19.4061247292246,40.10025));
#209904=CARTESIAN_POINT('Ctrl Pts',(59.9048758468125,19.3555723159016,40.1599500538468));
#209905=CARTESIAN_POINT('Ctrl Pts',(59.8620015382151,19.3668135526103,40.100244835349));
#209906=CARTESIAN_POINT('Ctrl Pts',(59.79096915834,19.357609838725,40.10025));
#209907=CARTESIAN_POINT('Ctrl Pts',(59.9061888791359,19.2705128813945,40.1202442001038));
#209908=CARTESIAN_POINT('Ctrl Pts',(59.8582551377157,19.303448093618,40.0633873868015));
#209909=CARTESIAN_POINT('Ctrl Pts',(59.7817014705984,19.3051157581411,40.0772271723538));
#209910=CARTESIAN_POINT('Ctrl Pts',(59.8700374834726,19.1466203444573,40.0045995998163));
#209911=CARTESIAN_POINT('Ctrl Pts',(59.8200494324146,19.2244111832563,39.9663485808318));
#209912=CARTESIAN_POINT('Ctrl Pts',(59.7316696194041,19.2239451174244,40.0101727202465));
#209913=CARTESIAN_POINT('Ctrl Pts',(59.8340873574359,19.1068608943535,39.9304654349858));
#209914=CARTESIAN_POINT('Ctrl Pts',(59.7849307811013,19.2088773592693,39.9051900162954));
#209915=CARTESIAN_POINT('Ctrl Pts',(59.692242551696,19.1948817636398,39.9671857458184));
#209916=CARTESIAN_POINT('Ctrl Pts',(59.7908376697914,19.0928077206404,39.8576902534424));
#209917=CARTESIAN_POINT('Ctrl Pts',(59.7518659300028,19.2142545736076,39.8573998014387));
#209918=CARTESIAN_POINT('Ctrl Pts',(59.6489943884567,19.1808295835774,39.92499));
#209919=CARTESIAN_POINT('Origin',(59.7752282754839,19.4061247292246,40.22725));
#209920=CARTESIAN_POINT('Origin',(0.0981128957140474,-0.301960443923713,
39.116));
#209921=CARTESIAN_POINT('Origin',(57.1650137687749,18.2401996527038,39.116));
#209922=CARTESIAN_POINT('Origin',(5.50785759597432E-15,5.64393089795711E-15,
40.22725));
#209923=CARTESIAN_POINT('Origin',(59.7658094374954,19.4351129318413,40.22725));
#209924=CARTESIAN_POINT('Ctrl Pts',(57.1650137687749,18.2401996527038,38.989));
#209925=CARTESIAN_POINT('Ctrl Pts',(57.12570981947,18.3611647704258,38.989));
#209926=CARTESIAN_POINT('Ctrl Pts',(57.1257686544592,18.3609836949479,39.1161901092325));
#209927=CARTESIAN_POINT('Ctrl Pts',(56.9585856505953,18.1733685221987,38.989));
#209928=CARTESIAN_POINT('Ctrl Pts',(56.9195342693658,18.2941737326422,38.989229898976));
#209929=CARTESIAN_POINT('Ctrl Pts',(56.9607434512663,18.307363756326,39.1161900493205));
#209930=CARTESIAN_POINT('Ctrl Pts',(56.7620685738646,18.109748568444,39.1034966344368));
#209931=CARTESIAN_POINT('Ctrl Pts',(56.7232097045345,18.2303834904104,39.1038314102557));
#209932=CARTESIAN_POINT('Ctrl Pts',(56.8036425617884,18.256318583299,39.2077528789596));
#209933=CARTESIAN_POINT('Ctrl Pts',(56.6526781108326,18.0743352474884,39.2875012672119));
#209934=CARTESIAN_POINT('Ctrl Pts',(56.6140134911409,18.1949032015564,39.2878045257868));
#209935=CARTESIAN_POINT('Ctrl Pts',(56.7161926934818,18.2279043987985,39.3549015295901));
#209936=CARTESIAN_POINT('Origin',(56.7552848242273,18.1070706485035,39.3548010137695));
#209937=CARTESIAN_POINT('Ctrl Pts',(59.5942745858238,19.6977666881838,39.8576902534424));
#209938=CARTESIAN_POINT('Ctrl Pts',(59.634130455146,19.5766071063161,39.8573998014387));
#209939=CARTESIAN_POINT('Ctrl Pts',(59.5312589135998,19.5431821162859,39.92499));
#209940=CARTESIAN_POINT('Ctrl Pts',(59.6375442153291,19.7118253299476,39.930498490249));
#209941=CARTESIAN_POINT('Ctrl Pts',(59.657733234755,19.6004058925617,39.9052171569797));
#209942=CARTESIAN_POINT('Ctrl Pts',(59.5745267832908,19.5572406993625,39.9672049726607));
#209943=CARTESIAN_POINT('Ctrl Pts',(59.68982858249,19.7007277907729,40.0043437678662));
#209944=CARTESIAN_POINT('Ctrl Pts',(59.6951745640082,19.6083614943627,39.9661628577643));
#209945=CARTESIAN_POINT('Ctrl Pts',(59.6233361049593,19.5568428722492,40.0100243556235));
#209946=CARTESIAN_POINT('Ctrl Pts',(59.7913053863693,19.6225475038102,40.1194874821987));
#209947=CARTESIAN_POINT('Ctrl Pts',(59.772067936249,19.5674227749664,40.062755148314));
#209948=CARTESIAN_POINT('Ctrl Pts',(59.7110541706151,19.5210053955052,40.0767884282377));
#209949=CARTESIAN_POINT('Ctrl Pts',(59.8408924241699,19.5524931121155,40.1599502015382));
#209950=CARTESIAN_POINT('Ctrl Pts',(59.8128277376098,19.5181549791671,40.100244945386));
#209951=CARTESIAN_POINT('Ctrl Pts',(59.749975597626,19.4837751174909,40.10025));
#209952=CARTESIAN_POINT('Ctrl Pts',(59.8682321556244,19.4684195516689,40.1599502534424));
#209953=CARTESIAN_POINT('Ctrl Pts',(59.8327559231849,19.4568831131876,40.10025));
#209954=CARTESIAN_POINT('Ctrl Pts',(59.7658094374954,19.4351129318413,40.10025));
#209955=CARTESIAN_POINT('Origin',(59.4920137553142,19.6639662938554,39.92499));
#209956=CARTESIAN_POINT('Origin',(56.5858547179605,18.0520194698706,39.6398955069319));
#209957=CARTESIAN_POINT('Origin',(56.4164246115666,17.9969682911404,39.92499));
#209958=CARTESIAN_POINT('Origin',(59.322583882151,19.6089151909096,39.6398955068279));
#209959=CARTESIAN_POINT('Origin',(59.1531540088002,19.5538640879525,39.3548010137695));
#209960=CARTESIAN_POINT('Ctrl Pts',(56.3138168485097,17.9642361803965,39.8576902534424));
#209961=CARTESIAN_POINT('Ctrl Pts',(56.2752137607568,18.0846218068688,39.8579948730703));
#209962=CARTESIAN_POINT('Ctrl Pts',(56.377179453281,18.1177524687099,39.92499));
#209963=CARTESIAN_POINT('Ctrl Pts',(56.2706044454597,17.9501961787615,39.9304020711229));
#209964=CARTESIAN_POINT('Ctrl Pts',(56.2513675234862,18.0608967538104,39.9058915297375));
#209965=CARTESIAN_POINT('Ctrl Pts',(56.3339654239817,18.103711379437,39.9671523786028));
#209966=CARTESIAN_POINT('Ctrl Pts',(56.2186079213555,17.961258833375,40.0043257306695));
#209967=CARTESIAN_POINT('Ctrl Pts',(56.2138593173292,18.0531413250547,39.9667894847838));
#209968=CARTESIAN_POINT('Ctrl Pts',(56.2854146278935,18.1041761987732,40.01001389752));
#209969=CARTESIAN_POINT('Ctrl Pts',(56.1179510603879,18.0394175380789,40.1195533054855));
#209970=CARTESIAN_POINT('Ctrl Pts',(56.1373490477008,18.094321865332,40.0630813209233));
#209971=CARTESIAN_POINT('Ctrl Pts',(56.1984140977479,18.1403075368572,40.076826594242));
#209972=CARTESIAN_POINT('Ctrl Pts',(56.0689198620977,18.109415362897,40.1599502027523));
#209973=CARTESIAN_POINT('Ctrl Pts',(56.0970362061477,18.1436123520178,40.1002552791541));
#209974=CARTESIAN_POINT('Ctrl Pts',(56.1599674935302,18.1777307632106,40.10025));
#209975=CARTESIAN_POINT('Ctrl Pts',(56.0417604764386,18.1930767435942,40.1599502534424));
#209976=CARTESIAN_POINT('Ctrl Pts',(56.0772424804487,18.2045954185338,40.10025));
#209977=CARTESIAN_POINT('Ctrl Pts',(56.144199857553,18.2263320786575,40.10025));
#209978=CARTESIAN_POINT('Origin',(56.144199857553,18.2263320786575,40.22725));
#209979=CARTESIAN_POINT('Ctrl Pts',(58.7434254837935,19.4207352200693,38.989));
#209980=CARTESIAN_POINT('Ctrl Pts',(58.7827292759118,19.2997705861181,38.989));
#209981=CARTESIAN_POINT('Ctrl Pts',(58.7826705983438,19.2999511771031,39.1161896013268));
#209982=CARTESIAN_POINT('Ctrl Pts',(58.949713783122,19.4879965013595,38.989));
#209983=CARTESIAN_POINT('Ctrl Pts',(58.9892635895134,19.3668771285518,38.9887769275436));
#209984=CARTESIAN_POINT('Ctrl Pts',(58.9476954469484,19.3535710010433,39.1161898821826));
#209985=CARTESIAN_POINT('Ctrl Pts',(59.1460976215391,19.552026077385,39.1034967087243));
#209986=CARTESIAN_POINT('Ctrl Pts',(59.185829577808,19.4307447900774,39.1031720232724));
#209987=CARTESIAN_POINT('Ctrl Pts',(59.1047962608428,19.4046161500175,39.207752961502));
#209988=CARTESIAN_POINT('Ctrl Pts',(59.2554138597574,19.5876674457071,39.2875012672119));
#209989=CARTESIAN_POINT('Ctrl Pts',(59.2953329133628,19.4663243070084,39.2872087095507));
#209990=CARTESIAN_POINT('Ctrl Pts',(59.1922458725045,19.4330302514106,39.3549017048229));
#209991=CARTESIAN_POINT('Origin',(58.7434254837935,19.4207352200693,39.116));
#209992=CARTESIAN_POINT('Origin',(5.72046327455653E-15,5.27083398054906E-15,
40.22725));
#209993=CARTESIAN_POINT('Origin',(56.1347810195644,18.2553202812742,40.22725));
#209994=CARTESIAN_POINT('Origin',(56.182627028633,18.588681363905,39.116));
#209995=CARTESIAN_POINT('Origin',(58.3616995707157,19.296759302446,39.1160373285272));
#209996=CARTESIAN_POINT('Ctrl Pts',(56.0323588238394,18.222012055021,40.1599502534424));
#209997=CARTESIAN_POINT('Ctrl Pts',(56.0678348753335,18.2335490499211,40.10025));
#209998=CARTESIAN_POINT('Ctrl Pts',(56.1347810195644,18.2553202812742,40.10025));
#209999=CARTESIAN_POINT('Ctrl Pts',(56.0052491386467,18.3053742463591,40.1599500566036));
#210000=CARTESIAN_POINT('Ctrl Pts',(56.048081262789,18.2942806848328,40.1002551305369));
#210001=CARTESIAN_POINT('Ctrl Pts',(56.1190241739986,18.3037418885561,40.10025));
#210002=CARTESIAN_POINT('Ctrl Pts',(56.0035251343647,18.3900709842064,40.1203070619046));
#210003=CARTESIAN_POINT('Ctrl Pts',(56.0514568378828,18.3574039607296,40.0637098684494));
#210004=CARTESIAN_POINT('Ctrl Pts',(56.1278011372726,18.3561185603235,40.0772636213363));
#210005=CARTESIAN_POINT('Ctrl Pts',(56.0390077039671,18.5134377270383,40.0046102245802));
#210006=CARTESIAN_POINT('Ctrl Pts',(56.0891934462337,18.4363968713613,39.9670001894019));
#210007=CARTESIAN_POINT('Ctrl Pts',(56.1770584756116,18.4370884086008,40.0101788811209));
#210008=CARTESIAN_POINT('Ctrl Pts',(56.0747542753111,18.5530236652636,39.9303710930186));
#210009=CARTESIAN_POINT('Ctrl Pts',(56.1242585025262,18.4521491348407,39.9058663574098));
#210010=CARTESIAN_POINT('Ctrl Pts',(56.2162483036945,18.4660698759066,39.9671344706357));
#210011=CARTESIAN_POINT('Ctrl Pts',(56.1179479440991,18.5670586829458,39.8576902534424));
#210012=CARTESIAN_POINT('Ctrl Pts',(56.1574782859,18.4469743395772,39.8579948730703));
#210013=CARTESIAN_POINT('Ctrl Pts',(56.2594439784241,18.4801050014183,39.92499));
#210014=CARTESIAN_POINT('Origin',(56.2201988201385,18.6008891789878,39.92499));
#210015=CARTESIAN_POINT('Origin',(58.3196542512034,19.283043599898,39.1925554488848));
#210016=CARTESIAN_POINT('Origin',(58.2418213702176,19.2577541638571,39.3343017080178));
#210017=CARTESIAN_POINT('Origin',(56.3896289265327,18.6559403576579,39.6398955069205));
#210018=CARTESIAN_POINT('Origin',(56.5590590327992,18.710991536351,39.3548010137695));
#210019=CARTESIAN_POINT('Ctrl Pts',(57.9280106456678,19.1557908785618,39.3978017080178));
#210020=CARTESIAN_POINT('Ctrl Pts',(57.9672558039534,19.0350067009923,39.3978017080178));
#210021=CARTESIAN_POINT('Ctrl Pts',(57.9672558039534,19.0350067009923,39.5248017080178));
#210022=CARTESIAN_POINT('Ctrl Pts',(58.0136880650213,19.1833829156704,39.3978017080178));
#210023=CARTESIAN_POINT('Ctrl Pts',(58.0527804636638,19.0627953474463,39.3980355775177));
#210024=CARTESIAN_POINT('Ctrl Pts',(58.0956618095403,19.076728341322,39.5248015517192));
#210025=CARTESIAN_POINT('Ctrl Pts',(58.0947019536607,19.2094750027313,39.3484893995498));
#210026=CARTESIAN_POINT('Ctrl Pts',(58.1340538395294,19.0892026680421,39.348943830342));
#210027=CARTESIAN_POINT('Ctrl Pts',(58.2170788227746,19.1161791203796,39.4508333155587));
#210028=CARTESIAN_POINT('Ctrl Pts',(58.1373965169896,19.2232259141432,39.2708017080178));
#210029=CARTESIAN_POINT('Ctrl Pts',(58.1769325318822,19.103134799738,39.2710850691866));
#210030=CARTESIAN_POINT('Ctrl Pts',(58.2810665285032,19.1369699862876,39.3343017080178));
#210031=CARTESIAN_POINT('Origin',(57.9280106456678,19.1557908785618,39.5248017080178));
#210032=CARTESIAN_POINT('Ctrl Pts',(56.4568070719814,18.6771643191703,39.2875012672119));
#210033=CARTESIAN_POINT('Ctrl Pts',(56.4963947983079,18.5568963159715,39.2878045257518));
#210034=CARTESIAN_POINT('Ctrl Pts',(56.5984571192852,18.5902571970793,39.3549015218345));
#210035=CARTESIAN_POINT('Ctrl Pts',(56.5661228951879,18.7128129802653,39.1034938540228));
#210036=CARTESIAN_POINT('Ctrl Pts',(56.6055928325719,18.5923766197456,39.1038286278815));
#210037=CARTESIAN_POINT('Ctrl Pts',(56.6859083114077,18.6186718120042,39.2077506434033));
#210038=CARTESIAN_POINT('Ctrl Pts',(56.7625049710037,18.7768537015935,38.989));
#210039=CARTESIAN_POINT('Ctrl Pts',(56.8019192501357,18.6561664154729,38.9892298954611));
#210040=CARTESIAN_POINT('Ctrl Pts',(56.8430104456831,18.6697173900106,39.1161900347285));
#210041=CARTESIAN_POINT('Ctrl Pts',(56.9687879773469,18.8441205405512,38.989));
#210042=CARTESIAN_POINT('Ctrl Pts',(57.0080919221123,18.7231554368006,38.989));
#210043=CARTESIAN_POINT('Ctrl Pts',(57.0080330916694,18.7233364982862,39.1161900945641));
#210044=CARTESIAN_POINT('Origin',(56.9687879773468,18.8441205405512,39.116));
#210045=CARTESIAN_POINT('Origin',(54.8193466381482,18.1457247135484,39.5248017080178));
#210046=CARTESIAN_POINT('Origin',(57.7842031819385,19.1090650011308,39.5248017080178));
#210047=CARTESIAN_POINT('Origin',(54.6058629360818,18.0763596539223,39.116));
#210048=CARTESIAN_POINT('Origin',(57.3504898524411,18.9681964166826,39.1160402713851));
#210049=CARTESIAN_POINT('Ctrl Pts',(57.5748148483578,19.0416371860871,39.2708017080178));
#210050=CARTESIAN_POINT('Ctrl Pts',(57.6147155869504,18.9204594407738,39.27051194648));
#210051=CARTESIAN_POINT('Ctrl Pts',(57.5096375484039,18.8863175164085,39.3343017080178));
#210052=CARTESIAN_POINT('Ctrl Pts',(57.617654601607,19.0554318862534,39.3487519301185));
#210053=CARTESIAN_POINT('Ctrl Pts',(57.6572916985381,18.9342932580151,39.3482879463994));
#210054=CARTESIAN_POINT('Ctrl Pts',(57.5738415009816,18.907178645177,39.4512271261639));
#210055=CARTESIAN_POINT('Ctrl Pts',(57.698814160686,19.0815664505361,39.3978017080178));
#210056=CARTESIAN_POINT('Ctrl Pts',(57.738049368389,18.9605330155748,39.3975673827378));
#210057=CARTESIAN_POINT('Ctrl Pts',(57.6954748424951,18.9466997135534,39.524801535518));
#210058=CARTESIAN_POINT('Ctrl Pts',(57.7842031819385,19.1090650011308,39.3978017080178));
#210059=CARTESIAN_POINT('Ctrl Pts',(57.8234483402241,18.9882808235613,39.3978017080178));
#210060=CARTESIAN_POINT('Ctrl Pts',(57.8234483402241,18.9882808235613,39.5248017080178));
#210061=CARTESIAN_POINT('Origin',(57.4703923901183,19.007101693978,39.3343017080178));
#210062=CARTESIAN_POINT('Origin',(57.3930236885618,18.9819630792876,39.1934008533553));
#210063=CARTESIAN_POINT('Origin',(60.1478239224126,12.4602215063114,39.192555449508));
#210064=CARTESIAN_POINT('Origin',(60.1910940874962,12.4693660187268,39.1160373285242));
#210065=CARTESIAN_POINT('Origin',(60.0677739512127,12.4432063593714,39.3343017080178));
#210066=CARTESIAN_POINT('Ctrl Pts',(59.9600752506739,12.4208962741579,39.2708017080178));
#210067=CARTESIAN_POINT('Ctrl Pts',(59.9342688867327,12.5446662374479,39.2710850691866));
#210068=CARTESIAN_POINT('Ctrl Pts',(60.0413691664789,12.5674311046646,39.3343017080178));
#210069=CARTESIAN_POINT('Ctrl Pts',(59.9160770362136,12.411425735194,39.3487519293518));
#210070=CARTESIAN_POINT('Ctrl Pts',(59.8900198101335,12.5352608058694,39.3492068662917));
#210071=CARTESIAN_POINT('Ctrl Pts',(59.9753363727294,12.5533954010678,39.4512271248731));
#210072=CARTESIAN_POINT('Ctrl Pts',(59.8327226933132,12.3934832896259,39.3978017080178));
#210073=CARTESIAN_POINT('Ctrl Pts',(59.8062838430906,12.517462176626,39.3980347781183));
#210074=CARTESIAN_POINT('Ctrl Pts',(59.8502383056106,12.5268049860494,39.5248015355195));
#210075=CARTESIAN_POINT('Ctrl Pts',(59.7450242491249,12.3746037924156,39.3978017080178));
#210076=CARTESIAN_POINT('Ctrl Pts',(59.7186194643911,12.4988285377088,39.3978017080178));
#210077=CARTESIAN_POINT('Ctrl Pts',(59.7186194643911,12.4988285377088,39.5248017080178));
#210078=CARTESIAN_POINT('Origin',(59.7450242491249,12.3746037924156,39.5248017080178));
#210079=CARTESIAN_POINT('Origin',(0.0660119618346401,-0.310561863232984,
39.116));
#210080=CARTESIAN_POINT('Origin',(60.5836663843183,12.5528626811439,39.116));
#210081=CARTESIAN_POINT('Origin',(0.0660119618346402,-0.310561863232984,
39.5248017080178));
#210082=CARTESIAN_POINT('Origin',(59.5971203935661,12.3431658574203,39.5248017080178));
#210083=CARTESIAN_POINT('Ctrl Pts',(61.1105274371643,12.6642893210134,39.2875012672119));
#210084=CARTESIAN_POINT('Ctrl Pts',(61.0844267845857,12.7893350777081,39.287208709576));
#210085=CARTESIAN_POINT('Ctrl Pts',(60.9785037674409,12.7666250679669,39.3549016990125));
#210086=CARTESIAN_POINT('Ctrl Pts',(60.9980344071778,12.6404971713765,39.103493917393));
#210087=CARTESIAN_POINT('Ctrl Pts',(60.9718026486744,12.7653958126118,39.1031692336348));
#210088=CARTESIAN_POINT('Ctrl Pts',(60.8885617651967,12.7475073053527,39.2077507202311));
#210089=CARTESIAN_POINT('Ctrl Pts',(60.7959446297927,12.5977561540106,38.989));
#210090=CARTESIAN_POINT('Ctrl Pts',(60.7696360759134,12.7224234952036,38.9887769311152));
#210091=CARTESIAN_POINT('Ctrl Pts',(60.7269846150093,12.7131630221032,39.1161898712895));
#210092=CARTESIAN_POINT('Ctrl Pts',(60.5836663843183,12.5528626811439,38.989));
#210093=CARTESIAN_POINT('Ctrl Pts',(60.5572221520605,12.6772730124465,38.989));
#210094=CARTESIAN_POINT('Ctrl Pts',(60.5572616290069,12.6770872880156,39.1161895903858));
#210095=CARTESIAN_POINT('Origin',(61.0050661295708,12.6424339620834,39.3548010137695));
#210096=CARTESIAN_POINT('Ctrl Pts',(59.5971203935661,12.3431658574203,39.3978017080178));
#210097=CARTESIAN_POINT('Ctrl Pts',(59.5707156088322,12.4673906027135,39.3978017080178));
#210098=CARTESIAN_POINT('Ctrl Pts',(59.5707156088322,12.4673906027135,39.5248017080178));
#210099=CARTESIAN_POINT('Ctrl Pts',(59.5091256622729,12.3242219811454,39.3978017080178));
#210100=CARTESIAN_POINT('Ctrl Pts',(59.4825873732131,12.4486583679636,39.3975666025021));
#210101=CARTESIAN_POINT('Ctrl Pts',(59.438651914001,12.4393195978187,39.5248015517177));
#210102=CARTESIAN_POINT('Ctrl Pts',(59.4259203549056,12.3063073021294,39.3484894016716));
#210103=CARTESIAN_POINT('Ctrl Pts',(59.399678430328,12.4310355281324,39.3480259000047));
#210104=CARTESIAN_POINT('Ctrl Pts',(59.313776274866,12.4127764613279,39.4508333188951));
#210105=CARTESIAN_POINT('Ctrl Pts',(59.3820708699072,12.2968658913796,39.2708017080178));
#210106=CARTESIAN_POINT('Ctrl Pts',(59.3560370505015,12.4217592664905,39.27051194648));
#210107=CARTESIAN_POINT('Ctrl Pts',(59.2479658375578,12.3987880210516,39.3343017080178));
#210108=CARTESIAN_POINT('Origin',(59.2743706222916,12.2745632757584,39.3343017080178));
#210109=CARTESIAN_POINT('Origin',(61.1793222555451,12.6794732450924,39.6398955068193));
#210110=CARTESIAN_POINT('Origin',(61.3535783813234,12.7165125280158,39.92499));
#210111=CARTESIAN_POINT('Origin',(59.1947980527947,12.2576496039896,39.193400853994));
#210112=CARTESIAN_POINT('Origin',(59.1510793400373,12.2483049653993,39.1160402713848));
#210113=CARTESIAN_POINT('Ctrl Pts',(61.5816197022699,13.0739701745317,40.1599502534424));
#210114=CARTESIAN_POINT('Ctrl Pts',(61.5451281645061,13.0662229071059,40.10025));
#210115=CARTESIAN_POINT('Ctrl Pts',(61.4762657165317,13.0516031943521,40.10025));
#210116=CARTESIAN_POINT('Ctrl Pts',(61.5999188988204,12.9877758510413,40.1599500538472));
#210117=CARTESIAN_POINT('Ctrl Pts',(61.5584544893695,13.0034370926703,40.100244835349));
#210118=CARTESIAN_POINT('Ctrl Pts',(61.4868491822358,13.0017087032037,40.10025));
#210119=CARTESIAN_POINT('Ctrl Pts',(61.5923336062397,12.9030451317653,40.1202442001039));
#210120=CARTESIAN_POINT('Ctrl Pts',(61.5481051179915,12.9408103617794,40.0633873868015));
#210121=CARTESIAN_POINT('Ctrl Pts',(61.4721451382827,12.9504709278431,40.0772271723536));
#210122=CARTESIAN_POINT('Ctrl Pts',(61.543429955208,12.7836101409423,40.0045995998162));
#210123=CARTESIAN_POINT('Ctrl Pts',(61.50184710076,12.8662000075457,39.9663485808317));
#210124=CARTESIAN_POINT('Ctrl Pts',(61.4139027244672,12.8749747009092,40.0101727202467));
#210125=CARTESIAN_POINT('Ctrl Pts',(61.5035207735038,12.7478263086943,39.9304654349859));
#210126=CARTESIAN_POINT('Ctrl Pts',(61.4652971063442,12.8544221781238,39.9051900162943));
#210127=CARTESIAN_POINT('Ctrl Pts',(61.3716536946539,12.8501918100163,39.9671857458174));
#210128=CARTESIAN_POINT('Ctrl Pts',(61.459039055521,12.7383709431243,39.8576902534424));
#210129=CARTESIAN_POINT('Ctrl Pts',(61.43297545991,12.8632261535947,39.8573998014387));
#210130=CARTESIAN_POINT('Ctrl Pts',(61.3271735965895,12.840737273309,39.92499));
#210131=CARTESIAN_POINT('Origin',(61.4762657165317,13.0516031943521,40.22725));
#210132=CARTESIAN_POINT('Origin',(0.0660119618346401,-0.310561863232984,
39.116));
#210133=CARTESIAN_POINT('Origin',(58.7584778814678,12.1649068885784,39.116));
#210134=CARTESIAN_POINT('Origin',(5.5033905580924E-15,5.66060211029175E-15,
40.22725));
#210135=CARTESIAN_POINT('Origin',(61.4699285681956,13.0814171332224,40.22725));
#210136=CARTESIAN_POINT('Ctrl Pts',(58.7584778814678,12.1649068885784,38.989));
#210137=CARTESIAN_POINT('Ctrl Pts',(58.7320335411742,12.2893177281492,38.989));
#210138=CARTESIAN_POINT('Ctrl Pts',(58.7320731263176,12.2891314946914,39.1161901092317));
#210139=CARTESIAN_POINT('Ctrl Pts',(58.5461948427484,12.1200194799672,38.989));
#210140=CARTESIAN_POINT('Ctrl Pts',(58.5199849720703,12.2442448876943,38.989229898976));
#210141=CARTESIAN_POINT('Ctrl Pts',(58.5623471386663,12.253055122593,39.1161900493197));
#210142=CARTESIAN_POINT('Ctrl Pts',(58.3441042111266,12.0772896710131,39.1034966344368));
#210143=CARTESIAN_POINT('Ctrl Pts',(58.3180679977636,12.2013256001478,39.103831410257));
#210144=CARTESIAN_POINT('Ctrl Pts',(58.4007711908128,12.2187110949216,39.2077528789602));
#210145=CARTESIAN_POINT('Ctrl Pts',(58.2316113004783,12.0535047649314,39.2875012672119));
#210146=CARTESIAN_POINT('Ctrl Pts',(58.205761272577,12.1774537884102,39.2878045257868));
#210147=CARTESIAN_POINT('Ctrl Pts',(58.3108302909892,12.1995935666429,39.3549015295897));
#210148=CARTESIAN_POINT('Origin',(58.3370777047236,12.0753355159225,39.3548010137695));
#210149=CARTESIAN_POINT('Ctrl Pts',(61.3267881959115,13.3605623192479,39.8576902534424));
#210150=CARTESIAN_POINT('Ctrl Pts',(61.3537611057085,13.2359003894743,39.8573998014387));
#210151=CARTESIAN_POINT('Ctrl Pts',(61.2479592423879,13.2134115091886,39.92499));
#210152=CARTESIAN_POINT('Ctrl Pts',(61.3712903180781,13.3700210384225,39.9304984902488));
#210153=CARTESIAN_POINT('Ctrl Pts',(61.3797222373778,13.257101641197,39.9052171569784));
#210154=CARTESIAN_POINT('Ctrl Pts',(61.2924596082479,13.2228703539488,39.9672049726591));
#210155=CARTESIAN_POINT('Ctrl Pts',(61.4221282572894,13.3535190881763,40.0043437678665));
#210156=CARTESIAN_POINT('Ctrl Pts',(61.4177900459395,13.2610999767695,39.9661628577646));
#210157=CARTESIAN_POINT('Ctrl Pts',(61.3409599630866,13.2173727427865,40.0100243556236));
#210158=CARTESIAN_POINT('Ctrl Pts',(61.5148770953648,13.2651598666395,40.1194874821984));
#210159=CARTESIAN_POINT('Ctrl Pts',(61.4899829268155,13.2123479779263,40.0627551483138));
#210160=CARTESIAN_POINT('Ctrl Pts',(61.4244514636298,13.1725625528863,40.0767884282376));
#210161=CARTESIAN_POINT('Ctrl Pts',(61.5568698122757,13.1903059833727,40.1599502015389));
#210162=CARTESIAN_POINT('Ctrl Pts',(61.5253695547392,13.1590895168683,40.1002449453881));
#210163=CARTESIAN_POINT('Ctrl Pts',(61.4592680512448,13.131467829277,40.10025));
#210164=CARTESIAN_POINT('Ctrl Pts',(61.5752716937453,13.103835206572,40.1599502534424));
#210165=CARTESIAN_POINT('Ctrl Pts',(61.5387839176329,13.0960702419672,40.10025));
#210166=CARTESIAN_POINT('Ctrl Pts',(61.4699285681956,13.0814171332224,40.10025));
#210167=CARTESIAN_POINT('Origin',(61.2215544576541,13.3376362544818,39.92499));
#210168=CARTESIAN_POINT('Origin',(58.1628213392008,12.0382961820508,39.6398955069312));
#210169=CARTESIAN_POINT('Origin',(57.9885649735461,12.0012568480852,39.92499));
#210170=CARTESIAN_POINT('Origin',(61.0472983318742,13.3005969715109,39.6398955068265));
#210171=CARTESIAN_POINT('Origin',(60.8730422059015,13.2635576885494,39.3548010137695));
#210172=CARTESIAN_POINT('Ctrl Pts',(57.8830978693157,11.9794294790605,39.8576902534424));
#210173=CARTESIAN_POINT('Ctrl Pts',(57.8572899778513,12.1031907419149,39.8579948730703));
#210174=CARTESIAN_POINT('Ctrl Pts',(57.9621601888122,12.1254815933784,39.92499));
#210175=CARTESIAN_POINT('Ctrl Pts',(57.8386546085357,11.9699833161083,39.930402071123));
#210176=CARTESIAN_POINT('Ctrl Pts',(57.8310944294252,12.0820882677175,39.9058915297371));
#210177=CARTESIAN_POINT('Ctrl Pts',(57.9177151970031,12.116034518736,39.967152378603));
#210178=CARTESIAN_POINT('Ctrl Pts',(57.7880992891176,11.9864204851022,40.0043257306694));
#210179=CARTESIAN_POINT('Ctrl Pts',(57.7929810340972,12.07829599916,39.9667894847842));
#210180=CARTESIAN_POINT('Ctrl Pts',(57.8694789541063,12.1215717318489,40.0100138975202));
#210181=CARTESIAN_POINT('Ctrl Pts',(57.6961636462599,12.0746725352383,40.1195533054856));
#210182=CARTESIAN_POINT('Ctrl Pts',(57.7211944343233,12.1272484490378,40.0630813209231));
#210183=CARTESIAN_POINT('Ctrl Pts',(57.7867317752137,12.1665991704017,40.0768265942418));
#210184=CARTESIAN_POINT('Ctrl Pts',(57.6547178110652,12.1494120604575,40.1599502027512));
#210185=CARTESIAN_POINT('Ctrl Pts',(57.6862546895629,12.1804827566577,40.1002552791553));
#210186=CARTESIAN_POINT('Ctrl Pts',(57.7524075778595,12.2078361528628,40.10025));
#210187=CARTESIAN_POINT('Ctrl Pts',(57.6364522029208,12.2354540642037,40.1599502534424));
#210188=CARTESIAN_POINT('Ctrl Pts',(57.6729438621908,12.243200759284,40.10025));
#210189=CARTESIAN_POINT('Ctrl Pts',(57.7418065394567,12.257819391976,40.10025));
#210190=CARTESIAN_POINT('Origin',(57.7418065394567,12.257819391976,40.22725));
#210191=CARTESIAN_POINT('Ctrl Pts',(60.4516424606491,13.1739864076099,38.989));
#210192=CARTESIAN_POINT('Ctrl Pts',(60.4780866951852,13.0495760655893,38.989));
#210193=CARTESIAN_POINT('Ctrl Pts',(60.4780472159571,13.0497618007542,39.116189601327));
#210194=CARTESIAN_POINT('Ctrl Pts',(60.6638314094603,13.2193162256446,38.989));
#210195=CARTESIAN_POINT('Ctrl Pts',(60.6905041359625,13.09472627695,38.9887769275436));
#210196=CARTESIAN_POINT('Ctrl Pts',(60.6477728389701,13.0858380958627,39.1161898821828));
#210197=CARTESIAN_POINT('Ctrl Pts',(60.8658323498481,13.2624673401125,39.1034967087243));
#210198=CARTESIAN_POINT('Ctrl Pts',(60.8926693037173,13.1376973240579,39.1031720232725));
#210199=CARTESIAN_POINT('Ctrl Pts',(60.8093487091504,13.1201821075159,39.2077529615018));
#210200=CARTESIAN_POINT('Ctrl Pts',(60.978275279735,13.2864868028988,39.2875012672119));
#210201=CARTESIAN_POINT('Ctrl Pts',(61.0052918407718,13.1616357172815,39.2872087095507));
#210202=CARTESIAN_POINT('Ctrl Pts',(60.8992893450416,13.1392995799678,39.354901704823));
#210203=CARTESIAN_POINT('Origin',(60.4516424606491,13.1739864076099,39.116));
#210204=CARTESIAN_POINT('Origin',(5.72205236298458E-15,5.26490342179783E-15,
40.22725));
#210205=CARTESIAN_POINT('Origin',(57.7354693911206,12.2876333308464,40.22725));
#210206=CARTESIAN_POINT('Origin',(59.4667368016504,12.9646382471638,39.116));
#210207=CARTESIAN_POINT('Origin',(60.0590486699124,13.090590866118,39.116037328527));
#210208=CARTESIAN_POINT('Ctrl Pts',(57.6301266171959,12.2652136052653,40.1599502534424));
#210209=CARTESIAN_POINT('Ctrl Pts',(57.6666142715157,12.2729791421547,40.10025));
#210210=CARTESIAN_POINT('Ctrl Pts',(57.7354693911206,12.2876333308464,40.10025));
#210211=CARTESIAN_POINT('Ctrl Pts',(57.6118791634503,12.3509528635298,40.1599500566038));
#210212=CARTESIAN_POINT('Ctrl Pts',(57.653317055794,12.3354428975785,40.1002551305378));
#210213=CARTESIAN_POINT('Ctrl Pts',(57.7248602994011,12.33743671835,40.10025));
#210214=CARTESIAN_POINT('Ctrl Pts',(57.6190178232952,12.4353658313036,40.1203070619047));
#210215=CARTESIAN_POINT('Ctrl Pts',(57.6632723181622,12.3978675338891,40.0637098684499));
#210216=CARTESIAN_POINT('Ctrl Pts',(57.7390640345626,12.388609022746,40.0772636213362));
#210217=CARTESIAN_POINT('Ctrl Pts',(57.6672013517154,12.5543478197367,40.0046102245801));
#210218=CARTESIAN_POINT('Ctrl Pts',(57.7090592089827,12.4724831634108,39.9670001894012));
#210219=CARTESIAN_POINT('Ctrl Pts',(57.7965151898612,12.4639865158414,40.0101788811209));
#210220=CARTESIAN_POINT('Ctrl Pts',(57.706889956891,12.5899803678805,39.9303710930187));
#210221=CARTESIAN_POINT('Ctrl Pts',(57.7455787351226,12.4844838378931,39.9058663574112));
#210222=CARTESIAN_POINT('Ctrl Pts',(57.8385197202051,12.4887127671316,39.9671344706359));
#210223=CARTESIAN_POINT('Ctrl Pts',(57.7513140650722,12.5994235324464,39.8576902534424));
#210224=CARTESIAN_POINT('Ctrl Pts',(57.7780756236497,12.4758649777945,39.8579948730703));
#210225=CARTESIAN_POINT('Ctrl Pts',(57.8829458346107,12.498155829258,39.92499));
#210226=CARTESIAN_POINT('Origin',(57.8565410498768,12.6223805745512,39.92499));
#210227=CARTESIAN_POINT('Origin',(60.0157999977491,13.0813452322602,39.1925554488844));
#210228=CARTESIAN_POINT('Origin',(59.9357500275435,13.0643300858374,39.3343017080178));
#210229=CARTESIAN_POINT('Origin',(58.0307974155297,12.6594199084523,39.6398955069217));
#210230=CARTESIAN_POINT('Origin',(58.2050537810543,12.6964592423885,39.3548010137695));
#210231=CARTESIAN_POINT('Ctrl Pts',(59.6130003254557,12.9957275188816,39.3978017080178));
#210232=CARTESIAN_POINT('Ctrl Pts',(59.6394051101895,12.8715027735884,39.3978017080178));
#210233=CARTESIAN_POINT('Ctrl Pts',(59.6394051101895,12.8715027735884,39.5248017080178));
#210234=CARTESIAN_POINT('Ctrl Pts',(59.7010925481784,13.0142126749437,39.3978017080178));
#210235=CARTESIAN_POINT('Ctrl Pts',(59.7273659613746,12.8901994296783,39.3980355775196));
#210236=CARTESIAN_POINT('Ctrl Pts',(59.7714687931893,12.8995737759683,39.5248015517192));
#210237=CARTESIAN_POINT('Ctrl Pts',(59.7843900000234,13.0316935695375,39.3484893995498));
#210238=CARTESIAN_POINT('Ctrl Pts',(59.8109544298265,12.9079667071261,39.348943830341));
#210239=CARTESIAN_POINT('Ctrl Pts',(59.896344400635,12.9261169057234,39.4508333155594));
#210240=CARTESIAN_POINT('Ctrl Pts',(59.8282880397057,13.0409063549231,39.2708017080178));
#210241=CARTESIAN_POINT('Ctrl Pts',(59.8550545325311,12.9173404733275,39.2710850691866));
#210242=CARTESIAN_POINT('Ctrl Pts',(59.9621548122773,12.9401053405442,39.3343017080178));
#210243=CARTESIAN_POINT('Origin',(59.6130003254557,12.9957275188816,39.5248017080178));
#210244=CARTESIAN_POINT('Ctrl Pts',(58.0998260601482,12.6735055745733,39.2875012672119));
#210245=CARTESIAN_POINT('Ctrl Pts',(58.1266254912132,12.5497583678823,39.2878045257519));
#210246=CARTESIAN_POINT('Ctrl Pts',(58.2316158657529,12.572268077024,39.3549015218347));
#210247=CARTESIAN_POINT('Ctrl Pts',(58.2122693395992,12.6975323335618,39.1034938540228));
#210248=CARTESIAN_POINT('Ctrl Pts',(58.2389340288488,12.5736300041238,39.1038286278811));
#210249=CARTESIAN_POINT('Ctrl Pts',(58.3215581271254,12.5913858949914,39.2077506434031));
#210250=CARTESIAN_POINT('Ctrl Pts',(58.4142696920429,12.7406947165192,38.989));
#210251=CARTESIAN_POINT('Ctrl Pts',(58.4408527990764,12.616548653953,38.9892298954611));
#210252=CARTESIAN_POINT('Ctrl Pts',(58.4831353553,12.6257301953092,39.1161900347289));
#210253=CARTESIAN_POINT('Ctrl Pts',(58.6264539577985,12.7860306150444,38.989));
#210254=CARTESIAN_POINT('Ctrl Pts',(58.6528982950381,12.6616197898418,38.989));
#210255=CARTESIAN_POINT('Ctrl Pts',(58.6528587129533,12.6618060089099,39.1161900945646));
#210256=CARTESIAN_POINT('Origin',(58.6264539577985,12.7860306150444,39.116));
#210257=CARTESIAN_POINT('Origin',(58.0246834617332,12.6581203474863,39.5248017080178));
#210258=CARTESIAN_POINT('Origin',(59.4650964698968,12.9642895838863,39.5248017080178));
#210259=CARTESIAN_POINT('Origin',(57.7988642628865,12.6101209950203,39.116));
#210260=CARTESIAN_POINT('Origin',(59.0190342907437,12.8695280801138,39.1160402713848));
#210261=CARTESIAN_POINT('Ctrl Pts',(59.2498070616281,12.9191181862038,39.2708017080178));
#210262=CARTESIAN_POINT('Ctrl Pts',(59.2768226963,12.7944335023701,39.27051194648));
#210263=CARTESIAN_POINT('Ctrl Pts',(59.1687514833562,12.7714622569312,39.3343017080178));
#210264=CARTESIAN_POINT('Ctrl Pts',(59.2938540730361,12.9283593439861,39.3487519301186));
#210265=CARTESIAN_POINT('Ctrl Pts',(59.3206115991492,12.8037411209992,39.3482879463993));
#210266=CARTESIAN_POINT('Ctrl Pts',(59.2347843016964,12.785497965755,39.4512271261639));
#210267=CARTESIAN_POINT('Ctrl Pts',(59.3773008374014,12.9458672564002,39.3978017080178));
#210268=CARTESIAN_POINT('Ctrl Pts',(59.4036696715717,12.8213956592928,39.3975673827383));
#210269=CARTESIAN_POINT('Ctrl Pts',(59.359882399582,12.812088387313,39.524801535518));
#210270=CARTESIAN_POINT('Ctrl Pts',(59.4650964698968,12.9642895838863,39.3978017080178));
#210271=CARTESIAN_POINT('Ctrl Pts',(59.4915012546307,12.8400648385931,39.3978017080178));
#210272=CARTESIAN_POINT('Ctrl Pts',(59.4915012546306,12.8400648385931,39.5248017080178));
#210273=CARTESIAN_POINT('Origin',(59.1423466986224,12.8956870022244,39.3343017080178));
#210274=CARTESIAN_POINT('Origin',(59.0627741301484,12.8787733309738,39.193400853354));
#210275=CARTESIAN_POINT('Origin',(61.1207756556245,6.10480350566312,39.1925554495082));
#210276=CARTESIAN_POINT('Origin',(61.1647646440471,6.10937495961979,39.1160373285255));
#210277=CARTESIAN_POINT('Origin',(61.0393856393805,6.09624906995156,39.3343017080178));
#210278=CARTESIAN_POINT('Ctrl Pts',(60.9299448846691,6.08531878138238,39.2708017080178));
#210279=CARTESIAN_POINT('Ctrl Pts',(60.9172173747511,6.21110821942853,39.2710850691866));
#210280=CARTESIAN_POINT('Ctrl Pts',(61.0261105245455,6.22255335066333,39.3343017080178));
#210281=CARTESIAN_POINT('Ctrl Pts',(60.8851977561471,6.08049918876568,39.3487519293518));
#210282=CARTESIAN_POINT('Ctrl Pts',(60.8722275639201,6.20637959976494,39.3492068662932));
#210283=CARTESIAN_POINT('Ctrl Pts',(60.9589723348255,6.21549684257569,39.4512271248742));
#210284=CARTESIAN_POINT('Ctrl Pts',(60.800424540796,6.07136793516269,39.3978017080178));
#210285=CARTESIAN_POINT('Ctrl Pts',(60.7870898478928,6.19743126523103,39.3980347781183));
#210286=CARTESIAN_POINT('Ctrl Pts',(60.8317801127809,6.20212840134595,39.5248015355195));
#210287=CARTESIAN_POINT('Ctrl Pts',(60.7112330730305,6.06175884541488,39.3978017080178));
#210288=CARTESIAN_POINT('Ctrl Pts',(60.6979579581955,6.18806312612664,39.3978017080178));
#210289=CARTESIAN_POINT('Ctrl Pts',(60.6979579581955,6.18806312612664,39.5248017080178));
#210290=CARTESIAN_POINT('Origin',(60.7112330730305,6.06175884541488,39.5248017080178));
#210291=CARTESIAN_POINT('Origin',(0.0331877870874813,-0.315760701779427,
39.116));
#210292=CARTESIAN_POINT('Origin',(61.5639141665613,6.15137923967592,39.116));
#210293=CARTESIAN_POINT('Origin',(0.0331877870874813,-0.315760701779427,
39.5248017080178));
#210294=CARTESIAN_POINT('Origin',(60.5608532912344,6.04595329344979,39.5248017080178));
#210295=CARTESIAN_POINT('Ctrl Pts',(62.099536274866,6.20712349654379,39.2875012672119));
#210296=CARTESIAN_POINT('Ctrl Pts',(62.0866494451786,6.33421250060427,39.287208709576));
#210297=CARTESIAN_POINT('Ctrl Pts',(61.9789328429853,6.32269886887908,39.3549016990127));
#210298=CARTESIAN_POINT('Ctrl Pts',(61.9851725366286,6.19522040634589,39.103493917393));
#210299=CARTESIAN_POINT('Ctrl Pts',(61.9721399414775,6.32217680516156,39.1031692336342));
#210300=CARTESIAN_POINT('Ctrl Pts',(61.8874852020945,6.31308733464671,39.207750720231));
#210301=CARTESIAN_POINT('Ctrl Pts',(61.7797221753254,6.17383766261649,38.989));
#210302=CARTESIAN_POINT('Ctrl Pts',(61.7665890280501,6.30057205577822,38.9887769311152));
#210303=CARTESIAN_POINT('Ctrl Pts',(61.7232032332894,6.29582060418239,39.1161898712899));
#210304=CARTESIAN_POINT('Ctrl Pts',(61.5639141665613,6.15137923967592,38.989));
#210305=CARTESIAN_POINT('Ctrl Pts',(61.5506192193202,6.27787221312686,38.989));
#210306=CARTESIAN_POINT('Ctrl Pts',(61.5506390665185,6.277683379649,39.1161895903862));
#210307=CARTESIAN_POINT('Origin',(61.992368188267,6.19641157197379,39.3548010137695));
#210308=CARTESIAN_POINT('Ctrl Pts',(60.5608532912344,6.04595329344978,39.3978017080178));
#210309=CARTESIAN_POINT('Ctrl Pts',(60.5475781763994,6.17225757416155,39.3978017080178));
#210310=CARTESIAN_POINT('Ctrl Pts',(60.5475781763994,6.17225757416155,39.5248017080178));
#210311=CARTESIAN_POINT('Ctrl Pts',(60.4713604300109,6.03631114774949,39.3978017080178));
#210312=CARTESIAN_POINT('Ctrl Pts',(60.457974664765,6.16283986559435,39.3975666025021));
#210313=CARTESIAN_POINT('Ctrl Pts',(60.413303721302,6.15814476024283,39.5248015517177));
#210314=CARTESIAN_POINT('Ctrl Pts',(60.3867383361559,6.02719193013296,39.3484894016716));
#210315=CARTESIAN_POINT('Ctrl Pts',(60.3736778173756,6.15397990991407,39.348025900005));
#210316=CARTESIAN_POINT('Ctrl Pts',(60.2863376507176,6.14480008848936,39.4508333188949));
#210317=CARTESIAN_POINT('Ctrl Pts',(60.3421421670676,6.02238575970194,39.2708017080178));
#210318=CARTESIAN_POINT('Ctrl Pts',(60.3293058762212,6.14931623097165,39.27051194648));
#210319=CARTESIAN_POINT('Ctrl Pts',(60.2194255397046,6.13776734223133,39.3343017080178));
#210320=CARTESIAN_POINT('Origin',(60.2327006545396,6.01146306151956,39.3343017080178));
#210321=CARTESIAN_POINT('Origin',(62.1695413802847,6.21503322485266,39.6398955068188));
#210322=CARTESIAN_POINT('Origin',(62.346714572097,6.2336548776654,39.92499));
#210323=CARTESIAN_POINT('Origin',(60.1517960317846,6.00295964302151,39.1934008539948));
#210324=CARTESIAN_POINT('Origin',(60.1073400339999,5.99823604520057,39.1160402713846));
#210325=CARTESIAN_POINT('Ctrl Pts',(62.6108711573006,6.56531752495217,40.1599502534424));
#210326=CARTESIAN_POINT('Ctrl Pts',(62.5737697140403,6.56142710223267,40.10025));
#210327=CARTESIAN_POINT('Ctrl Pts',(62.5037563256536,6.55408556365861,40.10025));
#210328=CARTESIAN_POINT('Ctrl Pts',(62.6200603487599,6.47768259608994,40.1599500538457));
#210329=CARTESIAN_POINT('Ctrl Pts',(62.5804601311999,6.49759225479877,40.100244835349));
#210330=CARTESIAN_POINT('Ctrl Pts',(62.5090664195357,6.50335812634666,40.10025));
#210331=CARTESIAN_POINT('Ctrl Pts',(62.6036598373291,6.39420891953678,40.1202442001038));
#210332=CARTESIAN_POINT('Ctrl Pts',(62.563621178826,6.43639040357846,40.0633873868017));
#210333=CARTESIAN_POINT('Ctrl Pts',(62.4890871199578,6.45393802799945,40.0772271723538));
#210334=CARTESIAN_POINT('Ctrl Pts',(62.5425397295636,6.28054002958054,40.0045995998163));
#210335=CARTESIAN_POINT('Ctrl Pts',(62.5098176621801,6.36702405212714,39.9663485808314));
#210336=CARTESIAN_POINT('Ctrl Pts',(62.4232722595963,6.38494336730895,40.0101727202465));
#210337=CARTESIAN_POINT('Ctrl Pts',(62.4991087455376,6.24912387034387,39.9304654349858));
#210338=CARTESIAN_POINT('Ctrl Pts',(62.4722367740482,6.35913125763675,39.9051900162951));
#210339=CARTESIAN_POINT('Ctrl Pts',(62.3786641568868,6.36471246584636,39.9671857458184));
#210340=CARTESIAN_POINT('Ctrl Pts',(62.4538823482276,6.24436990787975,39.8576902534424));
#210341=CARTESIAN_POINT('Ctrl Pts',(62.4410124550019,6.37126553603986,39.8573998014387));
#210342=CARTESIAN_POINT('Ctrl Pts',(62.333439457262,6.35995915837717,39.92499));
#210343=CARTESIAN_POINT('Origin',(62.5037563256536,6.55408556365861,40.22725));
#210344=CARTESIAN_POINT('Origin',(0.0331877870874813,-0.315760701779427,
39.116));
#210345=CARTESIAN_POINT('Origin',(59.7081718144893,5.95633285891129,39.116));
#210346=CARTESIAN_POINT('Origin',(5.50069060731754E-15,5.67764892858605E-15,
40.22725));
#210347=CARTESIAN_POINT('Origin',(62.5005702980932,6.58439859102944,40.22725));
#210348=CARTESIAN_POINT('Ctrl Pts',(59.7081718144893,5.95633285891129,38.989));
#210349=CARTESIAN_POINT('Ctrl Pts',(59.6948768129328,6.08282634913909,38.989));
#210350=CARTESIAN_POINT('Ctrl Pts',(59.6948967145276,6.08263699811301,39.1161901092323));
#210351=CARTESIAN_POINT('Ctrl Pts',(59.4923596726254,5.93388096803602,38.989));
#210352=CARTESIAN_POINT('Ctrl Pts',(59.4792784733323,6.06016553348709,38.9892298989766));
#210353=CARTESIAN_POINT('Ctrl Pts',(59.5223294958631,6.06449945282184,39.1161900493208));
#210354=CARTESIAN_POINT('Ctrl Pts',(59.286909633363,5.9125094606103,39.1034966344368));
#210355=CARTESIAN_POINT('Ctrl Pts',(59.2739813341599,6.03858743331972,39.1038314102557));
#210356=CARTESIAN_POINT('Ctrl Pts',(59.3580487495156,6.04723285085683,39.207752878959));
#210357=CARTESIAN_POINT('Ctrl Pts',(59.1725467709678,5.90061356181176,39.2875012672119));
#210358=CARTESIAN_POINT('Ctrl Pts',(59.1597945531718,6.02658564326341,39.2878045257868));
#210359=CARTESIAN_POINT('Ctrl Pts',(59.2666022295038,6.03762143444225,39.3549015295899));
#210360=CARTESIAN_POINT('Origin',(59.2797173540687,5.91130048050262,39.3548010137695));
#210361=CARTESIAN_POINT('Ctrl Pts',(62.3873926810692,6.8769768336648,39.8576902534424));
#210362=CARTESIAN_POINT('Ctrl Pts',(62.4011871104969,6.75017837817518,39.8573998014387));
#210363=CARTESIAN_POINT('Ctrl Pts',(62.293614112757,6.73887200051248,39.92499));
#210364=CARTESIAN_POINT('Ctrl Pts',(62.4326397213342,6.88173199854398,39.9304984902491));
#210365=CARTESIAN_POINT('Ctrl Pts',(62.4292221586334,6.76854981002337,39.9052171569783));
#210366=CARTESIAN_POINT('Ctrl Pts',(62.3388594194624,6.74362747387312,39.9672049726603));
#210367=CARTESIAN_POINT('Ctrl Pts',(62.4814742414947,6.86000643604644,40.0043437678662));
#210368=CARTESIAN_POINT('Ctrl Pts',(62.4674993676295,6.76854707276755,39.9661628577643));
#210369=CARTESIAN_POINT('Ctrl Pts',(62.3865194274378,6.73309031164093,40.0100243556236));
#210370=CARTESIAN_POINT('Ctrl Pts',(62.5644789380884,6.76243636205616,40.1194874821987));
#210371=CARTESIAN_POINT('Ctrl Pts',(62.5342007968288,6.71251593157812,40.062755148314));
#210372=CARTESIAN_POINT('Ctrl Pts',(62.4648696125156,6.67979835840173,40.0767884282376));
#210373=CARTESIAN_POINT('Ctrl Pts',(62.5984172531148,6.68360310202725,40.1599502015393));
#210374=CARTESIAN_POINT('Ctrl Pts',(62.5638265480141,6.65585031610542,40.1002449453885));
#210375=CARTESIAN_POINT('Ctrl Pts',(62.4951999029147,6.63528943158872,40.10025));
#210376=CARTESIAN_POINT('Ctrl Pts',(62.6076796697355,6.595682500798,40.1599502534424));
#210377=CARTESIAN_POINT('Ctrl Pts',(62.570580117661,6.59177408464689,40.10025));
#210378=CARTESIAN_POINT('Ctrl Pts',(62.5005702980932,6.58439859102943,40.10025));
#210379=CARTESIAN_POINT('Origin',(62.280338997922,6.86517628122425,39.92499));
#210380=CARTESIAN_POINT('Origin',(59.1025439185016,5.89267880207663,39.6398955069327));
#210381=CARTESIAN_POINT('Origin',(58.9253704827881,5.87405712357789,39.92499));
#210382=CARTESIAN_POINT('Origin',(62.1031658061007,6.84655462836685,39.6398955068273));
#210383=CARTESIAN_POINT('Origin',(61.925992614092,6.82793297553265,39.3548010137695));
#210384=CARTESIAN_POINT('Ctrl Pts',(58.8181995570486,5.863373641495,39.8576902534424));
#210385=CARTESIAN_POINT('Ctrl Pts',(58.8054696185321,5.98915458643714,39.8579948730703));
#210386=CARTESIAN_POINT('Ctrl Pts',(58.9120953679531,6.00036140428966,39.92499));
#210387=CARTESIAN_POINT('Ctrl Pts',(58.773012368204,5.85862481136378,39.9304020711231));
#210388=CARTESIAN_POINT('Ctrl Pts',(58.7772117628619,5.97090589422245,39.9058915297374));
#210389=CARTESIAN_POINT('Ctrl Pts',(58.8669063622644,5.99561184840434,39.967152378603));
#210390=CARTESIAN_POINT('Ctrl Pts',(58.7244521481309,5.88025640567497,40.0043257306692));
#210391=CARTESIAN_POINT('Ctrl Pts',(58.7389107566974,5.97111833475309,39.9667894847835));
#210392=CARTESIAN_POINT('Ctrl Pts',(58.8195131589314,6.00616078842818,40.0100138975201));
#210393=CARTESIAN_POINT('Ctrl Pts',(58.642244989525,5.97763489331366,40.1195533054858));
#210394=CARTESIAN_POINT('Ctrl Pts',(58.6726343357866,6.02730636094531,40.0630813209236));
#210395=CARTESIAN_POINT('Ctrl Pts',(58.7419259266988,6.0595909974108,40.0768265942419));
#210396=CARTESIAN_POINT('Ctrl Pts',(58.6088386066683,6.05629725705552,40.1599502027516));
#210397=CARTESIAN_POINT('Ctrl Pts',(58.6434504949707,6.08390124328528,40.1002552791541));
#210398=CARTESIAN_POINT('Ctrl Pts',(58.7121001992962,6.10418993496954,40.10025));
#210399=CARTESIAN_POINT('Ctrl Pts',(58.5996668978649,6.14377718965243,40.1599502534424));
#210400=CARTESIAN_POINT('Ctrl Pts',(58.6367684021393,6.14766703046091,40.10025));
#210401=CARTESIAN_POINT('Ctrl Pts',(58.7067819056644,6.15500747092236,40.10025));
#210402=CARTESIAN_POINT('Origin',(58.7067819056644,6.15500747092236,40.22725));
#210403=CARTESIAN_POINT('Ctrl Pts',(61.4975385923863,6.78290064323477,38.989));
#210404=CARTESIAN_POINT('Ctrl Pts',(61.5108335407727,6.65640765888665,38.989));
#210405=CARTESIAN_POINT('Ctrl Pts',(61.5108136924274,6.65659650327793,39.116189601327));
#210406=CARTESIAN_POINT('Ctrl Pts',(61.7133034041536,6.80580235504169,38.989));
#210407=CARTESIAN_POINT('Ctrl Pts',(61.7268068187943,6.67910686400998,38.9887769275436));
#210408=CARTESIAN_POINT('Ctrl Pts',(61.6833805404067,6.67473401011636,39.1161898821828));
#210409=CARTESIAN_POINT('Ctrl Pts',(61.9187082819379,6.82760223531297,39.1034967087243));
#210410=CARTESIAN_POINT('Ctrl Pts',(61.9323562021249,6.70071049691167,39.1031720232729));
#210411=CARTESIAN_POINT('Ctrl Pts',(61.8476612078252,6.69200060426922,39.2077529615018));
#210412=CARTESIAN_POINT('Ctrl Pts',(62.0330459552233,6.83973663030176,39.2875012672119));
#210413=CARTESIAN_POINT('Ctrl Pts',(62.0468640245951,6.71274549238693,39.2872087095507));
#210414=CARTESIAN_POINT('Ctrl Pts',(61.939107459519,6.70161199275173,39.354901704823));
#210415=CARTESIAN_POINT('Origin',(61.4975385923863,6.78290064323477,39.116));
#210416=CARTESIAN_POINT('Origin',(5.72301283402738E-15,5.25883924629658E-15,
40.22725));
#210417=CARTESIAN_POINT('Origin',(58.703595878104,6.18532049829319,40.22725));
#210418=CARTESIAN_POINT('Origin',(61.5094129706999,6.78414869068668,39.116));
#210419=CARTESIAN_POINT('Origin',(61.0983782637174,6.7409991768779,39.1160373285268));
#210420=CARTESIAN_POINT('Ctrl Pts',(58.5964866834552,6.17403490858941,40.1599502534424));
#210421=CARTESIAN_POINT('Ctrl Pts',(58.6335861742243,6.17794390662092,40.10025));
#210422=CARTESIAN_POINT('Ctrl Pts',(58.703595878104,6.18532049829319,40.10025));
#210423=CARTESIAN_POINT('Ctrl Pts',(58.5873013840786,6.26121185652462,40.1599500566038));
#210424=CARTESIAN_POINT('Ctrl Pts',(58.626891042407,6.24145541658181,40.1002551305375));
#210425=CARTESIAN_POINT('Ctrl Pts',(58.6982507756596,6.23596000968308,40.10025));
#210426=CARTESIAN_POINT('Ctrl Pts',(58.6032244953991,6.34441620808525,40.1203070619047));
#210427=CARTESIAN_POINT('Ctrl Pts',(58.6433169201086,6.3024974759265,40.0637098684499));
#210428=CARTESIAN_POINT('Ctrl Pts',(58.7177256636153,6.28536729223241,40.0772636213363));
#210429=CARTESIAN_POINT('Ctrl Pts',(58.6635810738165,6.45770985055596,40.0046102245801));
#210430=CARTESIAN_POINT('Ctrl Pts',(58.6966524426407,6.371918319887,39.9670001894012));
#210431=CARTESIAN_POINT('Ctrl Pts',(58.7827411889911,6.35432657855734,40.0101788811209));
#210432=CARTESIAN_POINT('Ctrl Pts',(58.7067768761601,6.48899861096476,39.9303710930187));
#210433=CARTESIAN_POINT('Ctrl Pts',(58.7342263230556,6.38003592347159,39.9058663574109));
#210434=CARTESIAN_POINT('Ctrl Pts',(58.8271002111738,6.37452670784879,39.9671344706364));
#210435=CARTESIAN_POINT('Ctrl Pts',(58.7519447039089,6.49374646112661,39.8576902534424));
#210436=CARTESIAN_POINT('Ctrl Pts',(58.7656442740271,6.36806742857246,39.8579948730703));
#210437=CARTESIAN_POINT('Ctrl Pts',(58.8722700234481,6.37927424642498,39.92499));
#210438=CARTESIAN_POINT('Origin',(58.8589949086131,6.50557852713675,39.92499));
#210439=CARTESIAN_POINT('Origin',(61.0544000804067,6.73632490881123,39.1925554488846));
#210440=CARTESIAN_POINT('Origin',(60.9730100652055,6.72777047351041,39.3343017080178));
#210441=CARTESIAN_POINT('Origin',(59.0361683443161,6.52420020557745,39.6398955069223));
#210442=CARTESIAN_POINT('Origin',(59.2133417798937,6.54282188406147,39.3548010137695));
#210443=CARTESIAN_POINT('Ctrl Pts',(60.6448574988555,6.69328024897373,39.3978017080178));
#210444=CARTESIAN_POINT('Ctrl Pts',(60.6581326136905,6.56697596826196,39.3978017080178));
#210445=CARTESIAN_POINT('Ctrl Pts',(60.6581326136905,6.56697596826196,39.5248017080178));
#210446=CARTESIAN_POINT('Ctrl Pts',(60.7343993681215,6.7024559967491,39.3978017080178));
#210447=CARTESIAN_POINT('Ctrl Pts',(60.747565938859,6.57637578951098,39.3980355775196));
#210448=CARTESIAN_POINT('Ctrl Pts',(60.7924070567583,6.58108878091632,39.5248015517192));
#210449=CARTESIAN_POINT('Ctrl Pts',(60.819067758858,6.71113417453909,39.3484893995498));
#210450=CARTESIAN_POINT('Ctrl Pts',(60.8325536871416,6.58530836180368,39.3489438303409));
#210451=CARTESIAN_POINT('Ctrl Pts',(60.9193730951232,6.59443344928337,39.4508333155592));
#210452=CARTESIAN_POINT('Ctrl Pts',(60.8636883187846,6.71570789669327,39.2708017080178));
#210453=CARTESIAN_POINT('Ctrl Pts',(60.8773920302462,6.59002106156384,39.2710850691866));
#210454=CARTESIAN_POINT('Ctrl Pts',(60.9862851800405,6.60146619279864,39.3343017080178));
#210455=CARTESIAN_POINT('Origin',(60.6448574988555,6.69328024897373,39.5248017080178));
#210456=CARTESIAN_POINT('Ctrl Pts',(59.1062911958297,6.53099325079975,39.2875012672119));
#210457=CARTESIAN_POINT('Ctrl Pts',(59.1200087114583,6.40512264090921,39.2878045257519));
#210458=CARTESIAN_POINT('Ctrl Pts',(59.2267768430461,6.41653455700044,39.3549015218347));
#210459=CARTESIAN_POINT('Ctrl Pts',(59.2206299794252,6.54313486548288,39.1034938540228));
#210460=CARTESIAN_POINT('Ctrl Pts',(59.2341972766244,6.41712406698054,39.1038286278808));
#210461=CARTESIAN_POINT('Ctrl Pts',(59.318224747433,6.42614611919662,39.2077506434031));
#210462=CARTESIAN_POINT('Ctrl Pts',(59.426035450364,6.56494601396981,38.989));
#210463=CARTESIAN_POINT('Ctrl Pts',(59.4394961352159,6.43870134519647,38.9892298954611));
#210464=CARTESIAN_POINT('Ctrl Pts',(59.48250679558,6.44341285848367,39.1161900347289));
#210465=CARTESIAN_POINT('Ctrl Pts',(59.6417962403144,6.58785426247015,38.989));
#210466=CARTESIAN_POINT('Ctrl Pts',(59.6550912403354,6.46136078685154,38.989));
#210467=CARTESIAN_POINT('Ctrl Pts',(59.6550713402783,6.46155012324659,39.1161900945646));
#210468=CARTESIAN_POINT('Origin',(59.6417962403144,6.58785426247015,39.116));
#210469=CARTESIAN_POINT('Origin',(60.0186752706393,6.62746584474012,39.5248017080178));
#210470=CARTESIAN_POINT('Origin',(60.4944777170595,6.67747469700864,39.5248017080178));
#210471=CARTESIAN_POINT('Origin',(59.7852323155142,6.60293000146354,39.116));
#210472=CARTESIAN_POINT('Origin',(60.04095383883,6.62985850077722,39.1160402713845));
#210473=CARTESIAN_POINT('Ctrl Pts',(60.275645989912,6.65505462397313,39.2708017080178));
#210474=CARTESIAN_POINT('Ctrl Pts',(60.2894805317163,6.52822907310695,39.27051194648));
#210475=CARTESIAN_POINT('Ctrl Pts',(60.1796001951996,6.51668018436665,39.3343017080178));
#210476=CARTESIAN_POINT('Ctrl Pts',(60.3204176712046,6.65964099131217,39.3487519301186));
#210477=CARTESIAN_POINT('Ctrl Pts',(60.3340024654441,6.53290851690509,39.3482879463988));
#210478=CARTESIAN_POINT('Ctrl Pts',(60.246738409926,6.52373669508256,39.4512271261639));
#210479=CARTESIAN_POINT('Ctrl Pts',(60.4052373806432,6.66833043150585,39.3978017080178));
#210480=CARTESIAN_POINT('Ctrl Pts',(60.4184509388162,6.54178440911706,39.3975673827397));
#210481=CARTESIAN_POINT('Ctrl Pts',(60.3739306632453,6.53710513959941,39.524801535518));
#210482=CARTESIAN_POINT('Ctrl Pts',(60.4944777170595,6.67747469700864,39.3978017080178));
#210483=CARTESIAN_POINT('Ctrl Pts',(60.5077528318945,6.55117041629687,39.3978017080178));
#210484=CARTESIAN_POINT('Ctrl Pts',(60.5077528318945,6.55117041629687,39.5248017080178));
#210485=CARTESIAN_POINT('Origin',(60.1663250803646,6.64298446507842,39.3343017080178));
#210486=CARTESIAN_POINT('Origin',(60.0854204586799,6.63448104699103,39.1934008533554));
#210487=CARTESIAN_POINT('Origin',(5.66467691768715E-15,1.86266069604307E-13,
2.53178198860262));
#210488=CARTESIAN_POINT('',(-0.0152399999993761,-59.0285534841294,2.65878198860221));
#210489=CARTESIAN_POINT('',(0.0152400000006239,-59.0285534841294,2.65878198860221));
#210490=CARTESIAN_POINT('Origin',(5.64679317051214E-15,1.85361349597066E-13,
2.65878198860263));
#210491=CARTESIAN_POINT('',(-0.015212193455297,-58.9208513795071,2.59908173515982));
#210492=CARTESIAN_POINT('Origin',(-0.015239999999376,-59.0285534841294,
2.5317819886022));
#210493=CARTESIAN_POINT('',(0.0152121934565426,-58.9208513795071,2.59908173515982));
#210494=CARTESIAN_POINT('Origin',(5.65519997554244E-15,1.85786641043733E-13,
2.59908173516023));
#210495=CARTESIAN_POINT('Origin',(0.0152400000006239,-59.0285534841294,
2.5317819886022));
#210496=CARTESIAN_POINT('Origin',(5.66467691768715E-15,1.86047439754084E-13,
2.53178198860262));
#210497=CARTESIAN_POINT('',(-0.0152661173102018,-62.9541448057646,2.59908173515979));
#210498=CARTESIAN_POINT('',(0.0152661173115319,-62.9541448057646,2.59908173515979));
#210499=CARTESIAN_POINT('Origin',(5.65519997554243E-15,1.8556801119351E-13,
2.59908173516023));
#210500=CARTESIAN_POINT('',(-0.0152399999993361,-62.8464427007194,2.65878198860218));
#210501=CARTESIAN_POINT('Origin',(-0.015239999999336,-62.8464427007194,
2.53178198860218));
#210502=CARTESIAN_POINT('',(0.0152400000006639,-62.8464427007194,2.65878198860218));
#210503=CARTESIAN_POINT('Origin',(5.64679317051213E-15,1.85142719746843E-13,
2.65878198860263));
#210504=CARTESIAN_POINT('Origin',(0.0152400000006639,-62.8464427007194,
2.53178198860217));
#210505=CARTESIAN_POINT('Origin',(3.5331177639001E-16,1.91577434745604E-13,
2.53178198860262));
#210506=CARTESIAN_POINT('',(-59.0285534841296,0.0152400000001907,2.65878198860261));
#210507=CARTESIAN_POINT('',(-59.0285534841296,-0.0152399999998093,2.65878198860261));
#210508=CARTESIAN_POINT('Origin',(3.17544282039971E-16,1.90690598485538E-13,
2.65878198860263));
#210509=CARTESIAN_POINT('',(-58.9208513795073,0.015212193456111,2.59908173516022));
#210510=CARTESIAN_POINT('Origin',(-59.0285534841296,0.0152400000001916,
2.53178198860261));
#210511=CARTESIAN_POINT('',(-58.9208513795073,-0.0152121934557287,2.59908173516022));
#210512=CARTESIAN_POINT('Origin',(3.34357892100574E-16,1.91107483127175E-13,
2.59908173516024));
#210513=CARTESIAN_POINT('Origin',(-59.0285534841296,-0.0152399999998084,
2.53178198860261));
#210514=CARTESIAN_POINT('Origin',(1.34681926167381E-16,1.91577434745604E-13,
2.53178198860262));
#210515=CARTESIAN_POINT('',(-62.9541448057648,0.0152661173110579,2.59908173516022));
#210516=CARTESIAN_POINT('',(-62.9541466567496,1.98817142546799E-13,2.59908173516022));
#210517=CARTESIAN_POINT('Origin',(1.15728041877948E-16,1.91107483127175E-13,
2.59908173516023));
#210518=CARTESIAN_POINT('',(-62.8464427007196,0.0152400000001907,2.65878198860261));
#210519=CARTESIAN_POINT('Origin',(-62.8464427007196,0.0152400000001916,
2.53178198860261));
#210520=CARTESIAN_POINT('',(-62.8464427007196,-0.0152399999998093,2.65878198860261));
#210521=CARTESIAN_POINT('Origin',(9.89144318173425E-17,1.90690598485538E-13,
2.65878198860263));
#210522=CARTESIAN_POINT('',(-62.9541448057648,-0.0152661173106757,2.59908173516022));
#210523=CARTESIAN_POINT('Origin',(-62.8464427007196,-0.0152399999998084,
2.5317819886026));
#210524=CARTESIAN_POINT('Origin',(1.15728041877948E-16,1.91107483127175E-13,
2.59908173516023));
#210525=CARTESIAN_POINT('Origin',(5.62443848654336E-15,1.89582053160455E-13,
2.81753198860262));
#210526=CARTESIAN_POINT('',(58.2189663438286,2.0114600153905E-13,2.18253198860263));
#210527=CARTESIAN_POINT('Origin',(5.71385722241845E-15,1.94016234460786E-13,
2.18253198860262));
#210528=CARTESIAN_POINT('',(57.6804558027693,1.98995629809826E-13,2.48103325581453));
#210529=CARTESIAN_POINT('Origin',(58.2189663438286,1.96711820238719E-13,
2.81753198860263));
#210530=CARTESIAN_POINT('',(-57.6804558027693,1.84867992695381E-13,2.48103325581451));
#210531=CARTESIAN_POINT('Origin',(5.67182319726696E-15,1.91931811252603E-13,
2.48103325581452));
#210532=CARTESIAN_POINT('Origin',(5.67182319726696E-15,1.91931811252603E-13,
2.48103325581452));
#210533=CARTESIAN_POINT('Origin',(5.62443848654336E-15,1.89582053160455E-13,
2.81753198860262));
#210534=CARTESIAN_POINT('',(58.8470884664677,1.99138501105563E-13,2.48103325581455));
#210535=CARTESIAN_POINT('Origin',(5.67182319726695E-15,1.91931811252603E-13,
2.48103325581454));
#210536=CARTESIAN_POINT('',(58.3085779254084,2.01156975792705E-13,2.18253198860263));
#210537=CARTESIAN_POINT('Origin',(58.3085779254084,1.96722794492374E-13,
2.81753198860263));
#210538=CARTESIAN_POINT('Origin',(5.71385722241845E-15,1.94016234460786E-13,
2.18253198860262));
#210539=CARTESIAN_POINT('Origin',(5.62443848654336E-15,1.89582053160455E-13,
2.81753198860262));
#210540=CARTESIAN_POINT('',(63.5664220745916,2.01800875993476E-13,2.18253198860263));
#210541=CARTESIAN_POINT('Origin',(5.71385722241845E-15,1.94016234460786E-13,
2.18253198860262));
#210542=CARTESIAN_POINT('',(63.0279115335323,1.99650504264252E-13,2.48103325581454));
#210543=CARTESIAN_POINT('Origin',(63.5664220745916,1.97366694693145E-13,
2.81753198860263));
#210544=CARTESIAN_POINT('',(-63.0279115335323,1.84213118240955E-13,2.48103325581452));
#210545=CARTESIAN_POINT('Origin',(5.67182319726696E-15,1.91931811252603E-13,
2.48103325581453));
#210546=CARTESIAN_POINT('Origin',(5.67182319726696E-15,1.91931811252603E-13,
2.48103325581453));
#210547=CARTESIAN_POINT('Origin',(5.62443848654336E-15,1.89582053160455E-13,
2.81753198860262));
#210548=CARTESIAN_POINT('',(64.1945441972308,1.99793375559989E-13,2.48103325581455));
#210549=CARTESIAN_POINT('Origin',(5.67182319726695E-15,1.91931811252603E-13,
2.48103325581454));
#210550=CARTESIAN_POINT('',(63.6560336561714,2.01811850247131E-13,2.18253198860263));
#210551=CARTESIAN_POINT('Origin',(63.6560336561714,1.973776689468E-13,2.81753198860263));
#210552=CARTESIAN_POINT('Origin',(5.71385722241845E-15,1.94016234460786E-13,
2.18253198860262));
#210553=CARTESIAN_POINT('Origin',(0.,-8.93279506303506E-14,42.7590319886026));
#210554=CARTESIAN_POINT('',(65.,1.88673894754252E-13,4.08753198860263));
#210555=CARTESIAN_POINT('Origin',(5.44560101479317E-15,1.80713690559794E-13,
4.08753198860262));
#210556=CARTESIAN_POINT('',(65.,1.90890985404417E-13,3.77003198860264));
#210557=CARTESIAN_POINT('',(65.,-8.13677464358929E-14,42.7590319886026));
#210558=CARTESIAN_POINT('Origin',(5.49031038273072E-15,1.82930781209959E-13,
3.77003198860263));
#210559=CARTESIAN_POINT('Origin',(5.71385722241845E-15,1.94016234460786E-13,
2.18253198860262));
#210560=CARTESIAN_POINT('',(64.008019903844,2.01854956130286E-13,2.18253198860263));
#210561=CARTESIAN_POINT('Origin',(5.49031038273072E-15,1.82930781209959E-13,
3.77003198860263));
#210562=CARTESIAN_POINT('',(62.9541448057648,-0.0152661173106757,2.59908173516024));
#210563=CARTESIAN_POINT('',(62.9541448057648,0.0152661173110579,2.59908173516024));
#210564=CARTESIAN_POINT('Origin',(-1.95097259456047E-16,1.91107483127175E-13,
2.59908173516023));
#210565=CARTESIAN_POINT('',(62.7644678366119,0.318045750793234,2.90134173516024));
#210566=CARTESIAN_POINT('Ctrl Pts',(62.9541448057648,0.0152661173110579,
2.59908173516025));
#210567=CARTESIAN_POINT('Ctrl Pts',(62.9541438736292,0.019087735244839,
2.59908174381684));
#210568=CARTESIAN_POINT('Ctrl Pts',(62.9540952129414,0.0228988721024147,
2.59915752000996));
#210569=CARTESIAN_POINT('Ctrl Pts',(62.9539999459718,0.0266975986405368,
2.59930729517471));
#210570=CARTESIAN_POINT('Ctrl Pts',(62.953449420412,0.0486495517943568,
2.60017281085929));
#210571=CARTESIAN_POINT('Ctrl Pts',(62.9513443281451,0.0701898812494245,
2.60350651800147));
#210572=CARTESIAN_POINT('Ctrl Pts',(62.94790035651,0.0909392844481384,2.60896880596674));
#210573=CARTESIAN_POINT('Ctrl Pts',(62.9465113235254,0.0993079960720901,
2.6111718723562));
#210574=CARTESIAN_POINT('Ctrl Pts',(62.9449047668207,0.107548428340682,
2.6137207657729));
#210575=CARTESIAN_POINT('Ctrl Pts',(62.9430957254317,0.115637319282417,
2.61659179896982));
#210576=CARTESIAN_POINT('Ctrl Pts',(62.9424282989905,0.118621628943673,
2.61765103591207));
#210577=CARTESIAN_POINT('Ctrl Pts',(62.9417332466658,0.121585194085759,
2.61875422455149));
#210578=CARTESIAN_POINT('Ctrl Pts',(62.941011293136,0.12452678807298,2.61990022440395));
#210579=CARTESIAN_POINT('Ctrl Pts',(62.9396576302675,0.13004227679902,2.62204897412732));
#210580=CARTESIAN_POINT('Ctrl Pts',(62.938209392844,0.135480523183793,2.62434823201769));
#210581=CARTESIAN_POINT('Ctrl Pts',(62.9366713579026,0.140833441493559,
2.62679048030304));
#210582=CARTESIAN_POINT('Ctrl Pts',(62.9312882356078,0.15956865557774,2.63533834930178));
#210583=CARTESIAN_POINT('Ctrl Pts',(62.9248050892389,0.177258600739159,
2.64563784783561));
#210584=CARTESIAN_POINT('Ctrl Pts',(62.9174267595942,0.193556601113839,
2.65736666737963));
#210585=CARTESIAN_POINT('Ctrl Pts',(62.9137375947719,0.201705601301178,
2.66323107715163));
#210586=CARTESIAN_POINT('Ctrl Pts',(62.9098246351408,0.209506615291594,
2.66945281780773));
#210587=CARTESIAN_POINT('Ctrl Pts',(62.9057134946881,0.216916308650584,
2.675991606312));
#210588=CARTESIAN_POINT('Ctrl Pts',(62.9036579244618,0.22062115533008,2.67926100056413));
#210589=CARTESIAN_POINT('Ctrl Pts',(62.9015528091474,0.224228171852737,
2.68260965685122));
#210590=CARTESIAN_POINT('Ctrl Pts',(62.8994013510256,0.227731941419725,
2.68603254012481));
#210591=CARTESIAN_POINT('Ctrl Pts',(62.8972498929038,0.231235710986713,
2.68945542339841));
#210592=CARTESIAN_POINT('Ctrl Pts',(62.8950520414621,0.23463611427692,2.69295261525384));
#210593=CARTESIAN_POINT('Ctrl Pts',(62.8928111037451,0.237927978231107,
2.69651891172098));
#210594=CARTESIAN_POINT('Ctrl Pts',(62.8927919932396,0.237956050936405,
2.69654932476087));
#210595=CARTESIAN_POINT('Ctrl Pts',(62.8927728797351,0.237984115711198,
2.69657974261145));
#210596=CARTESIAN_POINT('Ctrl Pts',(62.8927537632335,0.238012172553033,
2.69661016526973));
#210597=CARTESIAN_POINT('Ctrl Pts',(62.8829906867849,0.252341211296434,
2.71214746101059));
#210598=CARTESIAN_POINT('Ctrl Pts',(62.8725309380421,0.264702219189649,
2.72880565567421));
#210599=CARTESIAN_POINT('Ctrl Pts',(62.8615664772847,0.275152816745564,
2.7462804001209));
#210600=CARTESIAN_POINT('Ctrl Pts',(62.850231205745,0.285956846571411,2.7643461288212));
#210601=CARTESIAN_POINT('Ctrl Pts',(62.8383556508913,0.2947193320565,2.78328592654098));
#210602=CARTESIAN_POINT('Ctrl Pts',(62.8261370346469,0.301453885679487,
2.80278753267434));
#210603=CARTESIAN_POINT('Ctrl Pts',(62.814150842194,0.308060333921697,2.82191817722369));
#210604=CARTESIAN_POINT('Ctrl Pts',(62.8018335935207,0.312715155745102,
2.84159092314712));
#210605=CARTESIAN_POINT('Ctrl Pts',(62.7893708783688,0.315383336840664,
2.86151233816558));
#210606=CARTESIAN_POINT('Ctrl Pts',(62.7811147664987,0.317150913275342,
2.87470957721006));
#210607=CARTESIAN_POINT('Ctrl Pts',(62.7727948225172,0.318045664008643,
2.88801594388191));
#210608=CARTESIAN_POINT('Ctrl Pts',(62.7644678366119,0.318045750793233,
2.90134173516024));
#210609=CARTESIAN_POINT('',(62.4081695979768,0.318048871877314,3.47153072139072));
#210610=CARTESIAN_POINT('',(62.7644678366119,0.318045750793234,2.90134173516024));
#210611=CARTESIAN_POINT('',(62.0995362748659,6.20712349654482,3.47153072139077));
#210612=CARTESIAN_POINT('Origin',(5.53234440788222E-15,1.85015204418142E-13,
3.47153072139072));
#210613=CARTESIAN_POINT('',(62.4538823482275,6.24436990788079,2.90134173516028));
#210614=CARTESIAN_POINT('',(62.0995362748659,6.20712349654482,3.47153072139077));
#210615=CARTESIAN_POINT('',(62.6108711573006,6.56531752495322,2.59908173516028));
#210616=CARTESIAN_POINT('Ctrl Pts',(62.4538823482275,6.24436990788079,2.90134173516029));
#210617=CARTESIAN_POINT('Ctrl Pts',(62.4661208561101,6.24565635961461,2.88164837656795));
#210618=CARTESIAN_POINT('Ctrl Pts',(62.4781153572946,6.24887816048076,2.86203734439279));
#210619=CARTESIAN_POINT('Ctrl Pts',(62.4897034690548,6.25393874389341,2.84277945978351));
#210620=CARTESIAN_POINT('Ctrl Pts',(62.5015244311521,6.25910101415356,2.823134609203));
#210621=CARTESIAN_POINT('Ctrl Pts',(62.5129234356942,6.26617675898121,2.80385576863699));
#210622=CARTESIAN_POINT('Ctrl Pts',(62.5237314369727,6.27511683300188,2.78521678518818));
#210623=CARTESIAN_POINT('Ctrl Pts',(62.5341195571992,6.2837095932512,2.76730190934976));
#210624=CARTESIAN_POINT('Ctrl Pts',(62.5439624606622,6.29402509233161,2.74997687280356));
#210625=CARTESIAN_POINT('Ctrl Pts',(62.5531007542683,6.30606398946803,2.73349253346358));
#210626=CARTESIAN_POINT('Ctrl Pts',(62.5601204743134,6.31531185249283,2.72082983599693));
#210627=CARTESIAN_POINT('Ctrl Pts',(62.5667243349244,6.32557753707723,2.70866321039474));
#210628=CARTESIAN_POINT('Ctrl Pts',(62.5728320301413,6.3368780377171,2.6971164533585));
#210629=CARTESIAN_POINT('Ctrl Pts',(62.5728480373212,6.33690765431395,2.69708619136755));
#210630=CARTESIAN_POINT('Ctrl Pts',(62.5728640408535,6.33693727882116,2.69705593387223));
#210631=CARTESIAN_POINT('Ctrl Pts',(62.5728800407364,6.33696691123596,2.69702568087575));
#210632=CARTESIAN_POINT('Ctrl Pts',(62.5745955535553,6.34014410870347,2.6937819444327));
#210633=CARTESIAN_POINT('Ctrl Pts',(62.5762674929177,6.34341121944338,2.69059266624704));
#210634=CARTESIAN_POINT('Ctrl Pts',(62.5778935423008,6.34676388583406,2.68746219342681));
#210635=CARTESIAN_POINT('Ctrl Pts',(62.5869421374019,6.36542071200083,2.67004182395935));
#210636=CARTESIAN_POINT('Ctrl Pts',(62.5945741278863,6.38672471011596,2.65443567877611));
#210637=CARTESIAN_POINT('Ctrl Pts',(62.6004109483577,6.40987366744549,2.64136852352728));
#210638=CARTESIAN_POINT('Ctrl Pts',(62.6030305942149,6.42026324006697,2.63550380329468));
#210639=CARTESIAN_POINT('Ctrl Pts',(62.605288967123,6.43102458681701,2.6301499745099));
#210640=CARTESIAN_POINT('Ctrl Pts',(62.6071534261453,6.44208677567884,2.62536981119258));
#210641=CARTESIAN_POINT('Ctrl Pts',(62.607963694818,6.44689425333237,2.62329241687077));
#210642=CARTESIAN_POINT('Ctrl Pts',(62.6086994224563,6.45175840518007,2.62132362131432));
#210643=CARTESIAN_POINT('Ctrl Pts',(62.6093578414453,6.45667331290448,2.61946873372352));
#210644=CARTESIAN_POINT('Ctrl Pts',(62.6116623079068,6.47387548993995,2.61297662715572));
#210645=CARTESIAN_POINT('Ctrl Pts',(62.6130197402063,6.49169942613424,2.60787989113974));
#210646=CARTESIAN_POINT('Ctrl Pts',(62.6133114945132,6.50989137546638,2.60440616886185));
#210647=CARTESIAN_POINT('Ctrl Pts',(62.6134573716667,6.51898735013245,2.6026693077229));
#210648=CARTESIAN_POINT('Ctrl Pts',(62.6133368299269,6.52817532814412,2.60133820040189));
#210649=CARTESIAN_POINT('Ctrl Pts',(62.6129350466932,6.53742359207021,2.60044130723589));
#210650=CARTESIAN_POINT('Ctrl Pts',(62.6127341550764,6.54204772403325,2.59999286065289));
#210651=CARTESIAN_POINT('Ctrl Pts',(62.6124629532086,6.5466869274878,2.59965296768517));
#210652=CARTESIAN_POINT('Ctrl Pts',(62.6121195889602,6.55133723782971,2.59942518630959));
#210653=CARTESIAN_POINT('Ctrl Pts',(62.6117762247118,6.55598754817163,2.59919740493401));
#210654=CARTESIAN_POINT('Ctrl Pts',(62.6113606963859,6.56064896522291,2.59908173791625));
#210655=CARTESIAN_POINT('Ctrl Pts',(62.6108711573006,6.56531752495321,2.59908173516029));
#210656=CARTESIAN_POINT('',(62.6076796697354,6.59568250079905,2.59908173516029));
#210657=CARTESIAN_POINT('Origin',(5.50063869163689E-15,1.85396353497297E-13,
2.59908173516023));
#210658=CARTESIAN_POINT('',(62.3873926810691,6.87697683366584,2.90134173516029));
#210659=CARTESIAN_POINT('Ctrl Pts',(62.6076796697354,6.59568250079905,2.5990817351603));
#210660=CARTESIAN_POINT('Ctrl Pts',(62.6072792748563,6.59948308607522,2.59908174381695));
#210661=CARTESIAN_POINT('Ctrl Pts',(62.6068325084578,6.60326825869941,2.59915752001001));
#210662=CARTESIAN_POINT('Ctrl Pts',(62.6063406883232,6.60703621730616,2.59930729517476));
#210663=CARTESIAN_POINT('Ctrl Pts',(62.6034985746712,6.62881036977247,2.60017281085931));
#210664=CARTESIAN_POINT('Ctrl Pts',(62.5991534367839,6.65001265698881,2.60350651800137));
#210665=CARTESIAN_POINT('Ctrl Pts',(62.5935594283559,6.67028839972278,2.60896880596642));
#210666=CARTESIAN_POINT('Ctrl Pts',(62.5913032360736,6.67846607318599,2.61117187235597));
#210667=CARTESIAN_POINT('Ctrl Pts',(62.5888441205329,6.68649343260138,2.6137207657728));
#210668=CARTESIAN_POINT('Ctrl Pts',(62.5861994699221,6.69434891543626,2.61659179896988));
#210669=CARTESIAN_POINT('Ctrl Pts',(62.5852237544099,6.69724711167669,2.61765103591213));
#210670=CARTESIAN_POINT('Ctrl Pts',(62.5842227327444,6.70012178934745,2.61875422455152));
#210671=CARTESIAN_POINT('Ctrl Pts',(62.5831972538526,6.702971804282,2.61990022440399));
#210672=CARTESIAN_POINT('Ctrl Pts',(62.5812744809303,6.70831558228429,2.62204897412736));
#210673=CARTESIAN_POINT('Ctrl Pts',(62.5792657255654,6.71357265535402,2.62434823201774));
#210674=CARTESIAN_POINT('Ctrl Pts',(62.5771765838154,6.71873548138833,2.62679048030309));
#210675=CARTESIAN_POINT('Ctrl Pts',(62.5698645876906,6.7368053725084,2.63533834930182));
#210676=CARTESIAN_POINT('Ctrl Pts',(62.5615678538928,6.75372073697221,2.64563784783566));
#210677=CARTESIAN_POINT('Ctrl Pts',(62.5525263385764,6.76915820973631,2.65736666737968));
#210678=CARTESIAN_POINT('Ctrl Pts',(62.5480055809182,6.77687694611836,2.66323107715169));
#210679=CARTESIAN_POINT('Ctrl Pts',(62.5432986288851,6.78422620968084,2.66945281780777));
#210680=CARTESIAN_POINT('Ctrl Pts',(62.5384354858299,6.79116558077052,2.67599160631204));
#210681=CARTESIAN_POINT('Ctrl Pts',(62.5360039143022,6.79463526631536,2.67926100056418));
#210682=CARTESIAN_POINT('Ctrl Pts',(62.5335332951358,6.79800247875529,2.68260965685127));
#210683=CARTESIAN_POINT('Ctrl Pts',(62.5310273792782,6.80126216569473,2.68603254012487));
#210684=CARTESIAN_POINT('Ctrl Pts',(62.5285214634206,6.80452185263417,2.68945542339846));
#210685=CARTESIAN_POINT('Ctrl Pts',(62.5259802131086,6.80767389012568,2.69295261525388));
#210686=CARTESIAN_POINT('Ctrl Pts',(62.5234074580025,6.81071347912885,2.69651891172102));
#210687=CARTESIAN_POINT('Ctrl Pts',(62.5233855177896,6.81073940045716,2.6965493247609));
#210688=CARTESIAN_POINT('Ctrl Pts',(62.5233635754231,6.81076531358493,2.69657974261149));
#210689=CARTESIAN_POINT('Ctrl Pts',(62.5233416309052,6.81079121850992,2.69661016526977));
#210690=CARTESIAN_POINT('Ctrl Pts',(62.5121342452098,6.82402124190313,2.71214746101212));
#210691=CARTESIAN_POINT('Ctrl Pts',(62.5004397189044,6.83522119344041,2.72880565567745));
#210692=CARTESIAN_POINT('Ctrl Pts',(62.4884429377063,6.84446844329644,2.74628040012597));
#210693=CARTESIAN_POINT('Ctrl Pts',(62.4760404333341,6.85402842900223,2.76434612882814));
#210694=CARTESIAN_POINT('Ctrl Pts',(62.4633140048689,6.86150157917582,2.78328592654992));
#210695=CARTESIAN_POINT('Ctrl Pts',(62.4504583709406,6.86692204702988,2.80278753268532));
#210696=CARTESIAN_POINT('Ctrl Pts',(62.4378472782206,6.87223940617952,2.82191817723646));
#210697=CARTESIAN_POINT('Ctrl Pts',(62.4251109433513,6.87558122532578,2.84159092316169));
#210698=CARTESIAN_POINT('Ctrl Pts',(62.4124375993863,6.87693208138216,2.86151233818192));
#210699=CARTESIAN_POINT('Ctrl Pts',(62.404041953316,6.87782697616073,2.87470957722106));
#210700=CARTESIAN_POINT('Ctrl Pts',(62.3956740599424,6.87784715439664,2.88801594388745));
#210701=CARTESIAN_POINT('Ctrl Pts',(62.3873926810691,6.87697683366584,2.9013417351603));
#210702=CARTESIAN_POINT('',(62.0330459552232,6.83973663030279,3.47153072139077));
#210703=CARTESIAN_POINT('',(62.3873926810691,6.87697683366584,2.90134173516029));
#210704=CARTESIAN_POINT('',(61.1105274371641,12.6642893210144,3.47153072139081));
#210705=CARTESIAN_POINT('Origin',(5.53234440788222E-15,1.85015204418142E-13,
3.47153072139072));
#210706=CARTESIAN_POINT('',(61.4590390555209,12.7383709431253,2.90134173516033));
#210707=CARTESIAN_POINT('',(61.1105274371641,12.6642893210143,3.47153072139081));
#210708=CARTESIAN_POINT('',(61.5816197022698,13.0739701745327,2.59908173516033));
#210709=CARTESIAN_POINT('Ctrl Pts',(61.4590390555209,12.7383709431253,2.90134173516033));
#210710=CARTESIAN_POINT('Ctrl Pts',(61.4710760487544,12.7409296199637,2.88164837656726));
#210711=CARTESIAN_POINT('Ctrl Pts',(61.4826680729132,12.7453875382444,2.86203734439139));
#210712=CARTESIAN_POINT('Ctrl Pts',(61.4936637287778,12.7516316867664,2.84277945978143));
#210713=CARTESIAN_POINT('Ctrl Pts',(61.5048803302309,12.7580013045727,2.82313460920026));
#210714=CARTESIAN_POINT('Ctrl Pts',(61.5154772731004,12.7662298081578,2.80385576863363));
#210715=CARTESIAN_POINT('Ctrl Pts',(61.5252915748184,12.7762506512828,2.78521678518427));
#210716=CARTESIAN_POINT('Ctrl Pts',(61.5347245998114,12.7858821937365,2.76730190934541));
#210717=CARTESIAN_POINT('Ctrl Pts',(61.5434353195528,12.7971700470073,2.74997687279882));
#210718=CARTESIAN_POINT('Ctrl Pts',(61.5512651452133,12.8100982055938,2.73349253345852));
#210719=CARTESIAN_POINT('Ctrl Pts',(61.5572797455861,12.8200291684051,2.7208298359937));
#210720=CARTESIAN_POINT('Ctrl Pts',(61.5627743733228,12.8309289078952,2.70866321039323));
#210721=CARTESIAN_POINT('Ctrl Pts',(61.5676673859796,12.8428059312037,2.69711645335854));
#210722=CARTESIAN_POINT('Ctrl Pts',(61.5676802096931,12.8428370587636,2.6970861913676));
#210723=CARTESIAN_POINT('Ctrl Pts',(61.5676930289522,12.8428681938093,2.69705593387227));
#210724=CARTESIAN_POINT('Ctrl Pts',(61.5677058437553,12.8428993363378,2.69702568087579));
#210725=CARTESIAN_POINT('Ctrl Pts',(61.5690798512467,12.8462384487039,2.69378194443274));
#210726=CARTESIAN_POINT('Ctrl Pts',(61.5704011254854,12.8496624271215,2.69059266624708));
#210727=CARTESIAN_POINT('Ctrl Pts',(61.5716678181342,12.8531666956981,2.68746219342685));
#210728=CARTESIAN_POINT('Ctrl Pts',(61.5787166747153,12.8726671535583,2.67004182396061));
#210729=CARTESIAN_POINT('Ctrl Pts',(61.5840799821727,12.894652206378,2.65443567877833));
#210730=CARTESIAN_POINT('Ctrl Pts',(61.5874651029949,12.9182844651696,2.64136852353006));
#210731=CARTESIAN_POINT('Ctrl Pts',(61.5889843920982,12.9288909501824,2.63550380329639));
#210732=CARTESIAN_POINT('Ctrl Pts',(61.5901055263651,12.9398294094002,2.63014997451068));
#210733=CARTESIAN_POINT('Ctrl Pts',(61.5908034580838,12.9510258874722,2.62536981119262));
#210734=CARTESIAN_POINT('Ctrl Pts',(61.5911067697685,12.9558917253993,2.62329241687082));
#210735=CARTESIAN_POINT('Ctrl Pts',(61.5913300246961,12.9608061353937,2.62132362131436));
#210736=CARTESIAN_POINT('Ctrl Pts',(61.5914710890455,12.9657629422644,2.61946873372356));
#210737=CARTESIAN_POINT('Ctrl Pts',(61.5919648142682,12.9831117663121,2.61297662715576));
#210738=CARTESIAN_POINT('Ctrl Pts',(61.5914517017518,13.0009799514312,2.60787989113978));
#210739=CARTESIAN_POINT('Ctrl Pts',(61.5898402812905,13.0191027399908,2.60440616886188));
#210740=CARTESIAN_POINT('Ctrl Pts',(61.5890345710599,13.0281641342706,2.60266930772293));
#210741=CARTESIAN_POINT('Ctrl Pts',(61.5879542844384,13.0372891795345,2.60133820040193));
#210742=CARTESIAN_POINT('Ctrl Pts',(61.5865879953992,13.0464447827192,2.60044130723593));
#210743=CARTESIAN_POINT('Ctrl Pts',(61.5859048508796,13.0510225843115,2.59999286065293));
#210744=CARTESIAN_POINT('Ctrl Pts',(61.5851502058761,13.0556080254097,2.59965296768521));
#210745=CARTESIAN_POINT('Ctrl Pts',(61.5843226328192,13.0601969695277,2.59942518630963));
#210746=CARTESIAN_POINT('Ctrl Pts',(61.5834950597624,13.0647859136458,2.59919740493405));
#210747=CARTESIAN_POINT('Ctrl Pts',(61.5825945569831,13.0693783604294,2.59908173791627));
#210748=CARTESIAN_POINT('Ctrl Pts',(61.5816197022698,13.0739701745327,2.59908173516033));
#210749=CARTESIAN_POINT('',(61.5752716937451,13.103835206573,2.59908173516034));
#210750=CARTESIAN_POINT('Origin',(5.50318346416883E-15,1.85380286435869E-13,
2.59908173516022));
#210751=CARTESIAN_POINT('',(61.3267881959113,13.3605623192489,2.90134173516034));
#210752=CARTESIAN_POINT('Ctrl Pts',(61.5752716937451,13.103835206573,2.59908173516033));
#210753=CARTESIAN_POINT('Ctrl Pts',(61.5744762229326,13.1075731191839,2.59908174381695));
#210754=CARTESIAN_POINT('Ctrl Pts',(61.5736362456896,13.1112908564314,2.59915752001006));
#210755=CARTESIAN_POINT('Ctrl Pts',(61.5727532608744,13.1149867645638,2.5993072951748));
#210756=CARTESIAN_POINT('Ctrl Pts',(61.5676506979228,13.1363445541687,2.60017281085922));
#210757=CARTESIAN_POINT('Ctrl Pts',(61.5611131206563,13.1569765024481,2.60350651800036));
#210758=CARTESIAN_POINT('Ctrl Pts',(61.5534303645638,13.1765564394347,2.60896880596388));
#210759=CARTESIAN_POINT('Ctrl Pts',(61.5503317322976,13.1844534784381,2.61117187235401));
#210760=CARTESIAN_POINT('Ctrl Pts',(61.5470470005041,13.1921798155733,2.61372076577171));
#210761=CARTESIAN_POINT('Ctrl Pts',(61.5435957160157,13.19971582399,2.61659179896991));
#210762=CARTESIAN_POINT('Ctrl Pts',(61.542322401576,13.2024961535651,2.61765103591216));
#210763=CARTESIAN_POINT('Ctrl Pts',(61.5410263779726,13.2052504481944,2.61875422455157));
#210764=CARTESIAN_POINT('Ctrl Pts',(61.53970860908,13.2079776587163,2.61990022440403));
#210765=CARTESIAN_POINT('Ctrl Pts',(61.5372377924063,13.2130911784448,2.62204897412741));
#210766=CARTESIAN_POINT('Ctrl Pts',(61.5346905274442,13.2181094806068,2.62434823201777));
#210767=CARTESIAN_POINT('Ctrl Pts',(61.5320731679599,13.2230256493632,2.62679048030312));
#210768=CARTESIAN_POINT('Ctrl Pts',(61.5229124097647,13.2402322400107,2.63533834930186));
#210769=CARTESIAN_POINT('Ctrl Pts',(61.5128929892898,13.2561876955041,2.6456378478357));
#210770=CARTESIAN_POINT('Ctrl Pts',(61.5022873490355,13.2705955044755,2.65736666737972));
#210771=CARTESIAN_POINT('Ctrl Pts',(61.4969845289084,13.2777994089612,2.66323107715172));
#210772=CARTESIAN_POINT('Ctrl Pts',(61.4915351548247,13.2846164020262,2.66945281780781));
#210773=CARTESIAN_POINT('Ctrl Pts',(61.4859732907799,13.2910094216448,2.67599160631208));
#210774=CARTESIAN_POINT('Ctrl Pts',(61.4831923587575,13.2942059314541,2.67926100056422));
#210775=CARTESIAN_POINT('Ctrl Pts',(61.4803833043595,13.2972964479271,2.68260965685131));
#210776=CARTESIAN_POINT('Ctrl Pts',(61.4775503861047,13.3002763384268,2.68603254012491));
#210777=CARTESIAN_POINT('Ctrl Pts',(61.4747174678498,13.3032562289264,2.6894554233985));
#210778=CARTESIAN_POINT('Ctrl Pts',(61.4718606611378,13.3061253662368,2.69295261525394));
#210779=CARTESIAN_POINT('Ctrl Pts',(61.4689842762858,13.3088793779158,2.69651891172108));
#210780=CARTESIAN_POINT('Ctrl Pts',(61.4689597467471,13.3089028638676,2.69654932476096));
#210781=CARTESIAN_POINT('Ctrl Pts',(61.4689352159238,13.3089263414387,2.69657974261154));
#210782=CARTESIAN_POINT('Ctrl Pts',(61.4689106838182,13.3089498106271,2.69661016526982));
#210783=CARTESIAN_POINT('Ctrl Pts',(61.45638177934,13.320935867764,2.71214746101229));
#210784=CARTESIAN_POINT('Ctrl Pts',(61.4435806031503,13.3308520539316,2.72880565567773));
#210785=CARTESIAN_POINT('Ctrl Pts',(61.4306829407578,13.3387946412825,2.74628040012638));
#210786=CARTESIAN_POINT('Ctrl Pts',(61.4173490879876,13.3470058416637,2.76434612882863));
#210787=CARTESIAN_POINT('Ctrl Pts',(61.4039112193257,13.3531077791283,2.78328592655052));
#210788=CARTESIAN_POINT('Ctrl Pts',(61.3905594167301,13.3571547734334,2.80278753268603));
#210789=CARTESIAN_POINT('Ctrl Pts',(61.3774615935149,13.3611247853911,2.82191817723731));
#210790=CARTESIAN_POINT('Ctrl Pts',(61.3644457144006,13.3631169881908,2.8415909231627));
#210791=CARTESIAN_POINT('Ctrl Pts',(61.3517005934322,13.3631357189472,2.86151233818308));
#210792=CARTESIAN_POINT('Ctrl Pts',(61.3432573976137,13.3631481274166,2.87470957722185));
#210793=CARTESIAN_POINT('Ctrl Pts',(61.3349332352358,13.3622935120789,2.88801594388787));
#210794=CARTESIAN_POINT('Ctrl Pts',(61.3267881959113,13.3605623192489,2.90134173516034));
#210795=CARTESIAN_POINT('',(60.9782752797348,13.2864868028998,3.47153072139082));
#210796=CARTESIAN_POINT('',(61.3267881959113,13.3605623192489,2.90134173516034));
#210797=CARTESIAN_POINT('',(59.4519788726607,18.9827025415099,3.47153072139086));
#210798=CARTESIAN_POINT('Origin',(5.53234440788222E-15,1.85015204418142E-13,
3.47153072139072));
#210799=CARTESIAN_POINT('',(59.7908376697911,19.0928077206414,2.90134173516037));
#210800=CARTESIAN_POINT('',(59.4519788726608,18.9827025415099,3.47153072139085));
#210801=CARTESIAN_POINT('',(59.8776671349985,19.4393816709759,2.59908173516037));
#210802=CARTESIAN_POINT('Ctrl Pts',(59.7908376697911,19.0928077206414,2.90134173516037));
#210803=CARTESIAN_POINT('Ctrl Pts',(59.8025412685588,19.0966105891856,2.88164837656655));
#210804=CARTESIAN_POINT('Ctrl Pts',(59.8136038110496,19.1022557829952,2.86203734438993));
#210805=CARTESIAN_POINT('Ctrl Pts',(59.8238865403117,19.1096150844288,2.84277945977927));
#210806=CARTESIAN_POINT('Ctrl Pts',(59.834375889688,19.1171222629157,2.82313460919731));
#210807=CARTESIAN_POINT('Ctrl Pts',(59.8440546685612,19.1264133720513,2.80385576862993));
#210808=CARTESIAN_POINT('Ctrl Pts',(59.8527677431752,19.1374051938265,2.78521678517989));
#210809=CARTESIAN_POINT('Ctrl Pts',(59.861142322739,19.1479699932901,2.76730190934029));
#210810=CARTESIAN_POINT('Ctrl Pts',(59.8686254222904,19.160106528669,2.74997687279304));
#210811=CARTESIAN_POINT('Ctrl Pts',(59.8750609947968,19.1737823050951,2.73349253345219));
#210812=CARTESIAN_POINT('Ctrl Pts',(59.8800045782769,19.1842875619858,2.72082983598967));
#210813=CARTESIAN_POINT('Ctrl Pts',(59.8843297728482,19.1957019365543,2.70866321039134));
#210814=CARTESIAN_POINT('Ctrl Pts',(59.8879544940744,19.2080253553781,2.69711645335858));
#210815=CARTESIAN_POINT('Ctrl Pts',(59.8879639938223,19.2080576528611,2.69708619136764));
#210816=CARTESIAN_POINT('Ctrl Pts',(59.8879734883577,19.2080899573232,2.69705593387232));
#210817=CARTESIAN_POINT('Ctrl Pts',(59.8879829776793,19.2081222687613,2.69702568087584));
#210818=CARTESIAN_POINT('Ctrl Pts',(59.8890004259296,19.211586712012,2.69378194443279));
#210819=CARTESIAN_POINT('Ctrl Pts',(59.8899565588875,19.2151300442834,2.69059266624713));
#210820=CARTESIAN_POINT('Ctrl Pts',(59.8908500166522,19.2187475215461,2.6874621934269));
#210821=CARTESIAN_POINT('Ctrl Pts',(59.895821905966,19.2388779600025,2.67004182396195));
#210822=CARTESIAN_POINT('Ctrl Pts',(59.8988577688777,19.2613031946872,2.6544356787807));
#210823=CARTESIAN_POINT('Ctrl Pts',(59.8997541019592,19.285159834968,2.64136852353302));
#210824=CARTESIAN_POINT('Ctrl Pts',(59.9001563886589,19.2958670255031,2.63550380329822));
#210825=CARTESIAN_POINT('Ctrl Pts',(59.9001280009025,19.3068627531405,2.63014997451153));
#210826=CARTESIAN_POINT('Ctrl Pts',(59.8996517586312,19.318070849466,2.62536981119268));
#210827=CARTESIAN_POINT('Ctrl Pts',(59.8994447901818,19.3229417365281,2.62329241687088));
#210828=CARTESIAN_POINT('Ctrl Pts',(59.899153126371,19.3278525613648,2.62132362131442));
#210829=CARTESIAN_POINT('Ctrl Pts',(59.8987752905501,19.3327969595686,2.61946873372361));
#210830=CARTESIAN_POINT('Ctrl Pts',(59.8974528651773,19.3501023532816,2.61297662715581));
#210831=CARTESIAN_POINT('Ctrl Pts',(59.895074829613,19.3678190197503,2.60787989113983));
#210832=CARTESIAN_POINT('Ctrl Pts',(59.8915778894434,19.3856740904734,2.60440616886193));
#210833=CARTESIAN_POINT('Ctrl Pts',(59.8898294193586,19.394601625835,2.60266930772298));
#210834=CARTESIAN_POINT('Ctrl Pts',(59.8878012237015,19.4035637624458,2.60133820040198));
#210835=CARTESIAN_POINT('Ctrl Pts',(59.8854853982054,19.4125263941846,2.60044130723597));
#210836=CARTESIAN_POINT('Ctrl Pts',(59.8843274854574,19.417007710054,2.59999286065297));
#210837=CARTESIAN_POINT('Ctrl Pts',(59.8830976653668,19.4214891497435,2.59965296768525));
#210838=CARTESIAN_POINT('Ctrl Pts',(59.881794950565,19.4259664502057,2.59942518630967));
#210839=CARTESIAN_POINT('Ctrl Pts',(59.8804922357633,19.4304437506678,2.59919740493409));
#210840=CARTESIAN_POINT('Ctrl Pts',(59.8791166246276,19.4349169113757,2.59908173791627));
#210841=CARTESIAN_POINT('Ctrl Pts',(59.8776671349985,19.4393816709759,2.59908173516038));
#210842=CARTESIAN_POINT('',(59.8682321556242,19.4684195516699,2.59908173516038));
#210843=CARTESIAN_POINT('Origin',(5.50739376141089E-15,1.85364573392646E-13,
2.59908173516024));
#210844=CARTESIAN_POINT('',(59.5942745858235,19.6977666881848,2.90134173516037));
#210845=CARTESIAN_POINT('Ctrl Pts',(59.8682321556242,19.4684195516699,2.59908173516038));
#210846=CARTESIAN_POINT('Ctrl Pts',(59.8670503242229,19.4720538382629,2.59908174381699));
#210847=CARTESIAN_POINT('Ctrl Pts',(59.8658263391019,19.4756634078263,2.59915752001009));
#210848=CARTESIAN_POINT('Ctrl Pts',(59.8645618637724,19.4792467723414,2.59930729517484));
#210849=CARTESIAN_POINT('Ctrl Pts',(59.8572547562677,19.4999541986781,2.60017281085934));
#210850=CARTESIAN_POINT('Ctrl Pts',(59.8485963666847,19.5197897600826,2.60350651800101));
#210851=CARTESIAN_POINT('Ctrl Pts',(59.8389090368088,19.5384593694391,2.60896880596543));
#210852=CARTESIAN_POINT('Ctrl Pts',(59.8350019138237,19.5459892523658,2.61117187235522));
#210853=CARTESIAN_POINT('Ctrl Pts',(59.8309275539881,19.5533299158494,2.61372076577242));
#210854=CARTESIAN_POINT('Ctrl Pts',(59.8267074486193,19.560463883758,2.61659179896997));
#210855=CARTESIAN_POINT('Ctrl Pts',(59.8251504859514,19.5630958847952,2.61765103591222));
#210856=CARTESIAN_POINT('Ctrl Pts',(59.823573659916,19.5656996197547,2.61875422455163));
#210857=CARTESIAN_POINT('Ctrl Pts',(59.8219780387744,19.5682741459747,2.6199002244041));
#210858=CARTESIAN_POINT('Ctrl Pts',(59.8189862491339,19.5731013826371,2.62204897412747));
#210859=CARTESIAN_POINT('Ctrl Pts',(59.8159283829426,19.5778259323228,2.62434823201784));
#210860=CARTESIAN_POINT('Ctrl Pts',(59.8128114820621,19.5824415812277,2.62679048030319));
#210861=CARTESIAN_POINT('Ctrl Pts',(59.8019023289803,19.5985963523947,2.63533834930192));
#210862=CARTESIAN_POINT('Ctrl Pts',(59.7902699966956,19.6134170876084,2.64563784783576));
#210863=CARTESIAN_POINT('Ctrl Pts',(59.7782164291175,19.626637377817,2.65736666737978));
#210864=CARTESIAN_POINT('Ctrl Pts',(59.7721896453285,19.6332475229213,2.66323107715179));
#210865=CARTESIAN_POINT('Ctrl Pts',(59.766057553677,19.6394575570863,2.66945281780788));
#210866=CARTESIAN_POINT('Ctrl Pts',(59.7598579055891,19.645234181973,2.67599160631215));
#210867=CARTESIAN_POINT('Ctrl Pts',(59.7567580815451,19.6481224944163,2.67926100056428));
#210868=CARTESIAN_POINT('Ctrl Pts',(59.7536413685033,19.6509024545773,2.68260965685137));
#210869=CARTESIAN_POINT('Ctrl Pts',(59.7505124858965,19.6535699003333,2.68603254012496));
#210870=CARTESIAN_POINT('Ctrl Pts',(59.7473836032896,19.6562373460892,2.68945542339855));
#210871=CARTESIAN_POINT('Ctrl Pts',(59.7442425399497,19.6587921483498,2.69295261525399));
#210872=CARTESIAN_POINT('Ctrl Pts',(59.7410940396263,19.6612304091763,2.69651891172113));
#210873=CARTESIAN_POINT('Ctrl Pts',(59.7410671895125,19.6612512024346,2.696549324761));
#210874=CARTESIAN_POINT('Ctrl Pts',(59.7410403389972,19.6612719872239,2.69657974261158));
#210875=CARTESIAN_POINT('Ctrl Pts',(59.7410134880829,19.6612927635423,2.69661016526986));
#210876=CARTESIAN_POINT('Ctrl Pts',(59.7273003341214,19.6719035326723,2.71214746101201));
#210877=CARTESIAN_POINT('Ctrl Pts',(59.713532760413,19.6804273096593,2.7288056556771));
#210878=CARTESIAN_POINT('Ctrl Pts',(59.6998755263147,19.686978213856,2.74628040012537));
#210879=CARTESIAN_POINT('Ctrl Pts',(59.6857564136279,19.6937506652828,2.7643461288272));
#210880=CARTESIAN_POINT('Ctrl Pts',(59.6717543328707,19.6984145359348,2.78328592654863));
#210881=CARTESIAN_POINT('Ctrl Pts',(59.6580526467514,19.7010437169746,2.80278753268367));
#210882=CARTESIAN_POINT('Ctrl Pts',(59.6446115955335,19.7036228854586,2.82191817723442));
#210883=CARTESIAN_POINT('Ctrl Pts',(59.63145877687,19.7042436449213,2.84159092315926));
#210884=CARTESIAN_POINT('Ctrl Pts',(59.6187815171109,19.7029300451599,2.8615123381791));
#210885=CARTESIAN_POINT('Ctrl Pts',(59.6103832769634,19.7020598313705,2.87470957721919));
#210886=CARTESIAN_POINT('Ctrl Pts',(59.6021940468451,19.7003397858036,2.88801594388655));
#210887=CARTESIAN_POINT('Ctrl Pts',(59.5942745858236,19.6977666881848,2.90134173516037));
#210888=CARTESIAN_POINT('',(59.2554138597571,19.5876674457081,3.47153072139086));
#210889=CARTESIAN_POINT('',(59.5942745858236,19.6977666881848,2.90134173516038));
#210890=CARTESIAN_POINT('',(57.1420619865021,25.0931373005748,3.4715307213909));
#210891=CARTESIAN_POINT('Origin',(5.53234440788222E-15,1.85015204418142E-13,
3.47153072139072));
#210892=CARTESIAN_POINT('',(57.467555354514,25.2380597013433,2.90134173516042));
#210893=CARTESIAN_POINT('',(57.1420619865021,25.0931373005748,3.4715307213909));
#210894=CARTESIAN_POINT('',(57.5176823163888,25.5918112338797,2.59908173516042));
#210895=CARTESIAN_POINT('Ctrl Pts',(57.467555354514,25.2380597013433,2.90134173516042));
#210896=CARTESIAN_POINT('Ctrl Pts',(57.478797331737,25.2430650965687,2.88164837656886));
#210897=CARTESIAN_POINT('Ctrl Pts',(57.4892091890277,25.2498357159813,2.86203734439446));
#210898=CARTESIAN_POINT('Ctrl Pts',(57.4986663319526,25.2582295402783,2.84277945978591));
#210899=CARTESIAN_POINT('Ctrl Pts',(57.5083135057439,25.2667920292256,2.82313460920596));
#210900=CARTESIAN_POINT('Ctrl Pts',(57.5169680778932,25.2770439485736,2.80385576864049));
#210901=CARTESIAN_POINT('Ctrl Pts',(57.5244844631338,25.2888863202969,2.78521678519216));
#210902=CARTESIAN_POINT('Ctrl Pts',(57.5317088436217,25.3002686266143,2.7673019093538));
#210903=CARTESIAN_POINT('Ctrl Pts',(57.5378823365782,25.3131208736774,2.74997687280763));
#210904=CARTESIAN_POINT('Ctrl Pts',(57.5428531464515,25.3273944332716,2.73349253346765));
#210905=CARTESIAN_POINT('Ctrl Pts',(57.5466715501072,25.3383588864538,2.72082983599959));
#210906=CARTESIAN_POINT('Ctrl Pts',(57.5497799237789,25.3501628378305,2.70866321039607));
#210907=CARTESIAN_POINT('Ctrl Pts',(57.552096640372,25.3627976342212,2.69711645335863));
#210908=CARTESIAN_POINT('Ctrl Pts',(57.5521027120731,25.3628307477693,2.69708619136769));
#210909=CARTESIAN_POINT('Ctrl Pts',(57.5521087778605,25.3628638677134,2.69705593387237));
#210910=CARTESIAN_POINT('Ctrl Pts',(57.5521148377337,25.3628969940503,2.69702568087589));
#210911=CARTESIAN_POINT('Ctrl Pts',(57.552764579367,25.3664488110204,2.69378194443284));
#210912=CARTESIAN_POINT('Ctrl Pts',(57.5533450954513,25.3700726756556,2.69059266624717));
#210913=CARTESIAN_POINT('Ctrl Pts',(57.5538555294217,25.3737637277665,2.68746219342694));
#210914=CARTESIAN_POINT('Ctrl Pts',(57.5566959784088,25.3943035935237,2.67004182396249));
#210915=CARTESIAN_POINT('Ctrl Pts',(57.5573711352259,25.4169233145106,2.65443567878163));
#210916=CARTESIAN_POINT('Ctrl Pts',(57.5557688601538,25.4407429579385,2.64136852353417));
#210917=CARTESIAN_POINT('Ctrl Pts',(57.5550497369124,25.4514335437747,2.63550380329893));
#210918=CARTESIAN_POINT('Ctrl Pts',(57.5538721381545,25.4623660683379,2.63014997451186));
#210919=CARTESIAN_POINT('Ctrl Pts',(57.5522269397031,25.4734629846669,2.62536981119271));
#210920=CARTESIAN_POINT('Ctrl Pts',(57.5515119587092,25.4782855544061,2.62329241687091));
#210921=CARTESIAN_POINT('Ctrl Pts',(57.5507085716896,25.4831389900605,2.62132362131444));
#210922=CARTESIAN_POINT('Ctrl Pts',(57.549815975347,25.4880168077358,2.61946873372364));
#210923=CARTESIAN_POINT('Ctrl Pts',(57.5466918881476,25.5050891695995,2.61297662715584));
#210924=CARTESIAN_POINT('Ctrl Pts',(57.5424749837907,25.5224602099123,2.60787989113986));
#210925=CARTESIAN_POINT('Ctrl Pts',(57.537130837121,25.5398519389078,2.60440616886196));
#210926=CARTESIAN_POINT('Ctrl Pts',(57.5344587637862,25.5485478034055,2.60266930772301));
#210927=CARTESIAN_POINT('Ctrl Pts',(57.5315048804296,25.557248840319,2.60133820040202));
#210928=CARTESIAN_POINT('Ctrl Pts',(57.5282648911454,25.565920304143,2.60044130723602));
#210929=CARTESIAN_POINT('Ctrl Pts',(57.5266448965033,25.5702560360551,2.59999286065302));
#210930=CARTESIAN_POINT('Ctrl Pts',(57.5249533754919,25.5745843747449,2.5996529676853));
#210931=CARTESIAN_POINT('Ctrl Pts',(57.5231897917613,25.5789009773103,2.59942518630972));
#210932=CARTESIAN_POINT('Ctrl Pts',(57.5214262080306,25.5832175798758,2.59919740493414));
#210933=CARTESIAN_POINT('Ctrl Pts',(57.5195905600219,25.5875224456232,2.59908173791633));
#210934=CARTESIAN_POINT('Ctrl Pts',(57.5176823163888,25.5918112338797,2.59908173516042));
#210935=CARTESIAN_POINT('',(57.5052637377732,25.61970381813,2.59908173516043));
#210936=CARTESIAN_POINT('Origin',(5.5132234544654E-15,1.85349386523019E-13,
2.59908173516024));
#210937=CARTESIAN_POINT('',(57.2088336324698,25.8191582032623,2.90134173516042));
#210938=CARTESIAN_POINT('Ctrl Pts',(57.5052637377732,25.61970381813,2.59908173516043));
#210939=CARTESIAN_POINT('Ctrl Pts',(57.5037084941754,25.6231946607006,2.59908174381704));
#210940=CARTESIAN_POINT('Ctrl Pts',(57.5021139114133,25.6266565153805,2.59915752001015));
#210941=CARTESIAN_POINT('Ctrl Pts',(57.5004817994259,25.6300880761868,2.5993072951749));
#210942=CARTESIAN_POINT('Ctrl Pts',(57.491050205568,25.649918264356,2.60017281085936));
#210943=CARTESIAN_POINT('Ctrl Pts',(57.4803658667979,25.6687401163214,2.60350651800076));
#210944=CARTESIAN_POINT('Ctrl Pts',(57.4687800995534,25.6862948498987,2.60896880596472));
#210945=CARTESIAN_POINT('Ctrl Pts',(57.4641072931055,25.6933750777783,2.61117187235469));
#210946=CARTESIAN_POINT('Ctrl Pts',(57.4592879447655,25.7002496417677,2.61372076577214));
#210947=CARTESIAN_POINT('Ctrl Pts',(57.4543452548724,25.7069034079253,2.61659179897001));
#210948=CARTESIAN_POINT('Ctrl Pts',(57.4525217023852,25.7093582436704,2.61765103591227));
#210949=CARTESIAN_POINT('Ctrl Pts',(57.4506813499537,25.711782891895,2.61875422455167));
#210950=CARTESIAN_POINT('Ctrl Pts',(57.4488253585222,25.7141765267651,2.61990022440414));
#210951=CARTESIAN_POINT('Ctrl Pts',(57.4453453745883,25.7186645921465,2.62204897412751));
#210952=CARTESIAN_POINT('Ctrl Pts',(57.4418104097896,25.7230436262008,2.62434823201787));
#210953=CARTESIAN_POINT('Ctrl Pts',(57.4382281169313,25.7273081852389,2.62679048030323));
#210954=CARTESIAN_POINT('Ctrl Pts',(57.425690091927,25.742234141872,2.63533834930196));
#210955=CARTESIAN_POINT('Ctrl Pts',(57.4125722940993,25.7557577777295,2.64563784783579));
#210956=CARTESIAN_POINT('Ctrl Pts',(57.3992028606062,25.7676457049092,2.65736666737981));
#210957=CARTESIAN_POINT('Ctrl Pts',(57.3925181438596,25.7735896684991,2.66323107715181));
#210958=CARTESIAN_POINT('Ctrl Pts',(57.3857705191197,25.7791247053302,2.66945281780792));
#210959=CARTESIAN_POINT('Ctrl Pts',(57.3790010116303,25.7842216455739,2.67599160631219));
#210960=CARTESIAN_POINT('Ctrl Pts',(57.3756162578857,25.7867701156958,2.67926100056433));
#210961=CARTESIAN_POINT('Ctrl Pts',(57.3722260335605,25.7892090617194,2.68260965685141));
#210962=CARTESIAN_POINT('Ctrl Pts',(57.3688354672942,25.7915348376378,2.686032540125));
#210963=CARTESIAN_POINT('Ctrl Pts',(57.3654449010279,25.7938606135562,2.6894554233986));
#210964=CARTESIAN_POINT('Ctrl Pts',(57.3620539952074,25.7960730898187,2.69295261525401));
#210965=CARTESIAN_POINT('Ctrl Pts',(57.358667875041,25.7981688856969,2.69651891172116));
#210966=CARTESIAN_POINT('Ctrl Pts',(57.3586389985276,25.7981867584464,2.69654932476104));
#210967=CARTESIAN_POINT('Ctrl Pts',(57.3586101225001,25.7982046227313,2.69657974261162));
#210968=CARTESIAN_POINT('Ctrl Pts',(57.3585812469612,25.79822247855,2.6966101652699));
#210969=CARTESIAN_POINT('Ctrl Pts',(57.3438340876997,25.8073417058671,2.7121474610132));
#210970=CARTESIAN_POINT('Ctrl Pts',(57.3292509568899,25.8143796853896,2.72880565567959));
#210971=CARTESIAN_POINT('Ctrl Pts',(57.3149837825992,25.819467133355,2.74628040012926));
#210972=CARTESIAN_POINT('Ctrl Pts',(57.3002341019478,25.8247266354324,2.76434612883259));
#210973=CARTESIAN_POINT('Ctrl Pts',(57.2858212188209,25.8279013409287,2.78328592655563));
#210974=CARTESIAN_POINT('Ctrl Pts',(57.2719197677172,25.8290839028449,2.80278753269232));
#210975=CARTESIAN_POINT('Ctrl Pts',(57.2582827514651,25.8302439699451,2.82191817724463));
#210976=CARTESIAN_POINT('Ctrl Pts',(57.2451370982851,25.8294864848992,2.84159092317108));
#210977=CARTESIAN_POINT('Ctrl Pts',(57.2326665944452,25.8268549466926,2.8615123381925));
#210978=CARTESIAN_POINT('Ctrl Pts',(57.224405322849,25.8251116448887,2.87470957722821));
#210979=CARTESIAN_POINT('Ctrl Pts',(57.2164407479128,25.8225450142724,2.88801594389109));
#210980=CARTESIAN_POINT('Ctrl Pts',(57.2088336324698,25.8191582032623,2.90134173516042));
#210981=CARTESIAN_POINT('',(56.8833377255394,25.6742415049982,3.4715307213909));
#210982=CARTESIAN_POINT('',(57.2088336324698,25.8191582032623,2.90134173516042));
#210983=CARTESIAN_POINT('',(54.2060847114741,30.9286463962981,3.47153072139094));
#210984=CARTESIAN_POINT('Origin',(5.53234440788222E-15,1.85015204418142E-13,
3.47153072139072));
#210985=CARTESIAN_POINT('',(54.5146464769138,31.1067982185537,2.90134173516046));
#210986=CARTESIAN_POINT('',(54.2060847114741,30.9286463962981,3.47153072139094));
#210987=CARTESIAN_POINT('',(54.5275217339719,31.4638515574743,2.59908173516046));
#210988=CARTESIAN_POINT('Ctrl Pts',(54.5146464769138,31.1067982185537,2.90134173516046));
#210989=CARTESIAN_POINT('Ctrl Pts',(54.525303663139,31.1129513003043,2.88164837656733));
#210990=CARTESIAN_POINT('Ctrl Pts',(54.5349507607441,31.1207731649985,2.8620373443914));
#210991=CARTESIAN_POINT('Ctrl Pts',(54.5434787028964,31.1301095476656,2.84277945978138));
#210992=CARTESIAN_POINT('Ctrl Pts',(54.5521780046493,31.1396335346547,2.82313460920006));
#210993=CARTESIAN_POINT('Ctrl Pts',(54.5597135487721,31.150733942044,2.80385576863327));
#210994=CARTESIAN_POINT('Ctrl Pts',(54.5659508935503,31.1632971162157,2.78521678518377));
#210995=CARTESIAN_POINT('Ctrl Pts',(54.5719459231381,31.1753722224597,2.76730190934466));
#210996=CARTESIAN_POINT('Ctrl Pts',(54.5767421714191,31.1887993693014,2.74997687279784));
#210997=CARTESIAN_POINT('Ctrl Pts',(54.5801937574258,31.2035143279612,2.73349253345734));
#210998=CARTESIAN_POINT('Ctrl Pts',(54.5828451460238,31.2148178485853,2.720829835993));
#210999=CARTESIAN_POINT('Ctrl Pts',(54.5847026428007,31.2268820502013,2.70866321039296));
#211000=CARTESIAN_POINT('Ctrl Pts',(54.5856859723272,31.2396897946772,2.69711645335866));
#211001=CARTESIAN_POINT('Ctrl Pts',(54.5856885494585,31.2397233614914,2.69708619136772));
#211002=CARTESIAN_POINT('Ctrl Pts',(54.5856911200402,31.2397569340484,2.6970559338724));
#211003=CARTESIAN_POINT('Ctrl Pts',(54.5856936840716,31.239790512345,2.69702568087591));
#211004=CARTESIAN_POINT('Ctrl Pts',(54.5859686003825,31.2433907885846,2.69378194443287));
#211005=CARTESIAN_POINT('Ctrl Pts',(54.5861671393376,31.2470554817643,2.69059266624722));
#211006=CARTESIAN_POINT('Ctrl Pts',(54.5862889570923,31.2507796687841,2.68746219342699));
#211007=CARTESIAN_POINT('Ctrl Pts',(54.5869668451995,31.2715039227795,2.67004182395885));
#211008=CARTESIAN_POINT('Ctrl Pts',(54.5852738987617,31.2940703036778,2.65443567877506));
#211009=CARTESIAN_POINT('Ctrl Pts',(54.5811905703952,31.3175919772612,2.64136852352592));
#211010=CARTESIAN_POINT('Ctrl Pts',(54.5793579160776,31.3281488300975,2.63550380329393));
#211011=CARTESIAN_POINT('Ctrl Pts',(54.5770440083376,31.3388983725536,2.63014997450966));
#211012=CARTESIAN_POINT('Ctrl Pts',(54.5742478788459,31.3497625287428,2.62536981119277));
#211013=CARTESIAN_POINT('Ctrl Pts',(54.5730327187888,31.3544839440758,2.62329241687097));
#211014=CARTESIAN_POINT('Ctrl Pts',(54.5717264106369,31.3592268152914,2.6213236213145));
#211015=CARTESIAN_POINT('Ctrl Pts',(54.5703288332447,31.3639846100471,2.6194687337237));
#211016=CARTESIAN_POINT('Ctrl Pts',(54.5654373123719,31.3806368916921,2.6129766271559));
#211017=CARTESIAN_POINT('Ctrl Pts',(54.5594277405091,31.3974719850964,2.60787989113992));
#211018=CARTESIAN_POINT('Ctrl Pts',(54.5522949389286,31.4142098249418,2.60440616886202));
#211019=CARTESIAN_POINT('Ctrl Pts',(54.5487285381383,31.4225787448645,2.60266930772307));
#211020=CARTESIAN_POINT('Ctrl Pts',(54.5448813304464,31.4309233516995,2.60133820040207));
#211021=CARTESIAN_POINT('Ctrl Pts',(54.5407526753747,31.4392086412365,2.60044130723607));
#211022=CARTESIAN_POINT('Ctrl Pts',(54.5386883478389,31.443351286005,2.59999286065307));
#211023=CARTESIAN_POINT('Ctrl Pts',(54.5365536585648,31.4474791015107,2.59965296768534));
#211024=CARTESIAN_POINT('Ctrl Pts',(54.5343485280976,31.4515877125784,2.59942518630976));
#211025=CARTESIAN_POINT('Ctrl Pts',(54.5321433976305,31.4556963236462,2.59919740493418));
#211026=CARTESIAN_POINT('Ctrl Pts',(54.5298678244924,31.4597857294232,2.59908173791641));
#211027=CARTESIAN_POINT('Ctrl Pts',(54.5275217339719,31.4638515574743,2.59908173516046));
#211028=CARTESIAN_POINT('',(54.5122556166611,31.490293248291,2.59908173516046));
#211029=CARTESIAN_POINT('Origin',(5.52060867199534E-15,1.8533489221751E-13,
2.59908173516022));
#211030=CARTESIAN_POINT('',(54.1966007261207,31.6576696180587,2.90134173516046));
#211031=CARTESIAN_POINT('Ctrl Pts',(54.512255616661,31.490293248291,2.59908173516046));
#211032=CARTESIAN_POINT('Ctrl Pts',(54.510344000441,31.4936024004374,2.59908174381707));
#211033=CARTESIAN_POINT('Ctrl Pts',(54.5083962906204,31.4968786114295,2.59915752001018));
#211034=CARTESIAN_POINT('Ctrl Pts',(54.5064144237355,31.5001207716287,2.59930729517493));
#211035=CARTESIAN_POINT('Ctrl Pts',(54.4949616780397,31.5188564579406,2.60017281085941));
#211036=CARTESIAN_POINT('Ctrl Pts',(54.4823684499332,31.5364583843193,2.60350651800095));
#211037=CARTESIAN_POINT('Ctrl Pts',(54.4690111814096,31.5527059087838,2.60896880596516));
#211038=CARTESIAN_POINT('Ctrl Pts',(54.4636238877448,31.5592589091567,2.61117187235503));
#211039=CARTESIAN_POINT('Ctrl Pts',(54.4581123526902,31.5655920544889,2.61372076577234));
#211040=CARTESIAN_POINT('Ctrl Pts',(54.4525012314184,31.5716927188401,2.61659179897004));
#211041=CARTESIAN_POINT('Ctrl Pts',(54.4504310683346,31.5739434935989,2.61765103591229));
#211042=CARTESIAN_POINT('Ctrl Pts',(54.4483473527933,31.5761624901353,2.6187542245517));
#211043=CARTESIAN_POINT('Ctrl Pts',(54.4462513257025,31.5783490084909,2.61990022440417));
#211044=CARTESIAN_POINT('Ctrl Pts',(54.4423212749073,31.5824487304078,2.62204897412754));
#211045=CARTESIAN_POINT('Ctrl Pts',(54.4383479413154,31.5864342712172,2.62434823201791));
#211046=CARTESIAN_POINT('Ctrl Pts',(54.4343395048294,31.5903010169872,2.62679048030327));
#211047=CARTESIAN_POINT('Ctrl Pts',(54.4203099771284,31.6038346271821,2.635338349302));
#211048=CARTESIAN_POINT('Ctrl Pts',(54.4058504350957,31.6159129958989,2.64563784783584));
#211049=CARTESIAN_POINT('Ctrl Pts',(54.3913116139985,31.6263383134319,2.65736666737986));
#211050=CARTESIAN_POINT('Ctrl Pts',(54.38404220345,31.6315509721985,2.66323107715186));
#211051=CARTESIAN_POINT('Ctrl Pts',(54.3767529740104,31.6363503686739,2.66945281780794));
#211052=CARTESIAN_POINT('Ctrl Pts',(54.3694877752603,31.6407117811307,2.67599160631221));
#211053=CARTESIAN_POINT('Ctrl Pts',(54.3658551758853,31.6428924873591,2.67926100056434));
#211054=CARTESIAN_POINT('Ctrl Pts',(54.3622285842838,31.6449636976424,2.68260965685144));
#211055=CARTESIAN_POINT('Ctrl Pts',(54.3586134821116,31.6469223220355,2.68603254012503));
#211056=CARTESIAN_POINT('Ctrl Pts',(54.3549983799395,31.6488809464286,2.68945542339863));
#211057=CARTESIAN_POINT('Ctrl Pts',(54.3513947831121,31.6507268563402,2.69295261525406));
#211058=CARTESIAN_POINT('Ctrl Pts',(54.3478081421437,31.6524572252918,2.6965189117212));
#211059=CARTESIAN_POINT('Ctrl Pts',(54.3477775556079,31.652471981715,2.69654932476109));
#211060=CARTESIAN_POINT('Ctrl Pts',(54.34774697044,31.6524867297707,2.69657974261167));
#211061=CARTESIAN_POINT('Ctrl Pts',(54.3477163866431,31.6525014694577,2.69661016526995));
#211062=CARTESIAN_POINT('Ctrl Pts',(54.3320967950474,31.6600292427972,2.7121474610112));
#211063=CARTESIAN_POINT('Ctrl Pts',(54.316857882972,31.6655043152778,2.72880565567527));
#211064=CARTESIAN_POINT('Ctrl Pts',(54.3021370826389,31.6690725678673,2.74628040012244));
#211065=CARTESIAN_POINT('Ctrl Pts',(54.2869184346136,31.6727614963899,2.76434612882311));
#211066=CARTESIAN_POINT('Ctrl Pts',(54.2722526596834,31.6744122539933,2.78328592654331));
#211067=CARTESIAN_POINT('Ctrl Pts',(54.258303750805,31.6741352403916,2.80278753267708));
#211068=CARTESIAN_POINT('Ctrl Pts',(54.244620179525,31.6738634961715,2.82191817722668));
#211069=CARTESIAN_POINT('Ctrl Pts',(54.2316257183574,31.6717360657839,2.84159092315034));
#211070=CARTESIAN_POINT('Ctrl Pts',(54.2194985998879,31.6678154208183,2.86151233816903));
#211071=CARTESIAN_POINT('Ctrl Pts',(54.2114648090554,31.6652181309789,2.87470957721245));
#211072=CARTESIAN_POINT('Ctrl Pts',(54.2038121508433,31.6618330358534,2.88801594388323));
#211073=CARTESIAN_POINT('Ctrl Pts',(54.1966007261207,31.6576696180587,2.90134173516047));
#211074=CARTESIAN_POINT('',(53.888035839597,31.4795232016792,3.47153072139094));
#211075=CARTESIAN_POINT('',(54.1966007261207,31.6576696180587,2.90134173516047));
#211076=CARTESIAN_POINT('',(50.6762142289948,36.4252947698681,3.47153072139098));
#211077=CARTESIAN_POINT('Origin',(5.53234440788222E-15,1.85015204418142E-13,
3.47153072139072));
#211078=CARTESIAN_POINT('',(50.9644637245892,36.6347241449657,2.90134173516049));
#211079=CARTESIAN_POINT('',(50.6762142289948,36.4252947698681,3.47153072139097));
#211080=CARTESIAN_POINT('',(50.9399462128201,36.991167339171,2.5990817351605));
#211081=CARTESIAN_POINT('Ctrl Pts',(50.9644637245892,36.6347241449657,2.90134173516049));
#211082=CARTESIAN_POINT('Ctrl Pts',(50.9744193574537,36.6419574987897,2.88164837656693));
#211083=CARTESIAN_POINT('Ctrl Pts',(50.9831959997526,36.6507449107785,2.86203734439056));
#211084=CARTESIAN_POINT('Ctrl Pts',(50.9907013072129,36.6609215604528,2.84277945978012));
#211085=CARTESIAN_POINT('Ctrl Pts',(50.9983574255566,36.6713026986887,2.82313460919836));
#211086=CARTESIAN_POINT('Ctrl Pts',(51.0046913806542,36.6831299757322,2.80385576863117));
#211087=CARTESIAN_POINT('Ctrl Pts',(51.0095813473151,36.6962763075863,2.7852167851813));
#211088=CARTESIAN_POINT('Ctrl Pts',(51.0142813432041,36.7089119163653,2.76730190934179));
#211089=CARTESIAN_POINT('Ctrl Pts',(51.0176477981096,36.7227668523545,2.74997687279462));
#211090=CARTESIAN_POINT('Ctrl Pts',(51.0195423439511,36.7377619899128,2.73349253345383));
#211091=CARTESIAN_POINT('Ctrl Pts',(51.0209976683244,36.7492807342429,2.72082983599076));
#211092=CARTESIAN_POINT('Ctrl Pts',(51.0215839370839,36.7614730081827,2.70866321039192));
#211093=CARTESIAN_POINT('Ctrl Pts',(51.0212231059805,36.7743133764174,2.69711645335871));
#211094=CARTESIAN_POINT('Ctrl Pts',(51.0212221603065,36.7743470287326,2.69708619136776));
#211095=CARTESIAN_POINT('Ctrl Pts',(51.0212212075184,36.7743806860746,2.69705593387243));
#211096=CARTESIAN_POINT('Ctrl Pts',(51.021220247616,36.77441434844,2.69702568087595));
#211097=CARTESIAN_POINT('Ctrl Pts',(51.021117326564,36.7780236385692,2.69378194443291));
#211098=CARTESIAN_POINT('Ctrl Pts',(51.0209317131555,36.7816890091481,2.69059266624725));
#211099=CARTESIAN_POINT('Ctrl Pts',(51.0206635800337,36.7854055281044,2.68746219342702));
#211100=CARTESIAN_POINT('Ctrl Pts',(51.0191714801765,36.8060871110679,2.67004182396082));
#211101=CARTESIAN_POINT('Ctrl Pts',(51.0151289787604,36.8283529098782,2.65443567877857));
#211102=CARTESIAN_POINT('Ctrl Pts',(51.008609334902,36.8513189052307,2.64136852353032));
#211103=CARTESIAN_POINT('Ctrl Pts',(51.0056832284522,36.8616263619856,2.63550380329661));
#211104=CARTESIAN_POINT('Ctrl Pts',(51.0022583633864,36.8720751481058,2.63014997451086));
#211105=CARTESIAN_POINT('Ctrl Pts',(50.9983419378324,36.8825875141944,2.62536981119277));
#211106=CARTESIAN_POINT('Ctrl Pts',(50.9966399122601,36.8871560463068,2.62329241687097));
#211107=CARTESIAN_POINT('Ctrl Pts',(50.9948449951613,36.8917363891939,2.62132362131452));
#211108=CARTESIAN_POINT('Ctrl Pts',(50.9929577488699,36.896322033635,2.61946873372372));
#211109=CARTESIAN_POINT('Ctrl Pts',(50.98635238685,36.9123717891789,2.61297662715592));
#211110=CARTESIAN_POINT('Ctrl Pts',(50.9786159896081,36.9284864868683,2.60787989113995));
#211111=CARTESIAN_POINT('Ctrl Pts',(50.9697726815835,36.9443870542878,2.60440616886205));
#211112=CARTESIAN_POINT('Ctrl Pts',(50.9653510275712,36.9523373379975,2.6026693077231));
#211113=CARTESIAN_POINT('Ctrl Pts',(50.9606526463565,36.9602340894952,2.6013382004021));
#211114=CARTESIAN_POINT('Ctrl Pts',(50.9556805599063,36.9680424293792,2.6004413072361));
#211115=CARTESIAN_POINT('Ctrl Pts',(50.9531945166812,36.9719465993212,2.5999928606531));
#211116=CARTESIAN_POINT('Ctrl Pts',(50.9506400472468,36.9758286664323,2.59965296768539));
#211117=CARTESIAN_POINT('Ctrl Pts',(50.948017529914,36.9796842711997,2.59942518630981));
#211118=CARTESIAN_POINT('Ctrl Pts',(50.9453950125812,36.9835398759671,2.59919740493423));
#211119=CARTESIAN_POINT('Ctrl Pts',(50.9427044459694,36.9873690173882,2.59908173791644));
#211120=CARTESIAN_POINT('Ctrl Pts',(50.9399462128201,36.991167339171,2.59908173516051));
#211121=CARTESIAN_POINT('',(50.9219998155899,37.0158684358562,2.5990817351605));
#211122=CARTESIAN_POINT('Origin',(5.52946850001198E-15,1.85321249278761E-13,
2.59908173516024));
#211123=CARTESIAN_POINT('',(50.5905785208484,37.1493329797263,2.90134173516049));
#211124=CARTESIAN_POINT('Ctrl Pts',(50.9219998155899,37.0158684358562,2.5990817351605));
#211125=CARTESIAN_POINT('Ctrl Pts',(50.919752770815,37.0189596418151,2.5990817438171));
#211126=CARTESIAN_POINT('Ctrl Pts',(50.9174732734523,37.0220143142661,2.59915752001021));
#211127=CARTESIAN_POINT('Ctrl Pts',(50.9151633654183,37.0250315520726,2.59930729517496));
#211128=CARTESIAN_POINT('Ctrl Pts',(50.9018149465624,37.0424674644278,2.60017281085949));
#211129=CARTESIAN_POINT('Ctrl Pts',(50.8874508031614,37.0586566148313,2.60350651800136));
#211130=CARTESIAN_POINT('Ctrl Pts',(50.8724683783874,37.0734189189052,2.6089688059661));
#211131=CARTESIAN_POINT('Ctrl Pts',(50.866425621823,37.0793728957275,2.61117187235576));
#211132=CARTESIAN_POINT('Ctrl Pts',(50.8602822855856,37.0850952351367,2.61372076577277));
#211133=CARTESIAN_POINT('Ctrl Pts',(50.8540642095546,37.0905759575257,2.61659179897008));
#211134=CARTESIAN_POINT('Ctrl Pts',(50.851770117014,37.092598011339,2.61765103591234));
#211135=CARTESIAN_POINT('Ctrl Pts',(50.8494658679866,37.0945870443968,2.61875422455173));
#211136=CARTESIAN_POINT('Ctrl Pts',(50.8471527697479,37.0965424902854,2.6199002244042));
#211137=CARTESIAN_POINT('Ctrl Pts',(50.8428157105504,37.1002089513264,2.62204897412757));
#211138=CARTESIAN_POINT('Ctrl Pts',(50.8384475408395,37.1037573324719,2.62434823201794));
#211139=CARTESIAN_POINT('Ctrl Pts',(50.8340568779948,37.1071839000979,2.62679048030329));
#211140=CARTESIAN_POINT('Ctrl Pts',(50.8186895580383,37.1191768867891,2.63533834930203));
#211141=CARTESIAN_POINT('Ctrl Pts',(50.803046693569,37.1296776552302,2.64563784783587));
#211142=CARTESIAN_POINT('Ctrl Pts',(50.7874977752343,37.1385261411559,2.65736666737988));
#211143=CARTESIAN_POINT('Ctrl Pts',(50.7797233160669,37.1429503841188,2.66323107715189));
#211144=CARTESIAN_POINT('Ctrl Pts',(50.7719723442506,37.1469615570465,2.66945281780798));
#211145=CARTESIAN_POINT('Ctrl Pts',(50.7642910532777,37.1505396571688,2.67599160631225));
#211146=CARTESIAN_POINT('Ctrl Pts',(50.7604504077912,37.1523287072299,2.67926100056438));
#211147=CARTESIAN_POINT('Ctrl Pts',(50.75662718261,37.1540094891596,2.68260965685147));
#211148=CARTESIAN_POINT('Ctrl Pts',(50.7528271523479,37.1555795029288,2.68603254012506));
#211149=CARTESIAN_POINT('Ctrl Pts',(50.7490271220858,37.1571495166979,2.68945542339865));
#211150=CARTESIAN_POINT('Ctrl Pts',(50.7452503160124,37.1586086360832,2.69295261525409));
#211151=CARTESIAN_POINT('Ctrl Pts',(50.7415024502312,37.159954619824,2.69651891172123));
#211152=CARTESIAN_POINT('Ctrl Pts',(50.7414704887853,37.1599660982464,2.69654932476111));
#211153=CARTESIAN_POINT('Ctrl Pts',(50.7414385295747,37.1599775684901,2.6965797426117));
#211154=CARTESIAN_POINT('Ctrl Pts',(50.7414065726022,37.1599890305542,2.69661016526998));
#211155=CARTESIAN_POINT('Ctrl Pts',(50.725085680185,37.1658428740571,2.7121474610108));
#211156=CARTESIAN_POINT('Ctrl Pts',(50.7093579475521,37.1696950534567,2.72880565567438));
#211157=CARTESIAN_POINT('Ctrl Pts',(50.6943448053442,37.1717050161482,2.74628040012103));
#211158=CARTESIAN_POINT('Ctrl Pts',(50.6788239286359,37.1737829544433,2.76434612882126));
#211159=CARTESIAN_POINT('Ctrl Pts',(50.6640659432,37.1738916781079,2.78328592654098));
#211160=CARTESIAN_POINT('Ctrl Pts',(50.6502224037102,37.1721581240066,2.80278753267426));
#211161=CARTESIAN_POINT('Ctrl Pts',(50.6366421974712,37.1704575457521,2.82191817722355));
#211162=CARTESIAN_POINT('Ctrl Pts',(50.6239412983508,37.1669834785941,2.8415909231469));
#211163=CARTESIAN_POINT('Ctrl Pts',(50.6122904324984,37.1618166822747,2.8615123381653));
#211164=CARTESIAN_POINT('Ctrl Pts',(50.6045721423274,37.1583938608507,2.87470957720995));
#211165=CARTESIAN_POINT('Ctrl Pts',(50.5973152449684,37.1542273890273,2.88801594388198));
#211166=CARTESIAN_POINT('Ctrl Pts',(50.5905785208484,37.1493329797263,2.90134173516049));
#211167=CARTESIAN_POINT('',(50.3023253561995,36.9399086546489,3.47153072139098));
#211168=CARTESIAN_POINT('',(50.5905785208484,37.1493329797263,2.90134173516049));
#211169=CARTESIAN_POINT('',(46.5911245387429,41.5228599914565,3.47153072139101));
#211170=CARTESIAN_POINT('Origin',(5.53234440788222E-15,1.85015204418142E-13,
3.47153072139072));
#211171=CARTESIAN_POINT('',(46.8559036426985,41.7612723673365,2.90134173516054));
#211172=CARTESIAN_POINT('',(46.5911245387429,41.5228599914565,3.47153072139101));
#211173=CARTESIAN_POINT('',(46.7942619810916,42.1132001506003,2.59908173516053));
#211174=CARTESIAN_POINT('Ctrl Pts',(46.8559036426985,41.7612723673365,2.90134173516054));
#211175=CARTESIAN_POINT('Ctrl Pts',(46.8650486462049,41.7695067430958,2.88164837656678));
#211176=CARTESIAN_POINT('Ctrl Pts',(46.8728586744677,41.7791634256546,2.86203734439022));
#211177=CARTESIAN_POINT('Ctrl Pts',(46.8792591175168,41.7900688448325,2.84277945977961));
#211178=CARTESIAN_POINT('Ctrl Pts',(46.8857881704163,41.8011933963921,2.82313460919779));
#211179=CARTESIAN_POINT('Ctrl Pts',(46.8908511403512,41.8136179609673,2.80385576863053));
#211180=CARTESIAN_POINT('Ctrl Pts',(46.8943401533968,41.8272034165405,2.78521678518062));
#211181=CARTESIAN_POINT('Ctrl Pts',(46.8976936214484,41.8402610894801,2.76730190934118));
#211182=CARTESIAN_POINT('Ctrl Pts',(46.8995933993941,41.8543920170382,2.74997687279408));
#211183=CARTESIAN_POINT('Ctrl Pts',(46.8999101480297,41.8695030436293,2.73349253345337));
#211184=CARTESIAN_POINT('Ctrl Pts',(46.9001534633402,41.8811108098929,2.72082983599048));
#211185=CARTESIAN_POINT('Ctrl Pts',(46.8994620807994,41.8932975750526,2.70866321039181));
#211186=CARTESIAN_POINT('Ctrl Pts',(46.8977610424072,41.9060298852857,2.69711645335875));
#211187=CARTESIAN_POINT('Ctrl Pts',(46.8977565842889,41.9060632544002,2.6970861913678));
#211188=CARTESIAN_POINT('Ctrl Pts',(46.8977521185701,41.9060966277702,2.69705593387247));
#211189=CARTESIAN_POINT('Ctrl Pts',(46.8977476452509,41.9061300053926,2.69702568087599));
#211190=CARTESIAN_POINT('Ctrl Pts',(46.8972680144604,41.9097087652734,2.69378194443295));
#211191=CARTESIAN_POINT('Ctrl Pts',(46.8967002823076,41.9133346546844,2.69059266624729));
#211192=CARTESIAN_POINT('Ctrl Pts',(46.8960451360319,41.9170027866178,2.68746219342706));
#211193=CARTESIAN_POINT('Ctrl Pts',(46.8923993959693,41.9374151067975,2.6700418239636));
#211194=CARTESIAN_POINT('Ctrl Pts',(46.8860516300673,41.959136374768,2.65443567878352));
#211195=CARTESIAN_POINT('Ctrl Pts',(46.8771671013007,41.9812950716377,2.64136852353652));
#211196=CARTESIAN_POINT('Ctrl Pts',(46.8731796017524,41.9912402016588,2.6355038033004));
#211197=CARTESIAN_POINT('Ctrl Pts',(46.8686813028982,42.0012737523567,2.63014997451258));
#211198=CARTESIAN_POINT('Ctrl Pts',(46.8636874904589,42.0113191526628,2.62536981119282));
#211199=CARTESIAN_POINT('Ctrl Pts',(46.8615172471196,42.0156847477608,2.62329241687102));
#211200=CARTESIAN_POINT('Ctrl Pts',(46.8592533865613,42.0200523791243,2.62132362131456));
#211201=CARTESIAN_POINT('Ctrl Pts',(46.856897148436,42.0244156319707,2.61946873372376));
#211202=CARTESIAN_POINT('Ctrl Pts',(46.8486503149976,42.0396870169331,2.61297662715596));
#211203=CARTESIAN_POINT('Ctrl Pts',(46.8392718539638,42.0549047629076,2.60787989113997));
#211204=CARTESIAN_POINT('Ctrl Pts',(46.8288149286284,42.069793847957,2.60440616886208));
#211205=CARTESIAN_POINT('Ctrl Pts',(46.8235864659607,42.0772383904817,2.60266930772313));
#211206=CARTESIAN_POINT('Ctrl Pts',(46.8180883876711,42.0846007681801,2.60133820040213));
#211207=CARTESIAN_POINT('Ctrl Pts',(46.8123273450619,42.0918466086054,2.60044130723613));
#211208=CARTESIAN_POINT('Ctrl Pts',(46.8094468237573,42.0954695288181,2.59999286065313));
#211209=CARTESIAN_POINT('Ctrl Pts',(46.8065005614644,42.0990633147949,2.59965296768541));
#211210=CARTESIAN_POINT('Ctrl Pts',(46.8034893901146,42.1026236704492,2.59942518630983));
#211211=CARTESIAN_POINT('Ctrl Pts',(46.8004782187648,42.1061840261036,2.59919740493425));
#211212=CARTESIAN_POINT('Ctrl Pts',(46.79740213709,42.1097109502941,2.59908173791642));
#211213=CARTESIAN_POINT('Ctrl Pts',(46.7942619810916,42.1132001506003,2.59908173516054));
#211214=CARTESIAN_POINT('',(46.7738319284257,42.1358900227698,2.59908173516053));
#211215=CARTESIAN_POINT('Origin',(5.53970586838553E-15,1.85308607181667E-13,
2.59908173516024));
#211216=CARTESIAN_POINT('',(46.4302753505424,42.2339804752704,2.90134173516054));
#211217=CARTESIAN_POINT('Ctrl Pts',(46.7738319284257,42.1358900227698,2.59908173516054));
#211218=CARTESIAN_POINT('Ctrl Pts',(46.7712740741886,42.1387294146417,2.59908174381718));
#211219=CARTESIAN_POINT('Ctrl Pts',(46.7686877639338,42.1415290809211,2.59915752001025));
#211220=CARTESIAN_POINT('Ctrl Pts',(46.7660751225865,42.1442883388461,2.599307295175));
#211221=CARTESIAN_POINT('Ctrl Pts',(46.750977278643,42.1602334457376,2.60017281085945));
#211222=CARTESIAN_POINT('Ctrl Pts',(46.7349995965107,42.1748324484442,2.6035065180008));
#211223=CARTESIAN_POINT('Ctrl Pts',(46.7185561660696,42.1879477932332,2.60896880596467));
#211224=CARTESIAN_POINT('Ctrl Pts',(46.711924152309,42.1932375134913,2.61117187235468));
#211225=CARTESIAN_POINT('Ctrl Pts',(46.7052163225641,42.1982863518313,2.61372076577218));
#211226=CARTESIAN_POINT('Ctrl Pts',(46.6984594183138,42.2030870843187,2.61659179897014));
#211227=CARTESIAN_POINT('Ctrl Pts',(46.6959665308744,42.2048582631418,2.61765103591239));
#211228=CARTESIAN_POINT('Ctrl Pts',(46.6934669941953,42.2065955404586,2.61875422455181));
#211229=CARTESIAN_POINT('Ctrl Pts',(46.6909621675971,42.2082984896057,2.61990022440427));
#211230=CARTESIAN_POINT('Ctrl Pts',(46.6862656177253,42.2114915192565,2.62204897412764));
#211231=CARTESIAN_POINT('Ctrl Pts',(46.681550470477,42.2145638639316,2.624348232018));
#211232=CARTESIAN_POINT('Ctrl Pts',(46.6768256862945,42.2175127112218,2.62679048030335));
#211233=CARTESIAN_POINT('Ctrl Pts',(46.6602889416558,42.2278336767375,2.63533834930209));
#211234=CARTESIAN_POINT('Ctrl Pts',(46.6436341412466,42.2366417962862,2.64563784783592));
#211235=CARTESIAN_POINT('Ctrl Pts',(46.6272454828773,42.2438165047412,2.65736666737994));
#211236=CARTESIAN_POINT('Ctrl Pts',(46.6190511536927,42.2474038589687,2.66323107715194));
#211237=CARTESIAN_POINT('Ctrl Pts',(46.610923360769,42.2505828610986,2.66945281780803));
#211238=CARTESIAN_POINT('Ctrl Pts',(46.6029101354045,42.2533384464727,2.6759916063123));
#211239=CARTESIAN_POINT('Ctrl Pts',(46.5989035227223,42.2547162391598,2.67926100056443));
#211240=CARTESIAN_POINT('Ctrl Pts',(46.5949255520165,42.2559881777373,2.68260965685152));
#211241=CARTESIAN_POINT('Ctrl Pts',(46.5909822275911,42.2571523794831,2.68603254012511));
#211242=CARTESIAN_POINT('Ctrl Pts',(46.5870389031658,42.2583165812289,2.68945542339871));
#211243=CARTESIAN_POINT('Ctrl Pts',(46.5831302673242,42.2593729236706,2.69295261525413));
#211244=CARTESIAN_POINT('Ctrl Pts',(46.5792622391319,42.2603197753209,2.69651891172127));
#211245=CARTESIAN_POINT('Ctrl Pts',(46.5792292529523,42.2603278499825,2.69654932476115));
#211246=CARTESIAN_POINT('Ctrl Pts',(46.5791962698506,42.2603359167438,2.69657974261174));
#211247=CARTESIAN_POINT('Ctrl Pts',(46.5791632898298,42.2603439756044,2.69661016527002));
#211248=CARTESIAN_POINT('Ctrl Pts',(46.5623199117,42.2644597533374,2.71214746101394));
#211249=CARTESIAN_POINT('Ctrl Pts',(46.5462756748362,42.2666468343723,2.72880565568106));
#211250=CARTESIAN_POINT('Ctrl Pts',(46.5311346778782,42.2670764855935,2.74628040013152));
#211251=CARTESIAN_POINT('Ctrl Pts',(46.5154816224569,42.2675206673336,2.76434612883585));
#211252=CARTESIAN_POINT('Ctrl Pts',(46.5007931180894,42.2660861658586,2.78328592655997));
#211253=CARTESIAN_POINT('Ctrl Pts',(46.4872066207018,42.2629150644369,2.80278753269777));
#211254=CARTESIAN_POINT('Ctrl Pts',(46.4738785670832,42.2598042840369,2.82191817725141));
#211255=CARTESIAN_POINT('Ctrl Pts',(46.4616103837171,42.2550216427124,2.84159092317923));
#211256=CARTESIAN_POINT('Ctrl Pts',(46.4505634198054,42.2486653035374,2.861512338202));
#211257=CARTESIAN_POINT('Ctrl Pts',(46.4432451935067,42.2444544516793,2.87470957723464));
#211258=CARTESIAN_POINT('Ctrl Pts',(46.4364635650945,42.2395522518996,2.88801594389437));
#211259=CARTESIAN_POINT('Ctrl Pts',(46.4302753505424,42.2339804752704,2.90134173516054));
#211260=CARTESIAN_POINT('',(46.1654920697611,41.9955727382253,3.47153072139101));
#211261=CARTESIAN_POINT('',(46.4302753505424,42.2339804752704,2.90134173516054));
#211262=CARTESIAN_POINT('',(41.995572738225,46.1654920697615,3.47153072139104));
#211263=CARTESIAN_POINT('Origin',(5.53234440788222E-15,1.85015204418142E-13,
3.47153072139072));
#211264=CARTESIAN_POINT('',(42.23398047527,46.4302753505428,2.90134173516057));
#211265=CARTESIAN_POINT('',(41.995572738225,46.1654920697615,3.47153072139105));
#211266=CARTESIAN_POINT('',(42.1358900227694,46.773831928426,2.59908173516056));
#211267=CARTESIAN_POINT('Ctrl Pts',(42.23398047527,46.4302753505428,2.90134173516057));
#211268=CARTESIAN_POINT('Ctrl Pts',(42.2422146548459,46.4394205306929,2.8816483765676));
#211269=CARTESIAN_POINT('Ctrl Pts',(42.2489725007683,46.4498406831863,2.86203734439182));
#211270=CARTESIAN_POINT('Ctrl Pts',(42.2541979548125,46.4613553898124,2.84277945978195));
#211271=CARTESIAN_POINT('Ctrl Pts',(42.2595284085979,46.4731014717802,2.82313460920104));
#211272=CARTESIAN_POINT('Ctrl Pts',(42.2632649224119,46.4859871977567,2.80385576863465));
#211273=CARTESIAN_POINT('Ctrl Pts',(42.2653147554854,46.4998629319539,2.78521678518551));
#211274=CARTESIAN_POINT('Ctrl Pts',(42.2672849544021,46.5131996064559,2.76730190934719));
#211275=CARTESIAN_POINT('Ctrl Pts',(42.2676972410237,46.5274517041822,2.7499768728011));
#211276=CARTESIAN_POINT('Ctrl Pts',(42.2664327220898,46.5425130602354,2.73349253346124));
#211277=CARTESIAN_POINT('Ctrl Pts',(42.2654613625243,46.5540826713185,2.72082983599553));
#211278=CARTESIAN_POINT('Ctrl Pts',(42.263499903615,46.5661304069514,2.70866321039422));
#211279=CARTESIAN_POINT('Ctrl Pts',(42.2604772948659,46.5786151613303,2.69711645335877));
#211280=CARTESIAN_POINT('Ctrl Pts',(42.2604693731474,46.578647881645,2.69708619136783));
#211281=CARTESIAN_POINT('Ctrl Pts',(42.2604614434252,46.5786806053975,2.69705593387251));
#211282=CARTESIAN_POINT('Ctrl Pts',(42.2604535056997,46.5787133325846,2.69702568087603));
#211283=CARTESIAN_POINT('Ctrl Pts',(42.2596024201061,46.5822223525749,2.69378194443298));
#211284=CARTESIAN_POINT('Ctrl Pts',(42.2586587894014,46.5857690348148,2.69059266624733));
#211285=CARTESIAN_POINT('Ctrl Pts',(42.2576238078915,46.5893485909043,2.6874621934271));
#211286=CARTESIAN_POINT('Ctrl Pts',(42.2518643711132,46.609268006656,2.67004182396018));
#211287=CARTESIAN_POINT('Ctrl Pts',(42.2432808881735,46.6302067610372,2.65443567877737));
#211288=CARTESIAN_POINT('Ctrl Pts',(42.2321288152501,46.6513153841123,2.64136852352879));
#211289=CARTESIAN_POINT('Ctrl Pts',(42.2271236104851,46.6607892264664,2.63550380329572));
#211290=CARTESIAN_POINT('Ctrl Pts',(42.2216011621494,46.6702976120529,2.63014997451052));
#211291=CARTESIAN_POINT('Ctrl Pts',(42.2155846760829,46.6797659870608,2.62536981119287));
#211292=CARTESIAN_POINT('Ctrl Pts',(42.2129699926169,46.6838808147709,2.62329241687107));
#211293=CARTESIAN_POINT('Ctrl Pts',(42.210261991929,46.6879878819276,2.6213236213146));
#211294=CARTESIAN_POINT('Ctrl Pts',(42.2074625774078,46.6920809384681,2.6194687337238));
#211295=CARTESIAN_POINT('Ctrl Pts',(42.1976646265838,46.7064066363597,2.612976627156));
#211296=CARTESIAN_POINT('Ctrl Pts',(42.1867468541396,46.7205607018097,2.60787989114002));
#211297=CARTESIAN_POINT('Ctrl Pts',(42.1747908797557,46.7342751765575,2.60440616886212));
#211298=CARTESIAN_POINT('Ctrl Pts',(42.1688128925637,46.7411324139315,2.60266930772318));
#211299=CARTESIAN_POINT('Ctrl Pts',(42.1625753552954,46.74787975408,2.60133820040217));
#211300=CARTESIAN_POINT('Ctrl Pts',(42.1560884757157,46.7544837081026,2.60044130723617));
#211301=CARTESIAN_POINT('Ctrl Pts',(42.1528450359258,46.7577856851138,2.59999286065317));
#211302=CARTESIAN_POINT('Ctrl Pts',(42.1495392606405,46.7610518156852,2.59965296768545));
#211303=CARTESIAN_POINT('Ctrl Pts',(42.1461724262973,46.7642779142249,2.59942518630987));
#211304=CARTESIAN_POINT('Ctrl Pts',(42.142805591954,46.7675040127646,2.59919740493429));
#211305=CARTESIAN_POINT('Ctrl Pts',(42.1393776974108,46.770690078005,2.59908173791647));
#211306=CARTESIAN_POINT('Ctrl Pts',(42.1358900227694,46.773831928426,2.59908173516057));
#211307=CARTESIAN_POINT('',(42.1132001506,46.7942619810919,2.59908173516056));
#211308=CARTESIAN_POINT('Origin',(5.55120861436579E-15,1.85297104435686E-13,
2.59908173516022));
#211309=CARTESIAN_POINT('',(41.7612723673362,46.8559036426988,2.90134173516057));
#211310=CARTESIAN_POINT('Ctrl Pts',(42.1132001506,46.7942619810919,2.59908173516057));
#211311=CARTESIAN_POINT('Ctrl Pts',(42.1103595112871,46.7968184499055,2.59908174381712));
#211312=CARTESIAN_POINT('Ctrl Pts',(42.1074947242966,46.7993324362836,2.59915752001029));
#211313=CARTESIAN_POINT('Ctrl Pts',(42.1046079742813,46.8018034833199,2.59930729517504));
#211314=CARTESIAN_POINT('Ctrl Pts',(42.0879261203895,46.8160830868189,2.60017281085934));
#211315=CARTESIAN_POINT('Ctrl Pts',(42.0705099543567,46.8289319920994,2.60350651799969));
#211316=CARTESIAN_POINT('Ctrl Pts',(42.0527856759152,46.8402566831411,2.60896880596189));
#211317=CARTESIAN_POINT('Ctrl Pts',(42.0456370666871,46.8448241915535,2.61117187235254));
#211318=CARTESIAN_POINT('Ctrl Pts',(42.0384382358194,46.8491442126957,2.613720765771));
#211319=CARTESIAN_POINT('Ctrl Pts',(42.031216533405,46.8532123574522,2.61659179897017));
#211320=CARTESIAN_POINT('Ctrl Pts',(42.0285521636633,46.8547132558792,2.61765103591242));
#211321=CARTESIAN_POINT('Ctrl Pts',(42.0258847247795,46.8561797434811,2.61875422455182));
#211322=CARTESIAN_POINT('Ctrl Pts',(42.0232156132261,46.8576115380196,2.61990022440429));
#211323=CARTESIAN_POINT('Ctrl Pts',(42.0182110290634,46.8602961527791,2.62204897412766));
#211324=CARTESIAN_POINT('Ctrl Pts',(42.0132005644175,46.8628587997327,2.62434823201803));
#211325=CARTESIAN_POINT('Ctrl Pts',(42.0081934246215,46.865297618499,2.62679048030338));
#211326=CARTESIAN_POINT('Ctrl Pts',(41.9906684353354,46.8738334841811,2.63533834930212));
#211327=CARTESIAN_POINT('Ctrl Pts',(41.9731841724648,46.8808524512365,2.64563784783596));
#211328=CARTESIAN_POINT('Ctrl Pts',(41.9561353316316,46.8862747746136,2.65736666737997));
#211329=CARTESIAN_POINT('Ctrl Pts',(41.9476109112151,46.8889859363021,2.66323107715198));
#211330=CARTESIAN_POINT('Ctrl Pts',(41.939195346984,46.8912979378216,2.66945281780806));
#211331=CARTESIAN_POINT('Ctrl Pts',(41.930937981802,46.8932008176776,2.67599160631233));
#211332=CARTESIAN_POINT('Ctrl Pts',(41.926809299211,46.8941522576056,2.67926100056447));
#211333=CARTESIAN_POINT('Ctrl Pts',(41.92272016646,46.8950014172057,2.68260965685155));
#211334=CARTESIAN_POINT('Ctrl Pts',(41.9186767517591,46.8957470516901,2.68603254012514));
#211335=CARTESIAN_POINT('Ctrl Pts',(41.9146333370581,46.8964926861746,2.68945542339874));
#211336=CARTESIAN_POINT('Ctrl Pts',(41.9106356952805,46.8971346781639,2.69295261525418));
#211337=CARTESIAN_POINT('Ctrl Pts',(41.9066898836034,46.897672023819,2.69651891172132));
#211338=CARTESIAN_POINT('Ctrl Pts',(41.9066562340936,46.8976766062521,2.6965493247612));
#211339=CARTESIAN_POINT('Ctrl Pts',(41.9066225884706,46.8976811811499,2.69657974261178));
#211340=CARTESIAN_POINT('Ctrl Pts',(41.9065889467375,46.8976857485122,2.69661016527006));
#211341=CARTESIAN_POINT('Ctrl Pts',(41.8894076224749,46.9000183671519,2.71214746101303));
#211342=CARTESIAN_POINT('Ctrl Pts',(41.8732226654007,46.9005163877046,2.72880565567905));
#211343=CARTESIAN_POINT('Ctrl Pts',(41.858119701627,46.8993610201074,2.74628040012834));
#211344=CARTESIAN_POINT('Ctrl Pts',(41.8425059656474,46.8981665787453,2.76434612883104));
#211345=CARTESIAN_POINT('Ctrl Pts',(41.8280478726794,46.8952045688309,2.7832859265534));
#211346=CARTESIAN_POINT('Ctrl Pts',(41.8148672739051,46.8906306633424,2.8027875326894));
#211347=CARTESIAN_POINT('Ctrl Pts',(41.8019373978546,46.8861437631608,2.82191817724083));
#211348=CARTESIAN_POINT('Ctrl Pts',(41.7902363430293,46.8801049472928,2.84159092316637));
#211349=CARTESIAN_POINT('Ctrl Pts',(41.7799143139083,46.8726287066489,2.86151233818688));
#211350=CARTESIAN_POINT('Ctrl Pts',(41.7730763314897,46.8676759593275,2.87470957722448));
#211351=CARTESIAN_POINT('Ctrl Pts',(41.7668442729546,46.8620917411126,2.8880159438893));
#211352=CARTESIAN_POINT('Ctrl Pts',(41.7612723673362,46.8559036426988,2.90134173516057));
#211353=CARTESIAN_POINT('',(41.5228599914562,46.5911245387433,3.47153072139105));
#211354=CARTESIAN_POINT('',(41.7612723673362,46.8559036426988,2.90134173516057));
#211355=CARTESIAN_POINT('',(36.9399086546485,50.3023253561998,3.47153072139107));
#211356=CARTESIAN_POINT('Origin',(5.53234440788222E-15,1.85015204418142E-13,
3.47153072139072));
#211357=CARTESIAN_POINT('',(37.149332979726,50.5905785208487,2.90134173516058));
#211358=CARTESIAN_POINT('',(36.9399086546485,50.3023253561998,3.47153072139107));
#211359=CARTESIAN_POINT('',(37.0158684358559,50.9219998155902,2.59908173516059));
#211360=CARTESIAN_POINT('Ctrl Pts',(37.149332979726,50.5905785208487,2.90134173516059));
#211361=CARTESIAN_POINT('Ctrl Pts',(37.1565661199776,50.6005343088823,2.88164837656743));
#211362=CARTESIAN_POINT('Ctrl Pts',(37.1621977431859,50.6116037659393,2.86203734439147));
#211363=CARTESIAN_POINT('Ctrl Pts',(37.1661909570576,50.6236016024789,2.84277945978143));
#211364=CARTESIAN_POINT('Ctrl Pts',(37.1702644101621,50.6358405223237,2.82313460920001));
#211365=CARTESIAN_POINT('Ctrl Pts',(37.172633529828,50.6490462309924,2.80385576863314));
#211366=CARTESIAN_POINT('Ctrl Pts',(37.1732217245288,50.6630602183675,2.78521678518356));
#211367=CARTESIAN_POINT('Ctrl Pts',(37.1737870683988,50.676529775037,2.76730190934436));
#211368=CARTESIAN_POINT('Ctrl Pts',(37.172707346597,50.6907468939687,2.74997687279745));
#211369=CARTESIAN_POINT('Ctrl Pts',(37.1698754144267,50.7055935641174,2.73349253345689));
#211370=CARTESIAN_POINT('Ctrl Pts',(37.1677000224033,50.7169982609366,2.72082983599275));
#211371=CARTESIAN_POINT('Ctrl Pts',(37.1644899772797,50.7287749695264,2.7086632103929));
#211372=CARTESIAN_POINT('Ctrl Pts',(37.1601789145086,50.7408753824655,2.69711645335879));
#211373=CARTESIAN_POINT('Ctrl Pts',(37.1601676159819,50.7409070954899,2.69708619136785));
#211374=CARTESIAN_POINT('Ctrl Pts',(37.160156309136,50.7409388110965,2.69705593387252));
#211375=CARTESIAN_POINT('Ctrl Pts',(37.1601449939716,50.7409705292824,2.69702568087604));
#211376=CARTESIAN_POINT('Ctrl Pts',(37.1589317782469,50.7443713638248,2.693781944433));
#211377=CARTESIAN_POINT('Ctrl Pts',(37.1576225876056,50.7477999807009,2.69059266624734));
#211378=CARTESIAN_POINT('Ctrl Pts',(37.1562191103355,50.7512517425808,2.6874621934271));
#211379=CARTESIAN_POINT('Ctrl Pts',(37.1484090784356,50.770460012616,2.67004182395759));
#211380=CARTESIAN_POINT('Ctrl Pts',(37.1376839208933,50.7903868440317,2.65443567877273));
#211381=CARTESIAN_POINT('Ctrl Pts',(37.1243864882577,50.8102141228191,2.64136852352296));
#211382=CARTESIAN_POINT('Ctrl Pts',(37.1184184163473,50.8191128801081,2.63550380329217));
#211383=CARTESIAN_POINT('Ctrl Pts',(37.1119323236298,50.8279919247225,2.63014997450893));
#211384=CARTESIAN_POINT('Ctrl Pts',(37.1049590818166,50.8367795369357,2.62536981119286));
#211385=CARTESIAN_POINT('Ctrl Pts',(37.101928605243,50.8405985143444,2.62329241687106));
#211386=CARTESIAN_POINT('Ctrl Pts',(37.0988061338478,50.844400019407,2.6213236213146));
#211387=CARTESIAN_POINT('Ctrl Pts',(37.0955942139021,50.8481780352576,2.61946873372381));
#211388=CARTESIAN_POINT('Ctrl Pts',(37.084352494092,50.8614010907344,2.61297662715601));
#211389=CARTESIAN_POINT('Ctrl Pts',(37.0720150276372,50.874336400757,2.60787989114004));
#211390=CARTESIAN_POINT('Ctrl Pts',(37.058690996362,50.886726006548,2.60440616886214));
#211391=CARTESIAN_POINT('Ctrl Pts',(37.0520289807243,50.8929208094435,2.60266930772319));
#211392=CARTESIAN_POINT('Ctrl Pts',(37.045120324241,50.8989791867715,2.60133820040219));
#211393=CARTESIAN_POINT('Ctrl Pts',(37.0379786793009,50.904868900089,2.60044130723619));
#211394=CARTESIAN_POINT('Ctrl Pts',(37.0344078568308,50.9078137567478,2.59999286065319));
#211395=CARTESIAN_POINT('Ctrl Pts',(37.030778787319,50.9107164475037,2.59965296768547));
#211396=CARTESIAN_POINT('Ctrl Pts',(37.0270931777238,50.913572943118,2.59942518630989));
#211397=CARTESIAN_POINT('Ctrl Pts',(37.0234075681286,50.9164294387324,2.59919740493431));
#211398=CARTESIAN_POINT('Ctrl Pts',(37.0196654174469,50.9192397378252,2.59908173791651));
#211399=CARTESIAN_POINT('Ctrl Pts',(37.0158684358559,50.9219998155902,2.59908173516059));
#211400=CARTESIAN_POINT('',(36.9911673391707,50.9399462128204,2.5990817351606));
#211401=CARTESIAN_POINT('Origin',(5.56385071146069E-15,1.85286867067313E-13,
2.59908173516024));
#211402=CARTESIAN_POINT('',(36.6347241449654,50.9644637245895,2.90134173516059));
#211403=CARTESIAN_POINT('Ctrl Pts',(36.9911673391707,50.9399462128204,2.5990817351606));
#211404=CARTESIAN_POINT('Ctrl Pts',(36.9880750374206,50.9421917493682,2.59908174381721));
#211405=CARTESIAN_POINT('Ctrl Pts',(36.9849631609003,50.9443925120842,2.59915752001032));
#211406=CARTESIAN_POINT('Ctrl Pts',(36.9818339300542,50.9465482749234,2.59930729517507));
#211407=CARTESIAN_POINT('Ctrl Pts',(36.9637508360889,50.9590059247118,2.60017281085961));
#211408=CARTESIAN_POINT('Ctrl Pts',(36.9450870013071,50.9699639572759,2.6035065180015));
#211409=CARTESIAN_POINT('Ctrl Pts',(36.9262760657608,50.9793739188888,2.60896880596628));
#211410=CARTESIAN_POINT('Ctrl Pts',(36.9186891827317,50.9831691728722,2.61117187235594));
#211411=CARTESIAN_POINT('Ctrl Pts',(36.9110782226465,50.9867130457562,2.61372076577293));
#211412=CARTESIAN_POINT('Ctrl Pts',(36.9034708445587,50.9900040313324,2.61659179897021));
#211413=CARTESIAN_POINT('Ctrl Pts',(36.9006641839072,50.9912182052061,2.61765103591246));
#211414=CARTESIAN_POINT('Ctrl Pts',(36.8978580678372,50.9923978359481,2.61875422455187));
#211415=CARTESIAN_POINT('Ctrl Pts',(36.8950539146733,50.9935427888373,2.61990022440433));
#211416=CARTESIAN_POINT('Ctrl Pts',(36.8897961274911,50.9956895755044,2.6220489741277));
#211417=CARTESIAN_POINT('Ctrl Pts',(36.8845452411468,50.9977144478402,2.62434823201806));
#211418=CARTESIAN_POINT('Ctrl Pts',(36.8793106050087,50.9996165178739,2.62679048030342));
#211419=CARTESIAN_POINT('Ctrl Pts',(36.8609893785252,51.0062737629918,2.63533834930215));
#211420=CARTESIAN_POINT('Ctrl Pts',(36.8428672144359,51.0114266762821,2.64563784783598));
#211421=CARTESIAN_POINT('Ctrl Pts',(36.8253449818067,51.0150372064715,2.65736666737999));
#211422=CARTESIAN_POINT('Ctrl Pts',(36.8165838654922,51.0168424715662,2.663231077152));
#211423=CARTESIAN_POINT('Ctrl Pts',(36.8079727326367,51.0182621417029,2.6694528178081));
#211424=CARTESIAN_POINT('Ctrl Pts',(36.7995616970579,51.0192914676908,2.67599160631236));
#211425=CARTESIAN_POINT('Ctrl Pts',(36.7953561792686,51.0198061306848,2.6792610005645));
#211426=CARTESIAN_POINT('Ctrl Pts',(36.7912006858666,51.0202232077372,2.68260965685158));
#211427=CARTESIAN_POINT('Ctrl Pts',(36.7871014813876,51.0205421056329,2.68603254012517));
#211428=CARTESIAN_POINT('Ctrl Pts',(36.7830022769086,51.0208610035285,2.68945542339877));
#211429=CARTESIAN_POINT('Ctrl Pts',(36.7789594281949,51.0210816112669,2.6929526152542));
#211430=CARTESIAN_POINT('Ctrl Pts',(36.7749790641715,51.0212035636553,2.69651891172134));
#211431=CARTESIAN_POINT('Ctrl Pts',(36.7749451200025,51.0212046036538,2.69654932476122));
#211432=CARTESIAN_POINT('Ctrl Pts',(36.7749111804867,51.0212056365646,2.6965797426118));
#211433=CARTESIAN_POINT('Ctrl Pts',(36.7748772456272,51.0212066623878,2.69661016527007));
#211434=CARTESIAN_POINT('Ctrl Pts',(36.7575462174171,51.0217305652763,2.71214746101103));
#211435=CARTESIAN_POINT('Ctrl Pts',(36.7413978659101,51.0205340689296,2.72880565567476));
#211436=CARTESIAN_POINT('Ctrl Pts',(36.7264984065534,51.0178063409637,2.74628040012157));
#211437=CARTESIAN_POINT('Ctrl Pts',(36.7110950573747,51.0149863630491,2.76434612882204));
#211438=CARTESIAN_POINT('Ctrl Pts',(36.6970257816983,51.0105292970963,2.78328592654201));
#211439=CARTESIAN_POINT('Ctrl Pts',(36.6843954909359,51.0046027002071,2.80278753267555));
#211440=CARTESIAN_POINT('Ctrl Pts',(36.6720054548804,50.9987888396615,2.82191817722516));
#211441=CARTESIAN_POINT('Ctrl Pts',(36.6609997278005,50.9915600117806,2.84159092314885));
#211442=CARTESIAN_POINT('Ctrl Pts',(36.6515157237802,50.9830457809249,2.86151233816758));
#211443=CARTESIAN_POINT('Ctrl Pts',(36.6452329036075,50.9774054014754,2.87470957721151));
#211444=CARTESIAN_POINT('Ctrl Pts',(36.6396186946865,50.9712003466878,2.88801594388282));
#211445=CARTESIAN_POINT('Ctrl Pts',(36.6347241449653,50.9644637245895,2.90134173516059));
#211446=CARTESIAN_POINT('',(36.4252947698678,50.6762142289951,3.47153072139107));
#211447=CARTESIAN_POINT('',(36.6347241449653,50.9644637245895,2.90134173516059));
#211448=CARTESIAN_POINT('',(31.4795232016789,53.8880358395973,3.4715307213911));
#211449=CARTESIAN_POINT('Origin',(5.53234440788222E-15,1.85015204418142E-13,
3.47153072139072));
#211450=CARTESIAN_POINT('',(31.6576696180583,54.196600726121,2.90134173516061));
#211451=CARTESIAN_POINT('',(31.4795232016789,53.8880358395973,3.4715307213911));
#211452=CARTESIAN_POINT('',(31.4902932482907,54.5122556166613,2.59908173516061));
#211453=CARTESIAN_POINT('Ctrl Pts',(31.6576696180583,54.196600726121,2.90134173516061));
#211454=CARTESIAN_POINT('Ctrl Pts',(31.6638224711871,54.2072580443423,2.8816483765657));
#211455=CARTESIAN_POINT('Ctrl Pts',(31.668266170439,54.2188555266763,2.862037344388));
#211456=CARTESIAN_POINT('Ctrl Pts',(31.6709833936512,54.2312050423228,2.84277945977631));
#211457=CARTESIAN_POINT('Ctrl Pts',(31.6737552164697,54.2438027078783,2.82313460919356));
#211458=CARTESIAN_POINT('Ctrl Pts',(31.6747309854164,54.2571837147323,2.80385576862544));
#211459=CARTESIAN_POINT('Ctrl Pts',(31.67385109736,54.2711824151075,2.78521678517473));
#211460=CARTESIAN_POINT('Ctrl Pts',(31.6730053921571,54.2846372786627,2.76730190933514));
#211461=CARTESIAN_POINT('Ctrl Pts',(31.6704454915897,54.2986636530692,2.74997687278792));
#211462=CARTESIAN_POINT('Ctrl Pts',(31.6660771734241,54.3131329740882,2.73349253344715));
#211463=CARTESIAN_POINT('Ctrl Pts',(31.6627215829937,54.324247804397,2.72082983598652));
#211464=CARTESIAN_POINT('Ctrl Pts',(31.6582981215828,54.3356244578582,2.70866321038996));
#211465=CARTESIAN_POINT('Ctrl Pts',(31.6527458376967,54.3472079546996,2.69711645335882));
#211466=CARTESIAN_POINT('Ctrl Pts',(31.6527312861508,54.3472383129791,2.69708619136788));
#211467=CARTESIAN_POINT('Ctrl Pts',(31.6527167260613,54.3472686729571,2.69705593387255));
#211468=CARTESIAN_POINT('Ctrl Pts',(31.6527021574293,54.3472990346307,2.69702568087607));
#211469=CARTESIAN_POINT('Ctrl Pts',(31.6511401038187,54.3505544234703,2.69378194443303));
#211470=CARTESIAN_POINT('Ctrl Pts',(31.6494796970076,54.3538274103386,2.69059266624737));
#211471=CARTESIAN_POINT('Ctrl Pts',(31.6477231007679,54.3571135597835,2.68746219342714));
#211472=CARTESIAN_POINT('Ctrl Pts',(31.637948042092,54.3754002342713,2.67004182395931));
#211473=CARTESIAN_POINT('Ctrl Pts',(31.6251987170208,54.3940968201815,2.65443567877578));
#211474=CARTESIAN_POINT('Ctrl Pts',(31.6099016141321,54.4124255228606,2.64136852352678));
#211475=CARTESIAN_POINT('Ctrl Pts',(31.6030360625184,54.4206516984424,2.6355038032945));
#211476=CARTESIAN_POINT('Ctrl Pts',(31.5956573884051,54.4288041214188,2.63014997450999));
#211477=CARTESIAN_POINT('Ctrl Pts',(31.5878037911381,54.4368146919238,2.62536981119289));
#211478=CARTESIAN_POINT('Ctrl Pts',(31.5843907239925,54.4402959775155,2.62329241687109));
#211479=CARTESIAN_POINT('Ctrl Pts',(31.58088799234,54.4437502703991,2.62132362131464));
#211480=CARTESIAN_POINT('Ctrl Pts',(31.5772987574367,54.4471718528274,2.61946873372384));
#211481=CARTESIAN_POINT('Ctrl Pts',(31.5647364352753,54.4591473913265,2.61297662715605));
#211482=CARTESIAN_POINT('Ctrl Pts',(31.5511144466741,54.4707222239583,2.60787989114006));
#211483=CARTESIAN_POINT('Ctrl Pts',(31.5365683393825,54.4816512176787,2.60440616886217));
#211484=CARTESIAN_POINT('Ctrl Pts',(31.5292952857367,54.4871157145388,2.60266930772322));
#211485=CARTESIAN_POINT('Ctrl Pts',(31.5217912027244,54.4924187521965,2.60133820040221));
#211486=CARTESIAN_POINT('Ctrl Pts',(31.5140730377803,54.4975296958775,2.60044130723621));
#211487=CARTESIAN_POINT('Ctrl Pts',(31.5102139553083,54.5000851677179,2.59999286065321));
#211488=CARTESIAN_POINT('Ctrl Pts',(31.5063013524149,54.5025926161709,2.59965296768549));
#211489=CARTESIAN_POINT('Ctrl Pts',(31.5023373478778,54.5050482124963,2.59942518630991));
#211490=CARTESIAN_POINT('Ctrl Pts',(31.4983733433407,54.5075038088217,2.59919740493433));
#211491=CARTESIAN_POINT('Ctrl Pts',(31.4943579363065,54.5099075515419,2.59908173791649));
#211492=CARTESIAN_POINT('Ctrl Pts',(31.4902932482907,54.5122556166613,2.59908173516061));
#211493=CARTESIAN_POINT('',(31.4638515574739,54.5275217339722,2.59908173516062));
#211494=CARTESIAN_POINT('Origin',(5.57749365020894E-15,1.85278007239296E-13,
2.59908173516024));
#211495=CARTESIAN_POINT('',(31.1067982185534,54.5146464769141,2.90134173516061));
#211496=CARTESIAN_POINT('Ctrl Pts',(31.4638515574739,54.5275217339722,2.59908173516061));
#211497=CARTESIAN_POINT('Ctrl Pts',(31.4605414731919,54.529431735686,2.59908174381718));
#211498=CARTESIAN_POINT('Ctrl Pts',(31.457216601512,54.5312951627229,2.59915752001034));
#211499=CARTESIAN_POINT('Ctrl Pts',(31.4538791743432,54.5331120223762,2.59930729517509));
#211500=CARTESIAN_POINT('Ctrl Pts',(31.4345929624716,54.5436112298317,2.60017281085957));
#211501=CARTESIAN_POINT('Ctrl Pts',(31.4148859438265,54.5525583311779,2.60350651800109));
#211502=CARTESIAN_POINT('Ctrl Pts',(31.3951944477277,54.5599504658509,2.60896880596526));
#211503=CARTESIAN_POINT('Ctrl Pts',(31.3872524143699,54.5629318838125,2.61117187235515));
#211504=CARTESIAN_POINT('Ctrl Pts',(31.3793127123325,54.5656607810288,2.61372076577249));
#211505=CARTESIAN_POINT('Ctrl Pts',(31.3714030065918,54.568138550701,2.61659179897022));
#211506=CARTESIAN_POINT('Ctrl Pts',(31.3684848053918,54.5690526972783,2.61765103591248));
#211507=CARTESIAN_POINT('Ctrl Pts',(31.3655707565306,54.5699325468792,2.61875422455188));
#211508=CARTESIAN_POINT('Ctrl Pts',(31.3626622846451,54.5707781137756,2.61990022440434));
#211509=CARTESIAN_POINT('Ctrl Pts',(31.3572088998599,54.5723635517065,2.62204897412771));
#211510=CARTESIAN_POINT('Ctrl Pts',(31.3517751216268,54.5738284644993,2.62434823201808));
#211511=CARTESIAN_POINT('Ctrl Pts',(31.3463703409155,54.5751729463231,2.62679048030343));
#211512=CARTESIAN_POINT('Ctrl Pts',(31.3274536084259,54.5798786327062,2.63533834930216));
#211513=CARTESIAN_POINT('Ctrl Pts',(31.3088920933401,54.5831090358349,2.645637847836));
#211514=CARTESIAN_POINT('Ctrl Pts',(31.2910884461624,54.5848682151125,2.65736666738002));
#211515=CARTESIAN_POINT('Ctrl Pts',(31.2821866225735,54.5857478047513,2.66323107715202));
#211516=CARTESIAN_POINT('Ctrl Pts',(31.273474266467,54.586259589302,2.66945281780811));
#211517=CARTESIAN_POINT('Ctrl Pts',(31.2650017135576,54.586404083911,2.67599160631237));
#211518=CARTESIAN_POINT('Ctrl Pts',(31.2607654371028,54.5864763312154,2.67926100056451));
#211519=CARTESIAN_POINT('Ctrl Pts',(31.2565891115051,54.5864567561366,2.6826096568516));
#211520=CARTESIAN_POINT('Ctrl Pts',(31.2524790289902,54.5863454235315,2.6860325401252));
#211521=CARTESIAN_POINT('Ctrl Pts',(31.2483689464753,54.5862340909263,2.68945542339879));
#211522=CARTESIAN_POINT('Ctrl Pts',(31.244325185122,54.5860308973891,2.69295261525422));
#211523=CARTESIAN_POINT('Ctrl Pts',(31.2403538784534,54.585736120375,2.69651891172136));
#211524=CARTESIAN_POINT('Ctrl Pts',(31.2403200115247,54.5857336065444,2.69654932476124));
#211525=CARTESIAN_POINT('Ctrl Pts',(31.2402861499645,54.5857310861514,2.69657974261182));
#211526=CARTESIAN_POINT('Ctrl Pts',(31.240252293776,54.5857285591963,2.6966101652701));
#211527=CARTESIAN_POINT('Ctrl Pts',(31.2229614439884,54.5844380063444,2.71214746101062));
#211528=CARTESIAN_POINT('Ctrl Pts',(31.2070266227655,54.5815601021627,2.72880565567384));
#211529=CARTESIAN_POINT('Ctrl Pts',(31.1924939094189,54.577289899386,2.7462804001201));
#211530=CARTESIAN_POINT('Ctrl Pts',(31.1774697093569,54.572875281187,2.76434612881997));
#211531=CARTESIAN_POINT('Ctrl Pts',(31.1639433968999,54.5669719917423,2.78328592653931));
#211532=CARTESIAN_POINT('Ctrl Pts',(31.1520017942572,54.5597576364874,2.8027875326722));
#211533=CARTESIAN_POINT('Ctrl Pts',(31.1402873460242,54.5526805134498,2.82191817722124));
#211534=CARTESIAN_POINT('Ctrl Pts',(31.1300975277384,54.5443408741059,2.84159092314435));
#211535=CARTESIAN_POINT('Ctrl Pts',(31.1215554575517,54.5348819367323,2.86151233816251));
#211536=CARTESIAN_POINT('Ctrl Pts',(31.1158966355205,54.5286157223332,2.87470957720811));
#211537=CARTESIAN_POINT('Ctrl Pts',(31.1109617866641,54.5218578148532,2.88801594388113));
#211538=CARTESIAN_POINT('Ctrl Pts',(31.1067982185534,54.514646476914,2.90134173516061));
#211539=CARTESIAN_POINT('',(30.9286463962977,54.2060847114744,3.4715307213911));
#211540=CARTESIAN_POINT('',(31.1067982185534,54.514646476914,2.90134173516061));
#211541=CARTESIAN_POINT('',(25.6742415049979,56.8833377255397,3.47153072139112));
#211542=CARTESIAN_POINT('Origin',(5.53234440788222E-15,1.85015204418142E-13,
3.47153072139072));
#211543=CARTESIAN_POINT('',(25.8191582032619,57.2088336324701,2.90134173516063));
#211544=CARTESIAN_POINT('',(25.6742415049979,56.8833377255397,3.47153072139112));
#211545=CARTESIAN_POINT('',(25.6197038181297,57.5052637377734,2.59908173516064));
#211546=CARTESIAN_POINT('Ctrl Pts',(25.8191582032619,57.2088336324701,2.90134173516064));
#211547=CARTESIAN_POINT('Ctrl Pts',(25.8241633573214,57.220075717069,2.88164837656632));
#211548=CARTESIAN_POINT('Ctrl Pts',(25.8273704465176,57.2320741602348,2.86203734438921));
#211549=CARTESIAN_POINT('Ctrl Pts',(25.8287819086042,57.2446400511088,2.84277945977808));
#211550=CARTESIAN_POINT('Ctrl Pts',(25.8302217324661,57.2574584397136,2.82313460919575));
#211551=CARTESIAN_POINT('Ctrl Pts',(25.8297934599651,57.2708681396401,2.80385576862801));
#211552=CARTESIAN_POINT('Ctrl Pts',(25.8274551293899,57.2846981803233,2.78521678517766));
#211553=CARTESIAN_POINT('Ctrl Pts',(25.8252076408377,57.2979909364628,2.76730190933808));
#211554=CARTESIAN_POINT('Ctrl Pts',(25.8211956083118,57.3116728904502,2.74997687279086));
#211555=CARTESIAN_POINT('Ctrl Pts',(25.8153387643597,57.3256063334298,2.73349253345006));
#211556=CARTESIAN_POINT('Ctrl Pts',(25.8108397400729,57.3363095208249,2.72082983598839));
#211557=CARTESIAN_POINT('Ctrl Pts',(25.8052513267427,57.3471614741653,2.70866321039087));
#211558=CARTESIAN_POINT('Ctrl Pts',(25.798518653724,57.3581011436976,2.69711645335884));
#211559=CARTESIAN_POINT('Ctrl Pts',(25.7985010085887,57.3581298146205,2.6970861913679));
#211560=CARTESIAN_POINT('Ctrl Pts',(25.798483354779,57.3581584863396,2.69705593387257));
#211561=CARTESIAN_POINT('Ctrl Pts',(25.7984656922965,57.3581871588521,2.69702568087609));
#211562=CARTESIAN_POINT('Ctrl Pts',(25.7965719149862,57.3612614352675,2.69378194443305));
#211563=CARTESIAN_POINT('Ctrl Pts',(25.7945784837697,57.364342932599,2.6905926662474));
#211564=CARTESIAN_POINT('Ctrl Pts',(25.7924880141965,57.3674274658678,2.68746219342717));
#211565=CARTESIAN_POINT('Ctrl Pts',(25.7808550263308,57.3845921921799,2.67004182395704));
#211566=CARTESIAN_POINT('Ctrl Pts',(25.7662212180005,57.4018536888811,2.65443567877168));
#211567=CARTESIAN_POINT('Ctrl Pts',(25.7490920431143,57.4184830023538,2.64136852352162));
#211568=CARTESIAN_POINT('Ctrl Pts',(25.7414042322205,57.4259464685231,2.63550380329137));
#211569=CARTESIAN_POINT('Ctrl Pts',(25.7332138190127,57.4332829502053,2.63014997450861));
#211570=CARTESIAN_POINT('Ctrl Pts',(25.724565911951,57.4404287135114,2.62536981119292));
#211571=CARTESIAN_POINT('Ctrl Pts',(25.7208076485113,57.4435341655925,2.62329241687112));
#211572=CARTESIAN_POINT('Ctrl Pts',(25.7169630332625,57.4466034003414,2.62132362131468));
#211573=CARTESIAN_POINT('Ctrl Pts',(25.7130358078104,57.4496310617744,2.61946873372388));
#211574=CARTESIAN_POINT('Ctrl Pts',(25.699290518728,57.46022787679,2.61297662715608));
#211575=CARTESIAN_POINT('Ctrl Pts',(25.6845332533381,57.4703154157424,2.60787989114009));
#211576=CARTESIAN_POINT('Ctrl Pts',(25.6689244402255,57.47966405705,2.60440616886219));
#211577=CARTESIAN_POINT('Ctrl Pts',(25.6611200336693,57.4843383777037,2.60266930772324));
#211578=CARTESIAN_POINT('Ctrl Pts',(25.6531027404319,57.4888279745008,2.60133820040224));
#211579=CARTESIAN_POINT('Ctrl Pts',(25.6448926173141,57.4931041519766,2.60044130723624));
#211580=CARTESIAN_POINT('Ctrl Pts',(25.6407875557553,57.4952422407145,2.59999286065324));
#211581=CARTESIAN_POINT('Ctrl Pts',(25.6366342867764,57.4973269747347,2.59965296768552));
#211582=CARTESIAN_POINT('Ctrl Pts',(25.6324353177606,57.4993547677438,2.59942518630994));
#211583=CARTESIAN_POINT('Ctrl Pts',(25.6282363487449,57.5013825607529,2.59919740493437));
#211584=CARTESIAN_POINT('Ctrl Pts',(25.6239916789979,57.5033534111923,2.59908173791663));
#211585=CARTESIAN_POINT('Ctrl Pts',(25.6197038181297,57.5052637377734,2.59908173516064));
#211586=CARTESIAN_POINT('',(25.5918112338793,57.5176823163891,2.59908173516065));
#211587=CARTESIAN_POINT('Origin',(5.59198795571863E-15,1.85270622021766E-13,
2.59908173516023));
#211588=CARTESIAN_POINT('',(25.2380597013429,57.4675553545143,2.90134173516064));
#211589=CARTESIAN_POINT('Ctrl Pts',(25.5918112338793,57.5176823163891,2.59908173516064));
#211590=CARTESIAN_POINT('Ctrl Pts',(25.5883196330413,57.5192358568903,2.59908174381722));
#211591=CARTESIAN_POINT('Ctrl Pts',(25.5848181941918,57.5207415321518,2.59915752001036));
#211592=CARTESIAN_POINT('Ctrl Pts',(25.5813091362507,57.5221995827245,2.59930729517511));
#211593=CARTESIAN_POINT('Ctrl Pts',(25.5610311102461,57.5306253163333,2.60017281085954));
#211594=CARTESIAN_POINT('Ctrl Pts',(25.5404968219579,57.5374634601473,2.6035065180007));
#211595=CARTESIAN_POINT('Ctrl Pts',(25.5201405094588,57.5427567781063,2.60896880596427));
#211596=CARTESIAN_POINT('Ctrl Pts',(25.5119303403515,57.5448916950066,2.61117187235438));
#211597=CARTESIAN_POINT('Ctrl Pts',(25.503748885399,57.546775718186,2.61372076577206));
#211598=CARTESIAN_POINT('Ctrl Pts',(25.4956235123965,57.548413124991,2.61659179897022));
#211599=CARTESIAN_POINT('Ctrl Pts',(25.492625743071,57.5490172286908,2.61765103591247));
#211600=CARTESIAN_POINT('Ctrl Pts',(25.4896356883477,57.5495876573341,2.61875422455189));
#211601=CARTESIAN_POINT('Ctrl Pts',(25.4866547635673,57.55012457403,2.61990022440435));
#211602=CARTESIAN_POINT('Ctrl Pts',(25.481065529604,57.5511312928347,2.62204897412772));
#211603=CARTESIAN_POINT('Ctrl Pts',(25.4755083930936,57.5520201961936,2.62434823201809));
#211604=CARTESIAN_POINT('Ctrl Pts',(25.4699926837176,57.5527923593832,2.62679048030344));
#211605=CARTESIAN_POINT('Ctrl Pts',(25.4506877009016,57.5554949305468,2.63533834930218));
#211606=CARTESIAN_POINT('Ctrl Pts',(25.4318901986628,57.5567674305413,2.64563784783603));
#211607=CARTESIAN_POINT('Ctrl Pts',(25.4140001974206,57.5566559849707,2.65736666738005));
#211608=CARTESIAN_POINT('Ctrl Pts',(25.4050551967996,57.5566002621854,2.66323107715206));
#211609=CARTESIAN_POINT('Ctrl Pts',(25.3963370718388,57.5561985539316,2.66945281780813));
#211610=CARTESIAN_POINT('Ctrl Pts',(25.3878958286612,57.5554566340483,2.6759916063124));
#211611=CARTESIAN_POINT('Ctrl Pts',(25.3836752070724,57.5550856741067,2.67926100056454));
#211612=CARTESIAN_POINT('Ctrl Pts',(25.3795238059763,57.5546296613654,2.68260965685163));
#211613=CARTESIAN_POINT('Ctrl Pts',(25.3754478763495,57.5540893180427,2.68603254012523));
#211614=CARTESIAN_POINT('Ctrl Pts',(25.3713719467228,57.55354897472,2.68945542339882));
#211615=CARTESIAN_POINT('Ctrl Pts',(25.3673715770255,57.5529242061382,2.69295261525425));
#211616=CARTESIAN_POINT('Ctrl Pts',(25.3634528381786,57.5522159293601,2.69651891172139));
#211617=CARTESIAN_POINT('Ctrl Pts',(25.3634194195433,57.5522098892426,2.69654932476127));
#211618=CARTESIAN_POINT('Ctrl Pts',(25.3633860069332,57.5522038431597,2.69657974261185));
#211619=CARTESIAN_POINT('Ctrl Pts',(25.3633526003511,57.5521977911121,2.69661016527013));
#211620=CARTESIAN_POINT('Ctrl Pts',(25.3462913711518,57.5491069220865,2.71214746101287));
#211621=CARTESIAN_POINT('Ctrl Pts',(25.3307446654463,57.5445791409893,2.72880565567863));
#211622=CARTESIAN_POINT('Ctrl Pts',(25.3167379215565,57.5388132486358,2.74628040012763));
#211623=CARTESIAN_POINT('Ctrl Pts',(25.3022574788892,57.5328523576317,2.7643461288303));
#211624=CARTESIAN_POINT('Ctrl Pts',(25.2894223267598,57.5255675223679,2.78328592655263));
#211625=CARTESIAN_POINT('Ctrl Pts',(25.2783002469335,57.5171444507308,2.8027875326886));
#211626=CARTESIAN_POINT('Ctrl Pts',(25.2673897324687,57.5088816036403,2.82191817724038));
#211627=CARTESIAN_POINT('Ctrl Pts',(25.2581274647585,57.499522523665,2.84159092316628));
#211628=CARTESIAN_POINT('Ctrl Pts',(25.2506209171144,57.4892225138682,2.86151233818717));
#211629=CARTESIAN_POINT('Ctrl Pts',(25.245648092468,57.4823991184802,2.8747095772247));
#211630=CARTESIAN_POINT('Ctrl Pts',(25.2414466709169,57.4751623993613,2.88801594388944));
#211631=CARTESIAN_POINT('Ctrl Pts',(25.2380597013429,57.4675553545143,2.90134173516063));
#211632=CARTESIAN_POINT('',(25.0931373005745,57.1420619865024,3.47153072139112));
#211633=CARTESIAN_POINT('',(25.2380597013429,57.4675553545143,2.90134173516064));
#211634=CARTESIAN_POINT('',(19.5876674457077,59.2554138597574,3.47153072139113));
#211635=CARTESIAN_POINT('Origin',(5.53234440788222E-15,1.85015204418142E-13,
3.47153072139072));
#211636=CARTESIAN_POINT('',(19.6977666881844,59.5942745858238,2.90134173516065));
#211637=CARTESIAN_POINT('',(19.5876674457077,59.2554138597574,3.47153072139113));
#211638=CARTESIAN_POINT('',(19.4684195516695,59.8682321556244,2.59908173516065));
#211639=CARTESIAN_POINT('Ctrl Pts',(19.6977666881844,59.5942745858238,2.90134173516065));
#211640=CARTESIAN_POINT('Ctrl Pts',(19.7015693056591,59.6059782661683,2.88164837656773));
#211641=CARTESIAN_POINT('Ctrl Pts',(19.7035046472595,59.6182462127114,2.862037344392));
#211642=CARTESIAN_POINT('Ctrl Pts',(19.7035948839467,59.6308908042823,2.84277945978218));
#211643=CARTESIAN_POINT('Ctrl Pts',(19.7036869338407,59.6437894749879,2.82313460920108));
#211644=CARTESIAN_POINT('Ctrl Pts',(19.7018593121356,59.6570809485078,2.80385576863451));
#211645=CARTESIAN_POINT('Ctrl Pts',(19.6980881582811,59.6705908046785,2.7852167851852));
#211646=CARTESIAN_POINT('Ctrl Pts',(19.6944635103351,59.6835758151839,2.76730190934623));
#211647=CARTESIAN_POINT('Ctrl Pts',(19.6890433025191,59.6967634464006,2.74997687279954));
#211648=CARTESIAN_POINT('Ctrl Pts',(19.6817621015892,59.7100083536232,2.73349253345916));
#211649=CARTESIAN_POINT('Ctrl Pts',(19.6761689356969,59.7201826317454,2.72082983599423));
#211650=CARTESIAN_POINT('Ctrl Pts',(19.6694767982722,59.7303909886949,2.70866321039365));
#211651=CARTESIAN_POINT('Ctrl Pts',(19.661637500694,59.740566973611,2.69711645335886));
#211652=CARTESIAN_POINT('Ctrl Pts',(19.6616169552931,59.7405936430526,2.69708619136792));
#211653=CARTESIAN_POINT('Ctrl Pts',(19.6615964011821,59.7406203123795,2.69705593387259));
#211654=CARTESIAN_POINT('Ctrl Pts',(19.6615758383628,59.7406469815888,2.69702568087611));
#211655=CARTESIAN_POINT('Ctrl Pts',(19.6593710859735,59.7435064631644,2.69378194443307));
#211656=CARTESIAN_POINT('Ctrl Pts',(19.6570664708011,59.7463627094293,2.69059266624741));
#211657=CARTESIAN_POINT('Ctrl Pts',(19.6546650315164,59.7492118317302,2.68746219342718));
#211658=CARTESIAN_POINT('Ctrl Pts',(19.6413015679148,59.765066549527,2.67004182396116));
#211659=CARTESIAN_POINT('Ctrl Pts',(19.6249436073983,59.780703836443,2.65443567877906));
#211660=CARTESIAN_POINT('Ctrl Pts',(19.6061700313475,59.7954515664656,2.64136852353089));
#211661=CARTESIAN_POINT('Ctrl Pts',(19.5977441904329,59.8020705519314,2.63550380329702));
#211662=CARTESIAN_POINT('Ctrl Pts',(19.5888317740052,59.8085107122966,2.63014997451115));
#211663=CARTESIAN_POINT('Ctrl Pts',(19.5794843054211,59.8147133779312,2.62536981119295));
#211664=CARTESIAN_POINT('Ctrl Pts',(19.5754220220079,59.817408972519,2.62329241687115));
#211665=CARTESIAN_POINT('Ctrl Pts',(19.571277645572,59.820059521955,2.62132362131469));
#211666=CARTESIAN_POINT('Ctrl Pts',(19.5670554570749,59.8226600907005,2.61946873372389));
#211667=CARTESIAN_POINT('Ctrl Pts',(19.5522777973353,59.8317620813097,2.61297662715609));
#211668=CARTESIAN_POINT('Ctrl Pts',(19.5365469388443,59.840251805395,2.60787989114011));
#211669=CARTESIAN_POINT('Ctrl Pts',(19.5200464333337,59.8479176686192,2.60440616886221));
#211670=CARTESIAN_POINT('Ctrl Pts',(19.5117961805784,59.8517506002313,2.60266930772326));
#211671=CARTESIAN_POINT('Ctrl Pts',(19.5033535162583,59.8553775672057,2.60133820040226));
#211672=CARTESIAN_POINT('Ctrl Pts',(19.4947413867938,59.8587721277811,2.60044130723625));
#211673=CARTESIAN_POINT('Ctrl Pts',(19.4904353220616,59.8604694080689,2.59999286065325));
#211674=CARTESIAN_POINT('Ctrl Pts',(19.4860868910813,59.8621085868741,2.59965296768554));
#211675=CARTESIAN_POINT('Ctrl Pts',(19.4816989623701,59.8636863596424,2.59942518630996));
#211676=CARTESIAN_POINT('Ctrl Pts',(19.4773110336589,59.8652641324107,2.59919740493438));
#211677=CARTESIAN_POINT('Ctrl Pts',(19.4728836066891,59.8667804975195,2.5990817379166));
#211678=CARTESIAN_POINT('Ctrl Pts',(19.4684195516695,59.8682321556244,2.59908173516065));
#211679=CARTESIAN_POINT('',(19.4393816709755,59.8776671349988,2.59908173516066));
#211680=CARTESIAN_POINT('Origin',(5.60717482534548E-15,1.85264792328712E-13,
2.59908173516023));
#211681=CARTESIAN_POINT('',(19.092807720641,59.7908376697914,2.90134173516065));
#211682=CARTESIAN_POINT('Ctrl Pts',(19.4393816709755,59.8776671349988,2.59908173516065));
#211683=CARTESIAN_POINT('Ctrl Pts',(19.435746808291,59.8788471933726,2.59908174381724));
#211684=CARTESIAN_POINT('Ctrl Pts',(19.4321071647686,59.8799786203653,2.59915752001037));
#211685=CARTESIAN_POINT('Ctrl Pts',(19.4284649220283,59.8810618871503,2.59930729517512));
#211686=CARTESIAN_POINT('Ctrl Pts',(19.4074172521858,59.8873218328124,2.60017281085955));
#211687=CARTESIAN_POINT('Ctrl Pts',(19.3862806722129,59.8919760989601,2.60350651800072));
#211688=CARTESIAN_POINT('Ctrl Pts',(19.3654825713317,59.8951126055062,2.6089688059643));
#211689=CARTESIAN_POINT('Ctrl Pts',(19.3570942188071,59.8963776307484,2.61117187235441));
#211690=CARTESIAN_POINT('Ctrl Pts',(19.3487606486731,59.8973961381381,2.61372076577208));
#211691=CARTESIAN_POINT('Ctrl Pts',(19.3405086316971,59.8981752423039,2.61659179897023));
#211692=CARTESIAN_POINT('Ctrl Pts',(19.3374641384343,59.8984626844396,2.61765103591249));
#211693=CARTESIAN_POINT('Ctrl Pts',(19.3344308375141,59.8987174423899,2.61875422455189));
#211694=CARTESIAN_POINT('Ctrl Pts',(19.3314101194744,59.8989398263135,2.61990022440436));
#211695=CARTESIAN_POINT('Ctrl Pts',(19.32574627315,59.8993567961702,2.62204897412773));
#211696=CARTESIAN_POINT('Ctrl Pts',(19.3201266635128,59.8996599510839,2.6243482320181));
#211697=CARTESIAN_POINT('Ctrl Pts',(19.3145604567382,59.8998513356578,2.62679048030346));
#211698=CARTESIAN_POINT('Ctrl Pts',(19.2950787330274,59.9005211816666,2.63533834930219));
#211699=CARTESIAN_POINT('Ctrl Pts',(19.2762511930037,59.8998218367508,2.64563784783603));
#211700=CARTESIAN_POINT('Ctrl Pts',(19.2584708442945,59.8978409873529,2.65736666738005));
#211701=CARTESIAN_POINT('Ctrl Pts',(19.2495806699398,59.896850562654,2.66323107715206));
#211702=CARTESIAN_POINT('Ctrl Pts',(19.2409522937263,59.8955397627953,2.66945281780814));
#211703=CARTESIAN_POINT('Ctrl Pts',(19.2326348443073,59.8939195570494,2.67599160631241));
#211704=CARTESIAN_POINT('Ctrl Pts',(19.2284761195978,59.8931094541765,2.67926100056455));
#211705=CARTESIAN_POINT('Ctrl Pts',(19.2243951266223,59.8922219999437,2.68260965685163));
#211706=CARTESIAN_POINT('Ctrl Pts',(19.2203980066217,59.891258566018,2.68603254012523));
#211707=CARTESIAN_POINT('Ctrl Pts',(19.2164008866211,59.8902951320923,2.68945542339882));
#211708=CARTESIAN_POINT('Ctrl Pts',(19.2124877374673,59.8892556335612,2.69295261525426));
#211709=CARTESIAN_POINT('Ctrl Pts',(19.208664500965,59.8881416170478,2.6965189117214));
#211710=CARTESIAN_POINT('Ctrl Pts',(19.2086318967648,59.8881321168201,2.69654932476128));
#211711=CARTESIAN_POINT('Ctrl Pts',(19.2085992991801,59.8881226112894,2.69657974261186));
#211712=CARTESIAN_POINT('Ctrl Pts',(19.208566708214,59.888113100457,2.69661016527014));
#211713=CARTESIAN_POINT('Ctrl Pts',(19.1919220260051,59.8832557794662,2.71214746101075));
#211714=CARTESIAN_POINT('Ctrl Pts',(19.1769337687821,59.8771277287724,2.72880565567407));
#211715=CARTESIAN_POINT('Ctrl Pts',(19.1636064551693,59.8699293191676,2.74628040012045));
#211716=CARTESIAN_POINT('Ctrl Pts',(19.1498284206598,59.86248746413,2.76434612882027));
#211717=CARTESIAN_POINT('Ctrl Pts',(19.137825053473,59.8539008972299,2.78328592653955));
#211718=CARTESIAN_POINT('Ctrl Pts',(19.1276443522983,59.8443613941499,2.80278753267238));
#211719=CARTESIAN_POINT('Ctrl Pts',(19.1176573094823,59.8350033524917,2.82191817722113));
#211720=CARTESIAN_POINT('Ctrl Pts',(19.109424071691,59.8247273719278,2.84159092314393));
#211721=CARTESIAN_POINT('Ctrl Pts',(19.1030352898954,59.8136991387748,2.86151233816177));
#211722=CARTESIAN_POINT('Ctrl Pts',(19.0988029459333,59.806393320938,2.87470957720763));
#211723=CARTESIAN_POINT('Ctrl Pts',(19.0953809833349,59.7987570771806,2.8880159438809));
#211724=CARTESIAN_POINT('Ctrl Pts',(19.092807720641,59.7908376697914,2.90134173516065));
#211725=CARTESIAN_POINT('',(18.9827025415095,59.451978872661,3.47153072139113));
#211726=CARTESIAN_POINT('',(19.092807720641,59.7908376697914,2.90134173516065));
#211727=CARTESIAN_POINT('',(13.2864868028994,60.978275279735,3.47153072139114));
#211728=CARTESIAN_POINT('Origin',(5.53234440788222E-15,1.85015204418142E-13,
3.47153072139072));
#211729=CARTESIAN_POINT('',(13.3605623192485,61.3267881959115,2.90134173516065));
#211730=CARTESIAN_POINT('',(13.2864868028994,60.978275279735,3.47153072139114));
#211731=CARTESIAN_POINT('',(13.1038352065726,61.5752716937453,2.59908173516066));
#211732=CARTESIAN_POINT('Ctrl Pts',(13.3605623192485,61.3267881959115,2.90134173516065));
#211733=CARTESIAN_POINT('Ctrl Pts',(13.3631207378658,61.3388252440315,2.88164837656783));
#211734=CARTESIAN_POINT('Ctrl Pts',(13.3637631278629,61.3512282837631,2.8620373443922));
#211735=CARTESIAN_POINT('Ctrl Pts',(13.3625311504985,61.3638130392405,2.84277945978247));
#211736=CARTESIAN_POINT('Ctrl Pts',(13.3612744179065,61.3766506715123,2.82313460920144));
#211737=CARTESIAN_POINT('Ctrl Pts',(13.3580674708028,61.3896782944613,2.80385576863494));
#211738=CARTESIAN_POINT('Ctrl Pts',(13.3529048112192,61.402719949309,2.7852167851857));
#211739=CARTESIAN_POINT('Ctrl Pts',(13.3479427162803,61.4152549476886,2.76730190934671));
#211740=CARTESIAN_POINT('Ctrl Pts',(13.3411737181046,61.4278037696881,2.74997687279999));
#211741=CARTESIAN_POINT('Ctrl Pts',(13.3325479345572,61.4402150271791,2.73349253345958));
#211742=CARTESIAN_POINT('Ctrl Pts',(13.3259219069559,61.4497489245058,2.7208298359945));
#211743=CARTESIAN_POINT('Ctrl Pts',(13.3181993658957,61.4592018401669,2.70866321039379));
#211744=CARTESIAN_POINT('Ctrl Pts',(13.3093393327442,61.4685026502441,2.69711645335887));
#211745=CARTESIAN_POINT('Ctrl Pts',(13.3093161121774,61.4685270260086,2.69708619136793));
#211746=CARTESIAN_POINT('Ctrl Pts',(13.3092928829602,61.4685514007484,2.69705593387261));
#211747=CARTESIAN_POINT('Ctrl Pts',(13.3092696450948,61.4685757744611,2.69702568087613));
#211748=CARTESIAN_POINT('Ctrl Pts',(13.3067780733549,61.4711891321183,2.69378194443309));
#211749=CARTESIAN_POINT('Ctrl Pts',(13.3041875240728,61.4737888336849,2.69059266624742));
#211750=CARTESIAN_POINT('Ctrl Pts',(13.301501425748,61.4763713294376,2.68746219342719));
#211751=CARTESIAN_POINT('Ctrl Pts',(13.2865538993128,61.4907423311159,2.67004182396279));
#211752=CARTESIAN_POINT('Ctrl Pts',(13.2686510078465,61.5045840828619,2.65443567878197));
#211753=CARTESIAN_POINT('Ctrl Pts',(13.248438717856,61.5172886502207,2.64136852353454));
#211754=CARTESIAN_POINT('Ctrl Pts',(13.2393671621987,61.5229906359903,2.63550380329926));
#211755=CARTESIAN_POINT('Ctrl Pts',(13.2298303888527,61.5284639152911,2.63014997451216));
#211756=CARTESIAN_POINT('Ctrl Pts',(13.2198857715705,61.533655525549,2.62536981119297));
#211757=CARTESIAN_POINT('Ctrl Pts',(13.215563975411,61.535911729145,2.62329241687117));
#211758=CARTESIAN_POINT('Ctrl Pts',(13.2111652444435,61.5381145532938,2.62132362131472));
#211759=CARTESIAN_POINT('Ctrl Pts',(13.2066943520822,61.5402595369764,2.61946873372392));
#211760=CARTESIAN_POINT('Ctrl Pts',(13.1910462288177,61.5477669798655,2.61297662715612));
#211761=CARTESIAN_POINT('Ctrl Pts',(13.1745141278034,61.55456587389,2.60787989114012));
#211762=CARTESIAN_POINT('Ctrl Pts',(13.1573027128859,61.5604649702292,2.60440616886222));
#211763=CARTESIAN_POINT('Ctrl Pts',(13.1486970054272,61.5634145183988,2.60266930772327));
#211764=CARTESIAN_POINT('Ctrl Pts',(13.1399214696215,61.5661391177413,2.60133820040227));
#211765=CARTESIAN_POINT('Ctrl Pts',(13.1310016901029,61.5686148699004,2.60044130723627));
#211766=CARTESIAN_POINT('Ctrl Pts',(13.1265418003436,61.5698527459799,2.59999286065327));
#211767=CARTESIAN_POINT('Ctrl Pts',(13.1220458496817,61.5710284103841,2.59965296768555));
#211768=CARTESIAN_POINT('Ctrl Pts',(13.1175170363402,61.572138876503,2.59942518630997));
#211769=CARTESIAN_POINT('Ctrl Pts',(13.1129882229987,61.5732493426219,2.59919740493439));
#211770=CARTESIAN_POINT('Ctrl Pts',(13.1084265466226,61.5742946087866,2.59908173791658));
#211771=CARTESIAN_POINT('Ctrl Pts',(13.1038352065726,61.5752716937454,2.59908173516066));
#211772=CARTESIAN_POINT('',(13.0739701745323,61.58161970227,2.59908173516067));
#211773=CARTESIAN_POINT('Origin',(5.62288786856779E-15,1.8526058203147E-13,
2.59908173516022));
#211774=CARTESIAN_POINT('',(12.7383709431249,61.4590390555211,2.90134173516066));
#211775=CARTESIAN_POINT('Ctrl Pts',(13.0739701745323,61.58161970227,2.59908173516067));
#211776=CARTESIAN_POINT('Ctrl Pts',(13.0702318743176,61.58241334955,2.59908174381723));
#211777=CARTESIAN_POINT('Ctrl Pts',(13.0664939028184,61.583158132123,2.59915752001038));
#211778=CARTESIAN_POINT('Ctrl Pts',(13.0627583804525,61.5838547466228,2.59930729517513));
#211779=CARTESIAN_POINT('Ctrl Pts',(13.0411716694464,61.5878803190637,2.6001728108596));
#211780=CARTESIAN_POINT('Ctrl Pts',(13.0196643745811,61.5902997144312,2.60350651800106));
#211781=CARTESIAN_POINT('Ctrl Pts',(12.9986523536623,61.5912450453421,2.60896880596512));
#211782=CARTESIAN_POINT('Ctrl Pts',(12.990177722267,61.5916263190448,2.61117187235505));
#211783=CARTESIAN_POINT('Ctrl Pts',(12.981783341291,61.5917681516649,2.61372076577245));
#211784=CARTESIAN_POINT('Ctrl Pts',(12.9734950911672,61.5916804171631,2.61659179897026));
#211785=CARTESIAN_POINT('Ctrl Pts',(12.9704372300723,61.5916480484586,2.61765103591252));
#211786=CARTESIAN_POINT('Ctrl Pts',(12.9673939164349,61.5915843445343,2.61875422455192));
#211787=CARTESIAN_POINT('Ctrl Pts',(12.9643665007549,61.5914897592008,2.61990022440438));
#211788=CARTESIAN_POINT('Ctrl Pts',(12.9586900963549,61.5913124117006,2.62204897412776));
#211789=CARTESIAN_POINT('Ctrl Pts',(12.95306958321,61.5910264967404,2.62434823201813));
#211790=CARTESIAN_POINT('Ctrl Pts',(12.9475138635632,61.5906350058493,2.62679048030348));
#211791=CARTESIAN_POINT('Ctrl Pts',(12.9280688447993,61.5892647877302,2.63533834930222));
#211792=CARTESIAN_POINT('Ctrl Pts',(12.9094175454592,61.5866012600732,2.64563784783605));
#211793=CARTESIAN_POINT('Ctrl Pts',(12.8919416545041,61.5827727094487,2.65736666738007));
#211794=CARTESIAN_POINT('Ctrl Pts',(12.8832037090265,61.5808584341364,2.66323107715207));
#211795=CARTESIAN_POINT('Ctrl Pts',(12.8747596158555,61.5786529040704,2.66945281780816));
#211796=CARTESIAN_POINT('Ctrl Pts',(12.8666570879116,61.576172163775,2.67599160631243));
#211797=CARTESIAN_POINT('Ctrl Pts',(12.8626058239396,61.5749317936274,2.67926100056456));
#211798=CARTESIAN_POINT('Ctrl Pts',(12.8586399512977,61.5736226210374,2.68260965685165));
#211799=CARTESIAN_POINT('Ctrl Pts',(12.8547654342064,61.5722466520924,2.68603254012524));
#211800=CARTESIAN_POINT('Ctrl Pts',(12.8508909171151,61.5708706831473,2.68945542339884));
#211801=CARTESIAN_POINT('Ctrl Pts',(12.8471078617859,61.5694278436304,2.69295261525427));
#211802=CARTESIAN_POINT('Ctrl Pts',(12.8434220158074,61.5679202927798,2.69651891172141));
#211803=CARTESIAN_POINT('Ctrl Pts',(12.8433905832605,61.5679074365283,2.69654932476129));
#211804=CARTESIAN_POINT('Ctrl Pts',(12.8433591578474,61.5678945756945,2.69657974261187));
#211805=CARTESIAN_POINT('Ctrl Pts',(12.8433277395707,61.5678817102798,2.69661016527015));
#211806=CARTESIAN_POINT('Ctrl Pts',(12.8272819669693,61.561311155148,2.71214746101265));
#211807=CARTESIAN_POINT('Ctrl Pts',(12.8130163727079,61.5536499750614,2.72880565567815));
#211808=CARTESIAN_POINT('Ctrl Pts',(12.8005145062065,61.5450979154849,2.74628040012685));
#211809=CARTESIAN_POINT('Ctrl Pts',(12.7875898348814,61.5362566309324,2.76434612882922));
#211810=CARTESIAN_POINT('Ctrl Pts',(12.7765497640381,61.5264624086165,2.78328592655123));
#211811=CARTESIAN_POINT('Ctrl Pts',(12.7674219834068,61.515910990882,2.80278753268687));
#211812=CARTESIAN_POINT('Ctrl Pts',(12.7584678323699,61.5055602833153,2.82191817723828));
#211813=CARTESIAN_POINT('Ctrl Pts',(12.7513538295739,61.4944799879523,2.84159092316381));
#211814=CARTESIAN_POINT('Ctrl Pts',(12.7461528104582,61.4828443590693,2.86151233818433));
#211815=CARTESIAN_POINT('Ctrl Pts',(12.7427073176334,61.4751361628607,2.87470957722279));
#211816=CARTESIAN_POINT('Ctrl Pts',(12.7401023057312,61.4671840587583,2.8880159438885));
#211817=CARTESIAN_POINT('Ctrl Pts',(12.7383709431249,61.4590390555211,2.90134173516065));
#211818=CARTESIAN_POINT('',(12.664289321014,61.1105274371643,3.47153072139115));
#211819=CARTESIAN_POINT('',(12.7383709431249,61.4590390555211,2.90134173516066));
#211820=CARTESIAN_POINT('',(6.8397366303024,62.0330459552234,3.47153072139115));
#211821=CARTESIAN_POINT('Origin',(5.53234440788222E-15,1.85015204418142E-13,
3.47153072139072));
#211822=CARTESIAN_POINT('',(6.87697683366544,62.3873926810693,2.90134173516067));
#211823=CARTESIAN_POINT('',(6.8397366303024,62.0330459552234,3.47153072139115));
#211824=CARTESIAN_POINT('',(6.59568250079865,62.6076796697356,2.59908173516067));
#211825=CARTESIAN_POINT('Ctrl Pts',(6.87697683366544,62.3873926810693,2.90134173516067));
#211826=CARTESIAN_POINT('Ctrl Pts',(6.87826302285572,62.3996312165481,2.88164837656554));
#211827=CARTESIAN_POINT('Ctrl Pts',(6.87760542308992,62.412033459171,2.86203734438761));
#211828=CARTESIAN_POINT('Ctrl Pts',(6.8750647294751,62.424420497342,2.8427794597757));
#211829=CARTESIAN_POINT('Ctrl Pts',(6.87247298342164,62.4370564393959,2.82313460919239));
#211830=CARTESIAN_POINT('Ctrl Pts',(6.86792184690156,62.4496774784122,2.80385576862372));
#211831=CARTESIAN_POINT('Ctrl Pts',(6.86142424476594,62.4621080448389,2.78521678517253));
#211832=CARTESIAN_POINT('Ctrl Pts',(6.85517906858305,62.4740556950285,2.76730190933172));
#211833=CARTESIAN_POINT('Ctrl Pts',(6.84713544260611,62.4858282202922,2.74997687278339));
#211834=CARTESIAN_POINT('Ctrl Pts',(6.83725958232828,62.4972698477185,2.73349253344165));
#211835=CARTESIAN_POINT('Ctrl Pts',(6.82967328916546,62.506058908871,2.72082983598302));
#211836=CARTESIAN_POINT('Ctrl Pts',(6.82100495424929,62.5146528151173,2.70866321038834));
#211837=CARTESIAN_POINT('Ctrl Pts',(6.8112212579066,62.52297654873,2.69711645335888));
#211838=CARTESIAN_POINT('Ctrl Pts',(6.8111956165833,62.5229983637513,2.69708619136794));
#211839=CARTESIAN_POINT('Ctrl Pts',(6.8111699667641,62.5230201768494,2.69705593387261));
#211840=CARTESIAN_POINT('Ctrl Pts',(6.81114430845136,62.5230419880219,2.69702568087613));
#211841=CARTESIAN_POINT('Ctrl Pts',(6.80839321554227,62.5253805892673,2.69378194443309));
#211842=CARTESIAN_POINT('Ctrl Pts',(6.80554511475049,62.5276952632613,2.69059266624743));
#211843=CARTESIAN_POINT('Ctrl Pts',(6.80260378684096,62.529982838102,2.6874621934272));
#211844=CARTESIAN_POINT('Ctrl Pts',(6.78623596579732,62.5427126719625,2.67004182396155));
#211845=CARTESIAN_POINT('Ctrl Pts',(6.7669842912032,62.5546072354118,2.65443567877975));
#211846=CARTESIAN_POINT('Ctrl Pts',(6.74555473734773,62.56512944621,2.64136852353176));
#211847=CARTESIAN_POINT('Ctrl Pts',(6.73593685681286,62.5698519601318,2.63550380329757));
#211848=CARTESIAN_POINT('Ctrl Pts',(6.72588021343625,62.5742983919729,2.63014997451141));
#211849=CARTESIAN_POINT('Ctrl Pts',(6.71544740276757,62.5784220664836,2.62536981119299));
#211850=CARTESIAN_POINT('Ctrl Pts',(6.71091344436492,62.5802141596492,2.62329241687119));
#211851=CARTESIAN_POINT('Ctrl Pts',(6.70630855228275,62.5819451239084,2.62132362131473));
#211852=CARTESIAN_POINT('Ctrl Pts',(6.70163794008956,62.583611021638,2.61946873372393));
#211853=CARTESIAN_POINT('Ctrl Pts',(6.68529079741337,62.5894416636915,2.61297662715612));
#211854=CARTESIAN_POINT('Ctrl Pts',(6.66813858303384,62.5944752375496,2.60787989114014));
#211855=CARTESIAN_POINT('Ctrl Pts',(6.65040483057318,62.5985429352698,2.60440616886224));
#211856=CARTESIAN_POINT('Ctrl Pts',(6.64153795434285,62.6005767841299,2.60266930772329));
#211857=CARTESIAN_POINT('Ctrl Pts',(6.63252569365822,62.6023691645601,2.60133820040229));
#211858=CARTESIAN_POINT('Ctrl Pts',(6.6233959910565,62.603898983444,2.60044130723629));
#211859=CARTESIAN_POINT('Ctrl Pts',(6.61883113975564,62.604663892886,2.59999286065329));
#211860=CARTESIAN_POINT('Ctrl Pts',(6.61423692798837,62.6053631620639,2.59965296768557));
#211861=CARTESIAN_POINT('Ctrl Pts',(6.60961684864331,62.6059941550342,2.59942518630999));
#211862=CARTESIAN_POINT('Ctrl Pts',(6.60499676929825,62.6066251480045,2.59919740493441));
#211863=CARTESIAN_POINT('Ctrl Pts',(6.6003508221967,62.6071878630702,2.59908173791661));
#211864=CARTESIAN_POINT('Ctrl Pts',(6.59568250079866,62.6076796697356,2.59908173516068));
#211865=CARTESIAN_POINT('',(6.56531752495282,62.6108711573008,2.59908173516067));
#211866=CARTESIAN_POINT('Origin',(5.63895492999586E-15,1.85258037258938E-13,
2.59908173516024));
#211867=CARTESIAN_POINT('',(6.24436990788039,62.4538823482277,2.90134173516068));
#211868=CARTESIAN_POINT('Ctrl Pts',(6.56531752495282,62.6108711573008,2.59908173516068));
#211869=CARTESIAN_POINT('Ctrl Pts',(6.56151674480724,62.6112696981213,2.59908174381733));
#211870=CARTESIAN_POINT('Ctrl Pts',(6.55772139932922,62.6116196762809,2.59915752001041));
#211871=CARTESIAN_POINT('Ctrl Pts',(6.5539335245026,62.6119220062411,2.59930729517515));
#211872=CARTESIAN_POINT('Ctrl Pts',(6.53204428085627,62.6136691004466,2.60017281085965));
#211873=CARTESIAN_POINT('Ctrl Pts',(6.51040190952201,62.6138271176317,2.60350651800131));
#211874=CARTESIAN_POINT('Ctrl Pts',(6.48940618066432,62.6125709156641,2.6089688059657));
#211875=CARTESIAN_POINT('Ctrl Pts',(6.48093812023298,62.6120642605131,2.6111718723555));
#211876=CARTESIAN_POINT('Ctrl Pts',(6.47257489900914,62.6113278644157,2.61372076577271));
#211877=CARTESIAN_POINT('Ctrl Pts',(6.46434122354008,62.6103742524842,2.61659179897029));
#211878=CARTESIAN_POINT('Ctrl Pts',(6.46130349717915,62.6100224275776,2.61765103591254));
#211879=CARTESIAN_POINT('Ctrl Pts',(6.45828351400561,62.6096409597324,2.61875422455194));
#211880=CARTESIAN_POINT('Ctrl Pts',(6.45528256968501,62.6092304414386,2.61990022440441));
#211881=CARTESIAN_POINT('Ctrl Pts',(6.44965579908389,62.6084607196377,2.62204897412778));
#211882=CARTESIAN_POINT('Ctrl Pts',(6.4440959619495,62.6075888673477,2.62434823201815));
#211883=CARTESIAN_POINT('Ctrl Pts',(6.43861159905745,62.6066187902476,2.6267904803035));
#211884=CARTESIAN_POINT('Ctrl Pts',(6.41941632893527,62.6032235203972,2.63533834930224));
#211885=CARTESIAN_POINT('Ctrl Pts',(6.4011456178173,62.5986249921654,2.64563784783608));
#211886=CARTESIAN_POINT('Ctrl Pts',(6.38416565413472,62.5929906867161,2.65736666738009));
#211887=CARTESIAN_POINT('Ctrl Pts',(6.37567567229344,62.5901735339914,2.66323107715209));
#211888=CARTESIAN_POINT('Ctrl Pts',(6.36750837741684,62.587097437967,2.66945281780817));
#211889=CARTESIAN_POINT('Ctrl Pts',(6.35970954393956,62.5837833426319,2.67599160631244));
#211890=CARTESIAN_POINT('Ctrl Pts',(6.35581012720092,62.5821262949644,2.67926100056457));
#211891=CARTESIAN_POINT('Ctrl Pts',(6.35200282582338,62.5804097475861,2.68260965685166));
#211892=CARTESIAN_POINT('Ctrl Pts',(6.34829336166143,62.5786363190255,2.68603254012526));
#211893=CARTESIAN_POINT('Ctrl Pts',(6.34458389749948,62.5768628904649,2.68945542339885));
#211894=CARTESIAN_POINT('Ctrl Pts',(6.3409723839406,62.5750325180137,2.69295261525428));
#211895=CARTESIAN_POINT('Ctrl Pts',(6.33746431138575,62.5731479498684,2.69651891172142));
#211896=CARTESIAN_POINT('Ctrl Pts',(6.3374343948739,62.573131878449,2.6965493247613));
#211897=CARTESIAN_POINT('Ctrl Pts',(6.33740448593562,62.5731158032181,2.69657974261189));
#211898=CARTESIAN_POINT('Ctrl Pts',(6.33737458457357,62.5730997241773,2.69661016527017));
#211899=CARTESIAN_POINT('Ctrl Pts',(6.32210352242475,62.5648879232823,2.71214746101204));
#211900=CARTESIAN_POINT('Ctrl Pts',(6.30871688796312,62.5557775512965,2.7288056556768));
#211901=CARTESIAN_POINT('Ctrl Pts',(6.29717744164003,62.5459655399043,2.74628040012473));
#211902=CARTESIAN_POINT('Ctrl Pts',(6.28524773890477,62.5358216928023,2.76434612882623));
#211903=CARTESIAN_POINT('Ctrl Pts',(6.27529192173244,62.5249271226219,2.78328592654731));
#211904=CARTESIAN_POINT('Ctrl Pts',(6.26731706751958,62.513479393776,2.802787532682));
#211905=CARTESIAN_POINT('Ctrl Pts',(6.25949391181462,62.5022494248212,2.82191817723251));
#211906=CARTESIAN_POINT('Ctrl Pts',(6.25357708651698,62.4904862126961,2.84159092315711));
#211907=CARTESIAN_POINT('Ctrl Pts',(6.24962081353417,62.4783706704707,2.86151233817672));
#211908=CARTESIAN_POINT('Ctrl Pts',(6.24699992138298,62.4703445484958,2.87470957721769));
#211909=CARTESIAN_POINT('Ctrl Pts',(6.24524040122966,62.4621637089592,2.88801594388596));
#211910=CARTESIAN_POINT('Ctrl Pts',(6.24436990788039,62.4538823482277,2.90134173516068));
#211911=CARTESIAN_POINT('',(6.20712349654444,62.0995362748661,3.47153072139115));
#211912=CARTESIAN_POINT('',(6.24436990788039,62.4538823482277,2.90134173516068));
#211913=CARTESIAN_POINT('',(0.318048871876918,62.408169597977,3.47153072139115));
#211914=CARTESIAN_POINT('Origin',(5.53234440788222E-15,1.85015204418142E-13,
3.47153072139072));
#211915=CARTESIAN_POINT('',(0.318045750792831,62.7644678366121,2.90134173516067));
#211916=CARTESIAN_POINT('',(0.318048871876917,62.408169597977,3.47153072139115));
#211917=CARTESIAN_POINT('',(0.0152661173106527,62.954144805765,2.59908173516067));
#211918=CARTESIAN_POINT('Ctrl Pts',(0.318045750792831,62.7644678366121,
2.90134173516066));
#211919=CARTESIAN_POINT('Ctrl Pts',(0.318045618797917,62.7767737714906,
2.88164837656858));
#211920=CARTESIAN_POINT('Ctrl Pts',(0.316095234070562,62.7890393354359,
2.86203734439368));
#211921=CARTESIAN_POINT('Ctrl Pts',(0.312273660577917,62.8010929413147,
2.84277945978465));
#211922=CARTESIAN_POINT('Ctrl Pts',(0.308375296776869,62.8133887511219,
2.82313460920437));
#211923=CARTESIAN_POINT('Ctrl Pts',(0.302529834047427,62.8254649274575,
2.80385576863857));
#211924=CARTESIAN_POINT('Ctrl Pts',(0.294768478452471,62.8371482135729,
2.78521678518996));
#211925=CARTESIAN_POINT('Ctrl Pts',(0.287308644486513,62.848377614614,2.76730190935162));
#211926=CARTESIAN_POINT('Ctrl Pts',(0.27807851836262,62.8592448608886,2.74997687280549));
#211927=CARTESIAN_POINT('Ctrl Pts',(0.267060783352071,62.8695915013832,
2.73349253346556));
#211928=CARTESIAN_POINT('Ctrl Pts',(0.258597341637146,62.8775394315783,
2.72082983599834));
#211929=CARTESIAN_POINT('Ctrl Pts',(0.249078184947951,62.8851801717842,
2.70866321039561));
#211930=CARTESIAN_POINT('Ctrl Pts',(0.238478017627659,62.892435632374,2.69711645335889));
#211931=CARTESIAN_POINT('Ctrl Pts',(0.238450236479551,62.8924546476422,
2.69708619136795));
#211932=CARTESIAN_POINT('Ctrl Pts',(0.238422447083127,62.8924736601097,
2.69705593387262));
#211933=CARTESIAN_POINT('Ctrl Pts',(0.238394649440964,62.8924926697744,
2.69702568087614));
#211934=CARTESIAN_POINT('Ctrl Pts',(0.2354141769123,62.8945308924034,2.6937819444331));
#211935=CARTESIAN_POINT('Ctrl Pts',(0.232339728999105,62.896535178772,2.69059266624743));
#211936=CARTESIAN_POINT('Ctrl Pts',(0.229175397308913,62.8985027695521,
2.6874621934272));
#211937=CARTESIAN_POINT('Ctrl Pts',(0.211566610931505,62.9094519648693,
2.67004182396259));
#211938=CARTESIAN_POINT('Ctrl Pts',(0.191177078587904,62.9192690206943,
2.6544356787816));
#211939=CARTESIAN_POINT('Ctrl Pts',(0.168765047547321,62.9274935913875,
2.64136852353408));
#211940=CARTESIAN_POINT('Ctrl Pts',(0.158706217644123,62.9311848926123,
2.63550380329897));
#211941=CARTESIAN_POINT('Ctrl Pts',(0.148239886923453,62.9345557609572,
2.63014997451202));
#211942=CARTESIAN_POINT('Ctrl Pts',(0.137433186922148,62.9375663198811,
2.62536981119296));
#211943=CARTESIAN_POINT('Ctrl Pts',(0.1327367412734,62.9388746680685,2.62329241687116));
#211944=CARTESIAN_POINT('Ctrl Pts',(0.127976140237888,62.9401148076315,
2.62132362131471));
#211945=CARTESIAN_POINT('Ctrl Pts',(0.123156980417348,62.941283367484,2.61946873372391));
#211946=CARTESIAN_POINT('Ctrl Pts',(0.106289921045458,62.9453733269675,
2.61297662715611));
#211947=CARTESIAN_POINT('Ctrl Pts',(0.0887055165508409,62.9485864317706,
2.60787989114013));
#211948=CARTESIAN_POINT('Ctrl Pts',(0.0706437212499503,62.9507781643244,
2.60440616886223));
#211949=CARTESIAN_POINT('Ctrl Pts',(0.0616128235995051,62.9518740306013,
2.60266930772328));
#211950=CARTESIAN_POINT('Ctrl Pts',(0.0524625782499263,62.9527145544239,
2.60133820040229));
#211951=CARTESIAN_POINT('Ctrl Pts',(0.043222979497305,62.9532816790169,
2.60044130723629));
#211952=CARTESIAN_POINT('Ctrl Pts',(0.0386031801209943,62.9535652413134,
2.59999286065329));
#211953=CARTESIAN_POINT('Ctrl Pts',(0.0339610423938989,62.9537804539257,
2.59965296768556));
#211954=CARTESIAN_POINT('Ctrl Pts',(0.0293003156013865,62.9539250604563,
2.59942518630998));
#211955=CARTESIAN_POINT('Ctrl Pts',(0.0246395888088739,62.954069666987,
2.59919740493441));
#211956=CARTESIAN_POINT('Ctrl Pts',(0.0199602729505793,62.9541436657298,
2.59908173791657));
#211957=CARTESIAN_POINT('Ctrl Pts',(0.0152661173106527,62.954144805765,
2.59908173516068));
#211958=CARTESIAN_POINT('',(-0.015266117311081,62.954144805765,2.59908173516067));
#211959=CARTESIAN_POINT('Origin',(-3.96846087890508E-17,1.90952070476508E-13,
2.59908173516023));
#211960=CARTESIAN_POINT('',(-0.318045750793258,62.7644678366121,2.90134173516066));
#211961=CARTESIAN_POINT('Ctrl Pts',(-0.015266117311081,62.954144805765,
2.59908173516068));
#211962=CARTESIAN_POINT('Ctrl Pts',(-0.0190877352448647,62.9541438736294,
2.59908174381727));
#211963=CARTESIAN_POINT('Ctrl Pts',(-0.022898872102443,62.9540952129416,
2.59915752001039));
#211964=CARTESIAN_POINT('Ctrl Pts',(-0.0266975986405677,62.953999945972,
2.59930729517514));
#211965=CARTESIAN_POINT('Ctrl Pts',(-0.0486495517927879,62.9534494204122,
2.60017281085966));
#211966=CARTESIAN_POINT('Ctrl Pts',(-0.0701898812463166,62.9513443281456,
2.60350651800143));
#211967=CARTESIAN_POINT('Ctrl Pts',(-0.0909392844436332,62.947900356511,
2.608968805966));
#211968=CARTESIAN_POINT('Ctrl Pts',(-0.099307996069169,62.9465113235261,
2.61117187235574));
#211969=CARTESIAN_POINT('Ctrl Pts',(-0.107548428339302,62.9449047668212,
2.61372076577286));
#211970=CARTESIAN_POINT('Ctrl Pts',(-0.115637319282522,62.9430957254319,
2.6165917989703));
#211971=CARTESIAN_POINT('Ctrl Pts',(-0.118621628943776,62.9424282989907,
2.61765103591255));
#211972=CARTESIAN_POINT('Ctrl Pts',(-0.12158519408586,62.9417332466659,
2.61875422455195));
#211973=CARTESIAN_POINT('Ctrl Pts',(-0.124526788073079,62.9410112931361,
2.61990022440441));
#211974=CARTESIAN_POINT('Ctrl Pts',(-0.130042276799115,62.9396576302677,
2.62204897412778));
#211975=CARTESIAN_POINT('Ctrl Pts',(-0.135480523183885,62.9382093928442,
2.62434823201817));
#211976=CARTESIAN_POINT('Ctrl Pts',(-0.140833441493647,62.9366713579028,
2.62679048030352));
#211977=CARTESIAN_POINT('Ctrl Pts',(-0.159568655577816,62.931288235608,
2.63533834930225));
#211978=CARTESIAN_POINT('Ctrl Pts',(-0.177258600739223,62.924805089239,
2.64563784783608));
#211979=CARTESIAN_POINT('Ctrl Pts',(-0.193556601113891,62.9174267595944,
2.65736666738009));
#211980=CARTESIAN_POINT('Ctrl Pts',(-0.201705601301226,62.913737594772,
2.66323107715209));
#211981=CARTESIAN_POINT('Ctrl Pts',(-0.209506615291636,62.909824635141,
2.66945281780818));
#211982=CARTESIAN_POINT('Ctrl Pts',(-0.216916308650622,62.9057134946883,
2.67599160631244));
#211983=CARTESIAN_POINT('Ctrl Pts',(-0.220621155330115,62.903657924462,
2.67926100056457));
#211984=CARTESIAN_POINT('Ctrl Pts',(-0.22422817185277,62.9015528091476,
2.68260965685166));
#211985=CARTESIAN_POINT('Ctrl Pts',(-0.227731941419756,62.8994013510258,
2.68603254012525));
#211986=CARTESIAN_POINT('Ctrl Pts',(-0.231235710986742,62.897249892904,
2.68945542339885));
#211987=CARTESIAN_POINT('Ctrl Pts',(-0.234636114276948,62.8950520414623,
2.69295261525428));
#211988=CARTESIAN_POINT('Ctrl Pts',(-0.237927978231133,62.8928111037453,
2.69651891172142));
#211989=CARTESIAN_POINT('Ctrl Pts',(-0.237956050936432,62.8927919932398,
2.6965493247613));
#211990=CARTESIAN_POINT('Ctrl Pts',(-0.237984115711227,62.8927728797353,
2.69657974261189));
#211991=CARTESIAN_POINT('Ctrl Pts',(-0.238012172553063,62.8927537632337,
2.69661016527017));
#211992=CARTESIAN_POINT('Ctrl Pts',(-0.25234121129623,62.8829906867852,
2.71214746101078));
#211993=CARTESIAN_POINT('Ctrl Pts',(-0.264702219189273,62.8725309380426,
2.72880565567411));
#211994=CARTESIAN_POINT('Ctrl Pts',(-0.275152816745077,62.8615664772854,
2.74628040012049));
#211995=CARTESIAN_POINT('Ctrl Pts',(-0.285956846570814,62.8502312057459,
2.76434612882047));
#211996=CARTESIAN_POINT('Ctrl Pts',(-0.294719332055858,62.8383556508924,
2.78328592653991));
#211997=CARTESIAN_POINT('Ctrl Pts',(-0.301453885678867,62.8261370346483,
2.80278753267292));
#211998=CARTESIAN_POINT('Ctrl Pts',(-0.308060333921113,62.8141508421955,
2.82191817722197));
#211999=CARTESIAN_POINT('Ctrl Pts',(-0.31271515574461,62.8018335935224,
2.8415909231451));
#212000=CARTESIAN_POINT('Ctrl Pts',(-0.315383336840319,62.7893708783707,
2.86151233816327));
#212001=CARTESIAN_POINT('Ctrl Pts',(-0.317150913275242,62.7811147665001,
2.87470957720864));
#212002=CARTESIAN_POINT('Ctrl Pts',(-0.318045664008668,62.7727948225179,
2.88801594388141));
#212003=CARTESIAN_POINT('Ctrl Pts',(-0.318045750793257,62.7644678366121,
2.90134173516066));
#212004=CARTESIAN_POINT('',(-0.318048871877343,62.408169597977,3.47153072139115));
#212005=CARTESIAN_POINT('',(-0.318045750793259,62.7644678366121,2.90134173516066));
#212006=CARTESIAN_POINT('',(-6.20712349654485,62.099536274866,3.47153072139116));
#212007=CARTESIAN_POINT('Origin',(5.53234440788222E-15,1.85015204418142E-13,
3.47153072139072));
#212008=CARTESIAN_POINT('',(-6.2443699078808,62.4538823482277,2.90134173516068));
#212009=CARTESIAN_POINT('',(-6.20712349654485,62.099536274866,3.47153072139115));
#212010=CARTESIAN_POINT('',(-6.56531752495323,62.6108711573007,2.59908173516067));
#212011=CARTESIAN_POINT('Ctrl Pts',(-6.2443699078808,62.4538823482277,2.90134173516068));
#212012=CARTESIAN_POINT('Ctrl Pts',(-6.24565635961481,62.4661208561115,
2.88164837656632));
#212013=CARTESIAN_POINT('Ctrl Pts',(-6.24887816048149,62.4781153572972,
2.86203734438916));
#212014=CARTESIAN_POINT('Ctrl Pts',(-6.25393874389503,62.4897034690586,
2.84277945977798));
#212015=CARTESIAN_POINT('Ctrl Pts',(-6.25910101415609,62.501524431157,2.82313460919551));
#212016=CARTESIAN_POINT('Ctrl Pts',(-6.26617675898503,62.5129234357001,
2.80385576862764));
#212017=CARTESIAN_POINT('Ctrl Pts',(-6.27511683300737,62.5237314369795,
2.78521678517717));
#212018=CARTESIAN_POINT('Ctrl Pts',(-6.28370959325826,62.5341195572068,
2.76730190933723));
#212019=CARTESIAN_POINT('Ctrl Pts',(-6.29402509234058,62.5439624606704,
2.74997687278967));
#212020=CARTESIAN_POINT('Ctrl Pts',(-6.30606398947926,62.553100754277,2.73349253344858));
#212021=CARTESIAN_POINT('Ctrl Pts',(-6.31531185250115,62.5601204743189,
2.72082983598746));
#212022=CARTESIAN_POINT('Ctrl Pts',(-6.32557753708182,62.566724334927,2.70866321039045));
#212023=CARTESIAN_POINT('Ctrl Pts',(-6.33687803771711,62.5728320301414,
2.69711645335888));
#212024=CARTESIAN_POINT('Ctrl Pts',(-6.33690765431396,62.5728480373213,
2.69708619136794));
#212025=CARTESIAN_POINT('Ctrl Pts',(-6.33693727882117,62.5728640408536,
2.69705593387261));
#212026=CARTESIAN_POINT('Ctrl Pts',(-6.33696691123597,62.5728800407365,
2.69702568087613));
#212027=CARTESIAN_POINT('Ctrl Pts',(-6.34014410870348,62.5745955535555,
2.69378194443309));
#212028=CARTESIAN_POINT('Ctrl Pts',(-6.34341121944339,62.5762674929179,
2.69059266624743));
#212029=CARTESIAN_POINT('Ctrl Pts',(-6.34676388583407,62.577893542301,2.6874621934272));
#212030=CARTESIAN_POINT('Ctrl Pts',(-6.36542071199959,62.5869421374014,
2.67004182396091));
#212031=CARTESIAN_POINT('Ctrl Pts',(-6.38672471011312,62.5945741278854,
2.6544356787786));
#212032=CARTESIAN_POINT('Ctrl Pts',(-6.40987366744084,62.6004109483567,
2.64136852353031));
#212033=CARTESIAN_POINT('Ctrl Pts',(-6.42026324006377,62.6030305942144,
2.63550380329668));
#212034=CARTESIAN_POINT('Ctrl Pts',(-6.43102458681537,62.6052889671229,
2.630149974511));
#212035=CARTESIAN_POINT('Ctrl Pts',(-6.44208677567886,62.6071534261455,
2.62536981119296));
#212036=CARTESIAN_POINT('Ctrl Pts',(-6.44689425333239,62.6079636948181,
2.62329241687116));
#212037=CARTESIAN_POINT('Ctrl Pts',(-6.45175840518009,62.6086994224564,
2.6213236213147));
#212038=CARTESIAN_POINT('Ctrl Pts',(-6.45667331290451,62.6093578414454,
2.6194687337239));
#212039=CARTESIAN_POINT('Ctrl Pts',(-6.47387548993997,62.611662307907,2.6129766271561));
#212040=CARTESIAN_POINT('Ctrl Pts',(-6.49169942613426,62.6130197402064,
2.60787989114011));
#212041=CARTESIAN_POINT('Ctrl Pts',(-6.5098913754664,62.6133114945134,2.60440616886222));
#212042=CARTESIAN_POINT('Ctrl Pts',(-6.51898735013247,62.6134573716668,
2.60266930772327));
#212043=CARTESIAN_POINT('Ctrl Pts',(-6.52817532814414,62.6133368299271,
2.60133820040228));
#212044=CARTESIAN_POINT('Ctrl Pts',(-6.53742359207023,62.6129350466934,
2.60044130723627));
#212045=CARTESIAN_POINT('Ctrl Pts',(-6.54204772403327,62.6127341550766,
2.59999286065327));
#212046=CARTESIAN_POINT('Ctrl Pts',(-6.54668692748782,62.6124629532087,
2.59965296768555));
#212047=CARTESIAN_POINT('Ctrl Pts',(-6.55133723782973,62.6121195889603,
2.59942518630998));
#212048=CARTESIAN_POINT('Ctrl Pts',(-6.55598754817164,62.611776224712,2.5991974049344));
#212049=CARTESIAN_POINT('Ctrl Pts',(-6.56064896522293,62.6113606963861,
2.59908173791658));
#212050=CARTESIAN_POINT('Ctrl Pts',(-6.56531752495323,62.6108711573007,
2.59908173516068));
#212051=CARTESIAN_POINT('',(-6.59568250079906,62.6076796697356,2.59908173516067));
#212052=CARTESIAN_POINT('Origin',(-2.34395632424774E-17,1.90952921843269E-13,
2.59908173516024));
#212053=CARTESIAN_POINT('',(-6.87697683366585,62.3873926810693,2.90134173516067));
#212054=CARTESIAN_POINT('Ctrl Pts',(-6.59568250079906,62.6076796697356,
2.59908173516068));
#212055=CARTESIAN_POINT('Ctrl Pts',(-6.59948308607524,62.6072792748565,
2.59908174381726));
#212056=CARTESIAN_POINT('Ctrl Pts',(-6.60326825869943,62.606832508458,2.59915752001039));
#212057=CARTESIAN_POINT('Ctrl Pts',(-6.60703621730618,62.6063406883234,
2.59930729517514));
#212058=CARTESIAN_POINT('Ctrl Pts',(-6.62881036976983,62.6034985746717,
2.60017281085959));
#212059=CARTESIAN_POINT('Ctrl Pts',(-6.65001265698364,62.5991534367851,
2.60350651800094));
#212060=CARTESIAN_POINT('Ctrl Pts',(-6.67028839971536,62.5935594283582,
2.60896880596481));
#212061=CARTESIAN_POINT('Ctrl Pts',(-6.67846607318115,62.5913032360753,
2.61117187235482));
#212062=CARTESIAN_POINT('Ctrl Pts',(-6.68649343259904,62.5888441205338,
2.61372076577233));
#212063=CARTESIAN_POINT('Ctrl Pts',(-6.6943489154363,62.5861994699222,2.61659179897028));
#212064=CARTESIAN_POINT('Ctrl Pts',(-6.69724711167674,62.5852237544101,
2.61765103591253));
#212065=CARTESIAN_POINT('Ctrl Pts',(-6.70012178934749,62.5842227327446,
2.61875422455194));
#212066=CARTESIAN_POINT('Ctrl Pts',(-6.70297180428205,62.5831972538527,
2.61990022440441));
#212067=CARTESIAN_POINT('Ctrl Pts',(-6.70831558228433,62.5812744809304,
2.62204897412778));
#212068=CARTESIAN_POINT('Ctrl Pts',(-6.71357265535406,62.5792657255655,
2.62434823201814));
#212069=CARTESIAN_POINT('Ctrl Pts',(-6.71873548138837,62.5771765838156,
2.62679048030349));
#212070=CARTESIAN_POINT('Ctrl Pts',(-6.73680537250844,62.5698645876908,
2.63533834930223));
#212071=CARTESIAN_POINT('Ctrl Pts',(-6.75372073697224,62.561567853893,2.64563784783606));
#212072=CARTESIAN_POINT('Ctrl Pts',(-6.76915820973634,62.5525263385766,
2.65736666738008));
#212073=CARTESIAN_POINT('Ctrl Pts',(-6.77687694611839,62.5480055809184,
2.66323107715209));
#212074=CARTESIAN_POINT('Ctrl Pts',(-6.78422620968087,62.5432986288853,
2.66945281780817));
#212075=CARTESIAN_POINT('Ctrl Pts',(-6.79116558077055,62.53843548583,2.67599160631244));
#212076=CARTESIAN_POINT('Ctrl Pts',(-6.79463526631539,62.5360039143024,
2.67926100056457));
#212077=CARTESIAN_POINT('Ctrl Pts',(-6.79800247875532,62.533533295136,2.68260965685166));
#212078=CARTESIAN_POINT('Ctrl Pts',(-6.80126216569475,62.5310273792784,
2.68603254012526));
#212079=CARTESIAN_POINT('Ctrl Pts',(-6.80452185263419,62.5285214634208,
2.68945542339885));
#212080=CARTESIAN_POINT('Ctrl Pts',(-6.80767389012568,62.5259802131088,
2.69295261525429));
#212081=CARTESIAN_POINT('Ctrl Pts',(-6.81071347912886,62.5234074580026,
2.69651891172143));
#212082=CARTESIAN_POINT('Ctrl Pts',(-6.81073940045717,62.5233855177898,
2.69654932476131));
#212083=CARTESIAN_POINT('Ctrl Pts',(-6.81076531358493,62.5233635754233,
2.69657974261189));
#212084=CARTESIAN_POINT('Ctrl Pts',(-6.81079121850992,62.5233416309053,
2.69661016527016));
#212085=CARTESIAN_POINT('Ctrl Pts',(-6.82402124190201,62.5121342452109,
2.71214746101119));
#212086=CARTESIAN_POINT('Ctrl Pts',(-6.83522119343849,62.5004397189066,
2.72880565567501));
#212087=CARTESIAN_POINT('Ctrl Pts',(-6.84446844329406,62.4884429377095,
2.74628040012191));
#212088=CARTESIAN_POINT('Ctrl Pts',(-6.85402842899935,62.4760404333385,
2.76434612882238));
#212089=CARTESIAN_POINT('Ctrl Pts',(-6.86150157917281,62.4633140048744,
2.78328592654235));
#212090=CARTESIAN_POINT('Ctrl Pts',(-6.86692204702709,62.4504583709472,
2.8027875326759));
#212091=CARTESIAN_POINT('Ctrl Pts',(-6.87223940617701,62.4378472782282,
2.82191817722543));
#212092=CARTESIAN_POINT('Ctrl Pts',(-6.87558122532386,62.4251109433598,
2.84159092314904));
#212093=CARTESIAN_POINT('Ctrl Pts',(-6.87693208138113,62.4124375993958,
2.86151233816768));
#212094=CARTESIAN_POINT('Ctrl Pts',(-6.8778269761607,62.4040419533223,2.87470957721161));
#212095=CARTESIAN_POINT('Ctrl Pts',(-6.87784715439696,62.3956740599456,
2.8880159438829));
#212096=CARTESIAN_POINT('Ctrl Pts',(-6.87697683366585,62.3873926810693,
2.90134173516067));
#212097=CARTESIAN_POINT('',(-6.83973663030281,62.0330459552234,3.47153072139115));
#212098=CARTESIAN_POINT('',(-6.87697683366585,62.3873926810693,2.90134173516067));
#212099=CARTESIAN_POINT('',(-12.6642893210144,61.1105274371642,3.47153072139114));
#212100=CARTESIAN_POINT('Origin',(5.53234440788222E-15,1.85015204418142E-13,
3.47153072139072));
#212101=CARTESIAN_POINT('',(-12.7383709431253,61.459039055521,2.90134173516066));
#212102=CARTESIAN_POINT('',(-12.6642893210144,61.1105274371642,3.47153072139114));
#212103=CARTESIAN_POINT('',(-13.0739701745327,61.5816197022699,2.59908173516066));
#212104=CARTESIAN_POINT('Ctrl Pts',(-12.7383709431253,61.459039055521,2.90134173516066));
#212105=CARTESIAN_POINT('Ctrl Pts',(-12.7409296199638,61.4710760487557,
2.88164837656569));
#212106=CARTESIAN_POINT('Ctrl Pts',(-12.7453875382449,61.4826680729157,
2.86203734438793));
#212107=CARTESIAN_POINT('Ctrl Pts',(-12.7516316867679,61.4936637287812,
2.84277945977618));
#212108=CARTESIAN_POINT('Ctrl Pts',(-12.7580013045751,61.5048803302354,
2.82313460919295));
#212109=CARTESIAN_POINT('Ctrl Pts',(-12.7662298081617,61.5154772731058,
2.80385576862436));
#212110=CARTESIAN_POINT('Ctrl Pts',(-12.7762506512886,61.5252915748246,
2.78521678517323));
#212111=CARTESIAN_POINT('Ctrl Pts',(-12.7858821937442,61.5347245998185,
2.76730190933241));
#212112=CARTESIAN_POINT('Ctrl Pts',(-12.7971700470174,61.5434353195605,
2.74997687278406));
#212113=CARTESIAN_POINT('Ctrl Pts',(-12.8100982056066,61.5512651452213,
2.7334925334423));
#212114=CARTESIAN_POINT('Ctrl Pts',(-12.8200291684145,61.5572797455911,
2.72082983598343));
#212115=CARTESIAN_POINT('Ctrl Pts',(-12.8309289079003,61.5627743733251,
2.70866321038853));
#212116=CARTESIAN_POINT('Ctrl Pts',(-12.8428059312037,61.5676673859797,
2.69711645335887));
#212117=CARTESIAN_POINT('Ctrl Pts',(-12.8428370587636,61.5676802096933,
2.69708619136793));
#212118=CARTESIAN_POINT('Ctrl Pts',(-12.8428681938093,61.5676930289523,
2.6970559338726));
#212119=CARTESIAN_POINT('Ctrl Pts',(-12.8428993363378,61.5677058437554,
2.69702568087612));
#212120=CARTESIAN_POINT('Ctrl Pts',(-12.8462384487039,61.5690798512469,
2.69378194443308));
#212121=CARTESIAN_POINT('Ctrl Pts',(-12.8496624271215,61.5704011254856,
2.69059266624742));
#212122=CARTESIAN_POINT('Ctrl Pts',(-12.8531666956981,61.5716678181343,
2.68746219342719));
#212123=CARTESIAN_POINT('Ctrl Pts',(-12.8726671535595,61.5787166747159,
2.67004182395993));
#212124=CARTESIAN_POINT('Ctrl Pts',(-12.8946522063806,61.5840799821735,
2.65443567877684));
#212125=CARTESIAN_POINT('Ctrl Pts',(-12.9182844651737,61.5874651029957,
2.64136852352809));
#212126=CARTESIAN_POINT('Ctrl Pts',(-12.9288909501853,61.5889843920987,
2.63550380329533));
#212127=CARTESIAN_POINT('Ctrl Pts',(-12.9398294094017,61.5901055263653,
2.63014997451039));
#212128=CARTESIAN_POINT('Ctrl Pts',(-12.9510258874722,61.5908034580839,
2.62536981119295));
#212129=CARTESIAN_POINT('Ctrl Pts',(-12.9558917253993,61.5911067697687,
2.62329241687115));
#212130=CARTESIAN_POINT('Ctrl Pts',(-12.9608061353937,61.5913300246962,
2.6213236213147));
#212131=CARTESIAN_POINT('Ctrl Pts',(-12.9657629422644,61.5914710890456,
2.6194687337239));
#212132=CARTESIAN_POINT('Ctrl Pts',(-12.9831117663121,61.5919648142684,
2.6129766271561));
#212133=CARTESIAN_POINT('Ctrl Pts',(-13.0009799514312,61.5914517017519,
2.60787989114012));
#212134=CARTESIAN_POINT('Ctrl Pts',(-13.0191027399908,61.5898402812907,
2.60440616886223));
#212135=CARTESIAN_POINT('Ctrl Pts',(-13.0281641342706,61.58903457106,2.60266930772328));
#212136=CARTESIAN_POINT('Ctrl Pts',(-13.0372891795345,61.5879542844385,
2.60133820040226));
#212137=CARTESIAN_POINT('Ctrl Pts',(-13.0464447827192,61.5865879953993,
2.60044130723626));
#212138=CARTESIAN_POINT('Ctrl Pts',(-13.0510225843115,61.5859048508797,
2.59999286065326));
#212139=CARTESIAN_POINT('Ctrl Pts',(-13.0556080254097,61.5851502058762,
2.59965296768554));
#212140=CARTESIAN_POINT('Ctrl Pts',(-13.0601969695277,61.5843226328194,
2.59942518630996));
#212141=CARTESIAN_POINT('Ctrl Pts',(-13.0647859136458,61.5834950597625,
2.59919740493438));
#212142=CARTESIAN_POINT('Ctrl Pts',(-13.0693783604294,61.5825945569832,
2.59908173791658));
#212143=CARTESIAN_POINT('Ctrl Pts',(-13.0739701745327,61.5816197022699,
2.59908173516066));
#212144=CARTESIAN_POINT('',(-13.103835206573,61.5752716937453,2.59908173516066));
#212145=CARTESIAN_POINT('Origin',(-7.37250181440781E-18,1.90955466615801E-13,
2.59908173516024));
#212146=CARTESIAN_POINT('',(-13.3605623192489,61.3267881959114,2.90134173516066));
#212147=CARTESIAN_POINT('Ctrl Pts',(-13.103835206573,61.5752716937453,2.59908173516067));
#212148=CARTESIAN_POINT('Ctrl Pts',(-13.107573119184,61.5744762229328,2.59908174381721));
#212149=CARTESIAN_POINT('Ctrl Pts',(-13.1112908564314,61.5736362456897,
2.59915752001038));
#212150=CARTESIAN_POINT('Ctrl Pts',(-13.1149867645638,61.5727532608745,
2.59930729517513));
#212151=CARTESIAN_POINT('Ctrl Pts',(-13.1363445541693,61.5676506979228,
2.60017281085957));
#212152=CARTESIAN_POINT('Ctrl Pts',(-13.1569765024492,61.5611131206561,
2.60350651800086));
#212153=CARTESIAN_POINT('Ctrl Pts',(-13.1765564394362,61.5534303645633,
2.60896880596463));
#212154=CARTESIAN_POINT('Ctrl Pts',(-13.1844534784391,61.5503317322973,
2.61117187235468));
#212155=CARTESIAN_POINT('Ctrl Pts',(-13.1921798155738,61.547047000504,2.61372076577224));
#212156=CARTESIAN_POINT('Ctrl Pts',(-13.1997158239901,61.5435957160158,
2.61659179897027));
#212157=CARTESIAN_POINT('Ctrl Pts',(-13.2024961535652,61.5423224015761,
2.61765103591252));
#212158=CARTESIAN_POINT('Ctrl Pts',(-13.2052504481945,61.5410263779727,
2.61875422455193));
#212159=CARTESIAN_POINT('Ctrl Pts',(-13.2079776587163,61.5397086090801,
2.6199002244044));
#212160=CARTESIAN_POINT('Ctrl Pts',(-13.2130911784448,61.5372377924064,
2.62204897412777));
#212161=CARTESIAN_POINT('Ctrl Pts',(-13.2181094806068,61.5346905274443,
2.62434823201813));
#212162=CARTESIAN_POINT('Ctrl Pts',(-13.2230256493633,61.53207316796,2.62679048030349));
#212163=CARTESIAN_POINT('Ctrl Pts',(-13.2402322400107,61.5229124097648,
2.63533834930222));
#212164=CARTESIAN_POINT('Ctrl Pts',(-13.2561876955041,61.5128929892898,
2.64563784783606));
#212165=CARTESIAN_POINT('Ctrl Pts',(-13.2705955044755,61.5022873490356,
2.65736666738007));
#212166=CARTESIAN_POINT('Ctrl Pts',(-13.2777994089612,61.4969845289085,
2.66323107715208));
#212167=CARTESIAN_POINT('Ctrl Pts',(-13.2846164020262,61.4915351548249,
2.66945281780817));
#212168=CARTESIAN_POINT('Ctrl Pts',(-13.2910094216448,61.48597329078,2.67599160631244));
#212169=CARTESIAN_POINT('Ctrl Pts',(-13.2942059314541,61.4831923587576,
2.67926100056457));
#212170=CARTESIAN_POINT('Ctrl Pts',(-13.2972964479272,61.4803833043596,
2.68260965685166));
#212171=CARTESIAN_POINT('Ctrl Pts',(-13.3002763384268,61.4775503861048,
2.68603254012525));
#212172=CARTESIAN_POINT('Ctrl Pts',(-13.3032562289264,61.47471746785,2.68945542339885));
#212173=CARTESIAN_POINT('Ctrl Pts',(-13.3061253662369,61.4718606611379,
2.69295261525427));
#212174=CARTESIAN_POINT('Ctrl Pts',(-13.3088793779158,61.468984276286,2.69651891172141));
#212175=CARTESIAN_POINT('Ctrl Pts',(-13.3089028638677,61.4689597467473,
2.69654932476129));
#212176=CARTESIAN_POINT('Ctrl Pts',(-13.3089263414387,61.4689352159239,
2.69657974261188));
#212177=CARTESIAN_POINT('Ctrl Pts',(-13.3089498106271,61.4689106838184,
2.69661016527015));
#212178=CARTESIAN_POINT('Ctrl Pts',(-13.3209358677632,61.4563817793409,
2.71214746101158));
#212179=CARTESIAN_POINT('Ctrl Pts',(-13.3308520539303,61.4435806031522,
2.72880565567585));
#212180=CARTESIAN_POINT('Ctrl Pts',(-13.338794641281,61.4306829407606,2.74628040012323));
#212181=CARTESIAN_POINT('Ctrl Pts',(-13.3470058416618,61.4173490879912,
2.76434612882423));
#212182=CARTESIAN_POINT('Ctrl Pts',(-13.3531077791265,61.4039112193301,
2.78328592654476));
#212183=CARTESIAN_POINT('Ctrl Pts',(-13.3571547734318,61.3905594167353,
2.80278753267888));
#212184=CARTESIAN_POINT('Ctrl Pts',(-13.3611247853898,61.3774615935208,
2.82191817722895));
#212185=CARTESIAN_POINT('Ctrl Pts',(-13.36311698819,61.3644457144072,2.8415909231531));
#212186=CARTESIAN_POINT('Ctrl Pts',(-13.3631357189472,61.3517005934394,
2.86151233817227));
#212187=CARTESIAN_POINT('Ctrl Pts',(-13.3631481274171,61.3432573976185,
2.87470957721469));
#212188=CARTESIAN_POINT('Ctrl Pts',(-13.3622935120794,61.3349332352382,
2.88801594388444));
#212189=CARTESIAN_POINT('Ctrl Pts',(-13.3605623192489,61.3267881959114,
2.90134173516065));
#212190=CARTESIAN_POINT('',(-13.2864868028998,60.9782752797349,3.47153072139114));
#212191=CARTESIAN_POINT('',(-13.3605623192489,61.3267881959114,2.90134173516066));
#212192=CARTESIAN_POINT('',(-18.9827025415099,59.4519788726608,3.47153072139113));
#212193=CARTESIAN_POINT('Origin',(5.53234440788222E-15,1.85015204418142E-13,
3.47153072139072));
#212194=CARTESIAN_POINT('',(-19.0928077206414,59.7908376697913,2.90134173516065));
#212195=CARTESIAN_POINT('',(-18.9827025415099,59.4519788726608,3.47153072139113));
#212196=CARTESIAN_POINT('',(-19.4393816709759,59.8776671349986,2.59908173516064));
#212197=CARTESIAN_POINT('Ctrl Pts',(-19.0928077206414,59.7908376697913,
2.90134173516065));
#212198=CARTESIAN_POINT('Ctrl Pts',(-19.0966105891852,59.802541268558,2.88164837656838));
#212199=CARTESIAN_POINT('Ctrl Pts',(-19.1022557829942,59.813603811048,2.86203734439329));
#212200=CARTESIAN_POINT('Ctrl Pts',(-19.109615084427,59.8238865403095,2.84277945978409));
#212201=CARTESIAN_POINT('Ctrl Pts',(-19.117122262913,59.834375889685,2.82313460920358));
#212202=CARTESIAN_POINT('Ctrl Pts',(-19.1264133720475,59.8440546685577,
2.80385576863757));
#212203=CARTESIAN_POINT('Ctrl Pts',(-19.1374051938214,59.8527677431713,
2.78521678518877));
#212204=CARTESIAN_POINT('Ctrl Pts',(-19.1479699932837,59.8611423227348,
2.76730190935032));
#212205=CARTESIAN_POINT('Ctrl Pts',(-19.1601065286611,59.8686254222859,
2.74997687280409));
#212206=CARTESIAN_POINT('Ctrl Pts',(-19.1737823050855,59.8750609947923,
2.73349253346408));
#212207=CARTESIAN_POINT('Ctrl Pts',(-19.1842875619788,59.8800045782744,
2.72082983599738));
#212208=CARTESIAN_POINT('Ctrl Pts',(-19.1957019365505,59.8843297728472,
2.70866321039513));
#212209=CARTESIAN_POINT('Ctrl Pts',(-19.2080253553781,59.8879544940745,
2.69711645335885));
#212210=CARTESIAN_POINT('Ctrl Pts',(-19.2080576528611,59.8879639938225,
2.69708619136791));
#212211=CARTESIAN_POINT('Ctrl Pts',(-19.2080899573232,59.8879734883578,
2.69705593387258));
#212212=CARTESIAN_POINT('Ctrl Pts',(-19.2081222687613,59.8879829776794,
2.6970256808761));
#212213=CARTESIAN_POINT('Ctrl Pts',(-19.211586712012,59.8890004259297,2.69378194443306));
#212214=CARTESIAN_POINT('Ctrl Pts',(-19.2151300442834,59.8899565588876,
2.6905926662474));
#212215=CARTESIAN_POINT('Ctrl Pts',(-19.2187475215461,59.8908500166523,
2.68746219342717));
#212216=CARTESIAN_POINT('Ctrl Pts',(-19.2388779600059,59.8958219059669,
2.67004182395933));
#212217=CARTESIAN_POINT('Ctrl Pts',(-19.2613031946947,59.8988577688788,
2.6544356787758));
#212218=CARTESIAN_POINT('Ctrl Pts',(-19.2851598349798,59.8997541019597,
2.6413685235268));
#212219=CARTESIAN_POINT('Ctrl Pts',(-19.2958670255112,59.900156388659,2.63550380329453));
#212220=CARTESIAN_POINT('Ctrl Pts',(-19.3068627531447,59.9001280009024,
2.63014997451003));
#212221=CARTESIAN_POINT('Ctrl Pts',(-19.318070849466,59.8996517586313,2.62536981119294));
#212222=CARTESIAN_POINT('Ctrl Pts',(-19.3229417365281,59.8994447901819,
2.62329241687114));
#212223=CARTESIAN_POINT('Ctrl Pts',(-19.3278525613648,59.899153126371,2.62132362131468));
#212224=CARTESIAN_POINT('Ctrl Pts',(-19.3327969595686,59.8987752905502,
2.61946873372389));
#212225=CARTESIAN_POINT('Ctrl Pts',(-19.3501023532817,59.8974528651774,
2.61297662715609));
#212226=CARTESIAN_POINT('Ctrl Pts',(-19.3678190197503,59.8950748296131,
2.6078798911401));
#212227=CARTESIAN_POINT('Ctrl Pts',(-19.3856740904735,59.8915778894435,
2.6044061688622));
#212228=CARTESIAN_POINT('Ctrl Pts',(-19.394601625835,59.8898294193587,2.60266930772325));
#212229=CARTESIAN_POINT('Ctrl Pts',(-19.4035637624458,59.8878012237016,
2.60133820040226));
#212230=CARTESIAN_POINT('Ctrl Pts',(-19.4125263941846,59.8854853982055,
2.60044130723625));
#212231=CARTESIAN_POINT('Ctrl Pts',(-19.417007710054,59.8843274854575,2.59999286065325));
#212232=CARTESIAN_POINT('Ctrl Pts',(-19.4214891497435,59.8830976653669,
2.59965296768552));
#212233=CARTESIAN_POINT('Ctrl Pts',(-19.4259664502057,59.8817949505652,
2.59942518630994));
#212234=CARTESIAN_POINT('Ctrl Pts',(-19.4304437506678,59.8804922357634,
2.59919740493436));
#212235=CARTESIAN_POINT('Ctrl Pts',(-19.4349169113758,59.8791166246277,
2.59908173791657));
#212236=CARTESIAN_POINT('Ctrl Pts',(-19.4393816709759,59.8776671349986,
2.59908173516064));
#212237=CARTESIAN_POINT('',(-19.4684195516699,59.8682321556243,2.59908173516065));
#212238=CARTESIAN_POINT('Origin',(8.34054140790947E-18,1.90959676913043E-13,
2.59908173516022));
#212239=CARTESIAN_POINT('',(-19.6977666881848,59.5942745858237,2.90134173516065));
#212240=CARTESIAN_POINT('Ctrl Pts',(-19.4684195516699,59.8682321556243,
2.59908173516064));
#212241=CARTESIAN_POINT('Ctrl Pts',(-19.4720538382629,59.8670503242231,
2.59908174381719));
#212242=CARTESIAN_POINT('Ctrl Pts',(-19.4756634078263,59.8658263391019,
2.59915752001037));
#212243=CARTESIAN_POINT('Ctrl Pts',(-19.4792467723414,59.8645618637724,
2.59930729517512));
#212244=CARTESIAN_POINT('Ctrl Pts',(-19.4999541986765,59.8572547562683,
2.60017281085956));
#212245=CARTESIAN_POINT('Ctrl Pts',(-19.5197897600796,59.8485963666861,
2.60350651800078));
#212246=CARTESIAN_POINT('Ctrl Pts',(-19.538459369435,59.838909036811,2.60896880596448));
#212247=CARTESIAN_POINT('Ctrl Pts',(-19.5459892523631,59.8350019138254,
2.61117187235455));
#212248=CARTESIAN_POINT('Ctrl Pts',(-19.5533299158481,59.830927553989,2.61372076577216));
#212249=CARTESIAN_POINT('Ctrl Pts',(-19.560463883758,59.8267074486194,2.61659179897023));
#212250=CARTESIAN_POINT('Ctrl Pts',(-19.5630958847952,59.8251504859515,
2.61765103591249));
#212251=CARTESIAN_POINT('Ctrl Pts',(-19.5656996197547,59.8235736599161,
2.61875422455189));
#212252=CARTESIAN_POINT('Ctrl Pts',(-19.5682741459747,59.8219780387745,
2.61990022440436));
#212253=CARTESIAN_POINT('Ctrl Pts',(-19.5731013826371,59.818986249134,2.62204897412773));
#212254=CARTESIAN_POINT('Ctrl Pts',(-19.5778259323228,59.8159283829427,
2.62434823201809));
#212255=CARTESIAN_POINT('Ctrl Pts',(-19.5824415812277,59.8128114820622,
2.62679048030344));
#212256=CARTESIAN_POINT('Ctrl Pts',(-19.5985963523948,59.8019023289804,
2.63533834930218));
#212257=CARTESIAN_POINT('Ctrl Pts',(-19.6134170876084,59.7902699966957,
2.64563784783603));
#212258=CARTESIAN_POINT('Ctrl Pts',(-19.626637377817,59.7782164291177,2.65736666738005));
#212259=CARTESIAN_POINT('Ctrl Pts',(-19.6332475229213,59.7721896453286,
2.66323107715205));
#212260=CARTESIAN_POINT('Ctrl Pts',(-19.6394575570863,59.7660575536772,
2.66945281780814));
#212261=CARTESIAN_POINT('Ctrl Pts',(-19.645234181973,59.7598579055892,2.67599160631241));
#212262=CARTESIAN_POINT('Ctrl Pts',(-19.6481224944163,59.7567580815452,
2.67926100056455));
#212263=CARTESIAN_POINT('Ctrl Pts',(-19.6509024545773,59.7536413685034,
2.68260965685163));
#212264=CARTESIAN_POINT('Ctrl Pts',(-19.6535699003333,59.7505124858966,
2.68603254012522));
#212265=CARTESIAN_POINT('Ctrl Pts',(-19.6562373460892,59.7473836032897,
2.68945542339882));
#212266=CARTESIAN_POINT('Ctrl Pts',(-19.6587921483498,59.7442425399498,
2.69295261525425));
#212267=CARTESIAN_POINT('Ctrl Pts',(-19.6612304091763,59.7410940396264,
2.69651891172139));
#212268=CARTESIAN_POINT('Ctrl Pts',(-19.6612512024346,59.7410671895126,
2.69654932476127));
#212269=CARTESIAN_POINT('Ctrl Pts',(-19.6612719872239,59.7410403389973,
2.69657974261185));
#212270=CARTESIAN_POINT('Ctrl Pts',(-19.6612927635423,59.741013488083,2.69661016527013));
#212271=CARTESIAN_POINT('Ctrl Pts',(-19.6719035326719,59.727300334122,2.71214746101175));
#212272=CARTESIAN_POINT('Ctrl Pts',(-19.6804273096587,59.7135327604141,
2.72880565567622));
#212273=CARTESIAN_POINT('Ctrl Pts',(-19.6869782138553,59.6998755263162,
2.74628040012384));
#212274=CARTESIAN_POINT('Ctrl Pts',(-19.693750665282,59.68575641363,2.76434612882499));
#212275=CARTESIAN_POINT('Ctrl Pts',(-19.698414535934,59.6717543328732,2.78328592654569));
#212276=CARTESIAN_POINT('Ctrl Pts',(-19.7010437169739,59.6580526467544,
2.80278753267999));
#212277=CARTESIAN_POINT('Ctrl Pts',(-19.7036228854582,59.6446115955367,
2.82191817723016));
#212278=CARTESIAN_POINT('Ctrl Pts',(-19.7042436449211,59.6314587768735,
2.84159092315442));
#212279=CARTESIAN_POINT('Ctrl Pts',(-19.7029300451602,59.6187815171146,
2.86151233817369));
#212280=CARTESIAN_POINT('Ctrl Pts',(-19.7020598313709,59.6103832769659,
2.87470957721564));
#212281=CARTESIAN_POINT('Ctrl Pts',(-19.7003397858039,59.6021940468463,
2.88801594388491));
#212282=CARTESIAN_POINT('Ctrl Pts',(-19.6977666881848,59.5942745858237,
2.90134173516065));
#212283=CARTESIAN_POINT('',(-19.5876674457081,59.2554138597572,3.47153072139113));
#212284=CARTESIAN_POINT('',(-19.6977666881848,59.5942745858237,2.90134173516065));
#212285=CARTESIAN_POINT('',(-25.0931373005748,57.1420619865022,3.47153072139111));
#212286=CARTESIAN_POINT('Origin',(5.53234440788222E-15,1.85015204418142E-13,
3.47153072139072));
#212287=CARTESIAN_POINT('',(-25.2380597013433,57.4675553545141,2.90134173516062));
#212288=CARTESIAN_POINT('',(-25.0931373005748,57.1420619865022,3.47153072139111));
#212289=CARTESIAN_POINT('',(-25.5918112338797,57.5176823163889,2.59908173516063));
#212290=CARTESIAN_POINT('Ctrl Pts',(-25.2380597013433,57.4675553545141,
2.90134173516062));
#212291=CARTESIAN_POINT('Ctrl Pts',(-25.2430650965697,57.4787973317385,
2.88164837656627));
#212292=CARTESIAN_POINT('Ctrl Pts',(-25.2498357159836,57.4892091890306,
2.86203734438913));
#212293=CARTESIAN_POINT('Ctrl Pts',(-25.2582295402822,57.4986663319565,
2.84277945977796));
#212294=CARTESIAN_POINT('Ctrl Pts',(-25.2667920292312,57.5083135057489,
2.82313460919546));
#212295=CARTESIAN_POINT('Ctrl Pts',(-25.2770439485811,57.5169680778989,
2.80385576862757));
#212296=CARTESIAN_POINT('Ctrl Pts',(-25.2888863203068,57.5244844631399,
2.78521678517707));
#212297=CARTESIAN_POINT('Ctrl Pts',(-25.3002686266263,57.531708843628,2.76730190933709));
#212298=CARTESIAN_POINT('Ctrl Pts',(-25.3131208736917,57.5378823365845,
2.74997687278951));
#212299=CARTESIAN_POINT('Ctrl Pts',(-25.3273944332885,57.5428531464575,
2.73349253344838));
#212300=CARTESIAN_POINT('Ctrl Pts',(-25.3383588864659,57.5466715501105,
2.72082983598732));
#212301=CARTESIAN_POINT('Ctrl Pts',(-25.350162837837,57.5497799237802,2.70866321039035));
#212302=CARTESIAN_POINT('Ctrl Pts',(-25.3627976342212,57.5520966403721,
2.69711645335883));
#212303=CARTESIAN_POINT('Ctrl Pts',(-25.3628307477693,57.5521027120731,
2.69708619136789));
#212304=CARTESIAN_POINT('Ctrl Pts',(-25.3628638677133,57.5521087778607,
2.69705593387256));
#212305=CARTESIAN_POINT('Ctrl Pts',(-25.3628969940503,57.5521148377338,
2.69702568087608));
#212306=CARTESIAN_POINT('Ctrl Pts',(-25.3664488110204,57.5527645793671,
2.69378194443304));
#212307=CARTESIAN_POINT('Ctrl Pts',(-25.3700726756556,57.5533450954514,
2.69059266624738));
#212308=CARTESIAN_POINT('Ctrl Pts',(-25.3737637277665,57.5538555294218,
2.68746219342715));
#212309=CARTESIAN_POINT('Ctrl Pts',(-25.394303593528,57.5566959784095,2.67004182395906));
#212310=CARTESIAN_POINT('Ctrl Pts',(-25.41692331452,57.5573711352263,2.65443567877532));
#212311=CARTESIAN_POINT('Ctrl Pts',(-25.4407429579534,57.5557688601529,
2.6413685235262));
#212312=CARTESIAN_POINT('Ctrl Pts',(-25.4514335437849,57.5550497369114,
2.63550380329415));
#212313=CARTESIAN_POINT('Ctrl Pts',(-25.462366068343,57.5538721381539,2.63014997450983));
#212314=CARTESIAN_POINT('Ctrl Pts',(-25.4734629846669,57.5522269397032,
2.6253698111929));
#212315=CARTESIAN_POINT('Ctrl Pts',(-25.4782855544061,57.5515119587093,
2.6232924168711));
#212316=CARTESIAN_POINT('Ctrl Pts',(-25.4831389900605,57.5507085716897,
2.62132362131465));
#212317=CARTESIAN_POINT('Ctrl Pts',(-25.4880168077359,57.549815975347,2.61946873372385));
#212318=CARTESIAN_POINT('Ctrl Pts',(-25.5050891695995,57.5466918881477,
2.61297662715605));
#212319=CARTESIAN_POINT('Ctrl Pts',(-25.5224602099123,57.5424749837908,
2.60787989114007));
#212320=CARTESIAN_POINT('Ctrl Pts',(-25.5398519389078,57.5371308371211,
2.60440616886217));
#212321=CARTESIAN_POINT('Ctrl Pts',(-25.5485478034055,57.5344587637863,
2.60266930772322));
#212322=CARTESIAN_POINT('Ctrl Pts',(-25.557248840319,57.5315048804297,2.60133820040223));
#212323=CARTESIAN_POINT('Ctrl Pts',(-25.565920304143,57.5282648911455,2.60044130723623));
#212324=CARTESIAN_POINT('Ctrl Pts',(-25.5702560360551,57.5266448965034,
2.59999286065323));
#212325=CARTESIAN_POINT('Ctrl Pts',(-25.5745843747449,57.524953375492,2.5996529676855));
#212326=CARTESIAN_POINT('Ctrl Pts',(-25.5789009773103,57.5231897917614,
2.59942518630992));
#212327=CARTESIAN_POINT('Ctrl Pts',(-25.5832175798758,57.5214262080307,
2.59919740493434));
#212328=CARTESIAN_POINT('Ctrl Pts',(-25.5875224456232,57.5195905600219,
2.59908173791657));
#212329=CARTESIAN_POINT('Ctrl Pts',(-25.5918112338797,57.5176823163889,
2.59908173516063));
#212330=CARTESIAN_POINT('',(-25.61970381813,57.5052637377733,2.59908173516063));
#212331=CARTESIAN_POINT('Origin',(2.35274110347535E-17,1.90965506606098E-13,
2.59908173516024));
#212332=CARTESIAN_POINT('',(-25.8191582032623,57.2088336324699,2.90134173516062));
#212333=CARTESIAN_POINT('Ctrl Pts',(-25.61970381813,57.5052637377733,2.59908173516064));
#212334=CARTESIAN_POINT('Ctrl Pts',(-25.6231946607006,57.5037084941755,
2.59908174381719));
#212335=CARTESIAN_POINT('Ctrl Pts',(-25.6266565153805,57.5021139114134,
2.59915752001035));
#212336=CARTESIAN_POINT('Ctrl Pts',(-25.6300880761868,57.500481799426,2.59930729517509));
#212337=CARTESIAN_POINT('Ctrl Pts',(-25.649918264359,57.4910502055666,2.60017281085968));
#212338=CARTESIAN_POINT('Ctrl Pts',(-25.668740116327,57.4803658667948,2.60350651800195));
#212339=CARTESIAN_POINT('Ctrl Pts',(-25.6862948499065,57.4687800995483,
2.60896880596735));
#212340=CARTESIAN_POINT('Ctrl Pts',(-25.6933750777833,57.4641072931021,
2.61117187235676));
#212341=CARTESIAN_POINT('Ctrl Pts',(-25.7002496417701,57.4592879447638,
2.61372076577339));
#212342=CARTESIAN_POINT('Ctrl Pts',(-25.7069034079253,57.4543452548725,
2.61659179897021));
#212343=CARTESIAN_POINT('Ctrl Pts',(-25.7093582436704,57.4525217023853,
2.61765103591246));
#212344=CARTESIAN_POINT('Ctrl Pts',(-25.711782891895,57.4506813499538,2.61875422455187));
#212345=CARTESIAN_POINT('Ctrl Pts',(-25.7141765267651,57.4488253585223,
2.61990022440433));
#212346=CARTESIAN_POINT('Ctrl Pts',(-25.7186645921465,57.4453453745884,
2.6220489741277));
#212347=CARTESIAN_POINT('Ctrl Pts',(-25.7230436262008,57.4418104097897,
2.62434823201807));
#212348=CARTESIAN_POINT('Ctrl Pts',(-25.7273081852388,57.4382281169314,
2.62679048030342));
#212349=CARTESIAN_POINT('Ctrl Pts',(-25.742234141872,57.4256900919271,2.63533834930216));
#212350=CARTESIAN_POINT('Ctrl Pts',(-25.7557577777295,57.4125722940994,
2.645637847836));
#212351=CARTESIAN_POINT('Ctrl Pts',(-25.7676457049092,57.3992028606062,
2.65736666738001));
#212352=CARTESIAN_POINT('Ctrl Pts',(-25.7735896684991,57.3925181438597,
2.66323107715202));
#212353=CARTESIAN_POINT('Ctrl Pts',(-25.7791247053302,57.3857705191198,
2.66945281780811));
#212354=CARTESIAN_POINT('Ctrl Pts',(-25.7842216455739,57.3790010116304,
2.67599160631238));
#212355=CARTESIAN_POINT('Ctrl Pts',(-25.7867701156958,57.3756162578857,
2.67926100056452));
#212356=CARTESIAN_POINT('Ctrl Pts',(-25.7892090617194,57.3722260335606,
2.68260965685161));
#212357=CARTESIAN_POINT('Ctrl Pts',(-25.7915348376378,57.3688354672943,
2.6860325401252));
#212358=CARTESIAN_POINT('Ctrl Pts',(-25.7938606135562,57.365444901028,2.6894554233988));
#212359=CARTESIAN_POINT('Ctrl Pts',(-25.7960730898187,57.3620539952075,
2.69295261525422));
#212360=CARTESIAN_POINT('Ctrl Pts',(-25.7981688856969,57.358667875041,2.69651891172136));
#212361=CARTESIAN_POINT('Ctrl Pts',(-25.7981867584464,57.3586389985277,
2.69654932476124));
#212362=CARTESIAN_POINT('Ctrl Pts',(-25.7982046227313,57.3586101225002,
2.69657974261182));
#212363=CARTESIAN_POINT('Ctrl Pts',(-25.7982224785501,57.3585812469613,
2.6966101652701));
#212364=CARTESIAN_POINT('Ctrl Pts',(-25.8073417058664,57.3438340877009,
2.71214746101221));
#212365=CARTESIAN_POINT('Ctrl Pts',(-25.8143796853885,57.3292509568922,
2.72880565567726));
#212366=CARTESIAN_POINT('Ctrl Pts',(-25.8194671333539,57.3149837826026,
2.74628040012549));
#212367=CARTESIAN_POINT('Ctrl Pts',(-25.8247266354312,57.3002341019522,
2.76434612882735));
#212368=CARTESIAN_POINT('Ctrl Pts',(-25.8279013409277,57.2858212188262,
2.78328592654881));
#212369=CARTESIAN_POINT('Ctrl Pts',(-25.8290839028445,57.2719197677234,
2.80278753268388));
#212370=CARTESIAN_POINT('Ctrl Pts',(-25.8302439699452,57.2582827514722,
2.82191817723466));
#212371=CARTESIAN_POINT('Ctrl Pts',(-25.8294864849001,57.2451370982929,
2.84159092315952));
#212372=CARTESIAN_POINT('Ctrl Pts',(-25.8268549466945,57.2326665944535,
2.86151233817938));
#212373=CARTESIAN_POINT('Ctrl Pts',(-25.8251116448906,57.2244053228544,
2.87470957721946));
#212374=CARTESIAN_POINT('Ctrl Pts',(-25.8225450142736,57.2164407479154,
2.88801594388681));
#212375=CARTESIAN_POINT('Ctrl Pts',(-25.8191582032623,57.2088336324699,
2.90134173516062));
#212376=CARTESIAN_POINT('',(-25.6742415049982,56.8833377255395,3.47153072139111));
#212377=CARTESIAN_POINT('',(-25.8191582032623,57.2088336324699,2.90134173516062));
#212378=CARTESIAN_POINT('',(-30.9286463962981,54.2060847114742,3.47153072139109));
#212379=CARTESIAN_POINT('Origin',(5.53234440788222E-15,1.85015204418142E-13,
3.47153072139072));
#212380=CARTESIAN_POINT('',(-31.1067982185537,54.5146464769138,2.90134173516061));
#212381=CARTESIAN_POINT('',(-30.9286463962981,54.2060847114742,3.47153072139109));
#212382=CARTESIAN_POINT('',(-31.4638515574743,54.527521733972,2.59908173516061));
#212383=CARTESIAN_POINT('Ctrl Pts',(-31.1067982185537,54.5146464769138,
2.90134173516061));
#212384=CARTESIAN_POINT('Ctrl Pts',(-31.1129513003036,54.5253036631384,
2.88164837656892));
#212385=CARTESIAN_POINT('Ctrl Pts',(-31.120773164997,54.534950760743,2.8620373443944));
#212386=CARTESIAN_POINT('Ctrl Pts',(-31.1301095476631,54.5434787028948,
2.84277945978573));
#212387=CARTESIAN_POINT('Ctrl Pts',(-31.1396335346515,54.5521780046474,
2.82313460920559));
#212388=CARTESIAN_POINT('Ctrl Pts',(-31.1507339420397,54.5597135487699,
2.80385576863993));
#212389=CARTESIAN_POINT('Ctrl Pts',(-31.1632971162103,54.565950893548,2.78521678519144));
#212390=CARTESIAN_POINT('Ctrl Pts',(-31.1753722224535,54.5719459231359,
2.76730190935284));
#212391=CARTESIAN_POINT('Ctrl Pts',(-31.1887993692945,54.5767421714171,
2.74997687280646));
#212392=CARTESIAN_POINT('Ctrl Pts',(-31.2035143279533,54.580193757424,2.73349253346629));
#212393=CARTESIAN_POINT('Ctrl Pts',(-31.2148178485797,54.5828451460231,
2.72082983599878));
#212394=CARTESIAN_POINT('Ctrl Pts',(-31.2268820501983,54.5847026428005,
2.70866321039578));
#212395=CARTESIAN_POINT('Ctrl Pts',(-31.2396897946772,54.5856859723273,
2.69711645335882));
#212396=CARTESIAN_POINT('Ctrl Pts',(-31.2397233614914,54.5856885494586,
2.69708619136788));
#212397=CARTESIAN_POINT('Ctrl Pts',(-31.2397569340484,54.5856911200402,
2.69705593387255));
#212398=CARTESIAN_POINT('Ctrl Pts',(-31.239790512345,54.5856936840717,2.69702568087608));
#212399=CARTESIAN_POINT('Ctrl Pts',(-31.2433907885846,54.5859686003826,
2.69378194443303));
#212400=CARTESIAN_POINT('Ctrl Pts',(-31.2470554817643,54.5861671393377,
2.69059266624736));
#212401=CARTESIAN_POINT('Ctrl Pts',(-31.2507796687841,54.5862889570924,
2.68746219342713));
#212402=CARTESIAN_POINT('Ctrl Pts',(-31.2715039227763,54.5869668451994,
2.67004182396171));
#212403=CARTESIAN_POINT('Ctrl Pts',(-31.2940703036708,54.5852738987623,
2.65443567878008));
#212404=CARTESIAN_POINT('Ctrl Pts',(-31.3175919772501,54.5811905703971,
2.64136852353218));
#212405=CARTESIAN_POINT('Ctrl Pts',(-31.32814883009,54.5793579160793,2.63550380329779));
#212406=CARTESIAN_POINT('Ctrl Pts',(-31.3388983725498,54.5770440083387,
2.63014997451145));
#212407=CARTESIAN_POINT('Ctrl Pts',(-31.3497625287429,54.574247878846,2.62536981119289));
#212408=CARTESIAN_POINT('Ctrl Pts',(-31.3544839440759,54.5730327187889,
2.62329241687109));
#212409=CARTESIAN_POINT('Ctrl Pts',(-31.3592268152914,54.5717264106369,
2.62132362131464));
#212410=CARTESIAN_POINT('Ctrl Pts',(-31.3639846100471,54.5703288332447,
2.61946873372384));
#212411=CARTESIAN_POINT('Ctrl Pts',(-31.3806368916921,54.5654373123719,
2.61297662715604));
#212412=CARTESIAN_POINT('Ctrl Pts',(-31.3974719850964,54.5594277405091,
2.60787989114006));
#212413=CARTESIAN_POINT('Ctrl Pts',(-31.4142098249418,54.5522949389286,
2.60440616886217));
#212414=CARTESIAN_POINT('Ctrl Pts',(-31.4225787448645,54.5487285381383,
2.60266930772322));
#212415=CARTESIAN_POINT('Ctrl Pts',(-31.4309233516995,54.5448813304464,
2.60133820040221));
#212416=CARTESIAN_POINT('Ctrl Pts',(-31.4392086412365,54.5407526753748,
2.60044130723621));
#212417=CARTESIAN_POINT('Ctrl Pts',(-31.443351286005,54.5386883478389,2.59999286065321));
#212418=CARTESIAN_POINT('Ctrl Pts',(-31.4474791015107,54.5365536585648,
2.59965296768548));
#212419=CARTESIAN_POINT('Ctrl Pts',(-31.4515877125784,54.5343485280977,
2.5994251863099));
#212420=CARTESIAN_POINT('Ctrl Pts',(-31.4556963236462,54.5321433976305,
2.59919740493432));
#212421=CARTESIAN_POINT('Ctrl Pts',(-31.4597857294232,54.5298678244925,
2.59908173791653));
#212422=CARTESIAN_POINT('Ctrl Pts',(-31.4638515574743,54.527521733972,2.59908173516061));
#212423=CARTESIAN_POINT('',(-31.490293248291,54.5122556166611,2.59908173516061));
#212424=CARTESIAN_POINT('Origin',(3.80217165444497E-17,1.90972891823628E-13,
2.59908173516022));
#212425=CARTESIAN_POINT('',(-31.6576696180587,54.1966007261208,2.9013417351606));
#212426=CARTESIAN_POINT('Ctrl Pts',(-31.490293248291,54.5122556166611,2.59908173516061));
#212427=CARTESIAN_POINT('Ctrl Pts',(-31.4936024004374,54.5103440004411,
2.59908174381717));
#212428=CARTESIAN_POINT('Ctrl Pts',(-31.4968786114295,54.5083962906205,
2.59915752001032));
#212429=CARTESIAN_POINT('Ctrl Pts',(-31.5001207716287,54.5064144237356,
2.59930729517507));
#212430=CARTESIAN_POINT('Ctrl Pts',(-31.5188564579396,54.4949616780404,
2.6001728108595));
#212431=CARTESIAN_POINT('Ctrl Pts',(-31.5364583843175,54.4823684499346,
2.60350651800074));
#212432=CARTESIAN_POINT('Ctrl Pts',(-31.5527059087812,54.4690111814119,
2.60896880596443));
#212433=CARTESIAN_POINT('Ctrl Pts',(-31.559258909155,54.4636238877464,2.61117187235451));
#212434=CARTESIAN_POINT('Ctrl Pts',(-31.5655920544881,54.458112352691,2.61372076577212));
#212435=CARTESIAN_POINT('Ctrl Pts',(-31.57169271884,54.4525012314185,2.6165917989702));
#212436=CARTESIAN_POINT('Ctrl Pts',(-31.5739434935988,54.4504310683346,
2.61765103591245));
#212437=CARTESIAN_POINT('Ctrl Pts',(-31.5761624901353,54.4483473527934,
2.61875422455185));
#212438=CARTESIAN_POINT('Ctrl Pts',(-31.5783490084909,54.4462513257026,
2.61990022440431));
#212439=CARTESIAN_POINT('Ctrl Pts',(-31.5824487304078,54.4423212749074,
2.62204897412768));
#212440=CARTESIAN_POINT('Ctrl Pts',(-31.5864342712172,54.4383479413155,
2.62434823201804));
#212441=CARTESIAN_POINT('Ctrl Pts',(-31.5903010169872,54.4343395048295,
2.6267904803034));
#212442=CARTESIAN_POINT('Ctrl Pts',(-31.603834627182,54.4203099771284,2.63533834930213));
#212443=CARTESIAN_POINT('Ctrl Pts',(-31.6159129958989,54.4058504350958,
2.64563784783597));
#212444=CARTESIAN_POINT('Ctrl Pts',(-31.6263383134319,54.3913116139986,
2.65736666737999));
#212445=CARTESIAN_POINT('Ctrl Pts',(-31.6315509721984,54.3840422034501,
2.66323107715199));
#212446=CARTESIAN_POINT('Ctrl Pts',(-31.6363503686739,54.3767529740104,
2.66945281780809));
#212447=CARTESIAN_POINT('Ctrl Pts',(-31.6407117811307,54.3694877752603,
2.67599160631236));
#212448=CARTESIAN_POINT('Ctrl Pts',(-31.6428924873591,54.3658551758853,
2.67926100056449));
#212449=CARTESIAN_POINT('Ctrl Pts',(-31.6449636976424,54.3622285842839,
2.68260965685157));
#212450=CARTESIAN_POINT('Ctrl Pts',(-31.6469223220355,54.3586134821117,
2.68603254012517));
#212451=CARTESIAN_POINT('Ctrl Pts',(-31.6488809464286,54.3549983799396,
2.68945542339876));
#212452=CARTESIAN_POINT('Ctrl Pts',(-31.6507268563402,54.3513947831121,
2.6929526152542));
#212453=CARTESIAN_POINT('Ctrl Pts',(-31.6524572252918,54.3478081421438,
2.69651891172134));
#212454=CARTESIAN_POINT('Ctrl Pts',(-31.652471981715,54.347777555608,2.69654932476122));
#212455=CARTESIAN_POINT('Ctrl Pts',(-31.6524867297707,54.3477469704401,
2.6965797426118));
#212456=CARTESIAN_POINT('Ctrl Pts',(-31.6525014694577,54.3477163866432,
2.69661016527008));
#212457=CARTESIAN_POINT('Ctrl Pts',(-31.6600292427979,54.332096795046,2.71214746101276));
#212458=CARTESIAN_POINT('Ctrl Pts',(-31.6655043152788,54.3168578829693,
2.72880565567847));
#212459=CARTESIAN_POINT('Ctrl Pts',(-31.6690725678682,54.3021370826349,
2.7462804001274));
#212460=CARTESIAN_POINT('Ctrl Pts',(-31.6727614963908,54.2869184346083,
2.76434612882998));
#212461=CARTESIAN_POINT('Ctrl Pts',(-31.6744122539938,54.2722526596768,
2.78328592655222));
#212462=CARTESIAN_POINT('Ctrl Pts',(-31.6741352403914,54.2583037507974,
2.80278753268809));
#212463=CARTESIAN_POINT('Ctrl Pts',(-31.6738634961706,54.2446201795163,
2.82191817723965));
#212464=CARTESIAN_POINT('Ctrl Pts',(-31.6717360657818,54.2316257183479,
2.84159092316531));
#212465=CARTESIAN_POINT('Ctrl Pts',(-31.6678154208149,54.2194985998778,
2.86151233818597));
#212466=CARTESIAN_POINT('Ctrl Pts',(-31.6652181309759,54.211464809049,2.87470957722388));
#212467=CARTESIAN_POINT('Ctrl Pts',(-31.6618330358515,54.2038121508403,
2.88801594388901));
#212468=CARTESIAN_POINT('Ctrl Pts',(-31.6576696180587,54.1966007261208,
2.9013417351606));
#212469=CARTESIAN_POINT('',(-31.4795232016792,53.8880358395971,3.47153072139108));
#212470=CARTESIAN_POINT('',(-31.6576696180587,54.1966007261208,2.90134173516061));
#212471=CARTESIAN_POINT('',(-36.4252947698681,50.6762142289948,3.47153072139106));
#212472=CARTESIAN_POINT('Origin',(5.53234440788222E-15,1.85015204418142E-13,
3.47153072139072));
#212473=CARTESIAN_POINT('',(-36.6347241449657,50.9644637245893,2.90134173516059));
#212474=CARTESIAN_POINT('',(-36.4252947698681,50.6762142289948,3.47153072139106));
#212475=CARTESIAN_POINT('',(-36.991167339171,50.9399462128202,2.59908173516058));
#212476=CARTESIAN_POINT('Ctrl Pts',(-36.6347241449657,50.9644637245893,
2.90134173516059));
#212477=CARTESIAN_POINT('Ctrl Pts',(-36.6419574987897,50.9744193574538,
2.88164837656681));
#212478=CARTESIAN_POINT('Ctrl Pts',(-36.6507449107787,50.9831959997528,
2.86203734439024));
#212479=CARTESIAN_POINT('Ctrl Pts',(-36.6609215604531,50.9907013072131,
2.84277945977961));
#212480=CARTESIAN_POINT('Ctrl Pts',(-36.6713026986892,50.9983574255568,
2.82313460919768));
#212481=CARTESIAN_POINT('Ctrl Pts',(-36.6831299757328,51.0046913806545,
2.80385576863033));
#212482=CARTESIAN_POINT('Ctrl Pts',(-36.6962763075871,51.0095813473154,
2.78521678518032));
#212483=CARTESIAN_POINT('Ctrl Pts',(-36.7089119163662,51.0142813432044,
2.76730190934075));
#212484=CARTESIAN_POINT('Ctrl Pts',(-36.7227668523555,51.0176477981099,
2.74997687279352));
#212485=CARTESIAN_POINT('Ctrl Pts',(-36.7377619899139,51.0195423439513,
2.73349253345269));
#212486=CARTESIAN_POINT('Ctrl Pts',(-36.7492807342437,51.0209976683244,
2.72082983599006));
#212487=CARTESIAN_POINT('Ctrl Pts',(-36.7614730081831,51.0215839370839,
2.70866321039163));
#212488=CARTESIAN_POINT('Ctrl Pts',(-36.7743133764174,51.0212231059805,
2.69711645335879));
#212489=CARTESIAN_POINT('Ctrl Pts',(-36.7743470287326,51.0212221603065,
2.69708619136785));
#212490=CARTESIAN_POINT('Ctrl Pts',(-36.7743806860745,51.0212212075184,
2.69705593387252));
#212491=CARTESIAN_POINT('Ctrl Pts',(-36.77441434844,51.0212202476161,2.69702568087604));
#212492=CARTESIAN_POINT('Ctrl Pts',(-36.7780236385692,51.021117326564,2.693781944433));
#212493=CARTESIAN_POINT('Ctrl Pts',(-36.7816890091481,51.0209317131555,
2.69059266624734));
#212494=CARTESIAN_POINT('Ctrl Pts',(-36.7854055281044,51.0206635800337,
2.68746219342711));
#212495=CARTESIAN_POINT('Ctrl Pts',(-36.8060871110679,51.0191714801765,
2.67004182396082));
#212496=CARTESIAN_POINT('Ctrl Pts',(-36.8283529098785,51.0151289787604,
2.6544356787785));
#212497=CARTESIAN_POINT('Ctrl Pts',(-36.851318905231,51.008609334902,2.64136852353021));
#212498=CARTESIAN_POINT('Ctrl Pts',(-36.8616263619858,51.0056832284522,
2.63550380329658));
#212499=CARTESIAN_POINT('Ctrl Pts',(-36.8720751481058,51.0022583633864,
2.63014997451091));
#212500=CARTESIAN_POINT('Ctrl Pts',(-36.8825875141944,50.9983419378325,
2.62536981119287));
#212501=CARTESIAN_POINT('Ctrl Pts',(-36.8871560463068,50.9966399122601,
2.62329241687107));
#212502=CARTESIAN_POINT('Ctrl Pts',(-36.8917363891939,50.9948449951613,
2.62132362131461));
#212503=CARTESIAN_POINT('Ctrl Pts',(-36.896322033635,50.9929577488699,2.61946873372381));
#212504=CARTESIAN_POINT('Ctrl Pts',(-36.9123717891789,50.9863523868501,
2.61297662715601));
#212505=CARTESIAN_POINT('Ctrl Pts',(-36.9284864868683,50.9786159896082,
2.60787989114004));
#212506=CARTESIAN_POINT('Ctrl Pts',(-36.9443870542878,50.9697726815835,
2.60440616886214));
#212507=CARTESIAN_POINT('Ctrl Pts',(-36.9523373379975,50.9653510275712,
2.6026693077232));
#212508=CARTESIAN_POINT('Ctrl Pts',(-36.9602340894951,50.9606526463566,
2.60133820040219));
#212509=CARTESIAN_POINT('Ctrl Pts',(-36.9680424293792,50.9556805599063,
2.60044130723619));
#212510=CARTESIAN_POINT('Ctrl Pts',(-36.9719465993212,50.9531945166812,
2.59999286065319));
#212511=CARTESIAN_POINT('Ctrl Pts',(-36.9758286664323,50.9506400472469,
2.59965296768546));
#212512=CARTESIAN_POINT('Ctrl Pts',(-36.9796842711996,50.9480175299141,
2.59942518630988));
#212513=CARTESIAN_POINT('Ctrl Pts',(-36.983539875967,50.9453950125813,2.5991974049343));
#212514=CARTESIAN_POINT('Ctrl Pts',(-36.9873690173881,50.9427044459694,
2.59908173791649));
#212515=CARTESIAN_POINT('Ctrl Pts',(-36.991167339171,50.9399462128202,2.59908173516058));
#212516=CARTESIAN_POINT('',(-37.0158684358562,50.92199981559,2.59908173516059));
#212517=CARTESIAN_POINT('Origin',(5.16646552926933E-17,1.90981751651644E-13,
2.59908173516023));
#212518=CARTESIAN_POINT('',(-37.1493329797263,50.5905785208484,2.90134173516058));
#212519=CARTESIAN_POINT('Ctrl Pts',(-37.0158684358562,50.92199981559,2.59908173516059));
#212520=CARTESIAN_POINT('Ctrl Pts',(-37.0189596418151,50.9197527708151,
2.59908174381714));
#212521=CARTESIAN_POINT('Ctrl Pts',(-37.0220143142661,50.9174732734523,
2.5991575200103));
#212522=CARTESIAN_POINT('Ctrl Pts',(-37.0250315520727,50.9151633654183,
2.59930729517505));
#212523=CARTESIAN_POINT('Ctrl Pts',(-37.0424674644257,50.9018149465641,
2.60017281085948));
#212524=CARTESIAN_POINT('Ctrl Pts',(-37.0586566148275,50.8874508031649,
2.60350651800064));
#212525=CARTESIAN_POINT('Ctrl Pts',(-37.0734189188999,50.8724683783928,
2.60896880596422));
#212526=CARTESIAN_POINT('Ctrl Pts',(-37.0793728957242,50.8664256218267,
2.61117187235434));
#212527=CARTESIAN_POINT('Ctrl Pts',(-37.085095235135,50.8602822855875,2.61372076577201));
#212528=CARTESIAN_POINT('Ctrl Pts',(-37.0905759575257,50.8540642095547,
2.61659179897017));
#212529=CARTESIAN_POINT('Ctrl Pts',(-37.092598011339,50.851770117014,2.61765103591242));
#212530=CARTESIAN_POINT('Ctrl Pts',(-37.0945870443968,50.8494658679866,
2.61875422455183));
#212531=CARTESIAN_POINT('Ctrl Pts',(-37.0965424902854,50.8471527697479,
2.6199002244043));
#212532=CARTESIAN_POINT('Ctrl Pts',(-37.1002089513264,50.8428157105504,
2.62204897412767));
#212533=CARTESIAN_POINT('Ctrl Pts',(-37.1037573324719,50.8384475408395,
2.62434823201804));
#212534=CARTESIAN_POINT('Ctrl Pts',(-37.107183900098,50.8340568779948,2.62679048030339));
#212535=CARTESIAN_POINT('Ctrl Pts',(-37.1191768867891,50.8186895580383,
2.63533834930213));
#212536=CARTESIAN_POINT('Ctrl Pts',(-37.1296776552302,50.8030466935691,
2.64563784783596));
#212537=CARTESIAN_POINT('Ctrl Pts',(-37.1385261411559,50.7874977752343,
2.65736666737998));
#212538=CARTESIAN_POINT('Ctrl Pts',(-37.1429503841188,50.7797233160669,
2.66323107715198));
#212539=CARTESIAN_POINT('Ctrl Pts',(-37.1469615570465,50.7719723442507,
2.66945281780807));
#212540=CARTESIAN_POINT('Ctrl Pts',(-37.1505396571688,50.7642910532777,
2.67599160631234));
#212541=CARTESIAN_POINT('Ctrl Pts',(-37.1523287072299,50.7604504077913,
2.67926100056447));
#212542=CARTESIAN_POINT('Ctrl Pts',(-37.1540094891596,50.7566271826101,
2.68260965685158));
#212543=CARTESIAN_POINT('Ctrl Pts',(-37.1555795029288,50.7528271523479,
2.68603254012517));
#212544=CARTESIAN_POINT('Ctrl Pts',(-37.1571495166979,50.7490271220858,
2.68945542339877));
#212545=CARTESIAN_POINT('Ctrl Pts',(-37.1586086360832,50.7452503160125,
2.6929526152542));
#212546=CARTESIAN_POINT('Ctrl Pts',(-37.159954619824,50.7415024502313,2.69651891172134));
#212547=CARTESIAN_POINT('Ctrl Pts',(-37.1599660982463,50.7414704887854,
2.69654932476122));
#212548=CARTESIAN_POINT('Ctrl Pts',(-37.15997756849,50.7414385295747,2.6965797426118));
#212549=CARTESIAN_POINT('Ctrl Pts',(-37.1599890305542,50.7414065726022,
2.69661016527007));
#212550=CARTESIAN_POINT('Ctrl Pts',(-37.1658428740569,50.7250856801856,
2.71214746101035));
#212551=CARTESIAN_POINT('Ctrl Pts',(-37.1696950534564,50.7093579475533,
2.7288056556733));
#212552=CARTESIAN_POINT('Ctrl Pts',(-37.171705016148,50.6943448053458,2.74628040011927));
#212553=CARTESIAN_POINT('Ctrl Pts',(-37.1737829544432,50.6788239286381,
2.76434612881873));
#212554=CARTESIAN_POINT('Ctrl Pts',(-37.1738916781079,50.6640659432027,
2.78328592653761));
#212555=CARTESIAN_POINT('Ctrl Pts',(-37.172158124007,50.6502224037134,2.80278753267004));
#212556=CARTESIAN_POINT('Ctrl Pts',(-37.1704575457528,50.6366421974747,
2.82191817721855));
#212557=CARTESIAN_POINT('Ctrl Pts',(-37.1669834785952,50.6239412983545,
2.84159092314111));
#212558=CARTESIAN_POINT('Ctrl Pts',(-37.1618166822764,50.6122904325024,
2.86151233815872));
#212559=CARTESIAN_POINT('Ctrl Pts',(-37.1583938608521,50.6045721423299,
2.87470957720556));
#212560=CARTESIAN_POINT('Ctrl Pts',(-37.1542273890282,50.5973152449696,
2.88801594387984));
#212561=CARTESIAN_POINT('Ctrl Pts',(-37.1493329797263,50.5905785208484,
2.90134173516058));
#212562=CARTESIAN_POINT('',(-36.9399086546489,50.3023253561995,3.47153072139106));
#212563=CARTESIAN_POINT('',(-37.1493329797263,50.5905785208484,2.90134173516058));
#212564=CARTESIAN_POINT('',(-41.5228599914565,46.591124538743,3.47153072139103));
#212565=CARTESIAN_POINT('Origin',(5.53234440788222E-15,1.85015204418142E-13,
3.47153072139072));
#212566=CARTESIAN_POINT('',(-41.7612723673365,46.8559036426985,2.90134173516056));
#212567=CARTESIAN_POINT('',(-41.5228599914565,46.591124538743,3.47153072139103));
#212568=CARTESIAN_POINT('',(-42.1132001506003,46.7942619810917,2.59908173516055));
#212569=CARTESIAN_POINT('Ctrl Pts',(-41.7612723673365,46.8559036426985,
2.90134173516056));
#212570=CARTESIAN_POINT('Ctrl Pts',(-41.7695067430953,46.8650486462049,
2.88164837656725));
#212571=CARTESIAN_POINT('Ctrl Pts',(-41.7791634256538,46.8728586744676,
2.86203734439113));
#212572=CARTESIAN_POINT('Ctrl Pts',(-41.7900688448314,46.8792591175166,
2.84277945978094));
#212573=CARTESIAN_POINT('Ctrl Pts',(-41.8011933963908,46.8857881704162,
2.82313460919932));
#212574=CARTESIAN_POINT('Ctrl Pts',(-41.8136179609658,46.890851140351,2.80385576863226));
#212575=CARTESIAN_POINT('Ctrl Pts',(-41.8272034165388,46.8943401533967,
2.78521678518251));
#212576=CARTESIAN_POINT('Ctrl Pts',(-41.8402610894785,46.8976936214484,
2.76730190934294));
#212577=CARTESIAN_POINT('Ctrl Pts',(-41.8543920170367,46.8995933993941,
2.7499768727957));
#212578=CARTESIAN_POINT('Ctrl Pts',(-41.8695030436278,46.8999101480298,
2.73349253345484));
#212579=CARTESIAN_POINT('Ctrl Pts',(-41.8811108098919,46.9001534633403,
2.72082983599143));
#212580=CARTESIAN_POINT('Ctrl Pts',(-41.8932975750521,46.8994620807995,
2.70866321039226));
#212581=CARTESIAN_POINT('Ctrl Pts',(-41.9060298852857,46.8977610424072,
2.69711645335876));
#212582=CARTESIAN_POINT('Ctrl Pts',(-41.9060632544001,46.897756584289,2.69708619136782));
#212583=CARTESIAN_POINT('Ctrl Pts',(-41.9060966277702,46.8977521185701,
2.69705593387249));
#212584=CARTESIAN_POINT('Ctrl Pts',(-41.9061300053926,46.8977476452509,
2.69702568087601));
#212585=CARTESIAN_POINT('Ctrl Pts',(-41.9097087652734,46.8972680144605,
2.69378194443296));
#212586=CARTESIAN_POINT('Ctrl Pts',(-41.9133346546844,46.8967002823077,
2.6905926662473));
#212587=CARTESIAN_POINT('Ctrl Pts',(-41.9170027866178,46.896045136032,2.68746219342707));
#212588=CARTESIAN_POINT('Ctrl Pts',(-41.9374151068008,46.8923993959688,
2.67004182396078));
#212589=CARTESIAN_POINT('Ctrl Pts',(-41.9591363747749,46.8860516300653,
2.65443567877847));
#212590=CARTESIAN_POINT('Ctrl Pts',(-41.9812950716484,46.8771671012965,
2.64136852353018));
#212591=CARTESIAN_POINT('Ctrl Pts',(-41.991240201666,46.8731796017492,2.63550380329656));
#212592=CARTESIAN_POINT('Ctrl Pts',(-42.0012737523602,46.8686813028964,
2.63014997451089));
#212593=CARTESIAN_POINT('Ctrl Pts',(-42.0113191526627,46.863687490459,2.62536981119286));
#212594=CARTESIAN_POINT('Ctrl Pts',(-42.0156847477607,46.8615172471197,
2.62329241687106));
#212595=CARTESIAN_POINT('Ctrl Pts',(-42.0200523791242,46.8592533865613,
2.62132362131461));
#212596=CARTESIAN_POINT('Ctrl Pts',(-42.0244156319706,46.8568971484361,
2.61946873372381));
#212597=CARTESIAN_POINT('Ctrl Pts',(-42.039687016933,46.8486503149977,2.612976627156));
#212598=CARTESIAN_POINT('Ctrl Pts',(-42.0549047629075,46.8392718539638,
2.60787989114001));
#212599=CARTESIAN_POINT('Ctrl Pts',(-42.0697938479569,46.8288149286284,
2.60440616886211));
#212600=CARTESIAN_POINT('Ctrl Pts',(-42.0772383904816,46.8235864659607,
2.60266930772316));
#212601=CARTESIAN_POINT('Ctrl Pts',(-42.0846007681801,46.8180883876711,
2.60133820040216));
#212602=CARTESIAN_POINT('Ctrl Pts',(-42.0918466086054,46.8123273450619,
2.60044130723616));
#212603=CARTESIAN_POINT('Ctrl Pts',(-42.095469528818,46.8094468237573,2.59999286065315));
#212604=CARTESIAN_POINT('Ctrl Pts',(-42.0990633147948,46.8065005614644,
2.59965296768544));
#212605=CARTESIAN_POINT('Ctrl Pts',(-42.1026236704492,46.8034893901146,
2.59942518630986));
#212606=CARTESIAN_POINT('Ctrl Pts',(-42.1061840261035,46.8004782187649,
2.59919740493428));
#212607=CARTESIAN_POINT('Ctrl Pts',(-42.109710950294,46.79740213709,2.5990817379165));
#212608=CARTESIAN_POINT('Ctrl Pts',(-42.1132001506003,46.7942619810917,
2.59908173516055));
#212609=CARTESIAN_POINT('',(-42.1358900227697,46.7738319284257,2.59908173516056));
#212610=CARTESIAN_POINT('Origin',(6.43067523875937E-17,1.90991989020018E-13,
2.59908173516023));
#212611=CARTESIAN_POINT('',(-42.2339804752703,46.4302753505425,2.90134173516055));
#212612=CARTESIAN_POINT('Ctrl Pts',(-42.1358900227697,46.7738319284257,
2.59908173516056));
#212613=CARTESIAN_POINT('Ctrl Pts',(-42.1387294146417,46.7712740741887,
2.59908174381715));
#212614=CARTESIAN_POINT('Ctrl Pts',(-42.141529080921,46.7686877639339,2.59915752001027));
#212615=CARTESIAN_POINT('Ctrl Pts',(-42.1442883388461,46.7660751225865,
2.59930729517502));
#212616=CARTESIAN_POINT('Ctrl Pts',(-42.1602334457364,46.7509772786441,
2.60017281085941));
#212617=CARTESIAN_POINT('Ctrl Pts',(-42.1748324484422,46.7349995965129,
2.60350651800036));
#212618=CARTESIAN_POINT('Ctrl Pts',(-42.1879477932305,46.7185561660731,
2.60896880596357));
#212619=CARTESIAN_POINT('Ctrl Pts',(-42.1932375134895,46.7119241523113,
2.61117187235383));
#212620=CARTESIAN_POINT('Ctrl Pts',(-42.1982863518305,46.7052163225653,
2.61372076577171));
#212621=CARTESIAN_POINT('Ctrl Pts',(-42.2030870843187,46.6984594183138,
2.61659179897015));
#212622=CARTESIAN_POINT('Ctrl Pts',(-42.2048582631418,46.6959665308744,
2.6176510359124));
#212623=CARTESIAN_POINT('Ctrl Pts',(-42.2065955404586,46.6934669941954,
2.6187542245518));
#212624=CARTESIAN_POINT('Ctrl Pts',(-42.2082984896057,46.6909621675971,
2.61990022440427));
#212625=CARTESIAN_POINT('Ctrl Pts',(-42.2114915192564,46.6862656177254,
2.62204897412764));
#212626=CARTESIAN_POINT('Ctrl Pts',(-42.2145638639316,46.681550470477,2.624348232018));
#212627=CARTESIAN_POINT('Ctrl Pts',(-42.2175127112218,46.6768256862946,
2.62679048030335));
#212628=CARTESIAN_POINT('Ctrl Pts',(-42.2278336767374,46.6602889416559,
2.63533834930209));
#212629=CARTESIAN_POINT('Ctrl Pts',(-42.2366417962861,46.6436341412466,
2.64563784783593));
#212630=CARTESIAN_POINT('Ctrl Pts',(-42.2438165047411,46.6272454828774,
2.65736666737995));
#212631=CARTESIAN_POINT('Ctrl Pts',(-42.2474038589686,46.6190511536928,
2.66323107715195));
#212632=CARTESIAN_POINT('Ctrl Pts',(-42.2505828610985,46.610923360769,2.66945281780804));
#212633=CARTESIAN_POINT('Ctrl Pts',(-42.2533384464727,46.6029101354046,
2.67599160631231));
#212634=CARTESIAN_POINT('Ctrl Pts',(-42.2547162391598,46.5989035227223,
2.67926100056444));
#212635=CARTESIAN_POINT('Ctrl Pts',(-42.2559881777373,46.5949255520165,
2.68260965685153));
#212636=CARTESIAN_POINT('Ctrl Pts',(-42.257152379483,46.5909822275912,2.68603254012512));
#212637=CARTESIAN_POINT('Ctrl Pts',(-42.2583165812288,46.5870389031658,
2.68945542339871));
#212638=CARTESIAN_POINT('Ctrl Pts',(-42.2593729236706,46.5831302673243,
2.69295261525415));
#212639=CARTESIAN_POINT('Ctrl Pts',(-42.2603197753209,46.5792622391319,
2.69651891172129));
#212640=CARTESIAN_POINT('Ctrl Pts',(-42.2603278499825,46.5792292529524,
2.69654932476117));
#212641=CARTESIAN_POINT('Ctrl Pts',(-42.2603359167438,46.5791962698506,
2.69657974261176));
#212642=CARTESIAN_POINT('Ctrl Pts',(-42.2603439756043,46.5791632898298,
2.69661016527004));
#212643=CARTESIAN_POINT('Ctrl Pts',(-42.2644597533368,46.5623199117021,
2.71214746101208));
#212644=CARTESIAN_POINT('Ctrl Pts',(-42.2666468343717,46.5462756748402,
2.72880565567704));
#212645=CARTESIAN_POINT('Ctrl Pts',(-42.2670764855933,46.5311346778838,
2.74628040012518));
#212646=CARTESIAN_POINT('Ctrl Pts',(-42.2675206673338,46.5154816224641,
2.76434612882708));
#212647=CARTESIAN_POINT('Ctrl Pts',(-42.2660861658596,46.5007931180981,
2.78328592654859));
#212648=CARTESIAN_POINT('Ctrl Pts',(-42.2629150644391,46.4872066207116,
2.80278753268372));
#212649=CARTESIAN_POINT('Ctrl Pts',(-42.2598042840403,46.473878567094,2.82191817723495));
#212650=CARTESIAN_POINT('Ctrl Pts',(-42.2550216427174,46.4616103837285,
2.8415909231603));
#212651=CARTESIAN_POINT('Ctrl Pts',(-42.2486653035442,46.4505634198172,
2.86151233818066));
#212652=CARTESIAN_POINT('Ctrl Pts',(-42.2444544516846,46.443245193514,2.8747095772203));
#212653=CARTESIAN_POINT('Ctrl Pts',(-42.2395522519026,46.4364635650978,
2.8880159438872));
#212654=CARTESIAN_POINT('Ctrl Pts',(-42.2339804752703,46.4302753505425,
2.90134173516055));
#212655=CARTESIAN_POINT('',(-41.9955727382253,46.1654920697612,3.47153072139103));
#212656=CARTESIAN_POINT('',(-42.2339804752703,46.4302753505425,2.90134173516055));
#212657=CARTESIAN_POINT('',(-46.1654920697614,41.995572738225,3.47153072139101));
#212658=CARTESIAN_POINT('Origin',(5.53234440788222E-15,1.85015204418142E-13,
3.47153072139072));
#212659=CARTESIAN_POINT('',(-46.4302753505427,42.2339804752701,2.90134173516052));
#212660=CARTESIAN_POINT('',(-46.1654920697614,41.995572738225,3.471530721391));
#212661=CARTESIAN_POINT('',(-46.7738319284259,42.1358900227694,2.59908173516052));
#212662=CARTESIAN_POINT('Ctrl Pts',(-46.4302753505427,42.2339804752701,
2.90134173516052));
#212663=CARTESIAN_POINT('Ctrl Pts',(-46.4394205306926,42.2422146548461,
2.88164837656763));
#212664=CARTESIAN_POINT('Ctrl Pts',(-46.4498406831858,42.2489725007686,
2.86203734439193));
#212665=CARTESIAN_POINT('Ctrl Pts',(-46.4613553898119,42.2541979548129,
2.84277945978213));
#212666=CARTESIAN_POINT('Ctrl Pts',(-46.4731014717798,42.2595284085983,
2.82313460920106));
#212667=CARTESIAN_POINT('Ctrl Pts',(-46.4859871977564,42.2632649224123,
2.80385576863452));
#212668=CARTESIAN_POINT('Ctrl Pts',(-46.4998629319538,42.2653147554857,
2.78521678518525));
#212669=CARTESIAN_POINT('Ctrl Pts',(-46.5131996064562,42.2672849544025,
2.76730190934637));
#212670=CARTESIAN_POINT('Ctrl Pts',(-46.5274517041831,42.2676972410239,
2.74997687279975));
#212671=CARTESIAN_POINT('Ctrl Pts',(-46.5425130602368,42.2664327220898,
2.73349253345943));
#212672=CARTESIAN_POINT('Ctrl Pts',(-46.5540826713195,42.2654613625242,
2.72082983599435));
#212673=CARTESIAN_POINT('Ctrl Pts',(-46.566130406952,42.2634999036149,2.70866321039363));
#212674=CARTESIAN_POINT('Ctrl Pts',(-46.5786151613303,42.2604772948659,
2.69711645335872));
#212675=CARTESIAN_POINT('Ctrl Pts',(-46.578647881645,42.2604693731475,2.69708619136778));
#212676=CARTESIAN_POINT('Ctrl Pts',(-46.5786806053975,42.2604614434252,
2.69705593387246));
#212677=CARTESIAN_POINT('Ctrl Pts',(-46.5787133325845,42.2604535056997,
2.69702568087598));
#212678=CARTESIAN_POINT('Ctrl Pts',(-46.5822223525748,42.2596024201062,
2.69378194443293));
#212679=CARTESIAN_POINT('Ctrl Pts',(-46.5857690348148,42.2586587894014,
2.69059266624727));
#212680=CARTESIAN_POINT('Ctrl Pts',(-46.5893485909042,42.2576238078915,
2.68746219342704));
#212681=CARTESIAN_POINT('Ctrl Pts',(-46.6092680066546,42.2518643711136,
2.67004182396129));
#212682=CARTESIAN_POINT('Ctrl Pts',(-46.6302067610343,42.2432808881746,
2.65443567877939));
#212683=CARTESIAN_POINT('Ctrl Pts',(-46.6513153841081,42.2321288152523,
2.64136852353134));
#212684=CARTESIAN_POINT('Ctrl Pts',(-46.6607892264636,42.2271236104868,
2.63550380329725));
#212685=CARTESIAN_POINT('Ctrl Pts',(-46.6702976120515,42.2216011621503,
2.63014997451117));
#212686=CARTESIAN_POINT('Ctrl Pts',(-46.6797659870608,42.2155846760829,
2.62536981119281));
#212687=CARTESIAN_POINT('Ctrl Pts',(-46.6838808147709,42.2129699926169,
2.62329241687101));
#212688=CARTESIAN_POINT('Ctrl Pts',(-46.6879878819276,42.210261991929,2.62132362131455));
#212689=CARTESIAN_POINT('Ctrl Pts',(-46.692080938468,42.2074625774078,2.61946873372376));
#212690=CARTESIAN_POINT('Ctrl Pts',(-46.7064066363596,42.1976646265838,
2.61297662715596));
#212691=CARTESIAN_POINT('Ctrl Pts',(-46.7205607018097,42.1867468541397,
2.60787989113998));
#212692=CARTESIAN_POINT('Ctrl Pts',(-46.7342751765575,42.1747908797557,
2.60440616886208));
#212693=CARTESIAN_POINT('Ctrl Pts',(-46.7411324139314,42.1688128925637,
2.60266930772313));
#212694=CARTESIAN_POINT('Ctrl Pts',(-46.74787975408,42.1625753552954,2.60133820040213));
#212695=CARTESIAN_POINT('Ctrl Pts',(-46.7544837081025,42.1560884757157,
2.60044130723612));
#212696=CARTESIAN_POINT('Ctrl Pts',(-46.7577856851138,42.1528450359258,
2.59999286065312));
#212697=CARTESIAN_POINT('Ctrl Pts',(-46.7610518156851,42.1495392606406,
2.59965296768541));
#212698=CARTESIAN_POINT('Ctrl Pts',(-46.7642779142248,42.1461724262973,
2.59942518630983));
#212699=CARTESIAN_POINT('Ctrl Pts',(-46.7675040127646,42.142805591954,2.59919740493425));
#212700=CARTESIAN_POINT('Ctrl Pts',(-46.770690078005,42.1393776974108,2.59908173791641));
#212701=CARTESIAN_POINT('Ctrl Pts',(-46.773831928426,42.1358900227694,2.59908173516052));
#212702=CARTESIAN_POINT('',(-46.7942619810919,42.1132001506,2.59908173516053));
#212703=CARTESIAN_POINT('Origin',(7.58094983678529E-17,1.91003491765998E-13,
2.59908173516023));
#212704=CARTESIAN_POINT('',(-46.8559036426987,41.7612723673362,2.90134173516051));
#212705=CARTESIAN_POINT('Ctrl Pts',(-46.7942619810919,42.1132001506,2.59908173516052));
#212706=CARTESIAN_POINT('Ctrl Pts',(-46.7968184499054,42.1103595112871,
2.5990817438171));
#212707=CARTESIAN_POINT('Ctrl Pts',(-46.7993324362835,42.1074947242967,
2.59915752001025));
#212708=CARTESIAN_POINT('Ctrl Pts',(-46.8018034833198,42.1046079742813,
2.599307295175));
#212709=CARTESIAN_POINT('Ctrl Pts',(-46.8160830868207,42.0879261203874,
2.60017281085942));
#212710=CARTESIAN_POINT('Ctrl Pts',(-46.8289319921028,42.0705099543521,
2.60350651800053));
#212711=CARTESIAN_POINT('Ctrl Pts',(-46.8402566831455,42.0527856759081,
2.60896880596404));
#212712=CARTESIAN_POINT('Ctrl Pts',(-46.8448241915563,42.0456370666824,
2.61117187235418));
#212713=CARTESIAN_POINT('Ctrl Pts',(-46.849144212697,42.0384382358171,2.61372076577189));
#212714=CARTESIAN_POINT('Ctrl Pts',(-46.8532123574521,42.0312165334051,
2.6165917989701));
#212715=CARTESIAN_POINT('Ctrl Pts',(-46.8547132558791,42.0285521636634,
2.61765103591236));
#212716=CARTESIAN_POINT('Ctrl Pts',(-46.8561797434811,42.0258847247796,
2.61875422455176));
#212717=CARTESIAN_POINT('Ctrl Pts',(-46.8576115380195,42.0232156132262,
2.61990022440423));
#212718=CARTESIAN_POINT('Ctrl Pts',(-46.860296152779,42.0182110290635,2.6220489741276));
#212719=CARTESIAN_POINT('Ctrl Pts',(-46.8628587997326,42.0132005644176,
2.62434823201797));
#212720=CARTESIAN_POINT('Ctrl Pts',(-46.8652976184989,42.0081934246215,
2.62679048030332));
#212721=CARTESIAN_POINT('Ctrl Pts',(-46.873833484181,41.9906684353355,2.63533834930206));
#212722=CARTESIAN_POINT('Ctrl Pts',(-46.8808524512365,41.9731841724648,
2.64563784783589));
#212723=CARTESIAN_POINT('Ctrl Pts',(-46.8862747746135,41.9561353316317,
2.65736666737991));
#212724=CARTESIAN_POINT('Ctrl Pts',(-46.888985936302,41.9476109112151,2.66323107715191));
#212725=CARTESIAN_POINT('Ctrl Pts',(-46.8912979378216,41.9391953469841,
2.669452817808));
#212726=CARTESIAN_POINT('Ctrl Pts',(-46.8932008176775,41.930937981802,2.67599160631227));
#212727=CARTESIAN_POINT('Ctrl Pts',(-46.8941522576055,41.926809299211,2.6792610005644));
#212728=CARTESIAN_POINT('Ctrl Pts',(-46.8950014172056,41.92272016646,2.68260965685149));
#212729=CARTESIAN_POINT('Ctrl Pts',(-46.8957470516901,41.9186767517591,
2.68603254012509));
#212730=CARTESIAN_POINT('Ctrl Pts',(-46.8964926861745,41.9146333370581,
2.68945542339868));
#212731=CARTESIAN_POINT('Ctrl Pts',(-46.8971346781638,41.9106356952805,
2.69295261525412));
#212732=CARTESIAN_POINT('Ctrl Pts',(-46.8976720238189,41.9066898836034,
2.69651891172126));
#212733=CARTESIAN_POINT('Ctrl Pts',(-46.897676606252,41.9066562340936,2.69654932476114));
#212734=CARTESIAN_POINT('Ctrl Pts',(-46.8976811811498,41.9066225884706,
2.69657974261172));
#212735=CARTESIAN_POINT('Ctrl Pts',(-46.8976857485122,41.9065889467375,
2.69661016527));
#212736=CARTESIAN_POINT('Ctrl Pts',(-46.9000183671518,41.8894076224752,
2.71214746101269));
#212737=CARTESIAN_POINT('Ctrl Pts',(-46.9005163877045,41.8732226654013,
2.72880565567839));
#212738=CARTESIAN_POINT('Ctrl Pts',(-46.8993610201073,41.858119701628,2.74628040012732));
#212739=CARTESIAN_POINT('Ctrl Pts',(-46.8981665787452,41.8425059656485,
2.76434612882993));
#212740=CARTESIAN_POINT('Ctrl Pts',(-46.8952045688308,41.8280478726805,
2.7832859265522));
#212741=CARTESIAN_POINT('Ctrl Pts',(-46.8906306633423,41.8148672739063,
2.80278753268811));
#212742=CARTESIAN_POINT('Ctrl Pts',(-46.8861437631607,41.8019373978555,
2.82191817723983));
#212743=CARTESIAN_POINT('Ctrl Pts',(-46.8801049472927,41.79023634303,2.84159092316567));
#212744=CARTESIAN_POINT('Ctrl Pts',(-46.8726287066487,41.7799143139087,
2.8615123381865));
#212745=CARTESIAN_POINT('Ctrl Pts',(-46.8676759593274,41.77307633149,2.87470957722421));
#212746=CARTESIAN_POINT('Ctrl Pts',(-46.8620917411125,41.7668442729548,
2.88801594388914));
#212747=CARTESIAN_POINT('Ctrl Pts',(-46.8559036426987,41.7612723673362,
2.90134173516052));
#212748=CARTESIAN_POINT('',(-46.5911245387432,41.5228599914562,3.471530721391));
#212749=CARTESIAN_POINT('',(-46.8559036426987,41.7612723673362,2.90134173516051));
#212750=CARTESIAN_POINT('',(-50.3023253561997,36.9399086546485,3.47153072139096));
#212751=CARTESIAN_POINT('Origin',(5.53234440788222E-15,1.85015204418142E-13,
3.47153072139072));
#212752=CARTESIAN_POINT('',(-50.5905785208486,37.149332979726,2.90134173516049));
#212753=CARTESIAN_POINT('',(-50.3023253561997,36.9399086546485,3.47153072139097));
#212754=CARTESIAN_POINT('',(-50.9219998155902,37.0158684358559,2.59908173516048));
#212755=CARTESIAN_POINT('Ctrl Pts',(-50.5905785208486,37.149332979726,2.90134173516048));
#212756=CARTESIAN_POINT('Ctrl Pts',(-50.600534308882,37.1565661199777,2.88164837656735));
#212757=CARTESIAN_POINT('Ctrl Pts',(-50.611603765939,37.1621977431861,2.86203734439141));
#212758=CARTESIAN_POINT('Ctrl Pts',(-50.6236016024787,37.1661909570579,
2.84277945978138));
#212759=CARTESIAN_POINT('Ctrl Pts',(-50.6358405223235,37.1702644101623,
2.82313460919987));
#212760=CARTESIAN_POINT('Ctrl Pts',(-50.6490462309923,37.1726335298282,
2.80385576863291));
#212761=CARTESIAN_POINT('Ctrl Pts',(-50.6630602183674,37.173221724529,2.78521678518325));
#212762=CARTESIAN_POINT('Ctrl Pts',(-50.6765297750374,37.1737870683989,
2.76730190934354));
#212763=CARTESIAN_POINT('Ctrl Pts',(-50.6907468939695,37.172707346597,2.74997687279617));
#212764=CARTESIAN_POINT('Ctrl Pts',(-50.7055935641188,37.1698754144265,
2.73349253345519));
#212765=CARTESIAN_POINT('Ctrl Pts',(-50.7169982609376,37.1677000224031,
2.72082983599163));
#212766=CARTESIAN_POINT('Ctrl Pts',(-50.7287749695268,37.1644899772796,
2.70866321039233));
#212767=CARTESIAN_POINT('Ctrl Pts',(-50.7408753824654,37.1601789145087,
2.69711645335869));
#212768=CARTESIAN_POINT('Ctrl Pts',(-50.7409070954898,37.160167615982,2.69708619136775));
#212769=CARTESIAN_POINT('Ctrl Pts',(-50.7409388110965,37.160156309136,2.69705593387243));
#212770=CARTESIAN_POINT('Ctrl Pts',(-50.7409705292823,37.1601449939716,
2.69702568087595));
#212771=CARTESIAN_POINT('Ctrl Pts',(-50.7443713638247,37.1589317782469,
2.6937819444329));
#212772=CARTESIAN_POINT('Ctrl Pts',(-50.7477999807009,37.1576225876056,
2.69059266624724));
#212773=CARTESIAN_POINT('Ctrl Pts',(-50.7512517425808,37.1562191103355,
2.68746219342701));
#212774=CARTESIAN_POINT('Ctrl Pts',(-50.7704600126106,37.1484090784377,
2.6700418239623));
#212775=CARTESIAN_POINT('Ctrl Pts',(-50.7903868440206,37.1376839208992,
2.65443567878123));
#212776=CARTESIAN_POINT('Ctrl Pts',(-50.8102141228026,37.1243864882687,
2.64136852353366));
#212777=CARTESIAN_POINT('Ctrl Pts',(-50.8191128800971,37.1184184163553,
2.63550380329865));
#212778=CARTESIAN_POINT('Ctrl Pts',(-50.827991924717,37.1119323236341,2.63014997451179));
#212779=CARTESIAN_POINT('Ctrl Pts',(-50.8367795369356,37.1049590818167,
2.6253698111928));
#212780=CARTESIAN_POINT('Ctrl Pts',(-50.8405985143443,37.1019286052431,
2.62329241687099));
#212781=CARTESIAN_POINT('Ctrl Pts',(-50.8444000194069,37.0988061338479,
2.62132362131454));
#212782=CARTESIAN_POINT('Ctrl Pts',(-50.8481780352574,37.0955942139022,
2.61946873372374));
#212783=CARTESIAN_POINT('Ctrl Pts',(-50.8614010907342,37.084352494092,2.61297662715593));
#212784=CARTESIAN_POINT('Ctrl Pts',(-50.8743364007569,37.0720150276372,
2.60787989113995));
#212785=CARTESIAN_POINT('Ctrl Pts',(-50.8867260065479,37.058690996362,2.60440616886204));
#212786=CARTESIAN_POINT('Ctrl Pts',(-50.8929208094434,37.0520289807244,
2.60266930772309));
#212787=CARTESIAN_POINT('Ctrl Pts',(-50.8989791867714,37.045120324241,2.6013382004021));
#212788=CARTESIAN_POINT('Ctrl Pts',(-50.9048689000889,37.0379786793009,
2.6004413072361));
#212789=CARTESIAN_POINT('Ctrl Pts',(-50.9078137567477,37.0344078568308,
2.59999286065309));
#212790=CARTESIAN_POINT('Ctrl Pts',(-50.9107164475036,37.030778787319,2.59965296768537));
#212791=CARTESIAN_POINT('Ctrl Pts',(-50.913572943118,37.0270931777238,2.59942518630979));
#212792=CARTESIAN_POINT('Ctrl Pts',(-50.9164294387324,37.0234075681287,
2.59919740493421));
#212793=CARTESIAN_POINT('Ctrl Pts',(-50.9192397378252,37.0196654174469,
2.59908173791642));
#212794=CARTESIAN_POINT('Ctrl Pts',(-50.9219998155902,37.0158684358559,
2.59908173516049));
#212795=CARTESIAN_POINT('',(-50.9399462128204,36.9911673391707,2.59908173516048));
#212796=CARTESIAN_POINT('Origin',(8.60468667414046E-17,1.91016133863093E-13,
2.59908173516023));
#212797=CARTESIAN_POINT('',(-50.9644637245895,36.6347241449654,2.90134173516048));
#212798=CARTESIAN_POINT('Ctrl Pts',(-50.9399462128204,36.9911673391707,
2.59908173516049));
#212799=CARTESIAN_POINT('Ctrl Pts',(-50.9421917493682,36.9880750374207,
2.59908174381708));
#212800=CARTESIAN_POINT('Ctrl Pts',(-50.9443925120841,36.9849631609003,
2.5991575200102));
#212801=CARTESIAN_POINT('Ctrl Pts',(-50.9465482749233,36.9818339300543,
2.59930729517495));
#212802=CARTESIAN_POINT('Ctrl Pts',(-50.9590059247116,36.9637508360892,
2.60017281085948));
#212803=CARTESIAN_POINT('Ctrl Pts',(-50.9699639572756,36.9450870013076,
2.60350651800129));
#212804=CARTESIAN_POINT('Ctrl Pts',(-50.9793739188884,36.9262760657615,
2.60896880596596));
#212805=CARTESIAN_POINT('Ctrl Pts',(-50.983169172872,36.9186891827322,2.61117187235565));
#212806=CARTESIAN_POINT('Ctrl Pts',(-50.9867130457561,36.9110782226467,
2.61372076577271));
#212807=CARTESIAN_POINT('Ctrl Pts',(-50.9900040313323,36.9034708445588,
2.61659179897008));
#212808=CARTESIAN_POINT('Ctrl Pts',(-50.991218205206,36.9006641839072,2.61765103591233));
#212809=CARTESIAN_POINT('Ctrl Pts',(-50.9923978359481,36.8978580678373,
2.61875422455174));
#212810=CARTESIAN_POINT('Ctrl Pts',(-50.9935427888372,36.8950539146734,
2.61990022440421));
#212811=CARTESIAN_POINT('Ctrl Pts',(-50.9956895755044,36.8897961274911,
2.62204897412758));
#212812=CARTESIAN_POINT('Ctrl Pts',(-50.9977144478401,36.8845452411468,
2.62434823201794));
#212813=CARTESIAN_POINT('Ctrl Pts',(-50.9996165178738,36.8793106050087,
2.62679048030329));
#212814=CARTESIAN_POINT('Ctrl Pts',(-51.0062737629918,36.8609893785252,
2.63533834930203));
#212815=CARTESIAN_POINT('Ctrl Pts',(-51.011426676282,36.8428672144359,2.64563784783588));
#212816=CARTESIAN_POINT('Ctrl Pts',(-51.0150372064714,36.8253449818068,
2.65736666737989));
#212817=CARTESIAN_POINT('Ctrl Pts',(-51.0168424715662,36.8165838654922,
2.66323107715189));
#212818=CARTESIAN_POINT('Ctrl Pts',(-51.0182621417029,36.8079727326367,
2.66945281780798));
#212819=CARTESIAN_POINT('Ctrl Pts',(-51.0192914676908,36.799561697058,2.67599160631225));
#212820=CARTESIAN_POINT('Ctrl Pts',(-51.0198061306847,36.7953561792686,
2.67926100056438));
#212821=CARTESIAN_POINT('Ctrl Pts',(-51.0202232077371,36.7912006858666,
2.68260965685147));
#212822=CARTESIAN_POINT('Ctrl Pts',(-51.0205421056328,36.7871014813876,
2.68603254012506));
#212823=CARTESIAN_POINT('Ctrl Pts',(-51.0208610035285,36.7830022769086,
2.68945542339865));
#212824=CARTESIAN_POINT('Ctrl Pts',(-51.0210816112668,36.778959428195,2.69295261525409));
#212825=CARTESIAN_POINT('Ctrl Pts',(-51.0212035636552,36.7749790641715,
2.69651891172123));
#212826=CARTESIAN_POINT('Ctrl Pts',(-51.0212046036537,36.7749451200025,
2.69654932476111));
#212827=CARTESIAN_POINT('Ctrl Pts',(-51.0212056365645,36.7749111804867,
2.69657974261169));
#212828=CARTESIAN_POINT('Ctrl Pts',(-51.0212066623877,36.7748772456272,
2.69661016526997));
#212829=CARTESIAN_POINT('Ctrl Pts',(-51.0217305652763,36.7575462174155,
2.71214746101237));
#212830=CARTESIAN_POINT('Ctrl Pts',(-51.0205340689294,36.7413978659071,
2.72880565567775));
#212831=CARTESIAN_POINT('Ctrl Pts',(-51.0178063409629,36.7264984065491,
2.74628040012634));
#212832=CARTESIAN_POINT('Ctrl Pts',(-51.0149863630479,36.7110950573693,
2.7643461288285));
#212833=CARTESIAN_POINT('Ctrl Pts',(-51.0105292970942,36.6970257816921,
2.7832859265503));
#212834=CARTESIAN_POINT('Ctrl Pts',(-51.0046027002041,36.6843954909291,
2.80278753268571));
#212835=CARTESIAN_POINT('Ctrl Pts',(-50.9987888396576,36.6720054548733,
2.82191817723679));
#212836=CARTESIAN_POINT('Ctrl Pts',(-50.9915600117756,36.6609997277932,
2.84159092316196));
#212837=CARTESIAN_POINT('Ctrl Pts',(-50.9830457809187,36.6515157237731,
2.86151233818214));
#212838=CARTESIAN_POINT('Ctrl Pts',(-50.9774054014708,36.6452329036033,
2.87470957722126));
#212839=CARTESIAN_POINT('Ctrl Pts',(-50.9712003466853,36.6396186946847,
2.88801594388765));
#212840=CARTESIAN_POINT('Ctrl Pts',(-50.9644637245895,36.6347241449654,
2.90134173516048));
#212841=CARTESIAN_POINT('',(-50.676214228995,36.4252947698678,3.47153072139096));
#212842=CARTESIAN_POINT('',(-50.9644637245895,36.6347241449654,2.90134173516049));
#212843=CARTESIAN_POINT('',(-53.8880358395972,31.4795232016788,3.47153072139093));
#212844=CARTESIAN_POINT('Origin',(5.53234440788222E-15,1.85015204418142E-13,
3.47153072139072));
#212845=CARTESIAN_POINT('',(-54.1966007261209,31.6576696180583,2.90134173516045));
#212846=CARTESIAN_POINT('',(-53.8880358395972,31.4795232016789,3.47153072139093));
#212847=CARTESIAN_POINT('',(-54.5122556166612,31.4902932482906,2.59908173516044));
#212848=CARTESIAN_POINT('Ctrl Pts',(-54.1966007261209,31.6576696180583,
2.90134173516045));
#212849=CARTESIAN_POINT('Ctrl Pts',(-54.2072580443415,31.6638224711873,
2.8816483765665));
#212850=CARTESIAN_POINT('Ctrl Pts',(-54.2188555266747,31.6682661704392,
2.86203734438975));
#212851=CARTESIAN_POINT('Ctrl Pts',(-54.2312050423205,31.6709833936514,
2.84277945977895));
#212852=CARTESIAN_POINT('Ctrl Pts',(-54.2438027078756,31.6737552164701,
2.82313460919676));
#212853=CARTESIAN_POINT('Ctrl Pts',(-54.2571837147291,31.6747309854169,
2.80385576862914));
#212854=CARTESIAN_POINT('Ctrl Pts',(-54.2711824151039,31.6738510973608,
2.7852167851789));
#212855=CARTESIAN_POINT('Ctrl Pts',(-54.2846372786593,31.6730053921579,
2.76730190933893));
#212856=CARTESIAN_POINT('Ctrl Pts',(-54.298663653066,31.6704454915906,2.74997687279134));
#212857=CARTESIAN_POINT('Ctrl Pts',(-54.3131329740852,31.6660771734251,
2.7334925334502));
#212858=CARTESIAN_POINT('Ctrl Pts',(-54.3242478043949,31.6627215829945,
2.72082983598842));
#212859=CARTESIAN_POINT('Ctrl Pts',(-54.3356244578571,31.6582981215833,
2.70866321039078));
#212860=CARTESIAN_POINT('Ctrl Pts',(-54.3472079546995,31.6527458376967,
2.69711645335865));
#212861=CARTESIAN_POINT('Ctrl Pts',(-54.347238312979,31.6527312861508,2.69708619136771));
#212862=CARTESIAN_POINT('Ctrl Pts',(-54.347268672957,31.6527167260613,2.69705593387238));
#212863=CARTESIAN_POINT('Ctrl Pts',(-54.3472990346306,31.6527021574293,
2.6970256808759));
#212864=CARTESIAN_POINT('Ctrl Pts',(-54.3505544234702,31.6511401038187,
2.69378194443285));
#212865=CARTESIAN_POINT('Ctrl Pts',(-54.3538274103385,31.6494796970076,
2.6905926662472));
#212866=CARTESIAN_POINT('Ctrl Pts',(-54.3571135597834,31.6477231007679,
2.68746219342697));
#212867=CARTESIAN_POINT('Ctrl Pts',(-54.3754002342689,31.6379480420932,
2.67004182396126));
#212868=CARTESIAN_POINT('Ctrl Pts',(-54.3940968201768,31.6251987170239,
2.65443567877941));
#212869=CARTESIAN_POINT('Ctrl Pts',(-54.4124255228538,31.6099016141377,
2.64136852353138));
#212870=CARTESIAN_POINT('Ctrl Pts',(-54.4206516984379,31.6030360625224,
2.63550380329723));
#212871=CARTESIAN_POINT('Ctrl Pts',(-54.4288041214165,31.5956573884073,
2.63014997451111));
#212872=CARTESIAN_POINT('Ctrl Pts',(-54.4368146919238,31.5878037911381,
2.62536981119271));
#212873=CARTESIAN_POINT('Ctrl Pts',(-54.4402959775154,31.5843907239925,
2.62329241687091));
#212874=CARTESIAN_POINT('Ctrl Pts',(-54.443750270399,31.58088799234,2.62132362131446));
#212875=CARTESIAN_POINT('Ctrl Pts',(-54.4471718528273,31.5772987574367,
2.61946873372366));
#212876=CARTESIAN_POINT('Ctrl Pts',(-54.4591473913264,31.5647364352753,
2.61297662715587));
#212877=CARTESIAN_POINT('Ctrl Pts',(-54.4707222239582,31.5511144466741,
2.60787989113988));
#212878=CARTESIAN_POINT('Ctrl Pts',(-54.4816512176786,31.5365683393824,
2.60440616886199));
#212879=CARTESIAN_POINT('Ctrl Pts',(-54.4871157145388,31.5292952857366,
2.60266930772304));
#212880=CARTESIAN_POINT('Ctrl Pts',(-54.4924187521964,31.5217912027244,
2.60133820040204));
#212881=CARTESIAN_POINT('Ctrl Pts',(-54.4975296958774,31.5140730377803,
2.60044130723604));
#212882=CARTESIAN_POINT('Ctrl Pts',(-54.5000851677178,31.5102139553083,
2.59999286065304));
#212883=CARTESIAN_POINT('Ctrl Pts',(-54.5025926161709,31.5063013524149,
2.59965296768532));
#212884=CARTESIAN_POINT('Ctrl Pts',(-54.5050482124962,31.5023373478778,
2.59942518630974));
#212885=CARTESIAN_POINT('Ctrl Pts',(-54.5075038088216,31.4983733433407,
2.59919740493416));
#212886=CARTESIAN_POINT('Ctrl Pts',(-54.5099075515418,31.4943579363065,
2.59908173791634));
#212887=CARTESIAN_POINT('Ctrl Pts',(-54.5122556166612,31.4902932482907,
2.59908173516044));
#212888=CARTESIAN_POINT('',(-54.5275217339721,31.4638515574739,2.59908173516044));
#212889=CARTESIAN_POINT('Origin',(9.49066947580433E-17,1.91029776801841E-13,
2.59908173516024));
#212890=CARTESIAN_POINT('',(-54.514646476914,31.1067982185534,2.90134173516043));
#212891=CARTESIAN_POINT('Ctrl Pts',(-54.5275217339721,31.4638515574739,
2.59908173516045));
#212892=CARTESIAN_POINT('Ctrl Pts',(-54.5294317356859,31.4605414731919,
2.59908174381707));
#212893=CARTESIAN_POINT('Ctrl Pts',(-54.5312951627229,31.457216601512,2.59915752001016));
#212894=CARTESIAN_POINT('Ctrl Pts',(-54.5331120223761,31.4538791743432,
2.59930729517491));
#212895=CARTESIAN_POINT('Ctrl Pts',(-54.5436112298317,31.4345929624713,
2.60017281085941));
#212896=CARTESIAN_POINT('Ctrl Pts',(-54.5525583311781,31.4148859438258,
2.60350651800102));
#212897=CARTESIAN_POINT('Ctrl Pts',(-54.5599504658512,31.3951944477268,
2.60896880596534));
#212898=CARTESIAN_POINT('Ctrl Pts',(-54.5629318838126,31.3872524143692,
2.61117187235517));
#212899=CARTESIAN_POINT('Ctrl Pts',(-54.5656607810288,31.3793127123322,
2.61372076577242));
#212900=CARTESIAN_POINT('Ctrl Pts',(-54.5681385507009,31.3714030065918,
2.61659179897004));
#212901=CARTESIAN_POINT('Ctrl Pts',(-54.5690526972783,31.3684848053918,
2.61765103591229));
#212902=CARTESIAN_POINT('Ctrl Pts',(-54.5699325468791,31.3655707565306,
2.6187542245517));
#212903=CARTESIAN_POINT('Ctrl Pts',(-54.5707781137756,31.3626622846451,
2.61990022440417));
#212904=CARTESIAN_POINT('Ctrl Pts',(-54.5723635517064,31.3572088998599,
2.62204897412754));
#212905=CARTESIAN_POINT('Ctrl Pts',(-54.5738284644992,31.3517751216268,
2.62434823201791));
#212906=CARTESIAN_POINT('Ctrl Pts',(-54.575172946323,31.3463703409155,2.62679048030326));
#212907=CARTESIAN_POINT('Ctrl Pts',(-54.5798786327061,31.3274536084259,
2.635338349302));
#212908=CARTESIAN_POINT('Ctrl Pts',(-54.5831090358349,31.3088920933401,
2.64563784783583));
#212909=CARTESIAN_POINT('Ctrl Pts',(-54.5848682151124,31.2910884461624,
2.65736666737985));
#212910=CARTESIAN_POINT('Ctrl Pts',(-54.5857478047512,31.2821866225735,
2.66323107715185));
#212911=CARTESIAN_POINT('Ctrl Pts',(-54.5862595893019,31.273474266467,2.66945281780794));
#212912=CARTESIAN_POINT('Ctrl Pts',(-54.5864040839109,31.2650017135575,
2.67599160631221));
#212913=CARTESIAN_POINT('Ctrl Pts',(-54.5864763312153,31.2607654371028,
2.67926100056434));
#212914=CARTESIAN_POINT('Ctrl Pts',(-54.5864567561366,31.2565891115051,
2.68260965685142));
#212915=CARTESIAN_POINT('Ctrl Pts',(-54.5863454235314,31.2524790289902,
2.68603254012502));
#212916=CARTESIAN_POINT('Ctrl Pts',(-54.5862340909262,31.2483689464753,
2.68945542339861));
#212917=CARTESIAN_POINT('Ctrl Pts',(-54.586030897389,31.244325185122,2.69295261525404));
#212918=CARTESIAN_POINT('Ctrl Pts',(-54.5857361203749,31.2403538784534,
2.69651891172118));
#212919=CARTESIAN_POINT('Ctrl Pts',(-54.5857336065443,31.2403200115247,
2.69654932476107));
#212920=CARTESIAN_POINT('Ctrl Pts',(-54.5857310861513,31.2402861499645,
2.69657974261165));
#212921=CARTESIAN_POINT('Ctrl Pts',(-54.5857285591962,31.2402522937759,
2.69661016526993));
#212922=CARTESIAN_POINT('Ctrl Pts',(-54.5844380063442,31.2229614439869,
2.71214746101179));
#212923=CARTESIAN_POINT('Ctrl Pts',(-54.5815601021621,31.2070266227627,
2.72880565567653));
#212924=CARTESIAN_POINT('Ctrl Pts',(-54.5772898993849,31.1924939094151,
2.74628040012444));
#212925=CARTESIAN_POINT('Ctrl Pts',(-54.5728752811852,31.1774697093521,
2.76434612882594));
#212926=CARTESIAN_POINT('Ctrl Pts',(-54.5669719917397,31.1639433968943,
2.78328592654701));
#212927=CARTESIAN_POINT('Ctrl Pts',(-54.5597576364838,31.1520017942511,
2.80278753268169));
#212928=CARTESIAN_POINT('Ctrl Pts',(-54.5526805134453,31.1402873460179,
2.82191817723222));
#212929=CARTESIAN_POINT('Ctrl Pts',(-54.5443408741004,31.130097527732,2.84159092315684));
#212930=CARTESIAN_POINT('Ctrl Pts',(-54.5348819367256,31.1215554575456,
2.86151233817648));
#212931=CARTESIAN_POINT('Ctrl Pts',(-54.5286157223284,31.1158966355169,
2.87470957721744));
#212932=CARTESIAN_POINT('Ctrl Pts',(-54.5218578148506,31.1109617866625,
2.88801594388571));
#212933=CARTESIAN_POINT('Ctrl Pts',(-54.514646476914,31.1067982185534,2.90134173516043));
#212934=CARTESIAN_POINT('',(-54.2060847114743,30.9286463962977,3.47153072139093));
#212935=CARTESIAN_POINT('',(-54.514646476914,31.1067982185534,2.90134173516043));
#212936=CARTESIAN_POINT('',(-56.8833377255396,25.6742415049979,3.47153072139089));
#212937=CARTESIAN_POINT('Origin',(5.53234440788222E-15,1.85015204418142E-13,
3.47153072139072));
#212938=CARTESIAN_POINT('',(-57.20883363247,25.8191582032619,2.90134173516041));
#212939=CARTESIAN_POINT('',(-56.8833377255396,25.6742415049979,3.47153072139089));
#212940=CARTESIAN_POINT('',(-57.5052637377733,25.6197038181296,2.5990817351604));
#212941=CARTESIAN_POINT('Ctrl Pts',(-57.20883363247,25.8191582032619,2.90134173516041));
#212942=CARTESIAN_POINT('Ctrl Pts',(-57.2200757170682,25.8241633573212,
2.88164837656715));
#212943=CARTESIAN_POINT('Ctrl Pts',(-57.2320741602334,25.8273704465174,
2.86203734439109));
#212944=CARTESIAN_POINT('Ctrl Pts',(-57.2446400511066,25.8287819086041,
2.84277945978095));
#212945=CARTESIAN_POINT('Ctrl Pts',(-57.2574584397107,25.8302217324662,
2.82313460919956));
#212946=CARTESIAN_POINT('Ctrl Pts',(-57.2708681396365,25.8297934599655,
2.80385576863272));
#212947=CARTESIAN_POINT('Ctrl Pts',(-57.2846981803189,25.8274551293907,
2.78521678518317));
#212948=CARTESIAN_POINT('Ctrl Pts',(-57.2979909364578,25.825207640839,2.7673019093442));
#212949=CARTESIAN_POINT('Ctrl Pts',(-57.3116728904446,25.8211956083136,
2.74997687279751));
#212950=CARTESIAN_POINT('Ctrl Pts',(-57.3256063334235,25.8153387643623,
2.73349253345713));
#212951=CARTESIAN_POINT('Ctrl Pts',(-57.3363095208206,25.810839740075,2.72082983599284));
#212952=CARTESIAN_POINT('Ctrl Pts',(-57.3471614741631,25.805251326744,2.70866321039285));
#212953=CARTESIAN_POINT('Ctrl Pts',(-57.3581011436975,25.798518653724,2.69711645335861));
#212954=CARTESIAN_POINT('Ctrl Pts',(-57.3581298146204,25.7985010085887,
2.69708619136767));
#212955=CARTESIAN_POINT('Ctrl Pts',(-57.3581584863395,25.798483354779,2.69705593387234));
#212956=CARTESIAN_POINT('Ctrl Pts',(-57.358187158852,25.7984656922965,2.69702568087586));
#212957=CARTESIAN_POINT('Ctrl Pts',(-57.3612614352675,25.7965719149862,
2.69378194443282));
#212958=CARTESIAN_POINT('Ctrl Pts',(-57.3643429325989,25.7945784837697,
2.69059266624716));
#212959=CARTESIAN_POINT('Ctrl Pts',(-57.3674274658677,25.7924880141965,
2.68746219342693));
#212960=CARTESIAN_POINT('Ctrl Pts',(-57.3845921921772,25.7808550263326,
2.67004182395949));
#212961=CARTESIAN_POINT('Ctrl Pts',(-57.4018536888757,25.766221218005,2.65443567877626));
#212962=CARTESIAN_POINT('Ctrl Pts',(-57.418483002346,25.7490920431222,2.64136852352743));
#212963=CARTESIAN_POINT('Ctrl Pts',(-57.425946468518,25.7414042322261,2.63550380329482));
#212964=CARTESIAN_POINT('Ctrl Pts',(-57.4332829502027,25.7332138190157,
2.63014997451002));
#212965=CARTESIAN_POINT('Ctrl Pts',(-57.4404287135112,25.724565911951,2.6253698111927));
#212966=CARTESIAN_POINT('Ctrl Pts',(-57.4435341655924,25.7208076485113,
2.6232924168709));
#212967=CARTESIAN_POINT('Ctrl Pts',(-57.4466034003413,25.7169630332624,
2.62132362131444));
#212968=CARTESIAN_POINT('Ctrl Pts',(-57.4496310617743,25.7130358078103,
2.61946873372364));
#212969=CARTESIAN_POINT('Ctrl Pts',(-57.4602278767899,25.699290518728,2.61297662715584));
#212970=CARTESIAN_POINT('Ctrl Pts',(-57.4703154157423,25.6845332533381,
2.60787989113985));
#212971=CARTESIAN_POINT('Ctrl Pts',(-57.4796640570499,25.6689244402255,
2.60440616886196));
#212972=CARTESIAN_POINT('Ctrl Pts',(-57.4843383777036,25.6611200336692,
2.60266930772301));
#212973=CARTESIAN_POINT('Ctrl Pts',(-57.4888279745007,25.6531027404319,
2.601338200402));
#212974=CARTESIAN_POINT('Ctrl Pts',(-57.4931041519765,25.6448926173141,
2.600441307236));
#212975=CARTESIAN_POINT('Ctrl Pts',(-57.4952422407144,25.6407875557552,
2.599992860653));
#212976=CARTESIAN_POINT('Ctrl Pts',(-57.4973269747346,25.6366342867764,
2.59965296768529));
#212977=CARTESIAN_POINT('Ctrl Pts',(-57.4993547677437,25.6324353177606,
2.59942518630971));
#212978=CARTESIAN_POINT('Ctrl Pts',(-57.5013825607528,25.6282363487448,
2.59919740493413));
#212979=CARTESIAN_POINT('Ctrl Pts',(-57.5033534111923,25.6239916789979,
2.59908173791629));
#212980=CARTESIAN_POINT('Ctrl Pts',(-57.5052637377733,25.6197038181296,
2.5990817351604));
#212981=CARTESIAN_POINT('',(-57.517682316389,25.5918112338793,2.5990817351604));
#212982=CARTESIAN_POINT('Origin',(1.02291912287982E-16,1.91044271107351E-13,
2.59908173516023));
#212983=CARTESIAN_POINT('',(-57.4675553545142,25.2380597013429,2.90134173516039));
#212984=CARTESIAN_POINT('Ctrl Pts',(-57.517682316389,25.5918112338793,2.59908173516041));
#212985=CARTESIAN_POINT('Ctrl Pts',(-57.5192358568902,25.5883196330413,
2.59908174381697));
#212986=CARTESIAN_POINT('Ctrl Pts',(-57.5207415321516,25.5848181941918,
2.59915752001012));
#212987=CARTESIAN_POINT('Ctrl Pts',(-57.5221995827244,25.5813091362507,
2.59930729517487));
#212988=CARTESIAN_POINT('Ctrl Pts',(-57.5306253163332,25.5610311102459,
2.60017281085931));
#212989=CARTESIAN_POINT('Ctrl Pts',(-57.5374634601473,25.5404968219576,
2.60350651800052));
#212990=CARTESIAN_POINT('Ctrl Pts',(-57.5427567781063,25.5201405094583,
2.60896880596417));
#212991=CARTESIAN_POINT('Ctrl Pts',(-57.5448916950066,25.5119303403511,
2.61117187235426));
#212992=CARTESIAN_POINT('Ctrl Pts',(-57.5467757181859,25.5037488853987,
2.6137207657719));
#212993=CARTESIAN_POINT('Ctrl Pts',(-57.5484131249909,25.4956235123964,
2.61659179897001));
#212994=CARTESIAN_POINT('Ctrl Pts',(-57.5490172286907,25.492625743071,2.61765103591227));
#212995=CARTESIAN_POINT('Ctrl Pts',(-57.549587657334,25.4896356883477,2.61875422455167));
#212996=CARTESIAN_POINT('Ctrl Pts',(-57.5501245740299,25.4866547635672,
2.61990022440413));
#212997=CARTESIAN_POINT('Ctrl Pts',(-57.5511312928346,25.4810655296039,
2.6220489741275));
#212998=CARTESIAN_POINT('Ctrl Pts',(-57.5520201961935,25.4755083930936,
2.62434823201787));
#212999=CARTESIAN_POINT('Ctrl Pts',(-57.5527923593831,25.4699926837176,
2.62679048030322));
#213000=CARTESIAN_POINT('Ctrl Pts',(-57.5554949305467,25.4506877009016,
2.63533834930196));
#213001=CARTESIAN_POINT('Ctrl Pts',(-57.5567674305412,25.4318901986627,
2.64563784783579));
#213002=CARTESIAN_POINT('Ctrl Pts',(-57.5566559849706,25.4140001974206,
2.6573666673798));
#213003=CARTESIAN_POINT('Ctrl Pts',(-57.5566002621853,25.4050551967995,
2.66323107715181));
#213004=CARTESIAN_POINT('Ctrl Pts',(-57.5561985539314,25.3963370718388,
2.66945281780789));
#213005=CARTESIAN_POINT('Ctrl Pts',(-57.5554566340482,25.3878958286612,
2.67599160631216));
#213006=CARTESIAN_POINT('Ctrl Pts',(-57.5550856741066,25.3836752070724,
2.67926100056429));
#213007=CARTESIAN_POINT('Ctrl Pts',(-57.5546296613653,25.3795238059763,
2.68260965685139));
#213008=CARTESIAN_POINT('Ctrl Pts',(-57.5540893180426,25.3754478763495,
2.68603254012499));
#213009=CARTESIAN_POINT('Ctrl Pts',(-57.5535489747199,25.3713719467228,
2.68945542339858));
#213010=CARTESIAN_POINT('Ctrl Pts',(-57.5529242061381,25.3673715770255,
2.69295261525401));
#213011=CARTESIAN_POINT('Ctrl Pts',(-57.55221592936,25.3634528381786,2.69651891172115));
#213012=CARTESIAN_POINT('Ctrl Pts',(-57.5522098892425,25.3634194195433,
2.69654932476103));
#213013=CARTESIAN_POINT('Ctrl Pts',(-57.5522038431596,25.3633860069332,
2.69657974261161));
#213014=CARTESIAN_POINT('Ctrl Pts',(-57.552197791112,25.3633526003511,2.69661016526989));
#213015=CARTESIAN_POINT('Ctrl Pts',(-57.5491069220866,25.3462913711527,
2.71214746101178));
#213016=CARTESIAN_POINT('Ctrl Pts',(-57.5445791409896,25.330744665448,2.72880565567655));
#213017=CARTESIAN_POINT('Ctrl Pts',(-57.5388132486367,25.3167379215589,
2.74628040012449));
#213018=CARTESIAN_POINT('Ctrl Pts',(-57.532852357633,25.3022574788921,2.76434612882608));
#213019=CARTESIAN_POINT('Ctrl Pts',(-57.5255675223698,25.2894223267632,
2.78328592654724));
#213020=CARTESIAN_POINT('Ctrl Pts',(-57.5171444507335,25.2783002469371,
2.80278753268202));
#213021=CARTESIAN_POINT('Ctrl Pts',(-57.5088816036436,25.2673897324725,
2.82191817723273));
#213022=CARTESIAN_POINT('Ctrl Pts',(-57.4995225236691,25.2581274647623,
2.84159092315754));
#213023=CARTESIAN_POINT('Ctrl Pts',(-57.4892225138731,25.2506209171179,
2.86151233817736));
#213024=CARTESIAN_POINT('Ctrl Pts',(-57.4823991184836,25.24564809247,2.87470957721803));
#213025=CARTESIAN_POINT('Ctrl Pts',(-57.475162399363,25.2414466709177,2.88801594388598));
#213026=CARTESIAN_POINT('Ctrl Pts',(-57.4675553545142,25.2380597013429,
2.9013417351604));
#213027=CARTESIAN_POINT('',(-57.1420619865023,25.0931373005744,3.47153072139088));
#213028=CARTESIAN_POINT('',(-57.4675553545142,25.2380597013429,2.90134173516039));
#213029=CARTESIAN_POINT('',(-59.2554138597572,19.5876674457077,3.47153072139085));
#213030=CARTESIAN_POINT('Origin',(5.53234440788222E-15,1.85015204418142E-13,
3.47153072139072));
#213031=CARTESIAN_POINT('',(-59.5942745858237,19.6977666881844,2.90134173516036));
#213032=CARTESIAN_POINT('',(-59.2554138597572,19.5876674457077,3.47153072139084));
#213033=CARTESIAN_POINT('',(-59.8682321556243,19.4684195516695,2.59908173516036));
#213034=CARTESIAN_POINT('Ctrl Pts',(-59.5942745858237,19.6977666881844,
2.90134173516036));
#213035=CARTESIAN_POINT('Ctrl Pts',(-59.6059782661689,19.701569305659,2.8816483765663));
#213036=CARTESIAN_POINT('Ctrl Pts',(-59.6182462127128,19.7035046472594,
2.86203734438945));
#213037=CARTESIAN_POINT('Ctrl Pts',(-59.6308908042844,19.7035948839464,
2.84277945977856));
#213038=CARTESIAN_POINT('Ctrl Pts',(-59.6437894749908,19.7036869338401,
2.82313460919653));
#213039=CARTESIAN_POINT('Ctrl Pts',(-59.6570809485114,19.7018593121346,
2.80385576862909));
#213040=CARTESIAN_POINT('Ctrl Pts',(-59.6705908046827,19.6980881582796,
2.785216785179));
#213041=CARTESIAN_POINT('Ctrl Pts',(-59.6835758151885,19.6944635103332,
2.76730190933965));
#213042=CARTESIAN_POINT('Ctrl Pts',(-59.6967634464057,19.6890433025166,
2.74997687279263));
#213043=CARTESIAN_POINT('Ctrl Pts',(-59.7100083536286,19.6817621015861,
2.733492533452));
#213044=CARTESIAN_POINT('Ctrl Pts',(-59.7201826317489,19.6761689356945,
2.72082983598954));
#213045=CARTESIAN_POINT('Ctrl Pts',(-59.7303909886966,19.6694767982707,
2.70866321039127));
#213046=CARTESIAN_POINT('Ctrl Pts',(-59.7405669736108,19.661637500694,2.69711645335857));
#213047=CARTESIAN_POINT('Ctrl Pts',(-59.7405936430525,19.6616169552931,
2.69708619136763));
#213048=CARTESIAN_POINT('Ctrl Pts',(-59.7406203123794,19.6615964011821,
2.6970559338723));
#213049=CARTESIAN_POINT('Ctrl Pts',(-59.7406469815886,19.6615758383628,
2.69702568087582));
#213050=CARTESIAN_POINT('Ctrl Pts',(-59.7435064631642,19.6593710859734,
2.69378194443278));
#213051=CARTESIAN_POINT('Ctrl Pts',(-59.7463627094291,19.6570664708011,
2.69059266624713));
#213052=CARTESIAN_POINT('Ctrl Pts',(-59.74921183173,19.6546650315164,2.6874621934269));
#213053=CARTESIAN_POINT('Ctrl Pts',(-59.7650665495267,19.641301567915,2.67004182396107));
#213054=CARTESIAN_POINT('Ctrl Pts',(-59.7807038364425,19.6249436073987,
2.65443567877911));
#213055=CARTESIAN_POINT('Ctrl Pts',(-59.795451566465,19.6061700313481,2.64136852353103));
#213056=CARTESIAN_POINT('Ctrl Pts',(-59.8020705519309,19.5977441904333,
2.63550380329699));
#213057=CARTESIAN_POINT('Ctrl Pts',(-59.8085107122963,19.5888317740054,
2.63014997451096));
#213058=CARTESIAN_POINT('Ctrl Pts',(-59.8147133779311,19.579484305421,2.62536981119264));
#213059=CARTESIAN_POINT('Ctrl Pts',(-59.8174089725189,19.5754220220078,
2.62329241687084));
#213060=CARTESIAN_POINT('Ctrl Pts',(-59.8200595219549,19.5712776455719,
2.62132362131439));
#213061=CARTESIAN_POINT('Ctrl Pts',(-59.8226600907004,19.5670554570749,
2.61946873372359));
#213062=CARTESIAN_POINT('Ctrl Pts',(-59.8317620813096,19.5522777973352,
2.6129766271558));
#213063=CARTESIAN_POINT('Ctrl Pts',(-59.8402518053949,19.5365469388443,
2.60787989113981));
#213064=CARTESIAN_POINT('Ctrl Pts',(-59.8479176686191,19.5200464333337,
2.60440616886191));
#213065=CARTESIAN_POINT('Ctrl Pts',(-59.8517506002312,19.5117961805783,
2.60266930772296));
#213066=CARTESIAN_POINT('Ctrl Pts',(-59.8553775672056,19.5033535162583,
2.60133820040197));
#213067=CARTESIAN_POINT('Ctrl Pts',(-59.858772127781,19.4947413867938,2.60044130723597));
#213068=CARTESIAN_POINT('Ctrl Pts',(-59.8604694080688,19.4904353220616,
2.59999286065296));
#213069=CARTESIAN_POINT('Ctrl Pts',(-59.862108586874,19.4860868910813,2.59965296768524));
#213070=CARTESIAN_POINT('Ctrl Pts',(-59.8636863596423,19.4816989623701,
2.59942518630966));
#213071=CARTESIAN_POINT('Ctrl Pts',(-59.8652641324106,19.4773110336588,
2.59919740493408));
#213072=CARTESIAN_POINT('Ctrl Pts',(-59.8667804975194,19.4728836066891,
2.59908173791629));
#213073=CARTESIAN_POINT('Ctrl Pts',(-59.8682321556243,19.4684195516695,
2.59908173516036));
#213074=CARTESIAN_POINT('',(-59.8776671349986,19.4393816709755,2.59908173516036));
#213075=CARTESIAN_POINT('Origin',(1.08121605342496E-16,1.91059457976978E-13,
2.59908173516023));
#213076=CARTESIAN_POINT('',(-59.7908376697913,19.092807720641,2.90134173516036));
#213077=CARTESIAN_POINT('Ctrl Pts',(-59.8776671349986,19.4393816709755,
2.59908173516036));
#213078=CARTESIAN_POINT('Ctrl Pts',(-59.8788471933725,19.435746808291,2.59908174381695));
#213079=CARTESIAN_POINT('Ctrl Pts',(-59.8799786203652,19.4321071647686,
2.59915752001008));
#213080=CARTESIAN_POINT('Ctrl Pts',(-59.8810618871502,19.4284649220283,
2.59930729517482));
#213081=CARTESIAN_POINT('Ctrl Pts',(-59.8873218328134,19.4074172521822,
2.6001728108594));
#213082=CARTESIAN_POINT('Ctrl Pts',(-59.8919760989615,19.3862806722057,
2.60350651800157));
#213083=CARTESIAN_POINT('Ctrl Pts',(-59.8951126055077,19.3654825713211,
2.60896880596681));
#213084=CARTESIAN_POINT('Ctrl Pts',(-59.8963776307491,19.3570942188,2.61117187235629));
#213085=CARTESIAN_POINT('Ctrl Pts',(-59.8973961381383,19.3487606486696,
2.61372076577302));
#213086=CARTESIAN_POINT('Ctrl Pts',(-59.8981752423037,19.340508631697,2.61659179896998));
#213087=CARTESIAN_POINT('Ctrl Pts',(-59.8984626844395,19.3374641384342,
2.61765103591223));
#213088=CARTESIAN_POINT('Ctrl Pts',(-59.8987174423897,19.334430837514,2.61875422455163));
#213089=CARTESIAN_POINT('Ctrl Pts',(-59.8989398263133,19.3314101194743,
2.61990022440409));
#213090=CARTESIAN_POINT('Ctrl Pts',(-59.8993567961701,19.3257462731499,
2.62204897412746));
#213091=CARTESIAN_POINT('Ctrl Pts',(-59.8996599510838,19.3201266635127,
2.62434823201782));
#213092=CARTESIAN_POINT('Ctrl Pts',(-59.8998513356577,19.3145604567382,
2.62679048030317));
#213093=CARTESIAN_POINT('Ctrl Pts',(-59.9005211816665,19.2950787330273,
2.63533834930191));
#213094=CARTESIAN_POINT('Ctrl Pts',(-59.8998218367506,19.2762511930036,
2.64563784783575));
#213095=CARTESIAN_POINT('Ctrl Pts',(-59.8978409873528,19.2584708442944,
2.65736666737977));
#213096=CARTESIAN_POINT('Ctrl Pts',(-59.8968505626539,19.2495806699398,
2.66323107715177));
#213097=CARTESIAN_POINT('Ctrl Pts',(-59.8955397627952,19.2409522937262,
2.66945281780786));
#213098=CARTESIAN_POINT('Ctrl Pts',(-59.8939195570493,19.2326348443073,
2.67599160631213));
#213099=CARTESIAN_POINT('Ctrl Pts',(-59.8931094541763,19.2284761195978,
2.67926100056426));
#213100=CARTESIAN_POINT('Ctrl Pts',(-59.8922219999436,19.2243951266223,
2.68260965685134));
#213101=CARTESIAN_POINT('Ctrl Pts',(-59.8912585660179,19.2203980066217,
2.68603254012494));
#213102=CARTESIAN_POINT('Ctrl Pts',(-59.8902951320921,19.2164008866211,
2.68945542339853));
#213103=CARTESIAN_POINT('Ctrl Pts',(-59.889255633561,19.2124877374673,2.69295261525395));
#213104=CARTESIAN_POINT('Ctrl Pts',(-59.8881416170477,19.208664500965,2.69651891172109));
#213105=CARTESIAN_POINT('Ctrl Pts',(-59.8881321168199,19.2086318967647,
2.69654932476097));
#213106=CARTESIAN_POINT('Ctrl Pts',(-59.8881226112893,19.2085992991801,
2.69657974261156));
#213107=CARTESIAN_POINT('Ctrl Pts',(-59.8881131004568,19.208566708214,2.69661016526983));
#213108=CARTESIAN_POINT('Ctrl Pts',(-59.8832557794656,19.1919220260032,
2.71214746101221));
#213109=CARTESIAN_POINT('Ctrl Pts',(-59.8771277287708,19.1769337687786,
2.72880565567756));
#213110=CARTESIAN_POINT('Ctrl Pts',(-59.8699293191651,19.1636064551647,
2.7462804001261));
#213111=CARTESIAN_POINT('Ctrl Pts',(-59.8624874641263,19.1498284206539,
2.7643461288283));
#213112=CARTESIAN_POINT('Ctrl Pts',(-59.8539008972247,19.1378250534663,
2.78328592655013));
#213113=CARTESIAN_POINT('Ctrl Pts',(-59.8443613941432,19.1276443522912,
2.80278753268557));
#213114=CARTESIAN_POINT('Ctrl Pts',(-59.8350033524835,19.117657309475,2.82191817723668));
#213115=CARTESIAN_POINT('Ctrl Pts',(-59.824727371918,19.1094240716838,2.84159092316188));
#213116=CARTESIAN_POINT('Ctrl Pts',(-59.8136991387633,19.1030352898888,
2.86151233818209));
#213117=CARTESIAN_POINT('Ctrl Pts',(-59.8063933209299,19.0988029459297,
2.87470957722119));
#213118=CARTESIAN_POINT('Ctrl Pts',(-59.7987570771764,19.0953809833336,
2.88801594388754));
#213119=CARTESIAN_POINT('Ctrl Pts',(-59.7908376697913,19.092807720641,2.90134173516036));
#213120=CARTESIAN_POINT('',(-59.4519788726609,18.9827025415095,3.47153072139084));
#213121=CARTESIAN_POINT('',(-59.7908376697913,19.092807720641,2.90134173516036));
#213122=CARTESIAN_POINT('',(-60.9782752797349,13.2864868028993,3.4715307213908));
#213123=CARTESIAN_POINT('Origin',(5.53234440788222E-15,1.85015204418142E-13,
3.47153072139072));
#213124=CARTESIAN_POINT('',(-61.3267881959114,13.3605623192485,2.90134173516031));
#213125=CARTESIAN_POINT('',(-60.9782752797349,13.2864868028994,3.4715307213908));
#213126=CARTESIAN_POINT('',(-61.5752716937452,13.1038352065726,2.59908173516031));
#213127=CARTESIAN_POINT('Ctrl Pts',(-61.3267881959114,13.3605623192485,
2.90134173516031));
#213128=CARTESIAN_POINT('Ctrl Pts',(-61.3388252440314,13.3631207378657,
2.88164837656731));
#213129=CARTESIAN_POINT('Ctrl Pts',(-61.3512282837632,13.3637631278628,
2.8620373443915));
#213130=CARTESIAN_POINT('Ctrl Pts',(-61.3638130392407,13.3625311504984,
2.8427794597816));
#213131=CARTESIAN_POINT('Ctrl Pts',(-61.3766506715126,13.3612744179064,
2.82313460920043));
#213132=CARTESIAN_POINT('Ctrl Pts',(-61.3896782944617,13.3580674708025,
2.80385576863379));
#213133=CARTESIAN_POINT('Ctrl Pts',(-61.4027199493095,13.3529048112189,
2.78521678518442));
#213134=CARTESIAN_POINT('Ctrl Pts',(-61.4152549476891,13.3479427162799,
2.7673019093454));
#213135=CARTESIAN_POINT('Ctrl Pts',(-61.4278037696887,13.3411737181041,
2.74997687279866));
#213136=CARTESIAN_POINT('Ctrl Pts',(-61.4402150271797,13.3325479345567,
2.73349253345823));
#213137=CARTESIAN_POINT('Ctrl Pts',(-61.4497489245061,13.3259219069554,
2.72082983599351));
#213138=CARTESIAN_POINT('Ctrl Pts',(-61.459201840167,13.3181993658954,2.70866321039313));
#213139=CARTESIAN_POINT('Ctrl Pts',(-61.4685026502439,13.3093393327442,
2.69711645335852));
#213140=CARTESIAN_POINT('Ctrl Pts',(-61.4685270260084,13.3093161121774,
2.69708619136758));
#213141=CARTESIAN_POINT('Ctrl Pts',(-61.4685514007483,13.3092928829602,
2.69705593387226));
#213142=CARTESIAN_POINT('Ctrl Pts',(-61.4685757744609,13.3092696450948,
2.69702568087578));
#213143=CARTESIAN_POINT('Ctrl Pts',(-61.4711891321181,13.3067780733548,
2.69378194443274));
#213144=CARTESIAN_POINT('Ctrl Pts',(-61.4737888336847,13.3041875240727,
2.69059266624707));
#213145=CARTESIAN_POINT('Ctrl Pts',(-61.4763713294375,13.301501425748,2.68746219342684));
#213146=CARTESIAN_POINT('Ctrl Pts',(-61.4907423311174,13.2865538993111,
2.67004182396047));
#213147=CARTESIAN_POINT('Ctrl Pts',(-61.5045840828649,13.2686510078425,
2.65443567877809));
#213148=CARTESIAN_POINT('Ctrl Pts',(-61.5172886502248,13.2484387178491,
2.64136852352976));
#213149=CARTESIAN_POINT('Ctrl Pts',(-61.5229906359929,13.2393671621939,
2.6355038032962));
#213150=CARTESIAN_POINT('Ctrl Pts',(-61.5284639152923,13.2298303888501,
2.63014997451059));
#213151=CARTESIAN_POINT('Ctrl Pts',(-61.5336555255488,13.2198857715704,
2.6253698111926));
#213152=CARTESIAN_POINT('Ctrl Pts',(-61.5359117291449,13.2155639754109,
2.6232924168708));
#213153=CARTESIAN_POINT('Ctrl Pts',(-61.5381145532937,13.2111652444434,
2.62132362131434));
#213154=CARTESIAN_POINT('Ctrl Pts',(-61.5402595369763,13.2066943520821,
2.61946873372354));
#213155=CARTESIAN_POINT('Ctrl Pts',(-61.5477669798653,13.1910462288177,
2.61297662715574));
#213156=CARTESIAN_POINT('Ctrl Pts',(-61.5545658738899,13.1745141278033,
2.60787989113976));
#213157=CARTESIAN_POINT('Ctrl Pts',(-61.560464970229,13.1573027128859,2.60440616886186));
#213158=CARTESIAN_POINT('Ctrl Pts',(-61.5634145183986,13.1486970054272,
2.60266930772291));
#213159=CARTESIAN_POINT('Ctrl Pts',(-61.5661391177411,13.1399214696215,
2.60133820040192));
#213160=CARTESIAN_POINT('Ctrl Pts',(-61.5686148699002,13.1310016901029,
2.60044130723592));
#213161=CARTESIAN_POINT('Ctrl Pts',(-61.5698527459798,13.1265418003436,
2.59999286065292));
#213162=CARTESIAN_POINT('Ctrl Pts',(-61.571028410384,13.1220458496817,2.59965296768519));
#213163=CARTESIAN_POINT('Ctrl Pts',(-61.5721388765028,13.1175170363402,
2.59942518630961));
#213164=CARTESIAN_POINT('Ctrl Pts',(-61.5732493426217,13.1129882229987,
2.59919740493403));
#213165=CARTESIAN_POINT('Ctrl Pts',(-61.5742946087864,13.1084265466226,
2.59908173791626));
#213166=CARTESIAN_POINT('Ctrl Pts',(-61.5752716937452,13.1038352065726,
2.59908173516031));
#213167=CARTESIAN_POINT('',(-61.5816197022698,13.0739701745323,2.59908173516031));
#213168=CARTESIAN_POINT('Origin',(1.12331902584552E-16,1.910751710202E-13,
2.59908173516024));
#213169=CARTESIAN_POINT('',(-61.4590390555209,12.7383709431249,2.90134173516031));
#213170=CARTESIAN_POINT('Ctrl Pts',(-61.5816197022698,13.0739701745323,
2.59908173516032));
#213171=CARTESIAN_POINT('Ctrl Pts',(-61.5824133495499,13.0702318743175,
2.59908174381692));
#213172=CARTESIAN_POINT('Ctrl Pts',(-61.5831581321229,13.0664939028184,
2.59915752001004));
#213173=CARTESIAN_POINT('Ctrl Pts',(-61.5838547466226,13.0627583804525,
2.59930729517479));
#213174=CARTESIAN_POINT('Ctrl Pts',(-61.5878803190636,13.0411716694462,
2.60017281085927));
#213175=CARTESIAN_POINT('Ctrl Pts',(-61.5902997144311,13.0196643745807,
2.60350651800077));
#213176=CARTESIAN_POINT('Ctrl Pts',(-61.591245045342,12.9986523536618,2.60896880596491));
#213177=CARTESIAN_POINT('Ctrl Pts',(-61.5916263190447,12.9901777222667,
2.61117187235481));
#213178=CARTESIAN_POINT('Ctrl Pts',(-61.5917681516647,12.9817833412908,
2.61372076577216));
#213179=CARTESIAN_POINT('Ctrl Pts',(-61.591680417163,12.9734950911671,2.61659179896992));
#213180=CARTESIAN_POINT('Ctrl Pts',(-61.5916480484584,12.9704372300723,
2.61765103591218));
#213181=CARTESIAN_POINT('Ctrl Pts',(-61.5915843445341,12.9673939164349,
2.61875422455157));
#213182=CARTESIAN_POINT('Ctrl Pts',(-61.5914897592007,12.9643665007549,
2.61990022440404));
#213183=CARTESIAN_POINT('Ctrl Pts',(-61.5913124117005,12.9586900963548,
2.62204897412741));
#213184=CARTESIAN_POINT('Ctrl Pts',(-61.5910264967403,12.9530695832099,
2.62434823201778));
#213185=CARTESIAN_POINT('Ctrl Pts',(-61.5906350058491,12.9475138635631,
2.62679048030314));
#213186=CARTESIAN_POINT('Ctrl Pts',(-61.5892647877301,12.9280688447993,
2.63533834930187));
#213187=CARTESIAN_POINT('Ctrl Pts',(-61.5866012600731,12.9094175454591,
2.6456378478357));
#213188=CARTESIAN_POINT('Ctrl Pts',(-61.5827727094485,12.891941654504,2.65736666737971));
#213189=CARTESIAN_POINT('Ctrl Pts',(-61.5808584341363,12.8832037090265,
2.66323107715172));
#213190=CARTESIAN_POINT('Ctrl Pts',(-61.5786529040703,12.8747596158555,
2.66945281780782));
#213191=CARTESIAN_POINT('Ctrl Pts',(-61.5761721637749,12.8666570879115,
2.67599160631208));
#213192=CARTESIAN_POINT('Ctrl Pts',(-61.5749317936272,12.8626058239395,
2.67926100056422));
#213193=CARTESIAN_POINT('Ctrl Pts',(-61.5736226210373,12.8586399512977,
2.6826096568513));
#213194=CARTESIAN_POINT('Ctrl Pts',(-61.5722466520922,12.8547654342064,
2.68603254012489));
#213195=CARTESIAN_POINT('Ctrl Pts',(-61.5708706831472,12.8508909171151,
2.68945542339849));
#213196=CARTESIAN_POINT('Ctrl Pts',(-61.5694278436302,12.8471078617859,
2.69295261525392));
#213197=CARTESIAN_POINT('Ctrl Pts',(-61.5679202927796,12.8434220158074,
2.69651891172106));
#213198=CARTESIAN_POINT('Ctrl Pts',(-61.5679074365282,12.8433905832605,
2.69654932476094));
#213199=CARTESIAN_POINT('Ctrl Pts',(-61.5678945756944,12.8433591578474,
2.69657974261152));
#213200=CARTESIAN_POINT('Ctrl Pts',(-61.5678817102797,12.8433277395707,
2.6966101652698));
#213201=CARTESIAN_POINT('Ctrl Pts',(-61.5613111551478,12.8272819669692,
2.71214746101236));
#213202=CARTESIAN_POINT('Ctrl Pts',(-61.5536499750612,12.8130163727078,
2.72880565567793));
#213203=CARTESIAN_POINT('Ctrl Pts',(-61.5450979154847,12.8005145062063,
2.74628040012671));
#213204=CARTESIAN_POINT('Ctrl Pts',(-61.5362566309321,12.7875898348812,
2.76434612882914));
#213205=CARTESIAN_POINT('Ctrl Pts',(-61.5264624086162,12.7765497640378,
2.78328592655121));
#213206=CARTESIAN_POINT('Ctrl Pts',(-61.5159109908817,12.7674219834065,
2.8027875326869));
#213207=CARTESIAN_POINT('Ctrl Pts',(-61.5055602833149,12.7584678323696,
2.82191817723834));
#213208=CARTESIAN_POINT('Ctrl Pts',(-61.4944799879519,12.7513538295737,
2.8415909231639));
#213209=CARTESIAN_POINT('Ctrl Pts',(-61.4828443590689,12.746152810458,2.86151233818444));
#213210=CARTESIAN_POINT('Ctrl Pts',(-61.4751361628604,12.7427073176333,
2.87470957722276));
#213211=CARTESIAN_POINT('Ctrl Pts',(-61.4671840587581,12.7401023057312,
2.8880159438883));
#213212=CARTESIAN_POINT('Ctrl Pts',(-61.4590390555209,12.7383709431249,
2.9013417351603));
#213213=CARTESIAN_POINT('',(-61.1105274371642,12.6642893210139,3.47153072139079));
#213214=CARTESIAN_POINT('',(-61.4590390555209,12.7383709431249,2.90134173516031));
#213215=CARTESIAN_POINT('',(-62.0330459552233,6.83973663030237,3.47153072139075));
#213216=CARTESIAN_POINT('Origin',(5.53234440788222E-15,1.85015204418142E-13,
3.47153072139072));
#213217=CARTESIAN_POINT('',(-62.3873926810692,6.87697683366542,2.90134173516027));
#213218=CARTESIAN_POINT('',(-62.0330459552233,6.83973663030238,3.47153072139076));
#213219=CARTESIAN_POINT('',(-62.6076796697355,6.59568250079864,2.59908173516026));
#213220=CARTESIAN_POINT('Ctrl Pts',(-62.3873926810692,6.87697683366542,
2.90134173516026));
#213221=CARTESIAN_POINT('Ctrl Pts',(-62.3996312165471,6.87826302285565,
2.88164837656657));
#213222=CARTESIAN_POINT('Ctrl Pts',(-62.412033459169,6.87760542309004,2.86203734439007));
#213223=CARTESIAN_POINT('Ctrl Pts',(-62.4244204973391,6.87506472947568,
2.84277945977952));
#213224=CARTESIAN_POINT('Ctrl Pts',(-62.4370564393921,6.87247298342269,
2.82313460919761));
#213225=CARTESIAN_POINT('Ctrl Pts',(-62.4496774784074,6.86792184690335,
2.80385576863027));
#213226=CARTESIAN_POINT('Ctrl Pts',(-62.4621080448333,6.86142424476877,
2.78521678518027));
#213227=CARTESIAN_POINT('Ctrl Pts',(-62.4740556950222,6.85517906858685,
2.76730190934053));
#213228=CARTESIAN_POINT('Ctrl Pts',(-62.4858282202851,6.84713544261114,
2.74997687279314));
#213229=CARTESIAN_POINT('Ctrl Pts',(-62.4972698477107,6.8372595823348,2.73349253345217));
#213230=CARTESIAN_POINT('Ctrl Pts',(-62.5060589088659,6.82967328917041,
2.72082983598962));
#213231=CARTESIAN_POINT('Ctrl Pts',(-62.5146528151147,6.82100495425208,
2.70866321039126));
#213232=CARTESIAN_POINT('Ctrl Pts',(-62.5229765487298,6.81122125790657,
2.69711645335848));
#213233=CARTESIAN_POINT('Ctrl Pts',(-62.5229983637511,6.81119561658327,
2.69708619136754));
#213234=CARTESIAN_POINT('Ctrl Pts',(-62.5230201768492,6.81116996676408,
2.69705593387221));
#213235=CARTESIAN_POINT('Ctrl Pts',(-62.5230419880218,6.81114430845134,
2.69702568087573));
#213236=CARTESIAN_POINT('Ctrl Pts',(-62.5253805892672,6.80839321554225,
2.69378194443269));
#213237=CARTESIAN_POINT('Ctrl Pts',(-62.5276952632611,6.80554511475047,
2.69059266624703));
#213238=CARTESIAN_POINT('Ctrl Pts',(-62.5299828381019,6.80260378684094,
2.6874621934268));
#213239=CARTESIAN_POINT('Ctrl Pts',(-62.5427126719616,6.7862359657982,2.6700418239621));
#213240=CARTESIAN_POINT('Ctrl Pts',(-62.5546072354103,6.76698429120527,
2.65443567878105));
#213241=CARTESIAN_POINT('Ctrl Pts',(-62.5651294462082,6.74555473735121,
2.64136852353349));
#213242=CARTESIAN_POINT('Ctrl Pts',(-62.5698519601306,6.73593685681528,
2.63550380329846));
#213243=CARTESIAN_POINT('Ctrl Pts',(-62.5742983919722,6.72588021343749,
2.63014997451158));
#213244=CARTESIAN_POINT('Ctrl Pts',(-62.5784220664834,6.71544740276753,
2.62536981119257));
#213245=CARTESIAN_POINT('Ctrl Pts',(-62.580214159649,6.71091344436488,2.62329241687077));
#213246=CARTESIAN_POINT('Ctrl Pts',(-62.5819451239082,6.70630855228272,
2.62132362131432));
#213247=CARTESIAN_POINT('Ctrl Pts',(-62.5836110216378,6.70163794008952,
2.61946873372352));
#213248=CARTESIAN_POINT('Ctrl Pts',(-62.5894416636914,6.68529079741334,
2.61297662715572));
#213249=CARTESIAN_POINT('Ctrl Pts',(-62.5944752375494,6.66813858303381,
2.60787989113972));
#213250=CARTESIAN_POINT('Ctrl Pts',(-62.5985429352697,6.65040483057315,
2.60440616886183));
#213251=CARTESIAN_POINT('Ctrl Pts',(-62.6005767841298,6.64153795434282,
2.60266930772288));
#213252=CARTESIAN_POINT('Ctrl Pts',(-62.6023691645599,6.63252569365819,
2.60133820040187));
#213253=CARTESIAN_POINT('Ctrl Pts',(-62.6038989834438,6.62339599105648,
2.60044130723587));
#213254=CARTESIAN_POINT('Ctrl Pts',(-62.6046638928858,6.61883113975562,
2.59999286065287));
#213255=CARTESIAN_POINT('Ctrl Pts',(-62.6053631620638,6.61423692798835,
2.59965296768515));
#213256=CARTESIAN_POINT('Ctrl Pts',(-62.6059941550341,6.60961684864329,
2.59942518630957));
#213257=CARTESIAN_POINT('Ctrl Pts',(-62.6066251480043,6.60499676929823,
2.59919740493399));
#213258=CARTESIAN_POINT('Ctrl Pts',(-62.6071878630701,6.60035082219668,
2.59908173791619));
#213259=CARTESIAN_POINT('Ctrl Pts',(-62.6076796697355,6.59568250079864,
2.59908173516027));
#213260=CARTESIAN_POINT('',(-62.6108711573006,6.5653175249528,2.59908173516027));
#213261=CARTESIAN_POINT('Origin',(1.148766751165E-16,1.91091238081628E-13,
2.59908173516023));
#213262=CARTESIAN_POINT('',(-62.4538823482276,6.24436990788037,2.90134173516026));
#213263=CARTESIAN_POINT('Ctrl Pts',(-62.6108711573006,6.5653175249528,2.59908173516027));
#213264=CARTESIAN_POINT('Ctrl Pts',(-62.6112696981211,6.56151674480722,
2.59908174381689));
#213265=CARTESIAN_POINT('Ctrl Pts',(-62.6116196762807,6.5577213993292,2.59915752000999));
#213266=CARTESIAN_POINT('Ctrl Pts',(-62.6119220062409,6.55393352450258,
2.59930729517474));
#213267=CARTESIAN_POINT('Ctrl Pts',(-62.6136691004464,6.53204428085739,
2.60017281085919));
#213268=CARTESIAN_POINT('Ctrl Pts',(-62.6138271176316,6.51040190952424,
2.60350651800055));
#213269=CARTESIAN_POINT('Ctrl Pts',(-62.6125709156642,6.48940618066758,
2.60896880596443));
#213270=CARTESIAN_POINT('Ctrl Pts',(-62.6120642605131,6.48093812023513,
2.61117187235443));
#213271=CARTESIAN_POINT('Ctrl Pts',(-62.6113278644157,6.4725748990102,2.61372076577192));
#213272=CARTESIAN_POINT('Ctrl Pts',(-62.610374252484,6.46434122354008,2.61659179896986));
#213273=CARTESIAN_POINT('Ctrl Pts',(-62.6100224275775,6.46130349717916,
2.61765103591212));
#213274=CARTESIAN_POINT('Ctrl Pts',(-62.6096409597322,6.45828351400561,
2.61875422455152));
#213275=CARTESIAN_POINT('Ctrl Pts',(-62.6092304414384,6.45528256968502,
2.61990022440398));
#213276=CARTESIAN_POINT('Ctrl Pts',(-62.6084607196375,6.4496557990839,2.62204897412735));
#213277=CARTESIAN_POINT('Ctrl Pts',(-62.6075888673476,6.4440959619495,2.62434823201773));
#213278=CARTESIAN_POINT('Ctrl Pts',(-62.6066187902475,6.43861159905745,
2.62679048030308));
#213279=CARTESIAN_POINT('Ctrl Pts',(-62.6032235203971,6.41941632893527,
2.63533834930182));
#213280=CARTESIAN_POINT('Ctrl Pts',(-62.5986249921653,6.40114561781729,
2.64563784783565));
#213281=CARTESIAN_POINT('Ctrl Pts',(-62.5929906867159,6.38416565413471,
2.65736666737967));
#213282=CARTESIAN_POINT('Ctrl Pts',(-62.5901735339912,6.37567567229342,
2.66323107715167));
#213283=CARTESIAN_POINT('Ctrl Pts',(-62.5870974379668,6.36750837741682,
2.66945281780776));
#213284=CARTESIAN_POINT('Ctrl Pts',(-62.5837833426318,6.35970954393955,
2.67599160631203));
#213285=CARTESIAN_POINT('Ctrl Pts',(-62.5821262949642,6.35581012720091,
2.67926100056416));
#213286=CARTESIAN_POINT('Ctrl Pts',(-62.580409747586,6.35200282582336,2.68260965685125));
#213287=CARTESIAN_POINT('Ctrl Pts',(-62.5786363190253,6.34829336166141,
2.68603254012485));
#213288=CARTESIAN_POINT('Ctrl Pts',(-62.5768628904647,6.34458389749946,
2.68945542339844));
#213289=CARTESIAN_POINT('Ctrl Pts',(-62.5750325180135,6.34097238394057,
2.69295261525388));
#213290=CARTESIAN_POINT('Ctrl Pts',(-62.5731479498682,6.33746431138572,
2.69651891172102));
#213291=CARTESIAN_POINT('Ctrl Pts',(-62.5731318784488,6.33743439487387,
2.6965493247609));
#213292=CARTESIAN_POINT('Ctrl Pts',(-62.5731158032179,6.3374044859356,2.69657974261148));
#213293=CARTESIAN_POINT('Ctrl Pts',(-62.5730997241771,6.33737458457355,
2.69661016526975));
#213294=CARTESIAN_POINT('Ctrl Pts',(-62.5648879232822,6.32210352242481,
2.71214746101154));
#213295=CARTESIAN_POINT('Ctrl Pts',(-62.5557775512964,6.30871688796325,
2.72880565567622));
#213296=CARTESIAN_POINT('Ctrl Pts',(-62.5459655399043,6.2971774416402,2.74628040012404));
#213297=CARTESIAN_POINT('Ctrl Pts',(-62.5358216928023,6.28524773890498,
2.76434612882545));
#213298=CARTESIAN_POINT('Ctrl Pts',(-62.524927122622,6.27529192173268,2.78328592654642));
#213299=CARTESIAN_POINT('Ctrl Pts',(-62.5134793937762,6.26731706751981,
2.802787532681));
#213300=CARTESIAN_POINT('Ctrl Pts',(-62.5022494248214,6.25949391181485,
2.82191817723141));
#213301=CARTESIAN_POINT('Ctrl Pts',(-62.4904862126964,6.25357708651719,
2.84159092315592));
#213302=CARTESIAN_POINT('Ctrl Pts',(-62.4783706704711,6.24962081353434,
2.86151233817543));
#213303=CARTESIAN_POINT('Ctrl Pts',(-62.470344548496,6.24699992138305,2.87470957721668));
#213304=CARTESIAN_POINT('Ctrl Pts',(-62.4621637089593,6.24524040122967,
2.88801594388524));
#213305=CARTESIAN_POINT('Ctrl Pts',(-62.4538823482276,6.24436990788038,
2.90134173516025));
#213306=CARTESIAN_POINT('',(-62.0995362748659,6.20712349654441,3.47153072139075));
#213307=CARTESIAN_POINT('',(-62.4538823482276,6.24436990788037,2.90134173516027));
#213308=CARTESIAN_POINT('',(-62.4081695979768,0.318048871877305,3.47153072139071));
#213309=CARTESIAN_POINT('Origin',(5.53234440788222E-15,1.85015204418142E-13,
3.47153072139072));
#213310=CARTESIAN_POINT('',(-62.7644678366119,0.318045750793233,2.90134173516022));
#213311=CARTESIAN_POINT('',(-62.4081695979768,0.318048871877314,3.47153072139071));
#213312=CARTESIAN_POINT('Ctrl Pts',(-62.7644678366119,0.318045750793234,
2.90134173516022));
#213313=CARTESIAN_POINT('Ctrl Pts',(-62.7767737714904,0.318045618798321,
2.88164837656814));
#213314=CARTESIAN_POINT('Ctrl Pts',(-62.7890393354357,0.316095234070967,
2.86203734439325));
#213315=CARTESIAN_POINT('Ctrl Pts',(-62.8010929413145,0.312273660578323,
2.84277945978422));
#213316=CARTESIAN_POINT('Ctrl Pts',(-62.8133887511217,0.308375296777275,
2.82313460920393));
#213317=CARTESIAN_POINT('Ctrl Pts',(-62.8254649274573,0.302529834047833,
2.80385576863813));
#213318=CARTESIAN_POINT('Ctrl Pts',(-62.8371482135727,0.294768478452875,
2.78521678518951));
#213319=CARTESIAN_POINT('Ctrl Pts',(-62.8483776146138,0.287308644486914,
2.76730190935116));
#213320=CARTESIAN_POINT('Ctrl Pts',(-62.8592448608884,0.278078518363015,
2.74997687280502));
#213321=CARTESIAN_POINT('Ctrl Pts',(-62.869591501383,0.267060783352459,
2.73349253346508));
#213322=CARTESIAN_POINT('Ctrl Pts',(-62.8775394315781,0.258597341637538,
2.72082983599787));
#213323=CARTESIAN_POINT('Ctrl Pts',(-62.885180171784,0.249078184948348,
2.70866321039515));
#213324=CARTESIAN_POINT('Ctrl Pts',(-62.8924356323738,0.238478017628062,
2.69711645335844));
#213325=CARTESIAN_POINT('Ctrl Pts',(-62.892454647642,0.238450236479951,
2.6970861913675));
#213326=CARTESIAN_POINT('Ctrl Pts',(-62.8924736601095,0.238422447083525,
2.69705593387217));
#213327=CARTESIAN_POINT('Ctrl Pts',(-62.8924926697742,0.23839464944136,
2.69702568087569));
#213328=CARTESIAN_POINT('Ctrl Pts',(-62.8945308924032,0.235414176912695,
2.69378194443264));
#213329=CARTESIAN_POINT('Ctrl Pts',(-62.8965351787718,0.232339728999503,
2.69059266624698));
#213330=CARTESIAN_POINT('Ctrl Pts',(-62.8985027695519,0.22917539730931,
2.68746219342675));
#213331=CARTESIAN_POINT('Ctrl Pts',(-62.9094519648697,0.211566610930952,
2.6700418239612));
#213332=CARTESIAN_POINT('Ctrl Pts',(-62.9192690206952,0.191177078586108,
2.65443567877947));
#213333=CARTESIAN_POINT('Ctrl Pts',(-62.9274935913887,0.168765047544095,
2.64136852353151));
#213334=CARTESIAN_POINT('Ctrl Pts',(-62.9311848926129,0.158706217641999,
2.63550380329723));
#213335=CARTESIAN_POINT('Ctrl Pts',(-62.9345557609574,0.148239886922536,
2.63014997451099));
#213336=CARTESIAN_POINT('Ctrl Pts',(-62.9375663198809,0.137433186922523,
2.6253698111925));
#213337=CARTESIAN_POINT('Ctrl Pts',(-62.9388746680683,0.132736741273776,
2.6232924168707));
#213338=CARTESIAN_POINT('Ctrl Pts',(-62.9401148076313,0.127976140238265,
2.62132362131425));
#213339=CARTESIAN_POINT('Ctrl Pts',(-62.9412833674838,0.123156980417726,
2.61946873372345));
#213340=CARTESIAN_POINT('Ctrl Pts',(-62.9453733269673,0.10628992104584,
2.61297662715565));
#213341=CARTESIAN_POINT('Ctrl Pts',(-62.9485864317704,0.0887055165512269,
2.60787989113966));
#213342=CARTESIAN_POINT('Ctrl Pts',(-62.9507781643242,0.070643721250341,
2.60440616886177));
#213343=CARTESIAN_POINT('Ctrl Pts',(-62.9518740306011,0.061612823599898,
2.60266930772282));
#213344=CARTESIAN_POINT('Ctrl Pts',(-62.9527145544237,0.0524625782503221,
2.60133820040182));
#213345=CARTESIAN_POINT('Ctrl Pts',(-62.9532816790167,0.0432229794977032,
2.60044130723581));
#213346=CARTESIAN_POINT('Ctrl Pts',(-62.9535652413132,0.0386031801213938,
2.59999286065281));
#213347=CARTESIAN_POINT('Ctrl Pts',(-62.9537804539255,0.0339610423942995,
2.5996529676851));
#213348=CARTESIAN_POINT('Ctrl Pts',(-62.9539250604562,0.0293003156017882,
2.59942518630953));
#213349=CARTESIAN_POINT('Ctrl Pts',(-62.9540696669868,0.0246395888092768,
2.59919740493395));
#213350=CARTESIAN_POINT('Ctrl Pts',(-62.9541436657296,0.0199602729509832,
2.59908173791615));
#213351=CARTESIAN_POINT('Ctrl Pts',(-62.9541448057648,0.0152661173110579,
2.59908173516022));
#213352=CARTESIAN_POINT('',(-62.2224557307631,1.90550834334536E-13,3.77003198860262));
#213353=CARTESIAN_POINT('',(-62.7644678366119,-0.318045750792855,2.90134173516021));
#213354=CARTESIAN_POINT('Ctrl Pts',(-62.9541448057648,-0.0152661173106757,
2.59908173516023));
#213355=CARTESIAN_POINT('Ctrl Pts',(-62.9541438736292,-0.0190877352444563,
2.59908174381683));
#213356=CARTESIAN_POINT('Ctrl Pts',(-62.9540952129414,-0.0228988721020315,
2.59915752000994));
#213357=CARTESIAN_POINT('Ctrl Pts',(-62.9539999459718,-0.0266975986401531,
2.59930729517469));
#213358=CARTESIAN_POINT('Ctrl Pts',(-62.9534494204121,-0.0486495517880578,
2.60017281085904));
#213359=CARTESIAN_POINT('Ctrl Pts',(-62.9513443281462,-0.0701898812374375,
2.60350651799966));
#213360=CARTESIAN_POINT('Ctrl Pts',(-62.9479003565128,-0.0909392844309831,
2.60896880596233));
#213361=CARTESIAN_POINT('Ctrl Pts',(-62.9465113235275,-0.0993079960606954,
2.6111718723528));
#213362=CARTESIAN_POINT('Ctrl Pts',(-62.9449047668219,-0.107548428334892,
2.61372076577099));
#213363=CARTESIAN_POINT('Ctrl Pts',(-62.9430957254317,-0.11563731928203,
2.61659179896983));
#213364=CARTESIAN_POINT('Ctrl Pts',(-62.9424282989905,-0.118621628943286,
2.61765103591208));
#213365=CARTESIAN_POINT('Ctrl Pts',(-62.9417332466658,-0.121585194085372,
2.61875422455148));
#213366=CARTESIAN_POINT('Ctrl Pts',(-62.941011293136,-0.124526788072593,
2.61990022440394));
#213367=CARTESIAN_POINT('Ctrl Pts',(-62.9396576302675,-0.130042276798633,
2.62204897412731));
#213368=CARTESIAN_POINT('Ctrl Pts',(-62.938209392844,-0.135480523183407,
2.62434823201768));
#213369=CARTESIAN_POINT('Ctrl Pts',(-62.9366713579026,-0.140833441493173,
2.62679048030304));
#213370=CARTESIAN_POINT('Ctrl Pts',(-62.9312882356078,-0.159568655577355,
2.63533834930178));
#213371=CARTESIAN_POINT('Ctrl Pts',(-62.9248050892389,-0.177258600738774,
2.64563784783561));
#213372=CARTESIAN_POINT('Ctrl Pts',(-62.9174267595942,-0.193556601113454,
2.65736666737962));
#213373=CARTESIAN_POINT('Ctrl Pts',(-62.9137375947719,-0.201705601300794,
2.66323107715163));
#213374=CARTESIAN_POINT('Ctrl Pts',(-62.9098246351408,-0.20950661529121,
2.66945281780772));
#213375=CARTESIAN_POINT('Ctrl Pts',(-62.9057134946881,-0.216916308650201,
2.67599160631199));
#213376=CARTESIAN_POINT('Ctrl Pts',(-62.9036579244618,-0.220621155329696,
2.67926100056413));
#213377=CARTESIAN_POINT('Ctrl Pts',(-62.9015528091474,-0.224228171852353,
2.68260965685121));
#213378=CARTESIAN_POINT('Ctrl Pts',(-62.8994013510256,-0.227731941419342,
2.68603254012481));
#213379=CARTESIAN_POINT('Ctrl Pts',(-62.8972498929038,-0.23123571098633,
2.6894554233984));
#213380=CARTESIAN_POINT('Ctrl Pts',(-62.8950520414621,-0.234636114276541,
2.69295261525383));
#213381=CARTESIAN_POINT('Ctrl Pts',(-62.8928111037451,-0.237927978230728,
2.69651891172097));
#213382=CARTESIAN_POINT('Ctrl Pts',(-62.8927919932396,-0.237956050936022,
2.69654932476085));
#213383=CARTESIAN_POINT('Ctrl Pts',(-62.8927728797351,-0.237984115710813,
2.69657974261143));
#213384=CARTESIAN_POINT('Ctrl Pts',(-62.8927537632335,-0.238012172552645,
2.69661016526971));
#213385=CARTESIAN_POINT('Ctrl Pts',(-62.8829906867838,-0.252341211297632,
2.71214746101229));
#213386=CARTESIAN_POINT('Ctrl Pts',(-62.8725309380398,-0.264702219192015,
2.72880565567787));
#213387=CARTESIAN_POINT('Ctrl Pts',(-62.861566477281,-0.275152816748675,
2.74628040012666));
#213388=CARTESIAN_POINT('Ctrl Pts',(-62.8502312057401,-0.285956846575219,
2.76434612882901));
#213389=CARTESIAN_POINT('Ctrl Pts',(-62.8383556508849,-0.294719332060581,
2.783285926551));
#213390=CARTESIAN_POINT('Ctrl Pts',(-62.8261370346392,-0.301453885683407,
2.80278753268661));
#213391=CARTESIAN_POINT('Ctrl Pts',(-62.8141508421851,-0.308060333925367,
2.82191817723792));
#213392=CARTESIAN_POINT('Ctrl Pts',(-62.8018335935106,-0.31271515574816,
2.84159092316334));
#213393=CARTESIAN_POINT('Ctrl Pts',(-62.7893708783575,-0.315383336842736,
2.86151233818375));
#213394=CARTESIAN_POINT('Ctrl Pts',(-62.7811147664911,-0.31715091327579,
2.87470957722226));
#213395=CARTESIAN_POINT('Ctrl Pts',(-62.7727948225133,-0.318045664008263,
2.88801594388801));
#213396=CARTESIAN_POINT('Ctrl Pts',(-62.7644678366119,-0.318045750792856,
2.90134173516021));
#213397=CARTESIAN_POINT('',(-62.4081695979768,-0.318048871876942,3.4715307213907));
#213398=CARTESIAN_POINT('',(-62.7644678366119,-0.318045750792856,2.90134173516021));
#213399=CARTESIAN_POINT('',(-62.0995362748658,-6.20712349654488,3.47153072139067));
#213400=CARTESIAN_POINT('Origin',(5.53234440788222E-15,1.85015204418142E-13,
3.47153072139072));
#213401=CARTESIAN_POINT('',(-62.4538823482275,-6.24436990788084,2.90134173516018));
#213402=CARTESIAN_POINT('',(-62.0995362748658,-6.20712349654488,3.47153072139066));
#213403=CARTESIAN_POINT('',(-62.6108711573005,-6.56531752495326,2.59908173516017));
#213404=CARTESIAN_POINT('Ctrl Pts',(-62.4538823482275,-6.24436990788084,
2.90134173516018));
#213405=CARTESIAN_POINT('Ctrl Pts',(-62.4661208561115,-6.24565635961485,
2.8816483765655));
#213406=CARTESIAN_POINT('Ctrl Pts',(-62.4781153572974,-6.24887816048161,
2.86203734438804));
#213407=CARTESIAN_POINT('Ctrl Pts',(-62.4897034690589,-6.25393874389528,
2.84277945977656));
#213408=CARTESIAN_POINT('Ctrl Pts',(-62.5015244311575,-6.25910101415649,
2.82313460919377));
#213409=CARTESIAN_POINT('Ctrl Pts',(-62.5129234357008,-6.26617675898563,
2.80385576862559));
#213410=CARTESIAN_POINT('Ctrl Pts',(-62.5237314369803,-6.27511683300826,
2.78521678517484));
#213411=CARTESIAN_POINT('Ctrl Pts',(-62.5341195572078,-6.28370959325942,
2.76730190933462));
#213412=CARTESIAN_POINT('Ctrl Pts',(-62.5439624606715,-6.29402509234208,
2.74997687278681));
#213413=CARTESIAN_POINT('Ctrl Pts',(-62.5531007542782,-6.30606398948117,
2.73349253344551));
#213414=CARTESIAN_POINT('Ctrl Pts',(-62.5601204743196,-6.31531185250257,
2.72082983598532));
#213415=CARTESIAN_POINT('Ctrl Pts',(-62.5667243349272,-6.32557753708262,
2.70866321038916));
#213416=CARTESIAN_POINT('Ctrl Pts',(-62.5728320301412,-6.33687803771715,
2.69711645335838));
#213417=CARTESIAN_POINT('Ctrl Pts',(-62.5728480373211,-6.33690765431399,
2.69708619136744));
#213418=CARTESIAN_POINT('Ctrl Pts',(-62.5728640408534,-6.3369372788212,
2.69705593387211));
#213419=CARTESIAN_POINT('Ctrl Pts',(-62.5728800407363,-6.33696691123601,
2.69702568087563));
#213420=CARTESIAN_POINT('Ctrl Pts',(-62.5745955535552,-6.34014410870351,
2.69378194443259));
#213421=CARTESIAN_POINT('Ctrl Pts',(-62.5762674929177,-6.34341121944343,
2.69059266624693));
#213422=CARTESIAN_POINT('Ctrl Pts',(-62.5778935423007,-6.34676388583411,
2.6874621934267));
#213423=CARTESIAN_POINT('Ctrl Pts',(-62.5869421374015,-6.36542071200024,
2.67004182395984));
#213424=CARTESIAN_POINT('Ctrl Pts',(-62.5945741278857,-6.38672471011456,
2.65443567877707));
#213425=CARTESIAN_POINT('Ctrl Pts',(-62.6004109483571,-6.40987366744317,
2.64136852352852));
#213426=CARTESIAN_POINT('Ctrl Pts',(-62.6030305942145,-6.42026324006541,
2.63550380329538));
#213427=CARTESIAN_POINT('Ctrl Pts',(-62.6052889671228,-6.43102458681625,
2.63014997451014));
#213428=CARTESIAN_POINT('Ctrl Pts',(-62.6071534261453,-6.44208677567895,
2.62536981119245));
#213429=CARTESIAN_POINT('Ctrl Pts',(-62.6079636948179,-6.44689425333248,
2.62329241687065));
#213430=CARTESIAN_POINT('Ctrl Pts',(-62.6086994224562,-6.45175840518017,
2.62132362131419));
#213431=CARTESIAN_POINT('Ctrl Pts',(-62.6093578414452,-6.45667331290459,
2.61946873372339));
#213432=CARTESIAN_POINT('Ctrl Pts',(-62.6116623079068,-6.47387548994004,
2.6129766271556));
#213433=CARTESIAN_POINT('Ctrl Pts',(-62.6130197402062,-6.49169942613433,
2.60787989113962));
#213434=CARTESIAN_POINT('Ctrl Pts',(-62.6133114945132,-6.50989137546646,
2.60440616886172));
#213435=CARTESIAN_POINT('Ctrl Pts',(-62.6134573716666,-6.51898735013253,
2.60266930772277));
#213436=CARTESIAN_POINT('Ctrl Pts',(-62.6133368299269,-6.52817532814419,
2.60133820040178));
#213437=CARTESIAN_POINT('Ctrl Pts',(-62.6129350466932,-6.53742359207027,
2.60044130723578));
#213438=CARTESIAN_POINT('Ctrl Pts',(-62.6127341550763,-6.54204772403331,
2.59999286065278));
#213439=CARTESIAN_POINT('Ctrl Pts',(-62.6124629532085,-6.54668692748786,
2.59965296768506));
#213440=CARTESIAN_POINT('Ctrl Pts',(-62.6121195889601,-6.55133723782977,
2.59942518630948));
#213441=CARTESIAN_POINT('Ctrl Pts',(-62.6117762247117,-6.55598754817168,
2.5991974049339));
#213442=CARTESIAN_POINT('Ctrl Pts',(-62.6113606963859,-6.56064896522296,
2.59908173791611));
#213443=CARTESIAN_POINT('Ctrl Pts',(-62.6108711573005,-6.56531752495326,
2.59908173516018));
#213444=CARTESIAN_POINT('',(-62.6076796697354,-6.5956825007991,2.59908173516018));
#213445=CARTESIAN_POINT('Origin',(1.14876675116497E-16,1.91123728172721E-13,
2.59908173516023));
#213446=CARTESIAN_POINT('',(-62.3873926810691,-6.87697683366589,2.90134173516017));
#213447=CARTESIAN_POINT('Ctrl Pts',(-62.6076796697354,-6.5956825007991,
2.59908173516018));
#213448=CARTESIAN_POINT('Ctrl Pts',(-62.6072792748562,-6.59948308607527,
2.59908174381681));
#213449=CARTESIAN_POINT('Ctrl Pts',(-62.6068325084578,-6.60326825869946,
2.59915752000989));
#213450=CARTESIAN_POINT('Ctrl Pts',(-62.6063406883232,-6.60703621730621,
2.59930729517464));
#213451=CARTESIAN_POINT('Ctrl Pts',(-62.6034985746717,-6.62881036976824,
2.60017281085903));
#213452=CARTESIAN_POINT('Ctrl Pts',(-62.5991534367856,-6.65001265698052,
2.60350651799994));
#213453=CARTESIAN_POINT('Ctrl Pts',(-62.5935594283592,-6.67028839971087,
2.60896880596309));
#213454=CARTESIAN_POINT('Ctrl Pts',(-62.591303236076,-6.67846607317822,
2.61117187235337));
#213455=CARTESIAN_POINT('Ctrl Pts',(-62.5888441205341,-6.68649343259762,
2.61372076577129));
#213456=CARTESIAN_POINT('Ctrl Pts',(-62.586199469922,-6.69434891543633,
2.61659179896978));
#213457=CARTESIAN_POINT('Ctrl Pts',(-62.5852237544099,-6.69724711167676,
2.61765103591203));
#213458=CARTESIAN_POINT('Ctrl Pts',(-62.5842227327444,-6.70012178934752,
2.61875422455144));
#213459=CARTESIAN_POINT('Ctrl Pts',(-62.5831972538525,-6.70297180428207,
2.6199002244039));
#213460=CARTESIAN_POINT('Ctrl Pts',(-62.5812744809302,-6.70831558228435,
2.62204897412727));
#213461=CARTESIAN_POINT('Ctrl Pts',(-62.5792657255653,-6.71357265535409,
2.62434823201763));
#213462=CARTESIAN_POINT('Ctrl Pts',(-62.5771765838154,-6.71873548138839,
2.62679048030299));
#213463=CARTESIAN_POINT('Ctrl Pts',(-62.5698645876906,-6.73680537250846,
2.63533834930172));
#213464=CARTESIAN_POINT('Ctrl Pts',(-62.5615678538927,-6.75372073697227,
2.64563784783556));
#213465=CARTESIAN_POINT('Ctrl Pts',(-62.5525263385764,-6.76915820973636,
2.65736666737958));
#213466=CARTESIAN_POINT('Ctrl Pts',(-62.5480055809182,-6.77687694611841,
2.66323107715158));
#213467=CARTESIAN_POINT('Ctrl Pts',(-62.5432986288851,-6.7842262096809,
2.66945281780768));
#213468=CARTESIAN_POINT('Ctrl Pts',(-62.5384354858298,-6.79116558077058,
2.67599160631195));
#213469=CARTESIAN_POINT('Ctrl Pts',(-62.5360039143022,-6.79463526631542,
2.67926100056409));
#213470=CARTESIAN_POINT('Ctrl Pts',(-62.5335332951357,-6.79800247875535,
2.68260965685116));
#213471=CARTESIAN_POINT('Ctrl Pts',(-62.5310273792781,-6.80126216569478,
2.68603254012475));
#213472=CARTESIAN_POINT('Ctrl Pts',(-62.5285214634206,-6.80452185263422,
2.68945542339835));
#213473=CARTESIAN_POINT('Ctrl Pts',(-62.5259802131086,-6.80767389012573,
2.69295261525378));
#213474=CARTESIAN_POINT('Ctrl Pts',(-62.5234074580024,-6.8107134791289,
2.69651891172092));
#213475=CARTESIAN_POINT('Ctrl Pts',(-62.5233855177896,-6.81073940045721,
2.6965493247608));
#213476=CARTESIAN_POINT('Ctrl Pts',(-62.5233635754231,-6.81076531358497,
2.69657974261138));
#213477=CARTESIAN_POINT('Ctrl Pts',(-62.5233416309051,-6.81079121850996,
2.69661016526966));
#213478=CARTESIAN_POINT('Ctrl Pts',(-62.5121342452089,-6.82402124190414,
2.71214746101314));
#213479=CARTESIAN_POINT('Ctrl Pts',(-62.5004397189026,-6.8352211934421,
2.72880565567975));
#213480=CARTESIAN_POINT('Ctrl Pts',(-62.4884429377036,-6.84446844329853,
2.74628040012967));
#213481=CARTESIAN_POINT('Ctrl Pts',(-62.4760404333306,-6.85402842900468,
2.76434612883316));
#213482=CARTESIAN_POINT('Ctrl Pts',(-62.4633140048645,-6.86150157917835,
2.78328592655637));
#213483=CARTESIAN_POINT('Ctrl Pts',(-62.4504583709352,-6.86692204703221,
2.80278753269324));
#213484=CARTESIAN_POINT('Ctrl Pts',(-62.4378472782144,-6.8722394061816,
2.82191817724563));
#213485=CARTESIAN_POINT('Ctrl Pts',(-62.4251109433444,-6.87558122532737,
2.84159092317214));
#213486=CARTESIAN_POINT('Ctrl Pts',(-62.4124375993787,-6.87693208138303,
2.86151233819362));
#213487=CARTESIAN_POINT('Ctrl Pts',(-62.4040419533109,-6.87782697616081,
2.87470957722888));
#213488=CARTESIAN_POINT('Ctrl Pts',(-62.3956740599399,-6.87784715439644,
2.8880159438913));
#213489=CARTESIAN_POINT('Ctrl Pts',(-62.3873926810691,-6.87697683366589,
2.90134173516017));
#213490=CARTESIAN_POINT('',(-62.0330459552232,-6.83973663030285,3.47153072139066));
#213491=CARTESIAN_POINT('',(-62.3873926810691,-6.87697683366589,2.90134173516017));
#213492=CARTESIAN_POINT('',(-61.110527437164,-12.6642893210144,3.47153072139062));
#213493=CARTESIAN_POINT('Origin',(5.53234440788222E-15,1.85015204418142E-13,
3.47153072139072));
#213494=CARTESIAN_POINT('',(-61.4590390555207,-12.7383709431253,2.90134173516013));
#213495=CARTESIAN_POINT('',(-61.110527437164,-12.6642893210144,3.47153072139062));
#213496=CARTESIAN_POINT('',(-61.5816197022697,-13.0739701745327,2.59908173516013));
#213497=CARTESIAN_POINT('Ctrl Pts',(-61.4590390555208,-12.7383709431253,
2.90134173516013));
#213498=CARTESIAN_POINT('Ctrl Pts',(-61.4710760487536,-12.7409296199635,
2.88164837656823));
#213499=CARTESIAN_POINT('Ctrl Pts',(-61.4826680729118,-12.7453875382437,
2.8620373443935));
#213500=CARTESIAN_POINT('Ctrl Pts',(-61.4936637287758,-12.7516316867652,
2.84277945978463));
#213501=CARTESIAN_POINT('Ctrl Pts',(-61.5048803302284,-12.7580013045708,
2.8231346092045));
#213502=CARTESIAN_POINT('Ctrl Pts',(-61.5154772730974,-12.7662298081553,
2.80385576863884));
#213503=CARTESIAN_POINT('Ctrl Pts',(-61.525291574815,-12.7762506512793,
2.78521678519036));
#213504=CARTESIAN_POINT('Ctrl Pts',(-61.5347245998078,-12.7858821937322,
2.76730190935215));
#213505=CARTESIAN_POINT('Ctrl Pts',(-61.543435319549,-12.7971700470021,
2.74997687280613));
#213506=CARTESIAN_POINT('Ctrl Pts',(-61.5512651452094,-12.8100982055875,
2.73349253346629));
#213507=CARTESIAN_POINT('Ctrl Pts',(-61.5572797455837,-12.8200291684005,
2.72082983599861));
#213508=CARTESIAN_POINT('Ctrl Pts',(-61.5627743733217,-12.8309289078927,
2.70866321039545));
#213509=CARTESIAN_POINT('Ctrl Pts',(-61.5676673859795,-12.8428059312037,
2.69711645335834));
#213510=CARTESIAN_POINT('Ctrl Pts',(-61.567680209693,-12.8428370587637,
2.6970861913674));
#213511=CARTESIAN_POINT('Ctrl Pts',(-61.5676930289521,-12.8428681938094,
2.69705593387208));
#213512=CARTESIAN_POINT('Ctrl Pts',(-61.5677058437552,-12.8428993363379,
2.6970256808756));
#213513=CARTESIAN_POINT('Ctrl Pts',(-61.5690798512466,-12.8462384487039,
2.69378194443255));
#213514=CARTESIAN_POINT('Ctrl Pts',(-61.5704011254853,-12.8496624271216,
2.69059266624688));
#213515=CARTESIAN_POINT('Ctrl Pts',(-61.5716678181341,-12.8531666956982,
2.68746219342665));
#213516=CARTESIAN_POINT('Ctrl Pts',(-61.5787166747154,-12.8726671535587,
2.67004182396012));
#213517=CARTESIAN_POINT('Ctrl Pts',(-61.5840799821728,-12.8946522063788,
2.65443567877762));
#213518=CARTESIAN_POINT('Ctrl Pts',(-61.587465102995,-12.9182844651708,
2.64136852352922));
#213519=CARTESIAN_POINT('Ctrl Pts',(-61.5889843920982,-12.9288909501833,
2.6355038032958));
#213520=CARTESIAN_POINT('Ctrl Pts',(-61.590105526365,-12.9398294094007,
2.63014997451031));
#213521=CARTESIAN_POINT('Ctrl Pts',(-61.5908034580837,-12.9510258874722,
2.62536981119243));
#213522=CARTESIAN_POINT('Ctrl Pts',(-61.5911067697684,-12.9558917253993,
2.62329241687063));
#213523=CARTESIAN_POINT('Ctrl Pts',(-61.591330024696,-12.9608061353937,
2.62132362131416));
#213524=CARTESIAN_POINT('Ctrl Pts',(-61.5914710890454,-12.9657629422644,
2.61946873372336));
#213525=CARTESIAN_POINT('Ctrl Pts',(-61.5919648142681,-12.9831117663121,
2.61297662715556));
#213526=CARTESIAN_POINT('Ctrl Pts',(-61.5914517017517,-13.0009799514312,
2.60787989113959));
#213527=CARTESIAN_POINT('Ctrl Pts',(-61.5898402812904,-13.0191027399908,
2.60440616886169));
#213528=CARTESIAN_POINT('Ctrl Pts',(-61.5890345710598,-13.0281641342706,
2.60266930772274));
#213529=CARTESIAN_POINT('Ctrl Pts',(-61.5879542844383,-13.0372891795346,
2.60133820040173));
#213530=CARTESIAN_POINT('Ctrl Pts',(-61.5865879953991,-13.0464447827192,
2.60044130723573));
#213531=CARTESIAN_POINT('Ctrl Pts',(-61.5859048508795,-13.0510225843115,
2.59999286065273));
#213532=CARTESIAN_POINT('Ctrl Pts',(-61.585150205876,-13.0556080254097,
2.599652967685));
#213533=CARTESIAN_POINT('Ctrl Pts',(-61.5843226328191,-13.0601969695278,
2.59942518630943));
#213534=CARTESIAN_POINT('Ctrl Pts',(-61.5834950597623,-13.0647859136458,
2.59919740493385));
#213535=CARTESIAN_POINT('Ctrl Pts',(-61.582594556983,-13.0693783604294,
2.59908173791607));
#213536=CARTESIAN_POINT('Ctrl Pts',(-61.5816197022697,-13.0739701745327,
2.59908173516013));
#213537=CARTESIAN_POINT('',(-61.575271693745,-13.103835206573,2.59908173516013));
#213538=CARTESIAN_POINT('Origin',(1.12331902584553E-16,1.91139795234149E-13,
2.59908173516023));
#213539=CARTESIAN_POINT('',(-61.3267881959112,-13.3605623192489,2.90134173516012));
#213540=CARTESIAN_POINT('Ctrl Pts',(-61.575271693745,-13.103835206573,2.59908173516014));
#213541=CARTESIAN_POINT('Ctrl Pts',(-61.5744762229325,-13.107573119184,
2.5990817438167));
#213542=CARTESIAN_POINT('Ctrl Pts',(-61.5736362456895,-13.1112908564314,
2.59915752000985));
#213543=CARTESIAN_POINT('Ctrl Pts',(-61.5727532608743,-13.1149867645638,
2.59930729517459));
#213544=CARTESIAN_POINT('Ctrl Pts',(-61.5676506979224,-13.1363445541701,
2.60017281085907));
#213545=CARTESIAN_POINT('Ctrl Pts',(-61.5611131206554,-13.1569765024506,
2.60350651800056));
#213546=CARTESIAN_POINT('Ctrl Pts',(-61.5534303645623,-13.1765564394382,
2.60896880596467));
#213547=CARTESIAN_POINT('Ctrl Pts',(-61.5503317322965,-13.1844534784405,
2.61117187235458));
#213548=CARTESIAN_POINT('Ctrl Pts',(-61.5470470005034,-13.1921798155745,
2.61372076577195));
#213549=CARTESIAN_POINT('Ctrl Pts',(-61.5435957160156,-13.19971582399,2.61659179896972));
#213550=CARTESIAN_POINT('Ctrl Pts',(-61.5423224015758,-13.2024961535652,
2.61765103591197));
#213551=CARTESIAN_POINT('Ctrl Pts',(-61.5410263779725,-13.2052504481945,
2.61875422455137));
#213552=CARTESIAN_POINT('Ctrl Pts',(-61.5397086090799,-13.2079776587163,
2.61990022440384));
#213553=CARTESIAN_POINT('Ctrl Pts',(-61.5372377924062,-13.2130911784448,
2.62204897412721));
#213554=CARTESIAN_POINT('Ctrl Pts',(-61.5346905274441,-13.2181094806068,
2.62434823201759));
#213555=CARTESIAN_POINT('Ctrl Pts',(-61.5320731679598,-13.2230256493633,
2.62679048030294));
#213556=CARTESIAN_POINT('Ctrl Pts',(-61.5229124097646,-13.2402322400107,
2.63533834930168));
#213557=CARTESIAN_POINT('Ctrl Pts',(-61.5128929892896,-13.2561876955041,
2.64563784783551));
#213558=CARTESIAN_POINT('Ctrl Pts',(-61.5022873490354,-13.2705955044755,
2.65736666737953));
#213559=CARTESIAN_POINT('Ctrl Pts',(-61.4969845289083,-13.2777994089612,
2.66323107715154));
#213560=CARTESIAN_POINT('Ctrl Pts',(-61.4915351548246,-13.2846164020263,
2.66945281780763));
#213561=CARTESIAN_POINT('Ctrl Pts',(-61.4859732907798,-13.2910094216448,
2.6759916063119));
#213562=CARTESIAN_POINT('Ctrl Pts',(-61.4831923587574,-13.2942059314541,
2.67926100056404));
#213563=CARTESIAN_POINT('Ctrl Pts',(-61.4803833043594,-13.2972964479272,
2.68260965685112));
#213564=CARTESIAN_POINT('Ctrl Pts',(-61.4775503861045,-13.3002763384268,
2.68603254012471));
#213565=CARTESIAN_POINT('Ctrl Pts',(-61.4747174678497,-13.3032562289265,
2.68945542339831));
#213566=CARTESIAN_POINT('Ctrl Pts',(-61.4718606611377,-13.3061253662369,
2.69295261525373));
#213567=CARTESIAN_POINT('Ctrl Pts',(-61.4689842762857,-13.3088793779159,
2.69651891172087));
#213568=CARTESIAN_POINT('Ctrl Pts',(-61.468959746747,-13.3089028638677,
2.69654932476075));
#213569=CARTESIAN_POINT('Ctrl Pts',(-61.4689352159237,-13.3089263414388,
2.69657974261133));
#213570=CARTESIAN_POINT('Ctrl Pts',(-61.4689106838181,-13.3089498106271,
2.69661016526961));
#213571=CARTESIAN_POINT('Ctrl Pts',(-61.4563817793397,-13.3209358677642,
2.71214746101225));
#213572=CARTESIAN_POINT('Ctrl Pts',(-61.4435806031499,-13.3308520539319,
2.7288056556779));
#213573=CARTESIAN_POINT('Ctrl Pts',(-61.4306829407573,-13.3387946412829,
2.74628040012677));
#213574=CARTESIAN_POINT('Ctrl Pts',(-61.4173490879869,-13.3470058416641,
2.76434612882926));
#213575=CARTESIAN_POINT('Ctrl Pts',(-61.4039112193248,-13.3531077791288,
2.7832859265514));
#213576=CARTESIAN_POINT('Ctrl Pts',(-61.390559416729,-13.3571547734338,
2.80278753268716));
#213577=CARTESIAN_POINT('Ctrl Pts',(-61.3774615935137,-13.3611247853914,
2.82191817723859));
#213578=CARTESIAN_POINT('Ctrl Pts',(-61.3644457143994,-13.3631169881911,
2.84159092316412));
#213579=CARTESIAN_POINT('Ctrl Pts',(-61.3517005934309,-13.3631357189473,
2.86151233818464));
#213580=CARTESIAN_POINT('Ctrl Pts',(-61.3432573976128,-13.3631481274167,
2.87470957722283));
#213581=CARTESIAN_POINT('Ctrl Pts',(-61.3349332352353,-13.3622935120789,
2.88801594388825));
#213582=CARTESIAN_POINT('Ctrl Pts',(-61.3267881959112,-13.3605623192489,
2.90134173516012));
#213583=CARTESIAN_POINT('',(-60.9782752797347,-13.2864868028998,3.47153072139061));
#213584=CARTESIAN_POINT('',(-61.3267881959112,-13.3605623192489,2.90134173516012));
#213585=CARTESIAN_POINT('',(-59.4519788726606,-18.98270254151,3.47153072139058));
#213586=CARTESIAN_POINT('Origin',(5.53234440788222E-15,1.85015204418142E-13,
3.47153072139072));
#213587=CARTESIAN_POINT('',(-59.790837669791,-19.0928077206414,2.90134173516009));
#213588=CARTESIAN_POINT('',(-59.4519788726606,-18.98270254151,3.47153072139058));
#213589=CARTESIAN_POINT('',(-59.8776671349984,-19.4393816709759,2.59908173516009));
#213590=CARTESIAN_POINT('Ctrl Pts',(-59.790837669791,-19.0928077206414,
2.90134173516009));
#213591=CARTESIAN_POINT('Ctrl Pts',(-59.8025412685584,-19.0966105891854,
2.88164837656674));
#213592=CARTESIAN_POINT('Ctrl Pts',(-59.813603811049,-19.1022557829948,
2.86203734439059));
#213593=CARTESIAN_POINT('Ctrl Pts',(-59.8238865403109,-19.1096150844282,
2.84277945978036));
#213594=CARTESIAN_POINT('Ctrl Pts',(-59.834375889687,-19.1171222629148,
2.82313460919879));
#213595=CARTESIAN_POINT('Ctrl Pts',(-59.84405466856,-19.1264133720502,2.80385576863178));
#213596=CARTESIAN_POINT('Ctrl Pts',(-59.8527677431739,-19.137405193825,
2.78521678518207));
#213597=CARTESIAN_POINT('Ctrl Pts',(-59.8611423227377,-19.1479699932883,
2.76730190934267));
#213598=CARTESIAN_POINT('Ctrl Pts',(-59.868625422289,-19.1601065286669,
2.74997687279559));
#213599=CARTESIAN_POINT('Ctrl Pts',(-59.8750609947955,-19.1737823050926,
2.73349253345488));
#213600=CARTESIAN_POINT('Ctrl Pts',(-59.8800045782761,-19.184287561984,
2.72082983599128));
#213601=CARTESIAN_POINT('Ctrl Pts',(-59.8843297728478,-19.1957019365533,
2.70866321039196));
#213602=CARTESIAN_POINT('Ctrl Pts',(-59.8879544940743,-19.2080253553781,
2.6971164533583));
#213603=CARTESIAN_POINT('Ctrl Pts',(-59.8879639938222,-19.2080576528611,
2.69708619136736));
#213604=CARTESIAN_POINT('Ctrl Pts',(-59.8879734883575,-19.2080899573232,
2.69705593387203));
#213605=CARTESIAN_POINT('Ctrl Pts',(-59.8879829776791,-19.2081222687614,
2.69702568087555));
#213606=CARTESIAN_POINT('Ctrl Pts',(-59.8890004259295,-19.2115867120121,
2.6937819444325));
#213607=CARTESIAN_POINT('Ctrl Pts',(-59.8899565588874,-19.2151300442834,
2.69059266624684));
#213608=CARTESIAN_POINT('Ctrl Pts',(-59.8908500166521,-19.2187475215461,
2.68746219342661));
#213609=CARTESIAN_POINT('Ctrl Pts',(-59.8958219059659,-19.2388779600028,
2.67004182396144));
#213610=CARTESIAN_POINT('Ctrl Pts',(-59.8988577688777,-19.2613031946878,
2.65443567878001));
#213611=CARTESIAN_POINT('Ctrl Pts',(-59.8997541019591,-19.2851598349689,
2.64136852353223));
#213612=CARTESIAN_POINT('Ctrl Pts',(-59.9001563886588,-19.2958670255037,
2.63550380329761));
#213613=CARTESIAN_POINT('Ctrl Pts',(-59.9001280009023,-19.3068627531409,
2.63014997451108));
#213614=CARTESIAN_POINT('Ctrl Pts',(-59.8996517586311,-19.3180708494661,
2.62536981119236));
#213615=CARTESIAN_POINT('Ctrl Pts',(-59.8994447901816,-19.3229417365282,
2.62329241687056));
#213616=CARTESIAN_POINT('Ctrl Pts',(-59.8991531263708,-19.3278525613649,
2.62132362131411));
#213617=CARTESIAN_POINT('Ctrl Pts',(-59.89877529055,-19.3327969595686,2.61946873372331));
#213618=CARTESIAN_POINT('Ctrl Pts',(-59.8974528651771,-19.3501023532817,
2.61297662715552));
#213619=CARTESIAN_POINT('Ctrl Pts',(-59.8950748296128,-19.3678190197503,
2.60787989113953));
#213620=CARTESIAN_POINT('Ctrl Pts',(-59.8915778894432,-19.3856740904735,
2.60440616886164));
#213621=CARTESIAN_POINT('Ctrl Pts',(-59.8898294193584,-19.3946016258351,
2.60266930772269));
#213622=CARTESIAN_POINT('Ctrl Pts',(-59.8878012237013,-19.4035637624459,
2.6013382004017));
#213623=CARTESIAN_POINT('Ctrl Pts',(-59.8854853982053,-19.4125263941846,
2.6004413072357));
#213624=CARTESIAN_POINT('Ctrl Pts',(-59.8843274854572,-19.417007710054,
2.5999928606527));
#213625=CARTESIAN_POINT('Ctrl Pts',(-59.8830976653666,-19.4214891497435,
2.59965296768497));
#213626=CARTESIAN_POINT('Ctrl Pts',(-59.8817949505649,-19.4259664502057,
2.59942518630939));
#213627=CARTESIAN_POINT('Ctrl Pts',(-59.8804922357631,-19.4304437506678,
2.59919740493381));
#213628=CARTESIAN_POINT('Ctrl Pts',(-59.8791166246274,-19.4349169113758,
2.59908173791598));
#213629=CARTESIAN_POINT('Ctrl Pts',(-59.8776671349984,-19.4393816709759,
2.59908173516009));
#213630=CARTESIAN_POINT('',(-59.868232155624,-19.4684195516699,2.59908173516009));
#213631=CARTESIAN_POINT('Origin',(1.08121605342496E-16,1.91155508277372E-13,
2.59908173516023));
#213632=CARTESIAN_POINT('',(-59.5942745858234,-19.6977666881848,2.90134173516009));
#213633=CARTESIAN_POINT('Ctrl Pts',(-59.868232155624,-19.4684195516699,
2.59908173516009));
#213634=CARTESIAN_POINT('Ctrl Pts',(-59.8670503242228,-19.4720538382629,
2.59908174381669));
#213635=CARTESIAN_POINT('Ctrl Pts',(-59.8658263391017,-19.4756634078263,
2.59915752000981));
#213636=CARTESIAN_POINT('Ctrl Pts',(-59.8645618637722,-19.4792467723414,
2.59930729517456));
#213637=CARTESIAN_POINT('Ctrl Pts',(-59.8572547562677,-19.4999541986775,
2.60017281085904));
#213638=CARTESIAN_POINT('Ctrl Pts',(-59.848596366685,-19.5197897600815,
2.60350651800056));
#213639=CARTESIAN_POINT('Ctrl Pts',(-59.8389090368093,-19.5384593694377,
2.60896880596472));
#213640=CARTESIAN_POINT('Ctrl Pts',(-59.8350019138241,-19.5459892523649,
2.61117187235461));
#213641=CARTESIAN_POINT('Ctrl Pts',(-59.8309275539882,-19.553329915849,
2.61372076577195));
#213642=CARTESIAN_POINT('Ctrl Pts',(-59.8267074486191,-19.560463883758,
2.61659179896968));
#213643=CARTESIAN_POINT('Ctrl Pts',(-59.8251504859513,-19.5630958847952,
2.61765103591193));
#213644=CARTESIAN_POINT('Ctrl Pts',(-59.8235736599158,-19.5656996197547,
2.61875422455134));
#213645=CARTESIAN_POINT('Ctrl Pts',(-59.8219780387742,-19.5682741459747,
2.6199002244038));
#213646=CARTESIAN_POINT('Ctrl Pts',(-59.8189862491337,-19.5731013826371,
2.62204897412717));
#213647=CARTESIAN_POINT('Ctrl Pts',(-59.8159283829424,-19.5778259323228,
2.62434823201754));
#213648=CARTESIAN_POINT('Ctrl Pts',(-59.8128114820619,-19.5824415812277,
2.62679048030289));
#213649=CARTESIAN_POINT('Ctrl Pts',(-59.8019023289802,-19.5985963523948,
2.63533834930163));
#213650=CARTESIAN_POINT('Ctrl Pts',(-59.7902699966955,-19.6134170876084,
2.64563784783547));
#213651=CARTESIAN_POINT('Ctrl Pts',(-59.7782164291174,-19.626637377817,
2.65736666737949));
#213652=CARTESIAN_POINT('Ctrl Pts',(-59.7721896453284,-19.6332475229213,
2.6632310771515));
#213653=CARTESIAN_POINT('Ctrl Pts',(-59.7660575536769,-19.6394575570863,
2.66945281780758));
#213654=CARTESIAN_POINT('Ctrl Pts',(-59.7598579055889,-19.645234181973,
2.67599160631185));
#213655=CARTESIAN_POINT('Ctrl Pts',(-59.7567580815449,-19.6481224944163,
2.67926100056399));
#213656=CARTESIAN_POINT('Ctrl Pts',(-59.7536413685032,-19.6509024545773,
2.68260965685108));
#213657=CARTESIAN_POINT('Ctrl Pts',(-59.7505124858963,-19.6535699003333,
2.68603254012467));
#213658=CARTESIAN_POINT('Ctrl Pts',(-59.7473836032895,-19.6562373460893,
2.68945542339827));
#213659=CARTESIAN_POINT('Ctrl Pts',(-59.7442425399495,-19.6587921483498,
2.6929526152537));
#213660=CARTESIAN_POINT('Ctrl Pts',(-59.7410940396261,-19.6612304091763,
2.69651891172084));
#213661=CARTESIAN_POINT('Ctrl Pts',(-59.7410671895124,-19.6612512024347,
2.69654932476071));
#213662=CARTESIAN_POINT('Ctrl Pts',(-59.741040338997,-19.6612719872239,
2.6965797426113));
#213663=CARTESIAN_POINT('Ctrl Pts',(-59.7410134880827,-19.6612927635423,
2.69661016526957));
#213664=CARTESIAN_POINT('Ctrl Pts',(-59.7273003341204,-19.6719035326729,
2.71214746101264));
#213665=CARTESIAN_POINT('Ctrl Pts',(-59.7135327604112,-19.6804273096603,
2.72880565567879));
#213666=CARTESIAN_POINT('Ctrl Pts',(-59.6998755263121,-19.6869782138572,
2.7462804001282));
#213667=CARTESIAN_POINT('Ctrl Pts',(-59.6857564136245,-19.6937506652841,
2.76434612883127));
#213668=CARTESIAN_POINT('Ctrl Pts',(-59.6717543328665,-19.698414535936,
2.78328592655404));
#213669=CARTESIAN_POINT('Ctrl Pts',(-59.6580526467464,-19.7010437169754,
2.80278753269046));
#213670=CARTESIAN_POINT('Ctrl Pts',(-59.6446115955276,-19.7036228854591,
2.82191817724254));
#213671=CARTESIAN_POINT('Ctrl Pts',(-59.6314587768635,-19.7042436449212,
2.84159092316874));
#213672=CARTESIAN_POINT('Ctrl Pts',(-59.6187815171037,-19.7029300451591,
2.86151233818992));
#213673=CARTESIAN_POINT('Ctrl Pts',(-59.6103832769587,-19.7020598313695,
2.87470957722636));
#213674=CARTESIAN_POINT('Ctrl Pts',(-59.6021940468427,-19.7003397858028,
2.88801594389));
#213675=CARTESIAN_POINT('Ctrl Pts',(-59.5942745858234,-19.6977666881848,
2.90134173516009));
#213676=CARTESIAN_POINT('',(-59.255413859757,-19.5876674457081,3.47153072139057));
#213677=CARTESIAN_POINT('',(-59.5942745858234,-19.6977666881848,2.90134173516009));
#213678=CARTESIAN_POINT('',(-57.1420619865019,-25.0931373005748,3.47153072139054));
#213679=CARTESIAN_POINT('Origin',(5.53234440788222E-15,1.85015204418142E-13,
3.47153072139072));
#213680=CARTESIAN_POINT('',(-57.4675553545138,-25.2380597013433,2.90134173516005));
#213681=CARTESIAN_POINT('',(-57.1420619865019,-25.0931373005748,3.47153072139053));
#213682=CARTESIAN_POINT('',(-57.5176823163886,-25.5918112338797,2.59908173516005));
#213683=CARTESIAN_POINT('Ctrl Pts',(-57.4675553545138,-25.2380597013433,
2.90134173516005));
#213684=CARTESIAN_POINT('Ctrl Pts',(-57.4787973317383,-25.2430650965696,
2.88164837656564));
#213685=CARTESIAN_POINT('Ctrl Pts',(-57.4892091890304,-25.2498357159834,
2.86203734438844));
#213686=CARTESIAN_POINT('Ctrl Pts',(-57.4986663319564,-25.2582295402821,
2.84277945977721));
#213687=CARTESIAN_POINT('Ctrl Pts',(-57.5083135057489,-25.2667920292311,
2.82313460919456));
#213688=CARTESIAN_POINT('Ctrl Pts',(-57.5169680778989,-25.2770439485812,
2.80385576862652));
#213689=CARTESIAN_POINT('Ctrl Pts',(-57.5244844631399,-25.2888863203071,
2.78521678517588));
#213690=CARTESIAN_POINT('Ctrl Pts',(-57.5317088436281,-25.3002686266268,
2.76730190933564));
#213691=CARTESIAN_POINT('Ctrl Pts',(-57.5378823365847,-25.3131208736925,
2.74997687278781));
#213692=CARTESIAN_POINT('Ctrl Pts',(-57.5428531464576,-25.3273944332896,
2.73349253344648));
#213693=CARTESIAN_POINT('Ctrl Pts',(-57.5466715501105,-25.3383588864668,
2.72082983598588));
#213694=CARTESIAN_POINT('Ctrl Pts',(-57.54977992378,-25.3501628378374,2.70866321038936));
#213695=CARTESIAN_POINT('Ctrl Pts',(-57.5520966403719,-25.3627976342212,
2.69711645335824));
#213696=CARTESIAN_POINT('Ctrl Pts',(-57.5521027120729,-25.3628307477693,
2.6970861913673));
#213697=CARTESIAN_POINT('Ctrl Pts',(-57.5521087778604,-25.3628638677133,
2.69705593387198));
#213698=CARTESIAN_POINT('Ctrl Pts',(-57.5521148377335,-25.3628969940503,
2.6970256808755));
#213699=CARTESIAN_POINT('Ctrl Pts',(-57.5527645793668,-25.3664488110204,
2.69378194443245));
#213700=CARTESIAN_POINT('Ctrl Pts',(-57.5533450954511,-25.3700726756556,
2.6905926662468));
#213701=CARTESIAN_POINT('Ctrl Pts',(-57.5538555294215,-25.3737637277665,
2.68746219342657));
#213702=CARTESIAN_POINT('Ctrl Pts',(-57.5566959784091,-25.3943035935275,
2.67004182395887));
#213703=CARTESIAN_POINT('Ctrl Pts',(-57.5573711352259,-25.416923314519,
2.65443567877544));
#213704=CARTESIAN_POINT('Ctrl Pts',(-57.5557688601527,-25.4407429579518,
2.6413685235265));
#213705=CARTESIAN_POINT('Ctrl Pts',(-57.5550497369112,-25.4514335437838,
2.63550380329411));
#213706=CARTESIAN_POINT('Ctrl Pts',(-57.5538721381537,-25.4623660683425,
2.63014997450951));
#213707=CARTESIAN_POINT('Ctrl Pts',(-57.5522269397029,-25.4734629846669,
2.62536981119234));
#213708=CARTESIAN_POINT('Ctrl Pts',(-57.551511958709,-25.478285554406,2.62329241687053));
#213709=CARTESIAN_POINT('Ctrl Pts',(-57.5507085716895,-25.4831389900605,
2.62132362131408));
#213710=CARTESIAN_POINT('Ctrl Pts',(-57.5498159753468,-25.4880168077358,
2.61946873372328));
#213711=CARTESIAN_POINT('Ctrl Pts',(-57.5466918881474,-25.5050891695994,
2.61297662715548));
#213712=CARTESIAN_POINT('Ctrl Pts',(-57.5424749837906,-25.5224602099123,
2.6078798911395));
#213713=CARTESIAN_POINT('Ctrl Pts',(-57.5371308371209,-25.5398519389078,
2.6044061688616));
#213714=CARTESIAN_POINT('Ctrl Pts',(-57.534458763786,-25.5485478034055,
2.60266930772265));
#213715=CARTESIAN_POINT('Ctrl Pts',(-57.5315048804294,-25.557248840319,
2.60133820040166));
#213716=CARTESIAN_POINT('Ctrl Pts',(-57.5282648911452,-25.565920304143,
2.60044130723566));
#213717=CARTESIAN_POINT('Ctrl Pts',(-57.5266448965032,-25.5702560360551,
2.59999286065266));
#213718=CARTESIAN_POINT('Ctrl Pts',(-57.5249533754917,-25.5745843747449,
2.59965296768492));
#213719=CARTESIAN_POINT('Ctrl Pts',(-57.5231897917611,-25.5789009773103,
2.59942518630934));
#213720=CARTESIAN_POINT('Ctrl Pts',(-57.5214262080304,-25.5832175798758,
2.59919740493376));
#213721=CARTESIAN_POINT('Ctrl Pts',(-57.5195905600217,-25.5875224456232,
2.59908173791597));
#213722=CARTESIAN_POINT('Ctrl Pts',(-57.5176823163886,-25.5918112338797,
2.59908173516005));
#213723=CARTESIAN_POINT('',(-57.505263737773,-25.61970381813,2.59908173516005));
#213724=CARTESIAN_POINT('Origin',(1.02291912287982E-16,1.91170695146999E-13,
2.59908173516023));
#213725=CARTESIAN_POINT('',(-57.2088336324697,-25.8191582032623,2.90134173516005));
#213726=CARTESIAN_POINT('Ctrl Pts',(-57.505263737773,-25.61970381813,2.59908173516005));
#213727=CARTESIAN_POINT('Ctrl Pts',(-57.5037084941752,-25.6231946607006,
2.59908174381664));
#213728=CARTESIAN_POINT('Ctrl Pts',(-57.5021139114131,-25.6266565153805,
2.59915752000977));
#213729=CARTESIAN_POINT('Ctrl Pts',(-57.5004817994257,-25.6300880761868,
2.59930729517452));
#213730=CARTESIAN_POINT('Ctrl Pts',(-57.4910502055666,-25.6499182643584,
2.60017281085909));
#213731=CARTESIAN_POINT('Ctrl Pts',(-57.4803658667951,-25.668740116326,
2.60350651800119));
#213732=CARTESIAN_POINT('Ctrl Pts',(-57.468780099549,-25.6862948499051,
2.60896880596634));
#213733=CARTESIAN_POINT('Ctrl Pts',(-57.4641072931024,-25.6933750777824,
2.61117187235585));
#213734=CARTESIAN_POINT('Ctrl Pts',(-57.4592879447638,-25.7002496417697,
2.61372076577263));
#213735=CARTESIAN_POINT('Ctrl Pts',(-57.4543452548722,-25.7069034079254,
2.61659179896964));
#213736=CARTESIAN_POINT('Ctrl Pts',(-57.452521702385,-25.7093582436704,
2.6176510359119));
#213737=CARTESIAN_POINT('Ctrl Pts',(-57.4506813499535,-25.7117828918951,
2.61875422455131));
#213738=CARTESIAN_POINT('Ctrl Pts',(-57.448825358522,-25.7141765267651,
2.61990022440377));
#213739=CARTESIAN_POINT('Ctrl Pts',(-57.4453453745881,-25.7186645921465,
2.62204897412714));
#213740=CARTESIAN_POINT('Ctrl Pts',(-57.4418104097894,-25.7230436262008,
2.62434823201751));
#213741=CARTESIAN_POINT('Ctrl Pts',(-57.4382281169311,-25.7273081852389,
2.62679048030286));
#213742=CARTESIAN_POINT('Ctrl Pts',(-57.4256900919268,-25.742234141872,
2.6353383493016));
#213743=CARTESIAN_POINT('Ctrl Pts',(-57.4125722940991,-25.7557577777295,
2.64563784783544));
#213744=CARTESIAN_POINT('Ctrl Pts',(-57.399202860606,-25.7676457049092,
2.65736666737945));
#213745=CARTESIAN_POINT('Ctrl Pts',(-57.3925181438594,-25.7735896684991,
2.66323107715146));
#213746=CARTESIAN_POINT('Ctrl Pts',(-57.3857705191195,-25.7791247053303,
2.66945281780755));
#213747=CARTESIAN_POINT('Ctrl Pts',(-57.3790010116301,-25.7842216455739,
2.67599160631182));
#213748=CARTESIAN_POINT('Ctrl Pts',(-57.3756162578855,-25.7867701156958,
2.67926100056395));
#213749=CARTESIAN_POINT('Ctrl Pts',(-57.3722260335603,-25.7892090617194,
2.68260965685103));
#213750=CARTESIAN_POINT('Ctrl Pts',(-57.368835467294,-25.7915348376378,
2.68603254012463));
#213751=CARTESIAN_POINT('Ctrl Pts',(-57.3654449010277,-25.7938606135562,
2.68945542339822));
#213752=CARTESIAN_POINT('Ctrl Pts',(-57.3620539952072,-25.7960730898187,
2.69295261525365));
#213753=CARTESIAN_POINT('Ctrl Pts',(-57.3586678750408,-25.7981688856969,
2.69651891172079));
#213754=CARTESIAN_POINT('Ctrl Pts',(-57.3586389985274,-25.7981867584464,
2.69654932476067));
#213755=CARTESIAN_POINT('Ctrl Pts',(-57.3586101224999,-25.7982046227313,
2.69657974261125));
#213756=CARTESIAN_POINT('Ctrl Pts',(-57.3585812469611,-25.79822247855,2.69661016526953));
#213757=CARTESIAN_POINT('Ctrl Pts',(-57.343834087701,-25.8073417058661,
2.71214746101119));
#213758=CARTESIAN_POINT('Ctrl Pts',(-57.3292509568927,-25.8143796853881,
2.72880565567573));
#213759=CARTESIAN_POINT('Ctrl Pts',(-57.3149837826035,-25.8194671333533,
2.74628040012341));
#213760=CARTESIAN_POINT('Ctrl Pts',(-57.3002341019535,-25.8247266354307,
2.76434612882476));
#213761=CARTESIAN_POINT('Ctrl Pts',(-57.285821218828,-25.8279013409272,
2.78328592654568));
#213762=CARTESIAN_POINT('Ctrl Pts',(-57.2719197677254,-25.8290839028441,
2.80278753268019));
#213763=CARTESIAN_POINT('Ctrl Pts',(-57.2582827514744,-25.830243969945,
2.82191817723063));
#213764=CARTESIAN_POINT('Ctrl Pts',(-57.2451370982952,-25.8294864849001,
2.84159092315515));
#213765=CARTESIAN_POINT('Ctrl Pts',(-57.2326665944559,-25.8268549466949,
2.8615123381747));
#213766=CARTESIAN_POINT('Ctrl Pts',(-57.2244053228559,-25.825111644891,
2.87470957721612));
#213767=CARTESIAN_POINT('Ctrl Pts',(-57.2164407479159,-25.8225450142739,
2.88801594388485));
#213768=CARTESIAN_POINT('Ctrl Pts',(-57.2088336324697,-25.8191582032623,
2.90134173516005));
#213769=CARTESIAN_POINT('',(-56.8833377255392,-25.6742415049982,3.47153072139053));
#213770=CARTESIAN_POINT('',(-57.2088336324697,-25.8191582032623,2.90134173516005));
#213771=CARTESIAN_POINT('',(-54.2060847114739,-30.9286463962981,3.47153072139049));
#213772=CARTESIAN_POINT('Origin',(5.53234440788222E-15,1.85015204418142E-13,
3.47153072139072));
#213773=CARTESIAN_POINT('',(-54.5146464769135,-31.1067982185537,2.90134173516001));
#213774=CARTESIAN_POINT('',(-54.2060847114739,-30.9286463962981,3.47153072139049));
#213775=CARTESIAN_POINT('',(-54.5275217339717,-31.4638515574743,2.59908173516001));
#213776=CARTESIAN_POINT('Ctrl Pts',(-54.5146464769135,-31.1067982185537,
2.90134173516001));
#213777=CARTESIAN_POINT('Ctrl Pts',(-54.525303663139,-31.1129513003045,
2.88164837656633));
#213778=CARTESIAN_POINT('Ctrl Pts',(-54.5349507607444,-31.120773164999,
2.86203734438985));
#213779=CARTESIAN_POINT('Ctrl Pts',(-54.5434787028968,-31.1301095476664,
2.84277945977932));
#213780=CARTESIAN_POINT('Ctrl Pts',(-54.5521780046499,-31.1396335346559,
2.82313460919749));
#213781=CARTESIAN_POINT('Ctrl Pts',(-54.5597135487728,-31.1507339420456,
2.80385576863023));
#213782=CARTESIAN_POINT('Ctrl Pts',(-54.565950893551,-31.1632971162178,
2.78521678518031));
#213783=CARTESIAN_POINT('Ctrl Pts',(-54.5719459231389,-31.1753722224622,
2.76730190934082));
#213784=CARTESIAN_POINT('Ctrl Pts',(-54.5767421714198,-31.1887993693045,
2.74997687279367));
#213785=CARTESIAN_POINT('Ctrl Pts',(-54.5801937574263,-31.2035143279648,
2.73349253345291));
#213786=CARTESIAN_POINT('Ctrl Pts',(-54.582845146024,-31.2148178485878,
2.72082983598999));
#213787=CARTESIAN_POINT('Ctrl Pts',(-54.5847026428005,-31.2268820502026,
2.70866321039129));
#213788=CARTESIAN_POINT('Ctrl Pts',(-54.585685972327,-31.2396897946772,
2.69711645335821));
#213789=CARTESIAN_POINT('Ctrl Pts',(-54.5856885494583,-31.2397233614914,
2.69708619136727));
#213790=CARTESIAN_POINT('Ctrl Pts',(-54.5856911200399,-31.2397569340484,
2.69705593387194));
#213791=CARTESIAN_POINT('Ctrl Pts',(-54.5856936840713,-31.239790512345,
2.69702568087546));
#213792=CARTESIAN_POINT('Ctrl Pts',(-54.5859686003823,-31.2433907885846,
2.69378194443242));
#213793=CARTESIAN_POINT('Ctrl Pts',(-54.5861671393374,-31.2470554817643,
2.69059266624676));
#213794=CARTESIAN_POINT('Ctrl Pts',(-54.5862889570921,-31.2507796687841,
2.68746219342653));
#213795=CARTESIAN_POINT('Ctrl Pts',(-54.5869668451991,-31.2715039227755,
2.67004182396178));
#213796=CARTESIAN_POINT('Ctrl Pts',(-54.5852738987621,-31.294070303669,
2.6544356787807));
#213797=CARTESIAN_POINT('Ctrl Pts',(-54.5811905703973,-31.3175919772474,
2.64136852353312));
#213798=CARTESIAN_POINT('Ctrl Pts',(-54.5793579160794,-31.3281488300881,
2.63550380329813));
#213799=CARTESIAN_POINT('Ctrl Pts',(-54.5770440083386,-31.3388983725489,
2.63014997451128));
#213800=CARTESIAN_POINT('Ctrl Pts',(-54.5742478788456,-31.3497625287429,
2.6253698111923));
#213801=CARTESIAN_POINT('Ctrl Pts',(-54.5730327187885,-31.3544839440759,
2.6232924168705));
#213802=CARTESIAN_POINT('Ctrl Pts',(-54.5717264106366,-31.3592268152914,
2.62132362131404));
#213803=CARTESIAN_POINT('Ctrl Pts',(-54.5703288332444,-31.3639846100471,
2.61946873372324));
#213804=CARTESIAN_POINT('Ctrl Pts',(-54.5654373123717,-31.3806368916921,
2.61297662715544));
#213805=CARTESIAN_POINT('Ctrl Pts',(-54.5594277405088,-31.3974719850964,
2.60787989113946));
#213806=CARTESIAN_POINT('Ctrl Pts',(-54.5522949389283,-31.4142098249418,
2.60440616886156));
#213807=CARTESIAN_POINT('Ctrl Pts',(-54.548728538138,-31.4225787448646,
2.60266930772261));
#213808=CARTESIAN_POINT('Ctrl Pts',(-54.5448813304461,-31.4309233516995,
2.60133820040161));
#213809=CARTESIAN_POINT('Ctrl Pts',(-54.5407526753744,-31.4392086412365,
2.60044130723561));
#213810=CARTESIAN_POINT('Ctrl Pts',(-54.5386883478386,-31.443351286005,
2.59999286065261));
#213811=CARTESIAN_POINT('Ctrl Pts',(-54.5365536585645,-31.4474791015107,
2.59965296768489));
#213812=CARTESIAN_POINT('Ctrl Pts',(-54.5343485280974,-31.4515877125784,
2.59942518630931));
#213813=CARTESIAN_POINT('Ctrl Pts',(-54.5321433976302,-31.4556963236462,
2.59919740493373));
#213814=CARTESIAN_POINT('Ctrl Pts',(-54.5298678244922,-31.4597857294232,
2.59908173791588));
#213815=CARTESIAN_POINT('Ctrl Pts',(-54.5275217339717,-31.4638515574743,
2.59908173516001));
#213816=CARTESIAN_POINT('',(-54.5122556166608,-31.490293248291,2.59908173516001));
#213817=CARTESIAN_POINT('Origin',(9.49066947580418E-17,1.91185189452508E-13,
2.59908173516023));
#213818=CARTESIAN_POINT('',(-54.1966007261205,-31.6576696180587,2.90134173516001));
#213819=CARTESIAN_POINT('Ctrl Pts',(-54.5122556166608,-31.490293248291,
2.59908173516001));
#213820=CARTESIAN_POINT('Ctrl Pts',(-54.5103440004408,-31.4936024004374,
2.5990817438166));
#213821=CARTESIAN_POINT('Ctrl Pts',(-54.5083962906202,-31.4968786114295,
2.59915752000972));
#213822=CARTESIAN_POINT('Ctrl Pts',(-54.5064144237353,-31.5001207716287,
2.59930729517447));
#213823=CARTESIAN_POINT('Ctrl Pts',(-54.4949616780389,-31.5188564579415,
2.60017281085899));
#213824=CARTESIAN_POINT('Ctrl Pts',(-54.4823684499318,-31.5364583843209,
2.6035065180008));
#213825=CARTESIAN_POINT('Ctrl Pts',(-54.4690111814076,-31.552705908786,
2.60896880596544));
#213826=CARTESIAN_POINT('Ctrl Pts',(-54.4636238877434,-31.5592589091581,
2.61117187235515));
#213827=CARTESIAN_POINT('Ctrl Pts',(-54.4581123526894,-31.5655920544896,
2.61372076577221));
#213828=CARTESIAN_POINT('Ctrl Pts',(-54.4525012314182,-31.5716927188401,
2.61659179896959));
#213829=CARTESIAN_POINT('Ctrl Pts',(-54.4504310683343,-31.5739434935989,
2.61765103591185));
#213830=CARTESIAN_POINT('Ctrl Pts',(-54.4483473527931,-31.5761624901353,
2.61875422455126));
#213831=CARTESIAN_POINT('Ctrl Pts',(-54.4462513257023,-31.578349008491,
2.61990022440373));
#213832=CARTESIAN_POINT('Ctrl Pts',(-54.4423212749071,-31.5824487304078,
2.6220489741271));
#213833=CARTESIAN_POINT('Ctrl Pts',(-54.4383479413152,-31.5864342712173,
2.62434823201746));
#213834=CARTESIAN_POINT('Ctrl Pts',(-54.4343395048292,-31.5903010169872,
2.62679048030282));
#213835=CARTESIAN_POINT('Ctrl Pts',(-54.4203099771281,-31.6038346271821,
2.63533834930155));
#213836=CARTESIAN_POINT('Ctrl Pts',(-54.4058504350955,-31.6159129958989,
2.64563784783538));
#213837=CARTESIAN_POINT('Ctrl Pts',(-54.3913116139983,-31.6263383134319,
2.6573666673794));
#213838=CARTESIAN_POINT('Ctrl Pts',(-54.3840422034498,-31.6315509721985,
2.6632310771514));
#213839=CARTESIAN_POINT('Ctrl Pts',(-54.3767529740101,-31.6363503686739,
2.66945281780751));
#213840=CARTESIAN_POINT('Ctrl Pts',(-54.36948777526,-31.6407117811307,2.67599160631178));
#213841=CARTESIAN_POINT('Ctrl Pts',(-54.365855175885,-31.6428924873591,
2.67926100056391));
#213842=CARTESIAN_POINT('Ctrl Pts',(-54.3622285842836,-31.6449636976424,
2.682609656851));
#213843=CARTESIAN_POINT('Ctrl Pts',(-54.3586134821114,-31.6469223220355,
2.68603254012459));
#213844=CARTESIAN_POINT('Ctrl Pts',(-54.3549983799392,-31.6488809464287,
2.68945542339819));
#213845=CARTESIAN_POINT('Ctrl Pts',(-54.3513947831118,-31.6507268563402,
2.69295261525361));
#213846=CARTESIAN_POINT('Ctrl Pts',(-54.3478081421435,-31.6524572252918,
2.69651891172075));
#213847=CARTESIAN_POINT('Ctrl Pts',(-54.3477775556076,-31.652471981715,
2.69654932476063));
#213848=CARTESIAN_POINT('Ctrl Pts',(-54.3477469704398,-31.6524867297707,
2.69657974261121));
#213849=CARTESIAN_POINT('Ctrl Pts',(-54.3477163866429,-31.6525014694577,
2.69661016526948));
#213850=CARTESIAN_POINT('Ctrl Pts',(-54.3320967950441,-31.6600292427987,
2.71214746101382));
#213851=CARTESIAN_POINT('Ctrl Pts',(-54.3168578829657,-31.66550431528,2.72880565568142));
#213852=CARTESIAN_POINT('Ctrl Pts',(-54.3021370826299,-31.6690725678695,
2.7462804001324));
#213853=CARTESIAN_POINT('Ctrl Pts',(-54.2869184346017,-31.672761496392,
2.76434612883701));
#213854=CARTESIAN_POINT('Ctrl Pts',(-54.272252659669,-31.6744122539947,
2.78328592656142));
#213855=CARTESIAN_POINT('Ctrl Pts',(-54.2583037507884,-31.6741352403914,
2.80278753269951));
#213856=CARTESIAN_POINT('Ctrl Pts',(-54.2446201795064,-31.6738634961698,
2.82191817725287));
#213857=CARTESIAN_POINT('Ctrl Pts',(-54.2316257183374,-31.67173606578,2.84159092318038));
#213858=CARTESIAN_POINT('Ctrl Pts',(-54.2194985998668,-31.6678154208116,
2.86151233820282));
#213859=CARTESIAN_POINT('Ctrl Pts',(-54.2114648090419,-31.6652181309731,
2.87470957723501));
#213860=CARTESIAN_POINT('Ctrl Pts',(-54.2038121508368,-31.6618330358498,
2.88801594389429));
#213861=CARTESIAN_POINT('Ctrl Pts',(-54.1966007261205,-31.6576696180587,
2.90134173516001));
#213862=CARTESIAN_POINT('',(-53.8880358395968,-31.4795232016792,3.47153072139049));
#213863=CARTESIAN_POINT('',(-54.1966007261205,-31.6576696180587,2.90134173516001));
#213864=CARTESIAN_POINT('',(-50.6762142289945,-36.4252947698681,3.47153072139046));
#213865=CARTESIAN_POINT('Origin',(5.53234440788222E-15,1.85015204418142E-13,
3.47153072139072));
#213866=CARTESIAN_POINT('',(-50.964463724589,-36.6347241449657,2.90134173515997));
#213867=CARTESIAN_POINT('',(-50.6762142289945,-36.4252947698681,3.47153072139045));
#213868=CARTESIAN_POINT('',(-50.9399462128199,-36.991167339171,2.59908173515996));
#213869=CARTESIAN_POINT('Ctrl Pts',(-50.964463724589,-36.6347241449657,
2.90134173515997));
#213870=CARTESIAN_POINT('Ctrl Pts',(-50.9744193574531,-36.6419574987894,
2.88164837656707));
#213871=CARTESIAN_POINT('Ctrl Pts',(-50.9831959997518,-36.6507449107779,
2.86203734439136));
#213872=CARTESIAN_POINT('Ctrl Pts',(-50.9907013072118,-36.6609215604517,
2.84277945978155));
#213873=CARTESIAN_POINT('Ctrl Pts',(-50.9983574255554,-36.6713026986872,
2.82313460920043));
#213874=CARTESIAN_POINT('Ctrl Pts',(-51.0046913806529,-36.6831299757302,
2.80385576863384));
#213875=CARTESIAN_POINT('Ctrl Pts',(-51.0095813473138,-36.6962763075836,
2.78521678518451));
#213876=CARTESIAN_POINT('Ctrl Pts',(-51.0142813432029,-36.708911916362,
2.76730190934553));
#213877=CARTESIAN_POINT('Ctrl Pts',(-51.0176477981085,-36.7227668523506,
2.74997687279883));
#213878=CARTESIAN_POINT('Ctrl Pts',(-51.0195423439502,-36.7377619899081,
2.73349253345843));
#213879=CARTESIAN_POINT('Ctrl Pts',(-51.0209976683239,-36.7492807342396,
2.72082983599352));
#213880=CARTESIAN_POINT('Ctrl Pts',(-51.0215839370837,-36.7614730081809,
2.70866321039295));
#213881=CARTESIAN_POINT('Ctrl Pts',(-51.0212231059802,-36.7743133764174,
2.69711645335817));
#213882=CARTESIAN_POINT('Ctrl Pts',(-51.0212221603062,-36.7743470287326,
2.69708619136723));
#213883=CARTESIAN_POINT('Ctrl Pts',(-51.0212212075181,-36.7743806860745,
2.6970559338719));
#213884=CARTESIAN_POINT('Ctrl Pts',(-51.0212202476158,-36.77441434844,2.69702568087542));
#213885=CARTESIAN_POINT('Ctrl Pts',(-51.0211173265637,-36.7780236385692,
2.69378194443237));
#213886=CARTESIAN_POINT('Ctrl Pts',(-51.0209317131552,-36.7816890091481,
2.69059266624672));
#213887=CARTESIAN_POINT('Ctrl Pts',(-51.0206635800334,-36.7854055281044,
2.68746219342649));
#213888=CARTESIAN_POINT('Ctrl Pts',(-51.0191714801761,-36.8060871110696,
2.67004182395884));
#213889=CARTESIAN_POINT('Ctrl Pts',(-51.0151289787594,-36.8283529098819,
2.65443567877545));
#213890=CARTESIAN_POINT('Ctrl Pts',(-51.0086093349001,-36.8513189052364,
2.64136852352653));
#213891=CARTESIAN_POINT('Ctrl Pts',(-51.0056832284506,-36.8616263619894,
2.6355038032941));
#213892=CARTESIAN_POINT('Ctrl Pts',(-51.0022583633854,-36.8720751481077,
2.63014997450945));
#213893=CARTESIAN_POINT('Ctrl Pts',(-50.9983419378322,-36.8825875141944,
2.62536981119224));
#213894=CARTESIAN_POINT('Ctrl Pts',(-50.9966399122598,-36.8871560463068,
2.62329241687044));
#213895=CARTESIAN_POINT('Ctrl Pts',(-50.994844995161,-36.8917363891939,
2.62132362131399));
#213896=CARTESIAN_POINT('Ctrl Pts',(-50.9929577488696,-36.896322033635,
2.61946873372319));
#213897=CARTESIAN_POINT('Ctrl Pts',(-50.9863523868497,-36.9123717891789,
2.61297662715539));
#213898=CARTESIAN_POINT('Ctrl Pts',(-50.9786159896078,-36.9284864868683,
2.6078798911394));
#213899=CARTESIAN_POINT('Ctrl Pts',(-50.9697726815832,-36.9443870542878,
2.60440616886151));
#213900=CARTESIAN_POINT('Ctrl Pts',(-50.9653510275709,-36.9523373379975,
2.60266930772256));
#213901=CARTESIAN_POINT('Ctrl Pts',(-50.9606526463563,-36.9602340894951,
2.60133820040158));
#213902=CARTESIAN_POINT('Ctrl Pts',(-50.955680559906,-36.9680424293792,
2.60044130723558));
#213903=CARTESIAN_POINT('Ctrl Pts',(-50.9531945166809,-36.9719465993212,
2.59999286065257));
#213904=CARTESIAN_POINT('Ctrl Pts',(-50.9506400472466,-36.9758286664323,
2.59965296768485));
#213905=CARTESIAN_POINT('Ctrl Pts',(-50.9480175299138,-36.9796842711996,
2.59942518630927));
#213906=CARTESIAN_POINT('Ctrl Pts',(-50.9453950125809,-36.983539875967,
2.59919740493369));
#213907=CARTESIAN_POINT('Ctrl Pts',(-50.9427044459691,-36.9873690173881,
2.59908173791591));
#213908=CARTESIAN_POINT('Ctrl Pts',(-50.9399462128199,-36.991167339171,
2.59908173515997));
#213909=CARTESIAN_POINT('',(-50.9219998155897,-37.0158684358562,2.59908173515996));
#213910=CARTESIAN_POINT('Origin',(8.60468667414046E-17,1.91198832391256E-13,
2.59908173516023));
#213911=CARTESIAN_POINT('',(-50.5905785208481,-37.1493329797263,2.90134173515997));
#213912=CARTESIAN_POINT('Ctrl Pts',(-50.9219998155897,-37.0158684358562,
2.59908173515997));
#213913=CARTESIAN_POINT('Ctrl Pts',(-50.9197527708147,-37.0189596418151,
2.59908174381654));
#213914=CARTESIAN_POINT('Ctrl Pts',(-50.917473273452,-37.0220143142661,
2.59915752000969));
#213915=CARTESIAN_POINT('Ctrl Pts',(-50.915163365418,-37.0250315520726,
2.59930729517444));
#213916=CARTESIAN_POINT('Ctrl Pts',(-50.9018149465594,-37.0424674644314,
2.60017281085915));
#213917=CARTESIAN_POINT('Ctrl Pts',(-50.8874508031551,-37.0586566148381,
2.60350651800223));
#213918=CARTESIAN_POINT('Ctrl Pts',(-50.8724683783777,-37.0734189189144,
2.608968805969));
#213919=CARTESIAN_POINT('Ctrl Pts',(-50.8664256218163,-37.0793728957335,
2.61117187235788));
#213920=CARTESIAN_POINT('Ctrl Pts',(-50.8602822855821,-37.0850952351395,
2.61372076577374));
#213921=CARTESIAN_POINT('Ctrl Pts',(-50.8540642095543,-37.0905759575257,
2.61659179896957));
#213922=CARTESIAN_POINT('Ctrl Pts',(-50.8517701170137,-37.092598011339,
2.61765103591182));
#213923=CARTESIAN_POINT('Ctrl Pts',(-50.8494658679863,-37.0945870443968,
2.61875422455122));
#213924=CARTESIAN_POINT('Ctrl Pts',(-50.8471527697476,-37.0965424902854,
2.61990022440369));
#213925=CARTESIAN_POINT('Ctrl Pts',(-50.84281571055,-37.1002089513264,2.62204897412706));
#213926=CARTESIAN_POINT('Ctrl Pts',(-50.8384475408392,-37.1037573324719,
2.62434823201744));
#213927=CARTESIAN_POINT('Ctrl Pts',(-50.8340568779945,-37.107183900098,
2.62679048030279));
#213928=CARTESIAN_POINT('Ctrl Pts',(-50.818689558038,-37.1191768867891,
2.63533834930153));
#213929=CARTESIAN_POINT('Ctrl Pts',(-50.8030466935687,-37.1296776552301,
2.64563784783535));
#213930=CARTESIAN_POINT('Ctrl Pts',(-50.787497775234,-37.1385261411559,
2.65736666737937));
#213931=CARTESIAN_POINT('Ctrl Pts',(-50.7797233160666,-37.1429503841188,
2.66323107715137));
#213932=CARTESIAN_POINT('Ctrl Pts',(-50.7719723442504,-37.1469615570464,
2.66945281780747));
#213933=CARTESIAN_POINT('Ctrl Pts',(-50.7642910532774,-37.1505396571688,
2.67599160631173));
#213934=CARTESIAN_POINT('Ctrl Pts',(-50.760450407791,-37.1523287072299,
2.67926100056387));
#213935=CARTESIAN_POINT('Ctrl Pts',(-50.7566271826098,-37.1540094891596,
2.68260965685095));
#213936=CARTESIAN_POINT('Ctrl Pts',(-50.7528271523476,-37.1555795029287,
2.68603254012454));
#213937=CARTESIAN_POINT('Ctrl Pts',(-50.7490271220855,-37.1571495166979,
2.68945542339814));
#213938=CARTESIAN_POINT('Ctrl Pts',(-50.7452503160122,-37.1586086360832,
2.69295261525356));
#213939=CARTESIAN_POINT('Ctrl Pts',(-50.7415024502309,-37.159954619824,
2.69651891172071));
#213940=CARTESIAN_POINT('Ctrl Pts',(-50.7414704887851,-37.1599660982464,
2.69654932476058));
#213941=CARTESIAN_POINT('Ctrl Pts',(-50.7414385295744,-37.15997756849,2.69657974261116));
#213942=CARTESIAN_POINT('Ctrl Pts',(-50.7414065726019,-37.1599890305542,
2.69661016526944));
#213943=CARTESIAN_POINT('Ctrl Pts',(-50.7250856801847,-37.1658428740571,
2.7121474610103));
#213944=CARTESIAN_POINT('Ctrl Pts',(-50.7093579475518,-37.1696950534567,
2.72880565567393));
#213945=CARTESIAN_POINT('Ctrl Pts',(-50.6943448053438,-37.1717050161482,
2.74628040012063));
#213946=CARTESIAN_POINT('Ctrl Pts',(-50.6788239286353,-37.1737829544433,
2.76434612882107));
#213947=CARTESIAN_POINT('Ctrl Pts',(-50.6640659431993,-37.1738916781079,
2.78328592654099));
#213948=CARTESIAN_POINT('Ctrl Pts',(-50.6502224037094,-37.1721581240065,
2.80278753267449));
#213949=CARTESIAN_POINT('Ctrl Pts',(-50.6366421974703,-37.1704575457519,
2.82191817722402));
#213950=CARTESIAN_POINT('Ctrl Pts',(-50.6239412983497,-37.1669834785938,
2.84159092314762));
#213951=CARTESIAN_POINT('Ctrl Pts',(-50.6122904324973,-37.1618166822743,
2.86151233816625));
#213952=CARTESIAN_POINT('Ctrl Pts',(-50.6045721423266,-37.1583938608503,
2.87470957721041));
#213953=CARTESIAN_POINT('Ctrl Pts',(-50.5973152449679,-37.1542273890271,
2.88801594388195));
#213954=CARTESIAN_POINT('Ctrl Pts',(-50.5905785208481,-37.1493329797263,
2.90134173515997));
#213955=CARTESIAN_POINT('',(-50.3023253561992,-36.9399086546488,3.47153072139045));
#213956=CARTESIAN_POINT('',(-50.5905785208481,-37.1493329797263,2.90134173515997));
#213957=CARTESIAN_POINT('',(-46.5911245387426,-41.5228599914565,3.47153072139042));
#213958=CARTESIAN_POINT('Origin',(5.53234440788222E-15,1.85015204418142E-13,
3.47153072139072));
#213959=CARTESIAN_POINT('',(-46.8559036426981,-41.7612723673365,2.90134173515993));
#213960=CARTESIAN_POINT('',(-46.5911245387426,-41.5228599914565,3.47153072139042));
#213961=CARTESIAN_POINT('',(-46.7942619810913,-42.1132001506003,2.59908173515993));
#213962=CARTESIAN_POINT('Ctrl Pts',(-46.8559036426982,-41.7612723673365,
2.90134173515993));
#213963=CARTESIAN_POINT('Ctrl Pts',(-46.865048646205,-41.7695067430963,
2.88164837656519));
#213964=CARTESIAN_POINT('Ctrl Pts',(-46.872858674468,-41.7791634256558,
2.86203734438765));
#213965=CARTESIAN_POINT('Ctrl Pts',(-46.8792591175172,-41.7900688448343,
2.84277945977611));
#213966=CARTESIAN_POINT('Ctrl Pts',(-46.8857881704169,-41.8011933963946,
2.82313460919348));
#213967=CARTESIAN_POINT('Ctrl Pts',(-46.8908511403517,-41.8136179609704,
2.80385576862546));
#213968=CARTESIAN_POINT('Ctrl Pts',(-46.8943401533973,-41.8272034165444,
2.78521678517485));
#213969=CARTESIAN_POINT('Ctrl Pts',(-46.8976936214487,-41.8402610894845,
2.76730190933515));
#213970=CARTESIAN_POINT('Ctrl Pts',(-46.8995933993942,-41.854392017043,
2.74997687278782));
#213971=CARTESIAN_POINT('Ctrl Pts',(-46.8999101480295,-41.8695030436346,
2.73349253344695));
#213972=CARTESIAN_POINT('Ctrl Pts',(-46.9001534633396,-41.8811108098966,
2.72082983598615));
#213973=CARTESIAN_POINT('Ctrl Pts',(-46.8994620807989,-41.8932975750545,
2.70866321038944));
#213974=CARTESIAN_POINT('Ctrl Pts',(-46.8977610424069,-41.9060298852857,
2.69711645335814));
#213975=CARTESIAN_POINT('Ctrl Pts',(-46.8977565842887,-41.9060632544001,
2.6970861913672));
#213976=CARTESIAN_POINT('Ctrl Pts',(-46.8977521185698,-41.9060966277702,
2.69705593387187));
#213977=CARTESIAN_POINT('Ctrl Pts',(-46.8977476452506,-41.9061300053925,
2.69702568087538));
#213978=CARTESIAN_POINT('Ctrl Pts',(-46.8972680144601,-41.9097087652733,
2.69378194443234));
#213979=CARTESIAN_POINT('Ctrl Pts',(-46.8967002823073,-41.9133346546844,
2.69059266624669));
#213980=CARTESIAN_POINT('Ctrl Pts',(-46.8960451360316,-41.9170027866178,
2.68746219342646));
#213981=CARTESIAN_POINT('Ctrl Pts',(-46.8923993959683,-41.9374151068017,
2.67004182395936));
#213982=CARTESIAN_POINT('Ctrl Pts',(-46.8860516300644,-41.959136374777,
2.65443567877639));
#213983=CARTESIAN_POINT('Ctrl Pts',(-46.8771671012949,-41.9812950716515,
2.64136852352772));
#213984=CARTESIAN_POINT('Ctrl Pts',(-46.8731796017479,-41.9912402016681,
2.6355038032948));
#213985=CARTESIAN_POINT('Ctrl Pts',(-46.8686813028956,-42.0012737523613,
2.63014997450974));
#213986=CARTESIAN_POINT('Ctrl Pts',(-46.8636874904586,-42.0113191526628,
2.6253698111922));
#213987=CARTESIAN_POINT('Ctrl Pts',(-46.8615172471193,-42.0156847477607,
2.6232924168704));
#213988=CARTESIAN_POINT('Ctrl Pts',(-46.859253386561,-42.0200523791242,
2.62132362131394));
#213989=CARTESIAN_POINT('Ctrl Pts',(-46.8568971484357,-42.0244156319706,
2.61946873372314));
#213990=CARTESIAN_POINT('Ctrl Pts',(-46.8486503149973,-42.0396870169331,
2.61297662715535));
#213991=CARTESIAN_POINT('Ctrl Pts',(-46.8392718539635,-42.0549047629075,
2.60787989113938));
#213992=CARTESIAN_POINT('Ctrl Pts',(-46.8288149286281,-42.0697938479569,
2.60440616886149));
#213993=CARTESIAN_POINT('Ctrl Pts',(-46.8235864659604,-42.0772383904816,
2.60266930772254));
#213994=CARTESIAN_POINT('Ctrl Pts',(-46.8180883876707,-42.0846007681801,
2.60133820040154));
#213995=CARTESIAN_POINT('Ctrl Pts',(-46.8123273450616,-42.0918466086054,
2.60044130723554));
#213996=CARTESIAN_POINT('Ctrl Pts',(-46.809446823757,-42.095469528818,2.59999286065254));
#213997=CARTESIAN_POINT('Ctrl Pts',(-46.8065005614641,-42.0990633147948,
2.59965296768481));
#213998=CARTESIAN_POINT('Ctrl Pts',(-46.8034893901143,-42.1026236704492,
2.59942518630923));
#213999=CARTESIAN_POINT('Ctrl Pts',(-46.8004782187645,-42.1061840261035,
2.59919740493365));
#214000=CARTESIAN_POINT('Ctrl Pts',(-46.7974021370897,-42.109710950294,
2.59908173791585));
#214001=CARTESIAN_POINT('Ctrl Pts',(-46.7942619810913,-42.1132001506003,
2.59908173515993));
#214002=CARTESIAN_POINT('',(-46.7738319284254,-42.1358900227697,2.59908173515994));
#214003=CARTESIAN_POINT('Origin',(7.58094983678529E-17,1.91211474488351E-13,
2.59908173516023));
#214004=CARTESIAN_POINT('',(-46.4302753505421,-42.2339804752703,2.90134173515993));
#214005=CARTESIAN_POINT('Ctrl Pts',(-46.7738319284254,-42.1358900227697,
2.59908173515993));
#214006=CARTESIAN_POINT('Ctrl Pts',(-46.7712740741883,-42.1387294146417,
2.5990817438165));
#214007=CARTESIAN_POINT('Ctrl Pts',(-46.7686877639335,-42.141529080921,
2.59915752000965));
#214008=CARTESIAN_POINT('Ctrl Pts',(-46.7660751225862,-42.1442883388461,
2.5993072951744));
#214009=CARTESIAN_POINT('Ctrl Pts',(-46.7509772786436,-42.1602334457366,
2.6001728108588));
#214010=CARTESIAN_POINT('Ctrl Pts',(-46.7349995965123,-42.1748324484425,
2.60350651799981));
#214011=CARTESIAN_POINT('Ctrl Pts',(-46.7185561660722,-42.1879477932309,
2.60896880596313));
#214012=CARTESIAN_POINT('Ctrl Pts',(-46.7119241523106,-42.1932375134898,
2.61117187235334));
#214013=CARTESIAN_POINT('Ctrl Pts',(-46.7052163225648,-42.1982863518306,
2.61372076577116));
#214014=CARTESIAN_POINT('Ctrl Pts',(-46.6984594183135,-42.2030870843186,
2.61659179896952));
#214015=CARTESIAN_POINT('Ctrl Pts',(-46.6959665308741,-42.2048582631417,
2.61765103591177));
#214016=CARTESIAN_POINT('Ctrl Pts',(-46.6934669941951,-42.2065955404585,
2.61875422455118));
#214017=CARTESIAN_POINT('Ctrl Pts',(-46.6909621675968,-42.2082984896056,
2.61990022440364));
#214018=CARTESIAN_POINT('Ctrl Pts',(-46.6862656177251,-42.2114915192564,
2.62204897412702));
#214019=CARTESIAN_POINT('Ctrl Pts',(-46.6815504704767,-42.2145638639315,
2.62434823201738));
#214020=CARTESIAN_POINT('Ctrl Pts',(-46.6768256862942,-42.2175127112217,
2.62679048030273));
#214021=CARTESIAN_POINT('Ctrl Pts',(-46.6602889416556,-42.2278336767374,
2.63533834930146));
#214022=CARTESIAN_POINT('Ctrl Pts',(-46.6436341412463,-42.2366417962861,
2.64563784783531));
#214023=CARTESIAN_POINT('Ctrl Pts',(-46.6272454828771,-42.2438165047411,
2.65736666737932));
#214024=CARTESIAN_POINT('Ctrl Pts',(-46.6190511536924,-42.2474038589686,
2.66323107715133));
#214025=CARTESIAN_POINT('Ctrl Pts',(-46.6109233607687,-42.2505828610985,
2.66945281780743));
#214026=CARTESIAN_POINT('Ctrl Pts',(-46.6029101354043,-42.2533384464727,
2.6759916063117));
#214027=CARTESIAN_POINT('Ctrl Pts',(-46.598903522722,-42.2547162391598,
2.67926100056383));
#214028=CARTESIAN_POINT('Ctrl Pts',(-46.5949255520162,-42.2559881777373,
2.68260965685092));
#214029=CARTESIAN_POINT('Ctrl Pts',(-46.5909822275908,-42.257152379483,
2.68603254012451));
#214030=CARTESIAN_POINT('Ctrl Pts',(-46.5870389031655,-42.2583165812288,
2.68945542339811));
#214031=CARTESIAN_POINT('Ctrl Pts',(-46.5831302673239,-42.2593729236706,
2.69295261525354));
#214032=CARTESIAN_POINT('Ctrl Pts',(-46.5792622391316,-42.2603197753209,
2.69651891172068));
#214033=CARTESIAN_POINT('Ctrl Pts',(-46.579229252952,-42.2603278499825,
2.69654932476056));
#214034=CARTESIAN_POINT('Ctrl Pts',(-46.5791962698503,-42.2603359167438,
2.69657974261114));
#214035=CARTESIAN_POINT('Ctrl Pts',(-46.5791632898295,-42.2603439756043,
2.69661016526942));
#214036=CARTESIAN_POINT('Ctrl Pts',(-46.5623199117004,-42.2644597533371,
2.71214746101271));
#214037=CARTESIAN_POINT('Ctrl Pts',(-46.5462756748372,-42.2666468343722,
2.7288056556791));
#214038=CARTESIAN_POINT('Ctrl Pts',(-46.5311346778796,-42.2670764855936,
2.74628040012878));
#214039=CARTESIAN_POINT('Ctrl Pts',(-46.515481622459,-42.2675206673339,
2.7643461288319));
#214040=CARTESIAN_POINT('Ctrl Pts',(-46.5007931180922,-42.2660861658594,
2.7832859265547));
#214041=CARTESIAN_POINT('Ctrl Pts',(-46.4872066207052,-42.2629150644383,
2.80278753269116));
#214042=CARTESIAN_POINT('Ctrl Pts',(-46.4738785670876,-42.259804284039,
2.82191817724294));
#214043=CARTESIAN_POINT('Ctrl Pts',(-46.4616103837222,-42.2550216427155,
2.84159092316883));
#214044=CARTESIAN_POINT('Ctrl Pts',(-46.4505634198111,-42.2486653035416,
2.86151233818969));
#214045=CARTESIAN_POINT('Ctrl Pts',(-46.44324519351,-42.2444544516826,2.87470957722616));
#214046=CARTESIAN_POINT('Ctrl Pts',(-46.4364635650958,-42.2395522519014,
2.88801594388982));
#214047=CARTESIAN_POINT('Ctrl Pts',(-46.4302753505421,-42.2339804752703,
2.90134173515993));
#214048=CARTESIAN_POINT('',(-46.1654920697608,-41.9955727382253,3.47153072139041));
#214049=CARTESIAN_POINT('',(-46.4302753505421,-42.2339804752703,2.90134173515993));
#214050=CARTESIAN_POINT('',(-41.9955727382247,-46.1654920697614,3.47153072139039));
#214051=CARTESIAN_POINT('Origin',(5.53234440788222E-15,1.85015204418142E-13,
3.47153072139072));
#214052=CARTESIAN_POINT('',(-42.2339804752697,-46.4302753505427,2.90134173515991));
#214053=CARTESIAN_POINT('',(-41.9955727382247,-46.1654920697614,3.47153072139039));
#214054=CARTESIAN_POINT('',(-42.1358900227691,-46.7738319284259,2.5990817351599));
#214055=CARTESIAN_POINT('Ctrl Pts',(-42.2339804752697,-46.4302753505427,
2.90134173515991));
#214056=CARTESIAN_POINT('Ctrl Pts',(-42.2422146548454,-46.4394205306916,
2.88164837656848));
#214057=CARTESIAN_POINT('Ctrl Pts',(-42.2489725007676,-46.4498406831839,
2.86203734439424));
#214058=CARTESIAN_POINT('Ctrl Pts',(-42.2541979548117,-46.4613553898089,
2.84277945978583));
#214059=CARTESIAN_POINT('Ctrl Pts',(-42.2595284085971,-46.4731014717758,
2.82313460920593));
#214060=CARTESIAN_POINT('Ctrl Pts',(-42.2632649224112,-46.4859871977515,
2.80385576864049));
#214061=CARTESIAN_POINT('Ctrl Pts',(-42.2653147554849,-46.4998629319478,
2.7852167851922));
#214062=CARTESIAN_POINT('Ctrl Pts',(-42.2672849544019,-46.5131996064496,
2.76730190935379));
#214063=CARTESIAN_POINT('Ctrl Pts',(-42.2676972410237,-46.5274517041758,
2.74997687280757));
#214064=CARTESIAN_POINT('Ctrl Pts',(-42.2664327220902,-46.5425130602287,
2.73349253346754));
#214065=CARTESIAN_POINT('Ctrl Pts',(-42.2654613625248,-46.5540826713139,
2.72082983599933));
#214066=CARTESIAN_POINT('Ctrl Pts',(-42.2634999036152,-46.566130406949,
2.70866321039567));
#214067=CARTESIAN_POINT('Ctrl Pts',(-42.2604772948656,-46.5786151613302,
2.69711645335811));
#214068=CARTESIAN_POINT('Ctrl Pts',(-42.2604693731471,-46.5786478816449,
2.69708619136717));
#214069=CARTESIAN_POINT('Ctrl Pts',(-42.2604614434249,-46.5786806053974,
2.69705593387185));
#214070=CARTESIAN_POINT('Ctrl Pts',(-42.2604535056994,-46.5787133325845,
2.69702568087537));
#214071=CARTESIAN_POINT('Ctrl Pts',(-42.2596024201058,-46.5822223525748,
2.69378194443233));
#214072=CARTESIAN_POINT('Ctrl Pts',(-42.2586587894011,-46.5857690348147,
2.69059266624667));
#214073=CARTESIAN_POINT('Ctrl Pts',(-42.2576238078912,-46.5893485909042,
2.68746219342644));
#214074=CARTESIAN_POINT('Ctrl Pts',(-42.2518643711134,-46.609268006654,
2.67004182396122));
#214075=CARTESIAN_POINT('Ctrl Pts',(-42.2432808881748,-46.630206761033,
2.65443567877976));
#214076=CARTESIAN_POINT('Ctrl Pts',(-42.232128815253,-46.6513153841061,
2.64136852353196));
#214077=CARTESIAN_POINT('Ctrl Pts',(-42.2271236104872,-46.6607892264622,
2.63550380329738));
#214078=CARTESIAN_POINT('Ctrl Pts',(-42.2216011621503,-46.6702976120509,
2.63014997451088));
#214079=CARTESIAN_POINT('Ctrl Pts',(-42.2155846760825,-46.6797659870608,
2.62536981119219));
#214080=CARTESIAN_POINT('Ctrl Pts',(-42.2129699926165,-46.6838808147709,
2.62329241687039));
#214081=CARTESIAN_POINT('Ctrl Pts',(-42.2102619919286,-46.6879878819275,
2.62132362131393));
#214082=CARTESIAN_POINT('Ctrl Pts',(-42.2074625774075,-46.692080938468,
2.61946873372313));
#214083=CARTESIAN_POINT('Ctrl Pts',(-42.1976646265834,-46.7064066363596,
2.61297662715533));
#214084=CARTESIAN_POINT('Ctrl Pts',(-42.1867468541393,-46.7205607018097,
2.60787989113935));
#214085=CARTESIAN_POINT('Ctrl Pts',(-42.1747908797553,-46.7342751765575,
2.60440616886145));
#214086=CARTESIAN_POINT('Ctrl Pts',(-42.1688128925633,-46.7411324139314,
2.6026693077225));
#214087=CARTESIAN_POINT('Ctrl Pts',(-42.1625753552951,-46.74787975408,2.60133820040151));
#214088=CARTESIAN_POINT('Ctrl Pts',(-42.1560884757153,-46.7544837081025,
2.6004413072355));
#214089=CARTESIAN_POINT('Ctrl Pts',(-42.1528450359255,-46.7577856851137,
2.5999928606525));
#214090=CARTESIAN_POINT('Ctrl Pts',(-42.1495392606402,-46.7610518156851,
2.59965296768478));
#214091=CARTESIAN_POINT('Ctrl Pts',(-42.1461724262969,-46.7642779142248,
2.5994251863092));
#214092=CARTESIAN_POINT('Ctrl Pts',(-42.1428055919536,-46.7675040127645,
2.59919740493363));
#214093=CARTESIAN_POINT('Ctrl Pts',(-42.1393776974104,-46.770690078005,
2.59908173791579));
#214094=CARTESIAN_POINT('Ctrl Pts',(-42.1358900227691,-46.7738319284259,
2.5990817351599));
#214095=CARTESIAN_POINT('',(-42.1132001505997,-46.7942619810918,2.5990817351599));
#214096=CARTESIAN_POINT('Origin',(6.43067523875891E-17,1.91222977234332E-13,
2.59908173516023));
#214097=CARTESIAN_POINT('',(-41.7612723673359,-46.8559036426987,2.9013417351599));
#214098=CARTESIAN_POINT('Ctrl Pts',(-42.1132001505997,-46.7942619810919,
2.5990817351599));
#214099=CARTESIAN_POINT('Ctrl Pts',(-42.1103595112868,-46.7968184499054,
2.59908174381644));
#214100=CARTESIAN_POINT('Ctrl Pts',(-42.1074947242963,-46.7993324362835,
2.59915752000963));
#214101=CARTESIAN_POINT('Ctrl Pts',(-42.104607974281,-46.8018034833198,
2.59930729517438));
#214102=CARTESIAN_POINT('Ctrl Pts',(-42.0879261203875,-46.8160830868203,
2.60017281085878));
#214103=CARTESIAN_POINT('Ctrl Pts',(-42.0705099543527,-46.828931992102,
2.60350651799972));
#214104=CARTESIAN_POINT('Ctrl Pts',(-42.0527856759093,-46.8402566831445,
2.60896880596294));
#214105=CARTESIAN_POINT('Ctrl Pts',(-42.0456370666831,-46.8448241915556,
2.61117187235319));
#214106=CARTESIAN_POINT('Ctrl Pts',(-42.0384382358172,-46.8491442126966,
2.61372076577107));
#214107=CARTESIAN_POINT('Ctrl Pts',(-42.0312165334047,-46.8532123574521,
2.61659179896951));
#214108=CARTESIAN_POINT('Ctrl Pts',(-42.028552163663,-46.8547132558791,
2.61765103591176));
#214109=CARTESIAN_POINT('Ctrl Pts',(-42.0258847247792,-46.8561797434811,
2.61875422455116));
#214110=CARTESIAN_POINT('Ctrl Pts',(-42.0232156132257,-46.8576115380195,
2.61990022440363));
#214111=CARTESIAN_POINT('Ctrl Pts',(-42.0182110290631,-46.860296152779,
2.622048974127));
#214112=CARTESIAN_POINT('Ctrl Pts',(-42.0132005644171,-46.8628587997326,
2.62434823201736));
#214113=CARTESIAN_POINT('Ctrl Pts',(-42.0081934246211,-46.8652976184989,
2.62679048030272));
#214114=CARTESIAN_POINT('Ctrl Pts',(-41.9906684353351,-46.873833484181,
2.63533834930145));
#214115=CARTESIAN_POINT('Ctrl Pts',(-41.9731841724644,-46.8808524512364,
2.6456378478353));
#214116=CARTESIAN_POINT('Ctrl Pts',(-41.9561353316313,-46.8862747746135,
2.65736666737931));
#214117=CARTESIAN_POINT('Ctrl Pts',(-41.9476109112147,-46.888985936302,
2.66323107715131));
#214118=CARTESIAN_POINT('Ctrl Pts',(-41.9391953469837,-46.8912979378215,
2.6694528178074));
#214119=CARTESIAN_POINT('Ctrl Pts',(-41.9309379818016,-46.8932008176775,
2.67599160631167));
#214120=CARTESIAN_POINT('Ctrl Pts',(-41.9268092992106,-46.8941522576055,
2.6792610005638));
#214121=CARTESIAN_POINT('Ctrl Pts',(-41.9227201664597,-46.8950014172056,
2.68260965685089));
#214122=CARTESIAN_POINT('Ctrl Pts',(-41.9186767517587,-46.89574705169,2.68603254012449));
#214123=CARTESIAN_POINT('Ctrl Pts',(-41.9146333370577,-46.8964926861745,
2.68945542339808));
#214124=CARTESIAN_POINT('Ctrl Pts',(-41.9106356952802,-46.8971346781638,
2.69295261525351));
#214125=CARTESIAN_POINT('Ctrl Pts',(-41.9066898836031,-46.8976720238189,
2.69651891172065));
#214126=CARTESIAN_POINT('Ctrl Pts',(-41.9066562340933,-46.897676606252,
2.69654932476053));
#214127=CARTESIAN_POINT('Ctrl Pts',(-41.9066225884702,-46.8976811811498,
2.69657974261112));
#214128=CARTESIAN_POINT('Ctrl Pts',(-41.9065889467371,-46.8976857485121,
2.6966101652694));
#214129=CARTESIAN_POINT('Ctrl Pts',(-41.8894076224763,-46.9000183671516,
2.71214746101077));
#214130=CARTESIAN_POINT('Ctrl Pts',(-41.8732226654037,-46.9005163877043,
2.72880565567496));
#214131=CARTESIAN_POINT('Ctrl Pts',(-41.8581197016315,-46.8993610201075,
2.74628040012227));
#214132=CARTESIAN_POINT('Ctrl Pts',(-41.8425059656531,-46.8981665787458,
2.76434612882316));
#214133=CARTESIAN_POINT('Ctrl Pts',(-41.8280478726861,-46.8952045688321,
2.7832859265436));
#214134=CARTESIAN_POINT('Ctrl Pts',(-41.8148672739126,-46.8906306633446,
2.80278753267762));
#214135=CARTESIAN_POINT('Ctrl Pts',(-41.8019373978624,-46.8861437631639,
2.82191817722768));
#214136=CARTESIAN_POINT('Ctrl Pts',(-41.7902363430373,-46.8801049472969,
2.84159092315182));
#214137=CARTESIAN_POINT('Ctrl Pts',(-41.7799143139161,-46.8726287066543,
2.86151233817099));
#214138=CARTESIAN_POINT('Ctrl Pts',(-41.7730763314944,-46.8676759593315,
2.87470957721359));
#214139=CARTESIAN_POINT('Ctrl Pts',(-41.7668442729565,-46.8620917411148,
2.88801594388352));
#214140=CARTESIAN_POINT('Ctrl Pts',(-41.7612723673359,-46.8559036426987,
2.90134173515991));
#214141=CARTESIAN_POINT('',(-41.5228599914559,-46.5911245387432,3.47153072139039));
#214142=CARTESIAN_POINT('',(-41.7612723673359,-46.8559036426987,2.9013417351599));
#214143=CARTESIAN_POINT('',(-36.9399086546482,-50.3023253561997,3.47153072139036));
#214144=CARTESIAN_POINT('Origin',(5.53234440788222E-15,1.85015204418142E-13,
3.47153072139072));
#214145=CARTESIAN_POINT('',(-37.1493329797256,-50.5905785208485,2.90134173515987));
#214146=CARTESIAN_POINT('',(-36.9399086546482,-50.3023253561997,3.47153072139036));
#214147=CARTESIAN_POINT('',(-37.0158684358555,-50.9219998155901,2.59908173515987));
#214148=CARTESIAN_POINT('Ctrl Pts',(-37.1493329797256,-50.5905785208486,
2.90134173515987));
#214149=CARTESIAN_POINT('Ctrl Pts',(-37.156566119977,-50.6005343088816,
2.88164837656766));
#214150=CARTESIAN_POINT('Ctrl Pts',(-37.1621977431852,-50.611603765938,
2.86203734439262));
#214151=CARTESIAN_POINT('Ctrl Pts',(-37.1661909570569,-50.623601602477,
2.84277945978346));
#214152=CARTESIAN_POINT('Ctrl Pts',(-37.1702644101613,-50.6358405223211,
2.82313460920288));
#214153=CARTESIAN_POINT('Ctrl Pts',(-37.1726335298273,-50.6490462309891,
2.8038557686368));
#214154=CARTESIAN_POINT('Ctrl Pts',(-37.1732217245285,-50.6630602183634,
2.78521678518795));
#214155=CARTESIAN_POINT('Ctrl Pts',(-37.1737870683987,-50.6765297750326,
2.76730190934898));
#214156=CARTESIAN_POINT('Ctrl Pts',(-37.1727073465972,-50.6907468939638,
2.74997687280227));
#214157=CARTESIAN_POINT('Ctrl Pts',(-37.1698754144273,-50.7055935641122,
2.73349253346184));
#214158=CARTESIAN_POINT('Ctrl Pts',(-37.167700022404,-50.716998260933,2.72082983599567));
#214159=CARTESIAN_POINT('Ctrl Pts',(-37.16448997728,-50.7287749695245,2.70866321039392));
#214160=CARTESIAN_POINT('Ctrl Pts',(-37.1601789145083,-50.7408753824654,
2.69711645335808));
#214161=CARTESIAN_POINT('Ctrl Pts',(-37.1601676159816,-50.7409070954897,
2.69708619136714));
#214162=CARTESIAN_POINT('Ctrl Pts',(-37.1601563091356,-50.7409388110964,
2.69705593387181));
#214163=CARTESIAN_POINT('Ctrl Pts',(-37.1601449939712,-50.7409705292823,
2.69702568087533));
#214164=CARTESIAN_POINT('Ctrl Pts',(-37.1589317782465,-50.7443713638247,
2.69378194443228));
#214165=CARTESIAN_POINT('Ctrl Pts',(-37.1576225876053,-50.7477999807008,
2.69059266624662));
#214166=CARTESIAN_POINT('Ctrl Pts',(-37.1562191103351,-50.7512517425807,
2.68746219342639));
#214167=CARTESIAN_POINT('Ctrl Pts',(-37.1484090784387,-50.7704600126073,
2.67004182396466));
#214168=CARTESIAN_POINT('Ctrl Pts',(-37.1376839209025,-50.7903868440138,
2.65443567878596));
#214169=CARTESIAN_POINT('Ctrl Pts',(-37.1243864882752,-50.8102141227924,
2.64136852353976));
#214170=CARTESIAN_POINT('Ctrl Pts',(-37.1184184163599,-50.8191128800903,
2.63550380330212));
#214171=CARTESIAN_POINT('Ctrl Pts',(-37.1119323236364,-50.8279919247136,
2.63014997451299));
#214172=CARTESIAN_POINT('Ctrl Pts',(-37.1049590818163,-50.8367795369355,
2.62536981119217));
#214173=CARTESIAN_POINT('Ctrl Pts',(-37.1019286052427,-50.8405985143442,
2.62329241687037));
#214174=CARTESIAN_POINT('Ctrl Pts',(-37.0988061338475,-50.8444000194069,
2.62132362131391));
#214175=CARTESIAN_POINT('Ctrl Pts',(-37.0955942139018,-50.8481780352574,
2.61946873372311));
#214176=CARTESIAN_POINT('Ctrl Pts',(-37.0843524940917,-50.8614010907342,
2.61297662715531));
#214177=CARTESIAN_POINT('Ctrl Pts',(-37.0720150276369,-50.8743364007569,
2.60787989113933));
#214178=CARTESIAN_POINT('Ctrl Pts',(-37.0586909963616,-50.8867260065479,
2.60440616886143));
#214179=CARTESIAN_POINT('Ctrl Pts',(-37.052028980724,-50.8929208094433,
2.60266930772248));
#214180=CARTESIAN_POINT('Ctrl Pts',(-37.0451203242406,-50.8989791867714,
2.60133820040147));
#214181=CARTESIAN_POINT('Ctrl Pts',(-37.0379786793005,-50.9048689000889,
2.60044130723546));
#214182=CARTESIAN_POINT('Ctrl Pts',(-37.0344078568305,-50.9078137567477,
2.59999286065246));
#214183=CARTESIAN_POINT('Ctrl Pts',(-37.0307787873186,-50.9107164475035,
2.59965296768475));
#214184=CARTESIAN_POINT('Ctrl Pts',(-37.0270931777235,-50.9135729431179,
2.59942518630917));
#214185=CARTESIAN_POINT('Ctrl Pts',(-37.0234075681283,-50.9164294387323,
2.59919740493359));
#214186=CARTESIAN_POINT('Ctrl Pts',(-37.0196654174466,-50.9192397378252,
2.59908173791576));
#214187=CARTESIAN_POINT('Ctrl Pts',(-37.0158684358555,-50.9219998155901,
2.59908173515987));
#214188=CARTESIAN_POINT('',(-36.9911673391703,-50.9399462128203,2.59908173515987));
#214189=CARTESIAN_POINT('Origin',(5.16646552926871E-17,1.91233214602705E-13,
2.59908173516024));
#214190=CARTESIAN_POINT('',(-36.634724144965,-50.9644637245894,2.90134173515987));
#214191=CARTESIAN_POINT('Ctrl Pts',(-36.9911673391703,-50.9399462128203,
2.59908173515988));
#214192=CARTESIAN_POINT('Ctrl Pts',(-36.9880750374203,-50.9421917493681,
2.59908174381648));
#214193=CARTESIAN_POINT('Ctrl Pts',(-36.9849631609,-50.9443925120841,2.5991575200096));
#214194=CARTESIAN_POINT('Ctrl Pts',(-36.9818339300539,-50.9465482749232,
2.59930729517435));
#214195=CARTESIAN_POINT('Ctrl Pts',(-36.9637508360892,-50.9590059247113,
2.60017281085885));
#214196=CARTESIAN_POINT('Ctrl Pts',(-36.945087001308,-50.9699639572751,
2.60350651800055));
#214197=CARTESIAN_POINT('Ctrl Pts',(-36.9262760657623,-50.9793739188877,
2.60896880596501));
#214198=CARTESIAN_POINT('Ctrl Pts',(-36.9186891827326,-50.9831691728715,
2.61117187235478));
#214199=CARTESIAN_POINT('Ctrl Pts',(-36.9110782226468,-50.9867130457558,
2.61372076577195));
#214200=CARTESIAN_POINT('Ctrl Pts',(-36.9034708445584,-50.9900040313322,
2.61659179896946));
#214201=CARTESIAN_POINT('Ctrl Pts',(-36.9006641839069,-50.9912182052059,
2.61765103591171));
#214202=CARTESIAN_POINT('Ctrl Pts',(-36.8978580678369,-50.992397835948,
2.61875422455112));
#214203=CARTESIAN_POINT('Ctrl Pts',(-36.8950539146731,-50.9935427888371,
2.61990022440358));
#214204=CARTESIAN_POINT('Ctrl Pts',(-36.8897961274908,-50.9956895755043,
2.62204897412696));
#214205=CARTESIAN_POINT('Ctrl Pts',(-36.8845452411465,-50.99771444784,2.62434823201732));
#214206=CARTESIAN_POINT('Ctrl Pts',(-36.8793106050084,-50.9996165178737,
2.62679048030267));
#214207=CARTESIAN_POINT('Ctrl Pts',(-36.8609893785248,-51.0062737629917,
2.63533834930141));
#214208=CARTESIAN_POINT('Ctrl Pts',(-36.8428672144356,-51.0114266762819,
2.64563784783525));
#214209=CARTESIAN_POINT('Ctrl Pts',(-36.8253449818064,-51.0150372064714,
2.65736666737927));
#214210=CARTESIAN_POINT('Ctrl Pts',(-36.8165838654919,-51.0168424715661,
2.66323107715127));
#214211=CARTESIAN_POINT('Ctrl Pts',(-36.8079727326363,-51.0182621417028,
2.66945281780736));
#214212=CARTESIAN_POINT('Ctrl Pts',(-36.7995616970576,-51.0192914676907,
2.67599160631163));
#214213=CARTESIAN_POINT('Ctrl Pts',(-36.7953561792682,-51.0198061306847,
2.67926100056377));
#214214=CARTESIAN_POINT('Ctrl Pts',(-36.7912006858663,-51.020223207737,
2.68260965685085));
#214215=CARTESIAN_POINT('Ctrl Pts',(-36.7871014813873,-51.0205421056327,
2.68603254012445));
#214216=CARTESIAN_POINT('Ctrl Pts',(-36.7830022769083,-51.0208610035284,
2.68945542339804));
#214217=CARTESIAN_POINT('Ctrl Pts',(-36.7789594281946,-51.0210816112668,
2.69295261525347));
#214218=CARTESIAN_POINT('Ctrl Pts',(-36.7749790641711,-51.0212035636552,
2.69651891172061));
#214219=CARTESIAN_POINT('Ctrl Pts',(-36.7749451200022,-51.0212046036537,
2.69654932476049));
#214220=CARTESIAN_POINT('Ctrl Pts',(-36.7749111804864,-51.0212056365644,
2.69657974261108));
#214221=CARTESIAN_POINT('Ctrl Pts',(-36.7748772456268,-51.0212066623876,
2.69661016526935));
#214222=CARTESIAN_POINT('Ctrl Pts',(-36.7575462174152,-51.0217305652762,
2.71214746101165));
#214223=CARTESIAN_POINT('Ctrl Pts',(-36.7413978659069,-51.0205340689294,
2.7288056556769));
#214224=CARTESIAN_POINT('Ctrl Pts',(-36.726498406549,-51.0178063409629,
2.74628040012535));
#214225=CARTESIAN_POINT('Ctrl Pts',(-36.7110950573694,-51.014986363048,
2.76434612882721));
#214226=CARTESIAN_POINT('Ctrl Pts',(-36.6970257816923,-51.0105292970946,
2.78328592654866));
#214227=CARTESIAN_POINT('Ctrl Pts',(-36.6843954909294,-51.0046027002046,
2.80278753268373));
#214228=CARTESIAN_POINT('Ctrl Pts',(-36.6720054548738,-50.9987888396584,
2.82191817723423));
#214229=CARTESIAN_POINT('Ctrl Pts',(-36.6609997277939,-50.9915600117767,
2.84159092315881));
#214230=CARTESIAN_POINT('Ctrl Pts',(-36.651515723774,-50.9830457809201,
2.86151233817839));
#214231=CARTESIAN_POINT('Ctrl Pts',(-36.6452329036036,-50.9774054014718,
2.87470957721854));
#214232=CARTESIAN_POINT('Ctrl Pts',(-36.6396186946846,-50.9712003466859,
2.88801594388598));
#214233=CARTESIAN_POINT('Ctrl Pts',(-36.634724144965,-50.9644637245894,
2.90134173515987));
#214234=CARTESIAN_POINT('',(-36.4252947698674,-50.6762142289949,3.47153072139035));
#214235=CARTESIAN_POINT('',(-36.634724144965,-50.9644637245894,2.90134173515987));
#214236=CARTESIAN_POINT('',(-31.4795232016785,-53.8880358395971,3.47153072139033));
#214237=CARTESIAN_POINT('Origin',(5.53234440788222E-15,1.85015204418142E-13,
3.47153072139072));
#214238=CARTESIAN_POINT('',(-31.6576696180579,-54.1966007261208,2.90134173515985));
#214239=CARTESIAN_POINT('',(-31.4795232016785,-53.8880358395971,3.47153072139033));
#214240=CARTESIAN_POINT('',(-31.4902932482903,-54.5122556166612,2.59908173515985));
#214241=CARTESIAN_POINT('Ctrl Pts',(-31.6576696180579,-54.1966007261208,
2.90134173515985));
#214242=CARTESIAN_POINT('Ctrl Pts',(-31.663822471187,-54.207258044342,2.8816483765649));
#214243=CARTESIAN_POINT('Ctrl Pts',(-31.668266170439,-54.2188555266759,
2.86203734438717));
#214244=CARTESIAN_POINT('Ctrl Pts',(-31.6709833936512,-54.2312050423224,
2.84277945977544));
#214245=CARTESIAN_POINT('Ctrl Pts',(-31.6737552164698,-54.2438027078782,
2.82313460919239));
#214246=CARTESIAN_POINT('Ctrl Pts',(-31.6747309854165,-54.2571837147324,
2.80385576862396));
#214247=CARTESIAN_POINT('Ctrl Pts',(-31.67385109736,-54.2711824151079,2.78521678517299));
#214248=CARTESIAN_POINT('Ctrl Pts',(-31.6730053921568,-54.2846372786638,
2.76730190933255));
#214249=CARTESIAN_POINT('Ctrl Pts',(-31.6704454915891,-54.2986636530711,
2.74997687278455));
#214250=CARTESIAN_POINT('Ctrl Pts',(-31.6660771734229,-54.3131329740909,
2.73349253344308));
#214251=CARTESIAN_POINT('Ctrl Pts',(-31.6627215829926,-54.3242478043988,
2.72082983598364));
#214252=CARTESIAN_POINT('Ctrl Pts',(-31.658298121582,-54.335624457859,2.7086632103882));
#214253=CARTESIAN_POINT('Ctrl Pts',(-31.6527458376963,-54.3472079546995,
2.69711645335805));
#214254=CARTESIAN_POINT('Ctrl Pts',(-31.6527312861504,-54.3472383129789,
2.69708619136711));
#214255=CARTESIAN_POINT('Ctrl Pts',(-31.6527167260609,-54.3472686729569,
2.69705593387179));
#214256=CARTESIAN_POINT('Ctrl Pts',(-31.6527021574289,-54.3472990346305,
2.69702568087531));
#214257=CARTESIAN_POINT('Ctrl Pts',(-31.6511401038183,-54.3505544234701,
2.69378194443226));
#214258=CARTESIAN_POINT('Ctrl Pts',(-31.6494796970072,-54.3538274103384,
2.6905926662466));
#214259=CARTESIAN_POINT('Ctrl Pts',(-31.6477231007675,-54.3571135597833,
2.68746219342637));
#214260=CARTESIAN_POINT('Ctrl Pts',(-31.6379480420931,-54.3754002342685,
2.67004182396106));
#214261=CARTESIAN_POINT('Ctrl Pts',(-31.6251987170241,-54.3940968201759,
2.65443567877953));
#214262=CARTESIAN_POINT('Ctrl Pts',(-31.6099016141384,-54.4124255228524,
2.64136852353169));
#214263=CARTESIAN_POINT('Ctrl Pts',(-31.6030360625228,-54.4206516984369,
2.6355038032972));
#214264=CARTESIAN_POINT('Ctrl Pts',(-31.5956573884073,-54.428804121416,
2.63014997451078));
#214265=CARTESIAN_POINT('Ctrl Pts',(-31.5878037911378,-54.4368146919236,
2.62536981119215));
#214266=CARTESIAN_POINT('Ctrl Pts',(-31.5843907239922,-54.4402959775153,
2.62329241687035));
#214267=CARTESIAN_POINT('Ctrl Pts',(-31.5808879923396,-54.4437502703989,
2.62132362131389));
#214268=CARTESIAN_POINT('Ctrl Pts',(-31.5772987574364,-54.4471718528272,
2.61946873372309));
#214269=CARTESIAN_POINT('Ctrl Pts',(-31.5647364352749,-54.4591473913263,
2.61297662715529));
#214270=CARTESIAN_POINT('Ctrl Pts',(-31.5511144466737,-54.4707222239581,
2.6078798911393));
#214271=CARTESIAN_POINT('Ctrl Pts',(-31.5365683393821,-54.4816512176785,
2.6044061688614));
#214272=CARTESIAN_POINT('Ctrl Pts',(-31.5292952857363,-54.4871157145387,
2.60266930772245));
#214273=CARTESIAN_POINT('Ctrl Pts',(-31.521791202724,-54.4924187521964,
2.60133820040144));
#214274=CARTESIAN_POINT('Ctrl Pts',(-31.51407303778,-54.4975296958773,2.60044130723544));
#214275=CARTESIAN_POINT('Ctrl Pts',(-31.5102139553079,-54.5000851677178,
2.59999286065244));
#214276=CARTESIAN_POINT('Ctrl Pts',(-31.5063013524145,-54.5025926161708,
2.59965296768472));
#214277=CARTESIAN_POINT('Ctrl Pts',(-31.5023373478775,-54.5050482124961,
2.59942518630914));
#214278=CARTESIAN_POINT('Ctrl Pts',(-31.4983733433404,-54.5075038088215,
2.59919740493356));
#214279=CARTESIAN_POINT('Ctrl Pts',(-31.4943579363061,-54.5099075515418,
2.59908173791574));
#214280=CARTESIAN_POINT('Ctrl Pts',(-31.4902932482903,-54.5122556166612,
2.59908173515985));
#214281=CARTESIAN_POINT('',(-31.4638515574735,-54.527521733972,2.59908173515985));
#214282=CARTESIAN_POINT('Origin',(3.80217165444466E-17,1.91242074430722E-13,
2.59908173516022));
#214283=CARTESIAN_POINT('',(-31.106798218553,-54.5146464769139,2.90134173515985));
#214284=CARTESIAN_POINT('Ctrl Pts',(-31.4638515574735,-54.527521733972,
2.59908173515985));
#214285=CARTESIAN_POINT('Ctrl Pts',(-31.4605414731915,-54.5294317356858,
2.59908174381641));
#214286=CARTESIAN_POINT('Ctrl Pts',(-31.4572166015116,-54.5312951627228,
2.59915752000956));
#214287=CARTESIAN_POINT('Ctrl Pts',(-31.4538791743428,-54.533112022376,
2.59930729517431));
#214288=CARTESIAN_POINT('Ctrl Pts',(-31.4345929624711,-54.5436112298315,
2.60017281085879));
#214289=CARTESIAN_POINT('Ctrl Pts',(-31.4148859438259,-54.5525583311778,
2.60350651800034));
#214290=CARTESIAN_POINT('Ctrl Pts',(-31.3951944477271,-54.5599504658508,
2.60896880596455));
#214291=CARTESIAN_POINT('Ctrl Pts',(-31.3872524143693,-54.5629318838124,
2.61117187235442));
#214292=CARTESIAN_POINT('Ctrl Pts',(-31.3793127123321,-54.5656607810286,
2.61372076577173));
#214293=CARTESIAN_POINT('Ctrl Pts',(-31.3714030065914,-54.5681385507008,
2.61659179896942));
#214294=CARTESIAN_POINT('Ctrl Pts',(-31.3684848053914,-54.5690526972782,
2.61765103591167));
#214295=CARTESIAN_POINT('Ctrl Pts',(-31.3655707565302,-54.569932546879,
2.61875422455108));
#214296=CARTESIAN_POINT('Ctrl Pts',(-31.3626622846448,-54.5707781137755,
2.61990022440354));
#214297=CARTESIAN_POINT('Ctrl Pts',(-31.3572088998595,-54.5723635517063,
2.62204897412691));
#214298=CARTESIAN_POINT('Ctrl Pts',(-31.3517751216265,-54.5738284644992,
2.62434823201728));
#214299=CARTESIAN_POINT('Ctrl Pts',(-31.3463703409152,-54.5751729463229,
2.62679048030263));
#214300=CARTESIAN_POINT('Ctrl Pts',(-31.3274536084255,-54.579878632706,
2.63533834930137));
#214301=CARTESIAN_POINT('Ctrl Pts',(-31.3088920933397,-54.5831090358348,
2.64563784783522));
#214302=CARTESIAN_POINT('Ctrl Pts',(-31.291088446162,-54.5848682151123,
2.65736666737923));
#214303=CARTESIAN_POINT('Ctrl Pts',(-31.2821866225732,-54.5857478047511,
2.66323107715124));
#214304=CARTESIAN_POINT('Ctrl Pts',(-31.2734742664667,-54.5862595893019,
2.66945281780732));
#214305=CARTESIAN_POINT('Ctrl Pts',(-31.2650017135572,-54.5864040839108,
2.67599160631159));
#214306=CARTESIAN_POINT('Ctrl Pts',(-31.2607654371024,-54.5864763312153,
2.67926100056373));
#214307=CARTESIAN_POINT('Ctrl Pts',(-31.2565891115048,-54.5864567561365,
2.68260965685083));
#214308=CARTESIAN_POINT('Ctrl Pts',(-31.2524790289898,-54.5863454235313,
2.68603254012442));
#214309=CARTESIAN_POINT('Ctrl Pts',(-31.2483689464749,-54.5862340909261,
2.68945542339802));
#214310=CARTESIAN_POINT('Ctrl Pts',(-31.2443251851216,-54.5860308973889,
2.69295261525344));
#214311=CARTESIAN_POINT('Ctrl Pts',(-31.240353878453,-54.5857361203748,
2.69651891172058));
#214312=CARTESIAN_POINT('Ctrl Pts',(-31.2403200115243,-54.5857336065442,
2.69654932476046));
#214313=CARTESIAN_POINT('Ctrl Pts',(-31.2402861499641,-54.5857310861512,
2.69657974261105));
#214314=CARTESIAN_POINT('Ctrl Pts',(-31.2402522937756,-54.5857285591961,
2.69661016526932));
#214315=CARTESIAN_POINT('Ctrl Pts',(-31.2229614439844,-54.584438006344,
2.71214746101312));
#214316=CARTESIAN_POINT('Ctrl Pts',(-31.2070266227583,-54.5815601021613,
2.72880565568009));
#214317=CARTESIAN_POINT('Ctrl Pts',(-31.1924939094092,-54.5772898993832,
2.74628040013039));
#214318=CARTESIAN_POINT('Ctrl Pts',(-31.1774697093447,-54.5728752811827,
2.76434612883432));
#214319=CARTESIAN_POINT('Ctrl Pts',(-31.1639433968857,-54.566971991736,
2.783285926558));
#214320=CARTESIAN_POINT('Ctrl Pts',(-31.1520017942418,-54.5597576364785,
2.80278753269533));
#214321=CARTESIAN_POINT('Ctrl Pts',(-31.1402873460082,-54.5526805134387,
2.82191817724808));
#214322=CARTESIAN_POINT('Ctrl Pts',(-31.1300975277222,-54.5443408740922,
2.84159092317495));
#214323=CARTESIAN_POINT('Ctrl Pts',(-31.1215554575361,-54.5348819367156,
2.86151233819678));
#214324=CARTESIAN_POINT('Ctrl Pts',(-31.1158966355112,-54.5286157223212,
2.8747095772309));
#214325=CARTESIAN_POINT('Ctrl Pts',(-31.1109617866599,-54.5218578148468,
2.88801594389215));
#214326=CARTESIAN_POINT('Ctrl Pts',(-31.106798218553,-54.5146464769139,
2.90134173515985));
#214327=CARTESIAN_POINT('',(-30.9286463962973,-54.2060847114743,3.47153072139033));
#214328=CARTESIAN_POINT('',(-31.106798218553,-54.5146464769139,2.90134173515985));
#214329=CARTESIAN_POINT('',(-25.6742415049975,-56.8833377255395,3.47153072139031));
#214330=CARTESIAN_POINT('Origin',(5.53234440788222E-15,1.85015204418142E-13,
3.47153072139072));
#214331=CARTESIAN_POINT('',(-25.8191582032616,-57.2088336324699,2.90134173515983));
#214332=CARTESIAN_POINT('',(-25.6742415049975,-56.8833377255395,3.47153072139031));
#214333=CARTESIAN_POINT('',(-25.6197038181293,-57.5052637377732,2.59908173515982));
#214334=CARTESIAN_POINT('Ctrl Pts',(-25.8191582032616,-57.2088336324699,
2.90134173515983));
#214335=CARTESIAN_POINT('Ctrl Pts',(-25.8241633573204,-57.2200757170667,
2.88164837656895));
#214336=CARTESIAN_POINT('Ctrl Pts',(-25.8273704465166,-57.2320741602303,
2.86203734439522));
#214337=CARTESIAN_POINT('Ctrl Pts',(-25.8287819086035,-57.2446400511018,
2.84277945978731));
#214338=CARTESIAN_POINT('Ctrl Pts',(-25.8302217324659,-57.2574584397044,
2.8231346092081));
#214339=CARTESIAN_POINT('Ctrl Pts',(-25.8297934599659,-57.2708681396284,
2.80385576864333));
#214340=CARTESIAN_POINT('Ctrl Pts',(-25.8274551293922,-57.284698180309,
2.78521678519563));
#214341=CARTESIAN_POINT('Ctrl Pts',(-25.8252076408415,-57.2979909364466,
2.76730190935802));
#214342=CARTESIAN_POINT('Ctrl Pts',(-25.8211956083174,-57.3116728904319,
2.74997687281252));
#214343=CARTESIAN_POINT('Ctrl Pts',(-25.8153387643678,-57.3256063334094,
2.7334925334731));
#214344=CARTESIAN_POINT('Ctrl Pts',(-25.8108397400796,-57.336309520811,
2.72082983600286));
#214345=CARTESIAN_POINT('Ctrl Pts',(-25.8052513267465,-57.3471614741582,
2.70866321039731));
#214346=CARTESIAN_POINT('Ctrl Pts',(-25.7985186537236,-57.3581011436974,
2.69711645335804));
#214347=CARTESIAN_POINT('Ctrl Pts',(-25.7985010085883,-57.3581298146203,
2.6970861913671));
#214348=CARTESIAN_POINT('Ctrl Pts',(-25.7984833547786,-57.3581584863394,
2.69705593387177));
#214349=CARTESIAN_POINT('Ctrl Pts',(-25.7984656922961,-57.3581871588519,
2.69702568087529));
#214350=CARTESIAN_POINT('Ctrl Pts',(-25.7965719149858,-57.3612614352674,
2.69378194443225));
#214351=CARTESIAN_POINT('Ctrl Pts',(-25.7945784837693,-57.3643429325988,
2.69059266624658));
#214352=CARTESIAN_POINT('Ctrl Pts',(-25.7924880141961,-57.3674274658676,
2.68746219342635));
#214353=CARTESIAN_POINT('Ctrl Pts',(-25.7808550263337,-57.3845921921749,
2.67004182396113));
#214354=CARTESIAN_POINT('Ctrl Pts',(-25.7662212180083,-57.4018536888712,
2.65443567877967));
#214355=CARTESIAN_POINT('Ctrl Pts',(-25.7490920431284,-57.4184830023395,
2.64136852353187));
#214356=CARTESIAN_POINT('Ctrl Pts',(-25.7414042322304,-57.4259464685137,
2.63550380329729));
#214357=CARTESIAN_POINT('Ctrl Pts',(-25.7332138190178,-57.4332829502006,
2.6301499745108));
#214358=CARTESIAN_POINT('Ctrl Pts',(-25.7245659119506,-57.4404287135112,
2.62536981119211));
#214359=CARTESIAN_POINT('Ctrl Pts',(-25.7208076485109,-57.4435341655923,
2.62329241687031));
#214360=CARTESIAN_POINT('Ctrl Pts',(-25.7169630332621,-57.4466034003412,
2.62132362131385));
#214361=CARTESIAN_POINT('Ctrl Pts',(-25.71303580781,-57.4496310617742,2.61946873372305));
#214362=CARTESIAN_POINT('Ctrl Pts',(-25.6992905187276,-57.4602278767898,
2.61297662715525));
#214363=CARTESIAN_POINT('Ctrl Pts',(-25.6845332533377,-57.4703154157422,
2.60787989113927));
#214364=CARTESIAN_POINT('Ctrl Pts',(-25.6689244402251,-57.4796640570498,
2.60440616886137));
#214365=CARTESIAN_POINT('Ctrl Pts',(-25.6611200336689,-57.4843383777035,
2.60266930772242));
#214366=CARTESIAN_POINT('Ctrl Pts',(-25.6531027404315,-57.4888279745006,
2.60133820040143));
#214367=CARTESIAN_POINT('Ctrl Pts',(-25.6448926173138,-57.4931041519764,
2.60044130723543));
#214368=CARTESIAN_POINT('Ctrl Pts',(-25.6407875557549,-57.4952422407143,
2.59999286065242));
#214369=CARTESIAN_POINT('Ctrl Pts',(-25.636634286776,-57.4973269747345,
2.5996529676847));
#214370=CARTESIAN_POINT('Ctrl Pts',(-25.6324353177602,-57.4993547677436,
2.59942518630912));
#214371=CARTESIAN_POINT('Ctrl Pts',(-25.6282363487445,-57.5013825607527,
2.59919740493354));
#214372=CARTESIAN_POINT('Ctrl Pts',(-25.6239916789975,-57.5033534111922,
2.59908173791572));
#214373=CARTESIAN_POINT('Ctrl Pts',(-25.6197038181293,-57.5052637377732,
2.59908173515983));
#214374=CARTESIAN_POINT('',(-25.5918112338789,-57.5176823163889,2.59908173515983));
#214375=CARTESIAN_POINT('Origin',(2.35274110347535E-17,1.91249459648252E-13,
2.59908173516024));
#214376=CARTESIAN_POINT('',(-25.2380597013425,-57.4675553545141,2.90134173515982));
#214377=CARTESIAN_POINT('Ctrl Pts',(-25.5918112338789,-57.5176823163889,
2.59908173515983));
#214378=CARTESIAN_POINT('Ctrl Pts',(-25.5883196330409,-57.5192358568901,
2.59908174381641));
#214379=CARTESIAN_POINT('Ctrl Pts',(-25.5848181941914,-57.5207415321516,
2.59915752000954));
#214380=CARTESIAN_POINT('Ctrl Pts',(-25.5813091362503,-57.5221995827243,
2.59930729517429));
#214381=CARTESIAN_POINT('Ctrl Pts',(-25.5610311102427,-57.5306253163343,
2.60017281085885));
#214382=CARTESIAN_POINT('Ctrl Pts',(-25.5404968219514,-57.5374634601491,
2.60350651800088));
#214383=CARTESIAN_POINT('Ctrl Pts',(-25.5201405094493,-57.5427567781085,
2.60896880596589));
#214384=CARTESIAN_POINT('Ctrl Pts',(-25.5119303403451,-57.5448916950078,
2.61117187235545));
#214385=CARTESIAN_POINT('Ctrl Pts',(-25.5037488853955,-57.5467757181864,
2.61372076577231));
#214386=CARTESIAN_POINT('Ctrl Pts',(-25.495623512396,-57.5484131249907,
2.61659179896943));
#214387=CARTESIAN_POINT('Ctrl Pts',(-25.4926257430706,-57.5490172286906,
2.61765103591169));
#214388=CARTESIAN_POINT('Ctrl Pts',(-25.4896356883473,-57.5495876573339,
2.61875422455109));
#214389=CARTESIAN_POINT('Ctrl Pts',(-25.4866547635669,-57.5501245740298,
2.61990022440355));
#214390=CARTESIAN_POINT('Ctrl Pts',(-25.4810655296035,-57.5511312928345,
2.62204897412692));
#214391=CARTESIAN_POINT('Ctrl Pts',(-25.4755083930932,-57.5520201961934,
2.62434823201729));
#214392=CARTESIAN_POINT('Ctrl Pts',(-25.4699926837172,-57.552792359383,
2.62679048030264));
#214393=CARTESIAN_POINT('Ctrl Pts',(-25.4506877009012,-57.5554949305466,
2.63533834930138));
#214394=CARTESIAN_POINT('Ctrl Pts',(-25.4318901986623,-57.5567674305411,
2.64563784783521));
#214395=CARTESIAN_POINT('Ctrl Pts',(-25.4140001974202,-57.5566559849705,
2.65736666737922));
#214396=CARTESIAN_POINT('Ctrl Pts',(-25.4050551967991,-57.5566002621852,
2.66323107715123));
#214397=CARTESIAN_POINT('Ctrl Pts',(-25.3963370718384,-57.5561985539314,
2.66945281780733));
#214398=CARTESIAN_POINT('Ctrl Pts',(-25.3878958286608,-57.5554566340481,
2.67599160631159));
#214399=CARTESIAN_POINT('Ctrl Pts',(-25.383675207072,-57.5550856741065,
2.67926100056373));
#214400=CARTESIAN_POINT('Ctrl Pts',(-25.3795238059759,-57.5546296613652,
2.6826096568508));
#214401=CARTESIAN_POINT('Ctrl Pts',(-25.3754478763491,-57.5540893180425,
2.6860325401244));
#214402=CARTESIAN_POINT('Ctrl Pts',(-25.3713719467224,-57.5535489747198,
2.68945542339799));
#214403=CARTESIAN_POINT('Ctrl Pts',(-25.3673715770251,-57.552924206138,
2.69295261525342));
#214404=CARTESIAN_POINT('Ctrl Pts',(-25.3634528381782,-57.5522159293599,
2.69651891172056));
#214405=CARTESIAN_POINT('Ctrl Pts',(-25.363419419543,-57.5522098892424,
2.69654932476044));
#214406=CARTESIAN_POINT('Ctrl Pts',(-25.3633860069328,-57.5522038431595,
2.69657974261102));
#214407=CARTESIAN_POINT('Ctrl Pts',(-25.3633526003507,-57.552197791112,
2.6966101652693));
#214408=CARTESIAN_POINT('Ctrl Pts',(-25.3462913711525,-57.5491069220865,
2.71214746101104));
#214409=CARTESIAN_POINT('Ctrl Pts',(-25.3307446654479,-57.5445791409897,
2.72880565567566));
#214410=CARTESIAN_POINT('Ctrl Pts',(-25.3167379215588,-57.5388132486368,
2.74628040012343));
#214411=CARTESIAN_POINT('Ctrl Pts',(-25.3022574788921,-57.5328523576332,
2.76434612882484));
#214412=CARTESIAN_POINT('Ctrl Pts',(-25.2894223267632,-57.5255675223701,
2.78328592654582));
#214413=CARTESIAN_POINT('Ctrl Pts',(-25.2783002469372,-57.5171444507339,
2.80278753268039));
#214414=CARTESIAN_POINT('Ctrl Pts',(-25.2673897324726,-57.5088816036442,
2.82191817723078));
#214415=CARTESIAN_POINT('Ctrl Pts',(-25.2581274647625,-57.4995225236699,
2.84159092315524));
#214416=CARTESIAN_POINT('Ctrl Pts',(-25.2506209171182,-57.4892225138741,
2.86151233817473));
#214417=CARTESIAN_POINT('Ctrl Pts',(-25.2456480924699,-57.4823991184843,
2.87470957721607));
#214418=CARTESIAN_POINT('Ctrl Pts',(-25.2414466709174,-57.4751623993634,
2.88801594388471));
#214419=CARTESIAN_POINT('Ctrl Pts',(-25.2380597013425,-57.4675553545141,
2.90134173515982));
#214420=CARTESIAN_POINT('',(-25.0931373005741,-57.1420619865022,3.47153072139031));
#214421=CARTESIAN_POINT('',(-25.2380597013425,-57.4675553545141,2.90134173515982));
#214422=CARTESIAN_POINT('',(-19.5876674457072,-59.2554138597571,3.4715307213903));
#214423=CARTESIAN_POINT('Origin',(5.53234440788222E-15,1.85015204418142E-13,
3.47153072139072));
#214424=CARTESIAN_POINT('',(-19.697766688184,-59.5942745858236,2.90134173515981));
#214425=CARTESIAN_POINT('',(-19.5876674457073,-59.2554138597571,3.4715307213903));
#214426=CARTESIAN_POINT('',(-19.4684195516691,-59.8682321556242,2.5990817351598));
#214427=CARTESIAN_POINT('Ctrl Pts',(-19.697766688184,-59.5942745858236,
2.90134173515981));
#214428=CARTESIAN_POINT('Ctrl Pts',(-19.7015693056586,-59.6059782661681,
2.8816483765668));
#214429=CARTESIAN_POINT('Ctrl Pts',(-19.703504647259,-59.6182462127113,
2.86203734439098));
#214430=CARTESIAN_POINT('Ctrl Pts',(-19.7035948839462,-59.6308908042823,
2.84277945978107));
#214431=CARTESIAN_POINT('Ctrl Pts',(-19.7036869338402,-59.6437894749879,
2.82313460919993));
#214432=CARTESIAN_POINT('Ctrl Pts',(-19.701859312135,-59.6570809485079,
2.80385576863333));
#214433=CARTESIAN_POINT('Ctrl Pts',(-19.6980881582805,-59.6705908046785,
2.78521678518401));
#214434=CARTESIAN_POINT('Ctrl Pts',(-19.6944635103345,-59.6835758151839,
2.76730190934502));
#214435=CARTESIAN_POINT('Ctrl Pts',(-19.6890433025185,-59.6967634464007,
2.74997687279832));
#214436=CARTESIAN_POINT('Ctrl Pts',(-19.6817621015886,-59.7100083536232,
2.73349253345792));
#214437=CARTESIAN_POINT('Ctrl Pts',(-19.6761689356963,-59.7201826317453,
2.72082983599314));
#214438=CARTESIAN_POINT('Ctrl Pts',(-19.6694767982717,-59.7303909886947,
2.70866321039269));
#214439=CARTESIAN_POINT('Ctrl Pts',(-19.6616375006935,-59.7405669736107,
2.69711645335803));
#214440=CARTESIAN_POINT('Ctrl Pts',(-19.6616169552926,-59.7405936430524,
2.69708619136709));
#214441=CARTESIAN_POINT('Ctrl Pts',(-19.6615964011816,-59.7406203123792,
2.69705593387176));
#214442=CARTESIAN_POINT('Ctrl Pts',(-19.6615758383624,-59.7406469815885,
2.69702568087528));
#214443=CARTESIAN_POINT('Ctrl Pts',(-19.659371085973,-59.7435064631641,
2.69378194443223));
#214444=CARTESIAN_POINT('Ctrl Pts',(-19.6570664708007,-59.746362709429,
2.69059266624656));
#214445=CARTESIAN_POINT('Ctrl Pts',(-19.654665031516,-59.7492118317299,
2.68746219342633));
#214446=CARTESIAN_POINT('Ctrl Pts',(-19.6413015679163,-59.7650665495245,
2.67004182396276));
#214447=CARTESIAN_POINT('Ctrl Pts',(-19.6249436074025,-59.7807038364384,
2.6544356787826));
#214448=CARTESIAN_POINT('Ctrl Pts',(-19.606170031355,-59.7954515664591,
2.64136852353555));
#214449=CARTESIAN_POINT('Ctrl Pts',(-19.5977441904381,-59.8020705519271,
2.63550380329953));
#214450=CARTESIAN_POINT('Ctrl Pts',(-19.5888317740078,-59.8085107122944,
2.6301499745118));
#214451=CARTESIAN_POINT('Ctrl Pts',(-19.5794843054207,-59.814713377931,
2.6253698111921));
#214452=CARTESIAN_POINT('Ctrl Pts',(-19.5754220220075,-59.8174089725188,
2.6232924168703));
#214453=CARTESIAN_POINT('Ctrl Pts',(-19.5712776455715,-59.8200595219548,
2.62132362131385));
#214454=CARTESIAN_POINT('Ctrl Pts',(-19.5670554570745,-59.8226600907003,
2.61946873372305));
#214455=CARTESIAN_POINT('Ctrl Pts',(-19.5522777973348,-59.8317620813095,
2.61297662715524));
#214456=CARTESIAN_POINT('Ctrl Pts',(-19.5365469388439,-59.8402518053948,
2.60787989113925));
#214457=CARTESIAN_POINT('Ctrl Pts',(-19.5200464333333,-59.847917668619,
2.60440616886135));
#214458=CARTESIAN_POINT('Ctrl Pts',(-19.5117961805779,-59.8517506002311,
2.60266930772241));
#214459=CARTESIAN_POINT('Ctrl Pts',(-19.5033535162579,-59.8553775672055,
2.60133820040141));
#214460=CARTESIAN_POINT('Ctrl Pts',(-19.4947413867934,-59.8587721277809,
2.60044130723541));
#214461=CARTESIAN_POINT('Ctrl Pts',(-19.4904353220612,-59.8604694080687,
2.59999286065241));
#214462=CARTESIAN_POINT('Ctrl Pts',(-19.4860868910809,-59.8621085868739,
2.59965296768468));
#214463=CARTESIAN_POINT('Ctrl Pts',(-19.4816989623697,-59.8636863596422,
2.5994251863091));
#214464=CARTESIAN_POINT('Ctrl Pts',(-19.4773110336585,-59.8652641324105,
2.59919740493352));
#214465=CARTESIAN_POINT('Ctrl Pts',(-19.4728836066887,-59.8667804975192,
2.59908173791576));
#214466=CARTESIAN_POINT('Ctrl Pts',(-19.4684195516691,-59.8682321556242,
2.59908173515981));
#214467=CARTESIAN_POINT('',(-19.4393816709751,-59.8776671349985,2.59908173515981));
#214468=CARTESIAN_POINT('Origin',(8.34054140790793E-18,1.91255289341306E-13,
2.59908173516022));
#214469=CARTESIAN_POINT('',(-19.0928077206406,-59.7908376697911,2.90134173515981));
#214470=CARTESIAN_POINT('Ctrl Pts',(-19.4393816709751,-59.8776671349985,
2.59908173515981));
#214471=CARTESIAN_POINT('Ctrl Pts',(-19.4357468082906,-59.8788471933724,
2.59908174381641));
#214472=CARTESIAN_POINT('Ctrl Pts',(-19.4321071647682,-59.879978620365,
2.59915752000953));
#214473=CARTESIAN_POINT('Ctrl Pts',(-19.4284649220279,-59.8810618871501,
2.59930729517428));
#214474=CARTESIAN_POINT('Ctrl Pts',(-19.4074172521841,-59.8873218328126,
2.60017281085876));
#214475=CARTESIAN_POINT('Ctrl Pts',(-19.3862806722099,-59.8919760989604,
2.6035065180003));
#214476=CARTESIAN_POINT('Ctrl Pts',(-19.3654825713274,-59.8951126055065,
2.60896880596449));
#214477=CARTESIAN_POINT('Ctrl Pts',(-19.3570942188041,-59.8963776307484,
2.61117187235437));
#214478=CARTESIAN_POINT('Ctrl Pts',(-19.3487606486714,-59.897396138138,
2.61372076577169));
#214479=CARTESIAN_POINT('Ctrl Pts',(-19.3405086316967,-59.8981752423036,
2.6165917989694));
#214480=CARTESIAN_POINT('Ctrl Pts',(-19.3374641384339,-59.8984626844394,
2.61765103591166));
#214481=CARTESIAN_POINT('Ctrl Pts',(-19.3344308375137,-59.8987174423896,
2.61875422455106));
#214482=CARTESIAN_POINT('Ctrl Pts',(-19.331410119474,-59.8989398263132,
2.61990022440352));
#214483=CARTESIAN_POINT('Ctrl Pts',(-19.3257462731495,-59.89935679617,2.62204897412689));
#214484=CARTESIAN_POINT('Ctrl Pts',(-19.3201266635123,-59.8996599510836,
2.62434823201726));
#214485=CARTESIAN_POINT('Ctrl Pts',(-19.3145604567378,-59.8998513356576,
2.62679048030262));
#214486=CARTESIAN_POINT('Ctrl Pts',(-19.295078733027,-59.9005211816664,
2.63533834930135));
#214487=CARTESIAN_POINT('Ctrl Pts',(-19.2762511930033,-59.8998218367505,
2.64563784783519));
#214488=CARTESIAN_POINT('Ctrl Pts',(-19.258470844294,-59.8978409873527,
2.6573666673792));
#214489=CARTESIAN_POINT('Ctrl Pts',(-19.2495806699394,-59.8968505626538,
2.66323107715121));
#214490=CARTESIAN_POINT('Ctrl Pts',(-19.2409522937258,-59.8955397627951,
2.66945281780731));
#214491=CARTESIAN_POINT('Ctrl Pts',(-19.2326348443069,-59.8939195570492,
2.67599160631158));
#214492=CARTESIAN_POINT('Ctrl Pts',(-19.2284761195974,-59.8931094541762,
2.67926100056371));
#214493=CARTESIAN_POINT('Ctrl Pts',(-19.2243951266219,-59.8922219999435,
2.6826096568508));
#214494=CARTESIAN_POINT('Ctrl Pts',(-19.2203980066213,-59.8912585660177,
2.68603254012439));
#214495=CARTESIAN_POINT('Ctrl Pts',(-19.2164008866207,-59.890295132092,
2.68945542339799));
#214496=CARTESIAN_POINT('Ctrl Pts',(-19.2124877374669,-59.8892556335609,
2.69295261525341));
#214497=CARTESIAN_POINT('Ctrl Pts',(-19.2086645009646,-59.8881416170476,
2.69651891172055));
#214498=CARTESIAN_POINT('Ctrl Pts',(-19.2086318967643,-59.8881321168198,
2.69654932476043));
#214499=CARTESIAN_POINT('Ctrl Pts',(-19.2085992991797,-59.8881226112892,
2.69657974261101));
#214500=CARTESIAN_POINT('Ctrl Pts',(-19.2085667082136,-59.8881131004567,
2.69661016526929));
#214501=CARTESIAN_POINT('Ctrl Pts',(-19.191922026002,-59.8832557794652,
2.7121474610124));
#214502=CARTESIAN_POINT('Ctrl Pts',(-19.1769337687768,-59.8771277287701,
2.7288056556786));
#214503=CARTESIAN_POINT('Ctrl Pts',(-19.1636064551624,-59.8699293191639,
2.74628040012806));
#214504=CARTESIAN_POINT('Ctrl Pts',(-19.1498284206512,-59.8624874641247,
2.76434612883123));
#214505=CARTESIAN_POINT('Ctrl Pts',(-19.1378250534633,-59.8539008972225,
2.7832859265541));
#214506=CARTESIAN_POINT('Ctrl Pts',(-19.1276443522881,-59.8443613941403,
2.80278753269061));
#214507=CARTESIAN_POINT('Ctrl Pts',(-19.1176573094717,-59.8350033524799,
2.82191817724284));
#214508=CARTESIAN_POINT('Ctrl Pts',(-19.1094240716806,-59.8247273719136,
2.8415909231692));
#214509=CARTESIAN_POINT('Ctrl Pts',(-19.1030352898857,-59.8136991387581,
2.86151233819053));
#214510=CARTESIAN_POINT('Ctrl Pts',(-19.0988029459279,-59.8063933209263,
2.87470957722669));
#214511=CARTESIAN_POINT('Ctrl Pts',(-19.0953809833327,-59.7987570771744,
2.88801594389002));
#214512=CARTESIAN_POINT('Ctrl Pts',(-19.0928077206406,-59.7908376697912,
2.90134173515981));
#214513=CARTESIAN_POINT('',(-18.9827025415091,-59.4519788726608,3.4715307213903));
#214514=CARTESIAN_POINT('',(-19.0928077206406,-59.7908376697911,2.90134173515981));
#214515=CARTESIAN_POINT('',(-13.2864868028989,-60.9782752797347,3.47153072139029));
#214516=CARTESIAN_POINT('Origin',(5.53234440788222E-15,1.85015204418142E-13,
3.47153072139072));
#214517=CARTESIAN_POINT('',(-13.360562319248,-61.3267881959112,2.90134173515981));
#214518=CARTESIAN_POINT('',(-13.2864868028989,-60.9782752797348,3.47153072139029));
#214519=CARTESIAN_POINT('',(-13.1038352065721,-61.5752716937451,2.5990817351598));
#214520=CARTESIAN_POINT('Ctrl Pts',(-13.360562319248,-61.3267881959112,
2.9013417351598));
#214521=CARTESIAN_POINT('Ctrl Pts',(-13.3631207378652,-61.3388252440305,
2.88164837656816));
#214522=CARTESIAN_POINT('Ctrl Pts',(-13.3637631278624,-61.3512282837613,
2.86203734439369));
#214523=CARTESIAN_POINT('Ctrl Pts',(-13.3625311504984,-61.363813039238,
2.84277945978507));
#214524=CARTESIAN_POINT('Ctrl Pts',(-13.3612744179067,-61.376650671509,
2.82313460920513));
#214525=CARTESIAN_POINT('Ctrl Pts',(-13.3580674708034,-61.3896782944572,
2.80385576863965));
#214526=CARTESIAN_POINT('Ctrl Pts',(-13.3529048112206,-61.4027199493042,
2.78521678519133));
#214527=CARTESIAN_POINT('Ctrl Pts',(-13.3479427162824,-61.415254947683,
2.76730190935321));
#214528=CARTESIAN_POINT('Ctrl Pts',(-13.3411737181076,-61.4278037696819,
2.74997687280727));
#214529=CARTESIAN_POINT('Ctrl Pts',(-13.3325479345614,-61.4402150271722,
2.73349253346748));
#214530=CARTESIAN_POINT('Ctrl Pts',(-13.325921906959,-61.4497489245011,
2.72082983599925));
#214531=CARTESIAN_POINT('Ctrl Pts',(-13.3181993658972,-61.4592018401645,
2.70866321039559));
#214532=CARTESIAN_POINT('Ctrl Pts',(-13.3093393327438,-61.4685026502438,
2.69711645335801));
#214533=CARTESIAN_POINT('Ctrl Pts',(-13.309316112177,-61.4685270260083,
2.69708619136707));
#214534=CARTESIAN_POINT('Ctrl Pts',(-13.3092928829598,-61.4685514007481,
2.69705593387175));
#214535=CARTESIAN_POINT('Ctrl Pts',(-13.3092696450943,-61.4685757744608,
2.69702568087527));
#214536=CARTESIAN_POINT('Ctrl Pts',(-13.3067780733544,-61.471189132118,
2.69378194443222));
#214537=CARTESIAN_POINT('Ctrl Pts',(-13.3041875240723,-61.4737888336846,
2.69059266624656));
#214538=CARTESIAN_POINT('Ctrl Pts',(-13.3015014257475,-61.4763713294374,
2.68746219342633));
#214539=CARTESIAN_POINT('Ctrl Pts',(-13.2865538993097,-61.4907423311182,
2.67004182395882));
#214540=CARTESIAN_POINT('Ctrl Pts',(-13.2686510078397,-61.5045840828665,
2.65443567877554));
#214541=CARTESIAN_POINT('Ctrl Pts',(-13.2484387178447,-61.5172886502272,
2.64136852352668));
#214542=CARTESIAN_POINT('Ctrl Pts',(-13.2393671621907,-61.5229906359943,
2.63550380329413));
#214543=CARTESIAN_POINT('Ctrl Pts',(-13.2298303888482,-61.5284639152929,
2.63014997450939));
#214544=CARTESIAN_POINT('Ctrl Pts',(-13.21988577157,-61.5336555255487,2.6253698111921));
#214545=CARTESIAN_POINT('Ctrl Pts',(-13.2155639754105,-61.5359117291448,
2.6232924168703));
#214546=CARTESIAN_POINT('Ctrl Pts',(-13.211165244443,-61.5381145532936,
2.62132362131384));
#214547=CARTESIAN_POINT('Ctrl Pts',(-13.2066943520817,-61.5402595369762,
2.61946873372304));
#214548=CARTESIAN_POINT('Ctrl Pts',(-13.1910462288172,-61.5477669798652,
2.61297662715524));
#214549=CARTESIAN_POINT('Ctrl Pts',(-13.1745141278029,-61.5545658738897,
2.60787989113926));
#214550=CARTESIAN_POINT('Ctrl Pts',(-13.1573027128855,-61.5604649702289,
2.60440616886136));
#214551=CARTESIAN_POINT('Ctrl Pts',(-13.1486970054267,-61.5634145183985,
2.60266930772241));
#214552=CARTESIAN_POINT('Ctrl Pts',(-13.1399214696211,-61.566139117741,
2.60133820040141));
#214553=CARTESIAN_POINT('Ctrl Pts',(-13.1310016901025,-61.5686148699001,
2.6004413072354));
#214554=CARTESIAN_POINT('Ctrl Pts',(-13.1265418003432,-61.5698527459796,
2.5999928606524));
#214555=CARTESIAN_POINT('Ctrl Pts',(-13.1220458496813,-61.5710284103838,
2.59965296768468));
#214556=CARTESIAN_POINT('Ctrl Pts',(-13.1175170363398,-61.5721388765027,
2.5994251863091));
#214557=CARTESIAN_POINT('Ctrl Pts',(-13.1129882229983,-61.5732493426216,
2.59919740493352));
#214558=CARTESIAN_POINT('Ctrl Pts',(-13.1084265466222,-61.5742946087863,
2.59908173791573));
#214559=CARTESIAN_POINT('Ctrl Pts',(-13.1038352065721,-61.5752716937451,
2.5990817351598));
#214560=CARTESIAN_POINT('',(-13.0739701745318,-61.5816197022697,2.5990817351598));
#214561=CARTESIAN_POINT('Origin',(-7.37250181440935E-18,1.91259499638548E-13,
2.59908173516023));
#214562=CARTESIAN_POINT('',(-12.7383709431244,-61.4590390555208,2.9013417351598));
#214563=CARTESIAN_POINT('Ctrl Pts',(-13.0739701745318,-61.5816197022697,
2.59908173515981));
#214564=CARTESIAN_POINT('Ctrl Pts',(-13.0702318743171,-61.5824133495498,
2.59908174381637));
#214565=CARTESIAN_POINT('Ctrl Pts',(-13.0664939028179,-61.5831581321227,
2.59915752000952));
#214566=CARTESIAN_POINT('Ctrl Pts',(-13.0627583804521,-61.5838547466225,
2.59930729517427));
#214567=CARTESIAN_POINT('Ctrl Pts',(-13.0411716694484,-61.587880319063,
2.60017281085864));
#214568=CARTESIAN_POINT('Ctrl Pts',(-13.0196643745854,-61.5902997144304,
2.60350651799945));
#214569=CARTESIAN_POINT('Ctrl Pts',(-12.9986523536689,-61.5912450453415,
2.60896880596243));
#214570=CARTESIAN_POINT('Ctrl Pts',(-12.9901777222712,-61.5916263190445,
2.61117187235278));
#214571=CARTESIAN_POINT('Ctrl Pts',(-12.9817833412928,-61.5917681516646,
2.6137207657708));
#214572=CARTESIAN_POINT('Ctrl Pts',(-12.9734950911667,-61.5916804171628,
2.6165917989694));
#214573=CARTESIAN_POINT('Ctrl Pts',(-12.9704372300718,-61.5916480484583,
2.61765103591165));
#214574=CARTESIAN_POINT('Ctrl Pts',(-12.9673939164345,-61.591584344534,
2.61875422455105));
#214575=CARTESIAN_POINT('Ctrl Pts',(-12.9643665007544,-61.5914897592006,
2.61990022440352));
#214576=CARTESIAN_POINT('Ctrl Pts',(-12.9586900963544,-61.5913124117003,
2.62204897412689));
#214577=CARTESIAN_POINT('Ctrl Pts',(-12.9530695832095,-61.5910264967401,
2.62434823201725));
#214578=CARTESIAN_POINT('Ctrl Pts',(-12.9475138635627,-61.590635005849,
2.6267904803026));
#214579=CARTESIAN_POINT('Ctrl Pts',(-12.9280688447988,-61.58926478773,2.63533834930134));
#214580=CARTESIAN_POINT('Ctrl Pts',(-12.9094175454587,-61.586601260073,
2.64563784783519));
#214581=CARTESIAN_POINT('Ctrl Pts',(-12.8919416545036,-61.5827727094484,
2.6573666673792));
#214582=CARTESIAN_POINT('Ctrl Pts',(-12.8832037090261,-61.5808584341362,
2.66323107715121));
#214583=CARTESIAN_POINT('Ctrl Pts',(-12.8747596158551,-61.5786529040702,
2.66945281780729));
#214584=CARTESIAN_POINT('Ctrl Pts',(-12.8666570879111,-61.5761721637748,
2.67599160631156));
#214585=CARTESIAN_POINT('Ctrl Pts',(-12.8626058239391,-61.5749317936271,
2.6792610005637));
#214586=CARTESIAN_POINT('Ctrl Pts',(-12.8586399512973,-61.5736226210371,
2.68260965685079));
#214587=CARTESIAN_POINT('Ctrl Pts',(-12.854765434206,-61.5722466520921,
2.68603254012439));
#214588=CARTESIAN_POINT('Ctrl Pts',(-12.8508909171147,-61.5708706831471,
2.68945542339798));
#214589=CARTESIAN_POINT('Ctrl Pts',(-12.8471078617854,-61.5694278436301,
2.69295261525342));
#214590=CARTESIAN_POINT('Ctrl Pts',(-12.8434220158069,-61.5679202927795,
2.69651891172056));
#214591=CARTESIAN_POINT('Ctrl Pts',(-12.8433905832601,-61.567907436528,
2.69654932476044));
#214592=CARTESIAN_POINT('Ctrl Pts',(-12.8433591578469,-61.5678945756942,
2.69657974261102));
#214593=CARTESIAN_POINT('Ctrl Pts',(-12.8433277395702,-61.5678817102795,
2.6966101652693));
#214594=CARTESIAN_POINT('Ctrl Pts',(-12.8272819669698,-61.5613111551481,
2.71214746101087));
#214595=CARTESIAN_POINT('Ctrl Pts',(-12.8130163727092,-61.553649975062,
2.72880565567529));
#214596=CARTESIAN_POINT('Ctrl Pts',(-12.8005145062083,-61.5450979154862,
2.74628040012284));
#214597=CARTESIAN_POINT('Ctrl Pts',(-12.7875898348838,-61.5362566309343,
2.76434612882401));
#214598=CARTESIAN_POINT('Ctrl Pts',(-12.7765497640409,-61.5264624086191,
2.78328592654474));
#214599=CARTESIAN_POINT('Ctrl Pts',(-12.7674219834097,-61.5159109908855,
2.80278753267906));
#214600=CARTESIAN_POINT('Ctrl Pts',(-12.7584678323728,-61.5055602833195,
2.82191817722935));
#214601=CARTESIAN_POINT('Ctrl Pts',(-12.7513538295766,-61.4944799879572,
2.84159092315374));
#214602=CARTESIAN_POINT('Ctrl Pts',(-12.7461528104605,-61.4828443590751,
2.86151233817315));
#214603=CARTESIAN_POINT('Ctrl Pts',(-12.7427073176343,-61.4751361628646,
2.874709577215));
#214604=CARTESIAN_POINT('Ctrl Pts',(-12.7401023057313,-61.4671840587602,
2.88801594388417));
#214605=CARTESIAN_POINT('Ctrl Pts',(-12.7383709431244,-61.4590390555208,
2.9013417351598));
#214606=CARTESIAN_POINT('',(-12.6642893210135,-61.1105274371641,3.47153072139029));
#214607=CARTESIAN_POINT('',(-12.7383709431244,-61.4590390555208,2.90134173515981));
#214608=CARTESIAN_POINT('',(-6.83973663030197,-62.0330459552231,3.47153072139028));
#214609=CARTESIAN_POINT('Origin',(5.53234440788222E-15,1.85015204418142E-13,
3.47153072139072));
#214610=CARTESIAN_POINT('',(-6.87697683366501,-62.387392681069,2.9013417351598));
#214611=CARTESIAN_POINT('',(-6.83973663030197,-62.0330459552231,3.47153072139028));
#214612=CARTESIAN_POINT('',(-6.59568250079822,-62.6076796697353,2.59908173515979));
#214613=CARTESIAN_POINT('Ctrl Pts',(-6.87697683366501,-62.387392681069,
2.9013417351598));
#214614=CARTESIAN_POINT('Ctrl Pts',(-6.87826302285514,-62.3996312165462,
2.88164837656717));
#214615=CARTESIAN_POINT('Ctrl Pts',(-6.87760542308965,-62.4120334591675,
2.86203734439173));
#214616=CARTESIAN_POINT('Ctrl Pts',(-6.87506472947562,-62.4244204973369,
2.84277945978219));
#214617=CARTESIAN_POINT('Ctrl Pts',(-6.87247298342297,-62.4370564393892,
2.82313460920135));
#214618=CARTESIAN_POINT('Ctrl Pts',(-6.8679218469042,-62.4496774784038,
2.80385576863502));
#214619=CARTESIAN_POINT('Ctrl Pts',(-6.86142424477042,-62.462108044829,
2.78521678518593));
#214620=CARTESIAN_POINT('Ctrl Pts',(-6.85517906858932,-62.4740556950172,
2.76730190934719));
#214621=CARTESIAN_POINT('Ctrl Pts',(-6.84713544261466,-62.4858282202794,
2.7499768728007));
#214622=CARTESIAN_POINT('Ctrl Pts',(-6.83725958233962,-62.4972698477045,
2.73349253346047));
#214623=CARTESIAN_POINT('Ctrl Pts',(-6.829673289174,-62.5060589088617,2.72082983599476));
#214624=CARTESIAN_POINT('Ctrl Pts',(-6.82100495425393,-62.5146528151126,
2.70866321039345));
#214625=CARTESIAN_POINT('Ctrl Pts',(-6.81122125790617,-62.5229765487296,
2.69711645335801));
#214626=CARTESIAN_POINT('Ctrl Pts',(-6.81119561658287,-62.522998363751,
2.69708619136706));
#214627=CARTESIAN_POINT('Ctrl Pts',(-6.81116996676367,-62.5230201768491,
2.69705593387174));
#214628=CARTESIAN_POINT('Ctrl Pts',(-6.81114430845093,-62.5230419880216,
2.69702568087526));
#214629=CARTESIAN_POINT('Ctrl Pts',(-6.80839321554184,-62.525380589267,
2.69378194443221));
#214630=CARTESIAN_POINT('Ctrl Pts',(-6.80554511475005,-62.5276952632609,
2.69059266624656));
#214631=CARTESIAN_POINT('Ctrl Pts',(-6.80260378684053,-62.5299828381017,
2.68746219342633));
#214632=CARTESIAN_POINT('Ctrl Pts',(-6.78623596579703,-62.542712671962,
2.67004182396084));
#214633=CARTESIAN_POINT('Ctrl Pts',(-6.76698429120308,-62.5546072354113,
2.65443567877915));
#214634=CARTESIAN_POINT('Ctrl Pts',(-6.74555473734785,-62.5651294462094,
2.64136852353122));
#214635=CARTESIAN_POINT('Ctrl Pts',(-6.73593685681281,-62.5698519601313,
2.6355038032969));
#214636=CARTESIAN_POINT('Ctrl Pts',(-6.72588021343601,-62.5742983919725,
2.63014997451062));
#214637=CARTESIAN_POINT('Ctrl Pts',(-6.71544740276711,-62.5784220664832,
2.6253698111921));
#214638=CARTESIAN_POINT('Ctrl Pts',(-6.71091344436447,-62.5802141596488,
2.6232924168703));
#214639=CARTESIAN_POINT('Ctrl Pts',(-6.7063085522823,-62.5819451239081,
2.62132362131385));
#214640=CARTESIAN_POINT('Ctrl Pts',(-6.70163794008911,-62.5836110216377,
2.61946873372305));
#214641=CARTESIAN_POINT('Ctrl Pts',(-6.68529079741292,-62.5894416636912,
2.61297662715525));
#214642=CARTESIAN_POINT('Ctrl Pts',(-6.66813858303339,-62.5944752375492,
2.60787989113926));
#214643=CARTESIAN_POINT('Ctrl Pts',(-6.65040483057274,-62.5985429352695,
2.60440616886136));
#214644=CARTESIAN_POINT('Ctrl Pts',(-6.64153795434241,-62.6005767841296,
2.60266930772241));
#214645=CARTESIAN_POINT('Ctrl Pts',(-6.63252569365778,-62.6023691645597,
2.6013382004014));
#214646=CARTESIAN_POINT('Ctrl Pts',(-6.62339599105606,-62.6038989834437,
2.6004413072354));
#214647=CARTESIAN_POINT('Ctrl Pts',(-6.6188311397552,-62.6046638928856,
2.59999286065239));
#214648=CARTESIAN_POINT('Ctrl Pts',(-6.61423692798793,-62.6053631620636,
2.59965296768467));
#214649=CARTESIAN_POINT('Ctrl Pts',(-6.60961684864287,-62.6059941550339,
2.59942518630909));
#214650=CARTESIAN_POINT('Ctrl Pts',(-6.60499676929781,-62.6066251480041,
2.59919740493351));
#214651=CARTESIAN_POINT('Ctrl Pts',(-6.60035082219627,-62.6071878630699,
2.59908173791564));
#214652=CARTESIAN_POINT('Ctrl Pts',(-6.59568250079822,-62.6076796697353,
2.5990817351598));
#214653=CARTESIAN_POINT('',(-6.56531752495238,-62.6108711573004,2.59908173515979));
#214654=CARTESIAN_POINT('Origin',(-2.34395632424767E-17,1.9126204441108E-13,
2.59908173516022));
#214655=CARTESIAN_POINT('',(-6.24436990787996,-62.4538823482274,2.9013417351598));
#214656=CARTESIAN_POINT('Ctrl Pts',(-6.56531752495238,-62.6108711573004,
2.5990817351598));
#214657=CARTESIAN_POINT('Ctrl Pts',(-6.5615167448068,-62.6112696981209,
2.59908174381637));
#214658=CARTESIAN_POINT('Ctrl Pts',(-6.55772139932878,-62.6116196762805,
2.59915752000953));
#214659=CARTESIAN_POINT('Ctrl Pts',(-6.55393352450217,-62.6119220062407,
2.59930729517428));
#214660=CARTESIAN_POINT('Ctrl Pts',(-6.53204428085601,-62.6136691004463,
2.60017281085877));
#214661=CARTESIAN_POINT('Ctrl Pts',(-6.51040190952193,-62.6138271176314,
2.60350651800037));
#214662=CARTESIAN_POINT('Ctrl Pts',(-6.4894061806644,-62.6125709156638,
2.60896880596468));
#214663=CARTESIAN_POINT('Ctrl Pts',(-6.48093812023291,-62.6120642605128,
2.61117187235451));
#214664=CARTESIAN_POINT('Ctrl Pts',(-6.47257489900891,-62.6113278644154,
2.61372076577177));
#214665=CARTESIAN_POINT('Ctrl Pts',(-6.46434122353971,-62.6103742524839,
2.61659179896939));
#214666=CARTESIAN_POINT('Ctrl Pts',(-6.46130349717878,-62.6100224275773,
2.61765103591164));
#214667=CARTESIAN_POINT('Ctrl Pts',(-6.45828351400523,-62.609640959732,
2.61875422455104));
#214668=CARTESIAN_POINT('Ctrl Pts',(-6.45528256968463,-62.6092304414382,
2.61990022440351));
#214669=CARTESIAN_POINT('Ctrl Pts',(-6.44965579908351,-62.6084607196374,
2.62204897412688));
#214670=CARTESIAN_POINT('Ctrl Pts',(-6.44409596194912,-62.6075888673474,
2.62434823201725));
#214671=CARTESIAN_POINT('Ctrl Pts',(-6.43861159905706,-62.6066187902473,
2.6267904803026));
#214672=CARTESIAN_POINT('Ctrl Pts',(-6.41941632893488,-62.6032235203969,
2.63533834930134));
#214673=CARTESIAN_POINT('Ctrl Pts',(-6.40114561781689,-62.5986249921651,
2.64563784783518));
#214674=CARTESIAN_POINT('Ctrl Pts',(-6.38416565413431,-62.5929906867157,
2.6573666673792));
#214675=CARTESIAN_POINT('Ctrl Pts',(-6.37567567229302,-62.590173533991,
2.66323107715121));
#214676=CARTESIAN_POINT('Ctrl Pts',(-6.36750837741642,-62.5870974379666,
2.66945281780729));
#214677=CARTESIAN_POINT('Ctrl Pts',(-6.35970954393914,-62.5837833426316,
2.67599160631156));
#214678=CARTESIAN_POINT('Ctrl Pts',(-6.3558101272005,-62.5821262949641,
2.6792610005637));
#214679=CARTESIAN_POINT('Ctrl Pts',(-6.35200282582295,-62.5804097475858,
2.68260965685079));
#214680=CARTESIAN_POINT('Ctrl Pts',(-6.348293361661,-62.5786363190252,2.68603254012438));
#214681=CARTESIAN_POINT('Ctrl Pts',(-6.34458389749905,-62.5768628904645,
2.68945542339798));
#214682=CARTESIAN_POINT('Ctrl Pts',(-6.34097238394016,-62.5750325180134,
2.69295261525342));
#214683=CARTESIAN_POINT('Ctrl Pts',(-6.33746431138531,-62.573147949868,
2.69651891172056));
#214684=CARTESIAN_POINT('Ctrl Pts',(-6.33743439487346,-62.5731318784487,
2.69654932476044));
#214685=CARTESIAN_POINT('Ctrl Pts',(-6.33740448593519,-62.5731158032177,
2.69657974261102));
#214686=CARTESIAN_POINT('Ctrl Pts',(-6.33737458457315,-62.5730997241769,
2.69661016526929));
#214687=CARTESIAN_POINT('Ctrl Pts',(-6.32210352242668,-62.5648879232833,
2.71214746100876));
#214688=CARTESIAN_POINT('Ctrl Pts',(-6.30871688796685,-62.555777551299,
2.72880565567079));
#214689=CARTESIAN_POINT('Ctrl Pts',(-6.29717744164499,-62.5459655399085,
2.74628040011576));
#214690=CARTESIAN_POINT('Ctrl Pts',(-6.28524773891098,-62.5358216928083,
2.76434612881422));
#214691=CARTESIAN_POINT('Ctrl Pts',(-6.2752919217393,-62.5249271226299,
2.78328592653204));
#214692=CARTESIAN_POINT('Ctrl Pts',(-6.26731706752645,-62.5134793937861,
2.80278753266338));
#214693=CARTESIAN_POINT('Ctrl Pts',(-6.25949391182138,-62.5022494248331,
2.8219181772109));
#214694=CARTESIAN_POINT('Ctrl Pts',(-6.25357708652309,-62.4904862127101,
2.84159092313247));
#214695=CARTESIAN_POINT('Ctrl Pts',(-6.24962081353905,-62.4783706704866,
2.86151233814911));
#214696=CARTESIAN_POINT('Ctrl Pts',(-6.24699992138491,-62.4703445485065,
2.87470957719884));
#214697=CARTESIAN_POINT('Ctrl Pts',(-6.24524040122981,-62.4621637089645,
2.88801594387607));
#214698=CARTESIAN_POINT('Ctrl Pts',(-6.24436990787996,-62.4538823482274,
2.90134173515979));
#214699=CARTESIAN_POINT('',(-6.207123496544,-62.0995362748658,3.47153072139028));
#214700=CARTESIAN_POINT('',(-6.24436990787996,-62.4538823482274,2.9013417351598));
#214701=CARTESIAN_POINT('',(-0.318048871876464,-62.4081695979766,3.47153072139028));
#214702=CARTESIAN_POINT('Origin',(5.53234440788222E-15,1.85015204418142E-13,
3.47153072139072));
#214703=CARTESIAN_POINT('',(-0.318045750792381,-62.7644678366118,2.9013417351598));
#214704=CARTESIAN_POINT('',(-0.31804887187647,-62.4081695979766,3.47153072139028));
#214705=CARTESIAN_POINT('Ctrl Pts',(-0.318045750792382,-62.7644678366118,
2.9013417351598));
#214706=CARTESIAN_POINT('Ctrl Pts',(-0.318045618797467,-62.7767737714908,
2.88164837656695));
#214707=CARTESIAN_POINT('Ctrl Pts',(-0.31609523406997,-62.7890393354365,
2.86203734439129));
#214708=CARTESIAN_POINT('Ctrl Pts',(-0.312273660577038,-62.8010929413157,
2.84277945978154));
#214709=CARTESIAN_POINT('Ctrl Pts',(-0.308375296775692,-62.8133887511234,
2.8231346092005));
#214710=CARTESIAN_POINT('Ctrl Pts',(-0.302529834045799,-62.8254649274595,
2.80385576863398));
#214711=CARTESIAN_POINT('Ctrl Pts',(-0.294768478450234,-62.8371482135753,
2.78521678518473));
#214712=CARTESIAN_POINT('Ctrl Pts',(-0.287308644483666,-62.8483776146167,
2.76730190934571));
#214713=CARTESIAN_POINT('Ctrl Pts',(-0.278078518359005,-62.8592448608917,
2.74997687279897));
#214714=CARTESIAN_POINT('Ctrl Pts',(-0.26706078334753,-62.8695915013867,
2.73349253345854));
#214715=CARTESIAN_POINT('Ctrl Pts',(-0.258597341633625,-62.8775394315804,
2.72082983599353));
#214716=CARTESIAN_POINT('Ctrl Pts',(-0.249078184945788,-62.885180171785,
2.70866321039287));
#214717=CARTESIAN_POINT('Ctrl Pts',(-0.238478017627207,-62.8924356323736,
2.69711645335801));
#214718=CARTESIAN_POINT('Ctrl Pts',(-0.238450236479097,-62.8924546476418,
2.69708619136707));
#214719=CARTESIAN_POINT('Ctrl Pts',(-0.238422447082671,-62.8924736601093,
2.69705593387174));
#214720=CARTESIAN_POINT('Ctrl Pts',(-0.238394649440506,-62.892492669774,
2.69702568087526));
#214721=CARTESIAN_POINT('Ctrl Pts',(-0.235414176911842,-62.894530892403,
2.69378194443221));
#214722=CARTESIAN_POINT('Ctrl Pts',(-0.232339728998653,-62.8965351787716,
2.69059266624654));
#214723=CARTESIAN_POINT('Ctrl Pts',(-0.229175397308462,-62.8985027695517,
2.68746219342631));
#214724=CARTESIAN_POINT('Ctrl Pts',(-0.211566610931929,-62.9094519648683,
2.67004182396257));
#214725=CARTESIAN_POINT('Ctrl Pts',(-0.191177078589483,-62.919269020693,
2.65443567878226));
#214726=CARTESIAN_POINT('Ctrl Pts',(-0.168765047550213,-62.9274935913859,
2.64136852353514));
#214727=CARTESIAN_POINT('Ctrl Pts',(-0.158706217646005,-62.9311848926112,
2.63550380329928));
#214728=CARTESIAN_POINT('Ctrl Pts',(-0.148239886924228,-62.9345557609565,
2.63014997451169));
#214729=CARTESIAN_POINT('Ctrl Pts',(-0.137433186921743,-62.9375663198807,
2.6253698111921));
#214730=CARTESIAN_POINT('Ctrl Pts',(-0.132736741272993,-62.9388746680681,
2.6232924168703));
#214731=CARTESIAN_POINT('Ctrl Pts',(-0.12797614023748,-62.9401148076311,
2.62132362131384));
#214732=CARTESIAN_POINT('Ctrl Pts',(-0.123156980416938,-62.9412833674836,
2.61946873372304));
#214733=CARTESIAN_POINT('Ctrl Pts',(-0.106289921045043,-62.9453733269671,
2.61297662715524));
#214734=CARTESIAN_POINT('Ctrl Pts',(-0.0887055165504184,-62.9485864317702,
2.60787989113925));
#214735=CARTESIAN_POINT('Ctrl Pts',(-0.0706437212495209,-62.950778164324,
2.60440616886136));
#214736=CARTESIAN_POINT('Ctrl Pts',(-0.0616128235990723,-62.9518740306009,
2.60266930772241));
#214737=CARTESIAN_POINT('Ctrl Pts',(-0.0524625782494904,-62.9527145544236,
2.60133820040141));
#214738=CARTESIAN_POINT('Ctrl Pts',(-0.0432229794968653,-62.9532816790165,
2.60044130723541));
#214739=CARTESIAN_POINT('Ctrl Pts',(-0.0386031801205529,-62.953565241313,
2.59999286065241));
#214740=CARTESIAN_POINT('Ctrl Pts',(-0.0339610423934555,-62.9537804539253,
2.59965296768468));
#214741=CARTESIAN_POINT('Ctrl Pts',(-0.0293003156009411,-62.953925060456,
2.5994251863091));
#214742=CARTESIAN_POINT('Ctrl Pts',(-0.0246395888084267,-62.9540696669866,
2.59919740493352));
#214743=CARTESIAN_POINT('Ctrl Pts',(-0.0199602729501303,-62.9541436657294,
2.5990817379157));
#214744=CARTESIAN_POINT('Ctrl Pts',(-0.0152661173102018,-62.9541448057646,
2.5990817351598));
#214745=CARTESIAN_POINT('',(0.318045750793708,-62.7644678366118,2.90134173515979));
#214746=CARTESIAN_POINT('Ctrl Pts',(0.0152661173115319,-62.9541448057646,
2.5990817351598));
#214747=CARTESIAN_POINT('Ctrl Pts',(0.0190877352453155,-62.954143873629,
2.59908174381636));
#214748=CARTESIAN_POINT('Ctrl Pts',(0.0228988721028936,-62.9540952129412,
2.59915752000952));
#214749=CARTESIAN_POINT('Ctrl Pts',(0.0266975986410181,-62.9539999459716,
2.59930729517427));
#214750=CARTESIAN_POINT('Ctrl Pts',(0.0486495517930506,-62.9534494204118,
2.60017281085878));
#214751=CARTESIAN_POINT('Ctrl Pts',(0.0701898812463959,-62.9513443281452,
2.60350651800049));
#214752=CARTESIAN_POINT('Ctrl Pts',(0.0909392844435494,-62.9479003565107,
2.60896880596498));
#214753=CARTESIAN_POINT('Ctrl Pts',(0.0993079960692669,-62.9465113235258,
2.61117187235474));
#214754=CARTESIAN_POINT('Ctrl Pts',(0.107548428339577,-62.9449047668209,
2.61372076577191));
#214755=CARTESIAN_POINT('Ctrl Pts',(0.115637319282967,-62.9430957254315,
2.61659179896941));
#214756=CARTESIAN_POINT('Ctrl Pts',(0.118621628944221,-62.9424282989903,
2.61765103591166));
#214757=CARTESIAN_POINT('Ctrl Pts',(0.121585194086305,-62.9417332466656,
2.61875422455107));
#214758=CARTESIAN_POINT('Ctrl Pts',(0.124526788073524,-62.9410112931357,
2.61990022440354));
#214759=CARTESIAN_POINT('Ctrl Pts',(0.13004227679956,-62.9396576302673,
2.62204897412691));
#214760=CARTESIAN_POINT('Ctrl Pts',(0.13548052318433,-62.9382093928438,
2.62434823201728));
#214761=CARTESIAN_POINT('Ctrl Pts',(0.140833441494092,-62.9366713579024,
2.62679048030263));
#214762=CARTESIAN_POINT('Ctrl Pts',(0.15956865557826,-62.9312882356076,
2.63533834930136));
#214763=CARTESIAN_POINT('Ctrl Pts',(0.177258600739667,-62.9248050892387,
2.64563784783519));
#214764=CARTESIAN_POINT('Ctrl Pts',(0.193556601114335,-62.917426759594,
2.6573666673792));
#214765=CARTESIAN_POINT('Ctrl Pts',(0.20170560130167,-62.9137375947717,
2.66323107715121));
#214766=CARTESIAN_POINT('Ctrl Pts',(0.20950661529208,-62.9098246351406,
2.66945281780729));
#214767=CARTESIAN_POINT('Ctrl Pts',(0.216916308651066,-62.9057134946879,
2.67599160631155));
#214768=CARTESIAN_POINT('Ctrl Pts',(0.220621155330559,-62.9036579244616,
2.67926100056369));
#214769=CARTESIAN_POINT('Ctrl Pts',(0.224228171853214,-62.9015528091472,
2.68260965685078));
#214770=CARTESIAN_POINT('Ctrl Pts',(0.2277319414202,-62.8994013510254,2.68603254012437));
#214771=CARTESIAN_POINT('Ctrl Pts',(0.231235710987187,-62.8972498929036,
2.68945542339796));
#214772=CARTESIAN_POINT('Ctrl Pts',(0.234636114277403,-62.8950520414619,
2.69295261525339));
#214773=CARTESIAN_POINT('Ctrl Pts',(0.237927978231588,-62.8928111037449,
2.69651891172053));
#214774=CARTESIAN_POINT('Ctrl Pts',(0.237956050936886,-62.8927919932394,
2.69654932476041));
#214775=CARTESIAN_POINT('Ctrl Pts',(0.23798411571168,-62.8927728797349,
2.696579742611));
#214776=CARTESIAN_POINT('Ctrl Pts',(0.238012172553516,-62.8927537632333,
2.69661016526928));
#214777=CARTESIAN_POINT('Ctrl Pts',(0.252341211298998,-62.8829906867833,
2.7121474610124));
#214778=CARTESIAN_POINT('Ctrl Pts',(0.26470221919375,-62.8725309380389,
2.72880565567861));
#214779=CARTESIAN_POINT('Ctrl Pts',(0.275152816750645,-62.8615664772797,
2.74628040012808));
#214780=CARTESIAN_POINT('Ctrl Pts',(0.285956846577482,-62.8502312057383,
2.76434612883121));
#214781=CARTESIAN_POINT('Ctrl Pts',(0.294719332062974,-62.8383556508826,
2.78328592655403));
#214782=CARTESIAN_POINT('Ctrl Pts',(0.301453885685765,-62.8261370346363,
2.8027875326905));
#214783=CARTESIAN_POINT('Ctrl Pts',(0.308060333927675,-62.8141508421817,
2.8219181772426));
#214784=CARTESIAN_POINT('Ctrl Pts',(0.312715155750267,-62.8018335935067,
2.84159092316882));
#214785=CARTESIAN_POINT('Ctrl Pts',(0.315383336844492,-62.7893708783531,
2.86151233819002));
#214786=CARTESIAN_POINT('Ctrl Pts',(0.317150913276949,-62.7811147664881,
2.87470957722633));
#214787=CARTESIAN_POINT('Ctrl Pts',(0.318045664009116,-62.7727948225118,
2.88801594388984));
#214788=CARTESIAN_POINT('Ctrl Pts',(0.318045750793708,-62.7644678366117,
2.90134173515979));
#214789=CARTESIAN_POINT('',(0.318048871877787,-62.4081695979766,3.47153072139028));
#214790=CARTESIAN_POINT('',(0.318045750793708,-62.7644678366118,2.90134173515979));
#214791=CARTESIAN_POINT('',(6.20712349654527,-62.0995362748656,3.47153072139028));
#214792=CARTESIAN_POINT('Origin',(5.53234440788222E-15,1.85015204418142E-13,
3.47153072139072));
#214793=CARTESIAN_POINT('',(6.24436990788122,-62.4538823482273,2.9013417351598));
#214794=CARTESIAN_POINT('',(6.20712349654526,-62.0995362748656,3.47153072139028));
#214795=CARTESIAN_POINT('',(6.56531752495365,-62.6108711573003,2.5990817351598));
#214796=CARTESIAN_POINT('Ctrl Pts',(6.24436990788123,-62.4538823482273,
2.9013417351598));
#214797=CARTESIAN_POINT('Ctrl Pts',(6.24565635961516,-62.4661208561104,
2.88164837656655));
#214798=CARTESIAN_POINT('Ctrl Pts',(6.24887816048156,-62.4781153572954,
2.86203734439049));
#214799=CARTESIAN_POINT('Ctrl Pts',(6.25393874389462,-62.4897034690562,
2.84277945978035));
#214800=CARTESIAN_POINT('Ctrl Pts',(6.25910101415518,-62.501524431154,2.82313460919898));
#214801=CARTESIAN_POINT('Ctrl Pts',(6.26617675898339,-62.5129234356965,
2.80385576863215));
#214802=CARTESIAN_POINT('Ctrl Pts',(6.27511683300479,-62.5237314369754,
2.78521678518261));
#214803=CARTESIAN_POINT('Ctrl Pts',(6.2837095932548,-62.5341195572022,2.76730190934353));
#214804=CARTESIAN_POINT('Ctrl Pts',(6.29402509233604,-62.5439624606655,
2.74997687279674));
#214805=CARTESIAN_POINT('Ctrl Pts',(6.30606398947345,-62.5531007542718,
2.73349253345627));
#214806=CARTESIAN_POINT('Ctrl Pts',(6.31531185249695,-62.5601204743155,
2.72082983599208));
#214807=CARTESIAN_POINT('Ctrl Pts',(6.3255775370797,-62.5667243349252,2.70866321039218));
#214808=CARTESIAN_POINT('Ctrl Pts',(6.33687803771754,-62.572832030141,2.69711645335801));
#214809=CARTESIAN_POINT('Ctrl Pts',(6.33690765431438,-62.5728480373209,
2.69708619136707));
#214810=CARTESIAN_POINT('Ctrl Pts',(6.3369372788216,-62.5728640408532,2.69705593387174));
#214811=CARTESIAN_POINT('Ctrl Pts',(6.3369669112364,-62.5728800407361,2.69702568087526));
#214812=CARTESIAN_POINT('Ctrl Pts',(6.34014410870391,-62.574595553555,2.69378194443222));
#214813=CARTESIAN_POINT('Ctrl Pts',(6.34341121944381,-62.5762674929175,
2.69059266624656));
#214814=CARTESIAN_POINT('Ctrl Pts',(6.34676388583449,-62.5778935423005,
2.68746219342633));
#214815=CARTESIAN_POINT('Ctrl Pts',(6.36542071199915,-62.5869421374006,
2.67004182396085));
#214816=CARTESIAN_POINT('Ctrl Pts',(6.38672471011157,-62.5945741278843,
2.65443567877916));
#214817=CARTESIAN_POINT('Ctrl Pts',(6.40987366743805,-62.6004109483555,
2.64136852353124));
#214818=CARTESIAN_POINT('Ctrl Pts',(6.42026324006196,-62.6030305942135,
2.63550380329691));
#214819=CARTESIAN_POINT('Ctrl Pts',(6.43102458681462,-62.6052889671223,
2.63014997451063));
#214820=CARTESIAN_POINT('Ctrl Pts',(6.44208677567923,-62.607153426145,2.6253698111921));
#214821=CARTESIAN_POINT('Ctrl Pts',(6.44689425333277,-62.6079636948177,
2.6232924168703));
#214822=CARTESIAN_POINT('Ctrl Pts',(6.45175840518046,-62.608699422456,2.62132362131385));
#214823=CARTESIAN_POINT('Ctrl Pts',(6.45667331290488,-62.609357841445,2.61946873372305));
#214824=CARTESIAN_POINT('Ctrl Pts',(6.47387548994035,-62.6116623079065,
2.61297662715525));
#214825=CARTESIAN_POINT('Ctrl Pts',(6.49169942613465,-62.613019740206,2.60787989113926));
#214826=CARTESIAN_POINT('Ctrl Pts',(6.5098913754668,-62.6133114945129,2.60440616886136));
#214827=CARTESIAN_POINT('Ctrl Pts',(6.51898735013288,-62.6134573716664,
2.60266930772241));
#214828=CARTESIAN_POINT('Ctrl Pts',(6.52817532814455,-62.6133368299267,
2.60133820040141));
#214829=CARTESIAN_POINT('Ctrl Pts',(6.53742359207063,-62.612935046693,2.60044130723541));
#214830=CARTESIAN_POINT('Ctrl Pts',(6.54204772403368,-62.6127341550761,
2.5999928606524));
#214831=CARTESIAN_POINT('Ctrl Pts',(6.54668692748823,-62.6124629532083,
2.59965296768468));
#214832=CARTESIAN_POINT('Ctrl Pts',(6.55133723783014,-62.6121195889599,
2.5994251863091));
#214833=CARTESIAN_POINT('Ctrl Pts',(6.55598754817206,-62.6117762247115,
2.59919740493352));
#214834=CARTESIAN_POINT('Ctrl Pts',(6.56064896522335,-62.6113606963857,
2.59908173791572));
#214835=CARTESIAN_POINT('Ctrl Pts',(6.56531752495365,-62.6108711573003,
2.5990817351598));
#214836=CARTESIAN_POINT('',(6.59568250079948,-62.6076796697351,2.5990817351598));
#214837=CARTESIAN_POINT('Origin',(5.63895492999586E-15,1.85567159826749E-13,
2.59908173516024));
#214838=CARTESIAN_POINT('',(6.87697683366627,-62.3873926810689,2.9013417351598));
#214839=CARTESIAN_POINT('Ctrl Pts',(6.59568250079948,-62.6076796697352,
2.59908173515981));
#214840=CARTESIAN_POINT('Ctrl Pts',(6.59948308607566,-62.607279274856,2.59908174381644));
#214841=CARTESIAN_POINT('Ctrl Pts',(6.60326825869985,-62.6068325084576,
2.59915752000952));
#214842=CARTESIAN_POINT('Ctrl Pts',(6.60703621730659,-62.606340688323,2.59930729517427));
#214843=CARTESIAN_POINT('Ctrl Pts',(6.62881036977196,-62.6034985746711,
2.60017281085879));
#214844=CARTESIAN_POINT('Ctrl Pts',(6.6500126569874,-62.599153436784,2.6035065180006));
#214845=CARTESIAN_POINT('Ctrl Pts',(6.67028839972057,-62.5935594283564,
2.60896880596523));
#214846=CARTESIAN_POINT('Ctrl Pts',(6.67846607318471,-62.5913032360739,
2.61117187235494));
#214847=CARTESIAN_POINT('Ctrl Pts',(6.68649343260099,-62.5888441205329,
2.61372076577201));
#214848=CARTESIAN_POINT('Ctrl Pts',(6.69434891543672,-62.5861994699218,
2.61659179896941));
#214849=CARTESIAN_POINT('Ctrl Pts',(6.69724711167715,-62.5852237544096,
2.61765103591166));
#214850=CARTESIAN_POINT('Ctrl Pts',(6.70012178934791,-62.5842227327442,
2.61875422455107));
#214851=CARTESIAN_POINT('Ctrl Pts',(6.70297180428246,-62.5831972538523,
2.61990022440353));
#214852=CARTESIAN_POINT('Ctrl Pts',(6.70831558228475,-62.58127448093,2.6220489741269));
#214853=CARTESIAN_POINT('Ctrl Pts',(6.71357265535448,-62.5792657255651,
2.62434823201727));
#214854=CARTESIAN_POINT('Ctrl Pts',(6.71873548138878,-62.5771765838151,
2.62679048030263));
#214855=CARTESIAN_POINT('Ctrl Pts',(6.73680537250885,-62.5698645876903,
2.63533834930136));
#214856=CARTESIAN_POINT('Ctrl Pts',(6.75372073697266,-62.5615678538925,
2.6456378478352));
#214857=CARTESIAN_POINT('Ctrl Pts',(6.76915820973675,-62.5525263385762,
2.65736666737921));
#214858=CARTESIAN_POINT('Ctrl Pts',(6.7768769461188,-62.548005580918,2.66323107715122));
#214859=CARTESIAN_POINT('Ctrl Pts',(6.78422620968128,-62.5432986288849,
2.6694528178073));
#214860=CARTESIAN_POINT('Ctrl Pts',(6.79116558077096,-62.5384354858296,
2.67599160631157));
#214861=CARTESIAN_POINT('Ctrl Pts',(6.7946352663158,-62.536003914302,2.6792610005637));
#214862=CARTESIAN_POINT('Ctrl Pts',(6.79800247875573,-62.5335332951355,
2.68260965685079));
#214863=CARTESIAN_POINT('Ctrl Pts',(6.80126216569517,-62.5310273792779,
2.68603254012438));
#214864=CARTESIAN_POINT('Ctrl Pts',(6.8045218526346,-62.5285214634203,2.68945542339798));
#214865=CARTESIAN_POINT('Ctrl Pts',(6.80767389012611,-62.5259802131084,
2.6929526152534));
#214866=CARTESIAN_POINT('Ctrl Pts',(6.81071347912929,-62.5234074580022,
2.69651891172054));
#214867=CARTESIAN_POINT('Ctrl Pts',(6.8107394004576,-62.5233855177894,2.69654932476042));
#214868=CARTESIAN_POINT('Ctrl Pts',(6.81076531358537,-62.5233635754229,
2.69657974261101));
#214869=CARTESIAN_POINT('Ctrl Pts',(6.81079121851035,-62.5233416309049,
2.69661016526929));
#214870=CARTESIAN_POINT('Ctrl Pts',(6.82402124190353,-62.5121342452096,
2.7121474610116));
#214871=CARTESIAN_POINT('Ctrl Pts',(6.83522119344078,-62.5004397189042,
2.72880565567688));
#214872=CARTESIAN_POINT('Ctrl Pts',(6.84446844329679,-62.4884429377061,
2.74628040012536));
#214873=CARTESIAN_POINT('Ctrl Pts',(6.85402842900256,-62.4760404333339,
2.7643461288275));
#214874=CARTESIAN_POINT('Ctrl Pts',(6.86150157917614,-62.4633140048688,
2.78328592654925));
#214875=CARTESIAN_POINT('Ctrl Pts',(6.86692204703019,-62.4504583709405,
2.80278753268463));
#214876=CARTESIAN_POINT('Ctrl Pts',(6.87223940617985,-62.4378472782204,
2.82191817723579));
#214877=CARTESIAN_POINT('Ctrl Pts',(6.87558122532613,-62.4251109433511,
2.84159092316106));
#214878=CARTESIAN_POINT('Ctrl Pts',(6.87693208138253,-62.4124375993861,
2.86151233818132));
#214879=CARTESIAN_POINT('Ctrl Pts',(6.87782697616112,-62.4040419533157,
2.87470957722049));
#214880=CARTESIAN_POINT('Ctrl Pts',(6.87784715439705,-62.3956740599421,
2.88801594388692));
#214881=CARTESIAN_POINT('Ctrl Pts',(6.87697683366627,-62.3873926810689,
2.90134173515981));
#214882=CARTESIAN_POINT('',(6.83973663030322,-62.033045955223,3.47153072139028));
#214883=CARTESIAN_POINT('',(6.87697683366627,-62.3873926810689,2.9013417351598));
#214884=CARTESIAN_POINT('',(12.6642893210148,-61.1105274371638,3.47153072139029));
#214885=CARTESIAN_POINT('Origin',(5.53234440788222E-15,1.85015204418142E-13,
3.47153072139072));
#214886=CARTESIAN_POINT('',(12.7383709431257,-61.4590390555205,2.90134173515981));
#214887=CARTESIAN_POINT('',(12.6642893210148,-61.1105274371638,3.47153072139029));
#214888=CARTESIAN_POINT('',(13.0739701745332,-61.5816197022694,2.59908173515981));
#214889=CARTESIAN_POINT('Ctrl Pts',(12.7383709431257,-61.4590390555205,
2.90134173515981));
#214890=CARTESIAN_POINT('Ctrl Pts',(12.740929619964,-61.471076048754,2.88164837656683));
#214891=CARTESIAN_POINT('Ctrl Pts',(12.7453875382446,-61.4826680729129,
2.86203734439105));
#214892=CARTESIAN_POINT('Ctrl Pts',(12.7516316867666,-61.4936637287773,
2.84277945978117));
#214893=CARTESIAN_POINT('Ctrl Pts',(12.7580013045728,-61.5048803302305,
2.82313460919998));
#214894=CARTESIAN_POINT('Ctrl Pts',(12.766229808158,-61.5154772731,2.80385576863331));
#214895=CARTESIAN_POINT('Ctrl Pts',(12.776250651283,-61.525291574818,2.78521678518393));
#214896=CARTESIAN_POINT('Ctrl Pts',(12.7858821937368,-61.5347245998112,
2.76730190934486));
#214897=CARTESIAN_POINT('Ctrl Pts',(12.7971700470077,-61.5434353195526,
2.74997687279808));
#214898=CARTESIAN_POINT('Ctrl Pts',(12.8100982055944,-61.5512651452132,
2.73349253345762));
#214899=CARTESIAN_POINT('Ctrl Pts',(12.8200291684057,-61.5572797455859,
2.72082983599294));
#214900=CARTESIAN_POINT('Ctrl Pts',(12.8309289078957,-61.5627743733226,
2.70866321039259));
#214901=CARTESIAN_POINT('Ctrl Pts',(12.8428059312041,-61.5676673859793,
2.69711645335802));
#214902=CARTESIAN_POINT('Ctrl Pts',(12.8428370587641,-61.5676802096928,
2.69708619136708));
#214903=CARTESIAN_POINT('Ctrl Pts',(12.8428681938098,-61.5676930289519,
2.69705593387175));
#214904=CARTESIAN_POINT('Ctrl Pts',(12.8428993363383,-61.567705843755,2.69702568087527));
#214905=CARTESIAN_POINT('Ctrl Pts',(12.8462384487043,-61.5690798512464,
2.69378194443223));
#214906=CARTESIAN_POINT('Ctrl Pts',(12.849662427122,-61.5704011254851,2.69059266624657));
#214907=CARTESIAN_POINT('Ctrl Pts',(12.8531666956986,-61.5716678181338,
2.68746219342633));
#214908=CARTESIAN_POINT('Ctrl Pts',(12.8726671535588,-61.578716674715,2.67004182396007));
#214909=CARTESIAN_POINT('Ctrl Pts',(12.8946522063786,-61.5840799821724,
2.65443567877777));
#214910=CARTESIAN_POINT('Ctrl Pts',(12.9182844651701,-61.5874651029946,
2.64136852352948));
#214911=CARTESIAN_POINT('Ctrl Pts',(12.928890950183,-61.5889843920979,2.63550380329583));
#214912=CARTESIAN_POINT('Ctrl Pts',(12.9398294094008,-61.5901055263647,
2.63014997451013));
#214913=CARTESIAN_POINT('Ctrl Pts',(12.9510258874727,-61.5908034580834,
2.62536981119208));
#214914=CARTESIAN_POINT('Ctrl Pts',(12.9558917253998,-61.5911067697682,
2.62329241687029));
#214915=CARTESIAN_POINT('Ctrl Pts',(12.9608061353942,-61.5913300246958,
2.62132362131383));
#214916=CARTESIAN_POINT('Ctrl Pts',(12.9657629422649,-61.5914710890451,
2.61946873372304));
#214917=CARTESIAN_POINT('Ctrl Pts',(12.9831117663126,-61.5919648142679,
2.61297662715524));
#214918=CARTESIAN_POINT('Ctrl Pts',(13.0009799514317,-61.5914517017514,
2.60787989113925));
#214919=CARTESIAN_POINT('Ctrl Pts',(13.0191027399913,-61.5898402812902,
2.60440616886136));
#214920=CARTESIAN_POINT('Ctrl Pts',(13.0281641342711,-61.5890345710596,
2.60266930772241));
#214921=CARTESIAN_POINT('Ctrl Pts',(13.037289179535,-61.587954284438,2.60133820040142));
#214922=CARTESIAN_POINT('Ctrl Pts',(13.0464447827197,-61.5865879953988,
2.60044130723542));
#214923=CARTESIAN_POINT('Ctrl Pts',(13.051022584312,-61.5859048508792,2.59999286065241));
#214924=CARTESIAN_POINT('Ctrl Pts',(13.0556080254101,-61.5851502058757,
2.59965296768469));
#214925=CARTESIAN_POINT('Ctrl Pts',(13.0601969695282,-61.5843226328189,
2.59942518630911));
#214926=CARTESIAN_POINT('Ctrl Pts',(13.0647859136462,-61.583495059762,2.59919740493353));
#214927=CARTESIAN_POINT('Ctrl Pts',(13.0693783604298,-61.5825945569828,
2.59908173791571));
#214928=CARTESIAN_POINT('Ctrl Pts',(13.0739701745332,-61.5816197022694,
2.59908173515981));
#214929=CARTESIAN_POINT('',(13.1038352065734,-61.5752716937448,2.59908173515981));
#214930=CARTESIAN_POINT('Origin',(5.62288786856779E-15,1.85564615054217E-13,
2.59908173516023));
#214931=CARTESIAN_POINT('',(13.3605623192493,-61.326788195911,2.90134173515982));
#214932=CARTESIAN_POINT('Ctrl Pts',(13.1038352065734,-61.5752716937448,
2.5990817351598));
#214933=CARTESIAN_POINT('Ctrl Pts',(13.1075731191844,-61.5744762229323,
2.59908174381639));
#214934=CARTESIAN_POINT('Ctrl Pts',(13.1112908564318,-61.5736362456893,
2.59915752000952));
#214935=CARTESIAN_POINT('Ctrl Pts',(13.1149867645642,-61.572753260874,2.59930729517427));
#214936=CARTESIAN_POINT('Ctrl Pts',(13.1363445541695,-61.5676506979224,
2.6001728108587));
#214937=CARTESIAN_POINT('Ctrl Pts',(13.1569765024491,-61.5611131206558,
2.60350651799992));
#214938=CARTESIAN_POINT('Ctrl Pts',(13.1765564394358,-61.5534303645632,
2.60896880596356));
#214939=CARTESIAN_POINT('Ctrl Pts',(13.184453478439,-61.5503317322971,2.61117187235366));
#214940=CARTESIAN_POINT('Ctrl Pts',(13.192179815574,-61.5470470005036,2.61372076577129));
#214941=CARTESIAN_POINT('Ctrl Pts',(13.1997158239905,-61.5435957160154,
2.61659179896941));
#214942=CARTESIAN_POINT('Ctrl Pts',(13.2024961535656,-61.5423224015756,
2.61765103591166));
#214943=CARTESIAN_POINT('Ctrl Pts',(13.2052504481949,-61.5410263779723,
2.61875422455106));
#214944=CARTESIAN_POINT('Ctrl Pts',(13.2079776587167,-61.5397086090796,
2.61990022440353));
#214945=CARTESIAN_POINT('Ctrl Pts',(13.2130911784452,-61.537237792406,2.6220489741269));
#214946=CARTESIAN_POINT('Ctrl Pts',(13.2181094806073,-61.5346905274439,
2.62434823201727));
#214947=CARTESIAN_POINT('Ctrl Pts',(13.2230256493637,-61.5320731679596,
2.62679048030262));
#214948=CARTESIAN_POINT('Ctrl Pts',(13.2402322400112,-61.5229124097644,
2.63533834930136));
#214949=CARTESIAN_POINT('Ctrl Pts',(13.2561876955045,-61.5128929892894,
2.6456378478352));
#214950=CARTESIAN_POINT('Ctrl Pts',(13.2705955044759,-61.5022873490352,
2.65736666737921));
#214951=CARTESIAN_POINT('Ctrl Pts',(13.2777994089617,-61.4969845289081,
2.66323107715122));
#214952=CARTESIAN_POINT('Ctrl Pts',(13.2846164020267,-61.4915351548244,
2.6694528178073));
#214953=CARTESIAN_POINT('Ctrl Pts',(13.2910094216452,-61.4859732907796,
2.67599160631157));
#214954=CARTESIAN_POINT('Ctrl Pts',(13.2942059314545,-61.4831923587572,
2.67926100056371));
#214955=CARTESIAN_POINT('Ctrl Pts',(13.2972964479276,-61.4803833043592,
2.6826096568508));
#214956=CARTESIAN_POINT('Ctrl Pts',(13.3002763384272,-61.4775503861043,
2.6860325401244));
#214957=CARTESIAN_POINT('Ctrl Pts',(13.3032562289269,-61.4747174678495,
2.68945542339799));
#214958=CARTESIAN_POINT('Ctrl Pts',(13.3061253662373,-61.4718606611374,
2.69295261525341));
#214959=CARTESIAN_POINT('Ctrl Pts',(13.3088793779163,-61.4689842762855,
2.69651891172055));
#214960=CARTESIAN_POINT('Ctrl Pts',(13.3089028638681,-61.4689597467468,
2.69654932476043));
#214961=CARTESIAN_POINT('Ctrl Pts',(13.3089263414392,-61.4689352159235,
2.69657974261101));
#214962=CARTESIAN_POINT('Ctrl Pts',(13.3089498106276,-61.4689106838179,
2.69661016526929));
#214963=CARTESIAN_POINT('Ctrl Pts',(13.3209358677647,-61.4563817793394,
2.71214746101209));
#214964=CARTESIAN_POINT('Ctrl Pts',(13.3308520539325,-61.4435806031494,
2.72880565567793));
#214965=CARTESIAN_POINT('Ctrl Pts',(13.3387946412835,-61.4306829407567,
2.746280400127));
#214966=CARTESIAN_POINT('Ctrl Pts',(13.3470058416648,-61.4173490879861,
2.76434612882973));
#214967=CARTESIAN_POINT('Ctrl Pts',(13.3531077791294,-61.4039112193238,
2.78328592655213));
#214968=CARTESIAN_POINT('Ctrl Pts',(13.3571547734345,-61.3905594167279,
2.80278753268816));
#214969=CARTESIAN_POINT('Ctrl Pts',(13.361124785392,-61.3774615935124,2.82191817723989));
#214970=CARTESIAN_POINT('Ctrl Pts',(13.3631169881916,-61.3644457143979,
2.84159092316572));
#214971=CARTESIAN_POINT('Ctrl Pts',(13.3631357189477,-61.3517005934293,
2.86151233818654));
#214972=CARTESIAN_POINT('Ctrl Pts',(13.3631481274169,-61.3432573976117,
2.87470957722401));
#214973=CARTESIAN_POINT('Ctrl Pts',(13.3622935120792,-61.3349332352346,
2.88801594388869));
#214974=CARTESIAN_POINT('Ctrl Pts',(13.3605623192493,-61.326788195911,2.90134173515982));
#214975=CARTESIAN_POINT('',(13.2864868029002,-60.9782752797345,3.47153072139029));
#214976=CARTESIAN_POINT('',(13.3605623192493,-61.326788195911,2.90134173515982));
#214977=CARTESIAN_POINT('',(18.9827025415103,-59.4519788726604,3.4715307213903));
#214978=CARTESIAN_POINT('Origin',(5.53234440788222E-15,1.85015204418142E-13,
3.47153072139072));
#214979=CARTESIAN_POINT('',(19.0928077206418,-59.7908376697908,2.90134173515982));
#214980=CARTESIAN_POINT('',(18.9827025415103,-59.4519788726604,3.4715307213903));
#214981=CARTESIAN_POINT('',(19.4393816709763,-59.8776671349981,2.59908173515982));
#214982=CARTESIAN_POINT('Ctrl Pts',(19.0928077206418,-59.7908376697907,
2.90134173515982));
#214983=CARTESIAN_POINT('Ctrl Pts',(19.0966105891854,-59.8025412685574,
2.88164837656781));
#214984=CARTESIAN_POINT('Ctrl Pts',(19.1022557829942,-59.8136038110473,
2.86203734439298));
#214985=CARTESIAN_POINT('Ctrl Pts',(19.1096150844268,-59.8238865403086,
2.84277945978402));
#214986=CARTESIAN_POINT('Ctrl Pts',(19.1171222629127,-59.8343758896842,
2.82313460920365));
#214987=CARTESIAN_POINT('Ctrl Pts',(19.1264133720472,-59.8440546685567,
2.80385576863777));
#214988=CARTESIAN_POINT('Ctrl Pts',(19.1374051938209,-59.8527677431703,
2.78521678518909));
#214989=CARTESIAN_POINT('Ctrl Pts',(19.1479699932833,-59.8611423227339,
2.76730190935045));
#214990=CARTESIAN_POINT('Ctrl Pts',(19.1601065286608,-59.8686254222852,
2.74997687280405));
#214991=CARTESIAN_POINT('Ctrl Pts',(19.1737823050853,-59.8750609947916,
2.73349253346387));
#214992=CARTESIAN_POINT('Ctrl Pts',(19.1842875619788,-59.8800045782738,
2.72082983599695));
#214993=CARTESIAN_POINT('Ctrl Pts',(19.1957019365507,-59.8843297728467,
2.7086632103945));
#214994=CARTESIAN_POINT('Ctrl Pts',(19.2080253553785,-59.887954494074,2.69711645335803));
#214995=CARTESIAN_POINT('Ctrl Pts',(19.2080576528615,-59.8879639938219,
2.69708619136709));
#214996=CARTESIAN_POINT('Ctrl Pts',(19.2080899573236,-59.8879734883573,
2.69705593387176));
#214997=CARTESIAN_POINT('Ctrl Pts',(19.2081222687617,-59.8879829776789,
2.69702568087529));
#214998=CARTESIAN_POINT('Ctrl Pts',(19.2115867120124,-59.8890004259292,
2.69378194443224));
#214999=CARTESIAN_POINT('Ctrl Pts',(19.2151300442838,-59.8899565588871,
2.69059266624658));
#215000=CARTESIAN_POINT('Ctrl Pts',(19.2187475215465,-59.8908500166518,
2.68746219342635));
#215001=CARTESIAN_POINT('Ctrl Pts',(19.238877960004,-59.8958219059659,2.67004182396045));
#215002=CARTESIAN_POINT('Ctrl Pts',(19.2613031946901,-59.8988577688777,
2.65443567877845));
#215003=CARTESIAN_POINT('Ctrl Pts',(19.2851598349722,-59.8997541019589,
2.64136852353034));
#215004=CARTESIAN_POINT('Ctrl Pts',(19.2958670255061,-59.9001563886585,
2.63550380329636));
#215005=CARTESIAN_POINT('Ctrl Pts',(19.3068627531423,-59.900128000902,2.63014997451039));
#215006=CARTESIAN_POINT('Ctrl Pts',(19.3180708494664,-59.8996517586308,
2.62536981119211));
#215007=CARTESIAN_POINT('Ctrl Pts',(19.3229417365285,-59.8994447901814,
2.62329241687031));
#215008=CARTESIAN_POINT('Ctrl Pts',(19.3278525613652,-59.8991531263706,
2.62132362131386));
#215009=CARTESIAN_POINT('Ctrl Pts',(19.332796959569,-59.8987752905497,2.61946873372306));
#215010=CARTESIAN_POINT('Ctrl Pts',(19.350102353282,-59.8974528651769,2.61297662715526));
#215011=CARTESIAN_POINT('Ctrl Pts',(19.3678190197507,-59.8950748296126,
2.60787989113928));
#215012=CARTESIAN_POINT('Ctrl Pts',(19.3856740904738,-59.891577889443,2.60440616886138));
#215013=CARTESIAN_POINT('Ctrl Pts',(19.3946016258354,-59.8898294193582,
2.60266930772243));
#215014=CARTESIAN_POINT('Ctrl Pts',(19.4035637624462,-59.8878012237011,
2.60133820040143));
#215015=CARTESIAN_POINT('Ctrl Pts',(19.412526394185,-59.885485398205,2.60044130723542));
#215016=CARTESIAN_POINT('Ctrl Pts',(19.4170077100544,-59.884327485457,2.59999286065242));
#215017=CARTESIAN_POINT('Ctrl Pts',(19.4214891497439,-59.8830976653664,
2.59965296768469));
#215018=CARTESIAN_POINT('Ctrl Pts',(19.4259664502061,-59.8817949505647,
2.59942518630911));
#215019=CARTESIAN_POINT('Ctrl Pts',(19.4304437506682,-59.8804922357629,
2.59919740493353));
#215020=CARTESIAN_POINT('Ctrl Pts',(19.4349169113761,-59.8791166246272,
2.59908173791573));
#215021=CARTESIAN_POINT('Ctrl Pts',(19.4393816709763,-59.8776671349981,
2.59908173515982));
#215022=CARTESIAN_POINT('',(19.4684195516703,-59.8682321556238,2.59908173515982));
#215023=CARTESIAN_POINT('Origin',(5.60717482534548E-15,1.85560404756975E-13,
2.59908173516023));
#215024=CARTESIAN_POINT('',(19.6977666881852,-59.5942745858232,2.90134173515982));
#215025=CARTESIAN_POINT('Ctrl Pts',(19.4684195516703,-59.8682321556238,
2.59908173515982));
#215026=CARTESIAN_POINT('Ctrl Pts',(19.4720538382633,-59.8670503242226,
2.59908174381642));
#215027=CARTESIAN_POINT('Ctrl Pts',(19.4756634078267,-59.8658263391015,
2.59915752000954));
#215028=CARTESIAN_POINT('Ctrl Pts',(19.4792467723418,-59.864561863772,2.59930729517429));
#215029=CARTESIAN_POINT('Ctrl Pts',(19.4999541986788,-59.8572547562672,
2.6001728108588));
#215030=CARTESIAN_POINT('Ctrl Pts',(19.5197897600835,-59.848596366684,2.60350651800055));
#215031=CARTESIAN_POINT('Ctrl Pts',(19.5384593694403,-59.8389090368079,
2.60896880596511));
#215032=CARTESIAN_POINT('Ctrl Pts',(19.5459892523667,-59.8350019138231,
2.61117187235484));
#215033=CARTESIAN_POINT('Ctrl Pts',(19.5533299158501,-59.8309275539876,
2.61372076577195));
#215034=CARTESIAN_POINT('Ctrl Pts',(19.5604638837584,-59.8267074486189,
2.61659179896939));
#215035=CARTESIAN_POINT('Ctrl Pts',(19.5630958847955,-59.825150485951,2.61765103591165));
#215036=CARTESIAN_POINT('Ctrl Pts',(19.5656996197551,-59.8235736599156,
2.61875422455105));
#215037=CARTESIAN_POINT('Ctrl Pts',(19.568274145975,-59.821978038774,2.61990022440351));
#215038=CARTESIAN_POINT('Ctrl Pts',(19.5731013826375,-59.8189862491335,
2.62204897412688));
#215039=CARTESIAN_POINT('Ctrl Pts',(19.5778259323232,-59.8159283829422,
2.62434823201726));
#215040=CARTESIAN_POINT('Ctrl Pts',(19.5824415812281,-59.8128114820617,
2.62679048030261));
#215041=CARTESIAN_POINT('Ctrl Pts',(19.5985963523951,-59.80190232898,2.63533834930135));
#215042=CARTESIAN_POINT('Ctrl Pts',(19.6134170876088,-59.7902699966952,
2.64563784783519));
#215043=CARTESIAN_POINT('Ctrl Pts',(19.6266373778174,-59.7782164291172,
2.65736666737921));
#215044=CARTESIAN_POINT('Ctrl Pts',(19.6332475229217,-59.7721896453281,
2.66323107715121));
#215045=CARTESIAN_POINT('Ctrl Pts',(19.6394575570867,-59.7660575536767,
2.6694528178073));
#215046=CARTESIAN_POINT('Ctrl Pts',(19.6452341819734,-59.7598579055887,
2.67599160631157));
#215047=CARTESIAN_POINT('Ctrl Pts',(19.6481224944167,-59.7567580815447,
2.67926100056371));
#215048=CARTESIAN_POINT('Ctrl Pts',(19.6509024545777,-59.7536413685029,
2.6826096568508));
#215049=CARTESIAN_POINT('Ctrl Pts',(19.6535699003337,-59.7505124858961,
2.68603254012439));
#215050=CARTESIAN_POINT('Ctrl Pts',(19.6562373460896,-59.7473836032892,
2.68945542339799));
#215051=CARTESIAN_POINT('Ctrl Pts',(19.6587921483502,-59.7442425399493,
2.69295261525343));
#215052=CARTESIAN_POINT('Ctrl Pts',(19.6612304091767,-59.7410940396259,
2.69651891172057));
#215053=CARTESIAN_POINT('Ctrl Pts',(19.661251202435,-59.7410671895121,2.69654932476045));
#215054=CARTESIAN_POINT('Ctrl Pts',(19.6612719872243,-59.7410403389968,
2.69657974261104));
#215055=CARTESIAN_POINT('Ctrl Pts',(19.6612927635427,-59.7410134880825,
2.69661016526931));
#215056=CARTESIAN_POINT('Ctrl Pts',(19.6719035326714,-59.7273003341226,
2.71214746100963));
#215057=CARTESIAN_POINT('Ctrl Pts',(19.6804273096576,-59.7135327604159,
2.72880565567262));
#215058=CARTESIAN_POINT('Ctrl Pts',(19.6869782138541,-59.6998755263192,
2.74628040011863));
#215059=CARTESIAN_POINT('Ctrl Pts',(19.6937506652805,-59.685756413634,2.76434612881815));
#215060=CARTESIAN_POINT('Ctrl Pts',(19.6984145359326,-59.6717543328784,
2.7832859265371));
#215061=CARTESIAN_POINT('Ctrl Pts',(19.7010437169731,-59.6580526467606,
2.80278753266961));
#215062=CARTESIAN_POINT('Ctrl Pts',(19.7036228854578,-59.6446115955438,
2.82191817721815));
#215063=CARTESIAN_POINT('Ctrl Pts',(19.7042436449215,-59.6314587768815,
2.84159092314074));
#215064=CARTESIAN_POINT('Ctrl Pts',(19.7029300451616,-59.6187815171233,
2.86151233815839));
#215065=CARTESIAN_POINT('Ctrl Pts',(19.7020598313726,-59.6103832769714,
2.87470957720509));
#215066=CARTESIAN_POINT('Ctrl Pts',(19.7003397858053,-59.6021940468487,
2.88801594387922));
#215067=CARTESIAN_POINT('Ctrl Pts',(19.6977666881852,-59.5942745858232,
2.90134173515983));
#215068=CARTESIAN_POINT('',(19.5876674457085,-59.2554138597567,3.4715307213903));
#215069=CARTESIAN_POINT('',(19.6977666881852,-59.5942745858232,2.90134173515982));
#215070=CARTESIAN_POINT('',(25.0931373005752,-57.1420619865017,3.47153072139032));
#215071=CARTESIAN_POINT('Origin',(5.53234440788222E-15,1.85015204418142E-13,
3.47153072139072));
#215072=CARTESIAN_POINT('',(25.2380597013437,-57.4675553545136,2.90134173515983));
#215073=CARTESIAN_POINT('',(25.0931373005752,-57.1420619865017,3.47153072139032));
#215074=CARTESIAN_POINT('',(25.5918112338801,-57.5176823163884,2.59908173515984));
#215075=CARTESIAN_POINT('Ctrl Pts',(25.2380597013437,-57.4675553545136,
2.90134173515984));
#215076=CARTESIAN_POINT('Ctrl Pts',(25.2430650965697,-57.4787973317373,
2.88164837656666));
#215077=CARTESIAN_POINT('Ctrl Pts',(25.249835715983,-57.4892091890288,2.86203734439068));
#215078=CARTESIAN_POINT('Ctrl Pts',(25.258229540281,-57.4986663319543,2.84277945978062));
#215079=CARTESIAN_POINT('Ctrl Pts',(25.2667920292293,-57.5083135057463,
2.82313460919922));
#215080=CARTESIAN_POINT('Ctrl Pts',(25.2770439485784,-57.5169680778959,
2.80385576863236));
#215081=CARTESIAN_POINT('Ctrl Pts',(25.288886320303,-57.5244844631367,2.78521678518279));
#215082=CARTESIAN_POINT('Ctrl Pts',(25.3002686266216,-57.5317088436247,
2.76730190934361));
#215083=CARTESIAN_POINT('Ctrl Pts',(25.3131208736859,-57.5378823365812,
2.74997687279672));
#215084=CARTESIAN_POINT('Ctrl Pts',(25.3273944332815,-57.5428531464543,
2.73349253345617));
#215085=CARTESIAN_POINT('Ctrl Pts',(25.338358886461,-57.5466715501085,2.72082983599201));
#215086=CARTESIAN_POINT('Ctrl Pts',(25.3501628378345,-57.5497799237791,
2.70866321039216));
#215087=CARTESIAN_POINT('Ctrl Pts',(25.3627976342216,-57.5520966403716,
2.69711645335804));
#215088=CARTESIAN_POINT('Ctrl Pts',(25.3628307477697,-57.5521027120726,
2.6970861913671));
#215089=CARTESIAN_POINT('Ctrl Pts',(25.3628638677137,-57.5521087778601,
2.69705593387177));
#215090=CARTESIAN_POINT('Ctrl Pts',(25.3628969940507,-57.5521148377332,
2.69702568087529));
#215091=CARTESIAN_POINT('Ctrl Pts',(25.3664488110208,-57.5527645793665,
2.69378194443225));
#215092=CARTESIAN_POINT('Ctrl Pts',(25.370072675656,-57.5533450954509,2.69059266624659));
#215093=CARTESIAN_POINT('Ctrl Pts',(25.3737637277669,-57.5538555294213,
2.68746219342636));
#215094=CARTESIAN_POINT('Ctrl Pts',(25.3943035935288,-57.556695978409,2.67004182395796));
#215095=CARTESIAN_POINT('Ctrl Pts',(25.4169233145212,-57.5573711352257,
2.65443567877397));
#215096=CARTESIAN_POINT('Ctrl Pts',(25.4407429579551,-57.5557688601523,
2.6413685235247));
#215097=CARTESIAN_POINT('Ctrl Pts',(25.4514335437862,-57.5550497369108,
2.63550380329293));
#215098=CARTESIAN_POINT('Ctrl Pts',(25.4623660683439,-57.5538721381532,
2.63014997450885));
#215099=CARTESIAN_POINT('Ctrl Pts',(25.4734629846673,-57.5522269397027,
2.62536981119211));
#215100=CARTESIAN_POINT('Ctrl Pts',(25.4782855544065,-57.5515119587087,
2.62329241687031));
#215101=CARTESIAN_POINT('Ctrl Pts',(25.483138990061,-57.5507085716892,2.62132362131385));
#215102=CARTESIAN_POINT('Ctrl Pts',(25.4880168077363,-57.5498159753465,
2.61946873372305));
#215103=CARTESIAN_POINT('Ctrl Pts',(25.5050891695999,-57.5466918881471,
2.61297662715526));
#215104=CARTESIAN_POINT('Ctrl Pts',(25.5224602099127,-57.5424749837903,
2.60787989113927));
#215105=CARTESIAN_POINT('Ctrl Pts',(25.5398519389082,-57.5371308371206,
2.60440616886138));
#215106=CARTESIAN_POINT('Ctrl Pts',(25.5485478034059,-57.5344587637858,
2.60266930772243));
#215107=CARTESIAN_POINT('Ctrl Pts',(25.5572488403194,-57.5315048804291,
2.60133820040144));
#215108=CARTESIAN_POINT('Ctrl Pts',(25.5659203041435,-57.528264891145,2.60044130723544));
#215109=CARTESIAN_POINT('Ctrl Pts',(25.5702560360555,-57.5266448965029,
2.59999286065244));
#215110=CARTESIAN_POINT('Ctrl Pts',(25.5745843747453,-57.5249533754915,
2.59965296768472));
#215111=CARTESIAN_POINT('Ctrl Pts',(25.5789009773107,-57.5231897917608,
2.59942518630914));
#215112=CARTESIAN_POINT('Ctrl Pts',(25.5832175798762,-57.5214262080301,
2.59919740493356));
#215113=CARTESIAN_POINT('Ctrl Pts',(25.5875224456236,-57.5195905600214,
2.5990817379158));
#215114=CARTESIAN_POINT('Ctrl Pts',(25.5918112338801,-57.5176823163884,
2.59908173515984));
#215115=CARTESIAN_POINT('',(25.6197038181304,-57.5052637377727,2.59908173515984));
#215116=CARTESIAN_POINT('Origin',(5.59198795571863E-15,1.8555457506392E-13,
2.59908173516024));
#215117=CARTESIAN_POINT('',(25.8191582032627,-57.2088336324694,2.90134173515984));
#215118=CARTESIAN_POINT('Ctrl Pts',(25.6197038181304,-57.5052637377727,
2.59908173515983));
#215119=CARTESIAN_POINT('Ctrl Pts',(25.623194660701,-57.5037084941749,2.59908174381647));
#215120=CARTESIAN_POINT('Ctrl Pts',(25.6266565153809,-57.5021139114129,
2.59915752000955));
#215121=CARTESIAN_POINT('Ctrl Pts',(25.6300880761872,-57.5004817994255,
2.5993072951743));
#215122=CARTESIAN_POINT('Ctrl Pts',(25.6499182643553,-57.4910502055681,
2.60017281085871));
#215123=CARTESIAN_POINT('Ctrl Pts',(25.6687401163196,-57.4803658667987,
2.60350651799978));
#215124=CARTESIAN_POINT('Ctrl Pts',(25.686294849896,-57.468780099555,2.60896880596317));
#215125=CARTESIAN_POINT('Ctrl Pts',(25.6933750777767,-57.4641072931065,
2.61117187235336));
#215126=CARTESIAN_POINT('Ctrl Pts',(25.7002496417671,-57.4592879447658,
2.61372076577113));
#215127=CARTESIAN_POINT('Ctrl Pts',(25.7069034079257,-57.4543452548719,
2.61659179896943));
#215128=CARTESIAN_POINT('Ctrl Pts',(25.7093582436708,-57.4525217023847,
2.61765103591169));
#215129=CARTESIAN_POINT('Ctrl Pts',(25.7117828918954,-57.4506813499532,
2.61875422455108));
#215130=CARTESIAN_POINT('Ctrl Pts',(25.7141765267655,-57.4488253585218,
2.61990022440354));
#215131=CARTESIAN_POINT('Ctrl Pts',(25.7186645921469,-57.4453453745878,
2.62204897412692));
#215132=CARTESIAN_POINT('Ctrl Pts',(25.7230436262012,-57.4418104097892,
2.6243482320173));
#215133=CARTESIAN_POINT('Ctrl Pts',(25.7273081852392,-57.4382281169308,
2.62679048030265));
#215134=CARTESIAN_POINT('Ctrl Pts',(25.7422341418724,-57.4256900919266,
2.63533834930139));
#215135=CARTESIAN_POINT('Ctrl Pts',(25.7557577777299,-57.4125722940988,
2.64563784783522));
#215136=CARTESIAN_POINT('Ctrl Pts',(25.7676457049096,-57.3992028606057,
2.65736666737924));
#215137=CARTESIAN_POINT('Ctrl Pts',(25.7735896684995,-57.3925181438591,
2.66323107715125));
#215138=CARTESIAN_POINT('Ctrl Pts',(25.7791247053306,-57.3857705191192,
2.66945281780733));
#215139=CARTESIAN_POINT('Ctrl Pts',(25.7842216455743,-57.3790010116299,
2.6759916063116));
#215140=CARTESIAN_POINT('Ctrl Pts',(25.7867701156962,-57.3756162578852,
2.67926100056373));
#215141=CARTESIAN_POINT('Ctrl Pts',(25.7892090617198,-57.37222603356,2.68260965685083));
#215142=CARTESIAN_POINT('Ctrl Pts',(25.7915348376382,-57.3688354672937,
2.68603254012442));
#215143=CARTESIAN_POINT('Ctrl Pts',(25.7938606135566,-57.3654449010275,
2.68945542339802));
#215144=CARTESIAN_POINT('Ctrl Pts',(25.7960730898191,-57.3620539952069,
2.69295261525343));
#215145=CARTESIAN_POINT('Ctrl Pts',(25.7981688856973,-57.3586678750405,
2.69651891172058));
#215146=CARTESIAN_POINT('Ctrl Pts',(25.7981867584468,-57.3586389985271,
2.69654932476046));
#215147=CARTESIAN_POINT('Ctrl Pts',(25.7982046227317,-57.3586101224996,
2.69657974261104));
#215148=CARTESIAN_POINT('Ctrl Pts',(25.7982224785504,-57.3585812469608,
2.69661016526931));
#215149=CARTESIAN_POINT('Ctrl Pts',(25.8073417058679,-57.3438340876984,
2.7121474610134));
#215150=CARTESIAN_POINT('Ctrl Pts',(25.8143796853907,-57.3292509568879,
2.7288056556807));
#215151=CARTESIAN_POINT('Ctrl Pts',(25.8194671333562,-57.3149837825966,
2.74628040013136));
#215152=CARTESIAN_POINT('Ctrl Pts',(25.8247266354337,-57.3002341019445,
2.76434612883568));
#215153=CARTESIAN_POINT('Ctrl Pts',(25.8279013409298,-57.2858212188169,
2.7832859265598));
#215154=CARTESIAN_POINT('Ctrl Pts',(25.8290839028457,-57.2719197677126,
2.80278753269758));
#215155=CARTESIAN_POINT('Ctrl Pts',(25.8302439699455,-57.25828275146,2.82191817725084));
#215156=CARTESIAN_POINT('Ctrl Pts',(25.8294864848991,-57.2451370982795,
2.84159092317825));
#215157=CARTESIAN_POINT('Ctrl Pts',(25.8268549466919,-57.2326665944393,
2.86151233820061));
#215158=CARTESIAN_POINT('Ctrl Pts',(25.825111644888,-57.2244053228451,2.87470957723346));
#215159=CARTESIAN_POINT('Ctrl Pts',(25.8225450142721,-57.2164407479107,
2.88801594389343));
#215160=CARTESIAN_POINT('Ctrl Pts',(25.8191582032627,-57.2088336324694,
2.90134173515983));
#215161=CARTESIAN_POINT('',(25.6742415049986,-56.883337725539,3.47153072139032));
#215162=CARTESIAN_POINT('',(25.8191582032627,-57.2088336324694,2.90134173515984));
#215163=CARTESIAN_POINT('',(30.9286463962985,-54.2060847114736,3.47153072139034));
#215164=CARTESIAN_POINT('Origin',(5.53234440788222E-15,1.85015204418142E-13,
3.47153072139072));
#215165=CARTESIAN_POINT('',(31.1067982185541,-54.5146464769132,2.90134173515985));
#215166=CARTESIAN_POINT('',(30.9286463962985,-54.2060847114736,3.47153072139034));
#215167=CARTESIAN_POINT('',(31.4638515574747,-54.5275217339714,2.59908173515985));
#215168=CARTESIAN_POINT('Ctrl Pts',(31.1067982185541,-54.5146464769132,
2.90134173515985));
#215169=CARTESIAN_POINT('Ctrl Pts',(31.1129513003042,-54.5253036631379,
2.8816483765679));
#215170=CARTESIAN_POINT('Ctrl Pts',(31.1207731649977,-54.5349507607426,
2.86203734439313));
#215171=CARTESIAN_POINT('Ctrl Pts',(31.1301095476641,-54.5434787028944,
2.84277945978422));
#215172=CARTESIAN_POINT('Ctrl Pts',(31.1396335346525,-54.5521780046471,
2.82313460920393));
#215173=CARTESIAN_POINT('Ctrl Pts',(31.1507339420409,-54.5597135487696,
2.80385576863812));
#215174=CARTESIAN_POINT('Ctrl Pts',(31.1632971162117,-54.5659508935477,
2.78521678518951));
#215175=CARTESIAN_POINT('Ctrl Pts',(31.1753722224549,-54.5719459231356,
2.7673019093509));
#215176=CARTESIAN_POINT('Ctrl Pts',(31.1887993692959,-54.5767421714167,
2.74997687280452));
#215177=CARTESIAN_POINT('Ctrl Pts',(31.2035143279548,-54.5801937574236,
2.73349253346437));
#215178=CARTESIAN_POINT('Ctrl Pts',(31.2148178485808,-54.5828451460226,
2.72082983599728));
#215179=CARTESIAN_POINT('Ctrl Pts',(31.2268820501991,-54.5847026428,2.70866321039468));
#215180=CARTESIAN_POINT('Ctrl Pts',(31.2396897946776,-54.5856859723267,
2.69711645335807));
#215181=CARTESIAN_POINT('Ctrl Pts',(31.2397233614918,-54.585688549458,2.69708619136713));
#215182=CARTESIAN_POINT('Ctrl Pts',(31.2397569340488,-54.5856911200396,
2.6970559338718));
#215183=CARTESIAN_POINT('Ctrl Pts',(31.2397905123454,-54.585693684071,2.69702568087532));
#215184=CARTESIAN_POINT('Ctrl Pts',(31.243390788585,-54.585968600382,2.69378194443227));
#215185=CARTESIAN_POINT('Ctrl Pts',(31.2470554817647,-54.5861671393371,
2.69059266624661));
#215186=CARTESIAN_POINT('Ctrl Pts',(31.2507796687845,-54.5862889570918,
2.68746219342638));
#215187=CARTESIAN_POINT('Ctrl Pts',(31.2715039227768,-54.5869668451988,
2.67004182396089));
#215188=CARTESIAN_POINT('Ctrl Pts',(31.2940703036714,-54.5852738987617,
2.6544356787792));
#215189=CARTESIAN_POINT('Ctrl Pts',(31.3175919772508,-54.5811905703965,
2.64136852353127));
#215190=CARTESIAN_POINT('Ctrl Pts',(31.3281488300906,-54.5793579160787,
2.63550380329693));
#215191=CARTESIAN_POINT('Ctrl Pts',(31.3388983725504,-54.577044008338,2.63014997451064));
#215192=CARTESIAN_POINT('Ctrl Pts',(31.3497625287433,-54.5742478788453,
2.62536981119211));
#215193=CARTESIAN_POINT('Ctrl Pts',(31.3544839440763,-54.5730327187882,
2.62329241687031));
#215194=CARTESIAN_POINT('Ctrl Pts',(31.3592268152919,-54.5717264106363,
2.62132362131385));
#215195=CARTESIAN_POINT('Ctrl Pts',(31.3639846100476,-54.5703288332441,
2.61946873372305));
#215196=CARTESIAN_POINT('Ctrl Pts',(31.3806368916926,-54.5654373123713,
2.61297662715526));
#215197=CARTESIAN_POINT('Ctrl Pts',(31.3974719850968,-54.5594277405085,
2.60787989113929));
#215198=CARTESIAN_POINT('Ctrl Pts',(31.4142098249423,-54.552294938928,2.6044061688614));
#215199=CARTESIAN_POINT('Ctrl Pts',(31.422578744865,-54.5487285381377,2.60266930772245));
#215200=CARTESIAN_POINT('Ctrl Pts',(31.4309233516999,-54.5448813304458,
2.60133820040145));
#215201=CARTESIAN_POINT('Ctrl Pts',(31.4392086412369,-54.5407526753742,
2.60044130723545));
#215202=CARTESIAN_POINT('Ctrl Pts',(31.4433512860054,-54.5386883478383,
2.59999286065245));
#215203=CARTESIAN_POINT('Ctrl Pts',(31.4474791015111,-54.5365536585642,
2.59965296768473));
#215204=CARTESIAN_POINT('Ctrl Pts',(31.4515877125788,-54.5343485280971,
2.59942518630915));
#215205=CARTESIAN_POINT('Ctrl Pts',(31.4556963236466,-54.5321433976299,
2.59919740493357));
#215206=CARTESIAN_POINT('Ctrl Pts',(31.4597857294236,-54.5298678244919,
2.59908173791582));
#215207=CARTESIAN_POINT('Ctrl Pts',(31.4638515574747,-54.5275217339714,
2.59908173515985));
#215208=CARTESIAN_POINT('',(31.4902932482914,-54.5122556166605,2.59908173515986));
#215209=CARTESIAN_POINT('Origin',(5.57749365020894E-15,1.8554718984639E-13,
2.59908173516024));
#215210=CARTESIAN_POINT('',(31.6576696180591,-54.1966007261202,2.90134173515985));
#215211=CARTESIAN_POINT('Ctrl Pts',(31.4902932482914,-54.5122556166605,
2.59908173515986));
#215212=CARTESIAN_POINT('Ctrl Pts',(31.4936024004378,-54.5103440004405,
2.59908174381646));
#215213=CARTESIAN_POINT('Ctrl Pts',(31.4968786114299,-54.5083962906199,
2.59915752000958));
#215214=CARTESIAN_POINT('Ctrl Pts',(31.5001207716291,-54.506414423735,2.59930729517433));
#215215=CARTESIAN_POINT('Ctrl Pts',(31.518856457946,-54.4949616780362,2.60017281085903));
#215216=CARTESIAN_POINT('Ctrl Pts',(31.536458384329,-54.482368449926,2.6035065180021));
#215217=CARTESIAN_POINT('Ctrl Pts',(31.552705908797,-54.4690111813986,2.60896880596886));
#215218=CARTESIAN_POINT('Ctrl Pts',(31.5592589091653,-54.4636238877371,
2.61117187235774));
#215219=CARTESIAN_POINT('Ctrl Pts',(31.5655920544933,-54.458112352686,2.61372076577361));
#215220=CARTESIAN_POINT('Ctrl Pts',(31.5716927188404,-54.4525012314179,
2.61659179896944));
#215221=CARTESIAN_POINT('Ctrl Pts',(31.5739434935992,-54.450431068334,2.61765103591169));
#215222=CARTESIAN_POINT('Ctrl Pts',(31.5761624901357,-54.4483473527928,
2.61875422455109));
#215223=CARTESIAN_POINT('Ctrl Pts',(31.5783490084913,-54.446251325702,2.61990022440356));
#215224=CARTESIAN_POINT('Ctrl Pts',(31.5824487304082,-54.4423212749068,
2.62204897412693));
#215225=CARTESIAN_POINT('Ctrl Pts',(31.5864342712176,-54.4383479413149,
2.62434823201731));
#215226=CARTESIAN_POINT('Ctrl Pts',(31.5903010169876,-54.4343395048289,
2.62679048030266));
#215227=CARTESIAN_POINT('Ctrl Pts',(31.6038346271824,-54.4203099771278,
2.6353383493014));
#215228=CARTESIAN_POINT('Ctrl Pts',(31.6159129958993,-54.4058504350952,
2.64563784783522));
#215229=CARTESIAN_POINT('Ctrl Pts',(31.6263383134323,-54.391311613998,2.65736666737924));
#215230=CARTESIAN_POINT('Ctrl Pts',(31.6315509721988,-54.3840422034495,
2.66323107715124));
#215231=CARTESIAN_POINT('Ctrl Pts',(31.6363503686743,-54.3767529740098,
2.66945281780734));
#215232=CARTESIAN_POINT('Ctrl Pts',(31.6407117811311,-54.3694877752597,
2.67599160631161));
#215233=CARTESIAN_POINT('Ctrl Pts',(31.6428924873595,-54.3658551758847,
2.67926100056374));
#215234=CARTESIAN_POINT('Ctrl Pts',(31.6449636976428,-54.3622285842833,
2.68260965685083));
#215235=CARTESIAN_POINT('Ctrl Pts',(31.6469223220359,-54.3586134821111,
2.68603254012442));
#215236=CARTESIAN_POINT('Ctrl Pts',(31.648880946429,-54.3549983799389,2.68945542339802));
#215237=CARTESIAN_POINT('Ctrl Pts',(31.6507268563406,-54.3513947831115,
2.69295261525345));
#215238=CARTESIAN_POINT('Ctrl Pts',(31.6524572252922,-54.3478081421432,
2.69651891172059));
#215239=CARTESIAN_POINT('Ctrl Pts',(31.6524719817154,-54.3477775556074,
2.69654932476047));
#215240=CARTESIAN_POINT('Ctrl Pts',(31.6524867297711,-54.3477469704395,
2.69657974261105));
#215241=CARTESIAN_POINT('Ctrl Pts',(31.6525014694581,-54.3477163866426,
2.69661016526933));
#215242=CARTESIAN_POINT('Ctrl Pts',(31.6600292427972,-54.3320967950475,
2.71214746100997));
#215243=CARTESIAN_POINT('Ctrl Pts',(31.6655043152777,-54.3168578829727,
2.72880565567334));
#215244=CARTESIAN_POINT('Ctrl Pts',(31.6690725678672,-54.3021370826402,
2.74628040011975));
#215245=CARTESIAN_POINT('Ctrl Pts',(31.6727614963898,-54.2869184346153,
2.76434612881985));
#215246=CARTESIAN_POINT('Ctrl Pts',(31.6744122539934,-54.2722526596854,
2.78328592653942));
#215247=CARTESIAN_POINT('Ctrl Pts',(31.674135240392,-54.2583037508073,2.80278753267255));
#215248=CARTESIAN_POINT('Ctrl Pts',(31.6738634961721,-54.2446201795274,
2.82191817722171));
#215249=CARTESIAN_POINT('Ctrl Pts',(31.6717360657848,-54.23162571836,2.84159092314493));
#215250=CARTESIAN_POINT('Ctrl Pts',(31.6678154208197,-54.2194985998906,
2.86151233816319));
#215251=CARTESIAN_POINT('Ctrl Pts',(31.6652181309801,-54.2114648090569,
2.87470957720832));
#215252=CARTESIAN_POINT('Ctrl Pts',(31.6618330358543,-54.2038121508437,
2.88801594388085));
#215253=CARTESIAN_POINT('Ctrl Pts',(31.6576696180591,-54.1966007261202,
2.90134173515986));
#215254=CARTESIAN_POINT('',(31.4795232016796,-53.8880358395965,3.47153072139034));
#215255=CARTESIAN_POINT('',(31.6576696180591,-54.1966007261202,2.90134173515985));
#215256=CARTESIAN_POINT('',(36.4252947698685,-50.6762142289942,3.47153072139037));
#215257=CARTESIAN_POINT('Origin',(5.53234440788222E-15,1.85015204418142E-13,
3.47153072139072));
#215258=CARTESIAN_POINT('',(36.634724144966,-50.9644637245887,2.90134173515987));
#215259=CARTESIAN_POINT('',(36.4252947698685,-50.6762142289942,3.47153072139037));
#215260=CARTESIAN_POINT('',(36.9911673391713,-50.9399462128196,2.59908173515987));
#215261=CARTESIAN_POINT('Ctrl Pts',(36.634724144966,-50.9644637245887,2.90134173515987));
#215262=CARTESIAN_POINT('Ctrl Pts',(36.6419574987901,-50.9744193574537,
2.88164837656548));
#215263=CARTESIAN_POINT('Ctrl Pts',(36.6507449107794,-50.9831959997529,
2.8620373443883));
#215264=CARTESIAN_POINT('Ctrl Pts',(36.6609215604541,-50.9907013072134,
2.8427794597771));
#215265=CARTESIAN_POINT('Ctrl Pts',(36.6713026986907,-50.9983574255574,
2.82313460919437));
#215266=CARTESIAN_POINT('Ctrl Pts',(36.683129975735,-51.0046913806552,2.80385576862625));
#215267=CARTESIAN_POINT('Ctrl Pts',(36.6962763075901,-51.0095813473161,
2.78521678517554));
#215268=CARTESIAN_POINT('Ctrl Pts',(36.7089119163701,-51.0142813432051,
2.76730190933505));
#215269=CARTESIAN_POINT('Ctrl Pts',(36.7227668523605,-51.0176477981104,
2.74997687278699));
#215270=CARTESIAN_POINT('Ctrl Pts',(36.7377619899201,-51.0195423439515,
2.73349253344545));
#215271=CARTESIAN_POINT('Ctrl Pts',(36.7492807342482,-51.0209976683241,
2.72082983598517));
#215272=CARTESIAN_POINT('Ctrl Pts',(36.7614730081857,-51.0215839370833,
2.70866321038893));
#215273=CARTESIAN_POINT('Ctrl Pts',(36.7743133764177,-51.0212231059799,
2.69711645335807));
#215274=CARTESIAN_POINT('Ctrl Pts',(36.7743470287329,-51.0212221603059,
2.69708619136713));
#215275=CARTESIAN_POINT('Ctrl Pts',(36.7743806860749,-51.0212212075178,
2.69705593387181));
#215276=CARTESIAN_POINT('Ctrl Pts',(36.7744143484403,-51.0212202476155,
2.69702568087533));
#215277=CARTESIAN_POINT('Ctrl Pts',(36.7780236385695,-51.0211173265635,
2.69378194443228));
#215278=CARTESIAN_POINT('Ctrl Pts',(36.7816890091485,-51.0209317131549,
2.69059266624663));
#215279=CARTESIAN_POINT('Ctrl Pts',(36.7854055281047,-51.0206635800331,
2.68746219342639));
#215280=CARTESIAN_POINT('Ctrl Pts',(36.806087111073,-51.0191714801756,2.67004182395614));
#215281=CARTESIAN_POINT('Ctrl Pts',(36.8283529098889,-51.015128978758,2.65443567877069));
#215282=CARTESIAN_POINT('Ctrl Pts',(36.851318905247,-51.0086093348969,2.64136852352057));
#215283=CARTESIAN_POINT('Ctrl Pts',(36.8616263619967,-51.0056832284481,
2.63550380329042));
#215284=CARTESIAN_POINT('Ctrl Pts',(36.8720751481116,-51.0022583633838,
2.63014997450773));
#215285=CARTESIAN_POINT('Ctrl Pts',(36.8825875141948,-50.9983419378318,
2.62536981119211));
#215286=CARTESIAN_POINT('Ctrl Pts',(36.8871560463072,-50.9966399122595,
2.62329241687032));
#215287=CARTESIAN_POINT('Ctrl Pts',(36.8917363891943,-50.9948449951607,
2.62132362131386));
#215288=CARTESIAN_POINT('Ctrl Pts',(36.8963220336354,-50.9929577488693,
2.61946873372307));
#215289=CARTESIAN_POINT('Ctrl Pts',(36.9123717891793,-50.9863523868494,
2.61297662715528));
#215290=CARTESIAN_POINT('Ctrl Pts',(36.9284864868687,-50.9786159896075,
2.60787989113931));
#215291=CARTESIAN_POINT('Ctrl Pts',(36.9443870542882,-50.9697726815829,
2.60440616886143));
#215292=CARTESIAN_POINT('Ctrl Pts',(36.9523373379979,-50.9653510275706,
2.60266930772248));
#215293=CARTESIAN_POINT('Ctrl Pts',(36.9602340894955,-50.960652646356,2.60133820040148));
#215294=CARTESIAN_POINT('Ctrl Pts',(36.9680424293796,-50.9556805599057,
2.60044130723547));
#215295=CARTESIAN_POINT('Ctrl Pts',(36.9719465993216,-50.9531945166806,
2.59999286065247));
#215296=CARTESIAN_POINT('Ctrl Pts',(36.9758286664326,-50.9506400472463,
2.59965296768476));
#215297=CARTESIAN_POINT('Ctrl Pts',(36.9796842712,-50.9480175299135,2.59942518630919));
#215298=CARTESIAN_POINT('Ctrl Pts',(36.9835398759674,-50.9453950125807,
2.59919740493361));
#215299=CARTESIAN_POINT('Ctrl Pts',(36.9873690173885,-50.9427044459688,
2.59908173791584));
#215300=CARTESIAN_POINT('Ctrl Pts',(36.9911673391713,-50.9399462128196,
2.59908173515988));
#215301=CARTESIAN_POINT('',(37.0158684358566,-50.9219998155894,2.59908173515989));
#215302=CARTESIAN_POINT('Origin',(5.56385071146069E-15,1.85538330018374E-13,
2.59908173516024));
#215303=CARTESIAN_POINT('',(37.1493329797267,-50.5905785208478,2.90134173515988));
#215304=CARTESIAN_POINT('Ctrl Pts',(37.0158684358566,-50.9219998155894,
2.59908173515989));
#215305=CARTESIAN_POINT('Ctrl Pts',(37.0189596418154,-50.9197527708144,
2.59908174381647));
#215306=CARTESIAN_POINT('Ctrl Pts',(37.0220143142664,-50.9174732734517,
2.5991575200096));
#215307=CARTESIAN_POINT('Ctrl Pts',(37.025031552073,-50.9151633654177,2.59930729517435));
#215308=CARTESIAN_POINT('Ctrl Pts',(37.0424674644288,-50.9018149465613,
2.60017281085891));
#215309=CARTESIAN_POINT('Ctrl Pts',(37.058656614833,-50.8874508031597,2.60350651800102));
#215310=CARTESIAN_POINT('Ctrl Pts',(37.0734189189074,-50.8724683783849,
2.60896880596616));
#215311=CARTESIAN_POINT('Ctrl Pts',(37.0793728957291,-50.8664256218212,
2.61117187235567));
#215312=CARTESIAN_POINT('Ctrl Pts',(37.0850952351376,-50.8602822855845,
2.61372076577245));
#215313=CARTESIAN_POINT('Ctrl Pts',(37.090575957526,-50.8540642095541,2.61659179896946));
#215314=CARTESIAN_POINT('Ctrl Pts',(37.0925980113393,-50.8517701170135,
2.61765103591172));
#215315=CARTESIAN_POINT('Ctrl Pts',(37.0945870443972,-50.849465867986,2.61875422455113));
#215316=CARTESIAN_POINT('Ctrl Pts',(37.0965424902857,-50.8471527697473,
2.61990022440359));
#215317=CARTESIAN_POINT('Ctrl Pts',(37.1002089513267,-50.8428157105498,
2.62204897412696));
#215318=CARTESIAN_POINT('Ctrl Pts',(37.1037573324722,-50.8384475408389,
2.62434823201734));
#215319=CARTESIAN_POINT('Ctrl Pts',(37.1071839000983,-50.8340568779942,
2.62679048030269));
#215320=CARTESIAN_POINT('Ctrl Pts',(37.1191768867895,-50.8186895580377,
2.63533834930143));
#215321=CARTESIAN_POINT('Ctrl Pts',(37.1296776552305,-50.8030466935685,
2.64563784783527));
#215322=CARTESIAN_POINT('Ctrl Pts',(37.1385261411562,-50.7874977752337,
2.65736666737928));
#215323=CARTESIAN_POINT('Ctrl Pts',(37.1429503841191,-50.7797233160663,
2.66323107715129));
#215324=CARTESIAN_POINT('Ctrl Pts',(37.1469615570468,-50.7719723442501,
2.66945281780737));
#215325=CARTESIAN_POINT('Ctrl Pts',(37.1505396571691,-50.7642910532771,
2.67599160631164));
#215326=CARTESIAN_POINT('Ctrl Pts',(37.1523287072303,-50.7604504077907,
2.67926100056378));
#215327=CARTESIAN_POINT('Ctrl Pts',(37.15400948916,-50.7566271826095,2.68260965685087));
#215328=CARTESIAN_POINT('Ctrl Pts',(37.1555795029291,-50.7528271523473,
2.68603254012446));
#215329=CARTESIAN_POINT('Ctrl Pts',(37.1571495166982,-50.7490271220852,
2.68945542339806));
#215330=CARTESIAN_POINT('Ctrl Pts',(37.1586086360836,-50.7452503160119,
2.69295261525348));
#215331=CARTESIAN_POINT('Ctrl Pts',(37.1599546198243,-50.7415024502306,
2.69651891172063));
#215332=CARTESIAN_POINT('Ctrl Pts',(37.1599660982467,-50.7414704887848,
2.69654932476051));
#215333=CARTESIAN_POINT('Ctrl Pts',(37.1599775684904,-50.7414385295741,
2.69657974261109));
#215334=CARTESIAN_POINT('Ctrl Pts',(37.1599890305545,-50.7414065726016,
2.69661016526937));
#215335=CARTESIAN_POINT('Ctrl Pts',(37.1658428740579,-50.7250856801833,
2.71214746101124));
#215336=CARTESIAN_POINT('Ctrl Pts',(37.1696950534575,-50.7093579475494,
2.72880565567602));
#215337=CARTESIAN_POINT('Ctrl Pts',(37.171705016149,-50.6943448053406,2.74628040012395));
#215338=CARTESIAN_POINT('Ctrl Pts',(37.173782954444,-50.6788239286313,2.76434612882549));
#215339=CARTESIAN_POINT('Ctrl Pts',(37.1738916781082,-50.6640659431946,
2.78328592654661));
#215340=CARTESIAN_POINT('Ctrl Pts',(37.1721581240063,-50.6502224037042,
2.80278753268133));
#215341=CARTESIAN_POINT('Ctrl Pts',(37.1704575457512,-50.6366421974646,
2.82191817723184));
#215342=CARTESIAN_POINT('Ctrl Pts',(37.1669834785924,-50.6239412983438,
2.84159092315645));
#215343=CARTESIAN_POINT('Ctrl Pts',(37.1618166822721,-50.6122904324912,
2.86151233817606));
#215344=CARTESIAN_POINT('Ctrl Pts',(37.1583938608486,-50.6045721423226,
2.87470957721698));
#215345=CARTESIAN_POINT('Ctrl Pts',(37.1542273890263,-50.5973152449659,
2.88801594388519));
#215346=CARTESIAN_POINT('Ctrl Pts',(37.1493329797266,-50.5905785208478,
2.90134173515986));
#215347=CARTESIAN_POINT('',(36.9399086546492,-50.3023253561989,3.47153072139037));
#215348=CARTESIAN_POINT('',(37.1493329797266,-50.5905785208478,2.90134173515989));
#215349=CARTESIAN_POINT('',(41.5228599914568,-46.5911245387423,3.4715307213904));
#215350=CARTESIAN_POINT('Origin',(5.53234440788222E-15,1.85015204418142E-13,
3.47153072139072));
#215351=CARTESIAN_POINT('',(41.7612723673368,-46.8559036426978,2.90134173515992));
#215352=CARTESIAN_POINT('',(41.5228599914568,-46.5911245387423,3.4715307213904));
#215353=CARTESIAN_POINT('',(42.1132001506006,-46.794261981091,2.59908173515991));
#215354=CARTESIAN_POINT('Ctrl Pts',(41.7612723673369,-46.8559036426978,
2.90134173515992));
#215355=CARTESIAN_POINT('Ctrl Pts',(41.7695067430959,-46.8650486462041,
2.88164837656661));
#215356=CARTESIAN_POINT('Ctrl Pts',(41.7791634256545,-46.8728586744666,
2.86203734439051));
#215357=CARTESIAN_POINT('Ctrl Pts',(41.7900688448321,-46.8792591175156,
2.84277945978033));
#215358=CARTESIAN_POINT('Ctrl Pts',(41.8011933963914,-46.8857881704151,
2.82313460919898));
#215359=CARTESIAN_POINT('Ctrl Pts',(41.8136179609662,-46.8908511403499,
2.80385576863217));
#215360=CARTESIAN_POINT('Ctrl Pts',(41.8272034165389,-46.8943401533956,
2.78521678518265));
#215361=CARTESIAN_POINT('Ctrl Pts',(41.8402610894779,-46.8976936214472,
2.76730190934385));
#215362=CARTESIAN_POINT('Ctrl Pts',(41.8543920170353,-46.899593399393,2.74997687279733));
#215363=CARTESIAN_POINT('Ctrl Pts',(41.8695030436256,-46.899910148029,2.73349253345709));
#215364=CARTESIAN_POINT('Ctrl Pts',(41.8811108098904,-46.9001534633397,
2.72082983599264));
#215365=CARTESIAN_POINT('Ctrl Pts',(41.8932975750515,-46.899462080799,2.7086632103925));
#215366=CARTESIAN_POINT('Ctrl Pts',(41.906029885286,-46.8977610424066,2.69711645335812));
#215367=CARTESIAN_POINT('Ctrl Pts',(41.9060632544005,-46.8977565842883,
2.69708619136718));
#215368=CARTESIAN_POINT('Ctrl Pts',(41.9060966277705,-46.8977521185695,
2.69705593387185));
#215369=CARTESIAN_POINT('Ctrl Pts',(41.9061300053929,-46.8977476452502,
2.69702568087537));
#215370=CARTESIAN_POINT('Ctrl Pts',(41.9097087652737,-46.8972680144598,
2.69378194443233));
#215371=CARTESIAN_POINT('Ctrl Pts',(41.9133346546847,-46.896700282307,2.69059266624667));
#215372=CARTESIAN_POINT('Ctrl Pts',(41.9170027866181,-46.8960451360313,
2.68746219342645));
#215373=CARTESIAN_POINT('Ctrl Pts',(41.9374151068032,-46.8923993959678,
2.67004182395839));
#215374=CARTESIAN_POINT('Ctrl Pts',(41.9591363747797,-46.8860516300634,
2.65443567877468));
#215375=CARTESIAN_POINT('Ctrl Pts',(41.9812950716555,-46.8771671012931,
2.64136852352558));
#215376=CARTESIAN_POINT('Ctrl Pts',(41.9912402016709,-46.8731796017465,
2.63550380329351));
#215377=CARTESIAN_POINT('Ctrl Pts',(42.0012737523628,-46.8686813028947,
2.63014997450917));
#215378=CARTESIAN_POINT('Ctrl Pts',(42.011319152663,-46.8636874904583,2.62536981119221));
#215379=CARTESIAN_POINT('Ctrl Pts',(42.015684747761,-46.861517247119,2.62329241687041));
#215380=CARTESIAN_POINT('Ctrl Pts',(42.0200523791245,-46.8592533865607,
2.62132362131396));
#215381=CARTESIAN_POINT('Ctrl Pts',(42.0244156319709,-46.8568971484354,
2.61946873372316));
#215382=CARTESIAN_POINT('Ctrl Pts',(42.0396870169334,-46.848650314997,2.61297662715536));
#215383=CARTESIAN_POINT('Ctrl Pts',(42.0549047629078,-46.8392718539632,
2.60787989113937));
#215384=CARTESIAN_POINT('Ctrl Pts',(42.0697938479572,-46.8288149286278,
2.60440616886147));
#215385=CARTESIAN_POINT('Ctrl Pts',(42.0772383904819,-46.8235864659601,
2.60266930772252));
#215386=CARTESIAN_POINT('Ctrl Pts',(42.0846007681804,-46.8180883876704,
2.60133820040152));
#215387=CARTESIAN_POINT('Ctrl Pts',(42.0918466086057,-46.8123273450613,
2.60044130723551));
#215388=CARTESIAN_POINT('Ctrl Pts',(42.0954695288184,-46.8094468237567,
2.59999286065251));
#215389=CARTESIAN_POINT('Ctrl Pts',(42.0990633147952,-46.8065005614637,
2.59965296768479));
#215390=CARTESIAN_POINT('Ctrl Pts',(42.1026236704495,-46.803489390114,2.59942518630921));
#215391=CARTESIAN_POINT('Ctrl Pts',(42.1061840261039,-46.8004782187642,
2.59919740493363));
#215392=CARTESIAN_POINT('Ctrl Pts',(42.1097109502944,-46.7974021370894,
2.59908173791584));
#215393=CARTESIAN_POINT('Ctrl Pts',(42.1132001506006,-46.794261981091,2.59908173515992));
#215394=CARTESIAN_POINT('',(42.1358900227701,-46.773831928425,2.59908173515991));
#215395=CARTESIAN_POINT('Origin',(5.55120861436579E-15,1.8552809265E-13,
2.59908173516023));
#215396=CARTESIAN_POINT('',(42.2339804752707,-46.4302753505418,2.90134173515992));
#215397=CARTESIAN_POINT('Ctrl Pts',(42.1358900227701,-46.773831928425,2.59908173515991));
#215398=CARTESIAN_POINT('Ctrl Pts',(42.138729414642,-46.771274074188,2.59908174381655));
#215399=CARTESIAN_POINT('Ctrl Pts',(42.1415290809214,-46.7686877639332,
2.59915752000963));
#215400=CARTESIAN_POINT('Ctrl Pts',(42.1442883388465,-46.7660751225859,
2.59930729517438));
#215401=CARTESIAN_POINT('Ctrl Pts',(42.1602334457314,-46.7509772786485,
2.60017281085848));
#215402=CARTESIAN_POINT('Ctrl Pts',(42.1748324484328,-46.734999596523,2.60350651799748));
#215403=CARTESIAN_POINT('Ctrl Pts',(42.1879477932176,-46.7185561660889,
2.60896880595744));
#215404=CARTESIAN_POINT('Ctrl Pts',(42.1932375134815,-46.7119241523218,
2.61117187234895));
#215405=CARTESIAN_POINT('Ctrl Pts',(42.1982863518268,-46.7052163225703,
2.61372076576869));
#215406=CARTESIAN_POINT('Ctrl Pts',(42.203087084319,-46.6984594183132,2.6165917989695));
#215407=CARTESIAN_POINT('Ctrl Pts',(42.2048582631421,-46.6959665308738,
2.61765103591176));
#215408=CARTESIAN_POINT('Ctrl Pts',(42.2065955404589,-46.6934669941947,
2.61875422455116));
#215409=CARTESIAN_POINT('Ctrl Pts',(42.208298489606,-46.6909621675965,2.61990022440363));
#215410=CARTESIAN_POINT('Ctrl Pts',(42.2114915192568,-46.6862656177247,
2.622048974127));
#215411=CARTESIAN_POINT('Ctrl Pts',(42.2145638639319,-46.6815504704764,
2.62434823201736));
#215412=CARTESIAN_POINT('Ctrl Pts',(42.2175127112221,-46.6768256862939,
2.62679048030272));
#215413=CARTESIAN_POINT('Ctrl Pts',(42.2278336767378,-46.6602889416552,
2.63533834930145));
#215414=CARTESIAN_POINT('Ctrl Pts',(42.2366417962865,-46.643634141246,2.6456378478353));
#215415=CARTESIAN_POINT('Ctrl Pts',(42.2438165047415,-46.6272454828767,
2.65736666737931));
#215416=CARTESIAN_POINT('Ctrl Pts',(42.247403858969,-46.6190511536921,2.66323107715132));
#215417=CARTESIAN_POINT('Ctrl Pts',(42.2505828610989,-46.6109233607684,
2.66945281780741));
#215418=CARTESIAN_POINT('Ctrl Pts',(42.253338446473,-46.6029101354039,2.67599160631168));
#215419=CARTESIAN_POINT('Ctrl Pts',(42.2547162391601,-46.5989035227217,
2.67926100056381));
#215420=CARTESIAN_POINT('Ctrl Pts',(42.2559881777376,-46.5949255520158,
2.6826096568509));
#215421=CARTESIAN_POINT('Ctrl Pts',(42.2571523794834,-46.5909822275905,
2.6860325401245));
#215422=CARTESIAN_POINT('Ctrl Pts',(42.2583165812292,-46.5870389031651,
2.68945542339809));
#215423=CARTESIAN_POINT('Ctrl Pts',(42.2593729236709,-46.5831302673236,
2.69295261525354));
#215424=CARTESIAN_POINT('Ctrl Pts',(42.2603197753212,-46.5792622391313,
2.69651891172068));
#215425=CARTESIAN_POINT('Ctrl Pts',(42.2603278499828,-46.5792292529517,
2.69654932476056));
#215426=CARTESIAN_POINT('Ctrl Pts',(42.2603359167441,-46.57919626985,2.69657974261114));
#215427=CARTESIAN_POINT('Ctrl Pts',(42.2603439756046,-46.5791632898291,
2.69661016526942));
#215428=CARTESIAN_POINT('Ctrl Pts',(42.264459753338,-46.562319911698,2.71214746101455));
#215429=CARTESIAN_POINT('Ctrl Pts',(42.266646834373,-46.5462756748331,2.72880565568302));
#215430=CARTESIAN_POINT('Ctrl Pts',(42.2670764855939,-46.531134677874,2.74628040013495));
#215431=CARTESIAN_POINT('Ctrl Pts',(42.2675206673338,-46.5154816224519,
2.76434612884054));
#215432=CARTESIAN_POINT('Ctrl Pts',(42.2660861658583,-46.5007931180837,
2.78328592656602));
#215433=CARTESIAN_POINT('Ctrl Pts',(42.2629150644359,-46.4872066206955,
2.80278753270522));
#215434=CARTESIAN_POINT('Ctrl Pts',(42.2598042840353,-46.4738785670766,
2.82191817725999));
#215435=CARTESIAN_POINT('Ctrl Pts',(42.25502164271,-46.4616103837102,2.84159092318895));
#215436=CARTESIAN_POINT('Ctrl Pts',(42.2486653035341,-46.4505634197984,
2.86151233821282));
#215437=CARTESIAN_POINT('Ctrl Pts',(42.2444544516768,-46.4432451935021,
2.87470957724171));
#215438=CARTESIAN_POINT('Ctrl Pts',(42.2395522518982,-46.436463565092,2.88801594389761));
#215439=CARTESIAN_POINT('Ctrl Pts',(42.2339804752707,-46.4302753505418,
2.90134173515992));
#215440=CARTESIAN_POINT('',(41.9955727382257,-46.1654920697605,3.4715307213904));
#215441=CARTESIAN_POINT('',(42.2339804752707,-46.4302753505418,2.90134173515992));
#215442=CARTESIAN_POINT('',(46.1654920697617,-41.9955727382244,3.47153072139043));
#215443=CARTESIAN_POINT('Origin',(5.53234440788222E-15,1.85015204418142E-13,
3.47153072139072));
#215444=CARTESIAN_POINT('',(46.430275350543,-42.2339804752694,2.90134173515995));
#215445=CARTESIAN_POINT('',(46.1654920697617,-41.9955727382244,3.47153072139043));
#215446=CARTESIAN_POINT('',(46.7738319284262,-42.1358900227688,2.59908173515994));
#215447=CARTESIAN_POINT('Ctrl Pts',(46.430275350543,-42.2339804752694,2.90134173515995));
#215448=CARTESIAN_POINT('Ctrl Pts',(46.4394205306929,-42.2422146548451,
2.88164837656735));
#215449=CARTESIAN_POINT('Ctrl Pts',(46.449840683186,-42.2489725007674,2.86203734439194));
#215450=CARTESIAN_POINT('Ctrl Pts',(46.4613553898119,-42.2541979548116,
2.84277945978242));
#215451=CARTESIAN_POINT('Ctrl Pts',(46.4731014717795,-42.259528408597,2.82313460920183));
#215452=CARTESIAN_POINT('Ctrl Pts',(46.4859871977557,-42.2632649224111,
2.80385576863575));
#215453=CARTESIAN_POINT('Ctrl Pts',(46.4998629319526,-42.2653147554846,
2.78521678518688));
#215454=CARTESIAN_POINT('Ctrl Pts',(46.5131996064543,-42.2672849544014,
2.76730190934884));
#215455=CARTESIAN_POINT('Ctrl Pts',(46.5274517041803,-42.2676972410231,
2.749976872803));
#215456=CARTESIAN_POINT('Ctrl Pts',(46.5425130602331,-42.2664327220894,
2.73349253346334));
#215457=CARTESIAN_POINT('Ctrl Pts',(46.554082671317,-42.265461362524,2.72082983599665));
#215458=CARTESIAN_POINT('Ctrl Pts',(46.5661304069508,-42.2634999036146,
2.70866321039442));
#215459=CARTESIAN_POINT('Ctrl Pts',(46.5786151613305,-42.2604772948653,
2.69711645335815));
#215460=CARTESIAN_POINT('Ctrl Pts',(46.5786478816452,-42.2604693731468,
2.69708619136721));
#215461=CARTESIAN_POINT('Ctrl Pts',(46.5786806053978,-42.2604614434245,
2.69705593387188));
#215462=CARTESIAN_POINT('Ctrl Pts',(46.5787133325848,-42.260453505699,2.6970256808754));
#215463=CARTESIAN_POINT('Ctrl Pts',(46.5822223525751,-42.2596024201055,
2.69378194443235));
#215464=CARTESIAN_POINT('Ctrl Pts',(46.5857690348151,-42.2586587894008,
2.69059266624671));
#215465=CARTESIAN_POINT('Ctrl Pts',(46.5893485909045,-42.2576238078908,
2.68746219342648));
#215466=CARTESIAN_POINT('Ctrl Pts',(46.6092680066585,-42.2518643711119,
2.67004182395757));
#215467=CARTESIAN_POINT('Ctrl Pts',(46.6302067610422,-42.2432808881709,
2.65443567877319));
#215468=CARTESIAN_POINT('Ctrl Pts',(46.6513153841198,-42.2321288152456,
2.64136852352369));
#215469=CARTESIAN_POINT('Ctrl Pts',(46.6607892264715,-42.2271236104816,
2.63550380329236));
#215470=CARTESIAN_POINT('Ctrl Pts',(46.6702976120556,-42.2216011621472,
2.63014997450866));
#215471=CARTESIAN_POINT('Ctrl Pts',(46.6797659870611,-42.2155846760822,
2.62536981119222));
#215472=CARTESIAN_POINT('Ctrl Pts',(46.6838808147712,-42.2129699926162,
2.62329241687042));
#215473=CARTESIAN_POINT('Ctrl Pts',(46.6879878819279,-42.2102619919283,
2.62132362131396));
#215474=CARTESIAN_POINT('Ctrl Pts',(46.6920809384683,-42.2074625774071,
2.61946873372316));
#215475=CARTESIAN_POINT('Ctrl Pts',(46.7064066363599,-42.1976646265831,
2.61297662715537));
#215476=CARTESIAN_POINT('Ctrl Pts',(46.72056070181,-42.186746854139,2.60787989113939));
#215477=CARTESIAN_POINT('Ctrl Pts',(46.7342751765578,-42.174790879755,2.60440616886149));
#215478=CARTESIAN_POINT('Ctrl Pts',(46.7411324139317,-42.168812892563,2.60266930772254));
#215479=CARTESIAN_POINT('Ctrl Pts',(46.7478797540803,-42.1625753552947,
2.60133820040155));
#215480=CARTESIAN_POINT('Ctrl Pts',(46.7544837081028,-42.156088475715,2.60044130723554));
#215481=CARTESIAN_POINT('Ctrl Pts',(46.7577856851141,-42.1528450359252,
2.59999286065254));
#215482=CARTESIAN_POINT('Ctrl Pts',(46.7610518156854,-42.1495392606399,
2.59965296768483));
#215483=CARTESIAN_POINT('Ctrl Pts',(46.7642779142252,-42.1461724262966,
2.59942518630925));
#215484=CARTESIAN_POINT('Ctrl Pts',(46.7675040127649,-42.1428055919533,
2.59919740493367));
#215485=CARTESIAN_POINT('Ctrl Pts',(46.7706900780053,-42.1393776974101,
2.59908173791585));
#215486=CARTESIAN_POINT('Ctrl Pts',(46.7738319284262,-42.1358900227688,
2.59908173515995));
#215487=CARTESIAN_POINT('',(46.7942619810922,-42.1132001505994,2.59908173515994));
#215488=CARTESIAN_POINT('Origin',(5.53970586838553E-15,1.8551658990402E-13,
2.59908173516022));
#215489=CARTESIAN_POINT('',(46.855903642699,-41.7612723673355,2.90134173515995));
#215490=CARTESIAN_POINT('Ctrl Pts',(46.7942619810922,-42.1132001505994,
2.59908173515994));
#215491=CARTESIAN_POINT('Ctrl Pts',(46.7968184499057,-42.1103595112864,
2.59908174381654));
#215492=CARTESIAN_POINT('Ctrl Pts',(46.7993324362838,-42.107494724296,2.59915752000967));
#215493=CARTESIAN_POINT('Ctrl Pts',(46.8018034833201,-42.1046079742807,
2.59930729517442));
#215494=CARTESIAN_POINT('Ctrl Pts',(46.8160830868215,-42.0879261203861,
2.60017281085887));
#215495=CARTESIAN_POINT('Ctrl Pts',(46.828931992104,-42.0705099543501,2.6035065180002));
#215496=CARTESIAN_POINT('Ctrl Pts',(46.840256683147,-42.0527856759055,2.60896880596406));
#215497=CARTESIAN_POINT('Ctrl Pts',(46.8448241915573,-42.0456370666804,
2.61117187235407));
#215498=CARTESIAN_POINT('Ctrl Pts',(46.8491442126976,-42.0384382358158,
2.61372076577158));
#215499=CARTESIAN_POINT('Ctrl Pts',(46.8532123574524,-42.0312165334044,
2.61659179896954));
#215500=CARTESIAN_POINT('Ctrl Pts',(46.8547132558794,-42.0285521636627,
2.61765103591179));
#215501=CARTESIAN_POINT('Ctrl Pts',(46.8561797434814,-42.0258847247789,
2.6187542245512));
#215502=CARTESIAN_POINT('Ctrl Pts',(46.8576115380198,-42.0232156132254,
2.61990022440366));
#215503=CARTESIAN_POINT('Ctrl Pts',(46.8602961527793,-42.0182110290628,
2.62204897412703));
#215504=CARTESIAN_POINT('Ctrl Pts',(46.8628587997329,-42.0132005644169,
2.6243482320174));
#215505=CARTESIAN_POINT('Ctrl Pts',(46.8652976184992,-42.0081934246209,
2.62679048030275));
#215506=CARTESIAN_POINT('Ctrl Pts',(46.8738334841813,-41.9906684353348,
2.63533834930149));
#215507=CARTESIAN_POINT('Ctrl Pts',(46.8808524512368,-41.9731841724641,
2.64563784783532));
#215508=CARTESIAN_POINT('Ctrl Pts',(46.8862747746138,-41.956135331631,2.65736666737934));
#215509=CARTESIAN_POINT('Ctrl Pts',(46.8889859363023,-41.9476109112144,
2.66323107715134));
#215510=CARTESIAN_POINT('Ctrl Pts',(46.8912979378218,-41.9391953469834,
2.66945281780743));
#215511=CARTESIAN_POINT('Ctrl Pts',(46.8932008176778,-41.9309379818013,
2.6759916063117));
#215512=CARTESIAN_POINT('Ctrl Pts',(46.8941522576058,-41.9268092992103,
2.67926100056383));
#215513=CARTESIAN_POINT('Ctrl Pts',(46.8950014172059,-41.9227201664594,
2.68260965685093));
#215514=CARTESIAN_POINT('Ctrl Pts',(46.8957470516903,-41.9186767517584,
2.68603254012452));
#215515=CARTESIAN_POINT('Ctrl Pts',(46.8964926861748,-41.9146333370574,
2.68945542339811));
#215516=CARTESIAN_POINT('Ctrl Pts',(46.8971346781641,-41.9106356952798,
2.69295261525355));
#215517=CARTESIAN_POINT('Ctrl Pts',(46.8976720238192,-41.9066898836027,
2.69651891172069));
#215518=CARTESIAN_POINT('Ctrl Pts',(46.8976766062523,-41.9066562340929,
2.69654932476057));
#215519=CARTESIAN_POINT('Ctrl Pts',(46.8976811811501,-41.9066225884699,
2.69657974261115));
#215520=CARTESIAN_POINT('Ctrl Pts',(46.8976857485125,-41.9065889467368,
2.69661016526943));
#215521=CARTESIAN_POINT('Ctrl Pts',(46.9000183671521,-41.8894076224748,
2.71214746101187));
#215522=CARTESIAN_POINT('Ctrl Pts',(46.9005163877047,-41.8732226654011,
2.7288056556773));
#215523=CARTESIAN_POINT('Ctrl Pts',(46.8993610201076,-41.858119701628,2.74628040012593));
#215524=CARTESIAN_POINT('Ctrl Pts',(46.8981665787456,-41.8425059656487,
2.76434612882826));
#215525=CARTESIAN_POINT('Ctrl Pts',(46.8952045688313,-41.8280478726808,
2.78328592655023));
#215526=CARTESIAN_POINT('Ctrl Pts',(46.890630663343,-41.8148672739068,2.80278753268583));
#215527=CARTESIAN_POINT('Ctrl Pts',(46.8861437631615,-41.8019373978561,
2.8219181772373));
#215528=CARTESIAN_POINT('Ctrl Pts',(46.8801049472937,-41.7902363430306,
2.84159092316289));
#215529=CARTESIAN_POINT('Ctrl Pts',(46.8726287066499,-41.7799143139093,
2.86151233818347));
#215530=CARTESIAN_POINT('Ctrl Pts',(46.8676759593283,-41.7730763314901,
2.87470957722199));
#215531=CARTESIAN_POINT('Ctrl Pts',(46.8620917411132,-41.7668442729545,
2.88801594388774));
#215532=CARTESIAN_POINT('Ctrl Pts',(46.855903642699,-41.7612723673355,2.90134173515995));
#215533=CARTESIAN_POINT('',(46.5911245387435,-41.5228599914555,3.47153072139043));
#215534=CARTESIAN_POINT('',(46.855903642699,-41.7612723673355,2.90134173515995));
#215535=CARTESIAN_POINT('',(50.3023253562,-36.9399086546478,3.47153072139046));
#215536=CARTESIAN_POINT('Origin',(5.53234440788222E-15,1.85015204418142E-13,
3.47153072139072));
#215537=CARTESIAN_POINT('',(50.5905785208489,-37.1493329797253,2.90134173515998));
#215538=CARTESIAN_POINT('',(50.3023253562,-36.9399086546478,3.47153072139047));
#215539=CARTESIAN_POINT('',(50.9219998155904,-37.0158684358552,2.59908173515998));
#215540=CARTESIAN_POINT('Ctrl Pts',(50.5905785208489,-37.1493329797253,
2.90134173515998));
#215541=CARTESIAN_POINT('Ctrl Pts',(50.6005343088832,-37.1565661199774,
2.88164837656534));
#215542=CARTESIAN_POINT('Ctrl Pts',(50.6116037659411,-37.162197743186,2.86203734438791));
#215543=CARTESIAN_POINT('Ctrl Pts',(50.6236016024818,-37.1661909570578,
2.84277945977646));
#215544=CARTESIAN_POINT('Ctrl Pts',(50.6358405223277,-37.1702644101623,
2.82313460919363));
#215545=CARTESIAN_POINT('Ctrl Pts',(50.6490462309976,-37.172633529828,2.80385576862541));
#215546=CARTESIAN_POINT('Ctrl Pts',(50.6630602183739,-37.1732217245284,
2.78521678517463));
#215547=CARTESIAN_POINT('Ctrl Pts',(50.6765297750448,-37.1737870683979,
2.76730190933408));
#215548=CARTESIAN_POINT('Ctrl Pts',(50.690746893978,-37.1727073465953,2.74997687278597));
#215549=CARTESIAN_POINT('Ctrl Pts',(50.7055935641283,-37.1698754144239,
2.7334925334444));
#215550=CARTESIAN_POINT('Ctrl Pts',(50.7169982609442,-37.1677000224006,
2.72082983598454));
#215551=CARTESIAN_POINT('Ctrl Pts',(50.7287749695304,-37.1644899772777,
2.7086632103887));
#215552=CARTESIAN_POINT('Ctrl Pts',(50.7408753824657,-37.1601789145079,
2.69711645335819));
#215553=CARTESIAN_POINT('Ctrl Pts',(50.7409070954901,-37.1601676159812,
2.69708619136725));
#215554=CARTESIAN_POINT('Ctrl Pts',(50.7409388110967,-37.1601563091353,
2.69705593387192));
#215555=CARTESIAN_POINT('Ctrl Pts',(50.7409705292826,-37.1601449939709,
2.69702568087544));
#215556=CARTESIAN_POINT('Ctrl Pts',(50.744371363825,-37.1589317782461,2.6937819444324));
#215557=CARTESIAN_POINT('Ctrl Pts',(50.7477999807011,-37.1576225876049,
2.69059266624673));
#215558=CARTESIAN_POINT('Ctrl Pts',(50.751251742581,-37.1562191103348,2.6874621934265));
#215559=CARTESIAN_POINT('Ctrl Pts',(50.7704600126089,-37.1484090784378,
2.67004182396362));
#215560=CARTESIAN_POINT('Ctrl Pts',(50.7903868440168,-37.1376839209007,
2.65443567878399));
#215561=CARTESIAN_POINT('Ctrl Pts',(50.8102141227966,-37.1243864882722,
2.64136852353726));
#215562=CARTESIAN_POINT('Ctrl Pts',(50.8191128800932,-37.1184184163576,
2.63550380330065));
#215563=CARTESIAN_POINT('Ctrl Pts',(50.8279919247152,-37.111932323635,2.6301499745124));
#215564=CARTESIAN_POINT('Ctrl Pts',(50.8367795369359,-37.104959081816,2.6253698111923));
#215565=CARTESIAN_POINT('Ctrl Pts',(50.8405985143445,-37.1019286052424,
2.62329241687049));
#215566=CARTESIAN_POINT('Ctrl Pts',(50.8444000194072,-37.0988061338472,
2.62132362131403));
#215567=CARTESIAN_POINT('Ctrl Pts',(50.8481780352577,-37.0955942139014,
2.61946873372323));
#215568=CARTESIAN_POINT('Ctrl Pts',(50.8614010907345,-37.0843524940913,
2.61297662715543));
#215569=CARTESIAN_POINT('Ctrl Pts',(50.8743364007572,-37.0720150276365,
2.60787989113944));
#215570=CARTESIAN_POINT('Ctrl Pts',(50.8867260065482,-37.0586909963613,
2.60440616886155));
#215571=CARTESIAN_POINT('Ctrl Pts',(50.8929208094436,-37.0520289807237,
2.6026693077226));
#215572=CARTESIAN_POINT('Ctrl Pts',(50.8989791867717,-37.0451203242403,
2.6013382004016));
#215573=CARTESIAN_POINT('Ctrl Pts',(50.9048689000892,-37.0379786793002,
2.6004413072356));
#215574=CARTESIAN_POINT('Ctrl Pts',(50.907813756748,-37.0344078568301,2.59999286065259));
#215575=CARTESIAN_POINT('Ctrl Pts',(50.9107164475038,-37.0307787873183,
2.59965296768487));
#215576=CARTESIAN_POINT('Ctrl Pts',(50.9135729431182,-37.0270931777231,
2.59942518630929));
#215577=CARTESIAN_POINT('Ctrl Pts',(50.9164294387326,-37.0234075681279,
2.59919740493371));
#215578=CARTESIAN_POINT('Ctrl Pts',(50.9192397378254,-37.0196654174462,
2.59908173791591));
#215579=CARTESIAN_POINT('Ctrl Pts',(50.9219998155904,-37.0158684358552,
2.59908173515998));
#215580=CARTESIAN_POINT('',(50.9399462128206,-36.9911673391699,2.59908173515998));
#215581=CARTESIAN_POINT('Origin',(5.52946850001198E-15,1.85503947806925E-13,
2.59908173516023));
#215582=CARTESIAN_POINT('',(50.9644637245897,-36.6347241449646,2.90134173515999));
#215583=CARTESIAN_POINT('Ctrl Pts',(50.9399462128206,-36.9911673391699,
2.59908173515998));
#215584=CARTESIAN_POINT('Ctrl Pts',(50.9421917493684,-36.9880750374199,
2.59908174381653));
#215585=CARTESIAN_POINT('Ctrl Pts',(50.9443925120844,-36.9849631608996,
2.5991575200097));
#215586=CARTESIAN_POINT('Ctrl Pts',(50.9465482749236,-36.9818339300535,
2.59930729517445));
#215587=CARTESIAN_POINT('Ctrl Pts',(50.9590059247082,-36.9637508360938,
2.60017281085871));
#215588=CARTESIAN_POINT('Ctrl Pts',(50.9699639572693,-36.945087001318,2.60350651799879));
#215589=CARTESIAN_POINT('Ctrl Pts',(50.9793739188802,-36.9262760657776,
2.60896880596056));
#215590=CARTESIAN_POINT('Ctrl Pts',(50.983169172867,-36.9186891827427,2.61117187235137));
#215591=CARTESIAN_POINT('Ctrl Pts',(50.9867130457539,-36.9110782226516,
2.61372076577008));
#215592=CARTESIAN_POINT('Ctrl Pts',(50.9900040313326,-36.9034708445581,
2.61659179896957));
#215593=CARTESIAN_POINT('Ctrl Pts',(50.9912182052063,-36.9006641839065,
2.61765103591182));
#215594=CARTESIAN_POINT('Ctrl Pts',(50.9923978359483,-36.8978580678366,
2.61875422455123));
#215595=CARTESIAN_POINT('Ctrl Pts',(50.9935427888375,-36.8950539146727,
2.6199002244037));
#215596=CARTESIAN_POINT('Ctrl Pts',(50.9956895755046,-36.8897961274904,
2.62204897412707));
#215597=CARTESIAN_POINT('Ctrl Pts',(50.9977144478404,-36.8845452411461,
2.62434823201743));
#215598=CARTESIAN_POINT('Ctrl Pts',(50.9996165178741,-36.879310605008,2.62679048030278));
#215599=CARTESIAN_POINT('Ctrl Pts',(51.006273762992,-36.8609893785245,2.63533834930152));
#215600=CARTESIAN_POINT('Ctrl Pts',(51.0114266762823,-36.8428672144352,
2.64563784783535));
#215601=CARTESIAN_POINT('Ctrl Pts',(51.0150372064717,-36.8253449818061,
2.65736666737937));
#215602=CARTESIAN_POINT('Ctrl Pts',(51.0168424715664,-36.8165838654915,
2.66323107715138));
#215603=CARTESIAN_POINT('Ctrl Pts',(51.0182621417031,-36.807972732636,2.66945281780747));
#215604=CARTESIAN_POINT('Ctrl Pts',(51.019291467691,-36.7995616970572,2.67599160631174));
#215605=CARTESIAN_POINT('Ctrl Pts',(51.019806130685,-36.7953561792679,2.67926100056388));
#215606=CARTESIAN_POINT('Ctrl Pts',(51.0202232077374,-36.7912006858659,
2.68260965685096));
#215607=CARTESIAN_POINT('Ctrl Pts',(51.0205421056331,-36.7871014813869,
2.68603254012456));
#215608=CARTESIAN_POINT('Ctrl Pts',(51.0208610035287,-36.7830022769079,
2.68945542339815));
#215609=CARTESIAN_POINT('Ctrl Pts',(51.0210816112671,-36.7789594281942,
2.6929526152536));
#215610=CARTESIAN_POINT('Ctrl Pts',(51.0212035636555,-36.7749790641708,
2.69651891172074));
#215611=CARTESIAN_POINT('Ctrl Pts',(51.021204603654,-36.7749451200018,2.69654932476061));
#215612=CARTESIAN_POINT('Ctrl Pts',(51.0212056365647,-36.774911180486,2.6965797426112));
#215613=CARTESIAN_POINT('Ctrl Pts',(51.0212066623879,-36.7748772456265,
2.69661016526947));
#215614=CARTESIAN_POINT('Ctrl Pts',(51.0217305652766,-36.7575462174142,
2.71214746101235));
#215615=CARTESIAN_POINT('Ctrl Pts',(51.0205340689296,-36.7413978659053,
2.72880565567827));
#215616=CARTESIAN_POINT('Ctrl Pts',(51.017806340963,-36.7264984065469,2.74628040012743));
#215617=CARTESIAN_POINT('Ctrl Pts',(51.0149863630479,-36.711095057367,2.76434612882988));
#215618=CARTESIAN_POINT('Ctrl Pts',(51.0105292970941,-36.6970257816896,
2.78328592655197));
#215619=CARTESIAN_POINT('Ctrl Pts',(51.0046027002038,-36.6843954909265,
2.80278753268768));
#215620=CARTESIAN_POINT('Ctrl Pts',(50.9987888396572,-36.6720054548709,
2.8219181772387));
#215621=CARTESIAN_POINT('Ctrl Pts',(50.9915600117752,-36.660999727791,2.84159092316381));
#215622=CARTESIAN_POINT('Ctrl Pts',(50.9830457809182,-36.6515157237711,
2.8615123381839));
#215623=CARTESIAN_POINT('Ctrl Pts',(50.9774054014705,-36.6452329036017,
2.87470957722229));
#215624=CARTESIAN_POINT('Ctrl Pts',(50.9712003466852,-36.6396186946836,
2.88801594388792));
#215625=CARTESIAN_POINT('Ctrl Pts',(50.9644637245897,-36.6347241449646,
2.90134173515999));
#215626=CARTESIAN_POINT('',(50.6762142289952,-36.4252947698671,3.47153072139047));
#215627=CARTESIAN_POINT('',(50.9644637245897,-36.6347241449646,2.90134173515999));
#215628=CARTESIAN_POINT('',(53.8880358395974,-31.4795232016781,3.4715307213905));
#215629=CARTESIAN_POINT('Origin',(5.53234440788222E-15,1.85015204418142E-13,
3.47153072139072));
#215630=CARTESIAN_POINT('',(54.1966007261211,-31.6576696180576,2.90134173516002));
#215631=CARTESIAN_POINT('',(53.8880358395974,-31.4795232016781,3.4715307213905));
#215632=CARTESIAN_POINT('',(54.5122556166615,-31.4902932482899,2.59908173516002));
#215633=CARTESIAN_POINT('Ctrl Pts',(54.1966007261211,-31.6576696180576,
2.90134173516003));
#215634=CARTESIAN_POINT('Ctrl Pts',(54.2072580443422,-31.6638224711865,
2.88164837656537));
#215635=CARTESIAN_POINT('Ctrl Pts',(54.2188555266759,-31.6682661704385,
2.86203734438793));
#215636=CARTESIAN_POINT('Ctrl Pts',(54.2312050423222,-31.6709833936507,
2.84277945977648));
#215637=CARTESIAN_POINT('Ctrl Pts',(54.2438027078777,-31.6737552164693,
2.82313460919376));
#215638=CARTESIAN_POINT('Ctrl Pts',(54.2571837147316,-31.674730985416,2.80385576862566));
#215639=CARTESIAN_POINT('Ctrl Pts',(54.2711824151068,-31.6738510973596,
2.78521678517498));
#215640=CARTESIAN_POINT('Ctrl Pts',(54.2846372786624,-31.6730053921566,
2.76730190933489));
#215641=CARTESIAN_POINT('Ctrl Pts',(54.2986636530693,-31.6704454915891,
2.74997687278722));
#215642=CARTESIAN_POINT('Ctrl Pts',(54.3131329740888,-31.6660771734233,
2.73349253344603));
#215643=CARTESIAN_POINT('Ctrl Pts',(54.3242478043974,-31.6627215829929,
2.72082983598559));
#215644=CARTESIAN_POINT('Ctrl Pts',(54.3356244578585,-31.658298121582,2.70866321038921));
#215645=CARTESIAN_POINT('Ctrl Pts',(54.3472079546998,-31.6527458376959,
2.69711645335823));
#215646=CARTESIAN_POINT('Ctrl Pts',(54.3472383129792,-31.65273128615,2.69708619136728));
#215647=CARTESIAN_POINT('Ctrl Pts',(54.3472686729573,-31.6527167260605,
2.69705593387196));
#215648=CARTESIAN_POINT('Ctrl Pts',(54.3472990346309,-31.6527021574285,
2.69702568087547));
#215649=CARTESIAN_POINT('Ctrl Pts',(54.3505544234705,-31.6511401038179,
2.69378194443243));
#215650=CARTESIAN_POINT('Ctrl Pts',(54.3538274103387,-31.6494796970068,
2.69059266624677));
#215651=CARTESIAN_POINT('Ctrl Pts',(54.3571135597836,-31.6477231007671,
2.68746219342654));
#215652=CARTESIAN_POINT('Ctrl Pts',(54.3754002342682,-31.637948042093,2.67004182396181));
#215653=CARTESIAN_POINT('Ctrl Pts',(54.394096820175,-31.6251987170246,2.65443567878073));
#215654=CARTESIAN_POINT('Ctrl Pts',(54.4124255228509,-31.6099016141395,
2.64136852353315));
#215655=CARTESIAN_POINT('Ctrl Pts',(54.4206516984361,-31.6030360625235,
2.63550380329814));
#215656=CARTESIAN_POINT('Ctrl Pts',(54.4288041214158,-31.5956573884075,
2.63014997451128));
#215657=CARTESIAN_POINT('Ctrl Pts',(54.436814691924,-31.5878037911374,2.62536981119229));
#215658=CARTESIAN_POINT('Ctrl Pts',(54.4402959775156,-31.5843907239917,
2.62329241687049));
#215659=CARTESIAN_POINT('Ctrl Pts',(54.4437502703992,-31.5808879923392,
2.62132362131404));
#215660=CARTESIAN_POINT('Ctrl Pts',(54.4471718528276,-31.577298757436,2.61946873372324));
#215661=CARTESIAN_POINT('Ctrl Pts',(54.4591473913267,-31.5647364352745,
2.61297662715544));
#215662=CARTESIAN_POINT('Ctrl Pts',(54.4707222239585,-31.5511144466733,
2.60787989113945));
#215663=CARTESIAN_POINT('Ctrl Pts',(54.4816512176788,-31.5365683393817,
2.60440616886156));
#215664=CARTESIAN_POINT('Ctrl Pts',(54.487115714539,-31.5292952857359,2.60266930772261));
#215665=CARTESIAN_POINT('Ctrl Pts',(54.4924187521967,-31.5217912027236,
2.60133820040162));
#215666=CARTESIAN_POINT('Ctrl Pts',(54.4975296958776,-31.5140730377796,
2.60044130723562));
#215667=CARTESIAN_POINT('Ctrl Pts',(54.5000851677181,-31.5102139553076,
2.59999286065261));
#215668=CARTESIAN_POINT('Ctrl Pts',(54.5025926161711,-31.5063013524142,
2.5996529676849));
#215669=CARTESIAN_POINT('Ctrl Pts',(54.5050482124964,-31.5023373478771,
2.59942518630932));
#215670=CARTESIAN_POINT('Ctrl Pts',(54.5075038088218,-31.49837334334,2.59919740493374));
#215671=CARTESIAN_POINT('Ctrl Pts',(54.5099075515421,-31.4943579363058,
2.59908173791587));
#215672=CARTESIAN_POINT('Ctrl Pts',(54.5122556166615,-31.4902932482899,
2.59908173516002));
#215673=CARTESIAN_POINT('',(54.5275217339723,-31.4638515574732,2.59908173516003));
#215674=CARTESIAN_POINT('Origin',(5.52060867199534E-15,1.85490304868177E-13,
2.59908173516022));
#215675=CARTESIAN_POINT('',(54.5146464769142,-31.1067982185526,2.90134173516002));
#215676=CARTESIAN_POINT('Ctrl Pts',(54.5275217339724,-31.4638515574732,
2.59908173516003));
#215677=CARTESIAN_POINT('Ctrl Pts',(54.5294317356861,-31.4605414731911,
2.59908174381663));
#215678=CARTESIAN_POINT('Ctrl Pts',(54.5312951627231,-31.4572166015113,
2.59915752000975));
#215679=CARTESIAN_POINT('Ctrl Pts',(54.5331120223763,-31.4538791743424,
2.5993072951745));
#215680=CARTESIAN_POINT('Ctrl Pts',(54.5436112298312,-31.434592962472,2.60017281085893));
#215681=CARTESIAN_POINT('Ctrl Pts',(54.552558331177,-31.414885943828,2.60350651800011));
#215682=CARTESIAN_POINT('Ctrl Pts',(54.5599504658498,-31.3951944477304,
2.60896880596372));
#215683=CARTESIAN_POINT('Ctrl Pts',(54.5629318838118,-31.3872524143714,
2.61117187235382));
#215684=CARTESIAN_POINT('Ctrl Pts',(54.5656607810285,-31.3793127123329,
2.61372076577147));
#215685=CARTESIAN_POINT('Ctrl Pts',(54.5681385507011,-31.3714030065911,
2.6165917989696));
#215686=CARTESIAN_POINT('Ctrl Pts',(54.5690526972785,-31.3684848053911,
2.61765103591185));
#215687=CARTESIAN_POINT('Ctrl Pts',(54.5699325468793,-31.3655707565299,
2.61875422455126));
#215688=CARTESIAN_POINT('Ctrl Pts',(54.5707781137758,-31.3626622846444,
2.61990022440373));
#215689=CARTESIAN_POINT('Ctrl Pts',(54.5723635517066,-31.3572088998592,
2.6220489741271));
#215690=CARTESIAN_POINT('Ctrl Pts',(54.5738284644995,-31.3517751216261,
2.62434823201746));
#215691=CARTESIAN_POINT('Ctrl Pts',(54.5751729463232,-31.3463703409148,
2.62679048030281));
#215692=CARTESIAN_POINT('Ctrl Pts',(54.5798786327063,-31.3274536084252,
2.63533834930155));
#215693=CARTESIAN_POINT('Ctrl Pts',(54.5831090358351,-31.3088920933393,
2.64563784783539));
#215694=CARTESIAN_POINT('Ctrl Pts',(54.5848682151126,-31.2910884461616,
2.65736666737941));
#215695=CARTESIAN_POINT('Ctrl Pts',(54.5857478047514,-31.2821866225728,
2.66323107715142));
#215696=CARTESIAN_POINT('Ctrl Pts',(54.5862595893022,-31.2734742664663,
2.66945281780751));
#215697=CARTESIAN_POINT('Ctrl Pts',(54.5864040839111,-31.2650017135568,
2.67599160631178));
#215698=CARTESIAN_POINT('Ctrl Pts',(54.5864763312156,-31.260765437102,2.67926100056391));
#215699=CARTESIAN_POINT('Ctrl Pts',(54.5864567561368,-31.2565891115044,
2.68260965685101));
#215700=CARTESIAN_POINT('Ctrl Pts',(54.5863454235316,-31.2524790289895,
2.6860325401246));
#215701=CARTESIAN_POINT('Ctrl Pts',(54.5862340909264,-31.2483689464745,
2.6894554233982));
#215702=CARTESIAN_POINT('Ctrl Pts',(54.5860308973892,-31.2443251851212,
2.69295261525362));
#215703=CARTESIAN_POINT('Ctrl Pts',(54.5857361203751,-31.2403538784526,
2.69651891172076));
#215704=CARTESIAN_POINT('Ctrl Pts',(54.5857336065445,-31.2403200115239,
2.69654932476065));
#215705=CARTESIAN_POINT('Ctrl Pts',(54.5857310861515,-31.2402861499638,
2.69657974261123));
#215706=CARTESIAN_POINT('Ctrl Pts',(54.5857285591964,-31.2402522937752,
2.69661016526951));
#215707=CARTESIAN_POINT('Ctrl Pts',(54.5844380063444,-31.2229614439857,
2.71214746101182));
#215708=CARTESIAN_POINT('Ctrl Pts',(54.5815601021622,-31.207026622761,2.7288056556771));
#215709=CARTESIAN_POINT('Ctrl Pts',(54.5772898993847,-31.192493909413,2.74628040012557));
#215710=CARTESIAN_POINT('Ctrl Pts',(54.5728752811848,-31.1774697093497,
2.76434612882767));
#215711=CARTESIAN_POINT('Ctrl Pts',(54.566971991739,-31.1639433968916,2.78328592654939));
#215712=CARTESIAN_POINT('Ctrl Pts',(54.5597576364827,-31.1520017942483,
2.80278753268472));
#215713=CARTESIAN_POINT('Ctrl Pts',(54.5526805134439,-31.1402873460149,
2.82191817723584));
#215714=CARTESIAN_POINT('Ctrl Pts',(54.5443408740986,-31.130097527729,2.84159092316106));
#215715=CARTESIAN_POINT('Ctrl Pts',(54.5348819367233,-31.1215554575426,
2.86151233818129));
#215716=CARTESIAN_POINT('Ctrl Pts',(54.5286157223268,-31.1158966355148,
2.87470957722054));
#215717=CARTESIAN_POINT('Ctrl Pts',(54.5218578148499,-31.1109617866612,
2.88801594388705));
#215718=CARTESIAN_POINT('Ctrl Pts',(54.5146464769142,-31.1067982185526,
2.90134173516002));
#215719=CARTESIAN_POINT('',(54.2060847114746,-30.928646396297,3.47153072139051));
#215720=CARTESIAN_POINT('',(54.5146464769142,-31.1067982185526,2.90134173516002));
#215721=CARTESIAN_POINT('',(56.8833377255397,-25.6742415049971,3.47153072139054));
#215722=CARTESIAN_POINT('Origin',(5.53234440788222E-15,1.85015204418142E-13,
3.47153072139072));
#215723=CARTESIAN_POINT('',(57.2088336324702,-25.8191582032612,2.90134173516006));
#215724=CARTESIAN_POINT('',(56.8833377255398,-25.6742415049971,3.47153072139054));
#215725=CARTESIAN_POINT('',(57.5052637377735,-25.6197038181289,2.59908173516006));
#215726=CARTESIAN_POINT('Ctrl Pts',(57.2088336324702,-25.8191582032612,
2.90134173516006));
#215727=CARTESIAN_POINT('Ctrl Pts',(57.220075717068,-25.8241633573203,2.88164837656754));
#215728=CARTESIAN_POINT('Ctrl Pts',(57.2320741602326,-25.8273704465165,
2.86203734439222));
#215729=CARTESIAN_POINT('Ctrl Pts',(57.2446400511053,-25.8287819086033,
2.84277945978278));
#215730=CARTESIAN_POINT('Ctrl Pts',(57.257458439709,-25.8302217324655,2.82313460920208));
#215731=CARTESIAN_POINT('Ctrl Pts',(57.2708681396342,-25.829793459965,2.80385576863588));
#215732=CARTESIAN_POINT('Ctrl Pts',(57.284698180316,-25.8274551293905,2.78521678518692));
#215733=CARTESIAN_POINT('Ctrl Pts',(57.2979909364545,-25.8252076408391,
2.76730190934833));
#215734=CARTESIAN_POINT('Ctrl Pts',(57.3116728904409,-25.8211956083142,
2.74997687280199));
#215735=CARTESIAN_POINT('Ctrl Pts',(57.3256063334194,-25.8153387643633,
2.73349253346188));
#215736=CARTESIAN_POINT('Ctrl Pts',(57.3363095208179,-25.8108397400758,
2.72082983599576));
#215737=CARTESIAN_POINT('Ctrl Pts',(57.3471614741618,-25.8052513267441,
2.70866321039406));
#215738=CARTESIAN_POINT('Ctrl Pts',(57.3581011436977,-25.7985186537232,
2.69711645335827));
#215739=CARTESIAN_POINT('Ctrl Pts',(57.3581298146206,-25.7985010085879,
2.69708619136733));
#215740=CARTESIAN_POINT('Ctrl Pts',(57.3581584863397,-25.7984833547782,
2.697055933872));
#215741=CARTESIAN_POINT('Ctrl Pts',(57.3581871588522,-25.7984656922957,
2.69702568087553));
#215742=CARTESIAN_POINT('Ctrl Pts',(57.3612614352676,-25.7965719149855,
2.69378194443248));
#215743=CARTESIAN_POINT('Ctrl Pts',(57.364342932599,-25.7945784837689,2.69059266624683));
#215744=CARTESIAN_POINT('Ctrl Pts',(57.3674274658679,-25.7924880141957,
2.68746219342659));
#215745=CARTESIAN_POINT('Ctrl Pts',(57.3845921921775,-25.7808550263318,
2.67004182395904));
#215746=CARTESIAN_POINT('Ctrl Pts',(57.4018536888761,-25.766221218004,2.65443567877572));
#215747=CARTESIAN_POINT('Ctrl Pts',(57.4184830023465,-25.7490920431211,
2.64136852352685));
#215748=CARTESIAN_POINT('Ctrl Pts',(57.4259464685184,-25.7414042322251,
2.63550380329434));
#215749=CARTESIAN_POINT('Ctrl Pts',(57.433282950203,-25.7332138190148,2.63014997450962));
#215750=CARTESIAN_POINT('Ctrl Pts',(57.4404287135114,-25.7245659119503,
2.62536981119236));
#215751=CARTESIAN_POINT('Ctrl Pts',(57.4435341655926,-25.7208076485105,
2.62329241687056));
#215752=CARTESIAN_POINT('Ctrl Pts',(57.4466034003415,-25.7169630332617,
2.6213236213141));
#215753=CARTESIAN_POINT('Ctrl Pts',(57.4496310617745,-25.7130358078096,
2.6194687337233));
#215754=CARTESIAN_POINT('Ctrl Pts',(57.4602278767901,-25.6992905187273,
2.6129766271555));
#215755=CARTESIAN_POINT('Ctrl Pts',(57.4703154157425,-25.6845332533373,
2.60787989113952));
#215756=CARTESIAN_POINT('Ctrl Pts',(57.47966405705,-25.6689244402248,2.60440616886163));
#215757=CARTESIAN_POINT('Ctrl Pts',(57.4843383777038,-25.6611200336685,
2.60266930772268));
#215758=CARTESIAN_POINT('Ctrl Pts',(57.4888279745008,-25.6531027404311,
2.60133820040167));
#215759=CARTESIAN_POINT('Ctrl Pts',(57.4931041519767,-25.6448926173134,
2.60044130723566));
#215760=CARTESIAN_POINT('Ctrl Pts',(57.4952422407146,-25.6407875557545,
2.59999286065266));
#215761=CARTESIAN_POINT('Ctrl Pts',(57.4973269747348,-25.6366342867756,
2.59965296768494));
#215762=CARTESIAN_POINT('Ctrl Pts',(57.4993547677439,-25.6324353177599,
2.59942518630936));
#215763=CARTESIAN_POINT('Ctrl Pts',(57.501382560753,-25.6282363487441,2.59919740493378));
#215764=CARTESIAN_POINT('Ctrl Pts',(57.5033534111924,-25.6239916789971,
2.599081737916));
#215765=CARTESIAN_POINT('Ctrl Pts',(57.5052637377735,-25.6197038181289,
2.59908173516006));
#215766=CARTESIAN_POINT('',(57.5176823163891,-25.5918112338785,2.59908173516007));
#215767=CARTESIAN_POINT('Origin',(5.5132234544654E-15,1.85475810562667E-13,
2.59908173516024));
#215768=CARTESIAN_POINT('',(57.4675553545143,-25.2380597013421,2.90134173516006));
#215769=CARTESIAN_POINT('Ctrl Pts',(57.5176823163891,-25.5918112338785,
2.59908173516007));
#215770=CARTESIAN_POINT('Ctrl Pts',(57.5192358568904,-25.5883196330406,
2.59908174381659));
#215771=CARTESIAN_POINT('Ctrl Pts',(57.5207415321518,-25.5848181941911,
2.59915752000978));
#215772=CARTESIAN_POINT('Ctrl Pts',(57.5221995827245,-25.5813091362499,
2.59930729517453));
#215773=CARTESIAN_POINT('Ctrl Pts',(57.5306253163349,-25.5610311102414,
2.60017281085912));
#215774=CARTESIAN_POINT('Ctrl Pts',(57.53746346015,-25.5404968219493,2.60350651800139));
#215775=CARTESIAN_POINT('Ctrl Pts',(57.5427567781094,-25.5201405094463,
2.60896880596683));
#215776=CARTESIAN_POINT('Ctrl Pts',(57.5448916950085,-25.5119303403429,
2.61117187235623));
#215777=CARTESIAN_POINT('Ctrl Pts',(57.5467757181868,-25.5037488853943,
2.61372076577285));
#215778=CARTESIAN_POINT('Ctrl Pts',(57.548413124991,-25.4956235123957,2.61659179896965));
#215779=CARTESIAN_POINT('Ctrl Pts',(57.5490172286909,-25.4926257430702,
2.61765103591191));
#215780=CARTESIAN_POINT('Ctrl Pts',(57.5495876573342,-25.4896356883469,
2.61875422455132));
#215781=CARTESIAN_POINT('Ctrl Pts',(57.5501245740301,-25.4866547635665,
2.61990022440379));
#215782=CARTESIAN_POINT('Ctrl Pts',(57.5511312928348,-25.4810655296032,
2.62204897412716));
#215783=CARTESIAN_POINT('Ctrl Pts',(57.5520201961937,-25.4755083930928,
2.62434823201752));
#215784=CARTESIAN_POINT('Ctrl Pts',(57.5527923593833,-25.4699926837168,
2.62679048030287));
#215785=CARTESIAN_POINT('Ctrl Pts',(57.5554949305468,-25.4506877009008,
2.63533834930161));
#215786=CARTESIAN_POINT('Ctrl Pts',(57.5567674305414,-25.4318901986619,
2.64563784783545));
#215787=CARTESIAN_POINT('Ctrl Pts',(57.5566559849708,-25.4140001974198,
2.65736666737946));
#215788=CARTESIAN_POINT('Ctrl Pts',(57.5566002621854,-25.4050551967988,
2.66323107715147));
#215789=CARTESIAN_POINT('Ctrl Pts',(57.5561985539316,-25.396337071838,2.66945281780755));
#215790=CARTESIAN_POINT('Ctrl Pts',(57.5554566340484,-25.3878958286604,
2.67599160631182));
#215791=CARTESIAN_POINT('Ctrl Pts',(57.5550856741068,-25.3836752070716,
2.67926100056396));
#215792=CARTESIAN_POINT('Ctrl Pts',(57.5546296613655,-25.3795238059755,
2.68260965685105));
#215793=CARTESIAN_POINT('Ctrl Pts',(57.5540893180428,-25.3754478763487,
2.68603254012464));
#215794=CARTESIAN_POINT('Ctrl Pts',(57.5535489747201,-25.371371946722,2.68945542339823));
#215795=CARTESIAN_POINT('Ctrl Pts',(57.5529242061383,-25.3673715770247,
2.69295261525366));
#215796=CARTESIAN_POINT('Ctrl Pts',(57.5522159293602,-25.3634528381778,
2.6965189117208));
#215797=CARTESIAN_POINT('Ctrl Pts',(57.5522098892427,-25.3634194195426,
2.69654932476068));
#215798=CARTESIAN_POINT('Ctrl Pts',(57.5522038431597,-25.3633860069324,
2.69657974261126));
#215799=CARTESIAN_POINT('Ctrl Pts',(57.5521977911122,-25.3633526003503,
2.69661016526954));
#215800=CARTESIAN_POINT('Ctrl Pts',(57.5491069220867,-25.3462913711517,
2.71214746101163));
#215801=CARTESIAN_POINT('Ctrl Pts',(57.5445791409897,-25.3307446654468,
2.72880565567666));
#215802=CARTESIAN_POINT('Ctrl Pts',(57.5388132486366,-25.3167379215575,
2.74628040012487));
#215803=CARTESIAN_POINT('Ctrl Pts',(57.5328523576328,-25.3022574788905,
2.76434612882686));
#215804=CARTESIAN_POINT('Ctrl Pts',(57.5255675223694,-25.2894223267614,
2.78328592654847));
#215805=CARTESIAN_POINT('Ctrl Pts',(57.5171444507328,-25.2783002469352,
2.80278753268369));
#215806=CARTESIAN_POINT('Ctrl Pts',(57.5088816036426,-25.2673897324705,
2.82191817723485));
#215807=CARTESIAN_POINT('Ctrl Pts',(57.4995225236678,-25.2581274647602,
2.84159092316011));
#215808=CARTESIAN_POINT('Ctrl Pts',(57.4892225138715,-25.2506209171159,
2.86151233818038));
#215809=CARTESIAN_POINT('Ctrl Pts',(57.4823991184825,-25.2456480924685,
2.87470957721994));
#215810=CARTESIAN_POINT('Ctrl Pts',(57.4751623993626,-25.2414466709166,
2.88801594388677));
#215811=CARTESIAN_POINT('Ctrl Pts',(57.4675553545144,-25.2380597013421,
2.90134173516006));
#215812=CARTESIAN_POINT('',(57.1420619865024,-25.0931373005737,3.47153072139055));
#215813=CARTESIAN_POINT('',(57.4675553545144,-25.2380597013421,2.90134173516006));
#215814=CARTESIAN_POINT('',(59.2554138597574,-19.5876674457069,3.47153072139059));
#215815=CARTESIAN_POINT('Origin',(5.53234440788222E-15,1.85015204418142E-13,
3.47153072139072));
#215816=CARTESIAN_POINT('',(59.5942745858238,-19.6977666881836,2.90134173516011));
#215817=CARTESIAN_POINT('',(59.2554138597574,-19.5876674457069,3.47153072139059));
#215818=CARTESIAN_POINT('',(59.8682321556244,-19.4684195516687,2.5990817351601));
#215819=CARTESIAN_POINT('Ctrl Pts',(59.5942745858238,-19.6977666881836,
2.90134173516011));
#215820=CARTESIAN_POINT('Ctrl Pts',(59.6059782661688,-19.7015693056584,
2.88164837656642));
#215821=CARTESIAN_POINT('Ctrl Pts',(59.6182462127124,-19.7035046472589,
2.86203734438993));
#215822=CARTESIAN_POINT('Ctrl Pts',(59.6308908042838,-19.703594883946,2.84277945977939));
#215823=CARTESIAN_POINT('Ctrl Pts',(59.6437894749899,-19.7036869338398,
2.82313460919753));
#215824=CARTESIAN_POINT('Ctrl Pts',(59.6570809485104,-19.7018593121344,
2.80385576863025));
#215825=CARTESIAN_POINT('Ctrl Pts',(59.6705908046816,-19.6980881582794,
2.78521678518031));
#215826=CARTESIAN_POINT('Ctrl Pts',(59.6835758151876,-19.694463510333,2.76730190934067));
#215827=CARTESIAN_POINT('Ctrl Pts',(59.696763446405,-19.6890433025163,2.74997687279338));
#215828=CARTESIAN_POINT('Ctrl Pts',(59.7100083536281,-19.6817621015857,
2.73349253345249));
#215829=CARTESIAN_POINT('Ctrl Pts',(59.7201826317487,-19.676168935694,2.72082983598977));
#215830=CARTESIAN_POINT('Ctrl Pts',(59.7303909886965,-19.6694767982701,
2.70866321039124));
#215831=CARTESIAN_POINT('Ctrl Pts',(59.740566973611,-19.6616375006931,2.69711645335832));
#215832=CARTESIAN_POINT('Ctrl Pts',(59.7405936430526,-19.6616169552923,
2.69708619136737));
#215833=CARTESIAN_POINT('Ctrl Pts',(59.7406203123795,-19.6615964011813,
2.69705593387205));
#215834=CARTESIAN_POINT('Ctrl Pts',(59.7406469815888,-19.661575838362,2.69702568087556));
#215835=CARTESIAN_POINT('Ctrl Pts',(59.7435064631644,-19.6593710859726,
2.69378194443252));
#215836=CARTESIAN_POINT('Ctrl Pts',(59.7463627094293,-19.6570664708003,
2.69059266624686));
#215837=CARTESIAN_POINT('Ctrl Pts',(59.7492118317302,-19.6546650315156,
2.68746219342663));
#215838=CARTESIAN_POINT('Ctrl Pts',(59.765066549526,-19.6413015679148,2.67004182396168));
#215839=CARTESIAN_POINT('Ctrl Pts',(59.7807038364411,-19.6249436073995,
2.65443567878043));
#215840=CARTESIAN_POINT('Ctrl Pts',(59.7954515664629,-19.6061700313502,
2.64136852353275));
#215841=CARTESIAN_POINT('Ctrl Pts',(59.8020705519296,-19.5977441904346,
2.63550380329795));
#215842=CARTESIAN_POINT('Ctrl Pts',(59.8085107122957,-19.5888317740057,
2.63014997451126));
#215843=CARTESIAN_POINT('Ctrl Pts',(59.8147133779312,-19.5794843054203,
2.62536981119241));
#215844=CARTESIAN_POINT('Ctrl Pts',(59.817408972519,-19.5754220220071,2.62329241687061));
#215845=CARTESIAN_POINT('Ctrl Pts',(59.820059521955,-19.5712776455712,2.62132362131414));
#215846=CARTESIAN_POINT('Ctrl Pts',(59.8226600907005,-19.5670554570741,
2.61946873372334));
#215847=CARTESIAN_POINT('Ctrl Pts',(59.8317620813098,-19.5522777973345,
2.61297662715554));
#215848=CARTESIAN_POINT('Ctrl Pts',(59.8402518053951,-19.5365469388435,
2.60787989113955));
#215849=CARTESIAN_POINT('Ctrl Pts',(59.8479176686193,-19.5200464333329,
2.60440616886165));
#215850=CARTESIAN_POINT('Ctrl Pts',(59.8517506002314,-19.5117961805776,
2.60266930772271));
#215851=CARTESIAN_POINT('Ctrl Pts',(59.8553775672057,-19.5033535162575,
2.60133820040171));
#215852=CARTESIAN_POINT('Ctrl Pts',(59.8587721277812,-19.494741386793,2.60044130723571));
#215853=CARTESIAN_POINT('Ctrl Pts',(59.8604694080689,-19.4904353220608,
2.5999928606527));
#215854=CARTESIAN_POINT('Ctrl Pts',(59.8621085868741,-19.4860868910805,
2.59965296768499));
#215855=CARTESIAN_POINT('Ctrl Pts',(59.8636863596424,-19.4816989623693,
2.59942518630941));
#215856=CARTESIAN_POINT('Ctrl Pts',(59.8652641324107,-19.4773110336581,
2.59919740493383));
#215857=CARTESIAN_POINT('Ctrl Pts',(59.8667804975195,-19.4728836066883,
2.59908173791605));
#215858=CARTESIAN_POINT('Ctrl Pts',(59.8682321556244,-19.4684195516687,
2.5990817351601));
#215859=CARTESIAN_POINT('',(59.8776671349988,-19.4393816709747,2.59908173516011));
#215860=CARTESIAN_POINT('Origin',(5.50739376141089E-15,1.8546062369304E-13,
2.59908173516023));
#215861=CARTESIAN_POINT('',(59.7908376697914,-19.0928077206402,2.90134173516011));
#215862=CARTESIAN_POINT('Ctrl Pts',(59.8776671349988,-19.4393816709747,
2.59908173516011));
#215863=CARTESIAN_POINT('Ctrl Pts',(59.8788471933727,-19.4357468082902,
2.59908174381669));
#215864=CARTESIAN_POINT('Ctrl Pts',(59.8799786203653,-19.4321071647678,
2.59915752000983));
#215865=CARTESIAN_POINT('Ctrl Pts',(59.8810618871504,-19.4284649220275,
2.59930729517458));
#215866=CARTESIAN_POINT('Ctrl Pts',(59.8873218328134,-19.4074172521818,
2.60017281085914));
#215867=CARTESIAN_POINT('Ctrl Pts',(59.8919760989615,-19.3862806722057,
2.60350651800119));
#215868=CARTESIAN_POINT('Ctrl Pts',(59.8951126055077,-19.3654825713214,
2.60896880596625));
#215869=CARTESIAN_POINT('Ctrl Pts',(59.8963776307492,-19.3570942188,2.61117187235579));
#215870=CARTESIAN_POINT('Ctrl Pts',(59.8973961381385,-19.3487606486692,
2.61372076577263));
#215871=CARTESIAN_POINT('Ctrl Pts',(59.8981752423039,-19.3405086316963,
2.61659179896971));
#215872=CARTESIAN_POINT('Ctrl Pts',(59.8984626844396,-19.3374641384334,
2.61765103591196));
#215873=CARTESIAN_POINT('Ctrl Pts',(59.8987174423899,-19.3344308375133,
2.61875422455137));
#215874=CARTESIAN_POINT('Ctrl Pts',(59.8989398263135,-19.3314101194736,
2.61990022440383));
#215875=CARTESIAN_POINT('Ctrl Pts',(59.8993567961702,-19.3257462731491,
2.6220489741272));
#215876=CARTESIAN_POINT('Ctrl Pts',(59.8996599510839,-19.3201266635119,
2.62434823201758));
#215877=CARTESIAN_POINT('Ctrl Pts',(59.8998513356578,-19.3145604567374,
2.62679048030293));
#215878=CARTESIAN_POINT('Ctrl Pts',(59.9005211816666,-19.2950787330265,
2.63533834930166));
#215879=CARTESIAN_POINT('Ctrl Pts',(59.8998218367508,-19.2762511930029,
2.64563784783549));
#215880=CARTESIAN_POINT('Ctrl Pts',(59.897840987353,-19.2584708442936,2.6573666673795));
#215881=CARTESIAN_POINT('Ctrl Pts',(59.8968505626541,-19.249580669939,2.66323107715151));
#215882=CARTESIAN_POINT('Ctrl Pts',(59.8955397627954,-19.2409522937254,
2.6694528178076));
#215883=CARTESIAN_POINT('Ctrl Pts',(59.8939195570494,-19.2326348443065,
2.67599160631187));
#215884=CARTESIAN_POINT('Ctrl Pts',(59.8931094541765,-19.228476119597,2.679261000564));
#215885=CARTESIAN_POINT('Ctrl Pts',(59.8922219999437,-19.2243951266215,
2.6826096568511));
#215886=CARTESIAN_POINT('Ctrl Pts',(59.891258566018,-19.2203980066209,2.68603254012469));
#215887=CARTESIAN_POINT('Ctrl Pts',(59.8902951320923,-19.2164008866203,
2.68945542339829));
#215888=CARTESIAN_POINT('Ctrl Pts',(59.8892556335612,-19.2124877374665,
2.69295261525372));
#215889=CARTESIAN_POINT('Ctrl Pts',(59.8881416170478,-19.2086645009642,
2.69651891172086));
#215890=CARTESIAN_POINT('Ctrl Pts',(59.8881321168201,-19.2086318967639,
2.69654932476074));
#215891=CARTESIAN_POINT('Ctrl Pts',(59.8881226112894,-19.2085992991793,
2.69657974261132));
#215892=CARTESIAN_POINT('Ctrl Pts',(59.888113100457,-19.2085667082132,2.69661016526959));
#215893=CARTESIAN_POINT('Ctrl Pts',(59.8832557794663,-19.1919220260043,
2.71214746101014));
#215894=CARTESIAN_POINT('Ctrl Pts',(59.8771277287724,-19.1769337687814,
2.72880565567341));
#215895=CARTESIAN_POINT('Ctrl Pts',(59.8699293191677,-19.1636064551686,
2.74628040011972));
#215896=CARTESIAN_POINT('Ctrl Pts',(59.8624874641301,-19.1498284206591,
2.76434612881963));
#215897=CARTESIAN_POINT('Ctrl Pts',(59.8539008972298,-19.1378250534723,
2.78328592653901));
#215898=CARTESIAN_POINT('Ctrl Pts',(59.8443613941499,-19.1276443522976,
2.80278753267194));
#215899=CARTESIAN_POINT('Ctrl Pts',(59.8350033524915,-19.1176573094815,
2.82191817722094));
#215900=CARTESIAN_POINT('Ctrl Pts',(59.8247273719274,-19.1094240716901,
2.84159092314401));
#215901=CARTESIAN_POINT('Ctrl Pts',(59.8136991387743,-19.1030352898944,
2.86151233816212));
#215902=CARTESIAN_POINT('Ctrl Pts',(59.8063933209376,-19.0988029459324,
2.87470957720769));
#215903=CARTESIAN_POINT('Ctrl Pts',(59.7987570771804,-19.0953809833341,
2.88801594388066));
#215904=CARTESIAN_POINT('Ctrl Pts',(59.7908376697914,-19.0928077206402,
2.90134173516011));
#215905=CARTESIAN_POINT('',(59.451978872661,-18.9827025415087,3.47153072139059));
#215906=CARTESIAN_POINT('',(59.7908376697914,-19.0928077206402,2.90134173516011));
#215907=CARTESIAN_POINT('',(60.978275279735,-13.2864868028986,3.47153072139063));
#215908=CARTESIAN_POINT('Origin',(5.53234440788222E-15,1.85015204418142E-13,
3.47153072139072));
#215909=CARTESIAN_POINT('',(61.3267881959115,-13.3605623192477,2.90134173516014));
#215910=CARTESIAN_POINT('',(60.978275279735,-13.2864868028986,3.47153072139063));
#215911=CARTESIAN_POINT('',(61.5752716937453,-13.1038352065718,2.59908173516015));
#215912=CARTESIAN_POINT('Ctrl Pts',(61.3267881959115,-13.3605623192477,
2.90134173516014));
#215913=CARTESIAN_POINT('Ctrl Pts',(61.3388252440308,-13.3631207378649,
2.88164837656838));
#215914=CARTESIAN_POINT('Ctrl Pts',(61.3512282837617,-13.363763127862,2.86203734439379));
#215915=CARTESIAN_POINT('Ctrl Pts',(61.3638130392384,-13.3625311504979,
2.84277945978506));
#215916=CARTESIAN_POINT('Ctrl Pts',(61.3766506715095,-13.3612744179062,
2.82313460920505));
#215917=CARTESIAN_POINT('Ctrl Pts',(61.3896782944578,-13.3580674708029,
2.80385576863951));
#215918=CARTESIAN_POINT('Ctrl Pts',(61.4027199493048,-13.35290481122,2.78521678519113));
#215919=CARTESIAN_POINT('Ctrl Pts',(61.4152549476837,-13.3479427162818,
2.767301909353));
#215920=CARTESIAN_POINT('Ctrl Pts',(61.4278037696825,-13.341173718107,2.74997687280706));
#215921=CARTESIAN_POINT('Ctrl Pts',(61.4402150271729,-13.3325479345607,
2.73349253346727));
#215922=CARTESIAN_POINT('Ctrl Pts',(61.4497489245016,-13.3259219069584,
2.72082983599924));
#215923=CARTESIAN_POINT('Ctrl Pts',(61.4592018401648,-13.3181993658968,
2.70866321039576));
#215924=CARTESIAN_POINT('Ctrl Pts',(61.468502650244,-13.3093393327434,2.69711645335836));
#215925=CARTESIAN_POINT('Ctrl Pts',(61.4685270260085,-13.3093161121766,
2.69708619136742));
#215926=CARTESIAN_POINT('Ctrl Pts',(61.4685514007484,-13.3092928829594,
2.69705593387209));
#215927=CARTESIAN_POINT('Ctrl Pts',(61.468575774461,-13.309269645094,2.69702568087561));
#215928=CARTESIAN_POINT('Ctrl Pts',(61.4711891321182,-13.3067780733541,
2.69378194443257));
#215929=CARTESIAN_POINT('Ctrl Pts',(61.4737888336848,-13.304187524072,2.6905926662469));
#215930=CARTESIAN_POINT('Ctrl Pts',(61.4763713294376,-13.3015014257472,
2.68746219342667));
#215931=CARTESIAN_POINT('Ctrl Pts',(61.4907423311174,-13.2865538993104,
2.67004182396043));
#215932=CARTESIAN_POINT('Ctrl Pts',(61.5045840828647,-13.2686510078419,
2.65443567877815));
#215933=CARTESIAN_POINT('Ctrl Pts',(61.5172886502247,-13.2484387178487,
2.64136852352988));
#215934=CARTESIAN_POINT('Ctrl Pts',(61.5229906359928,-13.2393671621934,
2.63550380329622));
#215935=CARTESIAN_POINT('Ctrl Pts',(61.5284639152923,-13.2298303888495,
2.63014997451051));
#215936=CARTESIAN_POINT('Ctrl Pts',(61.5336555255489,-13.2198857715696,
2.62536981119244));
#215937=CARTESIAN_POINT('Ctrl Pts',(61.535911729145,-13.2155639754102,2.62329241687064));
#215938=CARTESIAN_POINT('Ctrl Pts',(61.5381145532938,-13.2111652444426,
2.62132362131419));
#215939=CARTESIAN_POINT('Ctrl Pts',(61.5402595369764,-13.2066943520814,
2.61946873372339));
#215940=CARTESIAN_POINT('Ctrl Pts',(61.5477669798654,-13.1910462288169,
2.61297662715559));
#215941=CARTESIAN_POINT('Ctrl Pts',(61.55456587389,-13.1745141278025,2.6078798911396));
#215942=CARTESIAN_POINT('Ctrl Pts',(61.5604649702292,-13.1573027128851,
2.6044061688617));
#215943=CARTESIAN_POINT('Ctrl Pts',(61.5634145183988,-13.1486970054264,
2.60266930772275));
#215944=CARTESIAN_POINT('Ctrl Pts',(61.5661391177412,-13.1399214696207,
2.60133820040177));
#215945=CARTESIAN_POINT('Ctrl Pts',(61.5686148699003,-13.1310016901021,
2.60044130723576));
#215946=CARTESIAN_POINT('Ctrl Pts',(61.5698527459799,-13.1265418003428,
2.59999286065276));
#215947=CARTESIAN_POINT('Ctrl Pts',(61.5710284103841,-13.1220458496809,
2.59965296768503));
#215948=CARTESIAN_POINT('Ctrl Pts',(61.572138876503,-13.1175170363394,2.59942518630945));
#215949=CARTESIAN_POINT('Ctrl Pts',(61.5732493426218,-13.1129882229979,
2.59919740493387));
#215950=CARTESIAN_POINT('Ctrl Pts',(61.5742946087865,-13.1084265466218,
2.59908173791606));
#215951=CARTESIAN_POINT('Ctrl Pts',(61.5752716937453,-13.1038352065718,
2.59908173516015));
#215952=CARTESIAN_POINT('',(61.5816197022699,-13.0739701745315,2.59908173516015));
#215953=CARTESIAN_POINT('Origin',(5.50318346416883E-15,1.85444910649818E-13,
2.59908173516024));
#215954=CARTESIAN_POINT('',(61.459039055521,-12.7383709431241,2.90134173516015));
#215955=CARTESIAN_POINT('Ctrl Pts',(61.58161970227,-13.0739701745315,2.59908173516016));
#215956=CARTESIAN_POINT('Ctrl Pts',(61.58241334955,-13.0702318743168,2.59908174381671));
#215957=CARTESIAN_POINT('Ctrl Pts',(61.583158132123,-13.0664939028176,2.59915752000987));
#215958=CARTESIAN_POINT('Ctrl Pts',(61.5838547466227,-13.0627583804517,
2.59930729517462));
#215959=CARTESIAN_POINT('Ctrl Pts',(61.5878803190637,-13.0411716694454,
2.60017281085909));
#215960=CARTESIAN_POINT('Ctrl Pts',(61.5902997144312,-13.0196643745799,
2.6035065180006));
#215961=CARTESIAN_POINT('Ctrl Pts',(61.5912450453421,-12.998652353661,2.60896880596475));
#215962=CARTESIAN_POINT('Ctrl Pts',(61.5916263190448,-12.9901777222658,
2.61117187235465));
#215963=CARTESIAN_POINT('Ctrl Pts',(61.5917681516648,-12.98178334129,2.613720765772));
#215964=CARTESIAN_POINT('Ctrl Pts',(61.5916804171631,-12.9734950911664,
2.61659179896975));
#215965=CARTESIAN_POINT('Ctrl Pts',(61.5916480484585,-12.9704372300715,
2.617651035912));
#215966=CARTESIAN_POINT('Ctrl Pts',(61.5915843445342,-12.9673939164341,
2.61875422455141));
#215967=CARTESIAN_POINT('Ctrl Pts',(61.5914897592008,-12.9643665007541,
2.61990022440388));
#215968=CARTESIAN_POINT('Ctrl Pts',(61.5913124117006,-12.9586900963541,
2.62204897412725));
#215969=CARTESIAN_POINT('Ctrl Pts',(61.5910264967404,-12.9530695832092,
2.62434823201762));
#215970=CARTESIAN_POINT('Ctrl Pts',(61.5906350058492,-12.9475138635623,
2.62679048030297));
#215971=CARTESIAN_POINT('Ctrl Pts',(61.5892647877302,-12.9280688447985,
2.63533834930171));
#215972=CARTESIAN_POINT('Ctrl Pts',(61.5866012600732,-12.9094175454583,
2.64563784783553));
#215973=CARTESIAN_POINT('Ctrl Pts',(61.5827727094487,-12.8919416545033,
2.65736666737954));
#215974=CARTESIAN_POINT('Ctrl Pts',(61.5808584341364,-12.8832037090257,
2.66323107715155));
#215975=CARTESIAN_POINT('Ctrl Pts',(61.5786529040704,-12.8747596158547,
2.66945281780765));
#215976=CARTESIAN_POINT('Ctrl Pts',(61.576172163775,-12.8666570879107,2.67599160631192));
#215977=CARTESIAN_POINT('Ctrl Pts',(61.5749317936273,-12.8626058239388,
2.67926100056405));
#215978=CARTESIAN_POINT('Ctrl Pts',(61.5736226210374,-12.8586399512969,
2.68260965685114));
#215979=CARTESIAN_POINT('Ctrl Pts',(61.5722466520923,-12.8547654342056,
2.68603254012473));
#215980=CARTESIAN_POINT('Ctrl Pts',(61.5708706831473,-12.8508909171143,
2.68945542339832));
#215981=CARTESIAN_POINT('Ctrl Pts',(61.5694278436303,-12.8471078617851,
2.69295261525376));
#215982=CARTESIAN_POINT('Ctrl Pts',(61.5679202927797,-12.8434220158066,
2.6965189117209));
#215983=CARTESIAN_POINT('Ctrl Pts',(61.5679074365282,-12.8433905832597,
2.69654932476078));
#215984=CARTESIAN_POINT('Ctrl Pts',(61.5678945756945,-12.8433591578466,
2.69657974261137));
#215985=CARTESIAN_POINT('Ctrl Pts',(61.5678817102797,-12.8433277395699,
2.69661016526964));
#215986=CARTESIAN_POINT('Ctrl Pts',(61.5613111551486,-12.8272819669702,
2.71214746101055));
#215987=CARTESIAN_POINT('Ctrl Pts',(61.5536499750629,-12.8130163727101,
2.72880565567422));
#215988=CARTESIAN_POINT('Ctrl Pts',(61.5450979154875,-12.8005145062095,
2.74628040012097));
#215989=CARTESIAN_POINT('Ctrl Pts',(61.5362566309361,-12.7875898348854,
2.76434612882128));
#215990=CARTESIAN_POINT('Ctrl Pts',(61.5264624086214,-12.7765497640427,
2.78328592654109));
#215991=CARTESIAN_POINT('Ctrl Pts',(61.5159109908884,-12.7674219834115,
2.80278753267447));
#215992=CARTESIAN_POINT('Ctrl Pts',(61.505560283323,-12.7584678323747,2.82191817722384));
#215993=CARTESIAN_POINT('Ctrl Pts',(61.4944799879613,-12.7513538295784,
2.84159092314728));
#215994=CARTESIAN_POINT('Ctrl Pts',(61.4828443590798,-12.7461528104621,
2.86151233816575));
#215995=CARTESIAN_POINT('Ctrl Pts',(61.475136162868,-12.7427073176349,2.87470957721014));
#215996=CARTESIAN_POINT('Ctrl Pts',(61.467184058762,-12.7401023057312,2.88801594388191));
#215997=CARTESIAN_POINT('Ctrl Pts',(61.459039055521,-12.7383709431241,2.90134173516015));
#215998=CARTESIAN_POINT('',(61.1105274371643,-12.6642893210132,3.47153072139064));
#215999=CARTESIAN_POINT('',(61.459039055521,-12.7383709431241,2.90134173516015));
#216000=CARTESIAN_POINT('',(62.0330459552233,-6.83973663030158,3.47153072139068));
#216001=CARTESIAN_POINT('Origin',(5.53234440788222E-15,1.85015204418142E-13,
3.47153072139072));
#216002=CARTESIAN_POINT('',(62.3873926810692,-6.87697683366461,2.90134173516019));
#216003=CARTESIAN_POINT('',(62.0330459552233,-6.83973663030158,3.47153072139067));
#216004=CARTESIAN_POINT('',(62.6076796697355,-6.59568250079781,2.59908173516019));
#216005=CARTESIAN_POINT('Ctrl Pts',(62.3873926810692,-6.87697683366461,
2.90134173516019));
#216006=CARTESIAN_POINT('Ctrl Pts',(62.3996312165471,-6.87826302285487,
2.88164837656645));
#216007=CARTESIAN_POINT('Ctrl Pts',(62.4120334591692,-6.87760542308927,
2.86203734438992));
#216008=CARTESIAN_POINT('Ctrl Pts',(62.4244204973392,-6.87506472947491,
2.84277945977932));
#216009=CARTESIAN_POINT('Ctrl Pts',(62.4370564393923,-6.8724729834219,2.82313460919733));
#216010=CARTESIAN_POINT('Ctrl Pts',(62.4496774784077,-6.86792184690252,
2.80385576862992));
#216011=CARTESIAN_POINT('Ctrl Pts',(62.4621080448336,-6.86142424476788,
2.78521678517985));
#216012=CARTESIAN_POINT('Ctrl Pts',(62.4740556950225,-6.85517906858589,
2.76730190934001));
#216013=CARTESIAN_POINT('Ctrl Pts',(62.4858282202855,-6.84713544261008,
2.74997687279252));
#216014=CARTESIAN_POINT('Ctrl Pts',(62.4972698477112,-6.83725958233362,
2.73349253345147));
#216015=CARTESIAN_POINT('Ctrl Pts',(62.5060589088662,-6.82967328916932,
2.72082983598914));
#216016=CARTESIAN_POINT('Ctrl Pts',(62.5146528151149,-6.82100495425111,
2.70866321039099));
#216017=CARTESIAN_POINT('Ctrl Pts',(62.5229765487298,-6.81122125790576,
2.6971164533584));
#216018=CARTESIAN_POINT('Ctrl Pts',(62.5229983637512,-6.81119561658246,
2.69708619136746));
#216019=CARTESIAN_POINT('Ctrl Pts',(62.5230201768493,-6.81116996676326,
2.69705593387214));
#216020=CARTESIAN_POINT('Ctrl Pts',(62.5230419880218,-6.81114430845053,
2.69702568087566));
#216021=CARTESIAN_POINT('Ctrl Pts',(62.5253805892672,-6.80839321554143,
2.69378194443261));
#216022=CARTESIAN_POINT('Ctrl Pts',(62.5276952632612,-6.80554511474964,
2.69059266624695));
#216023=CARTESIAN_POINT('Ctrl Pts',(62.5299828381019,-6.80260378684012,
2.68746219342672));
#216024=CARTESIAN_POINT('Ctrl Pts',(62.5427126719616,-6.78623596579746,
2.67004182396211));
#216025=CARTESIAN_POINT('Ctrl Pts',(62.5546072354103,-6.76698429120464,
2.65443567878113));
#216026=CARTESIAN_POINT('Ctrl Pts',(62.5651294462081,-6.74555473735071,
2.64136852353361));
#216027=CARTESIAN_POINT('Ctrl Pts',(62.5698519601306,-6.73593685681467,
2.6355038032985));
#216028=CARTESIAN_POINT('Ctrl Pts',(62.5742983919722,-6.72588021343676,
2.63014997451154));
#216029=CARTESIAN_POINT('Ctrl Pts',(62.5784220664835,-6.71544740276666,
2.62536981119248));
#216030=CARTESIAN_POINT('Ctrl Pts',(62.5802141596491,-6.71091344436403,
2.62329241687068));
#216031=CARTESIAN_POINT('Ctrl Pts',(62.5819451239083,-6.70630855228186,
2.62132362131423));
#216032=CARTESIAN_POINT('Ctrl Pts',(62.5836110216379,-6.70163794008866,
2.61946873372343));
#216033=CARTESIAN_POINT('Ctrl Pts',(62.5894416636914,-6.68529079741248,
2.61297662715563));
#216034=CARTESIAN_POINT('Ctrl Pts',(62.5944752375495,-6.66813858303296,
2.60787989113965));
#216035=CARTESIAN_POINT('Ctrl Pts',(62.5985429352697,-6.65040483057231,
2.60440616886175));
#216036=CARTESIAN_POINT('Ctrl Pts',(62.6005767841298,-6.64153795434199,
2.6026693077228));
#216037=CARTESIAN_POINT('Ctrl Pts',(62.6023691645599,-6.63252569365736,
2.6013382004018));
#216038=CARTESIAN_POINT('Ctrl Pts',(62.6038989834439,-6.62339599105565,
2.6004413072358));
#216039=CARTESIAN_POINT('Ctrl Pts',(62.6046638928858,-6.61883113975479,
2.59999286065279));
#216040=CARTESIAN_POINT('Ctrl Pts',(62.6053631620638,-6.61423692798752,
2.59965296768508));
#216041=CARTESIAN_POINT('Ctrl Pts',(62.6059941550341,-6.60961684864246,
2.5994251863095));
#216042=CARTESIAN_POINT('Ctrl Pts',(62.6066251480044,-6.60499676929741,
2.59919740493392));
#216043=CARTESIAN_POINT('Ctrl Pts',(62.6071878630701,-6.60035082219586,
2.59908173791609));
#216044=CARTESIAN_POINT('Ctrl Pts',(62.6076796697355,-6.59568250079782,
2.5990817351602));
#216045=CARTESIAN_POINT('',(62.6108711573006,-6.56531752495198,2.5990817351602));
#216046=CARTESIAN_POINT('Origin',(5.50063869163689E-15,1.8542884358839E-13,
2.59908173516023));
#216047=CARTESIAN_POINT('',(62.4538823482276,-6.24436990787956,2.9013417351602));
#216048=CARTESIAN_POINT('Ctrl Pts',(62.6108711573006,-6.56531752495198,
2.59908173516019));
#216049=CARTESIAN_POINT('Ctrl Pts',(62.6112696981211,-6.56151674480639,
2.59908174381683));
#216050=CARTESIAN_POINT('Ctrl Pts',(62.6116196762807,-6.55772139932838,
2.59915752000993));
#216051=CARTESIAN_POINT('Ctrl Pts',(62.6119220062409,-6.55393352450177,
2.59930729517467));
#216052=CARTESIAN_POINT('Ctrl Pts',(62.6136691004465,-6.53204428085526,
2.60017281085918));
#216053=CARTESIAN_POINT('Ctrl Pts',(62.6138271176316,-6.51040190952082,
2.60350651800088));
#216054=CARTESIAN_POINT('Ctrl Pts',(62.612570915664,-6.48940618066297,2.60896880596535));
#216055=CARTESIAN_POINT('Ctrl Pts',(62.6120642605129,-6.48093812023183,
2.61117187235511));
#216056=CARTESIAN_POINT('Ctrl Pts',(62.6113278644156,-6.47257489900818,
2.61372076577227));
#216057=CARTESIAN_POINT('Ctrl Pts',(62.6103742524841,-6.46434122353931,
2.61659179896978));
#216058=CARTESIAN_POINT('Ctrl Pts',(62.6100224275775,-6.46130349717838,
2.61765103591203));
#216059=CARTESIAN_POINT('Ctrl Pts',(62.6096409597323,-6.45828351400483,
2.61875422455144));
#216060=CARTESIAN_POINT('Ctrl Pts',(62.6092304414385,-6.45528256968424,
2.61990022440391));
#216061=CARTESIAN_POINT('Ctrl Pts',(62.6084607196376,-6.44965579908311,
2.62204897412728));
#216062=CARTESIAN_POINT('Ctrl Pts',(62.6075888673476,-6.44409596194872,
2.62434823201764));
#216063=CARTESIAN_POINT('Ctrl Pts',(62.6066187902475,-6.43861159905666,
2.626790480303));
#216064=CARTESIAN_POINT('Ctrl Pts',(62.6032235203971,-6.41941632893448,
2.63533834930173));
#216065=CARTESIAN_POINT('Ctrl Pts',(62.5986249921653,-6.40114561781649,
2.64563784783558));
#216066=CARTESIAN_POINT('Ctrl Pts',(62.5929906867159,-6.38416565413391,
2.6573666673796));
#216067=CARTESIAN_POINT('Ctrl Pts',(62.5901735339913,-6.37567567229262,
2.66323107715161));
#216068=CARTESIAN_POINT('Ctrl Pts',(62.5870974379669,-6.36750837741602,
2.66945281780769));
#216069=CARTESIAN_POINT('Ctrl Pts',(62.5837833426318,-6.35970954393874,
2.67599160631196));
#216070=CARTESIAN_POINT('Ctrl Pts',(62.5821262949643,-6.3558101272001,2.67926100056409));
#216071=CARTESIAN_POINT('Ctrl Pts',(62.580409747586,-6.35200282582255,2.68260965685118));
#216072=CARTESIAN_POINT('Ctrl Pts',(62.5786363190254,-6.3482933616606,2.68603254012478));
#216073=CARTESIAN_POINT('Ctrl Pts',(62.5768628904648,-6.34458389749865,
2.68945542339837));
#216074=CARTESIAN_POINT('Ctrl Pts',(62.5750325180136,-6.34097238393975,
2.6929526152538));
#216075=CARTESIAN_POINT('Ctrl Pts',(62.5731479498683,-6.3374643113849,2.69651891172094));
#216076=CARTESIAN_POINT('Ctrl Pts',(62.5731318784489,-6.33743439487305,
2.69654932476082));
#216077=CARTESIAN_POINT('Ctrl Pts',(62.573115803218,-6.33740448593478,2.69657974261141));
#216078=CARTESIAN_POINT('Ctrl Pts',(62.5730997241771,-6.33737458457273,
2.69661016526968));
#216079=CARTESIAN_POINT('Ctrl Pts',(62.564887923282,-6.32210352242355,2.71214746101192));
#216080=CARTESIAN_POINT('Ctrl Pts',(62.555777551296,-6.30871688796164,2.7288056556771));
#216081=CARTESIAN_POINT('Ctrl Pts',(62.5459655399035,-6.29717744163835,
2.74628040012548));
#216082=CARTESIAN_POINT('Ctrl Pts',(62.5358216928012,-6.2852477389029,2.76434612882741));
#216083=CARTESIAN_POINT('Ctrl Pts',(62.5249271226206,-6.27529192173046,
2.78328592654895));
#216084=CARTESIAN_POINT('Ctrl Pts',(62.5134793937744,-6.2673170675176,2.8027875326841));
#216085=CARTESIAN_POINT('Ctrl Pts',(62.5022494248193,-6.25949391181267,
2.82191817723497));
#216086=CARTESIAN_POINT('Ctrl Pts',(62.4904862126941,-6.25357708651515,
2.84159092315994));
#216087=CARTESIAN_POINT('Ctrl Pts',(62.4783706704684,-6.24962081353253,
2.8615123381799));
#216088=CARTESIAN_POINT('Ctrl Pts',(62.4703445484942,-6.24699992138176,
2.87470957721967));
#216089=CARTESIAN_POINT('Ctrl Pts',(62.4621637089584,-6.24524040122871,
2.88801594388671));
#216090=CARTESIAN_POINT('Ctrl Pts',(62.4538823482276,-6.24436990787956,
2.9013417351602));
#216091=CARTESIAN_POINT('',(62.099536274866,-6.20712349654361,3.47153072139068));
#216092=CARTESIAN_POINT('',(62.4538823482276,-6.24436990787956,2.9013417351602));
#216093=CARTESIAN_POINT('',(62.4081695979768,-0.318048871876943,3.47153072139072));
#216094=CARTESIAN_POINT('Origin',(5.53234440788222E-15,1.85015204418142E-13,
3.47153072139072));
#216095=CARTESIAN_POINT('',(62.7644678366119,-0.318045750792856,2.90134173516023));
#216096=CARTESIAN_POINT('',(62.4081695979768,-0.318048871876944,3.47153072139072));
#216097=CARTESIAN_POINT('Ctrl Pts',(62.7644678366119,-0.318045750792856,
2.90134173516023));
#216098=CARTESIAN_POINT('Ctrl Pts',(62.7767737714904,-0.318045618797943,
2.88164837656825));
#216099=CARTESIAN_POINT('Ctrl Pts',(62.7890393354356,-0.316095234070607,
2.86203734439344));
#216100=CARTESIAN_POINT('Ctrl Pts',(62.8010929413143,-0.312273660577998,
2.8427794597845));
#216101=CARTESIAN_POINT('Ctrl Pts',(62.8133887511215,-0.308375296776985,
2.8231346092043));
#216102=CARTESIAN_POINT('Ctrl Pts',(62.8254649274571,-0.302529834047596,
2.80385576863858));
#216103=CARTESIAN_POINT('Ctrl Pts',(62.8371482135724,-0.294768478452709,
2.78521678519004));
#216104=CARTESIAN_POINT('Ctrl Pts',(62.8483776146134,-0.287308644486815,
2.76730190935176));
#216105=CARTESIAN_POINT('Ctrl Pts',(62.859244860888,-0.278078518363,2.74997687280568));
#216106=CARTESIAN_POINT('Ctrl Pts',(62.8695915013826,-0.267060783352544,
2.73349253346579));
#216107=CARTESIAN_POINT('Ctrl Pts',(62.8775394315778,-0.258597341637506,
2.72082983599833));
#216108=CARTESIAN_POINT('Ctrl Pts',(62.8851801717839,-0.24907818494816,
2.70866321039538));
#216109=CARTESIAN_POINT('Ctrl Pts',(62.8924356323738,-0.238478017627679,
2.69711645335845));
#216110=CARTESIAN_POINT('Ctrl Pts',(62.892454647642,-0.238450236479571,
2.69708619136751));
#216111=CARTESIAN_POINT('Ctrl Pts',(62.8924736601095,-0.238422447083147,
2.69705593387219));
#216112=CARTESIAN_POINT('Ctrl Pts',(62.8924926697742,-0.238394649440984,
2.69702568087571));
#216113=CARTESIAN_POINT('Ctrl Pts',(62.8945308924032,-0.23541417691232,
2.69378194443266));
#216114=CARTESIAN_POINT('Ctrl Pts',(62.8965351787718,-0.232339728999126,
2.690592666247));
#216115=CARTESIAN_POINT('Ctrl Pts',(62.8985027695519,-0.229175397308934,
2.68746219342677));
#216116=CARTESIAN_POINT('Ctrl Pts',(62.9094519648695,-0.211566610930916,
2.67004182396156));
#216117=CARTESIAN_POINT('Ctrl Pts',(62.9192690206948,-0.191177078586518,
2.65443567878009));
#216118=CARTESIAN_POINT('Ctrl Pts',(62.9274935913882,-0.168765047545019,
2.64136852353229));
#216119=CARTESIAN_POINT('Ctrl Pts',(62.9311848926126,-0.158706217642537,
2.63550380329772));
#216120=CARTESIAN_POINT('Ctrl Pts',(62.9345557609572,-0.148239886922649,
2.63014997451123));
#216121=CARTESIAN_POINT('Ctrl Pts',(62.9375663198809,-0.137433186922181,
2.62536981119254));
#216122=CARTESIAN_POINT('Ctrl Pts',(62.9388746680683,-0.132736741273433,
2.62329241687074));
#216123=CARTESIAN_POINT('Ctrl Pts',(62.9401148076313,-0.127976140237919,
2.62132362131427));
#216124=CARTESIAN_POINT('Ctrl Pts',(62.9412833674838,-0.123156980417379,
2.61946873372348));
#216125=CARTESIAN_POINT('Ctrl Pts',(62.9453733269673,-0.106289921045488,
2.61297662715568));
#216126=CARTESIAN_POINT('Ctrl Pts',(62.9485864317704,-0.0887055165508694,
2.60787989113969));
#216127=CARTESIAN_POINT('Ctrl Pts',(62.9507781643242,-0.0706437212499775,
2.60440616886179));
#216128=CARTESIAN_POINT('Ctrl Pts',(62.9518740306011,-0.0616128235995317,
2.60266930772284));
#216129=CARTESIAN_POINT('Ctrl Pts',(62.9527145544237,-0.0524625782499523,
2.60133820040185));
#216130=CARTESIAN_POINT('Ctrl Pts',(62.9532816790167,-0.0432229794973303,
2.60044130723585));
#216131=CARTESIAN_POINT('Ctrl Pts',(62.9535652413132,-0.0386031801210193,
2.59999286065284));
#216132=CARTESIAN_POINT('Ctrl Pts',(62.9537804539255,-0.0339610423939235,
2.59965296768511));
#216133=CARTESIAN_POINT('Ctrl Pts',(62.9539250604562,-0.0293003156014106,
2.59942518630953));
#216134=CARTESIAN_POINT('Ctrl Pts',(62.9540696669868,-0.0246395888088978,
2.59919740493395));
#216135=CARTESIAN_POINT('Ctrl Pts',(62.9541436657296,-0.0199602729506026,
2.59908173791615));
#216136=CARTESIAN_POINT('Ctrl Pts',(62.9541448057648,-0.0152661173106757,
2.59908173516024));
#216137=CARTESIAN_POINT('Origin',(5.71385722241845E-15,1.94016234460786E-13,
2.18253198860262));
#216138=CARTESIAN_POINT('',(-59.1088767419348,0.316922544675878,2.90134173516022));
#216139=CARTESIAN_POINT('Ctrl Pts',(-58.9208513795073,0.015212193456111,
2.59908173516023));
#216140=CARTESIAN_POINT('Ctrl Pts',(-58.9208504012364,0.0190220008287343,
2.59908174371509));
#216141=CARTESIAN_POINT('Ctrl Pts',(-58.9208964366351,0.0228214099819142,
2.59915764355889));
#216142=CARTESIAN_POINT('Ctrl Pts',(-58.9209883940807,0.0266084895331968,
2.59930765775276));
#216143=CARTESIAN_POINT('Ctrl Pts',(-58.9215313038857,0.0489671208155431,
2.60019333020889));
#216144=CARTESIAN_POINT('Ctrl Pts',(-58.9236732325291,0.0708986527649559,
2.60365973324157));
#216145=CARTESIAN_POINT('Ctrl Pts',(-58.9271900305707,0.0919988953574036,
2.6093417708256));
#216146=CARTESIAN_POINT('Ctrl Pts',(-58.9285037892495,0.0998812435911596,
2.61146439091957));
#216147=CARTESIAN_POINT('Ctrl Pts',(-58.93000918782,0.107647933248718,2.61389584429379));
#216148=CARTESIAN_POINT('Ctrl Pts',(-58.9316938830317,0.115279202947081,
2.6166160438525));
#216149=CARTESIAN_POINT('Ctrl Pts',(-58.933008366749,0.121233502390386,
2.61873848000773));
#216150=CARTESIAN_POINT('Ctrl Pts',(-58.9344322364591,0.127104908280178,
2.62103707099785));
#216151=CARTESIAN_POINT('Ctrl Pts',(-58.9359598525093,0.13288357827324,
2.62350262767649));
#216152=CARTESIAN_POINT('Ctrl Pts',(-58.9413065086848,0.153108923248959,
2.63213207605176));
#216153=CARTESIAN_POINT('Ctrl Pts',(-58.9479240485795,0.172198253417896,
2.64280685971912));
#216154=CARTESIAN_POINT('Ctrl Pts',(-58.9555707636545,0.189729578870957,
2.65513293646081));
#216155=CARTESIAN_POINT('Ctrl Pts',(-58.959394121192,0.198495241597488,
2.66129597483166));
#216156=CARTESIAN_POINT('Ctrl Pts',(-58.9634747743348,0.206871403160735,
2.66787183533849));
#216157=CARTESIAN_POINT('Ctrl Pts',(-58.9677825146336,0.2148053148634,2.67481125953859));
#216158=CARTESIAN_POINT('Ctrl Pts',(-58.9720718502312,0.222705329147818,
2.68172103524077));
#216159=CARTESIAN_POINT('Ctrl Pts',(-58.9765861722458,0.23016705507937,
2.68899101329786));
#216160=CARTESIAN_POINT('Ctrl Pts',(-58.9812961520165,0.237137844566841,
2.69657334701272));
#216161=CARTESIAN_POINT('Ctrl Pts',(-58.9813163616197,0.237167754862984,
2.69660588132569));
#216162=CARTESIAN_POINT('Ctrl Pts',(-58.9813365744745,0.237197656536892,
2.69663842081378));
#216163=CARTESIAN_POINT('Ctrl Pts',(-58.9813567905789,0.237227549588143,
2.69667096547378));
#216164=CARTESIAN_POINT('Ctrl Pts',(-58.9908903168205,0.251324537971825,
2.71201840157859));
#216165=CARTESIAN_POINT('Ctrl Pts',(-59.0011093202319,0.263501580511345,
2.7284564593918));
#216166=CARTESIAN_POINT('Ctrl Pts',(-59.011829410383,0.273820596507998,
2.74568723186633));
#216167=CARTESIAN_POINT('Ctrl Pts',(-59.0229394763206,0.28451499800261,
2.76354482593972));
#216168=CARTESIAN_POINT('Ctrl Pts',(-59.034588573653,0.29321400956702,2.78225519316684));
#216169=CARTESIAN_POINT('Ctrl Pts',(-59.0465875206362,0.299936893970986,
2.8015122308497));
#216170=CARTESIAN_POINT('Ctrl Pts',(-59.0584152157231,0.306563827729856,
2.82049442739634));
#216171=CARTESIAN_POINT('Ctrl Pts',(-59.0705837677918,0.311270560392258,
2.84000929088533));
#216172=CARTESIAN_POINT('Ctrl Pts',(-59.082913990599,0.314027284734976,
2.85976644340804));
#216173=CARTESIAN_POINT('Ctrl Pts',(-59.0915108413181,0.31594932199406,
2.87354148166398));
#216174=CARTESIAN_POINT('Ctrl Pts',(-59.1001863397057,0.316922445687917,
2.88743438345212));
#216175=CARTESIAN_POINT('Ctrl Pts',(-59.1088767419348,0.316922544675878,
2.90134173516022));
#216176=CARTESIAN_POINT('',(-59.4651754363832,0.316925998273232,3.47153072139072));
#216177=CARTESIAN_POINT('',(-59.1088767419348,0.316922544675878,2.90134173516022));
#216178=CARTESIAN_POINT('',(-59.1725467709678,5.90061356181237,3.47153072139075));
#216179=CARTESIAN_POINT('Origin',(5.53234440788222E-15,1.85015204418142E-13,
3.47153072139072));
#216180=CARTESIAN_POINT('',(-58.8181995570485,5.8633736414956,2.90134173516027));
#216181=CARTESIAN_POINT('',(-59.1725467709678,5.90061356181236,3.47153072139076));
#216182=CARTESIAN_POINT('',(-58.5996668978649,6.14377718965303,2.59908173516027));
#216183=CARTESIAN_POINT('Ctrl Pts',(-58.8181995570485,5.8633736414956,2.90134173516027));
#216184=CARTESIAN_POINT('Ctrl Pts',(-58.8060365798454,5.8620954050285,2.88176998919727));
#216185=CARTESIAN_POINT('Ctrl Pts',(-58.7937272422245,5.86273454612513,
2.86226752356565));
#216186=CARTESIAN_POINT('Ctrl Pts',(-58.7814443761798,5.86523378400462,
2.84310370499784));
#216187=CARTESIAN_POINT('Ctrl Pts',(-58.7689396367193,5.86777816724704,
2.8235937178835));
#216188=CARTESIAN_POINT('Ctrl Pts',(-58.7564614161378,5.87225032431066,
2.80443322636623));
#216189=CARTESIAN_POINT('Ctrl Pts',(-58.7441787427581,5.8786413544399,2.78589323877821));
#216190=CARTESIAN_POINT('Ctrl Pts',(-58.7324160859235,5.88476180492377,
2.7681381861952));
#216191=CARTESIAN_POINT('Ctrl Pts',(-58.7208319573114,5.89264238981991,
2.750950951982));
#216192=CARTESIAN_POINT('Ctrl Pts',(-58.7095754394624,5.90232005416046,
2.73457771434575));
#216193=CARTESIAN_POINT('Ctrl Pts',(-58.7006223753279,5.91001735013374,
2.7215549795523));
#216194=CARTESIAN_POINT('Ctrl Pts',(-58.6918764318946,5.91885232406616,
2.70904711159798));
#216195=CARTESIAN_POINT('Ctrl Pts',(-58.6834178317481,5.92886364759531,
2.69718956158341));
#216196=CARTESIAN_POINT('Ctrl Pts',(-58.6833947425173,5.92889097525654,
2.69715719432358));
#216197=CARTESIAN_POINT('Ctrl Pts',(-58.683371655605,5.92891831167209,2.69712483219024));
#216198=CARTESIAN_POINT('Ctrl Pts',(-58.6833485710132,5.92894565684157,
2.69709247518652));
#216199=CARTESIAN_POINT('Ctrl Pts',(-58.6787531612542,5.93438921243197,
2.69065122242277));
#216200=CARTESIAN_POINT('Ctrl Pts',(-58.6742527563956,5.94021607194757,
2.68442464469429));
#216201=CARTESIAN_POINT('Ctrl Pts',(-58.6698707672381,5.94639317576856,
2.67844505923581));
#216202=CARTESIAN_POINT('Ctrl Pts',(-58.6611744062938,5.95865206607762,
2.6665781577957));
#216203=CARTESIAN_POINT('Ctrl Pts',(-58.6529445485198,5.97229179622498,
2.65568445664175));
#216204=CARTESIAN_POINT('Ctrl Pts',(-58.6453649253901,5.98706231730018,
2.64601906229516));
#216205=CARTESIAN_POINT('Ctrl Pts',(-58.6396802080428,5.99814020810658,
2.63877001653522));
#216206=CARTESIAN_POINT('Ctrl Pts',(-58.6343612468744,6.00985416873249,
2.63221189387604));
#216207=CARTESIAN_POINT('Ctrl Pts',(-58.6294855649109,6.02209871088772,
2.62645231033236));
#216208=CARTESIAN_POINT('Ctrl Pts',(-58.6276571841746,6.02669041419593,
2.62429246650348));
#216209=CARTESIAN_POINT('Ctrl Pts',(-58.6258911397673,6.03135673055019,
2.62224491711748));
#216210=CARTESIAN_POINT('Ctrl Pts',(-58.6241915206271,6.03609209717129,
2.620315336726));
#216211=CARTESIAN_POINT('Ctrl Pts',(-58.6182428536364,6.05266588034514,
2.61356180535581));
#216212=CARTESIAN_POINT('Ctrl Pts',(-58.6131078911177,6.07008552874948,
2.60825339735349));
#216213=CARTESIAN_POINT('Ctrl Pts',(-58.6089619925611,6.08811254303241,
2.60463337987613));
#216214=CARTESIAN_POINT('Ctrl Pts',(-58.6068890432827,6.09712605017387,
2.60282337113744));
#216215=CARTESIAN_POINT('Ctrl Pts',(-58.6050633610079,6.10629139889381,
2.60143545939118));
#216216=CARTESIAN_POINT('Ctrl Pts',(-58.6035068699781,6.11557877725394,
2.600500050346));
#216217=CARTESIAN_POINT('Ctrl Pts',(-58.6027286244632,6.120222466434,2.6000323458234));
#216218=CARTESIAN_POINT('Ctrl Pts',(-58.6020176767849,6.12489666302712,
2.59967776696069));
#216219=CARTESIAN_POINT('Ctrl Pts',(-58.6013767677628,6.12959764057339,
2.59944011429163));
#216220=CARTESIAN_POINT('Ctrl Pts',(-58.6007358587407,6.13429861811967,
2.59920246162257));
#216221=CARTESIAN_POINT('Ctrl Pts',(-58.600164990065,6.13902637679624,2.5990817379131));
#216222=CARTESIAN_POINT('Ctrl Pts',(-58.5996668978649,6.14377718965303,
2.59908173516027));
#216223=CARTESIAN_POINT('',(-58.5964866834551,6.17403490859001,2.59908173516028));
#216224=CARTESIAN_POINT('Origin',(3.34731138317026E-16,1.91114605089249E-13,
2.59908173516024));
#216225=CARTESIAN_POINT('',(-58.7519447039088,6.49374646112719,2.90134173516027));
#216226=CARTESIAN_POINT('Ctrl Pts',(-58.5964866834551,6.17403490859001,
2.59908173516027));
#216227=CARTESIAN_POINT('Ctrl Pts',(-58.5960874772333,6.17782374318206,
2.59908174371516));
#216228=CARTESIAN_POINT('Ctrl Pts',(-58.5957361140451,6.18160715078384,
2.59915764355894));
#216229=CARTESIAN_POINT('Ctrl Pts',(-58.5954317101325,6.18538309648757,
2.59930765775281));
#216230=CARTESIAN_POINT('Ctrl Pts',(-58.5936345324521,6.20767599437474,
2.60019333020889));
#216231=CARTESIAN_POINT('Ctrl Pts',(-58.5934722580544,6.22971127560576,
2.60365973324126));
#216232=CARTESIAN_POINT('Ctrl Pts',(-58.5947642147754,6.25106353435537,
2.60934177082473));
#216233=CARTESIAN_POINT('Ctrl Pts',(-58.5952468467989,6.25904002743775,
2.61146439091893));
#216234=CARTESIAN_POINT('Ctrl Pts',(-58.595932158504,6.26692152735706,2.61389584429345));
#216235=CARTESIAN_POINT('Ctrl Pts',(-58.5968099398848,6.27468709076421,
2.61661604385256));
#216236=CARTESIAN_POINT('Ctrl Pts',(-58.5974948289522,6.28074617289512,
2.61873848000779));
#216237=CARTESIAN_POINT('Ctrl Pts',(-58.5982971695201,6.2867342495218,2.62103707099791));
#216238=CARTESIAN_POINT('Ctrl Pts',(-58.5992123816356,6.2926409427142,2.62350262767655));
#216239=CARTESIAN_POINT('Ctrl Pts',(-58.6024156240399,6.31331436888757,
2.63213207605182));
#216240=CARTESIAN_POINT('Ctrl Pts',(-58.6070015340112,6.33299084698429,
2.64280685971917));
#216241=CARTESIAN_POINT('Ctrl Pts',(-58.6127738370723,6.35122543337802,
2.65513293646087));
#216242=CARTESIAN_POINT('Ctrl Pts',(-58.6156599886029,6.36034272657488,
2.66129597483171));
#216243=CARTESIAN_POINT('Ctrl Pts',(-58.6188427402045,6.36909954705081,
2.66787183533855));
#216244=CARTESIAN_POINT('Ctrl Pts',(-58.6222975626532,6.37744027742862,
2.67481125953864));
#216245=CARTESIAN_POINT('Ctrl Pts',(-58.6257376244687,6.38574537226665,
2.68172103524082));
#216246=CARTESIAN_POINT('Ctrl Pts',(-58.6294472538099,6.3936380972257,2.6889910132979));
#216247=CARTESIAN_POINT('Ctrl Pts',(-58.6334027859058,6.40106302694644,
2.69657334701276));
#216248=CARTESIAN_POINT('Ctrl Pts',(-58.6334197583214,6.40109488586962,
2.69660588132573));
#216249=CARTESIAN_POINT('Ctrl Pts',(-58.633436734872,6.40112673655768,2.69663842081382));
#216250=CARTESIAN_POINT('Ctrl Pts',(-58.6334537155557,6.40115857900999,
2.69667096547382));
#216251=CARTESIAN_POINT('Ctrl Pts',(-58.6414614796113,6.41617486746512,
2.7120184015799));
#216252=CARTESIAN_POINT('Ctrl Pts',(-58.6503516547099,6.42935337961519,
2.72845645939456));
#216253=CARTESIAN_POINT('Ctrl Pts',(-58.6599343882018,6.44073642151277,
2.74568723187065));
#216254=CARTESIAN_POINT('Ctrl Pts',(-58.6698657226828,6.45253355607693,
2.7635448259456));
#216255=CARTESIAN_POINT('Ctrl Pts',(-58.6805417107313,6.46240257578875,
2.78225519317439));
#216256=CARTESIAN_POINT('Ctrl Pts',(-58.6917721934532,6.47034286301753,
2.80151223085897));
#216257=CARTESIAN_POINT('Ctrl Pts',(-58.7028423919877,6.47816982453123,
2.82049442740706));
#216258=CARTESIAN_POINT('Ctrl Pts',(-58.7144522959237,6.48412273326722,
2.84000929089754));
#216259=CARTESIAN_POINT('Ctrl Pts',(-58.726426816322,6.48815321522669,2.85976644342169));
#216260=CARTESIAN_POINT('Ctrl Pts',(-58.7347756649898,6.49096333895761,
2.87354148167318));
#216261=CARTESIAN_POINT('Ctrl Pts',(-58.7433019189624,6.49283796829162,
2.88743438345675));
#216262=CARTESIAN_POINT('Ctrl Pts',(-58.7519447039089,6.49374646112717,
2.90134173516027));
#216263=CARTESIAN_POINT('',(-59.1062911958297,6.53099325080035,3.47153072139076));
#216264=CARTESIAN_POINT('',(-58.7519447039089,6.4937464611272,2.90134173516027));
#216265=CARTESIAN_POINT('',(-58.2316113004782,12.053504764932,3.4715307213908));
#216266=CARTESIAN_POINT('Origin',(5.53234440788222E-15,1.85015204418142E-13,
3.47153072139072));
#216267=CARTESIAN_POINT('',(-57.8830978693156,11.979429479061,2.90134173516031));
#216268=CARTESIAN_POINT('',(-58.2316113004781,12.053504764932,3.4715307213908));
#216269=CARTESIAN_POINT('',(-57.6364522029208,12.2354540642043,2.59908173516031));
#216270=CARTESIAN_POINT('Ctrl Pts',(-57.8830978693156,11.979429479061,2.90134173516031));
#216271=CARTESIAN_POINT('Ctrl Pts',(-57.8711351342684,11.9768868675913,
2.88176998919809));
#216272=CARTESIAN_POINT('Ctrl Pts',(-57.8588264200507,11.9762358312607,
2.86226752356722));
#216273=CARTESIAN_POINT('Ctrl Pts',(-57.8463495993371,11.9774374689412,
2.84310370500015));
#216274=CARTESIAN_POINT('Ctrl Pts',(-57.8336474016779,11.9786608125864,
2.8235937178865));
#216275=CARTESIAN_POINT('Ctrl Pts',(-57.8207700703895,11.9818041414837,
2.80443322636989));
#216276=CARTESIAN_POINT('Ctrl Pts',(-57.8078866382221,11.9868762719075,
2.78589323878247));
#216277=CARTESIAN_POINT('Ctrl Pts',(-57.7955486571692,11.99173366148,2.76813818619992));
#216278=CARTESIAN_POINT('Ctrl Pts',(-57.7832042421973,11.9983602045449,
2.75095095198714));
#216279=CARTESIAN_POINT('Ctrl Pts',(-57.7709977973496,12.0068082271144,
2.73457771435122));
#216280=CARTESIAN_POINT('Ctrl Pts',(-57.7612891925164,12.0135275064601,
2.72155497955582));
#216281=CARTESIAN_POINT('Ctrl Pts',(-57.7516676540268,12.0213998814549,
2.70904711159967));
#216282=CARTESIAN_POINT('Ctrl Pts',(-57.7422089227118,12.0304721974328,
2.69718956158346));
#216283=CARTESIAN_POINT('Ctrl Pts',(-57.7421831034479,12.0304969619084,
2.69715719432363));
#216284=CARTESIAN_POINT('Ctrl Pts',(-57.7421572855746,12.0305217353328,
2.69712483219029));
#216285=CARTESIAN_POINT('Ctrl Pts',(-57.7421314690941,12.0305465177056,
2.69709247518657));
#216286=CARTESIAN_POINT('Ctrl Pts',(-57.7369922269699,12.0354799018088,
2.69065122242283));
#216287=CARTESIAN_POINT('Ctrl Pts',(-57.7319074031292,12.0408044207743,
2.68442464469433));
#216288=CARTESIAN_POINT('Ctrl Pts',(-57.726903735797,12.0464896431815,2.67844505923586));
#216289=CARTESIAN_POINT('Ctrl Pts',(-57.7169736114625,12.0577723607613,
2.66657815779574));
#216290=CARTESIAN_POINT('Ctrl Pts',(-57.7073630976788,12.0704771166537,
2.65568445664181));
#216291=CARTESIAN_POINT('Ctrl Pts',(-57.698281056648,12.0843744369111,2.64601906229522));
#216292=CARTESIAN_POINT('Ctrl Pts',(-57.6914695258749,12.0947974271042,
2.63877001653528));
#216293=CARTESIAN_POINT('Ctrl Pts',(-57.6849552602293,12.105891234591,2.63221189387608));
#216294=CARTESIAN_POINT('Ctrl Pts',(-57.6788263845868,12.1175590523201,
2.6264523103324));
#216295=CARTESIAN_POINT('Ctrl Pts',(-57.6765280562209,12.1219344839685,
2.62429246650352));
#216296=CARTESIAN_POINT('Ctrl Pts',(-57.674283923512,12.1263906358456,2.62224491711752));
#216297=CARTESIAN_POINT('Ctrl Pts',(-57.6720986344673,12.130922403056,2.62031533672604));
#216298=CARTESIAN_POINT('Ctrl Pts',(-57.6644501228111,12.1467835882925,
2.61356180535585));
#216299=CARTESIAN_POINT('Ctrl Pts',(-57.6575224410761,12.1635710602992,
2.60825339735355));
#216300=CARTESIAN_POINT('Ctrl Pts',(-57.6515149180852,12.1810659563067,
2.60463337987618));
#216301=CARTESIAN_POINT('Ctrl Pts',(-57.6485111565898,12.1898134043104,
2.6028233711375));
#216302=CARTESIAN_POINT('Ctrl Pts',(-57.6457374357765,12.1987377085285,
2.60143545939121));
#216303=CARTESIAN_POINT('Ctrl Pts',(-57.6432186759796,12.2078115120428,
2.60050005034603));
#216304=CARTESIAN_POINT('Ctrl Pts',(-57.6419592960812,12.2123484137999,
2.60003234582343));
#216305=CARTESIAN_POINT('Ctrl Pts',(-57.6407636564617,12.2169226903867,
2.59967776696073));
#216306=CARTESIAN_POINT('Ctrl Pts',(-57.6396348724476,12.221530922251,2.59944011429167));
#216307=CARTESIAN_POINT('Ctrl Pts',(-57.6385060884334,12.2261391541152,
2.59920246162261));
#216308=CARTESIAN_POINT('Ctrl Pts',(-57.637444161687,12.2307813416097,2.59908173791317));
#216309=CARTESIAN_POINT('Ctrl Pts',(-57.6364522029208,12.2354540642043,
2.59908173516031));
#216310=CARTESIAN_POINT('',(-57.6301266171958,12.2652136052659,2.59908173516031));
#216311=CARTESIAN_POINT('Origin',(3.35846787602729E-16,1.91121649021616E-13,
2.59908173516024));
#216312=CARTESIAN_POINT('',(-57.7513140650721,12.599423532447,2.9013417351603));
#216313=CARTESIAN_POINT('Ctrl Pts',(-57.6301266171958,12.2652136052659,
2.59908173516031));
#216314=CARTESIAN_POINT('Ctrl Pts',(-57.62933355681,12.2689399558127,2.5990817437152));
#216315=CARTESIAN_POINT('Ctrl Pts',(-57.6285886446436,12.2726659100577,
2.59915764355898));
#216316=CARTESIAN_POINT('Ctrl Pts',(-57.6278912144856,12.2763893518626,
2.59930765775284));
#216317=CARTESIAN_POINT('Ctrl Pts',(-57.6237736395748,12.2983722707008,
2.60019333020891));
#216318=CARTESIAN_POINT('Ctrl Pts',(-57.6213089400485,12.3202698780616,
2.6036597332411));
#216319=CARTESIAN_POINT('Ctrl Pts',(-57.620361900501,12.3416402131538,2.6093417708243));
#216320=CARTESIAN_POINT('Ctrl Pts',(-57.6200081180516,12.3496234589568,
2.61146439091861));
#216321=CARTESIAN_POINT('Ctrl Pts',(-57.6198658344726,12.3575334177749,
2.6138958442933));
#216322=CARTESIAN_POINT('Ctrl Pts',(-57.6199270848658,12.3653481937526,
2.61661604385262));
#216323=CARTESIAN_POINT('Ctrl Pts',(-57.6199748754952,12.3714456739993,
2.61873848000785));
#216324=CARTESIAN_POINT('Ctrl Pts',(-57.6201468963099,12.3774848147423,
2.62103707099796));
#216325=CARTESIAN_POINT('Ctrl Pts',(-57.6204396772352,12.3834548161674,
2.62350262767661));
#216326=CARTESIAN_POINT('Ctrl Pts',(-57.6214644104741,12.4043498211551,
2.63213207605187));
#216327=CARTESIAN_POINT('Ctrl Pts',(-57.6239684463328,12.424397867568,2.64280685971922));
#216328=CARTESIAN_POINT('Ctrl Pts',(-57.6278030948197,12.443135932958,2.65513293646092));
#216329=CARTESIAN_POINT('Ctrl Pts',(-57.6297204190631,12.452504965653,2.66129597483176));
#216330=CARTESIAN_POINT('Ctrl Pts',(-57.631970398231,12.461546503484,2.66787183533859));
#216331=CARTESIAN_POINT('Ctrl Pts',(-57.634534451072,12.4702026697495,2.67481125953868));
#216332=CARTESIAN_POINT('Ctrl Pts',(-57.6370875490681,12.4788218527842,
2.68172103524086));
#216333=CARTESIAN_POINT('Ctrl Pts',(-57.6399518422608,12.4870591024244,
2.68899101329793));
#216334=CARTESIAN_POINT('Ctrl Pts',(-57.6431095890443,12.4948568232947,
2.69657334701279));
#216335=CARTESIAN_POINT('Ctrl Pts',(-57.6431231383189,12.4948902817918,
2.69660588132577));
#216336=CARTESIAN_POINT('Ctrl Pts',(-57.6431366925668,12.4949237325312,
2.69663842081385));
#216337=CARTESIAN_POINT('Ctrl Pts',(-57.643150251786,12.494957175512,2.69667096547386));
#216338=CARTESIAN_POINT('Ctrl Pts',(-57.6495445189162,12.5107282424394,
2.71201840158057));
#216339=CARTESIAN_POINT('Ctrl Pts',(-57.6570084630825,12.5247638376628,
2.72845645939596));
#216340=CARTESIAN_POINT('Ctrl Pts',(-57.6653488494813,12.537086190472,2.74568723187283));
#216341=CARTESIAN_POINT('Ctrl Pts',(-57.6739926427264,12.5498568062306,
2.7635448259486));
#216342=CARTESIAN_POINT('Ctrl Pts',(-57.6835785531314,12.5607877070446,
2.78225519317828));
#216343=CARTESIAN_POINT('Ctrl Pts',(-57.6939175280725,12.5698584016499,
2.80151223086376));
#216344=CARTESIAN_POINT('Ctrl Pts',(-57.7041089426426,12.5787996370904,
2.82049442741271));
#216345=CARTESIAN_POINT('Ctrl Pts',(-57.7150329979085,12.5859335005865,
2.84000929090405));
#216346=CARTESIAN_POINT('Ctrl Pts',(-57.7265206205463,12.5911935813594,
2.85976644342905));
#216347=CARTESIAN_POINT('Ctrl Pts',(-57.734529995431,12.5948610032589,2.87354148167813));
#216348=CARTESIAN_POINT('Ctrl Pts',(-57.7428135895673,12.5976165994018,
2.88743438345924));
#216349=CARTESIAN_POINT('Ctrl Pts',(-57.7513140650721,12.599423532447,2.9013417351603));
#216350=CARTESIAN_POINT('',(-58.0998260601481,12.6735055745739,3.4715307213908));
#216351=CARTESIAN_POINT('',(-57.7513140650721,12.599423532447,2.9013417351603));
#216352=CARTESIAN_POINT('',(-56.6526781108324,18.074335247489,3.47153072139084));
#216353=CARTESIAN_POINT('Origin',(5.53234440788222E-15,1.85015204418142E-13,
3.47153072139072));
#216354=CARTESIAN_POINT('',(-56.3138168485096,17.9642361803971,2.90134173516035));
#216355=CARTESIAN_POINT('',(-56.6526781108324,18.074335247489,3.47153072139084));
#216356=CARTESIAN_POINT('',(-56.0417604764384,18.1930767435948,2.59908173516036));
#216357=CARTESIAN_POINT('Ctrl Pts',(-56.3138168485096,17.9642361803971,
2.90134173516035));
#216358=CARTESIAN_POINT('Ctrl Pts',(-56.3021854218461,17.9604570513083,
2.88176998919808));
#216359=CARTESIAN_POINT('Ctrl Pts',(-56.2900121878799,17.958522970441,2.86226752356716));
#216360=CARTESIAN_POINT('Ctrl Pts',(-56.2774781111554,17.958413842529,2.84310370500003));
#216361=CARTESIAN_POINT('Ctrl Pts',(-56.2647176232329,17.9583027433683,
2.82359371788659));
#216362=CARTESIAN_POINT('Ctrl Pts',(-56.2515822679736,17.9600828051304,
2.80443322637017));
#216363=CARTESIAN_POINT('Ctrl Pts',(-56.2382392305972,17.9637804645268,
2.78589323878292));
#216364=CARTESIAN_POINT('Ctrl Pts',(-56.2254611028283,17.9673215746115,
2.76813818620094));
#216365=CARTESIAN_POINT('Ctrl Pts',(-56.2124916494903,17.9726214740528,
2.75095095198868));
#216366=CARTESIAN_POINT('Ctrl Pts',(-56.1994690140083,17.9797472965484,
2.73457771435322));
#216367=CARTESIAN_POINT('Ctrl Pts',(-56.1891112379835,17.9854149414352,
2.72155497955712));
#216368=CARTESIAN_POINT('Ctrl Pts',(-56.1787195200274,17.9922384661037,
2.70904711160031));
#216369=CARTESIAN_POINT('Ctrl Pts',(-56.1683642893843,18.0002723763371,
2.6971895615835));
#216370=CARTESIAN_POINT('Ctrl Pts',(-56.1683360229684,18.0002943063023,
2.69715719432367));
#216371=CARTESIAN_POINT('Ctrl Pts',(-56.1683077570002,18.0003162453126,
2.69712483219033));
#216372=CARTESIAN_POINT('Ctrl Pts',(-56.1682794914817,18.000338193368,2.69709247518661));
#216373=CARTESIAN_POINT('Ctrl Pts',(-56.1626527236046,18.0047073547952,
2.69065122242287));
#216374=CARTESIAN_POINT('Ctrl Pts',(-56.1570391911759,18.0094711966667,
2.68442464469436));
#216375=CARTESIAN_POINT('Ctrl Pts',(-56.1514686668952,18.0146022491738,
2.67844505923589));
#216376=CARTESIAN_POINT('Ctrl Pts',(-56.1404135756907,18.0247851782094,
2.66657815779577));
#216377=CARTESIAN_POINT('Ctrl Pts',(-56.1295277006975,18.0364157638827,
2.65568445664184));
#216378=CARTESIAN_POINT('Ctrl Pts',(-56.1190427465077,18.0492876213733,
2.64601906229525));
#216379=CARTESIAN_POINT('Ctrl Pts',(-56.1111790308653,18.0589415144913,
2.63877001653531));
#216380=CARTESIAN_POINT('Ctrl Pts',(-56.1035408324002,18.0692936227627,
2.63221189387612));
#216381=CARTESIAN_POINT('Ctrl Pts',(-56.0962259123228,18.080256881013,2.62645231033244));
#216382=CARTESIAN_POINT('Ctrl Pts',(-56.0934828172938,18.0843681028569,
2.62429246650356));
#216383=CARTESIAN_POINT('Ctrl Pts',(-56.0907851834709,18.0885652677243,
2.62224491711756));
#216384=CARTESIAN_POINT('Ctrl Pts',(-56.0881381670059,18.0928437845341,
2.62031533672608));
#216385=CARTESIAN_POINT('Ctrl Pts',(-56.0788736093784,18.1078185933685,
2.61356180535589));
#216386=CARTESIAN_POINT('Ctrl Pts',(-56.0702291095578,18.1237899619214,
2.60825339735359));
#216387=CARTESIAN_POINT('Ctrl Pts',(-56.0624257818118,18.1405610619117,
2.60463337987622));
#216388=CARTESIAN_POINT('Ctrl Pts',(-56.0585241179387,18.1489466119069,
2.60282337113754));
#216389=CARTESIAN_POINT('Ctrl Pts',(-56.0548327480526,18.1575320950786,
2.60143545939126));
#216390=CARTESIAN_POINT('Ctrl Pts',(-56.0513793155481,18.1662929092569,
2.60050005034608));
#216391=CARTESIAN_POINT('Ctrl Pts',(-56.0496525992959,18.170673316346,2.60003234582348));
#216392=CARTESIAN_POINT('Ctrl Pts',(-56.0479853674132,18.1750975561951,
2.59967776696078));
#216393=CARTESIAN_POINT('Ctrl Pts',(-56.0463810756008,18.1795625536246,
2.59944011429172));
#216394=CARTESIAN_POINT('Ctrl Pts',(-56.0447767837884,18.1840275510541,
2.59920246162266));
#216395=CARTESIAN_POINT('Ctrl Pts',(-56.0432354336628,18.1885333065889,
2.59908173791323));
#216396=CARTESIAN_POINT('Ctrl Pts',(-56.0417604764384,18.1930767435948,
2.59908173516036));
#216397=CARTESIAN_POINT('',(-56.0323588238392,18.2220120550216,2.59908173516035));
#216398=CARTESIAN_POINT('Origin',(3.37692616670652E-16,1.9112853774948E-13,
2.59908173516024));
#216399=CARTESIAN_POINT('',(-56.1179479440989,18.5670586829464,2.90134173516035));
#216400=CARTESIAN_POINT('Ctrl Pts',(-56.0323588238392,18.2220120550216,
2.59908173516036));
#216401=CARTESIAN_POINT('Ctrl Pts',(-56.0311805982249,18.2256350948468,
2.59908174371523));
#216402=CARTESIAN_POINT('Ctrl Pts',(-56.0300502984939,18.2292627734005,
2.59915764355901));
#216403=CARTESIAN_POINT('Ctrl Pts',(-56.0289674832814,18.232892916499,2.59930765775288));
#216404=CARTESIAN_POINT('Ctrl Pts',(-56.0225746241525,18.2543250068297,
2.60019333020893));
#216405=CARTESIAN_POINT('Ctrl Pts',(-56.0178345032614,18.2758450255522,
2.60365973324109));
#216406=CARTESIAN_POINT('Ctrl Pts',(-56.0146588434089,18.296999299124,2.60934177082421));
#216407=CARTESIAN_POINT('Ctrl Pts',(-56.0134725226011,18.3049018315356,
2.61146439091855));
#216408=CARTESIAN_POINT('Ctrl Pts',(-56.0125042026266,18.3127535860879,
2.61389584429327));
#216409=CARTESIAN_POINT('Ctrl Pts',(-56.01174825096,18.3205319543147,2.61661604385263));
#216410=CARTESIAN_POINT('Ctrl Pts',(-56.0111584195474,18.3266010274078,
2.61873848000787));
#216411=CARTESIAN_POINT('Ctrl Pts',(-56.0106982359127,18.3326250661773,
2.62103707099799));
#216412=CARTESIAN_POINT('Ctrl Pts',(-56.0103653778789,18.3385929672501,
2.62350262767664));
#216413=CARTESIAN_POINT('Ctrl Pts',(-56.0092003747605,18.3594806210049,
2.6321320760519));
#216414=CARTESIAN_POINT('Ctrl Pts',(-56.0095951017657,18.3796805851421,
2.64280685971925));
#216415=CARTESIAN_POINT('Ctrl Pts',(-56.0114500824671,18.3987168313629,
2.65513293646094));
#216416=CARTESIAN_POINT('Ctrl Pts',(-56.0123775728178,18.4082349544732,
2.66129597483179));
#216417=CARTESIAN_POINT('Ctrl Pts',(-56.0136701283094,18.4174621486788,
2.66787183533863));
#216418=CARTESIAN_POINT('Ctrl Pts',(-56.0153153192431,18.426338912063,2.67481125953872));
#216419=CARTESIAN_POINT('Ctrl Pts',(-56.016953481144,18.4351777497213,2.6817210352409));
#216420=CARTESIAN_POINT('Ctrl Pts',(-56.0189410563924,18.4436692750118,
2.688991013298));
#216421=CARTESIAN_POINT('Ctrl Pts',(-56.0212664209291,18.4517543535699,
2.69657334701286));
#216422=CARTESIAN_POINT('Ctrl Pts',(-56.0212763986141,18.4517890450628,
2.69660588132583));
#216423=CARTESIAN_POINT('Ctrl Pts',(-56.021286382056,18.4518237293603,2.69663842081391));
#216424=CARTESIAN_POINT('Ctrl Pts',(-56.021296371253,18.4518584064613,2.69667096547392));
#216425=CARTESIAN_POINT('Ctrl Pts',(-56.0260070845284,18.4682114607492,
2.7120184015792));
#216426=CARTESIAN_POINT('Ctrl Pts',(-56.0319630212272,18.4829503621257,
2.72845645939294));
#216427=CARTESIAN_POINT('Ctrl Pts',(-56.0389696815128,18.4960770195692,
2.74568723186805));
#216428=CARTESIAN_POINT('Ctrl Pts',(-56.046231230313,18.5096811989822,2.76354482594212));
#216429=CARTESIAN_POINT('Ctrl Pts',(-56.0546220378327,18.5215542196609,
2.78225519317));
#216430=CARTESIAN_POINT('Ctrl Pts',(-56.0639562290182,18.5316559412141,
2.80151223085363));
#216431=CARTESIAN_POINT('Ctrl Pts',(-56.0731572003518,18.5416134885349,
2.82049442740119));
#216432=CARTESIAN_POINT('Ctrl Pts',(-56.0832757207105,18.5498501466901,
2.84000929089115));
#216433=CARTESIAN_POINT('Ctrl Pts',(-56.0941505847886,18.5562821957317,
2.8597664434148));
#216434=CARTESIAN_POINT('Ctrl Pts',(-56.1017327335067,18.5607667347609,
2.87354148166857));
#216435=CARTESIAN_POINT('Ctrl Pts',(-56.10968291102,18.5643731068268,2.88743438345449));
#216436=CARTESIAN_POINT('Ctrl Pts',(-56.1179479440989,18.5670586829464,
2.90134173516035));
#216437=CARTESIAN_POINT('',(-56.4568070719812,18.6771643191708,3.47153072139084));
#216438=CARTESIAN_POINT('',(-56.1179479440989,18.5670586829464,2.90134173516035));
#216439=CARTESIAN_POINT('',(-54.4530463244694,23.8971395307767,3.47153072139088));
#216440=CARTESIAN_POINT('Origin',(5.53234440788222E-15,1.85015204418142E-13,
3.47153072139072));
#216441=CARTESIAN_POINT('',(-54.1275498658875,23.7522229508827,2.90134173516039));
#216442=CARTESIAN_POINT('',(-54.4530463244694,23.8971395307767,3.47153072139088));
#216443=CARTESIAN_POINT('',(-53.8330634946839,23.9513722670364,2.5990817351604));
#216444=CARTESIAN_POINT('Ctrl Pts',(-54.1275498658875,23.7522229508827,
2.90134173516039));
#216445=CARTESIAN_POINT('Ctrl Pts',(-54.1163771839517,23.7472487091033,
2.88176998919681));
#216446=CARTESIAN_POINT('Ctrl Pts',(-54.1044728027349,23.7440527738937,
2.86226752356458));
#216447=CARTESIAN_POINT('Ctrl Pts',(-54.0920187959662,23.7426340760174,
2.84310370499621));
#216448=CARTESIAN_POINT('Ctrl Pts',(-54.0793398243553,23.7411897512767,
2.82359371788141));
#216449=CARTESIAN_POINT('Ctrl Pts',(-54.0660903588249,23.7415870431748,
2.80443322636371));
#216450=CARTESIAN_POINT('Ctrl Pts',(-54.0524339053478,23.7438697192146,
2.78589323877531));
#216451=CARTESIAN_POINT('Ctrl Pts',(-54.0393556307033,23.7460557526692,
2.76813818619207));
#216452=CARTESIAN_POINT('Ctrl Pts',(-54.0259032350424,23.749970941681,2.75095095197868));
#216453=CARTESIAN_POINT('Ctrl Pts',(-54.012207087644,23.7556964921021,2.73457771434229));
#216454=CARTESIAN_POINT('Ctrl Pts',(-54.0013136223926,23.7602504066258,
2.72155497955013));
#216455=CARTESIAN_POINT('Ctrl Pts',(-53.9902655788102,23.7659503210024,
2.70904711159702));
#216456=CARTESIAN_POINT('Ctrl Pts',(-53.9791273029164,23.772857804287,2.69718956158354));
#216457=CARTESIAN_POINT('Ctrl Pts',(-53.9790968990413,23.7728766594726,
2.69715719432371));
#216458=CARTESIAN_POINT('Ctrl Pts',(-53.979066494666,23.7728955237005,2.69712483219037));
#216459=CARTESIAN_POINT('Ctrl Pts',(-53.9790360897925,23.7729143969709,
2.69709247518665));
#216460=CARTESIAN_POINT('Ctrl Pts',(-53.9729834442088,23.7766714662754,
2.69065122242291));
#216461=CARTESIAN_POINT('Ctrl Pts',(-53.966902706228,23.7808224374043,2.68442464469441));
#216462=CARTESIAN_POINT('Ctrl Pts',(-53.9608263568287,23.7853431031263,
2.67844505923594));
#216463=CARTESIAN_POINT('Ctrl Pts',(-53.9487674206469,23.7943146773162,
2.66657815779582));
#216464=CARTESIAN_POINT('Ctrl Pts',(-53.9367254523685,23.80474366564,2.65568445664189));
#216465=CARTESIAN_POINT('Ctrl Pts',(-53.924952460372,23.8164490335996,2.64601906229531));
#216466=CARTESIAN_POINT('Ctrl Pts',(-53.9161227163745,23.8252280595693,
2.63877001653537));
#216467=CARTESIAN_POINT('Ctrl Pts',(-53.9074442707905,23.8347250487607,
2.63221189387617));
#216468=CARTESIAN_POINT('Ctrl Pts',(-53.8990234500734,23.8448636317806,
2.62645231033249));
#216469=CARTESIAN_POINT('Ctrl Pts',(-53.8958656423045,23.848665600413,2.62429246650361));
#216470=CARTESIAN_POINT('Ctrl Pts',(-53.8927440632083,23.8525577932541,
2.62224491711761));
#216471=CARTESIAN_POINT('Ctrl Pts',(-53.8896643205892,23.8565361833379,
2.62031533672612));
#216472=CARTESIAN_POINT('Ctrl Pts',(-53.8788852214227,23.8704605486311,
2.61356180535593));
#216473=CARTESIAN_POINT('Ctrl Pts',(-53.8686186144654,23.8854408280738,
2.60825339735363));
#216474=CARTESIAN_POINT('Ctrl Pts',(-53.8591049768559,23.901304384366,2.60463337987626));
#216475=CARTESIAN_POINT('Ctrl Pts',(-53.8543481580512,23.9092361625121,
2.60282337113758));
#216476=CARTESIAN_POINT('Ctrl Pts',(-53.8497795825132,23.9173887602871,
2.6014354593913));
#216477=CARTESIAN_POINT('Ctrl Pts',(-53.8454293138303,23.9257405998159,
2.60050005034611));
#216478=CARTESIAN_POINT('Ctrl Pts',(-53.8432541794888,23.9299165195804,
2.60003234582352));
#216479=CARTESIAN_POINT('Ctrl Pts',(-53.8411336218843,23.934142249794,2.5996777669608));
#216480=CARTESIAN_POINT('Ctrl Pts',(-53.8390713992305,23.9384150933427,
2.59944011429174));
#216481=CARTESIAN_POINT('Ctrl Pts',(-53.8370091765767,23.9426879368913,
2.59920246162268));
#216482=CARTESIAN_POINT('Ctrl Pts',(-53.8350052904264,23.9470078944659,
2.59908173791324));
#216483=CARTESIAN_POINT('Ctrl Pts',(-53.8330634946839,23.9513722670364,
2.59908173516039));
#216484=CARTESIAN_POINT('',(-53.8206887816837,23.9791663275012,2.59908173516039));
#216485=CARTESIAN_POINT('Origin',(3.40248402231255E-16,1.91135195798496E-13,
2.59908173516024));
#216486=CARTESIAN_POINT('',(-53.8697418420146,24.3312692531087,2.90134173516039));
#216487=CARTESIAN_POINT('Ctrl Pts',(-53.8206887816837,23.9791663275012,
2.59908173516039));
#216488=CARTESIAN_POINT('Ctrl Pts',(-53.8191382997273,23.9826463618224,
2.59908174371529));
#216489=CARTESIAN_POINT('Ctrl Pts',(-53.817634996232,23.9861360190795,2.59915764355906));
#216490=CARTESIAN_POINT('Ctrl Pts',(-53.816178659515,23.9896330908641,2.59930765775292));
#216491=CARTESIAN_POINT('Ctrl Pts',(-53.8075805576711,24.0102795382192,
2.60019333020891));
#216492=CARTESIAN_POINT('Ctrl Pts',(-53.8006169491722,24.0311861904733,
2.60365973324058));
#216493=CARTESIAN_POINT('Ctrl Pts',(-53.7952474622088,24.0518926318752,
2.60934177082291));
#216494=CARTESIAN_POINT('Ctrl Pts',(-53.793241600621,24.0596278690981,2.61146439091757));
#216495=CARTESIAN_POINT('Ctrl Pts',(-53.791457853367,24.0673353939202,2.61389584429274));
#216496=CARTESIAN_POINT('Ctrl Pts',(-53.7898929820049,24.0749921329677,
2.61661604385268));
#216497=CARTESIAN_POINT('Ctrl Pts',(-53.7886719908666,24.0809663048721,
2.61873848000792));
#216498=CARTESIAN_POINT('Ctrl Pts',(-53.7875846446508,24.0869092410388,
2.62103707099803));
#216499=CARTESIAN_POINT('Ctrl Pts',(-53.78662979452,24.0928096561863,2.62350262767668));
#216500=CARTESIAN_POINT('Ctrl Pts',(-53.7832878190623,24.1134611092026,
2.63213207605195));
#216501=CARTESIAN_POINT('Ctrl Pts',(-53.7815689125024,24.1335916760301,
2.6428068597193));
#216502=CARTESIAN_POINT('Ctrl Pts',(-53.7814239018616,24.1527175379843,
2.655132936461));
#216503=CARTESIAN_POINT('Ctrl Pts',(-53.7813513965412,24.1622804689615,
2.66129597483185));
#216504=CARTESIAN_POINT('Ctrl Pts',(-53.7816723668479,24.1715922244709,
2.66787183533867));
#216505=CARTESIAN_POINT('Ctrl Pts',(-53.7823806708182,24.1805923292966,
2.67481125953876));
#216506=CARTESIAN_POINT('Ctrl Pts',(-53.7830859485794,24.1895539814234,
2.68172103524095));
#216507=CARTESIAN_POINT('Ctrl Pts',(-53.7841750295932,24.1982067474363,
2.68899101329804));
#216508=CARTESIAN_POINT('Ctrl Pts',(-53.7856425347025,24.2064906018697,
2.6965733470129));
#216509=CARTESIAN_POINT('Ctrl Pts',(-53.7856488314803,24.206526146271,2.69660588132587));
#216510=CARTESIAN_POINT('Ctrl Pts',(-53.7856551347356,24.2065616841181,
2.69663842081396));
#216511=CARTESIAN_POINT('Ctrl Pts',(-53.7856614444666,24.2065972154097,
2.69667096547396));
#216512=CARTESIAN_POINT('Ctrl Pts',(-53.7886369923274,24.2233530895752,
2.71201840157957));
#216513=CARTESIAN_POINT('Ctrl Pts',(-53.7930196670707,24.2386338146185,
2.72845645939369));
#216514=CARTESIAN_POINT('Ctrl Pts',(-53.7986158348079,24.2524209582917,
2.74568723186921));
#216515=CARTESIAN_POINT('Ctrl Pts',(-53.8044155801161,24.2667096511237,
2.76354482594357));
#216516=CARTESIAN_POINT('Ctrl Pts',(-53.8115193533084,24.2793947083685,
2.78225519317175));
#216517=CARTESIAN_POINT('Ctrl Pts',(-53.8197464933879,24.2904167802946,
2.80151223085569));
#216518=CARTESIAN_POINT('Ctrl Pts',(-53.8278562137185,24.3012815425233,
2.82049442740332));
#216519=CARTESIAN_POINT('Ctrl Pts',(-53.8370583385447,24.3105307527869,
2.84000929089333));
#216520=CARTESIAN_POINT('Ctrl Pts',(-53.8472012967776,24.3180642992209,
2.85976644341703));
#216521=CARTESIAN_POINT('Ctrl Pts',(-53.8542731477182,24.3233168218295,
2.87354148167009));
#216522=CARTESIAN_POINT('Ctrl Pts',(-53.8618028047969,24.3277344576498,
2.88743438345526));
#216523=CARTESIAN_POINT('Ctrl Pts',(-53.8697418420146,24.3312692531087,
2.90134173516039));
#216524=CARTESIAN_POINT('',(-54.1952354911873,24.4761921430391,3.47153072139088));
#216525=CARTESIAN_POINT('',(-53.8697418420146,24.3312692531087,2.90134173516039));
#216526=CARTESIAN_POINT('',(-51.6568155675429,29.4581217525673,3.47153072139092));
#216527=CARTESIAN_POINT('Origin',(5.53234440788222E-15,1.85015204418142E-13,
3.47153072139072));
#216528=CARTESIAN_POINT('',(-51.3482501200167,29.2799753962461,2.90134173516043));
#216529=CARTESIAN_POINT('',(-51.6568155675429,29.4581217525673,3.47153072139092));
#216530=CARTESIAN_POINT('',(-51.0345602039888,29.4472515437734,2.59908173516043));
#216531=CARTESIAN_POINT('Ctrl Pts',(-51.3482501200167,29.2799753962461,
2.90134173516043));
#216532=CARTESIAN_POINT('Ctrl Pts',(-51.3376585930506,29.2738605406102,
2.88176998919663));
#216533=CARTESIAN_POINT('Ctrl Pts',(-51.3261534914758,29.2694377663933,
2.86226752356419));
#216534=CARTESIAN_POINT('Ctrl Pts',(-51.313916003368,29.2667250421033,2.84310370499561));
#216535=CARTESIAN_POINT('Ctrl Pts',(-51.3014574615356,29.2639633161063,
2.82359371788049));
#216536=CARTESIAN_POINT('Ctrl Pts',(-51.2882390496519,29.2629734853269,
2.80443322636248));
#216537=CARTESIAN_POINT('Ctrl Pts',(-51.2744188030369,29.263816168533,2.7858932387738));
#216538=CARTESIAN_POINT('Ctrl Pts',(-51.2611836698312,29.264623174717,2.7681381861901));
#216539=CARTESIAN_POINT('Ctrl Pts',(-51.2473957191101,29.2671107576683,
2.75095095197629));
#216540=CARTESIAN_POINT('Ctrl Pts',(-51.2331761176528,29.2713733056852,
2.73457771433953));
#216541=CARTESIAN_POINT('Ctrl Pts',(-51.2218663142576,29.2747635962062,
2.72155497954838));
#216542=CARTESIAN_POINT('Ctrl Pts',(-51.2102829897242,29.2792774508374,
2.70904711159621));
#216543=CARTESIAN_POINT('Ctrl Pts',(-51.1984837018592,29.2849828273428,
2.69718956158358));
#216544=CARTESIAN_POINT('Ctrl Pts',(-51.1984514936361,29.2849984011674,
2.69715719432375));
#216545=CARTESIAN_POINT('Ctrl Pts',(-51.1984192839704,29.2850139839325,
2.69712483219041));
#216546=CARTESIAN_POINT('Ctrl Pts',(-51.198387072864,29.2850295756385,2.69709247518669));
#216547=CARTESIAN_POINT('Ctrl Pts',(-51.1919748636254,29.2881333895826,
2.69065122242294));
#216548=CARTESIAN_POINT('Ctrl Pts',(-51.1854935419303,29.2916260110607,
2.68442464469444));
#216549=CARTESIAN_POINT('Ctrl Pts',(-51.1789779411679,29.2954867606378,
2.67844505923596));
#216550=CARTESIAN_POINT('Ctrl Pts',(-51.1660472802371,29.303148685538,2.66657815779585));
#216551=CARTESIAN_POINT('Ctrl Pts',(-51.152981152998,29.3122618143336,2.65568445664191));
#216552=CARTESIAN_POINT('Ctrl Pts',(-51.1400491105586,29.3226724463013,
2.64601906229532));
#216553=CARTESIAN_POINT('Ctrl Pts',(-51.130350078729,29.330480420277,2.63877001653539));
#216554=CARTESIAN_POINT('Ctrl Pts',(-51.1207264688922,29.3390182393876,
2.6322118938762));
#216555=CARTESIAN_POINT('Ctrl Pts',(-51.1112920078093,29.3482210667398,
2.62645231033252));
#216556=CARTESIAN_POINT('Ctrl Pts',(-51.1077540849032,29.3516721269969,
2.62429246650364));
#216557=CARTESIAN_POINT('Ctrl Pts',(-51.1042427612074,29.3552167041325,
2.62224491711764));
#216558=CARTESIAN_POINT('Ctrl Pts',(-51.100764034739,29.3588513794159,2.62031533672616));
#216559=CARTESIAN_POINT('Ctrl Pts',(-51.0885884920994,29.3715727429078,
2.61356180535597));
#216560=CARTESIAN_POINT('Ctrl Pts',(-51.0768122610998,29.3853978061641,
2.60825339735367));
#216561=CARTESIAN_POINT('Ctrl Pts',(-51.0656925470314,29.4001800143157,
2.6046333798763));
#216562=CARTESIAN_POINT('Ctrl Pts',(-51.0601326899972,29.4075711183915,
2.60282337113762));
#216563=CARTESIAN_POINT('Ctrl Pts',(-51.0547369630769,29.4152015092025,
2.60143545939133));
#216564=CARTESIAN_POINT('Ctrl Pts',(-51.0495375206696,29.4230528695804,
2.60050005034615));
#216565=CARTESIAN_POINT('Ctrl Pts',(-51.046937799466,29.4269785497693,2.60003234582355));
#216566=CARTESIAN_POINT('Ctrl Pts',(-51.0443871494124,29.430959472363,2.59967776696084));
#216567=CARTESIAN_POINT('Ctrl Pts',(-51.0418895900602,29.4349933478627,
2.59944011429178));
#216568=CARTESIAN_POINT('Ctrl Pts',(-51.039392030708,29.4390272233624,2.59920246162272));
#216569=CARTESIAN_POINT('Ctrl Pts',(-51.0369475635291,29.4431140526175,
2.59908173791332));
#216570=CARTESIAN_POINT('Ctrl Pts',(-51.0345602039888,29.4472515437734,
2.59908173516043));
#216571=CARTESIAN_POINT('',(-51.0193480105329,29.4735998357337,2.59908173516043));
#216572=CARTESIAN_POINT('Origin',(3.434861425631E-16,1.91141550221685E-13,
2.59908173516024));
#216573=CARTESIAN_POINT('',(-51.031327575341,29.8289013456885,2.90134173516044));
#216574=CARTESIAN_POINT('Ctrl Pts',(-51.0193480105329,29.4735998357337,
2.59908173516043));
#216575=CARTESIAN_POINT('Ctrl Pts',(-51.0174422596392,29.4768987365664,
2.59908174371533));
#216576=CARTESIAN_POINT('Ctrl Pts',(-51.0155824228873,29.4802121391118,
2.5991576435591));
#216577=CARTESIAN_POINT('Ctrl Pts',(-51.0137685205956,29.4835378249322,
2.59930765775296));
#216578=CARTESIAN_POINT('Ctrl Pts',(-51.0030593786377,29.5031724225187,
2.60019333020908));
#216579=CARTESIAN_POINT('Ctrl Pts',(-50.9939485772814,29.5232366506522,
2.60365973324168));
#216580=CARTESIAN_POINT('Ctrl Pts',(-50.9864440924292,29.5432683957837,
2.60934177082554));
#216581=CARTESIAN_POINT('Ctrl Pts',(-50.9836406667025,29.5507515889354,
2.61146439091959));
#216582=CARTESIAN_POINT('Ctrl Pts',(-50.9810610352785,29.5582304387677,
2.6138958442939));
#216583=CARTESIAN_POINT('Ctrl Pts',(-50.9787043892802,29.5656816597958,
2.61661604385273));
#216584=CARTESIAN_POINT('Ctrl Pts',(-50.9768656158506,29.5714954762341,
2.61873848000796));
#216585=CARTESIAN_POINT('Ctrl Pts',(-50.9751630202463,29.5772921977456,
2.62103707099807));
#216586=CARTESIAN_POINT('Ctrl Pts',(-50.9735966395564,29.5830604807848,
2.62350262767672));
#216587=CARTESIAN_POINT('Ctrl Pts',(-50.9681143071419,29.6032494714219,
2.63213207605199));
#216588=CARTESIAN_POINT('Ctrl Pts',(-50.9643005997168,29.6230900862367,
2.64280685971934));
#216589=CARTESIAN_POINT('Ctrl Pts',(-50.9621571865007,29.6420960169786,
2.65513293646104));
#216590=CARTESIAN_POINT('Ctrl Pts',(-50.9610854798927,29.6515989823495,
2.66129597483189));
#216591=CARTESIAN_POINT('Ctrl Pts',(-50.9604313483968,29.6608932776209,
2.66787183533872));
#216592=CARTESIAN_POINT('Ctrl Pts',(-50.9601950050771,29.6699181168562,
2.67481125953881));
#216593=CARTESIAN_POINT('Ctrl Pts',(-50.9599596715278,29.6789043977155,
2.68172103524099));
#216594=CARTESIAN_POINT('Ctrl Pts',(-50.9601383261075,29.6876236029356,
2.68899101329808));
#216595=CARTESIAN_POINT('Ctrl Pts',(-50.9607318934965,29.6960154736015,
2.69657334701294));
#216596=CARTESIAN_POINT('Ctrl Pts',(-50.9607344403782,29.6960514814794,
2.69660588132591));
#216597=CARTESIAN_POINT('Ctrl Pts',(-50.960736994387,29.6960874835161,2.696638420814));
#216598=CARTESIAN_POINT('Ctrl Pts',(-50.9607395555213,29.69612347971,2.69667096547401));
#216599=CARTESIAN_POINT('Ctrl Pts',(-50.9619473372423,29.713098592887,2.71201840157792));
#216600=CARTESIAN_POINT('Ctrl Pts',(-50.964708732528,29.728753722774,2.72845645939011));
#216601=CARTESIAN_POINT('Ctrl Pts',(-50.968833094931,29.743050297844,2.74568723186355));
#216602=CARTESIAN_POINT('Ctrl Pts',(-50.973107493523,29.7578669541847,2.76354482593593));
#216603=CARTESIAN_POINT('Ctrl Pts',(-50.9788464019613,29.771225067853,2.78225519316198));
#216604=CARTESIAN_POINT('Ctrl Pts',(-50.9858763526649,29.7830467300249,
2.80151223084375));
#216605=CARTESIAN_POINT('Ctrl Pts',(-50.9928059701984,29.7946996705526,
2.82049442738965));
#216606=CARTESIAN_POINT('Ctrl Pts',(-51.0009908790854,29.8048600966415,
2.8400092908779));
#216607=CARTESIAN_POINT('Ctrl Pts',(-51.0102908030987,29.8134126013573,
2.8597664433999));
#216608=CARTESIAN_POINT('Ctrl Pts',(-51.0167748755856,29.8193755598118,
2.87354148165858));
#216609=CARTESIAN_POINT('Ctrl Pts',(-51.0238015157341,29.8245560588468,
2.88743438344952));
#216610=CARTESIAN_POINT('Ctrl Pts',(-51.031327575341,29.8289013456885,2.90134173516043));
#216611=CARTESIAN_POINT('',(-51.3398895692699,30.0070536838157,3.47153072139092));
#216612=CARTESIAN_POINT('',(-51.031327575341,29.8289013456885,2.90134173516044));
#216613=CARTESIAN_POINT('',(-48.2946219293748,34.6963546279285,3.47153072139096));
#216614=CARTESIAN_POINT('Origin',(5.53234440788222E-15,1.85015204418142E-13,
3.47153072139072));
#216615=CARTESIAN_POINT('',(-48.0063682005189,34.4869303039396,2.90134173516046));
#216616=CARTESIAN_POINT('',(-48.2946219293748,34.6963546279284,3.47153072139096));
#216617=CARTESIAN_POINT('',(-47.6769115920306,34.6205005703634,2.59908173516047));
#216618=CARTESIAN_POINT('Ctrl Pts',(-48.0063682005189,34.4869303039396,
2.90134173516046));
#216619=CARTESIAN_POINT('Ctrl Pts',(-47.9964738715098,34.479741830086,2.88176998919909));
#216620=CARTESIAN_POINT('Ctrl Pts',(-47.985494101879,34.4741406737021,2.86226752356907));
#216621=CARTESIAN_POINT('Ctrl Pts',(-47.9736072089144,34.4701636441736,
2.84310370500279));
#216622=CARTESIAN_POINT('Ctrl Pts',(-47.9615055952539,34.4661147749682,
2.82359371788992));
#216623=CARTESIAN_POINT('Ctrl Pts',(-47.9484630607056,34.4637486663041,
2.80443322637404));
#216624=CARTESIAN_POINT('Ctrl Pts',(-47.9346304384691,34.463142124062,2.78589323878727));
#216625=CARTESIAN_POINT('Ctrl Pts',(-47.9213834535936,34.4625612612459,
2.76813818620531));
#216626=CARTESIAN_POINT('Ctrl Pts',(-47.907411011488,34.4635939836559,2.75095095199305));
#216627=CARTESIAN_POINT('Ctrl Pts',(-47.8928237489035,34.4663468278986,
2.73457771435755));
#216628=CARTESIAN_POINT('Ctrl Pts',(-47.8812215199315,34.4685363496847,
2.72155497955993));
#216629=CARTESIAN_POINT('Ctrl Pts',(-47.8692298237685,34.4718146898359,
2.70904711160169));
#216630=CARTESIAN_POINT('Ctrl Pts',(-47.8568987993929,34.4762554502657,
2.6971895615836));
#216631=CARTESIAN_POINT('Ctrl Pts',(-47.8568651397019,34.4762675720992,
2.69715719432378));
#216632=CARTESIAN_POINT('Ctrl Pts',(-47.8568314776416,34.4762797026734,
2.69712483219044));
#216633=CARTESIAN_POINT('Ctrl Pts',(-47.8567978132139,34.4762918419889,
2.69709247518672));
#216634=CARTESIAN_POINT('Ctrl Pts',(-47.8500962938266,34.4787083945376,
2.69065122242297));
#216635=CARTESIAN_POINT('Ctrl Pts',(-47.843285399134,34.4815044004731,2.68442464469447));
#216636=CARTESIAN_POINT('Ctrl Pts',(-47.836401933294,34.4846629347251,2.678445059236));
#216637=CARTESIAN_POINT('Ctrl Pts',(-47.8227412186412,34.4909312646828,
2.66657815779588));
#216638=CARTESIAN_POINT('Ctrl Pts',(-47.8087940876657,34.4986286886042,
2.65568445664195));
#216639=CARTESIAN_POINT('Ctrl Pts',(-47.7948446809467,34.5076305235176,
2.64601906229537));
#216640=CARTESIAN_POINT('Ctrl Pts',(-47.7843826259074,34.5143818997027,
2.63877001653543));
#216641=CARTESIAN_POINT('Ctrl Pts',(-47.7739192901009,34.5218670065995,
2.63221189387623));
#216642=CARTESIAN_POINT('Ctrl Pts',(-47.7635745545821,34.5300332501818,
2.62645231033255));
#216643=CARTESIAN_POINT('Ctrl Pts',(-47.7596952787625,34.5330955915252,
2.62429246650367));
#216644=CARTESIAN_POINT('Ctrl Pts',(-47.7558326812644,34.5362537178264,
2.62224491711768));
#216645=CARTESIAN_POINT('Ctrl Pts',(-47.7519930846017,34.5395048560464,
2.6203153367262));
#216646=CARTESIAN_POINT('Ctrl Pts',(-47.7385544962822,34.5508838398164,
2.61356180535601));
#216647=CARTESIAN_POINT('Ctrl Pts',(-47.7253976640914,34.5634022166003,
2.6082533973537));
#216648=CARTESIAN_POINT('Ctrl Pts',(-47.7127937034783,34.5769411196454,
2.60463337987634));
#216649=CARTESIAN_POINT('Ctrl Pts',(-47.7064917231718,34.5837105711679,
2.60282337113765));
#216650=CARTESIAN_POINT('Ctrl Pts',(-47.7003279615826,34.5907351548565,
2.60143545939137));
#216651=CARTESIAN_POINT('Ctrl Pts',(-47.69433631163,34.598000014936,2.60050005034618));
#216652=CARTESIAN_POINT('Ctrl Pts',(-47.6913404866537,34.6016324449758,
2.60003234582359));
#216653=CARTESIAN_POINT('Ctrl Pts',(-47.6883876896069,34.6053249441285,
2.59967776696089));
#216654=CARTESIAN_POINT('Ctrl Pts',(-47.6854821573391,34.6090756555952,
2.59944011429183));
#216655=CARTESIAN_POINT('Ctrl Pts',(-47.6825766250713,34.6128263670618,
2.59920246162277));
#216656=CARTESIAN_POINT('Ctrl Pts',(-47.6797183589578,34.6166352918409,
2.59908173791336));
#216657=CARTESIAN_POINT('Ctrl Pts',(-47.6769115920305,34.6205005703634,
2.59908173516047));
#216658=CARTESIAN_POINT('',(-47.6590285860937,34.6451144164185,2.59908173516047));
#216659=CARTESIAN_POINT('Origin',(3.4737036430558E-16,1.91147531398658E-13,
2.59908173516024));
#216660=CARTESIAN_POINT('',(-47.6338034047601,34.999721753026,2.90134173516047));
#216661=CARTESIAN_POINT('Ctrl Pts',(-47.6590285860937,34.6451144164185,
2.59908173516047));
#216662=CARTESIAN_POINT('Ctrl Pts',(-47.6567884460683,34.648196040315,2.59908174371537));
#216663=CARTESIAN_POINT('Ctrl Pts',(-47.6545924528205,34.651296885817,2.59915764355913));
#216664=CARTESIAN_POINT('Ctrl Pts',(-47.6524408584473,34.6544147487634,
2.599307657753));
#216665=CARTESIAN_POINT('Ctrl Pts',(-47.6397380079787,34.6728223758155,
2.60019333020899));
#216666=CARTESIAN_POINT('Ctrl Pts',(-47.6285798336134,34.6918243519402,
2.60365973324072));
#216667=CARTESIAN_POINT('Ctrl Pts',(-47.6190225715802,34.710961928804,2.60934177082314));
#216668=CARTESIAN_POINT('Ctrl Pts',(-47.615452296631,34.7181110904602,2.61146439091776));
#216669=CARTESIAN_POINT('Ctrl Pts',(-47.6121050440164,34.7252793254648,
2.61389584429288));
#216670=CARTESIAN_POINT('Ctrl Pts',(-47.6089824432867,34.7324433913425,
2.61661604385275));
#216671=CARTESIAN_POINT('Ctrl Pts',(-47.6065460335524,34.7380331549252,
2.61873848000798));
#216672=CARTESIAN_POINT('Ctrl Pts',(-47.6042468425534,34.7436201516877,
2.6210370709981));
#216673=CARTESIAN_POINT('Ctrl Pts',(-47.602086092899,34.7491931041024,2.62350262767674));
#216674=CARTESIAN_POINT('Ctrl Pts',(-47.5945234691089,34.7686984375539,
2.63213207605201));
#216675=CARTESIAN_POINT('Ctrl Pts',(-47.5886567445952,34.7880317224284,
2.64280685971936));
#216676=CARTESIAN_POINT('Ctrl Pts',(-47.5845384124876,34.8067094890034,
2.65513293646106));
#216677=CARTESIAN_POINT('Ctrl Pts',(-47.5824792464338,34.8160483722909,
2.66129597483191));
#216678=CARTESIAN_POINT('Ctrl Pts',(-47.5808571799367,34.8252233770803,
2.66787183533875));
#216679=CARTESIAN_POINT('Ctrl Pts',(-47.579678778754,34.834174072698,2.67481125953884));
#216680=CARTESIAN_POINT('Ctrl Pts',(-47.5785054122578,34.8430865267163,
2.68172103524103));
#216681=CARTESIAN_POINT('Ctrl Pts',(-47.5777716830264,34.8517766417065,
2.68899101329812));
#216682=CARTESIAN_POINT('Ctrl Pts',(-47.5774848094465,34.8601845855139,
2.69657334701298));
#216683=CARTESIAN_POINT('Ctrl Pts',(-47.577483578528,34.8602206623585,2.69660588132595));
#216684=CARTESIAN_POINT('Ctrl Pts',(-47.5774823553081,34.8602567341388,
2.69663842081403));
#216685=CARTESIAN_POINT('Ctrl Pts',(-47.5774811397854,34.8602928008533,
2.69667096547404));
#216686=CARTESIAN_POINT('Ctrl Pts',(-47.5769079226575,34.8773011701528,
2.71201840157922));
#216687=CARTESIAN_POINT('Ctrl Pts',(-47.5780177840617,34.8931591840073,
2.72845645939285));
#216688=CARTESIAN_POINT('Ctrl Pts',(-47.5806251537543,34.9078085542082,
2.74568723186784));
#216689=CARTESIAN_POINT('Ctrl Pts',(-47.5833273744258,34.9229908396723,
2.7635448259414));
#216690=CARTESIAN_POINT('Ctrl Pts',(-47.5876385414298,34.9368756554767,
2.78225519316872));
#216691=CARTESIAN_POINT('Ctrl Pts',(-47.5933942811485,34.9493673872906,
2.80151223085178));
#216692=CARTESIAN_POINT('Ctrl Pts',(-47.5990678735466,34.9616808340626,
2.82049442739819));
#216693=CARTESIAN_POINT('Ctrl Pts',(-47.6061458909216,34.972641156222,2.84000929088694));
#216694=CARTESIAN_POINT('Ctrl Pts',(-47.6145008888038,34.9821189161873,
2.85976644340938));
#216695=CARTESIAN_POINT('Ctrl Pts',(-47.6203261419784,34.9887269790624,
2.87354148166497));
#216696=CARTESIAN_POINT('Ctrl Pts',(-47.6267727798526,34.9946135826766,
2.88743438345274));
#216697=CARTESIAN_POINT('Ctrl Pts',(-47.6338034047602,34.999721753026,2.90134173516047));
#216698=CARTESIAN_POINT('',(-47.9220530736689,35.2091516650527,3.47153072139096));
#216699=CARTESIAN_POINT('',(-47.6338034047601,34.999721753026,2.90134173516047));
#216700=CARTESIAN_POINT('',(-44.4033023070491,39.554446981307,3.47153072139099));
#216701=CARTESIAN_POINT('Origin',(5.53234440788222E-15,1.85015204418142E-13,
3.47153072139072));
#216702=CARTESIAN_POINT('',(-44.1385184650378,39.3160391863689,2.9013417351605));
#216703=CARTESIAN_POINT('',(-44.4033023070491,39.554446981307,3.47153072139099));
#216704=CARTESIAN_POINT('',(-43.7969047596348,39.4144401478989,2.5990817351605));
#216705=CARTESIAN_POINT('Ctrl Pts',(-44.1385184650378,39.3160391863689,
2.9013417351605));
#216706=CARTESIAN_POINT('Ctrl Pts',(-44.1294297383223,39.30785585272,2.88176998919681));
#216707=CARTESIAN_POINT('Ctrl Pts',(-44.1190955972863,39.3011376816097,
2.86226752356449));
#216708=CARTESIAN_POINT('Ctrl Pts',(-44.1076895347485,39.2959399200101,
2.84310370499602));
#216709=CARTESIAN_POINT('Ctrl Pts',(-44.0960774370682,39.2906482678547,
2.82359371788097));
#216710=CARTESIAN_POINT('Ctrl Pts',(-44.0833536765897,39.2869318048881,
2.80443322636304));
#216711=CARTESIAN_POINT('Ctrl Pts',(-44.0696602318316,39.2848826826031,
2.78589323877442));
#216712=CARTESIAN_POINT('Ctrl Pts',(-44.0565465320208,39.2829203148427,
2.76813818619067));
#216713=CARTESIAN_POINT('Ctrl Pts',(-44.0425426835264,39.2824868619908,
2.75095095197682));
#216714=CARTESIAN_POINT('Ctrl Pts',(-44.0277475809121,39.2836998417248,
2.73457771434002));
#216715=CARTESIAN_POINT('Ctrl Pts',(-44.0159800428216,39.284664605917,2.72155497954872));
#216716=CARTESIAN_POINT('Ctrl Pts',(-44.0037113585722,39.2866715134056,
2.70904711159642));
#216717=CARTESIAN_POINT('Ctrl Pts',(-43.9909836989806,39.2897990038552,
2.69718956158366));
#216718=CARTESIAN_POINT('Ctrl Pts',(-43.9909489566042,39.2898075408882,
2.69715719432383));
#216719=CARTESIAN_POINT('Ctrl Pts',(-43.990914210958,39.2898160863664,2.69712483219049));
#216720=CARTESIAN_POINT('Ctrl Pts',(-43.9908794620435,39.2898246402906,
2.69709247518676));
#216721=CARTESIAN_POINT('Ctrl Pts',(-43.9839620557563,39.2915274551885,
2.69065122242303));
#216722=CARTESIAN_POINT('Ctrl Pts',(-43.9768962096537,39.2935962119552,
2.68442464469453));
#216723=CARTESIAN_POINT('Ctrl Pts',(-43.9697202954283,39.2960179253199,
2.67844505923606));
#216724=CARTESIAN_POINT('Ctrl Pts',(-43.955479196702,39.3008239832004,2.66657815779594));
#216725=CARTESIAN_POINT('Ctrl Pts',(-43.9408038696757,39.3070213676603,
2.655684456642));
#216726=CARTESIAN_POINT('Ctrl Pts',(-43.9259899312961,39.3145157795323,
2.64601906229541));
#216727=CARTESIAN_POINT('Ctrl Pts',(-43.9148794775114,39.3201365884364,
2.63877001653547));
#216728=CARTESIAN_POINT('Ctrl Pts',(-43.9036910542319,39.3264869747219,
2.63221189387627));
#216729=CARTESIAN_POINT('Ctrl Pts',(-43.8925493833644,39.3335271634608,
2.6264523103326));
#216730=CARTESIAN_POINT('Ctrl Pts',(-43.888371256789,39.3361672342378,2.62429246650372));
#216731=CARTESIAN_POINT('Ctrl Pts',(-43.8841997049151,39.3389043086121,
2.62224491711771));
#216732=CARTESIAN_POINT('Ctrl Pts',(-43.8800413054826,39.341736289618,2.62031533672623));
#216733=CARTESIAN_POINT('Ctrl Pts',(-43.865486907469,39.3516482231388,2.61356180535604));
#216734=CARTESIAN_POINT('Ctrl Pts',(-43.8510936230937,39.3627227594944,
2.60825339735373));
#216735=CARTESIAN_POINT('Ctrl Pts',(-43.8371435075661,39.374870022378,2.60463337987637));
#216736=CARTESIAN_POINT('Ctrl Pts',(-43.8301684498022,39.3809436538199,
2.60282337113768));
#216737=CARTESIAN_POINT('Ctrl Pts',(-43.8233041850059,39.3872854675772,
2.6014354593914));
#216738=CARTESIAN_POINT('Ctrl Pts',(-43.8165859732786,39.393884232031,2.60050005034622));
#216739=CARTESIAN_POINT('Ctrl Pts',(-43.813226867415,39.397183614258,2.60003234582362));
#216740=CARTESIAN_POINT('Ctrl Pts',(-43.8099042748374,39.4005472341764,
2.59967776696092));
#216741=CARTESIAN_POINT('Ctrl Pts',(-43.8066226032736,39.4039736880302,
2.59944011429186));
#216742=CARTESIAN_POINT('Ctrl Pts',(-43.8033409317098,39.4074001418841,
2.5992024616228));
#216743=CARTESIAN_POINT('Ctrl Pts',(-43.8001001824232,39.4108894308103,
2.59908173791338));
#216744=CARTESIAN_POINT('Ctrl Pts',(-43.7969047596348,39.4144401478989,
2.5990817351605));
#216745=CARTESIAN_POINT('',(-43.7765468711724,39.4370498736008,2.5990817351605));
#216746=CARTESIAN_POINT('Origin',(3.51858511112454E-16,1.91153073798388E-13,
2.59908173516023));
#216747=CARTESIAN_POINT('',(-43.7143933160625,39.7870778846747,2.9013417351605));
#216748=CARTESIAN_POINT('Ctrl Pts',(-43.7765468711724,39.4370498736008,
2.5990817351605));
#216749=CARTESIAN_POINT('Ctrl Pts',(-43.7739968854581,39.4398804576448,
2.59908174371538));
#216750=CARTESIAN_POINT('Ctrl Pts',(-43.771488795476,39.4427347725911,2.59915764355917));
#216751=CARTESIAN_POINT('Ctrl Pts',(-43.7690230823394,39.4456106527047,
2.59930765775303));
#216752=CARTESIAN_POINT('Ctrl Pts',(-43.7544656984466,39.4625896314113,
2.60019333020903));
#216753=CARTESIAN_POINT('Ctrl Pts',(-43.7413824023646,39.4803211659033,
2.60365973324078));
#216754=CARTESIAN_POINT('Ctrl Pts',(-43.7298770745125,39.4983548992053,
2.60934177082323));
#216755=CARTESIAN_POINT('Ctrl Pts',(-43.7255790670215,39.505091701652,2.61146439091784));
#216756=CARTESIAN_POINT('Ctrl Pts',(-43.7215008664177,39.5118707851432,
2.61389584429295));
#216757=CARTESIAN_POINT('Ctrl Pts',(-43.7176465228246,39.5186692048627,
2.6166160438528));
#216758=CARTESIAN_POINT('Ctrl Pts',(-43.7146391706003,39.5239736729702,
2.61873848000803));
#216759=CARTESIAN_POINT('Ctrl Pts',(-43.7117685746243,39.529289732678,2.62103707099814));
#216760=CARTESIAN_POINT('Ctrl Pts',(-43.7090371296309,39.5346062960354,
2.62350262767678));
#216761=CARTESIAN_POINT('Ctrl Pts',(-43.699477072154,39.5532142677863,2.63213207605205));
#216762=CARTESIAN_POINT('Ctrl Pts',(-43.6916216076132,39.5718284032055,
2.6428068597194));
#216763=CARTESIAN_POINT('Ctrl Pts',(-43.6855734779224,39.5899733680945,
2.6551329364611));
#216764=CARTESIAN_POINT('Ctrl Pts',(-43.682549413077,39.599045850539,2.66129597483194));
#216765=CARTESIAN_POINT('Ctrl Pts',(-43.6799771832788,39.6080010415739,
2.66787183533878));
#216766=CARTESIAN_POINT('Ctrl Pts',(-43.677869635043,39.6167795278797,2.67481125953887));
#216767=CARTESIAN_POINT('Ctrl Pts',(-43.6757710912487,39.6255205083456,
2.68172103524106));
#216768=CARTESIAN_POINT('Ctrl Pts',(-43.6741330170973,39.6340863223877,
2.68899101329813));
#216769=CARTESIAN_POINT('Ctrl Pts',(-43.6729688455954,39.6424182201447,
2.69657334701299));
#216770=CARTESIAN_POINT('Ctrl Pts',(-43.6729638503629,39.6424539706906,
2.69660588132596));
#216771=CARTESIAN_POINT('Ctrl Pts',(-43.6729588633162,39.6424897170046,
2.69663842081405));
#216772=CARTESIAN_POINT('Ctrl Pts',(-43.672953884454,39.6425254590851,2.69667096547406));
#216773=CARTESIAN_POINT('Ctrl Pts',(-43.6706059487636,39.659380737255,2.71201840158148));
#216774=CARTESIAN_POINT('Ctrl Pts',(-43.6700521164124,39.6752678913595,
2.72845645939766));
#216775=CARTESIAN_POINT('Ctrl Pts',(-43.6711139265066,39.6901095551267,
2.74568723187539));
#216776=CARTESIAN_POINT('Ctrl Pts',(-43.6722143631627,39.7054911294186,
2.76354482595175));
#216777=CARTESIAN_POINT('Ctrl Pts',(-43.6750505546851,39.7197505224127,
2.78225519318207));
#216778=CARTESIAN_POINT('Ctrl Pts',(-43.6794690223308,39.7327754618416,
2.8015122308682));
#216779=CARTESIAN_POINT('Ctrl Pts',(-43.683824428529,39.7456145061593,2.82049442741723));
#216780=CARTESIAN_POINT('Ctrl Pts',(-43.6897180061537,39.7572546408068,
2.84000929090864));
#216781=CARTESIAN_POINT('Ctrl Pts',(-43.697036538801,39.7675538157007,2.85976644343369));
#216782=CARTESIAN_POINT('Ctrl Pts',(-43.7021391499695,39.7747345836734,
2.87354148168132));
#216783=CARTESIAN_POINT('Ctrl Pts',(-43.7079351548543,39.781262797003,2.88743438346094));
#216784=CARTESIAN_POINT('Ctrl Pts',(-43.7143933160625,39.7870778846747,
2.9013417351605));
#216785=CARTESIAN_POINT('',(-43.9791725362585,40.0254908126588,3.471530721391));
#216786=CARTESIAN_POINT('',(-43.7143933160625,39.7870778846747,2.90134173516051));
#216787=CARTESIAN_POINT('',(-40.025490812659,43.9791725362583,3.47153072139102));
#216788=CARTESIAN_POINT('Origin',(5.53234440788222E-15,1.85015204418142E-13,
3.47153072139072));
#216789=CARTESIAN_POINT('',(-39.7870778846749,43.7143933160623,2.90134173516053));
#216790=CARTESIAN_POINT('',(-40.025490812659,43.9791725362582,3.47153072139102));
#216791=CARTESIAN_POINT('',(-39.437049873601,43.7765468711722,2.59908173516053));
#216792=CARTESIAN_POINT('Ctrl Pts',(-39.7870778846749,43.7143933160623,
2.90134173516053));
#216793=CARTESIAN_POINT('Ctrl Pts',(-39.7788943382465,43.7053047809347,
2.8817699891974));
#216794=CARTESIAN_POINT('Ctrl Pts',(-39.769319048819,43.6975432007871,2.86226752356563));
#216795=CARTESIAN_POINT('Ctrl Pts',(-39.7585187839181,43.6911816548805,
2.8431037049977));
#216796=CARTESIAN_POINT('Ctrl Pts',(-39.7475234267921,43.6847051962234,
2.82359371788292));
#216797=CARTESIAN_POINT('Ctrl Pts',(-39.7352578445677,43.6796790973,2.80443322636524));
#216798=CARTESIAN_POINT('Ctrl Pts',(-39.7218536055365,43.6762098455838,
2.78589323877684));
#216799=CARTESIAN_POINT('Ctrl Pts',(-39.7090168672317,43.6728874729903,
2.76813818619297));
#216800=CARTESIAN_POINT('Ctrl Pts',(-39.6951350414451,43.6709925938754,
2.75095095197898));
#216801=CARTESIAN_POINT('Ctrl Pts',(-39.6802941970433,43.6706524194393,
2.73457771434204));
#216802=CARTESIAN_POINT('Ctrl Pts',(-39.6684902774387,43.6703818558792,
2.72155497955002));
#216803=CARTESIAN_POINT('Ctrl Pts',(-39.6560790233689,43.6710953426077,
2.70904711159703));
#216804=CARTESIAN_POINT('Ctrl Pts',(-39.643094175457,43.6728752976394,2.69718956158366));
#216805=CARTESIAN_POINT('Ctrl Pts',(-39.6430587310401,43.6728801563384,
2.69715719432384));
#216806=CARTESIAN_POINT('Ctrl Pts',(-39.6430232824884,43.6728850230946,
2.6971248321905));
#216807=CARTESIAN_POINT('Ctrl Pts',(-39.6429878298037,43.6728898979089,
2.69709247518678));
#216808=CARTESIAN_POINT('Ctrl Pts',(-39.6359303251673,43.6738603187596,
2.69065122242303));
#216809=CARTESIAN_POINT('Ctrl Pts',(-39.6286869425433,43.6751791606255,
2.68442464469454));
#216810=CARTESIAN_POINT('Ctrl Pts',(-39.6212972007503,43.6768375203045,
2.67844505923606));
#216811=CARTESIAN_POINT('Ctrl Pts',(-39.6066317464083,43.680128649932,2.66657815779595));
#216812=CARTESIAN_POINT('Ctrl Pts',(-39.5913890092851,43.6847580950894,
2.65568445664202));
#216813=CARTESIAN_POINT('Ctrl Pts',(-39.5758728438538,43.6906629735752,
2.64601906229543));
#216814=CARTESIAN_POINT('Ctrl Pts',(-39.5642357197804,43.6950916324396,
2.63877001653549));
#216815=CARTESIAN_POINT('Ctrl Pts',(-39.5524447917348,43.7002377219528,
2.63221189387629));
#216816=CARTESIAN_POINT('Ctrl Pts',(-39.540628255996,43.7060747220671,2.62645231033261));
#216817=CARTESIAN_POINT('Ctrl Pts',(-39.5361970550939,43.70826359711,2.62429246650373));
#216818=CARTESIAN_POINT('Ctrl Pts',(-39.5317622532395,43.7105496315976,
2.62224491711774));
#216819=CARTESIAN_POINT('Ctrl Pts',(-39.5273306113316,43.712931427613,2.62031533672625));
#216820=CARTESIAN_POINT('Ctrl Pts',(-39.5118198646542,43.7212677136667,
2.61356180535607));
#216821=CARTESIAN_POINT('Ctrl Pts',(-39.4963478239301,43.7307770746562,
2.60825339735376));
#216822=CARTESIAN_POINT('Ctrl Pts',(-39.4812043938728,43.7413996094243,
2.60463337987639));
#216823=CARTESIAN_POINT('Ctrl Pts',(-39.4736326788442,43.7467108768083,
2.60282337113771));
#216824=CARTESIAN_POINT('Ctrl Pts',(-39.4661431171622,43.7523004383957,
2.60143545939144));
#216825=CARTESIAN_POINT('Ctrl Pts',(-39.4587719497939,43.7581608097797,
2.60050005034626));
#216826=CARTESIAN_POINT('Ctrl Pts',(-39.4550863661098,43.7610909954717,
2.60003234582367));
#216827=CARTESIAN_POINT('Ctrl Pts',(-39.4514303810208,43.764088883632,2.59967776696095));
#216828=CARTESIAN_POINT('Ctrl Pts',(-39.4478085248414,43.7671535389277,
2.59944011429189));
#216829=CARTESIAN_POINT('Ctrl Pts',(-39.444186668662,43.7702181942233,2.59920246162283));
#216830=CARTESIAN_POINT('Ctrl Pts',(-39.4405989425298,43.7733496179168,
2.59908173791343));
#216831=CARTESIAN_POINT('Ctrl Pts',(-39.437049873601,43.7765468711722,2.59908173516054));
#216832=CARTESIAN_POINT('',(-39.4144401478992,43.7969047596346,2.59908173516053));
#216833=CARTESIAN_POINT('Origin',(3.56901409908097E-16,1.91158116697184E-13,
2.59908173516024));
#216834=CARTESIAN_POINT('',(-39.3160391863692,44.1385184650376,2.90134173516053));
#216835=CARTESIAN_POINT('Ctrl Pts',(-39.4144401478992,43.7969047596346,
2.59908173516053));
#216836=CARTESIAN_POINT('Ctrl Pts',(-39.4116082546731,43.799453291355,2.59908174371542));
#216837=CARTESIAN_POINT('Ctrl Pts',(-39.4088155471153,43.8020298032738,
2.5991576435592));
#216838=CARTESIAN_POINT('Ctrl Pts',(-39.4060627300845,43.8046321918102,
2.59930765775307));
#216839=CARTESIAN_POINT('Ctrl Pts',(-39.3898103065118,43.8199964969273,
2.60019333020906));
#216840=CARTESIAN_POINT('Ctrl Pts',(-39.374945232043,43.8362633193841,2.60365973324077));
#216841=CARTESIAN_POINT('Ctrl Pts',(-39.3616178931518,43.8529956277683,
2.60934177082315));
#216842=CARTESIAN_POINT('Ctrl Pts',(-39.3566392429883,43.8592462611882,
2.61146439091779));
#216843=CARTESIAN_POINT('Ctrl Pts',(-39.3518747760143,43.8655619201089,
2.61389584429293));
#216844=CARTESIAN_POINT('Ctrl Pts',(-39.3473309185526,43.8719202087612,
2.61661604385284));
#216845=CARTESIAN_POINT('Ctrl Pts',(-39.3437855730188,43.8768812645309,
2.61873848000807));
#216846=CARTESIAN_POINT('Ctrl Pts',(-39.3403750229161,43.8818681433213,
2.62103707099818));
#216847=CARTESIAN_POINT('Ctrl Pts',(-39.3371028088665,43.8868700682407,
2.62350262767683));
#216848=CARTESIAN_POINT('Ctrl Pts',(-39.3256500596931,43.9043768054586,
2.6321320760521));
#216849=CARTESIAN_POINT('Ctrl Pts',(-39.3158919212385,43.9220678510596,
2.64280685971945));
#216850=CARTESIAN_POINT('Ctrl Pts',(-39.3079802585391,43.9394812142302,
2.65513293646114));
#216851=CARTESIAN_POINT('Ctrl Pts',(-39.3040244271894,43.9481878958155,
2.66129597483199));
#216852=CARTESIAN_POINT('Ctrl Pts',(-39.3005302159781,43.9568251581489,
2.66787183533882));
#216853=CARTESIAN_POINT('Ctrl Pts',(-39.2975166114287,43.9653352562099,
2.67481125953891));
#216854=CARTESIAN_POINT('Ctrl Pts',(-39.2945158824213,43.9738089951123,
2.6817210352411));
#216855=CARTESIAN_POINT('Ctrl Pts',(-39.291991410433,43.982156659355,2.68899101329819));
#216856=CARTESIAN_POINT('Ctrl Pts',(-39.2899626959158,43.9903212250463,
2.69657334701305));
#216857=CARTESIAN_POINT('Ctrl Pts',(-39.2899539910981,43.9903562576029,
2.69660588132602));
#216858=CARTESIAN_POINT('Ctrl Pts',(-39.2899452948636,43.9903912868066,
2.69663842081411));
#216859=CARTESIAN_POINT('Ctrl Pts',(-39.2899366072115,43.9904263126555,
2.69667096547411));
#216860=CARTESIAN_POINT('Ctrl Pts',(-39.2858396774342,44.0069438297351,
2.71201840157854));
#216861=CARTESIAN_POINT('Ctrl Pts',(-39.2836282192305,44.0226860610995,
2.72845645939131));
#216862=CARTESIAN_POINT('Ctrl Pts',(-39.2831328363115,44.0375574100545,
2.74568723186538));
#216863=CARTESIAN_POINT('Ctrl Pts',(-39.2826194323367,44.0529697494231,
2.76354482593832));
#216864=CARTESIAN_POINT('Ctrl Pts',(-39.2839495744673,44.0674474907097,
2.78225519316498));
#216865=CARTESIAN_POINT('Ctrl Pts',(-39.2869823603806,44.0808629337889,
2.80151223084737));
#216866=CARTESIAN_POINT('Ctrl Pts',(-39.289971861634,44.0940869083944,2.82049442739379));
#216867=CARTESIAN_POINT('Ctrl Pts',(-39.2946164282351,44.1062793237782,
2.84000929088258));
#216868=CARTESIAN_POINT('Ctrl Pts',(-39.3008183122678,44.1172870736854,
2.85976644340509));
#216869=CARTESIAN_POINT('Ctrl Pts',(-39.305142376159,44.1249618727701,2.8735414816621));
#216870=CARTESIAN_POINT('Ctrl Pts',(-39.3102242458182,44.1320601713533,
2.88743438345134));
#216871=CARTESIAN_POINT('Ctrl Pts',(-39.3160391863692,44.1385184650376,
2.90134173516053));
#216872=CARTESIAN_POINT('',(-39.5544469813073,44.4033023070489,3.47153072139102));
#216873=CARTESIAN_POINT('',(-39.3160391863692,44.1385184650376,2.90134173516054));
#216874=CARTESIAN_POINT('',(-35.209151665053,47.9220530736687,3.47153072139105));
#216875=CARTESIAN_POINT('Origin',(5.53234440788222E-15,1.85015204418142E-13,
3.47153072139072));
#216876=CARTESIAN_POINT('',(-34.9997217530263,47.63380340476,2.90134173516056));
#216877=CARTESIAN_POINT('',(-35.209151665053,47.9220530736687,3.47153072139105));
#216878=CARTESIAN_POINT('',(-34.6451144164188,47.6590285860936,2.59908173516056));
#216879=CARTESIAN_POINT('Ctrl Pts',(-34.9997217530262,47.63380340476,2.90134173516056));
#216880=CARTESIAN_POINT('Ctrl Pts',(-34.9925330475312,47.6239092440466,
2.88176998919708));
#216881=CARTESIAN_POINT('Ctrl Pts',(-34.983821518586,47.6151892923579,2.86226752356497));
#216882=CARTESIAN_POINT('Ctrl Pts',(-34.9737453812837,47.6077336605724,
2.8431037049967));
#216883=CARTESIAN_POINT('Ctrl Pts',(-34.9634872321452,47.6001433528501,
2.82359371788197));
#216884=CARTESIAN_POINT('Ctrl Pts',(-34.9518142124603,47.5938626849615,
2.80443322636432));
#216885=CARTESIAN_POINT('Ctrl Pts',(-34.9388460388037,47.589011313662,2.78589323877598));
#216886=CARTESIAN_POINT('Ctrl Pts',(-34.9264269039965,47.584365336845,2.76813818619268));
#216887=CARTESIAN_POINT('Ctrl Pts',(-34.9128191931065,47.5810297921593,
2.75095095197925));
#216888=CARTESIAN_POINT('Ctrl Pts',(-34.8980952063149,47.5791401905754,
2.73457771434281));
#216889=CARTESIAN_POINT('Ctrl Pts',(-34.88638423141,47.5776372636139,2.72155497955052));
#216890=CARTESIAN_POINT('Ctrl Pts',(-34.8739663878171,47.5770495124722,
2.7090471115973));
#216891=CARTESIAN_POINT('Ctrl Pts',(-34.8608666162964,47.577462430526,2.69718956158371));
#216892=CARTESIAN_POINT('Ctrl Pts',(-34.8608308581753,47.5774635576581,
2.69715719432388));
#216893=CARTESIAN_POINT('Ctrl Pts',(-34.8607950951,47.5774646923711,2.69712483219054));
#216894=CARTESIAN_POINT('Ctrl Pts',(-34.8607593270719,47.577465834666,2.69709247518681));
#216895=CARTESIAN_POINT('Ctrl Pts',(-34.8536390475841,47.5776932293355,
2.69065122242307));
#216896=CARTESIAN_POINT('Ctrl Pts',(-34.8462974884545,47.5782477067932,
2.68442464469458));
#216897=CARTESIAN_POINT('Ctrl Pts',(-34.8387748826515,47.5791245434507,
2.67844505923611));
#216898=CARTESIAN_POINT('Ctrl Pts',(-34.8238457504804,47.5808646865203,
2.66657815779599));
#216899=CARTESIAN_POINT('Ctrl Pts',(-34.8082026058779,47.5838754712052,
2.65568445664205));
#216900=CARTESIAN_POINT('Ctrl Pts',(-34.7921542117505,47.5881261212206,
2.64601906229547));
#216901=CARTESIAN_POINT('Ctrl Pts',(-34.780117916155,47.5913141087321,2.63877001653553));
#216902=CARTESIAN_POINT('Ctrl Pts',(-34.7678536672182,47.5951995198394,
2.63221189387632));
#216903=CARTESIAN_POINT('Ctrl Pts',(-34.7554917310465,47.5997693799344,
2.62645231033264));
#216904=CARTESIAN_POINT('Ctrl Pts',(-34.7508560049822,47.60148307747,2.62429246650376));
#216905=CARTESIAN_POINT('Ctrl Pts',(-34.7462065417643,47.6032930257988,
2.62224491711777));
#216906=CARTESIAN_POINT('Ctrl Pts',(-34.7415502113773,47.605198541368,2.62031533672629));
#216907=CARTESIAN_POINT('Ctrl Pts',(-34.7252530550225,47.6118678458601,
2.6135618053561));
#216908=CARTESIAN_POINT('Ctrl Pts',(-34.7088717728655,47.6197078449347,
2.6082533973538));
#216909=CARTESIAN_POINT('Ctrl Pts',(-34.6927009428672,47.6286892688734,
2.60463337987643));
#216910=CARTESIAN_POINT('Ctrl Pts',(-34.684615527868,47.6331799808427,2.60282337113774));
#216911=CARTESIAN_POINT('Ctrl Pts',(-34.6765827265055,47.6379560498536,
2.60143545939147));
#216912=CARTESIAN_POINT('Ctrl Pts',(-34.6686393635484,47.6430138207125,
2.60050005034628));
#216913=CARTESIAN_POINT('Ctrl Pts',(-34.6646676820698,47.645542706142,2.60003234582369));
#216914=CARTESIAN_POINT('Ctrl Pts',(-34.6607183602073,47.6481420170542,
2.59967776696097));
#216915=CARTESIAN_POINT('Ctrl Pts',(-34.6567960012265,47.6508112967869,
2.59944011429191));
#216916=CARTESIAN_POINT('Ctrl Pts',(-34.6528736422457,47.6534805765195,
2.59920246162285));
#216917=CARTESIAN_POINT('Ctrl Pts',(-34.6489782471461,47.6562198264472,
2.59908173791348));
#216918=CARTESIAN_POINT('Ctrl Pts',(-34.6451144164188,47.6590285860936,
2.59908173516056));
#216919=CARTESIAN_POINT('',(-34.6205005703637,47.6769115920304,2.59908173516056));
#216920=CARTESIAN_POINT('Origin',(3.62443809638014E-16,1.9116260484399E-13,
2.59908173516024));
#216921=CARTESIAN_POINT('',(-34.4869303039399,48.0063682005187,2.90134173516056));
#216922=CARTESIAN_POINT('Ctrl Pts',(-34.6205005703637,47.6769115920304,
2.59908173516056));
#216923=CARTESIAN_POINT('Ctrl Pts',(-34.6174177964407,47.6791501491803,
2.59908174371546));
#216924=CARTESIAN_POINT('Ctrl Pts',(-34.6143710687957,47.6814206292679,
2.59915764355922));
#216925=CARTESIAN_POINT('Ctrl Pts',(-34.61136130831,47.6837210139136,2.59930765775308));
#216926=CARTESIAN_POINT('Ctrl Pts',(-34.5935919100066,47.6973023109027,
2.6001933302093));
#216927=CARTESIAN_POINT('Ctrl Pts',(-34.5771079220135,47.7119261986175,
2.60365973324256));
#216928=CARTESIAN_POINT('Ctrl Pts',(-34.5621045891938,47.7271737594161,
2.60934177082752));
#216929=CARTESIAN_POINT('Ctrl Pts',(-34.5564998434951,47.7328697405577,
2.61146439092112));
#216930=CARTESIAN_POINT('Ctrl Pts',(-34.5511013106521,47.7386527792229,
2.61389584429479));
#216931=CARTESIAN_POINT('Ctrl Pts',(-34.5459177227788,47.744501274063,2.61661604385282));
#216932=CARTESIAN_POINT('Ctrl Pts',(-34.5418732274829,47.7490645631296,
2.61873848000805));
#216933=CARTESIAN_POINT('Ctrl Pts',(-34.537960089954,47.7536676237151,2.62103707099818));
#216934=CARTESIAN_POINT('Ctrl Pts',(-34.5341829579102,47.7583001080604,
2.62350262767682));
#216935=CARTESIAN_POINT('Ctrl Pts',(-34.5209629957568,47.7745138032688,
2.63213207605209));
#216936=CARTESIAN_POINT('Ctrl Pts',(-34.5094090955955,47.7910879322539,
2.64280685971945));
#216937=CARTESIAN_POINT('Ctrl Pts',(-34.4997205817196,47.8075789092552,
2.65513293646115));
#216938=CARTESIAN_POINT('Ctrl Pts',(-34.4948763247817,47.8158243977558,
2.661295974832));
#216939=CARTESIAN_POINT('Ctrl Pts',(-34.4904984154664,47.8240490997342,
2.66787183533883));
#216940=CARTESIAN_POINT('Ctrl Pts',(-34.4866117722854,47.8321975711351,
2.67481125953893));
#216941=CARTESIAN_POINT('Ctrl Pts',(-34.4827417346799,47.8403112284174,
2.68172103524111));
#216942=CARTESIAN_POINT('Ctrl Pts',(-34.4793585234982,47.8483492841045,
2.68899101329819));
#216943=CARTESIAN_POINT('Ctrl Pts',(-34.4764874929864,47.8562570650397,
2.69657334701305));
#216944=CARTESIAN_POINT('Ctrl Pts',(-34.4764751739553,47.8562909957832,
2.69660588132602));
#216945=CARTESIAN_POINT('Ctrl Pts',(-34.4764628638109,47.8563249240892,
2.69663842081411));
#216946=CARTESIAN_POINT('Ctrl Pts',(-34.4764505625524,47.8563588499558,
2.69667096547411));
#216947=CARTESIAN_POINT('Ctrl Pts',(-34.4706495255077,47.8723576365753,
2.71201840157889));
#216948=CARTESIAN_POINT('Ctrl Pts',(-34.4668046706504,47.8877824700219,
2.72845645939207));
#216949=CARTESIAN_POINT('Ctrl Pts',(-34.4647575222379,47.9025205705564,
2.74568723186657));
#216950=CARTESIAN_POINT('Ctrl Pts',(-34.4626359025942,47.9177948141892,
2.76354482593998));
#216951=CARTESIAN_POINT('Ctrl Pts',(-34.4624454220188,47.9323322826072,
2.78225519316713));
#216952=CARTESIAN_POINT('Ctrl Pts',(-34.4640592983646,47.9459912469369,
2.80151223085002));
#216953=CARTESIAN_POINT('Ctrl Pts',(-34.4656501410737,47.9594552671979,
2.82049442739673));
#216954=CARTESIAN_POINT('Ctrl Pts',(-34.4689948098096,47.9720663806638,
2.8400092908858));
#216955=CARTESIAN_POINT('Ctrl Pts',(-34.4740120960911,47.9836621023726,
2.85976644340858));
#216956=CARTESIAN_POINT('Ctrl Pts',(-34.4775102373536,47.9917468458577,
2.87354148166445));
#216957=CARTESIAN_POINT('Ctrl Pts',(-34.4818222937561,47.9993374592438,
2.88743438345252));
#216958=CARTESIAN_POINT('Ctrl Pts',(-34.4869303039399,48.0063682005187,
2.90134173516055));
#216959=CARTESIAN_POINT('',(-34.6963546279287,48.2946219293746,3.47153072139105));
#216960=CARTESIAN_POINT('',(-34.4869303039399,48.0063682005187,2.90134173516056));
#216961=CARTESIAN_POINT('',(-30.007053683816,51.3398895692697,3.47153072139107));
#216962=CARTESIAN_POINT('Origin',(5.53234440788222E-15,1.85015204418142E-13,
3.47153072139072));
#216963=CARTESIAN_POINT('',(-29.8289013456888,51.0313275753409,2.90134173516058));
#216964=CARTESIAN_POINT('',(-30.007053683816,51.3398895692697,3.47153072139107));
#216965=CARTESIAN_POINT('',(-29.473599835734,51.0193480105328,2.59908173516058));
#216966=CARTESIAN_POINT('Ctrl Pts',(-29.8289013456888,51.0313275753409,
2.90134173516058));
#216967=CARTESIAN_POINT('Ctrl Pts',(-29.8227862420895,51.0207361915371,
2.88176998919749));
#216968=CARTESIAN_POINT('Ctrl Pts',(-29.8150339189614,51.0111534059229,
2.86226752356577));
#216969=CARTESIAN_POINT('Ctrl Pts',(-29.8057923055269,51.0026853737207,
2.84310370499788));
#216970=CARTESIAN_POINT('Ctrl Pts',(-29.7963837548049,50.994064377933,2.82359371788349));
#216971=CARTESIAN_POINT('Ctrl Pts',(-29.7854311897062,50.9865979533909,
2.80443322636617));
#216972=CARTESIAN_POINT('Ctrl Pts',(-29.7730411634487,50.9804176151473,
2.78589323877811));
#216973=CARTESIAN_POINT('Ctrl Pts',(-29.7611756987788,50.9744989364009,
2.7681381861951));
#216974=CARTESIAN_POINT('Ctrl Pts',(-29.7479911917134,50.9697592710701,
2.7509509519819));
#216975=CARTESIAN_POINT('Ctrl Pts',(-29.7335453816122,50.9663409452088,
2.73457771434565));
#216976=CARTESIAN_POINT('Ctrl Pts',(-29.7220556592981,50.9636221212279,
2.72155497955235));
#216977=CARTESIAN_POINT('Ctrl Pts',(-29.7097672786746,50.9617395717404,
2.70904711159817));
#216978=CARTESIAN_POINT('Ctrl Pts',(-29.6966961073823,50.9607809287996,
2.69718956158373));
#216979=CARTESIAN_POINT('Ctrl Pts',(-29.6966604273306,50.9607783120158,
2.6971571943239));
#216980=CARTESIAN_POINT('Ctrl Pts',(-29.6966247415593,50.9607757022533,
2.69712483219056));
#216981=CARTESIAN_POINT('Ctrl Pts',(-29.6965890500698,50.9607730995136,
2.69709247518683));
#216982=CARTESIAN_POINT('Ctrl Pts',(-29.6894840070028,50.9602549766185,
2.6906512224231));
#216983=CARTESIAN_POINT('Ctrl Pts',(-29.6821247070256,50.9600390146968,
2.6844246446946));
#216984=CARTESIAN_POINT('Ctrl Pts',(-29.6745516564559,50.9601247215271,
2.67844505923613));
#216985=CARTESIAN_POINT('Ctrl Pts',(-29.6595224131521,50.9602948126671,
2.66657815779601));
#216986=CARTESIAN_POINT('Ctrl Pts',(-29.6436502506361,50.9616539500925,
2.65568445664207));
#216987=CARTESIAN_POINT('Ctrl Pts',(-29.6272454573769,50.9642038006262,
2.64601906229549));
#216988=CARTESIAN_POINT('Ctrl Pts',(-29.6149418624325,50.9661161885266,
2.63877001653555));
#216989=CARTESIAN_POINT('Ctrl Pts',(-29.6023386622825,50.9686983518508,
2.63221189387636));
#216990=CARTESIAN_POINT('Ctrl Pts',(-29.5895667656375,50.971951003583,2.62645231033268));
#216991=CARTESIAN_POINT('Ctrl Pts',(-29.5847773043957,50.9731707479826,
2.6242924665038));
#216992=CARTESIAN_POINT('Ctrl Pts',(-29.5799641203064,50.9744847799798,
2.6222449171178));
#216993=CARTESIAN_POINT('Ctrl Pts',(-29.5751341171702,50.9758931378755,
2.62031533672632));
#216994=CARTESIAN_POINT('Ctrl Pts',(-29.5582291061936,50.9808223905105,
2.61356180535613));
#216995=CARTESIAN_POINT('Ctrl Pts',(-29.5411180593589,50.9869071309996,
2.60825339735382));
#216996=CARTESIAN_POINT('Ctrl Pts',(-29.524097000417,50.9941490417487,2.60463337987645));
#216997=CARTESIAN_POINT('Ctrl Pts',(-29.5155864709461,50.9977699971232,
2.60282337113777));
#216998=CARTESIAN_POINT('Ctrl Pts',(-29.5070984389558,51.0016802459462,
2.6014354593915));
#216999=CARTESIAN_POINT('Ctrl Pts',(-29.4986699095566,51.0058800022841,
2.60050005034631));
#217000=CARTESIAN_POINT('Ctrl Pts',(-29.494455644857,51.007979880453,2.60003234582372));
#217001=CARTESIAN_POINT('Ctrl Pts',(-29.4902562558177,51.0101521355229,
2.59967776696102));
#217002=CARTESIAN_POINT('Ctrl Pts',(-29.4860763682213,51.0123967945052,
2.59944011429196));
#217003=CARTESIAN_POINT('Ctrl Pts',(-29.481896480625,51.0146414534876,2.5992024616229));
#217004=CARTESIAN_POINT('Ctrl Pts',(-29.4777360953218,51.0169585178539,
2.59908173791349));
#217005=CARTESIAN_POINT('Ctrl Pts',(-29.473599835734,51.0193480105328,2.59908173516058));
#217006=CARTESIAN_POINT('',(-29.4472515437738,51.0345602039887,2.59908173516058));
#217007=CARTESIAN_POINT('Origin',(3.68424986610942E-16,1.91166489065733E-13,
2.59908173516024));
#217008=CARTESIAN_POINT('',(-29.2799753962465,51.3482501200166,2.90134173516058));
#217009=CARTESIAN_POINT('Ctrl Pts',(-29.4472515437738,51.0345602039887,
2.59908173516058));
#217010=CARTESIAN_POINT('Ctrl Pts',(-29.4439516646701,51.0364642604676,
2.5990817437155));
#217011=CARTESIAN_POINT('Ctrl Pts',(-29.4406842975234,51.0384038328689,
2.59915764355925));
#217012=CARTESIAN_POINT('Ctrl Pts',(-29.4374505691487,51.0403770101285,
2.59930765775312));
#217013=CARTESIAN_POINT('Ctrl Pts',(-29.4183588813685,51.0520264994517,
2.60019333020917));
#217014=CARTESIAN_POINT('Ctrl Pts',(-29.4004365818796,51.0648472300434,
2.60365973324133));
#217015=CARTESIAN_POINT('Ctrl Pts',(-29.3839216347905,51.0784429877824,
2.60934177082445));
#217016=CARTESIAN_POINT('Ctrl Pts',(-29.3777522003165,51.0835219102907,
2.61146439091879));
#217017=CARTESIAN_POINT('Ctrl Pts',(-29.3717787490535,51.0887089685256,
2.6138958442935));
#217018=CARTESIAN_POINT('Ctrl Pts',(-29.3660122232361,51.0939835922269,
2.61661604385286));
#217019=CARTESIAN_POINT('Ctrl Pts',(-29.3615128905151,51.0980991182406,
2.61873848000809));
#217020=CARTESIAN_POINT('Ctrl Pts',(-29.3571400387136,51.1022679285262,
2.62103707099819));
#217021=CARTESIAN_POINT('Ctrl Pts',(-29.3528993717246,51.1064802178294,
2.62350262767684));
#217022=CARTESIAN_POINT('Ctrl Pts',(-29.3380570372632,51.1212232303906,
2.6321320760521));
#217023=CARTESIAN_POINT('Ctrl Pts',(-29.324833962343,51.1364988531344,2.64280685971946));
#217024=CARTESIAN_POINT('Ctrl Pts',(-29.3134747466761,51.1518867653714,
2.65513293646116));
#217025=CARTESIAN_POINT('Ctrl Pts',(-29.3077951388427,51.1595807214899,
2.66129597483201));
#217026=CARTESIAN_POINT('Ctrl Pts',(-29.3025814967141,51.1673027515572,
2.66787183533885));
#217027=CARTESIAN_POINT('Ctrl Pts',(-29.2978643977776,51.1750003199402,
2.67481125953895));
#217028=CARTESIAN_POINT('Ctrl Pts',(-29.2931674525158,51.1826650006753,
2.68172103524113));
#217029=CARTESIAN_POINT('Ctrl Pts',(-29.2889625693103,51.1903053811865,
2.68899101329822));
#217030=CARTESIAN_POINT('Ctrl Pts',(-29.2852806784151,51.197869738063,2.69657334701308));
#217031=CARTESIAN_POINT('Ctrl Pts',(-29.2852648801404,51.1979021952409,
2.69660588132605));
#217032=CARTESIAN_POINT('Ctrl Pts',(-29.2852490909586,51.1979346509236,
2.69663842081414));
#217033=CARTESIAN_POINT('Ctrl Pts',(-29.285233310869,51.1979671051091,2.69667096547414));
#217034=CARTESIAN_POINT('Ctrl Pts',(-29.2777917239323,51.2132718752146,
2.71201840157962));
#217035=CARTESIAN_POINT('Ctrl Pts',(-29.2723555974557,51.2282103130406,
2.7284564593936));
#217036=CARTESIAN_POINT('Ctrl Pts',(-29.268779112536,51.2426536914413,2.74568723186895));
#217037=CARTESIAN_POINT('Ctrl Pts',(-29.2650725221322,51.2576224915288,
2.76354482594299));
#217038=CARTESIAN_POINT('Ctrl Pts',(-29.2633635057959,51.2720604115324,
2.78225519317082));
#217039=CARTESIAN_POINT('Ctrl Pts',(-29.2635407906072,51.2858132466409,
2.8015122308544));
#217040=CARTESIAN_POINT('Ctrl Pts',(-29.2637155451665,51.2993697979339,
2.82049442740137));
#217041=CARTESIAN_POINT('Ctrl Pts',(-29.2657236711467,51.3122614394839,
2.8400092908907));
#217042=CARTESIAN_POINT('Ctrl Pts',(-29.2695013892387,51.3243180878406,
2.85976644341372));
#217043=CARTESIAN_POINT('Ctrl Pts',(-29.2721352815049,51.3327241975842,
2.87354148166792));
#217044=CARTESIAN_POINT('Ctrl Pts',(-29.2756302808585,51.3407239614242,
2.88743438345427));
#217045=CARTESIAN_POINT('Ctrl Pts',(-29.2799753962465,51.3482501200166,
2.90134173516058));
#217046=CARTESIAN_POINT('',(-29.4581217525676,51.6568155675428,3.47153072139108));
#217047=CARTESIAN_POINT('',(-29.2799753962465,51.3482501200166,2.90134173516058));
#217048=CARTESIAN_POINT('',(-24.4761921430394,54.1952354911873,3.4715307213911));
#217049=CARTESIAN_POINT('Origin',(5.53234440788222E-15,1.85015204418142E-13,
3.47153072139072));
#217050=CARTESIAN_POINT('',(-24.331269253109,53.8697418420146,2.9013417351606));
#217051=CARTESIAN_POINT('',(-24.4761921430394,54.1952354911873,3.4715307213911));
#217052=CARTESIAN_POINT('',(-23.9791663275016,53.8206887816837,2.59908173516061));
#217053=CARTESIAN_POINT('Ctrl Pts',(-24.331269253109,53.8697418420146,2.9013417351606));
#217054=CARTESIAN_POINT('Ctrl Pts',(-24.32629474976,53.8585692765371,2.881769989197));
#217055=CARTESIAN_POINT('Ctrl Pts',(-24.319586568523,53.8482286480016,2.86226752356478));
#217056=CARTESIAN_POINT('Ctrl Pts',(-24.3112807320066,53.8388409929152,
2.8431037049964));
#217057=CARTESIAN_POINT('Ctrl Pts',(-24.3028248617511,53.8292837624956,
2.8235937178814));
#217058=CARTESIAN_POINT('Ctrl Pts',(-24.292712749833,53.8207133850096,2.80443322636351));
#217059=CARTESIAN_POINT('Ctrl Pts',(-24.2810366186942,53.8132717929009,
2.78589323877493));
#217060=CARTESIAN_POINT('Ctrl Pts',(-24.2698548246746,53.8061452585079,
2.76813818619129));
#217061=CARTESIAN_POINT('Ctrl Pts',(-24.2572379736511,53.8000534012972,
2.75095095197752));
#217062=CARTESIAN_POINT('Ctrl Pts',(-24.2432286115574,53.7951438030521,
2.7345777143408));
#217063=CARTESIAN_POINT('Ctrl Pts',(-24.2320860256382,53.7912388700573,
2.72155497954925));
#217064=CARTESIAN_POINT('Ctrl Pts',(-24.2200617420557,53.7880821478308,
2.7090471115967));
#217065=CARTESIAN_POINT('Ctrl Pts',(-24.2071623814825,53.7857624469883,
2.69718956158374));
#217066=CARTESIAN_POINT('Ctrl Pts',(-24.2071271704182,53.7857561149585,
2.69715719432391));
#217067=CARTESIAN_POINT('Ctrl Pts',(-24.2070919529318,53.7857497893138,
2.69712483219057));
#217068=CARTESIAN_POINT('Ctrl Pts',(-24.2070567290244,53.7857434700556,
2.69709247518685));
#217069=CARTESIAN_POINT('Ctrl Pts',(-24.2000447667167,53.7844855062587,
2.69065122242311));
#217070=CARTESIAN_POINT('Ctrl Pts',(-24.1927483559227,53.7835014710817,
2.68442464469462));
#217071=CARTESIAN_POINT('Ctrl Pts',(-24.1852078325131,53.7827951090626,
2.67844505923615));
#217072=CARTESIAN_POINT('Ctrl Pts',(-24.1702431416111,53.7813932847189,
2.66657815779603));
#217073=CARTESIAN_POINT('Ctrl Pts',(-24.1543158599157,53.7810858838908,
2.6556844566421));
#217074=CARTESIAN_POINT('Ctrl Pts',(-24.1377344018726,53.781906998247,2.64601906229551));
#217075=CARTESIAN_POINT('Ctrl Pts',(-24.1252983083403,53.7825228340141,
2.63877001653557));
#217076=CARTESIAN_POINT('Ctrl Pts',(-24.1124942402751,53.7837734588335,
2.63221189387637));
#217077=CARTESIAN_POINT('Ctrl Pts',(-24.0994523147292,53.7856732654699,
2.62645231033269));
#217078=CARTESIAN_POINT('Ctrl Pts',(-24.0945615926495,53.7863856929585,
2.6242924665038));
#217079=CARTESIAN_POINT('Ctrl Pts',(-24.089637421941,53.7871894118147,2.62224491711781));
#217080=CARTESIAN_POINT('Ctrl Pts',(-24.0846866645808,53.7880851817731,
2.62031533672632));
#217081=CARTESIAN_POINT('Ctrl Pts',(-24.06735901382,53.7912203766274,2.61356180535613));
#217082=CARTESIAN_POINT('Ctrl Pts',(-24.0497056745176,53.7954831928409,
2.60825339735384));
#217083=CARTESIAN_POINT('Ctrl Pts',(-24.0320208729158,53.8009062465108,
2.60463337987647));
#217084=CARTESIAN_POINT('Ctrl Pts',(-24.023178472115,53.8036177733458,2.60282337113778));
#217085=CARTESIAN_POINT('Ctrl Pts',(-24.0143282061515,53.8066193604765,
2.6014354593915));
#217086=CARTESIAN_POINT('Ctrl Pts',(-24.0055068550422,53.809915088884,2.60050005034632));
#217087=CARTESIAN_POINT('Ctrl Pts',(-24.0010961794875,53.8115629530877,
2.60003234582373));
#217088=CARTESIAN_POINT('Ctrl Pts',(-23.9966927326565,53.8132843526341,
2.59967776696101));
#217089=CARTESIAN_POINT('Ctrl Pts',(-23.9923011121677,53.8150797979126,
2.59944011429195));
#217090=CARTESIAN_POINT('Ctrl Pts',(-23.987909491679,53.8168752431911,2.59920246162289));
#217091=CARTESIAN_POINT('Ctrl Pts',(-23.9835296982243,53.8187447357541,
2.59908173791349));
#217092=CARTESIAN_POINT('Ctrl Pts',(-23.9791663275016,53.8206887816837,
2.59908173516061));
#217093=CARTESIAN_POINT('',(-23.9513722670367,53.8330634946838,2.5990817351606));
#217094=CARTESIAN_POINT('Origin',(3.74779409800327E-16,1.91169726806065E-13,
2.59908173516024));
#217095=CARTESIAN_POINT('',(-23.752222950883,54.1275498658874,2.9013417351606));
#217096=CARTESIAN_POINT('Ctrl Pts',(-23.9513722670367,53.8330634946838,
2.5990817351606));
#217097=CARTESIAN_POINT('Ctrl Pts',(-23.9478914369184,53.8346121892504,
2.5990817437155));
#217098=CARTESIAN_POINT('Ctrl Pts',(-23.9444392282283,53.8361996036044,
2.59915764355927));
#217099=CARTESIAN_POINT('Ctrl Pts',(-23.9410169613692,53.8378239549349,
2.59930765775313));
#217100=CARTESIAN_POINT('Ctrl Pts',(-23.9208121566366,53.8474140023513,
2.60019333020913));
#217101=CARTESIAN_POINT('Ctrl Pts',(-23.9016479061139,53.8582911092149,
2.60365973324093));
#217102=CARTESIAN_POINT('Ctrl Pts',(-23.8838022859705,53.8700861059294,
2.60934177082346));
#217103=CARTESIAN_POINT('Ctrl Pts',(-23.877135756338,53.8744923240646,2.61146439091803));
#217104=CARTESIAN_POINT('Ctrl Pts',(-23.8706528330389,53.8790265713715,
2.61389584429309));
#217105=CARTESIAN_POINT('Ctrl Pts',(-23.8643665485424,53.883669534051,2.61661604385287));
#217106=CARTESIAN_POINT('Ctrl Pts',(-23.8594616740271,53.8872922064475,
2.6187384800081));
#217107=CARTESIAN_POINT('Ctrl Pts',(-23.8546770178326,53.8909810920752,
2.62103707099821));
#217108=CARTESIAN_POINT('Ctrl Pts',(-23.8500192775333,53.8947270356133,
2.62350262767686));
#217109=CARTESIAN_POINT('Ctrl Pts',(-23.8337171864861,53.9078378379965,
2.63213207605213));
#217110=CARTESIAN_POINT('Ctrl Pts',(-23.818969811583,53.9216475915795,2.64280685971948));
#217111=CARTESIAN_POINT('Ctrl Pts',(-23.806064348069,53.9357638458657,2.65513293646118));
#217112=CARTESIAN_POINT('Ctrl Pts',(-23.7996116163121,53.9428219730087,
2.66129597483203));
#217113=CARTESIAN_POINT('Ctrl Pts',(-23.7936193631243,53.9499567269876,
2.66787183533887));
#217114=CARTESIAN_POINT('Ctrl Pts',(-23.7881234899554,53.9571190561827,
2.67481125953896));
#217115=CARTESIAN_POINT('Ctrl Pts',(-23.7826510977526,53.9642507845245,
2.68172103524115));
#217116=CARTESIAN_POINT('Ctrl Pts',(-23.7776706121036,53.9714097802522,
2.68899101329824));
#217117=CARTESIAN_POINT('Ctrl Pts',(-23.773218200392,53.978547836393,2.6965733470131));
#217118=CARTESIAN_POINT('Ctrl Pts',(-23.773199095963,53.9785784643977,2.69660588132608));
#217119=CARTESIAN_POINT('Ctrl Pts',(-23.7731800007333,53.9786090918658,
2.69663842081416));
#217120=CARTESIAN_POINT('Ctrl Pts',(-23.7731609147026,53.9786397187955,
2.69667096547416));
#217121=CARTESIAN_POINT('Ctrl Pts',(-23.7641603094577,53.9930827901226,
2.71201840158019));
#217122=CARTESIAN_POINT('Ctrl Pts',(-23.757192470701,54.007371163677,2.72845645939479));
#217123=CARTESIAN_POINT('Ctrl Pts',(-23.7521258339913,54.0213615752674,
2.74568723187081));
#217124=CARTESIAN_POINT('Ctrl Pts',(-23.7468748830075,54.0358609305036,
2.76354482594575));
#217125=CARTESIAN_POINT('Ctrl Pts',(-23.7436660552509,54.05004111722,2.78225519317455));
#217126=CARTESIAN_POINT('Ctrl Pts',(-23.7424048061584,54.0637371441683,
2.80151223085914));
#217127=CARTESIAN_POINT('Ctrl Pts',(-23.7411615579203,54.0772376980811,
2.82049442740744));
#217128=CARTESIAN_POINT('Ctrl Pts',(-23.7418111396966,54.0902686241933,
2.84000929089815));
#217129=CARTESIAN_POINT('Ctrl Pts',(-23.7443079001293,54.1026541040363,
2.85976644342254));
#217130=CARTESIAN_POINT('Ctrl Pts',(-23.7460486859244,54.1112894809403,
2.87354148167386));
#217131=CARTESIAN_POINT('Ctrl Pts',(-23.7486883362847,54.1196107481466,
2.88743438345726));
#217132=CARTESIAN_POINT('Ctrl Pts',(-23.7522229508831,54.1275498658874,
2.9013417351606));
#217133=CARTESIAN_POINT('',(-23.8971395307771,54.4530463244693,3.4715307213911));
#217134=CARTESIAN_POINT('',(-23.752222950883,54.1275498658874,2.9013417351606));
#217135=CARTESIAN_POINT('',(-18.6771643191712,56.4568070719812,3.47153072139111));
#217136=CARTESIAN_POINT('Origin',(5.53234440788222E-15,1.85015204418142E-13,
3.47153072139072));
#217137=CARTESIAN_POINT('',(-18.5670586829468,56.1179479440989,2.90134173516062));
#217138=CARTESIAN_POINT('',(-18.6771643191712,56.4568070719812,3.47153072139112));
#217139=CARTESIAN_POINT('',(-18.2220120550219,56.0323588238392,2.59908173516062));
#217140=CARTESIAN_POINT('Ctrl Pts',(-18.5670586829468,56.1179479440989,
2.90134173516062));
#217141=CARTESIAN_POINT('Ctrl Pts',(-18.5632792815475,56.1063166059136,
2.88176998919699));
#217142=CARTESIAN_POINT('Ctrl Pts',(-18.5576887384392,56.0953314285471,
2.86226752356472));
#217143=CARTESIAN_POINT('Ctrl Pts',(-18.5504096793241,56.0851270036903,
2.84310370499631));
#217144=CARTESIAN_POINT('Ctrl Pts',(-18.5429991338194,56.0747382496557,
2.82359371788145));
#217145=CARTESIAN_POINT('Ctrl Pts',(-18.5338382654968,56.0651578180751,
2.80443322636368));
#217146=CARTESIAN_POINT('Ctrl Pts',(-18.5230039556137,56.0565365037418,
2.78589323877522));
#217147=CARTESIAN_POINT('Ctrl Pts',(-18.5126283423204,56.0482801935046,
2.76813818619188));
#217148=CARTESIAN_POINT('Ctrl Pts',(-18.5007173801999,56.0409028880764,
2.7509509519784));
#217149=CARTESIAN_POINT('Ctrl Pts',(-18.4872979556178,56.0345558080332,
2.73457771434192));
#217150=CARTESIAN_POINT('Ctrl Pts',(-18.476624586595,56.0295075492868,2.72155497954998));
#217151=CARTESIAN_POINT('Ctrl Pts',(-18.4649961406192,56.02511124003,2.70904711159707));
#217152=CARTESIAN_POINT('Ctrl Pts',(-18.4524099188568,56.0214558964135,
2.69718956158377));
#217153=CARTESIAN_POINT('Ctrl Pts',(-18.4523755625598,56.0214459185128,
2.69715719432394));
#217154=CARTESIAN_POINT('Ctrl Pts',(-18.4523411992083,56.0214359462908,
2.6971248321906));
#217155=CARTESIAN_POINT('Ctrl Pts',(-18.4523068288036,56.0214259797493,
2.69709247518687));
#217156=CARTESIAN_POINT('Ctrl Pts',(-18.4454647717816,56.0194419575651,
2.69065122242314));
#217157=CARTESIAN_POINT('Ctrl Pts',(-18.4383111911742,56.0177006304281,
2.68442464469464));
#217158=CARTESIAN_POINT('Ctrl Pts',(-18.4308858104772,56.0162099386099,
2.67844505923617));
#217159=CARTESIAN_POINT('Ctrl Pts',(-18.4161496282622,56.0132515574634,
2.66657815779605));
#217160=CARTESIAN_POINT('Ctrl Pts',(-18.4003417300186,56.0112809863295,
2.65568445664211));
#217161=CARTESIAN_POINT('Ctrl Pts',(-18.3837652771157,56.0103643682073,
2.64601906229553));
#217162=CARTESIAN_POINT('Ctrl Pts',(-18.3713329374386,56.0096769046157,
2.63877001653558));
#217163=CARTESIAN_POINT('Ctrl Pts',(-18.3584682855075,56.009582288823,2.63221189387638));
#217164=CARTESIAN_POINT('Ctrl Pts',(-18.3452992211262,56.0101084356845,
2.6264523103327));
#217165=CARTESIAN_POINT('Ctrl Pts',(-18.3403608219832,56.0103057407576,
2.62429246650382));
#217166=CARTESIAN_POINT('Ctrl Pts',(-18.3353796149,56.0105903407607,2.62224491711782));
#217167=CARTESIAN_POINT('Ctrl Pts',(-18.3303623448494,56.0109637085387,
2.62031533672634));
#217168=CARTESIAN_POINT('Ctrl Pts',(-18.3128018996724,56.0122704957615,
2.61356180535615));
#217169=CARTESIAN_POINT('Ctrl Pts',(-18.2947996815818,56.014664683393,2.60825339735385));
#217170=CARTESIAN_POINT('Ctrl Pts',(-18.2766448957073,56.0182094638728,
2.60463337987648));
#217171=CARTESIAN_POINT('Ctrl Pts',(-18.2675675027701,56.0199818541128,
2.6028233711378));
#217172=CARTESIAN_POINT('Ctrl Pts',(-18.2584519681994,56.0220418935344,
2.60143545939152));
#217173=CARTESIAN_POINT('Ctrl Pts',(-18.2493344439487,56.0243974853215,
2.60050005034633));
#217174=CARTESIAN_POINT('Ctrl Pts',(-18.2447756818233,56.025575281215,2.60003234582374));
#217175=CARTESIAN_POINT('Ctrl Pts',(-18.2402164222855,56.0268269652242,
2.59967776696103));
#217176=CARTESIAN_POINT('Ctrl Pts',(-18.2356611844174,56.0281535255247,
2.59944011429197));
#217177=CARTESIAN_POINT('Ctrl Pts',(-18.2311059465494,56.0294800858251,
2.59920246162291));
#217178=CARTESIAN_POINT('Ctrl Pts',(-18.2265547308768,56.030881524033,2.59908173791348));
#217179=CARTESIAN_POINT('Ctrl Pts',(-18.2220120550219,56.0323588238392,
2.59908173516062));
#217180=CARTESIAN_POINT('',(-18.1930767435952,56.0417604764384,2.59908173516062));
#217181=CARTESIAN_POINT('Origin',(3.81437458815951E-16,1.91172282591625E-13,
2.59908173516023));
#217182=CARTESIAN_POINT('',(-17.9642361803975,56.3138168485096,2.90134173516061));
#217183=CARTESIAN_POINT('Ctrl Pts',(-18.1930767435952,56.0417604764384,
2.59908173516062));
#217184=CARTESIAN_POINT('Ctrl Pts',(-18.1894530991653,56.042936841271,2.59908174371553));
#217185=CARTESIAN_POINT('Ctrl Pts',(-18.1858538720526,56.0441547055337,
2.59915764355928));
#217186=CARTESIAN_POINT('Ctrl Pts',(-18.1822805617811,56.045412434202,2.59930765775314));
#217187=CARTESIAN_POINT('Ctrl Pts',(-18.1611840081645,56.0528379691456,
2.60019333020911));
#217188=CARTESIAN_POINT('Ctrl Pts',(-18.1409877741468,56.0616522804226,
2.6036597332407));
#217189=CARTESIAN_POINT('Ctrl Pts',(-18.1220070012975,56.0715172876609,
2.60934177082289));
#217190=CARTESIAN_POINT('Ctrl Pts',(-18.1149164164007,56.0752025259747,
2.6114643909176));
#217191=CARTESIAN_POINT('Ctrl Pts',(-18.10799504933,56.0790342841908,2.61389584429285));
#217192=CARTESIAN_POINT('Ctrl Pts',(-18.1012578800032,56.0829947165772,
2.61661604385289));
#217193=CARTESIAN_POINT('Ctrl Pts',(-18.0960012025252,56.0860848445997,
2.61873848000813));
#217194=CARTESIAN_POINT('Ctrl Pts',(-18.0908571636321,56.0892533893667,
2.62103707099824));
#217195=CARTESIAN_POINT('Ctrl Pts',(-18.0858333812,56.0924919457983,2.62350262767689));
#217196=CARTESIAN_POINT('Ctrl Pts',(-18.0682501426879,56.1038268933091,
2.63213207605216));
#217197=CARTESIAN_POINT('Ctrl Pts',(-18.0521400431274,56.1160194751812,
2.64280685971951));
#217198=CARTESIAN_POINT('Ctrl Pts',(-18.0378297267253,56.1287094108805,
2.65513293646121));
#217199=CARTESIAN_POINT('Ctrl Pts',(-18.0306745685242,56.1350543787301,
2.66129597483206));
#217200=CARTESIAN_POINT('Ctrl Pts',(-18.0239693566573,56.141523686763,2.6678718353389));
#217201=CARTESIAN_POINT('Ctrl Pts',(-18.0177549231924,56.1480723047927,
2.67481125953899));
#217202=CARTESIAN_POINT('Ctrl Pts',(-18.0115670407226,56.154592944033,2.68172103524118));
#217203=CARTESIAN_POINT('Ctrl Pts',(-18.0058655198732,56.1611921195218,
2.68899101329827));
#217204=CARTESIAN_POINT('Ctrl Pts',(-18.0006913688997,56.1678256688902,
2.69657334701313));
#217205=CARTESIAN_POINT('Ctrl Pts',(-18.0006691676285,56.1678541321548,
2.6966058813261));
#217206=CARTESIAN_POINT('Ctrl Pts',(-18.0006469755623,56.1678825958475,
2.69663842081419));
#217207=CARTESIAN_POINT('Ctrl Pts',(-18.000624792701,56.1679110599662,2.69667096547419));
#217208=CARTESIAN_POINT('Ctrl Pts',(-17.9901637816629,56.1813341912024,
2.71201840157986));
#217209=CARTESIAN_POINT('Ctrl Pts',(-17.9817405717259,56.1948159540735,
2.72845645939404));
#217210=CARTESIAN_POINT('Ctrl Pts',(-17.9752392943583,56.2082001169759,
2.74568723186962));
#217211=CARTESIAN_POINT('Ctrl Pts',(-17.9685015133122,56.2220711693896,
2.76354482594404));
#217212=CARTESIAN_POINT('Ctrl Pts',(-17.9638280307234,56.2358382617248,
2.78225519317228));
#217213=CARTESIAN_POINT('Ctrl Pts',(-17.9611420662355,56.2493274239746,
2.80151223085629));
#217214=CARTESIAN_POINT('Ctrl Pts',(-17.9584944364875,56.2626240656124,
2.82049442740399));
#217215=CARTESIAN_POINT('Ctrl Pts',(-17.9577783571051,56.2756515067325,
2.84000929089407));
#217216=CARTESIAN_POINT('Ctrl Pts',(-17.9589668048478,56.2882301201518,
2.85976644341784));
#217217=CARTESIAN_POINT('Ctrl Pts',(-17.9597954117585,56.2970001532227,
2.8735414816707));
#217218=CARTESIAN_POINT('Ctrl Pts',(-17.9615507925646,56.3055517542533,
2.88743438345568));
#217219=CARTESIAN_POINT('Ctrl Pts',(-17.9642361803975,56.3138168485096,
2.9013417351606));
#217220=CARTESIAN_POINT('',(-18.0743352474894,56.6526781108324,3.47153072139111));
#217221=CARTESIAN_POINT('',(-17.9642361803975,56.3138168485096,2.90134173516061));
#217222=CARTESIAN_POINT('',(-12.6735055745743,58.0998260601481,3.47153072139113));
#217223=CARTESIAN_POINT('Origin',(5.53234440788222E-15,1.85015204418142E-13,
3.47153072139072));
#217224=CARTESIAN_POINT('',(-12.5994235324474,57.7513140650721,2.90134173516064));
#217225=CARTESIAN_POINT('',(-12.6735055745743,58.0998260601481,3.47153072139113));
#217226=CARTESIAN_POINT('',(-12.2652136052663,57.6301266171959,2.59908173516063));
#217227=CARTESIAN_POINT('Ctrl Pts',(-12.5994235324474,57.7513140650721,
2.90134173516064));
#217228=CARTESIAN_POINT('Ctrl Pts',(-12.5968806409108,57.7393513895546,
2.88176998919802));
#217229=CARTESIAN_POINT('Ctrl Pts',(-12.5924689870918,57.7278420192598,
2.86226752356677));
#217230=CARTESIAN_POINT('Ctrl Pts',(-12.5862964562735,57.7169326264472,
2.84310370499932));
#217231=CARTESIAN_POINT('Ctrl Pts',(-12.5800124270075,57.7058261701611,
2.82359371788539));
#217232=CARTESIAN_POINT('Ctrl Pts',(-12.5719031706713,57.6953406496997,
2.80443322636852));
#217233=CARTESIAN_POINT('Ctrl Pts',(-12.5620293850107,57.685634070066,2.78589323878086));
#217234=CARTESIAN_POINT('Ctrl Pts',(-12.5525736298349,57.6763384418474,
2.76813818619826));
#217235=CARTESIAN_POINT('Ctrl Pts',(-12.5414990556115,57.667756515504,2.75095095198544));
#217236=CARTESIAN_POINT('Ctrl Pts',(-12.5288165945656,57.6600414936,2.73457771434951));
#217237=CARTESIAN_POINT('Ctrl Pts',(-12.5187293821024,57.65390521888,2.72155497955484));
#217238=CARTESIAN_POINT('Ctrl Pts',(-12.5076241774191,57.648317489476,2.70904711159938));
#217239=CARTESIAN_POINT('Ctrl Pts',(-12.495488991745,57.6433665517942,2.69718956158379));
#217240=CARTESIAN_POINT('Ctrl Pts',(-12.49545586663,57.6433530373425,2.69715719432396));
#217241=CARTESIAN_POINT('Ctrl Pts',(-12.4954227339057,57.6433395278011,
2.69712483219062));
#217242=CARTESIAN_POINT('Ctrl Pts',(-12.4953895935729,57.6433260231718,
2.6970924751869));
#217243=CARTESIAN_POINT('Ctrl Pts',(-12.4887924048451,57.6406376799627,
2.69065122242315));
#217244=CARTESIAN_POINT('Ctrl Pts',(-12.4818600305505,57.6381581392101,
2.68442464469466));
#217245=CARTESIAN_POINT('Ctrl Pts',(-12.4746311465908,57.6358994499242,
2.67844505923618));
#217246=CARTESIAN_POINT('Ctrl Pts',(-12.4602849257588,57.6314169246178,
2.66657815779607));
#217247=CARTESIAN_POINT('Ctrl Pts',(-12.4447696056082,57.6278047731679,
2.65568445664213));
#217248=CARTESIAN_POINT('Ctrl Pts',(-12.4283797729325,57.6251604652273,
2.64601906229555));
#217249=CARTESIAN_POINT('Ctrl Pts',(-12.4160873984258,57.6231772342719,
2.63877001653561));
#217250=CARTESIAN_POINT('Ctrl Pts',(-12.4033031104474,57.6217384144976,
2.63221189387641));
#217251=CARTESIAN_POINT('Ctrl Pts',(-12.3901511902558,57.6208851370091,
2.62645231033273));
#217252=CARTESIAN_POINT('Ctrl Pts',(-12.3852192201839,57.6205651579509,
2.62429246650384));
#217253=CARTESIAN_POINT('Ctrl Pts',(-12.3802355518734,57.6203275209639,
2.62224491711784));
#217254=CARTESIAN_POINT('Ctrl Pts',(-12.3752067393931,57.6201743958659,
2.62031533672636));
#217255=CARTESIAN_POINT('Ctrl Pts',(-12.3576058957119,57.6196384580229,
2.61356180535617));
#217256=CARTESIAN_POINT('Ctrl Pts',(-12.3394520349016,57.6201377858516,
2.60825339735387));
#217257=CARTESIAN_POINT('Ctrl Pts',(-12.3210261723876,57.6217654557846,
2.6046333798765));
#217258=CARTESIAN_POINT('Ctrl Pts',(-12.3118132411305,57.6225792907512,
2.60282337113782));
#217259=CARTESIAN_POINT('Ctrl Pts',(-12.302532309657,57.6236752122408,2.60143545939154));
#217260=CARTESIAN_POINT('Ctrl Pts',(-12.2932185057685,57.6250648590508,
2.60050005034635));
#217261=CARTESIAN_POINT('Ctrl Pts',(-12.2885616038243,57.6257596824558,
2.60003234582376));
#217262=CARTESIAN_POINT('Ctrl Pts',(-12.2838964837812,57.626527937216,2.59967776696105));
#217263=CARTESIAN_POINT('Ctrl Pts',(-12.2792275366732,57.6273710784661,
2.59944011429199));
#217264=CARTESIAN_POINT('Ctrl Pts',(-12.2745585895652,57.6282142197163,
2.59920246162293));
#217265=CARTESIAN_POINT('Ctrl Pts',(-12.2698858157461,57.6291322491188,
2.59908173791354));
#217266=CARTESIAN_POINT('Ctrl Pts',(-12.2652136052663,57.6301266171959,
2.59908173516064));
#217267=CARTESIAN_POINT('',(-12.2354540642047,57.6364522029208,2.59908173516064));
#217268=CARTESIAN_POINT('Origin',(3.88326186679512E-16,1.91174128420693E-13,
2.59908173516024));
#217269=CARTESIAN_POINT('',(-11.9794294790614,57.8830978693157,2.90134173516063));
#217270=CARTESIAN_POINT('Ctrl Pts',(-12.2354540642047,57.6364522029208,
2.59908173516064));
#217271=CARTESIAN_POINT('Ctrl Pts',(-12.2317273068699,57.63724334952,2.59908174371556));
#217272=CARTESIAN_POINT('Ctrl Pts',(-12.2280204952201,57.638078320516,2.59915764355931));
#217273=CARTESIAN_POINT('Ctrl Pts',(-12.2243352914713,57.6389556465835,
2.59930765775318));
#217274=CARTESIAN_POINT('Ctrl Pts',(-12.2025781272232,57.6441353133407,
2.60019333020927));
#217275=CARTESIAN_POINT('Ctrl Pts',(-12.1815711838732,57.6507902575936,
2.60365973324169));
#217276=CARTESIAN_POINT('Ctrl Pts',(-12.1616632156344,57.6586171922739,
2.60934177082526));
#217277=CARTESIAN_POINT('Ctrl Pts',(-12.1542262614087,57.6615410745228,
2.61146439091942));
#217278=CARTESIAN_POINT('Ctrl Pts',(-12.1469422825158,57.6646283621018,
2.61389584429389));
#217279=CARTESIAN_POINT('Ctrl Pts',(-12.1398280421989,57.6678628728675,
2.61661604385293));
#217280=CARTESIAN_POINT('Ctrl Pts',(-12.1342771550166,57.6703866004267,
2.61873848000816));
#217281=CARTESIAN_POINT('Ctrl Pts',(-12.1288300925915,57.6730000890934,
2.62103707099826));
#217282=CARTESIAN_POINT('Ctrl Pts',(-12.1234953096383,57.6756957761166,
2.62350262767691));
#217283=CARTESIAN_POINT('Ctrl Pts',(-12.104823569302,57.685130680698,2.63213207605218));
#217284=CARTESIAN_POINT('Ctrl Pts',(-12.0875272507061,57.6955725063807,
2.64280685971954));
#217285=CARTESIAN_POINT('Ctrl Pts',(-12.071968868237,57.7066970899021,2.65513293646124));
#217286=CARTESIAN_POINT('Ctrl Pts',(-12.0641896770024,57.7122593816628,
2.66129597483209));
#217287=CARTESIAN_POINT('Ctrl Pts',(-12.0568449701605,57.717992364657,2.66787183533892));
#217288=CARTESIAN_POINT('Ctrl Pts',(-12.0499800630333,57.7238555234918,
2.67481125953901));
#217289=CARTESIAN_POINT('Ctrl Pts',(-12.0431444860318,57.7296936321426,
2.68172103524119));
#217290=CARTESIAN_POINT('Ctrl Pts',(-12.0367843970375,57.735660685445,2.68899101329828));
#217291=CARTESIAN_POINT('Ctrl Pts',(-12.0309451958829,57.7417170494859,
2.69657334701314));
#217292=CARTESIAN_POINT('Ctrl Pts',(-12.0309201410113,57.741743036161,2.69660588132611));
#217293=CARTESIAN_POINT('Ctrl Pts',(-12.0308950952495,57.741769024224,2.6966384208142));
#217294=CARTESIAN_POINT('Ctrl Pts',(-12.0308700585976,57.7417950136728,
2.6966709654742));
#217295=CARTESIAN_POINT('Ctrl Pts',(-12.0190632547925,57.7540511381832,
2.71201840157942));
#217296=CARTESIAN_POINT('Ctrl Pts',(-12.009276960126,57.7665785813559,2.72845645939309));
#217297=CARTESIAN_POINT('Ctrl Pts',(-12.0014122714559,57.7792098558806,
2.74568723186812));
#217298=CARTESIAN_POINT('Ctrl Pts',(-11.9932614808867,57.7923006313189,
2.76354482594205));
#217299=CARTESIAN_POINT('Ctrl Pts',(-11.9871745471191,57.8055037941284,
2.78225519316977));
#217300=CARTESIAN_POINT('Ctrl Pts',(-11.9830932952248,57.8186383015954,
2.80151223085323));
#217301=CARTESIAN_POINT('Ctrl Pts',(-11.9790702919525,57.8315853501699,
2.82049442740046));
#217302=CARTESIAN_POINT('Ctrl Pts',(-11.9769963969271,57.8444665749267,
2.84000929089006));
#217303=CARTESIAN_POINT('Ctrl Pts',(-11.9768635110977,57.8571005080016,
2.85976644341336));
#217304=CARTESIAN_POINT('Ctrl Pts',(-11.9767708607331,57.8659091109217,
2.87354148166769));
#217305=CARTESIAN_POINT('Ctrl Pts',(-11.9776227396652,57.8745973526462,
2.88743438345419));
#217306=CARTESIAN_POINT('Ctrl Pts',(-11.9794294790615,57.8830978693157,
2.90134173516063));
#217307=CARTESIAN_POINT('',(-12.0535047649324,58.2316113004782,3.47153072139112));
#217308=CARTESIAN_POINT('',(-11.9794294790614,57.8830978693157,2.90134173516064));
#217309=CARTESIAN_POINT('',(-6.53099325080075,59.1062911958298,3.47153072139113));
#217310=CARTESIAN_POINT('Origin',(5.53234440788222E-15,1.85015204418142E-13,
3.47153072139072));
#217311=CARTESIAN_POINT('',(-6.4937464611276,58.751944703909,2.90134173516065));
#217312=CARTESIAN_POINT('',(-6.53099325080075,59.1062911958298,3.47153072139113));
#217313=CARTESIAN_POINT('',(-6.1740349085904,58.5964866834552,2.59908173516065));
#217314=CARTESIAN_POINT('Ctrl Pts',(-6.4937464611276,58.751944703909,2.90134173516065));
#217315=CARTESIAN_POINT('Ctrl Pts',(-6.49246793990533,58.7397817566342,
2.88176998919662));
#217316=CARTESIAN_POINT('Ctrl Pts',(-6.48928351037726,58.7278742924791,
2.86226752356397));
#217317=CARTESIAN_POINT('Ctrl Pts',(-6.4842851353939,58.7163794573001,2.84310370499519));
#217318=CARTESIAN_POINT('Ctrl Pts',(-6.47919647150507,58.7046769834205,
2.82359371787983));
#217319=CARTESIAN_POINT('Ctrl Pts',(-6.47222767386301,58.6934012556334,
2.8044332263616));
#217320=CARTESIAN_POINT('Ctrl Pts',(-6.46342259168489,58.6827157580163,
2.78589323877272));
#217321=CARTESIAN_POINT('Ctrl Pts',(-6.45499029385684,58.6724826566635,
2.76813818618886));
#217322=CARTESIAN_POINT('Ctrl Pts',(-6.4448734428809,58.662790134785,2.7509509519749));
#217323=CARTESIAN_POINT('Ctrl Pts',(-6.43306689706553,58.6537916984143,
2.73457771433802));
#217324=CARTESIAN_POINT('Ctrl Pts',(-6.42367635877643,58.6466346380341,
2.72155497954749));
#217325=CARTESIAN_POINT('Ctrl Pts',(-6.4132160663368,58.6399167088188,2.70904711159589));
#217326=CARTESIAN_POINT('Ctrl Pts',(-6.40166487239057,58.6337244205834,
2.69718956158378));
#217327=CARTESIAN_POINT('Ctrl Pts',(-6.40163334138329,58.633707517648,2.69715719432396));
#217328=CARTESIAN_POINT('Ctrl Pts',(-6.40160180229505,58.6336906188005,
2.69712483219062));
#217329=CARTESIAN_POINT('Ctrl Pts',(-6.40157025512662,58.6336737240429,
2.6970924751869));
#217330=CARTESIAN_POINT('Ctrl Pts',(-6.39529021487341,58.6303105138596,
2.69065122242315));
#217331=CARTESIAN_POINT('Ctrl Pts',(-6.38865499943491,58.6271199258589,
2.68442464469466));
#217332=CARTESIAN_POINT('Ctrl Pts',(-6.38170181337804,58.6241179857778,
2.67844505923619));
#217333=CARTESIAN_POINT('Ctrl Pts',(-6.36790273412669,58.6181604277967,
2.66657815779607));
#217334=CARTESIAN_POINT('Ctrl Pts',(-6.35284998116341,58.612946271518,2.65568445664214));
#217335=CARTESIAN_POINT('Ctrl Pts',(-6.33682633915145,58.6086032453502,
2.64601906229556));
#217336=CARTESIAN_POINT('Ctrl Pts',(-6.32480860764249,58.6053459757243,
2.63877001653562));
#217337=CARTESIAN_POINT('Ctrl Pts',(-6.31224475095125,58.602578715979,2.63221189387642));
#217338=CARTESIAN_POINT('Ctrl Pts',(-6.2992540701391,58.6003553628272,2.62645231033274));
#217339=CARTESIAN_POINT('Ctrl Pts',(-6.29438256483455,58.5995216053953,
2.62429246650386));
#217340=CARTESIAN_POINT('Ctrl Pts',(-6.28945103740957,58.5987643350185,
2.62224491711786));
#217341=CARTESIAN_POINT('Ctrl Pts',(-6.28446577922136,58.5980863947152,
2.62031533672637));
#217342=CARTESIAN_POINT('Ctrl Pts',(-6.26701737556263,58.5957136036536,
2.61356180535618));
#217343=CARTESIAN_POINT('Ctrl Pts',(-6.24891076953076,58.5943126009393,
2.60825339735388));
#217344=CARTESIAN_POINT('Ctrl Pts',(-6.23041570798265,58.5940053272332,
2.60463337987651));
#217345=CARTESIAN_POINT('Ctrl Pts',(-6.2211681772086,58.5938516903802,2.60282337113783));
#217346=CARTESIAN_POINT('Ctrl Pts',(-6.21182353265963,58.5939714867927,
2.60143545939156));
#217347=CARTESIAN_POINT('Ctrl Pts',(-6.20241549311782,58.5943799633644,
2.60050005034637));
#217348=CARTESIAN_POINT('Ctrl Pts',(-6.19771147334692,58.5945842016503,
2.60003234582378));
#217349=CARTESIAN_POINT('Ctrl Pts',(-6.19299160483011,58.5948606100014,
2.59967776696106));
#217350=CARTESIAN_POINT('Ctrl Pts',(-6.18826010244368,58.5952110945693,
2.599440114292));
#217351=CARTESIAN_POINT('Ctrl Pts',(-6.18352860005725,58.5955615791371,
2.59920246162294));
#217352=CARTESIAN_POINT('Ctrl Pts',(-6.17878546397933,58.5959861416121,
2.59908173791359));
#217353=CARTESIAN_POINT('Ctrl Pts',(-6.1740349085904,58.5964866834552,2.59908173516065));
#217354=CARTESIAN_POINT('',(-6.14377718965342,58.599666897865,2.59908173516065));
#217355=CARTESIAN_POINT('Origin',(3.95370119046986E-16,1.91175244069979E-13,
2.59908173516024));
#217356=CARTESIAN_POINT('',(-5.863373641496,58.8181995570487,2.90134173516065));
#217357=CARTESIAN_POINT('Ctrl Pts',(-6.14377718965342,58.599666897865,2.59908173516065));
#217358=CARTESIAN_POINT('Ctrl Pts',(-6.13998815054705,58.6000641582632,
2.59908174371554));
#217359=CARTESIAN_POINT('Ctrl Pts',(-6.13621436696423,58.6005070878752,
2.59915764355931));
#217360=CARTESIAN_POINT('Ctrl Pts',(-6.13245764560145,58.6009943991741,
2.59930765775317));
#217361=CARTESIAN_POINT('Ctrl Pts',(-6.11027824677063,58.6038714482308,
2.60019333020922));
#217362=CARTESIAN_POINT('Ctrl Pts',(-6.08869075055971,58.6082941124961,
2.60365973324127));
#217363=CARTESIAN_POINT('Ctrl Pts',(-6.06807370280082,58.613997221082,2.60934177082423));
#217364=CARTESIAN_POINT('Ctrl Pts',(-6.06037186006897,58.6161277126016,
2.61146439091863));
#217365=CARTESIAN_POINT('Ctrl Pts',(-6.05280507414697,58.6184367045764,
2.61389584429346));
#217366=CARTESIAN_POINT('Ctrl Pts',(-6.04539170794193,58.6209098557465,
2.61661604385295));
#217367=CARTESIAN_POINT('Ctrl Pts',(-6.03960742773695,58.6228395323551,
2.61873848000818));
#217368=CARTESIAN_POINT('Ctrl Pts',(-6.03391702093564,58.6248693309928,
2.6210370709983));
#217369=CARTESIAN_POINT('Ctrl Pts',(-6.02832968645963,58.6269926140966,
2.62350262767695));
#217370=CARTESIAN_POINT('Ctrl Pts',(-6.00877401579357,58.6344241049596,
2.63213207605221));
#217371=CARTESIAN_POINT('Ctrl Pts',(-5.99048098024846,58.6430007716256,
2.64280685971957));
#217372=CARTESIAN_POINT('Ctrl Pts',(-5.97384499260641,58.652438119704,2.65513293646127));
#217373=CARTESIAN_POINT('Ctrl Pts',(-5.96552699878538,58.6571567937432,
2.66129597483211));
#217374=CARTESIAN_POINT('Ctrl Pts',(-5.95762326711374,58.6620906399374,
2.66787183533894));
#217375=CARTESIAN_POINT('Ctrl Pts',(-5.95018309968312,58.6672041015821,
2.67481125953903));
#217376=CARTESIAN_POINT('Ctrl Pts',(-5.942774720162,58.6722957161035,2.68172103524121));
#217377=CARTESIAN_POINT('Ctrl Pts',(-5.93582574548873,58.6775652709346,
2.6889910132983));
#217378=CARTESIAN_POINT('Ctrl Pts',(-5.92938546966289,58.6829780948562,
2.69657334701315));
#217379=CARTESIAN_POINT('Ctrl Pts',(-5.92935783569725,58.6830013202264,
2.69660588132613));
#217380=CARTESIAN_POINT('Ctrl Pts',(-5.92933021064649,58.6830245479291,
2.69663842081421));
#217381=CARTESIAN_POINT('Ctrl Pts',(-5.92930259451082,58.6830477779622,
2.69667096547422));
#217382=CARTESIAN_POINT('Ctrl Pts',(-5.91627935575166,58.6940026150824,
2.71201840157949));
#217383=CARTESIAN_POINT('Ctrl Pts',(-5.90523719704773,58.7054384852681,
2.72845645939321));
#217384=CARTESIAN_POINT('Ctrl Pts',(-5.89609526424982,58.7171784805286,
2.74568723186831));
#217385=CARTESIAN_POINT('Ctrl Pts',(-5.8866207659247,58.7293455537166,2.7635448259422));
#217386=CARTESIAN_POINT('Ctrl Pts',(-5.87918707069841,58.741840130386,2.78225519316988));
#217387=CARTESIAN_POINT('Ctrl Pts',(-5.87375524644771,58.7544760786581,
2.80151223085331));
#217388=CARTESIAN_POINT('Ctrl Pts',(-5.86840094651688,58.766931683596,2.82049442740043));
#217389=CARTESIAN_POINT('Ctrl Pts',(-5.8649919578766,58.7795255625957,2.84000929088992));
#217390=CARTESIAN_POINT('Ctrl Pts',(-5.86353919440033,58.7920763953117,
2.85976644341311));
#217391=CARTESIAN_POINT('Ctrl Pts',(-5.86252630185741,58.8008270591832,
2.87354148166754));
#217392=CARTESIAN_POINT('Ctrl Pts',(-5.86246534555161,58.8095567514062,
2.88743438345412));
#217393=CARTESIAN_POINT('Ctrl Pts',(-5.863373641496,58.8181995570487,2.90134173516065));
#217394=CARTESIAN_POINT('',(-5.90061356181277,59.1725467709679,3.47153072139113));
#217395=CARTESIAN_POINT('',(-5.863373641496,58.8181995570487,2.90134173516065));
#217396=CARTESIAN_POINT('',(-0.316925998273249,59.4651754363834,3.47153072139114));
#217397=CARTESIAN_POINT('Origin',(5.53234440788222E-15,1.85015204418142E-13,
3.47153072139072));
#217398=CARTESIAN_POINT('',(-0.316922544675889,59.108876741935,2.90134173516065));
#217399=CARTESIAN_POINT('',(-0.316925998273249,59.4651754363834,3.47153072139114));
#217400=CARTESIAN_POINT('',(-0.0152121934561199,58.9208513795075,2.59908173516064));
#217401=CARTESIAN_POINT('Ctrl Pts',(-0.316922544675889,59.108876741935,
2.90134173516064));
#217402=CARTESIAN_POINT('Ctrl Pts',(-0.316922401514067,59.0966467827009,
2.88176998919896));
#217403=CARTESIAN_POINT('Ctrl Pts',(-0.315000085554109,59.0844716853568,
2.86226752356863));
#217404=CARTESIAN_POINT('Ctrl Pts',(-0.311230629649539,59.0725173476332,
2.84310370500206));
#217405=CARTESIAN_POINT('Ctrl Pts',(-0.30739308360589,59.060347070915,2.82359371788902));
#217406=CARTESIAN_POINT('Ctrl Pts',(-0.301641096265653,59.0484046750375,
2.80443322637298));
#217407=CARTESIAN_POINT('Ctrl Pts',(-0.29400118789602,59.0368573319866,
2.78589323878608));
#217408=CARTESIAN_POINT('Ctrl Pts',(-0.286684733438416,59.0257988735011,
2.76813818620413));
#217409=CARTESIAN_POINT('Ctrl Pts',(-0.277636448050035,59.0151019493871,
2.75095095199189));
#217410=CARTESIAN_POINT('Ctrl Pts',(-0.266835172456312,59.0049186873026,
2.73457771435643));
#217411=CARTESIAN_POINT('Ctrl Pts',(-0.258244193038573,58.9968192555073,
2.72155497955927));
#217412=CARTESIAN_POINT('Ctrl Pts',(-0.248543417988618,58.9890447295132,
2.70904711160149));
#217413=CARTESIAN_POINT('Ctrl Pts',(-0.237702773059694,58.9816789347252,
2.6971895615838));
#217414=CARTESIAN_POINT('Ctrl Pts',(-0.237673181620435,58.9816588284981,
2.69715719432397));
#217415=CARTESIAN_POINT('Ctrl Pts',(-0.237643581717174,58.9816387254918,
2.69712483219063));
#217416=CARTESIAN_POINT('Ctrl Pts',(-0.237613973350488,58.9816186257084,
2.69709247518691));
#217417=CARTESIAN_POINT('Ctrl Pts',(-0.231719887006982,58.9776173965854,
2.69065122242317));
#217418=CARTESIAN_POINT('Ctrl Pts',(-0.225454527233559,58.9737507180864,
2.68442464469466));
#217419=CARTESIAN_POINT('Ctrl Pts',(-0.218853219640928,58.9700384170938,
2.67844505923619));
#217420=CARTESIAN_POINT('Ctrl Pts',(-0.205752467570126,58.9626710986901,
2.66657815779607));
#217421=CARTESIAN_POINT('Ctrl Pts',(-0.191327202905629,58.9559120649698,
2.65568445664213));
#217422=CARTESIAN_POINT('Ctrl Pts',(-0.175845309932447,58.9499179036783,
2.64601906229555));
#217423=CARTESIAN_POINT('Ctrl Pts',(-0.164233890202561,58.9454222827096,
2.63877001653561));
#217424=CARTESIAN_POINT('Ctrl Pts',(-0.152028117041498,58.9413569016701,
2.63221189387641));
#217425=CARTESIAN_POINT('Ctrl Pts',(-0.139341004226338,58.9377878323774,
2.62645231033273));
#217426=CARTESIAN_POINT('Ctrl Pts',(-0.134583336920653,58.9364494313926,
2.62429246650385));
#217427=CARTESIAN_POINT('Ctrl Pts',(-0.129757981227663,58.935180824439,
2.62224491711786));
#217428=CARTESIAN_POINT('Ctrl Pts',(-0.124870896863517,58.9339854965862,
2.62031533672638));
#217429=CARTESIAN_POINT('Ctrl Pts',(-0.107766101589008,58.9298018491014,
2.61356180535619));
#217430=CARTESIAN_POINT('Ctrl Pts',(-0.0899051301002618,58.9265158655231,
2.60825339735388));
#217431=CARTESIAN_POINT('Ctrl Pts',(-0.0715435052827858,58.9242770147328,
2.60463337987651));
#217432=CARTESIAN_POINT('Ctrl Pts',(-0.0623626928740478,58.9231575893377,
2.60282337113783));
#217433=CARTESIAN_POINT('Ctrl Pts',(-0.0530567171307718,58.9222999481583,
2.60143545939156));
#217434=CARTESIAN_POINT('Ctrl Pts',(-0.0436575183856266,58.921722779137,
2.60050005034638));
#217435=CARTESIAN_POINT('Ctrl Pts',(-0.038957919013054,58.9214341946264,
2.60003234582378));
#217436=CARTESIAN_POINT('Ctrl Pts',(-0.0342350138896582,58.9212157281807,
2.59967776696107));
#217437=CARTESIAN_POINT('Ctrl Pts',(-0.0294927955550828,58.9210697160841,
2.59944011429201));
#217438=CARTESIAN_POINT('Ctrl Pts',(-0.0247505772205072,58.9209237039874,
2.59920246162295));
#217439=CARTESIAN_POINT('Ctrl Pts',(-0.0199890456752399,58.9208501479393,
2.59908173791352));
#217440=CARTESIAN_POINT('Ctrl Pts',(-0.0152121934561203,58.9208513795075,
2.59908173516065));
#217441=CARTESIAN_POINT('',(0.0152121934557198,58.9208513795075,2.59908173516064));
#217442=CARTESIAN_POINT('Origin',(4.02492081121313E-16,1.91175617316195E-13,
2.59908173516023));
#217443=CARTESIAN_POINT('',(0.316922544675488,59.108876741935,2.90134173516064));
#217444=CARTESIAN_POINT('Ctrl Pts',(0.0152121934557198,58.9208513795075,
2.59908173516065));
#217445=CARTESIAN_POINT('Ctrl Pts',(0.0190220008283435,58.9208504012366,
2.59908174371555));
#217446=CARTESIAN_POINT('Ctrl Pts',(0.0228214099815236,58.9208964366353,
2.59915764355931));
#217447=CARTESIAN_POINT('Ctrl Pts',(0.0266084895328065,58.9209883940809,
2.59930765775317));
#217448=CARTESIAN_POINT('Ctrl Pts',(0.048967120812902,58.9215313038858,
2.60019333020922));
#217449=CARTESIAN_POINT('Ctrl Pts',(0.070898652760156,58.9236732325288,
2.6036597332413));
#217450=CARTESIAN_POINT('Ctrl Pts',(0.0919988953506439,58.9271900305698,
2.60934177082431));
#217451=CARTESIAN_POINT('Ctrl Pts',(0.0998812435866003,58.9285037892489,
2.6114643909187));
#217452=CARTESIAN_POINT('Ctrl Pts',(0.107647933246302,58.9300091878198,
2.61389584429349));
#217453=CARTESIAN_POINT('Ctrl Pts',(0.115279202946735,58.9316938830319,
2.61661604385294));
#217454=CARTESIAN_POINT('Ctrl Pts',(0.121233502390038,58.9330083667492,
2.61873848000818));
#217455=CARTESIAN_POINT('Ctrl Pts',(0.127104908279827,58.9344322364593,
2.6210370709983));
#217456=CARTESIAN_POINT('Ctrl Pts',(0.132883578272888,58.9359598525095,
2.62350262767694));
#217457=CARTESIAN_POINT('Ctrl Pts',(0.1531089232486,58.9413065086851,2.63213207605221));
#217458=CARTESIAN_POINT('Ctrl Pts',(0.17219825341753,58.9479240485797,2.64280685971956));
#217459=CARTESIAN_POINT('Ctrl Pts',(0.189729578870585,58.9555707636547,
2.65513293646126));
#217460=CARTESIAN_POINT('Ctrl Pts',(0.198495241597112,58.9593941211922,
2.6612959748321));
#217461=CARTESIAN_POINT('Ctrl Pts',(0.206871403160357,58.963474774335,2.66787183533893));
#217462=CARTESIAN_POINT('Ctrl Pts',(0.214805314863019,58.9677825146338,
2.67481125953902));
#217463=CARTESIAN_POINT('Ctrl Pts',(0.222705329147433,58.9720718502314,
2.68172103524121));
#217464=CARTESIAN_POINT('Ctrl Pts',(0.230167055078982,58.976586172246,2.68899101329828));
#217465=CARTESIAN_POINT('Ctrl Pts',(0.23713784456645,58.9812961520167,2.69657334701314));
#217466=CARTESIAN_POINT('Ctrl Pts',(0.237167754862593,58.9813163616199,
2.69660588132611));
#217467=CARTESIAN_POINT('Ctrl Pts',(0.237197656536502,58.9813365744747,
2.6966384208142));
#217468=CARTESIAN_POINT('Ctrl Pts',(0.237227549587754,58.9813567905791,
2.69667096547421));
#217469=CARTESIAN_POINT('Ctrl Pts',(0.251324537972172,58.9908903168212,
2.71201840157982));
#217470=CARTESIAN_POINT('Ctrl Pts',(0.263501580512235,59.0011093202332,
2.72845645939393));
#217471=CARTESIAN_POINT('Ctrl Pts',(0.273820596509237,59.0118294103849,
2.74568723186944));
#217472=CARTESIAN_POINT('Ctrl Pts',(0.284514998004185,59.0229394763231,
2.76354482594379));
#217473=CARTESIAN_POINT('Ctrl Pts',(0.293214009568733,59.0345885736561,
2.78225519317196));
#217474=CARTESIAN_POINT('Ctrl Pts',(0.299936893972635,59.04658752064,2.80151223085589));
#217475=CARTESIAN_POINT('Ctrl Pts',(0.3065638277314,59.0584152157275,2.82049442740346));
#217476=CARTESIAN_POINT('Ctrl Pts',(0.311270560393525,59.0705837677967,
2.8400092908934));
#217477=CARTESIAN_POINT('Ctrl Pts',(0.314027284735791,59.0829139906045,
2.85976644341704));
#217478=CARTESIAN_POINT('Ctrl Pts',(0.315949321994076,59.0915108413219,
2.87354148167017));
#217479=CARTESIAN_POINT('Ctrl Pts',(0.316922445687527,59.1001863397077,
2.88743438345543));
#217480=CARTESIAN_POINT('Ctrl Pts',(0.316922544675488,59.108876741935,2.90134173516064));
#217481=CARTESIAN_POINT('',(0.316925998272844,59.4651754363834,3.47153072139114));
#217482=CARTESIAN_POINT('',(0.316922544675488,59.108876741935,2.90134173516064));
#217483=CARTESIAN_POINT('',(5.90061356181238,59.1725467709679,3.47153072139113));
#217484=CARTESIAN_POINT('Origin',(5.53234440788222E-15,1.85015204418142E-13,
3.47153072139072));
#217485=CARTESIAN_POINT('',(5.86337364149561,58.8181995570487,2.90134173516065));
#217486=CARTESIAN_POINT('',(5.90061356181238,59.1725467709679,3.47153072139113));
#217487=CARTESIAN_POINT('',(6.14377718965303,58.599666897865,2.59908173516064));
#217488=CARTESIAN_POINT('Ctrl Pts',(5.86337364149561,58.8181995570487,2.90134173516065));
#217489=CARTESIAN_POINT('Ctrl Pts',(5.86209540502863,58.8060365798462,2.88176998919861));
#217490=CARTESIAN_POINT('Ctrl Pts',(5.86273454612518,58.7937272422258,2.86226752356793));
#217491=CARTESIAN_POINT('Ctrl Pts',(5.86523378400438,58.7814443761818,2.84310370500102));
#217492=CARTESIAN_POINT('Ctrl Pts',(5.86777816724649,58.768939636722,2.82359371788768));
#217493=CARTESIAN_POINT('Ctrl Pts',(5.8722503243096,58.7564614161411,2.80443322637135));
#217494=CARTESIAN_POINT('Ctrl Pts',(5.87864135443809,58.744178742762,2.78589323878419));
#217495=CARTESIAN_POINT('Ctrl Pts',(5.88476180492122,58.732416085928,2.76813818620209));
#217496=CARTESIAN_POINT('Ctrl Pts',(5.89264238981639,58.7208319573166,2.75095095198971));
#217497=CARTESIAN_POINT('Ctrl Pts',(5.90232005415578,58.7095754394681,2.73457771435415));
#217498=CARTESIAN_POINT('Ctrl Pts',(5.91001735013015,58.7006223753317,2.72155497955782));
#217499=CARTESIAN_POINT('Ctrl Pts',(5.91885232406413,58.6918764318965,2.7090471116008));
#217500=CARTESIAN_POINT('Ctrl Pts',(5.92886364759533,58.6834178317482,2.6971895615838));
#217501=CARTESIAN_POINT('Ctrl Pts',(5.92889097525656,58.6833947425175,2.69715719432397));
#217502=CARTESIAN_POINT('Ctrl Pts',(5.92891831167211,58.6833716556052,2.69712483219063));
#217503=CARTESIAN_POINT('Ctrl Pts',(5.92894565684159,58.6833485710134,2.6970924751869));
#217504=CARTESIAN_POINT('Ctrl Pts',(5.93438921243199,58.6787531612544,2.69065122242316));
#217505=CARTESIAN_POINT('Ctrl Pts',(5.94021607194757,58.6742527563958,2.68442464469467));
#217506=CARTESIAN_POINT('Ctrl Pts',(5.94639317576856,58.6698707672383,2.6784450592362));
#217507=CARTESIAN_POINT('Ctrl Pts',(5.95865206607762,58.661174406294,2.66657815779608));
#217508=CARTESIAN_POINT('Ctrl Pts',(5.97229179622498,58.65294454852,2.65568445664214));
#217509=CARTESIAN_POINT('Ctrl Pts',(5.98706231730018,58.6453649253903,2.64601906229556));
#217510=CARTESIAN_POINT('Ctrl Pts',(5.99814020810658,58.639680208043,2.63877001653562));
#217511=CARTESIAN_POINT('Ctrl Pts',(6.0098541687325,58.6343612468746,2.63221189387641));
#217512=CARTESIAN_POINT('Ctrl Pts',(6.02209871088772,58.6294855649111,2.62645231033273));
#217513=CARTESIAN_POINT('Ctrl Pts',(6.02669041419593,58.6276571841747,2.62429246650385));
#217514=CARTESIAN_POINT('Ctrl Pts',(6.03135673055019,58.6258911397674,2.62224491711786));
#217515=CARTESIAN_POINT('Ctrl Pts',(6.03609209717129,58.6241915206272,2.62031533672638));
#217516=CARTESIAN_POINT('Ctrl Pts',(6.05266588034514,58.6182428536365,2.61356180535619));
#217517=CARTESIAN_POINT('Ctrl Pts',(6.07008552874948,58.6131078911179,2.60825339735388));
#217518=CARTESIAN_POINT('Ctrl Pts',(6.08811254303241,58.6089619925612,2.60463337987651));
#217519=CARTESIAN_POINT('Ctrl Pts',(6.09712605017387,58.6068890432829,2.60282337113783));
#217520=CARTESIAN_POINT('Ctrl Pts',(6.10629139889382,58.6050633610081,2.60143545939155));
#217521=CARTESIAN_POINT('Ctrl Pts',(6.11557877725394,58.6035068699783,2.60050005034636));
#217522=CARTESIAN_POINT('Ctrl Pts',(6.120222466434,58.6027286244634,2.60003234582377));
#217523=CARTESIAN_POINT('Ctrl Pts',(6.12489666302712,58.602017676785,2.59967776696106));
#217524=CARTESIAN_POINT('Ctrl Pts',(6.12959764057339,58.6013767677629,2.599440114292));
#217525=CARTESIAN_POINT('Ctrl Pts',(6.13429861811967,58.6007358587408,2.59920246162294));
#217526=CARTESIAN_POINT('Ctrl Pts',(6.13902637679625,58.6001649900653,2.59908173791355));
#217527=CARTESIAN_POINT('Ctrl Pts',(6.14377718965303,58.599666897865,2.59908173516065));
#217528=CARTESIAN_POINT('',(6.17403490859001,58.5964866834553,2.59908173516065));
#217529=CARTESIAN_POINT('Origin',(5.66232193761676E-15,1.85922536175558E-13,
2.59908173516024));
#217530=CARTESIAN_POINT('',(6.49374646112721,58.7519447039091,2.90134173516065));
#217531=CARTESIAN_POINT('Ctrl Pts',(6.17403490859001,58.5964866834553,2.59908173516065));
#217532=CARTESIAN_POINT('Ctrl Pts',(6.17782374318207,58.5960874772335,2.59908174371556));
#217533=CARTESIAN_POINT('Ctrl Pts',(6.18160715078386,58.5957361140453,2.59915764355931));
#217534=CARTESIAN_POINT('Ctrl Pts',(6.18538309648759,58.5954317101327,2.59930765775318));
#217535=CARTESIAN_POINT('Ctrl Pts',(6.20767599437387,58.5936345324523,2.60019333020923));
#217536=CARTESIAN_POINT('Ctrl Pts',(6.22971127560402,58.5934722580546,2.60365973324136));
#217537=CARTESIAN_POINT('Ctrl Pts',(6.25106353435283,58.5947642147754,2.60934177082444));
#217538=CARTESIAN_POINT('Ctrl Pts',(6.25904002743607,58.595246846799,2.6114643909188));
#217539=CARTESIAN_POINT('Ctrl Pts',(6.26692152735623,58.5959321585041,2.61389584429355));
#217540=CARTESIAN_POINT('Ctrl Pts',(6.27468709076422,58.596809939885,2.61661604385295));
#217541=CARTESIAN_POINT('Ctrl Pts',(6.28074617289512,58.5974948289523,2.61873848000818));
#217542=CARTESIAN_POINT('Ctrl Pts',(6.2867342495218,58.5982971695203,2.62103707099828));
#217543=CARTESIAN_POINT('Ctrl Pts',(6.2926409427142,58.5992123816358,2.62350262767693));
#217544=CARTESIAN_POINT('Ctrl Pts',(6.31331436888758,58.6024156240401,2.63213207605219));
#217545=CARTESIAN_POINT('Ctrl Pts',(6.33299084698429,58.6070015340114,2.64280685971955));
#217546=CARTESIAN_POINT('Ctrl Pts',(6.35122543337802,58.6127738370725,2.65513293646125));
#217547=CARTESIAN_POINT('Ctrl Pts',(6.36034272657489,58.615659988603,2.6612959748321));
#217548=CARTESIAN_POINT('Ctrl Pts',(6.36909954705082,58.6188427402047,2.66787183533892));
#217549=CARTESIAN_POINT('Ctrl Pts',(6.37744027742863,58.6222975626534,2.67481125953901));
#217550=CARTESIAN_POINT('Ctrl Pts',(6.38574537226666,58.6257376244688,2.6817210352412));
#217551=CARTESIAN_POINT('Ctrl Pts',(6.39363809722571,58.6294472538101,2.68899101329829));
#217552=CARTESIAN_POINT('Ctrl Pts',(6.40106302694645,58.6334027859059,2.69657334701315));
#217553=CARTESIAN_POINT('Ctrl Pts',(6.40109488586963,58.6334197583216,2.69660588132612));
#217554=CARTESIAN_POINT('Ctrl Pts',(6.40112673655769,58.6334367348722,2.6966384208142));
#217555=CARTESIAN_POINT('Ctrl Pts',(6.40115857901,58.6334537155559,2.69667096547421));
#217556=CARTESIAN_POINT('Ctrl Pts',(6.41617486746507,58.6414614796115,2.71201840158023));
#217557=CARTESIAN_POINT('Ctrl Pts',(6.42935337961508,58.65035165471,2.72845645939482));
#217558=CARTESIAN_POINT('Ctrl Pts',(6.4407364215126,58.6599343882018,2.74568723187084));
#217559=CARTESIAN_POINT('Ctrl Pts',(6.45253355607674,58.6698657226829,2.76354482594574));
#217560=CARTESIAN_POINT('Ctrl Pts',(6.46240257578854,58.6805417107313,2.78225519317451));
#217561=CARTESIAN_POINT('Ctrl Pts',(6.47034286301732,58.6917721934532,2.80151223085904));
#217562=CARTESIAN_POINT('Ctrl Pts',(6.47816982453107,58.7028423919878,2.82049442740721));
#217563=CARTESIAN_POINT('Ctrl Pts',(6.48412273326709,58.7144522959238,2.84000929089776));
#217564=CARTESIAN_POINT('Ctrl Pts',(6.48815321522661,58.7264268163221,2.85976644342199));
#217565=CARTESIAN_POINT('Ctrl Pts',(6.49096333895756,58.7347756649899,2.8735414816735));
#217566=CARTESIAN_POINT('Ctrl Pts',(6.49283796829161,58.7433019189626,2.8874343834571));
#217567=CARTESIAN_POINT('Ctrl Pts',(6.49374646112721,58.7519447039091,2.90134173516065));
#217568=CARTESIAN_POINT('',(6.53099325080036,59.1062911958298,3.47153072139114));
#217569=CARTESIAN_POINT('',(6.49374646112721,58.7519447039091,2.90134173516065));
#217570=CARTESIAN_POINT('',(12.053504764932,58.2316113004783,3.47153072139113));
#217571=CARTESIAN_POINT('Origin',(5.53234440788222E-15,1.85015204418142E-13,
3.47153072139072));
#217572=CARTESIAN_POINT('',(11.9794294790611,57.8830978693158,2.90134173516064));
#217573=CARTESIAN_POINT('',(12.053504764932,58.2316113004783,3.47153072139113));
#217574=CARTESIAN_POINT('',(12.2354540642043,57.6364522029209,2.59908173516063));
#217575=CARTESIAN_POINT('Ctrl Pts',(11.9794294790611,57.8830978693158,2.90134173516064));
#217576=CARTESIAN_POINT('Ctrl Pts',(11.9768868675913,57.8711351342684,2.88176998919826));
#217577=CARTESIAN_POINT('Ctrl Pts',(11.9762358312606,57.8588264200507,2.86226752356724));
#217578=CARTESIAN_POINT('Ctrl Pts',(11.9774374689412,57.8463495993369,2.84310370500002));
#217579=CARTESIAN_POINT('Ctrl Pts',(11.9786608125865,57.8336474016777,2.82359371788621));
#217580=CARTESIAN_POINT('Ctrl Pts',(11.9818041414838,57.8207700703892,2.80443322636944));
#217581=CARTESIAN_POINT('Ctrl Pts',(11.9868762719078,57.8078866382217,2.78589323878188));
#217582=CARTESIAN_POINT('Ctrl Pts',(11.9917336614803,57.7955486571686,2.76813818619916));
#217583=CARTESIAN_POINT('Ctrl Pts',(11.9983602045454,57.7832042421965,2.75095095198623));
#217584=CARTESIAN_POINT('Ctrl Pts',(12.0068082271151,57.7709977973487,2.73457771435019));
#217585=CARTESIAN_POINT('Ctrl Pts',(12.0135275064606,57.7612891925159,2.72155497955527));
#217586=CARTESIAN_POINT('Ctrl Pts',(12.0213998814552,57.7516676540266,2.70904711159958));
#217587=CARTESIAN_POINT('Ctrl Pts',(12.0304721974328,57.742208922712,2.69718956158378));
#217588=CARTESIAN_POINT('Ctrl Pts',(12.0304969619084,57.742183103448,2.69715719432395));
#217589=CARTESIAN_POINT('Ctrl Pts',(12.0305217353328,57.7421572855747,2.69712483219061));
#217590=CARTESIAN_POINT('Ctrl Pts',(12.0305465177057,57.7421314690942,2.69709247518689));
#217591=CARTESIAN_POINT('Ctrl Pts',(12.0354799018088,57.7369922269701,2.69065122242315));
#217592=CARTESIAN_POINT('Ctrl Pts',(12.0408044207743,57.7319074031294,2.68442464469465));
#217593=CARTESIAN_POINT('Ctrl Pts',(12.0464896431816,57.7269037357971,2.67844505923618));
#217594=CARTESIAN_POINT('Ctrl Pts',(12.0577723607613,57.7169736114626,2.66657815779606));
#217595=CARTESIAN_POINT('Ctrl Pts',(12.0704771166537,57.7073630976789,2.65568445664212));
#217596=CARTESIAN_POINT('Ctrl Pts',(12.0843744369111,57.6982810566481,2.64601906229554));
#217597=CARTESIAN_POINT('Ctrl Pts',(12.0947974271042,57.691469525875,2.6387700165356));
#217598=CARTESIAN_POINT('Ctrl Pts',(12.105891234591,57.6849552602295,2.6322118938764));
#217599=CARTESIAN_POINT('Ctrl Pts',(12.1175590523201,57.678826384587,2.62645231033272));
#217600=CARTESIAN_POINT('Ctrl Pts',(12.1219344839685,57.676528056221,2.62429246650384));
#217601=CARTESIAN_POINT('Ctrl Pts',(12.1263906358456,57.6742839235121,2.62224491711785));
#217602=CARTESIAN_POINT('Ctrl Pts',(12.130922403056,57.6720986344675,2.62031533672637));
#217603=CARTESIAN_POINT('Ctrl Pts',(12.1467835882925,57.6644501228113,2.61356180535618));
#217604=CARTESIAN_POINT('Ctrl Pts',(12.1635710602992,57.6575224410762,2.60825339735387));
#217605=CARTESIAN_POINT('Ctrl Pts',(12.1810659563067,57.6515149180854,2.6046333798765));
#217606=CARTESIAN_POINT('Ctrl Pts',(12.1898134043104,57.6485111565899,2.60282337113781));
#217607=CARTESIAN_POINT('Ctrl Pts',(12.1987377085285,57.6457374357766,2.60143545939154));
#217608=CARTESIAN_POINT('Ctrl Pts',(12.2078115120428,57.6432186759798,2.60050005034636));
#217609=CARTESIAN_POINT('Ctrl Pts',(12.2123484137999,57.6419592960813,2.60003234582376));
#217610=CARTESIAN_POINT('Ctrl Pts',(12.2169226903867,57.6407636564619,2.59967776696105));
#217611=CARTESIAN_POINT('Ctrl Pts',(12.221530922251,57.6396348724477,2.59944011429199));
#217612=CARTESIAN_POINT('Ctrl Pts',(12.2261391541152,57.6385060884335,2.59920246162293));
#217613=CARTESIAN_POINT('Ctrl Pts',(12.2307813416097,57.6374441616871,2.59908173791356));
#217614=CARTESIAN_POINT('Ctrl Pts',(12.2354540642043,57.6364522029209,2.59908173516064));
#217615=CARTESIAN_POINT('',(12.2652136052659,57.630126617196,2.59908173516063));
#217616=CARTESIAN_POINT('Origin',(5.66936586998423E-15,1.85921420526272E-13,
2.59908173516023));
#217617=CARTESIAN_POINT('',(12.599423532447,57.7513140650722,2.90134173516063));
#217618=CARTESIAN_POINT('Ctrl Pts',(12.2652136052659,57.630126617196,2.59908173516064));
#217619=CARTESIAN_POINT('Ctrl Pts',(12.2689399558127,57.6293335568101,2.59908174371554));
#217620=CARTESIAN_POINT('Ctrl Pts',(12.2726659100577,57.6285886446437,2.59915764355929));
#217621=CARTESIAN_POINT('Ctrl Pts',(12.2763893518626,57.6278912144858,2.59930765775316));
#217622=CARTESIAN_POINT('Ctrl Pts',(12.2983722707008,57.623773639575,2.60019333020922));
#217623=CARTESIAN_POINT('Ctrl Pts',(12.3202698780615,57.6213089400487,2.60365973324141));
#217624=CARTESIAN_POINT('Ctrl Pts',(12.3416402131536,57.6203619005011,2.60934177082459));
#217625=CARTESIAN_POINT('Ctrl Pts',(12.3496234589567,57.6200081180517,2.61146439091891));
#217626=CARTESIAN_POINT('Ctrl Pts',(12.3575334177749,57.6198658344727,2.6138958442936));
#217627=CARTESIAN_POINT('Ctrl Pts',(12.3653481937526,57.6199270848659,2.61661604385293));
#217628=CARTESIAN_POINT('Ctrl Pts',(12.3714456739993,57.6199748754953,2.61873848000816));
#217629=CARTESIAN_POINT('Ctrl Pts',(12.3774848147423,57.62014689631,2.62103707099827));
#217630=CARTESIAN_POINT('Ctrl Pts',(12.3834548161673,57.6204396772354,2.62350262767692));
#217631=CARTESIAN_POINT('Ctrl Pts',(12.404349821155,57.6214644104742,2.63213207605218));
#217632=CARTESIAN_POINT('Ctrl Pts',(12.4243978675679,57.6239684463329,2.64280685971954));
#217633=CARTESIAN_POINT('Ctrl Pts',(12.443135932958,57.6278030948198,2.65513293646124));
#217634=CARTESIAN_POINT('Ctrl Pts',(12.452504965653,57.6297204190633,2.66129597483208));
#217635=CARTESIAN_POINT('Ctrl Pts',(12.461546503484,57.6319703982312,2.66787183533892));
#217636=CARTESIAN_POINT('Ctrl Pts',(12.4702026697495,57.6345344510721,2.67481125953901));
#217637=CARTESIAN_POINT('Ctrl Pts',(12.4788218527842,57.6370875490683,2.6817210352412));
#217638=CARTESIAN_POINT('Ctrl Pts',(12.4870591024244,57.6399518422609,2.68899101329827));
#217639=CARTESIAN_POINT('Ctrl Pts',(12.4948568232946,57.6431095890445,2.69657334701313));
#217640=CARTESIAN_POINT('Ctrl Pts',(12.4948902817918,57.6431231383191,2.6966058813261));
#217641=CARTESIAN_POINT('Ctrl Pts',(12.4949237325312,57.643136692567,2.69663842081419));
#217642=CARTESIAN_POINT('Ctrl Pts',(12.494957175512,57.6431502517861,2.69667096547419));
#217643=CARTESIAN_POINT('Ctrl Pts',(12.5107282424387,57.6495445189161,2.7120184015802));
#217644=CARTESIAN_POINT('Ctrl Pts',(12.5247638376615,57.657008463082,2.72845645939476));
#217645=CARTESIAN_POINT('Ctrl Pts',(12.5370861904703,57.6653488494803,2.74568723187076));
#217646=CARTESIAN_POINT('Ctrl Pts',(12.5498568062284,57.6739926427249,2.76354482594561));
#217647=CARTESIAN_POINT('Ctrl Pts',(12.5607877070422,57.6835785531293,2.7822551931743));
#217648=CARTESIAN_POINT('Ctrl Pts',(12.5698584016474,57.6939175280698,2.80151223085877));
#217649=CARTESIAN_POINT('Ctrl Pts',(12.5787996370878,57.7041089426393,2.8204944274068));
#217650=CARTESIAN_POINT('Ctrl Pts',(12.585933500584,57.7150329979046,2.84000929089722));
#217651=CARTESIAN_POINT('Ctrl Pts',(12.5911935813573,57.7265206205418,2.85976644342131));
#217652=CARTESIAN_POINT('Ctrl Pts',(12.5948610032578,57.7345299954279,2.87354148167304));
#217653=CARTESIAN_POINT('Ctrl Pts',(12.5976165994014,57.7428135895658,2.88743438345685));
#217654=CARTESIAN_POINT('Ctrl Pts',(12.599423532447,57.7513140650722,2.90134173516062));
#217655=CARTESIAN_POINT('',(12.6735055745739,58.0998260601482,3.47153072139113));
#217656=CARTESIAN_POINT('',(12.599423532447,57.7513140650722,2.90134173516063));
#217657=CARTESIAN_POINT('',(18.074335247489,56.6526781108326,3.47153072139111));
#217658=CARTESIAN_POINT('Origin',(5.53234440788222E-15,1.85015204418142E-13,
3.47153072139072));
#217659=CARTESIAN_POINT('',(17.9642361803971,56.3138168485097,2.90134173516062));
#217660=CARTESIAN_POINT('',(18.074335247489,56.6526781108326,3.47153072139112));
#217661=CARTESIAN_POINT('',(18.1930767435948,56.0417604764385,2.59908173516062));
#217662=CARTESIAN_POINT('Ctrl Pts',(17.9642361803971,56.3138168485097,2.90134173516062));
#217663=CARTESIAN_POINT('Ctrl Pts',(17.9604570513084,56.3021854218465,2.8817699891988));
#217664=CARTESIAN_POINT('Ctrl Pts',(17.9585229704411,56.2900121878806,2.86226752356833));
#217665=CARTESIAN_POINT('Ctrl Pts',(17.9584138425289,56.2774781111564,2.84310370500163));
#217666=CARTESIAN_POINT('Ctrl Pts',(17.9583027433682,56.2647176232342,2.82359371788858));
#217667=CARTESIAN_POINT('Ctrl Pts',(17.9600828051301,56.2515822679753,2.80443322637254));
#217668=CARTESIAN_POINT('Ctrl Pts',(17.9637804645263,56.2382392305991,2.78589323878563));
#217669=CARTESIAN_POINT('Ctrl Pts',(17.9673215746107,56.2254611028304,2.76813818620392));
#217670=CARTESIAN_POINT('Ctrl Pts',(17.9726214740518,56.2124916494927,2.7509509519919));
#217671=CARTESIAN_POINT('Ctrl Pts',(17.979747296547,56.1994690140109,2.73457771435663));
#217672=CARTESIAN_POINT('Ctrl Pts',(17.9854149414341,56.1891112379853,2.7215549795594));
#217673=CARTESIAN_POINT('Ctrl Pts',(17.9922384661031,56.1787195200284,2.70904711160154));
#217674=CARTESIAN_POINT('Ctrl Pts',(18.0002723763371,56.1683642893845,2.69718956158378));
#217675=CARTESIAN_POINT('Ctrl Pts',(18.0002943063023,56.1683360229685,2.69715719432395));
#217676=CARTESIAN_POINT('Ctrl Pts',(18.0003162453126,56.1683077570003,2.6971248321906));
#217677=CARTESIAN_POINT('Ctrl Pts',(18.000338193368,56.1682794914818,2.69709247518688));
#217678=CARTESIAN_POINT('Ctrl Pts',(18.0047073547953,56.1626527236047,2.69065122242314));
#217679=CARTESIAN_POINT('Ctrl Pts',(18.0094711966667,56.157039191176,2.68442464469463));
#217680=CARTESIAN_POINT('Ctrl Pts',(18.0146022491738,56.1514686668953,2.67844505923616));
#217681=CARTESIAN_POINT('Ctrl Pts',(18.0247851782094,56.1404135756909,2.66657815779605));
#217682=CARTESIAN_POINT('Ctrl Pts',(18.0364157638827,56.1295277006976,2.65568445664212));
#217683=CARTESIAN_POINT('Ctrl Pts',(18.0492876213733,56.1190427465078,2.64601906229553));
#217684=CARTESIAN_POINT('Ctrl Pts',(18.0589415144913,56.1111790308655,2.63877001653559));
#217685=CARTESIAN_POINT('Ctrl Pts',(18.0692936227627,56.1035408324003,2.63221189387639));
#217686=CARTESIAN_POINT('Ctrl Pts',(18.080256881013,56.0962259123229,2.62645231033271));
#217687=CARTESIAN_POINT('Ctrl Pts',(18.0843681028569,56.0934828172939,2.62429246650383));
#217688=CARTESIAN_POINT('Ctrl Pts',(18.0885652677243,56.090785183471,2.62224491711783));
#217689=CARTESIAN_POINT('Ctrl Pts',(18.0928437845341,56.088138167006,2.62031533672635));
#217690=CARTESIAN_POINT('Ctrl Pts',(18.1078185933686,56.0788736093786,2.61356180535616));
#217691=CARTESIAN_POINT('Ctrl Pts',(18.1237899619214,56.0702291095579,2.60825339735387));
#217692=CARTESIAN_POINT('Ctrl Pts',(18.1405610619117,56.0624257818119,2.6046333798765));
#217693=CARTESIAN_POINT('Ctrl Pts',(18.1489466119069,56.0585241179389,2.60282337113782));
#217694=CARTESIAN_POINT('Ctrl Pts',(18.1575320950786,56.0548327480527,2.60143545939154));
#217695=CARTESIAN_POINT('Ctrl Pts',(18.1662929092569,56.0513793155482,2.60050005034635));
#217696=CARTESIAN_POINT('Ctrl Pts',(18.170673316346,56.049652599296,2.60003234582376));
#217697=CARTESIAN_POINT('Ctrl Pts',(18.1750975561951,56.0479853674133,2.59967776696105));
#217698=CARTESIAN_POINT('Ctrl Pts',(18.1795625536246,56.0463810756009,2.59944011429199));
#217699=CARTESIAN_POINT('Ctrl Pts',(18.1840275510541,56.0447767837885,2.59920246162293));
#217700=CARTESIAN_POINT('Ctrl Pts',(18.1885333065889,56.043235433663,2.59908173791354));
#217701=CARTESIAN_POINT('Ctrl Pts',(18.1930767435948,56.0417604764385,2.59908173516063));
#217702=CARTESIAN_POINT('',(18.2220120550216,56.0323588238393,2.59908173516062));
#217703=CARTESIAN_POINT('Origin',(5.6762545978478E-15,1.85919574697204E-13,
2.59908173516023));
#217704=CARTESIAN_POINT('',(18.5670586829464,56.117947944099,2.90134173516062));
#217705=CARTESIAN_POINT('Ctrl Pts',(18.2220120550216,56.0323588238393,2.59908173516063));
#217706=CARTESIAN_POINT('Ctrl Pts',(18.2256350948468,56.031180598225,2.59908174371555));
#217707=CARTESIAN_POINT('Ctrl Pts',(18.2292627734005,56.030050298494,2.59915764355929));
#217708=CARTESIAN_POINT('Ctrl Pts',(18.232892916499,56.0289674832815,2.59930765775315));
#217709=CARTESIAN_POINT('Ctrl Pts',(18.2543250068308,56.0225746241523,2.60019333020925));
#217710=CARTESIAN_POINT('Ctrl Pts',(18.2758450255544,56.0178345032611,2.60365973324173));
#217711=CARTESIAN_POINT('Ctrl Pts',(18.2969992991273,56.0146588434085,2.60934177082538));
#217712=CARTESIAN_POINT('Ctrl Pts',(18.3049018315378,56.0134725226009,2.61146439091951));
#217713=CARTESIAN_POINT('Ctrl Pts',(18.312753586089,56.0125042026267,2.61389584429393));
#217714=CARTESIAN_POINT('Ctrl Pts',(18.3205319543147,56.0117482509602,2.61661604385292));
#217715=CARTESIAN_POINT('Ctrl Pts',(18.3266010274077,56.0111584195475,2.61873848000815));
#217716=CARTESIAN_POINT('Ctrl Pts',(18.3326250661772,56.0106982359128,2.62103707099826));
#217717=CARTESIAN_POINT('Ctrl Pts',(18.3385929672501,56.010365377879,2.62350262767691));
#217718=CARTESIAN_POINT('Ctrl Pts',(18.3594806210049,56.0092003747606,2.63213207605218));
#217719=CARTESIAN_POINT('Ctrl Pts',(18.3796805851421,56.0095951017658,2.64280685971953));
#217720=CARTESIAN_POINT('Ctrl Pts',(18.3987168313629,56.0114500824672,2.65513293646122));
#217721=CARTESIAN_POINT('Ctrl Pts',(18.4082349544733,56.012377572818,2.66129597483207));
#217722=CARTESIAN_POINT('Ctrl Pts',(18.4174621486788,56.0136701283095,2.6678718353389));
#217723=CARTESIAN_POINT('Ctrl Pts',(18.426338912063,56.0153153192432,2.67481125953899));
#217724=CARTESIAN_POINT('Ctrl Pts',(18.4351777497213,56.0169534811442,2.68172103524118));
#217725=CARTESIAN_POINT('Ctrl Pts',(18.4436692750119,56.0189410563925,2.68899101329826));
#217726=CARTESIAN_POINT('Ctrl Pts',(18.4517543535699,56.0212664209292,2.69657334701312));
#217727=CARTESIAN_POINT('Ctrl Pts',(18.4517890450628,56.0212763986143,2.69660588132609));
#217728=CARTESIAN_POINT('Ctrl Pts',(18.4518237293603,56.0212863820561,2.69663842081418));
#217729=CARTESIAN_POINT('Ctrl Pts',(18.4518584064613,56.0212963712531,2.69667096547418));
#217730=CARTESIAN_POINT('Ctrl Pts',(18.4682114607491,56.0260070845285,2.71201840157933));
#217731=CARTESIAN_POINT('Ctrl Pts',(18.4829503621255,56.0319630212272,2.72845645939292));
#217732=CARTESIAN_POINT('Ctrl Pts',(18.496077019569,56.0389696815127,2.74568723186786));
#217733=CARTESIAN_POINT('Ctrl Pts',(18.5096811989819,56.0462312303128,2.76354482594163));
#217734=CARTESIAN_POINT('Ctrl Pts',(18.5215542196605,56.0546220378322,2.78225519316918));
#217735=CARTESIAN_POINT('Ctrl Pts',(18.5316559412137,56.0639562290176,2.80151223085247));
#217736=CARTESIAN_POINT('Ctrl Pts',(18.5416134885343,56.0731572003508,2.82049442739942));
#217737=CARTESIAN_POINT('Ctrl Pts',(18.5498501466894,56.0832757207091,2.84000929088874));
#217738=CARTESIAN_POINT('Ctrl Pts',(18.5562821957309,56.0941505847868,2.85976644341176));
#217739=CARTESIAN_POINT('Ctrl Pts',(18.5607667347605,56.1017327335055,2.87354148166662));
#217740=CARTESIAN_POINT('Ctrl Pts',(18.5643731068268,56.1096829110195,2.88743438345364));
#217741=CARTESIAN_POINT('Ctrl Pts',(18.5670586829464,56.117947944099,2.90134173516062));
#217742=CARTESIAN_POINT('',(18.6771643191709,56.4568070719813,3.47153072139112));
#217743=CARTESIAN_POINT('',(18.5670586829464,56.117947944099,2.90134173516062));
#217744=CARTESIAN_POINT('',(23.8971395307767,54.4530463244695,3.4715307213911));
#217745=CARTESIAN_POINT('Origin',(5.53234440788222E-15,1.85015204418142E-13,
3.47153072139072));
#217746=CARTESIAN_POINT('',(23.7522229508827,54.1275498658876,2.90134173516061));
#217747=CARTESIAN_POINT('',(23.8971395307767,54.4530463244695,3.4715307213911));
#217748=CARTESIAN_POINT('',(23.9513722670364,53.833063494684,2.59908173516061));
#217749=CARTESIAN_POINT('Ctrl Pts',(23.7522229508827,54.1275498658876,2.90134173516061));
#217750=CARTESIAN_POINT('Ctrl Pts',(23.7472487091033,54.1163771839518,2.88176998919702));
#217751=CARTESIAN_POINT('Ctrl Pts',(23.7440527738937,54.1044728027351,2.8622675235648));
#217752=CARTESIAN_POINT('Ctrl Pts',(23.7426340760174,54.0920187959664,2.84310370499643));
#217753=CARTESIAN_POINT('Ctrl Pts',(23.7411897512766,54.0793398243554,2.8235937178816));
#217754=CARTESIAN_POINT('Ctrl Pts',(23.7415870431748,54.0660903588251,2.80443322636387));
#217755=CARTESIAN_POINT('Ctrl Pts',(23.7438697192146,54.0524339053479,2.78589323877544));
#217756=CARTESIAN_POINT('Ctrl Pts',(23.7460557526692,54.0393556307033,2.76813818619217));
#217757=CARTESIAN_POINT('Ctrl Pts',(23.749970941681,54.0259032350424,2.75095095197874));
#217758=CARTESIAN_POINT('Ctrl Pts',(23.7556964921022,54.0122070876439,2.73457771434232));
#217759=CARTESIAN_POINT('Ctrl Pts',(23.7602504066259,54.0013136223926,2.72155497955023));
#217760=CARTESIAN_POINT('Ctrl Pts',(23.7659503210024,53.9902655788103,2.70904711159718));
#217761=CARTESIAN_POINT('Ctrl Pts',(23.772857804287,53.9791273029166,2.69718956158376));
#217762=CARTESIAN_POINT('Ctrl Pts',(23.7728766594726,53.9790968990415,2.69715719432393));
#217763=CARTESIAN_POINT('Ctrl Pts',(23.7728955237005,53.9790664946661,2.69712483219059));
#217764=CARTESIAN_POINT('Ctrl Pts',(23.7729143969709,53.9790360897926,2.69709247518687));
#217765=CARTESIAN_POINT('Ctrl Pts',(23.7766714662753,53.9729834442089,2.69065122242313));
#217766=CARTESIAN_POINT('Ctrl Pts',(23.7808224374043,53.9669027062281,2.68442464469463));
#217767=CARTESIAN_POINT('Ctrl Pts',(23.7853431031263,53.9608263568288,2.67844505923616));
#217768=CARTESIAN_POINT('Ctrl Pts',(23.7943146773162,53.948767420647,2.66657815779604));
#217769=CARTESIAN_POINT('Ctrl Pts',(23.8047436656399,53.9367254523687,2.6556844566421));
#217770=CARTESIAN_POINT('Ctrl Pts',(23.8164490335996,53.9249524603721,2.64601906229552));
#217771=CARTESIAN_POINT('Ctrl Pts',(23.8252280595693,53.9161227163746,2.63877001653558));
#217772=CARTESIAN_POINT('Ctrl Pts',(23.8347250487607,53.9074442707907,2.63221189387639));
#217773=CARTESIAN_POINT('Ctrl Pts',(23.8448636317806,53.8990234500736,2.62645231033271));
#217774=CARTESIAN_POINT('Ctrl Pts',(23.848665600413,53.8958656423046,2.62429246650383));
#217775=CARTESIAN_POINT('Ctrl Pts',(23.8525577932542,53.8927440632084,2.62224491711782));
#217776=CARTESIAN_POINT('Ctrl Pts',(23.8565361833379,53.8896643205894,2.62031533672634));
#217777=CARTESIAN_POINT('Ctrl Pts',(23.8704605486311,53.8788852214228,2.61356180535615));
#217778=CARTESIAN_POINT('Ctrl Pts',(23.8854408280738,53.8686186144655,2.60825339735384));
#217779=CARTESIAN_POINT('Ctrl Pts',(23.901304384366,53.859104976856,2.60463337987647));
#217780=CARTESIAN_POINT('Ctrl Pts',(23.9092361625121,53.8543481580513,2.60282337113779));
#217781=CARTESIAN_POINT('Ctrl Pts',(23.9173887602871,53.8497795825133,2.60143545939151));
#217782=CARTESIAN_POINT('Ctrl Pts',(23.9257405998159,53.8454293138304,2.60050005034632));
#217783=CARTESIAN_POINT('Ctrl Pts',(23.9299165195804,53.8432541794889,2.60003234582373));
#217784=CARTESIAN_POINT('Ctrl Pts',(23.934142249794,53.8411336218844,2.59967776696103));
#217785=CARTESIAN_POINT('Ctrl Pts',(23.9384150933427,53.8390713992306,2.59944011429197));
#217786=CARTESIAN_POINT('Ctrl Pts',(23.9426879368913,53.8370091765768,2.59920246162291));
#217787=CARTESIAN_POINT('Ctrl Pts',(23.9470078944659,53.8350052904266,2.59908173791346));
#217788=CARTESIAN_POINT('Ctrl Pts',(23.9513722670364,53.833063494684,2.59908173516062));
#217789=CARTESIAN_POINT('',(23.9791663275012,53.8206887816839,2.59908173516061));
#217790=CARTESIAN_POINT('Origin',(5.68291264686342E-15,1.85917018911644E-13,
2.59908173516024));
#217791=CARTESIAN_POINT('',(24.3312692531087,53.8697418420147,2.90134173516062));
#217792=CARTESIAN_POINT('Ctrl Pts',(23.9791663275012,53.8206887816838,2.59908173516062));
#217793=CARTESIAN_POINT('Ctrl Pts',(23.9826463618224,53.8191382997274,2.59908174371552));
#217794=CARTESIAN_POINT('Ctrl Pts',(23.9861360190795,53.8176349962321,2.59915764355927));
#217795=CARTESIAN_POINT('Ctrl Pts',(23.9896330908641,53.8161786595151,2.59930765775314));
#217796=CARTESIAN_POINT('Ctrl Pts',(24.0102795382193,53.8075805576712,2.60019333020912));
#217797=CARTESIAN_POINT('Ctrl Pts',(24.0311861904735,53.8006169491722,2.60365973324083));
#217798=CARTESIAN_POINT('Ctrl Pts',(24.0518926318755,53.7952474622088,2.60934177082319));
#217799=CARTESIAN_POINT('Ctrl Pts',(24.0596278690982,53.7932416006211,2.61146439091783));
#217800=CARTESIAN_POINT('Ctrl Pts',(24.0673353939203,53.7914578533671,2.61389584429299));
#217801=CARTESIAN_POINT('Ctrl Pts',(24.0749921329676,53.789892982005,2.6166160438529));
#217802=CARTESIAN_POINT('Ctrl Pts',(24.0809663048721,53.7886719908667,2.61873848000813));
#217803=CARTESIAN_POINT('Ctrl Pts',(24.0869092410387,53.7875846446509,2.62103707099824));
#217804=CARTESIAN_POINT('Ctrl Pts',(24.0928096561863,53.7866297945201,2.62350262767689));
#217805=CARTESIAN_POINT('Ctrl Pts',(24.1134611092026,53.7832878190624,2.63213207605215));
#217806=CARTESIAN_POINT('Ctrl Pts',(24.1335916760301,53.7815689125025,2.64280685971951));
#217807=CARTESIAN_POINT('Ctrl Pts',(24.1527175379843,53.7814239018617,2.65513293646121));
#217808=CARTESIAN_POINT('Ctrl Pts',(24.1622804689615,53.7813513965413,2.66129597483206));
#217809=CARTESIAN_POINT('Ctrl Pts',(24.1715922244709,53.781672366848,2.66787183533889));
#217810=CARTESIAN_POINT('Ctrl Pts',(24.1805923292966,53.7823806708183,2.67481125953899));
#217811=CARTESIAN_POINT('Ctrl Pts',(24.1895539814234,53.7830859485795,2.68172103524117));
#217812=CARTESIAN_POINT('Ctrl Pts',(24.1982067474363,53.7841750295933,2.68899101329827));
#217813=CARTESIAN_POINT('Ctrl Pts',(24.2064906018697,53.7856425347027,2.69657334701313));
#217814=CARTESIAN_POINT('Ctrl Pts',(24.206526146271,53.7856488314805,2.6966058813261));
#217815=CARTESIAN_POINT('Ctrl Pts',(24.2065616841181,53.7856551347357,2.69663842081418));
#217816=CARTESIAN_POINT('Ctrl Pts',(24.2065972154097,53.7856614444667,2.69667096547419));
#217817=CARTESIAN_POINT('Ctrl Pts',(24.2233530895743,53.7886369923274,2.71201840157898));
#217818=CARTESIAN_POINT('Ctrl Pts',(24.2386338146169,53.7930196670704,2.72845645939216));
#217819=CARTESIAN_POINT('Ctrl Pts',(24.2524209582896,53.7986158348071,2.74568723186666));
#217820=CARTESIAN_POINT('Ctrl Pts',(24.2667096511209,53.8044155801148,2.76354482593984));
#217821=CARTESIAN_POINT('Ctrl Pts',(24.2793947083652,53.8115193533064,2.78225519316674));
#217822=CARTESIAN_POINT('Ctrl Pts',(24.2904167802911,53.8197464933851,2.80151223084937));
#217823=CARTESIAN_POINT('Ctrl Pts',(24.3012815425194,53.8278562137149,2.82049442739556));
#217824=CARTESIAN_POINT('Ctrl Pts',(24.3105307527829,53.8370583385401,2.84000929088409));
#217825=CARTESIAN_POINT('Ctrl Pts',(24.318064299217,53.847201296772,2.85976644340634));
#217826=CARTESIAN_POINT('Ctrl Pts',(24.3233168218273,53.8542731477143,2.87354148166297));
#217827=CARTESIAN_POINT('Ctrl Pts',(24.3277344576489,53.8618028047949,2.88743438345181));
#217828=CARTESIAN_POINT('Ctrl Pts',(24.3312692531087,53.8697418420148,2.90134173516062));
#217829=CARTESIAN_POINT('',(24.4761921430391,54.1952354911874,3.4715307213911));
#217830=CARTESIAN_POINT('',(24.3312692531087,53.8697418420147,2.90134173516061));
#217831=CARTESIAN_POINT('',(29.4581217525673,51.656815567543,3.47153072139109));
#217832=CARTESIAN_POINT('Origin',(5.53234440788222E-15,1.85015204418142E-13,
3.47153072139072));
#217833=CARTESIAN_POINT('',(29.2799753962461,51.3482501200168,2.90134173516058));
#217834=CARTESIAN_POINT('',(29.4581217525673,51.656815567543,3.47153072139109));
#217835=CARTESIAN_POINT('',(29.4472515437734,51.0345602039889,2.59908173516059));
#217836=CARTESIAN_POINT('Ctrl Pts',(29.2799753962461,51.3482501200168,2.90134173516059));
#217837=CARTESIAN_POINT('Ctrl Pts',(29.2738605406109,51.337658593052,2.88176998919915));
#217838=CARTESIAN_POINT('Ctrl Pts',(29.2694377663943,51.3261534914787,2.86226752356906));
#217839=CARTESIAN_POINT('Ctrl Pts',(29.2667250421043,51.3139160033725,2.84310370500273));
#217840=CARTESIAN_POINT('Ctrl Pts',(29.2639633161072,51.3014574615418,2.8235937178899));
#217841=CARTESIAN_POINT('Ctrl Pts',(29.2629734853273,51.2882390496599,2.80443322637407));
#217842=CARTESIAN_POINT('Ctrl Pts',(29.2638161685324,51.274418803047,2.78589323878736));
#217843=CARTESIAN_POINT('Ctrl Pts',(29.2646231747155,51.2611836698432,2.76813818620555));
#217844=CARTESIAN_POINT('Ctrl Pts',(29.2671107576654,51.2473957191241,2.75095095199344));
#217845=CARTESIAN_POINT('Ctrl Pts',(29.2713733056804,51.2331761176688,2.73457771435808));
#217846=CARTESIAN_POINT('Ctrl Pts',(29.274763596202,51.2218663142685,2.72155497956031));
#217847=CARTESIAN_POINT('Ctrl Pts',(29.2792774508348,51.2102829897298,2.70904711160195));
#217848=CARTESIAN_POINT('Ctrl Pts',(29.2849828273429,51.1984837018593,2.69718956158373));
#217849=CARTESIAN_POINT('Ctrl Pts',(29.2849984011674,51.1984514936362,2.69715719432391));
#217850=CARTESIAN_POINT('Ctrl Pts',(29.2850139839325,51.1984192839705,2.69712483219057));
#217851=CARTESIAN_POINT('Ctrl Pts',(29.2850295756385,51.1983870728641,2.69709247518685));
#217852=CARTESIAN_POINT('Ctrl Pts',(29.2881333895826,51.1919748636255,2.69065122242311));
#217853=CARTESIAN_POINT('Ctrl Pts',(29.2916260110607,51.1854935419304,2.68442464469461));
#217854=CARTESIAN_POINT('Ctrl Pts',(29.2954867606378,51.178977941168,2.67844505923613));
#217855=CARTESIAN_POINT('Ctrl Pts',(29.3031486855379,51.1660472802372,2.66657815779602));
#217856=CARTESIAN_POINT('Ctrl Pts',(29.3122618143336,51.1529811529981,2.65568445664209));
#217857=CARTESIAN_POINT('Ctrl Pts',(29.3226724463013,51.1400491105587,2.6460190622955));
#217858=CARTESIAN_POINT('Ctrl Pts',(29.330480420277,51.1303500787291,2.63877001653556));
#217859=CARTESIAN_POINT('Ctrl Pts',(29.3390182393876,51.1207264688923,2.63221189387636));
#217860=CARTESIAN_POINT('Ctrl Pts',(29.3482210667398,51.1112920078094,2.62645231033268));
#217861=CARTESIAN_POINT('Ctrl Pts',(29.3516721269969,51.1077540849033,2.6242924665038));
#217862=CARTESIAN_POINT('Ctrl Pts',(29.3552167041325,51.1042427612075,2.6222449171178));
#217863=CARTESIAN_POINT('Ctrl Pts',(29.3588513794159,51.1007640347391,2.62031533672632));
#217864=CARTESIAN_POINT('Ctrl Pts',(29.3715727429078,51.0885884920995,2.61356180535613));
#217865=CARTESIAN_POINT('Ctrl Pts',(29.3853978061641,51.0768122610999,2.60825339735383));
#217866=CARTESIAN_POINT('Ctrl Pts',(29.4001800143157,51.0656925470315,2.60463337987646));
#217867=CARTESIAN_POINT('Ctrl Pts',(29.4075711183915,51.0601326899973,2.60282337113778));
#217868=CARTESIAN_POINT('Ctrl Pts',(29.4152015092025,51.054736963077,2.60143545939149));
#217869=CARTESIAN_POINT('Ctrl Pts',(29.4230528695803,51.0495375206697,2.60050005034631));
#217870=CARTESIAN_POINT('Ctrl Pts',(29.4269785497693,51.046937799466,2.60003234582371));
#217871=CARTESIAN_POINT('Ctrl Pts',(29.430959472363,51.0443871494125,2.59967776696101));
#217872=CARTESIAN_POINT('Ctrl Pts',(29.4349933478627,51.0418895900603,2.59944011429195));
#217873=CARTESIAN_POINT('Ctrl Pts',(29.4390272233624,51.0393920307081,2.59920246162289));
#217874=CARTESIAN_POINT('Ctrl Pts',(29.4431140526175,51.0369475635292,2.59908173791351));
#217875=CARTESIAN_POINT('Ctrl Pts',(29.4472515437734,51.0345602039889,2.59908173516059));
#217876=CARTESIAN_POINT('',(29.4735998357337,51.019348010533,2.59908173516059));
#217877=CARTESIAN_POINT('Origin',(5.68926707005281E-15,1.85913781171312E-13,
2.59908173516024));
#217878=CARTESIAN_POINT('',(29.8289013456884,51.0313275753411,2.90134173516059));
#217879=CARTESIAN_POINT('Ctrl Pts',(29.4735998357337,51.019348010533,2.59908173516059));
#217880=CARTESIAN_POINT('Ctrl Pts',(29.4768987365664,51.0174422596393,2.59908174371551));
#217881=CARTESIAN_POINT('Ctrl Pts',(29.4802121391118,51.0155824228874,2.59915764355925));
#217882=CARTESIAN_POINT('Ctrl Pts',(29.4835378249322,51.0137685205957,2.59930765775312));
#217883=CARTESIAN_POINT('Ctrl Pts',(29.5031724225188,51.0030593786377,2.60019333020924));
#217884=CARTESIAN_POINT('Ctrl Pts',(29.5232366506524,50.9939485772814,2.60365973324187));
#217885=CARTESIAN_POINT('Ctrl Pts',(29.543268395784,50.9864440924292,2.60934177082577));
#217886=CARTESIAN_POINT('Ctrl Pts',(29.5507515889356,50.9836406667026,2.6114643909198));
#217887=CARTESIAN_POINT('Ctrl Pts',(29.5582304387678,50.9810610352786,2.61389584429407));
#217888=CARTESIAN_POINT('Ctrl Pts',(29.5656816597958,50.9787043892803,2.61661604385287));
#217889=CARTESIAN_POINT('Ctrl Pts',(29.571495476234,50.9768656158507,2.6187384800081));
#217890=CARTESIAN_POINT('Ctrl Pts',(29.5772921977456,50.9751630202464,2.62103707099821));
#217891=CARTESIAN_POINT('Ctrl Pts',(29.5830604807848,50.9735966395565,2.62350262767686));
#217892=CARTESIAN_POINT('Ctrl Pts',(29.6032494714218,50.968114307142,2.63213207605213));
#217893=CARTESIAN_POINT('Ctrl Pts',(29.6230900862367,50.9643005997169,2.64280685971949));
#217894=CARTESIAN_POINT('Ctrl Pts',(29.6420960169785,50.9621571865008,2.65513293646119));
#217895=CARTESIAN_POINT('Ctrl Pts',(29.6515989823495,50.9610854798928,2.66129597483204));
#217896=CARTESIAN_POINT('Ctrl Pts',(29.6608932776209,50.9604313483969,2.66787183533886));
#217897=CARTESIAN_POINT('Ctrl Pts',(29.6699181168562,50.9601950050772,2.67481125953896));
#217898=CARTESIAN_POINT('Ctrl Pts',(29.6789043977155,50.9599596715279,2.68172103524114));
#217899=CARTESIAN_POINT('Ctrl Pts',(29.6876236029356,50.9601383261076,2.68899101329823));
#217900=CARTESIAN_POINT('Ctrl Pts',(29.6960154736015,50.9607318934966,2.69657334701309));
#217901=CARTESIAN_POINT('Ctrl Pts',(29.6960514814794,50.9607344403783,2.69660588132607));
#217902=CARTESIAN_POINT('Ctrl Pts',(29.6960874835161,50.9607369943871,2.69663842081415));
#217903=CARTESIAN_POINT('Ctrl Pts',(29.69612347971,50.9607395555214,2.69667096547416));
#217904=CARTESIAN_POINT('Ctrl Pts',(29.7130985928877,50.9619473372424,2.71201840157874));
#217905=CARTESIAN_POINT('Ctrl Pts',(29.7287537227754,50.9647087325283,2.72845645939168));
#217906=CARTESIAN_POINT('Ctrl Pts',(29.7430502978459,50.9688330949316,2.74568723186593));
#217907=CARTESIAN_POINT('Ctrl Pts',(29.7578669541872,50.9731074935238,2.76354482593901));
#217908=CARTESIAN_POINT('Ctrl Pts',(29.7712250678558,50.9788464019624,2.78225519316582));
#217909=CARTESIAN_POINT('Ctrl Pts',(29.7830467300279,50.9858763526664,2.80151223084835));
#217910=CARTESIAN_POINT('Ctrl Pts',(29.7946996705556,50.9928059702003,2.82049442739468));
#217911=CARTESIAN_POINT('Ctrl Pts',(29.8048600966444,51.0009908790876,2.84000929088337));
#217912=CARTESIAN_POINT('Ctrl Pts',(29.81341260136,51.0102908031014,2.85976644340578));
#217913=CARTESIAN_POINT('Ctrl Pts',(29.8193755598134,51.0167748755875,2.87354148166258));
#217914=CARTESIAN_POINT('Ctrl Pts',(29.8245560588475,51.0238015157352,2.8874343834516));
#217915=CARTESIAN_POINT('Ctrl Pts',(29.8289013456884,51.0313275753411,2.90134173516059));
#217916=CARTESIAN_POINT('',(30.0070536838157,51.3398895692699,3.47153072139108));
#217917=CARTESIAN_POINT('',(29.8289013456884,51.0313275753411,2.90134173516059));
#217918=CARTESIAN_POINT('',(34.6963546279284,48.2946219293749,3.47153072139107));
#217919=CARTESIAN_POINT('Origin',(5.53234440788222E-15,1.85015204418142E-13,
3.47153072139072));
#217920=CARTESIAN_POINT('',(34.4869303039396,48.006368200519,2.90134173516058));
#217921=CARTESIAN_POINT('',(34.6963546279284,48.2946219293749,3.47153072139107));
#217922=CARTESIAN_POINT('',(34.6205005703634,47.6769115920306,2.59908173516057));
#217923=CARTESIAN_POINT('Ctrl Pts',(34.4869303039396,48.006368200519,2.90134173516058));
#217924=CARTESIAN_POINT('Ctrl Pts',(34.4797418300859,47.9964738715098,2.88176998919899));
#217925=CARTESIAN_POINT('Ctrl Pts',(34.4741406737019,47.9854941018789,2.86226752356877));
#217926=CARTESIAN_POINT('Ctrl Pts',(34.4701636441734,47.9736072089142,2.84310370500229));
#217927=CARTESIAN_POINT('Ctrl Pts',(34.466114774968,47.9615055952534,2.82359371788922));
#217928=CARTESIAN_POINT('Ctrl Pts',(34.4637486663039,47.948463060705,2.80443322637314));
#217929=CARTESIAN_POINT('Ctrl Pts',(34.4631421240619,47.9346304384684,2.7858932387862));
#217930=CARTESIAN_POINT('Ctrl Pts',(34.4625612612459,47.9213834535926,2.76813818620404));
#217931=CARTESIAN_POINT('Ctrl Pts',(34.463593983656,47.9074110114868,2.75095095199161));
#217932=CARTESIAN_POINT('Ctrl Pts',(34.4663468278988,47.8928237489021,2.73457771435597));
#217933=CARTESIAN_POINT('Ctrl Pts',(34.4685363496849,47.8812215199305,2.72155497955895));
#217934=CARTESIAN_POINT('Ctrl Pts',(34.4718146898361,47.8692298237681,2.70904711160129));
#217935=CARTESIAN_POINT('Ctrl Pts',(34.4762554502657,47.856898799393,2.69718956158372));
#217936=CARTESIAN_POINT('Ctrl Pts',(34.4762675720992,47.856865139702,2.69715719432389));
#217937=CARTESIAN_POINT('Ctrl Pts',(34.4762797026733,47.8568314776417,2.69712483219055));
#217938=CARTESIAN_POINT('Ctrl Pts',(34.4762918419889,47.856797813214,2.69709247518683));
#217939=CARTESIAN_POINT('Ctrl Pts',(34.4787083945376,47.8500962938267,2.69065122242308));
#217940=CARTESIAN_POINT('Ctrl Pts',(34.4815044004731,47.8432853991341,2.68442464469459));
#217941=CARTESIAN_POINT('Ctrl Pts',(34.4846629347251,47.836401933294,2.67844505923611));
#217942=CARTESIAN_POINT('Ctrl Pts',(34.4909312646828,47.8227412186413,2.66657815779599));
#217943=CARTESIAN_POINT('Ctrl Pts',(34.4986286886042,47.8087940876658,2.65568445664205));
#217944=CARTESIAN_POINT('Ctrl Pts',(34.5076305235176,47.7948446809468,2.64601906229547));
#217945=CARTESIAN_POINT('Ctrl Pts',(34.5143818997026,47.7843826259075,2.63877001653553));
#217946=CARTESIAN_POINT('Ctrl Pts',(34.5218670065994,47.7739192901009,2.63221189387634));
#217947=CARTESIAN_POINT('Ctrl Pts',(34.5300332501818,47.7635745545821,2.62645231033266));
#217948=CARTESIAN_POINT('Ctrl Pts',(34.5330955915252,47.7596952787626,2.62429246650378));
#217949=CARTESIAN_POINT('Ctrl Pts',(34.5362537178264,47.7558326812645,2.62224491711778));
#217950=CARTESIAN_POINT('Ctrl Pts',(34.5395048560464,47.7519930846018,2.6203153367263));
#217951=CARTESIAN_POINT('Ctrl Pts',(34.5508838398164,47.7385544962823,2.61356180535611));
#217952=CARTESIAN_POINT('Ctrl Pts',(34.5634022166002,47.7253976640915,2.60825339735381));
#217953=CARTESIAN_POINT('Ctrl Pts',(34.5769411196453,47.7127937034784,2.60463337987644));
#217954=CARTESIAN_POINT('Ctrl Pts',(34.5837105711679,47.7064917231719,2.60282337113776));
#217955=CARTESIAN_POINT('Ctrl Pts',(34.5907351548565,47.7003279615827,2.60143545939147));
#217956=CARTESIAN_POINT('Ctrl Pts',(34.598000014936,47.6943363116301,2.60050005034629));
#217957=CARTESIAN_POINT('Ctrl Pts',(34.6016324449757,47.6913404866537,2.60003234582369));
#217958=CARTESIAN_POINT('Ctrl Pts',(34.6053249441285,47.688387689607,2.59967776696099));
#217959=CARTESIAN_POINT('Ctrl Pts',(34.6090756555951,47.6854821573392,2.59944011429193));
#217960=CARTESIAN_POINT('Ctrl Pts',(34.6128263670618,47.6825766250714,2.59920246162287));
#217961=CARTESIAN_POINT('Ctrl Pts',(34.6166352918409,47.6797183589579,2.5990817379135));
#217962=CARTESIAN_POINT('Ctrl Pts',(34.6205005703634,47.6769115920306,2.59908173516058));
#217963=CARTESIAN_POINT('',(34.6451144164185,47.6590285860938,2.59908173516057));
#217964=CARTESIAN_POINT('Origin',(5.69524824702573E-15,1.85909896949569E-13,
2.59908173516024));
#217965=CARTESIAN_POINT('',(34.9997217530259,47.6338034047602,2.90134173516056));
#217966=CARTESIAN_POINT('Ctrl Pts',(34.6451144164185,47.6590285860938,2.59908173516057));
#217967=CARTESIAN_POINT('Ctrl Pts',(34.648196040315,47.6567884460683,2.59908174371547));
#217968=CARTESIAN_POINT('Ctrl Pts',(34.651296885817,47.6545924528205,2.59915764355924));
#217969=CARTESIAN_POINT('Ctrl Pts',(34.6544147487634,47.6524408584473,2.5993076577531));
#217970=CARTESIAN_POINT('Ctrl Pts',(34.672822375816,47.6397380079784,2.60019333020912));
#217971=CARTESIAN_POINT('Ctrl Pts',(34.6918243519411,47.6285798336129,2.603659733241));
#217972=CARTESIAN_POINT('Ctrl Pts',(34.7109619288054,47.6190225715796,2.60934177082367));
#217973=CARTESIAN_POINT('Ctrl Pts',(34.7181110904612,47.6154522966306,2.61146439091819));
#217974=CARTESIAN_POINT('Ctrl Pts',(34.7252793254653,47.6121050440163,2.61389584429317));
#217975=CARTESIAN_POINT('Ctrl Pts',(34.7324433913425,47.6089824432868,2.61661604385286));
#217976=CARTESIAN_POINT('Ctrl Pts',(34.7380331549252,47.6065460335524,2.61873848000809));
#217977=CARTESIAN_POINT('Ctrl Pts',(34.7436201516877,47.6042468425534,2.62103707099821));
#217978=CARTESIAN_POINT('Ctrl Pts',(34.7491931041024,47.6020860928991,2.62350262767686));
#217979=CARTESIAN_POINT('Ctrl Pts',(34.768698437554,47.594523469109,2.63213207605212));
#217980=CARTESIAN_POINT('Ctrl Pts',(34.7880317224284,47.5886567445953,2.64280685971947));
#217981=CARTESIAN_POINT('Ctrl Pts',(34.8067094890034,47.5845384124877,2.65513293646117));
#217982=CARTESIAN_POINT('Ctrl Pts',(34.8160483722909,47.5824792464338,2.66129597483202));
#217983=CARTESIAN_POINT('Ctrl Pts',(34.8252233770803,47.5808571799368,2.66787183533885));
#217984=CARTESIAN_POINT('Ctrl Pts',(34.8341740726979,47.5796787787541,2.67481125953894));
#217985=CARTESIAN_POINT('Ctrl Pts',(34.8430865267162,47.5785054122579,2.68172103524112));
#217986=CARTESIAN_POINT('Ctrl Pts',(34.8517766417065,47.5777716830265,2.68899101329822));
#217987=CARTESIAN_POINT('Ctrl Pts',(34.8601845855138,47.5774848094466,2.69657334701308));
#217988=CARTESIAN_POINT('Ctrl Pts',(34.8602206623585,47.5774835785281,2.69660588132605));
#217989=CARTESIAN_POINT('Ctrl Pts',(34.8602567341388,47.5774823553082,2.69663842081414));
#217990=CARTESIAN_POINT('Ctrl Pts',(34.8602928008533,47.5774811397855,2.69667096547414));
#217991=CARTESIAN_POINT('Ctrl Pts',(34.8773011701531,47.5769079226576,2.71201840157965));
#217992=CARTESIAN_POINT('Ctrl Pts',(34.8931591840079,47.5780177840619,2.72845645939364));
#217993=CARTESIAN_POINT('Ctrl Pts',(34.907808554209,47.5806251537546,2.74568723186902));
#217994=CARTESIAN_POINT('Ctrl Pts',(34.9229908396734,47.5833273744263,2.76354482594315));
#217995=CARTESIAN_POINT('Ctrl Pts',(34.9368756554781,47.5876385414306,2.78225519317108));
#217996=CARTESIAN_POINT('Ctrl Pts',(34.9493673872922,47.5933942811496,2.80151223085477));
#217997=CARTESIAN_POINT('Ctrl Pts',(34.9616808340646,47.5990678735481,2.82049442740203));
#217998=CARTESIAN_POINT('Ctrl Pts',(34.9726411562242,47.6061458909237,2.84000929089166));
#217999=CARTESIAN_POINT('Ctrl Pts',(34.9821189161897,47.6145008888064,2.85976644341498));
#218000=CARTESIAN_POINT('Ctrl Pts',(34.9887269790637,47.6203261419803,2.87354148166876));
#218001=CARTESIAN_POINT('Ctrl Pts',(34.9946135826771,47.6267727798537,2.88743438345469));
#218002=CARTESIAN_POINT('Ctrl Pts',(34.9997217530259,47.6338034047602,2.90134173516057));
#218003=CARTESIAN_POINT('',(35.2091516650527,47.922053073669,3.47153072139106));
#218004=CARTESIAN_POINT('',(34.9997217530259,47.6338034047602,2.90134173516056));
#218005=CARTESIAN_POINT('',(39.554446981307,44.4033023070492,3.47153072139104));
#218006=CARTESIAN_POINT('Origin',(5.53234440788222E-15,1.85015204418142E-13,
3.47153072139072));
#218007=CARTESIAN_POINT('',(39.3160391863689,44.1385184650378,2.90134173516055));
#218008=CARTESIAN_POINT('',(39.554446981307,44.4033023070492,3.47153072139104));
#218009=CARTESIAN_POINT('',(39.4144401478989,43.7969047596349,2.59908173516054));
#218010=CARTESIAN_POINT('Ctrl Pts',(39.3160391863689,44.1385184650378,2.90134173516055));
#218011=CARTESIAN_POINT('Ctrl Pts',(39.3078558527201,44.1294297383226,2.88176998919738));
#218012=CARTESIAN_POINT('Ctrl Pts',(39.30113768161,44.1190955972869,2.86226752356559));
#218013=CARTESIAN_POINT('Ctrl Pts',(39.2959399200105,44.1076895347495,2.84310370499762));
#218014=CARTESIAN_POINT('Ctrl Pts',(39.2906482678552,44.0960774370696,2.8235937178831));
#218015=CARTESIAN_POINT('Ctrl Pts',(39.2869318048885,44.0833536765915,2.80443322636566));
#218016=CARTESIAN_POINT('Ctrl Pts',(39.2848826826034,44.0696602318339,2.78589323877748));
#218017=CARTESIAN_POINT('Ctrl Pts',(39.2829203148429,44.0565465320237,2.76813818619431));
#218018=CARTESIAN_POINT('Ctrl Pts',(39.2824868619908,44.0425426835299,2.75095095198097));
#218019=CARTESIAN_POINT('Ctrl Pts',(39.2836998417244,44.0277475809163,2.73457771434461));
#218020=CARTESIAN_POINT('Ctrl Pts',(39.2846646059165,44.0159800428246,2.72155497955166));
#218021=CARTESIAN_POINT('Ctrl Pts',(39.2866715134052,44.0037113585737,2.70904711159781));
#218022=CARTESIAN_POINT('Ctrl Pts',(39.2897990038552,43.9909836989807,2.69718956158368));
#218023=CARTESIAN_POINT('Ctrl Pts',(39.2898075408882,43.9909489566043,2.69715719432385));
#218024=CARTESIAN_POINT('Ctrl Pts',(39.2898160863664,43.990914210958,2.69712483219051));
#218025=CARTESIAN_POINT('Ctrl Pts',(39.2898246402906,43.9908794620436,2.69709247518679));
#218026=CARTESIAN_POINT('Ctrl Pts',(39.2915274551884,43.9839620557564,2.69065122242305));
#218027=CARTESIAN_POINT('Ctrl Pts',(39.2935962119552,43.9768962096538,2.68442464469456));
#218028=CARTESIAN_POINT('Ctrl Pts',(39.2960179253199,43.9697202954283,2.67844505923608));
#218029=CARTESIAN_POINT('Ctrl Pts',(39.3008239832004,43.955479196702,2.66657815779597));
#218030=CARTESIAN_POINT('Ctrl Pts',(39.3070213676603,43.9408038696757,2.65568445664204));
#218031=CARTESIAN_POINT('Ctrl Pts',(39.3145157795323,43.9259899312962,2.64601906229545));
#218032=CARTESIAN_POINT('Ctrl Pts',(39.3201365884363,43.9148794775115,2.63877001653551));
#218033=CARTESIAN_POINT('Ctrl Pts',(39.3264869747219,43.903691054232,2.63221189387631));
#218034=CARTESIAN_POINT('Ctrl Pts',(39.3335271634607,43.8925493833644,2.62645231033263));
#218035=CARTESIAN_POINT('Ctrl Pts',(39.3361672342378,43.888371256789,2.62429246650375));
#218036=CARTESIAN_POINT('Ctrl Pts',(39.338904308612,43.8841997049151,2.62224491711776));
#218037=CARTESIAN_POINT('Ctrl Pts',(39.341736289618,43.8800413054827,2.62031533672627));
#218038=CARTESIAN_POINT('Ctrl Pts',(39.3516482231388,43.865486907469,2.61356180535609));
#218039=CARTESIAN_POINT('Ctrl Pts',(39.3627227594944,43.8510936230938,2.60825339735378));
#218040=CARTESIAN_POINT('Ctrl Pts',(39.374870022378,43.8371435075661,2.60463337987641));
#218041=CARTESIAN_POINT('Ctrl Pts',(39.3809436538198,43.8301684498023,2.60282337113772));
#218042=CARTESIAN_POINT('Ctrl Pts',(39.3872854675771,43.8233041850059,2.60143545939144));
#218043=CARTESIAN_POINT('Ctrl Pts',(39.393884232031,43.8165859732787,2.60050005034625));
#218044=CARTESIAN_POINT('Ctrl Pts',(39.3971836142579,43.8132268674151,2.60003234582366));
#218045=CARTESIAN_POINT('Ctrl Pts',(39.4005472341763,43.8099042748374,2.59967776696096));
#218046=CARTESIAN_POINT('Ctrl Pts',(39.4039736880302,43.8066226032737,2.5994401142919));
#218047=CARTESIAN_POINT('Ctrl Pts',(39.4074001418841,43.8033409317099,2.59920246162284));
#218048=CARTESIAN_POINT('Ctrl Pts',(39.4108894308102,43.8001001824233,2.59908173791343));
#218049=CARTESIAN_POINT('Ctrl Pts',(39.4144401478989,43.7969047596349,2.59908173516055));
#218050=CARTESIAN_POINT('',(39.4370498736007,43.7765468711725,2.59908173516054));
#218051=CARTESIAN_POINT('Origin',(5.70079064675565E-15,1.85905408802762E-13,
2.59908173516024));
#218052=CARTESIAN_POINT('',(39.7870778846746,43.7143933160626,2.90134173516054));
#218053=CARTESIAN_POINT('Ctrl Pts',(39.4370498736007,43.7765468711725,2.59908173516055));
#218054=CARTESIAN_POINT('Ctrl Pts',(39.4398804576448,43.7739968854582,2.59908174371544));
#218055=CARTESIAN_POINT('Ctrl Pts',(39.4427347725911,43.771488795476,2.59915764355922));
#218056=CARTESIAN_POINT('Ctrl Pts',(39.4456106527046,43.7690230823394,2.59930765775308));
#218057=CARTESIAN_POINT('Ctrl Pts',(39.4625896314097,43.7544656984479,2.600193330209));
#218058=CARTESIAN_POINT('Ctrl Pts',(39.4803211659001,43.7413824023669,2.6036597332402));
#218059=CARTESIAN_POINT('Ctrl Pts',(39.4983548992005,43.7298770745156,2.60934177082175));
#218060=CARTESIAN_POINT('Ctrl Pts',(39.5050917016488,43.7255790670235,2.61146439091671));
#218061=CARTESIAN_POINT('Ctrl Pts',(39.5118707851416,43.7215008664186,2.61389584429233));
#218062=CARTESIAN_POINT('Ctrl Pts',(39.5186692048627,43.7176465228246,2.61661604385282));
#218063=CARTESIAN_POINT('Ctrl Pts',(39.5239736729701,43.7146391706004,2.61873848000805));
#218064=CARTESIAN_POINT('Ctrl Pts',(39.5292897326779,43.7117685746244,2.62103707099818));
#218065=CARTESIAN_POINT('Ctrl Pts',(39.5346062960353,43.709037129631,2.62350262767683));
#218066=CARTESIAN_POINT('Ctrl Pts',(39.5532142677863,43.6994770721541,2.6321320760521));
#218067=CARTESIAN_POINT('Ctrl Pts',(39.5718284032055,43.6916216076132,2.64280685971944));
#218068=CARTESIAN_POINT('Ctrl Pts',(39.5899733680945,43.6855734779225,2.65513293646114));
#218069=CARTESIAN_POINT('Ctrl Pts',(39.599045850539,43.6825494130771,2.66129597483199));
#218070=CARTESIAN_POINT('Ctrl Pts',(39.6080010415738,43.6799771832789,2.66787183533882));
#218071=CARTESIAN_POINT('Ctrl Pts',(39.6167795278796,43.6778696350431,2.67481125953892));
#218072=CARTESIAN_POINT('Ctrl Pts',(39.6255205083456,43.6757710912488,2.6817210352411));
#218073=CARTESIAN_POINT('Ctrl Pts',(39.6340863223877,43.6741330170974,2.68899101329819));
#218074=CARTESIAN_POINT('Ctrl Pts',(39.6424182201447,43.6729688455955,2.69657334701305));
#218075=CARTESIAN_POINT('Ctrl Pts',(39.6424539706905,43.672963850363,2.69660588132602));
#218076=CARTESIAN_POINT('Ctrl Pts',(39.6424897170046,43.6729588633163,2.69663842081411));
#218077=CARTESIAN_POINT('Ctrl Pts',(39.6425254590851,43.6729538844541,2.69667096547411));
#218078=CARTESIAN_POINT('Ctrl Pts',(39.6593807372542,43.6706059487638,2.71201840158091));
#218079=CARTESIAN_POINT('Ctrl Pts',(39.6752678913581,43.6700521164126,2.72845645939637));
#218080=CARTESIAN_POINT('Ctrl Pts',(39.6901095551247,43.6711139265067,2.74568723187333));
#218081=CARTESIAN_POINT('Ctrl Pts',(39.7054911294161,43.6722143631628,2.76354482594909));
#218082=CARTESIAN_POINT('Ctrl Pts',(39.7197505224098,43.6750505546849,2.78225519317877));
#218083=CARTESIAN_POINT('Ctrl Pts',(39.7327754618385,43.6794690223303,2.80151223086424));
#218084=CARTESIAN_POINT('Ctrl Pts',(39.7456145061562,43.6838244285283,2.82049442741313));
#218085=CARTESIAN_POINT('Ctrl Pts',(39.7572546408038,43.6897180061528,2.84000929090442));
#218086=CARTESIAN_POINT('Ctrl Pts',(39.767553815698,43.6970365387998,2.85976644342937));
#218087=CARTESIAN_POINT('Ctrl Pts',(39.7747345836717,43.7021391499686,2.87354148167843));
#218088=CARTESIAN_POINT('Ctrl Pts',(39.7812627970021,43.7079351548539,2.88743438345951));
#218089=CARTESIAN_POINT('Ctrl Pts',(39.7870778846746,43.7143933160626,2.90134173516054));
#218090=CARTESIAN_POINT('',(40.0254908126588,43.9791725362585,3.47153072139104));
#218091=CARTESIAN_POINT('',(39.7870778846746,43.7143933160626,2.90134173516055));
#218092=CARTESIAN_POINT('',(43.9791725362582,40.0254908126591,3.47153072139101));
#218093=CARTESIAN_POINT('Origin',(5.53234440788222E-15,1.85015204418142E-13,
3.47153072139072));
#218094=CARTESIAN_POINT('',(43.7143933160623,39.787077884675,2.90134173516052));
#218095=CARTESIAN_POINT('',(43.9791725362582,40.0254908126591,3.47153072139101));
#218096=CARTESIAN_POINT('',(43.7765468711722,39.4370498736011,2.59908173516051));
#218097=CARTESIAN_POINT('Ctrl Pts',(43.7143933160623,39.787077884675,2.90134173516052));
#218098=CARTESIAN_POINT('Ctrl Pts',(43.7053047809347,39.7788943382461,2.88176998919692));
#218099=CARTESIAN_POINT('Ctrl Pts',(43.697543200787,39.7693190488182,2.8622675235647));
#218100=CARTESIAN_POINT('Ctrl Pts',(43.6911816548804,39.7585187839169,2.84310370499633));
#218101=CARTESIAN_POINT('Ctrl Pts',(43.6847051962234,39.7475234267907,2.8235937178814));
#218102=CARTESIAN_POINT('Ctrl Pts',(43.6796790972999,39.7352578445662,2.80443322636358));
#218103=CARTESIAN_POINT('Ctrl Pts',(43.6762098455837,39.7218536055349,2.78589323877506));
#218104=CARTESIAN_POINT('Ctrl Pts',(43.6728874729904,39.7090168672304,2.76813818619159));
#218105=CARTESIAN_POINT('Ctrl Pts',(43.6709925938755,39.6951350414441,2.75095095197799));
#218106=CARTESIAN_POINT('Ctrl Pts',(43.6706524194393,39.6802941970427,2.73457771434141));
#218107=CARTESIAN_POINT('Ctrl Pts',(43.6703818558792,39.6684902774383,2.72155497954961));
#218108=CARTESIAN_POINT('Ctrl Pts',(43.6710953426077,39.6560790233687,2.70904711159683));
#218109=CARTESIAN_POINT('Ctrl Pts',(43.6728752976394,39.6430941754571,2.69718956158366));
#218110=CARTESIAN_POINT('Ctrl Pts',(43.6728801563384,39.6430587310402,2.69715719432383));
#218111=CARTESIAN_POINT('Ctrl Pts',(43.6728850230946,39.6430232824885,2.69712483219048));
#218112=CARTESIAN_POINT('Ctrl Pts',(43.6728898979089,39.6429878298037,2.69709247518676));
#218113=CARTESIAN_POINT('Ctrl Pts',(43.6738603187595,39.6359303251674,2.69065122242302));
#218114=CARTESIAN_POINT('Ctrl Pts',(43.6751791606255,39.6286869425433,2.68442464469454));
#218115=CARTESIAN_POINT('Ctrl Pts',(43.6768375203044,39.6212972007503,2.67844505923606));
#218116=CARTESIAN_POINT('Ctrl Pts',(43.6801286499319,39.6066317464083,2.66657815779595));
#218117=CARTESIAN_POINT('Ctrl Pts',(43.6847580950893,39.5913890092851,2.65568445664201));
#218118=CARTESIAN_POINT('Ctrl Pts',(43.6906629735752,39.5758728438539,2.64601906229542));
#218119=CARTESIAN_POINT('Ctrl Pts',(43.6950916324396,39.5642357197805,2.63877001653548));
#218120=CARTESIAN_POINT('Ctrl Pts',(43.7002377219528,39.5524447917348,2.63221189387629));
#218121=CARTESIAN_POINT('Ctrl Pts',(43.7060747220671,39.540628255996,2.62645231033261));
#218122=CARTESIAN_POINT('Ctrl Pts',(43.70826359711,39.536197055094,2.62429246650373));
#218123=CARTESIAN_POINT('Ctrl Pts',(43.7105496315976,39.5317622532395,2.62224491711773));
#218124=CARTESIAN_POINT('Ctrl Pts',(43.7129314276129,39.5273306113317,2.62031533672625));
#218125=CARTESIAN_POINT('Ctrl Pts',(43.7212677136666,39.5118198646543,2.61356180535606));
#218126=CARTESIAN_POINT('Ctrl Pts',(43.7307770746562,39.4963478239302,2.60825339735375));
#218127=CARTESIAN_POINT('Ctrl Pts',(43.7413996094243,39.4812043938729,2.60463337987638));
#218128=CARTESIAN_POINT('Ctrl Pts',(43.7467108768083,39.4736326788442,2.6028233711377));
#218129=CARTESIAN_POINT('Ctrl Pts',(43.7523004383956,39.4661431171622,2.60143545939142));
#218130=CARTESIAN_POINT('Ctrl Pts',(43.7581608097796,39.4587719497939,2.60050005034623));
#218131=CARTESIAN_POINT('Ctrl Pts',(43.7610909954716,39.4550863661098,2.60003234582364));
#218132=CARTESIAN_POINT('Ctrl Pts',(43.764088883632,39.4514303810209,2.59967776696093));
#218133=CARTESIAN_POINT('Ctrl Pts',(43.7671535389276,39.4478085248415,2.59944011429187));
#218134=CARTESIAN_POINT('Ctrl Pts',(43.7702181942233,39.4441866686621,2.59920246162281));
#218135=CARTESIAN_POINT('Ctrl Pts',(43.7733496179168,39.4405989425298,2.59908173791339));
#218136=CARTESIAN_POINT('Ctrl Pts',(43.7765468711722,39.4370498736011,2.59908173516052));
#218137=CARTESIAN_POINT('',(43.7969047596346,39.4144401478992,2.59908173516051));
#218138=CARTESIAN_POINT('Origin',(5.7058335455513E-15,1.85900365903967E-13,
2.59908173516024));
#218139=CARTESIAN_POINT('',(44.1385184650375,39.3160391863693,2.90134173516051));
#218140=CARTESIAN_POINT('Ctrl Pts',(43.7969047596346,39.4144401478992,2.59908173516051));
#218141=CARTESIAN_POINT('Ctrl Pts',(43.799453291355,39.4116082546732,2.59908174371542));
#218142=CARTESIAN_POINT('Ctrl Pts',(43.8020298032738,39.4088155471154,2.59915764355919));
#218143=CARTESIAN_POINT('Ctrl Pts',(43.8046321918101,39.4060627300845,2.59930765775305));
#218144=CARTESIAN_POINT('Ctrl Pts',(43.8199964969283,39.3898103065108,2.6001933302091));
#218145=CARTESIAN_POINT('Ctrl Pts',(43.8362633193862,39.374945232041,2.60365973324122));
#218146=CARTESIAN_POINT('Ctrl Pts',(43.8529956277716,39.3616178931491,2.60934177082429));
#218147=CARTESIAN_POINT('Ctrl Pts',(43.8592462611905,39.3566392429866,2.61146439091865));
#218148=CARTESIAN_POINT('Ctrl Pts',(43.86556192011,39.3518747760135,2.6138958442934));
#218149=CARTESIAN_POINT('Ctrl Pts',(43.8719202087612,39.3473309185527,2.61661604385281));
#218150=CARTESIAN_POINT('Ctrl Pts',(43.8768812645308,39.3437855730189,2.61873848000804));
#218151=CARTESIAN_POINT('Ctrl Pts',(43.8818681433212,39.3403750229161,2.62103707099816));
#218152=CARTESIAN_POINT('Ctrl Pts',(43.8868700682407,39.3371028088665,2.6235026276768));
#218153=CARTESIAN_POINT('Ctrl Pts',(43.9043768054586,39.3256500596931,2.63213207605207));
#218154=CARTESIAN_POINT('Ctrl Pts',(43.9220678510596,39.3158919212386,2.64280685971942));
#218155=CARTESIAN_POINT('Ctrl Pts',(43.9394812142302,39.3079802585392,2.65513293646112));
#218156=CARTESIAN_POINT('Ctrl Pts',(43.9481878958155,39.3040244271895,2.66129597483196));
#218157=CARTESIAN_POINT('Ctrl Pts',(43.9568251581489,39.3005302159781,2.6678718353388));
#218158=CARTESIAN_POINT('Ctrl Pts',(43.9653352562098,39.2975166114287,2.67481125953889));
#218159=CARTESIAN_POINT('Ctrl Pts',(43.9738089951123,39.2945158824213,2.68172103524107));
#218160=CARTESIAN_POINT('Ctrl Pts',(43.982156659355,39.291991410433,2.68899101329814));
#218161=CARTESIAN_POINT('Ctrl Pts',(43.9903212250463,39.2899626959158,2.69657334701299));
#218162=CARTESIAN_POINT('Ctrl Pts',(43.9903562576029,39.2899539910981,2.69660588132597));
#218163=CARTESIAN_POINT('Ctrl Pts',(43.9903912868066,39.2899452948636,2.69663842081406));
#218164=CARTESIAN_POINT('Ctrl Pts',(43.9904263126554,39.2899366072115,2.69667096547406));
#218165=CARTESIAN_POINT('Ctrl Pts',(44.0069438297388,39.2858396774333,2.71201840158195));
#218166=CARTESIAN_POINT('Ctrl Pts',(44.0226860611066,39.2836282192295,2.72845645939866));
#218167=CARTESIAN_POINT('Ctrl Pts',(44.0375574100645,39.2831328363111,2.74568723187695));
#218168=CARTESIAN_POINT('Ctrl Pts',(44.0529697494363,39.282619432337,2.76354482595429));
#218169=CARTESIAN_POINT('Ctrl Pts',(44.0674474907255,39.283949574469,2.78225519318566));
#218170=CARTESIAN_POINT('Ctrl Pts',(44.0808629338068,39.2869823603845,2.80151223087286));
#218171=CARTESIAN_POINT('Ctrl Pts',(44.094086908414,39.28997186164,2.82049442742354));
#218172=CARTESIAN_POINT('Ctrl Pts',(44.1062793237989,39.2946164282438,2.84000929091666));
#218173=CARTESIAN_POINT('Ctrl Pts',(44.1172870737068,39.3008183122797,2.8597664434434));
#218174=CARTESIAN_POINT('Ctrl Pts',(44.1249618727833,39.3051423761684,2.87354148168786));
#218175=CARTESIAN_POINT('Ctrl Pts',(44.1320601713592,39.3102242458236,2.88743438346422));
#218176=CARTESIAN_POINT('Ctrl Pts',(44.1385184650375,39.3160391863692,2.90134173516051));
#218177=CARTESIAN_POINT('',(44.4033023070489,39.5544469813073,3.471530721391));
#218178=CARTESIAN_POINT('',(44.1385184650375,39.3160391863692,2.90134173516052));
#218179=CARTESIAN_POINT('',(47.9220530736687,35.209151665053,3.47153072139097));
#218180=CARTESIAN_POINT('Origin',(5.53234440788222E-15,1.85015204418142E-13,
3.47153072139072));
#218181=CARTESIAN_POINT('',(47.6338034047599,34.9997217530263,2.90134173516048));
#218182=CARTESIAN_POINT('',(47.9220530736687,35.209151665053,3.47153072139097));
#218183=CARTESIAN_POINT('',(47.6590285860935,34.6451144164188,2.59908173516048));
#218184=CARTESIAN_POINT('Ctrl Pts',(47.6338034047599,34.9997217530263,2.90134173516048));
#218185=CARTESIAN_POINT('Ctrl Pts',(47.6239092440469,34.992533047532,2.88176998919812));
#218186=CARTESIAN_POINT('Ctrl Pts',(47.6151892923585,34.9838215185875,2.86226752356711));
#218187=CARTESIAN_POINT('Ctrl Pts',(47.6077336605733,34.9737453812859,2.84310370499989));
#218188=CARTESIAN_POINT('Ctrl Pts',(47.6001433528511,34.9634872321481,2.82359371788591));
#218189=CARTESIAN_POINT('Ctrl Pts',(47.5938626849626,34.9518142124638,2.80443322636898));
#218190=CARTESIAN_POINT('Ctrl Pts',(47.5890113136631,34.9388460388079,2.78589323878128));
#218191=CARTESIAN_POINT('Ctrl Pts',(47.5843653368459,34.926426904001,2.76813818619804));
#218192=CARTESIAN_POINT('Ctrl Pts',(47.5810297921601,34.9128191931112,2.75095095198462));
#218193=CARTESIAN_POINT('Ctrl Pts',(47.5791401905759,34.8980952063199,2.73457771434816));
#218194=CARTESIAN_POINT('Ctrl Pts',(47.5776372636139,34.8863842314135,2.72155497955392));
#218195=CARTESIAN_POINT('Ctrl Pts',(47.5770495124721,34.873966387819,2.70904711159887));
#218196=CARTESIAN_POINT('Ctrl Pts',(47.5774624305259,34.8608666162964,2.69718956158364));
#218197=CARTESIAN_POINT('Ctrl Pts',(47.5774635576581,34.8608308581754,2.69715719432381));
#218198=CARTESIAN_POINT('Ctrl Pts',(47.577464692371,34.8607950951,2.69712483219046));
#218199=CARTESIAN_POINT('Ctrl Pts',(47.5774658346659,34.8607593270719,2.69709247518674));
#218200=CARTESIAN_POINT('Ctrl Pts',(47.5776932293355,34.8536390475842,2.690651222423));
#218201=CARTESIAN_POINT('Ctrl Pts',(47.5782477067931,34.8462974884545,2.6844246446945));
#218202=CARTESIAN_POINT('Ctrl Pts',(47.5791245434507,34.8387748826515,2.67844505923603));
#218203=CARTESIAN_POINT('Ctrl Pts',(47.5808646865202,34.8238457504805,2.66657815779591));
#218204=CARTESIAN_POINT('Ctrl Pts',(47.5838754712052,34.808202605878,2.65568445664198));
#218205=CARTESIAN_POINT('Ctrl Pts',(47.5881261212205,34.7921542117506,2.64601906229539));
#218206=CARTESIAN_POINT('Ctrl Pts',(47.591314108732,34.780117916155,2.63877001653545));
#218207=CARTESIAN_POINT('Ctrl Pts',(47.5951995198393,34.7678536672182,2.63221189387625));
#218208=CARTESIAN_POINT('Ctrl Pts',(47.5997693799344,34.7554917310466,2.62645231033257));
#218209=CARTESIAN_POINT('Ctrl Pts',(47.60148307747,34.7508560049822,2.62429246650369));
#218210=CARTESIAN_POINT('Ctrl Pts',(47.6032930257987,34.7462065417644,2.62224491711769));
#218211=CARTESIAN_POINT('Ctrl Pts',(47.6051985413679,34.7415502113773,2.62031533672621));
#218212=CARTESIAN_POINT('Ctrl Pts',(47.6118678458601,34.7252530550225,2.61356180535602));
#218213=CARTESIAN_POINT('Ctrl Pts',(47.6197078449347,34.7088717728655,2.60825339735371));
#218214=CARTESIAN_POINT('Ctrl Pts',(47.6286892688733,34.6927009428672,2.60463337987634));
#218215=CARTESIAN_POINT('Ctrl Pts',(47.6331799808426,34.6846155278681,2.60282337113766));
#218216=CARTESIAN_POINT('Ctrl Pts',(47.6379560498536,34.6765827265055,2.60143545939139));
#218217=CARTESIAN_POINT('Ctrl Pts',(47.6430138207125,34.6686393635484,2.6005000503462));
#218218=CARTESIAN_POINT('Ctrl Pts',(47.6455427061419,34.6646676820698,2.6000323458236));
#218219=CARTESIAN_POINT('Ctrl Pts',(47.6481420170542,34.6607183602073,2.59967776696091));
#218220=CARTESIAN_POINT('Ctrl Pts',(47.6508112967868,34.6567960012265,2.59944011429185));
#218221=CARTESIAN_POINT('Ctrl Pts',(47.6534805765195,34.6528736422458,2.59920246162279));
#218222=CARTESIAN_POINT('Ctrl Pts',(47.6562198264472,34.6489782471461,2.59908173791339));
#218223=CARTESIAN_POINT('Ctrl Pts',(47.6590285860935,34.6451144164188,2.59908173516049));
#218224=CARTESIAN_POINT('',(47.6769115920304,34.6205005703637,2.59908173516048));
#218225=CARTESIAN_POINT('Origin',(5.71032169235817E-15,1.85894823504237E-13,
2.59908173516024));
#218226=CARTESIAN_POINT('',(48.0063682005187,34.4869303039399,2.90134173516047));
#218227=CARTESIAN_POINT('Ctrl Pts',(47.6769115920304,34.6205005703637,2.59908173516048));
#218228=CARTESIAN_POINT('Ctrl Pts',(47.6791501491803,34.6174177964407,2.59908174371533));
#218229=CARTESIAN_POINT('Ctrl Pts',(47.6814206292678,34.6143710687957,2.59915764355915));
#218230=CARTESIAN_POINT('Ctrl Pts',(47.6837210139136,34.61136130831,2.59930765775302));
#218231=CARTESIAN_POINT('Ctrl Pts',(47.6973023109003,34.5935919100098,2.60019333020907));
#218232=CARTESIAN_POINT('Ctrl Pts',(47.7119261986122,34.5771079220194,2.60365973324124));
#218233=CARTESIAN_POINT('Ctrl Pts',(47.7271737594079,34.5621045892019,2.60934177082439));
#218234=CARTESIAN_POINT('Ctrl Pts',(47.7328697405521,34.5564998435003,2.61146439091872));
#218235=CARTESIAN_POINT('Ctrl Pts',(47.7386527792201,34.5511013106546,2.61389584429343));
#218236=CARTESIAN_POINT('Ctrl Pts',(47.744501274063,34.5459177227788,2.61661604385277));
#218237=CARTESIAN_POINT('Ctrl Pts',(47.7490645631296,34.541873227483,2.618738480008));
#218238=CARTESIAN_POINT('Ctrl Pts',(47.7536676237151,34.537960089954,2.62103707099811));
#218239=CARTESIAN_POINT('Ctrl Pts',(47.7583001080603,34.5341829579102,2.62350262767675));
#218240=CARTESIAN_POINT('Ctrl Pts',(47.7745138032687,34.5209629957568,2.63213207605202));
#218241=CARTESIAN_POINT('Ctrl Pts',(47.7910879322539,34.5094090955955,2.64280685971938));
#218242=CARTESIAN_POINT('Ctrl Pts',(47.8075789092551,34.4997205817196,2.65513293646107));
#218243=CARTESIAN_POINT('Ctrl Pts',(47.8158243977558,34.4948763247817,2.66129597483192));
#218244=CARTESIAN_POINT('Ctrl Pts',(47.8240490997342,34.4904984154664,2.66787183533875));
#218245=CARTESIAN_POINT('Ctrl Pts',(47.8321975711351,34.4866117722855,2.67481125953884));
#218246=CARTESIAN_POINT('Ctrl Pts',(47.8403112284174,34.4827417346799,2.68172103524103));
#218247=CARTESIAN_POINT('Ctrl Pts',(47.8483492841045,34.4793585234982,2.68899101329811));
#218248=CARTESIAN_POINT('Ctrl Pts',(47.8562570650397,34.4764874929865,2.69657334701297));
#218249=CARTESIAN_POINT('Ctrl Pts',(47.8562909957831,34.4764751739553,2.69660588132594));
#218250=CARTESIAN_POINT('Ctrl Pts',(47.8563249240891,34.4764628638109,2.69663842081403));
#218251=CARTESIAN_POINT('Ctrl Pts',(47.8563588499558,34.4764505625524,2.69667096547403));
#218252=CARTESIAN_POINT('Ctrl Pts',(47.8723576365775,34.4706495255069,2.71201840158102));
#218253=CARTESIAN_POINT('Ctrl Pts',(47.8877824700263,34.4668046706493,2.72845645939671));
#218254=CARTESIAN_POINT('Ctrl Pts',(47.9025205705626,34.4647575222371,2.7456872318739));
#218255=CARTESIAN_POINT('Ctrl Pts',(47.9177948141974,34.4626359025937,2.76354482595019));
#218256=CARTESIAN_POINT('Ctrl Pts',(47.9323322826173,34.4624454220191,2.78225519318044));
#218257=CARTESIAN_POINT('Ctrl Pts',(47.9459912469484,34.4640592983662,2.80151223086651));
#218258=CARTESIAN_POINT('Ctrl Pts',(47.9594552672108,34.4656501410767,2.82049442741633));
#218259=CARTESIAN_POINT('Ctrl Pts',(47.972066380678,34.4689948098143,2.84000929090859));
#218260=CARTESIAN_POINT('Ctrl Pts',(47.9836621023876,34.474012096098,2.8597664434345));
#218261=CARTESIAN_POINT('Ctrl Pts',(47.9917468458671,34.4775102373592,2.87354148168186));
#218262=CARTESIAN_POINT('Ctrl Pts',(47.9993374592481,34.4818222937595,2.88743438346119));
#218263=CARTESIAN_POINT('Ctrl Pts',(48.0063682005187,34.4869303039399,2.90134173516047));
#218264=CARTESIAN_POINT('',(48.2946219293746,34.6963546279288,3.47153072139097));
#218265=CARTESIAN_POINT('',(48.0063682005187,34.4869303039399,2.90134173516048));
#218266=CARTESIAN_POINT('',(51.3398895692697,30.007053683816,3.47153072139094));
#218267=CARTESIAN_POINT('Origin',(5.53234440788222E-15,1.85015204418142E-13,
3.47153072139072));
#218268=CARTESIAN_POINT('',(51.0313275753408,29.8289013456888,2.90134173516045));
#218269=CARTESIAN_POINT('',(51.3398895692697,30.007053683816,3.47153072139094));
#218270=CARTESIAN_POINT('',(51.0193480105327,29.473599835734,2.59908173516044));
#218271=CARTESIAN_POINT('Ctrl Pts',(51.0313275753408,29.8289013456888,2.90134173516045));
#218272=CARTESIAN_POINT('Ctrl Pts',(51.0207361915367,29.8227862420893,2.88176998919671));
#218273=CARTESIAN_POINT('Ctrl Pts',(51.0111534059222,29.8150339189608,2.86226752356434));
#218274=CARTESIAN_POINT('Ctrl Pts',(51.0026853737198,29.8057923055259,2.84310370499583));
#218275=CARTESIAN_POINT('Ctrl Pts',(50.9940643779319,29.7963837548036,2.82359371788082));
#218276=CARTESIAN_POINT('Ctrl Pts',(50.9865979533897,29.7854311897043,2.80443322636292));
#218277=CARTESIAN_POINT('Ctrl Pts',(50.980417615146,29.7730411634463,2.78589323877433));
#218278=CARTESIAN_POINT('Ctrl Pts',(50.9744989363996,29.7611756987759,2.76813818619093));
#218279=CARTESIAN_POINT('Ctrl Pts',(50.9697592710689,29.74799119171,2.75095095197738));
#218280=CARTESIAN_POINT('Ctrl Pts',(50.9663409452077,29.7335453816081,2.73457771434086));
#218281=CARTESIAN_POINT('Ctrl Pts',(50.9636221212274,29.7220556592952,2.72155497954923));
#218282=CARTESIAN_POINT('Ctrl Pts',(50.9617395717402,29.709767278673,2.70904711159661));
#218283=CARTESIAN_POINT('Ctrl Pts',(50.9607809287995,29.6966961073823,2.69718956158359));
#218284=CARTESIAN_POINT('Ctrl Pts',(50.9607783120157,29.6966604273306,2.69715719432376));
#218285=CARTESIAN_POINT('Ctrl Pts',(50.9607757022532,29.6966247415593,2.69712483219041));
#218286=CARTESIAN_POINT('Ctrl Pts',(50.9607730995135,29.6965890500699,2.69709247518669));
#218287=CARTESIAN_POINT('Ctrl Pts',(50.9602549766184,29.6894840070028,2.69065122242295));
#218288=CARTESIAN_POINT('Ctrl Pts',(50.9600390146967,29.6821247070257,2.68442464469445));
#218289=CARTESIAN_POINT('Ctrl Pts',(50.960124721527,29.674551656456,2.67844505923598));
#218290=CARTESIAN_POINT('Ctrl Pts',(50.960294812667,29.6595224131521,2.66657815779586));
#218291=CARTESIAN_POINT('Ctrl Pts',(50.9616539500924,29.6436502506362,2.65568445664193));
#218292=CARTESIAN_POINT('Ctrl Pts',(50.9642038006262,29.627245457377,2.64601906229534));
#218293=CARTESIAN_POINT('Ctrl Pts',(50.9661161885265,29.6149418624326,2.6387700165354));
#218294=CARTESIAN_POINT('Ctrl Pts',(50.9686983518507,29.6023386622825,2.63221189387621));
#218295=CARTESIAN_POINT('Ctrl Pts',(50.9719510035829,29.5895667656375,2.62645231033253));
#218296=CARTESIAN_POINT('Ctrl Pts',(50.9731707479825,29.5847773043957,2.62429246650365));
#218297=CARTESIAN_POINT('Ctrl Pts',(50.9744847799798,29.5799641203064,2.62224491711765));
#218298=CARTESIAN_POINT('Ctrl Pts',(50.9758931378754,29.5751341171702,2.62031533672617));
#218299=CARTESIAN_POINT('Ctrl Pts',(50.9808223905104,29.5582291061936,2.61356180535598));
#218300=CARTESIAN_POINT('Ctrl Pts',(50.9869071309995,29.5411180593589,2.60825339735368));
#218301=CARTESIAN_POINT('Ctrl Pts',(50.9941490417486,29.5240970004171,2.60463337987631));
#218302=CARTESIAN_POINT('Ctrl Pts',(50.9977699971231,29.5155864709462,2.60282337113763));
#218303=CARTESIAN_POINT('Ctrl Pts',(51.0016802459462,29.5070984389558,2.60143545939135));
#218304=CARTESIAN_POINT('Ctrl Pts',(51.005880002284,29.4986699095566,2.60050005034617));
#218305=CARTESIAN_POINT('Ctrl Pts',(51.0079798804529,29.4944556448571,2.60003234582357));
#218306=CARTESIAN_POINT('Ctrl Pts',(51.0101521355228,29.4902562558177,2.59967776696086));
#218307=CARTESIAN_POINT('Ctrl Pts',(51.0123967945051,29.4860763682213,2.5994401142918));
#218308=CARTESIAN_POINT('Ctrl Pts',(51.0146414534875,29.481896480625,2.59920246162274));
#218309=CARTESIAN_POINT('Ctrl Pts',(51.0169585178538,29.4777360953218,2.59908173791333));
#218310=CARTESIAN_POINT('Ctrl Pts',(51.0193480105327,29.473599835734,2.59908173516044));
#218311=CARTESIAN_POINT('',(51.0345602039887,29.4472515437738,2.59908173516044));
#218312=CARTESIAN_POINT('Origin',(5.71420591410065E-15,1.85888842327264E-13,
2.59908173516023));
#218313=CARTESIAN_POINT('',(51.3482501200165,29.2799753962465,2.90134173516044));
#218314=CARTESIAN_POINT('Ctrl Pts',(51.0345602039887,29.4472515437738,2.59908173516044));
#218315=CARTESIAN_POINT('Ctrl Pts',(51.0364642604675,29.4439516646701,2.59908174371532));
#218316=CARTESIAN_POINT('Ctrl Pts',(51.0384038328688,29.4406842975235,2.5991576435591));
#218317=CARTESIAN_POINT('Ctrl Pts',(51.0403770101285,29.4374505691487,2.59930765775297));
#218318=CARTESIAN_POINT('Ctrl Pts',(51.0520264994527,29.4183588813669,2.6001933302091));
#218319=CARTESIAN_POINT('Ctrl Pts',(51.0648472300456,29.4004365818765,2.60365973324178));
#218320=CARTESIAN_POINT('Ctrl Pts',(51.0784429877858,29.3839216347863,2.60934177082578));
#218321=CARTESIAN_POINT('Ctrl Pts',(51.0835219102931,29.3777522003137,2.61146439091977));
#218322=CARTESIAN_POINT('Ctrl Pts',(51.0887089685267,29.3717787490522,2.613895844294));
#218323=CARTESIAN_POINT('Ctrl Pts',(51.0939835922269,29.366012223236,2.61661604385274));
#218324=CARTESIAN_POINT('Ctrl Pts',(51.0980991182406,29.361512890515,2.61873848000797));
#218325=CARTESIAN_POINT('Ctrl Pts',(51.1022679285261,29.3571400387136,2.62103707099808));
#218326=CARTESIAN_POINT('Ctrl Pts',(51.1064802178293,29.3528993717246,2.62350262767673));
#218327=CARTESIAN_POINT('Ctrl Pts',(51.1212232303905,29.3380570372631,2.63213207605199));
#218328=CARTESIAN_POINT('Ctrl Pts',(51.1364988531343,29.3248339623429,2.64280685971935));
#218329=CARTESIAN_POINT('Ctrl Pts',(51.1518867653713,29.3134747466761,2.65513293646105));
#218330=CARTESIAN_POINT('Ctrl Pts',(51.1595807214898,29.3077951388427,2.66129597483189));
#218331=CARTESIAN_POINT('Ctrl Pts',(51.1673027515571,29.3025814967141,2.66787183533873));
#218332=CARTESIAN_POINT('Ctrl Pts',(51.1750003199401,29.2978643977776,2.67481125953882));
#218333=CARTESIAN_POINT('Ctrl Pts',(51.1826650006752,29.2931674525158,2.681721035241));
#218334=CARTESIAN_POINT('Ctrl Pts',(51.1903053811865,29.2889625693103,2.68899101329808));
#218335=CARTESIAN_POINT('Ctrl Pts',(51.1978697380629,29.2852806784151,2.69657334701294));
#218336=CARTESIAN_POINT('Ctrl Pts',(51.1979021952408,29.2852648801404,2.69660588132591));
#218337=CARTESIAN_POINT('Ctrl Pts',(51.1979346509235,29.2852490909586,2.696638420814));
#218338=CARTESIAN_POINT('Ctrl Pts',(51.1979671051091,29.285233310869,2.69667096547401));
#218339=CARTESIAN_POINT('Ctrl Pts',(51.2132718752135,29.2777917239328,2.71201840157856));
#218340=CARTESIAN_POINT('Ctrl Pts',(51.2282103130388,29.2723555974563,2.72845645939148));
#218341=CARTESIAN_POINT('Ctrl Pts',(51.2426536914386,29.2687791125366,2.7456872318657));
#218342=CARTESIAN_POINT('Ctrl Pts',(51.2576224915253,29.2650725221328,2.76354482593858));
#218343=CARTESIAN_POINT('Ctrl Pts',(51.2720604115281,29.2633635057962,2.78225519316517));
#218344=CARTESIAN_POINT('Ctrl Pts',(51.285813246636,29.2635407906071,2.80151223084747));
#218345=CARTESIAN_POINT('Ctrl Pts',(51.2993697979284,29.263715545166,2.82049442739328));
#218346=CARTESIAN_POINT('Ctrl Pts',(51.3122614394779,29.2657236711455,2.84000929088141));
#218347=CARTESIAN_POINT('Ctrl Pts',(51.3243180878342,29.2695013892367,2.85976644340326));
#218348=CARTESIAN_POINT('Ctrl Pts',(51.3327241975802,29.2721352815031,2.87354148166084));
#218349=CARTESIAN_POINT('Ctrl Pts',(51.3407239614222,29.2756302808574,2.88743438345066));
#218350=CARTESIAN_POINT('Ctrl Pts',(51.3482501200165,29.2799753962465,2.90134173516044));
#218351=CARTESIAN_POINT('',(51.6568155675427,29.4581217525676,3.47153072139093));
#218352=CARTESIAN_POINT('',(51.3482501200165,29.2799753962465,2.90134173516044));
#218353=CARTESIAN_POINT('',(54.1952354911872,24.4761921430395,3.4715307213909));
#218354=CARTESIAN_POINT('Origin',(5.53234440788222E-15,1.85015204418142E-13,
3.47153072139072));
#218355=CARTESIAN_POINT('',(53.8697418420145,24.3312692531091,2.90134173516041));
#218356=CARTESIAN_POINT('',(54.1952354911872,24.4761921430394,3.4715307213909));
#218357=CARTESIAN_POINT('',(53.8206887816836,23.9791663275016,2.5990817351604));
#218358=CARTESIAN_POINT('Ctrl Pts',(53.8697418420145,24.3312692531091,2.90134173516041));
#218359=CARTESIAN_POINT('Ctrl Pts',(53.8585692765374,24.3262947497599,2.88176998919737));
#218360=CARTESIAN_POINT('Ctrl Pts',(53.8482286480022,24.3195865685231,2.86226752356569));
#218361=CARTESIAN_POINT('Ctrl Pts',(53.838840992916,24.311280732007,2.84310370499783));
#218362=CARTESIAN_POINT('Ctrl Pts',(53.8292837624968,24.3028248617519,2.82359371788356));
#218363=CARTESIAN_POINT('Ctrl Pts',(53.820713385011,24.2927127498343,2.80443322636636));
#218364=CARTESIAN_POINT('Ctrl Pts',(53.8132717929024,24.2810366186963,2.78589323877841));
#218365=CARTESIAN_POINT('Ctrl Pts',(53.8061452585096,24.2698548246775,2.76813818619556));
#218366=CARTESIAN_POINT('Ctrl Pts',(53.800053401299,24.2572379736549,2.75095095198253));
#218367=CARTESIAN_POINT('Ctrl Pts',(53.7951438030538,24.2432286115624,2.73457771434643));
#218368=CARTESIAN_POINT('Ctrl Pts',(53.7912388700582,24.2320860256417,2.72155497955279));
#218369=CARTESIAN_POINT('Ctrl Pts',(53.788082147831,24.2200617420577,2.70904711159829));
#218370=CARTESIAN_POINT('Ctrl Pts',(53.7857624469883,24.2071623814825,2.69718956158356));
#218371=CARTESIAN_POINT('Ctrl Pts',(53.7857561149585,24.2071271704182,2.69715719432374));
#218372=CARTESIAN_POINT('Ctrl Pts',(53.7857497893137,24.2070919529318,2.69712483219039));
#218373=CARTESIAN_POINT('Ctrl Pts',(53.7857434700555,24.2070567290244,2.69709247518667));
#218374=CARTESIAN_POINT('Ctrl Pts',(53.7844855062586,24.2000447667167,2.69065122242293));
#218375=CARTESIAN_POINT('Ctrl Pts',(53.7835014710816,24.1927483559227,2.68442464469441));
#218376=CARTESIAN_POINT('Ctrl Pts',(53.7827951090625,24.1852078325131,2.67844505923594));
#218377=CARTESIAN_POINT('Ctrl Pts',(53.7813932847188,24.1702431416111,2.66657815779583));
#218378=CARTESIAN_POINT('Ctrl Pts',(53.7810858838907,24.1543158599158,2.6556844566419));
#218379=CARTESIAN_POINT('Ctrl Pts',(53.7819069982469,24.1377344018726,2.64601906229531));
#218380=CARTESIAN_POINT('Ctrl Pts',(53.782522834014,24.1252983083403,2.63877001653537));
#218381=CARTESIAN_POINT('Ctrl Pts',(53.7837734588334,24.1124942402751,2.63221189387617));
#218382=CARTESIAN_POINT('Ctrl Pts',(53.7856732654698,24.0994523147292,2.62645231033249));
#218383=CARTESIAN_POINT('Ctrl Pts',(53.7863856929584,24.0945615926495,2.62429246650361));
#218384=CARTESIAN_POINT('Ctrl Pts',(53.7871894118146,24.089637421941,2.62224491711761));
#218385=CARTESIAN_POINT('Ctrl Pts',(53.788085181773,24.0846866645808,2.62031533672613));
#218386=CARTESIAN_POINT('Ctrl Pts',(53.7912203766273,24.06735901382,2.61356180535594));
#218387=CARTESIAN_POINT('Ctrl Pts',(53.7954831928409,24.0497056745176,2.60825339735364));
#218388=CARTESIAN_POINT('Ctrl Pts',(53.8009062465108,24.0320208729158,2.60463337987627));
#218389=CARTESIAN_POINT('Ctrl Pts',(53.8036177733457,24.023178472115,2.60282337113758));
#218390=CARTESIAN_POINT('Ctrl Pts',(53.8066193604764,24.0143282061515,2.60143545939131));
#218391=CARTESIAN_POINT('Ctrl Pts',(53.8099150888839,24.0055068550422,2.60050005034612));
#218392=CARTESIAN_POINT('Ctrl Pts',(53.8115629530876,24.0010961794876,2.60003234582353));
#218393=CARTESIAN_POINT('Ctrl Pts',(53.813284352634,23.9966927326565,2.59967776696082));
#218394=CARTESIAN_POINT('Ctrl Pts',(53.8150797979125,23.9923011121677,2.59944011429176));
#218395=CARTESIAN_POINT('Ctrl Pts',(53.816875243191,23.987909491679,2.5992024616227));
#218396=CARTESIAN_POINT('Ctrl Pts',(53.818744735754,23.9835296982243,2.59908173791327));
#218397=CARTESIAN_POINT('Ctrl Pts',(53.8206887816836,23.9791663275016,2.59908173516041));
#218398=CARTESIAN_POINT('',(53.8330634946837,23.9513722670367,2.5990817351604));
#218399=CARTESIAN_POINT('Origin',(5.71744365443249E-15,1.85882487904075E-13,
2.59908173516024));
#218400=CARTESIAN_POINT('',(54.1275498658873,23.752222950883,2.9013417351604));
#218401=CARTESIAN_POINT('Ctrl Pts',(53.8330634946837,23.9513722670367,2.59908173516041));
#218402=CARTESIAN_POINT('Ctrl Pts',(53.8346121892503,23.9478914369184,2.59908174371528));
#218403=CARTESIAN_POINT('Ctrl Pts',(53.8361996036043,23.9444392282283,2.59915764355907));
#218404=CARTESIAN_POINT('Ctrl Pts',(53.8378239549348,23.9410169613692,2.59930765775294));
#218405=CARTESIAN_POINT('Ctrl Pts',(53.8474140023518,23.9208121566354,2.600193330209));
#218406=CARTESIAN_POINT('Ctrl Pts',(53.8582911092161,23.9016479061115,2.60365973324117));
#218407=CARTESIAN_POINT('Ctrl Pts',(53.8700861059314,23.8838022859672,2.60934177082432));
#218408=CARTESIAN_POINT('Ctrl Pts',(53.874492324066,23.8771357563359,2.61146439091865));
#218409=CARTESIAN_POINT('Ctrl Pts',(53.8790265713722,23.8706528330379,2.61389584429335));
#218410=CARTESIAN_POINT('Ctrl Pts',(53.8836695340509,23.8643665485424,2.61661604385269));
#218411=CARTESIAN_POINT('Ctrl Pts',(53.8872922064474,23.8594616740271,2.61873848000792));
#218412=CARTESIAN_POINT('Ctrl Pts',(53.8909810920751,23.8546770178326,2.62103707099804));
#218413=CARTESIAN_POINT('Ctrl Pts',(53.8947270356132,23.8500192775333,2.62350262767669));
#218414=CARTESIAN_POINT('Ctrl Pts',(53.9078378379965,23.8337171864861,2.63213207605195));
#218415=CARTESIAN_POINT('Ctrl Pts',(53.9216475915795,23.818969811583,2.6428068597193));
#218416=CARTESIAN_POINT('Ctrl Pts',(53.9357638458656,23.806064348069,2.655132936461));
#218417=CARTESIAN_POINT('Ctrl Pts',(53.9428219730086,23.7996116163121,2.66129597483185));
#218418=CARTESIAN_POINT('Ctrl Pts',(53.9499567269876,23.7936193631243,2.66787183533868));
#218419=CARTESIAN_POINT('Ctrl Pts',(53.9571190561826,23.7881234899554,2.67481125953877));
#218420=CARTESIAN_POINT('Ctrl Pts',(53.9642507845244,23.7826510977526,2.68172103524096));
#218421=CARTESIAN_POINT('Ctrl Pts',(53.9714097802521,23.7776706121036,2.68899101329806));
#218422=CARTESIAN_POINT('Ctrl Pts',(53.9785478363929,23.773218200392,2.69657334701291));
#218423=CARTESIAN_POINT('Ctrl Pts',(53.9785784643976,23.773199095963,2.69660588132589));
#218424=CARTESIAN_POINT('Ctrl Pts',(53.9786090918658,23.7731800007334,2.69663842081398));
#218425=CARTESIAN_POINT('Ctrl Pts',(53.9786397187954,23.7731609147026,2.69667096547398));
#218426=CARTESIAN_POINT('Ctrl Pts',(53.9930827901208,23.7641603094588,2.71201840157812));
#218427=CARTESIAN_POINT('Ctrl Pts',(54.0073711636735,23.7571924707026,2.72845645939056));
#218428=CARTESIAN_POINT('Ctrl Pts',(54.0213615752623,23.7521258339931,2.74568723186427));
#218429=CARTESIAN_POINT('Ctrl Pts',(54.0358609304966,23.7468748830093,2.76354482593661));
#218430=CARTESIAN_POINT('Ctrl Pts',(54.0500411172113,23.7436660552523,2.78225519316262));
#218431=CARTESIAN_POINT('Ctrl Pts',(54.0637371441579,23.7424048061589,2.80151223084434));
#218432=CARTESIAN_POINT('Ctrl Pts',(54.0772376980691,23.74116155792,2.82049442738965));
#218433=CARTESIAN_POINT('Ctrl Pts',(54.0902686241798,23.7418111396949,2.84000929087727));
#218434=CARTESIAN_POINT('Ctrl Pts',(54.1026541040215,23.7443079001259,2.85976644339863));
#218435=CARTESIAN_POINT('Ctrl Pts',(54.1112894809308,23.746048685921,2.87354148165772));
#218436=CARTESIAN_POINT('Ctrl Pts',(54.1196107481421,23.7486883362824,2.88743438344908));
#218437=CARTESIAN_POINT('Ctrl Pts',(54.1275498658873,23.752222950883,2.9013417351604));
#218438=CARTESIAN_POINT('',(54.4530463244692,23.8971395307771,3.47153072139089));
#218439=CARTESIAN_POINT('',(54.1275498658873,23.752222950883,2.9013417351604));
#218440=CARTESIAN_POINT('',(56.4568070719811,18.6771643191712,3.47153072139086));
#218441=CARTESIAN_POINT('Origin',(5.53234440788222E-15,1.85015204418142E-13,
3.47153072139072));
#218442=CARTESIAN_POINT('',(56.1179479440988,18.5670586829468,2.90134173516037));
#218443=CARTESIAN_POINT('',(56.4568070719811,18.6771643191712,3.47153072139086));
#218444=CARTESIAN_POINT('',(56.0323588238391,18.2220120550219,2.59908173516037));
#218445=CARTESIAN_POINT('Ctrl Pts',(56.1179479440988,18.5670586829468,2.90134173516037));
#218446=CARTESIAN_POINT('Ctrl Pts',(56.1063166059132,18.5632792815473,2.88176998919632));
#218447=CARTESIAN_POINT('Ctrl Pts',(56.0953314285466,18.5576887384388,2.86226752356364));
#218448=CARTESIAN_POINT('Ctrl Pts',(56.0851270036896,18.5504096793235,2.84310370499483));
#218449=CARTESIAN_POINT('Ctrl Pts',(56.0747382496548,18.5429991338186,2.82359371787964));
#218450=CARTESIAN_POINT('Ctrl Pts',(56.0651578180741,18.5338382654957,2.80443322636156));
#218451=CARTESIAN_POINT('Ctrl Pts',(56.0565365037408,18.5230039556123,2.78589323877282));
#218452=CARTESIAN_POINT('Ctrl Pts',(56.0482801935035,18.5126283423189,2.76813818618936));
#218453=CARTESIAN_POINT('Ctrl Pts',(56.0409028880753,18.5007173801981,2.75095095197577));
#218454=CARTESIAN_POINT('Ctrl Pts',(56.0345558080321,18.4872979556158,2.73457771433922));
#218455=CARTESIAN_POINT('Ctrl Pts',(56.0295075492861,18.4766245865935,2.72155497954816));
#218456=CARTESIAN_POINT('Ctrl Pts',(56.0251112400296,18.4649961406184,2.70904711159607));
#218457=CARTESIAN_POINT('Ctrl Pts',(56.0214558964134,18.4524099188568,2.69718956158351));
#218458=CARTESIAN_POINT('Ctrl Pts',(56.0214459185126,18.4523755625597,2.69715719432368));
#218459=CARTESIAN_POINT('Ctrl Pts',(56.0214359462907,18.4523411992083,2.69712483219034));
#218460=CARTESIAN_POINT('Ctrl Pts',(56.0214259797492,18.4523068288036,2.69709247518662));
#218461=CARTESIAN_POINT('Ctrl Pts',(56.019441957565,18.4454647717816,2.69065122242288));
#218462=CARTESIAN_POINT('Ctrl Pts',(56.017700630428,18.4383111911741,2.68442464469438));
#218463=CARTESIAN_POINT('Ctrl Pts',(56.0162099386098,18.4308858104772,2.67844505923591));
#218464=CARTESIAN_POINT('Ctrl Pts',(56.0132515574632,18.4161496282621,2.66657815779579));
#218465=CARTESIAN_POINT('Ctrl Pts',(56.0112809863294,18.4003417300186,2.65568445664185));
#218466=CARTESIAN_POINT('Ctrl Pts',(56.0103643682072,18.3837652771157,2.64601906229527));
#218467=CARTESIAN_POINT('Ctrl Pts',(56.0096769046155,18.3713329374386,2.63877001653533));
#218468=CARTESIAN_POINT('Ctrl Pts',(56.0095822888229,18.3584682855075,2.63221189387613));
#218469=CARTESIAN_POINT('Ctrl Pts',(56.0101084356844,18.3452992211262,2.62645231033245));
#218470=CARTESIAN_POINT('Ctrl Pts',(56.0103057407575,18.3403608219831,2.62429246650357));
#218471=CARTESIAN_POINT('Ctrl Pts',(56.0105903407606,18.3353796149,2.62224491711757));
#218472=CARTESIAN_POINT('Ctrl Pts',(56.0109637085386,18.3303623448494,2.62031533672609));
#218473=CARTESIAN_POINT('Ctrl Pts',(56.0122704957614,18.3128018996724,2.6135618053559));
#218474=CARTESIAN_POINT('Ctrl Pts',(56.0146646833929,18.2947996815818,2.60825339735361));
#218475=CARTESIAN_POINT('Ctrl Pts',(56.0182094638727,18.2766448957073,2.60463337987624));
#218476=CARTESIAN_POINT('Ctrl Pts',(56.0199818541126,18.2675675027701,2.60282337113756));
#218477=CARTESIAN_POINT('Ctrl Pts',(56.0220418935343,18.2584519681994,2.60143545939127));
#218478=CARTESIAN_POINT('Ctrl Pts',(56.0243974853213,18.2493344439487,2.60050005034609));
#218479=CARTESIAN_POINT('Ctrl Pts',(56.0255752812149,18.2447756818233,2.6000323458235));
#218480=CARTESIAN_POINT('Ctrl Pts',(56.0268269652241,18.2402164222855,2.59967776696078));
#218481=CARTESIAN_POINT('Ctrl Pts',(56.0281535255245,18.2356611844174,2.59944011429172));
#218482=CARTESIAN_POINT('Ctrl Pts',(56.029480085825,18.2311059465494,2.59920246162266));
#218483=CARTESIAN_POINT('Ctrl Pts',(56.0308815240328,18.2265547308768,2.59908173791323));
#218484=CARTESIAN_POINT('Ctrl Pts',(56.0323588238391,18.2220120550219,2.59908173516037));
#218485=CARTESIAN_POINT('',(56.0417604764383,18.1930767435952,2.59908173516037));
#218486=CARTESIAN_POINT('Origin',(5.71999943999309E-15,1.85875829855059E-13,
2.59908173516024));
#218487=CARTESIAN_POINT('',(56.3138168485095,17.9642361803975,2.90134173516037));
#218488=CARTESIAN_POINT('Ctrl Pts',(56.0417604764383,18.1930767435951,2.59908173516037));
#218489=CARTESIAN_POINT('Ctrl Pts',(56.0429368412708,18.1894530991653,2.59908174371526));
#218490=CARTESIAN_POINT('Ctrl Pts',(56.0441547055336,18.1858538720526,2.59915764355904));
#218491=CARTESIAN_POINT('Ctrl Pts',(56.0454124342019,18.1822805617811,2.5993076577529));
#218492=CARTESIAN_POINT('Ctrl Pts',(56.0528379691459,18.1611840081634,2.60019333020892));
#218493=CARTESIAN_POINT('Ctrl Pts',(56.0616522804234,18.1409877741446,2.60365973324084));
#218494=CARTESIAN_POINT('Ctrl Pts',(56.0715172876624,18.1220070012944,2.60934177082357));
#218495=CARTESIAN_POINT('Ctrl Pts',(56.0752025259757,18.1149164163987,2.61146439091806));
#218496=CARTESIAN_POINT('Ctrl Pts',(56.0790342841913,18.107995049329,2.61389584429301));
#218497=CARTESIAN_POINT('Ctrl Pts',(56.0829947165771,18.1012578800032,2.61661604385265));
#218498=CARTESIAN_POINT('Ctrl Pts',(56.0860848445996,18.0960012025252,2.61873848000788));
#218499=CARTESIAN_POINT('Ctrl Pts',(56.0892533893666,18.090857163632,2.621037070998));
#218500=CARTESIAN_POINT('Ctrl Pts',(56.0924919457982,18.0858333812,2.62350262767665));
#218501=CARTESIAN_POINT('Ctrl Pts',(56.103826893309,18.0682501426879,2.63213207605191));
#218502=CARTESIAN_POINT('Ctrl Pts',(56.1160194751811,18.0521400431274,2.64280685971927));
#218503=CARTESIAN_POINT('Ctrl Pts',(56.1287094108803,18.0378297267253,2.65513293646097));
#218504=CARTESIAN_POINT('Ctrl Pts',(56.13505437873,18.0306745685242,2.66129597483182));
#218505=CARTESIAN_POINT('Ctrl Pts',(56.1415236867628,18.0239693566572,2.66787183533864));
#218506=CARTESIAN_POINT('Ctrl Pts',(56.1480723047925,18.0177549231924,2.67481125953873));
#218507=CARTESIAN_POINT('Ctrl Pts',(56.1545929440329,18.0115670407226,2.68172103524091));
#218508=CARTESIAN_POINT('Ctrl Pts',(56.1611921195217,18.0058655198732,2.68899101329801));
#218509=CARTESIAN_POINT('Ctrl Pts',(56.1678256688901,18.0006913688997,2.69657334701286));
#218510=CARTESIAN_POINT('Ctrl Pts',(56.1678541321547,18.0006691676285,2.69660588132584));
#218511=CARTESIAN_POINT('Ctrl Pts',(56.1678825958474,18.0006469755623,2.69663842081393));
#218512=CARTESIAN_POINT('Ctrl Pts',(56.1679110599661,18.000624792701,2.69667096547393));
#218513=CARTESIAN_POINT('Ctrl Pts',(56.1813341912022,17.990163781663,2.71201840157953));
#218514=CARTESIAN_POINT('Ctrl Pts',(56.1948159540733,17.9817405717259,2.72845645939364));
#218515=CARTESIAN_POINT('Ctrl Pts',(56.2082001169757,17.9752392943583,2.74568723186914));
#218516=CARTESIAN_POINT('Ctrl Pts',(56.2220711693892,17.9685015133122,2.76354482594343));
#218517=CARTESIAN_POINT('Ctrl Pts',(56.2358382617244,17.9638280307234,2.78225519317152));
#218518=CARTESIAN_POINT('Ctrl Pts',(56.2493274239741,17.9611420662354,2.80151223085537));
#218519=CARTESIAN_POINT('Ctrl Pts',(56.2626240656117,17.9584944364873,2.82049442740277));
#218520=CARTESIAN_POINT('Ctrl Pts',(56.2756515067316,17.9577783571049,2.84000929089254));
#218521=CARTESIAN_POINT('Ctrl Pts',(56.2882301201508,17.9589668048475,2.859766443416));
#218522=CARTESIAN_POINT('Ctrl Pts',(56.297000153222,17.9597954117583,2.87354148166938));
#218523=CARTESIAN_POINT('Ctrl Pts',(56.3055517542529,17.9615507925644,2.8874343834549));
#218524=CARTESIAN_POINT('Ctrl Pts',(56.3138168485095,17.9642361803975,2.90134173516036));
#218525=CARTESIAN_POINT('',(56.6526781108323,18.0743352474894,3.47153072139086));
#218526=CARTESIAN_POINT('',(56.3138168485095,17.9642361803975,2.90134173516037));
#218527=CARTESIAN_POINT('',(58.099826060148,12.6735055745743,3.47153072139082));
#218528=CARTESIAN_POINT('Origin',(5.53234440788222E-15,1.85015204418142E-13,
3.47153072139072));
#218529=CARTESIAN_POINT('',(57.751314065072,12.5994235324474,2.90134173516033));
#218530=CARTESIAN_POINT('',(58.099826060148,12.6735055745743,3.47153072139082));
#218531=CARTESIAN_POINT('',(57.6301266171957,12.2652136052663,2.59908173516032));
#218532=CARTESIAN_POINT('Ctrl Pts',(57.751314065072,12.5994235324474,2.90134173516032));
#218533=CARTESIAN_POINT('Ctrl Pts',(57.739351389555,12.596880640911,2.88176998919846));
#218534=CARTESIAN_POINT('Ctrl Pts',(57.7278420192606,12.5924689870922,2.86226752356795));
#218535=CARTESIAN_POINT('Ctrl Pts',(57.7169326264483,12.5862964562743,2.8431037050012));
#218536=CARTESIAN_POINT('Ctrl Pts',(57.7058261701626,12.5800124270087,2.82359371788796));
#218537=CARTESIAN_POINT('Ctrl Pts',(57.6953406497014,12.5719031706729,2.80443322637173));
#218538=CARTESIAN_POINT('Ctrl Pts',(57.685634070068,12.562029385013,2.78589323878465));
#218539=CARTESIAN_POINT('Ctrl Pts',(57.6763384418496,12.5525736298376,2.76813818620248));
#218540=CARTESIAN_POINT('Ctrl Pts',(57.6677565155063,12.5414990556149,2.75095095199004));
#218541=CARTESIAN_POINT('Ctrl Pts',(57.6600414936023,12.5288165945697,2.73457771435441));
#218542=CARTESIAN_POINT('Ctrl Pts',(57.6539052188813,12.5187293821054,2.72155497955787));
#218543=CARTESIAN_POINT('Ctrl Pts',(57.6483174894765,12.5076241774207,2.70904711160065));
#218544=CARTESIAN_POINT('Ctrl Pts',(57.643366551794,12.495488991745,2.69718956158348));
#218545=CARTESIAN_POINT('Ctrl Pts',(57.6433530373424,12.49545586663,2.69715719432365));
#218546=CARTESIAN_POINT('Ctrl Pts',(57.643339527801,12.4954227339057,2.69712483219031));
#218547=CARTESIAN_POINT('Ctrl Pts',(57.6433260231716,12.4953895935729,2.69709247518659));
#218548=CARTESIAN_POINT('Ctrl Pts',(57.6406376799625,12.4887924048451,2.69065122242284));
#218549=CARTESIAN_POINT('Ctrl Pts',(57.63815813921,12.4818600305504,2.68442464469433));
#218550=CARTESIAN_POINT('Ctrl Pts',(57.6358994499241,12.4746311465908,2.67844505923586));
#218551=CARTESIAN_POINT('Ctrl Pts',(57.6314169246176,12.4602849257588,2.66657815779574));
#218552=CARTESIAN_POINT('Ctrl Pts',(57.6278047731677,12.4447696056082,2.65568445664181));
#218553=CARTESIAN_POINT('Ctrl Pts',(57.6251604652272,12.4283797729325,2.64601906229522));
#218554=CARTESIAN_POINT('Ctrl Pts',(57.6231772342717,12.4160873984258,2.63877001653528));
#218555=CARTESIAN_POINT('Ctrl Pts',(57.6217384144975,12.4033031104474,2.63221189387609));
#218556=CARTESIAN_POINT('Ctrl Pts',(57.620885137009,12.3901511902558,2.62645231033241));
#218557=CARTESIAN_POINT('Ctrl Pts',(57.6205651579508,12.3852192201839,2.62429246650353));
#218558=CARTESIAN_POINT('Ctrl Pts',(57.6203275209637,12.3802355518734,2.62224491711753));
#218559=CARTESIAN_POINT('Ctrl Pts',(57.6201743958657,12.375206739393,2.62031533672604));
#218560=CARTESIAN_POINT('Ctrl Pts',(57.6196384580227,12.3576058957119,2.61356180535586));
#218561=CARTESIAN_POINT('Ctrl Pts',(57.6201377858514,12.3394520349016,2.60825339735356));
#218562=CARTESIAN_POINT('Ctrl Pts',(57.6217654557845,12.3210261723876,2.60463337987619));
#218563=CARTESIAN_POINT('Ctrl Pts',(57.622579290751,12.3118132411305,2.6028233711375));
#218564=CARTESIAN_POINT('Ctrl Pts',(57.6236752122407,12.302532309657,2.60143545939122));
#218565=CARTESIAN_POINT('Ctrl Pts',(57.6250648590507,12.2932185057685,2.60050005034604));
#218566=CARTESIAN_POINT('Ctrl Pts',(57.6257596824557,12.2885616038243,2.60003234582344));
#218567=CARTESIAN_POINT('Ctrl Pts',(57.6265279372158,12.2838964837812,2.59967776696074));
#218568=CARTESIAN_POINT('Ctrl Pts',(57.627371078466,12.2792275366732,2.59944011429168));
#218569=CARTESIAN_POINT('Ctrl Pts',(57.6282142197161,12.2745585895652,2.59920246162262));
#218570=CARTESIAN_POINT('Ctrl Pts',(57.6291322491186,12.2698858157461,2.5990817379132));
#218571=CARTESIAN_POINT('Ctrl Pts',(57.6301266171957,12.2652136052663,2.59908173516033));
#218572=CARTESIAN_POINT('',(57.6364522029207,12.2354540642047,2.59908173516032));
#218573=CARTESIAN_POINT('Origin',(5.72184526906101E-15,1.85868941127195E-13,
2.59908173516024));
#218574=CARTESIAN_POINT('',(57.8830978693156,11.9794294790614,2.90134173516032));
#218575=CARTESIAN_POINT('Ctrl Pts',(57.6364522029207,12.2354540642047,2.59908173516033));
#218576=CARTESIAN_POINT('Ctrl Pts',(57.6372433495199,12.2317273068699,2.59908174371527));
#218577=CARTESIAN_POINT('Ctrl Pts',(57.6380783205158,12.2280204952201,2.59915764355899));
#218578=CARTESIAN_POINT('Ctrl Pts',(57.6389556465834,12.2243352914713,2.59930765775286));
#218579=CARTESIAN_POINT('Ctrl Pts',(57.6441353133405,12.2025781272235,2.60019333020894));
#218580=CARTESIAN_POINT('Ctrl Pts',(57.6507902575933,12.1815711838737,2.6036597332413));
#218581=CARTESIAN_POINT('Ctrl Pts',(57.6586171922735,12.1616632156351,2.60934177082476));
#218582=CARTESIAN_POINT('Ctrl Pts',(57.6615410745225,12.1542262614092,2.61146439091896));
#218583=CARTESIAN_POINT('Ctrl Pts',(57.6646283621015,12.146942282516,2.61389584429349));
#218584=CARTESIAN_POINT('Ctrl Pts',(57.6678628728673,12.1398280421989,2.6166160438526));
#218585=CARTESIAN_POINT('Ctrl Pts',(57.6703866004265,12.1342771550166,2.61873848000783));
#218586=CARTESIAN_POINT('Ctrl Pts',(57.6730000890932,12.1288300925915,2.62103707099796));
#218587=CARTESIAN_POINT('Ctrl Pts',(57.6756957761165,12.1234953096383,2.62350262767661));
#218588=CARTESIAN_POINT('Ctrl Pts',(57.6851306806979,12.104823569302,2.63213207605187));
#218589=CARTESIAN_POINT('Ctrl Pts',(57.6955725063806,12.0875272507062,2.64280685971922));
#218590=CARTESIAN_POINT('Ctrl Pts',(57.7066970899019,12.071968868237,2.65513293646092));
#218591=CARTESIAN_POINT('Ctrl Pts',(57.7122593816626,12.0641896770024,2.66129597483177));
#218592=CARTESIAN_POINT('Ctrl Pts',(57.7179923646568,12.0568449701605,2.6678718353386));
#218593=CARTESIAN_POINT('Ctrl Pts',(57.7238555234916,12.0499800630333,2.67481125953869));
#218594=CARTESIAN_POINT('Ctrl Pts',(57.7296936321425,12.0431444860318,2.68172103524088));
#218595=CARTESIAN_POINT('Ctrl Pts',(57.7356606854448,12.0367843970375,2.68899101329797));
#218596=CARTESIAN_POINT('Ctrl Pts',(57.7417170494857,12.0309451958829,2.69657334701283));
#218597=CARTESIAN_POINT('Ctrl Pts',(57.7417430361608,12.0309201410113,2.6966058813258));
#218598=CARTESIAN_POINT('Ctrl Pts',(57.7417690242238,12.0308950952495,2.69663842081389));
#218599=CARTESIAN_POINT('Ctrl Pts',(57.7417950136727,12.0308700585976,2.69667096547389));
#218600=CARTESIAN_POINT('Ctrl Pts',(57.7540511381823,12.0190632547933,2.71201840157817));
#218601=CARTESIAN_POINT('Ctrl Pts',(57.7665785813542,12.0092769601272,2.72845645939077));
#218602=CARTESIAN_POINT('Ctrl Pts',(57.7792098558781,12.0014122714574,2.74568723186465));
#218603=CARTESIAN_POINT('Ctrl Pts',(57.7923006313156,11.9932614808885,2.76354482593735));
#218604=CARTESIAN_POINT('Ctrl Pts',(57.8055037941242,11.9871745471209,2.78225519316374));
#218605=CARTESIAN_POINT('Ctrl Pts',(57.8186383015904,11.9830932952263,2.80151223084585));
#218606=CARTESIAN_POINT('Ctrl Pts',(57.8315853501642,11.9790702919537,2.82049442739185));
#218607=CARTESIAN_POINT('Ctrl Pts',(57.8444665749203,11.9769963969278,2.84000929088019));
#218608=CARTESIAN_POINT('Ctrl Pts',(57.8571005079945,11.9768635110977,2.85976644340226));
#218609=CARTESIAN_POINT('Ctrl Pts',(57.865909110917,11.9767708607326,2.87354148166013));
#218610=CARTESIAN_POINT('Ctrl Pts',(57.8745973526438,11.9776227396647,2.88743438345024));
#218611=CARTESIAN_POINT('Ctrl Pts',(57.8830978693156,11.9794294790614,2.90134173516032));
#218612=CARTESIAN_POINT('',(58.2316113004781,12.0535047649324,3.47153072139081));
#218613=CARTESIAN_POINT('',(57.8830978693156,11.9794294790614,2.90134173516032));
#218614=CARTESIAN_POINT('',(59.1062911958296,6.53099325080074,3.47153072139077));
#218615=CARTESIAN_POINT('Origin',(5.53234440788222E-15,1.85015204418142E-13,
3.47153072139072));
#218616=CARTESIAN_POINT('',(58.7519447039088,6.49374646112759,2.90134173516028));
#218617=CARTESIAN_POINT('',(59.1062911958296,6.53099325080074,3.47153072139077));
#218618=CARTESIAN_POINT('',(58.5964866834551,6.17403490859039,2.59908173516028));
#218619=CARTESIAN_POINT('Ctrl Pts',(58.7519447039088,6.49374646112759,2.90134173516028));
#218620=CARTESIAN_POINT('Ctrl Pts',(58.7397817566352,6.49246793990547,2.88176998919804));
#218621=CARTESIAN_POINT('Ctrl Pts',(58.7278742924811,6.48928351037784,2.86226752356716));
#218622=CARTESIAN_POINT('Ctrl Pts',(58.7163794573031,6.48428513539526,2.84310370500006));
#218623=CARTESIAN_POINT('Ctrl Pts',(58.7046769834245,6.47919647150722,2.82359371788643));
#218624=CARTESIAN_POINT('Ctrl Pts',(58.6934012556383,6.47222767386629,2.80443322636984));
#218625=CARTESIAN_POINT('Ctrl Pts',(58.6827157580219,6.46342259168963,2.78589323878244));
#218626=CARTESIAN_POINT('Ctrl Pts',(58.6724826566698,6.45499029386298,2.76813818619996));
#218627=CARTESIAN_POINT('Ctrl Pts',(58.662790134792,6.44487344288875,2.75095095198725));
#218628=CARTESIAN_POINT('Ctrl Pts',(58.6537916984216,6.43306689707541,2.73457771435139));
#218629=CARTESIAN_POINT('Ctrl Pts',(58.6466346380387,6.42367635878376,2.72155497955592));
#218630=CARTESIAN_POINT('Ctrl Pts',(58.6399167088208,6.41321606634085,2.7090471115997));
#218631=CARTESIAN_POINT('Ctrl Pts',(58.6337244205833,6.40166487239056,2.69718956158343));
#218632=CARTESIAN_POINT('Ctrl Pts',(58.6337075176479,6.40163334138328,2.6971571943236));
#218633=CARTESIAN_POINT('Ctrl Pts',(58.6336906188004,6.40160180229503,2.69712483219026));
#218634=CARTESIAN_POINT('Ctrl Pts',(58.6336737240427,6.4015702551266,2.69709247518654));
#218635=CARTESIAN_POINT('Ctrl Pts',(58.6303105138594,6.39529021487339,2.69065122242279));
#218636=CARTESIAN_POINT('Ctrl Pts',(58.6271199258587,6.3886549994349,2.6844246446943));
#218637=CARTESIAN_POINT('Ctrl Pts',(58.6241179857776,6.38170181337803,2.67844505923582));
#218638=CARTESIAN_POINT('Ctrl Pts',(58.6181604277966,6.36790273412668,2.66657815779571));
#218639=CARTESIAN_POINT('Ctrl Pts',(58.6129462715178,6.3528499811634,2.65568445664178));
#218640=CARTESIAN_POINT('Ctrl Pts',(58.60860324535,6.33682633915144,2.6460190622952));
#218641=CARTESIAN_POINT('Ctrl Pts',(58.6053459757242,6.32480860764248,2.63877001653526));
#218642=CARTESIAN_POINT('Ctrl Pts',(58.6025787159788,6.31224475095124,2.63221189387606));
#218643=CARTESIAN_POINT('Ctrl Pts',(58.600355362827,6.29925407013909,2.62645231033238));
#218644=CARTESIAN_POINT('Ctrl Pts',(58.5995216053951,6.29438256483454,2.6242924665035));
#218645=CARTESIAN_POINT('Ctrl Pts',(58.5987643350184,6.28945103740957,2.6222449171175));
#218646=CARTESIAN_POINT('Ctrl Pts',(58.5980863947151,6.28446577922136,2.62031533672602));
#218647=CARTESIAN_POINT('Ctrl Pts',(58.5957136036535,6.26701737556262,2.61356180535583));
#218648=CARTESIAN_POINT('Ctrl Pts',(58.5943126009392,6.24891076953075,2.60825339735352));
#218649=CARTESIAN_POINT('Ctrl Pts',(58.5940053272331,6.23041570798264,2.60463337987615));
#218650=CARTESIAN_POINT('Ctrl Pts',(58.59385169038,6.22116817720859,2.60282337113747));
#218651=CARTESIAN_POINT('Ctrl Pts',(58.5939714867925,6.21182353265962,2.60143545939119));
#218652=CARTESIAN_POINT('Ctrl Pts',(58.5943799633642,6.20241549311782,2.600500050346));
#218653=CARTESIAN_POINT('Ctrl Pts',(58.5945842016501,6.19771147334691,2.60003234582341));
#218654=CARTESIAN_POINT('Ctrl Pts',(58.5948606100012,6.19299160483011,2.5996777669607));
#218655=CARTESIAN_POINT('Ctrl Pts',(58.5952110945691,6.18826010244367,2.59944011429164));
#218656=CARTESIAN_POINT('Ctrl Pts',(58.595561579137,6.18352860005724,2.59920246162258));
#218657=CARTESIAN_POINT('Ctrl Pts',(58.5959861416118,6.17878546397932,2.59908173791315));
#218658=CARTESIAN_POINT('Ctrl Pts',(58.5964866834551,6.17403490859039,2.59908173516029));
#218659=CARTESIAN_POINT('',(58.5996668978648,6.14377718965341,2.59908173516028));
#218660=CARTESIAN_POINT('Origin',(5.72296091834672E-15,1.85861897194828E-13,
2.59908173516023));
#218661=CARTESIAN_POINT('',(58.8181995570485,5.86337364149599,2.90134173516027));
#218662=CARTESIAN_POINT('Ctrl Pts',(58.5996668978648,6.14377718965341,2.59908173516029));
#218663=CARTESIAN_POINT('Ctrl Pts',(58.600064158263,6.13998815054705,2.59908174371518));
#218664=CARTESIAN_POINT('Ctrl Pts',(58.6005070878751,6.13621436696423,2.59915764355894));
#218665=CARTESIAN_POINT('Ctrl Pts',(58.6009943991739,6.13245764560146,2.5993076577528));
#218666=CARTESIAN_POINT('Ctrl Pts',(58.6038714482307,6.11027824676951,2.60019333020889));
#218667=CARTESIAN_POINT('Ctrl Pts',(58.6082941124964,6.0886907505575,2.60365973324126));
#218668=CARTESIAN_POINT('Ctrl Pts',(58.6139972210827,6.06807370279766,2.60934177082473));
#218669=CARTESIAN_POINT('Ctrl Pts',(58.6161277126021,6.0603718600669,2.61146439091893));
#218670=CARTESIAN_POINT('Ctrl Pts',(58.6184367045766,6.05280507414597,2.61389584429346));
#218671=CARTESIAN_POINT('Ctrl Pts',(58.6209098557463,6.04539170794194,2.61661604385258));
#218672=CARTESIAN_POINT('Ctrl Pts',(58.6228395323549,6.03960742773696,2.61873848000781));
#218673=CARTESIAN_POINT('Ctrl Pts',(58.6248693309927,6.03391702093566,2.62103707099793));
#218674=CARTESIAN_POINT('Ctrl Pts',(58.6269926140964,6.02832968645964,2.62350262767658));
#218675=CARTESIAN_POINT('Ctrl Pts',(58.6344241049594,6.00877401579358,2.63213207605185));
#218676=CARTESIAN_POINT('Ctrl Pts',(58.6430007716254,5.99048098024846,2.64280685971919));
#218677=CARTESIAN_POINT('Ctrl Pts',(58.6524381197038,5.97384499260641,2.65513293646089));
#218678=CARTESIAN_POINT('Ctrl Pts',(58.657156793743,5.96552699878538,2.66129597483174));
#218679=CARTESIAN_POINT('Ctrl Pts',(58.6620906399372,5.95762326711374,2.66787183533857));
#218680=CARTESIAN_POINT('Ctrl Pts',(58.667204101582,5.95018309968312,2.67481125953866));
#218681=CARTESIAN_POINT('Ctrl Pts',(58.6722957161033,5.942774720162,2.68172103524084));
#218682=CARTESIAN_POINT('Ctrl Pts',(58.6775652709345,5.93582574548871,2.68899101329792));
#218683=CARTESIAN_POINT('Ctrl Pts',(58.682978094856,5.92938546966287,2.69657334701278));
#218684=CARTESIAN_POINT('Ctrl Pts',(58.6830013202262,5.92935783569723,2.69660588132575));
#218685=CARTESIAN_POINT('Ctrl Pts',(58.6830245479289,5.92933021064647,2.69663842081383));
#218686=CARTESIAN_POINT('Ctrl Pts',(58.6830477779621,5.92930259451081,2.69667096547384));
#218687=CARTESIAN_POINT('Ctrl Pts',(58.6940026150825,5.91627935575131,2.71201840157951));
#218688=CARTESIAN_POINT('Ctrl Pts',(58.7054384852685,5.90523719704714,2.7284564593937));
#218689=CARTESIAN_POINT('Ctrl Pts',(58.7171784805293,5.8960952642491,2.74568723186929));
#218690=CARTESIAN_POINT('Ctrl Pts',(58.7293455537178,5.8866207659238,2.76354482594377));
#218691=CARTESIAN_POINT('Ctrl Pts',(58.7418401303876,5.87918707069746,2.78225519317208));
#218692=CARTESIAN_POINT('Ctrl Pts',(58.7544760786601,5.87375524644683,2.80151223085615));
#218693=CARTESIAN_POINT('Ctrl Pts',(58.7669316835984,5.86840094651606,2.82049442740392));
#218694=CARTESIAN_POINT('Ctrl Pts',(58.7795255625985,5.86499195787596,2.84000929089408));
#218695=CARTESIAN_POINT('Ctrl Pts',(58.7920763953149,5.86353919439998,2.85976644341793));
#218696=CARTESIAN_POINT('Ctrl Pts',(58.8008270591852,5.86252630185742,2.87354148167065));
#218697=CARTESIAN_POINT('Ctrl Pts',(58.8095567514071,5.86246534555174,2.88743438345549));
#218698=CARTESIAN_POINT('Ctrl Pts',(58.8181995570485,5.86337364149599,2.90134173516027));
#218699=CARTESIAN_POINT('',(59.1725467709677,5.90061356181276,3.47153072139077));
#218700=CARTESIAN_POINT('',(58.8181995570485,5.86337364149599,2.90134173516028));
#218701=CARTESIAN_POINT('',(59.4651754363832,0.316925998273232,3.47153072139073));
#218702=CARTESIAN_POINT('Origin',(5.53234440788222E-15,1.85015204418142E-13,
3.47153072139072));
#218703=CARTESIAN_POINT('',(59.1088767419348,0.316922544675878,2.90134173516024));
#218704=CARTESIAN_POINT('',(59.4651754363832,0.316925998273232,3.47153072139073));
#218705=CARTESIAN_POINT('',(58.9208513795073,0.0152121934561109,2.59908173516024));
#218706=CARTESIAN_POINT('Ctrl Pts',(59.1088767419348,0.316922544675878,
2.90134173516024));
#218707=CARTESIAN_POINT('Ctrl Pts',(59.0966467827006,0.316922401514052,
2.88176998919844));
#218708=CARTESIAN_POINT('Ctrl Pts',(59.0844716853565,0.315000085554071,
2.86226752356799));
#218709=CARTESIAN_POINT('Ctrl Pts',(59.0725173476328,0.311230629649457,
2.84310370500131));
#218710=CARTESIAN_POINT('Ctrl Pts',(59.0603470709145,0.307393083605762,
2.82359371788815));
#218711=CARTESIAN_POINT('Ctrl Pts',(59.048404675037,0.301641096265457,2.804433226372));
#218712=CARTESIAN_POINT('Ctrl Pts',(59.036857331986,0.294001187895731,2.785893238785));
#218713=CARTESIAN_POINT('Ctrl Pts',(59.0257988735004,0.286684733438041,
2.76813818620296));
#218714=CARTESIAN_POINT('Ctrl Pts',(59.0151019493863,0.277636448049551,
2.75095095199063));
#218715=CARTESIAN_POINT('Ctrl Pts',(59.0049186873018,0.266835172455698,
2.7345777143551));
#218716=CARTESIAN_POINT('Ctrl Pts',(58.9968192555067,0.258244193038107,
2.72155497955828));
#218717=CARTESIAN_POINT('Ctrl Pts',(58.9890447295129,0.248543417988351,
2.7090471116008));
#218718=CARTESIAN_POINT('Ctrl Pts',(58.981678934725,0.237702773059678,2.69718956158338));
#218719=CARTESIAN_POINT('Ctrl Pts',(58.9816588284979,0.23767318162042,2.69715719432356));
#218720=CARTESIAN_POINT('Ctrl Pts',(58.9816387254916,0.23764358171716,2.69712483219022));
#218721=CARTESIAN_POINT('Ctrl Pts',(58.9816186257082,0.237613973350474,
2.6970924751865));
#218722=CARTESIAN_POINT('Ctrl Pts',(58.9776173965852,0.231719887006966,
2.69065122242275));
#218723=CARTESIAN_POINT('Ctrl Pts',(58.9737507180862,0.225454527233545,
2.68442464469425));
#218724=CARTESIAN_POINT('Ctrl Pts',(58.9700384170936,0.218853219640912,
2.67844505923578));
#218725=CARTESIAN_POINT('Ctrl Pts',(58.9626710986899,0.20575246757011,2.66657815779566));
#218726=CARTESIAN_POINT('Ctrl Pts',(58.9559120649696,0.191327202905614,
2.65568445664172));
#218727=CARTESIAN_POINT('Ctrl Pts',(58.9499179036781,0.175845309932433,
2.64601906229514));
#218728=CARTESIAN_POINT('Ctrl Pts',(58.9454222827095,0.164233890202547,
2.6387700165352));
#218729=CARTESIAN_POINT('Ctrl Pts',(58.9413569016699,0.152028117041484,
2.632211893876));
#218730=CARTESIAN_POINT('Ctrl Pts',(58.9377878323772,0.139341004226325,
2.62645231033232));
#218731=CARTESIAN_POINT('Ctrl Pts',(58.9364494313924,0.13458333692064,2.62429246650344));
#218732=CARTESIAN_POINT('Ctrl Pts',(58.9351808244388,0.12975798122765,2.62224491711744));
#218733=CARTESIAN_POINT('Ctrl Pts',(58.933985496586,0.124870896863504,2.62031533672596));
#218734=CARTESIAN_POINT('Ctrl Pts',(58.9298018491012,0.107766101588996,
2.61356180535577));
#218735=CARTESIAN_POINT('Ctrl Pts',(58.9265158655229,0.0899051301002505,
2.60825339735347));
#218736=CARTESIAN_POINT('Ctrl Pts',(58.9242770147326,0.0715435052827752,
2.6046333798761));
#218737=CARTESIAN_POINT('Ctrl Pts',(58.9231575893375,0.0623626928740375,
2.60282337113742));
#218738=CARTESIAN_POINT('Ctrl Pts',(58.9222999481582,0.0530567171307616,
2.60143545939114));
#218739=CARTESIAN_POINT('Ctrl Pts',(58.9217227791368,0.0436575183856167,
2.60050005034595));
#218740=CARTESIAN_POINT('Ctrl Pts',(58.9214341946262,0.0389579190130443,
2.60003234582336));
#218741=CARTESIAN_POINT('Ctrl Pts',(58.9212157281805,0.0342350138896486,
2.59967776696065));
#218742=CARTESIAN_POINT('Ctrl Pts',(58.9210697160839,0.0294927955550733,
2.59944011429159));
#218743=CARTESIAN_POINT('Ctrl Pts',(58.9209237039872,0.024750577220498,
2.59920246162253));
#218744=CARTESIAN_POINT('Ctrl Pts',(58.9208501479391,0.0199890456752306,
2.5990817379131));
#218745=CARTESIAN_POINT('Ctrl Pts',(58.9208513795073,0.0152121934561115,
2.59908173516024));
#218746=CARTESIAN_POINT('',(58.9208533432504,1.98323206572159E-13,2.59908173516024));
#218747=CARTESIAN_POINT('Origin',(4.7062627014205E-16,1.91107483127175E-13,
2.59908173516023));
#218748=CARTESIAN_POINT('',(58.6605641730809,2.0120008167586E-13,2.18253198860263));
#218749=CARTESIAN_POINT('',(58.9208513795073,-0.0152121934557287,2.59908173516024));
#218750=CARTESIAN_POINT('Origin',(4.7062627014205E-16,1.91107483127175E-13,
2.59908173516023));
#218751=CARTESIAN_POINT('',(59.1088767419348,-0.316922544675487,2.90134173516023));
#218752=CARTESIAN_POINT('Ctrl Pts',(58.9208513795073,-0.0152121934557287,
2.59908173516024));
#218753=CARTESIAN_POINT('Ctrl Pts',(58.9208504012364,-0.0190220008283522,
2.59908174371513));
#218754=CARTESIAN_POINT('Ctrl Pts',(58.9208964366351,-0.022821409981532,
2.5991576435589));
#218755=CARTESIAN_POINT('Ctrl Pts',(58.9209883940807,-0.0266084895328146,
2.59930765775277));
#218756=CARTESIAN_POINT('Ctrl Pts',(58.9215313038857,-0.0489671208145109,
2.60019333020887));
#218757=CARTESIAN_POINT('Ctrl Pts',(58.9236732325289,-0.070898652763302,
2.60365973324139));
#218758=CARTESIAN_POINT('Ctrl Pts',(58.9271900305704,-0.0919988953551827,
2.60934177082511));
#218759=CARTESIAN_POINT('Ctrl Pts',(58.9285037892493,-0.0998812435895791,
2.61146439091921));
#218760=CARTESIAN_POINT('Ctrl Pts',(58.9300091878199,-0.107647933247761,
2.61389584429359));
#218761=CARTESIAN_POINT('Ctrl Pts',(58.9316938830317,-0.115279202946726,
2.61661604385252));
#218762=CARTESIAN_POINT('Ctrl Pts',(58.933008366749,-0.12123350239003,2.61873848000775));
#218763=CARTESIAN_POINT('Ctrl Pts',(58.9344322364591,-0.12710490827982,
2.62103707099787));
#218764=CARTESIAN_POINT('Ctrl Pts',(58.9359598525093,-0.132883578272882,
2.62350262767652));
#218765=CARTESIAN_POINT('Ctrl Pts',(58.9413065086849,-0.153108923248597,
2.63213207605179));
#218766=CARTESIAN_POINT('Ctrl Pts',(58.9479240485795,-0.172198253417529,
2.64280685971914));
#218767=CARTESIAN_POINT('Ctrl Pts',(58.9555707636545,-0.189729578870587,
2.65513293646084));
#218768=CARTESIAN_POINT('Ctrl Pts',(58.959394121192,-0.198495241597116,
2.66129597483169));
#218769=CARTESIAN_POINT('Ctrl Pts',(58.9634747743348,-0.206871403160361,
2.66787183533852));
#218770=CARTESIAN_POINT('Ctrl Pts',(58.9677825146337,-0.214805314863025,
2.67481125953861));
#218771=CARTESIAN_POINT('Ctrl Pts',(58.9720718502312,-0.222705329147438,
2.68172103524079));
#218772=CARTESIAN_POINT('Ctrl Pts',(58.9765861722458,-0.230167055078992,
2.68899101329788));
#218773=CARTESIAN_POINT('Ctrl Pts',(58.9812961520165,-0.23713784456646,
2.69657334701273));
#218774=CARTESIAN_POINT('Ctrl Pts',(58.9813163616197,-0.237167754862604,
2.69660588132571));
#218775=CARTESIAN_POINT('Ctrl Pts',(58.9813365744745,-0.237197656536514,
2.6966384208138));
#218776=CARTESIAN_POINT('Ctrl Pts',(58.9813567905789,-0.237227549587767,
2.69667096547381));
#218777=CARTESIAN_POINT('Ctrl Pts',(58.9908903168207,-0.251324537971755,
2.71201840157895));
#218778=CARTESIAN_POINT('Ctrl Pts',(59.0011093202324,-0.263501580511499,
2.72845645939253));
#218779=CARTESIAN_POINT('Ctrl Pts',(59.0118294103837,-0.273820596508295,
2.74568723186747));
#218780=CARTESIAN_POINT('Ctrl Pts',(59.0229394763216,-0.284514998003045,
2.76354482594125));
#218781=CARTESIAN_POINT('Ctrl Pts',(59.0345885736542,-0.293214009567509,
2.78225519316881));
#218782=CARTESIAN_POINT('Ctrl Pts',(59.0465875206378,-0.299936893971445,
2.80151223085212));
#218783=CARTESIAN_POINT('Ctrl Pts',(59.0584152157249,-0.306563827730263,
2.82049442739912));
#218784=CARTESIAN_POINT('Ctrl Pts',(59.0705837677937,-0.311270560392544,
2.84000929088849));
#218785=CARTESIAN_POINT('Ctrl Pts',(59.0829139906012,-0.314027284735069,
2.85976644341157));
#218786=CARTESIAN_POINT('Ctrl Pts',(59.0915108413196,-0.315949321993822,
2.87354148166636));
#218787=CARTESIAN_POINT('Ctrl Pts',(59.1001863397065,-0.316922445687508,
2.88743438345332));
#218788=CARTESIAN_POINT('Ctrl Pts',(59.1088767419348,-0.316922544675462,
2.90134173516024));
#218789=CARTESIAN_POINT('',(59.4651754363832,-0.316925998272862,3.47153072139072));
#218790=CARTESIAN_POINT('',(59.1088767419348,-0.3169225446755,2.90134173516023));
#218791=CARTESIAN_POINT('',(59.1725467709678,-5.90061356181158,3.47153072139069));
#218792=CARTESIAN_POINT('Origin',(5.53234440788222E-15,1.85015204418142E-13,
3.47153072139072));
#218793=CARTESIAN_POINT('',(58.8181995570486,-5.86337364149481,2.90134173516019));
#218794=CARTESIAN_POINT('',(59.1725467709678,-5.90061356181158,3.47153072139069));
#218795=CARTESIAN_POINT('',(58.5996668978649,-6.14377718965223,2.5990817351602));
#218796=CARTESIAN_POINT('Ctrl Pts',(58.8181995570486,-5.86337364149481,
2.9013417351602));
#218797=CARTESIAN_POINT('Ctrl Pts',(58.8060365798459,-5.86209540502774,
2.88176998919788));
#218798=CARTESIAN_POINT('Ctrl Pts',(58.7937272422254,-5.86273454612429,
2.86226752356692));
#218799=CARTESIAN_POINT('Ctrl Pts',(58.7814443761811,-5.86523378400357,
2.84310370499975));
#218800=CARTESIAN_POINT('Ctrl Pts',(58.7689396367211,-5.86777816724576,
2.82359371788606));
#218801=CARTESIAN_POINT('Ctrl Pts',(58.75646141614,-5.87225032430905,2.80443322636941));
#218802=CARTESIAN_POINT('Ctrl Pts',(58.7441787427607,-5.8786413544378,2.78589323878195));
#218803=CARTESIAN_POINT('Ctrl Pts',(58.7324160859264,-5.88476180492122,
2.76813818619945));
#218804=CARTESIAN_POINT('Ctrl Pts',(58.7208319573147,-5.89264238981678,
2.75095095198671));
#218805=CARTESIAN_POINT('Ctrl Pts',(58.709575439466,-5.90232005415664,2.73457771435083));
#218806=CARTESIAN_POINT('Ctrl Pts',(58.7006223753302,-5.91001735013063,
2.72155497955553));
#218807=CARTESIAN_POINT('Ctrl Pts',(58.6918764318957,-5.91885232406405,
2.70904711159948));
#218808=CARTESIAN_POINT('Ctrl Pts',(58.6834178317481,-5.92886364759452,
2.69718956158335));
#218809=CARTESIAN_POINT('Ctrl Pts',(58.6833947425173,-5.92889097525576,
2.69715719432352));
#218810=CARTESIAN_POINT('Ctrl Pts',(58.683371655605,-5.92891831167131,2.69712483219017));
#218811=CARTESIAN_POINT('Ctrl Pts',(58.6833485710132,-5.92894565684079,
2.69709247518645));
#218812=CARTESIAN_POINT('Ctrl Pts',(58.6787531612542,-5.93438921243119,
2.69065122242271));
#218813=CARTESIAN_POINT('Ctrl Pts',(58.6742527563957,-5.94021607194678,
2.68442464469422));
#218814=CARTESIAN_POINT('Ctrl Pts',(58.6698707672382,-5.94639317576777,
2.67844505923575));
#218815=CARTESIAN_POINT('Ctrl Pts',(58.6611744062939,-5.95865206607682,
2.66657815779563));
#218816=CARTESIAN_POINT('Ctrl Pts',(58.6529445485199,-5.97229179622419,
2.65568445664168));
#218817=CARTESIAN_POINT('Ctrl Pts',(58.6453649253902,-5.98706231729939,
2.6460190622951));
#218818=CARTESIAN_POINT('Ctrl Pts',(58.6396802080429,-5.99814020810579,
2.63877001653516));
#218819=CARTESIAN_POINT('Ctrl Pts',(58.6343612468745,-6.0098541687317,2.63221189387596));
#218820=CARTESIAN_POINT('Ctrl Pts',(58.6294855649109,-6.02209871088692,
2.62645231033228));
#218821=CARTESIAN_POINT('Ctrl Pts',(58.6276571841746,-6.02669041419513,
2.6242924665034));
#218822=CARTESIAN_POINT('Ctrl Pts',(58.6258911397673,-6.0313567305494,2.62224491711741));
#218823=CARTESIAN_POINT('Ctrl Pts',(58.6241915206271,-6.0360920971705,2.62031533672592));
#218824=CARTESIAN_POINT('Ctrl Pts',(58.6182428536364,-6.05266588034435,
2.61356180535573));
#218825=CARTESIAN_POINT('Ctrl Pts',(58.6131078911178,-6.07008552874868,
2.60825339735344));
#218826=CARTESIAN_POINT('Ctrl Pts',(58.6089619925611,-6.08811254303161,
2.60463337987607));
#218827=CARTESIAN_POINT('Ctrl Pts',(58.6068890432828,-6.09712605017307,
2.60282337113739));
#218828=CARTESIAN_POINT('Ctrl Pts',(58.6050633610079,-6.10629139889302,
2.6014354593911));
#218829=CARTESIAN_POINT('Ctrl Pts',(58.6035068699781,-6.11557877725314,
2.60050005034591));
#218830=CARTESIAN_POINT('Ctrl Pts',(58.6027286244632,-6.1202224664332,2.60003234582332));
#218831=CARTESIAN_POINT('Ctrl Pts',(58.6020176767849,-6.12489666302632,
2.59967776696062));
#218832=CARTESIAN_POINT('Ctrl Pts',(58.6013767677628,-6.1295976405726,2.59944011429156));
#218833=CARTESIAN_POINT('Ctrl Pts',(58.6007358587407,-6.13429861811887,
2.5992024616225));
#218834=CARTESIAN_POINT('Ctrl Pts',(58.6001649900651,-6.13902637679545,
2.59908173791307));
#218835=CARTESIAN_POINT('Ctrl Pts',(58.5996668978649,-6.14377718965223,
2.5990817351602));
#218836=CARTESIAN_POINT('',(58.5964866834552,-6.17403490858921,2.59908173516019));
#218837=CARTESIAN_POINT('Origin',(5.72296091834672E-15,1.85847653270679E-13,
2.59908173516024));
#218838=CARTESIAN_POINT('',(58.7519447039089,-6.49374646112641,2.90134173516019));
#218839=CARTESIAN_POINT('Ctrl Pts',(58.5964866834552,-6.17403490858921,
2.5990817351602));
#218840=CARTESIAN_POINT('Ctrl Pts',(58.5960874772333,-6.17782374318127,
2.5990817437151));
#218841=CARTESIAN_POINT('Ctrl Pts',(58.5957361140452,-6.18160715078305,
2.59915764355886));
#218842=CARTESIAN_POINT('Ctrl Pts',(58.5954317101325,-6.18538309648678,
2.59930765775272));
#218843=CARTESIAN_POINT('Ctrl Pts',(58.5936345324522,-6.20767599437294,
2.60019333020876));
#218844=CARTESIAN_POINT('Ctrl Pts',(58.5934722580545,-6.22971127560298,
2.60365973324086));
#218845=CARTESIAN_POINT('Ctrl Pts',(58.5947642147753,-6.25106353435168,
2.60934177082389));
#218846=CARTESIAN_POINT('Ctrl Pts',(58.5952468467988,-6.25904002743504,
2.61146439091827));
#218847=CARTESIAN_POINT('Ctrl Pts',(58.595932158504,-6.26692152735531,2.61389584429305));
#218848=CARTESIAN_POINT('Ctrl Pts',(58.5968099398849,-6.2746870907634,2.61661604385248));
#218849=CARTESIAN_POINT('Ctrl Pts',(58.5974948289522,-6.28074617289431,
2.61873848000772));
#218850=CARTESIAN_POINT('Ctrl Pts',(58.5982971695202,-6.28673424952099,
2.62103707099783));
#218851=CARTESIAN_POINT('Ctrl Pts',(58.5992123816357,-6.29264094271338,
2.62350262767647));
#218852=CARTESIAN_POINT('Ctrl Pts',(58.6024156240399,-6.31331436888676,
2.63213207605174));
#218853=CARTESIAN_POINT('Ctrl Pts',(58.6070015340113,-6.33299084698348,
2.6428068597191));
#218854=CARTESIAN_POINT('Ctrl Pts',(58.6127738370724,-6.35122543337721,
2.6551329364608));
#218855=CARTESIAN_POINT('Ctrl Pts',(58.6156599886029,-6.36034272657408,
2.66129597483165));
#218856=CARTESIAN_POINT('Ctrl Pts',(58.6188427402045,-6.36909954705002,
2.66787183533847));
#218857=CARTESIAN_POINT('Ctrl Pts',(58.6222975626533,-6.37744027742783,
2.67481125953856));
#218858=CARTESIAN_POINT('Ctrl Pts',(58.6257376244687,-6.38574537226586,
2.68172103524075));
#218859=CARTESIAN_POINT('Ctrl Pts',(58.62944725381,-6.3936380972249,2.68899101329783));
#218860=CARTESIAN_POINT('Ctrl Pts',(58.6334027859058,-6.40106302694565,
2.69657334701269));
#218861=CARTESIAN_POINT('Ctrl Pts',(58.6334197583214,-6.40109488586883,
2.69660588132566));
#218862=CARTESIAN_POINT('Ctrl Pts',(58.6334367348721,-6.40112673655689,
2.69663842081375));
#218863=CARTESIAN_POINT('Ctrl Pts',(58.6334537155558,-6.4011585790092,2.69667096547375));
#218864=CARTESIAN_POINT('Ctrl Pts',(58.6414614796112,-6.41617486746407,
2.71201840157957));
#218865=CARTESIAN_POINT('Ctrl Pts',(58.6503516547096,-6.42935337961396,
2.72845645939393));
#218866=CARTESIAN_POINT('Ctrl Pts',(58.6599343882013,-6.44073642151141,
2.74568723186971));
#218867=CARTESIAN_POINT('Ctrl Pts',(58.6698657226822,-6.45253355607543,
2.7635448259443));
#218868=CARTESIAN_POINT('Ctrl Pts',(58.6805417107305,-6.46240257578718,
2.78225519317272));
#218869=CARTESIAN_POINT('Ctrl Pts',(58.691772193452,-6.47034286301596,2.80151223085691));
#218870=CARTESIAN_POINT('Ctrl Pts',(58.7028423919864,-6.47816982452966,
2.82049442740461));
#218871=CARTESIAN_POINT('Ctrl Pts',(58.7144522959221,-6.4841227332657,2.84000929089469));
#218872=CARTESIAN_POINT('Ctrl Pts',(58.7264268163201,-6.48815321522529,
2.85976644341845));
#218873=CARTESIAN_POINT('Ctrl Pts',(58.7347756649885,-6.49096333895657,
2.87354148167098));
#218874=CARTESIAN_POINT('Ctrl Pts',(58.7433019189618,-6.49283796829079,
2.88743438345561));
#218875=CARTESIAN_POINT('Ctrl Pts',(58.7519447039089,-6.49374646112638,
2.90134173516019));
#218876=CARTESIAN_POINT('',(59.1062911958297,-6.53099325079957,3.47153072139068));
#218877=CARTESIAN_POINT('',(58.7519447039089,-6.49374646112642,2.90134173516019));
#218878=CARTESIAN_POINT('',(58.2316113004783,-12.0535047649312,3.47153072139065));
#218879=CARTESIAN_POINT('Origin',(5.53234440788222E-15,1.85015204418142E-13,
3.47153072139072));
#218880=CARTESIAN_POINT('',(57.8830978693157,-11.9794294790603,2.90134173516016));
#218881=CARTESIAN_POINT('',(58.2316113004783,-12.0535047649312,3.47153072139065));
#218882=CARTESIAN_POINT('',(57.6364522029208,-12.2354540642035,2.59908173516015));
#218883=CARTESIAN_POINT('Ctrl Pts',(57.8830978693157,-11.9794294790603,
2.90134173516015));
#218884=CARTESIAN_POINT('Ctrl Pts',(57.8711351342685,-11.9768868675905,
2.88176998919795));
#218885=CARTESIAN_POINT('Ctrl Pts',(57.8588264200508,-11.9762358312599,
2.86226752356711));
#218886=CARTESIAN_POINT('Ctrl Pts',(57.8463495993372,-11.9774374689404,
2.84310370500005));
#218887=CARTESIAN_POINT('Ctrl Pts',(57.8336474016781,-11.9786608125856,
2.8235937178864));
#218888=CARTESIAN_POINT('Ctrl Pts',(57.8207700703897,-11.9818041414829,
2.8044332263698));
#218889=CARTESIAN_POINT('Ctrl Pts',(57.8078866382223,-11.9868762719067,
2.78589323878238));
#218890=CARTESIAN_POINT('Ctrl Pts',(57.7955486571693,-11.9917336614792,
2.7681381861998));
#218891=CARTESIAN_POINT('Ctrl Pts',(57.7832042421973,-11.9983602045441,
2.75095095198698));
#218892=CARTESIAN_POINT('Ctrl Pts',(57.7709977973496,-12.0068082271136,
2.73457771435104));
#218893=CARTESIAN_POINT('Ctrl Pts',(57.7612891925165,-12.0135275064593,
2.72155497955564));
#218894=CARTESIAN_POINT('Ctrl Pts',(57.7516676540269,-12.0213998814541,
2.7090471115995));
#218895=CARTESIAN_POINT('Ctrl Pts',(57.7422089227119,-12.030472197432,2.6971895615833));
#218896=CARTESIAN_POINT('Ctrl Pts',(57.7421831034479,-12.0304969619077,
2.69715719432347));
#218897=CARTESIAN_POINT('Ctrl Pts',(57.7421572855747,-12.030521735332,2.69712483219013));
#218898=CARTESIAN_POINT('Ctrl Pts',(57.7421314690942,-12.0305465177049,
2.69709247518641));
#218899=CARTESIAN_POINT('Ctrl Pts',(57.73699222697,-12.035479901808,2.69065122242267));
#218900=CARTESIAN_POINT('Ctrl Pts',(57.7319074031293,-12.0408044207735,
2.68442464469416));
#218901=CARTESIAN_POINT('Ctrl Pts',(57.726903735797,-12.0464896431808,2.67844505923569));
#218902=CARTESIAN_POINT('Ctrl Pts',(57.7169736114625,-12.0577723607605,
2.66657815779557));
#218903=CARTESIAN_POINT('Ctrl Pts',(57.7073630976789,-12.070477116653,2.65568445664164));
#218904=CARTESIAN_POINT('Ctrl Pts',(57.6982810566481,-12.0843744369104,
2.64601906229505));
#218905=CARTESIAN_POINT('Ctrl Pts',(57.691469525875,-12.0947974271034,2.63877001653511));
#218906=CARTESIAN_POINT('Ctrl Pts',(57.6849552602294,-12.1058912345902,
2.63221189387592));
#218907=CARTESIAN_POINT('Ctrl Pts',(57.6788263845869,-12.1175590523193,
2.62645231033224));
#218908=CARTESIAN_POINT('Ctrl Pts',(57.676528056221,-12.1219344839678,2.62429246650336));
#218909=CARTESIAN_POINT('Ctrl Pts',(57.6742839235121,-12.1263906358448,
2.62224491711736));
#218910=CARTESIAN_POINT('Ctrl Pts',(57.6720986344674,-12.1309224030552,
2.62031533672588));
#218911=CARTESIAN_POINT('Ctrl Pts',(57.6644501228112,-12.1467835882917,
2.61356180535569));
#218912=CARTESIAN_POINT('Ctrl Pts',(57.6575224410762,-12.1635710602984,
2.60825339735338));
#218913=CARTESIAN_POINT('Ctrl Pts',(57.6515149180853,-12.1810659563059,
2.60463337987601));
#218914=CARTESIAN_POINT('Ctrl Pts',(57.6485111565899,-12.1898134043097,
2.60282337113733));
#218915=CARTESIAN_POINT('Ctrl Pts',(57.6457374357766,-12.1987377085277,
2.60143545939106));
#218916=CARTESIAN_POINT('Ctrl Pts',(57.6432186759797,-12.207811512042,2.60050005034587));
#218917=CARTESIAN_POINT('Ctrl Pts',(57.6419592960813,-12.2123484137991,
2.60003234582328));
#218918=CARTESIAN_POINT('Ctrl Pts',(57.6407636564618,-12.216922690386,2.59967776696058));
#218919=CARTESIAN_POINT('Ctrl Pts',(57.6396348724477,-12.2215309222502,
2.59944011429152));
#218920=CARTESIAN_POINT('Ctrl Pts',(57.6385060884335,-12.2261391541144,
2.59920246162246));
#218921=CARTESIAN_POINT('Ctrl Pts',(57.637444161687,-12.2307813416089,2.59908173791303));
#218922=CARTESIAN_POINT('Ctrl Pts',(57.6364522029208,-12.2354540642035,
2.59908173516016));
#218923=CARTESIAN_POINT('',(57.6301266171959,-12.2652136052652,2.59908173516015));
#218924=CARTESIAN_POINT('Origin',(5.72184526906101E-15,1.85840609338312E-13,
2.59908173516024));
#218925=CARTESIAN_POINT('',(57.7513140650722,-12.5994235324463,2.90134173516015));
#218926=CARTESIAN_POINT('Ctrl Pts',(57.6301266171959,-12.2652136052652,
2.59908173516016));
#218927=CARTESIAN_POINT('Ctrl Pts',(57.6293335568101,-12.268939955812,2.59908174371505));
#218928=CARTESIAN_POINT('Ctrl Pts',(57.6285886446437,-12.272665910057,2.59915764355882));
#218929=CARTESIAN_POINT('Ctrl Pts',(57.6278912144857,-12.2763893518618,
2.59930765775268));
#218930=CARTESIAN_POINT('Ctrl Pts',(57.6237736395747,-12.2983722707009,
2.60019333020878));
#218931=CARTESIAN_POINT('Ctrl Pts',(57.6213089400484,-12.3202698780625,
2.60365973324121));
#218932=CARTESIAN_POINT('Ctrl Pts',(57.6203619005009,-12.3416402131555,
2.60934177082479));
#218933=CARTESIAN_POINT('Ctrl Pts',(57.6200081180516,-12.3496234589577,
2.61146439091895));
#218934=CARTESIAN_POINT('Ctrl Pts',(57.6198658344727,-12.3575334177749,
2.61389584429341));
#218935=CARTESIAN_POINT('Ctrl Pts',(57.6199270848659,-12.3653481937518,
2.61661604385244));
#218936=CARTESIAN_POINT('Ctrl Pts',(57.6199748754953,-12.3714456739986,
2.61873848000767));
#218937=CARTESIAN_POINT('Ctrl Pts',(57.62014689631,-12.3774848147415,2.62103707099779));
#218938=CARTESIAN_POINT('Ctrl Pts',(57.6204396772353,-12.3834548161666,
2.62350262767644));
#218939=CARTESIAN_POINT('Ctrl Pts',(57.6214644104742,-12.4043498211543,
2.6321320760517));
#218940=CARTESIAN_POINT('Ctrl Pts',(57.6239684463329,-12.4243978675672,
2.64280685971906));
#218941=CARTESIAN_POINT('Ctrl Pts',(57.6278030948198,-12.4431359329572,
2.65513293646075));
#218942=CARTESIAN_POINT('Ctrl Pts',(57.6297204190632,-12.4525049656522,
2.6612959748316));
#218943=CARTESIAN_POINT('Ctrl Pts',(57.6319703982311,-12.4615465034833,
2.66787183533843));
#218944=CARTESIAN_POINT('Ctrl Pts',(57.6345344510721,-12.4702026697488,
2.67481125953852));
#218945=CARTESIAN_POINT('Ctrl Pts',(57.6370875490682,-12.4788218527834,
2.68172103524071));
#218946=CARTESIAN_POINT('Ctrl Pts',(57.6399518422609,-12.4870591024237,
2.68899101329778));
#218947=CARTESIAN_POINT('Ctrl Pts',(57.6431095890444,-12.4948568232939,
2.69657334701264));
#218948=CARTESIAN_POINT('Ctrl Pts',(57.6431231383191,-12.4948902817911,
2.69660588132561));
#218949=CARTESIAN_POINT('Ctrl Pts',(57.6431366925669,-12.4949237325305,
2.6966384208137));
#218950=CARTESIAN_POINT('Ctrl Pts',(57.6431502517861,-12.4949571755113,
2.69667096547371));
#218951=CARTESIAN_POINT('Ctrl Pts',(57.6495445189161,-12.510728242438,2.71201840157977));
#218952=CARTESIAN_POINT('Ctrl Pts',(57.657008463082,-12.5247638376608,2.72845645939442));
#218953=CARTESIAN_POINT('Ctrl Pts',(57.6653488494803,-12.5370861904697,
2.74568723187049));
#218954=CARTESIAN_POINT('Ctrl Pts',(57.673992642725,-12.5498568062279,2.76354482594546));
#218955=CARTESIAN_POINT('Ctrl Pts',(57.6835785531295,-12.5607877070417,
2.78225519317428));
#218956=CARTESIAN_POINT('Ctrl Pts',(57.69391752807,-12.5698584016469,2.80151223085888));
#218957=CARTESIAN_POINT('Ctrl Pts',(57.7041089426397,-12.5787996370874,
2.82049442740705));
#218958=CARTESIAN_POINT('Ctrl Pts',(57.715032997905,-12.5859335005836,2.8400092908976));
#218959=CARTESIAN_POINT('Ctrl Pts',(57.7265206205423,-12.5911935813568,
2.85976644342183));
#218960=CARTESIAN_POINT('Ctrl Pts',(57.7345299954283,-12.5948610032571,
2.87354148167323));
#218961=CARTESIAN_POINT('Ctrl Pts',(57.742813589566,-12.5976165994007,2.88743438345671));
#218962=CARTESIAN_POINT('Ctrl Pts',(57.7513140650722,-12.5994235324462,
2.90134173516015));
#218963=CARTESIAN_POINT('',(58.0998260601482,-12.6735055745731,3.47153072139064));
#218964=CARTESIAN_POINT('',(57.7513140650722,-12.5994235324462,2.90134173516015));
#218965=CARTESIAN_POINT('',(56.6526781108326,-18.0743352474882,3.4715307213906));
#218966=CARTESIAN_POINT('Origin',(5.53234440788222E-15,1.85015204418142E-13,
3.47153072139072));
#218967=CARTESIAN_POINT('',(56.3138168485097,-17.9642361803963,2.90134173516012));
#218968=CARTESIAN_POINT('',(56.6526781108326,-18.0743352474882,3.4715307213906));
#218969=CARTESIAN_POINT('',(56.0417604764386,-18.193076743594,2.59908173516011));
#218970=CARTESIAN_POINT('Ctrl Pts',(56.3138168485097,-17.9642361803963,
2.90134173516011));
#218971=CARTESIAN_POINT('Ctrl Pts',(56.3021854218467,-17.9604570513074,
2.88176998919846));
#218972=CARTESIAN_POINT('Ctrl Pts',(56.2900121878809,-17.95852297044,2.86226752356817));
#218973=CARTESIAN_POINT('Ctrl Pts',(56.2774781111569,-17.9584138425278,
2.84310370500164));
#218974=CARTESIAN_POINT('Ctrl Pts',(56.2647176232347,-17.958302743367,2.82359371788856));
#218975=CARTESIAN_POINT('Ctrl Pts',(56.2515822679757,-17.9600828051289,
2.80443322637249));
#218976=CARTESIAN_POINT('Ctrl Pts',(56.2382392305995,-17.9637804645252,
2.78589323878555));
#218977=CARTESIAN_POINT('Ctrl Pts',(56.2254611028306,-17.9673215746097,
2.76813818620352));
#218978=CARTESIAN_POINT('Ctrl Pts',(56.2124916494926,-17.9726214740509,
2.7509509519912));
#218979=CARTESIAN_POINT('Ctrl Pts',(56.1994690140106,-17.9797472965464,
2.73457771435566));
#218980=CARTESIAN_POINT('Ctrl Pts',(56.1891112379851,-17.9854149414334,
2.72155497955859));
#218981=CARTESIAN_POINT('Ctrl Pts',(56.1787195200283,-17.9922384661024,
2.70904711160088));
#218982=CARTESIAN_POINT('Ctrl Pts',(56.1683642893845,-18.0002723763363,
2.69718956158326));
#218983=CARTESIAN_POINT('Ctrl Pts',(56.1683360229685,-18.0002943063015,
2.69715719432343));
#218984=CARTESIAN_POINT('Ctrl Pts',(56.1683077570003,-18.0003162453118,
2.69712483219009));
#218985=CARTESIAN_POINT('Ctrl Pts',(56.1682794914818,-18.0003381933673,
2.69709247518637));
#218986=CARTESIAN_POINT('Ctrl Pts',(56.1626527236048,-18.0047073547945,
2.69065122242262));
#218987=CARTESIAN_POINT('Ctrl Pts',(56.157039191176,-18.009471196666,2.68442464469411));
#218988=CARTESIAN_POINT('Ctrl Pts',(56.1514686668953,-18.0146022491731,
2.67844505923564));
#218989=CARTESIAN_POINT('Ctrl Pts',(56.1404135756909,-18.0247851782086,
2.66657815779552));
#218990=CARTESIAN_POINT('Ctrl Pts',(56.1295277006976,-18.036415763882,2.6556844566416));
#218991=CARTESIAN_POINT('Ctrl Pts',(56.1190427465078,-18.0492876213726,
2.64601906229501));
#218992=CARTESIAN_POINT('Ctrl Pts',(56.1111790308655,-18.0589415144906,
2.63877001653507));
#218993=CARTESIAN_POINT('Ctrl Pts',(56.1035408324003,-18.069293622762,2.63221189387587));
#218994=CARTESIAN_POINT('Ctrl Pts',(56.096225912323,-18.0802568810123,2.62645231033219));
#218995=CARTESIAN_POINT('Ctrl Pts',(56.0934828172939,-18.0843681028561,
2.62429246650331));
#218996=CARTESIAN_POINT('Ctrl Pts',(56.090785183471,-18.0885652677235,2.62224491711732));
#218997=CARTESIAN_POINT('Ctrl Pts',(56.088138167006,-18.0928437845334,2.62031533672584));
#218998=CARTESIAN_POINT('Ctrl Pts',(56.0788736093786,-18.1078185933678,
2.61356180535565));
#218999=CARTESIAN_POINT('Ctrl Pts',(56.0702291095579,-18.1237899619206,
2.60825339735334));
#219000=CARTESIAN_POINT('Ctrl Pts',(56.0624257818119,-18.1405610619109,
2.60463337987597));
#219001=CARTESIAN_POINT('Ctrl Pts',(56.0585241179389,-18.1489466119061,
2.60282337113729));
#219002=CARTESIAN_POINT('Ctrl Pts',(56.0548327480528,-18.1575320950778,
2.60143545939101));
#219003=CARTESIAN_POINT('Ctrl Pts',(56.0513793155483,-18.1662929092561,
2.60050005034582));
#219004=CARTESIAN_POINT('Ctrl Pts',(56.049652599296,-18.1706733163452,2.60003234582323));
#219005=CARTESIAN_POINT('Ctrl Pts',(56.0479853674133,-18.1750975561943,
2.59967776696052));
#219006=CARTESIAN_POINT('Ctrl Pts',(56.046381075601,-18.1795625536238,2.59944011429146));
#219007=CARTESIAN_POINT('Ctrl Pts',(56.0447767837886,-18.1840275510534,
2.5992024616224));
#219008=CARTESIAN_POINT('Ctrl Pts',(56.0432354336629,-18.1885333065881,
2.59908173791296));
#219009=CARTESIAN_POINT('Ctrl Pts',(56.0417604764386,-18.193076743594,2.59908173516011));
#219010=CARTESIAN_POINT('',(56.0323588238394,-18.2220120550208,2.59908173516011));
#219011=CARTESIAN_POINT('Origin',(5.71999943999309E-15,1.85833720610448E-13,
2.59908173516024));
#219012=CARTESIAN_POINT('',(56.1179479440991,-18.5670586829457,2.90134173516011));
#219013=CARTESIAN_POINT('Ctrl Pts',(56.0323588238394,-18.2220120550208,
2.59908173516011));
#219014=CARTESIAN_POINT('Ctrl Pts',(56.031180598225,-18.225635094846,2.59908174371501));
#219015=CARTESIAN_POINT('Ctrl Pts',(56.030050298494,-18.2292627733998,2.59915764355878));
#219016=CARTESIAN_POINT('Ctrl Pts',(56.0289674832815,-18.2328929164982,
2.59930765775265));
#219017=CARTESIAN_POINT('Ctrl Pts',(56.0225746241531,-18.2543250068274,
2.60019333020864));
#219018=CARTESIAN_POINT('Ctrl Pts',(56.0178345032622,-18.2758450255484,
2.60365973324037));
#219019=CARTESIAN_POINT('Ctrl Pts',(56.0146588434097,-18.2969992991187,
2.60934177082277));
#219020=CARTESIAN_POINT('Ctrl Pts',(56.0134725226016,-18.3049018315318,
2.6114643909174));
#219021=CARTESIAN_POINT('Ctrl Pts',(56.0125042026269,-18.3127535860857,
2.61389584429253));
#219022=CARTESIAN_POINT('Ctrl Pts',(56.0117482509602,-18.320531954314,2.61661604385242));
#219023=CARTESIAN_POINT('Ctrl Pts',(56.0111584195475,-18.326601027407,2.61873848000765));
#219024=CARTESIAN_POINT('Ctrl Pts',(56.0106982359128,-18.3326250661765,
2.62103707099775));
#219025=CARTESIAN_POINT('Ctrl Pts',(56.010365377879,-18.3385929672493,2.6235026276764));
#219026=CARTESIAN_POINT('Ctrl Pts',(56.0092003747606,-18.3594806210041,
2.63213207605167));
#219027=CARTESIAN_POINT('Ctrl Pts',(56.0095951017658,-18.3796805851414,
2.64280685971903));
#219028=CARTESIAN_POINT('Ctrl Pts',(56.0114500824673,-18.3987168313621,
2.65513293646072));
#219029=CARTESIAN_POINT('Ctrl Pts',(56.012377572818,-18.4082349544725,2.66129597483157));
#219030=CARTESIAN_POINT('Ctrl Pts',(56.0136701283095,-18.417462148678,2.6678718353384));
#219031=CARTESIAN_POINT('Ctrl Pts',(56.0153153192432,-18.4263389120622,
2.67481125953849));
#219032=CARTESIAN_POINT('Ctrl Pts',(56.0169534811442,-18.4351777497205,
2.68172103524067));
#219033=CARTESIAN_POINT('Ctrl Pts',(56.0189410563926,-18.4436692750111,
2.68899101329776));
#219034=CARTESIAN_POINT('Ctrl Pts',(56.0212664209293,-18.4517543535692,
2.69657334701262));
#219035=CARTESIAN_POINT('Ctrl Pts',(56.0212763986143,-18.451789045062,2.69660588132559));
#219036=CARTESIAN_POINT('Ctrl Pts',(56.0212863820562,-18.4518237293595,
2.69663842081367));
#219037=CARTESIAN_POINT('Ctrl Pts',(56.0212963712531,-18.4518584064605,
2.69667096547368));
#219038=CARTESIAN_POINT('Ctrl Pts',(56.0260070845286,-18.4682114607488,
2.71201840157927));
#219039=CARTESIAN_POINT('Ctrl Pts',(56.0319630212276,-18.4829503621255,
2.72845645939336));
#219040=CARTESIAN_POINT('Ctrl Pts',(56.0389696815133,-18.4960770195693,
2.74568723186885));
#219041=CARTESIAN_POINT('Ctrl Pts',(56.0462312303137,-18.5096811989825,
2.7635448259432));
#219042=CARTESIAN_POINT('Ctrl Pts',(56.0546220378335,-18.5215542196613,
2.78225519317137));
#219043=CARTESIAN_POINT('Ctrl Pts',(56.0639562290192,-18.5316559412145,
2.8015122308553));
#219044=CARTESIAN_POINT('Ctrl Pts',(56.0731572003529,-18.5416134885352,
2.82049442740297));
#219045=CARTESIAN_POINT('Ctrl Pts',(56.0832757207117,-18.5498501466904,
2.84000929089302));
#219046=CARTESIAN_POINT('Ctrl Pts',(56.0941505847899,-18.5562821957318,
2.85976644341677));
#219047=CARTESIAN_POINT('Ctrl Pts',(56.1017327335077,-18.5607667347606,
2.87354148166982));
#219048=CARTESIAN_POINT('Ctrl Pts',(56.1096829110206,-18.5643731068263,
2.88743438345499));
#219049=CARTESIAN_POINT('Ctrl Pts',(56.1179479440991,-18.5670586829457,
2.90134173516011));
#219050=CARTESIAN_POINT('',(56.4568070719814,-18.6771643191701,3.4715307213906));
#219051=CARTESIAN_POINT('',(56.1179479440991,-18.5670586829457,2.90134173516011));
#219052=CARTESIAN_POINT('',(54.4530463244696,-23.897139530776,3.47153072139056));
#219053=CARTESIAN_POINT('Origin',(5.53234440788222E-15,1.85015204418142E-13,
3.47153072139072));
#219054=CARTESIAN_POINT('',(54.1275498658877,-23.7522229508819,2.90134173516007));
#219055=CARTESIAN_POINT('',(54.4530463244695,-23.897139530776,3.47153072139056));
#219056=CARTESIAN_POINT('',(53.8330634946841,-23.9513722670356,2.59908173516007));
#219057=CARTESIAN_POINT('Ctrl Pts',(54.1275498658877,-23.7522229508819,
2.90134173516007));
#219058=CARTESIAN_POINT('Ctrl Pts',(54.1163771839526,-23.7472487091029,
2.8817699891978));
#219059=CARTESIAN_POINT('Ctrl Pts',(54.1044728027367,-23.7440527738934,
2.86226752356688));
#219060=CARTESIAN_POINT('Ctrl Pts',(54.0920187959689,-23.742634076017,2.84310370499975));
#219061=CARTESIAN_POINT('Ctrl Pts',(54.0793398243589,-23.7411897512761,
2.82359371788624));
#219062=CARTESIAN_POINT('Ctrl Pts',(54.0660903588296,-23.7415870431739,
2.80443322636975));
#219063=CARTESIAN_POINT('Ctrl Pts',(54.0524339053535,-23.743869719213,2.78589323878245));
#219064=CARTESIAN_POINT('Ctrl Pts',(54.03935563071,-23.746055752667,2.7681381862003));
#219065=CARTESIAN_POINT('Ctrl Pts',(54.0259032350502,-23.7499709416779,
2.75095095198788));
#219066=CARTESIAN_POINT('Ctrl Pts',(54.0122070876528,-23.7556964920978,
2.73457771435229));
#219067=CARTESIAN_POINT('Ctrl Pts',(54.0013136223986,-23.7602504066221,
2.72155497955642));
#219068=CARTESIAN_POINT('Ctrl Pts',(53.9902655788133,-23.7659503209998,
2.70904711159983));
#219069=CARTESIAN_POINT('Ctrl Pts',(53.9791273029166,-23.7728578042863,
2.69718956158322));
#219070=CARTESIAN_POINT('Ctrl Pts',(53.9790968990415,-23.7728766594719,
2.69715719432339));
#219071=CARTESIAN_POINT('Ctrl Pts',(53.9790664946662,-23.7728955236998,
2.69712483219005));
#219072=CARTESIAN_POINT('Ctrl Pts',(53.9790360897926,-23.7729143969702,
2.69709247518633));
#219073=CARTESIAN_POINT('Ctrl Pts',(53.972983444209,-23.7766714662746,2.69065122242259));
#219074=CARTESIAN_POINT('Ctrl Pts',(53.9669027062282,-23.7808224374036,
2.6844246446941));
#219075=CARTESIAN_POINT('Ctrl Pts',(53.9608263568289,-23.7853431031255,
2.67844505923562));
#219076=CARTESIAN_POINT('Ctrl Pts',(53.9487674206471,-23.7943146773155,
2.6665781577955));
#219077=CARTESIAN_POINT('Ctrl Pts',(53.9367254523687,-23.8047436656392,
2.65568445664157));
#219078=CARTESIAN_POINT('Ctrl Pts',(53.9249524603721,-23.8164490335988,
2.64601906229499));
#219079=CARTESIAN_POINT('Ctrl Pts',(53.9161227163747,-23.8252280595685,
2.63877001653505));
#219080=CARTESIAN_POINT('Ctrl Pts',(53.9074442707907,-23.83472504876,2.63221189387585));
#219081=CARTESIAN_POINT('Ctrl Pts',(53.8990234500736,-23.8448636317798,
2.62645231033217));
#219082=CARTESIAN_POINT('Ctrl Pts',(53.8958656423047,-23.8486656004123,
2.62429246650329));
#219083=CARTESIAN_POINT('Ctrl Pts',(53.8927440632084,-23.8525577932534,
2.62224491711729));
#219084=CARTESIAN_POINT('Ctrl Pts',(53.8896643205894,-23.8565361833372,
2.6203153367258));
#219085=CARTESIAN_POINT('Ctrl Pts',(53.8788852214228,-23.8704605486303,
2.61356180535561));
#219086=CARTESIAN_POINT('Ctrl Pts',(53.8686186144656,-23.8854408280731,
2.60825339735331));
#219087=CARTESIAN_POINT('Ctrl Pts',(53.8591049768561,-23.9013043843653,
2.60463337987594));
#219088=CARTESIAN_POINT('Ctrl Pts',(53.8543481580514,-23.9092361625114,
2.60282337113726));
#219089=CARTESIAN_POINT('Ctrl Pts',(53.8497795825134,-23.9173887602863,
2.60143545939098));
#219090=CARTESIAN_POINT('Ctrl Pts',(53.8454293138304,-23.9257405998152,
2.6005000503458));
#219091=CARTESIAN_POINT('Ctrl Pts',(53.843254179489,-23.9299165195797,2.60003234582321));
#219092=CARTESIAN_POINT('Ctrl Pts',(53.8411336218844,-23.9341422497933,
2.59967776696049));
#219093=CARTESIAN_POINT('Ctrl Pts',(53.8390713992306,-23.9384150933419,
2.59944011429143));
#219094=CARTESIAN_POINT('Ctrl Pts',(53.8370091765769,-23.9426879368906,
2.59920246162237));
#219095=CARTESIAN_POINT('Ctrl Pts',(53.8350052904266,-23.9470078944651,
2.59908173791295));
#219096=CARTESIAN_POINT('Ctrl Pts',(53.8330634946841,-23.9513722670356,
2.59908173516008));
#219097=CARTESIAN_POINT('',(53.8206887816839,-23.9791663275005,2.59908173516007));
#219098=CARTESIAN_POINT('Origin',(5.71744365443249E-15,1.85827062561433E-13,
2.59908173516024));
#219099=CARTESIAN_POINT('',(53.8697418420148,-24.331269253108,2.90134173516007));
#219100=CARTESIAN_POINT('Ctrl Pts',(53.8206887816839,-23.9791663275005,
2.59908173516008));
#219101=CARTESIAN_POINT('Ctrl Pts',(53.8191382997274,-23.9826463618216,
2.59908174371494));
#219102=CARTESIAN_POINT('Ctrl Pts',(53.8176349962322,-23.9861360190788,
2.59915764355873));
#219103=CARTESIAN_POINT('Ctrl Pts',(53.8161786595152,-23.9896330908633,
2.5993076577526));
#219104=CARTESIAN_POINT('Ctrl Pts',(53.8075805576709,-24.0102795382194,
2.60019333020862));
#219105=CARTESIAN_POINT('Ctrl Pts',(53.8006169491717,-24.0311861904745,
2.60365973324056));
#219106=CARTESIAN_POINT('Ctrl Pts',(53.7952474622082,-24.0518926318772,
2.60934177082334));
#219107=CARTESIAN_POINT('Ctrl Pts',(53.7932416006208,-24.0596278690992,
2.61146439091781));
#219108=CARTESIAN_POINT('Ctrl Pts',(53.791457853367,-24.0673353939204,2.61389584429273));
#219109=CARTESIAN_POINT('Ctrl Pts',(53.7898929820051,-24.0749921329669,
2.61661604385235));
#219110=CARTESIAN_POINT('Ctrl Pts',(53.7886719908667,-24.0809663048713,
2.61873848000758));
#219111=CARTESIAN_POINT('Ctrl Pts',(53.7875846446509,-24.086909241038,2.62103707099769));
#219112=CARTESIAN_POINT('Ctrl Pts',(53.7866297945202,-24.0928096561855,
2.62350262767634));
#219113=CARTESIAN_POINT('Ctrl Pts',(53.7832878190625,-24.1134611092019,
2.63213207605161));
#219114=CARTESIAN_POINT('Ctrl Pts',(53.7815689125025,-24.1335916760293,
2.64280685971896));
#219115=CARTESIAN_POINT('Ctrl Pts',(53.7814239018617,-24.1527175379836,
2.65513293646066));
#219116=CARTESIAN_POINT('Ctrl Pts',(53.7813513965413,-24.1622804689607,
2.66129597483151));
#219117=CARTESIAN_POINT('Ctrl Pts',(53.7816723668481,-24.1715922244702,
2.66787183533835));
#219118=CARTESIAN_POINT('Ctrl Pts',(53.7823806708184,-24.1805923292959,
2.67481125953844));
#219119=CARTESIAN_POINT('Ctrl Pts',(53.7830859485795,-24.1895539814227,
2.68172103524063));
#219120=CARTESIAN_POINT('Ctrl Pts',(53.7841750295933,-24.1982067474356,
2.68899101329771));
#219121=CARTESIAN_POINT('Ctrl Pts',(53.7856425347027,-24.206490601869,2.69657334701257));
#219122=CARTESIAN_POINT('Ctrl Pts',(53.7856488314805,-24.2065261462703,
2.69660588132554));
#219123=CARTESIAN_POINT('Ctrl Pts',(53.7856551347357,-24.2065616841174,
2.69663842081363));
#219124=CARTESIAN_POINT('Ctrl Pts',(53.7856614444667,-24.206597215409,2.69667096547363));
#219125=CARTESIAN_POINT('Ctrl Pts',(53.7886369923276,-24.2233530895744,
2.71201840157921));
#219126=CARTESIAN_POINT('Ctrl Pts',(53.7930196670709,-24.2386338146178,
2.7284564593933));
#219127=CARTESIAN_POINT('Ctrl Pts',(53.798615834808,-24.2524209582909,2.74568723186877));
#219128=CARTESIAN_POINT('Ctrl Pts',(53.8044155801162,-24.2667096511229,
2.76354482594304));
#219129=CARTESIAN_POINT('Ctrl Pts',(53.8115193533084,-24.2793947083677,
2.78225519317111));
#219130=CARTESIAN_POINT('Ctrl Pts',(53.8197464933878,-24.2904167802938,
2.80151223085494));
#219131=CARTESIAN_POINT('Ctrl Pts',(53.8278562137183,-24.3012815425224,
2.82049442740233));
#219132=CARTESIAN_POINT('Ctrl Pts',(53.8370583385443,-24.3105307527859,
2.84000929089209));
#219133=CARTESIAN_POINT('Ctrl Pts',(53.8472012967771,-24.3180642992199,
2.85976644341553));
#219134=CARTESIAN_POINT('Ctrl Pts',(53.8542731477179,-24.3233168218286,
2.87354148166897));
#219135=CARTESIAN_POINT('Ctrl Pts',(53.8618028047968,-24.327734457649,2.88743438345454));
#219136=CARTESIAN_POINT('Ctrl Pts',(53.8697418420148,-24.331269253108,2.90134173516007));
#219137=CARTESIAN_POINT('',(54.1952354911875,-24.4761921430384,3.47153072139056));
#219138=CARTESIAN_POINT('',(53.8697418420148,-24.331269253108,2.90134173516007));
#219139=CARTESIAN_POINT('',(51.6568155675431,-29.4581217525665,3.47153072139052));
#219140=CARTESIAN_POINT('Origin',(5.53234440788222E-15,1.85015204418142E-13,
3.47153072139072));
#219141=CARTESIAN_POINT('',(51.3482501200169,-29.2799753962454,2.90134173516004));
#219142=CARTESIAN_POINT('',(51.6568155675431,-29.4581217525665,3.47153072139052));
#219143=CARTESIAN_POINT('',(51.0345602039891,-29.4472515437727,2.59908173516003));
#219144=CARTESIAN_POINT('Ctrl Pts',(51.3482501200169,-29.2799753962454,
2.90134173516004));
#219145=CARTESIAN_POINT('Ctrl Pts',(51.3376585930517,-29.2738605406098,
2.88176998919757));
#219146=CARTESIAN_POINT('Ctrl Pts',(51.3261534914777,-29.269437766393,2.86226752356645));
#219147=CARTESIAN_POINT('Ctrl Pts',(51.3139160033708,-29.266725042103,2.84310370499914));
#219148=CARTESIAN_POINT('Ctrl Pts',(51.3014574615393,-29.2639633161059,
2.82359371788522));
#219149=CARTESIAN_POINT('Ctrl Pts',(51.2882390496566,-29.2629734853262,
2.80443322636835));
#219150=CARTESIAN_POINT('Ctrl Pts',(51.2744188030426,-29.2638161685318,
2.78589323878069));
#219151=CARTESIAN_POINT('Ctrl Pts',(51.2611836698378,-29.2646231747154,
2.76813818619779));
#219152=CARTESIAN_POINT('Ctrl Pts',(51.2473957191175,-29.267110757666,2.75095095198469));
#219153=CARTESIAN_POINT('Ctrl Pts',(51.2331761176611,-29.271373305682,2.73457771434851));
#219154=CARTESIAN_POINT('Ctrl Pts',(51.2218663142633,-29.2747635962033,
2.72155497955398));
#219155=CARTESIAN_POINT('Ctrl Pts',(51.2102829897272,-29.2792774508354,
2.70904711159866));
#219156=CARTESIAN_POINT('Ctrl Pts',(51.1984837018595,-29.2849828273421,
2.69718956158318));
#219157=CARTESIAN_POINT('Ctrl Pts',(51.1984514936364,-29.2849984011667,
2.69715719432336));
#219158=CARTESIAN_POINT('Ctrl Pts',(51.1984192839706,-29.2850139839317,
2.69712483219002));
#219159=CARTESIAN_POINT('Ctrl Pts',(51.1983870728642,-29.2850295756377,
2.6970924751863));
#219160=CARTESIAN_POINT('Ctrl Pts',(51.1919748636256,-29.2881333895818,
2.69065122242256));
#219161=CARTESIAN_POINT('Ctrl Pts',(51.1854935419305,-29.29162601106,2.68442464469405));
#219162=CARTESIAN_POINT('Ctrl Pts',(51.1789779411681,-29.2954867606371,
2.67844505923558));
#219163=CARTESIAN_POINT('Ctrl Pts',(51.1660472802373,-29.3031486855372,
2.66657815779546));
#219164=CARTESIAN_POINT('Ctrl Pts',(51.1529811529982,-29.3122618143328,
2.65568445664152));
#219165=CARTESIAN_POINT('Ctrl Pts',(51.1400491105588,-29.3226724463005,
2.64601906229494));
#219166=CARTESIAN_POINT('Ctrl Pts',(51.1303500787293,-29.3304804202763,
2.638770016535));
#219167=CARTESIAN_POINT('Ctrl Pts',(51.1207264688924,-29.3390182393868,
2.63221189387581));
#219168=CARTESIAN_POINT('Ctrl Pts',(51.1112920078095,-29.3482210667391,
2.62645231033213));
#219169=CARTESIAN_POINT('Ctrl Pts',(51.1077540849034,-29.3516721269962,
2.62429246650325));
#219170=CARTESIAN_POINT('Ctrl Pts',(51.1042427612076,-29.3552167041318,
2.62224491711724));
#219171=CARTESIAN_POINT('Ctrl Pts',(51.1007640347392,-29.3588513794152,
2.62031533672576));
#219172=CARTESIAN_POINT('Ctrl Pts',(51.0885884920996,-29.371572742907,2.61356180535557));
#219173=CARTESIAN_POINT('Ctrl Pts',(51.0768122611,-29.3853978061634,2.60825339735327));
#219174=CARTESIAN_POINT('Ctrl Pts',(51.0656925470316,-29.4001800143149,
2.6046333798759));
#219175=CARTESIAN_POINT('Ctrl Pts',(51.0601326899974,-29.4075711183907,
2.60282337113721));
#219176=CARTESIAN_POINT('Ctrl Pts',(51.0547369630771,-29.4152015092018,
2.60143545939095));
#219177=CARTESIAN_POINT('Ctrl Pts',(51.0495375206698,-29.4230528695796,
2.60050005034576));
#219178=CARTESIAN_POINT('Ctrl Pts',(51.0469377994662,-29.4269785497685,
2.60003234582316));
#219179=CARTESIAN_POINT('Ctrl Pts',(51.0443871494126,-29.4309594723622,
2.59967776696045));
#219180=CARTESIAN_POINT('Ctrl Pts',(51.0418895900604,-29.4349933478619,
2.59944011429139));
#219181=CARTESIAN_POINT('Ctrl Pts',(51.0393920307082,-29.4390272233617,
2.59920246162233));
#219182=CARTESIAN_POINT('Ctrl Pts',(51.0369475635293,-29.4431140526167,
2.59908173791293));
#219183=CARTESIAN_POINT('Ctrl Pts',(51.0345602039891,-29.4472515437727,
2.59908173516004));
#219184=CARTESIAN_POINT('',(51.0193480105331,-29.4735998357329,2.59908173516003));
#219185=CARTESIAN_POINT('Origin',(5.71420591410065E-15,1.85820708138243E-13,
2.59908173516023));
#219186=CARTESIAN_POINT('',(51.0313275753413,-29.8289013456877,2.90134173516003));
#219187=CARTESIAN_POINT('Ctrl Pts',(51.0193480105332,-29.4735998357329,
2.59908173516004));
#219188=CARTESIAN_POINT('Ctrl Pts',(51.0174422596394,-29.4768987365657,
2.59908174371493));
#219189=CARTESIAN_POINT('Ctrl Pts',(51.0155824228875,-29.4802121391111,
2.59915764355871));
#219190=CARTESIAN_POINT('Ctrl Pts',(51.0137685205959,-29.4835378249314,
2.59930765775257));
#219191=CARTESIAN_POINT('Ctrl Pts',(51.003059378638,-29.5031724225179,2.60019333020868));
#219192=CARTESIAN_POINT('Ctrl Pts',(50.9939485772817,-29.5232366506513,
2.60365973324125));
#219193=CARTESIAN_POINT('Ctrl Pts',(50.9864440924295,-29.5432683957827,
2.60934177082507));
#219194=CARTESIAN_POINT('Ctrl Pts',(50.9836406667028,-29.5507515889345,
2.61146439091913));
#219195=CARTESIAN_POINT('Ctrl Pts',(50.9810610352787,-29.5582304387669,
2.61389584429345));
#219196=CARTESIAN_POINT('Ctrl Pts',(50.9787043892804,-29.565681659795,2.61661604385232));
#219197=CARTESIAN_POINT('Ctrl Pts',(50.9768656158508,-29.5714954762333,
2.61873848000755));
#219198=CARTESIAN_POINT('Ctrl Pts',(50.9751630202465,-29.5772921977449,
2.62103707099767));
#219199=CARTESIAN_POINT('Ctrl Pts',(50.9735966395567,-29.583060480784,2.62350262767631));
#219200=CARTESIAN_POINT('Ctrl Pts',(50.9681143071422,-29.6032494714211,
2.63213207605158));
#219201=CARTESIAN_POINT('Ctrl Pts',(50.964300599717,-29.623090086236,2.64280685971894));
#219202=CARTESIAN_POINT('Ctrl Pts',(50.9621571865009,-29.6420960169778,
2.65513293646064));
#219203=CARTESIAN_POINT('Ctrl Pts',(50.9610854798929,-29.6515989823488,
2.66129597483149));
#219204=CARTESIAN_POINT('Ctrl Pts',(50.960431348397,-29.6608932776201,2.66787183533831));
#219205=CARTESIAN_POINT('Ctrl Pts',(50.9601950050773,-29.6699181168554,
2.6748112595384));
#219206=CARTESIAN_POINT('Ctrl Pts',(50.959959671528,-29.6789043977148,2.68172103524059));
#219207=CARTESIAN_POINT('Ctrl Pts',(50.9601383261077,-29.6876236029349,
2.68899101329768));
#219208=CARTESIAN_POINT('Ctrl Pts',(50.9607318934967,-29.6960154736008,
2.69657334701254));
#219209=CARTESIAN_POINT('Ctrl Pts',(50.9607344403784,-29.6960514814787,
2.69660588132551));
#219210=CARTESIAN_POINT('Ctrl Pts',(50.9607369943872,-29.6960874835153,
2.69663842081359));
#219211=CARTESIAN_POINT('Ctrl Pts',(50.9607395555215,-29.6961234797093,
2.6966709654736));
#219212=CARTESIAN_POINT('Ctrl Pts',(50.9619473372425,-29.7130985928864,
2.71201840157765));
#219213=CARTESIAN_POINT('Ctrl Pts',(50.9647087325282,-29.7287537227736,
2.72845645938998));
#219214=CARTESIAN_POINT('Ctrl Pts',(50.9688330949313,-29.7430502978437,
2.74568723186358));
#219215=CARTESIAN_POINT('Ctrl Pts',(50.9731074935233,-29.7578669541845,
2.76354482593602));
#219216=CARTESIAN_POINT('Ctrl Pts',(50.9788464019616,-29.7712250678528,
2.78225519316214));
#219217=CARTESIAN_POINT('Ctrl Pts',(50.9858763526652,-29.7830467300247,
2.80151223084397));
#219218=CARTESIAN_POINT('Ctrl Pts',(50.9928059701987,-29.7946996705523,
2.82049442738972));
#219219=CARTESIAN_POINT('Ctrl Pts',(51.0009908790856,-29.8048600966411,
2.84000929087781));
#219220=CARTESIAN_POINT('Ctrl Pts',(51.0102908030989,-29.8134126013568,
2.85976644339964));
#219221=CARTESIAN_POINT('Ctrl Pts',(51.0167748755858,-29.8193755598113,
2.87354148165827));
#219222=CARTESIAN_POINT('Ctrl Pts',(51.0238015157343,-29.8245560588462,
2.88743438344917));
#219223=CARTESIAN_POINT('Ctrl Pts',(51.0313275753413,-29.8289013456877,
2.90134173516003));
#219224=CARTESIAN_POINT('',(51.3398895692701,-30.007053683815,3.47153072139052));
#219225=CARTESIAN_POINT('',(51.0313275753413,-29.8289013456877,2.90134173516003));
#219226=CARTESIAN_POINT('',(48.2946219293751,-34.6963546279277,3.47153072139049));
#219227=CARTESIAN_POINT('Origin',(5.53234440788222E-15,1.85015204418142E-13,
3.47153072139072));
#219228=CARTESIAN_POINT('',(48.0063682005191,-34.4869303039389,2.90134173516));
#219229=CARTESIAN_POINT('',(48.2946219293751,-34.6963546279277,3.47153072139049));
#219230=CARTESIAN_POINT('',(47.6769115920308,-34.6205005703627,2.59908173516));
#219231=CARTESIAN_POINT('Ctrl Pts',(48.0063682005191,-34.4869303039389,
2.90134173516));
#219232=CARTESIAN_POINT('Ctrl Pts',(47.9964738715105,-34.4797418300855,
2.88176998919937));
#219233=CARTESIAN_POINT('Ctrl Pts',(47.9854941018801,-34.4741406737017,
2.86226752357008));
#219234=CARTESIAN_POINT('Ctrl Pts',(47.9736072089161,-34.4701636441732,
2.84310370500451));
#219235=CARTESIAN_POINT('Ctrl Pts',(47.961505595256,-34.4661147749679,2.82359371789228));
#219236=CARTESIAN_POINT('Ctrl Pts',(47.9484630607083,-34.4637486663037,
2.80443322637702));
#219237=CARTESIAN_POINT('Ctrl Pts',(47.9346304384724,-34.4631421240614,
2.78589323879081));
#219238=CARTESIAN_POINT('Ctrl Pts',(47.9213834535972,-34.462561261245,2.76813818620915));
#219239=CARTESIAN_POINT('Ctrl Pts',(47.9074110114921,-34.4635939836547,
2.75095095199715));
#219240=CARTESIAN_POINT('Ctrl Pts',(47.8928237489081,-34.4663468278971,
2.73457771436186));
#219241=CARTESIAN_POINT('Ctrl Pts',(47.8812215199347,-34.4685363496832,
2.72155497956252));
#219242=CARTESIAN_POINT('Ctrl Pts',(47.8692298237703,-34.4718146898347,
2.70904711160269));
#219243=CARTESIAN_POINT('Ctrl Pts',(47.8568987993932,-34.476255450265,2.69718956158315));
#219244=CARTESIAN_POINT('Ctrl Pts',(47.8568651397022,-34.4762675720985,
2.69715719432332));
#219245=CARTESIAN_POINT('Ctrl Pts',(47.8568314776419,-34.4762797026727,
2.69712483218998));
#219246=CARTESIAN_POINT('Ctrl Pts',(47.8567978132142,-34.4762918419882,
2.69709247518626));
#219247=CARTESIAN_POINT('Ctrl Pts',(47.8500962938269,-34.4787083945369,
2.69065122242252));
#219248=CARTESIAN_POINT('Ctrl Pts',(47.8432853991343,-34.4815044004724,
2.68442464469402));
#219249=CARTESIAN_POINT('Ctrl Pts',(47.8364019332942,-34.4846629347244,
2.67844505923554));
#219250=CARTESIAN_POINT('Ctrl Pts',(47.8227412186415,-34.4909312646821,
2.66657815779542));
#219251=CARTESIAN_POINT('Ctrl Pts',(47.808794087666,-34.4986286886035,2.65568445664149));
#219252=CARTESIAN_POINT('Ctrl Pts',(47.794844680947,-34.5076305235169,2.64601906229491));
#219253=CARTESIAN_POINT('Ctrl Pts',(47.7843826259077,-34.5143818997019,
2.63877001653497));
#219254=CARTESIAN_POINT('Ctrl Pts',(47.7739192901011,-34.5218670065987,
2.63221189387577));
#219255=CARTESIAN_POINT('Ctrl Pts',(47.7635745545823,-34.5300332501811,
2.62645231033209));
#219256=CARTESIAN_POINT('Ctrl Pts',(47.7596952787628,-34.5330955915245,
2.62429246650321));
#219257=CARTESIAN_POINT('Ctrl Pts',(47.7558326812647,-34.5362537178257,
2.62224491711721));
#219258=CARTESIAN_POINT('Ctrl Pts',(47.751993084602,-34.5395048560457,2.62031533672573));
#219259=CARTESIAN_POINT('Ctrl Pts',(47.7385544962824,-34.5508838398157,
2.61356180535554));
#219260=CARTESIAN_POINT('Ctrl Pts',(47.7253976640916,-34.5634022165996,
2.60825339735323));
#219261=CARTESIAN_POINT('Ctrl Pts',(47.7127937034786,-34.5769411196446,
2.60463337987586));
#219262=CARTESIAN_POINT('Ctrl Pts',(47.7064917231721,-34.5837105711672,
2.60282337113718));
#219263=CARTESIAN_POINT('Ctrl Pts',(47.7003279615829,-34.5907351548558,
2.6014354593909));
#219264=CARTESIAN_POINT('Ctrl Pts',(47.6943363116302,-34.5980000149353,
2.60050005034571));
#219265=CARTESIAN_POINT('Ctrl Pts',(47.6913404866539,-34.601632444975,2.60003234582311));
#219266=CARTESIAN_POINT('Ctrl Pts',(47.6883876896072,-34.6053249441278,
2.59967776696041));
#219267=CARTESIAN_POINT('Ctrl Pts',(47.6854821573394,-34.6090756555945,
2.59944011429135));
#219268=CARTESIAN_POINT('Ctrl Pts',(47.6825766250716,-34.6128263670611,
2.59920246162229));
#219269=CARTESIAN_POINT('Ctrl Pts',(47.679718358958,-34.6166352918402,2.59908173791286));
#219270=CARTESIAN_POINT('Ctrl Pts',(47.6769115920308,-34.6205005703627,
2.59908173516));
#219271=CARTESIAN_POINT('',(47.659028586094,-34.6451144164178,2.59908173516));
#219272=CARTESIAN_POINT('Origin',(5.71032169235817E-15,1.8581472696127E-13,
2.59908173516024));
#219273=CARTESIAN_POINT('',(47.6338034047604,-34.9997217530253,2.90134173515999));
#219274=CARTESIAN_POINT('Ctrl Pts',(47.659028586094,-34.6451144164178,2.59908173516));
#219275=CARTESIAN_POINT('Ctrl Pts',(47.6567884460685,-34.6481960403143,
2.59908174371483));
#219276=CARTESIAN_POINT('Ctrl Pts',(47.6545924528207,-34.6512968858163,
2.59915764355865));
#219277=CARTESIAN_POINT('Ctrl Pts',(47.6524408584475,-34.6544147487627,
2.59930765775252));
#219278=CARTESIAN_POINT('Ctrl Pts',(47.6397380079788,-34.6728223758151,
2.60019333020852));
#219279=CARTESIAN_POINT('Ctrl Pts',(47.6285798336134,-34.69182435194,2.60365973324032));
#219280=CARTESIAN_POINT('Ctrl Pts',(47.6190225715801,-34.710961928804,2.60934177082287));
#219281=CARTESIAN_POINT('Ctrl Pts',(47.615452296631,-34.71811109046,2.61146439091744));
#219282=CARTESIAN_POINT('Ctrl Pts',(47.6121050440166,-34.7252793254644,
2.6138958442925));
#219283=CARTESIAN_POINT('Ctrl Pts',(47.608982443287,-34.7324433913419,2.61661604385228));
#219284=CARTESIAN_POINT('Ctrl Pts',(47.6065460335526,-34.7380331549245,
2.61873848000751));
#219285=CARTESIAN_POINT('Ctrl Pts',(47.6042468425536,-34.743620151687,2.62103707099763));
#219286=CARTESIAN_POINT('Ctrl Pts',(47.6020860928993,-34.7491931041017,
2.62350262767627));
#219287=CARTESIAN_POINT('Ctrl Pts',(47.5945234691092,-34.7686984375533,
2.63213207605154));
#219288=CARTESIAN_POINT('Ctrl Pts',(47.5886567445954,-34.7880317224277,
2.64280685971889));
#219289=CARTESIAN_POINT('Ctrl Pts',(47.5845384124878,-34.8067094890027,
2.65513293646059));
#219290=CARTESIAN_POINT('Ctrl Pts',(47.582479246434,-34.8160483722902,2.66129597483144));
#219291=CARTESIAN_POINT('Ctrl Pts',(47.580857179937,-34.8252233770796,2.66787183533828));
#219292=CARTESIAN_POINT('Ctrl Pts',(47.5796787787543,-34.8341740726973,
2.67481125953837));
#219293=CARTESIAN_POINT('Ctrl Pts',(47.578505412258,-34.8430865267156,2.68172103524056));
#219294=CARTESIAN_POINT('Ctrl Pts',(47.5777716830267,-34.8517766417058,
2.68899101329765));
#219295=CARTESIAN_POINT('Ctrl Pts',(47.5774848094468,-34.8601845855132,
2.6965733470125));
#219296=CARTESIAN_POINT('Ctrl Pts',(47.5774835785283,-34.8602206623578,
2.69660588132548));
#219297=CARTESIAN_POINT('Ctrl Pts',(47.5774823553084,-34.8602567341381,
2.69663842081356));
#219298=CARTESIAN_POINT('Ctrl Pts',(47.5774811397857,-34.8602928008526,
2.69667096547357));
#219299=CARTESIAN_POINT('Ctrl Pts',(47.5769079226578,-34.8773011701513,
2.71201840157807));
#219300=CARTESIAN_POINT('Ctrl Pts',(47.578017784062,-34.8931591840051,2.72845645939092));
#219301=CARTESIAN_POINT('Ctrl Pts',(47.5806251537543,-34.9078085542054,
2.74568723186507));
#219302=CARTESIAN_POINT('Ctrl Pts',(47.5833273744258,-34.922990839669,2.76354482593811));
#219303=CARTESIAN_POINT('Ctrl Pts',(47.5876385414295,-34.9368756554732,
2.78225519316489));
#219304=CARTESIAN_POINT('Ctrl Pts',(47.5933942811479,-34.9493673872869,
2.80151223084739));
#219305=CARTESIAN_POINT('Ctrl Pts',(47.599067873546,-34.9616808340591,2.8204944273939));
#219306=CARTESIAN_POINT('Ctrl Pts',(47.6061458909209,-34.9726411562187,
2.84000929088276));
#219307=CARTESIAN_POINT('Ctrl Pts',(47.6145008888029,-34.9821189161845,
2.85976644340536));
#219308=CARTESIAN_POINT('Ctrl Pts',(47.6203261419778,-34.9887269790603,
2.87354148166211));
#219309=CARTESIAN_POINT('Ctrl Pts',(47.6267727798524,-34.9946135826752,
2.88743438345107));
#219310=CARTESIAN_POINT('Ctrl Pts',(47.6338034047604,-34.9997217530253,
2.90134173515999));
#219311=CARTESIAN_POINT('',(47.9220530736691,-35.209151665052,3.47153072139048));
#219312=CARTESIAN_POINT('',(47.6338034047604,-34.9997217530253,2.90134173515999));
#219313=CARTESIAN_POINT('',(44.4033023070494,-39.5544469813064,3.47153072139045));
#219314=CARTESIAN_POINT('Origin',(5.53234440788222E-15,1.85015204418142E-13,
3.47153072139072));
#219315=CARTESIAN_POINT('',(44.1385184650381,-39.3160391863683,2.90134173515996));
#219316=CARTESIAN_POINT('',(44.4033023070494,-39.5544469813064,3.47153072139045));
#219317=CARTESIAN_POINT('',(43.7969047596351,-39.4144401478983,2.59908173515996));
#219318=CARTESIAN_POINT('Ctrl Pts',(44.1385184650381,-39.3160391863683,
2.90134173515997));
#219319=CARTESIAN_POINT('Ctrl Pts',(44.1294297383231,-39.3078558527201,
2.88176998919776));
#219320=CARTESIAN_POINT('Ctrl Pts',(44.1190955972879,-39.3011376816103,
2.8622675235669));
#219321=CARTESIAN_POINT('Ctrl Pts',(44.1076895347511,-39.2959399200109,
2.84310370499984));
#219322=CARTESIAN_POINT('Ctrl Pts',(44.0960774370719,-39.2906482678558,
2.82359371788642));
#219323=CARTESIAN_POINT('Ctrl Pts',(44.0833536765948,-39.2869318048891,
2.80443322637003));
#219324=CARTESIAN_POINT('Ctrl Pts',(44.0696602318382,-39.2848826826036,
2.78589323878281));
#219325=CARTESIAN_POINT('Ctrl Pts',(44.0565465320292,-39.2829203148429,
2.76813818620078));
#219326=CARTESIAN_POINT('Ctrl Pts',(44.0425426835367,-39.2824868619903,
2.75095095198847));
#219327=CARTESIAN_POINT('Ctrl Pts',(44.0277475809245,-39.2836998417232,
2.73457771435298));
#219328=CARTESIAN_POINT('Ctrl Pts',(44.0159800428303,-39.284664605915,2.72155497955682));
#219329=CARTESIAN_POINT('Ctrl Pts',(44.0037113585768,-39.2866715134038,
2.70904711159996));
#219330=CARTESIAN_POINT('Ctrl Pts',(43.9909836989808,-39.2897990038545,
2.69718956158311));
#219331=CARTESIAN_POINT('Ctrl Pts',(43.9909489566045,-39.2898075408876,
2.69715719432328));
#219332=CARTESIAN_POINT('Ctrl Pts',(43.9909142109582,-39.2898160863657,
2.69712483218994));
#219333=CARTESIAN_POINT('Ctrl Pts',(43.9908794620438,-39.28982464029,2.69709247518622));
#219334=CARTESIAN_POINT('Ctrl Pts',(43.9839620557566,-39.2915274551878,
2.69065122242248));
#219335=CARTESIAN_POINT('Ctrl Pts',(43.976896209654,-39.2935962119545,2.68442464469397));
#219336=CARTESIAN_POINT('Ctrl Pts',(43.9697202954285,-39.2960179253192,
2.67844505923549));
#219337=CARTESIAN_POINT('Ctrl Pts',(43.9554791967022,-39.3008239831998,
2.66657815779538));
#219338=CARTESIAN_POINT('Ctrl Pts',(43.9408038696759,-39.3070213676597,
2.65568445664144));
#219339=CARTESIAN_POINT('Ctrl Pts',(43.9259899312963,-39.3145157795317,
2.64601906229486));
#219340=CARTESIAN_POINT('Ctrl Pts',(43.9148794775117,-39.3201365884357,
2.63877001653492));
#219341=CARTESIAN_POINT('Ctrl Pts',(43.9036910542322,-39.3264869747212,
2.63221189387573));
#219342=CARTESIAN_POINT('Ctrl Pts',(43.8925493833646,-39.3335271634601,
2.62645231033205));
#219343=CARTESIAN_POINT('Ctrl Pts',(43.8883712567893,-39.3361672342372,
2.62429246650317));
#219344=CARTESIAN_POINT('Ctrl Pts',(43.8841997049153,-39.3389043086114,
2.62224491711717));
#219345=CARTESIAN_POINT('Ctrl Pts',(43.8800413054829,-39.3417362896173,
2.62031533672569));
#219346=CARTESIAN_POINT('Ctrl Pts',(43.8654869074692,-39.3516482231381,
2.6135618053555));
#219347=CARTESIAN_POINT('Ctrl Pts',(43.851093623094,-39.3627227594938,2.6082533973532));
#219348=CARTESIAN_POINT('Ctrl Pts',(43.8371435075663,-39.3748700223774,
2.60463337987583));
#219349=CARTESIAN_POINT('Ctrl Pts',(43.8301684498025,-39.3809436538192,
2.60282337113715));
#219350=CARTESIAN_POINT('Ctrl Pts',(43.8233041850061,-39.3872854675765,
2.60143545939088));
#219351=CARTESIAN_POINT('Ctrl Pts',(43.8165859732789,-39.3938842320304,
2.60050005034569));
#219352=CARTESIAN_POINT('Ctrl Pts',(43.8132268674153,-39.3971836142573,
2.6000323458231));
#219353=CARTESIAN_POINT('Ctrl Pts',(43.8099042748376,-39.4005472341757,
2.59967776696038));
#219354=CARTESIAN_POINT('Ctrl Pts',(43.8066226032739,-39.4039736880296,
2.59944011429132));
#219355=CARTESIAN_POINT('Ctrl Pts',(43.8033409317101,-39.4074001418835,
2.59920246162226));
#219356=CARTESIAN_POINT('Ctrl Pts',(43.8001001824234,-39.4108894308096,
2.5990817379128));
#219357=CARTESIAN_POINT('Ctrl Pts',(43.7969047596351,-39.4144401478983,
2.59908173515997));
#219358=CARTESIAN_POINT('',(43.7765468711727,-39.4370498736001,2.59908173515996));
#219359=CARTESIAN_POINT('Origin',(5.7058335455513E-15,1.8580918456154E-13,
2.59908173516024));
#219360=CARTESIAN_POINT('',(43.7143933160628,-39.787077884674,2.90134173515997));
#219361=CARTESIAN_POINT('Ctrl Pts',(43.7765468711727,-39.4370498736001,
2.59908173515997));
#219362=CARTESIAN_POINT('Ctrl Pts',(43.7739968854584,-39.4398804576441,
2.59908174371481));
#219363=CARTESIAN_POINT('Ctrl Pts',(43.7714887954762,-39.4427347725904,
2.59915764355863));
#219364=CARTESIAN_POINT('Ctrl Pts',(43.7690230823397,-39.445610652704,2.59930765775249));
#219365=CARTESIAN_POINT('Ctrl Pts',(43.7544656984445,-39.4625896314133,
2.60019333020863));
#219366=CARTESIAN_POINT('Ctrl Pts',(43.7413824023606,-39.4803211659083,
2.60365973324136));
#219367=CARTESIAN_POINT('Ctrl Pts',(43.7298770745073,-39.4983548992134,
2.60934177082543));
#219368=CARTESIAN_POINT('Ctrl Pts',(43.7255790670182,-39.5050917016572,
2.6114643909194));
#219369=CARTESIAN_POINT('Ctrl Pts',(43.7215008664163,-39.5118707851455,
2.61389584429358));
#219370=CARTESIAN_POINT('Ctrl Pts',(43.7176465228248,-39.5186692048621,
2.61661604385227));
#219371=CARTESIAN_POINT('Ctrl Pts',(43.7146391706006,-39.5239736729695,
2.6187384800075));
#219372=CARTESIAN_POINT('Ctrl Pts',(43.7117685746246,-39.5292897326773,
2.62103707099761));
#219373=CARTESIAN_POINT('Ctrl Pts',(43.7090371296312,-39.5346062960347,
2.62350262767626));
#219374=CARTESIAN_POINT('Ctrl Pts',(43.6994770721543,-39.5532142677857,
2.63213207605152));
#219375=CARTESIAN_POINT('Ctrl Pts',(43.6916216076134,-39.5718284032049,
2.64280685971888));
#219376=CARTESIAN_POINT('Ctrl Pts',(43.6855734779227,-39.5899733680939,
2.65513293646057));
#219377=CARTESIAN_POINT('Ctrl Pts',(43.6825494130773,-39.5990458505383,
2.66129597483142));
#219378=CARTESIAN_POINT('Ctrl Pts',(43.6799771832791,-39.6080010415732,
2.66787183533825));
#219379=CARTESIAN_POINT('Ctrl Pts',(43.6778696350433,-39.616779527879,2.67481125953834));
#219380=CARTESIAN_POINT('Ctrl Pts',(43.675771091249,-39.625520508345,2.68172103524052));
#219381=CARTESIAN_POINT('Ctrl Pts',(43.6741330170976,-39.634086322387,2.68899101329759));
#219382=CARTESIAN_POINT('Ctrl Pts',(43.6729688455957,-39.6424182201441,
2.69657334701245));
#219383=CARTESIAN_POINT('Ctrl Pts',(43.6729638503632,-39.6424539706899,
2.69660588132542));
#219384=CARTESIAN_POINT('Ctrl Pts',(43.6729588633165,-39.6424897170039,
2.6966384208135));
#219385=CARTESIAN_POINT('Ctrl Pts',(43.6729538844543,-39.6425254590845,
2.69667096547351));
#219386=CARTESIAN_POINT('Ctrl Pts',(43.6706059487642,-39.6593807372523,
2.71201840157909));
#219387=CARTESIAN_POINT('Ctrl Pts',(43.6700521164129,-39.675267891355,2.72845645939318));
#219388=CARTESIAN_POINT('Ctrl Pts',(43.6711139265067,-39.6901095551206,
2.74568723186866));
#219389=CARTESIAN_POINT('Ctrl Pts',(43.6722143631624,-39.7054911294111,
2.76354482594304));
#219390=CARTESIAN_POINT('Ctrl Pts',(43.675050554684,-39.719750522404,2.78225519317123));
#219391=CARTESIAN_POINT('Ctrl Pts',(43.6794690223286,-39.7327754618321,
2.80151223085518));
#219392=CARTESIAN_POINT('Ctrl Pts',(43.6838244285259,-39.7456145061494,
2.8204944274028));
#219393=CARTESIAN_POINT('Ctrl Pts',(43.6897180061495,-39.7572546407968,
2.8400092908928));
#219394=CARTESIAN_POINT('Ctrl Pts',(43.6970365387954,-39.767553815691,2.85976644341649));
#219395=CARTESIAN_POINT('Ctrl Pts',(43.7021391499654,-39.7747345836671,
2.87354148166958));
#219396=CARTESIAN_POINT('Ctrl Pts',(43.7079351548522,-39.7812627969998,
2.88743438345479));
#219397=CARTESIAN_POINT('Ctrl Pts',(43.7143933160628,-39.787077884674,2.90134173515996));
#219398=CARTESIAN_POINT('',(43.9791725362587,-40.0254908126581,3.47153072139045));
#219399=CARTESIAN_POINT('',(43.7143933160628,-39.787077884674,2.90134173515997));
#219400=CARTESIAN_POINT('',(40.0254908126594,-43.9791725362576,3.47153072139042));
#219401=CARTESIAN_POINT('Origin',(5.53234440788222E-15,1.85015204418142E-13,
3.47153072139072));
#219402=CARTESIAN_POINT('',(39.7870778846752,-43.7143933160617,2.90134173515994));
#219403=CARTESIAN_POINT('',(40.0254908126594,-43.9791725362576,3.47153072139042));
#219404=CARTESIAN_POINT('',(39.4370498736014,-43.7765468711716,2.59908173515993));
#219405=CARTESIAN_POINT('Ctrl Pts',(39.7870778846752,-43.7143933160617,
2.90134173515994));
#219406=CARTESIAN_POINT('Ctrl Pts',(39.7788943382472,-43.7053047809349,
2.8817699891982));
#219407=CARTESIAN_POINT('Ctrl Pts',(39.7693190488203,-43.6975432007878,
2.86226752356781));
#219408=CARTESIAN_POINT('Ctrl Pts',(39.7585187839203,-43.6911816548816,
2.84310370500119));
#219409=CARTESIAN_POINT('Ctrl Pts',(39.7475234267954,-43.6847051962249,
2.82359371788803));
#219410=CARTESIAN_POINT('Ctrl Pts',(39.7352578445723,-43.6796790973015,
2.80443322637188));
#219411=CARTESIAN_POINT('Ctrl Pts',(39.7218536055427,-43.6762098455851,
2.78589323878489));
#219412=CARTESIAN_POINT('Ctrl Pts',(39.7090168672396,-43.6728874729914,
2.76813818620265));
#219413=CARTESIAN_POINT('Ctrl Pts',(39.6951350414549,-43.670992593876,2.75095095199014));
#219414=CARTESIAN_POINT('Ctrl Pts',(39.6802941970553,-43.670652419439,2.73457771435445));
#219415=CARTESIAN_POINT('Ctrl Pts',(39.6684902774472,-43.6703818558782,
2.72155497955776));
#219416=CARTESIAN_POINT('Ctrl Pts',(39.6560790233735,-43.6710953426065,
2.70904711160041));
#219417=CARTESIAN_POINT('Ctrl Pts',(39.6430941754573,-43.6728752976388,
2.6971895615831));
#219418=CARTESIAN_POINT('Ctrl Pts',(39.6430587310404,-43.6728801563378,
2.69715719432327));
#219419=CARTESIAN_POINT('Ctrl Pts',(39.6430232824887,-43.672885023094,2.69712483218993));
#219420=CARTESIAN_POINT('Ctrl Pts',(39.642987829804,-43.6728898979083,2.69709247518621));
#219421=CARTESIAN_POINT('Ctrl Pts',(39.6359303251676,-43.673860318759,2.69065122242247));
#219422=CARTESIAN_POINT('Ctrl Pts',(39.6286869425436,-43.6751791606249,
2.68442464469395));
#219423=CARTESIAN_POINT('Ctrl Pts',(39.6212972007506,-43.6768375203038,
2.67844505923548));
#219424=CARTESIAN_POINT('Ctrl Pts',(39.6066317464086,-43.6801286499313,
2.66657815779536));
#219425=CARTESIAN_POINT('Ctrl Pts',(39.5913890092854,-43.6847580950887,
2.65568445664143));
#219426=CARTESIAN_POINT('Ctrl Pts',(39.5758728438542,-43.6906629735746,
2.64601906229485));
#219427=CARTESIAN_POINT('Ctrl Pts',(39.5642357197808,-43.695091632439,2.63877001653491));
#219428=CARTESIAN_POINT('Ctrl Pts',(39.5524447917351,-43.7002377219522,
2.63221189387571));
#219429=CARTESIAN_POINT('Ctrl Pts',(39.5406282559963,-43.7060747220665,
2.62645231033202));
#219430=CARTESIAN_POINT('Ctrl Pts',(39.5361970550943,-43.7082635971094,
2.62429246650314));
#219431=CARTESIAN_POINT('Ctrl Pts',(39.5317622532398,-43.7105496315969,
2.62224491711714));
#219432=CARTESIAN_POINT('Ctrl Pts',(39.527330611332,-43.7129314276123,2.62031533672566));
#219433=CARTESIAN_POINT('Ctrl Pts',(39.5118198646546,-43.721267713666,2.61356180535547));
#219434=CARTESIAN_POINT('Ctrl Pts',(39.4963478239305,-43.7307770746556,
2.60825339735317));
#219435=CARTESIAN_POINT('Ctrl Pts',(39.4812043938732,-43.7413996094237,
2.6046333798758));
#219436=CARTESIAN_POINT('Ctrl Pts',(39.4736326788445,-43.7467108768077,
2.60282337113712));
#219437=CARTESIAN_POINT('Ctrl Pts',(39.4661431171625,-43.752300438395,2.60143545939084));
#219438=CARTESIAN_POINT('Ctrl Pts',(39.4587719497942,-43.758160809779,2.60050005034565));
#219439=CARTESIAN_POINT('Ctrl Pts',(39.4550863661101,-43.761090995471,2.60003234582306));
#219440=CARTESIAN_POINT('Ctrl Pts',(39.4514303810211,-43.7640888836314,
2.59967776696035));
#219441=CARTESIAN_POINT('Ctrl Pts',(39.4478085248418,-43.767153538927,2.59944011429129));
#219442=CARTESIAN_POINT('Ctrl Pts',(39.4441866686624,-43.7702181942226,
2.59920246162223));
#219443=CARTESIAN_POINT('Ctrl Pts',(39.4405989425301,-43.7733496179162,
2.59908173791281));
#219444=CARTESIAN_POINT('Ctrl Pts',(39.4370498736014,-43.7765468711716,
2.59908173515994));
#219445=CARTESIAN_POINT('',(39.4144401478995,-43.796904759634,2.59908173515993));
#219446=CARTESIAN_POINT('Origin',(5.70079064675565E-15,1.85804141662745E-13,
2.59908173516024));
#219447=CARTESIAN_POINT('',(39.3160391863695,-44.1385184650369,2.90134173515993));
#219448=CARTESIAN_POINT('Ctrl Pts',(39.4144401478995,-43.796904759634,2.59908173515994));
#219449=CARTESIAN_POINT('Ctrl Pts',(39.4116082546734,-43.7994532913544,
2.59908174371479));
#219450=CARTESIAN_POINT('Ctrl Pts',(39.4088155471157,-43.8020298032732,
2.5991576435586));
#219451=CARTESIAN_POINT('Ctrl Pts',(39.4060627300848,-43.8046321918096,
2.59930765775247));
#219452=CARTESIAN_POINT('Ctrl Pts',(39.3898103065133,-43.8199964969256,
2.6001933302084));
#219453=CARTESIAN_POINT('Ctrl Pts',(39.3749452320453,-43.8362633193812,
2.60365973323969));
#219454=CARTESIAN_POINT('Ctrl Pts',(39.3616178931548,-43.8529956277642,
2.60934177082139));
#219455=CARTESIAN_POINT('Ctrl Pts',(39.3566392429903,-43.8592462611853,
2.6114643909163));
#219456=CARTESIAN_POINT('Ctrl Pts',(39.3518747760154,-43.8655619201071,
2.61389584429184));
#219457=CARTESIAN_POINT('Ctrl Pts',(39.347330918553,-43.8719202087606,2.61661604385224));
#219458=CARTESIAN_POINT('Ctrl Pts',(39.3437855730191,-43.8768812645303,
2.61873848000747));
#219459=CARTESIAN_POINT('Ctrl Pts',(39.3403750229164,-43.8818681433207,
2.62103707099758));
#219460=CARTESIAN_POINT('Ctrl Pts',(39.3371028088668,-43.8868700682401,
2.62350262767623));
#219461=CARTESIAN_POINT('Ctrl Pts',(39.3256500596934,-43.904376805458,2.63213207605149));
#219462=CARTESIAN_POINT('Ctrl Pts',(39.3158919212388,-43.922067851059,2.64280685971885));
#219463=CARTESIAN_POINT('Ctrl Pts',(39.3079802585394,-43.9394812142296,
2.65513293646054));
#219464=CARTESIAN_POINT('Ctrl Pts',(39.3040244271897,-43.9481878958149,
2.66129597483139));
#219465=CARTESIAN_POINT('Ctrl Pts',(39.3005302159784,-43.9568251581483,
2.66787183533822));
#219466=CARTESIAN_POINT('Ctrl Pts',(39.297516611429,-43.9653352562093,2.67481125953831));
#219467=CARTESIAN_POINT('Ctrl Pts',(39.2945158824216,-43.9738089951117,
2.68172103524049));
#219468=CARTESIAN_POINT('Ctrl Pts',(39.2919914104334,-43.9821566593544,
2.68899101329759));
#219469=CARTESIAN_POINT('Ctrl Pts',(39.2899626959162,-43.9903212250457,
2.69657334701244));
#219470=CARTESIAN_POINT('Ctrl Pts',(39.2899539910984,-43.9903562576023,
2.69660588132542));
#219471=CARTESIAN_POINT('Ctrl Pts',(39.289945294864,-43.990391286806,2.6966384208135));
#219472=CARTESIAN_POINT('Ctrl Pts',(39.2899366072118,-43.9904263126548,
2.69667096547351));
#219473=CARTESIAN_POINT('Ctrl Pts',(39.2858396774343,-44.0069438297352,
2.71201840157866));
#219474=CARTESIAN_POINT('Ctrl Pts',(39.2836282192306,-44.0226860611004,
2.72845645939226));
#219475=CARTESIAN_POINT('Ctrl Pts',(39.2831328363118,-44.0375574100559,
2.74568723186722));
#219476=CARTESIAN_POINT('Ctrl Pts',(39.2826194323372,-44.0529697494253,
2.76354482594117));
#219477=CARTESIAN_POINT('Ctrl Pts',(39.2839495744681,-44.0674474907124,
2.78225519316891));
#219478=CARTESIAN_POINT('Ctrl Pts',(39.2869823603819,-44.0808629337922,
2.80151223085242));
#219479=CARTESIAN_POINT('Ctrl Pts',(39.2899718616358,-44.0940869083981,
2.82049442739997));
#219480=CARTESIAN_POINT('Ctrl Pts',(39.2946164282376,-44.1062793237822,
2.84000929088993));
#219481=CARTESIAN_POINT('Ctrl Pts',(39.300818312271,-44.1172870736897,2.85976644341359));
#219482=CARTESIAN_POINT('Ctrl Pts',(39.3051423761616,-44.1249618727725,
2.87354148166762));
#219483=CARTESIAN_POINT('Ctrl Pts',(39.3102242458198,-44.132060171354,2.8874343834538));
#219484=CARTESIAN_POINT('Ctrl Pts',(39.3160391863695,-44.1385184650369,
2.90134173515994));
#219485=CARTESIAN_POINT('',(39.5544469813076,-44.4033023070483,3.47153072139042));
#219486=CARTESIAN_POINT('',(39.3160391863695,-44.1385184650369,2.90134173515993));
#219487=CARTESIAN_POINT('',(35.2091516650533,-47.9220530736681,3.47153072139039));
#219488=CARTESIAN_POINT('Origin',(5.53234440788222E-15,1.85015204418142E-13,
3.47153072139072));
#219489=CARTESIAN_POINT('',(34.9997217530266,-47.6338034047594,2.90134173515991));
#219490=CARTESIAN_POINT('',(35.2091516650533,-47.9220530736681,3.47153072139039));
#219491=CARTESIAN_POINT('',(34.6451144164191,-47.659028586093,2.5990817351599));
#219492=CARTESIAN_POINT('Ctrl Pts',(34.9997217530266,-47.6338034047594,
2.90134173515991));
#219493=CARTESIAN_POINT('Ctrl Pts',(34.9925330475321,-47.6239092440466,
2.88176998919768));
#219494=CARTESIAN_POINT('Ctrl Pts',(34.9838215185876,-47.6151892923583,
2.86226752356681));
#219495=CARTESIAN_POINT('Ctrl Pts',(34.9737453812861,-47.6077336605731,
2.84310370499972));
#219496=CARTESIAN_POINT('Ctrl Pts',(34.9634872321484,-47.6001433528511,
2.82359371788609));
#219497=CARTESIAN_POINT('Ctrl Pts',(34.9518142124644,-47.5938626849626,
2.80443322636949));
#219498=CARTESIAN_POINT('Ctrl Pts',(34.9388460388088,-47.5890113136631,
2.78589323878208));
#219499=CARTESIAN_POINT('Ctrl Pts',(34.9264269040025,-47.5843653368459,
2.76813818619949));
#219500=CARTESIAN_POINT('Ctrl Pts',(34.9128191931135,-47.5810297921601,
2.75095095198667));
#219501=CARTESIAN_POINT('Ctrl Pts',(34.898095206323,-47.5791401905757,2.73457771435072));
#219502=CARTESIAN_POINT('Ctrl Pts',(34.8863842314158,-47.5776372636135,
2.72155497955536));
#219503=CARTESIAN_POINT('Ctrl Pts',(34.8739663878203,-47.5770495124715,
2.70904711159925));
#219504=CARTESIAN_POINT('Ctrl Pts',(34.8608666162967,-47.5774624305254,
2.69718956158306));
#219505=CARTESIAN_POINT('Ctrl Pts',(34.8608308581757,-47.5774635576576,
2.69715719432324));
#219506=CARTESIAN_POINT('Ctrl Pts',(34.8607950951003,-47.5774646923705,
2.69712483218989));
#219507=CARTESIAN_POINT('Ctrl Pts',(34.8607593270722,-47.5774658346654,
2.69709247518617));
#219508=CARTESIAN_POINT('Ctrl Pts',(34.8536390475845,-47.577693229335,2.69065122242243));
#219509=CARTESIAN_POINT('Ctrl Pts',(34.8462974884548,-47.5782477067926,
2.68442464469393));
#219510=CARTESIAN_POINT('Ctrl Pts',(34.8387748826518,-47.5791245434502,
2.67844505923545));
#219511=CARTESIAN_POINT('Ctrl Pts',(34.8238457504807,-47.5808646865197,
2.66657815779533));
#219512=CARTESIAN_POINT('Ctrl Pts',(34.8082026058782,-47.5838754712046,
2.65568445664141));
#219513=CARTESIAN_POINT('Ctrl Pts',(34.7921542117508,-47.58812612122,2.64601906229482));
#219514=CARTESIAN_POINT('Ctrl Pts',(34.7801179161553,-47.5913141087315,
2.63877001653488));
#219515=CARTESIAN_POINT('Ctrl Pts',(34.7678536672185,-47.5951995198388,
2.63221189387568));
#219516=CARTESIAN_POINT('Ctrl Pts',(34.7554917310468,-47.5997693799338,
2.626452310332));
#219517=CARTESIAN_POINT('Ctrl Pts',(34.7508560049825,-47.6014830774695,
2.62429246650311));
#219518=CARTESIAN_POINT('Ctrl Pts',(34.7462065417646,-47.6032930257982,
2.62224491711712));
#219519=CARTESIAN_POINT('Ctrl Pts',(34.7415502113776,-47.6051985413674,
2.62031533672564));
#219520=CARTESIAN_POINT('Ctrl Pts',(34.7252530550228,-47.6118678458595,
2.61356180535545));
#219521=CARTESIAN_POINT('Ctrl Pts',(34.7088717728658,-47.6197078449341,
2.60825339735313));
#219522=CARTESIAN_POINT('Ctrl Pts',(34.6927009428675,-47.6286892688728,
2.60463337987577));
#219523=CARTESIAN_POINT('Ctrl Pts',(34.6846155278684,-47.6331799808421,
2.60282337113708));
#219524=CARTESIAN_POINT('Ctrl Pts',(34.6765827265058,-47.6379560498531,
2.60143545939082));
#219525=CARTESIAN_POINT('Ctrl Pts',(34.6686393635487,-47.6430138207119,
2.60050005034563));
#219526=CARTESIAN_POINT('Ctrl Pts',(34.6646676820701,-47.6455427061414,
2.60003234582304));
#219527=CARTESIAN_POINT('Ctrl Pts',(34.6607183602076,-47.6481420170537,
2.59967776696033));
#219528=CARTESIAN_POINT('Ctrl Pts',(34.6567960012268,-47.6508112967863,
2.59944011429127));
#219529=CARTESIAN_POINT('Ctrl Pts',(34.6528736422461,-47.653480576519,2.59920246162221));
#219530=CARTESIAN_POINT('Ctrl Pts',(34.6489782471464,-47.6562198264466,
2.59908173791277));
#219531=CARTESIAN_POINT('Ctrl Pts',(34.6451144164191,-47.659028586093,2.59908173515991));
#219532=CARTESIAN_POINT('',(34.620500570364,-47.6769115920298,2.5990817351599));
#219533=CARTESIAN_POINT('Origin',(5.69524824702573E-15,1.85799653515938E-13,
2.59908173516023));
#219534=CARTESIAN_POINT('',(34.4869303039402,-48.0063682005181,2.90134173515989));
#219535=CARTESIAN_POINT('Ctrl Pts',(34.620500570364,-47.6769115920298,2.59908173515991));
#219536=CARTESIAN_POINT('Ctrl Pts',(34.617417796441,-47.6791501491797,2.59908174371474));
#219537=CARTESIAN_POINT('Ctrl Pts',(34.614371068796,-47.6814206292673,2.59915764355858));
#219538=CARTESIAN_POINT('Ctrl Pts',(34.6113613083103,-47.6837210139131,
2.59930765775244));
#219539=CARTESIAN_POINT('Ctrl Pts',(34.5935919100092,-47.6973023109004,
2.60019333020854));
#219540=CARTESIAN_POINT('Ctrl Pts',(34.577107922018,-47.7119261986131,2.60365973324102));
#219541=CARTESIAN_POINT('Ctrl Pts',(34.5621045891999,-47.7271737594097,
2.60934177082469));
#219542=CARTESIAN_POINT('Ctrl Pts',(34.5564998434991,-47.7328697405531,
2.61146439091881));
#219543=CARTESIAN_POINT('Ctrl Pts',(34.5511013106542,-47.7386527792204,
2.61389584429323));
#219544=CARTESIAN_POINT('Ctrl Pts',(34.5459177227791,-47.7445012740624,
2.6166160438522));
#219545=CARTESIAN_POINT('Ctrl Pts',(34.5418732274832,-47.7490645631291,
2.61873848000743));
#219546=CARTESIAN_POINT('Ctrl Pts',(34.5379600899543,-47.7536676237146,
2.62103707099754));
#219547=CARTESIAN_POINT('Ctrl Pts',(34.5341829579105,-47.7583001080598,
2.62350262767619));
#219548=CARTESIAN_POINT('Ctrl Pts',(34.5209629957571,-47.7745138032682,
2.63213207605145));
#219549=CARTESIAN_POINT('Ctrl Pts',(34.5094090955958,-47.7910879322534,
2.6428068597188));
#219550=CARTESIAN_POINT('Ctrl Pts',(34.4997205817199,-47.8075789092546,
2.6551329364605));
#219551=CARTESIAN_POINT('Ctrl Pts',(34.494876324782,-47.8158243977553,2.66129597483135));
#219552=CARTESIAN_POINT('Ctrl Pts',(34.4904984154667,-47.8240490997336,
2.66787183533818));
#219553=CARTESIAN_POINT('Ctrl Pts',(34.4866117722857,-47.8321975711346,
2.67481125953827));
#219554=CARTESIAN_POINT('Ctrl Pts',(34.4827417346802,-47.8403112284169,
2.68172103524046));
#219555=CARTESIAN_POINT('Ctrl Pts',(34.4793585234985,-47.8483492841039,
2.68899101329756));
#219556=CARTESIAN_POINT('Ctrl Pts',(34.4764874929868,-47.8562570650391,
2.69657334701241));
#219557=CARTESIAN_POINT('Ctrl Pts',(34.4764751739556,-47.8562909957826,
2.69660588132538));
#219558=CARTESIAN_POINT('Ctrl Pts',(34.4764628638112,-47.8563249240885,
2.69663842081347));
#219559=CARTESIAN_POINT('Ctrl Pts',(34.4764505625528,-47.8563588499552,
2.69667096547348));
#219560=CARTESIAN_POINT('Ctrl Pts',(34.4706495255088,-47.8723576365726,
2.71201840157626));
#219561=CARTESIAN_POINT('Ctrl Pts',(34.4668046706517,-47.8877824700173,
2.72845645938716));
#219562=CARTESIAN_POINT('Ctrl Pts',(34.464757522239,-47.90252057055,2.7456872318592));
#219563=CARTESIAN_POINT('Ctrl Pts',(34.4626359025951,-47.9177948141809,
2.76354482592991));
#219564=CARTESIAN_POINT('Ctrl Pts',(34.462445422019,-47.9323322825973,2.78225519315416));
#219565=CARTESIAN_POINT('Ctrl Pts',(34.4640592983636,-47.9459912469255,
2.80151223083409));
#219566=CARTESIAN_POINT('Ctrl Pts',(34.4656501410715,-47.9594552671851,
2.82049442737791));
#219567=CARTESIAN_POINT('Ctrl Pts',(34.4689948098058,-47.97206638065,2.84000929086404));
#219568=CARTESIAN_POINT('Ctrl Pts',(34.4740120960853,-47.983662102358,2.85976644338393));
#219569=CARTESIAN_POINT('Ctrl Pts',(34.4775102373488,-47.9917468458484,
2.87354148164767));
#219570=CARTESIAN_POINT('Ctrl Pts',(34.4818222937534,-47.9993374592392,
2.88743438344379));
#219571=CARTESIAN_POINT('Ctrl Pts',(34.4869303039402,-48.0063682005181,
2.90134173515989));
#219572=CARTESIAN_POINT('',(34.6963546279291,-48.2946219293741,3.47153072139039));
#219573=CARTESIAN_POINT('',(34.4869303039402,-48.0063682005181,2.90134173515989));
#219574=CARTESIAN_POINT('',(30.0070536838164,-51.3398895692692,3.47153072139037));
#219575=CARTESIAN_POINT('Origin',(5.53234440788222E-15,1.85015204418142E-13,
3.47153072139072));
#219576=CARTESIAN_POINT('',(29.8289013456892,-51.0313275753403,2.90134173515987));
#219577=CARTESIAN_POINT('',(30.0070536838164,-51.3398895692692,3.47153072139037));
#219578=CARTESIAN_POINT('',(29.4735998357344,-51.0193480105322,2.59908173515988));
#219579=CARTESIAN_POINT('Ctrl Pts',(29.8289013456892,-51.0313275753403,
2.90134173515987));
#219580=CARTESIAN_POINT('Ctrl Pts',(29.82278624209,-51.0207361915368,2.8817699891973));
#219581=CARTESIAN_POINT('Ctrl Pts',(29.8150339189621,-51.0111534059229,
2.8622675235661));
#219582=CARTESIAN_POINT('Ctrl Pts',(29.8057923055279,-51.0026853737208,
2.84310370499869));
#219583=CARTESIAN_POINT('Ctrl Pts',(29.7963837548063,-50.9940643779333,
2.82359371788484));
#219584=CARTESIAN_POINT('Ctrl Pts',(29.785431189708,-50.9865979533913,2.80443322636804));
#219585=CARTESIAN_POINT('Ctrl Pts',(29.7730411634511,-50.9804176151478,
2.78589323878044));
#219586=CARTESIAN_POINT('Ctrl Pts',(29.7611756987818,-50.9744989364014,
2.76813818619798));
#219587=CARTESIAN_POINT('Ctrl Pts',(29.747991191717,-50.9697592710706,2.75095095198528));
#219588=CARTESIAN_POINT('Ctrl Pts',(29.7335453816165,-50.9663409452091,
2.73457771434945));
#219589=CARTESIAN_POINT('Ctrl Pts',(29.7220556593013,-50.9636221212278,
2.72155497955453));
#219590=CARTESIAN_POINT('Ctrl Pts',(29.7097672786764,-50.9617395717399,
2.70904711159883));
#219591=CARTESIAN_POINT('Ctrl Pts',(29.6966961073826,-50.960780928799,2.69718956158301));
#219592=CARTESIAN_POINT('Ctrl Pts',(29.6966604273309,-50.9607783120152,
2.69715719432319));
#219593=CARTESIAN_POINT('Ctrl Pts',(29.6966247415596,-50.9607757022527,
2.69712483218985));
#219594=CARTESIAN_POINT('Ctrl Pts',(29.6965890500702,-50.960773099513,2.69709247518613));
#219595=CARTESIAN_POINT('Ctrl Pts',(29.6894840070031,-50.9602549766179,
2.69065122242238));
#219596=CARTESIAN_POINT('Ctrl Pts',(29.682124707026,-50.9600390146962,2.68442464469389));
#219597=CARTESIAN_POINT('Ctrl Pts',(29.6745516564563,-50.9601247215265,
2.67844505923542));
#219598=CARTESIAN_POINT('Ctrl Pts',(29.6595224131524,-50.9602948126665,
2.6665781577953));
#219599=CARTESIAN_POINT('Ctrl Pts',(29.6436502506365,-50.9616539500919,
2.65568445664136));
#219600=CARTESIAN_POINT('Ctrl Pts',(29.6272454573773,-50.9642038006257,
2.64601906229478));
#219601=CARTESIAN_POINT('Ctrl Pts',(29.6149418624329,-50.966116188526,2.63877001653484));
#219602=CARTESIAN_POINT('Ctrl Pts',(29.6023386622828,-50.9686983518502,
2.63221189387565));
#219603=CARTESIAN_POINT('Ctrl Pts',(29.5895667656379,-50.9719510035824,
2.62645231033197));
#219604=CARTESIAN_POINT('Ctrl Pts',(29.584777304396,-50.973170747982,2.62429246650308));
#219605=CARTESIAN_POINT('Ctrl Pts',(29.5799641203068,-50.9744847799793,
2.62224491711709));
#219606=CARTESIAN_POINT('Ctrl Pts',(29.5751341171706,-50.9758931378749,
2.62031533672561));
#219607=CARTESIAN_POINT('Ctrl Pts',(29.5582291061939,-50.9808223905099,
2.61356180535542));
#219608=CARTESIAN_POINT('Ctrl Pts',(29.5411180593592,-50.986907130999,2.60825339735312));
#219609=CARTESIAN_POINT('Ctrl Pts',(29.5240970004174,-50.9941490417481,
2.60463337987575));
#219610=CARTESIAN_POINT('Ctrl Pts',(29.5155864709465,-50.9977699971226,
2.60282337113707));
#219611=CARTESIAN_POINT('Ctrl Pts',(29.5070984389562,-51.0016802459457,
2.60143545939079));
#219612=CARTESIAN_POINT('Ctrl Pts',(29.498669909557,-51.0058800022835,2.6005000503456));
#219613=CARTESIAN_POINT('Ctrl Pts',(29.4944556448574,-51.0079798804524,
2.60003234582301));
#219614=CARTESIAN_POINT('Ctrl Pts',(29.490256255818,-51.0101521355223,2.59967776696029));
#219615=CARTESIAN_POINT('Ctrl Pts',(29.4860763682217,-51.0123967945046,
2.59944011429123));
#219616=CARTESIAN_POINT('Ctrl Pts',(29.4818964806253,-51.014641453487,2.59920246162217));
#219617=CARTESIAN_POINT('Ctrl Pts',(29.4777360953222,-51.0169585178533,
2.59908173791271));
#219618=CARTESIAN_POINT('Ctrl Pts',(29.4735998357344,-51.0193480105322,
2.59908173515988));
#219619=CARTESIAN_POINT('',(29.4472515437741,-51.0345602039881,2.59908173515987));
#219620=CARTESIAN_POINT('Origin',(5.68926707005281E-15,1.85795769294195E-13,
2.59908173516024));
#219621=CARTESIAN_POINT('',(29.2799753962469,-51.348250120016,2.90134173515988));
#219622=CARTESIAN_POINT('Ctrl Pts',(29.4472515437741,-51.0345602039881,
2.59908173515988));
#219623=CARTESIAN_POINT('Ctrl Pts',(29.4439516646705,-51.036464260467,2.59908174371475));
#219624=CARTESIAN_POINT('Ctrl Pts',(29.4406842975238,-51.0384038328683,
2.59915764355853));
#219625=CARTESIAN_POINT('Ctrl Pts',(29.437450569149,-51.0403770101279,2.59930765775239));
#219626=CARTESIAN_POINT('Ctrl Pts',(29.4183588813692,-51.0520264994509,
2.60019333020843));
#219627=CARTESIAN_POINT('Ctrl Pts',(29.4004365818807,-51.0648472300424,
2.60365973324047));
#219628=CARTESIAN_POINT('Ctrl Pts',(29.3839216347919,-51.078442987781,2.60934177082339));
#219629=CARTESIAN_POINT('Ctrl Pts',(29.3777522003175,-51.0835219102896,
2.61146439091781));
#219630=CARTESIAN_POINT('Ctrl Pts',(29.3717787490542,-51.0887089685247,
2.61389584429265));
#219631=CARTESIAN_POINT('Ctrl Pts',(29.3660122232364,-51.0939835922264,
2.61661604385216));
#219632=CARTESIAN_POINT('Ctrl Pts',(29.3615128905154,-51.0980991182401,
2.61873848000739));
#219633=CARTESIAN_POINT('Ctrl Pts',(29.357140038714,-51.1022679285256,2.62103707099751));
#219634=CARTESIAN_POINT('Ctrl Pts',(29.352899371725,-51.1064802178288,2.62350262767616));
#219635=CARTESIAN_POINT('Ctrl Pts',(29.3380570372635,-51.12122323039,2.63213207605142));
#219636=CARTESIAN_POINT('Ctrl Pts',(29.3248339623433,-51.1364988531338,
2.64280685971877));
#219637=CARTESIAN_POINT('Ctrl Pts',(29.3134747466765,-51.1518867653708,
2.65513293646047));
#219638=CARTESIAN_POINT('Ctrl Pts',(29.307795138843,-51.1595807214893,2.66129597483132));
#219639=CARTESIAN_POINT('Ctrl Pts',(29.3025814967145,-51.1673027515566,
2.66787183533815));
#219640=CARTESIAN_POINT('Ctrl Pts',(29.297864397778,-51.1750003199397,2.67481125953824));
#219641=CARTESIAN_POINT('Ctrl Pts',(29.2931674525162,-51.1826650006747,
2.68172103524043));
#219642=CARTESIAN_POINT('Ctrl Pts',(29.2889625693107,-51.190305381186,2.68899101329752));
#219643=CARTESIAN_POINT('Ctrl Pts',(29.2852806784154,-51.1978697380624,
2.69657334701238));
#219644=CARTESIAN_POINT('Ctrl Pts',(29.2852648801408,-51.1979021952403,
2.69660588132535));
#219645=CARTESIAN_POINT('Ctrl Pts',(29.2852490909589,-51.197934650923,2.69663842081344));
#219646=CARTESIAN_POINT('Ctrl Pts',(29.2852333108693,-51.1979671051086,
2.69667096547344));
#219647=CARTESIAN_POINT('Ctrl Pts',(29.2777917239327,-51.213271875214,2.71201840157896));
#219648=CARTESIAN_POINT('Ctrl Pts',(29.272355597456,-51.2282103130401,2.72845645939298));
#219649=CARTESIAN_POINT('Ctrl Pts',(29.2687791125364,-51.2426536914408,
2.74568723186839));
#219650=CARTESIAN_POINT('Ctrl Pts',(29.2650725221326,-51.2576224915284,
2.76354482594258));
#219651=CARTESIAN_POINT('Ctrl Pts',(29.2633635057963,-51.2720604115321,
2.78225519317057));
#219652=CARTESIAN_POINT('Ctrl Pts',(29.2635407906078,-51.2858132466407,
2.80151223085432));
#219653=CARTESIAN_POINT('Ctrl Pts',(29.2637155451671,-51.2993697979339,
2.82049442740165));
#219654=CARTESIAN_POINT('Ctrl Pts',(29.2657236711474,-51.3122614394841,
2.84000929089134));
#219655=CARTESIAN_POINT('Ctrl Pts',(29.2695013892396,-51.324318087841,2.85976644341472));
#219656=CARTESIAN_POINT('Ctrl Pts',(29.2721352815056,-51.3327241975843,
2.87354148166836));
#219657=CARTESIAN_POINT('Ctrl Pts',(29.2756302808591,-51.3407239614239,
2.88743438345414));
#219658=CARTESIAN_POINT('Ctrl Pts',(29.2799753962468,-51.348250120016,2.90134173515988));
#219659=CARTESIAN_POINT('',(29.458121752568,-51.6568155675422,3.47153072139037));
#219660=CARTESIAN_POINT('',(29.2799753962469,-51.348250120016,2.90134173515988));
#219661=CARTESIAN_POINT('',(24.4761921430398,-54.1952354911867,3.47153072139034));
#219662=CARTESIAN_POINT('Origin',(5.53234440788222E-15,1.85015204418142E-13,
3.47153072139072));
#219663=CARTESIAN_POINT('',(24.3312692531094,-53.869741842014,2.90134173515986));
#219664=CARTESIAN_POINT('',(24.4761921430398,-54.1952354911867,3.47153072139034));
#219665=CARTESIAN_POINT('',(23.979166327502,-53.8206887816831,2.59908173515986));
#219666=CARTESIAN_POINT('Ctrl Pts',(24.3312692531094,-53.869741842014,2.90134173515986));
#219667=CARTESIAN_POINT('Ctrl Pts',(24.3262947497604,-53.8585692765372,
2.88176998919721));
#219668=CARTESIAN_POINT('Ctrl Pts',(24.3195865685237,-53.8482286480022,
2.86226752356593));
#219669=CARTESIAN_POINT('Ctrl Pts',(24.3112807320078,-53.8388409929162,
2.84310370499844));
#219670=CARTESIAN_POINT('Ctrl Pts',(24.3028248617529,-53.8292837624971,
2.82359371788458));
#219671=CARTESIAN_POINT('Ctrl Pts',(24.2927127498357,-53.8207133850115,
2.80443322636777));
#219672=CARTESIAN_POINT('Ctrl Pts',(24.281036618698,-53.813271792903,2.78589323878017));
#219673=CARTESIAN_POINT('Ctrl Pts',(24.2698548246797,-53.8061452585103,
2.76813818619776));
#219674=CARTESIAN_POINT('Ctrl Pts',(24.2572379736576,-53.8000534012996,
2.75095095198512));
#219675=CARTESIAN_POINT('Ctrl Pts',(24.2432286115656,-53.7951438030544,
2.73457771434934));
#219676=CARTESIAN_POINT('Ctrl Pts',(24.2320860256442,-53.7912388700583,
2.72155497955446));
#219677=CARTESIAN_POINT('Ctrl Pts',(24.2200617420592,-53.7880821478308,
2.7090471115988));
#219678=CARTESIAN_POINT('Ctrl Pts',(24.2071623814828,-53.7857624469878,
2.69718956158302));
#219679=CARTESIAN_POINT('Ctrl Pts',(24.2071271704186,-53.785756114958,2.69715719432319));
#219680=CARTESIAN_POINT('Ctrl Pts',(24.2070919529321,-53.7857497893133,
2.69712483218985));
#219681=CARTESIAN_POINT('Ctrl Pts',(24.2070567290248,-53.7857434700551,
2.69709247518612));
#219682=CARTESIAN_POINT('Ctrl Pts',(24.2000447667171,-53.7844855062582,
2.69065122242238));
#219683=CARTESIAN_POINT('Ctrl Pts',(24.192748355923,-53.7835014710811,2.68442464469388));
#219684=CARTESIAN_POINT('Ctrl Pts',(24.1852078325135,-53.7827951090621,
2.67844505923541));
#219685=CARTESIAN_POINT('Ctrl Pts',(24.1702431416115,-53.7813932847184,
2.66657815779529));
#219686=CARTESIAN_POINT('Ctrl Pts',(24.1543158599161,-53.7810858838903,
2.65568445664136));
#219687=CARTESIAN_POINT('Ctrl Pts',(24.137734401873,-53.7819069982464,2.64601906229478));
#219688=CARTESIAN_POINT('Ctrl Pts',(24.1252983083406,-53.7825228340135,
2.63877001653484));
#219689=CARTESIAN_POINT('Ctrl Pts',(24.1124942402755,-53.7837734588329,
2.63221189387564));
#219690=CARTESIAN_POINT('Ctrl Pts',(24.0994523147296,-53.7856732654693,
2.62645231033196));
#219691=CARTESIAN_POINT('Ctrl Pts',(24.0945615926499,-53.786385692958,2.62429246650308));
#219692=CARTESIAN_POINT('Ctrl Pts',(24.0896374219413,-53.7871894118142,
2.62224491711709));
#219693=CARTESIAN_POINT('Ctrl Pts',(24.0846866645811,-53.7880851817726,
2.6203153367256));
#219694=CARTESIAN_POINT('Ctrl Pts',(24.0673590138204,-53.7912203766269,
2.61356180535542));
#219695=CARTESIAN_POINT('Ctrl Pts',(24.0497056745179,-53.7954831928404,
2.6082533973531));
#219696=CARTESIAN_POINT('Ctrl Pts',(24.0320208729162,-53.8009062465103,
2.60463337987573));
#219697=CARTESIAN_POINT('Ctrl Pts',(24.0231784721153,-53.8036177733453,
2.60282337113705));
#219698=CARTESIAN_POINT('Ctrl Pts',(24.0143282061519,-53.806619360476,2.60143545939077));
#219699=CARTESIAN_POINT('Ctrl Pts',(24.0055068550426,-53.8099150888835,
2.60050005034559));
#219700=CARTESIAN_POINT('Ctrl Pts',(24.0010961794879,-53.8115629530872,
2.60003234582299));
#219701=CARTESIAN_POINT('Ctrl Pts',(23.9966927326568,-53.8132843526336,
2.59967776696028));
#219702=CARTESIAN_POINT('Ctrl Pts',(23.9923011121681,-53.8150797979121,
2.59944011429122));
#219703=CARTESIAN_POINT('Ctrl Pts',(23.9879094916794,-53.8168752431906,
2.59920246162216));
#219704=CARTESIAN_POINT('Ctrl Pts',(23.9835296982247,-53.8187447357535,
2.59908173791273));
#219705=CARTESIAN_POINT('Ctrl Pts',(23.979166327502,-53.8206887816831,2.59908173515986));
#219706=CARTESIAN_POINT('',(23.9513722670371,-53.8330634946833,2.59908173515986));
#219707=CARTESIAN_POINT('Origin',(5.68291264686342E-15,1.85792531553863E-13,
2.59908173516024));
#219708=CARTESIAN_POINT('',(23.7522229508834,-54.1275498658869,2.90134173515986));
#219709=CARTESIAN_POINT('Ctrl Pts',(23.9513722670371,-53.8330634946833,
2.59908173515986));
#219710=CARTESIAN_POINT('Ctrl Pts',(23.9478914369187,-53.8346121892499,
2.59908174371477));
#219711=CARTESIAN_POINT('Ctrl Pts',(23.9444392282286,-53.8361996036039,
2.59915764355854));
#219712=CARTESIAN_POINT('Ctrl Pts',(23.9410169613696,-53.8378239549344,
2.5993076577524));
#219713=CARTESIAN_POINT('Ctrl Pts',(23.9208121566327,-53.8474140023528,
2.60019333020859));
#219714=CARTESIAN_POINT('Ctrl Pts',(23.9016479061061,-53.858291109219,2.60365973324168));
#219715=CARTESIAN_POINT('Ctrl Pts',(23.8838022859594,-53.8700861059364,
2.60934177082638));
#219716=CARTESIAN_POINT('Ctrl Pts',(23.877135756331,-53.8744923240693,2.61146439092009));
#219717=CARTESIAN_POINT('Ctrl Pts',(23.8706528330356,-53.8790265713737,
2.61389584429392));
#219718=CARTESIAN_POINT('Ctrl Pts',(23.8643665485428,-53.8836695340505,
2.61661604385215));
#219719=CARTESIAN_POINT('Ctrl Pts',(23.8594616740275,-53.887292206447,2.61873848000738));
#219720=CARTESIAN_POINT('Ctrl Pts',(23.8546770178329,-53.8909810920747,
2.62103707099751));
#219721=CARTESIAN_POINT('Ctrl Pts',(23.8500192775337,-53.8947270356128,
2.62350262767616));
#219722=CARTESIAN_POINT('Ctrl Pts',(23.8337171864864,-53.907837837996,2.63213207605142));
#219723=CARTESIAN_POINT('Ctrl Pts',(23.8189698115833,-53.921647591579,2.64280685971878));
#219724=CARTESIAN_POINT('Ctrl Pts',(23.8060643480694,-53.9357638458652,
2.65513293646048));
#219725=CARTESIAN_POINT('Ctrl Pts',(23.7996116163124,-53.9428219730082,
2.66129597483132));
#219726=CARTESIAN_POINT('Ctrl Pts',(23.7936193631247,-53.9499567269871,
2.66787183533814));
#219727=CARTESIAN_POINT('Ctrl Pts',(23.7881234899558,-53.9571190561822,
2.67481125953823));
#219728=CARTESIAN_POINT('Ctrl Pts',(23.7826510977529,-53.964250784524,2.68172103524042));
#219729=CARTESIAN_POINT('Ctrl Pts',(23.777670612104,-53.9714097802517,2.68899101329751));
#219730=CARTESIAN_POINT('Ctrl Pts',(23.7732182003924,-53.9785478363925,
2.69657334701237));
#219731=CARTESIAN_POINT('Ctrl Pts',(23.7731990959634,-53.9785784643972,
2.69660588132534));
#219732=CARTESIAN_POINT('Ctrl Pts',(23.7731800007337,-53.9786090918653,
2.69663842081342));
#219733=CARTESIAN_POINT('Ctrl Pts',(23.773160914703,-53.978639718795,2.69667096547343));
#219734=CARTESIAN_POINT('Ctrl Pts',(23.7641603094591,-53.9930827901205,
2.7120184015777));
#219735=CARTESIAN_POINT('Ctrl Pts',(23.7571924707029,-54.0073711636733,
2.72845645939029));
#219736=CARTESIAN_POINT('Ctrl Pts',(23.7521258339934,-54.0213615752622,
2.74568723186417));
#219737=CARTESIAN_POINT('Ctrl Pts',(23.7468748830096,-54.0358609304967,
2.76354482593678));
#219738=CARTESIAN_POINT('Ctrl Pts',(23.7436660552526,-54.0500411172115,
2.78225519316308));
#219739=CARTESIAN_POINT('Ctrl Pts',(23.7424048061593,-54.0637371441584,
2.8015122308451));
#219740=CARTESIAN_POINT('Ctrl Pts',(23.7411615579205,-54.0772376980698,
2.82049442739081));
#219741=CARTESIAN_POINT('Ctrl Pts',(23.7418111396955,-54.0902686241807,
2.84000929087886));
#219742=CARTESIAN_POINT('Ctrl Pts',(23.7443079001267,-54.1026541040226,
2.85976644340064));
#219743=CARTESIAN_POINT('Ctrl Pts',(23.7460486859218,-54.1112894809313,
2.87354148165889));
#219744=CARTESIAN_POINT('Ctrl Pts',(23.7486883362831,-54.1196107481421,
2.88743438344939));
#219745=CARTESIAN_POINT('Ctrl Pts',(23.7522229508834,-54.1275498658869,
2.90134173515986));
#219746=CARTESIAN_POINT('',(23.8971395307774,-54.4530463244688,3.47153072139034));
#219747=CARTESIAN_POINT('',(23.7522229508834,-54.1275498658869,2.90134173515986));
#219748=CARTESIAN_POINT('',(18.6771643191716,-56.4568070719807,3.47153072139033));
#219749=CARTESIAN_POINT('Origin',(5.53234440788222E-15,1.85015204418142E-13,
3.47153072139072));
#219750=CARTESIAN_POINT('',(18.5670586829472,-56.1179479440984,2.90134173515985));
#219751=CARTESIAN_POINT('',(18.6771643191716,-56.4568070719807,3.47153072139033));
#219752=CARTESIAN_POINT('',(18.2220120550223,-56.0323588238387,2.59908173515985));
#219753=CARTESIAN_POINT('Ctrl Pts',(18.5670586829472,-56.1179479440984,
2.90134173515985));
#219754=CARTESIAN_POINT('Ctrl Pts',(18.5632792815482,-56.1063166059137,
2.88176998919726));
#219755=CARTESIAN_POINT('Ctrl Pts',(18.5576887384403,-56.0953314285478,
2.86226752356603));
#219756=CARTESIAN_POINT('Ctrl Pts',(18.5504096793258,-56.0851270036914,
2.8431037049986));
#219757=CARTESIAN_POINT('Ctrl Pts',(18.5429991338217,-56.0747382496572,
2.82359371788465));
#219758=CARTESIAN_POINT('Ctrl Pts',(18.5338382654998,-56.065157818077,2.80443322636776));
#219759=CARTESIAN_POINT('Ctrl Pts',(18.5230039556175,-56.0565365037439,
2.78589323878008));
#219760=CARTESIAN_POINT('Ctrl Pts',(18.5126283423249,-56.0482801935068,
2.76813818619733));
#219761=CARTESIAN_POINT('Ctrl Pts',(18.5007173802052,-56.0409028880787,
2.75095095198438));
#219762=CARTESIAN_POINT('Ctrl Pts',(18.4872979556241,-56.0345558080355,
2.73457771434832));
#219763=CARTESIAN_POINT('Ctrl Pts',(18.4766245865996,-56.0295075492879,
2.7215549795538));
#219764=CARTESIAN_POINT('Ctrl Pts',(18.4649961406218,-56.0251112400301,
2.70904711159847));
#219765=CARTESIAN_POINT('Ctrl Pts',(18.4524099188571,-56.021455896413,2.69718956158299));
#219766=CARTESIAN_POINT('Ctrl Pts',(18.4523755625601,-56.0214459185123,
2.69715719432317));
#219767=CARTESIAN_POINT('Ctrl Pts',(18.4523411992087,-56.0214359462903,
2.69712483218983));
#219768=CARTESIAN_POINT('Ctrl Pts',(18.4523068288039,-56.0214259797488,
2.69709247518611));
#219769=CARTESIAN_POINT('Ctrl Pts',(18.4454647717819,-56.0194419575647,
2.69065122242236));
#219770=CARTESIAN_POINT('Ctrl Pts',(18.4383111911745,-56.0177006304276,
2.68442464469387));
#219771=CARTESIAN_POINT('Ctrl Pts',(18.4308858104775,-56.0162099386094,
2.6784450592354));
#219772=CARTESIAN_POINT('Ctrl Pts',(18.4161496282625,-56.0132515574629,
2.66657815779528));
#219773=CARTESIAN_POINT('Ctrl Pts',(18.4003417300189,-56.011280986329,2.65568445664134));
#219774=CARTESIAN_POINT('Ctrl Pts',(18.3837652771161,-56.0103643682068,
2.64601906229475));
#219775=CARTESIAN_POINT('Ctrl Pts',(18.371332937439,-56.0096769046152,2.63877001653481));
#219776=CARTESIAN_POINT('Ctrl Pts',(18.3584682855079,-56.0095822888225,
2.63221189387562));
#219777=CARTESIAN_POINT('Ctrl Pts',(18.3452992211265,-56.010108435684,2.62645231033194));
#219778=CARTESIAN_POINT('Ctrl Pts',(18.3403608219835,-56.0103057407571,
2.62429246650306));
#219779=CARTESIAN_POINT('Ctrl Pts',(18.3353796149004,-56.0105903407603,
2.62224491711705));
#219780=CARTESIAN_POINT('Ctrl Pts',(18.3303623448498,-56.0109637085382,
2.62031533672557));
#219781=CARTESIAN_POINT('Ctrl Pts',(18.3128018996728,-56.012270495761,2.61356180535538));
#219782=CARTESIAN_POINT('Ctrl Pts',(18.2947996815822,-56.0146646833925,
2.60825339735308));
#219783=CARTESIAN_POINT('Ctrl Pts',(18.2766448957077,-56.0182094638723,
2.60463337987572));
#219784=CARTESIAN_POINT('Ctrl Pts',(18.2675675027704,-56.0199818541123,
2.60282337113703));
#219785=CARTESIAN_POINT('Ctrl Pts',(18.2584519681998,-56.022041893534,2.60143545939075));
#219786=CARTESIAN_POINT('Ctrl Pts',(18.2493344439491,-56.024397485321,2.60050005034556));
#219787=CARTESIAN_POINT('Ctrl Pts',(18.2447756818237,-56.0255752812145,
2.60003234582297));
#219788=CARTESIAN_POINT('Ctrl Pts',(18.2402164222858,-56.0268269652237,
2.59967776696028));
#219789=CARTESIAN_POINT('Ctrl Pts',(18.2356611844178,-56.0281535255242,
2.59944011429122));
#219790=CARTESIAN_POINT('Ctrl Pts',(18.2311059465498,-56.0294800858246,
2.59920246162216));
#219791=CARTESIAN_POINT('Ctrl Pts',(18.2265547308772,-56.0308815240325,
2.59908173791271));
#219792=CARTESIAN_POINT('Ctrl Pts',(18.2220120550223,-56.0323588238387,
2.59908173515985));
#219793=CARTESIAN_POINT('',(18.1930767435955,-56.0417604764379,2.59908173515985));
#219794=CARTESIAN_POINT('Origin',(5.6762545978478E-15,1.85789975768303E-13,
2.59908173516024));
#219795=CARTESIAN_POINT('',(17.9642361803979,-56.3138168485091,2.90134173515985));
#219796=CARTESIAN_POINT('Ctrl Pts',(18.1930767435955,-56.0417604764379,
2.59908173515985));
#219797=CARTESIAN_POINT('Ctrl Pts',(18.1894530991656,-56.0429368412704,
2.59908174371471));
#219798=CARTESIAN_POINT('Ctrl Pts',(18.185853872053,-56.0441547055333,2.59915764355852));
#219799=CARTESIAN_POINT('Ctrl Pts',(18.1822805617814,-56.0454124342016,
2.59930765775238));
#219800=CARTESIAN_POINT('Ctrl Pts',(18.161184008162,-56.0528379691462,2.60019333020848));
#219801=CARTESIAN_POINT('Ctrl Pts',(18.1409877741415,-56.0616522804246,
2.60365973324091));
#219802=CARTESIAN_POINT('Ctrl Pts',(18.1220070012899,-56.0715172876645,
2.60934177082451));
#219803=CARTESIAN_POINT('Ctrl Pts',(18.1149164163959,-56.0752025259771,
2.61146439091866));
#219804=CARTESIAN_POINT('Ctrl Pts',(18.1079950493278,-56.0790342841918,
2.61389584429311));
#219805=CARTESIAN_POINT('Ctrl Pts',(18.1012578800036,-56.0829947165767,
2.61661604385213));
#219806=CARTESIAN_POINT('Ctrl Pts',(18.0960012025255,-56.0860848445992,
2.61873848000736));
#219807=CARTESIAN_POINT('Ctrl Pts',(18.0908571636324,-56.0892533893662,
2.62103707099748));
#219808=CARTESIAN_POINT('Ctrl Pts',(18.0858333812004,-56.0924919457979,
2.62350262767612));
#219809=CARTESIAN_POINT('Ctrl Pts',(18.0682501426882,-56.1038268933086,
2.63213207605139));
#219810=CARTESIAN_POINT('Ctrl Pts',(18.0521400431278,-56.1160194751807,
2.64280685971874));
#219811=CARTESIAN_POINT('Ctrl Pts',(18.0378297267257,-56.12870941088,2.65513293646044));
#219812=CARTESIAN_POINT('Ctrl Pts',(18.0306745685246,-56.1350543787296,
2.66129597483129));
#219813=CARTESIAN_POINT('Ctrl Pts',(18.0239693566576,-56.1415236867625,
2.66787183533812));
#219814=CARTESIAN_POINT('Ctrl Pts',(18.0177549231928,-56.1480723047922,
2.67481125953821));
#219815=CARTESIAN_POINT('Ctrl Pts',(18.011567040723,-56.1545929440325,2.6817210352404));
#219816=CARTESIAN_POINT('Ctrl Pts',(18.0058655198736,-56.1611921195213,
2.68899101329749));
#219817=CARTESIAN_POINT('Ctrl Pts',(18.0006913689001,-56.1678256688897,
2.69657334701235));
#219818=CARTESIAN_POINT('Ctrl Pts',(18.0006691676289,-56.1678541321544,
2.69660588132532));
#219819=CARTESIAN_POINT('Ctrl Pts',(18.0006469755627,-56.167882595847,2.69663842081341));
#219820=CARTESIAN_POINT('Ctrl Pts',(18.0006247927013,-56.1679110599657,
2.69667096547341));
#219821=CARTESIAN_POINT('Ctrl Pts',(17.9901637816639,-56.1813341912011,
2.71201840157821));
#219822=CARTESIAN_POINT('Ctrl Pts',(17.9817405717272,-56.1948159540715,
2.7284564593914));
#219823=CARTESIAN_POINT('Ctrl Pts',(17.9752392943597,-56.2082001169732,
2.74568723186593));
#219824=CARTESIAN_POINT('Ctrl Pts',(17.9685015133137,-56.2220711693861,
2.76354482593923));
#219825=CARTESIAN_POINT('Ctrl Pts',(17.9638280307249,-56.2358382617205,
2.78225519316626));
#219826=CARTESIAN_POINT('Ctrl Pts',(17.9611420662366,-56.2493274239697,
2.80151223084904));
#219827=CARTESIAN_POINT('Ctrl Pts',(17.9584944364883,-56.2626240656068,
2.82049442739549));
#219828=CARTESIAN_POINT('Ctrl Pts',(17.9577783571054,-56.2756515067261,
2.8400092908843));
#219829=CARTESIAN_POINT('Ctrl Pts',(17.9589668048474,-56.2882301201448,
2.85976644340682));
#219830=CARTESIAN_POINT('Ctrl Pts',(17.9597954117579,-56.297000153218,2.87354148166304));
#219831=CARTESIAN_POINT('Ctrl Pts',(17.9615507925642,-56.3055517542508,
2.88743438345146));
#219832=CARTESIAN_POINT('Ctrl Pts',(17.9642361803979,-56.3138168485091,
2.90134173515985));
#219833=CARTESIAN_POINT('',(18.0743352474898,-56.652678110832,3.47153072139033));
#219834=CARTESIAN_POINT('',(17.9642361803979,-56.3138168485091,2.90134173515984));
#219835=CARTESIAN_POINT('',(12.6735055745747,-58.0998260601477,3.47153072139032));
#219836=CARTESIAN_POINT('Origin',(5.53234440788222E-15,1.85015204418142E-13,
3.47153072139072));
#219837=CARTESIAN_POINT('',(12.5994235324478,-57.7513140650717,2.90134173515983));
#219838=CARTESIAN_POINT('',(12.6735055745747,-58.0998260601477,3.47153072139032));
#219839=CARTESIAN_POINT('',(12.2652136052667,-57.6301266171954,2.59908173515984));
#219840=CARTESIAN_POINT('Ctrl Pts',(12.5994235324478,-57.7513140650717,
2.90134173515983));
#219841=CARTESIAN_POINT('Ctrl Pts',(12.5968806409114,-57.7393513895545,
2.88176998919773));
#219842=CARTESIAN_POINT('Ctrl Pts',(12.5924689870926,-57.72784201926,2.86226752356698));
#219843=CARTESIAN_POINT('Ctrl Pts',(12.5862964562745,-57.7169326264476,
2.84310370500001));
#219844=CARTESIAN_POINT('Ctrl Pts',(12.5800124270088,-57.7058261701617,
2.82359371788647));
#219845=CARTESIAN_POINT('Ctrl Pts',(12.5719031706729,-57.6953406497004,
2.80443322636996));
#219846=CARTESIAN_POINT('Ctrl Pts',(12.5620293850127,-57.6856340700669,
2.78589323878263));
#219847=CARTESIAN_POINT('Ctrl Pts',(12.552573629837,-57.6763384418483,2.76813818620015));
#219848=CARTESIAN_POINT('Ctrl Pts',(12.5414990556139,-57.6677565155049,
2.75095095198743));
#219849=CARTESIAN_POINT('Ctrl Pts',(12.5288165945683,-57.6600414936009,
2.73457771435156));
#219850=CARTESIAN_POINT('Ctrl Pts',(12.5187293821045,-57.6539052188803,
2.72155497955587));
#219851=CARTESIAN_POINT('Ctrl Pts',(12.5076241774204,-57.6483174894759,
2.70904711159944));
#219852=CARTESIAN_POINT('Ctrl Pts',(12.4954889917454,-57.6433665517937,
2.69718956158298));
#219853=CARTESIAN_POINT('Ctrl Pts',(12.4954558666304,-57.6433530373421,
2.69715719432315));
#219854=CARTESIAN_POINT('Ctrl Pts',(12.4954227339061,-57.6433395278007,
2.69712483218981));
#219855=CARTESIAN_POINT('Ctrl Pts',(12.4953895935733,-57.6433260231713,
2.69709247518609));
#219856=CARTESIAN_POINT('Ctrl Pts',(12.4887924048456,-57.6406376799622,
2.69065122242235));
#219857=CARTESIAN_POINT('Ctrl Pts',(12.4818600305509,-57.6381581392096,
2.68442464469384));
#219858=CARTESIAN_POINT('Ctrl Pts',(12.4746311465912,-57.6358994499237,
2.67844505923537));
#219859=CARTESIAN_POINT('Ctrl Pts',(12.4602849257593,-57.6314169246173,
2.66657815779526));
#219860=CARTESIAN_POINT('Ctrl Pts',(12.4447696056087,-57.6278047731674,
2.65568445664133));
#219861=CARTESIAN_POINT('Ctrl Pts',(12.428379772933,-57.6251604652268,2.64601906229475));
#219862=CARTESIAN_POINT('Ctrl Pts',(12.4160873984262,-57.6231772342714,
2.63877001653481));
#219863=CARTESIAN_POINT('Ctrl Pts',(12.4033031104479,-57.6217384144971,
2.63221189387561));
#219864=CARTESIAN_POINT('Ctrl Pts',(12.3901511902562,-57.6208851370086,
2.62645231033193));
#219865=CARTESIAN_POINT('Ctrl Pts',(12.3852192201843,-57.6205651579504,
2.62429246650305));
#219866=CARTESIAN_POINT('Ctrl Pts',(12.3802355518738,-57.6203275209634,
2.62224491711704));
#219867=CARTESIAN_POINT('Ctrl Pts',(12.3752067393935,-57.6201743958654,
2.62031533672556));
#219868=CARTESIAN_POINT('Ctrl Pts',(12.3576058957123,-57.6196384580224,
2.61356180535537));
#219869=CARTESIAN_POINT('Ctrl Pts',(12.339452034902,-57.6201377858511,2.60825339735307));
#219870=CARTESIAN_POINT('Ctrl Pts',(12.321026172388,-57.6217654557842,2.60463337987571));
#219871=CARTESIAN_POINT('Ctrl Pts',(12.3118132411309,-57.6225792907507,
2.60282337113702));
#219872=CARTESIAN_POINT('Ctrl Pts',(12.3025323096574,-57.6236752122404,
2.60143545939074));
#219873=CARTESIAN_POINT('Ctrl Pts',(12.293218505769,-57.6250648590504,2.60050005034555));
#219874=CARTESIAN_POINT('Ctrl Pts',(12.2885616038247,-57.6257596824554,
2.60003234582296));
#219875=CARTESIAN_POINT('Ctrl Pts',(12.2838964837817,-57.6265279372155,
2.59967776696024));
#219876=CARTESIAN_POINT('Ctrl Pts',(12.2792275366736,-57.6273710784657,
2.59944011429118));
#219877=CARTESIAN_POINT('Ctrl Pts',(12.2745585895656,-57.6282142197158,
2.59920246162212));
#219878=CARTESIAN_POINT('Ctrl Pts',(12.2698858157465,-57.6291322491183,
2.5990817379127));
#219879=CARTESIAN_POINT('Ctrl Pts',(12.2652136052667,-57.6301266171954,
2.59908173515984));
#219880=CARTESIAN_POINT('',(12.2354540642051,-57.6364522029204,2.59908173515984));
#219881=CARTESIAN_POINT('Origin',(5.66936586998424E-15,1.85788129939235E-13,
2.59908173516024));
#219882=CARTESIAN_POINT('',(11.9794294790619,-57.8830978693153,2.90134173515983));
#219883=CARTESIAN_POINT('Ctrl Pts',(12.2354540642051,-57.6364522029204,
2.59908173515984));
#219884=CARTESIAN_POINT('Ctrl Pts',(12.2317273068703,-57.6372433495196,
2.59908174371473));
#219885=CARTESIAN_POINT('Ctrl Pts',(12.2280204952205,-57.6380783205155,
2.5991576435585));
#219886=CARTESIAN_POINT('Ctrl Pts',(12.2243352914717,-57.6389556465831,
2.59930765775236));
#219887=CARTESIAN_POINT('Ctrl Pts',(12.2025781272246,-57.64413531334,2.60019333020842));
#219888=CARTESIAN_POINT('Ctrl Pts',(12.1815711838755,-57.6507902575926,
2.60365973324057));
#219889=CARTESIAN_POINT('Ctrl Pts',(12.1616632156375,-57.6586171922724,
2.6093417708237));
#219890=CARTESIAN_POINT('Ctrl Pts',(12.1542262614109,-57.6615410745216,
2.61146439091804));
#219891=CARTESIAN_POINT('Ctrl Pts',(12.146942282517,-57.6646283621009,2.61389584429276));
#219892=CARTESIAN_POINT('Ctrl Pts',(12.1398280421993,-57.667862872867,2.61661604385213));
#219893=CARTESIAN_POINT('Ctrl Pts',(12.134277155017,-57.6703866004262,2.61873848000736));
#219894=CARTESIAN_POINT('Ctrl Pts',(12.1288300925919,-57.6730000890929,
2.62103707099748));
#219895=CARTESIAN_POINT('Ctrl Pts',(12.1234953096387,-57.6756957761162,
2.62350262767613));
#219896=CARTESIAN_POINT('Ctrl Pts',(12.1048235693024,-57.6851306806976,
2.63213207605139));
#219897=CARTESIAN_POINT('Ctrl Pts',(12.0875272507065,-57.6955725063803,
2.64280685971875));
#219898=CARTESIAN_POINT('Ctrl Pts',(12.0719688682374,-57.7066970899016,
2.65513293646045));
#219899=CARTESIAN_POINT('Ctrl Pts',(12.0641896770028,-57.7122593816623,
2.6612959748313));
#219900=CARTESIAN_POINT('Ctrl Pts',(12.0568449701609,-57.7179923646565,
2.66787183533812));
#219901=CARTESIAN_POINT('Ctrl Pts',(12.0499800630337,-57.7238555234913,
2.67481125953821));
#219902=CARTESIAN_POINT('Ctrl Pts',(12.0431444860322,-57.7296936321422,
2.68172103524039));
#219903=CARTESIAN_POINT('Ctrl Pts',(12.0367843970379,-57.7356606854445,
2.68899101329748));
#219904=CARTESIAN_POINT('Ctrl Pts',(12.0309451958833,-57.7417170494854,
2.69657334701234));
#219905=CARTESIAN_POINT('Ctrl Pts',(12.0309201410117,-57.7417430361605,
2.69660588132531));
#219906=CARTESIAN_POINT('Ctrl Pts',(12.0308950952499,-57.7417690242235,
2.6966384208134));
#219907=CARTESIAN_POINT('Ctrl Pts',(12.030870058598,-57.7417950136724,2.69667096547341));
#219908=CARTESIAN_POINT('Ctrl Pts',(12.0190632547926,-57.7540511381831,
2.71201840157904));
#219909=CARTESIAN_POINT('Ctrl Pts',(12.0092769601259,-57.7665785813561,
2.72845645939319));
#219910=CARTESIAN_POINT('Ctrl Pts',(12.0014122714556,-57.7792098558812,
2.74568723186873));
#219911=CARTESIAN_POINT('Ctrl Pts',(11.9932614808864,-57.7923006313198,
2.7635448259431));
#219912=CARTESIAN_POINT('Ctrl Pts',(11.9871745471188,-57.8055037941296,
2.78225519317128));
#219913=CARTESIAN_POINT('Ctrl Pts',(11.9830932952246,-57.8186383015968,
2.80151223085522));
#219914=CARTESIAN_POINT('Ctrl Pts',(11.9790702919523,-57.8315853501716,
2.82049442740278));
#219915=CARTESIAN_POINT('Ctrl Pts',(11.9769963969271,-57.8444665749285,
2.84000929089272));
#219916=CARTESIAN_POINT('Ctrl Pts',(11.976863511098,-57.8571005080036,2.85976644341635));
#219917=CARTESIAN_POINT('Ctrl Pts',(11.9767708607336,-57.8659091109228,
2.87354148166945));
#219918=CARTESIAN_POINT('Ctrl Pts',(11.9776227396658,-57.8745973526465,
2.88743438345466));
#219919=CARTESIAN_POINT('Ctrl Pts',(11.9794294790619,-57.8830978693152,
2.90134173515983));
#219920=CARTESIAN_POINT('',(12.0535047649328,-58.2316113004778,3.47153072139032));
#219921=CARTESIAN_POINT('',(11.9794294790618,-57.8830978693153,2.90134173515983));
#219922=CARTESIAN_POINT('',(6.53099325080115,-59.1062911958294,3.47153072139031));
#219923=CARTESIAN_POINT('Origin',(5.53234440788222E-15,1.85015204418142E-13,
3.47153072139072));
#219924=CARTESIAN_POINT('',(6.493746461128,-58.7519447039086,2.90134173515983));
#219925=CARTESIAN_POINT('',(6.53099325080115,-59.1062911958294,3.47153072139031));
#219926=CARTESIAN_POINT('',(6.17403490859079,-58.5964866834548,2.59908173515983));
#219927=CARTESIAN_POINT('Ctrl Pts',(6.49374646112799,-58.7519447039086,
2.90134173515983));
#219928=CARTESIAN_POINT('Ctrl Pts',(6.49246793990574,-58.7397817566341,
2.88176998919634));
#219929=CARTESIAN_POINT('Ctrl Pts',(6.48928351037779,-58.7278742924794,
2.86226752356423));
#219930=CARTESIAN_POINT('Ctrl Pts',(6.48428513539465,-58.7163794573007,
2.84310370499596));
#219931=CARTESIAN_POINT('Ctrl Pts',(6.47919647150606,-58.7046769834214,
2.82359371788115));
#219932=CARTESIAN_POINT('Ctrl Pts',(6.47222767386437,-58.6934012556346,
2.80443322636344));
#219933=CARTESIAN_POINT('Ctrl Pts',(6.46342259168671,-58.6827157580177,
2.78589323877503));
#219934=CARTESIAN_POINT('Ctrl Pts',(6.45499029385914,-58.6724826566651,
2.76813818619166));
#219935=CARTESIAN_POINT('Ctrl Pts',(6.44487344288378,-58.6627901347869,
2.75095095197815));
#219936=CARTESIAN_POINT('Ctrl Pts',(6.43306689706911,-58.6537916984163,
2.73457771434164));
#219937=CARTESIAN_POINT('Ctrl Pts',(6.42367635877919,-58.6466346380352,
2.72155497954951));
#219938=CARTESIAN_POINT('Ctrl Pts',(6.41321606633851,-58.6399167088191,
2.70904711159642));
#219939=CARTESIAN_POINT('Ctrl Pts',(6.40166487239097,-58.633724420583,2.69718956158297));
#219940=CARTESIAN_POINT('Ctrl Pts',(6.40163334138369,-58.6337075176476,
2.69715719432314));
#219941=CARTESIAN_POINT('Ctrl Pts',(6.40160180229544,-58.6336906188001,
2.6971248321898));
#219942=CARTESIAN_POINT('Ctrl Pts',(6.40157025512701,-58.6336737240425,
2.69709247518608));
#219943=CARTESIAN_POINT('Ctrl Pts',(6.3952902148738,-58.6303105138591,2.69065122242233));
#219944=CARTESIAN_POINT('Ctrl Pts',(6.3886549994353,-58.6271199258585,2.68442464469384));
#219945=CARTESIAN_POINT('Ctrl Pts',(6.38170181337843,-58.6241179857774,
2.67844505923537));
#219946=CARTESIAN_POINT('Ctrl Pts',(6.36790273412708,-58.6181604277963,
2.66657815779525));
#219947=CARTESIAN_POINT('Ctrl Pts',(6.3528499811638,-58.6129462715176,2.65568445664132));
#219948=CARTESIAN_POINT('Ctrl Pts',(6.33682633915184,-58.6086032453497,
2.64601906229474));
#219949=CARTESIAN_POINT('Ctrl Pts',(6.32480860764288,-58.6053459757239,
2.6387700165348));
#219950=CARTESIAN_POINT('Ctrl Pts',(6.31224475095164,-58.6025787159785,
2.6322118938756));
#219951=CARTESIAN_POINT('Ctrl Pts',(6.29925407013949,-58.6003553628267,
2.62645231033192));
#219952=CARTESIAN_POINT('Ctrl Pts',(6.29438256483494,-58.5995216053948,
2.62429246650304));
#219953=CARTESIAN_POINT('Ctrl Pts',(6.28945103740996,-58.5987643350181,
2.62224491711704));
#219954=CARTESIAN_POINT('Ctrl Pts',(6.28446577922175,-58.5980863947148,
2.62031533672556));
#219955=CARTESIAN_POINT('Ctrl Pts',(6.26701737556302,-58.5957136036532,
2.61356180535537));
#219956=CARTESIAN_POINT('Ctrl Pts',(6.24891076953115,-58.5943126009389,
2.60825339735306));
#219957=CARTESIAN_POINT('Ctrl Pts',(6.23041570798304,-58.5940053272328,
2.60463337987569));
#219958=CARTESIAN_POINT('Ctrl Pts',(6.22116817720899,-58.5938516903798,
2.60282337113701));
#219959=CARTESIAN_POINT('Ctrl Pts',(6.21182353266003,-58.5939714867922,
2.60143545939073));
#219960=CARTESIAN_POINT('Ctrl Pts',(6.20241549311822,-58.594379963364,2.60050005034555));
#219961=CARTESIAN_POINT('Ctrl Pts',(6.19771147334731,-58.5945842016499,
2.60003234582295));
#219962=CARTESIAN_POINT('Ctrl Pts',(6.19299160483051,-58.5948606100009,
2.59967776696025));
#219963=CARTESIAN_POINT('Ctrl Pts',(6.18826010244408,-58.5952110945688,
2.59944011429119));
#219964=CARTESIAN_POINT('Ctrl Pts',(6.18352860005764,-58.5955615791367,
2.59920246162213));
#219965=CARTESIAN_POINT('Ctrl Pts',(6.17878546397971,-58.5959861416116,
2.59908173791268));
#219966=CARTESIAN_POINT('Ctrl Pts',(6.17403490859079,-58.5964866834548,
2.59908173515983));
#219967=CARTESIAN_POINT('',(6.14377718965381,-58.5996668978646,2.59908173515983));
#219968=CARTESIAN_POINT('Origin',(5.66232193761676E-15,1.85787014289949E-13,
2.59908173516024));
#219969=CARTESIAN_POINT('',(5.8633736414964,-58.8181995570482,2.90134173515983));
#219970=CARTESIAN_POINT('Ctrl Pts',(6.14377718965381,-58.5996668978646,
2.59908173515983));
#219971=CARTESIAN_POINT('Ctrl Pts',(6.13998815054745,-58.6000641582627,
2.59908174371469));
#219972=CARTESIAN_POINT('Ctrl Pts',(6.13621436696463,-58.6005070878748,
2.5991576435585));
#219973=CARTESIAN_POINT('Ctrl Pts',(6.13245764560185,-58.6009943991737,
2.59930765775236));
#219974=CARTESIAN_POINT('Ctrl Pts',(6.11027824677107,-58.6038714482303,
2.6001933302084));
#219975=CARTESIAN_POINT('Ctrl Pts',(6.08869075056017,-58.6082941124956,
2.60365973324044));
#219976=CARTESIAN_POINT('Ctrl Pts',(6.06807370280131,-58.6139972210815,
2.60934177082338));
#219977=CARTESIAN_POINT('Ctrl Pts',(6.06037186006944,-58.6161277126012,
2.6114643909178));
#219978=CARTESIAN_POINT('Ctrl Pts',(6.05280507414744,-58.618436704576,2.61389584429262));
#219979=CARTESIAN_POINT('Ctrl Pts',(6.04539170794238,-58.6209098557461,
2.61661604385212));
#219980=CARTESIAN_POINT('Ctrl Pts',(6.03960742773739,-58.6228395323547,
2.61873848000735));
#219981=CARTESIAN_POINT('Ctrl Pts',(6.03391702093609,-58.6248693309924,
2.62103707099746));
#219982=CARTESIAN_POINT('Ctrl Pts',(6.02832968646007,-58.6269926140961,
2.62350262767611));
#219983=CARTESIAN_POINT('Ctrl Pts',(6.008774015794,-58.6344241049591,2.63213207605137));
#219984=CARTESIAN_POINT('Ctrl Pts',(5.99048098024888,-58.6430007716252,
2.64280685971873));
#219985=CARTESIAN_POINT('Ctrl Pts',(5.97384499260682,-58.6524381197036,
2.65513293646042));
#219986=CARTESIAN_POINT('Ctrl Pts',(5.9655269987858,-58.6571567937428,2.66129597483127));
#219987=CARTESIAN_POINT('Ctrl Pts',(5.95762326711415,-58.662090639937,2.6678718353381));
#219988=CARTESIAN_POINT('Ctrl Pts',(5.95018309968352,-58.6672041015817,
2.67481125953819));
#219989=CARTESIAN_POINT('Ctrl Pts',(5.9427747201624,-58.672295716103,2.68172103524038));
#219990=CARTESIAN_POINT('Ctrl Pts',(5.93582574548912,-58.6775652709342,
2.68899101329747));
#219991=CARTESIAN_POINT('Ctrl Pts',(5.92938546966327,-58.6829780948558,
2.69657334701233));
#219992=CARTESIAN_POINT('Ctrl Pts',(5.92935783569763,-58.683001320226,2.6966058813253));
#219993=CARTESIAN_POINT('Ctrl Pts',(5.92933021064688,-58.6830245479287,
2.69663842081338));
#219994=CARTESIAN_POINT('Ctrl Pts',(5.92930259451121,-58.6830477779618,
2.69667096547339));
#219995=CARTESIAN_POINT('Ctrl Pts',(5.91627935575179,-58.6940026150822,
2.71201840157897));
#219996=CARTESIAN_POINT('Ctrl Pts',(5.90523719704766,-58.7054384852681,
2.72845645939305));
#219997=CARTESIAN_POINT('Ctrl Pts',(5.89609526424964,-58.7171784805289,
2.74568723186852));
#219998=CARTESIAN_POINT('Ctrl Pts',(5.88662076592438,-58.7293455537172,
2.76354482594282));
#219999=CARTESIAN_POINT('Ctrl Pts',(5.87918707069805,-58.7418401303869,
2.78225519317093));
#220000=CARTESIAN_POINT('Ctrl Pts',(5.87375524644739,-58.7544760786592,
2.8015122308548));
#220001=CARTESIAN_POINT('Ctrl Pts',(5.86840094651664,-58.7669316835973,
2.82049442740227));
#220002=CARTESIAN_POINT('Ctrl Pts',(5.86499195787649,-58.7795255625973,
2.84000929089211));
#220003=CARTESIAN_POINT('Ctrl Pts',(5.86353919440045,-58.7920763953135,
2.85976644341564));
#220004=CARTESIAN_POINT('Ctrl Pts',(5.86252630185777,-58.8008270591842,
2.87354148166896));
#220005=CARTESIAN_POINT('Ctrl Pts',(5.86246534555209,-58.8095567514065,
2.88743438345442));
#220006=CARTESIAN_POINT('Ctrl Pts',(5.86337364149643,-58.8181995570482,
2.90134173515983));
#220007=CARTESIAN_POINT('',(5.90061356181316,-59.1725467709675,3.47153072139031));
#220008=CARTESIAN_POINT('',(5.86337364149639,-58.8181995570482,2.90134173515982));
#220009=CARTESIAN_POINT('',(0.316925998273675,-59.465175436383,3.4715307213903));
#220010=CARTESIAN_POINT('Origin',(5.53234440788222E-15,1.85015204418142E-13,
3.47153072139072));
#220011=CARTESIAN_POINT('',(0.316922544676313,-59.1088767419346,2.90134173515982));
#220012=CARTESIAN_POINT('',(0.316925998273675,-59.465175436383,3.47153072139031));
#220013=CARTESIAN_POINT('Ctrl Pts',(0.316922544676314,-59.1088767419346,
2.90134173515982));
#220014=CARTESIAN_POINT('Ctrl Pts',(0.316922401514487,-59.0966467827005,
2.88176998919813));
#220015=CARTESIAN_POINT('Ctrl Pts',(0.315000085554525,-59.0844716853564,
2.8622675235678));
#220016=CARTESIAN_POINT('Ctrl Pts',(0.311230629649952,-59.0725173476328,
2.84310370500122));
#220017=CARTESIAN_POINT('Ctrl Pts',(0.307393083606301,-59.0603470709146,
2.82359371788818));
#220018=CARTESIAN_POINT('Ctrl Pts',(0.301641096266063,-59.0484046750371,
2.80443322637214));
#220019=CARTESIAN_POINT('Ctrl Pts',(0.294001187896427,-59.0368573319862,
2.78589323878523));
#220020=CARTESIAN_POINT('Ctrl Pts',(0.286684733438826,-59.0257988735007,
2.76813818620329));
#220021=CARTESIAN_POINT('Ctrl Pts',(0.277636448050448,-59.0151019493867,
2.75095095199105));
#220022=CARTESIAN_POINT('Ctrl Pts',(0.26683517245673,-59.0049186873022,
2.7345777143556));
#220023=CARTESIAN_POINT('Ctrl Pts',(0.258244193038992,-58.9968192555069,
2.72155497955845));
#220024=CARTESIAN_POINT('Ctrl Pts',(0.248543417989038,-58.9890447295128,
2.70904711160066));
#220025=CARTESIAN_POINT('Ctrl Pts',(0.237702773060113,-58.9816789347248,
2.69718956158297));
#220026=CARTESIAN_POINT('Ctrl Pts',(0.237673181620855,-58.9816588284977,
2.69715719432314));
#220027=CARTESIAN_POINT('Ctrl Pts',(0.237643581717596,-58.9816387254914,
2.6971248321898));
#220028=CARTESIAN_POINT('Ctrl Pts',(0.23761397335091,-58.981618625708,2.69709247518608));
#220029=CARTESIAN_POINT('Ctrl Pts',(0.231719887007404,-58.977617396585,
2.69065122242234));
#220030=CARTESIAN_POINT('Ctrl Pts',(0.225454527233984,-58.973750718086,
2.68442464469383));
#220031=CARTESIAN_POINT('Ctrl Pts',(0.218853219641353,-58.9700384170934,
2.67844505923535));
#220032=CARTESIAN_POINT('Ctrl Pts',(0.20575246757055,-58.9626710986897,
2.66657815779524));
#220033=CARTESIAN_POINT('Ctrl Pts',(0.191327202906053,-58.9559120649694,
2.65568445664132));
#220034=CARTESIAN_POINT('Ctrl Pts',(0.175845309932871,-58.9499179036779,
2.64601906229473));
#220035=CARTESIAN_POINT('Ctrl Pts',(0.164233890202985,-58.9454222827093,
2.63877001653479));
#220036=CARTESIAN_POINT('Ctrl Pts',(0.152028117041922,-58.9413569016697,
2.63221189387559));
#220037=CARTESIAN_POINT('Ctrl Pts',(0.139341004226762,-58.937787832377,
2.62645231033191));
#220038=CARTESIAN_POINT('Ctrl Pts',(0.134583336921077,-58.9364494313922,
2.62429246650303));
#220039=CARTESIAN_POINT('Ctrl Pts',(0.129757981228087,-58.9351808244386,
2.62224491711703));
#220040=CARTESIAN_POINT('Ctrl Pts',(0.124870896863941,-58.9339854965858,
2.62031533672554));
#220041=CARTESIAN_POINT('Ctrl Pts',(0.107766101589432,-58.929801849101,
2.61356180535535));
#220042=CARTESIAN_POINT('Ctrl Pts',(0.0899051301006859,-58.9265158655227,
2.60825339735305));
#220043=CARTESIAN_POINT('Ctrl Pts',(0.0715435052832096,-58.9242770147324,
2.60463337987569));
#220044=CARTESIAN_POINT('Ctrl Pts',(0.0623626928744716,-58.9231575893373,
2.602823371137));
#220045=CARTESIAN_POINT('Ctrl Pts',(0.0530567171311952,-58.922299948158,
2.60143545939073));
#220046=CARTESIAN_POINT('Ctrl Pts',(0.0436575183860499,-58.9217227791367,
2.60050005034554));
#220047=CARTESIAN_POINT('Ctrl Pts',(0.0389579190134772,-58.921434194626,
2.60003234582295));
#220048=CARTESIAN_POINT('Ctrl Pts',(0.0342350138900813,-58.9212157281803,
2.59967776696023));
#220049=CARTESIAN_POINT('Ctrl Pts',(0.0294927955555056,-58.9210697160837,
2.59944011429117));
#220050=CARTESIAN_POINT('Ctrl Pts',(0.02475057722093,-58.9209237039871,
2.59920246162211));
#220051=CARTESIAN_POINT('Ctrl Pts',(0.0199890456756626,-58.920850147939,
2.5990817379127));
#220052=CARTESIAN_POINT('Ctrl Pts',(0.015212193456543,-58.9208513795071,
2.59908173515982));
#220053=CARTESIAN_POINT('',(-0.316922544675051,-59.1088767419346,2.90134173515982));
#220054=CARTESIAN_POINT('Ctrl Pts',(-0.015212193455297,-58.9208513795071,
2.59908173515982));
#220055=CARTESIAN_POINT('Ctrl Pts',(-0.0190220008279213,-58.9208504012362,
2.59908174371469));
#220056=CARTESIAN_POINT('Ctrl Pts',(-0.022821409981102,-58.9208964366349,
2.59915764355849));
#220057=CARTESIAN_POINT('Ctrl Pts',(-0.0266084895323855,-58.9209883940805,
2.59930765775236));
#220058=CARTESIAN_POINT('Ctrl Pts',(-0.0489671208120116,-58.9215313038854,
2.60019333020838));
#220059=CARTESIAN_POINT('Ctrl Pts',(-0.0708986527588113,-58.9236732325283,
2.60365973324034));
#220060=CARTESIAN_POINT('Ctrl Pts',(-0.0919988953488922,-58.9271900305692,
2.60934177082313));
#220061=CARTESIAN_POINT('Ctrl Pts',(-0.0998812435853016,-58.9285037892484,
2.6114643909176));
#220062=CARTESIAN_POINT('Ctrl Pts',(-0.107647933245444,-58.9300091878193,
2.61389584429252));
#220063=CARTESIAN_POINT('Ctrl Pts',(-0.115279202946303,-58.9316938830315,
2.61661604385212));
#220064=CARTESIAN_POINT('Ctrl Pts',(-0.121233502389606,-58.9330083667488,
2.61873848000735));
#220065=CARTESIAN_POINT('Ctrl Pts',(-0.127104908279396,-58.9344322364589,
2.62103707099747));
#220066=CARTESIAN_POINT('Ctrl Pts',(-0.132883578272457,-58.9359598525091,
2.62350262767611));
#220067=CARTESIAN_POINT('Ctrl Pts',(-0.15310892324817,-58.9413065086847,
2.63213207605138));
#220068=CARTESIAN_POINT('Ctrl Pts',(-0.172198253417102,-58.9479240485793,
2.64280685971873));
#220069=CARTESIAN_POINT('Ctrl Pts',(-0.189729578870158,-58.9555707636543,
2.65513293646042));
#220070=CARTESIAN_POINT('Ctrl Pts',(-0.198495241596686,-58.9593941211918,
2.66129597483127));
#220071=CARTESIAN_POINT('Ctrl Pts',(-0.206871403159931,-58.9634747743346,
2.6678718353381));
#220072=CARTESIAN_POINT('Ctrl Pts',(-0.214805314862594,-58.9677825146335,
2.67481125953819));
#220073=CARTESIAN_POINT('Ctrl Pts',(-0.222705329147009,-58.972071850231,
2.68172103524038));
#220074=CARTESIAN_POINT('Ctrl Pts',(-0.230167055078558,-58.9765861722456,
2.68899101329746));
#220075=CARTESIAN_POINT('Ctrl Pts',(-0.237137844566027,-58.9812961520163,
2.69657334701232));
#220076=CARTESIAN_POINT('Ctrl Pts',(-0.23716775486217,-58.9813163616195,
2.69660588132529));
#220077=CARTESIAN_POINT('Ctrl Pts',(-0.237197656536079,-58.9813365744743,
2.69663842081338));
#220078=CARTESIAN_POINT('Ctrl Pts',(-0.23722754958733,-58.9813567905787,
2.69667096547338));
#220079=CARTESIAN_POINT('Ctrl Pts',(-0.251324537971816,-58.9908903168209,
2.71201840157907));
#220080=CARTESIAN_POINT('Ctrl Pts',(-0.26350158051193,-59.0011093202329,
2.72845645939327));
#220081=CARTESIAN_POINT('Ctrl Pts',(-0.273820596508964,-59.0118294103847,
2.74568723186887));
#220082=CARTESIAN_POINT('Ctrl Pts',(-0.284514998003945,-59.0229394763229,
2.76354482594332));
#220083=CARTESIAN_POINT('Ctrl Pts',(-0.293214009568506,-59.034588573656,
2.78225519317159));
#220084=CARTESIAN_POINT('Ctrl Pts',(-0.2999368939724,-59.04658752064,2.80151223085562));
#220085=CARTESIAN_POINT('Ctrl Pts',(-0.306563827731156,-59.0584152157275,
2.82049442740328));
#220086=CARTESIAN_POINT('Ctrl Pts',(-0.311270560393252,-59.0705837677968,
2.84000929089333));
#220087=CARTESIAN_POINT('Ctrl Pts',(-0.314027284735468,-59.0829139906047,
2.85976644341707));
#220088=CARTESIAN_POINT('Ctrl Pts',(-0.315949321993669,-59.0915108413219,
2.87354148166992));
#220089=CARTESIAN_POINT('Ctrl Pts',(-0.316922445687073,-59.1001863397075,
2.88743438345489));
#220090=CARTESIAN_POINT('Ctrl Pts',(-0.316922544675027,-59.1088767419346,
2.90134173515982));
#220091=CARTESIAN_POINT('',(-0.316925998272418,-59.465175436383,3.47153072139031));
#220092=CARTESIAN_POINT('',(-0.316922544675064,-59.1088767419346,2.90134173515982));
#220093=CARTESIAN_POINT('',(-5.90061356181196,-59.1725467709676,3.47153072139031));
#220094=CARTESIAN_POINT('Origin',(5.53234440788222E-15,1.85015204418142E-13,
3.47153072139072));
#220095=CARTESIAN_POINT('',(-5.8633736414952,-58.8181995570483,2.90134173515982));
#220096=CARTESIAN_POINT('',(-5.90061356181196,-59.1725467709676,3.47153072139031));
#220097=CARTESIAN_POINT('',(-6.14377718965262,-58.5996668978647,2.59908173515982));
#220098=CARTESIAN_POINT('Ctrl Pts',(-5.8633736414952,-58.8181995570483,
2.90134173515982));
#220099=CARTESIAN_POINT('Ctrl Pts',(-5.86209540502805,-58.8060365798449,
2.88176998919624));
#220100=CARTESIAN_POINT('Ctrl Pts',(-5.86273454612475,-58.7937272422236,
2.86226752356404));
#220101=CARTESIAN_POINT('Ctrl Pts',(-5.86523378400442,-58.7814443761786,
2.84310370499567));
#220102=CARTESIAN_POINT('Ctrl Pts',(-5.86777816724702,-58.7689396367177,
2.82359371788075));
#220103=CARTESIAN_POINT('Ctrl Pts',(-5.87225032431096,-58.7564614161358,
2.80443322636292));
#220104=CARTESIAN_POINT('Ctrl Pts',(-5.87864135444063,-58.7441787427558,
2.7858932387744));
#220105=CARTESIAN_POINT('Ctrl Pts',(-5.88476180492493,-58.7324160859207,
2.76813818619086));
#220106=CARTESIAN_POINT('Ctrl Pts',(-5.89264238982162,-58.7208319573083,
2.75095095197719));
#220107=CARTESIAN_POINT('Ctrl Pts',(-5.90232005416286,-58.7095754394589,
2.73457771434054));
#220108=CARTESIAN_POINT('Ctrl Pts',(-5.91001735013549,-58.7006223753256,
2.72155497954881));
#220109=CARTESIAN_POINT('Ctrl Pts',(-5.91885232406698,-58.6918764318934,
2.70904711159609));
#220110=CARTESIAN_POINT('Ctrl Pts',(-5.92886364759491,-58.6834178317479,
2.69718956158297));
#220111=CARTESIAN_POINT('Ctrl Pts',(-5.92889097525615,-58.6833947425171,
2.69715719432314));
#220112=CARTESIAN_POINT('Ctrl Pts',(-5.92891831167169,-58.6833716556048,
2.6971248321898));
#220113=CARTESIAN_POINT('Ctrl Pts',(-5.92894565684117,-58.683348571013,
2.69709247518608));
#220114=CARTESIAN_POINT('Ctrl Pts',(-5.93438921243157,-58.678753161254,
2.69065122242233));
#220115=CARTESIAN_POINT('Ctrl Pts',(-5.94021607194716,-58.6742527563955,
2.68442464469383));
#220116=CARTESIAN_POINT('Ctrl Pts',(-5.94639317576815,-58.6698707672379,
2.67844505923536));
#220117=CARTESIAN_POINT('Ctrl Pts',(-5.95865206607721,-58.6611744062937,
2.66657815779524));
#220118=CARTESIAN_POINT('Ctrl Pts',(-5.97229179622458,-58.6529445485197,
2.65568445664132));
#220119=CARTESIAN_POINT('Ctrl Pts',(-5.98706231729978,-58.64536492539,2.64601906229473));
#220120=CARTESIAN_POINT('Ctrl Pts',(-5.99814020810618,-58.6396802080427,
2.63877001653479));
#220121=CARTESIAN_POINT('Ctrl Pts',(-6.00985416873209,-58.6343612468743,
2.63221189387559));
#220122=CARTESIAN_POINT('Ctrl Pts',(-6.02209871088731,-58.6294855649107,
2.62645231033191));
#220123=CARTESIAN_POINT('Ctrl Pts',(-6.02669041419552,-58.6276571841744,
2.62429246650303));
#220124=CARTESIAN_POINT('Ctrl Pts',(-6.03135673054979,-58.6258911397671,
2.62224491711703));
#220125=CARTESIAN_POINT('Ctrl Pts',(-6.03609209717089,-58.6241915206269,
2.62031533672554));
#220126=CARTESIAN_POINT('Ctrl Pts',(-6.05266588034474,-58.6182428536362,
2.61356180535535));
#220127=CARTESIAN_POINT('Ctrl Pts',(-6.07008552874908,-58.6131078911175,
2.60825339735306));
#220128=CARTESIAN_POINT('Ctrl Pts',(-6.088112543032,-58.6089619925609,2.60463337987569));
#220129=CARTESIAN_POINT('Ctrl Pts',(-6.09712605017347,-58.6068890432826,
2.60282337113701));
#220130=CARTESIAN_POINT('Ctrl Pts',(-6.10629139889341,-58.6050633610077,
2.60143545939073));
#220131=CARTESIAN_POINT('Ctrl Pts',(-6.11557877725353,-58.6035068699779,
2.60050005034554));
#220132=CARTESIAN_POINT('Ctrl Pts',(-6.12022246643359,-58.602728624463,
2.60003234582295));
#220133=CARTESIAN_POINT('Ctrl Pts',(-6.12489666302672,-58.6020176767847,
2.59967776696024));
#220134=CARTESIAN_POINT('Ctrl Pts',(-6.12959764057299,-58.6013767677626,
2.59944011429119));
#220135=CARTESIAN_POINT('Ctrl Pts',(-6.13429861811926,-58.6007358587405,
2.59920246162213));
#220136=CARTESIAN_POINT('Ctrl Pts',(-6.13902637679584,-58.6001649900649,
2.59908173791266));
#220137=CARTESIAN_POINT('Ctrl Pts',(-6.14377718965262,-58.5996668978647,
2.59908173515982));
#220138=CARTESIAN_POINT('',(-6.17403490858961,-58.5964866834549,2.59908173515982));
#220139=CARTESIAN_POINT('Origin',(3.95370119046988E-16,1.9103972218437E-13,
2.59908173516024));
#220140=CARTESIAN_POINT('',(-6.4937464611268,-58.7519447039087,2.90134173515982));
#220141=CARTESIAN_POINT('Ctrl Pts',(-6.17403490858961,-58.5964866834549,
2.59908173515983));
#220142=CARTESIAN_POINT('Ctrl Pts',(-6.17782374318166,-58.5960874772331,
2.5990817437147));
#220143=CARTESIAN_POINT('Ctrl Pts',(-6.18160715078344,-58.595736114045,
2.5991576435585));
#220144=CARTESIAN_POINT('Ctrl Pts',(-6.18538309648717,-58.5954317101323,
2.59930765775236));
#220145=CARTESIAN_POINT('Ctrl Pts',(-6.20767599437393,-58.593634532452,
2.60019333020843));
#220146=CARTESIAN_POINT('Ctrl Pts',(-6.22971127560455,-58.5934722580542,
2.60365973324068));
#220147=CARTESIAN_POINT('Ctrl Pts',(-6.2510635343538,-58.5947642147752,
2.60934177082398));
#220148=CARTESIAN_POINT('Ctrl Pts',(-6.25904002743657,-58.5952468467987,
2.61146439091825));
#220149=CARTESIAN_POINT('Ctrl Pts',(-6.26692152735626,-58.5959321585038,
2.61389584429287));
#220150=CARTESIAN_POINT('Ctrl Pts',(-6.27468709076379,-58.5968099398847,
2.61661604385211));
#220151=CARTESIAN_POINT('Ctrl Pts',(-6.2807461728947,-58.597494828952,2.61873848000734));
#220152=CARTESIAN_POINT('Ctrl Pts',(-6.28673424952138,-58.59829716952,2.62103707099745));
#220153=CARTESIAN_POINT('Ctrl Pts',(-6.29264094271378,-58.5992123816355,
2.6235026276761));
#220154=CARTESIAN_POINT('Ctrl Pts',(-6.31331436888716,-58.6024156240397,
2.63213207605136));
#220155=CARTESIAN_POINT('Ctrl Pts',(-6.33299084698388,-58.6070015340111,
2.64280685971873));
#220156=CARTESIAN_POINT('Ctrl Pts',(-6.35122543337761,-58.6127738370721,
2.65513293646043));
#220157=CARTESIAN_POINT('Ctrl Pts',(-6.36034272657447,-58.6156599886027,
2.66129597483128));
#220158=CARTESIAN_POINT('Ctrl Pts',(-6.36909954705041,-58.6188427402043,
2.6678718353381));
#220159=CARTESIAN_POINT('Ctrl Pts',(-6.37744027742822,-58.6222975626531,
2.67481125953819));
#220160=CARTESIAN_POINT('Ctrl Pts',(-6.38574537226625,-58.6257376244685,
2.68172103524038));
#220161=CARTESIAN_POINT('Ctrl Pts',(-6.39363809722528,-58.6294472538098,
2.68899101329747));
#220162=CARTESIAN_POINT('Ctrl Pts',(-6.40106302694602,-58.6334027859056,
2.69657334701232));
#220163=CARTESIAN_POINT('Ctrl Pts',(-6.40109488586921,-58.6334197583212,
2.6966058813253));
#220164=CARTESIAN_POINT('Ctrl Pts',(-6.40112673655726,-58.6334367348719,
2.69663842081339));
#220165=CARTESIAN_POINT('Ctrl Pts',(-6.40115857900958,-58.6334537155556,
2.69667096547339));
#220166=CARTESIAN_POINT('Ctrl Pts',(-6.41617486746338,-58.6414614796105,
2.71201840157812));
#220167=CARTESIAN_POINT('Ctrl Pts',(-6.42935337961243,-58.6503516547081,
2.72845645939122));
#220168=CARTESIAN_POINT('Ctrl Pts',(-6.44073642150931,-58.6599343881991,
2.74568723186565));
#220169=CARTESIAN_POINT('Ctrl Pts',(-6.45253355607274,-58.6698657226791,
2.76354482593886));
#220170=CARTESIAN_POINT('Ctrl Pts',(-6.46240257578417,-58.6805417107265,
2.78225519316581));
#220171=CARTESIAN_POINT('Ctrl Pts',(-6.47034286301293,-58.6917721934471,
2.80151223084849));
#220172=CARTESIAN_POINT('Ctrl Pts',(-6.4781698245267,-58.7028423919807,
2.82049442739492));
#220173=CARTESIAN_POINT('Ctrl Pts',(-6.48412273326305,-58.7144522959155,
2.84000929088371));
#220174=CARTESIAN_POINT('Ctrl Pts',(-6.48815321522321,-58.7264268163128,
2.85976644340622));
#220175=CARTESIAN_POINT('Ctrl Pts',(-6.49096333895585,-58.7347756649834,
2.87354148166263));
#220176=CARTESIAN_POINT('Ctrl Pts',(-6.49283796829092,-58.7433019189591,
2.88743438345124));
#220177=CARTESIAN_POINT('Ctrl Pts',(-6.49374646112681,-58.7519447039087,
2.90134173515981));
#220178=CARTESIAN_POINT('',(-6.53099325079995,-59.1062911958295,3.47153072139031));
#220179=CARTESIAN_POINT('',(-6.49374646112681,-58.7519447039087,2.90134173515982));
#220180=CARTESIAN_POINT('',(-12.0535047649316,-58.231611300478,3.47153072139032));
#220181=CARTESIAN_POINT('Origin',(5.53234440788222E-15,1.85015204418142E-13,
3.47153072139072));
#220182=CARTESIAN_POINT('',(-11.9794294790606,-57.8830978693155,2.90134173515983));
#220183=CARTESIAN_POINT('',(-12.0535047649316,-58.231611300478,3.47153072139032));
#220184=CARTESIAN_POINT('',(-12.2354540642039,-57.6364522029206,2.59908173515983));
#220185=CARTESIAN_POINT('Ctrl Pts',(-11.9794294790606,-57.8830978693155,
2.90134173515983));
#220186=CARTESIAN_POINT('Ctrl Pts',(-11.9768868675909,-57.8711351342679,
2.8817699891971));
#220187=CARTESIAN_POINT('Ctrl Pts',(-11.9762358312604,-57.8588264200499,
2.86226752356573));
#220188=CARTESIAN_POINT('Ctrl Pts',(-11.9774374689411,-57.8463495993359,
2.84310370499817));
#220189=CARTESIAN_POINT('Ctrl Pts',(-11.9786608125864,-57.8336474016765,
2.82359371788415));
#220190=CARTESIAN_POINT('Ctrl Pts',(-11.9818041414839,-57.8207700703878,
2.80443322636717));
#220191=CARTESIAN_POINT('Ctrl Pts',(-11.986876271908,-57.8078866382202,
2.78589323877943));
#220192=CARTESIAN_POINT('Ctrl Pts',(-11.9917336614806,-57.7955486571671,
2.76813818619671));
#220193=CARTESIAN_POINT('Ctrl Pts',(-11.9983602045457,-57.783204242195,
2.75095095198379));
#220194=CARTESIAN_POINT('Ctrl Pts',(-12.0068082271156,-57.7709977973472,
2.73457771434777));
#220195=CARTESIAN_POINT('Ctrl Pts',(-12.0135275064609,-57.7612891925148,
2.72155497955344));
#220196=CARTESIAN_POINT('Ctrl Pts',(-12.0213998814552,-57.751667654026,
2.70904711159829));
#220197=CARTESIAN_POINT('Ctrl Pts',(-12.0304721974324,-57.7422089227117,
2.69718956158298));
#220198=CARTESIAN_POINT('Ctrl Pts',(-12.030496961908,-57.7421831034477,
2.69715719432316));
#220199=CARTESIAN_POINT('Ctrl Pts',(-12.0305217353324,-57.7421572855745,
2.69712483218981));
#220200=CARTESIAN_POINT('Ctrl Pts',(-12.0305465177052,-57.7421314690939,
2.69709247518609));
#220201=CARTESIAN_POINT('Ctrl Pts',(-12.0354799018083,-57.7369922269698,
2.69065122242235));
#220202=CARTESIAN_POINT('Ctrl Pts',(-12.0408044207739,-57.7319074031291,
2.68442464469384));
#220203=CARTESIAN_POINT('Ctrl Pts',(-12.0464896431811,-57.7269037357968,
2.67844505923537));
#220204=CARTESIAN_POINT('Ctrl Pts',(-12.0577723607609,-57.7169736114624,
2.66657815779526));
#220205=CARTESIAN_POINT('Ctrl Pts',(-12.0704771166533,-57.7073630976787,
2.65568445664133));
#220206=CARTESIAN_POINT('Ctrl Pts',(-12.0843744369107,-57.6982810566479,
2.64601906229474));
#220207=CARTESIAN_POINT('Ctrl Pts',(-12.0947974271037,-57.6914695258748,
2.6387700165348));
#220208=CARTESIAN_POINT('Ctrl Pts',(-12.1058912345906,-57.6849552602292,
2.6322118938756));
#220209=CARTESIAN_POINT('Ctrl Pts',(-12.1175590523197,-57.6788263845867,
2.62645231033191));
#220210=CARTESIAN_POINT('Ctrl Pts',(-12.1219344839681,-57.6765280562207,
2.62429246650303));
#220211=CARTESIAN_POINT('Ctrl Pts',(-12.1263906358452,-57.6742839235119,
2.62224491711704));
#220212=CARTESIAN_POINT('Ctrl Pts',(-12.1309224030556,-57.6720986344672,
2.62031533672556));
#220213=CARTESIAN_POINT('Ctrl Pts',(-12.146783588292,-57.664450122811,2.61356180535537));
#220214=CARTESIAN_POINT('Ctrl Pts',(-12.1635710602988,-57.657522441076,
2.60825339735306));
#220215=CARTESIAN_POINT('Ctrl Pts',(-12.1810659563062,-57.6515149180851,
2.6046333798757));
#220216=CARTESIAN_POINT('Ctrl Pts',(-12.18981340431,-57.6485111565897,2.60282337113701));
#220217=CARTESIAN_POINT('Ctrl Pts',(-12.1987377085281,-57.6457374357763,
2.60143545939073));
#220218=CARTESIAN_POINT('Ctrl Pts',(-12.2078115120423,-57.6432186759795,
2.60050005034555));
#220219=CARTESIAN_POINT('Ctrl Pts',(-12.2123484137995,-57.6419592960811,
2.60003234582295));
#220220=CARTESIAN_POINT('Ctrl Pts',(-12.2169226903863,-57.6407636564616,
2.59967776696024));
#220221=CARTESIAN_POINT('Ctrl Pts',(-12.2215309222505,-57.6396348724474,
2.59944011429118));
#220222=CARTESIAN_POINT('Ctrl Pts',(-12.2261391541148,-57.6385060884332,
2.59920246162212));
#220223=CARTESIAN_POINT('Ctrl Pts',(-12.2307813416093,-57.6374441616868,
2.5990817379127));
#220224=CARTESIAN_POINT('Ctrl Pts',(-12.2354540642039,-57.6364522029206,
2.59908173515984));
#220225=CARTESIAN_POINT('',(-12.2652136052655,-57.6301266171957,2.59908173515984));
#220226=CARTESIAN_POINT('Origin',(3.88326186679512E-16,1.91040837833656E-13,
2.59908173516024));
#220227=CARTESIAN_POINT('',(-12.5994235324466,-57.7513140650719,2.90134173515983));
#220228=CARTESIAN_POINT('Ctrl Pts',(-12.2652136052655,-57.6301266171957,
2.59908173515984));
#220229=CARTESIAN_POINT('Ctrl Pts',(-12.2689399558123,-57.6293335568098,
2.59908174371468));
#220230=CARTESIAN_POINT('Ctrl Pts',(-12.2726659100573,-57.6285886446434,
2.5991576435585));
#220231=CARTESIAN_POINT('Ctrl Pts',(-12.2763893518622,-57.6278912144855,
2.59930765775236));
#220232=CARTESIAN_POINT('Ctrl Pts',(-12.2983722706983,-57.6237736395751,
2.60019333020834));
#220233=CARTESIAN_POINT('Ctrl Pts',(-12.3202698780571,-57.6213089400488,
2.60365973323998));
#220234=CARTESIAN_POINT('Ctrl Pts',(-12.3416402131473,-57.6203619005011,
2.60934177082223));
#220235=CARTESIAN_POINT('Ctrl Pts',(-12.3496234589524,-57.6200081180515,
2.61146439091692));
#220236=CARTESIAN_POINT('Ctrl Pts',(-12.3575334177725,-57.6198658344725,
2.61389584429214));
#220237=CARTESIAN_POINT('Ctrl Pts',(-12.3653481937522,-57.6199270848657,
2.61661604385214));
#220238=CARTESIAN_POINT('Ctrl Pts',(-12.3714456739989,-57.6199748754951,
2.61873848000737));
#220239=CARTESIAN_POINT('Ctrl Pts',(-12.3774848147419,-57.6201468963097,
2.62103707099747));
#220240=CARTESIAN_POINT('Ctrl Pts',(-12.3834548161669,-57.6204396772351,
2.62350262767612));
#220241=CARTESIAN_POINT('Ctrl Pts',(-12.4043498211546,-57.6214644104739,
2.63213207605139));
#220242=CARTESIAN_POINT('Ctrl Pts',(-12.4243978675675,-57.6239684463326,
2.64280685971874));
#220243=CARTESIAN_POINT('Ctrl Pts',(-12.4431359329576,-57.6278030948195,
2.65513293646044));
#220244=CARTESIAN_POINT('Ctrl Pts',(-12.4525049656526,-57.629720419063,
2.66129597483128));
#220245=CARTESIAN_POINT('Ctrl Pts',(-12.4615465034836,-57.6319703982309,
2.66787183533812));
#220246=CARTESIAN_POINT('Ctrl Pts',(-12.4702026697491,-57.6345344510719,
2.67481125953822));
#220247=CARTESIAN_POINT('Ctrl Pts',(-12.4788218527838,-57.637087549068,
2.6817210352404));
#220248=CARTESIAN_POINT('Ctrl Pts',(-12.487059102424,-57.6399518422607,
2.68899101329748));
#220249=CARTESIAN_POINT('Ctrl Pts',(-12.4948568232942,-57.6431095890442,
2.69657334701234));
#220250=CARTESIAN_POINT('Ctrl Pts',(-12.4948902817914,-57.6431231383188,
2.69660588132531));
#220251=CARTESIAN_POINT('Ctrl Pts',(-12.4949237325308,-57.6431366925667,
2.6966384208134));
#220252=CARTESIAN_POINT('Ctrl Pts',(-12.4949571755116,-57.6431502517858,
2.6966709654734));
#220253=CARTESIAN_POINT('Ctrl Pts',(-12.5107282424373,-57.6495445189154,
2.71201840157843));
#220254=CARTESIAN_POINT('Ctrl Pts',(-12.5247638376593,-57.6570084630808,
2.72845645939189));
#220255=CARTESIAN_POINT('Ctrl Pts',(-12.5370861904675,-57.6653488494784,
2.74568723186669));
#220256=CARTESIAN_POINT('Ctrl Pts',(-12.549856806225,-57.6739926427224,
2.76354482594026));
#220257=CARTESIAN_POINT('Ctrl Pts',(-12.5607877070384,-57.683578553126,
2.78225519316758));
#220258=CARTESIAN_POINT('Ctrl Pts',(-12.5698584016435,-57.6939175280655,
2.80151223085064));
#220259=CARTESIAN_POINT('Ctrl Pts',(-12.5787996370839,-57.7041089426343,
2.82049442739735));
#220260=CARTESIAN_POINT('Ctrl Pts',(-12.5859335005802,-57.7150329978987,
2.84000929088641));
#220261=CARTESIAN_POINT('Ctrl Pts',(-12.5911935813539,-57.7265206205349,
2.85976644340919));
#220262=CARTESIAN_POINT('Ctrl Pts',(-12.5948610032559,-57.7345299954231,
2.87354148166462));
#220263=CARTESIAN_POINT('Ctrl Pts',(-12.5976165994005,-57.7428135895632,
2.88743438345224));
#220264=CARTESIAN_POINT('Ctrl Pts',(-12.5994235324466,-57.7513140650719,
2.90134173515982));
#220265=CARTESIAN_POINT('',(-12.6735055745735,-58.0998260601479,3.47153072139032));
#220266=CARTESIAN_POINT('',(-12.5994235324466,-57.7513140650719,2.90134173515983));
#220267=CARTESIAN_POINT('',(-18.0743352474886,-56.6526781108323,3.47153072139033));
#220268=CARTESIAN_POINT('Origin',(5.53234440788222E-15,1.85015204418142E-13,
3.47153072139072));
#220269=CARTESIAN_POINT('',(-17.9642361803967,-56.3138168485095,2.90134173515983));
#220270=CARTESIAN_POINT('',(-18.0743352474886,-56.6526781108323,3.47153072139033));
#220271=CARTESIAN_POINT('',(-18.1930767435944,-56.0417604764383,2.59908173515983));
#220272=CARTESIAN_POINT('Ctrl Pts',(-17.9642361803967,-56.3138168485095,
2.90134173515983));
#220273=CARTESIAN_POINT('Ctrl Pts',(-17.9604570513079,-56.3021854218459,
2.88176998919747));
#220274=CARTESIAN_POINT('Ctrl Pts',(-17.9585229704406,-56.2900121878797,
2.86226752356647));
#220275=CARTESIAN_POINT('Ctrl Pts',(-17.9584138425285,-56.2774781111551,
2.84310370499926));
#220276=CARTESIAN_POINT('Ctrl Pts',(-17.9583027433679,-56.2647176232326,
2.8235937178857));
#220277=CARTESIAN_POINT('Ctrl Pts',(-17.96008280513,-56.2515822679732,2.80443322636917));
#220278=CARTESIAN_POINT('Ctrl Pts',(-17.9637804645265,-56.2382392305966,
2.78589323878182));
#220279=CARTESIAN_POINT('Ctrl Pts',(-17.9673215746112,-56.2254611028276,
2.76813818619968));
#220280=CARTESIAN_POINT('Ctrl Pts',(-17.9726214740526,-56.2124916494895,
2.75095095198728));
#220281=CARTESIAN_POINT('Ctrl Pts',(-17.9797472965484,-56.1994690140074,
2.7345777143517));
#220282=CARTESIAN_POINT('Ctrl Pts',(-17.9854149414351,-56.1891112379828,
2.72155497955596));
#220283=CARTESIAN_POINT('Ctrl Pts',(-17.9922384661036,-56.1787195200271,
2.70904711159949));
#220284=CARTESIAN_POINT('Ctrl Pts',(-18.0002723763367,-56.1683642893842,
2.69718956158298));
#220285=CARTESIAN_POINT('Ctrl Pts',(-18.0002943063019,-56.1683360229683,
2.69715719432316));
#220286=CARTESIAN_POINT('Ctrl Pts',(-18.0003162453122,-56.168307757,2.69712483218981));
#220287=CARTESIAN_POINT('Ctrl Pts',(-18.0003381933676,-56.1682794914815,
2.69709247518609));
#220288=CARTESIAN_POINT('Ctrl Pts',(-18.0047073547948,-56.1626527236045,
2.69065122242235));
#220289=CARTESIAN_POINT('Ctrl Pts',(-18.0094711966663,-56.1570391911757,
2.68442464469385));
#220290=CARTESIAN_POINT('Ctrl Pts',(-18.0146022491734,-56.1514686668951,
2.67844505923538));
#220291=CARTESIAN_POINT('Ctrl Pts',(-18.024785178209,-56.1404135756906,
2.66657815779526));
#220292=CARTESIAN_POINT('Ctrl Pts',(-18.0364157638823,-56.1295277006974,
2.65568445664133));
#220293=CARTESIAN_POINT('Ctrl Pts',(-18.049287621373,-56.1190427465076,
2.64601906229474));
#220294=CARTESIAN_POINT('Ctrl Pts',(-18.0589415144909,-56.1111790308652,
2.6387700165348));
#220295=CARTESIAN_POINT('Ctrl Pts',(-18.0692936227623,-56.1035408324,2.6322118938756));
#220296=CARTESIAN_POINT('Ctrl Pts',(-18.0802568810126,-56.0962259123227,
2.62645231033192));
#220297=CARTESIAN_POINT('Ctrl Pts',(-18.0843681028565,-56.0934828172937,
2.62429246650304));
#220298=CARTESIAN_POINT('Ctrl Pts',(-18.0885652677239,-56.0907851834708,
2.62224491711704));
#220299=CARTESIAN_POINT('Ctrl Pts',(-18.0928437845337,-56.0881381670058,
2.62031533672556));
#220300=CARTESIAN_POINT('Ctrl Pts',(-18.1078185933682,-56.0788736093783,
2.61356180535537));
#220301=CARTESIAN_POINT('Ctrl Pts',(-18.123789961921,-56.0702291095577,
2.60825339735306));
#220302=CARTESIAN_POINT('Ctrl Pts',(-18.1405610619113,-56.0624257818116,
2.60463337987569));
#220303=CARTESIAN_POINT('Ctrl Pts',(-18.1489466119065,-56.0585241179386,
2.60282337113701));
#220304=CARTESIAN_POINT('Ctrl Pts',(-18.1575320950781,-56.0548327480525,
2.60143545939074));
#220305=CARTESIAN_POINT('Ctrl Pts',(-18.1662929092565,-56.051379315548,
2.60050005034556));
#220306=CARTESIAN_POINT('Ctrl Pts',(-18.1706733163456,-56.0496525992958,
2.60003234582296));
#220307=CARTESIAN_POINT('Ctrl Pts',(-18.1750975561947,-56.0479853674131,
2.59967776696025));
#220308=CARTESIAN_POINT('Ctrl Pts',(-18.1795625536242,-56.0463810756007,
2.59944011429119));
#220309=CARTESIAN_POINT('Ctrl Pts',(-18.1840275510537,-56.0447767837883,
2.59920246162213));
#220310=CARTESIAN_POINT('Ctrl Pts',(-18.1885333065885,-56.0432354336627,
2.59908173791271));
#220311=CARTESIAN_POINT('Ctrl Pts',(-18.1930767435944,-56.0417604764383,
2.59908173515984));
#220312=CARTESIAN_POINT('',(-18.2220120550212,-56.0323588238391,2.59908173515983));
#220313=CARTESIAN_POINT('Origin',(3.81437458815951E-16,1.91042683662724E-13,
2.59908173516023));
#220314=CARTESIAN_POINT('',(-18.567058682946,-56.1179479440988,2.90134173515983));
#220315=CARTESIAN_POINT('Ctrl Pts',(-18.2220120550212,-56.0323588238391,
2.59908173515984));
#220316=CARTESIAN_POINT('Ctrl Pts',(-18.2256350948464,-56.0311805982248,
2.59908174371473));
#220317=CARTESIAN_POINT('Ctrl Pts',(-18.2292627734001,-56.0300502984937,
2.5991576435585));
#220318=CARTESIAN_POINT('Ctrl Pts',(-18.2328929164986,-56.0289674832812,
2.59930765775237));
#220319=CARTESIAN_POINT('Ctrl Pts',(-18.2543250068291,-56.0225746241524,
2.60019333020841));
#220320=CARTESIAN_POINT('Ctrl Pts',(-18.2758450255513,-56.0178345032614,
2.6036597332405));
#220321=CARTESIAN_POINT('Ctrl Pts',(-18.2969992991229,-56.0146588434089,
2.60934177082352));
#220322=CARTESIAN_POINT('Ctrl Pts',(-18.3049018315347,-56.013472522601,
2.6114643909179));
#220323=CARTESIAN_POINT('Ctrl Pts',(-18.3127535860873,-56.0125042026265,
2.61389584429268));
#220324=CARTESIAN_POINT('Ctrl Pts',(-18.3205319543143,-56.0117482509599,
2.61661604385212));
#220325=CARTESIAN_POINT('Ctrl Pts',(-18.3266010274073,-56.0111584195472,
2.61873848000736));
#220326=CARTESIAN_POINT('Ctrl Pts',(-18.3326250661768,-56.0106982359126,
2.62103707099747));
#220327=CARTESIAN_POINT('Ctrl Pts',(-18.3385929672496,-56.0103653778788,
2.62350262767612));
#220328=CARTESIAN_POINT('Ctrl Pts',(-18.3594806210044,-56.0092003747603,
2.63213207605138));
#220329=CARTESIAN_POINT('Ctrl Pts',(-18.3796805851417,-56.0095951017655,
2.64280685971873));
#220330=CARTESIAN_POINT('Ctrl Pts',(-18.3987168313625,-56.011450082467,
2.65513293646043));
#220331=CARTESIAN_POINT('Ctrl Pts',(-18.4082349544728,-56.0123775728177,
2.66129597483128));
#220332=CARTESIAN_POINT('Ctrl Pts',(-18.4174621486784,-56.0136701283092,
2.66787183533812));
#220333=CARTESIAN_POINT('Ctrl Pts',(-18.4263389120626,-56.0153153192429,
2.67481125953821));
#220334=CARTESIAN_POINT('Ctrl Pts',(-18.4351777497209,-56.0169534811439,
2.6817210352404));
#220335=CARTESIAN_POINT('Ctrl Pts',(-18.4436692750114,-56.0189410563923,
2.68899101329748));
#220336=CARTESIAN_POINT('Ctrl Pts',(-18.4517543535695,-56.021266420929,
2.69657334701234));
#220337=CARTESIAN_POINT('Ctrl Pts',(-18.4517890450624,-56.021276398614,
2.69660588132531));
#220338=CARTESIAN_POINT('Ctrl Pts',(-18.4518237293599,-56.0212863820559,
2.6966384208134));
#220339=CARTESIAN_POINT('Ctrl Pts',(-18.4518584064609,-56.0212963712528,
2.6966709654734));
#220340=CARTESIAN_POINT('Ctrl Pts',(-18.4682114607484,-56.0260070845282,
2.71201840157833));
#220341=CARTESIAN_POINT('Ctrl Pts',(-18.4829503621247,-56.0319630212268,
2.72845645939167));
#220342=CARTESIAN_POINT('Ctrl Pts',(-18.4960770195681,-56.0389696815121,
2.74568723186634));
#220343=CARTESIAN_POINT('Ctrl Pts',(-18.5096811989808,-56.0462312303121,
2.76354482593977));
#220344=CARTESIAN_POINT('Ctrl Pts',(-18.5215542196593,-56.0546220378313,
2.78225519316695));
#220345=CARTESIAN_POINT('Ctrl Pts',(-18.5316559412124,-56.0639562290164,
2.80151223084986));
#220346=CARTESIAN_POINT('Ctrl Pts',(-18.5416134885329,-56.0731572003494,
2.8204944273964));
#220347=CARTESIAN_POINT('Ctrl Pts',(-18.549850146688,-56.0832757207075,
2.84000929088528));
#220348=CARTESIAN_POINT('Ctrl Pts',(-18.5562821957296,-56.0941505847849,
2.85976644340788));
#220349=CARTESIAN_POINT('Ctrl Pts',(-18.5607667347597,-56.101732733504,
2.87354148166375));
#220350=CARTESIAN_POINT('Ctrl Pts',(-18.5643731068262,-56.1096829110186,
2.88743438345181));
#220351=CARTESIAN_POINT('Ctrl Pts',(-18.567058682946,-56.1179479440988,
2.90134173515983));
#220352=CARTESIAN_POINT('',(-18.6771643191705,-56.4568070719811,3.47153072139032));
#220353=CARTESIAN_POINT('',(-18.567058682946,-56.1179479440988,2.90134173515984));
#220354=CARTESIAN_POINT('',(-23.8971395307763,-54.4530463244693,3.47153072139034));
#220355=CARTESIAN_POINT('Origin',(5.53234440788222E-15,1.85015204418142E-13,
3.47153072139072));
#220356=CARTESIAN_POINT('',(-23.7522229508823,-54.1275498658874,2.90134173515985));
#220357=CARTESIAN_POINT('',(-23.8971395307763,-54.4530463244693,3.47153072139034));
#220358=CARTESIAN_POINT('',(-23.951372267036,-53.8330634946838,2.59908173515985));
#220359=CARTESIAN_POINT('Ctrl Pts',(-23.7522229508823,-54.1275498658874,
2.90134173515985));
#220360=CARTESIAN_POINT('Ctrl Pts',(-23.7472487091031,-54.1163771839526,
2.88176998919785));
#220361=CARTESIAN_POINT('Ctrl Pts',(-23.7440527738936,-54.1044728027369,
2.86226752356721));
#220362=CARTESIAN_POINT('Ctrl Pts',(-23.7426340760171,-54.0920187959693,
2.84310370500034));
#220363=CARTESIAN_POINT('Ctrl Pts',(-23.7411897512761,-54.0793398243594,
2.82359371788689));
#220364=CARTESIAN_POINT('Ctrl Pts',(-23.7415870431738,-54.0660903588301,
2.80443322637046));
#220365=CARTESIAN_POINT('Ctrl Pts',(-23.7438697192129,-54.052433905354,
2.78589323878321));
#220366=CARTESIAN_POINT('Ctrl Pts',(-23.746055752667,-54.0393556307103,
2.76813818620075));
#220367=CARTESIAN_POINT('Ctrl Pts',(-23.749970941678,-54.0259032350503,
2.75095095198804));
#220368=CARTESIAN_POINT('Ctrl Pts',(-23.755696492098,-54.0122070876526,
2.73457771435218));
#220369=CARTESIAN_POINT('Ctrl Pts',(-23.7602504066224,-54.0013136223984,
2.72155497955627));
#220370=CARTESIAN_POINT('Ctrl Pts',(-23.7659503210002,-53.9902655788131,
2.70904711159964));
#220371=CARTESIAN_POINT('Ctrl Pts',(-23.7728578042866,-53.9791273029163,
2.697189561583));
#220372=CARTESIAN_POINT('Ctrl Pts',(-23.7728766594722,-53.9790968990412,
2.69715719432317));
#220373=CARTESIAN_POINT('Ctrl Pts',(-23.7728955237001,-53.9790664946659,
2.69712483218983));
#220374=CARTESIAN_POINT('Ctrl Pts',(-23.7729143969706,-53.9790360897924,
2.69709247518611));
#220375=CARTESIAN_POINT('Ctrl Pts',(-23.776671466275,-53.9729834442087,
2.69065122242236));
#220376=CARTESIAN_POINT('Ctrl Pts',(-23.780822437404,-53.9669027062279,
2.68442464469386));
#220377=CARTESIAN_POINT('Ctrl Pts',(-23.7853431031259,-53.9608263568286,
2.67844505923539));
#220378=CARTESIAN_POINT('Ctrl Pts',(-23.7943146773159,-53.9487674206468,
2.66657815779527));
#220379=CARTESIAN_POINT('Ctrl Pts',(-23.8047436656396,-53.9367254523684,
2.65568445664134));
#220380=CARTESIAN_POINT('Ctrl Pts',(-23.8164490335992,-53.9249524603718,
2.64601906229476));
#220381=CARTESIAN_POINT('Ctrl Pts',(-23.8252280595689,-53.9161227163744,
2.63877001653482));
#220382=CARTESIAN_POINT('Ctrl Pts',(-23.8347250487603,-53.9074442707904,
2.63221189387562));
#220383=CARTESIAN_POINT('Ctrl Pts',(-23.8448636317802,-53.8990234500733,
2.62645231033194));
#220384=CARTESIAN_POINT('Ctrl Pts',(-23.8486656004127,-53.8958656423044,
2.62429246650306));
#220385=CARTESIAN_POINT('Ctrl Pts',(-23.8525577932538,-53.8927440632082,
2.62224491711707));
#220386=CARTESIAN_POINT('Ctrl Pts',(-23.8565361833376,-53.8896643205891,
2.62031533672558));
#220387=CARTESIAN_POINT('Ctrl Pts',(-23.8704605486307,-53.8788852214226,
2.6135618053554));
#220388=CARTESIAN_POINT('Ctrl Pts',(-23.8854408280735,-53.8686186144653,
2.60825339735309));
#220389=CARTESIAN_POINT('Ctrl Pts',(-23.9013043843656,-53.8591049768558,
2.60463337987572));
#220390=CARTESIAN_POINT('Ctrl Pts',(-23.9092361625117,-53.8543481580511,
2.60282337113704));
#220391=CARTESIAN_POINT('Ctrl Pts',(-23.9173887602867,-53.8497795825131,
2.60143545939075));
#220392=CARTESIAN_POINT('Ctrl Pts',(-23.9257405998156,-53.8454293138302,
2.60050005034556));
#220393=CARTESIAN_POINT('Ctrl Pts',(-23.92991651958,-53.8432541794887,2.60003234582297));
#220394=CARTESIAN_POINT('Ctrl Pts',(-23.9341422497936,-53.8411336218842,
2.59967776696026));
#220395=CARTESIAN_POINT('Ctrl Pts',(-23.9384150933423,-53.8390713992304,
2.5994401142912));
#220396=CARTESIAN_POINT('Ctrl Pts',(-23.942687936891,-53.8370091765766,
2.59920246162214));
#220397=CARTESIAN_POINT('Ctrl Pts',(-23.9470078944655,-53.8350052904263,
2.59908173791272));
#220398=CARTESIAN_POINT('Ctrl Pts',(-23.951372267036,-53.8330634946838,
2.59908173515985));
#220399=CARTESIAN_POINT('',(-23.9791663275009,-53.8206887816836,2.59908173515985));
#220400=CARTESIAN_POINT('Origin',(3.74779409800327E-16,1.91045239448285E-13,
2.59908173516024));
#220401=CARTESIAN_POINT('',(-24.3312692531083,-53.8697418420145,2.90134173515984));
#220402=CARTESIAN_POINT('Ctrl Pts',(-23.9791663275009,-53.8206887816836,
2.59908173515985));
#220403=CARTESIAN_POINT('Ctrl Pts',(-23.982646361822,-53.8191382997272,
2.59908174371477));
#220404=CARTESIAN_POINT('Ctrl Pts',(-23.9861360190791,-53.8176349962319,
2.59915764355852));
#220405=CARTESIAN_POINT('Ctrl Pts',(-23.9896330908637,-53.8161786595149,
2.59930765775239));
#220406=CARTESIAN_POINT('Ctrl Pts',(-24.0102795382214,-53.80758055767,2.60019333020848));
#220407=CARTESIAN_POINT('Ctrl Pts',(-24.031186190478,-53.8006169491704,
2.60365973324088));
#220408=CARTESIAN_POINT('Ctrl Pts',(-24.0518926318823,-53.7952474622067,
2.60934177082442));
#220409=CARTESIAN_POINT('Ctrl Pts',(-24.0596278691027,-53.7932416006198,
2.61146439091859));
#220410=CARTESIAN_POINT('Ctrl Pts',(-24.0673353939223,-53.7914578533664,
2.61389584429308));
#220411=CARTESIAN_POINT('Ctrl Pts',(-24.0749921329673,-53.7898929820048,
2.61661604385214));
#220412=CARTESIAN_POINT('Ctrl Pts',(-24.0809663048717,-53.7886719908665,
2.61873848000737));
#220413=CARTESIAN_POINT('Ctrl Pts',(-24.0869092410384,-53.7875846446507,
2.62103707099748));
#220414=CARTESIAN_POINT('Ctrl Pts',(-24.0928096561859,-53.7866297945199,
2.62350262767613));
#220415=CARTESIAN_POINT('Ctrl Pts',(-24.1134611092023,-53.7832878190622,
2.63213207605139));
#220416=CARTESIAN_POINT('Ctrl Pts',(-24.1335916760297,-53.7815689125022,
2.64280685971875));
#220417=CARTESIAN_POINT('Ctrl Pts',(-24.152717537984,-53.7814239018615,
2.65513293646044));
#220418=CARTESIAN_POINT('Ctrl Pts',(-24.1622804689611,-53.7813513965411,
2.66129597483129));
#220419=CARTESIAN_POINT('Ctrl Pts',(-24.1715922244705,-53.7816723668478,
2.66787183533813));
#220420=CARTESIAN_POINT('Ctrl Pts',(-24.1805923292962,-53.7823806708181,
2.67481125953822));
#220421=CARTESIAN_POINT('Ctrl Pts',(-24.1895539814231,-53.7830859485793,
2.6817210352404));
#220422=CARTESIAN_POINT('Ctrl Pts',(-24.198206747436,-53.784175029593,2.68899101329747));
#220423=CARTESIAN_POINT('Ctrl Pts',(-24.2064906018693,-53.7856425347024,
2.69657334701233));
#220424=CARTESIAN_POINT('Ctrl Pts',(-24.2065261462707,-53.7856488314802,
2.6966058813253));
#220425=CARTESIAN_POINT('Ctrl Pts',(-24.2065616841178,-53.7856551347354,
2.69663842081339));
#220426=CARTESIAN_POINT('Ctrl Pts',(-24.2065972154094,-53.7856614444664,
2.6966709654734));
#220427=CARTESIAN_POINT('Ctrl Pts',(-24.2233530895763,-53.7886369923275,
2.71201840158033));
#220428=CARTESIAN_POINT('Ctrl Pts',(-24.2386338146209,-53.7930196670714,
2.72845645939597));
#220429=CARTESIAN_POINT('Ctrl Pts',(-24.252420958295,-53.7986158348092,
2.74568723187311));
#220430=CARTESIAN_POINT('Ctrl Pts',(-24.266709651128,-53.8044155801181,
2.76354482594914));
#220431=CARTESIAN_POINT('Ctrl Pts',(-24.2793947083735,-53.8115193533113,
2.78225519317911));
#220432=CARTESIAN_POINT('Ctrl Pts',(-24.2904167803,-53.8197464933919,2.80151223086488));
#220433=CARTESIAN_POINT('Ctrl Pts',(-24.3012815425289,-53.8278562137235,
2.82049442741405));
#220434=CARTESIAN_POINT('Ctrl Pts',(-24.3105307527925,-53.8370583385507,
2.84000929090562));
#220435=CARTESIAN_POINT('Ctrl Pts',(-24.3180642992262,-53.8472012967848,
2.85976644343084));
#220436=CARTESIAN_POINT('Ctrl Pts',(-24.3233168218323,-53.8542731477233,
2.87354148167919));
#220437=CARTESIAN_POINT('Ctrl Pts',(-24.3277344576507,-53.8618028047995,
2.88743438345954));
#220438=CARTESIAN_POINT('Ctrl Pts',(-24.3312692531083,-53.8697418420145,
2.90134173515984));
#220439=CARTESIAN_POINT('',(-24.4761921430387,-54.1952354911872,3.47153072139034));
#220440=CARTESIAN_POINT('',(-24.3312692531083,-53.8697418420145,2.90134173515984));
#220441=CARTESIAN_POINT('',(-29.4581217525669,-51.6568155675428,3.47153072139036));
#220442=CARTESIAN_POINT('Origin',(5.53234440788222E-15,1.85015204418142E-13,
3.47153072139072));
#220443=CARTESIAN_POINT('',(-29.2799753962458,-51.3482501200166,2.90134173515987));
#220444=CARTESIAN_POINT('',(-29.4581217525669,-51.6568155675428,3.47153072139035));
#220445=CARTESIAN_POINT('',(-29.4472515437731,-51.0345602039888,2.59908173515987));
#220446=CARTESIAN_POINT('Ctrl Pts',(-29.2799753962458,-51.3482501200166,
2.90134173515987));
#220447=CARTESIAN_POINT('Ctrl Pts',(-29.2738605406103,-51.3376585930513,
2.88176998919738));
#220448=CARTESIAN_POINT('Ctrl Pts',(-29.2694377663935,-51.3261534914773,
2.86226752356625));
#220449=CARTESIAN_POINT('Ctrl Pts',(-29.2667250421036,-51.3139160033703,
2.84310370499892));
#220450=CARTESIAN_POINT('Ctrl Pts',(-29.2639633161065,-51.3014574615389,
2.82359371788513));
#220451=CARTESIAN_POINT('Ctrl Pts',(-29.2629734853268,-51.2882390496563,
2.80443322636838));
#220452=CARTESIAN_POINT('Ctrl Pts',(-29.2638161685324,-51.2744188030425,
2.78589323878084));
#220453=CARTESIAN_POINT('Ctrl Pts',(-29.2646231747158,-51.2611836698379,
2.76813818619833));
#220454=CARTESIAN_POINT('Ctrl Pts',(-29.2671107576663,-51.247395719118,
2.75095095198559));
#220455=CARTESIAN_POINT('Ctrl Pts',(-29.2713733056821,-51.233176117662,
2.73457771434972));
#220456=CARTESIAN_POINT('Ctrl Pts',(-29.2747635962034,-51.2218663142638,
2.7215549795547));
#220457=CARTESIAN_POINT('Ctrl Pts',(-29.2792774508355,-51.2102829897273,
2.70904711159891));
#220458=CARTESIAN_POINT('Ctrl Pts',(-29.2849828273425,-51.1984837018591,
2.69718956158302));
#220459=CARTESIAN_POINT('Ctrl Pts',(-29.2849984011671,-51.1984514936361,
2.69715719432319));
#220460=CARTESIAN_POINT('Ctrl Pts',(-29.2850139839321,-51.1984192839703,
2.69712483218985));
#220461=CARTESIAN_POINT('Ctrl Pts',(-29.2850295756381,-51.1983870728639,
2.69709247518613));
#220462=CARTESIAN_POINT('Ctrl Pts',(-29.2881333895822,-51.1919748636253,
2.69065122242239));
#220463=CARTESIAN_POINT('Ctrl Pts',(-29.2916260110603,-51.1854935419302,
2.68442464469389));
#220464=CARTESIAN_POINT('Ctrl Pts',(-29.2954867606375,-51.1789779411678,
2.67844505923542));
#220465=CARTESIAN_POINT('Ctrl Pts',(-29.3031486855376,-51.166047280237,
2.6665781577953));
#220466=CARTESIAN_POINT('Ctrl Pts',(-29.3122618143332,-51.1529811529979,
2.65568445664136));
#220467=CARTESIAN_POINT('Ctrl Pts',(-29.3226724463009,-51.1400491105585,
2.64601906229477));
#220468=CARTESIAN_POINT('Ctrl Pts',(-29.3304804202767,-51.130350078729,
2.63877001653483));
#220469=CARTESIAN_POINT('Ctrl Pts',(-29.3390182393872,-51.1207264688921,
2.63221189387563));
#220470=CARTESIAN_POINT('Ctrl Pts',(-29.3482210667394,-51.1112920078092,
2.62645231033195));
#220471=CARTESIAN_POINT('Ctrl Pts',(-29.3516721269965,-51.1077540849031,
2.62429246650307));
#220472=CARTESIAN_POINT('Ctrl Pts',(-29.3552167041322,-51.1042427612073,
2.62224491711707));
#220473=CARTESIAN_POINT('Ctrl Pts',(-29.3588513794155,-51.1007640347389,
2.62031533672559));
#220474=CARTESIAN_POINT('Ctrl Pts',(-29.3715727429074,-51.0885884920993,
2.6135618053554));
#220475=CARTESIAN_POINT('Ctrl Pts',(-29.3853978061638,-51.0768122610997,
2.6082533973531));
#220476=CARTESIAN_POINT('Ctrl Pts',(-29.4001800143153,-51.0656925470313,
2.60463337987573));
#220477=CARTESIAN_POINT('Ctrl Pts',(-29.4075711183911,-51.0601326899971,
2.60282337113705));
#220478=CARTESIAN_POINT('Ctrl Pts',(-29.4152015092021,-51.0547369630768,
2.60143545939077));
#220479=CARTESIAN_POINT('Ctrl Pts',(-29.42305286958,-51.0495375206695,2.60050005034558));
#220480=CARTESIAN_POINT('Ctrl Pts',(-29.4269785497689,-51.0469377994659,
2.60003234582299));
#220481=CARTESIAN_POINT('Ctrl Pts',(-29.4309594723626,-51.0443871494124,
2.59967776696029));
#220482=CARTESIAN_POINT('Ctrl Pts',(-29.4349933478623,-51.0418895900601,
2.59944011429123));
#220483=CARTESIAN_POINT('Ctrl Pts',(-29.439027223362,-51.0393920307079,
2.59920246162217));
#220484=CARTESIAN_POINT('Ctrl Pts',(-29.4431140526171,-51.036947563529,
2.59908173791276));
#220485=CARTESIAN_POINT('Ctrl Pts',(-29.4472515437731,-51.0345602039888,
2.59908173515987));
#220486=CARTESIAN_POINT('',(-29.4735998357333,-51.0193480105328,2.59908173515987));
#220487=CARTESIAN_POINT('Origin',(3.68424986610945E-16,1.91048477188617E-13,
2.59908173516023));
#220488=CARTESIAN_POINT('',(-29.8289013456881,-51.031327575341,2.90134173515987));
#220489=CARTESIAN_POINT('Ctrl Pts',(-29.4735998357333,-51.0193480105328,
2.59908173515987));
#220490=CARTESIAN_POINT('Ctrl Pts',(-29.4768987365661,-51.0174422596391,
2.59908174371478));
#220491=CARTESIAN_POINT('Ctrl Pts',(-29.4802121391114,-51.0155824228872,
2.59915764355853));
#220492=CARTESIAN_POINT('Ctrl Pts',(-29.4835378249318,-51.0137685205955,
2.5993076577524));
#220493=CARTESIAN_POINT('Ctrl Pts',(-29.5031724225193,-51.0030593786371,
2.60019333020856));
#220494=CARTESIAN_POINT('Ctrl Pts',(-29.5232366506538,-50.9939485772804,
2.60365973324146));
#220495=CARTESIAN_POINT('Ctrl Pts',(-29.5432683957864,-50.986444092428,
2.60934177082582));
#220496=CARTESIAN_POINT('Ctrl Pts',(-29.550751588937,-50.9836406667018,
2.61146439091966));
#220497=CARTESIAN_POINT('Ctrl Pts',(-29.5582304387683,-50.9810610352781,
2.61389584429368));
#220498=CARTESIAN_POINT('Ctrl Pts',(-29.5656816597954,-50.9787043892801,
2.61661604385215));
#220499=CARTESIAN_POINT('Ctrl Pts',(-29.5714954762337,-50.9768656158505,
2.61873848000738));
#220500=CARTESIAN_POINT('Ctrl Pts',(-29.5772921977452,-50.9751630202462,
2.62103707099751));
#220501=CARTESIAN_POINT('Ctrl Pts',(-29.5830604807844,-50.9735966395564,
2.62350262767616));
#220502=CARTESIAN_POINT('Ctrl Pts',(-29.6032494714215,-50.9681143071419,
2.63213207605142));
#220503=CARTESIAN_POINT('Ctrl Pts',(-29.6230900862363,-50.9643005997167,
2.64280685971877));
#220504=CARTESIAN_POINT('Ctrl Pts',(-29.6420960169782,-50.9621571865007,
2.65513293646047));
#220505=CARTESIAN_POINT('Ctrl Pts',(-29.6515989823491,-50.9610854798926,
2.66129597483132));
#220506=CARTESIAN_POINT('Ctrl Pts',(-29.6608932776205,-50.9604313483967,
2.66787183533815));
#220507=CARTESIAN_POINT('Ctrl Pts',(-29.6699181168558,-50.9601950050771,
2.67481125953824));
#220508=CARTESIAN_POINT('Ctrl Pts',(-29.6789043977152,-50.9599596715277,
2.68172103524042));
#220509=CARTESIAN_POINT('Ctrl Pts',(-29.6876236029352,-50.9601383261074,
2.68899101329751));
#220510=CARTESIAN_POINT('Ctrl Pts',(-29.6960154736012,-50.9607318934964,
2.69657334701236));
#220511=CARTESIAN_POINT('Ctrl Pts',(-29.6960514814791,-50.9607344403781,
2.69660588132534));
#220512=CARTESIAN_POINT('Ctrl Pts',(-29.6960874835157,-50.9607369943869,
2.69663842081342));
#220513=CARTESIAN_POINT('Ctrl Pts',(-29.6961234797097,-50.9607395555212,
2.69667096547343));
#220514=CARTESIAN_POINT('Ctrl Pts',(-29.7130985928885,-50.9619473372423,
2.71201840157905));
#220515=CARTESIAN_POINT('Ctrl Pts',(-29.7287537227772,-50.9647087325284,
2.7284564593932));
#220516=CARTESIAN_POINT('Ctrl Pts',(-29.7430502978486,-50.9688330949321,
2.74568723186873));
#220517=CARTESIAN_POINT('Ctrl Pts',(-29.7578669541906,-50.9731074935248,
2.76354482594296));
#220518=CARTESIAN_POINT('Ctrl Pts',(-29.7712250678598,-50.978846401964,
2.78225519317099));
#220519=CARTESIAN_POINT('Ctrl Pts',(-29.7830467300322,-50.9858763526687,
2.80151223085477));
#220520=CARTESIAN_POINT('Ctrl Pts',(-29.79469967056,-50.9928059702031,2.8204944274019));
#220521=CARTESIAN_POINT('Ctrl Pts',(-29.8048600966487,-51.000990879091,
2.84000929089138));
#220522=CARTESIAN_POINT('Ctrl Pts',(-29.813412601364,-51.0102908031055,
2.85976644341455));
#220523=CARTESIAN_POINT('Ctrl Pts',(-29.8193755598157,-51.0167748755905,
2.87354148166824));
#220524=CARTESIAN_POINT('Ctrl Pts',(-29.8245560588483,-51.0238015157366,
2.88743438345408));
#220525=CARTESIAN_POINT('Ctrl Pts',(-29.8289013456881,-51.031327575341,
2.90134173515987));
#220526=CARTESIAN_POINT('',(-30.0070536838153,-51.3398895692698,3.47153072139036));
#220527=CARTESIAN_POINT('',(-29.8289013456881,-51.031327575341,2.90134173515987));
#220528=CARTESIAN_POINT('',(-34.6963546279281,-48.2946219293748,3.47153072139038));
#220529=CARTESIAN_POINT('Origin',(5.53234440788222E-15,1.85015204418142E-13,
3.47153072139072));
#220530=CARTESIAN_POINT('',(-34.4869303039392,-48.0063682005188,2.90134173515989));
#220531=CARTESIAN_POINT('',(-34.6963546279281,-48.2946219293748,3.47153072139038));
#220532=CARTESIAN_POINT('',(-34.620500570363,-47.6769115920305,2.5990817351599));
#220533=CARTESIAN_POINT('Ctrl Pts',(-34.4869303039392,-48.0063682005188,
2.90134173515989));
#220534=CARTESIAN_POINT('Ctrl Pts',(-34.479741830085,-47.9964738715085,
2.88176998919639));
#220535=CARTESIAN_POINT('Ctrl Pts',(-34.4741406737007,-47.9854941018764,
2.86226752356426));
#220536=CARTESIAN_POINT('Ctrl Pts',(-34.4701636441721,-47.9736072089104,
2.84310370499598));
#220537=CARTESIAN_POINT('Ctrl Pts',(-34.4661147749668,-47.9615055952483,
2.8235937178812));
#220538=CARTESIAN_POINT('Ctrl Pts',(-34.4637486663029,-47.9484630606985,
2.80443322636351));
#220539=CARTESIAN_POINT('Ctrl Pts',(-34.4631421240615,-47.9346304384603,
2.78589323877512));
#220540=CARTESIAN_POINT('Ctrl Pts',(-34.4625612612459,-47.9213834535833,
2.76813818619183));
#220541=CARTESIAN_POINT('Ctrl Pts',(-34.4635939836568,-47.9074110114761,
2.75095095197838));
#220542=CARTESIAN_POINT('Ctrl Pts',(-34.4663468279008,-47.89282374889,2.73457771434193));
#220543=CARTESIAN_POINT('Ctrl Pts',(-34.4685363496869,-47.8812215199222,
2.72155497954972));
#220544=CARTESIAN_POINT('Ctrl Pts',(-34.4718146898373,-47.8692298237637,
2.70904711159655));
#220545=CARTESIAN_POINT('Ctrl Pts',(-34.4762554502653,-47.8568987993929,
2.69718956158302));
#220546=CARTESIAN_POINT('Ctrl Pts',(-34.4762675720988,-47.8568651397018,
2.6971571943232));
#220547=CARTESIAN_POINT('Ctrl Pts',(-34.476279702673,-47.8568314776415,
2.69712483218986));
#220548=CARTESIAN_POINT('Ctrl Pts',(-34.4762918419885,-47.8567978132139,
2.69709247518615));
#220549=CARTESIAN_POINT('Ctrl Pts',(-34.4787083945372,-47.8500962938265,
2.6906512224224));
#220550=CARTESIAN_POINT('Ctrl Pts',(-34.4815044004727,-47.843285399134,
2.68442464469391));
#220551=CARTESIAN_POINT('Ctrl Pts',(-34.4846629347248,-47.8364019332939,
2.67844505923543));
#220552=CARTESIAN_POINT('Ctrl Pts',(-34.4909312646825,-47.8227412186412,
2.66657815779531));
#220553=CARTESIAN_POINT('Ctrl Pts',(-34.4986286886039,-47.8087940876657,
2.65568445664138));
#220554=CARTESIAN_POINT('Ctrl Pts',(-34.5076305235173,-47.7948446809466,
2.64601906229479));
#220555=CARTESIAN_POINT('Ctrl Pts',(-34.5143818997023,-47.7843826259073,
2.63877001653485));
#220556=CARTESIAN_POINT('Ctrl Pts',(-34.5218670065991,-47.7739192901008,
2.63221189387566));
#220557=CARTESIAN_POINT('Ctrl Pts',(-34.5300332501815,-47.763574554582,
2.62645231033198));
#220558=CARTESIAN_POINT('Ctrl Pts',(-34.5330955915248,-47.7596952787624,
2.6242924665031));
#220559=CARTESIAN_POINT('Ctrl Pts',(-34.5362537178261,-47.7558326812644,
2.6222449171171));
#220560=CARTESIAN_POINT('Ctrl Pts',(-34.5395048560461,-47.7519930846016,
2.62031533672562));
#220561=CARTESIAN_POINT('Ctrl Pts',(-34.5508838398161,-47.7385544962821,
2.61356180535543));
#220562=CARTESIAN_POINT('Ctrl Pts',(-34.5634022165999,-47.7253976640913,
2.60825339735312));
#220563=CARTESIAN_POINT('Ctrl Pts',(-34.576941119645,-47.7127937034783,
2.60463337987576));
#220564=CARTESIAN_POINT('Ctrl Pts',(-34.5837105711675,-47.7064917231718,
2.60282337113707));
#220565=CARTESIAN_POINT('Ctrl Pts',(-34.5907351548561,-47.7003279615826,
2.6014354593908));
#220566=CARTESIAN_POINT('Ctrl Pts',(-34.5980000149356,-47.6943363116299,
2.60050005034561));
#220567=CARTESIAN_POINT('Ctrl Pts',(-34.6016324449754,-47.6913404866536,
2.60003234582302));
#220568=CARTESIAN_POINT('Ctrl Pts',(-34.6053249441282,-47.6883876896068,
2.59967776696031));
#220569=CARTESIAN_POINT('Ctrl Pts',(-34.6090756555948,-47.6854821573391,
2.59944011429125));
#220570=CARTESIAN_POINT('Ctrl Pts',(-34.6128263670615,-47.6825766250713,
2.59920246162219));
#220571=CARTESIAN_POINT('Ctrl Pts',(-34.6166352918405,-47.6797183589577,
2.59908173791276));
#220572=CARTESIAN_POINT('Ctrl Pts',(-34.620500570363,-47.6769115920305,
2.5990817351599));
#220573=CARTESIAN_POINT('',(-34.6451144164181,-47.6590285860937,2.59908173515989));
#220574=CARTESIAN_POINT('Origin',(3.62443809638016E-16,1.91052361410359E-13,
2.59908173516024));
#220575=CARTESIAN_POINT('',(-34.9997217530256,-47.6338034047601,2.9013417351599));
#220576=CARTESIAN_POINT('Ctrl Pts',(-34.6451144164181,-47.6590285860937,
2.59908173515989));
#220577=CARTESIAN_POINT('Ctrl Pts',(-34.6481960403147,-47.6567884460682,
2.59908174371476));
#220578=CARTESIAN_POINT('Ctrl Pts',(-34.6512968858166,-47.6545924528204,
2.59915764355856));
#220579=CARTESIAN_POINT('Ctrl Pts',(-34.654414748763,-47.6524408584472,
2.59930765775242));
#220580=CARTESIAN_POINT('Ctrl Pts',(-34.672822375818,-47.6397380079767,
2.60019333020855));
#220581=CARTESIAN_POINT('Ctrl Pts',(-34.6918243519456,-47.62857983361,2.60365973324119));
#220582=CARTESIAN_POINT('Ctrl Pts',(-34.7109619288123,-47.6190225715758,
2.60934177082513));
#220583=CARTESIAN_POINT('Ctrl Pts',(-34.7181110904657,-47.6154522966282,
2.61146439091915));
#220584=CARTESIAN_POINT('Ctrl Pts',(-34.7252793254674,-47.6121050440151,
2.61389584429341));
#220585=CARTESIAN_POINT('Ctrl Pts',(-34.7324433913422,-47.6089824432867,
2.61661604385218));
#220586=CARTESIAN_POINT('Ctrl Pts',(-34.7380331549248,-47.6065460335523,
2.61873848000741));
#220587=CARTESIAN_POINT('Ctrl Pts',(-34.7436201516873,-47.6042468425533,
2.62103707099753));
#220588=CARTESIAN_POINT('Ctrl Pts',(-34.7491931041021,-47.602086092899,
2.62350262767618));
#220589=CARTESIAN_POINT('Ctrl Pts',(-34.7686984375536,-47.5945234691089,
2.63213207605145));
#220590=CARTESIAN_POINT('Ctrl Pts',(-34.788031722428,-47.5886567445951,
2.64280685971879));
#220591=CARTESIAN_POINT('Ctrl Pts',(-34.8067094890031,-47.5845384124875,
2.65513293646049));
#220592=CARTESIAN_POINT('Ctrl Pts',(-34.8160483722906,-47.5824792464337,
2.66129597483134));
#220593=CARTESIAN_POINT('Ctrl Pts',(-34.8252233770799,-47.5808571799367,
2.66787183533817));
#220594=CARTESIAN_POINT('Ctrl Pts',(-34.8341740726976,-47.579678778754,
2.67481125953826));
#220595=CARTESIAN_POINT('Ctrl Pts',(-34.8430865267159,-47.5785054122577,
2.68172103524045));
#220596=CARTESIAN_POINT('Ctrl Pts',(-34.8517766417061,-47.5777716830264,
2.68899101329754));
#220597=CARTESIAN_POINT('Ctrl Pts',(-34.8601845855135,-47.5774848094464,
2.6965733470124));
#220598=CARTESIAN_POINT('Ctrl Pts',(-34.8602206623581,-47.577483578528,
2.69660588132537));
#220599=CARTESIAN_POINT('Ctrl Pts',(-34.8602567341385,-47.577482355308,
2.69663842081345));
#220600=CARTESIAN_POINT('Ctrl Pts',(-34.8602928008529,-47.5774811397854,
2.69667096547346));
#220601=CARTESIAN_POINT('Ctrl Pts',(-34.8773011701517,-47.5769079226575,
2.71201840157799));
#220602=CARTESIAN_POINT('Ctrl Pts',(-34.8931591840055,-47.5780177840616,
2.72845645939089));
#220603=CARTESIAN_POINT('Ctrl Pts',(-34.9078085542059,-47.580625153754,
2.74568723186509));
#220604=CARTESIAN_POINT('Ctrl Pts',(-34.9229908396696,-47.5833273744254,
2.76354482593811));
#220605=CARTESIAN_POINT('Ctrl Pts',(-34.9368756554737,-47.5876385414291,
2.78225519316485));
#220606=CARTESIAN_POINT('Ctrl Pts',(-34.9493673872874,-47.5933942811475,
2.80151223084732));
#220607=CARTESIAN_POINT('Ctrl Pts',(-34.9616808340595,-47.5990678735455,
2.82049442739359));
#220608=CARTESIAN_POINT('Ctrl Pts',(-34.972641156219,-47.6061458909203,
2.84000929088222));
#220609=CARTESIAN_POINT('Ctrl Pts',(-34.9821189161847,-47.6145008888021,
2.85976644340457));
#220610=CARTESIAN_POINT('Ctrl Pts',(-34.9887269790606,-47.6203261419772,
2.87354148166155));
#220611=CARTESIAN_POINT('Ctrl Pts',(-34.9946135826755,-47.6267727798519,
2.88743438345074));
#220612=CARTESIAN_POINT('Ctrl Pts',(-34.9997217530256,-47.6338034047601,
2.90134173515989));
#220613=CARTESIAN_POINT('',(-35.2091516650524,-47.9220530736688,3.47153072139038));
#220614=CARTESIAN_POINT('',(-34.9997217530256,-47.6338034047601,2.9013417351599));
#220615=CARTESIAN_POINT('',(-39.5544469813067,-44.4033023070491,3.47153072139041));
#220616=CARTESIAN_POINT('Origin',(5.53234440788222E-15,1.85015204418142E-13,
3.47153072139072));
#220617=CARTESIAN_POINT('',(-39.3160391863686,-44.1385184650377,2.90134173515991));
#220618=CARTESIAN_POINT('',(-39.5544469813067,-44.4033023070491,3.47153072139041));
#220619=CARTESIAN_POINT('',(-39.4144401478986,-43.7969047596348,2.59908173515993));
#220620=CARTESIAN_POINT('Ctrl Pts',(-39.3160391863686,-44.1385184650377,
2.90134173515992));
#220621=CARTESIAN_POINT('Ctrl Pts',(-39.3078558527196,-44.1294297383224,
2.88176998919639));
#220622=CARTESIAN_POINT('Ctrl Pts',(-39.3011376816092,-44.1190955972866,
2.86226752356423));
#220623=CARTESIAN_POINT('Ctrl Pts',(-39.2959399200097,-44.107689534749,
2.84310370499592));
#220624=CARTESIAN_POINT('Ctrl Pts',(-39.2906482678543,-44.0960774370687,
2.82359371788089));
#220625=CARTESIAN_POINT('Ctrl Pts',(-39.2869318048876,-44.0833536765902,
2.80443322636297));
#220626=CARTESIAN_POINT('Ctrl Pts',(-39.2848826826026,-44.0696602318321,
2.78589323877437));
#220627=CARTESIAN_POINT('Ctrl Pts',(-39.2829203148422,-44.0565465320211,
2.76813818619038));
#220628=CARTESIAN_POINT('Ctrl Pts',(-39.2824868619903,-44.0425426835265,
2.75095095197631));
#220629=CARTESIAN_POINT('Ctrl Pts',(-39.2836998417244,-44.027747580912,
2.73457771433931));
#220630=CARTESIAN_POINT('Ctrl Pts',(-39.2846646059167,-44.0159800428215,
2.72155497954806));
#220631=CARTESIAN_POINT('Ctrl Pts',(-39.2866715134052,-44.0037113585721,
2.70904711159579));
#220632=CARTESIAN_POINT('Ctrl Pts',(-39.2897990038549,-43.9909836989805,
2.69718956158308));
#220633=CARTESIAN_POINT('Ctrl Pts',(-39.2898075408879,-43.9909489566042,
2.69715719432325));
#220634=CARTESIAN_POINT('Ctrl Pts',(-39.2898160863661,-43.9909142109579,
2.6971248321899));
#220635=CARTESIAN_POINT('Ctrl Pts',(-39.2898246402903,-43.9908794620435,
2.69709247518618));
#220636=CARTESIAN_POINT('Ctrl Pts',(-39.2915274551881,-43.9839620557563,
2.69065122242244));
#220637=CARTESIAN_POINT('Ctrl Pts',(-39.2935962119549,-43.9768962096537,
2.68442464469393));
#220638=CARTESIAN_POINT('Ctrl Pts',(-39.2960179253196,-43.9697202954282,
2.67844505923546));
#220639=CARTESIAN_POINT('Ctrl Pts',(-39.3008239832001,-43.9554791967019,
2.66657815779534));
#220640=CARTESIAN_POINT('Ctrl Pts',(-39.30702136766,-43.9408038696756,2.65568445664141));
#220641=CARTESIAN_POINT('Ctrl Pts',(-39.314515779532,-43.925989931296,2.64601906229483));
#220642=CARTESIAN_POINT('Ctrl Pts',(-39.320136588436,-43.9148794775113,
2.63877001653489));
#220643=CARTESIAN_POINT('Ctrl Pts',(-39.3264869747216,-43.9036910542319,
2.63221189387569));
#220644=CARTESIAN_POINT('Ctrl Pts',(-39.3335271634604,-43.8925493833643,
2.62645231033201));
#220645=CARTESIAN_POINT('Ctrl Pts',(-39.3361672342375,-43.888371256789,
2.62429246650313));
#220646=CARTESIAN_POINT('Ctrl Pts',(-39.3389043086117,-43.884199704915,
2.62224491711713));
#220647=CARTESIAN_POINT('Ctrl Pts',(-39.3417362896177,-43.8800413054826,
2.62031533672564));
#220648=CARTESIAN_POINT('Ctrl Pts',(-39.3516482231385,-43.8654869074689,
2.61356180535546));
#220649=CARTESIAN_POINT('Ctrl Pts',(-39.3627227594941,-43.8510936230937,
2.60825339735315));
#220650=CARTESIAN_POINT('Ctrl Pts',(-39.3748700223777,-43.837143507566,
2.60463337987578));
#220651=CARTESIAN_POINT('Ctrl Pts',(-39.3809436538195,-43.8301684498022,
2.6028233711371));
#220652=CARTESIAN_POINT('Ctrl Pts',(-39.3872854675768,-43.8233041850058,
2.60143545939083));
#220653=CARTESIAN_POINT('Ctrl Pts',(-39.3938842320307,-43.8165859732786,
2.60050005034564));
#220654=CARTESIAN_POINT('Ctrl Pts',(-39.3971836142576,-43.8132268674149,
2.60003234582305));
#220655=CARTESIAN_POINT('Ctrl Pts',(-39.400547234176,-43.8099042748373,
2.59967776696034));
#220656=CARTESIAN_POINT('Ctrl Pts',(-39.4039736880299,-43.8066226032736,
2.59944011429128));
#220657=CARTESIAN_POINT('Ctrl Pts',(-39.4074001418838,-43.8033409317098,
2.59920246162222));
#220658=CARTESIAN_POINT('Ctrl Pts',(-39.4108894308099,-43.8001001824231,
2.59908173791277));
#220659=CARTESIAN_POINT('Ctrl Pts',(-39.4144401478986,-43.7969047596348,
2.59908173515992));
#220660=CARTESIAN_POINT('',(-39.4370498736004,-43.7765468711724,2.59908173515992));
#220661=CARTESIAN_POINT('Origin',(3.56901409908096E-16,1.91056849557166E-13,
2.59908173516024));
#220662=CARTESIAN_POINT('',(-39.7870778846743,-43.7143933160625,2.90134173515992));
#220663=CARTESIAN_POINT('Ctrl Pts',(-39.4370498736004,-43.7765468711724,
2.59908173515992));
#220664=CARTESIAN_POINT('Ctrl Pts',(-39.4398804576444,-43.7739968854581,
2.59908174371479));
#220665=CARTESIAN_POINT('Ctrl Pts',(-39.4427347725907,-43.7714887954759,
2.59915764355859));
#220666=CARTESIAN_POINT('Ctrl Pts',(-39.4456106527043,-43.7690230823394,
2.59930765775246));
#220667=CARTESIAN_POINT('Ctrl Pts',(-39.462589631414,-43.7544656984439,
2.60019333020861));
#220668=CARTESIAN_POINT('Ctrl Pts',(-39.4803211659094,-43.7413824023598,
2.60365973324145));
#220669=CARTESIAN_POINT('Ctrl Pts',(-39.4983548992148,-43.7298770745062,
2.60934177082573));
#220670=CARTESIAN_POINT('Ctrl Pts',(-39.5050917016582,-43.7255790670175,
2.61146439091961));
#220671=CARTESIAN_POINT('Ctrl Pts',(-39.5118707851462,-43.7215008664158,
2.61389584429367));
#220672=CARTESIAN_POINT('Ctrl Pts',(-39.5186692048624,-43.7176465228245,
2.6166160438522));
#220673=CARTESIAN_POINT('Ctrl Pts',(-39.5239736729698,-43.7146391706003,
2.61873848000744));
#220674=CARTESIAN_POINT('Ctrl Pts',(-39.5292897326776,-43.7117685746243,
2.62103707099755));
#220675=CARTESIAN_POINT('Ctrl Pts',(-39.534606296035,-43.7090371296309,
2.62350262767619));
#220676=CARTESIAN_POINT('Ctrl Pts',(-39.553214267786,-43.6994770721539,
2.63213207605146));
#220677=CARTESIAN_POINT('Ctrl Pts',(-39.5718284032052,-43.6916216076131,
2.64280685971882));
#220678=CARTESIAN_POINT('Ctrl Pts',(-39.5899733680942,-43.6855734779223,
2.65513293646052));
#220679=CARTESIAN_POINT('Ctrl Pts',(-39.5990458505387,-43.682549413077,
2.66129597483137));
#220680=CARTESIAN_POINT('Ctrl Pts',(-39.6080010415735,-43.6799771832788,
2.6678718353382));
#220681=CARTESIAN_POINT('Ctrl Pts',(-39.6167795278794,-43.677869635043,
2.67481125953829));
#220682=CARTESIAN_POINT('Ctrl Pts',(-39.6255205083453,-43.6757710912487,
2.68172103524048));
#220683=CARTESIAN_POINT('Ctrl Pts',(-39.6340863223874,-43.6741330170973,
2.68899101329756));
#220684=CARTESIAN_POINT('Ctrl Pts',(-39.6424182201444,-43.6729688455954,
2.69657334701241));
#220685=CARTESIAN_POINT('Ctrl Pts',(-39.6424539706902,-43.6729638503629,
2.69660588132539));
#220686=CARTESIAN_POINT('Ctrl Pts',(-39.6424897170043,-43.6729588633161,
2.69663842081348));
#220687=CARTESIAN_POINT('Ctrl Pts',(-39.6425254590848,-43.672953884454,
2.69667096547348));
#220688=CARTESIAN_POINT('Ctrl Pts',(-39.6593807372517,-43.670605948764,
2.71201840157821));
#220689=CARTESIAN_POINT('Ctrl Pts',(-39.6752678913536,-43.6700521164126,
2.72845645939134));
#220690=CARTESIAN_POINT('Ctrl Pts',(-39.6901095551185,-43.6711139265061,
2.74568723186578));
#220691=CARTESIAN_POINT('Ctrl Pts',(-39.7054911294082,-43.6722143631616,
2.76354482593897));
#220692=CARTESIAN_POINT('Ctrl Pts',(-39.7197505224005,-43.6750505546826,
2.78225519316589));
#220693=CARTESIAN_POINT('Ctrl Pts',(-39.7327754618281,-43.6794690223266,
2.80151223084853));
#220694=CARTESIAN_POINT('Ctrl Pts',(-39.7456145061449,-43.6838244285232,
2.82049442739476));
#220695=CARTESIAN_POINT('Ctrl Pts',(-39.7572546407919,-43.689718006146,
2.84000929088333));
#220696=CARTESIAN_POINT('Ctrl Pts',(-39.7675538156858,-43.697036538791,
2.85976644340562));
#220697=CARTESIAN_POINT('Ctrl Pts',(-39.7747345836642,-43.7021391499619,
2.87354148166226));
#220698=CARTESIAN_POINT('Ctrl Pts',(-39.7812627969987,-43.7079351548501,
2.88743438345111));
#220699=CARTESIAN_POINT('Ctrl Pts',(-39.7870778846743,-43.7143933160625,
2.90134173515992));
#220700=CARTESIAN_POINT('',(-40.0254908126584,-43.9791725362584,3.47153072139041));
#220701=CARTESIAN_POINT('',(-39.7870778846743,-43.7143933160625,2.90134173515992));
#220702=CARTESIAN_POINT('',(-43.9791725362579,-40.025490812659,3.47153072139043));
#220703=CARTESIAN_POINT('Origin',(5.53234440788222E-15,1.85015204418142E-13,
3.47153072139072));
#220704=CARTESIAN_POINT('',(-43.714393316062,-39.7870778846749,2.90134173515995));
#220705=CARTESIAN_POINT('',(-43.9791725362579,-40.025490812659,3.47153072139043));
#220706=CARTESIAN_POINT('',(-43.7765468711719,-39.437049873601,2.59908173515996));
#220707=CARTESIAN_POINT('Ctrl Pts',(-43.714393316062,-39.7870778846749,
2.90134173515995));
#220708=CARTESIAN_POINT('Ctrl Pts',(-43.7053047809348,-39.7788943382464,
2.88176998919728));
#220709=CARTESIAN_POINT('Ctrl Pts',(-43.6975432007875,-39.769319048819,
2.86226752356597));
#220710=CARTESIAN_POINT('Ctrl Pts',(-43.691181654881,-39.7585187839184,
2.84310370499846));
#220711=CARTESIAN_POINT('Ctrl Pts',(-43.6847051962242,-39.7475234267928,
2.82359371788444));
#220712=CARTESIAN_POINT('Ctrl Pts',(-43.6796790973008,-39.735257844569,
2.80443322636747));
#220713=CARTESIAN_POINT('Ctrl Pts',(-43.6762098455845,-39.7218536055386,
2.78589323877973));
#220714=CARTESIAN_POINT('Ctrl Pts',(-43.672887472991,-39.7090168672348,
2.76813818619693));
#220715=CARTESIAN_POINT('Ctrl Pts',(-43.6709925938758,-39.6951350414494,
2.75095095198392));
#220716=CARTESIAN_POINT('Ctrl Pts',(-43.6706524194392,-39.6802941970489,
2.73457771434783));
#220717=CARTESIAN_POINT('Ctrl Pts',(-43.6703818558787,-39.6684902774427,
2.72155497955352));
#220718=CARTESIAN_POINT('Ctrl Pts',(-43.6710953426071,-39.656079023371,
2.70904711159839));
#220719=CARTESIAN_POINT('Ctrl Pts',(-43.6728752976391,-39.643094175457,
2.6971895615831));
#220720=CARTESIAN_POINT('Ctrl Pts',(-43.6728801563381,-39.6430587310401,
2.69715719432327));
#220721=CARTESIAN_POINT('Ctrl Pts',(-43.6728850230943,-39.6430232824884,
2.69712483218993));
#220722=CARTESIAN_POINT('Ctrl Pts',(-43.6728898979086,-39.6429878298036,
2.69709247518621));
#220723=CARTESIAN_POINT('Ctrl Pts',(-43.6738603187593,-39.6359303251673,
2.69065122242247));
#220724=CARTESIAN_POINT('Ctrl Pts',(-43.6751791606252,-39.6286869425433,
2.68442464469396));
#220725=CARTESIAN_POINT('Ctrl Pts',(-43.6768375203041,-39.6212972007503,
2.67844505923549));
#220726=CARTESIAN_POINT('Ctrl Pts',(-43.6801286499316,-39.6066317464083,
2.66657815779537));
#220727=CARTESIAN_POINT('Ctrl Pts',(-43.684758095089,-39.591389009285,2.65568445664145));
#220728=CARTESIAN_POINT('Ctrl Pts',(-43.6906629735749,-39.5758728438538,
2.64601906229486));
#220729=CARTESIAN_POINT('Ctrl Pts',(-43.6950916324393,-39.5642357197804,
2.63877001653492));
#220730=CARTESIAN_POINT('Ctrl Pts',(-43.7002377219525,-39.5524447917348,
2.63221189387572));
#220731=CARTESIAN_POINT('Ctrl Pts',(-43.7060747220668,-39.540628255996,
2.62645231033204));
#220732=CARTESIAN_POINT('Ctrl Pts',(-43.7082635971097,-39.5361970550939,
2.62429246650316));
#220733=CARTESIAN_POINT('Ctrl Pts',(-43.7105496315973,-39.5317622532394,
2.62224491711717));
#220734=CARTESIAN_POINT('Ctrl Pts',(-43.7129314276126,-39.5273306113316,
2.62031533672568));
#220735=CARTESIAN_POINT('Ctrl Pts',(-43.7212677136663,-39.5118198646542,
2.6135618053555));
#220736=CARTESIAN_POINT('Ctrl Pts',(-43.7307770746559,-39.4963478239301,
2.60825339735318));
#220737=CARTESIAN_POINT('Ctrl Pts',(-43.741399609424,-39.4812043938728,
2.60463337987581));
#220738=CARTESIAN_POINT('Ctrl Pts',(-43.746710876808,-39.4736326788442,
2.60282337113713));
#220739=CARTESIAN_POINT('Ctrl Pts',(-43.7523004383953,-39.4661431171622,
2.60143545939086));
#220740=CARTESIAN_POINT('Ctrl Pts',(-43.7581608097794,-39.4587719497939,
2.60050005034567));
#220741=CARTESIAN_POINT('Ctrl Pts',(-43.7610909954714,-39.4550863661097,
2.60003234582308));
#220742=CARTESIAN_POINT('Ctrl Pts',(-43.7640888836317,-39.4514303810208,
2.59967776696037));
#220743=CARTESIAN_POINT('Ctrl Pts',(-43.7671535389273,-39.4478085248414,
2.59944011429131));
#220744=CARTESIAN_POINT('Ctrl Pts',(-43.770218194223,-39.444186668662,2.59920246162225));
#220745=CARTESIAN_POINT('Ctrl Pts',(-43.7733496179165,-39.4405989425297,
2.59908173791279));
#220746=CARTESIAN_POINT('Ctrl Pts',(-43.7765468711719,-39.437049873601,
2.59908173515996));
#220747=CARTESIAN_POINT('',(-43.7969047596343,-39.4144401478991,2.59908173515995));
#220748=CARTESIAN_POINT('Origin',(3.51858511112452E-16,1.91061892455961E-13,
2.59908173516024));
#220749=CARTESIAN_POINT('',(-44.1385184650372,-39.3160391863692,2.90134173515995));
#220750=CARTESIAN_POINT('Ctrl Pts',(-43.7969047596343,-39.4144401478991,
2.59908173515995));
#220751=CARTESIAN_POINT('Ctrl Pts',(-43.7994532913547,-39.4116082546731,
2.59908174371483));
#220752=CARTESIAN_POINT('Ctrl Pts',(-43.8020298032735,-39.4088155471153,
2.59915764355862));
#220753=CARTESIAN_POINT('Ctrl Pts',(-43.8046321918099,-39.4060627300844,
2.59930765775248));
#220754=CARTESIAN_POINT('Ctrl Pts',(-43.8199964969259,-39.3898103065129,
2.60019333020841));
#220755=CARTESIAN_POINT('Ctrl Pts',(-43.8362633193816,-39.3749452320449,
2.60365973323973));
#220756=CARTESIAN_POINT('Ctrl Pts',(-43.8529956277646,-39.3616178931544,
2.60934177082144));
#220757=CARTESIAN_POINT('Ctrl Pts',(-43.8592462611857,-39.35663924299,2.61146439091634));
#220758=CARTESIAN_POINT('Ctrl Pts',(-43.8655619201074,-39.3518747760151,
2.61389584429187));
#220759=CARTESIAN_POINT('Ctrl Pts',(-43.8719202087609,-39.3473309185526,
2.61661604385226));
#220760=CARTESIAN_POINT('Ctrl Pts',(-43.8768812645306,-39.3437855730188,
2.61873848000749));
#220761=CARTESIAN_POINT('Ctrl Pts',(-43.881868143321,-39.340375022916,2.6210370709976));
#220762=CARTESIAN_POINT('Ctrl Pts',(-43.8868700682404,-39.3371028088665,
2.62350262767625));
#220763=CARTESIAN_POINT('Ctrl Pts',(-43.9043768054583,-39.325650059693,
2.63213207605151));
#220764=CARTESIAN_POINT('Ctrl Pts',(-43.9220678510593,-39.3158919212385,
2.64280685971886));
#220765=CARTESIAN_POINT('Ctrl Pts',(-43.9394812142299,-39.3079802585391,
2.65513293646056));
#220766=CARTESIAN_POINT('Ctrl Pts',(-43.9481878958152,-39.3040244271894,
2.6612959748314));
#220767=CARTESIAN_POINT('Ctrl Pts',(-43.9568251581486,-39.3005302159781,
2.66787183533823));
#220768=CARTESIAN_POINT('Ctrl Pts',(-43.9653352562096,-39.2975166114286,
2.67481125953832));
#220769=CARTESIAN_POINT('Ctrl Pts',(-43.973808995112,-39.2945158824213,
2.6817210352405));
#220770=CARTESIAN_POINT('Ctrl Pts',(-43.9821566593547,-39.291991410433,
2.6889910132976));
#220771=CARTESIAN_POINT('Ctrl Pts',(-43.990321225046,-39.2899626959158,
2.69657334701245));
#220772=CARTESIAN_POINT('Ctrl Pts',(-43.9903562576026,-39.2899539910981,
2.69660588132543));
#220773=CARTESIAN_POINT('Ctrl Pts',(-43.9903912868063,-39.2899452948636,
2.69663842081351));
#220774=CARTESIAN_POINT('Ctrl Pts',(-43.9904263126551,-39.2899366072114,
2.69667096547352));
#220775=CARTESIAN_POINT('Ctrl Pts',(-44.0069438297366,-39.2858396774337,
2.71201840157964));
#220776=CARTESIAN_POINT('Ctrl Pts',(-44.0226860611028,-39.2836282192298,
2.72845645939433));
#220777=CARTESIAN_POINT('Ctrl Pts',(-44.0375574100593,-39.2831328363111,
2.74568723187047));
#220778=CARTESIAN_POINT('Ctrl Pts',(-44.0529697494292,-39.2826194323365,
2.76354482594518));
#220779=CARTESIAN_POINT('Ctrl Pts',(-44.0674474907168,-39.2839495744676,
2.78225519317373));
#220780=CARTESIAN_POINT('Ctrl Pts',(-44.080862933797,-39.2869823603817,
2.80151223085806));
#220781=CARTESIAN_POINT('Ctrl Pts',(-44.0940869084027,-39.2899718616359,
2.82049442740554));
#220782=CARTESIAN_POINT('Ctrl Pts',(-44.1062793237865,-39.2946164282379,
2.84000929089538));
#220783=CARTESIAN_POINT('Ctrl Pts',(-44.1172870736935,-39.3008183122717,
2.8597664434189));
#220784=CARTESIAN_POINT('Ctrl Pts',(-44.1249618727751,-39.3051423761621,
2.87354148167119));
#220785=CARTESIAN_POINT('Ctrl Pts',(-44.1320601713554,-39.3102242458199,
2.8874343834556));
#220786=CARTESIAN_POINT('Ctrl Pts',(-44.1385184650372,-39.3160391863692,
2.90134173515995));
#220787=CARTESIAN_POINT('',(-44.4033023070486,-39.5544469813073,3.47153072139044));
#220788=CARTESIAN_POINT('',(-44.1385184650372,-39.3160391863692,2.90134173515995));
#220789=CARTESIAN_POINT('',(-47.9220530736684,-35.209151665053,3.47153072139047));
#220790=CARTESIAN_POINT('Origin',(5.53234440788222E-15,1.85015204418142E-13,
3.47153072139072));
#220791=CARTESIAN_POINT('',(-47.6338034047597,-34.9997217530262,2.90134173515998));
#220792=CARTESIAN_POINT('',(-47.9220530736684,-35.209151665053,3.47153072139047));
#220793=CARTESIAN_POINT('',(-47.6590285860933,-34.6451144164188,2.59908173515998));
#220794=CARTESIAN_POINT('Ctrl Pts',(-47.6338034047597,-34.9997217530262,
2.90134173515998));
#220795=CARTESIAN_POINT('Ctrl Pts',(-47.6239092440466,-34.9925330475314,
2.8817699891971));
#220796=CARTESIAN_POINT('Ctrl Pts',(-47.6151892923582,-34.9838215185865,
2.86226752356558));
#220797=CARTESIAN_POINT('Ctrl Pts',(-47.6077336605729,-34.9737453812845,
2.84310370499787));
#220798=CARTESIAN_POINT('Ctrl Pts',(-47.6001433528508,-34.9634872321464,
2.82359371788377));
#220799=CARTESIAN_POINT('Ctrl Pts',(-47.5938626849622,-34.9518142124621,
2.80443322636672));
#220800=CARTESIAN_POINT('Ctrl Pts',(-47.5890113136627,-34.938846038806,
2.78589323877891));
#220801=CARTESIAN_POINT('Ctrl Pts',(-47.5843653368456,-34.9264269039996,
2.76813818619628));
#220802=CARTESIAN_POINT('Ctrl Pts',(-47.5810297921599,-34.9128191931104,
2.75095095198344));
#220803=CARTESIAN_POINT('Ctrl Pts',(-47.5791401905757,-34.8980952063196,
2.73457771434749));
#220804=CARTESIAN_POINT('Ctrl Pts',(-47.5776372636137,-34.8863842314133,
2.72155497955331));
#220805=CARTESIAN_POINT('Ctrl Pts',(-47.5770495124718,-34.8739663878189,
2.70904711159831));
#220806=CARTESIAN_POINT('Ctrl Pts',(-47.5774624305257,-34.8608666162964,
2.69718956158313));
#220807=CARTESIAN_POINT('Ctrl Pts',(-47.5774635576578,-34.8608308581753,
2.6971571943233));
#220808=CARTESIAN_POINT('Ctrl Pts',(-47.5774646923707,-34.8607950951,2.69712483218996));
#220809=CARTESIAN_POINT('Ctrl Pts',(-47.5774658346656,-34.8607593270719,
2.69709247518623));
#220810=CARTESIAN_POINT('Ctrl Pts',(-47.5776932293352,-34.8536390475841,
2.69065122242249));
#220811=CARTESIAN_POINT('Ctrl Pts',(-47.5782477067929,-34.8462974884545,
2.684424644694));
#220812=CARTESIAN_POINT('Ctrl Pts',(-47.5791245434504,-34.8387748826514,
2.67844505923552));
#220813=CARTESIAN_POINT('Ctrl Pts',(-47.58086468652,-34.8238457504804,2.66657815779541));
#220814=CARTESIAN_POINT('Ctrl Pts',(-47.5838754712049,-34.8082026058779,
2.65568445664148));
#220815=CARTESIAN_POINT('Ctrl Pts',(-47.5881261212203,-34.7921542117505,
2.64601906229489));
#220816=CARTESIAN_POINT('Ctrl Pts',(-47.5913141087318,-34.780117916155,
2.63877001653495));
#220817=CARTESIAN_POINT('Ctrl Pts',(-47.5951995198391,-34.7678536672182,
2.63221189387577));
#220818=CARTESIAN_POINT('Ctrl Pts',(-47.5997693799341,-34.7554917310465,
2.62645231033209));
#220819=CARTESIAN_POINT('Ctrl Pts',(-47.6014830774698,-34.7508560049821,
2.62429246650321));
#220820=CARTESIAN_POINT('Ctrl Pts',(-47.6032930257985,-34.7462065417643,
2.62224491711719));
#220821=CARTESIAN_POINT('Ctrl Pts',(-47.6051985413677,-34.7415502113772,
2.62031533672571));
#220822=CARTESIAN_POINT('Ctrl Pts',(-47.6118678458598,-34.7252530550225,
2.61356180535552));
#220823=CARTESIAN_POINT('Ctrl Pts',(-47.6197078449344,-34.7088717728654,
2.60825339735324));
#220824=CARTESIAN_POINT('Ctrl Pts',(-47.6286892688731,-34.6927009428671,
2.60463337987587));
#220825=CARTESIAN_POINT('Ctrl Pts',(-47.6331799808424,-34.684615527868,
2.60282337113719));
#220826=CARTESIAN_POINT('Ctrl Pts',(-47.6379560498533,-34.6765827265055,
2.6014354593909));
#220827=CARTESIAN_POINT('Ctrl Pts',(-47.6430138207122,-34.6686393635484,
2.60050005034571));
#220828=CARTESIAN_POINT('Ctrl Pts',(-47.6455427061417,-34.6646676820698,
2.60003234582312));
#220829=CARTESIAN_POINT('Ctrl Pts',(-47.6481420170539,-34.6607183602072,
2.5996777669604));
#220830=CARTESIAN_POINT('Ctrl Pts',(-47.6508112967866,-34.6567960012265,
2.59944011429134));
#220831=CARTESIAN_POINT('Ctrl Pts',(-47.6534805765192,-34.6528736422457,
2.59920246162228));
#220832=CARTESIAN_POINT('Ctrl Pts',(-47.6562198264469,-34.648978247146,
2.59908173791283));
#220833=CARTESIAN_POINT('Ctrl Pts',(-47.6590285860933,-34.6451144164188,
2.59908173515999));
#220834=CARTESIAN_POINT('',(-47.6769115920301,-34.6205005703637,2.59908173515998));
#220835=CARTESIAN_POINT('Origin',(3.4737036430558E-16,1.91067434855691E-13,
2.59908173516024));
#220836=CARTESIAN_POINT('',(-48.0063682005184,-34.4869303039399,2.90134173515999));
#220837=CARTESIAN_POINT('Ctrl Pts',(-47.6769115920301,-34.6205005703637,
2.59908173515998));
#220838=CARTESIAN_POINT('Ctrl Pts',(-47.67915014918,-34.6174177964407,2.59908174371487));
#220839=CARTESIAN_POINT('Ctrl Pts',(-47.6814206292676,-34.6143710687956,
2.59915764355865));
#220840=CARTESIAN_POINT('Ctrl Pts',(-47.6837210139133,-34.61136130831,2.59930765775252));
#220841=CARTESIAN_POINT('Ctrl Pts',(-47.6973023109009,-34.5935919100086,
2.60019333020864));
#220842=CARTESIAN_POINT('Ctrl Pts',(-47.7119261986139,-34.5771079220171,
2.60365973324122));
#220843=CARTESIAN_POINT('Ctrl Pts',(-47.7271737594107,-34.5621045891988,
2.60934177082506));
#220844=CARTESIAN_POINT('Ctrl Pts',(-47.7328697405539,-34.5564998434983,
2.61146439091911));
#220845=CARTESIAN_POINT('Ctrl Pts',(-47.7386527792209,-34.5511013106536,
2.61389584429342));
#220846=CARTESIAN_POINT('Ctrl Pts',(-47.7445012740627,-34.5459177227787,
2.61661604385227));
#220847=CARTESIAN_POINT('Ctrl Pts',(-47.7490645631293,-34.5418732274829,
2.6187384800075));
#220848=CARTESIAN_POINT('Ctrl Pts',(-47.7536676237148,-34.537960089954,
2.62103707099762));
#220849=CARTESIAN_POINT('Ctrl Pts',(-47.7583001080601,-34.5341829579102,
2.62350262767627));
#220850=CARTESIAN_POINT('Ctrl Pts',(-47.7745138032685,-34.5209629957568,
2.63213207605153));
#220851=CARTESIAN_POINT('Ctrl Pts',(-47.7910879322537,-34.5094090955954,
2.64280685971889));
#220852=CARTESIAN_POINT('Ctrl Pts',(-47.8075789092549,-34.4997205817196,
2.65513293646059));
#220853=CARTESIAN_POINT('Ctrl Pts',(-47.8158243977556,-34.4948763247816,
2.66129597483143));
#220854=CARTESIAN_POINT('Ctrl Pts',(-47.8240490997339,-34.4904984154664,
2.66787183533825));
#220855=CARTESIAN_POINT('Ctrl Pts',(-47.8321975711348,-34.4866117722854,
2.67481125953835));
#220856=CARTESIAN_POINT('Ctrl Pts',(-47.8403112284171,-34.4827417346799,
2.68172103524053));
#220857=CARTESIAN_POINT('Ctrl Pts',(-47.8483492841042,-34.4793585234982,
2.68899101329763));
#220858=CARTESIAN_POINT('Ctrl Pts',(-47.8562570650394,-34.4764874929864,
2.69657334701249));
#220859=CARTESIAN_POINT('Ctrl Pts',(-47.8562909957829,-34.4764751739553,
2.69660588132546));
#220860=CARTESIAN_POINT('Ctrl Pts',(-47.8563249240889,-34.4764628638109,
2.69663842081354));
#220861=CARTESIAN_POINT('Ctrl Pts',(-47.8563588499555,-34.4764505625524,
2.69667096547355));
#220862=CARTESIAN_POINT('Ctrl Pts',(-47.872357636575,-34.4706495255077,
2.71201840157839));
#220863=CARTESIAN_POINT('Ctrl Pts',(-47.8877824700218,-34.4668046706503,
2.72845645939164));
#220864=CARTESIAN_POINT('Ctrl Pts',(-47.9025205705563,-34.4647575222378,
2.74568723186622));
#220865=CARTESIAN_POINT('Ctrl Pts',(-47.917794814189,-34.4626359025941,
2.76354482593952));
#220866=CARTESIAN_POINT('Ctrl Pts',(-47.932332282607,-34.4624454220187,
2.78225519316656));
#220867=CARTESIAN_POINT('Ctrl Pts',(-47.9459912469366,-34.4640592983644,
2.80151223084933));
#220868=CARTESIAN_POINT('Ctrl Pts',(-47.9594552671974,-34.4656501410735,
2.82049442739569));
#220869=CARTESIAN_POINT('Ctrl Pts',(-47.9720663806631,-34.4689948098093,
2.8400092908844));
#220870=CARTESIAN_POINT('Ctrl Pts',(-47.9836621023717,-34.4740120960907,
2.85976644340683));
#220871=CARTESIAN_POINT('Ctrl Pts',(-47.9917468458571,-34.4775102373532,
2.87354148166309));
#220872=CARTESIAN_POINT('Ctrl Pts',(-47.9993374592434,-34.4818222937559,
2.88743438345156));
#220873=CARTESIAN_POINT('Ctrl Pts',(-48.0063682005184,-34.4869303039399,
2.90134173515999));
#220874=CARTESIAN_POINT('',(-48.2946219293743,-34.6963546279287,3.47153072139047));
#220875=CARTESIAN_POINT('',(-48.0063682005184,-34.4869303039399,2.90134173515999));
#220876=CARTESIAN_POINT('',(-51.3398895692695,-30.007053683816,3.4715307213905));
#220877=CARTESIAN_POINT('Origin',(5.53234440788222E-15,1.85015204418142E-13,
3.47153072139072));
#220878=CARTESIAN_POINT('',(-51.0313275753406,-29.8289013456888,2.90134173516002));
#220879=CARTESIAN_POINT('',(-51.3398895692695,-30.007053683816,3.4715307213905));
#220880=CARTESIAN_POINT('',(-51.0193480105325,-29.473599835734,2.59908173516003));
#220881=CARTESIAN_POINT('Ctrl Pts',(-51.0313275753406,-29.8289013456888,
2.90134173516002));
#220882=CARTESIAN_POINT('Ctrl Pts',(-51.0207361915371,-29.8227862420897,
2.8817699891976));
#220883=CARTESIAN_POINT('Ctrl Pts',(-51.0111534059233,-29.8150339189619,
2.86226752356654));
#220884=CARTESIAN_POINT('Ctrl Pts',(-51.0026853737213,-29.8057923055278,
2.84310370499927));
#220885=CARTESIAN_POINT('Ctrl Pts',(-50.9940643779338,-29.7963837548062,
2.82359371788554));
#220886=CARTESIAN_POINT('Ctrl Pts',(-50.9865979533919,-29.7854311897081,
2.80443322636885));
#220887=CARTESIAN_POINT('Ctrl Pts',(-50.9804176151483,-29.7730411634513,
2.78589323878137));
#220888=CARTESIAN_POINT('Ctrl Pts',(-50.9744989364019,-29.761175698782,
2.76813818619886));
#220889=CARTESIAN_POINT('Ctrl Pts',(-50.9697592710711,-29.7479911917172,
2.75095095198612));
#220890=CARTESIAN_POINT('Ctrl Pts',(-50.9663409452096,-29.7335453816167,
2.73457771435025));
#220891=CARTESIAN_POINT('Ctrl Pts',(-50.9636221212281,-29.7220556593013,
2.7215549795551));
#220892=CARTESIAN_POINT('Ctrl Pts',(-50.9617395717402,-29.7097672786763,
2.70904711159918));
#220893=CARTESIAN_POINT('Ctrl Pts',(-50.9607809287993,-29.6966961073822,
2.69718956158317));
#220894=CARTESIAN_POINT('Ctrl Pts',(-50.9607783120155,-29.6966604273305,
2.69715719432334));
#220895=CARTESIAN_POINT('Ctrl Pts',(-50.960775702253,-29.6966247415593,
2.69712483219));
#220896=CARTESIAN_POINT('Ctrl Pts',(-50.9607730995133,-29.6965890500698,
2.69709247518628));
#220897=CARTESIAN_POINT('Ctrl Pts',(-50.9602549766182,-29.6894840070028,
2.69065122242254));
#220898=CARTESIAN_POINT('Ctrl Pts',(-50.9600390146965,-29.6821247070256,
2.68442464469403));
#220899=CARTESIAN_POINT('Ctrl Pts',(-50.9601247215267,-29.6745516564559,
2.67844505923556));
#220900=CARTESIAN_POINT('Ctrl Pts',(-50.9602948126667,-29.6595224131521,
2.66657815779545));
#220901=CARTESIAN_POINT('Ctrl Pts',(-50.9616539500922,-29.6436502506361,
2.65568445664151));
#220902=CARTESIAN_POINT('Ctrl Pts',(-50.964203800626,-29.6272454573769,
2.64601906229493));
#220903=CARTESIAN_POINT('Ctrl Pts',(-50.9661161885263,-29.6149418624325,
2.63877001653499));
#220904=CARTESIAN_POINT('Ctrl Pts',(-50.9686983518505,-29.6023386622825,
2.63221189387579));
#220905=CARTESIAN_POINT('Ctrl Pts',(-50.9719510035827,-29.5895667656375,
2.62645231033211));
#220906=CARTESIAN_POINT('Ctrl Pts',(-50.9731707479823,-29.5847773043956,
2.62429246650323));
#220907=CARTESIAN_POINT('Ctrl Pts',(-50.9744847799795,-29.5799641203064,
2.62224491711723));
#220908=CARTESIAN_POINT('Ctrl Pts',(-50.9758931378752,-29.5751341171702,
2.62031533672575));
#220909=CARTESIAN_POINT('Ctrl Pts',(-50.9808223905102,-29.5582291061935,
2.61356180535556));
#220910=CARTESIAN_POINT('Ctrl Pts',(-50.9869071309993,-29.5411180593588,
2.60825339735326));
#220911=CARTESIAN_POINT('Ctrl Pts',(-50.9941490417484,-29.524097000417,
2.60463337987589));
#220912=CARTESIAN_POINT('Ctrl Pts',(-50.9977699971229,-29.5155864709461,
2.60282337113721));
#220913=CARTESIAN_POINT('Ctrl Pts',(-51.0016802459459,-29.5070984389558,
2.60143545939093));
#220914=CARTESIAN_POINT('Ctrl Pts',(-51.0058800022838,-29.4986699095566,
2.60050005034575));
#220915=CARTESIAN_POINT('Ctrl Pts',(-51.0079798804527,-29.494455644857,
2.60003234582315));
#220916=CARTESIAN_POINT('Ctrl Pts',(-51.0101521355226,-29.4902562558177,
2.59967776696044));
#220917=CARTESIAN_POINT('Ctrl Pts',(-51.0123967945049,-29.4860763682213,
2.59944011429138));
#220918=CARTESIAN_POINT('Ctrl Pts',(-51.0146414534873,-29.4818964806249,
2.59920246162232));
#220919=CARTESIAN_POINT('Ctrl Pts',(-51.0169585178536,-29.4777360953218,
2.59908173791288));
#220920=CARTESIAN_POINT('Ctrl Pts',(-51.0193480105325,-29.473599835734,
2.59908173516002));
#220921=CARTESIAN_POINT('',(-51.0345602039884,-29.4472515437738,2.59908173516002));
#220922=CARTESIAN_POINT('Origin',(3.43486142563102E-16,1.91073416032664E-13,
2.59908173516024));
#220923=CARTESIAN_POINT('',(-51.3482501200163,-29.2799753962465,2.90134173516002));
#220924=CARTESIAN_POINT('Ctrl Pts',(-51.0345602039884,-29.4472515437738,
2.59908173516002));
#220925=CARTESIAN_POINT('Ctrl Pts',(-51.0364642604673,-29.4439516646701,
2.59908174371488));
#220926=CARTESIAN_POINT('Ctrl Pts',(-51.0384038328686,-29.4406842975234,
2.59915764355868));
#220927=CARTESIAN_POINT('Ctrl Pts',(-51.0403770101282,-29.4374505691487,
2.59930765775255));
#220928=CARTESIAN_POINT('Ctrl Pts',(-51.0520264994499,-29.418358881371,
2.60019333020849));
#220929=CARTESIAN_POINT('Ctrl Pts',(-51.0648472300398,-29.4004365818843,
2.60365973323985));
#220930=CARTESIAN_POINT('Ctrl Pts',(-51.0784429877767,-29.383921634797,
2.60934177082164));
#220931=CARTESIAN_POINT('Ctrl Pts',(-51.0835219102868,-29.3777522003207,
2.61146439091651));
#220932=CARTESIAN_POINT('Ctrl Pts',(-51.0887089685234,-29.3717787490555,
2.61389584429199));
#220933=CARTESIAN_POINT('Ctrl Pts',(-51.0939835922267,-29.366012223236,
2.61661604385232));
#220934=CARTESIAN_POINT('Ctrl Pts',(-51.0980991182404,-29.361512890515,
2.61873848000755));
#220935=CARTESIAN_POINT('Ctrl Pts',(-51.1022679285259,-29.3571400387136,
2.62103707099765));
#220936=CARTESIAN_POINT('Ctrl Pts',(-51.1064802178291,-29.3528993717246,
2.6235026276763));
#220937=CARTESIAN_POINT('Ctrl Pts',(-51.1212232303903,-29.3380570372631,
2.63213207605156));
#220938=CARTESIAN_POINT('Ctrl Pts',(-51.1364988531341,-29.3248339623429,
2.64280685971893));
#220939=CARTESIAN_POINT('Ctrl Pts',(-51.1518867653711,-29.3134747466761,
2.65513293646063));
#220940=CARTESIAN_POINT('Ctrl Pts',(-51.1595807214896,-29.3077951388426,
2.66129597483147));
#220941=CARTESIAN_POINT('Ctrl Pts',(-51.1673027515569,-29.3025814967141,
2.6678718353383));
#220942=CARTESIAN_POINT('Ctrl Pts',(-51.1750003199399,-29.2978643977776,
2.67481125953839));
#220943=CARTESIAN_POINT('Ctrl Pts',(-51.182665000675,-29.2931674525158,
2.68172103524058));
#220944=CARTESIAN_POINT('Ctrl Pts',(-51.1903053811862,-29.2889625693103,
2.68899101329765));
#220945=CARTESIAN_POINT('Ctrl Pts',(-51.1978697380627,-29.2852806784151,
2.69657334701251));
#220946=CARTESIAN_POINT('Ctrl Pts',(-51.1979021952406,-29.2852648801404,
2.69660588132548));
#220947=CARTESIAN_POINT('Ctrl Pts',(-51.1979346509233,-29.2852490909586,
2.69663842081357));
#220948=CARTESIAN_POINT('Ctrl Pts',(-51.1979671051089,-29.285233310869,
2.69667096547357));
#220949=CARTESIAN_POINT('Ctrl Pts',(-51.2132718752151,-29.2777917239319,
2.71201840157988));
#220950=CARTESIAN_POINT('Ctrl Pts',(-51.2282103130419,-29.2723555974551,
2.72845645939479));
#220951=CARTESIAN_POINT('Ctrl Pts',(-51.2426536914433,-29.2687791125354,
2.74568723187116));
#220952=CARTESIAN_POINT('Ctrl Pts',(-51.2576224915316,-29.2650725221316,
2.7635448259463));
#220953=CARTESIAN_POINT('Ctrl Pts',(-51.2720604115359,-29.2633635057956,
2.78225519317531));
#220954=CARTESIAN_POINT('Ctrl Pts',(-51.285813246645,-29.2635407906074,
2.80151223086009));
#220955=CARTESIAN_POINT('Ctrl Pts',(-51.2993697979386,-29.2637155451671,
2.82049442740827));
#220956=CARTESIAN_POINT('Ctrl Pts',(-51.3122614394892,-29.2657236711479,
2.84000929089882));
#220957=CARTESIAN_POINT('Ctrl Pts',(-51.3243180878463,-29.2695013892407,
2.85976644342305));
#220958=CARTESIAN_POINT('Ctrl Pts',(-51.3327241975877,-29.2721352815066,
2.87354148167401));
#220959=CARTESIAN_POINT('Ctrl Pts',(-51.3407239614257,-29.2756302808596,
2.88743438345704));
#220960=CARTESIAN_POINT('Ctrl Pts',(-51.3482501200163,-29.2799753962465,
2.90134173516001));
#220961=CARTESIAN_POINT('',(-51.6568155675425,-29.4581217525676,3.47153072139051));
#220962=CARTESIAN_POINT('',(-51.3482501200163,-29.2799753962465,2.90134173516002));
#220963=CARTESIAN_POINT('',(-54.195235491187,-24.4761921430394,3.47153072139054));
#220964=CARTESIAN_POINT('Origin',(5.53234440788222E-15,1.85015204418142E-13,
3.47153072139072));
#220965=CARTESIAN_POINT('',(-53.8697418420143,-24.331269253109,2.90134173516006));
#220966=CARTESIAN_POINT('',(-54.195235491187,-24.4761921430394,3.47153072139055));
#220967=CARTESIAN_POINT('',(-53.8206887816834,-23.9791663275016,2.59908173516006));
#220968=CARTESIAN_POINT('Ctrl Pts',(-53.8697418420143,-24.331269253109,
2.90134173516006));
#220969=CARTESIAN_POINT('Ctrl Pts',(-53.8585692765376,-24.32629474976,2.88176998919761));
#220970=CARTESIAN_POINT('Ctrl Pts',(-53.8482286480027,-24.3195865685234,
2.86226752356651));
#220971=CARTESIAN_POINT('Ctrl Pts',(-53.8388409929167,-24.3112807320076,
2.84310370499922));
#220972=CARTESIAN_POINT('Ctrl Pts',(-53.8292837624978,-24.3028248617528,
2.82359371788556));
#220973=CARTESIAN_POINT('Ctrl Pts',(-53.8207133850122,-24.2927127498358,
2.80443322636894));
#220974=CARTESIAN_POINT('Ctrl Pts',(-53.8132717929037,-24.2810366186984,
2.78589323878152));
#220975=CARTESIAN_POINT('Ctrl Pts',(-53.806145258511,-24.2698548246802,
2.76813818619927));
#220976=CARTESIAN_POINT('Ctrl Pts',(-53.8000534013004,-24.2572379736583,
2.75095095198677));
#220977=CARTESIAN_POINT('Ctrl Pts',(-53.7951438030552,-24.2432286115666,
2.73457771435111));
#220978=CARTESIAN_POINT('Ctrl Pts',(-53.7912388700589,-24.2320860256448,
2.72155497955566));
#220979=CARTESIAN_POINT('Ctrl Pts',(-53.7880821478312,-24.2200617420593,
2.70904711159946));
#220980=CARTESIAN_POINT('Ctrl Pts',(-53.7857624469881,-24.2071623814824,
2.69718956158321));
#220981=CARTESIAN_POINT('Ctrl Pts',(-53.7857561149583,-24.2071271704182,
2.69715719432338));
#220982=CARTESIAN_POINT('Ctrl Pts',(-53.7857497893135,-24.2070919529317,
2.69712483219004));
#220983=CARTESIAN_POINT('Ctrl Pts',(-53.7857434700554,-24.2070567290244,
2.69709247518632));
#220984=CARTESIAN_POINT('Ctrl Pts',(-53.7844855062584,-24.2000447667167,
2.69065122242259));
#220985=CARTESIAN_POINT('Ctrl Pts',(-53.7835014710814,-24.1927483559227,
2.68442464469408));
#220986=CARTESIAN_POINT('Ctrl Pts',(-53.7827951090624,-24.1852078325131,
2.67844505923561));
#220987=CARTESIAN_POINT('Ctrl Pts',(-53.7813932847187,-24.1702431416111,
2.66657815779549));
#220988=CARTESIAN_POINT('Ctrl Pts',(-53.7810858838905,-24.1543158599158,
2.65568445664155));
#220989=CARTESIAN_POINT('Ctrl Pts',(-53.7819069982467,-24.1377344018726,
2.64601906229496));
#220990=CARTESIAN_POINT('Ctrl Pts',(-53.7825228340138,-24.1252983083403,
2.63877001653502));
#220991=CARTESIAN_POINT('Ctrl Pts',(-53.7837734588332,-24.1124942402751,
2.63221189387583));
#220992=CARTESIAN_POINT('Ctrl Pts',(-53.7856732654696,-24.0994523147292,
2.62645231033215));
#220993=CARTESIAN_POINT('Ctrl Pts',(-53.7863856929583,-24.0945615926495,
2.62429246650327));
#220994=CARTESIAN_POINT('Ctrl Pts',(-53.7871894118144,-24.089637421941,
2.62224491711727));
#220995=CARTESIAN_POINT('Ctrl Pts',(-53.7880851817728,-24.0846866645808,
2.62031533672578));
#220996=CARTESIAN_POINT('Ctrl Pts',(-53.7912203766271,-24.06735901382,2.61356180535559));
#220997=CARTESIAN_POINT('Ctrl Pts',(-53.7954831928407,-24.0497056745176,
2.6082533973533));
#220998=CARTESIAN_POINT('Ctrl Pts',(-53.8009062465106,-24.0320208729158,
2.60463337987593));
#220999=CARTESIAN_POINT('Ctrl Pts',(-53.8036177733455,-24.023178472115,
2.60282337113724));
#221000=CARTESIAN_POINT('Ctrl Pts',(-53.8066193604762,-24.0143282061515,
2.60143545939096));
#221001=CARTESIAN_POINT('Ctrl Pts',(-53.8099150888837,-24.0055068550422,
2.60050005034577));
#221002=CARTESIAN_POINT('Ctrl Pts',(-53.8115629530875,-24.0010961794875,
2.60003234582318));
#221003=CARTESIAN_POINT('Ctrl Pts',(-53.8132843526338,-23.9966927326564,
2.59967776696048));
#221004=CARTESIAN_POINT('Ctrl Pts',(-53.8150797979123,-23.9923011121677,
2.59944011429142));
#221005=CARTESIAN_POINT('Ctrl Pts',(-53.8168752431908,-23.987909491679,
2.59920246162236));
#221006=CARTESIAN_POINT('Ctrl Pts',(-53.8187447357538,-23.9835296982243,
2.59908173791293));
#221007=CARTESIAN_POINT('Ctrl Pts',(-53.8206887816834,-23.9791663275016,
2.59908173516006));
#221008=CARTESIAN_POINT('',(-53.8330634946836,-23.9513722670367,2.59908173516006));
#221009=CARTESIAN_POINT('Origin',(3.40248402231257E-16,1.91079770455854E-13,
2.59908173516024));
#221010=CARTESIAN_POINT('',(-54.1275498658872,-23.752222950883,2.90134173516006));
#221011=CARTESIAN_POINT('Ctrl Pts',(-53.8330634946836,-23.9513722670367,
2.59908173516006));
#221012=CARTESIAN_POINT('Ctrl Pts',(-53.8346121892501,-23.9478914369183,
2.59908174371493));
#221013=CARTESIAN_POINT('Ctrl Pts',(-53.8361996036041,-23.9444392282282,
2.59915764355872));
#221014=CARTESIAN_POINT('Ctrl Pts',(-53.8378239549346,-23.9410169613692,
2.59930765775258));
#221015=CARTESIAN_POINT('Ctrl Pts',(-53.8474140023514,-23.9208121566358,
2.60019333020862));
#221016=CARTESIAN_POINT('Ctrl Pts',(-53.8582911092154,-23.9016479061124,
2.60365973324066));
#221017=CARTESIAN_POINT('Ctrl Pts',(-53.8700861059304,-23.8838022859684,
2.60934177082359));
#221018=CARTESIAN_POINT('Ctrl Pts',(-53.8744923240653,-23.8771357563367,
2.61146439091801));
#221019=CARTESIAN_POINT('Ctrl Pts',(-53.8790265713717,-23.8706528330382,
2.61389584429284));
#221020=CARTESIAN_POINT('Ctrl Pts',(-53.8836695340507,-23.8643665485424,
2.61661604385234));
#221021=CARTESIAN_POINT('Ctrl Pts',(-53.8872922064472,-23.8594616740271,
2.61873848000757));
#221022=CARTESIAN_POINT('Ctrl Pts',(-53.8909810920749,-23.8546770178325,
2.62103707099769));
#221023=CARTESIAN_POINT('Ctrl Pts',(-53.894727035613,-23.8500192775333,
2.62350262767634));
#221024=CARTESIAN_POINT('Ctrl Pts',(-53.9078378379963,-23.833717186486,
2.63213207605161));
#221025=CARTESIAN_POINT('Ctrl Pts',(-53.9216475915793,-23.8189698115829,
2.64280685971896));
#221026=CARTESIAN_POINT('Ctrl Pts',(-53.9357638458654,-23.806064348069,
2.65513293646066));
#221027=CARTESIAN_POINT('Ctrl Pts',(-53.9428219730085,-23.799611616312,
2.66129597483151));
#221028=CARTESIAN_POINT('Ctrl Pts',(-53.9499567269874,-23.7936193631243,
2.66787183533834));
#221029=CARTESIAN_POINT('Ctrl Pts',(-53.9571190561825,-23.7881234899554,
2.67481125953843));
#221030=CARTESIAN_POINT('Ctrl Pts',(-53.9642507845242,-23.7826510977525,
2.68172103524061));
#221031=CARTESIAN_POINT('Ctrl Pts',(-53.9714097802519,-23.7776706121036,
2.68899101329771));
#221032=CARTESIAN_POINT('Ctrl Pts',(-53.9785478363928,-23.773218200392,
2.69657334701256));
#221033=CARTESIAN_POINT('Ctrl Pts',(-53.9785784643974,-23.773199095963,
2.69660588132554));
#221034=CARTESIAN_POINT('Ctrl Pts',(-53.9786090918656,-23.7731800007333,
2.69663842081363));
#221035=CARTESIAN_POINT('Ctrl Pts',(-53.9786397187952,-23.7731609147026,
2.69667096547363));
#221036=CARTESIAN_POINT('Ctrl Pts',(-53.993082790121,-23.7641603094586,
2.71201840157815));
#221037=CARTESIAN_POINT('Ctrl Pts',(-54.007371163674,-23.7571924707023,
2.72845645939101));
#221038=CARTESIAN_POINT('Ctrl Pts',(-54.0213615752631,-23.7521258339928,
2.74568723186518));
#221039=CARTESIAN_POINT('Ctrl Pts',(-54.0358609304978,-23.746874883009,
2.76354482593813));
#221040=CARTESIAN_POINT('Ctrl Pts',(-54.0500411172129,-23.7436660552521,
2.78225519316479));
#221041=CARTESIAN_POINT('Ctrl Pts',(-54.0637371441599,-23.7424048061589,
2.80151223084718));
#221042=CARTESIAN_POINT('Ctrl Pts',(-54.0772376980716,-23.7411615579202,
2.82049442739336));
#221043=CARTESIAN_POINT('Ctrl Pts',(-54.0902686241828,-23.7418111396954,
2.84000929088188));
#221044=CARTESIAN_POINT('Ctrl Pts',(-54.1026541040249,-23.7443079001269,
2.85976644340412));
#221045=CARTESIAN_POINT('Ctrl Pts',(-54.1112894809329,-23.746048685922,
2.87354148166129));
#221046=CARTESIAN_POINT('Ctrl Pts',(-54.119610748143,-23.748688336283,2.8874343834507));
#221047=CARTESIAN_POINT('Ctrl Pts',(-54.1275498658872,-23.752222950883,
2.90134173516006));
#221048=CARTESIAN_POINT('',(-54.4530463244691,-23.8971395307771,3.47153072139055));
#221049=CARTESIAN_POINT('',(-54.1275498658872,-23.752222950883,2.90134173516006));
#221050=CARTESIAN_POINT('',(-56.456807071981,-18.6771643191712,3.47153072139058));
#221051=CARTESIAN_POINT('Origin',(5.53234440788222E-15,1.85015204418142E-13,
3.47153072139072));
#221052=CARTESIAN_POINT('',(-56.1179479440987,-18.5670586829468,2.9013417351601));
#221053=CARTESIAN_POINT('',(-56.456807071981,-18.6771643191712,3.47153072139059));
#221054=CARTESIAN_POINT('',(-56.032358823839,-18.2220120550219,2.5990817351601));
#221055=CARTESIAN_POINT('Ctrl Pts',(-56.1179479440987,-18.5670586829468,
2.9013417351601));
#221056=CARTESIAN_POINT('Ctrl Pts',(-56.106316605913,-18.5632792815474,
2.88176998919588));
#221057=CARTESIAN_POINT('Ctrl Pts',(-56.0953314285462,-18.5576887384388,
2.86226752356303));
#221058=CARTESIAN_POINT('Ctrl Pts',(-56.0851270036891,-18.5504096793234,
2.84310370499407));
#221059=CARTESIAN_POINT('Ctrl Pts',(-56.0747382496542,-18.5429991338184,
2.82359371787864));
#221060=CARTESIAN_POINT('Ctrl Pts',(-56.0651578180735,-18.5338382654954,
2.80443322636034));
#221061=CARTESIAN_POINT('Ctrl Pts',(-56.05653650374,-18.5230039556117,2.7858932387714));
#221062=CARTESIAN_POINT('Ctrl Pts',(-56.0482801935027,-18.512628342318,
2.76813818618766));
#221063=CARTESIAN_POINT('Ctrl Pts',(-56.0409028880744,-18.500717380197,
2.75095095197381));
#221064=CARTESIAN_POINT('Ctrl Pts',(-56.0345558080313,-18.4872979556143,
2.73457771433704));
#221065=CARTESIAN_POINT('Ctrl Pts',(-56.0295075492856,-18.4766245865924,
2.72155497954667));
#221066=CARTESIAN_POINT('Ctrl Pts',(-56.0251112400293,-18.4649961406178,
2.70904711159522));
#221067=CARTESIAN_POINT('Ctrl Pts',(-56.0214558964132,-18.4524099188568,
2.69718956158324));
#221068=CARTESIAN_POINT('Ctrl Pts',(-56.0214459185125,-18.4523755625598,
2.69715719432342));
#221069=CARTESIAN_POINT('Ctrl Pts',(-56.0214359462906,-18.4523411992083,
2.69712483219007));
#221070=CARTESIAN_POINT('Ctrl Pts',(-56.021425979749,-18.4523068288036,
2.69709247518635));
#221071=CARTESIAN_POINT('Ctrl Pts',(-56.0194419575649,-18.4454647717816,
2.69065122242261));
#221072=CARTESIAN_POINT('Ctrl Pts',(-56.0177006304279,-18.4383111911741,
2.68442464469413));
#221073=CARTESIAN_POINT('Ctrl Pts',(-56.0162099386096,-18.4308858104772,
2.67844505923565));
#221074=CARTESIAN_POINT('Ctrl Pts',(-56.0132515574631,-18.4161496282621,
2.66657815779553));
#221075=CARTESIAN_POINT('Ctrl Pts',(-56.0112809863292,-18.4003417300186,
2.65568445664159));
#221076=CARTESIAN_POINT('Ctrl Pts',(-56.010364368207,-18.3837652771157,
2.64601906229501));
#221077=CARTESIAN_POINT('Ctrl Pts',(-56.0096769046154,-18.3713329374386,
2.63877001653507));
#221078=CARTESIAN_POINT('Ctrl Pts',(-56.0095822888227,-18.3584682855075,
2.63221189387587));
#221079=CARTESIAN_POINT('Ctrl Pts',(-56.0101084356843,-18.3452992211262,
2.62645231033219));
#221080=CARTESIAN_POINT('Ctrl Pts',(-56.0103057407573,-18.3403608219831,
2.6242924665033));
#221081=CARTESIAN_POINT('Ctrl Pts',(-56.0105903407605,-18.3353796149,2.62224491711731));
#221082=CARTESIAN_POINT('Ctrl Pts',(-56.0109637085384,-18.3303623448494,
2.62031533672582));
#221083=CARTESIAN_POINT('Ctrl Pts',(-56.0122704957612,-18.3128018996725,
2.61356180535563));
#221084=CARTESIAN_POINT('Ctrl Pts',(-56.0146646833927,-18.2947996815818,
2.60825339735333));
#221085=CARTESIAN_POINT('Ctrl Pts',(-56.0182094638726,-18.2766448957073,
2.60463337987597));
#221086=CARTESIAN_POINT('Ctrl Pts',(-56.0199818541125,-18.26756750277,2.60282337113728));
#221087=CARTESIAN_POINT('Ctrl Pts',(-56.0220418935342,-18.2584519681994,
2.601435459391));
#221088=CARTESIAN_POINT('Ctrl Pts',(-56.0243974853212,-18.2493344439487,
2.60050005034582));
#221089=CARTESIAN_POINT('Ctrl Pts',(-56.0255752812147,-18.2447756818233,
2.60003234582322));
#221090=CARTESIAN_POINT('Ctrl Pts',(-56.0268269652239,-18.2402164222855,
2.59967776696052));
#221091=CARTESIAN_POINT('Ctrl Pts',(-56.0281535255244,-18.2356611844174,
2.59944011429146));
#221092=CARTESIAN_POINT('Ctrl Pts',(-56.0294800858248,-18.2311059465494,
2.5992024616224));
#221093=CARTESIAN_POINT('Ctrl Pts',(-56.0308815240327,-18.2265547308768,
2.59908173791298));
#221094=CARTESIAN_POINT('Ctrl Pts',(-56.032358823839,-18.2220120550219,
2.5990817351601));
#221095=CARTESIAN_POINT('',(-56.0417604764382,-18.1930767435951,2.5990817351601));
#221096=CARTESIAN_POINT('Origin',(3.37692616670652E-16,1.91086428504869E-13,
2.59908173516024));
#221097=CARTESIAN_POINT('',(-56.3138168485094,-17.9642361803975,2.9013417351601));
#221098=CARTESIAN_POINT('Ctrl Pts',(-56.0417604764382,-18.1930767435951,
2.59908173516011));
#221099=CARTESIAN_POINT('Ctrl Pts',(-56.0429368412707,-18.1894530991653,
2.59908174371499));
#221100=CARTESIAN_POINT('Ctrl Pts',(-56.0441547055335,-18.1858538720526,
2.59915764355877));
#221101=CARTESIAN_POINT('Ctrl Pts',(-56.0454124342018,-18.1822805617811,
2.59930765775263));
#221102=CARTESIAN_POINT('Ctrl Pts',(-56.0528379691454,-18.1611840081647,
2.6001933302086));
#221103=CARTESIAN_POINT('Ctrl Pts',(-56.0616522804222,-18.140987774147,
2.60365973324016));
#221104=CARTESIAN_POINT('Ctrl Pts',(-56.0715172876605,-18.1220070012978,
2.60934177082228));
#221105=CARTESIAN_POINT('Ctrl Pts',(-56.0752025259743,-18.1149164164009,
2.61146439091702));
#221106=CARTESIAN_POINT('Ctrl Pts',(-56.0790342841905,-18.10799504933,2.61389584429231));
#221107=CARTESIAN_POINT('Ctrl Pts',(-56.082994716577,-18.1012578800032,
2.6166160438524));
#221108=CARTESIAN_POINT('Ctrl Pts',(-56.0860848445995,-18.0960012025251,
2.61873848000763));
#221109=CARTESIAN_POINT('Ctrl Pts',(-56.0892533893664,-18.090857163632,
2.62103707099775));
#221110=CARTESIAN_POINT('Ctrl Pts',(-56.0924919457981,-18.0858333812,2.62350262767639));
#221111=CARTESIAN_POINT('Ctrl Pts',(-56.1038268933089,-18.0682501426878,
2.63213207605166));
#221112=CARTESIAN_POINT('Ctrl Pts',(-56.116019475181,-18.0521400431274,
2.64280685971901));
#221113=CARTESIAN_POINT('Ctrl Pts',(-56.1287094108802,-18.0378297267253,
2.6551329364607));
#221114=CARTESIAN_POINT('Ctrl Pts',(-56.1350543787298,-18.0306745685242,
2.66129597483155));
#221115=CARTESIAN_POINT('Ctrl Pts',(-56.1415236867627,-18.0239693566572,
2.66787183533838));
#221116=CARTESIAN_POINT('Ctrl Pts',(-56.1480723047924,-18.0177549231924,
2.67481125953847));
#221117=CARTESIAN_POINT('Ctrl Pts',(-56.1545929440327,-18.0115670407226,
2.68172103524065));
#221118=CARTESIAN_POINT('Ctrl Pts',(-56.1611921195216,-18.0058655198732,
2.68899101329776));
#221119=CARTESIAN_POINT('Ctrl Pts',(-56.1678256688899,-18.0006913688997,
2.69657334701261));
#221120=CARTESIAN_POINT('Ctrl Pts',(-56.1678541321546,-18.0006691676285,
2.69660588132558));
#221121=CARTESIAN_POINT('Ctrl Pts',(-56.1678825958473,-18.0006469755623,
2.69663842081367));
#221122=CARTESIAN_POINT('Ctrl Pts',(-56.1679110599659,-18.000624792701,
2.69667096547367));
#221123=CARTESIAN_POINT('Ctrl Pts',(-56.1813341912018,-17.9901637816632,
2.71201840157894));
#221124=CARTESIAN_POINT('Ctrl Pts',(-56.1948159540726,-17.9817405717263,
2.72845645939267));
#221125=CARTESIAN_POINT('Ctrl Pts',(-56.2082001169746,-17.9752392943588,
2.74568723186776));
#221126=CARTESIAN_POINT('Ctrl Pts',(-56.2220711693879,-17.9685015133128,
2.7635448259417));
#221127=CARTESIAN_POINT('Ctrl Pts',(-56.2358382617228,-17.963828030724,
2.78225519316943));
#221128=CARTESIAN_POINT('Ctrl Pts',(-56.2493274239724,-17.9611420662359,
2.80151223085291));
#221129=CARTESIAN_POINT('Ctrl Pts',(-56.2626240656099,-17.9584944364878,
2.82049442740019));
#221130=CARTESIAN_POINT('Ctrl Pts',(-56.2756515067297,-17.9577783571051,
2.84000929088984));
#221131=CARTESIAN_POINT('Ctrl Pts',(-56.2882301201489,-17.9589668048476,
2.85976644341319));
#221132=CARTESIAN_POINT('Ctrl Pts',(-56.2970001532207,-17.9597954117582,
2.87354148166741));
#221133=CARTESIAN_POINT('Ctrl Pts',(-56.3055517542522,-17.9615507925643,
2.88743438345378));
#221134=CARTESIAN_POINT('Ctrl Pts',(-56.3138168485093,-17.9642361803975,
2.9013417351601));
#221135=CARTESIAN_POINT('',(-56.6526781108322,-18.0743352474894,3.47153072139059));
#221136=CARTESIAN_POINT('',(-56.3138168485094,-17.9642361803975,2.90134173516011));
#221137=CARTESIAN_POINT('',(-58.0998260601479,-12.6735055745743,3.47153072139063));
#221138=CARTESIAN_POINT('Origin',(5.53234440788222E-15,1.85015204418142E-13,
3.47153072139072));
#221139=CARTESIAN_POINT('',(-57.7513140650719,-12.5994235324474,2.90134173516015));
#221140=CARTESIAN_POINT('',(-58.0998260601479,-12.6735055745743,3.47153072139063));
#221141=CARTESIAN_POINT('',(-57.6301266171956,-12.2652136052663,2.59908173516014));
#221142=CARTESIAN_POINT('Ctrl Pts',(-57.7513140650719,-12.5994235324474,
2.90134173516015));
#221143=CARTESIAN_POINT('Ctrl Pts',(-57.7393513895546,-12.596880640911,
2.88176998919789));
#221144=CARTESIAN_POINT('Ctrl Pts',(-57.72784201926,-12.5924689870921,2.86226752356699));
#221145=CARTESIAN_POINT('Ctrl Pts',(-57.7169326264476,-12.5862964562739,
2.84310370499987));
#221146=CARTESIAN_POINT('Ctrl Pts',(-57.7058261701616,-12.5800124270081,
2.82359371788624));
#221147=CARTESIAN_POINT('Ctrl Pts',(-57.6953406497003,-12.5719031706721,
2.80443322636963));
#221148=CARTESIAN_POINT('Ctrl Pts',(-57.6856340700667,-12.5620293850118,
2.78589323878222));
#221149=CARTESIAN_POINT('Ctrl Pts',(-57.6763384418482,-12.5525736298361,
2.7681381861997));
#221150=CARTESIAN_POINT('Ctrl Pts',(-57.6677565155047,-12.541499055613,
2.75095095198695));
#221151=CARTESIAN_POINT('Ctrl Pts',(-57.6600414936007,-12.5288165945673,
2.73457771435106));
#221152=CARTESIAN_POINT('Ctrl Pts',(-57.6539052188803,-12.5187293821036,
2.72155497955566));
#221153=CARTESIAN_POINT('Ctrl Pts',(-57.648317489476,-12.5076241774198,
2.70904711159951));
#221154=CARTESIAN_POINT('Ctrl Pts',(-57.6433665517939,-12.495488991745,
2.69718956158329));
#221155=CARTESIAN_POINT('Ctrl Pts',(-57.6433530373423,-12.49545586663,2.69715719432346));
#221156=CARTESIAN_POINT('Ctrl Pts',(-57.6433395278009,-12.4954227339057,
2.69712483219012));
#221157=CARTESIAN_POINT('Ctrl Pts',(-57.6433260231715,-12.4953895935729,
2.6970924751864));
#221158=CARTESIAN_POINT('Ctrl Pts',(-57.6406376799624,-12.4887924048451,
2.69065122242266));
#221159=CARTESIAN_POINT('Ctrl Pts',(-57.6381581392099,-12.4818600305505,
2.68442464469416));
#221160=CARTESIAN_POINT('Ctrl Pts',(-57.635899449924,-12.4746311465908,
2.67844505923568));
#221161=CARTESIAN_POINT('Ctrl Pts',(-57.6314169246175,-12.4602849257589,
2.66657815779556));
#221162=CARTESIAN_POINT('Ctrl Pts',(-57.6278047731676,-12.4447696056083,
2.65568445664162));
#221163=CARTESIAN_POINT('Ctrl Pts',(-57.625160465227,-12.4283797729326,
2.64601906229503));
#221164=CARTESIAN_POINT('Ctrl Pts',(-57.6231772342716,-12.4160873984258,
2.63877001653509));
#221165=CARTESIAN_POINT('Ctrl Pts',(-57.6217384144973,-12.4033031104475,
2.63221189387591));
#221166=CARTESIAN_POINT('Ctrl Pts',(-57.6208851370088,-12.3901511902558,
2.62645231033223));
#221167=CARTESIAN_POINT('Ctrl Pts',(-57.6205651579507,-12.3852192201839,
2.62429246650335));
#221168=CARTESIAN_POINT('Ctrl Pts',(-57.6203275209636,-12.3802355518734,
2.62224491711735));
#221169=CARTESIAN_POINT('Ctrl Pts',(-57.6201743958656,-12.3752067393931,
2.62031533672586));
#221170=CARTESIAN_POINT('Ctrl Pts',(-57.6196384580226,-12.3576058957119,
2.61356180535568));
#221171=CARTESIAN_POINT('Ctrl Pts',(-57.6201377858513,-12.3394520349017,
2.60825339735338));
#221172=CARTESIAN_POINT('Ctrl Pts',(-57.6217654557844,-12.3210261723876,
2.60463337987601));
#221173=CARTESIAN_POINT('Ctrl Pts',(-57.6225792907509,-12.3118132411305,
2.60282337113733));
#221174=CARTESIAN_POINT('Ctrl Pts',(-57.6236752122406,-12.302532309657,
2.60143545939105));
#221175=CARTESIAN_POINT('Ctrl Pts',(-57.6250648590506,-12.2932185057686,
2.60050005034586));
#221176=CARTESIAN_POINT('Ctrl Pts',(-57.6257596824556,-12.2885616038243,
2.60003234582327));
#221177=CARTESIAN_POINT('Ctrl Pts',(-57.6265279372157,-12.2838964837813,
2.59967776696056));
#221178=CARTESIAN_POINT('Ctrl Pts',(-57.6273710784659,-12.2792275366732,
2.5994401142915));
#221179=CARTESIAN_POINT('Ctrl Pts',(-57.628214219716,-12.2745585895652,
2.59920246162244));
#221180=CARTESIAN_POINT('Ctrl Pts',(-57.6291322491185,-12.2698858157461,
2.59908173791297));
#221181=CARTESIAN_POINT('Ctrl Pts',(-57.6301266171956,-12.2652136052663,
2.59908173516014));
#221182=CARTESIAN_POINT('',(-57.6364522029206,-12.2354540642047,2.59908173516014));
#221183=CARTESIAN_POINT('Origin',(3.35846787602732E-16,1.91093317232733E-13,
2.59908173516024));
#221184=CARTESIAN_POINT('',(-57.8830978693155,-11.9794294790614,2.90134173516013));
#221185=CARTESIAN_POINT('Ctrl Pts',(-57.6364522029206,-12.2354540642047,
2.59908173516014));
#221186=CARTESIAN_POINT('Ctrl Pts',(-57.6372433495198,-12.2317273068699,
2.59908174371504));
#221187=CARTESIAN_POINT('Ctrl Pts',(-57.6380783205157,-12.2280204952201,
2.59915764355881));
#221188=CARTESIAN_POINT('Ctrl Pts',(-57.6389556465833,-12.2243352914713,
2.59930765775268));
#221189=CARTESIAN_POINT('Ctrl Pts',(-57.6441353133411,-12.2025781272208,
2.60019333020887));
#221190=CARTESIAN_POINT('Ctrl Pts',(-57.6507902575949,-12.1815711838685,
2.60365973324197));
#221191=CARTESIAN_POINT('Ctrl Pts',(-57.6586171922763,-12.1616632156277,
2.60934177082667));
#221192=CARTESIAN_POINT('Ctrl Pts',(-57.6615410745244,-12.1542262614044,
2.61146439092037));
#221193=CARTESIAN_POINT('Ctrl Pts',(-57.6646283621025,-12.1469422825137,
2.61389584429419));
#221194=CARTESIAN_POINT('Ctrl Pts',(-57.6678628728672,-12.1398280421989,
2.61661604385241));
#221195=CARTESIAN_POINT('Ctrl Pts',(-57.6703866004264,-12.1342771550166,
2.61873848000764));
#221196=CARTESIAN_POINT('Ctrl Pts',(-57.6730000890932,-12.1288300925915,
2.62103707099777));
#221197=CARTESIAN_POINT('Ctrl Pts',(-57.6756957761164,-12.1234953096383,
2.62350262767642));
#221198=CARTESIAN_POINT('Ctrl Pts',(-57.6851306806978,-12.104823569302,
2.63213207605169));
#221199=CARTESIAN_POINT('Ctrl Pts',(-57.6955725063805,-12.0875272507062,
2.64280685971904));
#221200=CARTESIAN_POINT('Ctrl Pts',(-57.7066970899018,-12.071968868237,
2.65513293646074));
#221201=CARTESIAN_POINT('Ctrl Pts',(-57.7122593816625,-12.0641896770024,
2.66129597483159));
#221202=CARTESIAN_POINT('Ctrl Pts',(-57.7179923646567,-12.0568449701606,
2.66787183533841));
#221203=CARTESIAN_POINT('Ctrl Pts',(-57.7238555234915,-12.0499800630333,
2.67481125953851));
#221204=CARTESIAN_POINT('Ctrl Pts',(-57.7296936321424,-12.0431444860318,
2.68172103524069));
#221205=CARTESIAN_POINT('Ctrl Pts',(-57.7356606854447,-12.0367843970375,
2.68899101329778));
#221206=CARTESIAN_POINT('Ctrl Pts',(-57.7417170494856,-12.0309451958829,
2.69657334701263));
#221207=CARTESIAN_POINT('Ctrl Pts',(-57.7417430361608,-12.0309201410113,
2.69660588132561));
#221208=CARTESIAN_POINT('Ctrl Pts',(-57.7417690242238,-12.0308950952495,
2.6966384208137));
#221209=CARTESIAN_POINT('Ctrl Pts',(-57.7417950136726,-12.0308700585976,
2.6966709654737));
#221210=CARTESIAN_POINT('Ctrl Pts',(-57.7540511381828,-12.0190632547927,
2.71201840157874));
#221211=CARTESIAN_POINT('Ctrl Pts',(-57.7665785813554,-12.0092769601263,
2.7284564593922));
#221212=CARTESIAN_POINT('Ctrl Pts',(-57.7792098558799,-12.0014122714562,
2.745687231867));
#221213=CARTESIAN_POINT('Ctrl Pts',(-57.792300631318,-11.9932614808871,
2.76354482594064));
#221214=CARTESIAN_POINT('Ctrl Pts',(-57.8055037941273,-11.9871745471194,
2.78225519316803));
#221215=CARTESIAN_POINT('Ctrl Pts',(-57.8186383015941,-11.9830932952251,
2.80151223085117));
#221216=CARTESIAN_POINT('Ctrl Pts',(-57.8315853501684,-11.9790702919526,
2.820494427398));
#221217=CARTESIAN_POINT('Ctrl Pts',(-57.8444665749249,-11.9769963969271,
2.8400092908872));
#221218=CARTESIAN_POINT('Ctrl Pts',(-57.8571005079996,-11.9768635110976,
2.8597664434101));
#221219=CARTESIAN_POINT('Ctrl Pts',(-57.8659091109203,-11.9767708607329,
2.87354148166534));
#221220=CARTESIAN_POINT('Ctrl Pts',(-57.8745973526454,-11.977622739665,
2.88743438345275));
#221221=CARTESIAN_POINT('Ctrl Pts',(-57.8830978693155,-11.9794294790614,
2.90134173516013));
#221222=CARTESIAN_POINT('',(-58.231611300478,-12.0535047649324,3.47153072139063));
#221223=CARTESIAN_POINT('',(-57.8830978693155,-11.9794294790614,2.90134173516013));
#221224=CARTESIAN_POINT('',(-59.1062911958296,-6.53099325080078,3.47153072139067));
#221225=CARTESIAN_POINT('Origin',(5.53234440788222E-15,1.85015204418142E-13,
3.47153072139072));
#221226=CARTESIAN_POINT('',(-58.7519447039088,-6.49374646112762,2.90134173516018));
#221227=CARTESIAN_POINT('',(-59.1062911958296,-6.53099325080078,3.47153072139067));
#221228=CARTESIAN_POINT('',(-58.596486683455,-6.17403490859042,2.59908173516019));
#221229=CARTESIAN_POINT('Ctrl Pts',(-58.7519447039088,-6.49374646112762,
2.90134173516018));
#221230=CARTESIAN_POINT('Ctrl Pts',(-58.7397817566354,-6.49246793990548,
2.88176998919848));
#221231=CARTESIAN_POINT('Ctrl Pts',(-58.7278742924817,-6.48928351037797,
2.86226752356812));
#221232=CARTESIAN_POINT('Ctrl Pts',(-58.716379457304,-6.48428513539561,
2.84310370500153));
#221233=CARTESIAN_POINT('Ctrl Pts',(-58.7046769834257,-6.47919647150781,
2.82359371788848));
#221234=CARTESIAN_POINT('Ctrl Pts',(-58.6934012556399,-6.47222767386725,
2.80443322637243));
#221235=CARTESIAN_POINT('Ctrl Pts',(-58.6827157580237,-6.46342259169109,
2.78589323878551));
#221236=CARTESIAN_POINT('Ctrl Pts',(-58.6724826566719,-6.45499029386492,
2.76813818620355));
#221237=CARTESIAN_POINT('Ctrl Pts',(-58.6627901347942,-6.44487344289129,
2.75095095199129));
#221238=CARTESIAN_POINT('Ctrl Pts',(-58.6537916984241,-6.43306689707866,
2.73457771435581));
#221239=CARTESIAN_POINT('Ctrl Pts',(-58.6466346380402,-6.42367635878618,
2.72155497955872));
#221240=CARTESIAN_POINT('Ctrl Pts',(-58.6399167088215,-6.4132160663422,
2.70904711160098));
#221241=CARTESIAN_POINT('Ctrl Pts',(-58.6337244205832,-6.40166487239058,
2.69718956158333));
#221242=CARTESIAN_POINT('Ctrl Pts',(-58.6337075176478,-6.4016333413833,
2.69715719432351));
#221243=CARTESIAN_POINT('Ctrl Pts',(-58.6336906188003,-6.40160180229505,
2.69712483219017));
#221244=CARTESIAN_POINT('Ctrl Pts',(-58.6336737240427,-6.40157025512662,
2.69709247518644));
#221245=CARTESIAN_POINT('Ctrl Pts',(-58.6303105138594,-6.39529021487341,
2.6906512224227));
#221246=CARTESIAN_POINT('Ctrl Pts',(-58.6271199258587,-6.38865499943493,
2.6844246446942));
#221247=CARTESIAN_POINT('Ctrl Pts',(-58.6241179857776,-6.38170181337806,
2.67844505923572));
#221248=CARTESIAN_POINT('Ctrl Pts',(-58.6181604277965,-6.36790273412671,
2.6665781577956));
#221249=CARTESIAN_POINT('Ctrl Pts',(-58.6129462715177,-6.35284998116343,
2.65568445664167));
#221250=CARTESIAN_POINT('Ctrl Pts',(-58.6086032453499,-6.33682633915147,
2.64601906229508));
#221251=CARTESIAN_POINT('Ctrl Pts',(-58.6053459757241,-6.3248086076425,
2.63877001653514));
#221252=CARTESIAN_POINT('Ctrl Pts',(-58.6025787159787,-6.31224475095126,
2.63221189387594));
#221253=CARTESIAN_POINT('Ctrl Pts',(-58.6003553628269,-6.29925407013912,
2.62645231033226));
#221254=CARTESIAN_POINT('Ctrl Pts',(-58.599521605395,-6.29438256483457,
2.62429246650338));
#221255=CARTESIAN_POINT('Ctrl Pts',(-58.5987643350183,-6.28945103740959,
2.62224491711737));
#221256=CARTESIAN_POINT('Ctrl Pts',(-58.598086394715,-6.28446577922139,
2.62031533672589));
#221257=CARTESIAN_POINT('Ctrl Pts',(-58.5957136036534,-6.26701737556265,
2.6135618053557));
#221258=CARTESIAN_POINT('Ctrl Pts',(-58.5943126009391,-6.24891076953078,
2.60825339735341));
#221259=CARTESIAN_POINT('Ctrl Pts',(-58.594005327233,-6.23041570798267,
2.60463337987604));
#221260=CARTESIAN_POINT('Ctrl Pts',(-58.59385169038,-6.22116817720862,2.60282337113736));
#221261=CARTESIAN_POINT('Ctrl Pts',(-58.5939714867924,-6.21182353265965,
2.60143545939109));
#221262=CARTESIAN_POINT('Ctrl Pts',(-58.5943799633642,-6.20241549311785,
2.60050005034591));
#221263=CARTESIAN_POINT('Ctrl Pts',(-58.5945842016501,-6.19771147334694,
2.60003234582332));
#221264=CARTESIAN_POINT('Ctrl Pts',(-58.5948606100011,-6.19299160483014,
2.5996777669606));
#221265=CARTESIAN_POINT('Ctrl Pts',(-58.5952110945691,-6.1882601024437,
2.59944011429154));
#221266=CARTESIAN_POINT('Ctrl Pts',(-58.595561579137,-6.18352860005727,
2.59920246162248));
#221267=CARTESIAN_POINT('Ctrl Pts',(-58.5959861416118,-6.17878546397934,
2.59908173791308));
#221268=CARTESIAN_POINT('Ctrl Pts',(-58.596486683455,-6.17403490859042,
2.59908173516019));
#221269=CARTESIAN_POINT('',(-58.5996668978648,-6.14377718965343,2.59908173516018));
#221270=CARTESIAN_POINT('Origin',(3.34731138317027E-16,1.911003611651E-13,
2.59908173516024));
#221271=CARTESIAN_POINT('',(-58.8181995570484,-5.86337364149602,2.90134173516017));
#221272=CARTESIAN_POINT('Ctrl Pts',(-58.5996668978648,-6.14377718965343,
2.59908173516018));
#221273=CARTESIAN_POINT('Ctrl Pts',(-58.600064158263,-6.13998815054707,
2.59908174371508));
#221274=CARTESIAN_POINT('Ctrl Pts',(-58.600507087875,-6.13621436696425,
2.59915764355885));
#221275=CARTESIAN_POINT('Ctrl Pts',(-58.6009943991739,-6.13245764560148,
2.59930765775272));
#221276=CARTESIAN_POINT('Ctrl Pts',(-58.6038714482307,-6.11027824676976,
2.60019333020879));
#221277=CARTESIAN_POINT('Ctrl Pts',(-58.6082941124962,-6.08869075055798,
2.60365973324109));
#221278=CARTESIAN_POINT('Ctrl Pts',(-58.6139972210824,-6.06807370279834,
2.60934177082446));
#221279=CARTESIAN_POINT('Ctrl Pts',(-58.6161277126019,-6.06037186006736,
2.6114643909187));
#221280=CARTESIAN_POINT('Ctrl Pts',(-58.6184367045765,-6.05280507414621,
2.61389584429328));
#221281=CARTESIAN_POINT('Ctrl Pts',(-58.6209098557463,-6.04539170794198,
2.61661604385248));
#221282=CARTESIAN_POINT('Ctrl Pts',(-58.6228395323549,-6.039607427737,2.61873848000771));
#221283=CARTESIAN_POINT('Ctrl Pts',(-58.6248693309926,-6.0339170209357,
2.62103707099782));
#221284=CARTESIAN_POINT('Ctrl Pts',(-58.6269926140963,-6.02832968645968,
2.62350262767646));
#221285=CARTESIAN_POINT('Ctrl Pts',(-58.6344241049593,-6.00877401579361,
2.63213207605173));
#221286=CARTESIAN_POINT('Ctrl Pts',(-58.6430007716254,-5.99048098024849,
2.64280685971909));
#221287=CARTESIAN_POINT('Ctrl Pts',(-58.6524381197038,-5.97384499260644,
2.65513293646079));
#221288=CARTESIAN_POINT('Ctrl Pts',(-58.657156793743,-5.96552699878541,
2.66129597483164));
#221289=CARTESIAN_POINT('Ctrl Pts',(-58.6620906399372,-5.95762326711377,
2.66787183533846));
#221290=CARTESIAN_POINT('Ctrl Pts',(-58.6672041015819,-5.95018309968314,
2.67481125953855));
#221291=CARTESIAN_POINT('Ctrl Pts',(-58.6722957161032,-5.94277472016202,
2.68172103524073));
#221292=CARTESIAN_POINT('Ctrl Pts',(-58.6775652709344,-5.93582574548874,
2.68899101329782));
#221293=CARTESIAN_POINT('Ctrl Pts',(-58.682978094856,-5.9293854696629,2.69657334701268));
#221294=CARTESIAN_POINT('Ctrl Pts',(-58.6830013202262,-5.92935783569726,
2.69660588132565));
#221295=CARTESIAN_POINT('Ctrl Pts',(-58.6830245479289,-5.9293302106465,
2.69663842081374));
#221296=CARTESIAN_POINT('Ctrl Pts',(-58.683047777962,-5.92930259451084,
2.69667096547375));
#221297=CARTESIAN_POINT('Ctrl Pts',(-58.694002615082,-5.91627935575193,
2.71201840157873));
#221298=CARTESIAN_POINT('Ctrl Pts',(-58.7054384852674,-5.90523719704818,
2.72845645939213));
#221299=CARTESIAN_POINT('Ctrl Pts',(-58.7171784805277,-5.89609526425038,
2.74568723186687));
#221300=CARTESIAN_POINT('Ctrl Pts',(-58.7293455537156,-5.88662076592534,
2.76354482594046));
#221301=CARTESIAN_POINT('Ctrl Pts',(-58.7418401303848,-5.87918707069908,
2.78225519316782));
#221302=CARTESIAN_POINT('Ctrl Pts',(-58.7544760786566,-5.87375524644833,
2.80151223085092));
#221303=CARTESIAN_POINT('Ctrl Pts',(-58.7669316835944,-5.86840094651743,
2.82049442739782));
#221304=CARTESIAN_POINT('Ctrl Pts',(-58.779525562594,-5.86499195787703,
2.84000929088709));
#221305=CARTESIAN_POINT('Ctrl Pts',(-58.7920763953099,-5.86353919440059,
2.85976644341007));
#221306=CARTESIAN_POINT('Ctrl Pts',(-58.8008270591819,-5.86252630185747,
2.87354148166533));
#221307=CARTESIAN_POINT('Ctrl Pts',(-58.8095567514054,-5.8624653455516,
2.88743438345277));
#221308=CARTESIAN_POINT('Ctrl Pts',(-58.8181995570484,-5.86337364149602,
2.90134173516017));
#221309=CARTESIAN_POINT('',(-59.1725467709677,-5.90061356181279,3.47153072139067));
#221310=CARTESIAN_POINT('',(-58.8181995570484,-5.86337364149602,2.90134173516017));
#221311=CARTESIAN_POINT('',(-59.4651754363832,-0.316925998272859,3.47153072139071));
#221312=CARTESIAN_POINT('Origin',(5.53234440788222E-15,1.85015204418142E-13,
3.47153072139072));
#221313=CARTESIAN_POINT('',(-59.1088767419348,-0.3169225446755,2.90134173516022));
#221314=CARTESIAN_POINT('',(-59.4651754363832,-0.316925998272862,3.47153072139071));
#221315=CARTESIAN_POINT('Ctrl Pts',(-59.1088767419348,-0.3169225446755,
2.90134173516022));
#221316=CARTESIAN_POINT('Ctrl Pts',(-59.0966467827004,-0.316922401513674,
2.88176998919804));
#221317=CARTESIAN_POINT('Ctrl Pts',(-59.084471685356,-0.315000085553621,
2.86226752356721));
#221318=CARTESIAN_POINT('Ctrl Pts',(-59.0725173476321,-0.311230629648864,
2.84310370500017));
#221319=CARTESIAN_POINT('Ctrl Pts',(-59.0603470709135,-0.307393083605022,
2.82359371788663));
#221320=CARTESIAN_POINT('Ctrl Pts',(-59.0484046750358,-0.301641096264493,
2.80443322637013));
#221321=CARTESIAN_POINT('Ctrl Pts',(-59.0368573319846,-0.294001187894466,
2.7858932387828));
#221322=CARTESIAN_POINT('Ctrl Pts',(-59.0257988734988,-0.286684733436473,
2.76813818620042));
#221323=CARTESIAN_POINT('Ctrl Pts',(-59.0151019493846,-0.277636448047603,
2.75095095198779));
#221324=CARTESIAN_POINT('Ctrl Pts',(-59.0049186872999,-0.26683517245329,
2.73457771435201));
#221325=CARTESIAN_POINT('Ctrl Pts',(-58.9968192555055,-0.2582441930362,
2.72155497955629));
#221326=CARTESIAN_POINT('Ctrl Pts',(-58.9890447295123,-0.248543417987119,
2.70904711159986));
#221327=CARTESIAN_POINT('Ctrl Pts',(-58.981678934725,-0.237702773059304,
2.69718956158338));
#221328=CARTESIAN_POINT('Ctrl Pts',(-58.9816588284979,-0.237673181620044,
2.69715719432355));
#221329=CARTESIAN_POINT('Ctrl Pts',(-58.9816387254916,-0.237643581716782,
2.69712483219021));
#221330=CARTESIAN_POINT('Ctrl Pts',(-58.9816186257082,-0.237613973350095,
2.69709247518649));
#221331=CARTESIAN_POINT('Ctrl Pts',(-58.9776173965852,-0.231719887006591,
2.69065122242275));
#221332=CARTESIAN_POINT('Ctrl Pts',(-58.9737507180862,-0.225454527233169,
2.68442464469424));
#221333=CARTESIAN_POINT('Ctrl Pts',(-58.9700384170936,-0.218853219640541,
2.67844505923577));
#221334=CARTESIAN_POINT('Ctrl Pts',(-58.9626710986899,-0.205752467569738,
2.66657815779565));
#221335=CARTESIAN_POINT('Ctrl Pts',(-58.9559120649696,-0.191327202905241,
2.65568445664172));
#221336=CARTESIAN_POINT('Ctrl Pts',(-58.9499179036781,-0.175845309932059,
2.64601906229514));
#221337=CARTESIAN_POINT('Ctrl Pts',(-58.9454222827095,-0.164233890202172,
2.6387700165352));
#221338=CARTESIAN_POINT('Ctrl Pts',(-58.9413569016699,-0.15202811704111,
2.632211893876));
#221339=CARTESIAN_POINT('Ctrl Pts',(-58.9377878323772,-0.139341004225949,
2.62645231033233));
#221340=CARTESIAN_POINT('Ctrl Pts',(-58.9364494313924,-0.134583336920264,
2.62429246650345));
#221341=CARTESIAN_POINT('Ctrl Pts',(-58.9351808244388,-0.129757981227273,
2.62224491711744));
#221342=CARTESIAN_POINT('Ctrl Pts',(-58.933985496586,-0.124870896863128,
2.62031533672596));
#221343=CARTESIAN_POINT('Ctrl Pts',(-58.9298018491012,-0.107766101588619,
2.61356180535577));
#221344=CARTESIAN_POINT('Ctrl Pts',(-58.9265158655229,-0.0899051300998722,
2.60825339735346));
#221345=CARTESIAN_POINT('Ctrl Pts',(-58.9242770147326,-0.0715435052823959,
2.60463337987609));
#221346=CARTESIAN_POINT('Ctrl Pts',(-58.9231575893375,-0.0623626928736577,
2.60282337113741));
#221347=CARTESIAN_POINT('Ctrl Pts',(-58.9222999481582,-0.0530567171303812,
2.60143545939113));
#221348=CARTESIAN_POINT('Ctrl Pts',(-58.9217227791368,-0.0436575183852358,
2.60050005034595));
#221349=CARTESIAN_POINT('Ctrl Pts',(-58.9214341946262,-0.0389579190126632,
2.60003234582335));
#221350=CARTESIAN_POINT('Ctrl Pts',(-58.9212157281805,-0.0342350138892673,
2.59967776696063));
#221351=CARTESIAN_POINT('Ctrl Pts',(-58.9210697160839,-0.0294927955546917,
2.59944011429157));
#221352=CARTESIAN_POINT('Ctrl Pts',(-58.9209237039872,-0.024750577220116,
2.59920246162251));
#221353=CARTESIAN_POINT('Ctrl Pts',(-58.9208501479391,-0.0199890456748488,
2.59908173791312));
#221354=CARTESIAN_POINT('Ctrl Pts',(-58.9208513795073,-0.0152121934557294,
2.59908173516023));
#221355=CARTESIAN_POINT('Origin',(5.49031038273072E-15,1.82930781209959E-13,
3.77003198860263));
#221356=CARTESIAN_POINT('',(56.875,1.74857057214726E-13,3.77003198860264));
#221357=CARTESIAN_POINT('',(-56.875,1.8989595988011E-13,3.77003198860262));
#221358=CARTESIAN_POINT('Origin',(5.49031038273072E-15,1.82930781209959E-13,
3.77003198860263));
#221359=CARTESIAN_POINT('',(-56.875,1.8989595988011E-13,3.77003198860262));
#221360=CARTESIAN_POINT('Origin',(5.49031038273072E-15,1.82930781209959E-13,
3.77003198860263));
#221361=CARTESIAN_POINT('Origin',(0.,-8.93279506303506E-14,42.7590319886026));
#221362=CARTESIAN_POINT('',(56.875,1.87678869229944E-13,4.08753198860264));
#221363=CARTESIAN_POINT('',(56.875,-8.23627719602001E-14,42.7590319886026));
#221364=CARTESIAN_POINT('Origin',(5.44560101479317E-15,1.80713690559794E-13,
4.08753198860262));
#221365=CARTESIAN_POINT('Origin',(60.4792282238308,1.82930781209959E-13,
3.77003198860263));
#221366=CARTESIAN_POINT('',(60.1802756340597,-6.00595296980763,3.77003198860259));
#221367=CARTESIAN_POINT('',(60.1803330762808,-6.00537737563893,3.77003198882083));
#221368=CARTESIAN_POINT('Origin',(5.49031038273072E-15,1.82930781209959E-13,
3.77003198860263));
#221369=CARTESIAN_POINT('',(59.7081718144893,-5.95633285891111,3.77003198860259));
#221370=CARTESIAN_POINT('',(59.70870646733,-5.95638905318906,3.77003198860259));
#221371=CARTESIAN_POINT('',(60.0036905223731,-0.317499999999817,3.77003198860263));
#221372=CARTESIAN_POINT('Origin',(5.49031038273072E-15,1.82930781209959E-13,
3.77003198860263));
#221373=CARTESIAN_POINT('',(60.4783948217626,-0.317500000025078,3.77003198860263));
#221374=CARTESIAN_POINT('',(60.4792282238308,-0.317499999999817,3.77003198860263));
#221375=CARTESIAN_POINT('',(60.4783917836885,-0.318078445377671,3.77003198902516));
#221376=CARTESIAN_POINT('Origin',(5.49031038273072E-15,1.82930781209959E-13,
3.77003198860263));
#221377=CARTESIAN_POINT('Origin',(5.49031038273072E-15,1.82930781209959E-13,
3.77003198860263));
#221378=CARTESIAN_POINT('Origin',(5.49031038273072E-15,1.82930781209959E-13,
3.77003198860263));
#221379=CARTESIAN_POINT('',(60.6410923272405,-0.318076890623181,3.48823028058481));
#221380=CARTESIAN_POINT('',(60.3421421673489,-6.02238575972983,3.48823028074801));
#221381=CARTESIAN_POINT('Origin',(5.52999282761009E-15,1.84898592019556E-13,
3.48823028058481));
#221382=CARTESIAN_POINT('',(60.3421421670676,-6.02238575970175,3.48823028058478));
#221383=CARTESIAN_POINT('',(60.4783917829566,-0.318078445373822,3.77003198860263));
#221384=CARTESIAN_POINT('Origin',(60.71525,1.85785428279622E-13,3.36123028058482));
#221385=CARTESIAN_POINT('',(61.0122769227456,-0.317499999999814,3.36123028058482));
#221386=CARTESIAN_POINT('',(60.7112330730305,-6.06175884541469,3.36123028058478));
#221387=CARTESIAN_POINT('Origin',(5.5478765747851E-15,1.85785428279622E-13,
3.36123028058482));
#221388=CARTESIAN_POINT('',(60.5608532912344,-6.0459532934496,3.36123028058478));
#221389=CARTESIAN_POINT('',(60.561380412237,-6.04600869609946,3.36123028058478));
#221390=CARTESIAN_POINT('',(60.8610688070707,-0.317499999999814,3.36123028058482));
#221391=CARTESIAN_POINT('Origin',(5.5478765747851E-15,1.85785428279622E-13,
3.36123028058482));
#221392=CARTESIAN_POINT('',(60.71525,-0.317499999999814,3.36123028058482));
#221393=CARTESIAN_POINT('Origin',(5.5478765747851E-15,1.85785428279622E-13,
3.36123028058482));
#221394=CARTESIAN_POINT('',(61.0917542093525,-6.10232411255987,3.77003198802717));
#221395=CARTESIAN_POINT('',(61.0918106390013,-6.10175915944532,3.77003198860259));
#221396=CARTESIAN_POINT('Origin',(5.49031038273072E-15,1.82930781209959E-13,
3.77003198860263));
#221397=CARTESIAN_POINT('',(60.9299448846691,-6.08531878138219,3.4882302805848));
#221398=CARTESIAN_POINT('',(61.0917542096815,-6.10232411260822,3.77003198860259));
#221399=CARTESIAN_POINT('',(61.2322532923707,-0.316930737397142,3.48823028042695));
#221400=CARTESIAN_POINT('Origin',(5.52999282761008E-15,1.84898592019556E-13,
3.48823028058484));
#221401=CARTESIAN_POINT('',(61.3949537495049,-0.316932243253077,3.77003198802708));
#221402=CARTESIAN_POINT('',(61.2322532920972,-0.316930737395729,3.48823028058484));
#221403=CARTESIAN_POINT('',(61.3949508163454,-0.317499999999817,3.77003198860263));
#221404=CARTESIAN_POINT('Origin',(5.49031038273072E-15,1.82930781209959E-13,
3.77003198860263));
#221405=CARTESIAN_POINT('Origin',(5.49031038273072E-15,1.82930781209959E-13,
3.77003198860263));
#221406=CARTESIAN_POINT('Origin',(62.2224557307631,1.82930781209959E-13,
3.77003198860263));
#221407=CARTESIAN_POINT('',(61.8696548221181,-0.317499999999817,3.77003198860263));
#221408=CARTESIAN_POINT('',(61.5639141665613,-6.15137923967574,3.77003198860259));
#221409=CARTESIAN_POINT('Origin',(5.49031038273072E-15,1.82930781209959E-13,
3.77003198860263));
#221410=CARTESIAN_POINT('',(61.0923331762718,-6.10181408032554,3.77003198860259));
#221411=CARTESIAN_POINT('',(62.2224557307631,-0.317499999999817,3.77003198860263));
#221412=CARTESIAN_POINT('Origin',(5.57972911860581E-15,1.8736496251029E-13,
3.13503198860263));
#221413=CARTESIAN_POINT('Origin',(59.7081714060831,-5.95632779542196,3.13502491541429));
#221414=CARTESIAN_POINT('Origin',(60.0036895869254,-0.317504993060329,3.13502491541433));
#221415=CARTESIAN_POINT('Origin',(5.57972911860581E-15,1.8736496251029E-13,
3.13503198860263));
#221416=CARTESIAN_POINT('Origin',(61.6018378049622,-6.15533145331055,3.2038202287229));
#221417=CARTESIAN_POINT('Origin',(61.9077842377864,-0.317533537011376,3.20381846780282));
#221418=CARTESIAN_POINT('Origin',(5.51210908043506E-15,1.8401175575949E-13,
3.61523028058481));
#221419=CARTESIAN_POINT('Origin',(60.7269085901928,-6.06344346747399,3.58781461834287));
#221420=CARTESIAN_POINT('Origin',(61.0281367271385,-0.317462907478312,3.58786945047018));
#221421=CARTESIAN_POINT('Origin',(5.51210908043507E-15,1.8401175575949E-13,
3.61523028058481));
#221422=CARTESIAN_POINT('Origin',(60.5450849487963,-6.04425010054694,3.58786923593026));
#221423=CARTESIAN_POINT('Origin',(60.8453028802691,-0.317545368445294,3.5878144026637));
#221424=CARTESIAN_POINT('Origin',(60.4792282238308,1.82930781209959E-13,
3.77003198860263));
#221425=CARTESIAN_POINT('',(58.7584778814678,-12.1649068885782,3.77003198860255));
#221426=CARTESIAN_POINT('',(59.6417962403144,-6.58785426246997,3.77003198860259));
#221427=CARTESIAN_POINT('Origin',(5.49031038273072E-15,1.82930781209959E-13,
3.77003198860263));
#221428=CARTESIAN_POINT('',(60.1139000598801,-6.63747437341682,3.77003198860259));
#221429=CARTESIAN_POINT('',(59.7852323155142,-6.60293000146336,3.77003198860259));
#221430=CARTESIAN_POINT('',(60.1138365744454,-6.63804933242006,3.77003198902532));
#221431=CARTESIAN_POINT('Origin',(5.49031038273072E-15,1.82930781209959E-13,
3.77003198860263));
#221432=CARTESIAN_POINT('',(59.2229260464988,-12.2630370254214,3.77003198882079));
#221433=CARTESIAN_POINT('Origin',(5.49031038273072E-15,1.82930781209959E-13,
3.77003198860263));
#221434=CARTESIAN_POINT('',(59.2228087529784,-12.2636034620779,3.77003198860255));
#221435=CARTESIAN_POINT('Origin',(5.49031038273072E-15,1.82930781209959E-13,
3.77003198860263));
#221436=CARTESIAN_POINT('',(58.7590037315227,-12.1650186614579,3.77003198860255));
#221437=CARTESIAN_POINT('Origin',(5.49031038273072E-15,1.82930781209959E-13,
3.77003198860263));
#221438=CARTESIAN_POINT('',(60.275645989912,-6.65505462397295,3.48823028058477));
#221439=CARTESIAN_POINT('',(60.1138365737176,-6.6380493323397,3.77003198860259));
#221440=CARTESIAN_POINT('',(59.3820708701841,-12.2968658914367,3.48823028074797));
#221441=CARTESIAN_POINT('Origin',(5.52999282761009E-15,1.84898592019556E-13,
3.48823028058481));
#221442=CARTESIAN_POINT('',(59.3820708699072,-12.2968658913794,3.48823028058473));
#221443=CARTESIAN_POINT('Origin',(60.71525,1.85785428279622E-13,3.36123028058482));
#221444=CARTESIAN_POINT('',(59.5971203935661,-12.3431658574201,3.36123028058474));
#221445=CARTESIAN_POINT('',(60.4944777170595,-6.67747469700845,3.36123028058478));
#221446=CARTESIAN_POINT('Origin',(5.5478765747851E-15,1.85785428279622E-13,
3.36123028058482));
#221447=CARTESIAN_POINT('',(60.6448574988555,-6.69328024897355,3.36123028058478));
#221448=CARTESIAN_POINT('',(60.0186752706393,-6.62746584473993,3.36123028058478));
#221449=CARTESIAN_POINT('',(59.7450242491249,-12.3746037924155,3.36123028058474));
#221450=CARTESIAN_POINT('Origin',(5.5478765747851E-15,1.85785428279622E-13,
3.36123028058482));
#221451=CARTESIAN_POINT('',(59.5976388357908,-12.3432760557168,3.36123028058474));
#221452=CARTESIAN_POINT('Origin',(5.5478765747851E-15,1.85785428279622E-13,
3.36123028058482));
#221453=CARTESIAN_POINT('',(59.9600752506739,-12.4208962741577,3.48823028058476));
#221454=CARTESIAN_POINT('',(60.8636883190564,-6.71570789672308,3.48823028042691));
#221455=CARTESIAN_POINT('Origin',(5.52999282761008E-15,1.84898592019556E-13,
3.48823028058484));
#221456=CARTESIAN_POINT('',(61.025497328658,-6.73271622308696,3.77003198802703));
#221457=CARTESIAN_POINT('',(60.8636883187846,-6.71570789669309,3.4882302805848));
#221458=CARTESIAN_POINT('',(61.0254350648263,-6.73328056300417,3.77003198860259));
#221459=CARTESIAN_POINT('Origin',(5.49031038273072E-15,1.82930781209959E-13,
3.77003198860263));
#221460=CARTESIAN_POINT('',(60.119335800013,-12.4541661686656,3.77003198860255));
#221461=CARTESIAN_POINT('Origin',(5.49031038273072E-15,1.82930781209959E-13,
3.77003198860263));
#221462=CARTESIAN_POINT('',(60.1192206258109,-12.4547221284034,3.77003198802712));
#221463=CARTESIAN_POINT('Origin',(5.49031038273072E-15,1.82930781209959E-13,
3.77003198860263));
#221464=CARTESIAN_POINT('',(60.1192206261331,-12.4547221284859,3.77003198860255));
#221465=CARTESIAN_POINT('Origin',(62.2224557307631,1.82930781209959E-13,
3.77003198860263));
#221466=CARTESIAN_POINT('',(61.4975385923863,-6.78290064323459,3.77003198860259));
#221467=CARTESIAN_POINT('',(61.5094129706999,-6.78414869068649,3.77003198860259));
#221468=CARTESIAN_POINT('',(60.5836663843183,-12.5528626811438,3.77003198860255));
#221469=CARTESIAN_POINT('Origin',(5.49031038273072E-15,1.82930781209959E-13,
3.77003198860263));
#221470=CARTESIAN_POINT('',(60.1198497339745,-12.4542754087014,3.77003198860255));
#221471=CARTESIAN_POINT('Origin',(5.57972911860581E-15,1.8736496251029E-13,
3.13503198860263));
#221472=CARTESIAN_POINT('Origin',(59.6417947880742,-6.58785913039715,3.13502491541431));
#221473=CARTESIAN_POINT('Origin',(58.7584780045776,-12.1649018101373,3.13502491541426));
#221474=CARTESIAN_POINT('Origin',(5.57972911860581E-15,1.8736496251029E-13,
3.13503198860263));
#221475=CARTESIAN_POINT('Origin',(61.5354556255543,-6.78691960575202,3.20381846780361));
#221476=CARTESIAN_POINT('Origin',(60.6209691542414,-12.5607573437831,3.20382022872141));
#221477=CARTESIAN_POINT('Origin',(5.51210908043506E-15,1.8401175575949E-13,
3.61523028058481));
#221478=CARTESIAN_POINT('Origin',(60.6606342988055,-6.69490116062973,3.5878694504686));
#221479=CARTESIAN_POINT('Origin',(59.7604378032109,-12.3779177236591,3.58781461833967));
#221480=CARTESIAN_POINT('Origin',(5.51210908043507E-15,1.8401175575949E-13,
3.61523028058481));
#221481=CARTESIAN_POINT('Origin',(60.4787934153613,-6.67587182881982,3.58781440266453));
#221482=CARTESIAN_POINT('Origin',(59.5816164638954,-12.3398237541814,3.58786923593063));
#221483=CARTESIAN_POINT('Origin',(60.4792282238308,1.82930781209959E-13,
3.77003198860263));
#221484=CARTESIAN_POINT('',(57.1650137687749,-18.2401996527036,3.77003198860251));
#221485=CARTESIAN_POINT('',(58.6264539577985,-12.7860306150442,3.77003198860254));
#221486=CARTESIAN_POINT('Origin',(5.49031038273072E-15,1.82930781209959E-13,
3.77003198860263));
#221487=CARTESIAN_POINT('',(59.0907848292992,-12.8847271885934,3.77003198860255));
#221488=CARTESIAN_POINT('',(57.7988642628865,-12.6101209950201,3.77003198860255));
#221489=CARTESIAN_POINT('',(59.0906615920636,-12.8852923618762,3.77003198902547));
#221490=CARTESIAN_POINT('Origin',(5.49031038273072E-15,1.82930781209959E-13,
3.77003198860263));
#221491=CARTESIAN_POINT('',(57.6166602457575,-18.3863402753478,3.77003198882074));
#221492=CARTESIAN_POINT('Origin',(5.49031038273072E-15,1.82930781209959E-13,
3.77003198860263));
#221493=CARTESIAN_POINT('',(57.6164843860299,-18.3868913484936,3.77003198860251));
#221494=CARTESIAN_POINT('Origin',(5.49031038273072E-15,1.82930781209959E-13,
3.77003198860263));
#221495=CARTESIAN_POINT('',(57.1655250547209,-18.2403657795778,3.77003198860251));
#221496=CARTESIAN_POINT('Origin',(5.49031038273072E-15,1.82930781209959E-13,
3.77003198860263));
#221497=CARTESIAN_POINT('',(59.2498070616281,-12.9191181862036,3.48823028058473));
#221498=CARTESIAN_POINT('',(59.0906615913479,-12.8852923617202,3.77003198860254));
#221499=CARTESIAN_POINT('',(57.7713971780683,-18.4366189871523,3.48823028074793));
#221500=CARTESIAN_POINT('Origin',(5.52999282761009E-15,1.84898592019556E-13,
3.48823028058481));
#221501=CARTESIAN_POINT('',(57.771397177799,-18.4366189870664,3.48823028058469));
#221502=CARTESIAN_POINT('Origin',(60.71525,1.85785428279622E-13,3.36123028058482));
#221503=CARTESIAN_POINT('',(57.9804289733666,-18.5051441132832,3.36123028058469));
#221504=CARTESIAN_POINT('',(59.4650964698968,-12.9642895838861,3.36123028058473));
#221505=CARTESIAN_POINT('Origin',(5.5478765747851E-15,1.85785428279622E-13,
3.36123028058482));
#221506=CARTESIAN_POINT('',(59.6130003254557,-12.9957275188814,3.36123028058473));
#221507=CARTESIAN_POINT('',(58.0246834617332,-12.6581203474861,3.36123028058474));
#221508=CARTESIAN_POINT('',(58.1242364370959,-18.5518699907141,3.36123028058469));
#221509=CARTESIAN_POINT('Origin',(5.5478765747851E-15,1.85785428279622E-13,
3.36123028058482));
#221510=CARTESIAN_POINT('',(57.9809330566519,-18.5053078998711,3.36123028058469));
#221511=CARTESIAN_POINT('Origin',(5.5478765747851E-15,1.85785428279622E-13,
3.36123028058482));
#221512=CARTESIAN_POINT('',(58.3332704847798,-18.6203878281138,3.48823028058472));
#221513=CARTESIAN_POINT('',(59.8282880399729,-13.0409063549811,3.48823028042686));
#221514=CARTESIAN_POINT('Origin',(5.52999282761008E-15,1.84898592019556E-13,
3.48823028058484));
#221515=CARTESIAN_POINT('',(59.9874327886719,-13.0747351550701,3.77003198802699));
#221516=CARTESIAN_POINT('',(59.8282880397057,-13.0409063549229,3.48823028058476));
#221517=CARTESIAN_POINT('',(59.9873118763437,-13.0752898951316,3.77003198860254));
#221518=CARTESIAN_POINT('Origin',(5.49031038273072E-15,1.82930781209959E-13,
3.77003198860263));
#221519=CARTESIAN_POINT('',(58.48818093722,-18.6701227271401,3.77003198860251));
#221520=CARTESIAN_POINT('Origin',(5.49031038273072E-15,1.82930781209959E-13,
3.77003198860263));
#221521=CARTESIAN_POINT('',(58.4880082803372,-18.6706636022899,3.77003198802708));
#221522=CARTESIAN_POINT('Origin',(5.49031038273072E-15,1.82930781209959E-13,
3.77003198860263));
#221523=CARTESIAN_POINT('',(58.488008280649,-18.6706636024057,3.77003198860251));
#221524=CARTESIAN_POINT('Origin',(62.2224557307631,1.82930781209959E-13,
3.77003198860263));
#221525=CARTESIAN_POINT('',(60.4516424606491,-13.1739864076097,3.77003198860254));
#221526=CARTESIAN_POINT('',(59.4667368016504,-12.9646382471636,3.77003198860254));
#221527=CARTESIAN_POINT('',(58.9396512752216,-18.8168143322217,3.7700319886025));
#221528=CARTESIAN_POINT('Origin',(5.49031038273072E-15,1.82930781209959E-13,
3.77003198860263));
#221529=CARTESIAN_POINT('',(58.4886806371044,-18.6702850894748,3.77003198860251));
#221530=CARTESIAN_POINT('Origin',(5.57972911860581E-15,1.8736496251029E-13,
3.13503198860263));
#221531=CARTESIAN_POINT('Origin',(58.626452004677,-12.7860353045039,3.13502491541425));
#221532=CARTESIAN_POINT('Origin',(57.165014422052,-18.2401946149514,3.13502491541418));
#221533=CARTESIAN_POINT('Origin',(5.57972911860581E-15,1.8736496251029E-13,
3.13503198860263));
#221534=CARTESIAN_POINT('Origin',(60.4889316843639,-13.1819467630394,3.20381846779961));
#221535=CARTESIAN_POINT('Origin',(58.9759244797151,-18.8285649482862,3.20382022872155));
#221536=CARTESIAN_POINT('Origin',(5.51210908043506E-15,1.8401175575949E-13,
3.61523028058481));
#221537=CARTESIAN_POINT('Origin',(59.6285212670395,-12.9989886756678,3.58786945047026));
#221538=CARTESIAN_POINT('Origin',(58.1392191539775,-18.5567769230171,3.58781461834326));
#221539=CARTESIAN_POINT('Origin',(5.51210908043507E-15,1.8401175575949E-13,
3.61523028058481));
#221540=CARTESIAN_POINT('Origin',(59.4496656337939,-12.9610560404244,3.58781440266666));
#221541=CARTESIAN_POINT('Origin',(57.9653593207604,-18.5001997164921,3.5878692359305));
#221542=CARTESIAN_POINT('Origin',(60.4792282238308,1.82930781209959E-13,
3.77003198860263));
#221543=CARTESIAN_POINT('',(54.9452378026832,-24.1156489724268,3.77003198860246));
#221544=CARTESIAN_POINT('',(56.9687879773468,-18.844120540551,3.7700319886025));
#221545=CARTESIAN_POINT('Origin',(5.49031038273072E-15,1.82930781209959E-13,
3.77003198860263));
#221546=CARTESIAN_POINT('',(57.4202585945868,-18.9908122363893,3.7700319886025));
#221547=CARTESIAN_POINT('',(54.6058629360818,-18.0763596539221,3.77003198860251));
#221548=CARTESIAN_POINT('',(57.4200769557625,-18.9913614317947,3.77003198902511));
#221549=CARTESIAN_POINT('Origin',(5.49031038273072E-15,1.82930781209959E-13,
3.77003198860263));
#221550=CARTESIAN_POINT('',(55.3791342583023,-24.3081989336284,3.7700319888207));
#221551=CARTESIAN_POINT('Origin',(5.49031038273072E-15,1.82930781209959E-13,
3.77003198860263));
#221552=CARTESIAN_POINT('',(55.3789017591236,-24.3087286055908,3.77003198860246));
#221553=CARTESIAN_POINT('Origin',(5.49031038273072E-15,1.82930781209959E-13,
3.77003198860263));
#221554=CARTESIAN_POINT('',(54.9457289227643,-24.1158676331749,3.77003198860246));
#221555=CARTESIAN_POINT('Origin',(5.49031038273072E-15,1.82930781209959E-13,
3.77003198860263));
#221556=CARTESIAN_POINT('',(57.5748148483578,-19.0416371860869,3.48823028058469));
#221557=CARTESIAN_POINT('',(57.4200769550675,-18.9913614315648,3.7700319886025));
#221558=CARTESIAN_POINT('',(55.5277679690275,-24.3743766271342,3.48823028074788));
#221559=CARTESIAN_POINT('Origin',(5.52999282761009E-15,1.84898592019556E-13,
3.48823028058481));
#221560=CARTESIAN_POINT('',(55.5277679687686,-24.3743766270205,3.48823028058465));
#221561=CARTESIAN_POINT('Origin',(60.71525,1.85785428279622E-13,3.36123028058482));
#221562=CARTESIAN_POINT('',(55.7284918401501,-24.4643761377908,3.36123028058465));
#221563=CARTESIAN_POINT('',(57.7842031819385,-19.1090650011306,3.36123028058469));
#221564=CARTESIAN_POINT('Origin',(5.5478765747851E-15,1.85785428279622E-13,
3.36123028058482));
#221565=CARTESIAN_POINT('',(57.9280106456678,-19.1557908785616,3.36123028058469));
#221566=CARTESIAN_POINT('',(54.8193466381482,-18.1457247135482,3.36123028058469));
#221567=CARTESIAN_POINT('',(55.8666273273836,-24.5258780191662,3.36123028058465));
#221568=CARTESIAN_POINT('Origin',(5.5478765747851E-15,1.85785428279622E-13,
3.36123028058482));
#221569=CARTESIAN_POINT('',(55.7289760416541,-24.4645917181899,3.36123028058465));
#221570=CARTESIAN_POINT('Origin',(5.5478765747851E-15,1.85785428279622E-13,
3.36123028058482));
#221571=CARTESIAN_POINT('',(56.0673542004329,-24.6158705164585,3.48823028058468));
#221572=CARTESIAN_POINT('',(58.1373965172492,-19.2232259142289,3.48823028042681));
#221573=CARTESIAN_POINT('Origin',(5.52999282761008E-15,1.84898592019556E-13,
3.48823028058484));
#221574=CARTESIAN_POINT('',(58.2921333818759,-19.27350455263,3.77003198802694));
#221575=CARTESIAN_POINT('',(58.1373965169896,-19.223225914143,3.48823028058471));
#221576=CARTESIAN_POINT('',(58.2919551457919,-19.2740436149875,3.7700319886025));
#221577=CARTESIAN_POINT('Origin',(5.49031038273072E-15,1.82930781209959E-13,
3.77003198860263));
#221578=CARTESIAN_POINT('',(56.2162173246401,-24.6815255140418,3.77003198860246));
#221579=CARTESIAN_POINT('Origin',(5.49031038273072E-15,1.82930781209959E-13,
3.77003198860263));
#221580=CARTESIAN_POINT('',(56.2159890767415,-24.6820453786623,3.77003198802704));
#221581=CARTESIAN_POINT('Origin',(5.49031038273072E-15,1.82930781209959E-13,
3.77003198860263));
#221582=CARTESIAN_POINT('',(56.2159890770395,-24.68204537881,3.77003198860246));
#221583=CARTESIAN_POINT('Origin',(62.2224557307631,1.82930781209959E-13,
3.77003198860263));
#221584=CARTESIAN_POINT('',(58.7434254837935,-19.4207352200692,3.7700319886025));
#221585=CARTESIAN_POINT('',(56.182627028633,-18.5886813639048,3.77003198860251));
#221586=CARTESIAN_POINT('',(56.6498810128385,-24.8746050278044,3.77003198860246));
#221587=CARTESIAN_POINT('Origin',(5.49031038273072E-15,1.82930781209959E-13,
3.77003198860263));
#221588=CARTESIAN_POINT('',(56.2166973156309,-24.6817392197996,3.77003198860246));
#221589=CARTESIAN_POINT('Origin',(5.57972911860581E-15,1.8736496251029E-13,
3.13503198860263));
#221590=CARTESIAN_POINT('Origin',(56.9687855447427,-18.8441250001647,3.13502491541417));
#221591=CARTESIAN_POINT('Origin',(54.94523897897,-24.115644030558,3.1350249154142));
#221592=CARTESIAN_POINT('Origin',(5.57972911860581E-15,1.8736496251029E-13,
3.13503198860263));
#221593=CARTESIAN_POINT('Origin',(58.7796783495195,-19.4325497530921,3.20381846780104));
#221594=CARTESIAN_POINT('Origin',(56.6847272350835,-24.8900828550879,3.20382022872263));
#221595=CARTESIAN_POINT('Origin',(5.51210908043506E-15,1.8401175575949E-13,
3.61523028058481));
#221596=CARTESIAN_POINT('Origin',(57.943105678202,-19.1606565505621,3.58786945047092));
#221597=CARTESIAN_POINT('Origin',(55.8810150532823,-24.5323241911522,3.58781461834182));
#221598=CARTESIAN_POINT('Origin',(5.51210908043507E-15,1.8401175575949E-13,
3.61523028058481));
#221599=CARTESIAN_POINT('Origin',(57.7691948748979,-19.1042362097742,3.58781440266462));
#221600=CARTESIAN_POINT('Origin',(55.7140215708763,-24.4578836192926,3.58786923593034));
#221601=CARTESIAN_POINT('Origin',(60.4792282238308,1.82930781209959E-13,
3.77003198860263));
#221602=CARTESIAN_POINT('',(52.123470313195,-29.7268821954841,3.77003198860243));
#221603=CARTESIAN_POINT('',(54.68696003433,-24.6957503380299,3.77003198860246));
#221604=CARTESIAN_POINT('Origin',(5.49031038273072E-15,1.82930781209959E-13,
3.77003198860263));
#221605=CARTESIAN_POINT('',(55.1206239907505,-24.8888299712403,3.77003198860246));
#221606=CARTESIAN_POINT('',(50.3447265545032,-22.7624634345039,3.77003198860247));
#221607=CARTESIAN_POINT('',(55.1203859404112,-24.8893571716688,3.77003198902525));
#221608=CARTESIAN_POINT('Origin',(5.49031038273072E-15,1.82930781209959E-13,
3.77003198860263));
#221609=CARTESIAN_POINT('',(52.5348628870842,-29.9637318775746,3.77003198882067));
#221610=CARTESIAN_POINT('Origin',(5.49031038273072E-15,1.82930781209959E-13,
3.77003198860263));
#221611=CARTESIAN_POINT('',(52.5345762957642,-29.9642343451567,3.77003198860242));
#221612=CARTESIAN_POINT('Origin',(5.49031038273072E-15,1.82930781209959E-13,
3.77003198860263));
#221613=CARTESIAN_POINT('',(52.123935886597,-29.7271509944131,3.77003198860243));
#221614=CARTESIAN_POINT('Origin',(5.49031038273072E-15,1.82930781209959E-13,
3.77003198860263));
#221615=CARTESIAN_POINT('',(55.2690209153043,-24.9555320242407,3.48823028058464));
#221616=CARTESIAN_POINT('',(55.1203859397437,-24.8893571713674,3.77003198860246));
#221617=CARTESIAN_POINT('',(52.6757649141856,-30.0450834961229,3.48823028074784));
#221618=CARTESIAN_POINT('Origin',(5.52999282761009E-15,1.84898592019556E-13,
3.48823028058481));
#221619=CARTESIAN_POINT('',(52.67576491394,-30.0450834959828,3.48823028058461));
#221620=CARTESIAN_POINT('Origin',(60.71525,1.85785428279622E-13,3.36123028058482));
#221621=CARTESIAN_POINT('',(52.8659816883963,-30.1555713378329,3.36123028058461));
#221622=CARTESIAN_POINT('',(55.470214071797,-25.0444775033939,3.36123028058465));
#221623=CARTESIAN_POINT('Origin',(5.5478765747851E-15,1.85785428279622E-13,
3.36123028058482));
#221624=CARTESIAN_POINT('',(55.6083495590305,-25.1059793847693,3.36123028058465));
#221625=CARTESIAN_POINT('',(50.5417021396889,-22.850162615334,3.36123028058466));
#221626=CARTESIAN_POINT('',(52.9969317578291,-30.2311753956704,3.36123028058461));
#221627=CARTESIAN_POINT('Origin',(5.5478765747851E-15,1.85785428279622E-13,
3.36123028058482));
#221628=CARTESIAN_POINT('',(52.866440703106,-30.1558363500991,3.36123028058461));
#221629=CARTESIAN_POINT('Origin',(5.5478765747851E-15,1.85785428279622E-13,
3.36123028058482));
#221630=CARTESIAN_POINT('',(53.1871522506179,-30.3416565762228,3.48823028058463));
#221631=CARTESIAN_POINT('',(55.8095395122503,-25.1949317876417,3.48823028042678));
#221632=CARTESIAN_POINT('Origin',(5.52999282761008E-15,1.84898592019556E-13,
3.48823028058484));
#221633=CARTESIAN_POINT('',(55.9581731633348,-25.2611094010713,3.7700319880269));
#221634=CARTESIAN_POINT('',(55.809539512001,-25.1949317875292,3.48823028058467));
#221635=CARTESIAN_POINT('',(55.9579395562869,-25.2616268796448,3.77003198860246));
#221636=CARTESIAN_POINT('Origin',(5.49031038273072E-15,1.82930781209959E-13,
3.77003198860263));
#221637=CARTESIAN_POINT('',(53.3283370710516,-30.4225123424703,3.77003198860242));
#221638=CARTESIAN_POINT('Origin',(5.49031038273072E-15,1.82930781209959E-13,
3.77003198860263));
#221639=CARTESIAN_POINT('',(53.328055732869,-30.4230055008159,3.770031988027));
#221640=CARTESIAN_POINT('Origin',(5.49031038273072E-15,1.82930781209959E-13,
3.77003198860263));
#221641=CARTESIAN_POINT('',(53.32805573315,-30.4230055009939,3.77003198860242));
#221642=CARTESIAN_POINT('Origin',(62.2224557307631,1.82930781209959E-13,
3.77003198860263));
#221643=CARTESIAN_POINT('',(56.3916032444854,-25.4547063934074,3.77003198860246));
#221644=CARTESIAN_POINT('',(51.7995637473369,-23.4101986852072,3.77003198860247));
#221645=CARTESIAN_POINT('',(53.7394427993291,-30.6598643453566,3.77003198860242));
#221646=CARTESIAN_POINT('Origin',(5.49031038273072E-15,1.82930781209959E-13,
3.77003198860263));
#221647=CARTESIAN_POINT('',(53.3287920942672,-30.4227750502462,3.77003198860242));
#221648=CARTESIAN_POINT('Origin',(5.57972911860581E-15,1.8736496251029E-13,
3.13503198860263));
#221649=CARTESIAN_POINT('Origin',(54.6869571488954,-24.6957545189369,3.13502491541414));
#221650=CARTESIAN_POINT('Origin',(52.1234719996039,-29.7268774036429,3.13502491541413));
#221651=CARTESIAN_POINT('Origin',(5.57972911860581E-15,1.8736496251029E-13,
3.13503198860263));
#221652=CARTESIAN_POINT('Origin',(56.426422558239,-25.470245661524,3.20381846780071));
#221653=CARTESIAN_POINT('Origin',(53.7724802568203,-30.6788998055451,3.20382022872057));
#221654=CARTESIAN_POINT('Origin',(5.51210908043506E-15,1.8401175575949E-13,
3.61523028058481));
#221655=CARTESIAN_POINT('Origin',(55.6228532981809,-25.1123962626636,3.58786945046893));
#221656=CARTESIAN_POINT('Origin',(53.0105668578093,-30.2390901817304,3.58781461833926));
#221657=CARTESIAN_POINT('Origin',(5.51210908043507E-15,1.8401175575949E-13,
3.61523028058481));
#221658=CARTESIAN_POINT('Origin',(55.4557927279746,-25.0381063693869,3.5878144026651));
#221659=CARTESIAN_POINT('Origin',(52.8522693417503,-30.1476018310214,3.58786923592679));
#221660=CARTESIAN_POINT('Origin',(60.4792282238308,1.82930781209959E-13,
3.77003198860263));
#221661=CARTESIAN_POINT('',(48.7306271754181,-35.0124214764577,3.77003198860239));
#221662=CARTESIAN_POINT('',(51.805970313195,-30.2768083268872,3.77003198860242));
#221663=CARTESIAN_POINT('Origin',(5.49031038273072E-15,1.82930781209959E-13,
3.77003198860263));
#221664=CARTESIAN_POINT('',(52.2170762957395,-30.5141604766039,3.77003198860242));
#221665=CARTESIAN_POINT('',(45.2006711678738,-26.4632370872581,3.77003198860245));
#221666=CARTESIAN_POINT('',(52.2167844420142,-30.5146599059371,3.77003198902529));
#221667=CARTESIAN_POINT('Origin',(5.49031038273072E-15,1.82930781209959E-13,
3.77003198860263));
#221668=CARTESIAN_POINT('',(49.1150085644485,-35.2909759047561,3.77003198882063));
#221669=CARTESIAN_POINT('Origin',(5.49031038273072E-15,1.82930781209959E-13,
3.77003198860263));
#221670=CARTESIAN_POINT('',(49.1146710209414,-35.2914456628179,3.77003198860239));
#221671=CARTESIAN_POINT('Origin',(5.49031038273072E-15,1.82930781209959E-13,
3.77003198860263));
#221672=CARTESIAN_POINT('',(48.7310621012213,-35.0127374685503,3.77003198860239));
#221673=CARTESIAN_POINT('Origin',(5.49031038273072E-15,1.82930781209959E-13,
3.77003198860263));
#221674=CARTESIAN_POINT('',(52.3576880233166,-30.596008831256,3.48823028058461));
#221675=CARTESIAN_POINT('',(52.2167844413819,-30.5146599055676,3.77003198860242));
#221676=CARTESIAN_POINT('',(49.2466351558313,-35.3866101429902,3.4882302807478));
#221677=CARTESIAN_POINT('Origin',(5.52999282761009E-15,1.84898592019556E-13,
3.48823028058481));
#221678=CARTESIAN_POINT('',(49.2466351556017,-35.3866101428252,3.48823028058457));
#221679=CARTESIAN_POINT('Origin',(60.71525,1.85785428279622E-13,3.36123028058482));
#221680=CARTESIAN_POINT('',(49.4242607783465,-35.5163757878388,3.36123028058458));
#221681=CARTESIAN_POINT('',(52.5484816883963,-30.7054974692361,3.36123028058461));
#221682=CARTESIAN_POINT('Origin',(5.5478765747851E-15,1.85785428279622E-13,
3.36123028058482));
#221683=CARTESIAN_POINT('',(52.6794317578291,-30.7811015270735,3.36123028058461));
#221684=CARTESIAN_POINT('',(45.3776875000007,-26.5654375142626,3.36123028058464));
#221685=CARTESIAN_POINT('',(49.5465907136149,-35.6052536882594,3.36123028058457));
#221686=CARTESIAN_POINT('Origin',(5.5478765747851E-15,1.85785428279622E-13,
3.36123028058482));
#221687=CARTESIAN_POINT('',(49.4246895772007,-35.5166873284423,3.36123028058458));
#221688=CARTESIAN_POINT('Origin',(5.5478765747851E-15,1.85785428279622E-13,
3.36123028058482));
#221689=CARTESIAN_POINT('',(49.7242207306179,-35.7350130971381,3.4882302805846));
#221690=CARTESIAN_POINT('',(52.8702215134581,-30.8905967160107,3.48823028042674));
#221691=CARTESIAN_POINT('Origin',(5.52999282761008E-15,1.84898592019556E-13,
3.48823028058484));
#221692=CARTESIAN_POINT('',(53.0111234896157,-30.9719482486873,3.77003198802686));
#221693=CARTESIAN_POINT('',(52.870221513222,-30.8905967158728,3.48823028058463));
#221694=CARTESIAN_POINT('',(53.0108370710516,-30.9724384738734,3.77003198860242));
#221695=CARTESIAN_POINT('Origin',(5.49031038273072E-15,1.82930781209959E-13,
3.77003198860263));
#221696=CARTESIAN_POINT('',(49.8561803968407,-35.8301837593547,3.77003198860238));
#221697=CARTESIAN_POINT('Origin',(5.49031038273072E-15,1.82930781209959E-13,
3.77003198860263));
#221698=CARTESIAN_POINT('',(49.8558490507741,-35.8306448082795,3.77003198802696));
#221699=CARTESIAN_POINT('Origin',(5.49031038273072E-15,1.82930781209959E-13,
3.77003198860263));
#221700=CARTESIAN_POINT('',(49.8558490510349,-35.8306448084859,3.77003198860238));
#221701=CARTESIAN_POINT('Origin',(62.2224557307631,1.82930781209959E-13,
3.77003198860263));
#221702=CARTESIAN_POINT('',(53.4219427993291,-31.2097904767597,3.77003198860242));
#221703=CARTESIAN_POINT('',(46.508091798073,-27.2180767400477,3.77003198860244));
#221704=CARTESIAN_POINT('',(50.2402240048087,-36.1092077731521,3.77003198860238));
#221705=CARTESIAN_POINT('Origin',(5.49031038273072E-15,1.82930781209959E-13,
3.77003198860263));
#221706=CARTESIAN_POINT('',(49.8566054669514,-35.8304925908675,3.77003198860238));
#221707=CARTESIAN_POINT('Origin',(5.57972911860581E-15,1.8736496251029E-13,
3.13503198860263));
#221708=CARTESIAN_POINT('Origin',(51.8059670065433,-30.2768121832808,3.13502491541412));
#221709=CARTESIAN_POINT('Origin',(48.7306293534724,-35.0124168871445,3.13502491541408));
#221710=CARTESIAN_POINT('Origin',(5.57972911860581E-15,1.8736496251029E-13,
3.13503198860263));
#221711=CARTESIAN_POINT('Origin',(53.4549470734263,-31.2288842284957,3.20381846780449));
#221712=CARTESIAN_POINT('Origin',(50.2710907322482,-36.1315923097636,3.20382022872168));
#221713=CARTESIAN_POINT('Origin',(5.51210908043506E-15,1.8401175575949E-13,
3.61523028058481));
#221714=CARTESIAN_POINT('Origin',(52.6931852975928,-30.7889993062039,3.5878694504706));
#221715=CARTESIAN_POINT('Origin',(49.5593237986642,-35.614550372339,3.58781461834505));
#221716=CARTESIAN_POINT('Origin',(5.51210908043507E-15,1.8401175575949E-13,
3.61523028058481));
#221717=CARTESIAN_POINT('Origin',(52.5348053110524,-30.6976537960595,3.58781440266643));
#221718=CARTESIAN_POINT('Origin',(49.4114565896706,-35.5070166082985,3.58786923592949));
#221719=CARTESIAN_POINT('Origin',(60.4792282238308,1.82930781209959E-13,
3.77003198860263));
#221720=CARTESIAN_POINT('',(44.8038810887679,-39.914357340915,3.77003198860236));
#221721=CARTESIAN_POINT('',(48.3573835402124,-35.5261472678858,3.77003198860239));
#221722=CARTESIAN_POINT('Origin',(5.49031038273072E-15,1.82930781209959E-13,
3.77003198860263));
#221723=CARTESIAN_POINT('',(48.7414273857065,-35.8051714542873,3.77003198860238));
#221724=CARTESIAN_POINT('',(39.3975469582356,-29.0164449471017,3.77003198860243));
#221725=CARTESIAN_POINT('',(48.7410849262051,-35.8056376406725,3.77003198902474));
#221726=CARTESIAN_POINT('Origin',(5.49031038273072E-15,1.82930781209959E-13,
3.77003198860263));
#221727=CARTESIAN_POINT('',(45.1570399300043,-40.2315646148135,3.77003198882059));
#221728=CARTESIAN_POINT('Origin',(5.49031038273072E-15,1.82930781209959E-13,
3.77003198860263));
#221729=CARTESIAN_POINT('',(45.1566551325076,-40.2319965165875,3.77003198860235));
#221730=CARTESIAN_POINT('Origin',(5.49031038273072E-15,1.82930781209959E-13,
3.77003198860263));
#221731=CARTESIAN_POINT('',(44.8042806018342,-39.9147170640957,3.77003198860236));
#221732=CARTESIAN_POINT('Origin',(5.49031038273072E-15,1.82930781209959E-13,
3.77003198860263));
#221733=CARTESIAN_POINT('',(48.8727133447948,-35.9012693628897,3.48823028058457));
#221734=CARTESIAN_POINT('',(48.7410849256156,-35.8056376402393,3.77003198860238));
#221735=CARTESIAN_POINT('',(45.2779489571888,-40.3404336840066,3.48823028074777));
#221736=CARTESIAN_POINT('Origin',(5.52999282761009E-15,1.84898592019556E-13,
3.48823028058481));
#221737=CARTESIAN_POINT('',(45.2779489569777,-40.3404336838186,3.48823028058454));
#221738=CARTESIAN_POINT('Origin',(60.71525,1.85785428279622E-13,3.36123028058482));
#221739=CARTESIAN_POINT('',(45.4410373245177,-40.4880553924336,3.36123028058454));
#221740=CARTESIAN_POINT('',(49.0510171431408,-36.0301015792669,3.36123028058457));
#221741=CARTESIAN_POINT('Origin',(5.5478765747851E-15,1.85785428279622E-13,
3.36123028058482));
#221742=CARTESIAN_POINT('',(49.1733470784092,-36.1189794796875,3.36123028058457));
#221743=CARTESIAN_POINT('',(39.5520252162596,-29.1286799712083,3.36123028058462));
#221744=CARTESIAN_POINT('',(45.5534068532516,-40.5892333705615,3.36123028058454));
#221745=CARTESIAN_POINT('Origin',(5.5478765747851E-15,1.85785428279622E-13,
3.36123028058482));
#221746=CARTESIAN_POINT('',(45.4414312095063,-40.4884100480704,3.36123028058454));
#221747=CARTESIAN_POINT('Origin',(5.5478765747851E-15,1.85785428279622E-13,
3.36123028058482));
#221748=CARTESIAN_POINT('',(45.7165002428312,-40.736849336529,3.48823028058456));
#221749=CARTESIAN_POINT('',(49.3516463039594,-36.2478178024862,3.48823028042671));
#221750=CARTESIAN_POINT('Origin',(5.52999282761008E-15,1.84898592019556E-13,
3.48823028058484));
#221751=CARTESIAN_POINT('',(49.4832728536536,-36.3434519499939,3.77003198802682));
#221752=CARTESIAN_POINT('',(49.351646303739,-36.2478178023243,3.48823028058459));
#221753=CARTESIAN_POINT('',(49.482936761635,-36.3439095507828,3.77003198860238));
#221754=CARTESIAN_POINT('Origin',(5.49031038273072E-15,1.82930781209959E-13,
3.77003198860263));
#221755=CARTESIAN_POINT('',(45.8377889771256,-40.8452921850237,3.77003198860235));
#221756=CARTESIAN_POINT('Origin',(5.49031038273072E-15,1.82930781209959E-13,
3.77003198860263));
#221757=CARTESIAN_POINT('',(45.8374112534718,-40.845716073179,3.77003198802693));
#221758=CARTESIAN_POINT('Origin',(5.49031038273072E-15,1.82930781209959E-13,
3.77003198860263));
#221759=CARTESIAN_POINT('',(45.8374112537096,-40.8457160734115,3.77003198860235));
#221760=CARTESIAN_POINT('Origin',(62.2224557307631,1.82930781209959E-13,
3.77003198860263));
#221761=CARTESIAN_POINT('',(49.866980369603,-36.6229335645802,3.77003198860238));
#221762=CARTESIAN_POINT('',(40.5385041740537,-29.8453988870281,3.77003198860243));
#221763=CARTESIAN_POINT('',(46.190562802649,-41.1629311642473,3.77003198860235));
#221764=CARTESIAN_POINT('Origin',(5.49031038273072E-15,1.82930781209959E-13,
3.77003198860263));
#221765=CARTESIAN_POINT('',(45.8381794369742,-40.8456437566505,3.77003198860235));
#221766=CARTESIAN_POINT('Origin',(5.57972911860581E-15,1.8736496251029E-13,
3.13503198860263));
#221767=CARTESIAN_POINT('Origin',(48.3573798485719,-35.5261507575143,3.1350249154141));
#221768=CARTESIAN_POINT('Origin',(44.8038837346045,-39.9143530044111,3.13502491541405));
#221769=CARTESIAN_POINT('Origin',(5.57972911860581E-15,1.8736496251029E-13,
3.13503198860263));
#221770=CARTESIAN_POINT('Origin',(49.8978080023041,-36.6453726047983,3.20381846780044));
#221771=CARTESIAN_POINT('Origin',(46.2189206177148,-41.188419527609,3.20382022872215));
#221772=CARTESIAN_POINT('Origin',(5.51210908043506E-15,1.8401175575949E-13,
3.61523028058481));
#221773=CARTESIAN_POINT('Origin',(49.1861997321271,-36.1282716303333,3.58786945047134));
#221774=CARTESIAN_POINT('Origin',(45.5650984170293,-40.5998100962466,3.58781461834286));
#221775=CARTESIAN_POINT('Origin',(5.51210908043507E-15,1.8401175575949E-13,
3.61523028058481));
#221776=CARTESIAN_POINT('Origin',(49.0382355735229,-36.0208713038475,3.58781440266324));
#221777=CARTESIAN_POINT('Origin',(45.4292815791815,-40.4774090812908,3.58786923592671));
#221778=CARTESIAN_POINT('Origin',(60.4792282238308,1.82930781209959E-13,
3.77003198860263));
#221779=CARTESIAN_POINT('',(40.3862543050944,-44.3789831537289,3.77003198860233));
#221780=CARTESIAN_POINT('',(44.37898315373,-40.3862543050931,3.77003198860235));
#221781=CARTESIAN_POINT('Origin',(5.49031038273072E-15,1.82930781209959E-13,
3.77003198860263));
#221782=CARTESIAN_POINT('',(44.7317571974364,-40.7038934808036,3.77003198860235));
#221783=CARTESIAN_POINT('',(33.1880655373225,-30.3099068238761,3.77003198860242));
#221784=CARTESIAN_POINT('',(44.7313678842181,-40.7043213166061,3.77003198902512));
#221785=CARTESIAN_POINT('Origin',(5.49031038273072E-15,1.82930781209959E-13,
3.77003198860263));
#221786=CARTESIAN_POINT('',(40.7043213163689,-44.7313678839549,3.77003198882056));
#221787=CARTESIAN_POINT('Origin',(5.49031038273072E-15,1.82930781209959E-13,
3.77003198860263));
#221788=CARTESIAN_POINT('',(40.7038934808044,-44.7317571974348,3.77003198860232));
#221789=CARTESIAN_POINT('Origin',(5.49031038273072E-15,1.82930781209959E-13,
3.77003198860263));
#221790=CARTESIAN_POINT('',(40.386614028275,-44.3793826667952,3.77003198860233));
#221791=CARTESIAN_POINT('Origin',(5.49031038273072E-15,1.82930781209959E-13,
3.77003198860263));
#221792=CARTESIAN_POINT('',(44.8522789915946,-40.8131880745599,3.48823028058453));
#221793=CARTESIAN_POINT('',(44.7313678836765,-40.7043213161132,3.77003198860235));
#221794=CARTESIAN_POINT('',(40.8131880747515,-44.8522789918026,3.48823028074774));
#221795=CARTESIAN_POINT('Origin',(5.52999282761009E-15,1.84898592019556E-13,
3.48823028058481));
#221796=CARTESIAN_POINT('',(40.8131880745612,-44.8522789915935,3.48823028058451));
#221797=CARTESIAN_POINT('Origin',(60.71525,1.85785428279622E-13,3.36123028058482));
#221798=CARTESIAN_POINT('',(40.959952356613,-45.0161393894786,3.36123028058451));
#221799=CARTESIAN_POINT('',(45.0161393894798,-40.9599523566118,3.36123028058454));
#221800=CARTESIAN_POINT('Origin',(5.5478765747851E-15,1.85785428279622E-13,
3.36123028058482));
#221801=CARTESIAN_POINT('',(45.1285089182138,-41.0611303347397,3.36123028058454));
#221802=CARTESIAN_POINT('',(33.3184119221875,-30.4272712359681,3.3612302805846));
#221803=CARTESIAN_POINT('',(41.0611303347409,-45.1285089182126,3.36123028058451));
#221804=CARTESIAN_POINT('Origin',(5.5478765747851E-15,1.85785428279622E-13,
3.36123028058482));
#221805=CARTESIAN_POINT('',(40.9603070122498,-45.0165332744673,3.36123028058451));
#221806=CARTESIAN_POINT('Origin',(5.5478765747851E-15,1.85785428279622E-13,
3.36123028058482));
#221807=CARTESIAN_POINT('',(41.2079002115913,-45.292364129855,3.48823028058453));
#221808=CARTESIAN_POINT('',(45.2923641300585,-41.2079002117741,3.48823028042666));
#221809=CARTESIAN_POINT('Origin',(5.52999282761008E-15,1.84898592019556E-13,
3.48823028058484));
#221810=CARTESIAN_POINT('',(45.4132731252663,-41.3167691863802,3.77003198802679));
#221811=CARTESIAN_POINT('',(45.2923641298562,-41.20790021159,3.48823028058456));
#221812=CARTESIAN_POINT('',(45.4128910420877,-41.3171891492018,3.77003198860235));
#221813=CARTESIAN_POINT('Origin',(5.49031038273072E-15,1.82930781209959E-13,
3.77003198860263));
#221814=CARTESIAN_POINT('',(41.3171891492031,-45.4128910420865,3.77003198860232));
#221815=CARTESIAN_POINT('Origin',(5.49031038273072E-15,1.82930781209959E-13,
3.77003198860263));
#221816=CARTESIAN_POINT('',(41.3167691863815,-45.4132731252652,3.7700319880269));
#221817=CARTESIAN_POINT('Origin',(5.49031038273072E-15,1.82930781209959E-13,
3.77003198860263));
#221818=CARTESIAN_POINT('',(41.3167691865937,-45.4132731255213,3.77003198860232));
#221819=CARTESIAN_POINT('Origin',(62.2224557307631,1.82930781209959E-13,
3.77003198860263));
#221820=CARTESIAN_POINT('',(45.7656648676111,-41.6348281284255,3.77003198860234));
#221821=CARTESIAN_POINT('',(34.1507877370015,-31.1767457860023,3.77003198860241));
#221822=CARTESIAN_POINT('',(41.6348281284267,-45.7656648676099,3.77003198860232));
#221823=CARTESIAN_POINT('Origin',(5.49031038273072E-15,1.82930781209959E-13,
3.77003198860263));
#221824=CARTESIAN_POINT('',(41.3175407208299,-45.4132815019352,3.77003198860232));
#221825=CARTESIAN_POINT('Origin',(5.57972911860581E-15,1.8736496251029E-13,
3.13503198860263));
#221826=CARTESIAN_POINT('Origin',(44.3789791175472,-40.3862573897237,3.13502491541404));
#221827=CARTESIAN_POINT('Origin',(40.3862573897248,-44.3789791175461,3.13502491541401));
#221828=CARTESIAN_POINT('Origin',(5.57972911860581E-15,1.8736496251029E-13,
3.13503198860263));
#221829=CARTESIAN_POINT('Origin',(45.7939781049198,-41.6603666103112,3.20381846780193));
#221830=CARTESIAN_POINT('Origin',(41.6603663369564,-45.793977801883,3.20382022871952));
#221831=CARTESIAN_POINT('Origin',(5.51210908043506E-15,1.8401175575949E-13,
3.61523028058481));
#221832=CARTESIAN_POINT('Origin',(45.1403198695222,-41.0717150501539,3.58786945047173));
#221833=CARTESIAN_POINT('Origin',(41.071652282027,-45.1402498046829,3.5878146183419));
#221834=CARTESIAN_POINT('Origin',(5.51210908043507E-15,1.8401175575949E-13,
3.61523028058481));
#221835=CARTESIAN_POINT('Origin',(45.0043926651417,-40.9494366077805,3.58781440266656));
#221836=CARTESIAN_POINT('Origin',(40.9493738530224,-45.0043225899478,3.58786923592653));
#221837=CARTESIAN_POINT('Origin',(60.4792282238308,1.82930781209959E-13,
3.77003198860263));
#221838=CARTESIAN_POINT('',(35.5261472678871,-48.3573835402113,3.7700319886023));
#221839=CARTESIAN_POINT('',(39.9143573409162,-44.8038810887668,3.77003198860232));
#221840=CARTESIAN_POINT('Origin',(5.49031038273072E-15,1.82930781209959E-13,
3.77003198860263));
#221841=CARTESIAN_POINT('',(40.2319965165892,-45.1566551325069,3.77003198860231));
#221842=CARTESIAN_POINT('',(26.8427652369017,-30.2864073093061,3.77003198860242));
#221843=CARTESIAN_POINT('',(40.2315646150508,-45.157039930268,3.7700319890254));
#221844=CARTESIAN_POINT('Origin',(5.49031038273072E-15,1.82930781209959E-13,
3.77003198860263));
#221845=CARTESIAN_POINT('',(35.8056376404645,-48.7410849259192,3.77003198882053));
#221846=CARTESIAN_POINT('Origin',(5.49031038273072E-15,1.82930781209959E-13,
3.77003198860263));
#221847=CARTESIAN_POINT('',(35.8051714542882,-48.741427385705,3.77003198860229));
#221848=CARTESIAN_POINT('Origin',(5.49031038273072E-15,1.82930781209959E-13,
3.77003198860263));
#221849=CARTESIAN_POINT('',(35.5264632599797,-48.3578184660146,3.77003198860229));
#221850=CARTESIAN_POINT('Origin',(5.49031038273072E-15,1.82930781209959E-13,
3.77003198860263));
#221851=CARTESIAN_POINT('',(40.3404336838198,-45.2779489569766,3.4882302805845));
#221852=CARTESIAN_POINT('',(40.2315646145633,-45.1570399297209,3.77003198860232));
#221853=CARTESIAN_POINT('',(35.9012693630584,-48.8727133450216,3.48823028074772));
#221854=CARTESIAN_POINT('Origin',(5.52999282761009E-15,1.84898592019556E-13,
3.48823028058481));
#221855=CARTESIAN_POINT('',(35.901269362891,-48.8727133447938,3.48823028058448));
#221856=CARTESIAN_POINT('Origin',(60.71525,1.85785428279622E-13,3.36123028058482));
#221857=CARTESIAN_POINT('',(36.0301015792682,-49.0510171431398,3.36123028058448));
#221858=CARTESIAN_POINT('',(40.4880553924349,-45.4410373245165,3.36123028058451));
#221859=CARTESIAN_POINT('Origin',(5.5478765747851E-15,1.85785428279622E-13,
3.36123028058482));
#221860=CARTESIAN_POINT('',(40.5892333705628,-45.5534068532505,3.3612302805845));
#221861=CARTESIAN_POINT('',(26.948440628206,-30.4037717213981,3.3612302805846));
#221862=CARTESIAN_POINT('',(36.1189794796889,-49.1733470784082,3.36123028058448));
#221863=CARTESIAN_POINT('Origin',(5.5478765747851E-15,1.85785428279622E-13,
3.36123028058482));
#221864=CARTESIAN_POINT('',(36.0304131198717,-49.0514459419939,3.36123028058447));
#221865=CARTESIAN_POINT('Origin',(5.5478765747851E-15,1.85785428279622E-13,
3.36123028058482));
#221866=CARTESIAN_POINT('',(36.2478178023256,-49.3516463037379,3.4882302805845));
#221867=CARTESIAN_POINT('',(40.7368493367122,-45.7165002430342,3.48823028042664));
#221868=CARTESIAN_POINT('Origin',(5.52999282761008E-15,1.84898592019556E-13,
3.48823028058484));
#221869=CARTESIAN_POINT('',(40.8457160731802,-45.8374112534706,3.77003198802676));
#221870=CARTESIAN_POINT('',(40.7368493365303,-45.71650024283,3.48823028058453));
#221871=CARTESIAN_POINT('',(40.8452921850249,-45.8377889771244,3.77003198860232));
#221872=CARTESIAN_POINT('Origin',(5.49031038273072E-15,1.82930781209959E-13,
3.77003198860263));
#221873=CARTESIAN_POINT('',(36.3439095507841,-49.482936761634,3.77003198860229));
#221874=CARTESIAN_POINT('Origin',(5.49031038273072E-15,1.82930781209959E-13,
3.77003198860263));
#221875=CARTESIAN_POINT('',(36.3434519499953,-49.4832728536526,3.77003198802686));
#221876=CARTESIAN_POINT('Origin',(5.49031038273072E-15,1.82930781209959E-13,
3.77003198860263));
#221877=CARTESIAN_POINT('',(36.3434519501796,-49.4832728539295,3.77003198860229));
#221878=CARTESIAN_POINT('Origin',(62.2224557307631,1.82930781209959E-13,
3.77003198860263));
#221879=CARTESIAN_POINT('',(41.1629311642486,-46.1905628026478,3.77003198860231));
#221880=CARTESIAN_POINT('',(27.6232705441551,-31.1532462714323,3.77003198860241));
#221881=CARTESIAN_POINT('',(36.6229335645815,-49.866980369602,3.77003198860229));
#221882=CARTESIAN_POINT('Origin',(5.49031038273072E-15,1.82930781209959E-13,
3.77003198860263));
#221883=CARTESIAN_POINT('',(36.3442183822969,-49.4833618317446,3.77003198860228));
#221884=CARTESIAN_POINT('Origin',(5.57972911860581E-15,1.8736496251029E-13,
3.13503198860263));
#221885=CARTESIAN_POINT('Origin',(39.9143530044124,-44.8038837346033,3.13502491541403));
#221886=CARTESIAN_POINT('Origin',(35.5261507575157,-48.3573798485708,3.13502491541401));
#221887=CARTESIAN_POINT('Origin',(5.57972911860581E-15,1.8736496251029E-13,
3.13503198860263));
#221888=CARTESIAN_POINT('Origin',(41.1884198004194,-46.21892092124,3.20381846780197));
#221889=CARTESIAN_POINT('Origin',(36.6453723646299,-49.8978076723495,3.20382022872569));
#221890=CARTESIAN_POINT('Origin',(5.51210908043506E-15,1.8401175575949E-13,
3.61523028058481));
#221891=CARTESIAN_POINT('Origin',(40.5998732162085,-45.5651681650769,3.58786945046948));
#221892=CARTESIAN_POINT('Origin',(36.1282165298264,-49.186123490054,3.58781461834262));
#221893=CARTESIAN_POINT('Origin',(5.51210908043507E-15,1.8401175575949E-13,
3.61523028058481));
#221894=CARTESIAN_POINT('Origin',(40.47747221295,-45.4293513150133,3.58781440266855));
#221895=CARTESIAN_POINT('Origin',(36.0208162177209,-49.0381593225528,3.58786923592943));
#221896=CARTESIAN_POINT('Origin',(60.4792282238308,1.82930781209959E-13,
3.77003198860263));
#221897=CARTESIAN_POINT('',(30.2768083268887,-51.8059703131941,3.77003198860227));
#221898=CARTESIAN_POINT('',(35.012421476459,-48.7306271754171,3.77003198860229));
#221899=CARTESIAN_POINT('Origin',(5.49031038273072E-15,1.82930781209959E-13,
3.77003198860263));
#221900=CARTESIAN_POINT('',(35.2914456628196,-49.1146710209409,3.77003198860229));
#221901=CARTESIAN_POINT('',(20.6381965522797,-28.9462038689909,3.77003198860243));
#221902=CARTESIAN_POINT('',(35.2909759049639,-49.1150085647348,3.77003198902485));
#221903=CARTESIAN_POINT('Origin',(5.49031038273072E-15,1.82930781209959E-13,
3.77003198860263));
#221904=CARTESIAN_POINT('',(30.5146599057598,-52.2167844417073,3.7700319888205));
#221905=CARTESIAN_POINT('Origin',(5.49031038273072E-15,1.82930781209959E-13,
3.77003198860263));
#221906=CARTESIAN_POINT('',(30.5141604766051,-52.217076295738,3.77003198860226));
#221907=CARTESIAN_POINT('Origin',(5.49031038273072E-15,1.82930781209959E-13,
3.77003198860263));
#221908=CARTESIAN_POINT('',(30.2770771258177,-51.8064358865961,3.77003198860227));
#221909=CARTESIAN_POINT('Origin',(5.49031038273072E-15,1.82930781209959E-13,
3.77003198860263));
#221910=CARTESIAN_POINT('',(35.3866101428265,-49.2466351556007,3.48823028058447));
#221911=CARTESIAN_POINT('',(35.2909759045368,-49.1150085641405,3.77003198860229));
#221912=CARTESIAN_POINT('',(30.5960088314001,-52.3576880235598,3.48823028074769));
#221913=CARTESIAN_POINT('Origin',(5.52999282761009E-15,1.84898592019556E-13,
3.48823028058481));
#221914=CARTESIAN_POINT('',(30.5960088312575,-52.3576880233157,3.48823028058445));
#221915=CARTESIAN_POINT('Origin',(60.71525,1.85785428279622E-13,3.36123028058482));
#221916=CARTESIAN_POINT('',(30.7054974692375,-52.5484816883954,3.36123028058446));
#221917=CARTESIAN_POINT('',(35.5163757878401,-49.4242607783455,3.36123028058448));
#221918=CARTESIAN_POINT('Origin',(5.5478765747851E-15,1.85785428279622E-13,
3.36123028058482));
#221919=CARTESIAN_POINT('',(35.6052536882608,-49.5465907136139,3.36123028058448));
#221920=CARTESIAN_POINT('',(20.7197400704249,-29.0584388930976,3.36123028058461));
#221921=CARTESIAN_POINT('',(30.781101527075,-52.6794317578282,3.36123028058446));
#221922=CARTESIAN_POINT('Origin',(5.5478765747851E-15,1.85785428279622E-13,
3.36123028058482));
#221923=CARTESIAN_POINT('',(30.7057624815037,-52.5489407031051,3.36123028058445));
#221924=CARTESIAN_POINT('Origin',(5.5478765747851E-15,1.85785428279622E-13,
3.36123028058482));
#221925=CARTESIAN_POINT('',(30.8905967158742,-52.870221513221,3.48823028058447));
#221926=CARTESIAN_POINT('',(35.7350130972991,-49.724220730839,3.48823028042661));
#221927=CARTESIAN_POINT('Origin',(5.52999282761008E-15,1.84898592019556E-13,
3.48823028058484));
#221928=CARTESIAN_POINT('',(35.8306448082808,-49.855849050773,3.77003198802673));
#221929=CARTESIAN_POINT('',(35.7350130971395,-49.7242207306169,3.4882302805845));
#221930=CARTESIAN_POINT('',(35.8301837593561,-49.8561803968397,3.77003198860229));
#221931=CARTESIAN_POINT('Origin',(5.49031038273072E-15,1.82930781209959E-13,
3.77003198860263));
#221932=CARTESIAN_POINT('',(30.9724384738749,-53.0108370710507,3.77003198860226));
#221933=CARTESIAN_POINT('Origin',(5.49031038273072E-15,1.82930781209959E-13,
3.77003198860263));
#221934=CARTESIAN_POINT('',(30.9719482486888,-53.0111234896148,3.77003198802684));
#221935=CARTESIAN_POINT('Origin',(5.49031038273072E-15,1.82930781209959E-13,
3.77003198860263));
#221936=CARTESIAN_POINT('',(30.9719482488431,-53.0111234899094,3.77003198860226));
#221937=CARTESIAN_POINT('Origin',(62.2224557307631,1.82930781209959E-13,
3.77003198860263));
#221938=CARTESIAN_POINT('',(36.1092077731534,-50.2402240048077,3.77003198860228));
#221939=CARTESIAN_POINT('',(21.2404668433939,-29.7751578089174,3.77003198860242));
#221940=CARTESIAN_POINT('',(31.2097904767612,-53.4219427993281,3.77003198860226));
#221941=CARTESIAN_POINT('Origin',(5.49031038273072E-15,1.82930781209959E-13,
3.77003198860263));
#221942=CARTESIAN_POINT('',(30.9727011816508,-53.0112920942662,3.77003198860226));
#221943=CARTESIAN_POINT('Origin',(5.57972911860581E-15,1.8736496251029E-13,
3.13503198860263));
#221944=CARTESIAN_POINT('Origin',(35.0124168871459,-48.7306293534713,3.13502491541405));
#221945=CARTESIAN_POINT('Origin',(30.2768121832823,-51.8059670065423,3.13502491541396));
#221946=CARTESIAN_POINT('Origin',(5.57972911860581E-15,1.8736496251029E-13,
3.13503198860263));
#221947=CARTESIAN_POINT('Origin',(36.1315925493471,-50.2710910626317,3.20381846780222));
#221948=CARTESIAN_POINT('Origin',(31.228884024128,-53.4549467201719,3.20382022872136));
#221949=CARTESIAN_POINT('Origin',(5.51210908043506E-15,1.8401175575949E-13,
3.61523028058481));
#221950=CARTESIAN_POINT('Origin',(35.6146058558668,-49.5593997624572,3.58786945047169));
#221951=CARTESIAN_POINT('Origin',(30.7889524770101,-52.6931037136105,3.58781461834191));
#221952=CARTESIAN_POINT('Origin',(5.51210908043507E-15,1.8401175575949E-13,
3.61523028058481));
#221953=CARTESIAN_POINT('Origin',(35.5070721047329,-49.4115325425344,3.58781440266241));
#221954=CARTESIAN_POINT('Origin',(30.6976069821031,-52.5347237197183,3.58786923592823));
#221955=CARTESIAN_POINT('Origin',(60.4792282238308,1.82930781209959E-13,
3.77003198860263));
#221956=CARTESIAN_POINT('',(24.6957503380314,-54.6869600343293,3.77003198860225));
#221957=CARTESIAN_POINT('',(29.7268821954856,-52.1234703131941,3.77003198860227));
#221958=CARTESIAN_POINT('Origin',(5.49031038273072E-15,1.82930781209959E-13,
3.77003198860263));
#221959=CARTESIAN_POINT('',(29.9642343451585,-52.5345762957638,3.77003198860226));
#221960=CARTESIAN_POINT('',(14.8448439902567,-26.3470240215573,3.77003198860244));
#221961=CARTESIAN_POINT('',(29.9637318777518,-52.5348628873914,3.77003198902526));
#221962=CARTESIAN_POINT('Origin',(5.49031038273072E-15,1.82930781209959E-13,
3.77003198860263));
#221963=CARTESIAN_POINT('',(24.8893571715245,-55.1203859400875,3.77003198882048));
#221964=CARTESIAN_POINT('Origin',(5.49031038273072E-15,1.82930781209959E-13,
3.77003198860263));
#221965=CARTESIAN_POINT('',(24.8888299712416,-55.1206239907492,3.77003198860224));
#221966=CARTESIAN_POINT('Origin',(5.49031038273072E-15,1.82930781209959E-13,
3.77003198860263));
#221967=CARTESIAN_POINT('',(24.6959689987794,-54.6874511544104,3.77003198860225));
#221968=CARTESIAN_POINT('Origin',(5.49031038273072E-15,1.82930781209959E-13,
3.77003198860263));
#221969=CARTESIAN_POINT('',(30.0450834959843,-52.675764913939,3.48823028058445));
#221970=CARTESIAN_POINT('',(29.9637318773888,-52.534862886755,3.77003198860227));
#221971=CARTESIAN_POINT('',(24.9555320243585,-55.2690209155612,3.48823028074766));
#221972=CARTESIAN_POINT('Origin',(5.52999282761009E-15,1.84898592019556E-13,
3.48823028058481));
#221973=CARTESIAN_POINT('',(24.9555320242422,-55.2690209153036,3.48823028058443));
#221974=CARTESIAN_POINT('Origin',(60.71525,1.85785428279622E-13,3.36123028058482));
#221975=CARTESIAN_POINT('',(25.0444775033954,-55.4702140717962,3.36123028058443));
#221976=CARTESIAN_POINT('',(30.1555713378344,-52.8659816883954,3.36123028058445));
#221977=CARTESIAN_POINT('Origin',(5.5478765747851E-15,1.85785428279622E-13,
3.36123028058482));
#221978=CARTESIAN_POINT('',(30.2311753956719,-52.9969317578282,3.36123028058445));
#221979=CARTESIAN_POINT('',(14.9038494342991,-26.4492244485618,3.36123028058463));
#221980=CARTESIAN_POINT('',(25.1059793847708,-55.6083495590297,3.36123028058443));
#221981=CARTESIAN_POINT('Origin',(5.5478765747851E-15,1.85785428279622E-13,
3.36123028058482));
#221982=CARTESIAN_POINT('',(25.0446930837944,-55.4706982733002,3.36123028058443));
#221983=CARTESIAN_POINT('Origin',(5.5478765747851E-15,1.85785428279622E-13,
3.36123028058482));
#221984=CARTESIAN_POINT('',(25.1949317875307,-55.8095395120002,3.48823028058446));
#221985=CARTESIAN_POINT('',(30.3416565763598,-53.1871522508545,3.48823028042659));
#221986=CARTESIAN_POINT('Origin',(5.52999282761008E-15,1.84898592019556E-13,
3.48823028058484));
#221987=CARTESIAN_POINT('',(30.4230055008174,-53.328055732868,3.7700319880267));
#221988=CARTESIAN_POINT('',(30.3416565762242,-53.187152250617,3.48823028058447));
#221989=CARTESIAN_POINT('',(30.4225123424717,-53.3283370710507,3.77003198860226));
#221990=CARTESIAN_POINT('Origin',(5.49031038273072E-15,1.82930781209959E-13,
3.77003198860263));
#221991=CARTESIAN_POINT('',(25.2616268796463,-55.9579395562862,3.77003198860224));
#221992=CARTESIAN_POINT('Origin',(5.49031038273072E-15,1.82930781209959E-13,
3.77003198860263));
#221993=CARTESIAN_POINT('',(25.2611094010728,-55.9581731633341,3.77003198802682));
#221994=CARTESIAN_POINT('Origin',(5.49031038273072E-15,1.82930781209959E-13,
3.77003198860263));
#221995=CARTESIAN_POINT('',(25.2611094011954,-55.9581731636432,3.77003198860224));
#221996=CARTESIAN_POINT('Origin',(62.2224557307631,1.82930781209959E-13,
3.77003198860263));
#221997=CARTESIAN_POINT('',(30.6598643453581,-53.7394427993281,3.77003198860226));
#221998=CARTESIAN_POINT('',(15.2806508669898,-27.1018636743469,3.77003198860244));
#221999=CARTESIAN_POINT('',(25.454706393409,-56.3916032444846,3.77003198860224));
#222000=CARTESIAN_POINT('Origin',(5.49031038273072E-15,1.82930781209959E-13,
3.77003198860263));
#222001=CARTESIAN_POINT('',(25.2618405854041,-55.958419547277,3.77003198860224));
#222002=CARTESIAN_POINT('Origin',(5.57972911860581E-15,1.8736496251029E-13,
3.13503198860263));
#222003=CARTESIAN_POINT('Origin',(29.7268774036444,-52.1234719996029,3.13502491541398));
#222004=CARTESIAN_POINT('Origin',(24.6957545189385,-54.6869571488945,3.13502491541394));
#222005=CARTESIAN_POINT('Origin',(5.57972911860581E-15,1.8736496251029E-13,
3.13503198860263));
#222006=CARTESIAN_POINT('Origin',(30.6789000092848,-53.7724806104344,3.20381846779911));
#222007=CARTESIAN_POINT('Origin',(25.4702454951989,-56.4264221855612,3.20382022872151));
#222008=CARTESIAN_POINT('Origin',(5.51210908043506E-15,1.8401175575949E-13,
3.61523028058481));
#222009=CARTESIAN_POINT('Origin',(30.2391374209345,-53.0106482050714,3.58786945046866));
#222010=CARTESIAN_POINT('Origin',(25.1123582178529,-55.6227672661395,3.58781461834242));
#222011=CARTESIAN_POINT('Origin',(5.51210908043507E-15,1.8401175575949E-13,
3.61523028058481));
#222012=CARTESIAN_POINT('Origin',(30.1476490842058,-52.852350679495,3.58781440266416));
#222013=CARTESIAN_POINT('Origin',(25.0380683404964,-55.4557066902189,3.58786923593021));
#222014=CARTESIAN_POINT('Origin',(60.4792282238308,1.82930781209959E-13,
3.77003198860263));
#222015=CARTESIAN_POINT('',(18.8441205405526,-56.9687879773462,3.77003198860223));
#222016=CARTESIAN_POINT('',(24.1156489724283,-54.9452378026824,3.77003198860224));
#222017=CARTESIAN_POINT('Origin',(5.49031038273072E-15,1.82930781209959E-13,
3.77003198860263));
#222018=CARTESIAN_POINT('',(24.3087286055926,-55.3789017591234,3.77003198860224));
#222019=CARTESIAN_POINT('',(9.71531210235053,-22.6015516358799,3.77003198860247));
#222020=CARTESIAN_POINT('',(24.3081989337723,-55.3791342586257,3.77003198902492));
#222021=CARTESIAN_POINT('Origin',(5.49031038273072E-15,1.82930781209959E-13,
3.77003198860263));
#222022=CARTESIAN_POINT('',(18.9913614316851,-57.4200769554257,3.77003198882047));
#222023=CARTESIAN_POINT('Origin',(5.49031038273072E-15,1.82930781209959E-13,
3.77003198860263));
#222024=CARTESIAN_POINT('',(18.9908122363906,-57.4202585945856,3.77003198860223));
#222025=CARTESIAN_POINT('Origin',(5.49031038273072E-15,1.82930781209959E-13,
3.77003198860263));
#222026=CARTESIAN_POINT('',(18.8442866674268,-56.9692992632922,3.77003198860223));
#222027=CARTESIAN_POINT('Origin',(5.49031038273072E-15,1.82930781209959E-13,
3.77003198860263));
#222028=CARTESIAN_POINT('',(24.374376627022,-55.5277679687678,3.48823028058442));
#222029=CARTESIAN_POINT('',(24.308198933478,-55.3791342579554,3.77003198860224));
#222030=CARTESIAN_POINT('',(19.0416371861772,-57.5748148486256,3.48823028074764));
#222031=CARTESIAN_POINT('Origin',(5.52999282761009E-15,1.84898592019556E-13,
3.48823028058481));
#222032=CARTESIAN_POINT('',(19.0416371860884,-57.5748148483572,3.48823028058441));
#222033=CARTESIAN_POINT('Origin',(60.71525,1.85785428279622E-13,3.36123028058482));
#222034=CARTESIAN_POINT('',(19.1090650011322,-57.7842031819379,3.36123028058441));
#222035=CARTESIAN_POINT('',(24.4643761377923,-55.7284918401494,3.36123028058443));
#222036=CARTESIAN_POINT('Origin',(5.5478765747851E-15,1.85785428279622E-13,
3.36123028058482));
#222037=CARTESIAN_POINT('',(24.5258780191677,-55.8666273273828,3.36123028058442));
#222038=CARTESIAN_POINT('',(9.75435829333414,-22.68925081671,3.36123028058466));
#222039=CARTESIAN_POINT('',(19.1557908785631,-57.9280106456672,3.36123028058441));
#222040=CARTESIAN_POINT('Origin',(5.5478765747851E-15,1.85785428279622E-13,
3.36123028058482));
#222041=CARTESIAN_POINT('',(19.1092287877201,-57.7847072652232,3.36123028058441));
#222042=CARTESIAN_POINT('Origin',(5.5478765747851E-15,1.85785428279622E-13,
3.36123028058482));
#222043=CARTESIAN_POINT('',(19.2232259141446,-58.137396516989,3.48823028058443));
#222044=CARTESIAN_POINT('',(24.6158705165699,-56.0673542006825,3.48823028042655));
#222045=CARTESIAN_POINT('Origin',(5.52999282761008E-15,1.84898592019556E-13,
3.48823028058484));
#222046=CARTESIAN_POINT('',(24.6820453786638,-56.2159890767406,3.77003198802669));
#222047=CARTESIAN_POINT('',(24.61587051646,-56.0673542004321,3.48823028058445));
#222048=CARTESIAN_POINT('',(24.6815255140433,-56.2162173246393,3.77003198860224));
#222049=CARTESIAN_POINT('Origin',(5.49031038273072E-15,1.82930781209959E-13,
3.77003198860263));
#222050=CARTESIAN_POINT('',(19.2740436149891,-58.2919551457913,3.77003198860222));
#222051=CARTESIAN_POINT('Origin',(5.49031038273072E-15,1.82930781209959E-13,
3.77003198860263));
#222052=CARTESIAN_POINT('',(19.2735045526316,-58.2921333818753,3.7700319880268));
#222053=CARTESIAN_POINT('Origin',(5.49031038273072E-15,1.82930781209959E-13,
3.77003198860263));
#222054=CARTESIAN_POINT('',(19.2735045527213,-58.2921333821955,3.77003198860222));
#222055=CARTESIAN_POINT('Origin',(62.2224557307631,1.82930781209959E-13,
3.77003198860263));
#222056=CARTESIAN_POINT('',(24.8746050278059,-56.6498810128377,3.77003198860224));
#222057=CARTESIAN_POINT('',(10.0037024164492,-23.2492868865832,3.77003198860246));
#222058=CARTESIAN_POINT('',(19.4207352200707,-58.7434254837928,3.77003198860222));
#222059=CARTESIAN_POINT('Origin',(5.49031038273072E-15,1.82930781209959E-13,
3.77003198860263));
#222060=CARTESIAN_POINT('',(19.2742059773237,-58.2924548456757,3.77003198860222));
#222061=CARTESIAN_POINT('Origin',(5.57972911860581E-15,1.8736496251029E-13,
3.13503198860263));
#222062=CARTESIAN_POINT('Origin',(24.1156440305597,-54.9452389789691,3.13502491541393));
#222063=CARTESIAN_POINT('Origin',(18.8441250001663,-56.968785544742,3.1350249154139));
#222064=CARTESIAN_POINT('Origin',(5.57972911860581E-15,1.8736496251029E-13,
3.13503198860263));
#222065=CARTESIAN_POINT('Origin',(24.8900830207518,-56.6847276080569,3.20381846780338));
#222066=CARTESIAN_POINT('Origin',(19.4325496266317,-58.7796779614975,3.20382022872089));
#222067=CARTESIAN_POINT('Origin',(5.51210908043506E-15,1.8401175575949E-13,
3.61523028058481));
#222068=CARTESIAN_POINT('Origin',(24.5323626684716,-55.8811008927591,3.58786945046644));
#222069=CARTESIAN_POINT('Origin',(19.1606277069622,-57.9430161406885,3.58781461834223));
#222070=CARTESIAN_POINT('Origin',(5.51210908043507E-15,1.8401175575949E-13,
3.61523028058481));
#222071=CARTESIAN_POINT('Origin',(24.4579221115133,-55.7141074023456,3.5878144026674));
#222072=CARTESIAN_POINT('Origin',(19.1042073825996,-57.7691053333649,3.5878692359277));
#222073=CARTESIAN_POINT('Origin',(60.4792282238308,1.82930781209959E-13,
3.77003198860263));
#222074=CARTESIAN_POINT('',(12.7860306150458,-58.626453957798,3.77003198860222));
#222075=CARTESIAN_POINT('',(18.2401996527051,-57.1650137687743,3.77003198860223));
#222076=CARTESIAN_POINT('Origin',(5.49031038273072E-15,1.82930781209959E-13,
3.77003198860263));
#222077=CARTESIAN_POINT('',(18.3868913484954,-57.6164843860299,3.77003198860223));
#222078=CARTESIAN_POINT('',(5.47329194811204,-17.8725121057136,3.7700319886025));
#222079=CARTESIAN_POINT('',(18.386340275457,-57.6166602460943,3.770031989025));
#222080=CARTESIAN_POINT('Origin',(5.49031038273072E-15,1.82930781209959E-13,
3.77003198860263));
#222081=CARTESIAN_POINT('',(12.8852923618023,-59.0906615917168,3.77003198882045));
#222082=CARTESIAN_POINT('Origin',(5.49031038273072E-15,1.82930781209959E-13,
3.77003198860263));
#222083=CARTESIAN_POINT('',(12.8847271885949,-59.0907848292981,3.77003198860221));
#222084=CARTESIAN_POINT('Origin',(5.49031038273072E-15,1.82930781209959E-13,
3.77003198860263));
#222085=CARTESIAN_POINT('',(12.7861423879254,-58.626979807853,3.77003198860222));
#222086=CARTESIAN_POINT('Origin',(5.49031038273072E-15,1.82930781209959E-13,
3.77003198860263));
#222087=CARTESIAN_POINT('',(18.4366189870679,-57.7713971777983,3.48823028058441));
#222088=CARTESIAN_POINT('',(18.3863402752344,-57.6166602453967,3.77003198860222));
#222089=CARTESIAN_POINT('',(12.9191181862654,-59.2498070619039,3.48823028074763));
#222090=CARTESIAN_POINT('Origin',(5.52999282761009E-15,1.84898592019556E-13,
3.48823028058481));
#222091=CARTESIAN_POINT('',(12.9191181862052,-59.2498070616276,3.4882302805844));
#222092=CARTESIAN_POINT('Origin',(60.71525,1.85785428279622E-13,3.36123028058482));
#222093=CARTESIAN_POINT('',(12.9642895838877,-59.4650964698963,3.3612302805844));
#222094=CARTESIAN_POINT('',(18.5051441132848,-57.980428973366,3.36123028058441));
#222095=CARTESIAN_POINT('Origin',(5.5478765747851E-15,1.85785428279622E-13,
3.36123028058482));
#222096=CARTESIAN_POINT('',(18.5518699907157,-58.1242364370953,3.36123028058441));
#222097=CARTESIAN_POINT('',(5.49583002221492,-17.9418771653397,3.36123028058469));
#222098=CARTESIAN_POINT('',(12.995727518883,-59.6130003254552,3.3612302805844));
#222099=CARTESIAN_POINT('Origin',(5.5478765747851E-15,1.85785428279622E-13,
3.36123028058482));
#222100=CARTESIAN_POINT('',(12.9643997821844,-59.465614912121,3.3612302805844));
#222101=CARTESIAN_POINT('Origin',(5.5478765747851E-15,1.85785428279622E-13,
3.36123028058482));
#222102=CARTESIAN_POINT('',(13.0409063549245,-59.8282880397052,3.48823028058442));
#222103=CARTESIAN_POINT('',(18.6203878281985,-58.3332704850397,3.48823028042654));
#222104=CARTESIAN_POINT('Origin',(5.52999282761008E-15,1.84898592019556E-13,
3.48823028058484));
#222105=CARTESIAN_POINT('',(18.6706636022915,-58.4880082803365,3.77003198802666));
#222106=CARTESIAN_POINT('',(18.6203878281154,-58.3332704847792,3.48823028058443));
#222107=CARTESIAN_POINT('',(18.6701227271417,-58.4881809372194,3.77003198860222));
#222108=CARTESIAN_POINT('Origin',(5.49031038273072E-15,1.82930781209959E-13,
3.77003198860263));
#222109=CARTESIAN_POINT('',(13.0752898951332,-59.9873118763432,3.77003198860221));
#222110=CARTESIAN_POINT('Origin',(5.49031038273072E-15,1.82930781209959E-13,
3.77003198860263));
#222111=CARTESIAN_POINT('',(13.0747351550717,-59.9874327886715,3.77003198802678));
#222112=CARTESIAN_POINT('Origin',(5.49031038273072E-15,1.82930781209959E-13,
3.77003198860263));
#222113=CARTESIAN_POINT('',(13.0747351551274,-59.9874327889994,3.77003198860221));
#222114=CARTESIAN_POINT('Origin',(62.2224557307631,1.82930781209959E-13,
3.77003198860263));
#222115=CARTESIAN_POINT('',(18.8168143322233,-58.9396512752209,3.77003198860221));
#222116=CARTESIAN_POINT('',(5.63975536249314,-18.3848338156963,3.7700319886025));
#222117=CARTESIAN_POINT('',(13.1739864076113,-60.4516424606486,3.7700319886022));
#222118=CARTESIAN_POINT('Origin',(5.49031038273072E-15,1.82930781209959E-13,
3.77003198860263));
#222119=CARTESIAN_POINT('',(13.075399135169,-59.9878258103048,3.77003198860221));
#222120=CARTESIAN_POINT('Origin',(5.57972911860581E-15,1.8736496251029E-13,
3.13503198860263));
#222121=CARTESIAN_POINT('Origin',(18.2401946149531,-57.1650144220513,3.13502491541393));
#222122=CARTESIAN_POINT('Origin',(12.7860353045056,-58.6264520046765,3.13502491541391));
#222123=CARTESIAN_POINT('Origin',(5.57972911860581E-15,1.8736496251029E-13,
3.13503198860263));
#222124=CARTESIAN_POINT('Origin',(18.828565074056,-58.9759248679618,3.20381846780251));
#222125=CARTESIAN_POINT('Origin',(13.1819466778355,-60.4889312852477,3.20382022871903));
#222126=CARTESIAN_POINT('Origin',(5.51210908043506E-15,1.8401175575949E-13,
3.61523028058481));
#222127=CARTESIAN_POINT('Origin',(18.5568062168847,-58.1393085451904,3.58786945047095));
#222128=CARTESIAN_POINT('Origin',(12.9989693492953,-59.6284292050465,3.58781461833786));
#222129=CARTESIAN_POINT('Origin',(5.51210908043507E-15,1.8401175575949E-13,
3.61523028058481));
#222130=CARTESIAN_POINT('Origin',(18.5002290260152,-57.9654487055678,3.58781440266512));
#222131=CARTESIAN_POINT('Origin',(12.9610367308101,-59.4495735695156,3.58786923592612));
#222132=CARTESIAN_POINT('Origin',(60.4792282238308,1.82930781209959E-13,
3.77003198860263));
#222133=CARTESIAN_POINT('',(6.58785426247156,-59.641796240314,3.77003198860221));
#222134=CARTESIAN_POINT('',(12.1649068885798,-58.7584778814673,3.77003198860222));
#222135=CARTESIAN_POINT('Origin',(5.49031038273072E-15,1.82930781209959E-13,
3.77003198860263));
#222136=CARTESIAN_POINT('',(12.2636034620796,-59.2228087529785,3.77003198860221));
#222137=CARTESIAN_POINT('',(2.30379013587727,-12.3655710936231,3.77003198860254));
#222138=CARTESIAN_POINT('',(12.2630370254948,-59.2229260468454,3.77003198902505));
#222139=CARTESIAN_POINT('Origin',(5.49031038273072E-15,1.82930781209959E-13,
3.77003198860263));
#222140=CARTESIAN_POINT('',(6.63804933238279,-60.113836574093,3.77003198882045));
#222141=CARTESIAN_POINT('Origin',(5.49031038273072E-15,1.82930781209959E-13,
3.77003198860263));
#222142=CARTESIAN_POINT('',(6.63747437341838,-60.1139000598791,3.77003198860221));
#222143=CARTESIAN_POINT('Origin',(5.49031038273072E-15,1.82930781209959E-13,
3.77003198860263));
#222144=CARTESIAN_POINT('',(6.58791045674951,-59.6423308931547,3.77003198860221));
#222145=CARTESIAN_POINT('Origin',(5.49031038273072E-15,1.82930781209959E-13,
3.77003198860263));
#222146=CARTESIAN_POINT('',(12.296865891381,-59.3820708699068,3.4882302805844));
#222147=CARTESIAN_POINT('',(12.2630370253463,-59.2229260461282,3.77003198860221));
#222148=CARTESIAN_POINT('',(6.65505462400559,-60.2756459901927,3.48823028074762));
#222149=CARTESIAN_POINT('Origin',(5.52999282761009E-15,1.84898592019556E-13,
3.48823028058481));
#222150=CARTESIAN_POINT('',(6.65505462397456,-60.2756459899116,3.48823028058439));
#222151=CARTESIAN_POINT('Origin',(60.71525,1.85785428279622E-13,3.36123028058482));
#222152=CARTESIAN_POINT('',(6.67747469701007,-60.4944777170591,3.36123028058439));
#222153=CARTESIAN_POINT('',(12.3431658574217,-59.5971203935656,3.3612302805844));
#222154=CARTESIAN_POINT('Origin',(5.5478765747851E-15,1.85785428279622E-13,
3.36123028058482));
#222155=CARTESIAN_POINT('',(12.3746037924171,-59.7450242491244,3.3612302805844));
#222156=CARTESIAN_POINT('',(2.31399271319981,-12.4135704460891,3.36123028058473));
#222157=CARTESIAN_POINT('',(6.69328024897516,-60.6448574988552,3.36123028058439));
#222158=CARTESIAN_POINT('Origin',(5.5478765747851E-15,1.85785428279622E-13,
3.36123028058482));
#222159=CARTESIAN_POINT('',(6.67753009965994,-60.4950048380617,3.36123028058439));
#222160=CARTESIAN_POINT('Origin',(5.5478765747851E-15,1.85785428279622E-13,
3.36123028058482));
#222161=CARTESIAN_POINT('',(6.71570789669471,-60.8636883187842,3.48823028058441));
#222162=CARTESIAN_POINT('',(12.4208962742148,-59.9600752509412,3.48823028042653));
#222163=CARTESIAN_POINT('Origin',(5.52999282761008E-15,1.84898592019556E-13,
3.48823028058484));
#222164=CARTESIAN_POINT('',(12.454722128405,-60.1192206258103,3.77003198802665));
#222165=CARTESIAN_POINT('',(12.4208962741593,-59.9600752506734,3.48823028058442));
#222166=CARTESIAN_POINT('',(12.4541661686672,-60.1193358000125,3.77003198860221));
#222167=CARTESIAN_POINT('Origin',(5.49031038273072E-15,1.82930781209959E-13,
3.77003198860263));
#222168=CARTESIAN_POINT('',(6.7332805630058,-61.025435064826,3.7700319886022));
#222169=CARTESIAN_POINT('Origin',(5.49031038273072E-15,1.82930781209959E-13,
3.77003198860263));
#222170=CARTESIAN_POINT('',(6.73271622308859,-61.0254973286577,3.77003198802678));
#222171=CARTESIAN_POINT('Origin',(5.49031038273072E-15,1.82930781209959E-13,
3.77003198860263));
#222172=CARTESIAN_POINT('',(6.7327162231097,-61.0254973289896,3.7700319886022));
#222173=CARTESIAN_POINT('Origin',(62.2224557307631,1.82930781209959E-13,
3.77003198860263));
#222174=CARTESIAN_POINT('',(12.5528626811454,-60.5836663843179,3.7700319886022));
#222175=CARTESIAN_POINT('',(2.3791451040456,-12.7200883457667,3.77003198860254));
#222176=CARTESIAN_POINT('',(6.78290064323623,-61.497538592386,3.7700319886022));
#222177=CARTESIAN_POINT('Origin',(5.49031038273072E-15,1.82930781209959E-13,
3.77003198860263));
#222178=CARTESIAN_POINT('',(6.73333548388602,-61.0259576020966,3.7700319886022));
#222179=CARTESIAN_POINT('Origin',(5.57972911860581E-15,1.8736496251029E-13,
3.13503198860263));
#222180=CARTESIAN_POINT('Origin',(12.1649018101392,-58.7584780045771,3.13502491541395));
#222181=CARTESIAN_POINT('Origin',(6.58785913039885,-59.6417947880739,3.1350249154139));
#222182=CARTESIAN_POINT('Origin',(5.57972911860581E-15,1.8736496251029E-13,
3.13503198860263));
#222183=CARTESIAN_POINT('Origin',(12.5607574282794,-60.6209695535071,3.20381846780018));
#222184=CARTESIAN_POINT('Origin',(6.78691956273308,-61.5354552197178,3.20382022872141));
#222185=CARTESIAN_POINT('Origin',(5.51210908043506E-15,1.8401175575949E-13,
3.61523028058481));
#222186=CARTESIAN_POINT('Origin',(12.3779375131254,-59.760529766771,3.5878694504689));
#222187=CARTESIAN_POINT('Origin',(6.69489156322728,-60.6605407209774,3.58781461834439));
#222188=CARTESIAN_POINT('Origin',(5.51210908043507E-15,1.8401175575949E-13,
3.61523028058481));
#222189=CARTESIAN_POINT('Origin',(12.3398435598856,-59.5817084227214,3.58781440266202));
#222190=CARTESIAN_POINT('Origin',(6.67586224832421,-60.4786998370195,3.58786923592969));
#222191=CARTESIAN_POINT('Origin',(60.4792282238308,1.82930781209959E-13,
3.77003198860263));
#222192=CARTESIAN_POINT('',(0.317500000000634,-60.0036905223729,3.77003198860221));
#222193=CARTESIAN_POINT('',(5.95633285891271,-59.708171814489,3.77003198860221));
#222194=CARTESIAN_POINT('Origin',(5.49031038273072E-15,1.82930781209959E-13,
3.77003198860263));
#222195=CARTESIAN_POINT('',(6.00595296980932,-60.18027563406,3.77003198860221));
#222196=CARTESIAN_POINT('',(0.34504741944992,-6.32035708677281,3.77003198860258));
#222197=CARTESIAN_POINT('',(6.00537737567573,-60.1803330766331,3.77003198902507));
#222198=CARTESIAN_POINT('Origin',(5.49031038273072E-15,1.82930781209959E-13,
3.77003198860263));
#222199=CARTESIAN_POINT('',(0.31807844537663,-60.4783917833344,3.77003198882044));
#222200=CARTESIAN_POINT('Origin',(5.49031038273072E-15,1.82930781209959E-13,
3.77003198860263));
#222201=CARTESIAN_POINT('',(0.317500000025924,-60.4783948217618,3.7700319886022));
#222202=CARTESIAN_POINT('Origin',(5.49031038273072E-15,1.82930781209959E-13,
3.77003198860263));
#222203=CARTESIAN_POINT('',(0.317500000000634,-60.0042281202308,3.77003198860221));
#222204=CARTESIAN_POINT('Origin',(5.49031038273072E-15,1.82930781209959E-13,
3.77003198860263));
#222205=CARTESIAN_POINT('',(6.02238575970337,-60.3421421670673,3.48823028058439));
#222206=CARTESIAN_POINT('',(6.00537737560301,-60.1803330759043,3.77003198860221));
#222207=CARTESIAN_POINT('',(0.318076890625489,-60.6410923275231,3.48823028074762));
#222208=CARTESIAN_POINT('Origin',(5.52999282761009E-15,1.84898592019556E-13,
3.48823028058481));
#222209=CARTESIAN_POINT('',(0.318076890624007,-60.6410923272403,3.48823028058439));
#222210=CARTESIAN_POINT('Origin',(60.71525,1.85785428279622E-13,3.36123028058482));
#222211=CARTESIAN_POINT('',(0.317500000000643,-60.8610688070705,3.36123028058439));
#222212=CARTESIAN_POINT('',(6.04595329345123,-60.5608532912341,3.36123028058439));
#222213=CARTESIAN_POINT('Origin',(5.5478765747851E-15,1.85785428279622E-13,
3.36123028058482));
#222214=CARTESIAN_POINT('',(6.06175884541631,-60.7112330730301,3.36123028058439));
#222215=CARTESIAN_POINT('',(0.347626240494121,-6.34489293004938,3.36123028058477));
#222216=CARTESIAN_POINT('',(0.317500000000645,-61.0122769227454,3.36123028058439));
#222217=CARTESIAN_POINT('Origin',(5.5478765747851E-15,1.85785428279622E-13,
3.36123028058482));
#222218=CARTESIAN_POINT('',(0.317500000000643,-60.8615988316029,3.36123028058439));
#222219=CARTESIAN_POINT('Origin',(5.5478765747851E-15,1.85785428279622E-13,
3.36123028058482));
#222220=CARTESIAN_POINT('',(0.316930737396561,-61.2322532920971,3.48823028058441));
#222221=CARTESIAN_POINT('',(6.08531878141099,-60.9299448849409,3.48823028042652));
#222222=CARTESIAN_POINT('Origin',(5.52999282761008E-15,1.84898592019556E-13,
3.48823028058484));
#222223=CARTESIAN_POINT('',(6.10232411256149,-61.0917542093521,3.77003198802665));
#222224=CARTESIAN_POINT('',(6.08531878138382,-60.9299448846688,3.48823028058441));
#222225=CARTESIAN_POINT('',(6.10175915944695,-61.0918106390009,3.7700319886022));
#222226=CARTESIAN_POINT('Origin',(5.49031038273072E-15,1.82930781209959E-13,
3.77003198860263));
#222227=CARTESIAN_POINT('',(0.317500000000649,-61.3949508163452,3.7700319886022));
#222228=CARTESIAN_POINT('Origin',(5.49031038273072E-15,1.82930781209959E-13,
3.77003198860263));
#222229=CARTESIAN_POINT('',(0.316932243253905,-61.3949537495048,3.77003198802678));
#222230=CARTESIAN_POINT('Origin',(5.49031038273072E-15,1.82930781209959E-13,
3.77003198860263));
#222231=CARTESIAN_POINT('',(0.316932243240209,-61.3949537498371,3.7700319886022));
#222232=CARTESIAN_POINT('Origin',(62.2224557307631,1.82930781209959E-13,
3.77003198860263));
#222233=CARTESIAN_POINT('',(6.15137923967738,-61.5639141665609,3.7700319886022));
#222234=CARTESIAN_POINT('',(0.364094271196581,-6.50157577599598,3.77003198860258));
#222235=CARTESIAN_POINT('',(0.317500000000654,-61.8696548221179,3.77003198860219));
#222236=CARTESIAN_POINT('Origin',(5.49031038273072E-15,1.82930781209959E-13,
3.77003198860263));
#222237=CARTESIAN_POINT('',(0.317500000000649,-61.3954762318971,3.7700319886022));
#222238=CARTESIAN_POINT('Origin',(5.57972911860581E-15,1.8736496251029E-13,
3.13503198860263));
#222239=CARTESIAN_POINT('Origin',(5.95632779542376,-59.7081714060827,3.13502491541391));
#222240=CARTESIAN_POINT('Origin',(0.317504993061173,-60.0036895869252,3.13502491541391));
#222241=CARTESIAN_POINT('Origin',(5.57972911860581E-15,1.8736496251029E-13,
3.13503198860263));
#222242=CARTESIAN_POINT('Origin',(6.15533149560982,-61.601838210872,3.20381846780011));
#222243=CARTESIAN_POINT('Origin',(0.317533536649249,-61.907783829675,3.20382022871824));
#222244=CARTESIAN_POINT('Origin',(5.51210908043506E-15,1.8401175575949E-13,
3.61523028058481));
#222245=CARTESIAN_POINT('Origin',(6.06345353572214,-60.727002118532,3.58786945046753));
#222246=CARTESIAN_POINT('Origin',(0.317463144197163,-61.0280426587402,3.58781461834126));
#222247=CARTESIAN_POINT('Origin',(5.51210908043507E-15,1.8401175575949E-13,
3.61523028058481));
#222248=CARTESIAN_POINT('Origin',(6.04426018543824,-60.5451784741221,3.58781440266149));
#222249=CARTESIAN_POINT('Origin',(0.317545622031384,-60.8452088131247,3.5878692359282));
#222250=CARTESIAN_POINT('Origin',(60.4792282238308,1.82930781209959E-13,
3.77003198860263));
#222251=CARTESIAN_POINT('',(-5.9563328589115,-59.7081718144891,3.77003198860221));
#222252=CARTESIAN_POINT('',(-0.317499999999366,-60.0036905223729,3.77003198860221));
#222253=CARTESIAN_POINT('Origin',(5.49031038273072E-15,1.82930781209959E-13,
3.77003198860263));
#222254=CARTESIAN_POINT('',(-0.317500000024619,-60.4783948217624,3.7700319886022));
#222255=CARTESIAN_POINT('',(-0.317499999999991,-4.53881144958709E-13,3.77003198860263));
#222256=CARTESIAN_POINT('',(-0.318078445377219,-60.4783917836887,3.77003198902499));
#222257=CARTESIAN_POINT('Origin',(5.49031038273072E-15,1.82930781209959E-13,
3.77003198860263));
#222258=CARTESIAN_POINT('',(-6.00537737563932,-60.1803330762805,3.77003198882045));
#222259=CARTESIAN_POINT('Origin',(5.49031038273072E-15,1.82930781209959E-13,
3.77003198860263));
#222260=CARTESIAN_POINT('',(-6.00595296980802,-60.1802756340595,3.77003198860221));
#222261=CARTESIAN_POINT('Origin',(5.49031038273072E-15,1.82930781209959E-13,
3.77003198860263));
#222262=CARTESIAN_POINT('',(-5.95638905318945,-59.7087064673298,3.77003198860221));
#222263=CARTESIAN_POINT('Origin',(5.49031038273072E-15,1.82930781209959E-13,
3.77003198860263));
#222264=CARTESIAN_POINT('',(-0.318076890622726,-60.6410923272404,3.48823028058439));
#222265=CARTESIAN_POINT('',(-0.318078445373366,-60.4783917829565,3.7700319886022));
#222266=CARTESIAN_POINT('',(-6.02238575973022,-60.3421421673487,3.48823028074762));
#222267=CARTESIAN_POINT('Origin',(5.52999282761009E-15,1.84898592019556E-13,
3.48823028058481));
#222268=CARTESIAN_POINT('',(-6.02238575970214,-60.3421421670674,3.48823028058439));
#222269=CARTESIAN_POINT('Origin',(60.71525,1.85785428279622E-13,3.36123028058482));
#222270=CARTESIAN_POINT('',(-6.04595329344999,-60.5608532912342,3.36123028058439));
#222271=CARTESIAN_POINT('',(-0.317499999999354,-60.8610688070705,3.36123028058439));
#222272=CARTESIAN_POINT('Origin',(5.5478765747851E-15,1.85785428279622E-13,
3.36123028058482));
#222273=CARTESIAN_POINT('',(-0.317499999999355,-61.0122769227454,3.36123028058439));
#222274=CARTESIAN_POINT('',(-0.317499999999991,-4.53498694770213E-13,3.36123028058482));
#222275=CARTESIAN_POINT('',(-6.06175884541508,-60.7112330730303,3.36123028058439));
#222276=CARTESIAN_POINT('Origin',(5.5478765747851E-15,1.85785428279622E-13,
3.36123028058482));
#222277=CARTESIAN_POINT('',(-6.04600869609986,-60.5613804122368,3.36123028058439));
#222278=CARTESIAN_POINT('Origin',(5.5478765747851E-15,1.85785428279622E-13,
3.36123028058482));
#222279=CARTESIAN_POINT('',(-6.08531878138258,-60.9299448846689,3.48823028058441));
#222280=CARTESIAN_POINT('',(-0.316930737396683,-61.2322532923705,3.48823028042652));
#222281=CARTESIAN_POINT('Origin',(5.52999282761008E-15,1.84898592019556E-13,
3.48823028058484));
#222282=CARTESIAN_POINT('',(-0.316932243252611,-61.3949537495047,3.77003198802664));
#222283=CARTESIAN_POINT('',(-0.316930737395267,-61.2322532920971,3.48823028058441));
#222284=CARTESIAN_POINT('',(-0.317499999999355,-61.3949508163452,3.7700319886022));
#222285=CARTESIAN_POINT('Origin',(5.49031038273072E-15,1.82930781209959E-13,
3.77003198860263));
#222286=CARTESIAN_POINT('',(-6.10175915944571,-61.0918106390011,3.7700319886022));
#222287=CARTESIAN_POINT('Origin',(5.49031038273072E-15,1.82930781209959E-13,
3.77003198860263));
#222288=CARTESIAN_POINT('',(-6.10232411256026,-61.0917542093523,3.77003198802677));
#222289=CARTESIAN_POINT('Origin',(5.49031038273072E-15,1.82930781209959E-13,
3.77003198860263));
#222290=CARTESIAN_POINT('',(-6.10232411260861,-61.0917542096813,3.7700319886022));
#222291=CARTESIAN_POINT('Origin',(62.2224557307631,1.82930781209959E-13,
3.77003198860263));
#222292=CARTESIAN_POINT('',(-0.317499999999346,-61.8696548221179,3.77003198860219));
#222293=CARTESIAN_POINT('',(-0.317499999999998,-4.72140483888146E-13,3.77003198860263));
#222294=CARTESIAN_POINT('',(-6.15137923967613,-61.5639141665611,3.7700319886022));
#222295=CARTESIAN_POINT('Origin',(5.49031038273072E-15,1.82930781209959E-13,
3.77003198860263));
#222296=CARTESIAN_POINT('',(-6.10181408032593,-61.0923331762716,3.7700319886022));
#222297=CARTESIAN_POINT('Origin',(5.57972911860581E-15,1.8736496251029E-13,
3.13503198860263));
#222298=CARTESIAN_POINT('Origin',(-0.317504993060079,-60.0036895869252,
3.13502491541387));
#222299=CARTESIAN_POINT('Origin',(-5.9563277954224,-59.7081714060829,3.13502491541391));
#222300=CARTESIAN_POINT('Origin',(5.57972911860581E-15,1.8736496251029E-13,
3.13503198860263));
#222301=CARTESIAN_POINT('Origin',(-0.317533537010846,-61.9077842377865,
3.20381846780275));
#222302=CARTESIAN_POINT('Origin',(-6.15533145331086,-61.6018378049613,3.20382022872096));
#222303=CARTESIAN_POINT('Origin',(5.51210908043506E-15,1.8401175575949E-13,
3.61523028058481));
#222304=CARTESIAN_POINT('Origin',(-0.31746290747785,-61.0281367271388,3.58786945046874));
#222305=CARTESIAN_POINT('Origin',(-6.06344346747435,-60.7269085901922,3.58781461834308));
#222306=CARTESIAN_POINT('Origin',(5.51210908043507E-15,1.8401175575949E-13,
3.61523028058481));
#222307=CARTESIAN_POINT('Origin',(-0.317545368444823,-60.8453028802683,
3.58781440266191));
#222308=CARTESIAN_POINT('Origin',(-6.0442501005473,-60.5450849487949,3.58786923592771));
#222309=CARTESIAN_POINT('Origin',(60.4792282238308,1.82930781209959E-13,
3.77003198860263));
#222310=CARTESIAN_POINT('',(-12.1649068885786,-58.7584778814676,3.77003198860222));
#222311=CARTESIAN_POINT('',(-6.58785426247035,-59.6417962403142,3.77003198860221));
#222312=CARTESIAN_POINT('Origin',(5.49031038273072E-15,1.82930781209959E-13,
3.77003198860263));
#222313=CARTESIAN_POINT('',(-6.63747437341721,-60.1139000598799,3.77003198860221));
#222314=CARTESIAN_POINT('',(0.345047419449671,6.32035708677198,3.77003198860267));
#222315=CARTESIAN_POINT('',(-6.63804933242046,-60.1138365744453,3.77003198902501));
#222316=CARTESIAN_POINT('Origin',(5.49031038273072E-15,1.82930781209959E-13,
3.77003198860263));
#222317=CARTESIAN_POINT('',(-12.2630370254217,-59.2229260464986,3.77003198882045));
#222318=CARTESIAN_POINT('Origin',(5.49031038273072E-15,1.82930781209959E-13,
3.77003198860263));
#222319=CARTESIAN_POINT('',(-12.2636034620782,-59.2228087529782,3.77003198860221));
#222320=CARTESIAN_POINT('Origin',(5.49031038273072E-15,1.82930781209959E-13,
3.77003198860263));
#222321=CARTESIAN_POINT('',(-12.1650186614582,-58.7590037315225,3.77003198860222));
#222322=CARTESIAN_POINT('Origin',(5.49031038273072E-15,1.82930781209959E-13,
3.77003198860263));
#222323=CARTESIAN_POINT('',(-6.65505462397334,-60.2756459899118,3.48823028058439));
#222324=CARTESIAN_POINT('',(-6.63804933234009,-60.1138365737174,3.77003198860221));
#222325=CARTESIAN_POINT('',(-12.296865891437,-59.3820708701839,3.48823028074763));
#222326=CARTESIAN_POINT('Origin',(5.52999282761009E-15,1.84898592019556E-13,
3.48823028058481));
#222327=CARTESIAN_POINT('',(-12.2968658913797,-59.382070869907,3.4882302805844));
#222328=CARTESIAN_POINT('Origin',(60.71525,1.85785428279622E-13,3.36123028058482));
#222329=CARTESIAN_POINT('',(-12.3431658574205,-59.5971203935659,3.3612302805844));
#222330=CARTESIAN_POINT('',(-6.67747469700884,-60.4944777170593,3.36123028058439));
#222331=CARTESIAN_POINT('Origin',(5.5478765747851E-15,1.85785428279622E-13,
3.36123028058482));
#222332=CARTESIAN_POINT('',(-6.69328024897394,-60.6448574988553,3.36123028058439));
#222333=CARTESIAN_POINT('',(0.347626240493851,6.34489293004856,3.36123028058486));
#222334=CARTESIAN_POINT('',(-12.3746037924158,-59.7450242491247,3.3612302805844));
#222335=CARTESIAN_POINT('Origin',(5.5478765747851E-15,1.85785428279622E-13,
3.36123028058482));
#222336=CARTESIAN_POINT('',(-12.3432760557172,-59.5976388357906,3.3612302805844));
#222337=CARTESIAN_POINT('Origin',(5.5478765747851E-15,1.85785428279622E-13,
3.36123028058482));
#222338=CARTESIAN_POINT('',(-12.420896274158,-59.9600752506736,3.48823028058442));
#222339=CARTESIAN_POINT('',(-6.71570789672347,-60.8636883190562,3.48823028042652));
#222340=CARTESIAN_POINT('Origin',(5.52999282761008E-15,1.84898592019556E-13,
3.48823028058484));
#222341=CARTESIAN_POINT('',(-6.73271622308735,-61.0254973286578,3.77003198802665));
#222342=CARTESIAN_POINT('',(-6.71570789669348,-60.8636883187843,3.48823028058441));
#222343=CARTESIAN_POINT('',(-6.73328056300457,-61.0254350648261,3.7700319886022));
#222344=CARTESIAN_POINT('Origin',(5.49031038273072E-15,1.82930781209959E-13,
3.77003198860263));
#222345=CARTESIAN_POINT('',(-12.4541661686659,-60.1193358000128,3.77003198860221));
#222346=CARTESIAN_POINT('Origin',(5.49031038273072E-15,1.82930781209959E-13,
3.77003198860263));
#222347=CARTESIAN_POINT('',(-12.4547221284037,-60.1192206258107,3.77003198802678));
#222348=CARTESIAN_POINT('Origin',(5.49031038273072E-15,1.82930781209959E-13,
3.77003198860263));
#222349=CARTESIAN_POINT('',(-12.4547221284862,-60.1192206261329,3.77003198860221));
#222350=CARTESIAN_POINT('Origin',(62.2224557307631,1.82930781209959E-13,
3.77003198860263));
#222351=CARTESIAN_POINT('',(-6.78290064323498,-61.4975385923861,3.7700319886022));
#222352=CARTESIAN_POINT('',(0.364094271196325,6.50157577599512,3.77003198860267));
#222353=CARTESIAN_POINT('',(-12.5528626811441,-60.5836663843181,3.7700319886022));
#222354=CARTESIAN_POINT('Origin',(5.49031038273072E-15,1.82930781209959E-13,
3.77003198860263));
#222355=CARTESIAN_POINT('',(-12.4542754087017,-60.1198497339743,3.7700319886022));
#222356=CARTESIAN_POINT('Origin',(5.57972911860581E-15,1.8736496251029E-13,
3.13503198860263));
#222357=CARTESIAN_POINT('Origin',(-6.58785913039748,-59.641794788074,3.13502491541394));
#222358=CARTESIAN_POINT('Origin',(-12.1649018101377,-58.7584780045774,3.1350249154139));
#222359=CARTESIAN_POINT('Origin',(5.57972911860581E-15,1.8736496251029E-13,
3.13503198860263));
#222360=CARTESIAN_POINT('Origin',(-6.78691960575311,-61.535455625553,3.20381846780075));
#222361=CARTESIAN_POINT('Origin',(-12.5607573437809,-60.6209691542415,3.2038202287205));
#222362=CARTESIAN_POINT('Origin',(5.51210908043506E-15,1.8401175575949E-13,
3.61523028058481));
#222363=CARTESIAN_POINT('Origin',(-6.69490116062999,-60.660634298804,3.58786945047091));
#222364=CARTESIAN_POINT('Origin',(-12.3779177236593,-59.7604378032097,3.58781461834093));
#222365=CARTESIAN_POINT('Origin',(5.51210908043507E-15,1.8401175575949E-13,
3.61523028058481));
#222366=CARTESIAN_POINT('Origin',(-6.67587182882074,-60.478793415361,3.58781440266411));
#222367=CARTESIAN_POINT('Origin',(-12.3398237541835,-59.5816164638921,3.58786923592573));
#222368=CARTESIAN_POINT('Origin',(60.4792282238308,1.82930781209959E-13,
3.77003198860263));
#222369=CARTESIAN_POINT('',(-18.240199652704,-57.1650137687747,3.77003198860223));
#222370=CARTESIAN_POINT('',(-12.7860306150445,-58.6264539577983,3.77003198860222));
#222371=CARTESIAN_POINT('Origin',(5.49031038273072E-15,1.82930781209959E-13,
3.77003198860263));
#222372=CARTESIAN_POINT('',(-12.8847271885938,-59.090784829299,3.77003198860221));
#222373=CARTESIAN_POINT('',(2.30379013587678,12.3655710936223,3.77003198860271));
#222374=CARTESIAN_POINT('',(-12.8852923618765,-59.090661592063,3.77003198902489));
#222375=CARTESIAN_POINT('Origin',(5.49031038273072E-15,1.82930781209959E-13,
3.77003198860263));
#222376=CARTESIAN_POINT('',(-18.3863402753482,-57.6166602457572,3.77003198882046));
#222377=CARTESIAN_POINT('Origin',(5.49031038273072E-15,1.82930781209959E-13,
3.77003198860263));
#222378=CARTESIAN_POINT('',(-18.386891348494,-57.6164843860297,3.77003198860222));
#222379=CARTESIAN_POINT('Origin',(5.49031038273072E-15,1.82930781209959E-13,
3.77003198860263));
#222380=CARTESIAN_POINT('',(-18.2403657795782,-57.1655250547206,3.77003198860222));
#222381=CARTESIAN_POINT('Origin',(5.49031038273072E-15,1.82930781209959E-13,
3.77003198860263));
#222382=CARTESIAN_POINT('',(-12.9191181862039,-59.2498070616279,3.4882302805844));
#222383=CARTESIAN_POINT('',(-12.8852923617205,-59.0906615913477,3.77003198860221));
#222384=CARTESIAN_POINT('',(-18.4366189871527,-57.771397178068,3.48823028074764));
#222385=CARTESIAN_POINT('Origin',(5.52999282761009E-15,1.84898592019556E-13,
3.48823028058481));
#222386=CARTESIAN_POINT('',(-18.4366189870667,-57.7713971777987,3.48823028058441));
#222387=CARTESIAN_POINT('Origin',(60.71525,1.85785428279622E-13,3.36123028058482));
#222388=CARTESIAN_POINT('',(-18.5051441132836,-57.9804289733664,3.36123028058441));
#222389=CARTESIAN_POINT('',(-12.9642895838864,-59.4650964698966,3.3612302805844));
#222390=CARTESIAN_POINT('Origin',(5.5478765747851E-15,1.85785428279622E-13,
3.36123028058482));
#222391=CARTESIAN_POINT('',(-12.9957275188818,-59.6130003254554,3.3612302805844));
#222392=CARTESIAN_POINT('',(2.31399271319931,12.4135704460882,3.3612302805849));
#222393=CARTESIAN_POINT('',(-18.5518699907145,-58.1242364370956,3.36123028058441));
#222394=CARTESIAN_POINT('Origin',(5.5478765747851E-15,1.85785428279622E-13,
3.36123028058482));
#222395=CARTESIAN_POINT('',(-18.5053078998715,-57.9809330566517,3.3612302805844));
#222396=CARTESIAN_POINT('Origin',(5.5478765747851E-15,1.85785428279622E-13,
3.36123028058482));
#222397=CARTESIAN_POINT('',(-18.6203878281142,-58.3332704847796,3.48823028058443));
#222398=CARTESIAN_POINT('',(-13.0409063549815,-59.8282880399726,3.48823028042653));
#222399=CARTESIAN_POINT('Origin',(5.52999282761008E-15,1.84898592019556E-13,
3.48823028058484));
#222400=CARTESIAN_POINT('',(-13.0747351550704,-59.9874327886717,3.77003198802665));
#222401=CARTESIAN_POINT('',(-13.0409063549232,-59.8282880397054,3.48823028058442));
#222402=CARTESIAN_POINT('',(-13.0752898951319,-59.9873118763435,3.77003198860221));
#222403=CARTESIAN_POINT('Origin',(5.49031038273072E-15,1.82930781209959E-13,
3.77003198860263));
#222404=CARTESIAN_POINT('',(-18.6701227271405,-58.4881809372197,3.77003198860222));
#222405=CARTESIAN_POINT('Origin',(5.49031038273072E-15,1.82930781209959E-13,
3.77003198860263));
#222406=CARTESIAN_POINT('',(-18.6706636022903,-58.4880082803369,3.77003198802679));
#222407=CARTESIAN_POINT('Origin',(5.49031038273072E-15,1.82930781209959E-13,
3.77003198860263));
#222408=CARTESIAN_POINT('',(-18.670663602406,-58.4880082806487,3.77003198860222));
#222409=CARTESIAN_POINT('Origin',(62.2224557307631,1.82930781209959E-13,
3.77003198860263));
#222410=CARTESIAN_POINT('',(-13.1739864076101,-60.4516424606488,3.7700319886022));
#222411=CARTESIAN_POINT('',(2.3791451040451,12.7200883457658,3.77003198860271));
#222412=CARTESIAN_POINT('',(-18.8168143322221,-58.9396512752213,3.77003198860221));
#222413=CARTESIAN_POINT('Origin',(5.49031038273072E-15,1.82930781209959E-13,
3.77003198860263));
#222414=CARTESIAN_POINT('',(-18.6702850894751,-58.4886806371042,3.77003198860221));
#222415=CARTESIAN_POINT('Origin',(5.57972911860581E-15,1.8736496251029E-13,
3.13503198860263));
#222416=CARTESIAN_POINT('Origin',(-12.7860353045042,-58.6264520046768,3.13502491541392));
#222417=CARTESIAN_POINT('Origin',(-18.2401946149518,-57.1650144220517,3.13502491541393));
#222418=CARTESIAN_POINT('Origin',(5.57972911860581E-15,1.8736496251029E-13,
3.13503198860263));
#222419=CARTESIAN_POINT('Origin',(-13.1819467630409,-60.4889316843646,3.20381846780152));
#222420=CARTESIAN_POINT('Origin',(-18.8285649482867,-58.9759244797155,3.20382022872249));
#222421=CARTESIAN_POINT('Origin',(5.51210908043506E-15,1.8401175575949E-13,
3.61523028058481));
#222422=CARTESIAN_POINT('Origin',(-12.9989886756684,-59.6285212670402,3.58786945046826));
#222423=CARTESIAN_POINT('Origin',(-18.556776923018,-58.1392191539787,3.58781461834011));
#222424=CARTESIAN_POINT('Origin',(5.51210908043507E-15,1.8401175575949E-13,
3.61523028058481));
#222425=CARTESIAN_POINT('Origin',(-12.9610560404233,-59.4496656337922,3.58781440266299));
#222426=CARTESIAN_POINT('Origin',(-18.5001997164934,-57.965359320759,3.58786923592875));
#222427=CARTESIAN_POINT('Origin',(60.4792282238308,1.82930781209959E-13,
3.77003198860263));
#222428=CARTESIAN_POINT('',(-24.1156489724272,-54.9452378026829,3.77003198860224));
#222429=CARTESIAN_POINT('',(-18.8441205405514,-56.9687879773466,3.77003198860223));
#222430=CARTESIAN_POINT('Origin',(5.49031038273072E-15,1.82930781209959E-13,
3.77003198860263));
#222431=CARTESIAN_POINT('',(-18.9908122363897,-57.4202585945866,3.77003198860222));
#222432=CARTESIAN_POINT('',(5.47329194811131,17.872512105713,3.77003198860275));
#222433=CARTESIAN_POINT('',(-18.9913614317952,-57.4200769557627,3.77003198902513));
#222434=CARTESIAN_POINT('Origin',(5.49031038273072E-15,1.82930781209959E-13,
3.77003198860263));
#222435=CARTESIAN_POINT('',(-24.3081989336288,-55.379134258302,3.77003198882047));
#222436=CARTESIAN_POINT('Origin',(5.49031038273072E-15,1.82930781209959E-13,
3.77003198860263));
#222437=CARTESIAN_POINT('',(-24.3087286055912,-55.3789017591234,3.77003198860224));
#222438=CARTESIAN_POINT('Origin',(5.49031038273072E-15,1.82930781209959E-13,
3.77003198860263));
#222439=CARTESIAN_POINT('',(-24.1158676331753,-54.9457289227641,3.77003198860224));
#222440=CARTESIAN_POINT('Origin',(5.49031038273072E-15,1.82930781209959E-13,
3.77003198860263));
#222441=CARTESIAN_POINT('',(-19.0416371860872,-57.5748148483576,3.48823028058441));
#222442=CARTESIAN_POINT('',(-18.9913614315652,-57.4200769550672,3.77003198860223));
#222443=CARTESIAN_POINT('',(-24.3743766271346,-55.5277679690272,3.48823028074766));
#222444=CARTESIAN_POINT('Origin',(5.52999282761009E-15,1.84898592019556E-13,
3.48823028058481));
#222445=CARTESIAN_POINT('',(-24.3743766270209,-55.5277679687683,3.48823028058442));
#222446=CARTESIAN_POINT('Origin',(60.71525,1.85785428279622E-13,3.36123028058482));
#222447=CARTESIAN_POINT('',(-24.4643761377912,-55.7284918401498,3.36123028058443));
#222448=CARTESIAN_POINT('',(-19.109065001131,-57.7842031819383,3.36123028058441));
#222449=CARTESIAN_POINT('Origin',(5.5478765747851E-15,1.85785428279622E-13,
3.36123028058482));
#222450=CARTESIAN_POINT('',(-19.155790878562,-57.9280106456676,3.36123028058441));
#222451=CARTESIAN_POINT('',(5.4958300222142,17.9418771653391,3.36123028058494));
#222452=CARTESIAN_POINT('',(-24.5258780191666,-55.8666273273833,3.36123028058442));
#222453=CARTESIAN_POINT('Origin',(5.5478765747851E-15,1.85785428279622E-13,
3.36123028058482));
#222454=CARTESIAN_POINT('',(-24.4645917181903,-55.7289760416539,3.36123028058442));
#222455=CARTESIAN_POINT('Origin',(5.5478765747851E-15,1.85785428279622E-13,
3.36123028058482));
#222456=CARTESIAN_POINT('',(-24.6158705164589,-56.0673542004326,3.48823028058445));
#222457=CARTESIAN_POINT('',(-19.2232259142293,-58.137396517249,3.48823028042654));
#222458=CARTESIAN_POINT('Origin',(5.52999282761008E-15,1.84898592019556E-13,
3.48823028058484));
#222459=CARTESIAN_POINT('',(-19.2735045526304,-58.2921333818756,3.77003198802666));
#222460=CARTESIAN_POINT('',(-19.2232259141434,-58.1373965169893,3.48823028058443));
#222461=CARTESIAN_POINT('',(-19.2740436149879,-58.2919551457917,3.77003198860222));
#222462=CARTESIAN_POINT('Origin',(5.49031038273072E-15,1.82930781209959E-13,
3.77003198860263));
#222463=CARTESIAN_POINT('',(-24.6815255140421,-56.2162173246398,3.77003198860223));
#222464=CARTESIAN_POINT('Origin',(5.49031038273072E-15,1.82930781209959E-13,
3.77003198860263));
#222465=CARTESIAN_POINT('',(-24.6820453786627,-56.2159890767412,3.77003198802681));
#222466=CARTESIAN_POINT('Origin',(5.49031038273072E-15,1.82930781209959E-13,
3.77003198860263));
#222467=CARTESIAN_POINT('',(-24.6820453788103,-56.2159890770392,3.77003198860223));
#222468=CARTESIAN_POINT('Origin',(62.2224557307631,1.82930781209959E-13,
3.77003198860263));
#222469=CARTESIAN_POINT('',(-19.4207352200695,-58.7434254837932,3.77003198860222));
#222470=CARTESIAN_POINT('',(5.6397553624924,18.3848338156956,3.77003198860276));
#222471=CARTESIAN_POINT('',(-24.8746050278048,-56.6498810128382,3.77003198860222));
#222472=CARTESIAN_POINT('Origin',(5.49031038273072E-15,1.82930781209959E-13,
3.77003198860263));
#222473=CARTESIAN_POINT('',(-24.6817392197999,-56.2166973156306,3.77003198860223));
#222474=CARTESIAN_POINT('Origin',(5.57972911860581E-15,1.8736496251029E-13,
3.13503198860263));
#222475=CARTESIAN_POINT('Origin',(-18.8441250001649,-56.9687855447424,3.13502491541394));
#222476=CARTESIAN_POINT('Origin',(-24.1156440305584,-54.9452389789697,3.13502491541395));
#222477=CARTESIAN_POINT('Origin',(5.57972911860581E-15,1.8736496251029E-13,
3.13503198860263));
#222478=CARTESIAN_POINT('Origin',(-19.4325497530904,-58.7796783495202,3.20381846780163));
#222479=CARTESIAN_POINT('Origin',(-24.8900828550892,-56.6847272350805,3.20382022871814));
#222480=CARTESIAN_POINT('Origin',(5.51210908043506E-15,1.8401175575949E-13,
3.61523028058481));
#222481=CARTESIAN_POINT('Origin',(-19.1606565505628,-57.9431056782031,3.58786945046785));
#222482=CARTESIAN_POINT('Origin',(-24.5323241911526,-55.881015053282,3.58781461834135));
#222483=CARTESIAN_POINT('Origin',(5.51210908043507E-15,1.8401175575949E-13,
3.61523028058481));
#222484=CARTESIAN_POINT('Origin',(-19.1042362097712,-57.7691948748994,3.58781440266517));
#222485=CARTESIAN_POINT('Origin',(-24.4578836192973,-55.7140215708735,3.58786923592871));
#222486=CARTESIAN_POINT('Origin',(60.4792282238308,1.82930781209959E-13,
3.77003198860263));
#222487=CARTESIAN_POINT('',(-29.7268821954845,-52.1234703131947,3.77003198860226));
#222488=CARTESIAN_POINT('',(-24.6957503380303,-54.6869600343298,3.77003198860224));
#222489=CARTESIAN_POINT('Origin',(5.49031038273072E-15,1.82930781209959E-13,
3.77003198860263));
#222490=CARTESIAN_POINT('',(-24.8888299712407,-55.1206239907502,3.77003198860224));
#222491=CARTESIAN_POINT('',(9.71531210234964,22.6015516358795,3.77003198860278));
#222492=CARTESIAN_POINT('',(-24.8893571716689,-55.1203859404104,3.77003198902472));
#222493=CARTESIAN_POINT('Origin',(5.49031038273072E-15,1.82930781209959E-13,
3.77003198860263));
#222494=CARTESIAN_POINT('',(-29.963731877575,-52.5348628870839,3.77003198882049));
#222495=CARTESIAN_POINT('Origin',(5.49031038273072E-15,1.82930781209959E-13,
3.77003198860263));
#222496=CARTESIAN_POINT('',(-29.964234345157,-52.5345762957639,3.77003198860226));
#222497=CARTESIAN_POINT('Origin',(5.49031038273072E-15,1.82930781209959E-13,
3.77003198860263));
#222498=CARTESIAN_POINT('',(-29.7271509944135,-52.1239358865967,3.77003198860226));
#222499=CARTESIAN_POINT('Origin',(5.49031038273072E-15,1.82930781209959E-13,
3.77003198860263));
#222500=CARTESIAN_POINT('',(-24.955532024241,-55.2690209153041,3.48823028058442));
#222501=CARTESIAN_POINT('',(-24.8893571713678,-55.1203859397435,3.77003198860224));
#222502=CARTESIAN_POINT('',(-30.0450834961233,-52.6757649141853,3.48823028074767));
#222503=CARTESIAN_POINT('Origin',(5.52999282761009E-15,1.84898592019556E-13,
3.48823028058481));
#222504=CARTESIAN_POINT('',(-30.0450834959832,-52.6757649139397,3.48823028058444));
#222505=CARTESIAN_POINT('Origin',(60.71525,1.85785428279622E-13,3.36123028058482));
#222506=CARTESIAN_POINT('',(-30.1555713378333,-52.865981688396,3.36123028058444));
#222507=CARTESIAN_POINT('',(-25.0444775033943,-55.4702140717967,3.36123028058442));
#222508=CARTESIAN_POINT('Origin',(5.5478765747851E-15,1.85785428279622E-13,
3.36123028058482));
#222509=CARTESIAN_POINT('',(-25.1059793847697,-55.6083495590302,3.36123028058442));
#222510=CARTESIAN_POINT('',(9.75435829333326,22.6892508167096,3.36123028058498));
#222511=CARTESIAN_POINT('',(-30.2311753956707,-52.9969317578288,3.36123028058444));
#222512=CARTESIAN_POINT('Origin',(5.5478765747851E-15,1.85785428279622E-13,
3.36123028058482));
#222513=CARTESIAN_POINT('',(-30.1558363500995,-52.8664407031057,3.36123028058444));
#222514=CARTESIAN_POINT('Origin',(5.5478765747851E-15,1.85785428279622E-13,
3.36123028058482));
#222515=CARTESIAN_POINT('',(-30.3416565762231,-53.1871522506176,3.48823028058446));
#222516=CARTESIAN_POINT('',(-25.1949317876421,-55.80953951225,3.48823028042655));
#222517=CARTESIAN_POINT('Origin',(5.52999282761008E-15,1.84898592019556E-13,
3.48823028058484));
#222518=CARTESIAN_POINT('',(-25.2611094010716,-55.9581731633345,3.77003198802667));
#222519=CARTESIAN_POINT('',(-25.1949317875296,-55.8095395120007,3.48823028058444));
#222520=CARTESIAN_POINT('',(-25.2616268796452,-55.9579395562867,3.77003198860223));
#222521=CARTESIAN_POINT('Origin',(5.49031038273072E-15,1.82930781209959E-13,
3.77003198860263));
#222522=CARTESIAN_POINT('',(-30.4225123424706,-53.3283370710513,3.77003198860225));
#222523=CARTESIAN_POINT('Origin',(5.49031038273072E-15,1.82930781209959E-13,
3.77003198860263));
#222524=CARTESIAN_POINT('',(-30.4230055008163,-53.3280557328687,3.77003198802683));
#222525=CARTESIAN_POINT('Origin',(5.49031038273072E-15,1.82930781209959E-13,
3.77003198860263));
#222526=CARTESIAN_POINT('',(-30.4230055009943,-53.3280557331497,3.77003198860225));
#222527=CARTESIAN_POINT('Origin',(62.2224557307631,1.82930781209959E-13,
3.77003198860263));
#222528=CARTESIAN_POINT('',(-25.4547063934078,-56.3916032444851,3.77003198860223));
#222529=CARTESIAN_POINT('',(10.0037024164483,23.2492868865828,3.77003198860279));
#222530=CARTESIAN_POINT('',(-30.659864345357,-53.7394427993287,3.77003198860225));
#222531=CARTESIAN_POINT('Origin',(5.49031038273072E-15,1.82930781209959E-13,
3.77003198860263));
#222532=CARTESIAN_POINT('',(-30.4227750502466,-53.3287920942669,3.77003198860225));
#222533=CARTESIAN_POINT('Origin',(5.57972911860581E-15,1.8736496251029E-13,
3.13503198860263));
#222534=CARTESIAN_POINT('Origin',(-24.6957545189372,-54.6869571488951,3.13502491541393));
#222535=CARTESIAN_POINT('Origin',(-29.7268774036433,-52.1234719996036,3.13502491541395));
#222536=CARTESIAN_POINT('Origin',(5.57972911860581E-15,1.8736496251029E-13,
3.13503198860263));
#222537=CARTESIAN_POINT('Origin',(-25.4702456615231,-56.4264225582405,3.20381846780269));
#222538=CARTESIAN_POINT('Origin',(-30.6788998055448,-53.7724802568237,3.20382022872574));
#222539=CARTESIAN_POINT('Origin',(5.51210908043506E-15,1.8401175575949E-13,
3.61523028058481));
#222540=CARTESIAN_POINT('Origin',(-25.1123962626642,-55.622853298181,3.58786945046793));
#222541=CARTESIAN_POINT('Origin',(-30.2390901817304,-53.0105668578083,3.58781461834049));
#222542=CARTESIAN_POINT('Origin',(5.51210908043507E-15,1.8401175575949E-13,
3.61523028058481));
#222543=CARTESIAN_POINT('Origin',(-25.038106369386,-55.4557927279741,3.58781440266369));
#222544=CARTESIAN_POINT('Origin',(-30.1476018310241,-52.852269341751,3.58786923593029));
#222545=CARTESIAN_POINT('Origin',(60.4792282238308,1.82930781209959E-13,
3.77003198860263));
#222546=CARTESIAN_POINT('',(-35.0124214764581,-48.7306271754178,3.77003198860228));
#222547=CARTESIAN_POINT('',(-30.2768083268876,-51.8059703131947,3.77003198860226));
#222548=CARTESIAN_POINT('Origin',(5.49031038273072E-15,1.82930781209959E-13,
3.77003198860263));
#222549=CARTESIAN_POINT('',(-30.5141604766043,-52.2170762957392,3.77003198860226));
#222550=CARTESIAN_POINT('',(14.8448439902557,26.347024021557,3.77003198860281));
#222551=CARTESIAN_POINT('',(-30.5146599059375,-52.216784442014,3.77003198902515));
#222552=CARTESIAN_POINT('Origin',(5.49031038273072E-15,1.82930781209959E-13,
3.77003198860263));
#222553=CARTESIAN_POINT('',(-35.2909759047564,-49.1150085644481,3.77003198882052));
#222554=CARTESIAN_POINT('Origin',(5.49031038273072E-15,1.82930781209959E-13,
3.77003198860263));
#222555=CARTESIAN_POINT('',(-35.2914456628182,-49.1146710209411,3.77003198860228));
#222556=CARTESIAN_POINT('Origin',(5.49031038273072E-15,1.82930781209959E-13,
3.77003198860263));
#222557=CARTESIAN_POINT('',(-35.0127374685506,-48.731062101221,3.77003198860228));
#222558=CARTESIAN_POINT('Origin',(5.49031038273072E-15,1.82930781209959E-13,
3.77003198860263));
#222559=CARTESIAN_POINT('',(-30.5960088312564,-52.3576880233163,3.48823028058444));
#222560=CARTESIAN_POINT('',(-30.514659905568,-52.2167844413816,3.77003198860226));
#222561=CARTESIAN_POINT('',(-35.3866101429905,-49.246635155831,3.48823028074769));
#222562=CARTESIAN_POINT('Origin',(5.52999282761009E-15,1.84898592019556E-13,
3.48823028058481));
#222563=CARTESIAN_POINT('',(-35.3866101428255,-49.2466351556014,3.48823028058446));
#222564=CARTESIAN_POINT('Origin',(60.71525,1.85785428279622E-13,3.36123028058482));
#222565=CARTESIAN_POINT('',(-35.5163757878391,-49.4242607783462,3.36123028058446));
#222566=CARTESIAN_POINT('',(-30.7054974692364,-52.548481688396,3.36123028058444));
#222567=CARTESIAN_POINT('Origin',(5.5478765747851E-15,1.85785428279622E-13,
3.36123028058482));
#222568=CARTESIAN_POINT('',(-30.7811015270739,-52.6794317578288,3.36123028058444));
#222569=CARTESIAN_POINT('',(14.903849434298,26.4492244485615,3.361230280585));
#222570=CARTESIAN_POINT('',(-35.6052536882598,-49.5465907136146,3.36123028058446));
#222571=CARTESIAN_POINT('Origin',(5.5478765747851E-15,1.85785428279622E-13,
3.36123028058482));
#222572=CARTESIAN_POINT('',(-35.5166873284426,-49.4246895772004,3.36123028058446));
#222573=CARTESIAN_POINT('Origin',(5.5478765747851E-15,1.85785428279622E-13,
3.36123028058482));
#222574=CARTESIAN_POINT('',(-35.7350130971385,-49.7242207306176,3.48823028058449));
#222575=CARTESIAN_POINT('',(-30.8905967160111,-52.8702215134578,3.48823028042657));
#222576=CARTESIAN_POINT('Origin',(5.52999282761008E-15,1.84898592019556E-13,
3.48823028058484));
#222577=CARTESIAN_POINT('',(-30.9719482486877,-53.0111234896154,3.7700319880267));
#222578=CARTESIAN_POINT('',(-30.8905967158731,-52.8702215132217,3.48823028058446));
#222579=CARTESIAN_POINT('',(-30.9724384738737,-53.0108370710513,3.77003198860225));
#222580=CARTESIAN_POINT('Origin',(5.49031038273072E-15,1.82930781209959E-13,
3.77003198860263));
#222581=CARTESIAN_POINT('',(-35.830183759355,-49.8561803968404,3.77003198860227));
#222582=CARTESIAN_POINT('Origin',(5.49031038273072E-15,1.82930781209959E-13,
3.77003198860263));
#222583=CARTESIAN_POINT('',(-35.8306448082798,-49.8558490507738,3.77003198802685));
#222584=CARTESIAN_POINT('Origin',(5.49031038273072E-15,1.82930781209959E-13,
3.77003198860263));
#222585=CARTESIAN_POINT('',(-35.8306448084862,-49.8558490510346,3.77003198860227));
#222586=CARTESIAN_POINT('Origin',(62.2224557307631,1.82930781209959E-13,
3.77003198860263));
#222587=CARTESIAN_POINT('',(-31.2097904767601,-53.4219427993288,3.77003198860225));
#222588=CARTESIAN_POINT('',(15.2806508669887,27.1018636743466,3.77003198860282));
#222589=CARTESIAN_POINT('',(-36.1092077731524,-50.2402240048084,3.77003198860227));
#222590=CARTESIAN_POINT('Origin',(5.49031038273072E-15,1.82930781209959E-13,
3.77003198860263));
#222591=CARTESIAN_POINT('',(-35.8304925908678,-49.8566054669511,3.77003198860227));
#222592=CARTESIAN_POINT('Origin',(5.57972911860581E-15,1.8736496251029E-13,
3.13503198860263));
#222593=CARTESIAN_POINT('Origin',(-30.2768121832811,-51.805967006543,3.13502491541393));
#222594=CARTESIAN_POINT('Origin',(-35.0124168871447,-48.7306293534721,3.135024915414));
#222595=CARTESIAN_POINT('Origin',(5.57972911860581E-15,1.8736496251029E-13,
3.13503198860263));
#222596=CARTESIAN_POINT('Origin',(-31.228884228498,-53.4549470734241,3.20381846780309));
#222597=CARTESIAN_POINT('Origin',(-36.1315923097639,-50.2710907322494,3.20382022872386));
#222598=CARTESIAN_POINT('Origin',(5.51210908043506E-15,1.8401175575949E-13,
3.61523028058481));
#222599=CARTESIAN_POINT('Origin',(-30.788999306205,-52.693185297594,3.58786945046744));
#222600=CARTESIAN_POINT('Origin',(-35.6145503723404,-49.5593237986655,3.58781461834121));
#222601=CARTESIAN_POINT('Origin',(5.51210908043507E-15,1.8401175575949E-13,
3.61523028058481));
#222602=CARTESIAN_POINT('Origin',(-30.6976537960623,-52.5348053110496,3.5878144026648));
#222603=CARTESIAN_POINT('Origin',(-35.5070166083019,-49.4114565896691,3.58786923593059));
#222604=CARTESIAN_POINT('Origin',(60.4792282238308,1.82930781209959E-13,
3.77003198860263));
#222605=CARTESIAN_POINT('',(-39.9143573409153,-44.8038810887676,3.77003198860231));
#222606=CARTESIAN_POINT('',(-35.5261472678861,-48.357383540212,3.77003198860228));
#222607=CARTESIAN_POINT('Origin',(5.49031038273072E-15,1.82930781209959E-13,
3.77003198860263));
#222608=CARTESIAN_POINT('',(-35.8051714542876,-48.7414273857062,3.77003198860228));
#222609=CARTESIAN_POINT('',(20.6381965522785,28.9462038689909,3.77003198860283));
#222610=CARTESIAN_POINT('',(-35.8056376406732,-48.7410849262054,3.77003198902507));
#222611=CARTESIAN_POINT('Origin',(5.49031038273072E-15,1.82930781209959E-13,
3.77003198860263));
#222612=CARTESIAN_POINT('',(-40.2315646148138,-45.157039930004,3.77003198882054));
#222613=CARTESIAN_POINT('Origin',(5.49031038273072E-15,1.82930781209959E-13,
3.77003198860263));
#222614=CARTESIAN_POINT('',(-40.2319965165878,-45.1566551325073,3.7700319886023));
#222615=CARTESIAN_POINT('Origin',(5.49031038273072E-15,1.82930781209959E-13,
3.77003198860263));
#222616=CARTESIAN_POINT('',(-39.914717064096,-44.8042806018339,3.77003198860231));
#222617=CARTESIAN_POINT('Origin',(5.49031038273072E-15,1.82930781209959E-13,
3.77003198860263));
#222618=CARTESIAN_POINT('',(-35.90126936289,-48.8727133447945,3.48823028058446));
#222619=CARTESIAN_POINT('',(-35.8056376402397,-48.7410849256153,3.77003198860228));
#222620=CARTESIAN_POINT('',(-40.3404336840069,-45.2779489571885,3.48823028074772));
#222621=CARTESIAN_POINT('Origin',(5.52999282761009E-15,1.84898592019556E-13,
3.48823028058481));
#222622=CARTESIAN_POINT('',(-40.3404336838189,-45.2779489569774,3.48823028058449));
#222623=CARTESIAN_POINT('Origin',(60.71525,1.85785428279622E-13,3.36123028058482));
#222624=CARTESIAN_POINT('',(-40.4880553924339,-45.4410373245173,3.36123028058449));
#222625=CARTESIAN_POINT('',(-36.0301015792672,-49.0510171431405,3.36123028058446));
#222626=CARTESIAN_POINT('Origin',(5.5478765747851E-15,1.85785428279622E-13,
3.36123028058482));
#222627=CARTESIAN_POINT('',(-36.1189794796879,-49.1733470784089,3.36123028058446));
#222628=CARTESIAN_POINT('',(20.7197400704237,29.0584388930976,3.36123028058502));
#222629=CARTESIAN_POINT('',(-40.5892333705619,-45.5534068532513,3.36123028058449));
#222630=CARTESIAN_POINT('Origin',(5.5478765747851E-15,1.85785428279622E-13,
3.36123028058482));
#222631=CARTESIAN_POINT('',(-40.4884100480707,-45.441431209506,3.36123028058449));
#222632=CARTESIAN_POINT('Origin',(5.5478765747851E-15,1.85785428279622E-13,
3.36123028058482));
#222633=CARTESIAN_POINT('',(-40.7368493365293,-45.7165002428309,3.48823028058451));
#222634=CARTESIAN_POINT('',(-36.2478178024865,-49.351646303959,3.4882302804266));
#222635=CARTESIAN_POINT('Origin',(5.52999282761008E-15,1.84898592019556E-13,
3.48823028058484));
#222636=CARTESIAN_POINT('',(-36.3434519499943,-49.4832728536533,3.77003198802672));
#222637=CARTESIAN_POINT('',(-36.2478178023246,-49.3516463037386,3.48823028058449));
#222638=CARTESIAN_POINT('',(-36.3439095507831,-49.4829367616347,3.77003198860228));
#222639=CARTESIAN_POINT('Origin',(5.49031038273072E-15,1.82930781209959E-13,
3.77003198860263));
#222640=CARTESIAN_POINT('',(-40.845292185024,-45.8377889771253,3.7700319886023));
#222641=CARTESIAN_POINT('Origin',(5.49031038273072E-15,1.82930781209959E-13,
3.77003198860263));
#222642=CARTESIAN_POINT('',(-40.8457160731793,-45.8374112534715,3.77003198802688));
#222643=CARTESIAN_POINT('Origin',(5.49031038273072E-15,1.82930781209959E-13,
3.77003198860263));
#222644=CARTESIAN_POINT('',(-40.8457160734119,-45.8374112537092,3.7700319886023));
#222645=CARTESIAN_POINT('Origin',(62.2224557307631,1.82930781209959E-13,
3.77003198860263));
#222646=CARTESIAN_POINT('',(-36.6229335645805,-49.8669803696027,3.77003198860227));
#222647=CARTESIAN_POINT('',(21.2404668433927,29.7751578089173,3.77003198860284));
#222648=CARTESIAN_POINT('',(-41.1629311642477,-46.1905628026487,3.7700319886023));
#222649=CARTESIAN_POINT('Origin',(5.49031038273072E-15,1.82930781209959E-13,
3.77003198860263));
#222650=CARTESIAN_POINT('',(-40.8456437566508,-45.8381794369739,3.7700319886023));
#222651=CARTESIAN_POINT('Origin',(5.57972911860581E-15,1.8736496251029E-13,
3.13503198860263));
#222652=CARTESIAN_POINT('Origin',(-35.5261507575146,-48.3573798485716,3.13502491541401));
#222653=CARTESIAN_POINT('Origin',(-39.9143530044114,-44.8038837346042,3.13502491541403));
#222654=CARTESIAN_POINT('Origin',(5.57972911860581E-15,1.8736496251029E-13,
3.13503198860263));
#222655=CARTESIAN_POINT('Origin',(-36.6453726047996,-49.8978080023045,3.20381846780233));
#222656=CARTESIAN_POINT('Origin',(-41.1884195276103,-46.218920617716,3.20382022872564));
#222657=CARTESIAN_POINT('Origin',(5.51210908043506E-15,1.8401175575949E-13,
3.61523028058481));
#222658=CARTESIAN_POINT('Origin',(-36.1282716303348,-49.1861997321284,3.5878694504674));
#222659=CARTESIAN_POINT('Origin',(-40.5998100962477,-45.5650984170299,3.58781461834035));
#222660=CARTESIAN_POINT('Origin',(5.51210908043507E-15,1.8401175575949E-13,
3.61523028058481));
#222661=CARTESIAN_POINT('Origin',(-36.020871303843,-49.0382355735282,3.5878144026659));
#222662=CARTESIAN_POINT('Origin',(-40.4774090812932,-45.4292815791794,3.58786923592717));
#222663=CARTESIAN_POINT('Origin',(60.4792282238308,1.82930781209959E-13,
3.77003198860263));
#222664=CARTESIAN_POINT('',(-44.3789831537292,-40.386254305094,3.77003198860234));
#222665=CARTESIAN_POINT('',(-40.3862543050934,-44.3789831537297,3.77003198860231));
#222666=CARTESIAN_POINT('Origin',(5.49031038273072E-15,1.82930781209959E-13,
3.77003198860263));
#222667=CARTESIAN_POINT('',(-40.7038934808039,-44.7317571974361,3.77003198860231));
#222668=CARTESIAN_POINT('',(26.8427652369004,30.2864073093063,3.77003198860284));
#222669=CARTESIAN_POINT('',(-40.7043213166062,-44.7313678842175,3.77003198902489));
#222670=CARTESIAN_POINT('Origin',(5.49031038273072E-15,1.82930781209959E-13,
3.77003198860263));
#222671=CARTESIAN_POINT('',(-44.7313678839552,-40.7043213163685,3.77003198882057));
#222672=CARTESIAN_POINT('Origin',(5.49031038273072E-15,1.82930781209959E-13,
3.77003198860263));
#222673=CARTESIAN_POINT('',(-44.7317571974351,-40.7038934808041,3.77003198860234));
#222674=CARTESIAN_POINT('Origin',(5.49031038273072E-15,1.82930781209959E-13,
3.77003198860263));
#222675=CARTESIAN_POINT('',(-44.3793826667955,-40.3866140282747,3.77003198860234));
#222676=CARTESIAN_POINT('Origin',(5.49031038273072E-15,1.82930781209959E-13,
3.77003198860263));
#222677=CARTESIAN_POINT('',(-40.8131880745603,-44.8522789915943,3.48823028058449));
#222678=CARTESIAN_POINT('',(-40.7043213161135,-44.7313678836761,3.77003198860231));
#222679=CARTESIAN_POINT('',(-44.8522789918029,-40.8131880747511,3.48823028074775));
#222680=CARTESIAN_POINT('Origin',(5.52999282761009E-15,1.84898592019556E-13,
3.48823028058481));
#222681=CARTESIAN_POINT('',(-44.8522789915938,-40.8131880745608,3.48823028058452));
#222682=CARTESIAN_POINT('Origin',(60.71525,1.85785428279622E-13,3.36123028058482));
#222683=CARTESIAN_POINT('',(-45.016139389479,-40.9599523566127,3.36123028058452));
#222684=CARTESIAN_POINT('',(-40.9599523566121,-45.0161393894795,3.36123028058449));
#222685=CARTESIAN_POINT('Origin',(5.5478765747851E-15,1.85785428279622E-13,
3.36123028058482));
#222686=CARTESIAN_POINT('',(-41.06113033474,-45.1285089182134,3.36123028058449));
#222687=CARTESIAN_POINT('',(26.9484406282047,30.4037717213984,3.36123028058503));
#222688=CARTESIAN_POINT('',(-45.1285089182129,-41.0611303347406,3.36123028058452));
#222689=CARTESIAN_POINT('Origin',(5.5478765747851E-15,1.85785428279622E-13,
3.36123028058482));
#222690=CARTESIAN_POINT('',(-45.0165332744676,-40.9603070122494,3.36123028058452));
#222691=CARTESIAN_POINT('Origin',(5.5478765747851E-15,1.85785428279622E-13,
3.36123028058482));
#222692=CARTESIAN_POINT('',(-45.2923641298554,-41.2079002115909,3.48823028058454));
#222693=CARTESIAN_POINT('',(-41.2079002117744,-45.2923641300582,3.48823028042662));
#222694=CARTESIAN_POINT('Origin',(5.52999282761008E-15,1.84898592019556E-13,
3.48823028058484));
#222695=CARTESIAN_POINT('',(-41.3167691863805,-45.413273125266,3.77003198802675));
#222696=CARTESIAN_POINT('',(-41.2079002115903,-45.2923641298559,3.48823028058452));
#222697=CARTESIAN_POINT('',(-41.3171891492021,-45.4128910420874,3.7700319886023));
#222698=CARTESIAN_POINT('Origin',(5.49031038273072E-15,1.82930781209959E-13,
3.77003198860263));
#222699=CARTESIAN_POINT('',(-45.4128910420869,-41.3171891492027,3.77003198860233));
#222700=CARTESIAN_POINT('Origin',(5.49031038273072E-15,1.82930781209959E-13,
3.77003198860263));
#222701=CARTESIAN_POINT('',(-45.4132731252655,-41.3167691863811,3.77003198802691));
#222702=CARTESIAN_POINT('Origin',(5.49031038273072E-15,1.82930781209959E-13,
3.77003198860263));
#222703=CARTESIAN_POINT('',(-45.4132731255216,-41.3167691865933,3.77003198860233));
#222704=CARTESIAN_POINT('Origin',(62.2224557307631,1.82930781209959E-13,
3.77003198860263));
#222705=CARTESIAN_POINT('',(-41.6348281284258,-45.7656648676108,3.7700319886023));
#222706=CARTESIAN_POINT('',(27.6232705441538,31.1532462714326,3.77003198860285));
#222707=CARTESIAN_POINT('',(-45.7656648676103,-41.6348281284264,3.77003198860233));
#222708=CARTESIAN_POINT('Origin',(5.49031038273072E-15,1.82930781209959E-13,
3.77003198860263));
#222709=CARTESIAN_POINT('',(-45.4132815019355,-41.3175407208296,3.77003198860233));
#222710=CARTESIAN_POINT('Origin',(5.57972911860581E-15,1.8736496251029E-13,
3.13503198860263));
#222711=CARTESIAN_POINT('Origin',(-40.3862573897238,-44.378979117547,3.13502491541399));
#222712=CARTESIAN_POINT('Origin',(-44.3789791175464,-40.3862573897246,3.13502491541403));
#222713=CARTESIAN_POINT('Origin',(5.57972911860581E-15,1.8736496251029E-13,
3.13503198860263));
#222714=CARTESIAN_POINT('Origin',(-41.6603666103058,-45.7939781049253,3.20381846780306));
#222715=CARTESIAN_POINT('Origin',(-45.7939778018807,-41.6603663369627,3.20382022872453));
#222716=CARTESIAN_POINT('Origin',(5.51210908043506E-15,1.8401175575949E-13,
3.61523028058481));
#222717=CARTESIAN_POINT('Origin',(-41.0717150501544,-45.1403198695221,3.58786945047096));
#222718=CARTESIAN_POINT('Origin',(-45.1402498046847,-41.071652282028,3.58781461833824));
#222719=CARTESIAN_POINT('Origin',(5.51210908043507E-15,1.8401175575949E-13,
3.61523028058481));
#222720=CARTESIAN_POINT('Origin',(-40.9494366077766,-45.0043926651437,3.58781440266436));
#222721=CARTESIAN_POINT('Origin',(-45.0043225899492,-40.9493738530207,3.5878692359261));
#222722=CARTESIAN_POINT('Origin',(60.4792282238308,1.82930781209959E-13,
3.77003198860263));
#222723=CARTESIAN_POINT('',(-48.3573835402116,-35.5261472678868,3.77003198860237));
#222724=CARTESIAN_POINT('',(-44.8038810887671,-39.9143573409159,3.77003198860234));
#222725=CARTESIAN_POINT('Origin',(5.49031038273072E-15,1.82930781209959E-13,
3.77003198860263));
#222726=CARTESIAN_POINT('',(-45.1566551325072,-40.2319965165888,3.77003198860234));
#222727=CARTESIAN_POINT('',(33.1880655373213,30.3099068238766,3.77003198860284));
#222728=CARTESIAN_POINT('',(-45.1570399302682,-40.2315646150503,3.77003198902526));
#222729=CARTESIAN_POINT('Origin',(5.49031038273072E-15,1.82930781209959E-13,
3.77003198860263));
#222730=CARTESIAN_POINT('',(-48.7410849259195,-35.8056376404641,3.77003198882061));
#222731=CARTESIAN_POINT('Origin',(5.49031038273072E-15,1.82930781209959E-13,
3.77003198860263));
#222732=CARTESIAN_POINT('',(-48.7414273857053,-35.8051714542879,3.77003198860237));
#222733=CARTESIAN_POINT('Origin',(5.49031038273072E-15,1.82930781209959E-13,
3.77003198860263));
#222734=CARTESIAN_POINT('',(-48.3578184660148,-35.5264632599794,3.77003198860237));
#222735=CARTESIAN_POINT('Origin',(5.49031038273072E-15,1.82930781209959E-13,
3.77003198860263));
#222736=CARTESIAN_POINT('',(-45.2779489569769,-40.3404336838195,3.48823028058452));
#222737=CARTESIAN_POINT('',(-45.1570399297212,-40.231564614563,3.77003198860234));
#222738=CARTESIAN_POINT('',(-48.8727133450219,-35.9012693630581,3.48823028074779));
#222739=CARTESIAN_POINT('Origin',(5.52999282761009E-15,1.84898592019556E-13,
3.48823028058481));
#222740=CARTESIAN_POINT('',(-48.8727133447941,-35.9012693628907,3.48823028058455));
#222741=CARTESIAN_POINT('Origin',(60.71525,1.85785428279622E-13,3.36123028058482));
#222742=CARTESIAN_POINT('',(-49.05101714314,-36.0301015792679,3.36123028058456));
#222743=CARTESIAN_POINT('',(-45.4410373245168,-40.4880553924345,3.36123028058453));
#222744=CARTESIAN_POINT('Origin',(5.5478765747851E-15,1.85785428279622E-13,
3.36123028058482));
#222745=CARTESIAN_POINT('',(-45.5534068532508,-40.5892333705625,3.36123028058452));
#222746=CARTESIAN_POINT('',(33.3184119221863,30.4272712359686,3.36123028058503));
#222747=CARTESIAN_POINT('',(-49.1733470784084,-36.1189794796885,3.36123028058456));
#222748=CARTESIAN_POINT('Origin',(5.5478765747851E-15,1.85785428279622E-13,
3.36123028058482));
#222749=CARTESIAN_POINT('',(-49.0514459419942,-36.0304131198714,3.36123028058456));
#222750=CARTESIAN_POINT('Origin',(5.5478765747851E-15,1.85785428279622E-13,
3.36123028058482));
#222751=CARTESIAN_POINT('',(-49.3516463037382,-36.2478178023253,3.48823028058458));
#222752=CARTESIAN_POINT('',(-45.7165002430345,-40.7368493367118,3.48823028042666));
#222753=CARTESIAN_POINT('Origin',(5.52999282761008E-15,1.84898592019556E-13,
3.48823028058484));
#222754=CARTESIAN_POINT('',(-45.8374112534709,-40.8457160731799,3.77003198802678));
#222755=CARTESIAN_POINT('',(-45.7165002428303,-40.7368493365299,3.48823028058455));
#222756=CARTESIAN_POINT('',(-45.8377889771247,-40.8452921850246,3.77003198860234));
#222757=CARTESIAN_POINT('Origin',(5.49031038273072E-15,1.82930781209959E-13,
3.77003198860263));
#222758=CARTESIAN_POINT('',(-49.4829367616343,-36.3439095507838,3.77003198860237));
#222759=CARTESIAN_POINT('Origin',(5.49031038273072E-15,1.82930781209959E-13,
3.77003198860263));
#222760=CARTESIAN_POINT('',(-49.4832728536529,-36.343451949995,3.77003198802694));
#222761=CARTESIAN_POINT('Origin',(5.49031038273072E-15,1.82930781209959E-13,
3.77003198860263));
#222762=CARTESIAN_POINT('',(-49.4832728539298,-36.3434519501792,3.77003198860237));
#222763=CARTESIAN_POINT('Origin',(62.2224557307631,1.82930781209959E-13,
3.77003198860263));
#222764=CARTESIAN_POINT('',(-46.1905628026481,-41.1629311642483,3.77003198860233));
#222765=CARTESIAN_POINT('',(34.1507877370002,31.1767457860028,3.77003198860285));
#222766=CARTESIAN_POINT('',(-49.8669803696023,-36.6229335645812,3.77003198860236));
#222767=CARTESIAN_POINT('Origin',(5.49031038273072E-15,1.82930781209959E-13,
3.77003198860263));
#222768=CARTESIAN_POINT('',(-49.4833618317449,-36.3442183822966,3.77003198860237));
#222769=CARTESIAN_POINT('Origin',(5.57972911860581E-15,1.8736496251029E-13,
3.13503198860263));
#222770=CARTESIAN_POINT('Origin',(-44.8038837346036,-39.9143530044121,3.13502491541405));
#222771=CARTESIAN_POINT('Origin',(-48.3573798485711,-35.5261507575154,3.13502491541409));
#222772=CARTESIAN_POINT('Origin',(5.57972911860581E-15,1.8736496251029E-13,
3.13503198860263));
#222773=CARTESIAN_POINT('Origin',(-46.2189209212445,-41.188419800416,3.20381846780359));
#222774=CARTESIAN_POINT('Origin',(-49.8978076723477,-36.6453723646279,3.20382022872044));
#222775=CARTESIAN_POINT('Origin',(5.51210908043506E-15,1.8401175575949E-13,
3.61523028058481));
#222776=CARTESIAN_POINT('Origin',(-45.5651681650776,-40.5998732162087,3.58786945046834));
#222777=CARTESIAN_POINT('Origin',(-49.1861234900546,-36.1282165298262,3.58781461834196));
#222778=CARTESIAN_POINT('Origin',(5.51210908043507E-15,1.8401175575949E-13,
3.61523028058481));
#222779=CARTESIAN_POINT('Origin',(-45.4293513150143,-40.4774722129462,3.58781440266486));
#222780=CARTESIAN_POINT('Origin',(-49.0381593225501,-36.0208162177263,3.58786923593133));
#222781=CARTESIAN_POINT('Origin',(60.4792282238308,1.82930781209959E-13,
3.77003198860263));
#222782=CARTESIAN_POINT('',(-51.8059703131944,-30.2768083268883,3.77003198860241));
#222783=CARTESIAN_POINT('',(-48.7306271754173,-35.0124214764587,3.77003198860237));
#222784=CARTESIAN_POINT('Origin',(5.49031038273072E-15,1.82930781209959E-13,
3.77003198860263));
#222785=CARTESIAN_POINT('',(-49.1146710209412,-35.2914456628193,3.77003198860238));
#222786=CARTESIAN_POINT('',(39.3975469582344,29.0164449471024,3.77003198860284));
#222787=CARTESIAN_POINT('',(-49.1150085647352,-35.2909759049636,3.77003198902498));
#222788=CARTESIAN_POINT('Origin',(5.49031038273072E-15,1.82930781209959E-13,
3.77003198860263));
#222789=CARTESIAN_POINT('',(-52.2167844417076,-30.5146599057594,3.77003198882065));
#222790=CARTESIAN_POINT('Origin',(5.49031038273072E-15,1.82930781209959E-13,
3.77003198860263));
#222791=CARTESIAN_POINT('',(-52.2170762957382,-30.5141604766047,3.77003198860241));
#222792=CARTESIAN_POINT('Origin',(5.49031038273072E-15,1.82930781209959E-13,
3.77003198860263));
#222793=CARTESIAN_POINT('',(-51.8064358865964,-30.2770771258173,3.77003198860241));
#222794=CARTESIAN_POINT('Origin',(5.49031038273072E-15,1.82930781209959E-13,
3.77003198860263));
#222795=CARTESIAN_POINT('',(-49.246635155601,-35.3866101428262,3.48823028058456));
#222796=CARTESIAN_POINT('',(-49.1150085641408,-35.2909759045365,3.77003198860237));
#222797=CARTESIAN_POINT('',(-52.3576880235601,-30.5960088313997,3.48823028074783));
#222798=CARTESIAN_POINT('Origin',(5.52999282761009E-15,1.84898592019556E-13,
3.48823028058481));
#222799=CARTESIAN_POINT('',(-52.357688023316,-30.5960088312571,3.48823028058459));
#222800=CARTESIAN_POINT('Origin',(60.71525,1.85785428279622E-13,3.36123028058482));
#222801=CARTESIAN_POINT('',(-52.5484816883957,-30.7054974692372,3.36123028058459));
#222802=CARTESIAN_POINT('',(-49.4242607783458,-35.5163757878398,3.36123028058456));
#222803=CARTESIAN_POINT('Origin',(5.5478765747851E-15,1.85785428279622E-13,
3.36123028058482));
#222804=CARTESIAN_POINT('',(-49.5465907136142,-35.6052536882604,3.36123028058456));
#222805=CARTESIAN_POINT('',(39.5520252162584,29.1286799712091,3.36123028058503));
#222806=CARTESIAN_POINT('',(-52.6794317578285,-30.7811015270746,3.36123028058459));
#222807=CARTESIAN_POINT('Origin',(5.5478765747851E-15,1.85785428279622E-13,
3.36123028058482));
#222808=CARTESIAN_POINT('',(-52.5489407031054,-30.7057624815034,3.36123028058459));
#222809=CARTESIAN_POINT('Origin',(5.5478765747851E-15,1.85785428279622E-13,
3.36123028058482));
#222810=CARTESIAN_POINT('',(-52.8702215132213,-30.8905967158739,3.48823028058462));
#222811=CARTESIAN_POINT('',(-49.7242207308393,-35.7350130972987,3.48823028042669));
#222812=CARTESIAN_POINT('Origin',(5.52999282761008E-15,1.84898592019556E-13,
3.48823028058484));
#222813=CARTESIAN_POINT('',(-49.8558490507733,-35.8306448082804,3.77003198802681));
#222814=CARTESIAN_POINT('',(-49.7242207306172,-35.7350130971391,3.48823028058458));
#222815=CARTESIAN_POINT('',(-49.85618039684,-35.8301837593557,3.77003198860237));
#222816=CARTESIAN_POINT('Origin',(5.49031038273072E-15,1.82930781209959E-13,
3.77003198860263));
#222817=CARTESIAN_POINT('',(-53.010837071051,-30.9724384738745,3.7700319886024));
#222818=CARTESIAN_POINT('Origin',(5.49031038273072E-15,1.82930781209959E-13,
3.77003198860263));
#222819=CARTESIAN_POINT('',(-53.0111234896151,-30.9719482486884,3.77003198802698));
#222820=CARTESIAN_POINT('Origin',(5.49031038273072E-15,1.82930781209959E-13,
3.77003198860263));
#222821=CARTESIAN_POINT('',(-53.0111234899097,-30.9719482488427,3.7700319886024));
#222822=CARTESIAN_POINT('Origin',(62.2224557307631,1.82930781209959E-13,
3.77003198860263));
#222823=CARTESIAN_POINT('',(-50.240224004808,-36.1092077731531,3.77003198860237));
#222824=CARTESIAN_POINT('',(40.5385041740525,29.8453988870289,3.77003198860284));
#222825=CARTESIAN_POINT('',(-53.4219427993284,-31.2097904767609,3.7700319886024));
#222826=CARTESIAN_POINT('Origin',(5.49031038273072E-15,1.82930781209959E-13,
3.77003198860263));
#222827=CARTESIAN_POINT('',(-53.0112920942665,-30.9727011816505,3.7700319886024));
#222828=CARTESIAN_POINT('Origin',(5.57972911860581E-15,1.8736496251029E-13,
3.13503198860263));
#222829=CARTESIAN_POINT('Origin',(-48.7306293534716,-35.0124168871455,3.13502491541407));
#222830=CARTESIAN_POINT('Origin',(-51.8059670065426,-30.2768121832819,3.13502491541411));
#222831=CARTESIAN_POINT('Origin',(5.57972911860581E-15,1.8736496251029E-13,
3.13503198860263));
#222832=CARTESIAN_POINT('Origin',(-50.2710910626254,-36.1315925493529,3.20381846779954));
#222833=CARTESIAN_POINT('Origin',(-53.4549467201712,-31.2288840241303,3.20382022872153));
#222834=CARTESIAN_POINT('Origin',(5.51210908043506E-15,1.8401175575949E-13,
3.61523028058481));
#222835=CARTESIAN_POINT('Origin',(-49.5593997624596,-35.6146058558681,3.58786945046727));
#222836=CARTESIAN_POINT('Origin',(-52.6931037136094,-30.7889524770089,3.58781461834492));
#222837=CARTESIAN_POINT('Origin',(5.51210908043507E-15,1.8401175575949E-13,
3.61523028058481));
#222838=CARTESIAN_POINT('Origin',(-49.4115325425325,-35.5070721047359,3.58781440266261));
#222839=CARTESIAN_POINT('Origin',(-52.5347237197169,-30.6976069821036,3.58786923592639));
#222840=CARTESIAN_POINT('Origin',(60.4792282238308,1.82930781209959E-13,
3.77003198860263));
#222841=CARTESIAN_POINT('',(-54.6869600343295,-24.695750338031,3.77003198860245));
#222842=CARTESIAN_POINT('',(-52.1234703131944,-29.7268821954852,3.77003198860241));
#222843=CARTESIAN_POINT('Origin',(5.49031038273072E-15,1.82930781209959E-13,
3.77003198860263));
#222844=CARTESIAN_POINT('',(-52.5345762957641,-29.9642343451581,3.77003198860241));
#222845=CARTESIAN_POINT('',(45.2006711678726,26.4632370872591,3.77003198860282));
#222846=CARTESIAN_POINT('',(-52.5348628873911,-29.9637318777511,3.77003198902505));
#222847=CARTESIAN_POINT('Origin',(5.49031038273072E-15,1.82930781209959E-13,
3.77003198860263));
#222848=CARTESIAN_POINT('',(-55.1203859400877,-24.8893571715241,3.77003198882068));
#222849=CARTESIAN_POINT('Origin',(5.49031038273072E-15,1.82930781209959E-13,
3.77003198860263));
#222850=CARTESIAN_POINT('',(-55.1206239907494,-24.8888299712412,3.77003198860244));
#222851=CARTESIAN_POINT('Origin',(5.49031038273072E-15,1.82930781209959E-13,
3.77003198860263));
#222852=CARTESIAN_POINT('',(-54.6874511544107,-24.6959689987791,3.77003198860245));
#222853=CARTESIAN_POINT('Origin',(5.49031038273072E-15,1.82930781209959E-13,
3.77003198860263));
#222854=CARTESIAN_POINT('',(-52.6757649139393,-30.0450834959839,3.48823028058459));
#222855=CARTESIAN_POINT('',(-52.5348628867552,-29.9637318773884,3.77003198860241));
#222856=CARTESIAN_POINT('',(-55.2690209155615,-24.9555320243581,3.48823028074786));
#222857=CARTESIAN_POINT('Origin',(5.52999282761009E-15,1.84898592019556E-13,
3.48823028058481));
#222858=CARTESIAN_POINT('',(-55.2690209153038,-24.9555320242418,3.48823028058463));
#222859=CARTESIAN_POINT('Origin',(60.71525,1.85785428279622E-13,3.36123028058482));
#222860=CARTESIAN_POINT('',(-55.4702140717965,-25.044477503395,3.36123028058463));
#222861=CARTESIAN_POINT('',(-52.8659816883957,-30.155571337834,3.3612302805846));
#222862=CARTESIAN_POINT('Origin',(5.5478765747851E-15,1.85785428279622E-13,
3.36123028058482));
#222863=CARTESIAN_POINT('',(-52.9969317578285,-30.2311753956715,3.3612302805846));
#222864=CARTESIAN_POINT('',(45.3776874999996,26.5654375142636,3.36123028058501));
#222865=CARTESIAN_POINT('',(-55.6083495590299,-25.1059793847704,3.36123028058463));
#222866=CARTESIAN_POINT('Origin',(5.5478765747851E-15,1.85785428279622E-13,
3.36123028058482));
#222867=CARTESIAN_POINT('',(-55.4706982733005,-25.0446930837941,3.36123028058463));
#222868=CARTESIAN_POINT('Origin',(5.5478765747851E-15,1.85785428279622E-13,
3.36123028058482));
#222869=CARTESIAN_POINT('',(-55.8095395120005,-25.1949317875303,3.48823028058465));
#222870=CARTESIAN_POINT('',(-53.1871522508548,-30.3416565763594,3.48823028042673));
#222871=CARTESIAN_POINT('Origin',(5.52999282761008E-15,1.84898592019556E-13,
3.48823028058484));
#222872=CARTESIAN_POINT('',(-53.3280557328683,-30.423005500817,3.77003198802685));
#222873=CARTESIAN_POINT('',(-53.1871522506172,-30.3416565762239,3.48823028058462));
#222874=CARTESIAN_POINT('',(-53.328337071051,-30.4225123424714,3.77003198860241));
#222875=CARTESIAN_POINT('Origin',(5.49031038273072E-15,1.82930781209959E-13,
3.77003198860263));
#222876=CARTESIAN_POINT('',(-55.9579395562864,-25.2616268796459,3.77003198860244));
#222877=CARTESIAN_POINT('Origin',(5.49031038273072E-15,1.82930781209959E-13,
3.77003198860263));
#222878=CARTESIAN_POINT('',(-55.9581731633343,-25.2611094010724,3.77003198802702));
#222879=CARTESIAN_POINT('Origin',(5.49031038273072E-15,1.82930781209959E-13,
3.77003198860263));
#222880=CARTESIAN_POINT('',(-55.9581731636435,-25.261109401195,3.77003198860244));
#222881=CARTESIAN_POINT('Origin',(62.2224557307631,1.82930781209959E-13,
3.77003198860263));
#222882=CARTESIAN_POINT('',(-53.7394427993284,-30.6598643453577,3.7700319886024));
#222883=CARTESIAN_POINT('',(46.5080917980719,27.2180767400487,3.77003198860282));
#222884=CARTESIAN_POINT('',(-56.3916032444849,-25.4547063934086,3.77003198860244));
#222885=CARTESIAN_POINT('Origin',(5.49031038273072E-15,1.82930781209959E-13,
3.77003198860263));
#222886=CARTESIAN_POINT('',(-55.9584195472773,-25.2618405854037,3.77003198860244));
#222887=CARTESIAN_POINT('Origin',(5.57972911860581E-15,1.8736496251029E-13,
3.13503198860263));
#222888=CARTESIAN_POINT('Origin',(-52.1234719996032,-29.726877403644,3.13502491541413));
#222889=CARTESIAN_POINT('Origin',(-54.6869571488948,-24.6957545189381,3.13502491541414));
#222890=CARTESIAN_POINT('Origin',(5.57972911860581E-15,1.8736496251029E-13,
3.13503198860263));
#222891=CARTESIAN_POINT('Origin',(-53.7724806104365,-30.6789000092851,3.20381846780326));
#222892=CARTESIAN_POINT('Origin',(-56.4264221855626,-25.4702454951955,3.20382022872092));
#222893=CARTESIAN_POINT('Origin',(5.51210908043506E-15,1.8401175575949E-13,
3.61523028058481));
#222894=CARTESIAN_POINT('Origin',(-53.0106482050715,-30.2391374209341,3.58786945046879));
#222895=CARTESIAN_POINT('Origin',(-55.6227672661396,-25.1123582178524,3.58781461834275));
#222896=CARTESIAN_POINT('Origin',(5.51210908043507E-15,1.8401175575949E-13,
3.61523028058481));
#222897=CARTESIAN_POINT('Origin',(-52.8523506794952,-30.1476490842058,3.58781440266405));
#222898=CARTESIAN_POINT('Origin',(-55.4557066902171,-25.0380683404975,3.58786923592836));
#222899=CARTESIAN_POINT('Origin',(60.4792282238308,1.82930781209959E-13,
3.77003198860263));
#222900=CARTESIAN_POINT('',(-56.9687879773465,-18.8441205405522,3.77003198860249));
#222901=CARTESIAN_POINT('',(-54.9452378026827,-24.1156489724279,3.77003198860245));
#222902=CARTESIAN_POINT('Origin',(5.49031038273072E-15,1.82930781209959E-13,
3.77003198860263));
#222903=CARTESIAN_POINT('',(-55.3789017591237,-24.3087286055922,3.77003198860245));
#222904=CARTESIAN_POINT('',(50.3447265545023,22.7624634345051,3.77003198860279));
#222905=CARTESIAN_POINT('',(-55.3791342586262,-24.308198933772,3.77003198902528));
#222906=CARTESIAN_POINT('Origin',(5.49031038273072E-15,1.82930781209959E-13,
3.77003198860263));
#222907=CARTESIAN_POINT('',(-57.420076955426,-18.9913614316847,3.77003198882073));
#222908=CARTESIAN_POINT('Origin',(5.49031038273072E-15,1.82930781209959E-13,
3.77003198860263));
#222909=CARTESIAN_POINT('',(-57.4202585945858,-18.9908122363903,3.77003198860249));
#222910=CARTESIAN_POINT('Origin',(5.49031038273072E-15,1.82930781209959E-13,
3.77003198860263));
#222911=CARTESIAN_POINT('',(-56.9692992632924,-18.8442866674264,3.77003198860249));
#222912=CARTESIAN_POINT('Origin',(5.49031038273072E-15,1.82930781209959E-13,
3.77003198860263));
#222913=CARTESIAN_POINT('',(-55.5277679687681,-24.3743766270217,3.48823028058463));
#222914=CARTESIAN_POINT('',(-55.3791342579556,-24.3081989334776,3.77003198860245));
#222915=CARTESIAN_POINT('',(-57.5748148486259,-19.0416371861768,3.4882302807479));
#222916=CARTESIAN_POINT('Origin',(5.52999282761009E-15,1.84898592019556E-13,
3.48823028058481));
#222917=CARTESIAN_POINT('',(-57.5748148483574,-19.041637186088,3.48823028058467));
#222918=CARTESIAN_POINT('Origin',(60.71525,1.85785428279622E-13,3.36123028058482));
#222919=CARTESIAN_POINT('',(-57.7842031819381,-19.1090650011318,3.36123028058467));
#222920=CARTESIAN_POINT('',(-55.7284918401496,-24.4643761377919,3.36123028058464));
#222921=CARTESIAN_POINT('Origin',(5.5478765747851E-15,1.85785428279622E-13,
3.36123028058482));
#222922=CARTESIAN_POINT('',(-55.8666273273831,-24.5258780191674,3.36123028058464));
#222923=CARTESIAN_POINT('',(50.541702139688,22.8501626153352,3.36123028058498));
#222924=CARTESIAN_POINT('',(-57.9280106456674,-19.1557908785628,3.36123028058467));
#222925=CARTESIAN_POINT('Origin',(5.5478765747851E-15,1.85785428279622E-13,
3.36123028058482));
#222926=CARTESIAN_POINT('',(-57.7847072652235,-19.1092287877198,3.36123028058467));
#222927=CARTESIAN_POINT('Origin',(5.5478765747851E-15,1.85785428279622E-13,
3.36123028058482));
#222928=CARTESIAN_POINT('',(-58.1373965169892,-19.2232259141442,3.4882302805847));
#222929=CARTESIAN_POINT('',(-56.0673542006828,-24.6158705165696,3.48823028042677));
#222930=CARTESIAN_POINT('Origin',(5.52999282761008E-15,1.84898592019556E-13,
3.48823028058484));
#222931=CARTESIAN_POINT('',(-56.2159890767409,-24.6820453786634,3.77003198802689));
#222932=CARTESIAN_POINT('',(-56.0673542004324,-24.6158705164596,3.48823028058466));
#222933=CARTESIAN_POINT('',(-56.2162173246396,-24.6815255140429,3.77003198860245));
#222934=CARTESIAN_POINT('Origin',(5.49031038273072E-15,1.82930781209959E-13,
3.77003198860263));
#222935=CARTESIAN_POINT('',(-58.2919551457915,-19.2740436149887,3.77003198860248));
#222936=CARTESIAN_POINT('Origin',(5.49031038273072E-15,1.82930781209959E-13,
3.77003198860263));
#222937=CARTESIAN_POINT('',(-58.2921333818755,-19.2735045526312,3.77003198802706));
#222938=CARTESIAN_POINT('Origin',(5.49031038273072E-15,1.82930781209959E-13,
3.77003198860263));
#222939=CARTESIAN_POINT('',(-58.2921333821958,-19.2735045527209,3.77003198860248));
#222940=CARTESIAN_POINT('Origin',(62.2224557307631,1.82930781209959E-13,
3.77003198860263));
#222941=CARTESIAN_POINT('',(-56.649881012838,-24.8746050278055,3.77003198860245));
#222942=CARTESIAN_POINT('',(51.799563747336,23.4101986852084,3.7700319886028));
#222943=CARTESIAN_POINT('',(-58.7434254837931,-19.4207352200704,3.77003198860248));
#222944=CARTESIAN_POINT('Origin',(5.49031038273072E-15,1.82930781209959E-13,
3.77003198860263));
#222945=CARTESIAN_POINT('',(-58.2924548456759,-19.2742059773234,3.77003198860248));
#222946=CARTESIAN_POINT('Origin',(5.57972911860581E-15,1.8736496251029E-13,
3.13503198860263));
#222947=CARTESIAN_POINT('Origin',(-54.9452389789694,-24.1156440305593,3.13502491541412));
#222948=CARTESIAN_POINT('Origin',(-56.9687855447422,-18.8441250001659,3.13502491541418));
#222949=CARTESIAN_POINT('Origin',(5.57972911860581E-15,1.8736496251029E-13,
3.13503198860263));
#222950=CARTESIAN_POINT('Origin',(-56.684727608054,-24.8900830207542,3.20381846780062));
#222951=CARTESIAN_POINT('Origin',(-58.7796779614966,-19.4325496266337,3.20382022872046));
#222952=CARTESIAN_POINT('Origin',(5.51210908043506E-15,1.8401175575949E-13,
3.61523028058481));
#222953=CARTESIAN_POINT('Origin',(-55.8811008927584,-24.5323626684708,3.58786945046843));
#222954=CARTESIAN_POINT('Origin',(-57.9430161406882,-19.1606277069616,3.58781461834337));
#222955=CARTESIAN_POINT('Origin',(5.51210908043507E-15,1.8401175575949E-13,
3.61523028058481));
#222956=CARTESIAN_POINT('Origin',(-55.7141074023436,-24.457922111514,3.58781440266405));
#222957=CARTESIAN_POINT('Origin',(-57.7691053333672,-19.1042073825995,3.58786923593191));
#222958=CARTESIAN_POINT('Origin',(60.4792282238308,1.82930781209959E-13,
3.77003198860263));
#222959=CARTESIAN_POINT('',(-58.6264539577983,-12.7860306150454,3.77003198860253));
#222960=CARTESIAN_POINT('',(-57.1650137687745,-18.2401996527048,3.77003198860249));
#222961=CARTESIAN_POINT('Origin',(5.49031038273072E-15,1.82930781209959E-13,
3.77003198860263));
#222962=CARTESIAN_POINT('',(-57.6164843860301,-18.386891348495,3.77003198860249));
#222963=CARTESIAN_POINT('',(54.6058629360811,18.0763596539235,3.77003198860276));
#222964=CARTESIAN_POINT('',(-57.6166602460947,-18.3863402754567,3.77003198902533));
#222965=CARTESIAN_POINT('Origin',(5.49031038273072E-15,1.82930781209959E-13,
3.77003198860263));
#222966=CARTESIAN_POINT('',(-59.090661591717,-12.8852923618019,3.77003198882077));
#222967=CARTESIAN_POINT('Origin',(5.49031038273072E-15,1.82930781209959E-13,
3.77003198860263));
#222968=CARTESIAN_POINT('',(-59.0907848292983,-12.8847271885945,3.77003198860253));
#222969=CARTESIAN_POINT('Origin',(5.49031038273072E-15,1.82930781209959E-13,
3.77003198860263));
#222970=CARTESIAN_POINT('',(-58.6269798078532,-12.786142387925,3.77003198860253));
#222971=CARTESIAN_POINT('Origin',(5.49031038273072E-15,1.82930781209959E-13,
3.77003198860263));
#222972=CARTESIAN_POINT('',(-57.7713971777986,-18.4366189870675,3.48823028058468));
#222973=CARTESIAN_POINT('',(-57.616660245397,-18.386340275234,3.77003198860249));
#222974=CARTESIAN_POINT('',(-59.2498070619041,-12.919118186265,3.48823028074795));
#222975=CARTESIAN_POINT('Origin',(5.52999282761009E-15,1.84898592019556E-13,
3.48823028058481));
#222976=CARTESIAN_POINT('',(-59.2498070616278,-12.9191181862048,3.48823028058471));
#222977=CARTESIAN_POINT('Origin',(60.71525,1.85785428279622E-13,3.36123028058482));
#222978=CARTESIAN_POINT('',(-59.4650964698965,-12.9642895838873,3.36123028058472));
#222979=CARTESIAN_POINT('',(-57.9804289733662,-18.5051441132844,3.36123028058468));
#222980=CARTESIAN_POINT('Origin',(5.5478765747851E-15,1.85785428279622E-13,
3.36123028058482));
#222981=CARTESIAN_POINT('',(-58.1242364370955,-18.5518699907153,3.36123028058468));
#222982=CARTESIAN_POINT('',(54.8193466381475,18.1457247135496,3.36123028058495));
#222983=CARTESIAN_POINT('',(-59.6130003254554,-12.9957275188826,3.36123028058472));
#222984=CARTESIAN_POINT('Origin',(5.5478765747851E-15,1.85785428279622E-13,
3.36123028058482));
#222985=CARTESIAN_POINT('',(-59.4656149121213,-12.964399782184,3.36123028058472));
#222986=CARTESIAN_POINT('Origin',(5.5478765747851E-15,1.85785428279622E-13,
3.36123028058482));
#222987=CARTESIAN_POINT('',(-59.8282880397054,-13.0409063549241,3.48823028058474));
#222988=CARTESIAN_POINT('',(-58.33327048504,-18.6203878281982,3.48823028042681));
#222989=CARTESIAN_POINT('Origin',(5.52999282761008E-15,1.84898592019556E-13,
3.48823028058484));
#222990=CARTESIAN_POINT('',(-58.4880082803367,-18.6706636022911,3.77003198802693));
#222991=CARTESIAN_POINT('',(-58.3332704847794,-18.620387828115,3.4882302805847));
#222992=CARTESIAN_POINT('',(-58.4881809372196,-18.6701227271413,3.77003198860249));
#222993=CARTESIAN_POINT('Origin',(5.49031038273072E-15,1.82930781209959E-13,
3.77003198860263));
#222994=CARTESIAN_POINT('',(-59.9873118763435,-13.0752898951328,3.77003198860253));
#222995=CARTESIAN_POINT('Origin',(5.49031038273072E-15,1.82930781209959E-13,
3.77003198860263));
#222996=CARTESIAN_POINT('',(-59.9874327886717,-13.0747351550713,3.7700319880271));
#222997=CARTESIAN_POINT('Origin',(5.49031038273072E-15,1.82930781209959E-13,
3.77003198860263));
#222998=CARTESIAN_POINT('',(-59.9874327889996,-13.074735155127,3.77003198860253));
#222999=CARTESIAN_POINT('Origin',(62.2224557307631,1.82930781209959E-13,
3.77003198860263));
#223000=CARTESIAN_POINT('',(-58.9396512752212,-18.8168143322229,3.77003198860249));
#223001=CARTESIAN_POINT('',(56.1826270286323,18.5886813639062,3.77003198860276));
#223002=CARTESIAN_POINT('',(-60.4516424606488,-13.1739864076109,3.77003198860253));
#223003=CARTESIAN_POINT('Origin',(5.49031038273072E-15,1.82930781209959E-13,
3.77003198860263));
#223004=CARTESIAN_POINT('',(-59.987825810305,-13.0753991351686,3.77003198860253));
#223005=CARTESIAN_POINT('Origin',(5.57972911860581E-15,1.8736496251029E-13,
3.13503198860263));
#223006=CARTESIAN_POINT('Origin',(-57.1650144220515,-18.2401946149528,3.13502491541416));
#223007=CARTESIAN_POINT('Origin',(-58.6264520046767,-12.7860353045052,3.13502491541418));
#223008=CARTESIAN_POINT('Origin',(5.57972911860581E-15,1.8736496251029E-13,
3.13503198860263));
#223009=CARTESIAN_POINT('Origin',(-58.9759248679613,-18.8285650740585,3.20381846780257));
#223010=CARTESIAN_POINT('Origin',(-60.4889312852508,-13.1819466778333,3.20382022872411));
#223011=CARTESIAN_POINT('Origin',(5.51210908043506E-15,1.8401175575949E-13,
3.61523028058481));
#223012=CARTESIAN_POINT('Origin',(-58.1393085451926,-18.556806216885,3.58786945046721));
#223013=CARTESIAN_POINT('Origin',(-59.6284292050451,-12.9989693492946,3.58781461834119));
#223014=CARTESIAN_POINT('Origin',(5.51210908043507E-15,1.8401175575949E-13,
3.61523028058481));
#223015=CARTESIAN_POINT('Origin',(-57.9654487055678,-18.5002290260137,3.58781440266419));
#223016=CARTESIAN_POINT('Origin',(-59.4495735695182,-12.9610367308095,3.58786923593005));
#223017=CARTESIAN_POINT('Origin',(60.4792282238308,1.82930781209959E-13,
3.77003198860263));
#223018=CARTESIAN_POINT('',(-59.6417962403142,-6.58785426247119,3.77003198860258));
#223019=CARTESIAN_POINT('',(-58.7584778814675,-12.1649068885794,3.77003198860253));
#223020=CARTESIAN_POINT('Origin',(5.49031038273072E-15,1.82930781209959E-13,
3.77003198860263));
#223021=CARTESIAN_POINT('',(-59.2228087529787,-12.2636034620792,3.77003198860253));
#223022=CARTESIAN_POINT('',(57.7988642628859,12.6101209950216,3.77003198860272));
#223023=CARTESIAN_POINT('',(-59.2229260468455,-12.2630370254944,3.7700319890253));
#223024=CARTESIAN_POINT('Origin',(5.49031038273072E-15,1.82930781209959E-13,
3.77003198860263));
#223025=CARTESIAN_POINT('',(-60.1138365740932,-6.63804933238242,3.77003198882081));
#223026=CARTESIAN_POINT('Origin',(5.49031038273072E-15,1.82930781209959E-13,
3.77003198860263));
#223027=CARTESIAN_POINT('',(-60.1139000598793,-6.63747437341801,3.77003198860257));
#223028=CARTESIAN_POINT('Origin',(5.49031038273072E-15,1.82930781209959E-13,
3.77003198860263));
#223029=CARTESIAN_POINT('',(-59.6423308931549,-6.58791045674914,3.77003198860258));
#223030=CARTESIAN_POINT('Origin',(5.49031038273072E-15,1.82930781209959E-13,
3.77003198860263));
#223031=CARTESIAN_POINT('',(-59.382070869907,-12.2968658913806,3.48823028058472));
#223032=CARTESIAN_POINT('',(-59.2229260461284,-12.2630370253459,3.77003198860253));
#223033=CARTESIAN_POINT('',(-60.2756459901929,-6.65505462400522,3.48823028074799));
#223034=CARTESIAN_POINT('Origin',(5.52999282761009E-15,1.84898592019556E-13,
3.48823028058481));
#223035=CARTESIAN_POINT('',(-60.2756459899118,-6.65505462397419,3.48823028058476));
#223036=CARTESIAN_POINT('Origin',(60.71525,1.85785428279622E-13,3.36123028058482));
#223037=CARTESIAN_POINT('',(-60.4944777170593,-6.67747469700969,3.36123028058476));
#223038=CARTESIAN_POINT('',(-59.5971203935658,-12.3431658574213,3.36123028058472));
#223039=CARTESIAN_POINT('Origin',(5.5478765747851E-15,1.85785428279622E-13,
3.36123028058482));
#223040=CARTESIAN_POINT('',(-59.7450242491247,-12.3746037924167,3.36123028058472));
#223041=CARTESIAN_POINT('',(58.0246834617327,12.6581203474876,3.36123028058491));
#223042=CARTESIAN_POINT('',(-60.6448574988554,-6.69328024897478,3.36123028058476));
#223043=CARTESIAN_POINT('Origin',(5.5478765747851E-15,1.85785428279622E-13,
3.36123028058482));
#223044=CARTESIAN_POINT('',(-60.4950048380619,-6.67753009965956,3.36123028058476));
#223045=CARTESIAN_POINT('Origin',(5.5478765747851E-15,1.85785428279622E-13,
3.36123028058482));
#223046=CARTESIAN_POINT('',(-60.8636883187844,-6.71570789669434,3.48823028058479));
#223047=CARTESIAN_POINT('',(-59.9600752509414,-12.4208962742144,3.48823028042685));
#223048=CARTESIAN_POINT('Origin',(5.52999282761008E-15,1.84898592019556E-13,
3.48823028058484));
#223049=CARTESIAN_POINT('',(-60.1192206258106,-12.4547221284046,3.77003198802697));
#223050=CARTESIAN_POINT('',(-59.9600752506736,-12.4208962741589,3.48823028058475));
#223051=CARTESIAN_POINT('',(-60.1193358000127,-12.4541661686668,3.77003198860253));
#223052=CARTESIAN_POINT('Origin',(5.49031038273072E-15,1.82930781209959E-13,
3.77003198860263));
#223053=CARTESIAN_POINT('',(-61.0254350648262,-6.73328056300543,3.77003198860258));
#223054=CARTESIAN_POINT('Origin',(5.49031038273072E-15,1.82930781209959E-13,
3.77003198860263));
#223055=CARTESIAN_POINT('',(-61.0254973286579,-6.73271622308821,3.77003198802715));
#223056=CARTESIAN_POINT('Origin',(5.49031038273072E-15,1.82930781209959E-13,
3.77003198860263));
#223057=CARTESIAN_POINT('',(-61.0254973289898,-6.73271622310933,3.77003198860258));
#223058=CARTESIAN_POINT('Origin',(62.2224557307631,1.82930781209959E-13,
3.77003198860263));
#223059=CARTESIAN_POINT('',(-60.5836663843181,-12.552862681145,3.77003198860253));
#223060=CARTESIAN_POINT('',(59.4667368016499,12.9646382471652,3.77003198860272));
#223061=CARTESIAN_POINT('',(-61.4975385923862,-6.78290064323585,3.77003198860257));
#223062=CARTESIAN_POINT('Origin',(5.49031038273072E-15,1.82930781209959E-13,
3.77003198860263));
#223063=CARTESIAN_POINT('',(-61.0259576020967,-6.73333548388565,3.77003198860257));
#223064=CARTESIAN_POINT('Origin',(5.57972911860581E-15,1.8736496251029E-13,
3.13503198860263));
#223065=CARTESIAN_POINT('Origin',(-58.7584780045773,-12.1649018101387,3.13502491541424));
#223066=CARTESIAN_POINT('Origin',(-59.6417947880741,-6.58785913039848,3.13502491541428));
#223067=CARTESIAN_POINT('Origin',(5.57972911860581E-15,1.8736496251029E-13,
3.13503198860263));
#223068=CARTESIAN_POINT('Origin',(-60.620969553509,-12.5607574282782,3.20381846780322));
#223069=CARTESIAN_POINT('Origin',(-61.5354552197175,-6.78691956273327,3.20382022872119));
#223070=CARTESIAN_POINT('Origin',(5.51210908043506E-15,1.8401175575949E-13,
3.61523028058481));
#223071=CARTESIAN_POINT('Origin',(-59.7605297667716,-12.3779375131251,3.58786945046874));
#223072=CARTESIAN_POINT('Origin',(-60.6605407209804,-6.69489156322718,3.58781461833949));
#223073=CARTESIAN_POINT('Origin',(5.51210908043507E-15,1.8401175575949E-13,
3.61523028058481));
#223074=CARTESIAN_POINT('Origin',(-59.5817084227228,-12.3398435598866,3.58781440266546));
#223075=CARTESIAN_POINT('Origin',(-60.4786998370192,-6.67586224832366,3.58786923592885));
#223076=CARTESIAN_POINT('Origin',(60.4792282238308,1.82930781209959E-13,
3.77003198860263));
#223077=CARTESIAN_POINT('',(-60.003690522373,-0.317499999999817,3.77003198860262));
#223078=CARTESIAN_POINT('',(-59.7081718144892,-5.95633285891234,3.77003198860258));
#223079=CARTESIAN_POINT('Origin',(5.49031038273072E-15,1.82930781209959E-13,
3.77003198860263));
#223080=CARTESIAN_POINT('',(-60.1802756340603,-6.00595296980896,3.77003198860258));
#223081=CARTESIAN_POINT('',(59.785232315514,6.60293000146494,3.77003198860268));
#223082=CARTESIAN_POINT('',(-60.1803330766332,-6.00537737567535,3.77003198902537));
#223083=CARTESIAN_POINT('Origin',(5.49031038273072E-15,1.82930781209959E-13,
3.77003198860263));
#223084=CARTESIAN_POINT('',(-60.4783917833346,-0.318078445375805,3.77003198882085));
#223085=CARTESIAN_POINT('Origin',(5.49031038273072E-15,1.82930781209959E-13,
3.77003198860263));
#223086=CARTESIAN_POINT('',(-60.478394821762,-0.317500000025102,3.77003198860262));
#223087=CARTESIAN_POINT('Origin',(5.49031038273072E-15,1.82930781209959E-13,
3.77003198860263));
#223088=CARTESIAN_POINT('',(-60.004228120231,-0.317499999999817,3.77003198860262));
#223089=CARTESIAN_POINT('Origin',(5.49031038273072E-15,1.82930781209959E-13,
3.77003198860263));
#223090=CARTESIAN_POINT('',(-60.3421421670675,-6.02238575970299,3.48823028058476));
#223091=CARTESIAN_POINT('',(-60.1803330759045,-6.00537737560264,3.77003198860258));
#223092=CARTESIAN_POINT('',(-60.6410923275232,-0.318076890624665,3.48823028074803));
#223093=CARTESIAN_POINT('Origin',(5.52999282761009E-15,1.84898592019556E-13,
3.48823028058481));
#223094=CARTESIAN_POINT('',(-60.6410923272405,-0.318076890623182,3.4882302805848));
#223095=CARTESIAN_POINT('Origin',(60.71525,1.85785428279622E-13,3.36123028058482));
#223096=CARTESIAN_POINT('',(-60.8610688070707,-0.317499999999814,3.36123028058481));
#223097=CARTESIAN_POINT('',(-60.5608532912343,-6.04595329345084,3.36123028058477));
#223098=CARTESIAN_POINT('Origin',(5.5478765747851E-15,1.85785428279622E-13,
3.36123028058482));
#223099=CARTESIAN_POINT('',(-60.7112330730303,-6.06175884541593,3.36123028058477));
#223100=CARTESIAN_POINT('',(60.0186752706391,6.62746584474152,3.36123028058487));
#223101=CARTESIAN_POINT('',(-61.0122769227456,-0.317499999999814,3.36123028058481));
#223102=CARTESIAN_POINT('Origin',(5.5478765747851E-15,1.85785428279622E-13,
3.36123028058482));
#223103=CARTESIAN_POINT('',(-60.8615988316031,-0.317499999999814,3.36123028058481));
#223104=CARTESIAN_POINT('Origin',(5.5478765747851E-15,1.85785428279622E-13,
3.36123028058482));
#223105=CARTESIAN_POINT('',(-61.2322532920972,-0.316930737395729,3.48823028058483));
#223106=CARTESIAN_POINT('',(-60.9299448849411,-6.08531878141062,3.4882302804269));
#223107=CARTESIAN_POINT('Origin',(5.52999282761008E-15,1.84898592019556E-13,
3.48823028058484));
#223108=CARTESIAN_POINT('',(-61.0917542093523,-6.10232411256111,3.77003198802702));
#223109=CARTESIAN_POINT('',(-60.929944884669,-6.08531878138344,3.48823028058479));
#223110=CARTESIAN_POINT('',(-61.0918106390011,-6.10175915944657,3.77003198860258));
#223111=CARTESIAN_POINT('Origin',(5.49031038273072E-15,1.82930781209959E-13,
3.77003198860263));
#223112=CARTESIAN_POINT('',(-61.3949508163453,-0.317499999999817,3.77003198860262));
#223113=CARTESIAN_POINT('Origin',(5.49031038273072E-15,1.82930781209959E-13,
3.77003198860263));
#223114=CARTESIAN_POINT('',(-61.394953749505,-0.316932243253074,3.77003198802719));
#223115=CARTESIAN_POINT('Origin',(5.49031038273072E-15,1.82930781209959E-13,
3.77003198860263));
#223116=CARTESIAN_POINT('',(-61.3949537498373,-0.316932243239378,3.77003198860262));
#223117=CARTESIAN_POINT('Origin',(62.2224557307631,1.82930781209959E-13,
3.77003198860263));
#223118=CARTESIAN_POINT('',(-61.5639141665611,-6.151379239677,3.77003198860258));
#223119=CARTESIAN_POINT('',(61.5094129706996,6.78414869068811,3.77003198860268));
#223120=CARTESIAN_POINT('',(-61.8696548221181,-0.317499999999817,3.77003198860262));
#223121=CARTESIAN_POINT('Origin',(5.49031038273072E-15,1.82930781209959E-13,
3.77003198860263));
#223122=CARTESIAN_POINT('',(-61.3954762318973,-0.317499999999817,3.77003198860261));
#223123=CARTESIAN_POINT('Origin',(5.57972911860581E-15,1.8736496251029E-13,
3.13503198860263));
#223124=CARTESIAN_POINT('Origin',(-59.7081714060829,-5.95632779542337,3.1350249154143));
#223125=CARTESIAN_POINT('Origin',(-60.0036895869254,-0.317504993060535,
3.13502491541431));
#223126=CARTESIAN_POINT('Origin',(5.57972911860581E-15,1.8736496251029E-13,
3.13503198860263));
#223127=CARTESIAN_POINT('Origin',(-61.6018382108717,-6.1553314956104,3.20381846779944));
#223128=CARTESIAN_POINT('Origin',(-61.9077838296769,-0.317533536648401,
3.20382022872143));
#223129=CARTESIAN_POINT('Origin',(5.51210908043506E-15,1.8401175575949E-13,
3.61523028058481));
#223130=CARTESIAN_POINT('Origin',(-60.7270021185311,-6.06345353572164,3.58786945047009));
#223131=CARTESIAN_POINT('Origin',(-61.0280426587404,-0.317463144196334,
3.58781461834189));
#223132=CARTESIAN_POINT('Origin',(5.51210908043507E-15,1.8401175575949E-13,
3.61523028058481));
#223133=CARTESIAN_POINT('Origin',(-60.5451784741226,-6.04426018543762,3.5878144026621));
#223134=CARTESIAN_POINT('Origin',(-60.845208813124,-0.317545622030571,3.5878692359272));
#223135=CARTESIAN_POINT('Origin',(60.4792282238308,1.82930781209959E-13,
3.77003198860263));
#223136=CARTESIAN_POINT('',(-59.7081718144893,5.95633285891189,3.77003198860266));
#223137=CARTESIAN_POINT('',(-60.003690522373,0.317500000000183,3.77003198860262));
#223138=CARTESIAN_POINT('Origin',(5.49031038273072E-15,1.82930781209959E-13,
3.77003198860263));
#223139=CARTESIAN_POINT('',(-60.4783948217626,0.317500000025444,3.77003198860262));
#223140=CARTESIAN_POINT('',(60.4792282238308,0.317500000000183,3.77003198860264));
#223141=CARTESIAN_POINT('',(-60.4783917836893,0.318078445378037,3.77003198902564));
#223142=CARTESIAN_POINT('Origin',(5.49031038273072E-15,1.82930781209959E-13,
3.77003198860263));
#223143=CARTESIAN_POINT('',(-60.1803330762807,6.00537737563972,3.7700319888209));
#223144=CARTESIAN_POINT('Origin',(5.49031038273072E-15,1.82930781209959E-13,
3.77003198860263));
#223145=CARTESIAN_POINT('',(-60.1802756340597,6.00595296980842,3.77003198860266));
#223146=CARTESIAN_POINT('Origin',(5.49031038273072E-15,1.82930781209959E-13,
3.77003198860263));
#223147=CARTESIAN_POINT('',(-59.7087064673299,5.95638905318984,3.77003198860266));
#223148=CARTESIAN_POINT('Origin',(5.49031038273072E-15,1.82930781209959E-13,
3.77003198860263));
#223149=CARTESIAN_POINT('',(-60.6410923272405,0.318076890623551,3.48823028058481));
#223150=CARTESIAN_POINT('',(-60.4783917829566,0.318078445374188,3.77003198860262));
#223151=CARTESIAN_POINT('',(-60.3421421673489,6.02238575973063,3.48823028074808));
#223152=CARTESIAN_POINT('Origin',(5.52999282761009E-15,1.84898592019556E-13,
3.48823028058481));
#223153=CARTESIAN_POINT('',(-60.3421421670675,6.02238575970255,3.48823028058485));
#223154=CARTESIAN_POINT('Origin',(60.71525,1.85785428279622E-13,3.36123028058482));
#223155=CARTESIAN_POINT('',(-60.5608532912344,6.04595329345039,3.36123028058485));
#223156=CARTESIAN_POINT('',(-60.8610688070707,0.317500000000186,3.36123028058481));
#223157=CARTESIAN_POINT('Origin',(5.5478765747851E-15,1.85785428279622E-13,
3.36123028058482));
#223158=CARTESIAN_POINT('',(-61.0122769227456,0.317500000000186,3.36123028058481));
#223159=CARTESIAN_POINT('',(60.71525,0.317500000000186,3.36123028058483));
#223160=CARTESIAN_POINT('',(-60.7112330730304,6.06175884541548,3.36123028058485));
#223161=CARTESIAN_POINT('Origin',(5.5478765747851E-15,1.85785428279622E-13,
3.36123028058482));
#223162=CARTESIAN_POINT('',(-60.5613804122369,6.04600869610026,3.36123028058485));
#223163=CARTESIAN_POINT('Origin',(5.5478765747851E-15,1.85785428279622E-13,
3.36123028058482));
#223164=CARTESIAN_POINT('',(-60.9299448846691,6.08531878138299,3.48823028058487));
#223165=CARTESIAN_POINT('',(-61.2322532923707,0.316930737397515,3.48823028042694));
#223166=CARTESIAN_POINT('Origin',(5.52999282761008E-15,1.84898592019556E-13,
3.48823028058484));
#223167=CARTESIAN_POINT('',(-61.3949537495049,0.316932243253443,3.77003198802707));
#223168=CARTESIAN_POINT('',(-61.2322532920972,0.316930737396099,3.48823028058484));
#223169=CARTESIAN_POINT('',(-61.3949508163453,0.317500000000183,3.77003198860262));
#223170=CARTESIAN_POINT('Origin',(5.49031038273072E-15,1.82930781209959E-13,
3.77003198860263));
#223171=CARTESIAN_POINT('',(-61.0918106390012,6.10175915944611,3.77003198860266));
#223172=CARTESIAN_POINT('Origin',(5.49031038273072E-15,1.82930781209959E-13,
3.77003198860263));
#223173=CARTESIAN_POINT('',(-61.0917542093524,6.10232411256066,3.77003198802724));
#223174=CARTESIAN_POINT('Origin',(5.49031038273072E-15,1.82930781209959E-13,
3.77003198860263));
#223175=CARTESIAN_POINT('',(-61.0917542096815,6.10232411260902,3.77003198860266));
#223176=CARTESIAN_POINT('Origin',(62.2224557307631,1.82930781209959E-13,
3.77003198860263));
#223177=CARTESIAN_POINT('',(-61.8696548221181,0.317500000000183,3.77003198860262));
#223178=CARTESIAN_POINT('',(62.2224557307631,0.317500000000183,3.77003198860264));
#223179=CARTESIAN_POINT('',(-61.5639141665612,6.15137923967653,3.77003198860266));
#223180=CARTESIAN_POINT('Origin',(5.49031038273072E-15,1.82930781209959E-13,
3.77003198860263));
#223181=CARTESIAN_POINT('',(-61.0923331762718,6.10181408032633,3.77003198860266));
#223182=CARTESIAN_POINT('Origin',(5.57972911860581E-15,1.8736496251029E-13,
3.13503198860263));
#223183=CARTESIAN_POINT('Origin',(-60.0036895869254,0.317504993060735,3.13502491541433));
#223184=CARTESIAN_POINT('Origin',(-59.708171406083,5.95632779542278,3.13502491541439));
#223185=CARTESIAN_POINT('Origin',(5.57972911860581E-15,1.8736496251029E-13,
3.13503198860263));
#223186=CARTESIAN_POINT('Origin',(-61.9077842377855,0.317533537011735,3.20381846780048));
#223187=CARTESIAN_POINT('Origin',(-61.6018378049612,6.15533145331065,3.2038202287209));
#223188=CARTESIAN_POINT('Origin',(5.51210908043506E-15,1.8401175575949E-13,
3.61523028058481));
#223189=CARTESIAN_POINT('Origin',(-61.0281367271391,0.317462907478675,3.58786945046904));
#223190=CARTESIAN_POINT('Origin',(-60.7269085901933,6.06344346747484,3.58781461834164));
#223191=CARTESIAN_POINT('Origin',(5.51210908043507E-15,1.8401175575949E-13,
3.61523028058481));
#223192=CARTESIAN_POINT('Origin',(-60.8453028802703,0.317545368445655,3.58781440266595));
#223193=CARTESIAN_POINT('Origin',(-60.5450849487958,6.0442501005477,3.587869235929));
#223194=CARTESIAN_POINT('Origin',(60.4792282238308,1.82930781209959E-13,
3.77003198860263));
#223195=CARTESIAN_POINT('',(-58.7584778814677,12.164906888579,3.77003198860271));
#223196=CARTESIAN_POINT('',(-59.6417962403143,6.58785426247075,3.77003198860266));
#223197=CARTESIAN_POINT('Origin',(5.49031038273072E-15,1.82930781209959E-13,
3.77003198860263));
#223198=CARTESIAN_POINT('',(-60.1139000598801,6.63747437341761,3.77003198860266));
#223199=CARTESIAN_POINT('',(59.8516078896891,-5.97140859790491,3.77003198860259));
#223200=CARTESIAN_POINT('',(-60.1138365744456,6.63804933242088,3.77003198902554));
#223201=CARTESIAN_POINT('Origin',(5.49031038273072E-15,1.82930781209959E-13,
3.77003198860263));
#223202=CARTESIAN_POINT('',(-59.2229260464987,12.2630370254221,3.77003198882094));
#223203=CARTESIAN_POINT('Origin',(5.49031038273072E-15,1.82930781209959E-13,
3.77003198860263));
#223204=CARTESIAN_POINT('',(-59.2228087529783,12.2636034620787,3.7700319886027));
#223205=CARTESIAN_POINT('Origin',(5.49031038273072E-15,1.82930781209959E-13,
3.77003198860263));
#223206=CARTESIAN_POINT('',(-58.7590037315226,12.1650186614586,3.77003198860271));
#223207=CARTESIAN_POINT('Origin',(5.49031038273072E-15,1.82930781209959E-13,
3.77003198860263));
#223208=CARTESIAN_POINT('',(-60.2756459899119,6.65505462397374,3.48823028058485));
#223209=CARTESIAN_POINT('',(-60.1138365737176,6.63804933234049,3.77003198860266));
#223210=CARTESIAN_POINT('',(-59.382070870184,12.2968658914375,3.48823028074812));
#223211=CARTESIAN_POINT('Origin',(5.52999282761009E-15,1.84898592019556E-13,
3.48823028058481));
#223212=CARTESIAN_POINT('',(-59.3820708699071,12.2968658913801,3.48823028058489));
#223213=CARTESIAN_POINT('Origin',(60.71525,1.85785428279622E-13,3.36123028058482));
#223214=CARTESIAN_POINT('',(-59.597120393566,12.3431658574209,3.3612302805849));
#223215=CARTESIAN_POINT('',(-60.4944777170594,6.67747469700925,3.36123028058485));
#223216=CARTESIAN_POINT('Origin',(5.5478765747851E-15,1.85785428279622E-13,
3.36123028058482));
#223217=CARTESIAN_POINT('',(-60.6448574988555,6.69328024897434,3.36123028058485));
#223218=CARTESIAN_POINT('',(60.0850508448142,-5.99594444118149,3.36123028058478));
#223219=CARTESIAN_POINT('',(-59.7450242491248,12.3746037924162,3.3612302805849));
#223220=CARTESIAN_POINT('Origin',(5.5478765747851E-15,1.85785428279622E-13,
3.36123028058482));
#223221=CARTESIAN_POINT('',(-59.5976388357907,12.3432760557176,3.3612302805849));
#223222=CARTESIAN_POINT('Origin',(5.5478765747851E-15,1.85785428279622E-13,
3.36123028058482));
#223223=CARTESIAN_POINT('',(-59.9600752506738,12.4208962741584,3.48823028058492));
#223224=CARTESIAN_POINT('',(-60.8636883190563,6.71570789672388,3.48823028042699));
#223225=CARTESIAN_POINT('Origin',(5.52999282761008E-15,1.84898592019556E-13,
3.48823028058484));
#223226=CARTESIAN_POINT('',(-61.0254973286579,6.73271622308775,3.77003198802711));
#223227=CARTESIAN_POINT('',(-60.8636883187845,6.71570789669389,3.48823028058488));
#223228=CARTESIAN_POINT('',(-61.0254350648263,6.73328056300497,3.77003198860266));
#223229=CARTESIAN_POINT('Origin',(5.49031038273072E-15,1.82930781209959E-13,
3.77003198860263));
#223230=CARTESIAN_POINT('',(-60.1193358000129,12.4541661686664,3.77003198860271));
#223231=CARTESIAN_POINT('Origin',(5.49031038273072E-15,1.82930781209959E-13,
3.77003198860263));
#223232=CARTESIAN_POINT('',(-60.1192206258108,12.4547221284042,3.77003198802728));
#223233=CARTESIAN_POINT('Origin',(5.49031038273072E-15,1.82930781209959E-13,
3.77003198860263));
#223234=CARTESIAN_POINT('',(-60.119220626133,12.4547221284867,3.77003198860271));
#223235=CARTESIAN_POINT('Origin',(62.2224557307631,1.82930781209959E-13,
3.77003198860263));
#223236=CARTESIAN_POINT('',(-61.4975385923863,6.78290064323539,3.77003198860267));
#223237=CARTESIAN_POINT('',(61.5757885448748,-6.15262728712807,3.77003198860259));
#223238=CARTESIAN_POINT('',(-60.5836663843182,12.5528626811445,3.77003198860271));
#223239=CARTESIAN_POINT('Origin',(5.49031038273072E-15,1.82930781209959E-13,
3.77003198860263));
#223240=CARTESIAN_POINT('',(-60.1198497339744,12.4542754087021,3.77003198860271));
#223241=CARTESIAN_POINT('Origin',(5.57972911860581E-15,1.8736496251029E-13,
3.13503198860263));
#223242=CARTESIAN_POINT('Origin',(-59.6417947880742,6.58785913039789,3.13502491541435));
#223243=CARTESIAN_POINT('Origin',(-58.7584780045775,12.1649018101381,3.1350249154144));
#223244=CARTESIAN_POINT('Origin',(5.57972911860581E-15,1.8736496251029E-13,
3.13503198860263));
#223245=CARTESIAN_POINT('Origin',(-61.5354556255549,6.78691960575353,3.20381846780464));
#223246=CARTESIAN_POINT('Origin',(-60.620969154241,12.5607573437829,3.20382022872046));
#223247=CARTESIAN_POINT('Origin',(5.51210908043506E-15,1.8401175575949E-13,
3.61523028058481));
#223248=CARTESIAN_POINT('Origin',(-60.6606342988042,6.69490116063041,3.5878694504714));
#223249=CARTESIAN_POINT('Origin',(-59.760437803209,12.3779177236595,3.58781461834269));
#223250=CARTESIAN_POINT('Origin',(5.51210908043507E-15,1.8401175575949E-13,
3.61523028058481));
#223251=CARTESIAN_POINT('Origin',(-60.4787934153616,6.67587182882183,3.58781440266543));
#223252=CARTESIAN_POINT('Origin',(-59.5816164638928,12.3398237541834,3.58786923592735));
#223253=CARTESIAN_POINT('Origin',(60.4792282238308,1.82930781209959E-13,
3.77003198860263));
#223254=CARTESIAN_POINT('',(-57.1650137687748,18.2401996527044,3.77003198860275));
#223255=CARTESIAN_POINT('',(-58.6264539577984,12.7860306150449,3.77003198860271));
#223256=CARTESIAN_POINT('Origin',(5.49031038273072E-15,1.82930781209959E-13,
3.77003198860263));
#223257=CARTESIAN_POINT('',(-59.0907848292991,12.8847271885942,3.77003198860271));
#223258=CARTESIAN_POINT('',(57.9308881865556,-11.9889972685545,3.77003198860255));
#223259=CARTESIAN_POINT('',(-59.090661592063,12.8852923618769,3.77003198902532));
#223260=CARTESIAN_POINT('Origin',(5.49031038273072E-15,1.82930781209959E-13,
3.77003198860263));
#223261=CARTESIAN_POINT('',(-57.6166602457573,18.3863402753485,3.77003198882099));
#223262=CARTESIAN_POINT('Origin',(5.49031038273072E-15,1.82930781209959E-13,
3.77003198860263));
#223263=CARTESIAN_POINT('',(-57.6164843860298,18.3868913484944,3.77003198860275));
#223264=CARTESIAN_POINT('Origin',(5.49031038273072E-15,1.82930781209959E-13,
3.77003198860263));
#223265=CARTESIAN_POINT('',(-57.1655250547207,18.2403657795786,3.77003198860275));
#223266=CARTESIAN_POINT('Origin',(5.49031038273072E-15,1.82930781209959E-13,
3.77003198860263));
#223267=CARTESIAN_POINT('',(-59.249807061628,12.9191181862044,3.48823028058489));
#223268=CARTESIAN_POINT('',(-59.0906615913478,12.8852923617209,3.77003198860271));
#223269=CARTESIAN_POINT('',(-57.7713971780681,18.4366189871531,3.48823028074816));
#223270=CARTESIAN_POINT('Origin',(5.52999282761009E-15,1.84898592019556E-13,
3.48823028058481));
#223271=CARTESIAN_POINT('',(-57.7713971777988,18.4366189870671,3.48823028058493));
#223272=CARTESIAN_POINT('Origin',(60.71525,1.85785428279622E-13,3.36123028058482));
#223273=CARTESIAN_POINT('',(-57.9804289733665,18.505144113284,3.36123028058494));
#223274=CARTESIAN_POINT('',(-59.4650964698967,12.9642895838869,3.3612302805849));
#223275=CARTESIAN_POINT('Origin',(5.5478765747851E-15,1.85785428279622E-13,
3.36123028058482));
#223276=CARTESIAN_POINT('',(-59.6130003254556,12.9957275188822,3.3612302805849));
#223277=CARTESIAN_POINT('',(58.1567073854023,-12.0369966210205,3.36123028058474));
#223278=CARTESIAN_POINT('',(-58.1242364370958,18.5518699907149,3.36123028058494));
#223279=CARTESIAN_POINT('Origin',(5.5478765747851E-15,1.85785428279622E-13,
3.36123028058482));
#223280=CARTESIAN_POINT('',(-57.9809330566518,18.5053078998719,3.36123028058494));
#223281=CARTESIAN_POINT('Origin',(5.5478765747851E-15,1.85785428279622E-13,
3.36123028058482));
#223282=CARTESIAN_POINT('',(-58.3332704847797,18.6203878281146,3.48823028058496));
#223283=CARTESIAN_POINT('',(-59.8282880399728,13.0409063549819,3.48823028042702));
#223284=CARTESIAN_POINT('Origin',(5.52999282761008E-15,1.84898592019556E-13,
3.48823028058484));
#223285=CARTESIAN_POINT('',(-59.9874327886718,13.0747351550709,3.77003198802716));
#223286=CARTESIAN_POINT('',(-59.8282880397056,13.0409063549237,3.48823028058492));
#223287=CARTESIAN_POINT('',(-59.9873118763436,13.0752898951323,3.77003198860271));
#223288=CARTESIAN_POINT('Origin',(5.49031038273072E-15,1.82930781209959E-13,
3.77003198860263));
#223289=CARTESIAN_POINT('',(-58.4881809372199,18.6701227271409,3.77003198860275));
#223290=CARTESIAN_POINT('Origin',(5.49031038273072E-15,1.82930781209959E-13,
3.77003198860263));
#223291=CARTESIAN_POINT('',(-58.488008280337,18.6706636022907,3.77003198802732));
#223292=CARTESIAN_POINT('Origin',(5.49031038273072E-15,1.82930781209959E-13,
3.77003198860263));
#223293=CARTESIAN_POINT('',(-58.4880082806488,18.6706636024064,3.77003198860275));
#223294=CARTESIAN_POINT('Origin',(62.2224557307631,1.82930781209959E-13,
3.77003198860263));
#223295=CARTESIAN_POINT('',(-60.451642460649,13.1739864076105,3.77003198860271));
#223296=CARTESIAN_POINT('',(59.5987607253196,-12.3435145206981,3.77003198860255));
#223297=CARTESIAN_POINT('',(-58.9396512752214,18.8168143322225,3.77003198860275));
#223298=CARTESIAN_POINT('Origin',(5.49031038273072E-15,1.82930781209959E-13,
3.77003198860263));
#223299=CARTESIAN_POINT('',(-58.4886806371043,18.6702850894755,3.77003198860275));
#223300=CARTESIAN_POINT('Origin',(5.57972911860581E-15,1.8736496251029E-13,
3.13503198860263));
#223301=CARTESIAN_POINT('Origin',(-58.6264520046769,12.7860353045046,3.13502491541439));
#223302=CARTESIAN_POINT('Origin',(-57.1650144220518,18.2401946149522,3.13502491541442));
#223303=CARTESIAN_POINT('Origin',(5.57972911860581E-15,1.8736496251029E-13,
3.13503198860263));
#223304=CARTESIAN_POINT('Origin',(-60.4889316843638,13.1819467630405,3.20381846779971));
#223305=CARTESIAN_POINT('Origin',(-58.9759244797154,18.8285649482883,3.20382022872347));
#223306=CARTESIAN_POINT('Origin',(5.51210908043506E-15,1.8401175575949E-13,
3.61523028058481));
#223307=CARTESIAN_POINT('Origin',(-59.6285212670405,12.9989886756689,3.58786945046839));
#223308=CARTESIAN_POINT('Origin',(-58.13921915398,18.5567769230188,3.5878146183382));
#223309=CARTESIAN_POINT('Origin',(5.51210908043507E-15,1.8401175575949E-13,
3.61523028058481));
#223310=CARTESIAN_POINT('Origin',(-59.4496656337924,12.9610560404238,3.58781440266355));
#223311=CARTESIAN_POINT('Origin',(-57.9653593207587,18.5001997164983,3.58786923593086));
#223312=CARTESIAN_POINT('Origin',(60.4792282238308,1.82930781209959E-13,
3.77003198860263));
#223313=CARTESIAN_POINT('',(-54.945237802683,24.1156489724276,3.77003198860279));
#223314=CARTESIAN_POINT('',(-56.9687879773467,18.8441205405518,3.77003198860275));
#223315=CARTESIAN_POINT('Origin',(5.49031038273072E-15,1.82930781209959E-13,
3.77003198860263));
#223316=CARTESIAN_POINT('',(-57.4202585945867,18.99081223639,3.77003198860275));
#223317=CARTESIAN_POINT('',(54.8020887275097,-17.472438766075,3.77003198860251));
#223318=CARTESIAN_POINT('',(-57.4200769557625,18.9913614317955,3.77003198902548));
#223319=CARTESIAN_POINT('Origin',(5.49031038273072E-15,1.82930781209959E-13,
3.77003198860263));
#223320=CARTESIAN_POINT('',(-55.3791342583021,24.3081989336292,3.77003198882103));
#223321=CARTESIAN_POINT('Origin',(5.49031038273072E-15,1.82930781209959E-13,
3.77003198860263));
#223322=CARTESIAN_POINT('',(-55.3789017591235,24.3087286055916,3.77003198860279));
#223323=CARTESIAN_POINT('Origin',(5.49031038273072E-15,1.82930781209959E-13,
3.77003198860263));
#223324=CARTESIAN_POINT('',(-54.9457289227642,24.1158676331756,3.77003198860279));
#223325=CARTESIAN_POINT('Origin',(5.49031038273072E-15,1.82930781209959E-13,
3.77003198860263));
#223326=CARTESIAN_POINT('',(-57.5748148483577,19.0416371860876,3.48823028058494));
#223327=CARTESIAN_POINT('',(-57.4200769550674,18.9913614315656,3.77003198860275));
#223328=CARTESIAN_POINT('',(-55.5277679690273,24.3743766271349,3.4882302807482));
#223329=CARTESIAN_POINT('Origin',(5.52999282761009E-15,1.84898592019556E-13,
3.48823028058481));
#223330=CARTESIAN_POINT('',(-55.5277679687684,24.3743766270213,3.48823028058497));
#223331=CARTESIAN_POINT('Origin',(60.71525,1.85785428279622E-13,3.36123028058482));
#223332=CARTESIAN_POINT('',(-55.7284918401499,24.4643761377916,3.36123028058498));
#223333=CARTESIAN_POINT('',(-57.7842031819384,19.1090650011314,3.36123028058494));
#223334=CARTESIAN_POINT('Origin',(5.5478765747851E-15,1.85785428279622E-13,
3.36123028058482));
#223335=CARTESIAN_POINT('',(-57.9280106456677,19.1557908785624,3.36123028058494));
#223336=CARTESIAN_POINT('',(55.0155724295761,-17.5418038257011,3.3612302805847));
#223337=CARTESIAN_POINT('',(-55.8666273273834,24.525878019167,3.36123028058498));
#223338=CARTESIAN_POINT('Origin',(5.5478765747851E-15,1.85785428279622E-13,
3.36123028058482));
#223339=CARTESIAN_POINT('',(-55.728976041654,24.4645917181906,3.36123028058498));
#223340=CARTESIAN_POINT('Origin',(5.5478765747851E-15,1.85785428279622E-13,
3.36123028058482));
#223341=CARTESIAN_POINT('',(-56.0673542004327,24.6158705164592,3.488230280585));
#223342=CARTESIAN_POINT('',(-58.1373965172491,19.2232259142297,3.48823028042707));
#223343=CARTESIAN_POINT('Origin',(5.52999282761008E-15,1.84898592019556E-13,
3.48823028058484));
#223344=CARTESIAN_POINT('',(-58.2921333818757,19.2735045526308,3.7700319880272));
#223345=CARTESIAN_POINT('',(-58.1373965169894,19.2232259141438,3.48823028058497));
#223346=CARTESIAN_POINT('',(-58.2919551457918,19.2740436149883,3.77003198860276));
#223347=CARTESIAN_POINT('Origin',(5.49031038273072E-15,1.82930781209959E-13,
3.77003198860263));
#223348=CARTESIAN_POINT('',(-56.2162173246399,24.6815255140425,3.77003198860279));
#223349=CARTESIAN_POINT('Origin',(5.49031038273072E-15,1.82930781209959E-13,
3.77003198860263));
#223350=CARTESIAN_POINT('',(-56.2159890767413,24.682045378663,3.77003198802737));
#223351=CARTESIAN_POINT('Origin',(5.49031038273072E-15,1.82930781209959E-13,
3.77003198860263));
#223352=CARTESIAN_POINT('',(-56.2159890770393,24.6820453788107,3.77003198860279));
#223353=CARTESIAN_POINT('Origin',(62.2224557307631,1.82930781209959E-13,
3.77003198860263));
#223354=CARTESIAN_POINT('',(-58.7434254837933,19.4207352200699,3.77003198860276));
#223355=CARTESIAN_POINT('',(56.3788528200609,-17.9847604760577,3.77003198860251));
#223356=CARTESIAN_POINT('',(-56.6498810128383,24.8746050278051,3.77003198860279));
#223357=CARTESIAN_POINT('Origin',(5.49031038273072E-15,1.82930781209959E-13,
3.77003198860263));
#223358=CARTESIAN_POINT('',(-56.2166973156307,24.6817392198003,3.77003198860279));
#223359=CARTESIAN_POINT('Origin',(5.57972911860581E-15,1.8736496251029E-13,
3.13503198860263));
#223360=CARTESIAN_POINT('Origin',(-56.9687855447426,18.8441250001653,3.13502491541443));
#223361=CARTESIAN_POINT('Origin',(-54.9452389789698,24.1156440305588,3.13502491541451));
#223362=CARTESIAN_POINT('Origin',(5.57972911860581E-15,1.8736496251029E-13,
3.13503198860263));
#223363=CARTESIAN_POINT('Origin',(-58.7796783495213,19.4325497530908,3.20381846780393));
#223364=CARTESIAN_POINT('Origin',(-56.6847272350798,24.8900828550892,3.2038202287169));
#223365=CARTESIAN_POINT('Origin',(5.51210908043506E-15,1.8401175575949E-13,
3.61523028058481));
#223366=CARTESIAN_POINT('Origin',(-57.9431056782028,19.1606565505631,3.58786945046924));
#223367=CARTESIAN_POINT('Origin',(-55.8810150532822,24.532324191153,3.58781461834167));
#223368=CARTESIAN_POINT('Origin',(5.51210908043507E-15,1.8401175575949E-13,
3.61523028058481));
#223369=CARTESIAN_POINT('Origin',(-57.7691948748981,19.1042362097749,3.58781440266532));
#223370=CARTESIAN_POINT('Origin',(-55.7140215708733,24.4578836192983,3.58786923592957));
#223371=CARTESIAN_POINT('Origin',(60.4792282238308,1.82930781209959E-13,
3.77003198860263));
#223372=CARTESIAN_POINT('',(-52.1234703131948,29.7268821954849,3.77003198860283));
#223373=CARTESIAN_POINT('',(-54.6869600343299,24.6957503380306,3.77003198860279));
#223374=CARTESIAN_POINT('Origin',(5.49031038273072E-15,1.82930781209959E-13,
3.77003198860263));
#223375=CARTESIAN_POINT('',(-55.1206239907504,24.888829971241,3.77003198860279));
#223376=CARTESIAN_POINT('',(50.603004322856,-22.1823620689011,3.77003198860248));
#223377=CARTESIAN_POINT('',(-55.1203859404111,24.8893571716696,3.77003198902569));
#223378=CARTESIAN_POINT('Origin',(5.49031038273072E-15,1.82930781209959E-13,
3.77003198860263));
#223379=CARTESIAN_POINT('',(-52.534862887084,29.9637318775753,3.77003198882107));
#223380=CARTESIAN_POINT('Origin',(5.49031038273072E-15,1.82930781209959E-13,
3.77003198860263));
#223381=CARTESIAN_POINT('',(-52.5345762957639,29.9642343451574,3.77003198860283));
#223382=CARTESIAN_POINT('Origin',(5.49031038273072E-15,1.82930781209959E-13,
3.77003198860263));
#223383=CARTESIAN_POINT('',(-52.1239358865968,29.7271509944138,3.77003198860283));
#223384=CARTESIAN_POINT('Origin',(5.49031038273072E-15,1.82930781209959E-13,
3.77003198860263));
#223385=CARTESIAN_POINT('',(-55.2690209153042,24.9555320242414,3.48823028058498));
#223386=CARTESIAN_POINT('',(-55.1203859397436,24.8893571713681,3.77003198860279));
#223387=CARTESIAN_POINT('',(-52.6757649141853,30.0450834961236,3.48823028074825));
#223388=CARTESIAN_POINT('Origin',(5.52999282761009E-15,1.84898592019556E-13,
3.48823028058481));
#223389=CARTESIAN_POINT('',(-52.6757649139398,30.0450834959835,3.48823028058502));
#223390=CARTESIAN_POINT('Origin',(60.71525,1.85785428279622E-13,3.36123028058482));
#223391=CARTESIAN_POINT('',(-52.8659816883961,30.1555713378337,3.36123028058502));
#223392=CARTESIAN_POINT('',(-55.4702140717968,25.0444775033946,3.36123028058499));
#223393=CARTESIAN_POINT('Origin',(5.5478765747851E-15,1.85785428279622E-13,
3.36123028058482));
#223394=CARTESIAN_POINT('',(-55.6083495590303,25.10597938477,3.36123028058499));
#223395=CARTESIAN_POINT('',(50.7999799080417,-22.2700612497312,3.36123028058467));
#223396=CARTESIAN_POINT('',(-52.9969317578289,30.2311753956711,3.36123028058502));
#223397=CARTESIAN_POINT('Origin',(5.5478765747851E-15,1.85785428279622E-13,
3.36123028058482));
#223398=CARTESIAN_POINT('',(-52.8664407031058,30.1558363500999,3.36123028058502));
#223399=CARTESIAN_POINT('Origin',(5.5478765747851E-15,1.85785428279622E-13,
3.36123028058482));
#223400=CARTESIAN_POINT('',(-53.1871522506177,30.3416565762235,3.48823028058504));
#223401=CARTESIAN_POINT('',(-55.8095395122501,25.1949317876425,3.48823028042712));
#223402=CARTESIAN_POINT('Origin',(5.52999282761008E-15,1.84898592019556E-13,
3.48823028058484));
#223403=CARTESIAN_POINT('',(-55.9581731633346,25.261109401072,3.77003198802724));
#223404=CARTESIAN_POINT('',(-55.8095395120008,25.19493178753,3.48823028058501));
#223405=CARTESIAN_POINT('',(-55.9579395562868,25.2616268796456,3.7700319886028));
#223406=CARTESIAN_POINT('Origin',(5.49031038273072E-15,1.82930781209959E-13,
3.77003198860263));
#223407=CARTESIAN_POINT('',(-53.3283370710514,30.422512342471,3.77003198860283));
#223408=CARTESIAN_POINT('Origin',(5.49031038273072E-15,1.82930781209959E-13,
3.77003198860263));
#223409=CARTESIAN_POINT('',(-53.3280557328688,30.4230055008167,3.77003198802741));
#223410=CARTESIAN_POINT('Origin',(5.49031038273072E-15,1.82930781209959E-13,
3.77003198860263));
#223411=CARTESIAN_POINT('',(-53.3280557331497,30.4230055009947,3.77003198860283));
#223412=CARTESIAN_POINT('Origin',(62.2224557307631,1.82930781209959E-13,
3.77003198860263));
#223413=CARTESIAN_POINT('',(-56.3916032444852,25.4547063934082,3.7700319886028));
#223414=CARTESIAN_POINT('',(52.0578415156897,-22.8300973196044,3.77003198860247));
#223415=CARTESIAN_POINT('',(-53.7394427993288,30.6598643453573,3.77003198860284));
#223416=CARTESIAN_POINT('Origin',(5.49031038273072E-15,1.82930781209959E-13,
3.77003198860263));
#223417=CARTESIAN_POINT('',(-53.3287920942669,30.422775050247,3.77003198860283));
#223418=CARTESIAN_POINT('Origin',(5.57972911860581E-15,1.8736496251029E-13,
3.13503198860263));
#223419=CARTESIAN_POINT('Origin',(-54.6869571488952,24.6957545189375,3.13502491541449));
#223420=CARTESIAN_POINT('Origin',(-52.1234719996037,29.7268774036436,3.13502491541452));
#223421=CARTESIAN_POINT('Origin',(5.57972911860581E-15,1.8736496251029E-13,
3.13503198860263));
#223422=CARTESIAN_POINT('Origin',(-56.4264225582392,25.4702456615255,3.20381846780165));
#223423=CARTESIAN_POINT('Origin',(-53.7724802568194,30.6788998055474,3.20382022872094));
#223424=CARTESIAN_POINT('Origin',(5.51210908043506E-15,1.8401175575949E-13,
3.61523028058481));
#223425=CARTESIAN_POINT('Origin',(-55.62285329818,25.112396262664,3.58786945047063));
#223426=CARTESIAN_POINT('Origin',(-53.0105668578065,30.2390901817298,3.58781461834535));
#223427=CARTESIAN_POINT('Origin',(5.51210908043507E-15,1.8401175575949E-13,
3.61523028058481));
#223428=CARTESIAN_POINT('Origin',(-55.4557927279724,25.0381063693915,3.58781440266499));
#223429=CARTESIAN_POINT('Origin',(-52.8522693417508,30.147601831022,3.58786923592841));
#223430=CARTESIAN_POINT('Origin',(60.4792282238308,1.82930781209959E-13,
3.77003198860263));
#223431=CARTESIAN_POINT('',(-48.7306271754178,35.0124214764584,3.77003198860287));
#223432=CARTESIAN_POINT('',(-51.8059703131948,30.276808326888,3.77003198860283));
#223433=CARTESIAN_POINT('Origin',(5.49031038273072E-15,1.82930781209959E-13,
3.77003198860263));
#223434=CARTESIAN_POINT('',(-52.2170762957392,30.5141604766046,3.77003198860283));
#223435=CARTESIAN_POINT('',(45.5181711678734,-25.9133109558552,3.77003198860245));
#223436=CARTESIAN_POINT('',(-52.2167844420139,30.5146599059378,3.77003198902559));
#223437=CARTESIAN_POINT('Origin',(5.49031038273072E-15,1.82930781209959E-13,
3.77003198860263));
#223438=CARTESIAN_POINT('',(-49.1150085644482,35.2909759047568,3.77003198882111));
#223439=CARTESIAN_POINT('Origin',(5.49031038273072E-15,1.82930781209959E-13,
3.77003198860263));
#223440=CARTESIAN_POINT('',(-49.1146710209412,35.2914456628186,3.77003198860286));
#223441=CARTESIAN_POINT('Origin',(5.49031038273072E-15,1.82930781209959E-13,
3.77003198860263));
#223442=CARTESIAN_POINT('',(-48.731062101221,35.012737468551,3.77003198860287));
#223443=CARTESIAN_POINT('Origin',(5.49031038273072E-15,1.82930781209959E-13,
3.77003198860263));
#223444=CARTESIAN_POINT('',(-52.3576880233164,30.5960088312567,3.48823028058502));
#223445=CARTESIAN_POINT('',(-52.2167844413817,30.5146599055683,3.77003198860283));
#223446=CARTESIAN_POINT('',(-49.2466351558311,35.3866101429909,3.48823028074828));
#223447=CARTESIAN_POINT('Origin',(5.52999282761009E-15,1.84898592019556E-13,
3.48823028058481));
#223448=CARTESIAN_POINT('',(-49.2466351556015,35.3866101428259,3.48823028058505));
#223449=CARTESIAN_POINT('Origin',(60.71525,1.85785428279622E-13,3.36123028058482));
#223450=CARTESIAN_POINT('',(-49.4242607783462,35.5163757878395,3.36123028058506));
#223451=CARTESIAN_POINT('',(-52.5484816883961,30.7054974692368,3.36123028058502));
#223452=CARTESIAN_POINT('Origin',(5.5478765747851E-15,1.85785428279622E-13,
3.36123028058482));
#223453=CARTESIAN_POINT('',(-52.6794317578289,30.7811015270742,3.36123028058502));
#223454=CARTESIAN_POINT('',(45.6951875000003,-26.0155113828597,3.36123028058464));
#223455=CARTESIAN_POINT('',(-49.5465907136146,35.6052536882601,3.36123028058506));
#223456=CARTESIAN_POINT('Origin',(5.5478765747851E-15,1.85785428279622E-13,
3.36123028058482));
#223457=CARTESIAN_POINT('',(-49.4246895772004,35.516687328443,3.36123028058506));
#223458=CARTESIAN_POINT('Origin',(5.5478765747851E-15,1.85785428279622E-13,
3.36123028058482));
#223459=CARTESIAN_POINT('',(-49.7242207306177,35.7350130971388,3.48823028058508));
#223460=CARTESIAN_POINT('',(-52.8702215134579,30.8905967160115,3.48823028042716));
#223461=CARTESIAN_POINT('Origin',(5.52999282761008E-15,1.84898592019556E-13,
3.48823028058484));
#223462=CARTESIAN_POINT('',(-53.0111234896155,30.971948248688,3.77003198802728));
#223463=CARTESIAN_POINT('',(-52.8702215132218,30.8905967158735,3.48823028058505));
#223464=CARTESIAN_POINT('',(-53.0108370710514,30.9724384738741,3.77003198860284));
#223465=CARTESIAN_POINT('Origin',(5.49031038273072E-15,1.82930781209959E-13,
3.77003198860263));
#223466=CARTESIAN_POINT('',(-49.8561803968405,35.8301837593554,3.77003198860287));
#223467=CARTESIAN_POINT('Origin',(5.49031038273072E-15,1.82930781209959E-13,
3.77003198860263));
#223468=CARTESIAN_POINT('',(-49.8558490507739,35.8306448082802,3.77003198802745));
#223469=CARTESIAN_POINT('Origin',(5.49031038273072E-15,1.82930781209959E-13,
3.77003198860263));
#223470=CARTESIAN_POINT('',(-49.8558490510346,35.8306448084866,3.77003198860287));
#223471=CARTESIAN_POINT('Origin',(62.2224557307631,1.82930781209959E-13,
3.77003198860263));
#223472=CARTESIAN_POINT('',(-53.4219427993288,31.2097904767605,3.77003198860284));
#223473=CARTESIAN_POINT('',(46.8255917980726,-26.6681506086448,3.77003198860245));
#223474=CARTESIAN_POINT('',(-50.2402240048085,36.1092077731528,3.77003198860287));
#223475=CARTESIAN_POINT('Origin',(5.49031038273072E-15,1.82930781209959E-13,
3.77003198860263));
#223476=CARTESIAN_POINT('',(-49.8566054669511,35.8304925908682,3.77003198860287));
#223477=CARTESIAN_POINT('Origin',(5.57972911860581E-15,1.8736496251029E-13,
3.13503198860263));
#223478=CARTESIAN_POINT('Origin',(-51.8059670065431,30.2768121832814,3.13502491541452));
#223479=CARTESIAN_POINT('Origin',(-48.7306293534722,35.012416887145,3.13502491541459));
#223480=CARTESIAN_POINT('Origin',(5.57972911860581E-15,1.8736496251029E-13,
3.13503198860263));
#223481=CARTESIAN_POINT('Origin',(-53.4549470734237,31.2288842284977,3.20381846780235));
#223482=CARTESIAN_POINT('Origin',(-50.2710907322488,36.131592309763,3.20382022872186));
#223483=CARTESIAN_POINT('Origin',(5.51210908043506E-15,1.8401175575949E-13,
3.61523028058481));
#223484=CARTESIAN_POINT('Origin',(-52.6931852975926,30.7889993062046,3.58786945047073));
#223485=CARTESIAN_POINT('Origin',(-49.5593237986663,35.6145503723413,3.58781461834041));
#223486=CARTESIAN_POINT('Origin',(5.51210908043507E-15,1.8401175575949E-13,
3.61523028058481));
#223487=CARTESIAN_POINT('Origin',(-52.5348053110472,30.6976537960624,3.58781440266096));
#223488=CARTESIAN_POINT('Origin',(-49.4114565896721,35.5070166082958,3.58786923592867));
#223489=CARTESIAN_POINT('Origin',(60.4792282238308,1.82930781209959E-13,
3.77003198860263));
#223490=CARTESIAN_POINT('',(-44.8038810887676,39.9143573409156,3.7700319886029));
#223491=CARTESIAN_POINT('',(-48.3573835402121,35.5261472678865,3.77003198860287));
#223492=CARTESIAN_POINT('Origin',(5.49031038273072E-15,1.82930781209959E-13,
3.77003198860263));
#223493=CARTESIAN_POINT('',(-48.7414273857063,35.805171454288,3.77003198860287));
#223494=CARTESIAN_POINT('',(39.7707905934409,-28.5027191556737,3.77003198860244));
#223495=CARTESIAN_POINT('',(-48.7410849262055,35.8056376406736,3.77003198902568));
#223496=CARTESIAN_POINT('Origin',(5.49031038273072E-15,1.82930781209959E-13,
3.77003198860263));
#223497=CARTESIAN_POINT('',(-45.157039930004,40.2315646148142,3.77003198882114));
#223498=CARTESIAN_POINT('Origin',(5.49031038273072E-15,1.82930781209959E-13,
3.77003198860263));
#223499=CARTESIAN_POINT('',(-45.1566551325073,40.2319965165881,3.7700319886029));
#223500=CARTESIAN_POINT('Origin',(5.49031038273072E-15,1.82930781209959E-13,
3.77003198860263));
#223501=CARTESIAN_POINT('',(-44.804280601834,39.9147170640963,3.7700319886029));
#223502=CARTESIAN_POINT('Origin',(5.49031038273072E-15,1.82930781209959E-13,
3.77003198860263));
#223503=CARTESIAN_POINT('',(-48.8727133447945,35.9012693628904,3.48823028058505));
#223504=CARTESIAN_POINT('',(-48.7410849256153,35.8056376402401,3.77003198860287));
#223505=CARTESIAN_POINT('',(-45.2779489571886,40.3404336840073,3.48823028074832));
#223506=CARTESIAN_POINT('Origin',(5.52999282761009E-15,1.84898592019556E-13,
3.48823028058481));
#223507=CARTESIAN_POINT('',(-45.2779489569775,40.3404336838192,3.48823028058509));
#223508=CARTESIAN_POINT('Origin',(60.71525,1.85785428279622E-13,3.36123028058482));
#223509=CARTESIAN_POINT('',(-45.4410373245174,40.4880553924343,3.36123028058509));
#223510=CARTESIAN_POINT('',(-49.0510171431405,36.0301015792676,3.36123028058506));
#223511=CARTESIAN_POINT('Origin',(5.5478765747851E-15,1.85785428279622E-13,
3.36123028058482));
#223512=CARTESIAN_POINT('',(-49.1733470784089,36.1189794796882,3.36123028058506));
#223513=CARTESIAN_POINT('',(39.9252688514649,-28.6149541797803,3.36123028058462));
#223514=CARTESIAN_POINT('',(-45.5534068532513,40.5892333705622,3.36123028058509));
#223515=CARTESIAN_POINT('Origin',(5.5478765747851E-15,1.85785428279622E-13,
3.36123028058482));
#223516=CARTESIAN_POINT('',(-45.441431209506,40.4884100480711,3.36123028058509));
#223517=CARTESIAN_POINT('Origin',(5.5478765747851E-15,1.85785428279622E-13,
3.36123028058482));
#223518=CARTESIAN_POINT('',(-45.7165002428309,40.7368493365297,3.48823028058512));
#223519=CARTESIAN_POINT('',(-49.3516463039591,36.2478178024869,3.48823028042719));
#223520=CARTESIAN_POINT('Origin',(5.52999282761008E-15,1.84898592019556E-13,
3.48823028058484));
#223521=CARTESIAN_POINT('',(-49.4832728536533,36.3434519499946,3.77003198802732));
#223522=CARTESIAN_POINT('',(-49.3516463037387,36.247817802325,3.48823028058509));
#223523=CARTESIAN_POINT('',(-49.4829367616348,36.3439095507835,3.77003198860287));
#223524=CARTESIAN_POINT('Origin',(5.49031038273072E-15,1.82930781209959E-13,
3.77003198860263));
#223525=CARTESIAN_POINT('',(-45.8377889771253,40.8452921850243,3.7700319886029));
#223526=CARTESIAN_POINT('Origin',(5.49031038273072E-15,1.82930781209959E-13,
3.77003198860263));
#223527=CARTESIAN_POINT('',(-45.8374112534715,40.8457160731797,3.77003198802748));
#223528=CARTESIAN_POINT('Origin',(5.49031038273072E-15,1.82930781209959E-13,
3.77003198860263));
#223529=CARTESIAN_POINT('',(-45.8374112537093,40.8457160734122,3.7700319886029));
#223530=CARTESIAN_POINT('Origin',(62.2224557307631,1.82930781209959E-13,
3.77003198860263));
#223531=CARTESIAN_POINT('',(-49.8669803696028,36.6229335645809,3.77003198860288));
#223532=CARTESIAN_POINT('',(40.911747809259,-29.3316730956001,3.77003198860243));
#223533=CARTESIAN_POINT('',(-46.1905628026487,41.162931164248,3.77003198860291));
#223534=CARTESIAN_POINT('Origin',(5.49031038273072E-15,1.82930781209959E-13,
3.77003198860263));
#223535=CARTESIAN_POINT('',(-45.838179436974,40.8456437566512,3.7700319886029));
#223536=CARTESIAN_POINT('Origin',(5.57972911860581E-15,1.8736496251029E-13,
3.13503198860263));
#223537=CARTESIAN_POINT('Origin',(-48.3573798485717,35.526150757515,3.13502491541459));
#223538=CARTESIAN_POINT('Origin',(-44.8038837346043,39.9143530044117,3.13502491541463));
#223539=CARTESIAN_POINT('Origin',(5.57972911860581E-15,1.8736496251029E-13,
3.13503198860263));
#223540=CARTESIAN_POINT('Origin',(-49.8978080023019,36.6453726048011,3.20381846780002));
#223541=CARTESIAN_POINT('Origin',(-46.2189206177177,41.1884195276069,3.20382022872409));
#223542=CARTESIAN_POINT('Origin',(5.51210908043506E-15,1.8401175575949E-13,
3.61523028058481));
#223543=CARTESIAN_POINT('Origin',(-49.1861997321276,36.1282716303346,3.58786945046978));
#223544=CARTESIAN_POINT('Origin',(-45.5650984170303,40.5998100962484,3.58781461834004));
#223545=CARTESIAN_POINT('Origin',(5.51210908043507E-15,1.8401175575949E-13,
3.61523028058481));
#223546=CARTESIAN_POINT('Origin',(-49.038235573526,36.0208713038445,3.58781440266443));
#223547=CARTESIAN_POINT('Origin',(-45.4292815791818,40.4774090812934,3.58786923593075));
#223548=CARTESIAN_POINT('Origin',(60.4792282238308,1.82930781209959E-13,
3.77003198860263));
#223549=CARTESIAN_POINT('',(-40.386254305094,44.3789831537295,3.77003198860293));
#223550=CARTESIAN_POINT('',(-44.3789831537298,40.3862543050938,3.7700319886029));
#223551=CARTESIAN_POINT('Origin',(5.49031038273072E-15,1.82930781209959E-13,
3.77003198860263));
#223552=CARTESIAN_POINT('',(-44.7317571974361,40.7038934808043,3.7700319886029));
#223553=CARTESIAN_POINT('',(33.61296347236,-29.838009859698,3.77003198860242));
#223554=CARTESIAN_POINT('',(-44.7313678842178,40.7043213166068,3.7700319890257));
#223555=CARTESIAN_POINT('Origin',(5.49031038273072E-15,1.82930781209959E-13,
3.77003198860263));
#223556=CARTESIAN_POINT('',(-40.7043213163686,44.7313678839555,3.77003198882117));
#223557=CARTESIAN_POINT('Origin',(5.49031038273072E-15,1.82930781209959E-13,
3.77003198860263));
#223558=CARTESIAN_POINT('',(-40.7038934808041,44.7317571974354,3.77003198860293));
#223559=CARTESIAN_POINT('Origin',(5.49031038273072E-15,1.82930781209959E-13,
3.77003198860263));
#223560=CARTESIAN_POINT('',(-40.3866140282747,44.3793826667959,3.77003198860293));
#223561=CARTESIAN_POINT('Origin',(5.49031038273072E-15,1.82930781209959E-13,
3.77003198860263));
#223562=CARTESIAN_POINT('',(-44.8522789915944,40.8131880745606,3.48823028058509));
#223563=CARTESIAN_POINT('',(-44.7313678836762,40.7043213161139,3.7700319886029));
#223564=CARTESIAN_POINT('',(-40.8131880747512,44.8522789918032,3.48823028074835));
#223565=CARTESIAN_POINT('Origin',(5.52999282761009E-15,1.84898592019556E-13,
3.48823028058481));
#223566=CARTESIAN_POINT('',(-40.8131880745609,44.8522789915941,3.48823028058512));
#223567=CARTESIAN_POINT('Origin',(60.71525,1.85785428279622E-13,3.36123028058482));
#223568=CARTESIAN_POINT('',(-40.9599523566127,45.0161393894793,3.36123028058512));
#223569=CARTESIAN_POINT('',(-45.0161393894795,40.9599523566124,3.3612302805851));
#223570=CARTESIAN_POINT('Origin',(5.5478765747851E-15,1.85785428279622E-13,
3.36123028058482));
#223571=CARTESIAN_POINT('',(-45.1285089182135,41.0611303347403,3.3612302805851));
#223572=CARTESIAN_POINT('',(33.743309857225,-29.95537427179,3.36123028058461));
#223573=CARTESIAN_POINT('',(-41.0611303347406,45.1285089182133,3.36123028058512));
#223574=CARTESIAN_POINT('Origin',(5.5478765747851E-15,1.85785428279622E-13,
3.36123028058482));
#223575=CARTESIAN_POINT('',(-40.9603070122495,45.0165332744679,3.36123028058512));
#223576=CARTESIAN_POINT('Origin',(5.5478765747851E-15,1.85785428279622E-13,
3.36123028058482));
#223577=CARTESIAN_POINT('',(-41.2079002115909,45.2923641298557,3.48823028058515));
#223578=CARTESIAN_POINT('',(-45.2923641300582,41.2079002117747,3.48823028042723));
#223579=CARTESIAN_POINT('Origin',(5.52999282761008E-15,1.84898592019556E-13,
3.48823028058484));
#223580=CARTESIAN_POINT('',(-45.413273125266,41.3167691863808,3.77003198802735));
#223581=CARTESIAN_POINT('',(-45.2923641298559,41.2079002115907,3.48823028058512));
#223582=CARTESIAN_POINT('',(-45.4128910420874,41.3171891492025,3.77003198860291));
#223583=CARTESIAN_POINT('Origin',(5.49031038273072E-15,1.82930781209959E-13,
3.77003198860263));
#223584=CARTESIAN_POINT('',(-41.3171891492027,45.4128910420872,3.77003198860294));
#223585=CARTESIAN_POINT('Origin',(5.49031038273072E-15,1.82930781209959E-13,
3.77003198860263));
#223586=CARTESIAN_POINT('',(-41.3167691863812,45.4132731252658,3.77003198802751));
#223587=CARTESIAN_POINT('Origin',(5.49031038273072E-15,1.82930781209959E-13,
3.77003198860263));
#223588=CARTESIAN_POINT('',(-41.3167691865933,45.4132731255219,3.77003198860294));
#223589=CARTESIAN_POINT('Origin',(62.2224557307631,1.82930781209959E-13,
3.77003198860263));
#223590=CARTESIAN_POINT('',(-45.7656648676108,41.6348281284261,3.77003198860291));
#223591=CARTESIAN_POINT('',(34.5756856720389,-30.7048488218242,3.77003198860241));
#223592=CARTESIAN_POINT('',(-41.6348281284264,45.7656648676106,3.77003198860294));
#223593=CARTESIAN_POINT('Origin',(5.49031038273072E-15,1.82930781209959E-13,
3.77003198860263));
#223594=CARTESIAN_POINT('',(-41.3175407208296,45.4132815019359,3.77003198860294));
#223595=CARTESIAN_POINT('Origin',(5.57972911860581E-15,1.8736496251029E-13,
3.13503198860263));
#223596=CARTESIAN_POINT('Origin',(-44.378979117547,40.3862573897242,3.1350249154146));
#223597=CARTESIAN_POINT('Origin',(-40.3862573897246,44.3789791175467,3.13502491541465));
#223598=CARTESIAN_POINT('Origin',(5.57972911860581E-15,1.8736496251029E-13,
3.13503198860263));
#223599=CARTESIAN_POINT('Origin',(-45.7939781049206,41.6603666103108,3.20381846780257));
#223600=CARTESIAN_POINT('Origin',(-41.6603663369642,45.7939778018766,3.20382022872076));
#223601=CARTESIAN_POINT('Origin',(5.51210908043506E-15,1.8401175575949E-13,
3.61523028058481));
#223602=CARTESIAN_POINT('Origin',(-45.1403198695224,41.0717150501549,3.58786945047098));
#223603=CARTESIAN_POINT('Origin',(-41.0716522820265,45.1402498046834,3.58781461834337));
#223604=CARTESIAN_POINT('Origin',(5.51210908043507E-15,1.8401175575949E-13,
3.61523028058481));
#223605=CARTESIAN_POINT('Origin',(-45.0043926651443,40.9494366077763,3.5878144026647));
#223606=CARTESIAN_POINT('Origin',(-40.9493738530234,45.0043225899479,3.58786923592787));
#223607=CARTESIAN_POINT('Origin',(60.4792282238308,1.82930781209959E-13,
3.77003198860263));
#223608=CARTESIAN_POINT('',(-35.5261472678868,48.3573835402119,3.77003198860296));
#223609=CARTESIAN_POINT('',(-39.9143573409159,44.8038810887674,3.77003198860293));
#223610=CARTESIAN_POINT('Origin',(5.49031038273072E-15,1.82930781209959E-13,
3.77003198860263));
#223611=CARTESIAN_POINT('',(-40.2319965165888,45.1566551325076,3.77003198860293));
#223612=CARTESIAN_POINT('',(27.3146622010794,-29.8615093742682,3.77003198860242));
#223613=CARTESIAN_POINT('',(-40.23156461505,45.1570399302682,3.77003198902564));
#223614=CARTESIAN_POINT('Origin',(5.49031038273072E-15,1.82930781209959E-13,
3.77003198860263));
#223615=CARTESIAN_POINT('',(-35.8056376404641,48.7410849259198,3.7700319888212));
#223616=CARTESIAN_POINT('Origin',(5.49031038273072E-15,1.82930781209959E-13,
3.77003198860263));
#223617=CARTESIAN_POINT('',(-35.8051714542879,48.7414273857056,3.77003198860296));
#223618=CARTESIAN_POINT('Origin',(5.49031038273072E-15,1.82930781209959E-13,
3.77003198860263));
#223619=CARTESIAN_POINT('',(-35.5264632599794,48.3578184660151,3.77003198860296));
#223620=CARTESIAN_POINT('Origin',(5.49031038273072E-15,1.82930781209959E-13,
3.77003198860263));
#223621=CARTESIAN_POINT('',(-40.3404336838195,45.2779489569772,3.48823028058512));
#223622=CARTESIAN_POINT('',(-40.231564614563,45.1570399297216,3.77003198860294));
#223623=CARTESIAN_POINT('',(-35.9012693630581,48.8727133450222,3.48823028074838));
#223624=CARTESIAN_POINT('Origin',(5.52999282761009E-15,1.84898592019556E-13,
3.48823028058481));
#223625=CARTESIAN_POINT('',(-35.9012693628907,48.8727133447944,3.48823028058514));
#223626=CARTESIAN_POINT('Origin',(60.71525,1.85785428279622E-13,3.36123028058482));
#223627=CARTESIAN_POINT('',(-36.0301015792679,49.0510171431404,3.36123028058515));
#223628=CARTESIAN_POINT('',(-40.4880553924345,45.4410373245172,3.36123028058512));
#223629=CARTESIAN_POINT('Origin',(5.5478765747851E-15,1.85785428279622E-13,
3.36123028058482));
#223630=CARTESIAN_POINT('',(-40.5892333705625,45.5534068532511,3.36123028058513));
#223631=CARTESIAN_POINT('',(27.4203375923837,-29.9788737863602,3.36123028058461));
#223632=CARTESIAN_POINT('',(-36.1189794796885,49.1733470784087,3.36123028058515));
#223633=CARTESIAN_POINT('Origin',(5.5478765747851E-15,1.85785428279622E-13,
3.36123028058482));
#223634=CARTESIAN_POINT('',(-36.0304131198714,49.0514459419945,3.36123028058515));
#223635=CARTESIAN_POINT('Origin',(5.5478765747851E-15,1.85785428279622E-13,
3.36123028058482));
#223636=CARTESIAN_POINT('',(-36.2478178023253,49.3516463037385,3.48823028058518));
#223637=CARTESIAN_POINT('',(-40.7368493367119,45.7165002430348,3.48823028042726));
#223638=CARTESIAN_POINT('Origin',(5.52999282761008E-15,1.84898592019556E-13,
3.48823028058484));
#223639=CARTESIAN_POINT('',(-40.8457160731799,45.8374112534712,3.77003198802738));
#223640=CARTESIAN_POINT('',(-40.7368493365299,45.7165002428307,3.48823028058515));
#223641=CARTESIAN_POINT('',(-40.8452921850246,45.8377889771251,3.77003198860294));
#223642=CARTESIAN_POINT('Origin',(5.49031038273072E-15,1.82930781209959E-13,
3.77003198860263));
#223643=CARTESIAN_POINT('',(-36.3439095507838,49.4829367616346,3.77003198860296));
#223644=CARTESIAN_POINT('Origin',(5.49031038273072E-15,1.82930781209959E-13,
3.77003198860263));
#223645=CARTESIAN_POINT('',(-36.343451949995,49.4832728536532,3.77003198802754));
#223646=CARTESIAN_POINT('Origin',(5.49031038273072E-15,1.82930781209959E-13,
3.77003198860263));
#223647=CARTESIAN_POINT('',(-36.3434519501792,49.4832728539301,3.77003198860296));
#223648=CARTESIAN_POINT('Origin',(62.2224557307631,1.82930781209959E-13,
3.77003198860263));
#223649=CARTESIAN_POINT('',(-41.1629311642483,46.1905628026485,3.77003198860294));
#223650=CARTESIAN_POINT('',(28.0951675083328,-30.7283483363944,3.77003198860241));
#223651=CARTESIAN_POINT('',(-36.6229335645812,49.8669803696026,3.77003198860297));
#223652=CARTESIAN_POINT('Origin',(5.49031038273072E-15,1.82930781209959E-13,
3.77003198860263));
#223653=CARTESIAN_POINT('',(-36.3442183822966,49.4833618317452,3.77003198860296));
#223654=CARTESIAN_POINT('Origin',(5.57972911860581E-15,1.8736496251029E-13,
3.13503198860263));
#223655=CARTESIAN_POINT('Origin',(-39.9143530044121,44.803883734604,3.13502491541464));
#223656=CARTESIAN_POINT('Origin',(-35.5261507575155,48.3573798485714,3.13502491541468));
#223657=CARTESIAN_POINT('Origin',(5.57972911860581E-15,1.8736496251029E-13,
3.13503198860263));
#223658=CARTESIAN_POINT('Origin',(-41.1884198004166,46.218920921244,3.2038184678044));
#223659=CARTESIAN_POINT('Origin',(-36.6453723646293,49.8978076723462,3.20382022872021));
#223660=CARTESIAN_POINT('Origin',(5.51210908043506E-15,1.8401175575949E-13,
3.61523028058481));
#223661=CARTESIAN_POINT('Origin',(-40.5998732162083,45.5651681650775,3.58786945047012));
#223662=CARTESIAN_POINT('Origin',(-36.1282165298269,49.1861234900557,3.58781461834067));
#223663=CARTESIAN_POINT('Origin',(5.51210908043507E-15,1.8401175575949E-13,
3.61523028058481));
#223664=CARTESIAN_POINT('Origin',(-40.4774722129442,45.4293513150162,3.58781440266541));
#223665=CARTESIAN_POINT('Origin',(-36.0208162177245,49.0381593225492,3.58786923592834));
#223666=CARTESIAN_POINT('Origin',(60.4792282238308,1.82930781209959E-13,
3.77003198860263));
#223667=CARTESIAN_POINT('',(-30.2768083268883,51.8059703131947,3.77003198860298));
#223668=CARTESIAN_POINT('',(-35.0124214764587,48.7306271754176,3.77003198860296));
#223669=CARTESIAN_POINT('Origin',(5.49031038273072E-15,1.82930781209959E-13,
3.77003198860263));
#223670=CARTESIAN_POINT('',(-35.2914456628193,49.1146710209415,3.77003198860296));
#223671=CARTESIAN_POINT('',(21.1519223437074,-28.572960233785,3.77003198860243));
#223672=CARTESIAN_POINT('',(-35.2909759049636,49.1150085647355,3.77003198902554));
#223673=CARTESIAN_POINT('Origin',(5.49031038273072E-15,1.82930781209959E-13,
3.77003198860263));
#223674=CARTESIAN_POINT('',(-30.5146599057594,52.2167844417079,3.77003198882123));
#223675=CARTESIAN_POINT('Origin',(5.49031038273072E-15,1.82930781209959E-13,
3.77003198860263));
#223676=CARTESIAN_POINT('',(-30.5141604766047,52.2170762957385,3.77003198860299));
#223677=CARTESIAN_POINT('Origin',(5.49031038273072E-15,1.82930781209959E-13,
3.77003198860263));
#223678=CARTESIAN_POINT('',(-30.2770771258173,51.8064358865967,3.77003198860298));
#223679=CARTESIAN_POINT('Origin',(5.49031038273072E-15,1.82930781209959E-13,
3.77003198860263));
#223680=CARTESIAN_POINT('',(-35.3866101428262,49.2466351556013,3.48823028058515));
#223681=CARTESIAN_POINT('',(-35.2909759045365,49.1150085641411,3.77003198860296));
#223682=CARTESIAN_POINT('',(-30.5960088313997,52.3576880235604,3.4882302807484));
#223683=CARTESIAN_POINT('Origin',(5.52999282761009E-15,1.84898592019556E-13,
3.48823028058481));
#223684=CARTESIAN_POINT('',(-30.5960088312571,52.3576880233163,3.48823028058517));
#223685=CARTESIAN_POINT('Origin',(60.71525,1.85785428279622E-13,3.36123028058482));
#223686=CARTESIAN_POINT('',(-30.7054974692372,52.5484816883959,3.36123028058518));
#223687=CARTESIAN_POINT('',(-35.5163757878398,49.4242607783461,3.36123028058515));
#223688=CARTESIAN_POINT('Origin',(5.5478765747851E-15,1.85785428279622E-13,
3.36123028058482));
#223689=CARTESIAN_POINT('',(-35.6052536882604,49.5465907136145,3.36123028058516));
#223690=CARTESIAN_POINT('',(21.2334658618526,-28.6851952578917,3.36123028058461));
#223691=CARTESIAN_POINT('',(-30.7811015270746,52.6794317578288,3.36123028058518));
#223692=CARTESIAN_POINT('Origin',(5.5478765747851E-15,1.85785428279622E-13,
3.36123028058482));
#223693=CARTESIAN_POINT('',(-30.7057624815034,52.5489407031057,3.36123028058518));
#223694=CARTESIAN_POINT('Origin',(5.5478765747851E-15,1.85785428279622E-13,
3.36123028058482));
#223695=CARTESIAN_POINT('',(-30.8905967158739,52.8702215132216,3.4882302805852));
#223696=CARTESIAN_POINT('',(-35.7350130972987,49.7242207308396,3.48823028042729));
#223697=CARTESIAN_POINT('Origin',(5.52999282761008E-15,1.84898592019556E-13,
3.48823028058484));
#223698=CARTESIAN_POINT('',(-35.8306448082804,49.8558490507736,3.77003198802741));
#223699=CARTESIAN_POINT('',(-35.7350130971392,49.7242207306175,3.48823028058518));
#223700=CARTESIAN_POINT('',(-35.8301837593557,49.8561803968403,3.77003198860297));
#223701=CARTESIAN_POINT('Origin',(5.49031038273072E-15,1.82930781209959E-13,
3.77003198860263));
#223702=CARTESIAN_POINT('',(-30.9724384738745,53.0108370710513,3.77003198860299));
#223703=CARTESIAN_POINT('Origin',(5.49031038273072E-15,1.82930781209959E-13,
3.77003198860263));
#223704=CARTESIAN_POINT('',(-30.9719482486884,53.0111234896154,3.77003198802757));
#223705=CARTESIAN_POINT('Origin',(5.49031038273072E-15,1.82930781209959E-13,
3.77003198860263));
#223706=CARTESIAN_POINT('',(-30.9719482488427,53.01112348991,3.77003198860299));
#223707=CARTESIAN_POINT('Origin',(62.2224557307631,1.82930781209959E-13,
3.77003198860263));
#223708=CARTESIAN_POINT('',(-36.1092077731531,50.2402240048083,3.77003198860297));
#223709=CARTESIAN_POINT('',(21.7541926348216,-29.4019141737115,3.77003198860242));
#223710=CARTESIAN_POINT('',(-31.2097904767608,53.4219427993287,3.77003198860299));
#223711=CARTESIAN_POINT('Origin',(5.49031038273072E-15,1.82930781209959E-13,
3.77003198860263));
#223712=CARTESIAN_POINT('',(-30.9727011816504,53.0112920942668,3.77003198860299));
#223713=CARTESIAN_POINT('Origin',(5.57972911860581E-15,1.8736496251029E-13,
3.13503198860263));
#223714=CARTESIAN_POINT('Origin',(-35.0124168871455,48.7306293534719,3.13502491541467));
#223715=CARTESIAN_POINT('Origin',(-30.2768121832819,51.8059670065428,3.13502491541469));
#223716=CARTESIAN_POINT('Origin',(5.57972911860581E-15,1.8736496251029E-13,
3.13503198860263));
#223717=CARTESIAN_POINT('Origin',(-36.1315925493535,50.2710910626265,3.20381846780134));
#223718=CARTESIAN_POINT('Origin',(-31.2288840241293,53.4549467201713,3.20382022872142));
#223719=CARTESIAN_POINT('Origin',(5.51210908043506E-15,1.8401175575949E-13,
3.61523028058481));
#223720=CARTESIAN_POINT('Origin',(-35.6146058558677,49.5593997624595,3.58786945046899));
#223721=CARTESIAN_POINT('Origin',(-30.7889524770103,52.6931037136122,3.58781461834046));
#223722=CARTESIAN_POINT('Origin',(5.51210908043507E-15,1.8401175575949E-13,
3.61523028058481));
#223723=CARTESIAN_POINT('Origin',(-35.5070721047356,49.411532542534,3.58781440266494));
#223724=CARTESIAN_POINT('Origin',(-30.6976069821026,52.5347237197209,3.58786923593167));
#223725=CARTESIAN_POINT('Origin',(60.4792282238308,1.82930781209959E-13,
3.77003198860263));
#223726=CARTESIAN_POINT('',(-24.695750338031,54.6869600343298,3.770031988603));
#223727=CARTESIAN_POINT('',(-29.7268821954852,52.1234703131947,3.77003198860298));
#223728=CARTESIAN_POINT('Origin',(5.49031038273072E-15,1.82930781209959E-13,
3.77003198860263));
#223729=CARTESIAN_POINT('',(-29.9642343451581,52.5345762957644,3.77003198860299));
#223730=CARTESIAN_POINT('',(15.3947701216595,-26.0295240215571,3.77003198860244));
#223731=CARTESIAN_POINT('',(-29.9637318777512,52.5348628873916,3.77003198902577));
#223732=CARTESIAN_POINT('Origin',(5.49031038273072E-15,1.82930781209959E-13,
3.77003198860263));
#223733=CARTESIAN_POINT('',(-24.8893571715241,55.120385940088,3.77003198882125));
#223734=CARTESIAN_POINT('Origin',(5.49031038273072E-15,1.82930781209959E-13,
3.77003198860263));
#223735=CARTESIAN_POINT('',(-24.8888299712412,55.1206239907497,3.77003198860301));
#223736=CARTESIAN_POINT('Origin',(5.49031038273072E-15,1.82930781209959E-13,
3.77003198860263));
#223737=CARTESIAN_POINT('',(-24.6959689987791,54.687451154411,3.770031988603));
#223738=CARTESIAN_POINT('Origin',(5.49031038273072E-15,1.82930781209959E-13,
3.77003198860263));
#223739=CARTESIAN_POINT('',(-30.0450834959839,52.6757649139396,3.48823028058517));
#223740=CARTESIAN_POINT('',(-29.9637318773884,52.5348628867555,3.77003198860299));
#223741=CARTESIAN_POINT('',(-24.9555320243581,55.2690209155618,3.48823028074843));
#223742=CARTESIAN_POINT('Origin',(5.52999282761009E-15,1.84898592019556E-13,
3.48823028058481));
#223743=CARTESIAN_POINT('',(-24.9555320242418,55.2690209153041,3.48823028058519));
#223744=CARTESIAN_POINT('Origin',(60.71525,1.85785428279622E-13,3.36123028058482));
#223745=CARTESIAN_POINT('',(-25.044477503395,55.4702140717967,3.3612302805852));
#223746=CARTESIAN_POINT('',(-30.155571337834,52.865981688396,3.36123028058518));
#223747=CARTESIAN_POINT('Origin',(5.5478765747851E-15,1.85785428279622E-13,
3.36123028058482));
#223748=CARTESIAN_POINT('',(-30.2311753956715,52.9969317578288,3.36123028058518));
#223749=CARTESIAN_POINT('',(15.4537755657018,-26.1317244485615,3.36123028058463));
#223750=CARTESIAN_POINT('',(-25.1059793847704,55.6083495590302,3.3612302805852));
#223751=CARTESIAN_POINT('Origin',(5.5478765747851E-15,1.85785428279622E-13,
3.36123028058482));
#223752=CARTESIAN_POINT('',(-25.0446930837941,55.4706982733008,3.3612302805852));
#223753=CARTESIAN_POINT('Origin',(5.5478765747851E-15,1.85785428279622E-13,
3.36123028058482));
#223754=CARTESIAN_POINT('',(-25.1949317875303,55.8095395120008,3.48823028058522));
#223755=CARTESIAN_POINT('',(-30.3416565763594,53.1871522508551,3.48823028042731));
#223756=CARTESIAN_POINT('Origin',(5.52999282761008E-15,1.84898592019556E-13,
3.48823028058484));
#223757=CARTESIAN_POINT('',(-30.423005500817,53.3280557328686,3.77003198802744));
#223758=CARTESIAN_POINT('',(-30.3416565762239,53.1871522506175,3.4882302805852));
#223759=CARTESIAN_POINT('',(-30.4225123424714,53.3283370710513,3.77003198860299));
#223760=CARTESIAN_POINT('Origin',(5.49031038273072E-15,1.82930781209959E-13,
3.77003198860263));
#223761=CARTESIAN_POINT('',(-25.2616268796459,55.9579395562867,3.77003198860301));
#223762=CARTESIAN_POINT('Origin',(5.49031038273072E-15,1.82930781209959E-13,
3.77003198860263));
#223763=CARTESIAN_POINT('',(-25.2611094010724,55.9581731633346,3.77003198802759));
#223764=CARTESIAN_POINT('Origin',(5.49031038273072E-15,1.82930781209959E-13,
3.77003198860263));
#223765=CARTESIAN_POINT('',(-25.261109401195,55.9581731636437,3.77003198860301));
#223766=CARTESIAN_POINT('Origin',(62.2224557307631,1.82930781209959E-13,
3.77003198860263));
#223767=CARTESIAN_POINT('',(-30.6598643453577,53.7394427993287,3.77003198860299));
#223768=CARTESIAN_POINT('',(15.8305769983926,-26.7843636743467,3.77003198860244));
#223769=CARTESIAN_POINT('',(-25.4547063934086,56.3916032444851,3.77003198860301));
#223770=CARTESIAN_POINT('Origin',(5.49031038273072E-15,1.82930781209959E-13,
3.77003198860263));
#223771=CARTESIAN_POINT('',(-25.2618405854037,55.9584195472775,3.77003198860301));
#223772=CARTESIAN_POINT('Origin',(5.57972911860581E-15,1.8736496251029E-13,
3.13503198860263));
#223773=CARTESIAN_POINT('Origin',(-29.7268774036442,52.1234719996035,3.13502491541469));
#223774=CARTESIAN_POINT('Origin',(-24.6957545189381,54.6869571488951,3.13502491541473));
#223775=CARTESIAN_POINT('Origin',(5.57972911860581E-15,1.8736496251029E-13,
3.13503198860263));
#223776=CARTESIAN_POINT('Origin',(-30.6789000092897,53.7724806104335,3.20381846780308));
#223777=CARTESIAN_POINT('Origin',(-25.4702454952008,56.4264221855609,3.2038202287226));
#223778=CARTESIAN_POINT('Origin',(5.51210908043506E-15,1.8401175575949E-13,
3.61523028058481));
#223779=CARTESIAN_POINT('Origin',(-30.2391374209354,53.010648205074,3.5878694504651));
#223780=CARTESIAN_POINT('Origin',(-25.1123582178531,55.6227672661415,3.58781461834012));
#223781=CARTESIAN_POINT('Origin',(5.51210908043507E-15,1.8401175575949E-13,
3.61523028058481));
#223782=CARTESIAN_POINT('Origin',(-30.1476490842064,52.8523506794932,3.58781440266171));
#223783=CARTESIAN_POINT('Origin',(-25.0380683404989,55.4557066902178,3.58786923593092));
#223784=CARTESIAN_POINT('Origin',(60.4792282238308,1.82930781209959E-13,
3.77003198860263));
#223785=CARTESIAN_POINT('',(-18.8441205405522,56.9687879773467,3.77003198860303));
#223786=CARTESIAN_POINT('',(-24.1156489724279,54.9452378026829,3.77003198860301));
#223787=CARTESIAN_POINT('Origin',(5.49031038273072E-15,1.82930781209959E-13,
3.77003198860263));
#223788=CARTESIAN_POINT('',(-24.3087286055922,55.378901759124,3.77003198860301));
#223789=CARTESIAN_POINT('',(10.2954134679533,-22.3432738675265,3.77003198860247));
#223790=CARTESIAN_POINT('',(-24.3081989337718,55.3791342586262,3.77003198902562));
#223791=CARTESIAN_POINT('Origin',(5.49031038273072E-15,1.82930781209959E-13,
3.77003198860263));
#223792=CARTESIAN_POINT('',(-18.9913614316847,57.4200769554262,3.77003198882127));
#223793=CARTESIAN_POINT('Origin',(5.49031038273072E-15,1.82930781209959E-13,
3.77003198860263));
#223794=CARTESIAN_POINT('',(-18.9908122363903,57.4202585945861,3.77003198860302));
#223795=CARTESIAN_POINT('Origin',(5.49031038273072E-15,1.82930781209959E-13,
3.77003198860263));
#223796=CARTESIAN_POINT('',(-18.8442866674264,56.9692992632927,3.77003198860302));
#223797=CARTESIAN_POINT('Origin',(5.49031038273072E-15,1.82930781209959E-13,
3.77003198860263));
#223798=CARTESIAN_POINT('',(-24.3743766270217,55.5277679687684,3.4882302805852));
#223799=CARTESIAN_POINT('',(-24.3081989334776,55.3791342579559,3.77003198860301));
#223800=CARTESIAN_POINT('',(-19.0416371861768,57.5748148486261,3.48823028074845));
#223801=CARTESIAN_POINT('Origin',(5.52999282761009E-15,1.84898592019556E-13,
3.48823028058481));
#223802=CARTESIAN_POINT('',(-19.041637186088,57.5748148483577,3.48823028058521));
#223803=CARTESIAN_POINT('Origin',(60.71525,1.85785428279622E-13,3.36123028058482));
#223804=CARTESIAN_POINT('',(-19.1090650011318,57.7842031819384,3.36123028058522));
#223805=CARTESIAN_POINT('',(-24.464376137792,55.7284918401499,3.3612302805852));
#223806=CARTESIAN_POINT('Origin',(5.5478765747851E-15,1.85785428279622E-13,
3.36123028058482));
#223807=CARTESIAN_POINT('',(-24.5258780191674,55.8666273273834,3.36123028058521));
#223808=CARTESIAN_POINT('',(10.3344596589369,-22.4309730483566,3.36123028058466));
#223809=CARTESIAN_POINT('',(-19.1557908785628,57.9280106456677,3.36123028058522));
#223810=CARTESIAN_POINT('Origin',(5.5478765747851E-15,1.85785428279622E-13,
3.36123028058482));
#223811=CARTESIAN_POINT('',(-19.1092287877198,57.7847072652237,3.36123028058521));
#223812=CARTESIAN_POINT('Origin',(5.5478765747851E-15,1.85785428279622E-13,
3.36123028058482));
#223813=CARTESIAN_POINT('',(-19.2232259141442,58.1373965169894,3.48823028058524));
#223814=CARTESIAN_POINT('',(-24.6158705165696,56.0673542006831,3.48823028042733));
#223815=CARTESIAN_POINT('Origin',(5.52999282761008E-15,1.84898592019556E-13,
3.48823028058484));
#223816=CARTESIAN_POINT('',(-24.6820453786634,56.2159890767412,3.77003198802746));
#223817=CARTESIAN_POINT('',(-24.6158705164596,56.0673542004326,3.48823028058523));
#223818=CARTESIAN_POINT('',(-24.6815255140429,56.2162173246398,3.77003198860301));
#223819=CARTESIAN_POINT('Origin',(5.49031038273072E-15,1.82930781209959E-13,
3.77003198860263));
#223820=CARTESIAN_POINT('',(-19.2740436149887,58.2919551457918,3.77003198860303));
#223821=CARTESIAN_POINT('Origin',(5.49031038273072E-15,1.82930781209959E-13,
3.77003198860263));
#223822=CARTESIAN_POINT('',(-19.2735045526312,58.2921333818758,3.77003198802761));
#223823=CARTESIAN_POINT('Origin',(5.49031038273072E-15,1.82930781209959E-13,
3.77003198860263));
#223824=CARTESIAN_POINT('',(-19.2735045527209,58.292133382196,3.77003198860303));
#223825=CARTESIAN_POINT('Origin',(62.2224557307631,1.82930781209959E-13,
3.77003198860263));
#223826=CARTESIAN_POINT('',(-24.8746050278055,56.6498810128383,3.77003198860302));
#223827=CARTESIAN_POINT('',(10.5838037820519,-22.9910091182298,3.77003198860247));
#223828=CARTESIAN_POINT('',(-19.4207352200703,58.7434254837933,3.77003198860304));
#223829=CARTESIAN_POINT('Origin',(5.49031038273072E-15,1.82930781209959E-13,
3.77003198860263));
#223830=CARTESIAN_POINT('',(-19.2742059773234,58.2924548456762,3.77003198860303));
#223831=CARTESIAN_POINT('Origin',(5.57972911860581E-15,1.8736496251029E-13,
3.13503198860263));
#223832=CARTESIAN_POINT('Origin',(-24.1156440305593,54.9452389789697,3.1350249154147));
#223833=CARTESIAN_POINT('Origin',(-18.844125000166,56.9687855447425,3.13502491541473));
#223834=CARTESIAN_POINT('Origin',(5.57972911860581E-15,1.8736496251029E-13,
3.13503198860263));
#223835=CARTESIAN_POINT('Origin',(-24.890083020755,56.6847276080529,3.20381846779927));
#223836=CARTESIAN_POINT('Origin',(-19.4325496266324,58.7796779614993,3.20382022872482));
#223837=CARTESIAN_POINT('Origin',(5.51210908043506E-15,1.8401175575949E-13,
3.61523028058481));
#223838=CARTESIAN_POINT('Origin',(-24.5323626684706,55.8811008927581,3.58786945047008));
#223839=CARTESIAN_POINT('Origin',(-19.160627706962,57.9430161406896,3.58781461834175));
#223840=CARTESIAN_POINT('Origin',(5.51210908043507E-15,1.8401175575949E-13,
3.61523028058481));
#223841=CARTESIAN_POINT('Origin',(-24.4579221115101,55.7141074023466,3.5878144026663));
#223842=CARTESIAN_POINT('Origin',(-19.1042073826016,57.769105333365,3.58786923592921));
#223843=CARTESIAN_POINT('Origin',(60.4792282238308,1.82930781209959E-13,
3.77003198860263));
#223844=CARTESIAN_POINT('',(-12.7860306150453,58.6264539577985,3.77003198860304));
#223845=CARTESIAN_POINT('',(-18.2401996527048,57.1650137687748,3.77003198860303));
#223846=CARTESIAN_POINT('Origin',(5.49031038273072E-15,1.82930781209959E-13,
3.77003198860263));
#223847=CARTESIAN_POINT('',(-18.386891348495,57.6164843860304,3.77003198860303));
#223848=CARTESIAN_POINT('',(6.07721283595923,-17.6762863142852,3.77003198860251));
#223849=CARTESIAN_POINT('',(-18.3863402754567,57.616660246095,3.77003198902593));
#223850=CARTESIAN_POINT('Origin',(5.49031038273072E-15,1.82930781209959E-13,
3.77003198860263));
#223851=CARTESIAN_POINT('',(-12.8852923618019,59.0906615917172,3.77003198882128));
#223852=CARTESIAN_POINT('Origin',(5.49031038273072E-15,1.82930781209959E-13,
3.77003198860263));
#223853=CARTESIAN_POINT('',(-12.8847271885945,59.0907848292986,3.77003198860304));
#223854=CARTESIAN_POINT('Origin',(5.49031038273072E-15,1.82930781209959E-13,
3.77003198860263));
#223855=CARTESIAN_POINT('',(-12.786142387925,58.6269798078534,3.77003198860304));
#223856=CARTESIAN_POINT('Origin',(5.49031038273072E-15,1.82930781209959E-13,
3.77003198860263));
#223857=CARTESIAN_POINT('',(-18.4366189870675,57.7713971777988,3.48823028058521));
#223858=CARTESIAN_POINT('',(-18.386340275234,57.6166602453972,3.77003198860303));
#223859=CARTESIAN_POINT('',(-12.919118186265,59.2498070619043,3.48823028074846));
#223860=CARTESIAN_POINT('Origin',(5.52999282761009E-15,1.84898592019556E-13,
3.48823028058481));
#223861=CARTESIAN_POINT('',(-12.9191181862048,59.2498070616281,3.48823028058522));
#223862=CARTESIAN_POINT('Origin',(60.71525,1.85785428279622E-13,3.36123028058482));
#223863=CARTESIAN_POINT('',(-12.9642895838873,59.4650964698968,3.36123028058523));
#223864=CARTESIAN_POINT('',(-18.5051441132844,57.9804289733665,3.36123028058522));
#223865=CARTESIAN_POINT('Origin',(5.5478765747851E-15,1.85785428279622E-13,
3.36123028058482));
#223866=CARTESIAN_POINT('',(-18.5518699907153,58.1242364370958,3.36123028058522));
#223867=CARTESIAN_POINT('',(6.0997509100621,-17.7456513739113,3.36123028058469));
#223868=CARTESIAN_POINT('',(-12.9957275188826,59.6130003254556,3.36123028058523));
#223869=CARTESIAN_POINT('Origin',(5.5478765747851E-15,1.85785428279622E-13,
3.36123028058482));
#223870=CARTESIAN_POINT('',(-12.964399782184,59.4656149121215,3.36123028058523));
#223871=CARTESIAN_POINT('Origin',(5.5478765747851E-15,1.85785428279622E-13,
3.36123028058482));
#223872=CARTESIAN_POINT('',(-13.0409063549241,59.8282880397056,3.48823028058526));
#223873=CARTESIAN_POINT('',(-18.6203878281982,58.3332704850402,3.48823028042735));
#223874=CARTESIAN_POINT('Origin',(5.52999282761008E-15,1.84898592019556E-13,
3.48823028058484));
#223875=CARTESIAN_POINT('',(-18.6706636022911,58.488008280337,3.77003198802748));
#223876=CARTESIAN_POINT('',(-18.620387828115,58.3332704847797,3.48823028058524));
#223877=CARTESIAN_POINT('',(-18.6701227271413,58.4881809372198,3.77003198860304));
#223878=CARTESIAN_POINT('Origin',(5.49031038273072E-15,1.82930781209959E-13,
3.77003198860263));
#223879=CARTESIAN_POINT('',(-13.0752898951327,59.9873118763437,3.77003198860305));
#223880=CARTESIAN_POINT('Origin',(5.49031038273072E-15,1.82930781209959E-13,
3.77003198860263));
#223881=CARTESIAN_POINT('',(-13.0747351550713,59.987432788672,3.77003198802762));
#223882=CARTESIAN_POINT('Origin',(5.49031038273072E-15,1.82930781209959E-13,
3.77003198860263));
#223883=CARTESIAN_POINT('',(-13.074735155127,59.9874327889998,3.77003198860305));
#223884=CARTESIAN_POINT('Origin',(62.2224557307631,1.82930781209959E-13,
3.77003198860263));
#223885=CARTESIAN_POINT('',(-18.8168143322229,58.9396512752214,3.77003198860304));
#223886=CARTESIAN_POINT('',(6.24367625034032,-18.1886080242679,3.7700319886025));
#223887=CARTESIAN_POINT('',(-13.1739864076109,60.451642460649,3.77003198860305));
#223888=CARTESIAN_POINT('Origin',(5.49031038273072E-15,1.82930781209959E-13,
3.77003198860263));
#223889=CARTESIAN_POINT('',(-13.0753991351685,59.9878258103052,3.77003198860304));
#223890=CARTESIAN_POINT('Origin',(5.57972911860581E-15,1.8736496251029E-13,
3.13503198860263));
#223891=CARTESIAN_POINT('Origin',(-18.2401946149527,57.1650144220518,3.13502491541473));
#223892=CARTESIAN_POINT('Origin',(-12.7860353045051,58.6264520046769,3.13502491541478));
#223893=CARTESIAN_POINT('Origin',(5.57972911860581E-15,1.8736496251029E-13,
3.13503198860263));
#223894=CARTESIAN_POINT('Origin',(-18.8285650740578,58.9759248679607,3.20381846780158));
#223895=CARTESIAN_POINT('Origin',(-13.1819466778329,60.48893128525,3.20382022872197));
#223896=CARTESIAN_POINT('Origin',(5.51210908043506E-15,1.8401175575949E-13,
3.61523028058481));
#223897=CARTESIAN_POINT('Origin',(-18.5568062168843,58.1393085451906,3.58786945047204));
#223898=CARTESIAN_POINT('Origin',(-12.9989693492947,59.6284292050461,3.58781461834054));
#223899=CARTESIAN_POINT('Origin',(5.51210908043507E-15,1.8401175575949E-13,
3.61523028058481));
#223900=CARTESIAN_POINT('Origin',(-18.5002290260139,57.9654487055657,3.58781440266093));
#223901=CARTESIAN_POINT('Origin',(-12.961036730812,59.4495735695173,3.58786923592967));
#223902=CARTESIAN_POINT('Origin',(60.4792282238308,1.82930781209959E-13,
3.77003198860263));
#223903=CARTESIAN_POINT('',(-6.58785426247116,59.6417962403144,3.77003198860304));
#223904=CARTESIAN_POINT('',(-12.1649068885794,58.7584778814678,3.77003198860304));
#223905=CARTESIAN_POINT('Origin',(5.49031038273072E-15,1.82930781209959E-13,
3.77003198860263));
#223906=CARTESIAN_POINT('',(-12.2636034620792,59.222808752979,3.77003198860304));
#223907=CARTESIAN_POINT('',(2.92491386234308,-12.2335471699534,3.77003198860254));
#223908=CARTESIAN_POINT('',(-12.2630370254944,59.222926046846,3.77003198902597));
#223909=CARTESIAN_POINT('Origin',(5.49031038273072E-15,1.82930781209959E-13,
3.77003198860263));
#223910=CARTESIAN_POINT('',(-6.63804933238239,60.1138365740934,3.77003198882129));
#223911=CARTESIAN_POINT('Origin',(5.49031038273072E-15,1.82930781209959E-13,
3.77003198860263));
#223912=CARTESIAN_POINT('',(-6.63747437341798,60.1139000598795,3.77003198860305));
#223913=CARTESIAN_POINT('Origin',(5.49031038273072E-15,1.82930781209959E-13,
3.77003198860263));
#223914=CARTESIAN_POINT('',(-6.58791045674911,59.6423308931551,3.77003198860304));
#223915=CARTESIAN_POINT('Origin',(5.49031038273072E-15,1.82930781209959E-13,
3.77003198860263));
#223916=CARTESIAN_POINT('',(-12.2968658913805,59.3820708699072,3.48823028058522));
#223917=CARTESIAN_POINT('',(-12.2630370253459,59.2229260461286,3.77003198860304));
#223918=CARTESIAN_POINT('',(-6.65505462400518,60.2756459901931,3.48823028074846));
#223919=CARTESIAN_POINT('Origin',(5.52999282761009E-15,1.84898592019556E-13,
3.48823028058481));
#223920=CARTESIAN_POINT('',(-6.65505462397415,60.2756459899121,3.48823028058523));
#223921=CARTESIAN_POINT('Origin',(60.71525,1.85785428279622E-13,3.36123028058482));
#223922=CARTESIAN_POINT('',(-6.67747469700966,60.4944777170595,3.36123028058524));
#223923=CARTESIAN_POINT('',(-12.3431658574213,59.5971203935661,3.36123028058523));
#223924=CARTESIAN_POINT('Origin',(5.5478765747851E-15,1.85785428279622E-13,
3.36123028058482));
#223925=CARTESIAN_POINT('',(-12.3746037924166,59.7450242491249,3.36123028058523));
#223926=CARTESIAN_POINT('',(2.93511643966565,-12.2815465224194,3.36123028058473));
#223927=CARTESIAN_POINT('',(-6.69328024897475,60.6448574988556,3.36123028058524));
#223928=CARTESIAN_POINT('Origin',(5.5478765747851E-15,1.85785428279622E-13,
3.36123028058482));
#223929=CARTESIAN_POINT('',(-6.67753009965953,60.4950048380621,3.36123028058524));
#223930=CARTESIAN_POINT('Origin',(5.5478765747851E-15,1.85785428279622E-13,
3.36123028058482));
#223931=CARTESIAN_POINT('',(-6.7157078966943,60.8636883187846,3.48823028058527));
#223932=CARTESIAN_POINT('',(-12.4208962742143,59.9600752509416,3.48823028042737));
#223933=CARTESIAN_POINT('Origin',(5.52999282761008E-15,1.84898592019556E-13,
3.48823028058484));
#223934=CARTESIAN_POINT('',(-12.4547221284046,60.1192206258108,3.77003198802749));
#223935=CARTESIAN_POINT('',(-12.4208962741589,59.9600752506738,3.48823028058526));
#223936=CARTESIAN_POINT('',(-12.4541661686668,60.119335800013,3.77003198860305));
#223937=CARTESIAN_POINT('Origin',(5.49031038273072E-15,1.82930781209959E-13,
3.77003198860263));
#223938=CARTESIAN_POINT('',(-6.73328056300539,61.0254350648264,3.77003198860305));
#223939=CARTESIAN_POINT('Origin',(5.49031038273072E-15,1.82930781209959E-13,
3.77003198860263));
#223940=CARTESIAN_POINT('',(-6.73271622308818,61.0254973286581,3.77003198802763));
#223941=CARTESIAN_POINT('Origin',(5.49031038273072E-15,1.82930781209959E-13,
3.77003198860263));
#223942=CARTESIAN_POINT('',(-6.73271622310929,61.02549732899,3.77003198860305));
#223943=CARTESIAN_POINT('Origin',(62.2224557307631,1.82930781209959E-13,
3.77003198860263));
#223944=CARTESIAN_POINT('',(-12.5528626811449,60.5836663843183,3.77003198860305));
#223945=CARTESIAN_POINT('',(3.00026883051142,-12.588064422097,3.77003198860254));
#223946=CARTESIAN_POINT('',(-6.78290064323581,61.4975385923864,3.77003198860306));
#223947=CARTESIAN_POINT('Origin',(5.49031038273072E-15,1.82930781209959E-13,
3.77003198860263));
#223948=CARTESIAN_POINT('',(-6.73333548388561,61.025957602097,3.77003198860305));
#223949=CARTESIAN_POINT('Origin',(5.57972911860581E-15,1.8736496251029E-13,
3.13503198860263));
#223950=CARTESIAN_POINT('Origin',(-12.1649018101387,58.7584780045775,3.13502491541476));
#223951=CARTESIAN_POINT('Origin',(-6.58785913039843,59.6417947880743,3.13502491541476));
#223952=CARTESIAN_POINT('Origin',(5.57972911860581E-15,1.8736496251029E-13,
3.13503198860263));
#223953=CARTESIAN_POINT('Origin',(-12.5607574282781,60.6209695535074,3.20381846780062));
#223954=CARTESIAN_POINT('Origin',(-6.78691956273312,61.5354552197182,3.20382022872275));
#223955=CARTESIAN_POINT('Origin',(5.51210908043506E-15,1.8401175575949E-13,
3.61523028058481));
#223956=CARTESIAN_POINT('Origin',(-12.3779375131253,59.7605297667728,3.58786945046749));
#223957=CARTESIAN_POINT('Origin',(-6.6948915632271,60.6605407209801,3.58781461834101));
#223958=CARTESIAN_POINT('Origin',(5.51210908043507E-15,1.8401175575949E-13,
3.61523028058481));
#223959=CARTESIAN_POINT('Origin',(-12.3398435598879,59.5817084227243,3.58781440266877));
#223960=CARTESIAN_POINT('Origin',(-6.67586224832368,60.4786998370192,3.58786923592871));
#223961=CARTESIAN_POINT('Origin',(60.4792282238308,1.82930781209959E-13,
3.77003198860263));
#223962=CARTESIAN_POINT('',(-0.317500000000204,60.0036905223732,3.77003198860305));
#223963=CARTESIAN_POINT('',(-5.9563328589123,59.7081718144894,3.77003198860304));
#223964=CARTESIAN_POINT('Origin',(5.49031038273072E-15,1.82930781209959E-13,
3.77003198860263));
#223965=CARTESIAN_POINT('',(-6.00595296980892,60.1802756340604,3.77003198860304));
#223966=CARTESIAN_POINT('',(0.9765688230087,-6.25398151259745,3.77003198860258));
#223967=CARTESIAN_POINT('',(-6.00537737567533,60.1803330766335,3.77003198902593));
#223968=CARTESIAN_POINT('Origin',(5.49031038273072E-15,1.82930781209959E-13,
3.77003198860263));
#223969=CARTESIAN_POINT('',(-0.3180784453762,60.4783917833348,3.77003198882129));
#223970=CARTESIAN_POINT('Origin',(5.49031038273072E-15,1.82930781209959E-13,
3.77003198860263));
#223971=CARTESIAN_POINT('',(-0.31750000002549,60.4783948217622,3.77003198860305));
#223972=CARTESIAN_POINT('Origin',(5.49031038273072E-15,1.82930781209959E-13,
3.77003198860263));
#223973=CARTESIAN_POINT('',(-0.317500000000204,60.0042281202312,3.77003198860305));
#223974=CARTESIAN_POINT('Origin',(5.49031038273072E-15,1.82930781209959E-13,
3.77003198860263));
#223975=CARTESIAN_POINT('',(-6.02238575970296,60.3421421670677,3.48823028058523));
#223976=CARTESIAN_POINT('',(-6.0053773756026,60.1803330759047,3.77003198860305));
#223977=CARTESIAN_POINT('',(-0.318076890625054,60.6410923275234,3.48823028074847));
#223978=CARTESIAN_POINT('Origin',(5.52999282761009E-15,1.84898592019556E-13,
3.48823028058481));
#223979=CARTESIAN_POINT('',(-0.318076890623573,60.6410923272407,3.48823028058523));
#223980=CARTESIAN_POINT('Origin',(60.71525,1.85785428279622E-13,3.36123028058482));
#223981=CARTESIAN_POINT('',(-0.317500000000207,60.8610688070709,3.36123028058524));
#223982=CARTESIAN_POINT('',(-6.04595329345081,60.5608532912345,3.36123028058524));
#223983=CARTESIAN_POINT('Origin',(5.5478765747851E-15,1.85785428279622E-13,
3.36123028058482));
#223984=CARTESIAN_POINT('',(-6.0617588454159,60.7112330730305,3.36123028058524));
#223985=CARTESIAN_POINT('',(0.97914764405288,-6.27851735587403,3.36123028058477));
#223986=CARTESIAN_POINT('',(-0.317500000000208,61.0122769227458,3.36123028058524));
#223987=CARTESIAN_POINT('Origin',(5.5478765747851E-15,1.85785428279622E-13,
3.36123028058482));
#223988=CARTESIAN_POINT('',(-0.317500000000207,60.8615988316033,3.36123028058524));
#223989=CARTESIAN_POINT('Origin',(5.5478765747851E-15,1.85785428279622E-13,
3.36123028058482));
#223990=CARTESIAN_POINT('',(-0.316930737396123,61.2322532920974,3.48823028058527));
#223991=CARTESIAN_POINT('',(-6.08531878141059,60.9299448849413,3.48823028042737));
#223992=CARTESIAN_POINT('Origin',(5.52999282761008E-15,1.84898592019556E-13,
3.48823028058484));
#223993=CARTESIAN_POINT('',(-6.10232411256108,61.0917542093525,3.7700319880275));
#223994=CARTESIAN_POINT('',(-6.08531878138341,60.9299448846692,3.48823028058527));
#223995=CARTESIAN_POINT('',(-6.10175915944654,61.0918106390013,3.77003198860305));
#223996=CARTESIAN_POINT('Origin',(5.49031038273072E-15,1.82930781209959E-13,
3.77003198860263));
#223997=CARTESIAN_POINT('',(-0.317500000000209,61.3949508163455,3.77003198860305));
#223998=CARTESIAN_POINT('Origin',(5.49031038273072E-15,1.82930781209959E-13,
3.77003198860263));
#223999=CARTESIAN_POINT('',(-0.316932243253465,61.3949537495052,3.77003198802764));
#224000=CARTESIAN_POINT('Origin',(5.49031038273072E-15,1.82930781209959E-13,
3.77003198860263));
#224001=CARTESIAN_POINT('',(-0.316932243239769,61.3949537498375,3.77003198860305));
#224002=CARTESIAN_POINT('Origin',(62.2224557307631,1.82930781209959E-13,
3.77003198860263));
#224003=CARTESIAN_POINT('',(-6.15137923967696,61.5639141665613,3.77003198860306));
#224004=CARTESIAN_POINT('',(0.995615674755347,-6.43520020182062,3.77003198860258));
#224005=CARTESIAN_POINT('',(-0.317500000000211,61.8696548221182,3.77003198860306));
#224006=CARTESIAN_POINT('Origin',(5.49031038273072E-15,1.82930781209959E-13,
3.77003198860263));
#224007=CARTESIAN_POINT('',(-0.317500000000209,61.3954762318975,3.77003198860305));
#224008=CARTESIAN_POINT('Origin',(5.57972911860581E-15,1.8736496251029E-13,
3.13503198860263));
#224009=CARTESIAN_POINT('Origin',(-5.95632779542334,59.7081714060832,3.13502491541474));
#224010=CARTESIAN_POINT('Origin',(-0.317504993060902,60.0036895869256,3.13502491541474));
#224011=CARTESIAN_POINT('Origin',(5.57972911860581E-15,1.8736496251029E-13,
3.13503198860263));
#224012=CARTESIAN_POINT('Origin',(-6.15533149561,61.6018382108726,3.20381846780166));
#224013=CARTESIAN_POINT('Origin',(-0.317533536648822,61.9077838296764,3.20382022872102));
#224014=CARTESIAN_POINT('Origin',(5.51210908043506E-15,1.8401175575949E-13,
3.61523028058481));
#224015=CARTESIAN_POINT('Origin',(-6.06345353572148,60.72700211853,3.58786945047319));
#224016=CARTESIAN_POINT('Origin',(-0.317463144196723,61.0280426587414,3.58781461834048));
#224017=CARTESIAN_POINT('Origin',(5.51210908043507E-15,1.8401175575949E-13,
3.61523028058481));
#224018=CARTESIAN_POINT('Origin',(-6.04426018543877,60.5451784741234,3.58781440266375));
#224019=CARTESIAN_POINT('Origin',(-0.317545622030984,60.8452088131242,3.58786923592738));
#224020=CARTESIAN_POINT('Origin',(60.4792282238308,1.82930781209959E-13,
3.77003198860263));
#224021=CARTESIAN_POINT('',(5.95633285891191,59.7081718144894,3.77003198860304));
#224022=CARTESIAN_POINT('',(0.317499999999796,60.0036905223732,3.77003198860305));
#224023=CARTESIAN_POINT('Origin',(5.49031038273072E-15,1.82930781209959E-13,
3.77003198860263));
#224024=CARTESIAN_POINT('',(0.317500000025055,60.4783948217628,3.77003198860305));
#224025=CARTESIAN_POINT('',(0.317500000000005,-2.71227701960981E-14,3.77003198860263));
#224026=CARTESIAN_POINT('',(0.318078445377653,60.4783917836891,3.77003198902584));
#224027=CARTESIAN_POINT('Origin',(5.49031038273072E-15,1.82930781209959E-13,
3.77003198860263));
#224028=CARTESIAN_POINT('',(6.00537737563974,60.1803330762809,3.77003198882129));
#224029=CARTESIAN_POINT('Origin',(5.49031038273072E-15,1.82930781209959E-13,
3.77003198860263));
#224030=CARTESIAN_POINT('',(6.00595296980844,60.1802756340599,3.77003198860305));
#224031=CARTESIAN_POINT('Origin',(5.49031038273072E-15,1.82930781209959E-13,
3.77003198860263));
#224032=CARTESIAN_POINT('',(5.95638905318986,59.7087064673301,3.77003198860304));
#224033=CARTESIAN_POINT('Origin',(5.49031038273072E-15,1.82930781209959E-13,
3.77003198860263));
#224034=CARTESIAN_POINT('',(0.31807689062316,60.6410923272407,3.48823028058523));
#224035=CARTESIAN_POINT('',(0.318078445373799,60.4783917829568,3.77003198860305));
#224036=CARTESIAN_POINT('',(6.02238575973065,60.3421421673491,3.48823028074847));
#224037=CARTESIAN_POINT('Origin',(5.52999282761009E-15,1.84898592019556E-13,
3.48823028058481));
#224038=CARTESIAN_POINT('',(6.02238575970257,60.3421421670677,3.48823028058523));
#224039=CARTESIAN_POINT('Origin',(60.71525,1.85785428279622E-13,3.36123028058482));
#224040=CARTESIAN_POINT('',(6.04595329345041,60.5608532912345,3.36123028058524));
#224041=CARTESIAN_POINT('',(0.317499999999793,60.8610688070709,3.36123028058524));
#224042=CARTESIAN_POINT('Origin',(5.5478765747851E-15,1.85785428279622E-13,
3.36123028058482));
#224043=CARTESIAN_POINT('',(0.317499999999792,61.0122769227458,3.36123028058524));
#224044=CARTESIAN_POINT('',(0.317500000000005,-2.50921887534909E-14,3.36123028058482));
#224045=CARTESIAN_POINT('',(6.0617588454155,60.7112330730306,3.36123028058524));
#224046=CARTESIAN_POINT('Origin',(5.5478765747851E-15,1.85785428279622E-13,
3.36123028058482));
#224047=CARTESIAN_POINT('',(6.04600869610028,60.5613804122371,3.36123028058524));
#224048=CARTESIAN_POINT('Origin',(5.5478765747851E-15,1.85785428279622E-13,
3.36123028058482));
#224049=CARTESIAN_POINT('',(6.08531878138301,60.9299448846692,3.48823028058527));
#224050=CARTESIAN_POINT('',(0.316930737397122,61.2322532923709,3.48823028042737));
#224051=CARTESIAN_POINT('Origin',(5.52999282761008E-15,1.84898592019556E-13,
3.48823028058484));
#224052=CARTESIAN_POINT('',(0.316932243253051,61.3949537495051,3.7700319880275));
#224053=CARTESIAN_POINT('',(0.316930737395706,61.2322532920974,3.48823028058527));
#224054=CARTESIAN_POINT('',(0.317499999999791,61.3949508163455,3.77003198860305));
#224055=CARTESIAN_POINT('Origin',(5.49031038273072E-15,1.82930781209959E-13,
3.77003198860263));
#224056=CARTESIAN_POINT('',(6.10175915944613,61.0918106390014,3.77003198860305));
#224057=CARTESIAN_POINT('Origin',(5.49031038273072E-15,1.82930781209959E-13,
3.77003198860263));
#224058=CARTESIAN_POINT('',(6.10232411256069,61.0917542093526,3.77003198802763));
#224059=CARTESIAN_POINT('Origin',(5.49031038273072E-15,1.82930781209959E-13,
3.77003198860263));
#224060=CARTESIAN_POINT('',(6.10232411260904,61.0917542096817,3.77003198860305));
#224061=CARTESIAN_POINT('Origin',(62.2224557307631,1.82930781209959E-13,
3.77003198860263));
#224062=CARTESIAN_POINT('',(0.31749999999979,61.8696548221183,3.77003198860306));
#224063=CARTESIAN_POINT('',(0.317500000000005,-3.32092165059103E-14,3.77003198860263));
#224064=CARTESIAN_POINT('',(6.15137923967656,61.5639141665614,3.77003198860306));
#224065=CARTESIAN_POINT('Origin',(5.49031038273072E-15,1.82930781209959E-13,
3.77003198860263));
#224066=CARTESIAN_POINT('',(6.10181408032636,61.0923331762719,3.77003198860305));
#224067=CARTESIAN_POINT('Origin',(5.57972911860581E-15,1.8736496251029E-13,
3.13503198860263));
#224068=CARTESIAN_POINT('Origin',(0.317504993060349,60.0036895869256,3.13502491541474));
#224069=CARTESIAN_POINT('Origin',(5.95632779542282,59.7081714060832,3.13502491541477));
#224070=CARTESIAN_POINT('Origin',(5.57972911860581E-15,1.8736496251029E-13,
3.13503198860263));
#224071=CARTESIAN_POINT('Origin',(0.317533537011351,61.9077842377866,3.20381846780236));
#224072=CARTESIAN_POINT('Origin',(6.15533145331141,61.6018378049635,3.20382022872551));
#224073=CARTESIAN_POINT('Origin',(5.51210908043506E-15,1.8401175575949E-13,
3.61523028058481));
#224074=CARTESIAN_POINT('Origin',(0.317462907478283,61.0281367271393,3.5878694504696));
#224075=CARTESIAN_POINT('Origin',(6.06344346747481,60.7269085901928,3.58781461834324));
#224076=CARTESIAN_POINT('Origin',(5.51210908043507E-15,1.8401175575949E-13,
3.61523028058481));
#224077=CARTESIAN_POINT('Origin',(0.31754536844525,60.84530288027,3.58781440266518));
#224078=CARTESIAN_POINT('Origin',(6.04425010054761,60.5450849487963,3.58786923593018));
#224079=CARTESIAN_POINT('Origin',(60.4792282238308,1.82930781209959E-13,
3.77003198860263));
#224080=CARTESIAN_POINT('',(12.164906888579,58.7584778814679,3.77003198860304));
#224081=CARTESIAN_POINT('',(6.58785426247077,59.6417962403145,3.77003198860304));
#224082=CARTESIAN_POINT('Origin',(5.49031038273072E-15,1.82930781209959E-13,
3.77003198860263));
#224083=CARTESIAN_POINT('',(6.63747437341763,60.1139000598802,3.77003198860305));
#224084=CARTESIAN_POINT('',(0.976568823008617,6.25398151259742,3.77003198860267));
#224085=CARTESIAN_POINT('',(6.63804933242087,60.1138365744455,3.77003198902578));
#224086=CARTESIAN_POINT('Origin',(5.49031038273072E-15,1.82930781209959E-13,
3.77003198860263));
#224087=CARTESIAN_POINT('',(12.2630370254222,59.2229260464989,3.77003198882128));
#224088=CARTESIAN_POINT('Origin',(5.49031038273072E-15,1.82930781209959E-13,
3.77003198860263));
#224089=CARTESIAN_POINT('',(12.2636034620787,59.2228087529784,3.77003198860304));
#224090=CARTESIAN_POINT('Origin',(5.49031038273072E-15,1.82930781209959E-13,
3.77003198860263));
#224091=CARTESIAN_POINT('',(12.1650186614586,58.7590037315228,3.77003198860304));
#224092=CARTESIAN_POINT('Origin',(5.49031038273072E-15,1.82930781209959E-13,
3.77003198860263));
#224093=CARTESIAN_POINT('',(6.65505462397376,60.2756459899121,3.48823028058523));
#224094=CARTESIAN_POINT('',(6.6380493323405,60.1138365737177,3.77003198860305));
#224095=CARTESIAN_POINT('',(12.2968658914375,59.3820708701842,3.48823028074845));
#224096=CARTESIAN_POINT('Origin',(5.52999282761009E-15,1.84898592019556E-13,
3.48823028058481));
#224097=CARTESIAN_POINT('',(12.2968658913801,59.3820708699073,3.48823028058522));
#224098=CARTESIAN_POINT('Origin',(60.71525,1.85785428279622E-13,3.36123028058482));
#224099=CARTESIAN_POINT('',(12.3431658574209,59.5971203935661,3.36123028058523));
#224100=CARTESIAN_POINT('',(6.67747469700926,60.4944777170596,3.36123028058524));
#224101=CARTESIAN_POINT('Origin',(5.5478765747851E-15,1.85785428279622E-13,
3.36123028058482));
#224102=CARTESIAN_POINT('',(6.69328024897435,60.6448574988556,3.36123028058524));
#224103=CARTESIAN_POINT('',(0.979147644052797,6.27851735587401,3.36123028058486));
#224104=CARTESIAN_POINT('',(12.3746037924162,59.745024249125,3.36123028058523));
#224105=CARTESIAN_POINT('Origin',(5.5478765747851E-15,1.85785428279622E-13,
3.36123028058482));
#224106=CARTESIAN_POINT('',(12.3432760557176,59.5976388357908,3.36123028058523));
#224107=CARTESIAN_POINT('Origin',(5.5478765747851E-15,1.85785428279622E-13,
3.36123028058482));
#224108=CARTESIAN_POINT('',(12.4208962741585,59.9600752506739,3.48823028058526));
#224109=CARTESIAN_POINT('',(6.7157078967239,60.8636883190565,3.48823028042737));
#224110=CARTESIAN_POINT('Origin',(5.52999282761008E-15,1.84898592019556E-13,
3.48823028058484));
#224111=CARTESIAN_POINT('',(6.73271622308777,61.0254973286581,3.7700319880275));
#224112=CARTESIAN_POINT('',(6.7157078966939,60.8636883187847,3.48823028058527));
#224113=CARTESIAN_POINT('',(6.73328056300499,61.0254350648264,3.77003198860305));
#224114=CARTESIAN_POINT('Origin',(5.49031038273072E-15,1.82930781209959E-13,
3.77003198860263));
#224115=CARTESIAN_POINT('',(12.4541661686664,60.1193358000131,3.77003198860305));
#224116=CARTESIAN_POINT('Origin',(5.49031038273072E-15,1.82930781209959E-13,
3.77003198860263));
#224117=CARTESIAN_POINT('',(12.4547221284042,60.119220625811,3.77003198802762));
#224118=CARTESIAN_POINT('Origin',(5.49031038273072E-15,1.82930781209959E-13,
3.77003198860263));
#224119=CARTESIAN_POINT('',(12.4547221284867,60.1192206261331,3.77003198860305));
#224120=CARTESIAN_POINT('Origin',(62.2224557307631,1.82930781209959E-13,
3.77003198860263));
#224121=CARTESIAN_POINT('',(6.78290064323541,61.4975385923864,3.77003198860306));
#224122=CARTESIAN_POINT('',(0.995615674755264,6.43520020182058,3.77003198860267));
#224123=CARTESIAN_POINT('',(12.5528626811445,60.5836663843184,3.77003198860305));
#224124=CARTESIAN_POINT('Origin',(5.49031038273072E-15,1.82930781209959E-13,
3.77003198860263));
#224125=CARTESIAN_POINT('',(12.4542754087022,60.1198497339746,3.77003198860305));
#224126=CARTESIAN_POINT('Origin',(5.57972911860581E-15,1.8736496251029E-13,
3.13503198860263));
#224127=CARTESIAN_POINT('Origin',(6.5878591303979,59.6417947880743,3.13502491541472));
#224128=CARTESIAN_POINT('Origin',(12.1649018101382,58.7584780045777,3.13502491541471));
#224129=CARTESIAN_POINT('Origin',(5.57972911860581E-15,1.8736496251029E-13,
3.13503198860263));
#224130=CARTESIAN_POINT('Origin',(6.7869196057536,61.5354556255538,3.20381846780299));
#224131=CARTESIAN_POINT('Origin',(12.5607573437845,60.6209691542431,3.20382022872538));
#224132=CARTESIAN_POINT('Origin',(5.51210908043506E-15,1.8401175575949E-13,
3.61523028058481));
#224133=CARTESIAN_POINT('Origin',(6.6949011606306,60.6606342988062,3.58786945046787));
#224134=CARTESIAN_POINT('Origin',(12.3779177236597,59.7604378032101,3.58781461834168));
#224135=CARTESIAN_POINT('Origin',(5.51210908043507E-15,1.8401175575949E-13,
3.61523028058481));
#224136=CARTESIAN_POINT('Origin',(6.67587182882186,60.4787934153623,3.58781440266664));
#224137=CARTESIAN_POINT('Origin',(12.3398237541835,59.5816164638945,3.5878692359302));
#224138=CARTESIAN_POINT('Origin',(60.4792282238308,1.82930781209959E-13,
3.77003198860263));
#224139=CARTESIAN_POINT('',(18.2401996527044,57.1650137687749,3.77003198860303));
#224140=CARTESIAN_POINT('',(12.786030615045,58.6264539577986,3.77003198860304));
#224141=CARTESIAN_POINT('Origin',(5.49031038273072E-15,1.82930781209959E-13,
3.77003198860263));
#224142=CARTESIAN_POINT('',(12.8847271885942,59.0907848292993,3.77003198860304));
#224143=CARTESIAN_POINT('',(2.92491386234291,12.2335471699534,3.77003198860271));
#224144=CARTESIAN_POINT('',(12.8852923618769,59.090661592063,3.77003198902557));
#224145=CARTESIAN_POINT('Origin',(5.49031038273072E-15,1.82930781209959E-13,
3.77003198860263));
#224146=CARTESIAN_POINT('',(18.3863402753486,57.6166602457575,3.77003198882127));
#224147=CARTESIAN_POINT('Origin',(5.49031038273072E-15,1.82930781209959E-13,
3.77003198860263));
#224148=CARTESIAN_POINT('',(18.3868913484944,57.6164843860299,3.77003198860303));
#224149=CARTESIAN_POINT('Origin',(5.49031038273072E-15,1.82930781209959E-13,
3.77003198860263));
#224150=CARTESIAN_POINT('',(18.2403657795786,57.1655250547209,3.77003198860303));
#224151=CARTESIAN_POINT('Origin',(5.49031038273072E-15,1.82930781209959E-13,
3.77003198860263));
#224152=CARTESIAN_POINT('',(12.9191181862044,59.2498070616282,3.48823028058522));
#224153=CARTESIAN_POINT('',(12.8852923617209,59.090661591348,3.77003198860304));
#224154=CARTESIAN_POINT('',(18.4366189871531,57.7713971780683,3.48823028074845));
#224155=CARTESIAN_POINT('Origin',(5.52999282761009E-15,1.84898592019556E-13,
3.48823028058481));
#224156=CARTESIAN_POINT('',(18.4366189870671,57.7713971777989,3.48823028058521));
#224157=CARTESIAN_POINT('Origin',(60.71525,1.85785428279622E-13,3.36123028058482));
#224158=CARTESIAN_POINT('',(18.505144113284,57.9804289733666,3.36123028058522));
#224159=CARTESIAN_POINT('',(12.9642895838869,59.4650964698968,3.36123028058523));
#224160=CARTESIAN_POINT('Origin',(5.5478765747851E-15,1.85785428279622E-13,
3.36123028058482));
#224161=CARTESIAN_POINT('',(12.9957275188822,59.6130003254557,3.36123028058523));
#224162=CARTESIAN_POINT('',(2.93511643966547,12.2815465224194,3.3612302805849));
#224163=CARTESIAN_POINT('',(18.5518699907149,58.1242364370959,3.36123028058522));
#224164=CARTESIAN_POINT('Origin',(5.5478765747851E-15,1.85785428279622E-13,
3.36123028058482));
#224165=CARTESIAN_POINT('',(18.505307899872,57.9809330566519,3.36123028058522));
#224166=CARTESIAN_POINT('Origin',(5.5478765747851E-15,1.85785428279622E-13,
3.36123028058482));
#224167=CARTESIAN_POINT('',(18.6203878281146,58.3332704847798,3.48823028058524));
#224168=CARTESIAN_POINT('',(13.0409063549819,59.8282880399729,3.48823028042736));
#224169=CARTESIAN_POINT('Origin',(5.52999282761008E-15,1.84898592019556E-13,
3.48823028058484));
#224170=CARTESIAN_POINT('',(13.0747351550709,59.987432788672,3.77003198802749));
#224171=CARTESIAN_POINT('',(13.0409063549237,59.8282880397057,3.48823028058526));
#224172=CARTESIAN_POINT('',(13.0752898951324,59.9873118763438,3.77003198860305));
#224173=CARTESIAN_POINT('Origin',(5.49031038273072E-15,1.82930781209959E-13,
3.77003198860263));
#224174=CARTESIAN_POINT('',(18.6701227271409,58.48818093722,3.77003198860304));
#224175=CARTESIAN_POINT('Origin',(5.49031038273072E-15,1.82930781209959E-13,
3.77003198860263));
#224176=CARTESIAN_POINT('',(18.6706636022907,58.4880082803372,3.77003198802761));
#224177=CARTESIAN_POINT('Origin',(5.49031038273072E-15,1.82930781209959E-13,
3.77003198860263));
#224178=CARTESIAN_POINT('',(18.6706636024065,58.488008280649,3.77003198860304));
#224179=CARTESIAN_POINT('Origin',(62.2224557307631,1.82930781209959E-13,
3.77003198860263));
#224180=CARTESIAN_POINT('',(13.1739864076105,60.4516424606491,3.77003198860305));
#224181=CARTESIAN_POINT('',(3.00026883051124,12.588064422097,3.77003198860271));
#224182=CARTESIAN_POINT('',(18.8168143322225,58.9396512752216,3.77003198860304));
#224183=CARTESIAN_POINT('Origin',(5.49031038273072E-15,1.82930781209959E-13,
3.77003198860263));
#224184=CARTESIAN_POINT('',(18.6702850894756,58.4886806371044,3.77003198860304));
#224185=CARTESIAN_POINT('Origin',(5.57972911860581E-15,1.8736496251029E-13,
3.13503198860263));
#224186=CARTESIAN_POINT('Origin',(12.7860353045046,58.626452004677,3.13502491541474));
#224187=CARTESIAN_POINT('Origin',(18.2401946149522,57.165014422052,3.13502491541474));
#224188=CARTESIAN_POINT('Origin',(5.57972911860581E-15,1.8736496251029E-13,
3.13503198860263));
#224189=CARTESIAN_POINT('Origin',(13.1819467630385,60.4889316843659,3.20381846780306));
#224190=CARTESIAN_POINT('Origin',(18.8285649482899,58.9759244797141,3.20382022872186));
#224191=CARTESIAN_POINT('Origin',(5.51210908043506E-15,1.8401175575949E-13,
3.61523028058481));
#224192=CARTESIAN_POINT('Origin',(12.9989886756684,59.6285212670385,3.5878694504728));
#224193=CARTESIAN_POINT('Origin',(18.5567769230182,58.1392191539783,3.58781461834213));
#224194=CARTESIAN_POINT('Origin',(5.51210908043507E-15,1.8401175575949E-13,
3.61523028058481));
#224195=CARTESIAN_POINT('Origin',(12.9610560404269,59.4496656337922,3.58781440266432));
#224196=CARTESIAN_POINT('Origin',(18.5001997164952,57.9653593207579,3.58786923592793));
#224197=CARTESIAN_POINT('Origin',(60.4792282238308,1.82930781209959E-13,
3.77003198860263));
#224198=CARTESIAN_POINT('',(24.1156489724276,54.9452378026831,3.77003198860301));
#224199=CARTESIAN_POINT('',(18.8441205405518,56.9687879773468,3.77003198860303));
#224200=CARTESIAN_POINT('Origin',(5.49031038273072E-15,1.82930781209959E-13,
3.77003198860263));
#224201=CARTESIAN_POINT('',(18.9908122363901,57.4202585945868,3.77003198860303));
#224202=CARTESIAN_POINT('',(6.07721283595898,17.6762863142852,3.77003198860275));
#224203=CARTESIAN_POINT('',(18.9913614317957,57.4200769557631,3.77003198902602));
#224204=CARTESIAN_POINT('Origin',(5.49031038273072E-15,1.82930781209959E-13,
3.77003198860263));
#224205=CARTESIAN_POINT('',(24.3081989336292,55.3791342583022,3.77003198882125));
#224206=CARTESIAN_POINT('Origin',(5.49031038273072E-15,1.82930781209959E-13,
3.77003198860263));
#224207=CARTESIAN_POINT('',(24.3087286055916,55.3789017591236,3.77003198860302));
#224208=CARTESIAN_POINT('Origin',(5.49031038273072E-15,1.82930781209959E-13,
3.77003198860263));
#224209=CARTESIAN_POINT('',(24.1158676331756,54.9457289227643,3.77003198860301));
#224210=CARTESIAN_POINT('Origin',(5.49031038273072E-15,1.82930781209959E-13,
3.77003198860263));
#224211=CARTESIAN_POINT('',(19.0416371860877,57.5748148483578,3.48823028058521));
#224212=CARTESIAN_POINT('',(18.9913614315656,57.4200769550675,3.77003198860303));
#224213=CARTESIAN_POINT('',(24.3743766271349,55.5277679690274,3.48823028074843));
#224214=CARTESIAN_POINT('Origin',(5.52999282761009E-15,1.84898592019556E-13,
3.48823028058481));
#224215=CARTESIAN_POINT('',(24.3743766270213,55.5277679687685,3.4882302805852));
#224216=CARTESIAN_POINT('Origin',(60.71525,1.85785428279622E-13,3.36123028058482));
#224217=CARTESIAN_POINT('',(24.4643761377916,55.72849184015,3.3612302805852));
#224218=CARTESIAN_POINT('',(19.1090650011314,57.7842031819385,3.36123028058522));
#224219=CARTESIAN_POINT('Origin',(5.5478765747851E-15,1.85785428279622E-13,
3.36123028058482));
#224220=CARTESIAN_POINT('',(19.1557908785624,57.9280106456678,3.36123028058522));
#224221=CARTESIAN_POINT('',(6.09975091006187,17.7456513739113,3.36123028058494));
#224222=CARTESIAN_POINT('',(24.525878019167,55.8666273273835,3.36123028058521));
#224223=CARTESIAN_POINT('Origin',(5.5478765747851E-15,1.85785428279622E-13,
3.36123028058482));
#224224=CARTESIAN_POINT('',(24.4645917181906,55.7289760416541,3.3612302805852));
#224225=CARTESIAN_POINT('Origin',(5.5478765747851E-15,1.85785428279622E-13,
3.36123028058482));
#224226=CARTESIAN_POINT('',(24.6158705164593,56.0673542004328,3.48823028058523));
#224227=CARTESIAN_POINT('',(19.2232259142297,58.1373965172492,3.48823028042735));
#224228=CARTESIAN_POINT('Origin',(5.52999282761008E-15,1.84898592019556E-13,
3.48823028058484));
#224229=CARTESIAN_POINT('',(19.2735045526308,58.2921333818758,3.77003198802748));
#224230=CARTESIAN_POINT('',(19.2232259141438,58.1373965169896,3.48823028058524));
#224231=CARTESIAN_POINT('',(19.2740436149883,58.2919551457919,3.77003198860303));
#224232=CARTESIAN_POINT('Origin',(5.49031038273072E-15,1.82930781209959E-13,
3.77003198860263));
#224233=CARTESIAN_POINT('',(24.6815255140425,56.21621732464,3.77003198860303));
#224234=CARTESIAN_POINT('Origin',(5.49031038273072E-15,1.82930781209959E-13,
3.77003198860263));
#224235=CARTESIAN_POINT('',(24.6820453786631,56.2159890767414,3.7700319880276));
#224236=CARTESIAN_POINT('Origin',(5.49031038273072E-15,1.82930781209959E-13,
3.77003198860263));
#224237=CARTESIAN_POINT('',(24.6820453788107,56.2159890770394,3.77003198860303));
#224238=CARTESIAN_POINT('Origin',(62.2224557307631,1.82930781209959E-13,
3.77003198860263));
#224239=CARTESIAN_POINT('',(19.42073522007,58.7434254837935,3.77003198860304));
#224240=CARTESIAN_POINT('',(6.24367625034007,18.1886080242679,3.77003198860276));
#224241=CARTESIAN_POINT('',(24.8746050278051,56.6498810128384,3.77003198860303));
#224242=CARTESIAN_POINT('Origin',(5.49031038273072E-15,1.82930781209959E-13,
3.77003198860263));
#224243=CARTESIAN_POINT('',(24.6817392198003,56.2166973156308,3.77003198860302));
#224244=CARTESIAN_POINT('Origin',(5.57972911860581E-15,1.8736496251029E-13,
3.13503198860263));
#224245=CARTESIAN_POINT('Origin',(18.8441250001652,56.9687855447427,3.13502491541475));
#224246=CARTESIAN_POINT('Origin',(24.1156440305588,54.9452389789699,3.13502491541474));
#224247=CARTESIAN_POINT('Origin',(5.57972911860581E-15,1.8736496251029E-13,
3.13503198860263));
#224248=CARTESIAN_POINT('Origin',(19.4325497530937,58.77967834952,3.20381846780313));
#224249=CARTESIAN_POINT('Origin',(24.8900828550905,56.6847272350808,3.20382022871978));
#224250=CARTESIAN_POINT('Origin',(5.51210908043506E-15,1.8401175575949E-13,
3.61523028058481));
#224251=CARTESIAN_POINT('Origin',(19.1606565505629,57.9431056782021,3.58786945047102));
#224252=CARTESIAN_POINT('Origin',(24.5323241911531,55.8810150532823,3.58781461834224));
#224253=CARTESIAN_POINT('Origin',(5.51210908043507E-15,1.8401175575949E-13,
3.61523028058481));
#224254=CARTESIAN_POINT('Origin',(19.1042362097724,57.7691948748974,3.58781440266281));
#224255=CARTESIAN_POINT('Origin',(24.4578836192999,55.7140215708719,3.58786923592786));
#224256=CARTESIAN_POINT('Origin',(60.4792282238308,1.82930781209959E-13,
3.77003198860263));
#224257=CARTESIAN_POINT('',(29.7268821954849,52.1234703131949,3.770031988603));
#224258=CARTESIAN_POINT('',(24.6957503380306,54.68696003433,3.77003198860302));
#224259=CARTESIAN_POINT('Origin',(5.49031038273072E-15,1.82930781209959E-13,
3.77003198860263));
#224260=CARTESIAN_POINT('',(24.8888299712411,55.1206239907505,3.77003198860301));
#224261=CARTESIAN_POINT('',(10.295413467953,22.3432738675266,3.77003198860278));
#224262=CARTESIAN_POINT('',(24.8893571716697,55.1203859404114,3.77003198902604));
#224263=CARTESIAN_POINT('Origin',(5.49031038273072E-15,1.82930781209959E-13,
3.77003198860263));
#224264=CARTESIAN_POINT('',(29.9637318775753,52.5348628870841,3.77003198882124));
#224265=CARTESIAN_POINT('Origin',(5.49031038273072E-15,1.82930781209959E-13,
3.77003198860263));
#224266=CARTESIAN_POINT('',(29.9642343451574,52.534576295764,3.770031988603));
#224267=CARTESIAN_POINT('Origin',(5.49031038273072E-15,1.82930781209959E-13,
3.77003198860263));
#224268=CARTESIAN_POINT('',(29.7271509944138,52.1239358865969,3.77003198860299));
#224269=CARTESIAN_POINT('Origin',(5.49031038273072E-15,1.82930781209959E-13,
3.77003198860263));
#224270=CARTESIAN_POINT('',(24.9555320242414,55.2690209153043,3.4882302805852));
#224271=CARTESIAN_POINT('',(24.8893571713682,55.1203859397437,3.77003198860302));
#224272=CARTESIAN_POINT('',(30.0450834961236,52.6757649141854,3.48823028074842));
#224273=CARTESIAN_POINT('Origin',(5.52999282761009E-15,1.84898592019556E-13,
3.48823028058481));
#224274=CARTESIAN_POINT('',(30.0450834959836,52.6757649139398,3.48823028058519));
#224275=CARTESIAN_POINT('Origin',(60.71525,1.85785428279622E-13,3.36123028058482));
#224276=CARTESIAN_POINT('',(30.1555713378337,52.8659816883962,3.36123028058519));
#224277=CARTESIAN_POINT('',(25.0444775033946,55.4702140717969,3.36123028058521));
#224278=CARTESIAN_POINT('Origin',(5.5478765747851E-15,1.85785428279622E-13,
3.36123028058482));
#224279=CARTESIAN_POINT('',(25.1059793847701,55.6083495590304,3.36123028058521));
#224280=CARTESIAN_POINT('',(10.3344596589366,22.4309730483567,3.36123028058497));
#224281=CARTESIAN_POINT('',(30.2311753956711,52.996931757829,3.36123028058519));
#224282=CARTESIAN_POINT('Origin',(5.5478765747851E-15,1.85785428279622E-13,
3.36123028058482));
#224283=CARTESIAN_POINT('',(30.1558363500999,52.8664407031059,3.36123028058519));
#224284=CARTESIAN_POINT('Origin',(5.5478765747851E-15,1.85785428279622E-13,
3.36123028058482));
#224285=CARTESIAN_POINT('',(30.3416565762235,53.1871522506177,3.48823028058522));
#224286=CARTESIAN_POINT('',(25.1949317876425,55.8095395122502,3.48823028042734));
#224287=CARTESIAN_POINT('Origin',(5.52999282761008E-15,1.84898592019556E-13,
3.48823028058484));
#224288=CARTESIAN_POINT('',(25.261109401072,55.9581731633347,3.77003198802746));
#224289=CARTESIAN_POINT('',(25.19493178753,55.8095395120009,3.48823028058523));
#224290=CARTESIAN_POINT('',(25.2616268796456,55.9579395562869,3.77003198860303));
#224291=CARTESIAN_POINT('Origin',(5.49031038273072E-15,1.82930781209959E-13,
3.77003198860263));
#224292=CARTESIAN_POINT('',(30.422512342471,53.3283370710515,3.77003198860301));
#224293=CARTESIAN_POINT('Origin',(5.49031038273072E-15,1.82930781209959E-13,
3.77003198860263));
#224294=CARTESIAN_POINT('',(30.4230055008167,53.3280557328689,3.77003198802758));
#224295=CARTESIAN_POINT('Origin',(5.49031038273072E-15,1.82930781209959E-13,
3.77003198860263));
#224296=CARTESIAN_POINT('',(30.4230055009947,53.3280557331498,3.77003198860301));
#224297=CARTESIAN_POINT('Origin',(62.2224557307631,1.82930781209959E-13,
3.77003198860263));
#224298=CARTESIAN_POINT('',(25.4547063934082,56.3916032444853,3.77003198860303));
#224299=CARTESIAN_POINT('',(10.5838037820516,22.9910091182299,3.77003198860279));
#224300=CARTESIAN_POINT('',(30.6598643453574,53.7394427993289,3.77003198860301));
#224301=CARTESIAN_POINT('Origin',(5.49031038273072E-15,1.82930781209959E-13,
3.77003198860263));
#224302=CARTESIAN_POINT('',(30.422775050247,53.328792094267,3.770031988603));
#224303=CARTESIAN_POINT('Origin',(5.57972911860581E-15,1.8736496251029E-13,
3.13503198860263));
#224304=CARTESIAN_POINT('Origin',(24.6957545189376,54.6869571488953,3.13502491541468));
#224305=CARTESIAN_POINT('Origin',(29.7268774036436,52.1234719996038,3.13502491541472));
#224306=CARTESIAN_POINT('Origin',(5.57972911860581E-15,1.8736496251029E-13,
3.13503198860263));
#224307=CARTESIAN_POINT('Origin',(25.4702456615188,56.4264225582421,3.20381846780199));
#224308=CARTESIAN_POINT('Origin',(30.678899805548,53.7724802568186,3.20382022872022));
#224309=CARTESIAN_POINT('Origin',(5.51210908043506E-15,1.8401175575949E-13,
3.61523028058481));
#224310=CARTESIAN_POINT('Origin',(25.112396262664,55.6228532981801,3.587869450471));
#224311=CARTESIAN_POINT('Origin',(30.2390901817309,53.0105668578086,3.5878146183411));
#224312=CARTESIAN_POINT('Origin',(5.51210908043507E-15,1.8401175575949E-13,
3.61523028058481));
#224313=CARTESIAN_POINT('Origin',(25.0381063693916,55.4557927279711,3.58781440266272));
#224314=CARTESIAN_POINT('Origin',(30.1476018310216,52.8522693417523,3.58786923593059));
#224315=CARTESIAN_POINT('Origin',(60.4792282238308,1.82930781209959E-13,
3.77003198860263));
#224316=CARTESIAN_POINT('',(35.0124214764584,48.7306271754179,3.77003198860297));
#224317=CARTESIAN_POINT('',(30.276808326888,51.8059703131949,3.77003198860299));
#224318=CARTESIAN_POINT('Origin',(5.49031038273072E-15,1.82930781209959E-13,
3.77003198860263));
#224319=CARTESIAN_POINT('',(30.5141604766046,52.2170762957393,3.770031988603));
#224320=CARTESIAN_POINT('',(15.3947701216591,26.0295240215572,3.77003198860281));
#224321=CARTESIAN_POINT('',(30.5146599059377,52.2167844420138,3.77003198902568));
#224322=CARTESIAN_POINT('Origin',(5.49031038273072E-15,1.82930781209959E-13,
3.77003198860263));
#224323=CARTESIAN_POINT('',(35.2909759047567,49.1150085644483,3.77003198882122));
#224324=CARTESIAN_POINT('Origin',(5.49031038273072E-15,1.82930781209959E-13,
3.77003198860263));
#224325=CARTESIAN_POINT('',(35.2914456628186,49.1146710209413,3.77003198860297));
#224326=CARTESIAN_POINT('Origin',(5.49031038273072E-15,1.82930781209959E-13,
3.77003198860263));
#224327=CARTESIAN_POINT('',(35.012737468551,48.7310621012211,3.77003198860297));
#224328=CARTESIAN_POINT('Origin',(5.49031038273072E-15,1.82930781209959E-13,
3.77003198860263));
#224329=CARTESIAN_POINT('',(30.5960088312567,52.3576880233165,3.48823028058518));
#224330=CARTESIAN_POINT('',(30.5146599055683,52.2167844413817,3.770031988603));
#224331=CARTESIAN_POINT('',(35.3866101429909,49.2466351558311,3.48823028074839));
#224332=CARTESIAN_POINT('Origin',(5.52999282761009E-15,1.84898592019556E-13,
3.48823028058481));
#224333=CARTESIAN_POINT('',(35.3866101428259,49.2466351556015,3.48823028058516));
#224334=CARTESIAN_POINT('Origin',(60.71525,1.85785428279622E-13,3.36123028058482));
#224335=CARTESIAN_POINT('',(35.5163757878395,49.4242607783463,3.36123028058517));
#224336=CARTESIAN_POINT('',(30.7054974692368,52.5484816883962,3.36123028058519));
#224337=CARTESIAN_POINT('Origin',(5.5478765747851E-15,1.85785428279622E-13,
3.36123028058482));
#224338=CARTESIAN_POINT('',(30.7811015270742,52.679431757829,3.36123028058519));
#224339=CARTESIAN_POINT('',(15.4537755657014,26.1317244485617,3.361230280585));
#224340=CARTESIAN_POINT('',(35.6052536882601,49.5465907136147,3.36123028058517));
#224341=CARTESIAN_POINT('Origin',(5.5478765747851E-15,1.85785428279622E-13,
3.36123028058482));
#224342=CARTESIAN_POINT('',(35.516687328443,49.4246895772005,3.36123028058516));
#224343=CARTESIAN_POINT('Origin',(5.5478765747851E-15,1.85785428279622E-13,
3.36123028058482));
#224344=CARTESIAN_POINT('',(35.7350130971388,49.7242207306177,3.48823028058519));
#224345=CARTESIAN_POINT('',(30.8905967160115,52.870221513458,3.48823028042732));
#224346=CARTESIAN_POINT('Origin',(5.52999282761008E-15,1.84898592019556E-13,
3.48823028058484));
#224347=CARTESIAN_POINT('',(30.971948248688,53.0111234896156,3.77003198802745));
#224348=CARTESIAN_POINT('',(30.8905967158735,52.8702215132218,3.48823028058522));
#224349=CARTESIAN_POINT('',(30.9724384738741,53.0108370710515,3.77003198860301));
#224350=CARTESIAN_POINT('Origin',(5.49031038273072E-15,1.82930781209959E-13,
3.77003198860263));
#224351=CARTESIAN_POINT('',(35.8301837593554,49.8561803968406,3.77003198860298));
#224352=CARTESIAN_POINT('Origin',(5.49031038273072E-15,1.82930781209959E-13,
3.77003198860263));
#224353=CARTESIAN_POINT('',(35.8306448082802,49.8558490507739,3.77003198802756));
#224354=CARTESIAN_POINT('Origin',(5.49031038273072E-15,1.82930781209959E-13,
3.77003198860263));
#224355=CARTESIAN_POINT('',(35.8306448084866,49.8558490510347,3.77003198860298));
#224356=CARTESIAN_POINT('Origin',(62.2224557307631,1.82930781209959E-13,
3.77003198860263));
#224357=CARTESIAN_POINT('',(31.2097904767605,53.4219427993289,3.77003198860301));
#224358=CARTESIAN_POINT('',(15.8305769983922,26.7843636743468,3.77003198860281));
#224359=CARTESIAN_POINT('',(36.1092077731528,50.2402240048086,3.77003198860298));
#224360=CARTESIAN_POINT('Origin',(5.49031038273072E-15,1.82930781209959E-13,
3.77003198860263));
#224361=CARTESIAN_POINT('',(35.8304925908681,49.8566054669512,3.77003198860297));
#224362=CARTESIAN_POINT('Origin',(5.57972911860581E-15,1.8736496251029E-13,
3.13503198860263));
#224363=CARTESIAN_POINT('Origin',(30.2768121832815,51.8059670065431,3.1350249154147));
#224364=CARTESIAN_POINT('Origin',(35.012416887145,48.7306293534723,3.13502491541466));
#224365=CARTESIAN_POINT('Origin',(5.57972911860581E-15,1.8736496251029E-13,
3.13503198860263));
#224366=CARTESIAN_POINT('Origin',(31.2288842284977,53.4549470734237,3.20381846780249));
#224367=CARTESIAN_POINT('Origin',(36.131592309765,50.2710907322454,3.20382022871924));
#224368=CARTESIAN_POINT('Origin',(5.51210908043506E-15,1.8401175575949E-13,
3.61523028058481));
#224369=CARTESIAN_POINT('Origin',(30.7889993062046,52.6931852975928,3.58786945047126));
#224370=CARTESIAN_POINT('Origin',(35.6145503723404,49.5593237986651,3.5878146183433));
#224371=CARTESIAN_POINT('Origin',(5.51210908043507E-15,1.8401175575949E-13,
3.61523028058481));
#224372=CARTESIAN_POINT('Origin',(30.6976537960638,52.5348053110502,3.58781440266714));
#224373=CARTESIAN_POINT('Origin',(35.5070166083019,49.4114565896684,3.58786923592972));
#224374=CARTESIAN_POINT('Origin',(60.4792282238308,1.82930781209959E-13,
3.77003198860263));
#224375=CARTESIAN_POINT('',(39.9143573409156,44.8038810887677,3.77003198860295));
#224376=CARTESIAN_POINT('',(35.5261472678865,48.3573835402122,3.77003198860297));
#224377=CARTESIAN_POINT('Origin',(5.49031038273072E-15,1.82930781209959E-13,
3.77003198860263));
#224378=CARTESIAN_POINT('',(35.8051714542879,48.7414273857063,3.77003198860297));
#224379=CARTESIAN_POINT('',(21.151922343707,28.5729602337853,3.77003198860282));
#224380=CARTESIAN_POINT('',(35.8056376406733,48.7410849262052,3.77003198902553));
#224381=CARTESIAN_POINT('Origin',(5.49031038273072E-15,1.82930781209959E-13,
3.77003198860263));
#224382=CARTESIAN_POINT('',(40.2315646148141,45.157039930004,3.77003198882119));
#224383=CARTESIAN_POINT('Origin',(5.49031038273072E-15,1.82930781209959E-13,
3.77003198860263));
#224384=CARTESIAN_POINT('',(40.2319965165881,45.1566551325074,3.77003198860295));
#224385=CARTESIAN_POINT('Origin',(5.49031038273072E-15,1.82930781209959E-13,
3.77003198860263));
#224386=CARTESIAN_POINT('',(39.9147170640963,44.804280601834,3.77003198860295));
#224387=CARTESIAN_POINT('Origin',(5.49031038273072E-15,1.82930781209959E-13,
3.77003198860263));
#224388=CARTESIAN_POINT('',(35.9012693628904,48.8727133447946,3.48823028058516));
#224389=CARTESIAN_POINT('',(35.80563764024,48.7410849256154,3.77003198860297));
#224390=CARTESIAN_POINT('',(40.3404336840073,45.2779489571886,3.48823028074837));
#224391=CARTESIAN_POINT('Origin',(5.52999282761009E-15,1.84898592019556E-13,
3.48823028058481));
#224392=CARTESIAN_POINT('',(40.3404336838192,45.2779489569775,3.48823028058513));
#224393=CARTESIAN_POINT('Origin',(60.71525,1.85785428279622E-13,3.36123028058482));
#224394=CARTESIAN_POINT('',(40.4880553924343,45.4410373245174,3.36123028058514));
#224395=CARTESIAN_POINT('',(36.0301015792676,49.0510171431406,3.36123028058517));
#224396=CARTESIAN_POINT('Origin',(5.5478765747851E-15,1.85785428279622E-13,
3.36123028058482));
#224397=CARTESIAN_POINT('',(36.1189794796882,49.173347078409,3.36123028058517));
#224398=CARTESIAN_POINT('',(21.2334658618522,28.685195257892,3.36123028058502));
#224399=CARTESIAN_POINT('',(40.5892333705622,45.5534068532514,3.36123028058514));
#224400=CARTESIAN_POINT('Origin',(5.5478765747851E-15,1.85785428279622E-13,
3.36123028058482));
#224401=CARTESIAN_POINT('',(40.488410048071,45.4414312095061,3.36123028058514));
#224402=CARTESIAN_POINT('Origin',(5.5478765747851E-15,1.85785428279622E-13,
3.36123028058482));
#224403=CARTESIAN_POINT('',(40.7368493365296,45.7165002428309,3.48823028058517));
#224404=CARTESIAN_POINT('',(36.2478178024869,49.3516463039592,3.4882302804273));
#224405=CARTESIAN_POINT('Origin',(5.52999282761008E-15,1.84898592019556E-13,
3.48823028058484));
#224406=CARTESIAN_POINT('',(36.3434519499946,49.4832728536534,3.77003198802742));
#224407=CARTESIAN_POINT('',(36.247817802325,49.3516463037387,3.48823028058519));
#224408=CARTESIAN_POINT('',(36.3439095507835,49.4829367616348,3.77003198860298));
#224409=CARTESIAN_POINT('Origin',(5.49031038273072E-15,1.82930781209959E-13,
3.77003198860263));
#224410=CARTESIAN_POINT('',(40.8452921850243,45.8377889771254,3.77003198860295));
#224411=CARTESIAN_POINT('Origin',(5.49031038273072E-15,1.82930781209959E-13,
3.77003198860263));
#224412=CARTESIAN_POINT('',(40.8457160731797,45.8374112534716,3.77003198802753));
#224413=CARTESIAN_POINT('Origin',(5.49031038273072E-15,1.82930781209959E-13,
3.77003198860263));
#224414=CARTESIAN_POINT('',(40.8457160734122,45.8374112537093,3.77003198860295));
#224415=CARTESIAN_POINT('Origin',(62.2224557307631,1.82930781209959E-13,
3.77003198860263));
#224416=CARTESIAN_POINT('',(36.6229335645808,49.8669803696028,3.77003198860298));
#224417=CARTESIAN_POINT('',(21.7541926348211,29.4019141737118,3.77003198860283));
#224418=CARTESIAN_POINT('',(41.162931164248,46.1905628026487,3.77003198860296));
#224419=CARTESIAN_POINT('Origin',(5.49031038273072E-15,1.82930781209959E-13,
3.77003198860263));
#224420=CARTESIAN_POINT('',(40.8456437566512,45.838179436974,3.77003198860295));
#224421=CARTESIAN_POINT('Origin',(5.57972911860581E-15,1.8736496251029E-13,
3.13503198860263));
#224422=CARTESIAN_POINT('Origin',(35.5261507575148,48.3573798485718,3.13502491541469));
#224423=CARTESIAN_POINT('Origin',(39.9143530044117,44.8038837346043,3.13502491541463));
#224424=CARTESIAN_POINT('Origin',(5.57972911860581E-15,1.8736496251029E-13,
3.13503198860263));
#224425=CARTESIAN_POINT('Origin',(36.6453726047997,49.8978080023046,3.20381846780288));
#224426=CARTESIAN_POINT('Origin',(41.188419527607,46.2189206177163,3.20382022872233));
#224427=CARTESIAN_POINT('Origin',(5.51210908043506E-15,1.8401175575949E-13,
3.61523028058481));
#224428=CARTESIAN_POINT('Origin',(36.1282716303338,49.1861997321267,3.58786945047242));
#224429=CARTESIAN_POINT('Origin',(40.5998100962474,45.5650984170292,3.58781461834315));
#224430=CARTESIAN_POINT('Origin',(5.51210908043507E-15,1.8401175575949E-13,
3.61523028058481));
#224431=CARTESIAN_POINT('Origin',(36.0208713038508,49.0382355735231,3.5878144026671));
#224432=CARTESIAN_POINT('Origin',(40.4774090812936,45.4292815791797,3.58786923592817));
#224433=CARTESIAN_POINT('Origin',(60.4792282238308,1.82930781209959E-13,
3.77003198860263));
#224434=CARTESIAN_POINT('',(44.3789831537295,40.3862543050941,3.77003198860292));
#224435=CARTESIAN_POINT('',(40.3862543050938,44.3789831537298,3.77003198860294));
#224436=CARTESIAN_POINT('Origin',(5.49031038273072E-15,1.82930781209959E-13,
3.77003198860263));
#224437=CARTESIAN_POINT('',(40.7038934808042,44.7317571974362,3.77003198860294));
#224438=CARTESIAN_POINT('',(27.314662201079,29.8615093742685,3.77003198860284));
#224439=CARTESIAN_POINT('',(40.7043213166065,44.7313678842176,3.77003198902556));
#224440=CARTESIAN_POINT('Origin',(5.49031038273072E-15,1.82930781209959E-13,
3.77003198860263));
#224441=CARTESIAN_POINT('',(44.7313678839555,40.7043213163686,3.77003198882116));
#224442=CARTESIAN_POINT('Origin',(5.49031038273072E-15,1.82930781209959E-13,
3.77003198860263));
#224443=CARTESIAN_POINT('',(44.7317571974354,40.7038934808041,3.77003198860292));
#224444=CARTESIAN_POINT('Origin',(5.49031038273072E-15,1.82930781209959E-13,
3.77003198860263));
#224445=CARTESIAN_POINT('',(44.3793826667958,40.3866140282747,3.77003198860292));
#224446=CARTESIAN_POINT('Origin',(5.49031038273072E-15,1.82930781209959E-13,
3.77003198860263));
#224447=CARTESIAN_POINT('',(40.8131880745606,44.8522789915944,3.48823028058513));
#224448=CARTESIAN_POINT('',(40.7043213161139,44.7313678836762,3.77003198860295));
#224449=CARTESIAN_POINT('',(44.8522789918032,40.8131880747512,3.48823028074834));
#224450=CARTESIAN_POINT('Origin',(5.52999282761009E-15,1.84898592019556E-13,
3.48823028058481));
#224451=CARTESIAN_POINT('',(44.8522789915941,40.8131880745609,3.4882302805851));
#224452=CARTESIAN_POINT('Origin',(60.71525,1.85785428279622E-13,3.36123028058482));
#224453=CARTESIAN_POINT('',(45.0161393894793,40.9599523566127,3.36123028058511));
#224454=CARTESIAN_POINT('',(40.9599523566124,45.0161393894796,3.36123028058514));
#224455=CARTESIAN_POINT('Origin',(5.5478765747851E-15,1.85785428279622E-13,
3.36123028058482));
#224456=CARTESIAN_POINT('',(41.0611303347403,45.1285089182135,3.36123028058514));
#224457=CARTESIAN_POINT('',(27.4203375923833,29.9788737863605,3.36123028058502));
#224458=CARTESIAN_POINT('',(45.1285089182132,41.0611303347406,3.36123028058511));
#224459=CARTESIAN_POINT('Origin',(5.5478765747851E-15,1.85785428279622E-13,
3.36123028058482));
#224460=CARTESIAN_POINT('',(45.0165332744679,40.9603070122495,3.36123028058511));
#224461=CARTESIAN_POINT('Origin',(5.5478765747851E-15,1.85785428279622E-13,
3.36123028058482));
#224462=CARTESIAN_POINT('',(45.2923641298556,41.207900211591,3.48823028058513));
#224463=CARTESIAN_POINT('',(41.2079002117747,45.2923641300583,3.48823028042727));
#224464=CARTESIAN_POINT('Origin',(5.52999282761008E-15,1.84898592019556E-13,
3.48823028058484));
#224465=CARTESIAN_POINT('',(41.3167691863808,45.4132731252661,3.77003198802739));
#224466=CARTESIAN_POINT('',(41.2079002115907,45.292364129856,3.48823028058516));
#224467=CARTESIAN_POINT('',(41.3171891492024,45.4128910420875,3.77003198860295));
#224468=CARTESIAN_POINT('Origin',(5.49031038273072E-15,1.82930781209959E-13,
3.77003198860263));
#224469=CARTESIAN_POINT('',(45.4128910420872,41.3171891492028,3.77003198860292));
#224470=CARTESIAN_POINT('Origin',(5.49031038273072E-15,1.82930781209959E-13,
3.77003198860263));
#224471=CARTESIAN_POINT('',(45.4132731252658,41.3167691863812,3.7700319880275));
#224472=CARTESIAN_POINT('Origin',(5.49031038273072E-15,1.82930781209959E-13,
3.77003198860263));
#224473=CARTESIAN_POINT('',(45.4132731255219,41.3167691865933,3.77003198860292));
#224474=CARTESIAN_POINT('Origin',(62.2224557307631,1.82930781209959E-13,
3.77003198860263));
#224475=CARTESIAN_POINT('',(41.6348281284261,45.7656648676109,3.77003198860295));
#224476=CARTESIAN_POINT('',(28.0951675083324,30.7283483363947,3.77003198860284));
#224477=CARTESIAN_POINT('',(45.7656648676106,41.6348281284264,3.77003198860293));
#224478=CARTESIAN_POINT('Origin',(5.49031038273072E-15,1.82930781209959E-13,
3.77003198860263));
#224479=CARTESIAN_POINT('',(45.4132815019358,41.3175407208296,3.77003198860292));
#224480=CARTESIAN_POINT('Origin',(5.57972911860581E-15,1.8736496251029E-13,
3.13503198860263));
#224481=CARTESIAN_POINT('Origin',(40.3862573897244,44.378979117547,3.13502491541459));
#224482=CARTESIAN_POINT('Origin',(44.3789791175466,40.3862573897247,3.13502491541461));
#224483=CARTESIAN_POINT('Origin',(5.57972911860581E-15,1.8736496251029E-13,
3.13503198860263));
#224484=CARTESIAN_POINT('Origin',(41.6603666103045,45.793978104926,3.20381846780249));
#224485=CARTESIAN_POINT('Origin',(45.7939778018837,41.6603663369562,3.20382022872035));
#224486=CARTESIAN_POINT('Origin',(5.51210908043506E-15,1.8401175575949E-13,
3.61523028058481));
#224487=CARTESIAN_POINT('Origin',(41.0717150501554,45.140319869523,3.58786945046952));
#224488=CARTESIAN_POINT('Origin',(45.1402498046841,41.0716522820273,3.58781461834098));
#224489=CARTESIAN_POINT('Origin',(5.51210908043507E-15,1.8401175575949E-13,
3.61523028058481));
#224490=CARTESIAN_POINT('Origin',(40.9494366077803,45.0043926651426,3.58781440266742));
#224491=CARTESIAN_POINT('Origin',(45.0043225899514,40.9493738530214,3.58786923593014));
#224492=CARTESIAN_POINT('Origin',(60.4792282238308,1.82930781209959E-13,
3.77003198860263));
#224493=CARTESIAN_POINT('',(48.3573835402119,35.5261472678868,3.77003198860288));
#224494=CARTESIAN_POINT('',(44.8038810887674,39.9143573409159,3.77003198860291));
#224495=CARTESIAN_POINT('Origin',(5.49031038273072E-15,1.82930781209959E-13,
3.77003198860263));
#224496=CARTESIAN_POINT('',(45.1566551325075,40.2319965165889,3.77003198860291));
#224497=CARTESIAN_POINT('',(33.6129634723596,29.8380098596984,3.77003198860284));
#224498=CARTESIAN_POINT('',(45.1570399302682,40.2315646150501,3.77003198902562));
#224499=CARTESIAN_POINT('Origin',(5.49031038273072E-15,1.82930781209959E-13,
3.77003198860263));
#224500=CARTESIAN_POINT('',(48.7410849259197,35.8056376404642,3.77003198882112));
#224501=CARTESIAN_POINT('Origin',(5.49031038273072E-15,1.82930781209959E-13,
3.77003198860263));
#224502=CARTESIAN_POINT('',(48.7414273857055,35.8051714542879,3.77003198860288));
#224503=CARTESIAN_POINT('Origin',(5.49031038273072E-15,1.82930781209959E-13,
3.77003198860263));
#224504=CARTESIAN_POINT('',(48.3578184660151,35.5264632599794,3.77003198860288));
#224505=CARTESIAN_POINT('Origin',(5.49031038273072E-15,1.82930781209959E-13,
3.77003198860263));
#224506=CARTESIAN_POINT('',(45.2779489569772,40.3404336838195,3.4882302805851));
#224507=CARTESIAN_POINT('',(45.1570399297215,40.231564614563,3.77003198860292));
#224508=CARTESIAN_POINT('',(48.8727133450222,35.9012693630581,3.4882302807483));
#224509=CARTESIAN_POINT('Origin',(5.52999282761009E-15,1.84898592019556E-13,
3.48823028058481));
#224510=CARTESIAN_POINT('',(48.8727133447943,35.9012693628907,3.48823028058507));
#224511=CARTESIAN_POINT('Origin',(60.71525,1.85785428279622E-13,3.36123028058482));
#224512=CARTESIAN_POINT('',(49.0510171431403,36.0301015792679,3.36123028058508));
#224513=CARTESIAN_POINT('',(45.4410373245171,40.4880553924346,3.3612302805851));
#224514=CARTESIAN_POINT('Origin',(5.5478765747851E-15,1.85785428279622E-13,
3.36123028058482));
#224515=CARTESIAN_POINT('',(45.5534068532511,40.5892333705625,3.36123028058511));
#224516=CARTESIAN_POINT('',(33.7433098572246,29.9553742717904,3.36123028058502));
#224517=CARTESIAN_POINT('',(49.1733470784087,36.1189794796885,3.36123028058508));
#224518=CARTESIAN_POINT('Origin',(5.5478765747851E-15,1.85785428279622E-13,
3.36123028058482));
#224519=CARTESIAN_POINT('',(49.0514459419945,36.0304131198714,3.36123028058508));
#224520=CARTESIAN_POINT('Origin',(5.5478765747851E-15,1.85785428279622E-13,
3.36123028058482));
#224521=CARTESIAN_POINT('',(49.3516463037384,36.2478178023253,3.4882302805851));
#224522=CARTESIAN_POINT('',(45.7165002430348,40.7368493367119,3.48823028042724));
#224523=CARTESIAN_POINT('Origin',(5.52999282761008E-15,1.84898592019556E-13,
3.48823028058484));
#224524=CARTESIAN_POINT('',(45.8374112534712,40.8457160731799,3.77003198802736));
#224525=CARTESIAN_POINT('',(45.7165002428306,40.73684933653,3.48823028058513));
#224526=CARTESIAN_POINT('',(45.8377889771251,40.8452921850246,3.77003198860292));
#224527=CARTESIAN_POINT('Origin',(5.49031038273072E-15,1.82930781209959E-13,
3.77003198860263));
#224528=CARTESIAN_POINT('',(49.4829367616345,36.3439095507838,3.77003198860289));
#224529=CARTESIAN_POINT('Origin',(5.49031038273072E-15,1.82930781209959E-13,
3.77003198860263));
#224530=CARTESIAN_POINT('',(49.4832728536532,36.343451949995,3.77003198802746));
#224531=CARTESIAN_POINT('Origin',(5.49031038273072E-15,1.82930781209959E-13,
3.77003198860263));
#224532=CARTESIAN_POINT('',(49.48327285393,36.3434519501792,3.77003198860289));
#224533=CARTESIAN_POINT('Origin',(62.2224557307631,1.82930781209959E-13,
3.77003198860263));
#224534=CARTESIAN_POINT('',(46.1905628026484,41.1629311642483,3.77003198860292));
#224535=CARTESIAN_POINT('',(34.5756856720385,30.7048488218246,3.77003198860284));
#224536=CARTESIAN_POINT('',(49.8669803696025,36.6229335645812,3.77003198860289));
#224537=CARTESIAN_POINT('Origin',(5.49031038273072E-15,1.82930781209959E-13,
3.77003198860263));
#224538=CARTESIAN_POINT('',(49.4833618317452,36.3442183822966,3.77003198860289));
#224539=CARTESIAN_POINT('Origin',(5.57972911860581E-15,1.8736496251029E-13,
3.13503198860263));
#224540=CARTESIAN_POINT('Origin',(44.8038837346038,39.9143530044123,3.13502491541461));
#224541=CARTESIAN_POINT('Origin',(48.3573798485713,35.5261507575156,3.13502491541455));
#224542=CARTESIAN_POINT('Origin',(5.57972911860581E-15,1.8736496251029E-13,
3.13503198860263));
#224543=CARTESIAN_POINT('Origin',(46.2189209212384,41.1884198004221,3.20381846780305));
#224544=CARTESIAN_POINT('Origin',(49.8978076723488,36.6453723646243,3.20382022871834));
#224545=CARTESIAN_POINT('Origin',(5.51210908043506E-15,1.8401175575949E-13,
3.61523028058481));
#224546=CARTESIAN_POINT('Origin',(45.5651681650784,40.5998732162089,3.58786945046786));
#224547=CARTESIAN_POINT('Origin',(49.1861234900541,36.1282165298258,3.58781461834413));
#224548=CARTESIAN_POINT('Origin',(5.51210908043507E-15,1.8401175575949E-13,
3.61523028058481));
#224549=CARTESIAN_POINT('Origin',(45.4293513150117,40.4774722129473,3.58781440266322));
#224550=CARTESIAN_POINT('Origin',(49.0381593225504,36.0208162177234,3.58786923592905));
#224551=CARTESIAN_POINT('Origin',(60.4792282238308,1.82930781209959E-13,
3.77003198860263));
#224552=CARTESIAN_POINT('',(51.8059703131946,30.2768083268883,3.77003198860285));
#224553=CARTESIAN_POINT('',(48.7306271754176,35.0124214764587,3.77003198860288));
#224554=CARTESIAN_POINT('Origin',(5.49031038273072E-15,1.82930781209959E-13,
3.77003198860263));
#224555=CARTESIAN_POINT('',(49.1146710209415,35.2914456628193,3.77003198860288));
#224556=CARTESIAN_POINT('',(39.7707905934405,28.5027191556742,3.77003198860283));
#224557=CARTESIAN_POINT('',(49.1150085647359,35.290975904964,3.77003198902583));
#224558=CARTESIAN_POINT('Origin',(5.49031038273072E-15,1.82930781209959E-13,
3.77003198860263));
#224559=CARTESIAN_POINT('',(52.2167844417078,30.5146599057594,3.77003198882108));
#224560=CARTESIAN_POINT('Origin',(5.49031038273072E-15,1.82930781209959E-13,
3.77003198860263));
#224561=CARTESIAN_POINT('',(52.2170762957385,30.5141604766047,3.77003198860285));
#224562=CARTESIAN_POINT('Origin',(5.49031038273072E-15,1.82930781209959E-13,
3.77003198860263));
#224563=CARTESIAN_POINT('',(51.8064358865966,30.2770771258173,3.77003198860285));
#224564=CARTESIAN_POINT('Origin',(5.49031038273072E-15,1.82930781209959E-13,
3.77003198860263));
#224565=CARTESIAN_POINT('',(49.2466351556012,35.3866101428262,3.48823028058506));
#224566=CARTESIAN_POINT('',(49.115008564141,35.2909759045365,3.77003198860288));
#224567=CARTESIAN_POINT('',(52.3576880235603,30.5960088313998,3.48823028074826));
#224568=CARTESIAN_POINT('Origin',(5.52999282761009E-15,1.84898592019556E-13,
3.48823028058481));
#224569=CARTESIAN_POINT('',(52.3576880233162,30.5960088312571,3.48823028058503));
#224570=CARTESIAN_POINT('Origin',(60.71525,1.85785428279622E-13,3.36123028058482));
#224571=CARTESIAN_POINT('',(52.5484816883959,30.7054974692372,3.36123028058504));
#224572=CARTESIAN_POINT('',(49.424260778346,35.5163757878398,3.36123028058507));
#224573=CARTESIAN_POINT('Origin',(5.5478765747851E-15,1.85785428279622E-13,
3.36123028058482));
#224574=CARTESIAN_POINT('',(49.5465907136144,35.6052536882604,3.36123028058507));
#224575=CARTESIAN_POINT('',(39.9252688514646,28.6149541797808,3.36123028058502));
#224576=CARTESIAN_POINT('',(52.6794317578287,30.7811015270746,3.36123028058504));
#224577=CARTESIAN_POINT('Origin',(5.5478765747851E-15,1.85785428279622E-13,
3.36123028058482));
#224578=CARTESIAN_POINT('',(52.5489407031056,30.7057624815034,3.36123028058504));
#224579=CARTESIAN_POINT('Origin',(5.5478765747851E-15,1.85785428279622E-13,
3.36123028058482));
#224580=CARTESIAN_POINT('',(52.8702215132216,30.8905967158739,3.48823028058506));
#224581=CARTESIAN_POINT('',(49.7242207308395,35.7350130972988,3.4882302804272));
#224582=CARTESIAN_POINT('Origin',(5.52999282761008E-15,1.84898592019556E-13,
3.48823028058484));
#224583=CARTESIAN_POINT('',(49.8558490507736,35.8306448082805,3.77003198802733));
#224584=CARTESIAN_POINT('',(49.7242207306174,35.7350130971392,3.4882302805851));
#224585=CARTESIAN_POINT('',(49.8561803968403,35.8301837593557,3.77003198860288));
#224586=CARTESIAN_POINT('Origin',(5.49031038273072E-15,1.82930781209959E-13,
3.77003198860263));
#224587=CARTESIAN_POINT('',(53.0108370710512,30.9724384738745,3.77003198860285));
#224588=CARTESIAN_POINT('Origin',(5.49031038273072E-15,1.82930781209959E-13,
3.77003198860263));
#224589=CARTESIAN_POINT('',(53.0111234896153,30.9719482486884,3.77003198802743));
#224590=CARTESIAN_POINT('Origin',(5.49031038273072E-15,1.82930781209959E-13,
3.77003198860263));
#224591=CARTESIAN_POINT('',(53.01112348991,30.9719482488427,3.77003198860285));
#224592=CARTESIAN_POINT('Origin',(62.2224557307631,1.82930781209959E-13,
3.77003198860263));
#224593=CARTESIAN_POINT('',(50.2402240048083,36.1092077731531,3.77003198860289));
#224594=CARTESIAN_POINT('',(40.9117478092586,29.3316730956006,3.77003198860284));
#224595=CARTESIAN_POINT('',(53.4219427993286,31.2097904767608,3.77003198860285));
#224596=CARTESIAN_POINT('Origin',(5.49031038273072E-15,1.82930781209959E-13,
3.77003198860263));
#224597=CARTESIAN_POINT('',(53.0112920942667,30.9727011816505,3.77003198860285));
#224598=CARTESIAN_POINT('Origin',(5.57972911860581E-15,1.8736496251029E-13,
3.13503198860263));
#224599=CARTESIAN_POINT('Origin',(48.7306293534718,35.0124168871457,3.13502491541459));
#224600=CARTESIAN_POINT('Origin',(51.8059670065428,30.276812183282,3.13502491541455));
#224601=CARTESIAN_POINT('Origin',(5.57972911860581E-15,1.8736496251029E-13,
3.13503198860263));
#224602=CARTESIAN_POINT('Origin',(50.2710910626284,36.1315925493517,3.20381846780242));
#224603=CARTESIAN_POINT('Origin',(53.4549467201727,31.2288840241313,3.20382022872574));
#224604=CARTESIAN_POINT('Origin',(5.51210908043506E-15,1.8401175575949E-13,
3.61523028058481));
#224605=CARTESIAN_POINT('Origin',(49.5593997624585,35.614605855867,3.58786945047113));
#224606=CARTESIAN_POINT('Origin',(52.6931037136114,30.78895247701,3.58781461834159));
#224607=CARTESIAN_POINT('Origin',(5.51210908043507E-15,1.8401175575949E-13,
3.61523028058481));
#224608=CARTESIAN_POINT('Origin',(49.4115325425393,35.5070721047293,3.5878144026661));
#224609=CARTESIAN_POINT('Origin',(52.5347237197189,30.6976069821031,3.58786923592938));
#224610=CARTESIAN_POINT('Origin',(60.4792282238308,1.82930781209959E-13,
3.77003198860263));
#224611=CARTESIAN_POINT('',(54.6869600343297,24.695750338031,3.77003198860281));
#224612=CARTESIAN_POINT('',(52.1234703131946,29.7268821954852,3.77003198860284));
#224613=CARTESIAN_POINT('Origin',(5.49031038273072E-15,1.82930781209959E-13,
3.77003198860263));
#224614=CARTESIAN_POINT('',(52.5345762957643,29.9642343451581,3.77003198860284));
#224615=CARTESIAN_POINT('',(45.518171167873,25.9133109558558,3.77003198860281));
#224616=CARTESIAN_POINT('',(52.5348628873916,29.9637318777512,3.77003198902563));
#224617=CARTESIAN_POINT('Origin',(5.49031038273072E-15,1.82930781209959E-13,
3.77003198860263));
#224618=CARTESIAN_POINT('',(55.1203859400879,24.8893571715241,3.77003198882105));
#224619=CARTESIAN_POINT('Origin',(5.49031038273072E-15,1.82930781209959E-13,
3.77003198860263));
#224620=CARTESIAN_POINT('',(55.1206239907496,24.8888299712412,3.77003198860281));
#224621=CARTESIAN_POINT('Origin',(5.49031038273072E-15,1.82930781209959E-13,
3.77003198860263));
#224622=CARTESIAN_POINT('',(54.6874511544109,24.6959689987791,3.77003198860281));
#224623=CARTESIAN_POINT('Origin',(5.49031038273072E-15,1.82930781209959E-13,
3.77003198860263));
#224624=CARTESIAN_POINT('',(52.6757649139395,30.0450834959839,3.48823028058503));
#224625=CARTESIAN_POINT('',(52.5348628867555,29.9637318773884,3.77003198860284));
#224626=CARTESIAN_POINT('',(55.2690209155617,24.9555320243581,3.48823028074822));
#224627=CARTESIAN_POINT('Origin',(5.52999282761009E-15,1.84898592019556E-13,
3.48823028058481));
#224628=CARTESIAN_POINT('',(55.269020915304,24.9555320242418,3.48823028058499));
#224629=CARTESIAN_POINT('Origin',(60.71525,1.85785428279622E-13,3.36123028058482));
#224630=CARTESIAN_POINT('',(55.4702140717966,25.044477503395,3.361230280585));
#224631=CARTESIAN_POINT('',(52.8659816883959,30.155571337834,3.36123028058503));
#224632=CARTESIAN_POINT('Origin',(5.5478765747851E-15,1.85785428279622E-13,
3.36123028058482));
#224633=CARTESIAN_POINT('',(52.9969317578287,30.2311753956715,3.36123028058503));
#224634=CARTESIAN_POINT('',(45.6951875,26.0155113828602,3.361230280585));
#224635=CARTESIAN_POINT('',(55.6083495590301,25.1059793847704,3.361230280585));
#224636=CARTESIAN_POINT('Origin',(5.5478765747851E-15,1.85785428279622E-13,
3.36123028058482));
#224637=CARTESIAN_POINT('',(55.4706982733007,25.0446930837941,3.361230280585));
#224638=CARTESIAN_POINT('Origin',(5.5478765747851E-15,1.85785428279622E-13,
3.36123028058482));
#224639=CARTESIAN_POINT('',(55.8095395120007,25.1949317875303,3.48823028058502));
#224640=CARTESIAN_POINT('',(53.187152250855,30.3416565763594,3.48823028042716));
#224641=CARTESIAN_POINT('Origin',(5.52999282761008E-15,1.84898592019556E-13,
3.48823028058484));
#224642=CARTESIAN_POINT('',(53.3280557328685,30.423005500817,3.77003198802729));
#224643=CARTESIAN_POINT('',(53.1871522506175,30.3416565762239,3.48823028058506));
#224644=CARTESIAN_POINT('',(53.3283370710512,30.4225123424714,3.77003198860285));
#224645=CARTESIAN_POINT('Origin',(5.49031038273072E-15,1.82930781209959E-13,
3.77003198860263));
#224646=CARTESIAN_POINT('',(55.9579395562866,25.2616268796459,3.77003198860281));
#224647=CARTESIAN_POINT('Origin',(5.49031038273072E-15,1.82930781209959E-13,
3.77003198860263));
#224648=CARTESIAN_POINT('',(55.9581731633345,25.2611094010724,3.77003198802739));
#224649=CARTESIAN_POINT('Origin',(5.49031038273072E-15,1.82930781209959E-13,
3.77003198860263));
#224650=CARTESIAN_POINT('',(55.9581731636437,25.261109401195,3.77003198860281));
#224651=CARTESIAN_POINT('Origin',(62.2224557307631,1.82930781209959E-13,
3.77003198860263));
#224652=CARTESIAN_POINT('',(53.7394427993286,30.6598643453577,3.77003198860285));
#224653=CARTESIAN_POINT('',(46.8255917980722,26.6681506086454,3.77003198860282));
#224654=CARTESIAN_POINT('',(56.391603244485,25.4547063934086,3.77003198860281));
#224655=CARTESIAN_POINT('Origin',(5.49031038273072E-15,1.82930781209959E-13,
3.77003198860263));
#224656=CARTESIAN_POINT('',(55.9584195472775,25.2618405854037,3.77003198860281));
#224657=CARTESIAN_POINT('Origin',(5.57972911860581E-15,1.8736496251029E-13,
3.13503198860263));
#224658=CARTESIAN_POINT('Origin',(52.1234719996034,29.7268774036441,3.13502491541453));
#224659=CARTESIAN_POINT('Origin',(54.6869571488949,24.6957545189382,3.13502491541452));
#224660=CARTESIAN_POINT('Origin',(5.57972911860581E-15,1.8736496251029E-13,
3.13503198860263));
#224661=CARTESIAN_POINT('Origin',(53.7724806104344,30.6789000092885,3.20381846780295));
#224662=CARTESIAN_POINT('Origin',(56.4264221855617,25.4702454951996,3.20382022872323));
#224663=CARTESIAN_POINT('Origin',(5.51210908043506E-15,1.8401175575949E-13,
3.61523028058481));
#224664=CARTESIAN_POINT('Origin',(53.0106482050721,30.2391374209343,3.58786945046861));
#224665=CARTESIAN_POINT('Origin',(55.62276726614,25.1123582178526,3.58781461834227));
#224666=CARTESIAN_POINT('Origin',(5.51210908043507E-15,1.8401175575949E-13,
3.61523028058481));
#224667=CARTESIAN_POINT('Origin',(52.8523506794959,30.1476490842084,3.58781440266723));
#224668=CARTESIAN_POINT('Origin',(55.4557066902163,25.0380683404988,3.58786923592829));
#224669=CARTESIAN_POINT('Origin',(60.4792282238308,1.82930781209959E-13,
3.77003198860263));
#224670=CARTESIAN_POINT('',(56.9687879773466,18.8441205405522,3.77003198860277));
#224671=CARTESIAN_POINT('',(54.9452378026828,24.1156489724279,3.7700319886028));
#224672=CARTESIAN_POINT('Origin',(5.49031038273072E-15,1.82930781209959E-13,
3.77003198860263));
#224673=CARTESIAN_POINT('',(55.3789017591239,24.3087286055922,3.7700319886028));
#224674=CARTESIAN_POINT('',(50.6030043228557,22.1823620689018,3.77003198860279));
#224675=CARTESIAN_POINT('',(55.3791342586263,24.3081989337719,3.77003198902557));
#224676=CARTESIAN_POINT('Origin',(5.49031038273072E-15,1.82930781209959E-13,
3.77003198860263));
#224677=CARTESIAN_POINT('',(57.4200769554261,18.9913614316847,3.770031988821));
#224678=CARTESIAN_POINT('Origin',(5.49031038273072E-15,1.82930781209959E-13,
3.77003198860263));
#224679=CARTESIAN_POINT('',(57.420258594586,18.9908122363903,3.77003198860277));
#224680=CARTESIAN_POINT('Origin',(5.49031038273072E-15,1.82930781209959E-13,
3.77003198860263));
#224681=CARTESIAN_POINT('',(56.9692992632926,18.8442866674264,3.77003198860277));
#224682=CARTESIAN_POINT('Origin',(5.49031038273072E-15,1.82930781209959E-13,
3.77003198860263));
#224683=CARTESIAN_POINT('',(55.5277679687683,24.3743766270217,3.48823028058499));
#224684=CARTESIAN_POINT('',(55.3791342579558,24.3081989334776,3.7700319886028));
#224685=CARTESIAN_POINT('',(57.574814848626,19.0416371861768,3.48823028074819));
#224686=CARTESIAN_POINT('Origin',(5.52999282761009E-15,1.84898592019556E-13,
3.48823028058481));
#224687=CARTESIAN_POINT('',(57.5748148483576,19.041637186088,3.48823028058495));
#224688=CARTESIAN_POINT('Origin',(60.71525,1.85785428279622E-13,3.36123028058482));
#224689=CARTESIAN_POINT('',(57.7842031819382,19.1090650011318,3.36123028058496));
#224690=CARTESIAN_POINT('',(55.7284918401498,24.464376137792,3.36123028058499));
#224691=CARTESIAN_POINT('Origin',(5.5478765747851E-15,1.85785428279622E-13,
3.36123028058482));
#224692=CARTESIAN_POINT('',(55.8666273273833,24.5258780191674,3.36123028058499));
#224693=CARTESIAN_POINT('',(50.7999799080414,22.2700612497319,3.36123028058498));
#224694=CARTESIAN_POINT('',(57.9280106456676,19.1557908785627,3.36123028058496));
#224695=CARTESIAN_POINT('Origin',(5.5478765747851E-15,1.85785428279622E-13,
3.36123028058482));
#224696=CARTESIAN_POINT('',(57.7847072652236,19.1092287877198,3.36123028058496));
#224697=CARTESIAN_POINT('Origin',(5.5478765747851E-15,1.85785428279622E-13,
3.36123028058482));
#224698=CARTESIAN_POINT('',(58.1373965169893,19.2232259141442,3.48823028058498));
#224699=CARTESIAN_POINT('',(56.067354200683,24.6158705165696,3.48823028042713));
#224700=CARTESIAN_POINT('Origin',(5.52999282761008E-15,1.84898592019556E-13,
3.48823028058484));
#224701=CARTESIAN_POINT('',(56.2159890767411,24.6820453786634,3.77003198802725));
#224702=CARTESIAN_POINT('',(56.0673542004326,24.6158705164596,3.48823028058502));
#224703=CARTESIAN_POINT('',(56.2162173246397,24.6815255140429,3.77003198860281));
#224704=CARTESIAN_POINT('Origin',(5.49031038273072E-15,1.82930781209959E-13,
3.77003198860263));
#224705=CARTESIAN_POINT('',(58.2919551457916,19.2740436149887,3.77003198860277));
#224706=CARTESIAN_POINT('Origin',(5.49031038273072E-15,1.82930781209959E-13,
3.77003198860263));
#224707=CARTESIAN_POINT('',(58.2921333818757,19.2735045526312,3.77003198802735));
#224708=CARTESIAN_POINT('Origin',(5.49031038273072E-15,1.82930781209959E-13,
3.77003198860263));
#224709=CARTESIAN_POINT('',(58.2921333821959,19.2735045527209,3.77003198860277));
#224710=CARTESIAN_POINT('Origin',(62.2224557307631,1.82930781209959E-13,
3.77003198860263));
#224711=CARTESIAN_POINT('',(56.6498810128382,24.8746050278055,3.77003198860281));
#224712=CARTESIAN_POINT('',(52.0578415156894,22.8300973196051,3.77003198860279));
#224713=CARTESIAN_POINT('',(58.7434254837932,19.4207352200703,3.77003198860277));
#224714=CARTESIAN_POINT('Origin',(5.49031038273072E-15,1.82930781209959E-13,
3.77003198860263));
#224715=CARTESIAN_POINT('',(58.2924548456761,19.2742059773234,3.77003198860277));
#224716=CARTESIAN_POINT('Origin',(5.57972911860581E-15,1.8736496251029E-13,
3.13503198860263));
#224717=CARTESIAN_POINT('Origin',(54.9452389789695,24.1156440305594,3.1350249154145));
#224718=CARTESIAN_POINT('Origin',(56.9687855447424,18.8441250001659,3.13502491541445));
#224719=CARTESIAN_POINT('Origin',(5.57972911860581E-15,1.8736496251029E-13,
3.13503198860263));
#224720=CARTESIAN_POINT('Origin',(56.6847276080577,24.8900830207505,3.20381846780404));
#224721=CARTESIAN_POINT('Origin',(58.7796779614983,19.4325496266339,3.20382022872385));
#224722=CARTESIAN_POINT('Origin',(5.51210908043506E-15,1.8401175575949E-13,
3.61523028058481));
#224723=CARTESIAN_POINT('Origin',(55.8811008927585,24.5323626684708,3.58786945046915));
#224724=CARTESIAN_POINT('Origin',(57.943016140689,19.1606277069619,3.58781461834233));
#224725=CARTESIAN_POINT('Origin',(5.51210908043507E-15,1.8401175575949E-13,
3.61523028058481));
#224726=CARTESIAN_POINT('Origin',(55.7141074023463,24.4579221115114,3.58781440266683));
#224727=CARTESIAN_POINT('Origin',(57.7691053333667,19.1042073826001,3.58786923593115));
#224728=CARTESIAN_POINT('Origin',(60.4792282238308,1.82930781209959E-13,
3.77003198860263));
#224729=CARTESIAN_POINT('',(58.6264539577984,12.7860306150453,3.77003198860272));
#224730=CARTESIAN_POINT('',(57.1650137687747,18.2401996527048,3.77003198860276));
#224731=CARTESIAN_POINT('Origin',(5.49031038273072E-15,1.82930781209959E-13,
3.77003198860263));
#224732=CARTESIAN_POINT('',(57.6164843860303,18.386891348495,3.77003198860276));
#224733=CARTESIAN_POINT('',(54.8020887275094,17.4724387660757,3.77003198860276));
#224734=CARTESIAN_POINT('',(57.6166602460946,18.3863402754566,3.77003198902546));
#224735=CARTESIAN_POINT('Origin',(5.49031038273072E-15,1.82930781209959E-13,
3.77003198860263));
#224736=CARTESIAN_POINT('',(59.0906615917171,12.8852923618019,3.77003198882096));
#224737=CARTESIAN_POINT('Origin',(5.49031038273072E-15,1.82930781209959E-13,
3.77003198860263));
#224738=CARTESIAN_POINT('',(59.0907848292984,12.8847271885945,3.77003198860272));
#224739=CARTESIAN_POINT('Origin',(5.49031038273072E-15,1.82930781209959E-13,
3.77003198860263));
#224740=CARTESIAN_POINT('',(58.6269798078533,12.786142387925,3.77003198860272));
#224741=CARTESIAN_POINT('Origin',(5.49031038273072E-15,1.82930781209959E-13,
3.77003198860263));
#224742=CARTESIAN_POINT('',(57.7713971777987,18.4366189870675,3.48823028058495));
#224743=CARTESIAN_POINT('',(57.6166602453971,18.386340275234,3.77003198860276));
#224744=CARTESIAN_POINT('',(59.2498070619042,12.919118186265,3.48823028074814));
#224745=CARTESIAN_POINT('Origin',(5.52999282761009E-15,1.84898592019556E-13,
3.48823028058481));
#224746=CARTESIAN_POINT('',(59.249807061628,12.9191181862048,3.48823028058491));
#224747=CARTESIAN_POINT('Origin',(60.71525,1.85785428279622E-13,3.36123028058482));
#224748=CARTESIAN_POINT('',(59.4650964698966,12.9642895838873,3.36123028058491));
#224749=CARTESIAN_POINT('',(57.9804289733663,18.5051441132844,3.36123028058495));
#224750=CARTESIAN_POINT('Origin',(5.5478765747851E-15,1.85785428279622E-13,
3.36123028058482));
#224751=CARTESIAN_POINT('',(58.1242364370956,18.5518699907153,3.36123028058495));
#224752=CARTESIAN_POINT('',(55.0155724295758,17.5418038257018,3.36123028058494));
#224753=CARTESIAN_POINT('',(59.6130003254555,12.9957275188826,3.36123028058491));
#224754=CARTESIAN_POINT('Origin',(5.5478765747851E-15,1.85785428279622E-13,
3.36123028058482));
#224755=CARTESIAN_POINT('',(59.4656149121214,12.964399782184,3.36123028058491));
#224756=CARTESIAN_POINT('Origin',(5.5478765747851E-15,1.85785428279622E-13,
3.36123028058482));
#224757=CARTESIAN_POINT('',(59.8282880397055,13.0409063549241,3.48823028058494));
#224758=CARTESIAN_POINT('',(58.3332704850401,18.6203878281981,3.48823028042708));
#224759=CARTESIAN_POINT('Origin',(5.52999282761008E-15,1.84898592019556E-13,
3.48823028058484));
#224760=CARTESIAN_POINT('',(58.4880082803368,18.6706636022911,3.77003198802721));
#224761=CARTESIAN_POINT('',(58.3332704847796,18.620387828115,3.48823028058497));
#224762=CARTESIAN_POINT('',(58.4881809372197,18.6701227271413,3.77003198860276));
#224763=CARTESIAN_POINT('Origin',(5.49031038273072E-15,1.82930781209959E-13,
3.77003198860263));
#224764=CARTESIAN_POINT('',(59.9873118763436,13.0752898951327,3.77003198860272));
#224765=CARTESIAN_POINT('Origin',(5.49031038273072E-15,1.82930781209959E-13,
3.77003198860263));
#224766=CARTESIAN_POINT('',(59.9874327886718,13.0747351550713,3.7700319880273));
#224767=CARTESIAN_POINT('Origin',(5.49031038273072E-15,1.82930781209959E-13,
3.77003198860263));
#224768=CARTESIAN_POINT('',(59.9874327889997,13.074735155127,3.77003198860272));
#224769=CARTESIAN_POINT('Origin',(62.2224557307631,1.82930781209959E-13,
3.77003198860263));
#224770=CARTESIAN_POINT('',(58.9396512752213,18.8168143322229,3.77003198860277));
#224771=CARTESIAN_POINT('',(56.3788528200606,17.9847604760584,3.77003198860276));
#224772=CARTESIAN_POINT('',(60.4516424606489,13.1739864076109,3.77003198860273));
#224773=CARTESIAN_POINT('Origin',(5.49031038273072E-15,1.82930781209959E-13,
3.77003198860263));
#224774=CARTESIAN_POINT('',(59.9878258103051,13.0753991351685,3.77003198860272));
#224775=CARTESIAN_POINT('Origin',(5.57972911860581E-15,1.8736496251029E-13,
3.13503198860263));
#224776=CARTESIAN_POINT('Origin',(57.1650144220517,18.2401946149527,3.13502491541448));
#224777=CARTESIAN_POINT('Origin',(58.6264520046768,12.7860353045052,3.13502491541442));
#224778=CARTESIAN_POINT('Origin',(5.57972911860581E-15,1.8736496251029E-13,
3.13503198860263));
#224779=CARTESIAN_POINT('Origin',(58.9759248679598,18.8285650740607,3.20381846780176));
#224780=CARTESIAN_POINT('Origin',(60.48893128525,13.1819466778333,3.20382022872223));
#224781=CARTESIAN_POINT('Origin',(5.51210908043506E-15,1.8401175575949E-13,
3.61523028058481));
#224782=CARTESIAN_POINT('Origin',(58.1393085451921,18.5568062168848,3.58786945046851));
#224783=CARTESIAN_POINT('Origin',(59.6284292050456,12.9989693492946,3.58781461834058));
#224784=CARTESIAN_POINT('Origin',(5.51210908043507E-15,1.8401175575949E-13,
3.61523028058481));
#224785=CARTESIAN_POINT('Origin',(57.9654487055676,18.5002290260159,3.58781440266516));
#224786=CARTESIAN_POINT('Origin',(59.4495735695174,12.9610367308101,3.58786923592919));
#224787=CARTESIAN_POINT('Origin',(60.4792282238308,1.82930781209959E-13,
3.77003198860263));
#224788=CARTESIAN_POINT('',(59.6417962403143,6.58785426247114,3.77003198860268));
#224789=CARTESIAN_POINT('',(58.7584778814676,12.1649068885794,3.77003198860272));
#224790=CARTESIAN_POINT('Origin',(5.49031038273072E-15,1.82930781209959E-13,
3.77003198860263));
#224791=CARTESIAN_POINT('',(59.2228087529788,12.2636034620792,3.77003198860272));
#224792=CARTESIAN_POINT('',(57.9308881865554,11.9889972685553,3.77003198860272));
#224793=CARTESIAN_POINT('',(59.2229260468459,12.2630370254944,3.77003198902565));
#224794=CARTESIAN_POINT('Origin',(5.49031038273072E-15,1.82930781209959E-13,
3.77003198860263));
#224795=CARTESIAN_POINT('',(60.1138365740932,6.63804933238237,3.77003198882092));
#224796=CARTESIAN_POINT('Origin',(5.49031038273072E-15,1.82930781209959E-13,
3.77003198860263));
#224797=CARTESIAN_POINT('',(60.1139000598794,6.63747437341796,3.77003198860268));
#224798=CARTESIAN_POINT('Origin',(5.49031038273072E-15,1.82930781209959E-13,
3.77003198860263));
#224799=CARTESIAN_POINT('',(59.6423308931549,6.58791045674909,3.77003198860268));
#224800=CARTESIAN_POINT('Origin',(5.49031038273072E-15,1.82930781209959E-13,
3.77003198860263));
#224801=CARTESIAN_POINT('',(59.3820708699071,12.2968658913805,3.4882302805849));
#224802=CARTESIAN_POINT('',(59.2229260461285,12.2630370253459,3.77003198860272));
#224803=CARTESIAN_POINT('',(60.2756459901929,6.65505462400517,3.48823028074809));
#224804=CARTESIAN_POINT('Origin',(5.52999282761009E-15,1.84898592019556E-13,
3.48823028058481));
#224805=CARTESIAN_POINT('',(60.2756459899119,6.65505462397414,3.48823028058486));
#224806=CARTESIAN_POINT('Origin',(60.71525,1.85785428279622E-13,3.36123028058482));
#224807=CARTESIAN_POINT('',(60.4944777170594,6.67747469700965,3.36123028058487));
#224808=CARTESIAN_POINT('',(59.5971203935659,12.3431658574213,3.36123028058491));
#224809=CARTESIAN_POINT('Origin',(5.5478765747851E-15,1.85785428279622E-13,
3.36123028058482));
#224810=CARTESIAN_POINT('',(59.7450242491248,12.3746037924166,3.36123028058491));
#224811=CARTESIAN_POINT('',(58.1567073854021,12.0369966210212,3.36123028058491));
#224812=CARTESIAN_POINT('',(60.6448574988554,6.69328024897474,3.36123028058487));
#224813=CARTESIAN_POINT('Origin',(5.5478765747851E-15,1.85785428279622E-13,
3.36123028058482));
#224814=CARTESIAN_POINT('',(60.495004838062,6.67753009965952,3.36123028058487));
#224815=CARTESIAN_POINT('Origin',(5.5478765747851E-15,1.85785428279622E-13,
3.36123028058482));
#224816=CARTESIAN_POINT('',(60.8636883187845,6.71570789669429,3.48823028058489));
#224817=CARTESIAN_POINT('',(59.9600752509415,12.4208962742143,3.48823028042704));
#224818=CARTESIAN_POINT('Origin',(5.52999282761008E-15,1.84898592019556E-13,
3.48823028058484));
#224819=CARTESIAN_POINT('',(60.1192206258106,12.4547221284046,3.77003198802716));
#224820=CARTESIAN_POINT('',(59.9600752506737,12.4208962741588,3.48823028058493));
#224821=CARTESIAN_POINT('',(60.1193358000128,12.4541661686668,3.77003198860272));
#224822=CARTESIAN_POINT('Origin',(5.49031038273072E-15,1.82930781209959E-13,
3.77003198860263));
#224823=CARTESIAN_POINT('',(61.0254350648262,6.73328056300537,3.77003198860268));
#224824=CARTESIAN_POINT('Origin',(5.49031038273072E-15,1.82930781209959E-13,
3.77003198860263));
#224825=CARTESIAN_POINT('',(61.025497328658,6.73271622308816,3.77003198802725));
#224826=CARTESIAN_POINT('Origin',(5.49031038273072E-15,1.82930781209959E-13,
3.77003198860263));
#224827=CARTESIAN_POINT('',(61.0254973289899,6.73271622310927,3.77003198860268));
#224828=CARTESIAN_POINT('Origin',(62.2224557307631,1.82930781209959E-13,
3.77003198860263));
#224829=CARTESIAN_POINT('',(60.5836663843182,12.5528626811449,3.77003198860272));
#224830=CARTESIAN_POINT('',(59.5987607253194,12.3435145206988,3.77003198860272));
#224831=CARTESIAN_POINT('',(61.4975385923862,6.78290064323579,3.77003198860268));
#224832=CARTESIAN_POINT('Origin',(5.49031038273072E-15,1.82930781209959E-13,
3.77003198860263));
#224833=CARTESIAN_POINT('',(61.0259576020968,6.73333548388559,3.77003198860268));
#224834=CARTESIAN_POINT('Origin',(5.57972911860581E-15,1.8736496251029E-13,
3.13503198860263));
#224835=CARTESIAN_POINT('Origin',(58.7584780045774,12.1649018101387,3.13502491541444));
#224836=CARTESIAN_POINT('Origin',(59.6417947880741,6.58785913039846,3.13502491541438));
#224837=CARTESIAN_POINT('Origin',(5.57972911860581E-15,1.8736496251029E-13,
3.13503198860263));
#224838=CARTESIAN_POINT('Origin',(60.6209695535092,12.560757428278,3.20381846780363));
#224839=CARTESIAN_POINT('Origin',(61.5354552197175,6.78691956273252,3.203820228721));
#224840=CARTESIAN_POINT('Origin',(5.51210908043506E-15,1.8401175575949E-13,
3.61523028058481));
#224841=CARTESIAN_POINT('Origin',(59.7605297667717,12.3779375131251,3.58786945046858));
#224842=CARTESIAN_POINT('Origin',(60.6605407209801,6.69489156322711,3.58781461834032));
#224843=CARTESIAN_POINT('Origin',(5.51210908043507E-15,1.8401175575949E-13,
3.61523028058481));
#224844=CARTESIAN_POINT('Origin',(59.5817084227231,12.3398435598876,3.58781440266648));
#224845=CARTESIAN_POINT('Origin',(60.478699837019,6.67586224832342,3.58786923592837));
#224846=CARTESIAN_POINT('Origin',(57.8669800961561,1.94016234460786E-13,
2.18253198860263));
#224847=CARTESIAN_POINT('Origin',(60.4792282238308,1.82930781209959E-13,
3.77003198860263));
#224848=CARTESIAN_POINT('',(60.0036905223731,0.317500000000183,3.77003198860264));
#224849=CARTESIAN_POINT('',(59.7081718144892,5.95633285891229,3.77003198860268));
#224850=CARTESIAN_POINT('Origin',(5.49031038273072E-15,1.82930781209959E-13,
3.77003198860263));
#224851=CARTESIAN_POINT('',(60.1802756340603,6.00595296980891,3.77003198860268));
#224852=CARTESIAN_POINT('',(59.851607889689,5.97140859790567,3.77003198860268));
#224853=CARTESIAN_POINT('',(60.1803330766335,6.00537737567532,3.77003198902561));
#224854=CARTESIAN_POINT('Origin',(5.49031038273072E-15,1.82930781209959E-13,
3.77003198860263));
#224855=CARTESIAN_POINT('',(60.4783917833346,0.318078445376176,3.77003198882088));
#224856=CARTESIAN_POINT('Origin',(5.49031038273072E-15,1.82930781209959E-13,
3.77003198860263));
#224857=CARTESIAN_POINT('',(60.478394821762,0.317500000025467,3.77003198860264));
#224858=CARTESIAN_POINT('Origin',(5.49031038273072E-15,1.82930781209959E-13,
3.77003198860263));
#224859=CARTESIAN_POINT('',(60.004228120231,0.317500000000183,3.77003198860264));
#224860=CARTESIAN_POINT('Origin',(5.49031038273072E-15,1.82930781209959E-13,
3.77003198860263));
#224861=CARTESIAN_POINT('',(60.3421421670675,6.02238575970295,3.48823028058486));
#224862=CARTESIAN_POINT('',(60.1803330759045,6.00537737560258,3.77003198860268));
#224863=CARTESIAN_POINT('',(60.6410923275233,0.318076890625034,3.48823028074806));
#224864=CARTESIAN_POINT('Origin',(5.52999282761009E-15,1.84898592019556E-13,
3.48823028058481));
#224865=CARTESIAN_POINT('',(60.6410923272405,0.318076890623551,3.48823028058482));
#224866=CARTESIAN_POINT('Origin',(60.71525,1.85785428279622E-13,3.36123028058482));
#224867=CARTESIAN_POINT('',(60.8610688070707,0.317500000000186,3.36123028058483));
#224868=CARTESIAN_POINT('',(60.5608532912343,6.04595329345079,3.36123028058486));
#224869=CARTESIAN_POINT('Origin',(5.5478765747851E-15,1.85785428279622E-13,
3.36123028058482));
#224870=CARTESIAN_POINT('',(60.7112330730304,6.06175884541589,3.36123028058486));
#224871=CARTESIAN_POINT('',(60.0850508448141,5.99594444118226,3.36123028058486));
#224872=CARTESIAN_POINT('',(61.0122769227456,0.317500000000186,3.36123028058483));
#224873=CARTESIAN_POINT('Origin',(5.5478765747851E-15,1.85785428279622E-13,
3.36123028058482));
#224874=CARTESIAN_POINT('',(60.8615988316031,0.317500000000186,3.36123028058483));
#224875=CARTESIAN_POINT('Origin',(5.5478765747851E-15,1.85785428279622E-13,
3.36123028058482));
#224876=CARTESIAN_POINT('',(61.2322532920972,0.316930737396099,3.48823028058485));
#224877=CARTESIAN_POINT('',(60.9299448849412,6.08531878141057,3.488230280427));
#224878=CARTESIAN_POINT('Origin',(5.52999282761008E-15,1.84898592019556E-13,
3.48823028058484));
#224879=CARTESIAN_POINT('',(61.0917542093523,6.10232411256106,3.77003198802712));
#224880=CARTESIAN_POINT('',(60.929944884669,6.08531878138339,3.48823028058489));
#224881=CARTESIAN_POINT('',(61.0918106390012,6.10175915944652,3.77003198860268));
#224882=CARTESIAN_POINT('Origin',(5.49031038273072E-15,1.82930781209959E-13,
3.77003198860263));
#224883=CARTESIAN_POINT('',(61.3949508163454,0.317500000000183,3.77003198860264));
#224884=CARTESIAN_POINT('Origin',(5.49031038273072E-15,1.82930781209959E-13,
3.77003198860263));
#224885=CARTESIAN_POINT('',(61.394953749505,0.316932243253439,3.77003198802722));
#224886=CARTESIAN_POINT('Origin',(5.49031038273072E-15,1.82930781209959E-13,
3.77003198860263));
#224887=CARTESIAN_POINT('',(61.3949537498373,0.316932243239743,3.77003198860264));
#224888=CARTESIAN_POINT('Origin',(62.2224557307631,1.82930781209959E-13,
3.77003198860263));
#224889=CARTESIAN_POINT('',(61.5639141665612,6.15137923967694,3.77003198860268));
#224890=CARTESIAN_POINT('',(61.5757885448747,6.15262728712883,3.77003198860268));
#224891=CARTESIAN_POINT('',(61.8696548221181,0.317500000000183,3.77003198860264));
#224892=CARTESIAN_POINT('Origin',(5.49031038273072E-15,1.82930781209959E-13,
3.77003198860263));
#224893=CARTESIAN_POINT('',(61.3954762318973,0.317500000000183,3.77003198860264));
#224894=CARTESIAN_POINT('Origin',(63.2144358269191,1.94016234460786E-13,
2.18253198860263));
#224895=CARTESIAN_POINT('Origin',(65.,1.80713690559794E-13,4.08753198860263));
#224896=CARTESIAN_POINT('Origin',(5.57972911860581E-15,1.8736496251029E-13,
3.13503198860263));
#224897=CARTESIAN_POINT('Origin',(59.708171406083,5.95632779542321,3.13502491541438));
#224898=CARTESIAN_POINT('Origin',(60.0036895869254,0.317504993060939,3.13502491541434));
#224899=CARTESIAN_POINT('Origin',(5.57972911860581E-15,1.8736496251029E-13,
3.13503198860263));
#224900=CARTESIAN_POINT('Origin',(61.6018382108745,6.15533149560987,3.20381846780522));
#224901=CARTESIAN_POINT('Origin',(61.9077838296783,0.317533536648817,3.20382022872431));
#224902=CARTESIAN_POINT('Origin',(5.51210908043506E-15,1.8401175575949E-13,
3.61523028058481));
#224903=CARTESIAN_POINT('Origin',(60.7270021185312,6.06345353572159,3.58786945047074));
#224904=CARTESIAN_POINT('Origin',(61.0280426587405,0.3174631441967,3.58781461834159));
#224905=CARTESIAN_POINT('Origin',(5.51210908043507E-15,1.8401175575949E-13,
3.61523028058481));
#224906=CARTESIAN_POINT('Origin',(60.5451784741228,6.04426018543852,3.58781440266261));
#224907=CARTESIAN_POINT('Origin',(60.8452088131258,0.317545622030932,3.58786923593057));
#224908=CARTESIAN_POINT('Origin',(58.2637721346185,-0.190499999999809,2.65878198860262));
#224909=CARTESIAN_POINT('',(59.0285534841296,0.0152400000001907,2.65878198860263));
#224910=CARTESIAN_POINT('',(62.8464427007196,0.0152400000001907,2.65878198860263));
#224911=CARTESIAN_POINT('',(58.2637721346185,0.0152400000001907,2.65878198860263));
#224912=CARTESIAN_POINT('',(62.8464427007196,-0.0152399999998093,2.65878198860263));
#224913=CARTESIAN_POINT('Origin',(-1.95097259456047E-16,1.90690598485538E-13,
2.65878198860263));
#224914=CARTESIAN_POINT('',(59.0285534841296,-0.0152399999998093,2.65878198860263));
#224915=CARTESIAN_POINT('',(58.9578504383728,-0.0152399999998093,2.65878198860263));
#224916=CARTESIAN_POINT('Origin',(4.7062627014205E-16,1.90690598485538E-13,
2.65878198860263));
#224917=CARTESIAN_POINT('Origin',(0.,-0.190500000000089,42.7590319886026));
#224918=CARTESIAN_POINT('',(60.0036905223731,-0.190499999999816,3.64303198860263));
#224919=CARTESIAN_POINT('',(59.5728760150042,-0.190499999999814,3.40423097483311));
#224920=CARTESIAN_POINT('Origin',(59.9654595002504,-0.190499999999813,3.20400220531706));
#224921=CARTESIAN_POINT('',(59.2165773020941,-0.19049999946855,2.83404198860262));
#224922=CARTESIAN_POINT('',(59.5728760150042,-0.190499999999814,3.4042309748331));
#224923=CARTESIAN_POINT('',(62.6567671111299,-0.190499999999809,2.83404198860262));
#224924=CARTESIAN_POINT('',(62.9165533988763,-0.190499999999811,2.83404198860262));
#224925=CARTESIAN_POINT('',(62.3004688883555,-0.190500000605564,3.4042309748331));
#224926=CARTESIAN_POINT('',(62.6567671111299,-0.190499999999811,2.83404198860262));
#224927=CARTESIAN_POINT('',(61.8696548221181,-0.190499999999816,3.64303198860263));
#224928=CARTESIAN_POINT('Origin',(61.9078859673766,-0.190499999999813,3.20400259788328));
#224929=CARTESIAN_POINT('',(61.4682752798284,-0.190500000711747,3.64303198860263));
#224930=CARTESIAN_POINT('',(5.50819412990574E-15,-0.190499999999816,3.64303198860262));
#224931=CARTESIAN_POINT('',(61.3422370451705,-0.190499999999815,3.42473028058486));
#224932=CARTESIAN_POINT('',(61.4682752798284,-0.190499999999816,3.64303198860263));
#224933=CARTESIAN_POINT('',(61.0122769227456,-0.190499999999813,3.23423028058482));
#224934=CARTESIAN_POINT('Origin',(61.0417043405089,-0.190499486622215,3.56425722717113));
#224935=CARTESIAN_POINT('',(60.8610688070707,-0.190499999999813,3.23423028058482));
#224936=CARTESIAN_POINT('',(5.56576032196012E-15,-0.190499999999813,3.23423028058481));
#224937=CARTESIAN_POINT('',(60.5311086139135,-0.190499999999815,3.42473028058481));
#224938=CARTESIAN_POINT('Origin',(60.83163848074,-0.190499486573319,3.56425909741097));
#224939=CARTESIAN_POINT('',(60.4050703266283,-0.190499999999816,3.64303198860263));
#224940=CARTESIAN_POINT('',(60.5311086139135,-0.190499999999815,3.42473028058481));
#224941=CARTESIAN_POINT('',(5.50819412990574E-15,-0.190499999999816,3.64303198860262));
#224942=CARTESIAN_POINT('Origin',(0.,0.190499999999911,42.7590319886026));
#224943=CARTESIAN_POINT('',(61.8696548221181,0.190500000000184,3.64303198860263));
#224944=CARTESIAN_POINT('',(62.3004688883555,0.190500000000186,3.4042309748331));
#224945=CARTESIAN_POINT('Origin',(61.9078859670888,0.190500000000187,3.20400259735841));
#224946=CARTESIAN_POINT('',(62.6567671111299,0.190500000452956,2.83404198860263));
#224947=CARTESIAN_POINT('',(62.3004688883555,0.190500000000186,3.4042309748331));
#224948=CARTESIAN_POINT('',(59.2165773020941,0.19050000000019,2.83404198860263));
#224949=CARTESIAN_POINT('',(0.,0.19050000000019,2.83404198860263));
#224950=CARTESIAN_POINT('',(59.5728760150042,0.190499999293458,3.40423097483312));
#224951=CARTESIAN_POINT('',(59.2165773020941,0.19050000000019,2.83404198860263));
#224952=CARTESIAN_POINT('',(60.0036905223731,0.190500000000184,3.64303198860263));
#224953=CARTESIAN_POINT('Origin',(59.9654594999465,0.190500000000187,3.20400220587196));
#224954=CARTESIAN_POINT('',(60.4050703266283,0.190499999258583,3.64303198860264));
#224955=CARTESIAN_POINT('',(60.4789282006569,0.190500000000184,3.64303198860263));
#224956=CARTESIAN_POINT('',(60.5311086139135,0.190500000000185,3.42473028058481));
#224957=CARTESIAN_POINT('',(60.4050703266283,0.190500000000184,3.64303198860263));
#224958=CARTESIAN_POINT('',(60.8610688070707,0.190500000000187,3.23423028058482));
#224959=CARTESIAN_POINT('Origin',(60.8316414495914,0.190499486502742,3.5642574300434));
#224960=CARTESIAN_POINT('',(61.0122769227456,0.190500000000187,3.23423028058482));
#224961=CARTESIAN_POINT('',(61.0128056337175,0.190500000000187,3.23423028058482));
#224962=CARTESIAN_POINT('',(61.3422370451705,0.190500000000185,3.42473028058486));
#224963=CARTESIAN_POINT('Origin',(61.04170717438,0.190499486688283,3.56425912918013));
#224964=CARTESIAN_POINT('',(61.4682752798284,0.190500000000184,3.64303198860263));
#224965=CARTESIAN_POINT('',(61.3422370451705,0.190500000000185,3.42473028058486));
#224966=CARTESIAN_POINT('',(61.8701762063762,0.190500000000184,3.64303198860263));
#224967=CARTESIAN_POINT('Origin',(58.2637721346185,0.0152400000001895,2.83404198860262));
#224968=CARTESIAN_POINT('Ctrl Pts',(62.6567671111299,0.19050000000019,2.83404198860263));
#224969=CARTESIAN_POINT('Ctrl Pts',(62.6673774406538,0.19050000000019,2.82419652440072));
#224970=CARTESIAN_POINT('Ctrl Pts',(62.6779562874464,0.18966280967327,2.81438790575662));
#224971=CARTESIAN_POINT('Ctrl Pts',(62.6884465439473,0.188003604115333,
2.80466781256922));
#224972=CARTESIAN_POINT('Ctrl Pts',(62.6985959295774,0.186398312858107,
2.79526356453104));
#224973=CARTESIAN_POINT('Ctrl Pts',(62.7086636500148,0.184023290311467,
2.78594102496265));
#224974=CARTESIAN_POINT('Ctrl Pts',(62.7185939622165,0.180846261210796,
2.77675109088818));
#224975=CARTESIAN_POINT('Ctrl Pts',(62.727987426086,0.177840987311745,2.76805797913727));
#224976=CARTESIAN_POINT('Ctrl Pts',(62.7372588214081,0.174117798731289,
2.75948271210212));
#224977=CARTESIAN_POINT('Ctrl Pts',(62.7463424082311,0.169611579426594,
2.7510857557328));
#224978=CARTESIAN_POINT('Ctrl Pts',(62.7547090486368,0.165461025548891,
2.74335155163331));
#224979=CARTESIAN_POINT('Ctrl Pts',(62.7629168328854,0.160645870588248,
2.73576818686008));
#224980=CARTESIAN_POINT('Ctrl Pts',(62.770889261081,0.155086395962765,2.72840626160565));
#224981=CARTESIAN_POINT('Ctrl Pts',(62.7732017594456,0.153473803705493,
2.72627084693725));
#224982=CARTESIAN_POINT('Ctrl Pts',(62.7754942590276,0.151798403770733,
2.72415424587544));
#224983=CARTESIAN_POINT('Ctrl Pts',(62.7777643638146,0.150057792857846,
2.72205867173257));
#224984=CARTESIAN_POINT('Ctrl Pts',(62.780225303358,0.148170858717228,2.71978693462861));
#224985=CARTESIAN_POINT('Ctrl Pts',(62.7826571567199,0.146210769553957,
2.71754411340762));
#224986=CARTESIAN_POINT('Ctrl Pts',(62.7850565204095,0.14417542182634,2.71533341844259));
#224987=CARTESIAN_POINT('Ctrl Pts',(62.791641592883,0.138589394016812,2.70926614876406));
#224988=CARTESIAN_POINT('Ctrl Pts',(62.7979456687654,0.132410786669233,
2.70347381860423));
#224989=CARTESIAN_POINT('Ctrl Pts',(62.8038680995982,0.125664597436926,
2.69804914171409));
#224990=CARTESIAN_POINT('Ctrl Pts',(62.8092868022739,0.119492200548509,
2.69308585687218));
#224991=CARTESIAN_POINT('Ctrl Pts',(62.8143744518939,0.11284434746039,2.68842799053199));
#224992=CARTESIAN_POINT('Ctrl Pts',(62.8190433630434,0.105708043833423,
2.6841476705423));
#224993=CARTESIAN_POINT('Ctrl Pts',(62.8213367169483,0.102202714803628,
2.68204519134565));
#224994=CARTESIAN_POINT('Ctrl Pts',(62.8235285419788,0.0985794274534579,
2.68003431778517));
#224995=CARTESIAN_POINT('Ctrl Pts',(62.8256051102647,0.0948363533474084,
2.67812693945267));
#224996=CARTESIAN_POINT('Ctrl Pts',(62.8259991188709,0.0941261414938091,
2.67776503299219));
#224997=CARTESIAN_POINT('Ctrl Pts',(62.8263888407139,0.0934111032314617,
2.6774065963994));
#224998=CARTESIAN_POINT('Ctrl Pts',(62.826774159152,0.0926913160162657,
2.67705178968871));
#224999=CARTESIAN_POINT('Ctrl Pts',(62.8271474363889,0.0919940221515445,
2.67670807068773));
#225000=CARTESIAN_POINT('Ctrl Pts',(62.8275165811343,0.0912922715312271,
2.67636775825281));
#225001=CARTESIAN_POINT('Ctrl Pts',(62.8278814873655,0.0905861384171377,
2.67603099699271));
#225002=CARTESIAN_POINT('Ctrl Pts',(62.8318581602824,0.0828908452420619,
2.67236104217145));
#225003=CARTESIAN_POINT('Ctrl Pts',(62.8353337180912,0.074669831663276,
2.66911440541491));
#225004=CARTESIAN_POINT('Ctrl Pts',(62.8381654210186,0.0660491922299371,
2.66646778189648));
#225005=CARTESIAN_POINT('Ctrl Pts',(62.8393612667489,0.0624086426656371,
2.66535009634991));
#225006=CARTESIAN_POINT('Ctrl Pts',(62.8404425512865,0.0586971697059423,
2.6643389791236));
#225007=CARTESIAN_POINT('Ctrl Pts',(62.8414000604479,0.0549254519866671,
2.66344564884808));
#225008=CARTESIAN_POINT('Ctrl Pts',(62.8430124819501,0.048573973592406,
2.661941302986));
#225009=CARTESIAN_POINT('Ctrl Pts',(62.8442717146911,0.042052924695462,
2.66077206705434));
#225010=CARTESIAN_POINT('Ctrl Pts',(62.8451307298764,0.0354197192408986,
2.65998225155728));
#225011=CARTESIAN_POINT('Ctrl Pts',(62.8453454836727,0.0337614178772578,
2.65978479768302));
#225012=CARTESIAN_POINT('Ctrl Pts',(62.8455349903695,0.0320960919387808,
2.65961098966636));
#225013=CARTESIAN_POINT('Ctrl Pts',(62.8456982067485,0.0304246312367792,
2.65946139030515));
#225014=CARTESIAN_POINT('Ctrl Pts',(62.845943031317,0.0279174401837767,
2.65923699126334));
#225015=CARTESIAN_POINT('Ctrl Pts',(62.8461286892223,0.0253964615341582,
2.65906707562455));
#225016=CARTESIAN_POINT('Ctrl Pts',(62.846253337618,0.0228647168033014,
2.65895332562933));
#225017=CARTESIAN_POINT('Ctrl Pts',(62.8463779860137,0.0203329720724447,
2.65883957563411));
#225018=CARTESIAN_POINT('Ctrl Pts',(62.8464416340693,0.0177904683743446,
2.65878198860262));
#225019=CARTESIAN_POINT('Ctrl Pts',(62.8464427007196,0.0152400000001907,
2.65878198860262));
#225020=CARTESIAN_POINT('Ctrl Pts',(59.0285534841296,0.015240000000191,
2.65878198860262));
#225021=CARTESIAN_POINT('Ctrl Pts',(59.0285496414744,0.0238699985094254,
2.65878198860262));
#225022=CARTESIAN_POINT('Ctrl Pts',(59.0292582026622,0.0324255116355521,
2.65945335517854));
#225023=CARTESIAN_POINT('Ctrl Pts',(59.0305954788489,0.0407807192227339,
2.66072561226598));
#225024=CARTESIAN_POINT('Ctrl Pts',(59.0314592220531,0.0461773260303339,
2.66154735980336));
#225025=CARTESIAN_POINT('Ctrl Pts',(59.0325843328198,0.0514905268410215,
2.66261895766881));
#225026=CARTESIAN_POINT('Ctrl Pts',(59.0339399880044,0.0566895722963242,
2.66391429251026));
#225027=CARTESIAN_POINT('Ctrl Pts',(59.0357368312948,0.063580609227557,
2.66563118464122));
#225028=CARTESIAN_POINT('Ctrl Pts',(59.0379438906768,0.0702685278902536,
2.66774105138698));
#225029=CARTESIAN_POINT('Ctrl Pts',(59.0405007795597,0.0766865040606001,
2.67016894181749));
#225030=CARTESIAN_POINT('Ctrl Pts',(59.0417792240012,0.0798954921457732,
2.67138288703274));
#225031=CARTESIAN_POINT('Ctrl Pts',(59.0431451240705,0.0830371938950924,
2.67267613167551));
#225032=CARTESIAN_POINT('Ctrl Pts',(59.0445909239228,0.0861046703639672,
2.67403835432553));
#225033=CARTESIAN_POINT('Ctrl Pts',(59.0453138238489,0.0876384085984046,
2.67471946565054));
#225034=CARTESIAN_POINT('Ctrl Pts',(59.0460566986719,0.089153606943806,
2.67541781389523));
#225035=CARTESIAN_POINT('Ctrl Pts',(59.0468186034775,0.0906495011922447,
2.67613207244169));
#225036=CARTESIAN_POINT('Ctrl Pts',(59.047009079679,0.0910234747543544,
2.67631063707831));
#225037=CARTESIAN_POINT('Ctrl Pts',(59.0472007452523,0.0913962421598847,
2.67649019601846));
#225038=CARTESIAN_POINT('Ctrl Pts',(59.0473935854286,0.0917677921728875,
2.67667072836657));
#225039=CARTESIAN_POINT('Ctrl Pts',(59.0479721059574,0.092882442211896,
2.67721232541091));
#225040=CARTESIAN_POINT('Ctrl Pts',(59.048561197931,0.0939861339739832,
2.67776268340048));
#225041=CARTESIAN_POINT('Ctrl Pts',(59.0491604624443,0.0950785796751064,
2.67832123541517));
#225042=CARTESIAN_POINT('Ctrl Pts',(59.0533816042975,0.102773626133288,
2.68225560368441));
#225043=CARTESIAN_POINT('Ctrl Pts',(59.0580834293365,0.10995882346637,2.68661792998879));
#225044=CARTESIAN_POINT('Ctrl Pts',(59.0631465696369,0.116642428646637,
2.69130986622563));
#225045=CARTESIAN_POINT('Ctrl Pts',(59.0656021872114,0.119883969936843,
2.69358545023044));
#225046=CARTESIAN_POINT('Ctrl Pts',(59.0681433715118,0.123007567718211,
2.69593918853465));
#225047=CARTESIAN_POINT('Ctrl Pts',(59.0707593633743,0.126014035556604,
2.69836306235476));
#225048=CARTESIAN_POINT('Ctrl Pts',(59.0747642641417,0.13061672776123,2.70207384382209));
#225049=CARTESIAN_POINT('Ctrl Pts',(59.0789414743143,0.134943070277463,
2.70594760814209));
#225050=CARTESIAN_POINT('Ctrl Pts',(59.0832455674828,0.138985142830926,
2.70995196345689));
#225051=CARTESIAN_POINT('Ctrl Pts',(59.0852444106167,0.140862302235665,
2.71181160678087));
#225052=CARTESIAN_POINT('Ctrl Pts',(59.0872703932641,0.142678271527306,
2.7136996277208));
#225053=CARTESIAN_POINT('Ctrl Pts',(59.0893195943183,0.144431197308928,
2.71561183138642));
#225054=CARTESIAN_POINT('Ctrl Pts',(59.0894766575049,0.144565552163213,
2.71575839426293));
#225055=CARTESIAN_POINT('Ctrl Pts',(59.0896338466133,0.14469956892598,2.7159050890319));
#225056=CARTESIAN_POINT('Ctrl Pts',(59.0897911602042,0.144833247843271,
2.71605191409893));
#225057=CARTESIAN_POINT('Ctrl Pts',(59.0920009418701,0.146711033602277,
2.71811436362734));
#225058=CARTESIAN_POINT('Ctrl Pts',(59.0942367399983,0.148520654545085,
2.7202009102694));
#225059=CARTESIAN_POINT('Ctrl Pts',(59.0964928714566,0.150262619641469,
2.72230624862163));
#225060=CARTESIAN_POINT('Ctrl Pts',(59.1045829576265,0.156508996679146,
2.72985561753101));
#225061=CARTESIAN_POINT('Ctrl Pts',(59.1129958342953,0.161935290146134,
2.73770089914346));
#225062=CARTESIAN_POINT('Ctrl Pts',(59.1216309196491,0.166622470788088,
2.74574823347109));
#225063=CARTESIAN_POINT('Ctrl Pts',(59.1311200109819,0.17177321144469,2.75459144547098));
#225064=CARTESIAN_POINT('Ctrl Pts',(59.1408779306752,0.17603186436329,2.76367911754385));
#225065=CARTESIAN_POINT('Ctrl Pts',(59.1508087658119,0.179468536018209,
2.77292162564885));
#225066=CARTESIAN_POINT('Ctrl Pts',(59.1615315754607,0.183179278918869,
2.78290121484987));
#225067=CARTESIAN_POINT('Ctrl Pts',(59.1724570142889,0.185932239425938,
2.79306229500547));
#225068=CARTESIAN_POINT('Ctrl Pts',(59.1834936683191,0.18776628610095,2.80331916685715));
#225069=CARTESIAN_POINT('Ctrl Pts',(59.1944377361589,0.189584947008325,
2.81348999409005));
#225070=CARTESIAN_POINT('Ctrl Pts',(59.2054925958133,0.19050000000019,2.82375635967032));
#225071=CARTESIAN_POINT('Ctrl Pts',(59.2165773020941,0.19050000000019,2.83404198860263));
#225072=CARTESIAN_POINT('Origin',(0.,-0.0152399999998105,2.83404198860262));
#225073=CARTESIAN_POINT('Ctrl Pts',(62.8464427007196,-0.0152399999998093,
2.65878198860262));
#225074=CARTESIAN_POINT('Ctrl Pts',(62.8464391086779,-0.0238289333902187,
2.65878198860262));
#225075=CARTESIAN_POINT('Ctrl Pts',(62.8457180711405,-0.0323412407622019,
2.65944603041843));
#225076=CARTESIAN_POINT('Ctrl Pts',(62.8443658068291,-0.040653113049866,
2.66070439264048));
#225077=CARTESIAN_POINT('Ctrl Pts',(62.843501774309,-0.0459640037531338,
2.66150842619576));
#225078=CARTESIAN_POINT('Ctrl Pts',(62.8423809556999,-0.0511932363888254,
2.66255428265356));
#225079=CARTESIAN_POINT('Ctrl Pts',(62.841033859251,-0.0563116129572788,
2.66381699700655));
#225080=CARTESIAN_POINT('Ctrl Pts',(62.8391953428955,-0.0632971699620584,
2.66554034873254));
#225081=CARTESIAN_POINT('Ctrl Pts',(62.8369299537504,-0.0700734120982055,
2.66766759643958));
#225082=CARTESIAN_POINT('Ctrl Pts',(62.8343031482014,-0.0765705776093055,
2.67012012783133));
#225083=CARTESIAN_POINT('Ctrl Pts',(62.8329897454269,-0.0798191603648555,
2.67134639352721));
#225084=CARTESIAN_POINT('Ctrl Pts',(62.8315859904681,-0.0829981827951411,
2.67265375584997));
#225085=CARTESIAN_POINT('Ctrl Pts',(62.8301000734874,-0.0861004173276881,
2.67403135126924));
#225086=CARTESIAN_POINT('Ctrl Pts',(62.8293571149971,-0.0876515345939617,
2.67472014897888));
#225087=CARTESIAN_POINT('Ctrl Pts',(62.8285936160519,-0.0891834722995234,
2.67542649668616));
#225088=CARTESIAN_POINT('Ctrl Pts',(62.82781060087,-0.0906954364276871,
2.67614899656085));
#225089=CARTESIAN_POINT('Ctrl Pts',(62.8276148470746,-0.091073427459728,
2.67632962152953));
#225090=CARTESIAN_POINT('Ctrl Pts',(62.8274178735164,-0.0914501705141547,
2.67651125590934));
#225091=CARTESIAN_POINT('Ctrl Pts',(62.8272196962038,-0.0918256539326625,
2.67669387767507));
#225092=CARTESIAN_POINT('Ctrl Pts',(62.8266251642659,-0.0929521041881856,
2.67724174297227));
#225093=CARTESIAN_POINT('Ctrl Pts',(62.826019798519,-0.0940672158684688,
2.67779849504731));
#225094=CARTESIAN_POINT('Ctrl Pts',(62.8254040313373,-0.095170690748659,
2.67836353617992));
#225095=CARTESIAN_POINT('Ctrl Pts',(62.8211486980557,-0.102796386827314,
2.68226832098888));
#225096=CARTESIAN_POINT('Ctrl Pts',(62.8164204928785,-0.109916699411195,
2.68659153751368));
#225097=CARTESIAN_POINT('Ctrl Pts',(62.8113377077397,-0.116542502759485,
2.69123699486152));
#225098=CARTESIAN_POINT('Ctrl Pts',(62.8088115774776,-0.119835508836209,
2.69354577441193));
#225099=CARTESIAN_POINT('Ctrl Pts',(62.8061972539433,-0.123006400629109,
2.69593478828097));
#225100=CARTESIAN_POINT('Ctrl Pts',(62.8035061084565,-0.126056303769779,
2.69839565261203));
#225101=CARTESIAN_POINT('Ctrl Pts',(62.7975690395531,-0.132784845643092,
2.70382468689029));
#225102=CARTESIAN_POINT('Ctrl Pts',(62.7912680187378,-0.138932019324493,
2.7096115581507));
#225103=CARTESIAN_POINT('Ctrl Pts',(62.7847385034067,-0.14444511341298,
2.71562701361751));
#225104=CARTESIAN_POINT('Ctrl Pts',(62.7823531891148,-0.146459116207277,
2.71782453535842));
#225105=CARTESIAN_POINT('Ctrl Pts',(62.7799396422115,-0.148396130390791,
2.72005051502386));
#225106=CARTESIAN_POINT('Ctrl Pts',(62.7775029828616,-0.150257579786298,
2.72229986760101));
#225107=CARTESIAN_POINT('Ctrl Pts',(62.7693185019449,-0.156509991333256,
2.72985520488842));
#225108=CARTESIAN_POINT('Ctrl Pts',(62.7608162581027,-0.161942805717608,
2.73770845534472));
#225109=CARTESIAN_POINT('Ctrl Pts',(62.7520965944504,-0.166635979460947,
2.74576706701628));
#225110=CARTESIAN_POINT('Ctrl Pts',(62.7425126511844,-0.171794333347877,
2.75462443584869));
#225111=CARTESIAN_POINT('Ctrl Pts',(62.7326655363513,-0.176059615357052,
2.76373036322983));
#225112=CARTESIAN_POINT('Ctrl Pts',(62.7226511116316,-0.179500292056274,
2.7729966463658));
#225113=CARTESIAN_POINT('Ctrl Pts',(62.7118651471245,-0.183206048282619,
2.78297683033192));
#225114=CARTESIAN_POINT('Ctrl Pts',(62.7008840239674,-0.185955767118741,
2.79314401478563));
#225115=CARTESIAN_POINT('Ctrl Pts',(62.6897991274287,-0.187785458034744,
2.80341452427555));
#225116=CARTESIAN_POINT('Ctrl Pts',(62.6788639144191,-0.189590441945804,
2.81354634721108));
#225117=CARTESIAN_POINT('Ctrl Pts',(62.6678262782739,-0.19049999999981,
2.82378004209077));
#225118=CARTESIAN_POINT('Ctrl Pts',(62.6567671111299,-0.190499999999811,
2.83404198860262));
#225119=CARTESIAN_POINT('Ctrl Pts',(59.2165773020941,-0.190499999999811,
2.83404198860262));
#225120=CARTESIAN_POINT('Ctrl Pts',(59.2059936184297,-0.19049999999981,
2.8242212644308));
#225121=CARTESIAN_POINT('Ctrl Pts',(59.1954479901471,-0.189665225488525,
2.81442815028649));
#225122=CARTESIAN_POINT('Ctrl Pts',(59.1849969778475,-0.188008762314082,
2.80471618166538));
#225123=CARTESIAN_POINT('Ctrl Pts',(59.1749056059515,-0.186409301377087,
2.79533842146494));
#225124=CARTESIAN_POINT('Ctrl Pts',(59.1649012152168,-0.184043455438379,
2.78603515650548));
#225125=CARTESIAN_POINT('Ctrl Pts',(59.1550396955556,-0.180877423727034,
2.77685887347105));
#225126=CARTESIAN_POINT('Ctrl Pts',(59.1457174710389,-0.177884532220033,
2.7681844121695));
#225127=CARTESIAN_POINT('Ctrl Pts',(59.1365220583474,-0.174176304387683,
2.75962261522018));
#225128=CARTESIAN_POINT('Ctrl Pts',(59.1275197082979,-0.169686797573322,
2.75123537702072));
#225129=CARTESIAN_POINT('Ctrl Pts',(59.1192286949278,-0.165552037114362,
2.74351087134539));
#225130=CARTESIAN_POINT('Ctrl Pts',(59.1111009786111,-0.160754293904838,
2.73593399450272));
#225131=CARTESIAN_POINT('Ctrl Pts',(59.1032135992748,-0.15521351501467,
2.72857657813005));
#225132=CARTESIAN_POINT('Ctrl Pts',(59.1008617419729,-0.15356136659691,
2.72638274508602));
#225133=CARTESIAN_POINT('Ctrl Pts',(59.0985314603587,-0.151842962928119,
2.72420861709732));
#225134=CARTESIAN_POINT('Ctrl Pts',(59.096225375957,-0.15005568617995,2.72205663736708));
#225135=CARTESIAN_POINT('Ctrl Pts',(59.0939428540559,-0.148286670996516,
2.71992664556747));
#225136=CARTESIAN_POINT('Ctrl Pts',(59.0916862380348,-0.146452235168713,
2.71782089927866));
#225137=CARTESIAN_POINT('Ctrl Pts',(59.0894604907299,-0.144552116609777,
2.71574387311227));
#225138=CARTESIAN_POINT('Ctrl Pts',(59.0893057166152,-0.144419986081231,
2.71559944077468));
#225139=CARTESIAN_POINT('Ctrl Pts',(59.0891510807051,-0.144287542501913,
2.7154551521605));
#225140=CARTESIAN_POINT('Ctrl Pts',(59.0889965840074,-0.14415478504376,
2.71531100781712));
#225141=CARTESIAN_POINT('Ctrl Pts',(59.0822228828154,-0.138334211749356,
2.70899119176068));
#225142=CARTESIAN_POINT('Ctrl Pts',(59.0757535782846,-0.131883990153991,
2.70298296066826));
#225143=CARTESIAN_POINT('Ctrl Pts',(59.0697047694308,-0.124808417215229,
2.69736727774127));
#225144=CARTESIAN_POINT('Ctrl Pts',(59.0640662283032,-0.118212753510043,
2.69213248525422));
#225145=CARTESIAN_POINT('Ctrl Pts',(59.0587927761314,-0.111072931137408,
2.68723866185464));
#225146=CARTESIAN_POINT('Ctrl Pts',(59.0540076654699,-0.10338954476835,
2.68278595829559));
#225147=CARTESIAN_POINT('Ctrl Pts',(59.0522572100838,-0.100578862632676,
2.68115710172796));
#225148=CARTESIAN_POINT('Ctrl Pts',(59.0505724231957,-0.0976954648437236,
2.67958763637796));
#225149=CARTESIAN_POINT('Ctrl Pts',(59.048960544286,-0.0947395585251538,
2.67808378645346));
#225150=CARTESIAN_POINT('Ctrl Pts',(59.0485729412563,-0.0940287618036577,
2.67772216078581));
#225151=CARTESIAN_POINT('Ctrl Pts',(59.0481896206934,-0.0933131922165624,
2.67736403603544));
#225152=CARTESIAN_POINT('Ctrl Pts',(59.0478106940136,-0.0925929271969761,
2.6770095693446));
#225153=CARTESIAN_POINT('Ctrl Pts',(59.0474436087926,-0.0918951704592519,
2.67666617973785));
#225154=CARTESIAN_POINT('Ctrl Pts',(59.0470806471271,-0.0911930071932342,
2.676326223141));
#225155=CARTESIAN_POINT('Ctrl Pts',(59.0467219102889,-0.0904865115876359,
2.67598984158754));
#225156=CARTESIAN_POINT('Ctrl Pts',(59.0427915336441,-0.0827460357496678,
2.672304392922));
#225157=CARTESIAN_POINT('Ctrl Pts',(59.039366072413,-0.0744802459940899,
2.66904964539953));
#225158=CARTESIAN_POINT('Ctrl Pts',(59.0365841602689,-0.0658168714606044,
2.66640203566702));
#225159=CARTESIAN_POINT('Ctrl Pts',(59.0354304183829,-0.0622239118141111,
2.66530399299418));
#225160=CARTESIAN_POINT('Ctrl Pts',(59.0343871039217,-0.0585629032862787,
2.66430995142239));
#225161=CARTESIAN_POINT('Ctrl Pts',(59.0334626554262,-0.054844071499784,
2.6634305347334));
#225162=CARTESIAN_POINT('Ctrl Pts',(59.0318859121827,-0.0485012163582169,
2.66193059792864));
#225163=CARTESIAN_POINT('Ctrl Pts',(59.0306571138137,-0.0419914004942296,
2.66076519817106));
#225164=CARTESIAN_POINT('Ctrl Pts',(59.0298212958157,-0.0353717968086348,
2.65997805604439));
#225165=CARTESIAN_POINT('Ctrl Pts',(59.0294033868167,-0.0320619949658374,
2.65958448498105));
#225166=CARTESIAN_POINT('Ctrl Pts',(59.0290851681639,-0.0287246785544886,
2.65928526260741));
#225167=CARTESIAN_POINT('Ctrl Pts',(59.0288723192866,-0.0253670368746793,
2.65908463971303));
#225168=CARTESIAN_POINT('Ctrl Pts',(59.0286594704093,-0.0220093951948699,
2.65888401681865));
#225169=CARTESIAN_POINT('Ctrl Pts',(59.0285519740191,-0.0186314705078166,
2.65878198860262));
#225170=CARTESIAN_POINT('Ctrl Pts',(59.0285534841296,-0.0152399999998093,
2.65878198860262));
#225171=CARTESIAN_POINT('Origin',(61.4240753804089,0.31749999970617,3.56647653909435));
#225172=CARTESIAN_POINT('Origin',(61.4683012396074,0.317551690013559,3.64299466007648));
#225173=CARTESIAN_POINT('Origin',(61.3422370451705,0.317500000000185,3.42473028058485));
#225174=CARTESIAN_POINT('Ctrl Pts',(61.2322532920972,0.316930737396099,
3.48823028058485));
#225175=CARTESIAN_POINT('Ctrl Pts',(61.2327440814646,0.190500000000179,
3.48794691941601));
#225176=CARTESIAN_POINT('Ctrl Pts',(61.3422370451705,0.190500000000185,
3.42473028058486));
#225177=CARTESIAN_POINT('Ctrl Pts',(61.1872475084174,0.317046579199821,
3.41028005925091));
#225178=CARTESIAN_POINT('Ctrl Pts',(61.1875064541755,0.1905000000014,3.40982512230973));
#225179=CARTESIAN_POINT('Ctrl Pts',(61.2747290395309,0.190500000000186,
3.30780486372821));
#225180=CARTESIAN_POINT('Ctrl Pts',(61.1019842137032,0.317266596913676,
3.36123028058482));
#225181=CARTESIAN_POINT('Ctrl Pts',(61.1018997758111,0.190500000000209,
3.36099721048472));
#225182=CARTESIAN_POINT('Ctrl Pts',(61.1468362071712,0.190500000000187,
3.23423045308393));
#225183=CARTESIAN_POINT('Ctrl Pts',(61.0122769227456,0.317500000000186,
3.36123028058482));
#225184=CARTESIAN_POINT('Ctrl Pts',(61.0122769227456,0.190500000000186,
3.36123028058482));
#225185=CARTESIAN_POINT('Ctrl Pts',(61.0122769227456,0.190500000000187,
3.23423028058482));
#225186=CARTESIAN_POINT('Origin',(61.0122769227456,0.317500000000187,3.23423028058482));
#225187=CARTESIAN_POINT('Origin',(5.50819412990574E-15,0.317500000000184,
3.64303198860263));
#225188=CARTESIAN_POINT('Origin',(61.8696548221181,0.317500000000184,3.64303198860263));
#225189=CARTESIAN_POINT('Origin',(5.56576032196012E-15,0.317500000000187,
3.23423028058482));
#225190=CARTESIAN_POINT('Origin',(60.8610688070707,0.317500000000187,3.23423028058482));
#225191=CARTESIAN_POINT('Ctrl Pts',(62.4081695979768,0.318048871877314,
3.47153072139072));
#225192=CARTESIAN_POINT('Ctrl Pts',(62.4086377819835,0.190309034175474,
3.47182327902663));
#225193=CARTESIAN_POINT('Ctrl Pts',(62.3003077603771,0.19050014212524,3.40413028959023));
#225194=CARTESIAN_POINT('Ctrl Pts',(62.2931881445372,0.317932489890133,
3.65553807120956));
#225195=CARTESIAN_POINT('Ctrl Pts',(62.2934975005737,0.190309294367812,
3.6558627549695));
#225196=CARTESIAN_POINT('Ctrl Pts',(62.2083564003272,0.190500141995652,
3.5512812683729));
#225197=CARTESIAN_POINT('Ctrl Pts',(62.0866281564673,0.317722686167576,
3.77003198860264));
#225198=CARTESIAN_POINT('Ctrl Pts',(62.0868143053088,0.190309769569989,
3.77025505748508));
#225199=CARTESIAN_POINT('Ctrl Pts',(62.0431695205372,0.19050014176205,3.64284211731158));
#225200=CARTESIAN_POINT('Ctrl Pts',(61.8696548221181,0.317500000000183,
3.77003198860264));
#225201=CARTESIAN_POINT('Ctrl Pts',(61.8696548221181,0.190310267889111,
3.77003198860264));
#225202=CARTESIAN_POINT('Ctrl Pts',(61.8696548221181,0.190500141514099,
3.6428423982169));
#225203=CARTESIAN_POINT('Origin',(62.3004688883555,0.317500000000185,3.4042309748331));
#225204=CARTESIAN_POINT('Ctrl Pts',(60.8610688070707,0.317500000000186,
3.36123028058482));
#225205=CARTESIAN_POINT('Ctrl Pts',(60.8610688070707,0.190500000000186,
3.36123028058482));
#225206=CARTESIAN_POINT('Ctrl Pts',(60.8610688070707,0.190500000000187,
3.23423028058482));
#225207=CARTESIAN_POINT('Ctrl Pts',(60.7710583184321,0.31773477376044,3.36123028058482));
#225208=CARTESIAN_POINT('Ctrl Pts',(60.7709717342409,0.190500000000059,
3.36146538610129));
#225209=CARTESIAN_POINT('Ctrl Pts',(60.7260547307357,0.190500000000187,
3.23423043688415));
#225210=CARTESIAN_POINT('Ctrl Pts',(60.6859465754578,0.317958617919221,
3.41054258693101));
#225211=CARTESIAN_POINT('Ctrl Pts',(60.6862105562578,0.190500000001745,
3.41100608859818));
#225212=CARTESIAN_POINT('Ctrl Pts',(60.598389295541,0.190500000000186,3.30819866970851));
#225213=CARTESIAN_POINT('Ctrl Pts',(60.6410923272405,0.318076890623551,
3.48823028058482));
#225214=CARTESIAN_POINT('Ctrl Pts',(60.6415942020421,0.190500000000185,
3.48852004212259));
#225215=CARTESIAN_POINT('Ctrl Pts',(60.5311086139135,0.190500000000185,
3.42473028058481));
#225216=CARTESIAN_POINT('Origin',(60.5311086139135,0.317500000000185,3.42473028058481));
#225217=CARTESIAN_POINT('Origin',(62.4786179998493,0.3174999999779,3.11913648178449));
#225218=CARTESIAN_POINT('Origin',(62.6567671111299,0.317500000000189,2.83404198860263));
#225219=CARTESIAN_POINT('Origin',(60.4497583458784,0.317499999994999,3.56563113460752));
#225220=CARTESIAN_POINT('Origin',(60.4050521322804,0.317550804320461,3.64299171721808));
#225221=CARTESIAN_POINT('Ctrl Pts',(62.9541448057648,0.0152661173110579,
2.59908173516024));
#225222=CARTESIAN_POINT('Ctrl Pts',(62.9168399481843,0.0152570710388248,
2.65878198860262));
#225223=CARTESIAN_POINT('Ctrl Pts',(62.8464427007196,0.0152400000001907,
2.65878198860262));
#225224=CARTESIAN_POINT('Ctrl Pts',(62.9541233134297,0.103381504925395,
2.59908193475635));
#225225=CARTESIAN_POINT('Ctrl Pts',(62.9168211560341,0.0794415635237661,
2.65878715325387));
#225226=CARTESIAN_POINT('Ctrl Pts',(62.8464212442881,0.0662446030561332,
2.65878198860262));
#225227=CARTESIAN_POINT('Ctrl Pts',(62.9290872705826,0.184683583687983,
2.63878778849892));
#225228=CARTESIAN_POINT('Ctrl Pts',(62.8936771137448,0.138547994784479,
2.69564460180121));
#225229=CARTESIAN_POINT('Ctrl Pts',(62.8213855864655,0.113305567451748,
2.6818048162489));
#225230=CARTESIAN_POINT('Ctrl Pts',(62.8564203507742,0.291340992631895,
2.75443238878626));
#225231=CARTESIAN_POINT('Ctrl Pts',(62.8329175802742,0.20191035119155,2.79268340777087));
#225232=CARTESIAN_POINT('Ctrl Pts',(62.7487193609389,0.175042741958035,
2.74885926835605));
#225233=CARTESIAN_POINT('Ctrl Pts',(62.8099434033762,0.318045276842822,
2.82856655361685));
#225234=CARTESIAN_POINT('Ctrl Pts',(62.7947175425004,0.205831635643201,
2.85384197230834));
#225235=CARTESIAN_POINT('Ctrl Pts',(62.7022409210441,0.190500000000191,
2.79184624278459));
#225236=CARTESIAN_POINT('Ctrl Pts',(62.7644678366119,0.318045750793234,
2.90134173516025));
#225237=CARTESIAN_POINT('Ctrl Pts',(62.7649326510149,0.190500000000187,
2.90163218716392));
#225238=CARTESIAN_POINT('Ctrl Pts',(62.6567671111299,0.19050000000019,2.83404198860263));
#225239=CARTESIAN_POINT('Origin',(62.8464427007196,0.0152400000001916,2.53178198860262));
#225240=CARTESIAN_POINT('Origin',(5.50819412990574E-15,0.317500000000184,
3.64303198860263));
#225241=CARTESIAN_POINT('Origin',(60.0036905223731,0.317500000000184,3.64303198860263));
#225242=CARTESIAN_POINT('Origin',(-1.95097259456047E-16,1.91577434745604E-13,
2.53178198860262));
#225243=CARTESIAN_POINT('Origin',(62.8464427007196,-0.0152399999998084,
2.53178198860262));
#225244=CARTESIAN_POINT('Ctrl Pts',(60.0036905223731,0.317500000000183,
3.77003198860264));
#225245=CARTESIAN_POINT('Ctrl Pts',(60.0036905223731,0.190309748265493,
3.77003198860264));
#225246=CARTESIAN_POINT('Ctrl Pts',(60.0036905223731,0.190500142289713,
3.64284187937064));
#225247=CARTESIAN_POINT('Ctrl Pts',(59.7867137603524,0.317270385524599,
3.77003198860264));
#225248=CARTESIAN_POINT('Ctrl Pts',(59.7869045527984,0.190310262476557,
3.76980208962932));
#225249=CARTESIAN_POINT('Ctrl Pts',(59.8301727552497,0.190500142032646,
3.6428419392832));
#225250=CARTESIAN_POINT('Ctrl Pts',(59.5801552670728,0.317049440713801,
3.65553535416585));
#225251=CARTESIAN_POINT('Ctrl Pts',(59.5804765271851,0.19031076108255,3.65520057834439));
#225252=CARTESIAN_POINT('Ctrl Pts',(59.6649871046547,0.19050014178529,3.55127910964224));
#225253=CARTESIAN_POINT('Ctrl Pts',(59.4651754363832,0.316925998273232,
3.47153072139074));
#225254=CARTESIAN_POINT('Ctrl Pts',(59.4656607446594,0.190311035335236,
3.47122746281584));
#225255=CARTESIAN_POINT('Ctrl Pts',(59.5730368716576,0.190500141647087,
3.40413045901283));
#225256=CARTESIAN_POINT('Origin',(59.5728760150042,0.317500000000185,3.40423097483311));
#225257=CARTESIAN_POINT('Ctrl Pts',(62.7644678366119,-0.318045750792856,
2.90134173516023));
#225258=CARTESIAN_POINT('Ctrl Pts',(62.7649326510148,-0.190499999999811,
2.90163218716391));
#225259=CARTESIAN_POINT('Ctrl Pts',(62.6567671111299,-0.190499999999811,
2.83404198860262));
#225260=CARTESIAN_POINT('Ctrl Pts',(62.8099640589334,-0.318045262794995,
2.82853349835363));
#225261=CARTESIAN_POINT('Ctrl Pts',(62.7947344577641,-0.205840330722858,
2.85381483162469));
#225262=CARTESIAN_POINT('Ctrl Pts',(62.7022616416345,-0.19049999999981,
2.79182701594314));
#225263=CARTESIAN_POINT('Ctrl Pts',(62.8562601188215,-0.291334117855231,
2.75468822073634));
#225264=CARTESIAN_POINT('Ctrl Pts',(62.8328016940824,-0.201836550627568,
2.79286913083857));
#225265=CARTESIAN_POINT('Ctrl Pts',(62.7485591297232,-0.175038734051986,
2.74900763297918));
#225266=CARTESIAN_POINT('Ctrl Pts',(62.928611257107,-0.185622189560187,
2.63954450640402));
#225267=CARTESIAN_POINT('Ctrl Pts',(62.8932808767899,-0.139140155999895,
2.69627684028843));
#225268=CARTESIAN_POINT('Ctrl Pts',(62.8209095783125,-0.113848895265506,
2.68224356036487));
#225269=CARTESIAN_POINT('Ctrl Pts',(62.9541233349674,-0.103673266462647,
2.59908178706356));
#225270=CARTESIAN_POINT('Ctrl Pts',(62.9168211653022,-0.0796882264535046,
2.65878704321517));
#225271=CARTESIAN_POINT('Ctrl Pts',(62.8464212664863,-0.0664134143649492,
2.65878198860262));
#225272=CARTESIAN_POINT('Ctrl Pts',(62.9541448057648,-0.0152661173106757,
2.59908173516024));
#225273=CARTESIAN_POINT('Ctrl Pts',(62.9168399481843,-0.0152570710384434,
2.65878198860262));
#225274=CARTESIAN_POINT('Ctrl Pts',(62.8464427007196,-0.0152399999998093,
2.65878198860262));
#225275=CARTESIAN_POINT('Origin',(62.6567671111299,-0.31749999999981,2.83404198860262));
#225276=CARTESIAN_POINT('Origin',(59.3947266586253,0.31749999997129,3.11913648167031));
#225277=CARTESIAN_POINT('Origin',(59.2165773020941,0.317500000000189,2.83404198860263));
#225278=CARTESIAN_POINT('Origin',(62.4786179998359,-0.317499999976169,3.1191364817761));
#225279=CARTESIAN_POINT('Origin',(62.3004688883555,-0.317499999999815,3.4042309748331));
#225280=CARTESIAN_POINT('Ctrl Pts',(59.1088767419348,0.316922544675878,
2.90134173516024));
#225281=CARTESIAN_POINT('Ctrl Pts',(59.1093642282367,0.190500000000189,
2.9010371155323));
#225282=CARTESIAN_POINT('Ctrl Pts',(59.2165773020941,0.19050000000019,2.83404198860262));
#225283=CARTESIAN_POINT('Ctrl Pts',(59.0634407053229,0.316922012809351,
2.82862991747967));
#225284=CARTESIAN_POINT('Ctrl Pts',(59.0793536643051,0.20569497374123,2.85314045886384));
#225285=CARTESIAN_POINT('Ctrl Pts',(59.1711393827298,0.19050000000019,2.79187960999874));
#225286=CARTESIAN_POINT('Ctrl Pts',(59.0174076205275,0.290332993455118,
2.7547062579332));
#225287=CARTESIAN_POINT('Ctrl Pts',(59.0412846811395,0.201480151666008,
2.79224250381903));
#225288=CARTESIAN_POINT('Ctrl Pts',(59.1251084688121,0.175054909459896,
2.7490180910826));
#225289=CARTESIAN_POINT('Ctrl Pts',(58.9458296250063,0.184894967401825,
2.63947868311706));
#225290=CARTESIAN_POINT('Ctrl Pts',(58.9812445774292,0.138672156931444,
2.69595066767909));
#225291=CARTESIAN_POINT('Ctrl Pts',(59.0535312451933,0.113807322597966,
2.68220539436061));
#225292=CARTESIAN_POINT('Ctrl Pts',(58.9208287018089,0.103171606455877,
2.59908178585054));
#225293=CARTESIAN_POINT('Ctrl Pts',(58.9581363848276,0.0793367652459778,
2.65877670944829));
#225294=CARTESIAN_POINT('Ctrl Pts',(59.0285307646513,0.0663350652345533,
2.65878198860262));
#225295=CARTESIAN_POINT('Ctrl Pts',(58.9208513795073,0.0152121934561115,
2.59908173516024));
#225296=CARTESIAN_POINT('Ctrl Pts',(58.9581562369413,0.0152218248292979,
2.65878198860262));
#225297=CARTESIAN_POINT('Ctrl Pts',(59.0285534841296,0.015240000000191,
2.65878198860262));
#225298=CARTESIAN_POINT('Origin',(59.0285534841296,0.0152400000001916,2.53178198860262));
#225299=CARTESIAN_POINT('Ctrl Pts',(61.8696548221181,-0.317499999999817,
3.77003198860264));
#225300=CARTESIAN_POINT('Ctrl Pts',(61.8696548221181,-0.19031025693103,
3.77003198860264));
#225301=CARTESIAN_POINT('Ctrl Pts',(61.8696548221181,-0.190500141530065,
3.64284238727555));
#225302=CARTESIAN_POINT('Ctrl Pts',(62.0866315324121,-0.317722689632047,
3.77003198860264));
#225303=CARTESIAN_POINT('Ctrl Pts',(62.0868176889517,-0.190309758575249,
3.77025506105891));
#225304=CARTESIAN_POINT('Ctrl Pts',(62.0431722165643,-0.190500141778049,
3.64284210641918));
#225305=CARTESIAN_POINT('Ctrl Pts',(62.2931898887681,-0.317932491655493,
3.65553527987835));
#225306=CARTESIAN_POINT('Ctrl Pts',(62.293499245807,-0.190309283352059,
3.65585996533076));
#225307=CARTESIAN_POINT('Ctrl Pts',(62.2083577878532,-0.190500142011671,
3.55127902710177));
#225308=CARTESIAN_POINT('Ctrl Pts',(62.4081695979768,-0.318048871876944,
3.47153072139071));
#225309=CARTESIAN_POINT('Ctrl Pts',(62.4086377820239,-0.190309023146102,
3.47182327905188));
#225310=CARTESIAN_POINT('Ctrl Pts',(62.3003077510784,-0.190500142141273,
3.40413028377964));
#225311=CARTESIAN_POINT('Origin',(61.8696548221181,-0.317499999999816,3.64303198860263));
#225312=CARTESIAN_POINT('Origin',(4.7062627014205E-16,1.91577434745604E-13,
2.53178198860262));
#225313=CARTESIAN_POINT('Origin',(59.0285534841296,-0.0152399999998084,
2.53178198860262));
#225314=CARTESIAN_POINT('Origin',(62.2224557307631,-0.317499999999816,3.64303198860263));
#225315=CARTESIAN_POINT('Origin',(61.4683012396074,-0.317551690013422,3.64299466007613));
#225316=CARTESIAN_POINT('Ctrl Pts',(58.9208513795073,-0.0152121934557287,
2.59908173516024));
#225317=CARTESIAN_POINT('Ctrl Pts',(58.9581562369414,-0.0152218248289162,
2.65878198860262));
#225318=CARTESIAN_POINT('Ctrl Pts',(59.0285534841296,-0.0152399999998093,
2.65878198860262));
#225319=CARTESIAN_POINT('Ctrl Pts',(58.9208288705618,-0.102871702177174,
2.59908193199893));
#225320=CARTESIAN_POINT('Ctrl Pts',(58.9581365422946,-0.0790852439331895,
2.65877685806655));
#225321=CARTESIAN_POINT('Ctrl Pts',(59.0285309330218,-0.0661608181923042,
2.65878198860262));
#225322=CARTESIAN_POINT('Ctrl Pts',(58.9453619764183,-0.183955833237358,
2.63872492669802));
#225323=CARTESIAN_POINT('Ctrl Pts',(58.9808530699761,-0.138075936735796,
2.69532212015275));
#225324=CARTESIAN_POINT('Ctrl Pts',(59.0530636028226,-0.113261762367989,
2.68176836726639));
#225325=CARTESIAN_POINT('Ctrl Pts',(59.0172303255293,-0.290319860890428,
2.75442176402246));
#225326=CARTESIAN_POINT('Ctrl Pts',(59.0411528690721,-0.201541405841727,
2.79203179920136));
#225327=CARTESIAN_POINT('Ctrl Pts',(59.1249311745757,-0.175047309550979,
2.74885310748172));
#225328=CARTESIAN_POINT('Ctrl Pts',(59.0634600627912,-0.316922027357153,
2.82866089558405));
#225329=CARTESIAN_POINT('Ctrl Pts',(59.0793694364684,-0.205687000367097,
2.85316563119185));
#225330=CARTESIAN_POINT('Ctrl Pts',(59.1711586818656,-0.19049999999981,
2.79189751796654));
#225331=CARTESIAN_POINT('Ctrl Pts',(59.1088767419348,-0.3169225446755,2.90134173516024));
#225332=CARTESIAN_POINT('Ctrl Pts',(59.1093642282367,-0.190499999999811,
2.9010371155323));
#225333=CARTESIAN_POINT('Ctrl Pts',(59.2165773020941,-0.190499999999811,
2.83404198860262));
#225334=CARTESIAN_POINT('Origin',(59.2165773020941,-0.31749999999981,2.83404198860262));
#225335=CARTESIAN_POINT('Origin',(61.4240753793285,-0.317499999994572,3.56647653971808));
#225336=CARTESIAN_POINT('Origin',(61.3422370451705,-0.317499999999815,3.42473028058486));
#225337=CARTESIAN_POINT('Origin',(59.3947266586072,-0.317499999969147,3.1191364816816));
#225338=CARTESIAN_POINT('Origin',(59.5728760150042,-0.317499999999815,3.4042309748331));
#225339=CARTESIAN_POINT('Ctrl Pts',(61.0122769227456,-0.317499999999814,
3.36123028058482));
#225340=CARTESIAN_POINT('Ctrl Pts',(61.0122769227456,-0.190499999999814,
3.36123028058482));
#225341=CARTESIAN_POINT('Ctrl Pts',(61.0122769227456,-0.190499999999813,
3.23423028058482));
#225342=CARTESIAN_POINT('Ctrl Pts',(61.1022873990971,-0.317265808076204,
3.36123028058482));
#225343=CARTESIAN_POINT('Ctrl Pts',(61.1022028716704,-0.190499999999688,
3.36099641108529));
#225344=CARTESIAN_POINT('Ctrl Pts',(61.1472909869838,-0.190499999999813,
3.23423043688437));
#225345=CARTESIAN_POINT('Ctrl Pts',(61.1873990841185,-0.317046189128919,
3.41054258905285));
#225346=CARTESIAN_POINT('Ctrl Pts',(61.1876587562326,-0.190500000001028,
3.41008815825968));
#225347=CARTESIAN_POINT('Ctrl Pts',(61.2749563897835,-0.190499999999814,
3.30819867304271));
#225348=CARTESIAN_POINT('Ctrl Pts',(61.2322532920972,-0.316930737395729,
3.48823028058483));
#225349=CARTESIAN_POINT('Ctrl Pts',(61.2327440814646,-0.190499999999809,
3.487946919416));
#225350=CARTESIAN_POINT('Ctrl Pts',(61.3422370451705,-0.190499999999815,
3.42473028058484));
#225351=CARTESIAN_POINT('Origin',(61.0122769227456,-0.317499999999813,3.23423028058482));
#225352=CARTESIAN_POINT('Ctrl Pts',(59.4651754363832,-0.316925998272862,
3.47153072139073));
#225353=CARTESIAN_POINT('Ctrl Pts',(59.4656607446034,-0.190311049924885,
3.47122746285078));
#225354=CARTESIAN_POINT('Ctrl Pts',(59.573036859247,-0.190500141624861,
3.4041304667679));
#225355=CARTESIAN_POINT('Ctrl Pts',(59.5801570044831,-0.317049442578994,
3.65553813457986));
#225356=CARTESIAN_POINT('Ctrl Pts',(59.5804782634893,-0.190310775687599,
3.65520336072057));
#225357=CARTESIAN_POINT('Ctrl Pts',(59.6649884842709,-0.190500141763048,
3.55128134519903));
#225358=CARTESIAN_POINT('Ctrl Pts',(59.7867171285936,-0.317270389088646,
3.77003198860264));
#225359=CARTESIAN_POINT('Ctrl Pts',(59.7869079131804,-0.190310277117966,
3.76980209314202));
#225360=CARTESIAN_POINT('Ctrl Pts',(59.8301754438931,-0.190500142010366,
3.6428419538746));
#225361=CARTESIAN_POINT('Ctrl Pts',(60.0036905223731,-0.317499999999817,
3.77003198860264));
#225362=CARTESIAN_POINT('Ctrl Pts',(60.0036905223731,-0.190309762954565,
3.77003198860264));
#225363=CARTESIAN_POINT('Ctrl Pts',(60.0036905223731,-0.19050014226739,
3.64284189403806));
#225364=CARTESIAN_POINT('Origin',(60.0036905223731,-0.317499999999816,3.64303198860263));
#225365=CARTESIAN_POINT('Origin',(60.71525,-0.317499999999813,3.23423028058482));
#225366=CARTESIAN_POINT('Origin',(60.8610688070707,-0.317499999999813,3.23423028058482));
#225367=CARTESIAN_POINT('Origin',(60.4792282238308,-0.317499999999816,3.64303198860263));
#225368=CARTESIAN_POINT('Origin',(60.4050521322803,-0.317550804320321,3.64299171721791));
#225369=CARTESIAN_POINT('Ctrl Pts',(60.6410923272405,-0.318076890623181,
3.48823028058482));
#225370=CARTESIAN_POINT('Ctrl Pts',(60.6415942020421,-0.190499999999815,
3.48852004212259));
#225371=CARTESIAN_POINT('Ctrl Pts',(60.5311086139135,-0.190499999999815,
3.42473028058481));
#225372=CARTESIAN_POINT('Ctrl Pts',(60.6860981505083,-0.317958218318571,
3.41028005848409));
#225373=CARTESIAN_POINT('Ctrl Pts',(60.6863613750299,-0.190499999999808,
3.41074404220335));
#225374=CARTESIAN_POINT('Ctrl Pts',(60.5986166446971,-0.190499999999814,
3.307804862439));
#225375=CARTESIAN_POINT('Ctrl Pts',(60.771361502534,-0.317733982967355,
3.36123028058482));
#225376=CARTESIAN_POINT('Ctrl Pts',(60.7712750141982,-0.190499999999842,
3.36146460586441));
#225377=CARTESIAN_POINT('Ctrl Pts',(60.7265095085039,-0.190499999999813,
3.23423045308464));
#225378=CARTESIAN_POINT('Ctrl Pts',(60.8610688070707,-0.317499999999814,
3.36123028058482));
#225379=CARTESIAN_POINT('Ctrl Pts',(60.8610688070707,-0.190499999999814,
3.36123028058482));
#225380=CARTESIAN_POINT('Ctrl Pts',(60.8610688070707,-0.190499999999813,
3.23423028058482));
#225381=CARTESIAN_POINT('Origin',(60.5311086139135,-0.317499999999815,3.42473028058481));
#225382=CARTESIAN_POINT('Origin',(60.4497583469872,-0.317500000300251,3.5656311352477));
#225383=CARTESIAN_POINT('Origin',(57.9645097668785,5.90076614434095,2.65878198860267));
#225384=CARTESIAN_POINT('',(58.7035958781039,6.18532049829418,2.65878198860267));
#225385=CARTESIAN_POINT('',(62.5005702980931,6.58439859103048,2.65878198860267));
#225386=CARTESIAN_POINT('',(57.9430040808458,6.10537907909402,2.65878198860267));
#225387=CARTESIAN_POINT('',(62.5037563256535,6.55408556365965,2.65878198860267));
#225388=CARTESIAN_POINT('Origin',(5.50059263827931E-15,1.84980347606071E-13,
2.65878198860263));
#225389=CARTESIAN_POINT('',(58.7067819056643,6.15500747092335,2.65878198860267));
#225390=CARTESIAN_POINT('',(58.63646617859,6.14761699020205,2.65878198860267));
#225391=CARTESIAN_POINT('Origin',(5.72291486498914E-15,1.85445891303602E-13,
2.65878198860263));
#225392=CARTESIAN_POINT('Origin',(0.019912672252488,-0.189456421067745,
42.7590319886026));
#225393=CARTESIAN_POINT('',(59.6948966996543,6.08263713962406,3.64303198860267));
#225394=CARTESIAN_POINT('',(59.2664422392336,6.03760476121538,3.40423097483316));
#225395=CARTESIAN_POINT('Origin',(59.6568751110701,6.07864090963233,3.20400220531864));
#225396=CARTESIAN_POINT('',(58.9120953678975,6.00036140481925,2.83404198860266));
#225397=CARTESIAN_POINT('',(59.2664422392336,6.03760476121538,3.40423097483316));
#225398=CARTESIAN_POINT('',(62.3334394572619,6.35995915837821,2.83404198860267));
#225399=CARTESIAN_POINT('',(62.5918026085422,6.38711421981435,2.83404198860267));
#225400=CARTESIAN_POINT('',(61.9790930734951,6.32271585208523,3.40423097483316));
#225401=CARTESIAN_POINT('',(62.3334394572619,6.35995915837821,2.83404198860267));
#225402=CARTESIAN_POINT('',(61.5506390517262,6.27768352038871,3.64303198860268));
#225403=CARTESIAN_POINT('Origin',(61.5886607627696,6.28167976325143,3.20400259788071));
#225404=CARTESIAN_POINT('',(61.1514583086406,6.23572793293823,3.64303198860268));
#225405=CARTESIAN_POINT('',(0.0199126722524935,-0.189456421067472,3.64303198860262));
#225406=CARTESIAN_POINT('',(61.0261105245454,6.22255335066435,3.4247302805849));
#225407=CARTESIAN_POINT('',(61.1514583085662,6.2357279336461,3.64303198860268));
#225408=CARTESIAN_POINT('',(60.6979579581954,6.18806312612766,3.23423028058487));
#225409=CARTESIAN_POINT('Origin',(60.7272241158227,6.19113963944967,3.56425722717094));
#225410=CARTESIAN_POINT('',(60.5475781763993,6.17225757416257,3.23423028058487));
#225411=CARTESIAN_POINT('',(0.0199126722524936,-0.189456421067469,3.23423028058481));
#225412=CARTESIAN_POINT('',(60.2194255397045,6.13776734223234,3.42473028058486));
#225413=CARTESIAN_POINT('Origin',(60.5183090188079,6.16918177799164,3.56425909741038));
#225414=CARTESIAN_POINT('',(60.0940777033447,6.12459275374953,3.64303198860267));
#225415=CARTESIAN_POINT('',(60.2194255397045,6.13776734223234,3.42473028058486));
#225416=CARTESIAN_POINT('',(0.0199126722524935,-0.189456421067472,3.64303198860262));
#225417=CARTESIAN_POINT('Origin',(-0.019912672252488,0.189456421067567,
42.7590319886026));
#225418=CARTESIAN_POINT('',(61.5108137072212,6.65659636252402,3.64303198860268));
#225419=CARTESIAN_POINT('',(61.9392677289269,6.70162869482191,3.40423097483315));
#225420=CARTESIAN_POINT('Origin',(61.5488354179799,6.66059260535681,3.20400259735912));
#225421=CARTESIAN_POINT('',(62.2936141127097,6.73887200096321,2.83404198860267));
#225422=CARTESIAN_POINT('',(61.9392677289269,6.70162869482191,3.40423097483315));
#225423=CARTESIAN_POINT('',(58.872270023448,6.37927424642597,2.83404198860267));
#225424=CARTESIAN_POINT('',(-0.019912672252488,0.189456421067845,2.83404198860263));
#225425=CARTESIAN_POINT('',(59.2266168948024,6.41651760264857,3.40423097483316));
#225426=CARTESIAN_POINT('',(58.872270023448,6.37927424642597,2.83404198860267));
#225427=CARTESIAN_POINT('',(59.6550713551493,6.46154998175937,3.64303198860268));
#225428=CARTESIAN_POINT('Origin',(59.6170497662628,6.45755375173588,3.20400220587344));
#225429=CARTESIAN_POINT('',(60.0542523589172,6.50350559514725,3.64303198860268));
#225430=CARTESIAN_POINT('',(60.1277056317065,6.51122584595726,3.64303198860268));
#225431=CARTESIAN_POINT('',(60.1796001951995,6.51668018436765,3.42473028058486));
#225432=CARTESIAN_POINT('',(60.0542523588397,6.50350559588484,3.64303198860268));
#225433=CARTESIAN_POINT('',(60.5077528318944,6.55117041629788,3.23423028058487));
#225434=CARTESIAN_POINT('Origin',(60.4784867342337,6.54809390915812,3.56425743004413));
#225435=CARTESIAN_POINT('',(60.6581326136904,6.56697596826297,3.23423028058487));
#225436=CARTESIAN_POINT('',(60.6586584283283,6.56703123360838,3.23423028058487));
#225437=CARTESIAN_POINT('',(60.9862851800404,6.60146619279966,3.42473028058489));
#225438=CARTESIAN_POINT('Origin',(60.6874016969832,6.57005175674002,3.56425912917906));
#225439=CARTESIAN_POINT('',(61.1116329640613,6.61464077578141,3.64303198860268));
#225440=CARTESIAN_POINT('',(60.9862851800404,6.60146619279966,3.42473028058489));
#225441=CARTESIAN_POINT('',(61.5113322352818,6.65665086201929,3.64303198860268));
#225442=CARTESIAN_POINT('Origin',(57.030176100279,11.9273822599896,2.65878198860271));
#225443=CARTESIAN_POINT('',(57.7354693911204,12.2876333308473,2.65878198860271));
#225444=CARTESIAN_POINT('',(61.4699285681954,13.0814171332235,2.65878198860272));
#225445=CARTESIAN_POINT('',(56.9874003490102,12.1286263473646,2.65878198860271));
#225446=CARTESIAN_POINT('',(61.4762657165316,13.0516031943531,2.65878198860272));
#225447=CARTESIAN_POINT('Origin',(5.50299975530876E-15,1.8496514966728E-13,
2.65878198860263));
#225448=CARTESIAN_POINT('',(57.7418065394566,12.257819391977,2.65878198860271));
#225449=CARTESIAN_POINT('',(57.672648524885,12.2431194021877,2.65878198860271));
#225450=CARTESIAN_POINT('Origin',(5.72166156020094E-15,1.85453804358607E-13,
2.65878198860263));
#225451=CARTESIAN_POINT('Origin',(0.0396071771007832,-0.186337117939879,
42.7590319886026));
#225452=CARTESIAN_POINT('',(58.7320730967338,12.2891316338726,3.64303198860272));
#225453=CARTESIAN_POINT('',(58.3106729199896,12.1995602612167,3.4042309748332));
#225454=CARTESIAN_POINT('Origin',(58.6946775141712,12.2811829574214,3.20400220531691));
#225455=CARTESIAN_POINT('',(57.9621601887016,12.1254815938992,2.83404198860271));
#225456=CARTESIAN_POINT('',(58.3106729199896,12.1995602612167,3.4042309748332));
#225457=CARTESIAN_POINT('',(61.3271735965893,12.84073727331,2.83404198860271));
#225458=CARTESIAN_POINT('',(61.581282930652,12.8947498796466,2.83404198860271));
#225459=CARTESIAN_POINT('',(60.9786613449626,12.7666587067856,3.4042309748332));
#225460=CARTESIAN_POINT('',(61.3271735965893,12.84073727331,2.83404198860271));
#225461=CARTESIAN_POINT('',(60.5572615995843,12.6770874264381,3.64303198860273));
#225462=CARTESIAN_POINT('Origin',(60.5946573025915,12.6850361284906,3.20400259788215));
#225463=CARTESIAN_POINT('',(60.164653163458,12.5936359264448,3.64303198860272));
#225464=CARTESIAN_POINT('',(0.0396071771007887,-0.186337117939606,3.64303198860262));
#225465=CARTESIAN_POINT('',(60.0413691664787,12.5674311046656,3.42473028058494));
#225466=CARTESIAN_POINT('',(60.16465316331,12.593635927141,3.64303198860272));
#225467=CARTESIAN_POINT('',(59.7186194643909,12.4988285377098,3.23423028058491));
#225468=CARTESIAN_POINT('Origin',(59.747403715734,12.5049473440523,3.56425722717254));
#225469=CARTESIAN_POINT('',(59.5707156088321,12.4673906027145,3.23423028058491));
#225470=CARTESIAN_POINT('',(0.0396071771007888,-0.186337117939603,3.23423028058481));
#225471=CARTESIAN_POINT('',(59.2479658375576,12.3987880210526,3.4247302805849));
#225472=CARTESIAN_POINT('Origin',(59.5419282989951,12.4612721960125,3.56425909740992));
#225473=CARTESIAN_POINT('',(59.124681789249,12.3725831876354,3.64303198860272));
#225474=CARTESIAN_POINT('',(59.2479658375576,12.3987880210526,3.4247302805849));
#225475=CARTESIAN_POINT('',(0.0396071771007887,-0.186337117939606,3.64303198860262));
#225476=CARTESIAN_POINT('Origin',(-0.0396071771007832,0.186337117939701,
42.7590319886026));
#225477=CARTESIAN_POINT('',(60.4780472453827,13.0497616623177,3.64303198860272));
#225478=CARTESIAN_POINT('',(60.8994469906352,13.1393329432572,3.4042309748332));
#225479=CARTESIAN_POINT('Origin',(60.5154429481088,13.0577103643104,3.20400259735752));
#225480=CARTESIAN_POINT('',(61.2479592422937,13.2134115096321,2.83404198860272));
#225481=CARTESIAN_POINT('',(60.8994469906352,13.1393329432572,3.4042309748332));
#225482=CARTESIAN_POINT('',(57.8829458346105,12.4981558292589,2.83404198860271));
#225483=CARTESIAN_POINT('',(-0.0396071771007831,0.186337117939978,2.83404198860263));
#225484=CARTESIAN_POINT('',(58.2314585659348,12.5722344964055,3.40423097483319));
#225485=CARTESIAN_POINT('',(57.8829458346105,12.4981558292589,2.83404198860271));
#225486=CARTESIAN_POINT('',(58.6528587425322,12.6618058697521,3.64303198860272));
#225487=CARTESIAN_POINT('Origin',(58.6154631596726,12.6538571932379,3.20400220587084));
#225488=CARTESIAN_POINT('',(59.0454674352017,12.7452574227893,3.64303198860272));
#225489=CARTESIAN_POINT('',(59.1177113373238,12.7606133389844,3.64303198860272));
#225490=CARTESIAN_POINT('',(59.1687514833561,12.7714622569322,3.4247302805849));
#225491=CARTESIAN_POINT('',(59.0454674350475,12.7452574235149,3.64303198860272));
#225492=CARTESIAN_POINT('',(59.4915012546305,12.8400648385941,3.23423028058491));
#225493=CARTESIAN_POINT('Origin',(59.4627170622781,12.8339460446679,3.5642574300432));
#225494=CARTESIAN_POINT('',(59.6394051101893,12.8715027735894,3.23423028058491));
#225495=CARTESIAN_POINT('',(59.639922267558,12.8716126987815,3.23423028058491));
#225496=CARTESIAN_POINT('',(59.9621548122771,12.9401053405452,3.42473028058493));
#225497=CARTESIAN_POINT('Origin',(59.6681923469394,12.8776211648734,3.5642591291771));
#225498=CARTESIAN_POINT('',(60.0854388091085,12.9663101630206,3.64303198860272));
#225499=CARTESIAN_POINT('',(59.9621548122771,12.9401053405452,3.42473028058493));
#225500=CARTESIAN_POINT('',(60.4785572361439,13.0498700642004,3.64303198860272));
#225501=CARTESIAN_POINT('Origin',(55.4710078899933,17.8233194796326,2.65878198860275));
#225502=CARTESIAN_POINT('',(56.1347810195642,18.2553202812751,2.65878198860275));
#225503=CARTESIAN_POINT('',(59.7658094374951,19.4351129318423,2.65878198860276));
#225504=CARTESIAN_POINT('',(55.4074307335706,18.0189898472952,2.65878198860275));
#225505=CARTESIAN_POINT('',(59.7752282754837,19.4061247292256,2.65878198860276));
#225506=CARTESIAN_POINT('Origin',(5.50698230308588E-15,1.84950286596632E-13,
2.65878198860263));
#225507=CARTESIAN_POINT('',(56.1441998575527,18.2263320786585,2.65878198860275));
#225508=CARTESIAN_POINT('',(56.0769572651639,18.2044836359655,2.65878198860275));
#225509=CARTESIAN_POINT('Origin',(5.71958798166808E-15,1.85461543059045E-13,
2.65878198860263));
#225510=CARTESIAN_POINT('Origin',(0.0588677374284276,-0.181176266354316,
42.7590319886026));
#225511=CARTESIAN_POINT('',(57.1257686104891,18.3609838302742,3.64303198860276));
#225512=CARTESIAN_POINT('',(56.7160396659414,18.227854826074,3.40423097483324));
#225513=CARTESIAN_POINT('Origin',(57.089408747774,18.3491697947258,3.20400220531851));
#225514=CARTESIAN_POINT('',(56.3771794531164,18.1177524692166,2.83404198860275));
#225515=CARTESIAN_POINT('',(56.7160396659414,18.227854826074,3.40423097483324));
#225516=CARTESIAN_POINT('',(59.6489943884564,19.1808295835784,2.83404198860276));
#225517=CARTESIAN_POINT('',(59.8960658302617,19.2611079613976,2.83404198860276));
#225518=CARTESIAN_POINT('',(59.3101346421294,19.0707273770999,3.40423097483324));
#225519=CARTESIAN_POINT('',(59.6489943884564,19.1808295835784,2.83404198860276));
#225520=CARTESIAN_POINT('',(58.9004061169357,18.9375985097924,3.64303198860277));
#225521=CARTESIAN_POINT('Origin',(58.9367660967588,18.9494125833916,3.20400259788259));
#225522=CARTESIAN_POINT('',(58.5186714879535,18.8135654093534,3.64303198860276));
#225523=CARTESIAN_POINT('',(0.0588677374284331,-0.181176266354043,3.64303198860263));
#225524=CARTESIAN_POINT('',(58.3988020033598,18.7746174535802,3.424730280585));
#225525=CARTESIAN_POINT('',(58.5186714877335,18.8135654100305,3.64303198860276));
#225526=CARTESIAN_POINT('',(58.08499127881,18.6726541682848,3.23423028058495));
#225527=CARTESIAN_POINT('Origin',(58.1129782575896,18.6817482287255,3.56425722717045));
#225528=CARTESIAN_POINT('',(57.9411838150807,18.6259282908539,3.23423028058495));
#225529=CARTESIAN_POINT('',(0.0588677374284332,-0.18117626635404,3.23423028058481));
#225530=CARTESIAN_POINT('',(57.6273730232605,18.523964983701,3.42473028058494));
#225531=CARTESIAN_POINT('Origin',(57.9131937527917,18.6168343081659,3.56425909741474));
#225532=CARTESIAN_POINT('',(57.5075034888353,18.485017010988,3.64303198860276));
#225533=CARTESIAN_POINT('',(57.6273730232605,18.523964983701,3.42473028058494));
#225534=CARTESIAN_POINT('',(0.0588677374284331,-0.181176266354043,3.64303198860263));
#225535=CARTESIAN_POINT('Origin',(-0.0588677374284276,0.181176266354137,
42.7590319886026));
#225536=CARTESIAN_POINT('',(58.7826706420788,19.2999510425009,3.64303198860277));
#225537=CARTESIAN_POINT('',(59.1923991670855,19.433079910384,3.40423097483324));
#225538=CARTESIAN_POINT('Origin',(58.8190306216281,19.311765116011,3.20400259735763));
#225539=CARTESIAN_POINT('',(59.5312589134598,19.5431821167169,2.83404198860276));
#225540=CARTESIAN_POINT('',(59.1923991670855,19.433079910384,3.40423097483324));
#225541=CARTESIAN_POINT('',(56.2594439784239,18.4801050014193,2.83404198860275));
#225542=CARTESIAN_POINT('',(-0.0588677374284273,0.181176266354414,2.83404198860262));
#225543=CARTESIAN_POINT('',(56.5983041913029,18.5902073581105,3.40423097483324));
#225544=CARTESIAN_POINT('',(56.2594439784239,18.4801050014193,2.83404198860275));
#225545=CARTESIAN_POINT('',(57.0080331356322,18.7233363629827,3.64303198860276));
#225546=CARTESIAN_POINT('Origin',(56.9716732726285,18.7115223273404,3.20400220587256));
#225547=CARTESIAN_POINT('',(57.3897680142076,18.8473695429911,3.64303198860276));
#225548=CARTESIAN_POINT('',(57.460011026353,18.8701928819397,3.64303198860276));
#225549=CARTESIAN_POINT('',(57.5096375484037,18.8863175164095,3.42473028058494));
#225550=CARTESIAN_POINT('',(57.3897680139784,18.8473695436964,3.64303198860276));
#225551=CARTESIAN_POINT('',(57.8234483402239,18.9882808235623,3.23423028058495));
#225552=CARTESIAN_POINT('Origin',(57.7954614188164,18.9791867816369,3.56425743004576));
#225553=CARTESIAN_POINT('',(57.9672558039532,19.0350067009933,3.23423028058495));
#225554=CARTESIAN_POINT('',(57.9677586379683,19.0351700816687,3.23423028058495));
#225555=CARTESIAN_POINT('',(58.281066528503,19.1369699862886,3.42473028058497));
#225556=CARTESIAN_POINT('Origin',(57.9952457951704,19.044100660709,3.564259129176));
#225557=CARTESIAN_POINT('',(58.4009360128767,19.1759179427389,3.64303198860277));
#225558=CARTESIAN_POINT('',(58.281066528503,19.1369699862886,3.42473028058497));
#225559=CARTESIAN_POINT('',(58.783166507975,19.3001121590972,3.64303198860277));
#225560=CARTESIAN_POINT('Origin',(53.3040877092102,23.5239806812874,2.65878198860279));
#225561=CARTESIAN_POINT('',(53.9190682401995,24.0229981225299,2.65878198860279));
#225562=CARTESIAN_POINT('',(57.4068835917979,25.575873566121,2.6587819886028));
#225563=CARTESIAN_POINT('',(53.2204057122638,23.7119335237428,2.65878198860279));
#225564=CARTESIAN_POINT('',(57.4192809246789,25.5480287005721,2.6587819886028));
#225565=CARTESIAN_POINT('Origin',(5.51249664798382E-15,1.8493592123704E-13,
2.65878198860263));
#225566=CARTESIAN_POINT('',(53.9314655730804,23.995153256981,2.65878198860279));
#225567=CARTESIAN_POINT('',(53.8668751267878,23.9663957374946,2.65878198860279));
#225568=CARTESIAN_POINT('Origin',(5.71671684795091E-15,1.85469022618095E-13,
2.65878198860263));
#225569=CARTESIAN_POINT('Origin',(0.0774833305059401,-0.174030409681005,
42.7590319886026));
#225570=CARTESIAN_POINT('',(54.8935822490122,24.2316692455485,3.6430319886028));
#225571=CARTESIAN_POINT('',(54.5000136127188,24.056441199033,3.40423097483328));
#225572=CARTESIAN_POINT('Origin',(54.8586564724108,24.2161192879489,3.20400220531754));
#225573=CARTESIAN_POINT('',(54.1745185417598,23.9115214570972,2.83404198860279));
#225574=CARTESIAN_POINT('',(54.5000136127188,24.056441199033,3.40423097483328));
#225575=CARTESIAN_POINT('',(57.317288315449,25.3107727110825,2.8340419886028));
#225576=CARTESIAN_POINT('',(57.5546148985775,25.4164373136776,2.8340419886028));
#225577=CARTESIAN_POINT('',(56.9917936927131,25.1658531674651,3.40423097483328));
#225578=CARTESIAN_POINT('',(57.317288315449,25.3107727110825,2.8340419886028));
#225579=CARTESIAN_POINT('',(56.5982254591675,24.9906253009261,3.64303198860281));
#225580=CARTESIAN_POINT('Origin',(56.6331513482583,25.0061753086093,3.20400259788195));
#225581=CARTESIAN_POINT('',(56.2315470018077,24.8273695326456,3.64303198860281));
#225582=CARTESIAN_POINT('',(0.0774833305059456,-0.174030409680732,3.64303198860263));
#225583=CARTESIAN_POINT('',(56.1164053447571,24.776105164832,3.42473028058504));
#225584=CARTESIAN_POINT('',(56.2315470015181,24.8273695332959,3.64303198860281));
#225585=CARTESIAN_POINT('',(55.8149717737126,24.641898292288,3.23423028058499));
#225586=CARTESIAN_POINT('Origin',(55.8418548487321,24.6538679703977,3.56425722716871));
#225587=CARTESIAN_POINT('',(55.6768362864792,24.5803964109126,3.23423028058499));
#225588=CARTESIAN_POINT('',(0.0774833305059457,-0.174030409680729,3.23423028058481));
#225589=CARTESIAN_POINT('',(55.3754026508175,24.4461895095991,3.42473028058498));
#225590=CARTESIAN_POINT('Origin',(55.6499501367166,24.568426487816,3.56425909741775));
#225591=CARTESIAN_POINT('',(55.260260945979,24.3949251197297,3.6430319886028));
#225592=CARTESIAN_POINT('',(55.3754026508175,24.4461895095991,3.42473028058498));
#225593=CARTESIAN_POINT('',(0.0774833305059456,-0.174030409680732,3.64303198860263));
#225594=CARTESIAN_POINT('Origin',(-0.0774833305059401,0.174030409680826,
42.7590319886026));
#225595=CARTESIAN_POINT('',(56.4432587981556,25.338686120288,3.64303198860281));
#225596=CARTESIAN_POINT('',(56.8368270314553,25.5139139873792,3.40423097483328));
#225597=CARTESIAN_POINT('Origin',(56.4781846869834,25.354236127854,3.20400259735723));
#225598=CARTESIAN_POINT('',(57.1623216542531,25.6588335308577,2.8340419886028));
#225599=CARTESIAN_POINT('',(56.8368270314553,25.5139139873792,3.40423097483328));
#225600=CARTESIAN_POINT('',(54.0195518809641,24.2595822759735,2.83404198860279));
#225601=CARTESIAN_POINT('',(-0.0774833305059396,0.174030409681103,2.83404198860262));
#225602=CARTESIAN_POINT('',(54.3450469519943,24.4045020177494,3.40423097483328));
#225603=CARTESIAN_POINT('',(54.0195518809641,24.2595822759735,2.83404198860279));
#225604=CARTESIAN_POINT('',(54.7386155880003,24.5797300649104,3.6430319886028));
#225605=CARTESIAN_POINT('Origin',(54.7036898111205,24.5641801071868,3.20400220587398));
#225606=CARTESIAN_POINT('',(55.1052942852688,24.7429859384141,3.64303198860281));
#225607=CARTESIAN_POINT('',(55.1727668102971,24.7730266428387,3.64303198860281));
#225608=CARTESIAN_POINT('',(55.2204359898056,24.794250328961,3.42473028058499));
#225609=CARTESIAN_POINT('',(55.1052942849672,24.7429859390916,3.64303198860281));
#225610=CARTESIAN_POINT('',(55.5218696254673,24.9284572302744,3.23423028058499));
#225611=CARTESIAN_POINT('Origin',(55.494986605568,24.9164875765746,3.56425743003997));
#225612=CARTESIAN_POINT('',(55.6600051127008,24.9899591116498,3.23423028058499));
#225613=CARTESIAN_POINT('',(55.6604881142076,24.9901741577757,3.23423028058499));
#225614=CARTESIAN_POINT('',(55.9614386837453,25.1241659841938,3.42473028058501));
#225615=CARTESIAN_POINT('Origin',(55.6868911941839,25.0019290044718,3.56425912917526));
#225616=CARTESIAN_POINT('',(56.0765803405063,25.1754303526578,3.64303198860281));
#225617=CARTESIAN_POINT('',(55.9614386837453,25.1241659841938,3.42473028058501));
#225618=CARTESIAN_POINT('',(56.4437351063763,25.3388981863709,3.64303198860281));
#225619=CARTESIAN_POINT('Origin',(50.5531567888875,28.9669082278886,2.65878198860283));
#225620=CARTESIAN_POINT('',(51.1126068659047,29.5274749692187,2.65878198860283));
#225621=CARTESIAN_POINT('',(54.4189959163063,31.4364195775137,2.65878198860284));
#225622=CARTESIAN_POINT('',(50.4502867888875,29.1450842944632,2.65878198860283));
#225623=CARTESIAN_POINT('',(54.4342359163063,31.4100231232064,2.65878198860284));
#225624=CARTESIAN_POINT('Origin',(5.51948237368594E-15,1.84922210978388E-13,
2.65878198860263));
#225625=CARTESIAN_POINT('',(51.1278468659047,29.5010785149114,2.65878198860283));
#225626=CARTESIAN_POINT('',(51.0666162321543,29.465726992033,2.65878198860283));
#225627=CARTESIAN_POINT('Origin',(5.71307961579125E-15,1.85476161088142E-13,
2.65878198860263));
#225628=CARTESIAN_POINT('Origin',(0.0952500000000002,-0.164977839421025,
42.7590319886026));
#225629=CARTESIAN_POINT('',(52.0599703131946,29.8368674217658,3.64303198860284));
#225630=CARTESIAN_POINT('',(51.6868740054943,29.6214601680814,3.40423097483331));
#225631=CARTESIAN_POINT('Origin',(52.0268612768246,29.8177519107051,3.20400220531536));
#225632=CARTESIAN_POINT('',(51.3783102685129,29.4433108120864,2.83404198860283));
#225633=CARTESIAN_POINT('',(51.6868740054943,29.6214601680814,3.40423097483331));
#225634=CARTESIAN_POINT('',(54.3576020372438,31.1634057161443,2.83404198860284));
#225635=CARTESIAN_POINT('',(54.582583561987,31.2932988600175,2.83404198860284));
#225636=CARTESIAN_POINT('',(54.0490387253004,30.985256604233,3.40423097483332));
#225637=CARTESIAN_POINT('',(54.3576020372438,31.1634057161443,2.83404198860284));
#225638=CARTESIAN_POINT('',(53.6759427993286,30.7698495716383,3.64303198860285));
#225639=CARTESIAN_POINT('Origin',(53.7090519423386,30.7889651442678,3.20400259788415));
#225640=CARTESIAN_POINT('',(53.3283379195024,30.5691597998769,3.64303198860284));
#225641=CARTESIAN_POINT('',(0.0952500000000057,-0.164977839420752,3.64303198860263));
#225642=CARTESIAN_POINT('',(53.2191856060845,30.5061406831646,3.42473028058507));
#225643=CARTESIAN_POINT('',(53.3283379191464,30.5691598004935,3.64303198860284));
#225644=CARTESIAN_POINT('',(52.9334317578287,30.3411606219521,3.23423028058503));
#225645=CARTESIAN_POINT('Origin',(52.9589163924918,30.3558747754324,3.56425722716898));
#225646=CARTESIAN_POINT('',(52.8024816883959,30.2655565641147,3.23423028058503));
#225647=CARTESIAN_POINT('',(0.0952500000000058,-0.164977839420749,3.23423028058481));
#225648=CARTESIAN_POINT('',(52.5167277788841,30.100576467536,3.42473028058502));
#225649=CARTESIAN_POINT('Origin',(52.7769940214379,30.2508418455893,3.5642590974096));
#225650=CARTESIAN_POINT('',(52.4075754202456,30.0375573238934,3.64303198860284));
#225651=CARTESIAN_POINT('',(52.5167277788841,30.100576467536,3.42473028058502));
#225652=CARTESIAN_POINT('',(0.0952500000000057,-0.164977839420752,3.64303198860263));
#225653=CARTESIAN_POINT('Origin',(-0.0952500000000002,0.164977839420846,
42.7590319886026));
#225654=CARTESIAN_POINT('',(53.4854427993286,31.0998052504802,3.64303198860285));
#225655=CARTESIAN_POINT('',(53.8585387249978,31.3152122835989,3.40423097483333));
#225656=CARTESIAN_POINT('Origin',(53.5185519420887,31.1189208229654,3.20400259735773));
#225657=CARTESIAN_POINT('',(54.1671020370177,31.4933613953778,2.83404198860284));
#225658=CARTESIAN_POINT('',(53.8585387249979,31.3152122835989,3.40423097483333));
#225659=CARTESIAN_POINT('',(51.1878102687785,29.7732664904683,2.83404198860283));
#225660=CARTESIAN_POINT('',(-0.0952499999999994,0.164977839421122,2.83404198860262));
#225661=CARTESIAN_POINT('',(51.4963740058474,29.9514158463116,3.40423097483332));
#225662=CARTESIAN_POINT('',(51.1878102687785,29.7732664904682,2.83404198860283));
#225663=CARTESIAN_POINT('',(51.8694703131946,30.1668231006077,3.64303198860284));
#225664=CARTESIAN_POINT('Origin',(51.8363612765612,30.1477075893948,3.20400220587076));
#225665=CARTESIAN_POINT('',(52.2170754206163,30.3675130020933,3.64303198860284));
#225666=CARTESIAN_POINT('',(52.2810382154239,30.4044419397496,3.64303198860284));
#225667=CARTESIAN_POINT('',(52.3262277788841,30.4305321463779,3.42473028058504));
#225668=CARTESIAN_POINT('',(52.2170754202456,30.3675130027353,3.64303198860284));
#225669=CARTESIAN_POINT('',(52.6119816883959,30.5955122429565,3.23423028058503));
#225670=CARTESIAN_POINT('Origin',(52.5864971060028,30.580798119516,3.56425743004708));
#225671=CARTESIAN_POINT('',(52.7429317578287,30.671116300794,3.23423028058504));
#225672=CARTESIAN_POINT('',(52.7433896349617,30.67138065628,3.23423028058504));
#225673=CARTESIAN_POINT('',(53.0286856060845,30.8360963620065,3.42473028058505));
#225674=CARTESIAN_POINT('Origin',(52.768419360041,30.6858309820707,3.5642591291773));
#225675=CARTESIAN_POINT('',(53.1378379191464,30.8991154793354,3.64303198860285));
#225676=CARTESIAN_POINT('',(53.0286856060845,30.8360963620065,3.42473028058505));
#225677=CARTESIAN_POINT('',(53.4858943313413,31.1000659426093,3.64303198860285));
#225678=CARTESIAN_POINT('Origin',(47.2483549038575,34.0924682662297,2.65878198860287));
#225679=CARTESIAN_POINT('',(47.7461450747864,34.7084426211234,2.65878198860287));
#225680=CARTESIAN_POINT('',(50.8348823336486,36.9525415975215,2.65878198860288));
#225681=CARTESIAN_POINT('',(47.1274239660509,34.2589154226524,2.65878198860287));
#225682=CARTESIAN_POINT('',(50.8527980281384,36.9278827595329,2.65878198860288));
#225683=CARTESIAN_POINT('Origin',(5.52786294311959E-15,1.84909306033141E-13,
2.65878198860263));
#225684=CARTESIAN_POINT('',(47.7640607692763,34.6837837831348,2.65878198860287));
#225685=CARTESIAN_POINT('',(47.706860803705,34.6422255755468,2.65878198860287));
#225686=CARTESIAN_POINT('Origin',(5.70871613546578E-15,1.85482880258616E-13,
2.65878198860263));
#225687=CARTESIAN_POINT('Origin',(0.111973090561716,-0.154117737428517,
42.7590319886026));
#225688=CARTESIAN_POINT('',(48.6559784483765,35.1151666347443,3.64303198860288));
#225689=CARTESIAN_POINT('',(48.3074421904918,34.8619402208393,3.40423097483335));
#225690=CARTESIAN_POINT('Origin',(48.6250489017664,35.0926950037602,3.2040022053186));
#225691=CARTESIAN_POINT('',(48.0191904763612,34.65251309241,2.83404198860287));
#225692=CARTESIAN_POINT('',(48.3074421904918,34.8619402208393,3.40423097483335));
#225693=CARTESIAN_POINT('',(50.8023624960591,36.6746059268181,2.83404198860288));
#225694=CARTESIAN_POINT('',(51.0125340177515,36.8273044755032,2.83404198860288));
#225695=CARTESIAN_POINT('',(50.5141111791245,36.4651790855638,3.40423097483335));
#225696=CARTESIAN_POINT('',(50.8023624960591,36.6746059268181,2.83404198860288));
#225697=CARTESIAN_POINT('',(50.1655752777671,36.2119529314387,3.64303198860289));
#225698=CARTESIAN_POINT('Origin',(50.1965049239958,36.2344246348,3.2040025978838));
#225699=CARTESIAN_POINT('',(49.8408524072786,35.9760279553333,3.64303198860289));
#225700=CARTESIAN_POINT('',(0.111973090561722,-0.154117737428244,3.64303198860263));
#225701=CARTESIAN_POINT('',(49.7388853330811,35.9019445403521,3.42473028058511));
#225702=CARTESIAN_POINT('',(49.8408524068603,35.9760279559089,3.64303198860289));
#225703=CARTESIAN_POINT('',(49.4719419865733,35.7079988465461,3.23423028058507));
#225704=CARTESIAN_POINT('Origin',(49.4957489658887,35.7252962640517,3.56425722717078));
#225705=CARTESIAN_POINT('',(49.3496120513049,35.6191209461254,3.23423028058507));
#225706=CARTESIAN_POINT('',(0.111973090561722,-0.154117737428241,3.23423028058481));
#225707=CARTESIAN_POINT('',(49.0826686475734,35.425175210744,3.42473028058506));
#225708=CARTESIAN_POINT('Origin',(49.3258021153704,35.60182264971,3.56425909741427));
#225709=CARTESIAN_POINT('',(48.9807015312178,35.3510917642536,3.64303198860288));
#225710=CARTESIAN_POINT('',(49.0826686475734,35.425175210744,3.42473028058506));
#225711=CARTESIAN_POINT('',(0.111973090561722,-0.154117737428244,3.64303198860263));
#225712=CARTESIAN_POINT('Origin',(-0.111973090561716,0.154117737428338,
42.7590319886026));
#225713=CARTESIAN_POINT('',(49.9416290966437,36.5201884062956,3.64303198860289));
#225714=CARTESIAN_POINT('',(50.2901649976455,36.7734145609101,3.40423097483336));
#225715=CARTESIAN_POINT('Origin',(49.9725587426394,36.5426601094876,3.20400259735887));
#225716=CARTESIAN_POINT('',(50.5784163146694,36.9828414020413,2.83404198860288));
#225717=CARTESIAN_POINT('',(50.2901649976455,36.7734145609101,3.40423097483336));
#225718=CARTESIAN_POINT('',(47.7952442955502,34.9607485668368,2.83404198860286));
#225719=CARTESIAN_POINT('',(-0.111973090561715,0.154117737428614,2.83404198860262));
#225720=CARTESIAN_POINT('',(48.0834960097835,35.1701756951247,3.40423097483336));
#225721=CARTESIAN_POINT('',(47.7952442955502,34.9607485668368,2.83404198860287));
#225722=CARTESIAN_POINT('',(48.432032267253,35.4234021096012,3.64303198860288));
#225723=CARTESIAN_POINT('Origin',(48.4011027203975,35.4009304784387,3.20400220587243));
#225724=CARTESIAN_POINT('',(48.7567553505302,35.6593272385106,3.64303198860288));
#225725=CARTESIAN_POINT('',(48.8165076253519,35.7027398082301,3.64303198860288));
#225726=CARTESIAN_POINT('',(48.85872246645,35.7334106856009,3.42473028058506));
#225727=CARTESIAN_POINT('',(48.7567553500944,35.6593272391105,3.64303198860288));
#225728=CARTESIAN_POINT('',(49.1256658701815,35.9273564209823,3.23423028058507));
#225729=CARTESIAN_POINT('Origin',(49.1018589397087,35.9100590388148,3.56425743004647));
#225730=CARTESIAN_POINT('',(49.2479958054498,36.0162343214029,3.23423028058507));
#225731=CARTESIAN_POINT('',(49.2484235416113,36.0165450899149,3.23423028058507));
#225732=CARTESIAN_POINT('',(49.5149391519577,36.2101800152089,3.4247302805851));
#225733=CARTESIAN_POINT('Origin',(49.2718056808886,36.0335325740073,3.56425912917859));
#225734=CARTESIAN_POINT('',(49.6169062257369,36.2842634307658,3.64303198860289));
#225735=CARTESIAN_POINT('',(49.5149391519577,36.2101800152089,3.4247302805851));
#225736=CARTESIAN_POINT('',(49.9420509053691,36.5204948682733,3.64303198860289));
#225737=CARTESIAN_POINT('Origin',(43.425890155147,38.8445040879384,2.6587819886029));
#225738=CARTESIAN_POINT('',(43.8565665267056,39.5091373124625,2.6587819886029));
#225739=CARTESIAN_POINT('',(46.6938111422604,42.0638038389703,2.65878198860292));
#225740=CARTESIAN_POINT('',(43.2882232241948,38.9973987043321,2.6587819886029));
#225741=CARTESIAN_POINT('',(46.7142062431422,42.0411527846897,2.65878198860292));
#225742=CARTESIAN_POINT('Origin',(5.5375465370123E-15,1.84897347790577E-13,
2.65878198860263));
#225743=CARTESIAN_POINT('',(43.8769616275874,39.4864862581819,2.6587819886029));
#225744=CARTESIAN_POINT('',(43.8244190249878,39.4391766863033,2.6587819886029));
#225745=CARTESIAN_POINT('Origin',(5.70367421417806E-15,1.85489106512878E-13,
2.65878198860263));
#225746=CARTESIAN_POINT('Origin',(0.127469380511363,-0.141569089253533,
42.7590319886026));
#225747=CARTESIAN_POINT('',(44.7189015017598,40.0087367337516,3.64303198860291));
#225748=CARTESIAN_POINT('',(44.398743929868,39.7204655612076,3.40423097483339));
#225749=CARTESIAN_POINT('Origin',(44.6904903154964,39.9831551867367,3.20400220531785));
#225750=CARTESIAN_POINT('',(44.1339623846891,39.4820551877881,2.8340419886029));
#225751=CARTESIAN_POINT('',(44.398743929868,39.7204655612076,3.40423097483339));
#225752=CARTESIAN_POINT('',(46.6905216402897,41.7839914803029,2.83404198860292));
#225753=CARTESIAN_POINT('',(46.8835804757584,41.9578224365464,2.83404198860292));
#225754=CARTESIAN_POINT('',(46.4257404601128,41.5455814340038,3.40423097483339));
#225755=CARTESIAN_POINT('',(46.6905216402897,41.7839914803029,2.83404198860291));
#225756=CARTESIAN_POINT('',(46.1055832156409,41.2573105570839,3.64303198860293));
#225757=CARTESIAN_POINT('Origin',(46.133994493411,41.2828921864918,3.20400259788132));
#225758=CARTESIAN_POINT('',(45.8073000862124,40.9887352200424,3.64303198860291));
#225759=CARTESIAN_POINT('',(0.127469380511368,-0.14156908925326,3.64303198860262));
#225760=CARTESIAN_POINT('',(45.7136354238375,40.9043991801906,3.42473028058514));
#225761=CARTESIAN_POINT('',(45.8073000857358,40.9887352205716,3.64303198860291));
#225762=CARTESIAN_POINT('',(45.4684272662435,40.6836127633981,3.23423028058511));
#225763=CARTESIAN_POINT('Origin',(45.4902957559646,40.7033039308034,3.56425722717177));
#225764=CARTESIAN_POINT('',(45.3560577375095,40.5824347852702,3.2342302805851));
#225765=CARTESIAN_POINT('',(0.127469380511368,-0.141569089253257,3.23423028058481));
#225766=CARTESIAN_POINT('',(45.1108495273512,40.3616483211486,3.4247302805851));
#225767=CARTESIAN_POINT('Origin',(45.3341863992351,40.5627424347172,3.56425909741047));
#225768=CARTESIAN_POINT('',(45.0171848263432,40.277312245553,3.64303198860291));
#225769=CARTESIAN_POINT('',(45.1108495273512,40.3616483211486,3.4247302805851));
#225770=CARTESIAN_POINT('',(0.127469380511368,-0.14156908925326,3.64303198860262));
#225771=CARTESIAN_POINT('Origin',(-0.127469380511363,0.141569089253354,
42.7590319886026));
#225772=CARTESIAN_POINT('',(45.8506444546181,41.5404487355908,3.64303198860292));
#225773=CARTESIAN_POINT('',(46.1708016986853,41.8287196129602,3.40423097483339));
#225774=CARTESIAN_POINT('Origin',(45.879055732176,41.5660303648075,3.20400259736081));
#225775=CARTESIAN_POINT('',(46.4355828789643,42.0671296591459,2.83404198860292));
#225776=CARTESIAN_POINT('',(46.1708016986853,41.8287196129602,3.40423097483339));
#225777=CARTESIAN_POINT('',(43.8790236240219,39.7651933659001,2.8340419886029));
#225778=CARTESIAN_POINT('',(-0.127469380511361,0.141569089253629,2.83404198860262));
#225779=CARTESIAN_POINT('',(44.1438051693184,40.0036037391891,3.4042309748334));
#225780=CARTESIAN_POINT('',(43.8790236240219,39.7651933659001,2.8340419886029));
#225781=CARTESIAN_POINT('',(44.4639627407371,40.2918749122585,3.64303198860291));
#225782=CARTESIAN_POINT('Origin',(44.435551554248,40.2662933650404,3.20400220587245));
#225783=CARTESIAN_POINT('',(44.7622460658166,40.5604504235089,3.64303198860292));
#225784=CARTESIAN_POINT('',(44.8171331622256,40.6098709880931,3.64303198860292));
#225785=CARTESIAN_POINT('',(44.8559107663285,40.6447864996555,3.4247302805851));
#225786=CARTESIAN_POINT('',(44.7622460653205,40.5604504240599,3.64303198860292));
#225787=CARTESIAN_POINT('',(45.1011189764868,40.8655729637771,3.23423028058511));
#225788=CARTESIAN_POINT('Origin',(45.0792505316455,40.8458818366205,3.56425743004429));
#225789=CARTESIAN_POINT('',(45.2134885052208,40.966750941905,3.23423028058511));
#225790=CARTESIAN_POINT('',(45.2138814140438,40.9671047185983,3.23423028058511));
#225791=CARTESIAN_POINT('',(45.4586966628148,41.1875373586975,3.42473028058513));
#225792=CARTESIAN_POINT('Origin',(45.2353597879082,40.9864432425615,3.56425912917935));
#225793=CARTESIAN_POINT('',(45.5523613247131,41.2718733990785,3.64303198860292));
#225794=CARTESIAN_POINT('',(45.4586966628148,41.1875373586975,3.42473028058513));
#225795=CARTESIAN_POINT('',(45.8510319186316,41.5407976097556,3.64303198860292));
#225796=CARTESIAN_POINT('Origin',(39.127642266445,43.1709513941246,2.65878198860293));
#225797=CARTESIAN_POINT('',(39.4864862581816,43.8769616275877,2.65878198860293));
#225798=CARTESIAN_POINT('',(42.0411527846894,46.7142062431425,2.65878198860295));
#225799=CARTESIAN_POINT('',(38.9747476500513,43.3086183250769,2.65878198860293));
#225800=CARTESIAN_POINT('',(42.06380383897,46.6938111422607,2.65878198860295));
#225801=CARTESIAN_POINT('Origin',(5.54842705988296E-15,1.84886467267707E-13,
2.65878198860263));
#225802=CARTESIAN_POINT('',(39.5091373124621,43.8565665267059,2.65878198860293));
#225803=CARTESIAN_POINT('',(39.4618277405835,43.8040239241062,2.65878198860293));
#225804=CARTESIAN_POINT('Origin',(5.69800909227282E-15,1.85494771634783E-13,
2.65878198860263));
#225805=CARTESIAN_POINT('Origin',(0.141569089253444,-0.127469380511452,
42.7590319886026));
#225806=CARTESIAN_POINT('',(40.2918749122581,44.4639627407374,3.64303198860293));
#225807=CARTESIAN_POINT('',(40.0036037397142,44.1438051688456,3.40423097483342));
#225808=CARTESIAN_POINT('Origin',(40.2662933652436,44.4355515544743,3.20400220531713));
#225809=CARTESIAN_POINT('',(39.7651933655048,43.8790236243779,2.83404198860293));
#225810=CARTESIAN_POINT('',(40.0036037397142,44.1438051688456,3.40423097483342));
#225811=CARTESIAN_POINT('',(42.0671296588095,46.4355828792673,2.83404198860295));
#225812=CARTESIAN_POINT('',(42.240960615053,46.628641714736,2.83404198860295));
#225813=CARTESIAN_POINT('',(41.8287196134096,46.1708016982807,3.40423097483344));
#225814=CARTESIAN_POINT('',(42.0671296588095,46.4355828792673,2.83404198860294));
#225815=CARTESIAN_POINT('',(41.5404487355905,45.8506444546185,3.64303198860296));
#225816=CARTESIAN_POINT('Origin',(41.566030364998,45.8790557323883,3.20400259788057));
#225817=CARTESIAN_POINT('',(41.2718733996072,45.5523613242371,3.64303198860294));
#225818=CARTESIAN_POINT('',(0.141569089253449,-0.127469380511178,3.64303198860262));
#225819=CARTESIAN_POINT('',(41.1875373586971,45.4586966628151,3.42473028058517));
#225820=CARTESIAN_POINT('',(41.2718733990782,45.5523613247134,3.64303198860294));
#225821=CARTESIAN_POINT('',(40.9667509419047,45.2134885052211,3.23423028058514));
#225822=CARTESIAN_POINT('Origin',(40.9864413462824,45.2353576819759,3.56425722717126));
#225823=CARTESIAN_POINT('',(40.8655729637768,45.1011189764871,3.23423028058513));
#225824=CARTESIAN_POINT('',(0.141569089253449,-0.127469380511176,3.23423028058481));
#225825=CARTESIAN_POINT('',(40.6447864996552,44.8559107663288,3.42473028058512));
#225826=CARTESIAN_POINT('Origin',(40.8458798501231,45.0792483253113,3.56425909741017));
#225827=CARTESIAN_POINT('',(40.5604504240596,44.7622460653208,3.64303198860294));
#225828=CARTESIAN_POINT('',(40.6447864996552,44.8559107663288,3.42473028058512));
#225829=CARTESIAN_POINT('',(0.141569089253449,-0.127469380511178,3.64303198860262));
#225830=CARTESIAN_POINT('Origin',(-0.141569089253444,0.127469380511273,
42.7590319886026));
#225831=CARTESIAN_POINT('',(41.2573105570836,46.1055832156412,3.64303198860295));
#225832=CARTESIAN_POINT('',(41.5455814344529,46.4257404597084,3.40423097483342));
#225833=CARTESIAN_POINT('Origin',(41.2828921862997,46.1339944931982,3.20400259735886));
#225834=CARTESIAN_POINT('',(41.7839914799664,46.6905216405928,2.83404198860295));
#225835=CARTESIAN_POINT('',(41.5455814344529,46.4257404597084,3.40423097483342));
#225836=CARTESIAN_POINT('',(39.4820551873929,44.133962385045,2.83404198860293));
#225837=CARTESIAN_POINT('',(-0.141569089253442,0.127469380511548,2.83404198860262));
#225838=CARTESIAN_POINT('',(39.7204655617325,44.3987439293954,3.40423097483342));
#225839=CARTESIAN_POINT('',(39.4820551873929,44.133962385045,2.83404198860293));
#225840=CARTESIAN_POINT('',(40.0087367337512,44.7189015017601,3.64303198860294));
#225841=CARTESIAN_POINT('Origin',(39.9831551865319,44.6904903152697,3.2040022058757));
#225842=CARTESIAN_POINT('',(40.2773122461039,45.0171848258472,3.64303198860295));
#225843=CARTESIAN_POINT('',(40.3267328095859,45.0720719232486,3.64303198860295));
#225844=CARTESIAN_POINT('',(40.3616483211483,45.1108495273515,3.42473028058513));
#225845=CARTESIAN_POINT('',(40.2773122455527,45.0171848263435,3.64303198860295));
#225846=CARTESIAN_POINT('',(40.5824347852699,45.3560577375099,3.23423028058514));
#225847=CARTESIAN_POINT('Origin',(40.5627444213189,45.3341886054746,3.56425743004301));
#225848=CARTESIAN_POINT('',(40.6836127633978,45.4684272662438,3.23423028058514));
#225849=CARTESIAN_POINT('',(40.6839665400911,45.4688201750668,3.23423028058514));
#225850=CARTESIAN_POINT('',(40.9043991801903,45.7136354238378,3.42473028058516));
#225851=CARTESIAN_POINT('Origin',(40.7033058269857,45.4902978619874,3.56425912917592));
#225852=CARTESIAN_POINT('',(40.9887352205713,45.8073000857361,3.64303198860295));
#225853=CARTESIAN_POINT('',(40.9043991801903,45.7136354238378,3.42473028058516));
#225854=CARTESIAN_POINT('',(41.2576594312484,46.1059706796547,3.64303198860295));
#225855=CARTESIAN_POINT('Origin',(34.4007037410862,47.0244087227344,2.65878198860296));
#225856=CARTESIAN_POINT('',(34.6837837831345,47.7640607692766,2.65878198860296));
#225857=CARTESIAN_POINT('',(36.9278827595326,50.8527980281387,2.65878198860298));
#225858=CARTESIAN_POINT('',(34.2342565846635,47.1453396605411,2.65878198860296));
#225859=CARTESIAN_POINT('',(36.9525415975211,50.8348823336489,2.65878198860298));
#225860=CARTESIAN_POINT('Origin',(5.5603853024461E-15,1.84876783673814E-13,
2.65878198860263));
#225861=CARTESIAN_POINT('',(34.7084426211231,47.7461450747867,2.65878198860296));
#225862=CARTESIAN_POINT('',(34.6668844135351,47.6889451092154,2.65878198860296));
#225863=CARTESIAN_POINT('Origin',(5.69178283801114E-15,1.85499813556071E-13,
2.65878198860263));
#225864=CARTESIAN_POINT('Origin',(0.154117737428428,-0.111973090561805,
42.7590319886026));
#225865=CARTESIAN_POINT('',(35.4234021096009,48.4320322672533,3.64303198860296));
#225866=CARTESIAN_POINT('',(35.1701756956958,48.0834960093686,3.40423097483345));
#225867=CARTESIAN_POINT('Origin',(35.4009304786174,48.4011027206441,3.20400220531654));
#225868=CARTESIAN_POINT('',(34.9607485664065,47.7952442958629,2.83404198860295));
#225869=CARTESIAN_POINT('',(35.1701756956958,48.0834960093686,3.40423097483344));
#225870=CARTESIAN_POINT('',(36.9828414016746,50.578416314936,2.83404198860297));
#225871=CARTESIAN_POINT('',(37.1355399503597,50.7885878366283,2.83404198860297));
#225872=CARTESIAN_POINT('',(36.7734145613994,50.29016499729,3.40423097483345));
#225873=CARTESIAN_POINT('',(36.9828414016746,50.5784163149359,2.83404198860297));
#225874=CARTESIAN_POINT('',(36.5201884062952,49.941629096644,3.64303198860299));
#225875=CARTESIAN_POINT('Origin',(36.542660109656,49.9725587428719,3.2040025978818));
#225876=CARTESIAN_POINT('',(36.2842634313411,49.616906225319,3.64303198860297));
#225877=CARTESIAN_POINT('',(0.154117737428433,-0.111973090561532,3.64303198860262));
#225878=CARTESIAN_POINT('',(36.2101800152086,49.514939151958,3.42473028058521));
#225879=CARTESIAN_POINT('',(36.2842634307655,49.6169062257372,3.64303198860297));
#225880=CARTESIAN_POINT('',(36.0162343214026,49.2479958054501,3.23423028058516));
#225881=CARTESIAN_POINT('Origin',(36.0335309082456,49.2718033882769,3.56425722717131));
#225882=CARTESIAN_POINT('',(35.927356420982,49.1256658701818,3.23423028058516));
#225883=CARTESIAN_POINT('',(0.154117737428433,-0.111973090561529,3.23423028058481));
#225884=CARTESIAN_POINT('',(35.7334106856005,48.8587224664503,3.42473028058515));
#225885=CARTESIAN_POINT('Origin',(35.9100572938233,49.1018565378139,3.5642590974097));
#225886=CARTESIAN_POINT('',(35.6593272391101,48.7567553500947,3.64303198860296));
#225887=CARTESIAN_POINT('',(35.7334106856005,48.8587224664503,3.42473028058515));
#225888=CARTESIAN_POINT('',(0.154117737428433,-0.111973090561532,3.64303198860262));
#225889=CARTESIAN_POINT('Origin',(-0.154117737428428,0.111973090561626,
42.7590319886026));
#225890=CARTESIAN_POINT('',(36.2119529314384,50.1655752777674,3.64303198860298));
#225891=CARTESIAN_POINT('',(36.4651790860528,50.5141111787692,3.40423097483345));
#225892=CARTESIAN_POINT('Origin',(36.2344246346307,50.1965049237635,3.2040025973597));
#225893=CARTESIAN_POINT('',(36.6746059264518,50.8023624963252,2.83404198860297));
#225894=CARTESIAN_POINT('',(36.4651790860528,50.5141111787692,3.40423097483345));
#225895=CARTESIAN_POINT('',(34.6525130919796,48.0191904766739,2.83404198860296));
#225896=CARTESIAN_POINT('',(-0.154117737428425,0.111973090561901,2.83404198860262));
#225897=CARTESIAN_POINT('',(34.8619402214104,48.3074421900769,3.40423097483345));
#225898=CARTESIAN_POINT('',(34.6525130919796,48.0191904766739,2.83404198860296));
#225899=CARTESIAN_POINT('',(35.115166634744,48.6559784483767,3.64303198860297));
#225900=CARTESIAN_POINT('Origin',(35.0926950035816,48.6250489015213,3.2040022058722));
#225901=CARTESIAN_POINT('',(35.3510917648536,48.9807015307819,3.64303198860298));
#225902=CARTESIAN_POINT('',(35.3945043333729,49.0404538064756,3.64303198860298));
#225903=CARTESIAN_POINT('',(35.4251752107437,49.0826686475737,3.42473028058515));
#225904=CARTESIAN_POINT('',(35.3510917642532,48.9807015312181,3.64303198860298));
#225905=CARTESIAN_POINT('',(35.6191209461251,49.3496120513052,3.23423028058516));
#225906=CARTESIAN_POINT('Origin',(35.6018243948128,49.3258045171784,3.56425743004293));
#225907=CARTESIAN_POINT('',(35.7079988465457,49.4719419865736,3.23423028058516));
#225908=CARTESIAN_POINT('',(35.7083096150578,49.472369722735,3.23423028058516));
#225909=CARTESIAN_POINT('',(35.9019445403517,49.7388853330814,3.42473028058518));
#225910=CARTESIAN_POINT('Origin',(35.7252979297061,49.4957512585779,3.56425912917861));
#225911=CARTESIAN_POINT('',(35.9760279559086,49.8408524068606,3.64303198860298));
#225912=CARTESIAN_POINT('',(35.9019445403517,49.7388853330814,3.42473028058518));
#225913=CARTESIAN_POINT('',(36.2122593934161,50.1659970864928,3.64303198860298));
#225914=CARTESIAN_POINT('Origin',(29.2968639067301,50.3626567888878,2.65878198860297));
#225915=CARTESIAN_POINT('',(29.501078514911,51.1278468659049,2.65878198860298));
#225916=CARTESIAN_POINT('',(31.410023123206,54.4342359163065,2.658781988603));
#225917=CARTESIAN_POINT('',(29.1186878401555,50.4655267888878,2.65878198860297));
#225918=CARTESIAN_POINT('',(31.4364195775134,54.4189959163065,2.658781988603));
#225919=CARTESIAN_POINT('Origin',(5.57329024769379E-15,1.8486840310438E-13,
2.65878198860263));
#225920=CARTESIAN_POINT('',(29.5274749692184,51.1126068659049,2.65878198860298));
#225921=CARTESIAN_POINT('',(29.49212344634,51.0513762321546,2.65878198860298));
#225922=CARTESIAN_POINT('Origin',(5.68506366753766E-15,1.85504177036396E-13,
2.65878198860263));
#225923=CARTESIAN_POINT('Origin',(0.164977839420936,-0.0952500000000889,
42.7590319886026));
#225924=CARTESIAN_POINT('',(30.1668231006074,51.8694703131949,3.64303198860299));
#225925=CARTESIAN_POINT('',(29.9514158469229,51.4963740054945,3.40423097483346));
#225926=CARTESIAN_POINT('Origin',(30.1477075895462,51.8363612768243,3.20400220531662));
#225927=CARTESIAN_POINT('',(29.7732664900075,51.1878102690446,2.83404198860297));
#225928=CARTESIAN_POINT('',(29.9514158469229,51.4963740054945,3.40423097483346));
#225929=CARTESIAN_POINT('',(31.4933613949858,54.1671020372441,2.834041988603));
#225930=CARTESIAN_POINT('',(31.623254538859,54.3920835619873,2.83404198860299));
#225931=CARTESIAN_POINT('',(31.3152122841225,53.8585387246956,3.40423097483348));
#225932=CARTESIAN_POINT('',(31.4933613949858,54.1671020372441,2.83404198860299));
#225933=CARTESIAN_POINT('',(31.0998052504799,53.4854427993289,3.64303198860301));
#225934=CARTESIAN_POINT('Origin',(31.1189208231087,53.5185519423378,3.2040025978818));
#225935=CARTESIAN_POINT('',(30.8991154799516,53.1378379187907,3.643031988603));
#225936=CARTESIAN_POINT('',(0.164977839420941,-0.0952499999998158,3.64303198860262));
#225937=CARTESIAN_POINT('',(30.8360963620061,53.0286856060848,3.42473028058523));
#225938=CARTESIAN_POINT('',(30.899115479335,53.1378379191467,3.643031988603));
#225939=CARTESIAN_POINT('',(30.6711163007936,52.742931757829,3.23423028058519));
#225940=CARTESIAN_POINT('Origin',(30.6858295650771,52.7684169058685,3.56425722717158));
#225941=CARTESIAN_POINT('',(30.5955122429562,52.6119816883962,3.23423028058518));
#225942=CARTESIAN_POINT('',(0.164977839420941,-0.095249999999813,3.23423028058481));
#225943=CARTESIAN_POINT('',(30.4305321463776,52.3262277788844,3.42473028058517));
#225944=CARTESIAN_POINT('Origin',(30.5807966351508,52.586494534866,3.56425909741312));
#225945=CARTESIAN_POINT('',(30.367513002735,52.2170754202459,3.64303198860299));
#225946=CARTESIAN_POINT('',(30.4305321463776,52.3262277788844,3.42473028058517));
#225947=CARTESIAN_POINT('',(0.164977839420941,-0.0952499999998158,3.64303198860262));
#225948=CARTESIAN_POINT('Origin',(-0.164977839420936,0.0952499999999103,
42.7590319886026));
#225949=CARTESIAN_POINT('',(30.769849571638,53.6759427993289,3.64303198860301));
#225950=CARTESIAN_POINT('',(30.9852566047567,54.0490387249981,3.40423097483348));
#225951=CARTESIAN_POINT('Origin',(30.7889651441231,53.709051942089,3.20400259735764));
#225952=CARTESIAN_POINT('',(31.1634057157522,54.3576020374702,2.83404198860299));
#225953=CARTESIAN_POINT('',(30.9852566047567,54.0490387249981,3.40423097483348));
#225954=CARTESIAN_POINT('',(29.443310811626,51.3783102687787,2.83404198860297));
#225955=CARTESIAN_POINT('',(-0.164977839420933,0.0952500000001842,2.83404198860262));
#225956=CARTESIAN_POINT('',(29.6214601686927,51.6868740051414,3.40423097483347));
#225957=CARTESIAN_POINT('',(29.443310811626,51.3783102687787,2.83404198860297));
#225958=CARTESIAN_POINT('',(29.8368674217655,52.0599703131949,3.643031988603));
#225959=CARTESIAN_POINT('Origin',(29.8177519105523,52.026861276561,3.20400220587187));
#225960=CARTESIAN_POINT('',(30.0375573245353,52.4075754198751,3.643031988603));
#225961=CARTESIAN_POINT('',(30.0744862609074,52.4715382154242,3.643031988603));
#225962=CARTESIAN_POINT('',(30.1005764675357,52.5167277788844,3.42473028058518));
#225963=CARTESIAN_POINT('',(30.0375573238931,52.4075754202459,3.643031988603));
#225964=CARTESIAN_POINT('',(30.2655565641143,52.8024816883962,3.23423028058519));
#225965=CARTESIAN_POINT('Origin',(30.2508433300764,52.776996592504,3.56425743004371));
#225966=CARTESIAN_POINT('',(30.3411606219517,52.933431757829,3.23423028058519));
#225967=CARTESIAN_POINT('',(30.3414249774377,52.933889634962,3.23423028058519));
#225968=CARTESIAN_POINT('',(30.5061406831642,53.2191856060848,3.42473028058522));
#225969=CARTESIAN_POINT('Origin',(30.355876192312,52.9589188467315,3.56425912917328));
#225970=CARTESIAN_POINT('',(30.5691598004931,53.3283379191467,3.643031988603));
#225971=CARTESIAN_POINT('',(30.5061406831642,53.2191856060848,3.42473028058522));
#225972=CARTESIAN_POINT('',(30.770110263767,53.6763943313416,3.64303198860301));
#225973=CARTESIAN_POINT('Origin',(23.8720415006489,53.1491210481986,2.65878198860299));
#225974=CARTESIAN_POINT('',(23.9951532569806,53.9314655730807,2.658781988603));
#225975=CARTESIAN_POINT('',(25.5480287005717,57.4192809246791,2.65878198860302));
#225976=CARTESIAN_POINT('',(23.6840886581935,53.232803045145,2.65878198860299));
#225977=CARTESIAN_POINT('',(25.5758735661207,57.4068835917982,2.65878198860302));
#225978=CARTESIAN_POINT('Origin',(5.58700050634535E-15,1.84861417378678E-13,
2.65878198860263));
#225979=CARTESIAN_POINT('',(24.0229981225296,53.9190682401997,2.658781988603));
#225980=CARTESIAN_POINT('',(23.9942406030432,53.8544777939071,2.658781988603));
#225981=CARTESIAN_POINT('Origin',(5.67792519749014E-15,1.85507814268556E-13,
2.65878198860263));
#225982=CARTESIAN_POINT('Origin',(0.174030409680916,-0.0774833305060288,
42.7590319886026));
#225983=CARTESIAN_POINT('',(24.57973006491,54.7386155880006,3.64303198860301));
#225984=CARTESIAN_POINT('',(24.4045020183944,54.3450469517072,3.40423097483348));
#225985=CARTESIAN_POINT('Origin',(24.5641801073106,54.7036898113997,3.20400220531693));
#225986=CARTESIAN_POINT('',(24.259582275487,54.0195518811808,2.834041988603));
#225987=CARTESIAN_POINT('',(24.4045020183944,54.3450469517072,3.40423097483348));
#225988=CARTESIAN_POINT('',(25.658833530444,57.1623216544373,2.83404198860302));
#225989=CARTESIAN_POINT('',(25.764498133039,57.3996482375659,2.83404198860302));
#225990=CARTESIAN_POINT('',(25.5139139879315,56.8368270312095,3.4042309748335));
#225991=CARTESIAN_POINT('',(25.658833530444,57.1623216544373,2.83404198860302));
#225992=CARTESIAN_POINT('',(25.3386861202876,56.4432587981559,3.64303198860302));
#225993=CARTESIAN_POINT('Origin',(25.3542361279708,56.478184687247,3.20400259788312));
#225994=CARTESIAN_POINT('',(25.1754303533072,56.0765803402172,3.64303198860302));
#225995=CARTESIAN_POINT('',(0.174030409680921,-0.0774833305057557,3.64303198860262));
#225996=CARTESIAN_POINT('',(25.1241659841934,55.9614386837455,3.42473028058525));
#225997=CARTESIAN_POINT('',(25.1754303526574,56.0765803405065,3.64303198860302));
#225998=CARTESIAN_POINT('',(24.9899591116494,55.660005112701,3.2342302805852));
#225999=CARTESIAN_POINT('Origin',(25.0019278517708,55.6868886053377,3.56425722717229));
#226000=CARTESIAN_POINT('',(24.928457230274,55.5218696254675,3.2342302805852));
#226001=CARTESIAN_POINT('',(0.174030409680921,-0.0774833305057528,3.23423028058481));
#226002=CARTESIAN_POINT('',(24.7942503289606,55.2204359898058,3.4247302805852));
#226003=CARTESIAN_POINT('Origin',(24.9164863691,55.4949838933624,3.564259097415));
#226004=CARTESIAN_POINT('',(24.7429859390912,55.1052942849674,3.64303198860301));
#226005=CARTESIAN_POINT('',(24.7942503289606,55.2204359898058,3.4247302805852));
#226006=CARTESIAN_POINT('',(0.174030409680921,-0.0774833305057557,3.64303198860263));
#226007=CARTESIAN_POINT('Origin',(-0.174030409680916,0.0774833305058502,
42.7590319886026));
#226008=CARTESIAN_POINT('',(24.9906253009257,56.5982254591678,3.64303198860303));
#226009=CARTESIAN_POINT('',(25.165853168017,56.9917936924675,3.4042309748335));
#226010=CARTESIAN_POINT('Origin',(25.0061753084924,56.633151347997,3.20400259736051));
#226011=CARTESIAN_POINT('',(25.3107727106687,57.3172883156333,2.83404198860302));
#226012=CARTESIAN_POINT('',(25.165853168017,56.9917936924675,3.4042309748335));
#226013=CARTESIAN_POINT('',(23.9115214566113,54.1745185419762,2.834041988603));
#226014=CARTESIAN_POINT('',(-0.174030409680912,0.0774833305061238,2.83404198860263));
#226015=CARTESIAN_POINT('',(24.0564411996779,54.5000136124318,3.40423097483349));
#226016=CARTESIAN_POINT('',(23.9115214566113,54.1745185419762,2.834041988603));
#226017=CARTESIAN_POINT('',(24.2316692455482,54.8935822490125,3.64303198860301));
#226018=CARTESIAN_POINT('Origin',(24.216119287825,54.8586564721335,3.20400220587276));
#226019=CARTESIAN_POINT('',(24.3949251204068,55.2602609456777,3.64303198860301));
#226020=CARTESIAN_POINT('',(24.4249658234765,55.3277334713092,3.64303198860301));
#226021=CARTESIAN_POINT('',(24.4461895095988,55.3754026508177,3.42473028058519));
#226022=CARTESIAN_POINT('',(24.3949251197294,55.2602609459793,3.64303198860301));
#226023=CARTESIAN_POINT('',(24.5803964109122,55.6768362864794,3.2342302805852));
#226024=CARTESIAN_POINT('Origin',(24.5684276954198,55.6499528488657,3.56425743004438));
#226025=CARTESIAN_POINT('',(24.6418982922876,55.8149717737129,3.23423028058521));
#226026=CARTESIAN_POINT('',(24.6421133384135,55.8154547752197,3.23423028058521));
#226027=CARTESIAN_POINT('',(24.7761051648316,56.1164053447574,3.42473028058522));
#226028=CARTESIAN_POINT('Origin',(24.6538691229768,55.8418574376299,3.56425912917584));
#226029=CARTESIAN_POINT('',(24.8273695332956,56.2315470015184,3.64303198860302));
#226030=CARTESIAN_POINT('',(24.7761051648316,56.1164053447574,3.42473028058522));
#226031=CARTESIAN_POINT('',(24.9908373670086,56.5987017673885,3.64303198860303));
#226032=CARTESIAN_POINT('Origin',(18.1856720123407,55.3532724151367,2.658781988603));
#226033=CARTESIAN_POINT('',(18.2263320786581,56.144199857553,2.65878198860301));
#226034=CARTESIAN_POINT('',(19.4061247292252,59.7752282754839,2.65878198860304));
#226035=CARTESIAN_POINT('',(17.9900016446781,55.4168495715594,2.658781988603));
#226036=CARTESIAN_POINT('',(19.4351129318419,59.7658094374954,2.65878198860304));
#226037=CARTESIAN_POINT('Origin',(5.60136586593794E-15,1.8485590303378E-13,
2.65878198860263));
#226038=CARTESIAN_POINT('',(18.2553202812748,56.1347810195644,2.65878198860301));
#226039=CARTESIAN_POINT('',(18.2334718385819,56.0675384271755,2.65878198860301));
#226040=CARTESIAN_POINT('Origin',(5.67044563844026E-15,1.85510685402273E-13,
2.65878198860263));
#226041=CARTESIAN_POINT('Origin',(0.181176266354227,-0.0588677374285163,
42.7590319886026));
#226042=CARTESIAN_POINT('',(18.7233363629823,57.0080331356325,3.64303198860302));
#226043=CARTESIAN_POINT('',(18.5902073587821,56.5983041910848,3.4042309748335));
#226044=CARTESIAN_POINT('Origin',(18.7115223274336,56.9716732729167,3.2040022053203));
#226045=CARTESIAN_POINT('',(18.4801050009137,56.2594439785883,2.83404198860301));
#226046=CARTESIAN_POINT('',(18.5902073587821,56.5983041910848,3.4042309748335));
#226047=CARTESIAN_POINT('',(19.5431821162865,59.5312589135998,2.83404198860303));
#226048=CARTESIAN_POINT('',(19.6234604941057,59.7783303554051,2.83404198860303));
#226049=CARTESIAN_POINT('',(19.4330799109591,59.1923991668988,3.40423097483352));
#226050=CARTESIAN_POINT('',(19.5431821162865,59.5312589135998,2.83404198860303));
#226051=CARTESIAN_POINT('',(19.2999510425005,58.7826706420791,3.64303198860304));
#226052=CARTESIAN_POINT('Origin',(19.3117651160994,58.8190306219014,3.20400259788138));
#226053=CARTESIAN_POINT('',(19.1759179434157,58.4009360126569,3.64303198860303));
#226054=CARTESIAN_POINT('',(0.181176266354232,-0.0588677374282432,3.64303198860263));
#226055=CARTESIAN_POINT('',(19.1369699862882,58.2810665285032,3.42473028058526));
#226056=CARTESIAN_POINT('',(19.1759179427385,58.4009360128769,3.64303198860303));
#226057=CARTESIAN_POINT('',(19.0350067009929,57.9672558039534,3.23423028058522));
#226058=CARTESIAN_POINT('Origin',(19.0440997849306,57.9952431000156,3.56425722717456));
#226059=CARTESIAN_POINT('',(18.9882808235619,57.8234483402241,3.23423028058522));
#226060=CARTESIAN_POINT('',(0.181176266354233,-0.0588677374282403,3.23423028058481));
#226061=CARTESIAN_POINT('',(18.8863175164091,57.5096375484039,3.42473028058521));
#226062=CARTESIAN_POINT('Origin',(18.9791858642781,57.7954585952479,3.56425909741103));
#226063=CARTESIAN_POINT('',(18.8473695436961,57.3897680139786,3.64303198860302));
#226064=CARTESIAN_POINT('',(18.8863175164091,57.5096375484039,3.42473028058521));
#226065=CARTESIAN_POINT('',(0.181176266354232,-0.0588677374282432,3.64303198860263));
#226066=CARTESIAN_POINT('Origin',(-0.181176266354227,0.0588677374283377,
42.7590319886026));
#226067=CARTESIAN_POINT('',(18.937598509792,58.9004061169359,3.64303198860304));
#226068=CARTESIAN_POINT('',(19.0707273776751,59.3101346419426,3.40423097483351));
#226069=CARTESIAN_POINT('Origin',(18.9494125833028,58.9367660964869,3.20400259736099));
#226070=CARTESIAN_POINT('',(19.1808295831469,59.6489943885967,2.83404198860303));
#226071=CARTESIAN_POINT('',(19.0707273776751,59.3101346419426,3.40423097483351));
#226072=CARTESIAN_POINT('',(18.1177524687105,56.377179453281,2.83404198860301));
#226073=CARTESIAN_POINT('',(-0.181176266354223,0.0588677374286111,2.83404198860262));
#226074=CARTESIAN_POINT('',(18.2278548267456,56.7160396657233,3.4042309748335));
#226075=CARTESIAN_POINT('',(18.1177524687105,56.377179453281,2.83404198860301));
#226076=CARTESIAN_POINT('',(18.3609838302739,57.1257686104893,3.64303198860302));
#226077=CARTESIAN_POINT('Origin',(18.3491697946318,57.0894087474861,3.20400220587187));
#226078=CARTESIAN_POINT('',(18.4850170116929,57.5075034886063,3.64303198860303));
#226079=CARTESIAN_POINT('',(18.5078403492309,57.5777465012101,3.64303198860303));
#226080=CARTESIAN_POINT('',(18.5239649837007,57.6273730232608,3.42473028058521));
#226081=CARTESIAN_POINT('',(18.4850170109876,57.5075034888355,3.64303198860303));
#226082=CARTESIAN_POINT('',(18.6259282908535,57.941183815081,3.23423028058522));
#226083=CARTESIAN_POINT('Origin',(18.6168352256576,57.9131965763127,3.56425743004216));
#226084=CARTESIAN_POINT('',(18.6726541682844,58.0849912788103,3.23423028058522));
#226085=CARTESIAN_POINT('',(18.6728175489599,58.0854941128254,3.23423028058522));
#226086=CARTESIAN_POINT('',(18.7746174535798,58.3988020033601,3.42473028058524));
#226087=CARTESIAN_POINT('Origin',(18.6817491043768,58.1129809527812,3.56425912918029));
#226088=CARTESIAN_POINT('',(18.8135654100301,58.5186714877338,3.64303198860303));
#226089=CARTESIAN_POINT('',(18.7746174535798,58.3988020033601,3.42473028058524));
#226090=CARTESIAN_POINT('',(18.9377596263884,58.9009019828321,3.64303198860304));
#226091=CARTESIAN_POINT('Origin',(12.3000564958688,56.9509617460777,2.65878198860302));
#226092=CARTESIAN_POINT('',(12.2578193919766,57.7418065394568,2.65878198860302));
#226093=CARTESIAN_POINT('',(13.0516031943527,61.4762657165318,2.65878198860305));
#226094=CARTESIAN_POINT('',(12.0988124084938,56.9937374973465,2.65878198860302));
#226095=CARTESIAN_POINT('',(13.0814171332231,61.4699285681957,2.65878198860305));
#226096=CARTESIAN_POINT('Origin',(5.61622893658571E-15,1.84851920486003E-13,
2.65878198860263));
#226097=CARTESIAN_POINT('',(12.2876333308469,57.7354693911207,2.65878198860302));
#226098=CARTESIAN_POINT('',(12.2729333410577,57.6663113765491,2.65878198860302));
#226099=CARTESIAN_POINT('Origin',(5.66270693800216E-15,1.85512758980806E-13,
2.65878198860263));
#226100=CARTESIAN_POINT('Origin',(0.18633711793979,-0.0396071771008719,
42.7590319886026));
#226101=CARTESIAN_POINT('',(12.6618058697518,58.6528587425324,3.64303198860303));
#226102=CARTESIAN_POINT('',(12.5722344970959,58.2314585657882,3.40423097483351));
#226103=CARTESIAN_POINT('Origin',(12.6538571933006,58.6154631599698,3.20400220531712));
#226104=CARTESIAN_POINT('',(12.4981558287383,57.8829458347213,2.83404198860302));
#226105=CARTESIAN_POINT('',(12.5722344970959,58.2314585657882,3.40423097483351));
#226106=CARTESIAN_POINT('',(13.2134115091892,61.247959242388,2.83404198860304));
#226107=CARTESIAN_POINT('',(13.2674241155258,61.5020685764507,2.83404198860305));
#226108=CARTESIAN_POINT('',(13.1393329438492,60.8994469905095,3.40423097483353));
#226109=CARTESIAN_POINT('',(13.2134115091892,61.247959242388,2.83404198860304));
#226110=CARTESIAN_POINT('',(13.0497616623173,60.478047245383,3.64303198860306));
#226111=CARTESIAN_POINT('Origin',(13.0577103643695,60.515442948389,3.20400259788024));
#226112=CARTESIAN_POINT('',(12.9663101637165,60.0854388089607,3.64303198860304));
#226113=CARTESIAN_POINT('',(0.186337117939796,-0.0396071771005988,3.64303198860263));
#226114=CARTESIAN_POINT('',(12.9401053405448,59.9621548122774,3.42473028058526));
#226115=CARTESIAN_POINT('',(12.9663101630202,60.0854388091087,3.64303198860304));
#226116=CARTESIAN_POINT('',(12.871502773589,59.6394051101896,3.23423028058523));
#226117=CARTESIAN_POINT('Origin',(12.8776205756132,59.6681895750061,3.56425722717471));
#226118=CARTESIAN_POINT('',(12.8400648385937,59.4915012546307,3.23423028058523));
#226119=CARTESIAN_POINT('',(0.186337117939796,-0.0396071771005959,3.23423028058481));
#226120=CARTESIAN_POINT('',(12.7714622569318,59.1687514833563,3.42473028058522));
#226121=CARTESIAN_POINT('Origin',(12.8339454274779,59.4627141582879,3.56425909740963));
#226122=CARTESIAN_POINT('',(12.7452574235146,59.0454674350477,3.64303198860304));
#226123=CARTESIAN_POINT('',(12.7714622569318,59.1687514833563,3.42473028058522));
#226124=CARTESIAN_POINT('',(0.186337117939796,-0.0396071771005988,3.64303198860263));
#226125=CARTESIAN_POINT('Origin',(-0.18633711793979,0.0396071771006933,
42.7590319886026));
#226126=CARTESIAN_POINT('',(12.6770874264377,60.5572615995845,3.64303198860305));
#226127=CARTESIAN_POINT('',(12.7666587073772,60.978661344837,3.40423097483353));
#226128=CARTESIAN_POINT('Origin',(12.6850361284308,60.5946573023123,3.20400259736161));
#226129=CARTESIAN_POINT('',(12.8407372728672,61.3271735966836,2.83404198860304));
#226130=CARTESIAN_POINT('',(12.7666587073772,60.978661344837,3.40423097483353));
#226131=CARTESIAN_POINT('',(12.125481593379,57.9621601888123,2.83404198860302));
#226132=CARTESIAN_POINT('',(-0.186337117939786,0.0396071771009666,2.83404198860262));
#226133=CARTESIAN_POINT('',(12.1995602619078,58.3106729198428,3.40423097483351));
#226134=CARTESIAN_POINT('',(12.125481593379,57.9621601888123,2.83404198860302));
#226135=CARTESIAN_POINT('',(12.2891316338722,58.732073096734,3.64303198860303));
#226136=CARTESIAN_POINT('Origin',(12.2811829573577,58.6946775138734,3.20400220587296));
#226137=CARTESIAN_POINT('',(12.3725831883598,59.1246817890952,3.64303198860304));
#226138=CARTESIAN_POINT('',(12.3879391031045,59.1969256915256,3.64303198860304));
#226139=CARTESIAN_POINT('',(12.3987880210522,59.2479658375578,3.42473028058521));
#226140=CARTESIAN_POINT('',(12.372583187635,59.1246817892492,3.64303198860304));
#226141=CARTESIAN_POINT('',(12.4673906027141,59.5707156088323,3.23423028058523));
#226142=CARTESIAN_POINT('Origin',(12.461272813341,59.5419312029578,3.56425743004745));
#226143=CARTESIAN_POINT('',(12.4988285377094,59.7186194643911,3.23423028058523));
#226144=CARTESIAN_POINT('',(12.4989384629016,59.7191366217598,3.23423028058523));
#226145=CARTESIAN_POINT('',(12.5674311046652,60.0413691664789,3.42473028058526));
#226146=CARTESIAN_POINT('Origin',(12.504947933183,59.7474064876941,3.56425912917753));
#226147=CARTESIAN_POINT('',(12.5936359271406,60.1646531633103,3.64303198860304));
#226148=CARTESIAN_POINT('',(12.5674311046652,60.0413691664789,3.42473028058526));
#226149=CARTESIAN_POINT('',(12.6771958283204,60.5577715903457,3.64303198860305));
#226150=CARTESIAN_POINT('Origin',(6.27967898647588,57.9246844223737,2.65878198860302));
#226151=CARTESIAN_POINT('',(6.15500747092297,58.7067819056645,2.65878198860303));
#226152=CARTESIAN_POINT('',(6.55408556365926,62.5037563256537,2.65878198860306));
#226153=CARTESIAN_POINT('',(6.07506605172282,57.9461901084064,2.65878198860302));
#226154=CARTESIAN_POINT('',(6.58439859103008,62.5005702980933,2.65878198860306));
#226155=CARTESIAN_POINT('Origin',(5.63142687537637E-15,1.84849513368974E-13,
2.65878198860263));
#226156=CARTESIAN_POINT('',(6.1853204982938,58.7035958781041,2.65878198860303));
#226157=CARTESIAN_POINT('',(6.1779300175725,58.6332801510297,2.65878198860303));
#226158=CARTESIAN_POINT('Origin',(5.65479388299727E-15,1.85514012285594E-13,
2.65878198860263));
#226159=CARTESIAN_POINT('Origin',(0.189456421067656,-0.0199126722525767,
42.7590319886026));
#226160=CARTESIAN_POINT('',(6.46154998175899,59.6550713551495,3.64303198860304));
#226161=CARTESIAN_POINT('',(6.41651760335031,59.2266168947288,3.40423097483351));
#226162=CARTESIAN_POINT('Origin',(6.45755375176729,59.6170497665656,3.20400220531847));
#226163=CARTESIAN_POINT('',(6.37927424589664,58.8722700235038,2.83404198860304));
#226164=CARTESIAN_POINT('',(6.41651760335031,59.2266168947288,3.40423097483351));
#226165=CARTESIAN_POINT('',(6.73887200051313,62.2936141127571,2.83404198860306));
#226166=CARTESIAN_POINT('',(6.76602706194927,62.5519772640374,2.83404198860306));
#226167=CARTESIAN_POINT('',(6.70162869542398,61.9392677288638,3.40423097483354));
#226168=CARTESIAN_POINT('',(6.73887200051313,62.2936141127571,2.83404198860306));
#226169=CARTESIAN_POINT('',(6.65659636252364,61.5108137072214,3.64303198860306));
#226170=CARTESIAN_POINT('Origin',(6.66059260538633,61.5488354182647,3.20400259788118));
#226171=CARTESIAN_POINT('',(6.61464077648901,61.111632963987,3.64303198860305));
#226172=CARTESIAN_POINT('',(0.189456421067662,-0.0199126722523036,3.64303198860263));
#226173=CARTESIAN_POINT('',(6.60146619279927,60.9862851800406,3.42473028058528));
#226174=CARTESIAN_POINT('',(6.61464077578103,61.1116329640614,3.64303198860305));
#226175=CARTESIAN_POINT('',(6.56697596826259,60.6581326136906,3.23423028058524));
#226176=CARTESIAN_POINT('Origin',(6.57005146045409,60.6873988786433,3.5642572271707));
#226177=CARTESIAN_POINT('',(6.55117041629749,60.5077528318946,3.23423028058524));
#226178=CARTESIAN_POINT('',(0.189456421067662,-0.0199126722523007,3.23423028058481));
#226179=CARTESIAN_POINT('',(6.51668018436727,60.1796001951997,3.42473028058523));
#226180=CARTESIAN_POINT('Origin',(6.54809359889897,60.4784837816403,3.56425909741505));
#226181=CARTESIAN_POINT('',(6.50350559588446,60.0542523588399,3.64303198860304));
#226182=CARTESIAN_POINT('',(6.51668018436727,60.1796001951997,3.42473028058523));
#226183=CARTESIAN_POINT('',(0.189456421067662,-0.0199126722523036,3.64303198860263));
#226184=CARTESIAN_POINT('Origin',(-0.189456421067656,0.0199126722523981,
42.7590319886026));
#226185=CARTESIAN_POINT('',(6.27768352038833,61.5506390517264,3.64303198860306));
#226186=CARTESIAN_POINT('',(6.32271585268621,61.9790930734321,3.40423097483353));
#226187=CARTESIAN_POINT('Origin',(6.28167976322103,61.5886607624844,3.20400259735781));
#226188=CARTESIAN_POINT('',(6.35995915792791,62.3334394573094,2.83404198860306));
#226189=CARTESIAN_POINT('',(6.32271585268621,61.9790930734321,3.40423097483353));
#226190=CARTESIAN_POINT('',(6.00036140429027,58.9120953679532,2.83404198860304));
#226191=CARTESIAN_POINT('',(-0.189456421067651,0.0199126722526713,2.83404198860263));
#226192=CARTESIAN_POINT('',(6.03760476191735,59.26644223916,3.40423097483352));
#226193=CARTESIAN_POINT('',(6.00036140429027,58.9120953679532,2.83404198860304));
#226194=CARTESIAN_POINT('',(6.08263713962368,59.6948966996544,3.64303198860304));
#226195=CARTESIAN_POINT('Origin',(6.07864090960019,59.656875110768,3.20400220587394));
#226196=CARTESIAN_POINT('',(6.12459275448634,60.0940777032674,3.64303198860305));
#226197=CARTESIAN_POINT('',(6.13231300382157,60.1675309762117,3.64303198860304));
#226198=CARTESIAN_POINT('',(6.13776734223196,60.2194255397047,3.42473028058523));
#226199=CARTESIAN_POINT('',(6.12459275374915,60.0940777033449,3.64303198860304));
#226200=CARTESIAN_POINT('',(6.17225757416218,60.5475781763996,3.23423028058524));
#226201=CARTESIAN_POINT('Origin',(6.16918208839113,60.518311971387,3.56425743004107));
#226202=CARTESIAN_POINT('',(6.18806312612727,60.6979579581956,3.23423028058524));
#226203=CARTESIAN_POINT('',(6.18811839147268,60.6984837728335,3.23423028058524));
#226204=CARTESIAN_POINT('',(6.22255335066396,61.0261105245456,3.42473028058526));
#226205=CARTESIAN_POINT('Origin',(6.19113993560424,60.7272269341776,3.56425912917774));
#226206=CARTESIAN_POINT('',(6.23572793364572,61.1514583085664,3.64303198860305));
#226207=CARTESIAN_POINT('',(6.22255335066396,61.0261105245456,3.42473028058526));
#226208=CARTESIAN_POINT('',(6.2777380198836,61.551157579787,3.64303198860306));
#226209=CARTESIAN_POINT('Origin',(0.190499999999802,58.2637721346187,2.65878198860302));
#226210=CARTESIAN_POINT('',(-0.0152400000002005,59.0285534841298,2.65878198860303));
#226211=CARTESIAN_POINT('',(-0.0152400000002138,62.8464427007198,2.65878198860306));
#226212=CARTESIAN_POINT('',(-0.0152400000001978,58.2637721346187,2.65878198860302));
#226213=CARTESIAN_POINT('',(0.0152399999997862,62.8464427007198,2.65878198860306));
#226214=CARTESIAN_POINT('Origin',(-4.80914138193527E-17,1.90543592639901E-13,
2.65878198860263));
#226215=CARTESIAN_POINT('',(0.0152399999997995,59.0285534841298,2.65878198860303));
#226216=CARTESIAN_POINT('',(0.0152399999997998,58.957850438373,2.65878198860303));
#226217=CARTESIAN_POINT('Origin',(3.94085276091011E-16,1.90767139479589E-13,
2.65878198860263));
#226218=CARTESIAN_POINT('Origin',(0.1905,-8.8662823435301E-14,42.7590319886026));
#226219=CARTESIAN_POINT('',(0.190499999999796,60.0036905223732,3.64303198860304));
#226220=CARTESIAN_POINT('',(0.190499999999798,59.5728760150044,3.40423097483352));
#226221=CARTESIAN_POINT('Origin',(0.190499999999796,59.9654595002493,3.20400220532009));
#226222=CARTESIAN_POINT('',(0.190499999468327,59.2165773020943,2.83404198860303));
#226223=CARTESIAN_POINT('',(0.190499999999798,59.5728760150044,3.40423097483352));
#226224=CARTESIAN_POINT('',(0.190499999999787,62.6567671111301,2.83404198860305));
#226225=CARTESIAN_POINT('',(0.190499999999786,62.9165533988765,2.83404198860306));
#226226=CARTESIAN_POINT('',(0.190500000604986,62.3004688883556,3.40423097483354));
#226227=CARTESIAN_POINT('',(0.190499999999787,62.6567671111301,2.83404198860305));
#226228=CARTESIAN_POINT('',(0.19049999999979,61.8696548221183,3.64303198860307));
#226229=CARTESIAN_POINT('Origin',(0.190499999999789,61.9078859673757,3.20400259788174));
#226230=CARTESIAN_POINT('',(0.190500000711646,61.4682752798286,3.64303198860306));
#226231=CARTESIAN_POINT('',(0.190500000000006,1.84482744665075E-13,3.64303198860263));
#226232=CARTESIAN_POINT('',(0.190499999999791,61.3422370451707,3.42473028058527));
#226233=CARTESIAN_POINT('',(0.190499999999791,61.4682752798286,3.64303198860306));
#226234=CARTESIAN_POINT('',(0.190499999999793,61.0122769227458,3.23423028058524));
#226235=CARTESIAN_POINT('Origin',(0.190499486622193,61.0417043405088,3.56425722717157));
#226236=CARTESIAN_POINT('',(0.190499999999793,60.8610688070709,3.23423028058524));
#226237=CARTESIAN_POINT('',(0.190500000000006,1.87337391734738E-13,3.23423028058481));
#226238=CARTESIAN_POINT('',(0.190499999999794,60.5311086139136,3.42473028058523));
#226239=CARTESIAN_POINT('Origin',(0.19049948657329,60.8316384807389,3.56425909740902));
#226240=CARTESIAN_POINT('',(0.190499999999795,60.4050703266284,3.64303198860304));
#226241=CARTESIAN_POINT('',(0.190499999999794,60.5311086139136,3.42473028058523));
#226242=CARTESIAN_POINT('',(0.190500000000006,1.84482744665075E-13,3.64303198860263));
#226243=CARTESIAN_POINT('Origin',(-0.1905,-8.99930778254002E-14,42.7590319886026));
#226244=CARTESIAN_POINT('',(-0.190500000000211,61.8696548221182,3.64303198860306));
#226245=CARTESIAN_POINT('',(-0.190500000000212,62.3004688883556,3.40423097483353));
#226246=CARTESIAN_POINT('Origin',(-0.190500000000211,61.9078859670883,3.20400259735724));
#226247=CARTESIAN_POINT('',(-0.190500000452774,62.6567671111301,2.83404198860305));
#226248=CARTESIAN_POINT('',(-0.190500000000212,62.3004688883556,3.40423097483353));
#226249=CARTESIAN_POINT('',(-0.190500000000202,59.2165773020943,2.83404198860303));
#226250=CARTESIAN_POINT('',(-0.190499999999994,1.83179523652187E-13,2.83404198860262));
#226251=CARTESIAN_POINT('',(-0.190499999294346,59.5728760150044,3.40423097483352));
#226252=CARTESIAN_POINT('',(-0.190500000000201,59.2165773020943,2.83404198860303));
#226253=CARTESIAN_POINT('',(-0.190500000000204,60.0036905223732,3.64303198860304));
#226254=CARTESIAN_POINT('Origin',(-0.190500000000204,59.9654594999458,3.20400220587403));
#226255=CARTESIAN_POINT('',(-0.190499999258359,60.4050703266284,3.64303198860304));
#226256=CARTESIAN_POINT('',(-0.190500000000206,60.478928200657,3.64303198860305));
#226257=CARTESIAN_POINT('',(-0.190500000000206,60.5311086139136,3.42473028058523));
#226258=CARTESIAN_POINT('',(-0.190500000000205,60.4050703266284,3.64303198860304));
#226259=CARTESIAN_POINT('',(-0.190500000000207,60.8610688070709,3.23423028058524));
#226260=CARTESIAN_POINT('Origin',(-0.190499486502772,60.8316414495897,3.56425743004083));
#226261=CARTESIAN_POINT('',(-0.190500000000207,61.0122769227458,3.23423028058524));
#226262=CARTESIAN_POINT('',(-0.190500000000207,61.0128056337177,3.23423028058524));
#226263=CARTESIAN_POINT('',(-0.190500000000209,61.3422370451707,3.42473028058527));
#226264=CARTESIAN_POINT('Origin',(-0.190499486688304,61.0417071743814,3.56425912917754));
#226265=CARTESIAN_POINT('',(-0.190500000000209,61.4682752798286,3.64303198860306));
#226266=CARTESIAN_POINT('',(-0.190500000000209,61.3422370451707,3.42473028058527));
#226267=CARTESIAN_POINT('',(-0.190500000000211,61.8701762063764,3.64303198860306));
#226268=CARTESIAN_POINT('Origin',(-5.90076614434095,57.9645097668786,2.65878198860302));
#226269=CARTESIAN_POINT('',(-6.18532049829418,58.7035958781041,2.65878198860303));
#226270=CARTESIAN_POINT('',(-6.58439859103049,62.5005702980932,2.65878198860306));
#226271=CARTESIAN_POINT('',(-6.10537907909402,57.943004080846,2.65878198860302));
#226272=CARTESIAN_POINT('',(-6.55408556365967,62.5037563256536,2.65878198860306));
#226273=CARTESIAN_POINT('Origin',(-3.27251186835855E-17,1.90544397953305E-13,
2.65878198860263));
#226274=CARTESIAN_POINT('',(-6.15500747092336,58.7067819056644,2.65878198860303));
#226275=CARTESIAN_POINT('',(-6.14761699020206,58.6364661785901,2.65878198860303));
#226276=CARTESIAN_POINT('Origin',(3.86084563605877E-16,1.90766720180015E-13,
2.65878198860263));
#226277=CARTESIAN_POINT('Origin',(0.189456421067656,0.0199126722523994,
42.7590319886026));
#226278=CARTESIAN_POINT('',(-6.08263713962407,59.6948966996544,3.64303198860304));
#226279=CARTESIAN_POINT('',(-6.03760476121539,59.2664422392338,3.40423097483352));
#226280=CARTESIAN_POINT('Origin',(-6.07864090963231,59.6568751110698,3.20400220532002));
#226281=CARTESIAN_POINT('',(-6.00036140481931,58.9120953678976,2.83404198860304));
#226282=CARTESIAN_POINT('',(-6.03760476121539,59.2664422392338,3.40423097483352));
#226283=CARTESIAN_POINT('',(-6.35995915837823,62.333439457262,2.83404198860306));
#226284=CARTESIAN_POINT('',(-6.38711421981437,62.5918026085423,2.83404198860306));
#226285=CARTESIAN_POINT('',(-6.32271585208448,61.9790930734953,3.40423097483354));
#226286=CARTESIAN_POINT('',(-6.35995915837823,62.3334394572621,2.83404198860306));
#226287=CARTESIAN_POINT('',(-6.27768352038873,61.5506390517263,3.64303198860306));
#226288=CARTESIAN_POINT('Origin',(-6.28167976325153,61.5886607627708,3.20400259788305));
#226289=CARTESIAN_POINT('',(-6.23572793293792,61.1514583086408,3.64303198860305));
#226290=CARTESIAN_POINT('',(0.189456421067662,0.0199126722526725,3.64303198860263));
#226291=CARTESIAN_POINT('',(-6.22255335066436,61.0261105245456,3.42473028058528));
#226292=CARTESIAN_POINT('',(-6.23572793364612,61.1514583085664,3.64303198860305));
#226293=CARTESIAN_POINT('',(-6.18806312612767,60.6979579581955,3.23423028058524));
#226294=CARTESIAN_POINT('Origin',(-6.19113963944983,60.7272241158243,3.56425722716837));
#226295=CARTESIAN_POINT('',(-6.17225757416258,60.5475781763995,3.23423028058524));
#226296=CARTESIAN_POINT('',(0.189456421067662,0.0199126722526753,3.23423028058481));
#226297=CARTESIAN_POINT('',(-6.13776734223235,60.2194255397047,3.42473028058522));
#226298=CARTESIAN_POINT('Origin',(-6.16918177799174,60.518309018809,3.5642590974125));
#226299=CARTESIAN_POINT('',(-6.12459275374954,60.0940777033448,3.64303198860304));
#226300=CARTESIAN_POINT('',(-6.13776734223235,60.2194255397047,3.42473028058522));
#226301=CARTESIAN_POINT('',(0.189456421067662,0.0199126722526725,3.64303198860263));
#226302=CARTESIAN_POINT('Origin',(-0.189456421067656,-0.019912672252578,
42.7590319886026));
#226303=CARTESIAN_POINT('',(-6.65659636252404,61.5108137072214,3.64303198860306));
#226304=CARTESIAN_POINT('',(-6.70162869482193,61.9392677289271,3.40423097483353));
#226305=CARTESIAN_POINT('Origin',(-6.66059260535667,61.5488354179786,3.20400259735651));
#226306=CARTESIAN_POINT('',(-6.73887200096381,62.2936141127098,2.83404198860306));
#226307=CARTESIAN_POINT('',(-6.70162869482193,61.9392677289271,3.40423097483353));
#226308=CARTESIAN_POINT('',(-6.37927424642597,58.8722700234482,2.83404198860303));
#226309=CARTESIAN_POINT('',(-0.18945642106765,-0.0199126722523048,2.83404198860263));
#226310=CARTESIAN_POINT('',(-6.41651760264873,59.2266168948026,3.40423097483352));
#226311=CARTESIAN_POINT('',(-6.37927424642597,58.8722700234482,2.83404198860304));
#226312=CARTESIAN_POINT('',(-6.46154998175939,59.6550713551494,3.64303198860304));
#226313=CARTESIAN_POINT('Origin',(-6.45755375173598,59.6170497662638,3.20400220587227));
#226314=CARTESIAN_POINT('',(-6.50350559514721,60.0542523589174,3.64303198860304));
#226315=CARTESIAN_POINT('',(-6.51122584595728,60.1277056317067,3.64303198860304));
#226316=CARTESIAN_POINT('',(-6.51668018436767,60.1796001951997,3.42473028058524));
#226317=CARTESIAN_POINT('',(-6.50350559588486,60.0542523588399,3.64303198860304));
#226318=CARTESIAN_POINT('',(-6.55117041629789,60.5077528318945,3.23423028058524));
#226319=CARTESIAN_POINT('Origin',(-6.54809390915841,60.4784867342365,3.56425743004926));
#226320=CARTESIAN_POINT('',(-6.56697596826298,60.6581326136906,3.23423028058524));
#226321=CARTESIAN_POINT('',(-6.5670312336084,60.6586584283285,3.23423028058524));
#226322=CARTESIAN_POINT('',(-6.60146619279967,60.9862851800406,3.42473028058526));
#226323=CARTESIAN_POINT('Origin',(-6.57005175674006,60.6874016969835,3.56425912917843));
#226324=CARTESIAN_POINT('',(-6.61464077578143,61.1116329640614,3.64303198860305));
#226325=CARTESIAN_POINT('',(-6.60146619279967,60.9862851800406,3.42473028058526));
#226326=CARTESIAN_POINT('',(-6.65665086201932,61.511332235282,3.64303198860306));
#226327=CARTESIAN_POINT('Origin',(-11.9273822599896,57.0301761002792,2.65878198860302));
#226328=CARTESIAN_POINT('',(-12.2876333308473,57.7354693911206,2.65878198860302));
#226329=CARTESIAN_POINT('',(-13.0814171332235,61.4699285681956,2.65878198860305));
#226330=CARTESIAN_POINT('',(-12.1286263473646,56.9874003490103,2.65878198860302));
#226331=CARTESIAN_POINT('',(-13.0516031943531,61.4762657165317,2.65878198860305));
#226332=CARTESIAN_POINT('Origin',(-1.75271798929331E-17,1.90546805070335E-13,
2.65878198860263));
#226333=CARTESIAN_POINT('',(-12.257819391977,57.7418065394567,2.65878198860302));
#226334=CARTESIAN_POINT('',(-12.2431194021877,57.6726485248851,2.65878198860302));
#226335=CARTESIAN_POINT('Origin',(3.78171508600985E-16,1.90765466875227E-13,
2.65878198860263));
#226336=CARTESIAN_POINT('Origin',(0.18633711793979,0.0396071771006945,42.7590319886026));
#226337=CARTESIAN_POINT('',(-12.2891316338726,58.7320730967339,3.64303198860303));
#226338=CARTESIAN_POINT('',(-12.1995602612167,58.3106729199897,3.4042309748335));
#226339=CARTESIAN_POINT('Origin',(-12.2811829574212,58.6946775141702,3.20400220531898));
#226340=CARTESIAN_POINT('',(-12.1254815938993,57.9621601887017,2.83404198860302));
#226341=CARTESIAN_POINT('',(-12.1995602612167,58.3106729199897,3.40423097483351));
#226342=CARTESIAN_POINT('',(-12.84073727331,61.3271735965895,2.83404198860304));
#226343=CARTESIAN_POINT('',(-12.8947498796467,61.5812829306521,2.83404198860305));
#226344=CARTESIAN_POINT('',(-12.766658706785,60.9786613449629,3.40423097483352));
#226345=CARTESIAN_POINT('',(-12.84073727331,61.3271735965895,2.83404198860304));
#226346=CARTESIAN_POINT('',(-12.6770874264381,60.5572615995845,3.64303198860306));
#226347=CARTESIAN_POINT('Origin',(-12.6850361284905,60.5946573025913,3.20400259788163));
#226348=CARTESIAN_POINT('',(-12.5936359264448,60.1646531634582,3.64303198860305));
#226349=CARTESIAN_POINT('',(0.186337117939795,0.0396071771009677,3.64303198860263));
#226350=CARTESIAN_POINT('',(-12.5674311046656,60.0413691664789,3.42473028058527));
#226351=CARTESIAN_POINT('',(-12.593635927141,60.1646531633102,3.64303198860304));
#226352=CARTESIAN_POINT('',(-12.4988285377098,59.7186194643911,3.23423028058523));
#226353=CARTESIAN_POINT('Origin',(-12.5049473440522,59.7474037157336,3.56425722717387));
#226354=CARTESIAN_POINT('',(-12.4673906027145,59.5707156088322,3.23423028058523));
#226355=CARTESIAN_POINT('',(0.186337117939795,0.0396071771009705,3.23423028058481));
#226356=CARTESIAN_POINT('',(-12.3987880210526,59.2479658375578,3.42473028058522));
#226357=CARTESIAN_POINT('Origin',(-12.4612721960129,59.5419282989965,3.56425909741342));
#226358=CARTESIAN_POINT('',(-12.3725831876354,59.1246817892492,3.64303198860304));
#226359=CARTESIAN_POINT('',(-12.3987880210526,59.2479658375578,3.42473028058522));
#226360=CARTESIAN_POINT('',(0.186337117939795,0.0396071771009677,3.64303198860263));
#226361=CARTESIAN_POINT('Origin',(-0.18633711793979,-0.0396071771008732,
42.7590319886026));
#226362=CARTESIAN_POINT('',(-13.0497616623177,60.4780472453829,3.64303198860305));
#226363=CARTESIAN_POINT('',(-13.1393329432572,60.8994469906353,3.40423097483352));
#226364=CARTESIAN_POINT('Origin',(-13.0577103643104,60.5154429481089,3.20400259735817));
#226365=CARTESIAN_POINT('',(-13.2134115096321,61.2479592422938,2.83404198860304));
#226366=CARTESIAN_POINT('',(-13.1393329432572,60.8994469906353,3.40423097483352));
#226367=CARTESIAN_POINT('',(-12.4981558292589,57.8829458346107,2.83404198860303));
#226368=CARTESIAN_POINT('',(-0.186337117939783,-0.0396071771005999,2.83404198860263));
#226369=CARTESIAN_POINT('',(-12.5722344964054,58.231458565935,3.40423097483351));
#226370=CARTESIAN_POINT('',(-12.4981558292589,57.8829458346107,2.83404198860303));
#226371=CARTESIAN_POINT('',(-12.6618058697522,58.6528587425324,3.64303198860303));
#226372=CARTESIAN_POINT('Origin',(-12.6538571932377,58.615463159672,3.20400220587252));
#226373=CARTESIAN_POINT('',(-12.7452574227899,59.0454674352017,3.64303198860304));
#226374=CARTESIAN_POINT('',(-12.7606133389844,59.1177113373239,3.64303198860304));
#226375=CARTESIAN_POINT('',(-12.7714622569322,59.1687514833562,3.42473028058522));
#226376=CARTESIAN_POINT('',(-12.745257423515,59.0454674350476,3.64303198860304));
#226377=CARTESIAN_POINT('',(-12.8400648385941,59.4915012546306,3.23423028058523));
#226378=CARTESIAN_POINT('Origin',(-12.8339460446679,59.4627170622779,3.56425743004263));
#226379=CARTESIAN_POINT('',(-12.8715027735894,59.6394051101895,3.23423028058523));
#226380=CARTESIAN_POINT('',(-12.8716126987815,59.6399222675582,3.23423028058523));
#226381=CARTESIAN_POINT('',(-12.9401053405452,59.9621548122773,3.42473028058525));
#226382=CARTESIAN_POINT('Origin',(-12.8776211648735,59.6681923469398,3.56425912917723));
#226383=CARTESIAN_POINT('',(-12.9663101630206,60.0854388091086,3.64303198860304));
#226384=CARTESIAN_POINT('',(-12.9401053405452,59.9621548122773,3.42473028058525));
#226385=CARTESIAN_POINT('',(-13.0498700642004,60.478557236144,3.64303198860305));
#226386=CARTESIAN_POINT('Origin',(-17.8233194796326,55.4710078899935,2.658781988603));
#226387=CARTESIAN_POINT('',(-18.2553202812751,56.1347810195643,2.658781988603));
#226388=CARTESIAN_POINT('',(-19.4351129318423,59.7658094374952,2.65878198860303));
#226389=CARTESIAN_POINT('',(-18.0189898472952,55.4074307335707,2.658781988603));
#226390=CARTESIAN_POINT('',(-19.4061247292256,59.7752282754838,2.65878198860303));
#226391=CARTESIAN_POINT('Origin',(-2.66410924515271E-18,1.90550787618112E-13,
2.65878198860263));
#226392=CARTESIAN_POINT('',(-18.2263320786585,56.1441998575529,2.658781988603));
#226393=CARTESIAN_POINT('',(-18.2044836359655,56.076957265164,2.658781988603));
#226394=CARTESIAN_POINT('Origin',(3.70432808162889E-16,1.90763393296694E-13,
2.65878198860263));
#226395=CARTESIAN_POINT('Origin',(0.181176266354227,0.0588677374283389,
42.7590319886026));
#226396=CARTESIAN_POINT('',(-18.3609838302743,57.1257686104892,3.64303198860302));
#226397=CARTESIAN_POINT('',(-18.227854826074,56.7160396659415,3.40423097483349));
#226398=CARTESIAN_POINT('Origin',(-18.3491697947259,57.0894087477744,3.20400220531829));
#226399=CARTESIAN_POINT('',(-18.1177524692165,56.3771794531165,2.834041988603));
#226400=CARTESIAN_POINT('',(-18.227854826074,56.7160396659415,3.4042309748335));
#226401=CARTESIAN_POINT('',(-19.1808295835784,59.6489943884565,2.83404198860303));
#226402=CARTESIAN_POINT('',(-19.2611079613977,59.8960658302619,2.83404198860303));
#226403=CARTESIAN_POINT('',(-19.0707273770998,59.3101346421295,3.40423097483351));
#226404=CARTESIAN_POINT('',(-19.1808295835784,59.6489943884565,2.83404198860302));
#226405=CARTESIAN_POINT('',(-18.9375985097924,58.9004061169358,3.64303198860304));
#226406=CARTESIAN_POINT('Origin',(-18.9494125833917,58.9367660967595,3.20400259788406));
#226407=CARTESIAN_POINT('',(-18.8135654093537,58.5186714879535,3.64303198860303));
#226408=CARTESIAN_POINT('',(0.181176266354232,0.0588677374286121,3.64303198860262));
#226409=CARTESIAN_POINT('',(-18.7746174535802,58.3988020033599,3.42473028058526));
#226410=CARTESIAN_POINT('',(-18.8135654100305,58.5186714877336,3.64303198860303));
#226411=CARTESIAN_POINT('',(-18.6726541682848,58.0849912788101,3.23423028058522));
#226412=CARTESIAN_POINT('Origin',(-18.6817482287253,58.1129782575892,3.56425722717134));
#226413=CARTESIAN_POINT('',(-18.6259282908539,57.9411838150808,3.23423028058522));
#226414=CARTESIAN_POINT('',(0.181176266354232,0.0588677374286149,3.23423028058481));
#226415=CARTESIAN_POINT('',(-18.523964983701,57.6273730232606,3.42473028058521));
#226416=CARTESIAN_POINT('Origin',(-18.6168343081645,57.9131937527875,3.56425909740641));
#226417=CARTESIAN_POINT('',(-18.485017010988,57.5075034888354,3.64303198860303));
#226418=CARTESIAN_POINT('',(-18.523964983701,57.6273730232606,3.42473028058521));
#226419=CARTESIAN_POINT('',(0.181176266354232,0.0588677374286121,3.64303198860263));
#226420=CARTESIAN_POINT('Origin',(-0.181176266354227,-0.0588677374285176,
42.7590319886026));
#226421=CARTESIAN_POINT('',(-19.2999510425009,58.7826706420789,3.64303198860303));
#226422=CARTESIAN_POINT('',(-19.433079910384,59.1923991670856,3.40423097483351));
#226423=CARTESIAN_POINT('Origin',(-19.3117651160115,58.8190306216296,3.20400259736054));
#226424=CARTESIAN_POINT('',(-19.5431821167169,59.5312589134599,2.83404198860303));
#226425=CARTESIAN_POINT('',(-19.433079910384,59.1923991670856,3.40423097483351));
#226426=CARTESIAN_POINT('',(-18.4801050014193,56.259443978424,2.834041988603));
#226427=CARTESIAN_POINT('',(-0.181176266354219,-0.0588677374282441,2.83404198860262));
#226428=CARTESIAN_POINT('',(-18.5902073581108,56.5983041913029,3.40423097483349));
#226429=CARTESIAN_POINT('',(-18.4801050014193,56.259443978424,2.834041988603));
#226430=CARTESIAN_POINT('',(-18.7233363629827,57.0080331356323,3.64303198860302));
#226431=CARTESIAN_POINT('Origin',(-18.7115223273403,56.9716732726283,3.20400220587359));
#226432=CARTESIAN_POINT('',(-18.8473695429914,57.3897680142076,3.64303198860302));
#226433=CARTESIAN_POINT('',(-18.8701928819397,57.4600110263531,3.64303198860303));
#226434=CARTESIAN_POINT('',(-18.8863175164095,57.5096375484038,3.42473028058521));
#226435=CARTESIAN_POINT('',(-18.8473695436964,57.3897680139785,3.64303198860302));
#226436=CARTESIAN_POINT('',(-18.9882808235623,57.823448340224,3.23423028058522));
#226437=CARTESIAN_POINT('Origin',(-18.9791867816366,57.7954614188155,3.56425743004422));
#226438=CARTESIAN_POINT('',(-19.0350067009933,57.9672558039533,3.23423028058522));
#226439=CARTESIAN_POINT('',(-19.0351700816687,57.9677586379684,3.23423028058522));
#226440=CARTESIAN_POINT('',(-19.1369699862886,58.2810665285031,3.42473028058524));
#226441=CARTESIAN_POINT('Origin',(-19.0441006607083,57.9952457951683,3.56425912918035));
#226442=CARTESIAN_POINT('',(-19.1759179427389,58.4009360128768,3.64303198860304));
#226443=CARTESIAN_POINT('',(-19.1369699862886,58.2810665285031,3.42473028058524));
#226444=CARTESIAN_POINT('',(-19.3001121590972,58.7831665079751,3.64303198860303));
#226445=CARTESIAN_POINT('Origin',(-23.5239806812874,53.3040877092103,2.65878198860298));
#226446=CARTESIAN_POINT('',(-24.0229981225299,53.9190682401996,2.65878198860299));
#226447=CARTESIAN_POINT('',(-25.5758735661211,57.406883591798,2.65878198860301));
#226448=CARTESIAN_POINT('',(-23.7119335237428,53.2204057122639,2.65878198860298));
#226449=CARTESIAN_POINT('',(-25.5480287005721,57.419280924679,2.65878198860301));
#226450=CARTESIAN_POINT('Origin',(1.17012503474363E-17,1.9055630196301E-13,
2.65878198860263));
#226451=CARTESIAN_POINT('',(-23.995153256981,53.9314655730805,2.65878198860299));
#226452=CARTESIAN_POINT('',(-23.9663957374946,53.8668751267879,2.65878198860299));
#226453=CARTESIAN_POINT('Origin',(3.62953249113008E-16,1.90760522162977E-13,
2.65878198860263));
#226454=CARTESIAN_POINT('Origin',(0.174030409680915,0.0774833305058514,
42.7590319886026));
#226455=CARTESIAN_POINT('',(-24.2316692455485,54.8935822490123,3.643031988603));
#226456=CARTESIAN_POINT('',(-24.056441199033,54.5000136127189,3.40423097483348));
#226457=CARTESIAN_POINT('Origin',(-24.2161192879492,54.8586564724116,3.20400220531659));
#226458=CARTESIAN_POINT('',(-23.9115214570978,54.1745185417596,2.83404198860299));
#226459=CARTESIAN_POINT('',(-24.056441199033,54.5000136127189,3.40423097483348));
#226460=CARTESIAN_POINT('',(-25.3107727110825,57.3172883154491,2.83404198860301));
#226461=CARTESIAN_POINT('',(-25.4164373136776,57.5546148985776,2.83404198860301));
#226462=CARTESIAN_POINT('',(-25.1658531674641,56.9917936927136,3.4042309748335));
#226463=CARTESIAN_POINT('',(-25.3107727110825,57.3172883154491,2.83404198860301));
#226464=CARTESIAN_POINT('',(-24.9906253009261,56.5982254591676,3.64303198860302));
#226465=CARTESIAN_POINT('Origin',(-25.0061753086091,56.6331513482581,3.20400259788199));
#226466=CARTESIAN_POINT('',(-24.8273695326455,56.2315470018078,3.64303198860301));
#226467=CARTESIAN_POINT('',(0.174030409680921,0.0774833305061245,3.64303198860263));
#226468=CARTESIAN_POINT('',(-24.776105164832,56.1164053447572,3.42473028058524));
#226469=CARTESIAN_POINT('',(-24.8273695332959,56.2315470015182,3.64303198860301));
#226470=CARTESIAN_POINT('',(-24.641898292288,55.8149717737127,3.2342302805852));
#226471=CARTESIAN_POINT('Origin',(-24.6538679703971,55.841854848731,3.56425722717164));
#226472=CARTESIAN_POINT('',(-24.5803964109126,55.6768362864792,3.2342302805852));
#226473=CARTESIAN_POINT('',(0.174030409680921,0.0774833305061274,3.23423028058481));
#226474=CARTESIAN_POINT('',(-24.4461895095991,55.3754026508176,3.42473028058519));
#226475=CARTESIAN_POINT('Origin',(-24.5684264878145,55.6499501367131,3.56425909741001));
#226476=CARTESIAN_POINT('',(-24.3949251197297,55.2602609459791,3.643031988603));
#226477=CARTESIAN_POINT('',(-24.4461895095991,55.3754026508176,3.42473028058519));
#226478=CARTESIAN_POINT('',(0.174030409680921,0.0774833305061245,3.64303198860262));
#226479=CARTESIAN_POINT('Origin',(-0.174030409680915,-0.07748333050603,
42.7590319886026));
#226480=CARTESIAN_POINT('',(-25.338686120288,56.4432587981557,3.64303198860301));
#226481=CARTESIAN_POINT('',(-25.5139139873792,56.8368270314554,3.40423097483349));
#226482=CARTESIAN_POINT('Origin',(-25.3542361278549,56.4781846869857,3.20400259736215));
#226483=CARTESIAN_POINT('',(-25.6588335308575,57.1623216542532,2.83404198860301));
#226484=CARTESIAN_POINT('',(-25.5139139873792,56.8368270314554,3.40423097483349));
#226485=CARTESIAN_POINT('',(-24.2595822759735,54.0195518809642,2.83404198860299));
#226486=CARTESIAN_POINT('',(-0.174030409680907,-0.0774833305057564,2.83404198860262));
#226487=CARTESIAN_POINT('',(-24.4045020177488,54.3450469519947,3.40423097483348));
#226488=CARTESIAN_POINT('',(-24.2595822759735,54.0195518809642,2.83404198860299));
#226489=CARTESIAN_POINT('',(-24.5797300649104,54.7386155880004,3.64303198860301));
#226490=CARTESIAN_POINT('Origin',(-24.5641801071872,54.7036898111215,3.20400220587239));
#226491=CARTESIAN_POINT('',(-24.7429859384138,55.105294285269,3.64303198860301));
#226492=CARTESIAN_POINT('',(-24.7730266428387,55.1727668102972,3.64303198860301));
#226493=CARTESIAN_POINT('',(-24.794250328961,55.2204359898057,3.42473028058518));
#226494=CARTESIAN_POINT('',(-24.7429859390916,55.1052942849672,3.64303198860301));
#226495=CARTESIAN_POINT('',(-24.9284572302744,55.5218696254674,3.2342302805852));
#226496=CARTESIAN_POINT('Origin',(-24.9164875765749,55.4949866055689,3.56425743004152));
#226497=CARTESIAN_POINT('',(-24.9899591116498,55.6600051127008,3.2342302805852));
#226498=CARTESIAN_POINT('',(-24.9901741577757,55.6604881142077,3.2342302805852));
#226499=CARTESIAN_POINT('',(-25.1241659841938,55.9614386837454,3.42473028058522));
#226500=CARTESIAN_POINT('Origin',(-25.0019290044706,55.6868911941813,3.56425912918012));
#226501=CARTESIAN_POINT('',(-25.1754303526578,56.0765803405064,3.64303198860301));
#226502=CARTESIAN_POINT('',(-25.1241659841938,55.9614386837454,3.42473028058522));
#226503=CARTESIAN_POINT('',(-25.3388981863709,56.4437351063764,3.64303198860301));
#226504=CARTESIAN_POINT('Origin',(-28.9669082278886,50.5531567888876,2.65878198860297));
#226505=CARTESIAN_POINT('',(-29.5274749692187,51.1126068659047,2.65878198860297));
#226506=CARTESIAN_POINT('',(-31.4364195775137,54.4189959163063,2.65878198860299));
#226507=CARTESIAN_POINT('',(-29.1450842944632,50.4502867888876,2.65878198860296));
#226508=CARTESIAN_POINT('',(-31.4100231232064,54.4342359163063,2.65878198860299));
#226509=CARTESIAN_POINT('Origin',(2.54115089989956E-17,1.90563287688712E-13,
2.65878198860263));
#226510=CARTESIAN_POINT('',(-29.5010785149114,51.1278468659047,2.65878198860297));
#226511=CARTESIAN_POINT('',(-29.465726992033,51.0666162321544,2.65878198860297));
#226512=CARTESIAN_POINT('Origin',(3.55814779065492E-16,1.90756884930817E-13,
2.65878198860263));
#226513=CARTESIAN_POINT('Origin',(0.164977839420935,0.0952499999999114,
42.7590319886026));
#226514=CARTESIAN_POINT('',(-29.8368674217658,52.0599703131947,3.64303198860298));
#226515=CARTESIAN_POINT('',(-29.6214601680814,51.6868740054943,3.40423097483346));
#226516=CARTESIAN_POINT('Origin',(-29.8177519107044,52.0268612768235,3.20400220531785));
#226517=CARTESIAN_POINT('',(-29.4433108120869,51.3783102685126,2.83404198860297));
#226518=CARTESIAN_POINT('',(-29.6214601680814,51.6868740054943,3.40423097483346));
#226519=CARTESIAN_POINT('',(-31.1634057161443,54.3576020372439,2.83404198860299));
#226520=CARTESIAN_POINT('',(-31.2932988600175,54.5825835619871,2.83404198860299));
#226521=CARTESIAN_POINT('',(-30.9852566042332,54.0490387253004,3.40423097483347));
#226522=CARTESIAN_POINT('',(-31.1634057161443,54.3576020372439,2.83404198860299));
#226523=CARTESIAN_POINT('',(-30.7698495716383,53.6759427993287,3.643031988603));
#226524=CARTESIAN_POINT('Origin',(-30.7889651442679,53.7090519423389,3.20400259788483));
#226525=CARTESIAN_POINT('',(-30.569159799877,53.3283379195024,3.64303198860299));
#226526=CARTESIAN_POINT('',(0.164977839420941,0.0952500000001846,3.64303198860263));
#226527=CARTESIAN_POINT('',(-30.5061406831646,53.2191856060846,3.42473028058522));
#226528=CARTESIAN_POINT('',(-30.5691598004935,53.3283379191465,3.64303198860299));
#226529=CARTESIAN_POINT('',(-30.3411606219521,52.9334317578288,3.23423028058518));
#226530=CARTESIAN_POINT('Origin',(-30.3558747754313,52.95891639249,3.56425722717323));
#226531=CARTESIAN_POINT('',(-30.2655565641147,52.802481688396,3.23423028058517));
#226532=CARTESIAN_POINT('',(0.164977839420941,0.0952500000001874,3.23423028058481));
#226533=CARTESIAN_POINT('',(-30.100576467536,52.5167277788842,3.42473028058516));
#226534=CARTESIAN_POINT('Origin',(-30.250841845591,52.7769940214409,3.56425909741636));
#226535=CARTESIAN_POINT('',(-30.0375573238934,52.4075754202457,3.64303198860298));
#226536=CARTESIAN_POINT('',(-30.100576467536,52.5167277788842,3.42473028058516));
#226537=CARTESIAN_POINT('',(0.164977839420941,0.0952500000001846,3.64303198860263));
#226538=CARTESIAN_POINT('Origin',(-0.164977839420935,-0.0952500000000901,
42.7590319886026));
#226539=CARTESIAN_POINT('',(-31.0998052504802,53.4854427993287,3.64303198860299));
#226540=CARTESIAN_POINT('',(-31.3152122835989,53.8585387249979,3.40423097483347));
#226541=CARTESIAN_POINT('Origin',(-31.1189208229661,53.5185519420901,3.20400259736088));
#226542=CARTESIAN_POINT('',(-31.4933613953777,54.1671020370178,2.83404198860299));
#226543=CARTESIAN_POINT('',(-31.3152122835989,53.8585387249979,3.40423097483347));
#226544=CARTESIAN_POINT('',(-29.7732664904682,51.1878102687785,2.83404198860297));
#226545=CARTESIAN_POINT('',(-0.164977839420927,-0.0952499999998162,2.83404198860262));
#226546=CARTESIAN_POINT('',(-29.9514158463113,51.4963740058476,3.40423097483345));
#226547=CARTESIAN_POINT('',(-29.7732664904682,51.1878102687785,2.83404198860297));
#226548=CARTESIAN_POINT('',(-30.1668231006077,51.8694703131947,3.64303198860298));
#226549=CARTESIAN_POINT('Origin',(-30.1477075893944,51.8363612765605,3.20400220587241));
#226550=CARTESIAN_POINT('',(-30.3675130020929,52.2170754206166,3.64303198860298));
#226551=CARTESIAN_POINT('',(-30.4044419397496,52.281038215424,3.64303198860298));
#226552=CARTESIAN_POINT('',(-30.4305321463779,52.3262277788842,3.42473028058517));
#226553=CARTESIAN_POINT('',(-30.3675130027353,52.2170754202457,3.64303198860298));
#226554=CARTESIAN_POINT('',(-30.5955122429565,52.611981688396,3.23423028058517));
#226555=CARTESIAN_POINT('Origin',(-30.580798119513,52.5864971059978,3.5642574300363));
#226556=CARTESIAN_POINT('',(-30.671116300794,52.7429317578288,3.23423028058517));
#226557=CARTESIAN_POINT('',(-30.6713806562799,52.7433896349617,3.23423028058517));
#226558=CARTESIAN_POINT('',(-30.8360963620065,53.0286856060846,3.4247302805852));
#226559=CARTESIAN_POINT('Origin',(-30.6858309820704,52.7684193600405,3.56425912917864));
#226560=CARTESIAN_POINT('',(-30.8991154793354,53.1378379191465,3.64303198860299));
#226561=CARTESIAN_POINT('',(-30.8360963620065,53.0286856060846,3.4247302805852));
#226562=CARTESIAN_POINT('',(-31.1000659426093,53.4858943313413,3.64303198860299));
#226563=CARTESIAN_POINT('Origin',(-34.0924682662297,47.2483549038576,2.65878198860294));
#226564=CARTESIAN_POINT('',(-34.7084426211234,47.7461450747865,2.65878198860295));
#226565=CARTESIAN_POINT('',(-36.9525415975215,50.8348823336486,2.65878198860297));
#226566=CARTESIAN_POINT('',(-34.2589154226524,47.1274239660509,2.65878198860294));
#226567=CARTESIAN_POINT('',(-36.9278827595329,50.8527980281385,2.65878198860297));
#226568=CARTESIAN_POINT('Origin',(3.83164542466812E-17,1.90571668258146E-13,
2.65878198860263));
#226569=CARTESIAN_POINT('',(-34.6837837831348,47.7640607692763,2.65878198860295));
#226570=CARTESIAN_POINT('',(-34.6422255755468,47.706860803705,2.65878198860295));
#226571=CARTESIAN_POINT('Origin',(3.49095608592005E-16,1.90752521450492E-13,
2.65878198860263));
#226572=CARTESIAN_POINT('Origin',(0.154117737428427,0.111973090561628,42.7590319886026));
#226573=CARTESIAN_POINT('',(-35.1151666347443,48.6559784483765,3.64303198860296));
#226574=CARTESIAN_POINT('',(-34.8619402208392,48.3074421904918,3.40423097483344));
#226575=CARTESIAN_POINT('Origin',(-35.0926950037607,48.6250489017672,3.20400220531682));
#226576=CARTESIAN_POINT('',(-34.6525130924105,48.0191904763608,2.83404198860294));
#226577=CARTESIAN_POINT('',(-34.8619402208392,48.3074421904918,3.40423097483344));
#226578=CARTESIAN_POINT('',(-36.674605926818,50.8023624960591,2.83404198860297));
#226579=CARTESIAN_POINT('',(-36.8273044755032,51.0125340177515,2.83404198860297));
#226580=CARTESIAN_POINT('',(-36.4651790855639,50.5141111791244,3.40423097483344));
#226581=CARTESIAN_POINT('',(-36.674605926818,50.8023624960591,2.83404198860296));
#226582=CARTESIAN_POINT('',(-36.2119529314387,50.1655752777672,3.64303198860298));
#226583=CARTESIAN_POINT('Origin',(-36.2344246347996,50.1965049239953,3.20400259788265));
#226584=CARTESIAN_POINT('',(-35.9760279553333,49.8408524072786,3.64303198860296));
#226585=CARTESIAN_POINT('',(0.154117737428432,0.111973090561901,3.64303198860263));
#226586=CARTESIAN_POINT('',(-35.9019445403521,49.7388853330811,3.42473028058518));
#226587=CARTESIAN_POINT('',(-35.9760279559089,49.8408524068604,3.64303198860296));
#226588=CARTESIAN_POINT('',(-35.7079988465461,49.4719419865733,3.23423028058515));
#226589=CARTESIAN_POINT('Origin',(-35.7252962640516,49.4957489658886,3.56425722717188));
#226590=CARTESIAN_POINT('',(-35.6191209461254,49.3496120513049,3.23423028058515));
#226591=CARTESIAN_POINT('',(0.154117737428432,0.111973090561904,3.23423028058481));
#226592=CARTESIAN_POINT('',(-35.425175210744,49.0826686475735,3.42473028058514));
#226593=CARTESIAN_POINT('Origin',(-35.6018226497097,49.3258021153701,3.56425909741368));
#226594=CARTESIAN_POINT('',(-35.3510917642536,48.9807015312178,3.64303198860296));
#226595=CARTESIAN_POINT('',(-35.425175210744,49.0826686475735,3.42473028058514));
#226596=CARTESIAN_POINT('',(0.154117737428432,0.111973090561901,3.64303198860263));
#226597=CARTESIAN_POINT('Origin',(-0.154117737428427,-0.111973090561806,
42.7590319886026));
#226598=CARTESIAN_POINT('',(-36.5201884062956,49.9416290966437,3.64303198860297));
#226599=CARTESIAN_POINT('',(-36.7734145609101,50.2901649976455,3.40423097483344));
#226600=CARTESIAN_POINT('Origin',(-36.5426601094868,49.9725587426385,3.20400259735612));
#226601=CARTESIAN_POINT('',(-36.9828414020409,50.5784163146698,2.83404198860296));
#226602=CARTESIAN_POINT('',(-36.7734145609101,50.2901649976455,3.40423097483344));
#226603=CARTESIAN_POINT('',(-34.9607485668368,47.7952442955502,2.83404198860294));
#226604=CARTESIAN_POINT('',(-0.154117737428418,-0.111973090561532,2.83404198860262));
#226605=CARTESIAN_POINT('',(-35.1701756951248,48.0834960097834,3.40423097483343));
#226606=CARTESIAN_POINT('',(-34.9607485668368,47.7952442955502,2.83404198860294));
#226607=CARTESIAN_POINT('',(-35.4234021096012,48.4320322672531,3.64303198860295));
#226608=CARTESIAN_POINT('Origin',(-35.4009304784384,48.4011027203971,3.20400220587326));
#226609=CARTESIAN_POINT('',(-35.6593272385106,48.7567553505302,3.64303198860296));
#226610=CARTESIAN_POINT('',(-35.7027398082301,48.8165076253519,3.64303198860296));
#226611=CARTESIAN_POINT('',(-35.7334106856009,48.85872246645,3.42473028058515));
#226612=CARTESIAN_POINT('',(-35.6593272391104,48.7567553500944,3.64303198860296));
#226613=CARTESIAN_POINT('',(-35.9273564209823,49.1256658701815,3.23423028058515));
#226614=CARTESIAN_POINT('Origin',(-35.9100590388141,49.1018589397078,3.56425743004463));
#226615=CARTESIAN_POINT('',(-36.0162343214029,49.2479958054499,3.23423028058515));
#226616=CARTESIAN_POINT('',(-36.0165450899149,49.2484235416113,3.23423028058515));
#226617=CARTESIAN_POINT('',(-36.2101800152089,49.5149391519577,3.42473028058518));
#226618=CARTESIAN_POINT('Origin',(-36.0335325740083,49.27180568089,3.56425912917508));
#226619=CARTESIAN_POINT('',(-36.2842634307658,49.616906225737,3.64303198860296));
#226620=CARTESIAN_POINT('',(-36.2101800152089,49.5149391519577,3.42473028058518));
#226621=CARTESIAN_POINT('',(-36.5204948682733,49.9420509053691,3.64303198860297));
#226622=CARTESIAN_POINT('Origin',(-38.8445040879384,43.4258901551471,2.65878198860291));
#226623=CARTESIAN_POINT('',(-39.5091373124624,43.8565665267056,2.65878198860292));
#226624=CARTESIAN_POINT('',(-42.0638038389703,46.6938111422604,2.65878198860294));
#226625=CARTESIAN_POINT('',(-38.9973987043321,43.2882232241948,2.65878198860291));
#226626=CARTESIAN_POINT('',(-42.0411527846897,46.7142062431422,2.65878198860294));
#226627=CARTESIAN_POINT('Origin',(5.02746968098277E-17,1.90581351852038E-13,
2.65878198860263));
#226628=CARTESIAN_POINT('',(-39.4864862581819,43.8769616275874,2.65878198860292));
#226629=CARTESIAN_POINT('',(-39.4391766863032,43.8244190249878,2.65878198860292));
#226630=CARTESIAN_POINT('Origin',(3.42869354330331E-16,1.90747479529204E-13,
2.65878198860263));
#226631=CARTESIAN_POINT('Origin',(0.141569089253443,0.127469380511274,42.7590319886026));
#226632=CARTESIAN_POINT('',(-40.0087367337515,44.7189015017598,3.64303198860293));
#226633=CARTESIAN_POINT('',(-39.7204655612076,44.3987439298681,3.4042309748334));
#226634=CARTESIAN_POINT('Origin',(-39.9831551867368,44.6904903154967,3.20400220531776));
#226635=CARTESIAN_POINT('',(-39.4820551877884,44.1339623846889,2.83404198860292));
#226636=CARTESIAN_POINT('',(-39.7204655612076,44.3987439298681,3.4042309748334));
#226637=CARTESIAN_POINT('',(-41.7839914803029,46.6905216402897,2.83404198860294));
#226638=CARTESIAN_POINT('',(-41.9578224365464,46.8835804757584,2.83404198860294));
#226639=CARTESIAN_POINT('',(-41.5455814340025,46.4257404601139,3.40423097483342));
#226640=CARTESIAN_POINT('',(-41.7839914803029,46.6905216402897,2.83404198860294));
#226641=CARTESIAN_POINT('',(-41.2573105570839,46.1055832156409,3.64303198860295));
#226642=CARTESIAN_POINT('Origin',(-41.2828921864922,46.1339944934115,3.20400259788282));
#226643=CARTESIAN_POINT('',(-40.9887352200424,45.8073000862123,3.64303198860294));
#226644=CARTESIAN_POINT('',(0.141569089253448,0.127469380511547,3.64303198860263));
#226645=CARTESIAN_POINT('',(-40.9043991801906,45.7136354238375,3.42473028058516));
#226646=CARTESIAN_POINT('',(-40.9887352205716,45.8073000857359,3.64303198860294));
#226647=CARTESIAN_POINT('',(-40.6836127633981,45.4684272662436,3.23423028058512));
#226648=CARTESIAN_POINT('Origin',(-40.7033039308037,45.490295755965,3.56425722717074));
#226649=CARTESIAN_POINT('',(-40.5824347852702,45.3560577375096,3.23423028058512));
#226650=CARTESIAN_POINT('',(0.141569089253449,0.12746938051155,3.23423028058481));
#226651=CARTESIAN_POINT('',(-40.3616483211486,45.1108495273513,3.42473028058512));
#226652=CARTESIAN_POINT('Origin',(-40.5627424347179,45.334186399236,3.56425909741268));
#226653=CARTESIAN_POINT('',(-40.277312245553,45.0171848263432,3.64303198860293));
#226654=CARTESIAN_POINT('',(-40.3616483211486,45.1108495273513,3.42473028058512));
#226655=CARTESIAN_POINT('',(0.141569089253448,0.127469380511547,3.64303198860263));
#226656=CARTESIAN_POINT('Origin',(-0.141569089253443,-0.127469380511452,
42.7590319886026));
#226657=CARTESIAN_POINT('',(-41.5404487355908,45.8506444546182,3.64303198860294));
#226658=CARTESIAN_POINT('',(-41.8287196129601,46.1708016986854,3.40423097483341));
#226659=CARTESIAN_POINT('Origin',(-41.5660303648069,45.8790557321753,3.20400259735887));
#226660=CARTESIAN_POINT('',(-42.0671296591458,46.4355828789644,2.83404198860293));
#226661=CARTESIAN_POINT('',(-41.8287196129601,46.1708016986854,3.40423097483341));
#226662=CARTESIAN_POINT('',(-39.7651933659001,43.879023624022,2.83404198860291));
#226663=CARTESIAN_POINT('',(-0.141569089253434,-0.127469380511178,2.83404198860262));
#226664=CARTESIAN_POINT('',(-40.00360373919,44.1438051693176,3.40423097483341));
#226665=CARTESIAN_POINT('',(-39.7651933659001,43.879023624022,2.83404198860291));
#226666=CARTESIAN_POINT('',(-40.2918749122584,44.4639627407371,3.64303198860293));
#226667=CARTESIAN_POINT('Origin',(-40.2662933650409,44.4355515542486,3.20400220587102));
#226668=CARTESIAN_POINT('',(-40.5604504235087,44.7622460658168,3.64303198860293));
#226669=CARTESIAN_POINT('',(-40.609870988093,44.8171331622256,3.64303198860293));
#226670=CARTESIAN_POINT('',(-40.6447864996555,44.8559107663285,3.42473028058512));
#226671=CARTESIAN_POINT('',(-40.5604504240599,44.7622460653205,3.64303198860293));
#226672=CARTESIAN_POINT('',(-40.8655729637771,45.1011189764869,3.23423028058512));
#226673=CARTESIAN_POINT('Origin',(-40.8458818366199,45.0792505316449,3.56425743004204));
#226674=CARTESIAN_POINT('',(-40.966750941905,45.2134885052208,3.23423028058512));
#226675=CARTESIAN_POINT('',(-40.9671047185982,45.2138814140438,3.23423028058512));
#226676=CARTESIAN_POINT('',(-41.1875373586974,45.4586966628148,3.42473028058515));
#226677=CARTESIAN_POINT('Origin',(-40.9864432425629,45.23535978791,3.56425912917542));
#226678=CARTESIAN_POINT('',(-41.2718733990785,45.5523613247131,3.64303198860294));
#226679=CARTESIAN_POINT('',(-41.1875373586974,45.4586966628148,3.42473028058515));
#226680=CARTESIAN_POINT('',(-41.5407976097556,45.8510319186317,3.64303198860294));
#226681=CARTESIAN_POINT('Origin',(-43.1709513941246,39.127642266445,2.65878198860289));
#226682=CARTESIAN_POINT('',(-43.8769616275876,39.4864862581816,2.65878198860289));
#226683=CARTESIAN_POINT('',(-46.7142062431425,42.0411527846894,2.65878198860291));
#226684=CARTESIAN_POINT('',(-43.3086183250768,38.9747476500513,2.65878198860289));
#226685=CARTESIAN_POINT('',(-46.6938111422606,42.06380383897,2.65878198860291));
#226686=CARTESIAN_POINT('Origin',(6.11552196804858E-17,1.90592232374909E-13,
2.65878198860263));
#226687=CARTESIAN_POINT('',(-43.8565665267058,39.5091373124622,2.65878198860289));
#226688=CARTESIAN_POINT('',(-43.8040239241062,39.4618277405835,2.65878198860289));
#226689=CARTESIAN_POINT('Origin',(3.37204232425085E-16,1.90741814407299E-13,
2.65878198860263));
#226690=CARTESIAN_POINT('Origin',(0.127469380511362,0.141569089253355,42.7590319886026));
#226691=CARTESIAN_POINT('',(-44.4639627407373,40.2918749122582,3.64303198860289));
#226692=CARTESIAN_POINT('',(-44.1438051688456,40.0036037397142,3.40423097483338));
#226693=CARTESIAN_POINT('Origin',(-44.4355515544742,40.2662933652435,3.20400220531717));
#226694=CARTESIAN_POINT('',(-43.8790236243777,39.7651933655051,2.83404198860289));
#226695=CARTESIAN_POINT('',(-44.1438051688456,40.0036037397142,3.40423097483338));
#226696=CARTESIAN_POINT('',(-46.4355828792672,42.0671296588095,2.8340419886029));
#226697=CARTESIAN_POINT('',(-46.6286417147359,42.240960615053,2.8340419886029));
#226698=CARTESIAN_POINT('',(-46.1708016982804,41.8287196134099,3.40423097483339));
#226699=CARTESIAN_POINT('',(-46.4355828792672,42.0671296588095,2.8340419886029));
#226700=CARTESIAN_POINT('',(-45.8506444546184,41.5404487355905,3.64303198860291));
#226701=CARTESIAN_POINT('Origin',(-45.879055732388,41.5660303649979,3.20400259787986));
#226702=CARTESIAN_POINT('',(-45.5523613242372,41.2718733996071,3.6430319886029));
#226703=CARTESIAN_POINT('',(0.127469380511367,0.141569089253628,3.64303198860262));
#226704=CARTESIAN_POINT('',(-45.458696662815,41.1875373586972,3.42473028058513));
#226705=CARTESIAN_POINT('',(-45.5523613247134,41.2718733990782,3.6430319886029));
#226706=CARTESIAN_POINT('',(-45.2134885052211,40.9667509419047,3.23423028058509));
#226707=CARTESIAN_POINT('Origin',(-45.2353576819753,40.986441346282,3.56425722717232));
#226708=CARTESIAN_POINT('',(-45.1011189764871,40.8655729637768,3.23423028058508));
#226709=CARTESIAN_POINT('',(0.127469380511367,0.141569089253631,3.23423028058481));
#226710=CARTESIAN_POINT('',(-44.8559107663287,40.6447864996552,3.42473028058509));
#226711=CARTESIAN_POINT('Origin',(-45.0792483253111,40.8458798501231,3.56425909740998));
#226712=CARTESIAN_POINT('',(-44.7622460653207,40.5604504240596,3.6430319886029));
#226713=CARTESIAN_POINT('',(-44.8559107663287,40.6447864996552,3.42473028058509));
#226714=CARTESIAN_POINT('',(0.127469380511367,0.141569089253628,3.64303198860262));
#226715=CARTESIAN_POINT('Origin',(-0.127469380511362,-0.141569089253534,
42.7590319886026));
#226716=CARTESIAN_POINT('',(-46.1055832156411,41.2573105570836,3.64303198860291));
#226717=CARTESIAN_POINT('',(-46.4257404597083,41.545581434453,3.40423097483338));
#226718=CARTESIAN_POINT('Origin',(-46.1339944931981,41.2828921862996,3.20400259735835));
#226719=CARTESIAN_POINT('',(-46.6905216405927,41.7839914799664,2.8340419886029));
#226720=CARTESIAN_POINT('',(-46.4257404597083,41.545581434453,3.40423097483338));
#226721=CARTESIAN_POINT('',(-44.1339623850449,39.482055187393,2.83404198860288));
#226722=CARTESIAN_POINT('',(-0.127469380511352,-0.141569089253259,2.83404198860262));
#226723=CARTESIAN_POINT('',(-44.3987439293959,39.720465561732,3.40423097483337));
#226724=CARTESIAN_POINT('',(-44.1339623850449,39.482055187393,2.83404198860288));
#226725=CARTESIAN_POINT('',(-44.7189015017601,40.0087367337513,3.6430319886029));
#226726=CARTESIAN_POINT('Origin',(-44.6904903152701,39.9831551865324,3.20400220587441));
#226727=CARTESIAN_POINT('',(-45.0171848258471,40.277312246104,3.6430319886029));
#226728=CARTESIAN_POINT('',(-45.0720719232486,40.3267328095859,3.6430319886029));
#226729=CARTESIAN_POINT('',(-45.1108495273515,40.3616483211483,3.42473028058508));
#226730=CARTESIAN_POINT('',(-45.0171848263434,40.2773122455527,3.6430319886029));
#226731=CARTESIAN_POINT('',(-45.3560577375098,40.5824347852699,3.23423028058509));
#226732=CARTESIAN_POINT('Origin',(-45.3341886054739,40.5627444213184,3.56425743004201));
#226733=CARTESIAN_POINT('',(-45.4684272662438,40.6836127633978,3.23423028058509));
#226734=CARTESIAN_POINT('',(-45.4688201750668,40.6839665400911,3.23423028058509));
#226735=CARTESIAN_POINT('',(-45.7136354238378,40.9043991801903,3.42473028058511));
#226736=CARTESIAN_POINT('Origin',(-45.4902978619855,40.7033058269841,3.56425912918036));
#226737=CARTESIAN_POINT('',(-45.8073000857361,40.9887352205713,3.64303198860291));
#226738=CARTESIAN_POINT('',(-45.7136354238378,40.9043991801903,3.42473028058511));
#226739=CARTESIAN_POINT('',(-46.1059706796546,41.2576594312484,3.64303198860291));
#226740=CARTESIAN_POINT('Origin',(-47.0244087227343,34.4007037410863,2.65878198860285));
#226741=CARTESIAN_POINT('',(-47.7640607692765,34.6837837831345,2.65878198860285));
#226742=CARTESIAN_POINT('',(-50.8527980281387,36.9278827595326,2.65878198860287));
#226743=CARTESIAN_POINT('',(-47.145339660541,34.2342565846636,2.65878198860285));
#226744=CARTESIAN_POINT('',(-50.8348823336488,36.9525415975211,2.65878198860287));
#226745=CARTESIAN_POINT('Origin',(7.08388135731919E-17,1.90604190617472E-13,
2.65878198860263));
#226746=CARTESIAN_POINT('',(-47.7461450747866,34.7084426211231,2.65878198860285));
#226747=CARTESIAN_POINT('',(-47.6889451092153,34.6668844135351,2.65878198860285));
#226748=CARTESIAN_POINT('Origin',(3.32162311137368E-16,1.90735588153037E-13,
2.65878198860263));
#226749=CARTESIAN_POINT('Origin',(0.111973090561715,0.154117737428339,42.7590319886026));
#226750=CARTESIAN_POINT('',(-48.4320322672532,35.4234021096009,3.64303198860286));
#226751=CARTESIAN_POINT('',(-48.0834960093685,35.1701756956958,3.40423097483334));
#226752=CARTESIAN_POINT('Origin',(-48.4011027206437,35.4009304786171,3.20400220531728));
#226753=CARTESIAN_POINT('',(-47.7952442958629,34.9607485664063,2.83404198860285));
#226754=CARTESIAN_POINT('',(-48.0834960093685,35.1701756956958,3.40423097483334));
#226755=CARTESIAN_POINT('',(-50.5784163149358,36.9828414016746,2.83404198860287));
#226756=CARTESIAN_POINT('',(-50.7885878366283,37.1355399503597,2.83404198860287));
#226757=CARTESIAN_POINT('',(-50.29016499729,36.7734145613993,3.40423097483335));
#226758=CARTESIAN_POINT('',(-50.5784163149359,36.9828414016746,2.83404198860287));
#226759=CARTESIAN_POINT('',(-49.9416290966439,36.5201884062952,3.64303198860288));
#226760=CARTESIAN_POINT('Origin',(-49.9725587428718,36.5426601096559,3.20400259788167));
#226761=CARTESIAN_POINT('',(-49.6169062253184,36.2842634313418,3.64303198860287));
#226762=CARTESIAN_POINT('',(0.111973090561721,0.154117737428612,3.64303198860263));
#226763=CARTESIAN_POINT('',(-49.5149391519579,36.2101800152086,3.42473028058509));
#226764=CARTESIAN_POINT('',(-49.6169062257371,36.2842634307655,3.64303198860287));
#226765=CARTESIAN_POINT('',(-49.2479958054501,36.0162343214026,3.23423028058506));
#226766=CARTESIAN_POINT('Origin',(-49.271803388277,36.0335309082457,3.56425722717104));
#226767=CARTESIAN_POINT('',(-49.1256658701817,35.927356420982,3.23423028058506));
#226768=CARTESIAN_POINT('',(0.111973090561721,0.154117737428615,3.23423028058481));
#226769=CARTESIAN_POINT('',(-48.8587224664502,35.7334106856006,3.42473028058505));
#226770=CARTESIAN_POINT('Origin',(-49.1018565378153,35.9100572938243,3.56425909741256));
#226771=CARTESIAN_POINT('',(-48.7567553500946,35.6593272391101,3.64303198860287));
#226772=CARTESIAN_POINT('',(-48.8587224664502,35.7334106856006,3.42473028058505));
#226773=CARTESIAN_POINT('',(0.111973090561721,0.154117737428612,3.64303198860263));
#226774=CARTESIAN_POINT('Origin',(-0.111973090561715,-0.154117737428517,
42.7590319886026));
#226775=CARTESIAN_POINT('',(-50.1655752777673,36.2119529314384,3.64303198860287));
#226776=CARTESIAN_POINT('',(-50.5141111787691,36.4651790860529,3.40423097483334));
#226777=CARTESIAN_POINT('Origin',(-50.1965049237621,36.2344246346297,3.20400259735654));
#226778=CARTESIAN_POINT('',(-50.8023624963254,36.6746059264515,2.83404198860287));
#226779=CARTESIAN_POINT('',(-50.5141111787691,36.4651790860529,3.40423097483334));
#226780=CARTESIAN_POINT('',(-48.0191904766738,34.6525130919796,2.83404198860285));
#226781=CARTESIAN_POINT('',(-0.111973090561705,-0.154117737428242,2.83404198860262));
#226782=CARTESIAN_POINT('',(-48.3074421900768,34.8619402214103,3.40423097483334));
#226783=CARTESIAN_POINT('',(-48.0191904766738,34.6525130919796,2.83404198860285));
#226784=CARTESIAN_POINT('',(-48.6559784483767,35.115166634744,3.64303198860286));
#226785=CARTESIAN_POINT('Origin',(-48.6250489015209,35.0926950035814,3.20400220587282));
#226786=CARTESIAN_POINT('',(-48.9807015307821,35.3510917648532,3.64303198860287));
#226787=CARTESIAN_POINT('',(-49.0404538064756,35.394504333373,3.64303198860286));
#226788=CARTESIAN_POINT('',(-49.0826686475736,35.4251752107437,3.42473028058505));
#226789=CARTESIAN_POINT('',(-48.980701531218,35.3510917642533,3.64303198860286));
#226790=CARTESIAN_POINT('',(-49.3496120513051,35.6191209461251,3.23423028058506));
#226791=CARTESIAN_POINT('Origin',(-49.3258045171776,35.6018243948123,3.56425743004168));
#226792=CARTESIAN_POINT('',(-49.4719419865735,35.7079988465457,3.23423028058506));
#226793=CARTESIAN_POINT('',(-49.4723697227349,35.7083096150578,3.23423028058506));
#226794=CARTESIAN_POINT('',(-49.7388853330813,35.9019445403517,3.42473028058508));
#226795=CARTESIAN_POINT('Origin',(-49.4957512585782,35.7252979297064,3.56425912917766));
#226796=CARTESIAN_POINT('',(-49.8408524068606,35.9760279559086,3.64303198860287));
#226797=CARTESIAN_POINT('',(-49.7388853330813,35.9019445403517,3.42473028058508));
#226798=CARTESIAN_POINT('',(-50.1659970864927,36.2122593934161,3.64303198860287));
#226799=CARTESIAN_POINT('Origin',(-50.3626567888877,29.2968639067301,2.65878198860282));
#226800=CARTESIAN_POINT('',(-51.1278468659049,29.501078514911,2.65878198860282));
#226801=CARTESIAN_POINT('',(-54.4342359163065,31.410023123206,2.65878198860283));
#226802=CARTESIAN_POINT('',(-50.4655267888877,29.1186878401555,2.65878198860282));
#226803=CARTESIAN_POINT('',(-54.4189959163065,31.4364195775134,2.65878198860283));
#226804=CARTESIAN_POINT('Origin',(7.92193830068373E-17,1.9061709556272E-13,
2.65878198860263));
#226805=CARTESIAN_POINT('',(-51.1126068659049,29.5274749692184,2.65878198860282));
#226806=CARTESIAN_POINT('',(-51.0513762321546,29.49212344634,2.65878198860282));
#226807=CARTESIAN_POINT('Origin',(3.27798830811897E-16,1.90728868982564E-13,
2.65878198860263));
#226808=CARTESIAN_POINT('Origin',(0.095249999999999,0.164977839420847,42.7590319886026));
#226809=CARTESIAN_POINT('',(-51.8694703131948,30.1668231006073,3.64303198860283));
#226810=CARTESIAN_POINT('',(-51.4963740054945,29.9514158469229,3.4042309748333));
#226811=CARTESIAN_POINT('Origin',(-51.8363612768229,30.1477075895454,3.20400220531979));
#226812=CARTESIAN_POINT('',(-51.1878102690446,29.7732664900073,2.83404198860282));
#226813=CARTESIAN_POINT('',(-51.4963740054945,29.9514158469229,3.4042309748333));
#226814=CARTESIAN_POINT('',(-54.167102037244,31.4933613949858,2.83404198860283));
#226815=CARTESIAN_POINT('',(-54.3920835619873,31.623254538859,2.83404198860283));
#226816=CARTESIAN_POINT('',(-53.8585387246954,31.3152122841228,3.40423097483331));
#226817=CARTESIAN_POINT('',(-54.167102037244,31.4933613949858,2.83404198860283));
#226818=CARTESIAN_POINT('',(-53.4854427993288,31.0998052504798,3.64303198860284));
#226819=CARTESIAN_POINT('Origin',(-53.5185519423381,31.1189208231089,3.20400259788301));
#226820=CARTESIAN_POINT('',(-53.1378379187908,30.8991154799513,3.64303198860283));
#226821=CARTESIAN_POINT('',(0.0952500000000046,0.16497783942112,3.64303198860263));
#226822=CARTESIAN_POINT('',(-53.0286856060847,30.8360963620061,3.42473028058505));
#226823=CARTESIAN_POINT('',(-53.1378379191466,30.899115479335,3.64303198860283));
#226824=CARTESIAN_POINT('',(-52.7429317578289,30.6711163007936,3.23423028058502));
#226825=CARTESIAN_POINT('Origin',(-52.7684169058678,30.6858295650768,3.56425722717264));
#226826=CARTESIAN_POINT('',(-52.6119816883961,30.5955122429562,3.23423028058502));
#226827=CARTESIAN_POINT('',(0.0952500000000046,0.164977839421123,3.23423028058481));
#226828=CARTESIAN_POINT('',(-52.3262277788843,30.4305321463775,3.42473028058501));
#226829=CARTESIAN_POINT('Origin',(-52.5864945348658,30.5807966351507,3.56425909741258));
#226830=CARTESIAN_POINT('',(-52.2170754202458,30.3675130027349,3.64303198860282));
#226831=CARTESIAN_POINT('',(-52.3262277788843,30.4305321463775,3.42473028058501));
#226832=CARTESIAN_POINT('',(0.0952500000000046,0.16497783942112,3.64303198860263));
#226833=CARTESIAN_POINT('Origin',(-0.095249999999999,-0.164977839421025,
42.7590319886026));
#226834=CARTESIAN_POINT('',(-53.6759427993288,30.769849571638,3.64303198860283));
#226835=CARTESIAN_POINT('',(-54.0490387249981,30.9852566047567,3.40423097483331));
#226836=CARTESIAN_POINT('Origin',(-53.7090519420892,30.7889651441233,3.20400259735861));
#226837=CARTESIAN_POINT('',(-54.3576020374704,31.1634057157518,2.83404198860283));
#226838=CARTESIAN_POINT('',(-54.0490387249981,30.9852566047567,3.40423097483331));
#226839=CARTESIAN_POINT('',(-51.3783102687787,29.443310811626,2.83404198860281));
#226840=CARTESIAN_POINT('',(-0.0952499999999886,-0.164977839420749,2.83404198860262));
#226841=CARTESIAN_POINT('',(-51.6868740051411,29.621460168693,3.4042309748333));
#226842=CARTESIAN_POINT('',(-51.3783102687787,29.443310811626,2.83404198860281));
#226843=CARTESIAN_POINT('',(-52.0599703131948,29.8368674217655,3.64303198860283));
#226844=CARTESIAN_POINT('Origin',(-52.0268612765603,29.817751910552,3.20400220587313));
#226845=CARTESIAN_POINT('',(-52.407575419875,30.0375573245353,3.64303198860283));
#226846=CARTESIAN_POINT('',(-52.4715382154241,30.0744862609074,3.64303198860283));
#226847=CARTESIAN_POINT('',(-52.5167277788843,30.1005764675357,3.42473028058501));
#226848=CARTESIAN_POINT('',(-52.4075754202458,30.0375573238931,3.64303198860283));
#226849=CARTESIAN_POINT('',(-52.8024816883961,30.2655565641143,3.23423028058502));
#226850=CARTESIAN_POINT('Origin',(-52.776996592507,30.2508433300782,3.56425743005036));
#226851=CARTESIAN_POINT('',(-52.9334317578289,30.3411606219517,3.23423028058502));
#226852=CARTESIAN_POINT('',(-52.9338896349619,30.3414249774377,3.23423028058502));
#226853=CARTESIAN_POINT('',(-53.2191856060847,30.5061406831642,3.42473028058504));
#226854=CARTESIAN_POINT('Origin',(-52.9589188467298,30.3558761923111,3.56425912917622));
#226855=CARTESIAN_POINT('',(-53.3283379191466,30.5691598004931,3.64303198860283));
#226856=CARTESIAN_POINT('',(-53.2191856060847,30.5061406831642,3.42473028058504));
#226857=CARTESIAN_POINT('',(-53.6763943313415,30.770110263767,3.64303198860283));
#226858=CARTESIAN_POINT('Origin',(-53.1491210481985,23.8720415006489,2.65878198860278));
#226859=CARTESIAN_POINT('',(-53.9314655730806,23.9951532569806,2.65878198860278));
#226860=CARTESIAN_POINT('',(-57.419280924679,25.5480287005717,2.65878198860279));
#226861=CARTESIAN_POINT('',(-53.2328030451449,23.6840886581935,2.65878198860278));
#226862=CARTESIAN_POINT('',(-57.4068835917981,25.5758735661207,2.65878198860279));
#226863=CARTESIAN_POINT('Origin',(8.62051087089598E-17,1.90630805821371E-13,
2.65878198860263));
#226864=CARTESIAN_POINT('',(-53.9190682401996,24.0229981225296,2.65878198860278));
#226865=CARTESIAN_POINT('',(-53.854477793907,23.9942406030432,2.65878198860278));
#226866=CARTESIAN_POINT('Origin',(3.24161598652235E-16,1.90721730512516E-13,
2.65878198860263));
#226867=CARTESIAN_POINT('Origin',(0.0774833305059389,0.174030409680827,
42.7590319886026));
#226868=CARTESIAN_POINT('',(-54.7386155880005,24.57973006491,3.64303198860279));
#226869=CARTESIAN_POINT('',(-54.3450469517071,24.4045020183944,3.40423097483326));
#226870=CARTESIAN_POINT('Origin',(-54.7036898113995,24.5641801073105,3.20400220531701));
#226871=CARTESIAN_POINT('',(-54.0195518811806,24.2595822754873,2.83404198860278));
#226872=CARTESIAN_POINT('',(-54.3450469517071,24.4045020183944,3.40423097483326));
#226873=CARTESIAN_POINT('',(-57.1623216544373,25.658833530444,2.83404198860279));
#226874=CARTESIAN_POINT('',(-57.3996482375658,25.7644981330391,2.83404198860279));
#226875=CARTESIAN_POINT('',(-56.8368270312095,25.5139139879314,3.40423097483327));
#226876=CARTESIAN_POINT('',(-57.1623216544372,25.658833530444,2.83404198860279));
#226877=CARTESIAN_POINT('',(-56.4432587981558,25.3386861202876,3.6430319886028));
#226878=CARTESIAN_POINT('Origin',(-56.4781846872464,25.3542361279706,3.20400259788151));
#226879=CARTESIAN_POINT('',(-56.076580340217,25.1754303533075,3.6430319886028));
#226880=CARTESIAN_POINT('',(0.0774833305059444,0.1740304096811,3.64303198860263));
#226881=CARTESIAN_POINT('',(-55.9614386837454,25.1241659841934,3.42473028058502));
#226882=CARTESIAN_POINT('',(-56.0765803405064,25.1754303526574,3.64303198860279));
#226883=CARTESIAN_POINT('',(-55.6600051127009,24.9899591116494,3.23423028058498));
#226884=CARTESIAN_POINT('Origin',(-55.6868886053398,25.0019278517718,3.56425722716828));
#226885=CARTESIAN_POINT('',(-55.5218696254674,24.928457230274,3.23423028058498));
#226886=CARTESIAN_POINT('',(0.0774833305059445,0.174030409681103,3.23423028058481));
#226887=CARTESIAN_POINT('',(-55.2204359898058,24.7942503289606,3.42473028058497));
#226888=CARTESIAN_POINT('Origin',(-55.49498389336,24.916486369099,3.56425909741029));
#226889=CARTESIAN_POINT('',(-55.1052942849673,24.7429859390912,3.64303198860279));
#226890=CARTESIAN_POINT('',(-55.2204359898058,24.7942503289606,3.42473028058497));
#226891=CARTESIAN_POINT('',(0.0774833305059444,0.1740304096811,3.64303198860263));
#226892=CARTESIAN_POINT('Origin',(-0.0774833305059389,-0.174030409681005,
42.7590319886026));
#226893=CARTESIAN_POINT('',(-56.5982254591677,24.9906253009257,3.64303198860279));
#226894=CARTESIAN_POINT('',(-56.9917936924674,25.165853168017,3.40423097483327));
#226895=CARTESIAN_POINT('Origin',(-56.6331513479964,25.0061753084922,3.20400259735894));
#226896=CARTESIAN_POINT('',(-57.317288315633,25.3107727106691,2.83404198860279));
#226897=CARTESIAN_POINT('',(-56.9917936924674,25.165853168017,3.40423097483326));
#226898=CARTESIAN_POINT('',(-54.1745185419761,23.9115214566113,2.83404198860277));
#226899=CARTESIAN_POINT('',(-0.0774833305059281,-0.174030409680729,2.83404198860262));
#226900=CARTESIAN_POINT('',(-54.5000136124314,24.0564411996785,3.40423097483327));
#226901=CARTESIAN_POINT('',(-54.1745185419761,23.9115214566113,2.83404198860278));
#226902=CARTESIAN_POINT('',(-54.8935822490124,24.2316692455482,3.64303198860279));
#226903=CARTESIAN_POINT('Origin',(-54.8586564721335,24.216119287825,3.2040022058723));
#226904=CARTESIAN_POINT('',(-55.2602609456777,24.3949251204066,3.64303198860279));
#226905=CARTESIAN_POINT('',(-55.3277334713091,24.4249658234765,3.64303198860279));
#226906=CARTESIAN_POINT('',(-55.3754026508176,24.4461895095988,3.42473028058497));
#226907=CARTESIAN_POINT('',(-55.2602609459792,24.3949251197294,3.64303198860279));
#226908=CARTESIAN_POINT('',(-55.6768362864793,24.5803964109122,3.23423028058498));
#226909=CARTESIAN_POINT('Origin',(-55.6499528488641,24.5684276954192,3.56425743004096));
#226910=CARTESIAN_POINT('',(-55.8149717737128,24.6418982922876,3.23423028058498));
#226911=CARTESIAN_POINT('',(-55.8154547752196,24.6421133384135,3.23423028058498));
#226912=CARTESIAN_POINT('',(-56.1164053447573,24.7761051648316,3.424730280585));
#226913=CARTESIAN_POINT('Origin',(-55.8418574376303,24.6538691229771,3.56425912917466));
#226914=CARTESIAN_POINT('',(-56.2315470015183,24.8273695332955,3.64303198860279));
#226915=CARTESIAN_POINT('',(-56.1164053447573,24.7761051648316,3.424730280585));
#226916=CARTESIAN_POINT('',(-56.5987017673884,24.9908373670086,3.64303198860279));
#226917=CARTESIAN_POINT('Origin',(-55.3532724151366,18.1856720123407,2.65878198860274));
#226918=CARTESIAN_POINT('',(-56.1441998575528,18.2263320786581,2.65878198860274));
#226919=CARTESIAN_POINT('',(-59.7752282754838,19.4061247292252,2.65878198860275));
#226920=CARTESIAN_POINT('',(-55.4168495715593,17.9900016446781,2.65878198860274));
#226921=CARTESIAN_POINT('',(-59.7658094374952,19.4351129318419,2.65878198860275));
#226922=CARTESIAN_POINT('Origin',(9.17194536069053E-17,1.90645171180964E-13,
2.65878198860263));
#226923=CARTESIAN_POINT('',(-56.1347810195643,18.2553202812748,2.65878198860274));
#226924=CARTESIAN_POINT('',(-56.0675384271754,18.2334718385818,2.65878198860274));
#226925=CARTESIAN_POINT('Origin',(3.21290464935061E-16,1.90714250953466E-13,
2.65878198860263));
#226926=CARTESIAN_POINT('Origin',(0.0588677374284264,0.181176266354138,
42.7590319886026));
#226927=CARTESIAN_POINT('',(-57.0080331356323,18.7233363629823,3.64303198860275));
#226928=CARTESIAN_POINT('',(-56.5983041910847,18.5902073587821,3.40423097483322));
#226929=CARTESIAN_POINT('Origin',(-56.9716732729175,18.7115223274339,3.204002205318));
#226930=CARTESIAN_POINT('',(-56.2594439785882,18.4801050009135,2.83404198860274));
#226931=CARTESIAN_POINT('',(-56.5983041910847,18.5902073587821,3.40423097483322));
#226932=CARTESIAN_POINT('',(-59.5312589135997,19.5431821162865,2.83404198860274));
#226933=CARTESIAN_POINT('',(-59.778330355405,19.6234604941057,2.83404198860274));
#226934=CARTESIAN_POINT('',(-59.1923991668985,19.4330799109595,3.40423097483322));
#226935=CARTESIAN_POINT('',(-59.5312589135997,19.5431821162865,2.83404198860274));
#226936=CARTESIAN_POINT('',(-58.7826706420789,19.2999510425005,3.64303198860276));
#226937=CARTESIAN_POINT('Origin',(-58.8190306219021,19.3117651160996,3.20400259788237));
#226938=CARTESIAN_POINT('',(-58.4009360126568,19.1759179434156,3.64303198860275));
#226939=CARTESIAN_POINT('',(0.0588677374284319,0.181176266354411,3.64303198860263));
#226940=CARTESIAN_POINT('',(-58.2810665285031,19.1369699862882,3.42473028058497));
#226941=CARTESIAN_POINT('',(-58.4009360128768,19.1759179427385,3.64303198860275));
#226942=CARTESIAN_POINT('',(-57.9672558039533,19.0350067009929,3.23423028058494));
#226943=CARTESIAN_POINT('Origin',(-57.9952431000166,19.044099784931,3.56425722717267));
#226944=CARTESIAN_POINT('',(-57.823448340224,18.9882808235619,3.23423028058494));
#226945=CARTESIAN_POINT('',(0.0588677374284319,0.181176266354414,3.23423028058481));
#226946=CARTESIAN_POINT('',(-57.5096375484038,18.8863175164091,3.42473028058494));
#226947=CARTESIAN_POINT('Origin',(-57.7954585952457,18.9791858642774,3.56425909740675));
#226948=CARTESIAN_POINT('',(-57.3897680139785,18.8473695436961,3.64303198860275));
#226949=CARTESIAN_POINT('',(-57.5096375484038,18.8863175164091,3.42473028058494));
#226950=CARTESIAN_POINT('',(0.0588677374284319,0.181176266354411,3.64303198860263));
#226951=CARTESIAN_POINT('Origin',(-0.0588677374284264,-0.181176266354316,
42.7590319886026));
#226952=CARTESIAN_POINT('',(-58.9004061169358,18.937598509792,3.64303198860275));
#226953=CARTESIAN_POINT('',(-59.3101346419425,19.0707273776751,3.40423097483323));
#226954=CARTESIAN_POINT('Origin',(-58.9367660964859,18.9494125833024,3.20400259735869));
#226955=CARTESIAN_POINT('',(-59.6489943885963,19.1808295831477,2.83404198860274));
#226956=CARTESIAN_POINT('',(-59.3101346419425,19.0707273776751,3.40423097483323));
#226957=CARTESIAN_POINT('',(-56.3771794532808,18.1177524687105,2.83404198860273));
#226958=CARTESIAN_POINT('',(-0.0588677374284154,-0.181176266354039,2.83404198860262));
#226959=CARTESIAN_POINT('',(-56.7160396657233,18.2278548267451,3.40423097483323));
#226960=CARTESIAN_POINT('',(-56.3771794532808,18.1177524687105,2.83404198860274));
#226961=CARTESIAN_POINT('',(-57.1257686104892,18.3609838302738,3.64303198860275));
#226962=CARTESIAN_POINT('Origin',(-57.0894087474844,18.3491697946313,3.20400220587492));
#226963=CARTESIAN_POINT('',(-57.5075034886063,18.4850170116926,3.64303198860275));
#226964=CARTESIAN_POINT('',(-57.57774650121,18.5078403492308,3.64303198860275));
#226965=CARTESIAN_POINT('',(-57.6273730232606,18.5239649837006,3.42473028058492));
#226966=CARTESIAN_POINT('',(-57.5075034888354,18.4850170109876,3.64303198860275));
#226967=CARTESIAN_POINT('',(-57.9411838150808,18.6259282908535,3.23423028058494));
#226968=CARTESIAN_POINT('Origin',(-57.913196576314,18.6168352256581,3.56425743004465));
#226969=CARTESIAN_POINT('',(-58.0849912788101,18.6726541682844,3.23423028058494));
#226970=CARTESIAN_POINT('',(-58.0854941128252,18.6728175489599,3.23423028058494));
#226971=CARTESIAN_POINT('',(-58.3988020033599,18.7746174535798,3.42473028058496));
#226972=CARTESIAN_POINT('Origin',(-58.1129809527837,18.6817491043776,3.56425912917502));
#226973=CARTESIAN_POINT('',(-58.5186714877337,18.8135654100301,3.64303198860275));
#226974=CARTESIAN_POINT('',(-58.3988020033599,18.7746174535798,3.42473028058496));
#226975=CARTESIAN_POINT('',(-58.900901982832,18.9377596263884,3.64303198860275));
#226976=CARTESIAN_POINT('Origin',(-56.9509617460775,12.3000564958688,2.6587819886027));
#226977=CARTESIAN_POINT('',(-57.7418065394567,12.2578193919766,2.6587819886027));
#226978=CARTESIAN_POINT('',(-61.4762657165316,13.0516031943527,2.6587819886027));
#226979=CARTESIAN_POINT('',(-56.9937374973464,12.0988124084938,2.6587819886027));
#226980=CARTESIAN_POINT('',(-61.4699285681955,13.081417133223,2.6587819886027));
#226981=CARTESIAN_POINT('Origin',(9.57020013840216E-17,1.90660034251612E-13,
2.65878198860263));
#226982=CARTESIAN_POINT('',(-57.7354693911205,12.2876333308469,2.6587819886027));
#226983=CARTESIAN_POINT('',(-57.6663113765489,12.2729333410577,2.6587819886027));
#226984=CARTESIAN_POINT('Origin',(3.19216886402203E-16,1.90706512253028E-13,
2.65878198860263));
#226985=CARTESIAN_POINT('Origin',(0.039607177100782,0.186337117939701,42.7590319886026));
#226986=CARTESIAN_POINT('',(-58.6528587425323,12.6618058697518,3.64303198860271));
#226987=CARTESIAN_POINT('',(-58.2314585657881,12.5722344970959,3.40423097483318));
#226988=CARTESIAN_POINT('Origin',(-58.6154631599687,12.6538571933004,3.20400220531852));
#226989=CARTESIAN_POINT('',(-57.882945834721,12.4981558287389,2.83404198860269));
#226990=CARTESIAN_POINT('',(-58.2314585657881,12.5722344970959,3.40423097483318));
#226991=CARTESIAN_POINT('',(-61.2479592423879,13.2134115091892,2.8340419886027));
#226992=CARTESIAN_POINT('',(-61.5020685764505,13.2674241155258,2.8340419886027));
#226993=CARTESIAN_POINT('',(-60.8994469905094,13.139332943849,3.40423097483318));
#226994=CARTESIAN_POINT('',(-61.2479592423878,13.2134115091892,2.8340419886027));
#226995=CARTESIAN_POINT('',(-60.4780472453828,13.0497616623173,3.64303198860271));
#226996=CARTESIAN_POINT('Origin',(-60.5154429483887,13.0577103643695,3.2040025978796));
#226997=CARTESIAN_POINT('',(-60.0854388089606,12.9663101637162,3.64303198860271));
#226998=CARTESIAN_POINT('',(0.0396071771007875,0.186337117939974,3.64303198860263));
#226999=CARTESIAN_POINT('',(-59.9621548122772,12.9401053405448,3.42473028058494));
#227000=CARTESIAN_POINT('',(-60.0854388091086,12.9663101630202,3.64303198860271));
#227001=CARTESIAN_POINT('',(-59.6394051101894,12.871502773589,3.2342302805849));
#227002=CARTESIAN_POINT('Origin',(-59.6681895750092,12.8776205756138,3.56425722716818));
#227003=CARTESIAN_POINT('',(-59.4915012546306,12.8400648385937,3.2342302805849));
#227004=CARTESIAN_POINT('',(0.0396071771007876,0.186337117939977,3.23423028058482));
#227005=CARTESIAN_POINT('',(-59.1687514833561,12.7714622569318,3.42473028058489));
#227006=CARTESIAN_POINT('Origin',(-59.46271415829,12.8339454274783,3.56425909741383));
#227007=CARTESIAN_POINT('',(-59.0454674350475,12.7452574235145,3.64303198860271));
#227008=CARTESIAN_POINT('',(-59.1687514833561,12.7714622569318,3.42473028058489));
#227009=CARTESIAN_POINT('',(0.0396071771007875,0.186337117939974,3.64303198860263));
#227010=CARTESIAN_POINT('Origin',(-0.039607177100782,-0.18633711793988,
42.7590319886026));
#227011=CARTESIAN_POINT('',(-60.5572615995844,12.6770874264377,3.64303198860271));
#227012=CARTESIAN_POINT('',(-60.9786613448368,12.7666587073772,3.40423097483318));
#227013=CARTESIAN_POINT('Origin',(-60.5946573023108,12.6850361284305,3.20400259735845));
#227014=CARTESIAN_POINT('',(-61.3271735966834,12.8407372728673,2.83404198860269));
#227015=CARTESIAN_POINT('',(-60.9786613448368,12.7666587073772,3.40423097483318));
#227016=CARTESIAN_POINT('',(-57.9621601888121,12.125481593379,2.83404198860269));
#227017=CARTESIAN_POINT('',(-0.0396071771007709,-0.186337117939602,2.83404198860262));
#227018=CARTESIAN_POINT('',(-58.3106729198428,12.1995602619073,3.40423097483318));
#227019=CARTESIAN_POINT('',(-57.9621601888121,12.125481593379,2.8340419886027));
#227020=CARTESIAN_POINT('',(-58.7320730967339,12.2891316338722,3.64303198860271));
#227021=CARTESIAN_POINT('Origin',(-58.6946775138721,12.2811829573574,3.2040022058751));
#227022=CARTESIAN_POINT('',(-59.1246817890948,12.3725831883607,3.6430319886027));
#227023=CARTESIAN_POINT('',(-59.1969256915255,12.3879391031045,3.64303198860271));
#227024=CARTESIAN_POINT('',(-59.2479658375577,12.3987880210522,3.42473028058489));
#227025=CARTESIAN_POINT('',(-59.1246817892491,12.372583187635,3.6430319886027));
#227026=CARTESIAN_POINT('',(-59.5707156088321,12.4673906027141,3.23423028058489));
#227027=CARTESIAN_POINT('Origin',(-59.5419312029586,12.4612728133412,3.5642574300495));
#227028=CARTESIAN_POINT('',(-59.718619464391,12.4988285377094,3.23423028058489));
#227029=CARTESIAN_POINT('',(-59.7191366217597,12.4989384629015,3.23423028058489));
#227030=CARTESIAN_POINT('',(-60.0413691664788,12.5674311046652,3.42473028058491));
#227031=CARTESIAN_POINT('Origin',(-59.7474064876925,12.5049479331827,3.56425912918016));
#227032=CARTESIAN_POINT('',(-60.1646531633101,12.5936359271406,3.64303198860271));
#227033=CARTESIAN_POINT('',(-60.0413691664788,12.5674311046652,3.42473028058491));
#227034=CARTESIAN_POINT('',(-60.5577715903455,12.6771958283204,3.64303198860271));
#227035=CARTESIAN_POINT('Origin',(-57.9246844223735,6.27967898647588,2.65878198860266));
#227036=CARTESIAN_POINT('',(-58.7067819056643,6.15500747092296,2.65878198860266));
#227037=CARTESIAN_POINT('',(-62.5037563256535,6.55408556365924,2.65878198860266));
#227038=CARTESIAN_POINT('',(-57.9461901084062,6.07506605172281,2.65878198860265));
#227039=CARTESIAN_POINT('',(-62.5005702980931,6.58439859103007,2.65878198860266));
#227040=CARTESIAN_POINT('Origin',(9.81091184134694E-17,1.90675232190402E-13,
2.65878198860263));
#227041=CARTESIAN_POINT('',(-58.7035958781039,6.18532049829379,2.65878198860266));
#227042=CARTESIAN_POINT('',(-58.6332801510296,6.17793001757249,2.65878198860266));
#227043=CARTESIAN_POINT('Origin',(3.17963581613999E-16,1.90698599198023E-13,
2.65878198860263));
#227044=CARTESIAN_POINT('Origin',(0.0199126722524868,0.189456421067567,
42.7590319886026));
#227045=CARTESIAN_POINT('',(-59.6550713551493,6.46154998175898,3.64303198860266));
#227046=CARTESIAN_POINT('',(-59.2266168947286,6.4165176033503,3.40423097483314));
#227047=CARTESIAN_POINT('Origin',(-59.6170497665662,6.45755375176737,3.20400220531682));
#227048=CARTESIAN_POINT('',(-58.8722700235037,6.37927424589668,2.83404198860265));
#227049=CARTESIAN_POINT('',(-59.2266168947286,6.4165176033503,3.40423097483314));
#227050=CARTESIAN_POINT('',(-62.293614112757,6.73887200051311,2.83404198860265));
#227051=CARTESIAN_POINT('',(-62.5519772640372,6.76602706194925,2.83404198860265));
#227052=CARTESIAN_POINT('',(-61.9392677288637,6.70162869542366,3.40423097483313));
#227053=CARTESIAN_POINT('',(-62.293614112757,6.73887200051311,2.83404198860265));
#227054=CARTESIAN_POINT('',(-61.5108137072212,6.65659636252362,3.64303198860267));
#227055=CARTESIAN_POINT('Origin',(-61.548835418265,6.66059260538636,3.20400259788154));
#227056=CARTESIAN_POINT('',(-61.1116329639869,6.61464077648907,3.64303198860266));
#227057=CARTESIAN_POINT('',(0.0199126722524923,0.18945642106784,3.64303198860263));
#227058=CARTESIAN_POINT('',(-60.9862851800405,6.60146619279925,3.42473028058489));
#227059=CARTESIAN_POINT('',(-61.1116329640613,6.61464077578101,3.64303198860266));
#227060=CARTESIAN_POINT('',(-60.6581326136904,6.56697596826257,3.23423028058485));
#227061=CARTESIAN_POINT('Origin',(-60.687398878641,6.57005146045385,3.56425722717401));
#227062=CARTESIAN_POINT('',(-60.5077528318944,6.55117041629748,3.23423028058485));
#227063=CARTESIAN_POINT('',(0.0199126722524923,0.189456421067843,3.23423028058482));
#227064=CARTESIAN_POINT('',(-60.1796001951996,6.51668018436725,3.42473028058484));
#227065=CARTESIAN_POINT('Origin',(-60.4784837816376,6.5480935988987,3.56425909740982));
#227066=CARTESIAN_POINT('',(-60.0542523588397,6.50350559588444,3.64303198860266));
#227067=CARTESIAN_POINT('',(-60.1796001951996,6.51668018436725,3.42473028058484));
#227068=CARTESIAN_POINT('',(0.0199126722524923,0.18945642106784,3.64303198860263));
#227069=CARTESIAN_POINT('Origin',(-0.0199126722524868,-0.189456421067745,
42.7590319886026));
#227070=CARTESIAN_POINT('',(-61.5506390517262,6.27768352038831,3.64303198860266));
#227071=CARTESIAN_POINT('',(-61.9790930734319,6.32271585268618,3.40423097483313));
#227072=CARTESIAN_POINT('Origin',(-61.5886607624842,6.28167976322102,3.20400259735761));
#227073=CARTESIAN_POINT('',(-62.3334394573092,6.35995915792815,2.83404198860265));
#227074=CARTESIAN_POINT('',(-61.9790930734319,6.32271585268619,3.40423097483313));
#227075=CARTESIAN_POINT('',(-58.9120953679531,6.00036140429027,2.83404198860265));
#227076=CARTESIAN_POINT('',(-0.0199126722524756,-0.189456421067467,2.83404198860262));
#227077=CARTESIAN_POINT('',(-59.2664422391598,6.03760476191725,3.40423097483313));
#227078=CARTESIAN_POINT('',(-58.912095367953,6.00036140429027,2.83404198860265));
#227079=CARTESIAN_POINT('',(-59.6948966996543,6.08263713962367,3.64303198860266));
#227080=CARTESIAN_POINT('Origin',(-59.6568751107688,6.07864090960027,3.20400220587169));
#227081=CARTESIAN_POINT('',(-60.0940777032672,6.12459275448651,3.64303198860266));
#227082=CARTESIAN_POINT('',(-60.1675309762115,6.13231300382155,3.64303198860266));
#227083=CARTESIAN_POINT('',(-60.2194255397045,6.13776734223194,3.42473028058484));
#227084=CARTESIAN_POINT('',(-60.0940777033447,6.12459275374913,3.64303198860266));
#227085=CARTESIAN_POINT('',(-60.5475781763994,6.17225757416217,3.23423028058485));
#227086=CARTESIAN_POINT('Origin',(-60.518311971389,6.16918208839134,3.56425743004515));
#227087=CARTESIAN_POINT('',(-60.6979579581954,6.18806312612726,3.23423028058485));
#227088=CARTESIAN_POINT('',(-60.6984837728333,6.18811839147267,3.23423028058485));
#227089=CARTESIAN_POINT('',(-61.0261105245454,6.22255335066394,3.42473028058488));
#227090=CARTESIAN_POINT('Origin',(-60.7272269341761,6.19113993560407,3.56425912918035));
#227091=CARTESIAN_POINT('',(-61.1514583085663,6.2357279336457,3.64303198860266));
#227092=CARTESIAN_POINT('',(-61.0261105245454,6.22255335066394,3.42473028058488));
#227093=CARTESIAN_POINT('',(-61.5511575797868,6.27773801988358,3.64303198860266));
#227094=CARTESIAN_POINT('Origin',(-58.2637721346185,0.190500000000191,2.65878198860262));
#227095=CARTESIAN_POINT('',(-58.2637721346185,-0.0152399999998093,2.65878198860261));
#227096=CARTESIAN_POINT('',(-58.9578504383728,0.0152400000001907,2.65878198860261));
#227097=CARTESIAN_POINT('Origin',(0.,0.190499999999911,42.7590319886026));
#227098=CARTESIAN_POINT('',(-60.0036905223731,0.190500000000184,3.64303198860262));
#227099=CARTESIAN_POINT('',(-59.5728760150042,0.190500000000185,3.4042309748331));
#227100=CARTESIAN_POINT('Origin',(-59.9654595002501,0.190500000000187,3.20400220531729));
#227101=CARTESIAN_POINT('',(-59.2165773020941,0.190499999468791,2.8340419886026));
#227102=CARTESIAN_POINT('',(-59.5728760150042,0.190500000000186,3.4042309748331));
#227103=CARTESIAN_POINT('',(-62.6567671111299,0.190500000000188,2.8340419886026));
#227104=CARTESIAN_POINT('',(-62.9165533988763,0.19050000000019,2.83404198860261));
#227105=CARTESIAN_POINT('',(-62.3004688883554,0.190500000605476,3.40423097483309));
#227106=CARTESIAN_POINT('',(-62.6567671111299,0.19050000000019,2.83404198860261));
#227107=CARTESIAN_POINT('',(-61.8696548221181,0.190500000000184,3.64303198860263));
#227108=CARTESIAN_POINT('Origin',(-61.9078859673764,0.190500000000187,3.20400259788294));
#227109=CARTESIAN_POINT('',(-61.4682752798284,0.190500000712183,3.64303198860261));
#227110=CARTESIAN_POINT('',(5.50819412990574E-15,0.190500000000184,3.64303198860262));
#227111=CARTESIAN_POINT('',(-61.3422370451705,0.190500000000185,3.42473028058485));
#227112=CARTESIAN_POINT('',(-61.4682752798284,0.190500000000184,3.64303198860261));
#227113=CARTESIAN_POINT('',(-61.0122769227456,0.190500000000187,3.23423028058481));
#227114=CARTESIAN_POINT('Origin',(-61.0417043405097,0.190499486622583,3.56425722716956));
#227115=CARTESIAN_POINT('',(-60.8610688070707,0.190500000000187,3.23423028058481));
#227116=CARTESIAN_POINT('',(5.56576032196012E-15,0.190500000000187,3.23423028058482));
#227117=CARTESIAN_POINT('',(-60.5311086139135,0.190500000000185,3.4247302805848));
#227118=CARTESIAN_POINT('Origin',(-60.8316384807435,0.190499486573693,3.56425909741752));
#227119=CARTESIAN_POINT('',(-60.4050703266282,0.190500000000184,3.64303198860261));
#227120=CARTESIAN_POINT('',(-60.5311086139135,0.190500000000185,3.4247302805848));
#227121=CARTESIAN_POINT('',(5.50819412990574E-15,0.190500000000184,3.64303198860263));
#227122=CARTESIAN_POINT('Origin',(0.,-0.190500000000089,42.7590319886026));
#227123=CARTESIAN_POINT('',(-61.8696548221181,-0.190499999999816,3.64303198860261));
#227124=CARTESIAN_POINT('',(-62.3004688883554,-0.190499999999815,3.40423097483308));
#227125=CARTESIAN_POINT('Origin',(-61.9078859670883,-0.190499999999813,
3.20400259735739));
#227126=CARTESIAN_POINT('',(-62.6567671111299,-0.190500000452382,2.8340419886026));
#227127=CARTESIAN_POINT('',(-62.3004688883554,-0.190499999999814,3.40423097483308));
#227128=CARTESIAN_POINT('',(-59.2165773020941,-0.190499999999811,2.83404198860261));
#227129=CARTESIAN_POINT('',(1.12442271988212E-14,-0.190499999999811,2.83404198860262));
#227130=CARTESIAN_POINT('',(-59.5728760150042,-0.190499999293226,3.4042309748331));
#227131=CARTESIAN_POINT('',(-59.2165773020941,-0.190499999999811,2.83404198860261));
#227132=CARTESIAN_POINT('',(-60.003690522373,-0.190499999999816,3.64303198860261));
#227133=CARTESIAN_POINT('Origin',(-59.9654594999467,-0.190499999999813,
3.20400220587133));
#227134=CARTESIAN_POINT('',(-60.4050703266283,-0.190499999257704,3.64303198860261));
#227135=CARTESIAN_POINT('',(-60.4789282006568,-0.190499999999816,3.64303198860261));
#227136=CARTESIAN_POINT('',(-60.5311086139135,-0.190499999999815,3.42473028058479));
#227137=CARTESIAN_POINT('',(-60.4050703266282,-0.190499999999816,3.64303198860261));
#227138=CARTESIAN_POINT('',(-60.8610688070707,-0.190499999999813,3.2342302805848));
#227139=CARTESIAN_POINT('Origin',(-60.8316414495926,-0.190499486502376,
3.56425743004576));
#227140=CARTESIAN_POINT('',(-61.0122769227456,-0.190499999999813,3.2342302805848));
#227141=CARTESIAN_POINT('',(-61.0128056337175,-0.190499999999813,3.2342302805848));
#227142=CARTESIAN_POINT('',(-61.3422370451705,-0.190499999999815,3.42473028058483));
#227143=CARTESIAN_POINT('Origin',(-61.0417071743823,-0.190499486687921,
3.56425912917566));
#227144=CARTESIAN_POINT('',(-61.4682752798284,-0.190499999999816,3.64303198860261));
#227145=CARTESIAN_POINT('',(-61.3422370451705,-0.190499999999815,3.42473028058483));
#227146=CARTESIAN_POINT('',(-61.8701762063762,-0.190499999999816,3.64303198860261));
#227147=CARTESIAN_POINT('Origin',(-57.9645097668784,-5.90076614434097,2.65878198860257));
#227148=CARTESIAN_POINT('',(-58.7035958781038,-6.1853204982942,2.65878198860257));
#227149=CARTESIAN_POINT('',(-62.500570298093,-6.58439859103053,2.65878198860257));
#227150=CARTESIAN_POINT('',(-57.9430040808457,-6.10537907909404,2.65878198860257));
#227151=CARTESIAN_POINT('',(-62.5037563256534,-6.5540855636597,2.65878198860257));
#227152=CARTESIAN_POINT('Origin',(9.81091184134687E-17,1.90705964780674E-13,
2.65878198860263));
#227153=CARTESIAN_POINT('',(-58.7067819056642,-6.15500747092338,2.65878198860257));
#227154=CARTESIAN_POINT('',(-58.6364661785899,-6.14761699020208,2.65878198860257));
#227155=CARTESIAN_POINT('Origin',(3.17963581613999E-16,1.90682597773053E-13,
2.65878198860263));
#227156=CARTESIAN_POINT('Origin',(-0.0199126722524893,0.189456421067567,
42.7590319886026));
#227157=CARTESIAN_POINT('',(-59.6948966996542,-6.08263713962411,3.64303198860258));
#227158=CARTESIAN_POINT('',(-59.2664422392335,-6.03760476121542,3.40423097483305));
#227159=CARTESIAN_POINT('Origin',(-59.656875111071,-6.07864090963248,3.20400220531675));
#227160=CARTESIAN_POINT('',(-58.9120953678974,-6.0003614048193,2.83404198860256));
#227161=CARTESIAN_POINT('',(-59.2664422392335,-6.03760476121542,3.40423097483305));
#227162=CARTESIAN_POINT('',(-62.3334394572618,-6.35995915837826,2.83404198860256));
#227163=CARTESIAN_POINT('',(-62.5918026085421,-6.3871142198144,2.83404198860256));
#227164=CARTESIAN_POINT('',(-61.9790930734951,-6.32271585208499,3.40423097483306));
#227165=CARTESIAN_POINT('',(-62.3334394572618,-6.35995915837826,2.83404198860256));
#227166=CARTESIAN_POINT('',(-61.5506390517261,-6.27768352038877,3.64303198860258));
#227167=CARTESIAN_POINT('Origin',(-61.5886607627703,-6.28167976325155,3.2040025978822));
#227168=CARTESIAN_POINT('',(-61.1514583086406,-6.23572793293815,3.64303198860257));
#227169=CARTESIAN_POINT('',(-0.0199126722524838,0.18945642106784,3.64303198860263));
#227170=CARTESIAN_POINT('',(-61.0261105245453,-6.22255335066439,3.4247302805848));
#227171=CARTESIAN_POINT('',(-61.1514583085662,-6.23572793364615,3.64303198860257));
#227172=CARTESIAN_POINT('',(-60.6979579581953,-6.1880631261277,3.23423028058476));
#227173=CARTESIAN_POINT('Origin',(-60.7272241158216,-6.19113963944962,3.56425722717282));
#227174=CARTESIAN_POINT('',(-60.5475781763993,-6.17225757416261,3.23423028058476));
#227175=CARTESIAN_POINT('',(-0.0199126722524838,0.189456421067843,3.23423028058482));
#227176=CARTESIAN_POINT('',(-60.2194255397045,-6.13776734223238,3.42473028058475));
#227177=CARTESIAN_POINT('Origin',(-60.5183090188083,-6.16918177799173,3.56425909741148));
#227178=CARTESIAN_POINT('',(-60.0940777033446,-6.12459275374958,3.64303198860258));
#227179=CARTESIAN_POINT('',(-60.2194255397045,-6.13776734223238,3.42473028058475));
#227180=CARTESIAN_POINT('',(-0.0199126722524838,0.18945642106784,3.64303198860263));
#227181=CARTESIAN_POINT('Origin',(0.0199126722524893,-0.189456421067745,
42.7590319886026));
#227182=CARTESIAN_POINT('',(-61.5108137072212,-6.65659636252408,3.64303198860257));
#227183=CARTESIAN_POINT('',(-61.9392677289269,-6.70162869482196,3.40423097483304));
#227184=CARTESIAN_POINT('Origin',(-61.548835417979,-6.66059260535676,3.20400259735693));
#227185=CARTESIAN_POINT('',(-62.2936141127096,-6.73887200096389,2.83404198860256));
#227186=CARTESIAN_POINT('',(-61.9392677289269,-6.70162869482196,3.40423097483304));
#227187=CARTESIAN_POINT('',(-58.872270023448,-6.37927424642599,2.83404198860256));
#227188=CARTESIAN_POINT('',(0.0199126722525006,-0.189456421067466,2.83404198860262));
#227189=CARTESIAN_POINT('',(-59.2266168948024,-6.41651760264851,3.40423097483305));
#227190=CARTESIAN_POINT('',(-58.872270023448,-6.379274246426,2.83404198860256));
#227191=CARTESIAN_POINT('',(-59.6550713551492,-6.46154998175942,3.64303198860257));
#227192=CARTESIAN_POINT('Origin',(-59.6170497662624,-6.45755375173588,3.20400220587399));
#227193=CARTESIAN_POINT('',(-60.0542523589172,-6.50350559514724,3.64303198860257));
#227194=CARTESIAN_POINT('',(-60.1277056317064,-6.51122584595731,3.64303198860257));
#227195=CARTESIAN_POINT('',(-60.1796001951995,-6.51668018436769,3.42473028058476));
#227196=CARTESIAN_POINT('',(-60.0542523588397,-6.50350559588489,3.64303198860257));
#227197=CARTESIAN_POINT('',(-60.5077528318943,-6.55117041629792,3.23423028058476));
#227198=CARTESIAN_POINT('Origin',(-60.4784867342349,-6.54809390915829,3.56425743004616));
#227199=CARTESIAN_POINT('',(-60.6581326136904,-6.56697596826301,3.23423028058476));
#227200=CARTESIAN_POINT('',(-60.6586584283283,-6.56703123360843,3.23423028058476));
#227201=CARTESIAN_POINT('',(-60.9862851800404,-6.60146619279971,3.42473028058479));
#227202=CARTESIAN_POINT('Origin',(-60.6874016969837,-6.57005175674012,3.56425912917731));
#227203=CARTESIAN_POINT('',(-61.1116329640612,-6.61464077578146,3.64303198860257));
#227204=CARTESIAN_POINT('',(-60.9862851800404,-6.60146619279971,3.42473028058479));
#227205=CARTESIAN_POINT('',(-61.5113322352818,-6.65665086201935,3.64303198860257));
#227206=CARTESIAN_POINT('Origin',(-57.0301761002789,-11.9273822599896,2.65878198860253));
#227207=CARTESIAN_POINT('',(-57.7354693911204,-12.2876333308473,2.65878198860253));
#227208=CARTESIAN_POINT('',(-61.4699285681953,-13.0814171332235,2.65878198860252));
#227209=CARTESIAN_POINT('',(-56.9874003490101,-12.1286263473646,2.65878198860253));
#227210=CARTESIAN_POINT('',(-61.4762657165315,-13.0516031943531,2.65878198860252));
#227211=CARTESIAN_POINT('Origin',(9.5702001384024E-17,1.90721162719465E-13,
2.65878198860263));
#227212=CARTESIAN_POINT('',(-57.7418065394565,-12.257819391977,2.65878198860253));
#227213=CARTESIAN_POINT('',(-57.6726485248849,-12.2431194021877,2.65878198860253));
#227214=CARTESIAN_POINT('Origin',(3.19216886402205E-16,1.90674684718048E-13,
2.65878198860263));
#227215=CARTESIAN_POINT('Origin',(-0.0396071771007845,0.1863371179397,42.7590319886026));
#227216=CARTESIAN_POINT('',(-58.7320730967337,-12.2891316338726,3.64303198860253));
#227217=CARTESIAN_POINT('',(-58.3106729199895,-12.1995602612167,3.40423097483302));
#227218=CARTESIAN_POINT('Origin',(-58.694677514171,-12.2811829574214,3.20400220531634));
#227219=CARTESIAN_POINT('',(-57.9621601887015,-12.1254815938993,2.83404198860251));
#227220=CARTESIAN_POINT('',(-58.3106729199895,-12.1995602612167,3.40423097483301));
#227221=CARTESIAN_POINT('',(-61.3271735965892,-12.8407372733101,2.83404198860251));
#227222=CARTESIAN_POINT('',(-61.5812829306519,-12.8947498796467,2.83404198860251));
#227223=CARTESIAN_POINT('',(-60.9786613449625,-12.7666587067857,3.404230974833));
#227224=CARTESIAN_POINT('',(-61.3271735965892,-12.8407372733101,2.83404198860251));
#227225=CARTESIAN_POINT('',(-60.5572615995842,-12.6770874264382,3.64303198860254));
#227226=CARTESIAN_POINT('Origin',(-60.594657302592,-12.6850361284908,3.20400259788303));
#227227=CARTESIAN_POINT('',(-60.1646531634579,-12.5936359264448,3.64303198860253));
#227228=CARTESIAN_POINT('',(-0.039607177100779,0.186337117939974,3.64303198860263));
#227229=CARTESIAN_POINT('',(-60.0413691664786,-12.5674311046657,3.42473028058475));
#227230=CARTESIAN_POINT('',(-60.1646531633099,-12.5936359271411,3.64303198860253));
#227231=CARTESIAN_POINT('',(-59.7186194643908,-12.4988285377098,3.23423028058472));
#227232=CARTESIAN_POINT('Origin',(-59.7474037157348,-12.5049473440525,3.56425722717003));
#227233=CARTESIAN_POINT('',(-59.570715608832,-12.4673906027145,3.23423028058472));
#227234=CARTESIAN_POINT('',(-0.0396071771007789,0.186337117939976,3.23423028058482));
#227235=CARTESIAN_POINT('',(-59.2479658375575,-12.3987880210526,3.42473028058471));
#227236=CARTESIAN_POINT('Origin',(-59.5419282989973,-12.4612721960131,3.56425909741388));
#227237=CARTESIAN_POINT('',(-59.1246817892489,-12.3725831876354,3.64303198860253));
#227238=CARTESIAN_POINT('',(-59.2479658375575,-12.3987880210526,3.42473028058471));
#227239=CARTESIAN_POINT('',(-0.039607177100779,0.186337117939974,3.64303198860263));
#227240=CARTESIAN_POINT('Origin',(0.0396071771007845,-0.186337117939879,
42.7590319886026));
#227241=CARTESIAN_POINT('',(-60.4780472453826,-13.0497616623178,3.64303198860253));
#227242=CARTESIAN_POINT('',(-60.8994469906351,-13.1393329432572,3.404230974833));
#227243=CARTESIAN_POINT('Origin',(-60.5154429481095,-13.0577103643106,3.20400259735919));
#227244=CARTESIAN_POINT('',(-61.2479592422936,-13.213411509632,2.83404198860251));
#227245=CARTESIAN_POINT('',(-60.8994469906351,-13.1393329432572,3.404230974833));
#227246=CARTESIAN_POINT('',(-57.8829458346104,-12.498155829259,2.83404198860252));
#227247=CARTESIAN_POINT('',(0.0396071771007956,-0.186337117939599,2.83404198860262));
#227248=CARTESIAN_POINT('',(-58.2314585659347,-12.5722344964057,3.404230974833));
#227249=CARTESIAN_POINT('',(-57.8829458346104,-12.498155829259,2.83404198860252));
#227250=CARTESIAN_POINT('',(-58.6528587425321,-12.6618058697522,3.64303198860253));
#227251=CARTESIAN_POINT('Origin',(-58.6154631596709,-12.6538571932375,3.20400220587388));
#227252=CARTESIAN_POINT('',(-59.0454674352016,-12.7452574227894,3.64303198860253));
#227253=CARTESIAN_POINT('',(-59.1177113373237,-12.7606133389845,3.64303198860253));
#227254=CARTESIAN_POINT('',(-59.168751483356,-12.7714622569322,3.42473028058471));
#227255=CARTESIAN_POINT('',(-59.0454674350473,-12.745257423515,3.64303198860253));
#227256=CARTESIAN_POINT('',(-59.4915012546304,-12.8400648385941,3.23423028058472));
#227257=CARTESIAN_POINT('Origin',(-59.4627170622801,-12.8339460446684,3.56425743004694));
#227258=CARTESIAN_POINT('',(-59.6394051101892,-12.8715027735894,3.23423028058472));
#227259=CARTESIAN_POINT('',(-59.6399222675579,-12.8716126987816,3.23423028058472));
#227260=CARTESIAN_POINT('',(-59.962154812277,-12.9401053405452,3.42473028058473));
#227261=CARTESIAN_POINT('Origin',(-59.6681923469391,-12.8776211648734,3.56425912917748));
#227262=CARTESIAN_POINT('',(-60.0854388091084,-12.9663101630206,3.64303198860253));
#227263=CARTESIAN_POINT('',(-59.962154812277,-12.9401053405452,3.42473028058473));
#227264=CARTESIAN_POINT('',(-60.4785572361438,-13.0498700642004,3.64303198860253));
#227265=CARTESIAN_POINT('Origin',(-55.4710078899932,-17.8233194796326,2.65878198860249));
#227266=CARTESIAN_POINT('',(-56.1347810195641,-18.2553202812751,2.65878198860248));
#227267=CARTESIAN_POINT('',(-59.765809437495,-19.4351129318423,2.65878198860248));
#227268=CARTESIAN_POINT('',(-55.4074307335705,-18.0189898472952,2.65878198860249));
#227269=CARTESIAN_POINT('',(-59.7752282754835,-19.4061247292256,2.65878198860248));
#227270=CARTESIAN_POINT('Origin',(9.1719453606903E-17,1.90736025790112E-13,
2.65878198860263));
#227271=CARTESIAN_POINT('',(-56.1441998575526,-18.2263320786585,2.65878198860248));
#227272=CARTESIAN_POINT('',(-56.0769572651637,-18.2044836359655,2.65878198860248));
#227273=CARTESIAN_POINT('Origin',(3.2129046493506E-16,1.9066694601761E-13,
2.65878198860263));
#227274=CARTESIAN_POINT('Origin',(-0.0588677374284288,0.181176266354137,
42.7590319886026));
#227275=CARTESIAN_POINT('',(-57.1257686104889,-18.3609838302743,3.64303198860249));
#227276=CARTESIAN_POINT('',(-56.7160396659413,-18.227854826074,3.40423097483297));
#227277=CARTESIAN_POINT('Origin',(-57.0894087477751,-18.3491697947262,3.2040022053157));
#227278=CARTESIAN_POINT('',(-56.3771794531163,-18.1177524692166,2.83404198860248));
#227279=CARTESIAN_POINT('',(-56.7160396659413,-18.227854826074,3.40423097483297));
#227280=CARTESIAN_POINT('',(-59.6489943884562,-19.1808295835785,2.83404198860248));
#227281=CARTESIAN_POINT('',(-59.8960658302616,-19.2611079613977,2.83404198860247));
#227282=CARTESIAN_POINT('',(-59.3101346421293,-19.0707273770996,3.40423097483296));
#227283=CARTESIAN_POINT('',(-59.6489943884562,-19.1808295835785,2.83404198860247));
#227284=CARTESIAN_POINT('',(-58.9004061169356,-18.9375985097924,3.64303198860249));
#227285=CARTESIAN_POINT('Origin',(-58.9367660967578,-18.9494125833913,3.20400259788049));
#227286=CARTESIAN_POINT('',(-58.5186714879534,-18.8135654093535,3.64303198860249));
#227287=CARTESIAN_POINT('',(-0.0588677374284233,0.18117626635441,3.64303198860263));
#227288=CARTESIAN_POINT('',(-58.3988020033597,-18.7746174535802,3.42473028058471));
#227289=CARTESIAN_POINT('',(-58.5186714877334,-18.8135654100305,3.64303198860249));
#227290=CARTESIAN_POINT('',(-58.0849912788099,-18.6726541682848,3.23423028058468));
#227291=CARTESIAN_POINT('Origin',(-58.1129782575883,-18.6817482287252,3.56425722717167));
#227292=CARTESIAN_POINT('',(-57.9411838150806,-18.6259282908539,3.23423028058468));
#227293=CARTESIAN_POINT('',(-0.0588677374284233,0.181176266354413,3.23423028058481));
#227294=CARTESIAN_POINT('',(-57.6273730232604,-18.523964983701,3.42473028058467));
#227295=CARTESIAN_POINT('Origin',(-57.9131937527887,-18.616834308165,3.56425909740917));
#227296=CARTESIAN_POINT('',(-57.5075034888351,-18.485017010988,3.64303198860249));
#227297=CARTESIAN_POINT('',(-57.6273730232604,-18.523964983701,3.42473028058467));
#227298=CARTESIAN_POINT('',(-0.0588677374284233,0.18117626635441,3.64303198860263));
#227299=CARTESIAN_POINT('Origin',(0.0588677374284288,-0.181176266354316,
42.7590319886026));
#227300=CARTESIAN_POINT('',(-58.7826706420787,-19.2999510425009,3.64303198860248));
#227301=CARTESIAN_POINT('',(-59.1923991670854,-19.433079910384,3.40423097483296));
#227302=CARTESIAN_POINT('Origin',(-58.8190306216284,-19.3117651160112,3.2040025973581));
#227303=CARTESIAN_POINT('',(-59.5312589134597,-19.5431821167168,2.83404198860247));
#227304=CARTESIAN_POINT('',(-59.1923991670854,-19.433079910384,3.40423097483296));
#227305=CARTESIAN_POINT('',(-56.2594439784237,-18.4801050014193,2.83404198860248));
#227306=CARTESIAN_POINT('',(0.0588677374284398,-0.181176266354035,2.83404198860262));
#227307=CARTESIAN_POINT('',(-56.5983041913028,-18.5902073581105,3.40423097483297));
#227308=CARTESIAN_POINT('',(-56.2594439784237,-18.4801050014193,2.83404198860248));
#227309=CARTESIAN_POINT('',(-57.0080331356321,-18.7233363629827,3.64303198860249));
#227310=CARTESIAN_POINT('Origin',(-56.9716732726287,-18.7115223273405,3.20400220587185));
#227311=CARTESIAN_POINT('',(-57.3897680142074,-18.8473695429911,3.64303198860249));
#227312=CARTESIAN_POINT('',(-57.4600110263529,-18.8701928819397,3.64303198860249));
#227313=CARTESIAN_POINT('',(-57.5096375484035,-18.8863175164095,3.42473028058467));
#227314=CARTESIAN_POINT('',(-57.3897680139783,-18.8473695436965,3.64303198860249));
#227315=CARTESIAN_POINT('',(-57.8234483402237,-18.9882808235623,3.23423028058468));
#227316=CARTESIAN_POINT('Origin',(-57.7954614188151,-18.9791867816366,3.56425743004336));
#227317=CARTESIAN_POINT('',(-57.967255803953,-19.0350067009933,3.23423028058468));
#227318=CARTESIAN_POINT('',(-57.9677586379681,-19.0351700816687,3.23423028058468));
#227319=CARTESIAN_POINT('',(-58.2810665285028,-19.1369699862886,3.4247302805847));
#227320=CARTESIAN_POINT('Origin',(-57.9952457951659,-19.0441006607077,3.56425912918371));
#227321=CARTESIAN_POINT('',(-58.4009360128765,-19.1759179427389,3.64303198860248));
#227322=CARTESIAN_POINT('',(-58.2810665285028,-19.1369699862886,3.4247302805847));
#227323=CARTESIAN_POINT('',(-58.7831665079749,-19.3001121590972,3.64303198860248));
#227324=CARTESIAN_POINT('Origin',(-53.30408770921,-23.5239806812874,2.65878198860245));
#227325=CARTESIAN_POINT('',(-53.9190682401993,-24.0229981225299,2.65878198860245));
#227326=CARTESIAN_POINT('',(-57.4068835917977,-25.575873566121,2.65878198860243));
#227327=CARTESIAN_POINT('',(-53.2204057122636,-23.7119335237428,2.65878198860245));
#227328=CARTESIAN_POINT('',(-57.4192809246787,-25.5480287005721,2.65878198860243));
#227329=CARTESIAN_POINT('Origin',(8.62051087089599E-17,1.90750391149705E-13,
2.65878198860263));
#227330=CARTESIAN_POINT('',(-53.9314655730802,-23.995153256981,2.65878198860245));
#227331=CARTESIAN_POINT('',(-53.8668751267876,-23.9663957374946,2.65878198860245));
#227332=CARTESIAN_POINT('Origin',(3.24161598652236E-16,1.9065946645856E-13,
2.65878198860263));
#227333=CARTESIAN_POINT('Origin',(-0.0774833305059413,0.174030409680826,
42.7590319886026));
#227334=CARTESIAN_POINT('',(-54.893582249012,-24.2316692455485,3.64303198860245));
#227335=CARTESIAN_POINT('',(-54.5000136127187,-24.056441199033,3.40423097483293));
#227336=CARTESIAN_POINT('Origin',(-54.858656472411,-24.2161192879491,3.20400220531633));
#227337=CARTESIAN_POINT('',(-54.1745185417597,-23.9115214570971,2.83404198860244));
#227338=CARTESIAN_POINT('',(-54.5000136127187,-24.056441199033,3.40423097483292));
#227339=CARTESIAN_POINT('',(-57.3172883154488,-25.3107727110825,2.83404198860243));
#227340=CARTESIAN_POINT('',(-57.5546148985774,-25.4164373136776,2.83404198860243));
#227341=CARTESIAN_POINT('',(-56.9917936927132,-25.1658531674645,3.40423097483292));
#227342=CARTESIAN_POINT('',(-57.3172883154488,-25.3107727110825,2.83404198860243));
#227343=CARTESIAN_POINT('',(-56.5982254591674,-24.9906253009261,3.64303198860245));
#227344=CARTESIAN_POINT('Origin',(-56.6331513482578,-25.0061753086091,3.204002597881));
#227345=CARTESIAN_POINT('',(-56.2315470018073,-24.827369532646,3.64303198860244));
#227346=CARTESIAN_POINT('',(-0.0774833305059357,0.174030409681099,3.64303198860263));
#227347=CARTESIAN_POINT('',(-56.116405344757,-24.776105164832,3.42473028058466));
#227348=CARTESIAN_POINT('',(-56.231547001518,-24.8273695332959,3.64303198860244));
#227349=CARTESIAN_POINT('',(-55.8149717737125,-24.641898292288,3.23423028058464));
#227350=CARTESIAN_POINT('Origin',(-55.8418548487312,-24.6538679703973,3.5642572271703));
#227351=CARTESIAN_POINT('',(-55.676836286479,-24.5803964109126,3.23423028058464));
#227352=CARTESIAN_POINT('',(-0.0774833305059357,0.174030409681102,3.23423028058481));
#227353=CARTESIAN_POINT('',(-55.3754026508173,-24.4461895095991,3.42473028058463));
#227354=CARTESIAN_POINT('Origin',(-55.6499501367103,-24.5684264878134,3.56425909740456));
#227355=CARTESIAN_POINT('',(-55.2602609459789,-24.3949251197297,3.64303198860245));
#227356=CARTESIAN_POINT('',(-55.3754026508173,-24.4461895095991,3.42473028058463));
#227357=CARTESIAN_POINT('',(-0.0774833305059357,0.174030409681099,3.64303198860263));
#227358=CARTESIAN_POINT('Origin',(0.0774833305059413,-0.174030409681004,
42.7590319886026));
#227359=CARTESIAN_POINT('',(-56.4432587981555,-25.338686120288,3.64303198860244));
#227360=CARTESIAN_POINT('',(-56.8368270314552,-25.5139139873792,3.40423097483292));
#227361=CARTESIAN_POINT('Origin',(-56.4781846869838,-25.3542361278542,3.20400259735806));
#227362=CARTESIAN_POINT('',(-57.1623216542527,-25.658833530858,2.83404198860243));
#227363=CARTESIAN_POINT('',(-56.8368270314552,-25.5139139873792,3.40423097483292));
#227364=CARTESIAN_POINT('',(-54.0195518809639,-24.2595822759735,2.83404198860244));
#227365=CARTESIAN_POINT('',(0.077483330505952,-0.174030409680723,2.83404198860262));
#227366=CARTESIAN_POINT('',(-54.3450469519943,-24.4045020177489,3.40423097483293));
#227367=CARTESIAN_POINT('',(-54.0195518809639,-24.2595822759735,2.83404198860244));
#227368=CARTESIAN_POINT('',(-54.7386155880002,-24.5797300649104,3.64303198860245));
#227369=CARTESIAN_POINT('Origin',(-54.7036898111213,-24.5641801071872,3.20400220587176));
#227370=CARTESIAN_POINT('',(-55.1052942852685,-24.7429859384143,3.64303198860244));
#227371=CARTESIAN_POINT('',(-55.1727668102969,-24.7730266428387,3.64303198860244));
#227372=CARTESIAN_POINT('',(-55.2204359898054,-24.794250328961,3.42473028058462));
#227373=CARTESIAN_POINT('',(-55.105294284967,-24.7429859390916,3.64303198860244));
#227374=CARTESIAN_POINT('',(-55.5218696254671,-24.9284572302744,3.23423028058463));
#227375=CARTESIAN_POINT('Origin',(-55.4949866055708,-24.9164875765759,3.56425743004543));
#227376=CARTESIAN_POINT('',(-55.6600051127006,-24.9899591116498,3.23423028058463));
#227377=CARTESIAN_POINT('',(-55.6604881142074,-24.9901741577757,3.23423028058463));
#227378=CARTESIAN_POINT('',(-55.9614386837451,-25.1241659841938,3.42473028058465));
#227379=CARTESIAN_POINT('Origin',(-55.6868911941847,-25.0019290044722,3.56425912917205));
#227380=CARTESIAN_POINT('',(-56.0765803405061,-25.1754303526578,3.64303198860244));
#227381=CARTESIAN_POINT('',(-55.9614386837451,-25.1241659841938,3.42473028058465));
#227382=CARTESIAN_POINT('',(-56.4437351063762,-25.3388981863709,3.64303198860244));
#227383=CARTESIAN_POINT('Origin',(-50.5531567888873,-28.9669082278885,2.65878198860241));
#227384=CARTESIAN_POINT('',(-51.1126068659045,-29.5274749692187,2.65878198860241));
#227385=CARTESIAN_POINT('',(-54.4189959163061,-31.4364195775137,2.65878198860239));
#227386=CARTESIAN_POINT('',(-50.4502867888873,-29.1450842944631,2.65878198860241));
#227387=CARTESIAN_POINT('',(-54.434235916306,-31.4100231232064,2.65878198860239));
#227388=CARTESIAN_POINT('Origin',(7.92193830068374E-17,1.90764101408356E-13,
2.65878198860263));
#227389=CARTESIAN_POINT('',(-51.1278468659044,-29.5010785149114,2.65878198860241));
#227390=CARTESIAN_POINT('',(-51.0666162321541,-29.465726992033,2.65878198860241));
#227391=CARTESIAN_POINT('Origin',(3.27798830811898E-16,1.90652327988513E-13,
2.65878198860263));
#227392=CARTESIAN_POINT('Origin',(-0.0952500000000014,0.164977839420845,
42.7590319886026));
#227393=CARTESIAN_POINT('',(-52.0599703131944,-29.8368674217658,3.64303198860241));
#227394=CARTESIAN_POINT('',(-51.686874005494,-29.6214601680814,3.40423097483289));
#227395=CARTESIAN_POINT('Origin',(-52.0268612768234,-29.8177519107044,3.20400220531693));
#227396=CARTESIAN_POINT('',(-51.3783102685124,-29.4433108120867,2.8340419886024));
#227397=CARTESIAN_POINT('',(-51.686874005494,-29.6214601680814,3.40423097483289));
#227398=CARTESIAN_POINT('',(-54.3576020372436,-31.1634057161443,2.83404198860239));
#227399=CARTESIAN_POINT('',(-54.5825835619868,-31.2932988600175,2.83404198860239));
#227400=CARTESIAN_POINT('',(-54.0490387253004,-30.9852566042326,3.40423097483288));
#227401=CARTESIAN_POINT('',(-54.3576020372436,-31.1634057161443,2.83404198860239));
#227402=CARTESIAN_POINT('',(-53.6759427993284,-30.7698495716384,3.64303198860241));
#227403=CARTESIAN_POINT('Origin',(-53.709051942338,-30.7889651442676,3.20400259788283));
#227404=CARTESIAN_POINT('',(-53.3283379195021,-30.5691597998771,3.64303198860241));
#227405=CARTESIAN_POINT('',(-0.0952499999999959,0.164977839421119,3.64303198860263));
#227406=CARTESIAN_POINT('',(-53.2191856060843,-30.5061406831646,3.42473028058463));
#227407=CARTESIAN_POINT('',(-53.3283379191462,-30.5691598004935,3.64303198860241));
#227408=CARTESIAN_POINT('',(-52.9334317578285,-30.3411606219521,3.2342302805846));
#227409=CARTESIAN_POINT('Origin',(-52.9589163924907,-30.3558747754319,3.56425722717026));
#227410=CARTESIAN_POINT('',(-52.8024816883957,-30.2655565641147,3.2342302805846));
#227411=CARTESIAN_POINT('',(-0.0952499999999958,0.164977839421121,3.23423028058481));
#227412=CARTESIAN_POINT('',(-52.5167277788839,-30.100576467536,3.42473028058458));
#227413=CARTESIAN_POINT('Origin',(-52.7769940214367,-30.2508418455888,3.56425909740749));
#227414=CARTESIAN_POINT('',(-52.4075754202454,-30.0375573238934,3.64303198860241));
#227415=CARTESIAN_POINT('',(-52.5167277788839,-30.100576467536,3.42473028058458));
#227416=CARTESIAN_POINT('',(-0.0952499999999959,0.164977839421119,3.64303198860263));
#227417=CARTESIAN_POINT('Origin',(0.0952500000000014,-0.164977839421024,
42.7590319886026));
#227418=CARTESIAN_POINT('',(-53.4854427993284,-31.0998052504802,3.6430319886024));
#227419=CARTESIAN_POINT('',(-53.8585387249976,-31.3152122835989,3.40423097483288));
#227420=CARTESIAN_POINT('Origin',(-53.5185519420882,-31.1189208229652,3.20400259735687));
#227421=CARTESIAN_POINT('',(-54.1671020370175,-31.4933613953778,2.83404198860239));
#227422=CARTESIAN_POINT('',(-53.8585387249976,-31.3152122835989,3.40423097483288));
#227423=CARTESIAN_POINT('',(-51.1878102687783,-29.7732664904682,2.8340419886024));
#227424=CARTESIAN_POINT('',(0.0952500000000119,-0.164977839420743,2.83404198860262));
#227425=CARTESIAN_POINT('',(-51.4963740058472,-29.9514158463116,3.40423097483288));
#227426=CARTESIAN_POINT('',(-51.1878102687783,-29.7732664904682,2.8340419886024));
#227427=CARTESIAN_POINT('',(-51.8694703131944,-30.1668231006077,3.64303198860241));
#227428=CARTESIAN_POINT('Origin',(-51.83636127656,-30.1477075893942,3.20400220587218));
#227429=CARTESIAN_POINT('',(-52.2170754206163,-30.3675130020929,3.64303198860241));
#227430=CARTESIAN_POINT('',(-52.2810382154237,-30.4044419397496,3.64303198860241));
#227431=CARTESIAN_POINT('',(-52.3262277788839,-30.4305321463779,3.42473028058459));
#227432=CARTESIAN_POINT('',(-52.2170754202454,-30.3675130027353,3.64303198860241));
#227433=CARTESIAN_POINT('',(-52.6119816883956,-30.5955122429565,3.2342302805846));
#227434=CARTESIAN_POINT('Origin',(-52.5864971059999,-30.5807981195144,3.56425743004055));
#227435=CARTESIAN_POINT('',(-52.7429317578285,-30.671116300794,3.23423028058459));
#227436=CARTESIAN_POINT('',(-52.7433896349615,-30.6713806562799,3.23423028058459));
#227437=CARTESIAN_POINT('',(-53.0286856060843,-30.8360963620065,3.42473028058461));
#227438=CARTESIAN_POINT('Origin',(-52.7684193600396,-30.68583098207,3.56425912917953));
#227439=CARTESIAN_POINT('',(-53.1378379191462,-30.8991154793354,3.6430319886024));
#227440=CARTESIAN_POINT('',(-53.0286856060843,-30.8360963620065,3.42473028058461));
#227441=CARTESIAN_POINT('',(-53.4858943313411,-31.1000659426093,3.6430319886024));
#227442=CARTESIAN_POINT('Origin',(-47.2483549038573,-34.0924682662297,2.65878198860237));
#227443=CARTESIAN_POINT('',(-47.7461450747862,-34.7084426211234,2.65878198860237));
#227444=CARTESIAN_POINT('',(-50.8348823336483,-36.9525415975214,2.65878198860236));
#227445=CARTESIAN_POINT('',(-47.1274239660506,-34.2589154226524,2.65878198860237));
#227446=CARTESIAN_POINT('',(-50.8527980281382,-36.9278827595329,2.65878198860236));
#227447=CARTESIAN_POINT('Origin',(7.08388135731921E-17,1.90777006353604E-13,
2.65878198860263));
#227448=CARTESIAN_POINT('',(-47.764060769276,-34.6837837831348,2.65878198860237));
#227449=CARTESIAN_POINT('',(-47.7068608037047,-34.6422255755468,2.65878198860237));
#227450=CARTESIAN_POINT('Origin',(3.32162311137369E-16,1.90645608818039E-13,
2.65878198860263));
#227451=CARTESIAN_POINT('Origin',(-0.111973090561717,0.154117737428337,
42.7590319886026));
#227452=CARTESIAN_POINT('',(-48.6559784483762,-35.1151666347443,3.64303198860237));
#227453=CARTESIAN_POINT('',(-48.3074421904915,-34.8619402208392,3.40423097483286));
#227454=CARTESIAN_POINT('Origin',(-48.6250489017663,-35.0926950037603,3.20400220531748));
#227455=CARTESIAN_POINT('',(-48.0191904763611,-34.6525130924096,2.83404198860237));
#227456=CARTESIAN_POINT('',(-48.3074421904915,-34.8619402208392,3.40423097483286));
#227457=CARTESIAN_POINT('',(-50.8023624960588,-36.674605926818,2.83404198860235));
#227458=CARTESIAN_POINT('',(-51.0125340177512,-36.8273044755032,2.83404198860235));
#227459=CARTESIAN_POINT('',(-50.514111179124,-36.4651790855641,3.40423097483284));
#227460=CARTESIAN_POINT('',(-50.8023624960588,-36.674605926818,2.83404198860235));
#227461=CARTESIAN_POINT('',(-50.1655752777668,-36.2119529314387,3.64303198860237));
#227462=CARTESIAN_POINT('Origin',(-50.1965049239947,-36.2344246347994,3.20400259788159));
#227463=CARTESIAN_POINT('',(-49.8408524072781,-35.9760279553335,3.64303198860237));
#227464=CARTESIAN_POINT('',(-0.111973090561712,0.15411773742861,3.64303198860263));
#227465=CARTESIAN_POINT('',(-49.7388853330808,-35.9019445403521,3.4247302805846));
#227466=CARTESIAN_POINT('',(-49.8408524068601,-35.9760279559089,3.64303198860236));
#227467=CARTESIAN_POINT('',(-49.471941986573,-35.707998846546,3.23423028058456));
#227468=CARTESIAN_POINT('Origin',(-49.495748965888,-35.7252962640513,3.5642572271713));
#227469=CARTESIAN_POINT('',(-49.3496120513046,-35.6191209461254,3.23423028058456));
#227470=CARTESIAN_POINT('',(-0.111973090561712,0.154117737428613,3.23423028058481));
#227471=CARTESIAN_POINT('',(-49.0826686475732,-35.425175210744,3.42473028058456));
#227472=CARTESIAN_POINT('Origin',(-49.3258021153687,-35.601822649709,3.56425909741072));
#227473=CARTESIAN_POINT('',(-48.9807015312175,-35.3510917642536,3.64303198860237));
#227474=CARTESIAN_POINT('',(-49.0826686475732,-35.425175210744,3.42473028058456));
#227475=CARTESIAN_POINT('',(-0.111973090561712,0.15411773742861,3.64303198860263));
#227476=CARTESIAN_POINT('Origin',(0.111973090561717,-0.154117737428516,
42.7590319886026));
#227477=CARTESIAN_POINT('',(-49.9416290966434,-36.5201884062956,3.64303198860236));
#227478=CARTESIAN_POINT('',(-50.2901649976452,-36.7734145609101,3.40423097483284));
#227479=CARTESIAN_POINT('Origin',(-49.9725587426394,-36.5426601094878,3.20400259735863));
#227480=CARTESIAN_POINT('',(-50.5784163146694,-36.982841402041,2.83404198860235));
#227481=CARTESIAN_POINT('',(-50.2901649976452,-36.7734145609101,3.40423097483284));
#227482=CARTESIAN_POINT('',(-47.7952442955499,-34.9607485668368,2.83404198860236));
#227483=CARTESIAN_POINT('',(0.111973090561728,-0.154117737428234,2.83404198860262));
#227484=CARTESIAN_POINT('',(-48.0834960097833,-35.1701756951246,3.40423097483285));
#227485=CARTESIAN_POINT('',(-47.7952442955499,-34.9607485668368,2.83404198860237));
#227486=CARTESIAN_POINT('',(-48.4320322672528,-35.4234021096012,3.64303198860237));
#227487=CARTESIAN_POINT('Origin',(-48.4011027203962,-35.400930478438,3.20400220587424));
#227488=CARTESIAN_POINT('',(-48.75675535053,-35.6593272385105,3.64303198860237));
#227489=CARTESIAN_POINT('',(-48.8165076253516,-35.7027398082301,3.64303198860237));
#227490=CARTESIAN_POINT('',(-48.8587224664497,-35.7334106856009,3.42473028058455));
#227491=CARTESIAN_POINT('',(-48.7567553500941,-35.6593272391104,3.64303198860237));
#227492=CARTESIAN_POINT('',(-49.1256658701812,-35.9273564209823,3.23423028058456));
#227493=CARTESIAN_POINT('Origin',(-49.1018589397083,-35.9100590388147,3.56425743004586));
#227494=CARTESIAN_POINT('',(-49.2479958054496,-36.0162343214029,3.23423028058455));
#227495=CARTESIAN_POINT('',(-49.248423541611,-36.0165450899149,3.23423028058455));
#227496=CARTESIAN_POINT('',(-49.5149391519574,-36.2101800152089,3.42473028058458));
#227497=CARTESIAN_POINT('Origin',(-49.2718056808885,-36.0335325740075,3.56425912917758));
#227498=CARTESIAN_POINT('',(-49.6169062257367,-36.2842634307658,3.64303198860236));
#227499=CARTESIAN_POINT('',(-49.5149391519574,-36.2101800152089,3.42473028058458));
#227500=CARTESIAN_POINT('',(-49.9420509053688,-36.5204948682733,3.64303198860236));
#227501=CARTESIAN_POINT('Origin',(-43.4258901551468,-38.8445040879383,2.65878198860234));
#227502=CARTESIAN_POINT('',(-43.8565665267053,-39.5091373124624,2.65878198860234));
#227503=CARTESIAN_POINT('',(-46.6938111422601,-42.0638038389702,2.65878198860232));
#227504=CARTESIAN_POINT('',(-43.2882232241945,-38.9973987043321,2.65878198860234));
#227505=CARTESIAN_POINT('',(-46.7142062431419,-42.0411527846897,2.65878198860232));
#227506=CARTESIAN_POINT('Origin',(6.11552196804844E-17,1.90788964596167E-13,
2.65878198860263));
#227507=CARTESIAN_POINT('',(-43.8769616275871,-39.4864862581819,2.65878198860234));
#227508=CARTESIAN_POINT('',(-43.8244190249875,-39.4391766863032,2.65878198860234));
#227509=CARTESIAN_POINT('Origin',(3.37204232425086E-16,1.90639382563777E-13,
2.65878198860263));
#227510=CARTESIAN_POINT('Origin',(-0.127469380511364,0.141569089253353,
42.7590319886026));
#227511=CARTESIAN_POINT('',(-44.7189015017595,-40.0087367337515,3.64303198860233));
#227512=CARTESIAN_POINT('',(-44.3987439298677,-39.7204655612076,3.40423097483282));
#227513=CARTESIAN_POINT('Origin',(-44.6904903154948,-39.9831551867354,3.20400220532103));
#227514=CARTESIAN_POINT('',(-44.1339623846888,-39.4820551877881,2.83404198860233));
#227515=CARTESIAN_POINT('',(-44.3987439298677,-39.7204655612076,3.40423097483282));
#227516=CARTESIAN_POINT('',(-46.6905216402894,-41.7839914803029,2.83404198860232));
#227517=CARTESIAN_POINT('',(-46.8835804757581,-41.9578224365464,2.83404198860231));
#227518=CARTESIAN_POINT('',(-46.4257404601132,-41.545581434003,3.40423097483281));
#227519=CARTESIAN_POINT('',(-46.6905216402894,-41.7839914803029,2.83404198860232));
#227520=CARTESIAN_POINT('',(-46.1055832156406,-41.2573105570839,3.64303198860234));
#227521=CARTESIAN_POINT('Origin',(-46.1339944934111,-41.2828921864921,3.20400259788175));
#227522=CARTESIAN_POINT('',(-45.8073000862121,-40.9887352200423,3.64303198860232));
#227523=CARTESIAN_POINT('',(-0.127469380511358,0.141569089253626,3.64303198860262));
#227524=CARTESIAN_POINT('',(-45.7136354238372,-40.9043991801905,3.42473028058455));
#227525=CARTESIAN_POINT('',(-45.8073000857355,-40.9887352205716,3.64303198860232));
#227526=CARTESIAN_POINT('',(-45.4684272662432,-40.6836127633981,3.23423028058452));
#227527=CARTESIAN_POINT('Origin',(-45.4902957559651,-40.703303930804,3.56425722716923));
#227528=CARTESIAN_POINT('',(-45.3560577375092,-40.5824347852702,3.23423028058452));
#227529=CARTESIAN_POINT('',(-0.127469380511358,0.141569089253629,3.23423028058481));
#227530=CARTESIAN_POINT('',(-45.1108495273509,-40.3616483211486,3.42473028058452));
#227531=CARTESIAN_POINT('Origin',(-45.3341863992363,-40.5627424347186,3.56425909741396));
#227532=CARTESIAN_POINT('',(-45.0171848263429,-40.277312245553,3.64303198860233));
#227533=CARTESIAN_POINT('',(-45.1108495273509,-40.3616483211486,3.42473028058452));
#227534=CARTESIAN_POINT('',(-0.127469380511358,0.141569089253626,3.64303198860262));
#227535=CARTESIAN_POINT('Origin',(0.127469380511364,-0.141569089253532,
42.7590319886026));
#227536=CARTESIAN_POINT('',(-45.8506444546178,-41.5404487355908,3.64303198860233));
#227537=CARTESIAN_POINT('',(-46.170801698685,-41.8287196129601,3.4042309748328));
#227538=CARTESIAN_POINT('Origin',(-45.8790557321755,-41.5660303648073,3.2040025973597));
#227539=CARTESIAN_POINT('',(-46.4355828789644,-42.0671296591455,2.83404198860231));
#227540=CARTESIAN_POINT('',(-46.170801698685,-41.8287196129601,3.4042309748328));
#227541=CARTESIAN_POINT('',(-43.8790236240217,-39.7651933659001,2.83404198860233));
#227542=CARTESIAN_POINT('',(0.127469380511373,-0.141569089253249,2.83404198860262));
#227543=CARTESIAN_POINT('',(-44.1438051693175,-40.0036037391897,3.40423097483282));
#227544=CARTESIAN_POINT('',(-43.8790236240217,-39.7651933659001,2.83404198860233));
#227545=CARTESIAN_POINT('',(-44.4639627407368,-40.2918749122584,3.64303198860234));
#227546=CARTESIAN_POINT('Origin',(-44.435551554248,-40.2662933650406,3.20400220587063));
#227547=CARTESIAN_POINT('',(-44.7622460658166,-40.5604504235085,3.64303198860233));
#227548=CARTESIAN_POINT('',(-44.8171331622253,-40.609870988093,3.64303198860233));
#227549=CARTESIAN_POINT('',(-44.8559107663282,-40.6447864996555,3.42473028058451));
#227550=CARTESIAN_POINT('',(-44.7622460653202,-40.5604504240599,3.64303198860233));
#227551=CARTESIAN_POINT('',(-45.1011189764865,-40.8655729637771,3.23423028058452));
#227552=CARTESIAN_POINT('Origin',(-45.0792505316448,-40.8458818366201,3.56425743004167));
#227553=CARTESIAN_POINT('',(-45.2134885052205,-40.966750941905,3.23423028058452));
#227554=CARTESIAN_POINT('',(-45.2138814140435,-40.9671047185982,3.23423028058452));
#227555=CARTESIAN_POINT('',(-45.4586966628145,-41.1875373586974,3.42473028058454));
#227556=CARTESIAN_POINT('Origin',(-45.2353597879101,-40.9864432425634,3.56425912917358));
#227557=CARTESIAN_POINT('',(-45.5523613247128,-41.2718733990784,3.64303198860233));
#227558=CARTESIAN_POINT('',(-45.4586966628145,-41.1875373586974,3.42473028058454));
#227559=CARTESIAN_POINT('',(-45.8510319186313,-41.5407976097556,3.64303198860233));
#227560=CARTESIAN_POINT('Origin',(-39.1276422664447,-43.1709513941245,2.65878198860231));
#227561=CARTESIAN_POINT('',(-39.4864862581813,-43.8769616275876,2.65878198860231));
#227562=CARTESIAN_POINT('',(-42.0411527846891,-46.7142062431424,2.65878198860229));
#227563=CARTESIAN_POINT('',(-38.974747650051,-43.3086183250768,2.65878198860231));
#227564=CARTESIAN_POINT('',(-42.0638038389696,-46.6938111422606,2.65878198860229));
#227565=CARTESIAN_POINT('Origin',(5.02746968098233E-17,1.90799845119038E-13,
2.65878198860263));
#227566=CARTESIAN_POINT('',(-39.5091373124618,-43.8565665267058,2.65878198860231));
#227567=CARTESIAN_POINT('',(-39.4618277405832,-43.8040239241061,2.65878198860231));
#227568=CARTESIAN_POINT('Origin',(3.4286935433033E-16,1.90633717441872E-13,
2.65878198860263));
#227569=CARTESIAN_POINT('Origin',(-0.141569089253445,0.127469380511272,
42.7590319886026));
#227570=CARTESIAN_POINT('',(-40.2918749122578,-44.4639627407373,3.64303198860231));
#227571=CARTESIAN_POINT('',(-40.0036037397139,-44.1438051688455,3.40423097483279));
#227572=CARTESIAN_POINT('Origin',(-40.2662933652432,-44.4355515544741,3.20400220531654));
#227573=CARTESIAN_POINT('',(-39.7651933655044,-43.8790236243779,2.8340419886023));
#227574=CARTESIAN_POINT('',(-40.0036037397139,-44.1438051688455,3.40423097483279));
#227575=CARTESIAN_POINT('',(-42.0671296588092,-46.4355828792672,2.83404198860229));
#227576=CARTESIAN_POINT('',(-42.2409606150526,-46.6286417147359,2.83404198860228));
#227577=CARTESIAN_POINT('',(-41.8287196134086,-46.1708016982812,3.40423097483278));
#227578=CARTESIAN_POINT('',(-42.0671296588092,-46.4355828792672,2.83404198860229));
#227579=CARTESIAN_POINT('',(-41.5404487355902,-45.8506444546184,3.64303198860231));
#227580=CARTESIAN_POINT('Origin',(-41.5660303649981,-45.8790557323884,3.20400259788069));
#227581=CARTESIAN_POINT('',(-41.2718733996069,-45.552361324237,3.6430319886023));
#227582=CARTESIAN_POINT('',(-0.141569089253439,0.127469380511545,3.64303198860263));
#227583=CARTESIAN_POINT('',(-41.1875373586968,-45.458696662815,3.42473028058453));
#227584=CARTESIAN_POINT('',(-41.2718733990778,-45.5523613247133,3.6430319886023));
#227585=CARTESIAN_POINT('',(-40.9667509419044,-45.213488505221,3.23423028058449));
#227586=CARTESIAN_POINT('Origin',(-40.9864413462824,-45.2353576819761,3.5642572271696));
#227587=CARTESIAN_POINT('',(-40.8655729637765,-45.1011189764871,3.23423028058449));
#227588=CARTESIAN_POINT('',(-0.141569089253439,0.127469380511548,3.23423028058481));
#227589=CARTESIAN_POINT('',(-40.6447864996549,-44.8559107663287,3.42473028058448));
#227590=CARTESIAN_POINT('Origin',(-40.8458798501217,-45.0792483253099,3.5642590974058));
#227591=CARTESIAN_POINT('',(-40.5604504240593,-44.7622460653207,3.64303198860231));
#227592=CARTESIAN_POINT('',(-40.6447864996549,-44.8559107663287,3.42473028058448));
#227593=CARTESIAN_POINT('',(-0.141569089253439,0.127469380511545,3.64303198860263));
#227594=CARTESIAN_POINT('Origin',(0.141569089253445,-0.127469380511451,
42.7590319886026));
#227595=CARTESIAN_POINT('',(-41.2573105570833,-46.1055832156411,3.6430319886023));
#227596=CARTESIAN_POINT('',(-41.5455814344526,-46.4257404597083,3.40423097483277));
#227597=CARTESIAN_POINT('Origin',(-41.282892186299,-46.1339944931978,3.20400259735698));
#227598=CARTESIAN_POINT('',(-41.7839914799663,-46.6905216405925,2.83404198860228));
#227599=CARTESIAN_POINT('',(-41.5455814344526,-46.4257404597083,3.40423097483277));
#227600=CARTESIAN_POINT('',(-39.4820551873926,-44.1339623850449,2.8340419886023));
#227601=CARTESIAN_POINT('',(0.141569089253454,-0.127469380511168,2.83404198860262));
#227602=CARTESIAN_POINT('',(-39.7204655617324,-44.3987439293951,3.40423097483279));
#227603=CARTESIAN_POINT('',(-39.4820551873926,-44.1339623850449,2.8340419886023));
#227604=CARTESIAN_POINT('',(-40.0087367337509,-44.71890150176,3.64303198860231));
#227605=CARTESIAN_POINT('Origin',(-39.9831551865321,-44.6904903152701,3.20400220587386));
#227606=CARTESIAN_POINT('',(-40.2773122461035,-45.0171848258472,3.6430319886023));
#227607=CARTESIAN_POINT('',(-40.3267328095855,-45.0720719232485,3.6430319886023));
#227608=CARTESIAN_POINT('',(-40.361648321148,-45.1108495273514,3.42473028058448));
#227609=CARTESIAN_POINT('',(-40.2773122455524,-45.0171848263434,3.6430319886023));
#227610=CARTESIAN_POINT('',(-40.5824347852696,-45.3560577375098,3.23423028058449));
#227611=CARTESIAN_POINT('Origin',(-40.5627444213187,-45.3341886054745,3.56425743004244));
#227612=CARTESIAN_POINT('',(-40.6836127633975,-45.4684272662438,3.23423028058449));
#227613=CARTESIAN_POINT('',(-40.6839665400907,-45.4688201750667,3.23423028058449));
#227614=CARTESIAN_POINT('',(-40.9043991801899,-45.7136354238377,3.4247302805845));
#227615=CARTESIAN_POINT('Origin',(-40.7033058269853,-45.4902978619871,3.56425912917549));
#227616=CARTESIAN_POINT('',(-40.988735220571,-45.807300085736,3.6430319886023));
#227617=CARTESIAN_POINT('',(-40.9043991801899,-45.7136354238377,3.4247302805845));
#227618=CARTESIAN_POINT('',(-41.2576594312481,-46.1059706796546,3.6430319886023));
#227619=CARTESIAN_POINT('Origin',(-34.4007037410859,-47.0244087227343,2.65878198860228));
#227620=CARTESIAN_POINT('',(-34.6837837831342,-47.7640607692764,2.65878198860228));
#227621=CARTESIAN_POINT('',(-36.9278827595322,-50.8527980281386,2.65878198860226));
#227622=CARTESIAN_POINT('',(-34.2342565846632,-47.1453396605409,2.65878198860228));
#227623=CARTESIAN_POINT('',(-36.9525415975208,-50.8348823336487,2.65878198860226));
#227624=CARTESIAN_POINT('Origin',(3.83164542466798E-17,1.90809528712931E-13,
2.65878198860263));
#227625=CARTESIAN_POINT('',(-34.7084426211227,-47.7461450747866,2.65878198860228));
#227626=CARTESIAN_POINT('',(-34.6668844135347,-47.6889451092152,2.65878198860228));
#227627=CARTESIAN_POINT('Origin',(3.49095608592005E-16,1.90628675520584E-13,
2.65878198860263));
#227628=CARTESIAN_POINT('Origin',(-0.154117737428428,0.111973090561625,
42.7590319886026));
#227629=CARTESIAN_POINT('',(-35.4234021096005,-48.4320322672532,3.64303198860228));
#227630=CARTESIAN_POINT('',(-35.1701756956954,-48.0834960093685,3.40423097483276));
#227631=CARTESIAN_POINT('Origin',(-35.400930478616,-48.4011027206425,3.20400220531938));
#227632=CARTESIAN_POINT('',(-34.9607485664058,-47.795244295863,2.83404198860228));
#227633=CARTESIAN_POINT('',(-35.1701756956954,-48.0834960093685,3.40423097483276));
#227634=CARTESIAN_POINT('',(-36.9828414016742,-50.5784163149358,2.83404198860225));
#227635=CARTESIAN_POINT('',(-37.1355399503593,-50.7885878366282,2.83404198860226));
#227636=CARTESIAN_POINT('',(-36.7734145613991,-50.2901649972899,3.40423097483274));
#227637=CARTESIAN_POINT('',(-36.9828414016742,-50.5784163149358,2.83404198860226));
#227638=CARTESIAN_POINT('',(-36.5201884062949,-49.9416290966439,3.64303198860227));
#227639=CARTESIAN_POINT('Origin',(-36.5426601096556,-49.9725587428718,3.20400259788141));
#227640=CARTESIAN_POINT('',(-36.2842634313412,-49.6169062253185,3.64303198860227));
#227641=CARTESIAN_POINT('',(-0.154117737428423,0.111973090561899,3.64303198860263));
#227642=CARTESIAN_POINT('',(-36.2101800152082,-49.5149391519578,3.42473028058449));
#227643=CARTESIAN_POINT('',(-36.2842634307651,-49.6169062257371,3.64303198860227));
#227644=CARTESIAN_POINT('',(-36.0162343214022,-49.24799580545,3.23423028058446));
#227645=CARTESIAN_POINT('Origin',(-36.0335309082464,-49.2718033882784,3.56425722716715));
#227646=CARTESIAN_POINT('',(-35.9273564209816,-49.1256658701816,3.23423028058446));
#227647=CARTESIAN_POINT('',(-0.154117737428423,0.111973090561901,3.23423028058481));
#227648=CARTESIAN_POINT('',(-35.7334106856002,-48.8587224664502,3.42473028058446));
#227649=CARTESIAN_POINT('Origin',(-35.9100572938239,-49.1018565378152,3.56425909741215));
#227650=CARTESIAN_POINT('',(-35.6593272391098,-48.7567553500946,3.64303198860228));
#227651=CARTESIAN_POINT('',(-35.7334106856002,-48.8587224664502,3.42473028058446));
#227652=CARTESIAN_POINT('',(-0.154117737428423,0.111973090561899,3.64303198860263));
#227653=CARTESIAN_POINT('Origin',(0.154117737428428,-0.111973090561804,
42.7590319886026));
#227654=CARTESIAN_POINT('',(-36.211952931438,-50.1655752777673,3.64303198860227));
#227655=CARTESIAN_POINT('',(-36.4651790860525,-50.5141111787691,3.40423097483274));
#227656=CARTESIAN_POINT('Origin',(-36.2344246346306,-50.1965049237636,3.20400259735939));
#227657=CARTESIAN_POINT('',(-36.6746059264515,-50.8023624963251,2.83404198860226));
#227658=CARTESIAN_POINT('',(-36.4651790860525,-50.5141111787691,3.40423097483274));
#227659=CARTESIAN_POINT('',(-34.6525130919793,-48.0191904766737,2.83404198860227));
#227660=CARTESIAN_POINT('',(0.154117737428437,-0.111973090561521,2.83404198860262));
#227661=CARTESIAN_POINT('',(-34.8619402214099,-48.3074421900768,3.40423097483277));
#227662=CARTESIAN_POINT('',(-34.6525130919793,-48.0191904766737,2.83404198860227));
#227663=CARTESIAN_POINT('',(-35.1151666347437,-48.6559784483766,3.64303198860228));
#227664=CARTESIAN_POINT('Origin',(-35.0926950035815,-48.6250489015215,3.20400220587083));
#227665=CARTESIAN_POINT('',(-35.3510917648527,-48.9807015307822,3.64303198860227));
#227666=CARTESIAN_POINT('',(-35.3945043333726,-49.0404538064755,3.64303198860227));
#227667=CARTESIAN_POINT('',(-35.4251752107434,-49.0826686475736,3.42473028058445));
#227668=CARTESIAN_POINT('',(-35.3510917642529,-48.980701531218,3.64303198860227));
#227669=CARTESIAN_POINT('',(-35.6191209461248,-49.3496120513051,3.23423028058446));
#227670=CARTESIAN_POINT('Origin',(-35.6018243948111,-49.3258045171764,3.56425743003822));
#227671=CARTESIAN_POINT('',(-35.7079988465454,-49.4719419865734,3.23423028058446));
#227672=CARTESIAN_POINT('',(-35.7083096150574,-49.4723697227349,3.23423028058446));
#227673=CARTESIAN_POINT('',(-35.9019445403514,-49.7388853330813,3.42473028058448));
#227674=CARTESIAN_POINT('Origin',(-35.7252979297054,-49.4957512585773,3.56425912917917));
#227675=CARTESIAN_POINT('',(-35.9760279559083,-49.8408524068605,3.64303198860227));
#227676=CARTESIAN_POINT('',(-35.9019445403514,-49.7388853330813,3.42473028058448));
#227677=CARTESIAN_POINT('',(-36.2122593934157,-50.1659970864927,3.64303198860227));
#227678=CARTESIAN_POINT('Origin',(-29.2968639067297,-50.3626567888876,2.65878198860226));
#227679=CARTESIAN_POINT('',(-29.5010785149107,-51.1278468659048,2.65878198860225));
#227680=CARTESIAN_POINT('',(-31.4100231232056,-54.4342359163064,2.65878198860223));
#227681=CARTESIAN_POINT('',(-29.1186878401551,-50.4655267888876,2.65878198860226));
#227682=CARTESIAN_POINT('',(-31.436419577513,-54.4189959163064,2.65878198860223));
#227683=CARTESIAN_POINT('Origin',(2.54115089989943E-17,1.90817909282364E-13,
2.65878198860263));
#227684=CARTESIAN_POINT('',(-29.527474969218,-51.1126068659048,2.65878198860225));
#227685=CARTESIAN_POINT('',(-29.4921234463396,-51.0513762321545,2.65878198860225));
#227686=CARTESIAN_POINT('Origin',(3.55814779065493E-16,1.90624312040259E-13,
2.65878198860263));
#227687=CARTESIAN_POINT('Origin',(-0.164977839420936,0.0952499999999092,
42.7590319886026));
#227688=CARTESIAN_POINT('',(-30.166823100607,-51.8694703131947,3.64303198860225));
#227689=CARTESIAN_POINT('',(-29.9514158469225,-51.4963740054944,3.40423097483274));
#227690=CARTESIAN_POINT('Origin',(-30.1477075895448,-51.8363612768224,3.20400220532004));
#227691=CARTESIAN_POINT('',(-29.7732664900078,-51.187810269044,2.83404198860225));
#227692=CARTESIAN_POINT('',(-29.9514158469225,-51.4963740054944,3.40423097483274));
#227693=CARTESIAN_POINT('',(-31.4933613949854,-54.1671020372439,2.83404198860223));
#227694=CARTESIAN_POINT('',(-31.6232545388586,-54.3920835619872,2.83404198860223));
#227695=CARTESIAN_POINT('',(-31.3152122841225,-53.8585387246953,3.40423097483272));
#227696=CARTESIAN_POINT('',(-31.4933613949854,-54.1671020372439,2.83404198860223));
#227697=CARTESIAN_POINT('',(-31.0998052504795,-53.4854427993288,3.64303198860225));
#227698=CARTESIAN_POINT('Origin',(-31.1189208231087,-53.5185519423383,3.20400259788257));
#227699=CARTESIAN_POINT('',(-30.899115479951,-53.1378379187907,3.64303198860225));
#227700=CARTESIAN_POINT('',(-0.164977839420931,0.0952500000001823,3.64303198860263));
#227701=CARTESIAN_POINT('',(-30.8360963620057,-53.0286856060847,3.42473028058447));
#227702=CARTESIAN_POINT('',(-30.8991154793346,-53.1378379191465,3.64303198860225));
#227703=CARTESIAN_POINT('',(-30.6711163007932,-52.7429317578288,3.23423028058444));
#227704=CARTESIAN_POINT('Origin',(-30.6858295650779,-52.7684169058702,3.56425722716709));
#227705=CARTESIAN_POINT('',(-30.5955122429558,-52.611981688396,3.23423028058444));
#227706=CARTESIAN_POINT('',(-0.164977839420931,0.0952500000001852,3.23423028058481));
#227707=CARTESIAN_POINT('',(-30.4305321463772,-52.3262277788842,3.42473028058445));
#227708=CARTESIAN_POINT('Origin',(-30.5807966351508,-52.5864945348665,3.56425909741311));
#227709=CARTESIAN_POINT('',(-30.3675130027346,-52.2170754202458,3.64303198860225));
#227710=CARTESIAN_POINT('',(-30.4305321463772,-52.3262277788842,3.42473028058445));
#227711=CARTESIAN_POINT('',(-0.164977839420931,0.0952500000001823,3.64303198860263));
#227712=CARTESIAN_POINT('Origin',(0.164977839420936,-0.0952500000000878,
42.7590319886026));
#227713=CARTESIAN_POINT('',(-30.7698495716376,-53.6759427993287,3.64303198860224));
#227714=CARTESIAN_POINT('',(-30.9852566047563,-54.049038724998,3.40423097483272));
#227715=CARTESIAN_POINT('Origin',(-30.7889651441224,-53.7090519420883,3.20400259735578));
#227716=CARTESIAN_POINT('',(-31.1634057157514,-54.3576020374703,2.83404198860223));
#227717=CARTESIAN_POINT('',(-30.9852566047563,-54.049038724998,3.40423097483272));
#227718=CARTESIAN_POINT('',(-29.4433108116256,-51.3783102687786,2.83404198860225));
#227719=CARTESIAN_POINT('',(0.164977839420945,-0.0952499999998041,2.83404198860262));
#227720=CARTESIAN_POINT('',(-29.6214601686928,-51.686874005141,3.40423097483274));
#227721=CARTESIAN_POINT('',(-29.4433108116256,-51.3783102687786,2.83404198860225));
#227722=CARTESIAN_POINT('',(-29.8368674217651,-52.0599703131947,3.64303198860225));
#227723=CARTESIAN_POINT('Origin',(-29.8177519105515,-52.0268612765601,3.20400220587275));
#227724=CARTESIAN_POINT('',(-30.0375573245347,-52.4075754198751,3.64303198860225));
#227725=CARTESIAN_POINT('',(-30.074486260907,-52.471538215424,3.64303198860225));
#227726=CARTESIAN_POINT('',(-30.1005764675353,-52.5167277788842,3.42473028058443));
#227727=CARTESIAN_POINT('',(-30.0375573238927,-52.4075754202458,3.64303198860225));
#227728=CARTESIAN_POINT('',(-30.2655565641139,-52.802481688396,3.23423028058444));
#227729=CARTESIAN_POINT('Origin',(-30.2508433300764,-52.7769965925045,3.56425743004421));
#227730=CARTESIAN_POINT('',(-30.3411606219514,-52.9334317578288,3.23423028058444));
#227731=CARTESIAN_POINT('',(-30.3414249774373,-52.9338896349618,3.23423028058444));
#227732=CARTESIAN_POINT('',(-30.5061406831638,-53.2191856060847,3.42473028058446));
#227733=CARTESIAN_POINT('Origin',(-30.3558761923104,-52.9589188467293,3.56425912917629));
#227734=CARTESIAN_POINT('',(-30.5691598004928,-53.3283379191465,3.64303198860225));
#227735=CARTESIAN_POINT('',(-30.5061406831638,-53.2191856060847,3.42473028058446));
#227736=CARTESIAN_POINT('',(-30.7701102637667,-53.6763943313414,3.64303198860224));
#227737=CARTESIAN_POINT('Origin',(-23.8720415006485,-53.1491210481984,2.65878198860224));
#227738=CARTESIAN_POINT('',(-23.9951532569802,-53.9314655730804,2.65878198860223));
#227739=CARTESIAN_POINT('',(-25.5480287005713,-57.4192809246789,2.65878198860221));
#227740=CARTESIAN_POINT('',(-23.6840886581931,-53.2328030451448,2.65878198860224));
#227741=CARTESIAN_POINT('',(-25.5758735661203,-57.406883591798,2.65878198860221));
#227742=CARTESIAN_POINT('Origin',(1.17012503474357E-17,1.90824895008066E-13,
2.65878198860263));
#227743=CARTESIAN_POINT('',(-24.0229981225292,-53.9190682401995,2.65878198860223));
#227744=CARTESIAN_POINT('',(-23.9942406030429,-53.8544777939069,2.65878198860223));
#227745=CARTESIAN_POINT('Origin',(3.6295324911301E-16,1.90620674808099E-13,
2.65878198860263));
#227746=CARTESIAN_POINT('Origin',(-0.174030409680916,0.077483330505849,
42.7590319886026));
#227747=CARTESIAN_POINT('',(-24.5797300649096,-54.7386155880004,3.64303198860224));
#227748=CARTESIAN_POINT('',(-24.4045020183941,-54.345046951707,3.40423097483272));
#227749=CARTESIAN_POINT('Origin',(-24.5641801073095,-54.7036898113979,3.20400220531965));
#227750=CARTESIAN_POINT('',(-24.259582275487,-54.0195518811804,2.83404198860223));
#227751=CARTESIAN_POINT('',(-24.4045020183941,-54.345046951707,3.40423097483272));
#227752=CARTESIAN_POINT('',(-25.6588335304436,-57.1623216544372,2.83404198860221));
#227753=CARTESIAN_POINT('',(-25.7644981330387,-57.3996482375657,2.83404198860221));
#227754=CARTESIAN_POINT('',(-25.5139139879318,-56.8368270312091,3.40423097483269));
#227755=CARTESIAN_POINT('',(-25.6588335304436,-57.1623216544371,2.83404198860221));
#227756=CARTESIAN_POINT('',(-25.3386861202872,-56.4432587981557,3.64303198860223));
#227757=CARTESIAN_POINT('Origin',(-25.3542361279701,-56.478184687246,3.20400259788053));
#227758=CARTESIAN_POINT('',(-25.1754303533071,-56.0765803402169,3.64303198860223));
#227759=CARTESIAN_POINT('',(-0.174030409680911,0.0774833305061222,3.64303198860263));
#227760=CARTESIAN_POINT('',(-25.1241659841931,-55.9614386837453,3.42473028058445));
#227761=CARTESIAN_POINT('',(-25.175430352657,-56.0765803405063,3.64303198860223));
#227762=CARTESIAN_POINT('',(-24.9899591116491,-55.6600051127008,3.23423028058442));
#227763=CARTESIAN_POINT('Origin',(-25.0019278517711,-55.6868886053389,3.56425722716884));
#227764=CARTESIAN_POINT('',(-24.9284572302736,-55.5218696254673,3.23423028058442));
#227765=CARTESIAN_POINT('',(-0.174030409680911,0.077483330506125,3.23423028058481));
#227766=CARTESIAN_POINT('',(-24.7942503289602,-55.2204359898057,3.42473028058442));
#227767=CARTESIAN_POINT('Origin',(-24.9164863690992,-55.4949838933612,3.56425909741228));
#227768=CARTESIAN_POINT('',(-24.7429859390908,-55.1052942849672,3.64303198860223));
#227769=CARTESIAN_POINT('',(-24.7942503289602,-55.2204359898057,3.42473028058442));
#227770=CARTESIAN_POINT('',(-0.174030409680911,0.0774833305061222,3.64303198860262));
#227771=CARTESIAN_POINT('Origin',(0.174030409680916,-0.0774833305060277,
42.7590319886026));
#227772=CARTESIAN_POINT('',(-24.9906253009254,-56.5982254591676,3.64303198860222));
#227773=CARTESIAN_POINT('',(-25.1658531680166,-56.9917936924673,3.40423097483269));
#227774=CARTESIAN_POINT('Origin',(-25.0061753084918,-56.6331513479964,3.20400259735859));
#227775=CARTESIAN_POINT('',(-25.3107727106681,-57.3172883156332,2.83404198860221));
#227776=CARTESIAN_POINT('',(-25.1658531680166,-56.9917936924673,3.40423097483269));
#227777=CARTESIAN_POINT('',(-23.911521456611,-54.174518541976,2.83404198860223));
#227778=CARTESIAN_POINT('',(0.174030409680924,-0.0774833305057438,2.83404198860262));
#227779=CARTESIAN_POINT('',(-24.0564411996779,-54.5000136124314,3.40423097483272));
#227780=CARTESIAN_POINT('',(-23.911521456611,-54.174518541976,2.83404198860223));
#227781=CARTESIAN_POINT('',(-24.2316692455478,-54.8935822490123,3.64303198860224));
#227782=CARTESIAN_POINT('Origin',(-24.2161192878243,-54.8586564721327,3.20400220587297));
#227783=CARTESIAN_POINT('',(-24.3949251204065,-55.2602609456775,3.64303198860224));
#227784=CARTESIAN_POINT('',(-24.4249658234761,-55.327733471309,3.64303198860224));
#227785=CARTESIAN_POINT('',(-24.4461895095984,-55.3754026508175,3.42473028058442));
#227786=CARTESIAN_POINT('',(-24.394925119729,-55.2602609459791,3.64303198860224));
#227787=CARTESIAN_POINT('',(-24.5803964109118,-55.6768362864792,3.23423028058442));
#227788=CARTESIAN_POINT('Origin',(-24.5684276954193,-55.6499528488651,3.56425743004285));
#227789=CARTESIAN_POINT('',(-24.6418982922872,-55.8149717737127,3.23423028058442));
#227790=CARTESIAN_POINT('',(-24.6421133384131,-55.8154547752195,3.23423028058442));
#227791=CARTESIAN_POINT('',(-24.7761051648312,-56.1164053447572,3.42473028058444));
#227792=CARTESIAN_POINT('Origin',(-24.6538691229758,-55.8418574376282,3.5642591291781));
#227793=CARTESIAN_POINT('',(-24.8273695332952,-56.2315470015182,3.64303198860223));
#227794=CARTESIAN_POINT('',(-24.7761051648312,-56.1164053447572,3.42473028058444));
#227795=CARTESIAN_POINT('',(-24.9908373670083,-56.5987017673883,3.64303198860222));
#227796=CARTESIAN_POINT('Origin',(-18.1856720123403,-55.3532724151365,2.65878198860223));
#227797=CARTESIAN_POINT('',(-18.2263320786577,-56.1441998575527,2.65878198860222));
#227798=CARTESIAN_POINT('',(-19.4061247292248,-59.7752282754837,2.6587819886022));
#227799=CARTESIAN_POINT('',(-17.9900016446778,-55.4168495715592,2.65878198860223));
#227800=CARTESIAN_POINT('',(-19.4351129318415,-59.7658094374951,2.6587819886022));
#227801=CARTESIAN_POINT('Origin',(-2.66410924515479E-18,1.90830409352964E-13,
2.65878198860263));
#227802=CARTESIAN_POINT('',(-18.2553202812744,-56.1347810195642,2.65878198860222));
#227803=CARTESIAN_POINT('',(-18.2334718385814,-56.0675384271753,2.65878198860222));
#227804=CARTESIAN_POINT('Origin',(3.7043280816289E-16,1.90617803674382E-13,
2.65878198860263));
#227805=CARTESIAN_POINT('Origin',(-0.181176266354227,0.0588677374283364,
42.7590319886026));
#227806=CARTESIAN_POINT('',(-18.7233363629819,-57.0080331356322,3.64303198860223));
#227807=CARTESIAN_POINT('',(-18.5902073587817,-56.5983041910846,3.4042309748327));
#227808=CARTESIAN_POINT('Origin',(-18.7115223274335,-56.9716732729172,3.2040022053177));
#227809=CARTESIAN_POINT('',(-18.4801050009129,-56.2594439785881,2.83404198860222));
#227810=CARTESIAN_POINT('',(-18.5902073587817,-56.5983041910846,3.4042309748327));
#227811=CARTESIAN_POINT('',(-19.5431821162861,-59.5312589135995,2.83404198860219));
#227812=CARTESIAN_POINT('',(-19.6234604941053,-59.7783303554049,2.83404198860219));
#227813=CARTESIAN_POINT('',(-19.4330799109586,-59.1923991668985,3.40423097483268));
#227814=CARTESIAN_POINT('',(-19.5431821162861,-59.5312589135995,2.83404198860219));
#227815=CARTESIAN_POINT('',(-19.2999510425001,-58.7826706420788,3.64303198860222));
#227816=CARTESIAN_POINT('Origin',(-19.3117651160993,-58.8190306219023,3.20400259788282));
#227817=CARTESIAN_POINT('',(-19.1759179434148,-58.4009360126568,3.64303198860221));
#227818=CARTESIAN_POINT('',(-0.181176266354222,0.0588677374286096,3.64303198860262));
#227819=CARTESIAN_POINT('',(-19.1369699862878,-58.281066528503,3.42473028058445));
#227820=CARTESIAN_POINT('',(-19.1759179427381,-58.4009360128767,3.64303198860221));
#227821=CARTESIAN_POINT('',(-19.0350067009925,-57.9672558039532,3.23423028058441));
#227822=CARTESIAN_POINT('Origin',(-19.0440997849304,-57.9952431000158,3.56425722717295));
#227823=CARTESIAN_POINT('',(-18.9882808235615,-57.8234483402239,3.23423028058441));
#227824=CARTESIAN_POINT('',(-0.181176266354222,0.0588677374286124,3.23423028058481));
#227825=CARTESIAN_POINT('',(-18.8863175164087,-57.5096375484037,3.4247302805844));
#227826=CARTESIAN_POINT('Origin',(-18.9791858642775,-57.7954585952473,3.56425909740992));
#227827=CARTESIAN_POINT('',(-18.8473695436957,-57.3897680139784,3.64303198860222));
#227828=CARTESIAN_POINT('',(-18.8863175164087,-57.5096375484037,3.4247302805844));
#227829=CARTESIAN_POINT('',(-0.181176266354222,0.0588677374286096,3.64303198860263));
#227830=CARTESIAN_POINT('Origin',(0.181176266354227,-0.0588677374285151,
42.7590319886026));
#227831=CARTESIAN_POINT('',(-18.9375985097916,-58.9004061169357,3.64303198860221));
#227832=CARTESIAN_POINT('',(-19.0707273776747,-59.3101346419424,3.40423097483268));
#227833=CARTESIAN_POINT('Origin',(-18.9494125833018,-58.9367660964848,3.20400259735645));
#227834=CARTESIAN_POINT('',(-19.1808295831472,-59.6489943885963,2.83404198860219));
#227835=CARTESIAN_POINT('',(-19.0707273776747,-59.3101346419424,3.40423097483268));
#227836=CARTESIAN_POINT('',(-18.1177524687101,-56.3771794532807,2.83404198860222));
#227837=CARTESIAN_POINT('',(0.181176266354235,-0.0588677374282309,2.83404198860262));
#227838=CARTESIAN_POINT('',(-18.2278548267447,-56.7160396657232,3.40423097483271));
#227839=CARTESIAN_POINT('',(-18.1177524687101,-56.3771794532807,2.83404198860222));
#227840=CARTESIAN_POINT('',(-18.3609838302735,-57.1257686104891,3.64303198860223));
#227841=CARTESIAN_POINT('Origin',(-18.3491697946312,-57.0894087474853,3.20400220587216));
#227842=CARTESIAN_POINT('',(-18.4850170116921,-57.5075034886062,3.64303198860222));
#227843=CARTESIAN_POINT('',(-18.5078403492304,-57.5777465012099,3.64303198860222));
#227844=CARTESIAN_POINT('',(-18.5239649837002,-57.6273730232605,3.4247302805844));
#227845=CARTESIAN_POINT('',(-18.4850170109872,-57.5075034888353,3.64303198860222));
#227846=CARTESIAN_POINT('',(-18.6259282908531,-57.9411838150807,3.23423028058441));
#227847=CARTESIAN_POINT('Origin',(-18.6168352256576,-57.9131965763137,3.56425743004373));
#227848=CARTESIAN_POINT('',(-18.672654168284,-58.08499127881,3.23423028058441));
#227849=CARTESIAN_POINT('',(-18.6728175489595,-58.0854941128251,3.23423028058441));
#227850=CARTESIAN_POINT('',(-18.7746174535794,-58.3988020033598,3.42473028058443));
#227851=CARTESIAN_POINT('Origin',(-18.6817491043762,-58.1129809527804,3.56425912918054));
#227852=CARTESIAN_POINT('',(-18.8135654100297,-58.5186714877335,3.64303198860222));
#227853=CARTESIAN_POINT('',(-18.7746174535794,-58.3988020033598,3.42473028058443));
#227854=CARTESIAN_POINT('',(-18.937759626388,-58.9009019828319,3.64303198860221));
#227855=CARTESIAN_POINT('Origin',(-12.3000564958684,-56.9509617460774,2.65878198860222));
#227856=CARTESIAN_POINT('',(-12.2578193919762,-57.7418065394565,2.65878198860222));
#227857=CARTESIAN_POINT('',(-13.0516031943522,-61.4762657165315,2.65878198860219));
#227858=CARTESIAN_POINT('',(-12.0988124084934,-56.9937374973463,2.65878198860222));
#227859=CARTESIAN_POINT('',(-13.0814171332226,-61.4699285681954,2.65878198860219));
#227860=CARTESIAN_POINT('Origin',(-1.75271798929367E-17,1.90834391900741E-13,
2.65878198860263));
#227861=CARTESIAN_POINT('',(-12.2876333308465,-57.7354693911204,2.65878198860222));
#227862=CARTESIAN_POINT('',(-12.2729333410573,-57.6663113765488,2.65878198860222));
#227863=CARTESIAN_POINT('Origin',(3.78171508600986E-16,1.90615730095849E-13,
2.65878198860263));
#227864=CARTESIAN_POINT('Origin',(-0.18633711793979,0.0396071771006919,
42.7590319886026));
#227865=CARTESIAN_POINT('',(-12.6618058697513,-58.6528587425322,3.64303198860222));
#227866=CARTESIAN_POINT('',(-12.5722344970954,-58.231458565788,3.40423097483269));
#227867=CARTESIAN_POINT('Origin',(-12.6538571933001,-58.6154631599695,3.20400220531593));
#227868=CARTESIAN_POINT('',(-12.4981558287385,-57.8829458347209,2.83404198860221));
#227869=CARTESIAN_POINT('',(-12.5722344970954,-58.231458565788,3.40423097483269));
#227870=CARTESIAN_POINT('',(-13.2134115091888,-61.2479592423877,2.83404198860219));
#227871=CARTESIAN_POINT('',(-13.2674241155254,-61.5020685764504,2.83404198860219));
#227872=CARTESIAN_POINT('',(-13.1393329438489,-60.8994469905092,3.40423097483268));
#227873=CARTESIAN_POINT('',(-13.2134115091888,-61.2479592423877,2.83404198860219));
#227874=CARTESIAN_POINT('',(-13.0497616623169,-60.4780472453827,3.64303198860221));
#227875=CARTESIAN_POINT('Origin',(-13.0577103643692,-60.5154429483892,3.20400259788019));
#227876=CARTESIAN_POINT('',(-12.966310163716,-60.0854388089605,3.64303198860221));
#227877=CARTESIAN_POINT('',(-0.186337117939785,0.0396071771009651,3.64303198860263));
#227878=CARTESIAN_POINT('',(-12.9401053405444,-59.9621548122771,3.42473028058443));
#227879=CARTESIAN_POINT('',(-12.9663101630198,-60.0854388091084,3.64303198860221));
#227880=CARTESIAN_POINT('',(-12.8715027735886,-59.6394051101893,3.2342302805844));
#227881=CARTESIAN_POINT('Origin',(-12.8776205756134,-59.6681895750089,3.5642572271675));
#227882=CARTESIAN_POINT('',(-12.8400648385932,-59.4915012546304,3.2342302805844));
#227883=CARTESIAN_POINT('',(-0.186337117939785,0.0396071771009679,3.23423028058481));
#227884=CARTESIAN_POINT('',(-12.7714622569314,-59.168751483356,3.42473028058439));
#227885=CARTESIAN_POINT('Origin',(-12.8339454274777,-59.4627141582888,3.56425909741086));
#227886=CARTESIAN_POINT('',(-12.7452574235141,-59.0454674350474,3.64303198860221));
#227887=CARTESIAN_POINT('',(-12.7714622569314,-59.168751483356,3.42473028058439));
#227888=CARTESIAN_POINT('',(-0.186337117939785,0.0396071771009651,3.64303198860263));
#227889=CARTESIAN_POINT('Origin',(0.18633711793979,-0.0396071771008706,
42.7590319886026));
#227890=CARTESIAN_POINT('',(-12.6770874264373,-60.5572615995843,3.6430319886022));
#227891=CARTESIAN_POINT('',(-12.7666587073768,-60.9786613448367,3.40423097483268));
#227892=CARTESIAN_POINT('Origin',(-12.6850361284299,-60.5946573023098,3.20400259735624));
#227893=CARTESIAN_POINT('',(-12.8407372728666,-61.3271735966833,2.83404198860219));
#227894=CARTESIAN_POINT('',(-12.7666587073768,-60.9786613448367,3.40423097483267));
#227895=CARTESIAN_POINT('',(-12.1254815933786,-57.962160188812,2.83404198860222));
#227896=CARTESIAN_POINT('',(0.186337117939797,-0.0396071771005863,2.83404198860263));
#227897=CARTESIAN_POINT('',(-12.1995602619071,-58.3106729198426,3.4042309748327));
#227898=CARTESIAN_POINT('',(-12.1254815933786,-57.962160188812,2.83404198860222));
#227899=CARTESIAN_POINT('',(-12.2891316338718,-58.7320730967337,3.64303198860222));
#227900=CARTESIAN_POINT('Origin',(-12.2811829573572,-58.6946775138729,3.20400220587262));
#227901=CARTESIAN_POINT('',(-12.37258318836,-59.1246817890948,3.64303198860221));
#227902=CARTESIAN_POINT('',(-12.387939103104,-59.1969256915253,3.64303198860221));
#227903=CARTESIAN_POINT('',(-12.3987880210518,-59.2479658375576,3.42473028058439));
#227904=CARTESIAN_POINT('',(-12.3725831876346,-59.124681789249,3.64303198860221));
#227905=CARTESIAN_POINT('',(-12.4673906027137,-59.570715608832,3.2342302805844));
#227906=CARTESIAN_POINT('Origin',(-12.4612728133404,-59.5419312029567,3.5642574300453));
#227907=CARTESIAN_POINT('',(-12.498828537709,-59.7186194643909,3.2342302805844));
#227908=CARTESIAN_POINT('',(-12.4989384629011,-59.7191366217596,3.2342302805844));
#227909=CARTESIAN_POINT('',(-12.5674311046648,-60.0413691664787,3.42473028058441));
#227910=CARTESIAN_POINT('Origin',(-12.5049479331826,-59.7474064876939,3.56425912917678));
#227911=CARTESIAN_POINT('',(-12.5936359271402,-60.16465316331,3.64303198860221));
#227912=CARTESIAN_POINT('',(-12.5674311046648,-60.0413691664787,3.42473028058441));
#227913=CARTESIAN_POINT('',(-12.67719582832,-60.5577715903454,3.6430319886022));
#227914=CARTESIAN_POINT('Origin',(-6.27967898647548,-57.9246844223734,2.65878198860221));
#227915=CARTESIAN_POINT('',(-6.15500747092256,-58.7067819056642,2.65878198860221));
#227916=CARTESIAN_POINT('',(-6.55408556365883,-62.5037563256533,2.65878198860218));
#227917=CARTESIAN_POINT('',(-6.07506605172241,-57.9461901084061,2.65878198860221));
#227918=CARTESIAN_POINT('',(-6.58439859102965,-62.500570298093,2.65878198860218));
#227919=CARTESIAN_POINT('Origin',(-3.27251186835868E-17,1.90836799017771E-13,
2.65878198860263));
#227920=CARTESIAN_POINT('',(-6.18532049829339,-58.7035958781038,2.65878198860221));
#227921=CARTESIAN_POINT('',(-6.17793001757209,-58.6332801510294,2.65878198860221));
#227922=CARTESIAN_POINT('Origin',(3.86084563605879E-16,1.90614476791061E-13,
2.65878198860263));
#227923=CARTESIAN_POINT('Origin',(-0.189456421067656,0.0199126722523968,
42.7590319886026));
#227924=CARTESIAN_POINT('',(-6.46154998175858,-59.6550713551491,3.64303198860221));
#227925=CARTESIAN_POINT('',(-6.4165176033499,-59.2266168947285,3.40423097483269));
#227926=CARTESIAN_POINT('Origin',(-6.45755375176689,-59.6170497665652,3.20400220531789));
#227927=CARTESIAN_POINT('',(-6.37927424589655,-58.8722700235035,2.8340419886022));
#227928=CARTESIAN_POINT('',(-6.4165176033499,-59.2266168947285,3.40423097483269));
#227929=CARTESIAN_POINT('',(-6.7388720005127,-62.2936141127568,2.83404198860218));
#227930=CARTESIAN_POINT('',(-6.76602706194884,-62.5519772640371,2.83404198860218));
#227931=CARTESIAN_POINT('',(-6.70162869542285,-61.9392677288636,3.40423097483267));
#227932=CARTESIAN_POINT('',(-6.7388720005127,-62.2936141127568,2.83404198860218));
#227933=CARTESIAN_POINT('',(-6.65659636252321,-61.5108137072211,3.6430319886022));
#227934=CARTESIAN_POINT('Origin',(-6.66059260538586,-61.5488354182639,3.20400259787953));
#227935=CARTESIAN_POINT('',(-6.61464077648837,-61.1116329639868,3.6430319886022));
#227936=CARTESIAN_POINT('',(-0.189456421067651,0.0199126722526699,3.64303198860263));
#227937=CARTESIAN_POINT('',(-6.60146619279885,-60.9862851800403,3.42473028058442));
#227938=CARTESIAN_POINT('',(-6.6146407757806,-61.1116329640611,3.6430319886022));
#227939=CARTESIAN_POINT('',(-6.56697596826216,-60.6581326136903,3.23423028058439));
#227940=CARTESIAN_POINT('Origin',(-6.5700514604535,-60.6873988786413,3.56425722717276));
#227941=CARTESIAN_POINT('',(-6.55117041629707,-60.5077528318942,3.23423028058439));
#227942=CARTESIAN_POINT('',(-0.189456421067651,0.0199126722526728,3.23423028058481));
#227943=CARTESIAN_POINT('',(-6.51668018436685,-60.1796001951994,3.42473028058439));
#227944=CARTESIAN_POINT('Origin',(-6.54809359889834,-60.478483781638,3.56425909741048));
#227945=CARTESIAN_POINT('',(-6.50350559588404,-60.0542523588396,3.64303198860221));
#227946=CARTESIAN_POINT('',(-6.51668018436685,-60.1796001951994,3.42473028058439));
#227947=CARTESIAN_POINT('',(-0.189456421067651,0.0199126722526699,3.64303198860263));
#227948=CARTESIAN_POINT('Origin',(0.189456421067656,-0.0199126722525754,
42.7590319886026));
#227949=CARTESIAN_POINT('',(-6.2776835203879,-61.5506390517261,3.64303198860219));
#227950=CARTESIAN_POINT('',(-6.32271585268578,-61.9790930734318,3.40423097483266));
#227951=CARTESIAN_POINT('Origin',(-6.28167976322058,-61.5886607624838,3.20400259735653));
#227952=CARTESIAN_POINT('',(-6.35995915792703,-62.3334394573091,2.83404198860218));
#227953=CARTESIAN_POINT('',(-6.32271585268577,-61.9790930734318,3.40423097483266));
#227954=CARTESIAN_POINT('',(-6.00036140428986,-58.9120953679529,2.8340419886022));
#227955=CARTESIAN_POINT('',(0.189456421067662,-0.0199126722522911,2.83404198860262));
#227956=CARTESIAN_POINT('',(-6.03760476191717,-59.2664422391596,3.40423097483269));
#227957=CARTESIAN_POINT('',(-6.00036140428986,-58.9120953679529,2.8340419886022));
#227958=CARTESIAN_POINT('',(-6.08263713962327,-59.6948966996541,3.64303198860221));
#227959=CARTESIAN_POINT('Origin',(-6.07864090959983,-59.6568751107683,3.20400220587196));
#227960=CARTESIAN_POINT('',(-6.12459275448642,-60.094077703267,3.6430319886022));
#227961=CARTESIAN_POINT('',(-6.13231300382116,-60.1675309762114,3.64303198860221));
#227962=CARTESIAN_POINT('',(-6.13776734223154,-60.2194255397044,3.42473028058439));
#227963=CARTESIAN_POINT('',(-6.12459275374873,-60.0940777033446,3.6430319886022));
#227964=CARTESIAN_POINT('',(-6.17225757416176,-60.5475781763992,3.23423028058439));
#227965=CARTESIAN_POINT('Origin',(-6.1691820883912,-60.5183119713912,3.56425743004905));
#227966=CARTESIAN_POINT('',(-6.18806312612685,-60.6979579581953,3.23423028058439));
#227967=CARTESIAN_POINT('',(-6.18811839147226,-60.6984837728332,3.23423028058439));
#227968=CARTESIAN_POINT('',(-6.22255335066353,-61.0261105245453,3.42473028058442));
#227969=CARTESIAN_POINT('Origin',(-6.19113993560378,-60.727226934177,3.56425912917781));
#227970=CARTESIAN_POINT('',(-6.23572793364529,-61.1514583085661,3.6430319886022));
#227971=CARTESIAN_POINT('',(-6.22255335066353,-61.0261105245453,3.42473028058442));
#227972=CARTESIAN_POINT('',(-6.27773801988317,-61.5511575797867,3.64303198860219));
#227973=CARTESIAN_POINT('Origin',(-0.190499999999384,-58.2637721346183,
2.65878198860221));
#227974=CARTESIAN_POINT('',(0.0152400000006159,-58.2637721346183,2.65878198860221));
#227975=CARTESIAN_POINT('',(-0.0152399999993768,-58.9578504383726,2.65878198860221));
#227976=CARTESIAN_POINT('Origin',(-0.1905,-9.13233322154995E-14,42.7590319886026));
#227977=CARTESIAN_POINT('',(-0.190499999999366,-60.0036905223729,3.64303198860221));
#227978=CARTESIAN_POINT('',(-0.19049999999937,-59.572876015004,3.40423097483269));
#227979=CARTESIAN_POINT('Origin',(-0.190499999999367,-59.9654595002501,
3.20400220531674));
#227980=CARTESIAN_POINT('',(-0.190499999467556,-59.2165773020939,2.8340419886022));
#227981=CARTESIAN_POINT('',(-0.19049999999937,-59.572876015004,3.40423097483268));
#227982=CARTESIAN_POINT('',(-0.190499999999337,-62.6567671111297,2.83404198860218));
#227983=CARTESIAN_POINT('',(-0.190499999999335,-62.9165533988761,2.83404198860218));
#227984=CARTESIAN_POINT('',(-0.19050000060547,-62.3004688883553,3.40423097483267));
#227985=CARTESIAN_POINT('',(-0.190499999999338,-62.6567671111297,2.83404198860218));
#227986=CARTESIAN_POINT('',(-0.190499999999346,-61.8696548221179,3.6430319886022));
#227987=CARTESIAN_POINT('Origin',(-0.190499999999346,-61.9078859673753,
3.20400259788085));
#227988=CARTESIAN_POINT('',(-0.190500000710895,-61.4682752798282,3.64303198860219));
#227989=CARTESIAN_POINT('',(-0.190499999999995,1.81822235884877E-13,3.64303198860263));
#227990=CARTESIAN_POINT('',(-0.190499999999352,-61.3422370451704,3.42473028058442));
#227991=CARTESIAN_POINT('',(-0.190499999999351,-61.4682752798282,3.64303198860219));
#227992=CARTESIAN_POINT('',(-0.190499999999355,-61.0122769227454,3.23423028058439));
#227993=CARTESIAN_POINT('Origin',(-0.190499486621758,-61.0417043405091,
3.56425722716995));
#227994=CARTESIAN_POINT('',(-0.190499999999357,-60.8610688070705,3.23423028058439));
#227995=CARTESIAN_POINT('',(-0.190499999999994,1.84676882954539E-13,3.23423028058481));
#227996=CARTESIAN_POINT('',(-0.19049999999936,-60.5311086139133,3.42473028058439));
#227997=CARTESIAN_POINT('Origin',(-0.190499486572858,-60.8316384807424,
3.5642590974155));
#227998=CARTESIAN_POINT('',(-0.190499999999362,-60.4050703266281,3.64303198860221));
#227999=CARTESIAN_POINT('',(-0.19049999999936,-60.5311086139133,3.42473028058439));
#228000=CARTESIAN_POINT('',(-0.190499999999995,1.81822235884877E-13,3.64303198860263));
#228001=CARTESIAN_POINT('Origin',(0.1905,-8.73325690452018E-14,42.7590319886026));
#228002=CARTESIAN_POINT('',(0.190500000000654,-61.8696548221179,3.64303198860219));
#228003=CARTESIAN_POINT('',(0.190500000000659,-62.3004688883553,3.40423097483266));
#228004=CARTESIAN_POINT('Origin',(0.190500000000654,-61.9078859670877,3.20400259735625));
#228005=CARTESIAN_POINT('',(0.190500000452861,-62.6567671111297,2.83404198860218));
#228006=CARTESIAN_POINT('',(0.190500000000658,-62.3004688883553,3.40423097483266));
#228007=CARTESIAN_POINT('',(0.190500000000626,-59.2165773020939,2.8340419886022));
#228008=CARTESIAN_POINT('',(0.190500000000006,1.97084259631206E-13,2.83404198860262));
#228009=CARTESIAN_POINT('',(0.190499999294164,-59.572876015004,3.40423097483268));
#228010=CARTESIAN_POINT('',(0.190500000000626,-59.2165773020939,2.8340419886022));
#228011=CARTESIAN_POINT('',(0.190500000000634,-60.0036905223729,3.64303198860221));
#228012=CARTESIAN_POINT('Origin',(0.190500000000634,-59.9654594999461,3.20400220587172));
#228013=CARTESIAN_POINT('',(0.190499999259116,-60.4050703266281,3.6430319886022));
#228014=CARTESIAN_POINT('',(0.190500000000639,-60.4789282006567,3.6430319886022));
#228015=CARTESIAN_POINT('',(0.19050000000064,-60.5311086139133,3.42473028058439));
#228016=CARTESIAN_POINT('',(0.190500000000638,-60.4050703266281,3.6430319886022));
#228017=CARTESIAN_POINT('',(0.190500000000643,-60.8610688070705,3.23423028058439));
#228018=CARTESIAN_POINT('Origin',(0.190499486503203,-60.8316414495922,3.5642574300447));
#228019=CARTESIAN_POINT('',(0.190500000000645,-61.0122769227454,3.23423028058439));
#228020=CARTESIAN_POINT('',(0.190500000000645,-61.0128056337173,3.23423028058439));
#228021=CARTESIAN_POINT('',(0.190500000000648,-61.3422370451704,3.42473028058441));
#228022=CARTESIAN_POINT('Origin',(0.190499486688746,-61.0417071743789,3.56425912918094));
#228023=CARTESIAN_POINT('',(0.190500000000649,-61.4682752798282,3.64303198860219));
#228024=CARTESIAN_POINT('',(0.190500000000648,-61.3422370451704,3.42473028058441));
#228025=CARTESIAN_POINT('',(0.190500000000654,-61.870176206376,3.64303198860219));
#228026=CARTESIAN_POINT('Origin',(5.90076614434134,-57.9645097668782,2.65878198860221));
#228027=CARTESIAN_POINT('',(6.18532049829458,-58.7035958781036,2.65878198860221));
#228028=CARTESIAN_POINT('',(6.58439859103091,-62.5005702980928,2.65878198860218));
#228029=CARTESIAN_POINT('',(6.10537907909441,-57.9430040808455,2.65878198860221));
#228030=CARTESIAN_POINT('',(6.55408556366009,-62.5037563256532,2.65878198860218));
#228031=CARTESIAN_POINT('Origin',(5.63142687537637E-15,1.85141914433439E-13,
2.65878198860263));
#228032=CARTESIAN_POINT('',(6.15500747092375,-58.706781905664,2.65878198860221));
#228033=CARTESIAN_POINT('',(6.14761699020245,-58.6364661785897,2.65878198860221));
#228034=CARTESIAN_POINT('Origin',(5.65479388299727E-15,1.8536176889664E-13,
2.65878198860263));
#228035=CARTESIAN_POINT('Origin',(-0.189456421067656,-0.0199126722525792,
42.7590319886026));
#228036=CARTESIAN_POINT('',(6.08263713962448,-59.694896699654,3.64303198860221));
#228037=CARTESIAN_POINT('',(6.03760476121579,-59.2664422392334,3.40423097483269));
#228038=CARTESIAN_POINT('Origin',(6.07864090963303,-59.6568751110724,3.20400220531323));
#228039=CARTESIAN_POINT('',(6.00036140481974,-58.9120953678972,2.83404198860221));
#228040=CARTESIAN_POINT('',(6.03760476121579,-59.2664422392333,3.40423097483269));
#228041=CARTESIAN_POINT('',(6.35995915837864,-62.3334394572616,2.83404198860219));
#228042=CARTESIAN_POINT('',(6.38711421981479,-62.5918026085419,2.83404198860219));
#228043=CARTESIAN_POINT('',(6.32271585208535,-61.9790930734949,3.40423097483267));
#228044=CARTESIAN_POINT('',(6.35995915837864,-62.3334394572616,2.83404198860219));
#228045=CARTESIAN_POINT('',(6.27768352038914,-61.5506390517259,3.6430319886022));
#228046=CARTESIAN_POINT('Origin',(6.28167976325193,-61.58866076277,3.20400259788151));
#228047=CARTESIAN_POINT('',(6.23572793293846,-61.1514583086404,3.6430319886022));
#228048=CARTESIAN_POINT('',(-0.18945642106765,-0.0199126722523061,3.64303198860263));
#228049=CARTESIAN_POINT('',(6.22255335066477,-61.0261105245452,3.42473028058442));
#228050=CARTESIAN_POINT('',(6.23572793364653,-61.151458308566,3.6430319886022));
#228051=CARTESIAN_POINT('',(6.18806312612808,-60.6979579581952,3.23423028058439));
#228052=CARTESIAN_POINT('Origin',(6.19113963945025,-60.727224115824,3.56425722716726));
#228053=CARTESIAN_POINT('',(6.17225757416298,-60.5475781763991,3.23423028058439));
#228054=CARTESIAN_POINT('',(-0.18945642106765,-0.0199126722523032,3.23423028058481));
#228055=CARTESIAN_POINT('',(6.13776734223276,-60.2194255397043,3.42473028058439));
#228056=CARTESIAN_POINT('Origin',(6.1691817779921,-60.518309018808,3.56425909741116));
#228057=CARTESIAN_POINT('',(6.12459275374995,-60.0940777033444,3.64303198860221));
#228058=CARTESIAN_POINT('',(6.13776734223276,-60.2194255397043,3.42473028058439));
#228059=CARTESIAN_POINT('',(-0.18945642106765,-0.0199126722523061,3.64303198860263));
#228060=CARTESIAN_POINT('Origin',(0.189456421067656,0.0199126722524006,
42.7590319886026));
#228061=CARTESIAN_POINT('',(6.65659636252446,-61.510813707221,3.64303198860219));
#228062=CARTESIAN_POINT('',(6.70162869482234,-61.9392677289267,3.40423097483266));
#228063=CARTESIAN_POINT('Origin',(6.66059260535715,-61.5488354179788,3.20400259735661));
#228064=CARTESIAN_POINT('',(6.73887200096456,-62.2936141127093,2.83404198860219));
#228065=CARTESIAN_POINT('',(6.70162869482234,-61.9392677289267,3.40423097483266));
#228066=CARTESIAN_POINT('',(6.37927424642637,-58.8722700234478,2.83404198860221));
#228067=CARTESIAN_POINT('',(0.189456421067661,0.019912672252685,2.83404198860263));
#228068=CARTESIAN_POINT('',(6.41651760264875,-59.2266168948022,3.40423097483269));
#228069=CARTESIAN_POINT('',(6.37927424642637,-58.8722700234478,2.83404198860221));
#228070=CARTESIAN_POINT('',(6.46154998175979,-59.655071355149,3.64303198860221));
#228071=CARTESIAN_POINT('Origin',(6.45755375173623,-59.617049766262,3.20400220587411));
#228072=CARTESIAN_POINT('',(6.50350559514774,-60.054252358917,3.64303198860221));
#228073=CARTESIAN_POINT('',(6.51122584595768,-60.1277056317062,3.64303198860221));
#228074=CARTESIAN_POINT('',(6.51668018436807,-60.1796001951993,3.42473028058439));
#228075=CARTESIAN_POINT('',(6.50350559588526,-60.0542523588395,3.64303198860221));
#228076=CARTESIAN_POINT('',(6.5511704162983,-60.5077528318941,3.23423028058439));
#228077=CARTESIAN_POINT('Origin',(6.54809390915869,-60.4784867342349,3.56425743004622));
#228078=CARTESIAN_POINT('',(6.56697596826339,-60.6581326136902,3.23423028058439));
#228079=CARTESIAN_POINT('',(6.5670312336088,-60.6586584283281,3.23423028058439));
#228080=CARTESIAN_POINT('',(6.60146619280008,-60.9862851800402,3.42473028058441));
#228081=CARTESIAN_POINT('Origin',(6.57005175674045,-60.687401696983,3.56425912917834));
#228082=CARTESIAN_POINT('',(6.61464077578184,-61.111632964061,3.6430319886022));
#228083=CARTESIAN_POINT('',(6.60146619280008,-60.9862851800402,3.42473028058441));
#228084=CARTESIAN_POINT('',(6.65665086201973,-61.5113322352816,3.64303198860219));
#228085=CARTESIAN_POINT('Origin',(11.92738225999,-57.0301761002787,2.65878198860222));
#228086=CARTESIAN_POINT('',(12.2876333308477,-57.7354693911201,2.65878198860222));
#228087=CARTESIAN_POINT('',(13.0814171332239,-61.4699285681951,2.65878198860219));
#228088=CARTESIAN_POINT('',(12.128626347365,-56.9874003490099,2.65878198860222));
#228089=CARTESIAN_POINT('',(13.0516031943535,-61.4762657165312,2.65878198860219));
#228090=CARTESIAN_POINT('Origin',(5.61622893658571E-15,1.8513950731641E-13,
2.65878198860263));
#228091=CARTESIAN_POINT('',(12.2578193919774,-57.7418065394563,2.65878198860222));
#228092=CARTESIAN_POINT('',(12.2431194021881,-57.6726485248847,2.65878198860222));
#228093=CARTESIAN_POINT('Origin',(5.66270693800216E-15,1.85363022201428E-13,
2.65878198860263));
#228094=CARTESIAN_POINT('Origin',(-0.18633711793979,-0.0396071771008745,
42.7590319886026));
#228095=CARTESIAN_POINT('',(12.289131633873,-58.7320730967335,3.64303198860222));
#228096=CARTESIAN_POINT('',(12.1995602612171,-58.3106729199893,3.4042309748327));
#228097=CARTESIAN_POINT('Origin',(12.2811829574217,-58.6946775141705,3.20400220531643));
#228098=CARTESIAN_POINT('',(12.1254815938998,-57.9621601887012,2.83404198860222));
#228099=CARTESIAN_POINT('',(12.1995602612171,-58.3106729199893,3.4042309748327));
#228100=CARTESIAN_POINT('',(12.8407372733105,-61.327173596589,2.83404198860219));
#228101=CARTESIAN_POINT('',(12.8947498796471,-61.5812829306517,2.83404198860219));
#228102=CARTESIAN_POINT('',(12.7666587067861,-60.9786613449623,3.40423097483267));
#228103=CARTESIAN_POINT('',(12.8407372733105,-61.327173596589,2.8340419886022));
#228104=CARTESIAN_POINT('',(12.6770874264386,-60.557261599584,3.64303198860221));
#228105=CARTESIAN_POINT('Origin',(12.6850361284912,-60.5946573025921,3.20400259788329));
#228106=CARTESIAN_POINT('',(12.5936359264454,-60.1646531634577,3.64303198860221));
#228107=CARTESIAN_POINT('',(-0.186337117939784,-0.0396071771006013,3.64303198860263));
#228108=CARTESIAN_POINT('',(12.5674311046661,-60.0413691664784,3.42473028058443));
#228109=CARTESIAN_POINT('',(12.5936359271415,-60.1646531633097,3.64303198860221));
#228110=CARTESIAN_POINT('',(12.4988285377103,-59.7186194643906,3.2342302805844));
#228111=CARTESIAN_POINT('Origin',(12.5049473440529,-59.7474037157344,3.56425722716985));
#228112=CARTESIAN_POINT('',(12.4673906027149,-59.5707156088318,3.2342302805844));
#228113=CARTESIAN_POINT('',(-0.186337117939784,-0.0396071771005985,3.23423028058481));
#228114=CARTESIAN_POINT('',(12.398788021053,-59.2479658375573,3.4247302805844));
#228115=CARTESIAN_POINT('Origin',(12.461272196013,-59.5419282989947,3.56425909740943));
#228116=CARTESIAN_POINT('',(12.3725831876358,-59.1246817892487,3.64303198860221));
#228117=CARTESIAN_POINT('',(12.398788021053,-59.2479658375573,3.4247302805844));
#228118=CARTESIAN_POINT('',(-0.186337117939784,-0.0396071771006013,3.64303198860263));
#228119=CARTESIAN_POINT('Origin',(0.18633711793979,0.0396071771006958,42.7590319886026));
#228120=CARTESIAN_POINT('',(13.0497616623182,-60.4780472453824,3.6430319886022));
#228121=CARTESIAN_POINT('',(13.1393329432576,-60.8994469906349,3.40423097483267));
#228122=CARTESIAN_POINT('Origin',(13.0577103643107,-60.5154429481078,3.20400259735575));
#228123=CARTESIAN_POINT('',(13.2134115096327,-61.2479592422933,2.8340419886022));
#228124=CARTESIAN_POINT('',(13.1393329432576,-60.8994469906349,3.40423097483267));
#228125=CARTESIAN_POINT('',(12.4981558292594,-57.8829458346102,2.83404198860222));
#228126=CARTESIAN_POINT('',(0.186337117939794,0.0396071771009801,2.83404198860263));
#228127=CARTESIAN_POINT('',(12.5722344964055,-58.2314585659346,3.4042309748327));
#228128=CARTESIAN_POINT('',(12.4981558292594,-57.8829458346102,2.83404198860222));
#228129=CARTESIAN_POINT('',(12.6618058697526,-58.6528587425319,3.64303198860222));
#228130=CARTESIAN_POINT('Origin',(12.653857193238,-58.6154631596709,3.20400220587288));
#228131=CARTESIAN_POINT('',(12.7452574227896,-59.0454674352014,3.64303198860221));
#228132=CARTESIAN_POINT('',(12.7606133389849,-59.1177113373235,3.64303198860221));
#228133=CARTESIAN_POINT('',(12.7714622569326,-59.1687514833557,3.4247302805844));
#228134=CARTESIAN_POINT('',(12.7452574235154,-59.0454674350471,3.64303198860221));
#228135=CARTESIAN_POINT('',(12.8400648385945,-59.4915012546302,3.2342302805844));
#228136=CARTESIAN_POINT('Origin',(12.8339460446681,-59.4627170622764,3.56425743004005));
#228137=CARTESIAN_POINT('',(12.8715027735898,-59.639405110189,3.2342302805844));
#228138=CARTESIAN_POINT('',(12.871612698782,-59.6399222675577,3.2342302805844));
#228139=CARTESIAN_POINT('',(12.9401053405456,-59.9621548122768,3.42473028058442));
#228140=CARTESIAN_POINT('Origin',(12.8776211648735,-59.6681923469374,3.56425912918013));
#228141=CARTESIAN_POINT('',(12.966310163021,-60.0854388091081,3.64303198860221));
#228142=CARTESIAN_POINT('',(12.9401053405456,-59.9621548122768,3.42473028058442));
#228143=CARTESIAN_POINT('',(13.0498700642008,-60.4785572361435,3.6430319886022));
#228144=CARTESIAN_POINT('Origin',(17.823319479633,-55.471007889993,2.65878198860223));
#228145=CARTESIAN_POINT('',(18.2553202812755,-56.1347810195638,2.65878198860223));
#228146=CARTESIAN_POINT('',(19.4351129318427,-59.7658094374947,2.6587819886022));
#228147=CARTESIAN_POINT('',(18.0189898472955,-55.4074307335703,2.65878198860223));
#228148=CARTESIAN_POINT('',(19.406124729226,-59.7752282754833,2.6587819886022));
#228149=CARTESIAN_POINT('Origin',(5.60136586593793E-15,1.85135524768633E-13,
2.65878198860263));
#228150=CARTESIAN_POINT('',(18.2263320786588,-56.1441998575524,2.65878198860223));
#228151=CARTESIAN_POINT('',(18.2044836359659,-56.0769572651635,2.65878198860223));
#228152=CARTESIAN_POINT('Origin',(5.67044563844026E-15,1.85365095779961E-13,
2.65878198860263));
#228153=CARTESIAN_POINT('Origin',(-0.181176266354226,-0.0588677374285187,
42.7590319886026));
#228154=CARTESIAN_POINT('',(18.3609838302746,-57.1257686104887,3.64303198860223));
#228155=CARTESIAN_POINT('',(18.2278548260744,-56.716039665941,3.40423097483271));
#228156=CARTESIAN_POINT('Origin',(18.3491697947263,-57.089408747774,3.20400220531739));
#228157=CARTESIAN_POINT('',(18.1177524692163,-56.3771794531162,2.83404198860223));
#228158=CARTESIAN_POINT('',(18.2278548260744,-56.716039665941,3.40423097483271));
#228159=CARTESIAN_POINT('',(19.1808295835788,-59.648994388456,2.83404198860221));
#228160=CARTESIAN_POINT('',(19.261107961398,-59.8960658302613,2.8340419886022));
#228161=CARTESIAN_POINT('',(19.0707273770999,-59.3101346421291,3.40423097483269));
#228162=CARTESIAN_POINT('',(19.1808295835788,-59.648994388456,2.83404198860221));
#228163=CARTESIAN_POINT('',(18.9375985097928,-58.9004061169353,3.64303198860222));
#228164=CARTESIAN_POINT('Origin',(18.9494125833922,-58.9367660967591,3.2040025978833));
#228165=CARTESIAN_POINT('',(18.8135654093539,-58.5186714879531,3.64303198860221));
#228166=CARTESIAN_POINT('',(-0.181176266354221,-0.0588677374282456,3.64303198860263));
#228167=CARTESIAN_POINT('',(18.7746174535806,-58.3988020033594,3.42473028058444));
#228168=CARTESIAN_POINT('',(18.8135654100308,-58.5186714877332,3.64303198860222));
#228169=CARTESIAN_POINT('',(18.6726541682852,-58.0849912788097,3.23423028058441));
#228170=CARTESIAN_POINT('Origin',(18.6817482287255,-58.1129782575881,3.56425722717241));
#228171=CARTESIAN_POINT('',(18.6259282908542,-57.9411838150804,3.23423028058441));
#228172=CARTESIAN_POINT('',(-0.181176266354221,-0.0588677374282427,3.23423028058481));
#228173=CARTESIAN_POINT('',(18.5239649837014,-57.6273730232602,3.4247302805844));
#228174=CARTESIAN_POINT('Origin',(18.6168343081654,-57.9131937527885,3.56425909740864));
#228175=CARTESIAN_POINT('',(18.4850170109884,-57.5075034888349,3.64303198860222));
#228176=CARTESIAN_POINT('',(18.5239649837014,-57.6273730232602,3.4247302805844));
#228177=CARTESIAN_POINT('',(-0.181176266354221,-0.0588677374282456,3.64303198860263));
#228178=CARTESIAN_POINT('Origin',(0.181176266354226,0.0588677374283401,
42.7590319886026));
#228179=CARTESIAN_POINT('',(19.2999510425012,-58.7826706420785,3.64303198860222));
#228180=CARTESIAN_POINT('',(19.4330799103844,-59.1923991670851,3.40423097483269));
#228181=CARTESIAN_POINT('Origin',(19.3117651160117,-58.8190306216285,3.20400259735858));
#228182=CARTESIAN_POINT('',(19.5431821167169,-59.5312589134596,2.83404198860221));
#228183=CARTESIAN_POINT('',(19.4330799103844,-59.1923991670851,3.40423097483269));
#228184=CARTESIAN_POINT('',(18.4801050014197,-56.2594439784235,2.83404198860223));
#228185=CARTESIAN_POINT('',(0.18117626635423,0.0588677374286242,2.83404198860263));
#228186=CARTESIAN_POINT('',(18.5902073581109,-56.5983041913025,3.40423097483271));
#228187=CARTESIAN_POINT('',(18.4801050014197,-56.2594439784235,2.83404198860223));
#228188=CARTESIAN_POINT('',(18.7233363629831,-57.0080331356318,3.64303198860223));
#228189=CARTESIAN_POINT('Origin',(18.7115223273407,-56.9716732726276,3.20400220587314));
#228190=CARTESIAN_POINT('',(18.8473695429913,-57.3897680142073,3.64303198860223));
#228191=CARTESIAN_POINT('',(18.8701928819401,-57.4600110263526,3.64303198860222));
#228192=CARTESIAN_POINT('',(18.8863175164099,-57.5096375484033,3.42473028058439));
#228193=CARTESIAN_POINT('',(18.8473695436968,-57.389768013978,3.64303198860223));
#228194=CARTESIAN_POINT('',(18.9882808235627,-57.8234483402235,3.23423028058441));
#228195=CARTESIAN_POINT('Origin',(18.979186781637,-57.7954614188149,3.5642574300438));
#228196=CARTESIAN_POINT('',(19.0350067009936,-57.9672558039528,3.23423028058441));
#228197=CARTESIAN_POINT('',(19.0351700816691,-57.9677586379679,3.23423028058441));
#228198=CARTESIAN_POINT('',(19.136969986289,-58.2810665285026,3.42473028058442));
#228199=CARTESIAN_POINT('Origin',(19.0441006607087,-57.9952457951678,3.56425912917952));
#228200=CARTESIAN_POINT('',(19.1759179427393,-58.4009360128763,3.64303198860222));
#228201=CARTESIAN_POINT('',(19.136969986289,-58.2810665285026,3.42473028058442));
#228202=CARTESIAN_POINT('',(19.3001121590976,-58.7831665079746,3.64303198860222));
#228203=CARTESIAN_POINT('Origin',(23.5239806812878,-53.3040877092098,2.65878198860225));
#228204=CARTESIAN_POINT('',(24.0229981225303,-53.919068240199,2.65878198860224));
#228205=CARTESIAN_POINT('',(25.5758735661215,-57.4068835917975,2.65878198860222));
#228206=CARTESIAN_POINT('',(23.7119335237431,-53.2204057122634,2.65878198860225));
#228207=CARTESIAN_POINT('',(25.5480287005725,-57.4192809246784,2.65878198860222));
#228208=CARTESIAN_POINT('Origin',(5.58700050634534E-15,1.85130010423735E-13,
2.65878198860263));
#228209=CARTESIAN_POINT('',(23.9951532569813,-53.93146557308,2.65878198860224));
#228210=CARTESIAN_POINT('',(23.966395737495,-53.8668751267874,2.65878198860224));
#228211=CARTESIAN_POINT('Origin',(5.67792519749014E-15,1.85367966913678E-13,
2.65878198860263));
#228212=CARTESIAN_POINT('Origin',(-0.174030409680915,-0.0774833305060312,
42.7590319886026));
#228213=CARTESIAN_POINT('',(24.2316692455489,-54.8935822490118,3.64303198860224));
#228214=CARTESIAN_POINT('',(24.0564411990333,-54.5000136127184,3.40423097483272));
#228215=CARTESIAN_POINT('Origin',(24.2161192879494,-54.8586564724106,3.20400220531692));
#228216=CARTESIAN_POINT('',(23.9115214570976,-54.1745185417594,2.83404198860224));
#228217=CARTESIAN_POINT('',(24.0564411990333,-54.5000136127184,3.40423097483272));
#228218=CARTESIAN_POINT('',(25.3107727110829,-57.3172883154485,2.83404198860222));
#228219=CARTESIAN_POINT('',(25.416437313678,-57.5546148985771,2.83404198860222));
#228220=CARTESIAN_POINT('',(25.1658531674655,-56.9917936927127,3.4042309748327));
#228221=CARTESIAN_POINT('',(25.3107727110829,-57.3172883154485,2.83404198860222));
#228222=CARTESIAN_POINT('',(24.9906253009265,-56.5982254591671,3.64303198860224));
#228223=CARTESIAN_POINT('Origin',(25.0061753086093,-56.6331513482572,3.2040025978802));
#228224=CARTESIAN_POINT('',(24.8273695326461,-56.2315470018072,3.64303198860223));
#228225=CARTESIAN_POINT('',(-0.174030409680909,-0.077483330505758,3.64303198860262));
#228226=CARTESIAN_POINT('',(24.7761051648324,-56.1164053447567,3.42473028058445));
#228227=CARTESIAN_POINT('',(24.8273695332963,-56.2315470015177,3.64303198860223));
#228228=CARTESIAN_POINT('',(24.6418982922884,-55.8149717737122,3.23423028058442));
#228229=CARTESIAN_POINT('Origin',(24.653867970398,-55.8418548487315,3.56425722716896));
#228230=CARTESIAN_POINT('',(24.5803964109129,-55.6768362864787,3.23423028058442));
#228231=CARTESIAN_POINT('',(-0.174030409680909,-0.0774833305057552,3.23423028058481));
#228232=CARTESIAN_POINT('',(24.4461895095995,-55.375402650817,3.42473028058442));
#228233=CARTESIAN_POINT('Origin',(24.5684264878159,-55.649950136715,3.56425909741445));
#228234=CARTESIAN_POINT('',(24.3949251197301,-55.2602609459786,3.64303198860224));
#228235=CARTESIAN_POINT('',(24.4461895095995,-55.375402650817,3.42473028058442));
#228236=CARTESIAN_POINT('',(-0.174030409680909,-0.077483330505758,3.64303198860263));
#228237=CARTESIAN_POINT('Origin',(0.174030409680915,0.0774833305058525,
42.7590319886026));
#228238=CARTESIAN_POINT('',(25.3386861202883,-56.4432587981552,3.64303198860224));
#228239=CARTESIAN_POINT('',(25.5139139873796,-56.8368270314549,3.4042309748327));
#228240=CARTESIAN_POINT('Origin',(25.3542361278552,-56.4781846869849,3.20400259736081));
#228241=CARTESIAN_POINT('',(25.6588335308581,-57.1623216542526,2.83404198860222));
#228242=CARTESIAN_POINT('',(25.5139139873796,-56.8368270314549,3.4042309748327));
#228243=CARTESIAN_POINT('',(24.2595822759739,-54.0195518809636,2.83404198860224));
#228244=CARTESIAN_POINT('',(0.174030409680918,0.0774833305061365,2.83404198860263));
#228245=CARTESIAN_POINT('',(24.4045020177497,-54.3450469519939,3.40423097483273));
#228246=CARTESIAN_POINT('',(24.2595822759739,-54.0195518809636,2.83404198860224));
#228247=CARTESIAN_POINT('',(24.5797300649108,-54.7386155879999,3.64303198860224));
#228248=CARTESIAN_POINT('Origin',(24.564180107187,-54.7036898111196,3.20400220587456));
#228249=CARTESIAN_POINT('',(24.7429859384147,-55.1052942852682,3.64303198860224));
#228250=CARTESIAN_POINT('',(24.773026642839,-55.1727668102967,3.64303198860224));
#228251=CARTESIAN_POINT('',(24.7942503289613,-55.2204359898052,3.42473028058442));
#228252=CARTESIAN_POINT('',(24.7429859390919,-55.1052942849667,3.64303198860224));
#228253=CARTESIAN_POINT('',(24.9284572302748,-55.5218696254668,3.23423028058442));
#228254=CARTESIAN_POINT('Origin',(24.9164875765751,-55.4949866055679,3.56425743004029));
#228255=CARTESIAN_POINT('',(24.9899591116502,-55.6600051127003,3.23423028058443));
#228256=CARTESIAN_POINT('',(24.9901741577761,-55.6604881142071,3.23423028058443));
#228257=CARTESIAN_POINT('',(25.1241659841942,-55.9614386837448,3.42473028058445));
#228258=CARTESIAN_POINT('Origin',(25.0019290044718,-55.6868911941825,3.564259129176));
#228259=CARTESIAN_POINT('',(25.1754303526582,-56.0765803405058,3.64303198860224));
#228260=CARTESIAN_POINT('',(25.1241659841942,-55.9614386837448,3.42473028058445));
#228261=CARTESIAN_POINT('',(25.3388981863712,-56.4437351063759,3.64303198860224));
#228262=CARTESIAN_POINT('Origin',(28.9669082278889,-50.553156788887,2.65878198860227));
#228263=CARTESIAN_POINT('',(29.5274749692191,-51.1126068659042,2.65878198860226));
#228264=CARTESIAN_POINT('',(31.4364195775141,-54.4189959163058,2.65878198860224));
#228265=CARTESIAN_POINT('',(29.1450842944635,-50.450286788887,2.65878198860227));
#228266=CARTESIAN_POINT('',(31.4100231232068,-54.4342359163058,2.65878198860224));
#228267=CARTESIAN_POINT('Origin',(5.57329024769379E-15,1.85123024698033E-13,
2.65878198860263));
#228268=CARTESIAN_POINT('',(29.5010785149117,-51.1278468659042,2.65878198860226));
#228269=CARTESIAN_POINT('',(29.4657269920333,-51.0666162321539,2.65878198860226));
#228270=CARTESIAN_POINT('Origin',(5.68506366753766E-15,1.85371604145838E-13,
2.65878198860263));
#228271=CARTESIAN_POINT('Origin',(-0.164977839420934,-0.0952500000000912,
42.7590319886026));
#228272=CARTESIAN_POINT('',(29.8368674217662,-52.0599703131941,3.64303198860226));
#228273=CARTESIAN_POINT('',(29.6214601680818,-51.6868740054938,3.40423097483274));
#228274=CARTESIAN_POINT('Origin',(29.8177519107049,-52.0268612768232,3.20400220531664));
#228275=CARTESIAN_POINT('',(29.4433108120869,-51.3783102685122,2.83404198860226));
#228276=CARTESIAN_POINT('',(29.6214601680818,-51.6868740054938,3.40423097483274));
#228277=CARTESIAN_POINT('',(31.1634057161447,-54.3576020372433,2.83404198860224));
#228278=CARTESIAN_POINT('',(31.2932988600179,-54.5825835619865,2.83404198860223));
#228279=CARTESIAN_POINT('',(30.9852566042328,-54.0490387253002,3.40423097483274));
#228280=CARTESIAN_POINT('',(31.1634057161447,-54.3576020372433,2.83404198860224));
#228281=CARTESIAN_POINT('',(30.7698495716387,-53.6759427993281,3.64303198860226));
#228282=CARTESIAN_POINT('Origin',(30.7889651442677,-53.7090519423374,3.20400259788206));
#228283=CARTESIAN_POINT('',(30.5691597998771,-53.328337919502,3.64303198860225));
#228284=CARTESIAN_POINT('',(-0.164977839420929,-0.0952499999998181,3.64303198860262));
#228285=CARTESIAN_POINT('',(30.506140683165,-53.219185606084,3.42473028058449));
#228286=CARTESIAN_POINT('',(30.5691598004939,-53.3283379191459,3.64303198860225));
#228287=CARTESIAN_POINT('',(30.3411606219525,-52.9334317578282,3.23423028058445));
#228288=CARTESIAN_POINT('Origin',(30.3558747754316,-52.9589163924893,3.56425722717266));
#228289=CARTESIAN_POINT('',(30.265556564115,-52.8024816883954,3.23423028058445));
#228290=CARTESIAN_POINT('',(-0.164977839420929,-0.0952499999998153,3.23423028058481));
#228291=CARTESIAN_POINT('',(30.1005764675364,-52.5167277788836,3.42473028058445));
#228292=CARTESIAN_POINT('Origin',(30.250841845591,-52.7769940214396,3.56425909741364));
#228293=CARTESIAN_POINT('',(30.0375573238938,-52.4075754202451,3.64303198860226));
#228294=CARTESIAN_POINT('',(30.1005764675364,-52.5167277788836,3.42473028058445));
#228295=CARTESIAN_POINT('',(-0.164977839420929,-0.0952499999998181,3.64303198860262));
#228296=CARTESIAN_POINT('Origin',(0.164977839420934,0.0952499999999126,
42.7590319886026));
#228297=CARTESIAN_POINT('',(31.0998052504806,-53.4854427993281,3.64303198860226));
#228298=CARTESIAN_POINT('',(31.3152122835993,-53.8585387249973,3.40423097483272));
#228299=CARTESIAN_POINT('Origin',(31.1189208229655,-53.5185519420876,3.20400259735637));
#228300=CARTESIAN_POINT('',(31.4933613953782,-54.1671020370171,2.83404198860224));
#228301=CARTESIAN_POINT('',(31.3152122835993,-53.8585387249973,3.40423097483272));
#228302=CARTESIAN_POINT('',(29.7732664904686,-51.1878102687779,2.83404198860226));
#228303=CARTESIAN_POINT('',(0.164977839420937,0.0952500000001963,2.83404198860262));
#228304=CARTESIAN_POINT('',(29.9514158463116,-51.4963740058471,3.40423097483275));
#228305=CARTESIAN_POINT('',(29.7732664904686,-51.1878102687779,2.83404198860226));
#228306=CARTESIAN_POINT('',(30.1668231006081,-51.8694703131941,3.64303198860227));
#228307=CARTESIAN_POINT('Origin',(30.1477075893944,-51.8363612765593,3.20400220587301));
#228308=CARTESIAN_POINT('',(30.3675130020933,-52.217075420616,3.64303198860227));
#228309=CARTESIAN_POINT('',(30.40444193975,-52.2810382154234,3.64303198860227));
#228310=CARTESIAN_POINT('',(30.4305321463783,-52.3262277788836,3.42473028058445));
#228311=CARTESIAN_POINT('',(30.3675130027357,-52.2170754202451,3.64303198860227));
#228312=CARTESIAN_POINT('',(30.5955122429569,-52.6119816883954,3.23423028058445));
#228313=CARTESIAN_POINT('Origin',(30.5807981195161,-52.586497106002,3.5642574300457));
#228314=CARTESIAN_POINT('',(30.6711163007943,-52.7429317578282,3.23423028058445));
#228315=CARTESIAN_POINT('',(30.6713806562803,-52.7433896349612,3.23423028058445));
#228316=CARTESIAN_POINT('',(30.8360963620068,-53.028685606084,3.42473028058447));
#228317=CARTESIAN_POINT('Origin',(30.6858309820709,-52.7684193600401,3.56425912917733));
#228318=CARTESIAN_POINT('',(30.8991154793358,-53.1378379191459,3.64303198860226));
#228319=CARTESIAN_POINT('',(30.8360963620068,-53.028685606084,3.42473028058447));
#228320=CARTESIAN_POINT('',(31.1000659426097,-53.4858943313408,3.64303198860226));
#228321=CARTESIAN_POINT('Origin',(34.09246826623,-47.248354903857,2.6587819886023));
#228322=CARTESIAN_POINT('',(34.7084426211237,-47.7461450747859,2.65878198860229));
#228323=CARTESIAN_POINT('',(36.9525415975218,-50.834882333648,2.65878198860227));
#228324=CARTESIAN_POINT('',(34.2589154226527,-47.1274239660504,2.6587819886023));
#228325=CARTESIAN_POINT('',(36.9278827595333,-50.8527980281379,2.65878198860227));
#228326=CARTESIAN_POINT('Origin',(5.5603853024461E-15,1.85114644128599E-13,
2.65878198860263));
#228327=CARTESIAN_POINT('',(34.6837837831351,-47.7640607692757,2.65878198860229));
#228328=CARTESIAN_POINT('',(34.6422255755471,-47.7068608037044,2.65878198860229));
#228329=CARTESIAN_POINT('Origin',(5.69178283801114E-15,1.85375967626163E-13,
2.65878198860263));
#228330=CARTESIAN_POINT('Origin',(-0.154117737428426,-0.111973090561807,
42.7590319886026));
#228331=CARTESIAN_POINT('',(35.1151666347447,-48.6559784483759,3.64303198860229));
#228332=CARTESIAN_POINT('',(34.8619402208396,-48.3074421904912,3.40423097483276));
#228333=CARTESIAN_POINT('Origin',(35.0926950037607,-48.6250489017661,3.20400220531733));
#228334=CARTESIAN_POINT('',(34.6525130924105,-48.0191904763605,2.83404198860228));
#228335=CARTESIAN_POINT('',(34.8619402208396,-48.3074421904912,3.40423097483276));
#228336=CARTESIAN_POINT('',(36.6746059268184,-50.8023624960585,2.83404198860226));
#228337=CARTESIAN_POINT('',(36.8273044755035,-51.0125340177509,2.83404198860226));
#228338=CARTESIAN_POINT('',(36.4651790855638,-50.5141111791242,3.40423097483275));
#228339=CARTESIAN_POINT('',(36.6746059268184,-50.8023624960585,2.83404198860226));
#228340=CARTESIAN_POINT('',(36.2119529314391,-50.1655752777666,3.64303198860229));
#228341=CARTESIAN_POINT('Origin',(36.2344246348003,-50.1965049239951,3.20400259788241));
#228342=CARTESIAN_POINT('',(35.9760279553338,-49.8408524072779,3.64303198860228));
#228343=CARTESIAN_POINT('',(-0.154117737428421,-0.111973090561534,3.64303198860262));
#228344=CARTESIAN_POINT('',(35.9019445403524,-49.7388853330806,3.42473028058451));
#228345=CARTESIAN_POINT('',(35.9760279559093,-49.8408524068598,3.64303198860228));
#228346=CARTESIAN_POINT('',(35.7079988465464,-49.4719419865727,3.23423028058448));
#228347=CARTESIAN_POINT('Origin',(35.7252962640508,-49.4957489658865,3.56425722717396));
#228348=CARTESIAN_POINT('',(35.6191209461258,-49.3496120513043,3.23423028058447));
#228349=CARTESIAN_POINT('',(-0.154117737428421,-0.111973090561531,3.23423028058481));
#228350=CARTESIAN_POINT('',(35.4251752107443,-49.0826686475729,3.42473028058447));
#228351=CARTESIAN_POINT('Origin',(35.6018226497107,-49.3258021153704,3.56425909741572));
#228352=CARTESIAN_POINT('',(35.3510917642539,-48.9807015312173,3.64303198860228));
#228353=CARTESIAN_POINT('',(35.4251752107443,-49.0826686475729,3.42473028058447));
#228354=CARTESIAN_POINT('',(-0.154117737428421,-0.111973090561534,3.64303198860262));
#228355=CARTESIAN_POINT('Origin',(0.154117737428426,0.111973090561629,42.7590319886026));
#228356=CARTESIAN_POINT('',(36.5201884062959,-49.9416290966431,3.64303198860228));
#228357=CARTESIAN_POINT('',(36.7734145609104,-50.2901649976449,3.40423097483275));
#228358=CARTESIAN_POINT('Origin',(36.5426601094879,-49.9725587426388,3.20400259735788));
#228359=CARTESIAN_POINT('',(36.9828414020409,-50.5784163146694,2.83404198860226));
#228360=CARTESIAN_POINT('',(36.7734145609104,-50.2901649976449,3.40423097483275));
#228361=CARTESIAN_POINT('',(34.9607485668371,-47.7952442955496,2.83404198860229));
#228362=CARTESIAN_POINT('',(0.154117737428429,0.111973090561912,2.83404198860262));
#228363=CARTESIAN_POINT('',(35.1701756951247,-48.0834960097832,3.40423097483277));
#228364=CARTESIAN_POINT('',(34.9607485668371,-47.7952442955496,2.83404198860229));
#228365=CARTESIAN_POINT('',(35.4234021096015,-48.4320322672525,3.6430319886023));
#228366=CARTESIAN_POINT('Origin',(35.4009304784387,-48.4011027203966,3.20400220587264));
#228367=CARTESIAN_POINT('',(35.6593272385107,-48.7567553505298,3.64303198860229));
#228368=CARTESIAN_POINT('',(35.7027398082304,-48.8165076253514,3.64303198860229));
#228369=CARTESIAN_POINT('',(35.7334106856012,-48.8587224664495,3.42473028058447));
#228370=CARTESIAN_POINT('',(35.6593272391108,-48.7567553500938,3.64303198860229));
#228371=CARTESIAN_POINT('',(35.9273564209826,-49.1256658701809,3.23423028058448));
#228372=CARTESIAN_POINT('Origin',(35.9100590388149,-49.1018589397078,3.56425743004547));
#228373=CARTESIAN_POINT('',(36.0162343214032,-49.2479958054493,3.23423028058448));
#228374=CARTESIAN_POINT('',(36.0165450899153,-49.2484235416107,3.23423028058448));
#228375=CARTESIAN_POINT('',(36.2101800152092,-49.5149391519571,3.4247302805845));
#228376=CARTESIAN_POINT('Origin',(36.0335325740078,-49.2718056808884,3.56425912917759));
#228377=CARTESIAN_POINT('',(36.2842634307661,-49.6169062257364,3.64303198860229));
#228378=CARTESIAN_POINT('',(36.2101800152092,-49.5149391519571,3.4247302805845));
#228379=CARTESIAN_POINT('',(36.5204948682736,-49.9420509053685,3.64303198860228));
#228380=CARTESIAN_POINT('Origin',(38.8445040879387,-43.4258901551464,2.65878198860232));
#228381=CARTESIAN_POINT('',(39.5091373124628,-43.856566526705,2.65878198860232));
#228382=CARTESIAN_POINT('',(42.0638038389706,-46.6938111422597,2.6587819886023));
#228383=CARTESIAN_POINT('',(38.9973987043324,-43.2882232241942,2.65878198860232));
#228384=CARTESIAN_POINT('',(42.04115278469,-46.7142062431416,2.6587819886023));
#228385=CARTESIAN_POINT('Origin',(5.54842705988295E-15,1.85104960534706E-13,
2.65878198860263));
#228386=CARTESIAN_POINT('',(39.4864862581822,-43.8769616275868,2.65878198860232));
#228387=CARTESIAN_POINT('',(39.4391766863035,-43.8244190249872,2.65878198860232));
#228388=CARTESIAN_POINT('Origin',(5.69800909227282E-15,1.85381009547451E-13,
2.65878198860263));
#228389=CARTESIAN_POINT('Origin',(-0.141569089253442,-0.127469380511453,
42.7590319886026));
#228390=CARTESIAN_POINT('',(40.0087367337519,-44.7189015017592,3.64303198860231));
#228391=CARTESIAN_POINT('',(39.7204655612079,-44.3987439298674,3.4042309748328));
#228392=CARTESIAN_POINT('Origin',(39.9831551867373,-44.6904903154961,3.20400220531642));
#228393=CARTESIAN_POINT('',(39.4820551877884,-44.1339623846885,2.83404198860231));
#228394=CARTESIAN_POINT('',(39.7204655612079,-44.3987439298674,3.4042309748328));
#228395=CARTESIAN_POINT('',(41.7839914803032,-46.690521640289,2.8340419886023));
#228396=CARTESIAN_POINT('',(41.9578224365467,-46.8835804757578,2.8340419886023));
#228397=CARTESIAN_POINT('',(41.5455814340034,-46.4257404601128,3.40423097483279));
#228398=CARTESIAN_POINT('',(41.7839914803032,-46.690521640289,2.8340419886023));
#228399=CARTESIAN_POINT('',(41.2573105570842,-46.1055832156402,3.64303198860232));
#228400=CARTESIAN_POINT('Origin',(41.2828921864925,-46.1339944934109,3.20400259788226));
#228401=CARTESIAN_POINT('',(40.9887352200427,-45.8073000862117,3.64303198860231));
#228402=CARTESIAN_POINT('',(-0.141569089253437,-0.12746938051118,3.64303198860262));
#228403=CARTESIAN_POINT('',(40.9043991801909,-45.7136354238369,3.42473028058453));
#228404=CARTESIAN_POINT('',(40.9887352205719,-45.8073000857352,3.64303198860231));
#228405=CARTESIAN_POINT('',(40.6836127633984,-45.4684272662429,3.2342302805845));
#228406=CARTESIAN_POINT('Origin',(40.7033039308027,-45.4902957559628,3.56425722717323));
#228407=CARTESIAN_POINT('',(40.5824347852705,-45.3560577375089,3.2342302805845));
#228408=CARTESIAN_POINT('',(-0.141569089253437,-0.127469380511178,3.23423028058481));
#228409=CARTESIAN_POINT('',(40.3616483211489,-45.1108495273506,3.4247302805845));
#228410=CARTESIAN_POINT('Origin',(40.5627424347182,-45.3341863992352,3.56425909741185));
#228411=CARTESIAN_POINT('',(40.2773122455534,-45.0171848263426,3.6430319886023));
#228412=CARTESIAN_POINT('',(40.3616483211489,-45.1108495273506,3.4247302805845));
#228413=CARTESIAN_POINT('',(-0.141569089253437,-0.12746938051118,3.64303198860262));
#228414=CARTESIAN_POINT('Origin',(0.141569089253442,0.127469380511275,42.7590319886026));
#228415=CARTESIAN_POINT('',(41.5404487355911,-45.8506444546175,3.64303198860231));
#228416=CARTESIAN_POINT('',(41.8287196129605,-46.1708016986847,3.40423097483278));
#228417=CARTESIAN_POINT('Origin',(41.5660303648061,-45.8790557321733,3.20400259735469));
#228418=CARTESIAN_POINT('',(42.0671296591466,-46.4355828789634,2.8340419886023));
#228419=CARTESIAN_POINT('',(41.8287196129605,-46.1708016986847,3.40423097483278));
#228420=CARTESIAN_POINT('',(39.7651933659004,-43.8790236240213,2.83404198860232));
#228421=CARTESIAN_POINT('',(0.141569089253444,0.127469380511558,2.83404198860262));
#228422=CARTESIAN_POINT('',(40.003603739189,-44.1438051693181,3.40423097483281));
#228423=CARTESIAN_POINT('',(39.7651933659004,-43.8790236240213,2.83404198860232));
#228424=CARTESIAN_POINT('',(40.2918749122587,-44.4639627407365,3.64303198860232));
#228425=CARTESIAN_POINT('Origin',(40.2662933650399,-44.4355515542465,3.20400220587391));
#228426=CARTESIAN_POINT('',(40.5604504235095,-44.7622460658158,3.64303198860232));
#228427=CARTESIAN_POINT('',(40.6098709880934,-44.817133162225,3.64303198860232));
#228428=CARTESIAN_POINT('',(40.6447864996558,-44.8559107663279,3.4247302805845));
#228429=CARTESIAN_POINT('',(40.5604504240602,-44.7622460653199,3.64303198860232));
#228430=CARTESIAN_POINT('',(40.8655729637774,-45.1011189764862,3.2342302805845));
#228431=CARTESIAN_POINT('Origin',(40.8458818366188,-45.0792505316427,3.56425743003812));
#228432=CARTESIAN_POINT('',(40.9667509419053,-45.2134885052202,3.2342302805845));
#228433=CARTESIAN_POINT('',(40.9671047185986,-45.2138814140432,3.2342302805845));
#228434=CARTESIAN_POINT('',(41.1875373586978,-45.4586966628142,3.42473028058452));
#228435=CARTESIAN_POINT('Origin',(40.9864432425628,-45.2353597879088,3.56425912917589));
#228436=CARTESIAN_POINT('',(41.2718733990788,-45.5523613247125,3.64303198860231));
#228437=CARTESIAN_POINT('',(41.1875373586978,-45.4586966628142,3.42473028058452));
#228438=CARTESIAN_POINT('',(41.5407976097559,-45.851031918631,3.64303198860231));
#228439=CARTESIAN_POINT('Origin',(43.1709513941248,-39.1276422664444,2.65878198860235));
#228440=CARTESIAN_POINT('',(43.8769616275879,-39.486486258181,2.65878198860235));
#228441=CARTESIAN_POINT('',(46.7142062431428,-42.0411527846888,2.65878198860233));
#228442=CARTESIAN_POINT('',(43.3086183250771,-38.9747476500507,2.65878198860235));
#228443=CARTESIAN_POINT('',(46.6938111422609,-42.0638038389693,2.65878198860233));
#228444=CARTESIAN_POINT('Origin',(5.5375465370123E-15,1.85094080011836E-13,
2.65878198860263));
#228445=CARTESIAN_POINT('',(43.8565665267061,-39.5091373124615,2.65878198860235));
#228446=CARTESIAN_POINT('',(43.8040239241064,-39.4618277405829,2.65878198860235));
#228447=CARTESIAN_POINT('Origin',(5.70367421417806E-15,1.85386674669356E-13,
2.65878198860263));
#228448=CARTESIAN_POINT('Origin',(-0.127469380511361,-0.141569089253534,
42.7590319886026));
#228449=CARTESIAN_POINT('',(44.4639627407376,-40.2918749122575,3.64303198860234));
#228450=CARTESIAN_POINT('',(44.1438051688458,-40.0036037397136,3.40423097483283));
#228451=CARTESIAN_POINT('Origin',(44.4355515544733,-40.2662933652418,3.2040022053198));
#228452=CARTESIAN_POINT('',(43.8790236243779,-39.7651933655044,2.83404198860234));
#228453=CARTESIAN_POINT('',(44.1438051688458,-40.0036037397136,3.40423097483283));
#228454=CARTESIAN_POINT('',(46.4355828792675,-42.0671296588088,2.83404198860233));
#228455=CARTESIAN_POINT('',(46.6286417147362,-42.2409606150523,2.83404198860233));
#228456=CARTESIAN_POINT('',(46.1708016982804,-41.8287196134095,3.4042309748328));
#228457=CARTESIAN_POINT('',(46.4355828792675,-42.0671296588088,2.83404198860233));
#228458=CARTESIAN_POINT('',(45.8506444546187,-41.5404487355899,3.64303198860235));
#228459=CARTESIAN_POINT('Origin',(45.8790557323885,-41.5660303649975,3.20400259788037));
#228460=CARTESIAN_POINT('',(45.5523613242375,-41.2718733996063,3.64303198860234));
#228461=CARTESIAN_POINT('',(-0.127469380511355,-0.141569089253261,3.64303198860262));
#228462=CARTESIAN_POINT('',(45.4586966628153,-41.1875373586965,3.42473028058456));
#228463=CARTESIAN_POINT('',(45.5523613247136,-41.2718733990775,3.64303198860234));
#228464=CARTESIAN_POINT('',(45.2134885052213,-40.9667509419041,3.23423028058453));
#228465=CARTESIAN_POINT('Origin',(45.2353576819761,-40.9864413462819,3.56425722717016));
#228466=CARTESIAN_POINT('',(45.1011189764874,-40.8655729637762,3.23423028058453));
#228467=CARTESIAN_POINT('',(-0.127469380511355,-0.141569089253258,3.23423028058481));
#228468=CARTESIAN_POINT('',(44.855910766329,-40.6447864996546,3.42473028058453));
#228469=CARTESIAN_POINT('Origin',(45.0792483253103,-40.8458798501214,3.5642590974069));
#228470=CARTESIAN_POINT('',(44.762246065321,-40.560450424059,3.64303198860234));
#228471=CARTESIAN_POINT('',(44.855910766329,-40.6447864996546,3.42473028058453));
#228472=CARTESIAN_POINT('',(-0.127469380511355,-0.141569089253261,3.64303198860262));
#228473=CARTESIAN_POINT('Origin',(0.127469380511361,0.141569089253356,42.7590319886026));
#228474=CARTESIAN_POINT('',(46.1055832156414,-41.257310557083,3.64303198860234));
#228475=CARTESIAN_POINT('',(46.4257404597086,-41.5455814344523,3.40423097483282));
#228476=CARTESIAN_POINT('Origin',(46.1339944931989,-41.2828921862993,3.20400259735935));
#228477=CARTESIAN_POINT('',(46.6905216405931,-41.7839914799656,2.83404198860233));
#228478=CARTESIAN_POINT('',(46.4257404597086,-41.5455814344523,3.40423097483282));
#228479=CARTESIAN_POINT('',(44.1339623850452,-39.4820551873923,2.83404198860234));
#228480=CARTESIAN_POINT('',(0.127469380511362,0.141569089253638,2.83404198860262));
#228481=CARTESIAN_POINT('',(44.3987439293953,-39.7204655617323,3.40423097483283));
#228482=CARTESIAN_POINT('',(44.1339623850452,-39.4820551873923,2.83404198860235));
#228483=CARTESIAN_POINT('',(44.7189015017603,-40.0087367337506,3.64303198860235));
#228484=CARTESIAN_POINT('Origin',(44.6904903152704,-39.9831551865318,3.20400220587396));
#228485=CARTESIAN_POINT('',(45.0171848258476,-40.2773122461031,3.64303198860235));
#228486=CARTESIAN_POINT('',(45.0720719232488,-40.3267328095852,3.64303198860235));
#228487=CARTESIAN_POINT('',(45.1108495273517,-40.3616483211477,3.42473028058454));
#228488=CARTESIAN_POINT('',(45.0171848263437,-40.2773122455521,3.64303198860235));
#228489=CARTESIAN_POINT('',(45.3560577375101,-40.5824347852693,3.23423028058454));
#228490=CARTESIAN_POINT('Origin',(45.3341886054736,-40.5627444213173,3.56425743003981));
#228491=CARTESIAN_POINT('',(45.4684272662441,-40.6836127633972,3.23423028058454));
#228492=CARTESIAN_POINT('',(45.468820175067,-40.6839665400904,3.23423028058454));
#228493=CARTESIAN_POINT('',(45.7136354238381,-40.9043991801896,3.42473028058456));
#228494=CARTESIAN_POINT('Origin',(45.4902978619872,-40.7033058269848,3.56425912917625));
#228495=CARTESIAN_POINT('',(45.8073000857364,-40.9887352205706,3.64303198860234));
#228496=CARTESIAN_POINT('',(45.7136354238381,-40.9043991801896,3.42473028058456));
#228497=CARTESIAN_POINT('',(46.1059706796549,-41.2576594312477,3.64303198860234));
#228498=CARTESIAN_POINT('Origin',(47.0244087227346,-34.4007037410856,2.65878198860239));
#228499=CARTESIAN_POINT('',(47.7640607692767,-34.6837837831338,2.65878198860238));
#228500=CARTESIAN_POINT('',(50.8527980281389,-36.9278827595319,2.65878198860237));
#228501=CARTESIAN_POINT('',(47.1453396605412,-34.2342565846629,2.65878198860239));
#228502=CARTESIAN_POINT('',(50.8348823336491,-36.9525415975204,2.65878198860237));
#228503=CARTESIAN_POINT('Origin',(5.52786294311959E-15,1.85082121769273E-13,
2.65878198860263));
#228504=CARTESIAN_POINT('',(47.7461450747869,-34.7084426211224,2.65878198860238));
#228505=CARTESIAN_POINT('',(47.6889451092156,-34.6668844135344,2.65878198860238));
#228506=CARTESIAN_POINT('Origin',(5.70871613546578E-15,1.85392900923618E-13,
2.65878198860263));
#228507=CARTESIAN_POINT('Origin',(-0.111973090561714,-0.154117737428518,
42.7590319886026));
#228508=CARTESIAN_POINT('',(48.4320322672535,-35.4234021096002,3.64303198860239));
#228509=CARTESIAN_POINT('',(48.0834960093688,-35.1701756956951,3.40423097483286));
#228510=CARTESIAN_POINT('Origin',(48.4011027206439,-35.4009304786163,3.20400220531683));
#228511=CARTESIAN_POINT('',(47.7952442958629,-34.960748566406,2.83404198860238));
#228512=CARTESIAN_POINT('',(48.0834960093688,-35.1701756956951,3.40423097483286));
#228513=CARTESIAN_POINT('',(50.5784163149361,-36.9828414016739,2.83404198860236));
#228514=CARTESIAN_POINT('',(50.7885878366285,-37.135539950359,2.83404198860236));
#228515=CARTESIAN_POINT('',(50.2901649972897,-36.7734145613994,3.40423097483285));
#228516=CARTESIAN_POINT('',(50.5784163149361,-36.9828414016739,2.83404198860236));
#228517=CARTESIAN_POINT('',(49.9416290966442,-36.5201884062945,3.64303198860239));
#228518=CARTESIAN_POINT('Origin',(49.9725587428726,-36.5426601096557,3.20400259788266));
#228519=CARTESIAN_POINT('',(49.6169062253194,-36.2842634313401,3.64303198860238));
#228520=CARTESIAN_POINT('',(-0.111973090561709,-0.154117737428245,3.64303198860263));
#228521=CARTESIAN_POINT('',(49.5149391519582,-36.2101800152079,3.42473028058461));
#228522=CARTESIAN_POINT('',(49.6169062257374,-36.2842634307648,3.64303198860238));
#228523=CARTESIAN_POINT('',(49.2479958054503,-36.0162343214019,3.23423028058457));
#228524=CARTESIAN_POINT('Origin',(49.2718033882774,-36.0335309082452,3.56425722717045));
#228525=CARTESIAN_POINT('',(49.1256658701819,-35.9273564209813,3.23423028058457));
#228526=CARTESIAN_POINT('',(-0.111973090561709,-0.154117737428242,3.23423028058481));
#228527=CARTESIAN_POINT('',(48.8587224664505,-35.7334106855999,3.42473028058457));
#228528=CARTESIAN_POINT('Origin',(49.1018565378152,-35.9100572938234,3.56425909741191));
#228529=CARTESIAN_POINT('',(48.7567553500948,-35.6593272391094,3.64303198860238));
#228530=CARTESIAN_POINT('',(48.8587224664505,-35.7334106855999,3.42473028058457));
#228531=CARTESIAN_POINT('',(-0.111973090561709,-0.154117737428245,3.64303198860263));
#228532=CARTESIAN_POINT('Origin',(0.111973090561714,0.15411773742834,42.7590319886026));
#228533=CARTESIAN_POINT('',(50.1655752777676,-36.2119529314377,3.64303198860238));
#228534=CARTESIAN_POINT('',(50.5141111787694,-36.4651790860522,3.40423097483286));
#228535=CARTESIAN_POINT('Origin',(50.1965049237626,-36.2344246346292,3.20400259735642));
#228536=CARTESIAN_POINT('',(50.8023624963256,-36.6746059264507,2.83404198860237));
#228537=CARTESIAN_POINT('',(50.5141111787694,-36.4651790860522,3.40423097483285));
#228538=CARTESIAN_POINT('',(48.0191904766741,-34.6525130919789,2.83404198860238));
#228539=CARTESIAN_POINT('',(0.111973090561715,0.154117737428622,2.83404198860262));
#228540=CARTESIAN_POINT('',(48.3074421900767,-34.8619402214102,3.40423097483287));
#228541=CARTESIAN_POINT('',(48.0191904766741,-34.6525130919789,2.83404198860238));
#228542=CARTESIAN_POINT('',(48.6559784483769,-35.1151666347433,3.64303198860239));
#228543=CARTESIAN_POINT('Origin',(48.6250489015204,-35.0926950035802,3.20400220587407));
#228544=CARTESIAN_POINT('',(48.9807015307823,-35.3510917648527,3.64303198860238));
#228545=CARTESIAN_POINT('',(49.0404538064758,-35.3945043333723,3.64303198860239));
#228546=CARTESIAN_POINT('',(49.0826686475739,-35.425175210743,3.42473028058457));
#228547=CARTESIAN_POINT('',(48.9807015312183,-35.3510917642526,3.64303198860239));
#228548=CARTESIAN_POINT('',(49.3496120513054,-35.6191209461244,3.23423028058457));
#228549=CARTESIAN_POINT('Origin',(49.325804517179,-35.6018243948125,3.56425743004393));
#228550=CARTESIAN_POINT('',(49.4719419865737,-35.707998846545,3.23423028058457));
#228551=CARTESIAN_POINT('',(49.4723697227352,-35.7083096150571,3.23423028058457));
#228552=CARTESIAN_POINT('',(49.7388853330816,-35.9019445403511,3.42473028058459));
#228553=CARTESIAN_POINT('Origin',(49.4957512585772,-35.7252979297049,3.56425912917973));
#228554=CARTESIAN_POINT('',(49.8408524068608,-35.9760279559079,3.64303198860239));
#228555=CARTESIAN_POINT('',(49.7388853330816,-35.9019445403511,3.42473028058459));
#228556=CARTESIAN_POINT('',(50.165997086493,-36.2122593934154,3.64303198860238));
#228557=CARTESIAN_POINT('Origin',(50.3626567888879,-29.2968639067293,2.65878198860242));
#228558=CARTESIAN_POINT('',(51.1278468659051,-29.5010785149103,2.65878198860242));
#228559=CARTESIAN_POINT('',(54.4342359163067,-31.4100231232053,2.65878198860241));
#228560=CARTESIAN_POINT('',(50.4655267888879,-29.1186878401547,2.65878198860242));
#228561=CARTESIAN_POINT('',(54.4189959163067,-31.4364195775126,2.65878198860241));
#228562=CARTESIAN_POINT('Origin',(5.51948237368594E-15,1.85069216824025E-13,
2.65878198860263));
#228563=CARTESIAN_POINT('',(51.1126068659051,-29.5274749692176,2.65878198860242));
#228564=CARTESIAN_POINT('',(51.0513762321548,-29.4921234463392,2.65878198860242));
#228565=CARTESIAN_POINT('Origin',(5.71307961579125E-15,1.85399620094091E-13,
2.65878198860263));
#228566=CARTESIAN_POINT('Origin',(-0.0952499999999979,-0.164977839421026,
42.7590319886026));
#228567=CARTESIAN_POINT('',(51.869470313195,-30.1668231006066,3.64303198860242));
#228568=CARTESIAN_POINT('',(51.4963740054947,-29.9514158469222,3.4042309748329));
#228569=CARTESIAN_POINT('Origin',(51.8363612768233,-30.1477075895448,3.20400220531909));
#228570=CARTESIAN_POINT('',(51.187810269045,-29.7732664900063,2.83404198860242));
#228571=CARTESIAN_POINT('',(51.4963740054947,-29.9514158469222,3.4042309748329));
#228572=CARTESIAN_POINT('',(54.1671020372442,-31.493361394985,2.8340419886024));
#228573=CARTESIAN_POINT('',(54.3920835619875,-31.6232545388582,2.8340419886024));
#228574=CARTESIAN_POINT('',(53.8585387246959,-31.3152122841216,3.40423097483289));
#228575=CARTESIAN_POINT('',(54.1671020372442,-31.493361394985,2.8340419886024));
#228576=CARTESIAN_POINT('',(53.4854427993291,-31.0998052504791,3.64303198860242));
#228577=CARTESIAN_POINT('Origin',(53.5185519423371,-31.1189208231074,3.20400259787966));
#228578=CARTESIAN_POINT('',(53.1378379187913,-30.8991154799502,3.64303198860242));
#228579=CARTESIAN_POINT('',(-0.0952499999999924,-0.164977839420753,3.64303198860263));
#228580=CARTESIAN_POINT('',(53.028685606085,-30.8360963620053,3.42473028058464));
#228581=CARTESIAN_POINT('',(53.1378379191468,-30.8991154793343,3.64303198860242));
#228582=CARTESIAN_POINT('',(52.7429317578291,-30.6711163007929,3.23423028058461));
#228583=CARTESIAN_POINT('Origin',(52.7684169058679,-30.685829565076,3.5642572271725));
#228584=CARTESIAN_POINT('',(52.6119816883963,-30.5955122429554,3.23423028058461));
#228585=CARTESIAN_POINT('',(-0.0952499999999923,-0.16497783942075,3.23423028058481));
#228586=CARTESIAN_POINT('',(52.3262277788845,-30.4305321463768,3.42473028058461));
#228587=CARTESIAN_POINT('Origin',(52.5864945348665,-30.5807966351502,3.56425909741314));
#228588=CARTESIAN_POINT('',(52.217075420246,-30.3675130027342,3.64303198860242));
#228589=CARTESIAN_POINT('',(52.3262277788845,-30.4305321463768,3.42473028058461));
#228590=CARTESIAN_POINT('',(-0.0952499999999924,-0.164977839420753,3.64303198860263));
#228591=CARTESIAN_POINT('Origin',(0.0952499999999979,0.164977839420847,
42.7590319886026));
#228592=CARTESIAN_POINT('',(53.675942799329,-30.7698495716372,3.64303198860242));
#228593=CARTESIAN_POINT('',(54.0490387249983,-30.9852566047559,3.40423097483289));
#228594=CARTESIAN_POINT('Origin',(53.7090519420895,-30.7889651441226,3.20400259735806));
#228595=CARTESIAN_POINT('',(54.3576020374704,-31.1634057157514,2.8340419886024));
#228596=CARTESIAN_POINT('',(54.0490387249983,-30.9852566047559,3.40423097483289));
#228597=CARTESIAN_POINT('',(51.3783102687789,-29.4433108116253,2.83404198860242));
#228598=CARTESIAN_POINT('',(0.0952499999999987,0.164977839421129,2.83404198860262));
#228599=CARTESIAN_POINT('',(51.6868740051417,-29.6214601686917,3.40423097483291));
#228600=CARTESIAN_POINT('',(51.3783102687789,-29.4433108116253,2.83404198860242));
#228601=CARTESIAN_POINT('',(52.059970313195,-29.8368674217647,3.64303198860242));
#228602=CARTESIAN_POINT('Origin',(52.0268612765608,-29.8177519105514,3.20400220587201));
#228603=CARTESIAN_POINT('',(52.4075754198753,-30.0375573245345,3.64303198860242));
#228604=CARTESIAN_POINT('',(52.4715382154243,-30.0744862609066,3.64303198860242));
#228605=CARTESIAN_POINT('',(52.5167277788845,-30.1005764675349,3.42473028058461));
#228606=CARTESIAN_POINT('',(52.407575420246,-30.0375573238923,3.64303198860242));
#228607=CARTESIAN_POINT('',(52.8024816883963,-30.2655565641136,3.23423028058461));
#228608=CARTESIAN_POINT('Origin',(52.7769965925028,-30.2508433300749,3.56425743003977));
#228609=CARTESIAN_POINT('',(52.9334317578291,-30.341160621951,3.23423028058461));
#228610=CARTESIAN_POINT('',(52.9338896349621,-30.341424977437,3.23423028058461));
#228611=CARTESIAN_POINT('',(53.219185606085,-30.5061406831635,3.42473028058463));
#228612=CARTESIAN_POINT('Origin',(52.9589188467291,-30.3558761923098,3.56425912917761));
#228613=CARTESIAN_POINT('',(53.3283379191468,-30.5691598004924,3.64303198860242));
#228614=CARTESIAN_POINT('',(53.219185606085,-30.5061406831635,3.42473028058463));
#228615=CARTESIAN_POINT('',(53.6763943313417,-30.7701102637663,3.64303198860242));
#228616=CARTESIAN_POINT('Origin',(53.1491210481986,-23.8720415006481,2.65878198860246));
#228617=CARTESIAN_POINT('',(53.9314655730807,-23.9951532569799,2.65878198860246));
#228618=CARTESIAN_POINT('',(57.4192809246792,-25.548028700571,2.65878198860245));
#228619=CARTESIAN_POINT('',(53.2328030451451,-23.6840886581928,2.65878198860246));
#228620=CARTESIAN_POINT('',(57.4068835917983,-25.5758735661199,2.65878198860245));
#228621=CARTESIAN_POINT('Origin',(5.51249664798382E-15,1.85055506565373E-13,
2.65878198860263));
#228622=CARTESIAN_POINT('',(53.9190682401998,-24.0229981225288,2.65878198860246));
#228623=CARTESIAN_POINT('',(53.8544777939072,-23.9942406030425,2.65878198860246));
#228624=CARTESIAN_POINT('Origin',(5.71671684795091E-15,1.85406758564139E-13,
2.65878198860263));
#228625=CARTESIAN_POINT('Origin',(-0.0774833305059378,-0.174030409681006,
42.7590319886026));
#228626=CARTESIAN_POINT('',(54.7386155880007,-24.5797300649093,3.64303198860246));
#228627=CARTESIAN_POINT('',(54.3450469517073,-24.4045020183937,3.40423097483294));
#228628=CARTESIAN_POINT('Origin',(54.7036898113994,-24.5641801073097,3.20400220531724));
#228629=CARTESIAN_POINT('',(54.0195518811808,-24.2595822754864,2.83404198860245));
#228630=CARTESIAN_POINT('',(54.3450469517073,-24.4045020183937,3.40423097483294));
#228631=CARTESIAN_POINT('',(57.1623216544374,-25.6588335304432,2.83404198860244));
#228632=CARTESIAN_POINT('',(57.399648237566,-25.7644981330383,2.83404198860244));
#228633=CARTESIAN_POINT('',(56.8368270312097,-25.5139139879307,3.40423097483294));
#228634=CARTESIAN_POINT('',(57.1623216544374,-25.6588335304432,2.83404198860244));
#228635=CARTESIAN_POINT('',(56.443258798156,-25.3386861202868,3.64303198860246));
#228636=CARTESIAN_POINT('Origin',(56.478184687247,-25.3542361279701,3.20400259788249));
#228637=CARTESIAN_POINT('',(56.0765803402173,-25.1754303533064,3.64303198860245));
#228638=CARTESIAN_POINT('',(-0.0774833305059323,-0.174030409680733,3.64303198860263));
#228639=CARTESIAN_POINT('',(55.9614386837456,-25.1241659841927,3.42473028058468));
#228640=CARTESIAN_POINT('',(56.0765803405066,-25.1754303526566,3.64303198860245));
#228641=CARTESIAN_POINT('',(55.6600051127011,-24.9899591116487,3.23423028058465));
#228642=CARTESIAN_POINT('Origin',(55.6868886053365,-25.0019278517695,3.56425722717436));
#228643=CARTESIAN_POINT('',(55.5218696254676,-24.9284572302733,3.23423028058465));
#228644=CARTESIAN_POINT('',(-0.0774833305059322,-0.17403040968073,3.23423028058481));
#228645=CARTESIAN_POINT('',(55.2204359898059,-24.7942503289599,3.42473028058464));
#228646=CARTESIAN_POINT('Origin',(55.4949838933612,-24.9164863690988,3.56425909741192));
#228647=CARTESIAN_POINT('',(55.1052942849675,-24.7429859390905,3.64303198860246));
#228648=CARTESIAN_POINT('',(55.2204359898059,-24.7942503289599,3.42473028058464));
#228649=CARTESIAN_POINT('',(-0.0774833305059323,-0.174030409680733,3.64303198860263));
#228650=CARTESIAN_POINT('Origin',(0.0774833305059378,0.174030409680827,
42.7590319886026));
#228651=CARTESIAN_POINT('',(56.5982254591679,-24.990625300925,3.64303198860246));
#228652=CARTESIAN_POINT('',(56.9917936924676,-25.1658531680162,3.40423097483293));
#228653=CARTESIAN_POINT('Origin',(56.6331513479955,-25.0061753084909,3.20400259735638));
#228654=CARTESIAN_POINT('',(57.3172883156333,-25.3107727106681,2.83404198860245));
#228655=CARTESIAN_POINT('',(56.9917936924676,-25.1658531680162,3.40423097483293));
#228656=CARTESIAN_POINT('',(54.1745185419763,-23.9115214566106,2.83404198860245));
#228657=CARTESIAN_POINT('',(0.0774833305059383,0.174030409681108,2.83404198860262));
#228658=CARTESIAN_POINT('',(54.5000136124319,-24.0564411996771,3.40423097483294));
#228659=CARTESIAN_POINT('',(54.1745185419763,-23.9115214566106,2.83404198860246));
#228660=CARTESIAN_POINT('',(54.8935822490125,-24.2316692455474,3.64303198860246));
#228661=CARTESIAN_POINT('Origin',(54.8586564721336,-24.2161192878243,3.20400220587174));
#228662=CARTESIAN_POINT('',(55.2602609456776,-24.3949251204063,3.64303198860247));
#228663=CARTESIAN_POINT('',(55.3277334713093,-24.4249658234757,3.64303198860246));
#228664=CARTESIAN_POINT('',(55.3754026508178,-24.446189509598,3.42473028058465));
#228665=CARTESIAN_POINT('',(55.2602609459794,-24.3949251197286,3.64303198860247));
#228666=CARTESIAN_POINT('',(55.6768362864795,-24.5803964109114,3.23423028058465));
#228667=CARTESIAN_POINT('Origin',(55.6499528488669,-24.5684276954195,3.56425743004579));
#228668=CARTESIAN_POINT('',(55.814971773713,-24.6418982922869,3.23423028058465));
#228669=CARTESIAN_POINT('',(55.8154547752198,-24.6421133384127,3.23423028058465));
#228670=CARTESIAN_POINT('',(56.1164053447575,-24.7761051648309,3.42473028058467));
#228671=CARTESIAN_POINT('Origin',(55.8418574376288,-24.6538691229756,3.56425912917798));
#228672=CARTESIAN_POINT('',(56.2315470015185,-24.8273695332948,3.64303198860246));
#228673=CARTESIAN_POINT('',(56.1164053447575,-24.7761051648309,3.42473028058467));
#228674=CARTESIAN_POINT('',(56.5987017673886,-24.9908373670079,3.64303198860246));
#228675=CARTESIAN_POINT('Origin',(55.3532724151367,-18.1856720123399,2.6587819886025));
#228676=CARTESIAN_POINT('',(56.144199857553,-18.2263320786573,2.6587819886025));
#228677=CARTESIAN_POINT('',(59.7752282754839,-19.4061247292244,2.65878198860249));
#228678=CARTESIAN_POINT('',(55.4168495715594,-17.9900016446774,2.6587819886025));
#228679=CARTESIAN_POINT('',(59.7658094374954,-19.4351129318411,2.65878198860249));
#228680=CARTESIAN_POINT('Origin',(5.50698230308587E-15,1.85041141205781E-13,
2.65878198860263));
#228681=CARTESIAN_POINT('',(56.1347810195644,-18.255320281274,2.6587819886025));
#228682=CARTESIAN_POINT('',(56.0675384271755,-18.2334718385811,2.6587819886025));
#228683=CARTESIAN_POINT('Origin',(5.71958798166808E-15,1.85414238123189E-13,
2.65878198860263));
#228684=CARTESIAN_POINT('Origin',(-0.0588677374284251,-0.181176266354317,
42.7590319886026));
#228685=CARTESIAN_POINT('',(57.0080331356325,-18.7233363629815,3.6430319886025));
#228686=CARTESIAN_POINT('',(56.5983041910848,-18.5902073587813,3.40423097483299));
#228687=CARTESIAN_POINT('Origin',(56.9716732729175,-18.7115223274331,3.20400220531805));
#228688=CARTESIAN_POINT('',(56.2594439785883,-18.4801050009127,2.8340419886025));
#228689=CARTESIAN_POINT('',(56.5983041910848,-18.5902073587813,3.40423097483299));
#228690=CARTESIAN_POINT('',(59.5312589135998,-19.5431821162857,2.83404198860249));
#228691=CARTESIAN_POINT('',(59.7783303554051,-19.6234604941049,2.83404198860249));
#228692=CARTESIAN_POINT('',(59.1923991668989,-19.4330799109579,3.40423097483297));
#228693=CARTESIAN_POINT('',(59.5312589135998,-19.5431821162857,2.83404198860249));
#228694=CARTESIAN_POINT('',(58.7826706420791,-19.2999510424997,3.6430319886025));
#228695=CARTESIAN_POINT('Origin',(58.8190306219008,-19.3117651160984,3.20400259787949));
#228696=CARTESIAN_POINT('',(58.400936012657,-19.1759179434147,3.6430319886025));
#228697=CARTESIAN_POINT('',(-0.0588677374284196,-0.181176266354044,3.64303198860263));
#228698=CARTESIAN_POINT('',(58.2810665285032,-19.1369699862874,3.42473028058473));
#228699=CARTESIAN_POINT('',(58.4009360128769,-19.1759179427377,3.6430319886025));
#228700=CARTESIAN_POINT('',(57.9672558039534,-19.0350067009921,3.23423028058469));
#228701=CARTESIAN_POINT('Origin',(57.9952431000169,-19.0440997849303,3.56425722717133));
#228702=CARTESIAN_POINT('',(57.8234483402241,-18.9882808235611,3.23423028058469));
#228703=CARTESIAN_POINT('',(-0.0588677374284196,-0.181176266354041,3.23423028058481));
#228704=CARTESIAN_POINT('',(57.5096375484039,-18.8863175164083,3.42473028058468));
#228705=CARTESIAN_POINT('Origin',(57.795458595248,-18.9791858642773,3.56425909741065));
#228706=CARTESIAN_POINT('',(57.3897680139787,-18.8473695436953,3.6430319886025));
#228707=CARTESIAN_POINT('',(57.5096375484039,-18.8863175164083,3.42473028058468));
#228708=CARTESIAN_POINT('',(-0.0588677374284196,-0.181176266354044,3.64303198860263));
#228709=CARTESIAN_POINT('Origin',(0.0588677374284251,0.181176266354138,
42.7590319886026));
#228710=CARTESIAN_POINT('',(58.9004061169359,-18.9375985097912,3.6430319886025));
#228711=CARTESIAN_POINT('',(59.3101346419426,-19.0707273776743,3.40423097483297));
#228712=CARTESIAN_POINT('Origin',(58.9367660964857,-18.9494125833016,3.20400259735816));
#228713=CARTESIAN_POINT('',(59.6489943885965,-19.1808295831467,2.83404198860249));
#228714=CARTESIAN_POINT('',(59.3101346419426,-19.0707273776743,3.40423097483297));
#228715=CARTESIAN_POINT('',(56.377179453281,-18.1177524687097,2.8340419886025));
#228716=CARTESIAN_POINT('',(0.0588677374284254,0.181176266354419,2.83404198860262));
#228717=CARTESIAN_POINT('',(56.7160396657232,-18.2278548267452,3.40423097483298));
#228718=CARTESIAN_POINT('',(56.377179453281,-18.1177524687097,2.83404198860249));
#228719=CARTESIAN_POINT('',(57.1257686104893,-18.3609838302731,3.6430319886025));
#228720=CARTESIAN_POINT('Origin',(57.0894087474848,-18.3491697946306,3.20400220587425));
#228721=CARTESIAN_POINT('',(57.5075034886063,-18.4850170116922,3.6430319886025));
#228722=CARTESIAN_POINT('',(57.5777465012101,-18.5078403492301,3.6430319886025));
#228723=CARTESIAN_POINT('',(57.6273730232608,-18.5239649836999,3.42473028058467));
#228724=CARTESIAN_POINT('',(57.5075034888355,-18.4850170109868,3.6430319886025));
#228725=CARTESIAN_POINT('',(57.941183815081,-18.6259282908527,3.23423028058469));
#228726=CARTESIAN_POINT('Origin',(57.9131965763133,-18.616835225657,3.56425743004289));
#228727=CARTESIAN_POINT('',(58.0849912788103,-18.6726541682836,3.23423028058469));
#228728=CARTESIAN_POINT('',(58.0854941128254,-18.6728175489591,3.23423028058469));
#228729=CARTESIAN_POINT('',(58.3988020033601,-18.774617453579,3.42473028058471));
#228730=CARTESIAN_POINT('Origin',(58.1129809527839,-18.6817491043768,3.5642591291744));
#228731=CARTESIAN_POINT('',(58.5186714877338,-18.8135654100293,3.64303198860251));
#228732=CARTESIAN_POINT('',(58.3988020033601,-18.774617453579,3.42473028058471));
#228733=CARTESIAN_POINT('',(58.9009019828321,-18.9377596263876,3.6430319886025));
#228734=CARTESIAN_POINT('Origin',(56.9509617460776,-12.3000564958681,2.65878198860254));
#228735=CARTESIAN_POINT('',(57.7418065394567,-12.2578193919758,2.65878198860254));
#228736=CARTESIAN_POINT('',(61.4762657165317,-13.0516031943519,2.65878198860254));
#228737=CARTESIAN_POINT('',(56.9937374973465,-12.0988124084931,2.65878198860254));
#228738=CARTESIAN_POINT('',(61.4699285681956,-13.0814171332223,2.65878198860254));
#228739=CARTESIAN_POINT('Origin',(5.50299975530876E-15,1.85026278135133E-13,
2.65878198860263));
#228740=CARTESIAN_POINT('',(57.7354693911206,-12.2876333308462,2.65878198860254));
#228741=CARTESIAN_POINT('',(57.666311376549,-12.2729333410569,2.65878198860254));
#228742=CARTESIAN_POINT('Origin',(5.72166156020094E-15,1.85421976823627E-13,
2.65878198860263));
#228743=CARTESIAN_POINT('Origin',(-0.0396071771007808,-0.18633711793988,
42.7590319886026));
#228744=CARTESIAN_POINT('',(58.6528587425324,-12.661805869751,3.64303198860255));
#228745=CARTESIAN_POINT('',(58.2314585657882,-12.5722344970951,3.40423097483302));
#228746=CARTESIAN_POINT('Origin',(58.6154631599697,-12.6538571932998,3.20400220531626));
#228747=CARTESIAN_POINT('',(57.8829458347212,-12.4981558287377,2.83404198860254));
#228748=CARTESIAN_POINT('',(58.2314585657882,-12.5722344970951,3.40423097483302));
#228749=CARTESIAN_POINT('',(61.2479592423879,-13.2134115091884,2.83404198860253));
#228750=CARTESIAN_POINT('',(61.5020685764506,-13.267424115525,2.83404198860253));
#228751=CARTESIAN_POINT('',(60.8994469905095,-13.1393329438485,3.40423097483302));
#228752=CARTESIAN_POINT('',(61.2479592423879,-13.2134115091884,2.83404198860253));
#228753=CARTESIAN_POINT('',(60.4780472453829,-13.0497616623165,3.64303198860255));
#228754=CARTESIAN_POINT('Origin',(60.51544294839,-13.057710364369,3.20400259788175));
#228755=CARTESIAN_POINT('',(60.0854388089606,-12.9663101637158,3.64303198860254));
#228756=CARTESIAN_POINT('',(-0.0396071771007753,-0.186337117939607,3.64303198860262));
#228757=CARTESIAN_POINT('',(59.9621548122773,-12.940105340544,3.42473028058477));
#228758=CARTESIAN_POINT('',(60.0854388091086,-12.9663101630194,3.64303198860254));
#228759=CARTESIAN_POINT('',(59.6394051101895,-12.8715027735882,3.23423028058473));
#228760=CARTESIAN_POINT('Origin',(59.6681895750078,-12.8776205756128,3.56425722717025));
#228761=CARTESIAN_POINT('',(59.4915012546306,-12.8400648385929,3.23423028058473));
#228762=CARTESIAN_POINT('',(-0.0396071771007752,-0.186337117939604,3.23423028058481));
#228763=CARTESIAN_POINT('',(59.1687514833562,-12.771462256931,3.42473028058473));
#228764=CARTESIAN_POINT('Origin',(59.462714158291,-12.8339454274777,3.56425909741496));
#228765=CARTESIAN_POINT('',(59.0454674350476,-12.7452574235138,3.64303198860254));
#228766=CARTESIAN_POINT('',(59.1687514833562,-12.771462256931,3.42473028058473));
#228767=CARTESIAN_POINT('',(-0.0396071771007753,-0.186337117939607,3.64303198860262));
#228768=CARTESIAN_POINT('Origin',(0.0396071771007808,0.186337117939701,
42.7590319886026));
#228769=CARTESIAN_POINT('',(60.5572615995845,-12.677087426437,3.64303198860255));
#228770=CARTESIAN_POINT('',(60.9786613448369,-12.7666587073764,3.40423097483302));
#228771=CARTESIAN_POINT('Origin',(60.594657302311,-12.6850361284297,3.20400259735834));
#228772=CARTESIAN_POINT('',(61.3271735966835,-12.8407372728664,2.83404198860253));
#228773=CARTESIAN_POINT('',(60.9786613448369,-12.7666587073764,3.40423097483302));
#228774=CARTESIAN_POINT('',(57.9621601888122,-12.1254815933782,2.83404198860254));
#228775=CARTESIAN_POINT('',(0.0396071771007809,0.186337117939981,2.83404198860263));
#228776=CARTESIAN_POINT('',(58.3106729198429,-12.1995602619066,3.40423097483303));
#228777=CARTESIAN_POINT('',(57.9621601888122,-12.1254815933782,2.83404198860254));
#228778=CARTESIAN_POINT('',(58.7320730967339,-12.2891316338714,3.64303198860255));
#228779=CARTESIAN_POINT('Origin',(58.6946775138721,-12.2811829573567,3.20400220587502));
#228780=CARTESIAN_POINT('',(59.1246817890951,-12.3725831883593,3.64303198860254));
#228781=CARTESIAN_POINT('',(59.1969256915255,-12.3879391031037,3.64303198860255));
#228782=CARTESIAN_POINT('',(59.2479658375578,-12.3987880210515,3.42473028058472));
#228783=CARTESIAN_POINT('',(59.1246817892492,-12.3725831876342,3.64303198860255));
#228784=CARTESIAN_POINT('',(59.5707156088322,-12.4673906027133,3.23423028058473));
#228785=CARTESIAN_POINT('Origin',(59.541931202957,-12.46127281334,3.5642574300457));
#228786=CARTESIAN_POINT('',(59.7186194643911,-12.4988285377087,3.23423028058473));
#228787=CARTESIAN_POINT('',(59.7191366217598,-12.4989384629008,3.23423028058473));
#228788=CARTESIAN_POINT('',(60.0413691664789,-12.5674311046645,3.42473028058476));
#228789=CARTESIAN_POINT('Origin',(59.7474064876929,-12.504947933182,3.56425912917895));
#228790=CARTESIAN_POINT('',(60.1646531633102,-12.5936359271399,3.64303198860255));
#228791=CARTESIAN_POINT('',(60.0413691664789,-12.5674311046645,3.42473028058476));
#228792=CARTESIAN_POINT('',(60.5577715903456,-12.6771958283196,3.64303198860255));
#228793=CARTESIAN_POINT('Origin',(57.9246844223736,-6.27967898647509,2.65878198860258));
#228794=CARTESIAN_POINT('',(58.7067819056644,-6.15500747092217,2.65878198860258));
#228795=CARTESIAN_POINT('',(62.5037563256536,-6.55408556365842,2.65878198860258));
#228796=CARTESIAN_POINT('',(57.9461901084063,-6.07506605172202,2.65878198860258));
#228797=CARTESIAN_POINT('',(62.5005702980932,-6.58439859102925,2.65878198860258));
#228798=CARTESIAN_POINT('Origin',(5.50059263827931E-15,1.85011080196342E-13,
2.65878198860263));
#228799=CARTESIAN_POINT('',(58.703595878104,-6.185320498293,2.65878198860258));
#228800=CARTESIAN_POINT('',(58.6332801510296,-6.1779300175717,2.65878198860258));
#228801=CARTESIAN_POINT('Origin',(5.72291486498914E-15,1.85429889878632E-13,
2.65878198860263));
#228802=CARTESIAN_POINT('Origin',(-0.0199126722524855,-0.189456421067746,
42.7590319886026));
#228803=CARTESIAN_POINT('',(59.6550713551494,-6.46154998175819,3.64303198860259));
#228804=CARTESIAN_POINT('',(59.2266168947287,-6.41651760334952,3.40423097483306));
#228805=CARTESIAN_POINT('Origin',(59.6170497665656,-6.4575537517665,3.20400220531816));
#228806=CARTESIAN_POINT('',(58.8722700235037,-6.37927424589621,2.83404198860258));
#228807=CARTESIAN_POINT('',(59.2266168947287,-6.41651760334952,3.40423097483306));
#228808=CARTESIAN_POINT('',(62.293614112757,-6.73887200051229,2.83404198860258));
#228809=CARTESIAN_POINT('',(62.5519772640373,-6.76602706194843,2.83404198860258));
#228810=CARTESIAN_POINT('',(61.9392677288638,-6.70162869542246,3.40423097483306));
#228811=CARTESIAN_POINT('',(62.293614112757,-6.73887200051229,2.83404198860258));
#228812=CARTESIAN_POINT('',(61.5108137072213,-6.65659636252282,3.64303198860259));
#228813=CARTESIAN_POINT('Origin',(61.5488354182641,-6.66059260538546,3.20400259787972));
#228814=CARTESIAN_POINT('',(61.1116329639869,-6.61464077648827,3.64303198860259));
#228815=CARTESIAN_POINT('',(-0.0199126722524799,-0.189456421067473,3.64303198860262));
#228816=CARTESIAN_POINT('',(60.9862851800405,-6.60146619279846,3.42473028058482));
#228817=CARTESIAN_POINT('',(61.1116329640613,-6.61464077578021,3.64303198860259));
#228818=CARTESIAN_POINT('',(60.6581326136905,-6.56697596826177,3.23423028058478));
#228819=CARTESIAN_POINT('Origin',(60.6873988786434,-6.5700514604533,3.56425722717));
#228820=CARTESIAN_POINT('',(60.5077528318945,-6.55117041629668,3.23423028058478));
#228821=CARTESIAN_POINT('',(-0.0199126722524799,-0.18945642106747,3.23423028058481));
#228822=CARTESIAN_POINT('',(60.1796001951996,-6.51668018436646,3.42473028058476));
#228823=CARTESIAN_POINT('Origin',(60.4784837816402,-6.54809359889815,3.56425909741463));
#228824=CARTESIAN_POINT('',(60.0542523588398,-6.50350559588366,3.64303198860259));
#228825=CARTESIAN_POINT('',(60.1796001951996,-6.51668018436646,3.42473028058476));
#228826=CARTESIAN_POINT('',(-0.0199126722524799,-0.189456421067473,3.64303198860262));
#228827=CARTESIAN_POINT('Origin',(0.0199126722524855,0.189456421067567,
42.7590319886026));
#228828=CARTESIAN_POINT('',(61.5506390517263,-6.27768352038751,3.64303198860259));
#228829=CARTESIAN_POINT('',(61.979093073432,-6.32271585268538,3.40423097483306));
#228830=CARTESIAN_POINT('Origin',(61.5886607624847,-6.28167976322025,3.20400259735804));
#228831=CARTESIAN_POINT('',(62.3334394573093,-6.35995915792693,2.83404198860258));
#228832=CARTESIAN_POINT('',(61.979093073432,-6.32271585268538,3.40423097483306));
#228833=CARTESIAN_POINT('',(58.9120953679531,-6.00036140428947,2.83404198860258));
#228834=CARTESIAN_POINT('',(0.0199126722524855,0.189456421067846,2.83404198860263));
#228835=CARTESIAN_POINT('',(59.2664422391598,-6.03760476191704,3.40423097483307));
#228836=CARTESIAN_POINT('',(58.9120953679531,-6.00036140428947,2.83404198860258));
#228837=CARTESIAN_POINT('',(59.6948966996543,-6.08263713962288,3.64303198860259));
#228838=CARTESIAN_POINT('Origin',(59.6568751107681,-6.0786409095994,3.20400220587286));
#228839=CARTESIAN_POINT('',(60.0940777032672,-6.12459275448601,3.64303198860259));
#228840=CARTESIAN_POINT('',(60.1675309762116,-6.13231300382077,3.64303198860259));
#228841=CARTESIAN_POINT('',(60.2194255397046,-6.13776734223115,3.42473028058478));
#228842=CARTESIAN_POINT('',(60.0940777033448,-6.12459275374834,3.64303198860259));
#228843=CARTESIAN_POINT('',(60.5475781763994,-6.17225757416137,3.23423028058478));
#228844=CARTESIAN_POINT('Origin',(60.5183119713881,-6.16918208839045,3.56425743004337));
#228845=CARTESIAN_POINT('',(60.6979579581955,-6.18806312612646,3.23423028058478));
#228846=CARTESIAN_POINT('',(60.6984837728334,-6.18811839147187,3.23423028058478));
#228847=CARTESIAN_POINT('',(61.0261105245455,-6.22255335066314,3.42473028058481));
#228848=CARTESIAN_POINT('Origin',(60.7272269341771,-6.1911399356034,3.56425912917777));
#228849=CARTESIAN_POINT('',(61.1514583085663,-6.2357279336449,3.64303198860259));
#228850=CARTESIAN_POINT('',(61.0261105245455,-6.22255335066314,3.42473028058481));
#228851=CARTESIAN_POINT('',(61.5511575797869,-6.27773801988278,3.64303198860259));
#228852=CARTESIAN_POINT('Origin',(57.9430040808458,6.10537907909402,2.83404198860266));
#228853=CARTESIAN_POINT('Ctrl Pts',(62.2936141127569,6.73887200051352,2.83404198860267));
#228854=CARTESIAN_POINT('Ctrl Pts',(62.3041663177857,6.73998108195344,2.82419652440025));
#228855=CARTESIAN_POINT('Ctrl Pts',(62.3147747227674,6.74025426844108,2.81438790575571));
#228856=CARTESIAN_POINT('Ctrl Pts',(62.3253809467532,6.73970068257604,2.8046678125679));
#228857=CARTESIAN_POINT('Ctrl Pts',(62.3356425316152,6.73916508495522,2.7952635645294));
#228858=CARTESIAN_POINT('Ctrl Pts',(62.345903357484,6.7378554363764,2.78594102496071));
#228859=CARTESIAN_POINT('Ctrl Pts',(62.3561113603665,6.73573381164759,2.77675109088598));
#228860=CARTESIAN_POINT('Ctrl Pts',(62.3657675025208,6.73372688529627,2.76805797913484));
#228861=CARTESIAN_POINT('Ctrl Pts',(62.3753772873503,6.73099321743756,2.75948271209948));
#228862=CARTESIAN_POINT('Ctrl Pts',(62.3848821415136,6.72746117704499,2.75108575572998));
#228863=CARTESIAN_POINT('Ctrl Pts',(62.3936367996066,6.72420791239975,2.74335155163028));
#228864=CARTESIAN_POINT('Ctrl Pts',(62.4023029415032,6.72027708243581,2.73576818685687));
#228865=CARTESIAN_POINT('Ctrl Pts',(62.4108128192423,6.71558140886142,2.72840626160229));
#228866=CARTESIAN_POINT('Ctrl Pts',(62.4132812112882,6.71421937245427,2.72627084693503));
#228867=CARTESIAN_POINT('Ctrl Pts',(62.4157362792969,6.71279278199471,2.72415424587436));
#228868=CARTESIAN_POINT('Ctrl Pts',(62.4181758915949,6.71129899689616,2.72205867173259));
#228869=CARTESIAN_POINT('Ctrl Pts',(62.4208205881801,6.70967963780687,2.71978693462864));
#228870=CARTESIAN_POINT('Ctrl Pts',(62.4234440047029,6.70798448411193,2.71754411340765));
#228871=CARTESIAN_POINT('Ctrl Pts',(62.4260429761973,6.70621108803143,2.71533341844262));
#228872=CARTESIAN_POINT('Ctrl Pts',(62.4331758738576,6.70134398857289,2.7092661487641));
#228873=CARTESIAN_POINT('Ctrl Pts',(62.4400912556838,6.69585818364714,2.70347381860428));
#228874=CARTESIAN_POINT('Ctrl Pts',(62.4466864116142,6.68976801333907,2.69804914171414));
#228875=CARTESIAN_POINT('Ctrl Pts',(62.4527206212313,6.68419583815009,2.69308585687209));
#228876=CARTESIAN_POINT('Ctrl Pts',(62.4584752900419,6.67811620689301,2.68842799053178));
#228877=CARTESIAN_POINT('Ctrl Pts',(62.4638645712592,6.67150703079137,2.684147670542));
#228878=CARTESIAN_POINT('Ctrl Pts',(62.4665117685881,6.66826062508035,2.68204519134548));
#228879=CARTESIAN_POINT('Ctrl Pts',(62.4690703232302,6.66488629457976,2.68003431778511));
#228880=CARTESIAN_POINT('Ctrl Pts',(62.4715267736419,6.6613807859173,2.67812693945273));
#228881=CARTESIAN_POINT('Ctrl Pts',(62.4719928611814,6.66071564979267,2.67776503299224));
#228882=CARTESIAN_POINT('Ctrl Pts',(62.472455189938,6.66004526561009,2.67740659639945));
#228883=CARTESIAN_POINT('Ctrl Pts',(62.4729136358129,6.65936969820877,2.67705178968876));
#228884=CARTESIAN_POINT('Ctrl Pts',(62.4733577552542,6.65871524228875,2.67670807068779));
#228885=CARTESIAN_POINT('Ctrl Pts',(62.4737982307,6.65805592206471,2.67636775825286));
#228886=CARTESIAN_POINT('Ctrl Pts',(62.474234948946,6.65739180030929,2.67603099699276));
#228887=CARTESIAN_POINT('Ctrl Pts',(62.4789942144025,6.65015433826444,2.67236104217156));
#228888=CARTESIAN_POINT('Ctrl Pts',(62.4833100626578,6.64234165497511,2.66911440541507));
#228889=CARTESIAN_POINT('Ctrl Pts',(62.4870273554125,6.63406423386216,2.66646778189666));
#228890=CARTESIAN_POINT('Ctrl Pts',(62.4885971912262,6.63056862752565,2.66535009635004));
#228891=CARTESIAN_POINT('Ctrl Pts',(62.490060506939,6.6269905114141,2.66433897912368));
#228892=CARTESIAN_POINT('Ctrl Pts',(62.4914070226221,6.6233395425202,2.66344564884813));
#228893=CARTESIAN_POINT('Ctrl Pts',(62.4936745213867,6.61719140213092,2.66194130298605));
#228894=CARTESIAN_POINT('Ctrl Pts',(62.4956084911391,6.61083770188544,2.66077206705439));
#228895=CARTESIAN_POINT('Ctrl Pts',(62.4971561593216,6.60433062536158,2.65998225155733));
#228896=CARTESIAN_POINT('Ctrl Pts',(62.4975430763672,6.60270385623062,2.65978479768306));
#228897=CARTESIAN_POINT('Ctrl Pts',(62.4979056188877,6.60106746196568,2.65961098966641));
#228898=CARTESIAN_POINT('Ctrl Pts',(62.4982426563689,6.59942221845757,2.6594613903052));
#228899=CARTESIAN_POINT('Ctrl Pts',(62.4987482125908,6.59695435319542,2.65923699126338));
#228900=CARTESIAN_POINT('Ctrl Pts',(62.4991963674669,6.59446659126617,2.6590670756246));
#228901=CARTESIAN_POINT('Ctrl Pts',(62.4995849724118,6.59196174500311,2.65895332562937));
#228902=CARTESIAN_POINT('Ctrl Pts',(62.4999735773567,6.58945689874005,2.65883957563415));
#228903=CARTESIAN_POINT('Ctrl Pts',(62.5003026407462,6.58693497617669,2.65878198860267));
#228904=CARTESIAN_POINT('Ctrl Pts',(62.5005702980931,6.58439859103048,2.65878198860267));
#228905=CARTESIAN_POINT('Ctrl Pts',(58.7035958781039,6.18532049829418,2.65878198860267));
#228906=CARTESIAN_POINT('Ctrl Pts',(58.702689976017,6.1939028191017,2.65878198860267));
#228907=CARTESIAN_POINT('Ctrl Pts',(58.7025003609929,6.20248552904377,2.65945335517858));
#228908=CARTESIAN_POINT('Ctrl Pts',(58.7029569544313,6.21093474935427,2.660725612266));
#228909=CARTESIAN_POINT('Ctrl Pts',(58.7032518669434,6.21639207873501,2.66154735980339));
#228910=CARTESIAN_POINT('Ctrl Pts',(58.7038154335198,6.22179377937528,2.66261895766886));
#228911=CARTESIAN_POINT('Ctrl Pts',(58.7046202140516,6.22710604846885,2.66391429251034));
#228912=CARTESIAN_POINT('Ctrl Pts',(58.7056869045457,6.23414715684661,2.6656311846413));
#228913=CARTESIAN_POINT('Ctrl Pts',(58.7071827955652,6.24102913891663,2.66774105138706));
#228914=CARTESIAN_POINT('Ctrl Pts',(58.709054816357,6.24767922440765,2.67016894181756));
#228915=CARTESIAN_POINT('Ctrl Pts',(58.7099908267528,6.25100426715316,2.67138288703282));
#228916=CARTESIAN_POINT('Ctrl Pts',(58.7110208470228,6.25427153376679,2.67267613167558));
#228917=CARTESIAN_POINT('Ctrl Pts',(58.7121380880307,6.25747333351535,2.6740383543256));
#228918=CARTESIAN_POINT('Ctrl Pts',(58.7126967085347,6.25907423338963,2.6747194656506));
#228919=CARTESIAN_POINT('Ctrl Pts',(58.7132771324571,6.2606587828836,2.67541781389529));
#228920=CARTESIAN_POINT('Ctrl Pts',(58.7138784999415,6.26222612320532,2.67613207244176));
#228921=CARTESIAN_POINT('Ctrl Pts',(58.7140288418126,6.26261795828575,2.67631063707837));
#228922=CARTESIAN_POINT('Ctrl Pts',(58.7141804926178,6.26300871814026,2.67649019601852));
#228923=CARTESIAN_POINT('Ctrl Pts',(58.7143334388435,6.2633983900507,2.67667072836663));
#228924=CARTESIAN_POINT('Ctrl Pts',(58.7147922775207,6.26456740578201,2.67721232541097));
#228925=CARTESIAN_POINT('Ctrl Pts',(58.715262775183,6.26572662828386,2.67776268340053));
#228926=CARTESIAN_POINT('Ctrl Pts',(58.7157445651923,6.2668757296518,2.67832123541522));
#228927=CARTESIAN_POINT('Ctrl Pts',(58.7191382318077,6.27496985131148,2.68225560368446));
#228928=CARTESIAN_POINT('Ctrl Pts',(58.7230632421217,6.28260716192764,2.68661792998883));
#228929=CARTESIAN_POINT('Ctrl Pts',(58.7274000190312,6.28978339589432,2.69130986622566));
#228930=CARTESIAN_POINT('Ctrl Pts',(58.729503351146,6.29326386161362,2.69358545023048));
#228931=CARTESIAN_POINT('Ctrl Pts',(58.731704109697,6.29663597408932,2.69593918853469));
#228932=CARTESIAN_POINT('Ctrl Pts',(58.7339915094193,6.29989941779164,2.6983630623548));
#228933=CARTESIAN_POINT('Ctrl Pts',(58.7374933585782,6.30489552208953,2.70207384382213));
#228934=CARTESIAN_POINT('Ctrl Pts',(58.7411954596217,6.30963480180888,2.70594760814213));
#228935=CARTESIAN_POINT('Ctrl Pts',(58.745053462885,6.31410463171063,2.70995196345693));
#228936=CARTESIAN_POINT('Ctrl Pts',(58.7468451395591,6.31618044384083,2.71181160678091));
#228937=CARTESIAN_POINT('Ctrl Pts',(58.7486702031823,6.31819823791544,2.71369962772084));
#228938=CARTESIAN_POINT('Ctrl Pts',(58.7505249478605,6.32015576082333,2.71561183138646));
#228939=CARTESIAN_POINT('Ctrl Pts',(58.750667106732,6.3203057972412,2.71575839426297));
#228940=CARTESIAN_POINT('Ctrl Pts',(58.7508094261759,6.32045551058207,2.71590508903194));
#228941=CARTESIAN_POINT('Ctrl Pts',(58.7509519047346,6.32060490094016,2.71605191409897));
#228942=CARTESIAN_POINT('Ctrl Pts',(58.7529532989256,6.32270338507401,2.71811436362738));
#228943=CARTESIAN_POINT('Ctrl Pts',(58.7549876922215,6.32473679726646,2.72020091026944));
#228944=CARTESIAN_POINT('Ctrl Pts',(58.757049379421,6.32670504965004,2.72230624862167));
#228945=CARTESIAN_POINT('Ctrl Pts',(58.7644422230598,6.33376285265589,2.72985561753118));
#228946=CARTESIAN_POINT('Ctrl Pts',(58.7722418109927,6.34003880538944,2.73770089914376));
#228947=CARTESIAN_POINT('Ctrl Pts',(58.780339648656,6.34560292136768,2.74574823347153));
#228948=CARTESIAN_POINT('Ctrl Pts',(58.7892383587479,6.35171732586275,2.75459144547133));
#228949=CARTESIAN_POINT('Ctrl Pts',(58.7984976730909,6.35697262978522,2.7636791175441));
#228950=CARTESIAN_POINT('Ctrl Pts',(58.8080148760667,6.36142852992898,2.77292162564898));
#228951=CARTESIAN_POINT('Ctrl Pts',(58.8182910667888,6.36623978380599,2.78290121484943));
#228952=CARTESIAN_POINT('Ctrl Pts',(58.828868892188,6.37011968263842,2.79306229500443));
#228953=CARTESIAN_POINT('Ctrl Pts',(58.8396533761915,6.37309732669917,2.8033191668555));
#228954=CARTESIAN_POINT('Ctrl Pts',(58.8503473894534,6.37604999138528,2.81348999408895));
#228955=CARTESIAN_POINT('Ctrl Pts',(58.8612460403474,6.3781155791126,2.82375635966979));
#228956=CARTESIAN_POINT('Ctrl Pts',(58.872270023448,6.37927424642597,2.83404198860267));
#228957=CARTESIAN_POINT('Origin',(0.00159301378019908,-0.0151565136852236,
2.83404198860262));
#228958=CARTESIAN_POINT('Ctrl Pts',(62.5037563256535,6.55408556365965,2.65878198860267));
#228959=CARTESIAN_POINT('Ctrl Pts',(62.5046505412978,6.54554330587399,2.65878198860267));
#228960=CARTESIAN_POINT('Ctrl Pts',(62.5048232320879,6.53700226086626,2.65944603041855));
#228961=CARTESIAN_POINT('Ctrl Pts',(62.5043472028589,6.52859457177385,2.66070439264073));
#228962=CARTESIAN_POINT('Ctrl Pts',(62.5040430428431,6.52322245869445,2.66150842619599));
#228963=CARTESIAN_POINT('Ctrl Pts',(62.5034749678471,6.51790471489591,2.66255428265372));
#228964=CARTESIAN_POINT('Ctrl Pts',(62.5026702669707,6.5126735674086,2.66381699700661));
#228965=CARTESIAN_POINT('Ctrl Pts',(62.5015720117389,6.50553410072667,2.66554034873261));
#228966=CARTESIAN_POINT('Ctrl Pts',(62.5000273428098,6.49855818190791,2.66766759643965));
#228967=CARTESIAN_POINT('Ctrl Pts',(62.4980940659029,6.49182203260195,2.6701201278314));
#228968=CARTESIAN_POINT('Ctrl Pts',(62.4971274274495,6.48845395794897,2.67134639352728));
#228969=CARTESIAN_POINT('Ctrl Pts',(62.4960636607366,6.48514561818754,2.67265375585004));
#228970=CARTESIAN_POINT('Ctrl Pts',(62.494910155573,6.48190505740182,2.67403135126931));
#228971=CARTESIAN_POINT('Ctrl Pts',(62.4943334029912,6.48028477700896,2.67472014897895));
#228972=CARTESIAN_POINT('Ctrl Pts',(62.4937342176674,6.47868142404699,2.67542649668624));
#228973=CARTESIAN_POINT('Ctrl Pts',(62.4931135352114,6.47709589524284,2.67614899656093));
#228974=CARTESIAN_POINT('Ctrl Pts',(62.4929583645974,6.47669951304181,2.6763296215296));
#228975=CARTESIAN_POINT('Ctrl Pts',(62.4928018504535,6.47630424448191,2.67651125590941));
#228976=CARTESIAN_POINT('Ctrl Pts',(62.4926440074817,6.47591010283092,2.67669387767514));
#228977=CARTESIAN_POINT('Ctrl Pts',(62.4921704785661,6.47472767787793,2.67724174297234));
#228978=CARTESIAN_POINT('Ctrl Pts',(62.4916849899864,6.47355539694487,2.67779849504738));
#228979=CARTESIAN_POINT('Ctrl Pts',(62.4911879405752,6.47239360181829,2.67836353617999));
#228980=CARTESIAN_POINT('Ctrl Pts',(62.4877530207469,6.46436487665183,2.68226832098905));
#228981=CARTESIAN_POINT('Ctrl Pts',(62.4837949925047,6.45678933786393,2.68659153751396));
#228982=CARTESIAN_POINT('Ctrl Pts',(62.4794326364365,6.44966853563983,2.69123699486192));
#228983=CARTESIAN_POINT('Ctrl Pts',(62.4772645574451,6.44612951648082,2.69354577441223));
#228984=CARTESIAN_POINT('Ctrl Pts',(62.4749960038951,6.44270272394358,2.69593478828115));
#228985=CARTESIAN_POINT('Ctrl Pts',(62.4726384024734,6.43938822718943,2.69839565261208));
#228986=CARTESIAN_POINT('Ctrl Pts',(62.4674371815967,6.43207595228373,2.70382468689034));
#228987=CARTESIAN_POINT('Ctrl Pts',(62.461813233051,6.42530381744009,2.70961155815075));
#228988=CARTESIAN_POINT('Ctrl Pts',(62.4558957623411,6.41913840445444,2.71562701361755));
#228989=CARTESIAN_POINT('Ctrl Pts',(62.4537340356675,6.41688610134083,2.71782453535845));
#228990=CARTESIAN_POINT('Ctrl Pts',(62.4515361835425,6.41470741397486,2.72005051502389));
#228991=CARTESIAN_POINT('Ctrl Pts',(62.4493074469123,6.41260146153657,2.72229986760102));
#228992=CARTESIAN_POINT('Ctrl Pts',(62.4418213564087,6.40552779014103,2.7298552048888));
#228993=CARTESIAN_POINT('Ctrl Pts',(62.4339335724862,6.39923601079887,2.7377084553455));
#228994=CARTESIAN_POINT('Ctrl Pts',(62.4257522463024,6.39365709371033,2.74576706701749));
#228995=CARTESIAN_POINT('Ctrl Pts',(62.4167599996846,6.38752520296385,2.7546244358503));
#228996=CARTESIAN_POINT('Ctrl Pts',(62.4074126717503,6.38225398283454,2.76373036323188));
#228997=CARTESIAN_POINT('Ctrl Pts',(62.3978127557445,6.37778536209576,2.77299664636831));
#228998=CARTESIAN_POINT('Ctrl Pts',(62.3874732348825,6.3729724660949,2.78297683033493));
#228999=CARTESIAN_POINT('Ctrl Pts',(62.3768396913508,6.36908997057773,2.79314401478916));
#229000=CARTESIAN_POINT('Ctrl Pts',(62.3660067738144,6.36611161569945,2.80341452427963));
#229001=CARTESIAN_POINT('Ctrl Pts',(62.3553201372418,6.36317347866838,2.81354634721382));
#229002=CARTESIAN_POINT('Ctrl Pts',(62.3444380411295,6.36111515612462,2.82378004209215));
#229003=CARTESIAN_POINT('Ctrl Pts',(62.3334394572619,6.35995915837821,2.83404198860267));
#229004=CARTESIAN_POINT('Ctrl Pts',(58.912095367953,6.00036140429066,2.83404198860266));
#229005=CARTESIAN_POINT('Ctrl Pts',(58.9015696628155,5.99925510810155,2.82422126443124));
#229006=CARTESIAN_POINT('Ctrl Pts',(58.8909945468916,5.99898299131213,2.81442815028733));
#229007=CARTESIAN_POINT('Ctrl Pts',(58.8804276387812,5.99953795195263,2.80471618166661));
#229008=CARTESIAN_POINT('Ctrl Pts',(58.8702243592828,6.00007381527864,2.79533842146637));
#229009=CARTESIAN_POINT('Ctrl Pts',(58.8600274754072,6.00138095727621,2.78603515650712));
#229010=CARTESIAN_POINT('Ctrl Pts',(58.8498890377533,6.00349883563876,2.77685887347287));
#229011=CARTESIAN_POINT('Ctrl Pts',(58.840305039008,6.00550089396986,2.76818441217135));
#229012=CARTESIAN_POINT('Ctrl Pts',(58.8307723843927,6.00822762538427,2.75962261522206));
#229013=CARTESIAN_POINT('Ctrl Pts',(58.8213500689105,6.01175153639394,2.75123537702261));
#229014=CARTESIAN_POINT('Ctrl Pts',(58.8126722744225,6.01499699931587,2.74351087134724));
#229015=CARTESIAN_POINT('Ctrl Pts',(58.8040875818613,6.01891888228952,2.73593399450453));
#229016=CARTESIAN_POINT('Ctrl Pts',(58.7956642413115,6.02360485257183,2.72857657813182));
#229017=CARTESIAN_POINT('Ctrl Pts',(58.7931525711942,6.02500211431843,2.7263827450872));
#229018=CARTESIAN_POINT('Ctrl Pts',(58.7906554330111,6.02646752363638,2.72420861709793));
#229019=CARTESIAN_POINT('Ctrl Pts',(58.7881751602884,6.02800395803723,2.72205663736713));
#229020=CARTESIAN_POINT('Ctrl Pts',(58.7857202298425,6.0295246938637,2.71992664556752));
#229021=CARTESIAN_POINT('Ctrl Pts',(58.783284225042,6.03111319985522,2.7178208992787));
#229022=CARTESIAN_POINT('Ctrl Pts',(58.7808720541407,6.03277025542048,2.71574387311232));
#229023=CARTESIAN_POINT('Ctrl Pts',(58.7807043164937,6.0328854838238,2.71559944077473));
#229024=CARTESIAN_POINT('Ctrl Pts',(58.7805366835715,6.03300103800929,2.71545515216055));
#229025=CARTESIAN_POINT('Ctrl Pts',(58.7803691562898,6.03311691890581,2.71531100781716));
#229026=CARTESIAN_POINT('Ctrl Pts',(58.7730241465597,6.03819756191456,2.70899119176059));
#229027=CARTESIAN_POINT('Ctrl Pts',(58.7659160498048,6.04393622206024,2.70298296066806));
#229028=CARTESIAN_POINT('Ctrl Pts',(58.7591607781926,6.05034076157619,2.69736727774097));
#229029=CARTESIAN_POINT('Ctrl Pts',(58.7528636909918,6.05631090550661,2.69213248525372));
#229030=CARTESIAN_POINT('Ctrl Pts',(58.7468728126818,6.06286038933392,2.68723866185397));
#229031=CARTESIAN_POINT('Ctrl Pts',(58.7413107827872,6.07000150504488,2.6827859582948));
#229032=CARTESIAN_POINT('Ctrl Pts',(58.7392761202949,6.07261381755777,2.68115710172747));
#229033=CARTESIAN_POINT('Ctrl Pts',(58.7372991657061,6.07530531160715,2.67958763637775));
#229034=CARTESIAN_POINT('Ctrl Pts',(58.735387140493,6.07807653793574,2.67808378645351));
#229035=CARTESIAN_POINT('Ctrl Pts',(58.7349273623043,6.07874292528938,2.67772216078586));
#229036=CARTESIAN_POINT('Ctrl Pts',(58.7344713442223,6.07941450700203,2.67736403603549));
#229037=CARTESIAN_POINT('Ctrl Pts',(58.7340192051468,6.08009121771094,2.67700956934465));
#229038=CARTESIAN_POINT('Ctrl Pts',(58.7335811954175,6.0807467812102,2.6766661797379));
#229039=CARTESIAN_POINT('Ctrl Pts',(58.7331468260468,6.08140715812726,2.67632622314104));
#229040=CARTESIAN_POINT('Ctrl Pts',(58.7327162055066,6.0820722852656,2.67598984158759));
#229041=CARTESIAN_POINT('Ctrl Pts',(58.7279982598322,6.08935952173602,2.67230439292219));
#229042=CARTESIAN_POINT('Ctrl Pts',(58.7237275533354,6.09722197243166,2.66904964539982));
#229043=CARTESIAN_POINT('Ctrl Pts',(58.7200553115705,6.10554709909129,2.66640203566737));
#229044=CARTESIAN_POINT('Ctrl Pts',(58.7185323234527,6.10899977726284,2.66530399299441));
#229045=CARTESIAN_POINT('Ctrl Pts',(58.7171120447817,6.11253167434587,2.66430995142251));
#229046=CARTESIAN_POINT('Ctrl Pts',(58.7158039367398,6.11613350280244,2.66343053473345));
#229047=CARTESIAN_POINT('Ctrl Pts',(58.7135728221602,6.12227679657168,2.66193059792869));
#229048=CARTESIAN_POINT('Ctrl Pts',(58.7116702942288,6.12862250657805,2.66076519817111));
#229049=CARTESIAN_POINT('Ctrl Pts',(58.7101471179289,6.13511848061118,2.65997805604443));
#229050=CARTESIAN_POINT('Ctrl Pts',(58.7093855297789,6.13836646762775,2.65958448498109));
#229051=CARTESIAN_POINT('Ctrl Pts',(58.7087202098052,6.14165223896383,2.65928526260745));
#229052=CARTESIAN_POINT('Ctrl Pts',(58.7081575578112,6.14496923836513,2.65908463971307));
#229053=CARTESIAN_POINT('Ctrl Pts',(58.7075949058173,6.14828623776644,2.6588840168187));
#229054=CARTESIAN_POINT('Ctrl Pts',(58.7071349090267,6.15163442139611,2.65878198860267));
#229055=CARTESIAN_POINT('Ctrl Pts',(58.7067819056643,6.15500747092335,2.65878198860267));
#229056=CARTESIAN_POINT('Origin',(56.9874003490102,12.1286263473646,2.83404198860271));
#229057=CARTESIAN_POINT('Ctrl Pts',(61.2479592423878,13.2134115091896,2.83404198860272));
#229058=CARTESIAN_POINT('Ctrl Pts',(61.2583377107544,13.215617520741,2.82419652440085));
#229059=CARTESIAN_POINT('Ctrl Pts',(61.2688594460195,13.2169980909549,2.81438790575682));
#229060=CARTESIAN_POINT('Ctrl Pts',(61.2794654334798,13.2175561899855,2.80466781256948));
#229061=CARTESIAN_POINT('Ctrl Pts',(61.2897267895022,13.2180961541209,2.79526356453138));
#229062=CARTESIAN_POINT('Ctrl Pts',(61.3000683010463,13.2178662282941,2.78594102496306));
#229063=CARTESIAN_POINT('Ctrl Pts',(61.310442153593,13.2168232529021,2.77675109088867));
#229064=CARTESIAN_POINT('Ctrl Pts',(61.3202551793171,13.2158366624039,2.76805797913786));
#229065=CARTESIAN_POINT('Ctrl Pts',(61.3300980668398,13.2141224659046,2.7594827121028));
#229066=CARTESIAN_POINT('Ctrl Pts',(61.3399200511715,13.2116033021985,2.75108575573356));
#229067=CARTESIAN_POINT('Ctrl Pts',(61.348966809085,13.2092829702345,2.74335155163417));
#229068=CARTESIAN_POINT('Ctrl Pts',(61.3579963605644,13.2062795322637,2.73576818686104));
#229069=CARTESIAN_POINT('Ctrl Pts',(61.3669504518452,13.2024991065236,2.72840626160669));
#229070=CARTESIAN_POINT('Ctrl Pts',(61.3695476933555,13.2014025487211,2.72627084693797));
#229071=CARTESIAN_POINT('Ctrl Pts',(61.3721384315549,13.2002403977588,2.72415424587585));
#229072=CARTESIAN_POINT('Ctrl Pts',(61.374720822464,13.1990098046949,2.72205867173268));
#229073=CARTESIAN_POINT('Ctrl Pts',(61.3775203002416,13.197675762694,2.71978693462871));
#229074=CARTESIAN_POINT('Ctrl Pts',(61.3803065372249,13.196264116926,2.71754411340771));
#229075=CARTESIAN_POINT('Ctrl Pts',(61.3830766416486,13.1947721021912,2.71533341844267));
#229076=CARTESIAN_POINT('Ctrl Pts',(61.3906792149762,13.1906772560438,2.70926614876414));
#229077=CARTESIAN_POINT('Ctrl Pts',(61.3981301363758,13.1859443571666,2.70347381860432));
#229078=CARTESIAN_POINT('Ctrl Pts',(61.4053257594953,13.1805769309631,2.69804914171418));
#229079=CARTESIAN_POINT('Ctrl Pts',(61.4119093639903,13.1756660273912,2.69308585687216));
#229080=CARTESIAN_POINT('Ctrl Pts',(61.4182680026355,13.1702212276777,2.68842799053186));
#229081=CARTESIAN_POINT('Ctrl Pts',(61.4243186078278,13.1642115906181,2.6841476705421));
#229082=CARTESIAN_POINT('Ctrl Pts',(61.4272906453329,13.1612596765259,2.68204519134556));
#229083=CARTESIAN_POINT('Ctrl Pts',(61.4301878975268,13.1581712727458,2.68003431778516));
#229084=CARTESIAN_POINT('Ctrl Pts',(61.4329973166795,13.1549417366132,2.67812693945276));
#229085=CARTESIAN_POINT('Ctrl Pts',(61.4335303765997,13.1543289635881,2.67776503299228));
#229086=CARTESIAN_POINT('Ctrl Pts',(61.4340602468995,13.1537105783546,2.67740659639948));
#229087=CARTESIAN_POINT('Ctrl Pts',(61.4345867973822,13.153086632425,2.67705178968879));
#229088=CARTESIAN_POINT('Ctrl Pts',(61.4350968931623,13.1524821848057,2.67670807068782));
#229089=CARTESIAN_POINT('Ctrl Pts',(61.4356038733673,13.1518725186283,2.6763677582529));
#229090=CARTESIAN_POINT('Ctrl Pts',(61.4361076188515,13.1512576844885,2.67603099699279));
#229091=CARTESIAN_POINT('Ctrl Pts',(61.4415973333393,13.1445573487226,2.67236104217168));
#229092=CARTESIAN_POINT('Ctrl Pts',(61.4467061867043,13.1372385931158,2.66911440541525));
#229093=CARTESIAN_POINT('Ctrl Pts',(61.4512683418492,13.1293950794811,2.66646778189688));
#229094=CARTESIAN_POINT('Ctrl Pts',(61.4531949682967,13.1260827149669,2.66535009635018));
#229095=CARTESIAN_POINT('Ctrl Pts',(61.4550242827915,13.1226771582923,2.66433897912377));
#229096=CARTESIAN_POINT('Ctrl Pts',(61.4567450522889,13.119186939003,2.66344564884816));
#229097=CARTESIAN_POINT('Ctrl Pts',(61.4596427851248,13.1133094969314,2.66194130298609));
#229098=CARTESIAN_POINT('Ctrl Pts',(61.4622303029113,13.1071927578069,2.66077206705443));
#229099=CARTESIAN_POINT('Ctrl Pts',(61.4644496675149,13.1008831031058,2.65998225155737));
#229100=CARTESIAN_POINT('Ctrl Pts',(61.4650045086658,13.0993056894305,2.6597847976831));
#229101=CARTESIAN_POINT('Ctrl Pts',(61.4655361149183,13.0977161555171,2.65961098966645));
#229102=CARTESIAN_POINT('Ctrl Pts',(61.4660432808485,13.0961151548351,2.65946139030524));
#229103=CARTESIAN_POINT('Ctrl Pts',(61.4668040297439,13.093713653812,2.65923699126343));
#229104=CARTESIAN_POINT('Ctrl Pts',(61.4675097715121,13.0912863650434,2.65906707562464));
#229105=CARTESIAN_POINT('Ctrl Pts',(61.4681580753691,13.088835860868,2.65895332562942));
#229106=CARTESIAN_POINT('Ctrl Pts',(61.4688063792261,13.0863853566926,2.6588395756342));
#229107=CARTESIAN_POINT('Ctrl Pts',(61.4693972526619,13.0839116459753,2.65878198860271));
#229108=CARTESIAN_POINT('Ctrl Pts',(61.4699285681954,13.0814171332235,2.65878198860271));
#229109=CARTESIAN_POINT('Ctrl Pts',(57.7354693911204,12.2876333308473,2.65878198860271));
#229110=CARTESIAN_POINT('Ctrl Pts',(57.7336713548546,12.2960739442509,2.65878198860271));
#229111=CARTESIAN_POINT('Ctrl Pts',(57.7325856410805,12.3045898170433,2.65945335517869));
#229112=CARTESIAN_POINT('Ctrl Pts',(57.7321565492375,12.3130404786518,2.66072561226624));
#229113=CARTESIAN_POINT('Ctrl Pts',(57.7318793999343,12.3184987389624,2.66154735980361));
#229114=CARTESIAN_POINT('Ctrl Pts',(57.7318752477671,12.3239297572691,2.662618957669));
#229115=CARTESIAN_POINT('Ctrl Pts',(57.7321203363021,12.3292970476686,2.66391429251038));
#229116=CARTESIAN_POINT('Ctrl Pts',(57.7324451871157,12.3364110836361,2.66563118464134));
#229117=CARTESIAN_POINT('Ctrl Pts',(57.7332135204776,12.3434117286777,2.66774105138709));
#229118=CARTESIAN_POINT('Ctrl Pts',(57.7343801629266,12.3502210637611,2.6701689418176));
#229119=CARTESIAN_POINT('Ctrl Pts',(57.7349634841511,12.3536257313029,2.67138288703285));
#229120=CARTESIAN_POINT('Ctrl Pts',(57.7356463395041,12.3569827659241,2.67267613167561));
#229121=CARTESIAN_POINT('Ctrl Pts',(57.7364227809415,12.3602838093643,2.67403835432563));
#229122=CARTESIAN_POINT('Ctrl Pts',(57.7368110016602,12.3619343310844,2.67471946565064));
#229123=CARTESIAN_POINT('Ctrl Pts',(57.737222615436,12.3635708710711,2.67541781389532));
#229124=CARTESIAN_POINT('Ctrl Pts',(57.7376568568912,12.3651924853575,2.67613207244178));
#229125=CARTESIAN_POINT('Ctrl Pts',(57.737765417255,12.3655978889291,2.6763106370784));
#229126=CARTESIAN_POINT('Ctrl Pts',(57.7378753917741,12.3660023599859,2.67649019601855));
#229127=CARTESIAN_POINT('Ctrl Pts',(57.7379867683384,12.3664058844668,2.67667072836666));
#229128=CARTESIAN_POINT('Ctrl Pts',(57.7383208980314,12.3676164579094,2.677212325411));
#229129=CARTESIAN_POINT('Ctrl Pts',(57.7386676465115,12.3688185104667,2.67776268340057));
#229130=CARTESIAN_POINT('Ctrl Pts',(57.7390266834246,12.3700116777064,2.67832123541526));
#229131=CARTESIAN_POINT('Ctrl Pts',(57.7415556930807,12.378416193677,2.68225560368456));
#229132=CARTESIAN_POINT('Ctrl Pts',(57.7446608854353,12.3864219416031,2.68661792998903));
#229133=CARTESIAN_POINT('Ctrl Pts',(57.7482237843187,12.3940121800353,2.69130986622596));
#229134=CARTESIAN_POINT('Ctrl Pts',(57.7499517864269,12.3976934374727,2.6935854502307));
#229135=CARTESIAN_POINT('Ctrl Pts',(57.7517880072572,12.4012771190727,2.69593918853482));
#229136=CARTESIAN_POINT('Ctrl Pts',(57.7537217536093,12.4047617836667,2.69836306235484));
#229137=CARTESIAN_POINT('Ctrl Pts',(57.7566821841675,12.4100965616936,2.70207384382218));
#229138=CARTESIAN_POINT('Ctrl Pts',(57.759868615088,12.4151968540757,2.70594760814218));
#229139=CARTESIAN_POINT('Ctrl Pts',(57.7632382593551,12.420045468934,2.70995196345698));
#229140=CARTESIAN_POINT('Ctrl Pts',(57.7648031395849,12.4222971907576,2.71181160678096));
#229141=CARTESIAN_POINT('Ctrl Pts',(57.7664072884048,12.424494702241,2.71369962772089));
#229142=CARTESIAN_POINT('Ctrl Pts',(57.7680472557362,12.4266353752445,2.71561183138651));
#229143=CARTESIAN_POINT('Ctrl Pts',(57.7681729527704,12.4267994493956,2.71575839426302));
#229144=CARTESIAN_POINT('Ctrl Pts',(57.768298843268,12.4269632190239,2.71590508903199));
#229145=CARTESIAN_POINT('Ctrl Pts',(57.7684249257697,12.4271266840708,2.71605191409901));
#229146=CARTESIAN_POINT('Ctrl Pts',(57.7701960047922,12.4294228751481,2.71811436362743));
#229147=CARTESIAN_POINT('Ctrl Pts',(57.7720067040171,12.4316578001007,2.72020091026949));
#229148=CARTESIAN_POINT('Ctrl Pts',(57.7738513586814,12.4338307751865,2.72230624862172));
#229149=CARTESIAN_POINT('Ctrl Pts',(57.7804659622463,12.4416226773929,2.72985561753045));
#229150=CARTESIAN_POINT('Ctrl Pts',(57.7875668075249,12.4486795287408,2.7377008991422));
#229151=CARTESIAN_POINT('Ctrl Pts',(57.7950386758926,12.4550596184357,2.74574823346909));
#229152=CARTESIAN_POINT('Ctrl Pts',(57.803249508613,12.4620706960736,2.75459144546791));
#229153=CARTESIAN_POINT('Ctrl Pts',(57.8119087706191,12.46826507279,2.76367911753964));
#229154=CARTESIAN_POINT('Ctrl Pts',(57.8209080689656,12.473691381648,2.77292162564346));
#229155=CARTESIAN_POINT('Ctrl Pts',(57.8306250526641,12.4795504333968,2.78290121484255));
#229156=CARTESIAN_POINT('Ctrl Pts',(57.840739371765,12.484514761571,2.79306229499614));
#229157=CARTESIAN_POINT('Ctrl Pts',(57.8511535286773,12.4886033793261,2.80331916684582));
#229158=CARTESIAN_POINT('Ctrl Pts',(57.8614803215165,12.4926576977804,2.81348999408244));
#229159=CARTESIAN_POINT('Ctrl Pts',(57.8721033557531,12.495851189233,2.82375635966655));
#229160=CARTESIAN_POINT('Ctrl Pts',(57.8829458346105,12.4981558292589,2.83404198860271));
#229161=CARTESIAN_POINT('Origin',(0.00316857416806278,-0.0149069694349949,
2.83404198860262));
#229162=CARTESIAN_POINT('Ctrl Pts',(61.4762657165316,13.0516031943531,2.65878198860271));
#229163=CARTESIAN_POINT('Ctrl Pts',(61.4780479426482,13.0432012029367,2.65878198860271));
#229164=CARTESIAN_POINT('Ctrl Pts',(61.4791124697294,13.0347249977703,2.65944603041856));
#229165=CARTESIAN_POINT('Ctrl Pts',(61.4795178910588,13.0263136082749,2.66070439264067));
#229166=CARTESIAN_POINT('Ctrl Pts',(61.4797769359881,13.0209391308139,2.66150842619593));
#229167=CARTESIAN_POINT('Ctrl Pts',(61.4797678285537,13.0155911381657,2.66255428265368));
#229168=CARTESIAN_POINT('Ctrl Pts',(61.4795143397208,13.0103045333055,2.6638169970066));
#229169=CARTESIAN_POINT('Ctrl Pts',(61.479168378327,13.0030893784374,2.6655403487326));
#229170=CARTESIAN_POINT('Ctrl Pts',(61.4783613533299,12.9959902125624,2.66766759643964));
#229171=CARTESIAN_POINT('Ctrl Pts',(61.4771427864515,12.989088882123,2.6701201278314));
#229172=CARTESIAN_POINT('Ctrl Pts',(61.4765335030122,12.9856382169033,2.67134639352728));
#229173=CARTESIAN_POINT('Ctrl Pts',(61.4758213793959,12.9822368066734,2.67265375585004));
#229174=CARTESIAN_POINT('Ctrl Pts',(61.4750129240934,12.9788934238966,2.67403135126932));
#229175=CARTESIAN_POINT('Ctrl Pts',(61.4746086964421,12.9772217325082,2.67472014897896));
#229176=CARTESIAN_POINT('Ctrl Pts',(61.4741803895393,12.9755645309604,2.67542649668625));
#229177=CARTESIAN_POINT('Ctrl Pts',(61.4737288401361,12.9739228088657,2.67614899656094));
#229178=CARTESIAN_POINT('Ctrl Pts',(61.4736159527854,12.973512378342,2.67632962152962));
#229179=CARTESIAN_POINT('Ctrl Pts',(61.4735016128575,12.9731029149217,2.67651125590943));
#229180=CARTESIAN_POINT('Ctrl Pts',(61.473385833587,12.9726944333366,2.67669387767516));
#229181=CARTESIAN_POINT('Ctrl Pts',(61.4730384957757,12.9714689885813,2.67724174297236));
#229182=CARTESIAN_POINT('Ctrl Pts',(61.4726782034777,12.9702523821507,2.6777984950474));
#229183=CARTESIAN_POINT('Ctrl Pts',(61.4723053176144,12.9690449956483,2.67836353618002));
#229184=CARTESIAN_POINT('Ctrl Pts',(61.46972844494,12.9607012057873,2.68226832098904));
#229185=CARTESIAN_POINT('Ctrl Pts',(61.4665839586185,12.9527534399839,2.68659153751391));
#229186=CARTESIAN_POINT('Ctrl Pts',(61.4629898265071,12.9452156558834,2.69123699486182));
#229187=CARTESIAN_POINT('Ctrl Pts',(61.4612035527134,12.9414693978764,2.69354577441217));
#229188=CARTESIAN_POINT('Ctrl Pts',(61.4593056238949,12.9378242492507,2.69593478828114));
#229189=CARTESIAN_POINT('Ctrl Pts',(61.4573073969127,12.9342814732029,2.69839565261212));
#229190=CARTESIAN_POINT('Ctrl Pts',(61.4528990097271,12.9264655800789,2.70382468689038));
#229191=CARTESIAN_POINT('Ctrl Pts',(61.4480137506082,12.9191426809995,2.70961155815079));
#229192=CARTESIAN_POINT('Ctrl Pts',(61.4427731575668,12.9123924986716,2.7156270136176));
#229193=CARTESIAN_POINT('Ctrl Pts',(61.4408587028414,12.9099265719429,2.71782453535851));
#229194=CARTESIAN_POINT('Ctrl Pts',(61.4389006256227,12.9075300815492,2.72005051502395));
#229195=CARTESIAN_POINT('Ctrl Pts',(61.436904230217,12.9052026993237,2.72229986760109));
#229196=CARTESIAN_POINT('Ctrl Pts',(61.4301985493013,12.8973852687042,2.72985520488861));
#229197=CARTESIAN_POINT('Ctrl Pts',(61.4230116455106,12.8903034584559,2.73770845534501));
#229198=CARTESIAN_POINT('Ctrl Pts',(61.415458293118,12.8838999218056,2.74576706701669));
#229199=CARTESIAN_POINT('Ctrl Pts',(61.407156264085,12.8768616764781,2.7546244358492));
#229200=CARTESIAN_POINT('Ctrl Pts',(61.398411134331,12.8706422708196,2.76373036323047));
#229201=CARTESIAN_POINT('Ctrl Pts',(61.3893309057286,12.8651946651853,2.77299664636657));
#229202=CARTESIAN_POINT('Ctrl Pts',(61.3795511104668,12.8593273605057,2.78297683033289));
#229203=CARTESIAN_POINT('Ctrl Pts',(61.3693816498896,12.8543546257408,2.79314401478682));
#229204=CARTESIAN_POINT('Ctrl Pts',(61.3589193990677,12.8502602383793,2.803414524277));
#229205=CARTESIAN_POINT('Ctrl Pts',(61.3485984239563,12.8462211390714,2.81354634721204));
#229206=CARTESIAN_POINT('Ctrl Pts',(61.3379910943966,12.8430366034498,2.82378004209126));
#229207=CARTESIAN_POINT('Ctrl Pts',(61.3271735965893,12.84073727331,2.83404198860272));
#229208=CARTESIAN_POINT('Ctrl Pts',(57.9621601888121,12.1254815933794,2.8340419886027));
#229209=CARTESIAN_POINT('Ctrl Pts',(57.9518077840282,12.1232811218135,2.82422126443033));
#229210=CARTESIAN_POINT('Ctrl Pts',(57.9413190436447,12.1219050950918,2.81442815028545));
#229211=CARTESIAN_POINT('Ctrl Pts',(57.9307520129786,12.1213524729337,2.80471618166379));
#229212=CARTESIAN_POINT('Ctrl Pts',(57.9205486151423,12.1208188676182,2.79533842146307));
#229213=CARTESIAN_POINT('Ctrl Pts',(57.9102709573187,12.1210529843537,2.78603515650333));
#229214=CARTESIAN_POINT('Ctrl Pts',(57.8999666805159,12.1220995054494,2.77685887346864));
#229215=CARTESIAN_POINT('Ctrl Pts',(57.8902259118376,12.1230887956349,2.76818441216703));
#229216=CARTESIAN_POINT('Ctrl Pts',(57.8804604570571,12.1248041559918,2.75962261521767));
#229217=CARTESIAN_POINT('Ctrl Pts',(57.8707214090023,12.1273238624908,2.75123537701818));
#229218=CARTESIAN_POINT('Ctrl Pts',(57.8617519091287,12.1296444699052,2.74351087134297));
#229219=CARTESIAN_POINT('Ctrl Pts',(57.8528042960114,12.1326475236727,2.73593399450044));
#229220=CARTESIAN_POINT('Ctrl Pts',(57.8439372821301,12.1364273448765,2.7285765781279));
#229221=CARTESIAN_POINT('Ctrl Pts',(57.8412933175829,12.1375544112589,2.72638274508463));
#229222=CARTESIAN_POINT('Ctrl Pts',(57.8386566820015,12.1387507708937,2.72420861709668));
#229223=CARTESIAN_POINT('Ctrl Pts',(57.8360293953471,12.1400195294492,2.72205663736717));
#229224=CARTESIAN_POINT('Ctrl Pts',(57.8334289530881,12.1412753244188,2.71992664556756));
#229225=CARTESIAN_POINT('Ctrl Pts',(57.8308402488866,12.14260049657,2.71782089927875));
#229226=CARTESIAN_POINT('Ctrl Pts',(57.8282680826381,12.143996334094,2.71574387311236));
#229227=CARTESIAN_POINT('Ctrl Pts',(57.8280892192276,12.1440933979056,2.71559944077477));
#229228=CARTESIAN_POINT('Ctrl Pts',(57.8279104259146,12.1441907966614,2.71545515216059));
#229229=CARTESIAN_POINT('Ctrl Pts',(57.8277317035128,12.144288531381,2.7153110078172));
#229230=CARTESIAN_POINT('Ctrl Pts',(57.8198958587085,12.1485735795159,2.70899119176064));
#229231=CARTESIAN_POINT('Ctrl Pts',(57.812226847525,12.1535378042503,2.70298296066811));
#229232=CARTESIAN_POINT('Ctrl Pts',(57.8048391253241,12.1592011408681,2.69736727774103));
#229233=CARTESIAN_POINT('Ctrl Pts',(57.7979524842552,12.1644803548773,2.69213248525373));
#229234=CARTESIAN_POINT('Ctrl Pts',(57.7913098171238,12.1703677426436,2.68723866185394));
#229235=CARTESIAN_POINT('Ctrl Pts',(57.7850318067596,12.1768883481381,2.68278595829474));
#229236=CARTESIAN_POINT('Ctrl Pts',(57.7827352293487,12.179273669986,2.68115710172745));
#229237=CARTESIAN_POINT('Ctrl Pts',(57.7804877669873,12.1817437717242,2.67958763637776));
#229238=CARTESIAN_POINT('Ctrl Pts',(57.7782965440189,12.1842999559277,2.67808378645355));
#229239=CARTESIAN_POINT('Ctrl Pts',(57.7777696280971,12.1849146328342,2.6777221607859));
#229240=CARTESIAN_POINT('Ctrl Pts',(57.7772459087255,12.1855348686826,2.67736403603553));
#229241=CARTESIAN_POINT('Ctrl Pts',(57.7767255109848,12.1861606108967,2.67700956934469));
#229242=CARTESIAN_POINT('Ctrl Pts',(57.7762213756734,12.1867667986667,2.67666617973794));
#229243=CARTESIAN_POINT('Ctrl Pts',(57.7757203576392,12.187378154007,2.67632622314108));
#229244=CARTESIAN_POINT('Ctrl Pts',(57.7752225713658,12.187994625406,2.67598984158763));
#229245=CARTESIAN_POINT('Ctrl Pts',(57.7697687474616,12.1947487820215,2.67230439292218));
#229246=CARTESIAN_POINT('Ctrl Pts',(57.764699586453,12.2021217510025,2.66904964539978));
#229247=CARTESIAN_POINT('Ctrl Pts',(57.7601772489165,12.2100174179589,2.6664020356673));
#229248=CARTESIAN_POINT('Ctrl Pts',(57.7583017007436,12.2132919863906,2.66530399299439));
#229249=CARTESIAN_POINT('Ctrl Pts',(57.7565200187333,12.2166560758248,2.66430995142252));
#229250=CARTESIAN_POINT('Ctrl Pts',(57.7548425830507,12.2201014385647,2.66343053473349));
#229251=CARTESIAN_POINT('Ctrl Pts',(57.7519815416931,12.2259778637495,2.66193059792872));
#229252=CARTESIAN_POINT('Ctrl Pts',(57.7494261286934,12.2320899429715,2.66076519817115));
#229253=CARTESIAN_POINT('Ctrl Pts',(57.7472322823296,12.2383911161014,2.65997805604447));
#229254=CARTESIAN_POINT('Ctrl Pts',(57.7461353591478,12.2415417026663,2.65958448498113));
#229255=CARTESIAN_POINT('Ctrl Pts',(57.745130227238,12.2447399293287,2.65928526260749));
#229256=CARTESIAN_POINT('Ctrl Pts',(57.7442239366605,12.247979944712,2.65908463971311));
#229257=CARTESIAN_POINT('Ctrl Pts',(57.7433176460829,12.2512199600952,2.65888401681874));
#229258=CARTESIAN_POINT('Ctrl Pts',(57.7425101887133,12.254501719267,2.65878198860271));
#229259=CARTESIAN_POINT('Ctrl Pts',(57.7418065394566,12.257819391977,2.65878198860271));
#229260=CARTESIAN_POINT('Origin',(55.4074307335706,18.0189898472952,2.83404198860275));
#229261=CARTESIAN_POINT('Ctrl Pts',(59.5312589135996,19.5431821162869,2.83404198860276));
#229262=CARTESIAN_POINT('Ctrl Pts',(59.5413499366335,19.5464608884258,2.82419652440055));
#229263=CARTESIAN_POINT('Ctrl Pts',(59.5516697238494,19.5489337165498,2.81438790575618));
#229264=CARTESIAN_POINT('Ctrl Pts',(59.562159273367,19.5505973858262,2.8046678125685));
#229265=CARTESIAN_POINT('Ctrl Pts',(59.5723079749865,19.5522069957576,2.79526356453009));
#229266=CARTESIAN_POINT('Ctrl Pts',(59.5826168684419,19.553059311798,2.78594102496147));
#229267=CARTESIAN_POINT('Ctrl Pts',(59.5930429125542,19.5531064127991,2.77675109088679));
#229268=CARTESIAN_POINT('Ctrl Pts',(59.6029053082857,19.5531509674457,2.76805797913568));
#229269=CARTESIAN_POINT('Ctrl Pts',(59.6128734577668,19.5524750234009,2.75948271210033));
#229270=CARTESIAN_POINT('Ctrl Pts',(59.6229049605519,19.5509963368653,2.75108575573083));
#229271=CARTESIAN_POINT('Ctrl Pts',(59.6321447001138,19.5496343596247,2.74335155163114));
#229272=CARTESIAN_POINT('Ctrl Pts',(59.6414387315215,19.5475912199412,2.73576818685772));
#229273=CARTESIAN_POINT('Ctrl Pts',(59.6507389334469,19.54476746117,2.72840626160314));
#229274=CARTESIAN_POINT('Ctrl Pts',(59.653436568497,19.54394839609,2.72627084693563));
#229275=CARTESIAN_POINT('Ctrl Pts',(59.6561345922141,19.5430634173954,2.7241542458747));
#229276=CARTESIAN_POINT('Ctrl Pts',(59.658831468516,19.542109499003,2.72205867173269));
#229277=CARTESIAN_POINT('Ctrl Pts',(59.6617550558218,19.5410753901338,2.71978693462873));
#229278=CARTESIAN_POINT('Ctrl Pts',(59.6646735866702,19.5399627185792,2.71754411340774));
#229279=CARTESIAN_POINT('Ctrl Pts',(59.6675844741794,19.5387684320157,2.71533341844271));
#229280=CARTESIAN_POINT('Ctrl Pts',(59.6755734277899,19.5354907031708,2.70926614876419));
#229281=CARTESIAN_POINT('Ctrl Pts',(59.683478254909,19.5315625649727,2.70347381860436));
#229282=CARTESIAN_POINT('Ctrl Pts',(59.6911955084649,19.5269766895185,2.69804914171422));
#229283=CARTESIAN_POINT('Ctrl Pts',(59.6982563764893,19.5227808624507,2.69308585687216));
#229284=CARTESIAN_POINT('Ctrl Pts',(59.7051493183936,19.5180305486458,2.68842799053182));
#229285=CARTESIAN_POINT('Ctrl Pts',(59.7117949558643,19.5126862934693,2.68414767054202));
#229286=CARTESIAN_POINT('Ctrl Pts',(59.7150592712806,19.5100612127846,2.68204519134552));
#229287=CARTESIAN_POINT('Ctrl Pts',(59.7182634781249,19.5072925729231,2.68003431778517));
#229288=CARTESIAN_POINT('Ctrl Pts',(59.7213950854346,19.5043743927941,2.6781269394528));
#229289=CARTESIAN_POINT('Ctrl Pts',(59.7219892774193,19.5038206965381,2.67776503299232));
#229290=CARTESIAN_POINT('Ctrl Pts',(59.7225808838923,19.5032610854118,2.67740659639953));
#229291=CARTESIAN_POINT('Ctrl Pts',(59.7231697699855,19.5026955970361,2.67705178968884));
#229292=CARTESIAN_POINT('Ctrl Pts',(59.7237402533883,19.5021477801721,2.67670807068786));
#229293=CARTESIAN_POINT('Ctrl Pts',(59.7243081837714,19.5015944476715,2.67636775825294));
#229294=CARTESIAN_POINT('Ctrl Pts',(59.724873437353,19.5010356373988,2.67603099699284));
#229295=CARTESIAN_POINT('Ctrl Pts',(59.7310334544114,19.4949458381924,2.67236104217166));
#229296=CARTESIAN_POINT('Ctrl Pts',(59.73687933922,19.4882011960857,2.66911440541519));
#229297=CARTESIAN_POINT('Ctrl Pts',(59.7422363728284,19.4808775251058,2.66646778189679));
#229298=CARTESIAN_POINT('Ctrl Pts',(59.744498681387,19.4777846933729,2.66535009635015));
#229299=CARTESIAN_POINT('Ctrl Pts',(59.7466739523113,19.4745890081272,2.66433897912378));
#229300=CARTESIAN_POINT('Ctrl Pts',(59.748750122512,19.4712977780157,2.66344564884821));
#229301=CARTESIAN_POINT('Ctrl Pts',(59.752246341252,19.465755428747,2.66194130298614));
#229302=CARTESIAN_POINT('Ctrl Pts',(59.7554590576862,19.4599426670173,2.66077206705447));
#229303=CARTESIAN_POINT('Ctrl Pts',(59.758325802888,19.4538995640364,2.65998225155741));
#229304=CARTESIAN_POINT('Ctrl Pts',(59.7590424891885,19.4523887882911,2.65978479768315));
#229305=CARTESIAN_POINT('Ctrl Pts',(59.7597373347835,19.4508635299954,2.65961098966649));
#229306=CARTESIAN_POINT('Ctrl Pts',(59.7604090725467,19.449324313038,2.65946139030529));
#229307=CARTESIAN_POINT('Ctrl Pts',(59.7614166791915,19.4470154876017,2.65923699126347));
#229308=CARTESIAN_POINT('Ctrl Pts',(59.7623722755974,19.4446752658775,2.65906707562469));
#229309=CARTESIAN_POINT('Ctrl Pts',(59.7632731754137,19.4423059520262,2.65895332562946));
#229310=CARTESIAN_POINT('Ctrl Pts',(59.76417407523,19.439936638175,2.65883957563424));
#229311=CARTESIAN_POINT('Ctrl Pts',(59.7650202849808,19.4375382417966,2.65878198860276));
#229312=CARTESIAN_POINT('Ctrl Pts',(59.7658094374968,19.4351129318428,2.65878198860276));
#229313=CARTESIAN_POINT('Ctrl Pts',(56.1347810195642,18.2553202812751,2.65878198860275));
#229314=CARTESIAN_POINT('Ctrl Pts',(56.1321105487811,18.2635267101474,2.65878198860275));
#229315=CARTESIAN_POINT('Ctrl Pts',(56.1301406315643,18.2718824441049,2.6594533551787));
#229316=CARTESIAN_POINT('Ctrl Pts',(56.1288305556598,18.2802419597938,2.66072561226618));
#229317=CARTESIAN_POINT('Ctrl Pts',(56.1279843810471,18.2856413491927,2.66154735980356));
#229318=CARTESIAN_POINT('Ctrl Pts',(56.1274125556283,18.2910421817935,2.66261895766898));
#229319=CARTESIAN_POINT('Ctrl Pts',(56.1270952669252,18.2964056883426,2.6639142925104));
#229320=CARTESIAN_POINT('Ctrl Pts',(56.1266747189247,18.3035147090331,2.66563118464136));
#229321=CARTESIAN_POINT('Ctrl Pts',(56.126707076608,18.3105573165143,2.66774105138712));
#229322=CARTESIAN_POINT('Ctrl Pts',(56.1271555587355,18.3174512966901,2.67016894181762));
#229323=CARTESIAN_POINT('Ctrl Pts',(56.1273797997992,18.320898286778,2.67138288703288));
#229324=CARTESIAN_POINT('Ctrl Pts',(56.127708008729,18.324308309033,2.67267613167564));
#229325=CARTESIAN_POINT('Ctrl Pts',(56.128135143741,18.3276724292421,2.67403835432566));
#229326=CARTESIAN_POINT('Ctrl Pts',(56.128348711247,18.3293544893466,2.67471946565067));
#229327=CARTESIAN_POINT('Ctrl Pts',(56.1285870051496,18.3310250895515,2.67541781389536));
#229328=CARTESIAN_POINT('Ctrl Pts',(56.1288493629352,18.3326832110572,2.67613207244182));
#229329=CARTESIAN_POINT('Ctrl Pts',(56.1289149523817,18.3330977414336,2.67631063707844));
#229330=CARTESIAN_POINT('Ctrl Pts',(56.1289820457109,18.3335114922231,2.67649019601858));
#229331=CARTESIAN_POINT('Ctrl Pts',(56.1290506323488,18.3339244481758,2.6766707283667));
#229332=CARTESIAN_POINT('Ctrl Pts',(56.1292563922628,18.3351633160338,2.67721232541104));
#229333=CARTESIAN_POINT('Ctrl Pts',(56.1294755925119,18.3363950287072,2.6777626834006));
#229334=CARTESIAN_POINT('Ctrl Pts',(56.1297079426452,18.3376191892287,2.67832123541529));
#229335=CARTESIAN_POINT('Ctrl Pts',(56.1313445869829,18.3462420178745,2.68225560368465));
#229336=CARTESIAN_POINT('Ctrl Pts',(56.1335959402409,18.3545284904609,2.68661792998919));
#229337=CARTESIAN_POINT('Ctrl Pts',(56.1363459252322,18.3624495731178,2.69130986622619));
#229338=CARTESIAN_POINT('Ctrl Pts',(56.1376796649813,18.3662912896467,2.69358545023088));
#229339=CARTESIAN_POINT('Ctrl Pts',(56.1391312300712,18.3700472768054,2.69593918853493));
#229340=CARTESIAN_POINT('Ctrl Pts',(56.1406901365234,18.3737149835765,2.69836306235489));
#229341=CARTESIAN_POINT('Ctrl Pts',(56.1430767133842,18.3793299863881,2.70207384382222));
#229342=CARTESIAN_POINT('Ctrl Pts',(56.1457125629779,18.3847354115623,2.70594760814222));
#229343=CARTESIAN_POINT('Ctrl Pts',(56.148556929721,18.3899096889381,2.70995196345702));
#229344=CARTESIAN_POINT('Ctrl Pts',(56.1498778683512,18.3923126501195,2.711811606781));
#229345=CARTESIAN_POINT('Ctrl Pts',(56.1512435269776,18.3946658026161,2.71369962772093));
#229346=CARTESIAN_POINT('Ctrl Pts',(56.152650749137,18.3969661720539,2.71561183138655));
#229347=CARTESIAN_POINT('Ctrl Pts',(56.1527586071708,18.3971424863074,2.71575839426306));
#229348=CARTESIAN_POINT('Ctrl Pts',(56.1528666894395,18.3973185179288,2.71590508903203));
#229349=CARTESIAN_POINT('Ctrl Pts',(56.1529749944979,18.3974942667072,2.71605191409906));
#229350=CARTESIAN_POINT('Ctrl Pts',(56.1544963540396,18.3999630071782,2.71811436362748));
#229351=CARTESIAN_POINT('Ctrl Pts',(56.1560635207938,18.4023749585854,2.72020091026954));
#229352=CARTESIAN_POINT('Ctrl Pts',(56.1576709325004,18.4047288488037,2.72230624862177));
#229353=CARTESIAN_POINT('Ctrl Pts',(56.1634348250117,18.4131694805009,2.72985561753108));
#229354=CARTESIAN_POINT('Ctrl Pts',(56.1697591292906,18.4209299141242,2.73770089914347));
#229355=CARTESIAN_POINT('Ctrl Pts',(56.1765231650109,18.4280560759389,2.74574823347102));
#229356=CARTESIAN_POINT('Ctrl Pts',(56.1839561607596,18.4358870118866,2.75459144547035));
#229357=CARTESIAN_POINT('Ctrl Pts',(56.1919204977439,18.44295259451,2.76367911754263));
#229358=CARTESIAN_POINT('Ctrl Pts',(56.2003032932669,18.4492898603071,2.77292162564701));
#229359=CARTESIAN_POINT('Ctrl Pts',(56.2093546086368,18.456132516931,2.78290121484645));
#229360=CARTESIAN_POINT('Ctrl Pts',(56.2188946068446,18.4621268842286,2.7930622950004));
#229361=CARTESIAN_POINT('Ctrl Pts',(56.2288243369853,18.4672816799261,2.80331916685042));
#229362=CARTESIAN_POINT('Ctrl Pts',(56.2386707668939,18.4723932321846,2.81348999408555));
#229363=CARTESIAN_POINT('Ctrl Pts',(56.2489017962819,18.4766796388001,2.82375635966813));
#229364=CARTESIAN_POINT('Ctrl Pts',(56.2594439784239,18.4801050014193,2.83404198860275));
#229365=CARTESIAN_POINT('Origin',(0.00470941899427448,-0.0144941013081504,
2.83404198860262));
#229366=CARTESIAN_POINT('Ctrl Pts',(59.7752282754837,19.4061247292256,2.65878198860276));
#229367=CARTESIAN_POINT('Ctrl Pts',(59.7778789856303,19.3979550581544,2.65878198860276));
#229368=CARTESIAN_POINT('Ctrl Pts',(59.7798236858212,19.3896365599065,2.65944603041863));
#229369=CARTESIAN_POINT('Ctrl Pts',(59.781106115828,19.3813136269513,2.66070439264079));
#229370=CARTESIAN_POINT('Ctrl Pts',(59.7819255275519,19.3759956690086,2.66150842619604));
#229371=CARTESIAN_POINT('Ctrl Pts',(59.7824754874621,19.3706760212378,2.66255428265377));
#229372=CARTESIAN_POINT('Ctrl Pts',(59.7827759879495,19.3653918801542,2.66381699700666));
#229373=CARTESIAN_POINT('Ctrl Pts',(59.783186110819,19.3581800878465,2.66554034873266));
#229374=CARTESIAN_POINT('Ctrl Pts',(59.7831255716887,19.3510354548622,2.6676675964397));
#229375=CARTESIAN_POINT('Ctrl Pts',(59.7826350657124,19.3440445557098,2.67012012783147));
#229376=CARTESIAN_POINT('Ctrl Pts',(59.7823898127243,19.3405491061336,2.67134639352735));
#229377=CARTESIAN_POINT('Ctrl Pts',(59.7820371343799,19.3370918919976,2.67265375585011));
#229378=CARTESIAN_POINT('Ctrl Pts',(59.7815825865439,19.3336823180311,2.67403135126939));
#229379=CARTESIAN_POINT('Ctrl Pts',(59.7813553126259,19.3319775310479,2.67472014897903));
#229380=CARTESIAN_POINT('Ctrl Pts',(59.7811025767643,19.3302846375612,2.67542649668632));
#229381=CARTESIAN_POINT('Ctrl Pts',(59.7808251076836,19.3286047092266,2.67614899656101));
#229382=CARTESIAN_POINT('Ctrl Pts',(59.7807557404135,19.328184727143,2.67632962152968));
#229383=CARTESIAN_POINT('Ctrl Pts',(59.7806848274338,19.3277655550292,2.67651125590949));
#229384=CARTESIAN_POINT('Ctrl Pts',(59.7806123803667,19.3273472089197,2.67669387767523));
#229385=CARTESIAN_POINT('Ctrl Pts',(59.7803950391653,19.3260921705914,2.67724174297243));
#229386=CARTESIAN_POINT('Ctrl Pts',(59.7801638905868,19.3248445680579,2.67779849504746));
#229387=CARTESIAN_POINT('Ctrl Pts',(59.7799192536869,19.3236048185588,2.67836353618008));
#229388=CARTESIAN_POINT('Ctrl Pts',(59.7782286609226,19.315037380311,2.68226832098912));
#229389=CARTESIAN_POINT('Ctrl Pts',(59.7759321681721,19.3068044648772,2.68659153751402));
#229390=CARTESIAN_POINT('Ctrl Pts',(59.7731456380809,19.2989322844403,2.69123699486196));
#229391=CARTESIAN_POINT('Ctrl Pts',(59.7717607402745,19.2950198323721,2.69354577441228));
#229392=CARTESIAN_POINT('Ctrl Pts',(59.7702542302928,19.2911962646692,2.69593478828122));
#229393=CARTESIAN_POINT('Ctrl Pts',(59.7686372707431,19.2874640247236,2.69839565261218));
#229394=CARTESIAN_POINT('Ctrl Pts',(59.765070016461,19.2792301459419,2.70382468689043));
#229395=CARTESIAN_POINT('Ctrl Pts',(59.7609769706902,19.2714367138416,2.70961155815084));
#229396=CARTESIAN_POINT('Ctrl Pts',(59.7564706723513,19.2641757185814,2.71562701361764));
#229397=CARTESIAN_POINT('Ctrl Pts',(59.7548244647406,19.2615231854469,2.71782453535854));
#229398=CARTESIAN_POINT('Ctrl Pts',(59.7531276155319,19.2589351484757,2.72005051502398));
#229399=CARTESIAN_POINT('Ctrl Pts',(59.7513854342766,19.2564118357497,2.72229986760111));
#229400=CARTESIAN_POINT('Ctrl Pts',(59.7455336317917,19.2479362953116,2.72985520488891));
#229401=CARTESIAN_POINT('Ctrl Pts',(59.7391263493541,19.2401420439515,2.73770845534564));
#229402=CARTESIAN_POINT('Ctrl Pts',(59.7322837268614,19.2329840462267,2.74576706701767));
#229403=CARTESIAN_POINT('Ctrl Pts',(59.72476287418,19.2251165588065,2.75462443585051));
#229404=CARTESIAN_POINT('Ctrl Pts',(59.7167157560775,19.2180171087286,2.76373036323212));
#229405=CARTESIAN_POINT('Ctrl Pts',(59.7082546997627,19.2116502033059,2.77299664636857));
#229406=CARTESIAN_POINT('Ctrl Pts',(59.6991417795841,19.2047927733655,2.78297683033519));
#229407=CARTESIAN_POINT('Ctrl Pts',(59.6895478206989,19.1987842816755,2.79314401478941));
#229408=CARTESIAN_POINT('Ctrl Pts',(59.6795708632003,19.1936187207957,2.80341452427985));
#229409=CARTESIAN_POINT('Ctrl Pts',(59.6697286283149,19.1885229124291,2.81354634721401));
#229410=CARTESIAN_POINT('Ctrl Pts',(59.6595122814319,19.1842470541691,2.8237800420923));
#229411=CARTESIAN_POINT('Ctrl Pts',(59.6489943884564,19.1808295835784,2.83404198860276));
#229412=CARTESIAN_POINT('Ctrl Pts',(56.3771794532807,18.1177524687109,2.83404198860275));
#229413=CARTESIAN_POINT('Ctrl Pts',(56.3671137719648,18.1144819305953,2.82422126443045));
#229414=CARTESIAN_POINT('Ctrl Pts',(56.3568263239572,18.1120170699781,2.81442815028565));
#229415=CARTESIAN_POINT('Ctrl Pts',(56.3463749453358,18.1103629196652,2.80471618166407));
#229416=CARTESIAN_POINT('Ctrl Pts',(56.3362832197241,18.1087656919995,2.79533842146335));
#229417=CARTESIAN_POINT('Ctrl Pts',(56.3260373921228,18.1079242184407,2.78603515650362));
#229418=CARTESIAN_POINT('Ctrl Pts',(56.3156801719846,18.107887916365,2.77685887346893));
#229419=CARTESIAN_POINT('Ctrl Pts',(56.3058893552734,18.1078535995344,2.76818441216724));
#229420=CARTESIAN_POINT('Ctrl Pts',(56.2959980926938,18.1085387949865,2.75962261521781));
#229421=CARTESIAN_POINT('Ctrl Pts',(56.286049015115,18.1100266905428,2.75123537701824));
#229422=CARTESIAN_POINT('Ctrl Pts',(56.2768860815732,18.1113970173888,2.74351087134289));
#229423=CARTESIAN_POINT('Ctrl Pts',(56.2676735798211,18.1134483398646,2.73593399450021));
#229424=CARTESIAN_POINT('Ctrl Pts',(56.2584600414676,18.1162805994777,2.72857657812754));
#229425=CARTESIAN_POINT('Ctrl Pts',(56.255712750318,18.1171251221214,2.72638274508441));
#229426=CARTESIAN_POINT('Ctrl Pts',(56.2529655048683,18.1180393245074,2.72420861709659));
#229427=CARTESIAN_POINT('Ctrl Pts',(56.2502199893832,18.1190265064342,2.72205663736722));
#229428=CARTESIAN_POINT('Ctrl Pts',(56.2475025263006,18.1200036017944,2.71992664556761));
#229429=CARTESIAN_POINT('Ctrl Pts',(56.244789485083,18.1210509212418,2.71782089927879));
#229430=CARTESIAN_POINT('Ctrl Pts',(56.242085504679,18.1221702476366,2.7157438731124));
#229431=CARTESIAN_POINT('Ctrl Pts',(56.2418974751699,18.1222480834051,2.71559944077481));
#229432=CARTESIAN_POINT('Ctrl Pts',(56.2417094803631,18.12232625961,2.71545515216063));
#229433=CARTESIAN_POINT('Ctrl Pts',(56.2415215209613,18.1224047773505,2.71531100781725));
#229434=CARTESIAN_POINT('Ctrl Pts',(56.2332806922381,18.1258472827277,2.7089911917607));
#229435=CARTESIAN_POINT('Ctrl Pts',(56.2251347899176,18.1299826829658,2.70298296066818));
#229436=CARTESIAN_POINT('Ctrl Pts',(56.2171955585582,18.1348427679843,2.69736727774111));
#229437=CARTESIAN_POINT('Ctrl Pts',(56.2097948151021,18.1393732118986,2.69213248525389));
#229438=CARTESIAN_POINT('Ctrl Pts',(56.2025731376006,18.1445340001514,2.68723866185417));
#229439=CARTESIAN_POINT('Ctrl Pts',(56.1956479299622,18.1503626543108,2.68278595829503));
#229440=CARTESIAN_POINT('Ctrl Pts',(56.1931145994154,18.1524948514087,2.68115710172765));
#229441=CARTESIAN_POINT('Ctrl Pts',(56.190621252949,18.1547164978844,2.67958763637787));
#229442=CARTESIAN_POINT('Ctrl Pts',(56.1881748397225,18.1570296338739,2.67808378645358));
#229443=CARTESIAN_POINT('Ctrl Pts',(56.1875865590689,18.1575858658044,2.67772216078593));
#229444=CARTESIAN_POINT('Ctrl Pts',(56.1870008763867,18.1581479603548,2.67736403603556));
#229445=CARTESIAN_POINT('Ctrl Pts',(56.1864179215672,18.1587158783115,2.67700956934472));
#229446=CARTESIAN_POINT('Ctrl Pts',(56.1858531840857,18.159266048832,2.67666617973797));
#229447=CARTESIAN_POINT('Ctrl Pts',(56.1852910066466,18.1598216844587,2.67632622314112));
#229448=CARTESIAN_POINT('Ctrl Pts',(56.1847315084904,18.1603827459286,2.67598984158766));
#229449=CARTESIAN_POINT('Ctrl Pts',(56.1786015595926,18.1665298227359,2.67230439292221));
#229450=CARTESIAN_POINT('Ctrl Pts',(56.172789482861,18.1733325302111,2.6690496453998));
#229451=CARTESIAN_POINT('Ctrl Pts',(56.1674665972293,18.1807122308847,2.66640203566733));
#229452=CARTESIAN_POINT('Ctrl Pts',(56.1652590378995,18.1837728127195,2.66530399299442));
#229453=CARTESIAN_POINT('Ctrl Pts',(56.1631354730308,18.1869322368373,2.66430995142256));
#229454=CARTESIAN_POINT('Ctrl Pts',(56.1611070880438,18.1901833857455,2.66343053473353));
#229455=CARTESIAN_POINT('Ctrl Pts',(56.157647466076,18.1957285590018,2.66193059792876));
#229456=CARTESIAN_POINT('Ctrl Pts',(56.1544671656478,18.2015400422205,2.66076519817119));
#229457=CARTESIAN_POINT('Ctrl Pts',(56.1516266854597,18.2075773774755,2.65997805604451));
#229458=CARTESIAN_POINT('Ctrl Pts',(56.1502064453657,18.210596045103,2.65958448498117));
#229459=CARTESIAN_POINT('Ctrl Pts',(56.1488725139556,18.2136716866512,2.65928526260753));
#229460=CARTESIAN_POINT('Ctrl Pts',(56.1476325143037,18.2167992197299,2.65908463971316));
#229461=CARTESIAN_POINT('Ctrl Pts',(56.1463925146518,18.2199267528085,2.65888401681878));
#229462=CARTESIAN_POINT('Ctrl Pts',(56.1452464433752,18.2231061318822,2.65878198860275));
#229463=CARTESIAN_POINT('Ctrl Pts',(56.1441998575527,18.2263320786585,2.65878198860275));
#229464=CARTESIAN_POINT('Origin',(53.2204057122638,23.7119335237428,2.83404198860279));
#229465=CARTESIAN_POINT('Ctrl Pts',(57.1623216544371,25.6588335304443,2.8340419886028));
#229466=CARTESIAN_POINT('Ctrl Pts',(57.1720146727781,25.663149140257,2.82419652440077));
#229467=CARTESIAN_POINT('Ctrl Pts',(57.1820194461961,25.6666871334688,2.8143879057565));
#229468=CARTESIAN_POINT('Ctrl Pts',(57.1922776320711,25.6694381454823,2.8046678125689));
#229469=CARTESIAN_POINT('Ctrl Pts',(57.2022024879886,25.6720997659865,2.79526356453055));
#229470=CARTESIAN_POINT('Ctrl Pts',(57.2123658169611,25.6740249857413,2.78594102496196));
#229471=CARTESIAN_POINT('Ctrl Pts',(57.2227298227175,25.6751616470872,2.77675109088729));
#229472=CARTESIAN_POINT('Ctrl Pts',(57.2325335339844,25.6762368587288,2.76805797913617));
#229473=CARTESIAN_POINT('Ctrl Pts',(57.2425177322919,25.676606572923,2.7594827121008));
#229474=CARTESIAN_POINT('Ctrl Pts',(57.2526488462863,25.6761845643574,2.75108575573128));
#229475=CARTESIAN_POINT('Ctrl Pts',(57.261980334976,25.675795863948,2.74335155163154));
#229476=CARTESIAN_POINT('Ctrl Pts',(57.2714370189586,25.6747354076181,2.73576818685809));
#229477=CARTESIAN_POINT('Ctrl Pts',(57.2809814365697,25.6728992535083,2.72840626160347));
#229478=CARTESIAN_POINT('Ctrl Pts',(57.2837499093069,25.6723666549987,2.72627084693586));
#229479=CARTESIAN_POINT('Ctrl Pts',(57.2865256584309,25.671768544583,2.72415424587485));
#229480=CARTESIAN_POINT('Ctrl Pts',(57.289307472586,25.6711017521907,2.72205867173275));
#229481=CARTESIAN_POINT('Ctrl Pts',(57.2923231379855,25.6703789063664,2.71978693462878));
#229482=CARTESIAN_POINT('Ctrl Pts',(57.2953419866643,25.6695773996876,2.71754411340779));
#229483=CARTESIAN_POINT('Ctrl Pts',(57.2983617649664,25.6686939261489,2.71533341844276));
#229484=CARTESIAN_POINT('Ctrl Pts',(57.3066495702123,25.6662692260896,2.70926614876423));
#229485=CARTESIAN_POINT('Ctrl Pts',(57.3149216961106,25.6631888860747,2.70347381860441));
#229486=CARTESIAN_POINT('Ctrl Pts',(57.323076028258,25.6594348051809,2.69804914171426));
#229487=CARTESIAN_POINT('Ctrl Pts',(57.3305367994641,25.6560000249768,2.69308585687221));
#229488=CARTESIAN_POINT('Ctrl Pts',(57.3378885241135,25.6519962425126,2.68842799053188));
#229489=CARTESIAN_POINT('Ctrl Pts',(57.3450563828676,25.6473759219974,2.6841476705421));
#229490=CARTESIAN_POINT('Ctrl Pts',(57.3485772116725,25.6451064356535,2.68204519134558));
#229491=CARTESIAN_POINT('Ctrl Pts',(57.3520532672065,25.6426878935082,2.68003431778521));
#229492=CARTESIAN_POINT('Ctrl Pts',(57.3554727521281,25.6401130415749,2.67812693945283));
#229493=CARTESIAN_POINT('Ctrl Pts',(57.3561215660858,25.6396244884999,2.67776503299235));
#229494=CARTESIAN_POINT('Ctrl Pts',(57.3567684269677,25.6391297826975,2.67740659639955));
#229495=CARTESIAN_POINT('Ctrl Pts',(57.3574131967122,25.6386289474846,2.67705178968887));
#229496=CARTESIAN_POINT('Ctrl Pts',(57.3580378174022,25.6381437633721,2.67670807068789));
#229497=CARTESIAN_POINT('Ctrl Pts',(57.3586604755991,25.637652826975,2.67636775825297));
#229498=CARTESIAN_POINT('Ctrl Pts',(57.3592810442415,25.6371561630117,2.67603099699287));
#229499=CARTESIAN_POINT('Ctrl Pts',(57.3660438734345,25.6317436214795,2.67236104217177));
#229500=CARTESIAN_POINT('Ctrl Pts',(57.3725627409489,25.6256469885836,2.66911440541536));
#229501=CARTESIAN_POINT('Ctrl Pts',(57.3786559602397,25.6189233999305,2.66646778189699));
#229502=CARTESIAN_POINT('Ctrl Pts',(57.3812291645836,25.6160839866904,2.66535009635028));
#229503=CARTESIAN_POINT('Ctrl Pts',(57.3837265592141,25.6131331854697,2.66433897912385));
#229504=CARTESIAN_POINT('Ctrl Pts',(57.3861353831632,25.6100770039414,2.66344564884824));
#229505=CARTESIAN_POINT('Ctrl Pts',(57.3901917825031,25.6049304706141,2.66194130298617));
#229506=CARTESIAN_POINT('Ctrl Pts',(57.3939944983914,25.5994853721131,2.66077206705451));
#229507=CARTESIAN_POINT('Ctrl Pts',(57.397477215531,25.5937750303531,2.65998225155745));
#229508=CARTESIAN_POINT('Ctrl Pts',(57.398347894816,25.5923474449131,2.65978479768319));
#229509=CARTESIAN_POINT('Ctrl Pts',(57.3991983668799,25.5909031732843,2.65961098966653));
#229510=CARTESIAN_POINT('Ctrl Pts',(57.4000273167765,25.5894426040344,2.65946139030532));
#229511=CARTESIAN_POINT('Ctrl Pts',(57.4012707416215,25.5872517501597,2.65923699126351));
#229512=CARTESIAN_POINT('Ctrl Pts',(57.4024657229508,25.5850242354387,2.65906707562473));
#229513=CARTESIAN_POINT('Ctrl Pts',(57.4036093482795,25.58276207061,2.65895332562951));
#229514=CARTESIAN_POINT('Ctrl Pts',(57.4047529736082,25.5804999057813,2.65883957563428));
#229515=CARTESIAN_POINT('Ctrl Pts',(57.4058452484196,25.5782031010733,2.6587819886028));
#229516=CARTESIAN_POINT('Ctrl Pts',(57.4068835917979,25.5758735661211,2.6587819886028));
#229517=CARTESIAN_POINT('Ctrl Pts',(53.9190682401995,24.0229981225299,2.65878198860279));
#229518=CARTESIAN_POINT('Ctrl Pts',(53.915554593136,24.0308804555186,2.65878198860279));
#229519=CARTESIAN_POINT('Ctrl Pts',(53.9127220553018,24.0389845034714,2.65945335517867));
#229520=CARTESIAN_POINT('Ctrl Pts',(53.9105453488017,24.0471612846371,2.66072561226602));
#229521=CARTESIAN_POINT('Ctrl Pts',(53.9091394197454,24.0524426462845,2.66154735980342));
#229522=CARTESIAN_POINT('Ctrl Pts',(53.9080061861139,24.0577541205273,2.66261895766892));
#229523=CARTESIAN_POINT('Ctrl Pts',(53.9071299964541,24.0630550795263,2.66391429251044));
#229524=CARTESIAN_POINT('Ctrl Pts',(53.9059686572515,24.0700811970213,2.6656311846414));
#229525=CARTESIAN_POINT('Ctrl Pts',(53.9052646847386,24.0770886066608,2.66774105138715));
#229526=CARTESIAN_POINT('Ctrl Pts',(53.9049900928804,24.0839917000394,2.67016894181766));
#229527=CARTESIAN_POINT('Ctrl Pts',(53.9048527969514,24.0874432467287,2.67138288703291));
#229528=CARTESIAN_POINT('Ctrl Pts',(53.9048227635323,24.0908688957001,2.67267613167568));
#229529=CARTESIAN_POINT('Ctrl Pts',(53.9048959123383,24.0942592346731,2.67403835432569));
#229530=CARTESIAN_POINT('Ctrl Pts',(53.9049324867413,24.0959544041596,2.6747194656507));
#229531=CARTESIAN_POINT('Ctrl Pts',(53.9049948499728,24.0976407611372,2.6754178138954));
#229532=CARTESIAN_POINT('Ctrl Pts',(53.9050824496422,24.099317223136,2.67613207244186));
#229533=CARTESIAN_POINT('Ctrl Pts',(53.9051043495595,24.0997363386357,2.67631063707847));
#229534=CARTESIAN_POINT('Ctrl Pts',(53.9051278266102,24.1001548360176,2.67649019601862));
#229535=CARTESIAN_POINT('Ctrl Pts',(53.9051528718723,24.1005726990103,2.67667072836673));
#229536=CARTESIAN_POINT('Ctrl Pts',(53.9052280076585,24.1018262879881,2.67721232541107));
#229537=CARTESIAN_POINT('Ctrl Pts',(53.9053172580728,24.1030741658758,2.67776268340064));
#229538=CARTESIAN_POINT('Ctrl Pts',(53.9054203757497,24.1043159075203,2.67832123541533));
#229539=CARTESIAN_POINT('Ctrl Pts',(53.906146723351,24.1130625753258,2.68225560368456));
#229540=CARTESIAN_POINT('Ctrl Pts',(53.9075195712149,24.1215389842443,2.68661792998894));
#229541=CARTESIAN_POINT('Ctrl Pts',(53.9094265129031,24.1297041260866,2.69130986622577));
#229542=CARTESIAN_POINT('Ctrl Pts',(53.9103513775612,24.133664211057,2.69358545023059));
#229543=CARTESIAN_POINT('Ctrl Pts',(53.91140238326,24.1375513523935,2.6959391885348));
#229544=CARTESIAN_POINT('Ctrl Pts',(53.9125693701071,24.1413619171793,2.69836306235492));
#229545=CARTESIAN_POINT('Ctrl Pts',(53.914355945435,24.1471956256297,2.70207384382226));
#229546=CARTESIAN_POINT('Ctrl Pts',(53.916412334782,24.1528469606267,2.70594760814226));
#229547=CARTESIAN_POINT('Ctrl Pts',(53.9187002605239,24.1582902100542,2.70995196345705));
#229548=CARTESIAN_POINT('Ctrl Pts',(53.9197627850745,24.1608180832479,2.71181160678103));
#229549=CARTESIAN_POINT('Ctrl Pts',(53.9208749910658,24.1633010951265,2.71369962772097));
#229550=CARTESIAN_POINT('Ctrl Pts',(53.9220340502326,24.1657359576697,2.71561183138659));
#229551=CARTESIAN_POINT('Ctrl Pts',(53.9221228875509,24.1659225802897,2.7157583942631));
#229552=CARTESIAN_POINT('Ctrl Pts',(53.9222119774187,24.1661089452649,2.71590508903207));
#229553=CARTESIAN_POINT('Ctrl Pts',(53.922301318421,24.1662950522344,2.71605191409909));
#229554=CARTESIAN_POINT('Ctrl Pts',(53.9235562901482,24.1689092940617,2.71811436362751));
#229555=CARTESIAN_POINT('Ctrl Pts',(53.9248627542249,24.1714718460794,2.72020091026957));
#229556=CARTESIAN_POINT('Ctrl Pts',(53.9262153118348,24.1739808617162,2.7223062486218));
#229557=CARTESIAN_POINT('Ctrl Pts',(53.9310653428794,24.1829777455763,2.72985561753096));
#229558=CARTESIAN_POINT('Ctrl Pts',(53.9365438157567,24.1913567365396,2.73770089914317));
#229559=CARTESIAN_POINT('Ctrl Pts',(53.9425259106379,24.1991508947534,2.74574823347055));
#229560=CARTESIAN_POINT('Ctrl Pts',(53.9490996319576,24.2077158916377,2.75459144546979));
#229561=CARTESIAN_POINT('Ctrl Pts',(53.9562817849767,24.2155752681661,2.76367911754196));
#229562=CARTESIAN_POINT('Ctrl Pts',(53.9639562340135,24.2227540584919,2.77292162564624));
#229563=CARTESIAN_POINT('Ctrl Pts',(53.9722427129493,24.2305053504132,2.78290121484572));
#229564=CARTESIAN_POINT('Ctrl Pts',(53.9811038680469,24.2374640812918,2.79306229499973));
#229565=CARTESIAN_POINT('Ctrl Pts',(53.9904403792142,24.2436285779114,2.8033191668498));
#229566=CARTESIAN_POINT('Ctrl Pts',(53.9996985666472,24.249741360739,2.81348999408515));
#229567=CARTESIAN_POINT('Ctrl Pts',(54.0094254978895,24.2550737197503,2.82375635966795));
#229568=CARTESIAN_POINT('Ctrl Pts',(54.0195518809641,24.2595822759735,2.83404198860279));
#229569=CARTESIAN_POINT('Origin',(0.00619866644047569,-0.013922432774286,
2.83404198860262));
#229570=CARTESIAN_POINT('Ctrl Pts',(57.4192809246789,25.5480287005721,2.6587819886028));
#229571=CARTESIAN_POINT('Ctrl Pts',(57.4227710771203,25.5401808584724,2.6587819886028));
#229572=CARTESIAN_POINT('Ctrl Pts',(57.4255746438785,25.5321112063512,2.65944603041859));
#229573=CARTESIAN_POINT('Ctrl Pts',(57.4277200319912,25.5239679177318,2.66070439264063));
#229574=CARTESIAN_POINT('Ctrl Pts',(57.4290908328636,25.518764743967,2.6615084261959));
#229575=CARTESIAN_POINT('Ctrl Pts',(57.4301938346425,25.5135317242471,2.66255428265371));
#229576=CARTESIAN_POINT('Ctrl Pts',(57.4310450321041,25.5083079410949,2.6638169970067));
#229577=CARTESIAN_POINT('Ctrl Pts',(57.4322067458449,25.5011785252534,2.66554034873269));
#229578=CARTESIAN_POINT('Ctrl Pts',(57.4328933558607,25.4940667032539,2.66766759643973));
#229579=CARTESIAN_POINT('Ctrl Pts',(57.4331362848728,25.4870628291426,2.67012012783149));
#229580=CARTESIAN_POINT('Ctrl Pts',(57.4332577493788,25.483560892087,2.67134639352736));
#229581=CARTESIAN_POINT('Ctrl Pts',(57.4332683803241,25.4800857520064,2.67265375585012));
#229582=CARTESIAN_POINT('Ctrl Pts',(57.4331727200758,25.4766473428561,2.6740313512694));
#229583=CARTESIAN_POINT('Ctrl Pts',(57.4331248899517,25.4749281382809,2.67472014897904));
#229584=CARTESIAN_POINT('Ctrl Pts',(57.4330504941582,25.4732181005506,2.67542649668632));
#229585=CARTESIAN_POINT('Ctrl Pts',(57.4329501454094,25.4715183716227,2.67614899656101));
#229586=CARTESIAN_POINT('Ctrl Pts',(57.4329250582222,25.4710934393907,2.67632962152968));
#229587=CARTESIAN_POINT('Ctrl Pts',(57.4328983491282,25.4706691511208,2.67651125590949));
#229588=CARTESIAN_POINT('Ctrl Pts',(57.4328700280096,25.4702455239745,2.67669387767523));
#229589=CARTESIAN_POINT('Ctrl Pts',(57.4327850646539,25.4689746425357,2.67724174297243));
#229590=CARTESIAN_POINT('Ctrl Pts',(57.432685592307,25.4677097128937,2.67779849504747));
#229591=CARTESIAN_POINT('Ctrl Pts',(57.4325718846637,25.4664511833529,2.67836353618008));
#229592=CARTESIAN_POINT('Ctrl Pts',(57.4317860942976,25.4577539633647,2.68226832098906));
#229593=CARTESIAN_POINT('Ctrl Pts',(57.4303627559732,25.4493260998451,2.68659153751387));
#229594=CARTESIAN_POINT('Ctrl Pts',(57.4284143577091,25.4412057723282,2.69123699486172));
#229595=CARTESIAN_POINT('Ctrl Pts',(57.42744600912,25.4371699918421,2.69354577441213));
#229596=CARTESIAN_POINT('Ctrl Pts',(57.4263474236138,25.4332098968698,2.69593478828116));
#229597=CARTESIAN_POINT('Ctrl Pts',(57.4251294472437,25.4293290842281,2.6983956526122));
#229598=CARTESIAN_POINT('Ctrl Pts',(57.4224424094497,25.4207674318877,2.70382468689046));
#229599=CARTESIAN_POINT('Ctrl Pts',(57.4191864212928,25.4125888532393,2.70961155815088));
#229600=CARTESIAN_POINT('Ctrl Pts',(57.4154637896041,25.4048965980306,2.71562701361769));
#229601=CARTESIAN_POINT('Ctrl Pts',(57.4141038653033,25.4020865201984,2.71782453535861));
#229602=CARTESIAN_POINT('Ctrl Pts',(57.4126868351396,25.3993352917243,2.72005051502405));
#229603=CARTESIAN_POINT('Ctrl Pts',(57.4112179557371,25.3966436944401,2.72229986760119));
#229604=CARTESIAN_POINT('Ctrl Pts',(57.406284145256,25.3876029039783,2.72985520488885));
#229605=CARTESIAN_POINT('Ctrl Pts',(57.4007266836991,25.379181606956,2.73770845534538));
#229606=CARTESIAN_POINT('Ctrl Pts',(57.3946697603107,25.3713475726778,2.74576706701718));
#229607=CARTESIAN_POINT('Ctrl Pts',(57.3880124840171,25.3627370410037,2.75462443584985));
#229608=CARTESIAN_POINT('Ctrl Pts',(57.3807515434763,25.3548353295672,2.76373036323127));
#229609=CARTESIAN_POINT('Ctrl Pts',(57.3730023605528,25.3476188815044,2.77299664636754));
#229610=CARTESIAN_POINT('Ctrl Pts',(57.364656158518,25.3398464577404,2.78297683033412));
#229611=CARTESIAN_POINT('Ctrl Pts',(57.3557428147462,25.3328680394176,2.79314401478833));
#229612=CARTESIAN_POINT('Ctrl Pts',(57.3463604602054,25.3266878999853,2.80341452427883));
#229613=CARTESIAN_POINT('Ctrl Pts',(57.33710479913,25.3205912133023,2.81354634721327));
#229614=CARTESIAN_POINT('Ctrl Pts',(57.3273913673572,25.3152708796012,2.82378004209189));
#229615=CARTESIAN_POINT('Ctrl Pts',(57.317288315449,25.3107727110825,2.8340419886028));
#229616=CARTESIAN_POINT('Ctrl Pts',(54.1745185419759,23.9115214566117,2.83404198860279));
#229617=CARTESIAN_POINT('Ctrl Pts',(54.164849865839,23.9072166846466,2.8242212644308));
#229618=CARTESIAN_POINT('Ctrl Pts',(54.1548764216408,23.9036899956627,2.8144281502863));
#229619=CARTESIAN_POINT('Ctrl Pts',(54.1446552025556,23.9009524404119,2.80471618166502));
#229620=CARTESIAN_POINT('Ctrl Pts',(54.1347857162263,23.8983090899566,2.79533842146448));
#229621=CARTESIAN_POINT('Ctrl Pts',(54.1246839742788,23.8964012454639,2.78603515650492));
#229622=CARTESIAN_POINT('Ctrl Pts',(54.1143872866766,23.89528251795,2.7768588734704));
#229623=CARTESIAN_POINT('Ctrl Pts',(54.1046536921696,23.8942249700856,2.76818441216881));
#229624=CARTESIAN_POINT('Ctrl Pts',(54.0947449925338,23.8938724934879,2.75962261521947));
#229625=CARTESIAN_POINT('Ctrl Pts',(54.0846948896071,23.8943122764064,2.75123537701999));
#229626=CARTESIAN_POINT('Ctrl Pts',(54.0754389134147,23.8947173090963,2.74351087134468));
#229627=CARTESIAN_POINT('Ctrl Pts',(54.0660624571252,23.8957944255618,2.73593399450204));
#229628=CARTESIAN_POINT('Ctrl Pts',(54.056603339754,23.8976480927549,2.7285765781294));
#229629=CARTESIAN_POINT('Ctrl Pts',(54.0537828218979,23.8982008188933,2.72638274508565));
#229630=CARTESIAN_POINT('Ctrl Pts',(54.0509550659748,23.8988228478381,2.72420861709723));
#229631=CARTESIAN_POINT('Ctrl Pts',(54.0481214021003,23.8995176373646,2.72205663736726));
#229632=CARTESIAN_POINT('Ctrl Pts',(54.0453166912883,23.9002053278541,2.71992664556764));
#229633=CARTESIAN_POINT('Ctrl Pts',(54.042509037702,23.9009633199468,2.71782089927883));
#229634=CARTESIAN_POINT('Ctrl Pts',(54.0397028685176,23.9017938716382,2.71574387311244));
#229635=CARTESIAN_POINT('Ctrl Pts',(54.0395077330006,23.9018516265785,2.71559944077485));
#229636=CARTESIAN_POINT('Ctrl Pts',(54.0393125964104,23.9019097237178,2.71545515216067));
#229637=CARTESIAN_POINT('Ctrl Pts',(54.0391174593312,23.9019681642225,2.71531100781729));
#229638=CARTESIAN_POINT('Ctrl Pts',(54.0305619349333,23.9045304100324,2.7089911917609));
#229639=CARTESIAN_POINT('Ctrl Pts',(54.0220283896864,23.9077916774637,2.70298296066853));
#229640=CARTESIAN_POINT('Ctrl Pts',(54.013624633049,23.9117952627743,2.69736727774157));
#229641=CARTESIAN_POINT('Ctrl Pts',(54.0057908713,23.9155273001022,2.69213248525463));
#229642=CARTESIAN_POINT('Ctrl Pts',(53.9980693056385,23.9199049461651,2.68723866185514));
#229643=CARTESIAN_POINT('Ctrl Pts',(53.9905727747503,23.9249777890345,2.68278595829617));
#229644=CARTESIAN_POINT('Ctrl Pts',(53.9878304467667,23.926833500585,2.68115710172839));
#229645=CARTESIAN_POINT('Ctrl Pts',(53.9851185338205,23.9287823509747,2.67958763637825));
#229646=CARTESIAN_POINT('Ctrl Pts',(53.9824437337507,23.9308270955486,2.67808378645362));
#229647=CARTESIAN_POINT('Ctrl Pts',(53.9818005336912,23.9313187883097,2.67772216078597));
#229648=CARTESIAN_POINT('Ctrl Pts',(53.9811593045604,23.9318165831367,2.6773640360356));
#229649=CARTESIAN_POINT('Ctrl Pts',(53.9805201796371,23.9323204546079,2.67700956934476));
#229650=CARTESIAN_POINT('Ctrl Pts',(53.9799010273677,23.9328085800956,2.67666617973801));
#229651=CARTESIAN_POINT('Ctrl Pts',(53.9792838498571,23.9333024083484,2.67632622314116));
#229652=CARTESIAN_POINT('Ctrl Pts',(53.9786687697971,23.9338019127825,2.6759898415877));
#229653=CARTESIAN_POINT('Ctrl Pts',(53.9719298569081,23.9392745611219,2.67230439292204));
#229654=CARTESIAN_POINT('Ctrl Pts',(53.9654385427822,23.945432475205,2.66904964539947));
#229655=CARTESIAN_POINT('Ctrl Pts',(53.9593734277039,23.9522153560514,2.66640203566691));
#229656=CARTESIAN_POINT('Ctrl Pts',(53.9568580436995,23.9550284189141,2.66530399299418));
#229657=CARTESIAN_POINT('Ctrl Pts',(53.9544158621939,23.9579485624032,2.66430995142248));
#229658=CARTESIAN_POINT('Ctrl Pts',(53.9520587513132,23.9609698772115,2.66343053473357));
#229659=CARTESIAN_POINT('Ctrl Pts',(53.9480384530775,23.9661230444607,2.6619305979288));
#229660=CARTESIAN_POINT('Ctrl Pts',(53.9442681092575,23.9715702598497,2.66076519817123));
#229661=CARTESIAN_POINT('Ctrl Pts',(53.9408121161403,23.9772776109213,2.65997805604455));
#229662=CARTESIAN_POINT('Ctrl Pts',(53.9390841195817,23.980131286457,2.65958448498121));
#229663=CARTESIAN_POINT('Ctrl Pts',(53.9374360035029,23.9830506455188,2.65928526260757));
#229664=CARTESIAN_POINT('Ctrl Pts',(53.9358758804724,23.9860314303859,2.6590846397132));
#229665=CARTESIAN_POINT('Ctrl Pts',(53.934315757442,23.9890122152531,2.65888401681882));
#229666=CARTESIAN_POINT('Ctrl Pts',(53.9328436288553,23.9920543802864,2.65878198860279));
#229667=CARTESIAN_POINT('Ctrl Pts',(53.9314655730804,23.995153256981,2.65878198860279));
#229668=CARTESIAN_POINT('Origin',(50.4502867888875,29.1450842944632,2.83404198860283));
#229669=CARTESIAN_POINT('Ctrl Pts',(54.1671020372438,31.4933613949861,2.83404198860284));
#229670=CARTESIAN_POINT('Ctrl Pts',(54.1762908521541,31.4986665597481,2.82419652440088));
#229671=CARTESIAN_POINT('Ctrl Pts',(54.1858709973828,31.5032309550536,2.81438790575673));
#229672=CARTESIAN_POINT('Ctrl Pts',(54.1957854287838,31.5070391691408,2.80466781256927));
#229673=CARTESIAN_POINT('Ctrl Pts',(54.2053777002009,31.5107236389466,2.79526356453105));
#229674=CARTESIAN_POINT('Ctrl Pts',(54.2152841131313,31.5137006693053,2.7859410249626));
#229675=CARTESIAN_POINT('Ctrl Pts',(54.2254725303159,31.5159144374965,2.77675109088808));
#229676=CARTESIAN_POINT('Ctrl Pts',(54.235110145606,31.5180085258893,2.76805797913714));
#229677=CARTESIAN_POINT('Ctrl Pts',(54.2450010037737,31.5194198476566,2.75948271210195));
#229678=CARTESIAN_POINT('Ctrl Pts',(54.2551207303723,31.5200591406751,2.75108575573259));
#229679=CARTESIAN_POINT('Ctrl Pts',(54.2644417304469,31.5206479757801,2.74335155163306));
#229680=CARTESIAN_POINT('Ctrl Pts',(54.2739574575954,31.5205818213853,2.73576818685979));
#229681=CARTESIAN_POINT('Ctrl Pts',(54.2836415202553,31.5197533892257,2.72840626160534));
#229682=CARTESIAN_POINT('Ctrl Pts',(54.2864504987137,31.5195130925472,2.72627084693712));
#229683=CARTESIAN_POINT('Ctrl Pts',(54.289273561557,31.5192084034332,2.7241542458755));
#229684=CARTESIAN_POINT('Ctrl Pts',(54.292109835428,31.5188360425581,2.7220586717328));
#229685=CARTESIAN_POINT('Ctrl Pts',(54.2951845386601,31.5184323794288,2.71978693462884));
#229686=CARTESIAN_POINT('Ctrl Pts',(54.2982706300314,31.5179508191006,2.71754411340784));
#229687=CARTESIAN_POINT('Ctrl Pts',(54.3013662138033,31.5173878381078,2.71533341844281));
#229688=CARTESIAN_POINT('Ctrl Pts',(54.3098620677559,31.5158427323553,2.70926614876428));
#229689=CARTESIAN_POINT('Ctrl Pts',(54.3184108612912,31.5136439393734,2.70347381860445));
#229690=CARTESIAN_POINT('Ctrl Pts',(54.3269129314607,31.5107627835359,2.69804914171431));
#229691=CARTESIAN_POINT('Ctrl Pts',(54.3346918640778,31.5081266823661,2.6930858568723));
#229692=CARTESIAN_POINT('Ctrl Pts',(54.3424218244385,31.5049132975211,2.68842799053201));
#229693=CARTESIAN_POINT('Ctrl Pts',(54.3500333719156,31.5010675328657,2.68414767054226));
#229694=CARTESIAN_POINT('Ctrl Pts',(54.3537721391719,31.4991785058298,2.6820451913457));
#229695=CARTESIAN_POINT('Ctrl Pts',(54.3574819590039,31.4971365594546,2.6800343177853));
#229696=CARTESIAN_POINT('Ctrl Pts',(54.3611518569451,31.4949332463336,2.67812693945288));
#229697=CARTESIAN_POINT('Ctrl Pts',(54.3618481843342,31.4945151891294,2.6777650329924));
#229698=CARTESIAN_POINT('Ctrl Pts',(54.3625432124817,31.494090808751,2.6774065963996));
#229699=CARTESIAN_POINT('Ctrl Pts',(54.3632368016453,31.4936601139564,2.67705178968892));
#229700=CARTESIAN_POINT('Ctrl Pts',(54.3639087161475,31.4932428783741,2.67670807068794));
#229701=CARTESIAN_POINT('Ctrl Pts',(54.3645792801848,31.4928197168825,2.67636775825302));
#229702=CARTESIAN_POINT('Ctrl Pts',(54.3652483648081,31.4923906407828,2.67603099699292));
#229703=CARTESIAN_POINT('Ctrl Pts',(54.372539911164,31.4877146578622,2.67236104217175));
#229704=CARTESIAN_POINT('Ctrl Pts',(54.3796603393079,31.4823328301627,2.66911440541529));
#229705=CARTESIAN_POINT('Ctrl Pts',(54.3864229856955,31.4762829888805,2.6664677818969));
#229706=CARTESIAN_POINT('Ctrl Pts',(54.3892788932593,31.473728103339,2.66535009635024));
#229707=CARTESIAN_POINT('Ctrl Pts',(54.3920710496176,31.4710545157391,2.66433897912386));
#229708=CARTESIAN_POINT('Ctrl Pts',(54.3947861357355,31.4682668669588,2.66344564884829));
#229709=CARTESIAN_POINT('Ctrl Pts',(54.3993582729152,31.4635725360689,2.66194130298621));
#229710=CARTESIAN_POINT('Ctrl Pts',(54.4037093249067,31.4585547584353,2.66077206705456));
#229711=CARTESIAN_POINT('Ctrl Pts',(54.4077698566065,31.4532397415957,2.6599822515575));
#229712=CARTESIAN_POINT('Ctrl Pts',(54.4087849895314,31.4519109873858,2.65978479768323));
#229713=CARTESIAN_POINT('Ctrl Pts',(54.4097817701143,31.4505635261659,2.65961098966658));
#229714=CARTESIAN_POINT('Ctrl Pts',(54.4107588499958,31.449197606926,2.65946139030537));
#229715=CARTESIAN_POINT('Ctrl Pts',(54.4122244698182,31.4471487280663,2.65923699126355));
#229716=CARTESIAN_POINT('Ctrl Pts',(54.4136457436054,31.445058325466,2.65906707562477));
#229717=CARTESIAN_POINT('Ctrl Pts',(54.4150195646481,31.442928094411,2.65895332562955));
#229718=CARTESIAN_POINT('Ctrl Pts',(54.4163933856907,31.4407978633561,2.65883957563432));
#229719=CARTESIAN_POINT('Ctrl Pts',(54.4177197583729,31.4386278145921,2.65878198860284));
#229720=CARTESIAN_POINT('Ctrl Pts',(54.4189959163063,31.4364195775137,2.65878198860284));
#229721=CARTESIAN_POINT('Ctrl Pts',(51.1126068659047,29.5274749692187,2.65878198860283));
#229722=CARTESIAN_POINT('Ctrl Pts',(51.108288538813,29.5349468458349,2.65878198860283));
#229723=CARTESIAN_POINT('Ctrl Pts',(51.1046244142386,29.5427104181385,2.65945335517877));
#229724=CARTESIAN_POINT('Ctrl Pts',(51.1016049255946,29.5506148782563,2.66072561226624));
#229725=CARTESIAN_POINT('Ctrl Pts',(51.099654645748,29.555720348448,2.66154735980362));
#229726=CARTESIAN_POINT('Ctrl Pts',(51.0979724198487,29.5608842707087,2.66261895766906));
#229727=CARTESIAN_POINT('Ctrl Pts',(51.0965469289497,29.5660646037407,2.6639142925105));
#229728=CARTESIAN_POINT('Ctrl Pts',(51.0946575224202,29.5729308384267,2.66563118464146));
#229729=CARTESIAN_POINT('Ctrl Pts',(51.0932249325813,29.579826275578,2.66774105138722));
#229730=CARTESIAN_POINT('Ctrl Pts',(51.0922302752234,29.5866628504239,2.67016894181773));
#229731=CARTESIAN_POINT('Ctrl Pts',(51.0917329465445,29.5900811378468,2.67138288703299));
#229732=CARTESIAN_POINT('Ctrl Pts',(51.0913449998289,29.5934848814075,2.67267613167574));
#229733=CARTESIAN_POINT('Ctrl Pts',(51.0910633609953,29.5968642938812,2.67403835432576));
#229734=CARTESIAN_POINT('Ctrl Pts',(51.0909225415785,29.598554000118,2.67471946565077));
#229735=CARTESIAN_POINT('Ctrl Pts',(51.0908082908743,29.6002376377884,2.67541781389546));
#229736=CARTESIAN_POINT('Ctrl Pts',(51.0907201726671,29.6019140726117,2.67613207244193));
#229737=CARTESIAN_POINT('Ctrl Pts',(51.0906981431153,29.6023331813176,2.67631063707854));
#229738=CARTESIAN_POINT('Ctrl Pts',(51.090677746668,29.6027518401471,2.67649019601869));
#229739=CARTESIAN_POINT('Ctrl Pts',(51.090658976153,29.6031700319853,2.6766707283668));
#229740=CARTESIAN_POINT('Ctrl Pts',(51.0906026646081,29.6044246074998,2.67721232541114));
#229741=CARTESIAN_POINT('Ctrl Pts',(51.0905609873413,29.6056749785905,2.6777626834007));
#229742=CARTESIAN_POINT('Ctrl Pts',(51.090533742783,29.6069206965766,2.67832123541539));
#229743=CARTESIAN_POINT('Ctrl Pts',(51.0903418356317,29.6156953732193,2.68225560368463));
#229744=CARTESIAN_POINT('Ctrl Pts',(51.0908211368931,29.6242688491604,2.686617929989));
#229745=CARTESIAN_POINT('Ctrl Pts',(51.091864142426,29.6325885911856,2.69130986622583));
#229746=CARTESIAN_POINT('Ctrl Pts',(51.0923699989825,29.6366236570776,2.69358545023065));
#229747=CARTESIAN_POINT('Ctrl Pts',(51.0930089302516,29.6405993642577,2.69593918853486));
#229748=CARTESIAN_POINT('Ctrl Pts',(51.0937712117414,29.6445110377127,2.69836306235497));
#229749=CARTESIAN_POINT('Ctrl Pts',(51.0949382114433,29.6504995364713,2.7020738438223));
#229750=CARTESIAN_POINT('Ctrl Pts',(51.0963926103116,29.6563348640822,2.7059476081423));
#229751=CARTESIAN_POINT('Ctrl Pts',(51.098099028059,29.6619874481817,2.7099519634571));
#229752=CARTESIAN_POINT('Ctrl Pts',(51.0988914972888,29.6646125374801,2.71181160678108));
#229753=CARTESIAN_POINT('Ctrl Pts',(51.0997380650833,29.6671982043429,2.71369962772101));
#229754=CARTESIAN_POINT('Ctrl Pts',(51.1006362623629,29.6697408831278,2.71561183138664));
#229755=CARTESIAN_POINT('Ctrl Pts',(51.1007051056453,29.669935769438,2.71575839426314));
#229756=CARTESIAN_POINT('Ctrl Pts',(51.100774227025,29.6701304259133,2.71590508903212));
#229757=CARTESIAN_POINT('Ctrl Pts',(51.1008436251324,29.6703248520471,2.71605191409914));
#229758=CARTESIAN_POINT('Ctrl Pts',(51.1018184593124,29.6730559530502,2.71811436362756));
#229759=CARTESIAN_POINT('Ctrl Pts',(51.1028499068178,29.675741029822,2.72020091026962));
#229760=CARTESIAN_POINT('Ctrl Pts',(51.1039327914267,29.6783776815771,2.72230624862184));
#229761=CARTESIAN_POINT('Ctrl Pts',(51.1078158230499,29.6878322458583,2.72985561753126));
#229762=CARTESIAN_POINT('Ctrl Pts',(51.1123884412305,29.6967379921835,2.73770089914375));
#229763=CARTESIAN_POINT('Ctrl Pts',(51.1175230541897,29.7051147523685,2.74574823347141));
#229764=CARTESIAN_POINT('Ctrl Pts',(51.1231654780142,29.7143199702913,2.75459144547089));
#229765=CARTESIAN_POINT('Ctrl Pts',(51.129486757897,29.722887031751,2.76367911754332));
#229766=CARTESIAN_POINT('Ctrl Pts',(51.1363687775784,29.7308286942766,2.77292162564785));
#229767=CARTESIAN_POINT('Ctrl Pts',(51.1437996316828,29.7394036967188,2.7829012148475));
#229768=CARTESIAN_POINT('Ctrl Pts',(51.1518848590008,29.7472505498668,2.79306229500166));
#229769=CARTESIAN_POINT('Ctrl Pts',(51.1605258584248,29.7543572078934,2.8033191668519));
#229770=CARTESIAN_POINT('Ctrl Pts',(51.1690943687425,29.7614042483616,2.81348999408657));
#229771=CARTESIAN_POINT('Ctrl Pts',(51.1782106315441,29.7677241373269,2.82375635966868));
#229772=CARTESIAN_POINT('Ctrl Pts',(51.1878102687784,29.7732664904682,2.83404198860283));
#229773=CARTESIAN_POINT('Origin',(0.00762000000000077,-0.0131982271534882,
2.83404198860262));
#229774=CARTESIAN_POINT('Ctrl Pts',(54.4342359163063,31.4100231232064,2.65878198860284));
#229775=CARTESIAN_POINT('Ctrl Pts',(54.4385272722025,31.4025830926773,2.65878198860284));
#229776=CARTESIAN_POINT('Ctrl Pts',(54.4421589890644,31.3948506994788,2.65944603041879));
#229777=CARTESIAN_POINT('Ctrl Pts',(54.4451438299621,31.3869762747681,2.6607043926411));
#229778=CARTESIAN_POINT('Ctrl Pts',(54.4470510012012,31.3819448922431,2.66150842619633));
#229779=CARTESIAN_POINT('Ctrl Pts',(54.4486949601302,31.3768558346346,2.66255428265399));
#229780=CARTESIAN_POINT('Ctrl Pts',(54.4500875286681,31.3717496422766,2.66381699700677));
#229781=CARTESIAN_POINT('Ctrl Pts',(54.4519881053013,31.3647807142731,2.66554034873277));
#229782=CARTESIAN_POINT('Ctrl Pts',(54.4534143418203,31.3577796218684,2.66766759643982));
#229783=CARTESIAN_POINT('Ctrl Pts',(54.4543880442396,31.3508395087087,2.67012012783158));
#229784=CARTESIAN_POINT('Ctrl Pts',(54.4548748954493,31.3473694521289,2.67134639352746));
#229785=CARTESIAN_POINT('Ctrl Pts',(54.4552487192094,31.3439144604656,2.67265375585022));
#229786=CARTESIAN_POINT('Ctrl Pts',(54.4555129946225,31.3404848880616,2.67403135126949));
#229787=CARTESIAN_POINT('Ctrl Pts',(54.4556451323291,31.3387701018596,2.67472014897913));
#229788=CARTESIAN_POINT('Ctrl Pts',(54.4557498916996,31.337061655417,2.67542649668642));
#229789=CARTESIAN_POINT('Ctrl Pts',(54.4558277627246,31.3353607484814,2.67614899656111));
#229790=CARTESIAN_POINT('Ctrl Pts',(54.4558472304809,31.3349355217475,2.67632962152979));
#229791=CARTESIAN_POINT('Ctrl Pts',(54.4558650179028,31.3345107659126,2.6765112559096));
#229792=CARTESIAN_POINT('Ctrl Pts',(54.4558811330249,31.3340864990772,2.67669387767533));
#229793=CARTESIAN_POINT('Ctrl Pts',(54.4559294783911,31.3328136985709,2.67724174297253));
#229794=CARTESIAN_POINT('Ctrl Pts',(54.4559627721159,31.3315453006542,2.67779849504757));
#229795=CARTESIAN_POINT('Ctrl Pts',(54.4559812395338,31.3302817797847,2.67836353618018));
#229796=CARTESIAN_POINT('Ctrl Pts',(54.4561088608496,31.321550066618,2.68226832098923));
#229797=CARTESIAN_POINT('Ctrl Pts',(54.4555742713438,31.3130195924487,2.68659153751413));
#229798=CARTESIAN_POINT('Ctrl Pts',(54.4544853519657,31.3047400858591,2.69123699486207));
#229799=CARTESIAN_POINT('Ctrl Pts',(54.4539441620239,31.3006251938109,2.69354577441238));
#229800=CARTESIAN_POINT('Ctrl Pts',(54.4532655373259,31.2965719591987,2.69593478828131));
#229801=CARTESIAN_POINT('Ctrl Pts',(54.4524598885395,31.2925850928565,2.69839565261226));
#229802=CARTESIAN_POINT('Ctrl Pts',(54.4506825069818,31.2837894702121,2.70382468689051));
#229803=CARTESIAN_POINT('Ctrl Pts',(54.4482992497266,31.2753153512349,2.70961155815092));
#229804=CARTESIAN_POINT('Ctrl Pts',(54.4454010706198,31.2672761140353,2.71562701361772));
#229805=CARTESIAN_POINT('Ctrl Pts',(54.444342329244,31.2643392793061,2.71782453535862));
#229806=CARTESIAN_POINT('Ctrl Pts',(54.4432206434043,31.2614550023641,2.72005051502406));
#229807=CARTESIAN_POINT('Ctrl Pts',(54.4420411592047,31.2586246102248,2.72229986760119));
#229808=CARTESIAN_POINT('Ctrl Pts',(54.4380793965872,31.2491176225312,2.729855204889));
#229809=CARTESIAN_POINT('Ctrl Pts',(54.4334326446224,31.2401615453387,2.73770845534573));
#229810=CARTESIAN_POINT('Ctrl Pts',(54.4282277812583,31.231737305826,2.74576706701775));
#229811=CARTESIAN_POINT('Ctrl Pts',(54.4225070198645,31.2224780686847,2.7546244358506));
#229812=CARTESIAN_POINT('Ctrl Pts',(54.4161118092692,31.2138606686935,2.76373036323222));
#229813=CARTESIAN_POINT('Ctrl Pts',(54.4091594014068,31.2058737429056,2.7729966463687));
#229814=CARTESIAN_POINT('Ctrl Pts',(54.4016713602519,31.1972714816195,2.78297683033537));
#229815=CARTESIAN_POINT('Ctrl Pts',(54.3935362880533,31.1893995936754,2.79314401478967));
#229816=CARTESIAN_POINT('Ctrl Pts',(54.3848513315099,31.1822725865916,2.80341452428021));
#229817=CARTESIAN_POINT('Ctrl Pts',(54.3762836512046,31.1752418181678,2.81354634721425));
#229818=CARTESIAN_POINT('Ctrl Pts',(54.3671795569335,31.1689352997153,2.82378004209244));
#229819=CARTESIAN_POINT('Ctrl Pts',(54.3576020372438,31.1634057161443,2.83404198860284));
#229820=CARTESIAN_POINT('Ctrl Pts',(51.3783102687784,29.4433108116264,2.83404198860283));
#229821=CARTESIAN_POINT('Ctrl Pts',(51.3691445298587,29.4380189697937,2.82422126443021));
#229822=CARTESIAN_POINT('Ctrl Pts',(51.3595943606106,29.4334690915853,2.81442815028509));
#229823=CARTESIAN_POINT('Ctrl Pts',(51.3497152868758,29.4296781246248,2.80471618166319));
#229824=CARTESIAN_POINT('Ctrl Pts',(51.3401761719858,29.4260176124805,2.79533842146225));
#229825=CARTESIAN_POINT('Ctrl Pts',(51.3303291924903,29.4230642997975,2.78603515650231));
#229826=CARTESIAN_POINT('Ctrl Pts',(51.3202058500874,29.4208754038582,2.77685887346742));
#229827=CARTESIAN_POINT('Ctrl Pts',(51.3106361210823,29.4188062116758,2.76818441216558));
#229828=CARTESIAN_POINT('Ctrl Pts',(51.3008185461766,29.4174199248361,2.75962261521601));
#229829=CARTESIAN_POINT('Ctrl Pts',(51.2907775289323,29.4168067767633,2.75123537701632));
#229830=CARTESIAN_POINT('Ctrl Pts',(51.2815299205009,29.4162420776746,2.74351087134085));
#229831=CARTESIAN_POINT('Ctrl Pts',(51.2720922400908,29.4163331870168,2.73593399449808));
#229832=CARTESIAN_POINT('Ctrl Pts',(51.2624911797709,29.4171879526247,2.72857657812533));
#229833=CARTESIAN_POINT('Ctrl Pts',(51.2596283373946,29.4174428264742,2.72638274508297));
#229834=CARTESIAN_POINT('Ctrl Pts',(51.2567510524865,29.4177658668981,2.72420861709592));
#229835=CARTESIAN_POINT('Ctrl Pts',(51.2538602864394,29.4181606517644,2.72205663736729));
#229836=CARTESIAN_POINT('Ctrl Pts',(51.2509990568967,29.4185514029024,2.71992664556768));
#229837=CARTESIAN_POINT('Ctrl Pts',(51.2481275521819,29.4190117629204,2.71782089927886));
#229838=CARTESIAN_POINT('Ctrl Pts',(51.245249939194,29.4195444402102,2.71574387311248));
#229839=CARTESIAN_POINT('Ctrl Pts',(51.2450498356145,29.4195814815471,2.71559944077488));
#229840=CARTESIAN_POINT('Ctrl Pts',(51.2448496951983,29.4196188630963,2.71545515216071));
#229841=CARTESIAN_POINT('Ctrl Pts',(51.2446495184043,29.4196565860788,2.71531100781732));
#229842=CARTESIAN_POINT('Ctrl Pts',(51.2358730344471,29.4213104998204,2.70899119176083));
#229843=CARTESIAN_POINT('Ctrl Pts',(51.2270453415808,29.4236619033166,2.70298296066837));
#229844=CARTESIAN_POINT('Ctrl Pts',(51.2182691329814,29.426765124801,2.69736727774133));
#229845=CARTESIAN_POINT('Ctrl Pts',(51.210088181272,29.4296578665608,2.69213248525424));
#229846=CARTESIAN_POINT('Ctrl Pts',(51.2019513265391,29.4332044080281,2.68723866185463));
#229847=CARTESIAN_POINT('Ctrl Pts',(51.1939656059618,29.4374658604801,2.68278595829557));
#229848=CARTESIAN_POINT('Ctrl Pts',(51.1910443260615,29.4390247549185,2.68115710172801));
#229849=CARTESIAN_POINT('Ctrl Pts',(51.1881435589221,29.4406794572088,2.67958763637807));
#229850=CARTESIAN_POINT('Ctrl Pts',(51.1852696776793,29.442433407717,2.67808378645363));
#229851=CARTESIAN_POINT('Ctrl Pts',(51.1845786052483,29.4428551742199,2.67772216078598));
#229852=CARTESIAN_POINT('Ctrl Pts',(51.1838888551095,29.443283215379,2.67736403603562));
#229853=CARTESIAN_POINT('Ctrl Pts',(51.1832005624688,29.4437175198436,2.67700956934477));
#229854=CARTESIAN_POINT('Ctrl Pts',(51.1825337789732,29.4441382522936,2.67666617973802));
#229855=CARTESIAN_POINT('Ctrl Pts',(51.1818683633172,29.4445648626868,2.67632622314117));
#229856=CARTESIAN_POINT('Ctrl Pts',(51.1812044402993,29.4449973374098,2.67598984158772));
#229857=CARTESIAN_POINT('Ctrl Pts',(51.1739303963595,29.4497355978005,2.67230439292217));
#229858=CARTESIAN_POINT('Ctrl Pts',(51.1668309650358,29.4551812510956,2.66904964539969));
#229859=CARTESIAN_POINT('Ctrl Pts',(51.1600900711812,29.4612929974521,2.66640203566718));
#229860=CARTESIAN_POINT('Ctrl Pts',(51.1572944215753,29.4638277208377,2.66530399299435));
#229861=CARTESIAN_POINT('Ctrl Pts',(51.1545603804838,29.4664765899956,2.66430995142256));
#229862=CARTESIAN_POINT('Ctrl Pts',(51.151900368709,29.4692349685474,2.66343053473359));
#229863=CARTESIAN_POINT('Ctrl Pts',(51.1473634414341,29.4739396706108,2.66193059792883));
#229864=CARTESIAN_POINT('Ctrl Pts',(51.1430443628984,29.4789629373384,2.66076519817126));
#229865=CARTESIAN_POINT('Ctrl Pts',(51.1390107214364,29.4842777732942,2.65997805604459));
#229866=CARTESIAN_POINT('Ctrl Pts',(51.1369939007054,29.486935191272,2.65958448498125));
#229867=CARTESIAN_POINT('Ctrl Pts',(51.1350496570625,29.4896662827383,2.65928526260761));
#229868=CARTESIAN_POINT('Ctrl Pts',(51.1331865036877,29.4924676612912,2.65908463971323));
#229869=CARTESIAN_POINT('Ctrl Pts',(51.1313233503128,29.495269039844,2.65888401681885));
#229870=CARTESIAN_POINT('Ctrl Pts',(51.1295412933646,29.49814066024,2.65878198860283));
#229871=CARTESIAN_POINT('Ctrl Pts',(51.1278468659047,29.5010785149114,2.65878198860283));
#229872=CARTESIAN_POINT('Origin',(47.1274239660509,34.2589154226524,2.83404198860286));
#229873=CARTESIAN_POINT('Ctrl Pts',(50.5784163149356,36.9828414016749,2.83404198860288));
#229874=CARTESIAN_POINT('Ctrl Pts',(50.5870002518361,36.9890779968908,2.82419652440103));
#229875=CARTESIAN_POINT('Ctrl Pts',(50.5960508067995,36.9946187858197,2.81438790575704));
#229876=CARTESIAN_POINT('Ctrl Pts',(50.6055128591414,36.99944247839,2.80466781256976));
#229877=CARTESIAN_POINT('Ctrl Pts',(50.614667451125,37.0041094296751,2.7952635645317));
#229878=CARTESIAN_POINT('Ctrl Pts',(50.6242084112801,37.0081056536701,2.78594102496345));
#229879=CARTESIAN_POINT('Ctrl Pts',(50.6341096134621,37.0113722741989,2.77675109088912));
#229880=CARTESIAN_POINT('Ctrl Pts',(50.6434755410454,37.0144622960723,2.76805797913836));
#229881=CARTESIAN_POINT('Ctrl Pts',(50.6531646927615,37.016899762676,2.75948271210336));
#229882=CARTESIAN_POINT('Ctrl Pts',(50.6631621581219,37.0185933530506,2.75108575573417));
#229883=CARTESIAN_POINT('Ctrl Pts',(50.6723705467539,37.0201532722693,2.74335155163484));
#229884=CARTESIAN_POINT('Ctrl Pts',(50.6818410607704,37.021082144611,2.73576818686177));
#229885=CARTESIAN_POINT('Ctrl Pts',(50.6915586678622,37.0212705108776,2.72840626160748));
#229886=CARTESIAN_POINT('Ctrl Pts',(50.6943773762862,37.0213251487712,2.72627084693853));
#229887=CARTESIAN_POINT('Ctrl Pts',(50.6972168227816,37.0213172191968,2.7241542458762));
#229888=CARTESIAN_POINT('Ctrl Pts',(50.7000764815586,37.0212433695026,2.72205867173281));
#229889=CARTESIAN_POINT('Ctrl Pts',(50.7031765355313,37.0211633116861,2.71978693462885));
#229890=CARTESIAN_POINT('Ctrl Pts',(50.7062960577322,37.0210069737843,2.71754411340786));
#229891=CARTESIAN_POINT('Ctrl Pts',(50.7094335311104,37.0207706534748,2.71533341844283));
#229892=CARTESIAN_POINT('Ctrl Pts',(50.718044351416,37.0201220705311,2.70926614876431));
#229893=CARTESIAN_POINT('Ctrl Pts',(50.7267761502172,37.0188289150183,2.70347381860448));
#229894=CARTESIAN_POINT('Ctrl Pts',(50.7355328079489,37.0168522507833,2.69804914171435));
#229895=CARTESIAN_POINT('Ctrl Pts',(50.7435446743633,37.015043710324,2.69308585687253));
#229896=CARTESIAN_POINT('Ctrl Pts',(50.7515681793718,37.0126559296151,2.68842799053241));
#229897=CARTESIAN_POINT('Ctrl Pts',(50.7595400218646,37.0096268558219,2.68414767054279));
#229898=CARTESIAN_POINT('Ctrl Pts',(50.7634557648561,37.0081389846695,2.68204519134607));
#229899=CARTESIAN_POINT('Ctrl Pts',(50.7673587034238,37.0064960060561,2.68003431778552));
#229900=CARTESIAN_POINT('Ctrl Pts',(50.771238806215,37.0046883717069,2.67812693945297));
#229901=CARTESIAN_POINT('Ctrl Pts',(50.7719750179269,37.0043453906958,2.67776503299249));
#229902=CARTESIAN_POINT('Ctrl Pts',(50.7727105984664,37.0039959853417,2.67740659639969));
#229903=CARTESIAN_POINT('Ctrl Pts',(50.7734454079409,37.0036401497476,2.677051789689));
#229904=CARTESIAN_POINT('Ctrl Pts',(50.7741572546194,37.0032954340158,2.67670807068803));
#229905=CARTESIAN_POINT('Ctrl Pts',(50.7748683776572,37.0029446836755,2.67636775825311));
#229906=CARTESIAN_POINT('Ctrl Pts',(50.7755786476302,37.0025878964871,2.67603099699301));
#229907=CARTESIAN_POINT('Ctrl Pts',(50.7833190234415,36.9986997032255,2.67236104217173));
#229908=CARTESIAN_POINT('Ctrl Pts',(50.7909629993143,36.9940916451527,2.66911440541517));
#229909=CARTESIAN_POINT('Ctrl Pts',(50.7983209798299,36.9887818345683,2.66646778189672));
#229910=CARTESIAN_POINT('Ctrl Pts',(50.8014283006924,36.9865394685862,2.66535009635016));
#229911=CARTESIAN_POINT('Ctrl Pts',(50.804484627329,36.9841723869924,2.66433897912387));
#229912=CARTESIAN_POINT('Ctrl Pts',(50.807476228564,36.9816838130236,2.66344564884836));
#229913=CARTESIAN_POINT('Ctrl Pts',(50.8125140102918,36.9774931166428,2.66194130298628));
#229914=CARTESIAN_POINT('Ctrl Pts',(50.8173657273503,36.9729576356983,2.66077206705461));
#229915=CARTESIAN_POINT('Ctrl Pts',(50.8219595855751,36.9680961762157,2.65998225155755));
#229916=CARTESIAN_POINT('Ctrl Pts',(50.8231080501312,36.966880811345,2.65978479768328));
#229917=CARTESIAN_POINT('Ctrl Pts',(50.8242402182964,36.9656449236012,2.65961098966662));
#229918=CARTESIAN_POINT('Ctrl Pts',(50.8253547230712,36.9643886196684,2.65946139030541));
#229919=CARTESIAN_POINT('Ctrl Pts',(50.8270264802334,36.9625041637692,2.6592369912636));
#229920=CARTESIAN_POINT('Ctrl Pts',(50.8286584747055,36.9605737761779,2.65906707562481));
#229921=CARTESIAN_POINT('Ctrl Pts',(50.8302474395914,36.9585988181539,2.65895332562959));
#229922=CARTESIAN_POINT('Ctrl Pts',(50.8318364044772,36.95662386013,2.65883957563436));
#229923=CARTESIAN_POINT('Ctrl Pts',(50.8333823430135,36.9546043428184,2.65878198860288));
#229924=CARTESIAN_POINT('Ctrl Pts',(50.8348823336486,36.9525415975215,2.65878198860288));
#229925=CARTESIAN_POINT('Ctrl Pts',(47.7461450747864,34.7084426211234,2.65878198860287));
#229926=CARTESIAN_POINT('Ctrl Pts',(47.7410693801618,34.715422177923,2.65878198860287));
#229927=CARTESIAN_POINT('Ctrl Pts',(47.7366138137628,34.7227602152544,2.65945335517884));
#229928=CARTESIAN_POINT('Ctrl Pts',(47.7327846251244,34.7303057514051,2.66072561226636));
#229929=CARTESIAN_POINT('Ctrl Pts',(47.7303113621616,34.7351793935413,2.66154735980373));
#229930=CARTESIAN_POINT('Ctrl Pts',(47.7280985748135,34.7401391868073,2.66261895766913));
#229931=CARTESIAN_POINT('Ctrl Pts',(47.7261394006518,34.7451421370596,2.66391429251051));
#229932=CARTESIAN_POINT('Ctrl Pts',(47.7235426275288,34.7517732610326,2.66563118464148));
#229933=CARTESIAN_POINT('Ctrl Pts',(47.721397116118,34.7584811778434,2.66774105138723));
#229934=CARTESIAN_POINT('Ctrl Pts',(47.7196932909345,34.7651763312118,2.67016894181774));
#229935=CARTESIAN_POINT('Ctrl Pts',(47.7188413783428,34.768523907896,2.671382887033));
#229936=CARTESIAN_POINT('Ctrl Pts',(47.7180997687562,34.7718684539193,2.67267613167576));
#229937=CARTESIAN_POINT('Ctrl Pts',(47.7174664279769,34.7751999143434,2.67403835432578));
#229938=CARTESIAN_POINT('Ctrl Pts',(47.7171497575873,34.7768656445554,2.67471946565078));
#229939=CARTESIAN_POINT('Ctrl Pts',(47.716860144702,34.778528116632,2.67541781389548));
#229940=CARTESIAN_POINT('Ctrl Pts',(47.7165972740597,34.7801861569092,2.67613207244195));
#229941=CARTESIAN_POINT('Ctrl Pts',(47.7165315563991,34.7806006669785,2.67631063707856));
#229942=CARTESIAN_POINT('Ctrl Pts',(47.7164675099217,34.7810149003419,2.67649019601871));
#229943=CARTESIAN_POINT('Ctrl Pts',(47.7164051292834,34.7814288392283,2.67667072836682));
#229944=CARTESIAN_POINT('Ctrl Pts',(47.7162179873684,34.7826706558876,2.67721232541116));
#229945=CARTESIAN_POINT('Ctrl Pts',(47.7160458390454,34.783909820854,2.67776268340072));
#229946=CARTESIAN_POINT('Ctrl Pts',(47.7158885307488,34.7851458668349,2.67832123541541));
#229947=CARTESIAN_POINT('Ctrl Pts',(47.7147804714199,34.7938524151214,2.68225560368475));
#229948=CARTESIAN_POINT('Ctrl Pts',(47.7143609747538,34.8024290252888,2.68661792998926));
#229949=CARTESIAN_POINT('Ctrl Pts',(47.7145286167447,34.8108122146624,2.69130986622623));
#229950=CARTESIAN_POINT('Ctrl Pts',(47.7146099229291,34.8148780524495,2.69358545023094));
#229951=CARTESIAN_POINT('Ctrl Pts',(47.7148297795039,34.8188987667931,2.69593918853502));
#229952=CARTESIAN_POINT('Ctrl Pts',(47.7151790039209,34.8228686918041,2.698363062355));
#229953=CARTESIAN_POINT('Ctrl Pts',(47.7157136421038,34.8289463696255,2.70207384382233));
#229954=CARTESIAN_POINT('Ctrl Pts',(47.7165501157951,34.8349017567798,2.70594760814235));
#229955=CARTESIAN_POINT('Ctrl Pts',(47.7176563296781,34.840701744657,2.70995196345714));
#229956=CARTESIAN_POINT('Ctrl Pts',(47.7181700611282,34.8433952890323,2.71181160678112));
#229957=CARTESIAN_POINT('Ctrl Pts',(47.7187417155521,34.8460552817721,2.71369962772105));
#229958=CARTESIAN_POINT('Ctrl Pts',(47.719369210107,34.8486779186779,2.71561183138667));
#229959=CARTESIAN_POINT('Ctrl Pts',(47.7194173050922,34.848878933463,2.71575839426318));
#229960=CARTESIAN_POINT('Ctrl Pts',(47.7194657006756,34.8490797487414,2.71590508903215));
#229961=CARTESIAN_POINT('Ctrl Pts',(47.7195143955479,34.849280363866,2.71605191409917));
#229962=CARTESIAN_POINT('Ctrl Pts',(47.7201984116934,34.8520984015308,2.71811436362759));
#229963=CARTESIAN_POINT('Ctrl Pts',(47.7209435418727,34.8548765847938,2.72020091026965));
#229964=CARTESIAN_POINT('Ctrl Pts',(47.7217448891703,34.8576119849588,2.72230624862188));
#229965=CARTESIAN_POINT('Ctrl Pts',(47.7246183780645,34.8674206434754,2.72985561753082));
#229966=CARTESIAN_POINT('Ctrl Pts',(47.7282350429865,34.8767555719414,2.7377008991428));
#229967=CARTESIAN_POINT('Ctrl Pts',(47.732465918129,34.8856231565591,2.74574823346993));
#229968=CARTESIAN_POINT('Ctrl Pts',(47.7371152248816,34.8953677412261,2.75459144546899));
#229969=CARTESIAN_POINT('Ctrl Pts',(47.7425063743624,34.9045486250985,2.76367911754097));
#229970=CARTESIAN_POINT('Ctrl Pts',(47.7485205638399,34.9131661493071,2.77292162564506));
#229971=CARTESIAN_POINT('Ctrl Pts',(47.7550143791199,34.9224709127488,2.7829012148444));
#229972=CARTESIAN_POINT('Ctrl Pts',(47.7622350952152,34.9311199164008,2.79306229499825));
#229973=CARTESIAN_POINT('Ctrl Pts',(47.7700859102974,34.9390908738021,2.80331916684818));
#229974=CARTESIAN_POINT('Ctrl Pts',(47.7778708651092,34.9469949630624,2.81348999408409));
#229975=CARTESIAN_POINT('Ctrl Pts',(47.7862765797887,34.954233139957,2.82375635966745));
#229976=CARTESIAN_POINT('Ctrl Pts',(47.7952442955502,34.9607485668368,2.83404198860287));
#229977=CARTESIAN_POINT('Origin',(0.00895784724493838,-0.012329418994088,
2.83404198860262));
#229978=CARTESIAN_POINT('Ctrl Pts',(50.8527980281385,36.9278827595329,2.65878198860288));
#229979=CARTESIAN_POINT('Ctrl Pts',(50.8578435704956,36.9209320551072,2.65878198860288));
#229980=CARTESIAN_POINT('Ctrl Pts',(50.8622636476106,36.9136216385509,2.65944603041873));
#229981=CARTESIAN_POINT('Ctrl Pts',(50.8660552387515,36.9061023515954,2.66070439264086));
#229982=CARTESIAN_POINT('Ctrl Pts',(50.8684778849907,36.9012978851886,2.66150842619611));
#229983=CARTESIAN_POINT('Ctrl Pts',(50.8706447895123,36.8964085464701,2.66255428265387));
#229984=CARTESIAN_POINT('Ctrl Pts',(50.8725634718546,36.8914758894169,2.66381699700678));
#229985=CARTESIAN_POINT('Ctrl Pts',(50.875182088265,36.8847438022849,2.66554034873278));
#229986=CARTESIAN_POINT('Ctrl Pts',(50.8773323251414,36.8779301449086,2.66766759643982));
#229987=CARTESIAN_POINT('Ctrl Pts',(50.8790261328805,36.8711298300324,2.67012012783159));
#229988=CARTESIAN_POINT('Ctrl Pts',(50.87987303675,36.8677296725944,2.67134639352747));
#229989=CARTESIAN_POINT('Ctrl Pts',(50.8806059576336,36.8643326829601,2.67265375585023));
#229990=CARTESIAN_POINT('Ctrl Pts',(50.8812272732515,36.8609495224154,2.67403135126951));
#229991=CARTESIAN_POINT('Ctrl Pts',(50.8815379310604,36.859257942143,2.67472014897915));
#229992=CARTESIAN_POINT('Ctrl Pts',(50.8818206978293,36.8575698050848,2.67542649668644));
#229993=CARTESIAN_POINT('Ctrl Pts',(50.8820759354568,36.855886355634,2.67614899656114));
#229994=CARTESIAN_POINT('Ctrl Pts',(50.8821397448637,36.8554654932713,2.67632962152981));
#229995=CARTESIAN_POINT('Ctrl Pts',(50.882201833919,36.8550449235852,2.67651125590961));
#229996=CARTESIAN_POINT('Ctrl Pts',(50.8822622087211,36.8546246654168,2.67669387767535));
#229997=CARTESIAN_POINT('Ctrl Pts',(50.8824433331273,36.8533638909117,2.67724174297255));
#229998=CARTESIAN_POINT('Ctrl Pts',(50.8826090281506,36.8521059215534,2.67779849504759));
#229999=CARTESIAN_POINT('Ctrl Pts',(50.8827594682968,36.8508512527542,2.67836353618021));
#230000=CARTESIAN_POINT('Ctrl Pts',(50.8837991030487,36.842180712886,2.68226832098921));
#230001=CARTESIAN_POINT('Ctrl Pts',(50.884159119436,36.8336410897273,2.68659153751404));
#230002=CARTESIAN_POINT('Ctrl Pts',(50.8839416093727,36.825293116072,2.69123699486192));
#230003=CARTESIAN_POINT('Ctrl Pts',(50.8838335074683,36.82114419608,2.69354577441229));
#230004=CARTESIAN_POINT('Ctrl Pts',(50.8835822787327,36.8170422299141,2.69593478828129));
#230005=CARTESIAN_POINT('Ctrl Pts',(50.8831977843866,36.8129929908133,2.6983956526123));
#230006=CARTESIAN_POINT('Ctrl Pts',(50.8823495324296,36.8040597645471,2.70382468689055));
#230007=CARTESIAN_POINT('Ctrl Pts',(50.8808651175412,36.7953829494618,2.70961155815097));
#230008=CARTESIAN_POINT('Ctrl Pts',(50.8788231440731,36.7870848098365,2.71562701361776));
#230009=CARTESIAN_POINT('Ctrl Pts',(50.8780771854145,36.7840533947863,2.71782453535866));
#230010=CARTESIAN_POINT('Ctrl Pts',(50.8772631333235,36.7810676701179,2.7200505150241));
#230011=CARTESIAN_POINT('Ctrl Pts',(50.8763859670025,36.7781294934921,2.72229986760123));
#230012=CARTESIAN_POINT('Ctrl Pts',(50.8734396581491,36.7682604691136,2.7298552048891));
#230013=CARTESIAN_POINT('Ctrl Pts',(50.8697545265637,36.7588677364069,2.7377084553459));
#230014=CARTESIAN_POINT('Ctrl Pts',(50.8654587487961,36.7499455893907,2.745767067018));
#230015=CARTESIAN_POINT('Ctrl Pts',(50.8607371801612,36.740139092922,2.75462443585091));
#230016=CARTESIAN_POINT('Ctrl Pts',(50.8552777667771,36.7309004184138,2.76373036323261));
#230017=CARTESIAN_POINT('Ctrl Pts',(50.8491983060112,36.7222305213312,2.77299664636915));
#230018=CARTESIAN_POINT('Ctrl Pts',(50.8426504662821,36.7128926706977,2.78297683033586));
#230019=CARTESIAN_POINT('Ctrl Pts',(50.8353827952099,36.7042135591838,2.79314401479019));
#230020=CARTESIAN_POINT('Ctrl Pts',(50.8274903908653,36.6962177694295,2.80341452428075));
#230021=CARTESIAN_POINT('Ctrl Pts',(50.8197045606282,36.6883299498348,2.81354634721465));
#230022=CARTESIAN_POINT('Ctrl Pts',(50.8113095502206,36.6811063421668,2.82378004209267));
#230023=CARTESIAN_POINT('Ctrl Pts',(50.8023624960591,36.6746059268181,2.83404198860288));
#230024=CARTESIAN_POINT('Ctrl Pts',(48.0191904766736,34.6525130919799,2.83404198860286));
#230025=CARTESIAN_POINT('Ctrl Pts',(48.010628096726,34.646292158807,2.824221264431));
#230026=CARTESIAN_POINT('Ctrl Pts',(48.0016058360822,34.6407689407924,2.81442815028663));
#230027=CARTESIAN_POINT('Ctrl Pts',(47.9921771448984,34.6359660967498,2.80471618166547));
#230028=CARTESIAN_POINT('Ctrl Pts',(47.9830729139875,34.6313285282538,2.79533842146496));
#230029=CARTESIAN_POINT('Ctrl Pts',(47.9735885825128,34.6273621044923,2.78603515650543));
#230030=CARTESIAN_POINT('Ctrl Pts',(47.9637494987682,34.6241270221294,2.77685887347094));
#230031=CARTESIAN_POINT('Ctrl Pts',(47.9544484832192,34.6210688561314,2.76818441216929));
#230032=CARTESIAN_POINT('Ctrl Pts',(47.9448295964494,34.618663947498,2.75962261521989));
#230033=CARTESIAN_POINT('Ctrl Pts',(47.9349076763743,34.6170045862121,2.75123537702035));
#230034=CARTESIAN_POINT('Ctrl Pts',(47.9257697544377,34.6154763423056,2.74351087134492));
#230035=CARTESIAN_POINT('Ctrl Pts',(47.916374251109,34.6145804463111,2.73593399450217));
#230036=CARTESIAN_POINT('Ctrl Pts',(47.9067364390668,34.6144269453422,2.72857657812942));
#230037=CARTESIAN_POINT('Ctrl Pts',(47.9038626380671,34.6143811744519,2.72638274508568));
#230038=CARTESIAN_POINT('Ctrl Pts',(47.9009673483059,34.6144016870566,2.72420861709728));
#230039=CARTESIAN_POINT('Ctrl Pts',(47.8980511519205,34.6144921419177,2.72205663736733));
#230040=CARTESIAN_POINT('Ctrl Pts',(47.8951647518766,34.6145816725529,2.71992664556772));
#230041=CARTESIAN_POINT('Ctrl Pts',(47.8922608568399,34.6147393566953,2.71782089927891));
#230042=CARTESIAN_POINT('Ctrl Pts',(47.8893433277785,34.6149683234597,2.71574387311252));
#230043=CARTESIAN_POINT('Ctrl Pts',(47.8891404485133,34.6149842453607,2.71559944077493));
#230044=CARTESIAN_POINT('Ctrl Pts',(47.8889374970514,34.6150005017597,2.71545515216075));
#230045=CARTESIAN_POINT('Ctrl Pts',(47.8887344737214,34.6150170939191,2.71531100781736));
#230046=CARTESIAN_POINT('Ctrl Pts',(47.8798331871999,34.6157445549672,2.70899119176091));
#230047=CARTESIAN_POINT('Ctrl Pts',(47.8708080647649,34.6171603320595,2.70298296066847));
#230048=CARTESIAN_POINT('Ctrl Pts',(47.8617555581815,34.6193291901737,2.69736727774146));
#230049=CARTESIAN_POINT('Ctrl Pts',(47.853317048731,34.6213509428812,2.69213248525445));
#230050=CARTESIAN_POINT('Ctrl Pts',(47.8448540540103,34.6240275231021,2.6872386618549));
#230051=CARTESIAN_POINT('Ctrl Pts',(47.83646663697,34.6274308957716,2.68278595829589));
#230052=CARTESIAN_POINT('Ctrl Pts',(47.8333984113064,34.6286758935244,2.68115710172822));
#230053=CARTESIAN_POINT('Ctrl Pts',(47.8303405713851,34.6300183184512,2.67958763637817));
#230054=CARTESIAN_POINT('Ctrl Pts',(47.827299095813,34.6314622582451,2.67808378645364));
#230055=CARTESIAN_POINT('Ctrl Pts',(47.8265677225447,34.6318094775277,2.67772216078599));
#230056=CARTESIAN_POINT('Ctrl Pts',(47.8258370084447,34.6321630753106,2.67736403603562));
#230057=CARTESIAN_POINT('Ctrl Pts',(47.8251070891649,34.6325230544378,2.67700956934478));
#230058=CARTESIAN_POINT('Ctrl Pts',(47.8243999798625,34.6328717842173,2.67666617973803));
#230059=CARTESIAN_POINT('Ctrl Pts',(47.8236936164943,34.6332265027182,2.67632622314117));
#230060=CARTESIAN_POINT('Ctrl Pts',(47.822988124598,34.6335872094466,2.67598984158772));
#230061=CARTESIAN_POINT('Ctrl Pts',(47.8152586455549,34.6375391685162,2.67230439292226));
#230062=CARTESIAN_POINT('Ctrl Pts',(47.8076288798887,34.6422128973063,2.66904964539986));
#230063=CARTESIAN_POINT('Ctrl Pts',(47.8002860619016,34.647586547601,2.6664020356674));
#230064=CARTESIAN_POINT('Ctrl Pts',(47.7972407764162,34.6498151605497,2.66530399299449));
#230065=CARTESIAN_POINT('Ctrl Pts',(47.7942448304652,34.6521637338115,2.66430995142263));
#230066=CARTESIAN_POINT('Ctrl Pts',(47.7913110614419,34.654628954734,2.6634305347336));
#230067=CARTESIAN_POINT('Ctrl Pts',(47.7863072126526,34.6588336459113,2.66193059792885));
#230068=CARTESIAN_POINT('Ctrl Pts',(47.7814867201293,34.6633779280161,2.66076519817129));
#230069=CARTESIAN_POINT('Ctrl Pts',(47.7769196237423,34.6682420184009,2.65997805604462));
#230070=CARTESIAN_POINT('Ctrl Pts',(47.7746360755487,34.6706740635933,2.65958448498128));
#230071=CARTESIAN_POINT('Ctrl Pts',(47.7724170058819,34.6731869650546,2.65928526260764));
#230072=CARTESIAN_POINT('Ctrl Pts',(47.7702712352611,34.6757782448035,2.65908463971327));
#230073=CARTESIAN_POINT('Ctrl Pts',(47.7681254646402,34.6783695245525,2.65888401681889));
#230074=CARTESIAN_POINT('Ctrl Pts',(47.7660530039194,34.6810391382372,2.65878198860287));
#230075=CARTESIAN_POINT('Ctrl Pts',(47.7640607692763,34.6837837831348,2.65878198860287));
#230076=CARTESIAN_POINT('Origin',(43.2882232241948,38.9973987043321,2.8340419886029));
#230077=CARTESIAN_POINT('Ctrl Pts',(46.435582879267,42.0671296588098,2.83404198860292));
#230078=CARTESIAN_POINT('Ctrl Pts',(46.4434678907493,42.0742293550379,2.82419652440087));
#230079=CARTESIAN_POINT('Ctrl Pts',(46.451889695674,42.0806858315475,2.81438790575664));
#230080=CARTESIAN_POINT('Ctrl Pts',(46.4607957007318,42.0864721532161,2.80466781256909));
#230081=CARTESIAN_POINT('Ctrl Pts',(46.469412313657,42.0920704538858,2.79526356453077));
#230082=CARTESIAN_POINT('Ctrl Pts',(46.4784832882813,42.0970420880508,2.78594102496224));
#230083=CARTESIAN_POINT('Ctrl Pts',(46.4879887958181,42.1013257711392,2.77675109088763));
#230084=CARTESIAN_POINT('Ctrl Pts',(46.4969804206325,42.1053778715667,2.76805797913658));
#230085=CARTESIAN_POINT('Ctrl Pts',(46.5063617095237,42.1088147776126,2.75948271210128));
#230086=CARTESIAN_POINT('Ctrl Pts',(46.5161273793239,42.1115441100125,2.75108575573183));
#230087=CARTESIAN_POINT('Ctrl Pts',(46.5251222674812,42.1140580225433,2.7433515516322));
#230088=CARTESIAN_POINT('Ctrl Pts',(46.534443807433,42.1159717447015,2.73576818685884));
#230089=CARTESIAN_POINT('Ctrl Pts',(46.5440884908204,42.1171748456138,2.72840626160431));
#230090=CARTESIAN_POINT('Ctrl Pts',(46.5468860468482,42.117523819455,2.72627084693645));
#230091=CARTESIAN_POINT('Ctrl Pts',(46.5497107674235,42.1178127362982,2.72415424587519));
#230092=CARTESIAN_POINT('Ctrl Pts',(46.5525624800841,42.1180382068977,2.72205867173285));
#230093=CARTESIAN_POINT('Ctrl Pts',(46.5556539199574,42.118282631524,2.71978693462889));
#230094=CARTESIAN_POINT('Ctrl Pts',(46.5587726948498,42.1184532289194,2.7175441134079));
#230095=CARTESIAN_POINT('Ctrl Pts',(46.5619176830194,42.1185461584681,2.71533341844287));
#230096=CARTESIAN_POINT('Ctrl Pts',(46.5705491277288,42.1188012043437,2.70926614876435));
#230097=CARTESIAN_POINT('Ctrl Pts',(46.5793682643811,42.1184278543823,2.70347381860453));
#230098=CARTESIAN_POINT('Ctrl Pts',(46.5882835699004,42.1173773384969,2.69804914171439));
#230099=CARTESIAN_POINT('Ctrl Pts',(46.5964405904275,42.1164161734956,2.6930858568724));
#230100=CARTESIAN_POINT('Ctrl Pts',(46.6046697328844,42.1148801579478,2.68842799053214));
#230101=CARTESIAN_POINT('Ctrl Pts',(46.612914529219,42.1127009621828,2.6841476705424));
#230102=CARTESIAN_POINT('Ctrl Pts',(46.6169643462455,42.1116305483417,2.68204519134583));
#230103=CARTESIAN_POINT('Ctrl Pts',(46.6210176421367,42.1104045383079,2.68003431778542));
#230104=CARTESIAN_POINT('Ctrl Pts',(46.6250654385592,42.109012387551,2.67812693945299));
#230105=CARTESIAN_POINT('Ctrl Pts',(46.6258334685044,42.1087482405046,2.67776503299251));
#230106=CARTESIAN_POINT('Ctrl Pts',(46.6266015422614,42.108477638333,2.67740659639971));
#230107=CARTESIAN_POINT('Ctrl Pts',(46.6273695213206,42.1082005605487,2.67705178968902));
#230108=CARTESIAN_POINT('Ctrl Pts',(46.6281135010342,42.1079321414452,2.67670807068805));
#230109=CARTESIAN_POINT('Ctrl Pts',(46.6288573918596,42.1076576451502,2.67636775825313));
#230110=CARTESIAN_POINT('Ctrl Pts',(46.6296010653159,42.1073770559081,2.67603099699302));
#230111=CARTESIAN_POINT('Ctrl Pts',(46.6377054654054,42.1043192521646,2.67236104217164));
#230112=CARTESIAN_POINT('Ctrl Pts',(46.6457892400078,42.1005354505673,2.66911440541501));
#230113=CARTESIAN_POINT('Ctrl Pts',(46.653661939077,42.0960238460767,2.66646778189653));
#230114=CARTESIAN_POINT('Ctrl Pts',(46.6569866287807,42.0941185674849,2.66535009635006));
#230115=CARTESIAN_POINT('Ctrl Pts',(46.6602736399414,42.0920839261384,2.66433897912384));
#230116=CARTESIAN_POINT('Ctrl Pts',(46.6635089796843,42.0899216923181,2.66344564884839));
#230117=CARTESIAN_POINT('Ctrl Pts',(46.6689572109695,42.0862805445928,2.66194130298631));
#230118=CARTESIAN_POINT('Ctrl Pts',(46.6742564366675,42.0822770520159,2.66077206705464));
#230119=CARTESIAN_POINT('Ctrl Pts',(46.679333290145,42.0779224130574,2.65998225155758));
#230120=CARTESIAN_POINT('Ctrl Pts',(46.6806025035143,42.0768337533177,2.65978479768331));
#230121=CARTESIAN_POINT('Ctrl Pts',(46.6818576549905,42.0757229796948,2.65961098966666));
#230122=CARTESIAN_POINT('Ctrl Pts',(46.683097373911,42.0745900553978,2.65946139030545));
#230123=CARTESIAN_POINT('Ctrl Pts',(46.6849569522919,42.0728906689523,2.65923699126363));
#230124=CARTESIAN_POINT('Ctrl Pts',(46.686781786976,42.0711414461005,2.65906707562485));
#230125=CARTESIAN_POINT('Ctrl Pts',(46.6885684866733,42.069343399161,2.65895332562962));
#230126=CARTESIAN_POINT('Ctrl Pts',(46.6903551863705,42.0675453522215,2.6588395756344));
#230127=CARTESIAN_POINT('Ctrl Pts',(46.692103753135,42.0656984926167,2.65878198860292));
#230128=CARTESIAN_POINT('Ctrl Pts',(46.6938111422604,42.0638038389703,2.65878198860292));
#230129=CARTESIAN_POINT('Ctrl Pts',(43.8565665267056,39.5091373124625,2.6587819886029));
#230130=CARTESIAN_POINT('Ctrl Pts',(43.8507890749209,39.5155480799603,2.6587819886029));
#230131=CARTESIAN_POINT('Ctrl Pts',(43.8455908828153,39.5223801852464,2.65945335517882));
#230132=CARTESIAN_POINT('Ctrl Pts',(43.8409939475747,39.5294841269563,2.66072561226625));
#230133=CARTESIAN_POINT('Ctrl Pts',(43.8380247990819,39.5340725443945,2.66154735980364));
#230134=CARTESIAN_POINT('Ctrl Pts',(43.8353056940461,39.5387738681333,2.6626189576691));
#230135=CARTESIAN_POINT('Ctrl Pts',(43.8328343017436,39.5435446222365,2.66391429251056));
#230136=CARTESIAN_POINT('Ctrl Pts',(43.8295586128169,39.5498679835146,2.66563118464153));
#230137=CARTESIAN_POINT('Ctrl Pts',(43.8267236865061,39.5563148866445,2.66774105138728));
#230138=CARTESIAN_POINT('Ctrl Pts',(43.8243293609623,39.5627952650341,2.67016894181779));
#230139=CARTESIAN_POINT('Ctrl Pts',(43.8231321981904,39.566035454229,2.67138288703305));
#230140=CARTESIAN_POINT('Ctrl Pts',(43.8220450509626,39.5692841591688,2.67267613167581));
#230141=CARTESIAN_POINT('Ctrl Pts',(43.8210669472518,39.5725311673657,2.67403835432583));
#230142=CARTESIAN_POINT('Ctrl Pts',(43.8205778953964,39.5741546714642,2.67471946565083));
#230143=CARTESIAN_POINT('Ctrl Pts',(43.8201160933895,39.5757777635549,2.67541781389553));
#230144=CARTESIAN_POINT('Ctrl Pts',(43.8196813503778,39.5773992434497,2.67613207244199));
#230145=CARTESIAN_POINT('Ctrl Pts',(43.8195726646249,39.5778046134234,2.6763106370786));
#230146=CARTESIAN_POINT('Ctrl Pts',(43.8194656698239,39.5782098828932,2.67649019601875));
#230147=CARTESIAN_POINT('Ctrl Pts',(43.8193603625175,39.5786150336268,2.67667072836686));
#230148=CARTESIAN_POINT('Ctrl Pts',(43.8190444405985,39.5798304858278,2.6772123254112));
#230149=CARTESIAN_POINT('Ctrl Pts',(43.8187437073124,39.5810448681192,2.67776268340076));
#230150=CARTESIAN_POINT('Ctrl Pts',(43.8184580587802,39.5822576997163,2.67832123541545));
#230151=CARTESIAN_POINT('Ctrl Pts',(43.8164459874035,39.5908007288813,2.6822556036847));
#230152=CARTESIAN_POINT('Ctrl Pts',(43.8151322889032,39.5992865061387,2.6866179299891));
#230153=CARTESIAN_POINT('Ctrl Pts',(43.8144227306312,39.6076412948833,2.69130986622595));
#230154=CARTESIAN_POINT('Ctrl Pts',(43.814078595636,39.6116933583963,2.69358545023075));
#230155=CARTESIAN_POINT('Ctrl Pts',(43.8138769687219,39.6157150281162,2.69593918853494));
#230156=CARTESIAN_POINT('Ctrl Pts',(43.8138093098903,39.6196997093544,2.69836306235503));
#230157=CARTESIAN_POINT('Ctrl Pts',(43.8137057289464,39.6257999779284,2.70207384382236));
#230158=CARTESIAN_POINT('Ctrl Pts',(43.8139151128799,39.6318101761583,2.70594760814237));
#230159=CARTESIAN_POINT('Ctrl Pts',(43.8144090029878,39.6376940219323,2.70995196345716));
#230160=CARTESIAN_POINT('Ctrl Pts',(43.8146383681089,39.6404265103487,2.71181160678114));
#230161=CARTESIAN_POINT('Ctrl Pts',(43.8149288459967,39.6431316855284,2.71369962772107));
#230162=CARTESIAN_POINT('Ctrl Pts',(43.8152787628653,39.6458055463963,2.71561183138669));
#230163=CARTESIAN_POINT('Ctrl Pts',(43.8153055826145,39.6460104872963,2.7157583942632));
#230164=CARTESIAN_POINT('Ctrl Pts',(43.8153327221694,39.6462152612036,2.71590508903217));
#230165=CARTESIAN_POINT('Ctrl Pts',(43.8153601802954,39.6464198673377,2.71605191409919));
#230166=CARTESIAN_POINT('Ctrl Pts',(43.8157458841823,39.6492939666539,2.71811436362761));
#230167=CARTESIAN_POINT('Ctrl Pts',(43.8161965332334,39.6521348180508,2.72020091026967));
#230168=CARTESIAN_POINT('Ctrl Pts',(43.816707563491,39.654938997009,2.7223062486219));
#230169=CARTESIAN_POINT('Ctrl Pts',(43.818540027111,39.6649942840467,2.72985561753114));
#230170=CARTESIAN_POINT('Ctrl Pts',(43.821161113837,39.6746561192247,2.73770089914344));
#230171=CARTESIAN_POINT('Ctrl Pts',(43.82444189681,39.6839173731633,2.74574823347091));
#230172=CARTESIAN_POINT('Ctrl Pts',(43.8280471477134,39.6940945608664,2.75459144547029));
#230173=CARTESIAN_POINT('Ctrl Pts',(43.8324491002309,39.703788679467,2.7636791175426));
#230174=CARTESIAN_POINT('Ctrl Pts',(43.8375295667867,39.7129876499604,2.77292162564703));
#230175=CARTESIAN_POINT('Ctrl Pts',(43.8430151956439,39.7229202294667,2.78290121484676));
#230176=CARTESIAN_POINT('Ctrl Pts',(43.8492922888407,39.7322766233291,2.79306229500101));
#230177=CARTESIAN_POINT('Ctrl Pts',(43.8562669044089,39.7410245486279,2.80331916685133));
#230178=CARTESIAN_POINT('Ctrl Pts',(43.8631830101192,39.7496990878222,2.81348999408622));
#230179=CARTESIAN_POINT('Ctrl Pts',(43.8707860819058,39.7577762496637,2.82375635966854));
#230180=CARTESIAN_POINT('Ctrl Pts',(43.8790236240219,39.7651933659001,2.8340419886029));
#230181=CARTESIAN_POINT('Origin',(0.0101975504409105,-0.0113255271400898,
2.83404198860262));
#230182=CARTESIAN_POINT('Ctrl Pts',(46.7142062431422,42.0411527846897,2.65878198860292));
#230183=CARTESIAN_POINT('Ctrl Pts',(46.7199506919426,42.0347675597391,2.65878198860292));
#230184=CARTESIAN_POINT('Ctrl Pts',(46.7251107020211,42.027959214278,2.65944603041874));
#230185=CARTESIAN_POINT('Ctrl Pts',(46.7296675019392,42.0208774479587,2.66070439264083));
#230186=CARTESIAN_POINT('Ctrl Pts',(46.7325790801594,42.0163525364098,2.66150842619609));
#230187=CARTESIAN_POINT('Ctrl Pts',(46.735245189214,42.0117164852,2.66255428265387));
#230188=CARTESIAN_POINT('Ctrl Pts',(46.7376689638753,42.0070114066747,2.66381699700683));
#230189=CARTESIAN_POINT('Ctrl Pts',(46.7409769299535,42.0005899185698,2.66554034873282));
#230190=CARTESIAN_POINT('Ctrl Pts',(46.7438276087421,41.9940383480778,2.66766759643986));
#230191=CARTESIAN_POINT('Ctrl Pts',(46.7462229640888,41.9874523371582,2.67012012783161));
#230192=CARTESIAN_POINT('Ctrl Pts',(46.7474206417622,41.9841593316984,2.67134639352748));
#230193=CARTESIAN_POINT('Ctrl Pts',(46.7485046297347,41.9808575622225,2.67265375585023));
#230194=CARTESIAN_POINT('Ctrl Pts',(46.7494761782933,41.9775578801519,2.67403135126951));
#230195=CARTESIAN_POINT('Ctrl Pts',(46.7499619525726,41.9759080391167,2.67472014897914));
#230196=CARTESIAN_POINT('Ctrl Pts',(46.7504196286881,41.9742587070257,2.67542649668643));
#230197=CARTESIAN_POINT('Ctrl Pts',(46.7508494364813,41.9726111592841,2.67614899656112));
#230198=CARTESIAN_POINT('Ctrl Pts',(46.7509568884295,41.9721992723487,2.67632962152979));
#230199=CARTESIAN_POINT('Ctrl Pts',(46.7510625988575,41.9717874966609,2.67651125590961));
#230200=CARTESIAN_POINT('Ctrl Pts',(46.7511665718606,41.971375851596,2.67669387767534));
#230201=CARTESIAN_POINT('Ctrl Pts',(46.7514784908699,41.9701409164014,2.67724174297254));
#230202=CARTESIAN_POINT('Ctrl Pts',(46.7517747718024,41.968907158177,2.67779849504757));
#230203=CARTESIAN_POINT('Ctrl Pts',(46.7520555364232,41.9676750878621,2.67836353618018));
#230204=CARTESIAN_POINT('Ctrl Pts',(46.7539957941554,41.9591607175414,2.68226832098922));
#230205=CARTESIAN_POINT('Ctrl Pts',(46.7552464720209,41.9507055072916,2.6865915375141));
#230206=CARTESIAN_POINT('Ctrl Pts',(46.755902754358,41.9423805287166,2.69123699486203));
#230207=CARTESIAN_POINT('Ctrl Pts',(46.7562289248781,41.9382430372166,2.69354577441237));
#230208=CARTESIAN_POINT('Ctrl Pts',(46.7564078446195,41.934137281497,2.69593478828134));
#230209=CARTESIAN_POINT('Ctrl Pts',(46.7564487173143,41.9300700339486,2.69839565261231));
#230210=CARTESIAN_POINT('Ctrl Pts',(46.7565388885838,41.9210970783571,2.70382468689057));
#230211=CARTESIAN_POINT('Ctrl Pts',(46.7559695796225,41.9123126321656,2.70961155815099));
#230212=CARTESIAN_POINT('Ctrl Pts',(46.7548061840817,41.9038465062687,2.71562701361779));
#230213=CARTESIAN_POINT('Ctrl Pts',(46.7543811810194,41.900753723715,2.7178245353587));
#230214=CARTESIAN_POINT('Ctrl Pts',(46.7538836816023,41.8976992635448,2.72005051502414));
#230215=CARTESIAN_POINT('Ctrl Pts',(46.7533184435777,41.8946854937103,2.72229986760127));
#230216=CARTESIAN_POINT('Ctrl Pts',(46.7514198688645,41.8845625597425,2.72985520488967));
#230217=CARTESIAN_POINT('Ctrl Pts',(46.748736732731,41.8748360802661,2.73770845534701));
#230218=CARTESIAN_POINT('Ctrl Pts',(46.7453971059998,41.8655137786555,2.74576706701967));
#230219=CARTESIAN_POINT('Ctrl Pts',(46.7417264606174,41.8552674648863,2.75462443585317));
#230220=CARTESIAN_POINT('Ctrl Pts',(46.7372626589195,41.8455087367117,2.76373036323547));
#230221=CARTESIAN_POINT('Ctrl Pts',(46.732122753094,41.8362508575405,2.77299664637264));
#230222=CARTESIAN_POINT('Ctrl Pts',(46.7265868542923,41.8262797250045,2.78297683034014));
#230223=CARTESIAN_POINT('Ctrl Pts',(46.720266210471,41.8168884800825,2.79314401479529));
#230224=CARTESIAN_POINT('Ctrl Pts',(46.713252829158,41.808111511203,2.80341452428671));
#230225=CARTESIAN_POINT('Ctrl Pts',(46.7063341521755,41.7994530610414,2.81354634721862));
#230226=CARTESIAN_POINT('Ctrl Pts',(46.6987402031235,41.7913915075168,2.82378004209465));
#230227=CARTESIAN_POINT('Ctrl Pts',(46.6905216402897,41.7839914803029,2.83404198860292));
#230228=CARTESIAN_POINT('Ctrl Pts',(44.1339623850447,39.4820551873932,2.8340419886029));
#230229=CARTESIAN_POINT('Ctrl Pts',(44.1260971752944,39.4749733207248,2.82422126443033));
#230230=CARTESIAN_POINT('Ctrl Pts',(44.1177016730292,39.4685372764357,2.81442815028527));
#230231=CARTESIAN_POINT('Ctrl Pts',(44.1088266671086,39.4627751762749,2.80471618166343));
#230232=CARTESIAN_POINT('Ctrl Pts',(44.100257068035,39.4572113615978,2.79533842146243));
#230233=CARTESIAN_POINT('Ctrl Pts',(44.0912392969003,39.4522752837263,2.78603515650242));
#230234=CARTESIAN_POINT('Ctrl Pts',(44.0817922708732,39.4480294591793,2.77685887346747));
#230235=CARTESIAN_POINT('Ctrl Pts',(44.0728618726522,39.4440158252724,2.76818441216543));
#230236=CARTESIAN_POINT('Ctrl Pts',(44.0635470605538,39.4406186435278,2.75962261521566));
#230237=CARTESIAN_POINT('Ctrl Pts',(44.0538529442796,39.4379312493386,2.75123537701578));
#230238=CARTESIAN_POINT('Ctrl Pts',(44.0449248258219,39.4354562043748,2.74351087134));
#230239=CARTESIAN_POINT('Ctrl Pts',(44.0356744386745,39.4335831186678,2.73593399449692));
#230240=CARTESIAN_POINT('Ctrl Pts',(44.0261054687948,39.4324230329116,2.72857657812389));
#230241=CARTESIAN_POINT('Ctrl Pts',(44.0232521951408,39.4320771187572,2.72638274508204));
#230242=CARTESIAN_POINT('Ctrl Pts',(44.0203706219312,39.4317948788026,2.72420861709549));
#230243=CARTESIAN_POINT('Ctrl Pts',(44.0174609456696,39.4315800126159,2.72205663736736));
#230244=CARTESIAN_POINT('Ctrl Pts',(44.0145809991274,39.4313673418319,2.71992664556775));
#230245=CARTESIAN_POINT('Ctrl Pts',(44.0116765294504,39.4312206224785,2.71782089927893));
#230246=CARTESIAN_POINT('Ctrl Pts',(44.0087510493745,39.4311433701096,2.71574387311255));
#230247=CARTESIAN_POINT('Ctrl Pts',(44.0085476172113,39.431137998131,2.71559944077495));
#230248=CARTESIAN_POINT('Ctrl Pts',(44.0083440782823,39.4311329512713,2.71545515216078));
#230249=CARTESIAN_POINT('Ctrl Pts',(44.0081404327824,39.4311282308204,2.71531100781739));
#230250=CARTESIAN_POINT('Ctrl Pts',(43.9992118680542,39.4309212689595,2.70899119176083));
#230251=CARTESIAN_POINT('Ctrl Pts',(43.9900881971803,39.4313859080979,2.70298296066829));
#230252=CARTESIAN_POINT('Ctrl Pts',(43.9808585737693,39.4325966403786,2.6973672777412));
#230253=CARTESIAN_POINT('Ctrl Pts',(43.9722549606524,39.4337252532881,2.69213248525396));
#230254=CARTESIAN_POINT('Ctrl Pts',(43.9635585482846,39.4355025470899,2.68723866185422));
#230255=CARTESIAN_POINT('Ctrl Pts',(43.9548613290769,39.438010551914,2.68278595829505));
#230256=CARTESIAN_POINT('Ctrl Pts',(43.9516797737733,39.4389280125252,2.6811571017277));
#230257=CARTESIAN_POINT('Ctrl Pts',(43.948498363405,39.4399434521997,2.67958763637796));
#230258=CARTESIAN_POINT('Ctrl Pts',(43.9453226165471,39.4410615611725,2.6780837864537));
#230259=CARTESIAN_POINT('Ctrl Pts',(43.9445589555201,39.4413304290278,2.67772216078605));
#230260=CARTESIAN_POINT('Ctrl Pts',(43.9437952833156,39.441605709343,2.67736403603568));
#230261=CARTESIAN_POINT('Ctrl Pts',(43.9430317345449,39.4418874191263,2.67700956934484));
#230262=CARTESIAN_POINT('Ctrl Pts',(43.9422920466734,39.4421603254788,2.67666617973809));
#230263=CARTESIAN_POINT('Ctrl Pts',(43.9415524746578,39.4424392657173,2.67632622314124));
#230264=CARTESIAN_POINT('Ctrl Pts',(43.9408131433999,39.4427242524727,2.67598984158778));
#230265=CARTESIAN_POINT('Ctrl Pts',(43.9327129150437,39.4458466117307,2.67230439292245));
#230266=CARTESIAN_POINT('Ctrl Pts',(43.9246364083441,39.4496972096652,2.66904964540014));
#230267=CARTESIAN_POINT('Ctrl Pts',(43.9167721156751,39.4542738890608,2.66640203566772));
#230268=CARTESIAN_POINT('Ctrl Pts',(43.9135105590952,39.4561719744227,2.6653039929947));
#230269=CARTESIAN_POINT('Ctrl Pts',(43.9102855324954,39.4581945203283,2.66430995142275));
#230270=CARTESIAN_POINT('Ctrl Pts',(43.9071101492109,39.4603395741453,2.66343053473365));
#230271=CARTESIAN_POINT('Ctrl Pts',(43.9016942021215,39.4639981869599,2.66193059792889));
#230272=CARTESIAN_POINT('Ctrl Pts',(43.8964251099356,39.4680136963363,2.66076519817133));
#230273=CARTESIAN_POINT('Ctrl Pts',(43.8913745966875,39.4723737491583,2.65997805604465));
#230274=CARTESIAN_POINT('Ctrl Pts',(43.8888493400635,39.4745537755693,2.65958448498131));
#230275=CARTESIAN_POINT('Ctrl Pts',(43.8863797569643,39.4768209551513,2.65928526260768));
#230276=CARTESIAN_POINT('Ctrl Pts',(43.8839748786094,39.479173745493,2.6590846397133));
#230277=CARTESIAN_POINT('Ctrl Pts',(43.8815700002544,39.4815265358348,2.65888401681892));
#230278=CARTESIAN_POINT('Ctrl Pts',(43.879229842074,39.483964893962,2.6587819886029));
#230279=CARTESIAN_POINT('Ctrl Pts',(43.8769616275874,39.4864862581819,2.6587819886029));
#230280=CARTESIAN_POINT('Origin',(38.9747476500513,43.3086183250769,2.83404198860292));
#230281=CARTESIAN_POINT('Ctrl Pts',(41.7839914803026,46.69052164029,2.83404198860295));
#230282=CARTESIAN_POINT('Ctrl Pts',(41.7910911765306,46.6984066517723,2.82419652440089));
#230283=CARTESIAN_POINT('Ctrl Pts',(41.7987919603591,46.7057080773548,2.81438790575666));
#230284=CARTESIAN_POINT('Ctrl Pts',(41.8070443420773,46.7123936319704,2.80466781256913));
#230285=CARTESIAN_POINT('Ctrl Pts',(41.8150285705293,46.7188619458709,2.79526356453088));
#230286=CARTESIAN_POINT('Ctrl Pts',(41.8235301761263,46.7247545199416,2.78594102496242));
#230287=CARTESIAN_POINT('Ctrl Pts',(41.8325358446879,46.7300083326612,2.77675109088789));
#230288=CARTESIAN_POINT('Ctrl Pts',(41.84105465261,46.7349781159828,2.76805797913695));
#230289=CARTESIAN_POINT('Ctrl Pts',(41.8500252953116,46.7393768060089,2.75948271210177));
#230290=CARTESIAN_POINT('Ctrl Pts',(41.8594521748292,46.7431119772975,2.75108575573242));
#230291=CARTESIAN_POINT('Ctrl Pts',(41.8681350126342,46.7465523401887,2.74335155163291));
#230292=CARTESIAN_POINT('Ctrl Pts',(41.8772054497783,46.7494299450231,2.73576818685966));
#230293=CARTESIAN_POINT('Ctrl Pts',(41.8866715402913,46.7516345991559,2.72840626160521));
#230294=CARTESIAN_POINT('Ctrl Pts',(41.8894172933155,46.7522740855145,2.72627084693707));
#230295=CARTESIAN_POINT('Ctrl Pts',(41.8921963397426,46.7528566833419,2.72415424587553));
#230296=CARTESIAN_POINT('Ctrl Pts',(41.8950088623279,46.753379003932,2.72205867173292));
#230297=CARTESIAN_POINT('Ctrl Pts',(41.8980578176395,46.7539452330338,2.71978693462894));
#230298=CARTESIAN_POINT('Ctrl Pts',(41.9011416752732,46.7544408966256,2.71754411340795));
#230299=CARTESIAN_POINT('Ctrl Pts',(41.9042597210856,46.7548620578768,2.71533341844291));
#230300=CARTESIAN_POINT('Ctrl Pts',(41.9128172222843,46.7560179382356,2.70926614876437));
#230301=CARTESIAN_POINT('Ctrl Pts',(41.921627072481,46.7565684843261,2.70347381860455));
#230302=CARTESIAN_POINT('Ctrl Pts',(41.9306033478349,46.7564556264621,2.6980491417144));
#230303=CARTESIAN_POINT('Ctrl Pts',(41.9388161524502,46.7563523676437,2.69308585687263));
#230304=CARTESIAN_POINT('Ctrl Pts',(41.9471607721481,46.7556849461649,2.68842799053256));
#230305=CARTESIAN_POINT('Ctrl Pts',(41.9555881906098,46.7543795041533,2.68414767054298));
#230306=CARTESIAN_POINT('Ctrl Pts',(41.9597277110291,46.7537382753015,2.68204519134619));
#230307=CARTESIAN_POINT('Ctrl Pts',(41.9638869554865,46.7529426662696,2.68003431778557));
#230308=CARTESIAN_POINT('Ctrl Pts',(41.9680580970364,46.7519812517997,2.67812693945295));
#230309=CARTESIAN_POINT('Ctrl Pts',(41.968849530518,46.7517988327684,2.67776503299247));
#230310=CARTESIAN_POINT('Ctrl Pts',(41.9696416823157,46.7516099985533,2.67740659639968));
#230311=CARTESIAN_POINT('Ctrl Pts',(41.9704344168203,46.751414714301,2.67705178968899));
#230312=CARTESIAN_POINT('Ctrl Pts',(41.9712023783716,46.7512255326816,2.67670807068802));
#230313=CARTESIAN_POINT('Ctrl Pts',(41.9719708867611,46.7510302978709,2.67636775825309));
#230314=CARTESIAN_POINT('Ctrl Pts',(41.9727398158587,46.7508289807696,2.67603099699299));
#230315=CARTESIAN_POINT('Ctrl Pts',(41.9811194467225,46.748635068482,2.67236104217173));
#230316=CARTESIAN_POINT('Ctrl Pts',(41.9895544525278,46.7457169794824,2.6691144054152));
#230317=CARTESIAN_POINT('Ctrl Pts',(41.9978556152118,46.742053011169,2.66646778189678));
#230318=CARTESIAN_POINT('Ctrl Pts',(42.001361247761,46.740505694598,2.6653500963502));
#230319=CARTESIAN_POINT('Ctrl Pts',(42.0048429302642,46.738825785455,2.66433897912389));
#230320=CARTESIAN_POINT('Ctrl Pts',(42.0082865614562,46.7370135816691,2.66344564884837));
#230321=CARTESIAN_POINT('Ctrl Pts',(42.0140855503366,46.7339618757758,2.6619413029863));
#230322=CARTESIAN_POINT('Ctrl Pts',(42.0197742252485,46.7305342346688,2.66077206705465));
#230323=CARTESIAN_POINT('Ctrl Pts',(42.0252784509104,46.7267341265711,2.6599822515576));
#230324=CARTESIAN_POINT('Ctrl Pts',(42.0266545073259,46.7257840995467,2.65978479768334));
#230325=CARTESIAN_POINT('Ctrl Pts',(42.0280188904107,46.7248106099128,2.65961098966668));
#230326=CARTESIAN_POINT('Ctrl Pts',(42.029370240857,46.7238134778072,2.65946139030547));
#230327=CARTESIAN_POINT('Ctrl Pts',(42.0313972665265,46.7223177796489,2.65923699126366));
#230328=CARTESIAN_POINT('Ctrl Pts',(42.0333949481518,46.720768886388,2.65906707562488));
#230329=CARTESIAN_POINT('Ctrl Pts',(42.0353598072046,46.7191674503113,2.65895332562965));
#230330=CARTESIAN_POINT('Ctrl Pts',(42.0373246662573,46.7175660142347,2.65883957563443));
#230331=CARTESIAN_POINT('Ctrl Pts',(42.0392567035874,46.7159120469178,2.65878198860295));
#230332=CARTESIAN_POINT('Ctrl Pts',(42.0411527846906,46.7142062431438,2.65878198860295));
#230333=CARTESIAN_POINT('Ctrl Pts',(39.4864862581816,43.8769616275877,2.65878198860293));
#230334=CARTESIAN_POINT('Ctrl Pts',(39.4800703482072,43.8827333680739,2.65878198860293));
#230335=CARTESIAN_POINT('Ctrl Pts',(39.4741864828752,43.8889846873401,2.65945335517889));
#230336=CARTESIAN_POINT('Ctrl Pts',(39.4688721660166,43.8955692023378,2.6607256122664));
#230337=CARTESIAN_POINT('Ctrl Pts',(39.4654396626065,43.8998221234159,2.66154735980377));
#230338=CARTESIAN_POINT('Ctrl Pts',(39.462244030967,43.9042134689402,2.66261895766919));
#230339=CARTESIAN_POINT('Ctrl Pts',(39.4592874976153,43.9086997575135,2.66391429251058));
#230340=CARTESIAN_POINT('Ctrl Pts',(39.4553687820182,43.9146460760273,2.66563118464155));
#230341=CARTESIAN_POINT('Ctrl Pts',(39.4518755008533,43.9207613318565,2.6677410513873));
#230342=CARTESIAN_POINT('Ctrl Pts',(39.4488169076809,43.9269559348856,2.67016894181782));
#230343=CARTESIAN_POINT('Ctrl Pts',(39.4472876110947,43.9300532364002,2.67138288703307));
#230344=CARTESIAN_POINT('Ctrl Pts',(39.4458668372381,43.9331705067654,2.67267613167583));
#230345=CARTESIAN_POINT('Ctrl Pts',(39.4445546869048,43.9362974878338,2.67403835432585));
#230346=CARTESIAN_POINT('Ctrl Pts',(39.4438986117382,43.9378609783681,2.67471946565086));
#230347=CARTESIAN_POINT('Ctrl Pts',(39.4432696802089,43.9394269075363,2.67541781389555));
#230348=CARTESIAN_POINT('Ctrl Pts',(39.4426678279634,43.9409940617757,2.67613207244201));
#230349=CARTESIAN_POINT('Ctrl Pts',(39.442517364902,43.9413858503355,2.67631063707863));
#230350=CARTESIAN_POINT('Ctrl Pts',(39.4423685940347,43.9417777156947,2.67649019601877));
#230351=CARTESIAN_POINT('Ctrl Pts',(39.4422215138293,43.9421696393593,2.67667072836689));
#230352=CARTESIAN_POINT('Ctrl Pts',(39.4417802732128,43.9433454103532,2.67721232541123));
#230353=CARTESIAN_POINT('Ctrl Pts',(39.4413542498604,43.9445217049431,2.67776268340079));
#230354=CARTESIAN_POINT('Ctrl Pts',(39.4409433907177,43.9456980341197,2.67832123541549));
#230355=CARTESIAN_POINT('Ctrl Pts',(39.4380493519682,43.9539839449482,2.6822556036848));
#230356=CARTESIAN_POINT('Ctrl Pts',(39.4358558447893,43.9622859173447,2.68661792998926));
#230357=CARTESIAN_POINT('Ctrl Pts',(39.4342768603234,43.9705207686467,2.69130986622619));
#230358=CARTESIAN_POINT('Ctrl Pts',(39.4335110545637,43.9745146626294,2.69358545023093));
#230359=CARTESIAN_POINT('Ctrl Pts',(39.4328901532274,43.9784932254702,2.69593918853504));
#230360=CARTESIAN_POINT('Ctrl Pts',(39.4324063524315,43.9824490059338,2.69836306235507));
#230361=CARTESIAN_POINT('Ctrl Pts',(39.4316656872152,43.9885050294414,2.70207384382239));
#230362=CARTESIAN_POINT('Ctrl Pts',(39.4312456873368,43.9945041897574,2.7059476081424));
#230363=CARTESIAN_POINT('Ctrl Pts',(39.4311218425061,44.0004074287825,2.70995196345719));
#230364=CARTESIAN_POINT('Ctrl Pts',(39.4310643283261,44.0031489235251,2.71181160678117));
#230365=CARTESIAN_POINT('Ctrl Pts',(39.4310704471411,44.0058696426793,2.7136996277211));
#230366=CARTESIAN_POINT('Ctrl Pts',(39.431138952561,44.0085654321303,2.71561183138673));
#230367=CARTESIAN_POINT('Ctrl Pts',(39.4311442032315,44.0087720537697,2.71575839426324));
#230368=CARTESIAN_POINT('Ctrl Pts',(39.4311497894112,44.0089785427601,2.7159050890322));
#230369=CARTESIAN_POINT('Ctrl Pts',(39.431155709954,44.009184898196,2.71605191409923));
#230370=CARTESIAN_POINT('Ctrl Pts',(39.4312388757299,44.0120835699301,2.71811436362764));
#230371=CARTESIAN_POINT('Ctrl Pts',(39.4313901062474,44.0149559644986,2.72020091026971));
#230372=CARTESIAN_POINT('Ctrl Pts',(39.4316052205105,44.0177981990786,2.72230624862194));
#230373=CARTESIAN_POINT('Ctrl Pts',(39.4323765820014,44.0279899468082,2.72985561753132));
#230374=CARTESIAN_POINT('Ctrl Pts',(39.4339733733565,44.0378728316098,2.73770089914377));
#230375=CARTESIAN_POINT('Ctrl Pts',(39.4362681192151,44.047426286633,2.7457482334714));
#230376=CARTESIAN_POINT('Ctrl Pts',(39.4387898143859,44.0579245739738,2.75459144547098));
#230377=CARTESIAN_POINT('Ctrl Pts',(39.442154341227,44.0680257165107,2.76367911754352));
#230378=CARTESIAN_POINT('Ctrl Pts',(39.4462454222063,44.0777053474432,2.77292162564817));
#230379=CARTESIAN_POINT('Ctrl Pts',(39.4506627629427,44.0881569195945,2.78290121484824));
#230380=CARTESIAN_POINT('Ctrl Pts',(39.4559274600944,44.0981181930583,2.79306229500285));
#230381=CARTESIAN_POINT('Ctrl Pts',(39.4619494608007,44.1075472421544,2.80331916685354));
#230382=CARTESIAN_POINT('Ctrl Pts',(39.4679209431084,44.1168971912164,2.81348999408771));
#230383=CARTESIAN_POINT('Ctrl Pts',(39.474638071157,44.1257248429294,2.8237563596693));
#230384=CARTESIAN_POINT('Ctrl Pts',(39.4820551873929,44.133962385045,2.83404198860293));
#230385=CARTESIAN_POINT('Origin',(0.0113255271402773,-0.0101975504407237,
2.83404198860262));
#230386=CARTESIAN_POINT('Ctrl Pts',(42.06380383897,46.6938111422607,2.65878198860295));
#230387=CARTESIAN_POINT('Ctrl Pts',(42.0701842568306,46.6880613546458,2.65878198860295));
#230388=CARTESIAN_POINT('Ctrl Pts',(42.0760276657225,46.6818296739374,2.6594460304188));
#230389=CARTESIAN_POINT('Ctrl Pts',(42.0812997491645,46.6752630175677,2.66070439264092));
#230390=CARTESIAN_POINT('Ctrl Pts',(42.084668359505,46.6710672367549,2.66150842619618));
#230391=CARTESIAN_POINT('Ctrl Pts',(42.0878044626438,46.6667352666012,2.66255428265393));
#230392=CARTESIAN_POINT('Ctrl Pts',(42.0907067742416,46.6623093164291,2.66381699700685));
#230393=CARTESIAN_POINT('Ctrl Pts',(42.0946678472191,46.6562687825186,2.66554034873284));
#230394=CARTESIAN_POINT('Ctrl Pts',(42.0981877352865,46.6500510792884,2.66766759643988));
#230395=CARTESIAN_POINT('Ctrl Pts',(42.1012583942265,46.643751530039,2.67012012783163));
#230396=CARTESIAN_POINT('Ctrl Pts',(42.1027937236965,46.6406017554143,2.67134639352751));
#230397=CARTESIAN_POINT('Ctrl Pts',(42.1042169023589,46.637431380974,2.67265375585027));
#230398=CARTESIAN_POINT('Ctrl Pts',(42.1055280393689,46.6342513293849,2.67403135126955));
#230399=CARTESIAN_POINT('Ctrl Pts',(42.1061836078739,46.6326613035904,2.67472014897919));
#230400=CARTESIAN_POINT('Ctrl Pts',(42.1068111789407,46.6310688468942,2.67542649668648));
#230401=CARTESIAN_POINT('Ctrl Pts',(42.1074108478354,46.6294752517396,2.67614899656117));
#230402=CARTESIAN_POINT('Ctrl Pts',(42.107560765059,46.629076852951,2.67632962152984));
#230403=CARTESIAN_POINT('Ctrl Pts',(42.1077089386741,46.628678382762,2.67651125590965));
#230404=CARTESIAN_POINT('Ctrl Pts',(42.1078553707282,46.6282798608701,2.67669387767539));
#230405=CARTESIAN_POINT('Ctrl Pts',(42.1082946668907,46.6270842951944,2.67724174297259));
#230406=CARTESIAN_POINT('Ctrl Pts',(42.1087182876164,46.6258882654173,2.67779849504762));
#230407=CARTESIAN_POINT('Ctrl Pts',(42.109126300596,46.6246922924068,2.67836353618024));
#230408=CARTESIAN_POINT('Ctrl Pts',(42.1119459234385,46.616427376857,2.68226832098914));
#230409=CARTESIAN_POINT('Ctrl Pts',(42.1140735600937,46.6081492165692,2.68659153751386));
#230410=CARTESIAN_POINT('Ctrl Pts',(42.1155964444647,46.5999384432824,2.69123699486161));
#230411=CARTESIAN_POINT('Ctrl Pts',(42.116353313817,46.5958577114966,2.6935457744121));
#230412=CARTESIAN_POINT('Ctrl Pts',(42.1169604217533,46.5917931497418,2.69593478828122));
#230413=CARTESIAN_POINT('Ctrl Pts',(42.1174262136792,46.5877524553607,2.69839565261236));
#230414=CARTESIAN_POINT('Ctrl Pts',(42.11845382024,46.5788380800231,2.70382468689062));
#230415=CARTESIAN_POINT('Ctrl Pts',(42.1188058546738,46.570042246956,2.70961155815103));
#230416=CARTESIAN_POINT('Ctrl Pts',(42.1185337834653,46.5615008914346,2.71562701361784));
#230417=CARTESIAN_POINT('Ctrl Pts',(42.1184343924219,46.5583806265504,2.71782453535875));
#230418=CARTESIAN_POINT('Ctrl Pts',(42.1182588963863,46.555290896183,2.72005051502419));
#230419=CARTESIAN_POINT('Ctrl Pts',(42.1180117795242,46.552234552633,2.72229986760133));
#230420=CARTESIAN_POINT('Ctrl Pts',(42.1171817401336,46.5419686180608,2.72985520488881));
#230421=CARTESIAN_POINT('Ctrl Pts',(42.1155299964535,46.5320149571611,2.73770845534515));
#230422=CARTESIAN_POINT('Ctrl Pts',(42.1131831104089,46.5223946380452,2.74576706701676));
#230423=CARTESIAN_POINT('Ctrl Pts',(42.1106036046389,46.511820767735,2.75462443584922));
#230424=CARTESIAN_POINT('Ctrl Pts',(42.107184320974,46.5016489045637,2.76373036323042));
#230425=CARTESIAN_POINT('Ctrl Pts',(42.103040283974,46.4919044745669,2.77299664636647));
#230426=CARTESIAN_POINT('Ctrl Pts',(42.0985769785671,46.4814093059446,2.78297683033278));
#230427=CARTESIAN_POINT('Ctrl Pts',(42.0932726122948,46.4714088200601,2.79314401478671));
#230428=CARTESIAN_POINT('Ctrl Pts',(42.0872150940887,46.4619468343642,2.80341452427691));
#230429=CARTESIAN_POINT('Ctrl Pts',(42.0812393728308,46.4526126174223,2.81354634721203));
#230430=CARTESIAN_POINT('Ctrl Pts',(42.0745296860258,46.4438014421038,2.82378004209136));
#230431=CARTESIAN_POINT('Ctrl Pts',(42.0671296588095,46.4355828792673,2.83404198860295));
#230432=CARTESIAN_POINT('Ctrl Pts',(39.7651933658998,43.8790236240223,2.83404198860292));
#230433=CARTESIAN_POINT('Ctrl Pts',(39.7581114992313,43.8711584142718,2.82422126443018));
#230434=CARTESIAN_POINT('Ctrl Pts',(39.7504347382248,43.8638800583564,2.81442815028494));
#230435=CARTESIAN_POINT('Ctrl Pts',(39.7422106539902,43.8572218328528,2.80471618166292));
#230436=CARTESIAN_POINT('Ctrl Pts',(39.734269577075,43.8507927303126,2.79533842146191));
#230437=CARTESIAN_POINT('Ctrl Pts',(39.7258171668685,43.8449410790334,2.78603515650188));
#230438=CARTESIAN_POINT('Ctrl Pts',(39.7168657021537,43.8397310304445,2.77685887346692));
#230439=CARTESIAN_POINT('Ctrl Pts',(39.7084037645731,43.8348059028418,2.76818441216503));
#230440=CARTESIAN_POINT('Ctrl Pts',(39.6994950821773,43.83045366822,2.7596226152154));
#230441=CARTESIAN_POINT('Ctrl Pts',(39.6901349804713,43.8267676847806,2.75123537701567));
#230442=CARTESIAN_POINT('Ctrl Pts',(39.6815144838276,43.8233729558699,2.74351087134018));
#230443=CARTESIAN_POINT('Ctrl Pts',(39.6725105620397,43.8205432023694,2.7359339944974));
#230444=CARTESIAN_POINT('Ctrl Pts',(39.6631152739599,43.8183892419678,2.72857657812464));
#230445=CARTESIAN_POINT('Ctrl Pts',(39.6603137887123,43.8177469744569,2.72638274508255));
#230446=CARTESIAN_POINT('Ctrl Pts',(39.6574775031707,43.8171650742228,2.72420861709576));
#230447=CARTESIAN_POINT('Ctrl Pts',(39.654606226052,43.8166472411073,2.72205663736739));
#230448=CARTESIAN_POINT('Ctrl Pts',(39.6517642863086,43.8161346989698,2.71992664556778));
#230449=CARTESIAN_POINT('Ctrl Pts',(39.6488910639689,43.8156851836084,2.71782089927897));
#230450=CARTESIAN_POINT('Ctrl Pts',(39.6459896850503,43.8153025584994,2.71574387311258));
#230451=CARTESIAN_POINT('Ctrl Pts',(39.6457879288345,43.8152759514976,2.71559944077499));
#230452=CARTESIAN_POINT('Ctrl Pts',(39.6455860324536,43.8152496566737,2.71545515216081));
#230453=CARTESIAN_POINT('Ctrl Pts',(39.6453839959665,43.8152236753308,2.71531100781743));
#230454=CARTESIAN_POINT('Ctrl Pts',(39.6365259762554,43.8140845580784,2.7089911917609));
#230455=CARTESIAN_POINT('Ctrl Pts',(39.6274037177901,43.8135929685792,2.70298296066839));
#230456=CARTESIAN_POINT('Ctrl Pts',(39.6180980992372,43.8138323099901,2.69736727774132));
#230457=CARTESIAN_POINT('Ctrl Pts',(39.6094236454403,43.8140554177823,2.69213248525419));
#230458=CARTESIAN_POINT('Ctrl Pts',(39.6005890951397,43.8149139527619,2.68723866185454));
#230459=CARTESIAN_POINT('Ctrl Pts',(39.5916773623189,43.8164991115146,2.68278595829545));
#230460=CARTESIAN_POINT('Ctrl Pts',(39.5884173351601,43.8170789830939,2.68115710172796));
#230461=CARTESIAN_POINT('Ctrl Pts',(39.5851472105417,43.8177563121468,2.67958763637809));
#230462=CARTESIAN_POINT('Ctrl Pts',(39.5818719865444,43.8185363400629,2.67808378645371));
#230463=CARTESIAN_POINT('Ctrl Pts',(39.5810844045886,43.8187239107184,2.67772216078606));
#230464=CARTESIAN_POINT('Ctrl Pts',(39.5802961412321,43.8189178575373,2.67736403603569));
#230465=CARTESIAN_POINT('Ctrl Pts',(39.5795073285708,43.8191182115053,2.67700956934485));
#230466=CARTESIAN_POINT('Ctrl Pts',(39.5787431663051,43.8193123044117,2.6766661797381));
#230467=CARTESIAN_POINT('Ctrl Pts',(39.577978488548,43.8195124102601,2.67632622314124));
#230468=CARTESIAN_POINT('Ctrl Pts',(39.5772134181964,43.8197185546681,2.67598984158779));
#230469=CARTESIAN_POINT('Ctrl Pts',(39.5688311883234,43.8219771048932,2.67230439292236));
#230470=CARTESIAN_POINT('Ctrl Pts',(39.5603964284877,43.8249623840155,2.66904964539998));
#230471=CARTESIAN_POINT('Ctrl Pts',(39.5520968239724,43.8286919494552,2.66640203566753));
#230472=CARTESIAN_POINT('Ctrl Pts',(39.5486547305949,43.8302387114097,2.6653039929946));
#230473=CARTESIAN_POINT('Ctrl Pts',(39.5452359574131,43.8319130705227,2.66430995142272));
#230474=CARTESIAN_POINT('Ctrl Pts',(39.5418537500316,43.8337144555752,2.66343053473367));
#230475=CARTESIAN_POINT('Ctrl Pts',(39.5360850428918,43.8367869054997,2.66193059792891));
#230476=CARTESIAN_POINT('Ctrl Pts',(39.5304250803199,43.8402296473865,2.66076519817135));
#230477=CARTESIAN_POINT('Ctrl Pts',(39.5249464846905,43.8440378929944,2.65997805604468));
#230478=CARTESIAN_POINT('Ctrl Pts',(39.5222071868758,43.8459420157983,2.65958448498134));
#230479=CARTESIAN_POINT('Ctrl Pts',(39.5195141476136,43.847938633807,2.65928526260771));
#230480=CARTESIAN_POINT('Ctrl Pts',(39.5168765098751,43.8500271570784,2.65908463971333));
#230481=CARTESIAN_POINT('Ctrl Pts',(39.5142388721366,43.8521156803497,2.65888401681895));
#230482=CARTESIAN_POINT('Ctrl Pts',(39.5116566557597,43.8542960677576,2.65878198860293));
#230483=CARTESIAN_POINT('Ctrl Pts',(39.5091373124622,43.8565665267059,2.65878198860293));
#230484=CARTESIAN_POINT('Origin',(34.2342565846635,47.1453396605411,2.83404198860295));
#230485=CARTESIAN_POINT('Ctrl Pts',(36.6746059268177,50.8023624960594,2.83404198860298));
#230486=CARTESIAN_POINT('Ctrl Pts',(36.6808425220336,50.8109464329599,2.82419652440128));
#230487=CARTESIAN_POINT('Ctrl Pts',(36.6877379133664,50.8190128116683,2.81438790575741));
#230488=CARTESIAN_POINT('Ctrl Pts',(36.6952462569238,50.8265243508953,2.80466781257023));
#230489=CARTESIAN_POINT('Ctrl Pts',(36.7025106240248,50.8337918098257,2.79526356453224));
#230490=CARTESIAN_POINT('Ctrl Pts',(36.7103497152242,50.8405407635273,2.78594102496402));
#230491=CARTESIAN_POINT('Ctrl Pts',(36.7187568768209,50.8467071440065,2.77675109088972));
#230492=CARTESIAN_POINT('Ctrl Pts',(36.7267095340082,50.8525401602359,2.76805797913899));
#230493=CARTESIAN_POINT('Ctrl Pts',(36.7351712462813,50.8578524412739,2.759482712104));
#230494=CARTESIAN_POINT('Ctrl Pts',(36.7441560526514,50.8625525281326,2.75108575573482));
#230495=CARTESIAN_POINT('Ctrl Pts',(36.752431709116,50.8668816480485,2.7433515516355));
#230496=CARTESIAN_POINT('Ctrl Pts',(36.7611516658447,50.8706916079184,2.73576818686243));
#230497=CARTESIAN_POINT('Ctrl Pts',(36.7703354510145,50.8738736606197,2.72840626160814));
#230498=CARTESIAN_POINT('Ctrl Pts',(36.7729993179912,50.8747966531497,2.72627084693901));
#230499=CARTESIAN_POINT('Ctrl Pts',(36.7757022424569,50.8756665488981,2.7241542458765));
#230500=CARTESIAN_POINT('Ctrl Pts',(36.7784447603818,50.8764799968255,2.72205867173293));
#230501=CARTESIAN_POINT('Ctrl Pts',(36.7814178261393,50.8773618266784,2.71978693462896));
#230502=CARTESIAN_POINT('Ctrl Pts',(36.7844329791247,50.8781771258726,2.71754411340797));
#230503=CARTESIAN_POINT('Ctrl Pts',(36.7874899206174,50.8789219044956,2.71533341844294));
#230504=CARTESIAN_POINT('Ctrl Pts',(36.7958797205316,50.8809659552705,2.70926614876441));
#230505=CARTESIAN_POINT('Ctrl Pts',(36.8045837617103,50.8824343655145,2.70347381860458));
#230506=CARTESIAN_POINT('Ctrl Pts',(36.8135226609478,50.8832604021664,2.69804914171444));
#230507=CARTESIAN_POINT('Ctrl Pts',(36.8217012684459,50.8840161808562,2.69308585687253));
#230508=CARTESIAN_POINT('Ctrl Pts',(36.8300699399858,50.8842246658556,2.68842799053233));
#230509=CARTESIAN_POINT('Ctrl Pts',(36.838587648015,50.883807280293,2.68414767054265));
#230510=CARTESIAN_POINT('Ctrl Pts',(36.8427715183746,50.8836022618681,2.68204519134601));
#230511=CARTESIAN_POINT('Ctrl Pts',(36.8469911418449,50.8832457706971,2.68003431778553));
#230512=CARTESIAN_POINT('Ctrl Pts',(36.8512399286217,50.8827256259727,2.67812693945304));
#230513=CARTESIAN_POINT('Ctrl Pts',(36.8520460945289,50.8826269335775,2.67776503299256));
#230514=CARTESIAN_POINT('Ctrl Pts',(36.8528536453865,50.8825219362261,2.67740659639976));
#230515=CARTESIAN_POINT('Ctrl Pts',(36.8536624499713,50.8824105850809,2.67705178968908));
#230516=CARTESIAN_POINT('Ctrl Pts',(36.8544459794128,50.882302713659,2.6767080706881));
#230517=CARTESIAN_POINT('Ctrl Pts',(36.8552306854278,50.8821888793659,2.67636775825318));
#230518=CARTESIAN_POINT('Ctrl Pts',(36.8560164456185,50.8820690400777,2.67603099699308));
#230519=CARTESIAN_POINT('Ctrl Pts',(36.8645794982675,50.8807630562082,2.67236104217187));
#230520=CARTESIAN_POINT('Ctrl Pts',(36.8732733195871,50.878742651,2.66911440541537));
#230521=CARTESIAN_POINT('Ctrl Pts',(36.8819119966105,50.8759664620671,2.66646778189695));
#230522=CARTESIAN_POINT('Ctrl Pts',(36.8855601635613,50.8747940602413,2.66535009635033));
#230523=CARTESIAN_POINT('Ctrl Pts',(36.8891983713647,50.873487288738,2.66433897912399));
#230524=CARTESIAN_POINT('Ctrl Pts',(36.8928125648617,50.8720449698706,2.66344564884844));
#230525=CARTESIAN_POINT('Ctrl Pts',(36.8988987764016,50.8696161409376,2.66194130298636));
#230526=CARTESIAN_POINT('Ctrl Pts',(36.9049145742147,50.8668019052538,2.6607720670547));
#230527=CARTESIAN_POINT('Ctrl Pts',(36.9107858666119,50.8635979627953,2.65998225155764));
#230528=CARTESIAN_POINT('Ctrl Pts',(36.9122536897112,50.8627969771806,2.65978479768337));
#230529=CARTESIAN_POINT('Ctrl Pts',(36.9137123559382,50.861971437292,2.65961098966672));
#230530=CARTESIAN_POINT('Ctrl Pts',(36.915160532232,50.861121022166,2.65946139030551));
#230531=CARTESIAN_POINT('Ctrl Pts',(36.9173327966728,50.859845399477,2.65923699126369));
#230532=CARTESIAN_POINT('Ctrl Pts',(36.9194814382216,50.8585138058059,2.65906707562491));
#230533=CARTESIAN_POINT('Ctrl Pts',(36.921602929223,50.8571265262611,2.65895332562968));
#230534=CARTESIAN_POINT('Ctrl Pts',(36.9237244202244,50.8557392467162,2.65883957563446));
#230535=CARTESIAN_POINT('Ctrl Pts',(36.9258187603129,50.8542962928972,2.65878198860298));
#230536=CARTESIAN_POINT('Ctrl Pts',(36.9278827595326,50.8527980281388,2.65878198860298));
#230537=CARTESIAN_POINT('Ctrl Pts',(34.6837837831345,47.7640607692766,2.65878198860296));
#230538=CARTESIAN_POINT('Ctrl Pts',(34.6767997090223,47.7691302463548,2.65878198860296));
#230539=CARTESIAN_POINT('Ctrl Pts',(34.6702946353236,47.7747322888391,2.65945335517902));
#230540=CARTESIAN_POINT('Ctrl Pts',(34.6643211616144,47.7807252358007,2.66072561226671));
#230541=CARTESIAN_POINT('Ctrl Pts',(34.6604629105129,47.784596064625,2.66154735980404));
#230542=CARTESIAN_POINT('Ctrl Pts',(34.656825764279,47.7886293194342,2.66261895766936));
#230543=CARTESIAN_POINT('Ctrl Pts',(34.6534164822763,47.792781989761,2.66391429251062));
#230544=CARTESIAN_POINT('Ctrl Pts',(34.6488976742769,47.7982861164004,2.66563118464159));
#230545=CARTESIAN_POINT('Ctrl Pts',(34.6447843113774,47.8040027249065,2.66774105138734));
#230546=CARTESIAN_POINT('Ctrl Pts',(34.6410949611633,47.809843683208,2.67016894181786));
#230547=CARTESIAN_POINT('Ctrl Pts',(34.6392502860562,47.8127641623587,2.67138288703311));
#230548=CARTESIAN_POINT('Ctrl Pts',(34.6375114518666,47.8157158446828,2.67267613167587));
#230549=CARTESIAN_POINT('Ctrl Pts',(34.6358796311044,47.8186885387639,2.67403835432589));
#230550=CARTESIAN_POINT('Ctrl Pts',(34.6350637207233,47.8201748858044,2.6747194656509));
#230551=CARTESIAN_POINT('Ctrl Pts',(34.6342745503772,47.8216664954026,2.6754178138956));
#230552=CARTESIAN_POINT('Ctrl Pts',(34.6335121829169,47.8231621539168,2.67613207244206));
#230553=CARTESIAN_POINT('Ctrl Pts',(34.6333215910518,47.8235360685453,2.67631063707867));
#230554=CARTESIAN_POINT('Ctrl Pts',(34.6331326740831,47.8239102364348,2.67649019601882));
#230555=CARTESIAN_POINT('Ctrl Pts',(34.63294543242,47.8242846390328,2.67667072836694));
#230556=CARTESIAN_POINT('Ctrl Pts',(34.6323837074307,47.8254078468266,2.67721232541128));
#230557=CARTESIAN_POINT('Ctrl Pts',(34.6318370616129,47.8265331659853,2.67776268340084));
#230558=CARTESIAN_POINT('Ctrl Pts',(34.6313054933184,47.8276601046328,2.67832123541553));
#230559=CARTESIAN_POINT('Ctrl Pts',(34.6275611948903,47.8355981149517,2.68225560368485));
#230560=CARTESIAN_POINT('Ctrl Pts',(34.6245119115566,47.8436253243401,2.68661792998933));
#230561=CARTESIAN_POINT('Ctrl Pts',(34.622080800581,47.8516500154454,2.69130986622627));
#230562=CARTESIAN_POINT('Ctrl Pts',(34.6209017143848,47.8555419819597,2.69358545023099));
#230563=CARTESIAN_POINT('Ctrl Pts',(34.6198683413513,47.8594338479544,2.69593918853509));
#230564=CARTESIAN_POINT('Ctrl Pts',(34.618973699214,47.8633173872851,2.6983630623551));
#230565=CARTESIAN_POINT('Ctrl Pts',(34.6176040646085,47.8692628146653,2.70207384382242));
#230566=CARTESIAN_POINT('Ctrl Pts',(34.6165592825246,47.8751852090115,2.70594760814242));
#230567=CARTESIAN_POINT('Ctrl Pts',(34.6158190596252,47.8810431641658,2.70995196345722));
#230568=CARTESIAN_POINT('Ctrl Pts',(34.6154752962814,47.8837636288445,2.71181160678119));
#230569=CARTESIAN_POINT('Ctrl Pts',(34.6151969889848,47.8864700832049,2.71369962772113));
#230570=CARTESIAN_POINT('Ctrl Pts',(34.6149833323962,47.8891582656054,2.71561183138676));
#230571=CARTESIAN_POINT('Ctrl Pts',(34.6149669564605,47.8893643041944,2.71575839426326));
#230572=CARTESIAN_POINT('Ctrl Pts',(34.6149509280617,47.8895702459312,2.71590508903223));
#230573=CARTESIAN_POINT('Ctrl Pts',(34.6149352461545,47.8897760897958,2.71605191409926));
#230574=CARTESIAN_POINT('Ctrl Pts',(34.6147149626377,47.8926675754935,2.71811436362768));
#230575=CARTESIAN_POINT('Ctrl Pts',(34.6145651177085,47.8955400426776,2.72020091026974));
#230576=CARTESIAN_POINT('Ctrl Pts',(34.6144819591403,47.8983891927626,2.72230624862197));
#230577=CARTESIAN_POINT('Ctrl Pts',(34.614183767304,47.9086057382621,2.72985561753074));
#230578=CARTESIAN_POINT('Ctrl Pts',(34.614738768508,47.9186013937325,2.73770089914255));
#230579=CARTESIAN_POINT('Ctrl Pts',(34.6160223355359,47.9283423801869,2.7457482334695));
#230580=CARTESIAN_POINT('Ctrl Pts',(34.6174328467539,47.9390467457313,2.75459144546827));
#230581=CARTESIAN_POINT('Ctrl Pts',(34.6197230854579,47.9494442419719,2.76367911753994));
#230582=CARTESIAN_POINT('Ctrl Pts',(34.6227799581206,47.9594984812804,2.7729216256437));
#230583=CARTESIAN_POINT('Ctrl Pts',(34.6260806134258,47.9703545364636,2.78290121484248));
#230584=CARTESIAN_POINT('Ctrl Pts',(34.6302752334074,47.9808115517308,2.79306229499576));
#230585=CARTESIAN_POINT('Ctrl Pts',(34.6352786409506,47.9908184179881,2.80331916684511));
#230586=CARTESIAN_POINT('Ctrl Pts',(34.6402400750473,48.0007413369228,2.81348999408205));
#230587=CARTESIAN_POINT('Ctrl Pts',(34.6459976650991,48.0102227609114,2.82375635966647));
#230588=CARTESIAN_POINT('Ctrl Pts',(34.6525130919796,48.0191904766739,2.83404198860296));
#230589=CARTESIAN_POINT('Origin',(0.0123294189942765,-0.00895784724475234,
2.83404198860262));
#230590=CARTESIAN_POINT('Ctrl Pts',(36.9525415975211,50.8348823336489,2.65878198860297));
#230591=CARTESIAN_POINT('Ctrl Pts',(36.9594880792487,50.8298309792461,2.65878198860297));
#230592=CARTESIAN_POINT('Ctrl Pts',(36.9659508653433,50.8242442388882,2.65944603041884));
#230593=CARTESIAN_POINT('Ctrl Pts',(36.9718804702599,50.8182646381295,2.660704392641));
#230594=CARTESIAN_POINT('Ctrl Pts',(36.975669205521,50.8144439579054,2.66150842619626));
#230595=CARTESIAN_POINT('Ctrl Pts',(36.9792409429416,50.8104635307793,2.662554282654));
#230596=CARTESIAN_POINT('Ctrl Pts',(36.9825899931428,50.8063652005967,2.6638169970069));
#230597=CARTESIAN_POINT('Ctrl Pts',(36.987160774675,50.8007718022342,2.6655403487329));
#230598=CARTESIAN_POINT('Ctrl Pts',(36.9913113073909,50.7949560887233,2.66766759643995));
#230599=CARTESIAN_POINT('Ctrl Pts',(36.9950236271423,50.7890120203241,2.67012012783171));
#230600=CARTESIAN_POINT('Ctrl Pts',(36.996879787018,50.7860399861245,2.67134639352759));
#230601=CARTESIAN_POINT('Ctrl Pts',(36.998626563727,50.7830357420057,2.67265375585035));
#230602=CARTESIAN_POINT('Ctrl Pts',(37.000262924097,50.7800101622087,2.67403135126963));
#230603=CARTESIAN_POINT('Ctrl Pts',(37.001081104282,50.7784973723102,2.67472014897927));
#230604=CARTESIAN_POINT('Ctrl Pts',(37.0018716945001,50.7769792382976,2.67542649668655));
#230605=CARTESIAN_POINT('Ctrl Pts',(37.0026346543984,50.7754570554921,2.67614899656125));
#230606=CARTESIAN_POINT('Ctrl Pts',(37.002825394373,50.7750765097907,2.67632962152992));
#230607=CARTESIAN_POINT('Ctrl Pts',(37.0030144077539,50.7746957108234,2.67651125590973));
#230608=CARTESIAN_POINT('Ctrl Pts',(37.0032016945189,50.7743146783937,2.67669387767546));
#230609=CARTESIAN_POINT('Ctrl Pts',(37.0037635548139,50.7731715811047,2.67724174297267));
#230610=CARTESIAN_POINT('Ctrl Pts',(37.0043098740556,50.7720263837273,2.6777984950477));
#230611=CARTESIAN_POINT('Ctrl Pts',(37.0048406651182,50.7708796113518,2.67836353618031));
#230612=CARTESIAN_POINT('Ctrl Pts',(37.0085087606933,50.7629547027167,2.6822683209893));
#230613=CARTESIAN_POINT('Ctrl Pts',(37.011490045306,50.7549442896469,2.68659153751414));
#230614=CARTESIAN_POINT('Ctrl Pts',(37.013862846671,50.7469376805981,2.69123699486201));
#230615=CARTESIAN_POINT('Ctrl Pts',(37.0150421224362,50.7429584178785,2.69354577441238));
#230616=CARTESIAN_POINT('Ctrl Pts',(37.0160707669658,50.738979582278,2.69593478828138));
#230617=CARTESIAN_POINT('Ctrl Pts',(37.0169563748089,50.7350097117579,2.69839565261239));
#230618=CARTESIAN_POINT('Ctrl Pts',(37.0189101579885,50.7262515844358,2.70382468689064));
#230619=CARTESIAN_POINT('Ctrl Pts',(37.0201796788545,50.717540733481,2.70961155815106));
#230620=CARTESIAN_POINT('Ctrl Pts',(37.0208019128474,50.7090177292134,2.71562701361786));
#230621=CARTESIAN_POINT('Ctrl Pts',(37.0210292227719,50.7059041682737,2.71782453535876));
#230622=CARTESIAN_POINT('Ctrl Pts',(37.0211776528892,50.7028130194417,2.72005051502421));
#230623=CARTESIAN_POINT('Ctrl Pts',(37.0212513646536,50.6997475881156,2.72229986760134));
#230624=CARTESIAN_POINT('Ctrl Pts',(37.0214989546703,50.6894511286653,2.72985520488865));
#230625=CARTESIAN_POINT('Ctrl Pts',(37.0208967002927,50.6793793407332,2.73770845534483));
#230626=CARTESIAN_POINT('Ctrl Pts',(37.0195682679088,50.6695664063405,2.74576706701628));
#230627=CARTESIAN_POINT('Ctrl Pts',(37.0181081633557,50.6587808290243,2.75462443584856));
#230628=CARTESIAN_POINT('Ctrl Pts',(37.0157708601105,50.6483072759169,2.76373036322957));
#230629=CARTESIAN_POINT('Ctrl Pts',(37.0126680948719,50.6381830571081,2.77299664636543));
#230630=CARTESIAN_POINT('Ctrl Pts',(37.009326283767,50.6272788396627,2.78297683033147));
#230631=CARTESIAN_POINT('Ctrl Pts',(37.0050963107899,50.6167786802315,2.7931440147851));
#230632=CARTESIAN_POINT('Ctrl Pts',(37.0000610231269,50.6067353452142,2.80341452427499));
#230633=CARTESIAN_POINT('Ctrl Pts',(36.9950937288478,50.5968276291287,2.81354634721077));
#230634=CARTESIAN_POINT('Ctrl Pts',(36.9893418170244,50.5873633690991,2.82378004209075));
#230635=CARTESIAN_POINT('Ctrl Pts',(36.9828414016746,50.578416314936,2.83404198860297));
#230636=CARTESIAN_POINT('Ctrl Pts',(34.9607485668365,47.7952442955505,2.83404198860296));
#230637=CARTESIAN_POINT('Ctrl Pts',(34.9545276336629,47.7866819156019,2.8242212644301));
#230638=CARTESIAN_POINT('Ctrl Pts',(34.9476537221154,47.7786409912509,2.81442815028473));
#230639=CARTESIAN_POINT('Ctrl Pts',(34.9401706643545,47.7711595893163,2.8047161816626));
#230640=CARTESIAN_POINT('Ctrl Pts',(34.9329451136982,47.7639356375058,2.7953384214615));
#230641=CARTESIAN_POINT('Ctrl Pts',(34.925150670795,47.7572325247347,2.7860351565014));
#230642=CARTESIAN_POINT('Ctrl Pts',(34.9167928415129,47.7511153344865,2.77685887346636));
#230643=CARTESIAN_POINT('Ctrl Pts',(34.9088920753314,47.7453326739165,2.76818441216439));
#230644=CARTESIAN_POINT('Ctrl Pts',(34.9004871280265,47.7400730704108,2.7596226152147));
#230645=CARTESIAN_POINT('Ctrl Pts',(34.8915635921215,47.735428882127,2.7512353770149));
#230646=CARTESIAN_POINT('Ctrl Pts',(34.8833451652565,47.7311516626297,2.74351087133933));
#230647=CARTESIAN_POINT('Ctrl Pts',(34.874686357679,47.7273962447071,2.73593399449646));
#230648=CARTESIAN_POINT('Ctrl Pts',(34.8655676881409,47.724272008901,2.72857657812362));
#230649=CARTESIAN_POINT('Ctrl Pts',(34.8628486849589,47.7233404248511,2.72638274508189));
#230650=CARTESIAN_POINT('Ctrl Pts',(34.8600887620239,47.7224652397585,2.72420861709545));
#230651=CARTESIAN_POINT('Ctrl Pts',(34.857287342362,47.7216501132022,2.72205663736741));
#230652=CARTESIAN_POINT('Ctrl Pts',(34.8545145463038,47.7208433152301,2.71992664556781));
#230653=CARTESIAN_POINT('Ctrl Pts',(34.8517040509267,47.720095928845,2.71782089927899));
#230654=CARTESIAN_POINT('Ctrl Pts',(34.84885856128,47.7194121231168,2.7157438731126));
#230655=CARTESIAN_POINT('Ctrl Pts',(34.8486606914949,47.7193645726037,2.71559944077501));
#230656=CARTESIAN_POINT('Ctrl Pts',(34.848462649681,47.7193173179072,2.71545515216084));
#230657=CARTESIAN_POINT('Ctrl Pts',(34.8482644357608,47.7192703603292,2.71531100781745));
#230658=CARTESIAN_POINT('Ctrl Pts',(34.8395740113843,47.7172115680924,2.70899119176087));
#230659=CARTESIAN_POINT('Ctrl Pts',(34.8305531107002,47.7157691359129,2.70298296066831));
#230660=CARTESIAN_POINT('Ctrl Pts',(34.8212734513094,47.7150344641794,2.6973672777412));
#230661=CARTESIAN_POINT('Ctrl Pts',(34.8126231959631,47.7143496224387,2.69213248525395));
#230662=CARTESIAN_POINT('Ctrl Pts',(34.8037473009111,47.7142799923074,2.68723866185419));
#230663=CARTESIAN_POINT('Ctrl Pts',(34.7947186932864,47.7149249376578,2.68278595829501));
#230664=CARTESIAN_POINT('Ctrl Pts',(34.7914159118127,47.7151608670108,2.68115710172771));
#230665=CARTESIAN_POINT('Ctrl Pts',(34.7880929011145,47.7154926644832,2.679587636378));
#230666=CARTESIAN_POINT('Ctrl Pts',(34.7847540840179,47.7159260651935,2.67808378645377));
#230667=CARTESIAN_POINT('Ctrl Pts',(34.7839512100461,47.7160302835857,2.67772216078612));
#230668=CARTESIAN_POINT('Ctrl Pts',(34.7831469919157,47.7161407719863,2.67736403603575));
#230669=CARTESIAN_POINT('Ctrl Pts',(34.7823415577603,47.716257575019,2.67700956934491));
#230670=CARTESIAN_POINT('Ctrl Pts',(34.7815612934223,47.7163707279569,2.67666617973816));
#230671=CARTESIAN_POINT('Ctrl Pts',(34.7807798878931,47.7164898070136,2.67632622314131));
#230672=CARTESIAN_POINT('Ctrl Pts',(34.7799974607188,47.7166148505128,2.67598984158786));
#230673=CARTESIAN_POINT('Ctrl Pts',(34.771425066794,47.7179848465561,2.67230439292247));
#230674=CARTESIAN_POINT('Ctrl Pts',(34.7627244668162,47.7200720995233,2.66904964540012));
#230675=CARTESIAN_POINT('Ctrl Pts',(34.7540804826589,47.7229136891076,2.66640203566768));
#230676=CARTESIAN_POINT('Ctrl Pts',(34.7504955647788,47.7240921810071,2.66530399299471));
#230677=CARTESIAN_POINT('Ctrl Pts',(34.7469205018091,47.7254000086987,2.66430995142279));
#230678=CARTESIAN_POINT('Ctrl Pts',(34.743368526502,47.7268379886355,2.66343053473372));
#230679=CARTESIAN_POINT('Ctrl Pts',(34.7373102624745,47.7292906132654,2.66193059792896));
#230680=CARTESIAN_POINT('Ctrl Pts',(34.731321441251,47.7321228682622,2.66076519817139));
#230681=CARTESIAN_POINT('Ctrl Pts',(34.7254747878806,47.7353375827203,2.65997805604471));
#230682=CARTESIAN_POINT('Ctrl Pts',(34.7225514611955,47.7369449399493,2.65958448498138));
#230683=CARTESIAN_POINT('Ctrl Pts',(34.7196644712719,47.7386491210201,2.65928526260774));
#230684=CARTESIAN_POINT('Ctrl Pts',(34.7168229726608,47.7404504949229,2.65908463971336));
#230685=CARTESIAN_POINT('Ctrl Pts',(34.7139814740498,47.7422518688257,2.65888401681898));
#230686=CARTESIAN_POINT('Ctrl Pts',(34.7111854907792,47.7441503967334,2.65878198860296));
#230687=CARTESIAN_POINT('Ctrl Pts',(34.7084426211231,47.7461450747867,2.65878198860296));
#230688=CARTESIAN_POINT('Origin',(29.1186878401555,50.4655267888878,2.83404198860297));
#230689=CARTESIAN_POINT('Ctrl Pts',(31.1634057161439,54.3576020372441,2.83404198860299));
#230690=CARTESIAN_POINT('Ctrl Pts',(31.1687108809056,54.3667908521539,2.824196524402));
#230691=CARTESIAN_POINT('Ctrl Pts',(31.1747253323925,54.3755338070552,2.81438790575873));
#230692=CARTESIAN_POINT('Ctrl Pts',(31.1814073748057,54.3837890328978,2.80466781257207));
#230693=CARTESIAN_POINT('Ctrl Pts',(31.1878722906296,54.3917760130573,2.7952635645345));
#230694=CARTESIAN_POINT('Ctrl Pts',(31.1949629807077,54.3993074034407,2.78594102496663));
#230695=CARTESIAN_POINT('Ctrl Pts',(31.2026795247177,54.4063187915243,2.77675109089263));
#230696=CARTESIAN_POINT('Ctrl Pts',(31.2099789001937,54.4129511329149,2.76805797914216));
#230697=CARTESIAN_POINT('Ctrl Pts',(31.2178389737478,54.4191188025019,2.75948271210739));
#230698=CARTESIAN_POINT('Ctrl Pts',(31.2262832675514,54.4247323097956,2.7510857557384));
#230699=CARTESIAN_POINT('Ctrl Pts',(31.2340610728514,54.4299027559922,2.7433515516393));
#230700=CARTESIAN_POINT('Ctrl Pts',(31.2423350114939,54.4346033281798,2.73576818686641));
#230701=CARTESIAN_POINT('Ctrl Pts',(31.2511358718481,54.4387279162142,2.7284062616123));
#230702=CARTESIAN_POINT('Ctrl Pts',(31.2536886668935,54.4399243024168,2.72627084694178));
#230703=CARTESIAN_POINT('Ctrl Pts',(31.2562858555919,54.4410719653267,2.7241542458779));
#230704=CARTESIAN_POINT('Ctrl Pts',(31.2589283212566,54.4421676282861,2.72205867173299));
#230705=CARTESIAN_POINT('Ctrl Pts',(31.2617929239294,54.4433553973776,2.71978693462901));
#230706=CARTESIAN_POINT('Ctrl Pts',(31.2647063376194,54.4444813995855,2.717544113408));
#230707=CARTESIAN_POINT('Ctrl Pts',(31.2676686823018,54.4455416356298,2.71533341844297));
#230708=CARTESIAN_POINT('Ctrl Pts',(31.2757988605279,54.4484514617728,2.70926614876443));
#230709=CARTESIAN_POINT('Ctrl Pts',(31.2843017293921,54.4508216479605,2.7034738186046));
#230710=CARTESIAN_POINT('Ctrl Pts',(31.2931053160624,54.4525775288977,2.69804914171446));
#230711=CARTESIAN_POINT('Ctrl Pts',(31.3011601199078,54.4541840646263,2.6930858568726));
#230712=CARTESIAN_POINT('Ctrl Pts',(31.3094611543727,54.4552661718987,2.68842799053244));
#230713=CARTESIAN_POINT('Ctrl Pts',(31.3179758301774,54.4557414157487,2.68414767054279));
#230714=CARTESIAN_POINT('Ctrl Pts',(31.3221582111184,54.4559748539754,2.68204519134609));
#230715=CARTESIAN_POINT('Ctrl Pts',(31.3263919825241,54.4560613864573,2.68003431778556));
#230716=CARTESIAN_POINT('Ctrl Pts',(31.3306718639313,54.4559882102926,2.67812693945302));
#230717=CARTESIAN_POINT('Ctrl Pts',(31.3314839297417,54.4559743258281,2.67776503299254));
#230718=CARTESIAN_POINT('Ctrl Pts',(31.332298031963,54.4559543157133,2.67740659639975));
#230719=CARTESIAN_POINT('Ctrl Pts',(31.3331140451957,54.4559281176617,2.67705178968906));
#230720=CARTESIAN_POINT('Ctrl Pts',(31.333904558015,54.4559027382991,2.67670807068809));
#230721=CARTESIAN_POINT('Ctrl Pts',(31.3346968642519,54.4558715517161,2.67636775825316));
#230722=CARTESIAN_POINT('Ctrl Pts',(31.3354908465828,54.4558345032253,2.67603099699306));
#230723=CARTESIAN_POINT('Ctrl Pts',(31.3441435024206,54.4554307564064,2.67236104217172));
#230724=CARTESIAN_POINT('Ctrl Pts',(31.3530008879293,54.4543301709716,2.66911440541512));
#230725=CARTESIAN_POINT('Ctrl Pts',(31.3618824321393,54.452472177926,2.66646778189666));
#230726=CARTESIAN_POINT('Ctrl Pts',(31.3656331634107,54.4516875359253,2.66535009635016));
#230727=CARTESIAN_POINT('Ctrl Pts',(31.3693880355479,54.4507682193237,2.66433897912391));
#230728=CARTESIAN_POINT('Ctrl Pts',(31.3731331934892,54.4497115877223,2.66344564884843));
#230729=CARTESIAN_POINT('Ctrl Pts',(31.3794399458813,54.4479322465077,2.66194130298636));
#230730=CARTESIAN_POINT('Ctrl Pts',(31.3857169562559,54.4457622496023,2.66077206705471));
#230731=CARTESIAN_POINT('Ctrl Pts',(31.3918909882808,54.4431895758478,2.65998225155765));
#230732=CARTESIAN_POINT('Ctrl Pts',(31.393434496287,54.4425464074092,2.65978479768339));
#230733=CARTESIAN_POINT('Ctrl Pts',(31.3949714642037,54.4418778620535,2.65961098966673));
#230734=CARTESIAN_POINT('Ctrl Pts',(31.3965005998225,54.441183481233,2.65946139030552));
#230735=CARTESIAN_POINT('Ctrl Pts',(31.3987943032508,54.4401419100023,2.65923699126371));
#230736=CARTESIAN_POINT('Ctrl Pts',(31.4010703637564,54.4390422051399,2.65906707562492));
#230737=CARTESIAN_POINT('Ctrl Pts',(31.4033252432071,54.4378842814516,2.6589533256297));
#230738=CARTESIAN_POINT('Ctrl Pts',(31.4055801226578,54.4367263577634,2.65883957563448));
#230739=CARTESIAN_POINT('Ctrl Pts',(31.4078138194781,54.4355102267488,2.658781988603));
#230740=CARTESIAN_POINT('Ctrl Pts',(31.4100231232069,54.434235916308,2.658781988603));
#230741=CARTESIAN_POINT('Ctrl Pts',(29.501078514911,51.1278468659049,2.65878198860297));
#230742=CARTESIAN_POINT('Ctrl Pts',(29.4936027956392,51.1321585373229,2.65878198860297));
#230743=CARTESIAN_POINT('Ctrl Pts',(29.4865477845229,51.1370499258751,2.65945335517901));
#230744=CARTESIAN_POINT('Ctrl Pts',(29.4799806005914,51.1423856448188,2.66072561226665));
#230745=CARTESIAN_POINT('Ctrl Pts',(29.4757388736044,51.1458319717794,2.66154735980399));
#230746=CARTESIAN_POINT('Ctrl Pts',(29.4717000621109,51.1494629466904,2.66261895766934));
#230747=CARTESIAN_POINT('Ctrl Pts',(29.4678753842639,51.1532365012462,2.66391429251063));
#230748=CARTESIAN_POINT('Ctrl Pts',(29.4628059928683,51.1582381316479,2.6656311846416));
#230749=CARTESIAN_POINT('Ctrl Pts',(29.4581176150989,51.1634934604717,2.66774105138736));
#230750=CARTESIAN_POINT('Ctrl Pts',(29.453837929136,51.1689167792842,2.67016894181786));
#230751=CARTESIAN_POINT('Ctrl Pts',(29.4516980861545,51.1716284386904,2.67138288703312));
#230752=CARTESIAN_POINT('Ctrl Pts',(29.4496602426632,51.1743821937241,2.67267613167588));
#230753=CARTESIAN_POINT('Ctrl Pts',(29.4477266300417,51.1771680313594,2.6740383543259));
#230754=CARTESIAN_POINT('Ctrl Pts',(29.446759823731,51.178560950177,2.67471946565091));
#230755=CARTESIAN_POINT('Ctrl Pts',(29.4458190608836,51.1799618978182,2.6754178138956));
#230756=CARTESIAN_POINT('Ctrl Pts',(29.4449045308659,51.1813696738594,2.67613207244206));
#230757=CARTESIAN_POINT('Ctrl Pts',(29.4446758983615,51.1817216178697,2.67631063707868));
#230758=CARTESIAN_POINT('Ctrl Pts',(29.4444489051053,51.182073988828,2.67649019601883));
#230759=CARTESIAN_POINT('Ctrl Pts',(29.4442235534434,51.1824267683261,2.67667072836694));
#230760=CARTESIAN_POINT('Ctrl Pts',(29.4435474984577,51.1834851068202,2.67721232541128));
#230761=CARTESIAN_POINT('Ctrl Pts',(29.4428862193406,51.1845471213154,2.67776268340085));
#230762=CARTESIAN_POINT('Ctrl Pts',(29.4422397658678,51.1856123224582,2.67832123541554));
#230763=CARTESIAN_POINT('Ctrl Pts',(29.4376862310783,51.1931154617652,2.68225560368482));
#230764=CARTESIAN_POINT('Ctrl Pts',(29.4338145801761,51.2007799603597,2.68661792998926));
#230765=CARTESIAN_POINT('Ctrl Pts',(29.4305579784513,51.208506571073,2.69130986622615));
#230766=CARTESIAN_POINT('Ctrl Pts',(29.4289785301339,51.2122539689196,2.69358545023091));
#230767=CARTESIAN_POINT('Ctrl Pts',(29.4275440072542,51.21601649797,2.69593918853506));
#230768=CARTESIAN_POINT('Ctrl Pts',(29.4262483256618,51.2197852472981,2.69836306235511));
#230769=CARTESIAN_POINT('Ctrl Pts',(29.4242647276705,51.2255549392046,2.70207384382244));
#230770=CARTESIAN_POINT('Ctrl Pts',(29.4226066102323,51.2313356805892,2.70594760814244));
#230771=CARTESIAN_POINT('Ctrl Pts',(29.4212581193013,51.2370841708901,2.70995196345724));
#230772=CARTESIAN_POINT('Ctrl Pts',(29.4206318731368,51.2397537995246,2.71181160678122));
#230773=CARTESIAN_POINT('Ctrl Pts',(29.4200721889214,51.2424163366107,2.71369962772114));
#230774=CARTESIAN_POINT('Ctrl Pts',(29.4195787111907,51.2450674596719,2.71561183138676));
#230775=CARTESIAN_POINT('Ctrl Pts',(29.419540888067,51.2452706578086,2.71575839426327));
#230776=CARTESIAN_POINT('Ctrl Pts',(29.4195034207002,51.2454737959511,2.71590508903225));
#230777=CARTESIAN_POINT('Ctrl Pts',(29.4194663081573,51.2456768729758,2.71605191409928));
#230778=CARTESIAN_POINT('Ctrl Pts',(29.4189449888201,51.2485294929148,2.71811436362769));
#230779=CARTESIAN_POINT('Ctrl Pts',(29.4184957101765,51.251370561363,2.72020091026976));
#230780=CARTESIAN_POINT('Ctrl Pts',(29.4181151898796,51.2541954110683,2.72230624862198));
#230781=CARTESIAN_POINT('Ctrl Pts',(29.4167507117684,51.2643248197285,2.72985561753095));
#230782=CARTESIAN_POINT('Ctrl Pts',(29.4162578421121,51.2743237313756,2.73770089914296));
#230783=CARTESIAN_POINT('Ctrl Pts',(29.4165161672808,51.2841455249762,2.74574823347012));
#230784=CARTESIAN_POINT('Ctrl Pts',(29.4168000406901,51.2949386894568,2.75459144546939));
#230785=CARTESIAN_POINT('Ctrl Pts',(29.4179908989232,51.3055186222579,2.76367911754159));
#230786=CARTESIAN_POINT('Ctrl Pts',(29.4199800715336,51.3158373135939,2.77292162564591));
#230787=CARTESIAN_POINT('Ctrl Pts',(29.4221278787387,51.3269789105989,2.78290121484585));
#230788=CARTESIAN_POINT('Ctrl Pts',(29.4252064644174,51.3378170984242,2.79306229500033));
#230789=CARTESIAN_POINT('Ctrl Pts',(29.4291364604194,51.3482921445236,2.80331916685089));
#230790=CARTESIAN_POINT('Ctrl Pts',(29.4330334877931,51.3586793157498,2.81348999408594));
#230791=CARTESIAN_POINT('Ctrl Pts',(29.4377684584844,51.368710631544,2.82375635966844));
#230792=CARTESIAN_POINT('Ctrl Pts',(29.443310811626,51.3783102687787,2.83404198860297));
#230793=CARTESIAN_POINT('Origin',(0.0131982271536777,-0.00761999999981537,
2.83404198860262));
#230794=CARTESIAN_POINT('Ctrl Pts',(31.4364195775134,54.4189959163066,2.658781988603));
#230795=CARTESIAN_POINT('Ctrl Pts',(31.443856016,54.414698338812,2.658781988603));
#230796=CARTESIAN_POINT('Ctrl Pts',(31.4508673716603,54.4098177483015,2.65944603041881));
#230797=CARTESIAN_POINT('Ctrl Pts',(31.4573895320587,54.4044907169113,2.66070439264087));
#230798=CARTESIAN_POINT('Ctrl Pts',(31.4615568820643,54.4010869974476,2.66150842619614));
#230799=CARTESIAN_POINT('Ctrl Pts',(31.4655251210645,54.3975017237413,2.66255428265392));
#230800=CARTESIAN_POINT('Ctrl Pts',(31.4692842169744,54.3937759157111,2.66381699700688));
#230801=CARTESIAN_POINT('Ctrl Pts',(31.4744146286224,54.3886909353395,2.66554034873288));
#230802=CARTESIAN_POINT('Ctrl Pts',(31.479150331882,54.3833409297223,2.66766759643993));
#230803=CARTESIAN_POINT('Ctrl Pts',(31.4834636394928,54.3778174666305,2.67012012783169));
#230804=CARTESIAN_POINT('Ctrl Pts',(31.4856202932981,54.3750557350846,2.67134639352757));
#230805=CARTESIAN_POINT('Ctrl Pts',(31.4876715300025,54.3722505364144,2.67265375585033));
#230806=CARTESIAN_POINT('Ctrl Pts',(31.4896151854259,54.369412577295,2.67403135126961));
#230807=CARTESIAN_POINT('Ctrl Pts',(31.4905870131376,54.3679935977353,2.67472014897925));
#230808=CARTESIAN_POINT('Ctrl Pts',(31.4915319606351,54.3665664194002,2.67542649668655));
#230809=CARTESIAN_POINT('Ctrl Pts',(31.4924498523887,54.3651323262971,2.67614899656124));
#230810=CARTESIAN_POINT('Ctrl Pts',(31.4926793253271,54.3647738030213,2.67632962152991));
#230811=CARTESIAN_POINT('Ctrl Pts',(31.4929071076039,54.3644148473888,2.67651125590973));
#230812=CARTESIAN_POINT('Ctrl Pts',(31.4931331971267,54.3640554790924,2.67669387767546));
#230813=CARTESIAN_POINT('Ctrl Pts',(31.4938114656952,54.3629773742031,2.67724174297266));
#230814=CARTESIAN_POINT('Ctrl Pts',(31.4944744978649,54.3618955562475,2.6777984950477));
#230815=CARTESIAN_POINT('Ctrl Pts',(31.4951222515527,54.3608105487852,2.67836353618032));
#230816=CARTESIAN_POINT('Ctrl Pts',(31.4995986314374,54.3533124740226,2.68226832098919));
#230817=CARTESIAN_POINT('Ctrl Pts',(31.5034009004293,54.3456575719331,2.68659153751388));
#230818=CARTESIAN_POINT('Ctrl Pts',(31.50659762188,54.337942849207,2.69123699486159));
#230819=CARTESIAN_POINT('Ctrl Pts',(31.5081863836663,54.3341086531882,2.6935457744121));
#230820=CARTESIAN_POINT('Ctrl Pts',(31.5096252947445,54.3302591366971,2.69593478828124));
#230821=CARTESIAN_POINT('Ctrl Pts',(31.5109210156001,54.3264035847698,2.69839565261241));
#230822=CARTESIAN_POINT('Ctrl Pts',(31.5137795693411,54.3178976613388,2.70382468689067));
#230823=CARTESIAN_POINT('Ctrl Pts',(31.515952667503,54.3093672304022,2.70961155815108));
#230824=CARTESIAN_POINT('Ctrl Pts',(31.5174623893715,54.3009559572069,2.71562701361788));
#230825=CARTESIAN_POINT('Ctrl Pts',(31.5180139098087,54.2978832130369,2.71782453535878));
#230826=CARTESIAN_POINT('Ctrl Pts',(31.5184846398474,54.2948245130136,2.72005051502421));
#230827=CARTESIAN_POINT('Ctrl Pts',(31.5188783726369,54.2917835794185,2.72229986760133));
#230828=CARTESIAN_POINT('Ctrl Pts',(31.5202008794132,54.2815694052532,2.72985520488948));
#230829=CARTESIAN_POINT('Ctrl Pts',(31.5206547127629,54.2714898389033,2.73770845534655));
#230830=CARTESIAN_POINT('Ctrl Pts',(31.5203592886226,54.2615918017952,2.74576706701893));
#230831=CARTESIAN_POINT('Ctrl Pts',(31.5200345824971,54.2507126865138,2.75462443585215));
#230832=CARTESIAN_POINT('Ctrl Pts',(31.5188048676544,54.2400521939087,2.76373036323415));
#230833=CARTESIAN_POINT('Ctrl Pts',(31.5167773687218,54.2296591093466,2.77299664637103));
#230834=CARTESIAN_POINT('Ctrl Pts',(31.5145936654999,54.2184653119648,2.78297683033819));
#230835=CARTESIAN_POINT('Ctrl Pts',(31.511484430286,54.2075805209297,2.793144014793));
#230836=CARTESIAN_POINT('Ctrl Pts',(31.5075265408301,54.1970658734701,2.80341452428409));
#230837=CARTESIAN_POINT('Ctrl Pts',(31.5036220962464,54.1866932092558,2.81354634721688));
#230838=CARTESIAN_POINT('Ctrl Pts',(31.498890978556,54.1766795569324,2.82378004209381));
#230839=CARTESIAN_POINT('Ctrl Pts',(31.4933613949858,54.1671020372441,2.834041988603));
#230840=CARTESIAN_POINT('Ctrl Pts',(29.7732664904679,51.1878102687787,2.83404198860297));
#230841=CARTESIAN_POINT('Ctrl Pts',(29.7679746486357,51.1786445298597,2.82422126443112));
#230842=CARTESIAN_POINT('Ctrl Pts',(29.7619788985611,51.1699291351237,2.81442815028676));
#230843=CARTESIAN_POINT('Ctrl Pts',(29.7553188532218,51.1617065245642,2.80471618166561));
#230844=CARTESIAN_POINT('Ctrl Pts',(29.74888799347,51.1537668706117,2.79533842146517));
#230845=CARTESIAN_POINT('Ctrl Pts',(29.7418369154183,51.1462857370554,2.78603515650572));
#230846=CARTESIAN_POINT('Ctrl Pts',(29.7341642916964,51.1393284263646,2.77685887347129));
#230847=CARTESIAN_POINT('Ctrl Pts',(29.7269112593623,51.1327515888669,2.76818441216977));
#230848=CARTESIAN_POINT('Ctrl Pts',(29.7191021335107,51.126642241794,2.75962261522049));
#230849=CARTESIAN_POINT('Ctrl Pts',(29.7107129315343,51.1210907313645,2.75123537702107));
#230850=CARTESIAN_POINT('Ctrl Pts',(29.7029866172533,51.1159778833925,2.74351087134582));
#230851=CARTESIAN_POINT('Ctrl Pts',(29.6947677915948,51.1113379461923,2.73593399450323));
#230852=CARTESIAN_POINT('Ctrl Pts',(29.6860256466511,51.1072776647628,2.72857657813064));
#230853=CARTESIAN_POINT('Ctrl Pts',(29.6834189154995,51.1060669708022,2.72638274508653));
#230854=CARTESIAN_POINT('Ctrl Pts',(29.6807655934612,51.1049080895607,2.72420861709776));
#230855=CARTESIAN_POINT('Ctrl Pts',(29.6780647241927,51.1038046002595,2.72205663736744));
#230856=CARTESIAN_POINT('Ctrl Pts',(29.6753914511536,51.1027123859002,2.71992664556783));
#230857=CARTESIAN_POINT('Ctrl Pts',(29.6726744751146,51.1016753170133,2.71782089927902));
#230858=CARTESIAN_POINT('Ctrl Pts',(29.6699160505199,51.1006978225843,2.71574387311263));
#230859=CARTESIAN_POINT('Ctrl Pts',(29.6697242350682,51.1006298495334,2.71559944077503));
#230860=CARTESIAN_POINT('Ctrl Pts',(29.6695322176089,51.1005621526965,2.71545515216086));
#230861=CARTESIAN_POINT('Ctrl Pts',(29.6693399979287,51.1004947333606,2.71531100781747));
#230862=CARTESIAN_POINT('Ctrl Pts',(29.6609123829951,51.0975388226979,2.70899119176098));
#230863=CARTESIAN_POINT('Ctrl Pts',(29.652091674968,51.095161351427,2.70298296066851));
#230864=CARTESIAN_POINT('Ctrl Pts',(29.6429396446297,51.0934607157664,2.69736727774148));
#230865=CARTESIAN_POINT('Ctrl Pts',(29.6344083617423,51.0918754277622,2.69213248525433));
#230866=CARTESIAN_POINT('Ctrl Pts',(29.6255883681029,51.0908783954021,2.68723866185465));
#230867=CARTESIAN_POINT('Ctrl Pts',(29.6165418049893,51.0905760611939,2.68278595829554));
#230868=CARTESIAN_POINT('Ctrl Pts',(29.613232455165,51.0904654634292,2.68115710172806));
#230869=CARTESIAN_POINT('Ctrl Pts',(29.6098929659868,51.0904480940786,2.67958763637819));
#230870=CARTESIAN_POINT('Ctrl Pts',(29.6065271365692,51.0905301191543,2.67808378645382));
#230871=CARTESIAN_POINT('Ctrl Pts',(29.6057177670366,51.0905498434447,2.67772216078617));
#230872=CARTESIAN_POINT('Ctrl Pts',(29.6049064053145,51.090575662893,2.6773640360358));
#230873=CARTESIAN_POINT('Ctrl Pts',(29.6040931741702,51.0906076352719,2.67700956934496));
#230874=CARTESIAN_POINT('Ctrl Pts',(29.6033053564992,51.090638608514,2.67666617973821));
#230875=CARTESIAN_POINT('Ctrl Pts',(29.6025157844404,51.0906753561241,2.67632622314135));
#230876=CARTESIAN_POINT('Ctrl Pts',(29.6017245728792,51.0907179287118,2.6759898415879));
#230877=CARTESIAN_POINT('Ctrl Pts',(29.5930559358439,51.0911843606099,2.6723043929224));
#230878=CARTESIAN_POINT('Ctrl Pts',(29.5841848213177,51.0923507190418,2.66904964539997));
#230879=CARTESIAN_POINT('Ctrl Pts',(29.5752911628173,51.0942731997207,2.66640203566747));
#230880=CARTESIAN_POINT('Ctrl Pts',(29.5716026975456,51.0950705097612,2.6653039929946));
#230881=CARTESIAN_POINT('Ctrl Pts',(29.5679105139263,51.0959974771976,2.66430995142277));
#230882=CARTESIAN_POINT('Ctrl Pts',(29.5642276868789,51.0970562972093,2.66343053473376));
#230883=CARTESIAN_POINT('Ctrl Pts',(29.5579462415721,51.098862225076,2.66193059792899));
#230884=CARTESIAN_POINT('Ctrl Pts',(29.5516941764754,51.1010529624043,2.66076519817142));
#230885=CARTESIAN_POINT('Ctrl Pts',(29.5455435225218,51.1036389246281,2.65997805604474));
#230886=CARTESIAN_POINT('Ctrl Pts',(29.542468195545,51.10493190574,2.6595844849814));
#230887=CARTESIAN_POINT('Ctrl Pts',(29.5394188854259,51.1063249785083,2.65928526260776));
#230888=CARTESIAN_POINT('Ctrl Pts',(29.5364046579957,51.1078194668133,2.65908463971338));
#230889=CARTESIAN_POINT('Ctrl Pts',(29.5333904305655,51.1093139551182,2.658884016819));
#230890=CARTESIAN_POINT('Ctrl Pts',(29.5304113137792,51.1109098228568,2.65878198860297));
#230891=CARTESIAN_POINT('Ctrl Pts',(29.5274749692184,51.1126068659049,2.65878198860297));
#230892=CARTESIAN_POINT('Origin',(23.6840886581935,53.232803045145,2.83404198860299));
#230893=CARTESIAN_POINT('Ctrl Pts',(25.3107727110821,57.3172883154492,2.83404198860302));
#230894=CARTESIAN_POINT('Ctrl Pts',(25.3150883208947,57.3269813337902,2.8241965244009));
#230895=CARTESIAN_POINT('Ctrl Pts',(25.3201559369473,57.3363050752418,2.81438790575658));
#230896=CARTESIAN_POINT('Ctrl Pts',(25.3259384683624,57.3452135417191,2.80466781256893));
#230897=CARTESIAN_POINT('Ctrl Pts',(25.3315331019393,57.3538325360824,2.79526356453053));
#230898=CARTESIAN_POINT('Ctrl Pts',(25.3377977038129,57.3620638476591,2.78594102496191));
#230899=CARTESIAN_POINT('Ctrl Pts',(25.3447390861665,57.3698434251128,2.77675109088721));
#230900=CARTESIAN_POINT('Ctrl Pts',(25.3513052064473,57.3772024263452,2.76805797913609));
#230901=CARTESIAN_POINT('Ctrl Pts',(25.3584775246731,57.384157910203,2.75948271210072));
#230902=CARTESIAN_POINT('Ctrl Pts',(25.3662887884618,57.3906233351713,2.7510857557312));
#230903=CARTESIAN_POINT('Ctrl Pts',(25.3734835273362,57.3965784591586,2.74335155163148));
#230904=CARTESIAN_POINT('Ctrl Pts',(25.3812207968911,57.4021181432118,2.73576818685804));
#230905=CARTESIAN_POINT('Ctrl Pts',(25.3895423083639,57.4071400767298,2.72840626160343));
#230906=CARTESIAN_POINT('Ctrl Pts',(25.3919560625166,57.4085967487446,2.72627084693591));
#230907=CARTESIAN_POINT('Ctrl Pts',(25.3944190600999,57.4100096047785,2.72415424587498));
#230908=CARTESIAN_POINT('Ctrl Pts',(25.3969325220924,57.4113754784548,2.72205867173297));
#230909=CARTESIAN_POINT('Ctrl Pts',(25.3996572764942,57.4128561733383,2.719786934629));
#230910=CARTESIAN_POINT('Ctrl Pts',(25.4024370309187,57.4142805418442,2.71754411340801));
#230911=CARTESIAN_POINT('Ctrl Pts',(25.4052723227226,57.4156446191419,2.71533341844298));
#230912=CARTESIAN_POINT('Ctrl Pts',(25.4130538033266,57.419388339989,2.70926614876445));
#230913=CARTESIAN_POINT('Ctrl Pts',(25.4212623406656,57.4226343338645,2.70347381860462));
#230914=CARTESIAN_POINT('Ctrl Pts',(25.4298341608309,57.4253008212881,2.69804914171448));
#230915=CARTESIAN_POINT('Ctrl Pts',(25.4376769109072,57.4277405125137,2.6930858568726));
#230916=CARTESIAN_POINT('Ctrl Pts',(25.4458193604265,57.4296843862654,2.68842799053242));
#230917=CARTESIAN_POINT('Ctrl Pts',(25.4542377154369,57.4310470526569,2.68414767054276));
#230918=CARTESIAN_POINT('Ctrl Pts',(25.4583727839184,57.4317163899371,2.68204519134607));
#230919=CARTESIAN_POINT('Ctrl Pts',(25.462574317174,57.4322449980039,2.68003431778555));
#230920=CARTESIAN_POINT('Ctrl Pts',(25.466838401935,57.4326195921324,2.67812693945303));
#230921=CARTESIAN_POINT('Ctrl Pts',(25.4676474704857,57.4326906677196,2.67776503299255));
#230922=CARTESIAN_POINT('Ctrl Pts',(25.4684592045964,57.4327558640765,2.67740659639976));
#230923=CARTESIAN_POINT('Ctrl Pts',(25.4692734860654,57.4328151061498,2.67705178968907));
#230924=CARTESIAN_POINT('Ctrl Pts',(25.4700623212384,57.4328724969082,2.67670807068809));
#230925=CARTESIAN_POINT('Ctrl Pts',(25.4708535470246,57.432924299722,2.67636775825317));
#230926=CARTESIAN_POINT('Ctrl Pts',(25.4716470524589,57.4329704479396,2.67603099699307));
#230927=CARTESIAN_POINT('Ctrl Pts',(25.4802945111773,57.4334733617059,2.67236104217173));
#230928=CARTESIAN_POINT('Ctrl Pts',(25.4892184175055,57.4333046542891,2.66911440541513));
#230929=CARTESIAN_POINT('Ctrl Pts',(25.4982455208449,57.4323852136915,2.66646778189668));
#230930=CARTESIAN_POINT('Ctrl Pts',(25.5020577226405,57.4319969282177,2.66535009635017));
#230931=CARTESIAN_POINT('Ctrl Pts',(25.5058881199468,57.4314751387429,2.66433897912392));
#230932=CARTESIAN_POINT('Ctrl Pts',(25.5097232095986,57.4308157710843,2.66344564884845));
#230933=CARTESIAN_POINT('Ctrl Pts',(25.516181404744,57.4297054124228,2.66194130298638));
#230934=CARTESIAN_POINT('Ctrl Pts',(25.5226508554408,57.4282034292358,2.66077206705473));
#230935=CARTESIAN_POINT('Ctrl Pts',(25.5290599831064,57.4262902109372,2.65998225155767));
#230936=CARTESIAN_POINT('Ctrl Pts',(25.5306622650228,57.4258119063626,2.65978479768341));
#230937=CARTESIAN_POINT('Ctrl Pts',(25.532260695287,57.4253076802627,2.65961098966675));
#230938=CARTESIAN_POINT('Ctrl Pts',(25.5338540367011,57.4247769415294,2.65946139030554));
#230939=CARTESIAN_POINT('Ctrl Pts',(25.5362440488221,57.4239808334294,2.65923699126373));
#230940=CARTESIAN_POINT('Ctrl Pts',(25.5386225912894,57.4231250659722,2.65906707562494));
#230941=CARTESIAN_POINT('Ctrl Pts',(25.5409861542582,57.4222091845949,2.65895332562972));
#230942=CARTESIAN_POINT('Ctrl Pts',(25.543349717227,57.4212933032176,2.6588395756345));
#230943=CARTESIAN_POINT('Ctrl Pts',(25.5456982979286,57.4203173191919,2.65878198860302));
#230944=CARTESIAN_POINT('Ctrl Pts',(25.5480287005724,57.4192809246807,2.65878198860302));
#230945=CARTESIAN_POINT('Ctrl Pts',(23.9951532569806,53.9314655730807,2.658781988603));
#230946=CARTESIAN_POINT('Ctrl Pts',(23.9872677980943,53.9349721992639,2.658781988603));
#230947=CARTESIAN_POINT('Ctrl Pts',(23.979740145739,53.9390993428072,2.65945335517894));
#230948=CARTESIAN_POINT('Ctrl Pts',(23.972651203027,53.9437193744794,2.6607256122664));
#230949=CARTESIAN_POINT('Ctrl Pts',(23.9680724734026,53.9467034408971,2.66154735980378));
#230950=CARTESIAN_POINT('Ctrl Pts',(23.9636762467129,53.9498923541891,2.66261895766923));
#230951=CARTESIAN_POINT('Ctrl Pts',(23.9594780769921,53.9532454491207,2.66391429251067));
#230952=CARTESIAN_POINT('Ctrl Pts',(23.9539136435132,53.9576897843755,2.66563118464163));
#230953=CARTESIAN_POINT('Ctrl Pts',(23.9487016177219,53.9624262550347,2.66774105138739));
#230954=CARTESIAN_POINT('Ctrl Pts',(23.9438784851452,53.9673725153422,2.6701689418179));
#230955=CARTESIAN_POINT('Ctrl Pts',(23.9414669188569,53.969845645496,2.67138288703315));
#230956=CARTESIAN_POINT('Ctrl Pts',(23.9391523931035,53.9723713025231,2.67267613167591));
#230957=CARTESIAN_POINT('Ctrl Pts',(23.9369381736874,53.9749397614924,2.67403835432593));
#230958=CARTESIAN_POINT('Ctrl Pts',(23.9358310639794,53.976223990977,2.67471946565094));
#230959=CARTESIAN_POINT('Ctrl Pts',(23.9347490158252,53.9775189275857,2.67541781389563));
#230960=CARTESIAN_POINT('Ctrl Pts',(23.9336923430325,53.9788233972651,2.67613207244209));
#230961=CARTESIAN_POINT('Ctrl Pts',(23.9334281748343,53.979149514685,2.6763106370787));
#230962=CARTESIAN_POINT('Ctrl Pts',(23.9331655922761,53.979476228062,2.67649019601885));
#230963=CARTESIAN_POINT('Ctrl Pts',(23.9329045996154,53.9798035193342,2.67667072836697));
#230964=CARTESIAN_POINT('Ctrl Pts',(23.9321216216332,53.9807853931505,2.6772123254113));
#230965=CARTESIAN_POINT('Ctrl Pts',(23.9313529543291,53.9817724673294,2.67776268340087));
#230966=CARTESIAN_POINT('Ctrl Pts',(23.9305986983576,53.9827642604007,2.67832123541556));
#230967=CARTESIAN_POINT('Ctrl Pts',(23.9252858166867,53.9897503227315,2.68225560368483));
#230968=CARTESIAN_POINT('Ctrl Pts',(23.9206342168334,53.9969681366817,2.68661792998925));
#230969=CARTESIAN_POINT('Ctrl Pts',(23.9165878043695,54.0043120126392,2.69130986622613));
#230970=CARTESIAN_POINT('Ctrl Pts',(23.914625298697,54.0078737845429,2.6935854502309));
#230971=CARTESIAN_POINT('Ctrl Pts',(23.9128053429042,54.0114657535934,2.69593918853507));
#230972=CARTESIAN_POINT('Ctrl Pts',(23.9111228176154,54.0150784217127,2.69836306235513));
#230973=CARTESIAN_POINT('Ctrl Pts',(23.9085469889529,54.0206091641934,2.70207384382246));
#230974=CARTESIAN_POINT('Ctrl Pts',(23.906293702842,54.0261849176041,2.70594760814246));
#230975=CARTESIAN_POINT('Ctrl Pts',(23.9043517182282,54.0317609613889,2.70995196345726));
#230976=CARTESIAN_POINT('Ctrl Pts',(23.903449850527,54.0343505049692,2.71181160678124));
#230977=CARTESIAN_POINT('Ctrl Pts',(23.9026149214104,54.0369399534677,2.71369962772117));
#230978=CARTESIAN_POINT('Ctrl Pts',(23.9018470291827,54.0395249709305,2.71561183138679));
#230979=CARTESIAN_POINT('Ctrl Pts',(23.9017881732691,54.0397231023335,2.7157583942633));
#230980=CARTESIAN_POINT('Ctrl Pts',(23.9017296774346,54.0399212112578,2.71590508903227));
#230981=CARTESIAN_POINT('Ctrl Pts',(23.9016715408688,54.0401192964882,2.7160519140993));
#230982=CARTESIAN_POINT('Ctrl Pts',(23.9008548973949,54.0429017967675,2.71811436362771));
#230983=CARTESIAN_POINT('Ctrl Pts',(23.9001111074278,54.0456803391392,2.72020091026977));
#230984=CARTESIAN_POINT('Ctrl Pts',(23.8994373944623,54.0484499388204,2.722306248622));
#230985=CARTESIAN_POINT('Ctrl Pts',(23.8970215795838,54.0583812307207,2.72985561753144));
#230986=CARTESIAN_POINT('Ctrl Pts',(23.8954862390501,54.0682738483763,2.73770089914397));
#230987=CARTESIAN_POINT('Ctrl Pts',(23.8947164920949,54.0780688394974,2.74574823347167));
#230988=CARTESIAN_POINT('Ctrl Pts',(23.8938706175192,54.0888325507453,2.75459144547126));
#230989=CARTESIAN_POINT('Ctrl Pts',(23.8939490479891,54.0994790041489,2.7636791175438));
#230990=CARTESIAN_POINT('Ctrl Pts',(23.8948487267558,54.1099490937706,2.77292162564846));
#230991=CARTESIAN_POINT('Ctrl Pts',(23.8958201540351,54.1212541629279,2.78290121484838));
#230992=CARTESIAN_POINT('Ctrl Pts',(23.8977489757816,54.1323547778562,2.79306229500283));
#230993=CARTESIAN_POINT('Ctrl Pts',(23.900562502383,54.1431832369997,2.80331916685335));
#230994=CARTESIAN_POINT('Ctrl Pts',(23.9033524263869,54.1539208564969,2.81348999408761));
#230995=CARTESIAN_POINT('Ctrl Pts',(23.9070129003886,54.1643921589027,2.82375635966928));
#230996=CARTESIAN_POINT('Ctrl Pts',(23.9115214566113,54.1745185419762,2.834041988603));
#230997=CARTESIAN_POINT('Origin',(0.0139224327744766,-0.00619866644029082,
2.83404198860263));
#230998=CARTESIAN_POINT('Ctrl Pts',(25.5758735661207,57.4068835917982,2.65878198860302));
#230999=CARTESIAN_POINT('Ctrl Pts',(25.5837184861914,57.4033868763696,2.65878198860302));
#231000=CARTESIAN_POINT('Ctrl Pts',(25.5912015935385,57.3992659084766,2.65944603041899));
#231001=CARTESIAN_POINT('Ctrl Pts',(25.5982448512655,57.3946498105247,2.66070439264133));
#231002=CARTESIAN_POINT('Ctrl Pts',(25.6027451576558,57.3917003436848,2.66150842619654));
#231003=CARTESIAN_POINT('Ctrl Pts',(25.6070664213777,57.3885495044082,2.66255428265417));
#231004=CARTESIAN_POINT('Ctrl Pts',(25.6111943775539,57.3852370392635,2.66381699700691));
#231005=CARTESIAN_POINT('Ctrl Pts',(25.6168282094541,57.3807161889919,2.6655403487329));
#231006=CARTESIAN_POINT('Ctrl Pts',(25.6220971979014,57.3758905070495,2.66766759643995));
#231007=CARTESIAN_POINT('Ctrl Pts',(25.6269642358706,57.3708481654826,2.67012012783171));
#231008=CARTESIAN_POINT('Ctrl Pts',(25.6293977548552,57.3683269946991,2.67134639352759));
#231009=CARTESIAN_POINT('Ctrl Pts',(25.6317309777765,57.3657515758213,2.67265375585036));
#231010=CARTESIAN_POINT('Ctrl Pts',(25.6339606331577,57.3631323306534,2.67403135126964));
#231011=CARTESIAN_POINT('Ctrl Pts',(25.6350754608483,57.3618227080694,2.67472014897928));
#231012=CARTESIAN_POINT('Ctrl Pts',(25.6361644125826,57.3605021218764,2.67542649668657));
#231013=CARTESIAN_POINT('Ctrl Pts',(25.6372271795775,57.3591718306998,2.67614899656126));
#231014=CARTESIAN_POINT('Ctrl Pts',(25.6374928713262,57.3588392579056,2.67632962152993));
#231015=CARTESIAN_POINT('Ctrl Pts',(25.6377569268685,57.358506078401,2.67651125590975));
#231016=CARTESIAN_POINT('Ctrl Pts',(25.638019342065,57.3581723115521,2.67669387767548));
#231017=CARTESIAN_POINT('Ctrl Pts',(25.6388065876546,57.3571710110053,2.67724174297269));
#231018=CARTESIAN_POINT('Ctrl Pts',(25.6395790684331,57.3561644250955,2.67779849504772));
#231019=CARTESIAN_POINT('Ctrl Pts',(25.6403366878211,57.3551530701152,2.67836353618034));
#231020=CARTESIAN_POINT('Ctrl Pts',(25.6455723078613,57.3481639797005,2.68226832098951));
#231021=CARTESIAN_POINT('Ctrl Pts',(25.650153902778,57.3409484572996,2.68659153751456));
#231022=CARTESIAN_POINT('Ctrl Pts',(25.6541395203654,57.333610145012,2.69123699486267));
#231023=CARTESIAN_POINT('Ctrl Pts',(25.6561203613657,57.3299630239487,2.69354577441286));
#231024=CARTESIAN_POINT('Ctrl Pts',(25.6579537739813,57.3262850026761,2.69593478828165));
#231025=CARTESIAN_POINT('Ctrl Pts',(25.6596454116603,57.3225860115761,2.69839565261244));
#231026=CARTESIAN_POINT('Ctrl Pts',(25.6633774170497,57.3144254847134,2.7038246868907));
#231027=CARTESIAN_POINT('Ctrl Pts',(25.6664302835893,57.3061689349814,2.70961155815111));
#231028=CARTESIAN_POINT('Ctrl Pts',(25.6688109525047,57.2979615485276,2.71562701361791));
#231029=CARTESIAN_POINT('Ctrl Pts',(25.6696806408813,57.2949632867554,2.71782453535882));
#231030=CARTESIAN_POINT('Ctrl Pts',(25.6704685134247,57.2919705472985,2.72005051502426));
#231031=CARTESIAN_POINT('Ctrl Pts',(25.6711779534203,57.2889874285392,2.72229986760139));
#231032=CARTESIAN_POINT('Ctrl Pts',(25.6735608872951,57.2789674482901,2.72985520488926));
#231033=CARTESIAN_POINT('Ctrl Pts',(25.6750658360792,57.2689905373625,2.73770845534603));
#231034=CARTESIAN_POINT('Ctrl Pts',(25.6758066569115,57.2591158425062,2.7457670670181));
#231035=CARTESIAN_POINT('Ctrl Pts',(25.6766209067623,57.2482623831247,2.75462443585101));
#231036=CARTESIAN_POINT('Ctrl Pts',(25.676512253336,57.2375317496112,2.76373036323268));
#231037=CARTESIAN_POINT('Ctrl Pts',(25.6755822344127,57.2269836681064,2.77299664636922));
#231038=CARTESIAN_POINT('Ctrl Pts',(25.6745805641841,57.2156229323763,2.78297683033602));
#231039=CARTESIAN_POINT('Ctrl Pts',(25.6726261321661,57.2044727657868,2.79314401479045));
#231040=CARTESIAN_POINT('Ctrl Pts',(25.6697890043839,57.1936020065639,2.80341452428115));
#231041=CARTESIAN_POINT('Ctrl Pts',(25.6669901874063,57.182878039296,2.81354634721492));
#231042=CARTESIAN_POINT('Ctrl Pts',(25.6633316989624,57.1724247063449,2.82378004209285));
#231043=CARTESIAN_POINT('Ctrl Pts',(25.658833530444,57.1623216544374,2.83404198860302));
#231044=CARTESIAN_POINT('Ctrl Pts',(24.2595822759732,54.0195518809643,2.83404198860301));
#231045=CARTESIAN_POINT('Ctrl Pts',(24.2552775040086,54.0098832048286,2.82422126443219));
#231046=CARTESIAN_POINT('Ctrl Pts',(24.2502256060994,54.0005888273964,2.81442815028887));
#231047=CARTESIAN_POINT('Ctrl Pts',(24.2444615420318,53.9917150968541,2.80471618166874));
#231048=CARTESIAN_POINT('Ctrl Pts',(24.2388958310297,53.9831467292698,2.79533842146893));
#231049=CARTESIAN_POINT('Ctrl Pts',(24.232665370916,53.9749695397932,2.78603515651008));
#231050=CARTESIAN_POINT('Ctrl Pts',(24.2257620156254,53.9672483344118,2.77685887347623));
#231051=CARTESIAN_POINT('Ctrl Pts',(24.2192361828786,53.9599493771943,2.76818441217506));
#231052=CARTESIAN_POINT('Ctrl Pts',(24.2121084368973,53.9530572218393,2.75962261522611));
#231053=CARTESIAN_POINT('Ctrl Pts',(24.2043454827017,53.9466592127743,2.75123537702697));
#231054=CARTESIAN_POINT('Ctrl Pts',(24.1971959321207,53.9407667537598,2.74351087135186));
#231055=CARTESIAN_POINT('Ctrl Pts',(24.1895071355548,53.9352931334051,2.73593399450939));
#231056=CARTESIAN_POINT('Ctrl Pts',(24.1812372959747,53.9303412916453,2.72857657813688));
#231057=CARTESIAN_POINT('Ctrl Pts',(24.178771396746,53.92886475239,2.72638274509066));
#231058=CARTESIAN_POINT('Ctrl Pts',(24.1762537459564,53.9274348719445,2.72420861709981));
#231059=CARTESIAN_POINT('Ctrl Pts',(24.1736830183708,53.9260551099578,2.72205663736747));
#231060=CARTESIAN_POINT('Ctrl Pts',(24.1711385572897,53.9246894457404,2.71992664556785));
#231061=CARTESIAN_POINT('Ctrl Pts',(24.1685448683468,53.9233740566952,2.71782089927904));
#231062=CARTESIAN_POINT('Ctrl Pts',(24.1659037306811,53.922113583199,2.71574387311265));
#231063=CARTESIAN_POINT('Ctrl Pts',(24.1657200711331,53.9220259323372,2.71559944077506));
#231064=CARTESIAN_POINT('Ctrl Pts',(24.1655361818118,53.9219385350608,2.71545515216088));
#231065=CARTESIAN_POINT('Ctrl Pts',(24.1653520623708,53.9218513926273,2.7153110078175));
#231066=CARTESIAN_POINT('Ctrl Pts',(24.1572795915927,53.9180307491144,2.708991191761));
#231067=CARTESIAN_POINT('Ctrl Pts',(24.1487557177455,53.9147442868249,2.70298296066853));
#231068=CARTESIAN_POINT('Ctrl Pts',(24.1398315880192,53.9120963197574,2.69736727774148));
#231069=CARTESIAN_POINT('Ctrl Pts',(24.1315127481111,53.9096279542368,2.6921324852544));
#231070=CARTESIAN_POINT('Ctrl Pts',(24.1228452895803,53.9077144433432,2.6872386618548));
#231071=CARTESIAN_POINT('Ctrl Pts',(24.1138798870163,53.9064681420133,2.68278595829574));
#231072=CARTESIAN_POINT('Ctrl Pts',(24.1106002267709,53.9060122288631,2.68115710172819));
#231073=CARTESIAN_POINT('Ctrl Pts',(24.1072808472552,53.9056458829918,2.67958763637825));
#231074=CARTESIAN_POINT('Ctrl Pts',(24.103924882248,53.9053756337488,2.67808378645381));
#231075=CARTESIAN_POINT('Ctrl Pts',(24.1031178847767,53.9053106478341,2.67772216078616));
#231076=CARTESIAN_POINT('Ctrl Pts',(24.1023082689118,53.9052515154468,2.67736403603579));
#231077=CARTESIAN_POINT('Ctrl Pts',(24.1014961507091,53.9051983068759,2.67700956934495));
#231078=CARTESIAN_POINT('Ctrl Pts',(24.1007094112003,53.9051467610728,2.6766661797382));
#231079=CARTESIAN_POINT('Ctrl Pts',(24.0999203233287,53.9051007746217,2.67632622314135));
#231080=CARTESIAN_POINT('Ctrl Pts',(24.0991289960601,53.9050604098636,2.67598984158789));
#231081=CARTESIAN_POINT('Ctrl Pts',(24.090459091316,53.9046181672911,2.67230439292245));
#231082=CARTESIAN_POINT('Ctrl Pts',(24.0815146560291,53.9048508523206,2.66904964540005));
#231083=CARTESIAN_POINT('Ctrl Pts',(24.0724687639696,53.9058331609933,2.66640203566758));
#231084=CARTESIAN_POINT('Ctrl Pts',(24.0687171629031,53.9062405536793,2.66530399299466));
#231085=CARTESIAN_POINT('Ctrl Pts',(24.0649483109702,53.9067765048113,2.6643099514228));
#231086=CARTESIAN_POINT('Ctrl Pts',(24.061174982006,53.9074445642444,2.66343053473376));
#231087=CARTESIAN_POINT('Ctrl Pts',(24.0547391762491,53.9085840092243,2.661930597929));
#231088=CARTESIAN_POINT('Ctrl Pts',(24.0482923662128,53.9101092267075,2.66076519817143));
#231089=CARTESIAN_POINT('Ctrl Pts',(24.0419050995277,53.9120381043536,2.65997805604476));
#231090=CARTESIAN_POINT('Ctrl Pts',(24.0387114661852,53.9130025431767,2.65958448498142));
#231091=CARTESIAN_POINT('Ctrl Pts',(24.0355332447503,53.9140692448459,2.65928526260778));
#231092=CARTESIAN_POINT('Ctrl Pts',(24.0323793130074,53.9152404736263,2.65908463971341));
#231093=CARTESIAN_POINT('Ctrl Pts',(24.0292253812646,53.9164117024068,2.65888401681903));
#231094=CARTESIAN_POINT('Ctrl Pts',(24.0260957707896,53.9176874253156,2.658781988603));
#231095=CARTESIAN_POINT('Ctrl Pts',(24.0229981225296,53.9190682401997,2.658781988603));
#231096=CARTESIAN_POINT('Origin',(17.9900016446781,55.4168495715594,2.834041988603));
#231097=CARTESIAN_POINT('Ctrl Pts',(19.180829583578,59.6489943884566,2.83404198860303));
#231098=CARTESIAN_POINT('Ctrl Pts',(19.1841083557167,59.65908541149,2.82419652440163));
#231099=CARTESIAN_POINT('Ctrl Pts',(19.1881736144722,59.6688877866282,2.81438790575802));
#231100=CARTESIAN_POINT('Ctrl Pts',(19.1929932802638,59.6783518907161,2.80466781257107));
#231101=CARTESIAN_POINT('Ctrl Pts',(19.1976563356165,59.6875084677763,2.79526356453326));
#231102=CARTESIAN_POINT('Ctrl Pts',(19.2030262129953,59.6963495165733,2.78594102496521));
#231103=CARTESIAN_POINT('Ctrl Pts',(19.2091163824534,59.7048120487176,2.77675109089105));
#231104=CARTESIAN_POINT('Ctrl Pts',(19.2148773077497,59.7128170830335,2.76805797914046));
#231105=CARTESIAN_POINT('Ctrl Pts',(19.2212832892262,59.7204841754248,2.7594827121056));
#231106=CARTESIAN_POINT('Ctrl Pts',(19.2283759411575,59.7277306815184,2.75108575573653));
#231107=CARTESIAN_POINT('Ctrl Pts',(19.2349087865398,59.7344052377112,2.74335155163732));
#231108=CARTESIAN_POINT('Ctrl Pts',(19.2420246158606,59.7407233396916,2.73576818686435));
#231109=CARTESIAN_POINT('Ctrl Pts',(19.2497756062286,59.7465875973385,2.72840626161014));
#231110=CARTESIAN_POINT('Ctrl Pts',(19.2520238738985,59.7482885955657,2.72627084694036));
#231111=CARTESIAN_POINT('Ctrl Pts',(19.2543256952557,59.7499511651806,2.72415424587721));
#231112=CARTESIAN_POINT('Ctrl Pts',(19.2566826155664,59.7515722847792,2.72205867173301));
#231113=CARTESIAN_POINT('Ctrl Pts',(19.2592376687177,59.7533296826515,2.71978693462903));
#231114=CARTESIAN_POINT('Ctrl Pts',(19.2618533083056,59.755036811776,2.71754411340803));
#231115=CARTESIAN_POINT('Ctrl Pts',(19.2645304831806,59.7566897852107,2.715333418443));
#231116=CARTESIAN_POINT('Ctrl Pts',(19.2718780106326,59.7612263837727,2.70926614876447));
#231117=CARTESIAN_POINT('Ctrl Pts',(19.2797022819936,59.7653126215478,2.70347381860464));
#231118=CARTESIAN_POINT('Ctrl Pts',(19.2879484209985,59.7688605008636,2.6980491417145));
#231119=CARTESIAN_POINT('Ctrl Pts',(19.2954931904947,59.7721066178187,2.69308585687256));
#231120=CARTESIAN_POINT('Ctrl Pts',(19.3033878446876,59.7748909605622,2.68842799053233));
#231121=CARTESIAN_POINT('Ctrl Pts',(19.3116176456448,59.7771261198371,2.68414767054262));
#231122=CARTESIAN_POINT('Ctrl Pts',(19.315660096991,59.7782240227715,2.68204519134601));
#231123=CARTESIAN_POINT('Ctrl Pts',(19.3197833592188,59.7791889148826,2.68003431778555));
#231124=CARTESIAN_POINT('Ctrl Pts',(19.3239849291286,59.7800071751725,2.67812693945308));
#231125=CARTESIAN_POINT('Ctrl Pts',(19.3247821360952,59.7801624320925,2.6777650329926));
#231126=CARTESIAN_POINT('Ctrl Pts',(19.3255826085666,59.7803121206161,2.6774065963998));
#231127=CARTESIAN_POINT('Ctrl Pts',(19.3263862368335,59.7804561537457,2.67705178968912));
#231128=CARTESIAN_POINT('Ctrl Pts',(19.3271647517172,59.7805956858399,2.67670807068814));
#231129=CARTESIAN_POINT('Ctrl Pts',(19.3279462282172,59.780729910488,2.67636775825322));
#231130=CARTESIAN_POINT('Ctrl Pts',(19.3287305629435,59.7808587498045,2.67603099699312));
#231131=CARTESIAN_POINT('Ctrl Pts',(19.3372780811749,59.7822628141275,2.67236104217182));
#231132=CARTESIAN_POINT('Ctrl Pts',(19.3461707361375,59.7830278331225,2.66911440541526));
#231133=CARTESIAN_POINT('Ctrl Pts',(19.3552444957729,59.7830570185565,2.66646778189681));
#231134=CARTESIAN_POINT('Ctrl Pts',(19.3590764008121,59.7830693437465,2.66535009635027));
#231135=CARTESIAN_POINT('Ctrl Pts',(19.3629403566533,59.7829507982332,2.66433897912399));
#231136=CARTESIAN_POINT('Ctrl Pts',(19.3668233599709,59.7826959186874,2.66344564884849));
#231137=CARTESIAN_POINT('Ctrl Pts',(19.3733622405322,59.7822667079009,2.66194130298641));
#231138=CARTESIAN_POINT('Ctrl Pts',(19.3799532508955,59.7814491944745,2.66077206705475));
#231139=CARTESIAN_POINT('Ctrl Pts',(19.3865272544576,59.7802163932511,2.65998225155769));
#231140=CARTESIAN_POINT('Ctrl Pts',(19.3881707553481,59.7799081929452,2.65978479768342));
#231141=CARTESIAN_POINT('Ctrl Pts',(19.3898131352235,59.7795738105079,2.65961098966677));
#231142=CARTESIAN_POINT('Ctrl Pts',(19.3914532254508,59.7792125287464,2.65946139030556));
#231143=CARTESIAN_POINT('Ctrl Pts',(19.3939133607917,59.7786706061042,2.65923699126375));
#231144=CARTESIAN_POINT('Ctrl Pts',(19.3963683254117,59.7780681520197,2.65906707562496));
#231145=CARTESIAN_POINT('Ctrl Pts',(19.3988146762082,59.7774043475415,2.65895332562974));
#231146=CARTESIAN_POINT('Ctrl Pts',(19.4012610270047,59.7767405430632,2.65883957563452));
#231147=CARTESIAN_POINT('Ctrl Pts',(19.4036987600453,59.7760153991104,2.65878198860303));
#231148=CARTESIAN_POINT('Ctrl Pts',(19.4061247292252,59.7752282754839,2.65878198860303));
#231149=CARTESIAN_POINT('Ctrl Pts',(18.2263320786581,56.144199857553,2.65878198860301));
#231150=CARTESIAN_POINT('Ctrl Pts',(18.2181232748938,56.1468630191717,2.65878198860301));
#231151=CARTESIAN_POINT('Ctrl Pts',(18.2102054558329,56.1501806998584,2.65945335517905));
#231152=CARTESIAN_POINT('Ctrl Pts',(18.2026724222794,56.1540344262263,2.6607256122667));
#231153=CARTESIAN_POINT('Ctrl Pts',(18.1978068555387,56.1565235380443,2.66154735980404));
#231154=CARTESIAN_POINT('Ctrl Pts',(18.1931013796334,56.1592354513152,2.66261895766939));
#231155=CARTESIAN_POINT('Ctrl Pts',(18.1885757140657,56.1621313494122,2.66391429251067));
#231156=CARTESIAN_POINT('Ctrl Pts',(18.1825772036012,56.165969696453,2.66563118464164));
#231157=CARTESIAN_POINT('Ctrl Pts',(18.1768986338333,56.1701354151838,2.6677410513874));
#231158=CARTESIAN_POINT('Ctrl Pts',(18.1715848978926,56.1745504247235,2.67016894181791));
#231159=CARTESIAN_POINT('Ctrl Pts',(18.1689280299223,56.1767579294933,2.67138288703317));
#231160=CARTESIAN_POINT('Ctrl Pts',(18.1663621803354,56.1790278168867,2.67267613167593));
#231161=CARTESIAN_POINT('Ctrl Pts',(18.1638916135759,56.1813507566161,2.67403835432595));
#231162=CARTESIAN_POINT('Ctrl Pts',(18.1626563301961,56.1825122264809,2.67471946565096));
#231163=CARTESIAN_POINT('Ctrl Pts',(18.1614448518812,56.1836869644606,2.67541781389565));
#231164=CARTESIAN_POINT('Ctrl Pts',(18.1602576134416,56.1848738357354,2.67613207244211));
#231165=CARTESIAN_POINT('Ctrl Pts',(18.1599608038317,56.1851705535541,2.67631063707873));
#231166=CARTESIAN_POINT('Ctrl Pts',(18.159665508881,56.1854680298098,2.67649019601887));
#231167=CARTESIAN_POINT('Ctrl Pts',(18.1593717347117,56.1857662469843,2.67667072836699));
#231168=CARTESIAN_POINT('Ctrl Pts',(18.1584904122037,56.1866608985079,2.67721232541133));
#231169=CARTESIAN_POINT('Ctrl Pts',(18.1576227783925,56.1875622177791,2.67776268340089));
#231170=CARTESIAN_POINT('Ctrl Pts',(18.1567689837085,56.1884697364866,2.67832123541558));
#231171=CARTESIAN_POINT('Ctrl Pts',(18.1507549641994,56.1948621810806,2.68225560368491));
#231172=CARTESIAN_POINT('Ctrl Pts',(18.1453743792964,56.2015542305064,2.68661792998941));
#231173=CARTESIAN_POINT('Ctrl Pts',(18.140582489435,56.2084349106665,2.69130986622636));
#231174=CARTESIAN_POINT('Ctrl Pts',(18.1382584280305,56.2117720331088,2.69358545023107));
#231175=CARTESIAN_POINT('Ctrl Pts',(18.136072979141,56.2151540877947,2.69593918853516));
#231176=CARTESIAN_POINT('Ctrl Pts',(18.134022044255,56.2185710935571,2.69836306235515));
#231177=CARTESIAN_POINT('Ctrl Pts',(18.1308822062392,56.22380229064,2.70207384382248));
#231178=CARTESIAN_POINT('Ctrl Pts',(18.1280584389298,56.2291119669557,2.70594760814247));
#231179=CARTESIAN_POINT('Ctrl Pts',(18.125544237423,56.2344544719218,2.70995196345727));
#231180=CARTESIAN_POINT('Ctrl Pts',(18.1243766292364,56.2369355588666,2.71181160678125));
#231181=CARTESIAN_POINT('Ctrl Pts',(18.1232756028766,56.2394235482377,2.71369962772118));
#231182=CARTESIAN_POINT('Ctrl Pts',(18.12224170934,56.2419141381099,2.7156118313868));
#231183=CARTESIAN_POINT('Ctrl Pts',(18.1221624654742,56.2421050320102,2.71575839426331));
#231184=CARTESIAN_POINT('Ctrl Pts',(18.1220835820645,56.2422959411933,2.71590508903228));
#231185=CARTESIAN_POINT('Ctrl Pts',(18.1220050584321,56.2424868643662,2.71605191409931));
#231186=CARTESIAN_POINT('Ctrl Pts',(18.1209020381385,56.2451687593305,2.71811436362772));
#231187=CARTESIAN_POINT('Ctrl Pts',(18.1198718859664,56.2478543333342,2.72020091026979));
#231188=CARTESIAN_POINT('Ctrl Pts',(18.1189123616725,56.2505383386776,2.72230624862202));
#231189=CARTESIAN_POINT('Ctrl Pts',(18.1154716782003,56.260162704504,2.72985561753083));
#231190=CARTESIAN_POINT('Ctrl Pts',(18.1129106883016,56.2698406425777,2.73770089914268));
#231191=CARTESIAN_POINT('Ctrl Pts',(18.1111213027312,56.2795015152455,2.74574823346968));
#231192=CARTESIAN_POINT('Ctrl Pts',(18.1091549477491,56.2901178437866,2.75459144546861));
#231193=CARTESIAN_POINT('Ctrl Pts',(18.1081200911551,56.3007141730203,2.76367911754047));
#231194=CARTESIAN_POINT('Ctrl Pts',(18.1079204190087,56.3112209484337,2.77292162564443));
#231195=CARTESIAN_POINT('Ctrl Pts',(18.1077048232014,56.3225656290393,2.78290121484364));
#231196=CARTESIAN_POINT('Ctrl Pts',(18.1084627484403,56.3338070504099,2.79306229499735));
#231197=CARTESIAN_POINT('Ctrl Pts',(18.1101289800542,56.3448702837326,2.80331916684715));
#231198=CARTESIAN_POINT('Ctrl Pts',(18.1117812336974,56.3558407078977,2.81348999408344));
#231199=CARTESIAN_POINT('Ctrl Pts',(18.1143271060909,56.3666372711378,2.82375635966719));
#231200=CARTESIAN_POINT('Ctrl Pts',(18.1177524687105,56.377179453281,2.83404198860301));
#231201=CARTESIAN_POINT('Origin',(0.014494101308342,-0.00470941899409004,
2.83404198860262));
#231202=CARTESIAN_POINT('Ctrl Pts',(19.4351129318419,59.7658094374954,2.65878198860303));
#231203=CARTESIAN_POINT('Ctrl Pts',(19.4432803829093,59.7631518948794,2.65878198860303));
#231204=CARTESIAN_POINT('Ctrl Pts',(19.4511532554518,59.7598356997915,2.6594460304189));
#231205=CARTESIAN_POINT('Ctrl Pts',(19.4586404431008,59.7559811102142,2.66070439264105));
#231206=CARTESIAN_POINT('Ctrl Pts',(19.4634243995787,59.7535182109732,2.6615084261963));
#231207=CARTESIAN_POINT('Ctrl Pts',(19.4680513433539,59.7508363273796,2.66255428265404));
#231208=CARTESIAN_POINT('Ctrl Pts',(19.4725029330461,59.7479734971808,2.66381699700693));
#231209=CARTESIAN_POINT('Ctrl Pts',(19.4785784597572,59.7440663083909,2.66554034873292));
#231210=CARTESIAN_POINT('Ctrl Pts',(19.4843230052521,59.7398178213045,2.66766759643996));
#231211=CARTESIAN_POINT('Ctrl Pts',(19.4896904492933,59.7353118462118,2.67012012783172));
#231212=CARTESIAN_POINT('Ctrl Pts',(19.4923741713139,59.7330588586655,2.67134639352759));
#231213=CARTESIAN_POINT('Ctrl Pts',(19.4949638171735,59.7307414364082,2.67265375585035));
#231214=CARTESIAN_POINT('Ctrl Pts',(19.4974550439415,59.72836960219,2.67403135126963));
#231215=CARTESIAN_POINT('Ctrl Pts',(19.4987006573255,59.7271836850809,2.67472014897927));
#231216=CARTESIAN_POINT('Ctrl Pts',(19.4999216825137,59.7259841596485,2.67542649668656));
#231217=CARTESIAN_POINT('Ctrl Pts',(19.5011176808521,59.7247722453469,2.67614899656125));
#231218=CARTESIAN_POINT('Ctrl Pts',(19.5014166804367,59.7244692667715,2.67632962152992));
#231219=CARTESIAN_POINT('Ctrl Pts',(19.5017141161967,59.7241655137792,2.67651125590973));
#231220=CARTESIAN_POINT('Ctrl Pts',(19.5020099819911,59.7238610051972,2.67669387767546));
#231221=CARTESIAN_POINT('Ctrl Pts',(19.5028975793744,59.7229474794513,2.67724174297267));
#231222=CARTESIAN_POINT('Ctrl Pts',(19.5037710453008,59.7220271539531,2.6777984950477));
#231223=CARTESIAN_POINT('Ctrl Pts',(19.5046302297524,59.7211005320716,2.67836353618032));
#231224=CARTESIAN_POINT('Ctrl Pts',(19.5105677273988,59.7146969999426,2.68226832098942));
#231225=CARTESIAN_POINT('Ctrl Pts',(19.5158784513273,59.7079999120045,2.6865915375144));
#231226=CARTESIAN_POINT('Ctrl Pts',(19.5206092977908,59.7011184102411,2.69123699486243));
#231227=CARTESIAN_POINT('Ctrl Pts',(19.5229605154971,59.6976983227543,2.69354577441269));
#231228=CARTESIAN_POINT('Ctrl Pts',(19.5251683423981,59.6942320938702,2.69593478828156));
#231229=CARTESIAN_POINT('Ctrl Pts',(19.5272373629643,59.6907301905173,2.69839565261244));
#231230=CARTESIAN_POINT('Ctrl Pts',(19.5318019313701,59.6830044686628,2.7038246868907));
#231231=CARTESIAN_POINT('Ctrl Pts',(19.5357011184427,59.6751122606221,2.70961155815111));
#231232=CARTESIAN_POINT('Ctrl Pts',(19.5389266512982,59.6671986827534,2.71562701361793));
#231233=CARTESIAN_POINT('Ctrl Pts',(19.5401049791264,59.6643077529625,2.71782453535883));
#231234=CARTESIAN_POINT('Ctrl Pts',(19.541201362078,59.6614137631516,2.72005051502428));
#231235=CARTESIAN_POINT('Ctrl Pts',(19.5422187365067,59.6585211429016,2.72229986760142));
#231236=CARTESIAN_POINT('Ctrl Pts',(19.5456359895577,59.6488051375692,2.72985520488895));
#231237=CARTESIAN_POINT('Ctrl Pts',(19.5481755652422,59.6390401911878,2.73770845534539));
#231238=CARTESIAN_POINT('Ctrl Pts',(19.5499445144591,59.6292970278069,2.7457670670171));
#231239=CARTESIAN_POINT('Ctrl Pts',(19.5518887991943,59.6185881370977,2.75462443584964));
#231240=CARTESIAN_POINT('Ctrl Pts',(19.552902397614,59.6079049297422,2.76373036323094));
#231241=CARTESIAN_POINT('Ctrl Pts',(19.5530800481819,59.5973174182832,2.77299664636706));
#231242=CARTESIAN_POINT('Ctrl Pts',(19.5532713854553,59.5859142148031,2.78297683033335));
#231243=CARTESIAN_POINT('Ctrl Pts',(19.5524931697994,59.574620836218,2.79314401478723));
#231244=CARTESIAN_POINT('Ctrl Pts',(19.5508078878564,59.5635130675447,2.80341452427733));
#231245=CARTESIAN_POINT('Ctrl Pts',(19.5491453629098,59.5525552912523,2.81354634721241));
#231246=CARTESIAN_POINT('Ctrl Pts',(19.5465995868775,59.5417768065764,2.82378004209164));
#231247=CARTESIAN_POINT('Ctrl Pts',(19.5431821162865,59.5312589135998,2.83404198860304));
#231248=CARTESIAN_POINT('Ctrl Pts',(18.4801050014189,56.2594439784241,2.83404198860301));
#231249=CARTESIAN_POINT('Ctrl Pts',(18.4768344633037,56.2493782971091,2.82422126443159));
#231250=CARTESIAN_POINT('Ctrl Pts',(18.4727817672096,56.2396067681233,2.81442815028768));
#231251=CARTESIAN_POINT('Ctrl Pts',(18.4679768367048,56.2301791400457,2.80471618166696));
#231252=CARTESIAN_POINT('Ctrl Pts',(18.4633372535458,56.2210759356572,2.79533842146675));
#231253=CARTESIAN_POINT('Ctrl Pts',(18.4579956735941,56.2122922812587,2.78603515650751));
#231254=CARTESIAN_POINT('Ctrl Pts',(18.4519372213388,56.203891776328,2.77685887347329));
#231255=CARTESIAN_POINT('Ctrl Pts',(18.4462100865676,56.1959506682931,2.76818441217179));
#231256=CARTESIAN_POINT('Ctrl Pts',(18.4398418135319,56.1883512165521,2.75962261522253));
#231257=CARTESIAN_POINT('Ctrl Pts',(18.4327901596667,56.1811768067775,2.75123537702312));
#231258=CARTESIAN_POINT('Ctrl Pts',(18.4262957047571,56.1745692957346,2.74351087134775));
#231259=CARTESIAN_POINT('Ctrl Pts',(18.419221177347,56.1683219623554,2.73593399450505));
#231260=CARTESIAN_POINT('Ctrl Pts',(18.4115142492222,56.1625328136801,2.72857657813234));
#231261=CARTESIAN_POINT('Ctrl Pts',(18.4092161988284,56.1608066064056,2.72638274508767));
#231262=CARTESIAN_POINT('Ctrl Pts',(18.4068618032004,56.1591213928279,2.72420861709834));
#231263=CARTESIAN_POINT('Ctrl Pts',(18.4044493827314,56.1574804751189,2.72205663736748));
#231264=CARTESIAN_POINT('Ctrl Pts',(18.4020616112563,56.1558563235463,2.71992664556786));
#231265=CARTESIAN_POINT('Ctrl Pts',(18.3996196264082,56.1542770260205,2.71782089927905));
#231266=CARTESIAN_POINT('Ctrl Pts',(18.3971247125286,56.1527473834686,2.71574387311266));
#231267=CARTESIAN_POINT('Ctrl Pts',(18.3969512210967,56.152641015117,2.71559944077507));
#231268=CARTESIAN_POINT('Ctrl Pts',(18.3967774746434,56.1525348749439,2.7154551521609));
#231269=CARTESIAN_POINT('Ctrl Pts',(18.3966034726925,56.1524289641635,2.71531100781751));
#231270=CARTESIAN_POINT('Ctrl Pts',(18.388974589749,56.1477854475703,2.70899119176095));
#231271=CARTESIAN_POINT('Ctrl Pts',(18.3808409394272,56.1436260014307,2.70298296066842));
#231272=CARTESIAN_POINT('Ctrl Pts',(18.3722424849456,56.1400597146375,2.69736727774133));
#231273=CARTESIAN_POINT('Ctrl Pts',(18.3642272309672,56.1367353155297,2.69213248525407));
#231274=CARTESIAN_POINT('Ctrl Pts',(18.355807270034,56.1339262909282,2.68723866185431));
#231275=CARTESIAN_POINT('Ctrl Pts',(18.3470212548457,56.1317496772148,2.68278595829514));
#231276=CARTESIAN_POINT('Ctrl Pts',(18.3438072168237,56.1309534437592,2.68115710172782));
#231277=CARTESIAN_POINT('Ctrl Pts',(18.3405443147877,56.1302421351292,2.6795876363781));
#231278=CARTESIAN_POINT('Ctrl Pts',(18.3372349828464,56.1296225724749,2.67808378645387));
#231279=CARTESIAN_POINT('Ctrl Pts',(18.3364391990694,56.1294735883543,2.67772216078622));
#231280=CARTESIAN_POINT('Ctrl Pts',(18.3356401993826,56.1293301519983,2.67736403603585));
#231281=CARTESIAN_POINT('Ctrl Pts',(18.3348380918585,56.1291923454417,2.67700956934501));
#231282=CARTESIAN_POINT('Ctrl Pts',(18.3340610501946,56.1290588453401,2.67666617973826));
#231283=CARTESIAN_POINT('Ctrl Pts',(18.333281091922,56.1289306286649,2.67632622314141));
#231284=CARTESIAN_POINT('Ctrl Pts',(18.3324983188931,56.128807768806,2.67598984158795));
#231285=CARTESIAN_POINT('Ctrl Pts',(18.3239221357308,56.127461697065,2.67230439292247));
#231286=CARTESIAN_POINT('Ctrl Pts',(18.3150023767875,56.1267581593461,2.66904964540004));
#231287=CARTESIAN_POINT('Ctrl Pts',(18.3059033598551,56.1267895336333,2.66640203566755));
#231288=CARTESIAN_POINT('Ctrl Pts',(18.3021297263205,56.1268025454853,2.66530399299466));
#231289=CARTESIAN_POINT('Ctrl Pts',(18.2983254984048,56.12694160832,2.66430995142282));
#231290=CARTESIAN_POINT('Ctrl Pts',(18.2945030089056,56.1272115877757,2.6634305347338));
#231291=CARTESIAN_POINT('Ctrl Pts',(18.2879833547333,56.1276720658711,2.66193059792904));
#231292=CARTESIAN_POINT('Ctrl Pts',(18.2814124323572,56.1285150529073,2.66076519817146));
#231293=CARTESIAN_POINT('Ctrl Pts',(18.2748585331713,56.1297657127891,2.65997805604477));
#231294=CARTESIAN_POINT('Ctrl Pts',(18.2715815835783,56.13039104273,2.65958448498143));
#231295=CARTESIAN_POINT('Ctrl Pts',(18.2683092720867,56.1311196862932,2.65928526260779));
#231296=CARTESIAN_POINT('Ctrl Pts',(18.2650501911674,56.1319548233215,2.65908463971341));
#231297=CARTESIAN_POINT('Ctrl Pts',(18.2617911102481,56.1327899603497,2.65888401681904));
#231298=CARTESIAN_POINT('Ctrl Pts',(18.2585452947514,56.1337315613411,2.65878198860301));
#231299=CARTESIAN_POINT('Ctrl Pts',(18.2553202812748,56.1347810195644,2.65878198860301));
#231300=CARTESIAN_POINT('Origin',(12.0988124084938,56.9937374973465,2.83404198860302));
#231301=CARTESIAN_POINT('Ctrl Pts',(12.8407372733096,61.3271735965896,2.83404198860304));
#231302=CARTESIAN_POINT('Ctrl Pts',(12.8429432848611,61.3375520649565,2.82419652440087));
#231303=CARTESIAN_POINT('Ctrl Pts',(12.8459616464944,61.347725676909,2.81438790575653));
#231304=CARTESIAN_POINT('Ctrl Pts',(12.8497656413963,61.3576417279037,2.80466781256891));
#231305=CARTESIAN_POINT('Ctrl Pts',(12.8534460291152,61.3672355662872,2.79526356453056));
#231306=CARTESIAN_POINT('Ctrl Pts',(12.8578623484999,61.3765894879247,2.785941024962));
#231307=CARTESIAN_POINT('Ctrl Pts',(12.8630345798925,61.3856422574874,2.77675109088739));
#231308=CARTESIAN_POINT('Ctrl Pts',(12.8679271923023,61.3942056200564,2.76805797913634));
#231309=CARTESIAN_POINT('Ctrl Pts',(12.8734966517572,61.4025003187132,2.75948271210106));
#231310=CARTESIAN_POINT('Ctrl Pts',(12.8797929832537,61.4104485116955,2.75108575573163));
#231311=CARTESIAN_POINT('Ctrl Pts',(12.8855923599243,61.4177693722601,2.74335155163202));
#231312=CARTESIAN_POINT('Ctrl Pts',(12.8920087864975,61.4247966697209,2.73576818685869));
#231313=CARTESIAN_POINT('Ctrl Pts',(12.8991043342901,61.431439001463,2.72840626160418));
#231314=CARTESIAN_POINT('Ctrl Pts',(12.9011624829819,61.4333656894067,2.72627084693641));
#231315=CARTESIAN_POINT('Ctrl Pts',(12.903277908872,61.4352597571387,2.72415424587524));
#231316=CARTESIAN_POINT('Ctrl Pts',(12.9054524645843,61.437118361331,2.72205867173299));
#231317=CARTESIAN_POINT('Ctrl Pts',(12.9078098227881,61.4391332077734,2.71978693462902));
#231318=CARTESIAN_POINT('Ctrl Pts',(12.9102326900447,61.4411043938525,2.71754411340803));
#231319=CARTESIAN_POINT('Ctrl Pts',(12.9127224163027,61.4430281531013,2.71533341844301));
#231320=CARTESIAN_POINT('Ctrl Pts',(12.9195554895544,61.4483079254552,2.70926614876448));
#231321=CARTESIAN_POINT('Ctrl Pts',(12.926909770583,61.4531896374538,2.70347381860465));
#231322=CARTESIAN_POINT('Ctrl Pts',(12.9347398820029,61.4575800373535,2.69804914171451));
#231323=CARTESIAN_POINT('Ctrl Pts',(12.9419040088454,61.4615970149014,2.69308585687261));
#231324=CARTESIAN_POINT('Ctrl Pts',(12.9494643722283,61.4651913207948,2.68842799053243));
#231325=CARTESIAN_POINT('Ctrl Pts',(12.9574154517105,61.4682744840804,2.68414767054275));
#231326=CARTESIAN_POINT('Ctrl Pts',(12.9613209959788,61.4697889238147,2.68204519134609));
#231327=CARTESIAN_POINT('Ctrl Pts',(12.9653208118552,61.4711795284102,2.68003431778559));
#231328=CARTESIAN_POINT('Ctrl Pts',(12.9694138336349,61.4724324898306,2.67812693945309));
#231329=CARTESIAN_POINT('Ctrl Pts',(12.970190444651,61.4726702270561,2.67776503299261));
#231330=CARTESIAN_POINT('Ctrl Pts',(12.9709708853391,61.4729027677277,2.67740659639981));
#231331=CARTESIAN_POINT('Ctrl Pts',(12.9717550556846,61.4731300138565,2.67705178968912));
#231332=CARTESIAN_POINT('Ctrl Pts',(12.9725147207069,61.4733501585437,2.67670807068815));
#231333=CARTESIAN_POINT('Ctrl Pts',(12.9732778859006,61.4735653344327,2.67636775825322));
#231334=CARTESIAN_POINT('Ctrl Pts',(12.9740444565835,61.4737754532576,2.67603099699312));
#231335=CARTESIAN_POINT('Ctrl Pts',(12.9823983859297,61.4760652849148,2.67236104217185));
#231336=CARTESIAN_POINT('Ctrl Pts',(12.9911623597379,61.4777556486133,2.66911440541531));
#231337=CARTESIAN_POINT('Ctrl Pts',(13.00018336166,61.4787331403172,2.66646778189688));
#231338=CARTESIAN_POINT('Ctrl Pts',(13.0039929867894,61.4791459411337,2.66535009635031));
#231339=CARTESIAN_POINT('Ctrl Pts',(13.0078481668565,61.4794319383913,2.66433897912401));
#231340=CARTESIAN_POINT('Ctrl Pts',(13.011736540843,61.479584339472,2.66344564884849));
#231341=CARTESIAN_POINT('Ctrl Pts',(13.0182844654763,61.4798409790836,2.66194130298642));
#231342=CARTESIAN_POINT('Ctrl Pts',(13.0249248230174,61.4797168922659,2.66077206705476));
#231343=CARTESIAN_POINT('Ctrl Pts',(13.0315916763176,61.4791780149469,2.6599822515577));
#231344=CARTESIAN_POINT('Ctrl Pts',(13.0332583896426,61.4790432956171,2.65978479768344));
#231345=CARTESIAN_POINT('Ctrl Pts',(13.0349267248715,61.4788824204062,2.65961098966678));
#231346=CARTESIAN_POINT('Ctrl Pts',(13.0365955947403,61.4786945538951,2.65946139030557));
#231347=CARTESIAN_POINT('Ctrl Pts',(13.0390988995433,61.4784127541283,2.65923699126376));
#231348=CARTESIAN_POINT('Ctrl Pts',(13.04160338921,61.4780702140294,2.65906707562498));
#231349=CARTESIAN_POINT('Ctrl Pts',(13.0441057251028,61.4776657592308,2.65895332562975));
#231350=CARTESIAN_POINT('Ctrl Pts',(13.0466080609957,61.4772613044323,2.65883957563453));
#231351=CARTESIAN_POINT('Ctrl Pts',(13.0491082380627,61.4767949453823,2.65878198860305));
#231352=CARTESIAN_POINT('Ctrl Pts',(13.0516031943527,61.4762657165318,2.65878198860305));
#231353=CARTESIAN_POINT('Ctrl Pts',(12.2578193919766,57.7418065394568,2.65878198860302));
#231354=CARTESIAN_POINT('Ctrl Pts',(12.249377180707,57.7435970583547,2.65878198860302));
#231355=CARTESIAN_POINT('Ctrl Pts',(12.2411559442237,57.7460689269806,2.65945335517902));
#231356=CARTESIAN_POINT('Ctrl Pts',(12.2332613533214,57.749114125811,2.6607256122666));
#231357=CARTESIAN_POINT('Ctrl Pts',(12.2281622576309,57.7510810117997,2.66154735980396));
#231358=CARTESIAN_POINT('Ctrl Pts',(12.223199086688,57.7532862127608,2.66261895766933));
#231359=CARTESIAN_POINT('Ctrl Pts',(12.2183955094118,57.755693185958,2.66391429251067));
#231360=CARTESIAN_POINT('Ctrl Pts',(12.2120286428976,57.7588834910513,2.66563118464164));
#231361=CARTESIAN_POINT('Ctrl Pts',(12.2059457447516,57.7624328173677,2.66774105138739));
#231362=CARTESIAN_POINT('Ctrl Pts',(12.2001996238499,57.7662682043711,2.6701689418179));
#231363=CARTESIAN_POINT('Ctrl Pts',(12.1973265633991,57.7681858978728,2.67138288703316));
#231364=CARTESIAN_POINT('Ctrl Pts',(12.1945375019637,57.7701751462712,2.67267613167592));
#231365=CARTESIAN_POINT('Ctrl Pts',(12.1918376559072,57.772227116147,2.67403835432593));
#231366=CARTESIAN_POINT('Ctrl Pts',(12.190487732879,57.7732531010849,2.67471946565094));
#231367=CARTESIAN_POINT('Ctrl Pts',(12.1891600976133,57.7742947697605,2.67541781389563));
#231368=CARTESIAN_POINT('Ctrl Pts',(12.1878553011596,57.7753510390206,2.6761320724421));
#231369=CARTESIAN_POINT('Ctrl Pts',(12.1875291020462,57.7756151063357,2.67631063707871));
#231370=CARTESIAN_POINT('Ctrl Pts',(12.1872043300163,57.7758800862579,2.67649019601886));
#231371=CARTESIAN_POINT('Ctrl Pts',(12.1868809929896,57.7761459620051,2.67667072836697));
#231372=CARTESIAN_POINT('Ctrl Pts',(12.1859109819096,57.7769435892467,2.67721232541131));
#231373=CARTESIAN_POINT('Ctrl Pts',(12.1849538875689,57.7777492785676,2.67776268340088));
#231374=CARTESIAN_POINT('Ctrl Pts',(12.1840099085256,57.7785625799464,2.67832123541557));
#231375=CARTESIAN_POINT('Ctrl Pts',(12.1773606420347,57.7842913698426,2.6822556036849));
#231376=CARTESIAN_POINT('Ctrl Pts',(12.1713100228962,57.7903843352501,2.68661792998939));
#231377=CARTESIAN_POINT('Ctrl Pts',(12.1658251565855,57.796726433441,2.69130986622634));
#231378=CARTESIAN_POINT('Ctrl Pts',(12.1631650023519,57.7998023442102,2.69358545023106));
#231379=CARTESIAN_POINT('Ctrl Pts',(12.1606380046011,57.8029374300327,2.69593918853516));
#231380=CARTESIAN_POINT('Ctrl Pts',(12.1582411305897,57.8061213360081,2.69836306235516));
#231381=CARTESIAN_POINT('Ctrl Pts',(12.1545716839429,57.8109956736034,2.70207384382249));
#231382=CARTESIAN_POINT('Ctrl Pts',(12.1512083732206,57.8159810988992,2.70594760814249));
#231383=CARTESIAN_POINT('Ctrl Pts',(12.1481495009385,57.8210315314443,2.70995196345728));
#231384=CARTESIAN_POINT('Ctrl Pts',(12.1467289448262,57.8233769784457,2.71181160678126));
#231385=CARTESIAN_POINT('Ctrl Pts',(12.1453738842984,57.8257362497573,2.71369962772119));
#231386=CARTESIAN_POINT('Ctrl Pts',(12.1440853170069,57.828105124615,2.71561183138682));
#231387=CARTESIAN_POINT('Ctrl Pts',(12.1439865534012,57.828286689539,2.71575839426332));
#231388=CARTESIAN_POINT('Ctrl Pts',(12.1438881466795,57.8284683073401,2.7159050890323));
#231389=CARTESIAN_POINT('Ctrl Pts',(12.143790096302,57.8286499766613,2.71605191409932));
#231390=CARTESIAN_POINT('Ctrl Pts',(12.1424127841096,57.8312018829081,2.71811436362774));
#231391=CARTESIAN_POINT('Ctrl Pts',(12.1411075562953,57.8337650648329,2.7202009102698));
#231392=CARTESIAN_POINT('Ctrl Pts',(12.1398727334219,57.8363340693142,2.72230624862203));
#231393=CARTESIAN_POINT('Ctrl Pts',(12.1354448782037,57.8455460625025,2.72985561753145));
#231394=CARTESIAN_POINT('Ctrl Pts',(12.1318862976809,57.8549032874811,2.73770089914395));
#231395=CARTESIAN_POINT('Ctrl Pts',(12.129096878378,57.8643241951544,2.74574823347162));
#231396=CARTESIAN_POINT('Ctrl Pts',(12.1260315867862,57.8746768262734,2.75459144547137));
#231397=CARTESIAN_POINT('Ctrl Pts',(12.1238947812338,57.8851069357383,2.76367911754407));
#231398=CARTESIAN_POINT('Ctrl Pts',(12.1225979458246,57.8955352825149,2.7729216256489));
#231399=CARTESIAN_POINT('Ctrl Pts',(12.1211976890438,57.9067952798761,2.78290121484937));
#231400=CARTESIAN_POINT('Ctrl Pts',(12.1207764137885,57.918054344326,2.79306229500438));
#231401=CARTESIAN_POINT('Ctrl Pts',(12.121277094834,57.9292311407304,2.80331916685547));
#231402=CARTESIAN_POINT('Ctrl Pts',(12.1217735756798,57.9403141752953,2.81348999408905));
#231403=CARTESIAN_POINT('Ctrl Pts',(12.1231769533538,57.9513177099582,2.82375635967002));
#231404=CARTESIAN_POINT('Ctrl Pts',(12.125481593379,57.9621601888123,2.83404198860303));
#231405=CARTESIAN_POINT('Origin',(0.0149069694351876,-0.00316857416787864,
2.83404198860262));
#231406=CARTESIAN_POINT('Ctrl Pts',(13.0814171332231,61.4699285681957,2.65878198860305));
#231407=CARTESIAN_POINT('Ctrl Pts',(13.0898176309846,61.4681393149851,2.65878198860305));
#231408=CARTESIAN_POINT('Ctrl Pts',(13.097994011884,61.4656642256292,2.65944603041891));
#231409=CARTESIAN_POINT('Ctrl Pts',(13.1058430982607,61.4626133761161,2.66070439264107));
#231410=CARTESIAN_POINT('Ctrl Pts',(13.1108582907973,61.4606640285138,2.66150842619632));
#231411=CARTESIAN_POINT('Ctrl Pts',(13.1157402208611,61.4584804838817,2.66255428265406));
#231412=CARTESIAN_POINT('Ctrl Pts',(13.1204666715205,61.4560986543958,2.66381699700696));
#231413=CARTESIAN_POINT('Ctrl Pts',(13.1269173283005,61.4528479350656,2.66554034873295));
#231414=CARTESIAN_POINT('Ctrl Pts',(13.1330744924004,61.4492231901486,2.66766759643999));
#231415=CARTESIAN_POINT('Ctrl Pts',(13.1388835356735,61.4453029499363,2.67012012783174));
#231416=CARTESIAN_POINT('Ctrl Pts',(13.1417880573101,61.4433428298302,2.67134639352762));
#231417=CARTESIAN_POINT('Ctrl Pts',(13.144605753406,61.4413087943566,2.67265375585038));
#231418=CARTESIAN_POINT('Ctrl Pts',(13.147331257159,61.4392103574001,2.67403135126966));
#231419=CARTESIAN_POINT('Ctrl Pts',(13.1486940090356,61.4381611389218,2.67472014897929));
#231420=CARTESIAN_POINT('Ctrl Pts',(13.1500337298701,61.4370958165019,2.67542649668658));
#231421=CARTESIAN_POINT('Ctrl Pts',(13.1513498559441,61.436015557062,2.67614899656127));
#231422=CARTESIAN_POINT('Ctrl Pts',(13.1516788874626,61.4357454922021,2.67632962152994));
#231423=CARTESIAN_POINT('Ctrl Pts',(13.1520064446718,61.4354744937033,2.67651125590976));
#231424=CARTESIAN_POINT('Ctrl Pts',(13.1523325194966,61.435202579648,2.67669387767549));
#231425=CARTESIAN_POINT('Ctrl Pts',(13.153310743971,61.4343868374822,2.67724174297269));
#231426=CARTESIAN_POINT('Ctrl Pts',(13.1542756251696,61.4335628556744,2.67779849504773));
#231427=CARTESIAN_POINT('Ctrl Pts',(13.1552269612802,61.4327311191549,2.67836353618034));
#231428=CARTESIAN_POINT('Ctrl Pts',(13.161801284066,61.4269833037496,2.68226832098935));
#231429=CARTESIAN_POINT('Ctrl Pts',(13.1677829516035,61.4208780249713,2.68659153751421));
#231430=CARTESIAN_POINT('Ctrl Pts',(13.1732071947994,61.4145287289055,2.69123699486212));
#231431=CARTESIAN_POINT('Ctrl Pts',(13.1759030287784,61.4113731461893,2.69354577441247));
#231432=CARTESIAN_POINT('Ctrl Pts',(13.1784610805514,61.4081566864227,2.69593478828145));
#231433=CARTESIAN_POINT('Ctrl Pts',(13.1808848153825,61.4048902384028,2.69839565261245));
#231434=CARTESIAN_POINT('Ctrl Pts',(13.1862319364381,61.397683966182,2.70382468689071));
#231435=CARTESIAN_POINT('Ctrl Pts',(13.1909347237342,61.3902425685154,2.70961155815112));
#231436=CARTESIAN_POINT('Ctrl Pts',(13.1949697809168,61.3827095020468,2.71562701361793));
#231437=CARTESIAN_POINT('Ctrl Pts',(13.1964438381903,61.3799575778689,2.71782453535884));
#231438=CARTESIAN_POINT('Ctrl Pts',(13.197836719349,61.3771940448621,2.72005051502428));
#231439=CARTESIAN_POINT('Ctrl Pts',(13.1991508816437,61.374423615274,2.72229986760141));
#231440=CARTESIAN_POINT('Ctrl Pts',(13.2035650137316,61.3651180354451,2.72985520488924));
#231441=CARTESIAN_POINT('Ctrl Pts',(13.207111392194,61.3556720404048,2.73770845534598));
#231442=CARTESIAN_POINT('Ctrl Pts',(13.2098890888177,61.3461671566351,2.745767067018));
#231443=CARTESIAN_POINT('Ctrl Pts',(13.2129421064468,61.3357201634447,2.75462443585087));
#231444=CARTESIAN_POINT('Ctrl Pts',(13.2150668515159,61.3252014297016,2.7637303632325));
#231445=CARTESIAN_POINT('Ctrl Pts',(13.216350225198,61.3146904872786,2.77299664636899));
#231446=CARTESIAN_POINT('Ctrl Pts',(13.2177324736418,61.3033697519308,2.78297683033573));
#231447=CARTESIAN_POINT('Ctrl Pts',(13.2181390006411,61.2920568939681,2.7931440147901));
#231448=CARTESIAN_POINT('Ctrl Pts',(13.2176240288385,61.2808338148818,2.80341452428073));
#231449=CARTESIAN_POINT('Ctrl Pts',(13.2171160108939,61.2697622852581,2.81354634721465));
#231450=CARTESIAN_POINT('Ctrl Pts',(13.2157108393287,61.2587767401939,2.82378004209273));
#231451=CARTESIAN_POINT('Ctrl Pts',(13.2134115091892,61.247959242388,2.83404198860305));
#231452=CARTESIAN_POINT('Ctrl Pts',(12.4981558292586,57.8829458346107,2.83404198860302));
#231453=CARTESIAN_POINT('Ctrl Pts',(12.4959553576928,57.8725934298276,2.82422126443134));
#231454=CARTESIAN_POINT('Ctrl Pts',(12.4929462656005,57.862451808205,2.81442815028716));
#231455=CARTESIAN_POINT('Ctrl Pts',(12.4891531124829,57.8525735736584,2.80471618166619));
#231456=CARTESIAN_POINT('Ctrl Pts',(12.4854904894114,57.8430352690781,2.79533842146582));
#231457=CARTESIAN_POINT('Ctrl Pts',(12.4810963130895,57.8337413853135,2.78603515650642));
#231458=CARTESIAN_POINT('Ctrl Pts',(12.4759491415405,57.8247536185236,2.77685887347205));
#231459=CARTESIAN_POINT('Ctrl Pts',(12.4710834524322,57.8162573641128,2.7681844121705));
#231460=CARTESIAN_POINT('Ctrl Pts',(12.4655444244746,57.8080338771694,2.75962261522118));
#231461=CARTESIAN_POINT('Ctrl Pts',(12.4592813303356,57.8001616710202,2.75123537702172));
#231462=CARTESIAN_POINT('Ctrl Pts',(12.4535131257047,57.7929115012227,2.74351087134634));
#231463=CARTESIAN_POINT('Ctrl Pts',(12.4471303774535,57.7859589019109,2.73593399450363));
#231464=CARTESIAN_POINT('Ctrl Pts',(12.4400707995019,57.7793958734444,2.72857657813092));
#231465=CARTESIAN_POINT('Ctrl Pts',(12.4379657758627,57.7774389108382,2.72638274508673));
#231466=CARTESIAN_POINT('Ctrl Pts',(12.4358004306464,57.7755168276804,2.72420861709788));
#231467=CARTESIAN_POINT('Ctrl Pts',(12.433572748276,57.7736327324863,2.72205663736748));
#231468=CARTESIAN_POINT('Ctrl Pts',(12.4313678273309,57.771767888103,2.71992664556787));
#231469=CARTESIAN_POINT('Ctrl Pts',(12.4291043014747,57.7699419852108,2.71782089927905));
#231470=CARTESIAN_POINT('Ctrl Pts',(12.4267829461797,57.768159932687,2.71574387311267));
#231471=CARTESIAN_POINT('Ctrl Pts',(12.4266215236723,57.7680360122397,2.71559944077507));
#231472=CARTESIAN_POINT('Ctrl Pts',(12.4264598236895,57.7679122920637,2.7154551521609));
#231473=CARTESIAN_POINT('Ctrl Pts',(12.4262978456307,57.7677887733172,2.71531100781751));
#231474=CARTESIAN_POINT('Ctrl Pts',(12.4191961341597,57.7623732589831,2.70899119176094));
#231475=CARTESIAN_POINT('Ctrl Pts',(12.4115418213385,57.7573864007559,2.7029829606684));
#231476=CARTESIAN_POINT('Ctrl Pts',(12.4033632485682,57.7529408672214,2.6973672777413));
#231477=CARTESIAN_POINT('Ctrl Pts',(12.3957393973198,57.7487968573387,2.69213248525403));
#231478=CARTESIAN_POINT('Ctrl Pts',(12.3876591848384,57.7451230952907,2.68723866185426));
#231479=CARTESIAN_POINT('Ctrl Pts',(12.3791488184472,57.7420400166291,2.68278595829508));
#231480=CARTESIAN_POINT('Ctrl Pts',(12.3760356163213,57.7409121865684,2.68115710172778));
#231481=CARTESIAN_POINT('Ctrl Pts',(12.3728649408021,57.7398637084259,2.67958763637807));
#231482=CARTESIAN_POINT('Ctrl Pts',(12.3696384996596,57.7389016204184,2.67808378645385));
#231483=CARTESIAN_POINT('Ctrl Pts',(12.3688626483506,57.7386702703931,2.6777221607862));
#231484=CARTESIAN_POINT('Ctrl Pts',(12.3680830188495,57.738444101587,2.67736403603583));
#231485=CARTESIAN_POINT('Ctrl Pts',(12.367299710062,57.7382232068823,2.67700956934499));
#231486=CARTESIAN_POINT('Ctrl Pts',(12.3665408796741,57.7380092151372,2.67666617973824));
#231487=CARTESIAN_POINT('Ctrl Pts',(12.3657785963866,57.7378001730067,2.67632622314139));
#231488=CARTESIAN_POINT('Ctrl Pts',(12.3650129538224,57.7375961641251,2.67598984158793));
#231489=CARTESIAN_POINT('Ctrl Pts',(12.3566244546995,57.7353610110593,2.67230439292252));
#231490=CARTESIAN_POINT('Ctrl Pts',(12.3478270988458,57.7337289586987,2.66904964540014));
#231491=CARTESIAN_POINT('Ctrl Pts',(12.3387746477744,57.732809054857,2.66640203566768));
#231492=CARTESIAN_POINT('Ctrl Pts',(12.3350203264901,57.7324275433144,2.66530399299474));
#231493=CARTESIAN_POINT('Ctrl Pts',(12.3312224025083,57.7321681942504,2.66430995142285));
#231494=CARTESIAN_POINT('Ctrl Pts',(12.3273926324687,57.7320371357771,2.66343053473379));
#231495=CARTESIAN_POINT('Ctrl Pts',(12.3208605605765,57.7318136018937,2.66193059792903));
#231496=CARTESIAN_POINT('Ctrl Pts',(12.3142375182613,57.7319651225405,2.66076519817146));
#231497=CARTESIAN_POINT('Ctrl Pts',(12.3075887924653,57.7325238621662,2.65997805604478));
#231498=CARTESIAN_POINT('Ctrl Pts',(12.3042644295673,57.7328032319791,2.65958448498144));
#231499=CARTESIAN_POINT('Ctrl Pts',(12.3009338801485,57.7331858342652,2.6592852626078));
#231500=CARTESIAN_POINT('Ctrl Pts',(12.2976053572253,57.7336757296052,2.65908463971342));
#231501=CARTESIAN_POINT('Ctrl Pts',(12.2942768343021,57.7341656249453,2.65888401681905));
#231502=CARTESIAN_POINT('Ctrl Pts',(12.2909503756177,57.734762787642,2.65878198860302));
#231503=CARTESIAN_POINT('Ctrl Pts',(12.2876333308469,57.7354693911207,2.65878198860302));
#231504=CARTESIAN_POINT('Origin',(6.07506605172281,57.9461901084064,2.83404198860303));
#231505=CARTESIAN_POINT('Ctrl Pts',(6.35995915837782,62.3334394572621,2.83404198860306));
#231506=CARTESIAN_POINT('Ctrl Pts',(6.36106823981771,62.3439916622907,2.82419652440113));
#231507=CARTESIAN_POINT('Ctrl Pts',(6.36300663452681,62.3544250468354,2.81438790575701));
#231508=CARTESIAN_POINT('Ctrl Pts',(6.36575328117443,62.3646844024064,2.80466781256959));
#231509=CARTESIAN_POINT('Ctrl Pts',(6.3684106781612,62.3746103900118,2.7952635645314));
#231510=CARTESIAN_POINT('Ctrl Pts',(6.37182505343177,62.3843747009663,2.785941024963));
#231511=CARTESIAN_POINT('Ctrl Pts',(6.37602267870884,62.3939185239092,2.77675109088852));
#231512=CARTESIAN_POINT('Ctrl Pts',(6.37999337374607,62.4029463927383,2.7680579791376));
#231513=CARTESIAN_POINT('Ctrl Pts',(6.38466529101529,62.411777819206,2.75948271210245));
#231514=CARTESIAN_POINT('Ctrl Pts',(6.39009631815072,62.4203406170109,2.75108575573312));
#231515=CARTESIAN_POINT('Ctrl Pts',(6.39509868692433,62.4282275730665,2.74335155163362));
#231516=CARTESIAN_POINT('Ctrl Pts',(6.40074541103664,62.4358870734658,2.73576818686039));
#231517=CARTESIAN_POINT('Ctrl Pts',(6.40710777594623,62.4432347045263,2.72840626160597));
#231518=CARTESIAN_POINT('Ctrl Pts',(6.40895325615472,62.4453659729923,2.7262708469376));
#231519=CARTESIAN_POINT('Ctrl Pts',(6.41085910953164,62.4474707870411,2.72415424587584));
#231520=CARTESIAN_POINT('Ctrl Pts',(6.41282747576062,62.4495465125726,2.72205867173302));
#231521=CARTESIAN_POINT('Ctrl Pts',(6.41496131130727,62.4517967325058,2.71978693462905));
#231522=CARTESIAN_POINT('Ctrl Pts',(6.41716486079182,62.4540103788123,2.71754411340805));
#231523=CARTESIAN_POINT('Ctrl Pts',(6.41943986047092,62.4561838467664,2.71533341844302));
#231524=CARTESIAN_POINT('Ctrl Pts',(6.4256836149418,62.4621489466213,2.70926614876449));
#231525=CARTESIAN_POINT('Ctrl Pts',(6.43248733059615,62.4677726477851,2.70347381860466));
#231526=CARTESIAN_POINT('Ctrl Pts',(6.43981562609173,62.4729574661288,2.69804914171452));
#231527=CARTESIAN_POINT('Ctrl Pts',(6.44652061860817,62.4777012934232,2.69308585687231));
#231528=CARTESIAN_POINT('Ctrl Pts',(6.45366385825839,62.4820661824992,2.68842799053185));
#231529=CARTESIAN_POINT('Ctrl Pts',(6.4612491025755,62.4859635700135,2.68414767054195));
#231530=CARTESIAN_POINT('Ctrl Pts',(6.46497494980508,62.4878779540288,2.68204519134558));
#231531=CARTESIAN_POINT('Ctrl Pts',(6.46880749650976,62.4896790353535,2.68003431778536));
#231532=CARTESIAN_POINT('Ctrl Pts',(6.47274712615552,62.4913529701967,2.6781269394531));
#231533=CARTESIAN_POINT('Ctrl Pts',(6.4734946325084,62.4916705830289,2.67776503299262));
#231534=CARTESIAN_POINT('Ctrl Pts',(6.47424649074168,62.491983428084,2.67740659639982));
#231535=CARTESIAN_POINT('Ctrl Pts',(6.4750026116314,62.4922913974559,2.67705178968914));
#231536=CARTESIAN_POINT('Ctrl Pts',(6.47573510374332,62.4925897427849,2.67670807068816));
#231537=CARTESIAN_POINT('Ctrl Pts',(6.47647159623327,62.4928835124028,2.67636775825324));
#231538=CARTESIAN_POINT('Ctrl Pts',(6.47721200416386,62.4931726086303,2.67603099699313));
#231539=CARTESIAN_POINT('Ctrl Pts',(6.4852808172263,62.4963231197467,2.67236104217204));
#231540=CARTESIAN_POINT('Ctrl Pts',(6.49382008994886,62.4989203081702,2.66911440541564));
#231541=CARTESIAN_POINT('Ctrl Pts',(6.50268949817238,62.5008353965403,2.66646778189727));
#231542=CARTESIAN_POINT('Ctrl Pts',(6.50643510434214,62.5016441502512,2.66535009635055));
#231543=CARTESIAN_POINT('Ctrl Pts',(6.5102392704761,62.5023315568341,2.66433897912412));
#231544=CARTESIAN_POINT('Ctrl Pts',(6.5140904132927,62.5028895688031,2.6634456488485));
#231545=CARTESIAN_POINT('Ctrl Pts',(6.52057564156552,62.5038292470157,2.66194130298643));
#231546=CARTESIAN_POINT('Ctrl Pts',(6.52719259313764,62.5043999463279,2.66077206705477));
#231547=CARTESIAN_POINT('Ctrl Pts',(6.53387925273587,62.5045608969645,2.6599822515577));
#231548=CARTESIAN_POINT('Ctrl Pts',(6.53555091763543,62.5046011346237,2.65978479768344));
#231549=CARTESIAN_POINT('Ctrl Pts',(6.53722692958795,62.5046155292218,2.65961098966678));
#231550=CARTESIAN_POINT('Ctrl Pts',(6.53890629461062,62.5046031362659,2.65946139030558));
#231551=CARTESIAN_POINT('Ctrl Pts',(6.54142534214461,62.5045845468321,2.65923699126377));
#231552=CARTESIAN_POINT('Ctrl Pts',(6.54395191714495,62.5045056736599,2.65906707562498));
#231553=CARTESIAN_POINT('Ctrl Pts',(6.54648282201853,62.5043649998327,2.65895332562976));
#231554=CARTESIAN_POINT('Ctrl Pts',(6.54901372689211,62.5042243260055,2.65883957563454));
#231555=CARTESIAN_POINT('Ctrl Pts',(6.5515489555224,62.5040218613863,2.65878198860305));
#231556=CARTESIAN_POINT('Ctrl Pts',(6.55408556365926,62.5037563256537,2.65878198860305));
#231557=CARTESIAN_POINT('Ctrl Pts',(6.15500747092297,58.7067819056645,2.65878198860303));
#231558=CARTESIAN_POINT('Ctrl Pts',(6.14642434678111,58.707680164542,2.65878198860303));
#231559=CARTESIAN_POINT('Ctrl Pts',(6.13798976646258,58.7092791387971,2.65945335517905));
#231560=CARTESIAN_POINT('Ctrl Pts',(6.12982011300103,58.7114824462546,2.66072561226666));
#231561=CARTESIAN_POINT('Ctrl Pts',(6.12454335512052,58.7129055567995,2.66154735980401));
#231562=CARTESIAN_POINT('Ctrl Pts',(6.11937686667978,58.7145798848073,2.66261895766938));
#231563=CARTESIAN_POINT('Ctrl Pts',(6.11434800669314,58.7164715618027,2.6639142925107));
#231564=CARTESIAN_POINT('Ctrl Pts',(6.10768254085114,58.7189788712983,2.66563118464167));
#231565=CARTESIAN_POINT('Ctrl Pts',(6.1012619598322,58.7218729180383,2.66774105138743));
#231566=CARTESIAN_POINT('Ctrl Pts',(6.09514640967254,58.7250866612028,2.67016894181794));
#231567=CARTESIAN_POINT('Ctrl Pts',(6.09208863459271,58.726693532785,2.67138288703319));
#231568=CARTESIAN_POINT('Ctrl Pts',(6.08910691884953,58.7283803475668,2.67267613167595));
#231569=CARTESIAN_POINT('Ctrl Pts',(6.08620737357446,58.7301388657776,2.67403835432597));
#231570=CARTESIAN_POINT('Ctrl Pts',(6.08475760093692,58.7310181248829,2.67471946565098));
#231571=CARTESIAN_POINT('Ctrl Pts',(6.08332835457025,58.7319153115145,2.67541781389566));
#231572=CARTESIAN_POINT('Ctrl Pts',(6.08192029572552,58.7328294060529,2.67613207244213));
#231573=CARTESIAN_POINT('Ctrl Pts',(6.08156828101434,58.7330579296875,2.67631063707874));
#231574=CARTESIAN_POINT('Ctrl Pts',(6.08121759017549,58.7332875101008,2.67649019601889));
#231575=CARTESIAN_POINT('Ctrl Pts',(6.08086823283962,58.7335181314303,2.676670728367));
#231576=CARTESIAN_POINT('Ctrl Pts',(6.07982016083201,58.7342099954188,2.67721232541134));
#231577=CARTESIAN_POINT('Ctrl Pts',(6.0787840920876,58.7349112274887,2.67776268340091));
#231578=CARTESIAN_POINT('Ctrl Pts',(6.07776027111701,58.7356214008388,2.6783212354156));
#231579=CARTESIAN_POINT('Ctrl Pts',(6.07054860839945,58.7406237702164,2.68225560368493));
#231580=CARTESIAN_POINT('Ctrl Pts',(6.06389424687488,58.7460508958015,2.68661792998942));
#231581=CARTESIAN_POINT('Ctrl Pts',(6.05777649745789,58.7517849266683,2.69130986622638));
#231582=CARTESIAN_POINT('Ctrl Pts',(6.05480939560164,58.7545659254423,2.69358545023109));
#231583=CARTESIAN_POINT('Ctrl Pts',(6.05196853530569,58.7574196937451,2.69593918853518));
#231584=CARTESIAN_POINT('Ctrl Pts',(6.04925198282213,58.7603356163933,2.69836306235517));
#231585=CARTESIAN_POINT('Ctrl Pts',(6.04509313076974,58.7647996902382,2.7020738438225));
#231586=CARTESIAN_POINT('Ctrl Pts',(6.04122712577058,58.7694062431513,2.7059476081425));
#231587=CARTESIAN_POINT('Ctrl Pts',(6.03765709635815,58.7741092696795,2.7099519634573));
#231588=CARTESIAN_POINT('Ctrl Pts',(6.03599915623014,58.7762933795294,2.71181160678127));
#231589=CARTESIAN_POINT('Ctrl Pts',(6.03440490786103,58.7784980841113,2.71369962772121));
#231590=CARTESIAN_POINT('Ctrl Pts',(6.03287578462737,58.7807192900659,2.71561183138683));
#231591=CARTESIAN_POINT('Ctrl Pts',(6.03275858335656,58.7808895367503,2.71575839426334));
#231592=CARTESIAN_POINT('Ctrl Pts',(6.03264173148759,58.7810598733267,2.71590508903231));
#231593=CARTESIAN_POINT('Ctrl Pts',(6.0325252286253,58.781230298389,2.71605191409933));
#231594=CARTESIAN_POINT('Ctrl Pts',(6.03088871465485,58.7836242566995,2.71811436362775));
#231595=CARTESIAN_POINT('Ctrl Pts',(6.02932271154744,58.7860369637879,2.72020091026982));
#231596=CARTESIAN_POINT('Ctrl Pts',(6.02782611907238,58.7884628208565,2.72230624862204));
#231597=CARTESIAN_POINT('Ctrl Pts',(6.02245960461739,58.7971615128796,2.72985561753055));
#231598=CARTESIAN_POINT('Ctrl Pts',(6.01794242202412,58.8060955050461,2.73770089914207));
#231599=CARTESIAN_POINT('Ctrl Pts',(6.01418353045067,58.8151732302872,2.74574823346872));
#231600=CARTESIAN_POINT('Ctrl Pts',(6.0100528862257,58.8251487383885,2.75459144546705));
#231601=CARTESIAN_POINT('Ctrl Pts',(6.00683754300386,58.8352983536201,2.76367911753826));
#231602=CARTESIAN_POINT('Ctrl Pts',(6.0044577527316,58.8455340166078,2.77292162564155));
#231603=CARTESIAN_POINT('Ctrl Pts',(6.00188817648357,58.8565859638331,2.78290121483949));
#231604=CARTESIAN_POINT('Ctrl Pts',(6.0002923163131,58.8677393146921,2.7930622949919));
#231605=CARTESIAN_POINT('Ctrl Pts',(5.99962196122217,58.8789072188539,2.80331916684039));
#231606=CARTESIAN_POINT('Ctrl Pts',(5.99895722972127,58.8899814357811,2.81348999407889));
#231607=CARTESIAN_POINT('Ctrl Pts',(5.99920273697632,58.901071384847,2.82375635966493));
#231608=CARTESIAN_POINT('Ctrl Pts',(6.00036140429027,58.9120953679532,2.83404198860304));
#231609=CARTESIAN_POINT('Origin',(0.0151565136854175,-0.00159301378001511,
2.83404198860263));
#231610=CARTESIAN_POINT('Ctrl Pts',(6.58439859103009,62.5005702980933,2.65878198860306));
#231611=CARTESIAN_POINT('Ctrl Pts',(6.59294009787473,62.4996689377207,2.65878198860306));
#231612=CARTESIAN_POINT('Ctrl Pts',(6.60133040499113,62.4980620716937,2.65944603041897));
#231613=CARTESIAN_POINT('Ctrl Pts',(6.60945539386287,62.4958483879903,2.66070439264121));
#231614=CARTESIAN_POINT('Ctrl Pts',(6.61464687495897,62.4944339494871,2.66150842619644));
#231615=CARTESIAN_POINT('Ctrl Pts',(6.61973030386368,62.4927726671883,2.66255428265414));
#231616=CARTESIAN_POINT('Ctrl Pts',(6.62467983150747,62.4908979342378,2.66381699700697));
#231617=CARTESIAN_POINT('Ctrl Pts',(6.63143494361075,62.4883392999285,2.66554034873297));
#231618=CARTESIAN_POINT('Ctrl Pts',(6.63793726713745,62.4853780106449,2.66766759644002));
#231619=CARTESIAN_POINT('Ctrl Pts',(6.64412426454875,62.4820864562851,2.67012012783178));
#231620=CARTESIAN_POINT('Ctrl Pts',(6.6472177632544,62.4804406791052,2.67134639352766));
#231621=CARTESIAN_POINT('Ctrl Pts',(6.65023263831854,62.4787123157336,2.67265375585042));
#231622=CARTESIAN_POINT('Ctrl Pts',(6.65316255786721,62.4769102669532,2.6740313512697));
#231623=CARTESIAN_POINT('Ctrl Pts',(6.65462751764154,62.4760092425631,2.67472014897934));
#231624=CARTESIAN_POINT('Ctrl Pts',(6.65607125586062,62.4750897950508,2.67542649668662));
#231625=CARTESIAN_POINT('Ctrl Pts',(6.65749308991742,62.4741530260212,2.67614899656132));
#231626=CARTESIAN_POINT('Ctrl Pts',(6.65784854843162,62.4739188337638,2.67632962152999));
#231627=CARTESIAN_POINT('Ctrl Pts',(6.65820263830483,62.4736835588748,2.6765112559098));
#231628=CARTESIAN_POINT('Ctrl Pts',(6.65855534961595,62.4734472184936,2.67669387767554));
#231629=CARTESIAN_POINT('Ctrl Pts',(6.65961348354928,62.4727381973497,2.67724174297274));
#231630=CARTESIAN_POINT('Ctrl Pts',(6.66065920857987,62.4720195869494,2.67779849504777));
#231631=CARTESIAN_POINT('Ctrl Pts',(6.66169227331198,62.4712918484712,2.67836353618039));
#231632=CARTESIAN_POINT('Ctrl Pts',(6.66883139158122,62.4662627240579,2.68226832098947));
#231633=CARTESIAN_POINT('Ctrl Pts',(6.67541846632676,62.4608161451509,2.68659153751441));
#231634=CARTESIAN_POINT('Ctrl Pts',(6.68147667711152,62.4550686189988,2.6912369948624));
#231635=CARTESIAN_POINT('Ctrl Pts',(6.68448759124189,62.4522121142781,2.69354577441268));
#231636=CARTESIAN_POINT('Ctrl Pts',(6.68736784133606,62.4492806638355,2.69593478828158));
#231637=CARTESIAN_POINT('Ctrl Pts',(6.69011973548588,62.4462854590371,2.69839565261248));
#231638=CARTESIAN_POINT('Ctrl Pts',(6.69619082501402,62.4396775898763,2.70382468689073));
#231639=CARTESIAN_POINT('Ctrl Pts',(6.70164568781196,62.4327685320939,2.70961155815115));
#231640=CARTESIAN_POINT('Ctrl Pts',(6.70644606039074,62.4256985108781,2.71562701361794));
#231641=CARTESIAN_POINT('Ctrl Pts',(6.70819969702964,62.4231157429703,2.71782453535885));
#231642=CARTESIAN_POINT('Ctrl Pts',(6.70987381569795,62.4205129446135,2.72005051502429));
#231643=CARTESIAN_POINT('Ctrl Pts',(6.71147036762155,62.4178950590937,2.72229986760143));
#231644=CARTESIAN_POINT('Ctrl Pts',(6.71683301659097,62.4091018586491,2.72985520488884));
#231645=CARTESIAN_POINT('Ctrl Pts',(6.72134734296653,62.4000783072495,2.73770845534518));
#231646=CARTESIAN_POINT('Ctrl Pts',(6.72510335397126,62.3909158405878,2.74576706701679));
#231647=CARTESIAN_POINT('Ctrl Pts',(6.72923165499421,62.3808452043611,2.7546244358492));
#231648=CARTESIAN_POINT('Ctrl Pts',(6.73244426756114,62.3706061896797,2.76373036323036));
#231649=CARTESIAN_POINT('Ctrl Pts',(6.73481930344695,62.3602869763786,2.77299664636633));
#231650=CARTESIAN_POINT('Ctrl Pts',(6.73737731885814,62.3491727415102,2.78297683033235));
#231651=CARTESIAN_POINT('Ctrl Pts',(6.73896413451822,62.3379643502106,2.79314401478594));
#231652=CARTESIAN_POINT('Ctrl Pts',(6.7396251149953,62.3267489231154,2.80341452427569));
#231653=CARTESIAN_POINT('Ctrl Pts',(6.74027717000429,62.3156849421522,2.81354634721137));
#231654=CARTESIAN_POINT('Ctrl Pts',(6.74002799825975,62.3046126966268,2.82378004209116));
#231655=CARTESIAN_POINT('Ctrl Pts',(6.73887200051313,62.2936141127571,2.83404198860306));
#231656=CARTESIAN_POINT('Ctrl Pts',(6.37927424642559,58.8722700234482,2.83404198860304));
#231657=CARTESIAN_POINT('Ctrl Pts',(6.37816795023625,58.8617443183085,2.82422126442954));
#231658=CARTESIAN_POINT('Ctrl Pts',(6.37623543038808,58.8513437177761,2.81442815028353));
#231659=CARTESIAN_POINT('Ctrl Pts',(6.37349561323624,58.8411231047638,2.80471618166077));
#231660=CARTESIAN_POINT('Ctrl Pts',(6.37085007871655,58.8312542036518,2.79533842145934));
#231661=CARTESIAN_POINT('Ctrl Pts',(6.36745144953932,58.8215519162556,2.78603515649892));
#231662=CARTESIAN_POINT('Ctrl Pts',(6.3632719521844,58.8120753594595,2.77685887346358));
#231663=CARTESIAN_POINT('Ctrl Pts',(6.3593210182466,58.8031170454137,2.76818441216155));
#231664=CARTESIAN_POINT('Ctrl Pts',(6.35467192211579,58.7943596215114,2.7596226152118));
#231665=CARTESIAN_POINT('Ctrl Pts',(6.34926600747212,58.7858758685252,2.75123537701197));
#231666=CARTESIAN_POINT('Ctrl Pts',(6.3442872507764,58.7780624743506,2.74351087133653));
#231667=CARTESIAN_POINT('Ctrl Pts',(6.33866621240896,58.7704807832391,2.7359339944938));
#231668=CARTESIAN_POINT('Ctrl Pts',(6.33233133084323,58.7632157808948,2.72857657812111));
#231669=CARTESIAN_POINT('Ctrl Pts',(6.33044239704028,58.7610495038516,2.72638274508025));
#231670=CARTESIAN_POINT('Ctrl Pts',(6.32848982621314,58.7589116098618,2.72420861709468));
#231671=CARTESIAN_POINT('Ctrl Pts',(6.32647128889819,58.7568049797266,2.72205663736749));
#231672=CARTESIAN_POINT('Ctrl Pts',(6.32447337605832,58.754719874158,2.71992664556788));
#231673=CARTESIAN_POINT('Ctrl Pts',(6.32241310885705,58.7526673708736,2.71782089927907));
#231674=CARTESIAN_POINT('Ctrl Pts',(6.32029074540099,58.7506524329183,2.71574387311269));
#231675=CARTESIAN_POINT('Ctrl Pts',(6.32014316039694,58.7505123180735,2.71559944077509));
#231676=CARTESIAN_POINT('Ctrl Pts',(6.31999527850335,58.7503723733989,2.71545515216091));
#231677=CARTESIAN_POINT('Ctrl Pts',(6.31984709900205,58.7502325999834,2.71531100781753));
#231678=CARTESIAN_POINT('Ctrl Pts',(6.31335036684085,58.7441044214169,2.708991191761));
#231679=CARTESIAN_POINT('Ctrl Pts',(6.30625925377316,58.7383447881643,2.70298296066851));
#231680=CARTESIAN_POINT('Ctrl Pts',(6.29859016886908,58.7330687140843,2.69736727774144));
#231681=CARTESIAN_POINT('Ctrl Pts',(6.2914412488604,58.7281504960661,2.69213248525422));
#231682=CARTESIAN_POINT('Ctrl Pts',(6.28378931332983,58.7236522470775,2.6872386618545));
#231683=CARTESIAN_POINT('Ctrl Pts',(6.2756478370909,58.7196964823227,2.68278595829534));
#231684=CARTESIAN_POINT('Ctrl Pts',(6.2726695797549,58.7182494123989,2.68115710172795));
#231685=CARTESIAN_POINT('Ctrl Pts',(6.26962586933679,58.7168752520898,2.67958763637816));
#231686=CARTESIAN_POINT('Ctrl Pts',(6.26651766855733,58.7155811795666,2.67808378645386));
#231687=CARTESIAN_POINT('Ctrl Pts',(6.26577025010559,58.7152699983559,2.67772216078621));
#231688=CARTESIAN_POINT('Ctrl Pts',(6.26501853257419,58.7149635750525,2.67736403603584));
#231689=CARTESIAN_POINT('Ctrl Pts',(6.26426260461821,58.7146620123683,2.677009569345));
#231690=CARTESIAN_POINT('Ctrl Pts',(6.26353029941086,58.714369873518,2.67666617973825));
#231691=CARTESIAN_POINT('Ctrl Pts',(6.26279404284356,58.7140822962416,2.6763262231414));
#231692=CARTESIAN_POINT('Ctrl Pts',(6.2620539192844,58.7137993735014,2.67598984158795));
#231693=CARTESIAN_POINT('Ctrl Pts',(6.25394501035235,58.7106996279154,2.67230439292247));
#231694=CARTESIAN_POINT('Ctrl Pts',(6.24536644325958,58.7081569420202,2.66904964540004));
#231695=CARTESIAN_POINT('Ctrl Pts',(6.23645973859704,58.7062958387087,2.66640203566755));
#231696=CARTESIAN_POINT('Ctrl Pts',(6.23276586269294,58.7055239836918,2.66530399299466));
#231697=CARTESIAN_POINT('Ctrl Pts',(6.22901585349541,58.7048690642117,2.66430995142282));
#231698=CARTESIAN_POINT('Ctrl Pts',(6.2252207626778,58.7043384037136,2.66343053473381));
#231699=CARTESIAN_POINT('Ctrl Pts',(6.21874783981216,58.7034333069353,2.66193059792904));
#231700=CARTESIAN_POINT('Ctrl Pts',(6.21214524099542,58.7028917011007,2.66076519817147));
#231701=CARTESIAN_POINT('Ctrl Pts',(6.20547453342055,58.7027523988022,2.65997805604479));
#231702=CARTESIAN_POINT('Ctrl Pts',(6.20213917963312,58.7026827476529,2.65958448498145));
#231703=CARTESIAN_POINT('Ctrl Pts',(6.1987868824835,58.702715116791,2.65928526260781));
#231704=CARTESIAN_POINT('Ctrl Pts',(6.19542538555007,58.702854403047,2.65908463971344));
#231705=CARTESIAN_POINT('Ctrl Pts',(6.19206388861665,58.7029936893031,2.65888401681906));
#231706=CARTESIAN_POINT('Ctrl Pts',(6.18869323212197,58.7032398710657,2.65878198860303));
#231707=CARTESIAN_POINT('Ctrl Pts',(6.1853204982938,58.7035958781041,2.65878198860303));
#231708=CARTESIAN_POINT('Origin',(-0.0152400000001978,58.2637721346187,
2.83404198860302));
#231709=CARTESIAN_POINT('Ctrl Pts',(-0.190500000000213,62.6567671111301,
2.83404198860305));
#231710=CARTESIAN_POINT('Ctrl Pts',(-0.190500000000213,62.6673774406539,
2.82419652440183));
#231711=CARTESIAN_POINT('Ctrl Pts',(-0.189662809673352,62.6779562874463,
2.8143879057583));
#231712=CARTESIAN_POINT('Ctrl Pts',(-0.188003604115546,62.6884465439469,
2.80466781257137));
#231713=CARTESIAN_POINT('Ctrl Pts',(-0.186398312858428,62.6985959295767,
2.79526356453354));
#231714=CARTESIAN_POINT('Ctrl Pts',(-0.184023290311945,62.7086636500138,
2.78594102496541));
#231715=CARTESIAN_POINT('Ctrl Pts',(-0.180846261211493,62.7185939622152,
2.77675109089116));
#231716=CARTESIAN_POINT('Ctrl Pts',(-0.17784098731263,62.7279874260844,
2.7680579791404));
#231717=CARTESIAN_POINT('Ctrl Pts',(-0.174117798732407,62.7372588214061,
2.75948271210536));
#231718=CARTESIAN_POINT('Ctrl Pts',(-0.169611579427998,62.7463424082288,
2.75108575573613));
#231719=CARTESIAN_POINT('Ctrl Pts',(-0.165461025550571,62.7547090486342,
2.74335155163674));
#231720=CARTESIAN_POINT('Ctrl Pts',(-0.160645870590254,62.7629168328825,
2.7357681868636));
#231721=CARTESIAN_POINT('Ctrl Pts',(-0.155086395965148,62.7708892610778,
2.72840626160927));
#231722=CARTESIAN_POINT('Ctrl Pts',(-0.153473803707152,62.7732017594436,
2.72627084693978));
#231723=CARTESIAN_POINT('Ctrl Pts',(-0.151798403771608,62.7754942590267,
2.72415424587693));
#231724=CARTESIAN_POINT('Ctrl Pts',(-0.150057792857872,62.7777643638148,
2.72205867173303));
#231725=CARTESIAN_POINT('Ctrl Pts',(-0.148170858717257,62.7802253033583,
2.71978693462905));
#231726=CARTESIAN_POINT('Ctrl Pts',(-0.146210769553988,62.7826571567201,
2.71754411340805));
#231727=CARTESIAN_POINT('Ctrl Pts',(-0.144175421826372,62.7850565204097,
2.71533341844303));
#231728=CARTESIAN_POINT('Ctrl Pts',(-0.138589394016844,62.7916415928832,
2.7092661487645));
#231729=CARTESIAN_POINT('Ctrl Pts',(-0.132410786669256,62.7979456687655,
2.70347381860466));
#231730=CARTESIAN_POINT('Ctrl Pts',(-0.125664597436947,62.8038680995983,
2.69804914171452));
#231731=CARTESIAN_POINT('Ctrl Pts',(-0.119492200548546,62.8092868022741,
2.69308585687263));
#231732=CARTESIAN_POINT('Ctrl Pts',(-0.112844347460444,62.8143744518941,
2.68842799053244));
#231733=CARTESIAN_POINT('Ctrl Pts',(-0.105708043833497,62.8190433630436,
2.68414767054277));
#231734=CARTESIAN_POINT('Ctrl Pts',(-0.102202714803686,62.8213367169485,
2.68204519134611));
#231735=CARTESIAN_POINT('Ctrl Pts',(-0.0985794274534979,62.823528541979,
2.68003431778561));
#231736=CARTESIAN_POINT('Ctrl Pts',(-0.0948363533474291,62.8256051102649,
2.67812693945311));
#231737=CARTESIAN_POINT('Ctrl Pts',(-0.0941261414938298,62.8259991188711,
2.67776503299263));
#231738=CARTESIAN_POINT('Ctrl Pts',(-0.093411103231482,62.8263888407141,
2.67740659639983));
#231739=CARTESIAN_POINT('Ctrl Pts',(-0.0926913160162859,62.8267741591522,
2.67705178968914));
#231740=CARTESIAN_POINT('Ctrl Pts',(-0.0919940221515648,62.8271474363891,
2.67670807068817));
#231741=CARTESIAN_POINT('Ctrl Pts',(-0.0912922715312481,62.8275165811345,
2.67636775825325));
#231742=CARTESIAN_POINT('Ctrl Pts',(-0.0905861384171587,62.8278814873657,
2.67603099699314));
#231743=CARTESIAN_POINT('Ctrl Pts',(-0.0828908452419837,62.8318581602827,
2.67236104217184));
#231744=CARTESIAN_POINT('Ctrl Pts',(-0.0746698316630847,62.8353337180915,
2.66911440541526));
#231745=CARTESIAN_POINT('Ctrl Pts',(-0.0660491922296248,62.8381654210189,
2.66646778189682));
#231746=CARTESIAN_POINT('Ctrl Pts',(-0.0624086426654321,62.8393612667491,
2.66535009635028));
#231747=CARTESIAN_POINT('Ctrl Pts',(-0.0586971697058494,62.8404425512867,
2.66433897912401));
#231748=CARTESIAN_POINT('Ctrl Pts',(-0.0549254519866898,62.8414000604481,
2.66344564884851));
#231749=CARTESIAN_POINT('Ctrl Pts',(-0.0485739735924291,62.8430124819503,
2.66194130298644));
#231750=CARTESIAN_POINT('Ctrl Pts',(-0.0420529246954851,62.8442717146913,
2.66077206705478));
#231751=CARTESIAN_POINT('Ctrl Pts',(-0.0354197192409215,62.8451307298766,
2.65998225155772));
#231752=CARTESIAN_POINT('Ctrl Pts',(-0.0337614178772805,62.8453454836729,
2.65978479768345));
#231753=CARTESIAN_POINT('Ctrl Pts',(-0.0320960919388032,62.8455349903697,
2.6596109896668));
#231754=CARTESIAN_POINT('Ctrl Pts',(-0.0304246312368016,62.8456982067487,
2.65946139030559));
#231755=CARTESIAN_POINT('Ctrl Pts',(-0.0279174401837993,62.8459430313172,
2.65923699126377));
#231756=CARTESIAN_POINT('Ctrl Pts',(-0.0253964615341803,62.8461286892225,
2.65906707562499));
#231757=CARTESIAN_POINT('Ctrl Pts',(-0.0228647168033238,62.8462533376182,
2.65895332562976));
#231758=CARTESIAN_POINT('Ctrl Pts',(-0.0203329720724672,62.8463779860139,
2.65883957563454));
#231759=CARTESIAN_POINT('Ctrl Pts',(-0.0177904683743677,62.8464416340695,
2.65878198860306));
#231760=CARTESIAN_POINT('Ctrl Pts',(-0.0152400000002138,62.8464427007198,
2.65878198860306));
#231761=CARTESIAN_POINT('Ctrl Pts',(-0.0152400000002007,59.0285534841298,
2.65878198860303));
#231762=CARTESIAN_POINT('Ctrl Pts',(-0.0238699985097207,59.0285496414746,
2.65878198860303));
#231763=CARTESIAN_POINT('Ctrl Pts',(-0.0324255116361278,59.0292582026624,
2.65945335517899));
#231764=CARTESIAN_POINT('Ctrl Pts',(-0.0407807192235719,59.0305954788492,
2.66072561226651));
#231765=CARTESIAN_POINT('Ctrl Pts',(-0.0461773260309337,59.0314592220534,
2.66154735980389));
#231766=CARTESIAN_POINT('Ctrl Pts',(-0.0514905268413882,59.0325843328201,
2.6626189576693));
#231767=CARTESIAN_POINT('Ctrl Pts',(-0.0566895722964677,59.0339399880046,
2.6639142925107));
#231768=CARTESIAN_POINT('Ctrl Pts',(-0.0635806092276745,59.035736831295,
2.66563118464166));
#231769=CARTESIAN_POINT('Ctrl Pts',(-0.070268527890346,59.037943890677,
2.66774105138742));
#231770=CARTESIAN_POINT('Ctrl Pts',(-0.0766865040606691,59.0405007795599,
2.67016894181792));
#231771=CARTESIAN_POINT('Ctrl Pts',(-0.0798954921458306,59.0417792240014,
2.67138288703317));
#231772=CARTESIAN_POINT('Ctrl Pts',(-0.0830371938951397,59.0431451240708,
2.67267613167594));
#231773=CARTESIAN_POINT('Ctrl Pts',(-0.0861046703640038,59.044590923923,
2.67403835432595));
#231774=CARTESIAN_POINT('Ctrl Pts',(-0.0876384085984359,59.0453138238491,
2.67471946565096));
#231775=CARTESIAN_POINT('Ctrl Pts',(-0.0891536069438316,59.046056698672,
2.67541781389565));
#231776=CARTESIAN_POINT('Ctrl Pts',(-0.0906495011922653,59.0468186034777,
2.67613207244211));
#231777=CARTESIAN_POINT('Ctrl Pts',(-0.0910234747543737,59.0470090796791,
2.67631063707872));
#231778=CARTESIAN_POINT('Ctrl Pts',(-0.0913962421599025,59.0472007452525,
2.67649019601887));
#231779=CARTESIAN_POINT('Ctrl Pts',(-0.091767792172904,59.0473935854288,
2.67667072836699));
#231780=CARTESIAN_POINT('Ctrl Pts',(-0.0928824422119088,59.0479721059576,
2.67721232541132));
#231781=CARTESIAN_POINT('Ctrl Pts',(-0.0939861339739926,59.0485611979311,
2.67776268340089));
#231782=CARTESIAN_POINT('Ctrl Pts',(-0.0950785796751122,59.0491604624445,
2.67832123541558));
#231783=CARTESIAN_POINT('Ctrl Pts',(-0.102773626133376,59.0533816042978,
2.68225560368486));
#231784=CARTESIAN_POINT('Ctrl Pts',(-0.10995882346653,59.0580834293368,
2.68661792998929));
#231785=CARTESIAN_POINT('Ctrl Pts',(-0.116642428646858,59.0631465696372,
2.69130986622618));
#231786=CARTESIAN_POINT('Ctrl Pts',(-0.119883969936987,59.0656021872117,
2.69358545023095));
#231787=CARTESIAN_POINT('Ctrl Pts',(-0.123007567718284,59.0681433715121,
2.69593918853511));
#231788=CARTESIAN_POINT('Ctrl Pts',(-0.126014035556611,59.0707593633745,
2.69836306235516));
#231789=CARTESIAN_POINT('Ctrl Pts',(-0.130616727761238,59.0747642641418,
2.70207384382249));
#231790=CARTESIAN_POINT('Ctrl Pts',(-0.134943070277467,59.0789414743145,
2.70594760814249));
#231791=CARTESIAN_POINT('Ctrl Pts',(-0.13898514283093,59.083245567483,2.70995196345729));
#231792=CARTESIAN_POINT('Ctrl Pts',(-0.14086230223567,59.0852444106169,
2.71181160678127));
#231793=CARTESIAN_POINT('Ctrl Pts',(-0.142678271527317,59.0872703932643,
2.7136996277212));
#231794=CARTESIAN_POINT('Ctrl Pts',(-0.14443119730894,59.0893195943185,
2.71561183138683));
#231795=CARTESIAN_POINT('Ctrl Pts',(-0.144565552163225,59.0894766575051,
2.71575839426334));
#231796=CARTESIAN_POINT('Ctrl Pts',(-0.14469956892599,59.0896338466135,
2.7159050890323));
#231797=CARTESIAN_POINT('Ctrl Pts',(-0.144833247843279,59.0897911602044,
2.71605191409933));
#231798=CARTESIAN_POINT('Ctrl Pts',(-0.146711033602286,59.0920009418703,
2.71811436362774));
#231799=CARTESIAN_POINT('Ctrl Pts',(-0.148520654545092,59.0942367399985,
2.72020091026981));
#231800=CARTESIAN_POINT('Ctrl Pts',(-0.150262619641474,59.0964928714568,
2.72230624862203));
#231801=CARTESIAN_POINT('Ctrl Pts',(-0.156508996678944,59.1045829576264,
2.72985561753118));
#231802=CARTESIAN_POINT('Ctrl Pts',(-0.16193529014577,59.112995834295,2.73770089914338));
#231803=CARTESIAN_POINT('Ctrl Pts',(-0.166622470787609,59.1216309196484,
2.74574823347074));
#231804=CARTESIAN_POINT('Ctrl Pts',(-0.171773211444,59.1311200109807,2.7545914454702));
#231805=CARTESIAN_POINT('Ctrl Pts',(-0.176031864362475,59.1408779306735,
2.7636791175426));
#231806=CARTESIAN_POINT('Ctrl Pts',(-0.179468536017355,59.1508087658097,
2.77292162564712));
#231807=CARTESIAN_POINT('Ctrl Pts',(-0.183179278917844,59.1615315754576,
2.78290121484728));
#231808=CARTESIAN_POINT('Ctrl Pts',(-0.185932239424909,59.1724570142849,
2.79306229500199));
#231809=CARTESIAN_POINT('Ctrl Pts',(-0.18776628610007,59.1834936683141,
2.80331916685278));
#231810=CARTESIAN_POINT('Ctrl Pts',(-0.189584947008031,59.1944377361557,
2.81348999408724));
#231811=CARTESIAN_POINT('Ctrl Pts',(-0.190500000000201,59.2054925958118,
2.82375635966911));
#231812=CARTESIAN_POINT('Ctrl Pts',(-0.190500000000201,59.2165773020943,
2.83404198860303));
#231813=CARTESIAN_POINT('Origin',(0.0152400000000056,1.8389786102284E-13,
2.83404198860262));
#231814=CARTESIAN_POINT('Ctrl Pts',(0.0152399999997862,62.8464427007198,
2.65878198860306));
#231815=CARTESIAN_POINT('Ctrl Pts',(0.0238289333901328,62.8464391086781,
2.65878198860306));
#231816=CARTESIAN_POINT('Ctrl Pts',(0.0323412407620547,62.8457180711407,
2.65944603041885));
#231817=CARTESIAN_POINT('Ctrl Pts',(0.040653113049661,62.8443658068293,
2.66070439264089));
#231818=CARTESIAN_POINT('Ctrl Pts',(0.0459640037530079,62.8435017743092,
2.66150842619617));
#231819=CARTESIAN_POINT('Ctrl Pts',(0.0511932363887765,62.8423809557001,
2.66255428265399));
#231820=CARTESIAN_POINT('Ctrl Pts',(0.0563116129573038,62.8410338592511,
2.66381699700699));
#231821=CARTESIAN_POINT('Ctrl Pts',(0.0632971699620762,62.8391953428956,
2.66554034873299));
#231822=CARTESIAN_POINT('Ctrl Pts',(0.0700734120982157,62.8369299537506,
2.66766759644002));
#231823=CARTESIAN_POINT('Ctrl Pts',(0.076570577609309,62.8343031482015,
2.67012012783177));
#231824=CARTESIAN_POINT('Ctrl Pts',(0.0798191603648557,62.832989745427,
2.67134639352765));
#231825=CARTESIAN_POINT('Ctrl Pts',(0.0829981827951369,62.8315859904682,
2.67265375585041));
#231826=CARTESIAN_POINT('Ctrl Pts',(0.0861004173276806,62.8301000734876,
2.67403135126968));
#231827=CARTESIAN_POINT('Ctrl Pts',(0.0876515345939525,62.8293571149973,
2.67472014897932));
#231828=CARTESIAN_POINT('Ctrl Pts',(0.0891834722995143,62.8285936160521,
2.6754264966866));
#231829=CARTESIAN_POINT('Ctrl Pts',(0.0906954364276764,62.8278106008702,
2.67614899656129));
#231830=CARTESIAN_POINT('Ctrl Pts',(0.091073427459717,62.8276148470748,
2.67632962152996));
#231831=CARTESIAN_POINT('Ctrl Pts',(0.091450170514143,62.8274178735166,
2.67651125590977));
#231832=CARTESIAN_POINT('Ctrl Pts',(0.0918256539326503,62.827219696204,
2.67669387767551));
#231833=CARTESIAN_POINT('Ctrl Pts',(0.0929521041881723,62.8266251642661,
2.67724174297271));
#231834=CARTESIAN_POINT('Ctrl Pts',(0.0940672158684541,62.8260197985192,
2.67779849504774));
#231835=CARTESIAN_POINT('Ctrl Pts',(0.0951706907486432,62.8254040313375,
2.67836353618035));
#231836=CARTESIAN_POINT('Ctrl Pts',(0.10279638682729,62.8211486980558,2.68226832098931));
#231837=CARTESIAN_POINT('Ctrl Pts',(0.109916699411163,62.8164204928787,
2.68659153751411));
#231838=CARTESIAN_POINT('Ctrl Pts',(0.116542502759446,62.8113377077399,
2.69123699486194));
#231839=CARTESIAN_POINT('Ctrl Pts',(0.119835508836179,62.8088115774778,
2.69354577441236));
#231840=CARTESIAN_POINT('Ctrl Pts',(0.123006400629086,62.8061972539435,
2.69593478828141));
#231841=CARTESIAN_POINT('Ctrl Pts',(0.126056303769763,62.8035061084567,
2.69839565261247));
#231842=CARTESIAN_POINT('Ctrl Pts',(0.132784845643074,62.7975690395534,
2.70382468689072));
#231843=CARTESIAN_POINT('Ctrl Pts',(0.138932019324473,62.791268018738,2.70961155815114));
#231844=CARTESIAN_POINT('Ctrl Pts',(0.144445113412958,62.7847385034069,
2.71562701361794));
#231845=CARTESIAN_POINT('Ctrl Pts',(0.146459116207259,62.782353189115,2.71782453535886));
#231846=CARTESIAN_POINT('Ctrl Pts',(0.148396130390776,62.7799396422117,
2.7200505150243));
#231847=CARTESIAN_POINT('Ctrl Pts',(0.150257579786286,62.7775029828618,
2.72229986760145));
#231848=CARTESIAN_POINT('Ctrl Pts',(0.156509991333296,62.769318501945,2.72985520488891));
#231849=CARTESIAN_POINT('Ctrl Pts',(0.161942805717688,62.7608162581027,
2.73770845534525));
#231850=CARTESIAN_POINT('Ctrl Pts',(0.166635979461053,62.7520965944503,
2.74576706701686));
#231851=CARTESIAN_POINT('Ctrl Pts',(0.171794333348015,62.7425126511841,
2.75462443584931));
#231852=CARTESIAN_POINT('Ctrl Pts',(0.176059615357206,62.732665536351,2.7637303632305));
#231853=CARTESIAN_POINT('Ctrl Pts',(0.179500292056429,62.7226511116311,
2.77299664636653));
#231854=CARTESIAN_POINT('Ctrl Pts',(0.18320604828279,62.7118651471238,2.78297683033276));
#231855=CARTESIAN_POINT('Ctrl Pts',(0.185955767118902,62.7008840239666,
2.79314401478659));
#231856=CARTESIAN_POINT('Ctrl Pts',(0.187785458034874,62.6897991274278,
2.80341452427665));
#231857=CARTESIAN_POINT('Ctrl Pts',(0.189590441945833,62.6788639144185,
2.81354634721193));
#231858=CARTESIAN_POINT('Ctrl Pts',(0.190499999999787,62.6678262782736,
2.82378004209139));
#231859=CARTESIAN_POINT('Ctrl Pts',(0.190499999999787,62.6567671111301,
2.83404198860305));
#231860=CARTESIAN_POINT('Ctrl Pts',(0.190499999999799,59.2165773020943,
2.83404198860303));
#231861=CARTESIAN_POINT('Ctrl Pts',(0.190499999999799,59.2059936184297,
2.82422126443103));
#231862=CARTESIAN_POINT('Ctrl Pts',(0.189665225488488,59.1954479901469,
2.81442815028654));
#231863=CARTESIAN_POINT('Ctrl Pts',(0.188008762313989,59.1849969778471,
2.80471618166525));
#231864=CARTESIAN_POINT('Ctrl Pts',(0.186409301376948,59.174905605951,2.79533842146469));
#231865=CARTESIAN_POINT('Ctrl Pts',(0.184043455438172,59.1649012152161,
2.78603515650511));
#231866=CARTESIAN_POINT('Ctrl Pts',(0.180877423726733,59.1550396955548,
2.77685887347056));
#231867=CARTESIAN_POINT('Ctrl Pts',(0.177884532219648,59.145717471038,2.76818441216891));
#231868=CARTESIAN_POINT('Ctrl Pts',(0.174176304387194,59.1365220583465,
2.75962261521951));
#231869=CARTESIAN_POINT('Ctrl Pts',(0.169686797572706,59.1275197082968,
2.75123537701997));
#231870=CARTESIAN_POINT('Ctrl Pts',(0.165552037113637,59.1192286949267,
2.74351087134457));
#231871=CARTESIAN_POINT('Ctrl Pts',(0.160754293903984,59.11110097861,2.73593399450185));
#231872=CARTESIAN_POINT('Ctrl Pts',(0.15521351501367,59.1032135992736,2.72857657812913));
#231873=CARTESIAN_POINT('Ctrl Pts',(0.153561366596213,59.1008617419722,
2.72638274508555));
#231874=CARTESIAN_POINT('Ctrl Pts',(0.151842962927752,59.0985314603585,
2.7242086170973));
#231875=CARTESIAN_POINT('Ctrl Pts',(0.150055686179941,59.0962253759572,
2.72205663736749));
#231876=CARTESIAN_POINT('Ctrl Pts',(0.148286670996507,59.0939428540561,
2.71992664556788));
#231877=CARTESIAN_POINT('Ctrl Pts',(0.146452235168703,59.091686238035,2.71782089927906));
#231878=CARTESIAN_POINT('Ctrl Pts',(0.144552116609766,59.0894604907301,
2.71574387311268));
#231879=CARTESIAN_POINT('Ctrl Pts',(0.144419986081219,59.0893057166154,
2.71559944077508));
#231880=CARTESIAN_POINT('Ctrl Pts',(0.144287542501899,59.0891510807053,
2.71545515216091));
#231881=CARTESIAN_POINT('Ctrl Pts',(0.144154785043744,59.0889965840076,
2.71531100781752));
#231882=CARTESIAN_POINT('Ctrl Pts',(0.138334211749285,59.0822228828155,
2.70899119176102));
#231883=CARTESIAN_POINT('Ctrl Pts',(0.131883990153856,59.0757535782846,
2.70298296066855));
#231884=CARTESIAN_POINT('Ctrl Pts',(0.124808417215017,59.0697047694308,
2.69736727774151));
#231885=CARTESIAN_POINT('Ctrl Pts',(0.118212753509691,59.0640662283032,
2.69213248525436));
#231886=CARTESIAN_POINT('Ctrl Pts',(0.111072931136892,59.0587927761312,
2.68723866185469));
#231887=CARTESIAN_POINT('Ctrl Pts',(0.103389544767648,59.0540076654697,
2.68278595829559));
#231888=CARTESIAN_POINT('Ctrl Pts',(0.100578862632195,59.0522572100837,
2.6811571017281));
#231889=CARTESIAN_POINT('Ctrl Pts',(0.0976954648434748,59.0505724231958,
2.67958763637823));
#231890=CARTESIAN_POINT('Ctrl Pts',(0.0947395585251495,59.0489605442862,
2.67808378645385));
#231891=CARTESIAN_POINT('Ctrl Pts',(0.0940287618036534,59.0485729412565,
2.6777221607862));
#231892=CARTESIAN_POINT('Ctrl Pts',(0.093313192216558,59.0481896206936,
2.67736403603583));
#231893=CARTESIAN_POINT('Ctrl Pts',(0.0925929271969717,59.0478106940138,
2.67700956934499));
#231894=CARTESIAN_POINT('Ctrl Pts',(0.0918951704592475,59.0474436087928,
2.67666617973824));
#231895=CARTESIAN_POINT('Ctrl Pts',(0.0911930071932301,59.0470806471273,
2.67632622314139));
#231896=CARTESIAN_POINT('Ctrl Pts',(0.0904865115876316,59.0467219102891,
2.67598984158794));
#231897=CARTESIAN_POINT('Ctrl Pts',(0.0827460357498814,59.0427915336444,
2.6723043929225));
#231898=CARTESIAN_POINT('Ctrl Pts',(0.0744802459945514,59.0393660724133,
2.66904964540011));
#231899=CARTESIAN_POINT('Ctrl Pts',(0.0658168714613306,59.0365841602693,
2.66640203566765));
#231900=CARTESIAN_POINT('Ctrl Pts',(0.0622239118146019,59.0354304183832,
2.66530399299472));
#231901=CARTESIAN_POINT('Ctrl Pts',(0.0585629032865241,59.0343871039219,
2.66430995142284));
#231902=CARTESIAN_POINT('Ctrl Pts',(0.0548440714997765,59.0334626554263,
2.6634305347338));
#231903=CARTESIAN_POINT('Ctrl Pts',(0.0485012163582087,59.0318859121829,
2.66193059792904));
#231904=CARTESIAN_POINT('Ctrl Pts',(0.0419914004942172,59.0306571138139,
2.66076519817147));
#231905=CARTESIAN_POINT('Ctrl Pts',(0.0353717968086142,59.029821295816,
2.65997805604479));
#231906=CARTESIAN_POINT('Ctrl Pts',(0.0320619949658128,59.0294033868171,
2.65958448498145));
#231907=CARTESIAN_POINT('Ctrl Pts',(0.0287246785544705,59.0290851681643,
2.65928526260781));
#231908=CARTESIAN_POINT('Ctrl Pts',(0.0253670368746644,59.0288723192869,
2.65908463971343));
#231909=CARTESIAN_POINT('Ctrl Pts',(0.0220093951948583,59.0286594704096,
2.65888401681906));
#231910=CARTESIAN_POINT('Ctrl Pts',(0.0186314705078071,59.0285519740193,
2.65878198860303));
#231911=CARTESIAN_POINT('Ctrl Pts',(0.0152399999997995,59.0285534841298,
2.65878198860303));
#231912=CARTESIAN_POINT('Origin',(-6.10537907909402,57.943004080846,2.83404198860303));
#231913=CARTESIAN_POINT('Ctrl Pts',(-6.73887200051354,62.2936141127571,
2.83404198860306));
#231914=CARTESIAN_POINT('Ctrl Pts',(-6.73998108195343,62.3041663177857,
2.82419652440124));
#231915=CARTESIAN_POINT('Ctrl Pts',(-6.74025426844111,62.314774722767,2.81438790575723));
#231916=CARTESIAN_POINT('Ctrl Pts',(-6.73970068257616,62.3253809467524,
2.80466781256989));
#231917=CARTESIAN_POINT('Ctrl Pts',(-6.73916508495544,62.3356425316142,
2.79526356453176));
#231918=CARTESIAN_POINT('Ctrl Pts',(-6.73785543637676,62.3459033574827,
2.7859410249634));
#231919=CARTESIAN_POINT('Ctrl Pts',(-6.73573381164817,62.3561113603648,
2.77675109088895));
#231920=CARTESIAN_POINT('Ctrl Pts',(-6.73372688529703,62.3657675025186,
2.76805797913806));
#231921=CARTESIAN_POINT('Ctrl Pts',(-6.73099321743857,62.3753772873478,
2.75948271210292));
#231922=CARTESIAN_POINT('Ctrl Pts',(-6.72746117704631,62.3848821415107,
2.7510857557336));
#231923=CARTESIAN_POINT('Ctrl Pts',(-6.72420791240138,62.3936367996034,
2.74335155163412));
#231924=CARTESIAN_POINT('Ctrl Pts',(-6.72027708243781,62.4023029414995,
2.7357681868609));
#231925=CARTESIAN_POINT('Ctrl Pts',(-6.71558140886385,62.4108128192383,
2.72840626160649));
#231926=CARTESIAN_POINT('Ctrl Pts',(-6.71421937245599,62.4132812112856,
2.72627084693795));
#231927=CARTESIAN_POINT('Ctrl Pts',(-6.71279278199563,62.4157362792957,
2.72415424587601));
#231928=CARTESIAN_POINT('Ctrl Pts',(-6.71129899689619,62.4181758915951,
2.72205867173302));
#231929=CARTESIAN_POINT('Ctrl Pts',(-6.7096796378069,62.4208205881803,2.71978693462904));
#231930=CARTESIAN_POINT('Ctrl Pts',(-6.70798448411195,62.4234440047031,
2.71754411340805));
#231931=CARTESIAN_POINT('Ctrl Pts',(-6.70621108803144,62.4260429761975,
2.71533341844301));
#231932=CARTESIAN_POINT('Ctrl Pts',(-6.70134398857289,62.4331758738577,
2.70926614876449));
#231933=CARTESIAN_POINT('Ctrl Pts',(-6.69585818364715,62.4400912556839,
2.70347381860466));
#231934=CARTESIAN_POINT('Ctrl Pts',(-6.68976801333909,62.4466864116143,
2.69804914171452));
#231935=CARTESIAN_POINT('Ctrl Pts',(-6.6841958381505,62.452720621231,2.69308585687282));
#231936=CARTESIAN_POINT('Ctrl Pts',(-6.67811620689388,62.4584752900412,
2.6884279905328));
#231937=CARTESIAN_POINT('Ctrl Pts',(-6.67150703079278,62.4638645712582,
2.68414767054326));
#231938=CARTESIAN_POINT('Ctrl Pts',(-6.66826062508134,62.4665117685875,
2.68204519134642));
#231939=CARTESIAN_POINT('Ctrl Pts',(-6.66488629458029,62.46907032323,2.68003431778574));
#231940=CARTESIAN_POINT('Ctrl Pts',(-6.66138078591733,62.471526773642,2.67812693945309));
#231941=CARTESIAN_POINT('Ctrl Pts',(-6.6607156497927,62.4719928611815,2.67776503299261));
#231942=CARTESIAN_POINT('Ctrl Pts',(-6.66004526561012,62.4724551899382,
2.67740659639981));
#231943=CARTESIAN_POINT('Ctrl Pts',(-6.6593696982088,62.472913635813,2.67705178968912));
#231944=CARTESIAN_POINT('Ctrl Pts',(-6.65871524228878,62.4733577552543,
2.67670807068815));
#231945=CARTESIAN_POINT('Ctrl Pts',(-6.65805592206474,62.4737982307001,
2.67636775825322));
#231946=CARTESIAN_POINT('Ctrl Pts',(-6.65739180030932,62.4742349489461,
2.67603099699312));
#231947=CARTESIAN_POINT('Ctrl Pts',(-6.65015433826405,62.4789942144028,
2.67236104217171));
#231948=CARTESIAN_POINT('Ctrl Pts',(-6.64234165497423,62.4833100626584,
2.66911440541505));
#231949=CARTESIAN_POINT('Ctrl Pts',(-6.63406423386074,62.4870273554133,
2.66646778189657));
#231950=CARTESIAN_POINT('Ctrl Pts',(-6.63056862752469,62.4885971912268,
2.66535009635012));
#231951=CARTESIAN_POINT('Ctrl Pts',(-6.62699051141362,62.4900605069393,
2.66433897912393));
#231952=CARTESIAN_POINT('Ctrl Pts',(-6.62333954252022,62.4914070226223,
2.6634456488485));
#231953=CARTESIAN_POINT('Ctrl Pts',(-6.61719140213093,62.4936745213869,
2.66194130298643));
#231954=CARTESIAN_POINT('Ctrl Pts',(-6.61083770188548,62.4956084911392,
2.66077206705477));
#231955=CARTESIAN_POINT('Ctrl Pts',(-6.60433062536177,62.4971561593227,
2.65998225155772));
#231956=CARTESIAN_POINT('Ctrl Pts',(-6.60270385623084,62.4975430763686,
2.65978479768346));
#231957=CARTESIAN_POINT('Ctrl Pts',(-6.60106746196587,62.497905618889,2.6596109896668));
#231958=CARTESIAN_POINT('Ctrl Pts',(-6.59942221845775,62.4982426563701,
2.65946139030559));
#231959=CARTESIAN_POINT('Ctrl Pts',(-6.59695435319557,62.4987482125918,
2.65923699126377));
#231960=CARTESIAN_POINT('Ctrl Pts',(-6.59446659126629,62.4991963674678,
2.65906707562499));
#231961=CARTESIAN_POINT('Ctrl Pts',(-6.5919617450032,62.4995849724125,2.65895332562977));
#231962=CARTESIAN_POINT('Ctrl Pts',(-6.58945689874012,62.4999735773573,
2.65883957563454));
#231963=CARTESIAN_POINT('Ctrl Pts',(-6.58693497617671,62.5003026407463,
2.65878198860306));
#231964=CARTESIAN_POINT('Ctrl Pts',(-6.58439859103049,62.5005702980932,
2.65878198860306));
#231965=CARTESIAN_POINT('Ctrl Pts',(-6.18532049829418,58.7035958781041,
2.65878198860303));
#231966=CARTESIAN_POINT('Ctrl Pts',(-6.19390281910233,58.7026899760171,
2.65878198860303));
#231967=CARTESIAN_POINT('Ctrl Pts',(-6.20248552904501,58.702500360993,2.65945335517904));
#231968=CARTESIAN_POINT('Ctrl Pts',(-6.21093474935611,58.7029569544316,
2.66072561226664));
#231969=CARTESIAN_POINT('Ctrl Pts',(-6.21639207873623,58.7032518669437,
2.661547359804));
#231970=CARTESIAN_POINT('Ctrl Pts',(-6.22179377937587,58.7038154335201,
2.66261895766937));
#231971=CARTESIAN_POINT('Ctrl Pts',(-6.22710604846885,58.7046202140518,
2.6639142925107));
#231972=CARTESIAN_POINT('Ctrl Pts',(-6.23414715684661,58.7056869045459,
2.66563118464166));
#231973=CARTESIAN_POINT('Ctrl Pts',(-6.24102913891663,58.7071827955654,
2.66774105138742));
#231974=CARTESIAN_POINT('Ctrl Pts',(-6.24767922440765,58.7090548163571,
2.67016894181793));
#231975=CARTESIAN_POINT('Ctrl Pts',(-6.25100426715316,58.709990826753,2.67138288703318));
#231976=CARTESIAN_POINT('Ctrl Pts',(-6.2542715337668,58.711020847023,2.67267613167594));
#231977=CARTESIAN_POINT('Ctrl Pts',(-6.25747333351535,58.7121380880309,
2.67403835432596));
#231978=CARTESIAN_POINT('Ctrl Pts',(-6.25907423338963,58.7126967085349,
2.67471946565097));
#231979=CARTESIAN_POINT('Ctrl Pts',(-6.26065878288361,58.7132771324573,
2.67541781389566));
#231980=CARTESIAN_POINT('Ctrl Pts',(-6.26222612320533,58.7138784999417,
2.67613207244212));
#231981=CARTESIAN_POINT('Ctrl Pts',(-6.26261795828575,58.7140288418128,
2.67631063707873));
#231982=CARTESIAN_POINT('Ctrl Pts',(-6.26300871814027,58.714180492618,2.67649019601888));
#231983=CARTESIAN_POINT('Ctrl Pts',(-6.26339839005071,58.7143334388437,
2.676670728367));
#231984=CARTESIAN_POINT('Ctrl Pts',(-6.26456740578202,58.7147922775209,
2.67721232541133));
#231985=CARTESIAN_POINT('Ctrl Pts',(-6.26572662828387,58.7152627751832,
2.6777626834009));
#231986=CARTESIAN_POINT('Ctrl Pts',(-6.26687572965181,58.7157445651925,
2.67832123541559));
#231987=CARTESIAN_POINT('Ctrl Pts',(-6.27496985131174,58.7191382318081,
2.68225560368494));
#231988=CARTESIAN_POINT('Ctrl Pts',(-6.28260716192813,58.7230632421221,
2.68661792998947));
#231989=CARTESIAN_POINT('Ctrl Pts',(-6.289783395895,58.7274000190317,2.69130986622646));
#231990=CARTESIAN_POINT('Ctrl Pts',(-6.29326386161406,58.7295033511465,
2.69358545023115));
#231991=CARTESIAN_POINT('Ctrl Pts',(-6.29663597408954,58.7317041096973,
2.69593918853521));
#231992=CARTESIAN_POINT('Ctrl Pts',(-6.29989941779165,58.7339915094195,
2.69836306235517));
#231993=CARTESIAN_POINT('Ctrl Pts',(-6.30489552208954,58.7374933585784,
2.7020738438225));
#231994=CARTESIAN_POINT('Ctrl Pts',(-6.30963480180889,58.7411954596219,
2.7059476081425));
#231995=CARTESIAN_POINT('Ctrl Pts',(-6.31410463171064,58.7450534628852,
2.7099519634573));
#231996=CARTESIAN_POINT('Ctrl Pts',(-6.31618044384085,58.7468451395593,
2.71181160678128));
#231997=CARTESIAN_POINT('Ctrl Pts',(-6.31819823791545,58.7486702031825,
2.71369962772121));
#231998=CARTESIAN_POINT('Ctrl Pts',(-6.32015576082334,58.7505249478607,
2.71561183138683));
#231999=CARTESIAN_POINT('Ctrl Pts',(-6.3203057972412,58.7506671067322,2.71575839426334));
#232000=CARTESIAN_POINT('Ctrl Pts',(-6.32045551058208,58.7508094261761,
2.71590508903231));
#232001=CARTESIAN_POINT('Ctrl Pts',(-6.32060490094017,58.7509519047348,
2.71605191409934));
#232002=CARTESIAN_POINT('Ctrl Pts',(-6.32270338507401,58.7529532989258,
2.71811436362775));
#232003=CARTESIAN_POINT('Ctrl Pts',(-6.32473679726646,58.7549876922217,
2.72020091026982));
#232004=CARTESIAN_POINT('Ctrl Pts',(-6.32670504965004,58.7570493794211,
2.72230624862204));
#232005=CARTESIAN_POINT('Ctrl Pts',(-6.33376285265597,58.76444222306,2.72985561753164));
#232006=CARTESIAN_POINT('Ctrl Pts',(-6.34003880538957,58.7722418109931,
2.73770089914433));
#232007=CARTESIAN_POINT('Ctrl Pts',(-6.34560292136785,58.7803396486564,
2.74574823347221));
#232008=CARTESIAN_POINT('Ctrl Pts',(-6.35171732586278,58.7892383587482,
2.75459144547185));
#232009=CARTESIAN_POINT('Ctrl Pts',(-6.35697262978514,58.798497673091,2.76367911754444));
#232010=CARTESIAN_POINT('Ctrl Pts',(-6.36142852992882,58.8080148760666,
2.77292162564914));
#232011=CARTESIAN_POINT('Ctrl Pts',(-6.3662397838055,58.8182910667879,2.78290121484888));
#232012=CARTESIAN_POINT('Ctrl Pts',(-6.37011968263775,58.8288688921864,
2.79306229500313));
#232013=CARTESIAN_POINT('Ctrl Pts',(-6.37309732669844,58.8396533761891,
2.80331916685345));
#232014=CARTESIAN_POINT('Ctrl Pts',(-6.37604999138494,58.8503473894518,
2.81348999408769));
#232015=CARTESIAN_POINT('Ctrl Pts',(-6.37811557911251,58.8612460403467,
2.82375635966934));
#232016=CARTESIAN_POINT('Ctrl Pts',(-6.37927424642597,58.8722700234482,
2.83404198860304));
#232017=CARTESIAN_POINT('Origin',(0.0151565136854187,0.00159301378038297,
2.83404198860263));
#232018=CARTESIAN_POINT('Ctrl Pts',(-6.55408556365967,62.5037563256536,
2.65878198860306));
#232019=CARTESIAN_POINT('Ctrl Pts',(-6.54554330587443,62.5046505412979,
2.65878198860306));
#232020=CARTESIAN_POINT('Ctrl Pts',(-6.53700226086713,62.504823232088,2.65944603041887));
#232021=CARTESIAN_POINT('Ctrl Pts',(-6.52859457177513,62.5043472028591,
2.66070439264094));
#232022=CARTESIAN_POINT('Ctrl Pts',(-6.52322245869536,62.5040430428433,
2.6615084261962));
#232023=CARTESIAN_POINT('Ctrl Pts',(-6.51790471489646,62.5034749678474,
2.66255428265399));
#232024=CARTESIAN_POINT('Ctrl Pts',(-6.5126735674088,62.5026702669709,2.66381699700695));
#232025=CARTESIAN_POINT('Ctrl Pts',(-6.50553410072683,62.5015720117391,
2.66554034873295));
#232026=CARTESIAN_POINT('Ctrl Pts',(-6.49855818190805,62.50002734281,2.66766759644));
#232027=CARTESIAN_POINT('Ctrl Pts',(-6.49182203260205,62.4980940659031,
2.67012012783176));
#232028=CARTESIAN_POINT('Ctrl Pts',(-6.48845395794905,62.4971274274497,
2.67134639352764));
#232029=CARTESIAN_POINT('Ctrl Pts',(-6.48514561818761,62.4960636607367,
2.6726537558504));
#232030=CARTESIAN_POINT('Ctrl Pts',(-6.48190505740187,62.4949101555731,
2.67403135126968));
#232031=CARTESIAN_POINT('Ctrl Pts',(-6.48028477700901,62.4943334029914,
2.67472014897932));
#232032=CARTESIAN_POINT('Ctrl Pts',(-6.47868142404703,62.4937342176675,
2.67542649668661));
#232033=CARTESIAN_POINT('Ctrl Pts',(-6.47709589524288,62.4931135352115,
2.67614899656131));
#232034=CARTESIAN_POINT('Ctrl Pts',(-6.47669951304184,62.4929583645975,
2.67632962152998));
#232035=CARTESIAN_POINT('Ctrl Pts',(-6.47630424448194,62.4928018504536,
2.67651125590979));
#232036=CARTESIAN_POINT('Ctrl Pts',(-6.47591010283095,62.4926440074818,
2.67669387767552));
#232037=CARTESIAN_POINT('Ctrl Pts',(-6.47472767787795,62.4921704785663,
2.67724174297273));
#232038=CARTESIAN_POINT('Ctrl Pts',(-6.47355539694488,62.4916849899866,
2.67779849504777));
#232039=CARTESIAN_POINT('Ctrl Pts',(-6.4723936018183,62.4911879405754,2.67836353618038));
#232040=CARTESIAN_POINT('Ctrl Pts',(-6.46436487665209,62.4877530207471,
2.68226832098932));
#232041=CARTESIAN_POINT('Ctrl Pts',(-6.45678933786442,62.4837949925051,
2.68659153751408));
#232042=CARTESIAN_POINT('Ctrl Pts',(-6.44966853564051,62.479432636437,2.69123699486188));
#232043=CARTESIAN_POINT('Ctrl Pts',(-6.44612951648126,62.4772645574456,
2.69354577441232));
#232044=CARTESIAN_POINT('Ctrl Pts',(-6.4427027239438,62.4749960038954,2.69593478828139));
#232045=CARTESIAN_POINT('Ctrl Pts',(-6.43938822718944,62.4726384024735,
2.69839565261248));
#232046=CARTESIAN_POINT('Ctrl Pts',(-6.43207595228374,62.4674371815969,
2.70382468689073));
#232047=CARTESIAN_POINT('Ctrl Pts',(-6.42530381744011,62.4618132330512,
2.70961155815114));
#232048=CARTESIAN_POINT('Ctrl Pts',(-6.41913840445445,62.4558957623412,
2.71562701361794));
#232049=CARTESIAN_POINT('Ctrl Pts',(-6.41688610134085,62.4537340356676,
2.71782453535884));
#232050=CARTESIAN_POINT('Ctrl Pts',(-6.41470741397488,62.4515361835427,
2.72005051502428));
#232051=CARTESIAN_POINT('Ctrl Pts',(-6.41260146153658,62.4493074469124,
2.72229986760141));
#232052=CARTESIAN_POINT('Ctrl Pts',(-6.40552779014104,62.4418213564088,
2.72985520488918));
#232053=CARTESIAN_POINT('Ctrl Pts',(-6.39923601079888,62.4339335724863,
2.73770845534586));
#232054=CARTESIAN_POINT('Ctrl Pts',(-6.39365709371034,62.4257522463025,
2.74576706701784));
#232055=CARTESIAN_POINT('Ctrl Pts',(-6.38752520296386,62.4167599996847,
2.75462443585064));
#232056=CARTESIAN_POINT('Ctrl Pts',(-6.38225398283455,62.4074126717503,
2.76373036323221));
#232057=CARTESIAN_POINT('Ctrl Pts',(-6.37778536209576,62.3978127557445,
2.77299664636864));
#232058=CARTESIAN_POINT('Ctrl Pts',(-6.37297246609489,62.3874732348825,
2.78297683033526));
#232059=CARTESIAN_POINT('Ctrl Pts',(-6.36908997057771,62.3768396913508,
2.79314401478951));
#232060=CARTESIAN_POINT('Ctrl Pts',(-6.36611161569943,62.3660067738143,
2.80341452428));
#232061=CARTESIAN_POINT('Ctrl Pts',(-6.36317347866837,62.3553201372418,
2.81354634721418));
#232062=CARTESIAN_POINT('Ctrl Pts',(-6.36111515612462,62.3444380411295,
2.82378004209251));
#232063=CARTESIAN_POINT('Ctrl Pts',(-6.35995915837823,62.3334394572621,
2.83404198860306));
#232064=CARTESIAN_POINT('Ctrl Pts',(-6.00036140429066,58.9120953679532,
2.83404198860303));
#232065=CARTESIAN_POINT('Ctrl Pts',(-5.99925510810147,58.9015696628149,
2.82422126443092));
#232066=CARTESIAN_POINT('Ctrl Pts',(-5.99898299131208,58.8909945468903,
2.8144281502863));
#232067=CARTESIAN_POINT('Ctrl Pts',(-5.99953795195273,58.8804276387792,
2.80471618166489));
#232068=CARTESIAN_POINT('Ctrl Pts',(-6.00007381527886,58.8702243592803,
2.79533842146428));
#232069=CARTESIAN_POINT('Ctrl Pts',(-6.00138095727663,58.8600274754043,
2.78603515650465));
#232070=CARTESIAN_POINT('Ctrl Pts',(-6.00349883563944,58.84988903775,2.77685887347006));
#232071=CARTESIAN_POINT('Ctrl Pts',(-6.00550089397075,58.8403050390046,
2.76818441216843));
#232072=CARTESIAN_POINT('Ctrl Pts',(-6.0082276253854,58.8307723843892,2.75962261521906));
#232073=CARTESIAN_POINT('Ctrl Pts',(-6.01175153639534,58.8213500689069,
2.75123537701956));
#232074=CARTESIAN_POINT('Ctrl Pts',(-6.01499699931747,58.8126722744189,
2.74351087134424));
#232075=CARTESIAN_POINT('Ctrl Pts',(-6.01891888229134,58.8040875818577,
2.7359339945016));
#232076=CARTESIAN_POINT('Ctrl Pts',(-6.02360485257387,58.795664241308,2.72857657812896));
#232077=CARTESIAN_POINT('Ctrl Pts',(-6.02500211431986,58.7931525711919,
2.72638274508544));
#232078=CARTESIAN_POINT('Ctrl Pts',(-6.02646752363713,58.79065543301,2.72420861709724));
#232079=CARTESIAN_POINT('Ctrl Pts',(-6.02800395803724,58.7881751602885,
2.72205663736749));
#232080=CARTESIAN_POINT('Ctrl Pts',(-6.02952469386371,58.7857202298426,
2.71992664556788));
#232081=CARTESIAN_POINT('Ctrl Pts',(-6.03111319985523,58.7832842250421,
2.71782089927907));
#232082=CARTESIAN_POINT('Ctrl Pts',(-6.03277025542048,58.7808720541409,
2.71574387311268));
#232083=CARTESIAN_POINT('Ctrl Pts',(-6.03288548382381,58.7807043164939,
2.71559944077509));
#232084=CARTESIAN_POINT('Ctrl Pts',(-6.03300103800929,58.7805366835716,
2.71545515216092));
#232085=CARTESIAN_POINT('Ctrl Pts',(-6.03311691890581,58.78036915629,2.71531100781753));
#232086=CARTESIAN_POINT('Ctrl Pts',(-6.03819756191452,58.7730241465599,
2.70899119176101));
#232087=CARTESIAN_POINT('Ctrl Pts',(-6.04393622206015,58.765916049805,2.70298296066851));
#232088=CARTESIAN_POINT('Ctrl Pts',(-6.05034076157604,58.759160778193,2.69736727774145));
#232089=CARTESIAN_POINT('Ctrl Pts',(-6.05631090550631,58.7528636909922,
2.69213248525432));
#232090=CARTESIAN_POINT('Ctrl Pts',(-6.06286038933342,58.7468728126824,
2.68723866185467));
#232091=CARTESIAN_POINT('Ctrl Pts',(-6.07000150504417,58.741310782788,2.68278595829558));
#232092=CARTESIAN_POINT('Ctrl Pts',(-6.07261381755728,58.7392761202954,
2.68115710172809));
#232093=CARTESIAN_POINT('Ctrl Pts',(-6.0753053116069,58.7372991657065,2.67958763637822));
#232094=CARTESIAN_POINT('Ctrl Pts',(-6.07807653793573,58.7353871404932,
2.67808378645384));
#232095=CARTESIAN_POINT('Ctrl Pts',(-6.07874292528937,58.7349273623045,
2.67772216078619));
#232096=CARTESIAN_POINT('Ctrl Pts',(-6.07941450700202,58.7344713442225,
2.67736403603582));
#232097=CARTESIAN_POINT('Ctrl Pts',(-6.08009121771093,58.734019205147,2.67700956934498));
#232098=CARTESIAN_POINT('Ctrl Pts',(-6.08074678121019,58.7335811954177,
2.67666617973823));
#232099=CARTESIAN_POINT('Ctrl Pts',(-6.08140715812725,58.7331468260469,
2.67632622314138));
#232100=CARTESIAN_POINT('Ctrl Pts',(-6.08207228526558,58.7327162055067,
2.67598984158792));
#232101=CARTESIAN_POINT('Ctrl Pts',(-6.08935952173624,58.7279982598322,
2.6723043929224));
#232102=CARTESIAN_POINT('Ctrl Pts',(-6.09722197243217,58.7237275533352,
2.66904964539994));
#232103=CARTESIAN_POINT('Ctrl Pts',(-6.1055470990921,58.7200553115704,2.66640203566744));
#232104=CARTESIAN_POINT('Ctrl Pts',(-6.10899977726339,58.7185323234527,
2.66530399299459));
#232105=CARTESIAN_POINT('Ctrl Pts',(-6.11253167434615,58.7171120447817,
2.66430995142278));
#232106=CARTESIAN_POINT('Ctrl Pts',(-6.11613350280244,58.71580393674,2.66343053473379));
#232107=CARTESIAN_POINT('Ctrl Pts',(-6.12227679657168,58.7135728221604,
2.66193059792903));
#232108=CARTESIAN_POINT('Ctrl Pts',(-6.12862250657805,58.711670294229,2.66076519817146));
#232109=CARTESIAN_POINT('Ctrl Pts',(-6.13511848061116,58.7101471179289,
2.65997805604479));
#232110=CARTESIAN_POINT('Ctrl Pts',(-6.13836646762772,58.7093855297788,
2.65958448498145));
#232111=CARTESIAN_POINT('Ctrl Pts',(-6.1416522389638,58.7087202098051,2.65928526260781));
#232112=CARTESIAN_POINT('Ctrl Pts',(-6.14496923836511,58.7081575578112,
2.65908463971344));
#232113=CARTESIAN_POINT('Ctrl Pts',(-6.14828623776642,58.7075949058173,
2.65888401681906));
#232114=CARTESIAN_POINT('Ctrl Pts',(-6.15163442139611,58.7071349090269,
2.65878198860303));
#232115=CARTESIAN_POINT('Ctrl Pts',(-6.15500747092336,58.7067819056644,
2.65878198860303));
#232116=CARTESIAN_POINT('Origin',(-12.1286263473646,56.9874003490103,2.83404198860302));
#232117=CARTESIAN_POINT('Ctrl Pts',(-13.2134115091896,61.2479592423879,
2.83404198860304));
#232118=CARTESIAN_POINT('Ctrl Pts',(-13.215617520741,61.2583377107545,2.82419652440144));
#232119=CARTESIAN_POINT('Ctrl Pts',(-13.2169980909549,61.2688594460195,
2.81438790575762));
#232120=CARTESIAN_POINT('Ctrl Pts',(-13.2175561899856,61.2794654334797,
2.80466781257047));
#232121=CARTESIAN_POINT('Ctrl Pts',(-13.218096154121,61.289726789502,2.7952635645325));
#232122=CARTESIAN_POINT('Ctrl Pts',(-13.2178662282942,61.3000683010459,
2.78594102496429));
#232123=CARTESIAN_POINT('Ctrl Pts',(-13.2168232529022,61.3104421535925,
2.77675109088998));
#232124=CARTESIAN_POINT('Ctrl Pts',(-13.2158366624041,61.3202551793165,
2.76805797913924));
#232125=CARTESIAN_POINT('Ctrl Pts',(-13.2141224659049,61.330098066839,2.75948271210423));
#232126=CARTESIAN_POINT('Ctrl Pts',(-13.2116033021988,61.3399200511706,
2.75108575573504));
#232127=CARTESIAN_POINT('Ctrl Pts',(-13.209282970235,61.3489668090839,2.74335155163569));
#232128=CARTESIAN_POINT('Ctrl Pts',(-13.2062795322643,61.3579963605632,
2.73576818686259));
#232129=CARTESIAN_POINT('Ctrl Pts',(-13.2024991065243,61.3669504518439,
2.72840626160828));
#232130=CARTESIAN_POINT('Ctrl Pts',(-13.2014025487215,61.3695476933546,
2.72627084693913));
#232131=CARTESIAN_POINT('Ctrl Pts',(-13.200240397759,61.3721384315545,2.7241542458766));
#232132=CARTESIAN_POINT('Ctrl Pts',(-13.1990098046949,61.3747208224641,
2.72205867173302));
#232133=CARTESIAN_POINT('Ctrl Pts',(-13.197675762694,61.3775203002418,2.71978693462904));
#232134=CARTESIAN_POINT('Ctrl Pts',(-13.196264116926,61.3803065372251,2.71754411340804));
#232135=CARTESIAN_POINT('Ctrl Pts',(-13.1947721021912,61.3830766416488,
2.71533341844301));
#232136=CARTESIAN_POINT('Ctrl Pts',(-13.1906772560438,61.3906792149762,
2.70926614876448));
#232137=CARTESIAN_POINT('Ctrl Pts',(-13.1859443571666,61.3981301363759,
2.70347381860465));
#232138=CARTESIAN_POINT('Ctrl Pts',(-13.1805769309631,61.4053257594954,
2.69804914171452));
#232139=CARTESIAN_POINT('Ctrl Pts',(-13.1756660273915,61.41190936399,2.69308585687282));
#232140=CARTESIAN_POINT('Ctrl Pts',(-13.1702212276784,61.4182680026348,
2.68842799053281));
#232141=CARTESIAN_POINT('Ctrl Pts',(-13.1642115906192,61.4243186078267,
2.68414767054327));
#232142=CARTESIAN_POINT('Ctrl Pts',(-13.1612596765268,61.4272906453322,
2.68204519134642));
#232143=CARTESIAN_POINT('Ctrl Pts',(-13.1581712727462,61.4301878975265,
2.68003431778575));
#232144=CARTESIAN_POINT('Ctrl Pts',(-13.1549417366132,61.4329973166797,
2.67812693945308));
#232145=CARTESIAN_POINT('Ctrl Pts',(-13.1543289635881,61.4335303765998,
2.6777650329926));
#232146=CARTESIAN_POINT('Ctrl Pts',(-13.1537105783546,61.4340602468996,
2.67740659639981));
#232147=CARTESIAN_POINT('Ctrl Pts',(-13.153086632425,61.4345867973823,2.67705178968912));
#232148=CARTESIAN_POINT('Ctrl Pts',(-13.1524821848057,61.4350968931624,
2.67670807068815));
#232149=CARTESIAN_POINT('Ctrl Pts',(-13.1518725186283,61.4356038733674,
2.67636775825323));
#232150=CARTESIAN_POINT('Ctrl Pts',(-13.1512576844885,61.4361076188516,
2.67603099699312));
#232151=CARTESIAN_POINT('Ctrl Pts',(-13.1445573487222,61.4415973333397,
2.67236104217181));
#232152=CARTESIAN_POINT('Ctrl Pts',(-13.137238593115,61.446706186705,2.66911440541524));
#232153=CARTESIAN_POINT('Ctrl Pts',(-13.1293950794799,61.45126834185,2.66646778189679));
#232154=CARTESIAN_POINT('Ctrl Pts',(-13.126082714966,61.4531949682972,2.66535009635026));
#232155=CARTESIAN_POINT('Ctrl Pts',(-13.1226771582919,61.4550242827918,
2.66433897912399));
#232156=CARTESIAN_POINT('Ctrl Pts',(-13.119186939003,61.456745052289,2.6634456488485));
#232157=CARTESIAN_POINT('Ctrl Pts',(-13.1133094969314,61.459642785125,2.66194130298642));
#232158=CARTESIAN_POINT('Ctrl Pts',(-13.1071927578069,61.4622303029114,
2.66077206705477));
#232159=CARTESIAN_POINT('Ctrl Pts',(-13.1008831031061,61.4644496675159,
2.65998225155771));
#232160=CARTESIAN_POINT('Ctrl Pts',(-13.0993056894308,61.4650045086671,
2.65978479768345));
#232161=CARTESIAN_POINT('Ctrl Pts',(-13.0977161555174,61.4655361149194,
2.65961098966679));
#232162=CARTESIAN_POINT('Ctrl Pts',(-13.0961151548353,61.4660432808496,
2.65946139030558));
#232163=CARTESIAN_POINT('Ctrl Pts',(-13.0937136538122,61.4668040297448,
2.65923699126377));
#232164=CARTESIAN_POINT('Ctrl Pts',(-13.0912863650436,61.467509771513,2.65906707562498));
#232165=CARTESIAN_POINT('Ctrl Pts',(-13.0888358608681,61.4681580753698,
2.65895332562976));
#232166=CARTESIAN_POINT('Ctrl Pts',(-13.0863853566927,61.4688063792266,
2.65883957563454));
#232167=CARTESIAN_POINT('Ctrl Pts',(-13.0839116459753,61.469397252662,2.65878198860305));
#232168=CARTESIAN_POINT('Ctrl Pts',(-13.0814171332235,61.4699285681956,
2.65878198860305));
#232169=CARTESIAN_POINT('Ctrl Pts',(-12.2876333308473,57.7354693911206,
2.65878198860303));
#232170=CARTESIAN_POINT('Ctrl Pts',(-12.2960739442508,57.7336713548548,
2.65878198860303));
#232171=CARTESIAN_POINT('Ctrl Pts',(-12.304589817043,57.7325856410806,2.65945335517899));
#232172=CARTESIAN_POINT('Ctrl Pts',(-12.3130404786514,57.7321565492377,
2.6607256122665));
#232173=CARTESIAN_POINT('Ctrl Pts',(-12.3184987389621,57.7318793999345,
2.66154735980387));
#232174=CARTESIAN_POINT('Ctrl Pts',(-12.3239297572689,57.7318752477673,
2.66261895766928));
#232175=CARTESIAN_POINT('Ctrl Pts',(-12.3292970476685,57.7321203363023,
2.66391429251067));
#232176=CARTESIAN_POINT('Ctrl Pts',(-12.336411083636,57.7324451871159,2.66563118464163));
#232177=CARTESIAN_POINT('Ctrl Pts',(-12.3434117286776,57.7332135204778,
2.66774105138739));
#232178=CARTESIAN_POINT('Ctrl Pts',(-12.3502210637611,57.7343801629267,
2.6701689418179));
#232179=CARTESIAN_POINT('Ctrl Pts',(-12.3536257313028,57.7349634841512,
2.67138288703315));
#232180=CARTESIAN_POINT('Ctrl Pts',(-12.356982765924,57.7356463395042,2.67267613167591));
#232181=CARTESIAN_POINT('Ctrl Pts',(-12.3602838093642,57.7364227809416,
2.67403835432593));
#232182=CARTESIAN_POINT('Ctrl Pts',(-12.3619343310843,57.7368110016603,
2.67471946565094));
#232183=CARTESIAN_POINT('Ctrl Pts',(-12.363570871071,57.7372226154361,2.67541781389564));
#232184=CARTESIAN_POINT('Ctrl Pts',(-12.3651924853575,57.7376568568913,
2.6761320724421));
#232185=CARTESIAN_POINT('Ctrl Pts',(-12.3655978889291,57.7377654172551,
2.67631063707871));
#232186=CARTESIAN_POINT('Ctrl Pts',(-12.3660023599859,57.7378753917742,
2.67649019601886));
#232187=CARTESIAN_POINT('Ctrl Pts',(-12.3664058844667,57.7379867683386,
2.67667072836698));
#232188=CARTESIAN_POINT('Ctrl Pts',(-12.3676164579094,57.7383208980315,
2.67721232541132));
#232189=CARTESIAN_POINT('Ctrl Pts',(-12.3688185104667,57.7386676465117,
2.67776268340088));
#232190=CARTESIAN_POINT('Ctrl Pts',(-12.3700116777064,57.7390266834248,
2.67832123541557));
#232191=CARTESIAN_POINT('Ctrl Pts',(-12.378416193677,57.7415556930809,2.68225560368487));
#232192=CARTESIAN_POINT('Ctrl Pts',(-12.3864219416031,57.7446608854355,
2.68661792998933));
#232193=CARTESIAN_POINT('Ctrl Pts',(-12.3940121800352,57.7482237843188,
2.69130986622625));
#232194=CARTESIAN_POINT('Ctrl Pts',(-12.3976934374727,57.7499517864271,
2.693585450231));
#232195=CARTESIAN_POINT('Ctrl Pts',(-12.4012771190727,57.7517880072573,
2.69593918853513));
#232196=CARTESIAN_POINT('Ctrl Pts',(-12.4047617836667,57.7537217536094,
2.69836306235516));
#232197=CARTESIAN_POINT('Ctrl Pts',(-12.4100965616936,57.7566821841676,
2.70207384382249));
#232198=CARTESIAN_POINT('Ctrl Pts',(-12.4151968540757,57.7598686150881,
2.7059476081425));
#232199=CARTESIAN_POINT('Ctrl Pts',(-12.420045468934,57.7632382593552,2.70995196345729));
#232200=CARTESIAN_POINT('Ctrl Pts',(-12.4222971907576,57.7648031395851,
2.71181160678127));
#232201=CARTESIAN_POINT('Ctrl Pts',(-12.424494702241,57.766407288405,2.7136996277212));
#232202=CARTESIAN_POINT('Ctrl Pts',(-12.4266353752445,57.7680472557364,
2.71561183138683));
#232203=CARTESIAN_POINT('Ctrl Pts',(-12.4267994493956,57.7681729527705,
2.71575839426333));
#232204=CARTESIAN_POINT('Ctrl Pts',(-12.4269632190239,57.7682988432681,
2.7159050890323));
#232205=CARTESIAN_POINT('Ctrl Pts',(-12.4271266840707,57.7684249257698,
2.71605191409933));
#232206=CARTESIAN_POINT('Ctrl Pts',(-12.4294228751481,57.7701960047924,
2.71811436362774));
#232207=CARTESIAN_POINT('Ctrl Pts',(-12.4316578001007,57.7720067040172,
2.72020091026981));
#232208=CARTESIAN_POINT('Ctrl Pts',(-12.4338307751865,57.7738513586815,
2.72230624862203));
#232209=CARTESIAN_POINT('Ctrl Pts',(-12.4416226773935,57.7804659622468,
2.72985561753126));
#232210=CARTESIAN_POINT('Ctrl Pts',(-12.4486795287418,57.787566807526,2.73770089914356));
#232211=CARTESIAN_POINT('Ctrl Pts',(-12.4550596184371,57.7950386758943,
2.74574823347101));
#232212=CARTESIAN_POINT('Ctrl Pts',(-12.4620706960754,57.8032495086153,
2.75459144547052));
#232213=CARTESIAN_POINT('Ctrl Pts',(-12.4682650727921,57.8119087706221,
2.76367911754298));
#232214=CARTESIAN_POINT('Ctrl Pts',(-12.4736913816503,57.8209080689694,
2.77292162564755));
#232215=CARTESIAN_POINT('Ctrl Pts',(-12.4795504333995,57.830625052669,2.7829012148477));
#232216=CARTESIAN_POINT('Ctrl Pts',(-12.4845147615739,57.8407393717711,
2.79306229500239));
#232217=CARTESIAN_POINT('Ctrl Pts',(-12.4886033793289,57.8511535286846,
2.80331916685316));
#232218=CARTESIAN_POINT('Ctrl Pts',(-12.4926576977819,57.8614803215215,
2.81348999408749));
#232219=CARTESIAN_POINT('Ctrl Pts',(-12.4958511892336,57.8721033557557,
2.82375635966924));
#232220=CARTESIAN_POINT('Ctrl Pts',(-12.4981558292589,57.8829458346107,
2.83404198860303));
#232221=CARTESIAN_POINT('Origin',(0.0149069694351899,0.00316857416824667,
2.83404198860263));
#232222=CARTESIAN_POINT('Ctrl Pts',(-13.0516031943531,61.4762657165317,
2.65878198860305));
#232223=CARTESIAN_POINT('Ctrl Pts',(-13.0432012029365,61.4780479426483,
2.65878198860305));
#232224=CARTESIAN_POINT('Ctrl Pts',(-13.0347249977699,61.4791124697295,
2.65944603041892));
#232225=CARTESIAN_POINT('Ctrl Pts',(-13.0263136082743,61.4795178910589,
2.6607043926411));
#232226=CARTESIAN_POINT('Ctrl Pts',(-13.0209391308134,61.4797769359882,
2.66150842619636));
#232227=CARTESIAN_POINT('Ctrl Pts',(-13.0155911381655,61.4797678285538,
2.66255428265409));
#232228=CARTESIAN_POINT('Ctrl Pts',(-13.0103045333054,61.479514339721,2.66381699700698));
#232229=CARTESIAN_POINT('Ctrl Pts',(-13.0030893784373,61.4791683783271,
2.66554034873298));
#232230=CARTESIAN_POINT('Ctrl Pts',(-12.9959902125623,61.47836135333,2.66766759644002));
#232231=CARTESIAN_POINT('Ctrl Pts',(-12.9890888821229,61.4771427864516,
2.67012012783178));
#232232=CARTESIAN_POINT('Ctrl Pts',(-12.9856382169032,61.4765335030124,
2.67134639352766));
#232233=CARTESIAN_POINT('Ctrl Pts',(-12.9822368066734,61.4758213793961,
2.67265375585042));
#232234=CARTESIAN_POINT('Ctrl Pts',(-12.9788934238966,61.4750129240935,
2.67403135126969));
#232235=CARTESIAN_POINT('Ctrl Pts',(-12.9772217325082,61.4746086964423,
2.67472014897933));
#232236=CARTESIAN_POINT('Ctrl Pts',(-12.9755645309604,61.4741803895394,
2.67542649668662));
#232237=CARTESIAN_POINT('Ctrl Pts',(-12.9739228088656,61.4737288401363,
2.67614899656131));
#232238=CARTESIAN_POINT('Ctrl Pts',(-12.9735123783419,61.4736159527855,
2.67632962152998));
#232239=CARTESIAN_POINT('Ctrl Pts',(-12.9731029149216,61.4735016128576,
2.67651125590979));
#232240=CARTESIAN_POINT('Ctrl Pts',(-12.9726944333366,61.4733858335872,
2.67669387767553));
#232241=CARTESIAN_POINT('Ctrl Pts',(-12.9714689885813,61.4730384957759,
2.67724174297273));
#232242=CARTESIAN_POINT('Ctrl Pts',(-12.9702523821507,61.4726782034779,
2.67779849504776));
#232243=CARTESIAN_POINT('Ctrl Pts',(-12.9690449956483,61.4723053176145,
2.67836353618037));
#232244=CARTESIAN_POINT('Ctrl Pts',(-12.9607012057874,61.4697284449401,
2.68226832098937));
#232245=CARTESIAN_POINT('Ctrl Pts',(-12.952753439984,61.4665839586187,2.68659153751421));
#232246=CARTESIAN_POINT('Ctrl Pts',(-12.9452156558836,61.4629898265073,
2.6912369948621));
#232247=CARTESIAN_POINT('Ctrl Pts',(-12.9414693978765,61.4612035527136,
2.69354577441247));
#232248=CARTESIAN_POINT('Ctrl Pts',(-12.9378242492508,61.4593056238951,
2.69593478828146));
#232249=CARTESIAN_POINT('Ctrl Pts',(-12.9342814732029,61.4573073969128,
2.69839565261247));
#232250=CARTESIAN_POINT('Ctrl Pts',(-12.9264655800789,61.4528990097272,
2.70382468689072));
#232251=CARTESIAN_POINT('Ctrl Pts',(-12.9191426809995,61.4480137506084,
2.70961155815114));
#232252=CARTESIAN_POINT('Ctrl Pts',(-12.9123924986716,61.4427731575669,
2.71562701361793));
#232253=CARTESIAN_POINT('Ctrl Pts',(-12.9099265719429,61.4408587028415,
2.71782453535884));
#232254=CARTESIAN_POINT('Ctrl Pts',(-12.9075300815492,61.4389006256228,
2.72005051502428));
#232255=CARTESIAN_POINT('Ctrl Pts',(-12.9052026993237,61.4369042302171,
2.72229986760142));
#232256=CARTESIAN_POINT('Ctrl Pts',(-12.8973852687042,61.4301985493014,
2.72985520488897));
#232257=CARTESIAN_POINT('Ctrl Pts',(-12.8903034584558,61.4230116455107,
2.73770845534543));
#232258=CARTESIAN_POINT('Ctrl Pts',(-12.8838999218055,61.415458293118,2.74576706701717));
#232259=CARTESIAN_POINT('Ctrl Pts',(-12.876861676478,61.407156264085,2.75462443584973));
#232260=CARTESIAN_POINT('Ctrl Pts',(-12.8706422708196,61.3984111343311,
2.76373036323104));
#232261=CARTESIAN_POINT('Ctrl Pts',(-12.8651946651853,61.3893309057287,
2.77299664636719));
#232262=CARTESIAN_POINT('Ctrl Pts',(-12.8593273605058,61.3795511104671,
2.78297683033348));
#232263=CARTESIAN_POINT('Ctrl Pts',(-12.8543546257409,61.3693816498899,
2.79314401478736));
#232264=CARTESIAN_POINT('Ctrl Pts',(-12.8502602383794,61.3589193990681,
2.80341452427745));
#232265=CARTESIAN_POINT('Ctrl Pts',(-12.8462211390715,61.3485984239567,
2.81354634721249));
#232266=CARTESIAN_POINT('Ctrl Pts',(-12.8430366034498,61.3379910943969,
2.82378004209168));
#232267=CARTESIAN_POINT('Ctrl Pts',(-12.84073727331,61.3271735965895,2.83404198860304));
#232268=CARTESIAN_POINT('Ctrl Pts',(-12.1254815933794,57.9621601888122,
2.83404198860302));
#232269=CARTESIAN_POINT('Ctrl Pts',(-12.1232811218133,57.9518077840276,
2.82422126442991));
#232270=CARTESIAN_POINT('Ctrl Pts',(-12.1219050950916,57.9413190436432,
2.8144281502843));
#232271=CARTESIAN_POINT('Ctrl Pts',(-12.1213524729335,57.9307520129763,
2.80471618166192));
#232272=CARTESIAN_POINT('Ctrl Pts',(-12.1208188676181,57.9205486151395,
2.79533842146069));
#232273=CARTESIAN_POINT('Ctrl Pts',(-12.1210529843538,57.9102709573153,
2.78603515650046));
#232274=CARTESIAN_POINT('Ctrl Pts',(-12.1220995054497,57.8999666805119,
2.7768588734653));
#232275=CARTESIAN_POINT('Ctrl Pts',(-12.1230887956355,57.8902259118332,
2.76818441216329));
#232276=CARTESIAN_POINT('Ctrl Pts',(-12.1248041559928,57.8804604570522,
2.75962261521355));
#232277=CARTESIAN_POINT('Ctrl Pts',(-12.1273238624922,57.8707214089969,
2.75123537701372));
#232278=CARTESIAN_POINT('Ctrl Pts',(-12.1296444699069,57.8617519091229,
2.74351087133818));
#232279=CARTESIAN_POINT('Ctrl Pts',(-12.132647523675,57.8528042960052,2.73593399449536));
#232280=CARTESIAN_POINT('Ctrl Pts',(-12.1364273448794,57.8439372821234,
2.72857657812257));
#232281=CARTESIAN_POINT('Ctrl Pts',(-12.1375544112609,57.8412933175785,
2.72638274508121));
#232282=CARTESIAN_POINT('Ctrl Pts',(-12.1387507708948,57.8386566819994,
2.72420861709514));
#232283=CARTESIAN_POINT('Ctrl Pts',(-12.1400195294492,57.8360293953472,
2.72205663736748));
#232284=CARTESIAN_POINT('Ctrl Pts',(-12.1412753244188,57.8334289530882,
2.71992664556787));
#232285=CARTESIAN_POINT('Ctrl Pts',(-12.14260049657,57.8308402488867,2.71782089927905));
#232286=CARTESIAN_POINT('Ctrl Pts',(-12.143996334094,57.8282680826383,2.71574387311267));
#232287=CARTESIAN_POINT('Ctrl Pts',(-12.1440933979056,57.8280892192277,
2.71559944077508));
#232288=CARTESIAN_POINT('Ctrl Pts',(-12.1441907966614,57.8279104259147,
2.7154551521609));
#232289=CARTESIAN_POINT('Ctrl Pts',(-12.144288531381,57.827731703513,2.71531100781751));
#232290=CARTESIAN_POINT('Ctrl Pts',(-12.1485735795159,57.8198958587086,
2.70899119176097));
#232291=CARTESIAN_POINT('Ctrl Pts',(-12.1535378042503,57.8122268475252,
2.70298296066845));
#232292=CARTESIAN_POINT('Ctrl Pts',(-12.1592011408681,57.8048391253243,
2.69736727774137));
#232293=CARTESIAN_POINT('Ctrl Pts',(-12.1644803548772,57.7979524842554,
2.69213248525412));
#232294=CARTESIAN_POINT('Ctrl Pts',(-12.1703677426435,57.791309817124,2.68723866185435));
#232295=CARTESIAN_POINT('Ctrl Pts',(-12.1768883481379,57.7850318067599,
2.68278595829518));
#232296=CARTESIAN_POINT('Ctrl Pts',(-12.1792736699859,57.782735229349,2.68115710172784));
#232297=CARTESIAN_POINT('Ctrl Pts',(-12.1817437717242,57.7804877669875,
2.6795876363781));
#232298=CARTESIAN_POINT('Ctrl Pts',(-12.1842999559277,57.778296544019,2.67808378645385));
#232299=CARTESIAN_POINT('Ctrl Pts',(-12.1849146328342,57.7777696280973,
2.67772216078621));
#232300=CARTESIAN_POINT('Ctrl Pts',(-12.1855348686826,57.7772459087257,
2.67736403603584));
#232301=CARTESIAN_POINT('Ctrl Pts',(-12.1861606108967,57.7767255109849,
2.677009569345));
#232302=CARTESIAN_POINT('Ctrl Pts',(-12.1867667986667,57.7762213756735,
2.67666617973824));
#232303=CARTESIAN_POINT('Ctrl Pts',(-12.1873781540071,57.7757203576394,
2.67632622314139));
#232304=CARTESIAN_POINT('Ctrl Pts',(-12.187994625406,57.7752225713659,2.67598984158794));
#232305=CARTESIAN_POINT('Ctrl Pts',(-12.1947487820216,57.7697687474617,
2.67230439292248));
#232306=CARTESIAN_POINT('Ctrl Pts',(-12.2021217510026,57.7646995864531,
2.66904964540006));
#232307=CARTESIAN_POINT('Ctrl Pts',(-12.210017417959,57.7601772489166,2.66640203566758));
#232308=CARTESIAN_POINT('Ctrl Pts',(-12.2132919863906,57.7583017007437,
2.66530399299468));
#232309=CARTESIAN_POINT('Ctrl Pts',(-12.2166560758249,57.7565200187334,
2.66430995142283));
#232310=CARTESIAN_POINT('Ctrl Pts',(-12.2201014385647,57.7548425830509,
2.6634305347338));
#232311=CARTESIAN_POINT('Ctrl Pts',(-12.2259778637495,57.7519815416932,
2.66193059792904));
#232312=CARTESIAN_POINT('Ctrl Pts',(-12.2320899429716,57.7494261286936,
2.66076519817147));
#232313=CARTESIAN_POINT('Ctrl Pts',(-12.2383911161013,57.7472322823297,
2.65997805604479));
#232314=CARTESIAN_POINT('Ctrl Pts',(-12.2415417026662,57.7461353591477,
2.65958448498145));
#232315=CARTESIAN_POINT('Ctrl Pts',(-12.2447399293287,57.745130227238,2.65928526260781));
#232316=CARTESIAN_POINT('Ctrl Pts',(-12.2479799447119,57.7442239366605,
2.65908463971343));
#232317=CARTESIAN_POINT('Ctrl Pts',(-12.2512199600952,57.7433176460829,
2.65888401681905));
#232318=CARTESIAN_POINT('Ctrl Pts',(-12.254501719267,57.7425101887134,2.65878198860303));
#232319=CARTESIAN_POINT('Ctrl Pts',(-12.257819391977,57.7418065394567,2.65878198860303));
#232320=CARTESIAN_POINT('Origin',(-18.0189898472952,55.4074307335707,2.83404198860299));
#232321=CARTESIAN_POINT('Ctrl Pts',(-19.5431821162869,59.5312589135997,
2.83404198860303));
#232322=CARTESIAN_POINT('Ctrl Pts',(-19.5464608884256,59.5413499366332,
2.82419652440135));
#232323=CARTESIAN_POINT('Ctrl Pts',(-19.5489337165496,59.5516697238485,
2.81438790575749));
#232324=CARTESIAN_POINT('Ctrl Pts',(-19.550597385826,59.5621592733657,2.80466781257031));
#232325=CARTESIAN_POINT('Ctrl Pts',(-19.5522069957574,59.5723079749848,
2.79526356453234));
#232326=CARTESIAN_POINT('Ctrl Pts',(-19.5530593117979,59.5826168684397,
2.78594102496414));
#232327=CARTESIAN_POINT('Ctrl Pts',(-19.5531064127991,59.5930429125516,
2.77675109088984));
#232328=CARTESIAN_POINT('Ctrl Pts',(-19.553150967446,59.6029053082826,2.76805797913912));
#232329=CARTESIAN_POINT('Ctrl Pts',(-19.5524750234014,59.6128734577632,
2.75948271210414));
#232330=CARTESIAN_POINT('Ctrl Pts',(-19.5509963368661,59.6229049605478,
2.75108575573497));
#232331=CARTESIAN_POINT('Ctrl Pts',(-19.5496343596258,59.6321447001092,
2.74335155163568));
#232332=CARTESIAN_POINT('Ctrl Pts',(-19.5475912199427,59.6414387315163,
2.73576818686263));
#232333=CARTESIAN_POINT('Ctrl Pts',(-19.544767461172,59.6507389334411,2.72840626160835));
#232334=CARTESIAN_POINT('Ctrl Pts',(-19.5439483960915,59.6534365684931,
2.72627084693917));
#232335=CARTESIAN_POINT('Ctrl Pts',(-19.5430634173963,59.6561345922123,
2.72415424587661));
#232336=CARTESIAN_POINT('Ctrl Pts',(-19.5421094990031,59.6588314685162,
2.722058671733));
#232337=CARTESIAN_POINT('Ctrl Pts',(-19.5410753901339,59.661755055822,2.71978693462902));
#232338=CARTESIAN_POINT('Ctrl Pts',(-19.5399627185792,59.6646735866704,
2.71754411340802));
#232339=CARTESIAN_POINT('Ctrl Pts',(-19.5387684320157,59.6675844741796,
2.71533341844299));
#232340=CARTESIAN_POINT('Ctrl Pts',(-19.5354907031708,59.67557342779,2.70926614876445));
#232341=CARTESIAN_POINT('Ctrl Pts',(-19.5315625649727,59.6834782549091,
2.70347381860463));
#232342=CARTESIAN_POINT('Ctrl Pts',(-19.5269766895185,59.691195508465,2.69804914171448));
#232343=CARTESIAN_POINT('Ctrl Pts',(-19.5227808624511,59.6982563764889,
2.69308585687276));
#232344=CARTESIAN_POINT('Ctrl Pts',(-19.5180305486465,59.7051493183928,
2.68842799053272));
#232345=CARTESIAN_POINT('Ctrl Pts',(-19.5126862934704,59.711794955863,2.68414767054316));
#232346=CARTESIAN_POINT('Ctrl Pts',(-19.5100612127855,59.7150592712798,
2.68204519134634));
#232347=CARTESIAN_POINT('Ctrl Pts',(-19.5072925729236,59.7182634781245,
2.68003431778569));
#232348=CARTESIAN_POINT('Ctrl Pts',(-19.5043743927941,59.7213950854346,
2.67812693945305));
#232349=CARTESIAN_POINT('Ctrl Pts',(-19.5038206965381,59.7219892774194,
2.67776503299257));
#232350=CARTESIAN_POINT('Ctrl Pts',(-19.5032610854118,59.7225808838924,
2.67740659639977));
#232351=CARTESIAN_POINT('Ctrl Pts',(-19.5026955970361,59.7231697699857,
2.67705178968908));
#232352=CARTESIAN_POINT('Ctrl Pts',(-19.5021477801721,59.7237402533885,
2.67670807068811));
#232353=CARTESIAN_POINT('Ctrl Pts',(-19.5015944476715,59.7243081837715,
2.67636775825318));
#232354=CARTESIAN_POINT('Ctrl Pts',(-19.5010356373988,59.7248734373531,
2.67603099699308));
#232355=CARTESIAN_POINT('Ctrl Pts',(-19.4949458381921,59.7310334544119,
2.67236104217171));
#232356=CARTESIAN_POINT('Ctrl Pts',(-19.488201196085,59.7368793392206,2.6691144054151));
#232357=CARTESIAN_POINT('Ctrl Pts',(-19.4808775251047,59.7422363728294,
2.66646778189663));
#232358=CARTESIAN_POINT('Ctrl Pts',(-19.4777846933722,59.7444986813877,
2.66535009635015));
#232359=CARTESIAN_POINT('Ctrl Pts',(-19.4745890081269,59.7466739523117,
2.66433897912392));
#232360=CARTESIAN_POINT('Ctrl Pts',(-19.4712977780157,59.7487501225121,
2.66344564884846));
#232361=CARTESIAN_POINT('Ctrl Pts',(-19.465755428747,59.7522463412521,2.66194130298639));
#232362=CARTESIAN_POINT('Ctrl Pts',(-19.4599426670173,59.7554590576863,
2.66077206705474));
#232363=CARTESIAN_POINT('Ctrl Pts',(-19.4538995640366,59.7583258028888,
2.65998225155768));
#232364=CARTESIAN_POINT('Ctrl Pts',(-19.4523887882915,59.7590424891894,
2.65978479768342));
#232365=CARTESIAN_POINT('Ctrl Pts',(-19.4508635299958,59.7597373347844,
2.65961098966676));
#232366=CARTESIAN_POINT('Ctrl Pts',(-19.4493243130383,59.7604090725475,
2.65946139030555));
#232367=CARTESIAN_POINT('Ctrl Pts',(-19.447015487602,59.7614166791923,2.65923699126374));
#232368=CARTESIAN_POINT('Ctrl Pts',(-19.4446752658777,59.762372275598,2.65906707562495));
#232369=CARTESIAN_POINT('Ctrl Pts',(-19.4423059520264,59.7632731754142,
2.65895332562973));
#232370=CARTESIAN_POINT('Ctrl Pts',(-19.4399366381751,59.7641740752304,
2.65883957563451));
#232371=CARTESIAN_POINT('Ctrl Pts',(-19.4375382417961,59.7650202849792,
2.65878198860303));
#232372=CARTESIAN_POINT('Ctrl Pts',(-19.4351129318423,59.7658094374952,
2.65878198860303));
#232373=CARTESIAN_POINT('Ctrl Pts',(-18.2553202812751,56.1347810195643,
2.658781988603));
#232374=CARTESIAN_POINT('Ctrl Pts',(-18.2635267101473,56.1321105487812,
2.658781988603));
#232375=CARTESIAN_POINT('Ctrl Pts',(-18.2718824441049,56.1301406315644,
2.65945335517894));
#232376=CARTESIAN_POINT('Ctrl Pts',(-18.2802419597937,56.1288305556599,
2.66072561226642));
#232377=CARTESIAN_POINT('Ctrl Pts',(-18.2856413491927,56.1279843810472,
2.66154735980379));
#232378=CARTESIAN_POINT('Ctrl Pts',(-18.2910421817934,56.1274125556284,
2.66261895766922));
#232379=CARTESIAN_POINT('Ctrl Pts',(-18.2964056883427,56.1270952669254,
2.66391429251064));
#232380=CARTESIAN_POINT('Ctrl Pts',(-18.3035147090331,56.1266747189249,
2.6656311846416));
#232381=CARTESIAN_POINT('Ctrl Pts',(-18.3105573165143,56.1267070766082,
2.66774105138735));
#232382=CARTESIAN_POINT('Ctrl Pts',(-18.3174512966901,56.1271555587356,
2.67016894181786));
#232383=CARTESIAN_POINT('Ctrl Pts',(-18.320898286778,56.1273797997993,2.67138288703311));
#232384=CARTESIAN_POINT('Ctrl Pts',(-18.324308309033,56.1277080087291,2.67267613167588));
#232385=CARTESIAN_POINT('Ctrl Pts',(-18.3276724292421,56.1281351437411,
2.6740383543259));
#232386=CARTESIAN_POINT('Ctrl Pts',(-18.3293544893466,56.1283487112471,
2.6747194656509));
#232387=CARTESIAN_POINT('Ctrl Pts',(-18.3310250895515,56.1285870051497,
2.67541781389559));
#232388=CARTESIAN_POINT('Ctrl Pts',(-18.3326832110572,56.1288493629354,
2.67613207244206));
#232389=CARTESIAN_POINT('Ctrl Pts',(-18.3330977414336,56.1289149523818,
2.67631063707867));
#232390=CARTESIAN_POINT('Ctrl Pts',(-18.3335114922231,56.128982045711,2.67649019601882));
#232391=CARTESIAN_POINT('Ctrl Pts',(-18.3339244481758,56.1290506323489,
2.67667072836693));
#232392=CARTESIAN_POINT('Ctrl Pts',(-18.3351633160338,56.1292563922629,
2.67721232541127));
#232393=CARTESIAN_POINT('Ctrl Pts',(-18.3363950287072,56.129475592512,2.67776268340084));
#232394=CARTESIAN_POINT('Ctrl Pts',(-18.3376191892287,56.1297079426454,
2.67832123541553));
#232395=CARTESIAN_POINT('Ctrl Pts',(-18.3462420178743,56.131344586983,2.68225560368481));
#232396=CARTESIAN_POINT('Ctrl Pts',(-18.3545284904605,56.1335959402409,
2.68661792998924));
#232397=CARTESIAN_POINT('Ctrl Pts',(-18.3624495731174,56.1363459252322,
2.69130986622614));
#232398=CARTESIAN_POINT('Ctrl Pts',(-18.3662912896464,56.1376796649813,
2.69358545023091));
#232399=CARTESIAN_POINT('Ctrl Pts',(-18.3700472768052,56.1391312300713,
2.69593918853507));
#232400=CARTESIAN_POINT('Ctrl Pts',(-18.3737149835765,56.1406901365235,
2.69836306235513));
#232401=CARTESIAN_POINT('Ctrl Pts',(-18.3793299863881,56.1430767133843,
2.70207384382246));
#232402=CARTESIAN_POINT('Ctrl Pts',(-18.3847354115624,56.145712562978,2.70594760814247));
#232403=CARTESIAN_POINT('Ctrl Pts',(-18.3899096889381,56.1485569297211,
2.70995196345727));
#232404=CARTESIAN_POINT('Ctrl Pts',(-18.3923126501195,56.1498778683514,
2.71181160678125));
#232405=CARTESIAN_POINT('Ctrl Pts',(-18.3946658026161,56.1512435269778,
2.71369962772117));
#232406=CARTESIAN_POINT('Ctrl Pts',(-18.396966172054,56.1526507491371,2.7156118313868));
#232407=CARTESIAN_POINT('Ctrl Pts',(-18.3971424863075,56.1527586071709,
2.71575839426331));
#232408=CARTESIAN_POINT('Ctrl Pts',(-18.3973185179288,56.1528666894396,
2.71590508903228));
#232409=CARTESIAN_POINT('Ctrl Pts',(-18.3974942667072,56.152974994498,2.7160519140993));
#232410=CARTESIAN_POINT('Ctrl Pts',(-18.3999630071782,56.1544963540397,
2.71811436362772));
#232411=CARTESIAN_POINT('Ctrl Pts',(-18.4023749585855,56.1560635207939,
2.72020091026978));
#232412=CARTESIAN_POINT('Ctrl Pts',(-18.4047288488037,56.1576709325005,
2.72230624862201));
#232413=CARTESIAN_POINT('Ctrl Pts',(-18.4131694805009,56.1634348250118,
2.72985561753131));
#232414=CARTESIAN_POINT('Ctrl Pts',(-18.4209299141242,56.1697591292907,
2.73770089914368));
#232415=CARTESIAN_POINT('Ctrl Pts',(-18.4280560759388,56.1765231650109,
2.74574823347121));
#232416=CARTESIAN_POINT('Ctrl Pts',(-18.4358870118864,56.1839561607596,
2.75459144547045));
#232417=CARTESIAN_POINT('Ctrl Pts',(-18.4429525945098,56.1919204977437,
2.76367911754261));
#232418=CARTESIAN_POINT('Ctrl Pts',(-18.4492898603068,56.2003032932666,
2.77292162564687));
#232419=CARTESIAN_POINT('Ctrl Pts',(-18.4561325169306,56.2093546086363,
2.78290121484599));
#232420=CARTESIAN_POINT('Ctrl Pts',(-18.462126884228,56.2188946068438,2.7930622949996));
#232421=CARTESIAN_POINT('Ctrl Pts',(-18.4672816799253,56.2288243369841,
2.80331916684929));
#232422=CARTESIAN_POINT('Ctrl Pts',(-18.4723932321842,56.2386707668931,
2.81348999408487));
#232423=CARTESIAN_POINT('Ctrl Pts',(-18.4766796388,56.2489017962816,2.82375635966791));
#232424=CARTESIAN_POINT('Ctrl Pts',(-18.4801050014193,56.259443978424,2.834041988603));
#232425=CARTESIAN_POINT('Origin',(0.0144941013083455,0.00470941899445838,
2.83404198860262));
#232426=CARTESIAN_POINT('Ctrl Pts',(-19.4061247292256,59.7752282754838,
2.65878198860303));
#232427=CARTESIAN_POINT('Ctrl Pts',(-19.3979550581546,59.7778789856304,
2.65878198860303));
#232428=CARTESIAN_POINT('Ctrl Pts',(-19.3896365599069,59.7798236858212,
2.65944603041887));
#232429=CARTESIAN_POINT('Ctrl Pts',(-19.3813136269518,59.7811061158281,
2.66070439264098));
#232430=CARTESIAN_POINT('Ctrl Pts',(-19.3759956690089,59.781925527552,2.66150842619625));
#232431=CARTESIAN_POINT('Ctrl Pts',(-19.3706760212379,59.7824754874622,
2.66255428265402));
#232432=CARTESIAN_POINT('Ctrl Pts',(-19.3653918801541,59.7827759879496,
2.66381699700696));
#232433=CARTESIAN_POINT('Ctrl Pts',(-19.3581800878464,59.7831861108191,
2.66554034873296));
#232434=CARTESIAN_POINT('Ctrl Pts',(-19.3510354548621,59.7831255716888,
2.66766759644));
#232435=CARTESIAN_POINT('Ctrl Pts',(-19.3440445557098,59.7826350657125,
2.67012012783176));
#232436=CARTESIAN_POINT('Ctrl Pts',(-19.3405491061336,59.7823898127244,
2.67134639352764));
#232437=CARTESIAN_POINT('Ctrl Pts',(-19.3370918919976,59.78203713438,2.6726537558504));
#232438=CARTESIAN_POINT('Ctrl Pts',(-19.3336823180311,59.781582586544,2.67403135126968));
#232439=CARTESIAN_POINT('Ctrl Pts',(-19.3319775310479,59.781355312626,2.67472014897931));
#232440=CARTESIAN_POINT('Ctrl Pts',(-19.3302846375612,59.7811025767644,
2.6754264966866));
#232441=CARTESIAN_POINT('Ctrl Pts',(-19.3286047092266,59.7808251076838,
2.67614899656129));
#232442=CARTESIAN_POINT('Ctrl Pts',(-19.328184727143,59.7807557404136,2.67632962152997));
#232443=CARTESIAN_POINT('Ctrl Pts',(-19.3277655550292,59.7806848274339,
2.67651125590978));
#232444=CARTESIAN_POINT('Ctrl Pts',(-19.3273472089198,59.7806123803668,
2.67669387767551));
#232445=CARTESIAN_POINT('Ctrl Pts',(-19.3260921705915,59.7803950391654,
2.67724174297271));
#232446=CARTESIAN_POINT('Ctrl Pts',(-19.3248445680579,59.7801638905869,
2.67779849504775));
#232447=CARTESIAN_POINT('Ctrl Pts',(-19.3236048185588,59.779919253687,2.67836353618036));
#232448=CARTESIAN_POINT('Ctrl Pts',(-19.3150373803112,59.7782286609228,
2.68226832098929));
#232449=CARTESIAN_POINT('Ctrl Pts',(-19.3068044648777,59.7759321681723,
2.68659153751405));
#232450=CARTESIAN_POINT('Ctrl Pts',(-19.298932284441,59.7731456380812,2.69123699486184));
#232451=CARTESIAN_POINT('Ctrl Pts',(-19.2950198323725,59.7717607402747,
2.69354577441228));
#232452=CARTESIAN_POINT('Ctrl Pts',(-19.2911962646694,59.770254230293,2.69593478828135));
#232453=CARTESIAN_POINT('Ctrl Pts',(-19.2874640247236,59.7686372707432,
2.69839565261244));
#232454=CARTESIAN_POINT('Ctrl Pts',(-19.2792301459419,59.7650700164611,
2.70382468689069));
#232455=CARTESIAN_POINT('Ctrl Pts',(-19.2714367138416,59.7609769706903,
2.70961155815111));
#232456=CARTESIAN_POINT('Ctrl Pts',(-19.2641757185814,59.7564706723514,
2.71562701361791));
#232457=CARTESIAN_POINT('Ctrl Pts',(-19.2615231854469,59.7548244647407,
2.71782453535881));
#232458=CARTESIAN_POINT('Ctrl Pts',(-19.2589351484757,59.753127615532,2.72005051502424));
#232459=CARTESIAN_POINT('Ctrl Pts',(-19.2564118357498,59.7513854342767,
2.72229986760136));
#232460=CARTESIAN_POINT('Ctrl Pts',(-19.2479362953115,59.7455336317917,
2.72985520488924));
#232461=CARTESIAN_POINT('Ctrl Pts',(-19.2401420439513,59.7391263493539,
2.73770845534603));
#232462=CARTESIAN_POINT('Ctrl Pts',(-19.2329840462263,59.732283726861,2.74576706701812));
#232463=CARTESIAN_POINT('Ctrl Pts',(-19.2251165588061,59.7247628741795,
2.75462443585104));
#232464=CARTESIAN_POINT('Ctrl Pts',(-19.2180171087281,59.7167157560768,
2.76373036323274));
#232465=CARTESIAN_POINT('Ctrl Pts',(-19.2116502033053,59.7082546997617,
2.77299664636931));
#232466=CARTESIAN_POINT('Ctrl Pts',(-19.2047927733647,59.6991417795828,
2.78297683033612));
#232467=CARTESIAN_POINT('Ctrl Pts',(-19.1987842816746,59.6895478206973,
2.79314401479056));
#232468=CARTESIAN_POINT('Ctrl Pts',(-19.1936187207948,59.6795708631985,
2.80341452428128));
#232469=CARTESIAN_POINT('Ctrl Pts',(-19.1885229124286,59.6697286283136,
2.81354634721501));
#232470=CARTESIAN_POINT('Ctrl Pts',(-19.1842470541688,59.6595122814313,
2.82378004209289));
#232471=CARTESIAN_POINT('Ctrl Pts',(-19.1808295835784,59.6489943884565,
2.83404198860303));
#232472=CARTESIAN_POINT('Ctrl Pts',(-18.1177524687109,56.3771794532808,
2.83404198860299));
#232473=CARTESIAN_POINT('Ctrl Pts',(-18.1144819305952,56.3671137719646,
2.8242212644304));
#232474=CARTESIAN_POINT('Ctrl Pts',(-18.112017069978,56.3568263239567,2.8144281502853));
#232475=CARTESIAN_POINT('Ctrl Pts',(-18.110362919665,56.346374945335,2.80471618166343));
#232476=CARTESIAN_POINT('Ctrl Pts',(-18.1087656919993,56.336283219723,2.79533842146253));
#232477=CARTESIAN_POINT('Ctrl Pts',(-18.1079242184406,56.3260373921216,
2.78603515650262));
#232478=CARTESIAN_POINT('Ctrl Pts',(-18.107887916365,56.3156801719831,2.77685887346776));
#232479=CARTESIAN_POINT('Ctrl Pts',(-18.1078535995344,56.3058893552718,
2.76818441216597));
#232480=CARTESIAN_POINT('Ctrl Pts',(-18.1085387949866,56.2959980926921,
2.75962261521643));
#232481=CARTESIAN_POINT('Ctrl Pts',(-18.1100266905431,56.2860490151131,
2.75123537701679));
#232482=CARTESIAN_POINT('Ctrl Pts',(-18.1113970173892,56.2768860815712,
2.7435108713414));
#232483=CARTESIAN_POINT('Ctrl Pts',(-18.1134483398652,56.2676735798191,
2.7359339944987));
#232484=CARTESIAN_POINT('Ctrl Pts',(-18.1162805994784,56.2584600414655,
2.72857657812602));
#232485=CARTESIAN_POINT('Ctrl Pts',(-18.1171251221219,56.2557127503167,
2.72638274508348));
#232486=CARTESIAN_POINT('Ctrl Pts',(-18.1180393245077,56.2529655048677,
2.72420861709626));
#232487=CARTESIAN_POINT('Ctrl Pts',(-18.1190265064342,56.2502199893833,
2.72205663736746));
#232488=CARTESIAN_POINT('Ctrl Pts',(-18.1200036017944,56.2475025263007,
2.71992664556785));
#232489=CARTESIAN_POINT('Ctrl Pts',(-18.1210509212418,56.2447894850831,
2.71782089927904));
#232490=CARTESIAN_POINT('Ctrl Pts',(-18.1221702476366,56.2420855046791,
2.71574387311265));
#232491=CARTESIAN_POINT('Ctrl Pts',(-18.1222480834051,56.24189747517,2.71559944077506));
#232492=CARTESIAN_POINT('Ctrl Pts',(-18.1223262596101,56.2417094803632,
2.71545515216088));
#232493=CARTESIAN_POINT('Ctrl Pts',(-18.1224047773506,56.2415215209615,
2.7153110078175));
#232494=CARTESIAN_POINT('Ctrl Pts',(-18.1258472827277,56.2332806922383,
2.70899119176101));
#232495=CARTESIAN_POINT('Ctrl Pts',(-18.1299826829657,56.2251347899179,
2.70298296066855));
#232496=CARTESIAN_POINT('Ctrl Pts',(-18.1348427679841,56.2171955585586,
2.69736727774152));
#232497=CARTESIAN_POINT('Ctrl Pts',(-18.1393732118984,56.2097948151027,
2.69213248525441));
#232498=CARTESIAN_POINT('Ctrl Pts',(-18.144534000151,56.2025731376012,2.68723866185478));
#232499=CARTESIAN_POINT('Ctrl Pts',(-18.1503626543103,56.195647929963,2.6827859582957));
#232500=CARTESIAN_POINT('Ctrl Pts',(-18.1524948514083,56.193114599416,2.68115710172816));
#232501=CARTESIAN_POINT('Ctrl Pts',(-18.1547164978842,56.1906212529493,
2.67958763637824));
#232502=CARTESIAN_POINT('Ctrl Pts',(-18.1570296338739,56.1881748397226,
2.67808378645381));
#232503=CARTESIAN_POINT('Ctrl Pts',(-18.1575858658044,56.187586559069,2.67772216078617));
#232504=CARTESIAN_POINT('Ctrl Pts',(-18.1581479603548,56.1870008763869,
2.6773640360358));
#232505=CARTESIAN_POINT('Ctrl Pts',(-18.1587158783115,56.1864179215673,
2.67700956934496));
#232506=CARTESIAN_POINT('Ctrl Pts',(-18.159266048832,56.1858531840859,2.67666617973821));
#232507=CARTESIAN_POINT('Ctrl Pts',(-18.1598216844587,56.1852910066467,
2.67632622314135));
#232508=CARTESIAN_POINT('Ctrl Pts',(-18.1603827459286,56.1847315084905,
2.6759898415879));
#232509=CARTESIAN_POINT('Ctrl Pts',(-18.1665298227359,56.1786015595926,
2.67230439292242));
#232510=CARTESIAN_POINT('Ctrl Pts',(-18.1733325302112,56.1727894828611,
2.6690496454));
#232511=CARTESIAN_POINT('Ctrl Pts',(-18.1807122308848,56.1674665972294,
2.66640203566752));
#232512=CARTESIAN_POINT('Ctrl Pts',(-18.1837728127196,56.1652590378996,
2.66530399299463));
#232513=CARTESIAN_POINT('Ctrl Pts',(-18.1869322368374,56.1631354730309,
2.66430995142278));
#232514=CARTESIAN_POINT('Ctrl Pts',(-18.1901833857455,56.161107088044,2.66343053473377));
#232515=CARTESIAN_POINT('Ctrl Pts',(-18.1957285590018,56.1576474660762,
2.661930597929));
#232516=CARTESIAN_POINT('Ctrl Pts',(-18.2015400422205,56.1544671656479,
2.66076519817144));
#232517=CARTESIAN_POINT('Ctrl Pts',(-18.2075773774754,56.1516266854597,
2.65997805604476));
#232518=CARTESIAN_POINT('Ctrl Pts',(-18.2105960451029,56.1502064453656,
2.65958448498142));
#232519=CARTESIAN_POINT('Ctrl Pts',(-18.2136716866512,56.1488725139555,
2.65928526260778));
#232520=CARTESIAN_POINT('Ctrl Pts',(-18.2167992197298,56.1476325143036,
2.65908463971341));
#232521=CARTESIAN_POINT('Ctrl Pts',(-18.2199267528084,56.1463925146518,
2.65888401681903));
#232522=CARTESIAN_POINT('Ctrl Pts',(-18.2231061318822,56.1452464433753,
2.658781988603));
#232523=CARTESIAN_POINT('Ctrl Pts',(-18.2263320786585,56.1441998575529,
2.658781988603));
#232524=CARTESIAN_POINT('Origin',(-23.7119335237428,53.2204057122639,2.83404198860298));
#232525=CARTESIAN_POINT('Ctrl Pts',(-25.6588335304443,57.1623216544372,
2.83404198860301));
#232526=CARTESIAN_POINT('Ctrl Pts',(-25.6631491402569,57.172014672778,2.82419652440111));
#232527=CARTESIAN_POINT('Ctrl Pts',(-25.6666871334687,57.1820194461959,
2.81438790575699));
#232528=CARTESIAN_POINT('Ctrl Pts',(-25.6694381454821,57.1922776320707,
2.80466781256952));
#232529=CARTESIAN_POINT('Ctrl Pts',(-25.6720997659863,57.2022024879881,
2.79526356453127));
#232530=CARTESIAN_POINT('Ctrl Pts',(-25.6740249857412,57.2123658169604,
2.78594102496278));
#232531=CARTESIAN_POINT('Ctrl Pts',(-25.675161647087,57.2227298227167,2.7767510908882));
#232532=CARTESIAN_POINT('Ctrl Pts',(-25.6762368587287,57.2325335339835,
2.76805797913715));
#232533=CARTESIAN_POINT('Ctrl Pts',(-25.6766065729229,57.2425177322909,
2.75948271210185));
#232534=CARTESIAN_POINT('Ctrl Pts',(-25.6761845643574,57.2526488462852,
2.7510857557324));
#232535=CARTESIAN_POINT('Ctrl Pts',(-25.6757958639481,57.2619803349748,
2.74335155163276));
#232536=CARTESIAN_POINT('Ctrl Pts',(-25.6747354076182,57.2714370189572,
2.73576818685939));
#232537=CARTESIAN_POINT('Ctrl Pts',(-25.6728992535085,57.2809814365682,
2.72840626160486));
#232538=CARTESIAN_POINT('Ctrl Pts',(-25.6723666549989,57.2837499093059,
2.72627084693685));
#232539=CARTESIAN_POINT('Ctrl Pts',(-25.6717685445831,57.2865256584305,
2.72415424587543));
#232540=CARTESIAN_POINT('Ctrl Pts',(-25.6711017521907,57.2893074725861,
2.72205867173295));
#232541=CARTESIAN_POINT('Ctrl Pts',(-25.6703789063664,57.2923231379857,
2.71978693462898));
#232542=CARTESIAN_POINT('Ctrl Pts',(-25.6695773996876,57.2953419866644,
2.71754411340799));
#232543=CARTESIAN_POINT('Ctrl Pts',(-25.6686939261489,57.2983617649665,
2.71533341844297));
#232544=CARTESIAN_POINT('Ctrl Pts',(-25.6662692260896,57.3066495702124,
2.70926614876445));
#232545=CARTESIAN_POINT('Ctrl Pts',(-25.6631888860747,57.3149216961107,
2.70347381860462));
#232546=CARTESIAN_POINT('Ctrl Pts',(-25.6594348051809,57.3230760282581,
2.69804914171448));
#232547=CARTESIAN_POINT('Ctrl Pts',(-25.656000024977,57.3305367994638,2.69308585687273));
#232548=CARTESIAN_POINT('Ctrl Pts',(-25.6519962425131,57.3378885241127,
2.68842799053268));
#232549=CARTESIAN_POINT('Ctrl Pts',(-25.6473759219982,57.3450563828664,
2.68414767054311));
#232550=CARTESIAN_POINT('Ctrl Pts',(-25.6451064356541,57.3485772116717,
2.68204519134631));
#232551=CARTESIAN_POINT('Ctrl Pts',(-25.6426878935085,57.3520532672062,
2.68003431778569));
#232552=CARTESIAN_POINT('Ctrl Pts',(-25.6401130415749,57.3554727521282,
2.67812693945307));
#232553=CARTESIAN_POINT('Ctrl Pts',(-25.6396244884999,57.3561215660859,
2.67776503299259));
#232554=CARTESIAN_POINT('Ctrl Pts',(-25.6391297826974,57.3567684269678,
2.67740659639979));
#232555=CARTESIAN_POINT('Ctrl Pts',(-25.6386289474846,57.3574131967123,
2.67705178968911));
#232556=CARTESIAN_POINT('Ctrl Pts',(-25.6381437633721,57.3580378174023,
2.67670807068813));
#232557=CARTESIAN_POINT('Ctrl Pts',(-25.637652826975,57.3586604755992,2.67636775825321));
#232558=CARTESIAN_POINT('Ctrl Pts',(-25.6371561630117,57.3592810442416,
2.67603099699311));
#232559=CARTESIAN_POINT('Ctrl Pts',(-25.6317436214791,57.366043873435,2.6723610421718));
#232560=CARTESIAN_POINT('Ctrl Pts',(-25.6256469885829,57.3725627409498,
2.66911440541522));
#232561=CARTESIAN_POINT('Ctrl Pts',(-25.6189233999294,57.3786559602409,
2.66646778189677));
#232562=CARTESIAN_POINT('Ctrl Pts',(-25.6160839866896,57.3812291645844,
2.66535009635023));
#232563=CARTESIAN_POINT('Ctrl Pts',(-25.6131331854692,57.3837265592146,
2.66433897912396));
#232564=CARTESIAN_POINT('Ctrl Pts',(-25.6100770039414,57.3861353831633,
2.66344564884847));
#232565=CARTESIAN_POINT('Ctrl Pts',(-25.6049304706141,57.3901917825032,
2.66194130298639));
#232566=CARTESIAN_POINT('Ctrl Pts',(-25.5994853721132,57.3939944983915,
2.66077206705474));
#232567=CARTESIAN_POINT('Ctrl Pts',(-25.5937750303535,57.3974772155319,
2.65998225155768));
#232568=CARTESIAN_POINT('Ctrl Pts',(-25.5923474449136,57.3983478948169,
2.65978479768341));
#232569=CARTESIAN_POINT('Ctrl Pts',(-25.5909031732847,57.3991983668808,
2.65961098966675));
#232570=CARTESIAN_POINT('Ctrl Pts',(-25.5894426040348,57.4000273167774,
2.65946139030554));
#232571=CARTESIAN_POINT('Ctrl Pts',(-25.58725175016,57.4012707416222,2.65923699126373));
#232572=CARTESIAN_POINT('Ctrl Pts',(-25.585024235439,57.4024657229514,2.65906707562494));
#232573=CARTESIAN_POINT('Ctrl Pts',(-25.5827620706102,57.40360934828,2.65895332562972));
#232574=CARTESIAN_POINT('Ctrl Pts',(-25.5804999057814,57.4047529736086,
2.65883957563449));
#232575=CARTESIAN_POINT('Ctrl Pts',(-25.5782031010741,57.4058452484213,
2.65878198860301));
#232576=CARTESIAN_POINT('Ctrl Pts',(-25.5758735661218,57.4068835917996,
2.65878198860301));
#232577=CARTESIAN_POINT('Ctrl Pts',(-24.0229981225299,53.9190682401996,
2.65878198860299));
#232578=CARTESIAN_POINT('Ctrl Pts',(-24.0308804555191,53.9155545931358,
2.65878198860299));
#232579=CARTESIAN_POINT('Ctrl Pts',(-24.0389845034724,53.9127220553016,
2.65945335517895));
#232580=CARTESIAN_POINT('Ctrl Pts',(-24.0471612846387,53.9105453488013,
2.66072561226648));
#232581=CARTESIAN_POINT('Ctrl Pts',(-24.0524426462856,53.9091394197453,
2.66154735980385));
#232582=CARTESIAN_POINT('Ctrl Pts',(-24.0577541205278,53.9080061861139,
2.66261895766927));
#232583=CARTESIAN_POINT('Ctrl Pts',(-24.0630550795263,53.9071299964542,
2.66391429251066));
#232584=CARTESIAN_POINT('Ctrl Pts',(-24.0700811970214,53.9059686572516,
2.66563118464163));
#232585=CARTESIAN_POINT('Ctrl Pts',(-24.0770886066608,53.9052646847387,
2.66774105138738));
#232586=CARTESIAN_POINT('Ctrl Pts',(-24.0839917000394,53.9049900928805,
2.67016894181789));
#232587=CARTESIAN_POINT('Ctrl Pts',(-24.0874432467287,53.9048527969514,
2.67138288703315));
#232588=CARTESIAN_POINT('Ctrl Pts',(-24.0908688957001,53.9048227635324,
2.67267613167591));
#232589=CARTESIAN_POINT('Ctrl Pts',(-24.0942592346731,53.9048959123384,
2.67403835432593));
#232590=CARTESIAN_POINT('Ctrl Pts',(-24.0959544041596,53.9049324867414,
2.67471946565094));
#232591=CARTESIAN_POINT('Ctrl Pts',(-24.0976407611372,53.9049948499729,
2.67541781389562));
#232592=CARTESIAN_POINT('Ctrl Pts',(-24.099317223136,53.9050824496423,2.67613207244208));
#232593=CARTESIAN_POINT('Ctrl Pts',(-24.0997363386357,53.9051043495596,
2.6763106370787));
#232594=CARTESIAN_POINT('Ctrl Pts',(-24.1001548360176,53.9051278266103,
2.67649019601884));
#232595=CARTESIAN_POINT('Ctrl Pts',(-24.1005726990102,53.9051528718724,
2.67667072836696));
#232596=CARTESIAN_POINT('Ctrl Pts',(-24.1018262879881,53.9052280076586,
2.67721232541129));
#232597=CARTESIAN_POINT('Ctrl Pts',(-24.1030741658757,53.9053172580729,
2.67776268340086));
#232598=CARTESIAN_POINT('Ctrl Pts',(-24.1043159075202,53.9054203757498,
2.67832123541555));
#232599=CARTESIAN_POINT('Ctrl Pts',(-24.113062575326,53.9061467233511,2.6822556036849));
#232600=CARTESIAN_POINT('Ctrl Pts',(-24.1215389842448,53.9075195712151,
2.68661792998942));
#232601=CARTESIAN_POINT('Ctrl Pts',(-24.1297041260874,53.9094265129033,
2.6913098662264));
#232602=CARTESIAN_POINT('Ctrl Pts',(-24.1336642110575,53.9103513775614,
2.69358545023109));
#232603=CARTESIAN_POINT('Ctrl Pts',(-24.1375513523937,53.9114023832601,
2.69593918853516));
#232604=CARTESIAN_POINT('Ctrl Pts',(-24.1413619171793,53.9125693701072,
2.69836306235513));
#232605=CARTESIAN_POINT('Ctrl Pts',(-24.1471956256297,53.9143559454351,
2.70207384382245));
#232606=CARTESIAN_POINT('Ctrl Pts',(-24.1528469606267,53.9164123347821,
2.70594760814245));
#232607=CARTESIAN_POINT('Ctrl Pts',(-24.1582902100542,53.9187002605239,
2.70995196345725));
#232608=CARTESIAN_POINT('Ctrl Pts',(-24.1608180832479,53.9197627850746,
2.71181160678123));
#232609=CARTESIAN_POINT('Ctrl Pts',(-24.1633010951265,53.9208749910659,
2.71369962772116));
#232610=CARTESIAN_POINT('Ctrl Pts',(-24.1657359576696,53.9220340502327,
2.71561183138678));
#232611=CARTESIAN_POINT('Ctrl Pts',(-24.1659225802897,53.922122887551,2.71575839426329));
#232612=CARTESIAN_POINT('Ctrl Pts',(-24.1661089452649,53.9222119774188,
2.71590508903226));
#232613=CARTESIAN_POINT('Ctrl Pts',(-24.1662950522344,53.9223013184211,
2.71605191409929));
#232614=CARTESIAN_POINT('Ctrl Pts',(-24.1689092940617,53.9235562901483,
2.7181143636277));
#232615=CARTESIAN_POINT('Ctrl Pts',(-24.1714718460794,53.924862754225,2.72020091026977));
#232616=CARTESIAN_POINT('Ctrl Pts',(-24.1739808617162,53.9262153118349,
2.72230624862199));
#232617=CARTESIAN_POINT('Ctrl Pts',(-24.1829777455765,53.9310653428796,
2.72985561753131));
#232618=CARTESIAN_POINT('Ctrl Pts',(-24.1913567365399,53.936543815757,2.73770089914369));
#232619=CARTESIAN_POINT('Ctrl Pts',(-24.1991508947539,53.9425259106384,
2.74574823347124));
#232620=CARTESIAN_POINT('Ctrl Pts',(-24.2077158916383,53.9490996319582,
2.75459144547067));
#232621=CARTESIAN_POINT('Ctrl Pts',(-24.2155752681668,53.9562817849775,
2.76367911754305));
#232622=CARTESIAN_POINT('Ctrl Pts',(-24.2227540584928,53.9639562340145,
2.77292162564753));
#232623=CARTESIAN_POINT('Ctrl Pts',(-24.2305053504141,53.9722427129505,
2.78290121484725));
#232624=CARTESIAN_POINT('Ctrl Pts',(-24.2374640812929,53.9811038680483,
2.79306229500149));
#232625=CARTESIAN_POINT('Ctrl Pts',(-24.2436285779125,53.9904403792159,
2.8033191668518));
#232626=CARTESIAN_POINT('Ctrl Pts',(-24.2497413607397,53.9996985666484,
2.81348999408656));
#232627=CARTESIAN_POINT('Ctrl Pts',(-24.2550737197506,54.0094254978901,
2.82375635966875));
#232628=CARTESIAN_POINT('Ctrl Pts',(-24.2595822759735,54.0195518809642,
2.83404198860299));
#232629=CARTESIAN_POINT('Origin',(0.0139224327744811,0.00619866644065959,
2.83404198860262));
#232630=CARTESIAN_POINT('Ctrl Pts',(-25.5480287005721,57.419280924679,2.65878198860301));
#232631=CARTESIAN_POINT('Ctrl Pts',(-25.5401808584718,57.4227710771206,
2.65878198860301));
#232632=CARTESIAN_POINT('Ctrl Pts',(-25.53211120635,57.425574643879,2.65944603041891));
#232633=CARTESIAN_POINT('Ctrl Pts',(-25.5239679177299,57.4277200319918,
2.66070439264113));
#232634=CARTESIAN_POINT('Ctrl Pts',(-25.5187647439657,57.4290908328639,
2.66150842619636));
#232635=CARTESIAN_POINT('Ctrl Pts',(-25.5135317242465,57.4301938346427,
2.66255428265407));
#232636=CARTESIAN_POINT('Ctrl Pts',(-25.5083079410949,57.4310450321042,
2.66381699700691));
#232637=CARTESIAN_POINT('Ctrl Pts',(-25.5011785252534,57.432206745845,2.6655403487329));
#232638=CARTESIAN_POINT('Ctrl Pts',(-25.4940667032539,57.4328933558608,
2.66766759643994));
#232639=CARTESIAN_POINT('Ctrl Pts',(-25.4870628291427,57.4331362848729,
2.67012012783169));
#232640=CARTESIAN_POINT('Ctrl Pts',(-25.483560892087,57.4332577493789,2.67134639352757));
#232641=CARTESIAN_POINT('Ctrl Pts',(-25.4800857520065,57.4332683803242,
2.67265375585033));
#232642=CARTESIAN_POINT('Ctrl Pts',(-25.4766473428561,57.4331727200759,
2.67403135126961));
#232643=CARTESIAN_POINT('Ctrl Pts',(-25.4749281382809,57.4331248899517,
2.67472014897925));
#232644=CARTESIAN_POINT('Ctrl Pts',(-25.4732181005507,57.4330504941582,
2.67542649668654));
#232645=CARTESIAN_POINT('Ctrl Pts',(-25.4715183716227,57.4329501454095,
2.67614899656123));
#232646=CARTESIAN_POINT('Ctrl Pts',(-25.4710934393907,57.4329250582223,
2.6763296215299));
#232647=CARTESIAN_POINT('Ctrl Pts',(-25.4706691511208,57.4328983491282,
2.67651125590971));
#232648=CARTESIAN_POINT('Ctrl Pts',(-25.4702455239745,57.4328700280097,
2.67669387767545));
#232649=CARTESIAN_POINT('Ctrl Pts',(-25.4689746425357,57.4327850646539,
2.67724174297265));
#232650=CARTESIAN_POINT('Ctrl Pts',(-25.4677097128937,57.4326855923071,
2.67779849504769));
#232651=CARTESIAN_POINT('Ctrl Pts',(-25.4664511833529,57.4325718846638,
2.6783635361803));
#232652=CARTESIAN_POINT('Ctrl Pts',(-25.4577539633644,57.4317860942977,
2.68226832098941));
#232653=CARTESIAN_POINT('Ctrl Pts',(-25.4493260998446,57.4303627559732,
2.68659153751438));
#232654=CARTESIAN_POINT('Ctrl Pts',(-25.4412057723274,57.428414357709,2.69123699486241));
#232655=CARTESIAN_POINT('Ctrl Pts',(-25.4371699918416,57.42744600912,2.69354577441267));
#232656=CARTESIAN_POINT('Ctrl Pts',(-25.4332098968695,57.4263474236139,
2.69593478828154));
#232657=CARTESIAN_POINT('Ctrl Pts',(-25.4293290842281,57.4251294472438,
2.69839565261242));
#232658=CARTESIAN_POINT('Ctrl Pts',(-25.4207674318877,57.4224424094498,
2.70382468689068));
#232659=CARTESIAN_POINT('Ctrl Pts',(-25.4125888532393,57.419186421293,2.70961155815109));
#232660=CARTESIAN_POINT('Ctrl Pts',(-25.4048965980306,57.4154637896042,
2.7156270136179));
#232661=CARTESIAN_POINT('Ctrl Pts',(-25.4020865201984,57.4141038653034,
2.71782453535881));
#232662=CARTESIAN_POINT('Ctrl Pts',(-25.3993352917243,57.4126868351397,
2.72005051502425));
#232663=CARTESIAN_POINT('Ctrl Pts',(-25.3966436944401,57.4112179557372,
2.72229986760139));
#232664=CARTESIAN_POINT('Ctrl Pts',(-25.3876029039784,57.4062841452561,
2.72985520488901));
#232665=CARTESIAN_POINT('Ctrl Pts',(-25.3791816069562,57.4007266836993,
2.73770845534555));
#232666=CARTESIAN_POINT('Ctrl Pts',(-25.3713475726781,57.3946697603111,
2.74576706701736));
#232667=CARTESIAN_POINT('Ctrl Pts',(-25.3627370410042,57.3880124840177,
2.75462443585));
#232668=CARTESIAN_POINT('Ctrl Pts',(-25.3548353295678,57.380751543477,2.7637303632314));
#232669=CARTESIAN_POINT('Ctrl Pts',(-25.3476188815051,57.3730023605538,
2.77299664636762));
#232670=CARTESIAN_POINT('Ctrl Pts',(-25.3398464577413,57.3646561585193,
2.78297683033401));
#232671=CARTESIAN_POINT('Ctrl Pts',(-25.3328680394185,57.3557428147478,
2.793144014788));
#232672=CARTESIAN_POINT('Ctrl Pts',(-25.3266878999863,57.3463604602072,
2.80341452427818));
#232673=CARTESIAN_POINT('Ctrl Pts',(-25.320591213303,57.3371047991314,2.81354634721299));
#232674=CARTESIAN_POINT('Ctrl Pts',(-25.3152708796015,57.327391367358,2.82378004209192));
#232675=CARTESIAN_POINT('Ctrl Pts',(-25.3107727110825,57.3172883154491,
2.83404198860301));
#232676=CARTESIAN_POINT('Ctrl Pts',(-23.9115214566117,54.174518541976,2.83404198860299));
#232677=CARTESIAN_POINT('Ctrl Pts',(-23.9072166846465,54.1648498658389,
2.82422126443081));
#232678=CARTESIAN_POINT('Ctrl Pts',(-23.9036899956625,54.1548764216405,
2.81442815028612));
#232679=CARTESIAN_POINT('Ctrl Pts',(-23.9009524404117,54.1446552025551,
2.80471618166465));
#232680=CARTESIAN_POINT('Ctrl Pts',(-23.8983090899564,54.1347857162257,
2.79533842146399));
#232681=CARTESIAN_POINT('Ctrl Pts',(-23.8964012454638,54.1246839742781,
2.78603515650431));
#232682=CARTESIAN_POINT('Ctrl Pts',(-23.8952825179499,54.1143872866757,
2.77685887346968));
#232683=CARTESIAN_POINT('Ctrl Pts',(-23.8942249700855,54.1046536921685,
2.76818441216801));
#232684=CARTESIAN_POINT('Ctrl Pts',(-23.8938724934879,54.0947449925327,
2.75962261521858));
#232685=CARTESIAN_POINT('Ctrl Pts',(-23.8943122764064,54.0846948896059,
2.75123537701903));
#232686=CARTESIAN_POINT('Ctrl Pts',(-23.8947173090964,54.0754389134133,
2.74351087134367));
#232687=CARTESIAN_POINT('Ctrl Pts',(-23.895794425562,54.0660624571237,2.73593399450098));
#232688=CARTESIAN_POINT('Ctrl Pts',(-23.8976480927552,54.0566033397524,
2.7285765781283));
#232689=CARTESIAN_POINT('Ctrl Pts',(-23.8982008188935,54.0537828218969,
2.72638274508499));
#232690=CARTESIAN_POINT('Ctrl Pts',(-23.8988228478382,54.0509550659744,
2.724208617097));
#232691=CARTESIAN_POINT('Ctrl Pts',(-23.8995176373646,54.0481214021003,
2.72205663736744));
#232692=CARTESIAN_POINT('Ctrl Pts',(-23.9002053278541,54.0453166912884,
2.71992664556783));
#232693=CARTESIAN_POINT('Ctrl Pts',(-23.9009633199468,54.0425090377021,
2.71782089927902));
#232694=CARTESIAN_POINT('Ctrl Pts',(-23.9017938716382,54.0397028685178,
2.71574387311264));
#232695=CARTESIAN_POINT('Ctrl Pts',(-23.9018516265785,54.0395077330007,
2.71559944077504));
#232696=CARTESIAN_POINT('Ctrl Pts',(-23.9019097237178,54.0393125964105,
2.71545515216087));
#232697=CARTESIAN_POINT('Ctrl Pts',(-23.9019681642225,54.0391174593313,
2.71531100781748));
#232698=CARTESIAN_POINT('Ctrl Pts',(-23.9045304100324,54.0305619349333,
2.708991191761));
#232699=CARTESIAN_POINT('Ctrl Pts',(-23.9077916774638,54.0220283896862,
2.70298296066855));
#232700=CARTESIAN_POINT('Ctrl Pts',(-23.9117952627745,54.0136246330487,
2.69736727774153));
#232701=CARTESIAN_POINT('Ctrl Pts',(-23.9155273001025,54.0057908712995,
2.69213248525441));
#232702=CARTESIAN_POINT('Ctrl Pts',(-23.9199049461656,53.9980693056377,
2.68723866185476));
#232703=CARTESIAN_POINT('Ctrl Pts',(-23.9249777890353,53.9905727747493,
2.68278595829567));
#232704=CARTESIAN_POINT('Ctrl Pts',(-23.9268335005856,53.987830446766,2.68115710172815));
#232705=CARTESIAN_POINT('Ctrl Pts',(-23.928782350975,53.9851185338202,2.67958763637824));
#232706=CARTESIAN_POINT('Ctrl Pts',(-23.9308270955486,53.9824437337508,
2.67808378645382));
#232707=CARTESIAN_POINT('Ctrl Pts',(-23.9313187883097,53.9818005336913,
2.67772216078618));
#232708=CARTESIAN_POINT('Ctrl Pts',(-23.9318165831367,53.9811593045605,
2.67736403603581));
#232709=CARTESIAN_POINT('Ctrl Pts',(-23.9323204546079,53.9805201796372,
2.67700956934497));
#232710=CARTESIAN_POINT('Ctrl Pts',(-23.9328085800956,53.9799010273677,
2.67666617973821));
#232711=CARTESIAN_POINT('Ctrl Pts',(-23.9333024083484,53.9792838498572,
2.67632622314136));
#232712=CARTESIAN_POINT('Ctrl Pts',(-23.9338019127824,53.9786687697972,
2.67598984158791));
#232713=CARTESIAN_POINT('Ctrl Pts',(-23.9392745611217,53.9719298569084,
2.67230439292238));
#232714=CARTESIAN_POINT('Ctrl Pts',(-23.9454324752045,53.9654385427828,
2.66904964539992));
#232715=CARTESIAN_POINT('Ctrl Pts',(-23.9522153560506,53.9593734277047,
2.66640203566742));
#232716=CARTESIAN_POINT('Ctrl Pts',(-23.9550284189135,53.9568580437001,
2.66530399299457));
#232717=CARTESIAN_POINT('Ctrl Pts',(-23.9579485624029,53.9544158621942,
2.66430995142276));
#232718=CARTESIAN_POINT('Ctrl Pts',(-23.9609698772114,53.9520587513133,
2.66343053473377));
#232719=CARTESIAN_POINT('Ctrl Pts',(-23.9661230444607,53.9480384530776,
2.661930597929));
#232720=CARTESIAN_POINT('Ctrl Pts',(-23.9715702598497,53.9442681092576,
2.66076519817143));
#232721=CARTESIAN_POINT('Ctrl Pts',(-23.9772776109214,53.9408121161407,
2.65997805604475));
#232722=CARTESIAN_POINT('Ctrl Pts',(-23.9801312864573,53.9390841195823,
2.65958448498141));
#232723=CARTESIAN_POINT('Ctrl Pts',(-23.983050645519,53.9374360035034,2.65928526260777));
#232724=CARTESIAN_POINT('Ctrl Pts',(-23.9860314303861,53.9358758804728,
2.65908463971339));
#232725=CARTESIAN_POINT('Ctrl Pts',(-23.9890122152532,53.9343157574423,
2.65888401681901));
#232726=CARTESIAN_POINT('Ctrl Pts',(-23.9920543802863,53.9328436288554,
2.65878198860299));
#232727=CARTESIAN_POINT('Ctrl Pts',(-23.995153256981,53.9314655730805,2.65878198860299));
#232728=CARTESIAN_POINT('Origin',(-29.1450842944632,50.4502867888876,2.83404198860296));
#232729=CARTESIAN_POINT('Ctrl Pts',(-31.4933613949861,54.1671020372439,
2.83404198860299));
#232730=CARTESIAN_POINT('Ctrl Pts',(-31.4986665597483,54.1762908521544,
2.82419652440102));
#232731=CARTESIAN_POINT('Ctrl Pts',(-31.5032309550538,54.1858709973833,
2.81438790575682));
#232732=CARTESIAN_POINT('Ctrl Pts',(-31.507039169141,54.1957854287845,2.80466781256928));
#232733=CARTESIAN_POINT('Ctrl Pts',(-31.5107236389469,54.2053777002017,
2.79526356453096));
#232734=CARTESIAN_POINT('Ctrl Pts',(-31.5137006693056,54.2152841131322,
2.7859410249624));
#232735=CARTESIAN_POINT('Ctrl Pts',(-31.5159144374967,54.2254725303169,
2.77675109088775));
#232736=CARTESIAN_POINT('Ctrl Pts',(-31.5180085258895,54.2351101456071,
2.76805797913666));
#232737=CARTESIAN_POINT('Ctrl Pts',(-31.5194198476568,54.245001003775,2.75948271210131));
#232738=CARTESIAN_POINT('Ctrl Pts',(-31.5200591406753,54.2551207303737,
2.7510857557318));
#232739=CARTESIAN_POINT('Ctrl Pts',(-31.5206479757801,54.2644417304484,
2.7433515516321));
#232740=CARTESIAN_POINT('Ctrl Pts',(-31.5205818213852,54.2739574575971,
2.73576818685868));
#232741=CARTESIAN_POINT('Ctrl Pts',(-31.5197533892255,54.2836415202572,
2.7284062616041));
#232742=CARTESIAN_POINT('Ctrl Pts',(-31.5195130925471,54.286450498715,2.72627084693634));
#232743=CARTESIAN_POINT('Ctrl Pts',(-31.5192084034331,54.2892735615577,
2.72415424587518));
#232744=CARTESIAN_POINT('Ctrl Pts',(-31.5188360425581,54.2921098354281,
2.72205867173294));
#232745=CARTESIAN_POINT('Ctrl Pts',(-31.5184323794288,54.2951845386602,
2.71978693462897));
#232746=CARTESIAN_POINT('Ctrl Pts',(-31.5179508191006,54.2982706300314,
2.71754411340797));
#232747=CARTESIAN_POINT('Ctrl Pts',(-31.5173878381078,54.3013662138034,
2.71533341844295));
#232748=CARTESIAN_POINT('Ctrl Pts',(-31.5158427323552,54.309862067756,2.70926614876442));
#232749=CARTESIAN_POINT('Ctrl Pts',(-31.5136439393734,54.3184108612912,
2.70347381860459));
#232750=CARTESIAN_POINT('Ctrl Pts',(-31.5107627835359,54.3269129314608,
2.69804914171445));
#232751=CARTESIAN_POINT('Ctrl Pts',(-31.5081266823661,54.3346918640778,
2.69308585687251));
#232752=CARTESIAN_POINT('Ctrl Pts',(-31.5049132975212,54.3424218244384,
2.68842799053229));
#232753=CARTESIAN_POINT('Ctrl Pts',(-31.5010675328659,54.3500333719153,
2.68414767054259));
#232754=CARTESIAN_POINT('Ctrl Pts',(-31.4991785058299,54.3537721391718,
2.68204519134596));
#232755=CARTESIAN_POINT('Ctrl Pts',(-31.4971365594547,54.3574819590038,
2.68003431778549));
#232756=CARTESIAN_POINT('Ctrl Pts',(-31.4949332463336,54.3611518569451,
2.67812693945301));
#232757=CARTESIAN_POINT('Ctrl Pts',(-31.4945151891294,54.3618481843342,
2.67776503299253));
#232758=CARTESIAN_POINT('Ctrl Pts',(-31.494090808751,54.3625432124818,2.67740659639973));
#232759=CARTESIAN_POINT('Ctrl Pts',(-31.4936601139564,54.3632368016453,
2.67705178968905));
#232760=CARTESIAN_POINT('Ctrl Pts',(-31.4932428783741,54.3639087161475,
2.67670807068807));
#232761=CARTESIAN_POINT('Ctrl Pts',(-31.4928197168825,54.3645792801848,
2.67636775825315));
#232762=CARTESIAN_POINT('Ctrl Pts',(-31.4923906407828,54.3652483648081,
2.67603099699304));
#232763=CARTESIAN_POINT('Ctrl Pts',(-31.4877146578621,54.3725399111642,
2.67236104217182));
#232764=CARTESIAN_POINT('Ctrl Pts',(-31.4823328301625,54.3796603393082,
2.66911440541531));
#232765=CARTESIAN_POINT('Ctrl Pts',(-31.4762829888801,54.386422985696,2.66646778189689));
#232766=CARTESIAN_POINT('Ctrl Pts',(-31.4737281033388,54.3892788932596,
2.66535009635029));
#232767=CARTESIAN_POINT('Ctrl Pts',(-31.471054515739,54.3920710496178,2.66433897912396));
#232768=CARTESIAN_POINT('Ctrl Pts',(-31.4682668669588,54.3947861357356,
2.66344564884842));
#232769=CARTESIAN_POINT('Ctrl Pts',(-31.4635725360689,54.3993582729153,
2.66194130298635));
#232770=CARTESIAN_POINT('Ctrl Pts',(-31.4585547584354,54.4037093249068,
2.6607720670547));
#232771=CARTESIAN_POINT('Ctrl Pts',(-31.4532397415958,54.4077698566067,
2.65998225155764));
#232772=CARTESIAN_POINT('Ctrl Pts',(-31.4519109873859,54.4087849895317,
2.65978479768338));
#232773=CARTESIAN_POINT('Ctrl Pts',(-31.450563526166,54.4097817701145,2.65961098966672));
#232774=CARTESIAN_POINT('Ctrl Pts',(-31.4491976069262,54.4107588499961,
2.65946139030551));
#232775=CARTESIAN_POINT('Ctrl Pts',(-31.4471487280664,54.4122244698184,
2.6592369912637));
#232776=CARTESIAN_POINT('Ctrl Pts',(-31.4450583254661,54.4136457436056,
2.65906707562491));
#232777=CARTESIAN_POINT('Ctrl Pts',(-31.4429280944111,54.4150195646482,
2.65895332562969));
#232778=CARTESIAN_POINT('Ctrl Pts',(-31.4407978633561,54.4163933856909,
2.65883957563447));
#232779=CARTESIAN_POINT('Ctrl Pts',(-31.438627814593,54.4177197583745,2.65878198860299));
#232780=CARTESIAN_POINT('Ctrl Pts',(-31.4364195775146,54.4189959163078,
2.65878198860299));
#232781=CARTESIAN_POINT('Ctrl Pts',(-29.5274749692187,51.1126068659047,
2.65878198860297));
#232782=CARTESIAN_POINT('Ctrl Pts',(-29.5349468458355,51.1082885388127,
2.65878198860297));
#232783=CARTESIAN_POINT('Ctrl Pts',(-29.5427104181398,51.104624414238,2.65945335517903));
#232784=CARTESIAN_POINT('Ctrl Pts',(-29.5506148782584,51.1016049255938,
2.66072561226672));
#232785=CARTESIAN_POINT('Ctrl Pts',(-29.5557203484494,51.0996546457476,
2.66154735980405));
#232786=CARTESIAN_POINT('Ctrl Pts',(-29.5608842707094,51.0979724198486,
2.66261895766938));
#232787=CARTESIAN_POINT('Ctrl Pts',(-29.5660646037407,51.0965469289498,
2.66391429251063));
#232788=CARTESIAN_POINT('Ctrl Pts',(-29.5729308384267,51.0946575224203,
2.6656311846416));
#232789=CARTESIAN_POINT('Ctrl Pts',(-29.579826275578,51.0932249325814,2.66774105138736));
#232790=CARTESIAN_POINT('Ctrl Pts',(-29.5866628504239,51.0922302752235,
2.67016894181786));
#232791=CARTESIAN_POINT('Ctrl Pts',(-29.5900811378468,51.0917329465446,
2.67138288703312));
#232792=CARTESIAN_POINT('Ctrl Pts',(-29.5934848814075,51.091344999829,2.67267613167588));
#232793=CARTESIAN_POINT('Ctrl Pts',(-29.5968642938812,51.0910633609954,
2.6740383543259));
#232794=CARTESIAN_POINT('Ctrl Pts',(-29.598554000118,51.0909225415785,2.6747194656509));
#232795=CARTESIAN_POINT('Ctrl Pts',(-29.6002376377884,51.0908082908744,
2.67541781389559));
#232796=CARTESIAN_POINT('Ctrl Pts',(-29.6019140726117,51.0907201726672,
2.67613207244205));
#232797=CARTESIAN_POINT('Ctrl Pts',(-29.6023331813176,51.0906981431154,
2.67631063707867));
#232798=CARTESIAN_POINT('Ctrl Pts',(-29.6027518401471,51.0906777466681,
2.67649019601882));
#232799=CARTESIAN_POINT('Ctrl Pts',(-29.6031700319853,51.0906589761531,
2.67667072836693));
#232800=CARTESIAN_POINT('Ctrl Pts',(-29.6044246074998,51.0906026646082,
2.67721232541127));
#232801=CARTESIAN_POINT('Ctrl Pts',(-29.6056749785905,51.0905609873414,
2.67776268340083));
#232802=CARTESIAN_POINT('Ctrl Pts',(-29.6069206965766,51.090533742783,2.67832123541552));
#232803=CARTESIAN_POINT('Ctrl Pts',(-29.6156953732194,51.0903418356318,
2.68225560368482));
#232804=CARTESIAN_POINT('Ctrl Pts',(-29.6242688491607,51.0908211368932,
2.68661792998926));
#232805=CARTESIAN_POINT('Ctrl Pts',(-29.632588591186,51.0918641424261,2.69130986622617));
#232806=CARTESIAN_POINT('Ctrl Pts',(-29.6366236570778,51.0923699989826,
2.69358545023092));
#232807=CARTESIAN_POINT('Ctrl Pts',(-29.6405993642578,51.0930089302517,
2.69593918853506));
#232808=CARTESIAN_POINT('Ctrl Pts',(-29.6445110377126,51.0937712117415,
2.6983630623551));
#232809=CARTESIAN_POINT('Ctrl Pts',(-29.6504995364713,51.0949382114433,
2.70207384382243));
#232810=CARTESIAN_POINT('Ctrl Pts',(-29.6563348640822,51.0963926103117,
2.70594760814243));
#232811=CARTESIAN_POINT('Ctrl Pts',(-29.6619874481817,51.0980990280591,
2.70995196345723));
#232812=CARTESIAN_POINT('Ctrl Pts',(-29.66461253748,51.0988914972889,2.71181160678121));
#232813=CARTESIAN_POINT('Ctrl Pts',(-29.6671982043428,51.0997380650834,
2.71369962772114));
#232814=CARTESIAN_POINT('Ctrl Pts',(-29.6697408831278,51.1006362623629,
2.71561183138676));
#232815=CARTESIAN_POINT('Ctrl Pts',(-29.669935769438,51.1007051056453,2.71575839426327));
#232816=CARTESIAN_POINT('Ctrl Pts',(-29.6701304259133,51.1007742270251,
2.71590508903224));
#232817=CARTESIAN_POINT('Ctrl Pts',(-29.670324852047,51.1008436251325,2.71605191409926));
#232818=CARTESIAN_POINT('Ctrl Pts',(-29.6730559530502,51.1018184593125,
2.71811436362768));
#232819=CARTESIAN_POINT('Ctrl Pts',(-29.675741029822,51.1028499068179,2.72020091026974));
#232820=CARTESIAN_POINT('Ctrl Pts',(-29.6783776815771,51.1039327914268,
2.72230624862197));
#232821=CARTESIAN_POINT('Ctrl Pts',(-29.687832245858,51.1078158230498,2.72985561753114));
#232822=CARTESIAN_POINT('Ctrl Pts',(-29.6967379921829,51.1123884412303,
2.73770089914337));
#232823=CARTESIAN_POINT('Ctrl Pts',(-29.7051147523676,51.1175230541893,
2.74574823347076));
#232824=CARTESIAN_POINT('Ctrl Pts',(-29.7143199702903,51.1231654780136,
2.75459144547006));
#232825=CARTESIAN_POINT('Ctrl Pts',(-29.7228870317499,51.1294867578963,
2.76367911754229));
#232826=CARTESIAN_POINT('Ctrl Pts',(-29.7308286942754,51.1363687775774,
2.77292162564662));
#232827=CARTESIAN_POINT('Ctrl Pts',(-29.7394036967177,51.1437996316818,
2.78290121484625));
#232828=CARTESIAN_POINT('Ctrl Pts',(-29.7472505498657,51.1518848589997,
2.79306229500039));
#232829=CARTESIAN_POINT('Ctrl Pts',(-29.7543572078924,51.1605258584237,
2.80331916685061));
#232830=CARTESIAN_POINT('Ctrl Pts',(-29.761404248361,51.1690943687417,2.81348999408575));
#232831=CARTESIAN_POINT('Ctrl Pts',(-29.7677241373266,51.1782106315437,
2.82375635966834));
#232832=CARTESIAN_POINT('Ctrl Pts',(-29.7732664904682,51.1878102687785,
2.83404198860297));
#232833=CARTESIAN_POINT('Origin',(0.0131982271536832,0.00762000000018464,
2.83404198860262));
#232834=CARTESIAN_POINT('Ctrl Pts',(-31.4100231232064,54.4342359163063,
2.65878198860299));
#232835=CARTESIAN_POINT('Ctrl Pts',(-31.402583092678,54.4385272722022,2.65878198860299));
#232836=CARTESIAN_POINT('Ctrl Pts',(-31.3948506994804,54.4421589890637,
2.6594460304188));
#232837=CARTESIAN_POINT('Ctrl Pts',(-31.3869762747706,54.4451438299612,
2.66070439264085));
#232838=CARTESIAN_POINT('Ctrl Pts',(-31.3819448922448,54.4470510012007,
2.66150842619612));
#232839=CARTESIAN_POINT('Ctrl Pts',(-31.3768558346355,54.44869496013,2.66255428265391));
#232840=CARTESIAN_POINT('Ctrl Pts',(-31.3717496422766,54.4500875286681,
2.66381699700688));
#232841=CARTESIAN_POINT('Ctrl Pts',(-31.3647807142731,54.4519881053014,
2.66554034873288));
#232842=CARTESIAN_POINT('Ctrl Pts',(-31.3577796218685,54.4534143418204,
2.66766759643993));
#232843=CARTESIAN_POINT('Ctrl Pts',(-31.3508395087087,54.4543880442397,
2.67012012783169));
#232844=CARTESIAN_POINT('Ctrl Pts',(-31.3473694521289,54.4548748954494,
2.67134639352757));
#232845=CARTESIAN_POINT('Ctrl Pts',(-31.3439144604656,54.4552487192095,
2.67265375585033));
#232846=CARTESIAN_POINT('Ctrl Pts',(-31.3404848880616,54.4555129946226,
2.67403135126961));
#232847=CARTESIAN_POINT('Ctrl Pts',(-31.3387701018596,54.4556451323291,
2.67472014897925));
#232848=CARTESIAN_POINT('Ctrl Pts',(-31.337061655417,54.4557498916997,2.67542649668654));
#232849=CARTESIAN_POINT('Ctrl Pts',(-31.3353607484814,54.4558277627247,
2.67614899656123));
#232850=CARTESIAN_POINT('Ctrl Pts',(-31.3349355217475,54.4558472304809,
2.6763296215299));
#232851=CARTESIAN_POINT('Ctrl Pts',(-31.3345107659126,54.4558650179029,
2.67651125590971));
#232852=CARTESIAN_POINT('Ctrl Pts',(-31.3340864990772,54.455881133025,2.67669387767544));
#232853=CARTESIAN_POINT('Ctrl Pts',(-31.3328136985709,54.4559294783912,
2.67724174297265));
#232854=CARTESIAN_POINT('Ctrl Pts',(-31.3315453006542,54.4559627721159,
2.67779849504768));
#232855=CARTESIAN_POINT('Ctrl Pts',(-31.3302817797847,54.4559812395338,
2.6783635361803));
#232856=CARTESIAN_POINT('Ctrl Pts',(-31.3215500666182,54.4561088608497,
2.68226832098925));
#232857=CARTESIAN_POINT('Ctrl Pts',(-31.3130195924491,54.4555742713439,
2.68659153751404));
#232858=CARTESIAN_POINT('Ctrl Pts',(-31.3047400858596,54.4544853519659,
2.69123699486187));
#232859=CARTESIAN_POINT('Ctrl Pts',(-31.3006251938113,54.453944162024,2.69354577441229));
#232860=CARTESIAN_POINT('Ctrl Pts',(-31.2965719591988,54.453265537326,2.69593478828134));
#232861=CARTESIAN_POINT('Ctrl Pts',(-31.2925850928565,54.4524598885396,
2.6983956526124));
#232862=CARTESIAN_POINT('Ctrl Pts',(-31.2837894702121,54.4506825069819,
2.70382468689065));
#232863=CARTESIAN_POINT('Ctrl Pts',(-31.2753153512349,54.4482992497267,
2.70961155815107));
#232864=CARTESIAN_POINT('Ctrl Pts',(-31.2672761140353,54.4454010706198,
2.71562701361788));
#232865=CARTESIAN_POINT('Ctrl Pts',(-31.2643392793061,54.4443423292442,
2.71782453535879));
#232866=CARTESIAN_POINT('Ctrl Pts',(-31.2614550023641,54.4432206434044,
2.72005051502424));
#232867=CARTESIAN_POINT('Ctrl Pts',(-31.2586246102248,54.4420411592048,
2.72229986760139));
#232868=CARTESIAN_POINT('Ctrl Pts',(-31.2491176225323,54.4380793965878,
2.72985520488848));
#232869=CARTESIAN_POINT('Ctrl Pts',(-31.2401615453407,54.4334326446238,
2.73770845534446));
#232870=CARTESIAN_POINT('Ctrl Pts',(-31.2317373058287,54.4282277812603,
2.74576706701568));
#232871=CARTESIAN_POINT('Ctrl Pts',(-31.2224780686882,54.4225070198673,
2.75462443584773));
#232872=CARTESIAN_POINT('Ctrl Pts',(-31.2138606686978,54.4161118092728,
2.7637303632285));
#232873=CARTESIAN_POINT('Ctrl Pts',(-31.2058737429104,54.4091594014113,
2.77299664636408));
#232874=CARTESIAN_POINT('Ctrl Pts',(-31.1972714816249,54.4016713602574,
2.78297683032974));
#232875=CARTESIAN_POINT('Ctrl Pts',(-31.1893995936812,54.3935362880598,
2.79314401478298));
#232876=CARTESIAN_POINT('Ctrl Pts',(-31.1822725865976,54.3848513315174,
2.80341452427241));
#232877=CARTESIAN_POINT('Ctrl Pts',(-31.1752418181714,54.37628365121,2.8135463472091));
#232878=CARTESIAN_POINT('Ctrl Pts',(-31.168935299717,54.3671795569364,2.82378004208997));
#232879=CARTESIAN_POINT('Ctrl Pts',(-31.1634057161443,54.3576020372439,
2.83404198860299));
#232880=CARTESIAN_POINT('Ctrl Pts',(-29.4433108116264,51.3783102687785,
2.83404198860296));
#232881=CARTESIAN_POINT('Ctrl Pts',(-29.4380189697941,51.3691445298594,
2.82422126443104));
#232882=CARTESIAN_POINT('Ctrl Pts',(-29.4334690915859,51.3595943606121,
2.81442815028661));
#232883=CARTESIAN_POINT('Ctrl Pts',(-29.4296781246256,51.349715286878,2.8047161816654));
#232884=CARTESIAN_POINT('Ctrl Pts',(-29.4260176124813,51.3401761719884,
2.79533842146481));
#232885=CARTESIAN_POINT('Ctrl Pts',(-29.4230642997983,51.3303291924932,
2.7860351565052));
#232886=CARTESIAN_POINT('Ctrl Pts',(-29.4208754038589,51.3202058500908,
2.77685887347063));
#232887=CARTESIAN_POINT('Ctrl Pts',(-29.4188062116764,51.3106361210858,
2.76818441216884));
#232888=CARTESIAN_POINT('Ctrl Pts',(-29.4174199248365,51.3008185461803,
2.75962261521931));
#232889=CARTESIAN_POINT('Ctrl Pts',(-29.4168067767635,51.2907775289361,
2.75123537701965));
#232890=CARTESIAN_POINT('Ctrl Pts',(-29.4162420776746,51.2815299205047,
2.74351087134404));
#232891=CARTESIAN_POINT('Ctrl Pts',(-29.4163331870167,51.2720922400945,
2.73593399450111));
#232892=CARTESIAN_POINT('Ctrl Pts',(-29.4171879526243,51.2624911797745,
2.7285765781282));
#232893=CARTESIAN_POINT('Ctrl Pts',(-29.417442826474,51.2596283373971,2.72638274508491));
#232894=CARTESIAN_POINT('Ctrl Pts',(-29.4177658668979,51.2567510524878,
2.72420861709695));
#232895=CARTESIAN_POINT('Ctrl Pts',(-29.4181606517644,51.2538602864394,
2.72205663736742));
#232896=CARTESIAN_POINT('Ctrl Pts',(-29.4185514029024,51.2509990568967,
2.71992664556781));
#232897=CARTESIAN_POINT('Ctrl Pts',(-29.4190117629203,51.2481275521819,
2.717820899279));
#232898=CARTESIAN_POINT('Ctrl Pts',(-29.4195444402101,51.245249939194,2.71574387311261));
#232899=CARTESIAN_POINT('Ctrl Pts',(-29.4195814815471,51.2450498356146,
2.71559944077502));
#232900=CARTESIAN_POINT('Ctrl Pts',(-29.4196188630963,51.2448496951984,
2.71545515216085));
#232901=CARTESIAN_POINT('Ctrl Pts',(-29.4196565860788,51.2446495184043,
2.71531100781746));
#232902=CARTESIAN_POINT('Ctrl Pts',(-29.4213104998203,51.235873034447,2.70899119176089));
#232903=CARTESIAN_POINT('Ctrl Pts',(-29.4236619033166,51.2270453415807,
2.70298296066835));
#232904=CARTESIAN_POINT('Ctrl Pts',(-29.4267651248011,51.2182691329811,
2.69736727774125));
#232905=CARTESIAN_POINT('Ctrl Pts',(-29.429657866561,51.2100881812714,2.69213248525397));
#232906=CARTESIAN_POINT('Ctrl Pts',(-29.4332044080285,51.2019513265382,
2.68723866185419));
#232907=CARTESIAN_POINT('Ctrl Pts',(-29.4374658604808,51.1939656059606,
2.682785958295));
#232908=CARTESIAN_POINT('Ctrl Pts',(-29.4390247549189,51.1910443260608,
2.6811571017277));
#232909=CARTESIAN_POINT('Ctrl Pts',(-29.4406794572091,51.1881435589218,
2.679587636378));
#232910=CARTESIAN_POINT('Ctrl Pts',(-29.4424334077169,51.1852696776794,
2.67808378645378));
#232911=CARTESIAN_POINT('Ctrl Pts',(-29.4428551742198,51.1845786052484,
2.67772216078613));
#232912=CARTESIAN_POINT('Ctrl Pts',(-29.443283215379,51.1838888551096,2.67736403603576));
#232913=CARTESIAN_POINT('Ctrl Pts',(-29.4437175198435,51.1832005624689,
2.67700956934492));
#232914=CARTESIAN_POINT('Ctrl Pts',(-29.4441382522935,51.1825337789733,
2.67666617973817));
#232915=CARTESIAN_POINT('Ctrl Pts',(-29.4445648626867,51.1818683633173,
2.67632622314131));
#232916=CARTESIAN_POINT('Ctrl Pts',(-29.4449973374098,51.1812044402994,
2.67598984158786));
#232917=CARTESIAN_POINT('Ctrl Pts',(-29.4497355978001,51.17393039636,2.67230439292256));
#232918=CARTESIAN_POINT('Ctrl Pts',(-29.4551812510948,51.1668309650368,
2.66904964540027));
#232919=CARTESIAN_POINT('Ctrl Pts',(-29.4612929974509,51.1600900711827,
2.66640203566786));
#232920=CARTESIAN_POINT('Ctrl Pts',(-29.4638277208368,51.1572944215763,
2.66530399299482));
#232921=CARTESIAN_POINT('Ctrl Pts',(-29.4664765899952,51.1545603804843,
2.66430995142285));
#232922=CARTESIAN_POINT('Ctrl Pts',(-29.4692349685474,51.1519003687091,
2.66343053473373));
#232923=CARTESIAN_POINT('Ctrl Pts',(-29.4739396706108,51.1473634414342,
2.66193059792897));
#232924=CARTESIAN_POINT('Ctrl Pts',(-29.4789629373384,51.1430443628985,
2.6607651981714));
#232925=CARTESIAN_POINT('Ctrl Pts',(-29.4842777732943,51.1390107214368,
2.65997805604472));
#232926=CARTESIAN_POINT('Ctrl Pts',(-29.4869351912723,51.1369939007059,
2.65958448498138));
#232927=CARTESIAN_POINT('Ctrl Pts',(-29.4896662827385,51.1350496570629,
2.65928526260775));
#232928=CARTESIAN_POINT('Ctrl Pts',(-29.4924676612913,51.133186503688,2.65908463971337));
#232929=CARTESIAN_POINT('Ctrl Pts',(-29.4952690398441,51.1313233503131,
2.65888401681899));
#232930=CARTESIAN_POINT('Ctrl Pts',(-29.49814066024,51.1295412933646,2.65878198860297));
#232931=CARTESIAN_POINT('Ctrl Pts',(-29.5010785149114,51.1278468659047,
2.65878198860297));
#232932=CARTESIAN_POINT('Origin',(-34.2589154226524,47.1274239660509,2.83404198860294));
#232933=CARTESIAN_POINT('Ctrl Pts',(-36.9828414016749,50.5784163149357,
2.83404198860297));
#232934=CARTESIAN_POINT('Ctrl Pts',(-36.989077996891,50.5870002518364,2.82419652440097));
#232935=CARTESIAN_POINT('Ctrl Pts',(-36.99461878582,50.5960508068001,2.81438790575681));
#232936=CARTESIAN_POINT('Ctrl Pts',(-36.9994424783905,50.6055128591422,
2.80466781256934));
#232937=CARTESIAN_POINT('Ctrl Pts',(-37.0041094296756,50.6146674511261,
2.79526356453112));
#232938=CARTESIAN_POINT('Ctrl Pts',(-37.0081056536707,50.6242084112814,
2.78594102496269));
#232939=CARTESIAN_POINT('Ctrl Pts',(-37.0113722741995,50.6341096134636,
2.77675109088818));
#232940=CARTESIAN_POINT('Ctrl Pts',(-37.0144622960728,50.6434755410471,
2.76805797913724));
#232941=CARTESIAN_POINT('Ctrl Pts',(-37.0168997626765,50.6531646927634,
2.75948271210207));
#232942=CARTESIAN_POINT('Ctrl Pts',(-37.0185933530511,50.663162158124,2.75108575573272));
#232943=CARTESIAN_POINT('Ctrl Pts',(-37.0201532722696,50.6723705467562,
2.74335155163321));
#232944=CARTESIAN_POINT('Ctrl Pts',(-37.0210821446113,50.681841060773,2.73576818685996));
#232945=CARTESIAN_POINT('Ctrl Pts',(-37.0212705108777,50.691558667865,2.72840626160552));
#232946=CARTESIAN_POINT('Ctrl Pts',(-37.0213251487713,50.6943773762881,
2.72627084693727));
#232947=CARTESIAN_POINT('Ctrl Pts',(-37.0213172191968,50.6972168227826,
2.72415424587563));
#232948=CARTESIAN_POINT('Ctrl Pts',(-37.0212433695026,50.7000764815586,
2.72205867173291));
#232949=CARTESIAN_POINT('Ctrl Pts',(-37.0211633116861,50.7031765355314,
2.71978693462894));
#232950=CARTESIAN_POINT('Ctrl Pts',(-37.0210069737843,50.7062960577322,
2.71754411340795));
#232951=CARTESIAN_POINT('Ctrl Pts',(-37.0207706534748,50.7094335311104,
2.71533341844292));
#232952=CARTESIAN_POINT('Ctrl Pts',(-37.0201220705311,50.718044351416,2.70926614876439));
#232953=CARTESIAN_POINT('Ctrl Pts',(-37.0188289150183,50.7267761502173,
2.70347381860456));
#232954=CARTESIAN_POINT('Ctrl Pts',(-37.0168522507833,50.735532807949,2.69804914171442));
#232955=CARTESIAN_POINT('Ctrl Pts',(-37.015043710324,50.7435446743633,2.69308585687257));
#232956=CARTESIAN_POINT('Ctrl Pts',(-37.0126559296151,50.7515681793719,
2.68842799053243));
#232957=CARTESIAN_POINT('Ctrl Pts',(-37.0096268558218,50.7595400218647,
2.68414767054279));
#232958=CARTESIAN_POINT('Ctrl Pts',(-37.0081389846695,50.7634557648562,
2.68204519134608));
#232959=CARTESIAN_POINT('Ctrl Pts',(-37.0064960060561,50.7673587034239,
2.68003431778554));
#232960=CARTESIAN_POINT('Ctrl Pts',(-37.0046883717069,50.771238806215,2.678126939453));
#232961=CARTESIAN_POINT('Ctrl Pts',(-37.0043453906958,50.7719750179269,
2.67776503299252));
#232962=CARTESIAN_POINT('Ctrl Pts',(-37.0039959853417,50.7727105984664,
2.67740659639972));
#232963=CARTESIAN_POINT('Ctrl Pts',(-37.0036401497476,50.7734454079409,
2.67705178968904));
#232964=CARTESIAN_POINT('Ctrl Pts',(-37.0032954340158,50.7741572546194,
2.67670807068806));
#232965=CARTESIAN_POINT('Ctrl Pts',(-37.0029446836755,50.7748683776572,
2.67636775825313));
#232966=CARTESIAN_POINT('Ctrl Pts',(-37.0025878964871,50.7755786476302,
2.67603099699303));
#232967=CARTESIAN_POINT('Ctrl Pts',(-36.9986997032254,50.7833190234416,
2.6723610421717));
#232968=CARTESIAN_POINT('Ctrl Pts',(-36.9940916451526,50.7909629993146,
2.6691144054151));
#232969=CARTESIAN_POINT('Ctrl Pts',(-36.9887818345681,50.7983209798302,
2.66646778189665));
#232970=CARTESIAN_POINT('Ctrl Pts',(-36.9865394685861,50.8014283006926,
2.66535009635014));
#232971=CARTESIAN_POINT('Ctrl Pts',(-36.9841723869924,50.8044846273291,
2.66433897912389));
#232972=CARTESIAN_POINT('Ctrl Pts',(-36.9816838130236,50.807476228564,2.66344564884841));
#232973=CARTESIAN_POINT('Ctrl Pts',(-36.9774931166428,50.8125140102919,
2.66194130298634));
#232974=CARTESIAN_POINT('Ctrl Pts',(-36.9729576356984,50.8173657273503,
2.66077206705468));
#232975=CARTESIAN_POINT('Ctrl Pts',(-36.9680961762159,50.8219595855753,
2.65998225155762));
#232976=CARTESIAN_POINT('Ctrl Pts',(-36.9668808113453,50.8231080501316,
2.65978479768336));
#232977=CARTESIAN_POINT('Ctrl Pts',(-36.9656449236015,50.8242402182967,
2.6596109896667));
#232978=CARTESIAN_POINT('Ctrl Pts',(-36.9643886196686,50.8253547230715,
2.65946139030549));
#232979=CARTESIAN_POINT('Ctrl Pts',(-36.9625041637694,50.8270264802337,
2.65923699126368));
#232980=CARTESIAN_POINT('Ctrl Pts',(-36.9605737761781,50.8286584747058,
2.65906707562489));
#232981=CARTESIAN_POINT('Ctrl Pts',(-36.9585988181541,50.8302474395916,
2.65895332562967));
#232982=CARTESIAN_POINT('Ctrl Pts',(-36.9566238601301,50.8318364044774,
2.65883957563445));
#232983=CARTESIAN_POINT('Ctrl Pts',(-36.9546043428184,50.8333823430136,
2.65878198860296));
#232984=CARTESIAN_POINT('Ctrl Pts',(-36.9525415975215,50.8348823336486,
2.65878198860296));
#232985=CARTESIAN_POINT('Ctrl Pts',(-34.7084426211234,47.7461450747865,
2.65878198860294));
#232986=CARTESIAN_POINT('Ctrl Pts',(-34.7154221779232,47.7410693801617,
2.65878198860294));
#232987=CARTESIAN_POINT('Ctrl Pts',(-34.7227602152549,47.7366138137626,
2.65945335517896));
#232988=CARTESIAN_POINT('Ctrl Pts',(-34.7303057514058,47.732784625124,2.66072561226656));
#232989=CARTESIAN_POINT('Ctrl Pts',(-34.7351793935418,47.7303113621614,
2.66154735980391));
#232990=CARTESIAN_POINT('Ctrl Pts',(-34.7401391868075,47.7280985748135,
2.66261895766927));
#232991=CARTESIAN_POINT('Ctrl Pts',(-34.7451421370596,47.7261394006519,
2.66391429251058));
#232992=CARTESIAN_POINT('Ctrl Pts',(-34.7517732610326,47.7235426275289,
2.66563118464155));
#232993=CARTESIAN_POINT('Ctrl Pts',(-34.7584811778433,47.721397116118,2.6677410513873));
#232994=CARTESIAN_POINT('Ctrl Pts',(-34.7651763312118,47.7196932909346,
2.67016894181781));
#232995=CARTESIAN_POINT('Ctrl Pts',(-34.768523907896,47.7188413783428,2.67138288703307));
#232996=CARTESIAN_POINT('Ctrl Pts',(-34.7718684539193,47.7180997687562,
2.67267613167583));
#232997=CARTESIAN_POINT('Ctrl Pts',(-34.7751999143434,47.717466427977,2.67403835432585));
#232998=CARTESIAN_POINT('Ctrl Pts',(-34.7768656445554,47.7171497575874,
2.67471946565086));
#232999=CARTESIAN_POINT('Ctrl Pts',(-34.7785281166319,47.7168601447021,
2.67541781389555));
#233000=CARTESIAN_POINT('Ctrl Pts',(-34.7801861569091,47.7165972740598,
2.67613207244201));
#233001=CARTESIAN_POINT('Ctrl Pts',(-34.7806006669785,47.7165315563992,
2.67631063707863));
#233002=CARTESIAN_POINT('Ctrl Pts',(-34.7810149003418,47.7164675099217,
2.67649019601877));
#233003=CARTESIAN_POINT('Ctrl Pts',(-34.7814288392283,47.7164051292834,
2.67667072836689));
#233004=CARTESIAN_POINT('Ctrl Pts',(-34.7826706558876,47.7162179873685,
2.67721232541123));
#233005=CARTESIAN_POINT('Ctrl Pts',(-34.783909820854,47.7160458390455,2.67776268340079));
#233006=CARTESIAN_POINT('Ctrl Pts',(-34.7851458668348,47.7158885307489,
2.67832123541548));
#233007=CARTESIAN_POINT('Ctrl Pts',(-34.7938524151213,47.7147804714199,
2.68225560368478));
#233008=CARTESIAN_POINT('Ctrl Pts',(-34.8024290252886,47.7143609747538,
2.68661792998924));
#233009=CARTESIAN_POINT('Ctrl Pts',(-34.8108122146621,47.7145286167447,
2.69130986622615));
#233010=CARTESIAN_POINT('Ctrl Pts',(-34.8148780524493,47.7146099229291,
2.6935854502309));
#233011=CARTESIAN_POINT('Ctrl Pts',(-34.818898766793,47.714829779504,2.69593918853504));
#233012=CARTESIAN_POINT('Ctrl Pts',(-34.8228686918041,47.715179003921,2.69836306235508));
#233013=CARTESIAN_POINT('Ctrl Pts',(-34.8289463696254,47.7157136421038,
2.70207384382241));
#233014=CARTESIAN_POINT('Ctrl Pts',(-34.8349017567798,47.7165501157952,
2.70594760814241));
#233015=CARTESIAN_POINT('Ctrl Pts',(-34.8407017446569,47.7176563296782,
2.70995196345721));
#233016=CARTESIAN_POINT('Ctrl Pts',(-34.8433952890323,47.7181700611283,
2.71181160678119));
#233017=CARTESIAN_POINT('Ctrl Pts',(-34.846055281772,47.7187417155522,2.71369962772112));
#233018=CARTESIAN_POINT('Ctrl Pts',(-34.8486779186779,47.7193692101071,
2.71561183138674));
#233019=CARTESIAN_POINT('Ctrl Pts',(-34.848878933463,47.7194173050923,2.71575839426325));
#233020=CARTESIAN_POINT('Ctrl Pts',(-34.8490797487414,47.7194657006757,
2.71590508903222));
#233021=CARTESIAN_POINT('Ctrl Pts',(-34.849280363866,47.719514395548,2.71605191409925));
#233022=CARTESIAN_POINT('Ctrl Pts',(-34.8520984015308,47.7201984116934,
2.71811436362766));
#233023=CARTESIAN_POINT('Ctrl Pts',(-34.8548765847938,47.7209435418727,
2.72020091026972));
#233024=CARTESIAN_POINT('Ctrl Pts',(-34.8576119849587,47.7217448891703,
2.72230624862195));
#233025=CARTESIAN_POINT('Ctrl Pts',(-34.8674206434757,47.7246183780647,
2.72985561753111));
#233026=CARTESIAN_POINT('Ctrl Pts',(-34.8767555719419,47.7282350429867,
2.73770089914333));
#233027=CARTESIAN_POINT('Ctrl Pts',(-34.88562315656,47.7324659181295,2.74574823347071));
#233028=CARTESIAN_POINT('Ctrl Pts',(-34.8953677412274,47.7371152248823,
2.75459144547016));
#233029=CARTESIAN_POINT('Ctrl Pts',(-34.9045486251,47.7425063743634,2.76367911754256));
#233030=CARTESIAN_POINT('Ctrl Pts',(-34.9131661493089,47.7485205638412,
2.77292162564708));
#233031=CARTESIAN_POINT('Ctrl Pts',(-34.9224709127513,47.7550143791218,
2.78290121484722));
#233032=CARTESIAN_POINT('Ctrl Pts',(-34.9311199164039,47.7622350952179,
2.7930622950019));
#233033=CARTESIAN_POINT('Ctrl Pts',(-34.9390908738055,47.7700859103008,
2.80331916685266));
#233034=CARTESIAN_POINT('Ctrl Pts',(-34.9469949630644,47.7778708651116,
2.81348999408713));
#233035=CARTESIAN_POINT('Ctrl Pts',(-34.9542331399579,47.78627657979,2.82375635966901));
#233036=CARTESIAN_POINT('Ctrl Pts',(-34.9607485668368,47.7952442955502,
2.83404198860294));
#233037=CARTESIAN_POINT('Origin',(0.0123294189942831,0.00895784724512226,
2.83404198860262));
#233038=CARTESIAN_POINT('Ctrl Pts',(-36.9278827595329,50.8527980281385,
2.65878198860296));
#233039=CARTESIAN_POINT('Ctrl Pts',(-36.9209320551072,50.8578435704956,
2.65878198860297));
#233040=CARTESIAN_POINT('Ctrl Pts',(-36.9136216385509,50.8622636476106,
2.6594460304188));
#233041=CARTESIAN_POINT('Ctrl Pts',(-36.9061023515955,50.8660552387515,
2.66070439264092));
#233042=CARTESIAN_POINT('Ctrl Pts',(-36.9012978851887,50.8684778849908,
2.66150842619618));
#233043=CARTESIAN_POINT('Ctrl Pts',(-36.8964085464701,50.8706447895124,
2.66255428265394));
#233044=CARTESIAN_POINT('Ctrl Pts',(-36.8914758894168,50.8725634718547,
2.66381699700687));
#233045=CARTESIAN_POINT('Ctrl Pts',(-36.8847438022849,50.8751820882651,
2.66554034873287));
#233046=CARTESIAN_POINT('Ctrl Pts',(-36.8779301449085,50.8773323251415,
2.66766759643992));
#233047=CARTESIAN_POINT('Ctrl Pts',(-36.8711298300324,50.8790261328805,
2.67012012783168));
#233048=CARTESIAN_POINT('Ctrl Pts',(-36.8677296725943,50.8798730367501,
2.67134639352755));
#233049=CARTESIAN_POINT('Ctrl Pts',(-36.8643326829601,50.8806059576337,
2.67265375585032));
#233050=CARTESIAN_POINT('Ctrl Pts',(-36.8609495224154,50.8812272732515,
2.6740313512696));
#233051=CARTESIAN_POINT('Ctrl Pts',(-36.859257942143,50.8815379310604,2.67472014897924));
#233052=CARTESIAN_POINT('Ctrl Pts',(-36.8575698050848,50.8818206978293,
2.67542649668652));
#233053=CARTESIAN_POINT('Ctrl Pts',(-36.855886355634,50.8820759354569,2.67614899656121));
#233054=CARTESIAN_POINT('Ctrl Pts',(-36.8554654932713,50.8821397448637,
2.67632962152989));
#233055=CARTESIAN_POINT('Ctrl Pts',(-36.8550449235851,50.882201833919,2.6765112559097));
#233056=CARTESIAN_POINT('Ctrl Pts',(-36.8546246654168,50.8822622087211,
2.67669387767543));
#233057=CARTESIAN_POINT('Ctrl Pts',(-36.8533638909116,50.8824433331273,
2.67724174297264));
#233058=CARTESIAN_POINT('Ctrl Pts',(-36.8521059215534,50.8826090281506,
2.67779849504767));
#233059=CARTESIAN_POINT('Ctrl Pts',(-36.8508512527542,50.8827594682968,
2.67836353618029));
#233060=CARTESIAN_POINT('Ctrl Pts',(-36.8421807128859,50.8837991030488,
2.68226832098931));
#233061=CARTESIAN_POINT('Ctrl Pts',(-36.8336410897272,50.8841591194361,
2.68659153751419));
#233062=CARTESIAN_POINT('Ctrl Pts',(-36.8252931160718,50.8839416093727,
2.69123699486211));
#233063=CARTESIAN_POINT('Ctrl Pts',(-36.8211441960798,50.8838335074683,
2.69354577441245));
#233064=CARTESIAN_POINT('Ctrl Pts',(-36.817042229914,50.8835822787328,2.69593478828141));
#233065=CARTESIAN_POINT('Ctrl Pts',(-36.8129929908132,50.8831977843867,
2.69839565261238));
#233066=CARTESIAN_POINT('Ctrl Pts',(-36.8040597645471,50.8823495324296,
2.70382468689064));
#233067=CARTESIAN_POINT('Ctrl Pts',(-36.7953829494618,50.8808651175413,
2.70961155815105));
#233068=CARTESIAN_POINT('Ctrl Pts',(-36.7870848098364,50.8788231440731,
2.71562701361785));
#233069=CARTESIAN_POINT('Ctrl Pts',(-36.7840533947862,50.8780771854145,
2.71782453535875));
#233070=CARTESIAN_POINT('Ctrl Pts',(-36.7810676701179,50.8772631333236,
2.72005051502419));
#233071=CARTESIAN_POINT('Ctrl Pts',(-36.7781294934921,50.8763859670026,
2.72229986760131));
#233072=CARTESIAN_POINT('Ctrl Pts',(-36.7682604691134,50.873439658149,2.72985520488929));
#233073=CARTESIAN_POINT('Ctrl Pts',(-36.7588677364065,50.8697545265635,
2.73770845534619));
#233074=CARTESIAN_POINT('Ctrl Pts',(-36.7499455893901,50.8654587487958,
2.7457670670184));
#233075=CARTESIAN_POINT('Ctrl Pts',(-36.7401390929213,50.8607371801608,
2.75462443585143));
#233076=CARTESIAN_POINT('Ctrl Pts',(-36.7309004184129,50.8552777667765,
2.76373036323325));
#233077=CARTESIAN_POINT('Ctrl Pts',(-36.7222305213302,50.8491983060104,
2.77299664636993));
#233078=CARTESIAN_POINT('Ctrl Pts',(-36.7128926706964,50.8426504662811,
2.78297683033686));
#233079=CARTESIAN_POINT('Ctrl Pts',(-36.7042135591824,50.8353827952087,
2.79314401479143));
#233080=CARTESIAN_POINT('Ctrl Pts',(-36.696217769428,50.8274903908639,2.80341452428226));
#233081=CARTESIAN_POINT('Ctrl Pts',(-36.6883299498338,50.8197045606271,
2.81354634721565));
#233082=CARTESIAN_POINT('Ctrl Pts',(-36.6811063421663,50.81130955022,2.82378004209319));
#233083=CARTESIAN_POINT('Ctrl Pts',(-36.674605926818,50.8023624960591,2.83404198860297));
#233084=CARTESIAN_POINT('Ctrl Pts',(-34.6525130919799,48.0191904766737,
2.83404198860294));
#233085=CARTESIAN_POINT('Ctrl Pts',(-34.6462921588072,48.0106280967263,
2.82422126443143));
#233086=CARTESIAN_POINT('Ctrl Pts',(-34.6407689407928,48.0016058360829,
2.81442815028741));
#233087=CARTESIAN_POINT('Ctrl Pts',(-34.6359660967503,47.9921771448995,
2.80471618166661));
#233088=CARTESIAN_POINT('Ctrl Pts',(-34.6313285282544,47.9830729139888,
2.79533842146634));
#233089=CARTESIAN_POINT('Ctrl Pts',(-34.6273621044929,47.9735885825143,
2.78603515650706));
#233090=CARTESIAN_POINT('Ctrl Pts',(-34.62412702213,47.9637494987701,2.77685887347279));
#233091=CARTESIAN_POINT('Ctrl Pts',(-34.621068856132,47.9544484832213,2.7681844121713));
#233092=CARTESIAN_POINT('Ctrl Pts',(-34.6186639474985,47.9448295964517,
2.75962261522204));
#233093=CARTESIAN_POINT('Ctrl Pts',(-34.6170045862125,47.9349076763769,
2.75123537702263));
#233094=CARTESIAN_POINT('Ctrl Pts',(-34.615476342306,47.9257697544405,2.7435108713473));
#233095=CARTESIAN_POINT('Ctrl Pts',(-34.6145804463113,47.9163742511121,
2.73593399450464));
#233096=CARTESIAN_POINT('Ctrl Pts',(-34.6144269453422,47.9067364390701,
2.72857657813196));
#233097=CARTESIAN_POINT('Ctrl Pts',(-34.6143811744519,47.9038626380693,
2.72638274508739));
#233098=CARTESIAN_POINT('Ctrl Pts',(-34.6144016870566,47.9009673483071,
2.72420861709817));
#233099=CARTESIAN_POINT('Ctrl Pts',(-34.6144921419176,47.8980511519206,
2.72205663736741));
#233100=CARTESIAN_POINT('Ctrl Pts',(-34.6145816725529,47.8951647518767,
2.7199266455678));
#233101=CARTESIAN_POINT('Ctrl Pts',(-34.6147393566953,47.8922608568399,
2.71782089927899));
#233102=CARTESIAN_POINT('Ctrl Pts',(-34.6149683234597,47.8893433277786,
2.71574387311261));
#233103=CARTESIAN_POINT('Ctrl Pts',(-34.6149842453607,47.8891404485134,
2.71559944077501));
#233104=CARTESIAN_POINT('Ctrl Pts',(-34.6150005017597,47.8889374970515,
2.71545515216083));
#233105=CARTESIAN_POINT('Ctrl Pts',(-34.6150170939191,47.8887344737214,
2.71531100781743));
#233106=CARTESIAN_POINT('Ctrl Pts',(-34.6157445549672,47.8798331871998,
2.70899119176089));
#233107=CARTESIAN_POINT('Ctrl Pts',(-34.6171603320595,47.8708080647646,
2.70298296066838));
#233108=CARTESIAN_POINT('Ctrl Pts',(-34.6193291901738,47.8617555581811,
2.69736727774131));
#233109=CARTESIAN_POINT('Ctrl Pts',(-34.6213509428814,47.85331704873,2.69213248525403));
#233110=CARTESIAN_POINT('Ctrl Pts',(-34.6240275231026,47.8448540540089,
2.68723866185425));
#233111=CARTESIAN_POINT('Ctrl Pts',(-34.6274308957724,47.8364666369681,
2.68278595829506));
#233112=CARTESIAN_POINT('Ctrl Pts',(-34.628675893525,47.8333984113051,2.68115710172776));
#233113=CARTESIAN_POINT('Ctrl Pts',(-34.6300183184515,47.8303405713845,
2.67958763637807));
#233114=CARTESIAN_POINT('Ctrl Pts',(-34.6314622582451,47.827299095813,2.67808378645385));
#233115=CARTESIAN_POINT('Ctrl Pts',(-34.6318094775277,47.8265677225447,
2.6777221607862));
#233116=CARTESIAN_POINT('Ctrl Pts',(-34.6321630753106,47.8258370084447,
2.67736403603583));
#233117=CARTESIAN_POINT('Ctrl Pts',(-34.6325230544378,47.8251070891649,
2.67700956934499));
#233118=CARTESIAN_POINT('Ctrl Pts',(-34.6328717842173,47.8243999798626,
2.67666617973824));
#233119=CARTESIAN_POINT('Ctrl Pts',(-34.6332265027182,47.8236936164944,
2.67632622314139));
#233120=CARTESIAN_POINT('Ctrl Pts',(-34.6335872094466,47.822988124598,2.67598984158793));
#233121=CARTESIAN_POINT('Ctrl Pts',(-34.6375391685163,47.8152586455548,
2.67230439292241));
#233122=CARTESIAN_POINT('Ctrl Pts',(-34.6422128973065,47.8076288798884,
2.66904964539994));
#233123=CARTESIAN_POINT('Ctrl Pts',(-34.6475865476013,47.8002860619011,
2.66640203566743));
#233124=CARTESIAN_POINT('Ctrl Pts',(-34.6498151605499,47.7972407764159,
2.66530399299458));
#233125=CARTESIAN_POINT('Ctrl Pts',(-34.6521637338116,47.7942448304651,
2.66430995142276));
#233126=CARTESIAN_POINT('Ctrl Pts',(-34.654628954734,47.7913110614419,2.66343053473377));
#233127=CARTESIAN_POINT('Ctrl Pts',(-34.6588336459112,47.7863072126526,
2.661930597929));
#233128=CARTESIAN_POINT('Ctrl Pts',(-34.6633779280161,47.7814867201294,
2.66076519817141));
#233129=CARTESIAN_POINT('Ctrl Pts',(-34.6682420184012,47.7769196237427,
2.65997805604472));
#233130=CARTESIAN_POINT('Ctrl Pts',(-34.6706740635937,47.7746360755494,
2.65958448498137));
#233131=CARTESIAN_POINT('Ctrl Pts',(-34.6731869650549,47.7724170058824,
2.65928526260773));
#233132=CARTESIAN_POINT('Ctrl Pts',(-34.6757782448038,47.7702712352615,
2.65908463971335));
#233133=CARTESIAN_POINT('Ctrl Pts',(-34.6783695245527,47.7681254646406,
2.65888401681897));
#233134=CARTESIAN_POINT('Ctrl Pts',(-34.6810391382372,47.7660530039194,
2.65878198860294));
#233135=CARTESIAN_POINT('Ctrl Pts',(-34.6837837831348,47.7640607692763,
2.65878198860294));
#233136=CARTESIAN_POINT('Origin',(-38.9973987043321,43.2882232241948,2.83404198860291));
#233137=CARTESIAN_POINT('Ctrl Pts',(-42.0671296588098,46.435582879267,2.83404198860294));
#233138=CARTESIAN_POINT('Ctrl Pts',(-42.0742293550376,46.443467890749,2.82419652440176));
#233139=CARTESIAN_POINT('Ctrl Pts',(-42.0806858315469,46.4518896956732,
2.81438790575831));
#233140=CARTESIAN_POINT('Ctrl Pts',(-42.0864721532152,46.4607957007304,
2.80466781257148));
#233141=CARTESIAN_POINT('Ctrl Pts',(-42.0920704538847,46.4694123136551,
2.79526356453374));
#233142=CARTESIAN_POINT('Ctrl Pts',(-42.0970420880496,46.4784832882788,
2.78594102496572));
#233143=CARTESIAN_POINT('Ctrl Pts',(-42.1013257711378,46.487988795815,2.77675109089158));
#233144=CARTESIAN_POINT('Ctrl Pts',(-42.1053778715653,46.4969804206287,
2.76805797914095));
#233145=CARTESIAN_POINT('Ctrl Pts',(-42.1088147776111,46.5063617095192,
2.75948271210603));
#233146=CARTESIAN_POINT('Ctrl Pts',(-42.1115441100112,46.5161273793187,
2.75108575573691));
#233147=CARTESIAN_POINT('Ctrl Pts',(-42.114058022542,46.5251222674751,2.74335155163766));
#233148=CARTESIAN_POINT('Ctrl Pts',(-42.1159717447004,46.5344438074261,
2.73576818686464));
#233149=CARTESIAN_POINT('Ctrl Pts',(-42.1171748456129,46.5440884908126,
2.72840626161042));
#233150=CARTESIAN_POINT('Ctrl Pts',(-42.1175238194546,46.5468860468431,
2.72627084694051));
#233151=CARTESIAN_POINT('Ctrl Pts',(-42.117812736298,46.5497107674209,2.72415424587722));
#233152=CARTESIAN_POINT('Ctrl Pts',(-42.1180382068977,46.5525624800842,
2.7220586717329));
#233153=CARTESIAN_POINT('Ctrl Pts',(-42.118282631524,46.5556539199574,2.71978693462893));
#233154=CARTESIAN_POINT('Ctrl Pts',(-42.1184532289195,46.5587726948499,
2.71754411340793));
#233155=CARTESIAN_POINT('Ctrl Pts',(-42.1185461584681,46.5619176830194,
2.7153334184429));
#233156=CARTESIAN_POINT('Ctrl Pts',(-42.1188012043436,46.5705491277289,
2.70926614876438));
#233157=CARTESIAN_POINT('Ctrl Pts',(-42.1184278543823,46.5793682643812,
2.70347381860455));
#233158=CARTESIAN_POINT('Ctrl Pts',(-42.1173773384969,46.5882835699004,
2.69804914171441));
#233159=CARTESIAN_POINT('Ctrl Pts',(-42.1164161734955,46.5964405904275,
2.6930858568724));
#233160=CARTESIAN_POINT('Ctrl Pts',(-42.1148801579477,46.6046697328845,
2.68842799053211));
#233161=CARTESIAN_POINT('Ctrl Pts',(-42.1127009621827,46.6129145292191,
2.68414767054235));
#233162=CARTESIAN_POINT('Ctrl Pts',(-42.1116305483417,46.6169643462456,
2.6820451913458));
#233163=CARTESIAN_POINT('Ctrl Pts',(-42.1104045383079,46.6210176421368,
2.68003431778541));
#233164=CARTESIAN_POINT('Ctrl Pts',(-42.1090123875509,46.6250654385593,
2.678126939453));
#233165=CARTESIAN_POINT('Ctrl Pts',(-42.1087482405045,46.6258334685044,
2.67776503299252));
#233166=CARTESIAN_POINT('Ctrl Pts',(-42.108477638333,46.6266015422614,2.67740659639973));
#233167=CARTESIAN_POINT('Ctrl Pts',(-42.1082005605487,46.6273695213206,
2.67705178968904));
#233168=CARTESIAN_POINT('Ctrl Pts',(-42.1079321414451,46.6281135010342,
2.67670807068807));
#233169=CARTESIAN_POINT('Ctrl Pts',(-42.1076576451502,46.6288573918597,
2.67636775825315));
#233170=CARTESIAN_POINT('Ctrl Pts',(-42.1073770559081,46.629601065316,2.67603099699304));
#233171=CARTESIAN_POINT('Ctrl Pts',(-42.1043192521646,46.6377054654054,
2.6723610421717));
#233172=CARTESIAN_POINT('Ctrl Pts',(-42.1005354505673,46.6457892400076,
2.6691144054151));
#233173=CARTESIAN_POINT('Ctrl Pts',(-42.0960238460768,46.6536619390768,
2.66646778189663));
#233174=CARTESIAN_POINT('Ctrl Pts',(-42.0941185674849,46.6569866287806,
2.66535009635013));
#233175=CARTESIAN_POINT('Ctrl Pts',(-42.0920839261384,46.6602736399414,
2.66433897912388));
#233176=CARTESIAN_POINT('Ctrl Pts',(-42.089921692318,46.6635089796844,2.66344564884841));
#233177=CARTESIAN_POINT('Ctrl Pts',(-42.0862805445927,46.6689572109695,
2.66194130298633));
#233178=CARTESIAN_POINT('Ctrl Pts',(-42.0822770520158,46.6742564366676,
2.66077206705466));
#233179=CARTESIAN_POINT('Ctrl Pts',(-42.0779224130575,46.6793332901452,
2.6599822515576));
#233180=CARTESIAN_POINT('Ctrl Pts',(-42.0768337533179,46.6806025035146,
2.65978479768333));
#233181=CARTESIAN_POINT('Ctrl Pts',(-42.0757229796949,46.6818576549907,
2.65961098966667));
#233182=CARTESIAN_POINT('Ctrl Pts',(-42.0745900553979,46.6830973739112,
2.65946139030547));
#233183=CARTESIAN_POINT('Ctrl Pts',(-42.0728906689524,46.6849569522921,
2.65923699126365));
#233184=CARTESIAN_POINT('Ctrl Pts',(-42.0711414461006,46.6867817869761,
2.65906707562487));
#233185=CARTESIAN_POINT('Ctrl Pts',(-42.0693433991611,46.6885684866734,
2.65895332562964));
#233186=CARTESIAN_POINT('Ctrl Pts',(-42.0675453522216,46.6903551863706,
2.65883957563442));
#233187=CARTESIAN_POINT('Ctrl Pts',(-42.0656984926167,46.692103753135,2.65878198860294));
#233188=CARTESIAN_POINT('Ctrl Pts',(-42.0638038389703,46.6938111422604,
2.65878198860294));
#233189=CARTESIAN_POINT('Ctrl Pts',(-39.5091373124624,43.8565665267056,
2.65878198860292));
#233190=CARTESIAN_POINT('Ctrl Pts',(-39.5155480799604,43.8507890749208,
2.65878198860291));
#233191=CARTESIAN_POINT('Ctrl Pts',(-39.5223801852468,43.8455908828151,
2.65945335517887));
#233192=CARTESIAN_POINT('Ctrl Pts',(-39.5294841269569,43.8409939475743,
2.66072561226636));
#233193=CARTESIAN_POINT('Ctrl Pts',(-39.5340725443949,43.8380247990817,
2.66154735980374));
#233194=CARTESIAN_POINT('Ctrl Pts',(-39.5387738681336,43.835305694046,2.66261895766918));
#233195=CARTESIAN_POINT('Ctrl Pts',(-39.5435446222367,43.8328343017436,
2.6639142925106));
#233196=CARTESIAN_POINT('Ctrl Pts',(-39.5498679835147,43.8295586128169,
2.66563118464156));
#233197=CARTESIAN_POINT('Ctrl Pts',(-39.5563148866446,43.8267236865061,
2.66774105138731));
#233198=CARTESIAN_POINT('Ctrl Pts',(-39.5627952650342,43.8243293609623,
2.67016894181781));
#233199=CARTESIAN_POINT('Ctrl Pts',(-39.566035454229,43.8231321981904,2.67138288703306));
#233200=CARTESIAN_POINT('Ctrl Pts',(-39.5692841591688,43.8220450509626,
2.67267613167582));
#233201=CARTESIAN_POINT('Ctrl Pts',(-39.5725311673657,43.8210669472518,
2.67403835432583));
#233202=CARTESIAN_POINT('Ctrl Pts',(-39.5741546714642,43.8205778953965,
2.67471946565084));
#233203=CARTESIAN_POINT('Ctrl Pts',(-39.5757777635549,43.8201160933895,
2.67541781389553));
#233204=CARTESIAN_POINT('Ctrl Pts',(-39.5773992434497,43.8196813503779,
2.67613207244199));
#233205=CARTESIAN_POINT('Ctrl Pts',(-39.5778046134234,43.819572664625,2.6763106370786));
#233206=CARTESIAN_POINT('Ctrl Pts',(-39.5782098828932,43.8194656698239,
2.67649019601875));
#233207=CARTESIAN_POINT('Ctrl Pts',(-39.5786150336268,43.8193603625176,
2.67667072836686));
#233208=CARTESIAN_POINT('Ctrl Pts',(-39.5798304858278,43.8190444405985,
2.6772123254112));
#233209=CARTESIAN_POINT('Ctrl Pts',(-39.5810448681192,43.8187437073124,
2.67776268340076));
#233210=CARTESIAN_POINT('Ctrl Pts',(-39.5822576997163,43.8184580587802,
2.67832123541545));
#233211=CARTESIAN_POINT('Ctrl Pts',(-39.5908007288816,43.8164459874034,
2.68225560368484));
#233212=CARTESIAN_POINT('Ctrl Pts',(-39.5992865061393,43.8151322889031,
2.68661792998942));
#233213=CARTESIAN_POINT('Ctrl Pts',(-39.6076412948842,43.8144227306311,
2.69130986622647));
#233214=CARTESIAN_POINT('Ctrl Pts',(-39.6116933583969,43.814078595636,2.69358545023111));
#233215=CARTESIAN_POINT('Ctrl Pts',(-39.6157150281164,43.8138769687219,
2.69593918853513));
#233216=CARTESIAN_POINT('Ctrl Pts',(-39.6196997093544,43.8138093098904,
2.69836306235505));
#233217=CARTESIAN_POINT('Ctrl Pts',(-39.6257999779284,43.8137057289464,
2.70207384382238));
#233218=CARTESIAN_POINT('Ctrl Pts',(-39.6318101761583,43.81391511288,2.70594760814237));
#233219=CARTESIAN_POINT('Ctrl Pts',(-39.6376940219322,43.8144090029878,
2.70995196345717));
#233220=CARTESIAN_POINT('Ctrl Pts',(-39.6404265103486,43.814638368109,2.71181160678115));
#233221=CARTESIAN_POINT('Ctrl Pts',(-39.6431316855283,43.8149288459967,
2.71369962772109));
#233222=CARTESIAN_POINT('Ctrl Pts',(-39.6458055463963,43.8152787628653,
2.71561183138671));
#233223=CARTESIAN_POINT('Ctrl Pts',(-39.6460104872963,43.8153055826146,
2.71575839426322));
#233224=CARTESIAN_POINT('Ctrl Pts',(-39.6462152612035,43.8153327221694,
2.71590508903219));
#233225=CARTESIAN_POINT('Ctrl Pts',(-39.6464198673376,43.8153601802954,
2.71605191409921));
#233226=CARTESIAN_POINT('Ctrl Pts',(-39.6492939666538,43.8157458841824,
2.71811436362762));
#233227=CARTESIAN_POINT('Ctrl Pts',(-39.6521348180508,43.8161965332334,
2.72020091026968));
#233228=CARTESIAN_POINT('Ctrl Pts',(-39.654938997009,43.816707563491,2.72230624862191));
#233229=CARTESIAN_POINT('Ctrl Pts',(-39.6649942840473,43.8185400271112,
2.72985561753159));
#233230=CARTESIAN_POINT('Ctrl Pts',(-39.6746561192258,43.8211611138373,
2.73770089914436));
#233231=CARTESIAN_POINT('Ctrl Pts',(-39.6839173731649,43.8244418968106,
2.74574823347232));
#233232=CARTESIAN_POINT('Ctrl Pts',(-39.6940945608685,43.8280471477143,
2.75459144547224));
#233233=CARTESIAN_POINT('Ctrl Pts',(-39.7037886794696,43.8324491002322,
2.76367911754513));
#233234=CARTESIAN_POINT('Ctrl Pts',(-39.7129876499635,43.8375295667884,
2.77292162565014));
#233235=CARTESIAN_POINT('Ctrl Pts',(-39.7229202294704,43.8430151956461,
2.7829012148506));
#233236=CARTESIAN_POINT('Ctrl Pts',(-39.7322766233333,43.8492922888436,
2.79306229500561));
#233237=CARTESIAN_POINT('Ctrl Pts',(-39.7410245486324,43.8562669044125,
2.8033191668567));
#233238=CARTESIAN_POINT('Ctrl Pts',(-39.749699087825,43.8631830101219,2.81348999408983));
#233239=CARTESIAN_POINT('Ctrl Pts',(-39.7577762496649,43.8707860819073,
2.82375635967035));
#233240=CARTESIAN_POINT('Ctrl Pts',(-39.7651933659001,43.879023624022,2.83404198860291));
#233241=CARTESIAN_POINT('Origin',(0.0113255271402848,0.0101975504410943,
2.83404198860262));
#233242=CARTESIAN_POINT('Ctrl Pts',(-42.0411527846897,46.7142062431422,
2.65878198860294));
#233243=CARTESIAN_POINT('Ctrl Pts',(-42.034767559739,46.7199506919427,2.65878198860294));
#233244=CARTESIAN_POINT('Ctrl Pts',(-42.0279592142777,46.7251107020213,
2.6594460304188));
#233245=CARTESIAN_POINT('Ctrl Pts',(-42.0208774479582,46.7296675019396,
2.66070439264095));
#233246=CARTESIAN_POINT('Ctrl Pts',(-42.0163525364096,46.7325790801595,
2.6615084261962));
#233247=CARTESIAN_POINT('Ctrl Pts',(-42.0117164851999,46.735245189214,2.66255428265394));
#233248=CARTESIAN_POINT('Ctrl Pts',(-42.0070114066749,46.7376689638752,
2.66381699700683));
#233249=CARTESIAN_POINT('Ctrl Pts',(-42.00058991857,46.7409769299535,2.66554034873283));
#233250=CARTESIAN_POINT('Ctrl Pts',(-41.994038348078,46.743827608742,2.66766759643987));
#233251=CARTESIAN_POINT('Ctrl Pts',(-41.9874523371583,46.7462229640888,
2.67012012783163));
#233252=CARTESIAN_POINT('Ctrl Pts',(-41.9841593316985,46.7474206417622,
2.67134639352751));
#233253=CARTESIAN_POINT('Ctrl Pts',(-41.9808575622225,46.7485046297347,
2.67265375585028));
#233254=CARTESIAN_POINT('Ctrl Pts',(-41.977557880152,46.7494761782933,2.67403135126956));
#233255=CARTESIAN_POINT('Ctrl Pts',(-41.9759080391167,46.7499619525726,
2.6747201489792));
#233256=CARTESIAN_POINT('Ctrl Pts',(-41.9742587070257,46.7504196286881,
2.67542649668649));
#233257=CARTESIAN_POINT('Ctrl Pts',(-41.9726111592841,46.7508494364813,
2.67614899656118));
#233258=CARTESIAN_POINT('Ctrl Pts',(-41.9721992723487,46.7509568884296,
2.67632962152986));
#233259=CARTESIAN_POINT('Ctrl Pts',(-41.9717874966609,46.7510625988575,
2.67651125590967));
#233260=CARTESIAN_POINT('Ctrl Pts',(-41.971375851596,46.7511665718606,2.67669387767541));
#233261=CARTESIAN_POINT('Ctrl Pts',(-41.9701409164014,46.7514784908699,
2.67724174297261));
#233262=CARTESIAN_POINT('Ctrl Pts',(-41.968907158177,46.7517747718024,2.67779849504765));
#233263=CARTESIAN_POINT('Ctrl Pts',(-41.9676750878621,46.7520555364233,
2.67836353618026));
#233264=CARTESIAN_POINT('Ctrl Pts',(-41.9591607175417,46.7539957941553,
2.68226832098917));
#233265=CARTESIAN_POINT('Ctrl Pts',(-41.9507055072921,46.7552464720208,
2.6865915375139));
#233266=CARTESIAN_POINT('Ctrl Pts',(-41.9423805287174,46.755902754358,2.69123699486167));
#233267=CARTESIAN_POINT('Ctrl Pts',(-41.9382430372171,46.7562289248781,
2.69354577441213));
#233268=CARTESIAN_POINT('Ctrl Pts',(-41.9341372814972,46.7564078446195,
2.69593478828123));
#233269=CARTESIAN_POINT('Ctrl Pts',(-41.9300700339485,46.7564487173143,
2.69839565261235));
#233270=CARTESIAN_POINT('Ctrl Pts',(-41.9210970783571,46.7565388885839,
2.7038246868906));
#233271=CARTESIAN_POINT('Ctrl Pts',(-41.9123126321656,46.7559695796225,
2.70961155815102));
#233272=CARTESIAN_POINT('Ctrl Pts',(-41.9038465062686,46.7548061840817,
2.71562701361782));
#233273=CARTESIAN_POINT('Ctrl Pts',(-41.900753723715,46.7543811810195,2.71782453535872));
#233274=CARTESIAN_POINT('Ctrl Pts',(-41.8976992635448,46.7538836816024,
2.72005051502417));
#233275=CARTESIAN_POINT('Ctrl Pts',(-41.8946854937103,46.7533184435778,
2.7222998676013));
#233276=CARTESIAN_POINT('Ctrl Pts',(-41.8845625597437,46.7514198688648,
2.72985520488883));
#233277=CARTESIAN_POINT('Ctrl Pts',(-41.8748360802685,46.7487367327317,
2.73770845534526));
#233278=CARTESIAN_POINT('Ctrl Pts',(-41.865513778659,46.7453971060011,2.74576706701696));
#233279=CARTESIAN_POINT('Ctrl Pts',(-41.8552674648909,46.7417264606194,
2.75462443584949));
#233280=CARTESIAN_POINT('Ctrl Pts',(-41.8455087367173,46.7372626589223,
2.76373036323078));
#233281=CARTESIAN_POINT('Ctrl Pts',(-41.836250857547,46.7321227530976,2.7729966463669));
#233282=CARTESIAN_POINT('Ctrl Pts',(-41.826279725012,46.726586854297,2.78297683033316));
#233283=CARTESIAN_POINT('Ctrl Pts',(-41.8168884800907,46.7202662104769,
2.79314401478702));
#233284=CARTESIAN_POINT('Ctrl Pts',(-41.8081115112118,46.7132528291651,
2.80341452427711));
#233285=CARTESIAN_POINT('Ctrl Pts',(-41.799453061047,46.7063341521808,2.81354634721222));
#233286=CARTESIAN_POINT('Ctrl Pts',(-41.7913915075194,46.6987402031264,
2.82378004209149));
#233287=CARTESIAN_POINT('Ctrl Pts',(-41.7839914803029,46.6905216402897,
2.83404198860294));
#233288=CARTESIAN_POINT('Ctrl Pts',(-39.4820551873932,44.1339623850447,
2.83404198860292));
#233289=CARTESIAN_POINT('Ctrl Pts',(-39.4749733207252,44.1260971752949,
2.82422126443095));
#233290=CARTESIAN_POINT('Ctrl Pts',(-39.4685372764365,44.1177016730302,
2.81442815028649));
#233291=CARTESIAN_POINT('Ctrl Pts',(-39.462775176276,44.1088266671103,2.80471618166523));
#233292=CARTESIAN_POINT('Ctrl Pts',(-39.4572113615991,44.1002570680371,
2.79533842146471));
#233293=CARTESIAN_POINT('Ctrl Pts',(-39.4522752837277,44.091239296903,2.78603515650518));
#233294=CARTESIAN_POINT('Ctrl Pts',(-39.4480294591808,44.0817922708765,
2.77685887347067));
#233295=CARTESIAN_POINT('Ctrl Pts',(-39.4440158252739,44.0728618726561,
2.76818441216905));
#233296=CARTESIAN_POINT('Ctrl Pts',(-39.4406186435293,44.0635470605582,
2.75962261521967));
#233297=CARTESIAN_POINT('Ctrl Pts',(-39.43793124934,44.0538529442847,2.75123537702016));
#233298=CARTESIAN_POINT('Ctrl Pts',(-39.4354562043761,44.0449248258277,
2.74351087134483));
#233299=CARTESIAN_POINT('Ctrl Pts',(-39.433583118669,44.035674438681,2.73593399450217));
#233300=CARTESIAN_POINT('Ctrl Pts',(-39.4324230329125,44.0261054688021,
2.72857657812951));
#233301=CARTESIAN_POINT('Ctrl Pts',(-39.4320771187576,44.0232521951457,
2.72638274508576));
#233302=CARTESIAN_POINT('Ctrl Pts',(-39.4317948788027,44.0203706219338,
2.72420861709734));
#233303=CARTESIAN_POINT('Ctrl Pts',(-39.4315800126158,44.0174609456696,
2.72205663736736));
#233304=CARTESIAN_POINT('Ctrl Pts',(-39.4313673418319,44.0145809991274,
2.71992664556775));
#233305=CARTESIAN_POINT('Ctrl Pts',(-39.4312206224784,44.0116765294505,
2.71782089927894));
#233306=CARTESIAN_POINT('Ctrl Pts',(-39.4311433701096,44.0087510493745,
2.71574387311255));
#233307=CARTESIAN_POINT('Ctrl Pts',(-39.4311379981309,44.0085476172114,
2.71559944077496));
#233308=CARTESIAN_POINT('Ctrl Pts',(-39.4311329512713,44.0083440782824,
2.71545515216079));
#233309=CARTESIAN_POINT('Ctrl Pts',(-39.4311282308204,44.0081404327825,
2.71531100781741));
#233310=CARTESIAN_POINT('Ctrl Pts',(-39.4309212689595,43.9992118680545,
2.70899119176099));
#233311=CARTESIAN_POINT('Ctrl Pts',(-39.4313859080979,43.9900881971808,
2.70298296066859));
#233312=CARTESIAN_POINT('Ctrl Pts',(-39.4325966403785,43.98085857377,2.69736727774161));
#233313=CARTESIAN_POINT('Ctrl Pts',(-39.4337252532879,43.9722549606535,
2.6921324852546));
#233314=CARTESIAN_POINT('Ctrl Pts',(-39.4355025470896,43.9635585482861,
2.68723866185504));
#233315=CARTESIAN_POINT('Ctrl Pts',(-39.4380105519135,43.9548613290787,
2.68278595829602));
#233316=CARTESIAN_POINT('Ctrl Pts',(-39.4389280125248,43.9516797737745,
2.68115710172835));
#233317=CARTESIAN_POINT('Ctrl Pts',(-39.4399434521994,43.9484983634056,
2.67958763637829));
#233318=CARTESIAN_POINT('Ctrl Pts',(-39.4410615611725,43.9453226165472,
2.67808378645375));
#233319=CARTESIAN_POINT('Ctrl Pts',(-39.4413304290277,43.9445589555201,
2.6777221607861));
#233320=CARTESIAN_POINT('Ctrl Pts',(-39.441605709343,43.9437952833156,2.67736403603573));
#233321=CARTESIAN_POINT('Ctrl Pts',(-39.4418874191263,43.943031734545,2.67700956934489));
#233322=CARTESIAN_POINT('Ctrl Pts',(-39.4421603254788,43.9422920466734,
2.67666617973814));
#233323=CARTESIAN_POINT('Ctrl Pts',(-39.4424392657172,43.9415524746579,
2.67632622314129));
#233324=CARTESIAN_POINT('Ctrl Pts',(-39.4427242524727,43.9408131433999,
2.67598984158783));
#233325=CARTESIAN_POINT('Ctrl Pts',(-39.445846611731,43.9327129150429,2.67230439292216));
#233326=CARTESIAN_POINT('Ctrl Pts',(-39.4496972096658,43.9246364083426,
2.66904964539959));
#233327=CARTESIAN_POINT('Ctrl Pts',(-39.454273889062,43.9167721156729,2.66640203566703));
#233328=CARTESIAN_POINT('Ctrl Pts',(-39.4561719744235,43.9135105590938,
2.66530399299431));
#233329=CARTESIAN_POINT('Ctrl Pts',(-39.4581945203288,43.9102855324947,
2.6643099514226));
#233330=CARTESIAN_POINT('Ctrl Pts',(-39.4603395741452,43.9071101492109,
2.6634305347337));
#233331=CARTESIAN_POINT('Ctrl Pts',(-39.4639981869599,43.9016942021215,
2.66193059792893));
#233332=CARTESIAN_POINT('Ctrl Pts',(-39.4680136963362,43.8964251099357,
2.66076519817136));
#233333=CARTESIAN_POINT('Ctrl Pts',(-39.4723737491581,43.8913745966874,
2.65997805604468));
#233334=CARTESIAN_POINT('Ctrl Pts',(-39.474553775569,43.8888493400633,2.65958448498134));
#233335=CARTESIAN_POINT('Ctrl Pts',(-39.476820955151,43.8863797569641,2.6592852626077));
#233336=CARTESIAN_POINT('Ctrl Pts',(-39.4791737454928,43.8839748786092,
2.65908463971332));
#233337=CARTESIAN_POINT('Ctrl Pts',(-39.4815265358346,43.8815700002543,
2.65888401681894));
#233338=CARTESIAN_POINT('Ctrl Pts',(-39.4839648939619,43.8792298420741,
2.65878198860292));
#233339=CARTESIAN_POINT('Ctrl Pts',(-39.4864862581819,43.8769616275874,
2.65878198860292));
#233340=CARTESIAN_POINT('Origin',(-43.3086183250768,38.9747476500513,2.83404198860288));
#233341=CARTESIAN_POINT('Ctrl Pts',(-46.6905216402899,41.7839914803026,
2.8340419886029));
#233342=CARTESIAN_POINT('Ctrl Pts',(-46.6984066517724,41.7910911765308,
2.82419652440036));
#233343=CARTESIAN_POINT('Ctrl Pts',(-46.705708077355,41.7987919603594,2.8143879057557));
#233344=CARTESIAN_POINT('Ctrl Pts',(-46.7123936319708,41.8070443420779,
2.80466781256778));
#233345=CARTESIAN_POINT('Ctrl Pts',(-46.7188619458713,41.8150285705302,
2.79526356452918));
#233346=CARTESIAN_POINT('Ctrl Pts',(-46.7247545199422,41.8235301761275,
2.7859410249604));
#233347=CARTESIAN_POINT('Ctrl Pts',(-46.7300083326618,41.8325358446895,
2.77675109088559));
#233348=CARTESIAN_POINT('Ctrl Pts',(-46.7349781159835,41.8410546526119,
2.76805797913439));
#233349=CARTESIAN_POINT('Ctrl Pts',(-46.7393768060097,41.8500252953139,
2.75948271209897));
#233350=CARTESIAN_POINT('Ctrl Pts',(-46.7431119772982,41.859452174832,2.75108575572942));
#233351=CARTESIAN_POINT('Ctrl Pts',(-46.7465523401895,41.8681350126375,
2.74335155162965));
#233352=CARTESIAN_POINT('Ctrl Pts',(-46.7494299450239,41.8772054497821,
2.73576818685618));
#233353=CARTESIAN_POINT('Ctrl Pts',(-46.7516345991567,41.8866715402957,
2.72840626160154));
#233354=CARTESIAN_POINT('Ctrl Pts',(-46.7522740855149,41.8894172933185,
2.72627084693461));
#233355=CARTESIAN_POINT('Ctrl Pts',(-46.752856683342,41.8921963397441,2.72415424587426));
#233356=CARTESIAN_POINT('Ctrl Pts',(-46.7533790039318,41.8950088623279,
2.72205867173281));
#233357=CARTESIAN_POINT('Ctrl Pts',(-46.7539452330337,41.8980578176395,
2.71978693462886));
#233358=CARTESIAN_POINT('Ctrl Pts',(-46.7544408966255,41.9011416752732,
2.71754411340787));
#233359=CARTESIAN_POINT('Ctrl Pts',(-46.7548620578768,41.9042597210856,
2.71533341844285));
#233360=CARTESIAN_POINT('Ctrl Pts',(-46.7560179382356,41.9128172222844,
2.70926614876433));
#233361=CARTESIAN_POINT('Ctrl Pts',(-46.756568484326,41.921627072481,2.70347381860451));
#233362=CARTESIAN_POINT('Ctrl Pts',(-46.756455626462,41.930603347835,2.69804914171437));
#233363=CARTESIAN_POINT('Ctrl Pts',(-46.7563523676437,41.9388161524504,
2.69308585687251));
#233364=CARTESIAN_POINT('Ctrl Pts',(-46.7556849461648,41.9471607721486,
2.68842799053235));
#233365=CARTESIAN_POINT('Ctrl Pts',(-46.7543795041531,41.9555881906104,
2.6841476705427));
#233366=CARTESIAN_POINT('Ctrl Pts',(-46.7537382753014,41.9597277110295,
2.68204519134602));
#233367=CARTESIAN_POINT('Ctrl Pts',(-46.7529426662695,41.9638869554867,
2.6800343177855));
#233368=CARTESIAN_POINT('Ctrl Pts',(-46.7519812517997,41.9680580970364,
2.67812693945298));
#233369=CARTESIAN_POINT('Ctrl Pts',(-46.7517988327683,41.968849530518,2.6777650329925));
#233370=CARTESIAN_POINT('Ctrl Pts',(-46.7516099985532,41.9696416823158,
2.6774065963997));
#233371=CARTESIAN_POINT('Ctrl Pts',(-46.7514147143009,41.9704344168203,
2.67705178968901));
#233372=CARTESIAN_POINT('Ctrl Pts',(-46.7512255326815,41.9712023783716,
2.67670807068804));
#233373=CARTESIAN_POINT('Ctrl Pts',(-46.7510302978708,41.9719708867612,
2.67636775825311));
#233374=CARTESIAN_POINT('Ctrl Pts',(-46.7508289807695,41.9727398158588,
2.676030996993));
#233375=CARTESIAN_POINT('Ctrl Pts',(-46.748635068482,41.9811194467226,2.67236104217174));
#233376=CARTESIAN_POINT('Ctrl Pts',(-46.7457169794823,41.9895544525279,
2.6691144054152));
#233377=CARTESIAN_POINT('Ctrl Pts',(-46.7420530111689,41.9978556152119,
2.66646778189676));
#233378=CARTESIAN_POINT('Ctrl Pts',(-46.740505694598,42.0013612477611,2.66535009635019));
#233379=CARTESIAN_POINT('Ctrl Pts',(-46.7388257854549,42.0048429302643,
2.66433897912389));
#233380=CARTESIAN_POINT('Ctrl Pts',(-46.7370135816691,42.0082865614563,
2.66344564884837));
#233381=CARTESIAN_POINT('Ctrl Pts',(-46.7339618757758,42.0140855503366,
2.6619413029863));
#233382=CARTESIAN_POINT('Ctrl Pts',(-46.7305342346688,42.0197742252486,
2.66077206705463));
#233383=CARTESIAN_POINT('Ctrl Pts',(-46.7267341265708,42.0252784509102,
2.65998225155757));
#233384=CARTESIAN_POINT('Ctrl Pts',(-46.7257840995463,42.0266545073256,
2.6597847976833));
#233385=CARTESIAN_POINT('Ctrl Pts',(-46.7248106099124,42.0280188904105,
2.65961098966665));
#233386=CARTESIAN_POINT('Ctrl Pts',(-46.7238134778068,42.0293702408568,
2.65946139030544));
#233387=CARTESIAN_POINT('Ctrl Pts',(-46.7223177796485,42.0313972665263,
2.65923699126362));
#233388=CARTESIAN_POINT('Ctrl Pts',(-46.7207688863877,42.0333949481517,
2.65906707562484));
#233389=CARTESIAN_POINT('Ctrl Pts',(-46.7191674503111,42.0353598072044,
2.65895332562961));
#233390=CARTESIAN_POINT('Ctrl Pts',(-46.7175660142345,42.0373246662572,
2.65883957563439));
#233391=CARTESIAN_POINT('Ctrl Pts',(-46.7159120469178,42.0392567035874,
2.6587819886029));
#233392=CARTESIAN_POINT('Ctrl Pts',(-46.7142062431438,42.0411527846906,
2.6587819886029));
#233393=CARTESIAN_POINT('Ctrl Pts',(-43.8769616275876,39.4864862581816,
2.65878198860288));
#233394=CARTESIAN_POINT('Ctrl Pts',(-43.8827333680737,39.4800703482073,
2.65878198860288));
#233395=CARTESIAN_POINT('Ctrl Pts',(-43.8889846873398,39.4741864828755,
2.65945335517881));
#233396=CARTESIAN_POINT('Ctrl Pts',(-43.8955692023373,39.4688721660169,
2.66072561226626));
#233397=CARTESIAN_POINT('Ctrl Pts',(-43.8998221234155,39.4654396626067,
2.66154735980364));
#233398=CARTESIAN_POINT('Ctrl Pts',(-43.90421346894,39.4622440309671,2.66261895766907));
#233399=CARTESIAN_POINT('Ctrl Pts',(-43.9086997575135,39.4592874976153,
2.66391429251051));
#233400=CARTESIAN_POINT('Ctrl Pts',(-43.9146460760272,39.4553687820182,
2.66563118464146));
#233401=CARTESIAN_POINT('Ctrl Pts',(-43.9207613318565,39.4518755008533,
2.66774105138722));
#233402=CARTESIAN_POINT('Ctrl Pts',(-43.9269559348856,39.4488169076809,
2.67016894181773));
#233403=CARTESIAN_POINT('Ctrl Pts',(-43.9300532364002,39.4472876110947,
2.67138288703298));
#233404=CARTESIAN_POINT('Ctrl Pts',(-43.9331705067653,39.4458668372382,
2.67267613167573));
#233405=CARTESIAN_POINT('Ctrl Pts',(-43.9362974878338,39.4445546869048,
2.67403835432575));
#233406=CARTESIAN_POINT('Ctrl Pts',(-43.937860978368,39.4438986117382,2.67471946565076));
#233407=CARTESIAN_POINT('Ctrl Pts',(-43.9394269075363,39.443269680209,2.67541781389545));
#233408=CARTESIAN_POINT('Ctrl Pts',(-43.9409940617757,39.4426678279634,
2.67613207244191));
#233409=CARTESIAN_POINT('Ctrl Pts',(-43.9413858503355,39.442517364902,2.67631063707853));
#233410=CARTESIAN_POINT('Ctrl Pts',(-43.9417777156946,39.4423685940347,
2.67649019601868));
#233411=CARTESIAN_POINT('Ctrl Pts',(-43.9421696393593,39.4422215138293,
2.67667072836679));
#233412=CARTESIAN_POINT('Ctrl Pts',(-43.9433454103532,39.4417802732128,
2.67721232541113));
#233413=CARTESIAN_POINT('Ctrl Pts',(-43.944521704943,39.4413542498604,2.6777626834007));
#233414=CARTESIAN_POINT('Ctrl Pts',(-43.9456980341197,39.4409433907177,
2.67832123541539));
#233415=CARTESIAN_POINT('Ctrl Pts',(-43.953983944948,39.4380493519682,2.68225560368463));
#233416=CARTESIAN_POINT('Ctrl Pts',(-43.9622859173443,39.4358558447894,
2.68661792998902));
#233417=CARTESIAN_POINT('Ctrl Pts',(-43.9705207686461,39.4342768603235,
2.69130986622586));
#233418=CARTESIAN_POINT('Ctrl Pts',(-43.974514662629,39.4335110545637,2.69358545023068));
#233419=CARTESIAN_POINT('Ctrl Pts',(-43.9784932254699,39.4328901532274,
2.69593918853489));
#233420=CARTESIAN_POINT('Ctrl Pts',(-43.9824490059337,39.4324063524315,
2.698363062355));
#233421=CARTESIAN_POINT('Ctrl Pts',(-43.9885050294413,39.4316656872153,
2.70207384382234));
#233422=CARTESIAN_POINT('Ctrl Pts',(-43.9945041897573,39.4312456873368,
2.70594760814234));
#233423=CARTESIAN_POINT('Ctrl Pts',(-44.0004074287825,39.4311218425062,
2.70995196345714));
#233424=CARTESIAN_POINT('Ctrl Pts',(-44.003148923525,39.4310643283261,2.71181160678112));
#233425=CARTESIAN_POINT('Ctrl Pts',(-44.0058696426793,39.4310704471412,
2.71369962772106));
#233426=CARTESIAN_POINT('Ctrl Pts',(-44.0085654321302,39.4311389525611,
2.71561183138668));
#233427=CARTESIAN_POINT('Ctrl Pts',(-44.0087720537697,39.4311442032316,
2.71575839426319));
#233428=CARTESIAN_POINT('Ctrl Pts',(-44.00897854276,39.4311497894113,2.71590508903216));
#233429=CARTESIAN_POINT('Ctrl Pts',(-44.009184898196,39.431155709954,2.71605191409918));
#233430=CARTESIAN_POINT('Ctrl Pts',(-44.01208356993,39.4312388757299,2.7181143636276));
#233431=CARTESIAN_POINT('Ctrl Pts',(-44.0149559644985,39.4313901062474,
2.72020091026966));
#233432=CARTESIAN_POINT('Ctrl Pts',(-44.0177981990785,39.4316052205106,
2.72230624862189));
#233433=CARTESIAN_POINT('Ctrl Pts',(-44.0279899468081,39.4323765820014,
2.72985561753128));
#233434=CARTESIAN_POINT('Ctrl Pts',(-44.0378728316098,39.4339733733566,
2.73770089914376));
#233435=CARTESIAN_POINT('Ctrl Pts',(-44.047426286633,39.4362681192151,2.7457482334714));
#233436=CARTESIAN_POINT('Ctrl Pts',(-44.0579245739736,39.4387898143859,
2.75459144547082));
#233437=CARTESIAN_POINT('Ctrl Pts',(-44.0680257165102,39.4421543412269,
2.76367911754317));
#233438=CARTESIAN_POINT('Ctrl Pts',(-44.0777053474426,39.4462454222061,
2.77292162564763));
#233439=CARTESIAN_POINT('Ctrl Pts',(-44.0881569195933,39.4506627629422,
2.78290121484711));
#233440=CARTESIAN_POINT('Ctrl Pts',(-44.0981181930565,39.4559274600935,
2.7930622950011));
#233441=CARTESIAN_POINT('Ctrl Pts',(-44.1075472421522,39.4619494607994,
2.80331916685116));
#233442=CARTESIAN_POINT('Ctrl Pts',(-44.1168971912149,39.4679209431074,
2.81348999408609));
#233443=CARTESIAN_POINT('Ctrl Pts',(-44.1257248429287,39.4746380711565,
2.82375635966846));
#233444=CARTESIAN_POINT('Ctrl Pts',(-44.1339623850449,39.482055187393,2.83404198860288));
#233445=CARTESIAN_POINT('Origin',(0.0101975504409187,0.0113255271404612,
2.83404198860262));
#233446=CARTESIAN_POINT('Ctrl Pts',(-46.6938111422607,42.06380383897,2.6587819886029));
#233447=CARTESIAN_POINT('Ctrl Pts',(-46.688061354646,42.0701842568303,2.6587819886029));
#233448=CARTESIAN_POINT('Ctrl Pts',(-46.6818296739378,42.076027665722,2.6594460304187));
#233449=CARTESIAN_POINT('Ctrl Pts',(-46.6752630175683,42.081299749164,2.66070439264073));
#233450=CARTESIAN_POINT('Ctrl Pts',(-46.6710672367553,42.0846683595047,
2.661508426196));
#233451=CARTESIAN_POINT('Ctrl Pts',(-46.6667352666014,42.0878044626436,
2.6625542826538));
#233452=CARTESIAN_POINT('Ctrl Pts',(-46.6623093164291,42.0907067742417,
2.66381699700679));
#233453=CARTESIAN_POINT('Ctrl Pts',(-46.6562687825186,42.0946678472191,
2.66554034873278));
#233454=CARTESIAN_POINT('Ctrl Pts',(-46.6500510792883,42.0981877352865,
2.66766759643983));
#233455=CARTESIAN_POINT('Ctrl Pts',(-46.6437515300389,42.1012583942265,
2.67012012783158));
#233456=CARTESIAN_POINT('Ctrl Pts',(-46.6406017554143,42.1027937236966,
2.67134639352746));
#233457=CARTESIAN_POINT('Ctrl Pts',(-46.637431380974,42.1042169023589,2.67265375585022));
#233458=CARTESIAN_POINT('Ctrl Pts',(-46.6342513293849,42.105528039369,2.6740313512695));
#233459=CARTESIAN_POINT('Ctrl Pts',(-46.6326613035903,42.106183607874,2.67472014897914));
#233460=CARTESIAN_POINT('Ctrl Pts',(-46.6310688468941,42.1068111789407,
2.67542649668642));
#233461=CARTESIAN_POINT('Ctrl Pts',(-46.6294752517396,42.1074108478354,
2.67614899656111));
#233462=CARTESIAN_POINT('Ctrl Pts',(-46.6290768529509,42.1075607650591,
2.67632962152979));
#233463=CARTESIAN_POINT('Ctrl Pts',(-46.628678382762,42.1077089386741,2.67651125590961));
#233464=CARTESIAN_POINT('Ctrl Pts',(-46.6282798608701,42.1078553707283,
2.67669387767534));
#233465=CARTESIAN_POINT('Ctrl Pts',(-46.6270842951944,42.1082946668907,
2.67724174297254));
#233466=CARTESIAN_POINT('Ctrl Pts',(-46.6258882654172,42.1087182876165,
2.67779849504758));
#233467=CARTESIAN_POINT('Ctrl Pts',(-46.6246922924067,42.109126300596,2.67836353618019));
#233468=CARTESIAN_POINT('Ctrl Pts',(-46.6164273768569,42.1119459234385,
2.68226832098911));
#233469=CARTESIAN_POINT('Ctrl Pts',(-46.6081492165691,42.1140735600938,
2.68659153751385));
#233470=CARTESIAN_POINT('Ctrl Pts',(-46.5999384432822,42.1155964444648,
2.69123699486162));
#233471=CARTESIAN_POINT('Ctrl Pts',(-46.5958577114965,42.116353313817,2.69354577441209));
#233472=CARTESIAN_POINT('Ctrl Pts',(-46.5917931497417,42.1169604217533,
2.69593478828119));
#233473=CARTESIAN_POINT('Ctrl Pts',(-46.5877524553606,42.1174262136792,
2.69839565261231));
#233474=CARTESIAN_POINT('Ctrl Pts',(-46.578838080023,42.11845382024,2.70382468689056));
#233475=CARTESIAN_POINT('Ctrl Pts',(-46.570042246956,42.1188058546738,2.70961155815098));
#233476=CARTESIAN_POINT('Ctrl Pts',(-46.5615008914345,42.1185337834653,
2.71562701361779));
#233477=CARTESIAN_POINT('Ctrl Pts',(-46.5583806265504,42.1184343924219,
2.7178245353587));
#233478=CARTESIAN_POINT('Ctrl Pts',(-46.555290896183,42.1182588963864,2.72005051502415));
#233479=CARTESIAN_POINT('Ctrl Pts',(-46.552234552633,42.1180117795243,2.72229986760129));
#233480=CARTESIAN_POINT('Ctrl Pts',(-46.5419686180608,42.1171817401336,
2.72985520488875));
#233481=CARTESIAN_POINT('Ctrl Pts',(-46.5320149571612,42.1155299964536,
2.73770845534509));
#233482=CARTESIAN_POINT('Ctrl Pts',(-46.5223946380453,42.113183110409,2.74576706701668));
#233483=CARTESIAN_POINT('Ctrl Pts',(-46.5118207677352,42.1106036046391,
2.75462443584913));
#233484=CARTESIAN_POINT('Ctrl Pts',(-46.5016489045639,42.1071843209742,
2.76373036323031));
#233485=CARTESIAN_POINT('Ctrl Pts',(-46.4919044745672,42.1030402839742,
2.77299664636633));
#233486=CARTESIAN_POINT('Ctrl Pts',(-46.481409305945,42.0985769785674,2.78297683033259));
#233487=CARTESIAN_POINT('Ctrl Pts',(-46.4714088200605,42.0932726122952,
2.79314401478644));
#233488=CARTESIAN_POINT('Ctrl Pts',(-46.4619468343647,42.0872150940891,
2.80341452427655));
#233489=CARTESIAN_POINT('Ctrl Pts',(-46.4526126174226,42.0812393728311,
2.8135463472118));
#233490=CARTESIAN_POINT('Ctrl Pts',(-46.443801442104,42.074529686026,2.82378004209123));
#233491=CARTESIAN_POINT('Ctrl Pts',(-46.4355828792672,42.0671296588095,
2.8340419886029));
#233492=CARTESIAN_POINT('Ctrl Pts',(-43.8790236240222,39.7651933658998,
2.83404198860289));
#233493=CARTESIAN_POINT('Ctrl Pts',(-43.8711584142718,39.7581114992313,
2.82422126443015));
#233494=CARTESIAN_POINT('Ctrl Pts',(-43.8638800583564,39.7504347382249,
2.81442815028492));
#233495=CARTESIAN_POINT('Ctrl Pts',(-43.8572218328527,39.7422106539902,
2.80471618166291));
#233496=CARTESIAN_POINT('Ctrl Pts',(-43.8507927303126,39.734269577075,2.79533842146186));
#233497=CARTESIAN_POINT('Ctrl Pts',(-43.8449410790333,39.7258171668685,
2.78603515650181));
#233498=CARTESIAN_POINT('Ctrl Pts',(-43.8397310304444,39.7168657021537,
2.77685887346682));
#233499=CARTESIAN_POINT('Ctrl Pts',(-43.8348059028416,39.708403764573,2.76818441216487));
#233500=CARTESIAN_POINT('Ctrl Pts',(-43.8304536682199,39.6994950821771,
2.75962261521518));
#233501=CARTESIAN_POINT('Ctrl Pts',(-43.8267676847805,39.6901349804711,
2.75123537701539));
#233502=CARTESIAN_POINT('Ctrl Pts',(-43.8233729558698,39.6815144838273,
2.74351087133981));
#233503=CARTESIAN_POINT('Ctrl Pts',(-43.8205432023692,39.6725105620392,
2.73593399449693));
#233504=CARTESIAN_POINT('Ctrl Pts',(-43.8183892419676,39.6631152739593,
2.72857657812408));
#233505=CARTESIAN_POINT('Ctrl Pts',(-43.8177469744568,39.6603137887119,
2.72638274508216));
#233506=CARTESIAN_POINT('Ctrl Pts',(-43.8171650742227,39.6574775031705,
2.72420861709555));
#233507=CARTESIAN_POINT('Ctrl Pts',(-43.8166472411072,39.654606226052,2.72205663736734));
#233508=CARTESIAN_POINT('Ctrl Pts',(-43.8161346989697,39.6517642863086,
2.71992664556774));
#233509=CARTESIAN_POINT('Ctrl Pts',(-43.8156851836083,39.648891063969,2.71782089927893));
#233510=CARTESIAN_POINT('Ctrl Pts',(-43.8153025584993,39.6459896850504,
2.71574387311254));
#233511=CARTESIAN_POINT('Ctrl Pts',(-43.8152759514976,39.6457879288346,
2.71559944077495));
#233512=CARTESIAN_POINT('Ctrl Pts',(-43.8152496566737,39.6455860324536,
2.71545515216077));
#233513=CARTESIAN_POINT('Ctrl Pts',(-43.8152236753307,39.6453839959665,
2.71531100781738));
#233514=CARTESIAN_POINT('Ctrl Pts',(-43.8140845580784,39.6365259762555,
2.70899119176088));
#233515=CARTESIAN_POINT('Ctrl Pts',(-43.8135929685791,39.6274037177902,
2.70298296066839));
#233516=CARTESIAN_POINT('Ctrl Pts',(-43.81383230999,39.6180980992373,2.69736727774133));
#233517=CARTESIAN_POINT('Ctrl Pts',(-43.8140554177822,39.6094236454405,
2.69213248525425));
#233518=CARTESIAN_POINT('Ctrl Pts',(-43.8149139527618,39.60058909514,2.68723866185465));
#233519=CARTESIAN_POINT('Ctrl Pts',(-43.8164991115145,39.5916773623193,
2.6827859582956));
#233520=CARTESIAN_POINT('Ctrl Pts',(-43.8170789830938,39.5884173351603,
2.68115710172805));
#233521=CARTESIAN_POINT('Ctrl Pts',(-43.8177563121467,39.5851472105418,
2.67958763637811));
#233522=CARTESIAN_POINT('Ctrl Pts',(-43.8185363400629,39.5818719865445,
2.67808378645368));
#233523=CARTESIAN_POINT('Ctrl Pts',(-43.8187239107183,39.5810844045887,
2.67772216078603));
#233524=CARTESIAN_POINT('Ctrl Pts',(-43.8189178575372,39.5802961412321,
2.67736403603566));
#233525=CARTESIAN_POINT('Ctrl Pts',(-43.8191182115052,39.5795073285708,
2.67700956934482));
#233526=CARTESIAN_POINT('Ctrl Pts',(-43.8193123044117,39.5787431663051,
2.67666617973807));
#233527=CARTESIAN_POINT('Ctrl Pts',(-43.81951241026,39.577978488548,2.67632622314121));
#233528=CARTESIAN_POINT('Ctrl Pts',(-43.819718554668,39.5772134181965,2.67598984158776));
#233529=CARTESIAN_POINT('Ctrl Pts',(-43.8219771048932,39.5688311883232,
2.67230439292224));
#233530=CARTESIAN_POINT('Ctrl Pts',(-43.8249623840156,39.5603964284873,
2.66904964539979));
#233531=CARTESIAN_POINT('Ctrl Pts',(-43.8286919494555,39.5520968239718,
2.6664020356673));
#233532=CARTESIAN_POINT('Ctrl Pts',(-43.8302387114098,39.5486547305946,
2.66530399299444));
#233533=CARTESIAN_POINT('Ctrl Pts',(-43.8319130705227,39.545235957413,2.66430995142263));
#233534=CARTESIAN_POINT('Ctrl Pts',(-43.8337144555752,39.5418537500316,
2.66343053473364));
#233535=CARTESIAN_POINT('Ctrl Pts',(-43.8367869054996,39.5360850428919,
2.66193059792888));
#233536=CARTESIAN_POINT('Ctrl Pts',(-43.8402296473865,39.5304250803199,
2.66076519817131));
#233537=CARTESIAN_POINT('Ctrl Pts',(-43.8440378929942,39.5249464846904,
2.65997805604464));
#233538=CARTESIAN_POINT('Ctrl Pts',(-43.845942015798,39.5222071868757,2.6595844849813));
#233539=CARTESIAN_POINT('Ctrl Pts',(-43.8479386338068,39.5195141476135,
2.65928526260766));
#233540=CARTESIAN_POINT('Ctrl Pts',(-43.8500271570782,39.516876509875,2.65908463971329));
#233541=CARTESIAN_POINT('Ctrl Pts',(-43.8521156803496,39.5142388721366,
2.65888401681891));
#233542=CARTESIAN_POINT('Ctrl Pts',(-43.8542960677575,39.5116566557598,
2.65878198860288));
#233543=CARTESIAN_POINT('Ctrl Pts',(-43.8565665267058,39.5091373124622,
2.65878198860288));
#233544=CARTESIAN_POINT('Origin',(-47.145339660541,34.2342565846636,2.83404198860285));
#233545=CARTESIAN_POINT('Ctrl Pts',(-50.8023624960593,36.6746059268177,
2.83404198860287));
#233546=CARTESIAN_POINT('Ctrl Pts',(-50.8109464329599,36.6808425220338,
2.82419652440154));
#233547=CARTESIAN_POINT('Ctrl Pts',(-50.8190128116684,36.6877379133665,
2.81438790575794));
#233548=CARTESIAN_POINT('Ctrl Pts',(-50.8265243508953,36.6952462569238,
2.80466781257097));
#233549=CARTESIAN_POINT('Ctrl Pts',(-50.8337918098257,36.7025106240248,
2.79526356453312));
#233550=CARTESIAN_POINT('Ctrl Pts',(-50.8405407635273,36.710349715224,2.78594102496499));
#233551=CARTESIAN_POINT('Ctrl Pts',(-50.8467071440063,36.7187568768206,
2.77675109089075));
#233552=CARTESIAN_POINT('Ctrl Pts',(-50.8525401602357,36.7267095340077,
2.76805797914004));
#233553=CARTESIAN_POINT('Ctrl Pts',(-50.8578524412736,36.7351712462807,
2.75948271210505));
#233554=CARTESIAN_POINT('Ctrl Pts',(-50.8625525281323,36.7441560526506,
2.75108575573587));
#233555=CARTESIAN_POINT('Ctrl Pts',(-50.8668816480481,36.752431709115,2.74335155163653));
#233556=CARTESIAN_POINT('Ctrl Pts',(-50.870691607918,36.7611516658436,2.73576818686343));
#233557=CARTESIAN_POINT('Ctrl Pts',(-50.8738736606193,36.7703354510133,
2.72840626160913));
#233558=CARTESIAN_POINT('Ctrl Pts',(-50.8747966531494,36.7729993179904,
2.72627084693963));
#233559=CARTESIAN_POINT('Ctrl Pts',(-50.8756665488979,36.7757022424564,
2.72415424587676));
#233560=CARTESIAN_POINT('Ctrl Pts',(-50.8764799968254,36.7784447603819,
2.72205867173284));
#233561=CARTESIAN_POINT('Ctrl Pts',(-50.8773618266783,36.7814178261393,
2.71978693462886));
#233562=CARTESIAN_POINT('Ctrl Pts',(-50.8781771258725,36.7844329791247,
2.71754411340786));
#233563=CARTESIAN_POINT('Ctrl Pts',(-50.8789219044955,36.7874899206174,
2.71533341844283));
#233564=CARTESIAN_POINT('Ctrl Pts',(-50.8809659552704,36.7958797205316,
2.7092661487643));
#233565=CARTESIAN_POINT('Ctrl Pts',(-50.8824343655145,36.8045837617103,
2.70347381860447));
#233566=CARTESIAN_POINT('Ctrl Pts',(-50.8832604021663,36.8135226609478,
2.69804914171433));
#233567=CARTESIAN_POINT('Ctrl Pts',(-50.8840161808561,36.821701268446,2.69308585687238));
#233568=CARTESIAN_POINT('Ctrl Pts',(-50.8842246658556,36.8300699399859,
2.68842799053215));
#233569=CARTESIAN_POINT('Ctrl Pts',(-50.8838072802929,36.8385876480152,
2.68414767054244));
#233570=CARTESIAN_POINT('Ctrl Pts',(-50.883602261868,36.8427715183747,2.68204519134583));
#233571=CARTESIAN_POINT('Ctrl Pts',(-50.8832457706971,36.8469911418449,
2.68003431778538));
#233572=CARTESIAN_POINT('Ctrl Pts',(-50.8827256259726,36.8512399286217,
2.67812693945291));
#233573=CARTESIAN_POINT('Ctrl Pts',(-50.8826269335774,36.8520460945289,
2.67776503299243));
#233574=CARTESIAN_POINT('Ctrl Pts',(-50.882521936226,36.8528536453865,2.67740659639964));
#233575=CARTESIAN_POINT('Ctrl Pts',(-50.8824105850808,36.8536624499713,
2.67705178968895));
#233576=CARTESIAN_POINT('Ctrl Pts',(-50.8823027136589,36.8544459794128,
2.67670807068798));
#233577=CARTESIAN_POINT('Ctrl Pts',(-50.8821888793658,36.8552306854278,
2.67636775825305));
#233578=CARTESIAN_POINT('Ctrl Pts',(-50.8820690400776,36.8560164456185,
2.67603099699295));
#233579=CARTESIAN_POINT('Ctrl Pts',(-50.8807630562081,36.8645794982675,
2.67236104217174));
#233580=CARTESIAN_POINT('Ctrl Pts',(-50.8787426509999,36.8732733195871,
2.66911440541524));
#233581=CARTESIAN_POINT('Ctrl Pts',(-50.875966462067,36.8819119966105,2.66646778189683));
#233582=CARTESIAN_POINT('Ctrl Pts',(-50.8747940602413,36.8855601635613,
2.66535009635021));
#233583=CARTESIAN_POINT('Ctrl Pts',(-50.8734872887379,36.8891983713647,
2.66433897912387));
#233584=CARTESIAN_POINT('Ctrl Pts',(-50.8720449698705,36.8928125648617,
2.66344564884832));
#233585=CARTESIAN_POINT('Ctrl Pts',(-50.8696161409375,36.8988987764016,
2.66194130298624));
#233586=CARTESIAN_POINT('Ctrl Pts',(-50.8668019052538,36.9049145742147,
2.66077206705458));
#233587=CARTESIAN_POINT('Ctrl Pts',(-50.8635979627953,36.9107858666119,
2.65998225155752));
#233588=CARTESIAN_POINT('Ctrl Pts',(-50.8627969771806,36.9122536897112,
2.65978479768326));
#233589=CARTESIAN_POINT('Ctrl Pts',(-50.861971437292,36.9137123559382,2.6596109896666));
#233590=CARTESIAN_POINT('Ctrl Pts',(-50.861121022166,36.9151605322321,2.65946139030539));
#233591=CARTESIAN_POINT('Ctrl Pts',(-50.8598453994769,36.9173327966729,
2.65923699126358));
#233592=CARTESIAN_POINT('Ctrl Pts',(-50.8585138058059,36.9194814382216,
2.65906707562479));
#233593=CARTESIAN_POINT('Ctrl Pts',(-50.857126526261,36.921602929223,2.65895332562957));
#233594=CARTESIAN_POINT('Ctrl Pts',(-50.8557392467161,36.9237244202245,
2.65883957563435));
#233595=CARTESIAN_POINT('Ctrl Pts',(-50.8542962928972,36.9258187603129,
2.65878198860287));
#233596=CARTESIAN_POINT('Ctrl Pts',(-50.8527980281387,36.9278827595326,
2.65878198860287));
#233597=CARTESIAN_POINT('Ctrl Pts',(-47.7640607692765,34.6837837831345,
2.65878198860285));
#233598=CARTESIAN_POINT('Ctrl Pts',(-47.7691302463546,34.6767997090225,
2.65878198860285));
#233599=CARTESIAN_POINT('Ctrl Pts',(-47.7747322888389,34.6702946353238,
2.65945335517889));
#233600=CARTESIAN_POINT('Ctrl Pts',(-47.7807252358003,34.6643211616146,
2.66072561226654));
#233601=CARTESIAN_POINT('Ctrl Pts',(-47.7845960646247,34.6604629105131,
2.66154735980388));
#233602=CARTESIAN_POINT('Ctrl Pts',(-47.788629319434,34.6568257642791,2.66261895766922));
#233603=CARTESIAN_POINT('Ctrl Pts',(-47.7927819897609,34.6534164822764,
2.66391429251049));
#233604=CARTESIAN_POINT('Ctrl Pts',(-47.7982861164003,34.648897674277,2.66563118464146));
#233605=CARTESIAN_POINT('Ctrl Pts',(-47.8040027249063,34.6447843113775,
2.66774105138722));
#233606=CARTESIAN_POINT('Ctrl Pts',(-47.8098436832079,34.6410949611633,
2.67016894181774));
#233607=CARTESIAN_POINT('Ctrl Pts',(-47.8127641623586,34.6392502860563,
2.67138288703299));
#233608=CARTESIAN_POINT('Ctrl Pts',(-47.8157158446827,34.6375114518667,
2.67267613167576));
#233609=CARTESIAN_POINT('Ctrl Pts',(-47.8186885387638,34.6358796311044,
2.67403835432578));
#233610=CARTESIAN_POINT('Ctrl Pts',(-47.8201748858043,34.6350637207233,
2.67471946565079));
#233611=CARTESIAN_POINT('Ctrl Pts',(-47.8216664954025,34.6342745503772,
2.67541781389548));
#233612=CARTESIAN_POINT('Ctrl Pts',(-47.8231621539167,34.6335121829169,
2.67613207244195));
#233613=CARTESIAN_POINT('Ctrl Pts',(-47.8235360685452,34.6333215910518,
2.67631063707856));
#233614=CARTESIAN_POINT('Ctrl Pts',(-47.8239102364347,34.6331326740832,
2.67649019601871));
#233615=CARTESIAN_POINT('Ctrl Pts',(-47.8242846390327,34.6329454324201,
2.67667072836683));
#233616=CARTESIAN_POINT('Ctrl Pts',(-47.8254078468265,34.6323837074307,
2.67721232541117));
#233617=CARTESIAN_POINT('Ctrl Pts',(-47.8265331659852,34.6318370616129,
2.67776268340073));
#233618=CARTESIAN_POINT('Ctrl Pts',(-47.8276601046327,34.6313054933185,
2.67832123541542));
#233619=CARTESIAN_POINT('Ctrl Pts',(-47.8355981149515,34.6275611948904,
2.68225560368471));
#233620=CARTESIAN_POINT('Ctrl Pts',(-47.8436253243399,34.6245119115567,
2.68661792998915));
#233621=CARTESIAN_POINT('Ctrl Pts',(-47.851650015445,34.6220808005811,2.69130986622604));
#233622=CARTESIAN_POINT('Ctrl Pts',(-47.8555419819595,34.6209017143849,
2.6935854502308));
#233623=CARTESIAN_POINT('Ctrl Pts',(-47.8594338479543,34.6198683413514,
2.69593918853494));
#233624=CARTESIAN_POINT('Ctrl Pts',(-47.863317387285,34.618973699214,2.69836306235499));
#233625=CARTESIAN_POINT('Ctrl Pts',(-47.8692628146652,34.6176040646085,
2.70207384382232));
#233626=CARTESIAN_POINT('Ctrl Pts',(-47.8751852090114,34.6165592825246,
2.70594760814232));
#233627=CARTESIAN_POINT('Ctrl Pts',(-47.8810431641657,34.6158190596253,
2.70995196345712));
#233628=CARTESIAN_POINT('Ctrl Pts',(-47.8837636288444,34.6154752962814,
2.7118116067811));
#233629=CARTESIAN_POINT('Ctrl Pts',(-47.8864700832048,34.6151969889848,
2.71369962772103));
#233630=CARTESIAN_POINT('Ctrl Pts',(-47.8891582656053,34.6149833323962,
2.71561183138665));
#233631=CARTESIAN_POINT('Ctrl Pts',(-47.8893643041943,34.6149669564605,
2.71575839426316));
#233632=CARTESIAN_POINT('Ctrl Pts',(-47.8895702459311,34.6149509280617,
2.71590508903212));
#233633=CARTESIAN_POINT('Ctrl Pts',(-47.8897760897957,34.6149352461545,
2.71605191409915));
#233634=CARTESIAN_POINT('Ctrl Pts',(-47.8926675754934,34.6147149626377,
2.71811436362756));
#233635=CARTESIAN_POINT('Ctrl Pts',(-47.8955400426775,34.6145651177085,
2.72020091026963));
#233636=CARTESIAN_POINT('Ctrl Pts',(-47.8983891927624,34.6144819591403,
2.72230624862186));
#233637=CARTESIAN_POINT('Ctrl Pts',(-47.9086057382621,34.614183767304,2.72985561753071));
#233638=CARTESIAN_POINT('Ctrl Pts',(-47.9186013937326,34.614738768508,2.73770089914259));
#233639=CARTESIAN_POINT('Ctrl Pts',(-47.9283423801871,34.616022335536,2.74574823346962));
#233640=CARTESIAN_POINT('Ctrl Pts',(-47.9390467457316,34.617432846754,2.75459144546848));
#233641=CARTESIAN_POINT('Ctrl Pts',(-47.9494442419723,34.619723085458,2.76367911754026));
#233642=CARTESIAN_POINT('Ctrl Pts',(-47.959498481281,34.6227799581208,2.77292162564413));
#233643=CARTESIAN_POINT('Ctrl Pts',(-47.9703545364643,34.6260806134262,
2.78290121484312));
#233644=CARTESIAN_POINT('Ctrl Pts',(-47.9808115517317,34.6302752334078,
2.79306229499661));
#233645=CARTESIAN_POINT('Ctrl Pts',(-47.9908184179891,34.6352786409512,
2.80331916684618));
#233646=CARTESIAN_POINT('Ctrl Pts',(-48.0007413369235,34.6402400750478,
2.81348999408273));
#233647=CARTESIAN_POINT('Ctrl Pts',(-48.0102227609117,34.6459976650994,
2.82375635966676));
#233648=CARTESIAN_POINT('Ctrl Pts',(-48.0191904766738,34.6525130919796,
2.83404198860285));
#233649=CARTESIAN_POINT('Origin',(0.00895784724494739,0.0123294189944604,
2.83404198860262));
#233650=CARTESIAN_POINT('Ctrl Pts',(-50.8348823336488,36.9525415975211,
2.65878198860287));
#233651=CARTESIAN_POINT('Ctrl Pts',(-50.8298309792461,36.9594880792486,
2.65878198860287));
#233652=CARTESIAN_POINT('Ctrl Pts',(-50.8242442388883,36.9659508653432,
2.65944603041871));
#233653=CARTESIAN_POINT('Ctrl Pts',(-50.8182646381297,36.9718804702597,
2.66070439264082));
#233654=CARTESIAN_POINT('Ctrl Pts',(-50.8144439579055,36.9756692055208,
2.66150842619607));
#233655=CARTESIAN_POINT('Ctrl Pts',(-50.8104635307793,36.9792409429415,
2.66255428265383));
#233656=CARTESIAN_POINT('Ctrl Pts',(-50.8063652005966,36.9825899931428,
2.66381699700674));
#233657=CARTESIAN_POINT('Ctrl Pts',(-50.8007718022341,36.987160774675,2.66554034873273));
#233658=CARTESIAN_POINT('Ctrl Pts',(-50.7949560887232,36.9913113073909,
2.66766759643977));
#233659=CARTESIAN_POINT('Ctrl Pts',(-50.789012020324,36.9950236271423,2.67012012783152));
#233660=CARTESIAN_POINT('Ctrl Pts',(-50.7860399861244,36.9968797870181,
2.6713463935274));
#233661=CARTESIAN_POINT('Ctrl Pts',(-50.7830357420056,36.998626563727,2.67265375585016));
#233662=CARTESIAN_POINT('Ctrl Pts',(-50.7800101622086,37.0002629240971,
2.67403135126944));
#233663=CARTESIAN_POINT('Ctrl Pts',(-50.7784973723101,37.0010811042821,
2.67472014897908));
#233664=CARTESIAN_POINT('Ctrl Pts',(-50.7769792382975,37.0018716945001,
2.67542649668636));
#233665=CARTESIAN_POINT('Ctrl Pts',(-50.775457055492,37.0026346543984,2.67614899656106));
#233666=CARTESIAN_POINT('Ctrl Pts',(-50.7750765097906,37.002825394373,2.67632962152973));
#233667=CARTESIAN_POINT('Ctrl Pts',(-50.7746957108233,37.003014407754,2.67651125590955));
#233668=CARTESIAN_POINT('Ctrl Pts',(-50.7743146783936,37.0032016945189,
2.67669387767528));
#233669=CARTESIAN_POINT('Ctrl Pts',(-50.7731715811046,37.0037635548139,
2.67724174297248));
#233670=CARTESIAN_POINT('Ctrl Pts',(-50.7720263837272,37.0043098740556,
2.67779849504752));
#233671=CARTESIAN_POINT('Ctrl Pts',(-50.7708796113517,37.0048406651183,
2.67836353618014));
#233672=CARTESIAN_POINT('Ctrl Pts',(-50.7629547027164,37.0085087606934,
2.68226832098921));
#233673=CARTESIAN_POINT('Ctrl Pts',(-50.7549442896465,37.0114900453061,
2.68659153751414));
#233674=CARTESIAN_POINT('Ctrl Pts',(-50.7469376805975,37.0138628466712,
2.69123699486213));
#233675=CARTESIAN_POINT('Ctrl Pts',(-50.7429584178781,37.0150421224363,
2.69354577441243));
#233676=CARTESIAN_POINT('Ctrl Pts',(-50.7389795822777,37.0160707669658,
2.69593478828134));
#233677=CARTESIAN_POINT('Ctrl Pts',(-50.7350097117578,37.0169563748089,
2.69839565261227));
#233678=CARTESIAN_POINT('Ctrl Pts',(-50.7262515844356,37.0189101579885,
2.70382468689053));
#233679=CARTESIAN_POINT('Ctrl Pts',(-50.7175407334809,37.0201796788545,
2.70961155815094));
#233680=CARTESIAN_POINT('Ctrl Pts',(-50.7090177292134,37.0208019128475,
2.71562701361775));
#233681=CARTESIAN_POINT('Ctrl Pts',(-50.7059041682737,37.0210292227719,
2.71782453535867));
#233682=CARTESIAN_POINT('Ctrl Pts',(-50.7028130194416,37.0211776528892,
2.72005051502411));
#233683=CARTESIAN_POINT('Ctrl Pts',(-50.6997475881155,37.0212513646536,
2.72229986760125));
#233684=CARTESIAN_POINT('Ctrl Pts',(-50.6894511286645,37.0214989546704,
2.7298552048891));
#233685=CARTESIAN_POINT('Ctrl Pts',(-50.6793793407316,37.0208967002927,
2.73770845534585));
#233686=CARTESIAN_POINT('Ctrl Pts',(-50.6695664063382,37.0195682679086,
2.74576706701788));
#233687=CARTESIAN_POINT('Ctrl Pts',(-50.6587808290213,37.0181081633553,
2.75462443585076));
#233688=CARTESIAN_POINT('Ctrl Pts',(-50.6483072759133,37.0157708601097,
2.7637303632324));
#233689=CARTESIAN_POINT('Ctrl Pts',(-50.6381830571039,37.0126680948707,
2.77299664636891));
#233690=CARTESIAN_POINT('Ctrl Pts',(-50.6272788396577,37.0093262837653,
2.78297683033572));
#233691=CARTESIAN_POINT('Ctrl Pts',(-50.6167786802258,37.0050963107875,
2.79314401479016));
#233692=CARTESIAN_POINT('Ctrl Pts',(-50.606735345208,37.0000610231238,2.80341452428089));
#233693=CARTESIAN_POINT('Ctrl Pts',(-50.5968276291246,36.9950937288454,
2.81354634721468));
#233694=CARTESIAN_POINT('Ctrl Pts',(-50.5873633690971,36.9893418170231,
2.82378004209264));
#233695=CARTESIAN_POINT('Ctrl Pts',(-50.5784163149359,36.9828414016746,
2.83404198860287));
#233696=CARTESIAN_POINT('Ctrl Pts',(-47.7952442955504,34.9607485668365,
2.83404198860285));
#233697=CARTESIAN_POINT('Ctrl Pts',(-47.7866819156023,34.9545276336633,
2.82422126443049));
#233698=CARTESIAN_POINT('Ctrl Pts',(-47.7786409912516,34.9476537221161,
2.81442815028562));
#233699=CARTESIAN_POINT('Ctrl Pts',(-47.7711595893173,34.9401706643557,
2.80471618166397));
#233700=CARTESIAN_POINT('Ctrl Pts',(-47.7639356375071,34.9329451136996,
2.79533842146316));
#233701=CARTESIAN_POINT('Ctrl Pts',(-47.7572325247361,34.9251506707967,
2.78603515650334));
#233702=CARTESIAN_POINT('Ctrl Pts',(-47.7511153344879,34.916792841515,2.77685887346856));
#233703=CARTESIAN_POINT('Ctrl Pts',(-47.745332673918,34.9088920753337,2.76818441216674));
#233704=CARTESIAN_POINT('Ctrl Pts',(-47.7400730704123,34.9004871280291,
2.75962261521719));
#233705=CARTESIAN_POINT('Ctrl Pts',(-47.7354288821284,34.8915635921244,
2.75123537701751));
#233706=CARTESIAN_POINT('Ctrl Pts',(-47.7311516626311,34.8833451652596,
2.743510871342));
#233707=CARTESIAN_POINT('Ctrl Pts',(-47.7273962447083,34.8746863576823,
2.73593399449919));
#233708=CARTESIAN_POINT('Ctrl Pts',(-47.7242720089021,34.8655676881445,
2.72857657812639));
#233709=CARTESIAN_POINT('Ctrl Pts',(-47.7233404248517,34.8628486849613,
2.72638274508368));
#233710=CARTESIAN_POINT('Ctrl Pts',(-47.7224652397587,34.8600887620252,
2.72420861709628));
#233711=CARTESIAN_POINT('Ctrl Pts',(-47.7216501132021,34.857287342362,2.72205663736731));
#233712=CARTESIAN_POINT('Ctrl Pts',(-47.72084331523,34.8545145463038,2.7199266455677));
#233713=CARTESIAN_POINT('Ctrl Pts',(-47.720095928845,34.8517040509267,2.71782089927888));
#233714=CARTESIAN_POINT('Ctrl Pts',(-47.7194121231167,34.8488585612801,
2.7157438731125));
#233715=CARTESIAN_POINT('Ctrl Pts',(-47.7193645726037,34.8486606914949,
2.7155994407749));
#233716=CARTESIAN_POINT('Ctrl Pts',(-47.7193173179071,34.848462649681,2.71545515216073));
#233717=CARTESIAN_POINT('Ctrl Pts',(-47.7192703603292,34.8482644357608,
2.71531100781734));
#233718=CARTESIAN_POINT('Ctrl Pts',(-47.7172115680923,34.8395740113844,
2.70899119176081));
#233719=CARTESIAN_POINT('Ctrl Pts',(-47.7157691359129,34.8305531107004,
2.70298296066831));
#233720=CARTESIAN_POINT('Ctrl Pts',(-47.7150344641794,34.8212734513097,
2.69736727774125));
#233721=CARTESIAN_POINT('Ctrl Pts',(-47.7143496224387,34.8126231959635,
2.69213248525408));
#233722=CARTESIAN_POINT('Ctrl Pts',(-47.7142799923073,34.8037473009117,
2.68723866185439));
#233723=CARTESIAN_POINT('Ctrl Pts',(-47.7149249376576,34.7947186932872,
2.68278595829527));
#233724=CARTESIAN_POINT('Ctrl Pts',(-47.7151608670106,34.7914159118132,
2.68115710172783));
#233725=CARTESIAN_POINT('Ctrl Pts',(-47.7154926644831,34.7880929011147,
2.679587636378));
#233726=CARTESIAN_POINT('Ctrl Pts',(-47.7159260651934,34.784754084018,2.67808378645366));
#233727=CARTESIAN_POINT('Ctrl Pts',(-47.7160302835856,34.7839512100461,
2.67772216078602));
#233728=CARTESIAN_POINT('Ctrl Pts',(-47.7161407719862,34.7831469919158,
2.67736403603564));
#233729=CARTESIAN_POINT('Ctrl Pts',(-47.7162575750189,34.7823415577604,
2.6770095693448));
#233730=CARTESIAN_POINT('Ctrl Pts',(-47.7163707279568,34.7815612934223,
2.67666617973805));
#233731=CARTESIAN_POINT('Ctrl Pts',(-47.7164898070135,34.7807798878932,
2.67632622314121));
#233732=CARTESIAN_POINT('Ctrl Pts',(-47.7166148505127,34.7799974607189,
2.67598984158775));
#233733=CARTESIAN_POINT('Ctrl Pts',(-47.717984846556,34.771425066794,2.67230439292235));
#233734=CARTESIAN_POINT('Ctrl Pts',(-47.7200720995232,34.7627244668161,
2.66904964539999));
#233735=CARTESIAN_POINT('Ctrl Pts',(-47.7229136891076,34.7540804826588,
2.66640203566754));
#233736=CARTESIAN_POINT('Ctrl Pts',(-47.724092181007,34.7504955647788,2.66530399299458));
#233737=CARTESIAN_POINT('Ctrl Pts',(-47.7254000086987,34.7469205018091,
2.66430995142268));
#233738=CARTESIAN_POINT('Ctrl Pts',(-47.7268379886354,34.7433685265021,
2.66343053473362));
#233739=CARTESIAN_POINT('Ctrl Pts',(-47.7292906132653,34.7373102624746,
2.66193059792886));
#233740=CARTESIAN_POINT('Ctrl Pts',(-47.7321228682621,34.731321441251,2.66076519817129));
#233741=CARTESIAN_POINT('Ctrl Pts',(-47.7353375827201,34.7254747878806,
2.65997805604461));
#233742=CARTESIAN_POINT('Ctrl Pts',(-47.7369449399491,34.7225514611954,
2.65958448498127));
#233743=CARTESIAN_POINT('Ctrl Pts',(-47.7386491210198,34.7196644712719,
2.65928526260763));
#233744=CARTESIAN_POINT('Ctrl Pts',(-47.7404504949227,34.7168229726608,
2.65908463971326));
#233745=CARTESIAN_POINT('Ctrl Pts',(-47.7422518688256,34.7139814740497,
2.65888401681888));
#233746=CARTESIAN_POINT('Ctrl Pts',(-47.7441503967333,34.7111854907793,
2.65878198860285));
#233747=CARTESIAN_POINT('Ctrl Pts',(-47.7461450747866,34.7084426211231,
2.65878198860285));
#233748=CARTESIAN_POINT('Origin',(-50.4655267888877,29.1186878401555,2.83404198860281));
#233749=CARTESIAN_POINT('Ctrl Pts',(-54.357602037244,31.1634057161439,2.83404198860283));
#233750=CARTESIAN_POINT('Ctrl Pts',(-54.3667908521538,31.1687108809056,
2.8241965244016));
#233751=CARTESIAN_POINT('Ctrl Pts',(-54.3755338070552,31.1747253323926,
2.81438790575814));
#233752=CARTESIAN_POINT('Ctrl Pts',(-54.3837890328979,31.1814073748059,
2.80466781257132));
#233753=CARTESIAN_POINT('Ctrl Pts',(-54.3917760130574,31.1878722906298,
2.79526356453362));
#233754=CARTESIAN_POINT('Ctrl Pts',(-54.3993074034408,31.194962980708,2.78594102496565));
#233755=CARTESIAN_POINT('Ctrl Pts',(-54.4063187915245,31.2026795247181,
2.77675109089157));
#233756=CARTESIAN_POINT('Ctrl Pts',(-54.4129511329153,31.2099789001943,
2.76805797914105));
#233757=CARTESIAN_POINT('Ctrl Pts',(-54.4191188025023,31.2178389737485,
2.75948271210624));
#233758=CARTESIAN_POINT('Ctrl Pts',(-54.424732309796,31.2262832675523,2.75108575573722));
#233759=CARTESIAN_POINT('Ctrl Pts',(-54.4299027559926,31.2340610728523,
2.74335155163808));
#233760=CARTESIAN_POINT('Ctrl Pts',(-54.4346033281803,31.242335011495,2.73576818686516));
#233761=CARTESIAN_POINT('Ctrl Pts',(-54.4387279162147,31.2511358718494,
2.72840626161101));
#233762=CARTESIAN_POINT('Ctrl Pts',(-54.439924302417,31.2536886668944,2.72627084694087));
#233763=CARTESIAN_POINT('Ctrl Pts',(-54.4410719653267,31.2562858555924,
2.72415424587736));
#233764=CARTESIAN_POINT('Ctrl Pts',(-54.4421676282859,31.2589283212566,
2.72205867173281));
#233765=CARTESIAN_POINT('Ctrl Pts',(-54.4433553973774,31.2617929239294,
2.71978693462883));
#233766=CARTESIAN_POINT('Ctrl Pts',(-54.4444813995854,31.2647063376194,
2.71754411340783));
#233767=CARTESIAN_POINT('Ctrl Pts',(-54.4455416356297,31.2676686823018,
2.7153334184428));
#233768=CARTESIAN_POINT('Ctrl Pts',(-54.4484514617727,31.2757988605279,
2.70926614876426));
#233769=CARTESIAN_POINT('Ctrl Pts',(-54.4508216479604,31.2843017293921,
2.70347381860443));
#233770=CARTESIAN_POINT('Ctrl Pts',(-54.4525775288976,31.2931053160624,
2.69804914171429));
#233771=CARTESIAN_POINT('Ctrl Pts',(-54.4541840646262,31.3011601199081,
2.69308585687222));
#233772=CARTESIAN_POINT('Ctrl Pts',(-54.4552661718987,31.3094611543733,
2.68842799053189));
#233773=CARTESIAN_POINT('Ctrl Pts',(-54.4557414157487,31.3179758301784,
2.68414767054209));
#233774=CARTESIAN_POINT('Ctrl Pts',(-54.4559748539753,31.3221582111191,
2.68204519134559));
#233775=CARTESIAN_POINT('Ctrl Pts',(-54.4560613864572,31.3263919825245,
2.68003431778523));
#233776=CARTESIAN_POINT('Ctrl Pts',(-54.4559882102925,31.3306718639313,
2.67812693945286));
#233777=CARTESIAN_POINT('Ctrl Pts',(-54.455974325828,31.3314839297417,2.67776503299238));
#233778=CARTESIAN_POINT('Ctrl Pts',(-54.4559543157132,31.332298031963,2.67740659639959));
#233779=CARTESIAN_POINT('Ctrl Pts',(-54.4559281176616,31.3331140451957,
2.6770517896889));
#233780=CARTESIAN_POINT('Ctrl Pts',(-54.455902738299,31.3339045580149,2.67670807068793));
#233781=CARTESIAN_POINT('Ctrl Pts',(-54.455871551716,31.3346968642519,2.676367758253));
#233782=CARTESIAN_POINT('Ctrl Pts',(-54.4558345032252,31.3354908465828,
2.6760309969929));
#233783=CARTESIAN_POINT('Ctrl Pts',(-54.4554307564063,31.34414350242,2.67236104217183));
#233784=CARTESIAN_POINT('Ctrl Pts',(-54.4543301709717,31.353000887928,2.66911440541543));
#233785=CARTESIAN_POINT('Ctrl Pts',(-54.4524721779263,31.3618824321374,
2.66646778189708));
#233786=CARTESIAN_POINT('Ctrl Pts',(-54.4516875359255,31.3656331634094,
2.66535009635034));
#233787=CARTESIAN_POINT('Ctrl Pts',(-54.4507682193238,31.3693880355472,
2.6643389791239));
#233788=CARTESIAN_POINT('Ctrl Pts',(-54.4497115877222,31.3731331934892,
2.66344564884827));
#233789=CARTESIAN_POINT('Ctrl Pts',(-54.4479322465076,31.3794399458813,
2.6619413029862));
#233790=CARTESIAN_POINT('Ctrl Pts',(-54.4457622496022,31.3857169562559,
2.66077206705454));
#233791=CARTESIAN_POINT('Ctrl Pts',(-54.4431895758471,31.3918909882805,
2.65998225155748));
#233792=CARTESIAN_POINT('Ctrl Pts',(-54.4425464074084,31.3934344962866,
2.65978479768321));
#233793=CARTESIAN_POINT('Ctrl Pts',(-54.4418778620527,31.3949714642033,
2.65961098966656));
#233794=CARTESIAN_POINT('Ctrl Pts',(-54.4411834812323,31.3965005998222,
2.65946139030535));
#233795=CARTESIAN_POINT('Ctrl Pts',(-54.4401419100017,31.3987943032506,
2.65923699126354));
#233796=CARTESIAN_POINT('Ctrl Pts',(-54.4390422051394,31.4010703637562,
2.65906707562476));
#233797=CARTESIAN_POINT('Ctrl Pts',(-54.4378842814512,31.4033252432069,
2.65895332562953));
#233798=CARTESIAN_POINT('Ctrl Pts',(-54.4367263577631,31.4055801226576,
2.65883957563431));
#233799=CARTESIAN_POINT('Ctrl Pts',(-54.4355102267473,31.4078138194773,
2.65878198860283));
#233800=CARTESIAN_POINT('Ctrl Pts',(-54.4342359163065,31.410023123206,2.65878198860283));
#233801=CARTESIAN_POINT('Ctrl Pts',(-51.1278468659049,29.501078514911,2.65878198860281));
#233802=CARTESIAN_POINT('Ctrl Pts',(-51.1321585373225,29.4936027956397,
2.65878198860281));
#233803=CARTESIAN_POINT('Ctrl Pts',(-51.1370499258744,29.4865477845238,
2.65945335517875));
#233804=CARTESIAN_POINT('Ctrl Pts',(-51.1423856448177,29.4799806005927,
2.66072561226622));
#233805=CARTESIAN_POINT('Ctrl Pts',(-51.1458319717786,29.4757388736053,
2.66154735980359));
#233806=CARTESIAN_POINT('Ctrl Pts',(-51.1494629466899,29.4717000621112,
2.66261895766902));
#233807=CARTESIAN_POINT('Ctrl Pts',(-51.1532365012461,29.4678753842639,
2.66391429251045));
#233808=CARTESIAN_POINT('Ctrl Pts',(-51.1582381316478,29.4628059928683,
2.66563118464141));
#233809=CARTESIAN_POINT('Ctrl Pts',(-51.1634934604717,29.4581176150989,
2.66774105138716));
#233810=CARTESIAN_POINT('Ctrl Pts',(-51.1689167792841,29.453837929136,2.67016894181767));
#233811=CARTESIAN_POINT('Ctrl Pts',(-51.1716284386903,29.4516980861545,
2.67138288703292));
#233812=CARTESIAN_POINT('Ctrl Pts',(-51.174382193724,29.4496602426632,2.67267613167568));
#233813=CARTESIAN_POINT('Ctrl Pts',(-51.1771680313593,29.4477266300417,
2.6740383543257));
#233814=CARTESIAN_POINT('Ctrl Pts',(-51.1785609501769,29.446759823731,2.67471946565071));
#233815=CARTESIAN_POINT('Ctrl Pts',(-51.1799618978181,29.4458190608836,
2.6754178138954));
#233816=CARTESIAN_POINT('Ctrl Pts',(-51.1813696738594,29.4449045308659,
2.67613207244186));
#233817=CARTESIAN_POINT('Ctrl Pts',(-51.1817216178697,29.4446758983615,
2.67631063707848));
#233818=CARTESIAN_POINT('Ctrl Pts',(-51.1820739888279,29.4444489051053,
2.67649019601863));
#233819=CARTESIAN_POINT('Ctrl Pts',(-51.182426768326,29.4442235534434,2.67667072836674));
#233820=CARTESIAN_POINT('Ctrl Pts',(-51.1834851068201,29.4435474984577,
2.67721232541108));
#233821=CARTESIAN_POINT('Ctrl Pts',(-51.1845471213153,29.4428862193406,
2.67776268340065));
#233822=CARTESIAN_POINT('Ctrl Pts',(-51.1856123224581,29.4422397658678,
2.67832123541534));
#233823=CARTESIAN_POINT('Ctrl Pts',(-51.1931154617651,29.4376862310783,
2.68225560368461));
#233824=CARTESIAN_POINT('Ctrl Pts',(-51.2007799603596,29.4338145801761,
2.68661792998903));
#233825=CARTESIAN_POINT('Ctrl Pts',(-51.2085065710728,29.4305579784513,
2.69130986622591));
#233826=CARTESIAN_POINT('Ctrl Pts',(-51.2122539689194,29.4289785301339,
2.6935854502307));
#233827=CARTESIAN_POINT('Ctrl Pts',(-51.2160164979699,29.4275440072542,
2.69593918853487));
#233828=CARTESIAN_POINT('Ctrl Pts',(-51.219785247298,29.4262483256618,2.69836306235495));
#233829=CARTESIAN_POINT('Ctrl Pts',(-51.2255549392045,29.4242647276705,
2.70207384382228));
#233830=CARTESIAN_POINT('Ctrl Pts',(-51.2313356805891,29.4226066102323,
2.70594760814228));
#233831=CARTESIAN_POINT('Ctrl Pts',(-51.23708417089,29.4212581193013,2.70995196345707));
#233832=CARTESIAN_POINT('Ctrl Pts',(-51.2397537995244,29.4206318731367,
2.71181160678105));
#233833=CARTESIAN_POINT('Ctrl Pts',(-51.2424163366106,29.4200721889214,
2.713699627721));
#233834=CARTESIAN_POINT('Ctrl Pts',(-51.2450674596718,29.4195787111907,
2.71561183138662));
#233835=CARTESIAN_POINT('Ctrl Pts',(-51.2452706578085,29.419540888067,2.71575839426313));
#233836=CARTESIAN_POINT('Ctrl Pts',(-51.245473795951,29.4195034207002,2.7159050890321));
#233837=CARTESIAN_POINT('Ctrl Pts',(-51.2456768729757,29.4194663081573,
2.71605191409912));
#233838=CARTESIAN_POINT('Ctrl Pts',(-51.2485294929147,29.4189449888201,
2.71811436362754));
#233839=CARTESIAN_POINT('Ctrl Pts',(-51.2513705613629,29.4184957101765,
2.7202009102696));
#233840=CARTESIAN_POINT('Ctrl Pts',(-51.2541954110682,29.4181151898796,
2.72230624862182));
#233841=CARTESIAN_POINT('Ctrl Pts',(-51.264324819729,29.4167507117684,2.72985561753119));
#233842=CARTESIAN_POINT('Ctrl Pts',(-51.2743237313766,29.416257842112,2.73770089914364));
#233843=CARTESIAN_POINT('Ctrl Pts',(-51.2841455249777,29.4165161672808,
2.74574823347125));
#233844=CARTESIAN_POINT('Ctrl Pts',(-51.2949386894587,29.4168000406903,
2.75459144547095));
#233845=CARTESIAN_POINT('Ctrl Pts',(-51.3055186222603,29.4179908989235,
2.7636791175436));
#233846=CARTESIAN_POINT('Ctrl Pts',(-51.3158373135967,29.4199800715341,
2.77292162564838));
#233847=CARTESIAN_POINT('Ctrl Pts',(-51.3269789106022,29.4221278787395,
2.78290121484878));
#233848=CARTESIAN_POINT('Ctrl Pts',(-51.3378170984279,29.4252064644185,
2.79306229500373));
#233849=CARTESIAN_POINT('Ctrl Pts',(-51.3482921445277,29.4291364604209,
2.80331916685476));
#233850=CARTESIAN_POINT('Ctrl Pts',(-51.3586793157524,29.4330334877944,
2.8134899940885));
#233851=CARTESIAN_POINT('Ctrl Pts',(-51.3687106315452,29.4377684584852,
2.82375635966964));
#233852=CARTESIAN_POINT('Ctrl Pts',(-51.3783102687786,29.443310811626,2.83404198860281));
#233853=CARTESIAN_POINT('Origin',(0.00762000000001041,0.0131982271538616,
2.83404198860262));
#233854=CARTESIAN_POINT('Ctrl Pts',(-54.4189959163065,31.4364195775134,
2.65878198860283));
#233855=CARTESIAN_POINT('Ctrl Pts',(-54.4146983388117,31.4438560160004,
2.65878198860283));
#233856=CARTESIAN_POINT('Ctrl Pts',(-54.4098177483009,31.4508673716611,
2.65944603041872));
#233857=CARTESIAN_POINT('Ctrl Pts',(-54.4044907169104,31.4573895320598,
2.66070439264092));
#233858=CARTESIAN_POINT('Ctrl Pts',(-54.4010869974469,31.4615568820651,
2.66150842619617));
#233859=CARTESIAN_POINT('Ctrl Pts',(-54.3975017237409,31.4655251210649,
2.6625542826539));
#233860=CARTESIAN_POINT('Ctrl Pts',(-54.3937759157109,31.4692842169745,
2.66381699700676));
#233861=CARTESIAN_POINT('Ctrl Pts',(-54.3886909353394,31.4744146286225,
2.66554034873276));
#233862=CARTESIAN_POINT('Ctrl Pts',(-54.3833409297222,31.4791503318821,
2.66766759643981));
#233863=CARTESIAN_POINT('Ctrl Pts',(-54.3778174666304,31.4834636394928,
2.67012012783157));
#233864=CARTESIAN_POINT('Ctrl Pts',(-54.3750557350845,31.4856202932981,
2.67134639352745));
#233865=CARTESIAN_POINT('Ctrl Pts',(-54.3722505364143,31.4876715300026,
2.67265375585021));
#233866=CARTESIAN_POINT('Ctrl Pts',(-54.3694125772949,31.4896151854259,
2.67403135126949));
#233867=CARTESIAN_POINT('Ctrl Pts',(-54.3679935977352,31.4905870131376,
2.67472014897913));
#233868=CARTESIAN_POINT('Ctrl Pts',(-54.3665664194001,31.4915319606351,
2.67542649668641));
#233869=CARTESIAN_POINT('Ctrl Pts',(-54.365132326297,31.4924498523887,2.6761489965611));
#233870=CARTESIAN_POINT('Ctrl Pts',(-54.3647738030212,31.4926793253271,
2.67632962152978));
#233871=CARTESIAN_POINT('Ctrl Pts',(-54.3644148473887,31.4929071076039,
2.67651125590959));
#233872=CARTESIAN_POINT('Ctrl Pts',(-54.3640554790923,31.4931331971267,
2.67669387767532));
#233873=CARTESIAN_POINT('Ctrl Pts',(-54.362977374203,31.4938114656952,2.67724174297252));
#233874=CARTESIAN_POINT('Ctrl Pts',(-54.3618955562474,31.4944744978649,
2.67779849504756));
#233875=CARTESIAN_POINT('Ctrl Pts',(-54.3608105487851,31.4951222515527,
2.67836353618017));
#233876=CARTESIAN_POINT('Ctrl Pts',(-54.3533124740222,31.4995986314376,
2.68226832098918));
#233877=CARTESIAN_POINT('Ctrl Pts',(-54.3456575719325,31.5034009004296,
2.68659153751403));
#233878=CARTESIAN_POINT('Ctrl Pts',(-54.3379428492061,31.5065976218803,
2.69123699486192));
#233879=CARTESIAN_POINT('Ctrl Pts',(-54.3341086531876,31.5081863836665,
2.69354577441228));
#233880=CARTESIAN_POINT('Ctrl Pts',(-54.3302591366968,31.5096252947446,
2.69593478828126));
#233881=CARTESIAN_POINT('Ctrl Pts',(-54.3264035847697,31.5109210156001,
2.69839565261225));
#233882=CARTESIAN_POINT('Ctrl Pts',(-54.3178976613387,31.5137795693411,
2.7038246868905));
#233883=CARTESIAN_POINT('Ctrl Pts',(-54.3093672304021,31.515952667503,2.70961155815091));
#233884=CARTESIAN_POINT('Ctrl Pts',(-54.3009559572068,31.5174623893716,
2.71562701361771));
#233885=CARTESIAN_POINT('Ctrl Pts',(-54.2978832130368,31.5180139098087,
2.71782453535861));
#233886=CARTESIAN_POINT('Ctrl Pts',(-54.2948245130135,31.5184846398475,
2.72005051502405));
#233887=CARTESIAN_POINT('Ctrl Pts',(-54.2917835794184,31.5188783726369,
2.72229986760117));
#233888=CARTESIAN_POINT('Ctrl Pts',(-54.2815694052537,31.5202008794131,
2.72985520488892));
#233889=CARTESIAN_POINT('Ctrl Pts',(-54.2714898389044,31.5206547127628,
2.73770845534556));
#233890=CARTESIAN_POINT('Ctrl Pts',(-54.2615918017967,31.5203592886226,
2.74576706701748));
#233891=CARTESIAN_POINT('Ctrl Pts',(-54.2507126865158,31.5200345824972,
2.75462443585025));
#233892=CARTESIAN_POINT('Ctrl Pts',(-54.2400521939113,31.5188048676547,
2.76373036323178));
#233893=CARTESIAN_POINT('Ctrl Pts',(-54.2296591093496,31.5167773687224,
2.77299664636818));
#233894=CARTESIAN_POINT('Ctrl Pts',(-54.2184653119684,31.5145936655007,
2.78297683033481));
#233895=CARTESIAN_POINT('Ctrl Pts',(-54.2075805209337,31.5114844302872,
2.79314401478908));
#233896=CARTESIAN_POINT('Ctrl Pts',(-54.1970658734745,31.5075265408318,
2.80341452427962));
#233897=CARTESIAN_POINT('Ctrl Pts',(-54.1866932092586,31.5036220962478,
2.81354634721382));
#233898=CARTESIAN_POINT('Ctrl Pts',(-54.1766795569337,31.4988909785568,
2.82378004209219));
#233899=CARTESIAN_POINT('Ctrl Pts',(-54.167102037244,31.4933613949858,2.83404198860283));
#233900=CARTESIAN_POINT('Ctrl Pts',(-51.1878102687787,29.7732664904679,
2.83404198860282));
#233901=CARTESIAN_POINT('Ctrl Pts',(-51.1786445298589,29.7679746486352,
2.82422126443019));
#233902=CARTESIAN_POINT('Ctrl Pts',(-51.1699291351222,29.7619788985602,
2.81442815028505));
#233903=CARTESIAN_POINT('Ctrl Pts',(-51.1617065245621,29.7553188532202,
2.80471618166315));
#233904=CARTESIAN_POINT('Ctrl Pts',(-51.1537668706094,29.7488879934681,
2.79533842146229));
#233905=CARTESIAN_POINT('Ctrl Pts',(-51.1462857370529,29.7418369154159,
2.78603515650242));
#233906=CARTESIAN_POINT('Ctrl Pts',(-51.1393284263618,29.7341642916936,
2.77685887346761));
#233907=CARTESIAN_POINT('Ctrl Pts',(-51.1327515888641,29.7269112593592,
2.76818441216595));
#233908=CARTESIAN_POINT('Ctrl Pts',(-51.1266422417913,29.7191021335073,
2.75962261521655));
#233909=CARTESIAN_POINT('Ctrl Pts',(-51.1210907313619,29.7107129315305,
2.75123537701703));
#233910=CARTESIAN_POINT('Ctrl Pts',(-51.11597788339,29.7029866172493,2.7435108713418));
#233911=CARTESIAN_POINT('Ctrl Pts',(-51.1113379461899,29.6947677915906,
2.73593399449926));
#233912=CARTESIAN_POINT('Ctrl Pts',(-51.1072776647607,29.6860256466467,
2.72857657812672));
#233913=CARTESIAN_POINT('Ctrl Pts',(-51.1060669708008,29.6834189154965,
2.72638274508388));
#233914=CARTESIAN_POINT('Ctrl Pts',(-51.1049080895599,29.6807655934596,
2.72420861709636));
#233915=CARTESIAN_POINT('Ctrl Pts',(-51.1038046002594,29.6780647241927,
2.72205663736728));
#233916=CARTESIAN_POINT('Ctrl Pts',(-51.1027123859001,29.6753914511536,
2.71992664556767));
#233917=CARTESIAN_POINT('Ctrl Pts',(-51.1016753170131,29.6726744751146,
2.71782089927885));
#233918=CARTESIAN_POINT('Ctrl Pts',(-51.1006978225842,29.6699160505199,
2.71574387311247));
#233919=CARTESIAN_POINT('Ctrl Pts',(-51.1006298495333,29.6697242350682,
2.71559944077487));
#233920=CARTESIAN_POINT('Ctrl Pts',(-51.1005621526964,29.6695322176089,
2.7154551521607));
#233921=CARTESIAN_POINT('Ctrl Pts',(-51.1004947333605,29.6693399979287,
2.71531100781731));
#233922=CARTESIAN_POINT('Ctrl Pts',(-51.0975388226978,29.6609123829952,
2.70899119176091));
#233923=CARTESIAN_POINT('Ctrl Pts',(-51.095161351427,29.6520916749682,2.70298296066852));
#233924=CARTESIAN_POINT('Ctrl Pts',(-51.0934607157664,29.6429396446301,
2.69736727774156));
#233925=CARTESIAN_POINT('Ctrl Pts',(-51.0918754277622,29.6344083617429,
2.69213248525455));
#233926=CARTESIAN_POINT('Ctrl Pts',(-51.0908783954021,29.6255883681038,
2.68723866185501));
#233927=CARTESIAN_POINT('Ctrl Pts',(-51.0905760611938,29.6165418049905,
2.68278595829599));
#233928=CARTESIAN_POINT('Ctrl Pts',(-51.0904654634291,29.6132324551658,
2.6811571017283));
#233929=CARTESIAN_POINT('Ctrl Pts',(-51.0904480940785,29.6098929659872,
2.67958763637823));
#233930=CARTESIAN_POINT('Ctrl Pts',(-51.0905301191542,29.6065271365691,
2.67808378645367));
#233931=CARTESIAN_POINT('Ctrl Pts',(-51.0905498434446,29.6057177670366,
2.67772216078603));
#233932=CARTESIAN_POINT('Ctrl Pts',(-51.0905756628929,29.6049064053145,
2.67736403603566));
#233933=CARTESIAN_POINT('Ctrl Pts',(-51.0906076352719,29.6040931741702,
2.67700956934482));
#233934=CARTESIAN_POINT('Ctrl Pts',(-51.0906386085139,29.6033053564991,
2.67666617973806));
#233935=CARTESIAN_POINT('Ctrl Pts',(-51.090675356124,29.6025157844404,2.67632622314122));
#233936=CARTESIAN_POINT('Ctrl Pts',(-51.0907179287117,29.6017245728792,
2.67598984158776));
#233937=CARTESIAN_POINT('Ctrl Pts',(-51.0911843606098,29.5930559358438,
2.67230439292223));
#233938=CARTESIAN_POINT('Ctrl Pts',(-51.0923507190417,29.5841848213175,
2.66904964539975));
#233939=CARTESIAN_POINT('Ctrl Pts',(-51.0942731997207,29.575291162817,2.66640203566724));
#233940=CARTESIAN_POINT('Ctrl Pts',(-51.0950705097612,29.5716026975454,
2.6653039929944));
#233941=CARTESIAN_POINT('Ctrl Pts',(-51.0959974771975,29.5679105139262,
2.6643099514226));
#233942=CARTESIAN_POINT('Ctrl Pts',(-51.0970562972092,29.5642276868789,
2.66343053473361));
#233943=CARTESIAN_POINT('Ctrl Pts',(-51.0988622250759,29.5579462415721,
2.66193059792884));
#233944=CARTESIAN_POINT('Ctrl Pts',(-51.1010529624042,29.5516941764754,
2.66076519817127));
#233945=CARTESIAN_POINT('Ctrl Pts',(-51.1036389246278,29.5455435225217,
2.65997805604458));
#233946=CARTESIAN_POINT('Ctrl Pts',(-51.1049319057396,29.5424681955448,
2.65958448498124));
#233947=CARTESIAN_POINT('Ctrl Pts',(-51.106324978508,29.5394188854257,2.6592852626076));
#233948=CARTESIAN_POINT('Ctrl Pts',(-51.107819466813,29.5364046579956,2.65908463971322));
#233949=CARTESIAN_POINT('Ctrl Pts',(-51.109313955118,29.5333904305654,2.65888401681884));
#233950=CARTESIAN_POINT('Ctrl Pts',(-51.1109098228568,29.5304113137792,
2.65878198860281));
#233951=CARTESIAN_POINT('Ctrl Pts',(-51.1126068659049,29.5274749692184,
2.65878198860281));
#233952=CARTESIAN_POINT('Origin',(-53.2328030451449,23.6840886581935,2.83404198860278));
#233953=CARTESIAN_POINT('Ctrl Pts',(-57.3172883154491,25.3107727110821,
2.83404198860279));
#233954=CARTESIAN_POINT('Ctrl Pts',(-57.3269813337898,25.3150883208946,
2.82419652440072));
#233955=CARTESIAN_POINT('Ctrl Pts',(-57.3363050752412,25.320155936947,2.81438790575652));
#233956=CARTESIAN_POINT('Ctrl Pts',(-57.3452135417184,25.325938468362,2.80466781256901));
#233957=CARTESIAN_POINT('Ctrl Pts',(-57.3538325360815,25.3315331019387,
2.79526356453079));
#233958=CARTESIAN_POINT('Ctrl Pts',(-57.3620638476581,25.3377977038122,
2.78594102496236));
#233959=CARTESIAN_POINT('Ctrl Pts',(-57.3698434251117,25.3447390861656,
2.77675109088786));
#233960=CARTESIAN_POINT('Ctrl Pts',(-57.377202426344,25.3513052064463,2.76805797913696));
#233961=CARTESIAN_POINT('Ctrl Pts',(-57.3841579102018,25.3584775246719,
2.75948271210182));
#233962=CARTESIAN_POINT('Ctrl Pts',(-57.3906233351701,25.3662887884603,
2.7510857557325));
#233963=CARTESIAN_POINT('Ctrl Pts',(-57.3965784591573,25.3734835273345,
2.74335155163304));
#233964=CARTESIAN_POINT('Ctrl Pts',(-57.4021181432104,25.381220796889,2.73576818685985));
#233965=CARTESIAN_POINT('Ctrl Pts',(-57.4071400767283,25.3895423083614,
2.72840626160544));
#233966=CARTESIAN_POINT('Ctrl Pts',(-57.4085967487436,25.3919560625149,
2.72627084693717));
#233967=CARTESIAN_POINT('Ctrl Pts',(-57.410009604778,25.3944190600991,2.7241542458755));
#233968=CARTESIAN_POINT('Ctrl Pts',(-57.4113754784548,25.3969325220924,
2.72205867173276));
#233969=CARTESIAN_POINT('Ctrl Pts',(-57.4128561733382,25.3996572764942,
2.71978693462878));
#233970=CARTESIAN_POINT('Ctrl Pts',(-57.4142805418441,25.4024370309187,
2.71754411340779));
#233971=CARTESIAN_POINT('Ctrl Pts',(-57.4156446191418,25.4052723227226,
2.71533341844275));
#233972=CARTESIAN_POINT('Ctrl Pts',(-57.4193883399888,25.4130538033265,
2.70926614876421));
#233973=CARTESIAN_POINT('Ctrl Pts',(-57.4226343338643,25.4212623406656,
2.70347381860439));
#233974=CARTESIAN_POINT('Ctrl Pts',(-57.4253008212879,25.4298341608309,
2.69804914171424));
#233975=CARTESIAN_POINT('Ctrl Pts',(-57.4277405125135,25.4376769109071,
2.69308585687241));
#233976=CARTESIAN_POINT('Ctrl Pts',(-57.4296843862653,25.4458193604263,
2.68842799053228));
#233977=CARTESIAN_POINT('Ctrl Pts',(-57.4310470526568,25.4542377154367,
2.68414767054265));
#233978=CARTESIAN_POINT('Ctrl Pts',(-57.431716389937,25.4583727839182,2.68204519134592));
#233979=CARTESIAN_POINT('Ctrl Pts',(-57.4322449980039,25.4625743171739,
2.68003431778535));
#233980=CARTESIAN_POINT('Ctrl Pts',(-57.4326195921323,25.466838401935,2.67812693945279));
#233981=CARTESIAN_POINT('Ctrl Pts',(-57.4326906677196,25.4676474704857,
2.67776503299231));
#233982=CARTESIAN_POINT('Ctrl Pts',(-57.4327558640764,25.4684592045964,
2.67740659639951));
#233983=CARTESIAN_POINT('Ctrl Pts',(-57.4328151061497,25.4692734860654,
2.67705178968882));
#233984=CARTESIAN_POINT('Ctrl Pts',(-57.4328724969081,25.4700623212384,
2.67670807068784));
#233985=CARTESIAN_POINT('Ctrl Pts',(-57.4329242997219,25.4708535470245,
2.67636775825292));
#233986=CARTESIAN_POINT('Ctrl Pts',(-57.4329704479395,25.4716470524589,
2.67603099699282));
#233987=CARTESIAN_POINT('Ctrl Pts',(-57.4334733617058,25.4802945111771,
2.67236104217153));
#233988=CARTESIAN_POINT('Ctrl Pts',(-57.433304654289,25.4892184175053,2.66911440541498));
#233989=CARTESIAN_POINT('Ctrl Pts',(-57.4323852136914,25.4982455208445,
2.66646778189654));
#233990=CARTESIAN_POINT('Ctrl Pts',(-57.4319969282176,25.5020577226402,
2.66535009634999));
#233991=CARTESIAN_POINT('Ctrl Pts',(-57.4314751387428,25.5058881199466,
2.66433897912371));
#233992=CARTESIAN_POINT('Ctrl Pts',(-57.4308157710841,25.5097232095986,
2.66344564884821));
#233993=CARTESIAN_POINT('Ctrl Pts',(-57.4297054124227,25.516181404744,2.66194130298614));
#233994=CARTESIAN_POINT('Ctrl Pts',(-57.4282034292357,25.5226508554408,
2.66077206705449));
#233995=CARTESIAN_POINT('Ctrl Pts',(-57.4262902109369,25.5290599831063,
2.65998225155744));
#233996=CARTESIAN_POINT('Ctrl Pts',(-57.4258119063623,25.5306622650227,
2.65978479768317));
#233997=CARTESIAN_POINT('Ctrl Pts',(-57.4253076802624,25.5322606952869,
2.65961098966652));
#233998=CARTESIAN_POINT('Ctrl Pts',(-57.4247769415291,25.533854036701,2.65946139030531));
#233999=CARTESIAN_POINT('Ctrl Pts',(-57.4239808334291,25.536244048822,2.6592369912635));
#234000=CARTESIAN_POINT('Ctrl Pts',(-57.423125065972,25.5386225912894,2.65906707562471));
#234001=CARTESIAN_POINT('Ctrl Pts',(-57.4222091845947,25.5409861542582,
2.65895332562949));
#234002=CARTESIAN_POINT('Ctrl Pts',(-57.4212933032174,25.543349717227,2.65883957563427));
#234003=CARTESIAN_POINT('Ctrl Pts',(-57.4203173191902,25.5456982979278,
2.65878198860279));
#234004=CARTESIAN_POINT('Ctrl Pts',(-57.419280924679,25.5480287005717,2.65878198860279));
#234005=CARTESIAN_POINT('Ctrl Pts',(-53.9314655730806,23.9951532569806,
2.65878198860278));
#234006=CARTESIAN_POINT('Ctrl Pts',(-53.9349721992637,23.9872677980945,
2.65878198860278));
#234007=CARTESIAN_POINT('Ctrl Pts',(-53.9390993428069,23.9797401457393,
2.65945335517867));
#234008=CARTESIAN_POINT('Ctrl Pts',(-53.943719374479,23.9726512030275,2.66072561226607));
#234009=CARTESIAN_POINT('Ctrl Pts',(-53.9467034408968,23.968072473403,2.66154735980347));
#234010=CARTESIAN_POINT('Ctrl Pts',(-53.9498923541889,23.963676246713,2.66261895766895));
#234011=CARTESIAN_POINT('Ctrl Pts',(-53.9532454491207,23.959478076992,2.66391429251045));
#234012=CARTESIAN_POINT('Ctrl Pts',(-53.9576897843755,23.9539136435132,
2.66563118464141));
#234013=CARTESIAN_POINT('Ctrl Pts',(-53.9624262550346,23.9487016177219,
2.66774105138716));
#234014=CARTESIAN_POINT('Ctrl Pts',(-53.9673725153422,23.9438784851452,
2.67016894181766));
#234015=CARTESIAN_POINT('Ctrl Pts',(-53.9698456454959,23.9414669188569,
2.67138288703291));
#234016=CARTESIAN_POINT('Ctrl Pts',(-53.972371302523,23.9391523931035,2.67267613167568));
#234017=CARTESIAN_POINT('Ctrl Pts',(-53.9749397614923,23.9369381736874,
2.67403835432569));
#234018=CARTESIAN_POINT('Ctrl Pts',(-53.9762239909769,23.9358310639794,
2.6747194656507));
#234019=CARTESIAN_POINT('Ctrl Pts',(-53.9775189275857,23.9347490158252,
2.67541781389539));
#234020=CARTESIAN_POINT('Ctrl Pts',(-53.9788233972651,23.9336923430325,
2.67613207244185));
#234021=CARTESIAN_POINT('Ctrl Pts',(-53.9791495146849,23.9334281748343,
2.67631063707846));
#234022=CARTESIAN_POINT('Ctrl Pts',(-53.979476228062,23.9331655922761,2.67649019601861));
#234023=CARTESIAN_POINT('Ctrl Pts',(-53.9798035193341,23.9329045996154,
2.67667072836672));
#234024=CARTESIAN_POINT('Ctrl Pts',(-53.9807853931504,23.9321216216332,
2.67721232541106));
#234025=CARTESIAN_POINT('Ctrl Pts',(-53.9817724673293,23.9313529543291,
2.67776268340063));
#234026=CARTESIAN_POINT('Ctrl Pts',(-53.9827642604006,23.9305986983576,
2.67832123541532));
#234027=CARTESIAN_POINT('Ctrl Pts',(-53.9897503227314,23.9252858166867,
2.68225560368453));
#234028=CARTESIAN_POINT('Ctrl Pts',(-53.9969681366814,23.9206342168335,
2.68661792998889));
#234029=CARTESIAN_POINT('Ctrl Pts',(-54.0043120126388,23.9165878043696,
2.6913098662257));
#234030=CARTESIAN_POINT('Ctrl Pts',(-54.0078737845426,23.9146252986971,
2.69358545023054));
#234031=CARTESIAN_POINT('Ctrl Pts',(-54.0114657535932,23.9128053429042,
2.69593918853477));
#234032=CARTESIAN_POINT('Ctrl Pts',(-54.0150784217126,23.9111228176154,
2.69836306235491));
#234033=CARTESIAN_POINT('Ctrl Pts',(-54.0206091641933,23.9085469889529,
2.70207384382224));
#234034=CARTESIAN_POINT('Ctrl Pts',(-54.026184917604,23.906293702842,2.70594760814225));
#234035=CARTESIAN_POINT('Ctrl Pts',(-54.0317609613888,23.9043517182282,
2.70995196345704));
#234036=CARTESIAN_POINT('Ctrl Pts',(-54.0343505049691,23.903449850527,2.71181160678102));
#234037=CARTESIAN_POINT('Ctrl Pts',(-54.0369399534675,23.9026149214104,
2.71369962772095));
#234038=CARTESIAN_POINT('Ctrl Pts',(-54.0395249709304,23.9018470291827,
2.71561183138658));
#234039=CARTESIAN_POINT('Ctrl Pts',(-54.0397231023334,23.9017881732691,
2.71575839426308));
#234040=CARTESIAN_POINT('Ctrl Pts',(-54.0399212112576,23.9017296774346,
2.71590508903205));
#234041=CARTESIAN_POINT('Ctrl Pts',(-54.040119296488,23.9016715408687,2.71605191409908));
#234042=CARTESIAN_POINT('Ctrl Pts',(-54.0429017967674,23.9008548973949,
2.71811436362749));
#234043=CARTESIAN_POINT('Ctrl Pts',(-54.0456803391391,23.9001111074278,
2.72020091026955));
#234044=CARTESIAN_POINT('Ctrl Pts',(-54.0484499388203,23.8994373944623,
2.72230624862178));
#234045=CARTESIAN_POINT('Ctrl Pts',(-54.0583812307207,23.8970215795837,
2.72985561753132));
#234046=CARTESIAN_POINT('Ctrl Pts',(-54.0682738483765,23.89548623905,2.73770089914395));
#234047=CARTESIAN_POINT('Ctrl Pts',(-54.0780688394977,23.8947164920949,
2.74574823347176));
#234048=CARTESIAN_POINT('Ctrl Pts',(-54.0888325507458,23.8938706175191,
2.75459144547153));
#234049=CARTESIAN_POINT('Ctrl Pts',(-54.0994790041496,23.8939490479891,
2.76367911754426));
#234050=CARTESIAN_POINT('Ctrl Pts',(-54.1099490937715,23.8948487267558,
2.77292162564911));
#234051=CARTESIAN_POINT('Ctrl Pts',(-54.1212541629292,23.8958201540353,
2.78290121484939));
#234052=CARTESIAN_POINT('Ctrl Pts',(-54.1323547778578,23.8977489757819,
2.7930622950042));
#234053=CARTESIAN_POINT('Ctrl Pts',(-54.1431832370017,23.9005625023835,
2.80331916685509));
#234054=CARTESIAN_POINT('Ctrl Pts',(-54.1539208564981,23.9033524263874,
2.81348999408871));
#234055=CARTESIAN_POINT('Ctrl Pts',(-54.1643921589032,23.9070129003889,
2.82375635966972));
#234056=CARTESIAN_POINT('Ctrl Pts',(-54.1745185419761,23.9115214566113,
2.83404198860278));
#234057=CARTESIAN_POINT('Origin',(0.00619866644048587,0.0139224327746604,
2.83404198860262));
#234058=CARTESIAN_POINT('Ctrl Pts',(-57.4068835917981,25.5758735661207,
2.65878198860279));
#234059=CARTESIAN_POINT('Ctrl Pts',(-57.4033868763699,25.5837184861905,
2.65878198860279));
#234060=CARTESIAN_POINT('Ctrl Pts',(-57.3992659084775,25.5912015935367,
2.6594460304186));
#234061=CARTESIAN_POINT('Ctrl Pts',(-57.3946498105263,25.598244851263,2.66070439264066));
#234062=CARTESIAN_POINT('Ctrl Pts',(-57.3917003436859,25.6027451576543,
2.66150842619593));
#234063=CARTESIAN_POINT('Ctrl Pts',(-57.3885495044087,25.607066421377,2.66255428265373));
#234064=CARTESIAN_POINT('Ctrl Pts',(-57.3852370392633,25.611194377554,2.6638169970067));
#234065=CARTESIAN_POINT('Ctrl Pts',(-57.3807161889918,25.6168282094542,
2.6655403487327));
#234066=CARTESIAN_POINT('Ctrl Pts',(-57.3758905070494,25.6220971979014,
2.66766759643975));
#234067=CARTESIAN_POINT('Ctrl Pts',(-57.3708481654825,25.6269642358706,
2.67012012783151));
#234068=CARTESIAN_POINT('Ctrl Pts',(-57.368326994699,25.6293977548552,2.67134639352739));
#234069=CARTESIAN_POINT('Ctrl Pts',(-57.3657515758212,25.6317309777765,
2.67265375585015));
#234070=CARTESIAN_POINT('Ctrl Pts',(-57.3631323306533,25.6339606331577,
2.67403135126943));
#234071=CARTESIAN_POINT('Ctrl Pts',(-57.3618227080693,25.6350754608483,
2.67472014897907));
#234072=CARTESIAN_POINT('Ctrl Pts',(-57.3605021218763,25.6361644125826,
2.67542649668636));
#234073=CARTESIAN_POINT('Ctrl Pts',(-57.3591718306997,25.6372271795775,
2.67614899656105));
#234074=CARTESIAN_POINT('Ctrl Pts',(-57.3588392579055,25.6374928713262,
2.67632962152972));
#234075=CARTESIAN_POINT('Ctrl Pts',(-57.3585060784009,25.6377569268684,
2.67651125590953));
#234076=CARTESIAN_POINT('Ctrl Pts',(-57.358172311552,25.638019342065,2.67669387767526));
#234077=CARTESIAN_POINT('Ctrl Pts',(-57.3571710110052,25.6388065876546,
2.67724174297247));
#234078=CARTESIAN_POINT('Ctrl Pts',(-57.3561644250954,25.6395790684331,
2.6777984950475));
#234079=CARTESIAN_POINT('Ctrl Pts',(-57.3551530701151,25.6403366878211,
2.67836353618012));
#234080=CARTESIAN_POINT('Ctrl Pts',(-57.3481639797007,25.645572307861,2.68226832098908));
#234081=CARTESIAN_POINT('Ctrl Pts',(-57.3409484573003,25.6501539027775,
2.68659153751388));
#234082=CARTESIAN_POINT('Ctrl Pts',(-57.333610145013,25.6541395203647,2.69123699486171));
#234083=CARTESIAN_POINT('Ctrl Pts',(-57.3299630239494,25.6561203613653,
2.69354577441212));
#234084=CARTESIAN_POINT('Ctrl Pts',(-57.3262850026764,25.6579537739811,
2.69593478828116));
#234085=CARTESIAN_POINT('Ctrl Pts',(-57.322586011576,25.6596454116602,2.69839565261221));
#234086=CARTESIAN_POINT('Ctrl Pts',(-57.3144254847133,25.6633774170497,
2.70382468689046));
#234087=CARTESIAN_POINT('Ctrl Pts',(-57.3061689349813,25.6664302835893,
2.70961155815087));
#234088=CARTESIAN_POINT('Ctrl Pts',(-57.2979615485275,25.6688109525047,
2.71562701361767));
#234089=CARTESIAN_POINT('Ctrl Pts',(-57.2949632867553,25.6696806408813,
2.71782453535858));
#234090=CARTESIAN_POINT('Ctrl Pts',(-57.2919705472984,25.6704685134247,
2.72005051502402));
#234091=CARTESIAN_POINT('Ctrl Pts',(-57.2889874285391,25.6711779534203,
2.72229986760115));
#234092=CARTESIAN_POINT('Ctrl Pts',(-57.2789674482906,25.673560887295,2.72985520488863));
#234093=CARTESIAN_POINT('Ctrl Pts',(-57.2689905373634,25.675065836079,2.73770845534497));
#234094=CARTESIAN_POINT('Ctrl Pts',(-57.2591158425076,25.6758066569114,
2.74576706701659));
#234095=CARTESIAN_POINT('Ctrl Pts',(-57.2482623831266,25.6766209067622,
2.75462443584905));
#234096=CARTESIAN_POINT('Ctrl Pts',(-57.2375317496135,25.676512253336,2.76373036323026));
#234097=CARTESIAN_POINT('Ctrl Pts',(-57.2269836681092,25.6755822344129,
2.77299664636632));
#234098=CARTESIAN_POINT('Ctrl Pts',(-57.2156229323795,25.6745805641845,
2.78297683033263));
#234099=CARTESIAN_POINT('Ctrl Pts',(-57.2044727657904,25.6726261321668,
2.79314401478657));
#234100=CARTESIAN_POINT('Ctrl Pts',(-57.1936020065678,25.6697890043849,
2.80341452427681));
#234101=CARTESIAN_POINT('Ctrl Pts',(-57.1828780392985,25.6669901874072,
2.81354634721189));
#234102=CARTESIAN_POINT('Ctrl Pts',(-57.1724247063461,25.6633316989629,
2.82378004209119));
#234103=CARTESIAN_POINT('Ctrl Pts',(-57.1623216544372,25.658833530444,2.83404198860278));
#234104=CARTESIAN_POINT('Ctrl Pts',(-54.0195518809642,24.2595822759732,
2.83404198860278));
#234105=CARTESIAN_POINT('Ctrl Pts',(-54.0098832048258,24.2552775040074,
2.82422126442931));
#234106=CARTESIAN_POINT('Ctrl Pts',(-54.0005888273912,24.2502256060967,
2.81442815028334));
#234107=CARTESIAN_POINT('Ctrl Pts',(-53.9917150968467,24.2444615420273,
2.80471618166061));
#234108=CARTESIAN_POINT('Ctrl Pts',(-53.9831467292612,24.2388958310238,
2.79533842145915));
#234109=CARTESIAN_POINT('Ctrl Pts',(-53.9749695397835,24.2326653709086,
2.7860351564987));
#234110=CARTESIAN_POINT('Ctrl Pts',(-53.9672483344011,24.2257620156162,
2.77685887346333));
#234111=CARTESIAN_POINT('Ctrl Pts',(-53.9599493771831,24.219236182868,2.76818441216119));
#234112=CARTESIAN_POINT('Ctrl Pts',(-53.9530572218277,24.2121084368851,
2.75962261521134));
#234113=CARTESIAN_POINT('Ctrl Pts',(-53.9466592127625,24.2043454826878,
2.75123537701141));
#234114=CARTESIAN_POINT('Ctrl Pts',(-53.9407667537481,24.1971959321054,
2.74351087133577));
#234115=CARTESIAN_POINT('Ctrl Pts',(-53.9352931333934,24.1895071355379,
2.73593399449286));
#234116=CARTESIAN_POINT('Ctrl Pts',(-53.930341291634,24.181237295956,2.72857657812));
#234117=CARTESIAN_POINT('Ctrl Pts',(-53.9288647523826,24.1787713967333,
2.72638274507943));
#234118=CARTESIAN_POINT('Ctrl Pts',(-53.9274348719409,24.1762537459499,
2.72420861709414));
#234119=CARTESIAN_POINT('Ctrl Pts',(-53.9260551099577,24.1736830183709,
2.72205663736723));
#234120=CARTESIAN_POINT('Ctrl Pts',(-53.9246894457403,24.1711385572897,
2.71992664556762));
#234121=CARTESIAN_POINT('Ctrl Pts',(-53.9233740566951,24.1685448683468,
2.71782089927881));
#234122=CARTESIAN_POINT('Ctrl Pts',(-53.9221135831989,24.1659037306811,
2.71574387311243));
#234123=CARTESIAN_POINT('Ctrl Pts',(-53.9220259323371,24.1657200711331,
2.71559944077483));
#234124=CARTESIAN_POINT('Ctrl Pts',(-53.9219385350607,24.1655361818119,
2.71545515216065));
#234125=CARTESIAN_POINT('Ctrl Pts',(-53.9218513926272,24.1653520623708,
2.71531100781727));
#234126=CARTESIAN_POINT('Ctrl Pts',(-53.9180307491143,24.1572795915927,
2.70899119176075));
#234127=CARTESIAN_POINT('Ctrl Pts',(-53.9147442868248,24.1487557177454,
2.70298296066826));
#234128=CARTESIAN_POINT('Ctrl Pts',(-53.9120963197572,24.1398315880191,
2.6973672777412));
#234129=CARTESIAN_POINT('Ctrl Pts',(-53.9096279542367,24.1315127481108,
2.69213248525402));
#234130=CARTESIAN_POINT('Ctrl Pts',(-53.9077144433429,24.1228452895799,
2.68723866185433));
#234131=CARTESIAN_POINT('Ctrl Pts',(-53.9064681420131,24.1138798870157,
2.6827859582952));
#234132=CARTESIAN_POINT('Ctrl Pts',(-53.9060122288629,24.1106002267705,
2.68115710172776));
#234133=CARTESIAN_POINT('Ctrl Pts',(-53.9056458829916,24.107280847255,2.67958763637793));
#234134=CARTESIAN_POINT('Ctrl Pts',(-53.9053756337487,24.103924882248,2.6780837864536));
#234135=CARTESIAN_POINT('Ctrl Pts',(-53.905310647834,24.1031178847767,2.67772216078595));
#234136=CARTESIAN_POINT('Ctrl Pts',(-53.9052515154467,24.1023082689118,
2.67736403603558));
#234137=CARTESIAN_POINT('Ctrl Pts',(-53.9051983068757,24.1014961507091,
2.67700956934474));
#234138=CARTESIAN_POINT('Ctrl Pts',(-53.9051467610726,24.1007094112003,
2.67666617973799));
#234139=CARTESIAN_POINT('Ctrl Pts',(-53.9051007746215,24.0999203233287,
2.67632622314114));
#234140=CARTESIAN_POINT('Ctrl Pts',(-53.9050604098635,24.0991289960601,
2.67598984158768));
#234141=CARTESIAN_POINT('Ctrl Pts',(-53.904618167291,24.0904590913162,2.67230439292231));
#234142=CARTESIAN_POINT('Ctrl Pts',(-53.9048508523205,24.0815146560294,
2.66904964539997));
#234143=CARTESIAN_POINT('Ctrl Pts',(-53.9058331609931,24.0724687639701,
2.66640203566752));
#234144=CARTESIAN_POINT('Ctrl Pts',(-53.9062405536792,24.0687171629035,
2.66530399299454));
#234145=CARTESIAN_POINT('Ctrl Pts',(-53.9067765048111,24.0649483109704,
2.66430995142262));
#234146=CARTESIAN_POINT('Ctrl Pts',(-53.9074445642443,24.061174982006,2.66343053473355));
#234147=CARTESIAN_POINT('Ctrl Pts',(-53.9085840092242,24.0547391762491,
2.66193059792878));
#234148=CARTESIAN_POINT('Ctrl Pts',(-53.9101092267074,24.0482923662128,
2.66076519817121));
#234149=CARTESIAN_POINT('Ctrl Pts',(-53.9120381043537,24.0419050995278,
2.65997805604453));
#234150=CARTESIAN_POINT('Ctrl Pts',(-53.9130025431768,24.0387114661853,
2.6595844849812));
#234151=CARTESIAN_POINT('Ctrl Pts',(-53.914069244846,24.0355332447503,2.65928526260756));
#234152=CARTESIAN_POINT('Ctrl Pts',(-53.9152404736264,24.0323793130075,
2.65908463971318));
#234153=CARTESIAN_POINT('Ctrl Pts',(-53.9164117024068,24.0292253812647,
2.6588840168188));
#234154=CARTESIAN_POINT('Ctrl Pts',(-53.9176874253155,24.0260957707896,
2.65878198860278));
#234155=CARTESIAN_POINT('Ctrl Pts',(-53.9190682401996,24.0229981225296,
2.65878198860278));
#234156=CARTESIAN_POINT('Origin',(-55.4168495715593,17.9900016446781,2.83404198860273));
#234157=CARTESIAN_POINT('Ctrl Pts',(-59.6489943884565,19.180829583578,2.83404198860275));
#234158=CARTESIAN_POINT('Ctrl Pts',(-59.6590854114905,19.1841083557169,
2.82419652440111));
#234159=CARTESIAN_POINT('Ctrl Pts',(-59.668887786629,19.1881736144725,2.81438790575719));
#234160=CARTESIAN_POINT('Ctrl Pts',(-59.6783518907173,19.1929932802644,
2.80466781256988));
#234161=CARTESIAN_POINT('Ctrl Pts',(-59.6875084677778,19.1976563356173,
2.79526356453173));
#234162=CARTESIAN_POINT('Ctrl Pts',(-59.696349516575,19.2030262129964,2.78594102496329));
#234163=CARTESIAN_POINT('Ctrl Pts',(-59.7048120487195,19.2091163824548,
2.77675109088875));
#234164=CARTESIAN_POINT('Ctrl Pts',(-59.7128170830356,19.2148773077515,
2.7680579791377));
#234165=CARTESIAN_POINT('Ctrl Pts',(-59.7204841754272,19.2212832892285,
2.75948271210239));
#234166=CARTESIAN_POINT('Ctrl Pts',(-59.727730681521,19.2283759411603,2.75108575573291));
#234167=CARTESIAN_POINT('Ctrl Pts',(-59.734405237714,19.2349087865432,2.74335155163326));
#234168=CARTESIAN_POINT('Ctrl Pts',(-59.7407233396947,19.2420246158646,
2.73576818685987));
#234169=CARTESIAN_POINT('Ctrl Pts',(-59.7465875973417,19.2497756062333,
2.72840626160534));
#234170=CARTESIAN_POINT('Ctrl Pts',(-59.7482885955677,19.2520238739017,
2.72627084693707));
#234171=CARTESIAN_POINT('Ctrl Pts',(-59.7499511651814,19.2543256952573,
2.72415424587541));
#234172=CARTESIAN_POINT('Ctrl Pts',(-59.751572284779,19.2566826155664,2.72205867173268));
#234173=CARTESIAN_POINT('Ctrl Pts',(-59.7533296826513,19.2592376687177,
2.71978693462871));
#234174=CARTESIAN_POINT('Ctrl Pts',(-59.7550368117758,19.2618533083055,
2.71754411340772));
#234175=CARTESIAN_POINT('Ctrl Pts',(-59.7566897852105,19.2645304831806,
2.7153334184427));
#234176=CARTESIAN_POINT('Ctrl Pts',(-59.7612263837726,19.2718780106326,
2.70926614876418));
#234177=CARTESIAN_POINT('Ctrl Pts',(-59.7653126215477,19.2797022819936,
2.70347381860435));
#234178=CARTESIAN_POINT('Ctrl Pts',(-59.7688605008635,19.2879484209985,
2.69804914171422));
#234179=CARTESIAN_POINT('Ctrl Pts',(-59.7721066178187,19.2954931904948,
2.6930858568722));
#234180=CARTESIAN_POINT('Ctrl Pts',(-59.7748909605621,19.3033878446879,
2.6884279905319));
#234181=CARTESIAN_POINT('Ctrl Pts',(-59.7771261198371,19.3116176456452,
2.68414767054214));
#234182=CARTESIAN_POINT('Ctrl Pts',(-59.7782240227714,19.3156600969913,
2.6820451913456));
#234183=CARTESIAN_POINT('Ctrl Pts',(-59.7791889148824,19.319783359219,2.68003431778522));
#234184=CARTESIAN_POINT('Ctrl Pts',(-59.7800071751723,19.3239849291286,
2.67812693945282));
#234185=CARTESIAN_POINT('Ctrl Pts',(-59.7801624320924,19.3247821360952,
2.67776503299234));
#234186=CARTESIAN_POINT('Ctrl Pts',(-59.780312120616,19.3255826085666,2.67740659639954));
#234187=CARTESIAN_POINT('Ctrl Pts',(-59.7804561537455,19.3263862368335,
2.67705178968885));
#234188=CARTESIAN_POINT('Ctrl Pts',(-59.7805956858398,19.3271647517172,
2.67670807068788));
#234189=CARTESIAN_POINT('Ctrl Pts',(-59.7807299104879,19.3279462282172,
2.67636775825295));
#234190=CARTESIAN_POINT('Ctrl Pts',(-59.7808587498043,19.3287305629435,
2.67603099699285));
#234191=CARTESIAN_POINT('Ctrl Pts',(-59.7822628141274,19.3372780811748,
2.6723610421716));
#234192=CARTESIAN_POINT('Ctrl Pts',(-59.7830278331223,19.3461707361373,
2.66911440541507));
#234193=CARTESIAN_POINT('Ctrl Pts',(-59.7830570185564,19.3552444957726,
2.66646778189664));
#234194=CARTESIAN_POINT('Ctrl Pts',(-59.7830693437464,19.3590764008119,
2.66535009635006));
#234195=CARTESIAN_POINT('Ctrl Pts',(-59.7829507982331,19.3629403566532,
2.66433897912374));
#234196=CARTESIAN_POINT('Ctrl Pts',(-59.7826959186873,19.3668233599709,
2.66344564884821));
#234197=CARTESIAN_POINT('Ctrl Pts',(-59.7822667079008,19.3733622405321,
2.66194130298614));
#234198=CARTESIAN_POINT('Ctrl Pts',(-59.7814491944743,19.3799532508955,
2.66077206705447));
#234199=CARTESIAN_POINT('Ctrl Pts',(-59.7802163932509,19.3865272544576,
2.65998225155741));
#234200=CARTESIAN_POINT('Ctrl Pts',(-59.7799081929451,19.3881707553481,
2.65978479768314));
#234201=CARTESIAN_POINT('Ctrl Pts',(-59.7795738105078,19.3898131352235,
2.65961098966648));
#234202=CARTESIAN_POINT('Ctrl Pts',(-59.7792125287463,19.3914532254508,
2.65946139030528));
#234203=CARTESIAN_POINT('Ctrl Pts',(-59.7786706061041,19.3939133607916,
2.65923699126346));
#234204=CARTESIAN_POINT('Ctrl Pts',(-59.7780681520195,19.3963683254117,
2.65906707562467));
#234205=CARTESIAN_POINT('Ctrl Pts',(-59.7774043475413,19.3988146762082,
2.65895332562945));
#234206=CARTESIAN_POINT('Ctrl Pts',(-59.7767405430631,19.4012610270047,
2.65883957563423));
#234207=CARTESIAN_POINT('Ctrl Pts',(-59.7760153991119,19.4036987600458,
2.65878198860274));
#234208=CARTESIAN_POINT('Ctrl Pts',(-59.7752282754854,19.4061247292258,
2.65878198860274));
#234209=CARTESIAN_POINT('Ctrl Pts',(-56.1441998575528,18.2263320786581,
2.65878198860274));
#234210=CARTESIAN_POINT('Ctrl Pts',(-56.1468630191714,18.2181232748943,
2.65878198860274));
#234211=CARTESIAN_POINT('Ctrl Pts',(-56.1501806998579,18.2102054558339,
2.65945335517868));
#234212=CARTESIAN_POINT('Ctrl Pts',(-56.1540344262254,18.2026724222809,
2.66072561226617));
#234213=CARTESIAN_POINT('Ctrl Pts',(-56.1565235380436,18.1978068555396,
2.66154735980354));
#234214=CARTESIAN_POINT('Ctrl Pts',(-56.1592354513148,18.1931013796338,
2.66261895766897));
#234215=CARTESIAN_POINT('Ctrl Pts',(-56.1621313494121,18.1885757140657,
2.66391429251038));
#234216=CARTESIAN_POINT('Ctrl Pts',(-56.1659696964528,18.1825772036012,
2.66563118464135));
#234217=CARTESIAN_POINT('Ctrl Pts',(-56.1701354151837,18.1768986338332,
2.6677410513871));
#234218=CARTESIAN_POINT('Ctrl Pts',(-56.1745504247233,18.1715848978926,
2.67016894181761));
#234219=CARTESIAN_POINT('Ctrl Pts',(-56.1767579294932,18.1689280299222,
2.67138288703287));
#234220=CARTESIAN_POINT('Ctrl Pts',(-56.1790278168866,18.1663621803354,
2.67267613167563));
#234221=CARTESIAN_POINT('Ctrl Pts',(-56.181350756616,18.1638916135758,2.67403835432565));
#234222=CARTESIAN_POINT('Ctrl Pts',(-56.1825122264807,18.1626563301961,
2.67471946565066));
#234223=CARTESIAN_POINT('Ctrl Pts',(-56.1836869644605,18.1614448518812,
2.67541781389535));
#234224=CARTESIAN_POINT('Ctrl Pts',(-56.1848738357353,18.1602576134416,
2.67613207244181));
#234225=CARTESIAN_POINT('Ctrl Pts',(-56.185170553554,18.1599608038317,2.67631063707843));
#234226=CARTESIAN_POINT('Ctrl Pts',(-56.1854680298097,18.159665508881,2.67649019601858));
#234227=CARTESIAN_POINT('Ctrl Pts',(-56.1857662469842,18.1593717347117,
2.67667072836669));
#234228=CARTESIAN_POINT('Ctrl Pts',(-56.1866608985078,18.1584904122037,
2.67721232541103));
#234229=CARTESIAN_POINT('Ctrl Pts',(-56.187562217779,18.1576227783924,2.67776268340059));
#234230=CARTESIAN_POINT('Ctrl Pts',(-56.1884697364865,18.1567689837085,
2.67832123541529));
#234231=CARTESIAN_POINT('Ctrl Pts',(-56.1948621810803,18.1507549641995,
2.68225560368456));
#234232=CARTESIAN_POINT('Ctrl Pts',(-56.201554230506,18.1453743792965,2.68661792998898));
#234233=CARTESIAN_POINT('Ctrl Pts',(-56.2084349106661,18.1405824894352,
2.69130986622586));
#234234=CARTESIAN_POINT('Ctrl Pts',(-56.2117720331085,18.1382584280306,
2.69358545023064));
#234235=CARTESIAN_POINT('Ctrl Pts',(-56.2151540877945,18.136072979141,2.6959391885348));
#234236=CARTESIAN_POINT('Ctrl Pts',(-56.2185710935569,18.134022044255,2.69836306235487));
#234237=CARTESIAN_POINT('Ctrl Pts',(-56.2238022906399,18.1308822062392,
2.7020738438222));
#234238=CARTESIAN_POINT('Ctrl Pts',(-56.2291119669556,18.1280584389298,
2.7059476081422));
#234239=CARTESIAN_POINT('Ctrl Pts',(-56.2344544719217,18.1255442374229,
2.70995196345699));
#234240=CARTESIAN_POINT('Ctrl Pts',(-56.2369355588664,18.1243766292364,
2.71181160678098));
#234241=CARTESIAN_POINT('Ctrl Pts',(-56.2394235482376,18.1232756028766,
2.71369962772091));
#234242=CARTESIAN_POINT('Ctrl Pts',(-56.2419141381098,18.12224170934,2.71561183138654));
#234243=CARTESIAN_POINT('Ctrl Pts',(-56.24210503201,18.1221624654742,2.71575839426304));
#234244=CARTESIAN_POINT('Ctrl Pts',(-56.2422959411932,18.1220835820645,
2.71590508903201));
#234245=CARTESIAN_POINT('Ctrl Pts',(-56.2424868643661,18.1220050584321,
2.71605191409903));
#234246=CARTESIAN_POINT('Ctrl Pts',(-56.2451687593304,18.1209020381385,
2.71811436362744));
#234247=CARTESIAN_POINT('Ctrl Pts',(-56.247854333334,18.1198718859664,2.72020091026951));
#234248=CARTESIAN_POINT('Ctrl Pts',(-56.2505383386774,18.1189123616724,
2.72230624862174));
#234249=CARTESIAN_POINT('Ctrl Pts',(-56.2601627045042,18.1154716782002,
2.72985561753078));
#234250=CARTESIAN_POINT('Ctrl Pts',(-56.2698406425782,18.1129106883014,
2.73770089914286));
#234251=CARTESIAN_POINT('Ctrl Pts',(-56.2795015152462,18.111121302731,2.7457482334701));
#234252=CARTESIAN_POINT('Ctrl Pts',(-56.2901178437877,18.1091549477489,
2.75459144546933));
#234253=CARTESIAN_POINT('Ctrl Pts',(-56.3007141730217,18.108120091155,2.76367911754151));
#234254=CARTESIAN_POINT('Ctrl Pts',(-56.3112209484354,18.1079204190086,
2.77292162564579));
#234255=CARTESIAN_POINT('Ctrl Pts',(-56.3225656290416,18.1077048232014,
2.78290121484551));
#234256=CARTESIAN_POINT('Ctrl Pts',(-56.3338070504127,18.1084627484405,
2.79306229499976));
#234257=CARTESIAN_POINT('Ctrl Pts',(-56.3448702837359,18.1101289800547,
2.80331916685008));
#234258=CARTESIAN_POINT('Ctrl Pts',(-56.3558407078999,18.1117812336979,
2.81348999408533));
#234259=CARTESIAN_POINT('Ctrl Pts',(-56.3666372711388,18.1143271060913,
2.82375635966801));
#234260=CARTESIAN_POINT('Ctrl Pts',(-56.3771794532808,18.1177524687105,
2.83404198860274));
#234261=CARTESIAN_POINT('Origin',(0.00470941899428508,0.0144941013085259,
2.83404198860262));
#234262=CARTESIAN_POINT('Ctrl Pts',(-59.7658094374952,19.4351129318419,
2.65878198860274));
#234263=CARTESIAN_POINT('Ctrl Pts',(-59.7631518948791,19.4432803829098,
2.65878198860274));
#234264=CARTESIAN_POINT('Ctrl Pts',(-59.759835699791,19.4511532554527,2.65944603041869));
#234265=CARTESIAN_POINT('Ctrl Pts',(-59.7559811102134,19.4586404431021,
2.66070439264099));
#234266=CARTESIAN_POINT('Ctrl Pts',(-59.7535182109726,19.4634243995795,
2.66150842619621));
#234267=CARTESIAN_POINT('Ctrl Pts',(-59.7508363273793,19.4680513433543,
2.66255428265387));
#234268=CARTESIAN_POINT('Ctrl Pts',(-59.7479734971807,19.472502933046,2.66381699700665));
#234269=CARTESIAN_POINT('Ctrl Pts',(-59.7440663083908,19.4785784597571,
2.66554034873265));
#234270=CARTESIAN_POINT('Ctrl Pts',(-59.7398178213044,19.484323005252,2.66766759643969));
#234271=CARTESIAN_POINT('Ctrl Pts',(-59.7353118462117,19.4896904492932,
2.67012012783145));
#234272=CARTESIAN_POINT('Ctrl Pts',(-59.7330588586654,19.4923741713139,
2.67134639352733));
#234273=CARTESIAN_POINT('Ctrl Pts',(-59.7307414364081,19.4949638171734,
2.67265375585009));
#234274=CARTESIAN_POINT('Ctrl Pts',(-59.7283696021899,19.4974550439414,
2.67403135126937));
#234275=CARTESIAN_POINT('Ctrl Pts',(-59.7271836850808,19.4987006573255,
2.67472014897901));
#234276=CARTESIAN_POINT('Ctrl Pts',(-59.7259841596484,19.4999216825137,
2.67542649668629));
#234277=CARTESIAN_POINT('Ctrl Pts',(-59.7247722453468,19.5011176808521,
2.67614899656099));
#234278=CARTESIAN_POINT('Ctrl Pts',(-59.7244692667715,19.5014166804367,
2.67632962152966));
#234279=CARTESIAN_POINT('Ctrl Pts',(-59.7241655137791,19.5017141161967,
2.67651125590947));
#234280=CARTESIAN_POINT('Ctrl Pts',(-59.7238610051971,19.5020099819911,
2.67669387767521));
#234281=CARTESIAN_POINT('Ctrl Pts',(-59.7229474794512,19.5028975793744,
2.67724174297241));
#234282=CARTESIAN_POINT('Ctrl Pts',(-59.722027153953,19.5037710453007,2.67779849504745));
#234283=CARTESIAN_POINT('Ctrl Pts',(-59.7211005320715,19.5046302297524,
2.67836353618006));
#234284=CARTESIAN_POINT('Ctrl Pts',(-59.7146969999424,19.5105677273987,
2.68226832098917));
#234285=CARTESIAN_POINT('Ctrl Pts',(-59.7079999120044,19.5158784513273,
2.68659153751416));
#234286=CARTESIAN_POINT('Ctrl Pts',(-59.7011184102409,19.5206092977908,
2.6912369948622));
#234287=CARTESIAN_POINT('Ctrl Pts',(-59.6976983227541,19.5229605154971,
2.69354577441244));
#234288=CARTESIAN_POINT('Ctrl Pts',(-59.69423209387,19.5251683423981,2.6959347882813));
#234289=CARTESIAN_POINT('Ctrl Pts',(-59.6907301905172,19.5272373629642,
2.69839565261216));
#234290=CARTESIAN_POINT('Ctrl Pts',(-59.6830044686627,19.5318019313701,
2.70382468689042));
#234291=CARTESIAN_POINT('Ctrl Pts',(-59.675112260622,19.5357011184427,2.70961155815083));
#234292=CARTESIAN_POINT('Ctrl Pts',(-59.6671986827532,19.5389266512982,
2.71562701361763));
#234293=CARTESIAN_POINT('Ctrl Pts',(-59.6643077529623,19.5401049791264,
2.71782453535853));
#234294=CARTESIAN_POINT('Ctrl Pts',(-59.6614137631514,19.5412013620779,
2.72005051502397));
#234295=CARTESIAN_POINT('Ctrl Pts',(-59.6585211429014,19.5422187365067,
2.7222998676011));
#234296=CARTESIAN_POINT('Ctrl Pts',(-59.6488051375685,19.5456359895577,
2.72985520488895));
#234297=CARTESIAN_POINT('Ctrl Pts',(-59.6390401911866,19.5481755652423,
2.73770845534571));
#234298=CARTESIAN_POINT('Ctrl Pts',(-59.6292970278052,19.5499445144592,
2.74576706701776));
#234299=CARTESIAN_POINT('Ctrl Pts',(-59.6185881370955,19.5518887991944,
2.75462443585063));
#234300=CARTESIAN_POINT('Ctrl Pts',(-59.6079049297395,19.552902397614,2.76373036323228));
#234301=CARTESIAN_POINT('Ctrl Pts',(-59.5973174182801,19.5530800481818,
2.77299664636878));
#234302=CARTESIAN_POINT('Ctrl Pts',(-59.5859142147994,19.553271385455,2.78297683033552));
#234303=CARTESIAN_POINT('Ctrl Pts',(-59.5746208362138,19.5524931697989,
2.79314401478987));
#234304=CARTESIAN_POINT('Ctrl Pts',(-59.5635130675402,19.5508078878557,
2.80341452428049));
#234305=CARTESIAN_POINT('Ctrl Pts',(-59.5525552912493,19.549145362909,2.8135463472144));
#234306=CARTESIAN_POINT('Ctrl Pts',(-59.5417768065748,19.546599586877,2.82378004209245));
#234307=CARTESIAN_POINT('Ctrl Pts',(-59.5312589135997,19.5431821162865,
2.83404198860274));
#234308=CARTESIAN_POINT('Ctrl Pts',(-56.259443978424,18.4801050014189,2.83404198860274));
#234309=CARTESIAN_POINT('Ctrl Pts',(-56.2493782971086,18.4768344633036,
2.82422126443099));
#234310=CARTESIAN_POINT('Ctrl Pts',(-56.2396067681225,18.4727817672093,
2.81442815028674));
#234311=CARTESIAN_POINT('Ctrl Pts',(-56.2301791400446,18.4679768367043,
2.80471618166571));
#234312=CARTESIAN_POINT('Ctrl Pts',(-56.2210759356559,18.4633372535452,
2.79533842146523));
#234313=CARTESIAN_POINT('Ctrl Pts',(-56.2122922812571,18.4579956735932,
2.78603515650573));
#234314=CARTESIAN_POINT('Ctrl Pts',(-56.2038917763263,18.4519372213376,
2.77685887347126));
#234315=CARTESIAN_POINT('Ctrl Pts',(-56.1959506682911,18.4462100865662,
2.76818441216954));
#234316=CARTESIAN_POINT('Ctrl Pts',(-56.18835121655,18.4398418135303,2.75962261522005));
#234317=CARTESIAN_POINT('Ctrl Pts',(-56.1811768067752,18.4327901596647,
2.75123537702043));
#234318=CARTESIAN_POINT('Ctrl Pts',(-56.1745692957322,18.4262957047547,
2.74351087134483));
#234319=CARTESIAN_POINT('Ctrl Pts',(-56.1683219623528,18.4192211773442,
2.7359339945019));
#234320=CARTESIAN_POINT('Ctrl Pts',(-56.1625328136775,18.411514249219,2.728576578129));
#234321=CARTESIAN_POINT('Ctrl Pts',(-56.1608066064038,18.4092161988262,
2.72638274508536));
#234322=CARTESIAN_POINT('Ctrl Pts',(-56.159121392827,18.4068618031993,2.72420861709706));
#234323=CARTESIAN_POINT('Ctrl Pts',(-56.1574804751187,18.4044493827313,
2.7220566373672));
#234324=CARTESIAN_POINT('Ctrl Pts',(-56.1558563235461,18.4020616112562,
2.71992664556759));
#234325=CARTESIAN_POINT('Ctrl Pts',(-56.1542770260203,18.3996196264082,
2.71782089927877));
#234326=CARTESIAN_POINT('Ctrl Pts',(-56.1527473834684,18.3971247125286,
2.71574387311239));
#234327=CARTESIAN_POINT('Ctrl Pts',(-56.1526410151169,18.3969512210967,
2.71559944077479));
#234328=CARTESIAN_POINT('Ctrl Pts',(-56.1525348749437,18.3967774746433,
2.71545515216062));
#234329=CARTESIAN_POINT('Ctrl Pts',(-56.1524289641634,18.3966034726925,
2.71531100781723));
#234330=CARTESIAN_POINT('Ctrl Pts',(-56.1477854475702,18.3889745897491,
2.70899119176072));
#234331=CARTESIAN_POINT('Ctrl Pts',(-56.1436260014307,18.3808409394273,
2.70298296066823));
#234332=CARTESIAN_POINT('Ctrl Pts',(-56.1400597146375,18.3722424849457,
2.69736727774118));
#234333=CARTESIAN_POINT('Ctrl Pts',(-56.1367353155297,18.3642272309675,
2.69213248525402));
#234334=CARTESIAN_POINT('Ctrl Pts',(-56.1339262909282,18.3558072700345,
2.68723866185434));
#234335=CARTESIAN_POINT('Ctrl Pts',(-56.1317496772148,18.3470212548464,
2.68278595829523));
#234336=CARTESIAN_POINT('Ctrl Pts',(-56.1309534437592,18.3438072168241,
2.68115710172778));
#234337=CARTESIAN_POINT('Ctrl Pts',(-56.1302421351291,18.3405443147879,
2.67958763637794));
#234338=CARTESIAN_POINT('Ctrl Pts',(-56.1296225724748,18.3372349828464,
2.67808378645359));
#234339=CARTESIAN_POINT('Ctrl Pts',(-56.1294735883542,18.3364391990694,
2.67772216078594));
#234340=CARTESIAN_POINT('Ctrl Pts',(-56.1293301519981,18.3356401993825,
2.67736403603557));
#234341=CARTESIAN_POINT('Ctrl Pts',(-56.1291923454416,18.3348380918585,
2.67700956934473));
#234342=CARTESIAN_POINT('Ctrl Pts',(-56.12905884534,18.3340610501946,2.67666617973798));
#234343=CARTESIAN_POINT('Ctrl Pts',(-56.1289306286648,18.333281091922,2.67632622314113));
#234344=CARTESIAN_POINT('Ctrl Pts',(-56.1288077688058,18.3324983188931,
2.67598984158768));
#234345=CARTESIAN_POINT('Ctrl Pts',(-56.1274616970648,18.3239221357307,
2.67230439292216));
#234346=CARTESIAN_POINT('Ctrl Pts',(-56.126758159346,18.3150023767874,2.6690496453997));
#234347=CARTESIAN_POINT('Ctrl Pts',(-56.1267895336332,18.3059033598549,
2.6664020356672));
#234348=CARTESIAN_POINT('Ctrl Pts',(-56.1268025454852,18.3021297263203,
2.66530399299434));
#234349=CARTESIAN_POINT('Ctrl Pts',(-56.1269416083199,18.2983254984047,
2.66430995142253));
#234350=CARTESIAN_POINT('Ctrl Pts',(-56.1272115877755,18.2945030089055,
2.66343053473353));
#234351=CARTESIAN_POINT('Ctrl Pts',(-56.127672065871,18.2879833547333,2.66193059792876));
#234352=CARTESIAN_POINT('Ctrl Pts',(-56.1285150529071,18.2814124323572,
2.66076519817119));
#234353=CARTESIAN_POINT('Ctrl Pts',(-56.1297657127887,18.2748585331712,
2.65997805604451));
#234354=CARTESIAN_POINT('Ctrl Pts',(-56.1303910427295,18.2715815835782,
2.65958448498116));
#234355=CARTESIAN_POINT('Ctrl Pts',(-56.1311196862928,18.2683092720866,
2.65928526260752));
#234356=CARTESIAN_POINT('Ctrl Pts',(-56.1319548233211,18.2650501911673,
2.65908463971314));
#234357=CARTESIAN_POINT('Ctrl Pts',(-56.1327899603494,18.261791110248,2.65888401681877));
#234358=CARTESIAN_POINT('Ctrl Pts',(-56.1337315613409,18.2585452947514,
2.65878198860274));
#234359=CARTESIAN_POINT('Ctrl Pts',(-56.1347810195643,18.2553202812748,
2.65878198860274));
#234360=CARTESIAN_POINT('Origin',(-56.9937374973464,12.0988124084938,2.83404198860269));
#234361=CARTESIAN_POINT('Ctrl Pts',(-61.3271735965894,12.8407372733096,
2.83404198860269));
#234362=CARTESIAN_POINT('Ctrl Pts',(-61.3375520649563,12.8429432848611,
2.8241965244006));
#234363=CARTESIAN_POINT('Ctrl Pts',(-61.3477256769088,12.8459616464943,
2.81438790575634));
#234364=CARTESIAN_POINT('Ctrl Pts',(-61.3576417279035,12.8497656413963,
2.80466781256877));
#234365=CARTESIAN_POINT('Ctrl Pts',(-61.367235566287,12.8534460291152,2.79526356453046));
#234366=CARTESIAN_POINT('Ctrl Pts',(-61.3765894879244,12.8578623484998,
2.78594102496194));
#234367=CARTESIAN_POINT('Ctrl Pts',(-61.3856422574871,12.8630345798924,
2.77675109088735));
#234368=CARTESIAN_POINT('Ctrl Pts',(-61.394205620056,12.8679271923021,2.76805797913634));
#234369=CARTESIAN_POINT('Ctrl Pts',(-61.4025003187128,12.873496651757,2.75948271210109));
#234370=CARTESIAN_POINT('Ctrl Pts',(-61.410448511695,12.8797929832534,2.75108575573169));
#234371=CARTESIAN_POINT('Ctrl Pts',(-61.4177693722596,12.885592359924,2.74335155163209));
#234372=CARTESIAN_POINT('Ctrl Pts',(-61.4247966697204,12.8920087864971,
2.73576818685876));
#234373=CARTESIAN_POINT('Ctrl Pts',(-61.4314390014625,12.8991043342896,
2.72840626160425));
#234374=CARTESIAN_POINT('Ctrl Pts',(-61.4333656894063,12.9011624829816,
2.72627084693634));
#234375=CARTESIAN_POINT('Ctrl Pts',(-61.4352597571384,12.9032779088719,
2.72415424587503));
#234376=CARTESIAN_POINT('Ctrl Pts',(-61.4371183613309,12.9054524645842,
2.72205867173264));
#234377=CARTESIAN_POINT('Ctrl Pts',(-61.4391332077732,12.9078098227881,
2.71978693462867));
#234378=CARTESIAN_POINT('Ctrl Pts',(-61.4411043938524,12.9102326900447,
2.71754411340768));
#234379=CARTESIAN_POINT('Ctrl Pts',(-61.4430281531012,12.9127224163027,
2.71533341844265));
#234380=CARTESIAN_POINT('Ctrl Pts',(-61.448307925455,12.9195554895544,2.70926614876412));
#234381=CARTESIAN_POINT('Ctrl Pts',(-61.4531896374536,12.926909770583,2.7034738186043));
#234382=CARTESIAN_POINT('Ctrl Pts',(-61.4575800373534,12.9347398820029,
2.69804914171416));
#234383=CARTESIAN_POINT('Ctrl Pts',(-61.4615970149014,12.9419040088456,
2.69308585687211));
#234384=CARTESIAN_POINT('Ctrl Pts',(-61.4651913207949,12.9494643722288,
2.68842799053179));
#234385=CARTESIAN_POINT('Ctrl Pts',(-61.4682744840805,12.9574154517112,
2.684147670542));
#234386=CARTESIAN_POINT('Ctrl Pts',(-61.4697889238147,12.9613209959793,
2.68204519134549));
#234387=CARTESIAN_POINT('Ctrl Pts',(-61.4711795284101,12.9653208118555,
2.68003431778512));
#234388=CARTESIAN_POINT('Ctrl Pts',(-61.4724324898305,12.9694138336349,
2.67812693945274));
#234389=CARTESIAN_POINT('Ctrl Pts',(-61.472670227056,12.970190444651,2.67776503299226));
#234390=CARTESIAN_POINT('Ctrl Pts',(-61.4729027677275,12.9709708853391,
2.67740659639946));
#234391=CARTESIAN_POINT('Ctrl Pts',(-61.4731300138563,12.9717550556846,
2.67705178968878));
#234392=CARTESIAN_POINT('Ctrl Pts',(-61.4733501585436,12.9725147207069,
2.6767080706878));
#234393=CARTESIAN_POINT('Ctrl Pts',(-61.4735653344326,12.9732778859006,
2.67636775825288));
#234394=CARTESIAN_POINT('Ctrl Pts',(-61.4737754532575,12.9740444565835,
2.67603099699278));
#234395=CARTESIAN_POINT('Ctrl Pts',(-61.4760652849146,12.9823983859294,
2.6723610421716));
#234396=CARTESIAN_POINT('Ctrl Pts',(-61.4777556486131,12.9911623597375,
2.66911440541513));
#234397=CARTESIAN_POINT('Ctrl Pts',(-61.478733140317,13.0001833616593,2.66646778189674));
#234398=CARTESIAN_POINT('Ctrl Pts',(-61.4791459411335,13.0039929867889,
2.66535009635009));
#234399=CARTESIAN_POINT('Ctrl Pts',(-61.4794319383912,13.0078481668563,
2.66433897912372));
#234400=CARTESIAN_POINT('Ctrl Pts',(-61.4795843394718,13.011736540843,2.66344564884815));
#234401=CARTESIAN_POINT('Ctrl Pts',(-61.4798409790835,13.0182844654763,
2.66194130298608));
#234402=CARTESIAN_POINT('Ctrl Pts',(-61.4797168922658,13.0249248230174,
2.66077206705441));
#234403=CARTESIAN_POINT('Ctrl Pts',(-61.4791780149463,13.0315916763175,
2.65998225155735));
#234404=CARTESIAN_POINT('Ctrl Pts',(-61.4790432956164,13.0332583896425,
2.65978479768309));
#234405=CARTESIAN_POINT('Ctrl Pts',(-61.4788824204055,13.0349267248714,
2.65961098966643));
#234406=CARTESIAN_POINT('Ctrl Pts',(-61.4786945538944,13.0365955947402,
2.65946139030523));
#234407=CARTESIAN_POINT('Ctrl Pts',(-61.4784127541277,13.0390988995432,
2.65923699126341));
#234408=CARTESIAN_POINT('Ctrl Pts',(-61.4780702140289,13.0416033892099,
2.65906707562463));
#234409=CARTESIAN_POINT('Ctrl Pts',(-61.4776657592304,13.0441057251027,
2.65895332562941));
#234410=CARTESIAN_POINT('Ctrl Pts',(-61.477261304432,13.0466080609956,2.65883957563418));
#234411=CARTESIAN_POINT('Ctrl Pts',(-61.4767949453822,13.0491082380627,
2.6587819886027));
#234412=CARTESIAN_POINT('Ctrl Pts',(-61.4762657165316,13.0516031943527,
2.6587819886027));
#234413=CARTESIAN_POINT('Ctrl Pts',(-57.7418065394566,12.2578193919766,
2.6587819886027));
#234414=CARTESIAN_POINT('Ctrl Pts',(-57.7435970583545,12.2493771807076,
2.6587819886027));
#234415=CARTESIAN_POINT('Ctrl Pts',(-57.74606892698,12.241155944225,2.65945335517859));
#234416=CARTESIAN_POINT('Ctrl Pts',(-57.7491141258101,12.2332613533232,
2.66072561226599));
#234417=CARTESIAN_POINT('Ctrl Pts',(-57.7510810117991,12.228162257632,2.66154735980339));
#234418=CARTESIAN_POINT('Ctrl Pts',(-57.7532862127603,12.2231990866885,
2.66261895766887));
#234419=CARTESIAN_POINT('Ctrl Pts',(-57.7556931859579,12.2183955094118,
2.66391429251036));
#234420=CARTESIAN_POINT('Ctrl Pts',(-57.7588834910512,12.2120286428976,
2.66563118464133));
#234421=CARTESIAN_POINT('Ctrl Pts',(-57.7624328173675,12.2059457447516,
2.66774105138708));
#234422=CARTESIAN_POINT('Ctrl Pts',(-57.7662682043709,12.2001996238499,
2.67016894181759));
#234423=CARTESIAN_POINT('Ctrl Pts',(-57.7681858978726,12.1973265633991,
2.67138288703284));
#234424=CARTESIAN_POINT('Ctrl Pts',(-57.770175146271,12.1945375019637,2.6726761316756));
#234425=CARTESIAN_POINT('Ctrl Pts',(-57.7722271161468,12.1918376559072,
2.67403835432562));
#234426=CARTESIAN_POINT('Ctrl Pts',(-57.7732531010847,12.190487732879,2.67471946565063));
#234427=CARTESIAN_POINT('Ctrl Pts',(-57.7742947697603,12.1891600976133,
2.67541781389532));
#234428=CARTESIAN_POINT('Ctrl Pts',(-57.7753510390205,12.1878553011596,
2.67613207244178));
#234429=CARTESIAN_POINT('Ctrl Pts',(-57.7756151063355,12.1875291020462,
2.6763106370784));
#234430=CARTESIAN_POINT('Ctrl Pts',(-57.7758800862578,12.1872043300163,
2.67649019601855));
#234431=CARTESIAN_POINT('Ctrl Pts',(-57.776145962005,12.1868809929896,2.67667072836666));
#234432=CARTESIAN_POINT('Ctrl Pts',(-57.7769435892465,12.1859109819096,
2.677212325411));
#234433=CARTESIAN_POINT('Ctrl Pts',(-57.7777492785674,12.1849538875689,
2.67776268340056));
#234434=CARTESIAN_POINT('Ctrl Pts',(-57.7785625799462,12.1840099085256,
2.67832123541525));
#234435=CARTESIAN_POINT('Ctrl Pts',(-57.7842913698424,12.1773606420349,
2.6822556036845));
#234436=CARTESIAN_POINT('Ctrl Pts',(-57.7903843352497,12.1713100228965,
2.6866179299889));
#234437=CARTESIAN_POINT('Ctrl Pts',(-57.7967264334405,12.1658251565858,
2.69130986622575));
#234438=CARTESIAN_POINT('Ctrl Pts',(-57.7998023442099,12.1631650023521,
2.69358545023055));
#234439=CARTESIAN_POINT('Ctrl Pts',(-57.8029374300324,12.1606380046012,
2.69593918853474));
#234440=CARTESIAN_POINT('Ctrl Pts',(-57.8061213360079,12.1582411305897,
2.69836306235483));
#234441=CARTESIAN_POINT('Ctrl Pts',(-57.8109956736033,12.1545716839429,
2.70207384382216));
#234442=CARTESIAN_POINT('Ctrl Pts',(-57.815981098899,12.1512083732206,2.70594760814216));
#234443=CARTESIAN_POINT('Ctrl Pts',(-57.8210315314441,12.1481495009385,
2.70995196345695));
#234444=CARTESIAN_POINT('Ctrl Pts',(-57.8233769784455,12.1467289448262,
2.71181160678094));
#234445=CARTESIAN_POINT('Ctrl Pts',(-57.8257362497572,12.1453738842984,
2.71369962772087));
#234446=CARTESIAN_POINT('Ctrl Pts',(-57.8281051246149,12.1440853170068,
2.7156118313865));
#234447=CARTESIAN_POINT('Ctrl Pts',(-57.8282866895389,12.1439865534012,
2.715758394263));
#234448=CARTESIAN_POINT('Ctrl Pts',(-57.8284683073399,12.1438881466795,
2.71590508903197));
#234449=CARTESIAN_POINT('Ctrl Pts',(-57.8286499766611,12.143790096302,2.71605191409899));
#234450=CARTESIAN_POINT('Ctrl Pts',(-57.8312018829079,12.1424127841096,
2.71811436362741));
#234451=CARTESIAN_POINT('Ctrl Pts',(-57.8337650648327,12.1411075562953,
2.72020091026947));
#234452=CARTESIAN_POINT('Ctrl Pts',(-57.8363340693141,12.1398727334219,
2.72230624862169));
#234453=CARTESIAN_POINT('Ctrl Pts',(-57.845546062502,12.1354448782039,2.72985561753081));
#234454=CARTESIAN_POINT('Ctrl Pts',(-57.8549032874801,12.1318862976812,
2.73770089914296));
#234455=CARTESIAN_POINT('Ctrl Pts',(-57.8643241951531,12.1290968783784,
2.74574823347028));
#234456=CARTESIAN_POINT('Ctrl Pts',(-57.8746768262717,12.1260315867866,
2.75459144546973));
#234457=CARTESIAN_POINT('Ctrl Pts',(-57.8851069357363,12.1238947812342,
2.76367911754212));
#234458=CARTESIAN_POINT('Ctrl Pts',(-57.8955352825126,12.1225979458249,
2.77292162564662));
#234459=CARTESIAN_POINT('Ctrl Pts',(-57.9067952798735,12.121197689044,2.78290121484685));
#234460=CARTESIAN_POINT('Ctrl Pts',(-57.9180543443232,12.1207764137886,
2.79306229500162));
#234461=CARTESIAN_POINT('Ctrl Pts',(-57.9292311407273,12.1212770948338,
2.80331916685248));
#234462=CARTESIAN_POINT('Ctrl Pts',(-57.9403141752932,12.1217735756795,
2.81348999408692));
#234463=CARTESIAN_POINT('Ctrl Pts',(-57.9513177099571,12.1231769533536,
2.82375635966879));
#234464=CARTESIAN_POINT('Ctrl Pts',(-57.9621601888121,12.125481593379,2.83404198860269));
#234465=CARTESIAN_POINT('Origin',(0.00316857416807368,0.0149069694353715,
2.83404198860262));
#234466=CARTESIAN_POINT('Ctrl Pts',(-61.4699285681955,13.081417133223,2.65878198860269));
#234467=CARTESIAN_POINT('Ctrl Pts',(-61.4681393149849,13.0898176309847,
2.65878198860269));
#234468=CARTESIAN_POINT('Ctrl Pts',(-61.465664225629,13.0979940118842,2.65944603041858));
#234469=CARTESIAN_POINT('Ctrl Pts',(-61.4626133761159,13.105843098261,2.66070439264076));
#234470=CARTESIAN_POINT('Ctrl Pts',(-61.4606640285136,13.1108582907975,
2.66150842619601));
#234471=CARTESIAN_POINT('Ctrl Pts',(-61.4584804838815,13.1157402208611,
2.66255428265373));
#234472=CARTESIAN_POINT('Ctrl Pts',(-61.4560986543957,13.1204666715204,
2.66381699700659));
#234473=CARTESIAN_POINT('Ctrl Pts',(-61.4528479350655,13.1269173283004,
2.66554034873259));
#234474=CARTESIAN_POINT('Ctrl Pts',(-61.4492231901485,13.1330744924003,
2.66766759643963));
#234475=CARTESIAN_POINT('Ctrl Pts',(-61.4453029499362,13.1388835356735,
2.67012012783139));
#234476=CARTESIAN_POINT('Ctrl Pts',(-61.4433428298301,13.14178805731,2.67134639352727));
#234477=CARTESIAN_POINT('Ctrl Pts',(-61.4413087943565,13.1446057534059,
2.67265375585004));
#234478=CARTESIAN_POINT('Ctrl Pts',(-61.4392103574,13.147331257159,2.67403135126932));
#234479=CARTESIAN_POINT('Ctrl Pts',(-61.4381611389217,13.1486940090355,
2.67472014897896));
#234480=CARTESIAN_POINT('Ctrl Pts',(-61.4370958165018,13.1500337298701,
2.67542649668624));
#234481=CARTESIAN_POINT('Ctrl Pts',(-61.4360155570619,13.1513498559441,
2.67614899656094));
#234482=CARTESIAN_POINT('Ctrl Pts',(-61.4357454922019,13.1516788874625,
2.67632962152961));
#234483=CARTESIAN_POINT('Ctrl Pts',(-61.4354744937032,13.1520064446718,
2.67651125590942));
#234484=CARTESIAN_POINT('Ctrl Pts',(-61.4352025796479,13.1523325194966,
2.67669387767516));
#234485=CARTESIAN_POINT('Ctrl Pts',(-61.4343868374821,13.1533107439709,
2.67724174297236));
#234486=CARTESIAN_POINT('Ctrl Pts',(-61.4335628556743,13.1542756251696,
2.6777984950474));
#234487=CARTESIAN_POINT('Ctrl Pts',(-61.4327311191547,13.1552269612802,
2.67836353618001));
#234488=CARTESIAN_POINT('Ctrl Pts',(-61.4269833037494,13.161801284066,2.68226832098907));
#234489=CARTESIAN_POINT('Ctrl Pts',(-61.420878024971,13.1677829516036,2.68659153751398));
#234490=CARTESIAN_POINT('Ctrl Pts',(-61.4145287289051,13.1732071947995,
2.69123699486195));
#234491=CARTESIAN_POINT('Ctrl Pts',(-61.411373146189,13.1759030287785,2.69354577441226));
#234492=CARTESIAN_POINT('Ctrl Pts',(-61.4081566864225,13.1784610805514,
2.69593478828118));
#234493=CARTESIAN_POINT('Ctrl Pts',(-61.4048902384027,13.1808848153825,
2.69839565261211));
#234494=CARTESIAN_POINT('Ctrl Pts',(-61.3976839661819,13.1862319364381,
2.70382468689037));
#234495=CARTESIAN_POINT('Ctrl Pts',(-61.3902425685153,13.1909347237342,
2.70961155815078));
#234496=CARTESIAN_POINT('Ctrl Pts',(-61.3827095020467,13.1949697809168,
2.71562701361759));
#234497=CARTESIAN_POINT('Ctrl Pts',(-61.3799575778687,13.1964438381903,
2.7178245353585));
#234498=CARTESIAN_POINT('Ctrl Pts',(-61.377194044862,13.197836719349,2.72005051502394));
#234499=CARTESIAN_POINT('Ctrl Pts',(-61.3744236152739,13.1991508816437,
2.72229986760107));
#234500=CARTESIAN_POINT('Ctrl Pts',(-61.3651180354454,13.2035650137314,
2.72985520488854));
#234501=CARTESIAN_POINT('Ctrl Pts',(-61.3556720404057,13.2071113921937,
2.73770845534488));
#234502=CARTESIAN_POINT('Ctrl Pts',(-61.3461671566365,13.2098890888172,
2.74576706701649));
#234503=CARTESIAN_POINT('Ctrl Pts',(-61.3357201634466,13.2129421064463,
2.75462443584895));
#234504=CARTESIAN_POINT('Ctrl Pts',(-61.3252014297039,13.2150668515154,
2.76373036323015));
#234505=CARTESIAN_POINT('Ctrl Pts',(-61.3146904872814,13.2163502251976,
2.77299664636619));
#234506=CARTESIAN_POINT('Ctrl Pts',(-61.3033697519341,13.2177324736415,
2.78297683033245));
#234507=CARTESIAN_POINT('Ctrl Pts',(-61.2920568939719,13.218139000641,2.79314401478632));
#234508=CARTESIAN_POINT('Ctrl Pts',(-61.2808338148861,13.2176240288386,
2.80341452427645));
#234509=CARTESIAN_POINT('Ctrl Pts',(-61.2697622852609,13.2171160108943,
2.81354634721166));
#234510=CARTESIAN_POINT('Ctrl Pts',(-61.2587767401952,13.215710839329,2.82378004209106));
#234511=CARTESIAN_POINT('Ctrl Pts',(-61.2479592423879,13.2134115091892,
2.8340419886027));
#234512=CARTESIAN_POINT('Ctrl Pts',(-57.8829458346106,12.4981558292586,
2.83404198860269));
#234513=CARTESIAN_POINT('Ctrl Pts',(-57.8725934298279,12.4959553576929,
2.82422126443142));
#234514=CARTESIAN_POINT('Ctrl Pts',(-57.8624518082056,12.4929462656008,
2.81442815028765));
#234515=CARTESIAN_POINT('Ctrl Pts',(-57.8525735736594,12.4891531124833,
2.80471618166709));
#234516=CARTESIAN_POINT('Ctrl Pts',(-57.8430352690793,12.4854904894119,
2.79533842146691));
#234517=CARTESIAN_POINT('Ctrl Pts',(-57.8337413853149,12.4810963130903,
2.7860351565077));
#234518=CARTESIAN_POINT('Ctrl Pts',(-57.8247536185252,12.4759491415414,
2.77685887347351));
#234519=CARTESIAN_POINT('Ctrl Pts',(-57.8162573641143,12.4710834524333,
2.76818441217196));
#234520=CARTESIAN_POINT('Ctrl Pts',(-57.8080338771709,12.4655444244758,
2.75962261522265));
#234521=CARTESIAN_POINT('Ctrl Pts',(-57.8001616710216,12.4592813303369,
2.75123537702318));
#234522=CARTESIAN_POINT('Ctrl Pts',(-57.7929115012241,12.453513125706,2.74351087134769));
#234523=CARTESIAN_POINT('Ctrl Pts',(-57.7859589019121,12.4471303774549,
2.73593399450487));
#234524=CARTESIAN_POINT('Ctrl Pts',(-57.7793958734455,12.4400707995033,
2.72857657813204));
#234525=CARTESIAN_POINT('Ctrl Pts',(-57.7774389108389,12.4379657758637,
2.72638274508736));
#234526=CARTESIAN_POINT('Ctrl Pts',(-57.7755168276806,12.4358004306468,
2.72420861709803));
#234527=CARTESIAN_POINT('Ctrl Pts',(-57.7736327324861,12.433572748276,2.72205663736716));
#234528=CARTESIAN_POINT('Ctrl Pts',(-57.7717678881028,12.4313678273309,
2.71992664556755));
#234529=CARTESIAN_POINT('Ctrl Pts',(-57.7699419852106,12.4291043014747,
2.71782089927873));
#234530=CARTESIAN_POINT('Ctrl Pts',(-57.7681599326868,12.4267829461797,
2.71574387311234));
#234531=CARTESIAN_POINT('Ctrl Pts',(-57.7680360122395,12.4266215236723,
2.71559944077475));
#234532=CARTESIAN_POINT('Ctrl Pts',(-57.7679122920635,12.4264598236895,
2.71545515216057));
#234533=CARTESIAN_POINT('Ctrl Pts',(-57.767788773317,12.4262978456306,2.71531100781719));
#234534=CARTESIAN_POINT('Ctrl Pts',(-57.762373258983,12.4191961341598,2.70899119176065));
#234535=CARTESIAN_POINT('Ctrl Pts',(-57.7573864007557,12.4115418213385,
2.70298296066813));
#234536=CARTESIAN_POINT('Ctrl Pts',(-57.7529408672213,12.4033632485683,
2.69736727774106));
#234537=CARTESIAN_POINT('Ctrl Pts',(-57.7487968573386,12.39573939732,2.69213248525386));
#234538=CARTESIAN_POINT('Ctrl Pts',(-57.7451230952907,12.3876591848387,
2.68723866185414));
#234539=CARTESIAN_POINT('Ctrl Pts',(-57.7420400166291,12.3791488184476,
2.682785958295));
#234540=CARTESIAN_POINT('Ctrl Pts',(-57.7409121865683,12.3760356163216,
2.68115710172761));
#234541=CARTESIAN_POINT('Ctrl Pts',(-57.7398637084258,12.3728649408022,
2.67958763637783));
#234542=CARTESIAN_POINT('Ctrl Pts',(-57.7389016204182,12.3696384996596,
2.67808378645353));
#234543=CARTESIAN_POINT('Ctrl Pts',(-57.7386702703929,12.3688626483506,
2.67772216078589));
#234544=CARTESIAN_POINT('Ctrl Pts',(-57.7384441015868,12.3680830188495,
2.67736403603552));
#234545=CARTESIAN_POINT('Ctrl Pts',(-57.7382232068821,12.367299710062,2.67700956934467));
#234546=CARTESIAN_POINT('Ctrl Pts',(-57.738009215137,12.3665408796741,2.67666617973792));
#234547=CARTESIAN_POINT('Ctrl Pts',(-57.7378001730066,12.3657785963866,
2.67632622314107));
#234548=CARTESIAN_POINT('Ctrl Pts',(-57.737596164125,12.3650129538224,2.67598984158762));
#234549=CARTESIAN_POINT('Ctrl Pts',(-57.7353610110592,12.3566244546995,
2.6723043929222));
#234550=CARTESIAN_POINT('Ctrl Pts',(-57.7337289586985,12.3478270988458,
2.66904964539982));
#234551=CARTESIAN_POINT('Ctrl Pts',(-57.7328090548569,12.3387746477743,
2.66640203566736));
#234552=CARTESIAN_POINT('Ctrl Pts',(-57.7324275433143,12.33502032649,2.66530399299442));
#234553=CARTESIAN_POINT('Ctrl Pts',(-57.7321681942503,12.3312224025083,
2.66430995142253));
#234554=CARTESIAN_POINT('Ctrl Pts',(-57.732037135777,12.3273926324687,2.66343053473348));
#234555=CARTESIAN_POINT('Ctrl Pts',(-57.7318136018935,12.3208605605765,
2.66193059792871));
#234556=CARTESIAN_POINT('Ctrl Pts',(-57.7319651225403,12.3142375182613,
2.66076519817114));
#234557=CARTESIAN_POINT('Ctrl Pts',(-57.7325238621659,12.3075887924653,
2.65997805604446));
#234558=CARTESIAN_POINT('Ctrl Pts',(-57.7328032319787,12.3042644295673,
2.65958448498112));
#234559=CARTESIAN_POINT('Ctrl Pts',(-57.7331858342648,12.3009338801485,
2.65928526260748));
#234560=CARTESIAN_POINT('Ctrl Pts',(-57.7336757296049,12.2976053572253,
2.6590846397131));
#234561=CARTESIAN_POINT('Ctrl Pts',(-57.734165624945,12.294276834302,2.65888401681872));
#234562=CARTESIAN_POINT('Ctrl Pts',(-57.7347627876418,12.2909503756177,
2.6587819886027));
#234563=CARTESIAN_POINT('Ctrl Pts',(-57.7354693911205,12.2876333308469,
2.6587819886027));
#234564=CARTESIAN_POINT('Origin',(-57.9461901084062,6.07506605172281,2.83404198860265));
#234565=CARTESIAN_POINT('Ctrl Pts',(-62.3334394572619,6.3599591583778,2.83404198860264));
#234566=CARTESIAN_POINT('Ctrl Pts',(-62.3439916622905,6.36106823981769,
2.82419652440062));
#234567=CARTESIAN_POINT('Ctrl Pts',(-62.3544250468353,6.3630066345268,2.81438790575644));
#234568=CARTESIAN_POINT('Ctrl Pts',(-62.3646844024063,6.36575328117444,
2.80466781256896));
#234569=CARTESIAN_POINT('Ctrl Pts',(-62.3746103900118,6.36841067816123,
2.79526356453073));
#234570=CARTESIAN_POINT('Ctrl Pts',(-62.3843747009663,6.37182505343183,
2.78594102496229));
#234571=CARTESIAN_POINT('Ctrl Pts',(-62.3939185239092,6.37602267870893,
2.77675109088779));
#234572=CARTESIAN_POINT('Ctrl Pts',(-62.4029463927384,6.37999337374618,
2.76805797913686));
#234573=CARTESIAN_POINT('Ctrl Pts',(-62.4117778192061,6.38466529101543,
2.7594827121017));
#234574=CARTESIAN_POINT('Ctrl Pts',(-62.420340617011,6.3900963181509,2.75108575573236));
#234575=CARTESIAN_POINT('Ctrl Pts',(-62.4282275730666,6.39509868692453,
2.74335155163287));
#234576=CARTESIAN_POINT('Ctrl Pts',(-62.4358870734659,6.40074541103687,
2.73576818685965));
#234577=CARTESIAN_POINT('Ctrl Pts',(-62.4432347045264,6.40710777594649,
2.72840626160522));
#234578=CARTESIAN_POINT('Ctrl Pts',(-62.4453659729924,6.40895325615489,
2.72627084693697));
#234579=CARTESIAN_POINT('Ctrl Pts',(-62.4474707870411,6.41085910953172,
2.72415424587532));
#234580=CARTESIAN_POINT('Ctrl Pts',(-62.4495465125725,6.41282747576061,
2.72205867173261));
#234581=CARTESIAN_POINT('Ctrl Pts',(-62.4517967325057,6.41496131130725,
2.71978693462864));
#234582=CARTESIAN_POINT('Ctrl Pts',(-62.4540103788122,6.4171648607918,2.71754411340765));
#234583=CARTESIAN_POINT('Ctrl Pts',(-62.4561838467663,6.4194398604709,2.71533341844262));
#234584=CARTESIAN_POINT('Ctrl Pts',(-62.4621489466211,6.42568361494178,
2.70926614876408));
#234585=CARTESIAN_POINT('Ctrl Pts',(-62.467772647785,6.43248733059613,2.70347381860426));
#234586=CARTESIAN_POINT('Ctrl Pts',(-62.4729574661286,6.43981562609172,
2.69804914171411));
#234587=CARTESIAN_POINT('Ctrl Pts',(-62.477701293423,6.44652061860809,2.69308585687195));
#234588=CARTESIAN_POINT('Ctrl Pts',(-62.4820661824989,6.45366385825823,
2.68842799053153));
#234589=CARTESIAN_POINT('Ctrl Pts',(-62.4859635700132,6.46124910257527,
2.68414767054166));
#234590=CARTESIAN_POINT('Ctrl Pts',(-62.4878779540286,6.46497494980492,
2.68204519134525));
#234591=CARTESIAN_POINT('Ctrl Pts',(-62.4896790353533,6.46880749650967,
2.68003431778498));
#234592=CARTESIAN_POINT('Ctrl Pts',(-62.4913529701965,6.47274712615551,
2.67812693945269));
#234593=CARTESIAN_POINT('Ctrl Pts',(-62.4916705830287,6.47349463250838,
2.67776503299221));
#234594=CARTESIAN_POINT('Ctrl Pts',(-62.4919834280838,6.47424649074166,
2.67740659639941));
#234595=CARTESIAN_POINT('Ctrl Pts',(-62.4922913974557,6.47500261163138,
2.67705178968873));
#234596=CARTESIAN_POINT('Ctrl Pts',(-62.4925897427848,6.4757351037433,2.67670807068775));
#234597=CARTESIAN_POINT('Ctrl Pts',(-62.4928835124027,6.47647159623325,
2.67636775825283));
#234598=CARTESIAN_POINT('Ctrl Pts',(-62.4931726086301,6.47721200416384,
2.67603099699273));
#234599=CARTESIAN_POINT('Ctrl Pts',(-62.4963231197466,6.48528081722631,
2.67236104217163));
#234600=CARTESIAN_POINT('Ctrl Pts',(-62.49892030817,6.49382008994889,2.66911440541521));
#234601=CARTESIAN_POINT('Ctrl Pts',(-62.5008353965401,6.50268949817244,
2.66646778189685));
#234602=CARTESIAN_POINT('Ctrl Pts',(-62.5016441502511,6.50643510434217,
2.66535009635013));
#234603=CARTESIAN_POINT('Ctrl Pts',(-62.502331556834,6.51023927047611,2.66433897912371));
#234604=CARTESIAN_POINT('Ctrl Pts',(-62.502889568803,6.51409041329268,2.6634456488481));
#234605=CARTESIAN_POINT('Ctrl Pts',(-62.5038292470155,6.5205756415655,2.66194130298603));
#234606=CARTESIAN_POINT('Ctrl Pts',(-62.5043999463277,6.52719259313761,
2.66077206705437));
#234607=CARTESIAN_POINT('Ctrl Pts',(-62.5045608969645,6.53387925273585,
2.6599822515573));
#234608=CARTESIAN_POINT('Ctrl Pts',(-62.5046011346237,6.53555091763541,
2.65978479768304));
#234609=CARTESIAN_POINT('Ctrl Pts',(-62.5046155292218,6.53722692958794,
2.65961098966639));
#234610=CARTESIAN_POINT('Ctrl Pts',(-62.5046031362659,6.53890629461061,
2.65946139030518));
#234611=CARTESIAN_POINT('Ctrl Pts',(-62.504584546832,6.5414253421446,2.65923699126337));
#234612=CARTESIAN_POINT('Ctrl Pts',(-62.5045056736598,6.54395191714494,
2.65906707562458));
#234613=CARTESIAN_POINT('Ctrl Pts',(-62.5043649998326,6.54648282201852,
2.65895332562936));
#234614=CARTESIAN_POINT('Ctrl Pts',(-62.5042243260054,6.5490137268921,2.65883957563414));
#234615=CARTESIAN_POINT('Ctrl Pts',(-62.5040218613861,6.55154895552238,
2.65878198860265));
#234616=CARTESIAN_POINT('Ctrl Pts',(-62.5037563256535,6.55408556365924,
2.65878198860265));
#234617=CARTESIAN_POINT('Ctrl Pts',(-58.7067819056643,6.15500747092296,
2.65878198860265));
#234618=CARTESIAN_POINT('Ctrl Pts',(-58.7076801645418,6.14642434678151,
2.65878198860265));
#234619=CARTESIAN_POINT('Ctrl Pts',(-58.7092791387968,6.13798976646338,
2.6594533551786));
#234620=CARTESIAN_POINT('Ctrl Pts',(-58.7114824462541,6.12982011300218,
2.6607256122661));
#234621=CARTESIAN_POINT('Ctrl Pts',(-58.7129055567991,6.12454335512125,
2.66154735980348));
#234622=CARTESIAN_POINT('Ctrl Pts',(-58.714579884807,6.1193768666801,2.66261895766891));
#234623=CARTESIAN_POINT('Ctrl Pts',(-58.7164715618025,6.11434800669306,
2.66391429251034));
#234624=CARTESIAN_POINT('Ctrl Pts',(-58.7189788712982,6.10768254085107,
2.6656311846413));
#234625=CARTESIAN_POINT('Ctrl Pts',(-58.7218729180382,6.10126195983215,
2.66774105138706));
#234626=CARTESIAN_POINT('Ctrl Pts',(-58.7250866612026,6.0951464096725,2.67016894181756));
#234627=CARTESIAN_POINT('Ctrl Pts',(-58.7266935327849,6.09208863459267,
2.67138288703281));
#234628=CARTESIAN_POINT('Ctrl Pts',(-58.7283803475666,6.0891069188495,2.67267613167557));
#234629=CARTESIAN_POINT('Ctrl Pts',(-58.7301388657773,6.08620737357443,
2.67403835432559));
#234630=CARTESIAN_POINT('Ctrl Pts',(-58.7310181248827,6.0847576009369,2.6747194656506));
#234631=CARTESIAN_POINT('Ctrl Pts',(-58.7319153115143,6.08332835457022,
2.67541781389528));
#234632=CARTESIAN_POINT('Ctrl Pts',(-58.7328294060527,6.0819202957255,2.67613207244175));
#234633=CARTESIAN_POINT('Ctrl Pts',(-58.7330579296874,6.08156828101432,
2.67631063707836));
#234634=CARTESIAN_POINT('Ctrl Pts',(-58.7332875101006,6.08121759017548,
2.67649019601851));
#234635=CARTESIAN_POINT('Ctrl Pts',(-58.7335181314301,6.08086823283961,
2.67667072836662));
#234636=CARTESIAN_POINT('Ctrl Pts',(-58.7342099954186,6.07982016083199,
2.67721232541096));
#234637=CARTESIAN_POINT('Ctrl Pts',(-58.7349112274885,6.07878409208758,
2.67776268340052));
#234638=CARTESIAN_POINT('Ctrl Pts',(-58.7356214008386,6.07776027111699,
2.67832123541521));
#234639=CARTESIAN_POINT('Ctrl Pts',(-58.7406237702161,6.07054860839961,
2.68225560368445));
#234640=CARTESIAN_POINT('Ctrl Pts',(-58.746050895801,6.06389424687519,2.68661792998883));
#234641=CARTESIAN_POINT('Ctrl Pts',(-58.7517849266677,6.05777649745833,
2.69130986622566));
#234642=CARTESIAN_POINT('Ctrl Pts',(-58.7545659254419,6.05480939560192,
2.69358545023047));
#234643=CARTESIAN_POINT('Ctrl Pts',(-58.7574196937447,6.05196853530582,
2.69593918853468));
#234644=CARTESIAN_POINT('Ctrl Pts',(-58.7603356163931,6.04925198282212,
2.69836306235479));
#234645=CARTESIAN_POINT('Ctrl Pts',(-58.7647996902381,6.04509313076973,
2.70207384382212));
#234646=CARTESIAN_POINT('Ctrl Pts',(-58.7694062431511,6.04122712577057,
2.70594760814212));
#234647=CARTESIAN_POINT('Ctrl Pts',(-58.7741092696793,6.03765709635814,
2.70995196345691));
#234648=CARTESIAN_POINT('Ctrl Pts',(-58.7762933795292,6.03599915623013,
2.71181160678089));
#234649=CARTESIAN_POINT('Ctrl Pts',(-58.7784980841112,6.03440490786102,
2.71369962772083));
#234650=CARTESIAN_POINT('Ctrl Pts',(-58.7807192900657,6.03287578462736,
2.71561183138645));
#234651=CARTESIAN_POINT('Ctrl Pts',(-58.7808895367502,6.03275858335655,
2.71575839426296));
#234652=CARTESIAN_POINT('Ctrl Pts',(-58.7810598733265,6.03264173148758,
2.71590508903193));
#234653=CARTESIAN_POINT('Ctrl Pts',(-58.7812302983888,6.03252522862529,
2.71605191409895));
#234654=CARTESIAN_POINT('Ctrl Pts',(-58.7836242566993,6.03088871465484,
2.71811436362737));
#234655=CARTESIAN_POINT('Ctrl Pts',(-58.7860369637877,6.02932271154743,
2.72020091026943));
#234656=CARTESIAN_POINT('Ctrl Pts',(-58.7884628208564,6.02782611907237,
2.72230624862166));
#234657=CARTESIAN_POINT('Ctrl Pts',(-58.7971615128801,6.02245960461699,
2.72985561753071));
#234658=CARTESIAN_POINT('Ctrl Pts',(-58.8060955050472,6.01794242202343,
2.7377008991428));
#234659=CARTESIAN_POINT('Ctrl Pts',(-58.815173230289,6.0141835304498,2.74574823347006));
#234660=CARTESIAN_POINT('Ctrl Pts',(-58.825148738391,6.01005288622463,2.75459144546905));
#234661=CARTESIAN_POINT('Ctrl Pts',(-58.8352983536234,6.00683754300273,
2.76367911754095));
#234662=CARTESIAN_POINT('Ctrl Pts',(-58.8455340166119,6.00445775273053,
2.77292162564495));
#234663=CARTESIAN_POINT('Ctrl Pts',(-58.8565859638382,6.00188817648251,
2.78290121484389));
#234664=CARTESIAN_POINT('Ctrl Pts',(-58.8677393146984,6.00029231631224,
2.79306229499733));
#234665=CARTESIAN_POINT('Ctrl Pts',(-58.8789072188612,5.99962196122167,
2.80331916684684));
#234666=CARTESIAN_POINT('Ctrl Pts',(-58.889981435786,5.99895722972136,2.81348999408311));
#234667=CARTESIAN_POINT('Ctrl Pts',(-58.9010713848493,5.99920273697657,
2.82375635966685));
#234668=CARTESIAN_POINT('Ctrl Pts',(-58.912095367953,6.00036140429026,2.83404198860265));
#234669=CARTESIAN_POINT('Origin',(0.00159301378021015,0.0151565136856013,
2.83404198860262));
#234670=CARTESIAN_POINT('Ctrl Pts',(-62.5005702980931,6.58439859103007,
2.65878198860265));
#234671=CARTESIAN_POINT('Ctrl Pts',(-62.4996689377206,6.59294009787421,
2.65878198860265));
#234672=CARTESIAN_POINT('Ctrl Pts',(-62.4980620716937,6.60133040499013,
2.65944603041847));
#234673=CARTESIAN_POINT('Ctrl Pts',(-62.4958483879906,6.60945539386143,
2.66070439264056));
#234674=CARTESIAN_POINT('Ctrl Pts',(-62.4944339494872,6.61464687495804,
2.66150842619583));
#234675=CARTESIAN_POINT('Ctrl Pts',(-62.4927726671883,6.61973030386325,
2.6625542826536));
#234676=CARTESIAN_POINT('Ctrl Pts',(-62.4908979342376,6.62467983150749,
2.66381699700655));
#234677=CARTESIAN_POINT('Ctrl Pts',(-62.4883392999283,6.63143494361077,
2.66554034873254));
#234678=CARTESIAN_POINT('Ctrl Pts',(-62.4853780106447,6.63793726713746,
2.66766759643958));
#234679=CARTESIAN_POINT('Ctrl Pts',(-62.4820864562849,6.64412426454875,
2.67012012783134));
#234680=CARTESIAN_POINT('Ctrl Pts',(-62.480440679105,6.6472177632544,2.67134639352722));
#234681=CARTESIAN_POINT('Ctrl Pts',(-62.4787123157334,6.65023263831855,
2.67265375584998));
#234682=CARTESIAN_POINT('Ctrl Pts',(-62.476910266953,6.65316255786721,2.67403135126925));
#234683=CARTESIAN_POINT('Ctrl Pts',(-62.4760092425629,6.65462751764154,
2.67472014897889));
#234684=CARTESIAN_POINT('Ctrl Pts',(-62.4750897950506,6.65607125586062,
2.67542649668618));
#234685=CARTESIAN_POINT('Ctrl Pts',(-62.474153026021,6.65749308991742,2.67614899656087));
#234686=CARTESIAN_POINT('Ctrl Pts',(-62.4739188337636,6.65784854843162,
2.67632962152955));
#234687=CARTESIAN_POINT('Ctrl Pts',(-62.4736835588747,6.65820263830483,
2.67651125590936));
#234688=CARTESIAN_POINT('Ctrl Pts',(-62.4734472184934,6.65855534961595,
2.67669387767509));
#234689=CARTESIAN_POINT('Ctrl Pts',(-62.4727381973496,6.65961348354928,
2.67724174297229));
#234690=CARTESIAN_POINT('Ctrl Pts',(-62.4720195869492,6.66065920857987,
2.67779849504733));
#234691=CARTESIAN_POINT('Ctrl Pts',(-62.4712918484711,6.66169227331197,
2.67836353617994));
#234692=CARTESIAN_POINT('Ctrl Pts',(-62.4662627240579,6.66883139158105,
2.68226832098894));
#234693=CARTESIAN_POINT('Ctrl Pts',(-62.460816145151,6.67541846632645,2.68659153751377));
#234694=CARTESIAN_POINT('Ctrl Pts',(-62.455068618999,6.68147667711109,2.69123699486165));
#234695=CARTESIAN_POINT('Ctrl Pts',(-62.4522121142781,6.68448759124161,
2.69354577441203));
#234696=CARTESIAN_POINT('Ctrl Pts',(-62.4492806638354,6.68736784133592,
2.69593478828104));
#234697=CARTESIAN_POINT('Ctrl Pts',(-62.4462854590369,6.69011973548587,
2.69839565261206));
#234698=CARTESIAN_POINT('Ctrl Pts',(-62.4396775898761,6.696190825014,2.70382468689032));
#234699=CARTESIAN_POINT('Ctrl Pts',(-62.4327685320937,6.70164568781193,
2.70961155815073));
#234700=CARTESIAN_POINT('Ctrl Pts',(-62.4256985108779,6.70644606039072,
2.71562701361754));
#234701=CARTESIAN_POINT('Ctrl Pts',(-62.4231157429701,6.70819969702963,
2.71782453535844));
#234702=CARTESIAN_POINT('Ctrl Pts',(-62.4205129446133,6.70987381569794,
2.72005051502389));
#234703=CARTESIAN_POINT('Ctrl Pts',(-62.4178950590935,6.71147036762155,
2.72229986760102));
#234704=CARTESIAN_POINT('Ctrl Pts',(-62.4091018586484,6.71683301659127,
2.72985520488883));
#234705=CARTESIAN_POINT('Ctrl Pts',(-62.4000783072482,6.72134734296704,
2.73770845534555));
#234706=CARTESIAN_POINT('Ctrl Pts',(-62.3909158405859,6.7251033539719,2.74576706701756));
#234707=CARTESIAN_POINT('Ctrl Pts',(-62.3808452043584,6.72923165499498,
2.7546244358504));
#234708=CARTESIAN_POINT('Ctrl Pts',(-62.3706061896764,6.73244426756195,
2.76373036323201));
#234709=CARTESIAN_POINT('Ctrl Pts',(-62.3602869763746,6.73481930344769,
2.77299664636847));
#234710=CARTESIAN_POINT('Ctrl Pts',(-62.3491727415053,6.73737731885886,
2.78297683033515));
#234711=CARTESIAN_POINT('Ctrl Pts',(-62.3379643502049,6.73896413451877,
2.79314401478945));
#234712=CARTESIAN_POINT('Ctrl Pts',(-62.326748923109,6.73962511499558,2.80341452427999));
#234713=CARTESIAN_POINT('Ctrl Pts',(-62.3156849421477,6.74027717000414,
2.81354634721404));
#234714=CARTESIAN_POINT('Ctrl Pts',(-62.3046126966243,6.74002799825949,
2.82378004209224));
#234715=CARTESIAN_POINT('Ctrl Pts',(-62.293614112757,6.73887200051311,2.83404198860265));
#234716=CARTESIAN_POINT('Ctrl Pts',(-58.872270023448,6.37927424642558,2.83404198860265));
#234717=CARTESIAN_POINT('Ctrl Pts',(-58.8617443183093,6.37816795023634,
2.82422126443007));
#234718=CARTESIAN_POINT('Ctrl Pts',(-58.8513437177779,6.3762354303884,2.81442815028499));
#234719=CARTESIAN_POINT('Ctrl Pts',(-58.8411231047665,6.37349561323695,
2.80471618166313));
#234720=CARTESIAN_POINT('Ctrl Pts',(-58.831254203655,6.37085007871755,2.79533842146225));
#234721=CARTESIAN_POINT('Ctrl Pts',(-58.8215519162594,6.3674514495407,2.78603515650236));
#234722=CARTESIAN_POINT('Ctrl Pts',(-58.8120753594638,6.36327195218627,
2.77685887346753));
#234723=CARTESIAN_POINT('Ctrl Pts',(-58.8031170454182,6.35932101824884,
2.76818441216578));
#234724=CARTESIAN_POINT('Ctrl Pts',(-58.7943596215162,6.35467192211847,
2.75962261521629));
#234725=CARTESIAN_POINT('Ctrl Pts',(-58.7858758685301,6.34926600747531,
2.75123537701669));
#234726=CARTESIAN_POINT('Ctrl Pts',(-58.7780624743556,6.34428725078,2.74351087134135));
#234727=CARTESIAN_POINT('Ctrl Pts',(-58.7704807832442,6.33866621241302,
2.73593399449869));
#234728=CARTESIAN_POINT('Ctrl Pts',(-58.7632157808999,6.33233133084779,
2.72857657812605));
#234729=CARTESIAN_POINT('Ctrl Pts',(-58.7610495038549,6.33044239704342,
2.72638274508339));
#234730=CARTESIAN_POINT('Ctrl Pts',(-58.7589116098633,6.32848982621476,
2.72420861709603));
#234731=CARTESIAN_POINT('Ctrl Pts',(-58.7568049797265,6.32647128889817,
2.72205663736711));
#234732=CARTESIAN_POINT('Ctrl Pts',(-58.7547198741578,6.32447337605831,
2.7199266455675));
#234733=CARTESIAN_POINT('Ctrl Pts',(-58.7526673708734,6.32241310885704,
2.71782089927869));
#234734=CARTESIAN_POINT('Ctrl Pts',(-58.7506524329181,6.32029074540098,
2.7157438731123));
#234735=CARTESIAN_POINT('Ctrl Pts',(-58.7505123180733,6.32014316039693,
2.71559944077471));
#234736=CARTESIAN_POINT('Ctrl Pts',(-58.7503723733987,6.31999527850334,
2.71545515216053));
#234737=CARTESIAN_POINT('Ctrl Pts',(-58.7502325999832,6.31984709900204,
2.71531100781714));
#234738=CARTESIAN_POINT('Ctrl Pts',(-58.7441044214168,6.31335036684086,
2.70899119176064));
#234739=CARTESIAN_POINT('Ctrl Pts',(-58.7383447881641,6.3062592537732,2.70298296066816));
#234740=CARTESIAN_POINT('Ctrl Pts',(-58.7330687140841,6.29859016886915,
2.69736727774112));
#234741=CARTESIAN_POINT('Ctrl Pts',(-58.728150496066,6.29144124886053,2.69213248525394));
#234742=CARTESIAN_POINT('Ctrl Pts',(-58.7236522470775,6.28378931333004,
2.68723866185425));
#234743=CARTESIAN_POINT('Ctrl Pts',(-58.7196964823227,6.27564783709119,
2.68278595829512));
#234744=CARTESIAN_POINT('Ctrl Pts',(-58.7182494123989,6.2726695797551,2.68115710172767));
#234745=CARTESIAN_POINT('Ctrl Pts',(-58.7168752520897,6.26962586933689,
2.67958763637783));
#234746=CARTESIAN_POINT('Ctrl Pts',(-58.7155811795664,6.26651766855731,
2.67808378645348));
#234747=CARTESIAN_POINT('Ctrl Pts',(-58.7152699983557,6.26577025010558,
2.67772216078583));
#234748=CARTESIAN_POINT('Ctrl Pts',(-58.7149635750523,6.26501853257418,
2.67736403603546));
#234749=CARTESIAN_POINT('Ctrl Pts',(-58.7146620123681,6.2642626046182,2.67700956934462));
#234750=CARTESIAN_POINT('Ctrl Pts',(-58.7143698735178,6.26353029941084,
2.67666617973787));
#234751=CARTESIAN_POINT('Ctrl Pts',(-58.7140822962414,6.26279404284355,
2.67632622314102));
#234752=CARTESIAN_POINT('Ctrl Pts',(-58.7137993735012,6.26205391928439,
2.67598984158756));
#234753=CARTESIAN_POINT('Ctrl Pts',(-58.7106996279152,6.25394501035232,
2.67230439292207));
#234754=CARTESIAN_POINT('Ctrl Pts',(-58.70815694202,6.24536644325953,2.66904964539964));
#234755=CARTESIAN_POINT('Ctrl Pts',(-58.7062958387084,6.23645973859696,
2.66640203566715));
#234756=CARTESIAN_POINT('Ctrl Pts',(-58.7055239836916,6.23276586269288,
2.66530399299427));
#234757=CARTESIAN_POINT('Ctrl Pts',(-58.7048690642115,6.22901585349537,
2.66430995142244));
#234758=CARTESIAN_POINT('Ctrl Pts',(-58.7043384037134,6.22522076267779,
2.66343053473343));
#234759=CARTESIAN_POINT('Ctrl Pts',(-58.7034333069351,6.21874783981215,
2.66193059792867));
#234760=CARTESIAN_POINT('Ctrl Pts',(-58.7028917011005,6.21214524099541,
2.66076519817109));
#234761=CARTESIAN_POINT('Ctrl Pts',(-58.7027523988019,6.20547453342054,
2.65997805604441));
#234762=CARTESIAN_POINT('Ctrl Pts',(-58.7026827476526,6.2021391796331,2.65958448498108));
#234763=CARTESIAN_POINT('Ctrl Pts',(-58.7027151167907,6.19878688248349,
2.65928526260744));
#234764=CARTESIAN_POINT('Ctrl Pts',(-58.7028544030468,6.19542538555006,
2.65908463971306));
#234765=CARTESIAN_POINT('Ctrl Pts',(-58.7029936893028,6.19206388861664,
2.65888401681868));
#234766=CARTESIAN_POINT('Ctrl Pts',(-58.7032398710655,6.18869323212196,
2.65878198860265));
#234767=CARTESIAN_POINT('Ctrl Pts',(-58.7035958781039,6.18532049829379,
2.65878198860265));
#234768=CARTESIAN_POINT('Origin',(-58.2637721346185,-0.0152399999998105,
2.83404198860261));
#234769=CARTESIAN_POINT('Ctrl Pts',(-62.6567671111299,-0.190499999999811,
2.8340419886026));
#234770=CARTESIAN_POINT('Ctrl Pts',(-62.667377440654,-0.19049999999981,
2.82419652440118));
#234771=CARTESIAN_POINT('Ctrl Pts',(-62.6779562874467,-0.189662809672919,
2.81438790575745));
#234772=CARTESIAN_POINT('Ctrl Pts',(-62.6884465439475,-0.188003604115047,
2.80466781257031));
#234773=CARTESIAN_POINT('Ctrl Pts',(-62.6985959295775,-0.186398312857871,
2.79526356453232));
#234774=CARTESIAN_POINT('Ctrl Pts',(-62.7086636500148,-0.184023290311302,
2.78594102496403));
#234775=CARTESIAN_POINT('Ctrl Pts',(-62.7185939622164,-0.180846261210727,
2.77675109088961));
#234776=CARTESIAN_POINT('Ctrl Pts',(-62.7279874260857,-0.177840987311753,
2.76805797913871));
#234777=CARTESIAN_POINT('Ctrl Pts',(-62.7372588214076,-0.174117798731389,
2.75948271210353));
#234778=CARTESIAN_POINT('Ctrl Pts',(-62.7463424082304,-0.169611579426802,
2.75108575573417));
#234779=CARTESIAN_POINT('Ctrl Pts',(-62.7547090486359,-0.165461025549195,
2.74335155163464));
#234780=CARTESIAN_POINT('Ctrl Pts',(-62.7629168328844,-0.16064587058866,
2.73576818686135));
#234781=CARTESIAN_POINT('Ctrl Pts',(-62.7708892610798,-0.155086395963295,
2.7284062616069));
#234782=CARTESIAN_POINT('Ctrl Pts',(-62.7732017594448,-0.153473803705747,
2.72627084693807));
#234783=CARTESIAN_POINT('Ctrl Pts',(-62.7754942590272,-0.151798403770687,
2.72415424587586));
#234784=CARTESIAN_POINT('Ctrl Pts',(-62.7777643638146,-0.150057792857475,
2.72205867173259));
#234785=CARTESIAN_POINT('Ctrl Pts',(-62.780225303358,-0.148170858716853,
2.7197869346286));
#234786=CARTESIAN_POINT('Ctrl Pts',(-62.7826571567199,-0.146210769553579,
2.7175441134076));
#234787=CARTESIAN_POINT('Ctrl Pts',(-62.7850565204095,-0.144175421825956,
2.71533341844257));
#234788=CARTESIAN_POINT('Ctrl Pts',(-62.791641592883,-0.138589394016422,
2.70926614876403));
#234789=CARTESIAN_POINT('Ctrl Pts',(-62.7979456687653,-0.132410786668851,
2.7034738186042));
#234790=CARTESIAN_POINT('Ctrl Pts',(-62.8038680995981,-0.125664597436552,
2.69804914171406));
#234791=CARTESIAN_POINT('Ctrl Pts',(-62.8092868022739,-0.119492200548109,
2.69308585687212));
#234792=CARTESIAN_POINT('Ctrl Pts',(-62.814374451894,-0.112844347459958,
2.68842799053189));
#234793=CARTESIAN_POINT('Ctrl Pts',(-62.8190433630435,-0.105708043832951,
2.68414767054218));
#234794=CARTESIAN_POINT('Ctrl Pts',(-62.8213367169484,-0.102202714803191,
2.68204519134556));
#234795=CARTESIAN_POINT('Ctrl Pts',(-62.8235285419788,-0.098579427453058,
2.68003431778509));
#234796=CARTESIAN_POINT('Ctrl Pts',(-62.8256051102647,-0.0948363533470471,
2.67812693945261));
#234797=CARTESIAN_POINT('Ctrl Pts',(-62.8259991188709,-0.0941261414934478,
2.67776503299213));
#234798=CARTESIAN_POINT('Ctrl Pts',(-62.8263888407139,-0.0934111032311,
2.67740659639934));
#234799=CARTESIAN_POINT('Ctrl Pts',(-62.826774159152,-0.0926913160159039,
2.67705178968865));
#234800=CARTESIAN_POINT('Ctrl Pts',(-62.8271474363889,-0.0919940221511827,
2.67670807068767));
#234801=CARTESIAN_POINT('Ctrl Pts',(-62.8275165811343,-0.0912922715308663,
2.67636775825275));
#234802=CARTESIAN_POINT('Ctrl Pts',(-62.8278814873655,-0.0905861384167767,
2.67603099699265));
#234803=CARTESIAN_POINT('Ctrl Pts',(-62.8318581602824,-0.0828908452418365,
2.67236104217145));
#234804=CARTESIAN_POINT('Ctrl Pts',(-62.8353337180911,-0.0746698316632022,
2.66911440541497));
#234805=CARTESIAN_POINT('Ctrl Pts',(-62.8381654210184,-0.0660491922300273,
2.66646778189657));
#234806=CARTESIAN_POINT('Ctrl Pts',(-62.8393612667488,-0.0624086426655782,
2.66535009634994));
#234807=CARTESIAN_POINT('Ctrl Pts',(-62.8404425512864,-0.0586971697057279,
2.66433897912359));
#234808=CARTESIAN_POINT('Ctrl Pts',(-62.8414000604479,-0.0549254519862922,
2.66344564884803));
#234809=CARTESIAN_POINT('Ctrl Pts',(-62.8430124819501,-0.0485739735920286,
2.66194130298596));
#234810=CARTESIAN_POINT('Ctrl Pts',(-62.8442717146911,-0.0420529246950825,
2.66077206705431));
#234811=CARTESIAN_POINT('Ctrl Pts',(-62.8451307298764,-0.0354197192405181,
2.65998225155726));
#234812=CARTESIAN_POINT('Ctrl Pts',(-62.8453454836727,-0.0337614178768769,
2.659784797683));
#234813=CARTESIAN_POINT('Ctrl Pts',(-62.8455349903695,-0.0320960919383993,
2.65961098966634));
#234814=CARTESIAN_POINT('Ctrl Pts',(-62.8456982067485,-0.0304246312363976,
2.65946139030513));
#234815=CARTESIAN_POINT('Ctrl Pts',(-62.845943031317,-0.027917440183395,
2.65923699126332));
#234816=CARTESIAN_POINT('Ctrl Pts',(-62.8461286892223,-0.0253964615337772,
2.65906707562454));
#234817=CARTESIAN_POINT('Ctrl Pts',(-62.846253337618,-0.0228647168029203,
2.65895332562931));
#234818=CARTESIAN_POINT('Ctrl Pts',(-62.8463779860137,-0.0203329720720634,
2.65883957563409));
#234819=CARTESIAN_POINT('Ctrl Pts',(-62.8464416340693,-0.0177904683739631,
2.65878198860261));
#234820=CARTESIAN_POINT('Ctrl Pts',(-62.8464427007196,-0.0152399999998093,
2.65878198860261));
#234821=CARTESIAN_POINT('Ctrl Pts',(-59.0285534841296,-0.0152399999998097,
2.65878198860261));
#234822=CARTESIAN_POINT('Ctrl Pts',(-59.0285496414744,-0.0238699985093663,
2.65878198860261));
#234823=CARTESIAN_POINT('Ctrl Pts',(-59.0292582026622,-0.0324255116358099,
2.65945335517858));
#234824=CARTESIAN_POINT('Ctrl Pts',(-59.0305954788491,-0.0407807192232887,
2.66072561226611));
#234825=CARTESIAN_POINT('Ctrl Pts',(-59.0314592220532,-0.0461773260306079,
2.66154735980347));
#234826=CARTESIAN_POINT('Ctrl Pts',(-59.0325843328199,-0.051490526841021,
2.66261895766888));
#234827=CARTESIAN_POINT('Ctrl Pts',(-59.0339399880044,-0.0566895722960612,
2.66391429251027));
#234828=CARTESIAN_POINT('Ctrl Pts',(-59.0357368312948,-0.0635806092272726,
2.66563118464123));
#234829=CARTESIAN_POINT('Ctrl Pts',(-59.0379438906768,-0.0702685278899484,
2.66774105138698));
#234830=CARTESIAN_POINT('Ctrl Pts',(-59.0405007795597,-0.0766865040602752,
2.67016894181749));
#234831=CARTESIAN_POINT('Ctrl Pts',(-59.0417792240012,-0.0798954921454386,
2.67138288703274));
#234832=CARTESIAN_POINT('Ctrl Pts',(-59.0431451240706,-0.0830371938947498,
2.6726761316755));
#234833=CARTESIAN_POINT('Ctrl Pts',(-59.0445909239228,-0.0861046703636156,
2.67403835432552));
#234834=CARTESIAN_POINT('Ctrl Pts',(-59.0453138238489,-0.0876384085980485,
2.67471946565053));
#234835=CARTESIAN_POINT('Ctrl Pts',(-59.0460566986718,-0.0891536069434453,
2.67541781389522));
#234836=CARTESIAN_POINT('Ctrl Pts',(-59.0468186034775,-0.0906495011918796,
2.67613207244168));
#234837=CARTESIAN_POINT('Ctrl Pts',(-59.047009079679,-0.0910234747539882,
2.67631063707829));
#234838=CARTESIAN_POINT('Ctrl Pts',(-59.0472007452523,-0.0913962421595167,
2.67649019601844));
#234839=CARTESIAN_POINT('Ctrl Pts',(-59.0473935854286,-0.0917677921725184,
2.67667072836655));
#234840=CARTESIAN_POINT('Ctrl Pts',(-59.0479721059574,-0.0928824422115236,
2.67721232541089));
#234841=CARTESIAN_POINT('Ctrl Pts',(-59.0485611979309,-0.0939861339736083,
2.67776268340046));
#234842=CARTESIAN_POINT('Ctrl Pts',(-59.0491604624443,-0.0950785796747284,
2.67832123541515));
#234843=CARTESIAN_POINT('Ctrl Pts',(-59.0533816042976,-0.102773626133062,
2.68225560368446));
#234844=CARTESIAN_POINT('Ctrl Pts',(-59.0580834293367,-0.109958823466275,
2.68661792998894));
#234845=CARTESIAN_POINT('Ctrl Pts',(-59.0631465696372,-0.116642428646653,
2.69130986622588));
#234846=CARTESIAN_POINT('Ctrl Pts',(-59.0656021872116,-0.119883969936718,
2.69358545023061));
#234847=CARTESIAN_POINT('Ctrl Pts',(-59.0681433715119,-0.123007567717954,
2.69593918853473));
#234848=CARTESIAN_POINT('Ctrl Pts',(-59.0707593633743,-0.126014035556225,
2.69836306235474));
#234849=CARTESIAN_POINT('Ctrl Pts',(-59.0747642641416,-0.130616727760851,
2.70207384382207));
#234850=CARTESIAN_POINT('Ctrl Pts',(-59.0789414743143,-0.134943070277078,
2.70594760814207));
#234851=CARTESIAN_POINT('Ctrl Pts',(-59.0832455674828,-0.138985142830541,
2.70995196345687));
#234852=CARTESIAN_POINT('Ctrl Pts',(-59.0852444106167,-0.140862302235282,
2.71181160678085));
#234853=CARTESIAN_POINT('Ctrl Pts',(-59.0872703932641,-0.142678271526929,
2.71369962772079));
#234854=CARTESIAN_POINT('Ctrl Pts',(-59.0893195943183,-0.144431197308552,
2.71561183138641));
#234855=CARTESIAN_POINT('Ctrl Pts',(-59.0894766575048,-0.144565552162836,
2.71575839426292));
#234856=CARTESIAN_POINT('Ctrl Pts',(-59.0896338466133,-0.144699568925602,
2.71590508903189));
#234857=CARTESIAN_POINT('Ctrl Pts',(-59.0897911602042,-0.144833247842891,
2.71605191409891));
#234858=CARTESIAN_POINT('Ctrl Pts',(-59.0920009418701,-0.146711033601897,
2.71811436362732));
#234859=CARTESIAN_POINT('Ctrl Pts',(-59.0942367399983,-0.148520654544703,
2.72020091026939));
#234860=CARTESIAN_POINT('Ctrl Pts',(-59.0964928714565,-0.150262619641085,
2.72230624862161));
#234861=CARTESIAN_POINT('Ctrl Pts',(-59.1045829576263,-0.156508996678588,
2.7298556175308));
#234862=CARTESIAN_POINT('Ctrl Pts',(-59.1129958342949,-0.161935290145438,
2.73770089914304));
#234863=CARTESIAN_POINT('Ctrl Pts',(-59.1216309196483,-0.166622470787294,
2.74574823347045));
#234864=CARTESIAN_POINT('Ctrl Pts',(-59.1311200109807,-0.171773211443692,
2.75459144546993));
#234865=CARTESIAN_POINT('Ctrl Pts',(-59.1408779306735,-0.176031864362169,
2.76367911754237));
#234866=CARTESIAN_POINT('Ctrl Pts',(-59.1508087658098,-0.179468536017047,
2.77292162564692));
#234867=CARTESIAN_POINT('Ctrl Pts',(-59.1615315754577,-0.183179278917524,
2.78290121484709));
#234868=CARTESIAN_POINT('Ctrl Pts',(-59.172457014285,-0.185932239424576,
2.79306229500181));
#234869=CARTESIAN_POINT('Ctrl Pts',(-59.1834936683142,-0.187766286099724,
2.80331916685261));
#234870=CARTESIAN_POINT('Ctrl Pts',(-59.1944377361557,-0.189584947007655,
2.81348999408699));
#234871=CARTESIAN_POINT('Ctrl Pts',(-59.2054925958117,-0.19049999999981,
2.82375635966878));
#234872=CARTESIAN_POINT('Ctrl Pts',(-59.2165773020941,-0.190499999999811,
2.83404198860261));
#234873=CARTESIAN_POINT('Origin',(1.12442271988212E-14,0.0152400000001895,
2.83404198860262));
#234874=CARTESIAN_POINT('Ctrl Pts',(-62.8464427007196,0.0152400000001907,
2.6587819886026));
#234875=CARTESIAN_POINT('Ctrl Pts',(-62.8464391086779,0.023828933390642,
2.6587819886026));
#234876=CARTESIAN_POINT('Ctrl Pts',(-62.8457180711405,0.0323412407626657,
2.65944603041842));
#234877=CARTESIAN_POINT('Ctrl Pts',(-62.8443658068291,0.0406531130503683,
2.66070439264048));
#234878=CARTESIAN_POINT('Ctrl Pts',(-62.8435017743089,0.0459640037535742,
2.66150842619575));
#234879=CARTESIAN_POINT('Ctrl Pts',(-62.8423809556999,0.0511932363892055,
2.66255428265354));
#234880=CARTESIAN_POINT('Ctrl Pts',(-62.841033859251,0.0563116129576012,
2.66381699700651));
#234881=CARTESIAN_POINT('Ctrl Pts',(-62.8391953428955,0.063297169962393,
2.66554034873251));
#234882=CARTESIAN_POINT('Ctrl Pts',(-62.8369299537504,0.0700734120985513,
2.66766759643955));
#234883=CARTESIAN_POINT('Ctrl Pts',(-62.8343031482014,0.0765705776096623,
2.6701201278313));
#234884=CARTESIAN_POINT('Ctrl Pts',(-62.8329897454269,0.0798191603652178,
2.67134639352718));
#234885=CARTESIAN_POINT('Ctrl Pts',(-62.8315859904681,0.0829981827955089,
2.67265375584994));
#234886=CARTESIAN_POINT('Ctrl Pts',(-62.8301000734874,0.0861004173280608,
2.67403135126922));
#234887=CARTESIAN_POINT('Ctrl Pts',(-62.8293571149971,0.0876515345943367,
2.67472014897886));
#234888=CARTESIAN_POINT('Ctrl Pts',(-62.8285936160519,0.0891834722999017,
2.67542649668614));
#234889=CARTESIAN_POINT('Ctrl Pts',(-62.82781060087,0.0906954364280678,
2.67614899656084));
#234890=CARTESIAN_POINT('Ctrl Pts',(-62.8276148470745,0.0910734274601094,
2.67632962152951));
#234891=CARTESIAN_POINT('Ctrl Pts',(-62.8274178735164,0.0914501705145361,
2.67651125590932));
#234892=CARTESIAN_POINT('Ctrl Pts',(-62.8272196962038,0.0918256539330444,
2.67669387767505));
#234893=CARTESIAN_POINT('Ctrl Pts',(-62.8266251642659,0.0929521041885693,
2.67724174297226));
#234894=CARTESIAN_POINT('Ctrl Pts',(-62.826019798519,0.0940672158688541,
2.67779849504729));
#234895=CARTESIAN_POINT('Ctrl Pts',(-62.8254040313373,0.0951706907490459,
2.6783635361799));
#234896=CARTESIAN_POINT('Ctrl Pts',(-62.8211486980556,0.102796386827685,
2.68226832098886));
#234897=CARTESIAN_POINT('Ctrl Pts',(-62.8164204928785,0.109916699411551,
2.68659153751365));
#234898=CARTESIAN_POINT('Ctrl Pts',(-62.8113377077397,0.116542502759829,
2.69123699486148));
#234899=CARTESIAN_POINT('Ctrl Pts',(-62.8088115774776,0.119835508836568,
2.6935457744119));
#234900=CARTESIAN_POINT('Ctrl Pts',(-62.8061972539433,0.123006400629482,
2.69593478828095));
#234901=CARTESIAN_POINT('Ctrl Pts',(-62.8035061084566,0.126056303770164,
2.69839565261202));
#234902=CARTESIAN_POINT('Ctrl Pts',(-62.7975690395532,0.132784845643478,
2.70382468689028));
#234903=CARTESIAN_POINT('Ctrl Pts',(-62.7912680187378,0.138932019324877,
2.70961155815069));
#234904=CARTESIAN_POINT('Ctrl Pts',(-62.7847385034067,0.144445113413363,
2.7156270136175));
#234905=CARTESIAN_POINT('Ctrl Pts',(-62.7823531891148,0.146459116207659,
2.7178245353584));
#234906=CARTESIAN_POINT('Ctrl Pts',(-62.7799396422115,0.148396130391172,
2.72005051502385));
#234907=CARTESIAN_POINT('Ctrl Pts',(-62.7775029828616,0.150257579786679,
2.72229986760099));
#234908=CARTESIAN_POINT('Ctrl Pts',(-62.7693185019449,0.156509991333616,
2.72985520488837));
#234909=CARTESIAN_POINT('Ctrl Pts',(-62.7608162581028,0.161942805717951,
2.73770845534464));
#234910=CARTESIAN_POINT('Ctrl Pts',(-62.7520965944505,0.166635979461278,
2.74576706701618));
#234911=CARTESIAN_POINT('Ctrl Pts',(-62.7425126511845,0.171794333348195,
2.75462443584854));
#234912=CARTESIAN_POINT('Ctrl Pts',(-62.7326655363515,0.176059615357362,
2.76373036322965));
#234913=CARTESIAN_POINT('Ctrl Pts',(-62.7226511116318,0.179500292056582,
2.77299664636558));
#234914=CARTESIAN_POINT('Ctrl Pts',(-62.7118651471247,0.183206048282925,
2.78297683033166));
#234915=CARTESIAN_POINT('Ctrl Pts',(-62.7008840239677,0.185955767119051,
2.79314401478533));
#234916=CARTESIAN_POINT('Ctrl Pts',(-62.689799127429,0.187785458035066,
2.80341452427521));
#234917=CARTESIAN_POINT('Ctrl Pts',(-62.6788639144194,0.189590441946164,
2.81354634721084));
#234918=CARTESIAN_POINT('Ctrl Pts',(-62.667826278274,0.190500000000189,
2.82378004209064));
#234919=CARTESIAN_POINT('Ctrl Pts',(-62.6567671111299,0.190500000000189,
2.83404198860261));
#234920=CARTESIAN_POINT('Ctrl Pts',(-59.2165773020941,0.190500000000189,
2.8340419886026));
#234921=CARTESIAN_POINT('Ctrl Pts',(-59.2059936184299,0.190500000000189,
2.82422126443094));
#234922=CARTESIAN_POINT('Ctrl Pts',(-59.1954479901474,0.189665225488926,
2.81442815028678));
#234923=CARTESIAN_POINT('Ctrl Pts',(-59.1849969778479,0.188008762314532,
2.80471618166582));
#234924=CARTESIAN_POINT('Ctrl Pts',(-59.174905605952,0.186409301377575,
2.79533842146548));
#234925=CARTESIAN_POINT('Ctrl Pts',(-59.1649012152174,0.184043455438921,
2.78603515650611));
#234926=CARTESIAN_POINT('Ctrl Pts',(-59.1550396955563,0.180877423727649,
2.77685887347177));
#234927=CARTESIAN_POINT('Ctrl Pts',(-59.1457174710397,0.17788453222071,
2.76818441217027));
#234928=CARTESIAN_POINT('Ctrl Pts',(-59.1365220583483,0.174176304388436,
2.75962261522101));
#234929=CARTESIAN_POINT('Ctrl Pts',(-59.1275197082988,0.169686797574166,
2.7512353770216));
#234930=CARTESIAN_POINT('Ctrl Pts',(-59.1192286949288,0.165552037115291,
2.74351087134631));
#234931=CARTESIAN_POINT('Ctrl Pts',(-59.1111009786121,0.160754293905865,
2.73593399450368));
#234932=CARTESIAN_POINT('Ctrl Pts',(-59.1032135992758,0.155213515015811,
2.72857657813105));
#234933=CARTESIAN_POINT('Ctrl Pts',(-59.1008617419736,0.153561366597817,
2.72638274508667));
#234934=CARTESIAN_POINT('Ctrl Pts',(-59.0985314603591,0.151842962928774,
2.72420861709764));
#234935=CARTESIAN_POINT('Ctrl Pts',(-59.096225375957,0.15005568618033,2.72205663736707));
#234936=CARTESIAN_POINT('Ctrl Pts',(-59.0939428540559,0.148286670996897,
2.71992664556746));
#234937=CARTESIAN_POINT('Ctrl Pts',(-59.0916862380348,0.146452235169095,
2.71782089927864));
#234938=CARTESIAN_POINT('Ctrl Pts',(-59.0894604907299,0.144552116610158,
2.71574387311226));
#234939=CARTESIAN_POINT('Ctrl Pts',(-59.0893057166152,0.144419986081611,
2.71559944077466));
#234940=CARTESIAN_POINT('Ctrl Pts',(-59.0891510807051,0.144287542502291,
2.71545515216049));
#234941=CARTESIAN_POINT('Ctrl Pts',(-59.0889965840074,0.144154785044136,
2.7153110078171));
#234942=CARTESIAN_POINT('Ctrl Pts',(-59.0822228828154,0.13833421174979,
2.70899119176073));
#234943=CARTESIAN_POINT('Ctrl Pts',(-59.0757535782847,0.131883990154492,
2.70298296066836));
#234944=CARTESIAN_POINT('Ctrl Pts',(-59.069704769431,0.124808417215811,
2.69736727774142));
#234945=CARTESIAN_POINT('Ctrl Pts',(-59.0640662283035,0.118212753510756,
2.69213248525446));
#234946=CARTESIAN_POINT('Ctrl Pts',(-59.0587927761317,0.111072931138274,
2.68723866185495));
#234947=CARTESIAN_POINT('Ctrl Pts',(-59.0540076654703,0.103389544769389,
2.68278595829597));
#234948=CARTESIAN_POINT('Ctrl Pts',(-59.052257210084,0.100578862633506,
2.6811571017282));
#234949=CARTESIAN_POINT('Ctrl Pts',(-59.0505724231959,0.0976954648443338,
2.67958763637807));
#234950=CARTESIAN_POINT('Ctrl Pts',(-59.048960544286,0.0947395585255326,
2.67808378645345));
#234951=CARTESIAN_POINT('Ctrl Pts',(-59.0485729412563,0.0940287618040365,
2.6777221607858));
#234952=CARTESIAN_POINT('Ctrl Pts',(-59.0481896206935,0.0933131922169409,
2.67736403603543));
#234953=CARTESIAN_POINT('Ctrl Pts',(-59.0478106940137,0.0925929271973547,
2.67700956934459));
#234954=CARTESIAN_POINT('Ctrl Pts',(-59.0474436087926,0.0918951704596305,
2.67666617973784));
#234955=CARTESIAN_POINT('Ctrl Pts',(-59.047080647127,0.0911930071936125,
2.67632622314099));
#234956=CARTESIAN_POINT('Ctrl Pts',(-59.0467219102889,0.0904865115880142,
2.67598984158753));
#234957=CARTESIAN_POINT('Ctrl Pts',(-59.042791533644,0.0827460357498325,
2.6723043929219));
#234958=CARTESIAN_POINT('Ctrl Pts',(-59.0393660724128,0.0744802459940113,
2.66904964539934));
#234959=CARTESIAN_POINT('Ctrl Pts',(-59.0365841602687,0.0658168714602655,
2.6664020356668));
#234960=CARTESIAN_POINT('Ctrl Pts',(-59.0354304183828,0.0622239118140033,
2.66530399299404));
#234961=CARTESIAN_POINT('Ctrl Pts',(-59.0343871039216,0.0585629032864118,
2.66430995142232));
#234962=CARTESIAN_POINT('Ctrl Pts',(-59.0334626554261,0.0548440715001653,
2.66343053473339));
#234963=CARTESIAN_POINT('Ctrl Pts',(-59.0318859121827,0.0485012163585984,
2.66193059792863));
#234964=CARTESIAN_POINT('Ctrl Pts',(-59.0306571138137,0.0419914004946155,
2.66076519817106));
#234965=CARTESIAN_POINT('Ctrl Pts',(-59.0298212958155,0.0353717968090289,
2.65997805604438));
#234966=CARTESIAN_POINT('Ctrl Pts',(-59.0294033868165,0.0320619949662357,
2.65958448498104));
#234967=CARTESIAN_POINT('Ctrl Pts',(-59.0290851681637,0.02872467855488,
2.65928526260739));
#234968=CARTESIAN_POINT('Ctrl Pts',(-59.0288723192864,0.025367036875067,
2.65908463971302));
#234969=CARTESIAN_POINT('Ctrl Pts',(-59.0286594704092,0.022009395195254,
2.65888401681864));
#234970=CARTESIAN_POINT('Ctrl Pts',(-59.0285519740191,0.0186314705081981,
2.65878198860261));
#234971=CARTESIAN_POINT('Ctrl Pts',(-59.0285534841296,0.0152400000001907,
2.65878198860261));
#234972=CARTESIAN_POINT('Origin',(-57.9430040808457,-6.10537907909404,2.83404198860257));
#234973=CARTESIAN_POINT('Ctrl Pts',(-62.2936141127569,-6.73887200051357,
2.83404198860256));
#234974=CARTESIAN_POINT('Ctrl Pts',(-62.3041663177858,-6.7399810819535,
2.82419652440043));
#234975=CARTESIAN_POINT('Ctrl Pts',(-62.3147747227674,-6.74025426844116,
2.81438790575611));
#234976=CARTESIAN_POINT('Ctrl Pts',(-62.3253809467531,-6.73970068257615,
2.80466781256847));
#234977=CARTESIAN_POINT('Ctrl Pts',(-62.3356425316152,-6.73916508495536,
2.7952635645301));
#234978=CARTESIAN_POINT('Ctrl Pts',(-62.3459033574839,-6.73785543637658,
2.7859410249615));
#234979=CARTESIAN_POINT('Ctrl Pts',(-62.3561113603662,-6.73573381164783,
2.77675109088682));
#234980=CARTESIAN_POINT('Ctrl Pts',(-62.3657675025203,-6.73372688529656,
2.7680579791357));
#234981=CARTESIAN_POINT('Ctrl Pts',(-62.3753772873497,-6.7309932174379,
2.75948271210035));
#234982=CARTESIAN_POINT('Ctrl Pts',(-62.3848821415129,-6.7274611770454,
2.75108575573083));
#234983=CARTESIAN_POINT('Ctrl Pts',(-62.3936367996058,-6.72420791240022,
2.74335155163112));
#234984=CARTESIAN_POINT('Ctrl Pts',(-62.4023029415022,-6.72027708243635,
2.73576818685769));
#234985=CARTESIAN_POINT('Ctrl Pts',(-62.4108128192413,-6.71558140886203,
2.72840626160309));
#234986=CARTESIAN_POINT('Ctrl Pts',(-62.4132812112875,-6.71421937245472,
2.72627084693553));
#234987=CARTESIAN_POINT('Ctrl Pts',(-62.4157362792965,-6.71279278199497,
2.72415424587456));
#234988=CARTESIAN_POINT('Ctrl Pts',(-62.4181758915949,-6.71129899689621,
2.72205867173251));
#234989=CARTESIAN_POINT('Ctrl Pts',(-62.42082058818,-6.70967963780692,2.71978693462854));
#234990=CARTESIAN_POINT('Ctrl Pts',(-62.4234440047028,-6.70798448411198,
2.71754411340754));
#234991=CARTESIAN_POINT('Ctrl Pts',(-62.4260429761973,-6.70621108803147,
2.71533341844251));
#234992=CARTESIAN_POINT('Ctrl Pts',(-62.4331758738575,-6.70134398857293,
2.70926614876399));
#234993=CARTESIAN_POINT('Ctrl Pts',(-62.4400912556837,-6.69585818364719,
2.70347381860416));
#234994=CARTESIAN_POINT('Ctrl Pts',(-62.4466864116141,-6.68976801333912,
2.69804914171402));
#234995=CARTESIAN_POINT('Ctrl Pts',(-62.4527206212311,-6.68419583815025,
2.69308585687207));
#234996=CARTESIAN_POINT('Ctrl Pts',(-62.4584752900415,-6.6781162068933,
2.68842799053184));
#234997=CARTESIAN_POINT('Ctrl Pts',(-62.4638645712588,-6.67150703079182,
2.68414767054212));
#234998=CARTESIAN_POINT('Ctrl Pts',(-62.4665117685878,-6.66826062508068,
2.68204519134551));
#234999=CARTESIAN_POINT('Ctrl Pts',(-62.46907032323,-6.66488629457996,2.68003431778505));
#235000=CARTESIAN_POINT('Ctrl Pts',(-62.4715267736418,-6.66138078591736,
2.67812693945259));
#235001=CARTESIAN_POINT('Ctrl Pts',(-62.4719928611813,-6.66071564979273,
2.67776503299211));
#235002=CARTESIAN_POINT('Ctrl Pts',(-62.4724551899379,-6.66004526561014,
2.67740659639931));
#235003=CARTESIAN_POINT('Ctrl Pts',(-62.4729136358128,-6.65936969820883,
2.67705178968862));
#235004=CARTESIAN_POINT('Ctrl Pts',(-62.4733577552541,-6.6587152422888,
2.67670807068765));
#235005=CARTESIAN_POINT('Ctrl Pts',(-62.4737982306998,-6.65805592206477,
2.67636775825272));
#235006=CARTESIAN_POINT('Ctrl Pts',(-62.4742349489458,-6.65739180030934,
2.67603099699262));
#235007=CARTESIAN_POINT('Ctrl Pts',(-62.4789942144024,-6.65015433826441,
2.67236104217138));
#235008=CARTESIAN_POINT('Ctrl Pts',(-62.4833100626577,-6.64234165497498,
2.66911440541486));
#235009=CARTESIAN_POINT('Ctrl Pts',(-62.4870273554126,-6.63406423386192,
2.66646778189644));
#235010=CARTESIAN_POINT('Ctrl Pts',(-62.4885971912262,-6.63056862752551,
2.66535009634985));
#235011=CARTESIAN_POINT('Ctrl Pts',(-62.4900605069389,-6.62699051141405,
2.66433897912353));
#235012=CARTESIAN_POINT('Ctrl Pts',(-62.491407022622,-6.62333954252025,
2.663445648848));
#235013=CARTESIAN_POINT('Ctrl Pts',(-62.4936745213867,-6.61719140213097,
2.66194130298593));
#235014=CARTESIAN_POINT('Ctrl Pts',(-62.495608491139,-6.6108377018855,2.66077206705428));
#235015=CARTESIAN_POINT('Ctrl Pts',(-62.497156159322,-6.6043306253617,2.65998225155722));
#235016=CARTESIAN_POINT('Ctrl Pts',(-62.4975430763677,-6.60270385623075,
2.65978479768295));
#235017=CARTESIAN_POINT('Ctrl Pts',(-62.4979056188881,-6.60106746196581,
2.6596109896663));
#235018=CARTESIAN_POINT('Ctrl Pts',(-62.4982426563693,-6.5994222184577,
2.65946139030509));
#235019=CARTESIAN_POINT('Ctrl Pts',(-62.4987482125911,-6.59695435319553,
2.65923699126328));
#235020=CARTESIAN_POINT('Ctrl Pts',(-62.4991963674672,-6.59446659126626,
2.65906707562449));
#235021=CARTESIAN_POINT('Ctrl Pts',(-62.499584972412,-6.59196174500319,
2.65895332562927));
#235022=CARTESIAN_POINT('Ctrl Pts',(-62.4999735773569,-6.58945689874012,
2.65883957563405));
#235023=CARTESIAN_POINT('Ctrl Pts',(-62.5003026407461,-6.58693497617675,
2.65878198860256));
#235024=CARTESIAN_POINT('Ctrl Pts',(-62.500570298093,-6.58439859103053,
2.65878198860256));
#235025=CARTESIAN_POINT('Ctrl Pts',(-58.7035958781038,-6.1853204982942,
2.65878198860256));
#235026=CARTESIAN_POINT('Ctrl Pts',(-58.7026899760169,-6.19390281910169,
2.65878198860256));
#235027=CARTESIAN_POINT('Ctrl Pts',(-58.7025003609928,-6.20248552904371,
2.65945335517847));
#235028=CARTESIAN_POINT('Ctrl Pts',(-58.7029569544313,-6.21093474935418,
2.66072561226587));
#235029=CARTESIAN_POINT('Ctrl Pts',(-58.7032518669434,-6.21639207873494,
2.66154735980326));
#235030=CARTESIAN_POINT('Ctrl Pts',(-58.7038154335198,-6.22179377937522,
2.66261895766873));
#235031=CARTESIAN_POINT('Ctrl Pts',(-58.7046202140516,-6.22710604846881,
2.66391429251021));
#235032=CARTESIAN_POINT('Ctrl Pts',(-58.7056869045457,-6.23414715684659,
2.66563118464117));
#235033=CARTESIAN_POINT('Ctrl Pts',(-58.7071827955652,-6.24102913891662,
2.66774105138693));
#235034=CARTESIAN_POINT('Ctrl Pts',(-58.7090548163569,-6.24767922440765,
2.67016894181744));
#235035=CARTESIAN_POINT('Ctrl Pts',(-58.7099908267528,-6.25100426715317,
2.67138288703269));
#235036=CARTESIAN_POINT('Ctrl Pts',(-58.7110208470228,-6.25427153376681,
2.67267613167545));
#235037=CARTESIAN_POINT('Ctrl Pts',(-58.7121380880307,-6.25747333351537,
2.67403835432547));
#235038=CARTESIAN_POINT('Ctrl Pts',(-58.7126967085347,-6.25907423338965,
2.67471946565048));
#235039=CARTESIAN_POINT('Ctrl Pts',(-58.7132771324571,-6.26065878288363,
2.67541781389518));
#235040=CARTESIAN_POINT('Ctrl Pts',(-58.7138784999415,-6.26222612320535,
2.67613207244164));
#235041=CARTESIAN_POINT('Ctrl Pts',(-58.7140288418126,-6.26261795828578,
2.67631063707825));
#235042=CARTESIAN_POINT('Ctrl Pts',(-58.7141804926178,-6.26300871814029,
2.6764901960184));
#235043=CARTESIAN_POINT('Ctrl Pts',(-58.7143334388435,-6.26339839005073,
2.67667072836651));
#235044=CARTESIAN_POINT('Ctrl Pts',(-58.7147922775207,-6.26456740578205,
2.67721232541085));
#235045=CARTESIAN_POINT('Ctrl Pts',(-58.715262775183,-6.2657266282839,2.67776268340042));
#235046=CARTESIAN_POINT('Ctrl Pts',(-58.7157445651923,-6.26687572965184,
2.67832123541511));
#235047=CARTESIAN_POINT('Ctrl Pts',(-58.7191382318077,-6.27496985131151,
2.68225560368434));
#235048=CARTESIAN_POINT('Ctrl Pts',(-58.7230632421216,-6.28260716192766,
2.68661792998871));
#235049=CARTESIAN_POINT('Ctrl Pts',(-58.7274000190311,-6.28978339589433,
2.69130986622554));
#235050=CARTESIAN_POINT('Ctrl Pts',(-58.729503351146,-6.29326386161364,
2.69358545023036));
#235051=CARTESIAN_POINT('Ctrl Pts',(-58.7317041096969,-6.29663597408935,
2.69593918853458));
#235052=CARTESIAN_POINT('Ctrl Pts',(-58.7339915094193,-6.29989941779167,
2.6983630623547));
#235053=CARTESIAN_POINT('Ctrl Pts',(-58.7374933585782,-6.30489552208956,
2.70207384382203));
#235054=CARTESIAN_POINT('Ctrl Pts',(-58.7411954596216,-6.30963480180892,
2.70594760814204));
#235055=CARTESIAN_POINT('Ctrl Pts',(-58.7450534628849,-6.31410463171066,
2.70995196345684));
#235056=CARTESIAN_POINT('Ctrl Pts',(-58.7468451395591,-6.31618044384087,
2.71181160678082));
#235057=CARTESIAN_POINT('Ctrl Pts',(-58.7486702031823,-6.31819823791547,
2.71369962772075));
#235058=CARTESIAN_POINT('Ctrl Pts',(-58.7505249478605,-6.32015576082336,
2.71561183138637));
#235059=CARTESIAN_POINT('Ctrl Pts',(-58.750667106732,-6.32030579724123,
2.71575839426288));
#235060=CARTESIAN_POINT('Ctrl Pts',(-58.7508094261758,-6.3204555105821,
2.71590508903185));
#235061=CARTESIAN_POINT('Ctrl Pts',(-58.7509519047345,-6.32060490094019,
2.71605191409887));
#235062=CARTESIAN_POINT('Ctrl Pts',(-58.7529532989256,-6.32270338507403,
2.71811436362729));
#235063=CARTESIAN_POINT('Ctrl Pts',(-58.7549876922214,-6.32473679726649,
2.72020091026935));
#235064=CARTESIAN_POINT('Ctrl Pts',(-58.7570493794209,-6.32670504965006,
2.72230624862158));
#235065=CARTESIAN_POINT('Ctrl Pts',(-58.7644422230593,-6.33376285265554,
2.7298556175307));
#235066=CARTESIAN_POINT('Ctrl Pts',(-58.7722418109919,-6.34003880538879,
2.73770089914288));
#235067=CARTESIAN_POINT('Ctrl Pts',(-58.7803396486547,-6.3456029213668,
2.74574823347021));
#235068=CARTESIAN_POINT('Ctrl Pts',(-58.7892383587461,-6.35171732586157,
2.75459144546946));
#235069=CARTESIAN_POINT('Ctrl Pts',(-58.7984976730884,-6.35697262978384,
2.76367911754164));
#235070=CARTESIAN_POINT('Ctrl Pts',(-58.8080148760636,-6.3614285299275,
2.77292162564593));
#235071=CARTESIAN_POINT('Ctrl Pts',(-58.8182910667848,-6.36623978380432,
2.78290121484556));
#235072=CARTESIAN_POINT('Ctrl Pts',(-58.8288688921832,-6.37011968263671,
2.79306229499971));
#235073=CARTESIAN_POINT('Ctrl Pts',(-58.8396533761857,-6.37309732669757,
2.80331916684993));
#235074=CARTESIAN_POINT('Ctrl Pts',(-58.8503473894494,-6.37604999138454,
2.81348999408516));
#235075=CARTESIAN_POINT('Ctrl Pts',(-58.8612460403454,-6.37811557911242,
2.82375635966784));
#235076=CARTESIAN_POINT('Ctrl Pts',(-58.872270023448,-6.37927424642599,
2.83404198860256));
#235077=CARTESIAN_POINT('Origin',(-0.00159301378018793,0.0151565136856025,
2.83404198860262));
#235078=CARTESIAN_POINT('Ctrl Pts',(-62.5037563256534,-6.5540855636597,
2.65878198860256));
#235079=CARTESIAN_POINT('Ctrl Pts',(-62.5046505412977,-6.54554330587448,
2.65878198860256));
#235080=CARTESIAN_POINT('Ctrl Pts',(-62.5048232320878,-6.53700226086719,
2.65944603041837));
#235081=CARTESIAN_POINT('Ctrl Pts',(-62.5043472028589,-6.5285945717752,
2.66070439264043));
#235082=CARTESIAN_POINT('Ctrl Pts',(-62.5040430428431,-6.5232224586954,
2.6615084261957));
#235083=CARTESIAN_POINT('Ctrl Pts',(-62.5034749678471,-6.51790471489647,
2.66255428265349));
#235084=CARTESIAN_POINT('Ctrl Pts',(-62.5026702669707,-6.51267356740878,
2.66381699700646));
#235085=CARTESIAN_POINT('Ctrl Pts',(-62.5015720117389,-6.50553410072683,
2.66554034873246));
#235086=CARTESIAN_POINT('Ctrl Pts',(-62.5000273428098,-6.49855818190805,
2.66766759643951));
#235087=CARTESIAN_POINT('Ctrl Pts',(-62.4980940659029,-6.49182203260206,
2.67012012783127));
#235088=CARTESIAN_POINT('Ctrl Pts',(-62.4971274274494,-6.48845395794907,
2.67134639352714));
#235089=CARTESIAN_POINT('Ctrl Pts',(-62.4960636607365,-6.48514561818763,
2.67265375584991));
#235090=CARTESIAN_POINT('Ctrl Pts',(-62.4949101555729,-6.4819050574019,
2.67403135126919));
#235091=CARTESIAN_POINT('Ctrl Pts',(-62.4943334029911,-6.48028477700904,
2.67472014897882));
#235092=CARTESIAN_POINT('Ctrl Pts',(-62.4937342176673,-6.47868142404706,
2.67542649668611));
#235093=CARTESIAN_POINT('Ctrl Pts',(-62.4931135352113,-6.47709589524291,
2.67614899656081));
#235094=CARTESIAN_POINT('Ctrl Pts',(-62.4929583645973,-6.47669951304187,
2.67632962152948));
#235095=CARTESIAN_POINT('Ctrl Pts',(-62.4928018504534,-6.47630424448198,
2.67651125590929));
#235096=CARTESIAN_POINT('Ctrl Pts',(-62.4926440074816,-6.47591010283098,
2.67669387767502));
#235097=CARTESIAN_POINT('Ctrl Pts',(-62.492170478566,-6.47472767787799,
2.67724174297223));
#235098=CARTESIAN_POINT('Ctrl Pts',(-62.4916849899864,-6.47355539694492,
2.67779849504726));
#235099=CARTESIAN_POINT('Ctrl Pts',(-62.4911879405752,-6.47239360181834,
2.67836353617988));
#235100=CARTESIAN_POINT('Ctrl Pts',(-62.4877530207469,-6.46436487665208,
2.68226832098884));
#235101=CARTESIAN_POINT('Ctrl Pts',(-62.4837949925048,-6.45678933786437,
2.68659153751363));
#235102=CARTESIAN_POINT('Ctrl Pts',(-62.4794326364367,-6.44966853564042,
2.69123699486146));
#235103=CARTESIAN_POINT('Ctrl Pts',(-62.4772645574453,-6.44612951648122,
2.69354577441187));
#235104=CARTESIAN_POINT('Ctrl Pts',(-62.4749960038951,-6.4427027239438,
2.69593478828092));
#235105=CARTESIAN_POINT('Ctrl Pts',(-62.4726384024733,-6.43938822718948,
2.69839565261198));
#235106=CARTESIAN_POINT('Ctrl Pts',(-62.4674371815967,-6.43207595228378,
2.70382468689023));
#235107=CARTESIAN_POINT('Ctrl Pts',(-62.4618132330509,-6.42530381744014,
2.70961155815065));
#235108=CARTESIAN_POINT('Ctrl Pts',(-62.455895762341,-6.41913840445449,
2.71562701361744));
#235109=CARTESIAN_POINT('Ctrl Pts',(-62.4537340356674,-6.41688610134088,
2.71782453535834));
#235110=CARTESIAN_POINT('Ctrl Pts',(-62.4515361835425,-6.41470741397492,
2.72005051502378));
#235111=CARTESIAN_POINT('Ctrl Pts',(-62.4493074469122,-6.41260146153662,
2.72229986760091));
#235112=CARTESIAN_POINT('Ctrl Pts',(-62.4418213564087,-6.40552779014116,
2.72985520488862));
#235113=CARTESIAN_POINT('Ctrl Pts',(-62.4339335724863,-6.39923601079906,
2.73770845534524));
#235114=CARTESIAN_POINT('Ctrl Pts',(-62.4257522463026,-6.39365709371056,
2.74576706701716));
#235115=CARTESIAN_POINT('Ctrl Pts',(-62.416759999685,-6.38752520296414,
2.75462443584989));
#235116=CARTESIAN_POINT('Ctrl Pts',(-62.4074126717507,-6.38225398283486,
2.76373036323139));
#235117=CARTESIAN_POINT('Ctrl Pts',(-62.3978127557451,-6.37778536209609,
2.77299664636773));
#235118=CARTESIAN_POINT('Ctrl Pts',(-62.3874732348832,-6.37297246609526,
2.78297683033423));
#235119=CARTESIAN_POINT('Ctrl Pts',(-62.3768396913517,-6.36908997057808,
2.79314401478834));
#235120=CARTESIAN_POINT('Ctrl Pts',(-62.3660067738154,-6.36611161569978,
2.80341452427867));
#235121=CARTESIAN_POINT('Ctrl Pts',(-62.3553201372425,-6.36317347866857,
2.81354634721315));
#235122=CARTESIAN_POINT('Ctrl Pts',(-62.3444380411298,-6.36111515612471,
2.82378004209176));
#235123=CARTESIAN_POINT('Ctrl Pts',(-62.3334394572619,-6.35995915837826,
2.83404198860256));
#235124=CARTESIAN_POINT('Ctrl Pts',(-58.9120953679529,-6.00036140429068,
2.83404198860256));
#235125=CARTESIAN_POINT('Ctrl Pts',(-58.9015696628148,-5.9992551081015,
2.82422126443049));
#235126=CARTESIAN_POINT('Ctrl Pts',(-58.8909945468901,-5.9989829913121,
2.81442815028591));
#235127=CARTESIAN_POINT('Ctrl Pts',(-58.8804276387791,-5.99953795195274,
2.80471618166455));
#235128=CARTESIAN_POINT('Ctrl Pts',(-58.8702243592803,-6.00007381527886,
2.79533842146398));
#235129=CARTESIAN_POINT('Ctrl Pts',(-58.8600274754043,-6.00138095727662,
2.7860351565044));
#235130=CARTESIAN_POINT('Ctrl Pts',(-58.8498890377501,-6.00349883563941,
2.77685887346985));
#235131=CARTESIAN_POINT('Ctrl Pts',(-58.8403050390047,-6.00550089397069,
2.76818441216827));
#235132=CARTESIAN_POINT('Ctrl Pts',(-58.8307723843893,-6.0082276253853,
2.75962261521893));
#235133=CARTESIAN_POINT('Ctrl Pts',(-58.8213500689071,-6.0117515363952,
2.75123537701946));
#235134=CARTESIAN_POINT('Ctrl Pts',(-58.8126722744191,-6.01499699931729,
2.74351087134419));
#235135=CARTESIAN_POINT('Ctrl Pts',(-58.804087581858,-6.01891888229111,
2.7359339945016));
#235136=CARTESIAN_POINT('Ctrl Pts',(-58.7956642413083,-6.02360485257358,
2.72857657812899));
#235137=CARTESIAN_POINT('Ctrl Pts',(-58.793152571192,-6.02500211431966,
2.7263827450853));
#235138=CARTESIAN_POINT('Ctrl Pts',(-58.7906554330099,-6.02646752363703,
2.72420861709694));
#235139=CARTESIAN_POINT('Ctrl Pts',(-58.7881751602883,-6.02800395803725,
2.72205663736702));
#235140=CARTESIAN_POINT('Ctrl Pts',(-58.7857202298424,-6.02952469386373,
2.71992664556741));
#235141=CARTESIAN_POINT('Ctrl Pts',(-58.7832842250419,-6.03111319985525,
2.7178208992786));
#235142=CARTESIAN_POINT('Ctrl Pts',(-58.7808720541407,-6.03277025542051,
2.71574387311221));
#235143=CARTESIAN_POINT('Ctrl Pts',(-58.7807043164936,-6.03288548382383,
2.71559944077462));
#235144=CARTESIAN_POINT('Ctrl Pts',(-58.7805366835714,-6.03300103800931,
2.71545515216044));
#235145=CARTESIAN_POINT('Ctrl Pts',(-58.7803691562897,-6.03311691890583,
2.71531100781706));
#235146=CARTESIAN_POINT('Ctrl Pts',(-58.7730241465597,-6.03819756191456,
2.70899119176053));
#235147=CARTESIAN_POINT('Ctrl Pts',(-58.7659160498048,-6.0439362220602,
2.70298296066802));
#235148=CARTESIAN_POINT('Ctrl Pts',(-58.7591607781927,-6.05034076157611,
2.69736727774095));
#235149=CARTESIAN_POINT('Ctrl Pts',(-58.7528636909919,-6.05631090550645,
2.69213248525377));
#235150=CARTESIAN_POINT('Ctrl Pts',(-58.746872812682,-6.06286038933366,
2.68723866185407));
#235151=CARTESIAN_POINT('Ctrl Pts',(-58.7413107827875,-6.0700015050445,
2.68278595829494));
#235152=CARTESIAN_POINT('Ctrl Pts',(-58.739276120295,-6.07261381755752,
2.68115710172752));
#235153=CARTESIAN_POINT('Ctrl Pts',(-58.7372991657062,-6.07530531160704,
2.67958763637771));
#235154=CARTESIAN_POINT('Ctrl Pts',(-58.735387140493,-6.07807653793576,
2.67808378645339));
#235155=CARTESIAN_POINT('Ctrl Pts',(-58.7349273623043,-6.0787429252894,
2.67772216078575));
#235156=CARTESIAN_POINT('Ctrl Pts',(-58.7344713442222,-6.07941450700205,
2.67736403603538));
#235157=CARTESIAN_POINT('Ctrl Pts',(-58.7340192051468,-6.08009121771096,
2.67700956934454));
#235158=CARTESIAN_POINT('Ctrl Pts',(-58.7335811954174,-6.08074678121022,
2.67666617973778));
#235159=CARTESIAN_POINT('Ctrl Pts',(-58.7331468260467,-6.08140715812728,
2.67632622314093));
#235160=CARTESIAN_POINT('Ctrl Pts',(-58.7327162055066,-6.08207228526562,
2.67598984158748));
#235161=CARTESIAN_POINT('Ctrl Pts',(-58.7279982598321,-6.08935952173613,
2.67230439292203));
#235162=CARTESIAN_POINT('Ctrl Pts',(-58.7237275533352,-6.09722197243188,
2.66904964539963));
#235163=CARTESIAN_POINT('Ctrl Pts',(-58.7200553115703,-6.10554709909163,
2.66640203566715));
#235164=CARTESIAN_POINT('Ctrl Pts',(-58.7185323234525,-6.10899977726308,
2.66530399299424));
#235165=CARTESIAN_POINT('Ctrl Pts',(-58.7171120447815,-6.112531674346,2.66430995142237));
#235166=CARTESIAN_POINT('Ctrl Pts',(-58.7158039367398,-6.11613350280247,
2.66343053473334));
#235167=CARTESIAN_POINT('Ctrl Pts',(-58.7135728221601,-6.1222767965717,
2.66193059792858));
#235168=CARTESIAN_POINT('Ctrl Pts',(-58.7116702942287,-6.12862250657808,
2.660765198171));
#235169=CARTESIAN_POINT('Ctrl Pts',(-58.7101471179288,-6.1351184806112,
2.65997805604432));
#235170=CARTESIAN_POINT('Ctrl Pts',(-58.7093855297788,-6.13836646762777,
2.65958448498099));
#235171=CARTESIAN_POINT('Ctrl Pts',(-58.7087202098051,-6.14165223896384,
2.65928526260735));
#235172=CARTESIAN_POINT('Ctrl Pts',(-58.7081575578111,-6.14496923836515,
2.65908463971297));
#235173=CARTESIAN_POINT('Ctrl Pts',(-58.7075949058172,-6.14828623776645,
2.65888401681859));
#235174=CARTESIAN_POINT('Ctrl Pts',(-58.7071349090266,-6.15163442139613,
2.65878198860256));
#235175=CARTESIAN_POINT('Ctrl Pts',(-58.7067819056642,-6.15500747092338,
2.65878198860256));
#235176=CARTESIAN_POINT('Origin',(-56.9874003490101,-12.1286263473646,2.83404198860252));
#235177=CARTESIAN_POINT('Ctrl Pts',(-61.2479592423877,-13.2134115091896,
2.83404198860251));
#235178=CARTESIAN_POINT('Ctrl Pts',(-61.2583377107547,-13.2156175207411,
2.82419652440056));
#235179=CARTESIAN_POINT('Ctrl Pts',(-61.26885944602,-13.2169980909551,2.81438790575639));
#235180=CARTESIAN_POINT('Ctrl Pts',(-61.2794654334806,-13.2175561899857,
2.80466781256888));
#235181=CARTESIAN_POINT('Ctrl Pts',(-61.2897267895032,-13.218096154121,
2.79526356453059));
#235182=CARTESIAN_POINT('Ctrl Pts',(-61.3000683010475,-13.2178662282941,
2.78594102496206));
#235183=CARTESIAN_POINT('Ctrl Pts',(-61.3104421535944,-13.216823252902,
2.77675109088744));
#235184=CARTESIAN_POINT('Ctrl Pts',(-61.3202551793187,-13.2158366624037,
2.76805797913636));
#235185=CARTESIAN_POINT('Ctrl Pts',(-61.3300980668416,-13.2141224659042,
2.75948271210104));
#235186=CARTESIAN_POINT('Ctrl Pts',(-61.3399200511735,-13.2116033021979,
2.75108575573156));
#235187=CARTESIAN_POINT('Ctrl Pts',(-61.3489668090872,-13.2092829702338,
2.74335155163188));
#235188=CARTESIAN_POINT('Ctrl Pts',(-61.357996360567,-13.2062795322627,
2.73576818685848));
#235189=CARTESIAN_POINT('Ctrl Pts',(-61.3669504518481,-13.2024991065223,
2.72840626160392));
#235190=CARTESIAN_POINT('Ctrl Pts',(-61.3695476933574,-13.2014025487201,
2.72627084693605));
#235191=CARTESIAN_POINT('Ctrl Pts',(-61.3721384315557,-13.2002403977583,
2.72415424587479));
#235192=CARTESIAN_POINT('Ctrl Pts',(-61.3747208224638,-13.1990098046949,
2.72205867173245));
#235193=CARTESIAN_POINT('Ctrl Pts',(-61.3775203002415,-13.197675762694,
2.71978693462848));
#235194=CARTESIAN_POINT('Ctrl Pts',(-61.3803065372248,-13.196264116926,
2.71754411340749));
#235195=CARTESIAN_POINT('Ctrl Pts',(-61.3830766416485,-13.1947721021912,
2.71533341844247));
#235196=CARTESIAN_POINT('Ctrl Pts',(-61.3906792149761,-13.1906772560438,
2.70926614876395));
#235197=CARTESIAN_POINT('Ctrl Pts',(-61.3981301363757,-13.1859443571666,
2.70347381860412));
#235198=CARTESIAN_POINT('Ctrl Pts',(-61.4053257594952,-13.1805769309632,
2.69804914171398));
#235199=CARTESIAN_POINT('Ctrl Pts',(-61.4119093639901,-13.1756660273913,
2.69308585687203));
#235200=CARTESIAN_POINT('Ctrl Pts',(-61.4182680026353,-13.1702212276778,
2.68842799053179));
#235201=CARTESIAN_POINT('Ctrl Pts',(-61.4243186078275,-13.1642115906183,
2.68414767054208));
#235202=CARTESIAN_POINT('Ctrl Pts',(-61.4272906453326,-13.1612596765261,
2.68204519134548));
#235203=CARTESIAN_POINT('Ctrl Pts',(-61.4301878975266,-13.1581712727459,
2.68003431778503));
#235204=CARTESIAN_POINT('Ctrl Pts',(-61.4329973166795,-13.1549417366132,
2.67812693945258));
#235205=CARTESIAN_POINT('Ctrl Pts',(-61.4335303765996,-13.1543289635881,
2.6777650329921));
#235206=CARTESIAN_POINT('Ctrl Pts',(-61.4340602468994,-13.1537105783546,
2.6774065963993));
#235207=CARTESIAN_POINT('Ctrl Pts',(-61.434586797382,-13.153086632425,2.67705178968862));
#235208=CARTESIAN_POINT('Ctrl Pts',(-61.4350968931622,-13.1524821848057,
2.67670807068764));
#235209=CARTESIAN_POINT('Ctrl Pts',(-61.4356038733672,-13.1518725186283,
2.67636775825272));
#235210=CARTESIAN_POINT('Ctrl Pts',(-61.4361076188514,-13.1512576844885,
2.67603099699261));
#235211=CARTESIAN_POINT('Ctrl Pts',(-61.4415973333394,-13.1445573487223,
2.67236104217134));
#235212=CARTESIAN_POINT('Ctrl Pts',(-61.4467061867047,-13.1372385931151,
2.6691144054148));
#235213=CARTESIAN_POINT('Ctrl Pts',(-61.4512683418497,-13.1293950794801,
2.66646778189636));
#235214=CARTESIAN_POINT('Ctrl Pts',(-61.453194968297,-13.1260827149662,
2.66535009634979));
#235215=CARTESIAN_POINT('Ctrl Pts',(-61.4550242827916,-13.122677158292,
2.6643389791235));
#235216=CARTESIAN_POINT('Ctrl Pts',(-61.4567450522888,-13.119186939003,
2.66344564884798));
#235217=CARTESIAN_POINT('Ctrl Pts',(-61.4596427851247,-13.1133094969314,
2.66194130298591));
#235218=CARTESIAN_POINT('Ctrl Pts',(-61.4622303029112,-13.1071927578069,
2.66077206705424));
#235219=CARTESIAN_POINT('Ctrl Pts',(-61.4644496675151,-13.1008831031059,
2.65998225155718));
#235220=CARTESIAN_POINT('Ctrl Pts',(-61.4650045086661,-13.0993056894307,
2.65978479768292));
#235221=CARTESIAN_POINT('Ctrl Pts',(-61.4655361149185,-13.0977161555173,
2.65961098966626));
#235222=CARTESIAN_POINT('Ctrl Pts',(-61.4660432808487,-13.0961151548352,
2.65946139030505));
#235223=CARTESIAN_POINT('Ctrl Pts',(-61.4668040297441,-13.0937136538121,
2.65923699126324));
#235224=CARTESIAN_POINT('Ctrl Pts',(-61.4675097715122,-13.0912863650435,
2.65906707562445));
#235225=CARTESIAN_POINT('Ctrl Pts',(-61.4681580753692,-13.0888358608681,
2.65895332562923));
#235226=CARTESIAN_POINT('Ctrl Pts',(-61.4688063792261,-13.0863853566926,
2.658839575634));
#235227=CARTESIAN_POINT('Ctrl Pts',(-61.4693972526618,-13.0839116459753,
2.65878198860252));
#235228=CARTESIAN_POINT('Ctrl Pts',(-61.4699285681953,-13.0814171332235,
2.65878198860252));
#235229=CARTESIAN_POINT('Ctrl Pts',(-57.7354693911204,-12.2876333308473,
2.65878198860252));
#235230=CARTESIAN_POINT('Ctrl Pts',(-57.7336713548546,-12.2960739442503,
2.65878198860252));
#235231=CARTESIAN_POINT('Ctrl Pts',(-57.7325856410806,-12.3045898170421,
2.65945335517841));
#235232=CARTESIAN_POINT('Ctrl Pts',(-57.7321565492375,-12.31304047865,2.66072561226578));
#235233=CARTESIAN_POINT('Ctrl Pts',(-57.7318793999343,-12.3184987389612,
2.66154735980318));
#235234=CARTESIAN_POINT('Ctrl Pts',(-57.7318752477671,-12.3239297572686,
2.66261895766868));
#235235=CARTESIAN_POINT('Ctrl Pts',(-57.7321203363021,-12.3292970476686,
2.66391429251019));
#235236=CARTESIAN_POINT('Ctrl Pts',(-57.7324451871156,-12.3364110836361,
2.66563118464116));
#235237=CARTESIAN_POINT('Ctrl Pts',(-57.7332135204776,-12.3434117286777,
2.66774105138691));
#235238=CARTESIAN_POINT('Ctrl Pts',(-57.7343801629265,-12.3502210637612,
2.67016894181741));
#235239=CARTESIAN_POINT('Ctrl Pts',(-57.734963484151,-12.3536257313029,
2.67138288703267));
#235240=CARTESIAN_POINT('Ctrl Pts',(-57.735646339504,-12.3569827659241,
2.67267613167543));
#235241=CARTESIAN_POINT('Ctrl Pts',(-57.7364227809414,-12.3602838093643,
2.67403835432544));
#235242=CARTESIAN_POINT('Ctrl Pts',(-57.7368110016601,-12.3619343310844,
2.67471946565045));
#235243=CARTESIAN_POINT('Ctrl Pts',(-57.7372226154359,-12.3635708710711,
2.67541781389514));
#235244=CARTESIAN_POINT('Ctrl Pts',(-57.7376568568911,-12.3651924853575,
2.6761320724416));
#235245=CARTESIAN_POINT('Ctrl Pts',(-57.7377654172549,-12.3655978889291,
2.67631063707821));
#235246=CARTESIAN_POINT('Ctrl Pts',(-57.737875391774,-12.3660023599859,
2.67649019601836));
#235247=CARTESIAN_POINT('Ctrl Pts',(-57.7379867683383,-12.3664058844668,
2.67667072836647));
#235248=CARTESIAN_POINT('Ctrl Pts',(-57.7383208980313,-12.3676164579094,
2.67721232541081));
#235249=CARTESIAN_POINT('Ctrl Pts',(-57.7386676465114,-12.3688185104667,
2.67776268340038));
#235250=CARTESIAN_POINT('Ctrl Pts',(-57.7390266834246,-12.3700116777064,
2.67832123541507));
#235251=CARTESIAN_POINT('Ctrl Pts',(-57.7415556930806,-12.3784161936769,
2.68225560368429));
#235252=CARTESIAN_POINT('Ctrl Pts',(-57.7446608854351,-12.3864219416028,
2.68661792998865));
#235253=CARTESIAN_POINT('Ctrl Pts',(-57.7482237843183,-12.3940121800348,
2.69130986622546));
#235254=CARTESIAN_POINT('Ctrl Pts',(-57.7499517864267,-12.3976934374724,
2.6935854502303));
#235255=CARTESIAN_POINT('Ctrl Pts',(-57.751788007257,-12.4012771190725,
2.69593918853452));
#235256=CARTESIAN_POINT('Ctrl Pts',(-57.7537217536092,-12.4047617836667,
2.69836306235466));
#235257=CARTESIAN_POINT('Ctrl Pts',(-57.7566821841673,-12.4100965616936,
2.70207384382199));
#235258=CARTESIAN_POINT('Ctrl Pts',(-57.7598686150879,-12.4151968540757,
2.70594760814199));
#235259=CARTESIAN_POINT('Ctrl Pts',(-57.7632382593549,-12.420045468934,
2.70995196345679));
#235260=CARTESIAN_POINT('Ctrl Pts',(-57.7648031395848,-12.4222971907576,
2.71181160678077));
#235261=CARTESIAN_POINT('Ctrl Pts',(-57.7664072884047,-12.424494702241,
2.7136996277207));
#235262=CARTESIAN_POINT('Ctrl Pts',(-57.7680472557361,-12.4266353752446,
2.71561183138632));
#235263=CARTESIAN_POINT('Ctrl Pts',(-57.7681729527703,-12.4267994493956,
2.71575839426283));
#235264=CARTESIAN_POINT('Ctrl Pts',(-57.7682988432679,-12.4269632190239,
2.7159050890318));
#235265=CARTESIAN_POINT('Ctrl Pts',(-57.7684249257696,-12.4271266840708,
2.71605191409882));
#235266=CARTESIAN_POINT('Ctrl Pts',(-57.7701960047921,-12.4294228751481,
2.71811436362724));
#235267=CARTESIAN_POINT('Ctrl Pts',(-57.772006704017,-12.4316578001007,
2.7202009102693));
#235268=CARTESIAN_POINT('Ctrl Pts',(-57.7738513586812,-12.4338307751865,
2.72230624862153));
#235269=CARTESIAN_POINT('Ctrl Pts',(-57.7804659622465,-12.4416226773934,
2.72985561753072));
#235270=CARTESIAN_POINT('Ctrl Pts',(-57.7875668075256,-12.4486795287417,
2.73770089914296));
#235271=CARTESIAN_POINT('Ctrl Pts',(-57.7950386758939,-12.4550596184369,
2.74574823347037));
#235272=CARTESIAN_POINT('Ctrl Pts',(-57.8032495086148,-12.4620706960752,
2.75459144546979));
#235273=CARTESIAN_POINT('Ctrl Pts',(-57.8119087706216,-12.4682650727919,
2.76367911754215));
#235274=CARTESIAN_POINT('Ctrl Pts',(-57.8209080689687,-12.47369138165,2.77292162564663));
#235275=CARTESIAN_POINT('Ctrl Pts',(-57.8306250526682,-12.4795504333992,
2.78290121484661));
#235276=CARTESIAN_POINT('Ctrl Pts',(-57.84073937177,-12.4845147615735,2.79306229500112));
#235277=CARTESIAN_POINT('Ctrl Pts',(-57.8511535286833,-12.4886033793286,
2.80331916685171));
#235278=CARTESIAN_POINT('Ctrl Pts',(-57.8614803215206,-12.4926576977817,
2.81348999408635));
#235279=CARTESIAN_POINT('Ctrl Pts',(-57.8721033557551,-12.4958511892335,
2.82375635966841));
#235280=CARTESIAN_POINT('Ctrl Pts',(-57.8829458346104,-12.498155829259,
2.83404198860252));
#235281=CARTESIAN_POINT('Origin',(-0.00316857416805164,0.0149069694353738,
2.83404198860262));
#235282=CARTESIAN_POINT('Ctrl Pts',(-61.4762657165315,-13.0516031943531,
2.65878198860251));
#235283=CARTESIAN_POINT('Ctrl Pts',(-61.4780479426481,-13.0432012029363,
2.65878198860251));
#235284=CARTESIAN_POINT('Ctrl Pts',(-61.4791124697294,-13.0347249977694,
2.65944603041843));
#235285=CARTESIAN_POINT('Ctrl Pts',(-61.4795178910587,-13.0263136082735,
2.6607043926407));
#235286=CARTESIAN_POINT('Ctrl Pts',(-61.479776935988,-13.0209391308129,
2.66150842619592));
#235287=CARTESIAN_POINT('Ctrl Pts',(-61.4797678285536,-13.0155911381653,
2.66255428265361));
#235288=CARTESIAN_POINT('Ctrl Pts',(-61.4795143397208,-13.0103045333056,
2.66381699700642));
#235289=CARTESIAN_POINT('Ctrl Pts',(-61.4791683783269,-13.0030893784374,
2.66554034873241));
#235290=CARTESIAN_POINT('Ctrl Pts',(-61.4783613533298,-12.9959902125624,
2.66766759643946));
#235291=CARTESIAN_POINT('Ctrl Pts',(-61.4771427864514,-12.989088882123,
2.67012012783122));
#235292=CARTESIAN_POINT('Ctrl Pts',(-61.4765335030122,-12.9856382169033,
2.6713463935271));
#235293=CARTESIAN_POINT('Ctrl Pts',(-61.4758213793958,-12.9822368066735,
2.67265375584987));
#235294=CARTESIAN_POINT('Ctrl Pts',(-61.4750129240933,-12.9788934238967,
2.67403135126914));
#235295=CARTESIAN_POINT('Ctrl Pts',(-61.474608696442,-12.9772217325083,
2.67472014897878));
#235296=CARTESIAN_POINT('Ctrl Pts',(-61.4741803895392,-12.9755645309605,
2.67542649668607));
#235297=CARTESIAN_POINT('Ctrl Pts',(-61.4737288401361,-12.9739228088657,
2.67614899656076));
#235298=CARTESIAN_POINT('Ctrl Pts',(-61.4736159527853,-12.973512378342,
2.67632962152944));
#235299=CARTESIAN_POINT('Ctrl Pts',(-61.4735016128574,-12.9731029149217,
2.67651125590925));
#235300=CARTESIAN_POINT('Ctrl Pts',(-61.473385833587,-12.9726944333366,
2.67669387767498));
#235301=CARTESIAN_POINT('Ctrl Pts',(-61.4730384957756,-12.9714689885814,
2.67724174297219));
#235302=CARTESIAN_POINT('Ctrl Pts',(-61.4726782034776,-12.9702523821508,
2.67779849504722));
#235303=CARTESIAN_POINT('Ctrl Pts',(-61.4723053176143,-12.9690449956483,
2.67836353617984));
#235304=CARTESIAN_POINT('Ctrl Pts',(-61.4697284449399,-12.9607012057873,
2.6822683209889));
#235305=CARTESIAN_POINT('Ctrl Pts',(-61.4665839586184,-12.9527534399837,
2.68659153751382));
#235306=CARTESIAN_POINT('Ctrl Pts',(-61.4629898265069,-12.9452156558832,
2.69123699486179));
#235307=CARTESIAN_POINT('Ctrl Pts',(-61.4612035527133,-12.9414693978763,
2.69354577441209));
#235308=CARTESIAN_POINT('Ctrl Pts',(-61.4593056238948,-12.9378242492507,
2.69593478828101));
#235309=CARTESIAN_POINT('Ctrl Pts',(-61.4573073969126,-12.934281473203,
2.69839565261194));
#235310=CARTESIAN_POINT('Ctrl Pts',(-61.452899009727,-12.9264655800789,
2.70382468689019));
#235311=CARTESIAN_POINT('Ctrl Pts',(-61.4480137506081,-12.9191426809996,
2.7096115581506));
#235312=CARTESIAN_POINT('Ctrl Pts',(-61.4427731575667,-12.9123924986716,
2.71562701361741));
#235313=CARTESIAN_POINT('Ctrl Pts',(-61.4408587028413,-12.9099265719429,
2.71782453535831));
#235314=CARTESIAN_POINT('Ctrl Pts',(-61.4389006256226,-12.9075300815492,
2.72005051502376));
#235315=CARTESIAN_POINT('Ctrl Pts',(-61.4369042302169,-12.9052026993237,
2.7222998676009));
#235316=CARTESIAN_POINT('Ctrl Pts',(-61.4301985493014,-12.8973852687044,
2.72985520488827));
#235317=CARTESIAN_POINT('Ctrl Pts',(-61.4230116455109,-12.8903034584562,
2.73770845534453));
#235318=CARTESIAN_POINT('Ctrl Pts',(-61.4154582931184,-12.883899921806,
2.74576706701605));
#235319=CARTESIAN_POINT('Ctrl Pts',(-61.4071562640857,-12.8768616764787,
2.7546244358484));
#235320=CARTESIAN_POINT('Ctrl Pts',(-61.3984111343319,-12.8706422708203,
2.76373036322949));
#235321=CARTESIAN_POINT('Ctrl Pts',(-61.3893309057297,-12.865194665186,
2.77299664636542));
#235322=CARTESIAN_POINT('Ctrl Pts',(-61.3795511104683,-12.8593273605066,
2.7829768303315));
#235323=CARTESIAN_POINT('Ctrl Pts',(-61.3693816498913,-12.8543546257416,
2.79314401478517));
#235324=CARTESIAN_POINT('Ctrl Pts',(-61.3589193990697,-12.8502602383802,
2.80341452427506));
#235325=CARTESIAN_POINT('Ctrl Pts',(-61.3485984239577,-12.8462211390719,
2.8135463472107));
#235326=CARTESIAN_POINT('Ctrl Pts',(-61.3379910943973,-12.84303660345,2.82378004209051));
#235327=CARTESIAN_POINT('Ctrl Pts',(-61.3271735965892,-12.8407372733101,
2.83404198860251));
#235328=CARTESIAN_POINT('Ctrl Pts',(-57.962160188812,-12.1254815933794,
2.83404198860251));
#235329=CARTESIAN_POINT('Ctrl Pts',(-57.9518077840286,-12.1232811218136,
2.82422126443056));
#235330=CARTESIAN_POINT('Ctrl Pts',(-57.9413190436454,-12.121905095092,
2.8144281502861));
#235331=CARTESIAN_POINT('Ctrl Pts',(-57.9307520129798,-12.1213524729338,
2.80471618166485));
#235332=CARTESIAN_POINT('Ctrl Pts',(-57.9205486151437,-12.1208188676182,
2.79533842146432));
#235333=CARTESIAN_POINT('Ctrl Pts',(-57.9102709573203,-12.1210529843537,
2.78603515650477));
#235334=CARTESIAN_POINT('Ctrl Pts',(-57.8999666805177,-12.1220995054492,
2.77685887347025));
#235335=CARTESIAN_POINT('Ctrl Pts',(-57.8902259118395,-12.1230887956347,
2.76818441216864));
#235336=CARTESIAN_POINT('Ctrl Pts',(-57.880460457059,-12.1248041559915,
2.75962261521927));
#235337=CARTESIAN_POINT('Ctrl Pts',(-57.8707214090042,-12.1273238624903,
2.75123537701976));
#235338=CARTESIAN_POINT('Ctrl Pts',(-57.8617519091305,-12.1296444699046,
2.7435108713444));
#235339=CARTESIAN_POINT('Ctrl Pts',(-57.852804296013,-12.1326475236721,
2.73593399450171));
#235340=CARTESIAN_POINT('Ctrl Pts',(-57.8439372821316,-12.1364273448759,
2.72857657812902));
#235341=CARTESIAN_POINT('Ctrl Pts',(-57.8412933175838,-12.1375544112584,
2.7263827450853));
#235342=CARTESIAN_POINT('Ctrl Pts',(-57.838656682002,-12.1387507708935,
2.72420861709692));
#235343=CARTESIAN_POINT('Ctrl Pts',(-57.836029395347,-12.1400195294493,
2.72205663736698));
#235344=CARTESIAN_POINT('Ctrl Pts',(-57.833428953088,-12.1412753244188,
2.71992664556737));
#235345=CARTESIAN_POINT('Ctrl Pts',(-57.8308402488865,-12.14260049657,2.71782089927855));
#235346=CARTESIAN_POINT('Ctrl Pts',(-57.828268082638,-12.143996334094,2.71574387311217));
#235347=CARTESIAN_POINT('Ctrl Pts',(-57.8280892192275,-12.1440933979056,
2.71559944077458));
#235348=CARTESIAN_POINT('Ctrl Pts',(-57.8279104259145,-12.1441907966614,
2.7154551521604));
#235349=CARTESIAN_POINT('Ctrl Pts',(-57.8277317035127,-12.144288531381,
2.71531100781701));
#235350=CARTESIAN_POINT('Ctrl Pts',(-57.8198958587084,-12.1485735795159,
2.70899119176053));
#235351=CARTESIAN_POINT('Ctrl Pts',(-57.8122268475251,-12.1535378042502,
2.70298296066807));
#235352=CARTESIAN_POINT('Ctrl Pts',(-57.8048391253242,-12.1592011408679,
2.69736727774104));
#235353=CARTESIAN_POINT('Ctrl Pts',(-57.7979524842555,-12.164480354877,
2.69213248525387));
#235354=CARTESIAN_POINT('Ctrl Pts',(-57.7913098171242,-12.1703677426431,
2.68723866185419));
#235355=CARTESIAN_POINT('Ctrl Pts',(-57.7850318067602,-12.1768883481373,
2.68278595829508));
#235356=CARTESIAN_POINT('Ctrl Pts',(-57.7827352293491,-12.1792736699855,
2.6811571017276));
#235357=CARTESIAN_POINT('Ctrl Pts',(-57.7804877669874,-12.181743771724,
2.67958763637773));
#235358=CARTESIAN_POINT('Ctrl Pts',(-57.7782965440187,-12.1842999559277,
2.67808378645336));
#235359=CARTESIAN_POINT('Ctrl Pts',(-57.777769628097,-12.1849146328342,
2.67772216078571));
#235360=CARTESIAN_POINT('Ctrl Pts',(-57.7772459087254,-12.1855348686826,
2.67736403603534));
#235361=CARTESIAN_POINT('Ctrl Pts',(-57.7767255109846,-12.1861606108967,
2.6770095693445));
#235362=CARTESIAN_POINT('Ctrl Pts',(-57.7762213756733,-12.1867667986667,
2.67666617973775));
#235363=CARTESIAN_POINT('Ctrl Pts',(-57.7757203576391,-12.1873781540071,
2.6763262231409));
#235364=CARTESIAN_POINT('Ctrl Pts',(-57.7752225713656,-12.187994625406,
2.67598984158744));
#235365=CARTESIAN_POINT('Ctrl Pts',(-57.7697687474615,-12.1947487820215,
2.67230439292199));
#235366=CARTESIAN_POINT('Ctrl Pts',(-57.7646995864529,-12.2021217510025,
2.66904964539959));
#235367=CARTESIAN_POINT('Ctrl Pts',(-57.7601772489164,-12.2100174179589,
2.66640203566711));
#235368=CARTESIAN_POINT('Ctrl Pts',(-57.7583017007435,-12.2132919863906,
2.6653039929942));
#235369=CARTESIAN_POINT('Ctrl Pts',(-57.7565200187332,-12.2166560758248,
2.66430995142233));
#235370=CARTESIAN_POINT('Ctrl Pts',(-57.7548425830506,-12.2201014385648,
2.6634305347333));
#235371=CARTESIAN_POINT('Ctrl Pts',(-57.751981541693,-12.2259778637496,
2.66193059792854));
#235372=CARTESIAN_POINT('Ctrl Pts',(-57.7494261286933,-12.2320899429716,
2.66076519817096));
#235373=CARTESIAN_POINT('Ctrl Pts',(-57.7472322823293,-12.2383911161013,
2.65997805604428));
#235374=CARTESIAN_POINT('Ctrl Pts',(-57.7461353591473,-12.2415417026662,
2.65958448498095));
#235375=CARTESIAN_POINT('Ctrl Pts',(-57.7451302272376,-12.2447399293286,
2.6592852626073));
#235376=CARTESIAN_POINT('Ctrl Pts',(-57.7442239366601,-12.2479799447119,
2.65908463971293));
#235377=CARTESIAN_POINT('Ctrl Pts',(-57.7433176460826,-12.2512199600951,
2.65888401681855));
#235378=CARTESIAN_POINT('Ctrl Pts',(-57.7425101887131,-12.254501719267,
2.65878198860252));
#235379=CARTESIAN_POINT('Ctrl Pts',(-57.7418065394565,-12.257819391977,
2.65878198860252));
#235380=CARTESIAN_POINT('Origin',(-55.4074307335705,-18.0189898472952,2.83404198860248));
#235381=CARTESIAN_POINT('Ctrl Pts',(-59.5312589135994,-19.5431821162869,
2.83404198860247));
#235382=CARTESIAN_POINT('Ctrl Pts',(-59.5413499366331,-19.5464608884257,
2.82419652440051));
#235383=CARTESIAN_POINT('Ctrl Pts',(-59.5516697238487,-19.5489337165497,
2.81438790575637));
#235384=CARTESIAN_POINT('Ctrl Pts',(-59.5621592733661,-19.5505973858261,
2.80466781256894));
#235385=CARTESIAN_POINT('Ctrl Pts',(-59.5723079749853,-19.5522069957575,
2.79526356453074));
#235386=CARTESIAN_POINT('Ctrl Pts',(-59.5826168684405,-19.553059311798,
2.78594102496233));
#235387=CARTESIAN_POINT('Ctrl Pts',(-59.5930429125526,-19.5531064127991,
2.77675109088785));
#235388=CARTESIAN_POINT('Ctrl Pts',(-59.6029053082839,-19.5531509674459,
2.76805797913694));
#235389=CARTESIAN_POINT('Ctrl Pts',(-59.6128734577647,-19.5524750234011,
2.75948271210179));
#235390=CARTESIAN_POINT('Ctrl Pts',(-59.6229049605496,-19.5509963368657,
2.75108575573247));
#235391=CARTESIAN_POINT('Ctrl Pts',(-59.6321447001112,-19.5496343596252,
2.74335155163298));
#235392=CARTESIAN_POINT('Ctrl Pts',(-59.6414387315187,-19.5475912199419,
2.73576818685976));
#235393=CARTESIAN_POINT('Ctrl Pts',(-59.6507389334438,-19.544767461171,
2.72840626160533));
#235394=CARTESIAN_POINT('Ctrl Pts',(-59.6534365684948,-19.5439483960908,
2.72627084693698));
#235395=CARTESIAN_POINT('Ctrl Pts',(-59.656134592213,-19.5430634173959,
2.72415424587524));
#235396=CARTESIAN_POINT('Ctrl Pts',(-59.6588314685159,-19.542109499003,
2.72205867173243));
#235397=CARTESIAN_POINT('Ctrl Pts',(-59.6617550558217,-19.5410753901339,
2.71978693462846));
#235398=CARTESIAN_POINT('Ctrl Pts',(-59.6646735866701,-19.5399627185792,
2.71754411340746));
#235399=CARTESIAN_POINT('Ctrl Pts',(-59.6675844741793,-19.5387684320157,
2.71533341844243));
#235400=CARTESIAN_POINT('Ctrl Pts',(-59.6755734277898,-19.5354907031708,
2.7092661487639));
#235401=CARTESIAN_POINT('Ctrl Pts',(-59.6834782549088,-19.5315625649727,
2.70347381860408));
#235402=CARTESIAN_POINT('Ctrl Pts',(-59.6911955084647,-19.5269766895185,
2.69804914171394));
#235403=CARTESIAN_POINT('Ctrl Pts',(-59.6982563764891,-19.5227808624508,
2.6930858568719));
#235404=CARTESIAN_POINT('Ctrl Pts',(-59.7051493183934,-19.5180305486459,
2.68842799053159));
#235405=CARTESIAN_POINT('Ctrl Pts',(-59.711794955864,-19.5126862934694,
2.68414767054182));
#235406=CARTESIAN_POINT('Ctrl Pts',(-59.7150592712804,-19.5100612127847,
2.68204519134529));
#235407=CARTESIAN_POINT('Ctrl Pts',(-59.7182634781247,-19.5072925729232,
2.68003431778491));
#235408=CARTESIAN_POINT('Ctrl Pts',(-59.7213950854344,-19.5043743927941,
2.67812693945252));
#235409=CARTESIAN_POINT('Ctrl Pts',(-59.7219892774192,-19.5038206965381,
2.67776503299204));
#235410=CARTESIAN_POINT('Ctrl Pts',(-59.7225808838921,-19.5032610854118,
2.67740659639924));
#235411=CARTESIAN_POINT('Ctrl Pts',(-59.7231697699854,-19.5026955970361,
2.67705178968855));
#235412=CARTESIAN_POINT('Ctrl Pts',(-59.7237402533882,-19.5021477801721,
2.67670807068758));
#235413=CARTESIAN_POINT('Ctrl Pts',(-59.7243081837712,-19.5015944476715,
2.67636775825266));
#235414=CARTESIAN_POINT('Ctrl Pts',(-59.7248734373528,-19.5010356373988,
2.67603099699255));
#235415=CARTESIAN_POINT('Ctrl Pts',(-59.7310334544115,-19.4949458381922,
2.67236104217125));
#235416=CARTESIAN_POINT('Ctrl Pts',(-59.7368793392202,-19.4882011960853,
2.66911440541469));
#235417=CARTESIAN_POINT('Ctrl Pts',(-59.7422363728288,-19.4808775251051,
2.66646778189624));
#235418=CARTESIAN_POINT('Ctrl Pts',(-59.7444986813872,-19.4777846933724,
2.6653500963497));
#235419=CARTESIAN_POINT('Ctrl Pts',(-59.7466739523113,-19.474589008127,
2.66433897912342));
#235420=CARTESIAN_POINT('Ctrl Pts',(-59.7487501225119,-19.4712977780157,
2.66344564884792));
#235421=CARTESIAN_POINT('Ctrl Pts',(-59.7522463412519,-19.465755428747,
2.66194130298585));
#235422=CARTESIAN_POINT('Ctrl Pts',(-59.755459057686,-19.4599426670173,
2.66077206705419));
#235423=CARTESIAN_POINT('Ctrl Pts',(-59.758325802888,-19.4538995640364,
2.65998225155713));
#235424=CARTESIAN_POINT('Ctrl Pts',(-59.7590424891884,-19.4523887882912,
2.65978479768286));
#235425=CARTESIAN_POINT('Ctrl Pts',(-59.7597373347835,-19.4508635299955,
2.65961098966621));
#235426=CARTESIAN_POINT('Ctrl Pts',(-59.7604090725467,-19.449324313038,
2.659461390305));
#235427=CARTESIAN_POINT('Ctrl Pts',(-59.7614166791914,-19.4470154876018,
2.65923699126319));
#235428=CARTESIAN_POINT('Ctrl Pts',(-59.7623722755973,-19.4446752658775,
2.6590670756244));
#235429=CARTESIAN_POINT('Ctrl Pts',(-59.7632731754136,-19.4423059520263,
2.65895332562918));
#235430=CARTESIAN_POINT('Ctrl Pts',(-59.7641740752299,-19.439936638175,
2.65883957563396));
#235431=CARTESIAN_POINT('Ctrl Pts',(-59.7650202849806,-19.4375382417966,
2.65878198860247));
#235432=CARTESIAN_POINT('Ctrl Pts',(-59.7658094374966,-19.4351129318429,
2.65878198860247));
#235433=CARTESIAN_POINT('Ctrl Pts',(-56.134781019564,-18.2553202812751,
2.65878198860248));
#235434=CARTESIAN_POINT('Ctrl Pts',(-56.1321105487809,-18.2635267101474,
2.65878198860248));
#235435=CARTESIAN_POINT('Ctrl Pts',(-56.1301406315641,-18.271882444105,
2.65945335517843));
#235436=CARTESIAN_POINT('Ctrl Pts',(-56.1288305556596,-18.2802419597938,
2.66072561226593));
#235437=CARTESIAN_POINT('Ctrl Pts',(-56.1279843810469,-18.2856413491928,
2.6615473598033));
#235438=CARTESIAN_POINT('Ctrl Pts',(-56.1274125556282,-18.2910421817935,
2.66261895766873));
#235439=CARTESIAN_POINT('Ctrl Pts',(-56.1270952669251,-18.2964056883427,
2.66391429251015));
#235440=CARTESIAN_POINT('Ctrl Pts',(-56.1266747189246,-18.3035147090331,
2.66563118464111));
#235441=CARTESIAN_POINT('Ctrl Pts',(-56.1267070766079,-18.3105573165144,
2.66774105138687));
#235442=CARTESIAN_POINT('Ctrl Pts',(-56.1271555587354,-18.3174512966901,
2.67016894181738));
#235443=CARTESIAN_POINT('Ctrl Pts',(-56.1273797997991,-18.320898286778,
2.67138288703263));
#235444=CARTESIAN_POINT('Ctrl Pts',(-56.1277080087289,-18.324308309033,
2.67267613167539));
#235445=CARTESIAN_POINT('Ctrl Pts',(-56.1281351437408,-18.3276724292421,
2.6740383543254));
#235446=CARTESIAN_POINT('Ctrl Pts',(-56.1283487112468,-18.3293544893466,
2.67471946565041));
#235447=CARTESIAN_POINT('Ctrl Pts',(-56.1285870051494,-18.3310250895515,
2.6754178138951));
#235448=CARTESIAN_POINT('Ctrl Pts',(-56.1288493629351,-18.3326832110572,
2.67613207244156));
#235449=CARTESIAN_POINT('Ctrl Pts',(-56.1289149523815,-18.3330977414336,
2.67631063707818));
#235450=CARTESIAN_POINT('Ctrl Pts',(-56.1289820457107,-18.3335114922231,
2.67649019601833));
#235451=CARTESIAN_POINT('Ctrl Pts',(-56.1290506323487,-18.3339244481758,
2.67667072836644));
#235452=CARTESIAN_POINT('Ctrl Pts',(-56.1292563922626,-18.3351633160338,
2.67721232541078));
#235453=CARTESIAN_POINT('Ctrl Pts',(-56.1294755925117,-18.3363950287072,
2.67776268340034));
#235454=CARTESIAN_POINT('Ctrl Pts',(-56.1297079426451,-18.3376191892287,
2.67832123541503));
#235455=CARTESIAN_POINT('Ctrl Pts',(-56.1313445869827,-18.3462420178744,
2.68225560368434));
#235456=CARTESIAN_POINT('Ctrl Pts',(-56.1335959402407,-18.3545284904606,
2.6866179299888));
#235457=CARTESIAN_POINT('Ctrl Pts',(-56.136345925232,-18.3624495731175,
2.69130986622573));
#235458=CARTESIAN_POINT('Ctrl Pts',(-56.1376796649811,-18.3662912896465,
2.69358545023047));
#235459=CARTESIAN_POINT('Ctrl Pts',(-56.139131230071,-18.3700472768053,
2.69593918853459));
#235460=CARTESIAN_POINT('Ctrl Pts',(-56.1406901365233,-18.3737149835765,
2.69836306235462));
#235461=CARTESIAN_POINT('Ctrl Pts',(-56.143076713384,-18.3793299863881,
2.70207384382195));
#235462=CARTESIAN_POINT('Ctrl Pts',(-56.1457125629777,-18.3847354115623,
2.70594760814195));
#235463=CARTESIAN_POINT('Ctrl Pts',(-56.1485569297208,-18.3899096889381,
2.70995196345674));
#235464=CARTESIAN_POINT('Ctrl Pts',(-56.1498778683511,-18.3923126501195,
2.71181160678072));
#235465=CARTESIAN_POINT('Ctrl Pts',(-56.1512435269775,-18.3946658026161,
2.71369962772066));
#235466=CARTESIAN_POINT('Ctrl Pts',(-56.1526507491369,-18.396966172054,
2.71561183138628));
#235467=CARTESIAN_POINT('Ctrl Pts',(-56.1527586071707,-18.3971424863075,
2.71575839426279));
#235468=CARTESIAN_POINT('Ctrl Pts',(-56.1528666894394,-18.3973185179288,
2.71590508903176));
#235469=CARTESIAN_POINT('Ctrl Pts',(-56.1529749944978,-18.3974942667072,
2.71605191409879));
#235470=CARTESIAN_POINT('Ctrl Pts',(-56.1544963540395,-18.3999630071782,
2.7181143636272));
#235471=CARTESIAN_POINT('Ctrl Pts',(-56.1560635207937,-18.4023749585854,
2.72020091026926));
#235472=CARTESIAN_POINT('Ctrl Pts',(-56.1576709325003,-18.4047288488037,
2.72230624862149));
#235473=CARTESIAN_POINT('Ctrl Pts',(-56.1634348250117,-18.4131694805011,
2.72985561753089));
#235474=CARTESIAN_POINT('Ctrl Pts',(-56.1697591292906,-18.4209299141244,
2.73770089914337));
#235475=CARTESIAN_POINT('Ctrl Pts',(-56.176523165011,-18.4280560759392,
2.74574823347102));
#235476=CARTESIAN_POINT('Ctrl Pts',(-56.18395616076,-18.4358870118871,2.75459144547062));
#235477=CARTESIAN_POINT('Ctrl Pts',(-56.1919204977445,-18.4429525945107,
2.76367911754316));
#235478=CARTESIAN_POINT('Ctrl Pts',(-56.2003032932677,-18.4492898603079,
2.77292162564782));
#235479=CARTESIAN_POINT('Ctrl Pts',(-56.2093546086383,-18.4561325169322,
2.78290121484784));
#235480=CARTESIAN_POINT('Ctrl Pts',(-56.2188946068467,-18.46212688423,2.79306229500239));
#235481=CARTESIAN_POINT('Ctrl Pts',(-56.228824336988,-18.4672816799275,
2.80331916685301));
#235482=CARTESIAN_POINT('Ctrl Pts',(-56.2386707668957,-18.4723932321854,
2.81348999408721));
#235483=CARTESIAN_POINT('Ctrl Pts',(-56.2489017962828,-18.4766796388004,
2.82375635966882));
#235484=CARTESIAN_POINT('Ctrl Pts',(-56.2594439784237,-18.4801050014193,
2.83404198860248));
#235485=CARTESIAN_POINT('Origin',(-0.00470941899426334,0.0144941013085293,
2.83404198860262));
#235486=CARTESIAN_POINT('Ctrl Pts',(-59.7752282754835,-19.4061247292256,
2.65878198860247));
#235487=CARTESIAN_POINT('Ctrl Pts',(-59.7778789856301,-19.3979550581547,
2.65878198860247));
#235488=CARTESIAN_POINT('Ctrl Pts',(-59.7798236858209,-19.3896365599071,
2.65944603041829));
#235489=CARTESIAN_POINT('Ctrl Pts',(-59.7811061158277,-19.3813136269522,
2.66070439264036));
#235490=CARTESIAN_POINT('Ctrl Pts',(-59.7819255275517,-19.3759956690092,
2.66150842619563));
#235491=CARTESIAN_POINT('Ctrl Pts',(-59.7824754874619,-19.370676021238,
2.66255428265342));
#235492=CARTESIAN_POINT('Ctrl Pts',(-59.7827759879494,-19.3653918801541,
2.66381699700638));
#235493=CARTESIAN_POINT('Ctrl Pts',(-59.7831861108188,-19.3581800878464,
2.66554034873238));
#235494=CARTESIAN_POINT('Ctrl Pts',(-59.7831255716885,-19.3510354548621,
2.66766759643942));
#235495=CARTESIAN_POINT('Ctrl Pts',(-59.7826350657123,-19.3440445557098,
2.67012012783117));
#235496=CARTESIAN_POINT('Ctrl Pts',(-59.7823898127242,-19.3405491061336,
2.67134639352705));
#235497=CARTESIAN_POINT('Ctrl Pts',(-59.7820371343798,-19.3370918919976,
2.67265375584981));
#235498=CARTESIAN_POINT('Ctrl Pts',(-59.7815825865437,-19.3336823180311,
2.67403135126909));
#235499=CARTESIAN_POINT('Ctrl Pts',(-59.7813553126257,-19.3319775310478,
2.67472014897873));
#235500=CARTESIAN_POINT('Ctrl Pts',(-59.7811025767641,-19.3302846375612,
2.67542649668602));
#235501=CARTESIAN_POINT('Ctrl Pts',(-59.7808251076835,-19.3286047092266,
2.67614899656071));
#235502=CARTESIAN_POINT('Ctrl Pts',(-59.7807557404133,-19.328184727143,
2.67632962152938));
#235503=CARTESIAN_POINT('Ctrl Pts',(-59.7806848274336,-19.3277655550292,
2.67651125590919));
#235504=CARTESIAN_POINT('Ctrl Pts',(-59.7806123803665,-19.3273472089197,
2.67669387767492));
#235505=CARTESIAN_POINT('Ctrl Pts',(-59.7803950391652,-19.3260921705914,
2.67724174297213));
#235506=CARTESIAN_POINT('Ctrl Pts',(-59.7801638905866,-19.3248445680579,
2.67779849504716));
#235507=CARTESIAN_POINT('Ctrl Pts',(-59.7799192536868,-19.3236048185588,
2.67836353617977));
#235508=CARTESIAN_POINT('Ctrl Pts',(-59.7782286609225,-19.3150373803111,
2.68226832098874));
#235509=CARTESIAN_POINT('Ctrl Pts',(-59.775932168172,-19.3068044648775,
2.68659153751355));
#235510=CARTESIAN_POINT('Ctrl Pts',(-59.7731456380809,-19.2989322844408,
2.69123699486139));
#235511=CARTESIAN_POINT('Ctrl Pts',(-59.7717607402744,-19.2950198323724,
2.6935457744118));
#235512=CARTESIAN_POINT('Ctrl Pts',(-59.7702542302927,-19.2911962646694,
2.69593478828083));
#235513=CARTESIAN_POINT('Ctrl Pts',(-59.7686372707429,-19.2874640247236,
2.69839565261188));
#235514=CARTESIAN_POINT('Ctrl Pts',(-59.7650700164609,-19.2792301459419,
2.70382468689013));
#235515=CARTESIAN_POINT('Ctrl Pts',(-59.76097697069,-19.2714367138416,2.70961155815055));
#235516=CARTESIAN_POINT('Ctrl Pts',(-59.7564706723511,-19.2641757185814,
2.71562701361736));
#235517=CARTESIAN_POINT('Ctrl Pts',(-59.7548244647405,-19.261523185447,
2.71782453535826));
#235518=CARTESIAN_POINT('Ctrl Pts',(-59.7531276155318,-19.2589351484757,
2.72005051502371));
#235519=CARTESIAN_POINT('Ctrl Pts',(-59.7513854342765,-19.2564118357498,
2.72229986760084));
#235520=CARTESIAN_POINT('Ctrl Pts',(-59.7455336317917,-19.2479362953117,
2.72985520488853));
#235521=CARTESIAN_POINT('Ctrl Pts',(-59.7391263493542,-19.2401420439518,
2.73770845534514));
#235522=CARTESIAN_POINT('Ctrl Pts',(-59.7322837268617,-19.2329840462271,
2.74576706701703));
#235523=CARTESIAN_POINT('Ctrl Pts',(-59.7247628741805,-19.225116558807,
2.75462443584975));
#235524=CARTESIAN_POINT('Ctrl Pts',(-59.7167157560781,-19.2180171087292,
2.76373036323122));
#235525=CARTESIAN_POINT('Ctrl Pts',(-59.7082546997633,-19.2116502033065,
2.77299664636754));
#235526=CARTESIAN_POINT('Ctrl Pts',(-59.6991417795849,-19.2047927733661,
2.78297683033402));
#235527=CARTESIAN_POINT('Ctrl Pts',(-59.6895478206998,-19.1987842816761,
2.7931440147881));
#235528=CARTESIAN_POINT('Ctrl Pts',(-59.6795708632013,-19.1936187207963,
2.8034145242784));
#235529=CARTESIAN_POINT('Ctrl Pts',(-59.6697286283156,-19.1885229124295,
2.81354634721295));
#235530=CARTESIAN_POINT('Ctrl Pts',(-59.6595122814322,-19.1842470541692,
2.82378004209163));
#235531=CARTESIAN_POINT('Ctrl Pts',(-59.6489943884562,-19.1808295835784,
2.83404198860248));
#235532=CARTESIAN_POINT('Ctrl Pts',(-56.3771794532806,-18.1177524687109,
2.83404198860248));
#235533=CARTESIAN_POINT('Ctrl Pts',(-56.3671137719635,-18.1144819305949,
2.82422126442906));
#235534=CARTESIAN_POINT('Ctrl Pts',(-56.3568263239547,-18.1120170699775,
2.81442815028313));
#235535=CARTESIAN_POINT('Ctrl Pts',(-56.3463749453321,-18.1103629196645,
2.80471618166045));
#235536=CARTESIAN_POINT('Ctrl Pts',(-56.3362832197196,-18.1087656919989,
2.79533842145905));
#235537=CARTESIAN_POINT('Ctrl Pts',(-56.3260373921176,-18.1079242184403,
2.78603515649865));
#235538=CARTESIAN_POINT('Ctrl Pts',(-56.3156801719786,-18.1078879163649,
2.77685887346334));
#235539=CARTESIAN_POINT('Ctrl Pts',(-56.305889355267,-18.1078535995346,
2.76818441216131));
#235540=CARTESIAN_POINT('Ctrl Pts',(-56.2959980926869,-18.108538794987,
2.75962261521157));
#235541=CARTESIAN_POINT('Ctrl Pts',(-56.2860490151076,-18.1100266905438,
2.75123537701174));
#235542=CARTESIAN_POINT('Ctrl Pts',(-56.2768860815655,-18.1113970173903,
2.74351087133627));
#235543=CARTESIAN_POINT('Ctrl Pts',(-56.2676735798131,-18.1134483398666,
2.7359339944935));
#235544=CARTESIAN_POINT('Ctrl Pts',(-56.2584600414594,-18.1162805994802,
2.72857657812077));
#235545=CARTESIAN_POINT('Ctrl Pts',(-56.2557127503125,-18.1171251221232,
2.72638274507984));
#235546=CARTESIAN_POINT('Ctrl Pts',(-56.2529655048655,-18.1180393245084,
2.72420861709419));
#235547=CARTESIAN_POINT('Ctrl Pts',(-56.250219989383,-18.1190265064342,
2.72205663736694));
#235548=CARTESIAN_POINT('Ctrl Pts',(-56.2475025263005,-18.1200036017944,
2.71992664556733));
#235549=CARTESIAN_POINT('Ctrl Pts',(-56.2447894850829,-18.1210509212418,
2.71782089927852));
#235550=CARTESIAN_POINT('Ctrl Pts',(-56.2420855046789,-18.1221702476366,
2.71574387311213));
#235551=CARTESIAN_POINT('Ctrl Pts',(-56.2418974751698,-18.1222480834051,
2.71559944077454));
#235552=CARTESIAN_POINT('Ctrl Pts',(-56.241709480363,-18.12232625961,2.71545515216036));
#235553=CARTESIAN_POINT('Ctrl Pts',(-56.2415215209612,-18.1224047773506,
2.71531100781698));
#235554=CARTESIAN_POINT('Ctrl Pts',(-56.2332806922381,-18.1258472827276,
2.70899119176049));
#235555=CARTESIAN_POINT('Ctrl Pts',(-56.2251347899176,-18.1299826829657,
2.70298296066802));
#235556=CARTESIAN_POINT('Ctrl Pts',(-56.2171955585584,-18.1348427679841,
2.69736727774099));
#235557=CARTESIAN_POINT('Ctrl Pts',(-56.2097948151024,-18.1393732118984,
2.69213248525389));
#235558=CARTESIAN_POINT('Ctrl Pts',(-56.202573137601,-18.144534000151,2.68723866185426));
#235559=CARTESIAN_POINT('Ctrl Pts',(-56.1956479299628,-18.1503626543102,
2.68278595829519));
#235560=CARTESIAN_POINT('Ctrl Pts',(-56.1931145994157,-18.1524948514083,
2.68115710172764));
#235561=CARTESIAN_POINT('Ctrl Pts',(-56.1906212529491,-18.1547164978841,
2.67958763637771));
#235562=CARTESIAN_POINT('Ctrl Pts',(-56.1881748397224,-18.1570296338739,
2.67808378645328));
#235563=CARTESIAN_POINT('Ctrl Pts',(-56.1875865590688,-18.1575858658044,
2.67772216078563));
#235564=CARTESIAN_POINT('Ctrl Pts',(-56.1870008763866,-18.1581479603548,
2.67736403603526));
#235565=CARTESIAN_POINT('Ctrl Pts',(-56.186417921567,-18.1587158783115,
2.67700956934442));
#235566=CARTESIAN_POINT('Ctrl Pts',(-56.1858531840856,-18.159266048832,
2.67666617973767));
#235567=CARTESIAN_POINT('Ctrl Pts',(-56.1852910066464,-18.1598216844587,
2.67632622314082));
#235568=CARTESIAN_POINT('Ctrl Pts',(-56.1847315084903,-18.1603827459286,
2.67598984158737));
#235569=CARTESIAN_POINT('Ctrl Pts',(-56.1786015595924,-18.1665298227359,
2.67230439292192));
#235570=CARTESIAN_POINT('Ctrl Pts',(-56.172789482861,-18.173332530211,2.66904964539951));
#235571=CARTESIAN_POINT('Ctrl Pts',(-56.1674665972293,-18.1807122308847,
2.66640203566705));
#235572=CARTESIAN_POINT('Ctrl Pts',(-56.1652590378994,-18.1837728127195,
2.66530399299413));
#235573=CARTESIAN_POINT('Ctrl Pts',(-56.1631354730307,-18.1869322368373,
2.66430995142227));
#235574=CARTESIAN_POINT('Ctrl Pts',(-56.1611070880437,-18.1901833857455,
2.66343053473324));
#235575=CARTESIAN_POINT('Ctrl Pts',(-56.1576474660759,-18.1957285590018,
2.66193059792848));
#235576=CARTESIAN_POINT('Ctrl Pts',(-56.1544671656476,-18.2015400422205,
2.66076519817091));
#235577=CARTESIAN_POINT('Ctrl Pts',(-56.1516266854594,-18.2075773774754,
2.65997805604424));
#235578=CARTESIAN_POINT('Ctrl Pts',(-56.1502064453653,-18.2105960451028,
2.6595844849809));
#235579=CARTESIAN_POINT('Ctrl Pts',(-56.1488725139552,-18.2136716866511,
2.65928526260726));
#235580=CARTESIAN_POINT('Ctrl Pts',(-56.1476325143033,-18.2167992197298,
2.65908463971288));
#235581=CARTESIAN_POINT('Ctrl Pts',(-56.1463925146515,-18.2199267528084,
2.65888401681851));
#235582=CARTESIAN_POINT('Ctrl Pts',(-56.145246443375,-18.2231061318822,
2.65878198860248));
#235583=CARTESIAN_POINT('Ctrl Pts',(-56.1441998575526,-18.2263320786585,
2.65878198860248));
#235584=CARTESIAN_POINT('Origin',(-53.2204057122636,-23.7119335237428,2.83404198860244));
#235585=CARTESIAN_POINT('Ctrl Pts',(-57.1623216544369,-25.6588335304443,
2.83404198860243));
#235586=CARTESIAN_POINT('Ctrl Pts',(-57.1720146727776,-25.6631491402568,
2.82419652440027));
#235587=CARTESIAN_POINT('Ctrl Pts',(-57.1820194461954,-25.6666871334686,
2.81438790575597));
#235588=CARTESIAN_POINT('Ctrl Pts',(-57.1922776320702,-25.669438145482,
2.80466781256838));
#235589=CARTESIAN_POINT('Ctrl Pts',(-57.2022024879876,-25.6720997659862,
2.79526356453007));
#235590=CARTESIAN_POINT('Ctrl Pts',(-57.2123658169601,-25.6740249857411,
2.78594102496156));
#235591=CARTESIAN_POINT('Ctrl Pts',(-57.2227298227165,-25.675161647087,
2.776751090887));
#235592=CARTESIAN_POINT('Ctrl Pts',(-57.2325335339833,-25.6762368587286,
2.76805797913601));
#235593=CARTESIAN_POINT('Ctrl Pts',(-57.2425177322908,-25.6766065729229,
2.75948271210079));
#235594=CARTESIAN_POINT('Ctrl Pts',(-57.2526488462851,-25.6761845643573,
2.75108575573142));
#235595=CARTESIAN_POINT('Ctrl Pts',(-57.2619803349747,-25.675795863948,
2.74335155163188));
#235596=CARTESIAN_POINT('Ctrl Pts',(-57.2714370189571,-25.6747354076182,
2.7357681868586));
#235597=CARTESIAN_POINT('Ctrl Pts',(-57.2809814365681,-25.6728992535085,
2.72840626160414));
#235598=CARTESIAN_POINT('Ctrl Pts',(-57.2837499093058,-25.6723666549989,
2.72627084693618));
#235599=CARTESIAN_POINT('Ctrl Pts',(-57.2865256584302,-25.6717685445831,
2.72415424587481));
#235600=CARTESIAN_POINT('Ctrl Pts',(-57.2893074725858,-25.6711017521907,
2.72205867173237));
#235601=CARTESIAN_POINT('Ctrl Pts',(-57.2923231379854,-25.6703789063664,
2.71978693462841));
#235602=CARTESIAN_POINT('Ctrl Pts',(-57.2953419866641,-25.6695773996876,
2.71754411340741));
#235603=CARTESIAN_POINT('Ctrl Pts',(-57.2983617649662,-25.6686939261489,
2.71533341844238));
#235604=CARTESIAN_POINT('Ctrl Pts',(-57.306649570212,-25.6662692260896,
2.70926614876386));
#235605=CARTESIAN_POINT('Ctrl Pts',(-57.3149216961104,-25.6631888860747,
2.70347381860404));
#235606=CARTESIAN_POINT('Ctrl Pts',(-57.3230760282578,-25.6594348051809,
2.6980491417139));
#235607=CARTESIAN_POINT('Ctrl Pts',(-57.3305367994637,-25.6560000249769,
2.69308585687203));
#235608=CARTESIAN_POINT('Ctrl Pts',(-57.3378885241128,-25.6519962425129,
2.68842799053186));
#235609=CARTESIAN_POINT('Ctrl Pts',(-57.3450563828667,-25.6473759219979,
2.6841476705422));
#235610=CARTESIAN_POINT('Ctrl Pts',(-57.3485772116718,-25.6451064356538,
2.68204519134552));
#235611=CARTESIAN_POINT('Ctrl Pts',(-57.3520532672061,-25.6426878935084,
2.680034317785));
#235612=CARTESIAN_POINT('Ctrl Pts',(-57.3554727521279,-25.6401130415749,
2.67812693945248));
#235613=CARTESIAN_POINT('Ctrl Pts',(-57.3561215660856,-25.6396244884999,
2.677765032992));
#235614=CARTESIAN_POINT('Ctrl Pts',(-57.3567684269675,-25.6391297826974,
2.6774065963992));
#235615=CARTESIAN_POINT('Ctrl Pts',(-57.357413196712,-25.6386289474846,
2.67705178968851));
#235616=CARTESIAN_POINT('Ctrl Pts',(-57.358037817402,-25.6381437633721,
2.67670807068754));
#235617=CARTESIAN_POINT('Ctrl Pts',(-57.3586604755989,-25.637652826975,
2.67636775825261));
#235618=CARTESIAN_POINT('Ctrl Pts',(-57.3592810442413,-25.6371561630117,
2.67603099699251));
#235619=CARTESIAN_POINT('Ctrl Pts',(-57.3660438734346,-25.6317436214792,
2.67236104217124));
#235620=CARTESIAN_POINT('Ctrl Pts',(-57.3725627409493,-25.625646988583,
2.6691144054147));
#235621=CARTESIAN_POINT('Ctrl Pts',(-57.3786559602403,-25.6189233999296,
2.66646778189627));
#235622=CARTESIAN_POINT('Ctrl Pts',(-57.381229164584,-25.6160839866898,
2.6653500963497));
#235623=CARTESIAN_POINT('Ctrl Pts',(-57.3837265592142,-25.6131331854693,
2.6643389791234));
#235624=CARTESIAN_POINT('Ctrl Pts',(-57.386135383163,-25.6100770039414,
2.66344564884788));
#235625=CARTESIAN_POINT('Ctrl Pts',(-57.3901917825028,-25.6049304706141,
2.66194130298581));
#235626=CARTESIAN_POINT('Ctrl Pts',(-57.3939944983912,-25.5994853721131,
2.66077206705415));
#235627=CARTESIAN_POINT('Ctrl Pts',(-57.3974772155311,-25.5937750303533,
2.65998225155709));
#235628=CARTESIAN_POINT('Ctrl Pts',(-57.3983478948161,-25.5923474449133,
2.65978479768283));
#235629=CARTESIAN_POINT('Ctrl Pts',(-57.39919836688,-25.5909031732844,2.65961098966617));
#235630=CARTESIAN_POINT('Ctrl Pts',(-57.4000273167766,-25.5894426040346,
2.65946139030496));
#235631=CARTESIAN_POINT('Ctrl Pts',(-57.4012707416215,-25.5872517501598,
2.65923699126315));
#235632=CARTESIAN_POINT('Ctrl Pts',(-57.4024657229508,-25.5850242354388,
2.65906707562436));
#235633=CARTESIAN_POINT('Ctrl Pts',(-57.4036093482795,-25.58276207061,2.65895332562914));
#235634=CARTESIAN_POINT('Ctrl Pts',(-57.4047529736081,-25.5804999057813,
2.65883957563392));
#235635=CARTESIAN_POINT('Ctrl Pts',(-57.405845248421,-25.578203101074,2.65878198860243));
#235636=CARTESIAN_POINT('Ctrl Pts',(-57.4068835917993,-25.5758735661218,
2.65878198860243));
#235637=CARTESIAN_POINT('Ctrl Pts',(-53.9190682401993,-24.0229981225299,
2.65878198860244));
#235638=CARTESIAN_POINT('Ctrl Pts',(-53.9155545931357,-24.0308804555188,
2.65878198860244));
#235639=CARTESIAN_POINT('Ctrl Pts',(-53.9127220553015,-24.0389845034719,
2.65945335517837));
#235640=CARTESIAN_POINT('Ctrl Pts',(-53.9105453488013,-24.0471612846379,
2.66072561226581));
#235641=CARTESIAN_POINT('Ctrl Pts',(-53.9091394197451,-24.0524426462851,
2.6615473598032));
#235642=CARTESIAN_POINT('Ctrl Pts',(-53.9080061861137,-24.0577541205276,
2.66261895766866));
#235643=CARTESIAN_POINT('Ctrl Pts',(-53.907129996454,-24.0630550795264,
2.66391429251012));
#235644=CARTESIAN_POINT('Ctrl Pts',(-53.9059686572513,-24.0700811970214,
2.66563118464108));
#235645=CARTESIAN_POINT('Ctrl Pts',(-53.9052646847384,-24.0770886066608,
2.66774105138683));
#235646=CARTESIAN_POINT('Ctrl Pts',(-53.9049900928802,-24.0839917000395,
2.67016894181734));
#235647=CARTESIAN_POINT('Ctrl Pts',(-53.9048527969511,-24.0874432467288,
2.67138288703259));
#235648=CARTESIAN_POINT('Ctrl Pts',(-53.9048227635321,-24.0908688957001,
2.67267613167535));
#235649=CARTESIAN_POINT('Ctrl Pts',(-53.9048959123381,-24.0942592346731,
2.67403835432537));
#235650=CARTESIAN_POINT('Ctrl Pts',(-53.9049324867411,-24.0959544041596,
2.67471946565037));
#235651=CARTESIAN_POINT('Ctrl Pts',(-53.9049948499726,-24.0976407611372,
2.67541781389506));
#235652=CARTESIAN_POINT('Ctrl Pts',(-53.905082449642,-24.099317223136,2.67613207244152));
#235653=CARTESIAN_POINT('Ctrl Pts',(-53.9051043495593,-24.0997363386357,
2.67631063707814));
#235654=CARTESIAN_POINT('Ctrl Pts',(-53.90512782661,-24.1001548360176,2.67649019601829));
#235655=CARTESIAN_POINT('Ctrl Pts',(-53.9051528718721,-24.1005726990102,
2.6766707283664));
#235656=CARTESIAN_POINT('Ctrl Pts',(-53.9052280076583,-24.1018262879881,
2.67721232541074));
#235657=CARTESIAN_POINT('Ctrl Pts',(-53.9053172580726,-24.1030741658757,
2.6777626834003));
#235658=CARTESIAN_POINT('Ctrl Pts',(-53.9054203757495,-24.1043159075202,
2.67832123541499));
#235659=CARTESIAN_POINT('Ctrl Pts',(-53.9061467233508,-24.1130625753257,
2.68225560368422));
#235660=CARTESIAN_POINT('Ctrl Pts',(-53.9075195712147,-24.1215389842443,
2.6866179299886));
#235661=CARTESIAN_POINT('Ctrl Pts',(-53.9094265129029,-24.1297041260866,
2.69130986622543));
#235662=CARTESIAN_POINT('Ctrl Pts',(-53.910351377561,-24.133664211057,2.69358545023025));
#235663=CARTESIAN_POINT('Ctrl Pts',(-53.9114023832598,-24.1375513523935,
2.69593918853446));
#235664=CARTESIAN_POINT('Ctrl Pts',(-53.9125693701069,-24.1413619171792,
2.69836306235458));
#235665=CARTESIAN_POINT('Ctrl Pts',(-53.9143559454348,-24.1471956256297,
2.70207384382191));
#235666=CARTESIAN_POINT('Ctrl Pts',(-53.9164123347818,-24.1528469606266,
2.7059476081419));
#235667=CARTESIAN_POINT('Ctrl Pts',(-53.9187002605237,-24.1582902100541,
2.7099519634567));
#235668=CARTESIAN_POINT('Ctrl Pts',(-53.9197627850744,-24.1608180832479,
2.71181160678068));
#235669=CARTESIAN_POINT('Ctrl Pts',(-53.9208749910656,-24.1633010951265,
2.71369962772062));
#235670=CARTESIAN_POINT('Ctrl Pts',(-53.9220340502325,-24.1657359576696,
2.71561183138624));
#235671=CARTESIAN_POINT('Ctrl Pts',(-53.9221228875507,-24.1659225802897,
2.71575839426275));
#235672=CARTESIAN_POINT('Ctrl Pts',(-53.9222119774185,-24.1661089452649,
2.71590508903172));
#235673=CARTESIAN_POINT('Ctrl Pts',(-53.9223013184208,-24.1662950522344,
2.71605191409874));
#235674=CARTESIAN_POINT('Ctrl Pts',(-53.9235562901481,-24.1689092940617,
2.71811436362715));
#235675=CARTESIAN_POINT('Ctrl Pts',(-53.9248627542248,-24.1714718460793,
2.72020091026922));
#235676=CARTESIAN_POINT('Ctrl Pts',(-53.9262153118346,-24.1739808617162,
2.72230624862144));
#235677=CARTESIAN_POINT('Ctrl Pts',(-53.9310653428794,-24.1829777455767,
2.72985561753085));
#235678=CARTESIAN_POINT('Ctrl Pts',(-53.9365438157569,-24.1913567365402,
2.73770089914333));
#235679=CARTESIAN_POINT('Ctrl Pts',(-53.9425259106384,-24.1991508947542,
2.74574823347098));
#235680=CARTESIAN_POINT('Ctrl Pts',(-53.9490996319585,-24.207715891639,
2.75459144547082));
#235681=CARTESIAN_POINT('Ctrl Pts',(-53.9562817849782,-24.2155752681679,
2.76367911754364));
#235682=CARTESIAN_POINT('Ctrl Pts',(-53.9639562340156,-24.2227540584941,
2.77292162564857));
#235683=CARTESIAN_POINT('Ctrl Pts',(-53.9722427129526,-24.2305053504162,
2.78290121484941));
#235684=CARTESIAN_POINT('Ctrl Pts',(-53.9811038680515,-24.2374640812955,
2.7930622950048));
#235685=CARTESIAN_POINT('Ctrl Pts',(-53.9904403792203,-24.2436285779155,
2.80331916685628));
#235686=CARTESIAN_POINT('Ctrl Pts',(-53.9996985666513,-24.2497413607414,
2.8134899940894));
#235687=CARTESIAN_POINT('Ctrl Pts',(-54.0094254978916,-24.2550737197513,
2.82375635966991));
#235688=CARTESIAN_POINT('Ctrl Pts',(-54.0195518809639,-24.2595822759735,
2.83404198860244));
#235689=CARTESIAN_POINT('Origin',(-0.00619866644046454,0.0139224327746649,
2.83404198860262));
#235690=CARTESIAN_POINT('Ctrl Pts',(-57.4192809246787,-25.5480287005721,
2.65878198860243));
#235691=CARTESIAN_POINT('Ctrl Pts',(-57.4227710771204,-25.5401808584717,
2.65878198860243));
#235692=CARTESIAN_POINT('Ctrl Pts',(-57.4255746438787,-25.5321112063499,
2.65944603041834));
#235693=CARTESIAN_POINT('Ctrl Pts',(-57.4277200319916,-25.5239679177298,
2.66070439264058));
#235694=CARTESIAN_POINT('Ctrl Pts',(-57.4290908328637,-25.5187647439657,
2.66150842619582));
#235695=CARTESIAN_POINT('Ctrl Pts',(-57.4301938346425,-25.5135317242465,
2.66255428265352));
#235696=CARTESIAN_POINT('Ctrl Pts',(-57.4310450321039,-25.508307941095,
2.66381699700635));
#235697=CARTESIAN_POINT('Ctrl Pts',(-57.4322067458447,-25.5011785252535,
2.66554034873234));
#235698=CARTESIAN_POINT('Ctrl Pts',(-57.4328933558605,-25.4940667032539,
2.66766759643938));
#235699=CARTESIAN_POINT('Ctrl Pts',(-57.4331362848726,-25.4870628291427,
2.67012012783114));
#235700=CARTESIAN_POINT('Ctrl Pts',(-57.4332577493786,-25.4835608920871,
2.67134639352702));
#235701=CARTESIAN_POINT('Ctrl Pts',(-57.4332683803239,-25.4800857520065,
2.67265375584979));
#235702=CARTESIAN_POINT('Ctrl Pts',(-57.4331727200756,-25.4766473428561,
2.67403135126906));
#235703=CARTESIAN_POINT('Ctrl Pts',(-57.4331248899515,-25.4749281382809,
2.6747201489787));
#235704=CARTESIAN_POINT('Ctrl Pts',(-57.433050494158,-25.4732181005507,
2.67542649668599));
#235705=CARTESIAN_POINT('Ctrl Pts',(-57.4329501454092,-25.4715183716227,
2.67614899656068));
#235706=CARTESIAN_POINT('Ctrl Pts',(-57.4329250582221,-25.4710934393907,
2.67632962152936));
#235707=CARTESIAN_POINT('Ctrl Pts',(-57.432898349128,-25.4706691511208,
2.67651125590916));
#235708=CARTESIAN_POINT('Ctrl Pts',(-57.4328700280094,-25.4702455239746,
2.6766938776749));
#235709=CARTESIAN_POINT('Ctrl Pts',(-57.4327850646537,-25.4689746425358,
2.6772417429721));
#235710=CARTESIAN_POINT('Ctrl Pts',(-57.4326855923069,-25.4677097128937,
2.67779849504714));
#235711=CARTESIAN_POINT('Ctrl Pts',(-57.4325718846635,-25.4664511833529,
2.67836353617975));
#235712=CARTESIAN_POINT('Ctrl Pts',(-57.4317860942974,-25.4577539633644,
2.68226832098887));
#235713=CARTESIAN_POINT('Ctrl Pts',(-57.430362755973,-25.4493260998445,
2.68659153751386));
#235714=CARTESIAN_POINT('Ctrl Pts',(-57.4284143577087,-25.4412057723273,
2.69123699486191));
#235715=CARTESIAN_POINT('Ctrl Pts',(-57.4274460091197,-25.4371699918415,
2.69354577441215));
#235716=CARTESIAN_POINT('Ctrl Pts',(-57.4263474236136,-25.4332098968695,
2.69593478828099));
#235717=CARTESIAN_POINT('Ctrl Pts',(-57.4251294472436,-25.4293290842281,
2.69839565261185));
#235718=CARTESIAN_POINT('Ctrl Pts',(-57.4224424094495,-25.4207674318877,
2.7038246868901));
#235719=CARTESIAN_POINT('Ctrl Pts',(-57.4191864212927,-25.4125888532393,
2.70961155815051));
#235720=CARTESIAN_POINT('Ctrl Pts',(-57.4154637896039,-25.4048965980306,
2.71562701361731));
#235721=CARTESIAN_POINT('Ctrl Pts',(-57.4141038653031,-25.4020865201984,
2.71782453535822));
#235722=CARTESIAN_POINT('Ctrl Pts',(-57.4126868351393,-25.3993352917243,
2.72005051502366));
#235723=CARTESIAN_POINT('Ctrl Pts',(-57.4112179557368,-25.3966436944401,
2.72229986760078));
#235724=CARTESIAN_POINT('Ctrl Pts',(-57.4062841452555,-25.3876029039779,
2.72985520488874));
#235725=CARTESIAN_POINT('Ctrl Pts',(-57.4007266836983,-25.3791816069552,
2.73770845534561));
#235726=CARTESIAN_POINT('Ctrl Pts',(-57.3946697603096,-25.3713475726768,
2.74576706701778));
#235727=CARTESIAN_POINT('Ctrl Pts',(-57.3880124840157,-25.3627370410024,
2.75462443585078));
#235728=CARTESIAN_POINT('Ctrl Pts',(-57.3807515434745,-25.3548353295657,
2.76373036323256));
#235729=CARTESIAN_POINT('Ctrl Pts',(-57.3730023605507,-25.3476188815027,
2.77299664636921));
#235730=CARTESIAN_POINT('Ctrl Pts',(-57.3646561585156,-25.3398464577386,
2.78297683033614));
#235731=CARTESIAN_POINT('Ctrl Pts',(-57.3557428147435,-25.3328680394157,
2.7931440147907));
#235732=CARTESIAN_POINT('Ctrl Pts',(-57.3463604602023,-25.3266878999834,
2.80341452428155));
#235733=CARTESIAN_POINT('Ctrl Pts',(-57.3371047991278,-25.3205912133012,
2.81354634721498));
#235734=CARTESIAN_POINT('Ctrl Pts',(-57.327391367356,-25.3152708796007,
2.82378004209258));
#235735=CARTESIAN_POINT('Ctrl Pts',(-57.3172883154488,-25.3107727110825,
2.83404198860243));
#235736=CARTESIAN_POINT('Ctrl Pts',(-54.1745185419758,-23.9115214566117,
2.83404198860244));
#235737=CARTESIAN_POINT('Ctrl Pts',(-54.1648498658387,-23.9072166846465,
2.8242212644303));
#235738=CARTESIAN_POINT('Ctrl Pts',(-54.1548764216403,-23.9036899956625,
2.81442815028565));
#235739=CARTESIAN_POINT('Ctrl Pts',(-54.144655202555,-23.9009524404118,
2.80471618166422));
#235740=CARTESIAN_POINT('Ctrl Pts',(-54.1347857162255,-23.8983090899564,
2.79533842146358));
#235741=CARTESIAN_POINT('Ctrl Pts',(-54.124683974278,-23.8964012454638,
2.78603515650393));
#235742=CARTESIAN_POINT('Ctrl Pts',(-54.1143872866757,-23.8952825179499,
2.77685887346932));
#235743=CARTESIAN_POINT('Ctrl Pts',(-54.1046536921685,-23.8942249700855,
2.76818441216765));
#235744=CARTESIAN_POINT('Ctrl Pts',(-54.0947449925326,-23.8938724934879,
2.75962261521823));
#235745=CARTESIAN_POINT('Ctrl Pts',(-54.0846948896058,-23.8943122764064,
2.75123537701868));
#235746=CARTESIAN_POINT('Ctrl Pts',(-54.0754389134133,-23.8947173090964,
2.74351087134334));
#235747=CARTESIAN_POINT('Ctrl Pts',(-54.0660624571237,-23.895794425562,
2.73593399450066));
#235748=CARTESIAN_POINT('Ctrl Pts',(-54.0566033397524,-23.8976480927551,
2.728576578128));
#235749=CARTESIAN_POINT('Ctrl Pts',(-54.0537828218968,-23.8982008188934,
2.7263827450846));
#235750=CARTESIAN_POINT('Ctrl Pts',(-54.0509550659742,-23.8988228478381,
2.72420861709654));
#235751=CARTESIAN_POINT('Ctrl Pts',(-54.0481214021001,-23.8995176373646,
2.72205663736691));
#235752=CARTESIAN_POINT('Ctrl Pts',(-54.0453166912881,-23.9002053278541,
2.7199266455673));
#235753=CARTESIAN_POINT('Ctrl Pts',(-54.0425090377018,-23.9009633199468,
2.71782089927848));
#235754=CARTESIAN_POINT('Ctrl Pts',(-54.0397028685175,-23.9017938716382,
2.7157438731121));
#235755=CARTESIAN_POINT('Ctrl Pts',(-54.0395077330004,-23.9018516265785,
2.7155994407745));
#235756=CARTESIAN_POINT('Ctrl Pts',(-54.0393125964103,-23.9019097237178,
2.71545515216033));
#235757=CARTESIAN_POINT('Ctrl Pts',(-54.039117459331,-23.9019681642225,
2.71531100781694));
#235758=CARTESIAN_POINT('Ctrl Pts',(-54.0305619349331,-23.9045304100324,
2.70899119176051));
#235759=CARTESIAN_POINT('Ctrl Pts',(-54.0220283896861,-23.9077916774637,
2.70298296066809));
#235760=CARTESIAN_POINT('Ctrl Pts',(-54.0136246330487,-23.9117952627744,
2.6973672777411));
#235761=CARTESIAN_POINT('Ctrl Pts',(-54.0057908712997,-23.9155273001022,
2.69213248525413));
#235762=CARTESIAN_POINT('Ctrl Pts',(-53.9980693056381,-23.9199049461652,
2.68723866185462));
#235763=CARTESIAN_POINT('Ctrl Pts',(-53.9905727747499,-23.9249777890347,
2.68278595829563));
#235764=CARTESIAN_POINT('Ctrl Pts',(-53.9878304467663,-23.9268335005851,
2.68115710172792));
#235765=CARTESIAN_POINT('Ctrl Pts',(-53.9851185338202,-23.9287823509747,
2.67958763637783));
#235766=CARTESIAN_POINT('Ctrl Pts',(-53.9824437337505,-23.9308270955486,
2.67808378645326));
#235767=CARTESIAN_POINT('Ctrl Pts',(-53.981800533691,-23.9313187883097,
2.67772216078561));
#235768=CARTESIAN_POINT('Ctrl Pts',(-53.9811593045602,-23.9318165831366,
2.67736403603524));
#235769=CARTESIAN_POINT('Ctrl Pts',(-53.9805201796369,-23.9323204546078,
2.6770095693444));
#235770=CARTESIAN_POINT('Ctrl Pts',(-53.9799010273675,-23.9328085800956,
2.67666617973765));
#235771=CARTESIAN_POINT('Ctrl Pts',(-53.9792838498569,-23.9333024083484,
2.6763262231408));
#235772=CARTESIAN_POINT('Ctrl Pts',(-53.978668769797,-23.9338019127824,
2.67598984158734));
#235773=CARTESIAN_POINT('Ctrl Pts',(-53.971929856908,-23.9392745611218,
2.67230439292171));
#235774=CARTESIAN_POINT('Ctrl Pts',(-53.9654385427822,-23.9454324752049,
2.66904964539916));
#235775=CARTESIAN_POINT('Ctrl Pts',(-53.9593734277039,-23.9522153560512,
2.66640203566662));
#235776=CARTESIAN_POINT('Ctrl Pts',(-53.9568580436994,-23.9550284189139,
2.66530399299386));
#235777=CARTESIAN_POINT('Ctrl Pts',(-53.9544158621937,-23.9579485624031,
2.66430995142214));
#235778=CARTESIAN_POINT('Ctrl Pts',(-53.952058751313,-23.9609698772114,
2.66343053473321));
#235779=CARTESIAN_POINT('Ctrl Pts',(-53.9480384530773,-23.9661230444607,
2.66193059792845));
#235780=CARTESIAN_POINT('Ctrl Pts',(-53.9442681092574,-23.9715702598497,
2.66076519817088));
#235781=CARTESIAN_POINT('Ctrl Pts',(-53.9408121161402,-23.9772776109212,
2.6599780560442));
#235782=CARTESIAN_POINT('Ctrl Pts',(-53.9390841195816,-23.980131286457,
2.65958448498087));
#235783=CARTESIAN_POINT('Ctrl Pts',(-53.9374360035028,-23.9830506455188,
2.65928526260722));
#235784=CARTESIAN_POINT('Ctrl Pts',(-53.9358758804723,-23.9860314303859,
2.65908463971285));
#235785=CARTESIAN_POINT('Ctrl Pts',(-53.9343157574418,-23.9890122152531,
2.65888401681847));
#235786=CARTESIAN_POINT('Ctrl Pts',(-53.9328436288551,-23.9920543802863,
2.65878198860244));
#235787=CARTESIAN_POINT('Ctrl Pts',(-53.9314655730802,-23.995153256981,
2.65878198860244));
#235788=CARTESIAN_POINT('Origin',(-50.4502867888873,-29.1450842944631,2.8340419886024));
#235789=CARTESIAN_POINT('Ctrl Pts',(-54.1671020372436,-31.4933613949861,
2.83404198860239));
#235790=CARTESIAN_POINT('Ctrl Pts',(-54.176290852154,-31.4986665597482,
2.82419652440023));
#235791=CARTESIAN_POINT('Ctrl Pts',(-54.1858709973829,-31.5032309550537,
2.81438790575588));
#235792=CARTESIAN_POINT('Ctrl Pts',(-54.1957854287842,-31.507039169141,
2.80466781256822));
#235793=CARTESIAN_POINT('Ctrl Pts',(-54.2053777002014,-31.5107236389468,
2.79526356452981));
#235794=CARTESIAN_POINT('Ctrl Pts',(-54.215284113132,-31.5137006693056,
2.78594102496119));
#235795=CARTESIAN_POINT('Ctrl Pts',(-54.2254725303168,-31.5159144374967,
2.77675109088649));
#235796=CARTESIAN_POINT('Ctrl Pts',(-54.2351101456071,-31.5180085258895,
2.76805797913536));
#235797=CARTESIAN_POINT('Ctrl Pts',(-54.2450010037751,-31.5194198476567,
2.75948271209998));
#235798=CARTESIAN_POINT('Ctrl Pts',(-54.2551207303739,-31.5200591406752,
2.75108575573045));
#235799=CARTESIAN_POINT('Ctrl Pts',(-54.2644417304488,-31.52064797578,2.74335155163073));
#235800=CARTESIAN_POINT('Ctrl Pts',(-54.2739574575976,-31.5205818213851,
2.7357681868573));
#235801=CARTESIAN_POINT('Ctrl Pts',(-54.2836415202578,-31.5197533892253,
2.7284062616027));
#235802=CARTESIAN_POINT('Ctrl Pts',(-54.2864504987153,-31.519513092547,
2.72627084693521));
#235803=CARTESIAN_POINT('Ctrl Pts',(-54.2892735615577,-31.519208403433,
2.72415424587431));
#235804=CARTESIAN_POINT('Ctrl Pts',(-54.2921098354277,-31.518836042558,
2.72205867173232));
#235805=CARTESIAN_POINT('Ctrl Pts',(-54.2951845386599,-31.5184323794287,
2.71978693462836));
#235806=CARTESIAN_POINT('Ctrl Pts',(-54.2982706300311,-31.5179508191006,
2.71754411340737));
#235807=CARTESIAN_POINT('Ctrl Pts',(-54.301366213803,-31.5173878381077,
2.71533341844234));
#235808=CARTESIAN_POINT('Ctrl Pts',(-54.3098620677557,-31.5158427323552,
2.70926614876382));
#235809=CARTESIAN_POINT('Ctrl Pts',(-54.3184108612909,-31.5136439393734,
2.70347381860399));
#235810=CARTESIAN_POINT('Ctrl Pts',(-54.3269129314605,-31.5107627835359,
2.69804914171385));
#235811=CARTESIAN_POINT('Ctrl Pts',(-54.3346918640777,-31.508126682366,
2.69308585687177));
#235812=CARTESIAN_POINT('Ctrl Pts',(-54.3424218244386,-31.504913297521,
2.68842799053142));
#235813=CARTESIAN_POINT('Ctrl Pts',(-54.3500333719158,-31.5010675328655,
2.68414767054161));
#235814=CARTESIAN_POINT('Ctrl Pts',(-54.3537721391719,-31.4991785058296,
2.68204519134513));
#235815=CARTESIAN_POINT('Ctrl Pts',(-54.3574819590038,-31.4971365594545,
2.6800343177848));
#235816=CARTESIAN_POINT('Ctrl Pts',(-54.3611518569448,-31.4949332463336,
2.67812693945244));
#235817=CARTESIAN_POINT('Ctrl Pts',(-54.3618481843339,-31.4945151891294,
2.67776503299196));
#235818=CARTESIAN_POINT('Ctrl Pts',(-54.3625432124815,-31.494090808751,
2.67740659639916));
#235819=CARTESIAN_POINT('Ctrl Pts',(-54.363236801645,-31.4936601139564,
2.67705178968848));
#235820=CARTESIAN_POINT('Ctrl Pts',(-54.3639087161472,-31.4932428783741,
2.6767080706875));
#235821=CARTESIAN_POINT('Ctrl Pts',(-54.3645792801846,-31.4928197168825,
2.67636775825258));
#235822=CARTESIAN_POINT('Ctrl Pts',(-54.3652483648078,-31.4923906407828,
2.67603099699248));
#235823=CARTESIAN_POINT('Ctrl Pts',(-54.3725399111639,-31.4877146578621,
2.67236104217126));
#235824=CARTESIAN_POINT('Ctrl Pts',(-54.3796603393079,-31.4823328301625,
2.66911440541476));
#235825=CARTESIAN_POINT('Ctrl Pts',(-54.3864229856956,-31.4762829888802,
2.66646778189635));
#235826=CARTESIAN_POINT('Ctrl Pts',(-54.3892788932593,-31.4737281033388,
2.66535009634973));
#235827=CARTESIAN_POINT('Ctrl Pts',(-54.3920710496174,-31.471054515739,
2.66433897912339));
#235828=CARTESIAN_POINT('Ctrl Pts',(-54.3947861357353,-31.4682668669588,
2.66344564884785));
#235829=CARTESIAN_POINT('Ctrl Pts',(-54.399358272915,-31.4635725360689,
2.66194130298577));
#235830=CARTESIAN_POINT('Ctrl Pts',(-54.4037093249065,-31.4585547584354,
2.66077206705411));
#235831=CARTESIAN_POINT('Ctrl Pts',(-54.4077698566061,-31.4532397415956,
2.65998225155705));
#235832=CARTESIAN_POINT('Ctrl Pts',(-54.4087849895311,-31.4519109873857,
2.65978479768278));
#235833=CARTESIAN_POINT('Ctrl Pts',(-54.4097817701139,-31.4505635261658,
2.65961098966613));
#235834=CARTESIAN_POINT('Ctrl Pts',(-54.4107588499955,-31.4491976069259,
2.65946139030492));
#235835=CARTESIAN_POINT('Ctrl Pts',(-54.4122244698178,-31.4471487280662,
2.65923699126311));
#235836=CARTESIAN_POINT('Ctrl Pts',(-54.4136457436051,-31.4450583254659,
2.65906707562432));
#235837=CARTESIAN_POINT('Ctrl Pts',(-54.4150195646478,-31.442928094411,
2.6589533256291));
#235838=CARTESIAN_POINT('Ctrl Pts',(-54.4163933856905,-31.440797863356,
2.65883957563387));
#235839=CARTESIAN_POINT('Ctrl Pts',(-54.4177197583742,-31.438627814593,
2.65878198860239));
#235840=CARTESIAN_POINT('Ctrl Pts',(-54.4189959163076,-31.4364195775146,
2.65878198860239));
#235841=CARTESIAN_POINT('Ctrl Pts',(-51.1126068659044,-29.5274749692187,
2.65878198860241));
#235842=CARTESIAN_POINT('Ctrl Pts',(-51.1082885388128,-29.5349468458348,
2.65878198860241));
#235843=CARTESIAN_POINT('Ctrl Pts',(-51.1046244142384,-29.5427104181385,
2.65945335517834));
#235844=CARTESIAN_POINT('Ctrl Pts',(-51.1016049255943,-29.5506148782564,
2.66072561226581));
#235845=CARTESIAN_POINT('Ctrl Pts',(-51.0996546457477,-29.555720348448,
2.66154735980319));
#235846=CARTESIAN_POINT('Ctrl Pts',(-51.0979724198485,-29.5608842707088,
2.66261895766863));
#235847=CARTESIAN_POINT('Ctrl Pts',(-51.0965469289495,-29.5660646037407,
2.66391429251007));
#235848=CARTESIAN_POINT('Ctrl Pts',(-51.09465752242,-29.5729308384268,2.66563118464103));
#235849=CARTESIAN_POINT('Ctrl Pts',(-51.0932249325811,-29.5798262755781,
2.66774105138678));
#235850=CARTESIAN_POINT('Ctrl Pts',(-51.0922302752232,-29.5866628504239,
2.67016894181728));
#235851=CARTESIAN_POINT('Ctrl Pts',(-51.0917329465442,-29.5900811378468,
2.67138288703254));
#235852=CARTESIAN_POINT('Ctrl Pts',(-51.0913449998287,-29.5934848814075,
2.67267613167529));
#235853=CARTESIAN_POINT('Ctrl Pts',(-51.0910633609951,-29.5968642938812,
2.67403835432531));
#235854=CARTESIAN_POINT('Ctrl Pts',(-51.0909225415783,-29.598554000118,
2.67471946565032));
#235855=CARTESIAN_POINT('Ctrl Pts',(-51.0908082908741,-29.6002376377884,
2.67541781389501));
#235856=CARTESIAN_POINT('Ctrl Pts',(-51.0907201726669,-29.6019140726117,
2.67613207244147));
#235857=CARTESIAN_POINT('Ctrl Pts',(-51.090698143115,-29.6023331813176,
2.67631063707808));
#235858=CARTESIAN_POINT('Ctrl Pts',(-51.0906777466678,-29.6027518401471,
2.67649019601823));
#235859=CARTESIAN_POINT('Ctrl Pts',(-51.0906589761528,-29.6031700319853,
2.67667072836634));
#235860=CARTESIAN_POINT('Ctrl Pts',(-51.0906026646079,-29.6044246074998,
2.67721232541068));
#235861=CARTESIAN_POINT('Ctrl Pts',(-51.0905609873411,-29.6056749785905,
2.67776268340025));
#235862=CARTESIAN_POINT('Ctrl Pts',(-51.0905337427828,-29.6069206965766,
2.67832123541494));
#235863=CARTESIAN_POINT('Ctrl Pts',(-51.0903418356315,-29.6156953732194,
2.68225560368422));
#235864=CARTESIAN_POINT('Ctrl Pts',(-51.0908211368928,-29.6242688491606,
2.68661792998866));
#235865=CARTESIAN_POINT('Ctrl Pts',(-51.0918641424258,-29.6325885911859,
2.69130986622556));
#235866=CARTESIAN_POINT('Ctrl Pts',(-51.0923699989822,-29.6366236570778,
2.69358545023033));
#235867=CARTESIAN_POINT('Ctrl Pts',(-51.0930089302514,-29.6405993642578,
2.69593918853448));
#235868=CARTESIAN_POINT('Ctrl Pts',(-51.0937712117412,-29.6445110377126,
2.69836306235454));
#235869=CARTESIAN_POINT('Ctrl Pts',(-51.094938211443,-29.6504995364713,
2.70207384382187));
#235870=CARTESIAN_POINT('Ctrl Pts',(-51.0963926103114,-29.6563348640822,
2.70594760814187));
#235871=CARTESIAN_POINT('Ctrl Pts',(-51.0980990280588,-29.6619874481817,
2.70995196345666));
#235872=CARTESIAN_POINT('Ctrl Pts',(-51.0988914972886,-29.66461253748,2.71181160678064));
#235873=CARTESIAN_POINT('Ctrl Pts',(-51.0997380650831,-29.6671982043428,
2.71369962772058));
#235874=CARTESIAN_POINT('Ctrl Pts',(-51.1006362623626,-29.6697408831278,
2.7156118313862));
#235875=CARTESIAN_POINT('Ctrl Pts',(-51.100705105645,-29.669935769438,2.71575839426271));
#235876=CARTESIAN_POINT('Ctrl Pts',(-51.1007742270248,-29.6701304259133,
2.71590508903168));
#235877=CARTESIAN_POINT('Ctrl Pts',(-51.1008436251322,-29.670324852047,
2.71605191409871));
#235878=CARTESIAN_POINT('Ctrl Pts',(-51.1018184593122,-29.6730559530502,
2.71811436362713));
#235879=CARTESIAN_POINT('Ctrl Pts',(-51.1028499068176,-29.675741029822,
2.72020091026919));
#235880=CARTESIAN_POINT('Ctrl Pts',(-51.1039327914265,-29.678377681577,
2.72230624862142));
#235881=CARTESIAN_POINT('Ctrl Pts',(-51.1078158230492,-29.6878322458573,
2.72985561753005));
#235882=CARTESIAN_POINT('Ctrl Pts',(-51.1123884412293,-29.6967379921816,
2.7377008991417));
#235883=CARTESIAN_POINT('Ctrl Pts',(-51.1175230541879,-29.7051147523657,
2.74574823346848));
#235884=CARTESIAN_POINT('Ctrl Pts',(-51.1231654780116,-29.7143199702877,
2.75459144546698));
#235885=CARTESIAN_POINT('Ctrl Pts',(-51.1294867578937,-29.7228870317466,
2.76367911753838));
#235886=CARTESIAN_POINT('Ctrl Pts',(-51.1363687775741,-29.7308286942717,
2.77292162564186));
#235887=CARTESIAN_POINT('Ctrl Pts',(-51.1437996316773,-29.739403696713,
2.78290121484013));
#235888=CARTESIAN_POINT('Ctrl Pts',(-51.1518848589938,-29.7472505498604,
2.79306229499288));
#235889=CARTESIAN_POINT('Ctrl Pts',(-51.1605258584163,-29.7543572078866,
2.80331916684171));
#235890=CARTESIAN_POINT('Ctrl Pts',(-51.1690943687365,-29.7614042483575,
2.81348999407958));
#235891=CARTESIAN_POINT('Ctrl Pts',(-51.1782106315408,-29.7677241373251,
2.82375635966496));
#235892=CARTESIAN_POINT('Ctrl Pts',(-51.1878102687782,-29.7732664904682,
2.8340419886024));
#235893=CARTESIAN_POINT('Origin',(-0.00761999999998962,0.0131982271538671,
2.83404198860262));
#235894=CARTESIAN_POINT('Ctrl Pts',(-54.4342359163061,-31.4100231232064,
2.65878198860239));
#235895=CARTESIAN_POINT('Ctrl Pts',(-54.4385272722018,-31.4025830926782,
2.65878198860239));
#235896=CARTESIAN_POINT('Ctrl Pts',(-54.4421589890632,-31.3948506994807,
2.65944603041817));
#235897=CARTESIAN_POINT('Ctrl Pts',(-54.4451438299607,-31.386976274771,
2.66070439264018));
#235898=CARTESIAN_POINT('Ctrl Pts',(-54.4470510012003,-31.3819448922451,
2.66150842619546));
#235899=CARTESIAN_POINT('Ctrl Pts',(-54.4486949601297,-31.3768558346356,
2.66255428265328));
#235900=CARTESIAN_POINT('Ctrl Pts',(-54.4500875286678,-31.3717496422766,
2.66381699700629));
#235901=CARTESIAN_POINT('Ctrl Pts',(-54.4519881053011,-31.3647807142731,
2.66554034873229));
#235902=CARTESIAN_POINT('Ctrl Pts',(-54.4534143418201,-31.3577796218685,
2.66766759643933));
#235903=CARTESIAN_POINT('Ctrl Pts',(-54.4543880442394,-31.3508395087087,
2.67012012783109));
#235904=CARTESIAN_POINT('Ctrl Pts',(-54.454874895449,-31.3473694521289,
2.67134639352697));
#235905=CARTESIAN_POINT('Ctrl Pts',(-54.4552487192092,-31.3439144604656,
2.67265375584973));
#235906=CARTESIAN_POINT('Ctrl Pts',(-54.4555129946223,-31.3404848880616,
2.67403135126901));
#235907=CARTESIAN_POINT('Ctrl Pts',(-54.4556451323288,-31.3387701018596,
2.67472014897865));
#235908=CARTESIAN_POINT('Ctrl Pts',(-54.4557498916994,-31.337061655417,
2.67542649668594));
#235909=CARTESIAN_POINT('Ctrl Pts',(-54.4558277627244,-31.3353607484814,
2.67614899656063));
#235910=CARTESIAN_POINT('Ctrl Pts',(-54.4558472304807,-31.3349355217476,
2.67632962152931));
#235911=CARTESIAN_POINT('Ctrl Pts',(-54.4558650179026,-31.3345107659126,
2.67651125590912));
#235912=CARTESIAN_POINT('Ctrl Pts',(-54.4558811330247,-31.3340864990772,
2.67669387767485));
#235913=CARTESIAN_POINT('Ctrl Pts',(-54.4559294783909,-31.3328136985709,
2.67724174297205));
#235914=CARTESIAN_POINT('Ctrl Pts',(-54.4559627721156,-31.3315453006542,
2.67779849504709));
#235915=CARTESIAN_POINT('Ctrl Pts',(-54.4559812395335,-31.3302817797847,
2.6783635361797));
#235916=CARTESIAN_POINT('Ctrl Pts',(-54.4561088608494,-31.3215500666183,
2.68226832098864));
#235917=CARTESIAN_POINT('Ctrl Pts',(-54.4555742713436,-31.3130195924492,
2.68659153751341));
#235918=CARTESIAN_POINT('Ctrl Pts',(-54.4544853519656,-31.3047400858598,
2.69123699486121));
#235919=CARTESIAN_POINT('Ctrl Pts',(-54.4539441620237,-31.3006251938114,
2.69354577441165));
#235920=CARTESIAN_POINT('Ctrl Pts',(-54.4532655373257,-31.2965719591989,
2.69593478828072));
#235921=CARTESIAN_POINT('Ctrl Pts',(-54.4524598885392,-31.2925850928566,
2.6983956526118));
#235922=CARTESIAN_POINT('Ctrl Pts',(-54.4506825069816,-31.2837894702122,
2.70382468689006));
#235923=CARTESIAN_POINT('Ctrl Pts',(-54.4482992497263,-31.2753153512349,
2.70961155815047));
#235924=CARTESIAN_POINT('Ctrl Pts',(-54.4454010706195,-31.2672761140353,
2.71562701361727));
#235925=CARTESIAN_POINT('Ctrl Pts',(-54.4443423292438,-31.2643392793062,
2.71782453535817));
#235926=CARTESIAN_POINT('Ctrl Pts',(-54.4432206434041,-31.2614550023641,
2.72005051502361));
#235927=CARTESIAN_POINT('Ctrl Pts',(-54.4420411592045,-31.2586246102248,
2.72229986760075));
#235928=CARTESIAN_POINT('Ctrl Pts',(-54.4380793965871,-31.2491176225315,
2.72985520488836));
#235929=CARTESIAN_POINT('Ctrl Pts',(-54.4334326446226,-31.2401615453393,
2.73770845534488));
#235930=CARTESIAN_POINT('Ctrl Pts',(-54.4282277812587,-31.2317373058268,
2.74576706701668));
#235931=CARTESIAN_POINT('Ctrl Pts',(-54.4225070198651,-31.2224780686857,
2.7546244358493));
#235932=CARTESIAN_POINT('Ctrl Pts',(-54.4161118092701,-31.2138606686948,
2.76373036323069));
#235933=CARTESIAN_POINT('Ctrl Pts',(-54.4091594014079,-31.205873742907,
2.77299664636691));
#235934=CARTESIAN_POINT('Ctrl Pts',(-54.4016713602533,-31.1972714816211,
2.7829768303333));
#235935=CARTESIAN_POINT('Ctrl Pts',(-54.3935362880549,-31.1893995936771,
2.79314401478729));
#235936=CARTESIAN_POINT('Ctrl Pts',(-54.3848513315118,-31.1822725865933,
2.80341452427751));
#235937=CARTESIAN_POINT('Ctrl Pts',(-54.3762836512059,-31.1752418181688,
2.81354634721231));
#235938=CARTESIAN_POINT('Ctrl Pts',(-54.3671795569341,-31.1689352997158,
2.82378004209125));
#235939=CARTESIAN_POINT('Ctrl Pts',(-54.3576020372436,-31.1634057161443,
2.83404198860239));
#235940=CARTESIAN_POINT('Ctrl Pts',(-51.3783102687782,-29.4433108116264,
2.8340419886024));
#235941=CARTESIAN_POINT('Ctrl Pts',(-51.3691445298591,-29.4380189697941,
2.82422126443045));
#235942=CARTESIAN_POINT('Ctrl Pts',(-51.3595943606117,-29.4334690915859,
2.814428150286));
#235943=CARTESIAN_POINT('Ctrl Pts',(-51.3497152868776,-29.4296781246256,
2.80471618166476));
#235944=CARTESIAN_POINT('Ctrl Pts',(-51.3401761719881,-29.4260176124814,
2.79533842146423));
#235945=CARTESIAN_POINT('Ctrl Pts',(-51.330329192493,-29.4230642997984,
2.78603515650469));
#235946=CARTESIAN_POINT('Ctrl Pts',(-51.3202058500907,-29.420875403859,
2.77685887347017));
#235947=CARTESIAN_POINT('Ctrl Pts',(-51.3106361210858,-29.4188062116765,
2.76818441216856));
#235948=CARTESIAN_POINT('Ctrl Pts',(-51.3008185461805,-29.4174199248366,
2.75962261521919));
#235949=CARTESIAN_POINT('Ctrl Pts',(-51.2907775289365,-29.4168067767636,
2.75123537701968));
#235950=CARTESIAN_POINT('Ctrl Pts',(-51.2815299205054,-29.4162420776746,
2.74351087134432));
#235951=CARTESIAN_POINT('Ctrl Pts',(-51.2720922400956,-29.4163331870166,
2.73593399450163));
#235952=CARTESIAN_POINT('Ctrl Pts',(-51.2624911797759,-29.4171879526242,
2.72857657812894));
#235953=CARTESIAN_POINT('Ctrl Pts',(-51.2596283373979,-29.4174428264738,
2.72638274508521));
#235954=CARTESIAN_POINT('Ctrl Pts',(-51.256751052488,-29.4177658668978,
2.72420861709681));
#235955=CARTESIAN_POINT('Ctrl Pts',(-51.2538602864392,-29.4181606517644,
2.72205663736687));
#235956=CARTESIAN_POINT('Ctrl Pts',(-51.2509990568964,-29.4185514029024,
2.71992664556726));
#235957=CARTESIAN_POINT('Ctrl Pts',(-51.2481275521816,-29.4190117629203,
2.71782089927845));
#235958=CARTESIAN_POINT('Ctrl Pts',(-51.2452499391937,-29.4195444402101,
2.71574387311206));
#235959=CARTESIAN_POINT('Ctrl Pts',(-51.2450498356143,-29.4195814815471,
2.71559944077446));
#235960=CARTESIAN_POINT('Ctrl Pts',(-51.2448496951981,-29.4196188630963,
2.71545515216028));
#235961=CARTESIAN_POINT('Ctrl Pts',(-51.244649518404,-29.4196565860788,
2.71531100781689));
#235962=CARTESIAN_POINT('Ctrl Pts',(-51.2358730344469,-29.4213104998203,
2.70899119176044));
#235963=CARTESIAN_POINT('Ctrl Pts',(-51.2270453415807,-29.4236619033165,
2.70298296066801));
#235964=CARTESIAN_POINT('Ctrl Pts',(-51.2182691329813,-29.426765124801,
2.697367277741));
#235965=CARTESIAN_POINT('Ctrl Pts',(-51.2100881812719,-29.4296578665607,
2.69213248525393));
#235966=CARTESIAN_POINT('Ctrl Pts',(-51.2019513265391,-29.433204408028,
2.68723866185434));
#235967=CARTESIAN_POINT('Ctrl Pts',(-51.1939656059618,-29.43746586048,2.68278595829528));
#235968=CARTESIAN_POINT('Ctrl Pts',(-51.1910443260614,-29.4390247549184,
2.68115710172768));
#235969=CARTESIAN_POINT('Ctrl Pts',(-51.188143558922,-29.4406794572088,
2.6795876363777));
#235970=CARTESIAN_POINT('Ctrl Pts',(-51.1852696776791,-29.4424334077169,
2.67808378645323));
#235971=CARTESIAN_POINT('Ctrl Pts',(-51.1845786052481,-29.4428551742199,
2.67772216078558));
#235972=CARTESIAN_POINT('Ctrl Pts',(-51.1838888551093,-29.443283215379,
2.67736403603521));
#235973=CARTESIAN_POINT('Ctrl Pts',(-51.1832005624686,-29.4437175198435,
2.67700956934437));
#235974=CARTESIAN_POINT('Ctrl Pts',(-51.1825337789729,-29.4441382522935,
2.67666617973762));
#235975=CARTESIAN_POINT('Ctrl Pts',(-51.181868363317,-29.4445648626868,
2.67632622314077));
#235976=CARTESIAN_POINT('Ctrl Pts',(-51.1812044402991,-29.4449973374098,
2.67598984158731));
#235977=CARTESIAN_POINT('Ctrl Pts',(-51.1739303963593,-29.4497355978005,
2.67230439292177));
#235978=CARTESIAN_POINT('Ctrl Pts',(-51.1668309650356,-29.4551812510955,
2.6690496453993));
#235979=CARTESIAN_POINT('Ctrl Pts',(-51.160090071181,-29.461292997452,2.6664020356668));
#235980=CARTESIAN_POINT('Ctrl Pts',(-51.1572944215751,-29.4638277208377,
2.66530399299396));
#235981=CARTESIAN_POINT('Ctrl Pts',(-51.1545603804836,-29.4664765899956,
2.66430995142216));
#235982=CARTESIAN_POINT('Ctrl Pts',(-51.1519003687088,-29.4692349685474,
2.66343053473318));
#235983=CARTESIAN_POINT('Ctrl Pts',(-51.1473634414339,-29.4739396706108,
2.66193059792842));
#235984=CARTESIAN_POINT('Ctrl Pts',(-51.1430443628982,-29.4789629373384,
2.66076519817084));
#235985=CARTESIAN_POINT('Ctrl Pts',(-51.1390107214362,-29.4842777732941,
2.65997805604417));
#235986=CARTESIAN_POINT('Ctrl Pts',(-51.1369939007052,-29.486935191272,
2.65958448498083));
#235987=CARTESIAN_POINT('Ctrl Pts',(-51.1350496570623,-29.4896662827383,
2.65928526260719));
#235988=CARTESIAN_POINT('Ctrl Pts',(-51.1331865036874,-29.4924676612912,
2.65908463971281));
#235989=CARTESIAN_POINT('Ctrl Pts',(-51.1313233503126,-29.495269039844,
2.65888401681843));
#235990=CARTESIAN_POINT('Ctrl Pts',(-51.1295412933643,-29.49814066024,2.65878198860241));
#235991=CARTESIAN_POINT('Ctrl Pts',(-51.1278468659044,-29.5010785149114,
2.65878198860241));
#235992=CARTESIAN_POINT('Origin',(-47.1274239660506,-34.2589154226524,2.83404198860237));
#235993=CARTESIAN_POINT('Ctrl Pts',(-50.5784163149354,-36.9828414016749,
2.83404198860235));
#235994=CARTESIAN_POINT('Ctrl Pts',(-50.5870002518359,-36.9890779968908,
2.82419652440062));
#235995=CARTESIAN_POINT('Ctrl Pts',(-50.5960508067993,-36.9946187858197,
2.81438790575672));
#235996=CARTESIAN_POINT('Ctrl Pts',(-50.6055128591412,-36.9994424783901,
2.80466781256952));
#235997=CARTESIAN_POINT('Ctrl Pts',(-50.6146674511248,-37.0041094296751,
2.7952635645315));
#235998=CARTESIAN_POINT('Ctrl Pts',(-50.6242084112798,-37.0081056536702,
2.78594102496327));
#235999=CARTESIAN_POINT('Ctrl Pts',(-50.6341096134618,-37.011372274199,
2.77675109088895));
#236000=CARTESIAN_POINT('Ctrl Pts',(-50.643475541045,-37.0144622960723,
2.7680579791382));
#236001=CARTESIAN_POINT('Ctrl Pts',(-50.653164692761,-37.016899762676,2.7594827121032));
#236002=CARTESIAN_POINT('Ctrl Pts',(-50.6631621581214,-37.0185933530506,
2.75108575573402));
#236003=CARTESIAN_POINT('Ctrl Pts',(-50.6723705467533,-37.0201532722692,
2.74335155163468));
#236004=CARTESIAN_POINT('Ctrl Pts',(-50.6818410607698,-37.021082144611,
2.73576818686159));
#236005=CARTESIAN_POINT('Ctrl Pts',(-50.6915586678615,-37.0212705108776,
2.7284062616073));
#236006=CARTESIAN_POINT('Ctrl Pts',(-50.6943773762856,-37.0213251487712,
2.72627084693823));
#236007=CARTESIAN_POINT('Ctrl Pts',(-50.6972168227812,-37.0213172191968,
2.72415424587578));
#236008=CARTESIAN_POINT('Ctrl Pts',(-50.7000764815583,-37.0212433695026,
2.72205867173228));
#236009=CARTESIAN_POINT('Ctrl Pts',(-50.703176535531,-37.021163311686,2.71978693462832));
#236010=CARTESIAN_POINT('Ctrl Pts',(-50.7062960577319,-37.0210069737843,
2.71754411340733));
#236011=CARTESIAN_POINT('Ctrl Pts',(-50.7094335311101,-37.0207706534748,
2.71533341844231));
#236012=CARTESIAN_POINT('Ctrl Pts',(-50.7180443514157,-37.0201220705311,
2.70926614876378));
#236013=CARTESIAN_POINT('Ctrl Pts',(-50.726776150217,-37.0188289150183,
2.70347381860395));
#236014=CARTESIAN_POINT('Ctrl Pts',(-50.7355328079487,-37.0168522507833,
2.69804914171382));
#236015=CARTESIAN_POINT('Ctrl Pts',(-50.7435446743631,-37.0150437103239,
2.69308585687193));
#236016=CARTESIAN_POINT('Ctrl Pts',(-50.7515681793717,-37.012655929615,
2.68842799053176));
#236017=CARTESIAN_POINT('Ctrl Pts',(-50.7595400218646,-37.0096268558217,
2.68414767054209));
#236018=CARTESIAN_POINT('Ctrl Pts',(-50.763455764856,-37.0081389846694,
2.68204519134543));
#236019=CARTESIAN_POINT('Ctrl Pts',(-50.7673587034236,-37.006496006056,
2.68003431778493));
#236020=CARTESIAN_POINT('Ctrl Pts',(-50.7712388062147,-37.0046883717069,
2.67812693945242));
#236021=CARTESIAN_POINT('Ctrl Pts',(-50.7719750179266,-37.0043453906957,
2.67776503299194));
#236022=CARTESIAN_POINT('Ctrl Pts',(-50.7727105984661,-37.0039959853417,
2.67740659639915));
#236023=CARTESIAN_POINT('Ctrl Pts',(-50.7734454079406,-37.0036401497476,
2.67705178968846));
#236024=CARTESIAN_POINT('Ctrl Pts',(-50.7741572546191,-37.0032954340158,
2.67670807068748));
#236025=CARTESIAN_POINT('Ctrl Pts',(-50.7748683776569,-37.0029446836755,
2.67636775825256));
#236026=CARTESIAN_POINT('Ctrl Pts',(-50.7755786476299,-37.0025878964871,
2.67603099699246));
#236027=CARTESIAN_POINT('Ctrl Pts',(-50.7833190234414,-36.9986997032254,
2.6723610421711));
#236028=CARTESIAN_POINT('Ctrl Pts',(-50.7909629993144,-36.9940916451525,
2.66911440541448));
#236029=CARTESIAN_POINT('Ctrl Pts',(-50.7983209798301,-36.9887818345679,
2.666467781896));
#236030=CARTESIAN_POINT('Ctrl Pts',(-50.8014283006924,-36.986539468586,
2.66535009634952));
#236031=CARTESIAN_POINT('Ctrl Pts',(-50.8044846273289,-36.9841723869923,
2.66433897912328));
#236032=CARTESIAN_POINT('Ctrl Pts',(-50.8074762285637,-36.9816838130236,
2.66344564884782));
#236033=CARTESIAN_POINT('Ctrl Pts',(-50.8125140102916,-36.9774931166427,
2.66194130298574));
#236034=CARTESIAN_POINT('Ctrl Pts',(-50.81736572735,-36.9729576356983,2.66077206705408));
#236035=CARTESIAN_POINT('Ctrl Pts',(-50.8219595855748,-36.9680961762157,
2.65998225155702));
#236036=CARTESIAN_POINT('Ctrl Pts',(-50.823108050131,-36.966880811345,2.65978479768275));
#236037=CARTESIAN_POINT('Ctrl Pts',(-50.8242402182961,-36.9656449236012,
2.65961098966609));
#236038=CARTESIAN_POINT('Ctrl Pts',(-50.8253547230709,-36.9643886196684,
2.65946139030488));
#236039=CARTESIAN_POINT('Ctrl Pts',(-50.8270264802332,-36.9625041637692,
2.65923699126307));
#236040=CARTESIAN_POINT('Ctrl Pts',(-50.8286584747053,-36.9605737761779,
2.65906707562428));
#236041=CARTESIAN_POINT('Ctrl Pts',(-50.8302474395911,-36.9585988181539,
2.65895332562906));
#236042=CARTESIAN_POINT('Ctrl Pts',(-50.831836404477,-36.95662386013,2.65883957563384));
#236043=CARTESIAN_POINT('Ctrl Pts',(-50.8333823430133,-36.9546043428184,
2.65878198860235));
#236044=CARTESIAN_POINT('Ctrl Pts',(-50.8348823336483,-36.9525415975215,
2.65878198860235));
#236045=CARTESIAN_POINT('Ctrl Pts',(-47.7461450747862,-34.7084426211234,
2.65878198860237));
#236046=CARTESIAN_POINT('Ctrl Pts',(-47.7410693801616,-34.7154221779229,
2.65878198860237));
#236047=CARTESIAN_POINT('Ctrl Pts',(-47.7366138137626,-34.7227602152543,
2.65945335517834));
#236048=CARTESIAN_POINT('Ctrl Pts',(-47.7327846251241,-34.730305751405,
2.66072561226586));
#236049=CARTESIAN_POINT('Ctrl Pts',(-47.7303113621613,-34.7351793935413,
2.66154735980324));
#236050=CARTESIAN_POINT('Ctrl Pts',(-47.7280985748133,-34.7401391868073,
2.66261895766866));
#236051=CARTESIAN_POINT('Ctrl Pts',(-47.7261394006516,-34.7451421370596,
2.66391429251006));
#236052=CARTESIAN_POINT('Ctrl Pts',(-47.7235426275286,-34.7517732610326,
2.66563118464103));
#236053=CARTESIAN_POINT('Ctrl Pts',(-47.7213971161177,-34.7584811778434,
2.66774105138679));
#236054=CARTESIAN_POINT('Ctrl Pts',(-47.7196932909343,-34.7651763312118,
2.67016894181729));
#236055=CARTESIAN_POINT('Ctrl Pts',(-47.7188413783425,-34.768523907896,
2.67138288703255));
#236056=CARTESIAN_POINT('Ctrl Pts',(-47.7180997687559,-34.7718684539193,
2.67267613167531));
#236057=CARTESIAN_POINT('Ctrl Pts',(-47.7174664279767,-34.7751999143434,
2.67403835432532));
#236058=CARTESIAN_POINT('Ctrl Pts',(-47.7171497575871,-34.7768656445554,
2.67471946565033));
#236059=CARTESIAN_POINT('Ctrl Pts',(-47.7168601447018,-34.7785281166319,
2.67541781389502));
#236060=CARTESIAN_POINT('Ctrl Pts',(-47.7165972740595,-34.7801861569091,
2.67613207244148));
#236061=CARTESIAN_POINT('Ctrl Pts',(-47.7165315563989,-34.7806006669784,
2.67631063707809));
#236062=CARTESIAN_POINT('Ctrl Pts',(-47.7164675099215,-34.7810149003418,
2.67649019601824));
#236063=CARTESIAN_POINT('Ctrl Pts',(-47.7164051292831,-34.7814288392283,
2.67667072836636));
#236064=CARTESIAN_POINT('Ctrl Pts',(-47.7162179873682,-34.7826706558876,
2.67721232541069));
#236065=CARTESIAN_POINT('Ctrl Pts',(-47.7160458390452,-34.783909820854,
2.67776268340026));
#236066=CARTESIAN_POINT('Ctrl Pts',(-47.7158885307486,-34.7851458668348,
2.67832123541495));
#236067=CARTESIAN_POINT('Ctrl Pts',(-47.7147804714197,-34.7938524151211,
2.68225560368418));
#236068=CARTESIAN_POINT('Ctrl Pts',(-47.7143609747536,-34.8024290252883,
2.68661792998856));
#236069=CARTESIAN_POINT('Ctrl Pts',(-47.7145286167444,-34.8108122146617,
2.69130986622539));
#236070=CARTESIAN_POINT('Ctrl Pts',(-47.7146099229288,-34.814878052449,
2.69358545023021));
#236071=CARTESIAN_POINT('Ctrl Pts',(-47.7148297795037,-34.8188987667929,
2.69593918853441));
#236072=CARTESIAN_POINT('Ctrl Pts',(-47.7151790039207,-34.8228686918041,
2.69836306235452));
#236073=CARTESIAN_POINT('Ctrl Pts',(-47.7157136421035,-34.8289463696254,
2.70207384382184));
#236074=CARTESIAN_POINT('Ctrl Pts',(-47.7165501157949,-34.8349017567798,
2.70594760814185));
#236075=CARTESIAN_POINT('Ctrl Pts',(-47.7176563296779,-34.8407017446569,
2.70995196345664));
#236076=CARTESIAN_POINT('Ctrl Pts',(-47.718170061128,-34.8433952890322,
2.71181160678062));
#236077=CARTESIAN_POINT('Ctrl Pts',(-47.7187417155519,-34.846055281772,
2.71369962772054));
#236078=CARTESIAN_POINT('Ctrl Pts',(-47.7193692101068,-34.8486779186779,
2.71561183138616));
#236079=CARTESIAN_POINT('Ctrl Pts',(-47.719417305092,-34.848878933463,2.71575839426267));
#236080=CARTESIAN_POINT('Ctrl Pts',(-47.7194657006753,-34.8490797487414,
2.71590508903165));
#236081=CARTESIAN_POINT('Ctrl Pts',(-47.7195143955476,-34.8492803638659,
2.71605191409867));
#236082=CARTESIAN_POINT('Ctrl Pts',(-47.7201984116931,-34.8520984015308,
2.71811436362709));
#236083=CARTESIAN_POINT('Ctrl Pts',(-47.7209435418724,-34.8548765847938,
2.72020091026915));
#236084=CARTESIAN_POINT('Ctrl Pts',(-47.72174488917,-34.8576119849587,2.72230624862138));
#236085=CARTESIAN_POINT('Ctrl Pts',(-47.7246183780643,-34.8674206434752,
2.72985561753025));
#236086=CARTESIAN_POINT('Ctrl Pts',(-47.7282350429861,-34.8767555719411,
2.73770089914216));
#236087=CARTESIAN_POINT('Ctrl Pts',(-47.7324659181287,-34.8856231565588,
2.74574823346921));
#236088=CARTESIAN_POINT('Ctrl Pts',(-47.7371152248811,-34.8953677412255,
2.75459144546802));
#236089=CARTESIAN_POINT('Ctrl Pts',(-47.7425063743617,-34.9045486250976,
2.76367911753973));
#236090=CARTESIAN_POINT('Ctrl Pts',(-47.7485205638389,-34.913166149306,
2.77292162564353));
#236091=CARTESIAN_POINT('Ctrl Pts',(-47.7550143791185,-34.9224709127472,
2.78290121484226));
#236092=CARTESIAN_POINT('Ctrl Pts',(-47.7622350952133,-34.9311199163988,
2.79306229499547));
#236093=CARTESIAN_POINT('Ctrl Pts',(-47.7700859102949,-34.9390908737997,
2.80331916684477));
#236094=CARTESIAN_POINT('Ctrl Pts',(-47.7778708651073,-34.9469949630609,
2.81348999408162));
#236095=CARTESIAN_POINT('Ctrl Pts',(-47.7862765797875,-34.9542331399563,
2.82375635966596));
#236096=CARTESIAN_POINT('Ctrl Pts',(-47.7952442955499,-34.9607485668368,
2.83404198860237));
#236097=CARTESIAN_POINT('Origin',(-0.00895784724492722,0.0123294189944669,
2.83404198860262));
#236098=CARTESIAN_POINT('Ctrl Pts',(-50.8527980281382,-36.9278827595329,
2.65878198860235));
#236099=CARTESIAN_POINT('Ctrl Pts',(-50.8578435704952,-36.9209320551073,
2.65878198860235));
#236100=CARTESIAN_POINT('Ctrl Pts',(-50.8622636476101,-36.9136216385511,
2.65944603041817));
#236101=CARTESIAN_POINT('Ctrl Pts',(-50.866055238751,-36.9061023515958,
2.66070439264024));
#236102=CARTESIAN_POINT('Ctrl Pts',(-50.8684778849904,-36.9012978851888,
2.66150842619551));
#236103=CARTESIAN_POINT('Ctrl Pts',(-50.870644789512,-36.8964085464702,
2.66255428265329));
#236104=CARTESIAN_POINT('Ctrl Pts',(-50.8725634718544,-36.8914758894167,
2.66381699700625));
#236105=CARTESIAN_POINT('Ctrl Pts',(-50.8751820882648,-36.8847438022848,
2.66554034873224));
#236106=CARTESIAN_POINT('Ctrl Pts',(-50.8773323251411,-36.8779301449084,
2.66766759643928));
#236107=CARTESIAN_POINT('Ctrl Pts',(-50.8790261328802,-36.8711298300323,
2.67012012783103));
#236108=CARTESIAN_POINT('Ctrl Pts',(-50.8798730367497,-36.8677296725943,
2.67134639352691));
#236109=CARTESIAN_POINT('Ctrl Pts',(-50.8806059576334,-36.86433268296,2.67265375584968));
#236110=CARTESIAN_POINT('Ctrl Pts',(-50.8812272732512,-36.8609495224153,
2.67403135126895));
#236111=CARTESIAN_POINT('Ctrl Pts',(-50.8815379310601,-36.859257942143,
2.67472014897859));
#236112=CARTESIAN_POINT('Ctrl Pts',(-50.881820697829,-36.8575698050847,
2.67542649668587));
#236113=CARTESIAN_POINT('Ctrl Pts',(-50.8820759354566,-36.8558863556339,
2.67614899656056));
#236114=CARTESIAN_POINT('Ctrl Pts',(-50.8821397448634,-36.8554654932712,
2.67632962152924));
#236115=CARTESIAN_POINT('Ctrl Pts',(-50.8822018339187,-36.8550449235851,
2.67651125590905));
#236116=CARTESIAN_POINT('Ctrl Pts',(-50.8822622087208,-36.8546246654167,
2.67669387767478));
#236117=CARTESIAN_POINT('Ctrl Pts',(-50.882443333127,-36.8533638909116,
2.67724174297199));
#236118=CARTESIAN_POINT('Ctrl Pts',(-50.8826090281503,-36.8521059215534,
2.67779849504702));
#236119=CARTESIAN_POINT('Ctrl Pts',(-50.8827594682965,-36.8508512527541,
2.67836353617963));
#236120=CARTESIAN_POINT('Ctrl Pts',(-50.8837991030485,-36.8421807128858,
2.68226832098869));
#236121=CARTESIAN_POINT('Ctrl Pts',(-50.8841591194358,-36.8336410897271,
2.6865915375136));
#236122=CARTESIAN_POINT('Ctrl Pts',(-50.8839416093724,-36.8252931160716,
2.69123699486157));
#236123=CARTESIAN_POINT('Ctrl Pts',(-50.883833507468,-36.8211441960797,
2.69354577441188));
#236124=CARTESIAN_POINT('Ctrl Pts',(-50.8835822787324,-36.8170422299139,
2.69593478828082));
#236125=CARTESIAN_POINT('Ctrl Pts',(-50.8831977843863,-36.8129929908132,
2.69839565261176));
#236126=CARTESIAN_POINT('Ctrl Pts',(-50.8823495324293,-36.8040597645471,
2.70382468689002));
#236127=CARTESIAN_POINT('Ctrl Pts',(-50.8808651175409,-36.7953829494618,
2.70961155815043));
#236128=CARTESIAN_POINT('Ctrl Pts',(-50.8788231440728,-36.7870848098364,
2.71562701361724));
#236129=CARTESIAN_POINT('Ctrl Pts',(-50.8780771854143,-36.7840533947862,
2.71782453535815));
#236130=CARTESIAN_POINT('Ctrl Pts',(-50.8772631333233,-36.7810676701179,
2.7200505150236));
#236131=CARTESIAN_POINT('Ctrl Pts',(-50.8763859670024,-36.7781294934921,
2.72229986760074));
#236132=CARTESIAN_POINT('Ctrl Pts',(-50.8734396581491,-36.7682604691141,
2.72985520488826));
#236133=CARTESIAN_POINT('Ctrl Pts',(-50.869754526564,-36.7588677364079,
2.73770845534467));
#236134=CARTESIAN_POINT('Ctrl Pts',(-50.8654587487966,-36.749945589392,
2.74576706701634));
#236135=CARTESIAN_POINT('Ctrl Pts',(-50.860737180162,-36.7401390929237,
2.75462443584886));
#236136=CARTESIAN_POINT('Ctrl Pts',(-50.8552777667782,-36.7309004184158,
2.76373036323012));
#236137=CARTESIAN_POINT('Ctrl Pts',(-50.8491983060126,-36.7222305213335,
2.77299664636622));
#236138=CARTESIAN_POINT('Ctrl Pts',(-50.8426504662838,-36.7128926707001,
2.78297683033255));
#236139=CARTESIAN_POINT('Ctrl Pts',(-50.835382795212,-36.7042135591864,
2.79314401478649));
#236140=CARTESIAN_POINT('Ctrl Pts',(-50.8274903908677,-36.6962177694322,
2.80341452427668));
#236141=CARTESIAN_POINT('Ctrl Pts',(-50.8197045606298,-36.6883299498364,
2.81354634721171));
#236142=CARTESIAN_POINT('Ctrl Pts',(-50.8113095502213,-36.6811063421674,
2.82378004209092));
#236143=CARTESIAN_POINT('Ctrl Pts',(-50.8023624960588,-36.674605926818,
2.83404198860235));
#236144=CARTESIAN_POINT('Ctrl Pts',(-48.0191904766733,-34.6525130919799,
2.83404198860237));
#236145=CARTESIAN_POINT('Ctrl Pts',(-48.0106280967249,-34.6462921588064,
2.82422126442958));
#236146=CARTESIAN_POINT('Ctrl Pts',(-48.0016058360802,-34.6407689407913,
2.8144281502843));
#236147=CARTESIAN_POINT('Ctrl Pts',(-47.9921771448955,-34.6359660967484,
2.80471618166224));
#236148=CARTESIAN_POINT('Ctrl Pts',(-47.9830729139841,-34.6313285282523,
2.79533842146122));
#236149=CARTESIAN_POINT('Ctrl Pts',(-47.9735885825087,-34.6273621044907,
2.78603515650119));
#236150=CARTESIAN_POINT('Ctrl Pts',(-47.9637494987635,-34.6241270221279,
2.77685887346622));
#236151=CARTESIAN_POINT('Ctrl Pts',(-47.9544484832141,-34.62106885613,2.76818441216434));
#236152=CARTESIAN_POINT('Ctrl Pts',(-47.9448295964439,-34.6186639474967,
2.75962261521474));
#236153=CARTESIAN_POINT('Ctrl Pts',(-47.9349076763684,-34.6170045862111,
2.75123537701502));
#236154=CARTESIAN_POINT('Ctrl Pts',(-47.9257697544315,-34.6154763423049,
2.74351087133956));
#236155=CARTESIAN_POINT('Ctrl Pts',(-47.9163742511026,-34.6145804463106,
2.73593399449679));
#236156=CARTESIAN_POINT('Ctrl Pts',(-47.9067364390602,-34.614426945342,
2.72857657812405));
#236157=CARTESIAN_POINT('Ctrl Pts',(-47.9038626380626,-34.6143811744519,
2.72638274508197));
#236158=CARTESIAN_POINT('Ctrl Pts',(-47.9009673483035,-34.6144016870566,
2.72420861709519));
#236159=CARTESIAN_POINT('Ctrl Pts',(-47.8980511519203,-34.6144921419176,
2.72205663736682));
#236160=CARTESIAN_POINT('Ctrl Pts',(-47.8951647518764,-34.6145816725528,
2.71992664556721));
#236161=CARTESIAN_POINT('Ctrl Pts',(-47.8922608568396,-34.6147393566953,
2.7178208992784));
#236162=CARTESIAN_POINT('Ctrl Pts',(-47.8893433277782,-34.6149683234597,
2.71574387311201));
#236163=CARTESIAN_POINT('Ctrl Pts',(-47.8891404485131,-34.6149842453607,
2.71559944077442));
#236164=CARTESIAN_POINT('Ctrl Pts',(-47.8889374970512,-34.6150005017597,
2.71545515216025));
#236165=CARTESIAN_POINT('Ctrl Pts',(-47.8887344737211,-34.6150170939191,
2.71531100781686));
#236166=CARTESIAN_POINT('Ctrl Pts',(-47.8798331871996,-34.6157445549671,
2.7089911917604));
#236167=CARTESIAN_POINT('Ctrl Pts',(-47.8708080647646,-34.6171603320595,
2.70298296066797));
#236168=CARTESIAN_POINT('Ctrl Pts',(-47.8617555581812,-34.6193291901737,
2.69736727774096));
#236169=CARTESIAN_POINT('Ctrl Pts',(-47.8533170487304,-34.6213509428812,
2.69213248525385));
#236170=CARTESIAN_POINT('Ctrl Pts',(-47.8448540540096,-34.6240275231022,
2.68723866185421));
#236171=CARTESIAN_POINT('Ctrl Pts',(-47.836466636969,-34.6274308957718,
2.68278595829513));
#236172=CARTESIAN_POINT('Ctrl Pts',(-47.8333984113057,-34.6286758935246,
2.68115710172758));
#236173=CARTESIAN_POINT('Ctrl Pts',(-47.8303405713846,-34.6300183184512,
2.67958763637765));
#236174=CARTESIAN_POINT('Ctrl Pts',(-47.8272990958127,-34.631462258245,
2.67808378645322));
#236175=CARTESIAN_POINT('Ctrl Pts',(-47.8265677225444,-34.6318094775277,
2.67772216078557));
#236176=CARTESIAN_POINT('Ctrl Pts',(-47.8258370084444,-34.6321630753106,
2.6773640360352));
#236177=CARTESIAN_POINT('Ctrl Pts',(-47.8251070891646,-34.6325230544378,
2.67700956934436));
#236178=CARTESIAN_POINT('Ctrl Pts',(-47.8243999798622,-34.6328717842173,
2.67666617973761));
#236179=CARTESIAN_POINT('Ctrl Pts',(-47.823693616494,-34.6332265027181,
2.67632622314076));
#236180=CARTESIAN_POINT('Ctrl Pts',(-47.8229881245977,-34.6335872094466,
2.6759898415873));
#236181=CARTESIAN_POINT('Ctrl Pts',(-47.8152586455542,-34.6375391685165,
2.67230439292162));
#236182=CARTESIAN_POINT('Ctrl Pts',(-47.8076288798874,-34.6422128973069,
2.66904964539903));
#236183=CARTESIAN_POINT('Ctrl Pts',(-47.8002860618999,-34.647586547602,
2.66640203566646));
#236184=CARTESIAN_POINT('Ctrl Pts',(-47.797240776415,-34.6498151605503,
2.66530399299375));
#236185=CARTESIAN_POINT('Ctrl Pts',(-47.7942448304645,-34.6521637338119,
2.66430995142206));
#236186=CARTESIAN_POINT('Ctrl Pts',(-47.7913110614416,-34.654628954734,
2.66343053473316));
#236187=CARTESIAN_POINT('Ctrl Pts',(-47.7863072126523,-34.6588336459112,
2.66193059792839));
#236188=CARTESIAN_POINT('Ctrl Pts',(-47.7814867201291,-34.6633779280161,
2.66076519817082));
#236189=CARTESIAN_POINT('Ctrl Pts',(-47.7769196237422,-34.668242018401,
2.65997805604413));
#236190=CARTESIAN_POINT('Ctrl Pts',(-47.7746360755487,-34.6706740635934,
2.65958448498079));
#236191=CARTESIAN_POINT('Ctrl Pts',(-47.7724170058818,-34.6731869650547,
2.65928526260715));
#236192=CARTESIAN_POINT('Ctrl Pts',(-47.770271235261,-34.6757782448036,
2.65908463971277));
#236193=CARTESIAN_POINT('Ctrl Pts',(-47.7681254646401,-34.6783695245525,
2.65888401681839));
#236194=CARTESIAN_POINT('Ctrl Pts',(-47.7660530039191,-34.6810391382372,
2.65878198860237));
#236195=CARTESIAN_POINT('Ctrl Pts',(-47.764060769276,-34.6837837831348,
2.65878198860237));
#236196=CARTESIAN_POINT('Origin',(-43.2882232241945,-38.9973987043321,2.83404198860233));
#236197=CARTESIAN_POINT('Ctrl Pts',(-46.4355828792667,-42.0671296588098,
2.83404198860232));
#236198=CARTESIAN_POINT('Ctrl Pts',(-46.4434678907489,-42.0742293550377,
2.82419652440029));
#236199=CARTESIAN_POINT('Ctrl Pts',(-46.4518896956734,-42.0806858315472,
2.81438790575613));
#236200=CARTESIAN_POINT('Ctrl Pts',(-46.4607957007311,-42.0864721532157,
2.80466781256868));
#236201=CARTESIAN_POINT('Ctrl Pts',(-46.4694123136561,-42.0920704538853,
2.79526356453048));
#236202=CARTESIAN_POINT('Ctrl Pts',(-46.4784832882803,-42.0970420880504,
2.78594102496209));
#236203=CARTESIAN_POINT('Ctrl Pts',(-46.487988795817,-42.1013257711387,
2.77675109088763));
#236204=CARTESIAN_POINT('Ctrl Pts',(-46.4969804206313,-42.1053778715663,
2.76805797913676));
#236205=CARTESIAN_POINT('Ctrl Pts',(-46.5063617095223,-42.1088147776121,
2.75948271210165));
#236206=CARTESIAN_POINT('Ctrl Pts',(-46.5161273793223,-42.1115441100122,
2.75108575573236));
#236207=CARTESIAN_POINT('Ctrl Pts',(-46.5251222674793,-42.1140580225429,
2.74335155163292));
#236208=CARTESIAN_POINT('Ctrl Pts',(-46.5344438074308,-42.1159717447012,
2.73576818685973));
#236209=CARTESIAN_POINT('Ctrl Pts',(-46.544088490818,-42.1171748456135,
2.72840626160534));
#236210=CARTESIAN_POINT('Ctrl Pts',(-46.5468860468465,-42.1175238194549,
2.72627084693694));
#236211=CARTESIAN_POINT('Ctrl Pts',(-46.5497107674225,-42.1178127362981,
2.72415424587514));
#236212=CARTESIAN_POINT('Ctrl Pts',(-46.5525624800838,-42.1180382068977,
2.72205867173227));
#236213=CARTESIAN_POINT('Ctrl Pts',(-46.5556539199571,-42.118282631524,
2.7197869346283));
#236214=CARTESIAN_POINT('Ctrl Pts',(-46.5587726948496,-42.1184532289194,
2.7175441134073));
#236215=CARTESIAN_POINT('Ctrl Pts',(-46.5619176830191,-42.1185461584681,
2.71533341844227));
#236216=CARTESIAN_POINT('Ctrl Pts',(-46.5705491277285,-42.1188012043436,
2.70926614876374));
#236217=CARTESIAN_POINT('Ctrl Pts',(-46.5793682643808,-42.1184278543823,
2.70347381860392));
#236218=CARTESIAN_POINT('Ctrl Pts',(-46.5882835699001,-42.1173773384969,
2.69804914171379));
#236219=CARTESIAN_POINT('Ctrl Pts',(-46.596440590427,-42.1164161734956,
2.69308585687187));
#236220=CARTESIAN_POINT('Ctrl Pts',(-46.6046697328839,-42.1148801579478,
2.68842799053166));
#236221=CARTESIAN_POINT('Ctrl Pts',(-46.6129145292183,-42.1127009621828,
2.68414767054197));
#236222=CARTESIAN_POINT('Ctrl Pts',(-46.6169643462449,-42.1116305483418,
2.68204519134533));
#236223=CARTESIAN_POINT('Ctrl Pts',(-46.6210176421363,-42.1104045383079,
2.68003431778485));
#236224=CARTESIAN_POINT('Ctrl Pts',(-46.6250654385589,-42.109012387551,
2.67812693945236));
#236225=CARTESIAN_POINT('Ctrl Pts',(-46.6258334685041,-42.1087482405045,
2.67776503299188));
#236226=CARTESIAN_POINT('Ctrl Pts',(-46.6266015422611,-42.1084776383329,
2.67740659639909));
#236227=CARTESIAN_POINT('Ctrl Pts',(-46.6273695213203,-42.1082005605487,
2.6770517896884));
#236228=CARTESIAN_POINT('Ctrl Pts',(-46.6281135010339,-42.1079321414451,
2.67670807068742));
#236229=CARTESIAN_POINT('Ctrl Pts',(-46.6288573918593,-42.1076576451502,
2.6763677582525));
#236230=CARTESIAN_POINT('Ctrl Pts',(-46.6296010653156,-42.1073770559081,
2.6760309969924));
#236231=CARTESIAN_POINT('Ctrl Pts',(-46.637705465405,-42.1043192521647,
2.67236104217107));
#236232=CARTESIAN_POINT('Ctrl Pts',(-46.6457892400072,-42.1005354505673,
2.66911440541448));
#236233=CARTESIAN_POINT('Ctrl Pts',(-46.6536619390764,-42.0960238460769,
2.66646778189602));
#236234=CARTESIAN_POINT('Ctrl Pts',(-46.6569866287802,-42.0941185674849,
2.6653500963495));
#236235=CARTESIAN_POINT('Ctrl Pts',(-46.660273639941,-42.0920839261384,
2.66433897912325));
#236236=CARTESIAN_POINT('Ctrl Pts',(-46.663508979684,-42.089921692318,2.66344564884777));
#236237=CARTESIAN_POINT('Ctrl Pts',(-46.6689572109692,-42.0862805445927,
2.66194130298569));
#236238=CARTESIAN_POINT('Ctrl Pts',(-46.6742564366672,-42.0822770520158,
2.66077206705403));
#236239=CARTESIAN_POINT('Ctrl Pts',(-46.6793332901452,-42.0779224130578,
2.65998225155697));
#236240=CARTESIAN_POINT('Ctrl Pts',(-46.6806025035146,-42.0768337533183,
2.65978479768271));
#236241=CARTESIAN_POINT('Ctrl Pts',(-46.6818576549907,-42.0757229796953,
2.65961098966605));
#236242=CARTESIAN_POINT('Ctrl Pts',(-46.6830973739112,-42.0745900553982,
2.65946139030484));
#236243=CARTESIAN_POINT('Ctrl Pts',(-46.684956952292,-42.0728906689527,
2.65923699126303));
#236244=CARTESIAN_POINT('Ctrl Pts',(-46.6867817869761,-42.0711414461008,
2.65906707562424));
#236245=CARTESIAN_POINT('Ctrl Pts',(-46.6885684866732,-42.0693433991612,
2.65895332562902));
#236246=CARTESIAN_POINT('Ctrl Pts',(-46.6903551863704,-42.0675453522217,
2.6588395756338));
#236247=CARTESIAN_POINT('Ctrl Pts',(-46.6921037531347,-42.0656984926166,
2.65878198860231));
#236248=CARTESIAN_POINT('Ctrl Pts',(-46.6938111422601,-42.0638038389702,
2.65878198860231));
#236249=CARTESIAN_POINT('Ctrl Pts',(-43.8565665267053,-39.5091373124624,
2.65878198860234));
#236250=CARTESIAN_POINT('Ctrl Pts',(-43.8507890749206,-39.5155480799602,
2.65878198860234));
#236251=CARTESIAN_POINT('Ctrl Pts',(-43.845590882815,-39.5223801852464,
2.65945335517826));
#236252=CARTESIAN_POINT('Ctrl Pts',(-43.8409939475743,-39.5294841269563,
2.6607256122657));
#236253=CARTESIAN_POINT('Ctrl Pts',(-43.8380247990816,-39.5340725443945,
2.66154735980308));
#236254=CARTESIAN_POINT('Ctrl Pts',(-43.8353056940458,-39.5387738681332,
2.66261895766853));
#236255=CARTESIAN_POINT('Ctrl Pts',(-43.8328343017434,-39.5435446222364,
2.66391429250998));
#236256=CARTESIAN_POINT('Ctrl Pts',(-43.8295586128166,-39.5498679835145,
2.66563118464094));
#236257=CARTESIAN_POINT('Ctrl Pts',(-43.8267236865058,-39.5563148866444,
2.6677410513867));
#236258=CARTESIAN_POINT('Ctrl Pts',(-43.824329360962,-39.5627952650341,
2.67016894181721));
#236259=CARTESIAN_POINT('Ctrl Pts',(-43.8231321981901,-39.5660354542289,
2.67138288703246));
#236260=CARTESIAN_POINT('Ctrl Pts',(-43.8220450509623,-39.5692841591687,
2.67267613167523));
#236261=CARTESIAN_POINT('Ctrl Pts',(-43.8210669472515,-39.5725311673656,
2.67403835432525));
#236262=CARTESIAN_POINT('Ctrl Pts',(-43.8205778953961,-39.5741546714641,
2.67471946565026));
#236263=CARTESIAN_POINT('Ctrl Pts',(-43.8201160933892,-39.5757777635548,
2.67541781389494));
#236264=CARTESIAN_POINT('Ctrl Pts',(-43.8196813503776,-39.5773992434496,
2.67613207244141));
#236265=CARTESIAN_POINT('Ctrl Pts',(-43.8195726646246,-39.5778046134233,
2.67631063707802));
#236266=CARTESIAN_POINT('Ctrl Pts',(-43.8194656698236,-39.5782098828931,
2.67649019601817));
#236267=CARTESIAN_POINT('Ctrl Pts',(-43.8193603625172,-39.5786150336268,
2.67667072836628));
#236268=CARTESIAN_POINT('Ctrl Pts',(-43.8190444405982,-39.5798304858277,
2.67721232541062));
#236269=CARTESIAN_POINT('Ctrl Pts',(-43.8187437073121,-39.5810448681191,
2.67776268340019));
#236270=CARTESIAN_POINT('Ctrl Pts',(-43.8184580587799,-39.5822576997162,
2.67832123541488));
#236271=CARTESIAN_POINT('Ctrl Pts',(-43.8164459874031,-39.5908007288813,
2.68225560368418));
#236272=CARTESIAN_POINT('Ctrl Pts',(-43.8151322889028,-39.5992865061389,
2.68661792998865));
#236273=CARTESIAN_POINT('Ctrl Pts',(-43.8144227306308,-39.6076412948836,
2.69130986622557));
#236274=CARTESIAN_POINT('Ctrl Pts',(-43.8140785956356,-39.6116933583964,
2.69358545023032));
#236275=CARTESIAN_POINT('Ctrl Pts',(-43.8138769687216,-39.6157150281162,
2.69593918853444));
#236276=CARTESIAN_POINT('Ctrl Pts',(-43.81380930989,-39.6196997093543,2.69836306235448));
#236277=CARTESIAN_POINT('Ctrl Pts',(-43.8137057289461,-39.6257999779283,
2.7020738438218));
#236278=CARTESIAN_POINT('Ctrl Pts',(-43.8139151128796,-39.6318101761582,
2.7059476081418));
#236279=CARTESIAN_POINT('Ctrl Pts',(-43.8144090029875,-39.6376940219322,
2.7099519634566));
#236280=CARTESIAN_POINT('Ctrl Pts',(-43.8146383681086,-39.6404265103486,
2.71181160678058));
#236281=CARTESIAN_POINT('Ctrl Pts',(-43.8149288459964,-39.6431316855283,
2.71369962772051));
#236282=CARTESIAN_POINT('Ctrl Pts',(-43.815278762865,-39.6458055463962,
2.71561183138613));
#236283=CARTESIAN_POINT('Ctrl Pts',(-43.8153055826142,-39.6460104872962,
2.71575839426264));
#236284=CARTESIAN_POINT('Ctrl Pts',(-43.8153327221691,-39.6462152612035,
2.71590508903161));
#236285=CARTESIAN_POINT('Ctrl Pts',(-43.8153601802951,-39.6464198673376,
2.71605191409863));
#236286=CARTESIAN_POINT('Ctrl Pts',(-43.815745884182,-39.6492939666538,
2.71811436362705));
#236287=CARTESIAN_POINT('Ctrl Pts',(-43.8161965332331,-39.6521348180507,
2.72020091026911));
#236288=CARTESIAN_POINT('Ctrl Pts',(-43.8167075634907,-39.6549389970089,
2.72230624862134));
#236289=CARTESIAN_POINT('Ctrl Pts',(-43.8185400271108,-39.6649942840468,
2.72985561753065));
#236290=CARTESIAN_POINT('Ctrl Pts',(-43.8211611138367,-39.6746561192248,
2.73770089914302));
#236291=CARTESIAN_POINT('Ctrl Pts',(-43.8244418968098,-39.6839173731636,
2.74574823347057));
#236292=CARTESIAN_POINT('Ctrl Pts',(-43.8280471477134,-39.694094560867,
2.75459144547026));
#236293=CARTESIAN_POINT('Ctrl Pts',(-43.8324491002311,-39.7037886794679,
2.76367911754291));
#236294=CARTESIAN_POINT('Ctrl Pts',(-43.8375295667871,-39.7129876499616,
2.77292162564768));
#236295=CARTESIAN_POINT('Ctrl Pts',(-43.8430151956447,-39.7229202294687,
2.78290121484821));
#236296=CARTESIAN_POINT('Ctrl Pts',(-43.8492922888422,-39.7322766233317,
2.7930622950033));
#236297=CARTESIAN_POINT('Ctrl Pts',(-43.8562669044111,-39.741024548631,
2.80331916685446));
#236298=CARTESIAN_POINT('Ctrl Pts',(-43.8631830101207,-39.7496990878241,
2.81348999408814));
#236299=CARTESIAN_POINT('Ctrl Pts',(-43.8707860819065,-39.7577762496645,
2.82375635966922));
#236300=CARTESIAN_POINT('Ctrl Pts',(-43.8790236240217,-39.7651933659001,
2.83404198860233));
#236301=CARTESIAN_POINT('Origin',(-0.0101975504408993,0.0113255271404686,
2.83404198860262));
#236302=CARTESIAN_POINT('Ctrl Pts',(-46.7142062431419,-42.0411527846897,
2.65878198860231));
#236303=CARTESIAN_POINT('Ctrl Pts',(-46.7199506919425,-42.0347675597389,
2.65878198860232));
#236304=CARTESIAN_POINT('Ctrl Pts',(-46.7251107020211,-42.0279592142775,
2.65944603041819));
#236305=CARTESIAN_POINT('Ctrl Pts',(-46.7296675019394,-42.0208774479579,
2.66070439264037));
#236306=CARTESIAN_POINT('Ctrl Pts',(-46.7325790801593,-42.0163525364093,
2.66150842619562));
#236307=CARTESIAN_POINT('Ctrl Pts',(-46.7352451892138,-42.0117164851998,
2.66255428265335));
#236308=CARTESIAN_POINT('Ctrl Pts',(-46.737668963875,-42.0070114066748,
2.66381699700623));
#236309=CARTESIAN_POINT('Ctrl Pts',(-46.7409769299532,-42.0005899185698,
2.66554034873222));
#236310=CARTESIAN_POINT('Ctrl Pts',(-46.7438276087417,-41.9940383480779,
2.66766759643927));
#236311=CARTESIAN_POINT('Ctrl Pts',(-46.7462229640885,-41.9874523371582,
2.67012012783103));
#236312=CARTESIAN_POINT('Ctrl Pts',(-46.7474206417619,-41.9841593316984,
2.67134639352691));
#236313=CARTESIAN_POINT('Ctrl Pts',(-46.7485046297344,-41.9808575622225,
2.67265375584967));
#236314=CARTESIAN_POINT('Ctrl Pts',(-46.749476178293,-41.9775578801519,
2.67403135126894));
#236315=CARTESIAN_POINT('Ctrl Pts',(-46.7499619525723,-41.9759080391167,
2.67472014897858));
#236316=CARTESIAN_POINT('Ctrl Pts',(-46.7504196286878,-41.9742587070257,
2.67542649668587));
#236317=CARTESIAN_POINT('Ctrl Pts',(-46.7508494364809,-41.9726111592841,
2.67614899656056));
#236318=CARTESIAN_POINT('Ctrl Pts',(-46.7509568884292,-41.9721992723487,
2.67632962152923));
#236319=CARTESIAN_POINT('Ctrl Pts',(-46.7510625988572,-41.9717874966608,
2.67651125590905));
#236320=CARTESIAN_POINT('Ctrl Pts',(-46.7511665718603,-41.9713758515959,
2.67669387767478));
#236321=CARTESIAN_POINT('Ctrl Pts',(-46.7514784908696,-41.9701409164013,
2.67724174297198));
#236322=CARTESIAN_POINT('Ctrl Pts',(-46.7517747718021,-41.968907158177,
2.67779849504701));
#236323=CARTESIAN_POINT('Ctrl Pts',(-46.7520555364229,-41.9676750878621,
2.67836353617963));
#236324=CARTESIAN_POINT('Ctrl Pts',(-46.7539957941551,-41.9591607175413,
2.68226832098868));
#236325=CARTESIAN_POINT('Ctrl Pts',(-46.7552464720206,-41.9507055072914,
2.6865915375136));
#236326=CARTESIAN_POINT('Ctrl Pts',(-46.7559027543577,-41.9423805287164,
2.69123699486156));
#236327=CARTESIAN_POINT('Ctrl Pts',(-46.7562289248778,-41.9382430372165,
2.69354577441186));
#236328=CARTESIAN_POINT('Ctrl Pts',(-46.7564078446192,-41.9341372814969,
2.69593478828079));
#236329=CARTESIAN_POINT('Ctrl Pts',(-46.756448717314,-41.9300700339485,
2.69839565261173));
#236330=CARTESIAN_POINT('Ctrl Pts',(-46.7565388885836,-41.921097078357,
2.70382468688998));
#236331=CARTESIAN_POINT('Ctrl Pts',(-46.7559695796222,-41.9123126321655,
2.7096115581504));
#236332=CARTESIAN_POINT('Ctrl Pts',(-46.7548061840814,-41.9038465062686,
2.7156270136172));
#236333=CARTESIAN_POINT('Ctrl Pts',(-46.7543811810191,-41.900753723715,
2.7178245353581));
#236334=CARTESIAN_POINT('Ctrl Pts',(-46.753883681602,-41.8976992635447,
2.72005051502353));
#236335=CARTESIAN_POINT('Ctrl Pts',(-46.7533184435774,-41.8946854937103,
2.72229986760065));
#236336=CARTESIAN_POINT('Ctrl Pts',(-46.7514198688642,-41.8845625597427,
2.72985520488882));
#236337=CARTESIAN_POINT('Ctrl Pts',(-46.7487367327308,-41.8748360802666,
2.73770845534592));
#236338=CARTESIAN_POINT('Ctrl Pts',(-46.7453971059997,-41.8655137786563,
2.74576706701833));
#236339=CARTESIAN_POINT('Ctrl Pts',(-46.7417264606175,-41.8552674648873,
2.75462443585157));
#236340=CARTESIAN_POINT('Ctrl Pts',(-46.7372626589198,-41.845508736713,
2.76373036323361));
#236341=CARTESIAN_POINT('Ctrl Pts',(-46.7321227530945,-41.8362508575421,
2.77299664637051));
#236342=CARTESIAN_POINT('Ctrl Pts',(-46.7265868542931,-41.8262797250063,
2.78297683033768));
#236343=CARTESIAN_POINT('Ctrl Pts',(-46.7202662104721,-41.8168884800845,
2.79314401479249));
#236344=CARTESIAN_POINT('Ctrl Pts',(-46.7132528291595,-41.8081115112052,
2.80341452428356));
#236345=CARTESIAN_POINT('Ctrl Pts',(-46.7063341521765,-41.7994530610428,
2.81354634721632));
#236346=CARTESIAN_POINT('Ctrl Pts',(-46.698740203124,-41.7913915075174,
2.8237800420932));
#236347=CARTESIAN_POINT('Ctrl Pts',(-46.6905216402894,-41.7839914803029,
2.83404198860232));
#236348=CARTESIAN_POINT('Ctrl Pts',(-44.1339623850444,-39.4820551873932,
2.83404198860233));
#236349=CARTESIAN_POINT('Ctrl Pts',(-44.1260971752942,-39.4749733207249,
2.82422126442994));
#236350=CARTESIAN_POINT('Ctrl Pts',(-44.1177016730292,-39.4685372764358,
2.81442815028504));
#236351=CARTESIAN_POINT('Ctrl Pts',(-44.1088266671088,-39.4627751762752,
2.80471618166336));
#236352=CARTESIAN_POINT('Ctrl Pts',(-44.1002570680353,-39.4572113615981,
2.79533842146256));
#236353=CARTESIAN_POINT('Ctrl Pts',(-44.0912392969009,-39.4522752837267,
2.78603515650274));
#236354=CARTESIAN_POINT('Ctrl Pts',(-44.0817922708741,-39.4480294591797,
2.77685887346798));
#236355=CARTESIAN_POINT('Ctrl Pts',(-44.0728618726534,-39.4440158252729,
2.76818441216621));
#236356=CARTESIAN_POINT('Ctrl Pts',(-44.0635470605553,-39.4406186435284,
2.75962261521671));
#236357=CARTESIAN_POINT('Ctrl Pts',(-44.0538529442815,-39.4379312493392,
2.75123537701709));
#236358=CARTESIAN_POINT('Ctrl Pts',(-44.0449248258243,-39.4354562043754,
2.74351087134168));
#236359=CARTESIAN_POINT('Ctrl Pts',(-44.0356744386774,-39.4335831186684,
2.73593399449895));
#236360=CARTESIAN_POINT('Ctrl Pts',(-44.0261054687983,-39.432423032912,
2.72857657812624));
#236361=CARTESIAN_POINT('Ctrl Pts',(-44.0232521951431,-39.4320771187574,
2.7263827450834));
#236362=CARTESIAN_POINT('Ctrl Pts',(-44.0203706219322,-39.4317948788026,
2.72420861709588));
#236363=CARTESIAN_POINT('Ctrl Pts',(-44.0174609456693,-39.4315800126158,
2.72205663736679));
#236364=CARTESIAN_POINT('Ctrl Pts',(-44.0145809991271,-39.4313673418319,
2.71992664556718));
#236365=CARTESIAN_POINT('Ctrl Pts',(-44.0116765294501,-39.4312206224784,
2.71782089927837));
#236366=CARTESIAN_POINT('Ctrl Pts',(-44.0087510493742,-39.4311433701096,
2.71574387311198));
#236367=CARTESIAN_POINT('Ctrl Pts',(-44.008547617211,-39.4311379981309,
2.71559944077439));
#236368=CARTESIAN_POINT('Ctrl Pts',(-44.0083440782821,-39.4311329512713,
2.71545515216021));
#236369=CARTESIAN_POINT('Ctrl Pts',(-44.0081404327822,-39.4311282308203,
2.71531100781682));
#236370=CARTESIAN_POINT('Ctrl Pts',(-43.9992118680541,-39.4309212689595,
2.70899119176038));
#236371=CARTESIAN_POINT('Ctrl Pts',(-43.9900881971804,-39.4313859080978,
2.70298296066795));
#236372=CARTESIAN_POINT('Ctrl Pts',(-43.9808585737696,-39.4325966403785,
2.69736727774094));
#236373=CARTESIAN_POINT('Ctrl Pts',(-43.972254960653,-39.4337252532879,
2.69213248525389));
#236374=CARTESIAN_POINT('Ctrl Pts',(-43.9635585482856,-39.4355025470896,
2.6872386618543));
#236375=CARTESIAN_POINT('Ctrl Pts',(-43.9548613290782,-39.4380105519135,
2.68278595829526));
#236376=CARTESIAN_POINT('Ctrl Pts',(-43.951679773774,-39.4389280125248,
2.68115710172762));
#236377=CARTESIAN_POINT('Ctrl Pts',(-43.9484983634052,-39.4399434521994,
2.67958763637761));
#236378=CARTESIAN_POINT('Ctrl Pts',(-43.9453226165469,-39.4410615611724,
2.6780837864531));
#236379=CARTESIAN_POINT('Ctrl Pts',(-43.9445589555198,-39.4413304290277,
2.67772216078546));
#236380=CARTESIAN_POINT('Ctrl Pts',(-43.9437952833153,-39.441605709343,
2.67736403603508));
#236381=CARTESIAN_POINT('Ctrl Pts',(-43.9430317345446,-39.4418874191262,
2.67700956934424));
#236382=CARTESIAN_POINT('Ctrl Pts',(-43.9422920466731,-39.4421603254787,
2.67666617973749));
#236383=CARTESIAN_POINT('Ctrl Pts',(-43.9415524746576,-39.4424392657172,
2.67632622314064));
#236384=CARTESIAN_POINT('Ctrl Pts',(-43.9408131433996,-39.4427242524727,
2.67598984158719));
#236385=CARTESIAN_POINT('Ctrl Pts',(-43.9327129150434,-39.4458466117307,
2.67230439292187));
#236386=CARTESIAN_POINT('Ctrl Pts',(-43.9246364083439,-39.449697209665,
2.66904964539958));
#236387=CARTESIAN_POINT('Ctrl Pts',(-43.9167721156749,-39.4542738890606,
2.66640203566717));
#236388=CARTESIAN_POINT('Ctrl Pts',(-43.913510559095,-39.4561719744226,
2.66530399299414));
#236389=CARTESIAN_POINT('Ctrl Pts',(-43.9102855324951,-39.4581945203282,
2.66430995142218));
#236390=CARTESIAN_POINT('Ctrl Pts',(-43.9071101492106,-39.4603395741452,
2.66343053473307));
#236391=CARTESIAN_POINT('Ctrl Pts',(-43.9016942021212,-39.4639981869598,
2.66193059792832));
#236392=CARTESIAN_POINT('Ctrl Pts',(-43.8964251099354,-39.4680136963362,
2.66076519817075));
#236393=CARTESIAN_POINT('Ctrl Pts',(-43.8913745966871,-39.4723737491581,
2.65997805604408));
#236394=CARTESIAN_POINT('Ctrl Pts',(-43.8888493400629,-39.474553775569,
2.65958448498075));
#236395=CARTESIAN_POINT('Ctrl Pts',(-43.8863797569638,-39.4768209551509,
2.65928526260711));
#236396=CARTESIAN_POINT('Ctrl Pts',(-43.8839748786089,-39.4791737454928,
2.65908463971274));
#236397=CARTESIAN_POINT('Ctrl Pts',(-43.881570000254,-39.4815265358346,
2.65888401681836));
#236398=CARTESIAN_POINT('Ctrl Pts',(-43.8792298420738,-39.4839648939619,
2.65878198860234));
#236399=CARTESIAN_POINT('Ctrl Pts',(-43.8769616275871,-39.4864862581818,
2.65878198860234));
#236400=CARTESIAN_POINT('Origin',(-38.974747650051,-43.3086183250768,2.83404198860231));
#236401=CARTESIAN_POINT('Ctrl Pts',(-41.7839914803023,-46.6905216402899,
2.83404198860228));
#236402=CARTESIAN_POINT('Ctrl Pts',(-41.7910911765302,-46.6984066517721,
2.82419652440022));
#236403=CARTESIAN_POINT('Ctrl Pts',(-41.7987919603585,-46.7057080773545,
2.81438790575603));
#236404=CARTESIAN_POINT('Ctrl Pts',(-41.8070443420767,-46.7123936319701,
2.80466781256855));
#236405=CARTESIAN_POINT('Ctrl Pts',(-41.8150285705287,-46.7188619458705,
2.79526356453034));
#236406=CARTESIAN_POINT('Ctrl Pts',(-41.8235301761256,-46.7247545199412,
2.78594102496193));
#236407=CARTESIAN_POINT('Ctrl Pts',(-41.8325358446871,-46.7300083326608,
2.77675109088745));
#236408=CARTESIAN_POINT('Ctrl Pts',(-41.8410546526091,-46.7349781159824,
2.76805797913658));
#236409=CARTESIAN_POINT('Ctrl Pts',(-41.8500252953107,-46.7393768060085,
2.75948271210147));
#236410=CARTESIAN_POINT('Ctrl Pts',(-41.8594521748282,-46.7431119772971,
2.75108575573218));
#236411=CARTESIAN_POINT('Ctrl Pts',(-41.8681350126332,-46.7465523401883,
2.74335155163274));
#236412=CARTESIAN_POINT('Ctrl Pts',(-41.8772054497772,-46.7494299450228,
2.73576818685956));
#236413=CARTESIAN_POINT('Ctrl Pts',(-41.8866715402901,-46.7516345991556,
2.72840626160516));
#236414=CARTESIAN_POINT('Ctrl Pts',(-41.8894172933146,-46.7522740855142,
2.72627084693681));
#236415=CARTESIAN_POINT('Ctrl Pts',(-41.892196339742,-46.7528566833417,
2.72415424587506));
#236416=CARTESIAN_POINT('Ctrl Pts',(-41.8950088623276,-46.7533790039319,
2.72205867173224));
#236417=CARTESIAN_POINT('Ctrl Pts',(-41.8980578176392,-46.7539452330337,
2.71978693462827));
#236418=CARTESIAN_POINT('Ctrl Pts',(-41.9011416752729,-46.7544408966255,
2.71754411340727));
#236419=CARTESIAN_POINT('Ctrl Pts',(-41.9042597210852,-46.7548620578767,
2.71533341844224));
#236420=CARTESIAN_POINT('Ctrl Pts',(-41.912817222284,-46.7560179382355,
2.70926614876371));
#236421=CARTESIAN_POINT('Ctrl Pts',(-41.9216270724807,-46.756568484326,
2.70347381860389));
#236422=CARTESIAN_POINT('Ctrl Pts',(-41.9306033478346,-46.756455626462,
2.69804914171375));
#236423=CARTESIAN_POINT('Ctrl Pts',(-41.9388161524499,-46.7563523676437,
2.69308585687201));
#236424=CARTESIAN_POINT('Ctrl Pts',(-41.9471607721478,-46.7556849461648,
2.68842799053196));
#236425=CARTESIAN_POINT('Ctrl Pts',(-41.9555881906094,-46.7543795041532,
2.68414767054239));
#236426=CARTESIAN_POINT('Ctrl Pts',(-41.9597277110287,-46.7537382753014,
2.68204519134558));
#236427=CARTESIAN_POINT('Ctrl Pts',(-41.9638869554862,-46.7529426662695,
2.68003431778494));
#236428=CARTESIAN_POINT('Ctrl Pts',(-41.9680580970361,-46.7519812517996,
2.67812693945231));
#236429=CARTESIAN_POINT('Ctrl Pts',(-41.9688495305177,-46.7517988327683,
2.67776503299183));
#236430=CARTESIAN_POINT('Ctrl Pts',(-41.9696416823154,-46.7516099985532,
2.67740659639904));
#236431=CARTESIAN_POINT('Ctrl Pts',(-41.97043441682,-46.7514147143009,2.67705178968835));
#236432=CARTESIAN_POINT('Ctrl Pts',(-41.9712023783712,-46.7512255326815,
2.67670807068737));
#236433=CARTESIAN_POINT('Ctrl Pts',(-41.9719708867608,-46.7510302978708,
2.67636775825245));
#236434=CARTESIAN_POINT('Ctrl Pts',(-41.9727398158584,-46.7508289807695,
2.67603099699235));
#236435=CARTESIAN_POINT('Ctrl Pts',(-41.9811194467226,-46.7486350684818,
2.67236104217089));
#236436=CARTESIAN_POINT('Ctrl Pts',(-41.9895544525284,-46.745716979482,
2.6691144054142));
#236437=CARTESIAN_POINT('Ctrl Pts',(-41.9978556152128,-46.7420530111683,
2.6664677818957));
#236438=CARTESIAN_POINT('Ctrl Pts',(-42.0013612477616,-46.7405056945975,
2.66535009634929));
#236439=CARTESIAN_POINT('Ctrl Pts',(-42.0048429302643,-46.7388257854547,
2.66433897912313));
#236440=CARTESIAN_POINT('Ctrl Pts',(-42.0082865614559,-46.7370135816691,
2.66344564884772));
#236441=CARTESIAN_POINT('Ctrl Pts',(-42.0140855503362,-46.7339618757757,
2.66194130298565));
#236442=CARTESIAN_POINT('Ctrl Pts',(-42.0197742252482,-46.7305342346688,
2.660772067054));
#236443=CARTESIAN_POINT('Ctrl Pts',(-42.0252784509102,-46.7267341265712,
2.65998225155694));
#236444=CARTESIAN_POINT('Ctrl Pts',(-42.0266545073257,-46.7257840995468,
2.65978479768268));
#236445=CARTESIAN_POINT('Ctrl Pts',(-42.0280188904105,-46.7248106099129,
2.65961098966602));
#236446=CARTESIAN_POINT('Ctrl Pts',(-42.0293702408568,-46.7238134778073,
2.65946139030481));
#236447=CARTESIAN_POINT('Ctrl Pts',(-42.0313972665263,-46.7223177796489,
2.659236991263));
#236448=CARTESIAN_POINT('Ctrl Pts',(-42.0333949481516,-46.720768886388,
2.65906707562421));
#236449=CARTESIAN_POINT('Ctrl Pts',(-42.0353598072043,-46.7191674503113,
2.65895332562899));
#236450=CARTESIAN_POINT('Ctrl Pts',(-42.037324666257,-46.7175660142346,
2.65883957563377));
#236451=CARTESIAN_POINT('Ctrl Pts',(-42.039256703587,-46.7159120469177,
2.65878198860228));
#236452=CARTESIAN_POINT('Ctrl Pts',(-42.0411527846902,-46.7142062431437,
2.65878198860228));
#236453=CARTESIAN_POINT('Ctrl Pts',(-39.4864862581813,-43.8769616275876,
2.6587819886023));
#236454=CARTESIAN_POINT('Ctrl Pts',(-39.4800703482071,-43.8827333680736,
2.6587819886023));
#236455=CARTESIAN_POINT('Ctrl Pts',(-39.4741864828754,-43.8889846873395,
2.65945335517821));
#236456=CARTESIAN_POINT('Ctrl Pts',(-39.4688721660169,-43.895569202337,
2.66072561226562));
#236457=CARTESIAN_POINT('Ctrl Pts',(-39.4654396626066,-43.8998221234152,
2.66154735980301));
#236458=CARTESIAN_POINT('Ctrl Pts',(-39.4622440309669,-43.9042134689398,
2.66261895766847));
#236459=CARTESIAN_POINT('Ctrl Pts',(-39.459287497615,-43.9086997575135,
2.66391429250995));
#236460=CARTESIAN_POINT('Ctrl Pts',(-39.4553687820178,-43.9146460760272,
2.66563118464091));
#236461=CARTESIAN_POINT('Ctrl Pts',(-39.4518755008529,-43.9207613318564,
2.66774105138666));
#236462=CARTESIAN_POINT('Ctrl Pts',(-39.4488169076805,-43.9269559348855,
2.67016894181717));
#236463=CARTESIAN_POINT('Ctrl Pts',(-39.4472876110943,-43.9300532364001,
2.67138288703242));
#236464=CARTESIAN_POINT('Ctrl Pts',(-39.4458668372378,-43.9331705067653,
2.67267613167517));
#236465=CARTESIAN_POINT('Ctrl Pts',(-39.4445546869045,-43.9362974878338,
2.67403835432519));
#236466=CARTESIAN_POINT('Ctrl Pts',(-39.4438986117378,-43.937860978368,
2.6747194656502));
#236467=CARTESIAN_POINT('Ctrl Pts',(-39.4432696802086,-43.9394269075363,
2.67541781389489));
#236468=CARTESIAN_POINT('Ctrl Pts',(-39.442667827963,-43.9409940617756,
2.67613207244135));
#236469=CARTESIAN_POINT('Ctrl Pts',(-39.4425173649017,-43.9413858503355,
2.67631063707797));
#236470=CARTESIAN_POINT('Ctrl Pts',(-39.4423685940344,-43.9417777156946,
2.67649019601812));
#236471=CARTESIAN_POINT('Ctrl Pts',(-39.4422215138289,-43.9421696393592,
2.67667072836623));
#236472=CARTESIAN_POINT('Ctrl Pts',(-39.4417802732125,-43.9433454103531,
2.67721232541057));
#236473=CARTESIAN_POINT('Ctrl Pts',(-39.44135424986,-43.944521704943,2.67776268340013));
#236474=CARTESIAN_POINT('Ctrl Pts',(-39.4409433907174,-43.9456980341196,
2.67832123541482));
#236475=CARTESIAN_POINT('Ctrl Pts',(-39.4380493519679,-43.9539839449479,
2.68225560368404));
#236476=CARTESIAN_POINT('Ctrl Pts',(-39.4358558447891,-43.9622859173441,
2.6866179299884));
#236477=CARTESIAN_POINT('Ctrl Pts',(-39.4342768603232,-43.9705207686459,
2.69130986622521));
#236478=CARTESIAN_POINT('Ctrl Pts',(-39.4335110545634,-43.9745146626289,
2.69358545023006));
#236479=CARTESIAN_POINT('Ctrl Pts',(-39.4328901532271,-43.9784932254698,
2.69593918853429));
#236480=CARTESIAN_POINT('Ctrl Pts',(-39.4324063524312,-43.9824490059337,
2.69836306235443));
#236481=CARTESIAN_POINT('Ctrl Pts',(-39.4316656872149,-43.9885050294413,
2.70207384382176));
#236482=CARTESIAN_POINT('Ctrl Pts',(-39.4312456873365,-43.9945041897572,
2.70594760814177));
#236483=CARTESIAN_POINT('Ctrl Pts',(-39.4311218425058,-44.0004074287824,
2.70995196345657));
#236484=CARTESIAN_POINT('Ctrl Pts',(-39.4310643283258,-44.003148923525,
2.71181160678055));
#236485=CARTESIAN_POINT('Ctrl Pts',(-39.4310704471408,-44.0058696426792,
2.71369962772048));
#236486=CARTESIAN_POINT('Ctrl Pts',(-39.4311389525607,-44.0085654321301,
2.7156118313861));
#236487=CARTESIAN_POINT('Ctrl Pts',(-39.4311442032312,-44.0087720537696,
2.71575839426261));
#236488=CARTESIAN_POINT('Ctrl Pts',(-39.4311497894109,-44.00897854276,2.71590508903158));
#236489=CARTESIAN_POINT('Ctrl Pts',(-39.4311557099537,-44.0091848981959,
2.71605191409861));
#236490=CARTESIAN_POINT('Ctrl Pts',(-39.4312388757296,-44.01208356993,2.71811436362702));
#236491=CARTESIAN_POINT('Ctrl Pts',(-39.4313901062471,-44.0149559644985,
2.72020091026908));
#236492=CARTESIAN_POINT('Ctrl Pts',(-39.4316052205102,-44.0177981990785,
2.72230624862131));
#236493=CARTESIAN_POINT('Ctrl Pts',(-39.432376582001,-44.0279899468077,
2.72985561753042));
#236494=CARTESIAN_POINT('Ctrl Pts',(-39.4339733733561,-44.037872831609,
2.73770089914259));
#236495=CARTESIAN_POINT('Ctrl Pts',(-39.4362681192145,-44.0474262866319,
2.74574823346991));
#236496=CARTESIAN_POINT('Ctrl Pts',(-39.4387898143852,-44.0579245739722,
2.75459144546905));
#236497=CARTESIAN_POINT('Ctrl Pts',(-39.4421543412261,-44.0680257165085,
2.76367911754111));
#236498=CARTESIAN_POINT('Ctrl Pts',(-39.446245422205,-44.0777053474406,
2.77292162564527));
#236499=CARTESIAN_POINT('Ctrl Pts',(-39.4506627629409,-44.0881569195912,
2.78290121484453));
#236500=CARTESIAN_POINT('Ctrl Pts',(-39.455927460092,-44.0981181930543,
2.7930622949983));
#236501=CARTESIAN_POINT('Ctrl Pts',(-39.4619494607976,-44.1075472421499,
2.80331916684814));
#236502=CARTESIAN_POINT('Ctrl Pts',(-39.467920943106,-44.1168971912135,
2.81348999408387));
#236503=CARTESIAN_POINT('Ctrl Pts',(-39.4746380711555,-44.125724842928,
2.82375635966706));
#236504=CARTESIAN_POINT('Ctrl Pts',(-39.4820551873926,-44.1339623850449,
2.8340419886023));
#236505=CARTESIAN_POINT('Origin',(-0.0113255271402662,0.0101975504411025,
2.83404198860262));
#236506=CARTESIAN_POINT('Ctrl Pts',(-42.0638038389696,-46.6938111422606,
2.65878198860228));
#236507=CARTESIAN_POINT('Ctrl Pts',(-42.0701842568304,-46.6880613546456,
2.65878198860228));
#236508=CARTESIAN_POINT('Ctrl Pts',(-42.0760276657224,-46.681829673937,
2.65944603041817));
#236509=CARTESIAN_POINT('Ctrl Pts',(-42.0812997491646,-46.6752630175671,
2.66070439264036));
#236510=CARTESIAN_POINT('Ctrl Pts',(-42.0846683595049,-46.6710672367545,
2.6615084261956));
#236511=CARTESIAN_POINT('Ctrl Pts',(-42.0878044626435,-46.6667352666009,
2.66255428265333));
#236512=CARTESIAN_POINT('Ctrl Pts',(-42.0907067742413,-46.6623093164291,
2.6638169970062));
#236513=CARTESIAN_POINT('Ctrl Pts',(-42.0946678472187,-46.6562687825186,
2.6655403487322));
#236514=CARTESIAN_POINT('Ctrl Pts',(-42.0981877352861,-46.6500510792883,
2.66766759643925));
#236515=CARTESIAN_POINT('Ctrl Pts',(-42.1012583942262,-46.6437515300389,
2.67012012783101));
#236516=CARTESIAN_POINT('Ctrl Pts',(-42.1027937236962,-46.6406017554143,
2.67134639352689));
#236517=CARTESIAN_POINT('Ctrl Pts',(-42.1042169023586,-46.637431380974,
2.67265375584965));
#236518=CARTESIAN_POINT('Ctrl Pts',(-42.1055280393686,-46.6342513293849,
2.67403135126893));
#236519=CARTESIAN_POINT('Ctrl Pts',(-42.1061836078736,-46.6326613035903,
2.67472014897856));
#236520=CARTESIAN_POINT('Ctrl Pts',(-42.1068111789403,-46.6310688468941,
2.67542649668585));
#236521=CARTESIAN_POINT('Ctrl Pts',(-42.107410847835,-46.6294752517396,
2.67614899656055));
#236522=CARTESIAN_POINT('Ctrl Pts',(-42.1075607650587,-46.6290768529509,
2.67632962152922));
#236523=CARTESIAN_POINT('Ctrl Pts',(-42.1077089386737,-46.628678382762,
2.67651125590904));
#236524=CARTESIAN_POINT('Ctrl Pts',(-42.1078553707279,-46.6282798608701,
2.67669387767477));
#236525=CARTESIAN_POINT('Ctrl Pts',(-42.1082946668904,-46.6270842951944,
2.67724174297197));
#236526=CARTESIAN_POINT('Ctrl Pts',(-42.1087182876161,-46.6258882654172,
2.67779849504701));
#236527=CARTESIAN_POINT('Ctrl Pts',(-42.1091263005957,-46.6246922924067,
2.67836353617962));
#236528=CARTESIAN_POINT('Ctrl Pts',(-42.1119459234382,-46.6164273768568,
2.68226832098856));
#236529=CARTESIAN_POINT('Ctrl Pts',(-42.1140735600934,-46.6081492165689,
2.68659153751333));
#236530=CARTESIAN_POINT('Ctrl Pts',(-42.1155964444645,-46.599938443282,
2.69123699486112));
#236531=CARTESIAN_POINT('Ctrl Pts',(-42.1163533138166,-46.5958577114964,
2.69354577441156));
#236532=CARTESIAN_POINT('Ctrl Pts',(-42.1169604217529,-46.5917931497416,
2.69593478828063));
#236533=CARTESIAN_POINT('Ctrl Pts',(-42.1174262136788,-46.5877524553606,
2.69839565261171));
#236534=CARTESIAN_POINT('Ctrl Pts',(-42.1184538202397,-46.5788380800229,
2.70382468688996));
#236535=CARTESIAN_POINT('Ctrl Pts',(-42.1188058546734,-46.5700422469559,
2.70961155815037));
#236536=CARTESIAN_POINT('Ctrl Pts',(-42.118533783465,-46.5615008914345,
2.71562701361717));
#236537=CARTESIAN_POINT('Ctrl Pts',(-42.1184343924215,-46.5583806265503,
2.71782453535807));
#236538=CARTESIAN_POINT('Ctrl Pts',(-42.118258896386,-46.5552908961829,
2.72005051502352));
#236539=CARTESIAN_POINT('Ctrl Pts',(-42.1180117795239,-46.5522345526329,
2.72229986760066));
#236540=CARTESIAN_POINT('Ctrl Pts',(-42.1171817401332,-46.5419686180612,
2.72985520488781));
#236541=CARTESIAN_POINT('Ctrl Pts',(-42.1155299964533,-46.532014957162,
2.73770845534385));
#236542=CARTESIAN_POINT('Ctrl Pts',(-42.1131831104089,-46.5223946380466,
2.74576706701515));
#236543=CARTESIAN_POINT('Ctrl Pts',(-42.1106036046392,-46.5118207677369,
2.75462443584726));
#236544=CARTESIAN_POINT('Ctrl Pts',(-42.1071843209746,-46.5016489045661,
2.7637303632281));
#236545=CARTESIAN_POINT('Ctrl Pts',(-42.103040283975,-46.4919044745698,
2.77299664636376));
#236546=CARTESIAN_POINT('Ctrl Pts',(-42.0985769785686,-46.4814093059481,
2.78297683032949));
#236547=CARTESIAN_POINT('Ctrl Pts',(-42.0932726122969,-46.4714088200642,
2.79314401478278));
#236548=CARTESIAN_POINT('Ctrl Pts',(-42.0872150940914,-46.4619468343687,
2.80341452427227));
#236549=CARTESIAN_POINT('Ctrl Pts',(-42.0812393728328,-46.4526126174252,
2.81354634720878));
#236550=CARTESIAN_POINT('Ctrl Pts',(-42.0745296860268,-46.4438014421052,
2.82378004208946));
#236551=CARTESIAN_POINT('Ctrl Pts',(-42.0671296588092,-46.4355828792672,
2.83404198860229));
#236552=CARTESIAN_POINT('Ctrl Pts',(-39.7651933658995,-43.8790236240221,
2.8340419886023));
#236553=CARTESIAN_POINT('Ctrl Pts',(-39.7581114992311,-43.8711584142718,
2.82422126442972));
#236554=CARTESIAN_POINT('Ctrl Pts',(-39.7504347382248,-43.8638800583566,
2.81442815028464));
#236555=CARTESIAN_POINT('Ctrl Pts',(-39.7422106539903,-43.857221832853,
2.80471618166279));
#236556=CARTESIAN_POINT('Ctrl Pts',(-39.7342695770751,-43.8507927303129,
2.79533842146186));
#236557=CARTESIAN_POINT('Ctrl Pts',(-39.7258171668688,-43.8449410790337,
2.78603515650193));
#236558=CARTESIAN_POINT('Ctrl Pts',(-39.7168657021541,-43.8397310304448,
2.77685887346705));
#236559=CARTESIAN_POINT('Ctrl Pts',(-39.7084037645735,-43.8348059028421,
2.76818441216518));
#236560=CARTESIAN_POINT('Ctrl Pts',(-39.6994950821778,-43.8304536682203,
2.75962261521558));
#236561=CARTESIAN_POINT('Ctrl Pts',(-39.6901349804719,-43.8267676847809,
2.75123537701587));
#236562=CARTESIAN_POINT('Ctrl Pts',(-39.6815144838282,-43.8233729558701,
2.74351087134036));
#236563=CARTESIAN_POINT('Ctrl Pts',(-39.6725105620403,-43.8205432023696,
2.73593399449755));
#236564=CARTESIAN_POINT('Ctrl Pts',(-39.6631152739606,-43.8183892419679,
2.72857657812477));
#236565=CARTESIAN_POINT('Ctrl Pts',(-39.6603137887126,-43.8177469744569,
2.72638274508242));
#236566=CARTESIAN_POINT('Ctrl Pts',(-39.6574775031707,-43.8171650742228,
2.72420861709538));
#236567=CARTESIAN_POINT('Ctrl Pts',(-39.6546062260517,-43.8166472411071,
2.72205663736677));
#236568=CARTESIAN_POINT('Ctrl Pts',(-39.6517642863082,-43.8161346989697,
2.71992664556715));
#236569=CARTESIAN_POINT('Ctrl Pts',(-39.6488910639686,-43.8156851836083,
2.71782089927834));
#236570=CARTESIAN_POINT('Ctrl Pts',(-39.64598968505,-43.8153025584993,2.71574387311195));
#236571=CARTESIAN_POINT('Ctrl Pts',(-39.6457879288342,-43.8152759514975,
2.71559944077436));
#236572=CARTESIAN_POINT('Ctrl Pts',(-39.6455860324533,-43.8152496566736,
2.71545515216019));
#236573=CARTESIAN_POINT('Ctrl Pts',(-39.6453839959662,-43.8152236753307,
2.7153110078168));
#236574=CARTESIAN_POINT('Ctrl Pts',(-39.6365259762553,-43.8140845580783,
2.70899119176042));
#236575=CARTESIAN_POINT('Ctrl Pts',(-39.6274037177902,-43.8135929685791,
2.70298296066806));
#236576=CARTESIAN_POINT('Ctrl Pts',(-39.6180980992375,-43.81383230999,2.69736727774111));
#236577=CARTESIAN_POINT('Ctrl Pts',(-39.6094236454411,-43.8140554177821,
2.69213248525421));
#236578=CARTESIAN_POINT('Ctrl Pts',(-39.6005890951409,-43.8149139527617,
2.68723866185477));
#236579=CARTESIAN_POINT('Ctrl Pts',(-39.5916773623205,-43.8164991115142,
2.68278595829582));
#236580=CARTESIAN_POINT('Ctrl Pts',(-39.588417335161,-43.8170789830935,
2.68115710172799));
#236581=CARTESIAN_POINT('Ctrl Pts',(-39.585147210542,-43.8177563121465,
2.6795876363778));
#236582=CARTESIAN_POINT('Ctrl Pts',(-39.5818719865441,-43.8185363400628,
2.67808378645312));
#236583=CARTESIAN_POINT('Ctrl Pts',(-39.5810844045883,-43.8187239107183,
2.67772216078547));
#236584=CARTESIAN_POINT('Ctrl Pts',(-39.5802961412317,-43.8189178575372,
2.6773640360351));
#236585=CARTESIAN_POINT('Ctrl Pts',(-39.5795073285704,-43.8191182115052,
2.67700956934426));
#236586=CARTESIAN_POINT('Ctrl Pts',(-39.5787431663048,-43.8193123044116,
2.67666617973751));
#236587=CARTESIAN_POINT('Ctrl Pts',(-39.5779784885477,-43.81951241026,2.67632622314066));
#236588=CARTESIAN_POINT('Ctrl Pts',(-39.5772134181961,-43.819718554668,
2.6759898415872));
#236589=CARTESIAN_POINT('Ctrl Pts',(-39.5688311883227,-43.8219771048932,
2.67230439292161));
#236590=CARTESIAN_POINT('Ctrl Pts',(-39.5603964284866,-43.8249623840156,
2.66904964539909));
#236591=CARTESIAN_POINT('Ctrl Pts',(-39.5520968239709,-43.8286919494557,
2.66640203566656));
#236592=CARTESIAN_POINT('Ctrl Pts',(-39.5486547305939,-43.83023871141,2.66530399299378));
#236593=CARTESIAN_POINT('Ctrl Pts',(-39.5452359574124,-43.8319130705228,
2.66430995142202));
#236594=CARTESIAN_POINT('Ctrl Pts',(-39.5418537500312,-43.8337144555751,
2.66343053473307));
#236595=CARTESIAN_POINT('Ctrl Pts',(-39.5360850428915,-43.8367869054996,
2.66193059792831));
#236596=CARTESIAN_POINT('Ctrl Pts',(-39.5304250803196,-43.8402296473864,
2.66076519817074));
#236597=CARTESIAN_POINT('Ctrl Pts',(-39.52494648469,-43.844037892994,2.65997805604407));
#236598=CARTESIAN_POINT('Ctrl Pts',(-39.5222071868751,-43.8459420157977,
2.65958448498073));
#236599=CARTESIAN_POINT('Ctrl Pts',(-39.519514147613,-43.8479386338065,
2.65928526260709));
#236600=CARTESIAN_POINT('Ctrl Pts',(-39.5168765098746,-43.850027157078,
2.65908463971271));
#236601=CARTESIAN_POINT('Ctrl Pts',(-39.5142388721361,-43.8521156803494,
2.65888401681833));
#236602=CARTESIAN_POINT('Ctrl Pts',(-39.5116566557594,-43.8542960677575,
2.6587819886023));
#236603=CARTESIAN_POINT('Ctrl Pts',(-39.5091373124618,-43.8565665267058,
2.6587819886023));
#236604=CARTESIAN_POINT('Origin',(-34.2342565846632,-47.1453396605409,2.83404198860228));
#236605=CARTESIAN_POINT('Ctrl Pts',(-36.6746059268174,-50.8023624960592,
2.83404198860226));
#236606=CARTESIAN_POINT('Ctrl Pts',(-36.6808425220334,-50.8109464329599,
2.82419652440042));
#236607=CARTESIAN_POINT('Ctrl Pts',(-36.6877379133663,-50.8190128116684,
2.81438790575641));
#236608=CARTESIAN_POINT('Ctrl Pts',(-36.6952462569237,-50.8265243508954,
2.8046678125691));
#236609=CARTESIAN_POINT('Ctrl Pts',(-36.7025106240248,-50.8337918098259,
2.795263564531));
#236610=CARTESIAN_POINT('Ctrl Pts',(-36.7103497152243,-50.8405407635276,
2.78594102496269));
#236611=CARTESIAN_POINT('Ctrl Pts',(-36.7187568768212,-50.8467071440068,
2.7767510908883));
#236612=CARTESIAN_POINT('Ctrl Pts',(-36.7267095340086,-50.8525401602362,
2.76805797913748));
#236613=CARTESIAN_POINT('Ctrl Pts',(-36.7351712462818,-50.8578524412743,
2.75948271210241));
#236614=CARTESIAN_POINT('Ctrl Pts',(-36.7441560526521,-50.8625525281331,
2.75108575573316));
#236615=CARTESIAN_POINT('Ctrl Pts',(-36.7524317091168,-50.8668816480489,
2.74335155163377));
#236616=CARTESIAN_POINT('Ctrl Pts',(-36.7611516658457,-50.8706916079189,
2.73576818686063));
#236617=CARTESIAN_POINT('Ctrl Pts',(-36.7703354510156,-50.8738736606201,
2.72840626160628));
#236618=CARTESIAN_POINT('Ctrl Pts',(-36.7729993179918,-50.8747966531499,
2.72627084693754));
#236619=CARTESIAN_POINT('Ctrl Pts',(-36.775702242457,-50.8756665488981,
2.72415424587541));
#236620=CARTESIAN_POINT('Ctrl Pts',(-36.7784447603815,-50.8764799968254,
2.72205867173221));
#236621=CARTESIAN_POINT('Ctrl Pts',(-36.7814178261389,-50.8773618266783,
2.71978693462824));
#236622=CARTESIAN_POINT('Ctrl Pts',(-36.7844329791243,-50.8781771258725,
2.71754411340724));
#236623=CARTESIAN_POINT('Ctrl Pts',(-36.7874899206171,-50.8789219044954,
2.71533341844221));
#236624=CARTESIAN_POINT('Ctrl Pts',(-36.7958797205313,-50.8809659552704,
2.70926614876368));
#236625=CARTESIAN_POINT('Ctrl Pts',(-36.80458376171,-50.8824343655144,2.70347381860386));
#236626=CARTESIAN_POINT('Ctrl Pts',(-36.8135226609474,-50.8832604021662,
2.69804914171372));
#236627=CARTESIAN_POINT('Ctrl Pts',(-36.8217012684456,-50.8840161808561,
2.69308585687176));
#236628=CARTESIAN_POINT('Ctrl Pts',(-36.8300699399856,-50.8842246658555,
2.68842799053152));
#236629=CARTESIAN_POINT('Ctrl Pts',(-36.8385876480148,-50.8838072802928,
2.68414767054181));
#236630=CARTESIAN_POINT('Ctrl Pts',(-36.8427715183743,-50.8836022618679,
2.6820451913452));
#236631=CARTESIAN_POINT('Ctrl Pts',(-36.8469911418446,-50.883245770697,
2.68003431778475));
#236632=CARTESIAN_POINT('Ctrl Pts',(-36.8512399286213,-50.8827256259725,
2.6781269394523));
#236633=CARTESIAN_POINT('Ctrl Pts',(-36.8520460945285,-50.8826269335773,
2.67776503299182));
#236634=CARTESIAN_POINT('Ctrl Pts',(-36.8528536453862,-50.8825219362259,
2.67740659639902));
#236635=CARTESIAN_POINT('Ctrl Pts',(-36.8536624499709,-50.8824105850807,
2.67705178968834));
#236636=CARTESIAN_POINT('Ctrl Pts',(-36.8544459794125,-50.8823027136588,
2.67670807068736));
#236637=CARTESIAN_POINT('Ctrl Pts',(-36.8552306854274,-50.8821888793658,
2.67636775825244));
#236638=CARTESIAN_POINT('Ctrl Pts',(-36.8560164456182,-50.8820690400776,
2.67603099699234));
#236639=CARTESIAN_POINT('Ctrl Pts',(-36.864579498267,-50.8807630562081,
2.67236104217116));
#236640=CARTESIAN_POINT('Ctrl Pts',(-36.8732733195866,-50.8787426509999,
2.66911440541469));
#236641=CARTESIAN_POINT('Ctrl Pts',(-36.8819119966099,-50.875966462067,
2.66646778189629));
#236642=CARTESIAN_POINT('Ctrl Pts',(-36.8855601635608,-50.8747940602413,
2.66535009634964));
#236643=CARTESIAN_POINT('Ctrl Pts',(-36.8891983713642,-50.8734872887379,
2.66433897912328));
#236644=CARTESIAN_POINT('Ctrl Pts',(-36.8928125648613,-50.8720449698705,
2.66344564884771));
#236645=CARTESIAN_POINT('Ctrl Pts',(-36.8988987764012,-50.8696161409375,
2.66194130298563));
#236646=CARTESIAN_POINT('Ctrl Pts',(-36.9049145742144,-50.8668019052537,
2.66077206705397));
#236647=CARTESIAN_POINT('Ctrl Pts',(-36.9107858666116,-50.8635979627952,
2.65998225155691));
#236648=CARTESIAN_POINT('Ctrl Pts',(-36.9122536897109,-50.8627969771806,
2.65978479768265));
#236649=CARTESIAN_POINT('Ctrl Pts',(-36.9137123559378,-50.8619714372919,
2.65961098966599));
#236650=CARTESIAN_POINT('Ctrl Pts',(-36.9151605322317,-50.8611210221659,
2.65946139030478));
#236651=CARTESIAN_POINT('Ctrl Pts',(-36.9173327966725,-50.8598453994769,
2.65923699126297));
#236652=CARTESIAN_POINT('Ctrl Pts',(-36.9194814382212,-50.8585138058058,
2.65906707562418));
#236653=CARTESIAN_POINT('Ctrl Pts',(-36.9216029292227,-50.857126526261,
2.65895332562896));
#236654=CARTESIAN_POINT('Ctrl Pts',(-36.9237244202241,-50.8557392467161,
2.65883957563374));
#236655=CARTESIAN_POINT('Ctrl Pts',(-36.9258187603126,-50.8542962928971,
2.65878198860226));
#236656=CARTESIAN_POINT('Ctrl Pts',(-36.9278827595322,-50.8527980281386,
2.65878198860226));
#236657=CARTESIAN_POINT('Ctrl Pts',(-34.6837837831342,-47.7640607692764,
2.65878198860228));
#236658=CARTESIAN_POINT('Ctrl Pts',(-34.6767997090226,-47.7691302463542,
2.65878198860228));
#236659=CARTESIAN_POINT('Ctrl Pts',(-34.6702946353243,-47.7747322888381,
2.65945335517822));
#236660=CARTESIAN_POINT('Ctrl Pts',(-34.6643211616154,-47.7807252357991,
2.66072561226571));
#236661=CARTESIAN_POINT('Ctrl Pts',(-34.6604629105134,-47.7845960646239,
2.66154735980309));
#236662=CARTESIAN_POINT('Ctrl Pts',(-34.656825764279,-47.7886293194336,
2.66261895766852));
#236663=CARTESIAN_POINT('Ctrl Pts',(-34.6534164822759,-47.792781989761,
2.66391429250994));
#236664=CARTESIAN_POINT('Ctrl Pts',(-34.6488976742765,-47.7982861164004,
2.66563118464091));
#236665=CARTESIAN_POINT('Ctrl Pts',(-34.6447843113771,-47.8040027249064,
2.66774105138666));
#236666=CARTESIAN_POINT('Ctrl Pts',(-34.6410949611629,-47.8098436832079,
2.67016894181716));
#236667=CARTESIAN_POINT('Ctrl Pts',(-34.6392502860558,-47.8127641623586,
2.67138288703241));
#236668=CARTESIAN_POINT('Ctrl Pts',(-34.6375114518663,-47.8157158446827,
2.67267613167517));
#236669=CARTESIAN_POINT('Ctrl Pts',(-34.635879631104,-47.8186885387638,
2.67403835432519));
#236670=CARTESIAN_POINT('Ctrl Pts',(-34.6350637207229,-47.8201748858043,
2.67471946565019));
#236671=CARTESIAN_POINT('Ctrl Pts',(-34.6342745503768,-47.8216664954025,
2.67541781389488));
#236672=CARTESIAN_POINT('Ctrl Pts',(-34.6335121829165,-47.8231621539166,
2.67613207244134));
#236673=CARTESIAN_POINT('Ctrl Pts',(-34.6333215910514,-47.8235360685451,
2.67631063707796));
#236674=CARTESIAN_POINT('Ctrl Pts',(-34.6331326740828,-47.8239102364347,
2.67649019601811));
#236675=CARTESIAN_POINT('Ctrl Pts',(-34.6329454324197,-47.8242846390326,
2.67667072836622));
#236676=CARTESIAN_POINT('Ctrl Pts',(-34.6323837074303,-47.8254078468265,
2.67721232541055));
#236677=CARTESIAN_POINT('Ctrl Pts',(-34.6318370616125,-47.8265331659851,
2.67776268340012));
#236678=CARTESIAN_POINT('Ctrl Pts',(-34.6313054933181,-47.8276601046326,
2.67832123541481));
#236679=CARTESIAN_POINT('Ctrl Pts',(-34.6275611948901,-47.8355981149513,
2.68225560368403));
#236680=CARTESIAN_POINT('Ctrl Pts',(-34.6245119115564,-47.8436253243396,
2.68661792998839));
#236681=CARTESIAN_POINT('Ctrl Pts',(-34.6220808005808,-47.8516500154446,
2.6913098662252));
#236682=CARTESIAN_POINT('Ctrl Pts',(-34.6209017143846,-47.8555419819592,
2.69358545023004));
#236683=CARTESIAN_POINT('Ctrl Pts',(-34.619868341351,-47.859433847954,2.69593918853427));
#236684=CARTESIAN_POINT('Ctrl Pts',(-34.6189736992136,-47.8633173872849,
2.69836306235441));
#236685=CARTESIAN_POINT('Ctrl Pts',(-34.6176040646081,-47.8692628146652,
2.70207384382174));
#236686=CARTESIAN_POINT('Ctrl Pts',(-34.6165592825242,-47.8751852090114,
2.70594760814175));
#236687=CARTESIAN_POINT('Ctrl Pts',(-34.6158190596249,-47.8810431641657,
2.70995196345655));
#236688=CARTESIAN_POINT('Ctrl Pts',(-34.615475296281,-47.8837636288444,
2.71181160678053));
#236689=CARTESIAN_POINT('Ctrl Pts',(-34.6151969889844,-47.8864700832047,
2.71369962772046));
#236690=CARTESIAN_POINT('Ctrl Pts',(-34.6149833323959,-47.8891582656052,
2.71561183138608));
#236691=CARTESIAN_POINT('Ctrl Pts',(-34.6149669564602,-47.8893643041943,
2.71575839426258));
#236692=CARTESIAN_POINT('Ctrl Pts',(-34.6149509280614,-47.8895702459311,
2.71590508903155));
#236693=CARTESIAN_POINT('Ctrl Pts',(-34.6149352461542,-47.8897760897956,
2.71605191409858));
#236694=CARTESIAN_POINT('Ctrl Pts',(-34.6147149626374,-47.8926675754933,
2.71811436362699));
#236695=CARTESIAN_POINT('Ctrl Pts',(-34.6145651177081,-47.8955400426775,
2.72020091026905));
#236696=CARTESIAN_POINT('Ctrl Pts',(-34.6144819591399,-47.8983891927624,
2.72230624862128));
#236697=CARTESIAN_POINT('Ctrl Pts',(-34.6141837673036,-47.9086057382627,
2.72985561753056));
#236698=CARTESIAN_POINT('Ctrl Pts',(-34.6147387685077,-47.9186013937337,
2.73770089914291));
#236699=CARTESIAN_POINT('Ctrl Pts',(-34.6160223355358,-47.9283423801887,
2.74574823347042));
#236700=CARTESIAN_POINT('Ctrl Pts',(-34.617432846754,-47.9390467457338,
2.75459144546981));
#236701=CARTESIAN_POINT('Ctrl Pts',(-34.6197230854582,-47.9494442419751,
2.76367911754214));
#236702=CARTESIAN_POINT('Ctrl Pts',(-34.6227799581214,-47.9594984812842,
2.77292162564658));
#236703=CARTESIAN_POINT('Ctrl Pts',(-34.6260806134271,-47.9703545364682,
2.78290121484624));
#236704=CARTESIAN_POINT('Ctrl Pts',(-34.6302752334093,-47.9808115517362,
2.79306229500042));
#236705=CARTESIAN_POINT('Ctrl Pts',(-34.6352786409533,-47.990818417994,
2.80331916685067));
#236706=CARTESIAN_POINT('Ctrl Pts',(-34.6402400750493,-48.0007413369266,
2.81348999408557));
#236707=CARTESIAN_POINT('Ctrl Pts',(-34.6459976651001,-48.0102227609131,
2.8237563596679));
#236708=CARTESIAN_POINT('Ctrl Pts',(-34.6525130919793,-48.0191904766737,
2.83404198860227));
#236709=CARTESIAN_POINT('Origin',(-0.0123294189942654,0.0089578472451312,
2.83404198860262));
#236710=CARTESIAN_POINT('Ctrl Pts',(-36.9525415975208,-50.8348823336487,
2.65878198860226));
#236711=CARTESIAN_POINT('Ctrl Pts',(-36.9594880792482,-50.829830979246,
2.65878198860226));
#236712=CARTESIAN_POINT('Ctrl Pts',(-36.9659508653429,-50.8242442388882,
2.65944603041811));
#236713=CARTESIAN_POINT('Ctrl Pts',(-36.9718804702594,-50.8182646381296,
2.66070439264023));
#236714=CARTESIAN_POINT('Ctrl Pts',(-36.9756692055205,-50.8144439579054,
2.66150842619549));
#236715=CARTESIAN_POINT('Ctrl Pts',(-36.9792409429412,-50.8104635307791,
2.66255428265325));
#236716=CARTESIAN_POINT('Ctrl Pts',(-36.9825899931424,-50.8063652005965,
2.66381699700618));
#236717=CARTESIAN_POINT('Ctrl Pts',(-36.9871607746746,-50.800771802234,
2.66554034873217));
#236718=CARTESIAN_POINT('Ctrl Pts',(-36.9913113073906,-50.7949560887231,
2.66766759643921));
#236719=CARTESIAN_POINT('Ctrl Pts',(-36.995023627142,-50.7890120203239,
2.67012012783097));
#236720=CARTESIAN_POINT('Ctrl Pts',(-36.9968797870177,-50.7860399861243,
2.67134639352685));
#236721=CARTESIAN_POINT('Ctrl Pts',(-36.9986265637267,-50.7830357420055,
2.6726537558496));
#236722=CARTESIAN_POINT('Ctrl Pts',(-37.0002629240967,-50.7800101622085,
2.67403135126888));
#236723=CARTESIAN_POINT('Ctrl Pts',(-37.0010811042817,-50.7784973723101,
2.67472014897852));
#236724=CARTESIAN_POINT('Ctrl Pts',(-37.0018716944997,-50.7769792382975,
2.67542649668581));
#236725=CARTESIAN_POINT('Ctrl Pts',(-37.0026346543981,-50.7754570554919,
2.6761489965605));
#236726=CARTESIAN_POINT('Ctrl Pts',(-37.0028253943726,-50.7750765097906,
2.67632962152917));
#236727=CARTESIAN_POINT('Ctrl Pts',(-37.0030144077536,-50.7746957108233,
2.67651125590898));
#236728=CARTESIAN_POINT('Ctrl Pts',(-37.0032016945186,-50.7743146783936,
2.67669387767471));
#236729=CARTESIAN_POINT('Ctrl Pts',(-37.0037635548135,-50.7731715811045,
2.67724174297192));
#236730=CARTESIAN_POINT('Ctrl Pts',(-37.0043098740552,-50.7720263837271,
2.67779849504695));
#236731=CARTESIAN_POINT('Ctrl Pts',(-37.0048406651179,-50.7708796113517,
2.67836353617956));
#236732=CARTESIAN_POINT('Ctrl Pts',(-37.008508760693,-50.7629547027164,
2.68226832098861));
#236733=CARTESIAN_POINT('Ctrl Pts',(-37.0114900453057,-50.7549442896465,
2.68659153751352));
#236734=CARTESIAN_POINT('Ctrl Pts',(-37.0138628466708,-50.7469376805976,
2.69123699486147));
#236735=CARTESIAN_POINT('Ctrl Pts',(-37.015042122436,-50.7429584178781,
2.69354577441179));
#236736=CARTESIAN_POINT('Ctrl Pts',(-37.0160707669655,-50.7389795822778,
2.69593478828072));
#236737=CARTESIAN_POINT('Ctrl Pts',(-37.0169563748086,-50.7350097117578,
2.69839565261167));
#236738=CARTESIAN_POINT('Ctrl Pts',(-37.0189101579882,-50.7262515844357,
2.70382468688992));
#236739=CARTESIAN_POINT('Ctrl Pts',(-37.0201796788541,-50.7175407334809,
2.70961155815034));
#236740=CARTESIAN_POINT('Ctrl Pts',(-37.0208019128471,-50.7090177292133,
2.71562701361713));
#236741=CARTESIAN_POINT('Ctrl Pts',(-37.0210292227715,-50.7059041682736,
2.71782453535804));
#236742=CARTESIAN_POINT('Ctrl Pts',(-37.0211776528888,-50.7028130194415,
2.72005051502349));
#236743=CARTESIAN_POINT('Ctrl Pts',(-37.0212513646532,-50.6997475881154,
2.72229986760063));
#236744=CARTESIAN_POINT('Ctrl Pts',(-37.02149895467,-50.6894511286646,2.72985520488837));
#236745=CARTESIAN_POINT('Ctrl Pts',(-37.0208967002923,-50.6793793407319,
2.73770845534507));
#236746=CARTESIAN_POINT('Ctrl Pts',(-37.0195682679083,-50.6695664063388,
2.74576706701705));
#236747=CARTESIAN_POINT('Ctrl Pts',(-37.0181081633552,-50.6587808290222,
2.75462443584983));
#236748=CARTESIAN_POINT('Ctrl Pts',(-37.0157708601097,-50.6483072759145,
2.76373036323138));
#236749=CARTESIAN_POINT('Ctrl Pts',(-37.0126680948709,-50.6381830571054,
2.77299664636776));
#236750=CARTESIAN_POINT('Ctrl Pts',(-37.0093262837658,-50.6272788396598,
2.78297683033423));
#236751=CARTESIAN_POINT('Ctrl Pts',(-37.0050963107884,-50.6167786802283,
2.79314401478829));
#236752=CARTESIAN_POINT('Ctrl Pts',(-37.0000610231249,-50.6067353452108,
2.80341452427853));
#236753=CARTESIAN_POINT('Ctrl Pts',(-36.9950937288462,-50.5968276291265,
2.813546347213));
#236754=CARTESIAN_POINT('Ctrl Pts',(-36.9893418170235,-50.5873633690981,
2.82378004209157));
#236755=CARTESIAN_POINT('Ctrl Pts',(-36.9828414016742,-50.5784163149358,
2.83404198860226));
#236756=CARTESIAN_POINT('Ctrl Pts',(-34.9607485668361,-47.7952442955503,
2.83404198860228));
#236757=CARTESIAN_POINT('Ctrl Pts',(-34.9545276336627,-47.7866819156019,
2.82422126442951));
#236758=CARTESIAN_POINT('Ctrl Pts',(-34.9476537221152,-47.7786409912508,
2.81442815028424));
#236759=CARTESIAN_POINT('Ctrl Pts',(-34.9401706643544,-47.7711595893163,
2.8047161816622));
#236760=CARTESIAN_POINT('Ctrl Pts',(-34.9329451136981,-47.7639356375059,
2.79533842146112));
#236761=CARTESIAN_POINT('Ctrl Pts',(-34.9251506707949,-47.7572325247348,
2.78603515650104));
#236762=CARTESIAN_POINT('Ctrl Pts',(-34.9167928415129,-47.7511153344865,
2.77685887346602));
#236763=CARTESIAN_POINT('Ctrl Pts',(-34.9088920753313,-47.7453326739165,
2.768184412164));
#236764=CARTESIAN_POINT('Ctrl Pts',(-34.9004871280264,-47.7400730704108,
2.75962261521426));
#236765=CARTESIAN_POINT('Ctrl Pts',(-34.8915635921214,-47.7354288821269,
2.75123537701441));
#236766=CARTESIAN_POINT('Ctrl Pts',(-34.8833451652563,-47.7311516626296,
2.74351087133876));
#236767=CARTESIAN_POINT('Ctrl Pts',(-34.8746863576787,-47.7273962447069,
2.73593399449582));
#236768=CARTESIAN_POINT('Ctrl Pts',(-34.8655676881406,-47.7242720089008,
2.72857657812293));
#236769=CARTESIAN_POINT('Ctrl Pts',(-34.8628486849585,-47.7233404248509,
2.7263827450812));
#236770=CARTESIAN_POINT('Ctrl Pts',(-34.8600887620236,-47.7224652397583,
2.72420861709476));
#236771=CARTESIAN_POINT('Ctrl Pts',(-34.8572873423617,-47.721650113202,
2.72205663736674));
#236772=CARTESIAN_POINT('Ctrl Pts',(-34.8545145463035,-47.7208433152299,
2.71992664556713));
#236773=CARTESIAN_POINT('Ctrl Pts',(-34.8517040509264,-47.7200959288449,
2.71782089927832));
#236774=CARTESIAN_POINT('Ctrl Pts',(-34.8488585612797,-47.7194121231166,
2.71574387311193));
#236775=CARTESIAN_POINT('Ctrl Pts',(-34.8486606914946,-47.7193645726036,
2.71559944077434));
#236776=CARTESIAN_POINT('Ctrl Pts',(-34.8484626496807,-47.719317317907,
2.71545515216016));
#236777=CARTESIAN_POINT('Ctrl Pts',(-34.8482644357605,-47.7192703603291,
2.71531100781677));
#236778=CARTESIAN_POINT('Ctrl Pts',(-34.8395740113843,-47.7172115680923,
2.70899119176037));
#236779=CARTESIAN_POINT('Ctrl Pts',(-34.8305531107004,-47.7157691359129,
2.70298296066798));
#236780=CARTESIAN_POINT('Ctrl Pts',(-34.8212734513098,-47.7150344641794,
2.69736727774102));
#236781=CARTESIAN_POINT('Ctrl Pts',(-34.8126231959641,-47.7143496224387,
2.69213248525406));
#236782=CARTESIAN_POINT('Ctrl Pts',(-34.8037473009127,-47.7142799923072,
2.68723866185455));
#236783=CARTESIAN_POINT('Ctrl Pts',(-34.7947186932886,-47.7149249376575,
2.68278595829557));
#236784=CARTESIAN_POINT('Ctrl Pts',(-34.791415911814,-47.7151608670104,
2.68115710172783));
#236785=CARTESIAN_POINT('Ctrl Pts',(-34.788092901115,-47.715492664483,2.67958763637771));
#236786=CARTESIAN_POINT('Ctrl Pts',(-34.7847540840176,-47.7159260651933,
2.67808378645311));
#236787=CARTESIAN_POINT('Ctrl Pts',(-34.7839512100458,-47.7160302835855,
2.67772216078546));
#236788=CARTESIAN_POINT('Ctrl Pts',(-34.7831469919154,-47.7161407719862,
2.6773640360351));
#236789=CARTESIAN_POINT('Ctrl Pts',(-34.78234155776,-47.7162575750188,2.67700956934426));
#236790=CARTESIAN_POINT('Ctrl Pts',(-34.781561293422,-47.7163707279567,
2.67666617973751));
#236791=CARTESIAN_POINT('Ctrl Pts',(-34.7807798878928,-47.7164898070135,
2.67632622314065));
#236792=CARTESIAN_POINT('Ctrl Pts',(-34.7799974607185,-47.7166148505127,
2.6759898415872));
#236793=CARTESIAN_POINT('Ctrl Pts',(-34.7714250667934,-47.717984846556,
2.6723043929217));
#236794=CARTESIAN_POINT('Ctrl Pts',(-34.7627244668153,-47.7200720995233,
2.66904964539926));
#236795=CARTESIAN_POINT('Ctrl Pts',(-34.7540804826577,-47.7229136891077,
2.66640203566677));
#236796=CARTESIAN_POINT('Ctrl Pts',(-34.750495564778,-47.7240921810072,
2.66530399299389));
#236797=CARTESIAN_POINT('Ctrl Pts',(-34.7469205018085,-47.7254000086987,
2.66430995142206));
#236798=CARTESIAN_POINT('Ctrl Pts',(-34.7433685265017,-47.7268379886353,
2.66343053473306));
#236799=CARTESIAN_POINT('Ctrl Pts',(-34.7373102624742,-47.7292906132653,
2.66193059792829));
#236800=CARTESIAN_POINT('Ctrl Pts',(-34.7313214412506,-47.732122868262,
2.66076519817072));
#236801=CARTESIAN_POINT('Ctrl Pts',(-34.72547478788,-47.7353375827197,2.65997805604404));
#236802=CARTESIAN_POINT('Ctrl Pts',(-34.7225514611947,-47.7369449399485,
2.65958448498071));
#236803=CARTESIAN_POINT('Ctrl Pts',(-34.7196644712712,-47.7386491210193,
2.65928526260706));
#236804=CARTESIAN_POINT('Ctrl Pts',(-34.7168229726602,-47.7404504949223,
2.65908463971268));
#236805=CARTESIAN_POINT('Ctrl Pts',(-34.7139814740492,-47.7422518688253,
2.6588840168183));
#236806=CARTESIAN_POINT('Ctrl Pts',(-34.7111854907789,-47.7441503967333,
2.65878198860228));
#236807=CARTESIAN_POINT('Ctrl Pts',(-34.7084426211227,-47.7461450747865,
2.65878198860228));
#236808=CARTESIAN_POINT('Origin',(-29.1186878401551,-50.4655267888876,2.83404198860226));
#236809=CARTESIAN_POINT('Ctrl Pts',(-31.1634057161435,-54.3576020372439,
2.83404198860223));
#236810=CARTESIAN_POINT('Ctrl Pts',(-31.1687108809055,-54.3667908521543,
2.8241965244008));
#236811=CARTESIAN_POINT('Ctrl Pts',(-31.1747253323927,-54.375533807056,
2.81438790575706));
#236812=CARTESIAN_POINT('Ctrl Pts',(-31.1814073748063,-54.3837890328989,
2.80466781256992));
#236813=CARTESIAN_POINT('Ctrl Pts',(-31.1878722906305,-54.3917760130587,
2.79526356453192));
#236814=CARTESIAN_POINT('Ctrl Pts',(-31.194962980709,-54.3993074034423,
2.78594102496363));
#236815=CARTESIAN_POINT('Ctrl Pts',(-31.2026795247195,-54.4063187915261,
2.77675109088922));
#236816=CARTESIAN_POINT('Ctrl Pts',(-31.209978900196,-54.4129511329169,
2.76805797913831));
#236817=CARTESIAN_POINT('Ctrl Pts',(-31.2178389737506,-54.4191188025041,
2.75948271210313));
#236818=CARTESIAN_POINT('Ctrl Pts',(-31.2262832675548,-54.4247323097978,
2.75108575573377));
#236819=CARTESIAN_POINT('Ctrl Pts',(-31.2340610728554,-54.4299027559945,
2.74335155163424));
#236820=CARTESIAN_POINT('Ctrl Pts',(-31.2423350114986,-54.4346033281822,
2.73576818686097));
#236821=CARTESIAN_POINT('Ctrl Pts',(-31.2511358718536,-54.4387279162167,
2.72840626160653));
#236822=CARTESIAN_POINT('Ctrl Pts',(-31.2536886668971,-54.4399243024183,
2.72627084693769));
#236823=CARTESIAN_POINT('Ctrl Pts',(-31.2562858555936,-54.4410719653272,
2.72415424587548));
#236824=CARTESIAN_POINT('Ctrl Pts',(-31.2589283212562,-54.4421676282858,
2.7220586717322));
#236825=CARTESIAN_POINT('Ctrl Pts',(-31.261792923929,-54.4433553973773,
2.71978693462822));
#236826=CARTESIAN_POINT('Ctrl Pts',(-31.264706337619,-54.4444813995853,
2.71754411340722));
#236827=CARTESIAN_POINT('Ctrl Pts',(-31.2676686823014,-54.4455416356296,
2.71533341844219));
#236828=CARTESIAN_POINT('Ctrl Pts',(-31.2757988605275,-54.4484514617727,
2.70926614876367));
#236829=CARTESIAN_POINT('Ctrl Pts',(-31.2843017293917,-54.4508216479603,
2.70347381860383));
#236830=CARTESIAN_POINT('Ctrl Pts',(-31.293105316062,-54.4525775288975,
2.69804914171369));
#236831=CARTESIAN_POINT('Ctrl Pts',(-31.3011601199073,-54.454184064626,
2.69308585687188));
#236832=CARTESIAN_POINT('Ctrl Pts',(-31.3094611543721,-54.4552661718985,
2.68842799053176));
#236833=CARTESIAN_POINT('Ctrl Pts',(-31.3179758301767,-54.4557414157485,
2.68414767054214));
#236834=CARTESIAN_POINT('Ctrl Pts',(-31.3221582111178,-54.4559748539752,
2.68204519134541));
#236835=CARTESIAN_POINT('Ctrl Pts',(-31.3263919825236,-54.4560613864571,
2.68003431778483));
#236836=CARTESIAN_POINT('Ctrl Pts',(-31.3306718639309,-54.4559882102924,
2.67812693945226));
#236837=CARTESIAN_POINT('Ctrl Pts',(-31.3314839297413,-54.4559743258279,
2.67776503299178));
#236838=CARTESIAN_POINT('Ctrl Pts',(-31.3322980319626,-54.4559543157131,
2.67740659639898));
#236839=CARTESIAN_POINT('Ctrl Pts',(-31.3331140451953,-54.4559281176615,
2.6770517896883));
#236840=CARTESIAN_POINT('Ctrl Pts',(-31.3339045580146,-54.4559027382989,
2.67670807068732));
#236841=CARTESIAN_POINT('Ctrl Pts',(-31.3346968642516,-54.455871551716,
2.6763677582524));
#236842=CARTESIAN_POINT('Ctrl Pts',(-31.3354908465824,-54.4558345032251,
2.6760309969923));
#236843=CARTESIAN_POINT('Ctrl Pts',(-31.3441435024202,-54.4554307564062,
2.67236104217099));
#236844=CARTESIAN_POINT('Ctrl Pts',(-31.3530008879288,-54.4543301709715,
2.66911440541442));
#236845=CARTESIAN_POINT('Ctrl Pts',(-31.3618824321387,-54.4524721779259,
2.66646778189597));
#236846=CARTESIAN_POINT('Ctrl Pts',(-31.3656331634102,-54.4516875359252,
2.66535009634944));
#236847=CARTESIAN_POINT('Ctrl Pts',(-31.3693880355474,-54.4507682193236,
2.66433897912317));
#236848=CARTESIAN_POINT('Ctrl Pts',(-31.3731331934888,-54.4497115877221,
2.66344564884767));
#236849=CARTESIAN_POINT('Ctrl Pts',(-31.3794399458809,-54.4479322465076,
2.6619413029856));
#236850=CARTESIAN_POINT('Ctrl Pts',(-31.3857169562555,-54.4457622496021,
2.66077206705395));
#236851=CARTESIAN_POINT('Ctrl Pts',(-31.3918909882804,-54.4431895758478,
2.65998225155689));
#236852=CARTESIAN_POINT('Ctrl Pts',(-31.3934344962867,-54.4425464074092,
2.65978479768263));
#236853=CARTESIAN_POINT('Ctrl Pts',(-31.3949714642034,-54.4418778620535,
2.65961098966597));
#236854=CARTESIAN_POINT('Ctrl Pts',(-31.3965005998222,-54.441183481233,
2.65946139030476));
#236855=CARTESIAN_POINT('Ctrl Pts',(-31.3987943032505,-54.4401419100023,
2.65923699126295));
#236856=CARTESIAN_POINT('Ctrl Pts',(-31.4010703637561,-54.4390422051398,
2.65906707562416));
#236857=CARTESIAN_POINT('Ctrl Pts',(-31.4033252432067,-54.4378842814516,
2.65895332562894));
#236858=CARTESIAN_POINT('Ctrl Pts',(-31.4055801226574,-54.4367263577633,
2.65883957563371));
#236859=CARTESIAN_POINT('Ctrl Pts',(-31.4078138194778,-54.4355102267487,
2.65878198860223));
#236860=CARTESIAN_POINT('Ctrl Pts',(-31.4100231232065,-54.4342359163079,
2.65878198860223));
#236861=CARTESIAN_POINT('Ctrl Pts',(-29.5010785149107,-51.1278468659048,
2.65878198860225));
#236862=CARTESIAN_POINT('Ctrl Pts',(-29.4936027956394,-51.1321585373224,
2.65878198860225));
#236863=CARTESIAN_POINT('Ctrl Pts',(-29.4865477845236,-51.1370499258742,
2.65945335517818));
#236864=CARTESIAN_POINT('Ctrl Pts',(-29.4799806005925,-51.1423856448174,
2.66072561226564));
#236865=CARTESIAN_POINT('Ctrl Pts',(-29.475738873605,-51.1458319717784,
2.66154735980303));
#236866=CARTESIAN_POINT('Ctrl Pts',(-29.4717000621109,-51.1494629466898,
2.66261895766849));
#236867=CARTESIAN_POINT('Ctrl Pts',(-29.4678753842635,-51.1532365012461,
2.66391429250995));
#236868=CARTESIAN_POINT('Ctrl Pts',(-29.4628059928679,-51.1582381316478,
2.66563118464092));
#236869=CARTESIAN_POINT('Ctrl Pts',(-29.4581176150985,-51.1634934604716,
2.66774105138667));
#236870=CARTESIAN_POINT('Ctrl Pts',(-29.4538379291356,-51.168916779284,
2.67016894181718));
#236871=CARTESIAN_POINT('Ctrl Pts',(-29.4516980861541,-51.1716284386902,
2.67138288703243));
#236872=CARTESIAN_POINT('Ctrl Pts',(-29.4496602426628,-51.174382193724,
2.6726761316752));
#236873=CARTESIAN_POINT('Ctrl Pts',(-29.4477266300414,-51.1771680313592,
2.67403835432521));
#236874=CARTESIAN_POINT('Ctrl Pts',(-29.4467598237306,-51.1785609501768,
2.67471946565022));
#236875=CARTESIAN_POINT('Ctrl Pts',(-29.4458190608833,-51.179961897818,
2.6754178138949));
#236876=CARTESIAN_POINT('Ctrl Pts',(-29.4449045308656,-51.1813696738592,
2.67613207244136));
#236877=CARTESIAN_POINT('Ctrl Pts',(-29.4446758983612,-51.1817216178695,
2.67631063707798));
#236878=CARTESIAN_POINT('Ctrl Pts',(-29.4444489051049,-51.1820739888278,
2.67649019601813));
#236879=CARTESIAN_POINT('Ctrl Pts',(-29.444223553443,-51.1824267683259,
2.67667072836624));
#236880=CARTESIAN_POINT('Ctrl Pts',(-29.4435474984573,-51.1834851068199,
2.67721232541058));
#236881=CARTESIAN_POINT('Ctrl Pts',(-29.4428862193402,-51.1845471213153,
2.67776268340015));
#236882=CARTESIAN_POINT('Ctrl Pts',(-29.4422397658675,-51.185612322458,
2.67832123541484));
#236883=CARTESIAN_POINT('Ctrl Pts',(-29.437686231078,-51.1931154617649,
2.68225560368405));
#236884=CARTESIAN_POINT('Ctrl Pts',(-29.4338145801759,-51.2007799603593,
2.6866179299884));
#236885=CARTESIAN_POINT('Ctrl Pts',(-29.4305579784511,-51.2085065710724,
2.69130986622519));
#236886=CARTESIAN_POINT('Ctrl Pts',(-29.4289785301336,-51.2122539689191,
2.69358545023003));
#236887=CARTESIAN_POINT('Ctrl Pts',(-29.4275440072539,-51.2160164979697,
2.69593918853426));
#236888=CARTESIAN_POINT('Ctrl Pts',(-29.4262483256615,-51.219785247298,
2.6983630623544));
#236889=CARTESIAN_POINT('Ctrl Pts',(-29.4242647276701,-51.2255549392044,
2.70207384382173));
#236890=CARTESIAN_POINT('Ctrl Pts',(-29.4226066102319,-51.231335680589,
2.70594760814172));
#236891=CARTESIAN_POINT('Ctrl Pts',(-29.4212581193009,-51.2370841708899,
2.70995196345652));
#236892=CARTESIAN_POINT('Ctrl Pts',(-29.4206318731364,-51.2397537995244,
2.71181160678049));
#236893=CARTESIAN_POINT('Ctrl Pts',(-29.4200721889211,-51.2424163366105,
2.71369962772043));
#236894=CARTESIAN_POINT('Ctrl Pts',(-29.4195787111903,-51.2450674596717,
2.71561183138605));
#236895=CARTESIAN_POINT('Ctrl Pts',(-29.4195408880667,-51.2452706578084,
2.71575839426256));
#236896=CARTESIAN_POINT('Ctrl Pts',(-29.4195034206998,-51.245473795951,
2.71590508903153));
#236897=CARTESIAN_POINT('Ctrl Pts',(-29.4194663081569,-51.2456768729756,
2.71605191409856));
#236898=CARTESIAN_POINT('Ctrl Pts',(-29.4189449888197,-51.2485294929146,
2.71811436362697));
#236899=CARTESIAN_POINT('Ctrl Pts',(-29.4184957101761,-51.2513705613628,
2.72020091026903));
#236900=CARTESIAN_POINT('Ctrl Pts',(-29.4181151898793,-51.2541954110681,
2.72230624862126));
#236901=CARTESIAN_POINT('Ctrl Pts',(-29.4167507117681,-51.264324819728,
2.72985561752999));
#236902=CARTESIAN_POINT('Ctrl Pts',(-29.4162578421117,-51.2743237313747,
2.73770089914175));
#236903=CARTESIAN_POINT('Ctrl Pts',(-29.4165161672804,-51.2841455249749,
2.74574823346864));
#236904=CARTESIAN_POINT('Ctrl Pts',(-29.4168000406897,-51.2949386894546,
2.75459144546713));
#236905=CARTESIAN_POINT('Ctrl Pts',(-29.4179908989225,-51.3055186222547,
2.7636791175385));
#236906=CARTESIAN_POINT('Ctrl Pts',(-29.4199800715326,-51.3158373135899,
2.77292162564196));
#236907=CARTESIAN_POINT('Ctrl Pts',(-29.4221278787371,-51.3269789105929,
2.78290121483999));
#236908=CARTESIAN_POINT('Ctrl Pts',(-29.4252064644148,-51.3378170984163,
2.79306229499247));
#236909=CARTESIAN_POINT('Ctrl Pts',(-29.4291364604156,-51.348292144514,
2.80331916684103));
#236910=CARTESIAN_POINT('Ctrl Pts',(-29.43303348779,-51.3586793157436,2.81348999407907));
#236911=CARTESIAN_POINT('Ctrl Pts',(-29.4377684584824,-51.3687106315409,
2.82375635966462));
#236912=CARTESIAN_POINT('Ctrl Pts',(-29.4433108116256,-51.3783102687786,
2.83404198860225));
#236913=CARTESIAN_POINT('Origin',(-0.0131982271536665,0.00762000000019421,
2.83404198860262));
#236914=CARTESIAN_POINT('Ctrl Pts',(-31.436419577513,-54.4189959163064,
2.65878198860223));
#236915=CARTESIAN_POINT('Ctrl Pts',(-31.4438560159997,-54.4146983388118,
2.65878198860223));
#236916=CARTESIAN_POINT('Ctrl Pts',(-31.45086737166,-54.4098177483013,2.65944603041804));
#236917=CARTESIAN_POINT('Ctrl Pts',(-31.4573895320584,-54.4044907169111,
2.66070439264011));
#236918=CARTESIAN_POINT('Ctrl Pts',(-31.461556882064,-54.4010869974475,
2.66150842619537));
#236919=CARTESIAN_POINT('Ctrl Pts',(-31.4655251210642,-54.3975017237412,
2.66255428265315));
#236920=CARTESIAN_POINT('Ctrl Pts',(-31.4692842169741,-54.3937759157109,
2.6638169970061));
#236921=CARTESIAN_POINT('Ctrl Pts',(-31.4744146286221,-54.3886909353394,
2.6655403487321));
#236922=CARTESIAN_POINT('Ctrl Pts',(-31.4791503318816,-54.3833409297222,
2.66766759643914));
#236923=CARTESIAN_POINT('Ctrl Pts',(-31.4834636394924,-54.3778174666303,
2.6701201278309));
#236924=CARTESIAN_POINT('Ctrl Pts',(-31.4856202932977,-54.3750557350844,
2.67134639352678));
#236925=CARTESIAN_POINT('Ctrl Pts',(-31.4876715300022,-54.3722505364143,
2.67265375584955));
#236926=CARTESIAN_POINT('Ctrl Pts',(-31.4896151854255,-54.3694125772948,
2.67403135126882));
#236927=CARTESIAN_POINT('Ctrl Pts',(-31.4905870131372,-54.3679935977351,
2.67472014897846));
#236928=CARTESIAN_POINT('Ctrl Pts',(-31.4915319606347,-54.3665664194,2.67542649668576));
#236929=CARTESIAN_POINT('Ctrl Pts',(-31.4924498523884,-54.3651323262969,
2.67614899656045));
#236930=CARTESIAN_POINT('Ctrl Pts',(-31.4926793253268,-54.3647738030211,
2.67632962152913));
#236931=CARTESIAN_POINT('Ctrl Pts',(-31.4929071076035,-54.3644148473886,
2.67651125590894));
#236932=CARTESIAN_POINT('Ctrl Pts',(-31.4931331971263,-54.3640554790922,
2.67669387767467));
#236933=CARTESIAN_POINT('Ctrl Pts',(-31.4938114656948,-54.3629773742029,
2.67724174297187));
#236934=CARTESIAN_POINT('Ctrl Pts',(-31.4944744978645,-54.3618955562473,
2.67779849504691));
#236935=CARTESIAN_POINT('Ctrl Pts',(-31.4951222515523,-54.360810548785,
2.67836353617953));
#236936=CARTESIAN_POINT('Ctrl Pts',(-31.4995986314372,-54.3533124740222,
2.68226832098851));
#236937=CARTESIAN_POINT('Ctrl Pts',(-31.5034009004291,-54.3456575719325,
2.68659153751332));
#236938=CARTESIAN_POINT('Ctrl Pts',(-31.5065976218799,-54.3379428492062,
2.69123699486118));
#236939=CARTESIAN_POINT('Ctrl Pts',(-31.5081863836661,-54.3341086531876,
2.69354577441158));
#236940=CARTESIAN_POINT('Ctrl Pts',(-31.5096252947442,-54.3302591366968,
2.6959347882806));
#236941=CARTESIAN_POINT('Ctrl Pts',(-31.5109210155997,-54.3264035847697,
2.69839565261164));
#236942=CARTESIAN_POINT('Ctrl Pts',(-31.5137795693408,-54.3178976613387,
2.7038246868899));
#236943=CARTESIAN_POINT('Ctrl Pts',(-31.5159526675026,-54.3093672304021,
2.70961155815031));
#236944=CARTESIAN_POINT('Ctrl Pts',(-31.5174623893712,-54.3009559572067,
2.71562701361712));
#236945=CARTESIAN_POINT('Ctrl Pts',(-31.5180139098084,-54.2978832130367,
2.71782453535803));
#236946=CARTESIAN_POINT('Ctrl Pts',(-31.5184846398471,-54.2948245130135,
2.72005051502347));
#236947=CARTESIAN_POINT('Ctrl Pts',(-31.5188783726365,-54.2917835794184,
2.72229986760061));
#236948=CARTESIAN_POINT('Ctrl Pts',(-31.5202008794128,-54.2815694052538,
2.72985520488829));
#236949=CARTESIAN_POINT('Ctrl Pts',(-31.5206547127626,-54.2714898389048,
2.73770845534488));
#236950=CARTESIAN_POINT('Ctrl Pts',(-31.5203592886225,-54.2615918017974,
2.74576706701677));
#236951=CARTESIAN_POINT('Ctrl Pts',(-31.5200345824971,-54.2507126865167,
2.75462443584947));
#236952=CARTESIAN_POINT('Ctrl Pts',(-31.5188048676548,-54.2400521939124,
2.76373036323094));
#236953=CARTESIAN_POINT('Ctrl Pts',(-31.5167773687225,-54.229659109351,
2.77299664636724));
#236954=CARTESIAN_POINT('Ctrl Pts',(-31.514593665501,-54.21846531197,2.7829768303337));
#236955=CARTESIAN_POINT('Ctrl Pts',(-31.5114844302875,-54.2075805209355,
2.79314401478776));
#236956=CARTESIAN_POINT('Ctrl Pts',(-31.5075265408322,-54.1970658734764,
2.80341452427803));
#236957=CARTESIAN_POINT('Ctrl Pts',(-31.5036220962481,-54.1866932092599,
2.81354634721262));
#236958=CARTESIAN_POINT('Ctrl Pts',(-31.4988909785568,-54.1766795569344,
2.82378004209134));
#236959=CARTESIAN_POINT('Ctrl Pts',(-31.4933613949854,-54.1671020372439,
2.83404198860223));
#236960=CARTESIAN_POINT('Ctrl Pts',(-29.7732664904675,-51.1878102687786,
2.83404198860225));
#236961=CARTESIAN_POINT('Ctrl Pts',(-29.7679746486351,-51.1786445298593,
2.82422126443012));
#236962=CARTESIAN_POINT('Ctrl Pts',(-29.7619788985604,-51.169929135123,
2.81442815028548));
#236963=CARTESIAN_POINT('Ctrl Pts',(-29.7553188532208,-51.1617065245633,
2.80471618166407));
#236964=CARTESIAN_POINT('Ctrl Pts',(-29.7488879934689,-51.1537668706107,
2.79533842146347));
#236965=CARTESIAN_POINT('Ctrl Pts',(-29.741836915417,-51.1462857370543,
2.78603515650385));
#236966=CARTESIAN_POINT('Ctrl Pts',(-29.734164291695,-51.1393284263634,
2.77685887346928));
#236967=CARTESIAN_POINT('Ctrl Pts',(-29.7269112593607,-51.1327515888657,
2.76818441216769));
#236968=CARTESIAN_POINT('Ctrl Pts',(-29.7191021335091,-51.1266422417928,
2.75962261521835));
#236969=CARTESIAN_POINT('Ctrl Pts',(-29.7107129315325,-51.1210907313634,
2.75123537701888));
#236970=CARTESIAN_POINT('Ctrl Pts',(-29.7029866172514,-51.1159778833914,
2.74351087134362));
#236971=CARTESIAN_POINT('Ctrl Pts',(-29.6947677915928,-51.1113379461912,
2.73593399450103));
#236972=CARTESIAN_POINT('Ctrl Pts',(-29.686025646649,-51.1072776647618,
2.72857657812844));
#236973=CARTESIAN_POINT('Ctrl Pts',(-29.6834189154979,-51.1060669708015,
2.72638274508483));
#236974=CARTESIAN_POINT('Ctrl Pts',(-29.6807655934602,-51.1049080895602,
2.72420861709655));
#236975=CARTESIAN_POINT('Ctrl Pts',(-29.6780647241923,-51.1038046002594,
2.72205663736672));
#236976=CARTESIAN_POINT('Ctrl Pts',(-29.6753914511533,-51.1027123859001,
2.71992664556711));
#236977=CARTESIAN_POINT('Ctrl Pts',(-29.6726744751142,-51.1016753170131,
2.71782089927829));
#236978=CARTESIAN_POINT('Ctrl Pts',(-29.6699160505195,-51.1006978225841,
2.7157438731119));
#236979=CARTESIAN_POINT('Ctrl Pts',(-29.6697242350678,-51.1006298495332,
2.71559944077431));
#236980=CARTESIAN_POINT('Ctrl Pts',(-29.6695322176085,-51.1005621526963,
2.71545515216013));
#236981=CARTESIAN_POINT('Ctrl Pts',(-29.6693399979284,-51.1004947333604,
2.71531100781675));
#236982=CARTESIAN_POINT('Ctrl Pts',(-29.6609123829947,-51.0975388226977,
2.70899119176026));
#236983=CARTESIAN_POINT('Ctrl Pts',(-29.6520916749676,-51.0951613514268,
2.70298296066779));
#236984=CARTESIAN_POINT('Ctrl Pts',(-29.6429396446294,-51.0934607157662,
2.69736727774075));
#236985=CARTESIAN_POINT('Ctrl Pts',(-29.6344083617419,-51.091875427762,
2.69213248525359));
#236986=CARTESIAN_POINT('Ctrl Pts',(-29.6255883681025,-51.0908783954019,
2.68723866185391));
#236987=CARTESIAN_POINT('Ctrl Pts',(-29.6165418049888,-51.0905760611937,
2.68278595829479));
#236988=CARTESIAN_POINT('Ctrl Pts',(-29.6132324551646,-51.090465463429,
2.68115710172733));
#236989=CARTESIAN_POINT('Ctrl Pts',(-29.6098929659864,-51.0904480940785,
2.67958763637747));
#236990=CARTESIAN_POINT('Ctrl Pts',(-29.6065271365688,-51.0905301191541,
2.6780837864531));
#236991=CARTESIAN_POINT('Ctrl Pts',(-29.6057177670362,-51.0905498434445,
2.67772216078545));
#236992=CARTESIAN_POINT('Ctrl Pts',(-29.6049064053142,-51.0905756628929,
2.67736403603509));
#236993=CARTESIAN_POINT('Ctrl Pts',(-29.6040931741699,-51.0906076352718,
2.67700956934425));
#236994=CARTESIAN_POINT('Ctrl Pts',(-29.6033053564988,-51.0906386085138,
2.67666617973749));
#236995=CARTESIAN_POINT('Ctrl Pts',(-29.60251578444,-51.0906753561239,2.67632622314064));
#236996=CARTESIAN_POINT('Ctrl Pts',(-29.6017245728789,-51.0907179287116,
2.67598984158719));
#236997=CARTESIAN_POINT('Ctrl Pts',(-29.5930559358434,-51.0911843606097,
2.67230439292164));
#236998=CARTESIAN_POINT('Ctrl Pts',(-29.5841848213171,-51.0923507190417,
2.66904964539915));
#236999=CARTESIAN_POINT('Ctrl Pts',(-29.5752911628165,-51.0942731997206,
2.66640203566664));
#237000=CARTESIAN_POINT('Ctrl Pts',(-29.5716026975449,-51.0950705097612,
2.66530399299381));
#237001=CARTESIAN_POINT('Ctrl Pts',(-29.5679105139258,-51.0959974771975,
2.66430995142202));
#237002=CARTESIAN_POINT('Ctrl Pts',(-29.5642276868785,-51.0970562972091,
2.66343053473304));
#237003=CARTESIAN_POINT('Ctrl Pts',(-29.5579462415717,-51.0988622250758,
2.66193059792828));
#237004=CARTESIAN_POINT('Ctrl Pts',(-29.551694176475,-51.1010529624041,
2.6607651981707));
#237005=CARTESIAN_POINT('Ctrl Pts',(-29.5455435225214,-51.1036389246279,
2.65997805604402));
#237006=CARTESIAN_POINT('Ctrl Pts',(-29.5424681955446,-51.1049319057398,
2.65958448498068));
#237007=CARTESIAN_POINT('Ctrl Pts',(-29.5394188854255,-51.1063249785082,
2.65928526260704));
#237008=CARTESIAN_POINT('Ctrl Pts',(-29.5364046579953,-51.1078194668131,
2.65908463971266));
#237009=CARTESIAN_POINT('Ctrl Pts',(-29.5333904305651,-51.109313955118,
2.65888401681828));
#237010=CARTESIAN_POINT('Ctrl Pts',(-29.5304113137788,-51.1109098228567,
2.65878198860225));
#237011=CARTESIAN_POINT('Ctrl Pts',(-29.527474969218,-51.1126068659048,
2.65878198860225));
#237012=CARTESIAN_POINT('Origin',(-23.6840886581931,-53.2328030451448,2.83404198860224));
#237013=CARTESIAN_POINT('Ctrl Pts',(-25.3107727110817,-57.317288315449,
2.83404198860221));
#237014=CARTESIAN_POINT('Ctrl Pts',(-25.3150883208942,-57.3269813337895,
2.82419652440052));
#237015=CARTESIAN_POINT('Ctrl Pts',(-25.3201559369465,-57.3363050752407,
2.81438790575664));
#237016=CARTESIAN_POINT('Ctrl Pts',(-25.3259384683613,-57.3452135417177,
2.80466781256942));
#237017=CARTESIAN_POINT('Ctrl Pts',(-25.3315331019378,-57.3538325360807,
2.7952635645314));
#237018=CARTESIAN_POINT('Ctrl Pts',(-25.3377977038111,-57.3620638476571,
2.78594102496314));
#237019=CARTESIAN_POINT('Ctrl Pts',(-25.3447390861644,-57.3698434251106,
2.77675109088879));
#237020=CARTESIAN_POINT('Ctrl Pts',(-25.3513052064448,-57.3772024263427,
2.76805797913801));
#237021=CARTESIAN_POINT('Ctrl Pts',(-25.3584775246701,-57.3841579102004,
2.75948271210298));
#237022=CARTESIAN_POINT('Ctrl Pts',(-25.3662887884584,-57.3906233351686,
2.75108575573376));
#237023=CARTESIAN_POINT('Ctrl Pts',(-25.3734835273323,-57.3965784591558,
2.74335155163439));
#237024=CARTESIAN_POINT('Ctrl Pts',(-25.3812207968865,-57.4021181432088,
2.73576818686127));
#237025=CARTESIAN_POINT('Ctrl Pts',(-25.3895423083587,-57.4071400767267,
2.72840626160694));
#237026=CARTESIAN_POINT('Ctrl Pts',(-25.3919560625129,-57.4085967487426,
2.72627084693796));
#237027=CARTESIAN_POINT('Ctrl Pts',(-25.3944190600979,-57.4100096047774,
2.72415424587559));
#237028=CARTESIAN_POINT('Ctrl Pts',(-25.396932522092,-57.4113754784547,
2.72205867173217));
#237029=CARTESIAN_POINT('Ctrl Pts',(-25.3996572764938,-57.4128561733381,
2.7197869346282));
#237030=CARTESIAN_POINT('Ctrl Pts',(-25.4024370309183,-57.414280541844,
2.7175441134072));
#237031=CARTESIAN_POINT('Ctrl Pts',(-25.4052723227222,-57.4156446191417,
2.71533341844218));
#237032=CARTESIAN_POINT('Ctrl Pts',(-25.4130538033262,-57.4193883399888,
2.70926614876365));
#237033=CARTESIAN_POINT('Ctrl Pts',(-25.4212623406652,-57.4226343338643,
2.70347381860382));
#237034=CARTESIAN_POINT('Ctrl Pts',(-25.4298341608305,-57.4253008212879,
2.69804914171368));
#237035=CARTESIAN_POINT('Ctrl Pts',(-25.4376769109069,-57.4277405125135,
2.69308585687178));
#237036=CARTESIAN_POINT('Ctrl Pts',(-25.4458193604262,-57.4296843862652,
2.6884279905316));
#237037=CARTESIAN_POINT('Ctrl Pts',(-25.4542377154367,-57.4310470526568,
2.68414767054192));
#237038=CARTESIAN_POINT('Ctrl Pts',(-25.4583727839181,-57.4317163899369,
2.68204519134526));
#237039=CARTESIAN_POINT('Ctrl Pts',(-25.4625743171737,-57.4322449980037,
2.68003431778476));
#237040=CARTESIAN_POINT('Ctrl Pts',(-25.4668384019346,-57.4326195921322,
2.67812693945226));
#237041=CARTESIAN_POINT('Ctrl Pts',(-25.4676474704853,-57.4326906677194,
2.67776503299178));
#237042=CARTESIAN_POINT('Ctrl Pts',(-25.4684592045961,-57.4327558640764,
2.67740659639898));
#237043=CARTESIAN_POINT('Ctrl Pts',(-25.469273486065,-57.4328151061496,
2.67705178968829));
#237044=CARTESIAN_POINT('Ctrl Pts',(-25.470062321238,-57.432872496908,2.67670807068732));
#237045=CARTESIAN_POINT('Ctrl Pts',(-25.4708535470242,-57.4329242997218,
2.67636775825239));
#237046=CARTESIAN_POINT('Ctrl Pts',(-25.4716470524585,-57.4329704479393,
2.67603099699229));
#237047=CARTESIAN_POINT('Ctrl Pts',(-25.4802945111768,-57.4334733617056,
2.67236104217099));
#237048=CARTESIAN_POINT('Ctrl Pts',(-25.489218417505,-57.4333046542889,
2.66911440541443));
#237049=CARTESIAN_POINT('Ctrl Pts',(-25.4982455208442,-57.4323852136913,
2.66646778189599));
#237050=CARTESIAN_POINT('Ctrl Pts',(-25.5020577226399,-57.4319969282175,
2.66535009634944));
#237051=CARTESIAN_POINT('Ctrl Pts',(-25.5058881199463,-57.4314751387427,
2.66433897912316));
#237052=CARTESIAN_POINT('Ctrl Pts',(-25.5097232095982,-57.430815771084,
2.66344564884766));
#237053=CARTESIAN_POINT('Ctrl Pts',(-25.5161814047437,-57.4297054124226,
2.66194130298559));
#237054=CARTESIAN_POINT('Ctrl Pts',(-25.5226508554405,-57.4282034292356,
2.66077206705393));
#237055=CARTESIAN_POINT('Ctrl Pts',(-25.5290599831059,-57.4262902109366,
2.65998225155687));
#237056=CARTESIAN_POINT('Ctrl Pts',(-25.5306622650222,-57.4258119063619,
2.6597847976826));
#237057=CARTESIAN_POINT('Ctrl Pts',(-25.5322606952865,-57.4253076802621,
2.65961098966595));
#237058=CARTESIAN_POINT('Ctrl Pts',(-25.5338540367005,-57.4247769415288,
2.65946139030474));
#237059=CARTESIAN_POINT('Ctrl Pts',(-25.5362440488216,-57.4239808334288,
2.65923699126293));
#237060=CARTESIAN_POINT('Ctrl Pts',(-25.5386225912889,-57.4231250659717,
2.65906707562414));
#237061=CARTESIAN_POINT('Ctrl Pts',(-25.5409861542577,-57.4222091845944,
2.65895332562892));
#237062=CARTESIAN_POINT('Ctrl Pts',(-25.5433497172266,-57.4212933032172,
2.65883957563369));
#237063=CARTESIAN_POINT('Ctrl Pts',(-25.5456982979275,-57.4203173191901,
2.65878198860221));
#237064=CARTESIAN_POINT('Ctrl Pts',(-25.5480287005713,-57.4192809246789,
2.65878198860221));
#237065=CARTESIAN_POINT('Ctrl Pts',(-23.9951532569802,-53.9314655730804,
2.65878198860223));
#237066=CARTESIAN_POINT('Ctrl Pts',(-23.9872677980937,-53.9349721992637,
2.65878198860223));
#237067=CARTESIAN_POINT('Ctrl Pts',(-23.9797401457382,-53.9390993428072,
2.6594533551782));
#237068=CARTESIAN_POINT('Ctrl Pts',(-23.9726512030262,-53.9437193744796,
2.66072561226572));
#237069=CARTESIAN_POINT('Ctrl Pts',(-23.968072473402,-53.9467034408971,
2.66154735980308));
#237070=CARTESIAN_POINT('Ctrl Pts',(-23.9636762467124,-53.949892354189,
2.6626189576685));
#237071=CARTESIAN_POINT('Ctrl Pts',(-23.9594780769918,-53.9532454491205,
2.66391429250989));
#237072=CARTESIAN_POINT('Ctrl Pts',(-23.9539136435129,-53.9576897843753,
2.66563118464085));
#237073=CARTESIAN_POINT('Ctrl Pts',(-23.9487016177216,-53.9624262550345,
2.66774105138661));
#237074=CARTESIAN_POINT('Ctrl Pts',(-23.9438784851449,-53.967372515342,
2.67016894181712));
#237075=CARTESIAN_POINT('Ctrl Pts',(-23.9414669188565,-53.9698456454958,
2.67138288703237));
#237076=CARTESIAN_POINT('Ctrl Pts',(-23.9391523931032,-53.9723713025228,
2.67267613167513));
#237077=CARTESIAN_POINT('Ctrl Pts',(-23.9369381736871,-53.9749397614921,
2.67403835432515));
#237078=CARTESIAN_POINT('Ctrl Pts',(-23.935831063979,-53.9762239909768,
2.67471946565016));
#237079=CARTESIAN_POINT('Ctrl Pts',(-23.9347490158249,-53.9775189275855,
2.67541781389485));
#237080=CARTESIAN_POINT('Ctrl Pts',(-23.9336923430321,-53.9788233972649,
2.67613207244132));
#237081=CARTESIAN_POINT('Ctrl Pts',(-23.9334281748339,-53.9791495146848,
2.67631063707793));
#237082=CARTESIAN_POINT('Ctrl Pts',(-23.9331655922757,-53.9794762280618,
2.67649019601808));
#237083=CARTESIAN_POINT('Ctrl Pts',(-23.932904599615,-53.9798035193339,
2.67667072836619));
#237084=CARTESIAN_POINT('Ctrl Pts',(-23.9321216216328,-53.9807853931503,
2.67721232541053));
#237085=CARTESIAN_POINT('Ctrl Pts',(-23.9313529543287,-53.9817724673291,
2.67776268340009));
#237086=CARTESIAN_POINT('Ctrl Pts',(-23.9305986983573,-53.9827642604005,
2.67832123541478));
#237087=CARTESIAN_POINT('Ctrl Pts',(-23.9252858166862,-53.9897503227314,
2.6822556036841));
#237088=CARTESIAN_POINT('Ctrl Pts',(-23.9206342168329,-53.9969681366816,
2.68661792998857));
#237089=CARTESIAN_POINT('Ctrl Pts',(-23.916587804369,-54.0043120126392,
2.69130986622551));
#237090=CARTESIAN_POINT('Ctrl Pts',(-23.9146252986966,-54.0078737845428,
2.69358545023024));
#237091=CARTESIAN_POINT('Ctrl Pts',(-23.9128053429038,-54.0114657535932,
2.69593918853435));
#237092=CARTESIAN_POINT('Ctrl Pts',(-23.911122817615,-54.0150784217124,
2.69836306235437));
#237093=CARTESIAN_POINT('Ctrl Pts',(-23.9085469889525,-54.0206091641931,
2.7020738438217));
#237094=CARTESIAN_POINT('Ctrl Pts',(-23.9062937028416,-54.0261849176039,
2.7059476081417));
#237095=CARTESIAN_POINT('Ctrl Pts',(-23.9043517182278,-54.0317609613886,
2.7099519634565));
#237096=CARTESIAN_POINT('Ctrl Pts',(-23.9034498505266,-54.0343505049689,
2.71181160678048));
#237097=CARTESIAN_POINT('Ctrl Pts',(-23.90261492141,-54.0369399534674,2.71369962772041));
#237098=CARTESIAN_POINT('Ctrl Pts',(-23.9018470291824,-54.0395249709302,
2.71561183138603));
#237099=CARTESIAN_POINT('Ctrl Pts',(-23.9017881732688,-54.0397231023333,
2.71575839426254));
#237100=CARTESIAN_POINT('Ctrl Pts',(-23.9017296774342,-54.0399212112575,
2.71590508903151));
#237101=CARTESIAN_POINT('Ctrl Pts',(-23.9016715408684,-54.0401192964879,
2.71605191409853));
#237102=CARTESIAN_POINT('Ctrl Pts',(-23.9008548973945,-54.0429017967672,
2.71811436362695));
#237103=CARTESIAN_POINT('Ctrl Pts',(-23.9001111074275,-54.045680339139,
2.72020091026901));
#237104=CARTESIAN_POINT('Ctrl Pts',(-23.899437394462,-54.0484499388202,
2.72230624862123));
#237105=CARTESIAN_POINT('Ctrl Pts',(-23.8970215795834,-54.0583812307203,
2.72985561753059));
#237106=CARTESIAN_POINT('Ctrl Pts',(-23.8954862390497,-54.0682738483759,
2.73770089914301));
#237107=CARTESIAN_POINT('Ctrl Pts',(-23.8947164920946,-54.0780688394969,
2.7457482334706));
#237108=CARTESIAN_POINT('Ctrl Pts',(-23.8938706175188,-54.0888325507449,
2.75459144547029));
#237109=CARTESIAN_POINT('Ctrl Pts',(-23.8939490479887,-54.0994790041486,
2.76367911754294));
#237110=CARTESIAN_POINT('Ctrl Pts',(-23.8948487267554,-54.1099490937704,
2.77292162564771));
#237111=CARTESIAN_POINT('Ctrl Pts',(-23.8958201540348,-54.1212541629284,
2.78290121484815));
#237112=CARTESIAN_POINT('Ctrl Pts',(-23.8977489757814,-54.1323547778572,
2.79306229500313));
#237113=CARTESIAN_POINT('Ctrl Pts',(-23.900562502383,-54.1431832370012,
2.8033191668542));
#237114=CARTESIAN_POINT('Ctrl Pts',(-23.903352426387,-54.1539208564978,
2.81348999408793));
#237115=CARTESIAN_POINT('Ctrl Pts',(-23.9070129003885,-54.164392158903,
2.82375635966906));
#237116=CARTESIAN_POINT('Ctrl Pts',(-23.911521456611,-54.174518541976,2.83404198860223));
#237117=CARTESIAN_POINT('Origin',(-0.0139224327744654,0.00619866644066967,
2.83404198860262));
#237118=CARTESIAN_POINT('Ctrl Pts',(-25.5758735661203,-57.406883591798,
2.65878198860221));
#237119=CARTESIAN_POINT('Ctrl Pts',(-25.58371848619,-57.4033868763698,2.65878198860221));
#237120=CARTESIAN_POINT('Ctrl Pts',(-25.5912015935362,-57.3992659084774,
2.65944603041801));
#237121=CARTESIAN_POINT('Ctrl Pts',(-25.5982448512625,-57.3946498105263,
2.66070439264004));
#237122=CARTESIAN_POINT('Ctrl Pts',(-25.6027451576538,-57.3917003436859,
2.66150842619531));
#237123=CARTESIAN_POINT('Ctrl Pts',(-25.6070664213765,-57.3885495044087,
2.66255428265311));
#237124=CARTESIAN_POINT('Ctrl Pts',(-25.6111943775536,-57.3852370392633,
2.66381699700609));
#237125=CARTESIAN_POINT('Ctrl Pts',(-25.6168282094538,-57.3807161889918,
2.66554034873209));
#237126=CARTESIAN_POINT('Ctrl Pts',(-25.622097197901,-57.3758905070493,
2.66766759643913));
#237127=CARTESIAN_POINT('Ctrl Pts',(-25.6269642358703,-57.3708481654824,
2.67012012783089));
#237128=CARTESIAN_POINT('Ctrl Pts',(-25.6293977548549,-57.3683269946989,
2.67134639352677));
#237129=CARTESIAN_POINT('Ctrl Pts',(-25.6317309777762,-57.3657515758211,
2.67265375584953));
#237130=CARTESIAN_POINT('Ctrl Pts',(-25.6339606331573,-57.3631323306532,
2.67403135126881));
#237131=CARTESIAN_POINT('Ctrl Pts',(-25.6350754608479,-57.3618227080692,
2.67472014897845));
#237132=CARTESIAN_POINT('Ctrl Pts',(-25.6361644125823,-57.3605021218762,
2.67542649668574));
#237133=CARTESIAN_POINT('Ctrl Pts',(-25.6372271795771,-57.3591718306996,
2.67614899656043));
#237134=CARTESIAN_POINT('Ctrl Pts',(-25.6374928713258,-57.3588392579054,
2.67632962152911));
#237135=CARTESIAN_POINT('Ctrl Pts',(-25.6377569268681,-57.3585060784008,
2.67651125590892));
#237136=CARTESIAN_POINT('Ctrl Pts',(-25.6380193420646,-57.3581723115519,
2.67669387767465));
#237137=CARTESIAN_POINT('Ctrl Pts',(-25.6388065876542,-57.3571710110051,
2.67724174297186));
#237138=CARTESIAN_POINT('Ctrl Pts',(-25.6395790684328,-57.3561644250953,
2.67779849504689));
#237139=CARTESIAN_POINT('Ctrl Pts',(-25.6403366878208,-57.355153070115,
2.67836353617951));
#237140=CARTESIAN_POINT('Ctrl Pts',(-25.6455723078605,-57.3481639797008,
2.68226832098838));
#237141=CARTESIAN_POINT('Ctrl Pts',(-25.6501539027769,-57.3409484573005,
2.68659153751308));
#237142=CARTESIAN_POINT('Ctrl Pts',(-25.6541395203641,-57.3336101450134,
2.6912369948608));
#237143=CARTESIAN_POINT('Ctrl Pts',(-25.6561203613648,-57.3299630239497,
2.69354577441131));
#237144=CARTESIAN_POINT('Ctrl Pts',(-25.6579537739807,-57.3262850026765,
2.69593478828045));
#237145=CARTESIAN_POINT('Ctrl Pts',(-25.6596454116599,-57.3225860115759,
2.69839565261162));
#237146=CARTESIAN_POINT('Ctrl Pts',(-25.6633774170493,-57.3144254847132,
2.70382468688988));
#237147=CARTESIAN_POINT('Ctrl Pts',(-25.6664302835889,-57.3061689349812,
2.70961155815029));
#237148=CARTESIAN_POINT('Ctrl Pts',(-25.6688109525044,-57.2979615485274,
2.7156270136171));
#237149=CARTESIAN_POINT('Ctrl Pts',(-25.669680640881,-57.2949632867553,
2.717824535358));
#237150=CARTESIAN_POINT('Ctrl Pts',(-25.6704685134243,-57.2919705472983,
2.72005051502344));
#237151=CARTESIAN_POINT('Ctrl Pts',(-25.67117795342,-57.2889874285391,2.72229986760058));
#237152=CARTESIAN_POINT('Ctrl Pts',(-25.6735608872947,-57.2789674482905,
2.72985520488809));
#237153=CARTESIAN_POINT('Ctrl Pts',(-25.6750658360787,-57.2689905373633,
2.73770845534447));
#237154=CARTESIAN_POINT('Ctrl Pts',(-25.6758066569111,-57.2591158425076,
2.74576706701612));
#237155=CARTESIAN_POINT('Ctrl Pts',(-25.6766209067619,-57.2482623831265,
2.75462443584862));
#237156=CARTESIAN_POINT('Ctrl Pts',(-25.6765122533357,-57.2375317496134,
2.76373036322987));
#237157=CARTESIAN_POINT('Ctrl Pts',(-25.6755822344126,-57.226983668109,
2.77299664636597));
#237158=CARTESIAN_POINT('Ctrl Pts',(-25.6745805641842,-57.2156229323793,
2.78297683033233));
#237159=CARTESIAN_POINT('Ctrl Pts',(-25.6726261321664,-57.2044727657902,
2.79314401478631));
#237160=CARTESIAN_POINT('Ctrl Pts',(-25.6697890043845,-57.1936020065676,
2.80341452427657));
#237161=CARTESIAN_POINT('Ctrl Pts',(-25.6669901874068,-57.1828780392983,
2.81354634721156));
#237162=CARTESIAN_POINT('Ctrl Pts',(-25.6633316989625,-57.1724247063459,
2.82378004209075));
#237163=CARTESIAN_POINT('Ctrl Pts',(-25.6588335304436,-57.1623216544371,
2.83404198860221));
#237164=CARTESIAN_POINT('Ctrl Pts',(-24.2595822759728,-54.0195518809641,
2.83404198860223));
#237165=CARTESIAN_POINT('Ctrl Pts',(-24.2552775040074,-54.0098832048265,
2.82422126442958));
#237166=CARTESIAN_POINT('Ctrl Pts',(-24.2502256060972,-54.0005888273926,
2.81442815028443));
#237167=CARTESIAN_POINT('Ctrl Pts',(-24.2444615420283,-53.9917150968488,
2.8047161816625));
#237168=CARTESIAN_POINT('Ctrl Pts',(-24.2388958310253,-53.9831467292637,
2.79533842146156));
#237169=CARTESIAN_POINT('Ctrl Pts',(-24.2326653709106,-53.9749695397864,
2.78603515650162));
#237170=CARTESIAN_POINT('Ctrl Pts',(-24.2257620156187,-53.9672483344043,
2.77685887346673));
#237171=CARTESIAN_POINT('Ctrl Pts',(-24.219236182871,-53.9599493771864,
2.76818441216492));
#237172=CARTESIAN_POINT('Ctrl Pts',(-24.2121084368886,-53.9530572218312,
2.75962261521538));
#237173=CARTESIAN_POINT('Ctrl Pts',(-24.2043454826918,-53.9466592127661,
2.75123537701573));
#237174=CARTESIAN_POINT('Ctrl Pts',(-24.1971959321099,-53.9407667537517,
2.74351087134032));
#237175=CARTESIAN_POINT('Ctrl Pts',(-24.189507135543,-53.935293133397,2.73593399449761));
#237176=CARTESIAN_POINT('Ctrl Pts',(-24.1812372959618,-53.9303412916376,
2.72857657812491));
#237177=CARTESIAN_POINT('Ctrl Pts',(-24.1787713967371,-53.9288647523849,
2.72638274508249));
#237178=CARTESIAN_POINT('Ctrl Pts',(-24.1762537459517,-53.9274348719419,
2.72420861709538));
#237179=CARTESIAN_POINT('Ctrl Pts',(-24.1736830183705,-53.9260551099576,
2.72205663736669));
#237180=CARTESIAN_POINT('Ctrl Pts',(-24.1711385572894,-53.9246894457401,
2.71992664556708));
#237181=CARTESIAN_POINT('Ctrl Pts',(-24.1685448683464,-53.9233740566949,
2.71782089927827));
#237182=CARTESIAN_POINT('Ctrl Pts',(-24.1659037306808,-53.9221135831988,
2.71574387311189));
#237183=CARTESIAN_POINT('Ctrl Pts',(-24.1657200711327,-53.922025932337,
2.71559944077429));
#237184=CARTESIAN_POINT('Ctrl Pts',(-24.1655361818115,-53.9219385350606,
2.71545515216012));
#237185=CARTESIAN_POINT('Ctrl Pts',(-24.1653520623704,-53.921851392627,
2.71531100781673));
#237186=CARTESIAN_POINT('Ctrl Pts',(-24.1572795915924,-53.9180307491142,
2.70899119176026));
#237187=CARTESIAN_POINT('Ctrl Pts',(-24.1487557177452,-53.9147442868247,
2.70298296066782));
#237188=CARTESIAN_POINT('Ctrl Pts',(-24.139831588019,-53.9120963197572,
2.6973672777408));
#237189=CARTESIAN_POINT('Ctrl Pts',(-24.1315127481107,-53.9096279542366,
2.69213248525367));
#237190=CARTESIAN_POINT('Ctrl Pts',(-24.1228452895799,-53.9077144433429,
2.68723866185402));
#237191=CARTESIAN_POINT('Ctrl Pts',(-24.1138798870158,-53.906468142013,
2.68278595829492));
#237192=CARTESIAN_POINT('Ctrl Pts',(-24.1106002267704,-53.9060122288629,
2.68115710172739));
#237193=CARTESIAN_POINT('Ctrl Pts',(-24.1072808472548,-53.9056458829916,
2.67958763637748));
#237194=CARTESIAN_POINT('Ctrl Pts',(-24.1039248822477,-53.9053756337486,
2.67808378645307));
#237195=CARTESIAN_POINT('Ctrl Pts',(-24.1031178847763,-53.9053106478339,
2.67772216078542));
#237196=CARTESIAN_POINT('Ctrl Pts',(-24.1023082689114,-53.9052515154466,
2.67736403603505));
#237197=CARTESIAN_POINT('Ctrl Pts',(-24.1014961507088,-53.9051983068757,
2.67700956934421));
#237198=CARTESIAN_POINT('Ctrl Pts',(-24.1007094112,-53.9051467610726,2.67666617973746));
#237199=CARTESIAN_POINT('Ctrl Pts',(-24.0999203233284,-53.9051007746215,
2.67632622314061));
#237200=CARTESIAN_POINT('Ctrl Pts',(-24.0991289960597,-53.9050604098634,
2.67598984158715));
#237201=CARTESIAN_POINT('Ctrl Pts',(-24.0904590913153,-53.9046181672909,
2.67230439292157));
#237202=CARTESIAN_POINT('Ctrl Pts',(-24.081514656028,-53.9048508523204,
2.66904964539907));
#237203=CARTESIAN_POINT('Ctrl Pts',(-24.0724687639682,-53.9058331609931,
2.66640203566655));
#237204=CARTESIAN_POINT('Ctrl Pts',(-24.0687171629021,-53.9062405536792,
2.66530399299374));
#237205=CARTESIAN_POINT('Ctrl Pts',(-24.0649483109695,-53.9067765048111,
2.66430995142197));
#237206=CARTESIAN_POINT('Ctrl Pts',(-24.0611749820056,-53.9074445642442,
2.66343053473301));
#237207=CARTESIAN_POINT('Ctrl Pts',(-24.0547391762487,-53.9085840092241,
2.66193059792825));
#237208=CARTESIAN_POINT('Ctrl Pts',(-24.0482923662124,-53.9101092267073,
2.66076519817067));
#237209=CARTESIAN_POINT('Ctrl Pts',(-24.0419050995274,-53.9120381043535,
2.65997805604399));
#237210=CARTESIAN_POINT('Ctrl Pts',(-24.0387114661849,-53.9130025431766,
2.65958448498065));
#237211=CARTESIAN_POINT('Ctrl Pts',(-24.0355332447499,-53.9140692448458,
2.65928526260701));
#237212=CARTESIAN_POINT('Ctrl Pts',(-24.0323793130071,-53.9152404736262,
2.65908463971264));
#237213=CARTESIAN_POINT('Ctrl Pts',(-24.0292253812643,-53.9164117024067,
2.65888401681826));
#237214=CARTESIAN_POINT('Ctrl Pts',(-24.0260957707892,-53.9176874253153,
2.65878198860223));
#237215=CARTESIAN_POINT('Ctrl Pts',(-24.0229981225292,-53.9190682401995,
2.65878198860223));
#237216=CARTESIAN_POINT('Origin',(-17.9900016446778,-55.4168495715592,2.83404198860222));
#237217=CARTESIAN_POINT('Ctrl Pts',(-19.1808295835776,-59.6489943884564,
2.83404198860219));
#237218=CARTESIAN_POINT('Ctrl Pts',(-19.1841083557165,-59.6590854114903,
2.82419652440032));
#237219=CARTESIAN_POINT('Ctrl Pts',(-19.1881736144721,-59.6688877866289,
2.81438790575622));
#237220=CARTESIAN_POINT('Ctrl Pts',(-19.1929932802641,-59.6783518907172,
2.80466781256879));
#237221=CARTESIAN_POINT('Ctrl Pts',(-19.197656335617,-59.6875084677777,
2.7952635645306));
#237222=CARTESIAN_POINT('Ctrl Pts',(-19.2030262129961,-59.6963495165751,
2.78594102496216));
#237223=CARTESIAN_POINT('Ctrl Pts',(-19.2091163824546,-59.7048120487197,
2.77675109088764));
#237224=CARTESIAN_POINT('Ctrl Pts',(-19.2148773077513,-59.7128170830358,
2.76805797913666));
#237225=CARTESIAN_POINT('Ctrl Pts',(-19.2212832892283,-59.7204841754274,
2.75948271210142));
#237226=CARTESIAN_POINT('Ctrl Pts',(-19.2283759411601,-59.7277306815212,
2.75108575573202));
#237227=CARTESIAN_POINT('Ctrl Pts',(-19.234908786543,-59.7344052377143,
2.74335155163246));
#237228=CARTESIAN_POINT('Ctrl Pts',(-19.2420246158643,-59.7407233396949,
2.73576818685916));
#237229=CARTESIAN_POINT('Ctrl Pts',(-19.249775606233,-59.7465875973418,
2.72840626160468));
#237230=CARTESIAN_POINT('Ctrl Pts',(-19.2520238739014,-59.7482885955678,
2.72627084693646));
#237231=CARTESIAN_POINT('Ctrl Pts',(-19.2543256952569,-59.7499511651814,
2.72415424587484));
#237232=CARTESIAN_POINT('Ctrl Pts',(-19.2566826155659,-59.7515722847789,
2.72205867173216));
#237233=CARTESIAN_POINT('Ctrl Pts',(-19.2592376687173,-59.7533296826512,
2.71978693462818));
#237234=CARTESIAN_POINT('Ctrl Pts',(-19.2618533083051,-59.7550368117758,
2.71754411340719));
#237235=CARTESIAN_POINT('Ctrl Pts',(-19.2645304831802,-59.7566897852104,
2.71533341844216));
#237236=CARTESIAN_POINT('Ctrl Pts',(-19.2718780106322,-59.7612263837724,
2.70926614876362));
#237237=CARTESIAN_POINT('Ctrl Pts',(-19.2797022819932,-59.7653126215476,
2.7034738186038));
#237238=CARTESIAN_POINT('Ctrl Pts',(-19.2879484209981,-59.7688605008634,
2.69804914171365));
#237239=CARTESIAN_POINT('Ctrl Pts',(-19.2954931904944,-59.7721066178185,
2.69308585687161));
#237240=CARTESIAN_POINT('Ctrl Pts',(-19.3033878446875,-59.774890960562,
2.6884279905313));
#237241=CARTESIAN_POINT('Ctrl Pts',(-19.3116176456448,-59.777126119837,
2.68414767054152));
#237242=CARTESIAN_POINT('Ctrl Pts',(-19.3156600969909,-59.7782240227713,
2.68204519134499));
#237243=CARTESIAN_POINT('Ctrl Pts',(-19.3197833592186,-59.7791889148824,
2.68003431778461));
#237244=CARTESIAN_POINT('Ctrl Pts',(-19.3239849291282,-59.7800071751722,
2.67812693945221));
#237245=CARTESIAN_POINT('Ctrl Pts',(-19.3247821360948,-59.7801624320923,
2.67776503299173));
#237246=CARTESIAN_POINT('Ctrl Pts',(-19.3255826085661,-59.7803121206159,
2.67740659639893));
#237247=CARTESIAN_POINT('Ctrl Pts',(-19.3263862368331,-59.7804561537454,
2.67705178968825));
#237248=CARTESIAN_POINT('Ctrl Pts',(-19.3271647517167,-59.7805956858397,
2.67670807068727));
#237249=CARTESIAN_POINT('Ctrl Pts',(-19.3279462282167,-59.7807299104878,
2.67636775825235));
#237250=CARTESIAN_POINT('Ctrl Pts',(-19.328730562943,-59.7808587498042,
2.67603099699224));
#237251=CARTESIAN_POINT('Ctrl Pts',(-19.3372780811741,-59.7822628141272,
2.6723610421711));
#237252=CARTESIAN_POINT('Ctrl Pts',(-19.3461707361363,-59.7830278331222,
2.66911440541466));
#237253=CARTESIAN_POINT('Ctrl Pts',(-19.3552444957713,-59.7830570185563,
2.66646778189628));
#237254=CARTESIAN_POINT('Ctrl Pts',(-19.3590764008109,-59.7830693437463,
2.6653500963496));
#237255=CARTESIAN_POINT('Ctrl Pts',(-19.3629403566525,-59.782950798233,
2.66433897912321));
#237256=CARTESIAN_POINT('Ctrl Pts',(-19.3668233599705,-59.7826959186871,
2.66344564884762));
#237257=CARTESIAN_POINT('Ctrl Pts',(-19.3733622405317,-59.7822667079006,
2.66194130298555));
#237258=CARTESIAN_POINT('Ctrl Pts',(-19.3799532508951,-59.7814491944742,
2.6607720670539));
#237259=CARTESIAN_POINT('Ctrl Pts',(-19.3865272544572,-59.7802163932508,
2.65998225155684));
#237260=CARTESIAN_POINT('Ctrl Pts',(-19.3881707553477,-59.779908192945,
2.65978479768258));
#237261=CARTESIAN_POINT('Ctrl Pts',(-19.3898131352231,-59.7795738105077,
2.65961098966592));
#237262=CARTESIAN_POINT('Ctrl Pts',(-19.3914532254503,-59.7792125287462,
2.65946139030472));
#237263=CARTESIAN_POINT('Ctrl Pts',(-19.3939133607912,-59.7786706061039,
2.6592369912629));
#237264=CARTESIAN_POINT('Ctrl Pts',(-19.3963683254113,-59.7780681520194,
2.65906707562412));
#237265=CARTESIAN_POINT('Ctrl Pts',(-19.3988146762077,-59.7774043475412,
2.6589533256289));
#237266=CARTESIAN_POINT('Ctrl Pts',(-19.4012610270042,-59.776740543063,
2.65883957563368));
#237267=CARTESIAN_POINT('Ctrl Pts',(-19.4036987600449,-59.7760153991101,
2.65878198860219));
#237268=CARTESIAN_POINT('Ctrl Pts',(-19.4061247292248,-59.7752282754837,
2.65878198860219));
#237269=CARTESIAN_POINT('Ctrl Pts',(-18.2263320786577,-56.1441998575527,
2.65878198860222));
#237270=CARTESIAN_POINT('Ctrl Pts',(-18.2181232748941,-56.1468630191712,
2.65878198860222));
#237271=CARTESIAN_POINT('Ctrl Pts',(-18.2102054558338,-56.1501806998576,
2.65945335517814));
#237272=CARTESIAN_POINT('Ctrl Pts',(-18.2026724222809,-56.1540344262251,
2.66072561226558));
#237273=CARTESIAN_POINT('Ctrl Pts',(-18.1978068555395,-56.1565235380433,
2.66154735980296));
#237274=CARTESIAN_POINT('Ctrl Pts',(-18.1931013796336,-56.1592354513146,
2.6626189576684));
#237275=CARTESIAN_POINT('Ctrl Pts',(-18.1885757140654,-56.1621313494119,
2.66391429250985));
#237276=CARTESIAN_POINT('Ctrl Pts',(-18.1825772036009,-56.1659696964527,
2.66563118464081));
#237277=CARTESIAN_POINT('Ctrl Pts',(-18.1768986338329,-56.1701354151835,
2.66774105138657));
#237278=CARTESIAN_POINT('Ctrl Pts',(-18.1715848978922,-56.1745504247232,
2.67016894181708));
#237279=CARTESIAN_POINT('Ctrl Pts',(-18.1689280299219,-56.1767579294931,
2.67138288703234));
#237280=CARTESIAN_POINT('Ctrl Pts',(-18.166362180335,-56.1790278168864,
2.6726761316751));
#237281=CARTESIAN_POINT('Ctrl Pts',(-18.1638916135754,-56.1813507566159,
2.67403835432512));
#237282=CARTESIAN_POINT('Ctrl Pts',(-18.1626563301957,-56.1825122264806,
2.67471946565013));
#237283=CARTESIAN_POINT('Ctrl Pts',(-18.1614448518808,-56.1836869644603,
2.67541781389482));
#237284=CARTESIAN_POINT('Ctrl Pts',(-18.1602576134412,-56.1848738357352,
2.67613207244129));
#237285=CARTESIAN_POINT('Ctrl Pts',(-18.1599608038313,-56.1851705535539,
2.6763106370779));
#237286=CARTESIAN_POINT('Ctrl Pts',(-18.1596655088806,-56.1854680298096,
2.67649019601805));
#237287=CARTESIAN_POINT('Ctrl Pts',(-18.1593717347113,-56.1857662469841,
2.67667072836617));
#237288=CARTESIAN_POINT('Ctrl Pts',(-18.1584904122033,-56.1866608985077,
2.6772123254105));
#237289=CARTESIAN_POINT('Ctrl Pts',(-18.157622778392,-56.1875622177789,
2.67776268340007));
#237290=CARTESIAN_POINT('Ctrl Pts',(-18.1567689837081,-56.1884697364864,
2.67832123541476));
#237291=CARTESIAN_POINT('Ctrl Pts',(-18.1507549641991,-56.1948621810802,
2.68225560368402));
#237292=CARTESIAN_POINT('Ctrl Pts',(-18.1453743792962,-56.2015542305059,
2.68661792998842));
#237293=CARTESIAN_POINT('Ctrl Pts',(-18.1405824894349,-56.2084349106659,
2.69130986622527));
#237294=CARTESIAN_POINT('Ctrl Pts',(-18.1382584280302,-56.2117720331083,
2.69358545023007));
#237295=CARTESIAN_POINT('Ctrl Pts',(-18.1360729791407,-56.2151540877943,
2.69593918853426));
#237296=CARTESIAN_POINT('Ctrl Pts',(-18.1340220442546,-56.2185710935568,
2.69836306235436));
#237297=CARTESIAN_POINT('Ctrl Pts',(-18.1308822062388,-56.2238022906398,
2.70207384382169));
#237298=CARTESIAN_POINT('Ctrl Pts',(-18.1280584389294,-56.2291119669555,
2.70594760814169));
#237299=CARTESIAN_POINT('Ctrl Pts',(-18.1255442374225,-56.2344544719216,
2.70995196345649));
#237300=CARTESIAN_POINT('Ctrl Pts',(-18.124376629236,-56.2369355588663,
2.71181160678047));
#237301=CARTESIAN_POINT('Ctrl Pts',(-18.1232756028762,-56.2394235482375,
2.7136996277204));
#237302=CARTESIAN_POINT('Ctrl Pts',(-18.1222417093396,-56.2419141381097,
2.71561183138601));
#237303=CARTESIAN_POINT('Ctrl Pts',(-18.1221624654738,-56.2421050320099,
2.71575839426252));
#237304=CARTESIAN_POINT('Ctrl Pts',(-18.1220835820641,-56.2422959411931,
2.7159050890315));
#237305=CARTESIAN_POINT('Ctrl Pts',(-18.1220050584317,-56.242486864366,
2.71605191409852));
#237306=CARTESIAN_POINT('Ctrl Pts',(-18.1209020381381,-56.2451687593303,
2.71811436362694));
#237307=CARTESIAN_POINT('Ctrl Pts',(-18.119871885966,-56.2478543333339,
2.720200910269));
#237308=CARTESIAN_POINT('Ctrl Pts',(-18.1189123616721,-56.2505383386773,
2.72230624862123));
#237309=CARTESIAN_POINT('Ctrl Pts',(-18.1154716781999,-56.2601627045038,
2.72985561753003));
#237310=CARTESIAN_POINT('Ctrl Pts',(-18.1129106883012,-56.2698406425774,
2.73770089914187));
#237311=CARTESIAN_POINT('Ctrl Pts',(-18.1111213027308,-56.2795015152452,
2.74574823346885));
#237312=CARTESIAN_POINT('Ctrl Pts',(-18.1091549477488,-56.2901178437861,
2.75459144546766));
#237313=CARTESIAN_POINT('Ctrl Pts',(-18.1081200911548,-56.3007141730196,
2.76367911753939));
#237314=CARTESIAN_POINT('Ctrl Pts',(-18.1079204190083,-56.3112209484329,
2.77292162564321));
#237315=CARTESIAN_POINT('Ctrl Pts',(-18.107704823201,-56.3225656290382,
2.78290121484209));
#237316=CARTESIAN_POINT('Ctrl Pts',(-18.1084627484398,-56.3338070504084,
2.79306229499546));
#237317=CARTESIAN_POINT('Ctrl Pts',(-18.1101289800536,-56.3448702837308,
2.80331916684491));
#237318=CARTESIAN_POINT('Ctrl Pts',(-18.1117812336968,-56.3558407078965,
2.81348999408167));
#237319=CARTESIAN_POINT('Ctrl Pts',(-18.1143271060903,-56.3666372711371,
2.82375635966592));
#237320=CARTESIAN_POINT('Ctrl Pts',(-18.1177524687101,-56.3771794532807,
2.83404198860222));
#237321=CARTESIAN_POINT('Origin',(-0.0144941013083308,0.00470941899446887,
2.83404198860262));
#237322=CARTESIAN_POINT('Ctrl Pts',(-19.4351129318415,-59.7658094374951,
2.65878198860219));
#237323=CARTESIAN_POINT('Ctrl Pts',(-19.4432803829093,-59.763151894879,
2.65878198860219));
#237324=CARTESIAN_POINT('Ctrl Pts',(-19.4511532554522,-59.7598356997909,
2.65944603041813));
#237325=CARTESIAN_POINT('Ctrl Pts',(-19.4586404431015,-59.7559811102133,
2.66070439264041));
#237326=CARTESIAN_POINT('Ctrl Pts',(-19.463424399579,-59.7535182109725,
2.66150842619564));
#237327=CARTESIAN_POINT('Ctrl Pts',(-19.4680513433539,-59.7508363273792,
2.66255428265332));
#237328=CARTESIAN_POINT('Ctrl Pts',(-19.4725029330457,-59.7479734971805,
2.66381699700611));
#237329=CARTESIAN_POINT('Ctrl Pts',(-19.4785784597568,-59.7440663083906,
2.66554034873211));
#237330=CARTESIAN_POINT('Ctrl Pts',(-19.4843230052517,-59.7398178213042,
2.66766759643915));
#237331=CARTESIAN_POINT('Ctrl Pts',(-19.4896904492929,-59.7353118462116,
2.67012012783091));
#237332=CARTESIAN_POINT('Ctrl Pts',(-19.4923741713135,-59.7330588586653,
2.67134639352678));
#237333=CARTESIAN_POINT('Ctrl Pts',(-19.4949638171731,-59.730741436408,
2.67265375584954));
#237334=CARTESIAN_POINT('Ctrl Pts',(-19.4974550439411,-59.7283696021898,
2.67403135126882));
#237335=CARTESIAN_POINT('Ctrl Pts',(-19.4987006573251,-59.7271836850806,
2.67472014897845));
#237336=CARTESIAN_POINT('Ctrl Pts',(-19.4999216825133,-59.7259841596483,
2.67542649668574));
#237337=CARTESIAN_POINT('Ctrl Pts',(-19.5011176808517,-59.7247722453467,
2.67614899656043));
#237338=CARTESIAN_POINT('Ctrl Pts',(-19.5014166804363,-59.7244692667714,
2.6763296215291));
#237339=CARTESIAN_POINT('Ctrl Pts',(-19.5017141161963,-59.724165513779,
2.67651125590891));
#237340=CARTESIAN_POINT('Ctrl Pts',(-19.5020099819907,-59.723861005197,
2.67669387767465));
#237341=CARTESIAN_POINT('Ctrl Pts',(-19.502897579374,-59.7229474794511,
2.67724174297185));
#237342=CARTESIAN_POINT('Ctrl Pts',(-19.5037710453003,-59.7220271539529,
2.67779849504688));
#237343=CARTESIAN_POINT('Ctrl Pts',(-19.504630229752,-59.7211005320714,
2.6783635361795));
#237344=CARTESIAN_POINT('Ctrl Pts',(-19.5105677273983,-59.7146969999424,
2.68226832098858));
#237345=CARTESIAN_POINT('Ctrl Pts',(-19.5158784513268,-59.7079999120044,
2.68659153751352));
#237346=CARTESIAN_POINT('Ctrl Pts',(-19.5206092977903,-59.701118410241,
2.69123699486152));
#237347=CARTESIAN_POINT('Ctrl Pts',(-19.5229605154966,-59.6976983227542,
2.6935457744118));
#237348=CARTESIAN_POINT('Ctrl Pts',(-19.5251683423977,-59.69423209387,2.6959347882807));
#237349=CARTESIAN_POINT('Ctrl Pts',(-19.5272373629638,-59.6907301905171,
2.69839565261161));
#237350=CARTESIAN_POINT('Ctrl Pts',(-19.5318019313697,-59.6830044686626,
2.70382468688987));
#237351=CARTESIAN_POINT('Ctrl Pts',(-19.5357011184423,-59.6751122606219,
2.70961155815028));
#237352=CARTESIAN_POINT('Ctrl Pts',(-19.5389266512978,-59.6671986827531,
2.71562701361709));
#237353=CARTESIAN_POINT('Ctrl Pts',(-19.540104979126,-59.6643077529622,
2.71782453535799));
#237354=CARTESIAN_POINT('Ctrl Pts',(-19.5412013620775,-59.6614137631514,
2.72005051502344));
#237355=CARTESIAN_POINT('Ctrl Pts',(-19.5422187365063,-59.6585211429013,
2.72229986760057));
#237356=CARTESIAN_POINT('Ctrl Pts',(-19.5456359895573,-59.6488051375689,
2.72985520488817));
#237357=CARTESIAN_POINT('Ctrl Pts',(-19.5481755652418,-59.6390401911872,
2.73770845534464));
#237358=CARTESIAN_POINT('Ctrl Pts',(-19.5499445144587,-59.6292970278062,
2.74576706701639));
#237359=CARTESIAN_POINT('Ctrl Pts',(-19.5518887991939,-59.6185881370968,
2.75462443584899));
#237360=CARTESIAN_POINT('Ctrl Pts',(-19.5529023976135,-59.6079049297411,
2.76373036323034));
#237361=CARTESIAN_POINT('Ctrl Pts',(-19.5530800481814,-59.597317418282,
2.77299664636654));
#237362=CARTESIAN_POINT('Ctrl Pts',(-19.5532713854547,-59.5859142148015,
2.782976830333));
#237363=CARTESIAN_POINT('Ctrl Pts',(-19.5524931697988,-59.5746208362162,
2.79314401478706));
#237364=CARTESIAN_POINT('Ctrl Pts',(-19.5508078878557,-59.5635130675428,
2.8034145242774));
#237365=CARTESIAN_POINT('Ctrl Pts',(-19.549145362909,-59.5525552912509,
2.81354634721213));
#237366=CARTESIAN_POINT('Ctrl Pts',(-19.5465995868768,-59.5417768065755,
2.82378004209104));
#237367=CARTESIAN_POINT('Ctrl Pts',(-19.5431821162861,-59.5312589135995,
2.8340419886022));
#237368=CARTESIAN_POINT('Ctrl Pts',(-18.4801050014185,-56.2594439784239,
2.83404198860221));
#237369=CARTESIAN_POINT('Ctrl Pts',(-18.476834463303,-56.2493782971079,
2.82422126442993));
#237370=CARTESIAN_POINT('Ctrl Pts',(-18.4727817672085,-56.2396067681213,
2.81442815028515));
#237371=CARTESIAN_POINT('Ctrl Pts',(-18.4679768367031,-56.2301791400429,
2.80471618166358));
#237372=CARTESIAN_POINT('Ctrl Pts',(-18.4633372535438,-56.2210759356541,
2.79533842146289));
#237373=CARTESIAN_POINT('Ctrl Pts',(-18.4579956735917,-56.2122922812552,
2.78603515650318));
#237374=CARTESIAN_POINT('Ctrl Pts',(-18.4519372213358,-56.2038917763242,
2.77685887346852));
#237375=CARTESIAN_POINT('Ctrl Pts',(-18.4462100865643,-56.1959506682892,
2.76818441216688));
#237376=CARTESIAN_POINT('Ctrl Pts',(-18.4398418135283,-56.1883512165481,
2.7596226152175));
#237377=CARTESIAN_POINT('Ctrl Pts',(-18.4327901596627,-56.1811768067735,
2.75123537701798));
#237378=CARTESIAN_POINT('Ctrl Pts',(-18.4262957047529,-56.1745692957308,
2.74351087134269));
#237379=CARTESIAN_POINT('Ctrl Pts',(-18.4192211773425,-56.1683219623517,
2.73593399450007));
#237380=CARTESIAN_POINT('Ctrl Pts',(-18.4115142492175,-56.1625328136766,
2.72857657812745));
#237381=CARTESIAN_POINT('Ctrl Pts',(-18.409216198825,-56.1608066064032,
2.72638274508417));
#237382=CARTESIAN_POINT('Ctrl Pts',(-18.4068618031985,-56.1591213928266,
2.72420861709621));
#237383=CARTESIAN_POINT('Ctrl Pts',(-18.4044493827309,-56.1574804751186,
2.72205663736669));
#237384=CARTESIAN_POINT('Ctrl Pts',(-18.4020616112558,-56.155856323546,
2.71992664556708));
#237385=CARTESIAN_POINT('Ctrl Pts',(-18.3996196264078,-56.1542770260202,
2.71782089927826));
#237386=CARTESIAN_POINT('Ctrl Pts',(-18.3971247125282,-56.1527473834683,
2.71574387311188));
#237387=CARTESIAN_POINT('Ctrl Pts',(-18.3969512210963,-56.1526410151168,
2.71559944077428));
#237388=CARTESIAN_POINT('Ctrl Pts',(-18.3967774746429,-56.1525348749436,
2.71545515216011));
#237389=CARTESIAN_POINT('Ctrl Pts',(-18.3966034726921,-56.1524289641632,
2.71531100781672));
#237390=CARTESIAN_POINT('Ctrl Pts',(-18.3889745897488,-56.1477854475701,
2.70899119176033));
#237391=CARTESIAN_POINT('Ctrl Pts',(-18.3808409394273,-56.1436260014307,
2.70298296066796));
#237392=CARTESIAN_POINT('Ctrl Pts',(-18.3722424849459,-56.1400597146376,
2.697367277741));
#237393=CARTESIAN_POINT('Ctrl Pts',(-18.364227230968,-56.1367353155299,
2.69213248525405));
#237394=CARTESIAN_POINT('Ctrl Pts',(-18.3558072700354,-56.1339262909285,
2.68723866185456));
#237395=CARTESIAN_POINT('Ctrl Pts',(-18.3470212548478,-56.1317496772151,
2.68278595829558));
#237396=CARTESIAN_POINT('Ctrl Pts',(-18.3438072168249,-56.1309534437593,
2.68115710172781));
#237397=CARTESIAN_POINT('Ctrl Pts',(-18.3405443147881,-56.1302421351291,
2.67958763637767));
#237398=CARTESIAN_POINT('Ctrl Pts',(-18.337234982846,-56.1296225724747,
2.67808378645305));
#237399=CARTESIAN_POINT('Ctrl Pts',(-18.3364391990691,-56.1294735883541,
2.6777221607854));
#237400=CARTESIAN_POINT('Ctrl Pts',(-18.3356401993822,-56.129330151998,
2.67736403603504));
#237401=CARTESIAN_POINT('Ctrl Pts',(-18.3348380918581,-56.1291923454415,
2.6770095693442));
#237402=CARTESIAN_POINT('Ctrl Pts',(-18.3340610501942,-56.1290588453398,
2.67666617973744));
#237403=CARTESIAN_POINT('Ctrl Pts',(-18.3332810919216,-56.1289306286647,
2.67632622314059));
#237404=CARTESIAN_POINT('Ctrl Pts',(-18.3324983188927,-56.1288077688057,
2.67598984158714));
#237405=CARTESIAN_POINT('Ctrl Pts',(-18.3239221357301,-56.1274616970647,
2.67230439292152));
#237406=CARTESIAN_POINT('Ctrl Pts',(-18.3150023767865,-56.1267581593458,
2.66904964539899));
#237407=CARTESIAN_POINT('Ctrl Pts',(-18.3059033598538,-56.126789533633,
2.66640203566646));
#237408=CARTESIAN_POINT('Ctrl Pts',(-18.3021297263195,-56.1268025454851,
2.66530399299368));
#237409=CARTESIAN_POINT('Ctrl Pts',(-18.2983254984041,-56.1269416083198,
2.66430995142194));
#237410=CARTESIAN_POINT('Ctrl Pts',(-18.2945030089052,-56.1272115877754,
2.663430534733));
#237411=CARTESIAN_POINT('Ctrl Pts',(-18.2879833547329,-56.1276720658709,
2.66193059792823));
#237412=CARTESIAN_POINT('Ctrl Pts',(-18.2814124323568,-56.128515052907,
2.66076519817066));
#237413=CARTESIAN_POINT('Ctrl Pts',(-18.2748585331707,-56.1297657127883,
2.65997805604398));
#237414=CARTESIAN_POINT('Ctrl Pts',(-18.2715815835777,-56.1303910427289,
2.65958448498064));
#237415=CARTESIAN_POINT('Ctrl Pts',(-18.2683092720861,-56.1311196862923,
2.659285262607));
#237416=CARTESIAN_POINT('Ctrl Pts',(-18.2650501911668,-56.1319548233207,
2.65908463971262));
#237417=CARTESIAN_POINT('Ctrl Pts',(-18.2617911102476,-56.1327899603491,
2.65888401681824));
#237418=CARTESIAN_POINT('Ctrl Pts',(-18.258545294751,-56.1337315613408,
2.65878198860222));
#237419=CARTESIAN_POINT('Ctrl Pts',(-18.2553202812744,-56.1347810195642,
2.65878198860222));
#237420=CARTESIAN_POINT('Origin',(-12.0988124084934,-56.9937374973463,2.83404198860222));
#237421=CARTESIAN_POINT('Ctrl Pts',(-12.8407372733092,-61.3271735965893,
2.83404198860219));
#237422=CARTESIAN_POINT('Ctrl Pts',(-12.8429432848606,-61.337552064956,
2.82419652440055));
#237423=CARTESIAN_POINT('Ctrl Pts',(-12.8459616464937,-61.3477256769082,
2.8143879057567));
#237424=CARTESIAN_POINT('Ctrl Pts',(-12.8497656413955,-61.3576417279025,
2.80466781256951));
#237425=CARTESIAN_POINT('Ctrl Pts',(-12.8534460291142,-61.3672355662858,
2.79526356453151));
#237426=CARTESIAN_POINT('Ctrl Pts',(-12.8578623484986,-61.376589487923,
2.78594102496326));
#237427=CARTESIAN_POINT('Ctrl Pts',(-12.863034579891,-61.3856422574855,
2.77675109088891));
#237428=CARTESIAN_POINT('Ctrl Pts',(-12.8679271923005,-61.3942056200541,
2.76805797913813));
#237429=CARTESIAN_POINT('Ctrl Pts',(-12.873496651755,-61.4025003187107,
2.75948271210308));
#237430=CARTESIAN_POINT('Ctrl Pts',(-12.8797929832512,-61.4104485116927,
2.75108575573384));
#237431=CARTESIAN_POINT('Ctrl Pts',(-12.8855923599214,-61.4177693722571,
2.74335155163446));
#237432=CARTESIAN_POINT('Ctrl Pts',(-12.8920087864941,-61.4247966697177,
2.73576818686133));
#237433=CARTESIAN_POINT('Ctrl Pts',(-12.8991043342861,-61.4314390014596,
2.72840626160699));
#237434=CARTESIAN_POINT('Ctrl Pts',(-12.9011624829791,-61.4333656894044,
2.72627084693799));
#237435=CARTESIAN_POINT('Ctrl Pts',(-12.9032779088704,-61.4352597571375,
2.7241542458756));
#237436=CARTESIAN_POINT('Ctrl Pts',(-12.9054524645838,-61.4371183613308,
2.72205867173216));
#237437=CARTESIAN_POINT('Ctrl Pts',(-12.9078098227877,-61.4391332077732,
2.71978693462818));
#237438=CARTESIAN_POINT('Ctrl Pts',(-12.9102326900442,-61.4411043938523,
2.71754411340719));
#237439=CARTESIAN_POINT('Ctrl Pts',(-12.9127224163023,-61.4430281531011,
2.71533341844216));
#237440=CARTESIAN_POINT('Ctrl Pts',(-12.9195554895539,-61.4483079254549,
2.70926614876362));
#237441=CARTESIAN_POINT('Ctrl Pts',(-12.9269097705826,-61.4531896374535,
2.70347381860379));
#237442=CARTESIAN_POINT('Ctrl Pts',(-12.9347398820024,-61.4575800373532,
2.69804914171365));
#237443=CARTESIAN_POINT('Ctrl Pts',(-12.9419040088448,-61.4615970149011,
2.69308585687183));
#237444=CARTESIAN_POINT('Ctrl Pts',(-12.9494643722276,-61.4651913207944,
2.68842799053171));
#237445=CARTESIAN_POINT('Ctrl Pts',(-12.9574154517097,-61.46827448408,2.68414767054209));
#237446=CARTESIAN_POINT('Ctrl Pts',(-12.9613209959781,-61.4697889238144,
2.68204519134536));
#237447=CARTESIAN_POINT('Ctrl Pts',(-12.9653208118547,-61.4711795284099,
2.68003431778479));
#237448=CARTESIAN_POINT('Ctrl Pts',(-12.9694138336344,-61.4724324898303,
2.67812693945222));
#237449=CARTESIAN_POINT('Ctrl Pts',(-12.9701904446506,-61.4726702270558,
2.67776503299174));
#237450=CARTESIAN_POINT('Ctrl Pts',(-12.9709708853386,-61.4729027677274,
2.67740659639895));
#237451=CARTESIAN_POINT('Ctrl Pts',(-12.9717550556842,-61.4731300138562,
2.67705178968826));
#237452=CARTESIAN_POINT('Ctrl Pts',(-12.9725147207064,-61.4733501585434,
2.67670807068729));
#237453=CARTESIAN_POINT('Ctrl Pts',(-12.9732778859002,-61.4735653344324,
2.67636775825236));
#237454=CARTESIAN_POINT('Ctrl Pts',(-12.974044456583,-61.4737754532573,
2.67603099699226));
#237455=CARTESIAN_POINT('Ctrl Pts',(-12.9823983859293,-61.4760652849145,
2.67236104217095));
#237456=CARTESIAN_POINT('Ctrl Pts',(-12.9911623597377,-61.477755648613,
2.66911440541437));
#237457=CARTESIAN_POINT('Ctrl Pts',(-13.0001833616598,-61.4787331403169,
2.66646778189593));
#237458=CARTESIAN_POINT('Ctrl Pts',(-13.0039929867891,-61.4791459411334,
2.6653500963494));
#237459=CARTESIAN_POINT('Ctrl Pts',(-13.0078481668562,-61.4794319383911,
2.66433897912312));
#237460=CARTESIAN_POINT('Ctrl Pts',(-13.0117365408425,-61.4795843394717,
2.66344564884763));
#237461=CARTESIAN_POINT('Ctrl Pts',(-13.0182844654758,-61.4798409790834,
2.66194130298556));
#237462=CARTESIAN_POINT('Ctrl Pts',(-13.024924823017,-61.4797168922657,
2.66077206705391));
#237463=CARTESIAN_POINT('Ctrl Pts',(-13.0315916763171,-61.4791780149466,
2.65998225155685));
#237464=CARTESIAN_POINT('Ctrl Pts',(-13.0332583896422,-61.4790432956168,
2.65978479768259));
#237465=CARTESIAN_POINT('Ctrl Pts',(-13.0349267248711,-61.478882420406,
2.65961098966593));
#237466=CARTESIAN_POINT('Ctrl Pts',(-13.0365955947398,-61.4786945538948,
2.65946139030472));
#237467=CARTESIAN_POINT('Ctrl Pts',(-13.0390988995429,-61.478412754128,
2.65923699126291));
#237468=CARTESIAN_POINT('Ctrl Pts',(-13.0416033892095,-61.4780702140291,
2.65906707562412));
#237469=CARTESIAN_POINT('Ctrl Pts',(-13.0441057251024,-61.4776657592306,
2.6589533256289));
#237470=CARTESIAN_POINT('Ctrl Pts',(-13.0466080609952,-61.477261304432,
2.65883957563368));
#237471=CARTESIAN_POINT('Ctrl Pts',(-13.0491082380622,-61.4767949453821,
2.65878198860219));
#237472=CARTESIAN_POINT('Ctrl Pts',(-13.0516031943522,-61.4762657165315,
2.65878198860219));
#237473=CARTESIAN_POINT('Ctrl Pts',(-12.2578193919762,-57.7418065394565,
2.65878198860222));
#237474=CARTESIAN_POINT('Ctrl Pts',(-12.249377180707,-57.7435970583544,
2.65878198860222));
#237475=CARTESIAN_POINT('Ctrl Pts',(-12.2411559442242,-57.74606892698,2.65945335517815));
#237476=CARTESIAN_POINT('Ctrl Pts',(-12.2332613533223,-57.7491141258102,
2.66072561226559));
#237477=CARTESIAN_POINT('Ctrl Pts',(-12.2281622576313,-57.7510810117991,
2.66154735980298));
#237478=CARTESIAN_POINT('Ctrl Pts',(-12.2231990866879,-57.7532862127603,
2.66261895766844));
#237479=CARTESIAN_POINT('Ctrl Pts',(-12.2183955094113,-57.7556931859578,
2.6639142925099));
#237480=CARTESIAN_POINT('Ctrl Pts',(-12.2120286428971,-57.7588834910511,
2.66563118464086));
#237481=CARTESIAN_POINT('Ctrl Pts',(-12.2059457447512,-57.7624328173674,
2.66774105138662));
#237482=CARTESIAN_POINT('Ctrl Pts',(-12.2001996238495,-57.7662682043708,
2.67016894181712));
#237483=CARTESIAN_POINT('Ctrl Pts',(-12.1973265633986,-57.7681858978725,
2.67138288703237));
#237484=CARTESIAN_POINT('Ctrl Pts',(-12.1945375019632,-57.7701751462709,
2.67267613167513));
#237485=CARTESIAN_POINT('Ctrl Pts',(-12.1918376559068,-57.7722271161467,
2.67403835432515));
#237486=CARTESIAN_POINT('Ctrl Pts',(-12.1904877328785,-57.7732531010846,
2.67471946565016));
#237487=CARTESIAN_POINT('Ctrl Pts',(-12.1891600976129,-57.7742947697602,
2.67541781389485));
#237488=CARTESIAN_POINT('Ctrl Pts',(-12.1878553011592,-57.7753510390204,
2.67613207244131));
#237489=CARTESIAN_POINT('Ctrl Pts',(-12.1875291020458,-57.7756151063354,
2.67631063707792));
#237490=CARTESIAN_POINT('Ctrl Pts',(-12.1872043300158,-57.7758800862576,
2.67649019601807));
#237491=CARTESIAN_POINT('Ctrl Pts',(-12.1868809929892,-57.7761459620048,
2.67667072836618));
#237492=CARTESIAN_POINT('Ctrl Pts',(-12.1859109819092,-57.7769435892464,
2.67721232541052));
#237493=CARTESIAN_POINT('Ctrl Pts',(-12.1849538875684,-57.7777492785673,
2.67776268340008));
#237494=CARTESIAN_POINT('Ctrl Pts',(-12.1840099085252,-57.7785625799461,
2.67832123541477));
#237495=CARTESIAN_POINT('Ctrl Pts',(-12.1773606420344,-57.7842913698423,
2.68225560368405));
#237496=CARTESIAN_POINT('Ctrl Pts',(-12.1713100228959,-57.7903843352496,
2.68661792998849));
#237497=CARTESIAN_POINT('Ctrl Pts',(-12.1658251565853,-57.7967264334405,
2.69130986622539));
#237498=CARTESIAN_POINT('Ctrl Pts',(-12.1631650023516,-57.7998023442098,
2.69358545023015));
#237499=CARTESIAN_POINT('Ctrl Pts',(-12.1606380046007,-57.8029374300324,
2.6959391885343));
#237500=CARTESIAN_POINT('Ctrl Pts',(-12.1582411305893,-57.8061213360078,
2.69836306235436));
#237501=CARTESIAN_POINT('Ctrl Pts',(-12.1545716839425,-57.8109956736032,
2.70207384382169));
#237502=CARTESIAN_POINT('Ctrl Pts',(-12.1512083732202,-57.8159810988989,
2.70594760814169));
#237503=CARTESIAN_POINT('Ctrl Pts',(-12.1481495009381,-57.821031531444,
2.70995196345648));
#237504=CARTESIAN_POINT('Ctrl Pts',(-12.1467289448258,-57.8233769784454,
2.71181160678046));
#237505=CARTESIAN_POINT('Ctrl Pts',(-12.145373884298,-57.8257362497571,
2.71369962772039));
#237506=CARTESIAN_POINT('Ctrl Pts',(-12.1440853170064,-57.8281051246148,
2.71561183138601));
#237507=CARTESIAN_POINT('Ctrl Pts',(-12.1439865534007,-57.8282866895388,
2.71575839426252));
#237508=CARTESIAN_POINT('Ctrl Pts',(-12.1438881466791,-57.8284683073398,
2.7159050890315));
#237509=CARTESIAN_POINT('Ctrl Pts',(-12.1437900963015,-57.828649976661,
2.71605191409852));
#237510=CARTESIAN_POINT('Ctrl Pts',(-12.1424127841092,-57.8312018829078,
2.71811436362694));
#237511=CARTESIAN_POINT('Ctrl Pts',(-12.1411075562949,-57.8337650648326,
2.720200910269));
#237512=CARTESIAN_POINT('Ctrl Pts',(-12.1398727334215,-57.836334069314,
2.72230624862123));
#237513=CARTESIAN_POINT('Ctrl Pts',(-12.1354448782036,-57.8455460625015,
2.72985561753008));
#237514=CARTESIAN_POINT('Ctrl Pts',(-12.1318862976811,-57.8549032874793,
2.73770089914196));
#237515=CARTESIAN_POINT('Ctrl Pts',(-12.1290968783783,-57.8643241951519,
2.74574823346899));
#237516=CARTESIAN_POINT('Ctrl Pts',(-12.1260315867866,-57.8746768262699,
2.75459144546788));
#237517=CARTESIAN_POINT('Ctrl Pts',(-12.1238947812343,-57.8851069357338,
2.76367911753968));
#237518=CARTESIAN_POINT('Ctrl Pts',(-12.1225979458249,-57.8955352825095,
2.77292162564359));
#237519=CARTESIAN_POINT('Ctrl Pts',(-12.121197689044,-57.9067952798691,
2.78290121484263));
#237520=CARTESIAN_POINT('Ctrl Pts',(-12.1207764137884,-57.9180543443175,
2.79306229499618));
#237521=CARTESIAN_POINT('Ctrl Pts',(-12.1212770948332,-57.9292311407204,
2.80331916684581));
#237522=CARTESIAN_POINT('Ctrl Pts',(-12.1217735756786,-57.9403141752886,
2.81348999408227));
#237523=CARTESIAN_POINT('Ctrl Pts',(-12.1231769533527,-57.9513177099548,
2.82375635966622));
#237524=CARTESIAN_POINT('Ctrl Pts',(-12.1254815933786,-57.962160188812,
2.83404198860222));
#237525=CARTESIAN_POINT('Origin',(-0.0149069694351764,0.00316857416825746,
2.83404198860263));
#237526=CARTESIAN_POINT('Ctrl Pts',(-13.0814171332226,-61.4699285681954,
2.65878198860219));
#237527=CARTESIAN_POINT('Ctrl Pts',(-13.0898176309841,-61.4681393149848,
2.65878198860219));
#237528=CARTESIAN_POINT('Ctrl Pts',(-13.0979940118835,-61.465664225629,
2.65944603041805));
#237529=CARTESIAN_POINT('Ctrl Pts',(-13.1058430982601,-61.4626133761159,
2.6607043926402));
#237530=CARTESIAN_POINT('Ctrl Pts',(-13.1108582907967,-61.4606640285136,
2.66150842619545));
#237531=CARTESIAN_POINT('Ctrl Pts',(-13.1157402208605,-61.4584804838815,
2.66255428265318));
#237532=CARTESIAN_POINT('Ctrl Pts',(-13.1204666715199,-61.4560986543956,
2.66381699700607));
#237533=CARTESIAN_POINT('Ctrl Pts',(-13.1269173282999,-61.4528479350654,
2.66554034873207));
#237534=CARTESIAN_POINT('Ctrl Pts',(-13.1330744923998,-61.4492231901484,
2.66766759643912));
#237535=CARTESIAN_POINT('Ctrl Pts',(-13.138883535673,-61.4453029499361,
2.67012012783089));
#237536=CARTESIAN_POINT('Ctrl Pts',(-13.1417880573096,-61.4433428298299,
2.67134639352677));
#237537=CARTESIAN_POINT('Ctrl Pts',(-13.1446057534055,-61.4413087943563,
2.67265375584954));
#237538=CARTESIAN_POINT('Ctrl Pts',(-13.1473312571585,-61.4392103573998,
2.67403135126882));
#237539=CARTESIAN_POINT('Ctrl Pts',(-13.1486940090351,-61.4381611389216,
2.67472014897846));
#237540=CARTESIAN_POINT('Ctrl Pts',(-13.1500337298696,-61.4370958165016,
2.67542649668575));
#237541=CARTESIAN_POINT('Ctrl Pts',(-13.1513498559436,-61.4360155570618,
2.67614899656044));
#237542=CARTESIAN_POINT('Ctrl Pts',(-13.1516788874621,-61.4357454922018,
2.67632962152912));
#237543=CARTESIAN_POINT('Ctrl Pts',(-13.1520064446714,-61.435474493703,
2.67651125590893));
#237544=CARTESIAN_POINT('Ctrl Pts',(-13.1523325194961,-61.4352025796478,
2.67669387767466));
#237545=CARTESIAN_POINT('Ctrl Pts',(-13.1533107439705,-61.434386837482,
2.67724174297187));
#237546=CARTESIAN_POINT('Ctrl Pts',(-13.1542756251691,-61.4335628556741,
2.6777984950469));
#237547=CARTESIAN_POINT('Ctrl Pts',(-13.1552269612797,-61.4327311191546,
2.67836353617952));
#237548=CARTESIAN_POINT('Ctrl Pts',(-13.1618012840654,-61.4269833037495,
2.68226832098846));
#237549=CARTESIAN_POINT('Ctrl Pts',(-13.1677829516028,-61.4208780249712,
2.68659153751323));
#237550=CARTESIAN_POINT('Ctrl Pts',(-13.1732071947986,-61.4145287289055,
2.69123699486104));
#237551=CARTESIAN_POINT('Ctrl Pts',(-13.1759030287778,-61.4113731461892,
2.69354577441147));
#237552=CARTESIAN_POINT('Ctrl Pts',(-13.1784610805508,-61.4081566864225,
2.69593478828053));
#237553=CARTESIAN_POINT('Ctrl Pts',(-13.180884815382,-61.4048902384026,
2.69839565261161));
#237554=CARTESIAN_POINT('Ctrl Pts',(-13.1862319364376,-61.3976839661817,
2.70382468688986));
#237555=CARTESIAN_POINT('Ctrl Pts',(-13.1909347237338,-61.3902425685151,
2.70961155815028));
#237556=CARTESIAN_POINT('Ctrl Pts',(-13.1949697809164,-61.3827095020465,
2.71562701361708));
#237557=CARTESIAN_POINT('Ctrl Pts',(-13.1964438381899,-61.3799575778686,
2.71782453535798));
#237558=CARTESIAN_POINT('Ctrl Pts',(-13.1978367193485,-61.3771940448618,
2.72005051502342));
#237559=CARTESIAN_POINT('Ctrl Pts',(-13.1991508816433,-61.3744236152738,
2.72229986760056));
#237560=CARTESIAN_POINT('Ctrl Pts',(-13.2035650137308,-61.3651180354455,
2.72985520488783));
#237561=CARTESIAN_POINT('Ctrl Pts',(-13.207111392193,-61.3556720404061,
2.73770845534397));
#237562=CARTESIAN_POINT('Ctrl Pts',(-13.2098890888166,-61.3461671566372,
2.74576706701538));
#237563=CARTESIAN_POINT('Ctrl Pts',(-13.2129421064456,-61.3357201634476,
2.75462443584761));
#237564=CARTESIAN_POINT('Ctrl Pts',(-13.2150668515147,-61.3252014297053,
2.76373036322859));
#237565=CARTESIAN_POINT('Ctrl Pts',(-13.216350225197,-61.3146904872831,
2.77299664636439));
#237566=CARTESIAN_POINT('Ctrl Pts',(-13.2177324736409,-61.3033697519362,
2.78297683033034));
#237567=CARTESIAN_POINT('Ctrl Pts',(-13.2181390006406,-61.2920568939744,
2.79314401478388));
#237568=CARTESIAN_POINT('Ctrl Pts',(-13.2176240288383,-61.2808338148888,
2.80341452427365));
#237569=CARTESIAN_POINT('Ctrl Pts',(-13.2171160108941,-61.2697622852627,
2.81354634720964));
#237570=CARTESIAN_POINT('Ctrl Pts',(-13.2157108393288,-61.2587767401961,
2.82378004208981));
#237571=CARTESIAN_POINT('Ctrl Pts',(-13.2134115091888,-61.2479592423877,
2.83404198860219));
#237572=CARTESIAN_POINT('Ctrl Pts',(-12.4981558292581,-57.8829458346105,
2.83404198860221));
#237573=CARTESIAN_POINT('Ctrl Pts',(-12.4959553576925,-57.8725934298276,
2.82422126443078));
#237574=CARTESIAN_POINT('Ctrl Pts',(-12.4929462656003,-57.8624518082052,
2.81442815028684));
#237575=CARTESIAN_POINT('Ctrl Pts',(-12.4891531124827,-57.8525735736588,
2.80471618166611));
#237576=CARTESIAN_POINT('Ctrl Pts',(-12.4854904894113,-57.8430352690787,
2.79533842146592));
#237577=CARTESIAN_POINT('Ctrl Pts',(-12.4810963130896,-57.8337413853143,
2.78603515650671));
#237578=CARTESIAN_POINT('Ctrl Pts',(-12.4759491415407,-57.8247536185246,
2.77685887347252));
#237579=CARTESIAN_POINT('Ctrl Pts',(-12.4710834524327,-57.8162573641139,
2.76818441217116));
#237580=CARTESIAN_POINT('Ctrl Pts',(-12.4655444244753,-57.8080338771707,
2.75962261522203));
#237581=CARTESIAN_POINT('Ctrl Pts',(-12.4592813303365,-57.8001616710216,
2.75123537702274));
#237582=CARTESIAN_POINT('Ctrl Pts',(-12.4535131257059,-57.7929115012243,
2.74351087134758));
#237583=CARTESIAN_POINT('Ctrl Pts',(-12.447130377455,-57.7859589019126,
2.73593399450508));
#237584=CARTESIAN_POINT('Ctrl Pts',(-12.4400707995038,-57.7793958734463,
2.72857657813254));
#237585=CARTESIAN_POINT('Ctrl Pts',(-12.4379657758639,-57.7774389108393,
2.72638274508753));
#237586=CARTESIAN_POINT('Ctrl Pts',(-12.4358004306468,-57.7755168276808,
2.72420861709787));
#237587=CARTESIAN_POINT('Ctrl Pts',(-12.4335727482756,-57.773632732486,
2.72205663736669));
#237588=CARTESIAN_POINT('Ctrl Pts',(-12.4313678273305,-57.7717678881027,
2.71992664556707));
#237589=CARTESIAN_POINT('Ctrl Pts',(-12.4291043014743,-57.7699419852105,
2.71782089927826));
#237590=CARTESIAN_POINT('Ctrl Pts',(-12.4267829461793,-57.7681599326867,
2.71574387311187));
#237591=CARTESIAN_POINT('Ctrl Pts',(-12.4266215236719,-57.7680360122394,
2.71559944077428));
#237592=CARTESIAN_POINT('Ctrl Pts',(-12.426459823689,-57.7679122920634,
2.7154551521601));
#237593=CARTESIAN_POINT('Ctrl Pts',(-12.4262978456302,-57.7677887733168,
2.71531100781672));
#237594=CARTESIAN_POINT('Ctrl Pts',(-12.4191961341595,-57.7623732589829,
2.70899119176029));
#237595=CARTESIAN_POINT('Ctrl Pts',(-12.4115418213384,-57.7573864007558,
2.70298296066787));
#237596=CARTESIAN_POINT('Ctrl Pts',(-12.4033632485683,-57.7529408672214,
2.69736727774088));
#237597=CARTESIAN_POINT('Ctrl Pts',(-12.3957393973204,-57.7487968573389,
2.69213248525393));
#237598=CARTESIAN_POINT('Ctrl Pts',(-12.3876591848397,-57.7451230952911,
2.68723866185445));
#237599=CARTESIAN_POINT('Ctrl Pts',(-12.3791488184491,-57.7420400166296,
2.68278595829548));
#237600=CARTESIAN_POINT('Ctrl Pts',(-12.3760356163224,-57.7409121865686,
2.68115710172774));
#237601=CARTESIAN_POINT('Ctrl Pts',(-12.3728649408024,-57.7398637084258,
2.67958763637763));
#237602=CARTESIAN_POINT('Ctrl Pts',(-12.3696384996592,-57.7389016204181,
2.67808378645303));
#237603=CARTESIAN_POINT('Ctrl Pts',(-12.3688626483502,-57.7386702703928,
2.67772216078539));
#237604=CARTESIAN_POINT('Ctrl Pts',(-12.3680830188491,-57.7384441015867,
2.67736403603501));
#237605=CARTESIAN_POINT('Ctrl Pts',(-12.3672997100616,-57.738223206882,
2.67700956934417));
#237606=CARTESIAN_POINT('Ctrl Pts',(-12.3665408796737,-57.7380092151369,
2.67666617973742));
#237607=CARTESIAN_POINT('Ctrl Pts',(-12.3657785963861,-57.7378001730064,
2.67632622314057));
#237608=CARTESIAN_POINT('Ctrl Pts',(-12.365012953822,-57.7375961641248,
2.67598984158712));
#237609=CARTESIAN_POINT('Ctrl Pts',(-12.3566244546988,-57.7353610110589,
2.67230439292157));
#237610=CARTESIAN_POINT('Ctrl Pts',(-12.3478270988448,-57.7337289586983,
2.66904964539909));
#237611=CARTESIAN_POINT('Ctrl Pts',(-12.338774647773,-57.7328090548566,
2.66640203566658));
#237612=CARTESIAN_POINT('Ctrl Pts',(-12.335020326489,-57.7324275433141,
2.66530399299375));
#237613=CARTESIAN_POINT('Ctrl Pts',(-12.3312224025075,-57.7321681942501,
2.66430995142196));
#237614=CARTESIAN_POINT('Ctrl Pts',(-12.3273926324683,-57.7320371357768,
2.66343053473299));
#237615=CARTESIAN_POINT('Ctrl Pts',(-12.320860560576,-57.7318136018934,
2.66193059792822));
#237616=CARTESIAN_POINT('Ctrl Pts',(-12.3142375182609,-57.7319651225402,
2.66076519817066));
#237617=CARTESIAN_POINT('Ctrl Pts',(-12.3075887924648,-57.7325238621654,
2.65997805604398));
#237618=CARTESIAN_POINT('Ctrl Pts',(-12.3042644295668,-57.732803231978,
2.65958448498064));
#237619=CARTESIAN_POINT('Ctrl Pts',(-12.300933880148,-57.7331858342642,
2.659285262607));
#237620=CARTESIAN_POINT('Ctrl Pts',(-12.2976053572248,-57.7336757296044,
2.65908463971263));
#237621=CARTESIAN_POINT('Ctrl Pts',(-12.2942768343016,-57.7341656249446,
2.65888401681825));
#237622=CARTESIAN_POINT('Ctrl Pts',(-12.2909503756172,-57.7347627876417,
2.65878198860222));
#237623=CARTESIAN_POINT('Ctrl Pts',(-12.2876333308465,-57.7354693911204,
2.65878198860222));
#237624=CARTESIAN_POINT('Origin',(-6.07506605172241,-57.9461901084061,2.83404198860221));
#237625=CARTESIAN_POINT('Ctrl Pts',(-6.35995915837739,-62.3334394572618,
2.83404198860218));
#237626=CARTESIAN_POINT('Ctrl Pts',(-6.36106823981726,-62.3439916622901,
2.82419652440029));
#237627=CARTESIAN_POINT('Ctrl Pts',(-6.36300663452631,-62.3544250468347,
2.81438790575626));
#237628=CARTESIAN_POINT('Ctrl Pts',(-6.36575328117388,-62.3646844024056,
2.80466781256893));
#237629=CARTESIAN_POINT('Ctrl Pts',(-6.3684106781606,-62.3746103900109,
2.79526356453085));
#237630=CARTESIAN_POINT('Ctrl Pts',(-6.3718250534311,-62.3843747009652,
2.78594102496257));
#237631=CARTESIAN_POINT('Ctrl Pts',(-6.37602267870808,-62.393918523908,
2.77675109088821));
#237632=CARTESIAN_POINT('Ctrl Pts',(-6.37999337374521,-62.4029463927371,
2.76805797913744));
#237633=CARTESIAN_POINT('Ctrl Pts',(-6.38466529101432,-62.4117778192047,
2.75948271210242));
#237634=CARTESIAN_POINT('Ctrl Pts',(-6.39009631814961,-62.4203406170095,
2.75108575573322));
#237635=CARTESIAN_POINT('Ctrl Pts',(-6.39509868692306,-62.428227573065,
2.74335155163389));
#237636=CARTESIAN_POINT('Ctrl Pts',(-6.40074541103519,-62.4358870734642,
2.73576818686081));
#237637=CARTESIAN_POINT('Ctrl Pts',(-6.40710777594456,-62.4432347045246,
2.7284062616065));
#237638=CARTESIAN_POINT('Ctrl Pts',(-6.40895325615343,-62.4453659729911,
2.72627084693766));
#237639=CARTESIAN_POINT('Ctrl Pts',(-6.41085910953077,-62.4474707870404,
2.72415424587543));
#237640=CARTESIAN_POINT('Ctrl Pts',(-6.41282747576019,-62.4495465125723,
2.72205867173214));
#237641=CARTESIAN_POINT('Ctrl Pts',(-6.41496131130683,-62.4517967325055,
2.71978693462817));
#237642=CARTESIAN_POINT('Ctrl Pts',(-6.41716486079139,-62.454010378812,
2.71754411340717));
#237643=CARTESIAN_POINT('Ctrl Pts',(-6.41943986047049,-62.4561838467661,
2.71533341844213));
#237644=CARTESIAN_POINT('Ctrl Pts',(-6.42568361494137,-62.4621489466209,
2.7092661487636));
#237645=CARTESIAN_POINT('Ctrl Pts',(-6.43248733059572,-62.4677726477848,
2.70347381860378));
#237646=CARTESIAN_POINT('Ctrl Pts',(-6.4398156260913,-62.4729574661285,
2.69804914171364));
#237647=CARTESIAN_POINT('Ctrl Pts',(-6.4465206186072,-62.4777012934225,
2.69308585687183));
#237648=CARTESIAN_POINT('Ctrl Pts',(-6.4536638582568,-62.4820661824982,
2.68842799053171));
#237649=CARTESIAN_POINT('Ctrl Pts',(-6.46124910257323,-62.4859635700123,
2.68414767054209));
#237650=CARTESIAN_POINT('Ctrl Pts',(-6.46497494980339,-62.4878779540279,
2.68204519134535));
#237651=CARTESIAN_POINT('Ctrl Pts',(-6.46880749650867,-62.4896790353529,
2.68003431778478));
#237652=CARTESIAN_POINT('Ctrl Pts',(-6.47274712615509,-62.4913529701964,
2.67812693945221));
#237653=CARTESIAN_POINT('Ctrl Pts',(-6.47349463250796,-62.4916705830285,
2.67776503299173));
#237654=CARTESIAN_POINT('Ctrl Pts',(-6.47424649074124,-62.4919834280837,
2.67740659639893));
#237655=CARTESIAN_POINT('Ctrl Pts',(-6.47500261163096,-62.4922913974556,
2.67705178968824));
#237656=CARTESIAN_POINT('Ctrl Pts',(-6.47573510374288,-62.4925897427846,
2.67670807068727));
#237657=CARTESIAN_POINT('Ctrl Pts',(-6.47647159623283,-62.4928835124025,
2.67636775825234));
#237658=CARTESIAN_POINT('Ctrl Pts',(-6.47721200416342,-62.49317260863,2.67603099699224));
#237659=CARTESIAN_POINT('Ctrl Pts',(-6.48528081722642,-62.4963231197466,
2.6723610421709));
#237660=CARTESIAN_POINT('Ctrl Pts',(-6.4938200899496,-62.4989203081702,
2.6691144054143));
#237661=CARTESIAN_POINT('Ctrl Pts',(-6.50268949817377,-62.5008353965404,
2.66646778189584));
#237662=CARTESIAN_POINT('Ctrl Pts',(-6.50643510434294,-62.5016441502511,
2.66535009634934));
#237663=CARTESIAN_POINT('Ctrl Pts',(-6.51023927047629,-62.5023315568339,
2.66433897912309));
#237664=CARTESIAN_POINT('Ctrl Pts',(-6.51409041329226,-62.5028895688028,
2.66344564884762));
#237665=CARTESIAN_POINT('Ctrl Pts',(-6.52057564156509,-62.5038292470154,
2.66194130298555));
#237666=CARTESIAN_POINT('Ctrl Pts',(-6.52719259313717,-62.5043999463276,
2.66077206705389));
#237667=CARTESIAN_POINT('Ctrl Pts',(-6.53387925273547,-62.5045608969653,
2.65998225155684));
#237668=CARTESIAN_POINT('Ctrl Pts',(-6.53555091763504,-62.5046011346247,
2.65978479768257));
#237669=CARTESIAN_POINT('Ctrl Pts',(-6.53722692958757,-62.5046155292228,
2.65961098966592));
#237670=CARTESIAN_POINT('Ctrl Pts',(-6.53890629461024,-62.5046031362668,
2.65946139030471));
#237671=CARTESIAN_POINT('Ctrl Pts',(-6.54142534214424,-62.5045845468328,
2.65923699126289));
#237672=CARTESIAN_POINT('Ctrl Pts',(-6.54395191714457,-62.5045056736604,
2.65906707562411));
#237673=CARTESIAN_POINT('Ctrl Pts',(-6.54648282201814,-62.504364999833,
2.65895332562888));
#237674=CARTESIAN_POINT('Ctrl Pts',(-6.54901372689171,-62.5042243260056,
2.65883957563366));
#237675=CARTESIAN_POINT('Ctrl Pts',(-6.55154895552196,-62.504021861386,
2.65878198860218));
#237676=CARTESIAN_POINT('Ctrl Pts',(-6.55408556365882,-62.5037563256533,
2.65878198860218));
#237677=CARTESIAN_POINT('Ctrl Pts',(-6.15500747092256,-58.7067819056642,
2.65878198860221));
#237678=CARTESIAN_POINT('Ctrl Pts',(-6.14642434678128,-58.7076801645416,
2.65878198860221));
#237679=CARTESIAN_POINT('Ctrl Pts',(-6.13798976646331,-58.7092791387966,
2.65945335517813));
#237680=CARTESIAN_POINT('Ctrl Pts',(-6.12982011300226,-58.7114824462538,
2.66072561226557));
#237681=CARTESIAN_POINT('Ctrl Pts',(-6.12454335512117,-58.7129055567988,
2.66154735980295));
#237682=CARTESIAN_POINT('Ctrl Pts',(-6.11937686667988,-58.7145798848068,
2.66261895766841));
#237683=CARTESIAN_POINT('Ctrl Pts',(-6.1143480066927,-58.7164715618023,
2.66391429250987));
#237684=CARTESIAN_POINT('Ctrl Pts',(-6.1076825408507,-58.718978871298,2.66563118464083));
#237685=CARTESIAN_POINT('Ctrl Pts',(-6.10126195983177,-58.721872918038,
2.66774105138658));
#237686=CARTESIAN_POINT('Ctrl Pts',(-6.09514640967211,-58.7250866612025,
2.67016894181709));
#237687=CARTESIAN_POINT('Ctrl Pts',(-6.09208863459227,-58.7266935327847,
2.67138288703234));
#237688=CARTESIAN_POINT('Ctrl Pts',(-6.08910691884909,-58.7283803475664,
2.6726761316751));
#237689=CARTESIAN_POINT('Ctrl Pts',(-6.08620737357403,-58.7301388657772,
2.67403835432512));
#237690=CARTESIAN_POINT('Ctrl Pts',(-6.08475760093649,-58.7310181248826,
2.67471946565013));
#237691=CARTESIAN_POINT('Ctrl Pts',(-6.08332835456981,-58.7319153115141,
2.67541781389482));
#237692=CARTESIAN_POINT('Ctrl Pts',(-6.08192029572508,-58.7328294060526,
2.67613207244128));
#237693=CARTESIAN_POINT('Ctrl Pts',(-6.0815682810139,-58.7330579296872,
2.6763106370779));
#237694=CARTESIAN_POINT('Ctrl Pts',(-6.08121759017506,-58.7332875101005,
2.67649019601804));
#237695=CARTESIAN_POINT('Ctrl Pts',(-6.08086823283919,-58.73351813143,2.67667072836616));
#237696=CARTESIAN_POINT('Ctrl Pts',(-6.07982016083158,-58.7342099954185,
2.67721232541049));
#237697=CARTESIAN_POINT('Ctrl Pts',(-6.07878409208716,-58.7349112274884,
2.67776268340006));
#237698=CARTESIAN_POINT('Ctrl Pts',(-6.07776027111658,-58.7356214008384,
2.67832123541475));
#237699=CARTESIAN_POINT('Ctrl Pts',(-6.07054860839913,-58.7406237702159,
2.68225560368402));
#237700=CARTESIAN_POINT('Ctrl Pts',(-6.06389424687466,-58.7460508958009,
2.68661792998844));
#237701=CARTESIAN_POINT('Ctrl Pts',(-6.05777649745776,-58.7517849266676,
2.69130986622532));
#237702=CARTESIAN_POINT('Ctrl Pts',(-6.0548093956014,-58.7545659254418,
2.6935854502301));
#237703=CARTESIAN_POINT('Ctrl Pts',(-6.05196853530536,-58.7574196937446,
2.69593918853427));
#237704=CARTESIAN_POINT('Ctrl Pts',(-6.04925198282171,-58.7603356163929,
2.69836306235434));
#237705=CARTESIAN_POINT('Ctrl Pts',(-6.04509313076931,-58.7647996902379,
2.70207384382167));
#237706=CARTESIAN_POINT('Ctrl Pts',(-6.04122712577015,-58.769406243151,
2.70594760814168));
#237707=CARTESIAN_POINT('Ctrl Pts',(-6.03765709635773,-58.7741092696791,
2.70995196345648));
#237708=CARTESIAN_POINT('Ctrl Pts',(-6.03599915622971,-58.776293379529,
2.71181160678046));
#237709=CARTESIAN_POINT('Ctrl Pts',(-6.03440490786061,-58.778498084111,
2.71369962772039));
#237710=CARTESIAN_POINT('Ctrl Pts',(-6.03287578462695,-58.7807192900656,
2.71561183138601));
#237711=CARTESIAN_POINT('Ctrl Pts',(-6.03275858335614,-58.78088953675,2.71575839426252));
#237712=CARTESIAN_POINT('Ctrl Pts',(-6.03264173148717,-58.7810598733264,
2.71590508903149));
#237713=CARTESIAN_POINT('Ctrl Pts',(-6.03252522862488,-58.7812302983887,
2.71605191409851));
#237714=CARTESIAN_POINT('Ctrl Pts',(-6.03088871465443,-58.7836242566992,
2.71811436362693));
#237715=CARTESIAN_POINT('Ctrl Pts',(-6.02932271154701,-58.7860369637875,
2.72020091026899));
#237716=CARTESIAN_POINT('Ctrl Pts',(-6.02782611907196,-58.7884628208562,
2.72230624862122));
#237717=CARTESIAN_POINT('Ctrl Pts',(-6.02245960461621,-58.7971615128805,
2.72985561753076));
#237718=CARTESIAN_POINT('Ctrl Pts',(-6.01794242202239,-58.8060955050482,
2.7377008991434));
#237719=CARTESIAN_POINT('Ctrl Pts',(-6.01418353044859,-58.8151732302906,
2.74574823347121));
#237720=CARTESIAN_POINT('Ctrl Pts',(-6.01005288622323,-58.8251487383934,
2.75459144547085));
#237721=CARTESIAN_POINT('Ctrl Pts',(-6.00683754300126,-58.8352983536265,
2.76367911754344));
#237722=CARTESIAN_POINT('Ctrl Pts',(-6.00445775272911,-58.8455340166158,
2.77292162564815));
#237723=CARTESIAN_POINT('Ctrl Pts',(-6.00188817648111,-58.8565859638431,
2.78290121484799));
#237724=CARTESIAN_POINT('Ctrl Pts',(-6.00029231631103,-58.8677393147042,
2.79306229500235));
#237725=CARTESIAN_POINT('Ctrl Pts',(-5.99962196122081,-58.878907218868,
2.80331916685278));
#237726=CARTESIAN_POINT('Ctrl Pts',(-5.99895722972104,-58.8899814357904,
2.81348999408696));
#237727=CARTESIAN_POINT('Ctrl Pts',(-5.99920273697641,-58.9010713848515,
2.82375635966856));
#237728=CARTESIAN_POINT('Ctrl Pts',(-6.00036140428986,-58.9120953679529,
2.8340419886022));
#237729=CARTESIAN_POINT('Origin',(-0.0151565136854063,0.00159301378039395,
2.83404198860262));
#237730=CARTESIAN_POINT('Ctrl Pts',(-6.58439859102965,-62.500570298093,
2.65878198860218));
#237731=CARTESIAN_POINT('Ctrl Pts',(-6.59294009787386,-62.4996689377204,
2.65878198860218));
#237732=CARTESIAN_POINT('Ctrl Pts',(-6.60133040498984,-62.4980620716936,
2.65944603041802));
#237733=CARTESIAN_POINT('Ctrl Pts',(-6.60945539386119,-62.4958483879904,
2.66070439264013));
#237734=CARTESIAN_POINT('Ctrl Pts',(-6.61464687495772,-62.494433949487,
2.6615084261954));
#237735=CARTESIAN_POINT('Ctrl Pts',(-6.61973030386286,-62.4927726671881,
2.66255428265316));
#237736=CARTESIAN_POINT('Ctrl Pts',(-6.62467983150704,-62.4908979342375,
2.66381699700609));
#237737=CARTESIAN_POINT('Ctrl Pts',(-6.63143494361032,-62.4883392999282,
2.66554034873209));
#237738=CARTESIAN_POINT('Ctrl Pts',(-6.63793726713702,-62.4853780106446,
2.66766759643914));
#237739=CARTESIAN_POINT('Ctrl Pts',(-6.64412426454832,-62.4820864562847,
2.6701201278309));
#237740=CARTESIAN_POINT('Ctrl Pts',(-6.64721776325397,-62.4804406791048,
2.67134639352678));
#237741=CARTESIAN_POINT('Ctrl Pts',(-6.65023263831811,-62.4787123157332,
2.67265375584954));
#237742=CARTESIAN_POINT('Ctrl Pts',(-6.65316255786678,-62.4769102669529,
2.67403135126882));
#237743=CARTESIAN_POINT('Ctrl Pts',(-6.65462751764111,-62.4760092425627,
2.67472014897846));
#237744=CARTESIAN_POINT('Ctrl Pts',(-6.65607125586019,-62.4750897950505,
2.67542649668575));
#237745=CARTESIAN_POINT('Ctrl Pts',(-6.65749308991699,-62.4741530260209,
2.67614899656044));
#237746=CARTESIAN_POINT('Ctrl Pts',(-6.65784854843119,-62.4739188337634,
2.67632962152911));
#237747=CARTESIAN_POINT('Ctrl Pts',(-6.65820263830441,-62.4736835588745,
2.67651125590892));
#237748=CARTESIAN_POINT('Ctrl Pts',(-6.65855534961552,-62.4734472184932,
2.67669387767466));
#237749=CARTESIAN_POINT('Ctrl Pts',(-6.65961348354886,-62.4727381973494,
2.67724174297186));
#237750=CARTESIAN_POINT('Ctrl Pts',(-6.66065920857944,-62.4720195869491,
2.6777984950469));
#237751=CARTESIAN_POINT('Ctrl Pts',(-6.66169227331155,-62.4712918484709,
2.67836353617951));
#237752=CARTESIAN_POINT('Ctrl Pts',(-6.66883139158055,-62.4662627240578,
2.68226832098846));
#237753=CARTESIAN_POINT('Ctrl Pts',(-6.67541846632588,-62.4608161451509,
2.68659153751324));
#237754=CARTESIAN_POINT('Ctrl Pts',(-6.68147667711047,-62.4550686189991,
2.69123699486105));
#237755=CARTESIAN_POINT('Ctrl Pts',(-6.68448759124107,-62.4522121142781,
2.69354577441148));
#237756=CARTESIAN_POINT('Ctrl Pts',(-6.68736784133544,-62.4492806638354,
2.69593478828053));
#237757=CARTESIAN_POINT('Ctrl Pts',(-6.69011973548545,-62.4462854590367,
2.6983956526116));
#237758=CARTESIAN_POINT('Ctrl Pts',(-6.69619082501359,-62.439677589876,
2.70382468688985));
#237759=CARTESIAN_POINT('Ctrl Pts',(-6.70164568781153,-62.4327685320935,
2.70961155815027));
#237760=CARTESIAN_POINT('Ctrl Pts',(-6.7064460603903,-62.4256985108777,
2.71562701361706));
#237761=CARTESIAN_POINT('Ctrl Pts',(-6.70819969702921,-62.4231157429699,
2.71782453535797));
#237762=CARTESIAN_POINT('Ctrl Pts',(-6.70987381569752,-62.4205129446132,
2.72005051502341));
#237763=CARTESIAN_POINT('Ctrl Pts',(-6.71147036762112,-62.4178950590934,
2.72229986760055));
#237764=CARTESIAN_POINT('Ctrl Pts',(-6.71683301659051,-62.4091018586488,
2.72985520488792));
#237765=CARTESIAN_POINT('Ctrl Pts',(-6.72134734296604,-62.4000783072493,
2.73770845534421));
#237766=CARTESIAN_POINT('Ctrl Pts',(-6.72510335397076,-62.3909158405876,
2.74576706701578));
#237767=CARTESIAN_POINT('Ctrl Pts',(-6.7292316549937,-62.3808452043609,
2.75462443584815));
#237768=CARTESIAN_POINT('Ctrl Pts',(-6.73244426756063,-62.3706061896796,
2.76373036322926));
#237769=CARTESIAN_POINT('Ctrl Pts',(-6.73481930344644,-62.3602869763785,
2.77299664636518));
#237770=CARTESIAN_POINT('Ctrl Pts',(-6.73737731885764,-62.3491727415103,
2.78297683033115));
#237771=CARTESIAN_POINT('Ctrl Pts',(-6.73896413451773,-62.3379643502107,
2.79314401478467));
#237772=CARTESIAN_POINT('Ctrl Pts',(-6.73962511499484,-62.3267489231156,
2.80341452427437));
#237773=CARTESIAN_POINT('Ctrl Pts',(-6.74027717000387,-62.3156849421522,
2.81354634721019));
#237774=CARTESIAN_POINT('Ctrl Pts',(-6.74002799825934,-62.3046126966266,
2.82378004209014));
#237775=CARTESIAN_POINT('Ctrl Pts',(-6.7388720005127,-62.2936141127568,
2.83404198860218));
#237776=CARTESIAN_POINT('Ctrl Pts',(-6.37927424642518,-58.8722700234479,
2.8340419886022));
#237777=CARTESIAN_POINT('Ctrl Pts',(-6.37816795023606,-58.8617443183103,
2.82422126443067));
#237778=CARTESIAN_POINT('Ctrl Pts',(-6.37623543038838,-58.8513437177799,
2.81442815028664));
#237779=CARTESIAN_POINT('Ctrl Pts',(-6.37349561323738,-58.8411231047696,
2.80471618166581));
#237780=CARTESIAN_POINT('Ctrl Pts',(-6.37085007871829,-58.8312542036587,
2.79533842146557));
#237781=CARTESIAN_POINT('Ctrl Pts',(-6.36745144954188,-58.8215519162637,
2.7860351565063));
#237782=CARTESIAN_POINT('Ctrl Pts',(-6.36327195218801,-58.8120753594687,
2.77685887347205));
#237783=CARTESIAN_POINT('Ctrl Pts',(-6.35932101825102,-58.8031170454234,
2.76818441217064));
#237784=CARTESIAN_POINT('Ctrl Pts',(-6.35467192212117,-58.7943596215217,
2.75962261522147));
#237785=CARTESIAN_POINT('Ctrl Pts',(-6.34926600747862,-58.7858758685359,
2.75123537702214));
#237786=CARTESIAN_POINT('Ctrl Pts',(-6.34428725078379,-58.7780624743614,
2.74351087134693));
#237787=CARTESIAN_POINT('Ctrl Pts',(-6.33866621241734,-58.7704807832501,
2.73593399450439));
#237788=CARTESIAN_POINT('Ctrl Pts',(-6.33233133085271,-58.7632157809058,
2.72857657813182));
#237789=CARTESIAN_POINT('Ctrl Pts',(-6.33044239704668,-58.7610495038588,
2.72638274508705));
#237790=CARTESIAN_POINT('Ctrl Pts',(-6.32848982621625,-58.7589116098652,
2.72420861709762));
#237791=CARTESIAN_POINT('Ctrl Pts',(-6.32647128889777,-58.7568049797263,
2.72205663736667));
#237792=CARTESIAN_POINT('Ctrl Pts',(-6.32447337605792,-58.7547198741576,
2.71992664556706));
#237793=CARTESIAN_POINT('Ctrl Pts',(-6.32241310885664,-58.7526673708732,
2.71782089927824));
#237794=CARTESIAN_POINT('Ctrl Pts',(-6.32029074540058,-58.7506524329179,
2.71574387311186));
#237795=CARTESIAN_POINT('Ctrl Pts',(-6.32014316039653,-58.7505123180731,
2.71559944077427));
#237796=CARTESIAN_POINT('Ctrl Pts',(-6.31999527850295,-58.7503723733985,
2.71545515216009));
#237797=CARTESIAN_POINT('Ctrl Pts',(-6.31984709900165,-58.750232599983,
2.7153110078167));
#237798=CARTESIAN_POINT('Ctrl Pts',(-6.31335036684049,-58.7441044214166,
2.70899119176023));
#237799=CARTESIAN_POINT('Ctrl Pts',(-6.30625925377286,-58.738344788164,
2.70298296066777));
#237800=CARTESIAN_POINT('Ctrl Pts',(-6.29859016886885,-58.733068714084,
2.69736727774074));
#237801=CARTESIAN_POINT('Ctrl Pts',(-6.29144124886036,-58.728150496066,
2.69213248525365));
#237802=CARTESIAN_POINT('Ctrl Pts',(-6.28378931333002,-58.7236522470775,
2.68723866185404));
#237803=CARTESIAN_POINT('Ctrl Pts',(-6.27564783709133,-58.7196964823228,
2.68278595829497));
#237804=CARTESIAN_POINT('Ctrl Pts',(-6.27266957975507,-58.7182494123989,
2.68115710172741));
#237805=CARTESIAN_POINT('Ctrl Pts',(-6.26962586933668,-58.7168752520896,
2.67958763637747));
#237806=CARTESIAN_POINT('Ctrl Pts',(-6.26651766855692,-58.7155811795663,
2.67808378645303));
#237807=CARTESIAN_POINT('Ctrl Pts',(-6.26577025010519,-58.7152699983555,
2.67772216078538));
#237808=CARTESIAN_POINT('Ctrl Pts',(-6.26501853257379,-58.7149635750522,
2.67736403603501));
#237809=CARTESIAN_POINT('Ctrl Pts',(-6.26426260461781,-58.714662012368,
2.67700956934417));
#237810=CARTESIAN_POINT('Ctrl Pts',(-6.26353029941046,-58.7143698735177,
2.67666617973742));
#237811=CARTESIAN_POINT('Ctrl Pts',(-6.26279404284316,-58.7140822962413,
2.67632622314057));
#237812=CARTESIAN_POINT('Ctrl Pts',(-6.262053919284,-58.713799373501,2.67598984158711));
#237813=CARTESIAN_POINT('Ctrl Pts',(-6.25394501035187,-58.7106996279151,
2.6723043929216));
#237814=CARTESIAN_POINT('Ctrl Pts',(-6.24536644325901,-58.7081569420198,
2.66904964539914));
#237815=CARTESIAN_POINT('Ctrl Pts',(-6.23645973859638,-58.7062958387083,
2.66640203566664));
#237816=CARTESIAN_POINT('Ctrl Pts',(-6.23276586269236,-58.7055239836914,
2.66530399299379));
#237817=CARTESIAN_POINT('Ctrl Pts',(-6.22901585349491,-58.7048690642114,
2.66430995142197));
#237818=CARTESIAN_POINT('Ctrl Pts',(-6.2252207626774,-58.7043384037132,
2.66343053473298));
#237819=CARTESIAN_POINT('Ctrl Pts',(-6.21874783981175,-58.703433306935,
2.66193059792822));
#237820=CARTESIAN_POINT('Ctrl Pts',(-6.21214524099502,-58.7028917011004,
2.66076519817064));
#237821=CARTESIAN_POINT('Ctrl Pts',(-6.20547453342013,-58.7027523988016,
2.65997805604397));
#237822=CARTESIAN_POINT('Ctrl Pts',(-6.20213917963269,-58.7026827476522,
2.65958448498063));
#237823=CARTESIAN_POINT('Ctrl Pts',(-6.19878688248308,-58.7027151167904,
2.65928526260699));
#237824=CARTESIAN_POINT('Ctrl Pts',(-6.19542538554965,-58.7028544030465,
2.65908463971261));
#237825=CARTESIAN_POINT('Ctrl Pts',(-6.19206388861623,-58.7029936893026,
2.65888401681823));
#237826=CARTESIAN_POINT('Ctrl Pts',(-6.18869323212156,-58.7032398710653,
2.65878198860221));
#237827=CARTESIAN_POINT('Ctrl Pts',(-6.18532049829339,-58.7035958781038,
2.65878198860221));
#237828=CARTESIAN_POINT('Origin',(0.0152400000006159,-58.2637721346183,
2.83404198860221));
#237829=CARTESIAN_POINT('Ctrl Pts',(0.190500000000662,-62.6567671111298,
2.83404198860218));
#237830=CARTESIAN_POINT('Ctrl Pts',(0.190500000000662,-62.6673774406536,
2.82419652440023));
#237831=CARTESIAN_POINT('Ctrl Pts',(0.189662809673738,-62.6779562874463,
2.81438790575611));
#237832=CARTESIAN_POINT('Ctrl Pts',(0.188003604115792,-62.6884465439472,
2.80466781256867));
#237833=CARTESIAN_POINT('Ctrl Pts',(0.186398312858558,-62.6985959295773,
2.79526356453047));
#237834=CARTESIAN_POINT('Ctrl Pts',(0.184023290311906,-62.7086636500147,
2.78594102496205));
#237835=CARTESIAN_POINT('Ctrl Pts',(0.180846261211217,-62.7185939622165,
2.77675109088756));
#237836=CARTESIAN_POINT('Ctrl Pts',(0.177840987312148,-62.727987426086,
2.76805797913663));
#237837=CARTESIAN_POINT('Ctrl Pts',(0.174117798731669,-62.7372588214081,
2.75948271210146));
#237838=CARTESIAN_POINT('Ctrl Pts',(0.169611579426945,-62.7463424082311,
2.75108575573212));
#237839=CARTESIAN_POINT('Ctrl Pts',(0.165461025549218,-62.7547090486368,
2.74335155163261));
#237840=CARTESIAN_POINT('Ctrl Pts',(0.160645870588547,-62.7629168328855,
2.73576818685937));
#237841=CARTESIAN_POINT('Ctrl Pts',(0.155086395963031,-62.770889261081,
2.72840626160493));
#237842=CARTESIAN_POINT('Ctrl Pts',(0.153473803705819,-62.7732017594456,
2.72627084693661));
#237843=CARTESIAN_POINT('Ctrl Pts',(0.151798403771124,-62.7754942590275,
2.7241542458749));
#237844=CARTESIAN_POINT('Ctrl Pts',(0.150057792858307,-62.7777643638144,
2.72205867173211));
#237845=CARTESIAN_POINT('Ctrl Pts',(0.148170858717691,-62.7802253033579,
2.71978693462815));
#237846=CARTESIAN_POINT('Ctrl Pts',(0.146210769554423,-62.7826571567197,
2.71754411340716));
#237847=CARTESIAN_POINT('Ctrl Pts',(0.144175421826809,-62.7850565204093,
2.71533341844214));
#237848=CARTESIAN_POINT('Ctrl Pts',(0.138589394017279,-62.7916415928828,
2.70926614876361));
#237849=CARTESIAN_POINT('Ctrl Pts',(0.132410786669697,-62.7979456687652,
2.70347381860378));
#237850=CARTESIAN_POINT('Ctrl Pts',(0.125664597437387,-62.803868099598,
2.69804914171364));
#237851=CARTESIAN_POINT('Ctrl Pts',(0.119492200549002,-62.8092868022737,
2.69308585687176));
#237852=CARTESIAN_POINT('Ctrl Pts',(0.112844347460919,-62.8143744518937,
2.68842799053158));
#237853=CARTESIAN_POINT('Ctrl Pts',(0.105708043833992,-62.8190433630432,
2.68414767054191));
#237854=CARTESIAN_POINT('Ctrl Pts',(0.102202714804165,-62.8213367169481,
2.68204519134525));
#237855=CARTESIAN_POINT('Ctrl Pts',(0.0985794274539604,-62.8235285419786,
2.68003431778474));
#237856=CARTESIAN_POINT('Ctrl Pts',(0.0948363533478736,-62.8256051102646,
2.67812693945223));
#237857=CARTESIAN_POINT('Ctrl Pts',(0.0941261414942743,-62.8259991188708,
2.67776503299174));
#237858=CARTESIAN_POINT('Ctrl Pts',(0.0934111032319262,-62.8263888407137,
2.67740659639895));
#237859=CARTESIAN_POINT('Ctrl Pts',(0.0926913160167301,-62.8267741591518,
2.67705178968826));
#237860=CARTESIAN_POINT('Ctrl Pts',(0.091994022152009,-62.8271474363887,
2.67670807068729));
#237861=CARTESIAN_POINT('Ctrl Pts',(0.0912922715316926,-62.8275165811341,
2.67636775825236));
#237862=CARTESIAN_POINT('Ctrl Pts',(0.0905861384176031,-62.8278814873653,
2.67603099699226));
#237863=CARTESIAN_POINT('Ctrl Pts',(0.0828908452424436,-62.8318581602823,
2.67236104217096));
#237864=CARTESIAN_POINT('Ctrl Pts',(0.0746698316635625,-62.8353337180911,
2.66911440541439));
#237865=CARTESIAN_POINT('Ctrl Pts',(0.0660491922301222,-62.8381654210185,
2.66646778189595));
#237866=CARTESIAN_POINT('Ctrl Pts',(0.0624086426659131,-62.8393612667487,
2.66535009634941));
#237867=CARTESIAN_POINT('Ctrl Pts',(0.0586971697063133,-62.8404425512863,
2.66433897912313));
#237868=CARTESIAN_POINT('Ctrl Pts',(0.054925451987136,-62.8414000604477,
2.66344564884763));
#237869=CARTESIAN_POINT('Ctrl Pts',(0.0485739735928758,-62.8430124819499,
2.66194130298556));
#237870=CARTESIAN_POINT('Ctrl Pts',(0.0420529246959322,-62.844271714691,
2.6607720670539));
#237871=CARTESIAN_POINT('Ctrl Pts',(0.0354197192413684,-62.8451307298762,
2.65998225155684));
#237872=CARTESIAN_POINT('Ctrl Pts',(0.0337614178777275,-62.8453454836725,
2.65978479768257));
#237873=CARTESIAN_POINT('Ctrl Pts',(0.032096091939252,-62.8455349903693,
2.65961098966591));
#237874=CARTESIAN_POINT('Ctrl Pts',(0.0304246312372505,-62.8456982067483,
2.65946139030471));
#237875=CARTESIAN_POINT('Ctrl Pts',(0.0279174401842483,-62.8459430313168,
2.65923699126289));
#237876=CARTESIAN_POINT('Ctrl Pts',(0.0253964615346301,-62.8461286892221,
2.65906707562411));
#237877=CARTESIAN_POINT('Ctrl Pts',(0.0228647168037737,-62.8462533376178,
2.65895332562888));
#237878=CARTESIAN_POINT('Ctrl Pts',(0.0203329720729172,-62.8463779860135,
2.65883957563366));
#237879=CARTESIAN_POINT('Ctrl Pts',(0.0177904683748175,-62.8464416340691,
2.65878198860218));
#237880=CARTESIAN_POINT('Ctrl Pts',(0.0152400000006639,-62.8464427007194,
2.65878198860218));
#237881=CARTESIAN_POINT('Ctrl Pts',(0.0152400000006241,-59.0285534841294,
2.6587819886022));
#237882=CARTESIAN_POINT('Ctrl Pts',(0.0238699985099668,-59.0285496414742,
2.6587819886022));
#237883=CARTESIAN_POINT('Ctrl Pts',(0.0324255116361993,-59.029258202662,
2.65945335517814));
#237884=CARTESIAN_POINT('Ctrl Pts',(0.0407807192234809,-59.0305954788488,
2.66072561226561));
#237885=CARTESIAN_POINT('Ctrl Pts',(0.0461773260310371,-59.031459222053,
2.66154735980299));
#237886=CARTESIAN_POINT('Ctrl Pts',(0.0514905268416817,-59.0325843328197,
2.66261895766844));
#237887=CARTESIAN_POINT('Ctrl Pts',(0.0566895722969428,-59.0339399880042,
2.66391429250988));
#237888=CARTESIAN_POINT('Ctrl Pts',(0.0635806092281412,-59.0357368312947,
2.66563118464085));
#237889=CARTESIAN_POINT('Ctrl Pts',(0.0702685278908046,-59.0379438906766,
2.6677410513866));
#237890=CARTESIAN_POINT('Ctrl Pts',(0.0766865040611197,-59.0405007795596,
2.67016894181711));
#237891=CARTESIAN_POINT('Ctrl Pts',(0.0798954921462772,-59.041779224001,
2.67138288703236));
#237892=CARTESIAN_POINT('Ctrl Pts',(0.0830371938955821,-59.0431451240704,
2.67267613167512));
#237893=CARTESIAN_POINT('Ctrl Pts',(0.0861046703644424,-59.0445909239226,
2.67403835432513));
#237894=CARTESIAN_POINT('Ctrl Pts',(0.0876384085988726,-59.0453138238487,
2.67471946565014));
#237895=CARTESIAN_POINT('Ctrl Pts',(0.0891536069442672,-59.0460566986717,
2.67541781389483));
#237896=CARTESIAN_POINT('Ctrl Pts',(0.090649501192699,-59.0468186034774,
2.67613207244129));
#237897=CARTESIAN_POINT('Ctrl Pts',(0.091023474754807,-59.0470090796788,
2.6763106370779));
#237898=CARTESIAN_POINT('Ctrl Pts',(0.0913962421603352,-59.0472007452521,
2.67649019601805));
#237899=CARTESIAN_POINT('Ctrl Pts',(0.0917677921733363,-59.0473935854284,
2.67667072836616));
#237900=CARTESIAN_POINT('Ctrl Pts',(0.0928824422123397,-59.0479721059572,
2.6772123254105));
#237901=CARTESIAN_POINT('Ctrl Pts',(0.0939861339744225,-59.0485611979308,
2.67776268340007));
#237902=CARTESIAN_POINT('Ctrl Pts',(0.0950785796755408,-59.0491604624442,
2.67832123541475));
#237903=CARTESIAN_POINT('Ctrl Pts',(0.102773626133754,-59.0533816042974,
2.68225560368401));
#237904=CARTESIAN_POINT('Ctrl Pts',(0.109958823466863,-59.0580834293363,
2.68661792998841));
#237905=CARTESIAN_POINT('Ctrl Pts',(0.116642428647153,-59.0631465696368,
2.69130986622527));
#237906=CARTESIAN_POINT('Ctrl Pts',(0.11988396993733,-59.0656021872113,
2.69358545023007));
#237907=CARTESIAN_POINT('Ctrl Pts',(0.123007567718671,-59.0681433715117,
2.69593918853425));
#237908=CARTESIAN_POINT('Ctrl Pts',(0.126014035557039,-59.0707593633742,
2.69836306235434));
#237909=CARTESIAN_POINT('Ctrl Pts',(0.130616727761666,-59.0747642641415,
2.70207384382167));
#237910=CARTESIAN_POINT('Ctrl Pts',(0.134943070277899,-59.0789414743142,
2.70594760814168));
#237911=CARTESIAN_POINT('Ctrl Pts',(0.138985142831362,-59.0832455674826,
2.70995196345647));
#237912=CARTESIAN_POINT('Ctrl Pts',(0.1408623022361,-59.0852444106165,2.71181160678045));
#237913=CARTESIAN_POINT('Ctrl Pts',(0.14267827152774,-59.087270393264,2.71369962772038));
#237914=CARTESIAN_POINT('Ctrl Pts',(0.14443119730936,-59.0893195943181,
2.715611831386));
#237915=CARTESIAN_POINT('Ctrl Pts',(0.144565552163647,-59.0894766575047,
2.71575839426251));
#237916=CARTESIAN_POINT('Ctrl Pts',(0.144699568926416,-59.0896338466132,
2.71590508903148));
#237917=CARTESIAN_POINT('Ctrl Pts',(0.144833247843708,-59.089791160204,
2.71605191409851));
#237918=CARTESIAN_POINT('Ctrl Pts',(0.146711033602715,-59.09200094187,2.71811436362692));
#237919=CARTESIAN_POINT('Ctrl Pts',(0.14852065454552,-59.0942367399981,
2.72020091026899));
#237920=CARTESIAN_POINT('Ctrl Pts',(0.150262619641901,-59.0964928714564,
2.72230624862121));
#237921=CARTESIAN_POINT('Ctrl Pts',(0.156508996679337,-59.104582957626,
2.72985561753033));
#237922=CARTESIAN_POINT('Ctrl Pts',(0.161935290146135,-59.1129958342945,
2.73770089914249));
#237923=CARTESIAN_POINT('Ctrl Pts',(0.166622470787953,-59.1216309196479,
2.74574823346981));
#237924=CARTESIAN_POINT('Ctrl Pts',(0.171773211444284,-59.1311200109801,
2.75459144546915));
#237925=CARTESIAN_POINT('Ctrl Pts',(0.176031864362722,-59.1408779306728,
2.76367911754144));
#237926=CARTESIAN_POINT('Ctrl Pts',(0.179468536017587,-59.1508087658088,
2.77292162564584));
#237927=CARTESIAN_POINT('Ctrl Pts',(0.183179278918004,-59.1615315754565,
2.78290121484572));
#237928=CARTESIAN_POINT('Ctrl Pts',(0.185932239425051,-59.1724570142834,
2.79306229500014));
#237929=CARTESIAN_POINT('Ctrl Pts',(0.187766286100246,-59.1834936683123,
2.80331916685064));
#237930=CARTESIAN_POINT('Ctrl Pts',(0.18958494700837,-59.1944377361543,
2.81348999408552));
#237931=CARTESIAN_POINT('Ctrl Pts',(0.190500000000626,-59.2054925958109,
2.82375635966784));
#237932=CARTESIAN_POINT('Ctrl Pts',(0.190500000000626,-59.2165773020939,
2.8340419886022));
#237933=CARTESIAN_POINT('Origin',(-0.0152399999999944,1.94929247519246E-13,
2.83404198860262));
#237934=CARTESIAN_POINT('Ctrl Pts',(-0.0152399999993361,-62.8464427007194,
2.65878198860218));
#237935=CARTESIAN_POINT('Ctrl Pts',(-0.023828933389605,-62.8464391086777,
2.65878198860218));
#237936=CARTESIAN_POINT('Ctrl Pts',(-0.0323412407614512,-62.8457180711403,
2.65944603041796));
#237937=CARTESIAN_POINT('Ctrl Pts',(-0.0406531130489861,-62.8443658068289,
2.66070439263997));
#237938=CARTESIAN_POINT('Ctrl Pts',(-0.0459640037523977,-62.8435017743088,
2.66150842619525));
#237939=CARTESIAN_POINT('Ctrl Pts',(-0.0511932363882295,-62.8423809556997,
2.66255428265307));
#237940=CARTESIAN_POINT('Ctrl Pts',(-0.0563116129568179,-62.8410338592508,
2.66381699700609));
#237941=CARTESIAN_POINT('Ctrl Pts',(-0.0632971699615973,-62.8391953428953,
2.66554034873208));
#237942=CARTESIAN_POINT('Ctrl Pts',(-0.070073412097744,-62.8369299537502,
2.66766759643912));
#237943=CARTESIAN_POINT('Ctrl Pts',(-0.0765705776088438,-62.8343031482012,
2.67012012783087));
#237944=CARTESIAN_POINT('Ctrl Pts',(-0.0798191603643938,-62.8329897454267,
2.67134639352674));
#237945=CARTESIAN_POINT('Ctrl Pts',(-0.08299818279468,-62.8315859904679,
2.6726537558495));
#237946=CARTESIAN_POINT('Ctrl Pts',(-0.0861004173272267,-62.8301000734872,
2.67403135126878));
#237947=CARTESIAN_POINT('Ctrl Pts',(-0.0876515345935001,-62.8293571149969,
2.67472014897841));
#237948=CARTESIAN_POINT('Ctrl Pts',(-0.0891834722990619,-62.8285936160518,
2.6754264966857));
#237949=CARTESIAN_POINT('Ctrl Pts',(-0.0906954364272254,-62.8278106008699,
2.67614899656039));
#237950=CARTESIAN_POINT('Ctrl Pts',(-0.0910734274592663,-62.8276148470744,
2.67632962152906));
#237951=CARTESIAN_POINT('Ctrl Pts',(-0.0914501705136929,-62.8274178735162,
2.67651125590887));
#237952=CARTESIAN_POINT('Ctrl Pts',(-0.0918256539322006,-62.8272196962036,
2.67669387767461));
#237953=CARTESIAN_POINT('Ctrl Pts',(-0.0929521041877236,-62.8266251642657,
2.67724174297181));
#237954=CARTESIAN_POINT('Ctrl Pts',(-0.0940672158680064,-62.8260197985188,
2.67779849504684));
#237955=CARTESIAN_POINT('Ctrl Pts',(-0.0951706907481964,-62.8254040313371,
2.67836353617946));
#237956=CARTESIAN_POINT('Ctrl Pts',(-0.10279638682687,-62.8211486980554,
2.68226832098843));
#237957=CARTESIAN_POINT('Ctrl Pts',(-0.109916699410765,-62.8164204928783,
2.68659153751325));
#237958=CARTESIAN_POINT('Ctrl Pts',(-0.116542502759065,-62.8113377077395,
2.6912369948611));
#237959=CARTESIAN_POINT('Ctrl Pts',(-0.119835508835773,-62.8088115774774,
2.6935457744115));
#237960=CARTESIAN_POINT('Ctrl Pts',(-0.123006400628657,-62.8061972539431,
2.69593478828053));
#237961=CARTESIAN_POINT('Ctrl Pts',(-0.126056303769311,-62.8035061084564,
2.69839565261158));
#237962=CARTESIAN_POINT('Ctrl Pts',(-0.132784845642624,-62.797569039553,
2.70382468688984));
#237963=CARTESIAN_POINT('Ctrl Pts',(-0.138932019324019,-62.7912680187376,
2.70961155815025));
#237964=CARTESIAN_POINT('Ctrl Pts',(-0.144445113412511,-62.7847385034066,
2.71562701361707));
#237965=CARTESIAN_POINT('Ctrl Pts',(-0.146459116206809,-62.7823531891146,
2.71782453535798));
#237966=CARTESIAN_POINT('Ctrl Pts',(-0.148396130390324,-62.7799396422113,
2.72005051502342));
#237967=CARTESIAN_POINT('Ctrl Pts',(-0.150257579785834,-62.7775029828614,
2.72229986760055));
#237968=CARTESIAN_POINT('Ctrl Pts',(-0.156509991333105,-62.7693185019443,
2.7298552048883));
#237969=CARTESIAN_POINT('Ctrl Pts',(-0.161942805717696,-62.7608162581016,
2.73770845534492));
#237970=CARTESIAN_POINT('Ctrl Pts',(-0.1666359794612,-62.7520965944487,
2.74576706701681));
#237971=CARTESIAN_POINT('Ctrl Pts',(-0.171794333348312,-62.742512651182,
2.75462443584957));
#237972=CARTESIAN_POINT('Ctrl Pts',(-0.176059615357581,-62.7326655363484,
2.76373036323109));
#237973=CARTESIAN_POINT('Ctrl Pts',(-0.179500292056813,-62.7226511116281,
2.77299664636747));
#237974=CARTESIAN_POINT('Ctrl Pts',(-0.183206048283218,-62.7118651471201,
2.78297683033417));
#237975=CARTESIAN_POINT('Ctrl Pts',(-0.185955767119278,-62.7008840239623,
2.7931440147885));
#237976=CARTESIAN_POINT('Ctrl Pts',(-0.187785458035107,-62.6897991274229,
2.80341452427914));
#237977=CARTESIAN_POINT('Ctrl Pts',(-0.189590441945618,-62.6788639144151,
2.81354634721326));
#237978=CARTESIAN_POINT('Ctrl Pts',(-0.190499999999338,-62.6678262782717,
2.82378004209157));
#237979=CARTESIAN_POINT('Ctrl Pts',(-0.190499999999338,-62.6567671111297,
2.83404198860218));
#237980=CARTESIAN_POINT('Ctrl Pts',(-0.190499999999374,-59.2165773020939,
2.8340419886022));
#237981=CARTESIAN_POINT('Ctrl Pts',(-0.190499999999374,-59.2059936184288,
2.82422126442975));
#237982=CARTESIAN_POINT('Ctrl Pts',(-0.189665225487999,-59.1954479901455,
2.8144281502848));
#237983=CARTESIAN_POINT('Ctrl Pts',(-0.188008762313356,-59.1849969778452,
2.80471618166307));
#237984=CARTESIAN_POINT('Ctrl Pts',(-0.186409301376204,-59.1749056059489,
2.79533842146223));
#237985=CARTESIAN_POINT('Ctrl Pts',(-0.184043455437269,-59.1649012152137,
2.78603515650239));
#237986=CARTESIAN_POINT('Ctrl Pts',(-0.180877423725614,-59.1550396955521,
2.77685887346759));
#237987=CARTESIAN_POINT('Ctrl Pts',(-0.177884532218364,-59.1457174710352,
2.76818441216581));
#237988=CARTESIAN_POINT('Ctrl Pts',(-0.174176304385712,-59.1365220583436,
2.75962261521629));
#237989=CARTESIAN_POINT('Ctrl Pts',(-0.169686797570988,-59.1275197082938,
2.75123537701665));
#237990=CARTESIAN_POINT('Ctrl Pts',(-0.165552037111723,-59.1192286949236,
2.7435108713412));
#237991=CARTESIAN_POINT('Ctrl Pts',(-0.16075429390185,-59.1111009786068,
2.73593399449844));
#237992=CARTESIAN_POINT('Ctrl Pts',(-0.15521351501129,-59.1032135992704,
2.7285765781257));
#237993=CARTESIAN_POINT('Ctrl Pts',(-0.153561366594434,-59.10086174197,
2.726382745083));
#237994=CARTESIAN_POINT('Ctrl Pts',(-0.151842962926626,-59.0985314603572,
2.72420861709562));
#237995=CARTESIAN_POINT('Ctrl Pts',(-0.150055686179522,-59.0962253759568,
2.72205663736666));
#237996=CARTESIAN_POINT('Ctrl Pts',(-0.148286670996087,-59.0939428540557,
2.71992664556705));
#237997=CARTESIAN_POINT('Ctrl Pts',(-0.146452235168283,-59.0916862380346,
2.71782089927824));
#237998=CARTESIAN_POINT('Ctrl Pts',(-0.144552116609346,-59.0894604907297,
2.71574387311185));
#237999=CARTESIAN_POINT('Ctrl Pts',(-0.1444199860808,-59.089305716615,2.71559944077426));
#238000=CARTESIAN_POINT('Ctrl Pts',(-0.144287542501481,-59.0891510807049,
2.71545515216009));
#238001=CARTESIAN_POINT('Ctrl Pts',(-0.144154785043327,-59.0889965840072,
2.7153110078167));
#238002=CARTESIAN_POINT('Ctrl Pts',(-0.138334211748957,-59.0822228828152,
2.7089911917603));
#238003=CARTESIAN_POINT('Ctrl Pts',(-0.131883990153634,-59.0757535782844,
2.70298296066791));
#238004=CARTESIAN_POINT('Ctrl Pts',(-0.124808417214922,-59.0697047694307,
2.69736727774094));
#238005=CARTESIAN_POINT('Ctrl Pts',(-0.118212753509866,-59.0640662283032,
2.69213248525398));
#238006=CARTESIAN_POINT('Ctrl Pts',(-0.111072931137383,-59.0587927761315,
2.68723866185448));
#238007=CARTESIAN_POINT('Ctrl Pts',(-0.103389544768496,-59.0540076654701,
2.68278595829549));
#238008=CARTESIAN_POINT('Ctrl Pts',(-0.100578862632642,-59.0522572100838,
2.68115710172775));
#238009=CARTESIAN_POINT('Ctrl Pts',(-0.0976954648434998,-59.0505724231957,
2.67958763637763));
#238010=CARTESIAN_POINT('Ctrl Pts',(-0.09473955852473,-59.0489605442858,
2.67808378645302));
#238011=CARTESIAN_POINT('Ctrl Pts',(-0.0940287618032339,-59.0485729412561,
2.67772216078538));
#238012=CARTESIAN_POINT('Ctrl Pts',(-0.0933131922161383,-59.0481896206933,
2.67736403603501));
#238013=CARTESIAN_POINT('Ctrl Pts',(-0.092592927196552,-59.0478106940135,
2.67700956934417));
#238014=CARTESIAN_POINT('Ctrl Pts',(-0.0918951704588278,-59.0474436087924,
2.67666617973741));
#238015=CARTESIAN_POINT('Ctrl Pts',(-0.0911930071928101,-59.0470806471269,
2.67632622314056));
#238016=CARTESIAN_POINT('Ctrl Pts',(-0.0904865115872116,-59.0467219102887,
2.67598984158711));
#238017=CARTESIAN_POINT('Ctrl Pts',(-0.0827460357491968,-59.0427915336439,
2.67230439292155));
#238018=CARTESIAN_POINT('Ctrl Pts',(-0.0744802459935639,-59.0393660724127,
2.66904964539906));
#238019=CARTESIAN_POINT('Ctrl Pts',(-0.0658168714600205,-59.0365841602687,
2.66640203566654));
#238020=CARTESIAN_POINT('Ctrl Pts',(-0.0622239118135767,-59.0354304183827,
2.66530399299372));
#238021=CARTESIAN_POINT('Ctrl Pts',(-0.0585629032857959,-59.0343871039215,
2.66430995142194));
#238022=CARTESIAN_POINT('Ctrl Pts',(-0.0548440714993542,-59.033462655426,
2.66343053473297));
#238023=CARTESIAN_POINT('Ctrl Pts',(-0.0485012163577858,-59.0318859121825,
2.66193059792821));
#238024=CARTESIAN_POINT('Ctrl Pts',(-0.0419914004938017,-59.0306571138135,
2.66076519817064));
#238025=CARTESIAN_POINT('Ctrl Pts',(-0.0353717968082149,-59.0298212958154,
2.65997805604397));
#238026=CARTESIAN_POINT('Ctrl Pts',(-0.0320619949654215,-59.0294033868163,
2.65958448498063));
#238027=CARTESIAN_POINT('Ctrl Pts',(-0.0287246785540649,-59.0290851681635,
2.65928526260699));
#238028=CARTESIAN_POINT('Ctrl Pts',(-0.0253670368742519,-59.0288723192862,
2.65908463971261));
#238029=CARTESIAN_POINT('Ctrl Pts',(-0.0220093951944389,-59.028659470409,
2.65888401681823));
#238030=CARTESIAN_POINT('Ctrl Pts',(-0.0186314705073835,-59.0285519740189,
2.6587819886022));
#238031=CARTESIAN_POINT('Ctrl Pts',(-0.0152399999993761,-59.0285534841294,
2.6587819886022));
#238032=CARTESIAN_POINT('Origin',(6.10537907909441,-57.9430040808455,2.83404198860222));
#238033=CARTESIAN_POINT('Ctrl Pts',(6.73887200051396,-62.2936141127567,
2.83404198860219));
#238034=CARTESIAN_POINT('Ctrl Pts',(6.73998108195386,-62.3041663177854,
2.82419652440036));
#238035=CARTESIAN_POINT('Ctrl Pts',(6.74025426844153,-62.3147747227668,
2.81438790575631));
#238036=CARTESIAN_POINT('Ctrl Pts',(6.73970068257657,-62.3253809467523,
2.80466781256892));
#238037=CARTESIAN_POINT('Ctrl Pts',(6.73916508495583,-62.3356425316141,
2.79526356453073));
#238038=CARTESIAN_POINT('Ctrl Pts',(6.73785543637712,-62.3459033574826,
2.7859410249623));
#238039=CARTESIAN_POINT('Ctrl Pts',(6.73573381164848,-62.3561113603647,
2.77675109088778));
#238040=CARTESIAN_POINT('Ctrl Pts',(6.7337268852973,-62.3657675025187,2.76805797913679));
#238041=CARTESIAN_POINT('Ctrl Pts',(6.73099321743878,-62.3753772873479,
2.75948271210155));
#238042=CARTESIAN_POINT('Ctrl Pts',(6.72746117704644,-62.3848821415109,
2.75108575573215));
#238043=CARTESIAN_POINT('Ctrl Pts',(6.72420791240144,-62.3936367996036,
2.74335155163256));
#238044=CARTESIAN_POINT('Ctrl Pts',(6.72027708243777,-62.4023029414998,
2.73576818685925));
#238045=CARTESIAN_POINT('Ctrl Pts',(6.71558140886371,-62.4108128192388,
2.72840626160476));
#238046=CARTESIAN_POINT('Ctrl Pts',(6.714219372456,-62.4132812112858,2.7262708469365));
#238047=CARTESIAN_POINT('Ctrl Pts',(6.71279278199583,-62.4157362792955,
2.72415424587485));
#238048=CARTESIAN_POINT('Ctrl Pts',(6.7112989968966,-62.4181758915947,2.72205867173213));
#238049=CARTESIAN_POINT('Ctrl Pts',(6.70967963780731,-62.4208205881799,
2.71978693462816));
#238050=CARTESIAN_POINT('Ctrl Pts',(6.70798448411237,-62.4234440047026,
2.71754411340717));
#238051=CARTESIAN_POINT('Ctrl Pts',(6.70621108803186,-62.4260429761971,
2.71533341844214));
#238052=CARTESIAN_POINT('Ctrl Pts',(6.70134398857332,-62.4331758738573,
2.70926614876362));
#238053=CARTESIAN_POINT('Ctrl Pts',(6.69585818364757,-62.4400912556835,
2.70347381860379));
#238054=CARTESIAN_POINT('Ctrl Pts',(6.68976801333951,-62.4466864116139,
2.69804914171366));
#238055=CARTESIAN_POINT('Ctrl Pts',(6.68419583815074,-62.4527206212308,
2.6930858568718));
#238056=CARTESIAN_POINT('Ctrl Pts',(6.67811620689392,-62.4584752900412,
2.68842799053166));
#238057=CARTESIAN_POINT('Ctrl Pts',(6.67150703079258,-62.4638645712583,
2.68414767054201));
#238058=CARTESIAN_POINT('Ctrl Pts',(6.66826062508132,-62.4665117685874,
2.68204519134531));
#238059=CARTESIAN_POINT('Ctrl Pts',(6.66488629458047,-62.4690703232298,
2.68003431778478));
#238060=CARTESIAN_POINT('Ctrl Pts',(6.66138078591774,-62.4715267736416,
2.67812693945224));
#238061=CARTESIAN_POINT('Ctrl Pts',(6.66071564979311,-62.4719928611811,
2.67776503299176));
#238062=CARTESIAN_POINT('Ctrl Pts',(6.66004526561052,-62.4724551899378,
2.67740659639896));
#238063=CARTESIAN_POINT('Ctrl Pts',(6.6593696982092,-62.4729136358126,2.67705178968828));
#238064=CARTESIAN_POINT('Ctrl Pts',(6.65871524228918,-62.4733577552539,
2.6767080706873));
#238065=CARTESIAN_POINT('Ctrl Pts',(6.65805592206515,-62.4737982306997,
2.67636775825238));
#238066=CARTESIAN_POINT('Ctrl Pts',(6.65739180030972,-62.4742349489457,
2.67603099699228));
#238067=CARTESIAN_POINT('Ctrl Pts',(6.65015433826464,-62.4789942144023,
2.67236104217096));
#238068=CARTESIAN_POINT('Ctrl Pts',(6.64234165497504,-62.4833100626577,
2.66911440541437));
#238069=CARTESIAN_POINT('Ctrl Pts',(6.63406423386179,-62.4870273554126,
2.66646778189592));
#238070=CARTESIAN_POINT('Ctrl Pts',(6.63056862752553,-62.4885971912262,
2.66535009634939));
#238071=CARTESIAN_POINT('Ctrl Pts',(6.62699051141425,-62.4900605069388,
2.66433897912313));
#238072=CARTESIAN_POINT('Ctrl Pts',(6.62333954252063,-62.4914070226218,
2.66344564884764));
#238073=CARTESIAN_POINT('Ctrl Pts',(6.61719140213135,-62.4936745213864,
2.66194130298556));
#238074=CARTESIAN_POINT('Ctrl Pts',(6.61083770188589,-62.4956084911388,
2.6607720670539));
#238075=CARTESIAN_POINT('Ctrl Pts',(6.60433062536211,-62.4971561593219,
2.65998225155684));
#238076=CARTESIAN_POINT('Ctrl Pts',(6.60270385623117,-62.4975430763676,
2.65978479768258));
#238077=CARTESIAN_POINT('Ctrl Pts',(6.60106746196622,-62.4979056188881,
2.65961098966592));
#238078=CARTESIAN_POINT('Ctrl Pts',(6.5994222184581,-62.4982426563693,2.65946139030471));
#238079=CARTESIAN_POINT('Ctrl Pts',(6.59695435319593,-62.498748212591,2.6592369912629));
#238080=CARTESIAN_POINT('Ctrl Pts',(6.59446659126666,-62.4991963674671,
2.65906707562411));
#238081=CARTESIAN_POINT('Ctrl Pts',(6.59196174500359,-62.4995849724119,
2.65895332562889));
#238082=CARTESIAN_POINT('Ctrl Pts',(6.58945689874051,-62.4999735773567,
2.65883957563366));
#238083=CARTESIAN_POINT('Ctrl Pts',(6.58693497617713,-62.5003026407459,
2.65878198860218));
#238084=CARTESIAN_POINT('Ctrl Pts',(6.58439859103091,-62.5005702980928,
2.65878198860218));
#238085=CARTESIAN_POINT('Ctrl Pts',(6.18532049829458,-58.7035958781036,
2.65878198860221));
#238086=CARTESIAN_POINT('Ctrl Pts',(6.19390281910186,-58.7026899760168,
2.65878198860221));
#238087=CARTESIAN_POINT('Ctrl Pts',(6.20248552904368,-58.7025003609926,
2.65945335517809));
#238088=CARTESIAN_POINT('Ctrl Pts',(6.21093474935395,-58.7029569544311,
2.66072561226544));
#238089=CARTESIAN_POINT('Ctrl Pts',(6.21639207873494,-58.7032518669431,
2.66154735980284));
#238090=CARTESIAN_POINT('Ctrl Pts',(6.22179377937545,-58.7038154335196,
2.66261895766835));
#238091=CARTESIAN_POINT('Ctrl Pts',(6.22710604846926,-58.7046202140514,
2.66391429250988));
#238092=CARTESIAN_POINT('Ctrl Pts',(6.23414715684702,-58.7056869045455,
2.66563118464085));
#238093=CARTESIAN_POINT('Ctrl Pts',(6.24102913891703,-58.707182795565,2.66774105138661));
#238094=CARTESIAN_POINT('Ctrl Pts',(6.24767922440805,-58.7090548163567,
2.67016894181711));
#238095=CARTESIAN_POINT('Ctrl Pts',(6.25100426715356,-58.7099908267526,
2.67138288703237));
#238096=CARTESIAN_POINT('Ctrl Pts',(6.2542715337672,-58.7110208470225,2.67267613167513));
#238097=CARTESIAN_POINT('Ctrl Pts',(6.25747333351575,-58.7121380880305,
2.67403835432515));
#238098=CARTESIAN_POINT('Ctrl Pts',(6.25907423339003,-58.7126967085345,
2.67471946565015));
#238099=CARTESIAN_POINT('Ctrl Pts',(6.260658782884,-58.7132771324568,2.67541781389484));
#238100=CARTESIAN_POINT('Ctrl Pts',(6.26222612320572,-58.7138784999413,
2.6761320724413));
#238101=CARTESIAN_POINT('Ctrl Pts',(6.26261795828615,-58.7140288418124,
2.67631063707792));
#238102=CARTESIAN_POINT('Ctrl Pts',(6.26300871814067,-58.7141804926176,
2.67649019601807));
#238103=CARTESIAN_POINT('Ctrl Pts',(6.26339839005111,-58.7143334388433,
2.67667072836618));
#238104=CARTESIAN_POINT('Ctrl Pts',(6.26456740578242,-58.7147922775205,
2.67721232541052));
#238105=CARTESIAN_POINT('Ctrl Pts',(6.26572662828427,-58.7152627751828,
2.67776268340008));
#238106=CARTESIAN_POINT('Ctrl Pts',(6.26687572965221,-58.7157445651921,
2.67832123541477));
#238107=CARTESIAN_POINT('Ctrl Pts',(6.27496985131181,-58.7191382318075,
2.68225560368397));
#238108=CARTESIAN_POINT('Ctrl Pts',(6.2826071619279,-58.7230632421214,2.6866179299883));
#238109=CARTESIAN_POINT('Ctrl Pts',(6.28978339589452,-58.7274000190308,
2.69130986622508));
#238110=CARTESIAN_POINT('Ctrl Pts',(6.29326386161389,-58.7295033511457,
2.69358545022994));
#238111=CARTESIAN_POINT('Ctrl Pts',(6.29663597408966,-58.7317041096967,
2.69593918853419));
#238112=CARTESIAN_POINT('Ctrl Pts',(6.29989941779204,-58.7339915094191,
2.69836306235435));
#238113=CARTESIAN_POINT('Ctrl Pts',(6.30489552208993,-58.737493358578,2.70207384382168));
#238114=CARTESIAN_POINT('Ctrl Pts',(6.30963480180928,-58.7411954596214,
2.70594760814168));
#238115=CARTESIAN_POINT('Ctrl Pts',(6.31410463171103,-58.7450534628847,
2.70995196345648));
#238116=CARTESIAN_POINT('Ctrl Pts',(6.31618044384124,-58.7468451395589,
2.71181160678046));
#238117=CARTESIAN_POINT('Ctrl Pts',(6.31819823791584,-58.7486702031821,
2.71369962772039));
#238118=CARTESIAN_POINT('Ctrl Pts',(6.32015576082374,-58.7505249478603,
2.71561183138601));
#238119=CARTESIAN_POINT('Ctrl Pts',(6.3203057972416,-58.7506671067318,2.71575839426252));
#238120=CARTESIAN_POINT('Ctrl Pts',(6.32045551058247,-58.7508094261756,
2.71590508903149));
#238121=CARTESIAN_POINT('Ctrl Pts',(6.32060490094057,-58.7509519047343,
2.71605191409852));
#238122=CARTESIAN_POINT('Ctrl Pts',(6.32270338507441,-58.7529532989254,
2.71811436362693));
#238123=CARTESIAN_POINT('Ctrl Pts',(6.32473679726686,-58.7549876922213,
2.72020091026899));
#238124=CARTESIAN_POINT('Ctrl Pts',(6.32670504965044,-58.7570493794207,
2.72230624862122));
#238125=CARTESIAN_POINT('Ctrl Pts',(6.3337628526565,-58.7644422230597,2.72985561753095));
#238126=CARTESIAN_POINT('Ctrl Pts',(6.34003880539021,-58.7722418109929,
2.73770089914377));
#238127=CARTESIAN_POINT('Ctrl Pts',(6.34560292136856,-58.7803396486564,
2.74574823347179));
#238128=CARTESIAN_POINT('Ctrl Pts',(6.35171732586367,-58.7892383587485,
2.75459144547171));
#238129=CARTESIAN_POINT('Ctrl Pts',(6.35697262978615,-58.7984976730916,
2.7636791175446));
#238130=CARTESIAN_POINT('Ctrl Pts',(6.3614285299299,-58.8080148760675,2.77292162564961));
#238131=CARTESIAN_POINT('Ctrl Pts',(6.36623978380681,-58.8182910667895,
2.78290121485001));
#238132=CARTESIAN_POINT('Ctrl Pts',(6.37011968263915,-58.8288688921888,
2.79306229500494));
#238133=CARTESIAN_POINT('Ctrl Pts',(6.37309732669983,-58.8396533761922,
2.80331916685595));
#238134=CARTESIAN_POINT('Ctrl Pts',(6.3760499913858,-58.8503473894538,2.8134899940891));
#238135=CARTESIAN_POINT('Ctrl Pts',(6.37811557911303,-58.8612460403475,
2.82375635966963));
#238136=CARTESIAN_POINT('Ctrl Pts',(6.37927424642637,-58.8722700234478,
2.83404198860221));
#238137=CARTESIAN_POINT('Origin',(-0.0151565136854075,-0.00159301378000414,
2.83404198860263));
#238138=CARTESIAN_POINT('Ctrl Pts',(6.55408556366009,-62.5037563256532,
2.65878198860219));
#238139=CARTESIAN_POINT('Ctrl Pts',(6.54554330587499,-62.5046505412975,
2.65878198860219));
#238140=CARTESIAN_POINT('Ctrl Pts',(6.53700226086782,-62.5048232320876,
2.65944603041798));
#238141=CARTESIAN_POINT('Ctrl Pts',(6.52859457177595,-62.5043472028587,
2.66070439264));
#238142=CARTESIAN_POINT('Ctrl Pts',(6.52322245869602,-62.5040430428429,
2.66150842619527));
#238143=CARTESIAN_POINT('Ctrl Pts',(6.51790471489697,-62.5034749678469,
2.66255428265308));
#238144=CARTESIAN_POINT('Ctrl Pts',(6.51267356740915,-62.5026702669704,
2.66381699700608));
#238145=CARTESIAN_POINT('Ctrl Pts',(6.50553410072719,-62.5015720117387,
2.66554034873208));
#238146=CARTESIAN_POINT('Ctrl Pts',(6.49855818190841,-62.5000273428096,
2.66766759643912));
#238147=CARTESIAN_POINT('Ctrl Pts',(6.49182203260243,-62.4980940659027,
2.67012012783088));
#238148=CARTESIAN_POINT('Ctrl Pts',(6.48845395794944,-62.4971274274492,
2.67134639352676));
#238149=CARTESIAN_POINT('Ctrl Pts',(6.48514561818799,-62.4960636607363,
2.67265375584952));
#238150=CARTESIAN_POINT('Ctrl Pts',(6.48190505740227,-62.4949101555727,
2.6740313512688));
#238151=CARTESIAN_POINT('Ctrl Pts',(6.4802847770094,-62.4943334029909,2.67472014897844));
#238152=CARTESIAN_POINT('Ctrl Pts',(6.47868142404743,-62.4937342176671,
2.67542649668573));
#238153=CARTESIAN_POINT('Ctrl Pts',(6.47709589524328,-62.4931135352111,
2.67614899656042));
#238154=CARTESIAN_POINT('Ctrl Pts',(6.47669951304224,-62.4929583645971,
2.6763296215291));
#238155=CARTESIAN_POINT('Ctrl Pts',(6.47630424448235,-62.4928018504532,
2.67651125590891));
#238156=CARTESIAN_POINT('Ctrl Pts',(6.47591010283135,-62.4926440074814,
2.67669387767464));
#238157=CARTESIAN_POINT('Ctrl Pts',(6.47472767787836,-62.4921704785658,
2.67724174297184));
#238158=CARTESIAN_POINT('Ctrl Pts',(6.47355539694529,-62.4916849899862,
2.67779849504688));
#238159=CARTESIAN_POINT('Ctrl Pts',(6.47239360181871,-62.491187940575,2.67836353617949));
#238160=CARTESIAN_POINT('Ctrl Pts',(6.46436487665244,-62.4877530207467,
2.68226832098846));
#238161=CARTESIAN_POINT('Ctrl Pts',(6.45678933786472,-62.4837949925046,
2.68659153751326));
#238162=CARTESIAN_POINT('Ctrl Pts',(6.44966853564076,-62.4794326364365,
2.6912369948611));
#238163=CARTESIAN_POINT('Ctrl Pts',(6.44612951648157,-62.4772645574451,
2.69354577441151));
#238164=CARTESIAN_POINT('Ctrl Pts',(6.44270272394416,-62.4749960038949,
2.69593478828055));
#238165=CARTESIAN_POINT('Ctrl Pts',(6.43938822718985,-62.4726384024731,
2.6983956526116));
#238166=CARTESIAN_POINT('Ctrl Pts',(6.43207595228416,-62.4674371815965,
2.70382468688986));
#238167=CARTESIAN_POINT('Ctrl Pts',(6.42530381744052,-62.4618132330507,
2.70961155815027));
#238168=CARTESIAN_POINT('Ctrl Pts',(6.41913840445487,-62.4558957623408,
2.71562701361707));
#238169=CARTESIAN_POINT('Ctrl Pts',(6.41688610134126,-62.4537340356672,
2.71782453535798));
#238170=CARTESIAN_POINT('Ctrl Pts',(6.41470741397529,-62.4515361835423,
2.72005051502342));
#238171=CARTESIAN_POINT('Ctrl Pts',(6.41260146153699,-62.449307446912,2.72229986760055));
#238172=CARTESIAN_POINT('Ctrl Pts',(6.40552779014133,-62.4418213564083,
2.72985520488845));
#238173=CARTESIAN_POINT('Ctrl Pts',(6.39923601079907,-62.4339335724856,
2.73770845534527));
#238174=CARTESIAN_POINT('Ctrl Pts',(6.39365709371045,-62.4257522463017,
2.74576706701739));
#238175=CARTESIAN_POINT('Ctrl Pts',(6.3875252029639,-62.4167599996838,2.75462443585034));
#238176=CARTESIAN_POINT('Ctrl Pts',(6.38225398283455,-62.4074126717492,
2.76373036323206));
#238177=CARTESIAN_POINT('Ctrl Pts',(6.37778536209574,-62.3978127557432,
2.77299664636864));
#238178=CARTESIAN_POINT('Ctrl Pts',(6.37297246609485,-62.387473234881,2.78297683033545));
#238179=CARTESIAN_POINT('Ctrl Pts',(6.36908997057768,-62.3768396913491,
2.79314401478987));
#238180=CARTESIAN_POINT('Ctrl Pts',(6.36611161569944,-62.3660067738125,
2.80341452428055));
#238181=CARTESIAN_POINT('Ctrl Pts',(6.3631734786686,-62.3553201372404,2.81354634721426));
#238182=CARTESIAN_POINT('Ctrl Pts',(6.36111515612499,-62.3444380411286,
2.82378004209212));
#238183=CARTESIAN_POINT('Ctrl Pts',(6.35995915837865,-62.3334394572617,
2.83404198860219));
#238184=CARTESIAN_POINT('Ctrl Pts',(6.00036140429106,-58.9120953679528,
2.83404198860221));
#238185=CARTESIAN_POINT('Ctrl Pts',(5.99925510810183,-58.9015696628141,
2.82422126442971));
#238186=CARTESIAN_POINT('Ctrl Pts',(5.99898299131244,-58.8909945468891,
2.8144281502847));
#238187=CARTESIAN_POINT('Ctrl Pts',(5.99953795195317,-58.8804276387775,
2.80471618166292));
#238188=CARTESIAN_POINT('Ctrl Pts',(6.00007381527937,-58.8702243592784,
2.79533842146204));
#238189=CARTESIAN_POINT('Ctrl Pts',(6.00138095727725,-58.8600274754021,
2.78603515650214));
#238190=CARTESIAN_POINT('Ctrl Pts',(6.00349883564024,-58.8498890377475,
2.7768588734673));
#238191=CARTESIAN_POINT('Ctrl Pts',(6.00550089397171,-58.8403050390018,
2.76818441216545));
#238192=CARTESIAN_POINT('Ctrl Pts',(6.00822762538657,-58.8307723843861,
2.75962261521585));
#238193=CARTESIAN_POINT('Ctrl Pts',(6.01175153639678,-58.8213500689036,
2.75123537701615));
#238194=CARTESIAN_POINT('Ctrl Pts',(6.01499699931917,-58.8126722744153,
2.74351087134063));
#238195=CARTESIAN_POINT('Ctrl Pts',(6.01891888229335,-58.804087581854,2.7359339944978));
#238196=CARTESIAN_POINT('Ctrl Pts',(6.02360485257626,-58.795664241304,2.728576578125));
#238197=CARTESIAN_POINT('Ctrl Pts',(6.02500211432165,-58.7931525711891,
2.72638274508255));
#238198=CARTESIAN_POINT('Ctrl Pts',(6.02646752363825,-58.7906554330084,
2.7242086170954));
#238199=CARTESIAN_POINT('Ctrl Pts',(6.02800395803762,-58.7881751602881,
2.72205663736668));
#238200=CARTESIAN_POINT('Ctrl Pts',(6.0295246938641,-58.7857202298422,2.71992664556707));
#238201=CARTESIAN_POINT('Ctrl Pts',(6.03111319985562,-58.7832842250417,
2.71782089927825));
#238202=CARTESIAN_POINT('Ctrl Pts',(6.03277025542088,-58.7808720541405,
2.71574387311186));
#238203=CARTESIAN_POINT('Ctrl Pts',(6.0328854838242,-58.7807043164934,2.71559944077427));
#238204=CARTESIAN_POINT('Ctrl Pts',(6.03300103800968,-58.7805366835712,
2.7154551521601));
#238205=CARTESIAN_POINT('Ctrl Pts',(6.0331169189062,-58.7803691562895,2.71531100781671));
#238206=CARTESIAN_POINT('Ctrl Pts',(6.03819756191484,-58.7730241465596,
2.70899119176029));
#238207=CARTESIAN_POINT('Ctrl Pts',(6.04393622206038,-58.7659160498048,
2.70298296066787));
#238208=CARTESIAN_POINT('Ctrl Pts',(6.05034076157616,-58.7591607781928,
2.69736727774089));
#238209=CARTESIAN_POINT('Ctrl Pts',(6.05631090550625,-58.7528636909923,
2.69213248525389));
#238210=CARTESIAN_POINT('Ctrl Pts',(6.06286038933315,-58.7468728126826,
2.68723866185436));
#238211=CARTESIAN_POINT('Ctrl Pts',(6.07000150504366,-58.7413107827882,
2.68278595829535));
#238212=CARTESIAN_POINT('Ctrl Pts',(6.07261381755706,-58.7392761202954,
2.68115710172766));
#238213=CARTESIAN_POINT('Ctrl Pts',(6.07530531160698,-58.7372991657063,
2.6795876363776));
#238214=CARTESIAN_POINT('Ctrl Pts',(6.07807653793614,-58.7353871404928,
2.67808378645304));
#238215=CARTESIAN_POINT('Ctrl Pts',(6.07874292528977,-58.734927362304,2.6777221607854));
#238216=CARTESIAN_POINT('Ctrl Pts',(6.07941450700242,-58.734471344222,2.67736403603502));
#238217=CARTESIAN_POINT('Ctrl Pts',(6.08009121771134,-58.7340192051466,
2.67700956934418));
#238218=CARTESIAN_POINT('Ctrl Pts',(6.0807467812106,-58.7335811954172,2.67666617973743));
#238219=CARTESIAN_POINT('Ctrl Pts',(6.08140715812765,-58.7331468260465,
2.67632622314058));
#238220=CARTESIAN_POINT('Ctrl Pts',(6.08207228526599,-58.7327162055063,
2.67598984158713));
#238221=CARTESIAN_POINT('Ctrl Pts',(6.08935952173666,-58.7279982598318,
2.6723043929216));
#238222=CARTESIAN_POINT('Ctrl Pts',(6.0972219724326,-58.7237275533348,2.66904964539913));
#238223=CARTESIAN_POINT('Ctrl Pts',(6.10554709909255,-58.7200553115699,
2.66640203566663));
#238224=CARTESIAN_POINT('Ctrl Pts',(6.10899977726383,-58.7185323234522,
2.66530399299378));
#238225=CARTESIAN_POINT('Ctrl Pts',(6.11253167434656,-58.7171120447813,
2.66430995142198));
#238226=CARTESIAN_POINT('Ctrl Pts',(6.11613350280284,-58.7158039367396,
2.66343053473299));
#238227=CARTESIAN_POINT('Ctrl Pts',(6.12227679657208,-58.7135728221599,
2.66193059792823));
#238228=CARTESIAN_POINT('Ctrl Pts',(6.12862250657844,-58.7116702942285,
2.66076519817065));
#238229=CARTESIAN_POINT('Ctrl Pts',(6.13511848061151,-58.7101471179282,
2.65997805604398));
#238230=CARTESIAN_POINT('Ctrl Pts',(6.13836646762804,-58.709385529778,2.65958448498064));
#238231=CARTESIAN_POINT('Ctrl Pts',(6.14165223896415,-58.7087202098044,
2.659285262607));
#238232=CARTESIAN_POINT('Ctrl Pts',(6.14496923836547,-58.7081575578105,
2.65908463971262));
#238233=CARTESIAN_POINT('Ctrl Pts',(6.14828623776679,-58.7075949058167,
2.65888401681824));
#238234=CARTESIAN_POINT('Ctrl Pts',(6.15163442139651,-58.7071349090265,
2.65878198860221));
#238235=CARTESIAN_POINT('Ctrl Pts',(6.15500747092375,-58.706781905664,2.65878198860221));
#238236=CARTESIAN_POINT('Origin',(12.128626347365,-56.9874003490099,2.83404198860222));
#238237=CARTESIAN_POINT('Ctrl Pts',(13.21341150919,-61.2479592423874,2.8340419886022));
#238238=CARTESIAN_POINT('Ctrl Pts',(13.2156175207415,-61.2583377107542,
2.82419652440026));
#238239=CARTESIAN_POINT('Ctrl Pts',(13.2169980909554,-61.2688594460194,
2.81438790575614));
#238240=CARTESIAN_POINT('Ctrl Pts',(13.217556189986,-61.2794654334799,2.80466781256871));
#238241=CARTESIAN_POINT('Ctrl Pts',(13.2180961541214,-61.2897267895024,
2.7952635645305));
#238242=CARTESIAN_POINT('Ctrl Pts',(13.2178662282945,-61.3000683010466,
2.78594102496207));
#238243=CARTESIAN_POINT('Ctrl Pts',(13.2168232529024,-61.3104421535934,
2.77675109088757));
#238244=CARTESIAN_POINT('Ctrl Pts',(13.2158366624042,-61.3202551793176,
2.76805797913662));
#238245=CARTESIAN_POINT('Ctrl Pts',(13.2141224659048,-61.3300980668404,
2.75948271210143));
#238246=CARTESIAN_POINT('Ctrl Pts',(13.2116033021986,-61.3399200511723,
2.75108575573207));
#238247=CARTESIAN_POINT('Ctrl Pts',(13.2092829702346,-61.3489668090859,
2.74335155163254));
#238248=CARTESIAN_POINT('Ctrl Pts',(13.2062795322636,-61.3579963605655,
2.73576818685928));
#238249=CARTESIAN_POINT('Ctrl Pts',(13.2024991065234,-61.3669504518464,
2.72840626160483));
#238250=CARTESIAN_POINT('Ctrl Pts',(13.201402548721,-61.3695476933562,2.72627084693655));
#238251=CARTESIAN_POINT('Ctrl Pts',(13.2002403977589,-61.372138431555,2.72415424587488));
#238252=CARTESIAN_POINT('Ctrl Pts',(13.1990098046953,-61.3747208224636,
2.72205867173214));
#238253=CARTESIAN_POINT('Ctrl Pts',(13.1976757626944,-61.3775203002413,
2.71978693462817));
#238254=CARTESIAN_POINT('Ctrl Pts',(13.1962641169264,-61.3803065372246,
2.71754411340718));
#238255=CARTESIAN_POINT('Ctrl Pts',(13.1947721021916,-61.3830766416483,
2.71533341844215));
#238256=CARTESIAN_POINT('Ctrl Pts',(13.1906772560442,-61.3906792149758,
2.70926614876363));
#238257=CARTESIAN_POINT('Ctrl Pts',(13.1859443571671,-61.3981301363755,
2.7034738186038));
#238258=CARTESIAN_POINT('Ctrl Pts',(13.1805769309636,-61.405325759495,2.69804914171366));
#238259=CARTESIAN_POINT('Ctrl Pts',(13.1756660273918,-61.4119093639898,
2.69308585687178));
#238260=CARTESIAN_POINT('Ctrl Pts',(13.1702212276784,-61.4182680026348,
2.6884279905316));
#238261=CARTESIAN_POINT('Ctrl Pts',(13.164211590619,-61.424318607827,2.68414767054194));
#238262=CARTESIAN_POINT('Ctrl Pts',(13.1612596765267,-61.4272906453322,
2.68204519134527));
#238263=CARTESIAN_POINT('Ctrl Pts',(13.1581712727464,-61.4301878975263,
2.68003431778476));
#238264=CARTESIAN_POINT('Ctrl Pts',(13.1549417366136,-61.4329973166792,
2.67812693945224));
#238265=CARTESIAN_POINT('Ctrl Pts',(13.1543289635885,-61.4335303765994,
2.67776503299176));
#238266=CARTESIAN_POINT('Ctrl Pts',(13.1537105783551,-61.4340602468992,
2.67740659639897));
#238267=CARTESIAN_POINT('Ctrl Pts',(13.1530866324255,-61.4345867973818,
2.67705178968828));
#238268=CARTESIAN_POINT('Ctrl Pts',(13.1524821848061,-61.4350968931619,
2.6767080706873));
#238269=CARTESIAN_POINT('Ctrl Pts',(13.1518725186287,-61.435603873367,2.67636775825238));
#238270=CARTESIAN_POINT('Ctrl Pts',(13.1512576844889,-61.4361076188512,
2.67603099699228));
#238271=CARTESIAN_POINT('Ctrl Pts',(13.1445573487226,-61.4415973333393,
2.67236104217094));
#238272=CARTESIAN_POINT('Ctrl Pts',(13.1372385931153,-61.4467061867047,
2.66911440541433));
#238273=CARTESIAN_POINT('Ctrl Pts',(13.1293950794801,-61.4512683418497,
2.66646778189587));
#238274=CARTESIAN_POINT('Ctrl Pts',(13.1260827149663,-61.4531949682969,
2.66535009634936));
#238275=CARTESIAN_POINT('Ctrl Pts',(13.1226771582923,-61.4550242827914,
2.66433897912312));
#238276=CARTESIAN_POINT('Ctrl Pts',(13.1191869390034,-61.4567450522886,
2.66344564884764));
#238277=CARTESIAN_POINT('Ctrl Pts',(13.1133094969318,-61.4596427851245,
2.66194130298557));
#238278=CARTESIAN_POINT('Ctrl Pts',(13.1071927578073,-61.462230302911,2.66077206705391));
#238279=CARTESIAN_POINT('Ctrl Pts',(13.1008831031064,-61.4644496675151,
2.65998225155685));
#238280=CARTESIAN_POINT('Ctrl Pts',(13.0993056894312,-61.4650045086662,
2.65978479768258));
#238281=CARTESIAN_POINT('Ctrl Pts',(13.0977161555177,-61.4655361149186,
2.65961098966593));
#238282=CARTESIAN_POINT('Ctrl Pts',(13.0961151548357,-61.4660432808488,
2.65946139030472));
#238283=CARTESIAN_POINT('Ctrl Pts',(13.0937136538126,-61.4668040297441,
2.6592369912629));
#238284=CARTESIAN_POINT('Ctrl Pts',(13.091286365044,-61.4675097715122,2.65906707562412));
#238285=CARTESIAN_POINT('Ctrl Pts',(13.0888358608685,-61.4681580753691,
2.65895332562889));
#238286=CARTESIAN_POINT('Ctrl Pts',(13.0863853566931,-61.468806379226,2.65883957563367));
#238287=CARTESIAN_POINT('Ctrl Pts',(13.0839116459757,-61.4693972526616,
2.65878198860219));
#238288=CARTESIAN_POINT('Ctrl Pts',(13.0814171332239,-61.4699285681951,
2.65878198860219));
#238289=CARTESIAN_POINT('Ctrl Pts',(12.2876333308477,-57.7354693911201,
2.65878198860222));
#238290=CARTESIAN_POINT('Ctrl Pts',(12.296073944251,-57.7336713548543,2.65878198860222));
#238291=CARTESIAN_POINT('Ctrl Pts',(12.3045898170431,-57.7325856410802,
2.65945335517815));
#238292=CARTESIAN_POINT('Ctrl Pts',(12.3130404786512,-57.7321565492372,
2.66072561226561));
#238293=CARTESIAN_POINT('Ctrl Pts',(12.3184987389622,-57.731879399934,2.66154735980299));
#238294=CARTESIAN_POINT('Ctrl Pts',(12.3239297572692,-57.7318752477668,
2.66261895766843));
#238295=CARTESIAN_POINT('Ctrl Pts',(12.3292970476689,-57.7321203363018,
2.66391429250987));
#238296=CARTESIAN_POINT('Ctrl Pts',(12.3364110836364,-57.7324451871154,
2.66563118464083));
#238297=CARTESIAN_POINT('Ctrl Pts',(12.343411728678,-57.7332135204773,2.66774105138659));
#238298=CARTESIAN_POINT('Ctrl Pts',(12.3502210637615,-57.7343801629263,
2.6701689418171));
#238299=CARTESIAN_POINT('Ctrl Pts',(12.3536257313032,-57.7349634841508,
2.67138288703235));
#238300=CARTESIAN_POINT('Ctrl Pts',(12.3569827659245,-57.7356463395037,
2.67267613167511));
#238301=CARTESIAN_POINT('Ctrl Pts',(12.3602838093647,-57.7364227809411,
2.67403835432513));
#238302=CARTESIAN_POINT('Ctrl Pts',(12.3619343310848,-57.7368110016598,
2.67471946565014));
#238303=CARTESIAN_POINT('Ctrl Pts',(12.3635708710714,-57.7372226154356,
2.67541781389483));
#238304=CARTESIAN_POINT('Ctrl Pts',(12.3651924853579,-57.7376568568908,
2.67613207244129));
#238305=CARTESIAN_POINT('Ctrl Pts',(12.3655978889295,-57.7377654172546,
2.67631063707791));
#238306=CARTESIAN_POINT('Ctrl Pts',(12.3660023599863,-57.7378753917738,
2.67649019601806));
#238307=CARTESIAN_POINT('Ctrl Pts',(12.3664058844672,-57.7379867683381,
2.67667072836617));
#238308=CARTESIAN_POINT('Ctrl Pts',(12.3676164579098,-57.7383208980311,
2.67721232541051));
#238309=CARTESIAN_POINT('Ctrl Pts',(12.3688185104671,-57.7386676465112,
2.67776268340007));
#238310=CARTESIAN_POINT('Ctrl Pts',(12.3700116777068,-57.7390266834243,
2.67832123541476));
#238311=CARTESIAN_POINT('Ctrl Pts',(12.3784161936774,-57.7415556930804,
2.68225560368407));
#238312=CARTESIAN_POINT('Ctrl Pts',(12.3864219416035,-57.744660885435,2.68661792998854));
#238313=CARTESIAN_POINT('Ctrl Pts',(12.3940121800357,-57.7482237843183,
2.69130986622547));
#238314=CARTESIAN_POINT('Ctrl Pts',(12.3976934374731,-57.7499517864266,
2.69358545023021));
#238315=CARTESIAN_POINT('Ctrl Pts',(12.4012771190731,-57.7517880072568,
2.69593918853433));
#238316=CARTESIAN_POINT('Ctrl Pts',(12.4047617836671,-57.7537217536089,
2.69836306235435));
#238317=CARTESIAN_POINT('Ctrl Pts',(12.410096561694,-57.7566821841671,2.70207384382168));
#238318=CARTESIAN_POINT('Ctrl Pts',(12.4151968540761,-57.7598686150877,
2.70594760814168));
#238319=CARTESIAN_POINT('Ctrl Pts',(12.4200454689344,-57.7632382593548,
2.70995196345648));
#238320=CARTESIAN_POINT('Ctrl Pts',(12.422297190758,-57.7648031395846,2.71181160678046));
#238321=CARTESIAN_POINT('Ctrl Pts',(12.4244947022414,-57.7664072884045,
2.7136996277204));
#238322=CARTESIAN_POINT('Ctrl Pts',(12.426635375245,-57.7680472557359,2.71561183138603));
#238323=CARTESIAN_POINT('Ctrl Pts',(12.426799449396,-57.76817295277,2.71575839426253));
#238324=CARTESIAN_POINT('Ctrl Pts',(12.4269632190243,-57.7682988432676,
2.7159050890315));
#238325=CARTESIAN_POINT('Ctrl Pts',(12.4271266840712,-57.7684249257693,
2.71605191409852));
#238326=CARTESIAN_POINT('Ctrl Pts',(12.4294228751485,-57.7701960047918,
2.71811436362694));
#238327=CARTESIAN_POINT('Ctrl Pts',(12.4316578001011,-57.7720067040167,
2.720200910269));
#238328=CARTESIAN_POINT('Ctrl Pts',(12.4338307751869,-57.773851358681,2.72230624862123));
#238329=CARTESIAN_POINT('Ctrl Pts',(12.4416226773939,-57.7804659622463,
2.72985561753044));
#238330=CARTESIAN_POINT('Ctrl Pts',(12.4486795287422,-57.7875668075255,
2.73770089914271));
#238331=CARTESIAN_POINT('Ctrl Pts',(12.4550596184374,-57.7950386758937,
2.74574823347014));
#238332=CARTESIAN_POINT('Ctrl Pts',(12.4620706960757,-57.8032495086148,
2.75459144546965));
#238333=CARTESIAN_POINT('Ctrl Pts',(12.4682650727925,-57.8119087706216,
2.7636791175421));
#238334=CARTESIAN_POINT('Ctrl Pts',(12.4736913816506,-57.8209080689689,
2.77292162564668));
#238335=CARTESIAN_POINT('Ctrl Pts',(12.4795504333999,-57.8306250526684,
2.78290121484682));
#238336=CARTESIAN_POINT('Ctrl Pts',(12.4845147615742,-57.8407393717705,
2.7930622950015));
#238337=CARTESIAN_POINT('Ctrl Pts',(12.4886033793293,-57.851153528684,2.80331916685226));
#238338=CARTESIAN_POINT('Ctrl Pts',(12.4926576977823,-57.861480321521,2.81348999408662));
#238339=CARTESIAN_POINT('Ctrl Pts',(12.495851189234,-57.8721033557552,2.8237563596684));
#238340=CARTESIAN_POINT('Ctrl Pts',(12.4981558292594,-57.8829458346102,
2.83404198860222));
#238341=CARTESIAN_POINT('Origin',(-0.0149069694351787,-0.00316857416786783,
2.83404198860263));
#238342=CARTESIAN_POINT('Ctrl Pts',(13.0516031943535,-61.4762657165312,
2.65878198860219));
#238343=CARTESIAN_POINT('Ctrl Pts',(13.0432012029372,-61.4780479426478,
2.65878198860219));
#238344=CARTESIAN_POINT('Ctrl Pts',(13.0347249977709,-61.479112469729,2.65944603041803));
#238345=CARTESIAN_POINT('Ctrl Pts',(13.0263136082755,-61.4795178910584,
2.66070439264014));
#238346=CARTESIAN_POINT('Ctrl Pts',(13.0209391308144,-61.4797769359878,
2.6615084261954));
#238347=CARTESIAN_POINT('Ctrl Pts',(13.0155911381662,-61.4797678285534,
2.66255428265317));
#238348=CARTESIAN_POINT('Ctrl Pts',(13.0103045333059,-61.4795143397205,
2.66381699700611));
#238349=CARTESIAN_POINT('Ctrl Pts',(13.0030893784378,-61.4791683783267,
2.66554034873211));
#238350=CARTESIAN_POINT('Ctrl Pts',(12.9959902125628,-61.4783613533296,
2.66766759643915));
#238351=CARTESIAN_POINT('Ctrl Pts',(12.9890888821234,-61.4771427864511,
2.67012012783091));
#238352=CARTESIAN_POINT('Ctrl Pts',(12.9856382169037,-61.4765335030119,
2.67134639352679));
#238353=CARTESIAN_POINT('Ctrl Pts',(12.9822368066739,-61.4758213793956,
2.67265375584955));
#238354=CARTESIAN_POINT('Ctrl Pts',(12.9788934238971,-61.4750129240931,
2.67403135126883));
#238355=CARTESIAN_POINT('Ctrl Pts',(12.9772217325087,-61.4746086964418,
2.67472014897847));
#238356=CARTESIAN_POINT('Ctrl Pts',(12.9755645309609,-61.474180389539,2.67542649668576));
#238357=CARTESIAN_POINT('Ctrl Pts',(12.9739228088661,-61.4737288401358,
2.67614899656045));
#238358=CARTESIAN_POINT('Ctrl Pts',(12.9735123783424,-61.473615952785,2.67632962152912));
#238359=CARTESIAN_POINT('Ctrl Pts',(12.9731029149221,-61.4735016128572,
2.67651125590894));
#238360=CARTESIAN_POINT('Ctrl Pts',(12.972694433337,-61.4733858335867,2.67669387767467));
#238361=CARTESIAN_POINT('Ctrl Pts',(12.9714689885818,-61.4730384957754,
2.67724174297187));
#238362=CARTESIAN_POINT('Ctrl Pts',(12.9702523821512,-61.4726782034774,
2.67779849504691));
#238363=CARTESIAN_POINT('Ctrl Pts',(12.9690449956487,-61.4723053176141,
2.67836353617952));
#238364=CARTESIAN_POINT('Ctrl Pts',(12.9607012057879,-61.4697284449397,
2.68226832098848));
#238365=CARTESIAN_POINT('Ctrl Pts',(12.9527534399846,-61.4665839586183,
2.68659153751326));
#238366=CARTESIAN_POINT('Ctrl Pts',(12.9452156558843,-61.462989826507,2.69123699486108));
#238367=CARTESIAN_POINT('Ctrl Pts',(12.9414693978771,-61.4612035527133,
2.6935457744115));
#238368=CARTESIAN_POINT('Ctrl Pts',(12.9378242492513,-61.4593056238946,
2.69593478828055));
#238369=CARTESIAN_POINT('Ctrl Pts',(12.9342814732034,-61.4573073969123,
2.69839565261162));
#238370=CARTESIAN_POINT('Ctrl Pts',(12.9264655800793,-61.4528990097267,
2.70382468688987));
#238371=CARTESIAN_POINT('Ctrl Pts',(12.919142681,-61.4480137506079,2.70961155815028));
#238372=CARTESIAN_POINT('Ctrl Pts',(12.912392498672,-61.4427731575664,2.71562701361708));
#238373=CARTESIAN_POINT('Ctrl Pts',(12.9099265719433,-61.4408587028411,
2.71782453535799));
#238374=CARTESIAN_POINT('Ctrl Pts',(12.9075300815496,-61.4389006256223,
2.72005051502344));
#238375=CARTESIAN_POINT('Ctrl Pts',(12.9052026993241,-61.4369042302167,
2.72229986760058));
#238376=CARTESIAN_POINT('Ctrl Pts',(12.8973852687049,-61.4301985493012,
2.72985520488788));
#238377=CARTESIAN_POINT('Ctrl Pts',(12.8903034584567,-61.4230116455107,
2.73770845534406));
#238378=CARTESIAN_POINT('Ctrl Pts',(12.8838999218066,-61.4154582931183,
2.74576706701549));
#238379=CARTESIAN_POINT('Ctrl Pts',(12.8768616764793,-61.4071562640856,
2.75462443584776));
#238380=CARTESIAN_POINT('Ctrl Pts',(12.870642270821,-61.398411134332,2.76373036322875));
#238381=CARTESIAN_POINT('Ctrl Pts',(12.8651946651867,-61.3893309057298,
2.77299664636458));
#238382=CARTESIAN_POINT('Ctrl Pts',(12.8593273605072,-61.3795511104685,
2.78297683033057));
#238383=CARTESIAN_POINT('Ctrl Pts',(12.8543546257423,-61.3693816498916,
2.79314401478415));
#238384=CARTESIAN_POINT('Ctrl Pts',(12.8502602383809,-61.3589193990701,
2.80341452427397));
#238385=CARTESIAN_POINT('Ctrl Pts',(12.8462211390724,-61.3485984239579,
2.81354634720985));
#238386=CARTESIAN_POINT('Ctrl Pts',(12.8430366034505,-61.3379910943972,
2.82378004208991));
#238387=CARTESIAN_POINT('Ctrl Pts',(12.8407372733105,-61.327173596589,2.8340419886022));
#238388=CARTESIAN_POINT('Ctrl Pts',(12.1254815933798,-57.9621601888118,
2.83404198860222));
#238389=CARTESIAN_POINT('Ctrl Pts',(12.123281121814,-57.9518077840283,2.82422126443027));
#238390=CARTESIAN_POINT('Ctrl Pts',(12.1219050950924,-57.9413190436452,
2.81442815028583));
#238391=CARTESIAN_POINT('Ctrl Pts',(12.1213524729342,-57.9307520129796,
2.8047161816646));
#238392=CARTESIAN_POINT('Ctrl Pts',(12.1208188676186,-57.9205486151435,
2.79533842146407));
#238393=CARTESIAN_POINT('Ctrl Pts',(12.1210529843541,-57.9102709573202,
2.78603515650452));
#238394=CARTESIAN_POINT('Ctrl Pts',(12.1220995054496,-57.8999666805176,
2.77685887347001));
#238395=CARTESIAN_POINT('Ctrl Pts',(12.123088795635,-57.8902259118393,2.76818441216839));
#238396=CARTESIAN_POINT('Ctrl Pts',(12.1248041559918,-57.8804604570588,
2.75962261521902));
#238397=CARTESIAN_POINT('Ctrl Pts',(12.1273238624907,-57.870721409004,2.7512353770195));
#238398=CARTESIAN_POINT('Ctrl Pts',(12.129644469905,-57.8617519091303,2.74351087134412));
#238399=CARTESIAN_POINT('Ctrl Pts',(12.1326475236725,-57.8528042960128,
2.73593399450142));
#238400=CARTESIAN_POINT('Ctrl Pts',(12.1364273448763,-57.8439372821313,
2.72857657812872));
#238401=CARTESIAN_POINT('Ctrl Pts',(12.1375544112588,-57.8412933175836,
2.726382745085));
#238402=CARTESIAN_POINT('Ctrl Pts',(12.1387507708939,-57.8386566820017,
2.72420861709662));
#238403=CARTESIAN_POINT('Ctrl Pts',(12.1400195294497,-57.8360293953468,
2.72205663736668));
#238404=CARTESIAN_POINT('Ctrl Pts',(12.1412753244192,-57.8334289530878,
2.71992664556707));
#238405=CARTESIAN_POINT('Ctrl Pts',(12.1426004965704,-57.8308402488863,
2.71782089927826));
#238406=CARTESIAN_POINT('Ctrl Pts',(12.1439963340944,-57.8282680826378,
2.71574387311187));
#238407=CARTESIAN_POINT('Ctrl Pts',(12.144093397906,-57.8280892192272,2.71559944077428));
#238408=CARTESIAN_POINT('Ctrl Pts',(12.1441907966618,-57.8279104259143,
2.7154551521601));
#238409=CARTESIAN_POINT('Ctrl Pts',(12.1442885313814,-57.8277317035125,
2.71531100781671));
#238410=CARTESIAN_POINT('Ctrl Pts',(12.1485735795163,-57.8198958587082,
2.70899119176024));
#238411=CARTESIAN_POINT('Ctrl Pts',(12.1535378042506,-57.8122268475249,
2.70298296066779));
#238412=CARTESIAN_POINT('Ctrl Pts',(12.1592011408683,-57.8048391253241,
2.69736727774077));
#238413=CARTESIAN_POINT('Ctrl Pts',(12.1644803548772,-57.7979524842555,
2.69213248525369));
#238414=CARTESIAN_POINT('Ctrl Pts',(12.1703677426432,-57.7913098171243,
2.68723866185408));
#238415=CARTESIAN_POINT('Ctrl Pts',(12.1768883481373,-57.7850318067603,
2.68278595829502));
#238416=CARTESIAN_POINT('Ctrl Pts',(12.1792736699857,-57.7827352293491,
2.68115710172745));
#238417=CARTESIAN_POINT('Ctrl Pts',(12.1817437717242,-57.7804877669873,
2.6795876363775));
#238418=CARTESIAN_POINT('Ctrl Pts',(12.1842999559281,-57.7782965440185,
2.67808378645305));
#238419=CARTESIAN_POINT('Ctrl Pts',(12.1849146328346,-57.7777696280968,
2.6777221607854));
#238420=CARTESIAN_POINT('Ctrl Pts',(12.185534868683,-57.7772459087252,2.67736403603503));
#238421=CARTESIAN_POINT('Ctrl Pts',(12.1861606108971,-57.7767255109844,
2.67700956934419));
#238422=CARTESIAN_POINT('Ctrl Pts',(12.1867667986671,-57.776221375673,2.67666617973744));
#238423=CARTESIAN_POINT('Ctrl Pts',(12.1873781540075,-57.7757203576389,
2.67632622314058));
#238424=CARTESIAN_POINT('Ctrl Pts',(12.1879946254064,-57.7752225713654,
2.67598984158713));
#238425=CARTESIAN_POINT('Ctrl Pts',(12.194748782022,-57.7697687474612,2.67230439292162));
#238426=CARTESIAN_POINT('Ctrl Pts',(12.2021217510032,-57.7646995864525,
2.66904964539918));
#238427=CARTESIAN_POINT('Ctrl Pts',(12.2100174179597,-57.760177248916,2.66640203566668));
#238428=CARTESIAN_POINT('Ctrl Pts',(12.2132919863912,-57.7583017007431,
2.66530399299382));
#238429=CARTESIAN_POINT('Ctrl Pts',(12.2166560758254,-57.7565200187329,
2.66430995142199));
#238430=CARTESIAN_POINT('Ctrl Pts',(12.2201014385652,-57.7548425830504,
2.663430534733));
#238431=CARTESIAN_POINT('Ctrl Pts',(12.22597786375,-57.7519815416927,2.66193059792823));
#238432=CARTESIAN_POINT('Ctrl Pts',(12.232089942972,-57.7494261286931,2.66076519817066));
#238433=CARTESIAN_POINT('Ctrl Pts',(12.2383911161017,-57.7472322823289,
2.65997805604398));
#238434=CARTESIAN_POINT('Ctrl Pts',(12.2415417026665,-57.7461353591468,
2.65958448498064));
#238435=CARTESIAN_POINT('Ctrl Pts',(12.244739929329,-57.7451302272372,2.659285262607));
#238436=CARTESIAN_POINT('Ctrl Pts',(12.2479799447123,-57.7442239366597,
2.65908463971263));
#238437=CARTESIAN_POINT('Ctrl Pts',(12.2512199600955,-57.7433176460823,
2.65888401681825));
#238438=CARTESIAN_POINT('Ctrl Pts',(12.2545017192674,-57.7425101887129,
2.65878198860222));
#238439=CARTESIAN_POINT('Ctrl Pts',(12.2578193919774,-57.7418065394563,
2.65878198860222));
#238440=CARTESIAN_POINT('Origin',(18.0189898472955,-55.4074307335703,2.83404198860224));
#238441=CARTESIAN_POINT('Ctrl Pts',(19.5431821162873,-59.5312589135992,
2.83404198860221));
#238442=CARTESIAN_POINT('Ctrl Pts',(19.5464608884259,-59.5413499366323,
2.82419652440104));
#238443=CARTESIAN_POINT('Ctrl Pts',(19.5489337165498,-59.5516697238472,
2.81438790575766));
#238444=CARTESIAN_POINT('Ctrl Pts',(19.5505973858262,-59.5621592733639,
2.80466781257095));
#238445=CARTESIAN_POINT('Ctrl Pts',(19.5522069957576,-59.5723079749825,
2.79526356453334));
#238446=CARTESIAN_POINT('Ctrl Pts',(19.5530593117982,-59.5826168684371,
2.78594102496549));
#238447=CARTESIAN_POINT('Ctrl Pts',(19.5531064127995,-59.5930429125485,
2.77675109089153));
#238448=CARTESIAN_POINT('Ctrl Pts',(19.5531509674465,-59.6029053082791,
2.76805797914111));
#238449=CARTESIAN_POINT('Ctrl Pts',(19.5524750234021,-59.6128734577593,
2.75948271210642));
#238450=CARTESIAN_POINT('Ctrl Pts',(19.5509963368671,-59.6229049605435,
2.7510857557375));
#238451=CARTESIAN_POINT('Ctrl Pts',(19.549634359627,-59.6321447001044,2.7433515516385));
#238452=CARTESIAN_POINT('Ctrl Pts',(19.5475912199442,-59.641438731511,2.73576818686571));
#238453=CARTESIAN_POINT('Ctrl Pts',(19.544767461174,-59.6507389334354,2.72840626161167));
#238454=CARTESIAN_POINT('Ctrl Pts',(19.543948396093,-59.6534365684892,2.72627084694109));
#238455=CARTESIAN_POINT('Ctrl Pts',(19.5430634173973,-59.6561345922101,
2.72415424587715));
#238456=CARTESIAN_POINT('Ctrl Pts',(19.5421094990035,-59.6588314685158,
2.72205867173219));
#238457=CARTESIAN_POINT('Ctrl Pts',(19.5410753901343,-59.6617550558215,
2.71978693462821));
#238458=CARTESIAN_POINT('Ctrl Pts',(19.5399627185796,-59.6646735866698,
2.7175441134072));
#238459=CARTESIAN_POINT('Ctrl Pts',(19.5387684320161,-59.6675844741791,
2.71533341844217));
#238460=CARTESIAN_POINT('Ctrl Pts',(19.5354907031712,-59.6755734277895,
2.70926614876364));
#238461=CARTESIAN_POINT('Ctrl Pts',(19.5315625649731,-59.6834782549086,
2.70347381860381));
#238462=CARTESIAN_POINT('Ctrl Pts',(19.5269766895189,-59.6911955084645,
2.69804914171367));
#238463=CARTESIAN_POINT('Ctrl Pts',(19.5227808624514,-59.6982563764886,
2.69308585687186));
#238464=CARTESIAN_POINT('Ctrl Pts',(19.5180305486467,-59.7051493183925,
2.68842799053174));
#238465=CARTESIAN_POINT('Ctrl Pts',(19.5126862934705,-59.7117949558629,
2.68414767054212));
#238466=CARTESIAN_POINT('Ctrl Pts',(19.5100612127856,-59.7150592712796,
2.68204519134539));
#238467=CARTESIAN_POINT('Ctrl Pts',(19.5072925729238,-59.7182634781242,
2.68003431778482));
#238468=CARTESIAN_POINT('Ctrl Pts',(19.5043743927945,-59.7213950854342,
2.67812693945226));
#238469=CARTESIAN_POINT('Ctrl Pts',(19.5038206965385,-59.7219892774189,
2.67776503299178));
#238470=CARTESIAN_POINT('Ctrl Pts',(19.5032610854122,-59.7225808838919,
2.67740659639898));
#238471=CARTESIAN_POINT('Ctrl Pts',(19.5026955970365,-59.7231697699851,
2.6770517896883));
#238472=CARTESIAN_POINT('Ctrl Pts',(19.5021477801725,-59.7237402533879,
2.67670807068732));
#238473=CARTESIAN_POINT('Ctrl Pts',(19.5015944476719,-59.724308183771,2.6763677582524));
#238474=CARTESIAN_POINT('Ctrl Pts',(19.5010356373992,-59.7248734373526,
2.67603099699229));
#238475=CARTESIAN_POINT('Ctrl Pts',(19.4949458381923,-59.7310334544116,
2.67236104217082));
#238476=CARTESIAN_POINT('Ctrl Pts',(19.488201196085,-59.7368793392205,2.66911440541411));
#238477=CARTESIAN_POINT('Ctrl Pts',(19.4808775251044,-59.7422363728294,
2.66646778189559));
#238478=CARTESIAN_POINT('Ctrl Pts',(19.4777846933721,-59.7444986813875,
2.6653500963492));
#238479=CARTESIAN_POINT('Ctrl Pts',(19.474589008127,-59.7466739523113,2.66433897912305));
#238480=CARTESIAN_POINT('Ctrl Pts',(19.4712977780161,-59.7487501225116,
2.66344564884766));
#238481=CARTESIAN_POINT('Ctrl Pts',(19.4657554287474,-59.7522463412516,
2.66194130298558));
#238482=CARTESIAN_POINT('Ctrl Pts',(19.4599426670177,-59.7554590576858,
2.66077206705392));
#238483=CARTESIAN_POINT('Ctrl Pts',(19.4538995640369,-59.758325802888,2.65998225155686));
#238484=CARTESIAN_POINT('Ctrl Pts',(19.4523887882917,-59.7590424891886,
2.6597847976826));
#238485=CARTESIAN_POINT('Ctrl Pts',(19.450863529996,-59.7597373347836,2.65961098966594));
#238486=CARTESIAN_POINT('Ctrl Pts',(19.4493243130385,-59.7604090725468,
2.65946139030473));
#238487=CARTESIAN_POINT('Ctrl Pts',(19.4470154876023,-59.7614166791915,
2.65923699126292));
#238488=CARTESIAN_POINT('Ctrl Pts',(19.444675265878,-59.7623722755973,2.65906707562413));
#238489=CARTESIAN_POINT('Ctrl Pts',(19.4423059520267,-59.7632731754136,
2.65895332562891));
#238490=CARTESIAN_POINT('Ctrl Pts',(19.4399366381754,-59.7641740752298,
2.65883957563368));
#238491=CARTESIAN_POINT('Ctrl Pts',(19.4375382417965,-59.7650202849787,
2.6587819886022));
#238492=CARTESIAN_POINT('Ctrl Pts',(19.4351129318427,-59.7658094374947,
2.6587819886022));
#238493=CARTESIAN_POINT('Ctrl Pts',(18.2553202812755,-56.1347810195638,
2.65878198860223));
#238494=CARTESIAN_POINT('Ctrl Pts',(18.2635267101475,-56.1321105487808,
2.65878198860223));
#238495=CARTESIAN_POINT('Ctrl Pts',(18.2718824441049,-56.130140631564,2.65945335517815));
#238496=CARTESIAN_POINT('Ctrl Pts',(18.2802419597936,-56.1288305556595,
2.66072561226558));
#238497=CARTESIAN_POINT('Ctrl Pts',(18.2856413491927,-56.1279843810467,
2.66154735980296));
#238498=CARTESIAN_POINT('Ctrl Pts',(18.2910421817936,-56.1274125556279,
2.6626189576684));
#238499=CARTESIAN_POINT('Ctrl Pts',(18.2964056883429,-56.1270952669248,
2.66391429250985));
#238500=CARTESIAN_POINT('Ctrl Pts',(18.3035147090334,-56.1266747189243,
2.66563118464082));
#238501=CARTESIAN_POINT('Ctrl Pts',(18.3105573165146,-56.1267070766077,
2.66774105138658));
#238502=CARTESIAN_POINT('Ctrl Pts',(18.3174512966904,-56.1271555587351,
2.67016894181709));
#238503=CARTESIAN_POINT('Ctrl Pts',(18.3208982867783,-56.1273797997988,
2.67138288703234));
#238504=CARTESIAN_POINT('Ctrl Pts',(18.3243083090333,-56.1277080087286,
2.67267613167511));
#238505=CARTESIAN_POINT('Ctrl Pts',(18.3276724292424,-56.1281351437406,
2.67403835432513));
#238506=CARTESIAN_POINT('Ctrl Pts',(18.329354489347,-56.1283487112466,2.67471946565014));
#238507=CARTESIAN_POINT('Ctrl Pts',(18.3310250895518,-56.1285870051492,
2.67541781389483));
#238508=CARTESIAN_POINT('Ctrl Pts',(18.3326832110576,-56.1288493629349,
2.6761320724413));
#238509=CARTESIAN_POINT('Ctrl Pts',(18.333097741434,-56.1289149523813,2.67631063707791));
#238510=CARTESIAN_POINT('Ctrl Pts',(18.3335114922235,-56.1289820457105,
2.67649019601806));
#238511=CARTESIAN_POINT('Ctrl Pts',(18.3339244481761,-56.1290506323485,
2.67667072836617));
#238512=CARTESIAN_POINT('Ctrl Pts',(18.3351633160341,-56.1292563922624,
2.67721232541051));
#238513=CARTESIAN_POINT('Ctrl Pts',(18.3363950287075,-56.1294755925115,
2.67776268340008));
#238514=CARTESIAN_POINT('Ctrl Pts',(18.337619189229,-56.1297079426449,2.67832123541478));
#238515=CARTESIAN_POINT('Ctrl Pts',(18.3462420178745,-56.1313445869825,
2.68225560368399));
#238516=CARTESIAN_POINT('Ctrl Pts',(18.3545284904606,-56.1335959402404,
2.68661792998835));
#238517=CARTESIAN_POINT('Ctrl Pts',(18.3624495731173,-56.1363459252316,
2.69130986622515));
#238518=CARTESIAN_POINT('Ctrl Pts',(18.3662912896465,-56.1376796649807,
2.69358545022999));
#238519=CARTESIAN_POINT('Ctrl Pts',(18.3700472768054,-56.1391312300707,
2.69593918853423));
#238520=CARTESIAN_POINT('Ctrl Pts',(18.3737149835769,-56.140690136523,2.69836306235437));
#238521=CARTESIAN_POINT('Ctrl Pts',(18.3793299863885,-56.1430767133838,
2.7020738438217));
#238522=CARTESIAN_POINT('Ctrl Pts',(18.3847354115627,-56.1457125629775,
2.7059476081417));
#238523=CARTESIAN_POINT('Ctrl Pts',(18.3899096889384,-56.1485569297206,
2.7099519634565));
#238524=CARTESIAN_POINT('Ctrl Pts',(18.3923126501199,-56.1498778683509,
2.71181160678048));
#238525=CARTESIAN_POINT('Ctrl Pts',(18.3946658026165,-56.1512435269773,
2.71369962772041));
#238526=CARTESIAN_POINT('Ctrl Pts',(18.3969661720543,-56.1526507491366,
2.71561183138603));
#238527=CARTESIAN_POINT('Ctrl Pts',(18.3971424863078,-56.1527586071704,
2.71575839426254));
#238528=CARTESIAN_POINT('Ctrl Pts',(18.3973185179292,-56.1528666894391,
2.71590508903151));
#238529=CARTESIAN_POINT('Ctrl Pts',(18.3974942667076,-56.1529749944975,
2.71605191409853));
#238530=CARTESIAN_POINT('Ctrl Pts',(18.3999630071785,-56.1544963540392,
2.71811436362695));
#238531=CARTESIAN_POINT('Ctrl Pts',(18.4023749585858,-56.1560635207934,
2.72020091026901));
#238532=CARTESIAN_POINT('Ctrl Pts',(18.404728848804,-56.1576709325,2.72230624862124));
#238533=CARTESIAN_POINT('Ctrl Pts',(18.4131694805012,-56.1634348250113,
2.72985561753041));
#238534=CARTESIAN_POINT('Ctrl Pts',(18.4209299141243,-56.16975912929,2.73770089914263));
#238535=CARTESIAN_POINT('Ctrl Pts',(18.4280560759389,-56.1765231650101,
2.74574823347001));
#238536=CARTESIAN_POINT('Ctrl Pts',(18.4358870118867,-56.183956160759,2.75459144546945));
#238537=CARTESIAN_POINT('Ctrl Pts',(18.4429525945103,-56.1919204977433,
2.76367911754183));
#238538=CARTESIAN_POINT('Ctrl Pts',(18.4492898603074,-56.2003032932664,
2.77292162564633));
#238539=CARTESIAN_POINT('Ctrl Pts',(18.4561325169318,-56.2093546086369,
2.78290121484639));
#238540=CARTESIAN_POINT('Ctrl Pts',(18.4621268842297,-56.2188946068453,
2.79306229500099));
#238541=CARTESIAN_POINT('Ctrl Pts',(18.4672816799273,-56.2288243369867,
2.80331916685167));
#238542=CARTESIAN_POINT('Ctrl Pts',(18.4723932321855,-56.2386707668947,
2.81348999408623));
#238543=CARTESIAN_POINT('Ctrl Pts',(18.4766796388007,-56.2489017962822,
2.82375635966821));
#238544=CARTESIAN_POINT('Ctrl Pts',(18.4801050014197,-56.2594439784235,
2.83404198860223));
#238545=CARTESIAN_POINT('Origin',(-0.0144941013083342,-0.00470941899407953,
2.83404198860263));
#238546=CARTESIAN_POINT('Ctrl Pts',(19.406124729226,-59.7752282754833,2.65878198860221));
#238547=CARTESIAN_POINT('Ctrl Pts',(19.3979550581551,-59.7778789856298,
2.65878198860221));
#238548=CARTESIAN_POINT('Ctrl Pts',(19.3896365599077,-59.7798236858206,
2.65944603041802));
#238549=CARTESIAN_POINT('Ctrl Pts',(19.3813136269528,-59.7811061158275,
2.66070439264007));
#238550=CARTESIAN_POINT('Ctrl Pts',(19.3759956690097,-59.7819255275515,
2.66150842619534));
#238551=CARTESIAN_POINT('Ctrl Pts',(19.3706760212385,-59.7824754874617,
2.66255428265314));
#238552=CARTESIAN_POINT('Ctrl Pts',(19.3653918801545,-59.7827759879491,
2.66381699700612));
#238553=CARTESIAN_POINT('Ctrl Pts',(19.3581800878468,-59.7831861108186,
2.66554034873212));
#238554=CARTESIAN_POINT('Ctrl Pts',(19.3510354548625,-59.7831255716882,
2.66766759643916));
#238555=CARTESIAN_POINT('Ctrl Pts',(19.3440445557102,-59.782635065712,2.67012012783092));
#238556=CARTESIAN_POINT('Ctrl Pts',(19.340549106134,-59.7823898127239,2.6713463935268));
#238557=CARTESIAN_POINT('Ctrl Pts',(19.337091891998,-59.7820371343795,2.67265375584956));
#238558=CARTESIAN_POINT('Ctrl Pts',(19.3336823180315,-59.7815825865435,
2.67403135126883));
#238559=CARTESIAN_POINT('Ctrl Pts',(19.3319775310482,-59.7813553126255,
2.67472014897847));
#238560=CARTESIAN_POINT('Ctrl Pts',(19.3302846375616,-59.7811025767638,
2.67542649668576));
#238561=CARTESIAN_POINT('Ctrl Pts',(19.328604709227,-59.7808251076832,2.67614899656045));
#238562=CARTESIAN_POINT('Ctrl Pts',(19.3281847271434,-59.7807557404131,
2.67632962152913));
#238563=CARTESIAN_POINT('Ctrl Pts',(19.3277655550296,-59.7806848274334,
2.67651125590894));
#238564=CARTESIAN_POINT('Ctrl Pts',(19.3273472089201,-59.7806123803663,
2.67669387767467));
#238565=CARTESIAN_POINT('Ctrl Pts',(19.3260921705918,-59.7803950391649,
2.67724174297187));
#238566=CARTESIAN_POINT('Ctrl Pts',(19.3248445680583,-59.7801638905864,
2.67779849504691));
#238567=CARTESIAN_POINT('Ctrl Pts',(19.3236048185592,-59.7799192536865,
2.67836353617952));
#238568=CARTESIAN_POINT('Ctrl Pts',(19.3150373803116,-59.7782286609223,
2.68226832098846));
#238569=CARTESIAN_POINT('Ctrl Pts',(19.306804464878,-59.7759321681718,2.68659153751323));
#238570=CARTESIAN_POINT('Ctrl Pts',(19.2989322844414,-59.7731456380807,
2.69123699486104));
#238571=CARTESIAN_POINT('Ctrl Pts',(19.2950198323729,-59.7717607402742,
2.69354577441147));
#238572=CARTESIAN_POINT('Ctrl Pts',(19.2911962646698,-59.7702542302925,
2.69593478828054));
#238573=CARTESIAN_POINT('Ctrl Pts',(19.287464024724,-59.7686372707427,2.69839565261162));
#238574=CARTESIAN_POINT('Ctrl Pts',(19.2792301459423,-59.7650700164607,
2.70382468688988));
#238575=CARTESIAN_POINT('Ctrl Pts',(19.271436713842,-59.7609769706898,2.70961155815029));
#238576=CARTESIAN_POINT('Ctrl Pts',(19.2641757185818,-59.7564706723509,
2.71562701361709));
#238577=CARTESIAN_POINT('Ctrl Pts',(19.2615231854473,-59.7548244647403,
2.717824535358));
#238578=CARTESIAN_POINT('Ctrl Pts',(19.2589351484761,-59.7531276155315,
2.72005051502344));
#238579=CARTESIAN_POINT('Ctrl Pts',(19.2564118357501,-59.7513854342762,
2.72229986760057));
#238580=CARTESIAN_POINT('Ctrl Pts',(19.247936295312,-59.7455336317913,2.72985520488834));
#238581=CARTESIAN_POINT('Ctrl Pts',(19.2401420439519,-59.7391263493537,
2.737708455345));
#238582=CARTESIAN_POINT('Ctrl Pts',(19.2329840462271,-59.732283726861,2.74576706701695));
#238583=CARTESIAN_POINT('Ctrl Pts',(19.2251165588069,-59.7247628741795,
2.75462443584974));
#238584=CARTESIAN_POINT('Ctrl Pts',(19.2180171087289,-59.7167157560769,
2.76373036323129));
#238585=CARTESIAN_POINT('Ctrl Pts',(19.2116502033062,-59.7082546997619,
2.77299664636771));
#238586=CARTESIAN_POINT('Ctrl Pts',(19.2047927733656,-59.6991417795832,
2.78297683033439));
#238587=CARTESIAN_POINT('Ctrl Pts',(19.1987842816755,-59.6895478206978,
2.79314401478871));
#238588=CARTESIAN_POINT('Ctrl Pts',(19.1936187207957,-59.6795708631991,
2.80341452427932));
#238589=CARTESIAN_POINT('Ctrl Pts',(19.1885229124293,-59.6697286283138,
2.8135463472134));
#238590=CARTESIAN_POINT('Ctrl Pts',(19.1842470541693,-59.6595122814311,
2.82378004209167));
#238591=CARTESIAN_POINT('Ctrl Pts',(19.1808295835788,-59.648994388456,2.83404198860221));
#238592=CARTESIAN_POINT('Ctrl Pts',(18.1177524687112,-56.3771794532803,
2.83404198860223));
#238593=CARTESIAN_POINT('Ctrl Pts',(18.1144819305957,-56.3671137719644,
2.82422126442995));
#238594=CARTESIAN_POINT('Ctrl Pts',(18.1120170699785,-56.3568263239569,
2.81442815028516));
#238595=CARTESIAN_POINT('Ctrl Pts',(18.1103629196655,-56.3463749453355,
2.8047161816636));
#238596=CARTESIAN_POINT('Ctrl Pts',(18.1087656919998,-56.3362832197238,
2.79533842146289));
#238597=CARTESIAN_POINT('Ctrl Pts',(18.1079242184411,-56.3260373921225,
2.78603515650317));
#238598=CARTESIAN_POINT('Ctrl Pts',(18.1078879163654,-56.3156801719843,
2.77685887346849));
#238599=CARTESIAN_POINT('Ctrl Pts',(18.1078535995348,-56.3058893552732,
2.76818441216681));
#238600=CARTESIAN_POINT('Ctrl Pts',(18.1085387949868,-56.2959980926936,
2.75962261521739));
#238601=CARTESIAN_POINT('Ctrl Pts',(18.1100266905431,-56.2860490151148,
2.75123537701784));
#238602=CARTESIAN_POINT('Ctrl Pts',(18.1113970173892,-56.276886081573,2.7435108713425));
#238603=CARTESIAN_POINT('Ctrl Pts',(18.113448339865,-56.2676735798209,2.73593399449985));
#238604=CARTESIAN_POINT('Ctrl Pts',(18.116280599478,-56.2584600414674,2.7285765781272));
#238605=CARTESIAN_POINT('Ctrl Pts',(18.1171251221217,-56.2557127503178,
2.726382745084));
#238606=CARTESIAN_POINT('Ctrl Pts',(18.1180393245077,-56.252965504868,2.72420861709613));
#238607=CARTESIAN_POINT('Ctrl Pts',(18.1190265064346,-56.2502199893828,
2.72205663736669));
#238608=CARTESIAN_POINT('Ctrl Pts',(18.1200036017947,-56.2475025263002,
2.71992664556708));
#238609=CARTESIAN_POINT('Ctrl Pts',(18.1210509212422,-56.2447894850826,
2.71782089927827));
#238610=CARTESIAN_POINT('Ctrl Pts',(18.122170247637,-56.2420855046787,2.71574387311188));
#238611=CARTESIAN_POINT('Ctrl Pts',(18.1222480834054,-56.2418974751695,
2.71559944077429));
#238612=CARTESIAN_POINT('Ctrl Pts',(18.1223262596104,-56.2417094803627,
2.71545515216011));
#238613=CARTESIAN_POINT('Ctrl Pts',(18.1224047773509,-56.241521520961,2.71531100781673));
#238614=CARTESIAN_POINT('Ctrl Pts',(18.1258472827279,-56.233280692238,2.70899119176036));
#238615=CARTESIAN_POINT('Ctrl Pts',(18.1299826829659,-56.2251347899177,
2.70298296066801));
#238616=CARTESIAN_POINT('Ctrl Pts',(18.1348427679842,-56.2171955585586,
2.69736727774107));
#238617=CARTESIAN_POINT('Ctrl Pts',(18.1393732118983,-56.209794815103,2.69213248525417));
#238618=CARTESIAN_POINT('Ctrl Pts',(18.1445340001506,-56.2025731376018,
2.68723866185472));
#238619=CARTESIAN_POINT('Ctrl Pts',(18.1503626543095,-56.1956479299638,
2.68278595829577));
#238620=CARTESIAN_POINT('Ctrl Pts',(18.1524948514079,-56.1931145994164,
2.68115710172794));
#238621=CARTESIAN_POINT('Ctrl Pts',(18.1547164978841,-56.1906212529493,
2.67958763637774));
#238622=CARTESIAN_POINT('Ctrl Pts',(18.1570296338743,-56.1881748397222,
2.67808378645306));
#238623=CARTESIAN_POINT('Ctrl Pts',(18.1575858658048,-56.1875865590686,
2.67772216078541));
#238624=CARTESIAN_POINT('Ctrl Pts',(18.1581479603552,-56.1870008763864,
2.67736403603504));
#238625=CARTESIAN_POINT('Ctrl Pts',(18.1587158783119,-56.1864179215668,
2.6770095693442));
#238626=CARTESIAN_POINT('Ctrl Pts',(18.1592660488324,-56.1858531840854,
2.67666617973745));
#238627=CARTESIAN_POINT('Ctrl Pts',(18.1598216844591,-56.1852910066462,
2.6763262231406));
#238628=CARTESIAN_POINT('Ctrl Pts',(18.160382745929,-56.1847315084901,2.67598984158714));
#238629=CARTESIAN_POINT('Ctrl Pts',(18.1665298227365,-56.178601559592,2.67230439292156));
#238630=CARTESIAN_POINT('Ctrl Pts',(18.1733325302119,-56.1727894828603,
2.66904964539906));
#238631=CARTESIAN_POINT('Ctrl Pts',(18.1807122308858,-56.1674665972284,
2.66640203566653));
#238632=CARTESIAN_POINT('Ctrl Pts',(18.1837728127204,-56.1652590378988,
2.66530399299373));
#238633=CARTESIAN_POINT('Ctrl Pts',(18.1869322368379,-56.1631354730303,
2.66430995142196));
#238634=CARTESIAN_POINT('Ctrl Pts',(18.1901833857459,-56.1611070880435,
2.663430534733));
#238635=CARTESIAN_POINT('Ctrl Pts',(18.1957285590022,-56.1576474660757,
2.66193059792824));
#238636=CARTESIAN_POINT('Ctrl Pts',(18.2015400422208,-56.1544671656474,
2.66076519817067));
#238637=CARTESIAN_POINT('Ctrl Pts',(18.2075773774756,-56.1516266854589,
2.659978056044));
#238638=CARTESIAN_POINT('Ctrl Pts',(18.210596045103,-56.1502064453646,2.65958448498066));
#238639=CARTESIAN_POINT('Ctrl Pts',(18.2136716866514,-56.1488725139546,
2.65928526260701));
#238640=CARTESIAN_POINT('Ctrl Pts',(18.21679921973,-56.1476325143028,2.65908463971264));
#238641=CARTESIAN_POINT('Ctrl Pts',(18.2199267528087,-56.146392514651,2.65888401681826));
#238642=CARTESIAN_POINT('Ctrl Pts',(18.2231061318825,-56.1452464433748,
2.65878198860223));
#238643=CARTESIAN_POINT('Ctrl Pts',(18.2263320786588,-56.1441998575524,
2.65878198860223));
#238644=CARTESIAN_POINT('Origin',(23.7119335237431,-53.2204057122634,2.83404198860225));
#238645=CARTESIAN_POINT('Ctrl Pts',(25.6588335304447,-57.1623216544366,
2.83404198860222));
#238646=CARTESIAN_POINT('Ctrl Pts',(25.6631491402573,-57.1720146727775,
2.82419652440011));
#238647=CARTESIAN_POINT('Ctrl Pts',(25.6666871334691,-57.1820194461955,
2.8143879057558));
#238648=CARTESIAN_POINT('Ctrl Pts',(25.6694381454826,-57.1922776320705,
2.80466781256816));
#238649=CARTESIAN_POINT('Ctrl Pts',(25.6720997659868,-57.202202487988,2.79526356452979));
#238650=CARTESIAN_POINT('Ctrl Pts',(25.6740249857416,-57.2123658169605,
2.78594102496119));
#238651=CARTESIAN_POINT('Ctrl Pts',(25.6751616470875,-57.222729822717,2.77675109088652));
#238652=CARTESIAN_POINT('Ctrl Pts',(25.6762368587291,-57.2325335339839,
2.76805797913539));
#238653=CARTESIAN_POINT('Ctrl Pts',(25.6766065729233,-57.2425177322914,
2.75948271210003));
#238654=CARTESIAN_POINT('Ctrl Pts',(25.6761845643577,-57.2526488462859,
2.75108575573051));
#238655=CARTESIAN_POINT('Ctrl Pts',(25.6757958639483,-57.2619803349756,
2.7433515516308));
#238656=CARTESIAN_POINT('Ctrl Pts',(25.6747354076184,-57.2714370189582,
2.73576818685737));
#238657=CARTESIAN_POINT('Ctrl Pts',(25.6728992535086,-57.2809814365693,
2.72840626160277));
#238658=CARTESIAN_POINT('Ctrl Pts',(25.6723666549991,-57.2837499093065,
2.7262708469352));
#238659=CARTESIAN_POINT('Ctrl Pts',(25.6717685445834,-57.2865256584304,
2.72415424587422));
#238660=CARTESIAN_POINT('Ctrl Pts',(25.6711017521911,-57.2893074725855,
2.72205867173215));
#238661=CARTESIAN_POINT('Ctrl Pts',(25.6703789063668,-57.2923231379851,
2.71978693462819));
#238662=CARTESIAN_POINT('Ctrl Pts',(25.669577399688,-57.2953419866638,2.7175441134072));
#238663=CARTESIAN_POINT('Ctrl Pts',(25.6686939261493,-57.2983617649659,
2.71533341844218));
#238664=CARTESIAN_POINT('Ctrl Pts',(25.66626922609,-57.3066495702118,2.70926614876366));
#238665=CARTESIAN_POINT('Ctrl Pts',(25.6631888860751,-57.3149216961102,
2.70347381860383));
#238666=CARTESIAN_POINT('Ctrl Pts',(25.6594348051813,-57.3230760282576,
2.69804914171369));
#238667=CARTESIAN_POINT('Ctrl Pts',(25.6560000249773,-57.3305367994634,
2.69308585687179));
#238668=CARTESIAN_POINT('Ctrl Pts',(25.6519962425132,-57.3378885241126,
2.68842799053161));
#238669=CARTESIAN_POINT('Ctrl Pts',(25.6473759219982,-57.3450563828665,
2.68414767054193));
#238670=CARTESIAN_POINT('Ctrl Pts',(25.6451064356542,-57.3485772116716,
2.68204519134528));
#238671=CARTESIAN_POINT('Ctrl Pts',(25.6426878935088,-57.3520532672058,
2.68003431778478));
#238672=CARTESIAN_POINT('Ctrl Pts',(25.6401130415753,-57.3554727521276,
2.67812693945227));
#238673=CARTESIAN_POINT('Ctrl Pts',(25.6396244885003,-57.3561215660853,
2.67776503299179));
#238674=CARTESIAN_POINT('Ctrl Pts',(25.6391297826978,-57.3567684269672,
2.677406596399));
#238675=CARTESIAN_POINT('Ctrl Pts',(25.6386289474849,-57.3574131967117,
2.67705178968831));
#238676=CARTESIAN_POINT('Ctrl Pts',(25.6381437633725,-57.3580378174017,
2.67670807068733));
#238677=CARTESIAN_POINT('Ctrl Pts',(25.6376528269754,-57.3586604755986,
2.67636775825241));
#238678=CARTESIAN_POINT('Ctrl Pts',(25.6371561630121,-57.359281044241,2.67603099699231));
#238679=CARTESIAN_POINT('Ctrl Pts',(25.6317436214796,-57.3660438734343,
2.67236104217107));
#238680=CARTESIAN_POINT('Ctrl Pts',(25.6256469885835,-57.372562740949,2.66911440541455));
#238681=CARTESIAN_POINT('Ctrl Pts',(25.6189233999302,-57.3786559602399,
2.66646778189613));
#238682=CARTESIAN_POINT('Ctrl Pts',(25.6160839866903,-57.3812291645836,
2.66535009634953));
#238683=CARTESIAN_POINT('Ctrl Pts',(25.6131331854698,-57.3837265592139,
2.66433897912321));
#238684=CARTESIAN_POINT('Ctrl Pts',(25.6100770039418,-57.3861353831627,
2.66344564884768));
#238685=CARTESIAN_POINT('Ctrl Pts',(25.6049304706145,-57.3901917825026,
2.6619413029856));
#238686=CARTESIAN_POINT('Ctrl Pts',(25.5994853721135,-57.3939944983909,
2.66077206705394));
#238687=CARTESIAN_POINT('Ctrl Pts',(25.5937750303537,-57.3974772155308,
2.65998225155688));
#238688=CARTESIAN_POINT('Ctrl Pts',(25.5923474449137,-57.3983478948158,
2.65978479768261));
#238689=CARTESIAN_POINT('Ctrl Pts',(25.5909031732848,-57.3991983668797,
2.65961098966596));
#238690=CARTESIAN_POINT('Ctrl Pts',(25.589442604035,-57.4000273167763,2.65946139030475));
#238691=CARTESIAN_POINT('Ctrl Pts',(25.5872517501602,-57.4012707416212,
2.65923699126293));
#238692=CARTESIAN_POINT('Ctrl Pts',(25.5850242354392,-57.4024657229505,
2.65906707562415));
#238693=CARTESIAN_POINT('Ctrl Pts',(25.5827620706104,-57.4036093482792,
2.65895332562892));
#238694=CARTESIAN_POINT('Ctrl Pts',(25.5804999057817,-57.4047529736078,
2.6588395756337));
#238695=CARTESIAN_POINT('Ctrl Pts',(25.5782031010737,-57.4058452484191,
2.65878198860222));
#238696=CARTESIAN_POINT('Ctrl Pts',(25.5758735661215,-57.4068835917975,
2.65878198860222));
#238697=CARTESIAN_POINT('Ctrl Pts',(24.0229981225303,-53.919068240199,2.65878198860225));
#238698=CARTESIAN_POINT('Ctrl Pts',(24.0308804555195,-53.9155545931353,
2.65878198860225));
#238699=CARTESIAN_POINT('Ctrl Pts',(24.0389845034728,-53.912722055301,2.65945335517821));
#238700=CARTESIAN_POINT('Ctrl Pts',(24.0471612846391,-53.9105453488008,
2.66072561226574));
#238701=CARTESIAN_POINT('Ctrl Pts',(24.052442646286,-53.9091394197447,2.66154735980311));
#238702=CARTESIAN_POINT('Ctrl Pts',(24.0577541205282,-53.9080061861133,
2.66261895766853));
#238703=CARTESIAN_POINT('Ctrl Pts',(24.0630550795267,-53.9071299964537,
2.66391429250993));
#238704=CARTESIAN_POINT('Ctrl Pts',(24.0700811970218,-53.9059686572511,
2.66563118464089));
#238705=CARTESIAN_POINT('Ctrl Pts',(24.0770886066612,-53.9052646847382,
2.66774105138665));
#238706=CARTESIAN_POINT('Ctrl Pts',(24.0839917000398,-53.90499009288,2.67016894181716));
#238707=CARTESIAN_POINT('Ctrl Pts',(24.0874432467291,-53.9048527969509,
2.67138288703242));
#238708=CARTESIAN_POINT('Ctrl Pts',(24.0908688957005,-53.9048227635318,
2.67267613167517));
#238709=CARTESIAN_POINT('Ctrl Pts',(24.0942592346735,-53.9048959123378,
2.67403835432519));
#238710=CARTESIAN_POINT('Ctrl Pts',(24.09595440416,-53.9049324867408,2.6747194656502));
#238711=CARTESIAN_POINT('Ctrl Pts',(24.0976407611376,-53.9049948499723,
2.67541781389489));
#238712=CARTESIAN_POINT('Ctrl Pts',(24.0993172231363,-53.9050824496417,
2.67613207244135));
#238713=CARTESIAN_POINT('Ctrl Pts',(24.099736338636,-53.9051043495591,2.67631063707797));
#238714=CARTESIAN_POINT('Ctrl Pts',(24.100154836018,-53.9051278266098,2.67649019601811));
#238715=CARTESIAN_POINT('Ctrl Pts',(24.1005726990106,-53.9051528718718,
2.67667072836623));
#238716=CARTESIAN_POINT('Ctrl Pts',(24.1018262879885,-53.9052280076581,
2.67721232541056));
#238717=CARTESIAN_POINT('Ctrl Pts',(24.1030741658761,-53.9053172580723,
2.67776268340013));
#238718=CARTESIAN_POINT('Ctrl Pts',(24.1043159075206,-53.9054203757492,
2.67832123541482));
#238719=CARTESIAN_POINT('Ctrl Pts',(24.1130625753261,-53.9061467233506,
2.68225560368406));
#238720=CARTESIAN_POINT('Ctrl Pts',(24.1215389842447,-53.9075195712144,
2.68661792998844));
#238721=CARTESIAN_POINT('Ctrl Pts',(24.129704126087,-53.9094265129026,2.69130986622527));
#238722=CARTESIAN_POINT('Ctrl Pts',(24.1336642110574,-53.9103513775608,
2.69358545023008));
#238723=CARTESIAN_POINT('Ctrl Pts',(24.1375513523939,-53.9114023832595,
2.69593918853428));
#238724=CARTESIAN_POINT('Ctrl Pts',(24.1413619171796,-53.9125693701067,
2.69836306235439));
#238725=CARTESIAN_POINT('Ctrl Pts',(24.1471956256301,-53.9143559454345,
2.70207384382172));
#238726=CARTESIAN_POINT('Ctrl Pts',(24.152846960627,-53.9164123347816,2.70594760814172));
#238727=CARTESIAN_POINT('Ctrl Pts',(24.1582902100545,-53.9187002605234,
2.70995196345652));
#238728=CARTESIAN_POINT('Ctrl Pts',(24.1608180832483,-53.9197627850741,
2.71181160678049));
#238729=CARTESIAN_POINT('Ctrl Pts',(24.1633010951269,-53.9208749910653,
2.71369962772043));
#238730=CARTESIAN_POINT('Ctrl Pts',(24.16573595767,-53.9220340502322,2.71561183138605));
#238731=CARTESIAN_POINT('Ctrl Pts',(24.1659225802901,-53.9221228875504,
2.71575839426256));
#238732=CARTESIAN_POINT('Ctrl Pts',(24.1661089452653,-53.9222119774183,
2.71590508903153));
#238733=CARTESIAN_POINT('Ctrl Pts',(24.1662950522348,-53.9223013184205,
2.71605191409855));
#238734=CARTESIAN_POINT('Ctrl Pts',(24.1689092940621,-53.9235562901478,
2.71811436362697));
#238735=CARTESIAN_POINT('Ctrl Pts',(24.1714718460797,-53.9248627542245,
2.72020091026904));
#238736=CARTESIAN_POINT('Ctrl Pts',(24.1739808617166,-53.9262153118344,
2.72230624862126));
#238737=CARTESIAN_POINT('Ctrl Pts',(24.182977745577,-53.9310653428792,2.72985561753067));
#238738=CARTESIAN_POINT('Ctrl Pts',(24.1913567365405,-53.9365438157566,
2.73770089914315));
#238739=CARTESIAN_POINT('Ctrl Pts',(24.1991508947546,-53.9425259106381,
2.7457482334708));
#238740=CARTESIAN_POINT('Ctrl Pts',(24.2077158916392,-53.9490996319581,
2.75459144547045));
#238741=CARTESIAN_POINT('Ctrl Pts',(24.2155752681679,-53.9562817849776,
2.76367911754305));
#238742=CARTESIAN_POINT('Ctrl Pts',(24.2227540584939,-53.9639562340148,
2.77292162564776));
#238743=CARTESIAN_POINT('Ctrl Pts',(24.2305053504156,-53.9722427129512,
2.78290121484794));
#238744=CARTESIAN_POINT('Ctrl Pts',(24.2374640812946,-53.9811038680495,
2.79306229500265));
#238745=CARTESIAN_POINT('Ctrl Pts',(24.2436285779143,-53.9904403792176,
2.80331916685344));
#238746=CARTESIAN_POINT('Ctrl Pts',(24.2497413607409,-53.9996985666494,
2.81348999408742));
#238747=CARTESIAN_POINT('Ctrl Pts',(24.2550737197513,-54.0094254978904,
2.82375635966881));
#238748=CARTESIAN_POINT('Ctrl Pts',(24.2595822759739,-54.0195518809636,
2.83404198860224));
#238749=CARTESIAN_POINT('Origin',(-0.0139224327744698,-0.00619866644028074,
2.83404198860263));
#238750=CARTESIAN_POINT('Ctrl Pts',(25.5480287005725,-57.4192809246784,
2.65878198860223));
#238751=CARTESIAN_POINT('Ctrl Pts',(25.5401808584723,-57.42277107712,2.65878198860223));
#238752=CARTESIAN_POINT('Ctrl Pts',(25.5321112063506,-57.4255746438783,
2.65944603041811));
#238753=CARTESIAN_POINT('Ctrl Pts',(25.5239679177307,-57.4277200319911,
2.6607043926403));
#238754=CARTESIAN_POINT('Ctrl Pts',(25.5187647439664,-57.4290908328633,
2.66150842619555));
#238755=CARTESIAN_POINT('Ctrl Pts',(25.513531724247,-57.4301938346421,2.66255428265327));
#238756=CARTESIAN_POINT('Ctrl Pts',(25.5083079410953,-57.4310450321036,
2.66381699700614));
#238757=CARTESIAN_POINT('Ctrl Pts',(25.5011785252538,-57.4322067458444,
2.66554034873214));
#238758=CARTESIAN_POINT('Ctrl Pts',(25.4940667032543,-57.4328933558602,
2.66766759643918));
#238759=CARTESIAN_POINT('Ctrl Pts',(25.4870628291431,-57.4331362848723,
2.67012012783094));
#238760=CARTESIAN_POINT('Ctrl Pts',(25.4835608920874,-57.4332577493783,
2.67134639352682));
#238761=CARTESIAN_POINT('Ctrl Pts',(25.4800857520069,-57.4332683803236,
2.67265375584958));
#238762=CARTESIAN_POINT('Ctrl Pts',(25.4766473428565,-57.4331727200753,
2.67403135126885));
#238763=CARTESIAN_POINT('Ctrl Pts',(25.4749281382813,-57.4331248899512,
2.67472014897849));
#238764=CARTESIAN_POINT('Ctrl Pts',(25.4732181005511,-57.4330504941577,
2.67542649668578));
#238765=CARTESIAN_POINT('Ctrl Pts',(25.4715183716231,-57.432950145409,2.67614899656047));
#238766=CARTESIAN_POINT('Ctrl Pts',(25.4710934393911,-57.4329250582218,
2.67632962152915));
#238767=CARTESIAN_POINT('Ctrl Pts',(25.4706691511212,-57.4328983491277,
2.67651125590896));
#238768=CARTESIAN_POINT('Ctrl Pts',(25.470245523975,-57.4328700280091,2.67669387767469));
#238769=CARTESIAN_POINT('Ctrl Pts',(25.4689746425362,-57.4327850646534,
2.6772417429719));
#238770=CARTESIAN_POINT('Ctrl Pts',(25.4677097128941,-57.4326855923066,
2.67779849504693));
#238771=CARTESIAN_POINT('Ctrl Pts',(25.4664511833533,-57.4325718846632,
2.67836353617954));
#238772=CARTESIAN_POINT('Ctrl Pts',(25.4577539633651,-57.4317860942972,
2.68226832098854));
#238773=CARTESIAN_POINT('Ctrl Pts',(25.4493260998455,-57.4303627559728,
2.68659153751337));
#238774=CARTESIAN_POINT('Ctrl Pts',(25.4412057723285,-57.4284143577086,
2.69123699486124));
#238775=CARTESIAN_POINT('Ctrl Pts',(25.4371699918424,-57.4274460091196,
2.69354577441162));
#238776=CARTESIAN_POINT('Ctrl Pts',(25.4332098968701,-57.4263474236134,
2.69593478828062));
#238777=CARTESIAN_POINT('Ctrl Pts',(25.4293290842285,-57.4251294472433,
2.69839565261164));
#238778=CARTESIAN_POINT('Ctrl Pts',(25.4207674318881,-57.4224424094492,
2.7038246868899));
#238779=CARTESIAN_POINT('Ctrl Pts',(25.4125888532397,-57.4191864212924,
2.70961155815031));
#238780=CARTESIAN_POINT('Ctrl Pts',(25.404896598031,-57.4154637896036,2.71562701361711));
#238781=CARTESIAN_POINT('Ctrl Pts',(25.4020865201988,-57.4141038653028,
2.71782453535801));
#238782=CARTESIAN_POINT('Ctrl Pts',(25.3993352917247,-57.4126868351391,
2.72005051502345));
#238783=CARTESIAN_POINT('Ctrl Pts',(25.3966436944405,-57.4112179557366,
2.72229986760058));
#238784=CARTESIAN_POINT('Ctrl Pts',(25.3876029039784,-57.4062841452553,
2.72985520488844));
#238785=CARTESIAN_POINT('Ctrl Pts',(25.3791816069559,-57.4007266836981,
2.73770845534522));
#238786=CARTESIAN_POINT('Ctrl Pts',(25.3713475726775,-57.3946697603096,
2.74576706701729));
#238787=CARTESIAN_POINT('Ctrl Pts',(25.3627370410033,-57.3880124840158,
2.7546244358502));
#238788=CARTESIAN_POINT('Ctrl Pts',(25.3548353295667,-57.3807515434748,
2.76373036323187));
#238789=CARTESIAN_POINT('Ctrl Pts',(25.3476188815037,-57.3730023605511,
2.7729966463684));
#238790=CARTESIAN_POINT('Ctrl Pts',(25.3398464577397,-57.3646561585162,
2.78297683033518));
#238791=CARTESIAN_POINT('Ctrl Pts',(25.3328680394168,-57.3557428147443,
2.79314401478959));
#238792=CARTESIAN_POINT('Ctrl Pts',(25.3266878999846,-57.3463604602032,
2.80341452428026));
#238793=CARTESIAN_POINT('Ctrl Pts',(25.3205912133021,-57.3371047991284,
2.81354634721407));
#238794=CARTESIAN_POINT('Ctrl Pts',(25.3152708796014,-57.3273913673561,
2.82378004209203));
#238795=CARTESIAN_POINT('Ctrl Pts',(25.3107727110829,-57.3172883154485,
2.83404198860222));
#238796=CARTESIAN_POINT('Ctrl Pts',(23.9115214566121,-54.1745185419755,
2.83404198860224));
#238797=CARTESIAN_POINT('Ctrl Pts',(23.9072166846467,-54.164849865838,2.82422126442961));
#238798=CARTESIAN_POINT('Ctrl Pts',(23.9036899956626,-54.1548764216391,
2.81442815028448));
#238799=CARTESIAN_POINT('Ctrl Pts',(23.9009524404117,-54.1446552025532,
2.80471618166257));
#238800=CARTESIAN_POINT('Ctrl Pts',(23.8983090899564,-54.1347857162234,
2.79533842146166));
#238801=CARTESIAN_POINT('Ctrl Pts',(23.8964012454638,-54.1246839742756,
2.78603515650173));
#238802=CARTESIAN_POINT('Ctrl Pts',(23.89528251795,-54.1143872866729,2.77685887346686));
#238803=CARTESIAN_POINT('Ctrl Pts',(23.8942249700856,-54.1046536921655,
2.76818441216505));
#238804=CARTESIAN_POINT('Ctrl Pts',(23.8938724934882,-54.0947449925294,
2.7596226152155));
#238805=CARTESIAN_POINT('Ctrl Pts',(23.8943122764069,-54.0846948896024,
2.75123537701584));
#238806=CARTESIAN_POINT('Ctrl Pts',(23.8947173090971,-54.0754389134097,
2.74351087134042));
#238807=CARTESIAN_POINT('Ctrl Pts',(23.8957944255629,-54.06606245712,2.7359339944977));
#238808=CARTESIAN_POINT('Ctrl Pts',(23.8976480927562,-54.0566033397486,
2.72857657812499));
#238809=CARTESIAN_POINT('Ctrl Pts',(23.8982008188944,-54.0537828218941,
2.72638274508255));
#238810=CARTESIAN_POINT('Ctrl Pts',(23.8988228478388,-54.0509550659728,
2.72420861709542));
#238811=CARTESIAN_POINT('Ctrl Pts',(23.899517637365,-54.0481214020998,2.72205663736671));
#238812=CARTESIAN_POINT('Ctrl Pts',(23.9002053278545,-54.0453166912879,
2.7199266455671));
#238813=CARTESIAN_POINT('Ctrl Pts',(23.9009633199472,-54.0425090377016,
2.71782089927828));
#238814=CARTESIAN_POINT('Ctrl Pts',(23.9017938716385,-54.0397028685172,
2.7157438731119));
#238815=CARTESIAN_POINT('Ctrl Pts',(23.9018516265789,-54.0395077330001,
2.71559944077431));
#238816=CARTESIAN_POINT('Ctrl Pts',(23.9019097237182,-54.03931259641,2.71545515216013));
#238817=CARTESIAN_POINT('Ctrl Pts',(23.9019681642229,-54.0391174593308,
2.71531100781674));
#238818=CARTESIAN_POINT('Ctrl Pts',(23.9045304100328,-54.0305619349328,
2.70899119176028));
#238819=CARTESIAN_POINT('Ctrl Pts',(23.9077916774642,-54.0220283896857,
2.70298296066784));
#238820=CARTESIAN_POINT('Ctrl Pts',(23.9117952627748,-54.0136246330482,
2.69736727774082));
#238821=CARTESIAN_POINT('Ctrl Pts',(23.9155273001028,-54.005790871299,2.69213248525371));
#238822=CARTESIAN_POINT('Ctrl Pts',(23.919904946166,-53.9980693056372,2.68723866185408));
#238823=CARTESIAN_POINT('Ctrl Pts',(23.9249777890357,-53.9905727747488,
2.682785958295));
#238824=CARTESIAN_POINT('Ctrl Pts',(23.9268335005859,-53.9878304467655,
2.68115710172746));
#238825=CARTESIAN_POINT('Ctrl Pts',(23.9287823509753,-53.9851185338197,
2.67958763637753));
#238826=CARTESIAN_POINT('Ctrl Pts',(23.930827095549,-53.9824437337503,2.67808378645311));
#238827=CARTESIAN_POINT('Ctrl Pts',(23.9313187883101,-53.9818005336907,
2.67772216078546));
#238828=CARTESIAN_POINT('Ctrl Pts',(23.931816583137,-53.98115930456,2.67736403603509));
#238829=CARTESIAN_POINT('Ctrl Pts',(23.9323204546083,-53.9805201796367,
2.67700956934425));
#238830=CARTESIAN_POINT('Ctrl Pts',(23.932808580096,-53.9799010273672,2.6766661797375));
#238831=CARTESIAN_POINT('Ctrl Pts',(23.9333024083488,-53.9792838498566,
2.67632622314065));
#238832=CARTESIAN_POINT('Ctrl Pts',(23.9338019127828,-53.9786687697967,
2.67598984158719));
#238833=CARTESIAN_POINT('Ctrl Pts',(23.939274561122,-53.971929856908,2.6723043929217));
#238834=CARTESIAN_POINT('Ctrl Pts',(23.9454324752048,-53.9654385427824,
2.66904964539926));
#238835=CARTESIAN_POINT('Ctrl Pts',(23.9522153560509,-53.9593734277043,
2.66640203566676));
#238836=CARTESIAN_POINT('Ctrl Pts',(23.9550284189138,-53.9568580436996,
2.66530399299388));
#238837=CARTESIAN_POINT('Ctrl Pts',(23.9579485624032,-53.9544158621937,
2.66430995142205));
#238838=CARTESIAN_POINT('Ctrl Pts',(23.9609698772118,-53.9520587513127,
2.66343053473304));
#238839=CARTESIAN_POINT('Ctrl Pts',(23.9661230444611,-53.948038453077,2.66193059792827));
#238840=CARTESIAN_POINT('Ctrl Pts',(23.9715702598501,-53.9442681092571,
2.6607651981707));
#238841=CARTESIAN_POINT('Ctrl Pts',(23.9772776109218,-53.9408121161402,
2.65997805604402));
#238842=CARTESIAN_POINT('Ctrl Pts',(23.9801312864576,-53.9390841195817,
2.65958448498067));
#238843=CARTESIAN_POINT('Ctrl Pts',(23.9830506455193,-53.9374360035028,
2.65928526260703));
#238844=CARTESIAN_POINT('Ctrl Pts',(23.9860314303864,-53.9358758804722,
2.65908463971265));
#238845=CARTESIAN_POINT('Ctrl Pts',(23.9890122152535,-53.9343157574417,
2.65888401681827));
#238846=CARTESIAN_POINT('Ctrl Pts',(23.9920543802867,-53.9328436288549,
2.65878198860225));
#238847=CARTESIAN_POINT('Ctrl Pts',(23.9951532569813,-53.93146557308,2.65878198860225));
#238848=CARTESIAN_POINT('Origin',(29.1450842944635,-50.450286788887,2.83404198860226));
#238849=CARTESIAN_POINT('Ctrl Pts',(31.4933613949865,-54.1671020372433,
2.83404198860224));
#238850=CARTESIAN_POINT('Ctrl Pts',(31.4986665597481,-54.1762908521529,
2.8241965244016));
#238851=CARTESIAN_POINT('Ctrl Pts',(31.5032309550532,-54.1858709973807,
2.81438790575866));
#238852=CARTESIAN_POINT('Ctrl Pts',(31.5070391691402,-54.1957854287807,
2.80466781257231));
#238853=CARTESIAN_POINT('Ctrl Pts',(31.5107236389459,-54.2053777001969,
2.79526356453497));
#238854=CARTESIAN_POINT('Ctrl Pts',(31.5137006693046,-54.2152841131264,
2.78594102496732));
#238855=CARTESIAN_POINT('Ctrl Pts',(31.5159144374958,-54.2254725303099,
2.77675109089352));
#238856=CARTESIAN_POINT('Ctrl Pts',(31.5180085258887,-54.235110145599,2.76805797914324));
#238857=CARTESIAN_POINT('Ctrl Pts',(31.5194198476562,-54.2450010037657,
2.75948271210865));
#238858=CARTESIAN_POINT('Ctrl Pts',(31.5200591406751,-54.2551207303631,
2.75108575573982));
#238859=CARTESIAN_POINT('Ctrl Pts',(31.5206479757804,-54.2644417304365,
2.7433515516409));
#238860=CARTESIAN_POINT('Ctrl Pts',(31.5205818213861,-54.2739574575838,
2.73576818686817));
#238861=CARTESIAN_POINT('Ctrl Pts',(31.5197533892272,-54.2836415202426,
2.7284062616142));
#238862=CARTESIAN_POINT('Ctrl Pts',(31.5195130925486,-54.286450498705,2.72627084694278));
#238863=CARTESIAN_POINT('Ctrl Pts',(31.5192084034342,-54.2892735615524,
2.72415424587802));
#238864=CARTESIAN_POINT('Ctrl Pts',(31.5188360425585,-54.2921098354275,
2.72205867173224));
#238865=CARTESIAN_POINT('Ctrl Pts',(31.5184323794292,-54.2951845386597,
2.71978693462826));
#238866=CARTESIAN_POINT('Ctrl Pts',(31.517950819101,-54.2982706300309,2.71754411340725));
#238867=CARTESIAN_POINT('Ctrl Pts',(31.5173878381082,-54.3013662138028,
2.71533341844222));
#238868=CARTESIAN_POINT('Ctrl Pts',(31.5158427323556,-54.3098620677554,
2.70926614876369));
#238869=CARTESIAN_POINT('Ctrl Pts',(31.5136439393738,-54.3184108612907,
2.70347381860385));
#238870=CARTESIAN_POINT('Ctrl Pts',(31.5107627835363,-54.3269129314602,
2.69804914171372));
#238871=CARTESIAN_POINT('Ctrl Pts',(31.5081266823665,-54.3346918640773,
2.69308585687172));
#238872=CARTESIAN_POINT('Ctrl Pts',(31.5049132975215,-54.342421824438,2.68842799053145));
#238873=CARTESIAN_POINT('Ctrl Pts',(31.5010675328661,-54.3500333719151,
2.6841476705417));
#238874=CARTESIAN_POINT('Ctrl Pts',(31.4991785058302,-54.3537721391714,
2.68204519134514));
#238875=CARTESIAN_POINT('Ctrl Pts',(31.497136559455,-54.3574819590034,2.68003431778473));
#238876=CARTESIAN_POINT('Ctrl Pts',(31.494933246334,-54.3611518569446,2.67812693945231));
#238877=CARTESIAN_POINT('Ctrl Pts',(31.4945151891298,-54.3618481843337,
2.67776503299183));
#238878=CARTESIAN_POINT('Ctrl Pts',(31.4940908087514,-54.3625432124812,
2.67740659639903));
#238879=CARTESIAN_POINT('Ctrl Pts',(31.4936601139568,-54.3632368016448,
2.67705178968835));
#238880=CARTESIAN_POINT('Ctrl Pts',(31.4932428783745,-54.363908716147,2.67670807068737));
#238881=CARTESIAN_POINT('Ctrl Pts',(31.4928197168828,-54.3645792801843,
2.67636775825245));
#238882=CARTESIAN_POINT('Ctrl Pts',(31.4923906407832,-54.3652483648075,
2.67603099699235));
#238883=CARTESIAN_POINT('Ctrl Pts',(31.4877146578622,-54.3725399111641,
2.67236104217089));
#238884=CARTESIAN_POINT('Ctrl Pts',(31.4823328301622,-54.3796603393086,
2.6691144054142));
#238885=CARTESIAN_POINT('Ctrl Pts',(31.4762829888794,-54.3864229856966,
2.66646778189569));
#238886=CARTESIAN_POINT('Ctrl Pts',(31.4737281033384,-54.3892788932598,
2.66535009634929));
#238887=CARTESIAN_POINT('Ctrl Pts',(31.4710545157389,-54.3920710496176,
2.66433897912312));
#238888=CARTESIAN_POINT('Ctrl Pts',(31.4682668669592,-54.394786135735,2.66344564884771));
#238889=CARTESIAN_POINT('Ctrl Pts',(31.4635725360693,-54.3993582729147,
2.66194130298563));
#238890=CARTESIAN_POINT('Ctrl Pts',(31.4585547584358,-54.4037093249062,
2.66077206705397));
#238891=CARTESIAN_POINT('Ctrl Pts',(31.4532397415961,-54.4077698566059,
2.6599822515569));
#238892=CARTESIAN_POINT('Ctrl Pts',(31.4519109873861,-54.4087849895309,
2.65978479768264));
#238893=CARTESIAN_POINT('Ctrl Pts',(31.4505635261662,-54.4097817701137,
2.65961098966598));
#238894=CARTESIAN_POINT('Ctrl Pts',(31.4491976069264,-54.4107588499952,
2.65946139030477));
#238895=CARTESIAN_POINT('Ctrl Pts',(31.4471487280666,-54.4122244698176,
2.65923699126296));
#238896=CARTESIAN_POINT('Ctrl Pts',(31.4450583254663,-54.4136457436048,
2.65906707562417));
#238897=CARTESIAN_POINT('Ctrl Pts',(31.4429280944114,-54.4150195646475,
2.65895332562895));
#238898=CARTESIAN_POINT('Ctrl Pts',(31.4407978633565,-54.4163933856902,
2.65883957563372));
#238899=CARTESIAN_POINT('Ctrl Pts',(31.4386278145925,-54.4177197583724,
2.65878198860224));
#238900=CARTESIAN_POINT('Ctrl Pts',(31.4364195775141,-54.4189959163058,
2.65878198860224));
#238901=CARTESIAN_POINT('Ctrl Pts',(29.5274749692191,-51.1126068659042,
2.65878198860226));
#238902=CARTESIAN_POINT('Ctrl Pts',(29.5349468458347,-51.1082885388127,
2.65878198860226));
#238903=CARTESIAN_POINT('Ctrl Pts',(29.5427104181378,-51.1046244142385,
2.65945335517811));
#238904=CARTESIAN_POINT('Ctrl Pts',(29.5506148782552,-51.1016049255946,
2.66072561226542));
#238905=CARTESIAN_POINT('Ctrl Pts',(29.5557203484474,-51.0996546457478,
2.66154735980284));
#238906=CARTESIAN_POINT('Ctrl Pts',(29.5608842707086,-51.0979724198483,
2.66261895766837));
#238907=CARTESIAN_POINT('Ctrl Pts',(29.5660646037411,-51.0965469289492,
2.66391429250994));
#238908=CARTESIAN_POINT('Ctrl Pts',(29.5729308384272,-51.0946575224197,
2.6656311846409));
#238909=CARTESIAN_POINT('Ctrl Pts',(29.5798262755784,-51.0932249325808,
2.66774105138665));
#238910=CARTESIAN_POINT('Ctrl Pts',(29.5866628504243,-51.0922302752229,
2.67016894181715));
#238911=CARTESIAN_POINT('Ctrl Pts',(29.5900811378472,-51.091732946544,2.6713828870324));
#238912=CARTESIAN_POINT('Ctrl Pts',(29.5934848814079,-51.0913449998284,
2.67267613167516));
#238913=CARTESIAN_POINT('Ctrl Pts',(29.5968642938815,-51.0910633609948,
2.67403835432518));
#238914=CARTESIAN_POINT('Ctrl Pts',(29.5985540001184,-51.090922541578,2.67471946565019));
#238915=CARTESIAN_POINT('Ctrl Pts',(29.6002376377887,-51.0908082908738,
2.67541781389487));
#238916=CARTESIAN_POINT('Ctrl Pts',(29.6019140726121,-51.0907201726666,
2.67613207244134));
#238917=CARTESIAN_POINT('Ctrl Pts',(29.6023331813179,-51.0906981431148,
2.67631063707795));
#238918=CARTESIAN_POINT('Ctrl Pts',(29.6027518401475,-51.0906777466675,
2.6764901960181));
#238919=CARTESIAN_POINT('Ctrl Pts',(29.6031700319857,-51.0906589761525,
2.67667072836621));
#238920=CARTESIAN_POINT('Ctrl Pts',(29.6044246075002,-51.0906026646076,
2.67721232541055));
#238921=CARTESIAN_POINT('Ctrl Pts',(29.6056749785909,-51.0905609873408,
2.67776268340011));
#238922=CARTESIAN_POINT('Ctrl Pts',(29.606920696577,-51.0905337427825,2.6783212354148));
#238923=CARTESIAN_POINT('Ctrl Pts',(29.6156953732195,-51.0903418356312,
2.68225560368394));
#238924=CARTESIAN_POINT('Ctrl Pts',(29.6242688491604,-51.0908211368925,
2.68661792998821));
#238925=CARTESIAN_POINT('Ctrl Pts',(29.6325885911854,-51.0918641424254,
2.69130986622492));
#238926=CARTESIAN_POINT('Ctrl Pts',(29.6366236570776,-51.0923699989819,
2.69358545022984));
#238927=CARTESIAN_POINT('Ctrl Pts',(29.6405993642579,-51.0930089302511,
2.69593918853416));
#238928=CARTESIAN_POINT('Ctrl Pts',(29.644511037713,-51.0937712117409,2.6983630623544));
#238929=CARTESIAN_POINT('Ctrl Pts',(29.6504995364717,-51.0949382114428,
2.70207384382173));
#238930=CARTESIAN_POINT('Ctrl Pts',(29.6563348640826,-51.0963926103111,
2.70594760814173));
#238931=CARTESIAN_POINT('Ctrl Pts',(29.661987448182,-51.0980990280585,2.70995196345653));
#238932=CARTESIAN_POINT('Ctrl Pts',(29.6646125374804,-51.0988914972883,
2.7118116067805));
#238933=CARTESIAN_POINT('Ctrl Pts',(29.6671982043432,-51.0997380650828,
2.71369962772044));
#238934=CARTESIAN_POINT('Ctrl Pts',(29.6697408831281,-51.1006362623624,
2.71561183138606));
#238935=CARTESIAN_POINT('Ctrl Pts',(29.6699357694383,-51.1007051056447,
2.71575839426257));
#238936=CARTESIAN_POINT('Ctrl Pts',(29.6701304259137,-51.1007742270245,
2.71590508903154));
#238937=CARTESIAN_POINT('Ctrl Pts',(29.6703248520474,-51.1008436251319,
2.71605191409856));
#238938=CARTESIAN_POINT('Ctrl Pts',(29.6730559530505,-51.1018184593119,
2.71811436362698));
#238939=CARTESIAN_POINT('Ctrl Pts',(29.6757410298223,-51.1028499068173,
2.72020091026904));
#238940=CARTESIAN_POINT('Ctrl Pts',(29.6783776815774,-51.1039327914262,
2.72230624862126));
#238941=CARTESIAN_POINT('Ctrl Pts',(29.6878322458588,-51.1078158230494,
2.72985561753074));
#238942=CARTESIAN_POINT('Ctrl Pts',(29.6967379921841,-51.1123884412301,
2.7377008991433));
#238943=CARTESIAN_POINT('Ctrl Pts',(29.7051147523691,-51.1175230541893,
2.74574823347104));
#238944=CARTESIAN_POINT('Ctrl Pts',(29.7143199702922,-51.123165478014,2.75459144547081));
#238945=CARTESIAN_POINT('Ctrl Pts',(29.7228870317522,-51.1294867578971,
2.76367911754355));
#238946=CARTESIAN_POINT('Ctrl Pts',(29.730828694278,-51.1363687775787,2.7729216256484));
#238947=CARTESIAN_POINT('Ctrl Pts',(29.7394036967208,-51.1437996316838,
2.78290121484885));
#238948=CARTESIAN_POINT('Ctrl Pts',(29.7472505498693,-51.1518848590025,
2.79306229500385));
#238949=CARTESIAN_POINT('Ctrl Pts',(29.7543572078963,-51.1605258584273,
2.80331916685492));
#238950=CARTESIAN_POINT('Ctrl Pts',(29.7614042483635,-51.1690943687441,
2.81348999408842));
#238951=CARTESIAN_POINT('Ctrl Pts',(29.7677241373279,-51.1782106315447,
2.82375635966932));
#238952=CARTESIAN_POINT('Ctrl Pts',(29.7732664904686,-51.1878102687779,
2.83404198860226));
#238953=CARTESIAN_POINT('Origin',(-0.0131982271536719,-0.00761999999980581,
2.83404198860262));
#238954=CARTESIAN_POINT('Ctrl Pts',(31.4100231232068,-54.4342359163058,
2.65878198860224));
#238955=CARTESIAN_POINT('Ctrl Pts',(31.4025830926779,-54.4385272722019,
2.65878198860224));
#238956=CARTESIAN_POINT('Ctrl Pts',(31.3948506994796,-54.4421589890636,
2.65944603041815));
#238957=CARTESIAN_POINT('Ctrl Pts',(31.3869762747692,-54.4451438299613,
2.66070439264038));
#238958=CARTESIAN_POINT('Ctrl Pts',(31.381944892244,-54.4470510012005,2.66150842619562));
#238959=CARTESIAN_POINT('Ctrl Pts',(31.3768558346353,-54.4486949601296,
2.66255428265332));
#238960=CARTESIAN_POINT('Ctrl Pts',(31.371749642277,-54.4500875286676,2.66381699700615));
#238961=CARTESIAN_POINT('Ctrl Pts',(31.3647807142735,-54.4519881053008,
2.66554034873215));
#238962=CARTESIAN_POINT('Ctrl Pts',(31.3577796218689,-54.4534143418198,
2.66766759643919));
#238963=CARTESIAN_POINT('Ctrl Pts',(31.3508395087091,-54.4543880442391,
2.67012012783095));
#238964=CARTESIAN_POINT('Ctrl Pts',(31.3473694521293,-54.4548748954487,
2.67134639352683));
#238965=CARTESIAN_POINT('Ctrl Pts',(31.343914460466,-54.4552487192089,2.67265375584959));
#238966=CARTESIAN_POINT('Ctrl Pts',(31.340484888062,-54.455512994622,2.67403135126887));
#238967=CARTESIAN_POINT('Ctrl Pts',(31.33877010186,-54.4556451323286,2.67472014897851));
#238968=CARTESIAN_POINT('Ctrl Pts',(31.3370616554174,-54.4557498916991,
2.6754264966858));
#238969=CARTESIAN_POINT('Ctrl Pts',(31.3353607484818,-54.4558277627241,
2.67614899656049));
#238970=CARTESIAN_POINT('Ctrl Pts',(31.3349355217479,-54.4558472304803,
2.67632962152916));
#238971=CARTESIAN_POINT('Ctrl Pts',(31.334510765913,-54.4558650179023,2.67651125590897));
#238972=CARTESIAN_POINT('Ctrl Pts',(31.3340864990776,-54.4558811330244,
2.67669387767471));
#238973=CARTESIAN_POINT('Ctrl Pts',(31.3328136985713,-54.4559294783906,
2.67724174297191));
#238974=CARTESIAN_POINT('Ctrl Pts',(31.3315453006546,-54.4559627721153,
2.67779849504695));
#238975=CARTESIAN_POINT('Ctrl Pts',(31.3302817797851,-54.4559812395332,
2.67836353617956));
#238976=CARTESIAN_POINT('Ctrl Pts',(31.3215500666185,-54.4561088608491,
2.68226832098858));
#238977=CARTESIAN_POINT('Ctrl Pts',(31.3130195924492,-54.4555742713433,
2.68659153751344));
#238978=CARTESIAN_POINT('Ctrl Pts',(31.3047400858596,-54.4544853519652,
2.69123699486134));
#238979=CARTESIAN_POINT('Ctrl Pts',(31.3006251938115,-54.4539441620234,
2.69354577441169));
#238980=CARTESIAN_POINT('Ctrl Pts',(31.2965719591991,-54.4532655373254,
2.69593478828066));
#238981=CARTESIAN_POINT('Ctrl Pts',(31.292585092857,-54.4524598885389,2.69839565261165));
#238982=CARTESIAN_POINT('Ctrl Pts',(31.2837894702125,-54.4506825069813,
2.7038246868899));
#238983=CARTESIAN_POINT('Ctrl Pts',(31.2753153512353,-54.4482992497261,
2.70961155815032));
#238984=CARTESIAN_POINT('Ctrl Pts',(31.2672761140357,-54.4454010706192,
2.71562701361713));
#238985=CARTESIAN_POINT('Ctrl Pts',(31.2643392793065,-54.4443423292436,
2.71782453535804));
#238986=CARTESIAN_POINT('Ctrl Pts',(31.2614550023645,-54.4432206434038,
2.72005051502348));
#238987=CARTESIAN_POINT('Ctrl Pts',(31.2586246102252,-54.4420411592042,
2.72229986760062));
#238988=CARTESIAN_POINT('Ctrl Pts',(31.2491176225324,-54.4380793965871,
2.72985520488787));
#238989=CARTESIAN_POINT('Ctrl Pts',(31.2401615453406,-54.4334326446229,
2.73770845534399));
#238990=CARTESIAN_POINT('Ctrl Pts',(31.2317373058284,-54.4282277812593,
2.74576706701537));
#238991=CARTESIAN_POINT('Ctrl Pts',(31.2224780686878,-54.422507019866,2.75462443584758));
#238992=CARTESIAN_POINT('Ctrl Pts',(31.2138606686971,-54.4161118092713,
2.76373036322853));
#238993=CARTESIAN_POINT('Ctrl Pts',(31.2058737429096,-54.4091594014095,
2.77299664636431));
#238994=CARTESIAN_POINT('Ctrl Pts',(31.1972714816238,-54.4016713602553,
2.78297683033026));
#238995=CARTESIAN_POINT('Ctrl Pts',(31.1893995936799,-54.3935362880573,
2.79314401478381));
#238996=CARTESIAN_POINT('Ctrl Pts',(31.1822725865963,-54.3848513315147,
2.8034145242736));
#238997=CARTESIAN_POINT('Ctrl Pts',(31.1752418181707,-54.3762836512078,
2.81354634720961));
#238998=CARTESIAN_POINT('Ctrl Pts',(31.1689352997168,-54.367179556935,2.82378004208982));
#238999=CARTESIAN_POINT('Ctrl Pts',(31.1634057161447,-54.3576020372433,
2.83404198860224));
#239000=CARTESIAN_POINT('Ctrl Pts',(29.4433108116267,-51.3783102687779,
2.83404198860226));
#239001=CARTESIAN_POINT('Ctrl Pts',(29.4380189697936,-51.3691445298574,
2.82422126442883));
#239002=CARTESIAN_POINT('Ctrl Pts',(29.4334690915849,-51.3595943606086,
2.8144281502829));
#239003=CARTESIAN_POINT('Ctrl Pts',(29.4296781246242,-51.3497152868729,
2.8047161816602));
#239004=CARTESIAN_POINT('Ctrl Pts',(29.4260176124798,-51.3401761719824,
2.79533842145879));
#239005=CARTESIAN_POINT('Ctrl Pts',(29.4230642997968,-51.3303291924862,
2.78603515649837));
#239006=CARTESIAN_POINT('Ctrl Pts',(29.4208754038576,-51.3202058500828,
2.77685887346304));
#239007=CARTESIAN_POINT('Ctrl Pts',(29.4188062116754,-51.3106361210773,
2.76818441216095));
#239008=CARTESIAN_POINT('Ctrl Pts',(29.4174199248358,-51.3008185461712,
2.75962261521114));
#239009=CARTESIAN_POINT('Ctrl Pts',(29.4168067767633,-51.2907775289265,
2.75123537701125));
#239010=CARTESIAN_POINT('Ctrl Pts',(29.4162420776748,-51.2815299204948,
2.74351087133569));
#239011=CARTESIAN_POINT('Ctrl Pts',(29.4163331870173,-51.2720922400845,
2.73593399449284));
#239012=CARTESIAN_POINT('Ctrl Pts',(29.4171879526255,-51.2624911797642,
2.72857657812005));
#239013=CARTESIAN_POINT('Ctrl Pts',(29.417442826475,-51.25962833739,2.72638274507929));
#239014=CARTESIAN_POINT('Ctrl Pts',(29.4177658668987,-51.2567510524839,
2.72420861709381));
#239015=CARTESIAN_POINT('Ctrl Pts',(29.4181606517648,-51.2538602864389,
2.72205663736673));
#239016=CARTESIAN_POINT('Ctrl Pts',(29.4185514029028,-51.2509990568961,
2.71992664556712));
#239017=CARTESIAN_POINT('Ctrl Pts',(29.4190117629207,-51.2481275521813,
2.71782089927831));
#239018=CARTESIAN_POINT('Ctrl Pts',(29.4195444402105,-51.2452499391934,
2.71574387311192));
#239019=CARTESIAN_POINT('Ctrl Pts',(29.4195814815475,-51.245049835614,2.71559944077433));
#239020=CARTESIAN_POINT('Ctrl Pts',(29.4196188630967,-51.2448496951978,
2.71545515216015));
#239021=CARTESIAN_POINT('Ctrl Pts',(29.4196565860791,-51.2446495184037,
2.71531100781677));
#239022=CARTESIAN_POINT('Ctrl Pts',(29.4213104998207,-51.2358730344466,
2.70899119176035));
#239023=CARTESIAN_POINT('Ctrl Pts',(29.4236619033169,-51.2270453415805,
2.70298296066795));
#239024=CARTESIAN_POINT('Ctrl Pts',(29.4267651248013,-51.2182691329812,
2.69736727774097));
#239025=CARTESIAN_POINT('Ctrl Pts',(29.4296578665609,-51.210088181272,2.692132485254));
#239026=CARTESIAN_POINT('Ctrl Pts',(29.4332044080281,-51.2019513265393,
2.6872386618545));
#239027=CARTESIAN_POINT('Ctrl Pts',(29.43746586048,-51.1939656059622,2.68278595829551));
#239028=CARTESIAN_POINT('Ctrl Pts',(29.4390247549185,-51.1910443260616,
2.68115710172778));
#239029=CARTESIAN_POINT('Ctrl Pts',(29.440679457209,-51.1881435589219,2.67958763637767));
#239030=CARTESIAN_POINT('Ctrl Pts',(29.4424334077173,-51.1852696776788,
2.67808378645308));
#239031=CARTESIAN_POINT('Ctrl Pts',(29.4428551742202,-51.1845786052478,
2.67772216078543));
#239032=CARTESIAN_POINT('Ctrl Pts',(29.4432832153794,-51.183888855109,2.67736403603506));
#239033=CARTESIAN_POINT('Ctrl Pts',(29.4437175198439,-51.1832005624683,
2.67700956934422));
#239034=CARTESIAN_POINT('Ctrl Pts',(29.4441382522939,-51.1825337789726,
2.67666617973747));
#239035=CARTESIAN_POINT('Ctrl Pts',(29.4445648626871,-51.1818683633167,
2.67632622314062));
#239036=CARTESIAN_POINT('Ctrl Pts',(29.4449973374101,-51.1812044402988,
2.67598984158716));
#239037=CARTESIAN_POINT('Ctrl Pts',(29.4497355978008,-51.173930396359,2.67230439292164));
#239038=CARTESIAN_POINT('Ctrl Pts',(29.4551812510958,-51.1668309650354,
2.66904964539918));
#239039=CARTESIAN_POINT('Ctrl Pts',(29.4612929974523,-51.1600900711809,
2.66640203566668));
#239040=CARTESIAN_POINT('Ctrl Pts',(29.463827720838,-51.1572944215749,2.66530399299383));
#239041=CARTESIAN_POINT('Ctrl Pts',(29.4664765899959,-51.1545603804833,
2.66430995142202));
#239042=CARTESIAN_POINT('Ctrl Pts',(29.4692349685477,-51.1519003687084,
2.66343053473303));
#239043=CARTESIAN_POINT('Ctrl Pts',(29.4739396706111,-51.1473634414336,
2.66193059792826));
#239044=CARTESIAN_POINT('Ctrl Pts',(29.4789629373388,-51.1430443628979,
2.6607651981707));
#239045=CARTESIAN_POINT('Ctrl Pts',(29.4842777732944,-51.1390107214358,
2.65997805604402));
#239046=CARTESIAN_POINT('Ctrl Pts',(29.4869351912722,-51.1369939007047,
2.65958448498068));
#239047=CARTESIAN_POINT('Ctrl Pts',(29.4896662827385,-51.1350496570618,
2.65928526260704));
#239048=CARTESIAN_POINT('Ctrl Pts',(29.4924676612914,-51.133186503687,2.65908463971266));
#239049=CARTESIAN_POINT('Ctrl Pts',(29.4952690398443,-51.1313233503122,
2.65888401681829));
#239050=CARTESIAN_POINT('Ctrl Pts',(29.4981406602403,-51.1295412933641,
2.65878198860226));
#239051=CARTESIAN_POINT('Ctrl Pts',(29.5010785149117,-51.1278468659042,
2.65878198860226));
#239052=CARTESIAN_POINT('Origin',(34.2589154226527,-47.1274239660504,2.83404198860229));
#239053=CARTESIAN_POINT('Ctrl Pts',(36.9828414016752,-50.5784163149351,
2.83404198860226));
#239054=CARTESIAN_POINT('Ctrl Pts',(36.9890779968915,-50.587000251836,2.82419652440071));
#239055=CARTESIAN_POINT('Ctrl Pts',(36.9946187858205,-50.5960508067997,
2.81438790575687));
#239056=CARTESIAN_POINT('Ctrl Pts',(36.999442478391,-50.6055128591417,2.80466781256964));
#239057=CARTESIAN_POINT('Ctrl Pts',(37.0041094296761,-50.6146674511255,
2.79526356453155));
#239058=CARTESIAN_POINT('Ctrl Pts',(37.0081056536712,-50.6242084112807,
2.78594102496317));
#239059=CARTESIAN_POINT('Ctrl Pts',(37.0113722741999,-50.6341096134627,
2.77675109088868));
#239060=CARTESIAN_POINT('Ctrl Pts',(37.0144622960732,-50.6434755410461,
2.7680579791377));
#239061=CARTESIAN_POINT('Ctrl Pts',(37.0168997626768,-50.6531646927622,
2.75948271210245));
#239062=CARTESIAN_POINT('Ctrl Pts',(37.0185933530513,-50.6631621581227,
2.75108575573304));
#239063=CARTESIAN_POINT('Ctrl Pts',(37.0201532722699,-50.6723705467548,
2.74335155163341));
#239064=CARTESIAN_POINT('Ctrl Pts',(37.0210821446115,-50.6818410607715,
2.73576818686005));
#239065=CARTESIAN_POINT('Ctrl Pts',(37.021270510878,-50.6915586678635,2.72840626160554));
#239066=CARTESIAN_POINT('Ctrl Pts',(37.0213251487715,-50.6943773762868,
2.72627084693704));
#239067=CARTESIAN_POINT('Ctrl Pts',(37.0213172191971,-50.6972168227817,
2.72415424587516));
#239068=CARTESIAN_POINT('Ctrl Pts',(37.021243369503,-50.700076481558,2.72205867173221));
#239069=CARTESIAN_POINT('Ctrl Pts',(37.0211633116864,-50.7031765355308,
2.71978693462824));
#239070=CARTESIAN_POINT('Ctrl Pts',(37.0210069737846,-50.7062960577316,
2.71754411340725));
#239071=CARTESIAN_POINT('Ctrl Pts',(37.0207706534752,-50.7094335311098,
2.71533341844222));
#239072=CARTESIAN_POINT('Ctrl Pts',(37.0201220705315,-50.7180443514155,
2.7092661487637));
#239073=CARTESIAN_POINT('Ctrl Pts',(37.0188289150186,-50.7267761502167,
2.70347381860387));
#239074=CARTESIAN_POINT('Ctrl Pts',(37.0168522507837,-50.7355328079483,
2.69804914171373));
#239075=CARTESIAN_POINT('Ctrl Pts',(37.0150437103243,-50.7435446743629,
2.69308585687179));
#239076=CARTESIAN_POINT('Ctrl Pts',(37.0126559296154,-50.7515681793716,
2.68842799053157));
#239077=CARTESIAN_POINT('Ctrl Pts',(37.009626855822,-50.7595400218646,2.68414767054186));
#239078=CARTESIAN_POINT('Ctrl Pts',(37.0081389846697,-50.7634557648559,
2.68204519134525));
#239079=CARTESIAN_POINT('Ctrl Pts',(37.0064960060564,-50.7673587034234,
2.68003431778479));
#239080=CARTESIAN_POINT('Ctrl Pts',(37.0046883717073,-50.7712388062144,
2.67812693945232));
#239081=CARTESIAN_POINT('Ctrl Pts',(37.0043453906961,-50.7719750179263,
2.67776503299184));
#239082=CARTESIAN_POINT('Ctrl Pts',(37.003995985342,-50.7727105984658,2.67740659639905));
#239083=CARTESIAN_POINT('Ctrl Pts',(37.003640149748,-50.7734454079403,2.67705178968836));
#239084=CARTESIAN_POINT('Ctrl Pts',(37.0032954340162,-50.7741572546188,
2.67670807068738));
#239085=CARTESIAN_POINT('Ctrl Pts',(37.0029446836758,-50.7748683776566,
2.67636775825246));
#239086=CARTESIAN_POINT('Ctrl Pts',(37.0025878964874,-50.7755786476296,
2.67603099699236));
#239087=CARTESIAN_POINT('Ctrl Pts',(36.9986997032259,-50.7833190234408,
2.67236104217115));
#239088=CARTESIAN_POINT('Ctrl Pts',(36.9940916451532,-50.7909629993134,
2.66911440541465));
#239089=CARTESIAN_POINT('Ctrl Pts',(36.988781834569,-50.7983209798289,2.66646778189624));
#239090=CARTESIAN_POINT('Ctrl Pts',(36.9865394685868,-50.8014283006915,
2.66535009634962));
#239091=CARTESIAN_POINT('Ctrl Pts',(36.9841723869929,-50.8044846273283,
2.66433897912328));
#239092=CARTESIAN_POINT('Ctrl Pts',(36.9816838130239,-50.8074762285634,
2.66344564884773));
#239093=CARTESIAN_POINT('Ctrl Pts',(36.9774931166431,-50.8125140102912,
2.66194130298565));
#239094=CARTESIAN_POINT('Ctrl Pts',(36.9729576356987,-50.8173657273497,
2.66077206705399));
#239095=CARTESIAN_POINT('Ctrl Pts',(36.9680961762161,-50.8219595855745,
2.65998225155693));
#239096=CARTESIAN_POINT('Ctrl Pts',(36.9668808113454,-50.8231080501307,
2.65978479768266));
#239097=CARTESIAN_POINT('Ctrl Pts',(36.9656449236016,-50.8242402182959,
2.65961098966601));
#239098=CARTESIAN_POINT('Ctrl Pts',(36.9643886196688,-50.8253547230707,
2.6594613903048));
#239099=CARTESIAN_POINT('Ctrl Pts',(36.9625041637695,-50.8270264802329,
2.65923699126298));
#239100=CARTESIAN_POINT('Ctrl Pts',(36.9605737761783,-50.828658474705,2.6590670756242));
#239101=CARTESIAN_POINT('Ctrl Pts',(36.9585988181543,-50.8302474395909,
2.65895332562898));
#239102=CARTESIAN_POINT('Ctrl Pts',(36.9566238601303,-50.8318364044767,
2.65883957563375));
#239103=CARTESIAN_POINT('Ctrl Pts',(36.9546043428198,-50.8333823430144,
2.65878198860227));
#239104=CARTESIAN_POINT('Ctrl Pts',(36.9525415975228,-50.8348823336494,
2.65878198860227));
#239105=CARTESIAN_POINT('Ctrl Pts',(34.7084426211237,-47.7461450747859,
2.65878198860229));
#239106=CARTESIAN_POINT('Ctrl Pts',(34.7154221779231,-47.7410693801614,
2.65878198860229));
#239107=CARTESIAN_POINT('Ctrl Pts',(34.7227602152543,-47.7366138137625,
2.65945335517822));
#239108=CARTESIAN_POINT('Ctrl Pts',(34.7303057514047,-47.7327846251242,
2.66072561226567));
#239109=CARTESIAN_POINT('Ctrl Pts',(34.7351793935412,-47.7303113621612,
2.66154735980305));
#239110=CARTESIAN_POINT('Ctrl Pts',(34.7401391868074,-47.7280985748131,
2.6626189576685));
#239111=CARTESIAN_POINT('Ctrl Pts',(34.7451421370599,-47.7261394006513,
2.66391429250994));
#239112=CARTESIAN_POINT('Ctrl Pts',(34.7517732610329,-47.7235426275283,
2.6656311846409));
#239113=CARTESIAN_POINT('Ctrl Pts',(34.7584811778437,-47.7213971161174,
2.66774105138666));
#239114=CARTESIAN_POINT('Ctrl Pts',(34.7651763312121,-47.719693290934,2.67016894181717));
#239115=CARTESIAN_POINT('Ctrl Pts',(34.7685239078963,-47.7188413783422,
2.67138288703242));
#239116=CARTESIAN_POINT('Ctrl Pts',(34.7718684539197,-47.7180997687556,
2.67267613167518));
#239117=CARTESIAN_POINT('Ctrl Pts',(34.7751999143437,-47.7174664279764,
2.6740383543252));
#239118=CARTESIAN_POINT('Ctrl Pts',(34.7768656445558,-47.7171497575867,
2.67471946565021));
#239119=CARTESIAN_POINT('Ctrl Pts',(34.7785281166323,-47.7168601447015,
2.6754178138949));
#239120=CARTESIAN_POINT('Ctrl Pts',(34.7801861569095,-47.7165972740592,
2.67613207244136));
#239121=CARTESIAN_POINT('Ctrl Pts',(34.7806006669788,-47.7165315563986,
2.67631063707798));
#239122=CARTESIAN_POINT('Ctrl Pts',(34.7810149003422,-47.7164675099211,
2.67649019601813));
#239123=CARTESIAN_POINT('Ctrl Pts',(34.7814288392286,-47.7164051292828,
2.67667072836624));
#239124=CARTESIAN_POINT('Ctrl Pts',(34.7826706558879,-47.7162179873678,
2.67721232541058));
#239125=CARTESIAN_POINT('Ctrl Pts',(34.7839098208543,-47.7160458390449,
2.67776268340014));
#239126=CARTESIAN_POINT('Ctrl Pts',(34.7851458668352,-47.7158885307483,
2.67832123541483));
#239127=CARTESIAN_POINT('Ctrl Pts',(34.7938524151216,-47.7147804714194,
2.68225560368412));
#239128=CARTESIAN_POINT('Ctrl Pts',(34.8024290252888,-47.7143609747532,
2.68661792998856));
#239129=CARTESIAN_POINT('Ctrl Pts',(34.8108122146623,-47.7145286167441,
2.69130986622546));
#239130=CARTESIAN_POINT('Ctrl Pts',(34.8148780524495,-47.7146099229285,
2.69358545023023));
#239131=CARTESIAN_POINT('Ctrl Pts',(34.8188987667933,-47.7148297795034,
2.69593918853438));
#239132=CARTESIAN_POINT('Ctrl Pts',(34.8228686918044,-47.7151790039204,
2.69836306235443));
#239133=CARTESIAN_POINT('Ctrl Pts',(34.8289463696258,-47.7157136421032,
2.70207384382176));
#239134=CARTESIAN_POINT('Ctrl Pts',(34.8349017567801,-47.7165501157946,
2.70594760814176));
#239135=CARTESIAN_POINT('Ctrl Pts',(34.8407017446573,-47.7176563296776,
2.70995196345656));
#239136=CARTESIAN_POINT('Ctrl Pts',(34.8433952890326,-47.7181700611277,
2.71181160678054));
#239137=CARTESIAN_POINT('Ctrl Pts',(34.8460552817724,-47.7187417155516,
2.71369962772047));
#239138=CARTESIAN_POINT('Ctrl Pts',(34.8486779186782,-47.7193692101065,
2.7156118313861));
#239139=CARTESIAN_POINT('Ctrl Pts',(34.8488789334633,-47.7194173050917,
2.7157583942626));
#239140=CARTESIAN_POINT('Ctrl Pts',(34.8490797487417,-47.719465700675,2.71590508903158));
#239141=CARTESIAN_POINT('Ctrl Pts',(34.8492803638663,-47.7195143955473,
2.7160519140986));
#239142=CARTESIAN_POINT('Ctrl Pts',(34.8520984015311,-47.7201984116928,
2.71811436362702));
#239143=CARTESIAN_POINT('Ctrl Pts',(34.8548765847941,-47.7209435418721,
2.72020091026908));
#239144=CARTESIAN_POINT('Ctrl Pts',(34.8576119849591,-47.7217448891697,
2.72230624862131));
#239145=CARTESIAN_POINT('Ctrl Pts',(34.8674206434762,-47.7246183780641,
2.7298556175306));
#239146=CARTESIAN_POINT('Ctrl Pts',(34.8767555719426,-47.7282350429863,
2.73770089914297));
#239147=CARTESIAN_POINT('Ctrl Pts',(34.8856231565607,-47.7324659181291,
2.7457482334705));
#239148=CARTESIAN_POINT('Ctrl Pts',(34.895367741228,-47.7371152248818,2.75459144546986));
#239149=CARTESIAN_POINT('Ctrl Pts',(34.9045486251005,-47.7425063743629,
2.76367911754215));
#239150=CARTESIAN_POINT('Ctrl Pts',(34.9131661493093,-47.7485205638406,
2.77292162564655));
#239151=CARTESIAN_POINT('Ctrl Pts',(34.9224709127511,-47.7550143791208,
2.78290121484603));
#239152=CARTESIAN_POINT('Ctrl Pts',(34.9311199164031,-47.7622350952164,
2.79306229500001));
#239153=CARTESIAN_POINT('Ctrl Pts',(34.9390908738043,-47.7700859102987,
2.80331916685007));
#239154=CARTESIAN_POINT('Ctrl Pts',(34.9469949630638,-47.7778708651099,
2.81348999408516));
#239155=CARTESIAN_POINT('Ctrl Pts',(34.9542331399578,-47.7862765797888,
2.8237563596677));
#239156=CARTESIAN_POINT('Ctrl Pts',(34.9607485668371,-47.7952442955496,
2.83404198860229));
#239157=CARTESIAN_POINT('Origin',(-0.0123294189942718,-0.00895784724474341,
2.83404198860262));
#239158=CARTESIAN_POINT('Ctrl Pts',(36.9278827595333,-50.8527980281379,
2.65878198860226));
#239159=CARTESIAN_POINT('Ctrl Pts',(36.9209320551072,-50.8578435704953,
2.65878198860226));
#239160=CARTESIAN_POINT('Ctrl Pts',(36.9136216385505,-50.8622636476104,
2.65944603041817));
#239161=CARTESIAN_POINT('Ctrl Pts',(36.9061023515947,-50.8660552387514,
2.6607043926404));
#239162=CARTESIAN_POINT('Ctrl Pts',(36.9012978851882,-50.8684778849905,
2.66150842619563));
#239163=CARTESIAN_POINT('Ctrl Pts',(36.8964085464701,-50.8706447895119,
2.66255428265333));
#239164=CARTESIAN_POINT('Ctrl Pts',(36.8914758894172,-50.8725634718541,
2.66381699700615));
#239165=CARTESIAN_POINT('Ctrl Pts',(36.8847438022852,-50.8751820882645,
2.66554034873215));
#239166=CARTESIAN_POINT('Ctrl Pts',(36.8779301449089,-50.8773323251408,
2.66766759643919));
#239167=CARTESIAN_POINT('Ctrl Pts',(36.8711298300327,-50.8790261328799,
2.67012012783095));
#239168=CARTESIAN_POINT('Ctrl Pts',(36.8677296725947,-50.8798730367495,
2.67134639352683));
#239169=CARTESIAN_POINT('Ctrl Pts',(36.8643326829605,-50.8806059576331,
2.6726537558496));
#239170=CARTESIAN_POINT('Ctrl Pts',(36.8609495224157,-50.8812272732509,
2.67403135126888));
#239171=CARTESIAN_POINT('Ctrl Pts',(36.8592579421434,-50.8815379310598,
2.67472014897852));
#239172=CARTESIAN_POINT('Ctrl Pts',(36.8575698050851,-50.8818206978287,
2.6754264966858));
#239173=CARTESIAN_POINT('Ctrl Pts',(36.8558863556343,-50.8820759354563,
2.6761489965605));
#239174=CARTESIAN_POINT('Ctrl Pts',(36.8554654932716,-50.8821397448631,
2.67632962152917));
#239175=CARTESIAN_POINT('Ctrl Pts',(36.8550449235855,-50.8822018339184,
2.67651125590898));
#239176=CARTESIAN_POINT('Ctrl Pts',(36.8546246654171,-50.8822622087205,
2.67669387767471));
#239177=CARTESIAN_POINT('Ctrl Pts',(36.853363890912,-50.8824433331267,2.67724174297192));
#239178=CARTESIAN_POINT('Ctrl Pts',(36.8521059215537,-50.88260902815,2.67779849504695));
#239179=CARTESIAN_POINT('Ctrl Pts',(36.8508512527545,-50.8827594682963,
2.67836353617957));
#239180=CARTESIAN_POINT('Ctrl Pts',(36.8421807128861,-50.8837991030482,
2.68226832098865));
#239181=CARTESIAN_POINT('Ctrl Pts',(36.8336410897273,-50.8841591194355,
2.68659153751359));
#239182=CARTESIAN_POINT('Ctrl Pts',(36.8252931160718,-50.8839416093721,
2.69123699486159));
#239183=CARTESIAN_POINT('Ctrl Pts',(36.8211441960799,-50.8838335074677,
2.69354577441187));
#239184=CARTESIAN_POINT('Ctrl Pts',(36.8170422299142,-50.8835822787321,
2.69593478828077));
#239185=CARTESIAN_POINT('Ctrl Pts',(36.8129929908136,-50.883197784386,2.69839565261167));
#239186=CARTESIAN_POINT('Ctrl Pts',(36.8040597645474,-50.882349532429,2.70382468688993));
#239187=CARTESIAN_POINT('Ctrl Pts',(36.7953829494622,-50.8808651175407,
2.70961155815034));
#239188=CARTESIAN_POINT('Ctrl Pts',(36.7870848098368,-50.8788231440725,
2.71562701361715));
#239189=CARTESIAN_POINT('Ctrl Pts',(36.7840533947866,-50.878077185414,2.71782453535805));
#239190=CARTESIAN_POINT('Ctrl Pts',(36.7810676701183,-50.877263133323,2.72005051502349));
#239191=CARTESIAN_POINT('Ctrl Pts',(36.7781294934924,-50.876385967002,2.72229986760062));
#239192=CARTESIAN_POINT('Ctrl Pts',(36.7682604691141,-50.8734396581486,
2.72985520488837));
#239193=CARTESIAN_POINT('Ctrl Pts',(36.7588677364076,-50.8697545265633,
2.73770845534504));
#239194=CARTESIAN_POINT('Ctrl Pts',(36.7499455893915,-50.8654587487958,
2.745767067017));
#239195=CARTESIAN_POINT('Ctrl Pts',(36.740139092923,-50.860737180161,2.75462443584979));
#239196=CARTESIAN_POINT('Ctrl Pts',(36.730900418415,-50.8552777667771,2.76373036323134));
#239197=CARTESIAN_POINT('Ctrl Pts',(36.7222305213324,-50.8491983060113,
2.77299664636773));
#239198=CARTESIAN_POINT('Ctrl Pts',(36.712892670699,-50.8426504662824,2.78297683033429));
#239199=CARTESIAN_POINT('Ctrl Pts',(36.7042135591852,-50.8353827952104,
2.79314401478846));
#239200=CARTESIAN_POINT('Ctrl Pts',(36.696217769431,-50.8274903908659,2.80341452427885));
#239201=CARTESIAN_POINT('Ctrl Pts',(36.6883299498358,-50.8197045606284,
2.81354634721317));
#239202=CARTESIAN_POINT('Ctrl Pts',(36.6811063421674,-50.8113095502205,
2.82378004209163));
#239203=CARTESIAN_POINT('Ctrl Pts',(36.6746059268184,-50.8023624960585,
2.83404198860227));
#239204=CARTESIAN_POINT('Ctrl Pts',(34.6525130919802,-48.0191904766731,
2.83404198860228));
#239205=CARTESIAN_POINT('Ctrl Pts',(34.646292158807,-48.0106280967249,2.82422126442986));
#239206=CARTESIAN_POINT('Ctrl Pts',(34.6407689407921,-48.0016058360806,
2.81442815028493));
#239207=CARTESIAN_POINT('Ctrl Pts',(34.6359660967493,-47.9921771448963,
2.80471618166322));
#239208=CARTESIAN_POINT('Ctrl Pts',(34.6313285282533,-47.9830729139852,
2.79533842146252));
#239209=CARTESIAN_POINT('Ctrl Pts',(34.6273621044917,-47.9735885825102,
2.78603515650279));
#239210=CARTESIAN_POINT('Ctrl Pts',(34.6241270221289,-47.9637494987653,
2.77685887346812));
#239211=CARTESIAN_POINT('Ctrl Pts',(34.6210688561311,-47.9544484832163,
2.76818441216655));
#239212=CARTESIAN_POINT('Ctrl Pts',(34.6186639474978,-47.9448295964466,
2.75962261521724));
#239213=CARTESIAN_POINT('Ctrl Pts',(34.617004586212,-47.9349076763715,2.7512353770178));
#239214=CARTESIAN_POINT('Ctrl Pts',(34.6154763423057,-47.9257697544352,
2.74351087134269));
#239215=CARTESIAN_POINT('Ctrl Pts',(34.6145804463112,-47.9163742511068,
2.73593399450026));
#239216=CARTESIAN_POINT('Ctrl Pts',(34.6144269453425,-47.906736439065,2.72857657812782));
#239217=CARTESIAN_POINT('Ctrl Pts',(34.6143811744522,-47.9038626380657,
2.72638274508443));
#239218=CARTESIAN_POINT('Ctrl Pts',(34.6144016870569,-47.9009673483049,
2.72420861709637));
#239219=CARTESIAN_POINT('Ctrl Pts',(34.6144921419179,-47.89805115192,2.72205663736675));
#239220=CARTESIAN_POINT('Ctrl Pts',(34.6145816725532,-47.8951647518761,
2.71992664556714));
#239221=CARTESIAN_POINT('Ctrl Pts',(34.6147393566956,-47.8922608568393,
2.71782089927832));
#239222=CARTESIAN_POINT('Ctrl Pts',(34.61496832346,-47.8893433277779,2.71574387311194));
#239223=CARTESIAN_POINT('Ctrl Pts',(34.614984245361,-47.8891404485128,2.71559944077434));
#239224=CARTESIAN_POINT('Ctrl Pts',(34.61500050176,-47.8889374970509,2.71545515216017));
#239225=CARTESIAN_POINT('Ctrl Pts',(34.6150170939194,-47.8887344737208,
2.71531100781678));
#239226=CARTESIAN_POINT('Ctrl Pts',(34.6157445549674,-47.8798331871994,
2.70899119176039));
#239227=CARTESIAN_POINT('Ctrl Pts',(34.6171603320598,-47.8708080647645,
2.70298296066801));
#239228=CARTESIAN_POINT('Ctrl Pts',(34.619329190174,-47.8617555581812,2.69736727774105));
#239229=CARTESIAN_POINT('Ctrl Pts',(34.6213509428814,-47.8533170487307,
2.69213248525409));
#239230=CARTESIAN_POINT('Ctrl Pts',(34.6240275231023,-47.8448540540101,
2.68723866185458));
#239231=CARTESIAN_POINT('Ctrl Pts',(34.6274308957717,-47.8364666369698,
2.68278595829559));
#239232=CARTESIAN_POINT('Ctrl Pts',(34.6286758935246,-47.8333984113061,
2.68115710172785));
#239233=CARTESIAN_POINT('Ctrl Pts',(34.6300183184514,-47.8303405713847,
2.67958763637774));
#239234=CARTESIAN_POINT('Ctrl Pts',(34.6314622582454,-47.8272990958124,
2.67808378645315));
#239235=CARTESIAN_POINT('Ctrl Pts',(34.631809477528,-47.8265677225441,2.6777221607855));
#239236=CARTESIAN_POINT('Ctrl Pts',(34.6321630753109,-47.8258370084441,
2.67736403603513));
#239237=CARTESIAN_POINT('Ctrl Pts',(34.6325230544381,-47.8251070891643,
2.67700956934429));
#239238=CARTESIAN_POINT('Ctrl Pts',(34.6328717842176,-47.824399979862,2.67666617973753));
#239239=CARTESIAN_POINT('Ctrl Pts',(34.6332265027185,-47.8236936164938,
2.67632622314069));
#239240=CARTESIAN_POINT('Ctrl Pts',(34.6335872094469,-47.8229881245974,
2.67598984158723));
#239241=CARTESIAN_POINT('Ctrl Pts',(34.6375391685168,-47.815258645554,2.67230439292157));
#239242=CARTESIAN_POINT('Ctrl Pts',(34.6422128973072,-47.8076288798872,
2.66904964539901));
#239243=CARTESIAN_POINT('Ctrl Pts',(34.6475865476022,-47.8002860618998,
2.66640203566645));
#239244=CARTESIAN_POINT('Ctrl Pts',(34.6498151605506,-47.7972407764148,
2.66530399299372));
#239245=CARTESIAN_POINT('Ctrl Pts',(34.6521637338121,-47.7942448304643,
2.664309951422));
#239246=CARTESIAN_POINT('Ctrl Pts',(34.6546289547343,-47.7913110614413,
2.66343053473309));
#239247=CARTESIAN_POINT('Ctrl Pts',(34.6588336459115,-47.786307212652,2.66193059792832));
#239248=CARTESIAN_POINT('Ctrl Pts',(34.6633779280164,-47.7814867201288,
2.66076519817074));
#239249=CARTESIAN_POINT('Ctrl Pts',(34.6682420184012,-47.7769196237418,
2.65997805604406));
#239250=CARTESIAN_POINT('Ctrl Pts',(34.6706740635937,-47.7746360755483,
2.65958448498072));
#239251=CARTESIAN_POINT('Ctrl Pts',(34.6731869650549,-47.7724170058814,
2.65928526260708));
#239252=CARTESIAN_POINT('Ctrl Pts',(34.6757782448039,-47.7702712352606,
2.6590846397127));
#239253=CARTESIAN_POINT('Ctrl Pts',(34.6783695245528,-47.7681254646397,
2.65888401681832));
#239254=CARTESIAN_POINT('Ctrl Pts',(34.6810391382375,-47.7660530039188,
2.65878198860229));
#239255=CARTESIAN_POINT('Ctrl Pts',(34.6837837831351,-47.7640607692758,
2.65878198860229));
#239256=CARTESIAN_POINT('Origin',(38.9973987043324,-43.2882232241942,2.83404198860232));
#239257=CARTESIAN_POINT('Ctrl Pts',(42.0671296588101,-46.4355828792663,
2.8340419886023));
#239258=CARTESIAN_POINT('Ctrl Pts',(42.0742293550387,-46.4434678907493,
2.82419652439974));
#239259=CARTESIAN_POINT('Ctrl Pts',(42.0806858315488,-46.4518896956746,
2.81438790575495));
#239260=CARTESIAN_POINT('Ctrl Pts',(42.0864721532177,-46.460795700733,2.80466781256683));
#239261=CARTESIAN_POINT('Ctrl Pts',(42.0920704538876,-46.4694123136587,
2.79526356452807));
#239262=CARTESIAN_POINT('Ctrl Pts',(42.0970420880529,-46.4784832882836,
2.78594102495908));
#239263=CARTESIAN_POINT('Ctrl Pts',(42.1013257711413,-46.487988795821,2.77675109088403));
#239264=CARTESIAN_POINT('Ctrl Pts',(42.1053778715689,-46.4969804206359,
2.76805797913257));
#239265=CARTESIAN_POINT('Ctrl Pts',(42.1088147776147,-46.5063617095277,
2.75948271209687));
#239266=CARTESIAN_POINT('Ctrl Pts',(42.1115441100145,-46.5161273793285,
2.75108575572704));
#239267=CARTESIAN_POINT('Ctrl Pts',(42.1140580225452,-46.5251222674863,
2.74335155162698));
#239268=CARTESIAN_POINT('Ctrl Pts',(42.1159717447032,-46.5344438074388,
2.73576818685323));
#239269=CARTESIAN_POINT('Ctrl Pts',(42.1171748456151,-46.5440884908269,
2.72840626159835));
#239270=CARTESIAN_POINT('Ctrl Pts',(42.1175238194559,-46.5468860468524,
2.72627084693231));
#239271=CARTESIAN_POINT('Ctrl Pts',(42.1178127362988,-46.5497107674253,
2.72415424587285));
#239272=CARTESIAN_POINT('Ctrl Pts',(42.1180382068981,-46.5525624800835,
2.72205867173227));
#239273=CARTESIAN_POINT('Ctrl Pts',(42.1182826315244,-46.5556539199568,
2.7197869346283));
#239274=CARTESIAN_POINT('Ctrl Pts',(42.1184532289198,-46.5587726948493,
2.7175441134073));
#239275=CARTESIAN_POINT('Ctrl Pts',(42.1185461584685,-46.5619176830188,
2.71533341844227));
#239276=CARTESIAN_POINT('Ctrl Pts',(42.118801204344,-46.5705491277282,2.70926614876372));
#239277=CARTESIAN_POINT('Ctrl Pts',(42.1184278543827,-46.5793682643805,
2.70347381860389));
#239278=CARTESIAN_POINT('Ctrl Pts',(42.1173773384973,-46.5882835698998,
2.69804914171374));
#239279=CARTESIAN_POINT('Ctrl Pts',(42.1164161734959,-46.5964405904273,
2.69308585687143));
#239280=CARTESIAN_POINT('Ctrl Pts',(42.114880157948,-46.6046697328847,2.68842799053089));
#239281=CARTESIAN_POINT('Ctrl Pts',(42.1127009621828,-46.6129145292198,
2.68414767054092));
#239282=CARTESIAN_POINT('Ctrl Pts',(42.1116305483418,-46.6169643462458,
2.68204519134462));
#239283=CARTESIAN_POINT('Ctrl Pts',(42.1104045383081,-46.6210176421365,
2.68003431778445));
#239284=CARTESIAN_POINT('Ctrl Pts',(42.1090123875514,-46.6250654385586,
2.67812693945225));
#239285=CARTESIAN_POINT('Ctrl Pts',(42.108748240505,-46.6258334685037,2.67776503299177));
#239286=CARTESIAN_POINT('Ctrl Pts',(42.1084776383334,-46.6266015422607,
2.67740659639897));
#239287=CARTESIAN_POINT('Ctrl Pts',(42.1082005605491,-46.6273695213199,
2.67705178968829));
#239288=CARTESIAN_POINT('Ctrl Pts',(42.1079321414455,-46.6281135010335,
2.67670807068731));
#239289=CARTESIAN_POINT('Ctrl Pts',(42.1076576451506,-46.628857391859,2.67636775825239));
#239290=CARTESIAN_POINT('Ctrl Pts',(42.1073770559085,-46.6296010653153,
2.67603099699229));
#239291=CARTESIAN_POINT('Ctrl Pts',(42.1043192521654,-46.6377054654036,
2.67236104217142));
#239292=CARTESIAN_POINT('Ctrl Pts',(42.1005354505687,-46.6457892400048,
2.6691144054152));
#239293=CARTESIAN_POINT('Ctrl Pts',(42.096023846079,-46.653661939073,2.66646778189694));
#239294=CARTESIAN_POINT('Ctrl Pts',(42.0941185674866,-46.6569866287779,
2.66535009635002));
#239295=CARTESIAN_POINT('Ctrl Pts',(42.0920839261394,-46.6602736399397,
2.66433897912343));
#239296=CARTESIAN_POINT('Ctrl Pts',(42.0899216923184,-46.6635089796837,
2.66344564884769));
#239297=CARTESIAN_POINT('Ctrl Pts',(42.0862805445931,-46.6689572109688,
2.66194130298562));
#239298=CARTESIAN_POINT('Ctrl Pts',(42.0822770520162,-46.6742564366669,
2.66077206705398));
#239299=CARTESIAN_POINT('Ctrl Pts',(42.0779224130576,-46.6793332901443,
2.65998225155693));
#239300=CARTESIAN_POINT('Ctrl Pts',(42.076833753318,-46.6806025035137,2.65978479768267));
#239301=CARTESIAN_POINT('Ctrl Pts',(42.0757229796951,-46.6818576549898,
2.65961098966601));
#239302=CARTESIAN_POINT('Ctrl Pts',(42.0745900553981,-46.6830973739104,
2.65946139030481));
#239303=CARTESIAN_POINT('Ctrl Pts',(42.0728906689526,-46.6849569522912,
2.659236991263));
#239304=CARTESIAN_POINT('Ctrl Pts',(42.0711414461008,-46.6867817869753,
2.65906707562422));
#239305=CARTESIAN_POINT('Ctrl Pts',(42.0693433991613,-46.6885684866726,
2.658953325629));
#239306=CARTESIAN_POINT('Ctrl Pts',(42.0675453522218,-46.6903551863698,
2.65883957563378));
#239307=CARTESIAN_POINT('Ctrl Pts',(42.065698492617,-46.6921037531344,2.6587819886023));
#239308=CARTESIAN_POINT('Ctrl Pts',(42.0638038389706,-46.6938111422597,
2.6587819886023));
#239309=CARTESIAN_POINT('Ctrl Pts',(39.5091373124628,-43.856566526705,2.65878198860232));
#239310=CARTESIAN_POINT('Ctrl Pts',(39.5155480799608,-43.8507890749201,
2.65878198860232));
#239311=CARTESIAN_POINT('Ctrl Pts',(39.5223801852471,-43.8455908828144,
2.65945335517828));
#239312=CARTESIAN_POINT('Ctrl Pts',(39.5294841269573,-43.8409939475736,
2.66072561226578));
#239313=CARTESIAN_POINT('Ctrl Pts',(39.5340725443953,-43.838024799081,2.66154735980316));
#239314=CARTESIAN_POINT('Ctrl Pts',(39.5387738681338,-43.8353056940454,
2.66261895766858));
#239315=CARTESIAN_POINT('Ctrl Pts',(39.5435446222369,-43.832834301743,2.66391429250998));
#239316=CARTESIAN_POINT('Ctrl Pts',(39.5498679835149,-43.8295586128163,
2.66563118464095));
#239317=CARTESIAN_POINT('Ctrl Pts',(39.5563148866448,-43.8267236865055,
2.6677410513867));
#239318=CARTESIAN_POINT('Ctrl Pts',(39.5627952650345,-43.8243293609617,
2.6701689418172));
#239319=CARTESIAN_POINT('Ctrl Pts',(39.5660354542293,-43.8231321981898,
2.67138288703246));
#239320=CARTESIAN_POINT('Ctrl Pts',(39.5692841591691,-43.8220450509619,
2.67267613167522));
#239321=CARTESIAN_POINT('Ctrl Pts',(39.572531167366,-43.8210669472512,2.67403835432524));
#239322=CARTESIAN_POINT('Ctrl Pts',(39.5741546714645,-43.8205778953958,
2.67471946565025));
#239323=CARTESIAN_POINT('Ctrl Pts',(39.5757777635552,-43.8201160933889,
2.67541781389493));
#239324=CARTESIAN_POINT('Ctrl Pts',(39.57739924345,-43.8196813503772,2.6761320724414));
#239325=CARTESIAN_POINT('Ctrl Pts',(39.5778046134237,-43.8195726646243,
2.67631063707801));
#239326=CARTESIAN_POINT('Ctrl Pts',(39.5782098828935,-43.8194656698232,
2.67649019601816));
#239327=CARTESIAN_POINT('Ctrl Pts',(39.5786150336271,-43.8193603625169,
2.67667072836627));
#239328=CARTESIAN_POINT('Ctrl Pts',(39.5798304858281,-43.8190444405979,
2.67721232541061));
#239329=CARTESIAN_POINT('Ctrl Pts',(39.5810448681194,-43.8187437073117,
2.67776268340017));
#239330=CARTESIAN_POINT('Ctrl Pts',(39.5822576997166,-43.8184580587796,
2.67832123541486));
#239331=CARTESIAN_POINT('Ctrl Pts',(39.5908007288818,-43.8164459874028,
2.6822556036842));
#239332=CARTESIAN_POINT('Ctrl Pts',(39.5992865061394,-43.8151322889025,
2.68661792998872));
#239333=CARTESIAN_POINT('Ctrl Pts',(39.6076412948842,-43.8144227306305,
2.69130986622569));
#239334=CARTESIAN_POINT('Ctrl Pts',(39.611693358397,-43.8140785956353,2.69358545023039));
#239335=CARTESIAN_POINT('Ctrl Pts',(39.6157150281166,-43.8138769687213,
2.69593918853448));
#239336=CARTESIAN_POINT('Ctrl Pts',(39.6196997093547,-43.8138093098897,
2.69836306235446));
#239337=CARTESIAN_POINT('Ctrl Pts',(39.6257999779287,-43.8137057289457,
2.70207384382179));
#239338=CARTESIAN_POINT('Ctrl Pts',(39.6318101761586,-43.8139151128793,
2.70594760814179));
#239339=CARTESIAN_POINT('Ctrl Pts',(39.6376940219325,-43.8144090029872,
2.70995196345659));
#239340=CARTESIAN_POINT('Ctrl Pts',(39.6404265103489,-43.8146383681083,
2.71181160678057));
#239341=CARTESIAN_POINT('Ctrl Pts',(39.6431316855286,-43.8149288459961,
2.7136996277205));
#239342=CARTESIAN_POINT('Ctrl Pts',(39.6458055463966,-43.8152787628647,
2.71561183138612));
#239343=CARTESIAN_POINT('Ctrl Pts',(39.6460104872966,-43.8153055826139,
2.71575839426263));
#239344=CARTESIAN_POINT('Ctrl Pts',(39.6462152612038,-43.8153327221687,
2.7159050890316));
#239345=CARTESIAN_POINT('Ctrl Pts',(39.6464198673379,-43.8153601802948,
2.71605191409863));
#239346=CARTESIAN_POINT('Ctrl Pts',(39.6492939666541,-43.8157458841817,
2.71811436362704));
#239347=CARTESIAN_POINT('Ctrl Pts',(39.6521348180511,-43.8161965332328,
2.7202009102691));
#239348=CARTESIAN_POINT('Ctrl Pts',(39.6549389970093,-43.8167075634904,
2.72230624862133));
#239349=CARTESIAN_POINT('Ctrl Pts',(39.6649942840471,-43.8185400271104,
2.72985561753061));
#239350=CARTESIAN_POINT('Ctrl Pts',(39.6746561192251,-43.8211611138364,
2.73770089914295));
#239351=CARTESIAN_POINT('Ctrl Pts',(39.6839173731638,-43.8244418968094,
2.74574823347047));
#239352=CARTESIAN_POINT('Ctrl Pts',(39.6940945608671,-43.828047147713,2.75459144547006));
#239353=CARTESIAN_POINT('Ctrl Pts',(39.7037886794679,-43.8324491002306,
2.76367911754261));
#239354=CARTESIAN_POINT('Ctrl Pts',(39.7129876499616,-43.8375295667866,
2.77292162564728));
#239355=CARTESIAN_POINT('Ctrl Pts',(39.7229202294684,-43.8430151956441,
2.78290121484759));
#239356=CARTESIAN_POINT('Ctrl Pts',(39.7322766233313,-43.8492922888414,
2.79306229500245));
#239357=CARTESIAN_POINT('Ctrl Pts',(39.7410245486304,-43.8562669044101,
2.80331916685339));
#239358=CARTESIAN_POINT('Ctrl Pts',(39.7496990878239,-43.8631830101199,
2.81348999408741));
#239359=CARTESIAN_POINT('Ctrl Pts',(39.7577762496646,-43.8707860819059,
2.82375635966885));
#239360=CARTESIAN_POINT('Ctrl Pts',(39.7651933659004,-43.8790236240213,
2.83404198860232));
#239361=CARTESIAN_POINT('Origin',(-0.0113255271402735,-0.0101975504407155,
2.83404198860262));
#239362=CARTESIAN_POINT('Ctrl Pts',(42.0411527846901,-46.7142062431416,
2.6587819886023));
#239363=CARTESIAN_POINT('Ctrl Pts',(42.0347675597393,-46.7199506919421,
2.6587819886023));
#239364=CARTESIAN_POINT('Ctrl Pts',(42.0279592142781,-46.7251107020207,
2.65944603041816));
#239365=CARTESIAN_POINT('Ctrl Pts',(42.0208774479585,-46.7296675019389,
2.66070439264032));
#239366=CARTESIAN_POINT('Ctrl Pts',(42.0163525364099,-46.7325790801589,
2.66150842619558));
#239367=CARTESIAN_POINT('Ctrl Pts',(42.0117164852002,-46.7352451892134,
2.66255428265334));
#239368=CARTESIAN_POINT('Ctrl Pts',(42.0070114066752,-46.7376689638746,
2.66381699700625));
#239369=CARTESIAN_POINT('Ctrl Pts',(42.0005899185702,-46.7409769299529,
2.66554034873225));
#239370=CARTESIAN_POINT('Ctrl Pts',(41.9940383480783,-46.7438276087414,
2.6676675964393));
#239371=CARTESIAN_POINT('Ctrl Pts',(41.9874523371586,-46.7462229640882,
2.67012012783106));
#239372=CARTESIAN_POINT('Ctrl Pts',(41.9841593316988,-46.7474206417616,
2.67134639352694));
#239373=CARTESIAN_POINT('Ctrl Pts',(41.9808575622229,-46.7485046297341,
2.6726537558497));
#239374=CARTESIAN_POINT('Ctrl Pts',(41.9775578801523,-46.7494761782927,
2.67403135126898));
#239375=CARTESIAN_POINT('Ctrl Pts',(41.9759080391171,-46.749961952572,2.67472014897862));
#239376=CARTESIAN_POINT('Ctrl Pts',(41.9742587070261,-46.7504196286874,
2.6754264966859));
#239377=CARTESIAN_POINT('Ctrl Pts',(41.9726111592845,-46.7508494364806,
2.67614899656059));
#239378=CARTESIAN_POINT('Ctrl Pts',(41.9721992723491,-46.7509568884289,
2.67632962152926));
#239379=CARTESIAN_POINT('Ctrl Pts',(41.9717874966612,-46.7510625988569,
2.67651125590908));
#239380=CARTESIAN_POINT('Ctrl Pts',(41.9713758515963,-46.75116657186,2.67669387767482));
#239381=CARTESIAN_POINT('Ctrl Pts',(41.9701409164017,-46.7514784908693,
2.67724174297202));
#239382=CARTESIAN_POINT('Ctrl Pts',(41.9689071581774,-46.7517747718017,
2.67779849504705));
#239383=CARTESIAN_POINT('Ctrl Pts',(41.9676750878625,-46.7520555364226,
2.67836353617967));
#239384=CARTESIAN_POINT('Ctrl Pts',(41.9591607175419,-46.7539957941547,
2.68226832098866));
#239385=CARTESIAN_POINT('Ctrl Pts',(41.9507055072921,-46.7552464720202,
2.6865915375135));
#239386=CARTESIAN_POINT('Ctrl Pts',(41.9423805287172,-46.7559027543574,
2.69123699486138));
#239387=CARTESIAN_POINT('Ctrl Pts',(41.9382430372171,-46.7562289248775,
2.69354577441174));
#239388=CARTESIAN_POINT('Ctrl Pts',(41.9341372814973,-46.7564078446189,
2.69593478828073));
#239389=CARTESIAN_POINT('Ctrl Pts',(41.9300700339489,-46.7564487173136,
2.69839565261173));
#239390=CARTESIAN_POINT('Ctrl Pts',(41.9210970783574,-46.7565388885832,
2.70382468688997));
#239391=CARTESIAN_POINT('Ctrl Pts',(41.9123126321659,-46.7559695796219,
2.70961155815039));
#239392=CARTESIAN_POINT('Ctrl Pts',(41.903846506269,-46.7548061840811,2.71562701361718));
#239393=CARTESIAN_POINT('Ctrl Pts',(41.9007537237153,-46.7543811810188,
2.71782453535808));
#239394=CARTESIAN_POINT('Ctrl Pts',(41.8976992635451,-46.7538836816017,
2.72005051502352));
#239395=CARTESIAN_POINT('Ctrl Pts',(41.8946854937106,-46.7533184435771,
2.72229986760064));
#239396=CARTESIAN_POINT('Ctrl Pts',(41.8845625597436,-46.751419868864,2.72985520488842));
#239397=CARTESIAN_POINT('Ctrl Pts',(41.8748360802679,-46.7487367327307,
2.73770845534509));
#239398=CARTESIAN_POINT('Ctrl Pts',(41.865513778658,-46.7453971059998,2.74576706701706));
#239399=CARTESIAN_POINT('Ctrl Pts',(41.8552674648894,-46.7417264606178,
2.75462443584986));
#239400=CARTESIAN_POINT('Ctrl Pts',(41.8455087367155,-46.7372626589204,
2.76373036323144));
#239401=CARTESIAN_POINT('Ctrl Pts',(41.8362508575448,-46.7321227530954,
2.77299664636788));
#239402=CARTESIAN_POINT('Ctrl Pts',(41.8262797250094,-46.7265868542943,
2.78297683033457));
#239403=CARTESIAN_POINT('Ctrl Pts',(41.8168884800878,-46.7202662104738,
2.7931440147889));
#239404=CARTESIAN_POINT('Ctrl Pts',(41.8081115112088,-46.7132528291616,
2.80341452427952));
#239405=CARTESIAN_POINT('Ctrl Pts',(41.7994530610451,-46.706334152178,2.81354634721356));
#239406=CARTESIAN_POINT('Ctrl Pts',(41.7913915075187,-46.6987402031246,
2.82378004209179));
#239407=CARTESIAN_POINT('Ctrl Pts',(41.7839914803032,-46.690521640289,2.8340419886023));
#239408=CARTESIAN_POINT('Ctrl Pts',(39.4820551873935,-44.1339623850441,
2.83404198860232));
#239409=CARTESIAN_POINT('Ctrl Pts',(39.4749733207249,-44.1260971752936,
2.82422126442949));
#239410=CARTESIAN_POINT('Ctrl Pts',(39.4685372764356,-44.1177016730281,
2.81442815028416));
#239411=CARTESIAN_POINT('Ctrl Pts',(39.4627751762747,-44.1088266671073,
2.80471618166206));
#239412=CARTESIAN_POINT('Ctrl Pts',(39.4572113615976,-44.1002570680336,
2.79533842146101));
#239413=CARTESIAN_POINT('Ctrl Pts',(39.4522752837261,-44.0912392968988,
2.78603515650095));
#239414=CARTESIAN_POINT('Ctrl Pts',(39.4480294591791,-44.0817922708717,
2.77685887346595));
#239415=CARTESIAN_POINT('Ctrl Pts',(39.4440158252724,-44.0728618726508,
2.76818441216407));
#239416=CARTESIAN_POINT('Ctrl Pts',(39.4406186435279,-44.0635470605525,
2.75962261521446));
#239417=CARTESIAN_POINT('Ctrl Pts',(39.4379312493388,-44.0538529442785,
2.75123537701474));
#239418=CARTESIAN_POINT('Ctrl Pts',(39.4354562043751,-44.0449248258212,
2.74351087133926));
#239419=CARTESIAN_POINT('Ctrl Pts',(39.4335831186682,-44.0356744386741,
2.73593399449648));
#239420=CARTESIAN_POINT('Ctrl Pts',(39.432423032912,-44.0261054687947,2.72857657812373));
#239421=CARTESIAN_POINT('Ctrl Pts',(39.4320771187575,-44.0232521951406,
2.72638274508174));
#239422=CARTESIAN_POINT('Ctrl Pts',(39.4317948788029,-44.0203706219308,
2.72420861709505));
#239423=CARTESIAN_POINT('Ctrl Pts',(39.4315800126161,-44.017460945669,2.72205663736677));
#239424=CARTESIAN_POINT('Ctrl Pts',(39.4313673418322,-44.0145809991268,
2.71992664556716));
#239425=CARTESIAN_POINT('Ctrl Pts',(39.4312206224788,-44.0116765294498,
2.71782089927835));
#239426=CARTESIAN_POINT('Ctrl Pts',(39.4311433701099,-44.0087510493739,
2.71574387311197));
#239427=CARTESIAN_POINT('Ctrl Pts',(39.4311379981313,-44.0085476172107,
2.71559944077438));
#239428=CARTESIAN_POINT('Ctrl Pts',(39.4311329512716,-44.0083440782818,
2.7154551521602));
#239429=CARTESIAN_POINT('Ctrl Pts',(39.4311282308207,-44.0081404327819,
2.71531100781681));
#239430=CARTESIAN_POINT('Ctrl Pts',(39.4309212689598,-43.9992118680539,
2.70899119176044));
#239431=CARTESIAN_POINT('Ctrl Pts',(39.4313859080982,-43.9900881971803,
2.70298296066808));
#239432=CARTESIAN_POINT('Ctrl Pts',(39.4325966403788,-43.9808585737695,
2.69736727774114));
#239433=CARTESIAN_POINT('Ctrl Pts',(39.4337252532882,-43.9722549606532,
2.69213248525424));
#239434=CARTESIAN_POINT('Ctrl Pts',(39.4355025470898,-43.9635585482861,
2.6872386618548));
#239435=CARTESIAN_POINT('Ctrl Pts',(39.4380105519135,-43.954861329079,2.68278595829586));
#239436=CARTESIAN_POINT('Ctrl Pts',(39.4389280125249,-43.9516797737744,
2.68115710172802));
#239437=CARTESIAN_POINT('Ctrl Pts',(39.4399434521997,-43.9484983634053,
2.67958763637782));
#239438=CARTESIAN_POINT('Ctrl Pts',(39.4410615611728,-43.9453226165465,
2.67808378645314));
#239439=CARTESIAN_POINT('Ctrl Pts',(39.4413304290281,-43.9445589555194,
2.67772216078549));
#239440=CARTESIAN_POINT('Ctrl Pts',(39.4416057093433,-43.9437952833149,
2.67736403603512));
#239441=CARTESIAN_POINT('Ctrl Pts',(39.4418874191266,-43.9430317345443,
2.67700956934428));
#239442=CARTESIAN_POINT('Ctrl Pts',(39.4421603254791,-43.9422920466728,
2.67666617973753));
#239443=CARTESIAN_POINT('Ctrl Pts',(39.4424392657175,-43.9415524746572,
2.67632622314068));
#239444=CARTESIAN_POINT('Ctrl Pts',(39.442724252473,-43.9408131433993,2.67598984158722));
#239445=CARTESIAN_POINT('Ctrl Pts',(39.4458466117312,-43.9327129150425,
2.67230439292165));
#239446=CARTESIAN_POINT('Ctrl Pts',(39.4496972096659,-43.9246364083424,
2.66904964539915));
#239447=CARTESIAN_POINT('Ctrl Pts',(39.454273889062,-43.9167721156729,2.66640203566663));
#239448=CARTESIAN_POINT('Ctrl Pts',(39.4561719744236,-43.9135105590935,
2.66530399299382));
#239449=CARTESIAN_POINT('Ctrl Pts',(39.458194520329,-43.9102855324943,2.66430995142205));
#239450=CARTESIAN_POINT('Ctrl Pts',(39.4603395741455,-43.9071101492102,
2.66343053473309));
#239451=CARTESIAN_POINT('Ctrl Pts',(39.4639981869602,-43.9016942021209,
2.66193059792833));
#239452=CARTESIAN_POINT('Ctrl Pts',(39.4680136963365,-43.896425109935,2.66076519817076));
#239453=CARTESIAN_POINT('Ctrl Pts',(39.4723737491582,-43.8913745966866,
2.65997805604408));
#239454=CARTESIAN_POINT('Ctrl Pts',(39.4745537755691,-43.8888493400624,
2.65958448498074));
#239455=CARTESIAN_POINT('Ctrl Pts',(39.4768209551511,-43.8863797569633,
2.6592852626071));
#239456=CARTESIAN_POINT('Ctrl Pts',(39.479173745493,-43.8839748786084,2.65908463971272));
#239457=CARTESIAN_POINT('Ctrl Pts',(39.4815265358348,-43.8815700002535,
2.65888401681834));
#239458=CARTESIAN_POINT('Ctrl Pts',(39.4839648939622,-43.8792298420734,
2.65878198860232));
#239459=CARTESIAN_POINT('Ctrl Pts',(39.4864862581822,-43.8769616275868,
2.65878198860232));
#239460=CARTESIAN_POINT('Origin',(43.3086183250771,-38.9747476500507,2.83404198860235));
#239461=CARTESIAN_POINT('Ctrl Pts',(46.6905216402902,-41.7839914803019,
2.83404198860233));
#239462=CARTESIAN_POINT('Ctrl Pts',(46.6984066517725,-41.7910911765299,
2.82419652440033));
#239463=CARTESIAN_POINT('Ctrl Pts',(46.7057080773549,-41.7987919603583,
2.81438790575617));
#239464=CARTESIAN_POINT('Ctrl Pts',(46.7123936319704,-41.8070443420764,
2.8046678125687));
#239465=CARTESIAN_POINT('Ctrl Pts',(46.7188619458709,-41.8150285705284,
2.79526356453048));
#239466=CARTESIAN_POINT('Ctrl Pts',(46.7247545199416,-41.8235301761253,
2.78594102496204));
#239467=CARTESIAN_POINT('Ctrl Pts',(46.7300083326611,-41.8325358446869,
2.77675109088754));
#239468=CARTESIAN_POINT('Ctrl Pts',(46.7349781159827,-41.8410546526089,
2.76805797913662));
#239469=CARTESIAN_POINT('Ctrl Pts',(46.7393768060089,-41.8500252953105,
2.75948271210145));
#239470=CARTESIAN_POINT('Ctrl Pts',(46.7431119772974,-41.8594521748281,
2.75108575573212));
#239471=CARTESIAN_POINT('Ctrl Pts',(46.7465523401886,-41.868135012633,2.74335155163261));
#239472=CARTESIAN_POINT('Ctrl Pts',(46.7494299450231,-41.8772054497771,
2.73576818685938));
#239473=CARTESIAN_POINT('Ctrl Pts',(46.7516345991559,-41.8866715402901,
2.72840626160495));
#239474=CARTESIAN_POINT('Ctrl Pts',(46.7522740855145,-41.8894172933145,
2.72627084693667));
#239475=CARTESIAN_POINT('Ctrl Pts',(46.752856683342,-41.8921963397418,2.72415424587501));
#239476=CARTESIAN_POINT('Ctrl Pts',(46.7533790039321,-41.8950088623273,
2.72205867173227));
#239477=CARTESIAN_POINT('Ctrl Pts',(46.753945233034,-41.8980578176389,2.7197869346283));
#239478=CARTESIAN_POINT('Ctrl Pts',(46.7544408966258,-41.9011416752726,
2.71754411340731));
#239479=CARTESIAN_POINT('Ctrl Pts',(46.7548620578771,-41.9042597210849,
2.71533341844229));
#239480=CARTESIAN_POINT('Ctrl Pts',(46.7560179382359,-41.9128172222837,
2.70926614876376));
#239481=CARTESIAN_POINT('Ctrl Pts',(46.7565684843263,-41.9216270724804,
2.70347381860393));
#239482=CARTESIAN_POINT('Ctrl Pts',(46.7564556264623,-41.9306033478343,
2.69804914171379));
#239483=CARTESIAN_POINT('Ctrl Pts',(46.756352367644,-41.9388161524498,2.69308585687191));
#239484=CARTESIAN_POINT('Ctrl Pts',(46.7556849461651,-41.9471607721479,
2.68842799053174));
#239485=CARTESIAN_POINT('Ctrl Pts',(46.7543795041534,-41.9555881906098,
2.68414767054208));
#239486=CARTESIAN_POINT('Ctrl Pts',(46.7537382753017,-41.9597277110289,
2.68204519134541));
#239487=CARTESIAN_POINT('Ctrl Pts',(46.7529426662698,-41.9638869554861,
2.6800343177849));
#239488=CARTESIAN_POINT('Ctrl Pts',(46.7519812518,-41.9680580970358,2.67812693945238));
#239489=CARTESIAN_POINT('Ctrl Pts',(46.7517988327686,-41.9688495305174,
2.6777650329919));
#239490=CARTESIAN_POINT('Ctrl Pts',(46.7516099985535,-41.9696416823151,
2.6774065963991));
#239491=CARTESIAN_POINT('Ctrl Pts',(46.7514147143012,-41.9704344168197,
2.67705178968841));
#239492=CARTESIAN_POINT('Ctrl Pts',(46.7512255326818,-41.9712023783709,
2.67670807068744));
#239493=CARTESIAN_POINT('Ctrl Pts',(46.7510302978711,-41.9719708867605,
2.67636775825252));
#239494=CARTESIAN_POINT('Ctrl Pts',(46.7508289807698,-41.9727398158581,
2.67603099699241));
#239495=CARTESIAN_POINT('Ctrl Pts',(46.7486350684823,-41.9811194467219,
2.67236104217115));
#239496=CARTESIAN_POINT('Ctrl Pts',(46.7457169794826,-41.9895544525272,
2.6691144054146));
#239497=CARTESIAN_POINT('Ctrl Pts',(46.7420530111692,-41.9978556152113,
2.66646778189617));
#239498=CARTESIAN_POINT('Ctrl Pts',(46.7405056945983,-42.0013612477604,
2.6653500963496));
#239499=CARTESIAN_POINT('Ctrl Pts',(46.7388257854552,-42.0048429302636,
2.6643389791233));
#239500=CARTESIAN_POINT('Ctrl Pts',(46.7370135816694,-42.0082865614556,
2.66344564884778));
#239501=CARTESIAN_POINT('Ctrl Pts',(46.733961875776,-42.0140855503359,2.66194130298571));
#239502=CARTESIAN_POINT('Ctrl Pts',(46.7305342346691,-42.0197742252479,
2.66077206705405));
#239503=CARTESIAN_POINT('Ctrl Pts',(46.7267341265709,-42.0252784509094,
2.65998225155699));
#239504=CARTESIAN_POINT('Ctrl Pts',(46.7257840995464,-42.0266545073248,
2.65978479768272));
#239505=CARTESIAN_POINT('Ctrl Pts',(46.7248106099125,-42.0280188904096,
2.65961098966606));
#239506=CARTESIAN_POINT('Ctrl Pts',(46.7238134778069,-42.029370240856,2.65946139030486));
#239507=CARTESIAN_POINT('Ctrl Pts',(46.7223177796487,-42.0313972665255,
2.65923699126304));
#239508=CARTESIAN_POINT('Ctrl Pts',(46.7207688863879,-42.0333949481509,
2.65906707562426));
#239509=CARTESIAN_POINT('Ctrl Pts',(46.7191674503113,-42.0353598072037,
2.65895332562904));
#239510=CARTESIAN_POINT('Ctrl Pts',(46.7175660142347,-42.0373246662565,
2.65883957563381));
#239511=CARTESIAN_POINT('Ctrl Pts',(46.7159120469168,-42.0392567035856,
2.65878198860233));
#239512=CARTESIAN_POINT('Ctrl Pts',(46.7142062431428,-42.0411527846888,
2.65878198860233));
#239513=CARTESIAN_POINT('Ctrl Pts',(43.8769616275879,-39.486486258181,2.65878198860235));
#239514=CARTESIAN_POINT('Ctrl Pts',(43.8827333680736,-39.4800703482071,
2.65878198860235));
#239515=CARTESIAN_POINT('Ctrl Pts',(43.8889846873393,-39.4741864828756,
2.65945335517819));
#239516=CARTESIAN_POINT('Ctrl Pts',(43.8955692023364,-39.4688721660173,
2.66072561226549));
#239517=CARTESIAN_POINT('Ctrl Pts',(43.8998221234149,-39.4654396626067,
2.6615473598029));
#239518=CARTESIAN_POINT('Ctrl Pts',(43.9042134689398,-39.4622440309668,
2.66261895766843));
#239519=CARTESIAN_POINT('Ctrl Pts',(43.9086997575137,-39.4592874976147,
2.66391429250999));
#239520=CARTESIAN_POINT('Ctrl Pts',(43.9146460760274,-39.4553687820175,
2.66563118464095));
#239521=CARTESIAN_POINT('Ctrl Pts',(43.9207613318567,-39.4518755008527,
2.6677410513867));
#239522=CARTESIAN_POINT('Ctrl Pts',(43.9269559348858,-39.4488169076803,
2.67016894181721));
#239523=CARTESIAN_POINT('Ctrl Pts',(43.9300532364004,-39.4472876110941,
2.67138288703246));
#239524=CARTESIAN_POINT('Ctrl Pts',(43.9331705067656,-39.4458668372375,
2.67267613167523));
#239525=CARTESIAN_POINT('Ctrl Pts',(43.936297487834,-39.4445546869042,2.67403835432524));
#239526=CARTESIAN_POINT('Ctrl Pts',(43.9378609783683,-39.4438986117375,
2.67471946565025));
#239527=CARTESIAN_POINT('Ctrl Pts',(43.9394269075365,-39.4432696802083,
2.67541781389495));
#239528=CARTESIAN_POINT('Ctrl Pts',(43.9409940617759,-39.4426678279627,
2.67613207244141));
#239529=CARTESIAN_POINT('Ctrl Pts',(43.9413858503357,-39.4425173649013,
2.67631063707802));
#239530=CARTESIAN_POINT('Ctrl Pts',(43.9417777156949,-39.4423685940341,
2.67649019601817));
#239531=CARTESIAN_POINT('Ctrl Pts',(43.9421696393595,-39.4422215138286,
2.67667072836629));
#239532=CARTESIAN_POINT('Ctrl Pts',(43.9433454103534,-39.4417802732122,
2.67721232541063));
#239533=CARTESIAN_POINT('Ctrl Pts',(43.9445217049433,-39.4413542498597,
2.67776268340019));
#239534=CARTESIAN_POINT('Ctrl Pts',(43.9456980341199,-39.440943390717,2.67832123541488));
#239535=CARTESIAN_POINT('Ctrl Pts',(43.9539839449481,-39.4380493519676,
2.68225560368406));
#239536=CARTESIAN_POINT('Ctrl Pts',(43.9622859173443,-39.4358558447888,
2.68661792998838));
#239537=CARTESIAN_POINT('Ctrl Pts',(43.970520768646,-39.4342768603229,2.69130986622514));
#239538=CARTESIAN_POINT('Ctrl Pts',(43.9745146626291,-39.4335110545631,
2.69358545023002));
#239539=CARTESIAN_POINT('Ctrl Pts',(43.9784932254701,-39.4328901532268,
2.69593918853429));
#239540=CARTESIAN_POINT('Ctrl Pts',(43.982449005934,-39.4324063524309,2.69836306235448));
#239541=CARTESIAN_POINT('Ctrl Pts',(43.9885050294416,-39.4316656872146,
2.70207384382181));
#239542=CARTESIAN_POINT('Ctrl Pts',(43.9945041897575,-39.4312456873362,
2.70594760814182));
#239543=CARTESIAN_POINT('Ctrl Pts',(44.0004074287827,-39.4311218425055,
2.70995196345661));
#239544=CARTESIAN_POINT('Ctrl Pts',(44.0031489235253,-39.4310643283254,
2.71181160678059));
#239545=CARTESIAN_POINT('Ctrl Pts',(44.0058696426795,-39.4310704471405,
2.71369962772052));
#239546=CARTESIAN_POINT('Ctrl Pts',(44.0085654321305,-39.4311389525604,
2.71561183138614));
#239547=CARTESIAN_POINT('Ctrl Pts',(44.0087720537699,-39.4311442032309,
2.71575839426265));
#239548=CARTESIAN_POINT('Ctrl Pts',(44.0089785427603,-39.4311497894106,
2.71590508903162));
#239549=CARTESIAN_POINT('Ctrl Pts',(44.0091848981962,-39.4311557099534,
2.71605191409865));
#239550=CARTESIAN_POINT('Ctrl Pts',(44.0120835699303,-39.4312388757292,
2.71811436362706));
#239551=CARTESIAN_POINT('Ctrl Pts',(44.0149559644988,-39.4313901062468,
2.72020091026913));
#239552=CARTESIAN_POINT('Ctrl Pts',(44.0177981990788,-39.4316052205099,
2.72230624862136));
#239553=CARTESIAN_POINT('Ctrl Pts',(44.0279899468077,-39.4323765820007,
2.72985561753024));
#239554=CARTESIAN_POINT('Ctrl Pts',(44.0378728316087,-39.4339733733557,
2.73770089914215));
#239555=CARTESIAN_POINT('Ctrl Pts',(44.0474262866313,-39.436268119214,2.7457482334692));
#239556=CARTESIAN_POINT('Ctrl Pts',(44.0579245739712,-39.4387898143846,
2.75459144546802));
#239557=CARTESIAN_POINT('Ctrl Pts',(44.0680257165073,-39.4421543412252,
2.76367911753975));
#239558=CARTESIAN_POINT('Ctrl Pts',(44.0777053474391,-39.4462454222039,
2.77292162564357));
#239559=CARTESIAN_POINT('Ctrl Pts',(44.0881569195892,-39.4506627629395,
2.78290121484227));
#239560=CARTESIAN_POINT('Ctrl Pts',(44.0981181930518,-39.4559274600901,
2.79306229499547));
#239561=CARTESIAN_POINT('Ctrl Pts',(44.107547242147,-39.4619494607953,2.80331916684474));
#239562=CARTESIAN_POINT('Ctrl Pts',(44.1168971912118,-39.4679209431042,
2.81348999408159));
#239563=CARTESIAN_POINT('Ctrl Pts',(44.1257248429274,-39.4746380711544,
2.82375635966594));
#239564=CARTESIAN_POINT('Ctrl Pts',(44.1339623850452,-39.4820551873923,
2.83404198860235));
#239565=CARTESIAN_POINT('Origin',(-0.0101975504409074,-0.0113255271400824,
2.83404198860262));
#239566=CARTESIAN_POINT('Ctrl Pts',(46.6938111422609,-42.0638038389693,
2.65878198860233));
#239567=CARTESIAN_POINT('Ctrl Pts',(46.6880613546461,-42.0701842568298,
2.65878198860233));
#239568=CARTESIAN_POINT('Ctrl Pts',(46.6818296739378,-42.0760276657216,
2.65944603041817));
#239569=CARTESIAN_POINT('Ctrl Pts',(46.6752630175681,-42.0812997491637,
2.66070439264027));
#239570=CARTESIAN_POINT('Ctrl Pts',(46.6710672367553,-42.0846683595042,
2.66150842619554));
#239571=CARTESIAN_POINT('Ctrl Pts',(46.6667352666015,-42.0878044626431,
2.66255428265332));
#239572=CARTESIAN_POINT('Ctrl Pts',(46.6623093164294,-42.090706774241,2.66381699700627));
#239573=CARTESIAN_POINT('Ctrl Pts',(46.6562687825188,-42.0946678472184,
2.66554034873227));
#239574=CARTESIAN_POINT('Ctrl Pts',(46.6500510792886,-42.0981877352858,
2.66766759643931));
#239575=CARTESIAN_POINT('Ctrl Pts',(46.6437515300392,-42.1012583942258,
2.67012012783107));
#239576=CARTESIAN_POINT('Ctrl Pts',(46.6406017554146,-42.1027937236959,
2.67134639352695));
#239577=CARTESIAN_POINT('Ctrl Pts',(46.6374313809743,-42.1042169023582,
2.67265375584971));
#239578=CARTESIAN_POINT('Ctrl Pts',(46.6342513293852,-42.1055280393683,
2.67403135126899));
#239579=CARTESIAN_POINT('Ctrl Pts',(46.6326613035906,-42.1061836078733,
2.67472014897863));
#239580=CARTESIAN_POINT('Ctrl Pts',(46.6310688468945,-42.10681117894,2.67542649668591));
#239581=CARTESIAN_POINT('Ctrl Pts',(46.6294752517399,-42.1074108478347,
2.6761489965606));
#239582=CARTESIAN_POINT('Ctrl Pts',(46.6290768529512,-42.1075607650584,
2.67632962152927));
#239583=CARTESIAN_POINT('Ctrl Pts',(46.6286783827623,-42.1077089386734,
2.67651125590908));
#239584=CARTESIAN_POINT('Ctrl Pts',(46.6282798608704,-42.1078553707275,
2.67669387767482));
#239585=CARTESIAN_POINT('Ctrl Pts',(46.6270842951947,-42.10829466689,2.67724174297202));
#239586=CARTESIAN_POINT('Ctrl Pts',(46.6258882654176,-42.1087182876158,
2.67779849504706));
#239587=CARTESIAN_POINT('Ctrl Pts',(46.6246922924071,-42.1091263005953,
2.67836353617967));
#239588=CARTESIAN_POINT('Ctrl Pts',(46.6164273768573,-42.1119459234378,
2.68226832098857));
#239589=CARTESIAN_POINT('Ctrl Pts',(46.6081492165695,-42.1140735600931,
2.68659153751328));
#239590=CARTESIAN_POINT('Ctrl Pts',(46.5999384432826,-42.1155964444641,
2.69123699486103));
#239591=CARTESIAN_POINT('Ctrl Pts',(46.5958577114969,-42.1163533138163,
2.69354577441151));
#239592=CARTESIAN_POINT('Ctrl Pts',(46.591793149742,-42.1169604217526,2.69593478828062));
#239593=CARTESIAN_POINT('Ctrl Pts',(46.5877524553609,-42.1174262136785,
2.69839565261175));
#239594=CARTESIAN_POINT('Ctrl Pts',(46.5788380800233,-42.1184538202393,
2.70382468689001));
#239595=CARTESIAN_POINT('Ctrl Pts',(46.5700422469563,-42.1188058546731,
2.70961155815042));
#239596=CARTESIAN_POINT('Ctrl Pts',(46.5615008914348,-42.1185337834646,
2.71562701361721));
#239597=CARTESIAN_POINT('Ctrl Pts',(46.5583806265506,-42.1184343924212,
2.71782453535811));
#239598=CARTESIAN_POINT('Ctrl Pts',(46.5552908961832,-42.1182588963856,
2.72005051502355));
#239599=CARTESIAN_POINT('Ctrl Pts',(46.5522345526332,-42.1180117795235,
2.72229986760067));
#239600=CARTESIAN_POINT('Ctrl Pts',(46.5419686180604,-42.1171817401327,
2.7298552048885));
#239601=CARTESIAN_POINT('Ctrl Pts',(46.5320149571602,-42.1155299964524,
2.73770845534523));
#239602=CARTESIAN_POINT('Ctrl Pts',(46.5223946380437,-42.1131831104076,
2.74576706701726));
#239603=CARTESIAN_POINT('Ctrl Pts',(46.5118207677331,-42.1106036046374,
2.75462443585012));
#239604=CARTESIAN_POINT('Ctrl Pts',(46.5016489045613,-42.1071843209722,
2.76373036323175));
#239605=CARTESIAN_POINT('Ctrl Pts',(46.4919044745642,-42.1030402839719,
2.77299664636825));
#239606=CARTESIAN_POINT('Ctrl Pts',(46.4814093059416,-42.0985769785647,
2.782976830335));
#239607=CARTESIAN_POINT('Ctrl Pts',(46.4714088200568,-42.0932726122921,
2.79314401478939));
#239608=CARTESIAN_POINT('Ctrl Pts',(46.4619468343607,-42.0872150940856,
2.80341452428007));
#239609=CARTESIAN_POINT('Ctrl Pts',(46.4526126174202,-42.0812393728283,
2.81354634721395));
#239610=CARTESIAN_POINT('Ctrl Pts',(46.4438014421029,-42.0745296860242,
2.823780042092));
#239611=CARTESIAN_POINT('Ctrl Pts',(46.4355828792675,-42.0671296588088,
2.83404198860233));
#239612=CARTESIAN_POINT('Ctrl Pts',(43.8790236240225,-39.7651933658992,
2.83404198860234));
#239613=CARTESIAN_POINT('Ctrl Pts',(43.8711584142724,-39.758111499231,2.82422126443014));
#239614=CARTESIAN_POINT('Ctrl Pts',(43.8638800583574,-39.750434738225,2.81442815028543));
#239615=CARTESIAN_POINT('Ctrl Pts',(43.8572218328541,-39.7422106539909,
2.80471618166395));
#239616=CARTESIAN_POINT('Ctrl Pts',(43.8507927303141,-39.734269577076,2.79533842146328));
#239617=CARTESIAN_POINT('Ctrl Pts',(43.844941079035,-39.72581716687,2.7860351565036));
#239618=CARTESIAN_POINT('Ctrl Pts',(43.8397310304462,-39.7168657021556,
2.77685887346896));
#239619=CARTESIAN_POINT('Ctrl Pts',(43.8348059028435,-39.7084037645753,
2.76818441216728));
#239620=CARTESIAN_POINT('Ctrl Pts',(43.8304536682217,-39.6994950821798,
2.75962261521785));
#239621=CARTESIAN_POINT('Ctrl Pts',(43.8267676847823,-39.6901349804742,
2.75123537701829));
#239622=CARTESIAN_POINT('Ctrl Pts',(43.8233729558715,-39.6815144838308,
2.74351087134292));
#239623=CARTESIAN_POINT('Ctrl Pts',(43.8205432023708,-39.6725105620432,
2.73593399450023));
#239624=CARTESIAN_POINT('Ctrl Pts',(43.818389241969,-39.6631152739638,2.72857657812754));
#239625=CARTESIAN_POINT('Ctrl Pts',(43.8177469744577,-39.6603137887146,
2.72638274508427));
#239626=CARTESIAN_POINT('Ctrl Pts',(43.8171650742233,-39.6574775031716,
2.72420861709632));
#239627=CARTESIAN_POINT('Ctrl Pts',(43.8166472411075,-39.6546062260514,
2.72205663736681));
#239628=CARTESIAN_POINT('Ctrl Pts',(43.81613469897,-39.6517642863079,2.71992664556719));
#239629=CARTESIAN_POINT('Ctrl Pts',(43.8156851836086,-39.6488910639683,
2.71782089927838));
#239630=CARTESIAN_POINT('Ctrl Pts',(43.8153025584996,-39.6459896850497,
2.71574387311199));
#239631=CARTESIAN_POINT('Ctrl Pts',(43.8152759514979,-39.6457879288339,
2.7155994407744));
#239632=CARTESIAN_POINT('Ctrl Pts',(43.815249656674,-39.6455860324529,2.71545515216022));
#239633=CARTESIAN_POINT('Ctrl Pts',(43.815223675331,-39.6453839959659,2.71531100781683));
#239634=CARTESIAN_POINT('Ctrl Pts',(43.8140845580787,-39.636525976255,2.70899119176047));
#239635=CARTESIAN_POINT('Ctrl Pts',(43.8135929685794,-39.6274037177899,
2.70298296066812));
#239636=CARTESIAN_POINT('Ctrl Pts',(43.8138323099903,-39.6180980992372,
2.69736727774118));
#239637=CARTESIAN_POINT('Ctrl Pts',(43.8140554177825,-39.6094236454406,
2.69213248525422));
#239638=CARTESIAN_POINT('Ctrl Pts',(43.814913952762,-39.6005890951404,2.68723866185471));
#239639=CARTESIAN_POINT('Ctrl Pts',(43.8164991115146,-39.5916773623198,
2.68278595829573));
#239640=CARTESIAN_POINT('Ctrl Pts',(43.8170789830939,-39.5884173351605,
2.68115710172796));
#239641=CARTESIAN_POINT('Ctrl Pts',(43.8177563121469,-39.5851472105415,
2.67958763637782));
#239642=CARTESIAN_POINT('Ctrl Pts',(43.8185363400632,-39.5818719865438,
2.6780837864532));
#239643=CARTESIAN_POINT('Ctrl Pts',(43.8187239107186,-39.581084404588,2.67772216078556));
#239644=CARTESIAN_POINT('Ctrl Pts',(43.8189178575375,-39.5802961412314,
2.67736403603519));
#239645=CARTESIAN_POINT('Ctrl Pts',(43.8191182115055,-39.5795073285701,
2.67700956934434));
#239646=CARTESIAN_POINT('Ctrl Pts',(43.819312304412,-39.5787431663045,2.67666617973759));
#239647=CARTESIAN_POINT('Ctrl Pts',(43.8195124102603,-39.5779784885473,
2.67632622314074));
#239648=CARTESIAN_POINT('Ctrl Pts',(43.8197185546683,-39.5772134181958,
2.67598984158729));
#239649=CARTESIAN_POINT('Ctrl Pts',(43.8219771048936,-39.5688311883222,
2.67230439292161));
#239650=CARTESIAN_POINT('Ctrl Pts',(43.8249623840161,-39.5603964284858,
2.66904964539902));
#239651=CARTESIAN_POINT('Ctrl Pts',(43.8286919494563,-39.55209682397,2.66640203566646));
#239652=CARTESIAN_POINT('Ctrl Pts',(43.8302387114105,-39.5486547305931,
2.66530399299374));
#239653=CARTESIAN_POINT('Ctrl Pts',(43.8319130705232,-39.5452359574119,
2.66430995142204));
#239654=CARTESIAN_POINT('Ctrl Pts',(43.8337144555754,-39.5418537500309,
2.66343053473314));
#239655=CARTESIAN_POINT('Ctrl Pts',(43.8367869054999,-39.5360850428912,
2.66193059792838));
#239656=CARTESIAN_POINT('Ctrl Pts',(43.8402296473868,-39.5304250803193,
2.6607651981708));
#239657=CARTESIAN_POINT('Ctrl Pts',(43.8440378929944,-39.5249464846897,
2.65997805604412));
#239658=CARTESIAN_POINT('Ctrl Pts',(43.8459420157982,-39.522207186875,2.65958448498078));
#239659=CARTESIAN_POINT('Ctrl Pts',(43.847938633807,-39.5195141476128,2.65928526260714));
#239660=CARTESIAN_POINT('Ctrl Pts',(43.8500271570784,-39.5168765098743,
2.65908463971276));
#239661=CARTESIAN_POINT('Ctrl Pts',(43.8521156803498,-39.5142388721359,
2.65888401681838));
#239662=CARTESIAN_POINT('Ctrl Pts',(43.8542960677578,-39.5116566557591,
2.65878198860235));
#239663=CARTESIAN_POINT('Ctrl Pts',(43.8565665267061,-39.5091373124615,
2.65878198860235));
#239664=CARTESIAN_POINT('Origin',(47.1453396605412,-34.2342565846629,2.83404198860238));
#239665=CARTESIAN_POINT('Ctrl Pts',(50.8023624960595,-36.674605926817,2.83404198860237));
#239666=CARTESIAN_POINT('Ctrl Pts',(50.8109464329605,-36.6808425220333,
2.82419652440019));
#239667=CARTESIAN_POINT('Ctrl Pts',(50.8190128116693,-36.6877379133664,
2.81438790575583));
#239668=CARTESIAN_POINT('Ctrl Pts',(50.8265243508966,-36.6952462569242,
2.80466781256817));
#239669=CARTESIAN_POINT('Ctrl Pts',(50.8337918098273,-36.7025106240256,
2.7952635645298));
#239670=CARTESIAN_POINT('Ctrl Pts',(50.8405407635291,-36.7103497152253,
2.78594102496122));
#239671=CARTESIAN_POINT('Ctrl Pts',(50.8467071440084,-36.7187568768225,
2.77675109088657));
#239672=CARTESIAN_POINT('Ctrl Pts',(50.8525401602379,-36.7267095340102,
2.7680579791355));
#239673=CARTESIAN_POINT('Ctrl Pts',(50.857852441276,-36.7351712462838,2.7594827121002));
#239674=CARTESIAN_POINT('Ctrl Pts',(50.8625525281348,-36.7441560526544,
2.75108575573074));
#239675=CARTESIAN_POINT('Ctrl Pts',(50.8668816480507,-36.7524317091195,
2.7433515516311));
#239676=CARTESIAN_POINT('Ctrl Pts',(50.8706916079206,-36.7611516658488,
2.73576818685773));
#239677=CARTESIAN_POINT('Ctrl Pts',(50.8738736606218,-36.7703354510192,
2.72840626160318));
#239678=CARTESIAN_POINT('Ctrl Pts',(50.8747966531511,-36.7729993179942,
2.72627084693553));
#239679=CARTESIAN_POINT('Ctrl Pts',(50.8756665488988,-36.775702242458,2.72415424587447));
#239680=CARTESIAN_POINT('Ctrl Pts',(50.8764799968257,-36.7784447603811,
2.72205867173233));
#239681=CARTESIAN_POINT('Ctrl Pts',(50.8773618266786,-36.7814178261386,
2.71978693462836));
#239682=CARTESIAN_POINT('Ctrl Pts',(50.8781771258728,-36.784432979124,2.71754411340736));
#239683=CARTESIAN_POINT('Ctrl Pts',(50.8789219044957,-36.7874899206167,
2.71533341844232));
#239684=CARTESIAN_POINT('Ctrl Pts',(50.8809659552707,-36.7958797205309,
2.70926614876379));
#239685=CARTESIAN_POINT('Ctrl Pts',(50.8824343655147,-36.8045837617096,
2.70347381860397));
#239686=CARTESIAN_POINT('Ctrl Pts',(50.8832604021666,-36.8135226609471,
2.69804914171382));
#239687=CARTESIAN_POINT('Ctrl Pts',(50.8840161808564,-36.8217012684451,
2.69308585687198));
#239688=CARTESIAN_POINT('Ctrl Pts',(50.8842246658558,-36.8300699399848,
2.68842799053184));
#239689=CARTESIAN_POINT('Ctrl Pts',(50.8838072802932,-36.8385876480139,
2.6841476705422));
#239690=CARTESIAN_POINT('Ctrl Pts',(50.8836022618683,-36.8427715183736,
2.68204519134548));
#239691=CARTESIAN_POINT('Ctrl Pts',(50.8832457706973,-36.846991141844,2.68003431778493));
#239692=CARTESIAN_POINT('Ctrl Pts',(50.8827256259729,-36.851239928621,2.67812693945238));
#239693=CARTESIAN_POINT('Ctrl Pts',(50.8826269335777,-36.8520460945281,
2.67776503299189));
#239694=CARTESIAN_POINT('Ctrl Pts',(50.8825219362263,-36.8528536453858,
2.6774065963991));
#239695=CARTESIAN_POINT('Ctrl Pts',(50.8824105850811,-36.8536624499706,
2.67705178968841));
#239696=CARTESIAN_POINT('Ctrl Pts',(50.8823027136591,-36.8544459794121,
2.67670807068744));
#239697=CARTESIAN_POINT('Ctrl Pts',(50.8821888793661,-36.855230685427,2.67636775825251));
#239698=CARTESIAN_POINT('Ctrl Pts',(50.8820690400779,-36.8560164456178,
2.67603099699241));
#239699=CARTESIAN_POINT('Ctrl Pts',(50.8807630562084,-36.8645794982668,
2.6723610421712));
#239700=CARTESIAN_POINT('Ctrl Pts',(50.8787426510002,-36.8732733195864,
2.6691144054147));
#239701=CARTESIAN_POINT('Ctrl Pts',(50.8759664620673,-36.8819119966098,
2.6664677818963));
#239702=CARTESIAN_POINT('Ctrl Pts',(50.8747940602416,-36.8855601635606,
2.66535009634968));
#239703=CARTESIAN_POINT('Ctrl Pts',(50.8734872887382,-36.889198371364,2.66433897912334));
#239704=CARTESIAN_POINT('Ctrl Pts',(50.8720449698708,-36.892812564861,2.66344564884779));
#239705=CARTESIAN_POINT('Ctrl Pts',(50.8696161409378,-36.8988987764009,
2.66194130298573));
#239706=CARTESIAN_POINT('Ctrl Pts',(50.8668019052541,-36.904914574214,2.66077206705407));
#239707=CARTESIAN_POINT('Ctrl Pts',(50.8635979627959,-36.9107858666114,
2.65998225155702));
#239708=CARTESIAN_POINT('Ctrl Pts',(50.8627969771814,-36.9122536897108,
2.65978479768276));
#239709=CARTESIAN_POINT('Ctrl Pts',(50.8619714372927,-36.9137123559378,
2.6596109896661));
#239710=CARTESIAN_POINT('Ctrl Pts',(50.8611210221666,-36.9151605322316,
2.65946139030489));
#239711=CARTESIAN_POINT('Ctrl Pts',(50.8598453994776,-36.9173327966724,
2.65923699126308));
#239712=CARTESIAN_POINT('Ctrl Pts',(50.8585138058065,-36.9194814382211,
2.65906707562429));
#239713=CARTESIAN_POINT('Ctrl Pts',(50.8571265262615,-36.9216029292225,
2.65895332562907));
#239714=CARTESIAN_POINT('Ctrl Pts',(50.8557392467166,-36.9237244202238,
2.65883957563385));
#239715=CARTESIAN_POINT('Ctrl Pts',(50.8542962928974,-36.9258187603122,
2.65878198860237));
#239716=CARTESIAN_POINT('Ctrl Pts',(50.8527980281389,-36.9278827595319,
2.65878198860237));
#239717=CARTESIAN_POINT('Ctrl Pts',(47.7640607692767,-34.6837837831338,
2.65878198860238));
#239718=CARTESIAN_POINT('Ctrl Pts',(47.7691302463544,-34.6767997090224,
2.65878198860238));
#239719=CARTESIAN_POINT('Ctrl Pts',(47.7747322888382,-34.6702946353242,
2.6594533551783));
#239720=CARTESIAN_POINT('Ctrl Pts',(47.7807252357991,-34.6643211616154,
2.66072561226574));
#239721=CARTESIAN_POINT('Ctrl Pts',(47.784596064624,-34.6604629105133,2.66154735980313));
#239722=CARTESIAN_POINT('Ctrl Pts',(47.7886293194338,-34.6568257642788,
2.66261895766859));
#239723=CARTESIAN_POINT('Ctrl Pts',(47.7927819897613,-34.6534164822756,
2.66391429251005));
#239724=CARTESIAN_POINT('Ctrl Pts',(47.7982861164007,-34.6488976742762,
2.66563118464101));
#239725=CARTESIAN_POINT('Ctrl Pts',(47.8040027249067,-34.6447843113767,
2.66774105138676));
#239726=CARTESIAN_POINT('Ctrl Pts',(47.8098436832082,-34.6410949611626,
2.67016894181727));
#239727=CARTESIAN_POINT('Ctrl Pts',(47.812764162359,-34.6392502860555,2.67138288703252));
#239728=CARTESIAN_POINT('Ctrl Pts',(47.815715844683,-34.6375114518659,2.67267613167528));
#239729=CARTESIAN_POINT('Ctrl Pts',(47.8186885387641,-34.6358796311037,
2.6740383543253));
#239730=CARTESIAN_POINT('Ctrl Pts',(47.8201748858046,-34.6350637207225,
2.67471946565031));
#239731=CARTESIAN_POINT('Ctrl Pts',(47.8216664954028,-34.6342745503765,
2.67541781389499));
#239732=CARTESIAN_POINT('Ctrl Pts',(47.8231621539169,-34.6335121829162,
2.67613207244145));
#239733=CARTESIAN_POINT('Ctrl Pts',(47.8235360685455,-34.6333215910511,
2.67631063707807));
#239734=CARTESIAN_POINT('Ctrl Pts',(47.823910236435,-34.6331326740824,2.67649019601822));
#239735=CARTESIAN_POINT('Ctrl Pts',(47.824284639033,-34.6329454324193,2.67667072836633));
#239736=CARTESIAN_POINT('Ctrl Pts',(47.8254078468268,-34.63238370743,2.67721232541067));
#239737=CARTESIAN_POINT('Ctrl Pts',(47.8265331659855,-34.6318370616122,
2.67776268340023));
#239738=CARTESIAN_POINT('Ctrl Pts',(47.827660104633,-34.6313054933178,2.67832123541492));
#239739=CARTESIAN_POINT('Ctrl Pts',(47.8355981149517,-34.6275611948897,
2.68225560368415));
#239740=CARTESIAN_POINT('Ctrl Pts',(47.8436253243399,-34.6245119115561,
2.68661792998852));
#239741=CARTESIAN_POINT('Ctrl Pts',(47.8516500154449,-34.6220808005804,
2.69130986622533));
#239742=CARTESIAN_POINT('Ctrl Pts',(47.8555419819595,-34.6209017143843,
2.69358545023017));
#239743=CARTESIAN_POINT('Ctrl Pts',(47.8594338479544,-34.6198683413507,
2.69593918853438));
#239744=CARTESIAN_POINT('Ctrl Pts',(47.8633173872852,-34.6189736992133,
2.69836306235451));
#239745=CARTESIAN_POINT('Ctrl Pts',(47.8692628146655,-34.6176040646078,
2.70207384382184));
#239746=CARTESIAN_POINT('Ctrl Pts',(47.8751852090117,-34.6165592825239,
2.70594760814184));
#239747=CARTESIAN_POINT('Ctrl Pts',(47.881043164166,-34.6158190596246,2.70995196345663));
#239748=CARTESIAN_POINT('Ctrl Pts',(47.8837636288447,-34.6154752962807,
2.71181160678061));
#239749=CARTESIAN_POINT('Ctrl Pts',(47.886470083205,-34.6151969889841,2.71369962772056));
#239750=CARTESIAN_POINT('Ctrl Pts',(47.8891582656056,-34.6149833323955,
2.71561183138618));
#239751=CARTESIAN_POINT('Ctrl Pts',(47.8893643041946,-34.6149669564598,
2.71575839426269));
#239752=CARTESIAN_POINT('Ctrl Pts',(47.8895702459314,-34.614950928061,2.71590508903166));
#239753=CARTESIAN_POINT('Ctrl Pts',(47.8897760897959,-34.6149352461538,
2.71605191409868));
#239754=CARTESIAN_POINT('Ctrl Pts',(47.8926675754936,-34.614714962637,2.7181143636271));
#239755=CARTESIAN_POINT('Ctrl Pts',(47.8955400426778,-34.6145651177078,
2.72020091026915));
#239756=CARTESIAN_POINT('Ctrl Pts',(47.8983891927627,-34.6144819591396,
2.72230624862138));
#239757=CARTESIAN_POINT('Ctrl Pts',(47.9086057382625,-34.6141837673033,
2.72985561753034));
#239758=CARTESIAN_POINT('Ctrl Pts',(47.9186013937331,-34.6147387685073,
2.73770089914233));
#239759=CARTESIAN_POINT('Ctrl Pts',(47.9283423801878,-34.6160223355353,
2.74574823346948));
#239760=CARTESIAN_POINT('Ctrl Pts',(47.9390467457327,-34.6174328467534,
2.75459144546866));
#239761=CARTESIAN_POINT('Ctrl Pts',(47.9494442419738,-34.6197230854575,
2.76367911754079));
#239762=CARTESIAN_POINT('Ctrl Pts',(47.9594984812827,-34.6227799581205,
2.77292162564502));
#239763=CARTESIAN_POINT('Ctrl Pts',(47.9703545364669,-34.6260806134262,
2.78290121484476));
#239764=CARTESIAN_POINT('Ctrl Pts',(47.980811551735,-34.6302752334083,2.79306229499904));
#239765=CARTESIAN_POINT('Ctrl Pts',(47.990818417993,-34.6352786409523,2.8033191668494));
#239766=CARTESIAN_POINT('Ctrl Pts',(48.000741336926,-34.6402400750484,2.81348999408475));
#239767=CARTESIAN_POINT('Ctrl Pts',(48.010222760913,-34.6459976650995,2.82375635966754));
#239768=CARTESIAN_POINT('Ctrl Pts',(48.019190476674,-34.6525130919789,2.83404198860238));
#239769=CARTESIAN_POINT('Origin',(-0.00895784724493606,-0.0123294189940815,
2.83404198860262));
#239770=CARTESIAN_POINT('Ctrl Pts',(50.8348823336491,-36.9525415975204,
2.65878198860237));
#239771=CARTESIAN_POINT('Ctrl Pts',(50.8298309792463,-36.9594880792479,
2.65878198860237));
#239772=CARTESIAN_POINT('Ctrl Pts',(50.8242442388885,-36.9659508653425,
2.65944603041822));
#239773=CARTESIAN_POINT('Ctrl Pts',(50.8182646381299,-36.971880470259,2.66070439264035));
#239774=CARTESIAN_POINT('Ctrl Pts',(50.8144439579057,-36.9756692055201,
2.66150842619561));
#239775=CARTESIAN_POINT('Ctrl Pts',(50.8104635307794,-36.9792409429409,
2.66255428265338));
#239776=CARTESIAN_POINT('Ctrl Pts',(50.8063652005968,-36.9825899931421,
2.66381699700631));
#239777=CARTESIAN_POINT('Ctrl Pts',(50.8007718022343,-36.9871607746743,
2.66554034873231));
#239778=CARTESIAN_POINT('Ctrl Pts',(50.7949560887234,-36.9913113073903,
2.66766759643936));
#239779=CARTESIAN_POINT('Ctrl Pts',(50.7890120203242,-36.9950236271417,
2.67012012783111));
#239780=CARTESIAN_POINT('Ctrl Pts',(50.7860399861246,-36.9968797870174,
2.67134639352699));
#239781=CARTESIAN_POINT('Ctrl Pts',(50.7830357420058,-36.9986265637263,
2.67265375584973));
#239782=CARTESIAN_POINT('Ctrl Pts',(50.7800101622088,-37.0002629240964,
2.67403135126901));
#239783=CARTESIAN_POINT('Ctrl Pts',(50.7784973723104,-37.0010811042814,
2.67472014897864));
#239784=CARTESIAN_POINT('Ctrl Pts',(50.7769792382978,-37.0018716944994,
2.67542649668593));
#239785=CARTESIAN_POINT('Ctrl Pts',(50.7754570554922,-37.0026346543977,
2.67614899656062));
#239786=CARTESIAN_POINT('Ctrl Pts',(50.7750765097909,-37.0028253943723,
2.67632962152929));
#239787=CARTESIAN_POINT('Ctrl Pts',(50.7746957108236,-37.0030144077533,
2.6765112559091));
#239788=CARTESIAN_POINT('Ctrl Pts',(50.7743146783939,-37.0032016945182,
2.67669387767484));
#239789=CARTESIAN_POINT('Ctrl Pts',(50.7731715811048,-37.0037635548132,
2.67724174297204));
#239790=CARTESIAN_POINT('Ctrl Pts',(50.7720263837274,-37.0043098740549,
2.67779849504707));
#239791=CARTESIAN_POINT('Ctrl Pts',(50.770879611352,-37.0048406651175,2.67836353617968));
#239792=CARTESIAN_POINT('Ctrl Pts',(50.7629547027166,-37.0085087606927,
2.68226832098876));
#239793=CARTESIAN_POINT('Ctrl Pts',(50.7549442896467,-37.0114900453054,
2.6865915375137));
#239794=CARTESIAN_POINT('Ctrl Pts',(50.7469376805977,-37.0138628466705,
2.6912369948617));
#239795=CARTESIAN_POINT('Ctrl Pts',(50.7429584178783,-37.0150421224356,
2.69354577441198));
#239796=CARTESIAN_POINT('Ctrl Pts',(50.738979582278,-37.0160707669651,2.69593478828088));
#239797=CARTESIAN_POINT('Ctrl Pts',(50.7350097117581,-37.0169563748082,
2.69839565261178));
#239798=CARTESIAN_POINT('Ctrl Pts',(50.7262515844359,-37.0189101579878,
2.70382468689004));
#239799=CARTESIAN_POINT('Ctrl Pts',(50.7175407334812,-37.0201796788538,
2.70961155815045));
#239800=CARTESIAN_POINT('Ctrl Pts',(50.7090177292136,-37.0208019128467,
2.71562701361724));
#239801=CARTESIAN_POINT('Ctrl Pts',(50.7059041682739,-37.0210292227711,
2.71782453535815));
#239802=CARTESIAN_POINT('Ctrl Pts',(50.7028130194419,-37.0211776528884,
2.72005051502358));
#239803=CARTESIAN_POINT('Ctrl Pts',(50.6997475881157,-37.0212513646528,
2.7222998676007));
#239804=CARTESIAN_POINT('Ctrl Pts',(50.6894511286644,-37.0214989546696,
2.72985520488877));
#239805=CARTESIAN_POINT('Ctrl Pts',(50.6793793407311,-37.0208967002918,
2.73770845534576));
#239806=CARTESIAN_POINT('Ctrl Pts',(50.6695664063374,-37.0195682679076,
2.74576706701804));
#239807=CARTESIAN_POINT('Ctrl Pts',(50.6587808290202,-37.0181081633542,
2.75462443585118));
#239808=CARTESIAN_POINT('Ctrl Pts',(50.6483072759119,-37.0157708601084,
2.76373036323309));
#239809=CARTESIAN_POINT('Ctrl Pts',(50.6381830571022,-37.0126680948693,
2.77299664636988));
#239810=CARTESIAN_POINT('Ctrl Pts',(50.6272788396558,-37.0093262837637,
2.78297683033696));
#239811=CARTESIAN_POINT('Ctrl Pts',(50.6167786802238,-37.0050963107858,
2.79314401479169));
#239812=CARTESIAN_POINT('Ctrl Pts',(50.6067353452058,-37.0000610231218,
2.80341452428271));
#239813=CARTESIAN_POINT('Ctrl Pts',(50.5968276291233,-36.9950937288437,
2.81354634721573));
#239814=CARTESIAN_POINT('Ctrl Pts',(50.5873633690966,-36.9893418170218,
2.82378004209291));
#239815=CARTESIAN_POINT('Ctrl Pts',(50.5784163149361,-36.9828414016739,
2.83404198860236));
#239816=CARTESIAN_POINT('Ctrl Pts',(47.7952442955506,-34.9607485668358,
2.83404198860238));
#239817=CARTESIAN_POINT('Ctrl Pts',(47.7866819156027,-34.9545276336627,
2.82422126443021));
#239818=CARTESIAN_POINT('Ctrl Pts',(47.7786409912522,-34.9476537221156,
2.81442815028553));
#239819=CARTESIAN_POINT('Ctrl Pts',(47.771159589318,-34.9401706643554,2.80471618166407));
#239820=CARTESIAN_POINT('Ctrl Pts',(47.7639356375079,-34.9329451136995,
2.79533842146349));
#239821=CARTESIAN_POINT('Ctrl Pts',(47.7572325247371,-34.9251506707969,
2.7860351565039));
#239822=CARTESIAN_POINT('Ctrl Pts',(47.751115334489,-34.9167928415154,2.77685887346935));
#239823=CARTESIAN_POINT('Ctrl Pts',(47.7453326739193,-34.9088920753345,
2.76818441216786));
#239824=CARTESIAN_POINT('Ctrl Pts',(47.7400730704137,-34.9004871280303,
2.75962261521862));
#239825=CARTESIAN_POINT('Ctrl Pts',(47.7354288821299,-34.891563592126,2.75123537701924));
#239826=CARTESIAN_POINT('Ctrl Pts',(47.7311516626327,-34.8833451652618,
2.74351087134415));
#239827=CARTESIAN_POINT('Ctrl Pts',(47.72739624471,-34.874686357685,2.73593399450172));
#239828=CARTESIAN_POINT('Ctrl Pts',(47.7242720089038,-34.8655676881479,
2.72857657812927));
#239829=CARTESIAN_POINT('Ctrl Pts',(47.7233404248529,-34.8628486849634,
2.72638274508542));
#239830=CARTESIAN_POINT('Ctrl Pts',(47.7224652397594,-34.8600887620259,
2.72420861709691));
#239831=CARTESIAN_POINT('Ctrl Pts',(47.7216501132023,-34.8572873423613,
2.72205663736684));
#239832=CARTESIAN_POINT('Ctrl Pts',(47.7208433152302,-34.8545145463031,
2.71992664556723));
#239833=CARTESIAN_POINT('Ctrl Pts',(47.7200959288452,-34.851704050926,2.71782089927842));
#239834=CARTESIAN_POINT('Ctrl Pts',(47.7194121231169,-34.8488585612793,
2.71574387311204));
#239835=CARTESIAN_POINT('Ctrl Pts',(47.7193645726039,-34.8486606914942,
2.71559944077444));
#239836=CARTESIAN_POINT('Ctrl Pts',(47.7193173179073,-34.8484626496803,
2.71545515216027));
#239837=CARTESIAN_POINT('Ctrl Pts',(47.7192703603294,-34.8482644357601,
2.71531100781688));
#239838=CARTESIAN_POINT('Ctrl Pts',(47.7172115680926,-34.8395740113841,
2.70899119176062));
#239839=CARTESIAN_POINT('Ctrl Pts',(47.7157691359132,-34.8305531107004,
2.70298296066836));
#239840=CARTESIAN_POINT('Ctrl Pts',(47.7150344641797,-34.8212734513101,
2.6973672777415));
#239841=CARTESIAN_POINT('Ctrl Pts',(47.714349622439,-34.8126231959648,2.69213248525475));
#239842=CARTESIAN_POINT('Ctrl Pts',(47.7142799923075,-34.8037473009138,
2.68723866185542));
#239843=CARTESIAN_POINT('Ctrl Pts',(47.7149249376576,-34.7947186932901,
2.68278595829657));
#239844=CARTESIAN_POINT('Ctrl Pts',(47.7151608670106,-34.7914159118149,
2.6811571017285));
#239845=CARTESIAN_POINT('Ctrl Pts',(47.7154926644832,-34.7880929011152,
2.67958763637807));
#239846=CARTESIAN_POINT('Ctrl Pts',(47.7159260651936,-34.7847540840173,
2.67808378645319));
#239847=CARTESIAN_POINT('Ctrl Pts',(47.7160302835858,-34.7839512100454,
2.67772216078554));
#239848=CARTESIAN_POINT('Ctrl Pts',(47.7161407719865,-34.7831469919151,
2.67736403603517));
#239849=CARTESIAN_POINT('Ctrl Pts',(47.7162575750191,-34.7823415577597,
2.67700956934433));
#239850=CARTESIAN_POINT('Ctrl Pts',(47.716370727957,-34.7815612934216,2.67666617973758));
#239851=CARTESIAN_POINT('Ctrl Pts',(47.7164898070138,-34.7807798878925,
2.67632622314073));
#239852=CARTESIAN_POINT('Ctrl Pts',(47.716614850513,-34.7799974607182,2.67598984158727));
#239853=CARTESIAN_POINT('Ctrl Pts',(47.7179848465564,-34.7714250667927,
2.67230439292165));
#239854=CARTESIAN_POINT('Ctrl Pts',(47.7200720995237,-34.7627244668144,
2.66904964539912));
#239855=CARTESIAN_POINT('Ctrl Pts',(47.7229136891083,-34.7540804826565,
2.66640203566659));
#239856=CARTESIAN_POINT('Ctrl Pts',(47.7240921810077,-34.7504955647771,
2.66530399299382));
#239857=CARTESIAN_POINT('Ctrl Pts',(47.7254000086991,-34.7469205018078,
2.66430995142208));
#239858=CARTESIAN_POINT('Ctrl Pts',(47.7268379886356,-34.7433685265014,
2.66343053473314));
#239859=CARTESIAN_POINT('Ctrl Pts',(47.7292906132656,-34.7373102624738,
2.66193059792838));
#239860=CARTESIAN_POINT('Ctrl Pts',(47.7321228682623,-34.7313214412503,
2.66076519817082));
#239861=CARTESIAN_POINT('Ctrl Pts',(47.7353375827199,-34.7254747878796,
2.65997805604414));
#239862=CARTESIAN_POINT('Ctrl Pts',(47.7369449399486,-34.7225514611942,
2.65958448498081));
#239863=CARTESIAN_POINT('Ctrl Pts',(47.7386491210195,-34.7196644712708,
2.65928526260716));
#239864=CARTESIAN_POINT('Ctrl Pts',(47.7404504949225,-34.7168229726598,
2.65908463971278));
#239865=CARTESIAN_POINT('Ctrl Pts',(47.7422518688255,-34.7139814740488,
2.65888401681841));
#239866=CARTESIAN_POINT('Ctrl Pts',(47.7441503967336,-34.7111854907786,
2.65878198860238));
#239867=CARTESIAN_POINT('Ctrl Pts',(47.7461450747869,-34.7084426211224,
2.65878198860238));
#239868=CARTESIAN_POINT('Origin',(50.4655267888879,-29.1186878401547,2.83404198860242));
#239869=CARTESIAN_POINT('Ctrl Pts',(54.3576020372442,-31.1634057161431,
2.8340419886024));
#239870=CARTESIAN_POINT('Ctrl Pts',(54.3667908521544,-31.1687108809051,
2.82419652440104));
#239871=CARTESIAN_POINT('Ctrl Pts',(54.3755338070561,-31.1747253323922,
2.81438790575739));
#239872=CARTESIAN_POINT('Ctrl Pts',(54.383789032899,-31.1814073748058,2.80466781257036));
#239873=CARTESIAN_POINT('Ctrl Pts',(54.3917760130587,-31.1878722906299,
2.79526356453248));
#239874=CARTESIAN_POINT('Ctrl Pts',(54.3993074034423,-31.1949629807083,
2.78594102496432));
#239875=CARTESIAN_POINT('Ctrl Pts',(54.406318791526,-31.2026795247186,2.77675109089004));
#239876=CARTESIAN_POINT('Ctrl Pts',(54.4129511329169,-31.209978900195,2.7680579791393));
#239877=CARTESIAN_POINT('Ctrl Pts',(54.4191188025039,-31.2178389737494,
2.75948271210427));
#239878=CARTESIAN_POINT('Ctrl Pts',(54.4247323097976,-31.2262832675534,
2.75108575573505));
#239879=CARTESIAN_POINT('Ctrl Pts',(54.4299027559943,-31.2340610728538,
2.74335155163568));
#239880=CARTESIAN_POINT('Ctrl Pts',(54.434603328182,-31.2423350114968,2.73576818686256));
#239881=CARTESIAN_POINT('Ctrl Pts',(54.4387279162163,-31.2511358718515,
2.72840626160824));
#239882=CARTESIAN_POINT('Ctrl Pts',(54.4399243024182,-31.2536886668956,
2.72627084693889));
#239883=CARTESIAN_POINT('Ctrl Pts',(54.4410719653274,-31.2562858555926,
2.72415424587617));
#239884=CARTESIAN_POINT('Ctrl Pts',(54.4421676282862,-31.2589283212559,
2.7220586717324));
#239885=CARTESIAN_POINT('Ctrl Pts',(54.4433553973777,-31.2617929239286,
2.71978693462842));
#239886=CARTESIAN_POINT('Ctrl Pts',(54.4444813995856,-31.2647063376186,
2.71754411340741));
#239887=CARTESIAN_POINT('Ctrl Pts',(54.4455416356299,-31.2676686823011,
2.71533341844237));
#239888=CARTESIAN_POINT('Ctrl Pts',(54.448451461773,-31.2757988605271,2.70926614876383));
#239889=CARTESIAN_POINT('Ctrl Pts',(54.4508216479607,-31.2843017293913,
2.703473818604));
#239890=CARTESIAN_POINT('Ctrl Pts',(54.4525775288979,-31.2931053160616,
2.69804914171385));
#239891=CARTESIAN_POINT('Ctrl Pts',(54.4541840646265,-31.3011601199073,
2.69308585687181));
#239892=CARTESIAN_POINT('Ctrl Pts',(54.455266171899,-31.3094611543724,2.6884279905315));
#239893=CARTESIAN_POINT('Ctrl Pts',(54.4557414157489,-31.3179758301775,
2.68414767054173));
#239894=CARTESIAN_POINT('Ctrl Pts',(54.4559748539755,-31.3221582111182,
2.68204519134519));
#239895=CARTESIAN_POINT('Ctrl Pts',(54.4560613864574,-31.3263919825236,
2.6800343177848));
#239896=CARTESIAN_POINT('Ctrl Pts',(54.4559882102927,-31.3306718639305,
2.67812693945239));
#239897=CARTESIAN_POINT('Ctrl Pts',(54.4559743258282,-31.3314839297409,
2.67776503299191));
#239898=CARTESIAN_POINT('Ctrl Pts',(54.4559543157135,-31.3322980319622,
2.67740659639912));
#239899=CARTESIAN_POINT('Ctrl Pts',(54.4559281176618,-31.333114045195,2.67705178968843));
#239900=CARTESIAN_POINT('Ctrl Pts',(54.4559027382993,-31.3339045580142,
2.67670807068745));
#239901=CARTESIAN_POINT('Ctrl Pts',(54.4558715517163,-31.3346968642512,
2.67636775825253));
#239902=CARTESIAN_POINT('Ctrl Pts',(54.4558345032255,-31.335490846582,2.67603099699243));
#239903=CARTESIAN_POINT('Ctrl Pts',(54.4554307564065,-31.3441435024193,
2.67236104217133));
#239904=CARTESIAN_POINT('Ctrl Pts',(54.454330170972,-31.3530008879274,2.66911440541493));
#239905=CARTESIAN_POINT('Ctrl Pts',(54.4524721779265,-31.3618824321368,
2.66646778189657));
#239906=CARTESIAN_POINT('Ctrl Pts',(54.4516875359257,-31.3656331634087,
2.66535009634985));
#239907=CARTESIAN_POINT('Ctrl Pts',(54.4507682193241,-31.3693880355465,
2.66433897912343));
#239908=CARTESIAN_POINT('Ctrl Pts',(54.4497115877225,-31.3731331934884,
2.66344564884782));
#239909=CARTESIAN_POINT('Ctrl Pts',(54.4479322465079,-31.3794399458806,
2.66194130298575));
#239910=CARTESIAN_POINT('Ctrl Pts',(54.4457622496024,-31.3857169562551,
2.6607720670541));
#239911=CARTESIAN_POINT('Ctrl Pts',(54.4431895758475,-31.3918909882798,
2.65998225155705));
#239912=CARTESIAN_POINT('Ctrl Pts',(54.4425464074088,-31.393434496286,2.65978479768278));
#239913=CARTESIAN_POINT('Ctrl Pts',(54.4418778620531,-31.3949714642027,
2.65961098966613));
#239914=CARTESIAN_POINT('Ctrl Pts',(54.4411834812327,-31.3965005998215,
2.65946139030492));
#239915=CARTESIAN_POINT('Ctrl Pts',(54.4401419100021,-31.3987943032499,
2.65923699126311));
#239916=CARTESIAN_POINT('Ctrl Pts',(54.4390422051397,-31.4010703637555,
2.65906707562433));
#239917=CARTESIAN_POINT('Ctrl Pts',(54.4378842814515,-31.4033252432062,
2.65895332562911));
#239918=CARTESIAN_POINT('Ctrl Pts',(54.4367263577634,-31.4055801226569,
2.65883957563389));
#239919=CARTESIAN_POINT('Ctrl Pts',(54.435510226749,-31.4078138194774,2.65878198860241));
#239920=CARTESIAN_POINT('Ctrl Pts',(54.4342359163082,-31.4100231232061,
2.65878198860241));
#239921=CARTESIAN_POINT('Ctrl Pts',(51.1278468659051,-29.5010785149103,
2.65878198860242));
#239922=CARTESIAN_POINT('Ctrl Pts',(51.1321585373228,-29.4936027956388,
2.65878198860242));
#239923=CARTESIAN_POINT('Ctrl Pts',(51.1370499258748,-29.4865477845228,
2.65945335517838));
#239924=CARTESIAN_POINT('Ctrl Pts',(51.1423856448182,-29.4799806005916,
2.6607256122659));
#239925=CARTESIAN_POINT('Ctrl Pts',(51.145831971779,-29.4757388736043,2.66154735980328));
#239926=CARTESIAN_POINT('Ctrl Pts',(51.1494629466903,-29.4717000621104,
2.66261895766869));
#239927=CARTESIAN_POINT('Ctrl Pts',(51.1532365012464,-29.4678753842631,
2.66391429251009));
#239928=CARTESIAN_POINT('Ctrl Pts',(51.1582381316481,-29.4628059928675,
2.66563118464105));
#239929=CARTESIAN_POINT('Ctrl Pts',(51.1634934604719,-29.4581176150981,
2.6677410513868));
#239930=CARTESIAN_POINT('Ctrl Pts',(51.1689167792843,-29.4538379291352,
2.6701689418173));
#239931=CARTESIAN_POINT('Ctrl Pts',(51.1716284386905,-29.4516980861538,
2.67138288703256));
#239932=CARTESIAN_POINT('Ctrl Pts',(51.1743821937243,-29.4496602426625,
2.67267613167532));
#239933=CARTESIAN_POINT('Ctrl Pts',(51.1771680313595,-29.447726630041,2.67403835432533));
#239934=CARTESIAN_POINT('Ctrl Pts',(51.1785609501771,-29.4467598237303,
2.67471946565034));
#239935=CARTESIAN_POINT('Ctrl Pts',(51.1799618978184,-29.4458190608829,
2.67541781389503));
#239936=CARTESIAN_POINT('Ctrl Pts',(51.1813696738596,-29.4449045308652,
2.67613207244149));
#239937=CARTESIAN_POINT('Ctrl Pts',(51.1817216178699,-29.4446758983608,
2.67631063707811));
#239938=CARTESIAN_POINT('Ctrl Pts',(51.1820739888281,-29.4444489051046,
2.67649019601825));
#239939=CARTESIAN_POINT('Ctrl Pts',(51.1824267683262,-29.4442235534427,
2.67667072836637));
#239940=CARTESIAN_POINT('Ctrl Pts',(51.1834851068202,-29.443547498457,2.6772123254107));
#239941=CARTESIAN_POINT('Ctrl Pts',(51.1845471213156,-29.4428862193398,
2.67776268340027));
#239942=CARTESIAN_POINT('Ctrl Pts',(51.1856123224583,-29.4422397658671,
2.67832123541496));
#239943=CARTESIAN_POINT('Ctrl Pts',(51.1931154617654,-29.4376862310775,
2.68225560368428));
#239944=CARTESIAN_POINT('Ctrl Pts',(51.20077996036,-29.4338145801753,2.68661792998877));
#239945=CARTESIAN_POINT('Ctrl Pts',(51.2085065710734,-29.4305579784505,
2.69130986622573));
#239946=CARTESIAN_POINT('Ctrl Pts',(51.2122539689199,-29.4289785301331,
2.69358545023045));
#239947=CARTESIAN_POINT('Ctrl Pts',(51.2160164979702,-29.4275440072535,
2.69593918853455));
#239948=CARTESIAN_POINT('Ctrl Pts',(51.2197852472983,-29.4262483256611,
2.69836306235455));
#239949=CARTESIAN_POINT('Ctrl Pts',(51.2255549392047,-29.4242647276697,
2.70207384382188));
#239950=CARTESIAN_POINT('Ctrl Pts',(51.2313356805893,-29.4226066102315,
2.70594760814189));
#239951=CARTESIAN_POINT('Ctrl Pts',(51.2370841708902,-29.4212581193005,
2.70995196345668));
#239952=CARTESIAN_POINT('Ctrl Pts',(51.2397537995246,-29.420631873136,2.71181160678066));
#239953=CARTESIAN_POINT('Ctrl Pts',(51.2424163366108,-29.4200721889207,
2.71369962772059));
#239954=CARTESIAN_POINT('Ctrl Pts',(51.245067459672,-29.4195787111899,2.71561183138621));
#239955=CARTESIAN_POINT('Ctrl Pts',(51.2452706578087,-29.4195408880663,
2.71575839426272));
#239956=CARTESIAN_POINT('Ctrl Pts',(51.2454737959512,-29.4195034206994,
2.7159050890317));
#239957=CARTESIAN_POINT('Ctrl Pts',(51.2456768729759,-29.4194663081565,
2.71605191409872));
#239958=CARTESIAN_POINT('Ctrl Pts',(51.2485294929149,-29.4189449888193,
2.71811436362714));
#239959=CARTESIAN_POINT('Ctrl Pts',(51.2513705613631,-29.4184957101758,
2.7202009102692));
#239960=CARTESIAN_POINT('Ctrl Pts',(51.2541954110684,-29.4181151898789,
2.72230624862143));
#239961=CARTESIAN_POINT('Ctrl Pts',(51.2643248197287,-29.4167507117677,
2.72985561753046));
#239962=CARTESIAN_POINT('Ctrl Pts',(51.2743237313758,-29.4162578421113,
2.73770089914254));
#239963=CARTESIAN_POINT('Ctrl Pts',(51.2841455249765,-29.4165161672801,
2.74574823346978));
#239964=CARTESIAN_POINT('Ctrl Pts',(51.2949386894568,-29.4168000406894,
2.75459144546882));
#239965=CARTESIAN_POINT('Ctrl Pts',(51.3055186222576,-29.4179908989224,
2.7636791175408));
#239966=CARTESIAN_POINT('Ctrl Pts',(51.3158373135934,-29.4199800715328,
2.77292162564486));
#239967=CARTESIAN_POINT('Ctrl Pts',(51.3269789105976,-29.4221278787377,
2.78290121484403));
#239968=CARTESIAN_POINT('Ctrl Pts',(51.337817098422,-29.4252064644161,2.79306229499769));
#239969=CARTESIAN_POINT('Ctrl Pts',(51.3482921445208,-29.4291364604176,
2.80331916684744));
#239970=CARTESIAN_POINT('Ctrl Pts',(51.358679315748,-29.4330334877915,2.81348999408344));
#239971=CARTESIAN_POINT('Ctrl Pts',(51.3687106315432,-29.4377684584832,
2.8237563596669));
#239972=CARTESIAN_POINT('Ctrl Pts',(51.3783102687789,-29.4433108116253,
2.83404198860242));
#239973=CARTESIAN_POINT('Origin',(-0.00761999999999908,-0.0131982271534827,
2.83404198860262));
#239974=CARTESIAN_POINT('Ctrl Pts',(54.4189959163067,-31.4364195775126,
2.65878198860241));
#239975=CARTESIAN_POINT('Ctrl Pts',(54.4146983388121,-31.4438560159993,
2.65878198860241));
#239976=CARTESIAN_POINT('Ctrl Pts',(54.4098177483016,-31.4508673716596,
2.65944603041822));
#239977=CARTESIAN_POINT('Ctrl Pts',(54.4044907169114,-31.457389532058,2.66070439264029));
#239978=CARTESIAN_POINT('Ctrl Pts',(54.4010869974477,-31.4615568820637,
2.66150842619556));
#239979=CARTESIAN_POINT('Ctrl Pts',(54.3975017237414,-31.4655251210639,
2.66255428265336));
#239980=CARTESIAN_POINT('Ctrl Pts',(54.3937759157111,-31.4692842169739,
2.66381699700634));
#239981=CARTESIAN_POINT('Ctrl Pts',(54.3886909353395,-31.4744146286218,
2.66554034873233));
#239982=CARTESIAN_POINT('Ctrl Pts',(54.3833409297224,-31.4791503318814,
2.66766759643937));
#239983=CARTESIAN_POINT('Ctrl Pts',(54.3778174666306,-31.4834636394921,
2.67012012783112));
#239984=CARTESIAN_POINT('Ctrl Pts',(54.3750557350847,-31.4856202932974,
2.671346393527));
#239985=CARTESIAN_POINT('Ctrl Pts',(54.3722505364145,-31.4876715300018,
2.67265375584976));
#239986=CARTESIAN_POINT('Ctrl Pts',(54.3694125772951,-31.4896151854252,
2.67403135126903));
#239987=CARTESIAN_POINT('Ctrl Pts',(54.3679935977354,-31.4905870131369,
2.67472014897867));
#239988=CARTESIAN_POINT('Ctrl Pts',(54.3665664194003,-31.4915319606344,
2.67542649668595));
#239989=CARTESIAN_POINT('Ctrl Pts',(54.3651323262972,-31.492449852388,2.67614899656064));
#239990=CARTESIAN_POINT('Ctrl Pts',(54.3647738030214,-31.4926793253264,
2.67632962152931));
#239991=CARTESIAN_POINT('Ctrl Pts',(54.3644148473889,-31.4929071076032,
2.67651125590913));
#239992=CARTESIAN_POINT('Ctrl Pts',(54.3640554790925,-31.493133197126,2.67669387767486));
#239993=CARTESIAN_POINT('Ctrl Pts',(54.3629773742032,-31.4938114656944,
2.67724174297206));
#239994=CARTESIAN_POINT('Ctrl Pts',(54.3618955562477,-31.4944744978642,
2.67779849504709));
#239995=CARTESIAN_POINT('Ctrl Pts',(54.3608105487854,-31.495122251552,2.67836353617971));
#239996=CARTESIAN_POINT('Ctrl Pts',(54.3533124740225,-31.4995986314368,
2.68226832098868));
#239997=CARTESIAN_POINT('Ctrl Pts',(54.3456575719328,-31.5034009004288,
2.6865915375135));
#239998=CARTESIAN_POINT('Ctrl Pts',(54.3379428492065,-31.5065976218795,
2.69123699486135));
#239999=CARTESIAN_POINT('Ctrl Pts',(54.3341086531879,-31.5081863836657,
2.69354577441175));
#240000=CARTESIAN_POINT('Ctrl Pts',(54.330259136697,-31.5096252947438,2.69593478828078));
#240001=CARTESIAN_POINT('Ctrl Pts',(54.3264035847699,-31.5109210155993,
2.69839565261182));
#240002=CARTESIAN_POINT('Ctrl Pts',(54.3178976613389,-31.5137795693404,
2.70382468689008));
#240003=CARTESIAN_POINT('Ctrl Pts',(54.3093672304023,-31.5159526675022,
2.70961155815049));
#240004=CARTESIAN_POINT('Ctrl Pts',(54.300955957207,-31.5174623893708,2.71562701361729));
#240005=CARTESIAN_POINT('Ctrl Pts',(54.2978832130371,-31.518013909808,2.7178245353582));
#240006=CARTESIAN_POINT('Ctrl Pts',(54.2948245130138,-31.5184846398467,
2.72005051502364));
#240007=CARTESIAN_POINT('Ctrl Pts',(54.2917835794187,-31.5188783726362,
2.72229986760077));
#240008=CARTESIAN_POINT('Ctrl Pts',(54.2815694052538,-31.5202008794124,
2.72985520488861));
#240009=CARTESIAN_POINT('Ctrl Pts',(54.2714898389045,-31.5206547127622,
2.73770845534536));
#240010=CARTESIAN_POINT('Ctrl Pts',(54.2615918017967,-31.520359288622,2.74576706701739));
#240011=CARTESIAN_POINT('Ctrl Pts',(54.2507126865157,-31.5200345824966,
2.75462443585027));
#240012=CARTESIAN_POINT('Ctrl Pts',(54.2400521939111,-31.518804867654,2.76373036323191));
#240013=CARTESIAN_POINT('Ctrl Pts',(54.2296591093493,-31.5167773687216,
2.77299664636842));
#240014=CARTESIAN_POINT('Ctrl Pts',(54.2184653119679,-31.5145936654999,
2.78297683033519));
#240015=CARTESIAN_POINT('Ctrl Pts',(54.2075805209331,-31.5114844302862,
2.7931440147896));
#240016=CARTESIAN_POINT('Ctrl Pts',(54.1970658734737,-31.5075265408307,
2.80341452428028));
#240017=CARTESIAN_POINT('Ctrl Pts',(54.1866932092582,-31.5036220962467,
2.81354634721413));
#240018=CARTESIAN_POINT('Ctrl Pts',(54.1766795569337,-31.4988909785559,
2.82378004209214));
#240019=CARTESIAN_POINT('Ctrl Pts',(54.1671020372442,-31.493361394985,2.83404198860241));
#240020=CARTESIAN_POINT('Ctrl Pts',(51.1878102687789,-29.7732664904671,
2.83404198860241));
#240021=CARTESIAN_POINT('Ctrl Pts',(51.1786445298598,-29.7679746486349,
2.82422126443058));
#240022=CARTESIAN_POINT('Ctrl Pts',(51.1699291351239,-29.7619788985604,
2.81442815028624));
#240023=CARTESIAN_POINT('Ctrl Pts',(51.1617065245643,-29.7553188532211,
2.80471618166512));
#240024=CARTESIAN_POINT('Ctrl Pts',(51.1537668706119,-29.7488879934693,
2.79533842146471));
#240025=CARTESIAN_POINT('Ctrl Pts',(51.1462857370556,-29.7418369154176,
2.78603515650528));
#240026=CARTESIAN_POINT('Ctrl Pts',(51.1393284263648,-29.7341642916958,
2.77685887347088));
#240027=CARTESIAN_POINT('Ctrl Pts',(51.1327515888671,-29.7269112593617,
2.76818441216939));
#240028=CARTESIAN_POINT('Ctrl Pts',(51.1266422417943,-29.7191021335102,
2.75962261522015));
#240029=CARTESIAN_POINT('Ctrl Pts',(51.1210907313648,-29.7107129315338,
2.75123537702076));
#240030=CARTESIAN_POINT('Ctrl Pts',(51.1159778833928,-29.7029866172529,
2.74351087134555));
#240031=CARTESIAN_POINT('Ctrl Pts',(51.1113379461926,-29.6947677915945,
2.73593399450301));
#240032=CARTESIAN_POINT('Ctrl Pts',(51.1072776647632,-29.6860256466508,
2.72857657813045));
#240033=CARTESIAN_POINT('Ctrl Pts',(51.1060669708024,-29.6834189154991,
2.72638274508621));
#240034=CARTESIAN_POINT('Ctrl Pts',(51.1049080895609,-29.6807655934606,
2.72420861709731));
#240035=CARTESIAN_POINT('Ctrl Pts',(51.1038046002597,-29.678064724192,2.72205663736687));
#240036=CARTESIAN_POINT('Ctrl Pts',(51.1027123859004,-29.6753914511529,
2.71992664556726));
#240037=CARTESIAN_POINT('Ctrl Pts',(51.1016753170134,-29.6726744751138,
2.71782089927846));
#240038=CARTESIAN_POINT('Ctrl Pts',(51.1006978225844,-29.6699160505192,
2.71574387311207));
#240039=CARTESIAN_POINT('Ctrl Pts',(51.1006298495335,-29.6697242350675,
2.71559944077448));
#240040=CARTESIAN_POINT('Ctrl Pts',(51.1005621526966,-29.6695322176081,
2.7154551521603));
#240041=CARTESIAN_POINT('Ctrl Pts',(51.1004947333607,-29.669339997928,2.71531100781691));
#240042=CARTESIAN_POINT('Ctrl Pts',(51.097538822698,-29.6609123829944,2.70899119176043));
#240043=CARTESIAN_POINT('Ctrl Pts',(51.0951613514272,-29.6520916749673,
2.70298296066797));
#240044=CARTESIAN_POINT('Ctrl Pts',(51.0934607157665,-29.642939644629,2.69736727774094));
#240045=CARTESIAN_POINT('Ctrl Pts',(51.0918754277624,-29.6344083617416,
2.69213248525382));
#240046=CARTESIAN_POINT('Ctrl Pts',(51.0908783954022,-29.6255883681023,
2.68723866185417));
#240047=CARTESIAN_POINT('Ctrl Pts',(51.090576061194,-29.6165418049887,2.68278595829508));
#240048=CARTESIAN_POINT('Ctrl Pts',(51.0904654634293,-29.6132324551644,
2.68115710172757));
#240049=CARTESIAN_POINT('Ctrl Pts',(51.0904480940788,-29.6098929659862,
2.67958763637767));
#240050=CARTESIAN_POINT('Ctrl Pts',(51.0905301191544,-29.6065271365684,
2.67808378645327));
#240051=CARTESIAN_POINT('Ctrl Pts',(51.0905498434448,-29.6057177670358,
2.67772216078562));
#240052=CARTESIAN_POINT('Ctrl Pts',(51.0905756628932,-29.6049064053138,
2.67736403603526));
#240053=CARTESIAN_POINT('Ctrl Pts',(51.0906076352721,-29.6040931741695,
2.67700956934442));
#240054=CARTESIAN_POINT('Ctrl Pts',(51.0906386085141,-29.6033053564984,
2.67666617973766));
#240055=CARTESIAN_POINT('Ctrl Pts',(51.0906753561242,-29.6025157844397,
2.67632622314081));
#240056=CARTESIAN_POINT('Ctrl Pts',(51.0907179287119,-29.6017245728785,
2.67598984158736));
#240057=CARTESIAN_POINT('Ctrl Pts',(51.09118436061,-29.5930559358433,2.67230439292193));
#240058=CARTESIAN_POINT('Ctrl Pts',(51.0923507190419,-29.5841848213173,
2.66904964539953));
#240059=CARTESIAN_POINT('Ctrl Pts',(51.0942731997207,-29.575291162817,2.66640203566706));
#240060=CARTESIAN_POINT('Ctrl Pts',(51.0950705097613,-29.5716026975451,
2.66530399299413));
#240061=CARTESIAN_POINT('Ctrl Pts',(51.0959974771977,-29.5679105139257,
2.66430995142226));
#240062=CARTESIAN_POINT('Ctrl Pts',(51.0970562972094,-29.5642276868782,
2.66343053473321));
#240063=CARTESIAN_POINT('Ctrl Pts',(51.0988622250761,-29.5579462415713,
2.66193059792844));
#240064=CARTESIAN_POINT('Ctrl Pts',(51.1010529624044,-29.5516941764747,
2.66076519817087));
#240065=CARTESIAN_POINT('Ctrl Pts',(51.1036389246282,-29.545543522521,2.65997805604419));
#240066=CARTESIAN_POINT('Ctrl Pts',(51.1049319057401,-29.5424681955442,
2.65958448498084));
#240067=CARTESIAN_POINT('Ctrl Pts',(51.1063249785084,-29.5394188854251,
2.6592852626072));
#240068=CARTESIAN_POINT('Ctrl Pts',(51.1078194668134,-29.5364046579949,
2.65908463971282));
#240069=CARTESIAN_POINT('Ctrl Pts',(51.1093139551183,-29.5333904305647,
2.65888401681845));
#240070=CARTESIAN_POINT('Ctrl Pts',(51.110909822857,-29.5304113137785,2.65878198860242));
#240071=CARTESIAN_POINT('Ctrl Pts',(51.1126068659051,-29.5274749692176,
2.65878198860242));
#240072=CARTESIAN_POINT('Origin',(53.2328030451451,-23.6840886581928,2.83404198860246));
#240073=CARTESIAN_POINT('Ctrl Pts',(57.3172883154493,-25.3107727110814,
2.83404198860245));
#240074=CARTESIAN_POINT('Ctrl Pts',(57.3269813337899,-25.3150883208938,
2.8241965244006));
#240075=CARTESIAN_POINT('Ctrl Pts',(57.3363050752412,-25.3201559369462,
2.81438790575656));
#240076=CARTESIAN_POINT('Ctrl Pts',(57.3452135417183,-25.3259384683611,
2.8046678125692));
#240077=CARTESIAN_POINT('Ctrl Pts',(57.3538325360813,-25.3315331019378,
2.79526356453103));
#240078=CARTESIAN_POINT('Ctrl Pts',(57.3620638476579,-25.3377977038112,
2.78594102496265));
#240079=CARTESIAN_POINT('Ctrl Pts',(57.3698434251114,-25.3447390861645,
2.77675109088818));
#240080=CARTESIAN_POINT('Ctrl Pts',(57.3772024263436,-25.3513052064451,
2.76805797913728));
#240081=CARTESIAN_POINT('Ctrl Pts',(57.3841579102014,-25.3584775246706,
2.75948271210214));
#240082=CARTESIAN_POINT('Ctrl Pts',(57.3906233351696,-25.366288788459,2.75108575573282));
#240083=CARTESIAN_POINT('Ctrl Pts',(57.3965784591568,-25.3734835273331,
2.74335155163333));
#240084=CARTESIAN_POINT('Ctrl Pts',(57.4021181432099,-25.3812207968876,
2.73576818686011));
#240085=CARTESIAN_POINT('Ctrl Pts',(57.4071400767279,-25.3895423083599,
2.72840626160569));
#240086=CARTESIAN_POINT('Ctrl Pts',(57.4085967487434,-25.3919560625136,
2.72627084693721));
#240087=CARTESIAN_POINT('Ctrl Pts',(57.4100096047779,-25.3944190600981,
2.72415424587533));
#240088=CARTESIAN_POINT('Ctrl Pts',(57.4113754784549,-25.3969325220916,
2.72205867173239));
#240089=CARTESIAN_POINT('Ctrl Pts',(57.4128561733383,-25.3996572764934,
2.71978693462842));
#240090=CARTESIAN_POINT('Ctrl Pts',(57.4142805418443,-25.4024370309179,
2.71754411340743));
#240091=CARTESIAN_POINT('Ctrl Pts',(57.4156446191419,-25.4052723227218,
2.71533341844241));
#240092=CARTESIAN_POINT('Ctrl Pts',(57.419388339989,-25.4130538033258,2.70926614876388));
#240093=CARTESIAN_POINT('Ctrl Pts',(57.4226343338645,-25.4212623406648,
2.70347381860405));
#240094=CARTESIAN_POINT('Ctrl Pts',(57.4253008212881,-25.4298341608302,
2.69804914171392));
#240095=CARTESIAN_POINT('Ctrl Pts',(57.4277405125136,-25.4376769109061,
2.69308585687228));
#240096=CARTESIAN_POINT('Ctrl Pts',(57.4296843862653,-25.445819360425,2.68842799053232));
#240097=CARTESIAN_POINT('Ctrl Pts',(57.4310470526568,-25.454237715435,2.68414767054283));
#240098=CARTESIAN_POINT('Ctrl Pts',(57.4317163899371,-25.4583727839168,
2.68204519134593));
#240099=CARTESIAN_POINT('Ctrl Pts',(57.432244998004,-25.4625743171729,2.68003431778521));
#240100=CARTESIAN_POINT('Ctrl Pts',(57.4326195921325,-25.4668384019343,
2.67812693945251));
#240101=CARTESIAN_POINT('Ctrl Pts',(57.4326906677197,-25.4676474704849,
2.67776503299203));
#240102=CARTESIAN_POINT('Ctrl Pts',(57.4327558640766,-25.4684592045957,
2.67740659639923));
#240103=CARTESIAN_POINT('Ctrl Pts',(57.4328151061498,-25.4692734860646,
2.67705178968855));
#240104=CARTESIAN_POINT('Ctrl Pts',(57.4328724969083,-25.4700623212376,
2.67670807068757));
#240105=CARTESIAN_POINT('Ctrl Pts',(57.4329242997221,-25.4708535470238,
2.67636775825265));
#240106=CARTESIAN_POINT('Ctrl Pts',(57.4329704479397,-25.4716470524582,
2.67603099699254));
#240107=CARTESIAN_POINT('Ctrl Pts',(57.433473361706,-25.4802945111768,2.6723610421711));
#240108=CARTESIAN_POINT('Ctrl Pts',(57.4333046542892,-25.4892184175053,
2.66911440541443));
#240109=CARTESIAN_POINT('Ctrl Pts',(57.4323852136915,-25.4982455208449,
2.66646778189593));
#240110=CARTESIAN_POINT('Ctrl Pts',(57.4319969282177,-25.5020577226402,
2.6653500963495));
#240111=CARTESIAN_POINT('Ctrl Pts',(57.431475138743,-25.5058881199463,2.66433897912333));
#240112=CARTESIAN_POINT('Ctrl Pts',(57.4308157710843,-25.5097232095978,
2.66344564884791));
#240113=CARTESIAN_POINT('Ctrl Pts',(57.4297054124229,-25.5161814047433,
2.66194130298583));
#240114=CARTESIAN_POINT('Ctrl Pts',(57.4282034292359,-25.5226508554401,
2.66077206705417));
#240115=CARTESIAN_POINT('Ctrl Pts',(57.4262902109374,-25.5290599831057,
2.65998225155711));
#240116=CARTESIAN_POINT('Ctrl Pts',(57.4258119063628,-25.5306622650221,
2.65978479768285));
#240117=CARTESIAN_POINT('Ctrl Pts',(57.425307680263,-25.5322606952863,2.65961098966619));
#240118=CARTESIAN_POINT('Ctrl Pts',(57.4247769415296,-25.5338540367004,
2.65946139030498));
#240119=CARTESIAN_POINT('Ctrl Pts',(57.4239808334296,-25.5362440488214,
2.65923699126317));
#240120=CARTESIAN_POINT('Ctrl Pts',(57.4231250659724,-25.5386225912887,
2.65906707562438));
#240121=CARTESIAN_POINT('Ctrl Pts',(57.422209184595,-25.5409861542575,2.65895332562915));
#240122=CARTESIAN_POINT('Ctrl Pts',(57.4212933032177,-25.5433497172263,
2.65883957563393));
#240123=CARTESIAN_POINT('Ctrl Pts',(57.4203173191904,-25.5456982979271,
2.65878198860245));
#240124=CARTESIAN_POINT('Ctrl Pts',(57.4192809246792,-25.548028700571,2.65878198860245));
#240125=CARTESIAN_POINT('Ctrl Pts',(53.9314655730807,-23.9951532569799,
2.65878198860246));
#240126=CARTESIAN_POINT('Ctrl Pts',(53.9349721992641,-23.9872677980933,
2.65878198860246));
#240127=CARTESIAN_POINT('Ctrl Pts',(53.9390993428075,-23.9797401457377,
2.65945335517843));
#240128=CARTESIAN_POINT('Ctrl Pts',(53.9437193744799,-23.9726512030256,
2.66072561226598));
#240129=CARTESIAN_POINT('Ctrl Pts',(53.9467034408975,-23.9680724734015,
2.66154735980335));
#240130=CARTESIAN_POINT('Ctrl Pts',(53.9498923541893,-23.9636762467119,
2.66261895766876));
#240131=CARTESIAN_POINT('Ctrl Pts',(53.9532454491209,-23.9594780769913,
2.66391429251014));
#240132=CARTESIAN_POINT('Ctrl Pts',(53.9576897843756,-23.9539136435124,
2.66563118464111));
#240133=CARTESIAN_POINT('Ctrl Pts',(53.9624262550348,-23.9487016177212,
2.66774105138686));
#240134=CARTESIAN_POINT('Ctrl Pts',(53.9673725153423,-23.9438784851445,
2.67016894181736));
#240135=CARTESIAN_POINT('Ctrl Pts',(53.9698456454961,-23.9414669188561,
2.67138288703262));
#240136=CARTESIAN_POINT('Ctrl Pts',(53.9723713025231,-23.9391523931028,
2.67267613167538));
#240137=CARTESIAN_POINT('Ctrl Pts',(53.9749397614924,-23.9369381736867,
2.67403835432539));
#240138=CARTESIAN_POINT('Ctrl Pts',(53.9762239909771,-23.9358310639786,
2.6747194656504));
#240139=CARTESIAN_POINT('Ctrl Pts',(53.9775189275858,-23.9347490158245,
2.67541781389509));
#240140=CARTESIAN_POINT('Ctrl Pts',(53.9788233972652,-23.9336923430317,
2.67613207244155));
#240141=CARTESIAN_POINT('Ctrl Pts',(53.979149514685,-23.9334281748335,2.67631063707816));
#240142=CARTESIAN_POINT('Ctrl Pts',(53.9794762280621,-23.9331655922753,
2.67649019601831));
#240143=CARTESIAN_POINT('Ctrl Pts',(53.9798035193342,-23.9329045996146,
2.67667072836642));
#240144=CARTESIAN_POINT('Ctrl Pts',(53.9807853931505,-23.9321216216325,
2.67721232541076));
#240145=CARTESIAN_POINT('Ctrl Pts',(53.9817724673294,-23.9313529543284,
2.67776268340033));
#240146=CARTESIAN_POINT('Ctrl Pts',(53.9827642604008,-23.9305986983569,
2.67832123541502));
#240147=CARTESIAN_POINT('Ctrl Pts',(53.9897503227318,-23.9252858166858,
2.68225560368437));
#240148=CARTESIAN_POINT('Ctrl Pts',(53.996968136682,-23.9206342168325,2.6866179299889));
#240149=CARTESIAN_POINT('Ctrl Pts',(54.0043120126398,-23.9165878043685,
2.6913098662259));
#240150=CARTESIAN_POINT('Ctrl Pts',(54.0078737845432,-23.9146252986961,
2.69358545023058));
#240151=CARTESIAN_POINT('Ctrl Pts',(54.0114657535936,-23.9128053429034,
2.69593918853464));
#240152=CARTESIAN_POINT('Ctrl Pts',(54.0150784217127,-23.9111228176146,
2.6983630623546));
#240153=CARTESIAN_POINT('Ctrl Pts',(54.0206091641934,-23.9085469889521,
2.70207384382192));
#240154=CARTESIAN_POINT('Ctrl Pts',(54.0261849176042,-23.9062937028413,
2.70594760814192));
#240155=CARTESIAN_POINT('Ctrl Pts',(54.0317609613889,-23.9043517182274,
2.70995196345672));
#240156=CARTESIAN_POINT('Ctrl Pts',(54.0343505049692,-23.9034498505262,
2.7118116067807));
#240157=CARTESIAN_POINT('Ctrl Pts',(54.0369399534677,-23.9026149214096,
2.71369962772063));
#240158=CARTESIAN_POINT('Ctrl Pts',(54.0395249709305,-23.901847029182,2.71561183138625));
#240159=CARTESIAN_POINT('Ctrl Pts',(54.0397231023336,-23.9017881732684,
2.71575839426276));
#240160=CARTESIAN_POINT('Ctrl Pts',(54.0399212112578,-23.9017296774338,
2.71590508903173));
#240161=CARTESIAN_POINT('Ctrl Pts',(54.0401192964882,-23.901671540868,2.71605191409876));
#240162=CARTESIAN_POINT('Ctrl Pts',(54.0429017967675,-23.9008548973942,
2.71811436362717));
#240163=CARTESIAN_POINT('Ctrl Pts',(54.0456803391393,-23.9001111074271,
2.72020091026924));
#240164=CARTESIAN_POINT('Ctrl Pts',(54.0484499388205,-23.8994373944616,
2.72230624862147));
#240165=CARTESIAN_POINT('Ctrl Pts',(54.0583812307202,-23.8970215795832,
2.72985561753049));
#240166=CARTESIAN_POINT('Ctrl Pts',(54.0682738483753,-23.8954862390495,
2.73770089914257));
#240167=CARTESIAN_POINT('Ctrl Pts',(54.0780688394959,-23.8947164920943,
2.74574823346979));
#240168=CARTESIAN_POINT('Ctrl Pts',(54.0888325507431,-23.8938706175186,
2.75459144546888));
#240169=CARTESIAN_POINT('Ctrl Pts',(54.0994790041462,-23.8939490479884,
2.7636791175409));
#240170=CARTESIAN_POINT('Ctrl Pts',(54.1099490937673,-23.8948487267548,
2.77292162564502));
#240171=CARTESIAN_POINT('Ctrl Pts',(54.121254162924,-23.8958201540339,2.78290121484429));
#240172=CARTESIAN_POINT('Ctrl Pts',(54.1323547778516,-23.89774897578,2.79306229499807));
#240173=CARTESIAN_POINT('Ctrl Pts',(54.1431832369946,-23.9005625023809,
2.80331916684792));
#240174=CARTESIAN_POINT('Ctrl Pts',(54.1539208564936,-23.903352426385,2.81348999408378));
#240175=CARTESIAN_POINT('Ctrl Pts',(54.1643921589012,-23.9070129003871,
2.82375635966709));
#240176=CARTESIAN_POINT('Ctrl Pts',(54.1745185419763,-23.9115214566106,
2.83404198860246));
#240177=CARTESIAN_POINT('Origin',(-0.00619866644047451,-0.0139224327742815,
2.83404198860262));
#240178=CARTESIAN_POINT('Ctrl Pts',(57.4068835917983,-25.5758735661199,
2.65878198860245));
#240179=CARTESIAN_POINT('Ctrl Pts',(57.4033868763699,-25.5837184861902,
2.65878198860245));
#240180=CARTESIAN_POINT('Ctrl Pts',(57.3992659084772,-25.5912015935368,
2.65944603041834));
#240181=CARTESIAN_POINT('Ctrl Pts',(57.3946498105256,-25.5982448512635,
2.66070439264055));
#240182=CARTESIAN_POINT('Ctrl Pts',(57.3917003436855,-25.6027451576543,
2.66150842619579));
#240183=CARTESIAN_POINT('Ctrl Pts',(57.3885495044085,-25.6070664213766,
2.66255428265351));
#240184=CARTESIAN_POINT('Ctrl Pts',(57.3852370392635,-25.6111943775533,
2.66381699700637));
#240185=CARTESIAN_POINT('Ctrl Pts',(57.380716188992,-25.6168282094534,2.66554034873237));
#240186=CARTESIAN_POINT('Ctrl Pts',(57.3758905070496,-25.6220971979007,
2.66766759643942));
#240187=CARTESIAN_POINT('Ctrl Pts',(57.3708481654826,-25.6269642358699,
2.67012012783117));
#240188=CARTESIAN_POINT('Ctrl Pts',(57.3683269946992,-25.6293977548545,
2.67134639352705));
#240189=CARTESIAN_POINT('Ctrl Pts',(57.3657515758214,-25.6317309777758,
2.67265375584981));
#240190=CARTESIAN_POINT('Ctrl Pts',(57.3631323306535,-25.6339606331569,
2.67403135126909));
#240191=CARTESIAN_POINT('Ctrl Pts',(57.3618227080695,-25.6350754608475,
2.67472014897872));
#240192=CARTESIAN_POINT('Ctrl Pts',(57.3605021218765,-25.6361644125819,
2.67542649668601));
#240193=CARTESIAN_POINT('Ctrl Pts',(57.3591718306998,-25.6372271795767,
2.67614899656071));
#240194=CARTESIAN_POINT('Ctrl Pts',(57.3588392579057,-25.6374928713254,
2.67632962152938));
#240195=CARTESIAN_POINT('Ctrl Pts',(57.3585060784011,-25.6377569268677,
2.67651125590919));
#240196=CARTESIAN_POINT('Ctrl Pts',(57.3581723115521,-25.6380193420642,
2.67669387767493));
#240197=CARTESIAN_POINT('Ctrl Pts',(57.3571710110054,-25.6388065876538,
2.67724174297213));
#240198=CARTESIAN_POINT('Ctrl Pts',(57.3561644250956,-25.6395790684324,
2.67779849504716));
#240199=CARTESIAN_POINT('Ctrl Pts',(57.3551530701153,-25.6403366878204,
2.67836353617978));
#240200=CARTESIAN_POINT('Ctrl Pts',(57.3481639797008,-25.6455723078603,
2.68226832098882));
#240201=CARTESIAN_POINT('Ctrl Pts',(57.3409484573002,-25.6501539027769,
2.68659153751371));
#240202=CARTESIAN_POINT('Ctrl Pts',(57.3336101450128,-25.6541395203642,
2.69123699486164));
#240203=CARTESIAN_POINT('Ctrl Pts',(57.3299630239493,-25.6561203613647,
2.69354577441197));
#240204=CARTESIAN_POINT('Ctrl Pts',(57.3262850026764,-25.6579537739804,
2.69593478828091));
#240205=CARTESIAN_POINT('Ctrl Pts',(57.3225860115762,-25.6596454116595,
2.69839565261187));
#240206=CARTESIAN_POINT('Ctrl Pts',(57.3144254847134,-25.6633774170489,
2.70382468689012));
#240207=CARTESIAN_POINT('Ctrl Pts',(57.3061689349815,-25.6664302835885,
2.70961155815053));
#240208=CARTESIAN_POINT('Ctrl Pts',(57.2979615485277,-25.668810952504,2.71562701361733));
#240209=CARTESIAN_POINT('Ctrl Pts',(57.2949632867555,-25.6696806408806,
2.71782453535824));
#240210=CARTESIAN_POINT('Ctrl Pts',(57.2919705472986,-25.6704685134239,
2.72005051502368));
#240211=CARTESIAN_POINT('Ctrl Pts',(57.2889874285393,-25.6711779534196,
2.72229986760081));
#240212=CARTESIAN_POINT('Ctrl Pts',(57.2789674482908,-25.6735608872942,
2.72985520488827));
#240213=CARTESIAN_POINT('Ctrl Pts',(57.2689905373637,-25.6750658360783,
2.7377084553446));
#240214=CARTESIAN_POINT('Ctrl Pts',(57.259115842508,-25.6758066569107,2.7457670670162));
#240215=CARTESIAN_POINT('Ctrl Pts',(57.248262383127,-25.6766209067615,2.75462443584864));
#240216=CARTESIAN_POINT('Ctrl Pts',(57.237531749614,-25.6765122533353,2.76373036322983));
#240217=CARTESIAN_POINT('Ctrl Pts',(57.2269836681097,-25.6755822344122,
2.77299664636587));
#240218=CARTESIAN_POINT('Ctrl Pts',(57.2156229323801,-25.6745805641838,
2.78297683033213));
#240219=CARTESIAN_POINT('Ctrl Pts',(57.2044727657911,-25.6726261321662,
2.79314401478602));
#240220=CARTESIAN_POINT('Ctrl Pts',(57.1936020065686,-25.6697890043843,
2.80341452427617));
#240221=CARTESIAN_POINT('Ctrl Pts',(57.1828780392991,-25.6669901874066,
2.81354634721137));
#240222=CARTESIAN_POINT('Ctrl Pts',(57.1724247063465,-25.6633316989623,
2.82378004209078));
#240223=CARTESIAN_POINT('Ctrl Pts',(57.1623216544374,-25.6588335304432,
2.83404198860244));
#240224=CARTESIAN_POINT('Ctrl Pts',(54.0195518809644,-24.2595822759724,
2.83404198860245));
#240225=CARTESIAN_POINT('Ctrl Pts',(54.0098832048281,-24.2552775040076,
2.82422126443109));
#240226=CARTESIAN_POINT('Ctrl Pts',(54.0005888273954,-24.2502256060981,
2.81442815028723));
#240227=CARTESIAN_POINT('Ctrl Pts',(53.9917150968526,-24.2444615420302,
2.80471618166656));
#240228=CARTESIAN_POINT('Ctrl Pts',(53.9831467292681,-24.2388958310277,
2.79533842146638));
#240229=CARTESIAN_POINT('Ctrl Pts',(53.9749695397912,-24.2326653709137,
2.78603515650717));
#240230=CARTESIAN_POINT('Ctrl Pts',(53.9672483344096,-24.2257620156227,
2.77685887347298));
#240231=CARTESIAN_POINT('Ctrl Pts',(53.9599493771919,-24.2192361828756,
2.76818441217154));
#240232=CARTESIAN_POINT('Ctrl Pts',(53.9530572218368,-24.2121084368938,
2.75962261522233));
#240233=CARTESIAN_POINT('Ctrl Pts',(53.9466592127717,-24.2043454826978,
2.75123537702297));
#240234=CARTESIAN_POINT('Ctrl Pts',(53.9407667537572,-24.1971959321165,
2.74351087134767));
#240235=CARTESIAN_POINT('Ctrl Pts',(53.9352931334024,-24.1895071355501,
2.73593399450503));
#240236=CARTESIAN_POINT('Ctrl Pts',(53.9303412916427,-24.1812372959695,
2.72857657813237));
#240237=CARTESIAN_POINT('Ctrl Pts',(53.9288647523883,-24.1787713967423,
2.72638274508749));
#240238=CARTESIAN_POINT('Ctrl Pts',(53.9274348719438,-24.1762537459541,
2.72420861709797));
#240239=CARTESIAN_POINT('Ctrl Pts',(53.9260551099579,-24.1736830183701,
2.72205663736691));
#240240=CARTESIAN_POINT('Ctrl Pts',(53.9246894457405,-24.171138557289,2.7199266455673));
#240241=CARTESIAN_POINT('Ctrl Pts',(53.9233740566952,-24.168544868346,2.71782089927849));
#240242=CARTESIAN_POINT('Ctrl Pts',(53.9221135831991,-24.1659037306804,
2.7157438731121));
#240243=CARTESIAN_POINT('Ctrl Pts',(53.9220259323373,-24.1657200711324,
2.71559944077451));
#240244=CARTESIAN_POINT('Ctrl Pts',(53.9219385350609,-24.1655361818111,
2.71545515216033));
#240245=CARTESIAN_POINT('Ctrl Pts',(53.9218513926274,-24.1653520623701,
2.71531100781694));
#240246=CARTESIAN_POINT('Ctrl Pts',(53.9180307491145,-24.1572795915921,
2.70899119176053));
#240247=CARTESIAN_POINT('Ctrl Pts',(53.9147442868251,-24.148755717745,2.70298296066814));
#240248=CARTESIAN_POINT('Ctrl Pts',(53.9120963197576,-24.1398315880188,
2.69736727774116));
#240249=CARTESIAN_POINT('Ctrl Pts',(53.9096279542371,-24.1315127481109,
2.6921324852542));
#240250=CARTESIAN_POINT('Ctrl Pts',(53.9077144433434,-24.1228452895803,
2.68723866185469));
#240251=CARTESIAN_POINT('Ctrl Pts',(53.9064681420135,-24.1138798870165,
2.6827859582957));
#240252=CARTESIAN_POINT('Ctrl Pts',(53.9060122288633,-24.1106002267708,
2.68115710172797));
#240253=CARTESIAN_POINT('Ctrl Pts',(53.9056458829919,-24.1072808472548,
2.67958763637787));
#240254=CARTESIAN_POINT('Ctrl Pts',(53.9053756337489,-24.1039248822473,
2.67808378645328));
#240255=CARTESIAN_POINT('Ctrl Pts',(53.9053106478341,-24.1031178847759,
2.67772216078563));
#240256=CARTESIAN_POINT('Ctrl Pts',(53.9052515154469,-24.102308268911,2.67736403603527));
#240257=CARTESIAN_POINT('Ctrl Pts',(53.9051983068759,-24.1014961507084,
2.67700956934443));
#240258=CARTESIAN_POINT('Ctrl Pts',(53.9051467610728,-24.1007094111996,
2.67666617973767));
#240259=CARTESIAN_POINT('Ctrl Pts',(53.9051007746217,-24.099920323328,2.67632622314082));
#240260=CARTESIAN_POINT('Ctrl Pts',(53.9050604098637,-24.0991289960593,
2.67598984158737));
#240261=CARTESIAN_POINT('Ctrl Pts',(53.9046181672912,-24.0904590913151,
2.67230439292184));
#240262=CARTESIAN_POINT('Ctrl Pts',(53.9048508523207,-24.0815146560279,
2.66904964539938));
#240263=CARTESIAN_POINT('Ctrl Pts',(53.9058331609934,-24.0724687639682,
2.66640203566687));
#240264=CARTESIAN_POINT('Ctrl Pts',(53.9062405536795,-24.0687171629019,
2.66530399299402));
#240265=CARTESIAN_POINT('Ctrl Pts',(53.9067765048114,-24.0649483109693,
2.66430995142222));
#240266=CARTESIAN_POINT('Ctrl Pts',(53.9074445642445,-24.0611749820052,
2.66343053473323));
#240267=CARTESIAN_POINT('Ctrl Pts',(53.9085840092244,-24.0547391762483,
2.66193059792847));
#240268=CARTESIAN_POINT('Ctrl Pts',(53.9101092267075,-24.0482923662121,
2.6607651981709));
#240269=CARTESIAN_POINT('Ctrl Pts',(53.9120381043535,-24.0419050995269,
2.65997805604422));
#240270=CARTESIAN_POINT('Ctrl Pts',(53.9130025431765,-24.0387114661843,
2.65958448498088));
#240271=CARTESIAN_POINT('Ctrl Pts',(53.9140692448457,-24.0355332447494,
2.65928526260724));
#240272=CARTESIAN_POINT('Ctrl Pts',(53.9152404736262,-24.0323793130066,
2.65908463971286));
#240273=CARTESIAN_POINT('Ctrl Pts',(53.9164117024067,-24.0292253812638,
2.65888401681848));
#240274=CARTESIAN_POINT('Ctrl Pts',(53.9176874253156,-24.0260957707889,
2.65878198860246));
#240275=CARTESIAN_POINT('Ctrl Pts',(53.9190682401998,-24.0229981225288,
2.65878198860246));
#240276=CARTESIAN_POINT('Origin',(55.4168495715594,-17.9900016446774,2.8340419886025));
#240277=CARTESIAN_POINT('Ctrl Pts',(59.6489943884567,-19.1808295835772,
2.83404198860249));
#240278=CARTESIAN_POINT('Ctrl Pts',(59.6590854114903,-19.184108355716,2.82419652440052));
#240279=CARTESIAN_POINT('Ctrl Pts',(59.6688877866288,-19.1881736144716,
2.81438790575639));
#240280=CARTESIAN_POINT('Ctrl Pts',(59.678351890717,-19.1929932802635,2.80466781256897));
#240281=CARTESIAN_POINT('Ctrl Pts',(59.6875084677774,-19.1976563356163,
2.79526356453078));
#240282=CARTESIAN_POINT('Ctrl Pts',(59.6963495165747,-19.2030262129955,
2.78594102496239));
#240283=CARTESIAN_POINT('Ctrl Pts',(59.7048120487193,-19.2091163824539,
2.77675109088793));
#240284=CARTESIAN_POINT('Ctrl Pts',(59.7128170830354,-19.2148773077506,
2.76805797913705));
#240285=CARTESIAN_POINT('Ctrl Pts',(59.720484175427,-19.2212832892275,2.75948271210193));
#240286=CARTESIAN_POINT('Ctrl Pts',(59.7277306815208,-19.2283759411593,
2.75108575573264));
#240287=CARTESIAN_POINT('Ctrl Pts',(59.7344052377139,-19.2349087865421,
2.74335155163319));
#240288=CARTESIAN_POINT('Ctrl Pts',(59.7407233396945,-19.2420246158633,
2.73576818686));
#240289=CARTESIAN_POINT('Ctrl Pts',(59.7465875973415,-19.2497756062319,
2.72840626160561));
#240290=CARTESIAN_POINT('Ctrl Pts',(59.7482885955677,-19.2520238739005,
2.72627084693717));
#240291=CARTESIAN_POINT('Ctrl Pts',(59.7499511651815,-19.2543256952563,
2.72415424587534));
#240292=CARTESIAN_POINT('Ctrl Pts',(59.7515722847792,-19.2566826155655,
2.72205867173244));
#240293=CARTESIAN_POINT('Ctrl Pts',(59.7533296826515,-19.2592376687169,
2.71978693462847));
#240294=CARTESIAN_POINT('Ctrl Pts',(59.755036811776,-19.2618533083047,2.71754411340748));
#240295=CARTESIAN_POINT('Ctrl Pts',(59.7566897852107,-19.2645304831798,
2.71533341844245));
#240296=CARTESIAN_POINT('Ctrl Pts',(59.7612263837727,-19.2718780106318,
2.70926614876392));
#240297=CARTESIAN_POINT('Ctrl Pts',(59.7653126215479,-19.2797022819928,
2.7034738186041));
#240298=CARTESIAN_POINT('Ctrl Pts',(59.7688605008636,-19.2879484209977,
2.69804914171396));
#240299=CARTESIAN_POINT('Ctrl Pts',(59.7721066178187,-19.2954931904938,
2.69308585687204));
#240300=CARTESIAN_POINT('Ctrl Pts',(59.7748909605622,-19.3033878446867,
2.68842799053184));
#240301=CARTESIAN_POINT('Ctrl Pts',(59.7771261198371,-19.3116176456438,
2.68414767054215));
#240302=CARTESIAN_POINT('Ctrl Pts',(59.7782240227715,-19.3156600969901,
2.68204519134551));
#240303=CARTESIAN_POINT('Ctrl Pts',(59.7791889148826,-19.319783359218,2.68003431778503));
#240304=CARTESIAN_POINT('Ctrl Pts',(59.7800071751725,-19.3239849291278,
2.67812693945254));
#240305=CARTESIAN_POINT('Ctrl Pts',(59.7801624320925,-19.3247821360944,
2.67776503299206));
#240306=CARTESIAN_POINT('Ctrl Pts',(59.7803121206161,-19.3255826085658,
2.67740659639927));
#240307=CARTESIAN_POINT('Ctrl Pts',(59.7804561537457,-19.3263862368327,
2.67705178968858));
#240308=CARTESIAN_POINT('Ctrl Pts',(59.78059568584,-19.3271647517164,2.6767080706876));
#240309=CARTESIAN_POINT('Ctrl Pts',(59.780729910488,-19.3279462282163,2.67636775825268));
#240310=CARTESIAN_POINT('Ctrl Pts',(59.7808587498045,-19.3287305629427,
2.67603099699257));
#240311=CARTESIAN_POINT('Ctrl Pts',(59.7822628141275,-19.337278081174,2.67236104217133));
#240312=CARTESIAN_POINT('Ctrl Pts',(59.7830278331225,-19.3461707361365,
2.6691144054148));
#240313=CARTESIAN_POINT('Ctrl Pts',(59.7830570185565,-19.3552444957717,
2.66646778189637));
#240314=CARTESIAN_POINT('Ctrl Pts',(59.7830693437465,-19.3590764008111,
2.66535009634979));
#240315=CARTESIAN_POINT('Ctrl Pts',(59.7829507982333,-19.3629403566523,
2.66433897912347));
#240316=CARTESIAN_POINT('Ctrl Pts',(59.7826959186874,-19.3668233599701,
2.66344564884794));
#240317=CARTESIAN_POINT('Ctrl Pts',(59.7822667079009,-19.3733622405313,
2.66194130298587));
#240318=CARTESIAN_POINT('Ctrl Pts',(59.7814491944745,-19.3799532508947,
2.66077206705421));
#240319=CARTESIAN_POINT('Ctrl Pts',(59.7802163932513,-19.3865272544568,
2.65998225155715));
#240320=CARTESIAN_POINT('Ctrl Pts',(59.7799081929455,-19.3881707553474,
2.65978479768288));
#240321=CARTESIAN_POINT('Ctrl Pts',(59.7795738105081,-19.3898131352228,
2.65961098966623));
#240322=CARTESIAN_POINT('Ctrl Pts',(59.7792125287466,-19.39145322545,2.65946139030502));
#240323=CARTESIAN_POINT('Ctrl Pts',(59.7786706061044,-19.3939133607909,
2.6592369912632));
#240324=CARTESIAN_POINT('Ctrl Pts',(59.7780681520198,-19.3963683254109,
2.65906707562442));
#240325=CARTESIAN_POINT('Ctrl Pts',(59.7774043475416,-19.3988146762074,
2.65895332562919));
#240326=CARTESIAN_POINT('Ctrl Pts',(59.7767405430633,-19.4012610270039,
2.65883957563397));
#240327=CARTESIAN_POINT('Ctrl Pts',(59.7760153991104,-19.4036987600445,
2.65878198860249));
#240328=CARTESIAN_POINT('Ctrl Pts',(59.7752282754839,-19.4061247292244,
2.65878198860249));
#240329=CARTESIAN_POINT('Ctrl Pts',(56.144199857553,-18.2263320786573,2.6587819886025));
#240330=CARTESIAN_POINT('Ctrl Pts',(56.1468630191715,-18.2181232748938,
2.6587819886025));
#240331=CARTESIAN_POINT('Ctrl Pts',(56.1501806998578,-18.2102054558336,
2.6594533551784));
#240332=CARTESIAN_POINT('Ctrl Pts',(56.1540344262252,-18.2026724222807,
2.66072561226582));
#240333=CARTESIAN_POINT('Ctrl Pts',(56.1565235380435,-18.1978068555392,
2.66154735980322));
#240334=CARTESIAN_POINT('Ctrl Pts',(56.1592354513148,-18.1931013796332,
2.66261895766869));
#240335=CARTESIAN_POINT('Ctrl Pts',(56.1621313494123,-18.1885757140648,
2.66391429251018));
#240336=CARTESIAN_POINT('Ctrl Pts',(56.165969696453,-18.1825772036004,2.66563118464114));
#240337=CARTESIAN_POINT('Ctrl Pts',(56.1701354151839,-18.1768986338324,
2.6677410513869));
#240338=CARTESIAN_POINT('Ctrl Pts',(56.1745504247235,-18.1715848978918,
2.6701689418174));
#240339=CARTESIAN_POINT('Ctrl Pts',(56.1767579294934,-18.1689280299214,
2.67138288703266));
#240340=CARTESIAN_POINT('Ctrl Pts',(56.1790278168867,-18.1663621803345,
2.67267613167542));
#240341=CARTESIAN_POINT('Ctrl Pts',(56.1813507566161,-18.163891613575,2.67403835432543));
#240342=CARTESIAN_POINT('Ctrl Pts',(56.1825122264809,-18.1626563301953,
2.67471946565044));
#240343=CARTESIAN_POINT('Ctrl Pts',(56.1836869644606,-18.1614448518804,
2.67541781389513));
#240344=CARTESIAN_POINT('Ctrl Pts',(56.1848738357354,-18.1602576134408,
2.67613207244159));
#240345=CARTESIAN_POINT('Ctrl Pts',(56.1851705535541,-18.1599608038309,
2.6763106370782));
#240346=CARTESIAN_POINT('Ctrl Pts',(56.1854680298098,-18.1596655088802,
2.67649019601836));
#240347=CARTESIAN_POINT('Ctrl Pts',(56.1857662469844,-18.1593717347109,
2.67667072836647));
#240348=CARTESIAN_POINT('Ctrl Pts',(56.186660898508,-18.1584904122029,2.6772123254108));
#240349=CARTESIAN_POINT('Ctrl Pts',(56.1875622177791,-18.1576227783917,
2.67776268340037));
#240350=CARTESIAN_POINT('Ctrl Pts',(56.1884697364867,-18.1567689837077,
2.67832123541506));
#240351=CARTESIAN_POINT('Ctrl Pts',(56.1948621810804,-18.1507549641988,
2.68225560368426));
#240352=CARTESIAN_POINT('Ctrl Pts',(56.2015542305059,-18.1453743792959,
2.68661792998861));
#240353=CARTESIAN_POINT('Ctrl Pts',(56.2084349106659,-18.1405824894347,
2.6913098662254));
#240354=CARTESIAN_POINT('Ctrl Pts',(56.2117720331084,-18.1382584280299,
2.69358545023025));
#240355=CARTESIAN_POINT('Ctrl Pts',(56.2151540877945,-18.1360729791403,
2.69593918853449));
#240356=CARTESIAN_POINT('Ctrl Pts',(56.2185710935571,-18.1340220442542,
2.69836306235464));
#240357=CARTESIAN_POINT('Ctrl Pts',(56.2238022906401,-18.1308822062384,
2.70207384382197));
#240358=CARTESIAN_POINT('Ctrl Pts',(56.2291119669557,-18.128058438929,2.70594760814197));
#240359=CARTESIAN_POINT('Ctrl Pts',(56.2344544719218,-18.1255442374222,
2.70995196345676));
#240360=CARTESIAN_POINT('Ctrl Pts',(56.2369355588666,-18.1243766292356,
2.71181160678074));
#240361=CARTESIAN_POINT('Ctrl Pts',(56.2394235482377,-18.1232756028758,
2.71369962772068));
#240362=CARTESIAN_POINT('Ctrl Pts',(56.2419141381099,-18.1222417093392,
2.7156118313863));
#240363=CARTESIAN_POINT('Ctrl Pts',(56.2421050320102,-18.1221624654734,
2.71575839426281));
#240364=CARTESIAN_POINT('Ctrl Pts',(56.2422959411933,-18.1220835820637,
2.71590508903178));
#240365=CARTESIAN_POINT('Ctrl Pts',(56.2424868643662,-18.1220050584313,
2.7160519140988));
#240366=CARTESIAN_POINT('Ctrl Pts',(56.2451687593305,-18.1209020381377,
2.71811436362722));
#240367=CARTESIAN_POINT('Ctrl Pts',(56.2478543333342,-18.1198718859656,
2.72020091026928));
#240368=CARTESIAN_POINT('Ctrl Pts',(56.2505383386776,-18.1189123616717,
2.72230624862151));
#240369=CARTESIAN_POINT('Ctrl Pts',(56.2601627045038,-18.1154716781996,
2.72985561753017));
#240370=CARTESIAN_POINT('Ctrl Pts',(56.2698406425773,-18.1129106883009,
2.73770089914185));
#240371=CARTESIAN_POINT('Ctrl Pts',(56.2795015152448,-18.1111213027306,
2.74574823346867));
#240372=CARTESIAN_POINT('Ctrl Pts',(56.2901178437854,-18.1091549477486,
2.75459144546718));
#240373=CARTESIAN_POINT('Ctrl Pts',(56.3007141730186,-18.1081200911546,
2.76367911753858));
#240374=CARTESIAN_POINT('Ctrl Pts',(56.3112209484315,-18.107920419008,2.77292162564207));
#240375=CARTESIAN_POINT('Ctrl Pts',(56.3225656290361,-18.1077048232006,
2.78290121484032));
#240376=CARTESIAN_POINT('Ctrl Pts',(56.3338070504056,-18.1084627484392,
2.79306229499306));
#240377=CARTESIAN_POINT('Ctrl Pts',(56.3448702837274,-18.1101289800527,
2.80331916684187));
#240378=CARTESIAN_POINT('Ctrl Pts',(56.3558407078943,-18.1117812336958,
2.81348999407971));
#240379=CARTESIAN_POINT('Ctrl Pts',(56.3666372711362,-18.1143271060896,
2.82375635966507));
#240380=CARTESIAN_POINT('Ctrl Pts',(56.377179453281,-18.1177524687097,2.8340419886025));
#240381=CARTESIAN_POINT('Origin',(-0.00470941899427373,-0.014494101308147,
2.83404198860262));
#240382=CARTESIAN_POINT('Ctrl Pts',(59.7658094374954,-19.4351129318411,
2.65878198860249));
#240383=CARTESIAN_POINT('Ctrl Pts',(59.7631518948793,-19.4432803829088,
2.65878198860249));
#240384=CARTESIAN_POINT('Ctrl Pts',(59.7598356997912,-19.4511532554516,
2.6594460304184));
#240385=CARTESIAN_POINT('Ctrl Pts',(59.7559811102138,-19.4586404431008,
2.66070439264065));
#240386=CARTESIAN_POINT('Ctrl Pts',(59.7535182109729,-19.4634243995784,
2.66150842619589));
#240387=CARTESIAN_POINT('Ctrl Pts',(59.7508363273795,-19.4680513433534,
2.66255428265358));
#240388=CARTESIAN_POINT('Ctrl Pts',(59.7479734971808,-19.4725029330453,
2.66381699700641));
#240389=CARTESIAN_POINT('Ctrl Pts',(59.7440663083909,-19.4785784597564,
2.6655403487324));
#240390=CARTESIAN_POINT('Ctrl Pts',(59.7398178213044,-19.4843230052513,
2.66766759643944));
#240391=CARTESIAN_POINT('Ctrl Pts',(59.7353118462118,-19.4896904492925,
2.6701201278312));
#240392=CARTESIAN_POINT('Ctrl Pts',(59.7330588586655,-19.4923741713131,
2.67134639352707));
#240393=CARTESIAN_POINT('Ctrl Pts',(59.7307414364082,-19.4949638171727,
2.67265375584983));
#240394=CARTESIAN_POINT('Ctrl Pts',(59.72836960219,-19.4974550439407,2.67403135126911));
#240395=CARTESIAN_POINT('Ctrl Pts',(59.7271836850809,-19.4987006573247,
2.67472014897875));
#240396=CARTESIAN_POINT('Ctrl Pts',(59.7259841596486,-19.4999216825129,
2.67542649668603));
#240397=CARTESIAN_POINT('Ctrl Pts',(59.724772245347,-19.5011176808513,2.67614899656072));
#240398=CARTESIAN_POINT('Ctrl Pts',(59.7244692667716,-19.5014166804359,
2.67632962152939));
#240399=CARTESIAN_POINT('Ctrl Pts',(59.7241655137792,-19.5017141161959,
2.67651125590921));
#240400=CARTESIAN_POINT('Ctrl Pts',(59.7238610051972,-19.5020099819903,
2.67669387767494));
#240401=CARTESIAN_POINT('Ctrl Pts',(59.7229474794513,-19.5028975793736,
2.67724174297214));
#240402=CARTESIAN_POINT('Ctrl Pts',(59.7220271539532,-19.5037710453,2.67779849504718));
#240403=CARTESIAN_POINT('Ctrl Pts',(59.7211005320716,-19.5046302297516,
2.67836353617979));
#240404=CARTESIAN_POINT('Ctrl Pts',(59.7146969999426,-19.510567727398,2.68226832098892));
#240405=CARTESIAN_POINT('Ctrl Pts',(59.7079999120045,-19.5158784513265,
2.68659153751391));
#240406=CARTESIAN_POINT('Ctrl Pts',(59.701118410241,-19.5206092977901,2.69123699486197));
#240407=CARTESIAN_POINT('Ctrl Pts',(59.6976983227542,-19.5229605154963,
2.6935457744122));
#240408=CARTESIAN_POINT('Ctrl Pts',(59.6942320938701,-19.5251683423973,
2.69593478828105));
#240409=CARTESIAN_POINT('Ctrl Pts',(59.6907301905173,-19.5272373629634,
2.6983956526119));
#240410=CARTESIAN_POINT('Ctrl Pts',(59.6830044686628,-19.5318019313693,
2.70382468689016));
#240411=CARTESIAN_POINT('Ctrl Pts',(59.6751122606221,-19.5357011184419,
2.70961155815057));
#240412=CARTESIAN_POINT('Ctrl Pts',(59.6671986827534,-19.5389266512974,
2.71562701361738));
#240413=CARTESIAN_POINT('Ctrl Pts',(59.6643077529624,-19.5401049791256,
2.71782453535829));
#240414=CARTESIAN_POINT('Ctrl Pts',(59.6614137631516,-19.5412013620772,
2.72005051502373));
#240415=CARTESIAN_POINT('Ctrl Pts',(59.6585211429015,-19.5422187365059,
2.72229986760086));
#240416=CARTESIAN_POINT('Ctrl Pts',(59.6488051375687,-19.545635989557,2.7298552048887));
#240417=CARTESIAN_POINT('Ctrl Pts',(59.6390401911867,-19.5481755652416,
2.73770845534541));
#240418=CARTESIAN_POINT('Ctrl Pts',(59.6292970278052,-19.5499445144585,
2.7457670670174));
#240419=CARTESIAN_POINT('Ctrl Pts',(59.6185881370953,-19.5518887991936,
2.75462443585027));
#240420=CARTESIAN_POINT('Ctrl Pts',(59.6079049297392,-19.5529023976132,
2.76373036323189));
#240421=CARTESIAN_POINT('Ctrl Pts',(59.5973174182796,-19.5530800481809,
2.7729966463684));
#240422=CARTESIAN_POINT('Ctrl Pts',(59.5859142147986,-19.5532713854541,
2.78297683033527));
#240423=CARTESIAN_POINT('Ctrl Pts',(59.5746208362127,-19.5524931697979,
2.7931440147898));
#240424=CARTESIAN_POINT('Ctrl Pts',(59.5635130675389,-19.5508078878546,
2.80341452428065));
#240425=CARTESIAN_POINT('Ctrl Pts',(59.5525552912484,-19.549145362908,2.81354634721434));
#240426=CARTESIAN_POINT('Ctrl Pts',(59.5417768065743,-19.546599586876,2.82378004209225));
#240427=CARTESIAN_POINT('Ctrl Pts',(59.5312589135998,-19.5431821162857,
2.83404198860249));
#240428=CARTESIAN_POINT('Ctrl Pts',(56.2594439784241,-18.4801050014181,
2.83404198860249));
#240429=CARTESIAN_POINT('Ctrl Pts',(56.2493782971089,-18.4768344633028,
2.8242212644309));
#240430=CARTESIAN_POINT('Ctrl Pts',(56.239606768123,-18.4727817672086,2.8144281502868));
#240431=CARTESIAN_POINT('Ctrl Pts',(56.2301791400452,-18.4679768367037,
2.80471618166591));
#240432=CARTESIAN_POINT('Ctrl Pts',(56.2210759356566,-18.4633372535447,
2.7953384214656));
#240433=CARTESIAN_POINT('Ctrl Pts',(56.212292281258,-18.4579956735929,2.78603515650626));
#240434=CARTESIAN_POINT('Ctrl Pts',(56.2038917763273,-18.4519372213374,
2.77685887347194));
#240435=CARTESIAN_POINT('Ctrl Pts',(56.1959506682923,-18.4462100865662,
2.76818441217041));
#240436=CARTESIAN_POINT('Ctrl Pts',(56.1883512165513,-18.4398418135305,
2.75962261522113));
#240437=CARTESIAN_POINT('Ctrl Pts',(56.1811768067767,-18.4327901596652,
2.75123537702169));
#240438=CARTESIAN_POINT('Ctrl Pts',(56.1745692957339,-18.4262957047555,
2.74351087134639));
#240439=CARTESIAN_POINT('Ctrl Pts',(56.1683219623547,-18.4192211773454,
2.73593399450374));
#240440=CARTESIAN_POINT('Ctrl Pts',(56.1625328136795,-18.4115142492207,
2.72857657813109));
#240441=CARTESIAN_POINT('Ctrl Pts',(56.1608066064052,-18.4092161988271,
2.72638274508666));
#240442=CARTESIAN_POINT('Ctrl Pts',(56.1591213928277,-18.4068618031994,
2.72420861709758));
#240443=CARTESIAN_POINT('Ctrl Pts',(56.1574804751189,-18.4044493827306,
2.72205663736696));
#240444=CARTESIAN_POINT('Ctrl Pts',(56.1558563235463,-18.4020616112555,
2.71992664556735));
#240445=CARTESIAN_POINT('Ctrl Pts',(56.1542770260205,-18.3996196264074,
2.71782089927853));
#240446=CARTESIAN_POINT('Ctrl Pts',(56.1527473834686,-18.3971247125278,
2.71574387311215));
#240447=CARTESIAN_POINT('Ctrl Pts',(56.152641015117,-18.3969512210959,2.71559944077456));
#240448=CARTESIAN_POINT('Ctrl Pts',(56.1525348749439,-18.3967774746426,
2.71545515216038));
#240449=CARTESIAN_POINT('Ctrl Pts',(56.1524289641635,-18.3966034726917,
2.71531100781699));
#240450=CARTESIAN_POINT('Ctrl Pts',(56.1477854475703,-18.3889745897483,
2.70899119176047));
#240451=CARTESIAN_POINT('Ctrl Pts',(56.1436260014308,-18.3808409394265,
2.70298296066796));
#240452=CARTESIAN_POINT('Ctrl Pts',(56.1400597146376,-18.3722424849449,
2.69736727774089));
#240453=CARTESIAN_POINT('Ctrl Pts',(56.1367353155298,-18.3642272309667,
2.6921324852537));
#240454=CARTESIAN_POINT('Ctrl Pts',(56.1339262909283,-18.3558072700336,
2.68723866185399));
#240455=CARTESIAN_POINT('Ctrl Pts',(56.1317496772149,-18.3470212548454,
2.68278595829485));
#240456=CARTESIAN_POINT('Ctrl Pts',(56.1309534437593,-18.3438072168233,
2.68115710172744));
#240457=CARTESIAN_POINT('Ctrl Pts',(56.1302421351292,-18.3405443147871,
2.67958763637763));
#240458=CARTESIAN_POINT('Ctrl Pts',(56.1296225724749,-18.3372349828457,
2.67808378645331));
#240459=CARTESIAN_POINT('Ctrl Pts',(56.1294735883543,-18.3364391990687,
2.67772216078566));
#240460=CARTESIAN_POINT('Ctrl Pts',(56.1293301519983,-18.3356401993818,
2.67736403603529));
#240461=CARTESIAN_POINT('Ctrl Pts',(56.1291923454417,-18.3348380918578,
2.67700956934445));
#240462=CARTESIAN_POINT('Ctrl Pts',(56.1290588453401,-18.3340610501939,
2.6766661797377));
#240463=CARTESIAN_POINT('Ctrl Pts',(56.128930628665,-18.3332810919213,2.67632622314085));
#240464=CARTESIAN_POINT('Ctrl Pts',(56.128807768806,-18.3324983188923,2.67598984158739));
#240465=CARTESIAN_POINT('Ctrl Pts',(56.127461697065,-18.3239221357301,2.67230439292194));
#240466=CARTESIAN_POINT('Ctrl Pts',(56.1267581593462,-18.3150023767869,
2.66904964539953));
#240467=CARTESIAN_POINT('Ctrl Pts',(56.1267895336333,-18.3059033598546,
2.66640203566706));
#240468=CARTESIAN_POINT('Ctrl Pts',(56.1268025454853,-18.3021297263199,
2.66530399299415));
#240469=CARTESIAN_POINT('Ctrl Pts',(56.12694160832,-18.2983254984041,2.66430995142229));
#240470=CARTESIAN_POINT('Ctrl Pts',(56.1272115877757,-18.2945030089048,
2.66343053473326));
#240471=CARTESIAN_POINT('Ctrl Pts',(56.1276720658711,-18.2879833547325,
2.6619305979285));
#240472=CARTESIAN_POINT('Ctrl Pts',(56.1285150529072,-18.2814124323565,
2.66076519817093));
#240473=CARTESIAN_POINT('Ctrl Pts',(56.1297657127889,-18.2748585331705,
2.65997805604425));
#240474=CARTESIAN_POINT('Ctrl Pts',(56.1303910427297,-18.2715815835775,
2.65958448498091));
#240475=CARTESIAN_POINT('Ctrl Pts',(56.131119686293,-18.2683092720859,2.65928526260727));
#240476=CARTESIAN_POINT('Ctrl Pts',(56.1319548233213,-18.2650501911666,
2.6590846397129));
#240477=CARTESIAN_POINT('Ctrl Pts',(56.1327899603496,-18.2617911102473,
2.65888401681852));
#240478=CARTESIAN_POINT('Ctrl Pts',(56.1337315613411,-18.2585452947506,
2.6587819886025));
#240479=CARTESIAN_POINT('Ctrl Pts',(56.1347810195644,-18.255320281274,2.6587819886025));
#240480=CARTESIAN_POINT('Origin',(56.9937374973465,-12.0988124084931,2.83404198860254));
#240481=CARTESIAN_POINT('Ctrl Pts',(61.3271735965895,-12.8407372733088,
2.83404198860254));
#240482=CARTESIAN_POINT('Ctrl Pts',(61.3375520649561,-12.8429432848602,
2.82419652440068));
#240483=CARTESIAN_POINT('Ctrl Pts',(61.3477256769083,-12.8459616464934,
2.81438790575667));
#240484=CARTESIAN_POINT('Ctrl Pts',(61.3576417279027,-12.8497656413952,
2.80466781256936));
#240485=CARTESIAN_POINT('Ctrl Pts',(61.367235566286,-12.853446029114,2.79526356453127));
#240486=CARTESIAN_POINT('Ctrl Pts',(61.3765894879233,-12.8578623484984,
2.78594102496298));
#240487=CARTESIAN_POINT('Ctrl Pts',(61.3856422574858,-12.8630345798908,
2.7767510908886));
#240488=CARTESIAN_POINT('Ctrl Pts',(61.3942056200545,-12.8679271923004,
2.7680579791378));
#240489=CARTESIAN_POINT('Ctrl Pts',(61.4025003187112,-12.873496651755,2.75948271210275));
#240490=CARTESIAN_POINT('Ctrl Pts',(61.4104485116933,-12.8797929832512,
2.75108575573353));
#240491=CARTESIAN_POINT('Ctrl Pts',(61.4177693722577,-12.8855923599215,
2.74335155163415));
#240492=CARTESIAN_POINT('Ctrl Pts',(61.4247966697184,-12.8920087864942,
2.73576818686103));
#240493=CARTESIAN_POINT('Ctrl Pts',(61.4314390014603,-12.8991043342864,
2.7284062616067));
#240494=CARTESIAN_POINT('Ctrl Pts',(61.4333656894049,-12.9011624829791,
2.7262708469379));
#240495=CARTESIAN_POINT('Ctrl Pts',(61.4352597571378,-12.9032779088702,
2.72415424587572));
#240496=CARTESIAN_POINT('Ctrl Pts',(61.437118361331,-12.9054524645835,2.72205867173248));
#240497=CARTESIAN_POINT('Ctrl Pts',(61.4391332077734,-12.9078098227873,
2.71978693462851));
#240498=CARTESIAN_POINT('Ctrl Pts',(61.4411043938525,-12.9102326900439,
2.71754411340752));
#240499=CARTESIAN_POINT('Ctrl Pts',(61.4430281531013,-12.9127224163019,
2.71533341844249));
#240500=CARTESIAN_POINT('Ctrl Pts',(61.4483079254551,-12.9195554895536,
2.70926614876396));
#240501=CARTESIAN_POINT('Ctrl Pts',(61.4531896374537,-12.9269097705822,
2.70347381860413));
#240502=CARTESIAN_POINT('Ctrl Pts',(61.4575800373535,-12.9347398820021,
2.698049141714));
#240503=CARTESIAN_POINT('Ctrl Pts',(61.4615970149013,-12.9419040088445,
2.69308585687216));
#240504=CARTESIAN_POINT('Ctrl Pts',(61.4651913207947,-12.9494643722274,
2.68842799053203));
#240505=CARTESIAN_POINT('Ctrl Pts',(61.4682744840803,-12.9574154517094,
2.68414767054239));
#240506=CARTESIAN_POINT('Ctrl Pts',(61.4697889238146,-12.9613209959778,
2.68204519134568));
#240507=CARTESIAN_POINT('Ctrl Pts',(61.4711795284101,-12.9653208118544,
2.68003431778513));
#240508=CARTESIAN_POINT('Ctrl Pts',(61.4724324898306,-12.9694138336341,
2.67812693945258));
#240509=CARTESIAN_POINT('Ctrl Pts',(61.4726702270561,-12.9701904446502,
2.6777650329921));
#240510=CARTESIAN_POINT('Ctrl Pts',(61.4729027677276,-12.9709708853383,
2.6774065963993));
#240511=CARTESIAN_POINT('Ctrl Pts',(61.4731300138564,-12.9717550556838,
2.67705178968862));
#240512=CARTESIAN_POINT('Ctrl Pts',(61.4733501585437,-12.9725147207061,
2.67670807068764));
#240513=CARTESIAN_POINT('Ctrl Pts',(61.4735653344327,-12.9732778858998,
2.67636775825272));
#240514=CARTESIAN_POINT('Ctrl Pts',(61.4737754532575,-12.9740444565827,
2.67603099699262));
#240515=CARTESIAN_POINT('Ctrl Pts',(61.4760652849148,-12.982398385929,2.67236104217127));
#240516=CARTESIAN_POINT('Ctrl Pts',(61.4777556486133,-12.9911623597375,
2.66911440541467));
#240517=CARTESIAN_POINT('Ctrl Pts',(61.4787331403172,-13.0001833616597,
2.66646778189621));
#240518=CARTESIAN_POINT('Ctrl Pts',(61.4791459411336,-13.0039929867889,
2.66535009634971));
#240519=CARTESIAN_POINT('Ctrl Pts',(61.4794319383913,-13.0078481668559,
2.66433897912346));
#240520=CARTESIAN_POINT('Ctrl Pts',(61.4795843394719,-13.0117365408422,
2.66344564884798));
#240521=CARTESIAN_POINT('Ctrl Pts',(61.4798409790836,-13.0182844654755,
2.66194130298591));
#240522=CARTESIAN_POINT('Ctrl Pts',(61.4797168922659,-13.0249248230166,
2.66077206705425));
#240523=CARTESIAN_POINT('Ctrl Pts',(61.4791780149469,-13.0315916763168,
2.65998225155719));
#240524=CARTESIAN_POINT('Ctrl Pts',(61.4790432956172,-13.0332583896419,
2.65978479768293));
#240525=CARTESIAN_POINT('Ctrl Pts',(61.4788824204063,-13.0349267248708,
2.65961098966627));
#240526=CARTESIAN_POINT('Ctrl Pts',(61.4786945538951,-13.0365955947395,
2.65946139030506));
#240527=CARTESIAN_POINT('Ctrl Pts',(61.4784127541283,-13.0390988995425,
2.65923699126325));
#240528=CARTESIAN_POINT('Ctrl Pts',(61.4780702140294,-13.0416033892092,
2.65906707562446));
#240529=CARTESIAN_POINT('Ctrl Pts',(61.4776657592308,-13.044105725102,2.65895332562924));
#240530=CARTESIAN_POINT('Ctrl Pts',(61.4772613044323,-13.0466080609949,
2.65883957563402));
#240531=CARTESIAN_POINT('Ctrl Pts',(61.4767949453823,-13.0491082380619,
2.65878198860253));
#240532=CARTESIAN_POINT('Ctrl Pts',(61.4762657165317,-13.0516031943519,
2.65878198860253));
#240533=CARTESIAN_POINT('Ctrl Pts',(57.7418065394567,-12.2578193919758,
2.65878198860254));
#240534=CARTESIAN_POINT('Ctrl Pts',(57.7435970583545,-12.2493771807069,
2.65878198860254));
#240535=CARTESIAN_POINT('Ctrl Pts',(57.7460689269801,-12.2411559442244,
2.65945335517842));
#240536=CARTESIAN_POINT('Ctrl Pts',(57.7491141258102,-12.2332613533226,
2.6607256122658));
#240537=CARTESIAN_POINT('Ctrl Pts',(57.7510810117991,-12.2281622576314,
2.6615473598032));
#240538=CARTESIAN_POINT('Ctrl Pts',(57.7532862127604,-12.2231990866879,
2.66261895766868));
#240539=CARTESIAN_POINT('Ctrl Pts',(57.755693185958,-12.2183955094111,2.66391429251019));
#240540=CARTESIAN_POINT('Ctrl Pts',(57.7588834910513,-12.2120286428969,
2.66563118464116));
#240541=CARTESIAN_POINT('Ctrl Pts',(57.7624328173676,-12.2059457447509,
2.66774105138691));
#240542=CARTESIAN_POINT('Ctrl Pts',(57.766268204371,-12.2001996238492,2.67016894181742));
#240543=CARTESIAN_POINT('Ctrl Pts',(57.7681858978727,-12.1973265633984,
2.67138288703268));
#240544=CARTESIAN_POINT('Ctrl Pts',(57.7701751462711,-12.1945375019629,
2.67267613167544));
#240545=CARTESIAN_POINT('Ctrl Pts',(57.7722271161469,-12.1918376559065,
2.67403835432546));
#240546=CARTESIAN_POINT('Ctrl Pts',(57.7732531010848,-12.1904877328782,
2.67471946565047));
#240547=CARTESIAN_POINT('Ctrl Pts',(57.7742947697605,-12.1891600976126,
2.67541781389516));
#240548=CARTESIAN_POINT('Ctrl Pts',(57.7753510390206,-12.1878553011589,
2.67613207244162));
#240549=CARTESIAN_POINT('Ctrl Pts',(57.7756151063356,-12.1875291020455,
2.67631063707824));
#240550=CARTESIAN_POINT('Ctrl Pts',(57.7758800862579,-12.1872043300155,
2.67649019601839));
#240551=CARTESIAN_POINT('Ctrl Pts',(57.7761459620051,-12.1868809929889,
2.6766707283665));
#240552=CARTESIAN_POINT('Ctrl Pts',(57.7769435892466,-12.1859109819089,
2.67721232541084));
#240553=CARTESIAN_POINT('Ctrl Pts',(57.7777492785675,-12.1849538875681,
2.6777626834004));
#240554=CARTESIAN_POINT('Ctrl Pts',(57.7785625799464,-12.1840099085249,
2.67832123541509));
#240555=CARTESIAN_POINT('Ctrl Pts',(57.7842913698424,-12.1773606420342,
2.68225560368432));
#240556=CARTESIAN_POINT('Ctrl Pts',(57.7903843352497,-12.1713100228958,
2.68661792998868));
#240557=CARTESIAN_POINT('Ctrl Pts',(57.7967264334405,-12.1658251565852,
2.69130986622549));
#240558=CARTESIAN_POINT('Ctrl Pts',(57.7998023442099,-12.1631650023514,
2.69358545023032));
#240559=CARTESIAN_POINT('Ctrl Pts',(57.8029374300325,-12.1606380046005,
2.69593918853454));
#240560=CARTESIAN_POINT('Ctrl Pts',(57.806121336008,-12.1582411305889,2.69836306235468));
#240561=CARTESIAN_POINT('Ctrl Pts',(57.8109956736034,-12.1545716839421,
2.70207384382201));
#240562=CARTESIAN_POINT('Ctrl Pts',(57.8159810988991,-12.1512083732199,
2.705947608142));
#240563=CARTESIAN_POINT('Ctrl Pts',(57.8210315314442,-12.1481495009378,
2.7099519634568));
#240564=CARTESIAN_POINT('Ctrl Pts',(57.8233769784456,-12.1467289448255,
2.71181160678078));
#240565=CARTESIAN_POINT('Ctrl Pts',(57.8257362497573,-12.1453738842977,
2.71369962772071));
#240566=CARTESIAN_POINT('Ctrl Pts',(57.828105124615,-12.1440853170061,2.71561183138634));
#240567=CARTESIAN_POINT('Ctrl Pts',(57.828286689539,-12.1439865534004,2.71575839426285));
#240568=CARTESIAN_POINT('Ctrl Pts',(57.82846830734,-12.1438881466788,2.71590508903182));
#240569=CARTESIAN_POINT('Ctrl Pts',(57.8286499766612,-12.1437900963012,
2.71605191409884));
#240570=CARTESIAN_POINT('Ctrl Pts',(57.831201882908,-12.1424127841089,2.71811436362725));
#240571=CARTESIAN_POINT('Ctrl Pts',(57.8337650648328,-12.1411075562946,
2.72020091026932));
#240572=CARTESIAN_POINT('Ctrl Pts',(57.8363340693142,-12.1398727334212,
2.72230624862154));
#240573=CARTESIAN_POINT('Ctrl Pts',(57.845546062502,-12.1354448782032,2.72985561753057));
#240574=CARTESIAN_POINT('Ctrl Pts',(57.85490328748,-12.1318862976806,2.73770089914263));
#240575=CARTESIAN_POINT('Ctrl Pts',(57.8643241951528,-12.1290968783778,
2.74574823346985));
#240576=CARTESIAN_POINT('Ctrl Pts',(57.8746768262713,-12.126031586786,2.75459144546915));
#240577=CARTESIAN_POINT('Ctrl Pts',(57.8851069357357,-12.1238947812336,
2.7636791175414));
#240578=CARTESIAN_POINT('Ctrl Pts',(57.8955352825119,-12.1225979458242,
2.77292162564575));
#240579=CARTESIAN_POINT('Ctrl Pts',(57.9067952798725,-12.1211976890434,
2.78290121484571));
#240580=CARTESIAN_POINT('Ctrl Pts',(57.9180543443219,-12.1207764137879,
2.7930622950002));
#240581=CARTESIAN_POINT('Ctrl Pts',(57.9292311407257,-12.121277094833,2.80331916685078));
#240582=CARTESIAN_POINT('Ctrl Pts',(57.9403141752922,-12.1217735756786,
2.81348999408573));
#240583=CARTESIAN_POINT('Ctrl Pts',(57.9513177099566,-12.1231769533527,
2.82375635966811));
#240584=CARTESIAN_POINT('Ctrl Pts',(57.9621601888122,-12.1254815933782,
2.83404198860254));
#240585=CARTESIAN_POINT('Origin',(-0.00316857416806234,-0.0149069694349926,
2.83404198860262));
#240586=CARTESIAN_POINT('Ctrl Pts',(61.4699285681956,-13.0814171332223,
2.65878198860253));
#240587=CARTESIAN_POINT('Ctrl Pts',(61.468139314985,-13.089817630984,2.65878198860253));
#240588=CARTESIAN_POINT('Ctrl Pts',(61.4656642256291,-13.0979940118835,
2.65944603041842));
#240589=CARTESIAN_POINT('Ctrl Pts',(61.4626133761159,-13.1058430982603,
2.66070439264062));
#240590=CARTESIAN_POINT('Ctrl Pts',(61.4606640285136,-13.1108582907967,
2.66150842619587));
#240591=CARTESIAN_POINT('Ctrl Pts',(61.4584804838816,-13.1157402208604,
2.66255428265359));
#240592=CARTESIAN_POINT('Ctrl Pts',(61.4560986543958,-13.1204666715196,
2.66381699700645));
#240593=CARTESIAN_POINT('Ctrl Pts',(61.4528479350655,-13.1269173282996,
2.66554034873245));
#240594=CARTESIAN_POINT('Ctrl Pts',(61.4492231901486,-13.1330744923996,
2.66766759643949));
#240595=CARTESIAN_POINT('Ctrl Pts',(61.4453029499363,-13.1388835356727,
2.67012012783125));
#240596=CARTESIAN_POINT('Ctrl Pts',(61.4433428298301,-13.1417880573093,
2.67134639352713));
#240597=CARTESIAN_POINT('Ctrl Pts',(61.4413087943566,-13.1446057534052,
2.67265375584989));
#240598=CARTESIAN_POINT('Ctrl Pts',(61.4392103574001,-13.1473312571582,
2.67403135126917));
#240599=CARTESIAN_POINT('Ctrl Pts',(61.4381611389218,-13.1486940090348,
2.67472014897881));
#240600=CARTESIAN_POINT('Ctrl Pts',(61.4370958165018,-13.1500337298693,
2.6754264966861));
#240601=CARTESIAN_POINT('Ctrl Pts',(61.436015557062,-13.1513498559433,2.67614899656079));
#240602=CARTESIAN_POINT('Ctrl Pts',(61.435745492202,-13.1516788874618,2.67632962152946));
#240603=CARTESIAN_POINT('Ctrl Pts',(61.4354744937032,-13.152006444671,2.67651125590927));
#240604=CARTESIAN_POINT('Ctrl Pts',(61.435202579648,-13.1523325194958,2.67669387767501));
#240605=CARTESIAN_POINT('Ctrl Pts',(61.4343868374822,-13.1533107439701,
2.67724174297221));
#240606=CARTESIAN_POINT('Ctrl Pts',(61.4335628556744,-13.1542756251688,
2.67779849504725));
#240607=CARTESIAN_POINT('Ctrl Pts',(61.4327311191548,-13.1552269612794,
2.67836353617986));
#240608=CARTESIAN_POINT('Ctrl Pts',(61.4269833037496,-13.1618012840651,
2.68226832098887));
#240609=CARTESIAN_POINT('Ctrl Pts',(61.4208780249712,-13.1677829516027,
2.68659153751371));
#240610=CARTESIAN_POINT('Ctrl Pts',(61.4145287289055,-13.1732071947985,
2.6912369948616));
#240611=CARTESIAN_POINT('Ctrl Pts',(61.4113731461892,-13.1759030287776,
2.69354577441197));
#240612=CARTESIAN_POINT('Ctrl Pts',(61.4081566864226,-13.1784610805506,
2.69593478828095));
#240613=CARTESIAN_POINT('Ctrl Pts',(61.4048902384028,-13.1808848153817,
2.69839565261195));
#240614=CARTESIAN_POINT('Ctrl Pts',(61.3976839661819,-13.1862319364373,
2.7038246868902));
#240615=CARTESIAN_POINT('Ctrl Pts',(61.3902425685154,-13.1909347237334,
2.70961155815062));
#240616=CARTESIAN_POINT('Ctrl Pts',(61.3827095020468,-13.194969780916,2.71562701361742));
#240617=CARTESIAN_POINT('Ctrl Pts',(61.3799575778688,-13.1964438381895,
2.71782453535832));
#240618=CARTESIAN_POINT('Ctrl Pts',(61.377194044862,-13.1978367193482,2.72005051502376));
#240619=CARTESIAN_POINT('Ctrl Pts',(61.374423615274,-13.1991508816429,2.7222998676009));
#240620=CARTESIAN_POINT('Ctrl Pts',(61.3651180354455,-13.2035650137305,
2.72985520488838));
#240621=CARTESIAN_POINT('Ctrl Pts',(61.3556720404057,-13.2071113921929,
2.73770845534476));
#240622=CARTESIAN_POINT('Ctrl Pts',(61.3461671566366,-13.2098890888164,
2.74576706701642));
#240623=CARTESIAN_POINT('Ctrl Pts',(61.3357201634468,-13.2129421064455,
2.75462443584889));
#240624=CARTESIAN_POINT('Ctrl Pts',(61.3252014297043,-13.2150668515146,
2.76373036323012));
#240625=CARTESIAN_POINT('Ctrl Pts',(61.3146904872818,-13.2163502251968,
2.77299664636617));
#240626=CARTESIAN_POINT('Ctrl Pts',(61.3033697519348,-13.2177324736407,
2.78297683033235));
#240627=CARTESIAN_POINT('Ctrl Pts',(61.2920568939728,-13.2181390006403,
2.7931440147861));
#240628=CARTESIAN_POINT('Ctrl Pts',(61.280833814887,-13.2176240288379,2.80341452427607));
#240629=CARTESIAN_POINT('Ctrl Pts',(61.2697622852616,-13.2171160108936,
2.8135463472114));
#240630=CARTESIAN_POINT('Ctrl Pts',(61.2587767401957,-13.2157108393283,
2.82378004209088));
#240631=CARTESIAN_POINT('Ctrl Pts',(61.2479592423879,-13.2134115091884,
2.83404198860253));
#240632=CARTESIAN_POINT('Ctrl Pts',(57.8829458346107,-12.4981558292578,
2.83404198860253));
#240633=CARTESIAN_POINT('Ctrl Pts',(57.8725934298275,-12.4959553576921,
2.82422126443084));
#240634=CARTESIAN_POINT('Ctrl Pts',(57.8624518082049,-12.4929462655998,
2.81442815028665));
#240635=CARTESIAN_POINT('Ctrl Pts',(57.8525735736582,-12.4891531124821,
2.80471618166567));
#240636=CARTESIAN_POINT('Ctrl Pts',(57.8430352690779,-12.4854904894106,
2.79533842146522));
#240637=CARTESIAN_POINT('Ctrl Pts',(57.8337413853132,-12.4810963130887,
2.78603515650575));
#240638=CARTESIAN_POINT('Ctrl Pts',(57.8247536185233,-12.4759491415396,
2.77685887347131));
#240639=CARTESIAN_POINT('Ctrl Pts',(57.8162573641123,-12.4710834524312,
2.76818441216959));
#240640=CARTESIAN_POINT('Ctrl Pts',(57.8080338771688,-12.4655444244735,
2.75962261522012));
#240641=CARTESIAN_POINT('Ctrl Pts',(57.8001616710194,-12.4592813303343,
2.7512353770205));
#240642=CARTESIAN_POINT('Ctrl Pts',(57.7929115012218,-12.4535131257032,
2.74351087134493));
#240643=CARTESIAN_POINT('Ctrl Pts',(57.7859589019098,-12.4471303774518,
2.73593399450203));
#240644=CARTESIAN_POINT('Ctrl Pts',(57.7793958734432,-12.4400707994999,
2.72857657812914));
#240645=CARTESIAN_POINT('Ctrl Pts',(57.7774389108374,-12.4379657758611,
2.72638274508539));
#240646=CARTESIAN_POINT('Ctrl Pts',(57.7755168276799,-12.4358004306452,
2.72420861709697));
#240647=CARTESIAN_POINT('Ctrl Pts',(57.7736327324862,-12.4335727482752,
2.722056637367));
#240648=CARTESIAN_POINT('Ctrl Pts',(57.7717678881029,-12.4313678273301,
2.71992664556739));
#240649=CARTESIAN_POINT('Ctrl Pts',(57.7699419852107,-12.429104301474,2.71782089927857));
#240650=CARTESIAN_POINT('Ctrl Pts',(57.7681599326869,-12.4267829461789,
2.71574387311219));
#240651=CARTESIAN_POINT('Ctrl Pts',(57.7680360122396,-12.4266215236716,
2.7155994407746));
#240652=CARTESIAN_POINT('Ctrl Pts',(57.7679122920636,-12.4264598236887,
2.71545515216042));
#240653=CARTESIAN_POINT('Ctrl Pts',(57.7677887733171,-12.4262978456299,
2.71531100781703));
#240654=CARTESIAN_POINT('Ctrl Pts',(57.7623732589831,-12.419196134159,2.70899119176049));
#240655=CARTESIAN_POINT('Ctrl Pts',(57.7573864007558,-12.4115418213378,
2.70298296066798));
#240656=CARTESIAN_POINT('Ctrl Pts',(57.7529408672214,-12.4033632485675,
2.6973672777409));
#240657=CARTESIAN_POINT('Ctrl Pts',(57.7487968573387,-12.3957393973193,
2.69213248525374));
#240658=CARTESIAN_POINT('Ctrl Pts',(57.7451230952908,-12.3876591848381,
2.68723866185406));
#240659=CARTESIAN_POINT('Ctrl Pts',(57.7420400166292,-12.3791488184471,
2.68278595829494));
#240660=CARTESIAN_POINT('Ctrl Pts',(57.7409121865684,-12.376035616321,2.68115710172751));
#240661=CARTESIAN_POINT('Ctrl Pts',(57.7398637084259,-12.3728649408015,
2.67958763637769));
#240662=CARTESIAN_POINT('Ctrl Pts',(57.7389016204183,-12.3696384996589,
2.67808378645336));
#240663=CARTESIAN_POINT('Ctrl Pts',(57.738670270393,-12.3688626483499,2.67772216078571));
#240664=CARTESIAN_POINT('Ctrl Pts',(57.7384441015869,-12.3680830188488,
2.67736403603534));
#240665=CARTESIAN_POINT('Ctrl Pts',(57.7382232068822,-12.3672997100613,
2.6770095693445));
#240666=CARTESIAN_POINT('Ctrl Pts',(57.7380092151371,-12.3665408796734,
2.67666617973775));
#240667=CARTESIAN_POINT('Ctrl Pts',(57.7378001730067,-12.3657785963858,
2.6763262231409));
#240668=CARTESIAN_POINT('Ctrl Pts',(57.737596164125,-12.3650129538217,2.67598984158744));
#240669=CARTESIAN_POINT('Ctrl Pts',(57.7353610110592,-12.3566244546987,
2.67230439292203));
#240670=CARTESIAN_POINT('Ctrl Pts',(57.7337289586986,-12.3478270988451,
2.66904964539965));
#240671=CARTESIAN_POINT('Ctrl Pts',(57.732809054857,-12.3387746477736,2.66640203566719));
#240672=CARTESIAN_POINT('Ctrl Pts',(57.7324275433144,-12.3350203264893,
2.66530399299425));
#240673=CARTESIAN_POINT('Ctrl Pts',(57.7321681942504,-12.3312224025075,
2.66430995142236));
#240674=CARTESIAN_POINT('Ctrl Pts',(57.7320371357771,-12.327392632468,2.66343053473331));
#240675=CARTESIAN_POINT('Ctrl Pts',(57.7318136018937,-12.3208605605757,
2.66193059792855));
#240676=CARTESIAN_POINT('Ctrl Pts',(57.7319651225404,-12.3142375182605,
2.66076519817097));
#240677=CARTESIAN_POINT('Ctrl Pts',(57.7325238621659,-12.3075887924645,
2.6599780560443));
#240678=CARTESIAN_POINT('Ctrl Pts',(57.7328032319787,-12.3042644295665,
2.65958448498096));
#240679=CARTESIAN_POINT('Ctrl Pts',(57.7331858342648,-12.3009338801477,
2.65928526260732));
#240680=CARTESIAN_POINT('Ctrl Pts',(57.7336757296049,-12.2976053572245,
2.65908463971294));
#240681=CARTESIAN_POINT('Ctrl Pts',(57.7341656249451,-12.2942768343013,
2.65888401681856));
#240682=CARTESIAN_POINT('Ctrl Pts',(57.7347627876419,-12.2909503756169,
2.65878198860254));
#240683=CARTESIAN_POINT('Ctrl Pts',(57.7354693911206,-12.2876333308462,
2.65878198860254));
#240684=CARTESIAN_POINT('Origin',(57.9461901084063,-6.07506605172202,2.83404198860258));
#240685=CARTESIAN_POINT('Ctrl Pts',(62.333439457262,-6.35995915837698,2.83404198860258));
#240686=CARTESIAN_POINT('Ctrl Pts',(62.3439916622904,-6.36106823981685,
2.82419652440068));
#240687=CARTESIAN_POINT('Ctrl Pts',(62.354425046835,-6.36300663452592,2.81438790575664));
#240688=CARTESIAN_POINT('Ctrl Pts',(62.3646844024059,-6.36575328117349,
2.8046678125693));
#240689=CARTESIAN_POINT('Ctrl Pts',(62.3746103900112,-6.36841067816022,
2.7952635645312));
#240690=CARTESIAN_POINT('Ctrl Pts',(62.3843747009655,-6.37182505343072,
2.7859410249629));
#240691=CARTESIAN_POINT('Ctrl Pts',(62.3939185239083,-6.37602267870771,
2.77675109088853));
#240692=CARTESIAN_POINT('Ctrl Pts',(62.4029463927375,-6.37999337374486,
2.76805797913774));
#240693=CARTESIAN_POINT('Ctrl Pts',(62.4117778192051,-6.38466529101398,
2.75948271210271));
#240694=CARTESIAN_POINT('Ctrl Pts',(62.4203406170099,-6.39009631814929,
2.7510857557335));
#240695=CARTESIAN_POINT('Ctrl Pts',(62.4282275730653,-6.39509868692276,
2.74335155163415));
#240696=CARTESIAN_POINT('Ctrl Pts',(62.4358870734646,-6.4007454110349,2.73576818686106));
#240697=CARTESIAN_POINT('Ctrl Pts',(62.443234704525,-6.4071077759443,2.72840626160674));
#240698=CARTESIAN_POINT('Ctrl Pts',(62.4453659729915,-6.40895325615313,
2.72627084693796));
#240699=CARTESIAN_POINT('Ctrl Pts',(62.4474707870407,-6.41085910953041,
2.72415424587578));
#240700=CARTESIAN_POINT('Ctrl Pts',(62.4495465125726,-6.41282747575978,
2.72205867173254));
#240701=CARTESIAN_POINT('Ctrl Pts',(62.4517967325057,-6.41496131130642,
2.71978693462857));
#240702=CARTESIAN_POINT('Ctrl Pts',(62.4540103788123,-6.41716486079098,
2.71754411340758));
#240703=CARTESIAN_POINT('Ctrl Pts',(62.4561838467663,-6.41943986047008,
2.71533341844254));
#240704=CARTESIAN_POINT('Ctrl Pts',(62.4621489466212,-6.42568361494097,
2.70926614876401));
#240705=CARTESIAN_POINT('Ctrl Pts',(62.467772647785,-6.43248733059531,2.70347381860418));
#240706=CARTESIAN_POINT('Ctrl Pts',(62.4729574661287,-6.43981562609089,
2.69804914171404));
#240707=CARTESIAN_POINT('Ctrl Pts',(62.4777012934231,-6.44652061860733,
2.69308585687183));
#240708=CARTESIAN_POINT('Ctrl Pts',(62.4820661824991,-6.45366385825755,
2.68842799053136));
#240709=CARTESIAN_POINT('Ctrl Pts',(62.4859635700134,-6.46124910257467,
2.68414767054146));
#240710=CARTESIAN_POINT('Ctrl Pts',(62.4878779540287,-6.46497494980425,
2.6820451913451));
#240711=CARTESIAN_POINT('Ctrl Pts',(62.4896790353534,-6.46880749650892,
2.68003431778487));
#240712=CARTESIAN_POINT('Ctrl Pts',(62.4913529701965,-6.47274712615468,
2.67812693945262));
#240713=CARTESIAN_POINT('Ctrl Pts',(62.4916705830287,-6.47349463250756,
2.67776503299213));
#240714=CARTESIAN_POINT('Ctrl Pts',(62.491983428084,-6.47424649074084,2.67740659639934));
#240715=CARTESIAN_POINT('Ctrl Pts',(62.4922913974558,-6.47500261163056,
2.67705178968865));
#240716=CARTESIAN_POINT('Ctrl Pts',(62.4925897427849,-6.47573510374248,
2.67670807068768));
#240717=CARTESIAN_POINT('Ctrl Pts',(62.4928835124027,-6.47647159623243,
2.67636775825275));
#240718=CARTESIAN_POINT('Ctrl Pts',(62.4931726086302,-6.47721200416302,
2.67603099699265));
#240719=CARTESIAN_POINT('Ctrl Pts',(62.4963231197466,-6.4852808172255,2.67236104217154));
#240720=CARTESIAN_POINT('Ctrl Pts',(62.4989203081701,-6.4938200899481,2.66911440541513));
#240721=CARTESIAN_POINT('Ctrl Pts',(62.5008353965402,-6.50268949817166,
2.66646778189676));
#240722=CARTESIAN_POINT('Ctrl Pts',(62.5016441502512,-6.50643510434138,
2.66535009635005));
#240723=CARTESIAN_POINT('Ctrl Pts',(62.502331556834,-6.5102392704753,2.66433897912363));
#240724=CARTESIAN_POINT('Ctrl Pts',(62.5028895688031,-6.51409041329186,
2.66344564884803));
#240725=CARTESIAN_POINT('Ctrl Pts',(62.5038292470156,-6.52057564156468,
2.66194130298595));
#240726=CARTESIAN_POINT('Ctrl Pts',(62.5043999463278,-6.5271925931368,2.66077206705429));
#240727=CARTESIAN_POINT('Ctrl Pts',(62.5045608969644,-6.53387925273503,
2.65998225155723));
#240728=CARTESIAN_POINT('Ctrl Pts',(62.5046011346236,-6.53555091763458,
2.65978479768296));
#240729=CARTESIAN_POINT('Ctrl Pts',(62.5046155292217,-6.53722692958711,
2.65961098966631));
#240730=CARTESIAN_POINT('Ctrl Pts',(62.5046031362658,-6.53890629460977,
2.6594613903051));
#240731=CARTESIAN_POINT('Ctrl Pts',(62.5045845468319,-6.54142534214377,
2.65923699126329));
#240732=CARTESIAN_POINT('Ctrl Pts',(62.5045056736598,-6.54395191714411,
2.6590670756245));
#240733=CARTESIAN_POINT('Ctrl Pts',(62.5043649998326,-6.54648282201769,
2.65895332562928));
#240734=CARTESIAN_POINT('Ctrl Pts',(62.5042243260054,-6.54901372689127,
2.65883957563406));
#240735=CARTESIAN_POINT('Ctrl Pts',(62.5040218613862,-6.55154895552156,
2.65878198860258));
#240736=CARTESIAN_POINT('Ctrl Pts',(62.5037563256536,-6.55408556365842,
2.65878198860258));
#240737=CARTESIAN_POINT('Ctrl Pts',(58.7067819056644,-6.15500747092217,
2.65878198860258));
#240738=CARTESIAN_POINT('Ctrl Pts',(58.7076801645418,-6.14642434678064,
2.65878198860258));
#240739=CARTESIAN_POINT('Ctrl Pts',(58.7092791387969,-6.13798976646243,
2.65945335517854));
#240740=CARTESIAN_POINT('Ctrl Pts',(58.7114824462542,-6.12982011300116,
2.66072561226605));
#240741=CARTESIAN_POINT('Ctrl Pts',(58.7129055567992,-6.12454335512034,
2.66154735980342));
#240742=CARTESIAN_POINT('Ctrl Pts',(58.7145798848071,-6.1193768666793,2.66261895766884));
#240743=CARTESIAN_POINT('Ctrl Pts',(58.7164715618025,-6.11434800669237,
2.66391429251023));
#240744=CARTESIAN_POINT('Ctrl Pts',(58.7189788712982,-6.10768254085036,
2.6656311846412));
#240745=CARTESIAN_POINT('Ctrl Pts',(58.7218729180382,-6.10126195983141,
2.66774105138695));
#240746=CARTESIAN_POINT('Ctrl Pts',(58.7250866612027,-6.09514640967174,
2.67016894181746));
#240747=CARTESIAN_POINT('Ctrl Pts',(58.7266935327849,-6.09208863459191,
2.67138288703272));
#240748=CARTESIAN_POINT('Ctrl Pts',(58.7283803475667,-6.08910691884873,
2.67267613167548));
#240749=CARTESIAN_POINT('Ctrl Pts',(58.7301388657774,-6.08620737357365,
2.6740383543255));
#240750=CARTESIAN_POINT('Ctrl Pts',(58.7310181248828,-6.08475760093612,
2.67471946565051));
#240751=CARTESIAN_POINT('Ctrl Pts',(58.7319153115143,-6.08332835456944,
2.6754178138952));
#240752=CARTESIAN_POINT('Ctrl Pts',(58.7328294060528,-6.08192029572471,
2.67613207244166));
#240753=CARTESIAN_POINT('Ctrl Pts',(58.7330579296874,-6.08156828101352,
2.67631063707827));
#240754=CARTESIAN_POINT('Ctrl Pts',(58.7332875101007,-6.08121759017468,
2.67649019601842));
#240755=CARTESIAN_POINT('Ctrl Pts',(58.7335181314302,-6.08086823283881,
2.67667072836654));
#240756=CARTESIAN_POINT('Ctrl Pts',(58.7342099954187,-6.0798201608312,2.67721232541088));
#240757=CARTESIAN_POINT('Ctrl Pts',(58.7349112274886,-6.07878409208678,
2.67776268340044));
#240758=CARTESIAN_POINT('Ctrl Pts',(58.7356214008386,-6.07776027111619,
2.67832123541513));
#240759=CARTESIAN_POINT('Ctrl Pts',(58.7406237702162,-6.07054860839873,
2.68225560368441));
#240760=CARTESIAN_POINT('Ctrl Pts',(58.7460508958012,-6.06389424687424,
2.68661792998885));
#240761=CARTESIAN_POINT('Ctrl Pts',(58.7517849266679,-6.05777649745733,
2.69130986622574));
#240762=CARTESIAN_POINT('Ctrl Pts',(58.7545659254421,-6.05480939560099,
2.69358545023051));
#240763=CARTESIAN_POINT('Ctrl Pts',(58.7574196937449,-6.05196853530496,
2.69593918853466));
#240764=CARTESIAN_POINT('Ctrl Pts',(58.7603356163932,-6.04925198282133,
2.69836306235472));
#240765=CARTESIAN_POINT('Ctrl Pts',(58.7647996902381,-6.04509313076893,
2.70207384382205));
#240766=CARTESIAN_POINT('Ctrl Pts',(58.7694062431512,-6.04122712576978,
2.70594760814205));
#240767=CARTESIAN_POINT('Ctrl Pts',(58.7741092696794,-6.03765709635735,
2.70995196345684));
#240768=CARTESIAN_POINT('Ctrl Pts',(58.7762933795293,-6.03599915622934,
2.71181160678082));
#240769=CARTESIAN_POINT('Ctrl Pts',(58.7784980841112,-6.03440490786023,
2.71369962772075));
#240770=CARTESIAN_POINT('Ctrl Pts',(58.7807192900658,-6.03287578462657,
2.71561183138637));
#240771=CARTESIAN_POINT('Ctrl Pts',(58.7808895367502,-6.03275858335576,
2.71575839426288));
#240772=CARTESIAN_POINT('Ctrl Pts',(58.7810598733266,-6.03264173148679,
2.71590508903186));
#240773=CARTESIAN_POINT('Ctrl Pts',(58.7812302983889,-6.0325252286245,2.71605191409888));
#240774=CARTESIAN_POINT('Ctrl Pts',(58.7836242566994,-6.03088871465405,
2.7181143636273));
#240775=CARTESIAN_POINT('Ctrl Pts',(58.7860369637878,-6.02932271154663,
2.72020091026936));
#240776=CARTESIAN_POINT('Ctrl Pts',(58.7884628208564,-6.02782611907157,
2.72230624862159));
#240777=CARTESIAN_POINT('Ctrl Pts',(58.7971615128805,-6.02245960461597,
2.72985561753093));
#240778=CARTESIAN_POINT('Ctrl Pts',(58.8060955050479,-6.01794242202224,
2.73770089914333));
#240779=CARTESIAN_POINT('Ctrl Pts',(58.8151732302901,-6.01418353044851,
2.74574823347091));
#240780=CARTESIAN_POINT('Ctrl Pts',(58.8251487383928,-6.01005288622314,
2.75459144547047));
#240781=CARTESIAN_POINT('Ctrl Pts',(58.8352983536258,-6.00683754300114,
2.76367911754297));
#240782=CARTESIAN_POINT('Ctrl Pts',(58.845534016615,-6.00445775272896,2.77292162564759));
#240783=CARTESIAN_POINT('Ctrl Pts',(58.8565859638426,-6.00188817648084,
2.78290121484763));
#240784=CARTESIAN_POINT('Ctrl Pts',(58.8677393147039,-6.00029231631069,
2.79306229500219));
#240785=CARTESIAN_POINT('Ctrl Pts',(58.8789072188679,-5.99962196122044,
2.80331916685283));
#240786=CARTESIAN_POINT('Ctrl Pts',(58.8899814357904,-5.99895722972064,
2.81348999408712));
#240787=CARTESIAN_POINT('Ctrl Pts',(58.9010713848516,-5.99920273697601,
2.82375635966883));
#240788=CARTESIAN_POINT('Ctrl Pts',(58.9120953679531,-6.00036140428947,
2.83404198860258));
#240789=CARTESIAN_POINT('Origin',(-0.00159301378019881,-0.0151565136852225,
2.83404198860262));
#240790=CARTESIAN_POINT('Ctrl Pts',(62.5005702980932,-6.58439859102925,
2.65878198860258));
#240791=CARTESIAN_POINT('Ctrl Pts',(62.4996689377206,-6.59294009787341,
2.65878198860258));
#240792=CARTESIAN_POINT('Ctrl Pts',(62.4980620716938,-6.60133040498934,
2.65944603041841));
#240793=CARTESIAN_POINT('Ctrl Pts',(62.4958483879906,-6.60945539386065,
2.6607043926405));
#240794=CARTESIAN_POINT('Ctrl Pts',(62.4944339494873,-6.61464687495722,
2.66150842619576));
#240795=CARTESIAN_POINT('Ctrl Pts',(62.4927726671884,-6.61973030386238,
2.66255428265352));
#240796=CARTESIAN_POINT('Ctrl Pts',(62.4908979342377,-6.62467983150659,
2.66381699700646));
#240797=CARTESIAN_POINT('Ctrl Pts',(62.4883392999284,-6.63143494360989,
2.66554034873245));
#240798=CARTESIAN_POINT('Ctrl Pts',(62.4853780106448,-6.63793726713659,
2.6676675964395));
#240799=CARTESIAN_POINT('Ctrl Pts',(62.482086456285,-6.6441242645479,2.67012012783126));
#240800=CARTESIAN_POINT('Ctrl Pts',(62.4804406791051,-6.64721776325356,
2.67134639352714));
#240801=CARTESIAN_POINT('Ctrl Pts',(62.4787123157335,-6.65023263831771,
2.6726537558499));
#240802=CARTESIAN_POINT('Ctrl Pts',(62.4769102669531,-6.65316255786638,
2.67403135126918));
#240803=CARTESIAN_POINT('Ctrl Pts',(62.476009242563,-6.65462751764071,2.67472014897882));
#240804=CARTESIAN_POINT('Ctrl Pts',(62.4750897950507,-6.65607125585979,
2.67542649668611));
#240805=CARTESIAN_POINT('Ctrl Pts',(62.474153026021,-6.65749308991659,2.6761489965608));
#240806=CARTESIAN_POINT('Ctrl Pts',(62.4739188337636,-6.65784854843079,
2.67632962152947));
#240807=CARTESIAN_POINT('Ctrl Pts',(62.4736835588747,-6.65820263830401,
2.67651125590929));
#240808=CARTESIAN_POINT('Ctrl Pts',(62.4734472184934,-6.65855534961512,
2.67669387767502));
#240809=CARTESIAN_POINT('Ctrl Pts',(62.4727381973496,-6.65961348354846,
2.67724174297222));
#240810=CARTESIAN_POINT('Ctrl Pts',(62.4720195869493,-6.66065920857905,
2.67779849504726));
#240811=CARTESIAN_POINT('Ctrl Pts',(62.4712918484711,-6.66169227331115,
2.67836353617988));
#240812=CARTESIAN_POINT('Ctrl Pts',(62.4662627240579,-6.66883139158019,
2.68226832098884));
#240813=CARTESIAN_POINT('Ctrl Pts',(62.4608161451511,-6.67541846632554,
2.68659153751365));
#240814=CARTESIAN_POINT('Ctrl Pts',(62.4550686189992,-6.68147667711015,
2.69123699486149));
#240815=CARTESIAN_POINT('Ctrl Pts',(62.4522121142783,-6.68448759124072,
2.6935457744119));
#240816=CARTESIAN_POINT('Ctrl Pts',(62.4492806638355,-6.68736784133507,
2.69593478828094));
#240817=CARTESIAN_POINT('Ctrl Pts',(62.4462854590369,-6.69011973548505,
2.69839565261199));
#240818=CARTESIAN_POINT('Ctrl Pts',(62.4396775898762,-6.69619082501318,
2.70382468689024));
#240819=CARTESIAN_POINT('Ctrl Pts',(62.4327685320937,-6.70164568781112,
2.70961155815066));
#240820=CARTESIAN_POINT('Ctrl Pts',(62.4256985108779,-6.7064460603899,2.71562701361746));
#240821=CARTESIAN_POINT('Ctrl Pts',(62.4231157429702,-6.70819969702881,
2.71782453535837));
#240822=CARTESIAN_POINT('Ctrl Pts',(62.4205129446134,-6.70987381569712,
2.72005051502381));
#240823=CARTESIAN_POINT('Ctrl Pts',(62.4178950590936,-6.71147036762072,
2.72229986760094));
#240824=CARTESIAN_POINT('Ctrl Pts',(62.4091018586485,-6.71683301659044,
2.72985520488873));
#240825=CARTESIAN_POINT('Ctrl Pts',(62.4000783072483,-6.7213473429662,2.73770845534544));
#240826=CARTESIAN_POINT('Ctrl Pts',(62.390915840586,-6.72510335397105,2.74576706701744));
#240827=CARTESIAN_POINT('Ctrl Pts',(62.3808452043586,-6.72923165499413,
2.75462443585026));
#240828=CARTESIAN_POINT('Ctrl Pts',(62.3706061896766,-6.7324442675611,2.76373036323186));
#240829=CARTESIAN_POINT('Ctrl Pts',(62.3602869763748,-6.73481930344685,
2.7729966463683));
#240830=CARTESIAN_POINT('Ctrl Pts',(62.3491727415056,-6.73737731885801,
2.78297683033495));
#240831=CARTESIAN_POINT('Ctrl Pts',(62.3379643502052,-6.73896413451793,
2.79314401478921));
#240832=CARTESIAN_POINT('Ctrl Pts',(62.3267489231093,-6.73962511499475,
2.80341452427971));
#240833=CARTESIAN_POINT('Ctrl Pts',(62.315684942148,-6.74027717000334,2.81354634721384));
#240834=CARTESIAN_POINT('Ctrl Pts',(62.3046126966245,-6.74002799825869,
2.82378004209211));
#240835=CARTESIAN_POINT('Ctrl Pts',(62.293614112757,-6.73887200051229,2.83404198860258));
#240836=CARTESIAN_POINT('Ctrl Pts',(58.8722700234481,-6.37927424642479,
2.83404198860258));
#240837=CARTESIAN_POINT('Ctrl Pts',(58.8617443183095,-6.37816795023556,
2.82422126443008));
#240838=CARTESIAN_POINT('Ctrl Pts',(58.8513437177781,-6.37623543038764,
2.81442815028507));
#240839=CARTESIAN_POINT('Ctrl Pts',(58.8411231047668,-6.37349561323622,
2.80471618166329));
#240840=CARTESIAN_POINT('Ctrl Pts',(58.8312542036553,-6.37085007871684,
2.79533842146247));
#240841=CARTESIAN_POINT('Ctrl Pts',(58.8215519162598,-6.36745144954003,
2.78603515650264));
#240842=CARTESIAN_POINT('Ctrl Pts',(58.8120753594642,-6.36327195218565,
2.77685887346786));
#240843=CARTESIAN_POINT('Ctrl Pts',(58.8031170454187,-6.35932101824826,
2.76818441216615));
#240844=CARTESIAN_POINT('Ctrl Pts',(58.7943596215167,-6.35467192211794,
2.7596226152167));
#240845=CARTESIAN_POINT('Ctrl Pts',(58.7858758685307,-6.34926600747485,
2.75123537701714));
#240846=CARTESIAN_POINT('Ctrl Pts',(58.7780624743562,-6.34428725077959,
2.74351087134184));
#240847=CARTESIAN_POINT('Ctrl Pts',(58.7704807832448,-6.33866621241268,
2.73593399449922));
#240848=CARTESIAN_POINT('Ctrl Pts',(58.7632157809005,-6.33233133084754,
2.72857657812661));
#240849=CARTESIAN_POINT('Ctrl Pts',(58.7610495038554,-6.33044239704299,
2.72638274508373));
#240850=CARTESIAN_POINT('Ctrl Pts',(58.7589116098636,-6.32848982621416,
2.72420861709617));
#240851=CARTESIAN_POINT('Ctrl Pts',(58.7568049797265,-6.32647128889738,
2.72205663736704));
#240852=CARTESIAN_POINT('Ctrl Pts',(58.7547198741578,-6.32447337605752,
2.71992664556743));
#240853=CARTESIAN_POINT('Ctrl Pts',(58.7526673708734,-6.32241310885625,
2.71782089927861));
#240854=CARTESIAN_POINT('Ctrl Pts',(58.7506524329181,-6.32029074540019,
2.71574387311223));
#240855=CARTESIAN_POINT('Ctrl Pts',(58.7505123180733,-6.32014316039614,
2.71559944077464));
#240856=CARTESIAN_POINT('Ctrl Pts',(58.7503723733987,-6.31999527850255,
2.71545515216046));
#240857=CARTESIAN_POINT('Ctrl Pts',(58.7502325999832,-6.31984709900125,
2.71531100781707));
#240858=CARTESIAN_POINT('Ctrl Pts',(58.7441044214169,-6.31335036684014,
2.70899119176064));
#240859=CARTESIAN_POINT('Ctrl Pts',(58.7383447881643,-6.30625925377255,
2.70298296066821));
#240860=CARTESIAN_POINT('Ctrl Pts',(58.7330687140844,-6.29859016886859,
2.69736727774122));
#240861=CARTESIAN_POINT('Ctrl Pts',(58.7281504960664,-6.29144124886016,
2.69213248525417));
#240862=CARTESIAN_POINT('Ctrl Pts',(58.7236522470779,-6.28378931332989,
2.68723866185458));
#240863=CARTESIAN_POINT('Ctrl Pts',(58.7196964823232,-6.27564783709128,
2.68278595829554));
#240864=CARTESIAN_POINT('Ctrl Pts',(58.7182494123992,-6.27266957975491,
2.68115710172791));
#240865=CARTESIAN_POINT('Ctrl Pts',(58.7168752520899,-6.2696258693364,2.67958763637791));
#240866=CARTESIAN_POINT('Ctrl Pts',(58.7155811795665,-6.26651766855652,
2.67808378645341));
#240867=CARTESIAN_POINT('Ctrl Pts',(58.7152699983558,-6.26577025010479,
2.67772216078576));
#240868=CARTESIAN_POINT('Ctrl Pts',(58.7149635750523,-6.26501853257339,
2.67736403603539));
#240869=CARTESIAN_POINT('Ctrl Pts',(58.7146620123682,-6.26426260461741,
2.67700956934455));
#240870=CARTESIAN_POINT('Ctrl Pts',(58.7143698735179,-6.26353029941006,
2.6766661797378));
#240871=CARTESIAN_POINT('Ctrl Pts',(58.7140822962415,-6.26279404284275,
2.67632622314095));
#240872=CARTESIAN_POINT('Ctrl Pts',(58.7137993735012,-6.26205391928359,
2.67598984158749));
#240873=CARTESIAN_POINT('Ctrl Pts',(58.7106996279153,-6.25394501035143,
2.67230439292196));
#240874=CARTESIAN_POINT('Ctrl Pts',(58.70815694202,-6.24536644325852,2.66904964539949));
#240875=CARTESIAN_POINT('Ctrl Pts',(58.7062958387084,-6.23645973859584,
2.66640203566698));
#240876=CARTESIAN_POINT('Ctrl Pts',(58.7055239836916,-6.23276586269187,
2.66530399299414));
#240877=CARTESIAN_POINT('Ctrl Pts',(58.7048690642116,-6.22901585349446,
2.66430995142234));
#240878=CARTESIAN_POINT('Ctrl Pts',(58.7043384037135,-6.225220762677,2.66343053473336));
#240879=CARTESIAN_POINT('Ctrl Pts',(58.7034333069352,-6.21874783981136,
2.66193059792859));
#240880=CARTESIAN_POINT('Ctrl Pts',(58.7028917011006,-6.21214524099463,
2.66076519817102));
#240881=CARTESIAN_POINT('Ctrl Pts',(58.7027523988018,-6.20547453341974,
2.65997805604434));
#240882=CARTESIAN_POINT('Ctrl Pts',(58.7026827476524,-6.2021391796323,2.659584484981));
#240883=CARTESIAN_POINT('Ctrl Pts',(58.7027151167905,-6.19878688248268,
2.65928526260736));
#240884=CARTESIAN_POINT('Ctrl Pts',(58.7028544030466,-6.19542538554926,
2.65908463971298));
#240885=CARTESIAN_POINT('Ctrl Pts',(58.7029936893027,-6.19206388861583,
2.6588840168186));
#240886=CARTESIAN_POINT('Ctrl Pts',(58.7032398710656,-6.18869323212117,
2.65878198860258));
#240887=CARTESIAN_POINT('Ctrl Pts',(58.703595878104,-6.185320498293,2.65878198860258));
#240888=CARTESIAN_POINT('Origin',(61.0544000815099,6.7363249086374,3.56647653909516));
#240889=CARTESIAN_POINT('Origin',(61.0983782637164,6.740999176878,3.64299466007777));
#240890=CARTESIAN_POINT('Origin',(60.9730100652054,6.72777047351143,3.42473028058489));
#240891=CARTESIAN_POINT('Ctrl Pts',(60.8636883187845,6.71570789669429,3.48823028058489));
#240892=CARTESIAN_POINT('Ctrl Pts',(60.8773920302461,6.59002106156485,3.48794691941605));
#240893=CARTESIAN_POINT('Ctrl Pts',(60.9862851800404,6.60146619279966,3.4247302805849));
#240894=CARTESIAN_POINT('Ctrl Pts',(60.818916972731,6.711118718498,3.4102800592509));
#240895=CARTESIAN_POINT('Ctrl Pts',(60.8324022194115,6.58529244190214,3.40982512230983));
#240896=CARTESIAN_POINT('Ctrl Pts',(60.9191469903166,6.59440968471161,3.30780486372849));
#240897=CARTESIAN_POINT('Ctrl Pts',(60.7340977611529,6.70242508976221,3.36123028058486));
#240898=CARTESIAN_POINT('Ctrl Pts',(60.7472645033903,6.57634410736716,3.36099721048503));
#240899=CARTESIAN_POINT('Ctrl Pts',(60.7919547682788,6.58104124348259,3.23423045308447));
#240900=CARTESIAN_POINT('Ctrl Pts',(60.6448574988554,6.69328024897474,3.36123028058487));
#240901=CARTESIAN_POINT('Ctrl Pts',(60.6581326136904,6.56697596826297,3.36123028058487));
#240902=CARTESIAN_POINT('Ctrl Pts',(60.6581326136904,6.56697596826297,3.23423028058486));
#240903=CARTESIAN_POINT('Origin',(60.6448574988554,6.69328024897474,3.23423028058487));
#240904=CARTESIAN_POINT('Origin',(-0.0331877870874745,0.315760701779611,
3.64303198860263));
#240905=CARTESIAN_POINT('Origin',(61.4975385923862,6.78290064323579,3.64303198860268));
#240906=CARTESIAN_POINT('Origin',(-0.0331877870874745,0.315760701779613,
3.23423028058482));
#240907=CARTESIAN_POINT('Origin',(60.4944777170594,6.67747469700965,3.23423028058487));
#240908=CARTESIAN_POINT('Ctrl Pts',(62.0330459552232,6.83973663030279,3.47153072139077));
#240909=CARTESIAN_POINT('Ctrl Pts',(62.0468640234019,6.71274550335245,3.47182327902667));
#240910=CARTESIAN_POINT('Ctrl Pts',(61.9391074687686,6.70161199370844,3.40413028959037));
#240911=CARTESIAN_POINT('Ctrl Pts',(61.9187065474465,6.82760205123589,3.65553807120964));
#240912=CARTESIAN_POINT('Ctrl Pts',(61.9323544653024,6.7007103254433,3.65586275496912));
#240913=CARTESIAN_POINT('Ctrl Pts',(61.847659827901,6.6920004592179,3.5512812683724));
#240914=CARTESIAN_POINT('Ctrl Pts',(61.7133000470646,6.80580199871493,3.77003198860268));
#240915=CARTESIAN_POINT('Ctrl Pts',(61.7268034525367,6.67910652125837,3.77025505748527));
#240916=CARTESIAN_POINT('Ctrl Pts',(61.683377859151,6.67473372828961,3.64284211731182));
#240917=CARTESIAN_POINT('Ctrl Pts',(61.4975385923862,6.78290064323579,3.77003198860269));
#240918=CARTESIAN_POINT('Ctrl Pts',(61.5108335396272,6.65640766978549,3.77003198860269));
#240919=CARTESIAN_POINT('Ctrl Pts',(61.510813692429,6.65659650326271,3.64284239821713));
#240920=CARTESIAN_POINT('Origin',(61.9259926140919,6.82793297553368,3.40423097483315));
#240921=CARTESIAN_POINT('Ctrl Pts',(60.4944777170594,6.67747469700965,3.36123028058487));
#240922=CARTESIAN_POINT('Ctrl Pts',(60.5077528318944,6.55117041629788,3.36123028058486));
#240923=CARTESIAN_POINT('Ctrl Pts',(60.5077528318944,6.55117041629788,3.23423028058486));
#240924=CARTESIAN_POINT('Ctrl Pts',(60.4049357747551,6.66829952659943,3.36123028058487));
#240925=CARTESIAN_POINT('Ctrl Pts',(60.4181493202572,6.54175270773023,3.36146538610217));
#240926=CARTESIAN_POINT('Ctrl Pts',(60.3734783767964,6.53705760237909,3.23423043688484));
#240927=CARTESIAN_POINT('Ctrl Pts',(60.3202668847283,6.65962554481729,3.41054258693106));
#240928=CARTESIAN_POINT('Ctrl Pts',(60.3338524728743,6.53289275205003,3.41100608859737));
#240929=CARTESIAN_POINT('Ctrl Pts',(60.2465123062132,6.52371293062576,3.30819866970803));
#240930=CARTESIAN_POINT('Ctrl Pts',(60.2756459899119,6.65505462397414,3.48823028058486));
#240931=CARTESIAN_POINT('Ctrl Pts',(60.2894805317162,6.52822907310797,3.48852004212264));
#240932=CARTESIAN_POINT('Ctrl Pts',(60.1796001951995,6.51668018436765,3.42473028058485));
#240933=CARTESIAN_POINT('Origin',(60.1663250803646,6.64298446507942,3.42473028058486));
#240934=CARTESIAN_POINT('Origin',(62.1031658061134,6.84655462836832,3.11913648178332));
#240935=CARTESIAN_POINT('Origin',(62.2803389979219,6.86517628122529,2.83404198860267));
#240936=CARTESIAN_POINT('Origin',(60.0854204576116,6.63448104656903,3.56563113460833));
#240937=CARTESIAN_POINT('Origin',(60.0409538388298,6.62985850077833,3.6429917172181));
#240938=CARTESIAN_POINT('Ctrl Pts',(62.6076796697354,6.59568250079905,2.59908173516028));
#240939=CARTESIAN_POINT('Ctrl Pts',(62.5705801176609,6.59177408464793,2.65878198860267));
#240940=CARTESIAN_POINT('Ctrl Pts',(62.5005702980931,6.58439859103048,2.65878198860267));
#240941=CARTESIAN_POINT('Ctrl Pts',(62.5984477290791,6.68331293653946,2.59908193475784));
#240942=CARTESIAN_POINT('Ctrl Pts',(62.5638523220891,6.65560500345248,2.65878715325336));
#240943=CARTESIAN_POINT('Ctrl Pts',(62.4952175264233,6.63512154272615,2.65878198860267));
#240944=CARTESIAN_POINT('Ctrl Pts',(62.5650504549418,6.76155265492292,2.63878778849877));
#240945=CARTESIAN_POINT('Ctrl Pts',(62.5346567608587,6.71196843232436,2.69564460180128));
#240946=CARTESIAN_POINT('Ctrl Pts',(62.4653998062676,6.67930776339589,2.68180481624896));
#240947=CARTESIAN_POINT('Ctrl Pts',(62.4816328770701,6.86003002196278,2.7544323887865));
#240948=CARTESIAN_POINT('Ctrl Pts',(62.4676069047243,6.76863258245059,2.79268340777084));
#240949=CARTESIAN_POINT('Ctrl Pts',(62.3866783619496,6.73311104631474,2.74885926835607));
#240950=CARTESIAN_POINT('Ctrl Pts',(62.4326191774618,6.88172985342194,2.82856655361678));
#240951=CARTESIAN_POINT('Ctrl Pts',(62.4292062449152,6.76853939445046,2.85384197230682));
#240952=CARTESIAN_POINT('Ctrl Pts',(62.3388388123819,6.74362530798272,2.79184624278386));
#240953=CARTESIAN_POINT('Ctrl Pts',(62.3873926810691,6.87697683366584,2.9013417351603));
#240954=CARTESIAN_POINT('Ctrl Pts',(62.4011871104969,6.75017837817621,2.90163218716397));
#240955=CARTESIAN_POINT('Ctrl Pts',(62.2936141127569,6.73887200051352,2.83404198860268));
#240956=CARTESIAN_POINT('Origin',(62.5005702980931,6.58439859103048,2.53178198860267));
#240957=CARTESIAN_POINT('Origin',(-0.0331877870874745,0.315760701779611,
3.64303198860263));
#240958=CARTESIAN_POINT('Origin',(59.6417962403143,6.58785426247114,3.64303198860268));
#240959=CARTESIAN_POINT('Origin',(5.50069060731754E-15,1.85865314505527E-13,
2.53178198860262));
#240960=CARTESIAN_POINT('Origin',(62.5037563256535,6.55408556365965,2.53178198860267));
#240961=CARTESIAN_POINT('Ctrl Pts',(59.6417962403143,6.58785426247114,3.77003198860268));
#240962=CARTESIAN_POINT('Ctrl Pts',(59.6550912418708,6.46136077224306,3.77003198860268));
#240963=CARTESIAN_POINT('Ctrl Pts',(59.655071340276,6.46155012326943,3.64284187937014));
#240964=CARTESIAN_POINT('Ctrl Pts',(59.4260321009469,6.56494565834894,3.77003198860269));
#240965=CARTESIAN_POINT('Ctrl Pts',(59.4394927947744,6.43870097938004,3.76980208963001));
#240966=CARTESIAN_POINT('Ctrl Pts',(59.4825041216653,6.44341257746694,3.64284193928327));
#240967=CARTESIAN_POINT('Ctrl Pts',(59.2206282517276,6.54313468201947,3.65553535416592));
#240968=CARTESIAN_POINT('Ctrl Pts',(59.2341955513569,6.41712387095898,3.6552005783454));
#240969=CARTESIAN_POINT('Ctrl Pts',(59.3182233753696,6.42614597500995,3.55127910964209));
#240970=CARTESIAN_POINT('Ctrl Pts',(59.1062911958296,6.53099325080074,3.47153072139077));
#240971=CARTESIAN_POINT('Ctrl Pts',(59.1200087130389,6.40512262640546,3.47122746281587));
#240972=CARTESIAN_POINT('Ctrl Pts',(59.2267768553867,6.41653455832048,3.40413045901259));
#240973=CARTESIAN_POINT('Origin',(59.2133417798936,6.54282188406246,3.40423097483315));
#240974=CARTESIAN_POINT('Ctrl Pts',(62.4538823482275,6.24436990788079,2.90134173516029));
#240975=CARTESIAN_POINT('Ctrl Pts',(62.4410124550018,6.3712655360409,2.90163218716396));
#240976=CARTESIAN_POINT('Ctrl Pts',(62.3334394572619,6.35995915837821,2.83404198860267));
#240977=CARTESIAN_POINT('Ctrl Pts',(62.4991292864731,6.24912604340928,2.82853349835366));
#240978=CARTESIAN_POINT('Ctrl Pts',(62.4722545055307,6.35912437831578,2.85381483162363));
#240979=CARTESIAN_POINT('Ctrl Pts',(62.3786847639679,6.3647146317389,2.79182701594255));
#240980=CARTESIAN_POINT('Ctrl Pts',(62.5423796567684,6.28053011789759,2.75468822073642));
#240981=CARTESIAN_POINT('Ctrl Pts',(62.509694696565,6.36708533499915,2.79286913083882));
#240982=CARTESIAN_POINT('Ctrl Pts',(62.4231124872028,6.38493060453726,2.74900763297914));
#240983=CARTESIAN_POINT('Ctrl Pts',(62.6032845425345,6.39322569848906,2.63954450640404));
#240984=CARTESIAN_POINT('Ctrl Pts',(62.5632890102007,6.43576006824464,2.69627684028838));
#240985=CARTESIAN_POINT('Ctrl Pts',(62.4886705126496,6.45334792019217,2.682243560365));
#240986=CARTESIAN_POINT('Ctrl Pts',(62.6200908675645,6.47739243510505,2.59908178706469));
#240987=CARTESIAN_POINT('Ctrl Pts',(62.5804859237117,6.49734694408369,2.65878704321546));
#240988=CARTESIAN_POINT('Ctrl Pts',(62.5090840872014,6.50319024212522,2.65878198860267));
#240989=CARTESIAN_POINT('Ctrl Pts',(62.6108711573006,6.56531752495321,2.59908173516028));
#240990=CARTESIAN_POINT('Ctrl Pts',(62.5737697140402,6.56142710223371,2.65878198860267));
#240991=CARTESIAN_POINT('Ctrl Pts',(62.5037563256535,6.55408556365965,2.65878198860267));
#240992=CARTESIAN_POINT('Origin',(62.3467145720969,6.23365487766644,2.83404198860265));
#240993=CARTESIAN_POINT('Origin',(59.0361683443304,6.52420020557803,3.11913648167145));
#240994=CARTESIAN_POINT('Origin',(58.858994908613,6.50557852713774,2.83404198860267));
#240995=CARTESIAN_POINT('Origin',(62.1695413802689,6.21503322485029,3.11913648177391));
#240996=CARTESIAN_POINT('Origin',(61.9923681882669,6.19641157197482,3.40423097483315));
#240997=CARTESIAN_POINT('Ctrl Pts',(58.7519447039088,6.49374646112759,2.90134173516028));
#240998=CARTESIAN_POINT('Ctrl Pts',(58.7656442740271,6.36806742857345,2.90103711553234));
#240999=CARTESIAN_POINT('Ctrl Pts',(58.872270023448,6.37927424642597,2.83404198860267));
#241000=CARTESIAN_POINT('Ctrl Pts',(58.7067576262547,6.48899657309085,2.82862991747966));
#241001=CARTESIAN_POINT('Ctrl Pts',(58.7342098038491,6.38004220452818,2.85314045886426));
#241002=CARTESIAN_POINT('Ctrl Pts',(58.8270810177598,6.37452469054069,2.79187960999899));
#241003=CARTESIAN_POINT('Ctrl Pts',(58.6637560248473,6.45774144355334,2.7547062579333));
#241004=CARTESIAN_POINT('Ctrl Pts',(58.6967899354326,6.3718711793815,2.79224250381907));
#241005=CARTESIAN_POINT('Ctrl Pts',(58.7829167175848,6.35435266912784,2.7490180910826));
#241006=CARTESIAN_POINT('Ctrl Pts',(58.6035914159081,6.3453990801634,2.63947868311704));
#241007=CARTESIAN_POINT('Ctrl Pts',(58.6436439608621,6.30313135363863,2.69595066767916));
#241008=CARTESIAN_POINT('Ctrl Pts',(58.7181337176191,6.28595874576536,2.6822053943607));
#241009=CARTESIAN_POINT('Ctrl Pts',(58.5872698677167,6.2615101002574,2.5990817858507));
#241010=CARTESIAN_POINT('Ctrl Pts',(58.626864594668,6.24170554357551,2.6587767094479));
#241011=CARTESIAN_POINT('Ctrl Pts',(58.6982323944353,6.23613328458279,2.65878198860267));
#241012=CARTESIAN_POINT('Ctrl Pts',(58.5964866834551,6.17403490859039,2.59908173516029));
#241013=CARTESIAN_POINT('Ctrl Pts',(58.6335861742242,6.17794390662191,2.65878198860267));
#241014=CARTESIAN_POINT('Ctrl Pts',(58.7035958781039,6.18532049829418,2.65878198860267));
#241015=CARTESIAN_POINT('Origin',(58.7035958781039,6.18532049829418,2.53178198860267));
#241016=CARTESIAN_POINT('Ctrl Pts',(61.5639141665612,6.15137923967694,3.77003198860268));
#241017=CARTESIAN_POINT('Ctrl Pts',(61.5506192181748,6.27787222402466,3.77003198860268));
#241018=CARTESIAN_POINT('Ctrl Pts',(61.5506390665201,6.27768337963378,3.64284238727605));
#241019=CARTESIAN_POINT('Ctrl Pts',(61.7797255331386,6.17383801205373,3.77003198860268));
#241020=CARTESIAN_POINT('Ctrl Pts',(61.7665923920123,6.30057242039952,3.77025506105794));
#241021=CARTESIAN_POINT('Ctrl Pts',(61.7232059145523,6.29582088597906,3.64284210641878));
#241022=CARTESIAN_POINT('Ctrl Pts',(61.9851742714891,6.19522058691261,3.65553527987838));
#241023=CARTESIAN_POINT('Ctrl Pts',(61.9721416759924,6.3221769985454,3.65585996533047));
#241024=CARTESIAN_POINT('Ctrl Pts',(61.8874865820178,6.31308747966704,3.55127902710209));
#241025=CARTESIAN_POINT('Ctrl Pts',(62.0995362748659,6.20712349654482,3.47153072139077));
#241026=CARTESIAN_POINT('Ctrl Pts',(62.086649444066,6.33421251157719,3.47182327905194));
#241027=CARTESIAN_POINT('Ctrl Pts',(61.9789328337399,6.32269886789189,3.40413028377994));
#241028=CARTESIAN_POINT('Origin',(61.5639141665612,6.15137923967694,3.64303198860268));
#241029=CARTESIAN_POINT('Origin',(5.72301283402738E-15,1.86330858203059E-13,
2.53178198860262));
#241030=CARTESIAN_POINT('Origin',(58.7067819056643,6.15500747092335,2.53178198860267));
#241031=CARTESIAN_POINT('Origin',(61.5757885448747,6.15262728712883,3.64303198860268));
#241032=CARTESIAN_POINT('Origin',(61.1647646440466,6.10937495962146,3.64299466007718));
#241033=CARTESIAN_POINT('Ctrl Pts',(58.5996668978648,6.14377718965341,2.59908173516029));
#241034=CARTESIAN_POINT('Ctrl Pts',(58.6367684021392,6.1476670304619,2.65878198860267));
#241035=CARTESIAN_POINT('Ctrl Pts',(58.7067819056643,6.15500747092335,2.65878198860267));
#241036=CARTESIAN_POINT('Ctrl Pts',(58.6088074259633,6.05659553606724,2.59908193199912));
#241037=CARTESIAN_POINT('Ctrl Pts',(58.6434243604386,6.08415140319833,2.65877685806568));
#241038=CARTESIAN_POINT('Ctrl Pts',(58.7120821529696,6.10436324506841,2.65878198860267));
#241039=CARTESIAN_POINT('Ctrl Pts',(58.6416817365139,5.97852000021532,2.63872492669802));
#241040=CARTESIAN_POINT('Ctrl Pts',(58.6721826510715,6.0278583913126,2.69532212015282));
#241041=CARTESIAN_POINT('Ctrl Pts',(58.7414038195495,6.06008468706708,2.68176836726643));
#241042=CARTESIAN_POINT('Ctrl Pts',(58.7242744516464,5.88025093392496,2.75442176402255));
#241043=CARTESIAN_POINT('Ctrl Pts',(58.738786069515,5.97104363802187,2.7920317992014));
#241044=CARTESIAN_POINT('Ctrl Pts',(58.8193360415244,6.00614981441045,2.74885310748176));
#241045=CARTESIAN_POINT('Ctrl Pts',(58.7730316211507,5.85862682030293,2.82866089558402));
#241046=CARTESIAN_POINT('Ctrl Pts',(58.7772266151797,5.97091547255876,2.85316563119283));
#241047=CARTESIAN_POINT('Ctrl Pts',(58.866925555678,5.99561386571439,2.79189751796684));
#241048=CARTESIAN_POINT('Ctrl Pts',(58.8181995570485,5.86337364149599,2.90134173516028));
#241049=CARTESIAN_POINT('Ctrl Pts',(58.805469618532,5.98915458643813,2.90103711553234));
#241050=CARTESIAN_POINT('Ctrl Pts',(58.912095367953,6.00036140429066,2.83404198860266));
#241051=CARTESIAN_POINT('Origin',(58.925370482788,5.87405712357889,2.83404198860266));
#241052=CARTESIAN_POINT('Origin',(61.1207756545816,6.10480350526345,3.56647653971745));
#241053=CARTESIAN_POINT('Origin',(61.0393856393804,6.09624906995258,3.4247302805849));
#241054=CARTESIAN_POINT('Origin',(59.1025439184834,5.89267880207675,3.11913648168135));
#241055=CARTESIAN_POINT('Origin',(59.2797173540686,5.91130048050361,3.40423097483316));
#241056=CARTESIAN_POINT('Ctrl Pts',(60.7112330730304,6.06175884541589,3.36123028058486));
#241057=CARTESIAN_POINT('Ctrl Pts',(60.6979579581954,6.18806312612766,3.36123028058486));
#241058=CARTESIAN_POINT('Ctrl Pts',(60.6979579581954,6.18806312612766,3.23423028058486));
#241059=CARTESIAN_POINT('Ctrl Pts',(60.8007259828526,6.07140041118264,3.36123028058486));
#241060=CARTESIAN_POINT('Ctrl Pts',(60.7873912833627,6.19746294737676,3.36099641108536));
#241061=CARTESIAN_POINT('Ctrl Pts',(60.8322324012627,6.20217593878197,3.23423043688433));
#241062=CARTESIAN_POINT('Ctrl Pts',(60.885348460727,6.0805154206754,3.4105425890529));
#241063=CARTESIAN_POINT('Ctrl Pts',(60.8723790316482,6.20639551966689,3.41008815825971));
#241064=CARTESIAN_POINT('Ctrl Pts',(60.9591984396287,6.21552060714914,3.30819867304265));
#241065=CARTESIAN_POINT('Ctrl Pts',(60.929944884669,6.08531878138339,3.48823028058488));
#241066=CARTESIAN_POINT('Ctrl Pts',(60.917217374751,6.21110821942954,3.48794691941605));
#241067=CARTESIAN_POINT('Ctrl Pts',(61.0261105245454,6.22255335066434,3.42473028058489));
#241068=CARTESIAN_POINT('Origin',(60.7112330730304,6.06175884541589,3.23423028058486));
#241069=CARTESIAN_POINT('Ctrl Pts',(59.1725467709677,5.90061356181275,3.47153072139077));
#241070=CARTESIAN_POINT('Ctrl Pts',(59.1597945546412,6.02658562874821,3.47122746285082));
#241071=CARTESIAN_POINT('Ctrl Pts',(59.2666022171587,6.0376214331677,3.40413046676795));
#241072=CARTESIAN_POINT('Ctrl Pts',(59.2869113614505,5.91250964036482,3.65553813457993));
#241073=CARTESIAN_POINT('Ctrl Pts',(59.2739830624778,6.03858760028864,3.65520336072117));
#241074=CARTESIAN_POINT('Ctrl Pts',(59.358050121575,6.04723299508908,3.55128134519901));
#241075=CARTESIAN_POINT('Ctrl Pts',(59.4923630227875,5.93388131656907,3.77003198860267));
#241076=CARTESIAN_POINT('Ctrl Pts',(59.4792818168371,6.06016587018187,3.76980209314199));
#241077=CARTESIAN_POINT('Ctrl Pts',(59.5223321697727,6.0644997338841,3.64284195387436));
#241078=CARTESIAN_POINT('Ctrl Pts',(59.7081718144892,5.95633285891229,3.77003198860268));
#241079=CARTESIAN_POINT('Ctrl Pts',(59.6948768144683,6.08282633453086,3.77003198860268));
#241080=CARTESIAN_POINT('Ctrl Pts',(59.6948967145252,6.08263699813584,3.64284189403812));
#241081=CARTESIAN_POINT('Origin',(59.7081718144892,5.95633285891229,3.64303198860268));
#241082=CARTESIAN_POINT('Origin',(60.0850508448141,5.99594444118226,3.23423028058486));
#241083=CARTESIAN_POINT('Origin',(60.5608532912343,6.0459532934508,3.23423028058486));
#241084=CARTESIAN_POINT('Origin',(59.851607889689,5.97140859790567,3.64303198860267));
#241085=CARTESIAN_POINT('Origin',(60.1073400339998,5.99823604520145,3.64299171721797));
#241086=CARTESIAN_POINT('Ctrl Pts',(60.3421421670675,6.02238575970294,3.48823028058486));
#241087=CARTESIAN_POINT('Ctrl Pts',(60.3293058762211,6.14931623097265,3.48852004212264));
#241088=CARTESIAN_POINT('Ctrl Pts',(60.2194255397045,6.13776734223234,3.42473028058486));
#241089=CARTESIAN_POINT('Ctrl Pts',(60.3868890390928,6.02720817145219,3.41028005848414));
#241090=CARTESIAN_POINT('Ctrl Pts',(60.373827809951,6.15399567476929,3.41074404220338));
#241091=CARTESIAN_POINT('Ctrl Pts',(60.2865637544299,6.14482385294816,3.30780486243867));
#241092=CARTESIAN_POINT('Ctrl Pts',(60.4716618705782,6.03634362557921,3.36123028058486));
#241093=CARTESIAN_POINT('Ctrl Pts',(60.4582762833197,6.16287156698257,3.36146460586438));
#241094=CARTESIAN_POINT('Ctrl Pts',(60.4137560077509,6.15819229746517,3.23423045308448));
#241095=CARTESIAN_POINT('Ctrl Pts',(60.5608532912343,6.04595329345079,3.36123028058486));
#241096=CARTESIAN_POINT('Ctrl Pts',(60.5475781763993,6.17225757416256,3.36123028058486));
#241097=CARTESIAN_POINT('Ctrl Pts',(60.5475781763993,6.17225757416256,3.23423028058486));
#241098=CARTESIAN_POINT('Origin',(60.2327006545395,6.01146306152057,3.42473028058486));
#241099=CARTESIAN_POINT('Origin',(60.1517960329189,6.00295964283199,3.56563113524772));
#241100=CARTESIAN_POINT('Origin',(60.0157999988651,13.0813452322047,3.56647653909476));
#241101=CARTESIAN_POINT('Origin',(60.0590486699122,13.0905908661185,3.64299466007602));
#241102=CARTESIAN_POINT('Origin',(59.9357500275433,13.0643300858384,3.42473028058494));
#241103=CARTESIAN_POINT('Ctrl Pts',(59.8282880397055,13.0409063549241,3.48823028058493));
#241104=CARTESIAN_POINT('Ctrl Pts',(59.8550545325309,12.9173404733284,3.48794691941609));
#241105=CARTESIAN_POINT('Ctrl Pts',(59.9621548122771,12.9401053405452,3.42473028058494));
#241106=CARTESIAN_POINT('Ctrl Pts',(59.7842416555147,13.0316624367245,3.41028005925099));
#241107=CARTESIAN_POINT('Ctrl Pts',(59.8108054559367,12.9079350417515,3.40982512230876));
#241108=CARTESIAN_POINT('Ctrl Pts',(59.896122018529,12.9260696369486,3.30780486372844));
#241109=CARTESIAN_POINT('Ctrl Pts',(59.7007958241042,13.014150410756,3.36123028058491));
#241110=CARTESIAN_POINT('Ctrl Pts',(59.7270694888849,12.8901364125065,3.36099721048557));
#241111=CARTESIAN_POINT('Ctrl Pts',(59.7710239514078,12.8994792219298,3.23423045308437));
#241112=CARTESIAN_POINT('Ctrl Pts',(59.6130003254555,12.9957275188826,3.36123028058491));
#241113=CARTESIAN_POINT('Ctrl Pts',(59.6394051101893,12.8715027735894,3.36123028058491));
#241114=CARTESIAN_POINT('Ctrl Pts',(59.6394051101893,12.8715027735894,3.23423028058491));
#241115=CARTESIAN_POINT('Origin',(59.6130003254555,12.9957275188826,3.23423028058491));
#241116=CARTESIAN_POINT('Origin',(-0.0660119618346332,0.310561863233167,
3.64303198860263));
#241117=CARTESIAN_POINT('Origin',(60.4516424606489,13.1739864076109,3.64303198860273));
#241118=CARTESIAN_POINT('Origin',(-0.0660119618346331,0.31056186323317,
3.23423028058482));
#241119=CARTESIAN_POINT('Origin',(59.4650964698966,12.9642895838873,3.23423028058491));
#241120=CARTESIAN_POINT('Ctrl Pts',(60.9782752797348,13.2864868028998,3.47153072139082));
#241121=CARTESIAN_POINT('Ctrl Pts',(61.0052918384389,13.1616357280627,3.47182327902673));
#241122=CARTESIAN_POINT('Ctrl Pts',(60.8992893541409,13.1392995818862,3.40413028959068));
#241123=CARTESIAN_POINT('Ctrl Pts',(60.8658306440996,13.262466975741,3.65553807120968));
#241124=CARTESIAN_POINT('Ctrl Pts',(60.8926675943301,13.1376969719809,3.65586275496942));
#241125=CARTESIAN_POINT('Ctrl Pts',(60.8093473519449,13.1201818190172,3.5512812683721));
#241126=CARTESIAN_POINT('Ctrl Pts',(60.6638281080081,13.2193155203585,3.77003198860273));
#241127=CARTESIAN_POINT('Ctrl Pts',(60.6905008239745,13.0947255842078,3.77025505748434));
#241128=CARTESIAN_POINT('Ctrl Pts',(60.6477702018641,13.0858375353128,3.64284211731209));
#241129=CARTESIAN_POINT('Ctrl Pts',(60.4516424606489,13.1739864076109,3.77003198860273));
#241130=CARTESIAN_POINT('Ctrl Pts',(60.4780866929066,13.0495760763091,3.77003198860273));
#241131=CARTESIAN_POINT('Ctrl Pts',(60.4780472159603,13.0497618007392,3.64284239821766));
#241132=CARTESIAN_POINT('Origin',(60.8730422059013,13.2635576885504,3.4042309748332));
#241133=CARTESIAN_POINT('Ctrl Pts',(59.4650964698966,12.9642895838873,3.36123028058491));
#241134=CARTESIAN_POINT('Ctrl Pts',(59.4915012546305,12.8400648385941,3.36123028058491));
#241135=CARTESIAN_POINT('Ctrl Pts',(59.4915012546305,12.8400648385941,3.23423028058491));
#241136=CARTESIAN_POINT('Ctrl Pts',(59.3770041141843,12.945804994394,3.36123028058491));
#241137=CARTESIAN_POINT('Ctrl Pts',(59.4033730190103,12.8213326038448,3.36146538610185));
#241138=CARTESIAN_POINT('Ctrl Pts',(59.3594375597985,12.8119938336991,3.23423043688462));
#241139=CARTESIAN_POINT('Ctrl Pts',(59.2937057271824,12.9283282206298,3.41054258693108));
#241140=CARTESIAN_POINT('Ctrl Pts',(59.3204640761277,12.8037097640123,3.41100608859742));
#241141=CARTESIAN_POINT('Ctrl Pts',(59.2345619206652,12.7854506972086,3.30819866970818));
#241142=CARTESIAN_POINT('Ctrl Pts',(59.2498070616279,12.9191181862048,3.48823028058491));
#241143=CARTESIAN_POINT('Ctrl Pts',(59.2768226962998,12.794433502371,3.48852004212269));
#241144=CARTESIAN_POINT('Ctrl Pts',(59.1687514833561,12.7714622569322,3.42473028058491));
#241145=CARTESIAN_POINT('Origin',(59.1423466986222,12.8956870022254,3.42473028058489));
#241146=CARTESIAN_POINT('Origin',(61.047298331885,13.3005969715169,3.11913648178364));
#241147=CARTESIAN_POINT('Origin',(61.2215544576539,13.3376362544828,2.83404198860272));
#241148=CARTESIAN_POINT('Origin',(59.062774129126,12.8787733304441,3.56563113460766));
#241149=CARTESIAN_POINT('Origin',(59.0190342907436,12.8695280801148,3.64299171721792));
#241150=CARTESIAN_POINT('Ctrl Pts',(61.5752716937451,13.103835206573,2.59908173516033));
#241151=CARTESIAN_POINT('Ctrl Pts',(61.5387839176328,13.0960702419682,2.65878198860271));
#241152=CARTESIAN_POINT('Ctrl Pts',(61.4699285681954,13.0814171332235,2.65878198860271));
#241153=CARTESIAN_POINT('Ctrl Pts',(61.5569304518428,13.1900205930481,2.59908193475691));
#241154=CARTESIAN_POINT('Ctrl Pts',(61.5254208297802,13.1588482421891,2.6587871532543));
#241155=CARTESIAN_POINT('Ctrl Pts',(61.4593031273756,13.1313027022857,2.65878198860271));
#241156=CARTESIAN_POINT('Ctrl Pts',(61.515537853938,13.2643407403243,2.63878778849882));
#241157=CARTESIAN_POINT('Ctrl Pts',(61.4904936222815,13.21185113915,2.69564460180118));
#241158=CARTESIAN_POINT('Ctrl Pts',(61.4250300340663,13.1721300657491,2.68180481624894));
#241159=CARTESIAN_POINT('Ctrl Pts',(61.4222835584426,13.3535591268198,2.75443238878654));
#241160=CARTESIAN_POINT('Ctrl Pts',(61.41788805574,13.261196258709,2.79268340777107));
#241161=CARTESIAN_POINT('Ctrl Pts',(61.3411158595757,13.2174099770541,2.74885926835619));
#241162=CARTESIAN_POINT('Ctrl Pts',(61.3712701109737,13.3700167576321,2.82856655361681));
#241163=CARTESIAN_POINT('Ctrl Pts',(61.3797074995622,13.257089619244,2.85384197230726));
#241164=CARTESIAN_POINT('Ctrl Pts',(61.2924393404513,13.2228660458967,2.79184624278457));
#241165=CARTESIAN_POINT('Ctrl Pts',(61.3267881959113,13.3605623192489,2.90134173516034));
#241166=CARTESIAN_POINT('Ctrl Pts',(61.3537611057083,13.2359003894753,2.90163218716401));
#241167=CARTESIAN_POINT('Ctrl Pts',(61.2479592423878,13.2134115091896,2.83404198860272));
#241168=CARTESIAN_POINT('Origin',(61.4699285681954,13.0814171332235,2.53178198860271));
#241169=CARTESIAN_POINT('Origin',(-0.0660119618346332,0.310561863233167,
3.64303198860263));
#241170=CARTESIAN_POINT('Origin',(58.6264539577984,12.7860306150453,3.64303198860272));
#241171=CARTESIAN_POINT('Origin',(5.5033905580924E-15,1.85848267687233E-13,
2.53178198860262));
#241172=CARTESIAN_POINT('Origin',(61.4762657165316,13.0516031943531,2.53178198860271));
#241173=CARTESIAN_POINT('Ctrl Pts',(58.6264539577984,12.7860306150453,3.77003198860273));
#241174=CARTESIAN_POINT('Ctrl Pts',(58.6528982980922,12.6616197754737,3.77003198860273));
#241175=CARTESIAN_POINT('Ctrl Pts',(58.6528587129485,12.6618060089323,3.64284187937009));
#241176=CARTESIAN_POINT('Ctrl Pts',(58.4142663981468,12.7406940127368,3.77003198860273));
#241177=CARTESIAN_POINT('Ctrl Pts',(58.4408495151723,12.6165479409686,3.76980208962847));
#241178=CARTESIAN_POINT('Ctrl Pts',(58.4831327254081,12.6257296363319,3.64284193928262));
#241179=CARTESIAN_POINT('Ctrl Pts',(58.2122676405433,12.6975319705099,3.65553535416594));
#241180=CARTESIAN_POINT('Ctrl Pts',(58.2389323335222,12.5736296288395,3.65520057834622));
#241181=CARTESIAN_POINT('Ctrl Pts',(58.3215567776491,12.5913856081747,3.55127910964279));
#241182=CARTESIAN_POINT('Ctrl Pts',(58.099826060148,12.6735055745743,3.4715307213908));
#241183=CARTESIAN_POINT('Ctrl Pts',(58.1266254943014,12.5497583536231,3.4712274628159));
#241184=CARTESIAN_POINT('Ctrl Pts',(58.2316158778881,12.5722680796267,3.40413045901257));
#241185=CARTESIAN_POINT('Origin',(58.2050537810542,12.6964592423895,3.4042309748332));
#241186=CARTESIAN_POINT('Ctrl Pts',(61.4590390555209,12.7383709431253,2.90134173516033));
#241187=CARTESIAN_POINT('Ctrl Pts',(61.4329754599099,12.8632261535957,2.901632187164));
#241188=CARTESIAN_POINT('Ctrl Pts',(61.3271735965893,12.84073727331,2.83404198860272));
#241189=CARTESIAN_POINT('Ctrl Pts',(61.5035409747666,12.7478306169684,2.82853349835365));
#241190=CARTESIAN_POINT('Ctrl Pts',(61.4653154597763,12.8544171899351,2.85381483162389));
#241191=CARTESIAN_POINT('Ctrl Pts',(61.3716739624483,12.8501961180701,2.79182701594252));
#241192=CARTESIAN_POINT('Ctrl Pts',(61.5432717953614,12.7835835513932,2.75468822073652));
#241193=CARTESIAN_POINT('Ctrl Pts',(61.501718402959,12.8662481012968,2.79286913083821));
#241194=CARTESIAN_POINT('Ctrl Pts',(61.4137451613974,12.8749453072905,2.74900763297923));
#241195=CARTESIAN_POINT('Ctrl Pts',(61.5920631419344,12.9020280679173,2.63954450640403));
#241196=CARTESIAN_POINT('Ctrl Pts',(61.5478406570046,12.9401487584128,2.69627684028883));
#241197=CARTESIAN_POINT('Ctrl Pts',(61.4717924962542,12.9498405053864,2.682243560365));
#241198=CARTESIAN_POINT('Ctrl Pts',(61.599979580521,12.9874904696722,2.5990817870642));
#241199=CARTESIAN_POINT('Ctrl Pts',(61.5585057825378,13.0031958218443,2.6587870432155));
#241200=CARTESIAN_POINT('Ctrl Pts',(61.4868843017925,13.0015435854426,2.65878198860271));
#241201=CARTESIAN_POINT('Ctrl Pts',(61.5816197022698,13.0739701745327,2.59908173516033));
#241202=CARTESIAN_POINT('Ctrl Pts',(61.5451281645059,13.0662229071069,2.65878198860271));
#241203=CARTESIAN_POINT('Ctrl Pts',(61.4762657165316,13.0516031943531,2.65878198860271));
#241204=CARTESIAN_POINT('Origin',(61.3535783813232,12.7165125280168,2.83404198860271));
#241205=CARTESIAN_POINT('Origin',(58.030797415544,12.6594199084572,3.11913648167168));
#241206=CARTESIAN_POINT('Origin',(57.8565410498767,12.6223805745521,2.83404198860271));
#241207=CARTESIAN_POINT('Origin',(61.1793222555328,12.6794732450928,3.11913648177592));
#241208=CARTESIAN_POINT('Origin',(61.0050661295706,12.6424339620844,3.4042309748332));
#241209=CARTESIAN_POINT('Ctrl Pts',(57.751314065072,12.5994235324474,2.90134173516033));
#241210=CARTESIAN_POINT('Ctrl Pts',(57.7780756236495,12.4758649777955,2.90103711553238));
#241211=CARTESIAN_POINT('Ctrl Pts',(57.8829458346105,12.4981558292589,2.83404198860271));
#241212=CARTESIAN_POINT('Ctrl Pts',(57.7068710254545,12.5899763290075,2.82862991747974));
#241213=CARTESIAN_POINT('Ctrl Pts',(57.7455616498589,12.4844883578131,2.85314045886506));
#241214=CARTESIAN_POINT('Ctrl Pts',(57.838500842801,12.4887087546165,2.79187961000003));
#241215=CARTESIAN_POINT('Ctrl Pts',(57.6673720419786,12.5543975270268,2.7547062579333));
#241216=CARTESIAN_POINT('Ctrl Pts',(57.709200876099,12.472450653056,2.79224250381909));
#241217=CARTESIAN_POINT('Ctrl Pts',(57.7966870296826,12.464030811219,2.74901809108272));
#241218=CARTESIAN_POINT('Ctrl Pts',(57.6192799956674,12.4363816727425,2.63947868311713));
#241219=CARTESIAN_POINT('Ctrl Pts',(57.6635313090893,12.3985321242202,2.69595066767919));
#241220=CARTESIAN_POINT('Ctrl Pts',(57.7394080294762,12.3892398894927,2.68220539436066));
#241221=CARTESIAN_POINT('Ctrl Pts',(57.6118166447795,12.3512461790954,2.59908178585092));
#241222=CARTESIAN_POINT('Ctrl Pts',(57.6532646075499,12.335688889809,2.65877670944976));
#241223=CARTESIAN_POINT('Ctrl Pts',(57.7248239067136,12.3376071226709,2.65878198860271));
#241224=CARTESIAN_POINT('Ctrl Pts',(57.6301266171957,12.2652136052663,2.59908173516033));
#241225=CARTESIAN_POINT('Ctrl Pts',(57.6666142715155,12.2729791421557,2.65878198860271));
#241226=CARTESIAN_POINT('Ctrl Pts',(57.7354693911205,12.2876333308473,2.65878198860271));
#241227=CARTESIAN_POINT('Origin',(57.7354693911204,12.2876333308473,2.53178198860271));
#241228=CARTESIAN_POINT('Ctrl Pts',(60.5836663843182,12.5528626811449,3.77003198860273));
#241229=CARTESIAN_POINT('Ctrl Pts',(60.5572221497821,12.6772730231653,3.77003198860273));
#241230=CARTESIAN_POINT('Ctrl Pts',(60.5572616290101,12.6770872880007,3.64284238727601));
#241231=CARTESIAN_POINT('Ctrl Pts',(60.7959479326852,12.5977568525213,3.77003198860273));
#241232=CARTESIAN_POINT('Ctrl Pts',(60.769639383333,12.7224242094582,3.77025506105854));
#241233=CARTESIAN_POINT('Ctrl Pts',(60.7269872521267,12.7131635826241,3.64284210641938));
#241234=CARTESIAN_POINT('Ctrl Pts',(60.9980361136598,12.6404975322979,3.65553527987845));
#241235=CARTESIAN_POINT('Ctrl Pts',(60.9718043534744,12.7653961862443,3.65585996532996));
#241236=CARTESIAN_POINT('Ctrl Pts',(60.8885631224033,12.7475075938201,3.55127902710167));
#241237=CARTESIAN_POINT('Ctrl Pts',(61.1105274371641,12.6642893210143,3.47153072139081));
#241238=CARTESIAN_POINT('Ctrl Pts',(61.0844267823321,12.789335088505,3.47182327905198));
#241239=CARTESIAN_POINT('Ctrl Pts',(60.978503758349,12.7666250660186,3.40413028377993));
#241240=CARTESIAN_POINT('Origin',(60.5836663843182,12.5528626811449,3.64303198860273));
#241241=CARTESIAN_POINT('Origin',(5.72205236298458E-15,1.8633692237856E-13,
2.53178198860262));
#241242=CARTESIAN_POINT('Origin',(57.7418065394566,12.257819391977,2.53178198860271));
#241243=CARTESIAN_POINT('Origin',(59.5987607253194,12.3435145206988,3.64303198860272));
#241244=CARTESIAN_POINT('Origin',(60.1910940874972,12.4693660187261,3.64299466007668));
#241245=CARTESIAN_POINT('Ctrl Pts',(57.6364522029207,12.2354540642047,2.59908173516033));
#241246=CARTESIAN_POINT('Ctrl Pts',(57.6729438621906,12.2432007592849,2.65878198860272));
#241247=CARTESIAN_POINT('Ctrl Pts',(57.7418065394566,12.257819391977,2.65878198860271));
#241248=CARTESIAN_POINT('Ctrl Pts',(57.6546556225249,12.1497054461945,2.59908193200013));
#241249=CARTESIAN_POINT('Ctrl Pts',(57.6862025493675,12.1807288143664,2.65877685806641));
#241250=CARTESIAN_POINT('Ctrl Pts',(57.7523715145553,12.2080066271961,2.65878198860271));
#241251=CARTESIAN_POINT('Ctrl Pts',(57.6955109599436,12.07549391746,2.63872492669823));
#241252=CARTESIAN_POINT('Ctrl Pts',(57.7206875210986,12.1277502414154,2.69532212015283));
#241253=CARTESIAN_POINT('Ctrl Pts',(57.786160923601,12.1670355805165,2.68176836726644));
#241254=CARTESIAN_POINT('Ctrl Pts',(57.7879231380266,11.9863964689866,2.75442176402243));
#241255=CARTESIAN_POINT('Ctrl Pts',(57.7928648378988,12.078208678266,2.79203179920148));
#241256=CARTESIAN_POINT('Ctrl Pts',(57.8693039540642,12.1215423041374,2.74885310748183));
#241257=CARTESIAN_POINT('Ctrl Pts',(57.8386735460214,11.9699873265231,2.8286608955842));
#241258=CARTESIAN_POINT('Ctrl Pts',(57.8311081991734,12.0820993460728,2.85316563119168));
#241259=CARTESIAN_POINT('Ctrl Pts',(57.9177340744074,12.1160385312531,2.79189751796631));
#241260=CARTESIAN_POINT('Ctrl Pts',(57.8830978693156,11.9794294790614,2.90134173516032));
#241261=CARTESIAN_POINT('Ctrl Pts',(57.8572899778511,12.1031907419159,2.90103711553238));
#241262=CARTESIAN_POINT('Ctrl Pts',(57.9621601888121,12.1254815933794,2.8340419886027));
#241263=CARTESIAN_POINT('Origin',(57.9885649735459,12.0012568480862,2.83404198860271));
#241264=CARTESIAN_POINT('Origin',(60.1478239214148,12.4602215058071,3.56647653971879));
#241265=CARTESIAN_POINT('Origin',(60.0677739512126,12.4432063593724,3.42473028058494));
#241266=CARTESIAN_POINT('Origin',(58.1628213391868,12.0382961820438,3.11913648168105));
#241267=CARTESIAN_POINT('Origin',(58.3370777047235,12.0753355159235,3.4042309748332));
#241268=CARTESIAN_POINT('Ctrl Pts',(59.7450242491248,12.3746037924166,3.36123028058491));
#241269=CARTESIAN_POINT('Ctrl Pts',(59.7186194643909,12.4988285377098,3.36123028058491));
#241270=CARTESIAN_POINT('Ctrl Pts',(59.7186194643909,12.4988285377098,3.23423028058491));
#241271=CARTESIAN_POINT('Ctrl Pts',(59.8330190893702,12.3935470970139,3.36123028058491));
#241272=CARTESIAN_POINT('Ctrl Pts',(59.8065803155747,12.5175251937986,3.360996411086));
#241273=CARTESIAN_POINT('Ctrl Pts',(59.850683147391,12.5268995400898,3.23423043688411));
#241274=CARTESIAN_POINT('Ctrl Pts',(59.9162252185215,12.4114576311017,3.41054258905295));
#241275=CARTESIAN_POINT('Ctrl Pts',(59.8901687840297,12.5352924712488,3.41008815825902));
#241276=CARTESIAN_POINT('Ctrl Pts',(59.975558754836,12.5534426698448,3.30819867304308));
#241277=CARTESIAN_POINT('Ctrl Pts',(59.9600752506737,12.4208962741589,3.48823028058493));
#241278=CARTESIAN_POINT('Ctrl Pts',(59.9342688867325,12.5446662374489,3.48794691941609));
#241279=CARTESIAN_POINT('Ctrl Pts',(60.0413691664787,12.5674311046656,3.42473028058495));
#241280=CARTESIAN_POINT('Origin',(59.7450242491248,12.3746037924166,3.23423028058491));
#241281=CARTESIAN_POINT('Ctrl Pts',(58.2316113004781,12.0535047649324,3.47153072139082));
#241282=CARTESIAN_POINT('Ctrl Pts',(58.2057612755555,12.1774537741287,3.47122746285087));
#241283=CARTESIAN_POINT('Ctrl Pts',(58.3108302788454,12.199593564085,3.40413046676797));
#241284=CARTESIAN_POINT('Ctrl Pts',(58.3441059109581,12.0772900304169,3.65553813457996));
#241285=CARTESIAN_POINT('Ctrl Pts',(58.3180696991549,12.2013259468569,3.65520336072245));
#241286=CARTESIAN_POINT('Ctrl Pts',(58.400772540275,12.218711381782,3.55128134519958));
#241287=CARTESIAN_POINT('Ctrl Pts',(58.5461981381264,12.1200201767777,3.77003198860273));
#241288=CARTESIAN_POINT('Ctrl Pts',(58.5199882620693,12.2442455720377,3.7698020931414));
#241289=CARTESIAN_POINT('Ctrl Pts',(58.562349768553,12.2530556816161,3.64284195387389));
#241290=CARTESIAN_POINT('Ctrl Pts',(58.7584778814676,12.1649068885794,3.77003198860273));
#241291=CARTESIAN_POINT('Ctrl Pts',(58.7320335442281,12.289317713782,3.77003198860273));
#241292=CARTESIAN_POINT('Ctrl Pts',(58.7320731263129,12.2891314947139,3.64284189403811));
#241293=CARTESIAN_POINT('Origin',(58.7584778814676,12.1649068885794,3.64303198860273));
#241294=CARTESIAN_POINT('Origin',(58.1567073854021,12.0369966210212,3.2342302805849));
#241295=CARTESIAN_POINT('Origin',(59.5971203935659,12.3431658574213,3.23423028058491));
#241296=CARTESIAN_POINT('Origin',(57.9308881865554,11.9889972685553,3.64303198860271));
#241297=CARTESIAN_POINT('Origin',(59.1510793400373,12.2483049654005,3.64299171721818));
#241298=CARTESIAN_POINT('Ctrl Pts',(59.3820708699071,12.2968658913805,3.4882302805849));
#241299=CARTESIAN_POINT('Ctrl Pts',(59.3560370505014,12.4217592664914,3.48852004212268));
#241300=CARTESIAN_POINT('Ctrl Pts',(59.2479658375576,12.3987880210526,3.4247302805849));
#241301=CARTESIAN_POINT('Ctrl Pts',(59.4260685345961,12.3063392072225,3.41028005848414));
#241302=CARTESIAN_POINT('Ctrl Pts',(59.3998259533503,12.4310668851196,3.41074404220356));
#241303=CARTESIAN_POINT('Ctrl Pts',(59.3139986558962,12.412823729876,3.30780486243865));
#241304=CARTESIAN_POINT('Ctrl Pts',(59.5094220566593,12.3242857901784,3.36123028058491));
#241305=CARTESIAN_POINT('Ctrl Pts',(59.4828840257734,12.4487214234142,3.36146460586404));
#241306=CARTESIAN_POINT('Ctrl Pts',(59.4390967537846,12.4394141514346,3.23423045308438));
#241307=CARTESIAN_POINT('Ctrl Pts',(59.5971203935659,12.3431658574213,3.36123028058491));
#241308=CARTESIAN_POINT('Ctrl Pts',(59.5707156088321,12.4673906027145,3.36123028058491));
#241309=CARTESIAN_POINT('Ctrl Pts',(59.5707156088321,12.4673906027145,3.23423028058491));
#241310=CARTESIAN_POINT('Origin',(59.2743706222915,12.2745632757594,3.4247302805849));
#241311=CARTESIAN_POINT('Origin',(59.194798053941,12.2576496039181,3.56563113524751));
#241312=CARTESIAN_POINT('Origin',(58.3196542523191,19.2830435999599,3.56647653909436));
#241313=CARTESIAN_POINT('Origin',(58.361699570716,19.2967593024467,3.6429946600746));
#241314=CARTESIAN_POINT('Origin',(58.2418213702174,19.2577541638581,3.42473028058498));
#241315=CARTESIAN_POINT('Ctrl Pts',(58.1373965169893,19.2232259141442,3.48823028058498));
#241316=CARTESIAN_POINT('Ctrl Pts',(58.1769325318819,19.103134799739,3.48794691941614));
#241317=CARTESIAN_POINT('Ctrl Pts',(58.281066528503,19.1369699862886,3.42473028058499));
#241318=CARTESIAN_POINT('Ctrl Pts',(58.0945576760632,19.2094285342456,3.410280059251));
#241319=CARTESIAN_POINT('Ctrl Pts',(58.1339089916607,19.089155604122,3.40982512231157));
#241320=CARTESIAN_POINT('Ctrl Pts',(58.2168625998345,19.1161088652887,3.30780486372925));
#241321=CARTESIAN_POINT('Ctrl Pts',(58.0133994748125,19.1832899764608,3.36123028058496));
#241322=CARTESIAN_POINT('Ctrl Pts',(58.0524922023746,19.0627016856749,3.36099721048456));
#241323=CARTESIAN_POINT('Ctrl Pts',(58.0952292882363,19.0765878066324,3.23423045308386));
#241324=CARTESIAN_POINT('Ctrl Pts',(57.9280106456676,19.1557908785627,3.36123028058496));
#241325=CARTESIAN_POINT('Ctrl Pts',(57.9672558039532,19.0350067009933,3.36123028058496));
#241326=CARTESIAN_POINT('Ctrl Pts',(57.9672558039532,19.0350067009933,3.23423028058496));
#241327=CARTESIAN_POINT('Origin',(57.9280106456676,19.1557908785627,3.23423028058496));
#241328=CARTESIAN_POINT('Origin',(-0.0981128957140405,0.301960443923895,
3.64303198860263));
#241329=CARTESIAN_POINT('Origin',(58.7434254837932,19.4207352200703,3.64303198860277));
#241330=CARTESIAN_POINT('Origin',(-0.0981128957140404,0.301960443923898,
3.23423028058482));
#241331=CARTESIAN_POINT('Origin',(57.7842031819383,19.1090650011318,3.23423028058496));
#241332=CARTESIAN_POINT('Ctrl Pts',(59.2554138597571,19.5876674457081,3.47153072139086));
#241333=CARTESIAN_POINT('Ctrl Pts',(59.2953329099159,19.4663243174863,3.47182327902676));
#241334=CARTESIAN_POINT('Ctrl Pts',(59.1922458813531,19.4330302542695,3.40413028959063));
#241335=CARTESIAN_POINT('Ctrl Pts',(59.1460959632229,19.5520255367076,3.6555380712097));
#241336=CARTESIAN_POINT('Ctrl Pts',(59.1858279145887,19.4307442612476,3.65586275496854));
#241337=CARTESIAN_POINT('Ctrl Pts',(59.1047949412317,19.4046157212337,3.55128126837225));
#241338=CARTESIAN_POINT('Ctrl Pts',(58.9497105734782,19.4879954548407,3.77003198860277));
#241339=CARTESIAN_POINT('Ctrl Pts',(58.9892603680798,19.3668760934059,3.77025505748615));
#241340=CARTESIAN_POINT('Ctrl Pts',(58.9476928828794,19.3535701679107,3.64284211731241));
#241341=CARTESIAN_POINT('Ctrl Pts',(58.7434254837932,19.4207352200703,3.77003198860277));
#241342=CARTESIAN_POINT('Ctrl Pts',(58.7827292725254,19.2997705965407,3.77003198860277));
#241343=CARTESIAN_POINT('Ctrl Pts',(58.7826705983486,19.2999511770886,3.64284239821754));
#241344=CARTESIAN_POINT('Origin',(59.1531540087999,19.5538640879535,3.40423097483324));
#241345=CARTESIAN_POINT('Ctrl Pts',(57.7842031819382,19.1090650011318,3.36123028058496));
#241346=CARTESIAN_POINT('Ctrl Pts',(57.8234483402239,18.9882808235623,3.36123028058496));
#241347=CARTESIAN_POINT('Ctrl Pts',(57.8234483402239,18.9882808235623,3.23423028058496));
#241348=CARTESIAN_POINT('Ctrl Pts',(57.6985255711019,19.0814735135848,3.36123028058496));
#241349=CARTESIAN_POINT('Ctrl Pts',(57.7377609320111,18.9604392969148,3.36146538610105));
#241350=CARTESIAN_POINT('Ctrl Pts',(57.6950423231338,18.9465591794949,3.23423043688411));
#241351=CARTESIAN_POINT('Ctrl Pts',(57.6175103216835,19.0553854270318,3.41054258693115));
#241352=CARTESIAN_POINT('Ctrl Pts',(57.6571482613586,18.9342466524541,3.41100608859817));
#241353=CARTESIAN_POINT('Ctrl Pts',(57.5736252790864,18.9071083904255,3.30819866970882));
#241354=CARTESIAN_POINT('Ctrl Pts',(57.5748148483576,19.041637186088,3.48823028058495));
#241355=CARTESIAN_POINT('Ctrl Pts',(57.6147155869502,18.9204594407748,3.48852004212273));
#241356=CARTESIAN_POINT('Ctrl Pts',(57.5096375484037,18.8863175164095,3.42473028058495));
#241357=CARTESIAN_POINT('Origin',(57.4703923901181,19.007101693979,3.42473028058494));
#241358=CARTESIAN_POINT('Origin',(59.3225838821626,19.6089151909161,3.11913648178297));
#241359=CARTESIAN_POINT('Origin',(59.4920137553139,19.6639662938564,2.83404198860276));
#241360=CARTESIAN_POINT('Origin',(57.3930236876037,18.9819630786539,3.56563113460818));
#241361=CARTESIAN_POINT('Origin',(57.3504898524409,18.9681964166835,3.64299171721781));
#241362=CARTESIAN_POINT('Ctrl Pts',(59.8682321556242,19.4684195516699,2.59908173516038));
#241363=CARTESIAN_POINT('Ctrl Pts',(59.8327559231846,19.4568831131886,2.65878198860276));
#241364=CARTESIAN_POINT('Ctrl Pts',(59.7658094374951,19.4351129318423,2.65878198860276));
#241365=CARTESIAN_POINT('Ctrl Pts',(59.8409825629599,19.5522156237496,2.5990819347567));
#241366=CARTESIAN_POINT('Ctrl Pts',(59.8129039518352,19.5179203859181,2.65878715325351));
#241367=CARTESIAN_POINT('Ctrl Pts',(59.7500277420787,19.4836145615372,2.65878198860276));
#241368=CARTESIAN_POINT('Ctrl Pts',(59.7920481472525,19.6218019328335,2.6387877884989));
#241369=CARTESIAN_POINT('Ctrl Pts',(59.7726277678661,19.5669820401374,2.6956446018013));
#241370=CARTESIAN_POINT('Ctrl Pts',(59.7116747787988,19.5206357546568,2.68180481624901));
#241371=CARTESIAN_POINT('Ctrl Pts',(59.6899788477097,19.700783843471,2.75443238878654));
#241372=CARTESIAN_POINT('Ctrl Pts',(59.6952619726971,19.6084674936732,2.79268340777105));
#241373=CARTESIAN_POINT('Ctrl Pts',(59.6234872553896,19.5568961981638,2.74885926835621));
#241374=CARTESIAN_POINT('Ctrl Pts',(59.6375245663856,19.7118189603904,2.82856655361687));
#241375=CARTESIAN_POINT('Ctrl Pts',(59.6577198343149,19.6003923959453,2.85384197230812));
#241376=CARTESIAN_POINT('Ctrl Pts',(59.5745070768392,19.5572342963493,2.79184624278451));
#241377=CARTESIAN_POINT('Ctrl Pts',(59.5942745858236,19.6977666881848,2.90134173516037));
#241378=CARTESIAN_POINT('Ctrl Pts',(59.6341304551457,19.5766071063171,2.90163218716404));
#241379=CARTESIAN_POINT('Ctrl Pts',(59.5312589135995,19.5431821162869,2.83404198860275));
#241380=CARTESIAN_POINT('Origin',(59.7658094374951,19.4351129318423,2.53178198860275));
#241381=CARTESIAN_POINT('Origin',(-0.0981128957140405,0.301960443923895,
3.64303198860263));
#241382=CARTESIAN_POINT('Origin',(56.9687879773466,18.8441205405522,3.64303198860276));
#241383=CARTESIAN_POINT('Origin',(5.50785759597432E-15,1.85831596474898E-13,
2.53178198860262));
#241384=CARTESIAN_POINT('Origin',(59.7752282754837,19.4061247292256,2.53178198860276));
#241385=CARTESIAN_POINT('Ctrl Pts',(56.9687879773466,18.8441205405522,3.77003198860277));
#241386=CARTESIAN_POINT('Ctrl Pts',(57.0080919266514,18.7231554228307,3.77003198860277));
#241387=CARTESIAN_POINT('Ctrl Pts',(57.0080330916623,18.7233364983081,3.64284187937081));
#241388=CARTESIAN_POINT('Ctrl Pts',(56.7625017687172,18.7768526573606,3.77003198860276));
#241389=CARTESIAN_POINT('Ctrl Pts',(56.801916058745,18.6561653631331,3.7698020896293));
#241390=CARTESIAN_POINT('Ctrl Pts',(56.8430078886249,18.6697165591961,3.64284193928345));
#241391=CARTESIAN_POINT('Ctrl Pts',(56.5661212433897,18.7128124416003,3.65553535416601));
#241392=CARTESIAN_POINT('Ctrl Pts',(56.6055911857651,18.5923760693057,3.65520057834411));
#241393=CARTESIAN_POINT('Ctrl Pts',(56.6859069993072,18.618671385701,3.55127910964192));
#241394=CARTESIAN_POINT('Ctrl Pts',(56.4568070719811,18.6771643191712,3.47153072139087));
#241395=CARTESIAN_POINT('Ctrl Pts',(56.4963948028695,18.5568963021135,3.47122746281597));
#241396=CARTESIAN_POINT('Ctrl Pts',(56.5984571310816,18.5902572009362,3.40413045901299));
#241397=CARTESIAN_POINT('Origin',(56.5590590327989,18.7109915363519,3.40423097483324));
#241398=CARTESIAN_POINT('Ctrl Pts',(59.7908376697911,19.0928077206414,2.90134173516038));
#241399=CARTESIAN_POINT('Ctrl Pts',(59.7518659300026,19.2142545736086,2.90163218716405));
#241400=CARTESIAN_POINT('Ctrl Pts',(59.6489943884564,19.1808295835784,2.83404198860276));
#241401=CARTESIAN_POINT('Ctrl Pts',(59.8341069976972,19.1068672906324,2.82853349835363));
#241402=CARTESIAN_POINT('Ctrl Pts',(59.7849495554008,19.2088743168611,2.85381483162395));
#241403=CARTESIAN_POINT('Ctrl Pts',(59.6922622581485,19.1948881666554,2.7918270159429));
#241404=CARTESIAN_POINT('Ctrl Pts',(59.8698829694068,19.1465773683628,2.75468822073666));
#241405=CARTESIAN_POINT('Ctrl Pts',(59.8199164124673,19.2244455609615,2.79286913083863));
#241406=CARTESIAN_POINT('Ctrl Pts',(59.7315159919505,19.2238994150015,2.74900763297922));
#241407=CARTESIAN_POINT('Ctrl Pts',(59.9060262085835,19.2694731179105,2.63954450640398));
#241408=CARTESIAN_POINT('Ctrl Pts',(59.8580612818573,19.3027624708831,2.69627684028865));
#241409=CARTESIAN_POINT('Ctrl Pts',(59.7814166574712,19.3044519280754,2.6822435603651));
#241410=CARTESIAN_POINT('Ctrl Pts',(59.9049660265691,19.3552948408466,2.59908178706338));
#241411=CARTESIAN_POINT('Ctrl Pts',(59.8620777700642,19.3665789650876,2.65878704321569));
#241412=CARTESIAN_POINT('Ctrl Pts',(59.7910213450144,19.35744929649,2.65878198860276));
#241413=CARTESIAN_POINT('Ctrl Pts',(59.8776671349985,19.4393816709759,2.59908173516038));
#241414=CARTESIAN_POINT('Ctrl Pts',(59.8421853116552,19.4278624395269,2.65878198860276));
#241415=CARTESIAN_POINT('Ctrl Pts',(59.7752282754837,19.4061247292256,2.65878198860276));
#241416=CARTESIAN_POINT('Origin',(59.688239546742,19.0600454060089,2.83404198860274));
#241417=CARTESIAN_POINT('Origin',(56.3896289265484,18.655940357665,3.1191364816716));
#241418=CARTESIAN_POINT('Origin',(56.2201988201383,18.6008891789888,2.83404198860276));
#241419=CARTESIAN_POINT('Origin',(59.5188096735651,19.004994303108,3.11913648177534));
#241420=CARTESIAN_POINT('Origin',(59.349379800228,18.949943200106,3.40423097483324));
#241421=CARTESIAN_POINT('Ctrl Pts',(56.1179479440988,18.5670586829468,2.90134173516037));
#241422=CARTESIAN_POINT('Ctrl Pts',(56.1574782858997,18.4469743395782,2.90103711553243));
#241423=CARTESIAN_POINT('Ctrl Pts',(56.2594439784239,18.4801050014193,2.83404198860275));
#241424=CARTESIAN_POINT('Ctrl Pts',(56.0747358697604,18.5530176696409,2.82862991747964));
#241425=CARTESIAN_POINT('Ctrl Pts',(56.124241038399,18.4521518441037,2.853140458864));
#241426=CARTESIAN_POINT('Ctrl Pts',(56.2162299491245,18.4660639121464,2.79187960999976));
#241427=CARTESIAN_POINT('Ctrl Pts',(56.0391722633447,18.5135050040177,2.75470625793355));
#241428=CARTESIAN_POINT('Ctrl Pts',(56.0893377355418,18.4363793473474,2.79224250381941));
#241429=CARTESIAN_POINT('Ctrl Pts',(56.17722474395,18.4371504234765,2.74901809108276));
#241430=CARTESIAN_POINT('Ctrl Pts',(56.0036796861845,18.3911086652348,2.63947868311697));
#241431=CARTESIAN_POINT('Ctrl Pts',(56.051644941423,18.3580919822894,2.69595066767905));
#241432=CARTESIAN_POINT('Ctrl Pts',(56.1280773042132,18.3567819283755,2.68220539436071));
#241433=CARTESIAN_POINT('Ctrl Pts',(56.0051563026341,18.3056594201307,2.59908178585071));
#241434=CARTESIAN_POINT('Ctrl Pts',(56.0480033886683,18.2945198471562,2.65877670944838));
#241435=CARTESIAN_POINT('Ctrl Pts',(56.1189701685708,18.3039075553121,2.65878198860275));
#241436=CARTESIAN_POINT('Ctrl Pts',(56.0323588238391,18.2220120550219,2.59908173516037));
#241437=CARTESIAN_POINT('Ctrl Pts',(56.0678348753332,18.233549049922,2.65878198860275));
#241438=CARTESIAN_POINT('Ctrl Pts',(56.1347810195642,18.2553202812751,2.65878198860275));
#241439=CARTESIAN_POINT('Origin',(56.1347810195642,18.2553202812751,2.53178198860275));
#241440=CARTESIAN_POINT('Ctrl Pts',(58.9396512752213,18.8168143322229,3.77003198860277));
#241441=CARTESIAN_POINT('Ctrl Pts',(58.9003474831029,18.9377789661741,3.77003198860277));
#241442=CARTESIAN_POINT('Ctrl Pts',(58.9004061606709,18.9375983751891,3.64284238727594));
#241443=CARTESIAN_POINT('Ctrl Pts',(59.1460772043121,18.8836520326596,3.77003198860278));
#241444=CARTESIAN_POINT('Ctrl Pts',(59.1068814887048,19.0048864565363,3.77025506105934));
#241445=CARTESIAN_POINT('Ctrl Pts',(59.0654310094281,18.9912181986574,3.64284210641901));
#241446=CARTESIAN_POINT('Ctrl Pts',(59.3425907075099,18.9472825415239,3.65553527987848));
#241447=CARTESIAN_POINT('Ctrl Pts',(59.3034471832918,19.0687550219942,3.65585996532983));
#241448=CARTESIAN_POINT('Ctrl Pts',(59.2225318234683,19.0422633471877,3.55127902710181));
#241449=CARTESIAN_POINT('Ctrl Pts',(59.4519788726607,18.9827025415099,3.47153072139086));
#241450=CARTESIAN_POINT('Ctrl Pts',(59.4129503580329,19.1043350338628,3.47182327905202));
#241451=CARTESIAN_POINT('Ctrl Pts',(59.3099814352093,19.070677448334,3.40413028377992));
#241452=CARTESIAN_POINT('Origin',(58.9396512752213,18.8168143322229,3.64303198860277));
#241453=CARTESIAN_POINT('Origin',(5.72046327455653E-15,1.86342852937311E-13,
2.53178198860262));
#241454=CARTESIAN_POINT('Origin',(56.1441998575527,18.2263320786585,2.53178198860275));
#241455=CARTESIAN_POINT('Origin',(56.3788528200606,17.9847604760584,3.64303198860276));
#241456=CARTESIAN_POINT('Origin',(58.557957308329,18.6927400943496,3.64299466007604));
#241457=CARTESIAN_POINT('Ctrl Pts',(56.0417604764383,18.1930767435951,2.59908173516037));
#241458=CARTESIAN_POINT('Ctrl Pts',(56.0772424804484,18.2045954185348,2.65878198860275));
#241459=CARTESIAN_POINT('Ctrl Pts',(56.1441998575527,18.2263320786585,2.65878198860275));
#241460=CARTESIAN_POINT('Ctrl Pts',(56.0688273470726,18.1097006409637,2.59908193199914));
#241461=CARTESIAN_POINT('Ctrl Pts',(56.0969586315475,18.143851611662,2.65877685806678));
#241462=CARTESIAN_POINT('Ctrl Pts',(56.1599138083653,18.1778965340264,2.65878198860275));
#241463=CARTESIAN_POINT('Ctrl Pts',(56.117216091734,18.0401661963853,2.63872492669811));
#241464=CARTESIAN_POINT('Ctrl Pts',(56.1367924598137,18.0947679219783,2.69532212015279));
#241465=CARTESIAN_POINT('Ctrl Pts',(56.1978007560413,18.1406818860298,2.68176836726648));
#241466=CARTESIAN_POINT('Ctrl Pts',(56.2184352456064,17.9612165360193,2.75442176402263));
#241467=CARTESIAN_POINT('Ctrl Pts',(56.2137528851844,18.0530423367035,2.79203179920163));
#241468=CARTESIAN_POINT('Ctrl Pts',(56.2852436625535,18.1041286397846,2.74885310748188));
#241469=CARTESIAN_POINT('Ctrl Pts',(56.2706228600014,17.9502021467128,2.82866089558414));
#241470=CARTESIAN_POINT('Ctrl Pts',(56.2513800597969,18.0609092108093,2.85316563119182));
#241471=CARTESIAN_POINT('Ctrl Pts',(56.3339837785515,18.1037173431993,2.79189751796638));
#241472=CARTESIAN_POINT('Ctrl Pts',(56.3138168485095,17.9642361803975,2.90134173516036));
#241473=CARTESIAN_POINT('Ctrl Pts',(56.2752137607566,18.0846218068697,2.90103711553242));
#241474=CARTESIAN_POINT('Ctrl Pts',(56.3771794532807,18.1177524687109,2.83404198860275));
#241475=CARTESIAN_POINT('Origin',(56.4164246115663,17.9969682911414,2.83404198860275));
#241476=CARTESIAN_POINT('Origin',(58.5158800426277,18.6791227120617,3.56647653971811));
#241477=CARTESIAN_POINT('Origin',(58.4380471616454,18.6538332760107,3.42473028058499));
#241478=CARTESIAN_POINT('Origin',(56.5858547179432,18.0520194698692,3.11913648168141));
#241479=CARTESIAN_POINT('Origin',(56.755284824227,18.1070706485045,3.40423097483324));
#241480=CARTESIAN_POINT('Ctrl Pts',(58.1242364370956,18.5518699907153,3.36123028058495));
#241481=CARTESIAN_POINT('Ctrl Pts',(58.08499127881,18.6726541682848,3.36123028058495));
#241482=CARTESIAN_POINT('Ctrl Pts',(58.08499127881,18.6726541682848,3.23423028058495));
#241483=CARTESIAN_POINT('Ctrl Pts',(58.2097691178803,18.5799074873345,3.36123028058495));
#241484=CARTESIAN_POINT('Ctrl Pts',(58.1705159385191,18.7004428147373,3.36099641108521));
#241485=CARTESIAN_POINT('Ctrl Pts',(58.2133972843954,18.7143758086141,3.23423043688441));
#241486=CARTESIAN_POINT('Ctrl Pts',(58.2906472745455,18.6064173144578,3.41054258905298));
#241487=CARTESIAN_POINT('Ctrl Pts',(58.2517893143876,18.726850135337,3.41008815826));
#241488=CARTESIAN_POINT('Ctrl Pts',(58.3348142976333,18.7538265876728,3.30819867304287));
#241489=CARTESIAN_POINT('Ctrl Pts',(58.3332704847796,18.620387828115,3.48823028058497));
#241490=CARTESIAN_POINT('Ctrl Pts',(58.2946680067388,18.7407822670305,3.48794691941613));
#241491=CARTESIAN_POINT('Ctrl Pts',(58.3988020033598,18.7746174535802,3.42473028058498));
#241492=CARTESIAN_POINT('Origin',(58.1242364370957,18.5518699907153,3.23423028058495));
#241493=CARTESIAN_POINT('Ctrl Pts',(56.6526781108323,18.0743352474894,3.47153072139085));
#241494=CARTESIAN_POINT('Ctrl Pts',(56.6140134955962,18.1949031876636,3.4712274628509));
#241495=CARTESIAN_POINT('Ctrl Pts',(56.7161926816712,18.227904394985,3.40413046676804));
#241496=CARTESIAN_POINT('Ctrl Pts',(56.7620702268163,18.1097491035594,3.65553813458));
#241497=CARTESIAN_POINT('Ctrl Pts',(56.7232113603703,18.2303840130651,3.65520336072255));
#241498=CARTESIAN_POINT('Ctrl Pts',(56.8036438738775,18.2563190096466,3.55128134519941));
#241499=CARTESIAN_POINT('Ctrl Pts',(56.9585888550845,18.1733695596525,3.77003198860277));
#241500=CARTESIAN_POINT('Ctrl Pts',(56.9195374698046,18.2941747571327,3.76980209314092));
#241501=CARTESIAN_POINT('Ctrl Pts',(56.9607460083083,18.3073645871834,3.64284195387411));
#241502=CARTESIAN_POINT('Ctrl Pts',(57.1650137687747,18.2401996527047,3.77003198860277));
#241503=CARTESIAN_POINT('Ctrl Pts',(57.1257098240091,18.3611647564558,3.77003198860277));
#241504=CARTESIAN_POINT('Ctrl Pts',(57.1257686544522,18.3609836949697,3.64284189403821));
#241505=CARTESIAN_POINT('Origin',(57.1650137687747,18.2401996527048,3.64303198860277));
#241506=CARTESIAN_POINT('Origin',(55.0155724295758,17.5418038257018,3.23423028058494));
#241507=CARTESIAN_POINT('Origin',(57.9804289733664,18.5051441132844,3.23423028058495));
#241508=CARTESIAN_POINT('Origin',(54.8020887275094,17.4724387660757,3.64303198860275));
#241509=CARTESIAN_POINT('Origin',(57.5467470426661,18.3641788932758,3.64299171721809));
#241510=CARTESIAN_POINT('Ctrl Pts',(57.7713971777987,18.4366189870675,3.48823028058495));
#241511=CARTESIAN_POINT('Ctrl Pts',(57.732451061807,18.5581069080663,3.48852004212273));
#241512=CARTESIAN_POINT('Ctrl Pts',(57.6273730232605,18.523964983701,3.42473028058495));
#241513=CARTESIAN_POINT('Ctrl Pts',(57.81416358753,18.4506394153714,3.41028005848421));
#241514=CARTESIAN_POINT('Ctrl Pts',(57.7750271733923,18.571940725309,3.4107440422031));
#241515=CARTESIAN_POINT('Ctrl Pts',(57.691576975838,18.5448261124695,3.30780486243884));
#241516=CARTESIAN_POINT('Ctrl Pts',(57.8951845615409,18.4772005006368,3.36123028058495));
#241517=CARTESIAN_POINT('Ctrl Pts',(57.8557848432471,18.5981804828671,3.36146460586464));
#241518=CARTESIAN_POINT('Ctrl Pts',(57.8132103173518,18.5843471808459,3.2342304530846));
#241519=CARTESIAN_POINT('Ctrl Pts',(57.9804289733664,18.5051441132844,3.36123028058495));
#241520=CARTESIAN_POINT('Ctrl Pts',(57.9411838150807,18.6259282908539,3.36123028058495));
#241521=CARTESIAN_POINT('Ctrl Pts',(57.9411838150807,18.6259282908539,3.23423028058495));
#241522=CARTESIAN_POINT('Origin',(57.6666181815461,18.4031808061315,3.42473028058494));
#241523=CARTESIAN_POINT('Origin',(57.5892494801763,18.378042190866,3.56563113524728));
#241524=CARTESIAN_POINT('Origin',(55.9845461696119,25.2734729067944,3.56647653909496));
#241525=CARTESIAN_POINT('Origin',(56.024927478051,25.291508405747,3.642994660078));
#241526=CARTESIAN_POINT('Origin',(55.9097831300746,25.2401862573144,3.42473028058502));
#241527=CARTESIAN_POINT('Ctrl Pts',(55.8095395120007,25.1949317875303,3.48823028058502));
#241528=CARTESIAN_POINT('Ctrl Pts',(55.8614118841079,25.0796311836956,3.48794691941618));
#241529=CARTESIAN_POINT('Ctrl Pts',(55.9614386837453,25.1241659841938,3.42473028058503));
#241530=CARTESIAN_POINT('Ctrl Pts',(55.768377565646,25.1767321129109,3.41028005925103));
#241531=CARTESIAN_POINT('Ctrl Pts',(55.8200852551805,25.0612313830313,3.40982512231043));
#241532=CARTESIAN_POINT('Ctrl Pts',(55.8997670518382,25.096708004599,3.30780486372873));
#241533=CARTESIAN_POINT('Ctrl Pts',(55.69039618079,25.142253402824,3.36123028058499));
#241534=CARTESIAN_POINT('Ctrl Pts',(55.7418796630224,25.0264120100475,3.36099721048512));
#241535=CARTESIAN_POINT('Ctrl Pts',(55.7829311357718,25.0446893032919,3.23423045308384));
#241536=CARTESIAN_POINT('Ctrl Pts',(55.6083495590301,25.1059793847704,3.361230280585));
#241537=CARTESIAN_POINT('Ctrl Pts',(55.6600051127008,24.9899591116498,3.36123028058499));
#241538=CARTESIAN_POINT('Ctrl Pts',(55.6600051127007,24.9899591116498,3.234230280585));
#241539=CARTESIAN_POINT('Origin',(55.6083495590301,25.1059793847704,3.234230280585));
#241540=CARTESIAN_POINT('Origin',(-0.129138884176561,0.29005068280171,3.64303198860263));
#241541=CARTESIAN_POINT('Origin',(56.391603244485,25.4547063934086,3.64303198860281));
#241542=CARTESIAN_POINT('Origin',(-0.129138884176561,0.290050682801712,
3.23423028058482));
#241543=CARTESIAN_POINT('Origin',(55.4702140717966,25.044477503395,3.234230280585));
#241544=CARTESIAN_POINT('Ctrl Pts',(56.8833377255394,25.6742415049982,3.47153072139089));
#241545=CARTESIAN_POINT('Ctrl Pts',(56.9357219056859,25.557735784097,3.4718232790268));
#241546=CARTESIAN_POINT('Ctrl Pts',(56.8366797759152,25.5138485805639,3.4041302895904));
#241547=CARTESIAN_POINT('Ctrl Pts',(56.7783442778561,25.6273680143726,3.65553807120976));
#241548=CARTESIAN_POINT('Ctrl Pts',(56.8305359187846,25.5109042502493,3.65586275496975));
#241549=CARTESIAN_POINT('Ctrl Pts',(56.75267802867,25.4764485929324,3.55128126837275));
#241550=CARTESIAN_POINT('Ctrl Pts',(56.589727673885,25.5431608329956,3.77003198860282));
#241551=CARTESIAN_POINT('Ctrl Pts',(56.6417212312943,25.4268390553474,3.77025505748559));
#241552=CARTESIAN_POINT('Ctrl Pts',(56.6017723050711,25.4092610357532,3.6428421173121));
#241553=CARTESIAN_POINT('Ctrl Pts',(56.391603244485,25.4547063934086,3.77003198860282));
#241554=CARTESIAN_POINT('Ctrl Pts',(56.4433359691576,25.3385127913797,3.77003198860282));
#241555=CARTESIAN_POINT('Ctrl Pts',(56.4432587405968,25.3386862495674,3.64284239821708));
#241556=CARTESIAN_POINT('Origin',(56.7851714777847,25.6299342604998,3.40423097483328));
#241557=CARTESIAN_POINT('Ctrl Pts',(55.4702140717966,25.044477503395,3.361230280585));
#241558=CARTESIAN_POINT('Ctrl Pts',(55.5218696254673,24.9284572302744,3.361230280585));
#241559=CARTESIAN_POINT('Ctrl Pts',(55.5218696254673,24.9284572302744,3.234230280585));
#241560=CARTESIAN_POINT('Ctrl Pts',(55.3878899076697,25.0080814159064,3.361230280585));
#241561=CARTESIAN_POINT('Ctrl Pts',(55.4395618538378,24.8918114493205,3.36146538610114));
#241562=CARTESIAN_POINT('Ctrl Pts',(55.3985281293136,24.8735420580979,3.23423043688406));
#241563=CARTESIAN_POINT('Ctrl Pts',(55.310045415862,24.9736678430967,3.41054258693119));
#241564=CARTESIAN_POINT('Ctrl Pts',(55.3621286647045,24.8573359723243,3.41100608859826));
#241565=CARTESIAN_POINT('Ctrl Pts',(55.2818999508935,24.82161584755,3.30819866970888));
#241566=CARTESIAN_POINT('Ctrl Pts',(55.269020915304,24.9555320242418,3.48823028058499));
#241567=CARTESIAN_POINT('Ctrl Pts',(55.3213695969755,24.8391888661847,3.48852004212277));
#241568=CARTESIAN_POINT('Ctrl Pts',(55.2204359898056,24.794250328961,3.42473028058498));
#241569=CARTESIAN_POINT('Origin',(55.168780436135,24.9102706020816,3.42473028058499));
#241570=CARTESIAN_POINT('Origin',(56.9479187893833,25.7023940320522,3.11913648178455));
#241571=CARTESIAN_POINT('Origin',(57.1106661007665,25.774853803565,2.8340419886028));
#241572=CARTESIAN_POINT('Origin',(55.0944632682972,24.8771824671427,3.56563113460844));
#241573=CARTESIAN_POINT('Origin',(55.0536014459541,24.8590452239602,3.64299171721836));
#241574=CARTESIAN_POINT('Ctrl Pts',(57.5052637377732,25.61970381813,2.59908173516042));
#241575=CARTESIAN_POINT('Ctrl Pts',(57.4711877340329,25.6045223014064,2.6587819886028));
#241576=CARTESIAN_POINT('Ctrl Pts',(57.4068835917979,25.5758735661211,2.6587819886028));
#241577=CARTESIAN_POINT('Ctrl Pts',(57.4694043465862,25.7001924885132,2.59908193475692));
#241578=CARTESIAN_POINT('Ctrl Pts',(57.4450643815391,25.6631501095112,2.65878715325466));
#241579=CARTESIAN_POINT('Ctrl Pts',(57.3861185493425,25.6224598624441,2.6587819886028));
#241580=CARTESIAN_POINT('Ctrl Pts',(57.4134642487754,25.7642825572403,2.63878778849882));
#241581=CARTESIAN_POINT('Ctrl Pts',(57.3998804953989,25.707732991239,2.69564460180121));
#241582=CARTESIAN_POINT('Ctrl Pts',(57.3441059191831,25.6552692732807,2.68180481624899));
#241583=CARTESIAN_POINT('Ctrl Pts',(57.3036982377901,25.8321626496793,2.75443238878672));
#241584=CARTESIAN_POINT('Ctrl Pts',(57.3186021074451,25.7409042554411,2.79268340777125));
#241585=CARTESIAN_POINT('Ctrl Pts',(57.252611247817,25.6821129719829,2.74885926835631));
#241586=CARTESIAN_POINT('Ctrl Pts',(57.2503778226942,25.8376543496547,2.8285665536168));
#241587=CARTESIAN_POINT('Ctrl Pts',(57.2821097063818,25.7289491719109,2.85384197230857));
#241588=CARTESIAN_POINT('Ctrl Pts',(57.2038640469265,25.677329395237,2.79184624278517));
#241589=CARTESIAN_POINT('Ctrl Pts',(57.2088336324698,25.8191582032623,2.90134173516043));
#241590=CARTESIAN_POINT('Ctrl Pts',(57.2611357920724,25.7028284190336,2.9016321871641));
#241591=CARTESIAN_POINT('Ctrl Pts',(57.1623216544371,25.6588335304443,2.83404198860281));
#241592=CARTESIAN_POINT('Origin',(57.4068835917979,25.5758735661211,2.53178198860279));
#241593=CARTESIAN_POINT('Origin',(-0.129138884176561,0.29005068280171,3.64303198860263));
#241594=CARTESIAN_POINT('Origin',(54.6869600343297,24.695750338031,3.64303198860281));
#241595=CARTESIAN_POINT('Origin',(5.51404277916147E-15,1.85815483521814E-13,
2.53178198860262));
#241596=CARTESIAN_POINT('Origin',(57.4192809246789,25.5480287005721,2.5317819886028));
#241597=CARTESIAN_POINT('Ctrl Pts',(54.6869600343297,24.695750338031,3.77003198860281));
#241598=CARTESIAN_POINT('Ctrl Pts',(54.7386929703524,24.579556261302,3.77003198860281));
#241599=CARTESIAN_POINT('Ctrl Pts',(54.738615530126,24.5797301948983,3.64284187937045));
#241600=CARTESIAN_POINT('Ctrl Pts',(54.4888352915928,24.6072881749597,3.77003198860281));
#241601=CARTESIAN_POINT('Ctrl Pts',(54.5406489234213,24.4913819335272,3.76980208962995));
#241602=CARTESIAN_POINT('Ctrl Pts',(54.5800991622565,24.5091541605505,3.64284193928275));
#241603=CARTESIAN_POINT('Ctrl Pts',(54.3002245846706,24.523071423676,3.65553535416607));
#241604=CARTESIAN_POINT('Ctrl Pts',(54.3520673354842,24.4074205468493,3.65520057834532));
#241605=CARTESIAN_POINT('Ctrl Pts',(54.4291945615844,24.4419671033155,3.55127910964304));
#241606=CARTESIAN_POINT('Ctrl Pts',(54.1952354911872,24.4761921430395,3.4715307213909));
#241607=CARTESIAN_POINT('Ctrl Pts',(54.2471777873471,24.3607210114366,3.471227462816));
#241608=CARTESIAN_POINT('Ctrl Pts',(54.3451938439593,24.404567574091,3.4041304590128));
#241609=CARTESIAN_POINT('Origin',(54.2933913980363,24.5205222915154,3.40423097483328));
#241610=CARTESIAN_POINT('Ctrl Pts',(57.467555354514,25.2380597013433,2.90134173516042));
#241611=CARTESIAN_POINT('Ctrl Pts',(57.4161024530843,25.3547675996718,2.9016321871641));
#241612=CARTESIAN_POINT('Ctrl Pts',(57.317288315449,25.3107727110825,2.8340419886028));
#241613=CARTESIAN_POINT('Ctrl Pts',(57.5091180232694,25.2565651278905,2.82853349835381));
#241614=CARTESIAN_POINT('Ctrl Pts',(57.4495672328897,25.3528749970544,2.85381483162391));
#241615=CARTESIAN_POINT('Ctrl Pts',(57.3588496371379,25.3292770036978,2.79182701594204));
#241616=CARTESIAN_POINT('Ctrl Pts',(57.5405471770611,25.2997972770058,2.7546882207365));
#241617=CARTESIAN_POINT('Ctrl Pts',(57.4827148996401,25.3720159720862,2.79286913083861));
#241618=CARTESIAN_POINT('Ctrl Pts',(57.3948558336735,25.3622324578623,2.74900763297944));
#241619=CARTESIAN_POINT('Ctrl Pts',(57.5636463159493,25.4257977880274,2.63954450640422));
#241620=CARTESIAN_POINT('Ctrl Pts',(57.5124644611998,25.4538910783599,2.6962768402887));
#241621=CARTESIAN_POINT('Ctrl Pts',(57.4360631077221,25.4475597357239,2.68224356036497));
#241622=CARTESIAN_POINT('Ctrl Pts',(57.5536211289093,25.5110385513886,2.59908178706382));
#241623=CARTESIAN_POINT('Ctrl Pts',(57.5097883065956,25.5177778164716,2.65878704321471));
#241624=CARTESIAN_POINT('Ctrl Pts',(57.4400754463057,25.5012707422385,2.6587819886028));
#241625=CARTESIAN_POINT('Ctrl Pts',(57.5176823163888,25.5918112338797,2.59908173516042));
#241626=CARTESIAN_POINT('Ctrl Pts',(57.4835989537477,25.5766462455179,2.6587819886028));
#241627=CARTESIAN_POINT('Ctrl Pts',(57.4192809246789,25.5480287005721,2.6587819886028));
#241628=CARTESIAN_POINT('Origin',(57.3689438691196,25.1947524379619,2.8340419886028));
#241629=CARTESIAN_POINT('Origin',(54.1306438627454,24.4480624203093,3.11913648167094));
#241630=CARTESIAN_POINT('Origin',(53.9678963272934,24.3756025490942,2.83404198860279));
#241631=CARTESIAN_POINT('Origin',(57.2061965577015,25.1222926664872,3.11913648177431));
#241632=CARTESIAN_POINT('Origin',(57.0434492461379,25.0498328948967,3.40423097483328));
#241633=CARTESIAN_POINT('Ctrl Pts',(53.8697418420145,24.3312692531091,2.90134173516041));
#241634=CARTESIAN_POINT('Ctrl Pts',(53.9216078643417,24.2159747902189,2.90103711553247));
#241635=CARTESIAN_POINT('Ctrl Pts',(54.0195518809641,24.2595822759735,2.83404198860279));
#241636=CARTESIAN_POINT('Ctrl Pts',(53.8282341734841,24.3127882662182,2.82862991747974));
#241637=CARTESIAN_POINT('Ctrl Pts',(53.8880114973698,24.2176496934292,2.85314045886379));
#241638=CARTESIAN_POINT('Ctrl Pts',(53.9780422761232,24.2411010091826,2.79187960999981));
#241639=CARTESIAN_POINT('Ctrl Pts',(53.7969955864427,24.2697746459844,2.75470625793349));
#241640=CARTESIAN_POINT('Ctrl Pts',(53.8549480733041,24.1983152114493,2.79224250381912));
#241641=CARTESIAN_POINT('Ctrl Pts',(53.9422730280819,24.2082687574725,2.7490180910828));
#241642=CARTESIAN_POINT('Ctrl Pts',(53.7744913425366,24.1443388226039,2.63947868311711));
#241643=CARTESIAN_POINT('Ctrl Pts',(53.825645022219,24.1165167429223,2.69595066767933));
#241644=CARTESIAN_POINT('Ctrl Pts',(53.9017956184508,24.1232032230476,2.68220539436075));
#241645=CARTESIAN_POINT('Ctrl Pts',(53.7848917482047,24.0595120258536,2.59908178585076));
#241646=CARTESIAN_POINT('Ctrl Pts',(53.8286685158637,24.0529122166846,2.65877670944865));
#241647=CARTESIAN_POINT('Ctrl Pts',(53.8982652496115,24.0696665464382,2.65878198860279));
#241648=CARTESIAN_POINT('Ctrl Pts',(53.8206887816836,23.9791663275016,2.59908173516041));
#241649=CARTESIAN_POINT('Ctrl Pts',(53.8547645473081,23.994348378682,2.65878198860279));
#241650=CARTESIAN_POINT('Ctrl Pts',(53.9190682401995,24.0229981225299,2.65878198860279));
#241651=CARTESIAN_POINT('Origin',(53.9190682401995,24.0229981225299,2.53178198860279));
#241652=CARTESIAN_POINT('Ctrl Pts',(56.6498810128382,24.8746050278055,3.77003198860281));
#241653=CARTESIAN_POINT('Ctrl Pts',(56.5981482837089,24.9907986398443,3.77003198860282));
#241654=CARTESIAN_POINT('Ctrl Pts',(56.5982255167331,24.9906251716318,3.64284238727617));
#241655=CARTESIAN_POINT('Ctrl Pts',(56.8481896769745,24.962653969475,3.77003198860281));
#241656=CARTESIAN_POINT('Ctrl Pts',(56.7965362315775,25.0791271905738,3.77025506105648));
#241657=CARTESIAN_POINT('Ctrl Pts',(56.7567415443552,25.0612010539389,3.64284210641936));
#241658=CARTESIAN_POINT('Ctrl Pts',(57.0369754593332,25.0464771582513,3.65553527987854));
#241659=CARTESIAN_POINT('Ctrl Pts',(56.9853490357203,25.1631925873308,3.65585996533124));
#241660=CARTESIAN_POINT('Ctrl Pts',(56.9076460727629,25.1283880784732,3.55127902710152));
#241661=CARTESIAN_POINT('Ctrl Pts',(57.1420619865021,25.0931373005748,3.4715307213909));
#241662=CARTESIAN_POINT('Ctrl Pts',(57.0905332166521,25.2100238867501,3.47182327905207));
#241663=CARTESIAN_POINT('Ctrl Pts',(56.9916465440541,25.1657874977297,3.40413028378006));
#241664=CARTESIAN_POINT('Origin',(56.6498810128382,24.8746050278055,3.64303198860281));
#241665=CARTESIAN_POINT('Origin',(5.71826297912856E-15,1.8634858490287E-13,
2.53178198860262));
#241666=CARTESIAN_POINT('Origin',(53.9314655730804,23.995153256981,2.53178198860279));
#241667=CARTESIAN_POINT('Origin',(52.0578415156894,22.8300973196051,3.64303198860279));
#241668=CARTESIAN_POINT('Origin',(56.2832472948513,24.7113125977908,3.64299466007434));
#241669=CARTESIAN_POINT('Ctrl Pts',(53.8330634946837,23.9513722670367,2.59908173516041));
#241670=CARTESIAN_POINT('Ctrl Pts',(53.867147095173,23.9665367208227,2.65878198860279));
#241671=CARTESIAN_POINT('Ctrl Pts',(53.9314655730804,23.995153256981,2.65878198860279));
#241672=CARTESIAN_POINT('Ctrl Pts',(53.8686972660497,23.871282165812,2.59908193199869));
#241673=CARTESIAN_POINT('Ctrl Pts',(53.8931046959184,23.9081865738553,2.65877685806683));
#241674=CARTESIAN_POINT('Ctrl Pts',(53.9521563342717,23.9486256024595,2.65878198860279));
#241675=CARTESIAN_POINT('Ctrl Pts',(53.9240892607412,23.8071866393156,2.63872492669835));
#241676=CARTESIAN_POINT('Ctrl Pts',(53.93785095296,23.8635355386145,2.69532212015295));
#241677=CARTESIAN_POINT('Ctrl Pts',(53.9937257232527,23.915575084618,2.68176836726654));
#241678=CARTESIAN_POINT('Ctrl Pts',(54.0330064121713,23.7392497560572,2.75442176402247));
#241679=CARTESIAN_POINT('Ctrl Pts',(54.018751292376,23.8300830854579,2.79203179920153));
#241680=CARTESIAN_POINT('Ctrl Pts',(54.0845104630313,23.8883623535218,2.7488531074819));
#241681=CARTESIAN_POINT('Ctrl Pts',(54.0860594545425,23.7337507958616,2.82866089558431));
#241682=CARTESIAN_POINT('Ctrl Pts',(54.0553500291274,23.8418399747432,2.85316563119239));
#241683=CARTESIAN_POINT('Ctrl Pts',(54.1330265677739,23.8930480394869,2.79189751796661));
#241684=CARTESIAN_POINT('Ctrl Pts',(54.1275498658873,23.752222950883,2.90134173516041));
#241685=CARTESIAN_POINT('Ctrl Pts',(54.0765745253536,23.8679139708571,2.90103711553246));
#241686=CARTESIAN_POINT('Ctrl Pts',(54.1745185419759,23.9115214566117,2.83404198860279));
#241687=CARTESIAN_POINT('Origin',(54.2261740956466,23.7955011834911,2.83404198860279));
#241688=CARTESIAN_POINT('Origin',(56.2428239368568,24.6933715410265,3.5664765397182));
#241689=CARTESIAN_POINT('Origin',(56.1680608984278,24.6600848917114,3.42473028058504));
#241690=CARTESIAN_POINT('Origin',(54.3889216310578,23.8679610547533,3.11913648168222));
#241691=CARTESIAN_POINT('Origin',(54.5516691663895,23.9404209259124,3.40423097483327));
#241692=CARTESIAN_POINT('Ctrl Pts',(55.8666273273833,24.5258780191674,3.36123028058499));
#241693=CARTESIAN_POINT('Ctrl Pts',(55.8149717737126,24.641898292288,3.36123028058499));
#241694=CARTESIAN_POINT('Ctrl Pts',(55.8149717737126,24.641898292288,3.23423028058499));
#241695=CARTESIAN_POINT('Ctrl Pts',(55.9487607347572,24.5627025231289,3.36123028058499));
#241696=CARTESIAN_POINT('Ctrl Pts',(55.897123215879,24.6784744708799,3.36099641108583));
#241697=CARTESIAN_POINT('Ctrl Pts',(55.9383132588164,24.6968134595447,3.23423043688445));
#241698=CARTESIAN_POINT('Ctrl Pts',(56.0264248009279,24.597521196072,3.41054258905304));
#241699=CARTESIAN_POINT('Ctrl Pts',(55.9751910510453,24.7132325104955,3.41008815826033));
#241700=CARTESIAN_POINT('Ctrl Pts',(56.0549414076397,24.7487396569153,3.3081986730433));
#241701=CARTESIAN_POINT('Ctrl Pts',(56.0673542004326,24.6158705164596,3.48823028058501));
#241702=CARTESIAN_POINT('Ctrl Pts',(56.0163785451197,24.7315703643338,3.48794691941618));
#241703=CARTESIAN_POINT('Ctrl Pts',(56.1164053447572,24.776105164832,3.42473028058503));
#241704=CARTESIAN_POINT('Origin',(55.8666273273833,24.5258780191674,3.23423028058499));
#241705=CARTESIAN_POINT('Ctrl Pts',(54.4530463244692,23.8971395307771,3.47153072139089));
#241706=CARTESIAN_POINT('Ctrl Pts',(54.4019907365351,24.0130054343465,3.47122746285094));
#241707=CARTESIAN_POINT('Ctrl Pts',(54.5001606088505,24.0565064908995,3.40413046676799));
#241708=CARTESIAN_POINT('Ctrl Pts',(54.5581374230425,23.9437939758158,3.65553813458006));
#241709=CARTESIAN_POINT('Ctrl Pts',(54.5068816478256,24.0597061770701,3.65520336072347));
#241710=CARTESIAN_POINT('Ctrl Pts',(54.5841625982694,24.0939065860605,3.55128134519988));
#241711=CARTESIAN_POINT('Ctrl Pts',(54.7469293531944,24.0276077026117,3.7700319886028));
#241712=CARTESIAN_POINT('Ctrl Pts',(54.6954643138422,24.1436691352881,3.76980209313998));
#241713=CARTESIAN_POINT('Ctrl Pts',(54.7350683949958,24.1610941752717,3.64284195387376));
#241714=CARTESIAN_POINT('Ctrl Pts',(54.9452378026828,24.1156489724279,3.77003198860281));
#241715=CARTESIAN_POINT('Ctrl Pts',(54.893504872635,24.2318430357372,3.77003198860282));
#241716=CARTESIAN_POINT('Ctrl Pts',(54.8935823068776,24.2316691155807,3.64284189403809));
#241717=CARTESIAN_POINT('Origin',(54.9452378026828,24.1156489724279,3.64303198860281));
#241718=CARTESIAN_POINT('Origin',(50.7999799080414,22.2700612497319,3.23423028058498));
#241719=CARTESIAN_POINT('Origin',(55.7284918401498,24.4643761377919,3.23423028058499));
#241720=CARTESIAN_POINT('Origin',(50.6030043228557,22.1823620689018,3.64303198860279));
#241721=CARTESIAN_POINT('Origin',(55.3119205422645,24.2788510342448,3.64299171721805));
#241722=CARTESIAN_POINT('Ctrl Pts',(55.5277679687683,24.3743766270217,3.48823028058498));
#241723=CARTESIAN_POINT('Ctrl Pts',(55.4763362579874,24.4911280468229,3.48852004212277));
#241724=CARTESIAN_POINT('Ctrl Pts',(55.3754026508175,24.4461895095991,3.42473028058498));
#241725=CARTESIAN_POINT('Ctrl Pts',(55.5688345658069,24.3927905570421,3.41028005848426));
#241726=CARTESIAN_POINT('Ctrl Pts',(55.517233105522,24.509336496484,3.41074404220322));
#241727=CARTESIAN_POINT('Ctrl Pts',(55.4370743056941,24.4736474994207,3.30780486243939));
#241728=CARTESIAN_POINT('Ctrl Pts',(55.6466353090193,24.4276751358089,3.36123028058499));
#241729=CARTESIAN_POINT('Ctrl Pts',(55.5948055748756,24.5438739850311,3.36146460586506));
#241730=CARTESIAN_POINT('Ctrl Pts',(55.55391025049,24.5256662135189,3.23423045308453));
#241731=CARTESIAN_POINT('Ctrl Pts',(55.7284918401498,24.464376137792,3.36123028058499));
#241732=CARTESIAN_POINT('Ctrl Pts',(55.6768362864792,24.5803964109126,3.36123028058499));
#241733=CARTESIAN_POINT('Ctrl Pts',(55.6768362864792,24.5803964109126,3.23423028058499));
#241734=CARTESIAN_POINT('Origin',(55.4270582044881,24.3301692364785,3.42473028058498));
#241735=CARTESIAN_POINT('Origin',(55.3527410377821,24.2970811017195,3.56563113524761));
#241736=CARTESIAN_POINT('Origin',(53.036059683551,30.9870007556513,3.56647653909479));
#241737=CARTESIAN_POINT('Origin',(53.0743345559679,31.0091584503691,3.64299466007737));
#241738=CARTESIAN_POINT('Origin',(52.9651856060845,30.9460815882871,3.42473028058506));
#241739=CARTESIAN_POINT('Ctrl Pts',(52.8702215132216,30.8905967158739,3.48823028058506));
#241740=CARTESIAN_POINT('Ctrl Pts',(52.9338619179795,30.7813498801535,3.48794691941622));
#241741=CARTESIAN_POINT('Ctrl Pts',(53.0286856060846,30.8360963620065,3.42473028058507));
#241742=CARTESIAN_POINT('Ctrl Pts',(52.8311874403365,30.8681941459775,3.41028005925108));
#241743=CARTESIAN_POINT('Ctrl Pts',(52.8946849835393,30.7587310665082,3.40982512231106));
#241744=CARTESIAN_POINT('Ctrl Pts',(52.9702219582397,30.8023423591854,3.30780486372904));
#241745=CARTESIAN_POINT('Ctrl Pts',(52.7572372522458,30.8257530395514,3.36123028058504));
#241746=CARTESIAN_POINT('Ctrl Pts',(52.820547425344,30.7159277273268,3.36099721048389));
#241747=CARTESIAN_POINT('Ctrl Pts',(52.8594635164579,30.7383959430077,3.23423045308414));
#241748=CARTESIAN_POINT('Ctrl Pts',(52.6794317578287,30.7811015270746,3.36123028058504));
#241749=CARTESIAN_POINT('Ctrl Pts',(52.7429317578287,30.671116300794,3.36123028058504));
#241750=CARTESIAN_POINT('Ctrl Pts',(52.7429317578287,30.671116300794,3.23423028058503));
#241751=CARTESIAN_POINT('Origin',(52.6794317578287,30.7811015270746,3.23423028058504));
#241752=CARTESIAN_POINT('Origin',(-0.158749999999995,0.274963065701743,
3.64303198860263));
#241753=CARTESIAN_POINT('Origin',(53.4219427993286,31.2097904767608,3.64303198860285));
#241754=CARTESIAN_POINT('Origin',(-0.158749999999995,0.274963065701746,
3.23423028058482));
#241755=CARTESIAN_POINT('Origin',(52.5484816883959,30.7054974692372,3.23423028058504));
#241756=CARTESIAN_POINT('Ctrl Pts',(53.888035839597,31.4795232016792,3.47153072139094));
#241757=CARTESIAN_POINT('Ctrl Pts',(53.9523112176912,31.3691313491577,3.47182327902685));
#241758=CARTESIAN_POINT('Ctrl Pts',(53.858399113013,31.3151318426937,3.40413028959057));
#241759=CARTESIAN_POINT('Ctrl Pts',(53.7885171709474,31.4219316852026,3.6555380712098));
#241760=CARTESIAN_POINT('Ctrl Pts',(53.8525966788902,31.3115614337853,3.65586275496962));
#241761=CARTESIAN_POINT('Ctrl Pts',(53.7787668993598,31.2691561625552,3.55128126837278));
#241762=CARTESIAN_POINT('Ctrl Pts',(53.6097358757352,31.3184699958133,3.77003198860286));
#241763=CARTESIAN_POINT('Ctrl Pts',(53.6736035436629,31.2082202476918,3.77025505748367));
#241764=CARTESIAN_POINT('Ctrl Pts',(53.6357108652104,31.1865627224602,3.64284211731176));
#241765=CARTESIAN_POINT('Ctrl Pts',(53.4219427993286,31.2097904767608,3.77003198860286));
#241766=CARTESIAN_POINT('Ctrl Pts',(53.485537665384,31.0996409376523,3.77003198860286));
#241767=CARTESIAN_POINT('Ctrl Pts',(53.4854427285717,31.0998053730349,3.64284239821734));
#241768=CARTESIAN_POINT('Origin',(53.7950387249979,31.4251975098795,3.40423097483333));
#241769=CARTESIAN_POINT('Ctrl Pts',(52.5484816883959,30.7054974692372,3.36123028058504));
#241770=CARTESIAN_POINT('Ctrl Pts',(52.6119816883959,30.5955122429565,3.36123028058503));
#241771=CARTESIAN_POINT('Ctrl Pts',(52.6119816883959,30.5955122429565,3.23423028058503));
#241772=CARTESIAN_POINT('Ctrl Pts',(52.4704129317475,30.6606955449586,3.36123028058504));
#241773=CARTESIAN_POINT('Ctrl Pts',(52.5339553345216,30.5504637065426,3.3614653861012));
#241774=CARTESIAN_POINT('Ctrl Pts',(52.4950560684217,30.5280052047893,3.23423043688428));
#241775=CARTESIAN_POINT('Ctrl Pts',(52.3965920780925,30.6183335281986,3.41054258693123));
#241776=CARTESIAN_POINT('Ctrl Pts',(52.4605500011269,30.5080831175481,3.41100608859759));
#241777=CARTESIAN_POINT('Ctrl Pts',(52.3844945583568,30.4641724871913,3.30819866970862));
#241778=CARTESIAN_POINT('Ctrl Pts',(52.3576880233162,30.5960088312571,3.48823028058503));
#241779=CARTESIAN_POINT('Ctrl Pts',(52.4219111049556,30.4857749404423,3.48852004212281));
#241780=CARTESIAN_POINT('Ctrl Pts',(52.3262277788841,30.4305321463779,3.42473028058503));
#241781=CARTESIAN_POINT('Origin',(52.2627277788841,30.5405173726585,3.42473028058503));
#241782=CARTESIAN_POINT('Origin',(53.9493203812233,31.5142720656054,3.11913648178361));
#241783=CARTESIAN_POINT('Origin',(54.1036020372438,31.6033466212668,2.83404198860284));
#241784=CARTESIAN_POINT('Origin',(52.1922763801647,30.4998422386367,3.5656311346083));
#241785=CARTESIAN_POINT('Origin',(52.1535342613179,30.4775331296741,3.64299171721819));
#241786=CARTESIAN_POINT('Ctrl Pts',(54.5122556166611,31.490293248291,2.59908173516046));
#241787=CARTESIAN_POINT('Ctrl Pts',(54.4799531854479,31.4716329851992,2.65878198860284));
#241788=CARTESIAN_POINT('Ctrl Pts',(54.4189959163063,31.4364195775137,2.65878198860284));
#241789=CARTESIAN_POINT('Ctrl Pts',(54.4681793099455,31.5665926662618,2.59908193475672));
#241790=CARTESIAN_POINT('Ctrl Pts',(54.4478446647267,31.5272089901455,2.65878715325372));
#241791=CARTESIAN_POINT('Ctrl Pts',(54.3934750329626,31.4805801312539,2.65878198860284));
#241792=CARTESIAN_POINT('Ctrl Pts',(54.4058464214486,31.6244843104271,2.6387877884991));
#241793=CARTESIAN_POINT('Ctrl Pts',(54.3982481205272,31.5668246399996,2.69564460180143));
#241794=CARTESIAN_POINT('Ctrl Pts',(54.3482630350908,31.5088182930362,2.68180481624906));
#241795=CARTESIAN_POINT('Ctrl Pts',(54.2895863184077,31.6805188761702,2.75443238878651));
#241796=CARTESIAN_POINT('Ctrl Pts',(54.3139476428151,31.5913182835557,2.7926834077711));
#241797=CARTESIAN_POINT('Ctrl Pts',(54.2544636505346,31.5259511417533,2.74885926835632));
#241798=CARTESIAN_POINT('Ctrl Pts',(54.2359839591651,31.680406990988,2.82856655361704));
#241799=CARTESIAN_POINT('Ctrl Pts',(54.2789047974504,31.5756141966208,2.85384197230815));
#241800=CARTESIAN_POINT('Ctrl Pts',(54.2064835118364,31.5160982999433,2.79184624278487));
#241801=CARTESIAN_POINT('Ctrl Pts',(54.1966007261207,31.6576696180587,2.90134173516047));
#241802=CARTESIAN_POINT('Ctrl Pts',(54.2607761425982,31.5474441649286,2.90163218716414));
#241803=CARTESIAN_POINT('Ctrl Pts',(54.1671020372438,31.4933613949861,2.83404198860285));
#241804=CARTESIAN_POINT('Origin',(54.4189959163063,31.4364195775137,2.53178198860284));
#241805=CARTESIAN_POINT('Origin',(-0.158749999999995,0.274963065701743,
3.64303198860263));
#241806=CARTESIAN_POINT('Origin',(51.8059703131946,30.2768083268883,3.64303198860284));
#241807=CARTESIAN_POINT('Origin',(5.52187834149254E-15,1.85800105364867E-13,
2.53178198860262));
#241808=CARTESIAN_POINT('Origin',(54.4342359163063,31.4100231232064,2.53178198860284));
#241809=CARTESIAN_POINT('Ctrl Pts',(51.8059703131946,30.2768083268883,3.77003198860285));
#241810=CARTESIAN_POINT('Ctrl Pts',(51.8695654390622,30.166658337772,3.77003198860285));
#241811=CARTESIAN_POINT('Ctrl Pts',(51.8694702420498,30.1668232238341,3.6428418793704));
#241812=CARTESIAN_POINT('Ctrl Pts',(51.6181777324915,30.1681210939092,3.77003198860285));
#241813=CARTESIAN_POINT('Ctrl Pts',(51.6818230251222,30.058265798306,3.76980208962999));
#241814=CARTESIAN_POINT('Ctrl Pts',(51.7191994478437,30.080064340051,3.64284193928282));
#241815=CARTESIAN_POINT('Ctrl Pts',(51.4394033023493,30.0646505034507,3.65553535416608));
#241816=CARTESIAN_POINT('Ctrl Pts',(51.5030508615805,29.955052217304,3.65520057834494));
#241817=CARTESIAN_POINT('Ctrl Pts',(51.5761444782068,29.9974715145366,3.55127910964311));
#241818=CARTESIAN_POINT('Ctrl Pts',(51.3398895692697,30.007053683816,3.47153072139095));
#241819=CARTESIAN_POINT('Ctrl Pts',(51.4036173400347,29.8976445635502,3.47122746281605));
#241820=CARTESIAN_POINT('Ctrl Pts',(51.4965132406194,29.95149639792,3.40413045901281));
#241821=CARTESIAN_POINT('Origin',(51.4328740054943,30.0614010732039,3.40423097483332));
#241822=CARTESIAN_POINT('Ctrl Pts',(54.5146464769138,31.1067982185537,2.90134173516046));
#241823=CARTESIAN_POINT('Ctrl Pts',(54.4512761425982,31.2174884860868,2.90163218716414));
#241824=CARTESIAN_POINT('Ctrl Pts',(54.3576020372438,31.1634057161443,2.83404198860284));
#241825=CARTESIAN_POINT('Ctrl Pts',(54.5540471172215,31.1295467523331,2.82853349835374));
#241826=CARTESIAN_POINT('Ctrl Pts',(54.4847554296818,31.2191042733499,2.85381483162335));
#241827=CARTESIAN_POINT('Ctrl Pts',(54.3970014563935,31.1861529813963,2.79182701594249));
#241828=CARTESIAN_POINT('Ctrl Pts',(54.5807851087096,31.1758273123592,2.75468822073668));
#241829=CARTESIAN_POINT('Ctrl Pts',(54.5157207333379,31.2416052667856,2.79286913083842));
#241830=CARTESIAN_POINT('Ctrl Pts',(54.4293656242358,31.2226915745262,2.74900763297926));
#241831=CARTESIAN_POINT('Ctrl Pts',(54.5905870683104,31.3035520968882,2.63954450640412));
#241832=CARTESIAN_POINT('Ctrl Pts',(54.5367490446513,31.3261415286127,2.69627684028892));
#241833=CARTESIAN_POINT('Ctrl Pts',(54.4614280312972,31.3118587536638,2.68224356036523));
#241834=CARTESIAN_POINT('Ctrl Pts',(54.5717067142914,31.3872779850337,2.59908178706453));
#241835=CARTESIAN_POINT('Ctrl Pts',(54.5274095677396,31.3893985541597,2.65878704321558));
#241836=CARTESIAN_POINT('Ctrl Pts',(54.4598040608963,31.3656949292502,2.65878198860284));
#241837=CARTESIAN_POINT('Ctrl Pts',(54.5275217339719,31.4638515574743,2.59908173516046));
#241838=CARTESIAN_POINT('Ctrl Pts',(54.4952102564865,31.4452069629856,2.65878198860284));
#241839=CARTESIAN_POINT('Ctrl Pts',(54.4342359163063,31.4100231232064,2.65878198860284));
#241840=CARTESIAN_POINT('Origin',(54.4211020372438,31.0534204898637,2.83404198860284));
#241841=CARTESIAN_POINT('Origin',(51.2785921372156,29.9723263949883,3.11913648167148));
#241842=CARTESIAN_POINT('Origin',(51.1243102687785,29.8832517167489,2.83404198860284));
#241843=CARTESIAN_POINT('Origin',(54.2668203811903,30.9643459342355,3.11913648177614));
#241844=CARTESIAN_POINT('Origin',(54.1125387249979,30.8752713784764,3.40423097483332));
#241845=CARTESIAN_POINT('Ctrl Pts',(51.0313275753408,29.8289013456888,2.90134173516045));
#241846=CARTESIAN_POINT('Ctrl Pts',(51.0949610232001,29.7196599535395,2.90103711553251));
#241847=CARTESIAN_POINT('Ctrl Pts',(51.1878102687784,29.7732664904682,2.83404198860283));
#241848=CARTESIAN_POINT('Ctrl Pts',(50.991979079321,29.8061828667727,2.82862991747972));
#241849=CARTESIAN_POINT('Ctrl Pts',(51.0613736255819,29.7178139048432,2.85314045886472));
#241850=CARTESIAN_POINT('Ctrl Pts',(51.148459876313,29.7505475307856,2.7918796099996));
#241851=CARTESIAN_POINT('Ctrl Pts',(50.9654077681508,29.7601395581527,2.75470625793362));
#241852=CARTESIAN_POINT('Ctrl Pts',(51.0305123301031,29.6951292702712,2.79224250381908));
#241853=CARTESIAN_POINT('Ctrl Pts',(51.1163184807723,29.7141562330558,2.74901809108276));
#241854=CARTESIAN_POINT('Ctrl Pts',(50.9561384187038,29.6330385513052,2.63947868311705));
#241855=CARTESIAN_POINT('Ctrl Pts',(51.009920072411,29.6107158994146,2.69595066767941));
#241856=CARTESIAN_POINT('Ctrl Pts',(51.0849545802162,29.6253256551031,2.68220539436086));
#241857=CARTESIAN_POINT('Ctrl Pts',(50.9753486645701,29.5497635830445,2.59908178585111));
#241858=CARTESIAN_POINT('Ctrl Pts',(51.0195754864254,29.5477758465711,2.65877670944928));
#241859=CARTESIAN_POINT('Ctrl Pts',(51.0870396576422,29.5717132339806,2.65878198860283));
#241860=CARTESIAN_POINT('Ctrl Pts',(51.0193480105327,29.473599835734,2.59908173516044));
#241861=CARTESIAN_POINT('Ctrl Pts',(51.0516501490686,29.4922606054649,2.65878198860283));
#241862=CARTESIAN_POINT('Ctrl Pts',(51.1126068659047,29.5274749692187,2.65878198860283));
#241863=CARTESIAN_POINT('Origin',(51.1126068659047,29.5274749692187,2.53178198860283));
#241864=CARTESIAN_POINT('Ctrl Pts',(53.7394427993286,30.6598643453577,3.77003198860285));
#241865=CARTESIAN_POINT('Ctrl Pts',(53.6758479277943,30.770013893956,3.77003198860286));
#241866=CARTESIAN_POINT('Ctrl Pts',(53.6759428700937,30.7698494490696,3.64284238727595));
#241867=CARTESIAN_POINT('Ctrl Pts',(53.927461487289,30.7681598456258,3.77003198860286));
#241868=CARTESIAN_POINT('Ctrl Pts',(53.8639162380539,30.8785957589617,3.77025506105754));
#241869=CARTESIAN_POINT('Ctrl Pts',(53.8262133418071,30.8566081460782,3.64284210641868));
#241870=CARTESIAN_POINT('Ctrl Pts',(54.1064511722693,30.8712573299213,3.65553527987854));
#241871=CARTESIAN_POINT('Ctrl Pts',(54.0429074791695,30.9819369489461,3.65585996533185));
#241872=CARTESIAN_POINT('Ctrl Pts',(53.9692682429978,30.9392009315198,3.5512790271026));
#241873=CARTESIAN_POINT('Ctrl Pts',(54.2060847114741,30.9286463962981,3.47153072139093));
#241874=CARTESIAN_POINT('Ctrl Pts',(54.1426202463872,31.039506442398,3.4718232790521));
#241875=CARTESIAN_POINT('Ctrl Pts',(54.0488992470932,30.9851759130204,3.40413028377995));
#241876=CARTESIAN_POINT('Origin',(53.7394427993286,30.6598643453577,3.64303198860285));
#241877=CARTESIAN_POINT('Origin',(5.71547558359784E-15,1.86354055474621E-13,
2.53178198860262));
#241878=CARTESIAN_POINT('Origin',(51.1278468659047,29.5010785149114,2.53178198860283));
#241879=CARTESIAN_POINT('Origin',(46.8255917980722,26.6681506086454,3.64303198860282));
#241880=CARTESIAN_POINT('Origin',(53.3918862459818,30.4591427892376,3.64299466007562));
#241881=CARTESIAN_POINT('Ctrl Pts',(51.0345602039887,29.4472515437738,2.59908173516044));
#241882=CARTESIAN_POINT('Ctrl Pts',(51.0668719738977,29.465895631477,2.65878198860283));
#241883=CARTESIAN_POINT('Ctrl Pts',(51.1278468659047,29.5010785149114,2.65878198860283));
#241884=CARTESIAN_POINT('Ctrl Pts',(51.0783704650305,29.371324927865,2.59908193199872));
#241885=CARTESIAN_POINT('Ctrl Pts',(51.0987866273845,29.4105784408362,2.65877685806679));
#241886=CARTESIAN_POINT('Ctrl Pts',(51.1532877451687,29.4569685172212,2.65878198860283));
#241887=CARTESIAN_POINT('Ctrl Pts',(51.1401588234664,29.3133705634513,2.63872492669832));
#241888=CARTESIAN_POINT('Ctrl Pts',(51.147955063845,29.3708492661237,2.6953221201529));
#241889=CARTESIAN_POINT('Ctrl Pts',(51.1980841325267,29.4284442379234,2.68176836726648));
#241890=CARTESIAN_POINT('Ctrl Pts',(51.255580653351,29.2571907880105,2.75442176402257));
#241891=CARTESIAN_POINT('Ctrl Pts',(51.2319089562575,29.3460364571626,2.79203179920163));
#241892=CARTESIAN_POINT('Ctrl Pts',(51.2912160489646,29.4108701703525,2.74885310748203));
#241893=CARTESIAN_POINT('Ctrl Pts',(51.3089178634639,29.2572675046847,2.8286608955843));
#241894=CARTESIAN_POINT('Ctrl Pts',(51.267078271731,29.3615545506877,2.85316563119254));
#241895=CARTESIAN_POINT('Ctrl Pts',(51.338976589856,29.4206015015123,2.79189751796631));
#241896=CARTESIAN_POINT('Ctrl Pts',(51.3482501200165,29.2799753962465,2.90134173516044));
#241897=CARTESIAN_POINT('Ctrl Pts',(51.2854610232001,29.3897042746976,2.9010371155325));
#241898=CARTESIAN_POINT('Ctrl Pts',(51.3783102687784,29.4433108116264,2.83404198860283));
#241899=CARTESIAN_POINT('Origin',(51.4418102687785,29.3333255853458,2.83404198860283));
#241900=CARTESIAN_POINT('Origin',(53.3535596824668,30.4370746239672,3.56647653971804));
#241901=CARTESIAN_POINT('Origin',(53.2826856060845,30.396155456884,3.42473028058507));
#241902=CARTESIAN_POINT('Origin',(51.5960921371718,29.4224002636282,3.11913648168176));
#241903=CARTESIAN_POINT('Origin',(51.7503740054943,29.5114749418008,3.40423097483332));
#241904=CARTESIAN_POINT('Ctrl Pts',(52.9969317578287,30.2311753956715,3.36123028058503));
#241905=CARTESIAN_POINT('Ctrl Pts',(52.9334317578287,30.3411606219521,3.36123028058504));
#241906=CARTESIAN_POINT('Ctrl Pts',(52.9334317578287,30.3411606219521,3.23423028058503));
#241907=CARTESIAN_POINT('Ctrl Pts',(53.0747660209942,30.2763834500021,3.36123028058503));
#241908=CARTESIAN_POINT('Ctrl Pts',(53.0113099140584,30.3861235964147,3.36099641108553));
#241909=CARTESIAN_POINT('Ctrl Pts',(53.0503573673275,30.4086676540714,3.23423043688406));
#241910=CARTESIAN_POINT('Ctrl Pts',(53.1483650929077,30.3191294881009,3.41054258905306));
#241911=CARTESIAN_POINT('Ctrl Pts',(53.0853168809886,30.4288515386958,3.41008815826037));
#241912=CARTESIAN_POINT('Ctrl Pts',(53.1609188493357,30.4725003554708,3.30819867304338));
#241913=CARTESIAN_POINT('Ctrl Pts',(53.1871522506175,30.3416565762239,3.48823028058505));
#241914=CARTESIAN_POINT('Ctrl Pts',(53.1243619179795,30.4513942013116,3.48794691941621));
#241915=CARTESIAN_POINT('Ctrl Pts',(53.2191856060846,30.5061406831646,3.42473028058506));
#241916=CARTESIAN_POINT('Origin',(52.9969317578287,30.2311753956715,3.23423028058503));
#241917=CARTESIAN_POINT('Ctrl Pts',(51.6568155675427,29.4581217525676,3.47153072139093));
#241918=CARTESIAN_POINT('Ctrl Pts',(51.5939283826162,29.5680161684459,3.47122746285098));
#241919=CARTESIAN_POINT('Ctrl Pts',(51.6870133715071,29.6215404675519,3.40413046676814));
#241920=CARTESIAN_POINT('Ctrl Pts',(51.7564542486376,29.515505630712,3.65553813458009));
#241921=CARTESIAN_POINT('Ctrl Pts',(51.6933631336487,29.6254251653805,3.65520336072143));
#241922=CARTESIAN_POINT('Ctrl Pts',(51.7666458147661,29.6675162799441,3.5512813451999));
#241923=CARTESIAN_POINT('Ctrl Pts',(51.9354510367811,29.6185943474767,3.77003198860285));
#241924=CARTESIAN_POINT('Ctrl Pts',(51.8721362050985,29.7286404220052,3.76980209314336));
#241925=CARTESIAN_POINT('Ctrl Pts',(51.9097019182966,29.7501097595411,3.64284195387409));
#241926=CARTESIAN_POINT('Ctrl Pts',(52.1234703131946,29.7268821954852,3.77003198860285));
#241927=CARTESIAN_POINT('Ctrl Pts',(52.059875194672,29.8370321718797,3.77003198860284));
#241928=CARTESIAN_POINT('Ctrl Pts',(52.0599703843284,29.8368672985585,3.64284189403835));
#241929=CARTESIAN_POINT('Origin',(52.1234703131946,29.7268821954852,3.64303198860285));
#241930=CARTESIAN_POINT('Origin',(45.6951875,26.0155113828602,3.234230280585));
#241931=CARTESIAN_POINT('Origin',(52.8659816883959,30.155571337834,3.23423028058503));
#241932=CARTESIAN_POINT('Origin',(45.518171167873,25.9133109558558,3.64303198860281));
#241933=CARTESIAN_POINT('Origin',(52.4710850656383,29.9275190026066,3.64299171721804));
#241934=CARTESIAN_POINT('Ctrl Pts',(52.6757649139395,30.0450834959839,3.48823028058502));
#241935=CARTESIAN_POINT('Ctrl Pts',(52.6124111049556,30.1558192616004,3.4885200421228));
#241936=CARTESIAN_POINT('Ctrl Pts',(52.5167277788841,30.100576467536,3.42473028058502));
#241937=CARTESIAN_POINT('Ctrl Pts',(52.7146817640555,30.0676891808481,3.41028005848428));
#241938=CARTESIAN_POINT('Ctrl Pts',(52.6511806140155,30.1782028480908,3.41074404220291));
#241939=CARTESIAN_POINT('Ctrl Pts',(52.5751914484999,30.1343304829265,3.30780486243907));
#241940=CARTESIAN_POINT('Ctrl Pts',(52.788409875246,30.1105150503714,3.36123028058503));
#241941=CARTESIAN_POINT('Ctrl Pts',(52.7247179826696,30.2206596676792,3.36146460586399));
#241942=CARTESIAN_POINT('Ctrl Pts',(52.6859499175234,30.1982769148323,3.23423045308413));
#241943=CARTESIAN_POINT('Ctrl Pts',(52.8659816883959,30.155571337834,3.36123028058503));
#241944=CARTESIAN_POINT('Ctrl Pts',(52.8024816883959,30.2655565641147,3.36123028058503));
#241945=CARTESIAN_POINT('Ctrl Pts',(52.8024816883959,30.2655565641147,3.23423028058503));
#241946=CARTESIAN_POINT('Origin',(52.5802277788841,29.9905912412554,3.42473028058502));
#241947=CARTESIAN_POINT('Origin',(52.5097763812721,29.9499161075317,3.56563113524805));
#241948=CARTESIAN_POINT('Origin',(49.5064990290884,36.3610285397823,3.56647653909451));
#241949=CARTESIAN_POINT('Origin',(49.5422481179706,36.3870656659281,3.64299466007424));
#241950=CARTESIAN_POINT('Origin',(49.4402904249165,36.3129251734945,3.4247302805851));
#241951=CARTESIAN_POINT('Ctrl Pts',(49.3516463037385,36.2478178023253,3.48823028058509));
#241952=CARTESIAN_POINT('Ctrl Pts',(49.4263574835551,36.1458216659128,3.48794691941626));
#241953=CARTESIAN_POINT('Ctrl Pts',(49.5149391519577,36.2101800152089,3.4247302805851));
#241954=CARTESIAN_POINT('Ctrl Pts',(49.3151677697919,36.2214577843991,3.41028005925111));
#241955=CARTESIAN_POINT('Ctrl Pts',(49.389759474291,36.1192316557425,3.40982512230885));
#241956=CARTESIAN_POINT('Ctrl Pts',(49.4603240281395,36.1704998050828,3.30780486372839));
#241957=CARTESIAN_POINT('Ctrl Pts',(49.2460589922039,36.1715192752743,3.36123028058507));
#241958=CARTESIAN_POINT('Ctrl Pts',(49.3205022166664,36.068913312703,3.36099721048721));
#241959=CARTESIAN_POINT('Ctrl Pts',(49.3568565533006,36.095326284347,3.23423045308392));
#241960=CARTESIAN_POINT('Ctrl Pts',(49.1733470784087,36.1189794796885,3.36123028058507));
#241961=CARTESIAN_POINT('Ctrl Pts',(49.2479958054498,36.0162343214029,3.36123028058507));
#241962=CARTESIAN_POINT('Ctrl Pts',(49.2479958054498,36.0162343214029,3.23423028058507));
#241963=CARTESIAN_POINT('Origin',(49.1733470784087,36.1189794796885,3.23423028058507));
#241964=CARTESIAN_POINT('Origin',(-0.186621817602855,0.256862895714229,
3.64303198860263));
#241965=CARTESIAN_POINT('Origin',(49.8669803696025,36.6229335645812,3.64303198860289));
#241966=CARTESIAN_POINT('Origin',(-0.186621817602855,0.256862895714232,
3.23423028058482));
#241967=CARTESIAN_POINT('Origin',(49.0510171431403,36.0301015792679,3.23423028058507));
#241968=CARTESIAN_POINT('Ctrl Pts',(50.3023253561995,36.9399086546489,3.47153072139097));
#241969=CARTESIAN_POINT('Ctrl Pts',(50.377787717749,36.8368401467435,3.47182327902688));
#241970=CARTESIAN_POINT('Ctrl Pts',(50.2900345588334,36.773319967242,3.40413028959026));
#241971=CARTESIAN_POINT('Ctrl Pts',(50.209371813944,36.8722300970252,3.65553807120984));
#241972=CARTESIAN_POINT('Ctrl Pts',(50.2846371204137,36.769162597888,3.65586275497155));
#241973=CARTESIAN_POINT('Ctrl Pts',(50.2156443459751,36.7192723137729,3.55128126837369));
#241974=CARTESIAN_POINT('Ctrl Pts',(50.0423845927715,36.7506474475471,3.7700319886029));
#241975=CARTESIAN_POINT('Ctrl Pts',(50.1174266236742,36.6476776482614,3.77025505748318));
#241976=CARTESIAN_POINT('Ctrl Pts',(50.0820053531117,36.6221779017691,3.64284211731108));
#241977=CARTESIAN_POINT('Ctrl Pts',(49.8669803696025,36.6229335645812,3.7700319886029));
#241978=CARTESIAN_POINT('Ctrl Pts',(49.9417406183807,36.520034909793,3.7700319886029));
#241979=CARTESIAN_POINT('Ctrl Pts',(49.9416290134639,36.5201885207827,3.64284239821673));
#241980=CARTESIAN_POINT('Origin',(50.2155162706044,36.8761597191957,3.40423097483336));
#241981=CARTESIAN_POINT('Ctrl Pts',(49.0510171431403,36.0301015792679,3.36123028058507));
#241982=CARTESIAN_POINT('Ctrl Pts',(49.1256658701815,35.9273564209823,3.36123028058507));
#241983=CARTESIAN_POINT('Ctrl Pts',(49.1256658701815,35.9273564209823,3.23423028058507));
#241984=CARTESIAN_POINT('Ctrl Pts',(48.9780591316061,35.9773846774559,3.36123028058507));
#241985=CARTESIAN_POINT('Ctrl Pts',(49.0527758071189,35.8743986902987,3.36146538610131));
#241986=CARTESIAN_POINT('Ctrl Pts',(49.0164371879466,35.8479971380607,3.23423043688408));
#241987=CARTESIAN_POINT('Ctrl Pts',(48.9090707128234,35.9275383438676,3.41054258693127));
#241988=CARTESIAN_POINT('Ctrl Pts',(48.9842025736675,35.8245773199113,3.41100608859846));
#241989=CARTESIAN_POINT('Ctrl Pts',(48.9131536812798,35.7729572780257,3.30819866970899));
#241990=CARTESIAN_POINT('Ctrl Pts',(48.8727133447943,35.9012693628907,3.48823028058506));
#241991=CARTESIAN_POINT('Ctrl Pts',(48.9481071848796,35.7983524848938,3.48852004212283));
#241992=CARTESIAN_POINT('Ctrl Pts',(48.85872246645,35.7334106856009,3.42473028058505));
#241993=CARTESIAN_POINT('Origin',(48.7840737394089,35.8361558438865,3.42473028058506));
#241994=CARTESIAN_POINT('Origin',(50.3596419293496,36.9808731396203,3.11913648178429));
#241995=CARTESIAN_POINT('Origin',(50.5037675878945,37.0855865599605,2.83404198860288));
#241996=CARTESIAN_POINT('Origin',(48.7182599900761,35.7883393560613,3.56563113460849));
#241997=CARTESIAN_POINT('Origin',(48.6820620414867,35.7621028045851,3.64299171721869));
#241998=CARTESIAN_POINT('Ctrl Pts',(50.9219998155899,37.0158684358562,2.5990817351605));
#241999=CARTESIAN_POINT('Ctrl Pts',(50.8918248691,36.9939338721436,2.65878198860288));
#242000=CARTESIAN_POINT('Ctrl Pts',(50.8348823336486,36.9525415975215,2.65878198860288));
#242001=CARTESIAN_POINT('Ctrl Pts',(50.8701895025858,37.0871426490245,2.59908193475663));
#242002=CARTESIAN_POINT('Ctrl Pts',(50.8540829678233,37.0458491715908,2.65878715325424));
#242003=CARTESIAN_POINT('Ctrl Pts',(50.8048852215549,36.9937925764104,2.65878198860288));
#242004=CARTESIAN_POINT('Ctrl Pts',(50.8021467555733,37.1382015956602,2.63878778849918));
#242005=CARTESIAN_POINT('Ctrl Pts',(50.8006171556815,37.0800635522215,2.69564460180147));
#242006=CARTESIAN_POINT('Ctrl Pts',(50.7569692080811,37.0171501059292,2.6818048162493));
#242007=CARTESIAN_POINT('Ctrl Pts',(50.6806663304944,37.181776708279,2.75443238878649));
#242008=CARTESIAN_POINT('Ctrl Pts',(50.7142182018865,37.0956112176475,2.7926834077711));
#242009=CARTESIAN_POINT('Ctrl Pts',(50.6618927960203,37.0243843935852,2.74885926835615));
#242010=CARTESIAN_POINT('Ctrl Pts',(50.6273693057705,37.1760624637761,2.8285665536171));
#242011=CARTESIAN_POINT('Ctrl Pts',(50.6810088489707,37.076330184568,2.85384197230783));
#242012=CARTESIAN_POINT('Ctrl Pts',(50.6152053999547,37.0095702365076,2.79184624278437));
#242013=CARTESIAN_POINT('Ctrl Pts',(50.5905785208484,37.1493329797263,2.9013417351605));
#242014=CARTESIAN_POINT('Ctrl Pts',(50.6659240749083,37.0464195108255,2.90163218716417));
#242015=CARTESIAN_POINT('Ctrl Pts',(50.5784163149356,36.9828414016749,2.83404198860288));
#242016=CARTESIAN_POINT('Origin',(50.8348823336486,36.9525415975215,2.53178198860288));
#242017=CARTESIAN_POINT('Origin',(-0.186621817602855,0.256862895714229,
3.64303198860263));
#242018=CARTESIAN_POINT('Origin',(48.3573835402119,35.5261472678868,3.64303198860288));
#242019=CARTESIAN_POINT('Origin',(5.53127843490691E-15,1.85785630490362E-13,
2.53178198860262));
#242020=CARTESIAN_POINT('Origin',(50.8527980281384,36.9278827595329,2.53178198860288));
#242021=CARTESIAN_POINT('Ctrl Pts',(48.3573835402119,35.5261472678868,3.77003198860288));
#242022=CARTESIAN_POINT('Ctrl Pts',(48.4321440944169,35.4232481927146,3.77003198860289));
#242023=CARTESIAN_POINT('Ctrl Pts',(48.4320321836173,35.4234022247158,3.64284187937085));
#242024=CARTESIAN_POINT('Ctrl Pts',(48.1819806163552,35.3984257650681,3.77003198860288));
#242025=CARTESIAN_POINT('Ctrl Pts',(48.2567602586451,35.2958250128978,3.76980208962949));
#242026=CARTESIAN_POINT('Ctrl Pts',(48.2916533613389,35.3214110399815,3.64284193928375));
#242027=CARTESIAN_POINT('Ctrl Pts',(48.0150011530601,35.2768349808768,3.65553535416611));
#242028=CARTESIAN_POINT('Ctrl Pts',(48.0897561847312,35.1744900671688,3.65520057834472));
#242029=CARTESIAN_POINT('Ctrl Pts',(48.1580153629278,35.2243173504725,3.55127910964188));
#242030=CARTESIAN_POINT('Ctrl Pts',(47.9220530736687,35.209151665053,3.47153072139098));
#242031=CARTESIAN_POINT('Ctrl Pts',(47.9968681042461,35.1070032653416,3.47122746281608));
#242032=CARTESIAN_POINT('Ctrl Pts',(48.0836260618766,35.1702703594595,3.40413045901306));
#242033=CARTESIAN_POINT('Origin',(48.0088472823272,35.2729208539817,3.40423097483335));
#242034=CARTESIAN_POINT('Ctrl Pts',(50.9644637245892,36.6347241449657,2.90134173516049));
#242035=CARTESIAN_POINT('Ctrl Pts',(50.8898702560317,36.7381840359687,2.90163218716417));
#242036=CARTESIAN_POINT('Ctrl Pts',(50.8023624960591,36.6746059268181,2.83404198860288));
#242037=CARTESIAN_POINT('Ctrl Pts',(51.0012706547893,36.6614665482799,2.82853349835375));
#242038=CARTESIAN_POINT('Ctrl Pts',(50.9229972443171,36.7432905102108,2.85381483162291));
#242039=CARTESIAN_POINT('Ctrl Pts',(50.8391683443882,36.7013469409085,2.79182701594282));
#242040=CARTESIAN_POINT('Ctrl Pts',(51.0230245369437,36.7102884597168,2.75468822073677));
#242041=CARTESIAN_POINT('Ctrl Pts',(50.9514409225353,36.768904996455,2.79286913083859));
#242042=CARTESIAN_POINT('Ctrl Pts',(50.8675358949426,36.7410683485314,2.74900763297934));
#242043=CARTESIAN_POINT('Ctrl Pts',(51.0194219249361,36.8383381382864,2.63954450640411));
#242044=CARTESIAN_POINT('Ctrl Pts',(50.9635175930192,36.8551762168621,2.6962768402889));
#242045=CARTESIAN_POINT('Ctrl Pts',(50.8901021525742,36.8330984946708,2.68224356036522));
#242046=CARTESIAN_POINT('Ctrl Pts',(50.9918932610486,36.9196318328646,2.59908178706433));
#242047=CARTESIAN_POINT('Ctrl Pts',(50.9476171190683,36.9171104726343,2.65878704321594));
#242048=CARTESIAN_POINT('Ctrl Pts',(50.8828596657515,36.8864699989243,2.65878198860288));
#242049=CARTESIAN_POINT('Ctrl Pts',(50.9399462128201,36.991167339171,2.5990817351605));
#242050=CARTESIAN_POINT('Ctrl Pts',(50.9097606317994,36.9692474126343,2.65878198860288));
#242051=CARTESIAN_POINT('Ctrl Pts',(50.8527980281385,36.9278827595329,2.65878198860288));
#242052=CARTESIAN_POINT('Origin',(50.8770112231002,36.5718607685324,2.83404198860286));
#242053=CARTESIAN_POINT('Origin',(47.8647214254968,35.1682072895727,3.11913648167076));
#242054=CARTESIAN_POINT('Origin',(47.720595568509,35.0634937251224,2.83404198860287));
#242055=CARTESIAN_POINT('Origin',(50.732885564516,36.4671473482239,3.11913648177603));
#242056=CARTESIAN_POINT('Origin',(50.5887599058101,36.3624339277676,3.40423097483335));
#242057=CARTESIAN_POINT('Ctrl Pts',(47.6338034047599,34.9997217530263,2.90134173516048));
#242058=CARTESIAN_POINT('Ctrl Pts',(47.7085070967803,34.8977303031705,2.90103711553254));
#242059=CARTESIAN_POINT('Ctrl Pts',(47.7952442955502,34.9607485668368,2.83404198860287));
#242060=CARTESIAN_POINT('Ctrl Pts',(47.5970451916064,34.9730146904951,2.82862991747981));
#242061=CARTESIAN_POINT('Ctrl Pts',(47.6752966590732,34.8923835282627,2.85314045886538));
#242062=CARTESIAN_POINT('Ctrl Pts',(47.7584842465947,34.9340408279391,2.79187960999998));
#242063=CARTESIAN_POINT('Ctrl Pts',(47.5754322771535,34.9244461536127,2.75470625793358));
#242064=CARTESIAN_POINT('Ctrl Pts',(47.6469756149923,34.8665972787025,2.7922425038192));
#242065=CARTESIAN_POINT('Ctrl Pts',(47.7303228514092,34.8944891948625,2.74901809108285));
#242066=CARTESIAN_POINT('Ctrl Pts',(47.5794993790985,34.7970725085259,2.63947868311716));
#242067=CARTESIAN_POINT('Ctrl Pts',(47.6353197637775,34.7804938560724,2.69595066767937));
#242068=CARTESIAN_POINT('Ctrl Pts',(47.7084160893875,34.8028668197836,2.68220539436084));
#242069=CARTESIAN_POINT('Ctrl Pts',(47.6073089936889,34.7162617467346,2.59908178585162));
#242070=CARTESIAN_POINT('Ctrl Pts',(47.6515013114269,34.7189078610138,2.65877670944829));
#242071=CARTESIAN_POINT('Ctrl Pts',(47.7160937685338,34.7497660430532,2.65878198860287));
#242072=CARTESIAN_POINT('Ctrl Pts',(47.6590285860935,34.6451144164188,2.59908173516048));
#242073=CARTESIAN_POINT('Ctrl Pts',(47.6892031885513,34.667049453402,2.65878198860287));
#242074=CARTESIAN_POINT('Ctrl Pts',(47.7461450747864,34.7084426211234,2.65878198860287));
#242075=CARTESIAN_POINT('Origin',(47.7461450747864,34.7084426211234,2.53178198860287));
#242076=CARTESIAN_POINT('Ctrl Pts',(50.2402240048083,36.1092077731531,3.77003198860289));
#242077=CARTESIAN_POINT('Ctrl Pts',(50.1654637495898,36.2121064368056,3.77003198860289));
#242078=CARTESIAN_POINT('Ctrl Pts',(50.1655753609565,36.2119528169383,3.64284238727618));
#242079=CARTESIAN_POINT('Ctrl Pts',(50.4158927445022,36.2365633238567,3.77003198860289));
#242080=CARTESIAN_POINT('Ctrl Pts',(50.341151906482,36.3397519704545,3.77025506105886));
#242081=CARTESIAN_POINT('Ctrl Pts',(50.3059538820309,36.3139437822109,3.64284210641865));
#242082=CARTESIAN_POINT('Ctrl Pts',(50.5831252836564,36.3578055460627,3.6555352798786));
#242083=CARTESIAN_POINT('Ctrl Pts',(50.5083605190613,36.4612367259645,3.65585996533031));
#242084=CARTESIAN_POINT('Ctrl Pts',(50.4395918165622,36.4110374247138,3.55127902710232));
#242085=CARTESIAN_POINT('Ctrl Pts',(50.6762142289948,36.4252947698681,3.47153072139098));
#242086=CARTESIAN_POINT('Ctrl Pts',(50.6015093986315,36.5289136700282,3.47182327905215));
#242087=CARTESIAN_POINT('Ctrl Pts',(50.5139808995222,36.4650842569434,3.4041302837801));
#242088=CARTESIAN_POINT('Origin',(50.2402240048083,36.1092077731531,3.64303198860289));
#242089=CARTESIAN_POINT('Origin',(5.7121316272531E-15,1.86359204715837E-13,
2.53178198860262));
#242090=CARTESIAN_POINT('Origin',(47.7640607692763,34.6837837831348,2.53178198860287));
#242091=CARTESIAN_POINT('Origin',(40.9117478092586,29.3316730956006,3.64303198860284));
#242092=CARTESIAN_POINT('Origin',(49.915552518433,35.8732562382983,3.64299466007548));
#242093=CARTESIAN_POINT('Ctrl Pts',(47.6769115920304,34.6205005703637,2.59908173516048));
#242094=CARTESIAN_POINT('Ctrl Pts',(47.7070975168463,34.6424200234577,2.65878198860287));
#242095=CARTESIAN_POINT('Ctrl Pts',(47.7640607692763,34.6837837831348,2.65878198860287));
#242096=CARTESIAN_POINT('Ctrl Pts',(47.7284183483602,34.549569307663,2.59908193199826));
#242097=CARTESIAN_POINT('Ctrl Pts',(47.744619559451,34.590741855859,2.65877685806643));
#242098=CARTESIAN_POINT('Ctrl Pts',(47.7939730310146,34.6425747206405,2.65878198860287));
#242099=CARTESIAN_POINT('Ctrl Pts',(47.7959261043553,34.4983910654768,2.63872492669804));
#242100=CARTESIAN_POINT('Ctrl Pts',(47.7976714756521,34.5563698228279,2.69532212015263));
#242101=CARTESIAN_POINT('Ctrl Pts',(47.8415056181567,34.6188891978603,2.68176836726639));
#242102=CARTESIAN_POINT('Ctrl Pts',(47.9165880269729,34.4545839152295,2.75442176402293));
#242103=CARTESIAN_POINT('Ctrl Pts',(47.8837591046489,34.5404685123899,2.79203179920204));
#242104=CARTESIAN_POINT('Ctrl Pts',(47.9359643384885,34.6111463389766,2.7488531074822));
#242105=CARTESIAN_POINT('Ctrl Pts',(47.9696250311907,34.4602354682512,2.8286608955841));
#242106=CARTESIAN_POINT('Ctrl Pts',(47.9171136764626,34.5595777906759,2.85316563119194));
#242107=CARTESIAN_POINT('Ctrl Pts',(47.9824460410473,34.6258166968299,2.79189751796707));
#242108=CARTESIAN_POINT('Ctrl Pts',(48.0063682005187,34.4869303039399,2.90134173516047));
#242109=CARTESIAN_POINT('Ctrl Pts',(47.9324532779037,34.5894948283136,2.90103711553254));
#242110=CARTESIAN_POINT('Ctrl Pts',(48.0191904766736,34.6525130919799,2.83404198860286));
#242111=CARTESIAN_POINT('Origin',(48.0938392037147,34.5497679336943,2.83404198860286));
#242112=CARTESIAN_POINT('Origin',(49.8797426632439,35.8473027479614,3.56647653971835));
#242113=CARTESIAN_POINT('Origin',(49.8135340601223,35.7991993820665,3.42473028058511));
#242114=CARTESIAN_POINT('Origin',(48.2379650606502,34.6544814981832,3.11913648168303));
#242115=CARTESIAN_POINT('Origin',(48.3820909175329,34.7591950625537,3.40423097483335));
#242116=CARTESIAN_POINT('Ctrl Pts',(49.5465907136144,35.6052536882605,3.36123028058507));
#242117=CARTESIAN_POINT('Ctrl Pts',(49.4719419865733,35.7079988465461,3.36123028058507));
#242118=CARTESIAN_POINT('Ctrl Pts',(49.4719419865733,35.7079988465461,3.23423028058507));
#242119=CARTESIAN_POINT('Ctrl Pts',(49.6192730640952,35.6583499840585,3.36123028058507));
#242120=CARTESIAN_POINT('Ctrl Pts',(49.5446936074896,35.7608559931228,3.36099641108551));
#242121=CARTESIAN_POINT('Ctrl Pts',(49.5811706590218,35.7873581223575,3.23423043688383));
#242122=CARTESIAN_POINT('Ctrl Pts',(49.6880007749183,35.7085550527735,3.41054258905307));
#242123=CARTESIAN_POINT('Ctrl Pts',(49.613828870366,35.8110857017915,3.41008815826029));
#242124=CARTESIAN_POINT('Ctrl Pts',(49.6844541394801,35.8623979633508,3.30819867304359));
#242125=CARTESIAN_POINT('Ctrl Pts',(49.7242207306175,35.7350130971392,3.48823028058509));
#242126=CARTESIAN_POINT('Ctrl Pts',(49.6503036646785,35.8375861910559,3.48794691941625));
#242127=CARTESIAN_POINT('Ctrl Pts',(49.7388853330811,35.9019445403521,3.4247302805851));
#242128=CARTESIAN_POINT('Origin',(49.5465907136144,35.6052536882604,3.23423028058507));
#242129=CARTESIAN_POINT('Ctrl Pts',(48.2946219293746,34.6963546279288,3.47153072139098));
#242130=CARTESIAN_POINT('Ctrl Pts',(48.2205921526138,34.7990735298986,3.47122746285102));
#242131=CARTESIAN_POINT('Ctrl Pts',(48.3075723994626,34.8620346481359,3.40413046676832));
#242132=CARTESIAN_POINT('Ctrl Pts',(48.3877165307493,34.7638392294026,3.65553813458009));
#242133=CARTESIAN_POINT('Ctrl Pts',(48.3134813154532,34.8665617960676,3.65520336072165));
#242134=CARTESIAN_POINT('Ctrl Pts',(48.3819628268506,34.916082457139,3.55128134519971));
#242135=CARTESIAN_POINT('Ctrl Pts',(48.554957050614,34.8850734745865,3.77003198860289));
#242136=CARTESIAN_POINT('Ctrl Pts',(48.4804861171424,34.9878985031416,3.76980209314062));
#242137=CARTESIAN_POINT('Ctrl Pts',(48.5156018845759,35.0131769156733,3.64284195387393));
#242138=CARTESIAN_POINT('Ctrl Pts',(48.7306271754176,35.0124214764587,3.77003198860288));
#242139=CARTESIAN_POINT('Ctrl Pts',(48.655866629847,35.1153205397466,3.77003198860288));
#242140=CARTESIAN_POINT('Ctrl Pts',(48.6559785319992,35.1151665196475,3.64284189403863));
#242141=CARTESIAN_POINT('Origin',(48.7306271754176,35.0124214764587,3.64303198860288));
#242142=CARTESIAN_POINT('Origin',(39.9252688514646,28.6149541797808,3.23423028058502));
#242143=CARTESIAN_POINT('Origin',(49.424260778346,35.5163757878398,3.23423028058507));
#242144=CARTESIAN_POINT('Origin',(39.7707905934405,28.5027191556742,3.64303198860283));
#242145=CARTESIAN_POINT('Origin',(49.0553654007526,35.2482948100398,3.64299171721812));
#242146=CARTESIAN_POINT('Ctrl Pts',(49.2466351556012,35.3866101428262,3.48823028058506));
#242147=CARTESIAN_POINT('Ctrl Pts',(49.1720533660031,35.4901170100369,3.48852004212285));
#242148=CARTESIAN_POINT('Ctrl Pts',(49.0826686475734,35.425175210744,3.42473028058506));
#242149=CARTESIAN_POINT('Ctrl Pts',(49.2829758776385,35.4131599099239,3.41028005848434));
#242150=CARTESIAN_POINT('Ctrl Pts',(49.2082707697383,35.5164304941074,3.41074404220394));
#242151=CARTESIAN_POINT('Ctrl Pts',(49.1372837917345,35.4648554356502,3.30780486243961));
#242152=CARTESIAN_POINT('Ctrl Pts',(49.3518235761936,35.4634578610135,3.36123028058507));
#242153=CARTESIAN_POINT('Ctrl Pts',(49.2769673468815,35.5663414789286,3.36146460586394));
#242154=CARTESIAN_POINT('Ctrl Pts',(49.2407512920129,35.5400289748689,3.2342304530846));
#242155=CARTESIAN_POINT('Ctrl Pts',(49.424260778346,35.5163757878398,3.36123028058507));
#242156=CARTESIAN_POINT('Ctrl Pts',(49.3496120513049,35.6191209461254,3.36123028058507));
#242157=CARTESIAN_POINT('Ctrl Pts',(49.3496120513049,35.6191209461254,3.23423028058507));
#242158=CARTESIAN_POINT('Origin',(49.1573173746146,35.3224300524584,3.42473028058506));
#242159=CARTESIAN_POINT('Origin',(49.0915036263521,35.2746135650472,3.56563113524886));
#242160=CARTESIAN_POINT('Origin',(45.434534811362,41.3366772861974,3.56647653909408));
#242161=CARTESIAN_POINT('Origin',(45.467366442211,41.3663085755643,3.64299466007437));
#242162=CARTESIAN_POINT('Origin',(45.3737170758072,41.2819167515331,3.42473028058513));
#242163=CARTESIAN_POINT('Ctrl Pts',(45.2923641298557,41.207900211591,3.48823028058513));
#242164=CARTESIAN_POINT('Ctrl Pts',(45.3773275334105,41.1142722655009,3.48794691941629));
#242165=CARTESIAN_POINT('Ctrl Pts',(45.4586966628148,41.1875373586975,3.42473028058514));
#242166=CARTESIAN_POINT('Ctrl Pts',(45.2588408013013,41.1778715515044,3.41028005925115));
#242167=CARTESIAN_POINT('Ctrl Pts',(45.3437094247747,41.0840023845244,3.40982512230998));
#242168=CARTESIAN_POINT('Ctrl Pts',(45.4085284377455,41.1423656859498,3.30780486372877));
#242169=CARTESIAN_POINT('Ctrl Pts',(45.1953306044445,41.1209827764382,3.36123028058511));
#242170=CARTESIAN_POINT('Ctrl Pts',(45.2800912647191,41.0267203359203,3.3609972104844));
#242171=CARTESIAN_POINT('Ctrl Pts',(45.3134855411616,41.0567886774839,3.23423045308378));
#242172=CARTESIAN_POINT('Ctrl Pts',(45.1285089182132,41.0611303347406,3.36123028058511));
#242173=CARTESIAN_POINT('Ctrl Pts',(45.2134885052208,40.966750941905,3.36123028058511));
#242174=CARTESIAN_POINT('Ctrl Pts',(45.2134885052208,40.966750941905,3.23423028058511));
#242175=CARTESIAN_POINT('Origin',(45.1285089182132,41.0611303347407,3.23423028058511));
#242176=CARTESIAN_POINT('Origin',(-0.212448967518932,0.235948482089256,
3.64303198860263));
#242177=CARTESIAN_POINT('Origin',(45.7656648676106,41.6348281284264,3.64303198860292));
#242178=CARTESIAN_POINT('Origin',(-0.212448967518932,0.235948482089259,
3.23423028058482));
#242179=CARTESIAN_POINT('Origin',(45.0161393894793,40.9599523566127,3.23423028058511));
#242180=CARTESIAN_POINT('Ctrl Pts',(46.1654920697611,41.9955727382253,3.47153072139101));
#242181=CARTESIAN_POINT('Ctrl Pts',(46.2513146333407,41.9009568150781,3.47182327902692));
#242182=CARTESIAN_POINT('Ctrl Pts',(46.1706818621617,41.8286119029178,3.4041302895905));
#242183=CARTESIAN_POINT('Ctrl Pts',(46.0801220723609,41.918548639894,3.65553807120987));
#242184=CARTESIAN_POINT('Ctrl Pts',(46.1657485549047,41.823913122127,3.65586275497073));
#242185=CARTESIAN_POINT('Ctrl Pts',(46.1023486848312,41.7670844335153,3.55128126837336));
#242186=CARTESIAN_POINT('Ctrl Pts',(45.9267584721668,41.7801771152782,3.77003198860294));
#242187=CARTESIAN_POINT('Ctrl Pts',(46.0121526898534,41.6856154234963,3.77025505748536));
#242188=CARTESIAN_POINT('Ctrl Pts',(45.9795909100358,41.6565528363061,3.64284211731136));
#242189=CARTESIAN_POINT('Ctrl Pts',(45.7656648676106,41.6348281284264,3.77003198860293));
#242190=CARTESIAN_POINT('Ctrl Pts',(45.8507714101807,41.5403077371542,3.77003198860292));
#242191=CARTESIAN_POINT('Ctrl Pts',(45.8506443599268,41.5404488407561,3.64284239821717));
#242192=CARTESIAN_POINT('Origin',(46.0858221116777,41.9230990057958,3.4042309748334));
#242193=CARTESIAN_POINT('Ctrl Pts',(45.0161393894793,40.9599523566127,3.36123028058511));
#242194=CARTESIAN_POINT('Ctrl Pts',(45.1011189764868,40.8655729637771,3.36123028058511));
#242195=CARTESIAN_POINT('Ctrl Pts',(45.1011189764868,40.8655729637771,3.23423028058511));
#242196=CARTESIAN_POINT('Ctrl Pts',(44.9490914662984,40.8998980546784,3.36123028058511));
#242197=CARTESIAN_POINT('Ctrl Pts',(45.0341638030238,40.8052862548076,3.36146538609985));
#242198=CARTESIAN_POINT('Ctrl Pts',(45.0007839642919,40.7752309130122,3.23423043688394));
#242199=CARTESIAN_POINT('Ctrl Pts',(44.885691333943,40.843113531121,3.41054258693128));
#242200=CARTESIAN_POINT('Ctrl Pts',(44.9711739721975,40.7485699563826,3.41100608859847));
#242201=CARTESIAN_POINT('Ctrl Pts',(44.9059100567345,40.6898060629491,3.3081986697091));
#242202=CARTESIAN_POINT('Ctrl Pts',(44.8522789915941,40.8131880745609,3.4882302805851));
#242203=CARTESIAN_POINT('Ctrl Pts',(44.9380175594362,40.718715788234,3.48852004212289));
#242204=CARTESIAN_POINT('Ctrl Pts',(44.8559107663285,40.6447864996555,3.4247302805851));
#242205=CARTESIAN_POINT('Origin',(44.7709311793209,40.7391658924911,3.4247302805851));
#242206=CARTESIAN_POINT('Origin',(46.2182127020614,42.0423040287743,3.11913648178372));
#242207=CARTESIAN_POINT('Origin',(46.3506032922594,42.1615090516455,2.83404198860292));
#242208=CARTESIAN_POINT('Origin',(44.7104761485842,40.6847319383097,3.5656311346084));
#242209=CARTESIAN_POINT('Origin',(44.6772189625508,40.6548553974686,3.64299171721753));
#242210=CARTESIAN_POINT('Ctrl Pts',(46.7738319284257,42.1358900227698,2.59908173516054));
#242211=CARTESIAN_POINT('Ctrl Pts',(46.7461150696872,42.1109214781064,2.65878198860292));
#242212=CARTESIAN_POINT('Ctrl Pts',(46.6938111422604,42.0638038389703,2.65878198860292));
#242213=CARTESIAN_POINT('Ctrl Pts',(46.7148552537637,42.2013581359408,2.59908193475748));
#242214=CARTESIAN_POINT('Ctrl Pts',(46.7031532960233,42.1586072771698,2.65878715325374));
#242215=CARTESIAN_POINT('Ctrl Pts',(46.6596664560525,42.1016932886501,2.65878198860292));
#242216=CARTESIAN_POINT('Ctrl Pts',(46.6418481388115,42.245024972543,2.63878778849886));
#242217=CARTESIAN_POINT('Ctrl Pts',(46.646403998566,42.1870455286636,2.69564460180144));
#242218=CARTESIAN_POINT('Ctrl Pts',(46.6095714048494,42.1199142759252,2.68180481624926));
#242219=CARTESIAN_POINT('Ctrl Pts',(46.5164783566527,42.2756632139847,2.75443238878691));
#242220=CARTESIAN_POINT('Ctrl Pts',(46.558853173705,42.1934768724826,2.79268340777122));
#242221=CARTESIAN_POINT('Ctrl Pts',(46.5142596423497,42.1171707421502,2.74885926835627));
#242222=CARTESIAN_POINT('Ctrl Pts',(46.4640705998045,42.2644092166193,2.82856655361689));
#242223=CARTESIAN_POINT('Ctrl Pts',(46.527841161857,42.1708301402926,2.85384197230662));
#242224=CARTESIAN_POINT('Ctrl Pts',(46.4693765057995,42.0975575768112,2.79184624278484));
#242225=CARTESIAN_POINT('Ctrl Pts',(46.4302753505424,42.2339804752704,2.90134173516054));
#242226=CARTESIAN_POINT('Ctrl Pts',(46.5159655405274,42.1395065321002,2.90163218716422));
#242227=CARTESIAN_POINT('Ctrl Pts',(46.435582879267,42.0671296588098,2.83404198860292));
#242228=CARTESIAN_POINT('Origin',(46.6938111422604,42.0638038389703,2.53178198860292));
#242229=CARTESIAN_POINT('Origin',(-0.212448967518932,0.235948482089256,
3.64303198860263));
#242230=CARTESIAN_POINT('Origin',(44.3789831537295,40.3862543050941,3.64303198860291));
#242231=CARTESIAN_POINT('Origin',(5.54214007001405E-15,1.85772217488052E-13,
2.53178198860262));
#242232=CARTESIAN_POINT('Origin',(46.7142062431422,42.0411527846897,2.53178198860292));
#242233=CARTESIAN_POINT('Ctrl Pts',(44.3789831537295,40.3862543050941,3.77003198860292));
#242234=CARTESIAN_POINT('Ctrl Pts',(44.4640900439956,40.2917335276664,3.77003198860292));
#242235=CARTESIAN_POINT('Ctrl Pts',(44.4639626455268,40.2918750180002,3.64284187937102));
#242236=CARTESIAN_POINT('Ctrl Pts',(44.2178916378581,40.2408978759484,3.77003198860292));
#242237=CARTESIAN_POINT('Ctrl Pts',(44.3029863283938,40.1466757825266,3.76980208962809));
#242238=CARTESIAN_POINT('Ctrl Pts',(44.3350138149322,40.1757689690794,3.64284193928359));
#242239=CARTESIAN_POINT('Ctrl Pts',(44.0645366033527,40.1025190721003,3.65553535416613));
#242240=CARTESIAN_POINT('Ctrl Pts',(44.1495800756941,40.0085488431226,3.65520057834485));
#242241=CARTESIAN_POINT('Ctrl Pts',(44.212256953616,40.0652381943521,3.55127910964236));
#242242=CARTESIAN_POINT('Ctrl Pts',(43.9791725362582,40.0254908126591,3.47153072139101));
#242243=CARTESIAN_POINT('Ctrl Pts',(44.0642551375171,39.9317222927449,3.47122746281612));
#242244=CARTESIAN_POINT('Ctrl Pts',(44.1439246138546,40.0037114790886,3.40413045901317));
#242245=CARTESIAN_POINT('Origin',(44.0588255818377,40.0979831325501,3.40423097483339));
#242246=CARTESIAN_POINT('Ctrl Pts',(46.8559036426985,41.7612723673365,2.90134173516054));
#242247=CARTESIAN_POINT('Ctrl Pts',(46.7709043015502,41.8563683535933,2.90163218716421));
#242248=CARTESIAN_POINT('Ctrl Pts',(46.6905216402897,41.7839914803029,2.83404198860292));
#242249=CARTESIAN_POINT('Ctrl Pts',(46.8897135983608,41.7917156448191,2.82853349835381));
#242250=CARTESIAN_POINT('Ctrl Pts',(46.8033160448221,41.8649095672142,2.85381483162275));
#242251=CARTESIAN_POINT('Ctrl Pts',(46.7243306652211,41.814433263085,2.79182701594198));
#242252=CARTESIAN_POINT('Ctrl Pts',(46.9062450310969,41.842544004588,2.7546882207368));
#242253=CARTESIAN_POINT('Ctrl Pts',(46.8289264627106,41.8933569085954,2.7928691308389));
#242254=CARTESIAN_POINT('Ctrl Pts',(46.7483907976682,41.8569022891471,2.74900763297958));
#242255=CARTESIAN_POINT('Ctrl Pts',(46.8892773184517,41.9695156381237,2.63954450640415));
#242256=CARTESIAN_POINT('Ctrl Pts',(46.8319191778368,41.9804178820379,2.69627684028872));
#242257=CARTESIAN_POINT('Ctrl Pts',(46.7612136652291,41.950787100749,2.68224356036506));
#242258=CARTESIAN_POINT('Ctrl Pts',(46.8534019544985,42.0474864684053,2.59908178706327));
#242259=CARTESIAN_POINT('Ctrl Pts',(46.8096319157677,42.0403508033704,2.65878704321586));
#242260=CARTESIAN_POINT('Ctrl Pts',(46.748432012186,42.0031091843004,2.65878198860292));
#242261=CARTESIAN_POINT('Ctrl Pts',(46.7942619810916,42.1132001506003,2.59908173516054));
#242262=CARTESIAN_POINT('Ctrl Pts',(46.7665330160779,42.0882450513177,2.65878198860292));
#242263=CARTESIAN_POINT('Ctrl Pts',(46.7142062431422,42.0411527846897,2.65878198860292));
#242264=CARTESIAN_POINT('Origin',(46.7755012272973,41.6896120874673,2.83404198860291));
#242265=CARTESIAN_POINT('Origin',(43.926434809502,39.9787779456778,3.11913648166835));
#242266=CARTESIAN_POINT('Origin',(43.7940440370144,39.8595727587358,2.83404198860291));
#242267=CARTESIAN_POINT('Origin',(46.6431106370583,41.5704070646225,3.11913648177571));
#242268=CARTESIAN_POINT('Origin',(46.5107200467156,41.4512020416176,3.40423097483339));
#242269=CARTESIAN_POINT('Ctrl Pts',(43.7143933160623,39.787077884675,2.90134173516052));
#242270=CARTESIAN_POINT('Ctrl Pts',(43.7993487829613,39.6934538167803,2.90103711553257));
#242271=CARTESIAN_POINT('Ctrl Pts',(43.8790236240219,39.7651933659001,2.8340419886029));
#242272=CARTESIAN_POINT('Ctrl Pts',(43.680628116452,39.7566748466924,2.8286299174798));
#242273=CARTESIAN_POINT('Ctrl Pts',(43.7668791656722,39.6846648960474,2.85314045886468));
#242274=CARTESIAN_POINT('Ctrl Pts',(43.8452566693654,39.7347894633637,2.79187960999967));
#242275=CARTESIAN_POINT('Ctrl Pts',(43.6642103943288,39.7061132086031,2.7547062579337));
#242276=CARTESIAN_POINT('Ctrl Pts',(43.7414086642733,39.6560595510442,2.79224250381923));
#242277=CARTESIAN_POINT('Ctrl Pts',(43.8213838166747,39.6925108309093,2.74901809108282));
#242278=CARTESIAN_POINT('Ctrl Pts',(43.6815693876451,39.579862457588,2.63947868311711));
#242279=CARTESIAN_POINT('Ctrl Pts',(43.7388169234803,39.5692094437566,2.69595066767941));
#242280=CARTESIAN_POINT('Ctrl Pts',(43.8091742082548,39.5991004926181,2.68220539436094));
#242281=CARTESIAN_POINT('Ctrl Pts',(43.7176736830026,39.5024012818818,2.59908178585113));
#242282=CARTESIAN_POINT('Ctrl Pts',(43.7613473163392,39.5096522555303,2.6587767094491));
#242283=CARTESIAN_POINT('Ctrl Pts',(43.8223603708606,39.5470931435004,2.6587819886029));
#242284=CARTESIAN_POINT('Ctrl Pts',(43.7765468711722,39.4370498736011,2.59908173516051));
#242285=CARTESIAN_POINT('Ctrl Pts',(43.8042633382929,39.4620188529812,2.6587819886029));
#242286=CARTESIAN_POINT('Ctrl Pts',(43.8565665267056,39.5091373124625,2.6587819886029));
#242287=CARTESIAN_POINT('Origin',(43.8565665267056,39.5091373124625,2.5317819886029));
#242288=CARTESIAN_POINT('Ctrl Pts',(46.1905628026484,41.1629311642483,3.77003198860293));
#242289=CARTESIAN_POINT('Ctrl Pts',(46.1054562527465,41.2574515636634,3.77003198860293));
#242290=CARTESIAN_POINT('Ctrl Pts',(46.1055833103431,41.2573104519064,3.64284238727623));
#242291=CARTESIAN_POINT('Ctrl Pts',(46.3519569306026,41.3079514313235,3.77003198860293));
#242292=CARTESIAN_POINT('Ctrl Pts',(46.2668393800555,41.4027622547774,3.77025506105961));
#242293=CARTESIAN_POINT('Ctrl Pts',(46.2345318643233,41.3734162510829,3.6428421064187));
#242294=CARTESIAN_POINT('Ctrl Pts',(46.5056000892405,41.4460100362752,3.65553527987858));
#242295=CARTESIAN_POINT('Ctrl Pts',(46.4204333915653,41.541059563398,3.65585996533035));
#242296=CARTESIAN_POINT('Ctrl Pts',(46.3572886670239,41.4839469723853,3.55127902710264));
#242297=CARTESIAN_POINT('Ctrl Pts',(46.5911245387429,41.5228599914565,3.47153072139101));
#242298=CARTESIAN_POINT('Ctrl Pts',(46.5059978248577,41.6181024753231,3.47182327905218));
#242299=CARTESIAN_POINT('Ctrl Pts',(46.4256208064858,41.5454735069379,3.40413028378015));
#242300=CARTESIAN_POINT('Origin',(46.1905628026484,41.1629311642483,3.64303198860293));
#242301=CARTESIAN_POINT('Origin',(5.70826774717982E-15,1.86363976210353E-13,
2.53178198860262));
#242302=CARTESIAN_POINT('Origin',(43.8769616275874,39.4864862581819,2.5317819886029));
#242303=CARTESIAN_POINT('Origin',(34.5756856720385,30.7048488218246,3.64303198860284));
#242304=CARTESIAN_POINT('Origin',(45.8923335519908,40.8943347850524,3.64299466007427));
#242305=CARTESIAN_POINT('Ctrl Pts',(43.7969047596346,39.4144401478992,2.59908173516051));
#242306=CARTESIAN_POINT('Ctrl Pts',(43.8246341160485,39.439394812269,2.6587819886029));
#242307=CARTESIAN_POINT('Ctrl Pts',(43.8769616275874,39.4864862581819,2.6587819886029));
#242308=CARTESIAN_POINT('Ctrl Pts',(43.8555436924523,39.3492813761648,2.59908193199951));
#242309=CARTESIAN_POINT('Ctrl Pts',(43.867352448424,39.3919218645341,2.65877685806761));
#242310=CARTESIAN_POINT('Ctrl Pts',(43.9110175468029,39.4486296259976,2.6587819886029));
#242311=CARTESIAN_POINT('Ctrl Pts',(43.9280312169045,39.3054399757364,2.63872492669796));
#242312=CARTESIAN_POINT('Ctrl Pts',(43.9237065964663,39.3632835603677,2.69532212015287));
#242313=CARTESIAN_POINT('Ctrl Pts',(43.9607655567553,39.4300423632766,2.68176836726652));
#242314=CARTESIAN_POINT('Ctrl Pts',(44.0526112349805,39.2744854109881,2.75442176402307));
#242315=CARTESIAN_POINT('Ctrl Pts',(44.0109847679687,39.3564679665378,2.79203179920179));
#242316=CARTESIAN_POINT('Ctrl Pts',(44.0555161714748,39.4322155454634,2.74885310748213));
#242317=CARTESIAN_POINT('Ctrl Pts',(44.1047669487876,39.2856498807577,2.82866089558405));
#242318=CARTESIAN_POINT('Ctrl Pts',(44.0421591564529,39.378959064333,2.85316563119197));
#242319=CARTESIAN_POINT('Ctrl Pts',(44.1002097724415,39.4516641984997,2.79189751796637));
#242320=CARTESIAN_POINT('Ctrl Pts',(44.1385184650375,39.3160391863692,2.90134173516051));
#242321=CARTESIAN_POINT('Ctrl Pts',(44.054287543984,39.4103156382734,2.90103711553257));
#242322=CARTESIAN_POINT('Ctrl Pts',(44.1339623850447,39.4820551873932,2.8340419886029));
#242323=CARTESIAN_POINT('Origin',(44.2189419720523,39.3876757945576,2.8340419886029));
#242324=CARTESIAN_POINT('Origin',(45.8594327453971,40.8647803215169,3.56647653971841));
#242325=CARTESIAN_POINT('Origin',(45.7986150108451,40.810019787355,3.42473028058514));
#242326=CARTESIAN_POINT('Origin',(44.3513327444871,39.5068809815264,3.11913648168166));
#242327=CARTESIAN_POINT('Origin',(44.4837235168756,39.626086168372,3.40423097483339));
#242328=CARTESIAN_POINT('Ctrl Pts',(45.5534068532511,40.5892333705625,3.36123028058511));
#242329=CARTESIAN_POINT('Ctrl Pts',(45.4684272662435,40.6836127633981,3.36123028058511));
#242330=CARTESIAN_POINT('Ctrl Pts',(45.4684272662435,40.6836127633981,3.23423028058511));
#242331=CARTESIAN_POINT('Ctrl Pts',(45.6201409680065,40.6496361736985,3.3612302805851));
#242332=CARTESIAN_POINT('Ctrl Pts',(45.5352552698624,40.7437849681305,3.36099641108467));
#242333=CARTESIAN_POINT('Ctrl Pts',(45.568762269447,40.7739548060672,3.23423043688378));
#242334=CARTESIAN_POINT('Ctrl Pts',(45.6832443225595,40.7067502157883,3.41054258905314));
#242335=CARTESIAN_POINT('Ctrl Pts',(45.5987613682814,40.8009661159843,3.41008815826067));
#242336=CARTESIAN_POINT('Ctrl Pts',(45.6636361529344,40.8593796344575,3.30819867304272));
#242337=CARTESIAN_POINT('Ctrl Pts',(45.7165002428306,40.73684933653,3.48823028058513));
#242338=CARTESIAN_POINT('Ctrl Pts',(45.6322662944332,40.831134086994,3.48794691941629));
#242339=CARTESIAN_POINT('Ctrl Pts',(45.7136354238375,40.9043991801906,3.42473028058514));
#242340=CARTESIAN_POINT('Origin',(45.5534068532511,40.5892333705625,3.23423028058511));
#242341=CARTESIAN_POINT('Ctrl Pts',(44.4033023070489,39.5544469813073,3.471530721391));
#242342=CARTESIAN_POINT('Ctrl Pts',(44.3189410241794,39.6488649595838,3.47122746285105));
#242343=CARTESIAN_POINT('Ctrl Pts',(44.3988635552004,39.7205730817654,3.40413046676823));
#242344=CARTESIAN_POINT('Ctrl Pts',(44.4888328647686,39.6312929306955,3.65553813458014));
#242345=CARTESIAN_POINT('Ctrl Pts',(44.4042668857097,39.7256930794157,3.65520336072211));
#242346=CARTESIAN_POINT('Ctrl Pts',(44.4671969296246,39.7821007282715,3.55128134519937));
#242347=CARTESIAN_POINT('Ctrl Pts',(44.6424847942248,39.769344436534,3.77003198860291));
#242348=CARTESIAN_POINT('Ctrl Pts',(44.5576736780983,39.8638218465938,3.76980209314121));
#242349=CARTESIAN_POINT('Ctrl Pts',(44.589954764068,39.8926323785408,3.64284195387446));
#242350=CARTESIAN_POINT('Ctrl Pts',(44.8038810887674,39.9143573409159,3.77003198860292));
#242351=CARTESIAN_POINT('Ctrl Pts',(44.7187742083304,40.0088781074273,3.77003198860292));
#242352=CARTESIAN_POINT('Ctrl Pts',(44.7189015969554,40.0087366280261,3.64284189403844));
#242353=CARTESIAN_POINT('Origin',(44.8038810887674,39.9143573409159,3.64303198860291));
#242354=CARTESIAN_POINT('Origin',(33.7433098572246,29.9553742717904,3.23423028058502));
#242355=CARTESIAN_POINT('Origin',(45.4410373245171,40.4880553924346,3.23423028058509));
#242356=CARTESIAN_POINT('Origin',(33.6129634723596,29.8380098596984,3.64303198860283));
#242357=CARTESIAN_POINT('Origin',(45.1021848870409,40.1828829233551,3.6429917172188));
#242358=CARTESIAN_POINT('Ctrl Pts',(45.2779489569772,40.3404336838195,3.48823028058509));
#242359=CARTESIAN_POINT('Ctrl Pts',(45.1929563204589,40.4355776097271,3.48852004212287));
#242360=CARTESIAN_POINT('Ctrl Pts',(45.1108495273512,40.3616483211486,3.42473028058509));
#242361=CARTESIAN_POINT('Ctrl Pts',(45.3113153943834,40.370636648342,3.41028005848439));
#242362=CARTESIAN_POINT('Ctrl Pts',(45.2262248134184,40.4655326953366,3.41074404220356));
#242363=CARTESIAN_POINT('Ctrl Pts',(45.1610177711079,40.4068200107225,3.30780486244019));
#242364=CARTESIAN_POINT('Ctrl Pts',(45.3745283705076,40.4278556061241,3.36123028058511));
#242365=CARTESIAN_POINT('Ctrl Pts',(45.289327944973,40.5223510101974,3.36146460586618));
#242366=CARTESIAN_POINT('Ctrl Pts',(45.2560606910586,40.4923970402279,3.23423045308455));
#242367=CARTESIAN_POINT('Ctrl Pts',(45.4410373245171,40.4880553924346,3.3612302805851));
#242368=CARTESIAN_POINT('Ctrl Pts',(45.3560577375096,40.5824347852702,3.3612302805851));
#242369=CARTESIAN_POINT('Ctrl Pts',(45.3560577375095,40.5824347852702,3.2342302805851));
#242370=CARTESIAN_POINT('Origin',(45.1958291143588,40.267268928313,3.4247302805851));
#242371=CARTESIAN_POINT('Origin',(45.1353740846431,40.2128349746518,3.56563113524746));
#242372=CARTESIAN_POINT('Origin',(40.8647803224535,45.8594327460082,3.56647653909442));
#242373=CARTESIAN_POINT('Origin',(40.8943347850519,45.8923335519907,3.64299466007502));
#242374=CARTESIAN_POINT('Origin',(40.8100197873546,45.7986150108454,3.42473028058516));
#242375=CARTESIAN_POINT('Ctrl Pts',(40.7368493365296,45.716500242831,3.48823028058516));
#242376=CARTESIAN_POINT('Ctrl Pts',(40.8311340869937,45.6322662944335,3.48794691941633));
#242377=CARTESIAN_POINT('Ctrl Pts',(40.9043991801903,45.7136354238378,3.42473028058517));
#242378=CARTESIAN_POINT('Ctrl Pts',(40.7066485019687,45.6831319408696,3.41028005925118));
#242379=CARTESIAN_POINT('Ctrl Pts',(40.8008642060138,45.5986481857971,3.40982512231093));
#242380=CARTESIAN_POINT('Ctrl Pts',(40.8592275074409,45.6634671987666,3.30780486372955));
#242381=CARTESIAN_POINT('Ctrl Pts',(40.6494327168507,45.619916185186,3.36123028058514));
#242382=CARTESIAN_POINT('Ctrl Pts',(40.7435821574131,45.535030025745,3.36099721048418));
#242383=CARTESIAN_POINT('Ctrl Pts',(40.773650498978,45.5684243021861,3.23423045308372));
#242384=CARTESIAN_POINT('Ctrl Pts',(40.5892333705622,45.5534068532514,3.36123028058514));
#242385=CARTESIAN_POINT('Ctrl Pts',(40.6836127633978,45.4684272662438,3.36123028058514));
#242386=CARTESIAN_POINT('Ctrl Pts',(40.6836127633978,45.4684272662438,3.23423028058514));
#242387=CARTESIAN_POINT('Origin',(40.5892333705622,45.5534068532514,3.23423028058513));
#242388=CARTESIAN_POINT('Origin',(-0.235948482089068,0.212448967519121,
3.64303198860263));
#242389=CARTESIAN_POINT('Origin',(41.162931164248,46.1905628026487,3.64303198860295));
#242390=CARTESIAN_POINT('Origin',(-0.235948482089068,0.212448967519124,
3.23423028058482));
#242391=CARTESIAN_POINT('Origin',(40.4880553924343,45.4410373245174,3.23423028058514));
#242392=CARTESIAN_POINT('Ctrl Pts',(41.5228599914562,46.5911245387432,3.47153072139104));
#242393=CARTESIAN_POINT('Ctrl Pts',(41.6181024670999,46.5059978322076,3.47182327902695));
#242394=CARTESIAN_POINT('Ctrl Pts',(41.5454735131716,46.4256208133853,3.40413028959057));
#242395=CARTESIAN_POINT('Ctrl Pts',(41.4460088704669,46.5055987918447,3.65553807120989));
#242396=CARTESIAN_POINT('Ctrl Pts',(41.5410583874239,46.4204321019804,3.65586275497117));
#242397=CARTESIAN_POINT('Ctrl Pts',(41.4839460439622,46.3572876358818,3.55128126837357));
#242398=CARTESIAN_POINT('Ctrl Pts',(41.3079491749525,46.3519544194664,3.77003198860296));
#242399=CARTESIAN_POINT('Ctrl Pts',(41.402759982507,46.2668368728718,3.77025505748482));
#242400=CARTESIAN_POINT('Ctrl Pts',(41.3734144470994,46.2345298607729,3.64284211731151));
#242401=CARTESIAN_POINT('Ctrl Pts',(41.162931164248,46.1905628026487,3.77003198860296));
#242402=CARTESIAN_POINT('Ctrl Pts',(41.2574515555201,46.1054562600787,3.77003198860296));
#242403=CARTESIAN_POINT('Ctrl Pts',(41.2573104519183,46.1055833103325,3.64284239821727));
#242404=CARTESIAN_POINT('Origin',(41.4512020416173,46.5107200467159,3.40423097483342));
#242405=CARTESIAN_POINT('Ctrl Pts',(40.4880553924343,45.4410373245174,3.36123028058514));
#242406=CARTESIAN_POINT('Ctrl Pts',(40.5824347852699,45.3560577375099,3.36123028058514));
#242407=CARTESIAN_POINT('Ctrl Pts',(40.5824347852699,45.3560577375099,3.23423028058514));
#242408=CARTESIAN_POINT('Ctrl Pts',(40.4276521486861,45.3743035899571,3.36123028058514));
#242409=CARTESIAN_POINT('Ctrl Pts',(40.5221480762948,45.2891025640481,3.36146538610193));
#242410=CARTESIAN_POINT('Ctrl Pts',(40.4920927345048,45.2557227253148,3.23423043688447));
#242411=CARTESIAN_POINT('Ctrl Pts',(40.370534927874,45.3112030195552,3.41054258693135));
#242412=CARTESIAN_POINT('Ctrl Pts',(40.4654317778751,45.226112733226,3.41100608859797));
#242413=CARTESIAN_POINT('Ctrl Pts',(40.4066678844421,45.1608488177577,3.30819866970886));
#242414=CARTESIAN_POINT('Ctrl Pts',(40.3404336838192,45.2779489569775,3.48823028058513));
#242415=CARTESIAN_POINT('Ctrl Pts',(40.4355776097268,45.1929563204592,3.48852004212291));
#242416=CARTESIAN_POINT('Ctrl Pts',(40.3616483211483,45.1108495273515,3.42473028058513));
#242417=CARTESIAN_POINT('Origin',(40.2672689283127,45.1958291143591,3.42473028058513));
#242418=CARTESIAN_POINT('Origin',(41.5704070646308,46.6431106370695,3.11913648178441));
#242419=CARTESIAN_POINT('Origin',(41.689612087467,46.7755012272976,2.83404198860295));
#242420=CARTESIAN_POINT('Origin',(40.2128349741391,45.135374083614,3.56563113460788));
#242421=CARTESIAN_POINT('Origin',(40.1828829233534,45.1021848870414,3.64299171721765));
#242422=CARTESIAN_POINT('Ctrl Pts',(42.1132001506,46.7942619810919,2.59908173516057));
#242423=CARTESIAN_POINT('Ctrl Pts',(42.0882450513174,46.7665330160782,2.65878198860295));
#242424=CARTESIAN_POINT('Ctrl Pts',(42.0411527846894,46.7142062431425,2.65878198860295));
#242425=CARTESIAN_POINT('Ctrl Pts',(42.0477032750705,46.8532067119189,2.59908193475557));
#242426=CARTESIAN_POINT('Ctrl Pts',(42.0405341034505,46.8094668591667,2.65878715325391));
#242427=CARTESIAN_POINT('Ctrl Pts',(42.0032346206986,46.7483190388774,2.65878198860295));
#242428=CARTESIAN_POINT('Ctrl Pts',(41.9705316734065,46.8890030154865,2.63878778849903));
#242429=CARTESIAN_POINT('Ctrl Pts',(41.9811230778542,46.8318174060856,2.69564460180121));
#242430=CARTESIAN_POINT('Ctrl Pts',(41.9515093836257,46.7612038509546,2.68180481624906));
#242431=CARTESIAN_POINT('Ctrl Pts',(41.8426461117367,46.906368706767,2.75443238878681));
#242432=CARTESIAN_POINT('Ctrl Pts',(41.8933796070866,46.8290619651514,2.79268340777156));
#242433=CARTESIAN_POINT('Ctrl Pts',(41.8570065263035,46.7485125544804,2.74885926835653));
#242434=CARTESIAN_POINT('Ctrl Pts',(41.7917018131131,46.889698257691,2.82856655361701));
#242435=CARTESIAN_POINT('Ctrl Pts',(41.8649047103987,46.80329765619,2.85384197230859));
#242436=CARTESIAN_POINT('Ctrl Pts',(41.8144193983038,46.7243152668223,2.79184624278478));
#242437=CARTESIAN_POINT('Ctrl Pts',(41.7612723673362,46.8559036426988,2.90134173516057));
#242438=CARTESIAN_POINT('Ctrl Pts',(41.856368353593,46.7709043015505,2.90163218716424));
#242439=CARTESIAN_POINT('Ctrl Pts',(41.7839914803026,46.69052164029,2.83404198860295));
#242440=CARTESIAN_POINT('Origin',(42.0411527846894,46.7142062431425,2.53178198860295));
#242441=CARTESIAN_POINT('Origin',(-0.235948482089068,0.212448967519121,
3.64303198860263));
#242442=CARTESIAN_POINT('Origin',(39.9143573409156,44.8038810887677,3.64303198860294));
#242443=CARTESIAN_POINT('Origin',(5.55434424446679E-15,1.857600133136E-13,
2.53178198860262));
#242444=CARTESIAN_POINT('Origin',(42.06380383897,46.6938111422607,2.53178198860295));
#242445=CARTESIAN_POINT('Ctrl Pts',(39.9143573409156,44.8038810887677,3.77003198860295));
#242446=CARTESIAN_POINT('Ctrl Pts',(40.0088781183435,44.7187741985014,3.77003198860295));
#242447=CARTESIAN_POINT('Ctrl Pts',(40.0087366280095,44.7189015969704,3.64284187937082));
#242448=CARTESIAN_POINT('Ctrl Pts',(39.7693421853883,44.6424822887499,3.77003198860294));
#242449=CARTESIAN_POINT('Ctrl Pts',(39.8638196089383,44.5576711710519,3.76980208962821));
#242450=CARTESIAN_POINT('Ctrl Pts',(39.8926305794718,44.5899527660329,3.64284193928301));
#242451=CARTESIAN_POINT('Ctrl Pts',(39.6312917695241,44.4888315723759,3.65553535416619));
#242452=CARTESIAN_POINT('Ctrl Pts',(39.7256919284542,44.404265585613,3.65520057834613));
#242453=CARTESIAN_POINT('Ctrl Pts',(39.78209980511,44.4671959043832,3.55127910964301));
#242454=CARTESIAN_POINT('Ctrl Pts',(39.554446981307,44.4033023070492,3.47153072139103));
#242455=CARTESIAN_POINT('Ctrl Pts',(39.6488649704636,44.3189410144585,3.47122746281614));
#242456=CARTESIAN_POINT('Ctrl Pts',(39.7205730900532,44.3988635644383,3.40413045901307));
#242457=CARTESIAN_POINT('Origin',(39.6260861683717,44.4837235168759,3.40423097483342));
#242458=CARTESIAN_POINT('Ctrl Pts',(42.2339804752701,46.4302753505428,2.90134173516057));
#242459=CARTESIAN_POINT('Ctrl Pts',(42.1395065320998,46.5159655405278,2.90163218716425));
#242460=CARTESIAN_POINT('Ctrl Pts',(42.0671296588095,46.4355828792673,2.83404198860295));
#242461=CARTESIAN_POINT('Ctrl Pts',(42.2644230274451,46.4640859592749,2.82853349835392));
#242462=CARTESIAN_POINT('Ctrl Pts',(42.1708479205161,46.5278479142008,2.85381483162254));
#242463=CARTESIAN_POINT('Ctrl Pts',(42.0975714415913,46.4693919041985,2.79182701594249));
#242464=CARTESIAN_POINT('Ctrl Pts',(42.2755508889262,46.51636388123,2.7546882207367));
#242465=CARTESIAN_POINT('Ctrl Pts',(42.1933444849786,46.5588164356976,2.7928691308386));
#242466=CARTESIAN_POINT('Ctrl Pts',(42.1170605480854,46.5141432491638,2.74900763297952));
#242467=CARTESIAN_POINT('Ctrl Pts',(42.2454039774545,46.6408663419436,2.63954450640431));
#242468=CARTESIAN_POINT('Ctrl Pts',(42.1872204559318,46.6457133039302,2.69627684028895));
#242469=CARTESIAN_POINT('Ctrl Pts',(42.1199995355541,46.608854104584,2.68224356036518));
#242470=CARTESIAN_POINT('Ctrl Pts',(42.2015749714292,46.7146600431957,2.59908178706372));
#242471=CARTESIAN_POINT('Ctrl Pts',(42.1587905896517,46.702988253195,2.65878704321409));
#242472=CARTESIAN_POINT('Ctrl Pts',(42.101818754756,46.6595535157377,2.65878198860295));
#242473=CARTESIAN_POINT('Ctrl Pts',(42.1358900227694,46.773831928426,2.59908173516057));
#242474=CARTESIAN_POINT('Ctrl Pts',(42.110921478106,46.7461150696875,2.65878198860295));
#242475=CARTESIAN_POINT('Ctrl Pts',(42.06380383897,46.6938111422607,2.65878198860295));
#242476=CARTESIAN_POINT('Origin',(42.1615090516451,46.3506032922597,2.83404198860294));
#242477=CARTESIAN_POINT('Origin',(39.5068809815356,44.3513327445017,3.11913648167102));
#242478=CARTESIAN_POINT('Origin',(39.3876757945573,44.2189419720526,2.83404198860293));
#242479=CARTESIAN_POINT('Origin',(42.0423040287647,46.2182127020528,3.11913648177573));
#242480=CARTESIAN_POINT('Origin',(41.9230990057955,46.0858221116781,3.40423097483343));
#242481=CARTESIAN_POINT('Ctrl Pts',(39.3160391863689,44.1385184650378,2.90134173516055));
#242482=CARTESIAN_POINT('Ctrl Pts',(39.4103156382731,44.0542875439843,2.90103711553261));
#242483=CARTESIAN_POINT('Ctrl Pts',(39.4820551873929,44.133962385045,2.83404198860293));
#242484=CARTESIAN_POINT('Ctrl Pts',(39.2856369388939,44.1047525536514,2.82862991747984));
#242485=CARTESIAN_POINT('Ctrl Pts',(39.3789425853234,44.0421527706804,2.85314045886445));
#242486=CARTESIAN_POINT('Ctrl Pts',(39.4516512848565,44.1001954303884,2.79187960999954));
#242487=CARTESIAN_POINT('Ctrl Pts',(39.2745942851002,44.0527517782419,2.75470625793367));
#242488=CARTESIAN_POINT('Ctrl Pts',(39.3566016867499,44.0110417363806,2.79224250381939));
#242489=CARTESIAN_POINT('Ctrl Pts',(39.4323285306302,44.0556530121007,2.7490180910829));
#242490=CARTESIAN_POINT('Ctrl Pts',(39.3050549810248,43.929007150946,2.63947868311719));
#242491=CARTESIAN_POINT('Ctrl Pts',(39.3631024520339,43.9243964923855,2.69595066767934));
#242492=CARTESIAN_POINT('Ctrl Pts',(39.4299498468378,43.961478133811,2.68220539436092));
#242493=CARTESIAN_POINT('Ctrl Pts',(39.3490583909342,43.8557442421763,2.59908178585127));
#242494=CARTESIAN_POINT('Ctrl Pts',(39.3917348424063,43.867520632012,2.65877670944998));
#242495=CARTESIAN_POINT('Ctrl Pts',(39.4485000225478,43.9111340157081,2.65878198860293));
#242496=CARTESIAN_POINT('Ctrl Pts',(39.4144401478989,43.7969047596349,2.59908173516055));
#242497=CARTESIAN_POINT('Ctrl Pts',(39.4393948122687,43.8246341160488,2.65878198860293));
#242498=CARTESIAN_POINT('Ctrl Pts',(39.4864862581816,43.8769616275877,2.65878198860293));
#242499=CARTESIAN_POINT('Origin',(39.4864862581816,43.8769616275877,2.53178198860293));
#242500=CARTESIAN_POINT('Ctrl Pts',(41.6348281284261,45.7656648676109,3.77003198860296));
#242501=CARTESIAN_POINT('Ctrl Pts',(41.540307729011,45.8507714175129,3.77003198860296));
#242502=CARTESIAN_POINT('Ctrl Pts',(41.540448840768,45.8506443599162,3.64284238727624));
#242503=CARTESIAN_POINT('Ctrl Pts',(41.7801793768013,45.926760978664,3.77003198860296));
#242504=CARTESIAN_POINT('Ctrl Pts',(41.6856176794258,46.0121552117493,3.77025506105888));
#242505=CARTESIAN_POINT('Ctrl Pts',(41.6565546403128,45.9795929135644,3.64284210641882));
#242506=CARTESIAN_POINT('Ctrl Pts',(41.9185498083239,46.0801233673962,3.65553527987865));
#242507=CARTESIAN_POINT('Ctrl Pts',(41.8239142817222,46.1657498592392,3.65585996533134));
#242508=CARTESIAN_POINT('Ctrl Pts',(41.7670853619627,46.1023497159527,3.55127902710263));
#242509=CARTESIAN_POINT('Ctrl Pts',(41.995572738225,46.1654920697614,3.47153072139104));
#242510=CARTESIAN_POINT('Ctrl Pts',(41.900956806909,46.2513146407506,3.47182327905221));
#242511=CARTESIAN_POINT('Ctrl Pts',(41.8286118967078,46.170681855241,3.40413028378016));
#242512=CARTESIAN_POINT('Origin',(41.6348281284261,45.7656648676109,3.64303198860296));
#242513=CARTESIAN_POINT('Origin',(5.70392627685665E-15,1.86368317680676E-13,
2.53178198860262));
#242514=CARTESIAN_POINT('Origin',(39.5091373124621,43.8565665267059,2.53178198860292));
#242515=CARTESIAN_POINT('Origin',(28.0951675083324,30.7283483363947,3.64303198860284));
#242516=CARTESIAN_POINT('Origin',(41.3663085755636,45.4673664422112,3.64299466007543));
#242517=CARTESIAN_POINT('Ctrl Pts',(39.4370498736007,43.7765468711725,2.59908173516055));
#242518=CARTESIAN_POINT('Ctrl Pts',(39.4620188529809,43.8042633382932,2.65878198860293));
#242519=CARTESIAN_POINT('Ctrl Pts',(39.5091373124622,43.8565665267059,2.65878198860293));
#242520=CARTESIAN_POINT('Ctrl Pts',(39.5021785224869,43.7178744835422,2.59908193199943));
#242521=CARTESIAN_POINT('Ctrl Pts',(39.509465444134,43.761515733968,2.65877685806608));
#242522=CARTESIAN_POINT('Ctrl Pts',(39.546963765375,43.8224770900137,2.65878198860293));
#242523=CARTESIAN_POINT('Ctrl Pts',(39.5788516269097,43.6818502604301,2.63872492669813));
#242524=CARTESIAN_POINT('Ctrl Pts',(39.5685043961838,43.7389249259239,2.69532212015309));
#242525=CARTESIAN_POINT('Ctrl Pts',(39.5983821485332,43.8091917332949,2.68176836726648));
#242526=CARTESIAN_POINT('Ctrl Pts',(39.7059848156962,43.6640874258691,2.75442176402296));
#242527=CARTESIAN_POINT('Ctrl Pts',(39.6560168722793,43.7412697217734,2.79203179920159));
#242528=CARTESIAN_POINT('Ctrl Pts',(39.6923865500763,43.8212571467116,2.74885310748224));
#242529=CARTESIAN_POINT('Ctrl Pts',(39.756687810178,43.6806424921201,2.82866089558422));
#242530=CARTESIAN_POINT('Ctrl Pts',(39.6846695243131,43.7668962219033,2.85316563119229));
#242531=CARTESIAN_POINT('Ctrl Pts',(39.7348023770065,43.8452710114193,2.79189751796648));
#242532=CARTESIAN_POINT('Ctrl Pts',(39.7870778846746,43.7143933160626,2.90134173516054));
#242533=CARTESIAN_POINT('Ctrl Pts',(39.69345381678,43.7993487829616,2.9010371155326));
#242534=CARTESIAN_POINT('Ctrl Pts',(39.7651933658998,43.8790236240223,2.83404198860292));
#242535=CARTESIAN_POINT('Origin',(39.8595727587354,43.7940440370147,2.83404198860294));
#242536=CARTESIAN_POINT('Origin',(41.3366772856877,45.4345348103664,3.56647653971819));
#242537=CARTESIAN_POINT('Origin',(41.2819167515328,45.3737170758075,3.42473028058517));
#242538=CARTESIAN_POINT('Origin',(39.9787779456606,43.926434809488,3.11913648168203));
#242539=CARTESIAN_POINT('Origin',(40.0979831325498,44.058825581838,3.40423097483342));
#242540=CARTESIAN_POINT('Ctrl Pts',(41.0611303347403,45.1285089182135,3.36123028058514));
#242541=CARTESIAN_POINT('Ctrl Pts',(40.9667509419047,45.2134885052211,3.36123028058514));
#242542=CARTESIAN_POINT('Ctrl Pts',(40.9667509419047,45.2134885052211,3.23423028058514));
#242543=CARTESIAN_POINT('Ctrl Pts',(41.121185060844,45.1955564429366,3.36123028058513));
#242544=CARTESIAN_POINT('Ctrl Pts',(41.0269231466356,45.2803165088396,3.36099641108276));
#242545=CARTESIAN_POINT('Ctrl Pts',(41.0570929845744,45.3138235084253,3.23423043688384));
#242546=CARTESIAN_POINT('Ctrl Pts',(41.1779726855671,45.2589537050066,3.41054258905318));
#242547=CARTESIAN_POINT('Ctrl Pts',(41.0841042944916,45.3438226072607,3.41008815826171));
#242548=CARTESIAN_POINT('Ctrl Pts',(41.1425178129631,45.408697391911,3.3081986730431));
#242549=CARTESIAN_POINT('Ctrl Pts',(41.2079002115907,45.292364129856,3.48823028058516));
#242550=CARTESIAN_POINT('Ctrl Pts',(41.1142722655005,45.3773275334108,3.48794691941632));
#242551=CARTESIAN_POINT('Ctrl Pts',(41.1875373586971,45.4586966628151,3.42473028058517));
#242552=CARTESIAN_POINT('Origin',(41.0611303347403,45.1285089182135,3.23423028058514));
#242553=CARTESIAN_POINT('Ctrl Pts',(40.0254908126588,43.9791725362585,3.47153072139104));
#242554=CARTESIAN_POINT('Ctrl Pts',(39.9317223035498,44.0642551277131,3.47122746285109));
#242555=CARTESIAN_POINT('Ctrl Pts',(40.0037114707677,44.1439246046466,3.40413046676837));
#242556=CARTESIAN_POINT('Ctrl Pts',(40.102520236037,44.0645378932555,3.65553813458016));
#242557=CARTESIAN_POINT('Ctrl Pts',(40.0085500157868,44.1495813562475,3.65520336072198));
#242558=CARTESIAN_POINT('Ctrl Pts',(40.0652391174801,44.2122579788868,3.55128134519927));
#242559=CARTESIAN_POINT('Ctrl Pts',(40.2409001323905,44.217894138564,3.77003198860295));
#242560=CARTESIAN_POINT('Ctrl Pts',(40.1466780419431,44.3029888158481,3.76980209314041));
#242561=CARTESIAN_POINT('Ctrl Pts',(40.1757707681154,44.3350158129976,3.64284195387457));
#242562=CARTESIAN_POINT('Ctrl Pts',(40.3862543050938,44.3789831537298,3.77003198860295));
#242563=CARTESIAN_POINT('Ctrl Pts',(40.2917335385825,44.4640900341667,3.77003198860295));
#242564=CARTESIAN_POINT('Ctrl Pts',(40.2918750179835,44.4639626455418,3.64284189403867));
#242565=CARTESIAN_POINT('Origin',(40.3862543050938,44.3789831537298,3.64303198860294));
#242566=CARTESIAN_POINT('Origin',(27.4203375923833,29.9788737863605,3.23423028058502));
#242567=CARTESIAN_POINT('Origin',(40.9599523566124,45.0161393894796,3.23423028058513));
#242568=CARTESIAN_POINT('Origin',(27.314662201079,29.8615093742685,3.64303198860283));
#242569=CARTESIAN_POINT('Origin',(40.6548553974681,44.6772189625517,3.64299171721807));
#242570=CARTESIAN_POINT('Ctrl Pts',(40.8131880745606,44.8522789915944,3.48823028058513));
#242571=CARTESIAN_POINT('Ctrl Pts',(40.7187157882337,44.9380175594365,3.4885200421229));
#242572=CARTESIAN_POINT('Ctrl Pts',(40.6447864996552,44.8559107663288,3.42473028058512));
#242573=CARTESIAN_POINT('Ctrl Pts',(40.8432146576636,44.8858042435441,3.41028005848437));
#242574=CARTESIAN_POINT('Ctrl Pts',(40.7486708738398,44.9712860523973,3.41074404220417));
#242575=CARTESIAN_POINT('Ctrl Pts',(40.6899581892278,44.9060790100841,3.30780486244021));
#242576=CARTESIAN_POINT('Ctrl Pts',(40.900100336764,44.9493173051411,3.36123028058514));
#242577=CARTESIAN_POINT('Ctrl Pts',(40.8054891887023,45.0343891839535,3.361464605865));
#242578=CARTESIAN_POINT('Ctrl Pts',(40.7755352187354,45.0011219300372,3.23423045308391));
#242579=CARTESIAN_POINT('Ctrl Pts',(40.9599523566124,45.0161393894796,3.36123028058514));
#242580=CARTESIAN_POINT('Ctrl Pts',(40.8655729637768,45.1011189764871,3.36123028058513));
#242581=CARTESIAN_POINT('Ctrl Pts',(40.8655729637768,45.1011189764871,3.23423028058514));
#242582=CARTESIAN_POINT('Origin',(40.7391658924908,44.7709311793212,3.42473028058512));
#242583=CARTESIAN_POINT('Origin',(40.6847319392794,44.7104761492012,3.5656311352478));
#242584=CARTESIAN_POINT('Origin',(35.8473027488291,49.8797426639498,3.5664765390943));
#242585=CARTESIAN_POINT('Origin',(35.8732562382986,49.915552518433,3.64299466007487));
#242586=CARTESIAN_POINT('Origin',(35.7991993820661,49.8135340601225,3.42473028058518));
#242587=CARTESIAN_POINT('Ctrl Pts',(35.7350130971388,49.7242207306177,3.48823028058519));
#242588=CARTESIAN_POINT('Ctrl Pts',(35.8375861910555,49.6503036646788,3.48794691941635));
#242589=CARTESIAN_POINT('Ctrl Pts',(35.9019445403517,49.7388853330814,3.4247302805852));
#242590=CARTESIAN_POINT('Ctrl Pts',(35.7084656432359,49.6878783768795,3.41028005925123));
#242591=CARTESIAN_POINT('Ctrl Pts',(35.8109961808893,49.6137056554185,3.40982512231065));
#242592=CARTESIAN_POINT('Ctrl Pts',(35.8622643302261,49.6842702092639,3.30780486372868));
#242593=CARTESIAN_POINT('Ctrl Pts',(35.6581711379713,49.6190282456269,3.36123028058517));
#242594=CARTESIAN_POINT('Ctrl Pts',(35.7606778378438,49.5444483977866,3.36099721048315));
#242595=CARTESIAN_POINT('Ctrl Pts',(35.7870908094894,49.5808027344238,3.23423045308355));
#242596=CARTESIAN_POINT('Ctrl Pts',(35.6052536882601,49.5465907136147,3.36123028058517));
#242597=CARTESIAN_POINT('Ctrl Pts',(35.7079988465457,49.4719419865736,3.36123028058517));
#242598=CARTESIAN_POINT('Ctrl Pts',(35.7079988465457,49.4719419865736,3.23423028058517));
#242599=CARTESIAN_POINT('Origin',(35.6052536882601,49.5465907136147,3.23423028058516));
#242600=CARTESIAN_POINT('Origin',(-0.256862895714041,0.186621817603044,
3.64303198860263));
#242601=CARTESIAN_POINT('Origin',(36.1092077731528,50.2402240048086,3.64303198860298));
#242602=CARTESIAN_POINT('Origin',(-0.256862895714041,0.186621817603046,
3.23423028058482));
#242603=CARTESIAN_POINT('Origin',(35.5163757878395,49.4242607783463,3.23423028058516));
#242604=CARTESIAN_POINT('Ctrl Pts',(36.4252947698678,50.6762142289951,3.47153072139107));
#242605=CARTESIAN_POINT('Ctrl Pts',(36.5289136610816,50.6015094050817,3.47182327902698));
#242606=CARTESIAN_POINT('Ctrl Pts',(36.465084262422,50.5139809070356,3.40413028959067));
#242607=CARTESIAN_POINT('Ctrl Pts',(36.3578045222551,50.5831238715081,3.65553807120993));
#242608=CARTESIAN_POINT('Ctrl Pts',(36.4612356912254,50.5083591136211,3.65586275497056));
#242609=CARTESIAN_POINT('Ctrl Pts',(36.41103660916,50.4395906940215,3.55128126837327));
#242610=CARTESIAN_POINT('Ctrl Pts',(36.2365613423282,50.4158900112697,3.77003198860299));
#242611=CARTESIAN_POINT('Ctrl Pts',(36.3397499727013,50.3411491755185,3.7702550574847));
#242612=CARTESIAN_POINT('Ctrl Pts',(36.3139421975383,50.3059517008892,3.64284211731151));
#242613=CARTESIAN_POINT('Ctrl Pts',(36.1092077731528,50.2402240048086,3.77003198860299));
#242614=CARTESIAN_POINT('Ctrl Pts',(36.2121064279405,50.1654637560307,3.77003198860299));
#242615=CARTESIAN_POINT('Ctrl Pts',(36.2119528169512,50.1655753609472,3.64284239821743));
#242616=CARTESIAN_POINT('Origin',(36.3624339277672,50.5887599058104,3.40423097483345));
#242617=CARTESIAN_POINT('Ctrl Pts',(35.5163757878395,49.4242607783463,3.36123028058516));
#242618=CARTESIAN_POINT('Ctrl Pts',(35.6191209461251,49.3496120513052,3.36123028058517));
#242619=CARTESIAN_POINT('Ctrl Pts',(35.6191209461251,49.3496120513052,3.23423028058516));
#242620=CARTESIAN_POINT('Ctrl Pts',(35.4632790141048,49.3515787599191,3.36123028058517));
#242621=CARTESIAN_POINT('Ctrl Pts',(35.5661632154422,49.2767219882436,3.36146538610113));
#242622=CARTESIAN_POINT('Ctrl Pts',(35.5397616632037,49.2403833690707,3.23423043688441));
#242623=CARTESIAN_POINT('Ctrl Pts',(35.4130704930569,49.282853485729,3.41054258693134));
#242624=CARTESIAN_POINT('Ctrl Pts',(35.5163418450526,49.2081487547905,3.41100608859837));
#242625=CARTESIAN_POINT('Ctrl Pts',(35.4647218031682,49.1370998624031,3.30819866970878));
#242626=CARTESIAN_POINT('Ctrl Pts',(35.3866101428259,49.2466351556015,3.48823028058516));
#242627=CARTESIAN_POINT('Ctrl Pts',(35.4901170100366,49.1720533660034,3.48852004212294));
#242628=CARTESIAN_POINT('Ctrl Pts',(35.4251752107437,49.0826686475737,3.42473028058516));
#242629=CARTESIAN_POINT('Origin',(35.3224300524581,49.1573173746149,3.42473028058515));
#242630=CARTESIAN_POINT('Origin',(36.4671473482298,50.7328855645265,3.11913648178361));
#242631=CARTESIAN_POINT('Origin',(36.5718607685321,50.8770112231005,2.83404198860297));
#242632=CARTESIAN_POINT('Origin',(35.2746135646412,49.091503625274,3.56563113460758));
#242633=CARTESIAN_POINT('Origin',(35.2482948100395,49.0553654007528,3.64299171721827));
#242634=CARTESIAN_POINT('Ctrl Pts',(36.9911673391707,50.9399462128204,2.59908173516059));
#242635=CARTESIAN_POINT('Ctrl Pts',(36.9692474126339,50.9097606317996,2.65878198860298));
#242636=CARTESIAN_POINT('Ctrl Pts',(36.9278827595326,50.8527980281388,2.65878198860298));
#242637=CARTESIAN_POINT('Ctrl Pts',(36.9198678602469,50.9917217504956,2.59908193475707));
#242638=CARTESIAN_POINT('Ctrl Pts',(36.91731002169,50.9474721267398,2.65878715325422));
#242639=CARTESIAN_POINT('Ctrl Pts',(36.8866065570942,50.8827604229952,2.65878198860298));
#242640=CARTESIAN_POINT('Ctrl Pts',(36.8393772800889,51.019255329238,2.63878778849925));
#242641=CARTESIAN_POINT('Ctrl Pts',(36.8558881875867,50.9634900918196,2.69564460180162));
#242642=CARTESIAN_POINT('Ctrl Pts',(36.8338178466775,50.8901678911827,2.68180481624929));
#242643=CARTESIAN_POINT('Ctrl Pts',(36.7103770798843,51.0231582082091,2.75443238878662));
#242644=CARTESIAN_POINT('Ctrl Pts',(36.7689134067396,50.9515780553178,2.79268340777113));
#242645=CARTESIAN_POINT('Ctrl Pts',(36.7411592876132,50.8676678805079,2.74885926835635));
#242646=CARTESIAN_POINT('Ctrl Pts',(36.6614543958831,51.0012539523494,2.82856655361719));
#242647=CARTESIAN_POINT('Ctrl Pts',(36.7432876021367,50.9229784487433,2.85384197230806));
#242648=CARTESIAN_POINT('Ctrl Pts',(36.7013347616507,50.8391515810788,2.79184624278497));
#242649=CARTESIAN_POINT('Ctrl Pts',(36.6347241449653,50.9644637245896,2.90134173516059));
#242650=CARTESIAN_POINT('Ctrl Pts',(36.7381840359683,50.889870256032,2.90163218716427));
#242651=CARTESIAN_POINT('Ctrl Pts',(36.6746059268177,50.8023624960594,2.83404198860298));
#242652=CARTESIAN_POINT('Origin',(36.9278827595326,50.8527980281388,2.53178198860298));
#242653=CARTESIAN_POINT('Origin',(-0.256862895714041,0.186621817603044,
3.64303198860263));
#242654=CARTESIAN_POINT('Origin',(35.0124214764584,48.7306271754179,3.64303198860296));
#242655=CARTESIAN_POINT('Origin',(5.56775724677592E-15,1.85749151678493E-13,
2.53178198860262));
#242656=CARTESIAN_POINT('Origin',(36.9525415975211,50.8348823336489,2.53178198860298));
#242657=CARTESIAN_POINT('Ctrl Pts',(35.0124214764584,48.7306271754179,3.77003198860297));
#242658=CARTESIAN_POINT('Ctrl Pts',(35.1153205516307,48.6558666212128,3.77003198860297));
#242659=CARTESIAN_POINT('Ctrl Pts',(35.1151665196294,48.6559785320124,3.64284187937079));
#242660=CARTESIAN_POINT('Ctrl Pts',(34.8850714976655,48.5549543235562,3.77003198860297));
#242661=CARTESIAN_POINT('Ctrl Pts',(34.987896539803,48.4804833899298,3.76980208963067));
#242662=CARTESIAN_POINT('Ctrl Pts',(35.0131753353112,48.5155997094322,3.64284193928456));
#242663=CARTESIAN_POINT('Ctrl Pts',(34.7638382096863,48.3877151240595,3.6555353541662));
#242664=CARTESIAN_POINT('Ctrl Pts',(34.8665607873066,48.3134799021725,3.65520057834321));
#242665=CARTESIAN_POINT('Ctrl Pts',(34.916081646202,48.3819617107295,3.55127910964134));
#242666=CARTESIAN_POINT('Ctrl Pts',(34.6963546279284,48.2946219293749,3.47153072139107));
#242667=CARTESIAN_POINT('Ctrl Pts',(34.7990735417351,48.2205921440832,3.47122746281618));
#242668=CARTESIAN_POINT('Ctrl Pts',(34.8620346554129,48.3075724095164,3.40413045901307));
#242669=CARTESIAN_POINT('Origin',(34.7591950625533,48.3820909175332,3.40423097483344));
#242670=CARTESIAN_POINT('Ctrl Pts',(37.149332979726,50.5905785208487,2.90134173516059));
#242671=CARTESIAN_POINT('Ctrl Pts',(37.0464195108252,50.6659240749086,2.90163218716426));
#242672=CARTESIAN_POINT('Ctrl Pts',(36.9828414016746,50.578416314936,2.83404198860297));
#242673=CARTESIAN_POINT('Ctrl Pts',(37.1760745934432,50.6273860247245,2.82853349835386));
#242674=CARTESIAN_POINT('Ctrl Pts',(37.0763471615769,50.6810174228649,2.85381483162332));
#242675=CARTESIAN_POINT('Ctrl Pts',(37.0095824157646,50.6152221632646,2.79182701594277));
#242676=CARTESIAN_POINT('Ctrl Pts',(37.1816769644886,50.6805407410142,2.75468822073683));
#242677=CARTESIAN_POINT('Ctrl Pts',(37.0954833955427,50.7141678268709,2.79286913083839));
#242678=CARTESIAN_POINT('Ctrl Pts',(37.0242869695753,50.6617655220318,2.74900763297936));
#242679=CARTESIAN_POINT('Ctrl Pts',(37.1386811500613,50.8012099538924,2.63954450640423));
#242680=CARTESIAN_POINT('Ctrl Pts',(37.0803097184695,50.7999485296222,2.69627684028912));
#242681=CARTESIAN_POINT('Ctrl Pts',(37.0173098767919,50.75626474932,2.68224356036539));
#242682=CARTESIAN_POINT('Ctrl Pts',(37.0873787017257,50.8700180268816,2.59908178706417));
#242683=CARTESIAN_POINT('Ctrl Pts',(37.0460487315411,50.8539379904897,2.65878704321598));
#242684=CARTESIAN_POINT('Ctrl Pts',(36.9939291606762,50.8047860147164,2.65878198860297));
#242685=CARTESIAN_POINT('Ctrl Pts',(37.0158684358559,50.9219998155902,2.59908173516059));
#242686=CARTESIAN_POINT('Ctrl Pts',(36.9939338721432,50.8918248691003,2.65878198860297));
#242687=CARTESIAN_POINT('Ctrl Pts',(36.9525415975211,50.8348823336489,2.65878198860297));
#242688=CARTESIAN_POINT('Origin',(37.0855865599602,50.5037675878948,2.83404198860297));
#242689=CARTESIAN_POINT('Origin',(34.6544814981904,48.2379650606703,3.11913648167033));
#242690=CARTESIAN_POINT('Origin',(34.549767933694,48.093839203715,2.83404198860297));
#242691=CARTESIAN_POINT('Origin',(36.9808731396113,50.3596419293399,3.11913648177612));
#242692=CARTESIAN_POINT('Origin',(36.8761597191953,50.2155162706046,3.40423097483345));
#242693=CARTESIAN_POINT('Ctrl Pts',(34.4869303039396,48.006368200519,2.90134173516058));
#242694=CARTESIAN_POINT('Ctrl Pts',(34.5894948283132,47.932453277904,2.90103711553263));
#242695=CARTESIAN_POINT('Ctrl Pts',(34.6525130919796,48.0191904766739,2.83404198860296));
#242696=CARTESIAN_POINT('Ctrl Pts',(34.460224101985,47.96960936212,2.82862991747999));
#242697=CARTESIAN_POINT('Ctrl Pts',(34.5595620694345,47.9171056031441,2.85314045886591));
#242698=CARTESIAN_POINT('Ctrl Pts',(34.6258053530818,47.9824304277183,2.79187961000031));
#242699=CARTESIAN_POINT('Ctrl Pts',(34.4546775021468,47.9167391807672,2.75470625793355));
#242700=CARTESIAN_POINT('Ctrl Pts',(34.5405955452484,47.8838297385499,2.79224250381907));
#242701=CARTESIAN_POINT('Ctrl Pts',(34.6112444014588,47.9361122396532,2.74901809108288));
#242702=CARTESIAN_POINT('Ctrl Pts',(34.4979061669209,47.7968564492225,2.63947868311738));
#242703=CARTESIAN_POINT('Ctrl Pts',(34.5561175928641,47.7983386612737,2.69595066767962));
#242704=CARTESIAN_POINT('Ctrl Pts',(34.6187227036514,47.8422046210395,2.682205394361));
#242705=CARTESIAN_POINT('Ctrl Pts',(34.5493265808152,47.7285944911493,2.59908178585215));
#242706=CARTESIAN_POINT('Ctrl Pts',(34.5905382782887,47.7447672725793,2.6587767094491));
#242707=CARTESIAN_POINT('Ctrl Pts',(34.6424336528586,47.7940753146444,2.65878198860296));
#242708=CARTESIAN_POINT('Ctrl Pts',(34.6205005703634,47.6769115920306,2.59908173516057));
#242709=CARTESIAN_POINT('Ctrl Pts',(34.6424200234574,47.7070975168467,2.65878198860296));
#242710=CARTESIAN_POINT('Ctrl Pts',(34.6837837831345,47.7640607692766,2.65878198860296));
#242711=CARTESIAN_POINT('Origin',(34.6837837831345,47.7640607692766,2.53178198860296));
#242712=CARTESIAN_POINT('Ctrl Pts',(36.6229335645808,49.8669803696028,3.77003198860299));
#242713=CARTESIAN_POINT('Ctrl Pts',(36.5200349009284,49.9417406248212,3.77003198860299));
#242714=CARTESIAN_POINT('Ctrl Pts',(36.5201885207956,49.9416290134546,3.64284238727641));
#242715=CARTESIAN_POINT('Ctrl Pts',(36.7506494346803,50.042387321932,3.77003198860298));
#242716=CARTESIAN_POINT('Ctrl Pts',(36.6476796282221,50.1174293675638,3.77025506106058));
#242717=CARTESIAN_POINT('Ctrl Pts',(36.6221794864693,50.0820075342373,3.64284210641899));
#242718=CARTESIAN_POINT('Ctrl Pts',(36.8722311236859,50.2093732240195,3.65553527987869));
#242719=CARTESIAN_POINT('Ctrl Pts',(36.7691636147942,50.2846385388115,3.65585996532951));
#242720=CARTESIAN_POINT('Ctrl Pts',(36.7192731293506,50.2156454684943,3.55127902710247));
#242721=CARTESIAN_POINT('Ctrl Pts',(36.9399086546485,50.3023253561998,3.47153072139107));
#242722=CARTESIAN_POINT('Ctrl Pts',(36.836840137845,50.3777877242642,3.47182327905223));
#242723=CARTESIAN_POINT('Ctrl Pts',(36.7733199617898,50.2900345513019,3.40413028378026));
#242724=CARTESIAN_POINT('Origin',(36.6229335645808,49.8669803696028,3.64303198860299));
#242725=CARTESIAN_POINT('Origin',(5.69915478234096E-15,1.86372181560749E-13,
2.53178198860262));
#242726=CARTESIAN_POINT('Origin',(34.7084426211231,47.7461450747867,2.53178198860296));
#242727=CARTESIAN_POINT('Origin',(21.7541926348211,29.4019141737118,3.64303198860283));
#242728=CARTESIAN_POINT('Origin',(36.3870656659268,49.5422481179705,3.64299466007604));
#242729=CARTESIAN_POINT('Ctrl Pts',(34.6451144164185,47.6590285860938,2.59908173516057));
#242730=CARTESIAN_POINT('Ctrl Pts',(34.6670494534017,47.6892031885516,2.65878198860296));
#242731=CARTESIAN_POINT('Ctrl Pts',(34.7084426211231,47.7461450747867,2.65878198860296));
#242732=CARTESIAN_POINT('Ctrl Pts',(34.7160192182667,47.6074854095247,2.59908193199937));
#242733=CARTESIAN_POINT('Ctrl Pts',(34.7187044685527,47.6516492793368,2.65877685806639));
#242734=CARTESIAN_POINT('Ctrl Pts',(34.7496251732007,47.7161963245904,2.65878198860296));
#242735=CARTESIAN_POINT('Ctrl Pts',(34.7960378560835,47.5796730526555,2.63872492669835));
#242736=CARTESIAN_POINT('Ctrl Pts',(34.7797813814945,47.6353534770324,2.69532212015306));
#242737=CARTESIAN_POINT('Ctrl Pts',(34.8021505789971,47.7083584310197,2.68176836726665));
#242738=CARTESIAN_POINT('Ctrl Pts',(34.9243313177594,47.5752965616148,2.75442176402279));
#242739=CARTESIAN_POINT('Ctrl Pts',(34.8665693571826,47.6468329724891,2.79203179920176));
#242740=CARTESIAN_POINT('Ctrl Pts',(34.8943788354696,47.7301838844735,2.74885310748212));
#242741=CARTESIAN_POINT('Ctrl Pts',(34.973026080298,47.5970608435769,2.82866089558435));
#242742=CARTESIAN_POINT('Ctrl Pts',(34.8923863483137,47.6753141056551,2.85316563119181));
#242743=CARTESIAN_POINT('Ctrl Pts',(34.934052171687,47.7584998599249,2.79189751796619));
#242744=CARTESIAN_POINT('Ctrl Pts',(34.9997217530259,47.6338034047602,2.90134173516057));
#242745=CARTESIAN_POINT('Ctrl Pts',(34.8977303031701,47.7085070967806,2.90103711553263));
#242746=CARTESIAN_POINT('Ctrl Pts',(34.9607485668365,47.7952442955505,2.83404198860296));
#242747=CARTESIAN_POINT('Origin',(35.0634937251221,47.7205955685093,2.83404198860295));
#242748=CARTESIAN_POINT('Origin',(36.361028539381,49.5064990280457,3.56647653971785));
#242749=CARTESIAN_POINT('Origin',(36.3129251734942,49.4402904249168,3.4247302805852));
#242750=CARTESIAN_POINT('Origin',(35.1682072895616,47.8647214254827,3.11913648168205));
#242751=CARTESIAN_POINT('Origin',(35.2729208539814,48.0088472823275,3.40423097483344));
#242752=CARTESIAN_POINT('Ctrl Pts',(36.1189794796882,49.173347078409,3.36123028058516));
#242753=CARTESIAN_POINT('Ctrl Pts',(36.0162343214026,49.2479958054501,3.36123028058517));
#242754=CARTESIAN_POINT('Ctrl Pts',(36.0162343214026,49.2479958054501,3.23423028058516));
#242755=CARTESIAN_POINT('Ctrl Pts',(36.1716968449925,49.2463047380085,3.36123028058516));
#242756=CARTESIAN_POINT('Ctrl Pts',(36.0690914679755,49.3207474263634,3.36099641108398));
#242757=CARTESIAN_POINT('Ctrl Pts',(36.0955935972127,49.3572244778968,3.23423043688375));
#242758=CARTESIAN_POINT('Ctrl Pts',(36.2215465627857,49.3152906263888,3.4105425890532));
#242759=CARTESIAN_POINT('Ctrl Pts',(36.1193211766499,49.3898826892493,3.41008815825999));
#242760=CARTESIAN_POINT('Ctrl Pts',(36.1706334382091,49.4605079583594,3.30819867304302));
#242761=CARTESIAN_POINT('Ctrl Pts',(36.247817802325,49.3516463037388,3.48823028058519));
#242762=CARTESIAN_POINT('Ctrl Pts',(36.1458216659124,49.4263574835553,3.48794691941635));
#242763=CARTESIAN_POINT('Ctrl Pts',(36.2101800152086,49.514939151958,3.4247302805852));
#242764=CARTESIAN_POINT('Origin',(36.1189794796882,49.173347078409,3.23423028058516));
#242765=CARTESIAN_POINT('Ctrl Pts',(35.2091516650527,47.922053073669,3.47153072139106));
#242766=CARTESIAN_POINT('Ctrl Pts',(35.1070032771118,47.9968680956255,3.47122746285111));
#242767=CARTESIAN_POINT('Ctrl Pts',(35.1702703521468,48.0836260518495,3.40413046676815));
#242768=CARTESIAN_POINT('Ctrl Pts',(35.2768360036064,48.0150025575608,3.65553813458022));
#242769=CARTESIAN_POINT('Ctrl Pts',(35.1744910995524,48.0897575808465,3.65520336072116));
#242770=CARTESIAN_POINT('Ctrl Pts',(35.2243181613716,48.1580164790724,3.55128134520005));
#242771=CARTESIAN_POINT('Ctrl Pts',(35.3984277477544,48.1819833392242,3.77003198860297));
#242772=CARTESIAN_POINT('Ctrl Pts',(35.2958269999286,48.2567629686463,3.76980209314327));
#242773=CARTESIAN_POINT('Ctrl Pts',(35.3214126203092,48.2916555365114,3.64284195387391));
#242774=CARTESIAN_POINT('Ctrl Pts',(35.5261472678865,48.3573835402122,3.77003198860298));
#242775=CARTESIAN_POINT('Ctrl Pts',(35.4232482045982,48.432144085783,3.77003198860298));
#242776=CARTESIAN_POINT('Ctrl Pts',(35.4234022246977,48.4320321836305,3.64284189403824));
#242777=CARTESIAN_POINT('Origin',(35.5261472678865,48.3573835402122,3.64303198860297));
#242778=CARTESIAN_POINT('Origin',(21.2334658618522,28.685195257892,3.23423028058501));
#242779=CARTESIAN_POINT('Origin',(36.0301015792676,49.0510171431406,3.23423028058516));
#242780=CARTESIAN_POINT('Origin',(21.151922343707,28.5729602337853,3.64303198860282));
#242781=CARTESIAN_POINT('Origin',(35.7621028045852,48.6820620414859,3.64299171721778));
#242782=CARTESIAN_POINT('Ctrl Pts',(35.9012693628904,48.8727133447946,3.48823028058515));
#242783=CARTESIAN_POINT('Ctrl Pts',(35.7983524848935,48.9481071848799,3.48852004212293));
#242784=CARTESIAN_POINT('Ctrl Pts',(35.7334106856005,48.8587224664503,3.42473028058515));
#242785=CARTESIAN_POINT('Ctrl Pts',(35.9276271141626,48.9091935744952,3.41028005848438));
#242786=CARTESIAN_POINT('Ctrl Pts',(35.8246659689632,48.9843245886195,3.41074404220615));
#242787=CARTESIAN_POINT('Ctrl Pts',(35.7730909105068,48.9133376106115,3.30780486244039));
#242788=CARTESIAN_POINT('Ctrl Pts',(35.9775622448338,48.9783048775141,3.36123028058516));
#242789=CARTESIAN_POINT('Ctrl Pts',(35.8745769537814,49.0530211657582,3.3614646058623));
#242790=CARTESIAN_POINT('Ctrl Pts',(35.8482644497253,49.0168051108897,3.23423045308385));
#242791=CARTESIAN_POINT('Ctrl Pts',(36.0301015792676,49.0510171431406,3.36123028058516));
#242792=CARTESIAN_POINT('Ctrl Pts',(35.927356420982,49.1256658701818,3.36123028058516));
#242793=CARTESIAN_POINT('Ctrl Pts',(35.927356420982,49.1256658701818,3.23423028058516));
#242794=CARTESIAN_POINT('Origin',(35.8361558438862,48.7840737394092,3.42473028058515));
#242795=CARTESIAN_POINT('Origin',(35.7883393569602,48.7182599907914,3.56563113524771));
#242796=CARTESIAN_POINT('Origin',(30.4370746247567,53.353559683258,3.56647653909472));
#242797=CARTESIAN_POINT('Origin',(30.4591427892367,53.3918862459819,3.64299466007685));
#242798=CARTESIAN_POINT('Origin',(30.3961554568836,53.2826856060848,3.42473028058522));
#242799=CARTESIAN_POINT('Ctrl Pts',(30.3416565762235,53.1871522506177,3.48823028058521));
#242800=CARTESIAN_POINT('Ctrl Pts',(30.4513942013112,53.1243619179798,3.48794691941637));
#242801=CARTESIAN_POINT('Ctrl Pts',(30.5061406831642,53.2191856060848,3.42473028058522));
#242802=CARTESIAN_POINT('Ctrl Pts',(30.3190533624383,53.1482340195359,3.41028005925124));
#242803=CARTESIAN_POINT('Ctrl Pts',(30.4287753876659,53.0851849835414,3.40982512231138));
#242804=CARTESIAN_POINT('Ctrl Pts',(30.4723866803445,53.1607219582423,3.30780486372914));
#242805=CARTESIAN_POINT('Ctrl Pts',(30.2762311741522,53.0745038491597,3.36123028058519));
#242806=CARTESIAN_POINT('Ctrl Pts',(30.3859720484839,53.0110474253434,3.36099721048323));
#242807=CARTESIAN_POINT('Ctrl Pts',(30.4084402641645,53.0499635164565,3.23423045308342));
#242808=CARTESIAN_POINT('Ctrl Pts',(30.2311753956711,52.996931757829,3.36123028058519));
#242809=CARTESIAN_POINT('Ctrl Pts',(30.3411606219517,52.933431757829,3.3612302805852));
#242810=CARTESIAN_POINT('Ctrl Pts',(30.3411606219517,52.933431757829,3.23423028058519));
#242811=CARTESIAN_POINT('Origin',(30.2311753956711,52.996931757829,3.23423028058518));
#242812=CARTESIAN_POINT('Origin',(-0.274963065701554,0.158750000000183,
3.64303198860263));
#242813=CARTESIAN_POINT('Origin',(30.6598643453574,53.7394427993289,3.64303198860301));
#242814=CARTESIAN_POINT('Origin',(-0.274963065701554,0.158750000000186,
3.23423028058481));
#242815=CARTESIAN_POINT('Origin',(30.1555713378337,52.8659816883962,3.23423028058518));
#242816=CARTESIAN_POINT('Ctrl Pts',(30.9286463962977,54.2060847114744,3.4715307213911));
#242817=CARTESIAN_POINT('Ctrl Pts',(31.0395064328261,54.1426202518669,3.47182327902701));
#242818=CARTESIAN_POINT('Ctrl Pts',(30.9851759176836,54.0488992551382,3.40413028959063));
#242819=CARTESIAN_POINT('Ctrl Pts',(30.8712564593359,54.1064496608377,3.65553807120995));
#242820=CARTESIAN_POINT('Ctrl Pts',(30.9819360667861,54.0429059732649,3.65586275496934));
#242821=CARTESIAN_POINT('Ctrl Pts',(30.9392002377703,53.9692670413566,3.55128126837215));
#242822=CARTESIAN_POINT('Ctrl Pts',(30.7681581606533,53.9274585619031,3.77003198860301));
#242823=CARTESIAN_POINT('Ctrl Pts',(30.8785940576189,53.8639133132292,3.77025505748627));
#242824=CARTESIAN_POINT('Ctrl Pts',(30.8566067980787,53.8262110069716,3.64284211731313));
#242825=CARTESIAN_POINT('Ctrl Pts',(30.6598643453574,53.7394427993289,3.77003198860301));
#242826=CARTESIAN_POINT('Ctrl Pts',(30.770013884466,53.6758479332734,3.77003198860301));
#242827=CARTESIAN_POINT('Ctrl Pts',(30.7698494490833,53.6759428700859,3.64284239821732));
#242828=CARTESIAN_POINT('Origin',(30.8752713784761,54.1125387249981,3.40423097483348));
#242829=CARTESIAN_POINT('Ctrl Pts',(30.1555713378337,52.8659816883962,3.36123028058519));
#242830=CARTESIAN_POINT('Ctrl Pts',(30.2655565641143,52.8024816883962,3.3612302805852));
#242831=CARTESIAN_POINT('Ctrl Pts',(30.2655565641143,52.8024816883962,3.23423028058519));
#242832=CARTESIAN_POINT('Ctrl Pts',(30.1103627734736,52.7881477055083,3.3612302805852));
#242833=CARTESIAN_POINT('Ctrl Pts',(30.2205080277004,52.724455334521,3.36146538609984));
#242834=CARTESIAN_POINT('Ctrl Pts',(30.1980495259467,52.6855560684213,3.23423043688359));
#242835=CARTESIAN_POINT('Ctrl Pts',(30.0676130472596,52.714550696011,3.41054258693135));
#242836=CARTESIAN_POINT('Ctrl Pts',(30.178127438708,52.6510500011272,3.4110060885991));
#242837=CARTESIAN_POINT('Ctrl Pts',(30.1342168083496,52.5749945583581,3.3081986697097));
#242838=CARTESIAN_POINT('Ctrl Pts',(30.0450834959835,52.6757649139398,3.48823028058518));
#242839=CARTESIAN_POINT('Ctrl Pts',(30.1558192616,52.6124111049559,3.48852004212296));
#242840=CARTESIAN_POINT('Ctrl Pts',(30.1005764675357,52.5167277788844,3.42473028058518));
#242841=CARTESIAN_POINT('Origin',(29.9905912412551,52.5802277788844,3.42473028058518));
#242842=CARTESIAN_POINT('Origin',(30.9643459342412,54.2668203812011,3.1191364817839));
#242843=CARTESIAN_POINT('Origin',(31.0534204898633,54.4211020372441,2.83404198860299));
#242844=CARTESIAN_POINT('Origin',(29.9499161072422,52.5097763801589,3.56563113460804));
#242845=CARTESIAN_POINT('Origin',(29.9275190026063,52.4710850656386,3.64299171721831));
#242846=CARTESIAN_POINT('Ctrl Pts',(31.4638515574739,54.5275217339722,2.59908173516061));
#242847=CARTESIAN_POINT('Ctrl Pts',(31.4452069629852,54.4952102564868,2.658781988603));
#242848=CARTESIAN_POINT('Ctrl Pts',(31.410023123206,54.4342359163066,2.658781988603));
#242849=CARTESIAN_POINT('Ctrl Pts',(31.3875306471682,54.5715608148716,2.59908193475593));
#242850=CARTESIAN_POINT('Ctrl Pts',(31.3896121658899,54.5272862282513,2.65878715325435));
#242851=CARTESIAN_POINT('Ctrl Pts',(31.3658411130341,54.4597196360203,2.65878198860299));
#242852=CARTESIAN_POINT('Ctrl Pts',(31.3046029601557,54.5905300051366,2.63878778849934));
#242853=CARTESIAN_POINT('Ctrl Pts',(31.3268524737457,54.536796115311,2.69564460180165));
#242854=CARTESIAN_POINT('Ctrl Pts',(31.3125672934291,54.4615686025422,2.6818048162492));
#242855=CARTESIAN_POINT('Ctrl Pts',(31.1759014746041,54.5809273110399,2.75443238878657));
#242856=CARTESIAN_POINT('Ctrl Pts',(31.2415992967183,54.5158579940077,2.79268340777109));
#242857=CARTESIAN_POINT('Ctrl Pts',(31.222768219186,54.4295063924932,2.74885926835648));
#242858=CARTESIAN_POINT('Ctrl Pts',(31.1295364123888,54.554029236008,2.82856655361725));
#242859=CARTESIAN_POINT('Ctrl Pts',(31.2191033458805,54.4847364330945,2.85384197230826));
#242860=CARTESIAN_POINT('Ctrl Pts',(31.1861426211015,54.3969835118375,2.79184624278637));
#242861=CARTESIAN_POINT('Ctrl Pts',(31.1067982185534,54.514646476914,2.90134173516061));
#242862=CARTESIAN_POINT('Ctrl Pts',(31.2174884860864,54.4512761425985,2.90163218716429));
#242863=CARTESIAN_POINT('Ctrl Pts',(31.1634057161439,54.3576020372441,2.83404198860299));
#242864=CARTESIAN_POINT('Origin',(31.410023123206,54.4342359163066,2.53178198860299));
#242865=CARTESIAN_POINT('Origin',(-0.274963065701554,0.158750000000183,
3.64303198860263));
#242866=CARTESIAN_POINT('Origin',(29.7268821954849,52.1234703131949,3.64303198860299));
#242867=CARTESIAN_POINT('Origin',(5.5822321212813E-15,1.85739751585078E-13,
2.53178198860262));
#242868=CARTESIAN_POINT('Origin',(31.4364195775134,54.4189959163065,2.531781988603));
#242869=CARTESIAN_POINT('Ctrl Pts',(29.7268821954848,52.1234703131949,3.770031988603));
#242870=CARTESIAN_POINT('Ctrl Pts',(29.8370321846009,52.0598751873275,3.770031988603));
#242871=CARTESIAN_POINT('Ctrl Pts',(29.8368672985391,52.0599703843396,3.64284187937097));
#242872=CARTESIAN_POINT('Ctrl Pts',(29.6185926664441,51.9354481180159,3.77003198860299));
#242873=CARTESIAN_POINT('Ctrl Pts',(29.7286387544923,51.8721332875977,3.76980208962975));
#242874=CARTESIAN_POINT('Ctrl Pts',(29.7501084151995,51.9096995898733,3.6428419392844));
#242875=CARTESIAN_POINT('Ctrl Pts',(29.5155047636219,51.7564527430638,3.65553535416625));
#242876=CARTESIAN_POINT('Ctrl Pts',(29.625424309881,51.6933616226671,3.65520057834456));
#242877=CARTESIAN_POINT('Ctrl Pts',(29.6675155901175,51.766644619996,3.55127910964152));
#242878=CARTESIAN_POINT('Ctrl Pts',(29.4581217525673,51.656815567543,3.47153072139108));
#242879=CARTESIAN_POINT('Ctrl Pts',(29.5680161811089,51.5939283753698,3.47122746281618));
#242880=CARTESIAN_POINT('Ctrl Pts',(29.6215404737379,51.6870133822662,3.40413045901316));
#242881=CARTESIAN_POINT('Origin',(29.5114749418004,51.7503740054945,3.40423097483347));
#242882=CARTESIAN_POINT('Ctrl Pts',(31.6576696180583,54.196600726121,2.90134173516062));
#242883=CARTESIAN_POINT('Ctrl Pts',(31.5474441649283,54.2607761425985,2.90163218716429));
#242884=CARTESIAN_POINT('Ctrl Pts',(31.4933613949858,54.1671020372441,2.834041988603));
#242885=CARTESIAN_POINT('Ctrl Pts',(31.6804173065992,54.2360018544275,2.82853349835383));
#242886=CARTESIAN_POINT('Ctrl Pts',(31.5756301844086,54.2789150989578,2.8538148316219));
#242887=CARTESIAN_POINT('Ctrl Pts',(31.5161086602376,54.2065014563934,2.79182701594197));
#242888=CARTESIAN_POINT('Ctrl Pts',(31.6804328064621,54.2894509908547,2.75468822073695));
#242889=CARTESIAN_POINT('Ctrl Pts',(31.5911964272961,54.3138841827107,2.79286913083871));
#242890=CARTESIAN_POINT('Ctrl Pts',(31.5258675551965,54.2543268901839,2.74900763297946));
#242891=CARTESIAN_POINT('Ctrl Pts',(31.6250591602192,54.4049648787501,2.63954450640416));
#242892=CARTESIAN_POINT('Ctrl Pts',(31.5671393481782,54.3976088886512,2.69627684028899));
#242893=CARTESIAN_POINT('Ctrl Pts',(31.5090508246495,54.3475791360318,2.68224356036534));
#242894=CARTESIAN_POINT('Ctrl Pts',(31.5668453499337,54.4680334478298,2.59908178706333));
#242895=CARTESIAN_POINT('Ctrl Pts',(31.5274226111438,54.4477213412904,2.65878704321649));
#242896=CARTESIAN_POINT('Ctrl Pts',(31.4807263372355,54.3933906465338,2.658781988603));
#242897=CARTESIAN_POINT('Ctrl Pts',(31.4902932482907,54.5122556166613,2.59908173516061));
#242898=CARTESIAN_POINT('Ctrl Pts',(31.4716329851988,54.4799531854482,2.65878198860299));
#242899=CARTESIAN_POINT('Ctrl Pts',(31.4364195775134,54.4189959163066,2.658781988603));
#242900=CARTESIAN_POINT('Origin',(31.6033466212664,54.1036020372441,2.83404198860299));
#242901=CARTESIAN_POINT('Origin',(29.4224002636359,51.5960921371862,3.11913648167172));
#242902=CARTESIAN_POINT('Origin',(29.3333255853454,51.4418102687787,2.83404198860297));
#242903=CARTESIAN_POINT('Origin',(31.514272065599,53.9493203812113,3.11913648177522));
#242904=CARTESIAN_POINT('Origin',(31.4251975098792,53.7950387249981,3.40423097483348));
#242905=CARTESIAN_POINT('Ctrl Pts',(29.2799753962461,51.3482501200168,2.90134173516059));
#242906=CARTESIAN_POINT('Ctrl Pts',(29.3897042746973,51.2854610232004,2.90103711553265));
#242907=CARTESIAN_POINT('Ctrl Pts',(29.443310811626,51.3783102687787,2.83404198860297));
#242908=CARTESIAN_POINT('Ctrl Pts',(29.2572578385501,51.3089010921304,2.82862991748004));
#242909=CARTESIAN_POINT('Ctrl Pts',(29.3615397594609,51.2670685993238,2.85314045886498));
#242910=CARTESIAN_POINT('Ctrl Pts',(29.4205918519436,51.3389598763138,2.79187960999971));
#242911=CARTESIAN_POINT('Ctrl Pts',(29.2572680623749,51.2557407616058,2.75470625793352));
#242912=CARTESIAN_POINT('Ctrl Pts',(29.3461554108687,51.2319924817691,2.79224250381934));
#242913=CARTESIAN_POINT('Ctrl Pts',(29.4109522357566,51.2913733902317,2.74901809108292));
#242914=CARTESIAN_POINT('Ctrl Pts',(29.3127910737013,51.1410333861059,2.63947868311743));
#242915=CARTESIAN_POINT('Ctrl Pts',(29.3705286780144,51.1485922293427,2.69595066767947));
#242916=CARTESIAN_POINT('Ctrl Pts',(29.4282055900902,51.1987619028148,2.68220539436099));
#242917=CARTESIAN_POINT('Ctrl Pts',(29.3710651187648,51.0785202710264,2.59908178585195));
#242918=CARTESIAN_POINT('Ctrl Pts',(29.4103605382587,51.0989122516748,2.65877670944929));
#242919=CARTESIAN_POINT('Ctrl Pts',(29.456817530672,51.1533747228786,2.65878198860297));
#242920=CARTESIAN_POINT('Ctrl Pts',(29.4472515437734,51.0345602039889,2.59908173516059));
#242921=CARTESIAN_POINT('Ctrl Pts',(29.4658956314766,51.066871973898,2.65878198860297));
#242922=CARTESIAN_POINT('Ctrl Pts',(29.501078514911,51.1278468659049,2.65878198860297));
#242923=CARTESIAN_POINT('Origin',(29.501078514911,51.1278468659049,2.53178198860297));
#242924=CARTESIAN_POINT('Ctrl Pts',(31.2097904767605,53.4219427993289,3.770031988603));
#242925=CARTESIAN_POINT('Ctrl Pts',(31.0996409281621,53.4855376708633,3.770031988603));
#242926=CARTESIAN_POINT('Ctrl Pts',(31.0998053730486,53.4854427285638,3.64284238727594));
#242927=CARTESIAN_POINT('Ctrl Pts',(31.3184716867865,53.6097387976567,3.77003198860301));
#242928=CARTESIAN_POINT('Ctrl Pts',(31.2082219299913,53.6736064794787,3.77025506106071));
#242929=CARTESIAN_POINT('Ctrl Pts',(31.1865640704871,53.6357132000298,3.64284210642032));
#242930=CARTESIAN_POINT('Ctrl Pts',(31.4219325588445,53.7885186806146,3.65553527987871));
#242931=CARTESIAN_POINT('Ctrl Pts',(31.3115622968574,53.8525981958205,3.65585996532953));
#242932=CARTESIAN_POINT('Ctrl Pts',(31.2691568563325,53.7787681009853,3.55127902710111));
#242933=CARTESIAN_POINT('Ctrl Pts',(31.4795232016789,53.8880358395973,3.4715307213911));
#242934=CARTESIAN_POINT('Ctrl Pts',(31.3691313396259,53.9523112232411,3.47182327905227));
#242935=CARTESIAN_POINT('Ctrl Pts',(31.3151318380581,53.858399104952,3.40413028378004));
#242936=CARTESIAN_POINT('Origin',(31.2097904767605,53.4219427993289,3.643031988603));
#242937=CARTESIAN_POINT('Origin',(5.69400554112516E-15,1.86375525517094E-13,
2.53178198860262));
#242938=CARTESIAN_POINT('Origin',(29.5274749692184,51.1126068659049,2.53178198860297));
#242939=CARTESIAN_POINT('Origin',(15.8305769983922,26.7843636743468,3.64303198860281));
#242940=CARTESIAN_POINT('Origin',(31.0091584503732,53.0743345559682,3.6429946600739));
#242941=CARTESIAN_POINT('Ctrl Pts',(29.4735998357337,51.019348010533,2.59908173516059));
#242942=CARTESIAN_POINT('Ctrl Pts',(29.4922606054645,51.0516501490689,2.65878198860298));
#242943=CARTESIAN_POINT('Ctrl Pts',(29.5274749692184,51.112606865905,2.65878198860297));
#242944=CARTESIAN_POINT('Ctrl Pts',(29.5495039426972,50.9754987628541,2.59908193199997));
#242945=CARTESIAN_POINT('Ctrl Pts',(29.5475581014581,51.0197013834526,2.65877685806694));
#242946=CARTESIAN_POINT('Ctrl Pts',(29.5715624158012,51.0871269269775,2.65878198860297));
#242947=CARTESIAN_POINT('Ctrl Pts',(29.6319914129671,50.9562029902291,2.63872492669847));
#242948=CARTESIAN_POINT('Ctrl Pts',(29.6100038038528,51.0098791271092,2.69532212015295));
#242949=CARTESIAN_POINT('Ctrl Pts',(29.6246193648995,51.0848223701589,2.68176836726675));
#242950=CARTESIAN_POINT('Ctrl Pts',(29.760039537519,50.9652607924607,2.75442176402272));
#242951=CARTESIAN_POINT('Ctrl Pts',(29.6951164119093,51.0303675504161,2.79203179920195));
#242952=CARTESIAN_POINT('Ctrl Pts',(29.7140610042231,51.1161687394136,2.74885310748206));
#242953=CARTESIAN_POINT('Ctrl Pts',(29.8061925581058,50.9919958361064,2.82866089558443));
#242954=CARTESIAN_POINT('Ctrl Pts',(29.7178148857791,51.0613912713631,2.85316563119302));
#242955=CARTESIAN_POINT('Ctrl Pts',(29.7505571803537,51.1484765898561,2.79189751796687));
#242956=CARTESIAN_POINT('Ctrl Pts',(29.8289013456884,51.0313275753411,2.90134173516059));
#242957=CARTESIAN_POINT('Ctrl Pts',(29.7196599535392,51.0949610232004,2.90103711553265));
#242958=CARTESIAN_POINT('Ctrl Pts',(29.7732664904679,51.1878102687787,2.83404198860297));
#242959=CARTESIAN_POINT('Origin',(29.8832517167485,51.1243102687787,2.83404198860297));
#242960=CARTESIAN_POINT('Origin',(30.9870007553607,53.0360596824713,3.56647653971874));
#242961=CARTESIAN_POINT('Origin',(30.9460815882867,52.9651856060848,3.42473028058523));
#242962=CARTESIAN_POINT('Origin',(29.972326394982,51.2785921372019,3.11913648168102));
#242963=CARTESIAN_POINT('Origin',(30.0614010732035,51.4328740054945,3.40423097483347));
#242964=CARTESIAN_POINT('Ctrl Pts',(30.7811015270742,52.679431757829,3.36123028058519));
#242965=CARTESIAN_POINT('Ctrl Pts',(30.6711163007936,52.742931757829,3.36123028058519));
#242966=CARTESIAN_POINT('Ctrl Pts',(30.6711163007936,52.742931757829,3.23423028058519));
#242967=CARTESIAN_POINT('Ctrl Pts',(30.8259039490946,52.757500212918,3.36123028058519));
#242968=CARTESIAN_POINT('Ctrl Pts',(30.7160792752564,52.8208099140555,3.36099641108374));
#242969=CARTESIAN_POINT('Ctrl Pts',(30.738623332912,52.8598573673263,3.23423043688369));
#242970=CARTESIAN_POINT('Ctrl Pts',(30.8682695960183,52.8313189037788,3.4105425890532));
#242971=CARTESIAN_POINT('Ctrl Pts',(30.758807217536,52.8948168809936,3.41008815826104));
#242972=CARTESIAN_POINT('Ctrl Pts',(30.8024560343135,52.9704188493381,3.30819867304328));
#242973=CARTESIAN_POINT('Ctrl Pts',(30.8905967158735,52.8702215132218,3.48823028058522));
#242974=CARTESIAN_POINT('Ctrl Pts',(30.7813498801531,52.9338619179798,3.48794691941637));
#242975=CARTESIAN_POINT('Ctrl Pts',(30.8360963620061,53.0286856060848,3.42473028058523));
#242976=CARTESIAN_POINT('Origin',(30.7811015270742,52.679431757829,3.23423028058519));
#242977=CARTESIAN_POINT('Ctrl Pts',(30.0070536838157,51.33988956927,3.47153072139108));
#242978=CARTESIAN_POINT('Ctrl Pts',(29.8976445761574,51.4036173326914,3.47122746285113));
#242979=CARTESIAN_POINT('Ctrl Pts',(29.9514963916953,51.4965132298825,3.40413046676816));
#242980=CARTESIAN_POINT('Ctrl Pts',(30.0646513737708,51.4394048060583,3.65553813458026));
#242981=CARTESIAN_POINT('Ctrl Pts',(29.9550530981048,51.503052357962,3.65520336072079));
#242982=CARTESIAN_POINT('Ctrl Pts',(29.997472204327,51.5761456730035,3.55128134519865));
#242983=CARTESIAN_POINT('Ctrl Pts',(30.1681227811157,51.6181806476923,3.77003198860299));
#242984=CARTESIAN_POINT('Ctrl Pts',(30.0582674911759,51.6818259279778,3.76980209314328));
#242985=CARTESIAN_POINT('Ctrl Pts',(30.0800656843521,51.7192017762862,3.6428419538755));
#242986=CARTESIAN_POINT('Ctrl Pts',(30.276808326888,51.8059703131949,3.77003198860299));
#242987=CARTESIAN_POINT('Ctrl Pts',(30.1666583504933,51.8695654317176,3.77003198860299));
#242988=CARTESIAN_POINT('Ctrl Pts',(30.1668232238147,51.8694702420611,3.64284189403824));
#242989=CARTESIAN_POINT('Origin',(30.276808326888,51.8059703131949,3.64303198860299));
#242990=CARTESIAN_POINT('Origin',(15.4537755657014,26.1317244485617,3.234230280585));
#242991=CARTESIAN_POINT('Origin',(30.7054974692368,52.5484816883962,3.23423028058518));
#242992=CARTESIAN_POINT('Origin',(15.3947701216591,26.0295240215572,3.64303198860281));
#242993=CARTESIAN_POINT('Origin',(30.4775331296737,52.1535342613183,3.64299171721843));
#242994=CARTESIAN_POINT('Ctrl Pts',(30.5960088312567,52.3576880233165,3.48823028058518));
#242995=CARTESIAN_POINT('Ctrl Pts',(30.4857749404419,52.4219111049559,3.48852004212296));
#242996=CARTESIAN_POINT('Ctrl Pts',(30.4305321463775,52.3262277788844,3.42473028058518));
#242997=CARTESIAN_POINT('Ctrl Pts',(30.6184089696598,52.3967235457371,3.41028005848445));
#242998=CARTESIAN_POINT('Ctrl Pts',(30.5081585269356,52.4606806140204,3.41074404220395));
#242999=CARTESIAN_POINT('Ctrl Pts',(30.4642861617693,52.3846914485024,3.30780486244026));
#243000=CARTESIAN_POINT('Ctrl Pts',(30.660846452162,52.4706758922788,3.36123028058519));
#243001=CARTESIAN_POINT('Ctrl Pts',(30.5506153465192,52.5342179826657,3.36146460586487));
#243002=CARTESIAN_POINT('Ctrl Pts',(30.5282325936728,52.495449917522,3.23423045308379));
#243003=CARTESIAN_POINT('Ctrl Pts',(30.7054974692368,52.5484816883962,3.36123028058519));
#243004=CARTESIAN_POINT('Ctrl Pts',(30.5955122429562,52.6119816883962,3.36123028058519));
#243005=CARTESIAN_POINT('Ctrl Pts',(30.5955122429562,52.6119816883962,3.23423028058519));
#243006=CARTESIAN_POINT('Origin',(30.5405173726582,52.2627277788844,3.42473028058517));
#243007=CARTESIAN_POINT('Origin',(30.4998422394564,52.1922763809702,3.56563113524778));
#243008=CARTESIAN_POINT('Origin',(24.6933715417281,56.2428239377268,3.56647653909482));
#243009=CARTESIAN_POINT('Origin',(24.711312597791,56.2832472948498,3.64299466007726));
#243010=CARTESIAN_POINT('Origin',(24.660084891711,56.168060898428,3.42473028058523));
#243011=CARTESIAN_POINT('Ctrl Pts',(24.6158705164593,56.0673542004328,3.48823028058523));
#243012=CARTESIAN_POINT('Ctrl Pts',(24.7315703643334,56.01637854512,3.48794691941639));
#243013=CARTESIAN_POINT('Ctrl Pts',(24.7761051648316,56.1164053447574,3.42473028058524));
#243014=CARTESIAN_POINT('Ctrl Pts',(24.5974591883329,56.0262864882908,3.41028005925126));
#243015=CARTESIAN_POINT('Ctrl Pts',(24.7131705636703,55.9750519161968,3.40982512231045));
#243016=CARTESIAN_POINT('Ctrl Pts',(24.7486471852376,56.0547337128522,3.30780486372799));
#243017=CARTESIAN_POINT('Ctrl Pts',(24.5625784858792,55.9484840819678,3.36123028058521));
#243018=CARTESIAN_POINT('Ctrl Pts',(24.6783511906842,55.8968463240315,3.36099721048404));
#243019=CARTESIAN_POINT('Ctrl Pts',(24.6966284839291,55.9378977967826,3.23423045308457));
#243020=CARTESIAN_POINT('Ctrl Pts',(24.525878019167,55.8666273273835,3.36123028058521));
#243021=CARTESIAN_POINT('Ctrl Pts',(24.6418982922876,55.8149717737129,3.36123028058521));
#243022=CARTESIAN_POINT('Ctrl Pts',(24.6418982922876,55.8149717737129,3.23423028058521));
#243023=CARTESIAN_POINT('Origin',(24.525878019167,55.8666273273835,3.23423028058521));
#243024=CARTESIAN_POINT('Origin',(-0.290050682801521,0.12913888417675,3.64303198860263));
#243025=CARTESIAN_POINT('Origin',(24.8746050278051,56.6498810128384,3.64303198860303));
#243026=CARTESIAN_POINT('Origin',(-0.29005068280152,0.129138884176753,3.23423028058481));
#243027=CARTESIAN_POINT('Origin',(24.4643761377916,55.72849184015,3.2342302805852));
#243028=CARTESIAN_POINT('Ctrl Pts',(25.0931373005745,57.1420619865024,3.47153072139112));
#243029=CARTESIAN_POINT('Ctrl Pts',(25.2100238766582,57.0905332211011,3.47182327902702));
#243030=CARTESIAN_POINT('Ctrl Pts',(25.1657875015263,56.9916465525422,3.40413028959063));
#243031=CARTESIAN_POINT('Ctrl Pts',(25.0464764504229,57.0369738651803,3.65553807120995));
#243032=CARTESIAN_POINT('Ctrl Pts',(25.1631918674189,56.9853474458578,3.65586275496902));
#243033=CARTESIAN_POINT('Ctrl Pts',(25.128387514131,56.9076448051904,3.55128126837224));
#243034=CARTESIAN_POINT('Ctrl Pts',(24.9626525995183,56.8481865914869,3.77003198860303));
#243035=CARTESIAN_POINT('Ctrl Pts',(25.0791258042763,56.7965331449332,3.77025505748708));
#243036=CARTESIAN_POINT('Ctrl Pts',(25.0611999573796,56.7567390814036,3.64284211731277));
#243037=CARTESIAN_POINT('Ctrl Pts',(24.8746050278051,56.6498810128384,3.77003198860303));
#243038=CARTESIAN_POINT('Ctrl Pts',(24.990798629834,56.5981482881658,3.77003198860303));
#243039=CARTESIAN_POINT('Ctrl Pts',(24.9906251716464,56.5982255167267,3.64284239821729));
#243040=CARTESIAN_POINT('Origin',(25.0498328948964,57.0434492461381,3.4042309748335));
#243041=CARTESIAN_POINT('Ctrl Pts',(24.4643761377916,55.72849184015,3.3612302805852));
#243042=CARTESIAN_POINT('Ctrl Pts',(24.5803964109122,55.6768362864794,3.36123028058521));
#243043=CARTESIAN_POINT('Ctrl Pts',(24.5803964109122,55.6768362864794,3.2342302805852));
#243044=CARTESIAN_POINT('Ctrl Pts',(24.427551097298,55.6463586582055,3.36123028058521));
#243045=CARTESIAN_POINT('Ctrl Pts',(24.5437506299578,55.5945285148468,3.36146538610306));
#243046=CARTESIAN_POINT('Ctrl Pts',(24.5254812387356,55.5534947903256,3.23423043688532));
#243047=CARTESIAN_POINT('Ctrl Pts',(24.3927285408587,55.5686962576416,3.41054258693139));
#243048=CARTESIAN_POINT('Ctrl Pts',(24.5092751529615,55.5170953257214,3.41100608859824));
#243049=CARTESIAN_POINT('Ctrl Pts',(24.4735550281879,55.4368666119059,3.3081986697084));
#243050=CARTESIAN_POINT('Ctrl Pts',(24.3743766270213,55.5277679687685,3.4882302805852));
#243051=CARTESIAN_POINT('Ctrl Pts',(24.4911280468225,55.4763362579877,3.48852004212298));
#243052=CARTESIAN_POINT('Ctrl Pts',(24.4461895095988,55.3754026508177,3.4247302805852));
#243053=CARTESIAN_POINT('Origin',(24.3301692364782,55.4270582044884,3.4247302805852));
#243054=CARTESIAN_POINT('Origin',(25.1222926664936,57.2061965577162,3.11913648178449));
#243055=CARTESIAN_POINT('Origin',(25.1947524379615,57.3689438691199,2.83404198860302));
#243056=CARTESIAN_POINT('Origin',(24.2970811015511,55.352741036646,3.56563113460901));
#243057=CARTESIAN_POINT('Origin',(24.2788510342448,55.3119205422648,3.64299171721853));
#243058=CARTESIAN_POINT('Ctrl Pts',(25.5918112338793,57.5176823163891,2.59908173516063));
#243059=CARTESIAN_POINT('Ctrl Pts',(25.5766462455175,57.483598953748,2.65878198860302));
#243060=CARTESIAN_POINT('Ctrl Pts',(25.5480287005717,57.4192809246791,2.65878198860302));
#243061=CARTESIAN_POINT('Ctrl Pts',(25.5113050800555,57.5535024391258,2.59908193475632));
#243062=CARTESIAN_POINT('Ctrl Pts',(25.5180031505025,57.5096879712802,2.65878715325401));
#243063=CARTESIAN_POINT('Ctrl Pts',(25.5014249500146,57.4400067642831,2.65878198860302));
#243064=CARTESIAN_POINT('Ctrl Pts',(25.4268488592818,57.5636994104963,2.63878778849911));
#243065=CARTESIAN_POINT('Ctrl Pts',(25.4545932086374,57.5125855880056,2.69564460180157));
#243066=CARTESIAN_POINT('Ctrl Pts',(25.4482497003385,57.4362769714773,2.68180481624919));
#243067=CARTESIAN_POINT('Ctrl Pts',(25.2998561687912,57.5406963524573,2.75443238878687));
#243068=CARTESIAN_POINT('Ctrl Pts',(25.3719956870768,57.4828507843377,2.7926834077713));
#243069=CARTESIAN_POINT('Ctrl Pts',(25.3622939683645,57.3950038423349,2.74885926835656));
#243070=CARTESIAN_POINT('Ctrl Pts',(25.2565567136862,57.5090991591924,2.82856655361708));
#243071=CARTESIAN_POINT('Ctrl Pts',(25.3528760603488,57.4495482434217,2.85384197230864));
#243072=CARTESIAN_POINT('Ctrl Pts',(25.3292685758746,57.3588307079384,2.79184624278516));
#243073=CARTESIAN_POINT('Ctrl Pts',(25.2380597013429,57.4675553545143,2.90134173516065));
#243074=CARTESIAN_POINT('Ctrl Pts',(25.3547675996714,57.4161024530846,2.90163218716432));
#243075=CARTESIAN_POINT('Ctrl Pts',(25.3107727110821,57.3172883154492,2.83404198860303));
#243076=CARTESIAN_POINT('Origin',(25.5480287005717,57.4192809246791,2.53178198860302));
#243077=CARTESIAN_POINT('Origin',(-0.290050682801521,0.12913888417675,3.64303198860263));
#243078=CARTESIAN_POINT('Origin',(24.1156489724276,54.9452378026831,3.64303198860301));
#243079=CARTESIAN_POINT('Origin',(5.59761027822878E-15,1.85731916022747E-13,
2.53178198860262));
#243080=CARTESIAN_POINT('Origin',(25.5758735661207,57.4068835917982,2.53178198860302));
#243081=CARTESIAN_POINT('Ctrl Pts',(24.1156489724276,54.9452378026831,3.77003198860302));
#243082=CARTESIAN_POINT('Ctrl Pts',(24.2318430491563,54.8935048666605,3.77003198860301));
#243083=CARTESIAN_POINT('Ctrl Pts',(24.2316691155602,54.8935823068868,3.64284187937092));
#243084=CARTESIAN_POINT('Ctrl Pts',(24.0276063358801,54.7469262747036,3.77003198860301));
#243085=CARTESIAN_POINT('Ctrl Pts',(24.1436677818719,54.6954612380267,3.7698020896317));
#243086=CARTESIAN_POINT('Ctrl Pts',(24.1610930816811,54.735065938806,3.64284193928378));
#243087=CARTESIAN_POINT('Ctrl Pts',(23.9437932708528,54.5581358350801,3.65553535416626));
#243088=CARTESIAN_POINT('Ctrl Pts',(24.0597054841979,54.5068800556897,3.6552005783446));
#243089=CARTESIAN_POINT('Ctrl Pts',(24.0939060249002,54.5841613379376,3.55127910964213));
#243090=CARTESIAN_POINT('Ctrl Pts',(23.8971395307767,54.4530463244695,3.4715307213911));
#243091=CARTESIAN_POINT('Ctrl Pts',(24.0130054476975,54.4019907306521,3.4712274628162));
#243092=CARTESIAN_POINT('Ctrl Pts',(24.056506495927,54.5001606201972,3.40413045901315));
#243093=CARTESIAN_POINT('Origin',(23.940420925912,54.5516691663897,3.40423097483348));
#243094=CARTESIAN_POINT('Ctrl Pts',(25.8191582032619,57.2088336324701,2.90134173516064));
#243095=CARTESIAN_POINT('Ctrl Pts',(25.7028284190332,57.2611357920727,2.90163218716432));
#243096=CARTESIAN_POINT('Ctrl Pts',(25.658833530444,57.1623216544374,2.83404198860302));
#243097=CARTESIAN_POINT('Ctrl Pts',(25.8376627381927,57.2503966981989,2.82853349835388));
#243098=CARTESIAN_POINT('Ctrl Pts',(25.7289639953178,57.2821216226341,2.85381483162346));
#243099=CARTESIAN_POINT('Ctrl Pts',(25.6773378230594,57.2038829761266,2.79182701594241));
#243100=CARTESIAN_POINT('Ctrl Pts',(25.8320911970514,57.3035546548414,2.75468822073695));
#243101=CARTESIAN_POINT('Ctrl Pts',(25.7407897001103,57.3185262575348,2.79286913083887));
#243102=CARTESIAN_POINT('Ctrl Pts',(25.6820441386715,57.2524664994801,2.74900763297955));
#243103=CARTESIAN_POINT('Ctrl Pts',(25.7649464042485,57.4126476234252,2.63954450640422));
#243104=CARTESIAN_POINT('Ctrl Pts',(25.7081127933386,57.3992776612639,2.69627684028889));
#243105=CARTESIAN_POINT('Ctrl Pts',(25.6555720179788,57.3434500727663,2.68224356036531));
#243106=CARTESIAN_POINT('Ctrl Pts',(25.7004590346999,57.4692856961532,2.5990817870655));
#243107=CARTESIAN_POINT('Ctrl Pts',(25.6633754510789,57.444964063152,2.65878704321591));
#243108=CARTESIAN_POINT('Ctrl Pts',(25.6226140882766,57.3860499078752,2.65878198860302));
#243109=CARTESIAN_POINT('Ctrl Pts',(25.6197038181297,57.5052637377734,2.59908173516064));
#243110=CARTESIAN_POINT('Ctrl Pts',(25.604522301406,57.4711877340332,2.65878198860302));
#243111=CARTESIAN_POINT('Ctrl Pts',(25.5758735661207,57.4068835917982,2.65878198860302));
#243112=CARTESIAN_POINT('Origin',(25.7748538035646,57.1106661007667,2.83404198860302));
#243113=CARTESIAN_POINT('Origin',(23.8679610547573,54.3889216310773,3.11913648167036));
#243114=CARTESIAN_POINT('Origin',(23.7955011834907,54.2261740956468,2.834041988603));
#243115=CARTESIAN_POINT('Origin',(25.7023940320475,56.9479187893683,3.11913648177501));
#243116=CARTESIAN_POINT('Origin',(25.6299342604994,56.785171477785,3.4042309748335));
#243117=CARTESIAN_POINT('Ctrl Pts',(23.7522229508827,54.1275498658876,2.90134173516062));
#243118=CARTESIAN_POINT('Ctrl Pts',(23.8679139708567,54.0765745253538,2.90103711553268));
#243119=CARTESIAN_POINT('Ctrl Pts',(23.9115214566113,54.1745185419762,2.834041988603));
#243120=CARTESIAN_POINT('Ctrl Pts',(23.733742935761,54.0860417646977,2.8286299174799));
#243121=CARTESIAN_POINT('Ctrl Pts',(23.8418262755866,54.0553388636012,2.85314045886498));
#243122=CARTESIAN_POINT('Ctrl Pts',(23.8930401898204,54.1330089371355,2.79187960999965));
#243123=CARTESIAN_POINT('Ctrl Pts',(23.7393098712349,54.0331737207071,2.75470625793376));
#243124=CARTESIAN_POINT('Ctrl Pts',(23.8301926567301,54.0188467943744,2.79224250381938));
#243125=CARTESIAN_POINT('Ctrl Pts',(23.8884275227223,54.0846755205376,2.74901809108294));
#243126=CARTESIAN_POINT('Ctrl Pts',(23.8065189073822,53.9248984592619,2.63947868311725));
#243127=CARTESIAN_POINT('Ctrl Pts',(23.8631501047898,53.9384511174158,2.69595066767948));
#243128=CARTESIAN_POINT('Ctrl Pts',(23.9152668978358,53.9943748351525,2.68220539436102));
#243129=CARTESIAN_POINT('Ctrl Pts',(23.8710081209825,53.8688190939459,2.59908178585064));
#243130=CARTESIAN_POINT('Ctrl Pts',(23.9079567336561,53.8932068550022,2.65877670945022));
#243131=CARTESIAN_POINT('Ctrl Pts',(23.9484663513836,53.9522270531159,2.658781988603));
#243132=CARTESIAN_POINT('Ctrl Pts',(23.9513722670364,53.833063494684,2.59908173516062));
#243133=CARTESIAN_POINT('Ctrl Pts',(23.9665367208223,53.8671470951733,2.658781988603));
#243134=CARTESIAN_POINT('Ctrl Pts',(23.9951532569806,53.9314655730807,2.658781988603));
#243135=CARTESIAN_POINT('Origin',(23.9951532569806,53.9314655730807,2.531781988603));
#243136=CARTESIAN_POINT('Ctrl Pts',(25.4547063934082,56.3916032444853,3.77003198860302));
#243137=CARTESIAN_POINT('Ctrl Pts',(25.338512781369,56.4433359736147,3.77003198860302));
#243138=CARTESIAN_POINT('Ctrl Pts',(25.3386862495819,56.4432587405904,3.64284238727598));
#243139=CARTESIAN_POINT('Ctrl Pts',(25.5431622092832,56.589730756554,3.77003198860303));
#243140=CARTESIAN_POINT('Ctrl Pts',(25.426840421557,56.6417243268787,3.7702550610602));
#243141=CARTESIAN_POINT('Ctrl Pts',(25.4092621323412,56.6017747680089,3.64284210642014));
#243142=CARTESIAN_POINT('Ctrl Pts',(25.6273687254288,56.778345870572,3.65553527987874));
#243143=CARTESIAN_POINT('Ctrl Pts',(25.510904950034,56.8305375176137,3.6558599653302));
#243144=CARTESIAN_POINT('Ctrl Pts',(25.4764491573042,56.7526792962305,3.55127902710133));
#243145=CARTESIAN_POINT('Ctrl Pts',(25.6742415049979,56.8833377255397,3.47153072139111));
#243146=CARTESIAN_POINT('Ctrl Pts',(25.5577357740375,56.935721910209,3.47182327905228));
#243147=CARTESIAN_POINT('Ctrl Pts',(25.5138485767963,56.8366797674139,3.40413028378006));
#243148=CARTESIAN_POINT('Origin',(25.4547063934082,56.3916032444853,3.64303198860302));
#243149=CARTESIAN_POINT('Origin',(5.68853496937358E-15,1.86378312912625E-13,
2.53178198860262));
#243150=CARTESIAN_POINT('Origin',(24.0229981225296,53.9190682401997,2.531781988603));
#243151=CARTESIAN_POINT('Origin',(10.5838037820516,22.9910091182299,3.64303198860278));
#243152=CARTESIAN_POINT('Origin',(25.2915084057467,56.0249274780507,3.64299466007881));
#243153=CARTESIAN_POINT('Ctrl Pts',(23.9791663275012,53.8206887816838,2.59908173516062));
#243154=CARTESIAN_POINT('Ctrl Pts',(23.9943483786816,53.8547645473083,2.658781988603));
#243155=CARTESIAN_POINT('Ctrl Pts',(24.0229981225296,53.9190682401997,2.658781988603));
#243156=CARTESIAN_POINT('Ctrl Pts',(24.0592381183002,53.785013884428,2.59908193199958));
#243157=CARTESIAN_POINT('Ctrl Pts',(24.052682504579,53.8287709626505,2.65877685806597));
#243158=CARTESIAN_POINT('Ctrl Pts',(24.069507432327,53.8983362760834,2.658781988603));
#243159=CARTESIAN_POINT('Ctrl Pts',(24.1432906710371,53.774446104571,2.63872492669847));
#243160=CARTESIAN_POINT('Ctrl Pts',(24.115812828244,53.8255298669652,2.69532212015298));
#243161=CARTESIAN_POINT('Ctrl Pts',(24.1225146216897,53.9015903052242,2.68176836726667));
#243162=CARTESIAN_POINT('Ctrl Pts',(24.2696905364172,53.7968389608978,2.75442176402277));
#243163=CARTESIAN_POINT('Ctrl Pts',(24.1983175571252,53.8548027426703,2.79203179920197));
#243164=CARTESIAN_POINT('Ctrl Pts',(24.2081897025475,53.9421141528987,2.74885310748219));
#243165=CARTESIAN_POINT('Ctrl Pts',(24.3127961529008,53.828251851494,2.82866089558446));
#243166=CARTESIAN_POINT('Ctrl Pts',(24.2176488245051,53.8880291490199,2.85316563119328));
#243167=CARTESIAN_POINT('Ctrl Pts',(24.241108858848,53.9780599067615,2.79189751796784));
#243168=CARTESIAN_POINT('Ctrl Pts',(24.3312692531087,53.8697418420147,2.90134173516062));
#243169=CARTESIAN_POINT('Ctrl Pts',(24.2159747902185,53.921607864342,2.90103711553268));
#243170=CARTESIAN_POINT('Ctrl Pts',(24.2595822759732,54.0195518809643,2.83404198860301));
#243171=CARTESIAN_POINT('Origin',(24.3756025490938,53.9678963272937,2.834041988603));
#243172=CARTESIAN_POINT('Origin',(25.2734729066204,55.9845461685094,3.56647653971757));
#243173=CARTESIAN_POINT('Origin',(25.2401862573141,55.9097831300749,3.42473028058525));
#243174=CARTESIAN_POINT('Origin',(24.4480624203051,54.1306438627325,3.1191364816796));
#243175=CARTESIAN_POINT('Origin',(24.5205222915151,54.2933913980366,3.40423097483349));
#243176=CARTESIAN_POINT('Ctrl Pts',(25.1059793847701,55.6083495590304,3.3612302805852));
#243177=CARTESIAN_POINT('Ctrl Pts',(24.9899591116494,55.660005112701,3.3612302805852));
#243178=CARTESIAN_POINT('Ctrl Pts',(24.9899591116494,55.660005112701,3.2342302805852));
#243179=CARTESIAN_POINT('Ctrl Pts',(25.142375998795,55.6906734752783,3.3612302805852));
#243180=CARTESIAN_POINT('Ctrl Pts',(25.0265352902397,55.7421565548659,3.36099641108629));
#243181=CARTESIAN_POINT('Ctrl Pts',(25.0448742789053,55.7833465978028,3.23423043688484));
#243182=CARTESIAN_POINT('Ctrl Pts',(25.1767934079544,55.7685161955958,3.41054258905326));
#243183=CARTESIAN_POINT('Ctrl Pts',(25.0612933298581,55.8202243900361,3.41008815825965));
#243184=CARTESIAN_POINT('Ctrl Pts',(25.0968004762779,55.8999747466307,3.30819867304262));
#243185=CARTESIAN_POINT('Ctrl Pts',(25.19493178753,55.8095395120009,3.48823028058524));
#243186=CARTESIAN_POINT('Ctrl Pts',(25.0796311836953,55.8614118841081,3.4879469194164));
#243187=CARTESIAN_POINT('Ctrl Pts',(25.1241659841935,55.9614386837455,3.42473028058525));
#243188=CARTESIAN_POINT('Origin',(25.10597938477,55.6083495590304,3.2342302805852));
#243189=CARTESIAN_POINT('Ctrl Pts',(24.4761921430391,54.1952354911874,3.4715307213911));
#243190=CARTESIAN_POINT('Ctrl Pts',(24.3607210247427,54.2471777813618,3.47122746285115));
#243191=CARTESIAN_POINT('Ctrl Pts',(24.4045675690227,54.3451938326304,3.40413046676837));
#243192=CARTESIAN_POINT('Ctrl Pts',(24.5230721320477,54.3002261711155,3.65553813458027));
#243193=CARTESIAN_POINT('Ctrl Pts',(24.4074212664101,54.3520689157434,3.65520336071997));
#243194=CARTESIAN_POINT('Ctrl Pts',(24.4419676644371,54.4291958219389,3.55128134519898));
#243195=CARTESIAN_POINT('Ctrl Pts',(24.607289548202,54.4888383671851,3.77003198860301));
#243196=CARTESIAN_POINT('Ctrl Pts',(24.4913833136911,54.5406519873239,3.76980209314289));
#243197=CARTESIAN_POINT('Ctrl Pts',(24.5091552540987,54.5801016184608,3.64284195387538));
#243198=CARTESIAN_POINT('Ctrl Pts',(24.6957503380306,54.68696003433,3.77003198860301));
#243199=CARTESIAN_POINT('Ctrl Pts',(24.5795562747216,54.7386929643777,3.77003198860301));
#243200=CARTESIAN_POINT('Ctrl Pts',(24.5797301948779,54.7386155301352,3.64284189403862));
#243201=CARTESIAN_POINT('Origin',(24.6957503380306,54.68696003433,3.64303198860301));
#243202=CARTESIAN_POINT('Origin',(10.3344596589366,22.4309730483567,3.23423028058497));
#243203=CARTESIAN_POINT('Origin',(25.0444775033946,55.4702140717969,3.2342302805852));
#243204=CARTESIAN_POINT('Origin',(10.295413467953,22.3432738675266,3.64303198860278));
#243205=CARTESIAN_POINT('Origin',(24.85904522396,55.0536014459541,3.64299171721827));
#243206=CARTESIAN_POINT('Ctrl Pts',(24.9555320242414,55.2690209153042,3.4882302805852));
#243207=CARTESIAN_POINT('Ctrl Pts',(24.8391888661843,55.3213695969758,3.48852004212297));
#243208=CARTESIAN_POINT('Ctrl Pts',(24.7942503289606,55.2204359898058,3.4247302805852));
#243209=CARTESIAN_POINT('Ctrl Pts',(24.9737291291703,55.3101840490933,3.41028005848448));
#243210=CARTESIAN_POINT('Ctrl Pts',(24.8573973158455,55.3622664445142,3.41074404220458));
#243211=CARTESIAN_POINT('Ctrl Pts',(24.821708318783,55.2821076446845,3.30780486243998));
#243212=CARTESIAN_POINT('Ctrl Pts',(25.0082040095654,55.3881672017732,3.36123028058521));
#243213=CARTESIAN_POINT('Ctrl Pts',(24.8919348043908,55.4398389138618,3.36146460586492));
#243214=CARTESIAN_POINT('Ctrl Pts',(24.8737270328797,55.3989435894769,3.23423045308494));
#243215=CARTESIAN_POINT('Ctrl Pts',(25.0444775033946,55.4702140717969,3.3612302805852));
#243216=CARTESIAN_POINT('Ctrl Pts',(24.928457230274,55.5218696254676,3.3612302805852));
#243217=CARTESIAN_POINT('Ctrl Pts',(24.928457230274,55.5218696254675,3.2342302805852));
#243218=CARTESIAN_POINT('Origin',(24.9102706020812,55.1687804361352,3.4247302805852));
#243219=CARTESIAN_POINT('Origin',(24.8771824678745,55.0944632691843,3.56563113524835));
#243220=CARTESIAN_POINT('Origin',(18.6791227126688,58.515880043567,3.56647653909436));
#243221=CARTESIAN_POINT('Origin',(18.6927400943491,58.5579573083292,3.64299466007643));
#243222=CARTESIAN_POINT('Origin',(18.6538332760103,58.4380471616457,3.42473028058524));
#243223=CARTESIAN_POINT('Ctrl Pts',(18.6203878281146,58.3332704847798,3.48823028058524));
#243224=CARTESIAN_POINT('Ctrl Pts',(18.7407822670301,58.294668006739,3.4879469194164));
#243225=CARTESIAN_POINT('Ctrl Pts',(18.7746174535798,58.3988020033601,3.42473028058524));
#243226=CARTESIAN_POINT('Ctrl Pts',(18.6063701040105,58.290503238026,3.41028005925128));
#243227=CARTESIAN_POINT('Ctrl Pts',(18.7268030714127,58.2516444665228,3.40982512231052));
#243228=CARTESIAN_POINT('Ctrl Pts',(18.7537563325803,58.3345980746929,3.30780486372867));
#243229=CARTESIAN_POINT('Ctrl Pts',(18.5798130476677,58.2094810151997,3.36123028058522));
#243230=CARTESIAN_POINT('Ctrl Pts',(18.7003491529667,58.1702276772278,3.36099721048497));
#243231=CARTESIAN_POINT('Ctrl Pts',(18.7142352739232,58.2129647630924,3.23423045308476));
#243232=CARTESIAN_POINT('Ctrl Pts',(18.5518699907149,58.1242364370959,3.36123028058522));
#243233=CARTESIAN_POINT('Ctrl Pts',(18.6726541682844,58.0849912788103,3.36123028058522));
#243234=CARTESIAN_POINT('Ctrl Pts',(18.6726541682844,58.0849912788103,3.23423028058522));
#243235=CARTESIAN_POINT('Origin',(18.5518699907149,58.1242364370959,3.23423028058522));
#243236=CARTESIAN_POINT('Origin',(-0.301960443923706,0.0981128957142288,
3.64303198860263));
#243237=CARTESIAN_POINT('Origin',(18.8168143322225,58.9396512752215,3.64303198860304));
#243238=CARTESIAN_POINT('Origin',(-0.301960443923706,0.0981128957142317,
3.23423028058481));
#243239=CARTESIAN_POINT('Origin',(18.505144113284,57.9804289733666,3.23423028058522));
#243240=CARTESIAN_POINT('Ctrl Pts',(18.9827025415095,59.451978872661,3.47153072139113));
#243241=CARTESIAN_POINT('Ctrl Pts',(19.1043350233606,59.4129503614029,3.47182327902704));
#243242=CARTESIAN_POINT('Ctrl Pts',(19.0706774512227,59.3099814440482,3.40413028959084));
#243243=CARTESIAN_POINT('Ctrl Pts',(18.9472820042048,59.3425890481026,3.65553807120996));
#243244=CARTESIAN_POINT('Ctrl Pts',(19.0687544722072,59.3034455268841,3.65586275497006));
#243245=CARTESIAN_POINT('Ctrl Pts',(19.0422629184333,59.2225305038464,3.55128126837233));
#243246=CARTESIAN_POINT('Ctrl Pts',(18.8836509927315,59.1460739925269,3.77003198860305));
#243247=CARTESIAN_POINT('Ctrl Pts',(19.0048854004761,59.1068782740652,3.77025505748499));
#243248=CARTESIAN_POINT('Ctrl Pts',(18.9912173655549,59.0654284453504,3.64284211731256));
#243249=CARTESIAN_POINT('Ctrl Pts',(18.8168143322225,58.9396512752215,3.77003198860304));
#243250=CARTESIAN_POINT('Ctrl Pts',(18.9377789557523,58.9003474864894,3.77003198860305));
#243251=CARTESIAN_POINT('Ctrl Pts',(18.9375983752043,58.9004061606661,3.64284239821769));
#243252=CARTESIAN_POINT('Origin',(18.9499432001057,59.3493798002282,3.40423097483351));
#243253=CARTESIAN_POINT('Ctrl Pts',(18.505144113284,57.9804289733666,3.36123028058522));
#243254=CARTESIAN_POINT('Ctrl Pts',(18.6259282908535,57.941183815081,3.36123028058522));
#243255=CARTESIAN_POINT('Ctrl Pts',(18.6259282908535,57.941183815081,3.23423028058522));
#243256=CARTESIAN_POINT('Ctrl Pts',(18.477106059509,57.8948964606934,3.36123028058522));
#243257=CARTESIAN_POINT('Ctrl Pts',(18.5980867642071,57.8554964068689,3.36146538610141));
#243258=CARTESIAN_POINT('Ctrl Pts',(18.5842066467862,57.8127777979911,3.23423043688481));
#243259=CARTESIAN_POINT('Ctrl Pts',(18.4505921960619,57.814019554574,3.41054258693141));
#243260=CARTESIAN_POINT('Ctrl Pts',(18.5718941197465,57.7748837362139,3.41100608859804));
#243261=CARTESIAN_POINT('Ctrl Pts',(18.5447558577167,57.6913607539433,3.3081986697087));
#243262=CARTESIAN_POINT('Ctrl Pts',(18.4366189870672,57.7713971777989,3.48823028058521));
#243263=CARTESIAN_POINT('Ctrl Pts',(18.5581069080659,57.7324510618073,3.48852004212299));
#243264=CARTESIAN_POINT('Ctrl Pts',(18.5239649837007,57.6273730232607,3.42473028058521));
#243265=CARTESIAN_POINT('Origin',(18.4031808061312,57.6666181815464,3.42473028058521));
#243266=CARTESIAN_POINT('Origin',(19.0049943031126,59.518809673581,3.11913648178592));
#243267=CARTESIAN_POINT('Origin',(19.0600454060086,59.6882395467423,2.83404198860303));
#243268=CARTESIAN_POINT('Origin',(18.3780421908163,57.5892494790278,3.56563113460797));
#243269=CARTESIAN_POINT('Origin',(18.3641788932756,57.5467470426664,3.64299171721853));
#243270=CARTESIAN_POINT('Ctrl Pts',(19.4393816709755,59.8776671349988,2.59908173516065));
#243271=CARTESIAN_POINT('Ctrl Pts',(19.4278624395265,59.8421853116555,2.65878198860303));
#243272=CARTESIAN_POINT('Ctrl Pts',(19.4061247292252,59.7752282754839,2.65878198860303));
#243273=CARTESIAN_POINT('Ctrl Pts',(19.3555723159021,59.9048758468124,2.59908193475641));
#243274=CARTESIAN_POINT('Ctrl Pts',(19.3668135526097,59.8620015382116,2.65878715325483));
#243275=CARTESIAN_POINT('Ctrl Pts',(19.3576098387255,59.7909691583393,2.65878198860303));
#243276=CARTESIAN_POINT('Ctrl Pts',(19.2705128813952,59.9061888791358,2.63878778849937));
#243277=CARTESIAN_POINT('Ctrl Pts',(19.3034480936186,59.8582551377154,2.69564460180157));
#243278=CARTESIAN_POINT('Ctrl Pts',(19.3051157581416,59.7817014705981,2.68180481624928));
#243279=CARTESIAN_POINT('Ctrl Pts',(19.1466203444579,59.8700374834727,2.75443238878662));
#243280=CARTESIAN_POINT('Ctrl Pts',(19.2244111832569,59.8200494324149,2.79268340777132));
#243281=CARTESIAN_POINT('Ctrl Pts',(19.2239451174252,59.7316696194044,2.74885926835648));
#243282=CARTESIAN_POINT('Ctrl Pts',(19.1068608943533,59.8340873574361,2.82856655361729));
#243283=CARTESIAN_POINT('Ctrl Pts',(19.2088773592693,59.7849307811039,2.85384197230968));
#243284=CARTESIAN_POINT('Ctrl Pts',(19.1948817636406,59.6922425516966,2.7918462427856));
#243285=CARTESIAN_POINT('Ctrl Pts',(19.092807720641,59.7908376697914,2.90134173516065));
#243286=CARTESIAN_POINT('Ctrl Pts',(19.2142545736082,59.7518659300028,2.90163218716432));
#243287=CARTESIAN_POINT('Ctrl Pts',(19.180829583578,59.6489943884566,2.83404198860303));
#243288=CARTESIAN_POINT('Origin',(19.4061247292252,59.7752282754839,2.53178198860303));
#243289=CARTESIAN_POINT('Origin',(-0.301960443923706,0.0981128957142288,
3.64303198860263));
#243290=CARTESIAN_POINT('Origin',(18.2401996527044,57.1650137687749,3.64303198860302));
#243291=CARTESIAN_POINT('Origin',(5.61372323131277E-15,1.8572573083956E-13,
2.53178198860262));
#243292=CARTESIAN_POINT('Origin',(19.4351129318419,59.7658094374954,2.53178198860303));
#243293=CARTESIAN_POINT('Ctrl Pts',(18.2401996527044,57.1650137687749,3.77003198860303));
#243294=CARTESIAN_POINT('Ctrl Pts',(18.3611647704259,57.12570981947,3.77003198860303));
#243295=CARTESIAN_POINT('Ctrl Pts',(18.3609836949485,57.1257686544592,3.64284187937102));
#243296=CARTESIAN_POINT('Ctrl Pts',(18.1733685221985,56.9585856505955,3.77003198860303));
#243297=CARTESIAN_POINT('Ctrl Pts',(18.2941737326411,56.9195342693639,3.76980208963088));
#243298=CARTESIAN_POINT('Ctrl Pts',(18.3073637563258,56.9607434512639,3.64284193928411));
#243299=CARTESIAN_POINT('Ctrl Pts',(18.1097485684436,56.7620685738649,3.65553535416627));
#243300=CARTESIAN_POINT('Ctrl Pts',(18.2303834904051,56.7232097045396,3.65520057834355));
#243301=CARTESIAN_POINT('Ctrl Pts',(18.2563185833005,56.8036425617911,3.55127910964214));
#243302=CARTESIAN_POINT('Ctrl Pts',(18.074335247489,56.6526781108326,3.47153072139112));
#243303=CARTESIAN_POINT('Ctrl Pts',(18.1949032015565,56.614013491141,3.47122746281622));
#243304=CARTESIAN_POINT('Ctrl Pts',(18.227904398799,56.7161926934813,3.40413045901321));
#243305=CARTESIAN_POINT('Origin',(18.1070706485041,56.7552848242273,3.4042309748335));
#243306=CARTESIAN_POINT('Ctrl Pts',(19.6977666881844,59.5942745858238,2.90134173516066));
#243307=CARTESIAN_POINT('Ctrl Pts',(19.5766071063167,59.6341304551459,2.90163218716433));
#243308=CARTESIAN_POINT('Ctrl Pts',(19.5431821162865,59.5312589135998,2.83404198860304));
#243309=CARTESIAN_POINT('Ctrl Pts',(19.711825329948,59.6375442153292,2.82853349835397));
#243310=CARTESIAN_POINT('Ctrl Pts',(19.6004058925608,59.6577332347587,2.85381483162415));
#243311=CARTESIAN_POINT('Ctrl Pts',(19.5572406993635,59.5745267832919,2.79182701594345));
#243312=CARTESIAN_POINT('Ctrl Pts',(19.7007277907734,59.68982858249,2.75468822073685));
#243313=CARTESIAN_POINT('Ctrl Pts',(19.6083614943633,59.6951745640079,2.79286913083897));
#243314=CARTESIAN_POINT('Ctrl Pts',(19.55684287225,59.6233361049592,2.74900763297965));
#243315=CARTESIAN_POINT('Ctrl Pts',(19.6225475038109,59.7913053863692,2.63954450640434));
#243316=CARTESIAN_POINT('Ctrl Pts',(19.5674227749671,59.7720679362492,2.69627684028884));
#243317=CARTESIAN_POINT('Ctrl Pts',(19.5210053955057,59.7110541706152,2.68224356036523));
#243318=CARTESIAN_POINT('Ctrl Pts',(19.5524931121161,59.84089242417,2.59908178706474));
#243319=CARTESIAN_POINT('Ctrl Pts',(19.5181549791683,59.8128277376115,2.65878704321603));
#243320=CARTESIAN_POINT('Ctrl Pts',(19.4837751174921,59.7499755976275,2.65878198860303));
#243321=CARTESIAN_POINT('Ctrl Pts',(19.4684195516695,59.8682321556244,2.59908173516065));
#243322=CARTESIAN_POINT('Ctrl Pts',(19.4568831131883,59.8327559231848,2.65878198860303));
#243323=CARTESIAN_POINT('Ctrl Pts',(19.4351129318419,59.7658094374954,2.65878198860303));
#243324=CARTESIAN_POINT('Origin',(19.663966293856,59.4920137553142,2.83404198860303));
#243325=CARTESIAN_POINT('Origin',(18.0520194698747,56.5858547179582,3.11913648167174));
#243326=CARTESIAN_POINT('Origin',(17.996968291141,56.4164246115666,2.83404198860302));
#243327=CARTESIAN_POINT('Origin',(19.6089151909119,59.3225838821511,3.11913648177552));
#243328=CARTESIAN_POINT('Origin',(19.5538640879531,59.1531540088001,3.40423097483351));
#243329=CARTESIAN_POINT('Ctrl Pts',(17.9642361803971,56.3138168485097,2.90134173516062));
#243330=CARTESIAN_POINT('Ctrl Pts',(18.0846218068694,56.2752137607568,2.90103711553268));
#243331=CARTESIAN_POINT('Ctrl Pts',(18.1177524687105,56.377179453281,2.83404198860301));
#243332=CARTESIAN_POINT('Ctrl Pts',(17.9501961787627,56.2706044454594,2.82862991748007));
#243333=CARTESIAN_POINT('Ctrl Pts',(18.060896753813,56.2513675234856,2.85314045886484));
#243334=CARTESIAN_POINT('Ctrl Pts',(18.1037113794376,56.3339654239819,2.79187961000007));
#243335=CARTESIAN_POINT('Ctrl Pts',(17.9612588333756,56.2186079213555,2.75470625793356));
#243336=CARTESIAN_POINT('Ctrl Pts',(18.0531413250553,56.2138593173288,2.79224250381926));
#243337=CARTESIAN_POINT('Ctrl Pts',(18.1041761987739,56.2854146278935,2.7490180910829));
#243338=CARTESIAN_POINT('Ctrl Pts',(18.0394175380795,56.1179510603879,2.63947868311746));
#243339=CARTESIAN_POINT('Ctrl Pts',(18.0943218653326,56.1373490477011,2.69595066767958));
#243340=CARTESIAN_POINT('Ctrl Pts',(18.1403075368578,56.1984140977479,2.68220539436108));
#243341=CARTESIAN_POINT('Ctrl Pts',(18.1094153628979,56.0689198620984,2.5990817858519));
#243342=CARTESIAN_POINT('Ctrl Pts',(18.1436123520193,56.09703620615,2.65877670944818));
#243343=CARTESIAN_POINT('Ctrl Pts',(18.1777307632123,56.1599674935334,2.65878198860301));
#243344=CARTESIAN_POINT('Ctrl Pts',(18.1930767435948,56.0417604764385,2.59908173516063));
#243345=CARTESIAN_POINT('Ctrl Pts',(18.2045954185344,56.0772424804486,2.65878198860301));
#243346=CARTESIAN_POINT('Ctrl Pts',(18.2263320786581,56.144199857553,2.65878198860301));
#243347=CARTESIAN_POINT('Origin',(18.2263320786581,56.144199857553,2.53178198860301));
#243348=CARTESIAN_POINT('Ctrl Pts',(19.42073522007,58.7434254837934,3.77003198860304));
#243349=CARTESIAN_POINT('Ctrl Pts',(19.2997705861191,58.7827292759117,3.77003198860304));
#243350=CARTESIAN_POINT('Ctrl Pts',(19.2999511771037,58.7826705983438,3.64284238727658));
#243351=CARTESIAN_POINT('Ctrl Pts',(19.4879965013588,58.9497137831224,3.77003198860305));
#243352=CARTESIAN_POINT('Ctrl Pts',(19.366877128552,58.9892635895157,3.77025506105909));
#243353=CARTESIAN_POINT('Ctrl Pts',(19.3535710010443,58.9476954469493,3.64284210642029));
#243354=CARTESIAN_POINT('Ctrl Pts',(19.5520260773861,59.1460976215389,3.65553527987872));
#243355=CARTESIAN_POINT('Ctrl Pts',(19.4307447900789,59.1858295778046,3.65585996533));
#243356=CARTESIAN_POINT('Ctrl Pts',(19.4046161500178,59.104796260842,3.55127902710136));
#243357=CARTESIAN_POINT('Ctrl Pts',(19.5876674457077,59.2554138597574,3.47153072139113));
#243358=CARTESIAN_POINT('Ctrl Pts',(19.4663243070093,59.2953329133627,3.4718232790523));
#243359=CARTESIAN_POINT('Ctrl Pts',(19.4330302514113,59.1922458725047,3.40413028378039));
#243360=CARTESIAN_POINT('Origin',(19.42073522007,58.7434254837934,3.64303198860304));
#243361=CARTESIAN_POINT('Origin',(5.68280300381509E-15,1.86380513208053E-13,
2.53178198860262));
#243362=CARTESIAN_POINT('Origin',(18.2553202812748,56.1347810195644,2.53178198860301));
#243363=CARTESIAN_POINT('Origin',(6.24367625034007,18.1886080242679,3.64303198860275));
#243364=CARTESIAN_POINT('Origin',(19.2967593024483,58.3616995707169,3.64299466007272));
#243365=CARTESIAN_POINT('Ctrl Pts',(18.2220120550216,56.0323588238393,2.59908173516063));
#243366=CARTESIAN_POINT('Ctrl Pts',(18.2335490499217,56.0678348753335,2.65878198860301));
#243367=CARTESIAN_POINT('Ctrl Pts',(18.2553202812748,56.1347810195644,2.65878198860301));
#243368=CARTESIAN_POINT('Ctrl Pts',(18.3053742463598,56.0052491386471,2.59908193200014));
#243369=CARTESIAN_POINT('Ctrl Pts',(18.2942806848333,56.0480812627894,2.65877685806711));
#243370=CARTESIAN_POINT('Ctrl Pts',(18.3037418885569,56.1190241739995,2.65878198860301));
#243371=CARTESIAN_POINT('Ctrl Pts',(18.3900709842071,56.0035251343647,2.63872492669841));
#243372=CARTESIAN_POINT('Ctrl Pts',(18.3574039607304,56.0514568378825,2.69532212015323));
#243373=CARTESIAN_POINT('Ctrl Pts',(18.356118560324,56.1278011372721,2.68176836726683));
#243374=CARTESIAN_POINT('Ctrl Pts',(18.5134377270388,56.0390077039671,2.75442176402285));
#243375=CARTESIAN_POINT('Ctrl Pts',(18.4363968713618,56.089193446234,2.79203179920166));
#243376=CARTESIAN_POINT('Ctrl Pts',(18.4370884086014,56.1770584756122,2.74885310748205));
#243377=CARTESIAN_POINT('Ctrl Pts',(18.5530236652641,56.0747542753111,2.82866089558444));
#243378=CARTESIAN_POINT('Ctrl Pts',(18.4521491348401,56.1242585025252,2.85316563119344));
#243379=CARTESIAN_POINT('Ctrl Pts',(18.4660698759072,56.2162483036944,2.79189751796711));
#243380=CARTESIAN_POINT('Ctrl Pts',(18.5670586829464,56.117947944099,2.90134173516062));
#243381=CARTESIAN_POINT('Ctrl Pts',(18.4469743395778,56.1574782858999,2.90103711553269));
#243382=CARTESIAN_POINT('Ctrl Pts',(18.4801050014189,56.2594439784241,2.83404198860301));
#243383=CARTESIAN_POINT('Origin',(18.6008891789884,56.2201988201385,2.83404198860301));
#243384=CARTESIAN_POINT('Origin',(19.2830435998982,58.3196542512025,3.56647653971879));
#243385=CARTESIAN_POINT('Origin',(19.2577541638577,58.2418213702176,3.42473028058526));
#243386=CARTESIAN_POINT('Origin',(18.6559403576614,56.3896289265331,3.1191364816817));
#243387=CARTESIAN_POINT('Origin',(18.7109915363516,56.5590590327992,3.4042309748335));
#243388=CARTESIAN_POINT('Ctrl Pts',(19.1557908785624,57.9280106456678,3.36123028058522));
#243389=CARTESIAN_POINT('Ctrl Pts',(19.0350067009929,57.9672558039534,3.36123028058522));
#243390=CARTESIAN_POINT('Ctrl Pts',(19.0350067009929,57.9672558039534,3.23423028058522));
#243391=CARTESIAN_POINT('Ctrl Pts',(19.1833829156708,58.0136880650214,3.36123028058522));
#243392=CARTESIAN_POINT('Ctrl Pts',(19.0627953474453,58.0527804636623,3.36099641108519));
#243393=CARTESIAN_POINT('Ctrl Pts',(19.0767283413219,58.0956618095378,3.23423043688451));
#243394=CARTESIAN_POINT('Ctrl Pts',(19.2094750027316,58.0947019536608,3.41054258905325));
#243395=CARTESIAN_POINT('Ctrl Pts',(19.0892026680436,58.1340538395318,3.41008815826041));
#243396=CARTESIAN_POINT('Ctrl Pts',(19.1161791203813,58.2170788227779,3.30819867304298));
#243397=CARTESIAN_POINT('Ctrl Pts',(19.2232259141438,58.1373965169896,3.48823028058524));
#243398=CARTESIAN_POINT('Ctrl Pts',(19.1031347997386,58.1769325318822,3.4879469194164));
#243399=CARTESIAN_POINT('Ctrl Pts',(19.1369699862882,58.2810665285032,3.42473028058525));
#243400=CARTESIAN_POINT('Origin',(19.1557908785624,57.9280106456678,3.23423028058522));
#243401=CARTESIAN_POINT('Ctrl Pts',(18.6771643191709,56.4568070719813,3.47153072139112));
#243402=CARTESIAN_POINT('Ctrl Pts',(18.556896315972,56.496394798308,3.47122746285117));
#243403=CARTESIAN_POINT('Ctrl Pts',(18.5902571970799,56.5984571192853,3.40413046676847));
#243404=CARTESIAN_POINT('Ctrl Pts',(18.7128129802638,56.5661228951886,3.65553813458026));
#243405=CARTESIAN_POINT('Ctrl Pts',(18.5923766197464,56.605592832572,3.65520336072198));
#243406=CARTESIAN_POINT('Ctrl Pts',(18.6186718120051,56.6859083114086,3.551281345199));
#243407=CARTESIAN_POINT('Ctrl Pts',(18.7768537015931,56.762504971004,3.77003198860303));
#243408=CARTESIAN_POINT('Ctrl Pts',(18.6561664154735,56.8019192501356,3.76980209314125));
#243409=CARTESIAN_POINT('Ctrl Pts',(18.669717390011,56.8430104456825,3.64284195387498));
#243410=CARTESIAN_POINT('Ctrl Pts',(18.8441205405518,56.9687879773468,3.77003198860303));
#243411=CARTESIAN_POINT('Ctrl Pts',(18.7231554368011,57.0080919221123,3.77003198860303));
#243412=CARTESIAN_POINT('Ctrl Pts',(18.7233364982868,57.0080330916693,3.64284189403878));
#243413=CARTESIAN_POINT('Origin',(18.8441205405518,56.9687879773468,3.64303198860303));
#243414=CARTESIAN_POINT('Origin',(6.09975091006187,17.7456513739113,3.23423028058494));
#243415=CARTESIAN_POINT('Origin',(19.1090650011314,57.7842031819385,3.23423028058522));
#243416=CARTESIAN_POINT('Origin',(6.07721283595898,17.6762863142852,3.64303198860275));
#243417=CARTESIAN_POINT('Origin',(18.9681964166833,57.3504898524409,3.64299171721779));
#243418=CARTESIAN_POINT('Ctrl Pts',(19.0416371860877,57.5748148483578,3.48823028058521));
#243419=CARTESIAN_POINT('Ctrl Pts',(18.9204594407744,57.6147155869504,3.48852004212298));
#243420=CARTESIAN_POINT('Ctrl Pts',(18.8863175164091,57.5096375484039,3.42473028058521));
#243421=CARTESIAN_POINT('Ctrl Pts',(19.055431886255,57.6176546016067,3.41028005848447));
#243422=CARTESIAN_POINT('Ctrl Pts',(18.9342932580184,57.6572916985394,3.41074404220401));
#243423=CARTESIAN_POINT('Ctrl Pts',(18.9071786451787,57.573841500985,3.30780486243988));
#243424=CARTESIAN_POINT('Ctrl Pts',(19.0815664505365,57.6988141606861,3.36123028058522));
#243425=CARTESIAN_POINT('Ctrl Pts',(18.9605330155752,57.7380493683874,3.36146460586551));
#243426=CARTESIAN_POINT('Ctrl Pts',(18.9466997135531,57.6954748424925,3.23423045308519));
#243427=CARTESIAN_POINT('Ctrl Pts',(19.1090650011314,57.7842031819385,3.36123028058522));
#243428=CARTESIAN_POINT('Ctrl Pts',(18.9882808235619,57.8234483402241,3.36123028058521));
#243429=CARTESIAN_POINT('Ctrl Pts',(18.9882808235619,57.8234483402241,3.23423028058522));
#243430=CARTESIAN_POINT('Origin',(19.0071016939786,57.4703923901183,3.42473028058521));
#243431=CARTESIAN_POINT('Origin',(18.9819630792876,57.3930236885637,3.5656311352486));
#243432=CARTESIAN_POINT('Origin',(12.4602215063116,60.1478239224139,3.5664765390944));
#243433=CARTESIAN_POINT('Origin',(12.4693660187271,60.1910940874977,3.6429946600763));
#243434=CARTESIAN_POINT('Origin',(12.443206359372,60.0677739512128,3.42473028058526));
#243435=CARTESIAN_POINT('Ctrl Pts',(12.4208962741585,59.9600752506739,3.48823028058526));
#243436=CARTESIAN_POINT('Ctrl Pts',(12.5446662374485,59.9342688867327,3.48794691941642));
#243437=CARTESIAN_POINT('Ctrl Pts',(12.5674311046652,60.0413691664789,3.42473028058527));
#243438=CARTESIAN_POINT('Ctrl Pts',(12.4114257351941,59.9160770362137,3.4102800592513));
#243439=CARTESIAN_POINT('Ctrl Pts',(12.5352608058697,59.8900198101371,3.40982512230947));
#243440=CARTESIAN_POINT('Ctrl Pts',(12.5533954010692,59.9753363727331,3.30780486372805));
#243441=CARTESIAN_POINT('Ctrl Pts',(12.393483289627,59.8327226933131,3.36123028058523));
#243442=CARTESIAN_POINT('Ctrl Pts',(12.5174621766264,59.806283843088,3.360997210486));
#243443=CARTESIAN_POINT('Ctrl Pts',(12.5268049860494,59.8502383056079,3.23423045308477));
#243444=CARTESIAN_POINT('Ctrl Pts',(12.3746037924162,59.745024249125,3.36123028058523));
#243445=CARTESIAN_POINT('Ctrl Pts',(12.4988285377094,59.7186194643911,3.36123028058523));
#243446=CARTESIAN_POINT('Ctrl Pts',(12.4988285377094,59.7186194643911,3.23423028058523));
#243447=CARTESIAN_POINT('Origin',(12.3746037924162,59.745024249125,3.23423028058523));
#243448=CARTESIAN_POINT('Origin',(-0.310561863232978,0.0660119618348215,
3.64303198860263));
#243449=CARTESIAN_POINT('Origin',(12.5528626811445,60.5836663843184,3.64303198860305));
#243450=CARTESIAN_POINT('Origin',(-0.310561863232978,0.0660119618348243,
3.23423028058481));
#243451=CARTESIAN_POINT('Origin',(12.3431658574209,59.5971203935661,3.23423028058523));
#243452=CARTESIAN_POINT('Ctrl Pts',(12.664289321014,61.1105274371643,3.47153072139115));
#243453=CARTESIAN_POINT('Ctrl Pts',(12.7893350777084,61.0844267845858,3.47182327902705));
#243454=CARTESIAN_POINT('Ctrl Pts',(12.7666250679676,60.9785037674411,3.40413028959073));
#243455=CARTESIAN_POINT('Ctrl Pts',(12.6404971713776,60.9980344071778,3.65553807121));
#243456=CARTESIAN_POINT('Ctrl Pts',(12.7653958126153,60.9718026486719,3.65586275496976));
#243457=CARTESIAN_POINT('Ctrl Pts',(12.7475073053531,60.8885617651958,3.55128126837296));
#243458=CARTESIAN_POINT('Ctrl Pts',(12.5977561540106,60.795944629793,3.77003198860306));
#243459=CARTESIAN_POINT('Ctrl Pts',(12.7224234952036,60.769636075915,3.77025505748515));
#243460=CARTESIAN_POINT('Ctrl Pts',(12.713163022104,60.7269846150103,3.64284211731234));
#243461=CARTESIAN_POINT('Ctrl Pts',(12.5528626811445,60.5836663843184,3.77003198860306));
#243462=CARTESIAN_POINT('Ctrl Pts',(12.6772730124468,60.5572221520606,3.77003198860306));
#243463=CARTESIAN_POINT('Ctrl Pts',(12.6770872880162,60.5572616290069,3.64284239821747));
#243464=CARTESIAN_POINT('Origin',(12.642433962084,61.0050661295708,3.40423097483353));
#243465=CARTESIAN_POINT('Ctrl Pts',(12.3431658574209,59.5971203935661,3.36123028058523));
#243466=CARTESIAN_POINT('Ctrl Pts',(12.4673906027141,59.5707156088323,3.36123028058523));
#243467=CARTESIAN_POINT('Ctrl Pts',(12.4673906027141,59.5707156088323,3.23423028058523));
#243468=CARTESIAN_POINT('Ctrl Pts',(12.3242219811461,59.5091256622729,3.36123028058523));
#243469=CARTESIAN_POINT('Ctrl Pts',(12.4486583679642,59.4825873732132,3.36146538610137));
#243470=CARTESIAN_POINT('Ctrl Pts',(12.4393195978193,59.4386519140009,3.23423043688482));
#243471=CARTESIAN_POINT('Ctrl Pts',(12.3063073021293,59.4259203549058,3.41054258693141));
#243472=CARTESIAN_POINT('Ctrl Pts',(12.4310355281324,59.399678430328,3.41100608859797));
#243473=CARTESIAN_POINT('Ctrl Pts',(12.4127764613285,59.3137762748663,3.30819866970841));
#243474=CARTESIAN_POINT('Ctrl Pts',(12.2968658913801,59.3820708699073,3.48823028058522));
#243475=CARTESIAN_POINT('Ctrl Pts',(12.4217592664911,59.3560370505016,3.48852004212301));
#243476=CARTESIAN_POINT('Ctrl Pts',(12.3987880210522,59.2479658375578,3.42473028058522));
#243477=CARTESIAN_POINT('Origin',(12.274563275759,59.2743706222917,3.42473028058521));
#243478=CARTESIAN_POINT('Origin',(12.6794732450923,61.1793222555443,3.11913648178318));
#243479=CARTESIAN_POINT('Origin',(12.7165125280164,61.3535783813234,2.83404198860304));
#243480=CARTESIAN_POINT('Origin',(12.2576496039892,59.1947980527949,3.56563113460905));
#243481=CARTESIAN_POINT('Origin',(12.2483049653996,59.1510793400373,3.64299171721803));
#243482=CARTESIAN_POINT('Ctrl Pts',(13.0739701745323,61.58161970227,2.59908173516066));
#243483=CARTESIAN_POINT('Ctrl Pts',(13.0662229071065,61.5451281645061,2.65878198860305));
#243484=CARTESIAN_POINT('Ctrl Pts',(13.0516031943527,61.4762657165318,2.65878198860305));
#243485=CARTESIAN_POINT('Ctrl Pts',(12.9877758510419,61.5999188988205,2.59908193475586));
#243486=CARTESIAN_POINT('Ctrl Pts',(13.0034370926712,61.55845448937,2.65878715325448));
#243487=CARTESIAN_POINT('Ctrl Pts',(13.0017087032042,61.4868491822359,2.65878198860305));
#243488=CARTESIAN_POINT('Ctrl Pts',(12.9030451317659,61.5923336062398,2.63878778849915));
#243489=CARTESIAN_POINT('Ctrl Pts',(12.9408103617799,61.5481051179918,2.69564460180149));
#243490=CARTESIAN_POINT('Ctrl Pts',(12.9504709278438,61.4721451382827,2.68180481624929));
#243491=CARTESIAN_POINT('Ctrl Pts',(12.7836101409429,61.543429955208,2.75443238878687));
#243492=CARTESIAN_POINT('Ctrl Pts',(12.8662000075465,61.5018471007597,2.79268340777146));
#243493=CARTESIAN_POINT('Ctrl Pts',(12.8749747009097,61.4139027244672,2.7488592683565));
#243494=CARTESIAN_POINT('Ctrl Pts',(12.7478263086954,61.5035207735038,2.82856655361713));
#243495=CARTESIAN_POINT('Ctrl Pts',(12.8544221781243,61.4652971063428,2.85384197230755));
#243496=CARTESIAN_POINT('Ctrl Pts',(12.8501918100168,61.3716536946531,2.79184624278469));
#243497=CARTESIAN_POINT('Ctrl Pts',(12.7383709431249,61.4590390555211,2.90134173516067));
#243498=CARTESIAN_POINT('Ctrl Pts',(12.8632261535953,61.4329754599101,2.90163218716434));
#243499=CARTESIAN_POINT('Ctrl Pts',(12.8407372733096,61.3271735965896,2.83404198860305));
#243500=CARTESIAN_POINT('Origin',(13.0516031943527,61.4762657165318,2.53178198860305));
#243501=CARTESIAN_POINT('Origin',(-0.310561863232978,0.0660119618348215,
3.64303198860263));
#243502=CARTESIAN_POINT('Origin',(12.164906888579,58.7584778814679,3.64303198860303));
#243503=CARTESIAN_POINT('Origin',(5.63039444364742E-15,1.85721263801678E-13,
2.53178198860262));
#243504=CARTESIAN_POINT('Origin',(13.0814171332231,61.4699285681957,2.53178198860305));
#243505=CARTESIAN_POINT('Ctrl Pts',(12.164906888579,58.7584778814679,3.77003198860304));
#243506=CARTESIAN_POINT('Ctrl Pts',(12.2893177281505,58.7320335411741,3.77003198860304));
#243507=CARTESIAN_POINT('Ctrl Pts',(12.289131494692,58.7320731263177,3.64284187937058));
#243508=CARTESIAN_POINT('Ctrl Pts',(12.1200194799684,58.5461948427483,3.77003198860304));
#243509=CARTESIAN_POINT('Ctrl Pts',(12.244244887697,58.5199849720738,3.76980208962962));
#243510=CARTESIAN_POINT('Ctrl Pts',(12.2530551225943,58.5623471386693,3.64284193928367));
#243511=CARTESIAN_POINT('Ctrl Pts',(12.0772896710124,58.3441042111269,3.65553535416629));
#243512=CARTESIAN_POINT('Ctrl Pts',(12.2013256001486,58.3180679977585,3.65520057834544));
#243513=CARTESIAN_POINT('Ctrl Pts',(12.2187110949215,58.4007711908097,3.5512791096424));
#243514=CARTESIAN_POINT('Ctrl Pts',(12.053504764932,58.2316113004783,3.47153072139112));
#243515=CARTESIAN_POINT('Ctrl Pts',(12.1774537884115,58.2057612725769,3.47122746281622));
#243516=CARTESIAN_POINT('Ctrl Pts',(12.1995935666436,58.3108302909898,3.40413045901298));
#243517=CARTESIAN_POINT('Origin',(12.0753355159231,58.3370777047237,3.40423097483351));
#243518=CARTESIAN_POINT('Ctrl Pts',(13.3605623192485,61.3267881959115,2.90134173516067));
#243519=CARTESIAN_POINT('Ctrl Pts',(13.2359003894749,61.3537611057085,2.90163218716434));
#243520=CARTESIAN_POINT('Ctrl Pts',(13.2134115091892,61.247959242388,2.83404198860305));
#243521=CARTESIAN_POINT('Ctrl Pts',(13.3700210384233,61.3712903180782,2.82853349835398));
#243522=CARTESIAN_POINT('Ctrl Pts',(13.2571016411965,61.3797222373777,2.85381483162378));
#243523=CARTESIAN_POINT('Ctrl Pts',(13.2228703539492,61.2924596082468,2.79182701594254));
#243524=CARTESIAN_POINT('Ctrl Pts',(13.3535190881771,61.4221282572892,2.75468822073686));
#243525=CARTESIAN_POINT('Ctrl Pts',(13.2610999767702,61.4177900459395,2.79286913083897));
#243526=CARTESIAN_POINT('Ctrl Pts',(13.2173727427873,61.3409599630867,2.74900763297962));
#243527=CARTESIAN_POINT('Ctrl Pts',(13.2651598666398,61.5148770953651,2.63954450640435));
#243528=CARTESIAN_POINT('Ctrl Pts',(13.2123479779269,61.4899829268156,2.69627684028887));
#243529=CARTESIAN_POINT('Ctrl Pts',(13.1725625528867,61.4244514636298,2.68224356036528));
#243530=CARTESIAN_POINT('Ctrl Pts',(13.1903059833735,61.5568698122757,2.59908178706413));
#243531=CARTESIAN_POINT('Ctrl Pts',(13.1590895168685,61.5253695547374,2.65878704321587));
#243532=CARTESIAN_POINT('Ctrl Pts',(13.1314678292776,61.4592680512445,2.65878198860305));
#243533=CARTESIAN_POINT('Ctrl Pts',(13.1038352065726,61.5752716937454,2.59908173516066));
#243534=CARTESIAN_POINT('Ctrl Pts',(13.0960702419678,61.538783917633,2.65878198860304));
#243535=CARTESIAN_POINT('Ctrl Pts',(13.0814171332231,61.4699285681957,2.65878198860305));
#243536=CARTESIAN_POINT('Origin',(13.3376362544824,61.2215544576541,2.83404198860303));
#243537=CARTESIAN_POINT('Origin',(12.0382961820467,58.1628213392049,3.11913648166998));
#243538=CARTESIAN_POINT('Origin',(12.0012568480858,57.9885649735462,2.83404198860302));
#243539=CARTESIAN_POINT('Origin',(13.3005969715131,61.0472983318734,3.11913648177627));
#243540=CARTESIAN_POINT('Origin',(13.26355768855,60.8730422059016,3.40423097483353));
#243541=CARTESIAN_POINT('Ctrl Pts',(11.9794294790611,57.8830978693158,2.90134173516064));
#243542=CARTESIAN_POINT('Ctrl Pts',(12.1031907419155,57.8572899778513,2.9010371155327));
#243543=CARTESIAN_POINT('Ctrl Pts',(12.125481593379,57.9621601888123,2.83404198860303));
#243544=CARTESIAN_POINT('Ctrl Pts',(11.9699833161086,57.8386546085358,2.82862991747999));
#243545=CARTESIAN_POINT('Ctrl Pts',(12.0820882677179,57.8310944294269,2.85314045886453));
#243546=CARTESIAN_POINT('Ctrl Pts',(12.1160345187366,57.9177151970034,2.79187960999944));
#243547=CARTESIAN_POINT('Ctrl Pts',(11.9864204851029,57.7880992891177,2.75470625793369));
#243548=CARTESIAN_POINT('Ctrl Pts',(12.0782959991609,57.7929810340976,2.79224250381943));
#243549=CARTESIAN_POINT('Ctrl Pts',(12.1215717318493,57.8694789541067,2.74901809108301));
#243550=CARTESIAN_POINT('Ctrl Pts',(12.0746725352387,57.6961636462599,2.63947868311736));
#243551=CARTESIAN_POINT('Ctrl Pts',(12.127248449038,57.7211944343231,2.69595066767949));
#243552=CARTESIAN_POINT('Ctrl Pts',(12.1665991704024,57.7867317752134,2.68220539436099));
#243553=CARTESIAN_POINT('Ctrl Pts',(12.1494120604582,57.6547178110654,2.59908178585209));
#243554=CARTESIAN_POINT('Ctrl Pts',(12.1804827566586,57.6862546895637,2.65877670944884));
#243555=CARTESIAN_POINT('Ctrl Pts',(12.2078361528635,57.7524075778605,2.65878198860302));
#243556=CARTESIAN_POINT('Ctrl Pts',(12.2354540642043,57.6364522029209,2.59908173516064));
#243557=CARTESIAN_POINT('Ctrl Pts',(12.2432007592846,57.6729438621908,2.65878198860302));
#243558=CARTESIAN_POINT('Ctrl Pts',(12.2578193919766,57.7418065394568,2.65878198860302));
#243559=CARTESIAN_POINT('Origin',(12.2578193919766,57.7418065394568,2.53178198860302));
#243560=CARTESIAN_POINT('Ctrl Pts',(13.1739864076105,60.4516424606491,3.77003198860306));
#243561=CARTESIAN_POINT('Ctrl Pts',(13.0495760655906,60.478086695185,3.77003198860305));
#243562=CARTESIAN_POINT('Ctrl Pts',(13.0497618007548,60.4780472159572,3.64284238727674));
#243563=CARTESIAN_POINT('Ctrl Pts',(13.2193162256457,60.6638314094602,3.77003198860306));
#243564=CARTESIAN_POINT('Ctrl Pts',(13.0947262769519,60.6905041359632,3.77025506105868));
#243565=CARTESIAN_POINT('Ctrl Pts',(13.0858380958638,60.6477728389727,3.64284210641966));
#243566=CARTESIAN_POINT('Ctrl Pts',(13.2624673401133,60.8658323498481,3.65553527987878));
#243567=CARTESIAN_POINT('Ctrl Pts',(13.1376973240562,60.8926693037166,3.65585996533079));
#243568=CARTESIAN_POINT('Ctrl Pts',(13.1201821075159,60.8093487091478,3.55127902710192));
#243569=CARTESIAN_POINT('Ctrl Pts',(13.2864868028994,60.978275279735,3.47153072139115));
#243570=CARTESIAN_POINT('Ctrl Pts',(13.1616357172828,61.0052918407717,3.47182327905231));
#243571=CARTESIAN_POINT('Ctrl Pts',(13.1392995799685,60.8992893450422,3.40413028378048));
#243572=CARTESIAN_POINT('Origin',(13.1739864076105,60.4516424606491,3.64303198860306));
#243573=CARTESIAN_POINT('Origin',(5.67687244506386E-15,1.86382102296481E-13,
2.53178198860262));
#243574=CARTESIAN_POINT('Origin',(12.2876333308469,57.7354693911207,2.53178198860302));
#243575=CARTESIAN_POINT('Origin',(3.00026883051124,12.588064422097,3.64303198860271));
#243576=CARTESIAN_POINT('Origin',(13.0905908661193,60.059048669913,3.64299466007489));
#243577=CARTESIAN_POINT('Ctrl Pts',(12.2652136052659,57.630126617196,2.59908173516064));
#243578=CARTESIAN_POINT('Ctrl Pts',(12.2729791421553,57.6666142715157,2.65878198860302));
#243579=CARTESIAN_POINT('Ctrl Pts',(12.2876333308469,57.7354693911207,2.65878198860302));
#243580=CARTESIAN_POINT('Ctrl Pts',(12.3509528635304,57.6118791634506,2.59908193199958));
#243581=CARTESIAN_POINT('Ctrl Pts',(12.3354428975797,57.6533170557974,2.65877685806754));
#243582=CARTESIAN_POINT('Ctrl Pts',(12.3374367183508,57.7248602994024,2.65878198860302));
#243583=CARTESIAN_POINT('Ctrl Pts',(12.4353658313041,57.6190178232952,2.63872492669831));
#243584=CARTESIAN_POINT('Ctrl Pts',(12.3978675338896,57.6632723181626,2.69532212015325));
#243585=CARTESIAN_POINT('Ctrl Pts',(12.3886090227466,57.739064034563,2.68176836726674));
#243586=CARTESIAN_POINT('Ctrl Pts',(12.5543478197373,57.6672013517155,2.75442176402297));
#243587=CARTESIAN_POINT('Ctrl Pts',(12.4724831634114,57.7090592089824,2.7920317992016));
#243588=CARTESIAN_POINT('Ctrl Pts',(12.463986515842,57.796515189861,2.74885310748216));
#243589=CARTESIAN_POINT('Ctrl Pts',(12.5899803678813,57.706889956891,2.82866089558436));
#243590=CARTESIAN_POINT('Ctrl Pts',(12.484483837894,57.7455787351211,2.85316563119316));
#243591=CARTESIAN_POINT('Ctrl Pts',(12.4887127671322,57.8385197202054,2.79189751796709));
#243592=CARTESIAN_POINT('Ctrl Pts',(12.599423532447,57.7513140650722,2.90134173516062));
#243593=CARTESIAN_POINT('Ctrl Pts',(12.4758649777951,57.7780756236498,2.90103711553269));
#243594=CARTESIAN_POINT('Ctrl Pts',(12.4981558292586,57.8829458346107,2.83404198860301));
#243595=CARTESIAN_POINT('Origin',(12.6223805745518,57.8565410498769,2.83404198860302));
#243596=CARTESIAN_POINT('Origin',(13.0813452322622,60.0157999977499,3.56647653971802));
#243597=CARTESIAN_POINT('Origin',(13.064330085838,59.9357500275435,3.42473028058526));
#243598=CARTESIAN_POINT('Origin',(12.6594199084546,58.0307974155296,3.11913648168123));
#243599=CARTESIAN_POINT('Origin',(12.6964592423891,58.2050537810544,3.40423097483351));
#243600=CARTESIAN_POINT('Ctrl Pts',(12.9957275188822,59.6130003254557,3.36123028058523));
#243601=CARTESIAN_POINT('Ctrl Pts',(12.871502773589,59.6394051101896,3.36123028058523));
#243602=CARTESIAN_POINT('Ctrl Pts',(12.871502773589,59.6394051101896,3.23423028058523));
#243603=CARTESIAN_POINT('Ctrl Pts',(13.0142126749434,59.7010925481787,3.36123028058523));
#243604=CARTESIAN_POINT('Ctrl Pts',(12.8901994296778,59.7273659613729,3.36099641108525));
#243605=CARTESIAN_POINT('Ctrl Pts',(12.8995737759687,59.7714687931883,3.2342304368846));
#243606=CARTESIAN_POINT('Ctrl Pts',(13.0316935695382,59.7843900000234,3.41054258905324));
#243607=CARTESIAN_POINT('Ctrl Pts',(12.9079667071289,59.8109544298286,3.41008815826004));
#243608=CARTESIAN_POINT('Ctrl Pts',(12.9261169057243,59.8963444006364,3.30819867304273));
#243609=CARTESIAN_POINT('Ctrl Pts',(13.0409063549237,59.8282880397057,3.48823028058525));
#243610=CARTESIAN_POINT('Ctrl Pts',(12.9173404733281,59.8550545325311,3.48794691941641));
#243611=CARTESIAN_POINT('Ctrl Pts',(12.9401053405448,59.9621548122774,3.42473028058526));
#243612=CARTESIAN_POINT('Origin',(12.9957275188822,59.6130003254557,3.23423028058523));
#243613=CARTESIAN_POINT('Ctrl Pts',(12.6735055745739,58.0998260601482,3.47153072139113));
#243614=CARTESIAN_POINT('Ctrl Pts',(12.5497583678832,58.1266254912132,3.47122746285118));
#243615=CARTESIAN_POINT('Ctrl Pts',(12.5722680770245,58.2316158657528,3.40413046676845));
#243616=CARTESIAN_POINT('Ctrl Pts',(12.6975323335625,58.2122693395992,3.65553813458025));
#243617=CARTESIAN_POINT('Ctrl Pts',(12.5736300041264,58.2389340288484,3.65520336072215));
#243618=CARTESIAN_POINT('Ctrl Pts',(12.5913858949922,58.3215581271264,3.55128134519927));
#243619=CARTESIAN_POINT('Ctrl Pts',(12.7406947165202,58.4142696920428,3.77003198860304));
#243620=CARTESIAN_POINT('Ctrl Pts',(12.6165486539543,58.4408527990764,3.76980209314164));
#243621=CARTESIAN_POINT('Ctrl Pts',(12.6257301953096,58.4831353552992,3.6428419538751));
#243622=CARTESIAN_POINT('Ctrl Pts',(12.786030615045,58.6264539577986,3.77003198860304));
#243623=CARTESIAN_POINT('Ctrl Pts',(12.6616197898427,58.6528982950381,3.77003198860304));
#243624=CARTESIAN_POINT('Ctrl Pts',(12.6618060089105,58.6528587129534,3.64284189403875));
#243625=CARTESIAN_POINT('Origin',(12.786030615045,58.6264539577986,3.64303198860304));
#243626=CARTESIAN_POINT('Origin',(2.93511643966546,12.2815465224194,3.2342302805849));
#243627=CARTESIAN_POINT('Origin',(12.9642895838869,59.4650964698968,3.23423028058523));
#243628=CARTESIAN_POINT('Origin',(2.92491386234291,12.2335471699534,3.64303198860271));
#243629=CARTESIAN_POINT('Origin',(12.8695280801142,59.0190342907438,3.64299171721836));
#243630=CARTESIAN_POINT('Ctrl Pts',(12.9191181862044,59.2498070616281,3.48823028058522));
#243631=CARTESIAN_POINT('Ctrl Pts',(12.7944335023706,59.2768226963,3.488520042123));
#243632=CARTESIAN_POINT('Ctrl Pts',(12.7714622569318,59.1687514833563,3.42473028058522));
#243633=CARTESIAN_POINT('Ctrl Pts',(12.9283593439854,59.2938540730364,3.4102800584845));
#243634=CARTESIAN_POINT('Ctrl Pts',(12.8037411209988,59.3206115991505,3.41074404220436));
#243635=CARTESIAN_POINT('Ctrl Pts',(12.7854979657562,59.2347843016993,3.30780486244024));
#243636=CARTESIAN_POINT('Ctrl Pts',(12.9458672564001,59.3773008374016,3.36123028058523));
#243637=CARTESIAN_POINT('Ctrl Pts',(12.8213956592925,59.4036696715712,3.36146460586425));
#243638=CARTESIAN_POINT('Ctrl Pts',(12.8120883873131,59.3598823995799,3.23423045308459));
#243639=CARTESIAN_POINT('Ctrl Pts',(12.9642895838869,59.4650964698969,3.36123028058523));
#243640=CARTESIAN_POINT('Ctrl Pts',(12.8400648385937,59.4915012546307,3.36123028058523));
#243641=CARTESIAN_POINT('Ctrl Pts',(12.8400648385937,59.4915012546307,3.23423028058523));
#243642=CARTESIAN_POINT('Origin',(12.895687002225,59.1423466986224,3.42473028058522));
#243643=CARTESIAN_POINT('Origin',(12.8787733309736,59.0627741301473,3.56563113524825));
#243644=CARTESIAN_POINT('Origin',(6.1048035056639,61.1207756556243,3.56647653909506));
#243645=CARTESIAN_POINT('Origin',(6.10937495961997,61.1647646440472,3.64299466007747));
#243646=CARTESIAN_POINT('Origin',(6.09624906995219,61.0393856393806,3.42473028058526));
#243647=CARTESIAN_POINT('Ctrl Pts',(6.08531878138301,60.9299448846692,3.48823028058527));
#243648=CARTESIAN_POINT('Ctrl Pts',(6.21110821942915,60.9172173747512,3.48794691941643));
#243649=CARTESIAN_POINT('Ctrl Pts',(6.22255335066396,61.0261105245456,3.42473028058528));
#243650=CARTESIAN_POINT('Ctrl Pts',(6.08049918876605,60.8851977561472,3.4102800592513));
#243651=CARTESIAN_POINT('Ctrl Pts',(6.20637959976662,60.8722275639182,3.40982512230992));
#243652=CARTESIAN_POINT('Ctrl Pts',(6.21549684257615,60.958972334824,3.3078048637285));
#243653=CARTESIAN_POINT('Ctrl Pts',(6.07136793516312,60.8004245407961,3.36123028058523));
#243654=CARTESIAN_POINT('Ctrl Pts',(6.19743126523161,60.7870898478944,3.36099721048525));
#243655=CARTESIAN_POINT('Ctrl Pts',(6.2021284013467,60.8317801127822,3.23423045308461));
#243656=CARTESIAN_POINT('Ctrl Pts',(6.0617588454155,60.7112330730306,3.36123028058524));
#243657=CARTESIAN_POINT('Ctrl Pts',(6.18806312612727,60.6979579581956,3.36123028058524));
#243658=CARTESIAN_POINT('Ctrl Pts',(6.18806312612727,60.6979579581956,3.23423028058524));
#243659=CARTESIAN_POINT('Origin',(6.0617588454155,60.7112330730306,3.23423028058524));
#243660=CARTESIAN_POINT('Origin',(-0.315760701779421,0.0331877870876628,
3.64303198860263));
#243661=CARTESIAN_POINT('Origin',(6.15137923967656,61.5639141665614,3.64303198860306));
#243662=CARTESIAN_POINT('Origin',(-0.315760701779421,0.0331877870876657,
3.23423028058481));
#243663=CARTESIAN_POINT('Origin',(6.04595329345041,60.5608532912345,3.23423028058524));
#243664=CARTESIAN_POINT('Ctrl Pts',(6.20712349654444,62.0995362748661,3.47153072139115));
#243665=CARTESIAN_POINT('Ctrl Pts',(6.33421250060471,62.0866494451787,3.47182327902705));
#243666=CARTESIAN_POINT('Ctrl Pts',(6.32269886887974,61.9789328429856,3.40413028959051));
#243667=CARTESIAN_POINT('Ctrl Pts',(6.19522040634608,61.9851725366288,3.65553807121));
#243668=CARTESIAN_POINT('Ctrl Pts',(6.3221768051615,61.9721399414754,3.65586275496991));
#243669=CARTESIAN_POINT('Ctrl Pts',(6.31308733464731,61.8874852020943,3.55128126837335));
#243670=CARTESIAN_POINT('Ctrl Pts',(6.17383766261686,61.7797221753255,3.77003198860307));
#243671=CARTESIAN_POINT('Ctrl Pts',(6.30057205577832,61.7665890280519,3.7702550574855));
#243672=CARTESIAN_POINT('Ctrl Pts',(6.29582060418308,61.7232032332899,3.64284211731174));
#243673=CARTESIAN_POINT('Ctrl Pts',(6.15137923967656,61.5639141665614,3.77003198860306));
#243674=CARTESIAN_POINT('Ctrl Pts',(6.2778722131273,61.5506192193204,3.77003198860306));
#243675=CARTESIAN_POINT('Ctrl Pts',(6.27768337964964,61.5506390665186,3.64284239821706));
#243676=CARTESIAN_POINT('Origin',(6.19641157197444,61.9923681882671,3.40423097483353));
#243677=CARTESIAN_POINT('Ctrl Pts',(6.04595329345041,60.5608532912346,3.36123028058524));
#243678=CARTESIAN_POINT('Ctrl Pts',(6.17225757416218,60.5475781763996,3.36123028058524));
#243679=CARTESIAN_POINT('Ctrl Pts',(6.17225757416218,60.5475781763996,3.23423028058524));
#243680=CARTESIAN_POINT('Ctrl Pts',(6.03631114774998,60.471360430011,3.36123028058524));
#243681=CARTESIAN_POINT('Ctrl Pts',(6.16283986559469,60.4579746647638,3.3614653861017));
#243682=CARTESIAN_POINT('Ctrl Pts',(6.15814476024342,60.4133037213019,3.23423043688466));
#243683=CARTESIAN_POINT('Ctrl Pts',(6.02719193013372,60.3867383361561,3.41054258693141));
#243684=CARTESIAN_POINT('Ctrl Pts',(6.15397990991439,60.3736778173775,3.41100608859788));
#243685=CARTESIAN_POINT('Ctrl Pts',(6.14480008849003,60.2863376507181,3.30819866970873));
#243686=CARTESIAN_POINT('Ctrl Pts',(6.02238575970256,60.3421421670677,3.48823028058523));
#243687=CARTESIAN_POINT('Ctrl Pts',(6.14931623097227,60.3293058762214,3.48852004212301));
#243688=CARTESIAN_POINT('Ctrl Pts',(6.13776734223196,60.2194255397047,3.42473028058523));
#243689=CARTESIAN_POINT('Origin',(6.01146306152019,60.2327006545397,3.42473028058523));
#243690=CARTESIAN_POINT('Origin',(6.2150332248564,62.1695413802855,3.11913648178491));
#243691=CARTESIAN_POINT('Origin',(6.23365487766605,62.3467145720971,2.83404198860306));
#243692=CARTESIAN_POINT('Origin',(6.00295964302148,60.1517960317852,3.56563113460852));
#243693=CARTESIAN_POINT('Origin',(5.99823604520098,60.107340034,3.64299171721827));
#243694=CARTESIAN_POINT('Ctrl Pts',(6.56531752495282,62.6108711573008,2.59908173516067));
#243695=CARTESIAN_POINT('Ctrl Pts',(6.56142710223332,62.5737697140404,2.65878198860305));
#243696=CARTESIAN_POINT('Ctrl Pts',(6.55408556365926,62.5037563256537,2.65878198860305));
#243697=CARTESIAN_POINT('Ctrl Pts',(6.47768259609056,62.6200603487597,2.59908193475804));
#243698=CARTESIAN_POINT('Ctrl Pts',(6.49759225479945,62.5804601312001,2.65878715325562));
#243699=CARTESIAN_POINT('Ctrl Pts',(6.50335812634732,62.5090664195359,2.65878198860305));
#243700=CARTESIAN_POINT('Ctrl Pts',(6.39420891953744,62.6036598373292,2.63878778849925));
#243701=CARTESIAN_POINT('Ctrl Pts',(6.43639040357906,62.5636211788261,2.69564460180146));
#243702=CARTESIAN_POINT('Ctrl Pts',(6.45393802800011,62.4890871199582,2.68180481624927));
#243703=CARTESIAN_POINT('Ctrl Pts',(6.28054002958118,62.5425397295637,2.7544323887868));
#243704=CARTESIAN_POINT('Ctrl Pts',(6.36702405212782,62.5098176621802,2.79268340777155));
#243705=CARTESIAN_POINT('Ctrl Pts',(6.38494336730958,62.4232722595961,2.74885926835655));
#243706=CARTESIAN_POINT('Ctrl Pts',(6.24912387034457,62.4991087455378,2.82856655361721));
#243707=CARTESIAN_POINT('Ctrl Pts',(6.35913125763789,62.4722367740494,2.85384197230859));
#243708=CARTESIAN_POINT('Ctrl Pts',(6.36471246584707,62.3786641568876,2.79184624278505));
#243709=CARTESIAN_POINT('Ctrl Pts',(6.24436990788039,62.4538823482277,2.90134173516068));
#243710=CARTESIAN_POINT('Ctrl Pts',(6.3712655360405,62.441012455002,2.90163218716435));
#243711=CARTESIAN_POINT('Ctrl Pts',(6.35995915837782,62.3334394572621,2.83404198860306));
#243712=CARTESIAN_POINT('Origin',(6.55408556365926,62.5037563256537,2.53178198860305));
#243713=CARTESIAN_POINT('Origin',(-0.315760701779421,0.0331877870876628,
3.64303198860263));
#243714=CARTESIAN_POINT('Origin',(5.95633285891191,59.7081718144894,3.64303198860304));
#243715=CARTESIAN_POINT('Origin',(5.64744126194172E-15,1.85718563850903E-13,
2.53178198860262));
#243716=CARTESIAN_POINT('Origin',(6.58439859103008,62.5005702980933,2.53178198860305));
#243717=CARTESIAN_POINT('Ctrl Pts',(5.95633285891191,59.7081718144894,3.77003198860305));
#243718=CARTESIAN_POINT('Ctrl Pts',(6.08282634913973,59.6948768129329,3.77003198860305));
#243719=CARTESIAN_POINT('Ctrl Pts',(6.08263699811363,59.6948967145278,3.64284187937077));
#243720=CARTESIAN_POINT('Ctrl Pts',(5.93388096803625,59.4923596726255,3.77003198860305));
#243721=CARTESIAN_POINT('Ctrl Pts',(6.0601655334876,59.4792784733333,3.76980208962958));
#243722=CARTESIAN_POINT('Ctrl Pts',(6.06449945282239,59.5223294958626,3.64284193928352));
#243723=CARTESIAN_POINT('Ctrl Pts',(5.91250946061108,59.2869096333632,3.6555353541663));
#243724=CARTESIAN_POINT('Ctrl Pts',(6.03858743332218,59.2739813341586,3.65520057834539));
#243725=CARTESIAN_POINT('Ctrl Pts',(6.04723285085753,59.3580487495165,3.55127910964277));
#243726=CARTESIAN_POINT('Ctrl Pts',(5.90061356181238,59.1725467709679,3.47153072139113));
#243727=CARTESIAN_POINT('Ctrl Pts',(6.02658564326405,59.159794553172,3.47122746281623));
#243728=CARTESIAN_POINT('Ctrl Pts',(6.03762143444287,59.266602229504,3.40413045901309));
#243729=CARTESIAN_POINT('Origin',(5.91130048050323,59.2797173540688,3.40423097483352));
#243730=CARTESIAN_POINT('Ctrl Pts',(6.87697683366544,62.3873926810693,2.90134173516067));
#243731=CARTESIAN_POINT('Ctrl Pts',(6.75017837817581,62.401187110497,2.90163218716435));
#243732=CARTESIAN_POINT('Ctrl Pts',(6.73887200051313,62.2936141127571,2.83404198860306));
#243733=CARTESIAN_POINT('Ctrl Pts',(6.88173199854461,62.4326397213344,2.82853349835381));
#243734=CARTESIAN_POINT('Ctrl Pts',(6.76854981002487,62.4292221586341,2.85381483162498));
#243735=CARTESIAN_POINT('Ctrl Pts',(6.74362747387393,62.3388594194642,2.79182701594424));
#243736=CARTESIAN_POINT('Ctrl Pts',(6.86000643604706,62.4814742414947,2.75468822073712));
#243737=CARTESIAN_POINT('Ctrl Pts',(6.76854707276813,62.4674993676284,2.79286913083863));
#243738=CARTESIAN_POINT('Ctrl Pts',(6.73309031164157,62.3865194274376,2.74900763297951));
#243739=CARTESIAN_POINT('Ctrl Pts',(6.76243636205683,62.5644789380886,2.63954450640411));
#243740=CARTESIAN_POINT('Ctrl Pts',(6.71251593157878,62.5342007968301,2.69627684028914));
#243741=CARTESIAN_POINT('Ctrl Pts',(6.67979835840238,62.464869612516,2.68224356036541));
#243742=CARTESIAN_POINT('Ctrl Pts',(6.68360310202785,62.5984172531145,2.59908178706448));
#243743=CARTESIAN_POINT('Ctrl Pts',(6.65585031610561,62.56382654801,2.65878704321526));
#243744=CARTESIAN_POINT('Ctrl Pts',(6.63528943158918,62.495199902913,2.65878198860306));
#243745=CARTESIAN_POINT('Ctrl Pts',(6.59568250079866,62.6076796697356,2.59908173516068));
#243746=CARTESIAN_POINT('Ctrl Pts',(6.59177408464754,62.5705801176612,2.65878198860306));
#243747=CARTESIAN_POINT('Ctrl Pts',(6.58439859103009,62.5005702980933,2.65878198860306));
#243748=CARTESIAN_POINT('Origin',(6.8651762812249,62.2803389979221,2.83404198860306));
#243749=CARTESIAN_POINT('Origin',(5.89267880207495,59.1025439185017,3.11913648167056));
#243750=CARTESIAN_POINT('Origin',(5.8740571235785,58.9253704827882,2.83404198860304));
#243751=CARTESIAN_POINT('Origin',(6.84655462836425,62.1031658061012,3.11913648177577));
#243752=CARTESIAN_POINT('Origin',(6.82793297553329,61.9259926140921,3.40423097483353));
#243753=CARTESIAN_POINT('Ctrl Pts',(5.86337364149561,58.8181995570487,2.90134173516065));
#243754=CARTESIAN_POINT('Ctrl Pts',(5.98915458643775,58.8054696185322,2.90103711553271));
#243755=CARTESIAN_POINT('Ctrl Pts',(6.00036140429027,58.9120953679532,2.83404198860304));
#243756=CARTESIAN_POINT('Ctrl Pts',(5.85862481136466,58.7730123682042,2.82862991748005));
#243757=CARTESIAN_POINT('Ctrl Pts',(5.97090589422292,58.7772117628631,2.85314045886508));
#243758=CARTESIAN_POINT('Ctrl Pts',(5.99561184840489,58.8669063622639,2.79187961000089));
#243759=CARTESIAN_POINT('Ctrl Pts',(5.8802564056756,58.7244521481309,2.75470625793363));
#243760=CARTESIAN_POINT('Ctrl Pts',(5.9711183347537,58.7389107566978,2.79224250381922));
#243761=CARTESIAN_POINT('Ctrl Pts',(6.00616078842873,58.8195131589312,2.74901809108296));
#243762=CARTESIAN_POINT('Ctrl Pts',(5.97763489331424,58.6422449895252,2.63947868311745));
#243763=CARTESIAN_POINT('Ctrl Pts',(6.02730636094599,58.6726343357865,2.69595066767966));
#243764=CARTESIAN_POINT('Ctrl Pts',(6.05959099741147,58.7419259266992,2.68220539436107));
#243765=CARTESIAN_POINT('Ctrl Pts',(6.05629725705618,58.6088386066686,2.59908178585166));
#243766=CARTESIAN_POINT('Ctrl Pts',(6.08390124328611,58.6434504949727,2.65877670944951));
#243767=CARTESIAN_POINT('Ctrl Pts',(6.10418993497023,58.7121001992973,2.65878198860303));
#243768=CARTESIAN_POINT('Ctrl Pts',(6.14377718965303,58.599666897865,2.59908173516065));
#243769=CARTESIAN_POINT('Ctrl Pts',(6.14766703046151,58.6367684021394,2.65878198860303));
#243770=CARTESIAN_POINT('Ctrl Pts',(6.15500747092297,58.7067819056645,2.65878198860303));
#243771=CARTESIAN_POINT('Origin',(6.15500747092297,58.7067819056645,2.53178198860303));
#243772=CARTESIAN_POINT('Ctrl Pts',(6.78290064323541,61.4975385923864,3.77003198860306));
#243773=CARTESIAN_POINT('Ctrl Pts',(6.65640765888743,61.5108335407728,3.77003198860306));
#243774=CARTESIAN_POINT('Ctrl Pts',(6.65659650327857,61.5108136924275,3.64284238727617));
#243775=CARTESIAN_POINT('Ctrl Pts',(6.80580235504208,61.7133034041537,3.77003198860307));
#243776=CARTESIAN_POINT('Ctrl Pts',(6.67910686401112,61.7268068187944,3.77025506105831));
#243777=CARTESIAN_POINT('Ctrl Pts',(6.67473401011702,61.6833805404071,3.64284210641898));
#243778=CARTESIAN_POINT('Ctrl Pts',(6.82760223531318,61.918708281938,3.65553527987875));
#243779=CARTESIAN_POINT('Ctrl Pts',(6.7007104969118,61.9323562021251,3.65585996533108));
#243780=CARTESIAN_POINT('Ctrl Pts',(6.69200060426984,61.8476612078251,3.5512790271024));
#243781=CARTESIAN_POINT('Ctrl Pts',(6.8397366303024,62.0330459552234,3.47153072139115));
#243782=CARTESIAN_POINT('Ctrl Pts',(6.71274549238771,62.0468640245952,3.47182327905232));
#243783=CARTESIAN_POINT('Ctrl Pts',(6.70161199275238,61.9391074595192,3.40413028378018));
#243784=CARTESIAN_POINT('Origin',(6.78290064323541,61.4975385923864,3.64303198860306));
#243785=CARTESIAN_POINT('Origin',(5.67080826956262E-15,1.86383062767523E-13,
2.53178198860262));
#243786=CARTESIAN_POINT('Origin',(6.1853204982938,58.7035958781041,2.53178198860303));
#243787=CARTESIAN_POINT('Origin',(0.995615674755264,6.43520020182058,3.64303198860267));
#243788=CARTESIAN_POINT('Origin',(6.74099917688016,61.0983782637181,3.64299466007516));
#243789=CARTESIAN_POINT('Ctrl Pts',(6.17403490859001,58.5964866834553,2.59908173516065));
#243790=CARTESIAN_POINT('Ctrl Pts',(6.17794390662153,58.6335861742244,2.65878198860303));
#243791=CARTESIAN_POINT('Ctrl Pts',(6.1853204982938,58.7035958781041,2.65878198860303));
#243792=CARTESIAN_POINT('Ctrl Pts',(6.26121185652527,58.5873013840791,2.59908193199986));
#243793=CARTESIAN_POINT('Ctrl Pts',(6.24145541658269,58.6268910424095,2.65877685806751));
#243794=CARTESIAN_POINT('Ctrl Pts',(6.23596000968385,58.6982507756613,2.65878198860303));
#243795=CARTESIAN_POINT('Ctrl Pts',(6.34441620808585,58.6032244953992,2.63872492669832));
#243796=CARTESIAN_POINT('Ctrl Pts',(6.30249747592707,58.643316920109,2.69532212015315));
#243797=CARTESIAN_POINT('Ctrl Pts',(6.285367292233,58.7177256636154,2.68176836726675));
#243798=CARTESIAN_POINT('Ctrl Pts',(6.45770985055657,58.6635810738167,2.75442176402299));
#243799=CARTESIAN_POINT('Ctrl Pts',(6.37191831988765,58.6966524426405,2.79203179920177));
#243800=CARTESIAN_POINT('Ctrl Pts',(6.35432657855797,58.7827411889912,2.74885310748218));
#243801=CARTESIAN_POINT('Ctrl Pts',(6.4889986109651,58.7067768761602,2.82866089558439));
#243802=CARTESIAN_POINT('Ctrl Pts',(6.38003592347226,58.7342263230563,2.85316563119207));
#243803=CARTESIAN_POINT('Ctrl Pts',(6.37452670784949,58.8271002111747,2.79189751796582));
#243804=CARTESIAN_POINT('Ctrl Pts',(6.49374646112722,58.7519447039091,2.90134173516067));
#243805=CARTESIAN_POINT('Ctrl Pts',(6.36806742857307,58.7656442740273,2.90103711553272));
#243806=CARTESIAN_POINT('Ctrl Pts',(6.37927424642559,58.8722700234482,2.83404198860304));
#243807=CARTESIAN_POINT('Origin',(6.50557852713736,58.8589949086133,2.83404198860304));
#243808=CARTESIAN_POINT('Origin',(6.73632490881142,61.0544000804066,3.56647653971863));
#243809=CARTESIAN_POINT('Origin',(6.72777047351104,60.9730100652056,3.42473028058528));
#243810=CARTESIAN_POINT('Origin',(6.52420020557758,59.0361683443166,3.11913648168054));
#243811=CARTESIAN_POINT('Origin',(6.54282188406209,59.2133417798938,3.40423097483352));
#243812=CARTESIAN_POINT('Ctrl Pts',(6.69328024897436,60.6448574988556,3.36123028058524));
#243813=CARTESIAN_POINT('Ctrl Pts',(6.56697596826259,60.6581326136906,3.36123028058524));
#243814=CARTESIAN_POINT('Ctrl Pts',(6.56697596826259,60.6581326136906,3.23423028058524));
#243815=CARTESIAN_POINT('Ctrl Pts',(6.70245599674977,60.7343993681216,3.36123028058524));
#243816=CARTESIAN_POINT('Ctrl Pts',(6.57637578951156,60.7475659388558,3.36099641108513));
#243817=CARTESIAN_POINT('Ctrl Pts',(6.58108878091668,60.7924070567558,3.23423043688444));
#243818=CARTESIAN_POINT('Ctrl Pts',(6.71113417453879,60.8190677588582,3.41054258905326));
#243819=CARTESIAN_POINT('Ctrl Pts',(6.58530836180227,60.8325536871463,3.41008815825976));
#243820=CARTESIAN_POINT('Ctrl Pts',(6.59443344928435,60.9193730951266,3.30819867304253));
#243821=CARTESIAN_POINT('Ctrl Pts',(6.7157078966939,60.8636883187847,3.48823028058527));
#243822=CARTESIAN_POINT('Ctrl Pts',(6.59002106156447,60.8773920302463,3.48794691941643));
#243823=CARTESIAN_POINT('Ctrl Pts',(6.60146619279927,60.9862851800406,3.42473028058528));
#243824=CARTESIAN_POINT('Origin',(6.69328024897435,60.6448574988556,3.23423028058524));
#243825=CARTESIAN_POINT('Ctrl Pts',(6.53099325080036,59.1062911958299,3.47153072139113));
#243826=CARTESIAN_POINT('Ctrl Pts',(6.4051226409098,59.1200087114584,3.47122746285118));
#243827=CARTESIAN_POINT('Ctrl Pts',(6.41653455700106,59.2267768430463,3.40413046676828));
#243828=CARTESIAN_POINT('Ctrl Pts',(6.54313486548357,59.2206299794253,3.65553813458027));
#243829=CARTESIAN_POINT('Ctrl Pts',(6.41712406698097,59.2341972766231,3.6552033607226));
#243830=CARTESIAN_POINT('Ctrl Pts',(6.42614611919713,59.3182247474321,3.55128134519992));
#243831=CARTESIAN_POINT('Ctrl Pts',(6.5649460139707,59.4260354503641,3.77003198860305));
#243832=CARTESIAN_POINT('Ctrl Pts',(6.43870134519751,59.439496135217,3.76980209314202));
#243833=CARTESIAN_POINT('Ctrl Pts',(6.44341285848436,59.4825067955809,3.64284195387452));
#243834=CARTESIAN_POINT('Ctrl Pts',(6.58785426247077,59.6417962403145,3.77003198860305));
#243835=CARTESIAN_POINT('Ctrl Pts',(6.46136078685214,59.6550912403355,3.77003198860305));
#243836=CARTESIAN_POINT('Ctrl Pts',(6.46155012324721,59.6550713402785,3.64284189403843));
#243837=CARTESIAN_POINT('Origin',(6.58785426247077,59.6417962403145,3.64303198860305));
#243838=CARTESIAN_POINT('Origin',(0.979147644052797,6.27851735587401,3.23423028058486));
#243839=CARTESIAN_POINT('Origin',(6.67747469700926,60.4944777170596,3.23423028058524));
#243840=CARTESIAN_POINT('Origin',(0.976568823008617,6.25398151259742,3.64303198860267));
#243841=CARTESIAN_POINT('Origin',(6.62985850077821,60.0409538388298,3.64299171721826));
#243842=CARTESIAN_POINT('Ctrl Pts',(6.65505462397376,60.2756459899121,3.48823028058522));
#243843=CARTESIAN_POINT('Ctrl Pts',(6.52822907310758,60.2894805317164,3.488520042123));
#243844=CARTESIAN_POINT('Ctrl Pts',(6.51668018436727,60.1796001951997,3.42473028058522));
#243845=CARTESIAN_POINT('Ctrl Pts',(6.65964099131244,60.3204176712047,3.41028005848447));
#243846=CARTESIAN_POINT('Ctrl Pts',(6.5329085169049,60.3340024654481,3.41074404220456));
#243847=CARTESIAN_POINT('Ctrl Pts',(6.52373669508342,60.2467384099283,3.3078048624401));
#243848=CARTESIAN_POINT('Ctrl Pts',(6.66833043150643,60.4052373806433,3.36123028058524));
#243849=CARTESIAN_POINT('Ctrl Pts',(6.54178440911712,60.4184509388135,3.36146460586437));
#243850=CARTESIAN_POINT('Ctrl Pts',(6.53710513959985,60.3739306632437,3.23423045308454));
#243851=CARTESIAN_POINT('Ctrl Pts',(6.67747469700926,60.4944777170596,3.36123028058524));
#243852=CARTESIAN_POINT('Ctrl Pts',(6.5511704162975,60.5077528318946,3.36123028058524));
#243853=CARTESIAN_POINT('Ctrl Pts',(6.55117041629749,60.5077528318946,3.23423028058524));
#243854=CARTESIAN_POINT('Origin',(6.64298446507904,60.1663250803647,3.42473028058523));
#243855=CARTESIAN_POINT('Origin',(6.63448104699032,60.0854204586813,3.56563113524822));
#243856=CARTESIAN_POINT('Origin',(-0.31749999970759,61.4240753804098,3.56647653909432));
#243857=CARTESIAN_POINT('Origin',(-0.317551690015093,61.4683012396087,3.6429946600749));
#243858=CARTESIAN_POINT('Origin',(-0.317500000000209,61.3422370451707,3.42473028058526));
#243859=CARTESIAN_POINT('Ctrl Pts',(-0.316930737396123,61.2322532920974,
3.48823028058527));
#243860=CARTESIAN_POINT('Ctrl Pts',(-0.190500000000209,61.2327440814647,
3.48794691941643));
#243861=CARTESIAN_POINT('Ctrl Pts',(-0.190500000000209,61.3422370451707,
3.42473028058528));
#243862=CARTESIAN_POINT('Ctrl Pts',(-0.317046579199837,61.1872475084176,
3.41028005925129));
#243863=CARTESIAN_POINT('Ctrl Pts',(-0.190500000001825,61.187506454177,
3.40982512230997));
#243864=CARTESIAN_POINT('Ctrl Pts',(-0.190500000000208,61.2747290395328,
3.30780486372837));
#243865=CARTESIAN_POINT('Ctrl Pts',(-0.317266596913697,61.1019842137034,
3.36123028058524));
#243866=CARTESIAN_POINT('Ctrl Pts',(-0.190500000000084,61.1018997758103,
3.36099721048488));
#243867=CARTESIAN_POINT('Ctrl Pts',(-0.190500000000208,61.14683620717,3.23423045308409));
#243868=CARTESIAN_POINT('Ctrl Pts',(-0.317500000000208,61.0122769227458,
3.36123028058524));
#243869=CARTESIAN_POINT('Ctrl Pts',(-0.190500000000207,61.0122769227458,
3.36123028058524));
#243870=CARTESIAN_POINT('Ctrl Pts',(-0.190500000000207,61.0122769227458,
3.23423028058524));
#243871=CARTESIAN_POINT('Origin',(-0.317500000000208,61.0122769227458,3.23423028058524));
#243872=CARTESIAN_POINT('Origin',(-0.317499999999994,1.82709072144943E-13,
3.64303198860263));
#243873=CARTESIAN_POINT('Origin',(-0.317500000000211,61.8696548221182,3.64303198860306));
#243874=CARTESIAN_POINT('Origin',(-0.317499999999994,1.85563719214605E-13,
3.23423028058481));
#243875=CARTESIAN_POINT('Origin',(-0.317500000000207,60.8610688070709,3.23423028058524));
#243876=CARTESIAN_POINT('Ctrl Pts',(-0.318048871877342,62.408169597977,
3.47153072139115));
#243877=CARTESIAN_POINT('Ctrl Pts',(-0.190309034175511,62.4086377819836,
3.47182327902706));
#243878=CARTESIAN_POINT('Ctrl Pts',(-0.190500142125266,62.3003077603773,
3.40413028959066));
#243879=CARTESIAN_POINT('Ctrl Pts',(-0.317932489890151,62.2931881445373,
3.65553807121));
#243880=CARTESIAN_POINT('Ctrl Pts',(-0.190309294367321,62.2934975005775,
3.65586275497125));
#243881=CARTESIAN_POINT('Ctrl Pts',(-0.19050014199568,62.2083564003277,
3.55128126837385));
#243882=CARTESIAN_POINT('Ctrl Pts',(-0.31772268616762,62.0866281564674,
3.77003198860307));
#243883=CARTESIAN_POINT('Ctrl Pts',(-0.190309769569843,62.0868143053063,
3.77025505748512));
#243884=CARTESIAN_POINT('Ctrl Pts',(-0.190500141762077,62.0431695205371,
3.64284211731146));
#243885=CARTESIAN_POINT('Ctrl Pts',(-0.31750000000021,61.8696548221183,
3.77003198860307));
#243886=CARTESIAN_POINT('Ctrl Pts',(-0.190310267889154,61.8696548221182,
3.77003198860307));
#243887=CARTESIAN_POINT('Ctrl Pts',(-0.190500141514125,61.8696548221183,
3.64284239821734));
#243888=CARTESIAN_POINT('Origin',(-0.317500000000212,62.3004688883556,3.40423097483353));
#243889=CARTESIAN_POINT('Ctrl Pts',(-0.317500000000207,60.8610688070709,
3.36123028058524));
#243890=CARTESIAN_POINT('Ctrl Pts',(-0.190500000000207,60.8610688070709,
3.36123028058524));
#243891=CARTESIAN_POINT('Ctrl Pts',(-0.190500000000207,60.8610688070709,
3.23423028058524));
#243892=CARTESIAN_POINT('Ctrl Pts',(-0.317734773760476,60.7710583184322,
3.36123028058524));
#243893=CARTESIAN_POINT('Ctrl Pts',(-0.190500000000322,60.7709717342392,
3.36146538610154));
#243894=CARTESIAN_POINT('Ctrl Pts',(-0.190500000000206,60.7260547307348,
3.23423043688425));
#243895=CARTESIAN_POINT('Ctrl Pts',(-0.31795861791923,60.685946575458,3.41054258693139));
#243896=CARTESIAN_POINT('Ctrl Pts',(-0.190499999999005,60.6862105562605,
3.41100608859939));
#243897=CARTESIAN_POINT('Ctrl Pts',(-0.190500000000206,60.5983892955427,
3.30819866970959));
#243898=CARTESIAN_POINT('Ctrl Pts',(-0.318076890623573,60.6410923272407,
3.48823028058523));
#243899=CARTESIAN_POINT('Ctrl Pts',(-0.190500000000212,60.6415942020423,
3.488520042123));
#243900=CARTESIAN_POINT('Ctrl Pts',(-0.190500000000206,60.5311086139136,
3.42473028058523));
#243901=CARTESIAN_POINT('Origin',(-0.317500000000206,60.5311086139136,3.42473028058523));
#243902=CARTESIAN_POINT('Origin',(-0.317499999976043,62.4786179998491,3.11913648178467));
#243903=CARTESIAN_POINT('Origin',(-0.317500000000213,62.6567671111301,2.83404198860305));
#243904=CARTESIAN_POINT('Origin',(-0.317499999993752,60.4497583458794,3.56563113460841));
#243905=CARTESIAN_POINT('Origin',(-0.317550804320552,60.4050521322805,3.64299171721841));
#243906=CARTESIAN_POINT('Ctrl Pts',(-0.015266117311081,62.954144805765,
2.59908173516067));
#243907=CARTESIAN_POINT('Ctrl Pts',(-0.0152570710388482,62.9168399481845,
2.65878198860306));
#243908=CARTESIAN_POINT('Ctrl Pts',(-0.0152400000002138,62.8464427007198,
2.65878198860306));
#243909=CARTESIAN_POINT('Ctrl Pts',(-0.103381504925414,62.9541233134301,
2.59908193475651));
#243910=CARTESIAN_POINT('Ctrl Pts',(-0.0794415635237897,62.9168211560343,
2.65878715325392));
#243911=CARTESIAN_POINT('Ctrl Pts',(-0.0662446030561493,62.8464212442882,
2.65878198860306));
#243912=CARTESIAN_POINT('Ctrl Pts',(-0.184683583688025,62.9290872705828,
2.63878778849938));
#243913=CARTESIAN_POINT('Ctrl Pts',(-0.138547994784516,62.893677113745,
2.69564460180164));
#243914=CARTESIAN_POINT('Ctrl Pts',(-0.113305567451785,62.8213855864657,
2.68180481624935));
#243915=CARTESIAN_POINT('Ctrl Pts',(-0.291340992631915,62.8564203507744,
2.75443238878668));
#243916=CARTESIAN_POINT('Ctrl Pts',(-0.201910351191571,62.8329175802744,
2.79268340777131));
#243917=CARTESIAN_POINT('Ctrl Pts',(-0.175042741958052,62.7487193609391,
2.74885926835647));
#243918=CARTESIAN_POINT('Ctrl Pts',(-0.318045276842852,62.8099434033763,
2.8285665536173));
#243919=CARTESIAN_POINT('Ctrl Pts',(-0.20583163564296,62.7947175425021,
2.85384197230965));
#243920=CARTESIAN_POINT('Ctrl Pts',(-0.190500000000215,62.7022409210456,
2.7918462427865));
#243921=CARTESIAN_POINT('Ctrl Pts',(-0.318045750793259,62.7644678366121,
2.90134173516068));
#243922=CARTESIAN_POINT('Ctrl Pts',(-0.19050000000021,62.764932651015,2.90163218716436));
#243923=CARTESIAN_POINT('Ctrl Pts',(-0.190500000000213,62.6567671111301,
2.83404198860306));
#243924=CARTESIAN_POINT('Origin',(-0.0152400000002138,62.8464427007198,
2.53178198860305));
#243925=CARTESIAN_POINT('Origin',(-0.317499999999994,1.82709072144943E-13,
3.64303198860263));
#243926=CARTESIAN_POINT('Origin',(-0.317500000000204,60.0036905223732,3.64303198860304));
#243927=CARTESIAN_POINT('Origin',(-3.02076666443335E-17,1.91412545152793E-13,
2.53178198860262));
#243928=CARTESIAN_POINT('Origin',(0.0152399999997862,62.8464427007198,2.53178198860306));
#243929=CARTESIAN_POINT('Ctrl Pts',(-0.317500000000204,60.0036905223732,
3.77003198860305));
#243930=CARTESIAN_POINT('Ctrl Pts',(-0.190309748265563,60.0036905223732,
3.77003198860305));
#243931=CARTESIAN_POINT('Ctrl Pts',(-0.190500142289733,60.0036905223732,
3.6428418793711));
#243932=CARTESIAN_POINT('Ctrl Pts',(-0.317270385524616,59.7867137603526,
3.77003198860305));
#243933=CARTESIAN_POINT('Ctrl Pts',(-0.190310262476488,59.7869045527981,
3.76980208962936));
#243934=CARTESIAN_POINT('Ctrl Pts',(-0.190500142032665,59.8301727552489,
3.64284193928328));
#243935=CARTESIAN_POINT('Ctrl Pts',(-0.317049440713829,59.580155267073,
3.65553535416627));
#243936=CARTESIAN_POINT('Ctrl Pts',(-0.190310761082532,59.5804765271859,
3.65520057834489));
#243937=CARTESIAN_POINT('Ctrl Pts',(-0.190500141785308,59.6649871046561,
3.55127910964259));
#243938=CARTESIAN_POINT('Ctrl Pts',(-0.316925998273249,59.4651754363834,
3.47153072139113));
#243939=CARTESIAN_POINT('Ctrl Pts',(-0.190311035335302,59.4656607446595,
3.47122746281624));
#243940=CARTESIAN_POINT('Ctrl Pts',(-0.190500141647104,59.5730368716577,
3.40413045901326));
#243941=CARTESIAN_POINT('Origin',(-0.317500000000203,59.5728760150044,3.40423097483352));
#243942=CARTESIAN_POINT('Ctrl Pts',(0.318045750792832,62.7644678366121,
2.90134173516067));
#243943=CARTESIAN_POINT('Ctrl Pts',(0.190499999999787,62.764932651015,2.90163218716435));
#243944=CARTESIAN_POINT('Ctrl Pts',(0.190499999999787,62.6567671111301,
2.83404198860305));
#243945=CARTESIAN_POINT('Ctrl Pts',(0.318045262794965,62.8099640589336,
2.82853349835403));
#243946=CARTESIAN_POINT('Ctrl Pts',(0.2058403307229,62.7947344577637,2.85381483162476));
#243947=CARTESIAN_POINT('Ctrl Pts',(0.190499999999787,62.7022616416342,
2.79182701594311));
#243948=CARTESIAN_POINT('Ctrl Pts',(0.291334117855211,62.8562601188217,
2.75468822073678));
#243949=CARTESIAN_POINT('Ctrl Pts',(0.201836550627546,62.8328016940826,
2.79286913083901));
#243950=CARTESIAN_POINT('Ctrl Pts',(0.175038734051964,62.7485591297234,
2.74900763297961));
#243951=CARTESIAN_POINT('Ctrl Pts',(0.185622189560167,62.9286112571072,
2.63954450640446));
#243952=CARTESIAN_POINT('Ctrl Pts',(0.139140155999877,62.8932808767901,
2.69627684028887));
#243953=CARTESIAN_POINT('Ctrl Pts',(0.113848895265485,62.8209095783127,
2.6822435603653));
#243954=CARTESIAN_POINT('Ctrl Pts',(0.103673266462632,62.9541233349678,
2.59908178706367));
#243955=CARTESIAN_POINT('Ctrl Pts',(0.0796882264534906,62.9168211653024,
2.65878704321514));
#243956=CARTESIAN_POINT('Ctrl Pts',(0.0664134143649273,62.8464212664865,
2.65878198860306));
#243957=CARTESIAN_POINT('Ctrl Pts',(0.0152661173106522,62.954144805765,
2.59908173516067));
#243958=CARTESIAN_POINT('Ctrl Pts',(0.0152570710384197,62.9168399481845,
2.65878198860306));
#243959=CARTESIAN_POINT('Ctrl Pts',(0.0152399999997859,62.8464427007198,
2.65878198860306));
#243960=CARTESIAN_POINT('Origin',(0.317499999999787,62.6567671111301,2.83404198860304));
#243961=CARTESIAN_POINT('Origin',(-0.317499999971749,59.394726658624,3.1191364816716));
#243962=CARTESIAN_POINT('Origin',(-0.317500000000201,59.2165773020943,2.83404198860304));
#243963=CARTESIAN_POINT('Origin',(0.31749999997701,62.4786179998349,3.11913648177581));
#243964=CARTESIAN_POINT('Origin',(0.317499999999788,62.3004688883556,3.40423097483353));
#243965=CARTESIAN_POINT('Ctrl Pts',(-0.316922544675889,59.108876741935,
2.90134173516064));
#243966=CARTESIAN_POINT('Ctrl Pts',(-0.190500000000207,59.1093642282368,
2.9010371155327));
#243967=CARTESIAN_POINT('Ctrl Pts',(-0.190500000000201,59.2165773020943,
2.83404198860303));
#243968=CARTESIAN_POINT('Ctrl Pts',(-0.316922012809374,59.0634407053231,
2.82862991748008));
#243969=CARTESIAN_POINT('Ctrl Pts',(-0.205694973740556,59.0793536643045,
2.85314045886453));
#243970=CARTESIAN_POINT('Ctrl Pts',(-0.190500000000201,59.1711393827296,
2.79187960999964));
#243971=CARTESIAN_POINT('Ctrl Pts',(-0.290332993455134,59.0174076205277,
2.7547062579336));
#243972=CARTESIAN_POINT('Ctrl Pts',(-0.20148015166603,59.0412846811397,
2.79224250381941));
#243973=CARTESIAN_POINT('Ctrl Pts',(-0.175054909459902,59.1251084688123,
2.74901809108301));
#243974=CARTESIAN_POINT('Ctrl Pts',(-0.18489496740184,58.9458296250065,
2.63947868311748));
#243975=CARTESIAN_POINT('Ctrl Pts',(-0.138672156931446,58.9812445774294,
2.69595066767951));
#243976=CARTESIAN_POINT('Ctrl Pts',(-0.113807322597986,59.0535312451935,
2.68220539436102));
#243977=CARTESIAN_POINT('Ctrl Pts',(-0.103171606455878,58.9208287018092,
2.59908178585124));
#243978=CARTESIAN_POINT('Ctrl Pts',(-0.0793367652459801,58.9581363848287,
2.65877670944864));
#243979=CARTESIAN_POINT('Ctrl Pts',(-0.0663350652345453,59.0285307646524,
2.65878198860303));
#243980=CARTESIAN_POINT('Ctrl Pts',(-0.0152121934561203,58.9208513795075,
2.59908173516065));
#243981=CARTESIAN_POINT('Ctrl Pts',(-0.0152218248293074,58.9581562369415,
2.65878198860303));
#243982=CARTESIAN_POINT('Ctrl Pts',(-0.0152400000002007,59.0285534841298,
2.65878198860303));
#243983=CARTESIAN_POINT('Origin',(-0.0152400000002004,59.0285534841298,
2.53178198860303));
#243984=CARTESIAN_POINT('Ctrl Pts',(0.31749999999979,61.8696548221183,3.77003198860307));
#243985=CARTESIAN_POINT('Ctrl Pts',(0.190310256931134,61.8696548221183,
3.77003198860307));
#243986=CARTESIAN_POINT('Ctrl Pts',(0.190500141530038,61.8696548221183,
3.64284238727611));
#243987=CARTESIAN_POINT('Ctrl Pts',(0.317722689632019,62.0866315324122,
3.77003198860307));
#243988=CARTESIAN_POINT('Ctrl Pts',(0.190309758575237,62.0868176889507,
3.77025506105805));
#243989=CARTESIAN_POINT('Ctrl Pts',(0.190500141778022,62.0431722165645,
3.64284210641846));
#243990=CARTESIAN_POINT('Ctrl Pts',(0.317932491655467,62.2931898887683,
3.65553527987874));
#243991=CARTESIAN_POINT('Ctrl Pts',(0.190309283349448,62.2934992458087,
3.65585996533256));
#243992=CARTESIAN_POINT('Ctrl Pts',(0.190500142011647,62.2083577878533,
3.55127902710321));
#243993=CARTESIAN_POINT('Ctrl Pts',(0.318048871876917,62.408169597977,3.47153072139115));
#243994=CARTESIAN_POINT('Ctrl Pts',(0.190309023146207,62.4086377820241,
3.47182327905231));
#243995=CARTESIAN_POINT('Ctrl Pts',(0.190500142141247,62.3003077510786,
3.40413028378014));
#243996=CARTESIAN_POINT('Origin',(0.31749999999979,61.8696548221183,3.64303198860307));
#243997=CARTESIAN_POINT('Origin',(4.1196902326603E-16,1.9163609199248E-13,
2.53178198860262));
#243998=CARTESIAN_POINT('Origin',(0.0152399999997996,59.0285534841298,2.53178198860303));
#243999=CARTESIAN_POINT('Origin',(0.317500000000005,-3.23223802458442E-14,
3.64303198860263));
#244000=CARTESIAN_POINT('Origin',(0.317551690013334,61.4683012396078,3.64299466007611));
#244001=CARTESIAN_POINT('Ctrl Pts',(0.0152121934557198,58.9208513795075,
2.59908173516065));
#244002=CARTESIAN_POINT('Ctrl Pts',(0.0152218248289066,58.9581562369415,
2.65878198860303));
#244003=CARTESIAN_POINT('Ctrl Pts',(0.0152399999997995,59.0285534841298,
2.65878198860303));
#244004=CARTESIAN_POINT('Ctrl Pts',(0.102871702177208,58.9208288705622,
2.59908193199955));
#244005=CARTESIAN_POINT('Ctrl Pts',(0.0790852439333024,58.9581365422945,
2.65877685806598));
#244006=CARTESIAN_POINT('Ctrl Pts',(0.0661608181923186,59.0285309330229,
2.65878198860303));
#244007=CARTESIAN_POINT('Ctrl Pts',(0.183955833237286,58.9453619764185,
2.63872492669837));
#244008=CARTESIAN_POINT('Ctrl Pts',(0.138075936735604,58.9808530699765,
2.6953221201532));
#244009=CARTESIAN_POINT('Ctrl Pts',(0.113261762367936,59.0530636028228,
2.68176836726675));
#244010=CARTESIAN_POINT('Ctrl Pts',(0.290319860890481,59.0172303255296,
2.75442176402292));
#244011=CARTESIAN_POINT('Ctrl Pts',(0.201541405841888,59.041152869072,2.79203179920166));
#244012=CARTESIAN_POINT('Ctrl Pts',(0.175047309551012,59.1249311745759,
2.74885310748217));
#244013=CARTESIAN_POINT('Ctrl Pts',(0.316922027357146,59.0634600627913,
2.82866089558442));
#244014=CARTESIAN_POINT('Ctrl Pts',(0.205687000365689,59.0793694364681,
2.8531656311923));
#244015=CARTESIAN_POINT('Ctrl Pts',(0.190499999999799,59.1711586818657,
2.79189751796687));
#244016=CARTESIAN_POINT('Ctrl Pts',(0.316922544675488,59.108876741935,2.90134173516064));
#244017=CARTESIAN_POINT('Ctrl Pts',(0.190499999999804,59.1093642282368,
2.9010371155327));
#244018=CARTESIAN_POINT('Ctrl Pts',(0.190499999999799,59.2165773020943,
2.83404198860303));
#244019=CARTESIAN_POINT('Origin',(0.317499999999799,59.2165773020943,2.83404198860303));
#244020=CARTESIAN_POINT('Origin',(0.317499999995335,61.4240753793297,3.56647653971789));
#244021=CARTESIAN_POINT('Origin',(0.317499999999791,61.3422370451707,3.42473028058527));
#244022=CARTESIAN_POINT('Origin',(0.317499999969512,59.3947266586068,3.11913648168234));
#244023=CARTESIAN_POINT('Origin',(0.317499999999798,59.5728760150044,3.40423097483352));
#244024=CARTESIAN_POINT('Ctrl Pts',(0.317499999999793,61.0122769227458,
3.36123028058524));
#244025=CARTESIAN_POINT('Ctrl Pts',(0.190499999999793,61.0122769227458,
3.36123028058524));
#244026=CARTESIAN_POINT('Ctrl Pts',(0.190499999999793,61.0122769227458,
3.23423028058524));
#244027=CARTESIAN_POINT('Ctrl Pts',(0.317265808076183,61.1022873990973,
3.36123028058524));
#244028=CARTESIAN_POINT('Ctrl Pts',(0.190499999999665,61.1022028716689,
3.36099641108502));
#244029=CARTESIAN_POINT('Ctrl Pts',(0.190499999999792,61.1472909869829,
3.23423043688409));
#244030=CARTESIAN_POINT('Ctrl Pts',(0.317046189128874,61.1873990841187,
3.41054258905327));
#244031=CARTESIAN_POINT('Ctrl Pts',(0.190499999999403,61.1876587562349,
3.41008815826007));
#244032=CARTESIAN_POINT('Ctrl Pts',(0.190499999999792,61.2749563897851,
3.30819867304325));
#244033=CARTESIAN_POINT('Ctrl Pts',(0.316930737395706,61.2322532920974,
3.48823028058526));
#244034=CARTESIAN_POINT('Ctrl Pts',(0.190499999999791,61.2327440814647,
3.48794691941642));
#244035=CARTESIAN_POINT('Ctrl Pts',(0.190499999999791,61.3422370451707,
3.42473028058527));
#244036=CARTESIAN_POINT('Origin',(0.317499999999793,61.0122769227458,3.23423028058524));
#244037=CARTESIAN_POINT('Ctrl Pts',(0.316925998272845,59.4651754363834,
3.47153072139113));
#244038=CARTESIAN_POINT('Ctrl Pts',(0.190311049925297,59.4656607446036,
3.47122746285118));
#244039=CARTESIAN_POINT('Ctrl Pts',(0.190500141624843,59.5730368592468,
3.40413046676854));
#244040=CARTESIAN_POINT('Ctrl Pts',(0.317049442578967,59.5801570044832,
3.6555381345803));
#244041=CARTESIAN_POINT('Ctrl Pts',(0.190310775691579,59.5804782634891,
3.65520336072179));
#244042=CARTESIAN_POINT('Ctrl Pts',(0.190500141763024,59.6649884842734,
3.55128134519974));
#244043=CARTESIAN_POINT('Ctrl Pts',(0.317270389088637,59.7867171285937,
3.77003198860305));
#244044=CARTESIAN_POINT('Ctrl Pts',(0.190310277118373,59.7869079131808,
3.76980209314153));
#244045=CARTESIAN_POINT('Ctrl Pts',(0.190500142010346,59.8301754438912,
3.64284195387455));
#244046=CARTESIAN_POINT('Ctrl Pts',(0.317499999999796,60.0036905223732,
3.77003198860305));
#244047=CARTESIAN_POINT('Ctrl Pts',(0.190309762954983,60.0036905223732,
3.77003198860305));
#244048=CARTESIAN_POINT('Ctrl Pts',(0.190500142267369,60.0036905223733,
3.64284189403892));
#244049=CARTESIAN_POINT('Origin',(0.317499999999796,60.0036905223732,3.64303198860304));
#244050=CARTESIAN_POINT('Origin',(0.317500000000005,-2.42053524934248E-14,
3.23423028058481));
#244051=CARTESIAN_POINT('Origin',(0.317499999999793,60.8610688070709,3.23423028058524));
#244052=CARTESIAN_POINT('Origin',(0.317500000000005,-2.62359339360319E-14,
3.64303198860263));
#244053=CARTESIAN_POINT('Origin',(0.317550804319973,60.4050521322806,3.64299171721856));
#244054=CARTESIAN_POINT('Ctrl Pts',(0.31807689062316,60.6410923272407,3.48823028058523));
#244055=CARTESIAN_POINT('Ctrl Pts',(0.190499999999794,60.6415942020423,
3.48852004212301));
#244056=CARTESIAN_POINT('Ctrl Pts',(0.190499999999794,60.5311086139136,
3.42473028058523));
#244057=CARTESIAN_POINT('Ctrl Pts',(0.317958218318559,60.6860981505086,
3.41028005848445));
#244058=CARTESIAN_POINT('Ctrl Pts',(0.190500000001774,60.6863613750278,
3.41074404220382));
#244059=CARTESIAN_POINT('Ctrl Pts',(0.190499999999794,60.5986166446954,
3.30780486243962));
#244060=CARTESIAN_POINT('Ctrl Pts',(0.317733982967334,60.7713615025342,
3.36123028058524));
#244061=CARTESIAN_POINT('Ctrl Pts',(0.190499999999791,60.7712750142,3.36146460586396));
#244062=CARTESIAN_POINT('Ctrl Pts',(0.190499999999794,60.7265095085055,
3.23423045308419));
#244063=CARTESIAN_POINT('Ctrl Pts',(0.317499999999793,60.8610688070709,
3.36123028058524));
#244064=CARTESIAN_POINT('Ctrl Pts',(0.190499999999793,60.8610688070709,
3.36123028058524));
#244065=CARTESIAN_POINT('Ctrl Pts',(0.190499999999793,60.8610688070709,
3.23423028058524));
#244066=CARTESIAN_POINT('Origin',(0.317499999999794,60.5311086139136,3.42473028058523));
#244067=CARTESIAN_POINT('Origin',(0.317500000301406,60.4497583469877,3.56563113524828));
#244068=CARTESIAN_POINT('Origin',(-6.73632490863879,61.0544000815117,3.5664765390945));
#244069=CARTESIAN_POINT('Origin',(-6.74099917687954,61.0983782637177,3.64299466007596));
#244070=CARTESIAN_POINT('Origin',(-6.72777047351144,60.9730100652056,3.42473028058526));
#244071=CARTESIAN_POINT('Ctrl Pts',(-6.7157078966943,60.8636883187846,3.48823028058527));
#244072=CARTESIAN_POINT('Ctrl Pts',(-6.59002106156486,60.8773920302462,
3.48794691941643));
#244073=CARTESIAN_POINT('Ctrl Pts',(-6.60146619279967,60.9862851800406,
3.42473028058528));
#244074=CARTESIAN_POINT('Ctrl Pts',(-6.71111871849844,60.8189169727311,
3.41028005925127));
#244075=CARTESIAN_POINT('Ctrl Pts',(-6.58529244190401,60.8324022194122,
3.40982512231045));
#244076=CARTESIAN_POINT('Ctrl Pts',(-6.5944096847118,60.9191469903184,3.30780486372902));
#244077=CARTESIAN_POINT('Ctrl Pts',(-6.70242508976228,60.7340977611531,
3.36123028058523));
#244078=CARTESIAN_POINT('Ctrl Pts',(-6.57634410736717,60.7472645033899,
3.36099721048488));
#244079=CARTESIAN_POINT('Ctrl Pts',(-6.58104124348246,60.7919547682776,
3.23423045308408));
#244080=CARTESIAN_POINT('Ctrl Pts',(-6.69328024897476,60.6448574988556,
3.36123028058524));
#244081=CARTESIAN_POINT('Ctrl Pts',(-6.56697596826299,60.6581326136906,
3.36123028058524));
#244082=CARTESIAN_POINT('Ctrl Pts',(-6.56697596826298,60.6581326136906,
3.23423028058524));
#244083=CARTESIAN_POINT('Origin',(-6.69328024897475,60.6448574988556,3.23423028058523));
#244084=CARTESIAN_POINT('Origin',(-0.315760701779421,-0.0331877870872973,
3.64303198860263));
#244085=CARTESIAN_POINT('Origin',(-6.78290064323581,61.4975385923864,3.64303198860306));
#244086=CARTESIAN_POINT('Origin',(-0.315760701779421,-0.0331877870872945,
3.23423028058481));
#244087=CARTESIAN_POINT('Origin',(-6.67747469700966,60.4944777170595,3.23423028058524));
#244088=CARTESIAN_POINT('Ctrl Pts',(-6.83973663030281,62.0330459552234,
3.47153072139115));
#244089=CARTESIAN_POINT('Ctrl Pts',(-6.71274550335253,62.0468640234021,
3.47182327902705));
#244090=CARTESIAN_POINT('Ctrl Pts',(-6.70161199370846,61.9391074687687,
3.40413028959077));
#244091=CARTESIAN_POINT('Ctrl Pts',(-6.82760205123568,61.9187065474467,
3.65553807120999));
#244092=CARTESIAN_POINT('Ctrl Pts',(-6.70071032543994,61.932354465303,3.65586275496994));
#244093=CARTESIAN_POINT('Ctrl Pts',(-6.69200045921793,61.8476598279012,
3.55128126837326));
#244094=CARTESIAN_POINT('Ctrl Pts',(-6.80580199871472,61.7133000470648,
3.77003198860307));
#244095=CARTESIAN_POINT('Ctrl Pts',(-6.67910652125809,61.7268034525367,
3.77025505748508));
#244096=CARTESIAN_POINT('Ctrl Pts',(-6.67473372828963,61.6833778591512,
3.64284211731167));
#244097=CARTESIAN_POINT('Ctrl Pts',(-6.78290064323581,61.4975385923864,
3.77003198860306));
#244098=CARTESIAN_POINT('Ctrl Pts',(-6.65640766978556,61.5108335396274,
3.77003198860306));
#244099=CARTESIAN_POINT('Ctrl Pts',(-6.65659650326273,61.5108136924291,
3.64284239821755));
#244100=CARTESIAN_POINT('Origin',(-6.8279329755337,61.9259926140921,3.40423097483353));
#244101=CARTESIAN_POINT('Ctrl Pts',(-6.67747469700966,60.4944777170595,
3.36123028058524));
#244102=CARTESIAN_POINT('Ctrl Pts',(-6.55117041629789,60.5077528318945,
3.36123028058524));
#244103=CARTESIAN_POINT('Ctrl Pts',(-6.55117041629789,60.5077528318945,
3.23423028058524));
#244104=CARTESIAN_POINT('Ctrl Pts',(-6.66829952659951,60.4049357747552,
3.36123028058523));
#244105=CARTESIAN_POINT('Ctrl Pts',(-6.54175270773032,60.4181493202568,
3.36146538610149));
#244106=CARTESIAN_POINT('Ctrl Pts',(-6.53705760237914,60.3734783767969,
3.23423043688413));
#244107=CARTESIAN_POINT('Ctrl Pts',(-6.65962554481719,60.3202668847284,
3.41054258693142));
#244108=CARTESIAN_POINT('Ctrl Pts',(-6.53289275205069,60.333852472875,3.41100608859868));
#244109=CARTESIAN_POINT('Ctrl Pts',(-6.52371293062573,60.246512306213,3.30819866970914));
#244110=CARTESIAN_POINT('Ctrl Pts',(-6.65505462397415,60.275645989912,3.48823028058522));
#244111=CARTESIAN_POINT('Ctrl Pts',(-6.52822907310798,60.2894805317163,
3.488520042123));
#244112=CARTESIAN_POINT('Ctrl Pts',(-6.51668018436767,60.1796001951997,
3.42473028058522));
#244113=CARTESIAN_POINT('Origin',(-6.64298446507943,60.1663250803647,3.42473028058523));
#244114=CARTESIAN_POINT('Origin',(-6.8465546283654,62.1031658061152,3.11913648178458));
#244115=CARTESIAN_POINT('Origin',(-6.86517628122531,62.2803389979221,2.83404198860306));
#244116=CARTESIAN_POINT('Origin',(-6.63448104656892,60.0854204576118,3.56563113460873));
#244117=CARTESIAN_POINT('Origin',(-6.62985850077851,60.0409538388298,3.6429917172183));
#244118=CARTESIAN_POINT('Ctrl Pts',(-6.59568250079906,62.6076796697356,
2.59908173516068));
#244119=CARTESIAN_POINT('Ctrl Pts',(-6.59177408464795,62.5705801176611,
2.65878198860306));
#244120=CARTESIAN_POINT('Ctrl Pts',(-6.58439859103049,62.5005702980932,
2.65878198860306));
#244121=CARTESIAN_POINT('Ctrl Pts',(-6.68331293653974,62.5984477290804,
2.59908193475628));
#244122=CARTESIAN_POINT('Ctrl Pts',(-6.65560500345282,62.5638523220918,
2.65878715325384));
#244123=CARTESIAN_POINT('Ctrl Pts',(-6.63512154272671,62.4952175264277,
2.65878198860306));
#244124=CARTESIAN_POINT('Ctrl Pts',(-6.76155265492276,62.5650504549419,
2.63878778849935));
#244125=CARTESIAN_POINT('Ctrl Pts',(-6.71196843232432,62.5346567608582,
2.69564460180145));
#244126=CARTESIAN_POINT('Ctrl Pts',(-6.6793077633958,62.4653998062674,2.68180481624927));
#244127=CARTESIAN_POINT('Ctrl Pts',(-6.86003002196296,62.4816328770703,
2.7544323887867));
#244128=CARTESIAN_POINT('Ctrl Pts',(-6.76863258245071,62.4676069047251,
2.79268340777157));
#244129=CARTESIAN_POINT('Ctrl Pts',(-6.73311104631486,62.3866783619501,
2.74885926835654));
#244130=CARTESIAN_POINT('Ctrl Pts',(-6.88172985342186,62.4326191774619,
2.82856655361726));
#244131=CARTESIAN_POINT('Ctrl Pts',(-6.76853939445094,62.4292062449167,
2.85384197230834));
#244132=CARTESIAN_POINT('Ctrl Pts',(-6.74362530798282,62.3388388123828,
2.79184624278531));
#244133=CARTESIAN_POINT('Ctrl Pts',(-6.87697683366585,62.3873926810693,
2.90134173516067));
#244134=CARTESIAN_POINT('Ctrl Pts',(-6.75017837817622,62.401187110497,2.90163218716435));
#244135=CARTESIAN_POINT('Ctrl Pts',(-6.73887200051354,62.2936141127571,
2.83404198860306));
#244136=CARTESIAN_POINT('Origin',(-6.58439859103049,62.5005702980932,2.53178198860305));
#244137=CARTESIAN_POINT('Origin',(-0.315760701779421,-0.0331877870872973,
3.64303198860263));
#244138=CARTESIAN_POINT('Origin',(-6.58785426247116,59.6417962403144,3.64303198860304));
#244139=CARTESIAN_POINT('Origin',(-1.29720108988942E-17,1.91413448435235E-13,
2.53178198860262));
#244140=CARTESIAN_POINT('Origin',(-6.55408556365967,62.5037563256536,2.53178198860305));
#244141=CARTESIAN_POINT('Ctrl Pts',(-6.58785426247116,59.6417962403144,
3.77003198860305));
#244142=CARTESIAN_POINT('Ctrl Pts',(-6.46136077224333,59.6550912418709,
3.77003198860305));
#244143=CARTESIAN_POINT('Ctrl Pts',(-6.46155012326944,59.6550713402761,
3.64284187937076));
#244144=CARTESIAN_POINT('Ctrl Pts',(-6.56494565834896,59.4260321009471,
3.77003198860305));
#244145=CARTESIAN_POINT('Ctrl Pts',(-6.43870097938028,59.4394927947741,
3.76980208962928));
#244146=CARTESIAN_POINT('Ctrl Pts',(-6.44341257746682,59.4825041216641,
3.64284193928295));
#244147=CARTESIAN_POINT('Ctrl Pts',(-6.54313468201896,59.2206282517278,
3.65553535416626));
#244148=CARTESIAN_POINT('Ctrl Pts',(-6.41712387096215,59.2341955513573,
3.6552005783464));
#244149=CARTESIAN_POINT('Ctrl Pts',(-6.4261459750101,59.3182233753711,3.55127910964297));
#244150=CARTESIAN_POINT('Ctrl Pts',(-6.53099325080075,59.1062911958298,
3.47153072139114));
#244151=CARTESIAN_POINT('Ctrl Pts',(-6.4051226264057,59.1200087130391,3.47122746281624));
#244152=CARTESIAN_POINT('Ctrl Pts',(-6.41653455832046,59.2267768553867,
3.40413045901309));
#244153=CARTESIAN_POINT('Origin',(-6.54282188406247,59.2133417798938,3.40423097483351));
#244154=CARTESIAN_POINT('Ctrl Pts',(-6.2443699078808,62.4538823482277,2.90134173516068));
#244155=CARTESIAN_POINT('Ctrl Pts',(-6.37126553604091,62.441012455002,2.90163218716435));
#244156=CARTESIAN_POINT('Ctrl Pts',(-6.35995915837823,62.3334394572621,
2.83404198860306));
#244157=CARTESIAN_POINT('Ctrl Pts',(-6.2491260434095,62.4991292864734,2.82853349835389));
#244158=CARTESIAN_POINT('Ctrl Pts',(-6.35912437831714,62.4722545055302,
2.85381483162355));
#244159=CARTESIAN_POINT('Ctrl Pts',(-6.36471463173889,62.3786847639678,
2.79182701594274));
#244160=CARTESIAN_POINT('Ctrl Pts',(-6.28053011789765,62.5423796567684,
2.75468822073702));
#244161=CARTESIAN_POINT('Ctrl Pts',(-6.36708533499892,62.5096946965653,
2.79286913083867));
#244162=CARTESIAN_POINT('Ctrl Pts',(-6.38493060453728,62.423112487203,2.74900763297952));
#244163=CARTESIAN_POINT('Ctrl Pts',(-6.39322569848903,62.6032845425348,
2.63954450640421));
#244164=CARTESIAN_POINT('Ctrl Pts',(-6.435760068245,62.5632890102009,2.69627684028913));
#244165=CARTESIAN_POINT('Ctrl Pts',(-6.45334792019218,62.4886705126497,
2.6822435603654));
#244166=CARTESIAN_POINT('Ctrl Pts',(-6.47739243510518,62.6200908675654,
2.59908178706386));
#244167=CARTESIAN_POINT('Ctrl Pts',(-6.49734694408372,62.5804859237138,
2.65878704321526));
#244168=CARTESIAN_POINT('Ctrl Pts',(-6.50319024212541,62.5090840872034,
2.65878198860306));
#244169=CARTESIAN_POINT('Ctrl Pts',(-6.56531752495323,62.6108711573007,
2.59908173516068));
#244170=CARTESIAN_POINT('Ctrl Pts',(-6.56142710223373,62.5737697140404,
2.65878198860306));
#244171=CARTESIAN_POINT('Ctrl Pts',(-6.55408556365967,62.5037563256536,
2.65878198860306));
#244172=CARTESIAN_POINT('Origin',(-6.23365487766645,62.3467145720971,2.83404198860306));
#244173=CARTESIAN_POINT('Origin',(-6.52420020557968,59.0361683443311,3.11913648167141));
#244174=CARTESIAN_POINT('Origin',(-6.50557852713774,58.8589949086132,2.83404198860304));
#244175=CARTESIAN_POINT('Origin',(-6.21503322485406,62.1695413802722,3.11913648177653));
#244176=CARTESIAN_POINT('Origin',(-6.19641157197484,61.9923681882671,3.40423097483353));
#244177=CARTESIAN_POINT('Ctrl Pts',(-6.4937464611276,58.751944703909,2.90134173516065));
#244178=CARTESIAN_POINT('Ctrl Pts',(-6.36806742857345,58.7656442740272,
2.90103711553271));
#244179=CARTESIAN_POINT('Ctrl Pts',(-6.37927424642597,58.8722700234482,
2.83404198860304));
#244180=CARTESIAN_POINT('Ctrl Pts',(-6.48899657309077,58.7067576262548,
2.82862991747987));
#244181=CARTESIAN_POINT('Ctrl Pts',(-6.38004220452892,58.7342098038493,
2.85314045886452));
#244182=CARTESIAN_POINT('Ctrl Pts',(-6.37452469054063,58.8270810177594,
2.79187960999977));
#244183=CARTESIAN_POINT('Ctrl Pts',(-6.45774144355337,58.6637560248476,
2.75470625793387));
#244184=CARTESIAN_POINT('Ctrl Pts',(-6.37187117938144,58.6967899354331,
2.79224250381965));
#244185=CARTESIAN_POINT('Ctrl Pts',(-6.3543526691279,58.7829167175853,2.749018091083));
#244186=CARTESIAN_POINT('Ctrl Pts',(-6.34539908016339,58.6035914159082,
2.6394786831172));
#244187=CARTESIAN_POINT('Ctrl Pts',(-6.30313135363873,58.6436439608619,
2.69595066767937));
#244188=CARTESIAN_POINT('Ctrl Pts',(-6.2859587457653,58.718133717619,2.68220539436104));
#244189=CARTESIAN_POINT('Ctrl Pts',(-6.26151010025748,58.5872698677177,
2.59908178585244));
#244190=CARTESIAN_POINT('Ctrl Pts',(-6.24170554357565,58.6268645946703,
2.65877670944895));
#244191=CARTESIAN_POINT('Ctrl Pts',(-6.23613328458301,58.6982323944376,
2.65878198860303));
#244192=CARTESIAN_POINT('Ctrl Pts',(-6.1740349085904,58.5964866834552,2.59908173516065));
#244193=CARTESIAN_POINT('Ctrl Pts',(-6.17794390662191,58.6335861742244,
2.65878198860303));
#244194=CARTESIAN_POINT('Ctrl Pts',(-6.18532049829418,58.7035958781041,
2.65878198860303));
#244195=CARTESIAN_POINT('Origin',(-6.18532049829418,58.7035958781041,2.53178198860303));
#244196=CARTESIAN_POINT('Ctrl Pts',(-6.15137923967696,61.5639141665613,
3.77003198860306));
#244197=CARTESIAN_POINT('Ctrl Pts',(-6.27787222402482,61.550619218175,3.77003198860306));
#244198=CARTESIAN_POINT('Ctrl Pts',(-6.2776833796338,61.5506390665203,3.64284238727629));
#244199=CARTESIAN_POINT('Ctrl Pts',(-6.1738380120536,61.7797255331388,3.77003198860307));
#244200=CARTESIAN_POINT('Ctrl Pts',(-6.30057242039907,61.7665923920111,
3.77025506105846));
#244201=CARTESIAN_POINT('Ctrl Pts',(-6.29582088597906,61.7232059145522,
3.64284210641876));
#244202=CARTESIAN_POINT('Ctrl Pts',(-6.19522058691297,61.9851742714892,
3.65553527987877));
#244203=CARTESIAN_POINT('Ctrl Pts',(-6.32217699854561,61.9721416759944,
3.65585996533129));
#244204=CARTESIAN_POINT('Ctrl Pts',(-6.31308747966707,61.887486582018,3.55127902710258));
#244205=CARTESIAN_POINT('Ctrl Pts',(-6.20712349654484,62.099536274866,3.47153072139116));
#244206=CARTESIAN_POINT('Ctrl Pts',(-6.33421251157735,62.0866494440661,
3.47182327905233));
#244207=CARTESIAN_POINT('Ctrl Pts',(-6.3226988678919,61.9789328337399,3.40413028378025));
#244208=CARTESIAN_POINT('Origin',(-6.15137923967696,61.5639141665613,3.64303198860306));
#244209=CARTESIAN_POINT('Origin',(4.05837671390568E-16,1.91635770661944E-13,
2.53178198860262));
#244210=CARTESIAN_POINT('Origin',(-6.15500747092336,58.7067819056644,2.53178198860303));
#244211=CARTESIAN_POINT('Origin',(0.995615674755347,-6.43520020182062,3.64303198860258));
#244212=CARTESIAN_POINT('Origin',(-6.10937495961934,61.1647646440485,3.64299466007523));
#244213=CARTESIAN_POINT('Ctrl Pts',(-6.14377718965342,58.599666897865,2.59908173516065));
#244214=CARTESIAN_POINT('Ctrl Pts',(-6.1476670304619,58.6367684021394,2.65878198860303));
#244215=CARTESIAN_POINT('Ctrl Pts',(-6.15500747092336,58.7067819056644,
2.65878198860303));
#244216=CARTESIAN_POINT('Ctrl Pts',(-6.05659553606712,58.6088074259633,
2.59908193199927));
#244217=CARTESIAN_POINT('Ctrl Pts',(-6.08415140319808,58.6434243604378,
2.65877685806593));
#244218=CARTESIAN_POINT('Ctrl Pts',(-6.10436324506824,58.7120821529689,
2.65878198860303));
#244219=CARTESIAN_POINT('Ctrl Pts',(-5.97852000021548,58.6416817365141,
2.63872492669843));
#244220=CARTESIAN_POINT('Ctrl Pts',(-6.02785839131291,58.6721826510723,
2.69532212015316));
#244221=CARTESIAN_POINT('Ctrl Pts',(-6.06008468706722,58.74140381955,2.68176836726669));
#244222=CARTESIAN_POINT('Ctrl Pts',(-5.8802509339248,58.7242744516465,2.75442176402287));
#244223=CARTESIAN_POINT('Ctrl Pts',(-5.97104363802158,58.7387860695145,
2.79203179920173));
#244224=CARTESIAN_POINT('Ctrl Pts',(-6.00614981441032,58.8193360415243,
2.74885310748223));
#244225=CARTESIAN_POINT('Ctrl Pts',(-5.85862682030282,58.7730316211509,
2.82866089558445));
#244226=CARTESIAN_POINT('Ctrl Pts',(-5.97091547255964,58.7772266151799,
2.85316563119314));
#244227=CARTESIAN_POINT('Ctrl Pts',(-5.99561386571444,58.8669255556785,
2.79189751796691));
#244228=CARTESIAN_POINT('Ctrl Pts',(-5.863373641496,58.8181995570487,2.90134173516065));
#244229=CARTESIAN_POINT('Ctrl Pts',(-5.98915458643814,58.8054696185322,
2.90103711553271));
#244230=CARTESIAN_POINT('Ctrl Pts',(-6.00036140429066,58.9120953679532,
2.83404198860303));
#244231=CARTESIAN_POINT('Origin',(-5.87405712357889,58.9253704827882,2.83404198860304));
#244232=CARTESIAN_POINT('Origin',(-6.10480350526266,61.1207756545815,3.56647653971801));
#244233=CARTESIAN_POINT('Origin',(-6.09624906995259,61.0393856393806,3.42473028058528));
#244234=CARTESIAN_POINT('Origin',(-5.89267880207494,59.102543918484,3.11913648168155));
#244235=CARTESIAN_POINT('Origin',(-5.91130048050362,59.2797173540687,3.40423097483352));
#244236=CARTESIAN_POINT('Ctrl Pts',(-6.0617588454159,60.7112330730305,3.36123028058524));
#244237=CARTESIAN_POINT('Ctrl Pts',(-6.18806312612767,60.6979579581956,
3.36123028058524));
#244238=CARTESIAN_POINT('Ctrl Pts',(-6.18806312612767,60.6979579581955,
3.23423028058524));
#244239=CARTESIAN_POINT('Ctrl Pts',(-6.0714004111828,60.8007259828527,3.36123028058523));
#244240=CARTESIAN_POINT('Ctrl Pts',(-6.19746294737662,60.7873912833601,
3.36099641108498));
#244241=CARTESIAN_POINT('Ctrl Pts',(-6.2021759387818,60.8322324012611,3.23423043688417));
#244242=CARTESIAN_POINT('Ctrl Pts',(-6.08051542067558,60.8853484607272,
3.41054258905327));
#244243=CARTESIAN_POINT('Ctrl Pts',(-6.20639551966748,60.8723790316521,
3.41008815825964));
#244244=CARTESIAN_POINT('Ctrl Pts',(-6.2155206071494,60.9591984396311,3.30819867304283));
#244245=CARTESIAN_POINT('Ctrl Pts',(-6.08531878138341,60.9299448846692,
3.48823028058526));
#244246=CARTESIAN_POINT('Ctrl Pts',(-6.21110821942955,60.9172173747512,
3.48794691941642));
#244247=CARTESIAN_POINT('Ctrl Pts',(-6.22255335066436,61.0261105245456,
3.42473028058527));
#244248=CARTESIAN_POINT('Origin',(-6.0617588454159,60.7112330730305,3.23423028058524));
#244249=CARTESIAN_POINT('Ctrl Pts',(-5.90061356181277,59.1725467709679,
3.47153072139113));
#244250=CARTESIAN_POINT('Ctrl Pts',(-6.02658562874803,59.1597945546414,
3.47122746285117));
#244251=CARTESIAN_POINT('Ctrl Pts',(-6.0376214331677,59.2666022171587,3.40413046676841));
#244252=CARTESIAN_POINT('Ctrl Pts',(-5.91250964036455,59.2869113614507,
3.65553813458027));
#244253=CARTESIAN_POINT('Ctrl Pts',(-6.03858760028769,59.2739830624797,
3.65520336072141));
#244254=CARTESIAN_POINT('Ctrl Pts',(-6.0472329950892,59.3580501215762,3.55128134519959));
#244255=CARTESIAN_POINT('Ctrl Pts',(-5.9338813165692,59.4923630227876,3.77003198860305));
#244256=CARTESIAN_POINT('Ctrl Pts',(-6.06016587018168,59.479281816836,3.76980209314187));
#244257=CARTESIAN_POINT('Ctrl Pts',(-6.06449973388402,59.522332169772,3.64284195387442));
#244258=CARTESIAN_POINT('Ctrl Pts',(-5.9563328589123,59.7081718144894,3.77003198860305));
#244259=CARTESIAN_POINT('Ctrl Pts',(-6.08282633453069,59.6948768144684,
3.77003198860305));
#244260=CARTESIAN_POINT('Ctrl Pts',(-6.08263699813586,59.6948967145254,
3.64284189403867));
#244261=CARTESIAN_POINT('Origin',(-5.9563328589123,59.7081718144894,3.64303198860304));
#244262=CARTESIAN_POINT('Origin',(0.97914764405288,-6.27851735587403,3.23423028058477));
#244263=CARTESIAN_POINT('Origin',(-6.04595329345081,60.5608532912345,3.23423028058524));
#244264=CARTESIAN_POINT('Origin',(0.9765688230087,-6.25398151259745,3.64303198860258));
#244265=CARTESIAN_POINT('Origin',(-5.99823604520139,60.1073400339999,3.64299171721827));
#244266=CARTESIAN_POINT('Ctrl Pts',(-6.02238575970296,60.3421421670677,
3.48823028058523));
#244267=CARTESIAN_POINT('Ctrl Pts',(-6.14931623097267,60.3293058762213,
3.48852004212301));
#244268=CARTESIAN_POINT('Ctrl Pts',(-6.13776734223235,60.2194255397047,
3.42473028058523));
#244269=CARTESIAN_POINT('Ctrl Pts',(-6.02720817145212,60.386889039093,3.41028005848448));
#244270=CARTESIAN_POINT('Ctrl Pts',(-6.15399567477082,60.3738278099536,
3.41074404220489));
#244271=CARTESIAN_POINT('Ctrl Pts',(-6.1448238529486,60.2865637544341,3.30780486244054));
#244272=CARTESIAN_POINT('Ctrl Pts',(-6.03634362557923,60.4716618705783,
3.36123028058524));
#244273=CARTESIAN_POINT('Ctrl Pts',(-6.16287156698234,60.4582762833179,
3.36146460586411));
#244274=CARTESIAN_POINT('Ctrl Pts',(-6.15819229746487,60.413756007748,3.23423045308427));
#244275=CARTESIAN_POINT('Ctrl Pts',(-6.04595329345081,60.5608532912345,
3.36123028058524));
#244276=CARTESIAN_POINT('Ctrl Pts',(-6.17225757416258,60.5475781763995,
3.36123028058524));
#244277=CARTESIAN_POINT('Ctrl Pts',(-6.17225757416258,60.5475781763995,
3.23423028058524));
#244278=CARTESIAN_POINT('Origin',(-6.01146306152058,60.2327006545397,3.42473028058522));
#244279=CARTESIAN_POINT('Origin',(-6.00295964283336,60.1517960329196,3.56563113524853));
#244280=CARTESIAN_POINT('Origin',(-13.0813452322045,60.0157999988659,3.5664765390947));
#244281=CARTESIAN_POINT('Origin',(-13.0905908661195,60.0590486699126,3.64299466007543));
#244282=CARTESIAN_POINT('Origin',(-13.0643300858384,59.9357500275434,3.42473028058525));
#244283=CARTESIAN_POINT('Ctrl Pts',(-13.0409063549241,59.8282880397056,
3.48823028058526));
#244284=CARTESIAN_POINT('Ctrl Pts',(-12.9173404733285,59.855054532531,3.48794691941642));
#244285=CARTESIAN_POINT('Ctrl Pts',(-12.9401053405452,59.9621548122773,
3.42473028058527));
#244286=CARTESIAN_POINT('Ctrl Pts',(-13.0316624367251,59.7842416555147,
3.41028005925126));
#244287=CARTESIAN_POINT('Ctrl Pts',(-12.9079350417501,59.8108054559368,
3.40982512231019));
#244288=CARTESIAN_POINT('Ctrl Pts',(-12.9260696369491,59.8961220185315,
3.30780486372868));
#244289=CARTESIAN_POINT('Ctrl Pts',(-13.0141504107549,59.7007958241046,
3.36123028058523));
#244290=CARTESIAN_POINT('Ctrl Pts',(-12.8901364125053,59.7270694888855,
3.36099721048454));
#244291=CARTESIAN_POINT('Ctrl Pts',(-12.8994792219294,59.7710239514062,
3.2342304530839));
#244292=CARTESIAN_POINT('Ctrl Pts',(-12.9957275188826,59.6130003254556,
3.36123028058523));
#244293=CARTESIAN_POINT('Ctrl Pts',(-12.8715027735894,59.6394051101895,
3.36123028058523));
#244294=CARTESIAN_POINT('Ctrl Pts',(-12.8715027735894,59.6394051101895,
3.23423028058523));
#244295=CARTESIAN_POINT('Origin',(-12.9957275188826,59.6130003254556,3.23423028058522));
#244296=CARTESIAN_POINT('Origin',(-0.310561863232978,-0.066011961834456,
3.64303198860263));
#244297=CARTESIAN_POINT('Origin',(-13.1739864076109,60.451642460649,3.64303198860305));
#244298=CARTESIAN_POINT('Origin',(-0.310561863232978,-0.0660119618344531,
3.23423028058481));
#244299=CARTESIAN_POINT('Origin',(-12.9642895838873,59.4650964698968,3.23423028058523));
#244300=CARTESIAN_POINT('Ctrl Pts',(-13.2864868028998,60.9782752797349,
3.47153072139114));
#244301=CARTESIAN_POINT('Ctrl Pts',(-13.1616357280625,61.005291838439,3.47182327902704));
#244302=CARTESIAN_POINT('Ctrl Pts',(-13.1392995818862,60.8992893541408,
3.40413028959089));
#244303=CARTESIAN_POINT('Ctrl Pts',(-13.2624669757411,60.8658306440997,
3.65553807120998));
#244304=CARTESIAN_POINT('Ctrl Pts',(-13.1376969719796,60.8926675943329,
3.65586275497022));
#244305=CARTESIAN_POINT('Ctrl Pts',(-13.1201818190176,60.8093473519467,
3.55128126837324));
#244306=CARTESIAN_POINT('Ctrl Pts',(-13.2193155203587,60.6638281080081,
3.77003198860305));
#244307=CARTESIAN_POINT('Ctrl Pts',(-13.0947255842073,60.690500823973,3.77025505748489));
#244308=CARTESIAN_POINT('Ctrl Pts',(-13.0858375353125,60.6477702018628,
3.64284211731156));
#244309=CARTESIAN_POINT('Ctrl Pts',(-13.1739864076109,60.451642460649,3.77003198860306));
#244310=CARTESIAN_POINT('Ctrl Pts',(-13.049576076309,60.4780866929068,3.77003198860306));
#244311=CARTESIAN_POINT('Ctrl Pts',(-13.0497618007392,60.4780472159605,
3.64284239821778));
#244312=CARTESIAN_POINT('Origin',(-13.2635576885504,60.8730422059015,3.40423097483352));
#244313=CARTESIAN_POINT('Ctrl Pts',(-12.9642895838873,59.4650964698968,
3.36123028058523));
#244314=CARTESIAN_POINT('Ctrl Pts',(-12.8400648385941,59.4915012546306,
3.36123028058523));
#244315=CARTESIAN_POINT('Ctrl Pts',(-12.8400648385941,59.4915012546306,
3.23423028058523));
#244316=CARTESIAN_POINT('Ctrl Pts',(-12.9458049943933,59.3770041141846,
3.36123028058523));
#244317=CARTESIAN_POINT('Ctrl Pts',(-12.8213326038438,59.4033730190078,
3.36146538610137));
#244318=CARTESIAN_POINT('Ctrl Pts',(-12.8119938336987,59.3594375597966,
3.23423043688395));
#244319=CARTESIAN_POINT('Ctrl Pts',(-12.9283282206289,59.2937057271827,
3.4105425869314));
#244320=CARTESIAN_POINT('Ctrl Pts',(-12.8037097640135,59.3204640761313,
3.41100608859929));
#244321=CARTESIAN_POINT('Ctrl Pts',(-12.7854506972092,59.2345619206681,
3.30819866970998));
#244322=CARTESIAN_POINT('Ctrl Pts',(-12.9191181862048,59.2498070616281,
3.48823028058521));
#244323=CARTESIAN_POINT('Ctrl Pts',(-12.794433502371,59.2768226962999,3.48852004212299));
#244324=CARTESIAN_POINT('Ctrl Pts',(-12.7714622569322,59.1687514833562,
3.42473028058521));
#244325=CARTESIAN_POINT('Origin',(-12.8956870022254,59.1423466986223,3.42473028058522));
#244326=CARTESIAN_POINT('Origin',(-13.300596971516,61.0472983318851,3.1191364817838));
#244327=CARTESIAN_POINT('Origin',(-13.3376362544828,61.221554457654,2.83404198860304));
#244328=CARTESIAN_POINT('Origin',(-12.8787733304452,59.0627741291259,3.56563113460799));
#244329=CARTESIAN_POINT('Origin',(-12.8695280801149,59.0190342907436,3.64299171721817));
#244330=CARTESIAN_POINT('Ctrl Pts',(-13.103835206573,61.5752716937453,2.59908173516067));
#244331=CARTESIAN_POINT('Ctrl Pts',(-13.0960702419682,61.5387839176329,
2.65878198860306));
#244332=CARTESIAN_POINT('Ctrl Pts',(-13.0814171332235,61.4699285681956,
2.65878198860305));
#244333=CARTESIAN_POINT('Ctrl Pts',(-13.1900205930482,61.5569304518442,
2.59908193475517));
#244334=CARTESIAN_POINT('Ctrl Pts',(-13.1588482421902,61.5254208297847,
2.65878715325409));
#244335=CARTESIAN_POINT('Ctrl Pts',(-13.1313027022865,61.4593031273797,
2.65878198860305));
#244336=CARTESIAN_POINT('Ctrl Pts',(-13.2643407403244,61.515537853938,2.63878778849929));
#244337=CARTESIAN_POINT('Ctrl Pts',(-13.2118511391497,61.4904936222811,
2.69564460180163));
#244338=CARTESIAN_POINT('Ctrl Pts',(-13.1721300657491,61.4250300340664,
2.68180481624929));
#244339=CARTESIAN_POINT('Ctrl Pts',(-13.3535591268197,61.4222835584428,
2.75443238878675));
#244340=CARTESIAN_POINT('Ctrl Pts',(-13.2611962587093,61.4178880557408,
2.79268340777125));
#244341=CARTESIAN_POINT('Ctrl Pts',(-13.2174099770541,61.3411158595758,
2.74885926835651));
#244342=CARTESIAN_POINT('Ctrl Pts',(-13.3700167576322,61.3712701109737,
2.82856655361722));
#244343=CARTESIAN_POINT('Ctrl Pts',(-13.2570896192445,61.3797074995631,
2.8538419723086));
#244344=CARTESIAN_POINT('Ctrl Pts',(-13.2228660458969,61.292439340452,2.79184624278546));
#244345=CARTESIAN_POINT('Ctrl Pts',(-13.3605623192489,61.3267881959114,
2.90134173516065));
#244346=CARTESIAN_POINT('Ctrl Pts',(-13.2359003894753,61.3537611057084,
2.90163218716433));
#244347=CARTESIAN_POINT('Ctrl Pts',(-13.2134115091896,61.2479592423879,
2.83404198860304));
#244348=CARTESIAN_POINT('Origin',(-13.0814171332235,61.4699285681956,2.53178198860305));
#244349=CARTESIAN_POINT('Origin',(-0.310561863232978,-0.066011961834456,
3.64303198860263));
#244350=CARTESIAN_POINT('Origin',(-12.7860306150453,58.6264539577985,3.64303198860303));
#244351=CARTESIAN_POINT('Origin',(4.07480739540194E-18,1.9141614838601E-13,
2.53178198860262));
#244352=CARTESIAN_POINT('Origin',(-13.0516031943531,61.4762657165317,2.53178198860305));
#244353=CARTESIAN_POINT('Ctrl Pts',(-12.7860306150453,58.6264539577985,
3.77003198860304));
#244354=CARTESIAN_POINT('Ctrl Pts',(-12.6616197754742,58.6528982980922,
3.77003198860304));
#244355=CARTESIAN_POINT('Ctrl Pts',(-12.6618060089323,58.6528587129487,
3.64284187937092));
#244356=CARTESIAN_POINT('Ctrl Pts',(-12.7406940127365,58.414266398147,3.77003198860304));
#244357=CARTESIAN_POINT('Ctrl Pts',(-12.6165479409684,58.4408495151706,
3.76980208962871));
#244358=CARTESIAN_POINT('Ctrl Pts',(-12.6257296363315,58.4831327254065,
3.64284193928292));
#244359=CARTESIAN_POINT('Ctrl Pts',(-12.6975319705105,58.2122676405433,
3.65553535416627));
#244360=CARTESIAN_POINT('Ctrl Pts',(-12.5736296288415,58.2389323335244,
3.65520057834584));
#244361=CARTESIAN_POINT('Ctrl Pts',(-12.5913856081751,58.3215567776511,
3.55127910964328));
#244362=CARTESIAN_POINT('Ctrl Pts',(-12.6735055745743,58.0998260601481,
3.47153072139113));
#244363=CARTESIAN_POINT('Ctrl Pts',(-12.5497583536236,58.1266254943014,
3.47122746281623));
#244364=CARTESIAN_POINT('Ctrl Pts',(-12.5722680796266,58.2316158778878,
3.40413045901317));
#244365=CARTESIAN_POINT('Origin',(-12.6964592423895,58.2050537810543,3.40423097483351));
#244366=CARTESIAN_POINT('Ctrl Pts',(-12.7383709431253,61.459039055521,2.90134173516066));
#244367=CARTESIAN_POINT('Ctrl Pts',(-12.8632261535957,61.43297545991,2.90163218716434));
#244368=CARTESIAN_POINT('Ctrl Pts',(-12.84073727331,61.3271735965895,2.83404198860304));
#244369=CARTESIAN_POINT('Ctrl Pts',(-12.7478306169676,61.503540974767,2.82853349835378));
#244370=CARTESIAN_POINT('Ctrl Pts',(-12.8544171899352,61.4653154597768,
2.85381483162427));
#244371=CARTESIAN_POINT('Ctrl Pts',(-12.8501961180702,61.371673962449,2.79182701594335));
#244372=CARTESIAN_POINT('Ctrl Pts',(-12.7835835513933,61.5432717953613,
2.75468822073712));
#244373=CARTESIAN_POINT('Ctrl Pts',(-12.8662481012967,61.5017184029585,
2.79286913083838));
#244374=CARTESIAN_POINT('Ctrl Pts',(-12.8749453072905,61.4137451613973,
2.74900763297951));
#244375=CARTESIAN_POINT('Ctrl Pts',(-12.9020280679172,61.5920631419348,
2.6395445064041));
#244376=CARTESIAN_POINT('Ctrl Pts',(-12.940148758413,61.5478406570054,2.69627684028927));
#244377=CARTESIAN_POINT('Ctrl Pts',(-12.9498405053864,61.4717924962547,
2.68224356036539));
#244378=CARTESIAN_POINT('Ctrl Pts',(-12.9874904696724,61.5999795805214,
2.59908178706412));
#244379=CARTESIAN_POINT('Ctrl Pts',(-13.0031958218445,61.5585057825391,
2.65878704321686));
#244380=CARTESIAN_POINT('Ctrl Pts',(-13.0015435854427,61.4868843017926,
2.65878198860305));
#244381=CARTESIAN_POINT('Ctrl Pts',(-13.0739701745327,61.5816197022699,
2.59908173516066));
#244382=CARTESIAN_POINT('Ctrl Pts',(-13.0662229071069,61.545128164506,2.65878198860305));
#244383=CARTESIAN_POINT('Ctrl Pts',(-13.0516031943531,61.4762657165317,
2.65878198860305));
#244384=CARTESIAN_POINT('Origin',(-12.7165125280168,61.3535783813233,2.83404198860304));
#244385=CARTESIAN_POINT('Origin',(-12.6594199084583,58.0307974155462,3.1191364816706));
#244386=CARTESIAN_POINT('Origin',(-12.6223805745521,57.8565410498768,2.83404198860303));
#244387=CARTESIAN_POINT('Origin',(-12.6794732450929,61.1793222555332,3.11913648177642));
#244388=CARTESIAN_POINT('Origin',(-12.6424339620844,61.0050661295708,3.40423097483352));
#244389=CARTESIAN_POINT('Ctrl Pts',(-12.5994235324474,57.7513140650721,
2.90134173516064));
#244390=CARTESIAN_POINT('Ctrl Pts',(-12.4758649777955,57.7780756236497,
2.9010371155327));
#244391=CARTESIAN_POINT('Ctrl Pts',(-12.4981558292589,57.8829458346107,
2.83404198860303));
#244392=CARTESIAN_POINT('Ctrl Pts',(-12.5899763290073,57.7068710254546,
2.82862991748001));
#244393=CARTESIAN_POINT('Ctrl Pts',(-12.4844883578139,57.7455616498605,
2.85314045886469));
#244394=CARTESIAN_POINT('Ctrl Pts',(-12.4887087546166,57.8385008428016,
2.79187960999965));
#244395=CARTESIAN_POINT('Ctrl Pts',(-12.5543975270268,57.6673720419788,
2.75470625793368));
#244396=CARTESIAN_POINT('Ctrl Pts',(-12.4724506530562,57.7092008760992,
2.79224250381918));
#244397=CARTESIAN_POINT('Ctrl Pts',(-12.4640308112191,57.7966870296831,
2.74901809108302));
#244398=CARTESIAN_POINT('Ctrl Pts',(-12.4363816727425,57.6192799956675,
2.63947868311738));
#244399=CARTESIAN_POINT('Ctrl Pts',(-12.39853212422,57.6635313090894,2.69595066767966));
#244400=CARTESIAN_POINT('Ctrl Pts',(-12.3892398894927,57.7394080294761,
2.682205394361));
#244401=CARTESIAN_POINT('Ctrl Pts',(-12.3512461790954,57.6118166447798,
2.59908178585153));
#244402=CARTESIAN_POINT('Ctrl Pts',(-12.3356888898091,57.6532646075497,
2.65877670944829));
#244403=CARTESIAN_POINT('Ctrl Pts',(-12.3376071226707,57.7248239067131,
2.65878198860303));
#244404=CARTESIAN_POINT('Ctrl Pts',(-12.2652136052663,57.6301266171959,
2.59908173516064));
#244405=CARTESIAN_POINT('Ctrl Pts',(-12.2729791421557,57.6666142715156,
2.65878198860303));
#244406=CARTESIAN_POINT('Ctrl Pts',(-12.2876333308473,57.7354693911206,
2.65878198860303));
#244407=CARTESIAN_POINT('Origin',(-12.2876333308473,57.7354693911206,2.53178198860303));
#244408=CARTESIAN_POINT('Ctrl Pts',(-12.5528626811449,60.5836663843183,
3.77003198860306));
#244409=CARTESIAN_POINT('Ctrl Pts',(-12.6772730231651,60.5572221497823,
3.77003198860306));
#244410=CARTESIAN_POINT('Ctrl Pts',(-12.6770872880007,60.5572616290102,
3.64284238727649));
#244411=CARTESIAN_POINT('Ctrl Pts',(-12.5977568525211,60.7959479326854,
3.77003198860306));
#244412=CARTESIAN_POINT('Ctrl Pts',(-12.7224242094581,60.769639383333,3.77025506105759));
#244413=CARTESIAN_POINT('Ctrl Pts',(-12.7131635826242,60.7269872521273,
3.64284210641873));
#244414=CARTESIAN_POINT('Ctrl Pts',(-12.6404975322968,60.9980361136602,
3.65553527987876));
#244415=CARTESIAN_POINT('Ctrl Pts',(-12.7653961862431,60.971804353475,3.65585996533132));
#244416=CARTESIAN_POINT('Ctrl Pts',(-12.74750759382,60.8885631224031,3.55127902710283));
#244417=CARTESIAN_POINT('Ctrl Pts',(-12.6642893210144,61.1105274371642,
3.47153072139114));
#244418=CARTESIAN_POINT('Ctrl Pts',(-12.7893350885049,61.0844267823323,
3.4718232790523));
#244419=CARTESIAN_POINT('Ctrl Pts',(-12.7666250660187,60.9785037583492,
3.40413028378034));
#244420=CARTESIAN_POINT('Origin',(-12.5528626811449,60.5836663843183,3.64303198860306));
#244421=CARTESIAN_POINT('Origin',(3.9977349588932E-16,1.91634810190902E-13,
2.53178198860262));
#244422=CARTESIAN_POINT('Origin',(-12.257819391977,57.7418065394567,2.53178198860302));
#244423=CARTESIAN_POINT('Origin',(3.00026883051142,-12.588064422097,3.64303198860254));
#244424=CARTESIAN_POINT('Origin',(-12.469366018725,60.1910940874988,3.64299466007543));
#244425=CARTESIAN_POINT('Ctrl Pts',(-12.2354540642047,57.6364522029208,
2.59908173516064));
#244426=CARTESIAN_POINT('Ctrl Pts',(-12.2432007592849,57.6729438621907,
2.65878198860303));
#244427=CARTESIAN_POINT('Ctrl Pts',(-12.257819391977,57.7418065394567,2.65878198860303));
#244428=CARTESIAN_POINT('Ctrl Pts',(-12.1497054461945,57.6546556225247,
2.59908193199989));
#244429=CARTESIAN_POINT('Ctrl Pts',(-12.1807288143667,57.686202549369,2.65877685806701));
#244430=CARTESIAN_POINT('Ctrl Pts',(-12.208006627196,57.7523715145547,2.65878198860303));
#244431=CARTESIAN_POINT('Ctrl Pts',(-12.0754939174599,57.6955109599437,
2.63872492669841));
#244432=CARTESIAN_POINT('Ctrl Pts',(-12.1277502414152,57.7206875210981,
2.69532212015305));
#244433=CARTESIAN_POINT('Ctrl Pts',(-12.1670355805165,57.7861609236009,
2.68176836726676));
#244434=CARTESIAN_POINT('Ctrl Pts',(-11.9863964689867,57.7879231380268,
2.75442176402287));
#244435=CARTESIAN_POINT('Ctrl Pts',(-12.0782086782662,57.7928648378996,
2.79203179920193));
#244436=CARTESIAN_POINT('Ctrl Pts',(-12.1215423041375,57.8693039540647,
2.74885310748215));
#244437=CARTESIAN_POINT('Ctrl Pts',(-11.9699873265232,57.8386735460215,
2.82866089558444));
#244438=CARTESIAN_POINT('Ctrl Pts',(-12.0820993460723,57.8311081991745,
2.85316563119132));
#244439=CARTESIAN_POINT('Ctrl Pts',(-12.1160385312532,57.9177340744078,
2.79189751796604));
#244440=CARTESIAN_POINT('Ctrl Pts',(-11.9794294790614,57.8830978693157,
2.90134173516063));
#244441=CARTESIAN_POINT('Ctrl Pts',(-12.1031907419159,57.8572899778512,
2.90103711553269));
#244442=CARTESIAN_POINT('Ctrl Pts',(-12.1254815933794,57.9621601888122,
2.83404198860302));
#244443=CARTESIAN_POINT('Origin',(-12.0012568480862,57.9885649735461,2.83404198860303));
#244444=CARTESIAN_POINT('Origin',(-12.4602215058063,60.1478239214158,3.56647653971874));
#244445=CARTESIAN_POINT('Origin',(-12.4432063593724,60.0677739512127,3.42473028058527));
#244446=CARTESIAN_POINT('Origin',(-12.0382961820438,58.1628213391883,3.11913648168055));
#244447=CARTESIAN_POINT('Origin',(-12.0753355159235,58.3370777047236,3.40423097483351));
#244448=CARTESIAN_POINT('Ctrl Pts',(-12.3746037924166,59.7450242491249,
3.36123028058523));
#244449=CARTESIAN_POINT('Ctrl Pts',(-12.4988285377098,59.7186194643911,
3.36123028058523));
#244450=CARTESIAN_POINT('Ctrl Pts',(-12.4988285377098,59.7186194643911,
3.23423028058523));
#244451=CARTESIAN_POINT('Ctrl Pts',(-12.3935470970146,59.8330190893701,
3.36123028058523));
#244452=CARTESIAN_POINT('Ctrl Pts',(-12.5175251937993,59.806580315575,3.3609964110852));
#244453=CARTESIAN_POINT('Ctrl Pts',(-12.5268995400898,59.850683147391,3.23423043688408));
#244454=CARTESIAN_POINT('Ctrl Pts',(-12.4114576311013,59.9162252185218,
3.41054258905328));
#244455=CARTESIAN_POINT('Ctrl Pts',(-12.5352924712483,59.8901687840295,
3.4100881582603));
#244456=CARTESIAN_POINT('Ctrl Pts',(-12.5534426698448,59.9755587548362,
3.30819867304362));
#244457=CARTESIAN_POINT('Ctrl Pts',(-12.4208962741589,59.9600752506738,
3.48823028058525));
#244458=CARTESIAN_POINT('Ctrl Pts',(-12.5446662374489,59.9342688867326,
3.48794691941641));
#244459=CARTESIAN_POINT('Ctrl Pts',(-12.5674311046656,60.0413691664789,
3.42473028058526));
#244460=CARTESIAN_POINT('Origin',(-12.3746037924166,59.7450242491249,3.23423028058523));
#244461=CARTESIAN_POINT('Ctrl Pts',(-12.0535047649324,58.2316113004782,
3.47153072139112));
#244462=CARTESIAN_POINT('Ctrl Pts',(-12.1774537741283,58.2057612755557,
3.47122746285117));
#244463=CARTESIAN_POINT('Ctrl Pts',(-12.1995935640849,58.3108302788452,
3.40413046676848));
#244464=CARTESIAN_POINT('Ctrl Pts',(-12.0772900304161,58.3441059109584,
3.65553813458028));
#244465=CARTESIAN_POINT('Ctrl Pts',(-12.2013259468593,58.3180696991587,
3.65520336072124));
#244466=CARTESIAN_POINT('Ctrl Pts',(-12.2187113817826,58.4007725402778,
3.55128134519947));
#244467=CARTESIAN_POINT('Ctrl Pts',(-12.1200201767772,58.5461981381267,
3.77003198860304));
#244468=CARTESIAN_POINT('Ctrl Pts',(-12.2442455720352,58.5199882620668,
3.7698020931422));
#244469=CARTESIAN_POINT('Ctrl Pts',(-12.2530556816156,58.5623497685507,
3.64284195387449));
#244470=CARTESIAN_POINT('Ctrl Pts',(-12.1649068885794,58.7584778814678,
3.77003198860304));
#244471=CARTESIAN_POINT('Ctrl Pts',(-12.2893177137816,58.7320335442283,
3.77003198860304));
#244472=CARTESIAN_POINT('Ctrl Pts',(-12.2891314947139,58.732073126313,3.64284189403881));
#244473=CARTESIAN_POINT('Origin',(-12.1649068885794,58.7584778814678,3.64303198860303));
#244474=CARTESIAN_POINT('Origin',(2.93511643966563,-12.2815465224194,3.23423028058473));
#244475=CARTESIAN_POINT('Origin',(-12.3431658574213,59.597120393566,3.23423028058523));
#244476=CARTESIAN_POINT('Origin',(2.92491386234308,-12.2335471699534,3.64303198860254));
#244477=CARTESIAN_POINT('Origin',(-12.2483049654,59.1510793400373,3.64299171721807));
#244478=CARTESIAN_POINT('Ctrl Pts',(-12.2968658913805,59.3820708699072,
3.48823028058522));
#244479=CARTESIAN_POINT('Ctrl Pts',(-12.4217592664914,59.3560370505015,
3.488520042123));
#244480=CARTESIAN_POINT('Ctrl Pts',(-12.3987880210526,59.2479658375578,
3.42473028058522));
#244481=CARTESIAN_POINT('Ctrl Pts',(-12.3063392072225,59.4260685345963,
3.41028005848446));
#244482=CARTESIAN_POINT('Ctrl Pts',(-12.4310668851206,59.3998259533514,
3.41074404220392));
#244483=CARTESIAN_POINT('Ctrl Pts',(-12.4128237298765,59.3139986558986,
3.30780486244002));
#244484=CARTESIAN_POINT('Ctrl Pts',(-12.3242857901776,59.5094220566596,
3.36123028058523));
#244485=CARTESIAN_POINT('Ctrl Pts',(-12.4487214234132,59.482884025773,3.36146460586469));
#244486=CARTESIAN_POINT('Ctrl Pts',(-12.4394141514343,59.439096753783,3.23423045308409));
#244487=CARTESIAN_POINT('Ctrl Pts',(-12.3431658574213,59.597120393566,3.36123028058523));
#244488=CARTESIAN_POINT('Ctrl Pts',(-12.4673906027145,59.5707156088322,
3.36123028058523));
#244489=CARTESIAN_POINT('Ctrl Pts',(-12.4673906027145,59.5707156088322,
3.23423028058523));
#244490=CARTESIAN_POINT('Origin',(-12.2745632757594,59.2743706222916,3.42473028058522));
#244491=CARTESIAN_POINT('Origin',(-12.2576496039195,59.1947980539417,3.56563113524832));
#244492=CARTESIAN_POINT('Origin',(-19.283043599957,58.3196542523189,3.56647653909532));
#244493=CARTESIAN_POINT('Origin',(-19.2967593024444,58.3616995707145,3.64299466007843));
#244494=CARTESIAN_POINT('Origin',(-19.2577541638581,58.2418213702175,3.42473028058524));
#244495=CARTESIAN_POINT('Ctrl Pts',(-19.2232259141442,58.1373965169894,
3.48823028058524));
#244496=CARTESIAN_POINT('Ctrl Pts',(-19.103134799739,58.176932531882,3.48794691941641));
#244497=CARTESIAN_POINT('Ctrl Pts',(-19.1369699862886,58.2810665285031,
3.42473028058526));
#244498=CARTESIAN_POINT('Ctrl Pts',(-19.2094285342454,58.0945576760634,
3.41028005925126));
#244499=CARTESIAN_POINT('Ctrl Pts',(-19.0891556041227,58.1339089916642,
3.40982512231099));
#244500=CARTESIAN_POINT('Ctrl Pts',(-19.1161088652899,58.2168625998383,
3.30780486372909));
#244501=CARTESIAN_POINT('Ctrl Pts',(-19.1832899764623,58.0133994748122,
3.36123028058522));
#244502=CARTESIAN_POINT('Ctrl Pts',(-19.0627016856748,58.0524922023721,
3.36099721048474));
#244503=CARTESIAN_POINT('Ctrl Pts',(-19.0765878066315,58.0952292882337,
3.23423045308334));
#244504=CARTESIAN_POINT('Ctrl Pts',(-19.1557908785627,57.9280106456677,
3.36123028058522));
#244505=CARTESIAN_POINT('Ctrl Pts',(-19.0350067009933,57.9672558039533,
3.36123028058521));
#244506=CARTESIAN_POINT('Ctrl Pts',(-19.0350067009933,57.9672558039533,
3.23423028058522));
#244507=CARTESIAN_POINT('Origin',(-19.1557908785627,57.9280106456677,3.23423028058521));
#244508=CARTESIAN_POINT('Origin',(-0.301960443923705,-0.0981128957138633,
3.64303198860263));
#244509=CARTESIAN_POINT('Origin',(-19.4207352200703,58.7434254837933,3.64303198860303));
#244510=CARTESIAN_POINT('Origin',(-0.301960443923705,-0.0981128957138604,
3.23423028058481));
#244511=CARTESIAN_POINT('Origin',(-19.1090650011318,57.7842031819384,3.23423028058521));
#244512=CARTESIAN_POINT('Ctrl Pts',(-19.5876674457081,59.2554138597572,
3.47153072139113));
#244513=CARTESIAN_POINT('Ctrl Pts',(-19.4663243174857,59.2953329099162,
3.47182327902703));
#244514=CARTESIAN_POINT('Ctrl Pts',(-19.4330302542693,59.1922458813527,
3.40413028959058));
#244515=CARTESIAN_POINT('Ctrl Pts',(-19.5520255367089,59.1460959632226,
3.65553807120998));
#244516=CARTESIAN_POINT('Ctrl Pts',(-19.4307442612511,59.185827914589,3.65586275496843));
#244517=CARTESIAN_POINT('Ctrl Pts',(-19.4046157212344,59.104794941234,3.5512812683721));
#244518=CARTESIAN_POINT('Ctrl Pts',(-19.4879954548414,58.9497105734781,
3.77003198860303));
#244519=CARTESIAN_POINT('Ctrl Pts',(-19.3668760934058,58.989260368079,3.77025505748724));
#244520=CARTESIAN_POINT('Ctrl Pts',(-19.35357016791,58.9476928828774,3.64284211731298));
#244521=CARTESIAN_POINT('Ctrl Pts',(-19.4207352200704,58.7434254837933,
3.77003198860303));
#244522=CARTESIAN_POINT('Ctrl Pts',(-19.2997705965402,58.7827292725257,
3.77003198860303));
#244523=CARTESIAN_POINT('Ctrl Pts',(-19.2999511770886,58.7826705983487,
3.64284239821721));
#244524=CARTESIAN_POINT('Origin',(-19.5538640879535,59.1531540088,3.40423097483351));
#244525=CARTESIAN_POINT('Ctrl Pts',(-19.1090650011318,57.7842031819384,
3.36123028058522));
#244526=CARTESIAN_POINT('Ctrl Pts',(-18.9882808235623,57.823448340224,3.36123028058521));
#244527=CARTESIAN_POINT('Ctrl Pts',(-18.9882808235623,57.823448340224,3.23423028058522));
#244528=CARTESIAN_POINT('Ctrl Pts',(-19.0814735135847,57.698525571102,3.36123028058522));
#244529=CARTESIAN_POINT('Ctrl Pts',(-18.9604392969147,57.7377609320132,
3.36146538610115));
#244530=CARTESIAN_POINT('Ctrl Pts',(-18.9465591794955,57.6950423231356,
3.2342304368842));
#244531=CARTESIAN_POINT('Ctrl Pts',(-19.0553854270309,57.6175103216839,
3.4105425869314));
#244532=CARTESIAN_POINT('Ctrl Pts',(-18.934246652453,57.6571482613565,3.41100608859792));
#244533=CARTESIAN_POINT('Ctrl Pts',(-18.9071083904249,57.5736252790843,
3.30819866970861));
#244534=CARTESIAN_POINT('Ctrl Pts',(-19.041637186088,57.5748148483577,3.48823028058522));
#244535=CARTESIAN_POINT('Ctrl Pts',(-18.9204594407748,57.6147155869503,
3.488520042123));
#244536=CARTESIAN_POINT('Ctrl Pts',(-18.8863175164095,57.5096375484038,
3.42473028058522));
#244537=CARTESIAN_POINT('Origin',(-19.007101693979,57.4703923901181,3.42473028058521));
#244538=CARTESIAN_POINT('Origin',(-19.6089151909145,59.3225838821627,3.11913648178295));
#244539=CARTESIAN_POINT('Origin',(-19.6639662938564,59.492013755314,2.83404198860302));
#244540=CARTESIAN_POINT('Origin',(-18.9819630786544,57.3930236876033,3.56563113460828));
#244541=CARTESIAN_POINT('Origin',(-18.968196416683,57.3504898524415,3.64299171721863));
#244542=CARTESIAN_POINT('Ctrl Pts',(-19.4684195516699,59.8682321556243,
2.59908173516064));
#244543=CARTESIAN_POINT('Ctrl Pts',(-19.4568831131886,59.8327559231847,
2.65878198860303));
#244544=CARTESIAN_POINT('Ctrl Pts',(-19.4351129318423,59.7658094374952,
2.65878198860303));
#244545=CARTESIAN_POINT('Ctrl Pts',(-19.5522156237501,59.8409825629609,
2.59908193475531));
#244546=CARTESIAN_POINT('Ctrl Pts',(-19.5179203859192,59.8129039518386,
2.65878715325381));
#244547=CARTESIAN_POINT('Ctrl Pts',(-19.4836145615383,59.7500277420819,
2.65878198860303));
#244548=CARTESIAN_POINT('Ctrl Pts',(-19.6218019328333,59.7920481472526,
2.63878778849926));
#244549=CARTESIAN_POINT('Ctrl Pts',(-19.5669820401371,59.7726277678656,
2.69564460180159));
#244550=CARTESIAN_POINT('Ctrl Pts',(-19.5206357546565,59.7116747787983,
2.6818048162492));
#244551=CARTESIAN_POINT('Ctrl Pts',(-19.7007838434712,59.6899788477098,
2.75443238878672));
#244552=CARTESIAN_POINT('Ctrl Pts',(-19.6084674936735,59.6952619726978,
2.79268340777122));
#244553=CARTESIAN_POINT('Ctrl Pts',(-19.556896198164,59.6234872553903,2.74885926835654));
#244554=CARTESIAN_POINT('Ctrl Pts',(-19.7118189603902,59.6375245663858,
2.82856655361718));
#244555=CARTESIAN_POINT('Ctrl Pts',(-19.6003923959449,59.6577198343146,
2.85384197230828));
#244556=CARTESIAN_POINT('Ctrl Pts',(-19.5572342963493,59.5745070768393,
2.7918462427852));
#244557=CARTESIAN_POINT('Ctrl Pts',(-19.6977666881848,59.5942745858237,
2.90134173516065));
#244558=CARTESIAN_POINT('Ctrl Pts',(-19.5766071063171,59.6341304551458,
2.90163218716432));
#244559=CARTESIAN_POINT('Ctrl Pts',(-19.5431821162869,59.5312589135997,
2.83404198860303));
#244560=CARTESIAN_POINT('Origin',(-19.4351129318423,59.7658094374952,2.53178198860302));
#244561=CARTESIAN_POINT('Origin',(-0.301960443923705,-0.0981128957138633,
3.64303198860263));
#244562=CARTESIAN_POINT('Origin',(-18.8441205405522,56.9687879773467,3.64303198860302));
#244563=CARTESIAN_POINT('Origin',(2.07460197300515E-17,1.91420615423891E-13,
2.53178198860262));
#244564=CARTESIAN_POINT('Origin',(-19.4061247292256,59.7752282754838,2.53178198860303));
#244565=CARTESIAN_POINT('Ctrl Pts',(-18.8441205405522,56.9687879773467,
3.77003198860302));
#244566=CARTESIAN_POINT('Ctrl Pts',(-18.7231554228303,57.0080919266517,
3.77003198860302));
#244567=CARTESIAN_POINT('Ctrl Pts',(-18.7233364983081,57.0080330916624,
3.64284187937061));
#244568=CARTESIAN_POINT('Ctrl Pts',(-18.7768526573589,56.7625017687178,
3.77003198860302));
#244569=CARTESIAN_POINT('Ctrl Pts',(-18.6561653631322,56.8019160587479,
3.76980208963145));
#244570=CARTESIAN_POINT('Ctrl Pts',(-18.6697165591968,56.8430078886273,
3.64284193928381));
#244571=CARTESIAN_POINT('Ctrl Pts',(-18.7128124416019,56.5661212433893,
3.65553535416627));
#244572=CARTESIAN_POINT('Ctrl Pts',(-18.5923760693072,56.6055911857614,
3.6552005783438));
#244573=CARTESIAN_POINT('Ctrl Pts',(-18.6186713857001,56.6859069993048,
3.55127910964221));
#244574=CARTESIAN_POINT('Ctrl Pts',(-18.6771643191712,56.4568070719812,
3.47153072139111));
#244575=CARTESIAN_POINT('Ctrl Pts',(-18.556896302113,56.4963948028698,3.47122746281622));
#244576=CARTESIAN_POINT('Ctrl Pts',(-18.5902572009363,56.5984571310821,
3.404130459013));
#244577=CARTESIAN_POINT('Origin',(-18.7109915363519,56.559059032799,3.4042309748335));
#244578=CARTESIAN_POINT('Ctrl Pts',(-19.0928077206414,59.7908376697913,
2.90134173516066));
#244579=CARTESIAN_POINT('Ctrl Pts',(-19.2142545736086,59.7518659300027,
2.90163218716433));
#244580=CARTESIAN_POINT('Ctrl Pts',(-19.1808295835784,59.6489943884565,
2.83404198860303));
#244581=CARTESIAN_POINT('Ctrl Pts',(-19.1068672906321,59.8341069976973,
2.82853349835402));
#244582=CARTESIAN_POINT('Ctrl Pts',(-19.2088743168605,59.7849495553999,
2.85381483162332));
#244583=CARTESIAN_POINT('Ctrl Pts',(-19.1948881666552,59.6922622581478,
2.79182701594224));
#244584=CARTESIAN_POINT('Ctrl Pts',(-19.1465773683631,59.8698829694069,
2.75468822073679));
#244585=CARTESIAN_POINT('Ctrl Pts',(-19.2244455609618,59.8199164124671,
2.7928691308392));
#244586=CARTESIAN_POINT('Ctrl Pts',(-19.2238994150016,59.7315159919506,
2.74900763297943));
#244587=CARTESIAN_POINT('Ctrl Pts',(-19.2694731179103,59.9060262085836,
2.63954450640438));
#244588=CARTESIAN_POINT('Ctrl Pts',(-19.3027624708828,59.8580612818576,
2.69627684028872));
#244589=CARTESIAN_POINT('Ctrl Pts',(-19.3044519280753,59.7814166574713,
2.68224356036543));
#244590=CARTESIAN_POINT('Ctrl Pts',(-19.3552948408467,59.9049660265688,
2.59908178706424));
#244591=CARTESIAN_POINT('Ctrl Pts',(-19.3665789650877,59.8620777700636,
2.65878704321562));
#244592=CARTESIAN_POINT('Ctrl Pts',(-19.3574492964903,59.7910213450153,
2.65878198860303));
#244593=CARTESIAN_POINT('Ctrl Pts',(-19.4393816709759,59.8776671349986,
2.59908173516064));
#244594=CARTESIAN_POINT('Ctrl Pts',(-19.4278624395269,59.8421853116554,
2.65878198860302));
#244595=CARTESIAN_POINT('Ctrl Pts',(-19.4061247292256,59.7752282754838,
2.65878198860303));
#244596=CARTESIAN_POINT('Origin',(-19.0600454060089,59.6882395467421,2.83404198860304));
#244597=CARTESIAN_POINT('Origin',(-18.655940357667,56.3896289265487,3.11913648167136));
#244598=CARTESIAN_POINT('Origin',(-18.6008891789888,56.2201988201384,2.83404198860301));
#244599=CARTESIAN_POINT('Origin',(-19.0049943031078,59.5188096735657,3.11913648177589));
#244600=CARTESIAN_POINT('Origin',(-18.949943200106,59.3493798002281,3.40423097483351));
#244601=CARTESIAN_POINT('Ctrl Pts',(-18.5670586829468,56.1179479440989,
2.90134173516062));
#244602=CARTESIAN_POINT('Ctrl Pts',(-18.4469743395782,56.1574782858998,
2.90103711553268));
#244603=CARTESIAN_POINT('Ctrl Pts',(-18.4801050014193,56.259443978424,2.834041988603));
#244604=CARTESIAN_POINT('Ctrl Pts',(-18.5530176696412,56.0747358697604,
2.8286299174799));
#244605=CARTESIAN_POINT('Ctrl Pts',(-18.452151844104,56.1242410383984,2.85314045886485));
#244606=CARTESIAN_POINT('Ctrl Pts',(-18.4660639121463,56.2162299491243,
2.79187961000028));
#244607=CARTESIAN_POINT('Ctrl Pts',(-18.5135050040177,56.0391722633448,
2.75470625793378));
#244608=CARTESIAN_POINT('Ctrl Pts',(-18.4363793473475,56.0893377355419,
2.79224250381961));
#244609=CARTESIAN_POINT('Ctrl Pts',(-18.4371504234766,56.1772247439502,
2.74901809108305));
#244610=CARTESIAN_POINT('Ctrl Pts',(-18.3911086652348,56.0036796861847,
2.63947868311724));
#244611=CARTESIAN_POINT('Ctrl Pts',(-18.3580919822893,56.0516449414231,
2.69595066767933));
#244612=CARTESIAN_POINT('Ctrl Pts',(-18.3567819283755,56.1280773042133,
2.68220539436091));
#244613=CARTESIAN_POINT('Ctrl Pts',(-18.3056594201307,56.0051563026342,
2.59908178585092));
#244614=CARTESIAN_POINT('Ctrl Pts',(-18.2945198471559,56.0480033886673,
2.65877670944816));
#244615=CARTESIAN_POINT('Ctrl Pts',(-18.3039075553121,56.1189701685708,
2.658781988603));
#244616=CARTESIAN_POINT('Ctrl Pts',(-18.2220120550219,56.0323588238392,
2.59908173516062));
#244617=CARTESIAN_POINT('Ctrl Pts',(-18.233549049922,56.0678348753333,2.65878198860301));
#244618=CARTESIAN_POINT('Ctrl Pts',(-18.2553202812751,56.1347810195643,
2.658781988603));
#244619=CARTESIAN_POINT('Origin',(-18.2553202812751,56.1347810195643,2.531781988603));
#244620=CARTESIAN_POINT('Ctrl Pts',(-18.8168143322229,58.9396512752214,
3.77003198860304));
#244621=CARTESIAN_POINT('Ctrl Pts',(-18.9377789661744,58.900347483103,3.77003198860304));
#244622=CARTESIAN_POINT('Ctrl Pts',(-18.9375983751891,58.900406160671,3.642842387276));
#244623=CARTESIAN_POINT('Ctrl Pts',(-18.8836520326609,59.1460772043118,
3.77003198860304));
#244624=CARTESIAN_POINT('Ctrl Pts',(-19.0048864565378,59.1068814887035,
3.77025506105942));
#244625=CARTESIAN_POINT('Ctrl Pts',(-18.9912181986572,59.0654310094274,
3.64284210641963));
#244626=CARTESIAN_POINT('Ctrl Pts',(-18.9472825415244,59.3425907075099,
3.65553527987875));
#244627=CARTESIAN_POINT('Ctrl Pts',(-19.0687550219954,59.3034471832927,
3.65585996533051));
#244628=CARTESIAN_POINT('Ctrl Pts',(-19.042263347188,59.2225318234693,3.55127902710181));
#244629=CARTESIAN_POINT('Ctrl Pts',(-18.9827025415099,59.4519788726608,
3.47153072139112));
#244630=CARTESIAN_POINT('Ctrl Pts',(-19.104335033863,59.412950358033,3.47182327905229));
#244631=CARTESIAN_POINT('Ctrl Pts',(-19.0706774483339,59.3099814352092,
3.40413028378007));
#244632=CARTESIAN_POINT('Origin',(-18.8168143322229,58.9396512752214,3.64303198860304));
#244633=CARTESIAN_POINT('Origin',(3.93842937138093E-16,1.91633221102474E-13,
2.53178198860262));
#244634=CARTESIAN_POINT('Origin',(-18.2263320786585,56.1441998575529,2.531781988603));
#244635=CARTESIAN_POINT('Origin',(6.24367625034032,-18.1886080242679,3.6430319886025));
#244636=CARTESIAN_POINT('Origin',(-18.6927400943494,58.5579573083284,3.64299466007759));
#244637=CARTESIAN_POINT('Ctrl Pts',(-18.1930767435952,56.0417604764384,
2.59908173516062));
#244638=CARTESIAN_POINT('Ctrl Pts',(-18.2045954185348,56.0772424804485,
2.65878198860301));
#244639=CARTESIAN_POINT('Ctrl Pts',(-18.2263320786585,56.1441998575529,
2.658781988603));
#244640=CARTESIAN_POINT('Ctrl Pts',(-18.1097006409637,56.068827347073,2.5990819319998));
#244641=CARTESIAN_POINT('Ctrl Pts',(-18.1438516116621,56.0969586315483,
2.65877685806732));
#244642=CARTESIAN_POINT('Ctrl Pts',(-18.177896534026,56.1599138083643,2.658781988603));
#244643=CARTESIAN_POINT('Ctrl Pts',(-18.0401661963854,56.1172160917341,
2.63872492669835));
#244644=CARTESIAN_POINT('Ctrl Pts',(-18.0947679219784,56.1367924598138,
2.69532212015302));
#244645=CARTESIAN_POINT('Ctrl Pts',(-18.1406818860299,56.1978007560414,
2.68176836726667));
#244646=CARTESIAN_POINT('Ctrl Pts',(-17.9612165360192,56.2184352456066,
2.75442176402289));
#244647=CARTESIAN_POINT('Ctrl Pts',(-18.0530423367033,56.2137528851845,
2.7920317992019));
#244648=CARTESIAN_POINT('Ctrl Pts',(-18.1041286397845,56.2852436625536,
2.74885310748219));
#244649=CARTESIAN_POINT('Ctrl Pts',(-17.9502021467132,56.2706228600013,
2.82866089558439));
#244650=CARTESIAN_POINT('Ctrl Pts',(-18.0609092108088,56.2513800597978,
2.85316563119196));
#244651=CARTESIAN_POINT('Ctrl Pts',(-18.1037173431993,56.3339837785517,
2.79189751796651));
#244652=CARTESIAN_POINT('Ctrl Pts',(-17.9642361803975,56.3138168485096,
2.9013417351606));
#244653=CARTESIAN_POINT('Ctrl Pts',(-18.0846218068697,56.2752137607567,
2.90103711553267));
#244654=CARTESIAN_POINT('Ctrl Pts',(-18.1177524687109,56.3771794532808,
2.83404198860299));
#244655=CARTESIAN_POINT('Origin',(-17.9969682911414,56.4164246115665,2.834041988603));
#244656=CARTESIAN_POINT('Origin',(-18.6791227120619,58.5158800426281,3.56647653971818));
#244657=CARTESIAN_POINT('Origin',(-18.6538332760107,58.4380471616456,3.42473028058526));
#244658=CARTESIAN_POINT('Origin',(-18.0520194698684,56.5858547179441,3.11913648168137));
#244659=CARTESIAN_POINT('Origin',(-18.1070706485045,56.7552848242271,3.4042309748335));
#244660=CARTESIAN_POINT('Ctrl Pts',(-18.5518699907153,58.1242364370958,
3.36123028058522));
#244661=CARTESIAN_POINT('Ctrl Pts',(-18.6726541682848,58.0849912788101,
3.36123028058522));
#244662=CARTESIAN_POINT('Ctrl Pts',(-18.6726541682848,58.0849912788101,
3.23423028058522));
#244663=CARTESIAN_POINT('Ctrl Pts',(-18.5799074873338,58.2097691178806,
3.36123028058522));
#244664=CARTESIAN_POINT('Ctrl Pts',(-18.7004428147365,58.1705159385199,
3.36099641108529));
#244665=CARTESIAN_POINT('Ctrl Pts',(-18.7143758086138,58.2133972843944,
3.23423043688374));
#244666=CARTESIAN_POINT('Ctrl Pts',(-18.6064173144572,58.2906472745458,
3.41054258905323));
#244667=CARTESIAN_POINT('Ctrl Pts',(-18.7268501353369,58.2517893143872,
3.41008815826052));
#244668=CARTESIAN_POINT('Ctrl Pts',(-18.7538265876733,58.3348142976348,
3.30819867304345));
#244669=CARTESIAN_POINT('Ctrl Pts',(-18.620387828115,58.3332704847797,3.48823028058524));
#244670=CARTESIAN_POINT('Ctrl Pts',(-18.7407822670305,58.2946680067389,
3.4879469194164));
#244671=CARTESIAN_POINT('Ctrl Pts',(-18.7746174535802,58.3988020033599,
3.42473028058525));
#244672=CARTESIAN_POINT('Origin',(-18.5518699907153,58.1242364370958,3.23423028058522));
#244673=CARTESIAN_POINT('Ctrl Pts',(-18.0743352474894,56.6526781108325,
3.47153072139111));
#244674=CARTESIAN_POINT('Ctrl Pts',(-18.1949031876636,56.6140134955963,
3.47122746285116));
#244675=CARTESIAN_POINT('Ctrl Pts',(-18.227904394985,56.7161926816712,3.40413046676836));
#244676=CARTESIAN_POINT('Ctrl Pts',(-18.1097491035603,56.7620702268162,
3.65553813458026));
#244677=CARTESIAN_POINT('Ctrl Pts',(-18.2303840130631,56.7232113603728,
3.65520336072152));
#244678=CARTESIAN_POINT('Ctrl Pts',(-18.2563190096467,56.803643873878,3.55128134519884));
#244679=CARTESIAN_POINT('Ctrl Pts',(-18.1733695596533,56.9585888550844,
3.77003198860302));
#244680=CARTESIAN_POINT('Ctrl Pts',(-18.2941747571319,56.9195374698037,
3.76980209314226));
#244681=CARTESIAN_POINT('Ctrl Pts',(-18.3073645871833,56.9607460083081,
3.64284195387558));
#244682=CARTESIAN_POINT('Ctrl Pts',(-18.2401996527048,57.1650137687748,
3.77003198860302));
#244683=CARTESIAN_POINT('Ctrl Pts',(-18.3611647564557,57.1257098240093,
3.77003198860303));
#244684=CARTESIAN_POINT('Ctrl Pts',(-18.3609836949697,57.1257686544523,
3.64284189403859));
#244685=CARTESIAN_POINT('Origin',(-18.2401996527048,57.1650137687748,3.64303198860302));
#244686=CARTESIAN_POINT('Origin',(6.09975091006211,-17.7456513739113,3.23423028058469));
#244687=CARTESIAN_POINT('Origin',(-18.5051441132844,57.9804289733665,3.23423028058522));
#244688=CARTESIAN_POINT('Origin',(6.07721283595922,-17.6762863142852,3.6430319886025));
#244689=CARTESIAN_POINT('Origin',(-18.3641788932754,57.5467470426661,3.64299171721799));
#244690=CARTESIAN_POINT('Ctrl Pts',(-18.4366189870675,57.7713971777988,
3.48823028058521));
#244691=CARTESIAN_POINT('Ctrl Pts',(-18.5581069080663,57.7324510618071,
3.48852004212298));
#244692=CARTESIAN_POINT('Ctrl Pts',(-18.523964983701,57.6273730232606,3.4247302805852));
#244693=CARTESIAN_POINT('Ctrl Pts',(-18.450639415372,57.8141635875299,3.4102800584845));
#244694=CARTESIAN_POINT('Ctrl Pts',(-18.5719407253105,57.7750271733958,
3.41074404220504));
#244695=CARTESIAN_POINT('Ctrl Pts',(-18.5448261124707,57.691576975842,3.30780486244105));
#244696=CARTESIAN_POINT('Ctrl Pts',(-18.4772005006358,57.8951845615414,
3.36123028058522));
#244697=CARTESIAN_POINT('Ctrl Pts',(-18.5981804828652,57.855784843245,3.36146460586404));
#244698=CARTESIAN_POINT('Ctrl Pts',(-18.584347180845,57.813210317349,3.23423045308373));
#244699=CARTESIAN_POINT('Ctrl Pts',(-18.5051441132844,57.9804289733665,
3.36123028058522));
#244700=CARTESIAN_POINT('Ctrl Pts',(-18.6259282908539,57.9411838150808,
3.36123028058522));
#244701=CARTESIAN_POINT('Ctrl Pts',(-18.6259282908539,57.9411838150808,
3.23423028058522));
#244702=CARTESIAN_POINT('Origin',(-18.4031808061315,57.6666181815462,3.42473028058521));
#244703=CARTESIAN_POINT('Origin',(-18.3780421908669,57.5892494801769,3.56563113524799));
#244704=CARTESIAN_POINT('Origin',(-25.2734729067966,55.9845461696125,3.56647653909435));
#244705=CARTESIAN_POINT('Origin',(-25.2915084057495,56.0249274780519,3.64299466007493));
#244706=CARTESIAN_POINT('Origin',(-25.2401862573144,55.9097831300747,3.42473028058522));
#244707=CARTESIAN_POINT('Ctrl Pts',(-25.1949317875303,55.8095395120008,
3.48823028058522));
#244708=CARTESIAN_POINT('Ctrl Pts',(-25.0796311836956,55.8614118841079,
3.48794691941638));
#244709=CARTESIAN_POINT('Ctrl Pts',(-25.1241659841938,55.9614386837454,
3.42473028058523));
#244710=CARTESIAN_POINT('Ctrl Pts',(-25.1767321129103,55.7683775656463,
3.41028005925127));
#244711=CARTESIAN_POINT('Ctrl Pts',(-25.0612313830298,55.8200852551871,
3.40982512230946));
#244712=CARTESIAN_POINT('Ctrl Pts',(-25.0967080045987,55.8997670518378,
3.30780486372847));
#244713=CARTESIAN_POINT('Ctrl Pts',(-25.1422534028245,55.6903961807898,
3.3612302805852));
#244714=CARTESIAN_POINT('Ctrl Pts',(-25.0264120100478,55.741879663018,3.36099721048499));
#244715=CARTESIAN_POINT('Ctrl Pts',(-25.0446893032921,55.7829311357722,
3.23423045308483));
#244716=CARTESIAN_POINT('Ctrl Pts',(-25.1059793847704,55.6083495590302,
3.3612302805852));
#244717=CARTESIAN_POINT('Ctrl Pts',(-24.9899591116498,55.6600051127008,
3.3612302805852));
#244718=CARTESIAN_POINT('Ctrl Pts',(-24.9899591116498,55.6600051127009,
3.2342302805852));
#244719=CARTESIAN_POINT('Origin',(-25.1059793847704,55.6083495590302,3.2342302805852));
#244720=CARTESIAN_POINT('Origin',(-0.29005068280152,-0.129138884176384,
3.64303198860263));
#244721=CARTESIAN_POINT('Origin',(-25.4547063934086,56.3916032444851,3.64303198860301));
#244722=CARTESIAN_POINT('Origin',(-0.29005068280152,-0.129138884176381,
3.23423028058481));
#244723=CARTESIAN_POINT('Origin',(-25.044477503395,55.4702140717967,3.2342302805852));
#244724=CARTESIAN_POINT('Ctrl Pts',(-25.6742415049982,56.8833377255395,
3.47153072139111));
#244725=CARTESIAN_POINT('Ctrl Pts',(-25.5577357840968,56.9357219056861,
3.47182327902701));
#244726=CARTESIAN_POINT('Ctrl Pts',(-25.5138485805638,56.8366797759151,
3.40413028959052));
#244727=CARTESIAN_POINT('Ctrl Pts',(-25.6273680143746,56.7783442778553,
3.65553807120996));
#244728=CARTESIAN_POINT('Ctrl Pts',(-25.5109042502522,56.8305359187867,
3.65586275497023));
#244729=CARTESIAN_POINT('Ctrl Pts',(-25.4764485929327,56.7526780286707,
3.55128126837251));
#244730=CARTESIAN_POINT('Ctrl Pts',(-25.5431608329951,56.5897276738853,
3.77003198860302));
#244731=CARTESIAN_POINT('Ctrl Pts',(-25.4268390553461,56.6417212312926,
3.7702550574865));
#244732=CARTESIAN_POINT('Ctrl Pts',(-25.409261035753,56.6017723050706,3.64284211731288));
#244733=CARTESIAN_POINT('Ctrl Pts',(-25.4547063934086,56.3916032444851,
3.77003198860302));
#244734=CARTESIAN_POINT('Ctrl Pts',(-25.3385127913796,56.4433359691578,
3.77003198860302));
#244735=CARTESIAN_POINT('Ctrl Pts',(-25.3386862495673,56.4432587405969,
3.6428423982171));
#244736=CARTESIAN_POINT('Origin',(-25.6299342604998,56.7851714777848,3.40423097483349));
#244737=CARTESIAN_POINT('Ctrl Pts',(-25.044477503395,55.4702140717967,3.3612302805852));
#244738=CARTESIAN_POINT('Ctrl Pts',(-24.9284572302744,55.5218696254674,
3.3612302805852));
#244739=CARTESIAN_POINT('Ctrl Pts',(-24.9284572302744,55.5218696254674,
3.2342302805852));
#244740=CARTESIAN_POINT('Ctrl Pts',(-25.008081415906,55.38788990767,3.3612302805852));
#244741=CARTESIAN_POINT('Ctrl Pts',(-24.8918114493206,55.4395618538373,
3.36146538610207));
#244742=CARTESIAN_POINT('Ctrl Pts',(-24.8735420580978,55.3985281293134,
3.234230436885));
#244743=CARTESIAN_POINT('Ctrl Pts',(-24.9736678430969,55.310045415862,3.41054258693138));
#244744=CARTESIAN_POINT('Ctrl Pts',(-24.8573359723256,55.3621286647047,
3.41100608859807));
#244745=CARTESIAN_POINT('Ctrl Pts',(-24.8216158475502,55.281899950894,3.30819866970868));
#244746=CARTESIAN_POINT('Ctrl Pts',(-24.9555320242418,55.2690209153041,
3.48823028058519));
#244747=CARTESIAN_POINT('Ctrl Pts',(-24.8391888661847,55.3213695969756,
3.48852004212297));
#244748=CARTESIAN_POINT('Ctrl Pts',(-24.794250328961,55.2204359898057,3.42473028058518));
#244749=CARTESIAN_POINT('Origin',(-24.9102706020816,55.1687804361351,3.42473028058517));
#244750=CARTESIAN_POINT('Origin',(-25.7023940320541,56.9479187893831,3.11913648178511));
#244751=CARTESIAN_POINT('Origin',(-25.774853803565,57.1106661007666,2.83404198860301));
#244752=CARTESIAN_POINT('Origin',(-24.8771824671419,55.0944632682977,3.56563113460869));
#244753=CARTESIAN_POINT('Origin',(-24.8590452239605,55.0536014459536,3.64299171721809));
#244754=CARTESIAN_POINT('Ctrl Pts',(-25.61970381813,57.5052637377733,2.59908173516063));
#244755=CARTESIAN_POINT('Ctrl Pts',(-25.6045223014064,57.471187734033,2.65878198860301));
#244756=CARTESIAN_POINT('Ctrl Pts',(-25.5758735661211,57.406883591798,2.65878198860301));
#244757=CARTESIAN_POINT('Ctrl Pts',(-25.7001924885134,57.4694043465871,
2.59908193475586));
#244758=CARTESIAN_POINT('Ctrl Pts',(-25.6631501095125,57.4450643815424,
2.65878715325347));
#244759=CARTESIAN_POINT('Ctrl Pts',(-25.6224598624455,57.3861185493459,
2.65878198860301));
#244760=CARTESIAN_POINT('Ctrl Pts',(-25.7642825572405,57.4134642487753,
2.63878778849914));
#244761=CARTESIAN_POINT('Ctrl Pts',(-25.7077329912391,57.3998804953988,
2.69564460180175));
#244762=CARTESIAN_POINT('Ctrl Pts',(-25.6552692732808,57.3441059191832,
2.68180481624934));
#244763=CARTESIAN_POINT('Ctrl Pts',(-25.8321626496791,57.3036982377904,
2.7544323887868));
#244764=CARTESIAN_POINT('Ctrl Pts',(-25.7409042554409,57.3186021074456,
2.792683407771));
#244765=CARTESIAN_POINT('Ctrl Pts',(-25.6821129719827,57.2526112478171,
2.74885926835637));
#244766=CARTESIAN_POINT('Ctrl Pts',(-25.8376543496551,57.2503778226941,
2.82856655361711));
#244767=CARTESIAN_POINT('Ctrl Pts',(-25.7289491719114,57.2821097063804,
2.85384197230861));
#244768=CARTESIAN_POINT('Ctrl Pts',(-25.6773293952369,57.2038640469265,
2.79184624278536));
#244769=CARTESIAN_POINT('Ctrl Pts',(-25.8191582032623,57.2088336324699,
2.90134173516062));
#244770=CARTESIAN_POINT('Ctrl Pts',(-25.7028284190336,57.2611357920725,
2.9016321871643));
#244771=CARTESIAN_POINT('Ctrl Pts',(-25.6588335304443,57.1623216544372,
2.83404198860301));
#244772=CARTESIAN_POINT('Origin',(-25.5758735661211,57.406883591798,2.531781988603));
#244773=CARTESIAN_POINT('Origin',(-0.29005068280152,-0.129138884176384,
3.64303198860263));
#244774=CARTESIAN_POINT('Origin',(-24.695750338031,54.6869600343298,3.643031988603));
#244775=CARTESIAN_POINT('Origin',(3.68589728140384E-17,1.91426800607079E-13,
2.53178198860262));
#244776=CARTESIAN_POINT('Origin',(-25.5480287005721,57.419280924679,2.53178198860301));
#244777=CARTESIAN_POINT('Ctrl Pts',(-24.695750338031,54.6869600343298,3.77003198860301));
#244778=CARTESIAN_POINT('Ctrl Pts',(-24.5795562613022,54.7386929703524,
3.77003198860301));
#244779=CARTESIAN_POINT('Ctrl Pts',(-24.5797301948983,54.7386155301261,
3.64284187937088));
#244780=CARTESIAN_POINT('Ctrl Pts',(-24.6072881749585,54.4888352915936,
3.770031988603));
#244781=CARTESIAN_POINT('Ctrl Pts',(-24.4913819335251,54.5406489234201,
3.7698020896306));
#244782=CARTESIAN_POINT('Ctrl Pts',(-24.5091541605498,54.5800991622551,
3.64284193928419));
#244783=CARTESIAN_POINT('Ctrl Pts',(-24.5230714236766,54.3002245846703,
3.65553535416623));
#244784=CARTESIAN_POINT('Ctrl Pts',(-24.40742054685,54.352067335487,3.65520057834444));
#244785=CARTESIAN_POINT('Ctrl Pts',(-24.4419671033163,54.4291945615863,
3.55127910964207));
#244786=CARTESIAN_POINT('Ctrl Pts',(-24.4761921430394,54.1952354911873,
3.47153072139109));
#244787=CARTESIAN_POINT('Ctrl Pts',(-24.3607210114368,54.2471777873471,
3.47122746281619));
#244788=CARTESIAN_POINT('Ctrl Pts',(-24.4045675740909,54.3451938439592,
3.40413045901312));
#244789=CARTESIAN_POINT('Origin',(-24.5205222915154,54.2933913980364,3.40423097483348));
#244790=CARTESIAN_POINT('Ctrl Pts',(-25.2380597013433,57.4675553545141,
2.90134173516062));
#244791=CARTESIAN_POINT('Ctrl Pts',(-25.3547675996718,57.4161024530844,
2.9016321871643));
#244792=CARTESIAN_POINT('Ctrl Pts',(-25.3107727110825,57.3172883154491,
2.83404198860301));
#244793=CARTESIAN_POINT('Ctrl Pts',(-25.2565651278915,57.5091180232692,
2.82853349835384));
#244794=CARTESIAN_POINT('Ctrl Pts',(-25.352874997054,57.4495672328903,2.8538148316236));
#244795=CARTESIAN_POINT('Ctrl Pts',(-25.3292770036983,57.3588496371392,
2.79182701594351));
#244796=CARTESIAN_POINT('Ctrl Pts',(-25.299797277006,57.5405471770609,2.75468822073698));
#244797=CARTESIAN_POINT('Ctrl Pts',(-25.3720159720864,57.4827148996386,
2.79286913083892));
#244798=CARTESIAN_POINT('Ctrl Pts',(-25.3622324578622,57.3948558336733,
2.7490076329796));
#244799=CARTESIAN_POINT('Ctrl Pts',(-25.4257977880273,57.5636463159496,
2.63954450640416));
#244800=CARTESIAN_POINT('Ctrl Pts',(-25.4538910783598,57.5124644612013,
2.69627684028882));
#244801=CARTESIAN_POINT('Ctrl Pts',(-25.447559735724,57.4360631077224,2.68224356036522));
#244802=CARTESIAN_POINT('Ctrl Pts',(-25.5110385513887,57.553621128909,2.59908178706464));
#244803=CARTESIAN_POINT('Ctrl Pts',(-25.5177778164714,57.5097883065936,
2.65878704321651));
#244804=CARTESIAN_POINT('Ctrl Pts',(-25.5012707422378,57.4400754463041,
2.65878198860301));
#244805=CARTESIAN_POINT('Ctrl Pts',(-25.5918112338797,57.5176823163889,
2.59908173516063));
#244806=CARTESIAN_POINT('Ctrl Pts',(-25.5766462455179,57.4835989537478,
2.658781988603));
#244807=CARTESIAN_POINT('Ctrl Pts',(-25.5480287005721,57.419280924679,2.65878198860301));
#244808=CARTESIAN_POINT('Origin',(-25.1947524379619,57.3689438691197,2.83404198860301));
#244809=CARTESIAN_POINT('Origin',(-24.448062420315,54.1306438627484,3.11913648166798));
#244810=CARTESIAN_POINT('Origin',(-24.3756025490941,53.9678963272935,2.83404198860299));
#244811=CARTESIAN_POINT('Origin',(-25.1222926664895,57.2061965577035,3.11913648177619));
#244812=CARTESIAN_POINT('Origin',(-25.0498328948967,57.0434492461379,3.40423097483349));
#244813=CARTESIAN_POINT('Ctrl Pts',(-24.331269253109,53.8697418420146,2.9013417351606));
#244814=CARTESIAN_POINT('Ctrl Pts',(-24.2159747902189,53.9216078643418,
2.90103711553266));
#244815=CARTESIAN_POINT('Ctrl Pts',(-24.2595822759735,54.0195518809642,
2.83404198860299));
#244816=CARTESIAN_POINT('Ctrl Pts',(-24.3127882662189,53.8282341734839,
2.82862991747986));
#244817=CARTESIAN_POINT('Ctrl Pts',(-24.2176496934283,53.8880114973694,
2.85314045886434));
#244818=CARTESIAN_POINT('Ctrl Pts',(-24.2411010091826,53.9780422761234,
2.79187960999972));
#244819=CARTESIAN_POINT('Ctrl Pts',(-24.2697746459842,53.796995586443,2.7547062579338));
#244820=CARTESIAN_POINT('Ctrl Pts',(-24.1983152114491,53.8549480733042,
2.79224250381927));
#244821=CARTESIAN_POINT('Ctrl Pts',(-24.2082687574725,53.9422730280822,
2.7490180910829));
#244822=CARTESIAN_POINT('Ctrl Pts',(-24.1443388226041,53.7744913425365,
2.63947868311718));
#244823=CARTESIAN_POINT('Ctrl Pts',(-24.1165167429224,53.8256450222191,
2.69595066767952));
#244824=CARTESIAN_POINT('Ctrl Pts',(-24.1232032230476,53.9017956184506,
2.68220539436103));
#244825=CARTESIAN_POINT('Ctrl Pts',(-24.0595120258535,53.7848917482051,
2.59908178585127));
#244826=CARTESIAN_POINT('Ctrl Pts',(-24.0529122166851,53.8286685158653,
2.65877670944914));
#244827=CARTESIAN_POINT('Ctrl Pts',(-24.0696665464387,53.8982652496131,
2.65878198860299));
#244828=CARTESIAN_POINT('Ctrl Pts',(-23.9791663275016,53.8206887816837,
2.5990817351606));
#244829=CARTESIAN_POINT('Ctrl Pts',(-23.994348378682,53.8547645473082,2.65878198860299));
#244830=CARTESIAN_POINT('Ctrl Pts',(-24.0229981225299,53.9190682401996,
2.65878198860299));
#244831=CARTESIAN_POINT('Origin',(-24.0229981225299,53.9190682401996,2.53178198860299));
#244832=CARTESIAN_POINT('Ctrl Pts',(-24.8746050278055,56.6498810128383,
3.77003198860302));
#244833=CARTESIAN_POINT('Ctrl Pts',(-24.9907986398446,56.5981482837088,
3.77003198860302));
#244834=CARTESIAN_POINT('Ctrl Pts',(-24.9906251716318,56.5982255167332,
3.64284238727605));
#244835=CARTESIAN_POINT('Ctrl Pts',(-24.9626539694726,56.8481896769757,
3.77003198860302));
#244836=CARTESIAN_POINT('Ctrl Pts',(-25.0791271905709,56.7965362315773,
3.77025506105699));
#244837=CARTESIAN_POINT('Ctrl Pts',(-25.0612010539378,56.7567415443529,
3.6428421064198));
#244838=CARTESIAN_POINT('Ctrl Pts',(-25.0464771582518,57.0369754593331,
3.6555352798787));
#244839=CARTESIAN_POINT('Ctrl Pts',(-25.1631925873306,56.9853490357227,
3.65585996533181));
#244840=CARTESIAN_POINT('Ctrl Pts',(-25.1283880784745,56.9076460727658,
3.5512790271019));
#244841=CARTESIAN_POINT('Ctrl Pts',(-25.0931373005748,57.1420619865022,
3.47153072139112));
#244842=CARTESIAN_POINT('Ctrl Pts',(-25.2100238867504,57.090533216652,3.47182327905228));
#244843=CARTESIAN_POINT('Ctrl Pts',(-25.1657874977295,56.991646544054,3.4041302837801));
#244844=CARTESIAN_POINT('Origin',(-24.8746050278055,56.6498810128383,3.64303198860302));
#244845=CARTESIAN_POINT('Origin',(3.8811097157961E-16,1.91631020807046E-13,
2.53178198860262));
#244846=CARTESIAN_POINT('Origin',(-23.995153256981,53.9314655730805,2.531781988603));
#244847=CARTESIAN_POINT('Origin',(10.5838037820519,-22.9910091182298,3.64303198860247));
#244848=CARTESIAN_POINT('Origin',(-24.7113125977919,56.2832472948497,3.64299466007609));
#244849=CARTESIAN_POINT('Ctrl Pts',(-23.9513722670367,53.8330634946838,
2.5990817351606));
#244850=CARTESIAN_POINT('Ctrl Pts',(-23.9665367208226,53.8671470951731,
2.65878198860298));
#244851=CARTESIAN_POINT('Ctrl Pts',(-23.995153256981,53.9314655730805,2.65878198860299));
#244852=CARTESIAN_POINT('Ctrl Pts',(-23.8712821658121,53.8686972660502,
2.5990819319995));
#244853=CARTESIAN_POINT('Ctrl Pts',(-23.9081865738555,53.8931046959191,
2.65877685806726));
#244854=CARTESIAN_POINT('Ctrl Pts',(-23.9486256024603,53.9521563342736,
2.65878198860299));
#244855=CARTESIAN_POINT('Ctrl Pts',(-23.8071866393157,53.9240892607411,
2.6387249266983));
#244856=CARTESIAN_POINT('Ctrl Pts',(-23.8635355386145,53.9378509529601,
2.69532212015307));
#244857=CARTESIAN_POINT('Ctrl Pts',(-23.915575084618,53.9937257232528,2.68176836726675));
#244858=CARTESIAN_POINT('Ctrl Pts',(-23.7392497560571,54.0330064121716,
2.75442176402291));
#244859=CARTESIAN_POINT('Ctrl Pts',(-23.8300830854579,54.0187512923761,
2.7920317992018));
#244860=CARTESIAN_POINT('Ctrl Pts',(-23.8883623535218,54.0845104630314,
2.74885310748208));
#244861=CARTESIAN_POINT('Ctrl Pts',(-23.7337507958627,54.086059454542,2.82866089558432));
#244862=CARTESIAN_POINT('Ctrl Pts',(-23.8418399747444,54.0553500291281,
2.85316563119161));
#244863=CARTESIAN_POINT('Ctrl Pts',(-23.8930480394869,54.1330265677741,
2.79189751796665));
#244864=CARTESIAN_POINT('Ctrl Pts',(-23.752222950883,54.1275498658874,2.90134173516061));
#244865=CARTESIAN_POINT('Ctrl Pts',(-23.8679139708571,54.0765745253537,
2.90103711553267));
#244866=CARTESIAN_POINT('Ctrl Pts',(-23.9115214566117,54.174518541976,2.83404198860299));
#244867=CARTESIAN_POINT('Origin',(-23.7955011834911,54.2261740956467,2.83404198860299));
#244868=CARTESIAN_POINT('Origin',(-24.6933715410266,56.2428239368568,3.56647653971843));
#244869=CARTESIAN_POINT('Origin',(-24.6600848917114,56.1680608984279,3.42473028058524));
#244870=CARTESIAN_POINT('Origin',(-23.8679610547528,54.3889216310619,3.11913648168028));
#244871=CARTESIAN_POINT('Origin',(-23.9404209259123,54.5516691663896,3.40423097483349));
#244872=CARTESIAN_POINT('Ctrl Pts',(-24.5258780191674,55.8666273273834,
3.3612302805852));
#244873=CARTESIAN_POINT('Ctrl Pts',(-24.641898292288,55.8149717737127,3.3612302805852));
#244874=CARTESIAN_POINT('Ctrl Pts',(-24.641898292288,55.8149717737127,3.2342302805852));
#244875=CARTESIAN_POINT('Ctrl Pts',(-24.5627025231274,55.948760734758,3.3612302805852));
#244876=CARTESIAN_POINT('Ctrl Pts',(-24.6784744708784,55.8971232158773,
3.36099641108608));
#244877=CARTESIAN_POINT('Ctrl Pts',(-24.6968134595438,55.9383132588145,
3.23423043688449));
#244878=CARTESIAN_POINT('Ctrl Pts',(-24.5975211960717,56.0264248009281,
3.41054258905324));
#244879=CARTESIAN_POINT('Ctrl Pts',(-24.7132325104962,55.9751910510484,
3.41008815825971));
#244880=CARTESIAN_POINT('Ctrl Pts',(-24.7487396569165,56.0549414076424,
3.3081986730429));
#244881=CARTESIAN_POINT('Ctrl Pts',(-24.6158705164596,56.0673542004327,
3.48823028058522));
#244882=CARTESIAN_POINT('Ctrl Pts',(-24.7315703643338,56.0163785451198,
3.48794691941638));
#244883=CARTESIAN_POINT('Ctrl Pts',(-24.776105164832,56.1164053447573,3.42473028058524));
#244884=CARTESIAN_POINT('Origin',(-24.5258780191674,55.8666273273834,3.2342302805852));
#244885=CARTESIAN_POINT('Ctrl Pts',(-23.8971395307771,54.4530463244693,
3.4715307213911));
#244886=CARTESIAN_POINT('Ctrl Pts',(-24.0130054343467,54.4019907365351,
3.47122746285114));
#244887=CARTESIAN_POINT('Ctrl Pts',(-24.0565064908996,54.5001606088507,
3.40413046676809));
#244888=CARTESIAN_POINT('Ctrl Pts',(-23.943793975817,54.558137423042,3.65553813458026));
#244889=CARTESIAN_POINT('Ctrl Pts',(-24.0597061770712,54.5068816478237,
3.65520336072303));
#244890=CARTESIAN_POINT('Ctrl Pts',(-24.0939065860602,54.5841625982689,
3.55128134519959));
#244891=CARTESIAN_POINT('Ctrl Pts',(-24.0276077026098,54.7469293531954,
3.770031988603));
#244892=CARTESIAN_POINT('Ctrl Pts',(-24.1436691352855,54.6954643138445,
3.76980209314153));
#244893=CARTESIAN_POINT('Ctrl Pts',(-24.161094175272,54.7350683949965,3.64284195387456));
#244894=CARTESIAN_POINT('Ctrl Pts',(-24.1156489724279,54.9452378026829,
3.77003198860301));
#244895=CARTESIAN_POINT('Ctrl Pts',(-24.2318430357374,54.893504872635,3.77003198860301));
#244896=CARTESIAN_POINT('Ctrl Pts',(-24.2316691155806,54.8935823068777,
3.6428418940381));
#244897=CARTESIAN_POINT('Origin',(-24.1156489724279,54.9452378026829,3.64303198860301));
#244898=CARTESIAN_POINT('Origin',(10.3344596589369,-22.4309730483566,3.23423028058466));
#244899=CARTESIAN_POINT('Origin',(-24.4643761377919,55.7284918401499,3.2342302805852));
#244900=CARTESIAN_POINT('Origin',(10.2954134679533,-22.3432738675265,3.64303198860247));
#244901=CARTESIAN_POINT('Origin',(-24.2788510342447,55.3119205422646,3.64299171721813));
#244902=CARTESIAN_POINT('Ctrl Pts',(-24.3743766270216,55.5277679687684,
3.4882302805852));
#244903=CARTESIAN_POINT('Ctrl Pts',(-24.4911280468228,55.4763362579875,
3.48852004212298));
#244904=CARTESIAN_POINT('Ctrl Pts',(-24.4461895095991,55.3754026508176,
3.42473028058519));
#244905=CARTESIAN_POINT('Ctrl Pts',(-24.3927905570427,55.5688345658067,
3.41028005848444));
#244906=CARTESIAN_POINT('Ctrl Pts',(-24.5093364964839,55.5172331055217,
3.41074404220413));
#244907=CARTESIAN_POINT('Ctrl Pts',(-24.4736474994205,55.4370743056939,
3.30780486243907));
#244908=CARTESIAN_POINT('Ctrl Pts',(-24.4276751358083,55.6466353090197,
3.3612302805852));
#244909=CARTESIAN_POINT('Ctrl Pts',(-24.5438739850314,55.5948055748758,
3.36146460586418));
#244910=CARTESIAN_POINT('Ctrl Pts',(-24.525666213519,55.5539102504903,3.23423045308528));
#244911=CARTESIAN_POINT('Ctrl Pts',(-24.4643761377919,55.7284918401499,
3.3612302805852));
#244912=CARTESIAN_POINT('Ctrl Pts',(-24.5803964109126,55.6768362864793,
3.36123028058519));
#244913=CARTESIAN_POINT('Ctrl Pts',(-24.5803964109126,55.6768362864792,
3.2342302805852));
#244914=CARTESIAN_POINT('Origin',(-24.3301692364785,55.4270582044882,3.42473028058519));
#244915=CARTESIAN_POINT('Origin',(-24.2970811017194,55.3527410377817,3.56563113524755));
#244916=CARTESIAN_POINT('Origin',(-30.9870007556519,53.0360596835511,3.56647653909477));
#244917=CARTESIAN_POINT('Origin',(-31.0091584503732,53.0743345559675,3.64299466007354));
#244918=CARTESIAN_POINT('Origin',(-30.9460815882871,52.9651856060846,3.4247302805852));
#244919=CARTESIAN_POINT('Ctrl Pts',(-30.8905967158739,52.8702215132216,
3.4882302805852));
#244920=CARTESIAN_POINT('Ctrl Pts',(-30.7813498801535,52.9338619179796,
3.48794691941636));
#244921=CARTESIAN_POINT('Ctrl Pts',(-30.8360963620065,53.0286856060846,
3.42473028058521));
#244922=CARTESIAN_POINT('Ctrl Pts',(-30.8681941459792,52.8311874403356,
3.41028005925123));
#244923=CARTESIAN_POINT('Ctrl Pts',(-30.7587310665078,52.89468498354,3.40982512231133));
#244924=CARTESIAN_POINT('Ctrl Pts',(-30.8023423591859,52.9702219582407,
3.3078048637286));
#244925=CARTESIAN_POINT('Ctrl Pts',(-30.8257530395495,52.757237252247,3.36123028058518));
#244926=CARTESIAN_POINT('Ctrl Pts',(-30.7159277273256,52.8205474253446,
3.36099721048368));
#244927=CARTESIAN_POINT('Ctrl Pts',(-30.7383959430073,52.8594635164573,
3.23423045308469));
#244928=CARTESIAN_POINT('Ctrl Pts',(-30.7811015270746,52.6794317578288,
3.36123028058517));
#244929=CARTESIAN_POINT('Ctrl Pts',(-30.671116300794,52.7429317578288,3.36123028058517));
#244930=CARTESIAN_POINT('Ctrl Pts',(-30.671116300794,52.7429317578288,3.23423028058518));
#244931=CARTESIAN_POINT('Origin',(-30.7811015270746,52.6794317578288,3.23423028058517));
#244932=CARTESIAN_POINT('Origin',(-0.274963065701553,-0.158749999999817,
3.64303198860263));
#244933=CARTESIAN_POINT('Origin',(-31.2097904767608,53.4219427993287,3.64303198860299));
#244934=CARTESIAN_POINT('Origin',(-0.274963065701553,-0.158749999999815,
3.23423028058481));
#244935=CARTESIAN_POINT('Origin',(-30.7054974692372,52.5484816883959,3.23423028058517));
#244936=CARTESIAN_POINT('Ctrl Pts',(-31.4795232016792,53.8880358395971,
3.47153072139108));
#244937=CARTESIAN_POINT('Ctrl Pts',(-31.3691313491574,53.9523112176915,
3.47182327902699));
#244938=CARTESIAN_POINT('Ctrl Pts',(-31.3151318426936,53.8583991130128,
3.40413028959054));
#244939=CARTESIAN_POINT('Ctrl Pts',(-31.4219316852005,53.7885171709487,
3.65553807120994));
#244940=CARTESIAN_POINT('Ctrl Pts',(-31.3115614337831,53.8525966788921,
3.65586275496921));
#244941=CARTESIAN_POINT('Ctrl Pts',(-31.2691561625559,53.7787668993609,
3.55128126837211));
#244942=CARTESIAN_POINT('Ctrl Pts',(-31.3184699958136,53.6097358757351,
3.770031988603));
#244943=CARTESIAN_POINT('Ctrl Pts',(-31.2082202476926,53.6736035436622,
3.77025505748471));
#244944=CARTESIAN_POINT('Ctrl Pts',(-31.1865627224596,53.6357108652094,
3.64284211731288));
#244945=CARTESIAN_POINT('Ctrl Pts',(-31.2097904767608,53.4219427993287,
3.770031988603));
#244946=CARTESIAN_POINT('Ctrl Pts',(-31.099640937652,53.4855376653843,3.770031988603));
#244947=CARTESIAN_POINT('Ctrl Pts',(-31.0998053730349,53.4854427285717,
3.64284239821717));
#244948=CARTESIAN_POINT('Origin',(-31.4251975098795,53.7950387249979,3.40423097483346));
#244949=CARTESIAN_POINT('Ctrl Pts',(-30.7054974692372,52.548481688396,3.36123028058517));
#244950=CARTESIAN_POINT('Ctrl Pts',(-30.5955122429565,52.611981688396,3.36123028058518));
#244951=CARTESIAN_POINT('Ctrl Pts',(-30.5955122429565,52.611981688396,3.23423028058518));
#244952=CARTESIAN_POINT('Ctrl Pts',(-30.6606955449566,52.4704129317487,
3.36123028058518));
#244953=CARTESIAN_POINT('Ctrl Pts',(-30.550463706539,52.5339553345181,3.36146538610162));
#244954=CARTESIAN_POINT('Ctrl Pts',(-30.5280052047886,52.4950560684206,
3.23423043688486));
#244955=CARTESIAN_POINT('Ctrl Pts',(-30.6183335281992,52.3965920780923,
3.41054258693136));
#244956=CARTESIAN_POINT('Ctrl Pts',(-30.5080831175509,52.460550001133,3.41100608859922));
#244957=CARTESIAN_POINT('Ctrl Pts',(-30.4641724871923,52.3844945583586,
3.30819866970894));
#244958=CARTESIAN_POINT('Ctrl Pts',(-30.5960088312571,52.3576880233162,
3.48823028058517));
#244959=CARTESIAN_POINT('Ctrl Pts',(-30.4857749404422,52.4219111049557,
3.48852004212295));
#244960=CARTESIAN_POINT('Ctrl Pts',(-30.4305321463779,52.3262277788842,
3.42473028058517));
#244961=CARTESIAN_POINT('Origin',(-30.5405173726585,52.2627277788841,3.42473028058517));
#244962=CARTESIAN_POINT('Origin',(-31.5142720656054,53.9493203812247,3.11913648178448));
#244963=CARTESIAN_POINT('Origin',(-31.6033466212668,54.1036020372439,2.83404198860299));
#244964=CARTESIAN_POINT('Origin',(-30.4998422386358,52.1922763801653,3.56563113460844));
#244965=CARTESIAN_POINT('Origin',(-30.4775331296739,52.1535342613182,3.64299171721854));
#244966=CARTESIAN_POINT('Ctrl Pts',(-31.490293248291,54.5122556166611,2.5990817351606));
#244967=CARTESIAN_POINT('Ctrl Pts',(-31.4716329851992,54.4799531854479,
2.65878198860299));
#244968=CARTESIAN_POINT('Ctrl Pts',(-31.4364195775137,54.4189959163064,
2.65878198860299));
#244969=CARTESIAN_POINT('Ctrl Pts',(-31.566592666262,54.4681793099462,2.59908193475589));
#244970=CARTESIAN_POINT('Ctrl Pts',(-31.5272089901455,54.4478446647271,
2.65878715325492));
#244971=CARTESIAN_POINT('Ctrl Pts',(-31.4805801312544,54.3934750329635,
2.65878198860299));
#244972=CARTESIAN_POINT('Ctrl Pts',(-31.6244843104272,54.4058464214487,
2.63878778849906));
#244973=CARTESIAN_POINT('Ctrl Pts',(-31.5668246399999,54.3982481205276,
2.69564460180167));
#244974=CARTESIAN_POINT('Ctrl Pts',(-31.5088182930362,54.3482630350912,
2.68180481624915));
#244975=CARTESIAN_POINT('Ctrl Pts',(-31.6805188761701,54.2895863184077,
2.75443238878683));
#244976=CARTESIAN_POINT('Ctrl Pts',(-31.5913182835554,54.313947642815,2.79268340777106));
#244977=CARTESIAN_POINT('Ctrl Pts',(-31.5259511417533,54.2544636505344,
2.74885926835652));
#244978=CARTESIAN_POINT('Ctrl Pts',(-31.6804069909878,54.2359839591654,
2.82856655361705));
#244979=CARTESIAN_POINT('Ctrl Pts',(-31.5756141966206,54.2789047974521,
2.8538419723087));
#244980=CARTESIAN_POINT('Ctrl Pts',(-31.5160982999436,54.2064835118371,
2.79184624278552));
#244981=CARTESIAN_POINT('Ctrl Pts',(-31.6576696180587,54.1966007261208,
2.9013417351606));
#244982=CARTESIAN_POINT('Ctrl Pts',(-31.5474441649286,54.2607761425983,
2.90163218716428));
#244983=CARTESIAN_POINT('Ctrl Pts',(-31.4933613949861,54.1671020372439,
2.83404198860299));
#244984=CARTESIAN_POINT('Origin',(-31.4364195775137,54.4189959163064,2.53178198860298));
#244985=CARTESIAN_POINT('Origin',(-0.274963065701553,-0.158749999999817,
3.64303198860263));
#244986=CARTESIAN_POINT('Origin',(-30.2768083268883,51.8059703131947,3.64303198860298));
#244987=CARTESIAN_POINT('Origin',(5.22371297615238E-17,1.9143463616941E-13,
2.53178198860262));
#244988=CARTESIAN_POINT('Origin',(-31.4100231232064,54.4342359163063,2.53178198860299));
#244989=CARTESIAN_POINT('Ctrl Pts',(-30.2768083268883,51.8059703131947,
3.77003198860299));
#244990=CARTESIAN_POINT('Ctrl Pts',(-30.1666583377716,51.8695654390624,
3.77003198860298));
#244991=CARTESIAN_POINT('Ctrl Pts',(-30.166823223834,51.8694702420499,3.6428418793701));
#244992=CARTESIAN_POINT('Ctrl Pts',(-30.16812109391,51.6181777324911,3.77003198860298));
#244993=CARTESIAN_POINT('Ctrl Pts',(-30.0582657983062,51.6818230251234,
3.76980208963163));
#244994=CARTESIAN_POINT('Ctrl Pts',(-30.0800643400516,51.7191994478449,
3.64284193928342));
#244995=CARTESIAN_POINT('Ctrl Pts',(-30.0646505034496,51.4394033023499,
3.65553535416622));
#244996=CARTESIAN_POINT('Ctrl Pts',(-29.9550522173019,51.5030508615802,
3.65520057834434));
#244997=CARTESIAN_POINT('Ctrl Pts',(-29.997471514536,51.5761444782058,3.55127910964262));
#244998=CARTESIAN_POINT('Ctrl Pts',(-30.007053683816,51.3398895692697,3.47153072139107));
#244999=CARTESIAN_POINT('Ctrl Pts',(-29.8976445635498,51.403617340035,3.47122746281617));
#245000=CARTESIAN_POINT('Ctrl Pts',(-29.9514963979201,51.4965132406197,
3.4041304590127));
#245001=CARTESIAN_POINT('Origin',(-30.0614010732039,51.4328740054943,3.40423097483345));
#245002=CARTESIAN_POINT('Ctrl Pts',(-31.1067982185537,54.5146464769138,
2.90134173516061));
#245003=CARTESIAN_POINT('Ctrl Pts',(-31.2174884860867,54.4512761425983,
2.90163218716428));
#245004=CARTESIAN_POINT('Ctrl Pts',(-31.1634057161443,54.3576020372439,
2.83404198860299));
#245005=CARTESIAN_POINT('Ctrl Pts',(-31.1295467523322,54.5540471172221,
2.82853349835397));
#245006=CARTESIAN_POINT('Ctrl Pts',(-31.2191042733515,54.4847554296828,
2.85381483162437));
#245007=CARTESIAN_POINT('Ctrl Pts',(-31.1861529813966,54.3970014563942,
2.79182701594386));
#245008=CARTESIAN_POINT('Ctrl Pts',(-31.1758273123591,54.5807851087098,
2.75468822073672));
#245009=CARTESIAN_POINT('Ctrl Pts',(-31.2416052667856,54.5157207333386,
2.79286913083887));
#245010=CARTESIAN_POINT('Ctrl Pts',(-31.2226915745265,54.4293656242365,
2.74900763297948));
#245011=CARTESIAN_POINT('Ctrl Pts',(-31.3035520968883,54.5905870683103,
2.63954450640437));
#245012=CARTESIAN_POINT('Ctrl Pts',(-31.3261415286126,54.5367490446508,
2.69627684028885));
#245013=CARTESIAN_POINT('Ctrl Pts',(-31.3118587536635,54.4614280312966,
2.6822435603653));
#245014=CARTESIAN_POINT('Ctrl Pts',(-31.3872779850338,54.5717067142919,
2.59908178706413));
#245015=CARTESIAN_POINT('Ctrl Pts',(-31.3893985541597,54.5274095677402,
2.65878704321626));
#245016=CARTESIAN_POINT('Ctrl Pts',(-31.3656949292513,54.4598040608986,
2.65878198860299));
#245017=CARTESIAN_POINT('Ctrl Pts',(-31.4638515574743,54.527521733972,2.5990817351606));
#245018=CARTESIAN_POINT('Ctrl Pts',(-31.4452069629856,54.4952102564866,
2.65878198860298));
#245019=CARTESIAN_POINT('Ctrl Pts',(-31.4100231232064,54.4342359163063,
2.65878198860299));
#245020=CARTESIAN_POINT('Origin',(-31.0534204898636,54.4211020372439,2.83404198860299));
#245021=CARTESIAN_POINT('Origin',(-29.9723263949899,51.2785921372171,3.11913648167029));
#245022=CARTESIAN_POINT('Origin',(-29.8832517167489,51.1243102687785,2.83404198860297));
#245023=CARTESIAN_POINT('Origin',(-30.9643459342328,54.2668203811892,3.11913648177482));
#245024=CARTESIAN_POINT('Origin',(-30.8752713784764,54.1125387249979,3.40423097483347));
#245025=CARTESIAN_POINT('Ctrl Pts',(-29.8289013456888,51.0313275753409,
2.90134173516058));
#245026=CARTESIAN_POINT('Ctrl Pts',(-29.7196599535395,51.0949610232002,
2.90103711553264));
#245027=CARTESIAN_POINT('Ctrl Pts',(-29.7732664904682,51.1878102687785,
2.83404198860297));
#245028=CARTESIAN_POINT('Ctrl Pts',(-29.8061828667728,50.991979079321,2.82862991747989));
#245029=CARTESIAN_POINT('Ctrl Pts',(-29.7178139048439,51.0613736255813,
2.8531404588653));
#245030=CARTESIAN_POINT('Ctrl Pts',(-29.7505475307857,51.1484598763132,
2.79187960999984));
#245031=CARTESIAN_POINT('Ctrl Pts',(-29.7601395581528,50.9654077681508,
2.7547062579337));
#245032=CARTESIAN_POINT('Ctrl Pts',(-29.695129270271,51.0305123301031,2.79224250381932));
#245033=CARTESIAN_POINT('Ctrl Pts',(-29.7141562330556,51.1163184807721,
2.74901809108292));
#245034=CARTESIAN_POINT('Ctrl Pts',(-29.6330385513051,50.9561384187039,
2.63947868311724));
#245035=CARTESIAN_POINT('Ctrl Pts',(-29.6107158994147,51.0099200724111,
2.69595066767946));
#245036=CARTESIAN_POINT('Ctrl Pts',(-29.6253256551032,51.0849545802165,
2.68220539436098));
#245037=CARTESIAN_POINT('Ctrl Pts',(-29.5497635830448,50.9753486645705,
2.59908178585179));
#245038=CARTESIAN_POINT('Ctrl Pts',(-29.5477758465718,51.019575486427,2.65877670944799));
#245039=CARTESIAN_POINT('Ctrl Pts',(-29.5717132339817,51.0870396576443,
2.65878198860297));
#245040=CARTESIAN_POINT('Ctrl Pts',(-29.473599835734,51.0193480105328,2.59908173516058));
#245041=CARTESIAN_POINT('Ctrl Pts',(-29.4922606054649,51.0516501490686,
2.65878198860297));
#245042=CARTESIAN_POINT('Ctrl Pts',(-29.5274749692187,51.1126068659047,
2.65878198860297));
#245043=CARTESIAN_POINT('Origin',(-29.5274749692187,51.1126068659048,2.53178198860297));
#245044=CARTESIAN_POINT('Ctrl Pts',(-30.6598643453577,53.7394427993287,
3.770031988603));
#245045=CARTESIAN_POINT('Ctrl Pts',(-30.7700138939558,53.6758479277944,
3.770031988603));
#245046=CARTESIAN_POINT('Ctrl Pts',(-30.7698494490696,53.6759428700938,
3.64284238727623));
#245047=CARTESIAN_POINT('Ctrl Pts',(-30.7681598456252,53.9274614872894,
3.770031988603));
#245048=CARTESIAN_POINT('Ctrl Pts',(-30.8785957589627,53.863916238056,3.7702550610604));
#245049=CARTESIAN_POINT('Ctrl Pts',(-30.8566081460792,53.8262133418089,
3.64284210641982));
#245050=CARTESIAN_POINT('Ctrl Pts',(-30.8712573299214,54.1064511722693,
3.6555352798787));
#245051=CARTESIAN_POINT('Ctrl Pts',(-30.9819369489455,54.0429074791663,
3.6558599653291));
#245052=CARTESIAN_POINT('Ctrl Pts',(-30.9392009315185,53.9692682429957,
3.55127902710151));
#245053=CARTESIAN_POINT('Ctrl Pts',(-30.9286463962981,54.2060847114742,
3.4715307213911));
#245054=CARTESIAN_POINT('Ctrl Pts',(-31.0395064423978,54.1426202463874,
3.47182327905226));
#245055=CARTESIAN_POINT('Ctrl Pts',(-30.9851759130205,54.0488992470934,
3.40413028378019));
#245056=CARTESIAN_POINT('Origin',(-30.6598643453577,53.7394427993287,3.643031988603));
#245057=CARTESIAN_POINT('Origin',(3.8264039982802E-16,1.91628233411515E-13,
2.53178198860262));
#245058=CARTESIAN_POINT('Origin',(-29.5010785149114,51.1278468659047,2.53178198860297));
#245059=CARTESIAN_POINT('Origin',(15.8305769983926,-26.7843636743467,3.64303198860244));
#245060=CARTESIAN_POINT('Origin',(-30.4591427892365,53.3918862459827,3.64299466007577));
#245061=CARTESIAN_POINT('Ctrl Pts',(-29.4472515437738,51.0345602039887,
2.59908173516058));
#245062=CARTESIAN_POINT('Ctrl Pts',(-29.4658956314769,51.0668719738978,
2.65878198860297));
#245063=CARTESIAN_POINT('Ctrl Pts',(-29.5010785149114,51.1278468659047,
2.65878198860297));
#245064=CARTESIAN_POINT('Ctrl Pts',(-29.3713249278652,51.0783704650312,
2.59908193199997));
#245065=CARTESIAN_POINT('Ctrl Pts',(-29.4105784408376,51.0987866273871,
2.65877685806747));
#245066=CARTESIAN_POINT('Ctrl Pts',(-29.4569685172222,51.1532877451704,
2.65878198860297));
#245067=CARTESIAN_POINT('Ctrl Pts',(-29.3133705634514,51.1401588234664,
2.63872492669834));
#245068=CARTESIAN_POINT('Ctrl Pts',(-29.3708492661237,51.1479550638448,
2.69532212015298));
#245069=CARTESIAN_POINT('Ctrl Pts',(-29.4284442379232,51.1980841325265,
2.68176836726662));
#245070=CARTESIAN_POINT('Ctrl Pts',(-29.2571907880104,51.2555806533512,
2.75442176402282));
#245071=CARTESIAN_POINT('Ctrl Pts',(-29.3460364571626,51.231908956258,2.79203179920187));
#245072=CARTESIAN_POINT('Ctrl Pts',(-29.4108701703527,51.291216048965,2.74885310748217));
#245073=CARTESIAN_POINT('Ctrl Pts',(-29.2572675046848,51.3089178634639,
2.82866089558435));
#245074=CARTESIAN_POINT('Ctrl Pts',(-29.3615545506875,51.2670782717307,
2.85316563119275));
#245075=CARTESIAN_POINT('Ctrl Pts',(-29.4206015015119,51.3389765898555,
2.79189751796689));
#245076=CARTESIAN_POINT('Ctrl Pts',(-29.2799753962465,51.3482501200166,
2.90134173516058));
#245077=CARTESIAN_POINT('Ctrl Pts',(-29.3897042746976,51.2854610232002,
2.90103711553264));
#245078=CARTESIAN_POINT('Ctrl Pts',(-29.4433108116264,51.3783102687785,
2.83404198860296));
#245079=CARTESIAN_POINT('Origin',(-29.3333255853457,51.4418102687785,2.83404198860297));
#245080=CARTESIAN_POINT('Origin',(-30.437074623967,53.3535596824666,3.56647653971834));
#245081=CARTESIAN_POINT('Origin',(-30.396155456884,53.2826856060846,3.42473028058522));
#245082=CARTESIAN_POINT('Origin',(-29.4224002636271,51.5960921371734,3.11913648168138));
#245083=CARTESIAN_POINT('Origin',(-29.5114749418008,51.7503740054943,3.40423097483346));
#245084=CARTESIAN_POINT('Ctrl Pts',(-30.2311753956715,52.9969317578288,
3.36123028058518));
#245085=CARTESIAN_POINT('Ctrl Pts',(-30.3411606219521,52.9334317578288,
3.36123028058518));
#245086=CARTESIAN_POINT('Ctrl Pts',(-30.3411606219521,52.9334317578288,
3.23423028058518));
#245087=CARTESIAN_POINT('Ctrl Pts',(-30.2763834500034,53.0747660209935,
3.36123028058517));
#245088=CARTESIAN_POINT('Ctrl Pts',(-30.3861235964137,53.0113099140535,
3.36099641108513));
#245089=CARTESIAN_POINT('Ctrl Pts',(-30.4086676540701,53.0503573673254,
3.23423043688446));
#245090=CARTESIAN_POINT('Ctrl Pts',(-30.3191294880994,53.1483650929086,
3.4105425890532));
#245091=CARTESIAN_POINT('Ctrl Pts',(-30.4288515386952,53.0853168809963,
3.41008815825925));
#245092=CARTESIAN_POINT('Ctrl Pts',(-30.4725003554725,53.1609188493387,
3.30819867304248));
#245093=CARTESIAN_POINT('Ctrl Pts',(-30.3416565762239,53.1871522506175,
3.4882302805852));
#245094=CARTESIAN_POINT('Ctrl Pts',(-30.4513942013116,53.1243619179796,
3.48794691941636));
#245095=CARTESIAN_POINT('Ctrl Pts',(-30.5061406831646,53.2191856060846,
3.42473028058521));
#245096=CARTESIAN_POINT('Origin',(-30.2311753956715,52.9969317578288,3.23423028058518));
#245097=CARTESIAN_POINT('Ctrl Pts',(-29.4581217525676,51.6568155675428,
3.47153072139108));
#245098=CARTESIAN_POINT('Ctrl Pts',(-29.5680161684457,51.5939283826163,
3.47122746285112));
#245099=CARTESIAN_POINT('Ctrl Pts',(-29.6215404675518,51.687013371507,3.40413046676838));
#245100=CARTESIAN_POINT('Ctrl Pts',(-29.5155056307129,51.7564542486371,
3.65553813458023));
#245101=CARTESIAN_POINT('Ctrl Pts',(-29.6254251653839,51.6933631336535,
3.65520336072106));
#245102=CARTESIAN_POINT('Ctrl Pts',(-29.6675162799456,51.7666458147686,
3.55128134519885));
#245103=CARTESIAN_POINT('Ctrl Pts',(-29.6185943474775,51.9354510367807,
3.77003198860299));
#245104=CARTESIAN_POINT('Ctrl Pts',(-29.7286404220038,51.8721362050945,
3.76980209314207));
#245105=CARTESIAN_POINT('Ctrl Pts',(-29.7501097595399,51.9097019182946,
3.64284195387509));
#245106=CARTESIAN_POINT('Ctrl Pts',(-29.7268821954852,52.1234703131947,
3.77003198860299));
#245107=CARTESIAN_POINT('Ctrl Pts',(-29.8370321718796,52.0598751946722,
3.77003198860299));
#245108=CARTESIAN_POINT('Ctrl Pts',(-29.8368672985585,52.0599703843284,
3.64284189403866));
#245109=CARTESIAN_POINT('Origin',(-29.7268821954852,52.1234703131947,3.64303198860299));
#245110=CARTESIAN_POINT('Origin',(15.4537755657018,-26.1317244485615,3.23423028058463));
#245111=CARTESIAN_POINT('Origin',(-30.155571337834,52.865981688396,3.23423028058518));
#245112=CARTESIAN_POINT('Origin',(15.3947701216595,-26.0295240215571,3.64303198860244));
#245113=CARTESIAN_POINT('Origin',(-29.9275190026067,52.4710850656384,3.64299171721842));
#245114=CARTESIAN_POINT('Ctrl Pts',(-30.0450834959839,52.6757649139396,
3.48823028058517));
#245115=CARTESIAN_POINT('Ctrl Pts',(-30.1558192616004,52.6124111049557,
3.48852004212295));
#245116=CARTESIAN_POINT('Ctrl Pts',(-30.100576467536,52.5167277788842,3.42473028058517));
#245117=CARTESIAN_POINT('Ctrl Pts',(-30.0676891808483,52.7146817640555,
3.41028005848446));
#245118=CARTESIAN_POINT('Ctrl Pts',(-30.1782028480936,52.6511806140212,
3.41074404220526));
#245119=CARTESIAN_POINT('Ctrl Pts',(-30.1343304829282,52.5751914485028,
3.30780486243987));
#245120=CARTESIAN_POINT('Ctrl Pts',(-30.1105150503705,52.7884098752467,
3.36123028058518));
#245121=CARTESIAN_POINT('Ctrl Pts',(-30.2206596676762,52.7247179826659,
3.36146460586334));
#245122=CARTESIAN_POINT('Ctrl Pts',(-30.198276914831,52.6859499175213,3.23423045308457));
#245123=CARTESIAN_POINT('Ctrl Pts',(-30.155571337834,52.865981688396,3.36123028058518));
#245124=CARTESIAN_POINT('Ctrl Pts',(-30.2655565641147,52.802481688396,3.36123028058518));
#245125=CARTESIAN_POINT('Ctrl Pts',(-30.2655565641147,52.802481688396,3.23423028058518));
#245126=CARTESIAN_POINT('Origin',(-29.9905912412554,52.5802277788842,3.42473028058516));
#245127=CARTESIAN_POINT('Origin',(-29.9499161075312,52.5097763812718,3.56563113524792));
#245128=CARTESIAN_POINT('Origin',(-36.3610285397818,49.5064990290886,3.56647653909468));
#245129=CARTESIAN_POINT('Origin',(-36.3870656659258,49.5422481179709,3.64299466007638));
#245130=CARTESIAN_POINT('Origin',(-36.3129251734945,49.4402904249166,3.42473028058517));
#245131=CARTESIAN_POINT('Ctrl Pts',(-36.2478178023253,49.3516463037385,
3.48823028058518));
#245132=CARTESIAN_POINT('Ctrl Pts',(-36.1458216659127,49.4263574835551,
3.48794691941634));
#245133=CARTESIAN_POINT('Ctrl Pts',(-36.2101800152089,49.5149391519577,
3.42473028058519));
#245134=CARTESIAN_POINT('Ctrl Pts',(-36.2214577843987,49.3151677697922,
3.41028005925121));
#245135=CARTESIAN_POINT('Ctrl Pts',(-36.119231655743,49.3897594742935,3.40982512230947));
#245136=CARTESIAN_POINT('Ctrl Pts',(-36.1704998050837,49.4603240281409,
3.30780486372769));
#245137=CARTESIAN_POINT('Ctrl Pts',(-36.1715192752718,49.2460589922057,
3.36123028058515));
#245138=CARTESIAN_POINT('Ctrl Pts',(-36.0689133127008,49.320502216666,3.36099721048578));
#245139=CARTESIAN_POINT('Ctrl Pts',(-36.0953262843463,49.3568565532997,
3.23423045308452));
#245140=CARTESIAN_POINT('Ctrl Pts',(-36.1189794796885,49.1733470784087,
3.36123028058515));
#245141=CARTESIAN_POINT('Ctrl Pts',(-36.0162343214029,49.2479958054499,
3.36123028058515));
#245142=CARTESIAN_POINT('Ctrl Pts',(-36.0162343214029,49.2479958054499,
3.23423028058515));
#245143=CARTESIAN_POINT('Origin',(-36.1189794796885,49.1733470784087,3.23423028058515));
#245144=CARTESIAN_POINT('Origin',(-0.256862895714039,-0.186621817602678,
3.64303198860262));
#245145=CARTESIAN_POINT('Origin',(-36.6229335645812,49.8669803696026,3.64303198860296));
#245146=CARTESIAN_POINT('Origin',(-0.256862895714039,-0.186621817602675,
3.23423028058481));
#245147=CARTESIAN_POINT('Origin',(-36.0301015792679,49.0510171431404,3.23423028058515));
#245148=CARTESIAN_POINT('Ctrl Pts',(-36.9399086546489,50.3023253561995,
3.47153072139106));
#245149=CARTESIAN_POINT('Ctrl Pts',(-36.836840146744,50.3777877177487,3.47182327902697));
#245150=CARTESIAN_POINT('Ctrl Pts',(-36.7733199672423,50.2900345588339,
3.40413028959065));
#245151=CARTESIAN_POINT('Ctrl Pts',(-36.8722300970236,50.2093718139452,
3.65553807120991));
#245152=CARTESIAN_POINT('Ctrl Pts',(-36.7691625978843,50.2846371204111,
3.65586275496825));
#245153=CARTESIAN_POINT('Ctrl Pts',(-36.7192723137702,50.2156443459715,
3.55128126837211));
#245154=CARTESIAN_POINT('Ctrl Pts',(-36.7506474475451,50.042384592773,3.77003198860298));
#245155=CARTESIAN_POINT('Ctrl Pts',(-36.6476776482601,50.1174266236792,
3.77025505748624));
#245156=CARTESIAN_POINT('Ctrl Pts',(-36.6221779017714,50.0820053531149,
3.64284211731276));
#245157=CARTESIAN_POINT('Ctrl Pts',(-36.6229335645812,49.8669803696026,
3.77003198860297));
#245158=CARTESIAN_POINT('Ctrl Pts',(-36.5200349097935,49.9417406183804,
3.77003198860298));
#245159=CARTESIAN_POINT('Ctrl Pts',(-36.5201885207827,49.9416290134639,
3.6428423982174));
#245160=CARTESIAN_POINT('Origin',(-36.8761597191957,50.2155162706044,3.40423097483344));
#245161=CARTESIAN_POINT('Ctrl Pts',(-36.0301015792679,49.0510171431404,
3.36123028058515));
#245162=CARTESIAN_POINT('Ctrl Pts',(-35.9273564209823,49.1256658701815,
3.36123028058514));
#245163=CARTESIAN_POINT('Ctrl Pts',(-35.9273564209823,49.1256658701815,
3.23423028058515));
#245164=CARTESIAN_POINT('Ctrl Pts',(-35.9773846774562,48.9780591316059,
3.36123028058515));
#245165=CARTESIAN_POINT('Ctrl Pts',(-35.8743986902969,49.0527758071183,
3.36146538610325));
#245166=CARTESIAN_POINT('Ctrl Pts',(-35.8479971380602,49.016437187946,3.23423043688466));
#245167=CARTESIAN_POINT('Ctrl Pts',(-35.927538343867,48.9090707128239,3.41054258693134));
#245168=CARTESIAN_POINT('Ctrl Pts',(-35.8245773199118,48.9842025736696,
3.41100608859765));
#245169=CARTESIAN_POINT('Ctrl Pts',(-35.7729572780264,48.9131536812808,
3.30819866970901));
#245170=CARTESIAN_POINT('Ctrl Pts',(-35.9012693628907,48.8727133447944,
3.48823028058515));
#245171=CARTESIAN_POINT('Ctrl Pts',(-35.7983524848938,48.9481071848797,
3.48852004212292));
#245172=CARTESIAN_POINT('Ctrl Pts',(-35.7334106856009,48.85872246645,3.42473028058514));
#245173=CARTESIAN_POINT('Origin',(-35.8361558438865,48.7840737394089,3.42473028058514));
#245174=CARTESIAN_POINT('Origin',(-36.9808731396222,50.3596419293465,3.11913648178346));
#245175=CARTESIAN_POINT('Origin',(-37.0855865599605,50.5037675878945,2.83404198860296));
#245176=CARTESIAN_POINT('Origin',(-35.7883393560616,48.7182599900759,3.56563113460856));
#245177=CARTESIAN_POINT('Origin',(-35.7621028045853,48.6820620414862,3.64299171721815));
#245178=CARTESIAN_POINT('Ctrl Pts',(-37.0158684358562,50.92199981559,2.59908173516058));
#245179=CARTESIAN_POINT('Ctrl Pts',(-36.9939338721435,50.8918248691,2.65878198860296));
#245180=CARTESIAN_POINT('Ctrl Pts',(-36.9525415975215,50.8348823336486,
2.65878198860296));
#245181=CARTESIAN_POINT('Ctrl Pts',(-37.0871426490251,50.8701895025862,
2.59908193475566));
#245182=CARTESIAN_POINT('Ctrl Pts',(-37.0458491715926,50.8540829678254,
2.6587871532543));
#245183=CARTESIAN_POINT('Ctrl Pts',(-36.9937925764114,50.8048852215561,
2.65878198860296));
#245184=CARTESIAN_POINT('Ctrl Pts',(-37.1382015956599,50.8021467555735,
2.63878778849934));
#245185=CARTESIAN_POINT('Ctrl Pts',(-37.0800635522212,50.8006171556815,
2.69564460180152));
#245186=CARTESIAN_POINT('Ctrl Pts',(-37.0171501059291,50.7569692080812,
2.68180481624921));
#245187=CARTESIAN_POINT('Ctrl Pts',(-37.1817767082792,50.6806663304943,
2.75443238878651));
#245188=CARTESIAN_POINT('Ctrl Pts',(-37.0956112176478,50.7142182018865,
2.7926834077713));
#245189=CARTESIAN_POINT('Ctrl Pts',(-37.0243843935852,50.6618927960202,
2.74885926835641));
#245190=CARTESIAN_POINT('Ctrl Pts',(-37.176062463776,50.6273693057705,2.82856655361725));
#245191=CARTESIAN_POINT('Ctrl Pts',(-37.0763301845674,50.6810088489708,
2.8538419723077));
#245192=CARTESIAN_POINT('Ctrl Pts',(-37.0095702365079,50.6152053999551,
2.79184624278479));
#245193=CARTESIAN_POINT('Ctrl Pts',(-37.1493329797263,50.5905785208484,
2.90134173516059));
#245194=CARTESIAN_POINT('Ctrl Pts',(-37.0464195108255,50.6659240749083,
2.90163218716426));
#245195=CARTESIAN_POINT('Ctrl Pts',(-36.9828414016749,50.5784163149357,
2.83404198860297));
#245196=CARTESIAN_POINT('Origin',(-36.9525415975215,50.8348823336486,2.53178198860296));
#245197=CARTESIAN_POINT('Origin',(-0.256862895714039,-0.186621817602678,
3.64303198860262));
#245198=CARTESIAN_POINT('Origin',(-35.5261472678868,48.3573835402119,3.64303198860295));
#245199=CARTESIAN_POINT('Origin',(6.67120042669033E-17,1.91444036262824E-13,
2.53178198860262));
#245200=CARTESIAN_POINT('Origin',(-36.9278827595329,50.8527980281385,2.53178198860296));
#245201=CARTESIAN_POINT('Ctrl Pts',(-35.5261472678868,48.3573835402119,
3.77003198860296));
#245202=CARTESIAN_POINT('Ctrl Pts',(-35.4232481927148,48.4321440944168,
3.77003198860297));
#245203=CARTESIAN_POINT('Ctrl Pts',(-35.4234022247158,48.4320321836174,
3.6428418793712));
#245204=CARTESIAN_POINT('Ctrl Pts',(-35.3984257650681,48.1819806163551,
3.77003198860296));
#245205=CARTESIAN_POINT('Ctrl Pts',(-35.2958250128973,48.2567602586438,
3.76980208962953));
#245206=CARTESIAN_POINT('Ctrl Pts',(-35.321411039981,48.2916533613383,3.6428419392844));
#245207=CARTESIAN_POINT('Ctrl Pts',(-35.2768349808748,48.0150011530616,
3.65553535416619));
#245208=CARTESIAN_POINT('Ctrl Pts',(-35.1744900671665,48.0897561847352,
3.65520057834429));
#245209=CARTESIAN_POINT('Ctrl Pts',(-35.224317350473,48.1580153629285,3.55127910964166));
#245210=CARTESIAN_POINT('Ctrl Pts',(-35.209151665053,47.9220530736687,3.47153072139105));
#245211=CARTESIAN_POINT('Ctrl Pts',(-35.1070032653418,47.996868104246,3.47122746281616));
#245212=CARTESIAN_POINT('Ctrl Pts',(-35.1702703594593,48.0836260618765,
3.40413045901328));
#245213=CARTESIAN_POINT('Origin',(-35.2729208539817,48.0088472823272,3.40423097483344));
#245214=CARTESIAN_POINT('Ctrl Pts',(-36.6347241449657,50.9644637245893,
2.90134173516059));
#245215=CARTESIAN_POINT('Ctrl Pts',(-36.7381840359687,50.8898702560318,
2.90163218716426));
#245216=CARTESIAN_POINT('Ctrl Pts',(-36.674605926818,50.8023624960591,2.83404198860297));
#245217=CARTESIAN_POINT('Ctrl Pts',(-36.6614665482801,51.0012706547893,
2.82853349835384));
#245218=CARTESIAN_POINT('Ctrl Pts',(-36.7432905102105,50.9229972443181,
2.85381483162359));
#245219=CARTESIAN_POINT('Ctrl Pts',(-36.7013469409081,50.8391683443878,
2.79182701594228));
#245220=CARTESIAN_POINT('Ctrl Pts',(-36.7102884597168,51.0230245369438,
2.75468822073687));
#245221=CARTESIAN_POINT('Ctrl Pts',(-36.768904996455,50.9514409225354,2.79286913083867));
#245222=CARTESIAN_POINT('Ctrl Pts',(-36.7410683485314,50.8675358949426,
2.74900763297943));
#245223=CARTESIAN_POINT('Ctrl Pts',(-36.8383381382864,51.0194219249362,
2.63954450640419));
#245224=CARTESIAN_POINT('Ctrl Pts',(-36.855176216862,50.9635175930193,2.69627684028899));
#245225=CARTESIAN_POINT('Ctrl Pts',(-36.8330984946708,50.8901021525742,
2.68224356036531));
#245226=CARTESIAN_POINT('Ctrl Pts',(-36.9196318328648,50.9918932610489,
2.59908178706395));
#245227=CARTESIAN_POINT('Ctrl Pts',(-36.9171104726355,50.9476171190701,
2.6587870432158));
#245228=CARTESIAN_POINT('Ctrl Pts',(-36.8864699989252,50.8828596657528,
2.65878198860296));
#245229=CARTESIAN_POINT('Ctrl Pts',(-36.991167339171,50.9399462128202,2.59908173516058));
#245230=CARTESIAN_POINT('Ctrl Pts',(-36.9692474126343,50.9097606317994,
2.65878198860296));
#245231=CARTESIAN_POINT('Ctrl Pts',(-36.9278827595329,50.8527980281385,
2.65878198860296));
#245232=CARTESIAN_POINT('Origin',(-36.5718607685324,50.8770112231003,2.83404198860297));
#245233=CARTESIAN_POINT('Origin',(-35.1682072895741,47.8647214254955,3.11913648167096));
#245234=CARTESIAN_POINT('Origin',(-35.0634937251224,47.7205955685091,2.83404198860295));
#245235=CARTESIAN_POINT('Origin',(-36.4671473482213,50.7328855645148,3.1191364817745));
#245236=CARTESIAN_POINT('Origin',(-36.3624339277676,50.5887599058101,3.40423097483344));
#245237=CARTESIAN_POINT('Ctrl Pts',(-34.9997217530263,47.63380340476,2.90134173516056));
#245238=CARTESIAN_POINT('Ctrl Pts',(-34.8977303031704,47.7085070967804,
2.90103711553262));
#245239=CARTESIAN_POINT('Ctrl Pts',(-34.9607485668368,47.7952442955502,
2.83404198860294));
#245240=CARTESIAN_POINT('Ctrl Pts',(-34.9730146904938,47.5970451916073,
2.82862991747985));
#245241=CARTESIAN_POINT('Ctrl Pts',(-34.8923835282622,47.6752966590749,
2.85314045886441));
#245242=CARTESIAN_POINT('Ctrl Pts',(-34.9340408279393,47.758484246595,2.79187960999962));
#245243=CARTESIAN_POINT('Ctrl Pts',(-34.9244461536127,47.5754322771536,
2.75470625793369));
#245244=CARTESIAN_POINT('Ctrl Pts',(-34.8665972787025,47.6469756149924,
2.79224250381933));
#245245=CARTESIAN_POINT('Ctrl Pts',(-34.8944891948624,47.7303228514093,
2.74901809108295));
#245246=CARTESIAN_POINT('Ctrl Pts',(-34.7970725085258,47.5794993790986,
2.63947868311719));
#245247=CARTESIAN_POINT('Ctrl Pts',(-34.7804938560724,47.6353197637776,
2.69595066767939));
#245248=CARTESIAN_POINT('Ctrl Pts',(-34.8028668197836,47.7084160893876,
2.6822053943609));
#245249=CARTESIAN_POINT('Ctrl Pts',(-34.7162617467346,47.607308993689,2.59908178585189));
#245250=CARTESIAN_POINT('Ctrl Pts',(-34.7189078610144,47.6515013114278,
2.65877670944888));
#245251=CARTESIAN_POINT('Ctrl Pts',(-34.7497660430534,47.7160937685341,
2.65878198860294));
#245252=CARTESIAN_POINT('Ctrl Pts',(-34.6451144164188,47.6590285860936,
2.59908173516056));
#245253=CARTESIAN_POINT('Ctrl Pts',(-34.667049453402,47.6892031885514,2.65878198860294));
#245254=CARTESIAN_POINT('Ctrl Pts',(-34.7084426211234,47.7461450747865,
2.65878198860294));
#245255=CARTESIAN_POINT('Origin',(-34.7084426211234,47.7461450747865,2.53178198860294));
#245256=CARTESIAN_POINT('Ctrl Pts',(-36.1092077731531,50.2402240048083,
3.77003198860298));
#245257=CARTESIAN_POINT('Ctrl Pts',(-36.2121064368056,50.1654637495898,
3.77003198860298));
#245258=CARTESIAN_POINT('Ctrl Pts',(-36.2119528169383,50.1655753609565,
3.64284238727626));
#245259=CARTESIAN_POINT('Ctrl Pts',(-36.2365633238548,50.4158927445036,
3.77003198860298));
#245260=CARTESIAN_POINT('Ctrl Pts',(-36.3397519704521,50.3411519064821,
3.77025506106023));
#245261=CARTESIAN_POINT('Ctrl Pts',(-36.313943782211,50.3059538820312,3.64284210641963));
#245262=CARTESIAN_POINT('Ctrl Pts',(-36.3578055460589,50.5831252836592,
3.65553527987867));
#245263=CARTESIAN_POINT('Ctrl Pts',(-36.4612367259606,50.5083605190664,
3.65585996532998));
#245264=CARTESIAN_POINT('Ctrl Pts',(-36.4110374247136,50.4395918165619,
3.55127902710161));
#245265=CARTESIAN_POINT('Ctrl Pts',(-36.4252947698681,50.6762142289948,
3.47153072139106));
#245266=CARTESIAN_POINT('Ctrl Pts',(-36.5289136700282,50.6015093986316,
3.47182327905222));
#245267=CARTESIAN_POINT('Ctrl Pts',(-36.4650842569434,50.5139808995223,
3.40413028378018));
#245268=CARTESIAN_POINT('Origin',(-36.1092077731531,50.2402240048083,3.64303198860298));
#245269=CARTESIAN_POINT('Origin',(3.77491158612227E-16,1.9162488945517E-13,
2.53178198860262));
#245270=CARTESIAN_POINT('Origin',(-34.6837837831348,47.7640607692763,2.53178198860295));
#245271=CARTESIAN_POINT('Origin',(21.7541926348216,-29.4019141737115,3.64303198860242));
#245272=CARTESIAN_POINT('Origin',(-35.8732562382987,49.9155525184325,3.64299466007571));
#245273=CARTESIAN_POINT('Ctrl Pts',(-34.6205005703637,47.6769115920304,
2.59908173516056));
#245274=CARTESIAN_POINT('Ctrl Pts',(-34.6424200234577,47.7070975168464,
2.65878198860294));
#245275=CARTESIAN_POINT('Ctrl Pts',(-34.6837837831348,47.7640607692763,
2.65878198860294));
#245276=CARTESIAN_POINT('Ctrl Pts',(-34.5495693076635,47.7284183483607,
2.59908193199947));
#245277=CARTESIAN_POINT('Ctrl Pts',(-34.5907418558606,47.7446195594533,
2.6587768580676));
#245278=CARTESIAN_POINT('Ctrl Pts',(-34.6425747206424,47.7939730310167,
2.65878198860294));
#245279=CARTESIAN_POINT('Ctrl Pts',(-34.4983910654767,47.7959261043557,
2.63872492669839));
#245280=CARTESIAN_POINT('Ctrl Pts',(-34.5563698228278,47.7976714756521,
2.69532212015316));
#245281=CARTESIAN_POINT('Ctrl Pts',(-34.6188891978598,47.8415056181568,
2.68176836726693));
#245282=CARTESIAN_POINT('Ctrl Pts',(-34.4545839152296,47.9165880269727,
2.75442176402273));
#245283=CARTESIAN_POINT('Ctrl Pts',(-34.5404685123898,47.883759104649,2.79203179920163));
#245284=CARTESIAN_POINT('Ctrl Pts',(-34.6111463389771,47.9359643384886,
2.74885310748182));
#245285=CARTESIAN_POINT('Ctrl Pts',(-34.4602354682505,47.9696250311914,
2.82866089558438));
#245286=CARTESIAN_POINT('Ctrl Pts',(-34.5595777906764,47.917113676462,2.85316563119214));
#245287=CARTESIAN_POINT('Ctrl Pts',(-34.6258166968302,47.9824460410478,
2.79189751796674));
#245288=CARTESIAN_POINT('Ctrl Pts',(-34.4869303039399,48.0063682005187,
2.90134173516055));
#245289=CARTESIAN_POINT('Ctrl Pts',(-34.5894948283136,47.9324532779038,
2.90103711553262));
#245290=CARTESIAN_POINT('Ctrl Pts',(-34.6525130919799,48.0191904766737,
2.83404198860294));
#245291=CARTESIAN_POINT('Origin',(-34.5497679336943,48.0938392037148,2.83404198860294));
#245292=CARTESIAN_POINT('Origin',(-35.8473027479613,49.8797426632452,3.56647653971789));
#245293=CARTESIAN_POINT('Origin',(-35.7991993820664,49.8135340601223,3.42473028058518));
#245294=CARTESIAN_POINT('Origin',(-34.6544814981826,48.2379650606549,3.11913648168096));
#245295=CARTESIAN_POINT('Origin',(-34.7591950625536,48.3820909175329,3.40423097483344));
#245296=CARTESIAN_POINT('Ctrl Pts',(-35.6052536882604,49.5465907136145,
3.36123028058515));
#245297=CARTESIAN_POINT('Ctrl Pts',(-35.707998846546,49.4719419865733,3.36123028058515));
#245298=CARTESIAN_POINT('Ctrl Pts',(-35.707998846546,49.4719419865733,3.23423028058515));
#245299=CARTESIAN_POINT('Ctrl Pts',(-35.6583499840569,49.6192730640963,
3.36123028058515));
#245300=CARTESIAN_POINT('Ctrl Pts',(-35.7608559931183,49.5446936074887,
3.36099641108576));
#245301=CARTESIAN_POINT('Ctrl Pts',(-35.7873581223564,49.5811706590203,
3.23423043688435));
#245302=CARTESIAN_POINT('Ctrl Pts',(-35.7085550527713,49.6880007749199,
3.4105425890532));
#245303=CARTESIAN_POINT('Ctrl Pts',(-35.8110857017895,49.6138288703731,
3.41008815825907));
#245304=CARTESIAN_POINT('Ctrl Pts',(-35.8623979633523,49.6844541394821,
3.30819867304266));
#245305=CARTESIAN_POINT('Ctrl Pts',(-35.7350130971391,49.7242207306175,
3.48823028058517));
#245306=CARTESIAN_POINT('Ctrl Pts',(-35.8375861910559,49.6503036646785,
3.48794691941633));
#245307=CARTESIAN_POINT('Ctrl Pts',(-35.9019445403521,49.7388853330811,
3.42473028058518));
#245308=CARTESIAN_POINT('Origin',(-35.6052536882604,49.5465907136145,3.23423028058515));
#245309=CARTESIAN_POINT('Ctrl Pts',(-34.6963546279287,48.2946219293746,
3.47153072139105));
#245310=CARTESIAN_POINT('Ctrl Pts',(-34.7990735298985,48.2205921526139,
3.4712274628511));
#245311=CARTESIAN_POINT('Ctrl Pts',(-34.8620346481358,48.3075723994625,
3.40413046676847));
#245312=CARTESIAN_POINT('Ctrl Pts',(-34.7638392294003,48.387716530751,3.65553813458021));
#245313=CARTESIAN_POINT('Ctrl Pts',(-34.8665617960676,48.3134813154541,
3.65520336072058));
#245314=CARTESIAN_POINT('Ctrl Pts',(-34.91608245714,48.3819628268521,3.55128134519854));
#245315=CARTESIAN_POINT('Ctrl Pts',(-34.8850734745832,48.5549570506165,
3.77003198860297));
#245316=CARTESIAN_POINT('Ctrl Pts',(-34.9878985031393,48.4804861171435,
3.76980209314202));
#245317=CARTESIAN_POINT('Ctrl Pts',(-35.0131769156724,48.5156018845747,
3.64284195387532));
#245318=CARTESIAN_POINT('Ctrl Pts',(-35.0124214764587,48.7306271754176,
3.77003198860296));
#245319=CARTESIAN_POINT('Ctrl Pts',(-35.1153205397465,48.6558666298471,
3.77003198860297));
#245320=CARTESIAN_POINT('Ctrl Pts',(-35.1151665196474,48.6559785319993,
3.64284189403885));
#245321=CARTESIAN_POINT('Origin',(-35.0124214764587,48.7306271754176,3.64303198860296));
#245322=CARTESIAN_POINT('Origin',(21.2334658618526,-28.6851952578917,3.23423028058461));
#245323=CARTESIAN_POINT('Origin',(-35.5163757878398,49.4242607783461,3.23423028058515));
#245324=CARTESIAN_POINT('Origin',(21.1519223437074,-28.572960233785,3.64303198860243));
#245325=CARTESIAN_POINT('Origin',(-35.2482948100393,49.0553654007527,3.6429917172178));
#245326=CARTESIAN_POINT('Ctrl Pts',(-35.3866101428262,49.2466351556013,
3.48823028058515));
#245327=CARTESIAN_POINT('Ctrl Pts',(-35.4901170100369,49.1720533660031,
3.48852004212293));
#245328=CARTESIAN_POINT('Ctrl Pts',(-35.425175210744,49.0826686475735,3.42473028058515));
#245329=CARTESIAN_POINT('Ctrl Pts',(-35.4131599099208,49.2829758776408,
3.41028005848442));
#245330=CARTESIAN_POINT('Ctrl Pts',(-35.5164304941051,49.2082707697419,
3.41074404220321));
#245331=CARTESIAN_POINT('Ctrl Pts',(-35.4648554356506,49.1372837917352,
3.30780486243953));
#245332=CARTESIAN_POINT('Ctrl Pts',(-35.4634578610114,49.3518235761952,
3.36123028058516));
#245333=CARTESIAN_POINT('Ctrl Pts',(-35.5663414789262,49.276967346882,3.36146460586564));
#245334=CARTESIAN_POINT('Ctrl Pts',(-35.5400289748685,49.2407512920126,
3.23423045308515));
#245335=CARTESIAN_POINT('Ctrl Pts',(-35.5163757878398,49.4242607783461,
3.36123028058515));
#245336=CARTESIAN_POINT('Ctrl Pts',(-35.6191209461254,49.3496120513049,
3.36123028058514));
#245337=CARTESIAN_POINT('Ctrl Pts',(-35.6191209461254,49.3496120513049,
3.23423028058515));
#245338=CARTESIAN_POINT('Origin',(-35.3224300524584,49.1573173746146,3.42473028058514));
#245339=CARTESIAN_POINT('Origin',(-35.2746135650455,49.0915036263509,3.56563113524782));
#245340=CARTESIAN_POINT('Origin',(-41.3366772861972,45.4345348113618,3.56647653909426));
#245341=CARTESIAN_POINT('Origin',(-41.3663085755642,45.467366442211,3.64299466007489));
#245342=CARTESIAN_POINT('Origin',(-41.2819167515331,45.3737170758072,3.42473028058515));
#245343=CARTESIAN_POINT('Ctrl Pts',(-41.2079002115909,45.2923641298557,
3.48823028058514));
#245344=CARTESIAN_POINT('Ctrl Pts',(-41.1142722655008,45.3773275334105,
3.4879469194163));
#245345=CARTESIAN_POINT('Ctrl Pts',(-41.1875373586974,45.4586966628148,
3.42473028058515));
#245346=CARTESIAN_POINT('Ctrl Pts',(-41.1778715515056,45.2588408013002,
3.41028005925117));
#245347=CARTESIAN_POINT('Ctrl Pts',(-41.0840023845225,45.3437094247737,
3.40982512230944));
#245348=CARTESIAN_POINT('Ctrl Pts',(-41.1423656859486,45.4085284377442,
3.30780486372889));
#245349=CARTESIAN_POINT('Ctrl Pts',(-41.1209827764377,45.195330604445,3.36123028058512));
#245350=CARTESIAN_POINT('Ctrl Pts',(-41.0267203359219,45.2800912647195,
3.36099721048581));
#245351=CARTESIAN_POINT('Ctrl Pts',(-41.0567886774847,45.3134855411626,
3.23423045308423));
#245352=CARTESIAN_POINT('Ctrl Pts',(-41.0611303347406,45.1285089182133,
3.36123028058512));
#245353=CARTESIAN_POINT('Ctrl Pts',(-40.966750941905,45.2134885052208,3.36123028058512));
#245354=CARTESIAN_POINT('Ctrl Pts',(-40.966750941905,45.2134885052208,3.23423028058512));
#245355=CARTESIAN_POINT('Origin',(-41.0611303347406,45.1285089182133,3.23423028058512));
#245356=CARTESIAN_POINT('Origin',(-0.235948482089066,-0.212448967518755,
3.64303198860262));
#245357=CARTESIAN_POINT('Origin',(-41.6348281284264,45.7656648676106,3.64303198860294));
#245358=CARTESIAN_POINT('Origin',(-0.235948482089066,-0.212448967518752,
3.23423028058481));
#245359=CARTESIAN_POINT('Origin',(-40.9599523566127,45.0161393894793,3.23423028058512));
#245360=CARTESIAN_POINT('Ctrl Pts',(-41.9955727382253,46.1654920697612,
3.47153072139103));
#245361=CARTESIAN_POINT('Ctrl Pts',(-41.9009568150781,46.2513146333408,
3.47182327902694));
#245362=CARTESIAN_POINT('Ctrl Pts',(-41.8286119029177,46.1706818621617,
3.4041302895905));
#245363=CARTESIAN_POINT('Ctrl Pts',(-41.9185486398936,46.0801220723613,
3.65553807120985));
#245364=CARTESIAN_POINT('Ctrl Pts',(-41.8239131221222,46.1657485549054,
3.65586275497224));
#245365=CARTESIAN_POINT('Ctrl Pts',(-41.7670844335152,46.1023486848312,
3.55128126837279));
#245366=CARTESIAN_POINT('Ctrl Pts',(-41.7801771152745,45.92675847217,3.77003198860295));
#245367=CARTESIAN_POINT('Ctrl Pts',(-41.6856154234933,46.0121526898589,
3.77025505748236));
#245368=CARTESIAN_POINT('Ctrl Pts',(-41.6565528363061,45.9795909100358,
3.64284211731202));
#245369=CARTESIAN_POINT('Ctrl Pts',(-41.6348281284264,45.7656648676106,
3.77003198860294));
#245370=CARTESIAN_POINT('Ctrl Pts',(-41.5403077371542,45.8507714101807,
3.77003198860294));
#245371=CARTESIAN_POINT('Ctrl Pts',(-41.5404488407561,45.8506443599269,
3.64284239821714));
#245372=CARTESIAN_POINT('Origin',(-41.9230990057958,46.0858221116778,3.40423097483341));
#245373=CARTESIAN_POINT('Ctrl Pts',(-40.9599523566127,45.0161393894793,
3.36123028058512));
#245374=CARTESIAN_POINT('Ctrl Pts',(-40.8655729637771,45.1011189764869,
3.36123028058512));
#245375=CARTESIAN_POINT('Ctrl Pts',(-40.8655729637771,45.1011189764869,
3.23423028058512));
#245376=CARTESIAN_POINT('Ctrl Pts',(-40.8998980546751,44.9490914663013,
3.36123028058512));
#245377=CARTESIAN_POINT('Ctrl Pts',(-40.8052862548003,45.034163803023,3.36146538610349));
#245378=CARTESIAN_POINT('Ctrl Pts',(-40.7752309130104,45.0007839642901,
3.23423043688437));
#245379=CARTESIAN_POINT('Ctrl Pts',(-40.8431135311196,44.8856913339442,
3.4105425869313));
#245380=CARTESIAN_POINT('Ctrl Pts',(-40.7485699563858,44.9711739722047,
3.41100608859769));
#245381=CARTESIAN_POINT('Ctrl Pts',(-40.6898060629513,44.9059100567371,
3.30819866970974));
#245382=CARTESIAN_POINT('Ctrl Pts',(-40.8131880745608,44.8522789915941,
3.48823028058512));
#245383=CARTESIAN_POINT('Ctrl Pts',(-40.7187157882339,44.9380175594362,
3.48852004212289));
#245384=CARTESIAN_POINT('Ctrl Pts',(-40.6447864996555,44.8559107663285,
3.42473028058512));
#245385=CARTESIAN_POINT('Origin',(-40.7391658924911,44.770931179321,3.42473028058512));
#245386=CARTESIAN_POINT('Origin',(-42.0423040287732,46.2182127020604,3.1191364817828));
#245387=CARTESIAN_POINT('Origin',(-42.1615090516454,46.3506032922594,2.83404198860293));
#245388=CARTESIAN_POINT('Origin',(-40.684731938309,44.710476148586,3.56563113460894));
#245389=CARTESIAN_POINT('Origin',(-40.6548553974685,44.677218962551,3.64299171721771));
#245390=CARTESIAN_POINT('Ctrl Pts',(-42.1358900227697,46.7738319284257,
2.59908173516055));
#245391=CARTESIAN_POINT('Ctrl Pts',(-42.1109214781063,46.7461150696872,
2.65878198860294));
#245392=CARTESIAN_POINT('Ctrl Pts',(-42.0638038389703,46.6938111422604,
2.65878198860294));
#245393=CARTESIAN_POINT('Ctrl Pts',(-42.2013581359411,46.7148552537641,
2.59908193475657));
#245394=CARTESIAN_POINT('Ctrl Pts',(-42.1586072771691,46.7031532960226,
2.65878715325504));
#245395=CARTESIAN_POINT('Ctrl Pts',(-42.1016932886506,46.6596664560533,
2.65878198860294));
#245396=CARTESIAN_POINT('Ctrl Pts',(-42.2450249725428,46.6418481388114,
2.6387877884991));
#245397=CARTESIAN_POINT('Ctrl Pts',(-42.1870455286633,46.6464039985658,
2.6956446018015));
#245398=CARTESIAN_POINT('Ctrl Pts',(-42.1199142759249,46.6095714048491,
2.6818048162493));
#245399=CARTESIAN_POINT('Ctrl Pts',(-42.2756632139848,46.5164783566528,
2.75443238878669));
#245400=CARTESIAN_POINT('Ctrl Pts',(-42.1934768724829,46.5588531737054,
2.7926834077712));
#245401=CARTESIAN_POINT('Ctrl Pts',(-42.1171707421505,46.5142596423501,
2.74885926835627));
#245402=CARTESIAN_POINT('Ctrl Pts',(-42.2644092166194,46.4640705998043,
2.82856655361705));
#245403=CARTESIAN_POINT('Ctrl Pts',(-42.1708301402953,46.5278411618568,
2.85384197230856));
#245404=CARTESIAN_POINT('Ctrl Pts',(-42.0975575768117,46.4693765058001,
2.79184624278606));
#245405=CARTESIAN_POINT('Ctrl Pts',(-42.2339804752703,46.4302753505425,
2.90134173516055));
#245406=CARTESIAN_POINT('Ctrl Pts',(-42.1395065321001,46.5159655405275,
2.90163218716423));
#245407=CARTESIAN_POINT('Ctrl Pts',(-42.0671296588098,46.435582879267,2.83404198860294));
#245408=CARTESIAN_POINT('Origin',(-42.0638038389703,46.6938111422604,2.53178198860293));
#245409=CARTESIAN_POINT('Origin',(-0.235948482089066,-0.212448967518755,
3.64303198860262));
#245410=CARTESIAN_POINT('Origin',(-40.386254305094,44.3789831537295,3.64303198860293));
#245411=CARTESIAN_POINT('Origin',(8.01250065760356E-17,1.91454897897931E-13,
2.53178198860262));
#245412=CARTESIAN_POINT('Origin',(-42.0411527846897,46.7142062431422,2.53178198860294));
#245413=CARTESIAN_POINT('Ctrl Pts',(-40.386254305094,44.3789831537295,3.77003198860293));
#245414=CARTESIAN_POINT('Ctrl Pts',(-40.2917335276657,44.4640900439962,
3.77003198860293));
#245415=CARTESIAN_POINT('Ctrl Pts',(-40.2918750180001,44.4639626455268,
3.64284187937025));
#245416=CARTESIAN_POINT('Ctrl Pts',(-40.2408978759463,44.2178916378598,
3.77003198860293));
#245417=CARTESIAN_POINT('Ctrl Pts',(-40.1466757825282,44.3029863283998,
3.76980208962917));
#245418=CARTESIAN_POINT('Ctrl Pts',(-40.1757689690817,44.3350138149348,
3.64284193928323));
#245419=CARTESIAN_POINT('Ctrl Pts',(-40.1025190720996,44.0645366033534,
3.65553535416617));
#245420=CARTESIAN_POINT('Ctrl Pts',(-40.0085488431153,44.1495800756908,
3.65520057834612));
#245421=CARTESIAN_POINT('Ctrl Pts',(-40.0652381943495,44.2122569536132,
3.55127910964266));
#245422=CARTESIAN_POINT('Ctrl Pts',(-40.025490812659,43.9791725362583,3.47153072139102));
#245423=CARTESIAN_POINT('Ctrl Pts',(-39.9317222927443,44.0642551375177,
3.47122746281612));
#245424=CARTESIAN_POINT('Ctrl Pts',(-40.003711479089,44.1439246138551,3.40413045901276));
#245425=CARTESIAN_POINT('Origin',(-40.0979831325501,44.0588255818378,3.4042309748334));
#245426=CARTESIAN_POINT('Ctrl Pts',(-41.7612723673365,46.8559036426985,
2.90134173516056));
#245427=CARTESIAN_POINT('Ctrl Pts',(-41.8563683535932,46.7709043015502,
2.90163218716423));
#245428=CARTESIAN_POINT('Ctrl Pts',(-41.7839914803029,46.6905216402897,
2.83404198860294));
#245429=CARTESIAN_POINT('Ctrl Pts',(-41.7917156448183,46.8897135983615,
2.82853349835382));
#245430=CARTESIAN_POINT('Ctrl Pts',(-41.8649095672149,46.8033160448246,
2.85381483162464));
#245431=CARTESIAN_POINT('Ctrl Pts',(-41.8144332630853,46.7243306652216,
2.79182701594319));
#245432=CARTESIAN_POINT('Ctrl Pts',(-41.8425440045881,46.9062450310967,
2.75468822073682));
#245433=CARTESIAN_POINT('Ctrl Pts',(-41.893356908596,46.8289264627106,2.79286913083891));
#245434=CARTESIAN_POINT('Ctrl Pts',(-41.8569022891475,46.7483907976684,
2.74900763297939));
#245435=CARTESIAN_POINT('Ctrl Pts',(-41.9695156381235,46.8892773184519,
2.63954450640417));
#245436=CARTESIAN_POINT('Ctrl Pts',(-41.9804178820373,46.8319191778368,
2.69627684028874));
#245437=CARTESIAN_POINT('Ctrl Pts',(-41.9507871007486,46.7612136652289,
2.68224356036528));
#245438=CARTESIAN_POINT('Ctrl Pts',(-42.0474864684049,46.8534019544978,
2.59908178706453));
#245439=CARTESIAN_POINT('Ctrl Pts',(-42.0403508033696,46.8096319157664,
2.65878704321511));
#245440=CARTESIAN_POINT('Ctrl Pts',(-42.0031091843005,46.7484320121859,
2.65878198860294));
#245441=CARTESIAN_POINT('Ctrl Pts',(-42.1132001506003,46.7942619810917,
2.59908173516055));
#245442=CARTESIAN_POINT('Ctrl Pts',(-42.0882450513177,46.7665330160779,
2.65878198860293));
#245443=CARTESIAN_POINT('Ctrl Pts',(-42.0411527846897,46.7142062431422,
2.65878198860294));
#245444=CARTESIAN_POINT('Origin',(-41.6896120874673,46.7755012272973,2.83404198860294));
#245445=CARTESIAN_POINT('Origin',(-39.978777945671,43.9264348095002,3.11913648167199));
#245446=CARTESIAN_POINT('Origin',(-39.8595727587357,43.7940440370144,2.83404198860291));
#245447=CARTESIAN_POINT('Origin',(-41.5704070646268,46.6431106370601,3.11913648177836));
#245448=CARTESIAN_POINT('Origin',(-41.4512020416176,46.5107200467157,3.40423097483342));
#245449=CARTESIAN_POINT('Ctrl Pts',(-39.7870778846749,43.7143933160623,
2.90134173516053));
#245450=CARTESIAN_POINT('Ctrl Pts',(-39.6934538167802,43.7993487829613,
2.90103711553259));
#245451=CARTESIAN_POINT('Ctrl Pts',(-39.7651933659001,43.879023624022,2.83404198860291));
#245452=CARTESIAN_POINT('Ctrl Pts',(-39.7566748466934,43.6806281164511,
2.82862991747978));
#245453=CARTESIAN_POINT('Ctrl Pts',(-39.6846648960477,43.76687916567,2.85314045886605));
#245454=CARTESIAN_POINT('Ctrl Pts',(-39.7347894633637,43.8452566693654,
2.79187960999937));
#245455=CARTESIAN_POINT('Ctrl Pts',(-39.7061132086031,43.6642103943288,
2.75470625793373));
#245456=CARTESIAN_POINT('Ctrl Pts',(-39.6560595510442,43.7414086642734,
2.79224250381934));
#245457=CARTESIAN_POINT('Ctrl Pts',(-39.6925108309095,43.8213838166748,
2.74901809108295));
#245458=CARTESIAN_POINT('Ctrl Pts',(-39.5798624575879,43.6815693876452,
2.63947868311711));
#245459=CARTESIAN_POINT('Ctrl Pts',(-39.5692094437565,43.7388169234803,
2.69595066767937));
#245460=CARTESIAN_POINT('Ctrl Pts',(-39.5991004926179,43.8091742082548,
2.68220539436085));
#245461=CARTESIAN_POINT('Ctrl Pts',(-39.5024012818819,43.7176736830028,
2.5990817858515));
#245462=CARTESIAN_POINT('Ctrl Pts',(-39.5096522555301,43.761347316339,2.6587767094482));
#245463=CARTESIAN_POINT('Ctrl Pts',(-39.5470931435014,43.8223603708617,
2.65878198860291));
#245464=CARTESIAN_POINT('Ctrl Pts',(-39.437049873601,43.7765468711722,2.59908173516053));
#245465=CARTESIAN_POINT('Ctrl Pts',(-39.4620188529811,43.8042633382929,
2.65878198860292));
#245466=CARTESIAN_POINT('Ctrl Pts',(-39.5091373124624,43.8565665267056,
2.65878198860292));
#245467=CARTESIAN_POINT('Origin',(-39.5091373124624,43.8565665267056,2.53178198860292));
#245468=CARTESIAN_POINT('Ctrl Pts',(-41.1629311642483,46.1905628026485,
3.77003198860295));
#245469=CARTESIAN_POINT('Ctrl Pts',(-41.2574515636632,46.1054562527467,
3.77003198860295));
#245470=CARTESIAN_POINT('Ctrl Pts',(-41.2573104519064,46.1055833103431,
3.6428423872765));
#245471=CARTESIAN_POINT('Ctrl Pts',(-41.307951431326,46.3519569306005,3.77003198860295));
#245472=CARTESIAN_POINT('Ctrl Pts',(-41.4027622547777,46.2668393800569,
3.77025506105729));
#245473=CARTESIAN_POINT('Ctrl Pts',(-41.3734162510841,46.2345318643247,
3.64284210641953));
#245474=CARTESIAN_POINT('Ctrl Pts',(-41.4460100362743,46.5056000892413,
3.65553527987864));
#245475=CARTESIAN_POINT('Ctrl Pts',(-41.5410595633947,46.4204333915661,
3.65585996533167));
#245476=CARTESIAN_POINT('Ctrl Pts',(-41.4839469723838,46.3572886670224,
3.55127902710186));
#245477=CARTESIAN_POINT('Ctrl Pts',(-41.5228599914565,46.591124538743,3.47153072139103));
#245478=CARTESIAN_POINT('Ctrl Pts',(-41.6181024753229,46.5059978248579,
3.47182327905219));
#245479=CARTESIAN_POINT('Ctrl Pts',(-41.545473506938,46.425620806486,3.40413028378029));
#245480=CARTESIAN_POINT('Origin',(-41.1629311642483,46.1905628026485,3.64303198860295));
#245481=CARTESIAN_POINT('Origin',(3.72719664096539E-16,1.91621025575097E-13,
2.53178198860262));
#245482=CARTESIAN_POINT('Origin',(-39.4864862581819,43.8769616275874,2.53178198860292));
#245483=CARTESIAN_POINT('Origin',(28.0951675083328,-30.7283483363944,3.64303198860241));
#245484=CARTESIAN_POINT('Origin',(-40.8943347850524,45.8923335519903,3.64299466007517));
#245485=CARTESIAN_POINT('Ctrl Pts',(-39.4144401478992,43.7969047596346,
2.59908173516053));
#245486=CARTESIAN_POINT('Ctrl Pts',(-39.439394812269,43.8246341160485,2.65878198860292));
#245487=CARTESIAN_POINT('Ctrl Pts',(-39.4864862581819,43.8769616275874,
2.65878198860292));
#245488=CARTESIAN_POINT('Ctrl Pts',(-39.3492813761645,43.8555436924523,
2.59908193199924));
#245489=CARTESIAN_POINT('Ctrl Pts',(-39.3919218645329,43.8673524484227,
2.65877685806688));
#245490=CARTESIAN_POINT('Ctrl Pts',(-39.4486296259964,43.9110175468016,
2.65878198860292));
#245491=CARTESIAN_POINT('Ctrl Pts',(-39.3054399757367,43.9280312169046,
2.63872492669844));
#245492=CARTESIAN_POINT('Ctrl Pts',(-39.3632835603679,43.923706596467,2.69532212015284));
#245493=CARTESIAN_POINT('Ctrl Pts',(-39.4300423632768,43.9607655567558,
2.68176836726669));
#245494=CARTESIAN_POINT('Ctrl Pts',(-39.2744854109877,44.0526112349805,
2.75442176402264));
#245495=CARTESIAN_POINT('Ctrl Pts',(-39.3564679665374,44.0109847679682,
2.79203179920206));
#245496=CARTESIAN_POINT('Ctrl Pts',(-39.4322155454631,44.0555161714744,
2.748853107482));
#245497=CARTESIAN_POINT('Ctrl Pts',(-39.285649880758,44.1047669487877,2.82866089558441));
#245498=CARTESIAN_POINT('Ctrl Pts',(-39.3789590643335,44.042159156452,2.8531656311921));
#245499=CARTESIAN_POINT('Ctrl Pts',(-39.4516641984998,44.1002097724416,
2.79189751796671));
#245500=CARTESIAN_POINT('Ctrl Pts',(-39.3160391863692,44.1385184650376,
2.90134173516053));
#245501=CARTESIAN_POINT('Ctrl Pts',(-39.4103156382734,44.054287543984,2.90103711553259));
#245502=CARTESIAN_POINT('Ctrl Pts',(-39.4820551873932,44.1339623850447,
2.83404198860292));
#245503=CARTESIAN_POINT('Origin',(-39.3876757945576,44.2189419720523,2.83404198860292));
#245504=CARTESIAN_POINT('Origin',(-40.8647803215171,45.8594327453968,3.56647653971846));
#245505=CARTESIAN_POINT('Origin',(-40.8100197873549,45.7986150108451,3.42473028058516));
#245506=CARTESIAN_POINT('Origin',(-39.5068809815279,44.3513327444866,3.11913648168124));
#245507=CARTESIAN_POINT('Origin',(-39.626086168372,44.4837235168756,3.4042309748334));
#245508=CARTESIAN_POINT('Ctrl Pts',(-40.5892333705625,45.5534068532511,
3.36123028058513));
#245509=CARTESIAN_POINT('Ctrl Pts',(-40.6836127633981,45.4684272662436,
3.36123028058513));
#245510=CARTESIAN_POINT('Ctrl Pts',(-40.6836127633981,45.4684272662436,
3.23423028058513));
#245511=CARTESIAN_POINT('Ctrl Pts',(-40.649636173697,45.6201409680079,3.36123028058513));
#245512=CARTESIAN_POINT('Ctrl Pts',(-40.7437849681275,45.5352552698608,
3.36099641108633));
#245513=CARTESIAN_POINT('Ctrl Pts',(-40.7739548060672,45.5687622694471,
3.23423043688415));
#245514=CARTESIAN_POINT('Ctrl Pts',(-40.7067502157893,45.6832443225586,
3.41054258905314));
#245515=CARTESIAN_POINT('Ctrl Pts',(-40.8009661159856,45.5987613682859,
3.41008815825837));
#245516=CARTESIAN_POINT('Ctrl Pts',(-40.8593796344574,45.6636361529343,
3.3081986730425));
#245517=CARTESIAN_POINT('Ctrl Pts',(-40.7368493365299,45.7165002428307,
3.48823028058515));
#245518=CARTESIAN_POINT('Ctrl Pts',(-40.8311340869939,45.6322662944332,
3.48794691941631));
#245519=CARTESIAN_POINT('Ctrl Pts',(-40.9043991801906,45.7136354238376,
3.42473028058516));
#245520=CARTESIAN_POINT('Origin',(-40.5892333705625,45.5534068532511,3.23423028058513));
#245521=CARTESIAN_POINT('Ctrl Pts',(-39.5544469813073,44.4033023070489,
3.47153072139102));
#245522=CARTESIAN_POINT('Ctrl Pts',(-39.6488649595839,44.3189410241794,
3.47122746285107));
#245523=CARTESIAN_POINT('Ctrl Pts',(-39.7205730817654,44.3988635552005,
3.4041304667682));
#245524=CARTESIAN_POINT('Ctrl Pts',(-39.631292930691,44.4888328647726,3.65553813458016));
#245525=CARTESIAN_POINT('Ctrl Pts',(-39.7256930794102,44.4042668857101,
3.65520336072188));
#245526=CARTESIAN_POINT('Ctrl Pts',(-39.7821007282713,44.4671969296244,
3.55128134519921));
#245527=CARTESIAN_POINT('Ctrl Pts',(-39.769344436532,44.6424847942267,3.77003198860293));
#245528=CARTESIAN_POINT('Ctrl Pts',(-39.8638218465944,44.5576736781012,
3.76980209314289));
#245529=CARTESIAN_POINT('Ctrl Pts',(-39.8926323785409,44.5899547640682,
3.64284195387469));
#245530=CARTESIAN_POINT('Ctrl Pts',(-39.9143573409159,44.8038810887674,
3.77003198860294));
#245531=CARTESIAN_POINT('Ctrl Pts',(-40.0088781074273,44.7187742083304,
3.77003198860294));
#245532=CARTESIAN_POINT('Ctrl Pts',(-40.0087366280261,44.7189015969554,
3.64284189403838));
#245533=CARTESIAN_POINT('Origin',(-39.9143573409159,44.8038810887674,3.64303198860294));
#245534=CARTESIAN_POINT('Origin',(27.4203375923837,-29.9788737863602,3.23423028058461));
#245535=CARTESIAN_POINT('Origin',(-40.4880553924346,45.4410373245172,3.23423028058512));
#245536=CARTESIAN_POINT('Origin',(27.3146622010794,-29.8615093742682,3.64303198860242));
#245537=CARTESIAN_POINT('Origin',(-40.1828829233545,45.102184887041,3.64299171721827));
#245538=CARTESIAN_POINT('Ctrl Pts',(-40.3404336838195,45.2779489569772,
3.48823028058512));
#245539=CARTESIAN_POINT('Ctrl Pts',(-40.435577609727,45.1929563204589,3.4885200421229));
#245540=CARTESIAN_POINT('Ctrl Pts',(-40.3616483211486,45.1108495273513,
3.42473028058512));
#245541=CARTESIAN_POINT('Ctrl Pts',(-40.3706366483438,45.3113153943819,
3.41028005848437));
#245542=CARTESIAN_POINT('Ctrl Pts',(-40.4655326953357,45.2262248134114,
3.41074404220252));
#245543=CARTESIAN_POINT('Ctrl Pts',(-40.4068200107207,45.161017771106,3.30780486243924));
#245544=CARTESIAN_POINT('Ctrl Pts',(-40.4278556061233,45.3745283705083,
3.36123028058512));
#245545=CARTESIAN_POINT('Ctrl Pts',(-40.5223510101983,45.2893279449781,
3.3614646058656));
#245546=CARTESIAN_POINT('Ctrl Pts',(-40.4923970402292,45.25606069106,3.23423045308495));
#245547=CARTESIAN_POINT('Ctrl Pts',(-40.4880553924346,45.4410373245172,
3.36123028058512));
#245548=CARTESIAN_POINT('Ctrl Pts',(-40.5824347852702,45.3560577375096,
3.36123028058512));
#245549=CARTESIAN_POINT('Ctrl Pts',(-40.5824347852702,45.3560577375096,
3.23423028058512));
#245550=CARTESIAN_POINT('Origin',(-40.267268928313,45.1958291143588,3.42473028058512));
#245551=CARTESIAN_POINT('Origin',(-40.2128349746541,45.1353740846429,3.56563113524829));
#245552=CARTESIAN_POINT('Origin',(-45.8594327460063,40.8647803224533,3.56647653909523));
#245553=CARTESIAN_POINT('Origin',(-45.8923335519879,40.8943347850518,3.64299466007835));
#245554=CARTESIAN_POINT('Origin',(-45.7986150108453,40.8100197873546,3.42473028058512));
#245555=CARTESIAN_POINT('Ctrl Pts',(-45.7165002428309,40.7368493365297,
3.48823028058511));
#245556=CARTESIAN_POINT('Ctrl Pts',(-45.6322662944335,40.8311340869937,
3.48794691941628));
#245557=CARTESIAN_POINT('Ctrl Pts',(-45.7136354238378,40.9043991801903,
3.42473028058512));
#245558=CARTESIAN_POINT('Ctrl Pts',(-45.6831319408669,40.7066485019717,
3.41028005925112));
#245559=CARTESIAN_POINT('Ctrl Pts',(-45.5986481857945,40.8008642060163,
3.40982512231164));
#245560=CARTESIAN_POINT('Ctrl Pts',(-45.6634671987684,40.8592275074426,
3.30780486372857));
#245561=CARTESIAN_POINT('Ctrl Pts',(-45.619916185183,40.649432716854,3.36123028058509));
#245562=CARTESIAN_POINT('Ctrl Pts',(-45.5350300257419,40.7435821574166,
3.36099721048318));
#245563=CARTESIAN_POINT('Ctrl Pts',(-45.5684243021846,40.7736504989767,
3.23423045308402));
#245564=CARTESIAN_POINT('Ctrl Pts',(-45.5534068532514,40.5892333705622,
3.36123028058509));
#245565=CARTESIAN_POINT('Ctrl Pts',(-45.4684272662438,40.6836127633978,
3.3612302805851));
#245566=CARTESIAN_POINT('Ctrl Pts',(-45.4684272662438,40.6836127633978,
3.23423028058509));
#245567=CARTESIAN_POINT('Origin',(-45.5534068532514,40.5892333705622,3.23423028058509));
#245568=CARTESIAN_POINT('Origin',(-0.212448967518931,-0.23594848208889,
3.64303198860262));
#245569=CARTESIAN_POINT('Origin',(-46.1905628026487,41.162931164248,3.64303198860291));
#245570=CARTESIAN_POINT('Origin',(-0.212448967518931,-0.235948482088887,
3.23423028058481));
#245571=CARTESIAN_POINT('Origin',(-45.4410373245174,40.4880553924343,3.23423028058509));
#245572=CARTESIAN_POINT('Ctrl Pts',(-46.5911245387432,41.5228599914562,
3.471530721391));
#245573=CARTESIAN_POINT('Ctrl Pts',(-46.5059978322078,41.6181024670996,
3.4718232790269));
#245574=CARTESIAN_POINT('Ctrl Pts',(-46.4256208133854,41.5454735131718,
3.40413028959072));
#245575=CARTESIAN_POINT('Ctrl Pts',(-46.5055987918433,41.4460088704684,
3.65553807120985));
#245576=CARTESIAN_POINT('Ctrl Pts',(-46.4204321019747,41.5410583874226,
3.65586275496986));
#245577=CARTESIAN_POINT('Ctrl Pts',(-46.357287635879,41.4839460439597,3.5512812683726));
#245578=CARTESIAN_POINT('Ctrl Pts',(-46.3519544194661,41.3079491749529,
3.77003198860292));
#245579=CARTESIAN_POINT('Ctrl Pts',(-46.266836872876,41.4027599825079,3.77025505748455));
#245580=CARTESIAN_POINT('Ctrl Pts',(-46.2345298607751,41.3734144471015,
3.64284211731201));
#245581=CARTESIAN_POINT('Ctrl Pts',(-46.1905628026487,41.162931164248,3.77003198860291));
#245582=CARTESIAN_POINT('Ctrl Pts',(-46.1054562600789,41.2574515555199,
3.77003198860291));
#245583=CARTESIAN_POINT('Ctrl Pts',(-46.1055833103324,41.2573104519183,
3.64284239821759));
#245584=CARTESIAN_POINT('Origin',(-46.5107200467159,41.4512020416173,3.40423097483338));
#245585=CARTESIAN_POINT('Ctrl Pts',(-45.4410373245174,40.4880553924343,
3.36123028058509));
#245586=CARTESIAN_POINT('Ctrl Pts',(-45.3560577375098,40.5824347852699,
3.36123028058509));
#245587=CARTESIAN_POINT('Ctrl Pts',(-45.3560577375098,40.5824347852699,
3.23423028058509));
#245588=CARTESIAN_POINT('Ctrl Pts',(-45.3743035899554,40.4276521486878,
3.36123028058509));
#245589=CARTESIAN_POINT('Ctrl Pts',(-45.2891025640467,40.5221480762966,
3.36146538610229));
#245590=CARTESIAN_POINT('Ctrl Pts',(-45.2557227253145,40.4920927345046,
3.23423043688486));
#245591=CARTESIAN_POINT('Ctrl Pts',(-45.3112030195546,40.3705349278746,
3.41054258693126));
#245592=CARTESIAN_POINT('Ctrl Pts',(-45.2261127332244,40.4654317778764,
3.41100608859753));
#245593=CARTESIAN_POINT('Ctrl Pts',(-45.160848817758,40.4066678844424,3.30819866970865));
#245594=CARTESIAN_POINT('Ctrl Pts',(-45.2779489569775,40.3404336838192,
3.48823028058509));
#245595=CARTESIAN_POINT('Ctrl Pts',(-45.1929563204591,40.4355776097268,
3.48852004212286));
#245596=CARTESIAN_POINT('Ctrl Pts',(-45.1108495273515,40.3616483211483,
3.42473028058508));
#245597=CARTESIAN_POINT('Origin',(-45.1958291143591,40.2672689283127,3.42473028058508));
#245598=CARTESIAN_POINT('Origin',(-46.6431106370687,41.5704070646328,3.11913648178481));
#245599=CARTESIAN_POINT('Origin',(-46.7755012272975,41.689612087467,2.83404198860289));
#245600=CARTESIAN_POINT('Origin',(-45.1353740836137,40.2128349741376,3.56563113460713));
#245601=CARTESIAN_POINT('Origin',(-45.1021848870412,40.1828829233542,3.64299171721822));
#245602=CARTESIAN_POINT('Ctrl Pts',(-46.7942619810919,42.1132001506,2.59908173516052));
#245603=CARTESIAN_POINT('Ctrl Pts',(-46.7665330160781,42.0882450513175,
2.6587819886029));
#245604=CARTESIAN_POINT('Ctrl Pts',(-46.7142062431425,42.0411527846894,
2.6587819886029));
#245605=CARTESIAN_POINT('Ctrl Pts',(-46.8532067119185,42.0477032750704,
2.59908193475599));
#245606=CARTESIAN_POINT('Ctrl Pts',(-46.8094668591651,42.0405341034491,
2.65878715325439));
#245607=CARTESIAN_POINT('Ctrl Pts',(-46.748319038876,42.0032346206976,2.6587819886029));
#245608=CARTESIAN_POINT('Ctrl Pts',(-46.8890030154866,41.9705316734064,
2.63878778849898));
#245609=CARTESIAN_POINT('Ctrl Pts',(-46.8318174060858,41.9811230778545,
2.69564460180142));
#245610=CARTESIAN_POINT('Ctrl Pts',(-46.7612038509552,41.951509383626,2.68180481624926));
#245611=CARTESIAN_POINT('Ctrl Pts',(-46.9063687067669,41.8426461117369,
2.75443238878675));
#245612=CARTESIAN_POINT('Ctrl Pts',(-46.829061965151,41.8933796070863,2.79268340777128));
#245613=CARTESIAN_POINT('Ctrl Pts',(-46.7485125544798,41.8570065263033,
2.74885926835625));
#245614=CARTESIAN_POINT('Ctrl Pts',(-46.8896982576903,41.7917018131138,
2.82856655361699));
#245615=CARTESIAN_POINT('Ctrl Pts',(-46.803297656188,41.8649047103983,2.85384197230712));
#245616=CARTESIAN_POINT('Ctrl Pts',(-46.7243152668219,41.8144193983035,
2.79184624278388));
#245617=CARTESIAN_POINT('Ctrl Pts',(-46.8559036426987,41.7612723673362,
2.90134173516052));
#245618=CARTESIAN_POINT('Ctrl Pts',(-46.7709043015504,41.856368353593,2.9016321871642));
#245619=CARTESIAN_POINT('Ctrl Pts',(-46.6905216402899,41.7839914803026,
2.8340419886029));
#245620=CARTESIAN_POINT('Origin',(-46.7142062431425,42.0411527846894,2.5317819886029));
#245621=CARTESIAN_POINT('Origin',(-0.212448967518931,-0.23594848208889,
3.64303198860262));
#245622=CARTESIAN_POINT('Origin',(-44.8038810887676,39.9143573409156,3.6430319886029));
#245623=CARTESIAN_POINT('Origin',(9.23291810287662E-17,1.91467102072384E-13,
2.53178198860262));
#245624=CARTESIAN_POINT('Origin',(-46.6938111422607,42.06380383897,2.53178198860291));
#245625=CARTESIAN_POINT('Ctrl Pts',(-44.8038810887676,39.9143573409156,
3.7700319886029));
#245626=CARTESIAN_POINT('Ctrl Pts',(-44.7187741985014,40.0088781183435,
3.77003198860291));
#245627=CARTESIAN_POINT('Ctrl Pts',(-44.7189015969704,40.0087366280095,
3.64284187937085));
#245628=CARTESIAN_POINT('Ctrl Pts',(-44.6424822887494,39.7693421853888,
3.7700319886029));
#245629=CARTESIAN_POINT('Ctrl Pts',(-44.5576711710503,39.8638196089388,
3.76980208962854));
#245630=CARTESIAN_POINT('Ctrl Pts',(-44.5899527660323,39.8926305794714,
3.64284193928371));
#245631=CARTESIAN_POINT('Ctrl Pts',(-44.4888315723752,39.6312917695248,
3.65553535416614));
#245632=CARTESIAN_POINT('Ctrl Pts',(-44.4042655856132,39.7256919284555,
3.65520057834546));
#245633=CARTESIAN_POINT('Ctrl Pts',(-44.4671959043838,39.7820998051106,
3.55127910964227));
#245634=CARTESIAN_POINT('Ctrl Pts',(-44.4033023070491,39.554446981307,3.47153072139098));
#245635=CARTESIAN_POINT('Ctrl Pts',(-44.3189410144585,39.6488649704636,
3.47122746281608));
#245636=CARTESIAN_POINT('Ctrl Pts',(-44.3988635644382,39.7205730900532,
3.40413045901305));
#245637=CARTESIAN_POINT('Origin',(-44.4837235168759,39.6260861683717,3.40423097483337));
#245638=CARTESIAN_POINT('Ctrl Pts',(-46.4302753505427,42.2339804752701,
2.90134173516052));
#245639=CARTESIAN_POINT('Ctrl Pts',(-46.5159655405277,42.1395065320999,
2.9016321871642));
#245640=CARTESIAN_POINT('Ctrl Pts',(-46.4355828792672,42.0671296588095,
2.8340419886029));
#245641=CARTESIAN_POINT('Ctrl Pts',(-46.4640859592741,42.2644230274459,
2.82853349835383));
#245642=CARTESIAN_POINT('Ctrl Pts',(-46.5278479142006,42.1708479205174,
2.85381483162313));
#245643=CARTESIAN_POINT('Ctrl Pts',(-46.4693919041987,42.0975714415916,
2.79182701594276));
#245644=CARTESIAN_POINT('Ctrl Pts',(-46.5163638812299,42.2755508889262,
2.75468822073671));
#245645=CARTESIAN_POINT('Ctrl Pts',(-46.5588164356976,42.1933444849783,
2.79286913083864));
#245646=CARTESIAN_POINT('Ctrl Pts',(-46.5141432491638,42.1170605480854,
2.7490076329795));
#245647=CARTESIAN_POINT('Ctrl Pts',(-46.6408663419435,42.2454039774545,
2.6395445064042));
#245648=CARTESIAN_POINT('Ctrl Pts',(-46.6457133039302,42.1872204559321,
2.69627684028881));
#245649=CARTESIAN_POINT('Ctrl Pts',(-46.6088541045839,42.1199995355541,
2.6822435603651));
#245650=CARTESIAN_POINT('Ctrl Pts',(-46.7146600431957,42.2015749714294,
2.59908178706335));
#245651=CARTESIAN_POINT('Ctrl Pts',(-46.7029882531945,42.1587905896511,
2.65878704321545));
#245652=CARTESIAN_POINT('Ctrl Pts',(-46.6595535157374,42.1018187547559,
2.6587819886029));
#245653=CARTESIAN_POINT('Ctrl Pts',(-46.773831928426,42.1358900227694,2.59908173516052));
#245654=CARTESIAN_POINT('Ctrl Pts',(-46.7461150696874,42.1109214781061,
2.6587819886029));
#245655=CARTESIAN_POINT('Ctrl Pts',(-46.6938111422607,42.06380383897,2.6587819886029));
#245656=CARTESIAN_POINT('Origin',(-46.3506032922596,42.1615090516451,2.83404198860289));
#245657=CARTESIAN_POINT('Origin',(-44.3513327444991,39.5068809815365,3.11913648167179));
#245658=CARTESIAN_POINT('Origin',(-44.2189419720525,39.3876757945573,2.83404198860289));
#245659=CARTESIAN_POINT('Origin',(-46.2182127020521,42.042304028765,3.11913648177552));
#245660=CARTESIAN_POINT('Origin',(-46.085822111678,41.9230990057955,3.40423097483339));
#245661=CARTESIAN_POINT('Ctrl Pts',(-44.1385184650378,39.3160391863689,
2.9013417351605));
#245662=CARTESIAN_POINT('Ctrl Pts',(-44.0542875439842,39.4103156382731,
2.90103711553256));
#245663=CARTESIAN_POINT('Ctrl Pts',(-44.1339623850449,39.482055187393,2.83404198860288));
#245664=CARTESIAN_POINT('Ctrl Pts',(-44.1047525536513,39.285636938894,2.82862991747977));
#245665=CARTESIAN_POINT('Ctrl Pts',(-44.042152770681,39.3789425853231,2.85314045886458));
#245666=CARTESIAN_POINT('Ctrl Pts',(-44.1001954303878,39.4516512848561,
2.79187961000011));
#245667=CARTESIAN_POINT('Ctrl Pts',(-44.0527517782421,39.2745942850999,
2.7547062579337));
#245668=CARTESIAN_POINT('Ctrl Pts',(-44.0110417363808,39.3566016867497,
2.79224250381919));
#245669=CARTESIAN_POINT('Ctrl Pts',(-44.0556530121008,39.4323285306301,
2.74901809108306));
#245670=CARTESIAN_POINT('Ctrl Pts',(-43.9290071509456,39.3050549810251,
2.63947868311709));
#245671=CARTESIAN_POINT('Ctrl Pts',(-43.9243964923851,39.3631024520343,
2.6959506676794));
#245672=CARTESIAN_POINT('Ctrl Pts',(-43.9614781338108,39.4299498468379,
2.68220539436068));
#245673=CARTESIAN_POINT('Ctrl Pts',(-43.8557442421764,39.349058390934,2.59908178585111));
#245674=CARTESIAN_POINT('Ctrl Pts',(-43.8675206320104,39.3917348424044,
2.65877670944926));
#245675=CARTESIAN_POINT('Ctrl Pts',(-43.9111340157076,39.4485000225472,
2.65878198860288));
#245676=CARTESIAN_POINT('Ctrl Pts',(-43.7969047596348,39.4144401478989,
2.5990817351605));
#245677=CARTESIAN_POINT('Ctrl Pts',(-43.8246341160487,39.4393948122688,
2.65878198860288));
#245678=CARTESIAN_POINT('Ctrl Pts',(-43.8769616275876,39.4864862581816,
2.65878198860288));
#245679=CARTESIAN_POINT('Origin',(-43.8769616275876,39.4864862581816,2.53178198860288));
#245680=CARTESIAN_POINT('Ctrl Pts',(-45.7656648676108,41.6348281284262,
3.77003198860292));
#245681=CARTESIAN_POINT('Ctrl Pts',(-45.850771417513,41.5403077290108,3.77003198860292));
#245682=CARTESIAN_POINT('Ctrl Pts',(-45.8506443599162,41.540448840768,3.64284238727584));
#245683=CARTESIAN_POINT('Ctrl Pts',(-45.926760978667,41.780179376798,3.77003198860292));
#245684=CARTESIAN_POINT('Ctrl Pts',(-46.0121552117534,41.6856176794229,
3.77025506105564));
#245685=CARTESIAN_POINT('Ctrl Pts',(-45.979592913563,41.6565546403116,3.64284210641854));
#245686=CARTESIAN_POINT('Ctrl Pts',(-46.0801233673956,41.9185498083246,
3.65553527987863));
#245687=CARTESIAN_POINT('Ctrl Pts',(-46.165749859238,41.8239142817211,3.65585996533324));
#245688=CARTESIAN_POINT('Ctrl Pts',(-46.1023497159542,41.7670853619641,
3.5512790271029));
#245689=CARTESIAN_POINT('Ctrl Pts',(-46.1654920697614,41.995572738225,3.47153072139099));
#245690=CARTESIAN_POINT('Ctrl Pts',(-46.2513146407508,41.9009568069088,
3.47182327905216));
#245691=CARTESIAN_POINT('Ctrl Pts',(-46.1706818552407,41.8286118967076,
3.40413028377992));
#245692=CARTESIAN_POINT('Origin',(-45.7656648676108,41.6348281284262,3.64303198860292));
#245693=CARTESIAN_POINT('Origin',(3.68378193773366E-16,1.91616684104774E-13,
2.53178198860262));
#245694=CARTESIAN_POINT('Origin',(-43.8565665267058,39.5091373124622,2.53178198860288));
#245695=CARTESIAN_POINT('Origin',(34.5756856720389,-30.7048488218242,3.64303198860241));
#245696=CARTESIAN_POINT('Origin',(-45.4673664422109,41.3663085755629,3.64299466007616));
#245697=CARTESIAN_POINT('Ctrl Pts',(-43.7765468711724,39.4370498736008,
2.5990817351605));
#245698=CARTESIAN_POINT('Ctrl Pts',(-43.8042633382931,39.4620188529809,
2.65878198860288));
#245699=CARTESIAN_POINT('Ctrl Pts',(-43.8565665267058,39.5091373124622,
2.65878198860288));
#245700=CARTESIAN_POINT('Ctrl Pts',(-43.717874483542,39.5021785224867,2.59908193199899));
#245701=CARTESIAN_POINT('Ctrl Pts',(-43.7615157339669,39.5094654441329,
2.65877685806683));
#245702=CARTESIAN_POINT('Ctrl Pts',(-43.822477090013,39.5469637653744,2.65878198860288));
#245703=CARTESIAN_POINT('Ctrl Pts',(-43.6818502604299,39.5788516269098,
2.63872492669802));
#245704=CARTESIAN_POINT('Ctrl Pts',(-43.7389249259236,39.5685043961838,
2.69532212015301));
#245705=CARTESIAN_POINT('Ctrl Pts',(-43.8091917332946,39.5983821485331,
2.6817683672665));
#245706=CARTESIAN_POINT('Ctrl Pts',(-43.6640874258692,39.7059848156962,
2.75442176402299));
#245707=CARTESIAN_POINT('Ctrl Pts',(-43.7412697217737,39.6560168722793,
2.79203179920158));
#245708=CARTESIAN_POINT('Ctrl Pts',(-43.8212571467117,39.6923865500764,
2.74885310748213));
#245709=CARTESIAN_POINT('Ctrl Pts',(-43.6806424921191,39.7566878101789,
2.82866089558412));
#245710=CARTESIAN_POINT('Ctrl Pts',(-43.7668962219017,39.684669524315,2.85316563119281));
#245711=CARTESIAN_POINT('Ctrl Pts',(-43.8452710114193,39.7348023770065,
2.79189751796631));
#245712=CARTESIAN_POINT('Ctrl Pts',(-43.7143933160625,39.7870778846747,
2.9013417351605));
#245713=CARTESIAN_POINT('Ctrl Pts',(-43.7993487829615,39.69345381678,2.90103711553256));
#245714=CARTESIAN_POINT('Ctrl Pts',(-43.8790236240222,39.7651933658998,
2.83404198860289));
#245715=CARTESIAN_POINT('Origin',(-43.7940440370146,39.8595727587355,2.83404198860289));
#245716=CARTESIAN_POINT('Origin',(-45.4345348103666,41.3366772856881,3.56647653971791));
#245717=CARTESIAN_POINT('Origin',(-45.3737170758075,41.2819167515328,3.42473028058513));
#245718=CARTESIAN_POINT('Origin',(-43.9264348094881,39.9787779456592,3.11913648168251));
#245719=CARTESIAN_POINT('Origin',(-44.058825581838,40.0979831325499,3.40423097483338));
#245720=CARTESIAN_POINT('Ctrl Pts',(-45.1285089182135,41.0611303347403,
3.36123028058509));
#245721=CARTESIAN_POINT('Ctrl Pts',(-45.2134885052211,40.9667509419047,
3.3612302805851));
#245722=CARTESIAN_POINT('Ctrl Pts',(-45.2134885052211,40.9667509419047,
3.23423028058509));
#245723=CARTESIAN_POINT('Ctrl Pts',(-45.1955564429365,41.121185060844,3.36123028058509));
#245724=CARTESIAN_POINT('Ctrl Pts',(-45.2803165088389,41.0269231466363,
3.36099641108286));
#245725=CARTESIAN_POINT('Ctrl Pts',(-45.3138235084265,41.0570929845756,
3.23423043688394));
#245726=CARTESIAN_POINT('Ctrl Pts',(-45.2589537050067,41.177972685567,3.41054258905313));
#245727=CARTESIAN_POINT('Ctrl Pts',(-45.3438226072599,41.0841042944923,
3.41008815826159));
#245728=CARTESIAN_POINT('Ctrl Pts',(-45.4086973919092,41.1425178129616,
3.30819867304353));
#245729=CARTESIAN_POINT('Ctrl Pts',(-45.2923641298559,41.2079002115907,
3.48823028058512));
#245730=CARTESIAN_POINT('Ctrl Pts',(-45.3773275334107,41.1142722655006,
3.48794691941628));
#245731=CARTESIAN_POINT('Ctrl Pts',(-45.4586966628151,41.1875373586972,
3.42473028058512));
#245732=CARTESIAN_POINT('Origin',(-45.1285089182135,41.0611303347403,3.23423028058509));
#245733=CARTESIAN_POINT('Ctrl Pts',(-43.9791725362585,40.0254908126588,
3.471530721391));
#245734=CARTESIAN_POINT('Ctrl Pts',(-44.064255127713,39.9317223035499,3.47122746285105));
#245735=CARTESIAN_POINT('Ctrl Pts',(-44.1439246046464,40.0037114707677,
3.40413046676838));
#245736=CARTESIAN_POINT('Ctrl Pts',(-44.0645378932546,40.102520236038,3.65553813458013));
#245737=CARTESIAN_POINT('Ctrl Pts',(-44.1495813562469,40.0085500157883,
3.65520336072072));
#245738=CARTESIAN_POINT('Ctrl Pts',(-44.2122579788868,40.0652391174802,
3.55128134519897));
#245739=CARTESIAN_POINT('Ctrl Pts',(-44.2178941385633,40.2409001323912,
3.77003198860291));
#245740=CARTESIAN_POINT('Ctrl Pts',(-44.3029888158473,40.1466780419432,
3.76980209314169));
#245741=CARTESIAN_POINT('Ctrl Pts',(-44.3350158129974,40.1757707681154,
3.64284195387508));
#245742=CARTESIAN_POINT('Ctrl Pts',(-44.3789831537298,40.3862543050938,
3.77003198860291));
#245743=CARTESIAN_POINT('Ctrl Pts',(-44.4640900341665,40.2917335385827,
3.77003198860291));
#245744=CARTESIAN_POINT('Ctrl Pts',(-44.4639626455417,40.2918750179836,
3.64284189403873));
#245745=CARTESIAN_POINT('Origin',(-44.3789831537298,40.3862543050938,3.64303198860291));
#245746=CARTESIAN_POINT('Origin',(33.743309857225,-29.95537427179,3.23423028058461));
#245747=CARTESIAN_POINT('Origin',(-45.0161393894795,40.9599523566124,3.23423028058509));
#245748=CARTESIAN_POINT('Origin',(33.61296347236,-29.838009859698,3.64303198860242));
#245749=CARTESIAN_POINT('Origin',(-44.6772189625502,40.6548553974686,3.64299171721674));
#245750=CARTESIAN_POINT('Ctrl Pts',(-44.8522789915944,40.8131880745606,
3.48823028058509));
#245751=CARTESIAN_POINT('Ctrl Pts',(-44.9380175594364,40.7187157882337,
3.48852004212287));
#245752=CARTESIAN_POINT('Ctrl Pts',(-44.8559107663287,40.6447864996552,
3.42473028058509));
#245753=CARTESIAN_POINT('Ctrl Pts',(-44.8858042435428,40.843214657665,3.41028005848434));
#245754=CARTESIAN_POINT('Ctrl Pts',(-44.9712860523935,40.7486708738403,
3.41074404220265));
#245755=CARTESIAN_POINT('Ctrl Pts',(-44.9060790100831,40.689958189227,3.30780486243972));
#245756=CARTESIAN_POINT('Ctrl Pts',(-44.9493173051407,40.9001003367644,
3.3612302805851));
#245757=CARTESIAN_POINT('Ctrl Pts',(-45.0343891839537,40.8054891887047,
3.36146460586606));
#245758=CARTESIAN_POINT('Ctrl Pts',(-45.0011219300378,40.775535218736,3.23423045308401));
#245759=CARTESIAN_POINT('Ctrl Pts',(-45.0161393894795,40.9599523566124,
3.36123028058509));
#245760=CARTESIAN_POINT('Ctrl Pts',(-45.1011189764871,40.8655729637768,
3.36123028058509));
#245761=CARTESIAN_POINT('Ctrl Pts',(-45.1011189764871,40.8655729637768,
3.23423028058509));
#245762=CARTESIAN_POINT('Origin',(-44.7709311793212,40.7391658924908,3.42473028058509));
#245763=CARTESIAN_POINT('Origin',(-44.7104761492019,40.6847319392793,3.56563113524801));
#245764=CARTESIAN_POINT('Origin',(-49.8797426639493,35.847302748828,3.56647653909474));
#245765=CARTESIAN_POINT('Origin',(-49.915552518432,35.8732562382988,3.64299466007634));
#245766=CARTESIAN_POINT('Origin',(-49.8135340601225,35.7991993820661,3.42473028058508));
#245767=CARTESIAN_POINT('Ctrl Pts',(-49.7242207306177,35.7350130971388,
3.48823028058508));
#245768=CARTESIAN_POINT('Ctrl Pts',(-49.6503036646787,35.8375861910556,
3.48794691941624));
#245769=CARTESIAN_POINT('Ctrl Pts',(-49.7388853330813,35.9019445403518,
3.42473028058509));
#245770=CARTESIAN_POINT('Ctrl Pts',(-49.6878783768796,35.7084656432358,
3.41028005925112));
#245771=CARTESIAN_POINT('Ctrl Pts',(-49.613705655414,35.8109961808853,3.40982512231007));
#245772=CARTESIAN_POINT('Ctrl Pts',(-49.6842702092612,35.8622643302242,
3.3078048637291));
#245773=CARTESIAN_POINT('Ctrl Pts',(-49.6190282456272,35.6581711379708,
3.36123028058506));
#245774=CARTESIAN_POINT('Ctrl Pts',(-49.5444483977897,35.760677837847,3.36099721048571));
#245775=CARTESIAN_POINT('Ctrl Pts',(-49.5808027344257,35.7870908094908,
3.23423045308381));
#245776=CARTESIAN_POINT('Ctrl Pts',(-49.5465907136146,35.6052536882601,
3.36123028058506));
#245777=CARTESIAN_POINT('Ctrl Pts',(-49.4719419865735,35.7079988465457,
3.36123028058506));
#245778=CARTESIAN_POINT('Ctrl Pts',(-49.4719419865735,35.7079988465457,
3.23423028058506));
#245779=CARTESIAN_POINT('Origin',(-49.5465907136146,35.6052536882601,3.23423028058506));
#245780=CARTESIAN_POINT('Origin',(-0.186621817602853,-0.256862895713863,
3.64303198860262));
#245781=CARTESIAN_POINT('Origin',(-50.2402240048085,36.1092077731528,3.64303198860287));
#245782=CARTESIAN_POINT('Origin',(-0.186621817602853,-0.25686289571386,
3.23423028058481));
#245783=CARTESIAN_POINT('Origin',(-49.4242607783462,35.5163757878395,3.23423028058505));
#245784=CARTESIAN_POINT('Ctrl Pts',(-50.676214228995,36.4252947698678,3.47153072139096));
#245785=CARTESIAN_POINT('Ctrl Pts',(-50.6015094050814,36.5289136610819,
3.47182327902686));
#245786=CARTESIAN_POINT('Ctrl Pts',(-50.5139809070353,36.4650842624218,
3.40413028959039));
#245787=CARTESIAN_POINT('Ctrl Pts',(-50.5831238715073,36.3578045222561,
3.65553807120982));
#245788=CARTESIAN_POINT('Ctrl Pts',(-50.5083591136207,36.4612356912264,
3.65586275496999));
#245789=CARTESIAN_POINT('Ctrl Pts',(-50.439590694023,36.4110366091612,3.55128126837341));
#245790=CARTESIAN_POINT('Ctrl Pts',(-50.4158900112687,36.2365613423295,
3.77003198860288));
#245791=CARTESIAN_POINT('Ctrl Pts',(-50.3411491755171,36.3397499727027,
3.77025505748535));
#245792=CARTESIAN_POINT('Ctrl Pts',(-50.3059517008877,36.3139421975373,
3.64284211731124));
#245793=CARTESIAN_POINT('Ctrl Pts',(-50.2402240048085,36.1092077731528,
3.77003198860288));
#245794=CARTESIAN_POINT('Ctrl Pts',(-50.1654637560305,36.2121064279407,
3.77003198860288));
#245795=CARTESIAN_POINT('Ctrl Pts',(-50.1655753609471,36.2119528169512,
3.64284239821701));
#245796=CARTESIAN_POINT('Origin',(-50.5887599058103,36.3624339277672,3.40423097483334));
#245797=CARTESIAN_POINT('Ctrl Pts',(-49.4242607783463,35.5163757878395,
3.36123028058505));
#245798=CARTESIAN_POINT('Ctrl Pts',(-49.3496120513051,35.6191209461251,
3.36123028058505));
#245799=CARTESIAN_POINT('Ctrl Pts',(-49.3496120513051,35.6191209461251,
3.23423028058505));
#245800=CARTESIAN_POINT('Ctrl Pts',(-49.3515787599192,35.4632790141046,
3.36123028058505));
#245801=CARTESIAN_POINT('Ctrl Pts',(-49.2767219882431,35.5661632154426,
3.3614653861002));
#245802=CARTESIAN_POINT('Ctrl Pts',(-49.2403833690702,35.5397616632035,
3.23423043688465));
#245803=CARTESIAN_POINT('Ctrl Pts',(-49.2828534857269,35.4130704930598,
3.41054258693124));
#245804=CARTESIAN_POINT('Ctrl Pts',(-49.2081487547882,35.5163418450556,
3.41100608859887));
#245805=CARTESIAN_POINT('Ctrl Pts',(-49.1370998624035,35.4647218031686,
3.30819866970857));
#245806=CARTESIAN_POINT('Ctrl Pts',(-49.2466351556014,35.3866101428259,
3.48823028058505));
#245807=CARTESIAN_POINT('Ctrl Pts',(-49.1720533660033,35.4901170100366,
3.48852004212283));
#245808=CARTESIAN_POINT('Ctrl Pts',(-49.0826686475736,35.4251752107437,
3.42473028058505));
#245809=CARTESIAN_POINT('Origin',(-49.1573173746148,35.3224300524581,3.42473028058505));
#245810=CARTESIAN_POINT('Origin',(-50.7328855645271,36.4671473482322,3.11913648178468));
#245811=CARTESIAN_POINT('Origin',(-50.8770112231004,36.5718607685321,2.83404198860286));
#245812=CARTESIAN_POINT('Origin',(-49.0915036252753,35.274613564645,3.5656311346094));
#245813=CARTESIAN_POINT('Origin',(-49.0553654007528,35.2482948100391,3.64299171721782));
#245814=CARTESIAN_POINT('Ctrl Pts',(-50.9399462128204,36.9911673391707,
2.59908173516048));
#245815=CARTESIAN_POINT('Ctrl Pts',(-50.9097606317996,36.969247412634,2.65878198860286));
#245816=CARTESIAN_POINT('Ctrl Pts',(-50.8527980281387,36.9278827595326,
2.65878198860287));
#245817=CARTESIAN_POINT('Ctrl Pts',(-50.9917217504959,36.9198678602472,
2.59908193475632));
#245818=CARTESIAN_POINT('Ctrl Pts',(-50.9474721267405,36.9173100216906,
2.65878715325524));
#245819=CARTESIAN_POINT('Ctrl Pts',(-50.8827604229953,36.8866065570943,
2.65878198860287));
#245820=CARTESIAN_POINT('Ctrl Pts',(-51.019255329238,36.839377280089,2.63878778849898));
#245821=CARTESIAN_POINT('Ctrl Pts',(-50.9634900918195,36.8558881875867,
2.69564460180132));
#245822=CARTESIAN_POINT('Ctrl Pts',(-50.8901678911826,36.8338178466775,
2.6818048162491));
#245823=CARTESIAN_POINT('Ctrl Pts',(-51.0231582082089,36.7103770798843,
2.75443238878668));
#245824=CARTESIAN_POINT('Ctrl Pts',(-50.9515780553177,36.7689134067396,
2.79268340777122));
#245825=CARTESIAN_POINT('Ctrl Pts',(-50.8676678805079,36.7411592876132,
2.74885926835633));
#245826=CARTESIAN_POINT('Ctrl Pts',(-51.0012539523497,36.6614543958828,
2.82856655361696));
#245827=CARTESIAN_POINT('Ctrl Pts',(-50.9229784487439,36.7432876021376,
2.85384197230838));
#245828=CARTESIAN_POINT('Ctrl Pts',(-50.8391515810796,36.7013347616514,
2.79184624278597));
#245829=CARTESIAN_POINT('Ctrl Pts',(-50.9644637245895,36.6347241449654,
2.90134173516048));
#245830=CARTESIAN_POINT('Ctrl Pts',(-50.8898702560319,36.7381840359683,
2.90163218716416));
#245831=CARTESIAN_POINT('Ctrl Pts',(-50.8023624960593,36.6746059268177,
2.83404198860287));
#245832=CARTESIAN_POINT('Origin',(-50.8527980281387,36.9278827595326,2.53178198860286));
#245833=CARTESIAN_POINT('Origin',(-0.186621817602853,-0.256862895713863,
3.64303198860262));
#245834=CARTESIAN_POINT('Origin',(-48.7306271754178,35.0124214764584,3.64303198860286));
#245835=CARTESIAN_POINT('Origin',(1.03190816135906E-16,1.91480515074693E-13,
2.53178198860262));
#245836=CARTESIAN_POINT('Origin',(-50.8348823336488,36.9525415975211,2.53178198860287));
#245837=CARTESIAN_POINT('Ctrl Pts',(-48.7306271754178,35.0124214764584,
3.77003198860287));
#245838=CARTESIAN_POINT('Ctrl Pts',(-48.6558666212127,35.1153205516307,
3.77003198860288));
#245839=CARTESIAN_POINT('Ctrl Pts',(-48.6559785320123,35.1151665196294,
3.64284187937076));
#245840=CARTESIAN_POINT('Ctrl Pts',(-48.5549543235562,34.8850714976654,
3.77003198860287));
#245841=CARTESIAN_POINT('Ctrl Pts',(-48.4804833899302,34.9878965398035,
3.7698020896276));
#245842=CARTESIAN_POINT('Ctrl Pts',(-48.5155997094332,35.013175335312,3.64284193928272));
#245843=CARTESIAN_POINT('Ctrl Pts',(-48.387715124058,34.7638382096883,3.65553535416607));
#245844=CARTESIAN_POINT('Ctrl Pts',(-48.3134799021678,34.8665607873114,
3.65520057834561));
#245845=CARTESIAN_POINT('Ctrl Pts',(-48.381961710728,34.9160816462009,3.55127910964313));
#245846=CARTESIAN_POINT('Ctrl Pts',(-48.2946219293748,34.6963546279284,
3.47153072139095));
#245847=CARTESIAN_POINT('Ctrl Pts',(-48.2205921440832,34.7990735417351,
3.47122746281605));
#245848=CARTESIAN_POINT('Ctrl Pts',(-48.3075724095163,34.8620346554129,
3.404130459013));
#245849=CARTESIAN_POINT('Origin',(-48.3820909175331,34.7591950625533,3.40423097483334));
#245850=CARTESIAN_POINT('Ctrl Pts',(-50.5905785208486,37.149332979726,2.90134173516048));
#245851=CARTESIAN_POINT('Ctrl Pts',(-50.6659240749085,37.0464195108252,
2.90163218716416));
#245852=CARTESIAN_POINT('Ctrl Pts',(-50.5784163149359,36.9828414016746,
2.83404198860287));
#245853=CARTESIAN_POINT('Ctrl Pts',(-50.6273860247241,37.1760745934437,
2.82853349835373));
#245854=CARTESIAN_POINT('Ctrl Pts',(-50.6810174228646,37.076347161577,2.85381483162311));
#245855=CARTESIAN_POINT('Ctrl Pts',(-50.6152221632643,37.0095824157645,
2.79182701594214));
#245856=CARTESIAN_POINT('Ctrl Pts',(-50.6805407410139,37.181676964489,2.75468822073675));
#245857=CARTESIAN_POINT('Ctrl Pts',(-50.7141678268708,37.095483395543,2.79286913083874));
#245858=CARTESIAN_POINT('Ctrl Pts',(-50.6617655220316,37.0242869695755,
2.74900763297951));
#245859=CARTESIAN_POINT('Ctrl Pts',(-50.8012099538927,37.138681150061,2.6395445064041));
#245860=CARTESIAN_POINT('Ctrl Pts',(-50.7999485296221,37.0803097184692,
2.69627684028872));
#245861=CARTESIAN_POINT('Ctrl Pts',(-50.7562647493201,37.0173098767918,
2.68224356036502));
#245862=CARTESIAN_POINT('Ctrl Pts',(-50.8700180268811,37.0873787017258,
2.59908178706437));
#245863=CARTESIAN_POINT('Ctrl Pts',(-50.8539379904871,37.0460487315396,
2.6587870432151));
#245864=CARTESIAN_POINT('Ctrl Pts',(-50.8047860147156,36.9939291606759,
2.65878198860286));
#245865=CARTESIAN_POINT('Ctrl Pts',(-50.9219998155902,37.0158684358559,
2.59908173516048));
#245866=CARTESIAN_POINT('Ctrl Pts',(-50.8918248691002,36.9939338721432,
2.65878198860286));
#245867=CARTESIAN_POINT('Ctrl Pts',(-50.8348823336488,36.9525415975211,
2.65878198860287));
#245868=CARTESIAN_POINT('Origin',(-50.5037675878947,37.0855865599602,2.83404198860287));
#245869=CARTESIAN_POINT('Origin',(-48.2379650606672,34.6544814981911,3.11913648167148));
#245870=CARTESIAN_POINT('Origin',(-48.093839203715,34.549767933694,2.83404198860285));
#245871=CARTESIAN_POINT('Origin',(-50.3596419293379,36.9808731396133,3.11913648177577));
#245872=CARTESIAN_POINT('Origin',(-50.2155162706046,36.8761597191953,3.40423097483335));
#245873=CARTESIAN_POINT('Ctrl Pts',(-48.0063682005189,34.4869303039396,
2.90134173516046));
#245874=CARTESIAN_POINT('Ctrl Pts',(-47.9324532779039,34.5894948283133,
2.90103711553253));
#245875=CARTESIAN_POINT('Ctrl Pts',(-48.0191904766738,34.6525130919796,
2.83404198860285));
#245876=CARTESIAN_POINT('Ctrl Pts',(-47.9696093621199,34.4602241019851,
2.82862991747992));
#245877=CARTESIAN_POINT('Ctrl Pts',(-47.917105603147,34.5595620694344,2.85314045886476));
#245878=CARTESIAN_POINT('Ctrl Pts',(-47.9824304277182,34.6258053530819,
2.79187961000006));
#245879=CARTESIAN_POINT('Ctrl Pts',(-47.9167391807671,34.4546775021468,
2.75470625793343));
#245880=CARTESIAN_POINT('Ctrl Pts',(-47.8838297385501,34.5405955452484,
2.79224250381911));
#245881=CARTESIAN_POINT('Ctrl Pts',(-47.9361122396531,34.6112444014589,
2.74901809108276));
#245882=CARTESIAN_POINT('Ctrl Pts',(-47.7968564492224,34.4979061669209,
2.63947868311727));
#245883=CARTESIAN_POINT('Ctrl Pts',(-47.7983386612733,34.5561175928641,
2.69595066767943));
#245884=CARTESIAN_POINT('Ctrl Pts',(-47.8422046210394,34.6187227036514,
2.6822053943609));
#245885=CARTESIAN_POINT('Ctrl Pts',(-47.7285944911489,34.549326580815,2.59908178585132));
#245886=CARTESIAN_POINT('Ctrl Pts',(-47.7447672725779,34.5905382782875,
2.65877670944887));
#245887=CARTESIAN_POINT('Ctrl Pts',(-47.7940753146439,34.6424336528583,
2.65878198860285));
#245888=CARTESIAN_POINT('Ctrl Pts',(-47.6769115920305,34.6205005703634,
2.59908173516047));
#245889=CARTESIAN_POINT('Ctrl Pts',(-47.7070975168465,34.6424200234574,
2.65878198860285));
#245890=CARTESIAN_POINT('Ctrl Pts',(-47.7640607692765,34.6837837831345,
2.65878198860285));
#245891=CARTESIAN_POINT('Origin',(-47.7640607692765,34.6837837831345,2.53178198860285));
#245892=CARTESIAN_POINT('Ctrl Pts',(-49.8669803696028,36.6229335645809,
3.77003198860288));
#245893=CARTESIAN_POINT('Ctrl Pts',(-49.9417406248213,36.5200349009283,
3.77003198860289));
#245894=CARTESIAN_POINT('Ctrl Pts',(-49.9416290134545,36.5201885207956,
3.64284238727612));
#245895=CARTESIAN_POINT('Ctrl Pts',(-50.0423873219327,36.7506494346794,
3.77003198860288));
#245896=CARTESIAN_POINT('Ctrl Pts',(-50.1174293675641,36.6476796282231,
3.77025506105648));
#245897=CARTESIAN_POINT('Ctrl Pts',(-50.0820075342365,36.6221794864687,
3.64284210641859));
#245898=CARTESIAN_POINT('Ctrl Pts',(-50.2093732240185,36.872231123687,3.65553527987858));
#245899=CARTESIAN_POINT('Ctrl Pts',(-50.2846385388092,36.7691636147952,
3.65585996533204));
#245900=CARTESIAN_POINT('Ctrl Pts',(-50.2156454684952,36.7192731293512,
3.55127902710267));
#245901=CARTESIAN_POINT('Ctrl Pts',(-50.3023253561997,36.9399086546485,
3.47153072139096));
#245902=CARTESIAN_POINT('Ctrl Pts',(-50.3777877242642,36.8368401378449,
3.47182327905213));
#245903=CARTESIAN_POINT('Ctrl Pts',(-50.2900345513017,36.7733199617897,
3.40413028378005));
#245904=CARTESIAN_POINT('Origin',(-49.8669803696028,36.6229335645809,3.64303198860288));
#245905=CARTESIAN_POINT('Origin',(3.64514313700082E-16,1.91611912610258E-13,
2.53178198860262));
#245906=CARTESIAN_POINT('Origin',(-47.7461450747866,34.7084426211231,2.53178198860285));
#245907=CARTESIAN_POINT('Origin',(40.911747809259,-29.3316730956001,3.64303198860243));
#245908=CARTESIAN_POINT('Origin',(-49.5422481179709,36.3870656659281,3.6429946600739));
#245909=CARTESIAN_POINT('Ctrl Pts',(-47.6590285860937,34.6451144164185,
2.59908173516047));
#245910=CARTESIAN_POINT('Ctrl Pts',(-47.6892031885515,34.6670494534017,
2.65878198860286));
#245911=CARTESIAN_POINT('Ctrl Pts',(-47.7461450747866,34.7084426211231,
2.65878198860285));
#245912=CARTESIAN_POINT('Ctrl Pts',(-47.6074854095247,34.7160192182667,
2.59908193199939));
#245913=CARTESIAN_POINT('Ctrl Pts',(-47.6516492793366,34.718704468553,2.65877685806607));
#245914=CARTESIAN_POINT('Ctrl Pts',(-47.7161963245898,34.7496251732003,
2.65878198860285));
#245915=CARTESIAN_POINT('Ctrl Pts',(-47.5796730526554,34.7960378560836,
2.63872492669829));
#245916=CARTESIAN_POINT('Ctrl Pts',(-47.6353534770329,34.7797813814945,
2.69532212015307));
#245917=CARTESIAN_POINT('Ctrl Pts',(-47.7083584310196,34.8021505789971,
2.68176836726655));
#245918=CARTESIAN_POINT('Ctrl Pts',(-47.5752965616147,34.9243313177595,
2.75442176402265));
#245919=CARTESIAN_POINT('Ctrl Pts',(-47.6468329724884,34.8665693571826,
2.7920317992015));
#245920=CARTESIAN_POINT('Ctrl Pts',(-47.7301838844734,34.8943788354696,
2.74885310748201));
#245921=CARTESIAN_POINT('Ctrl Pts',(-47.5970608435764,34.9730260802987,
2.82866089558427));
#245922=CARTESIAN_POINT('Ctrl Pts',(-47.6753141056554,34.8923863483139,
2.85316563119179));
#245923=CARTESIAN_POINT('Ctrl Pts',(-47.7584998599246,34.9340521716868,
2.79189751796643));
#245924=CARTESIAN_POINT('Ctrl Pts',(-47.6338034047601,34.999721753026,2.90134173516047));
#245925=CARTESIAN_POINT('Ctrl Pts',(-47.7085070967805,34.8977303031701,
2.90103711553253));
#245926=CARTESIAN_POINT('Ctrl Pts',(-47.7952442955504,34.9607485668365,
2.83404198860285));
#245927=CARTESIAN_POINT('Origin',(-47.7205955685092,35.0634937251221,2.83404198860286));
#245928=CARTESIAN_POINT('Origin',(-49.5064990280443,36.3610285393819,3.56647653971805));
#245929=CARTESIAN_POINT('Origin',(-49.4402904249167,36.3129251734942,3.42473028058509));
#245930=CARTESIAN_POINT('Origin',(-47.8647214254834,35.1682072895626,3.11913648168123));
#245931=CARTESIAN_POINT('Origin',(-48.0088472823274,35.2729208539814,3.40423097483334));
#245932=CARTESIAN_POINT('Ctrl Pts',(-49.1733470784089,36.1189794796882,
3.36123028058506));
#245933=CARTESIAN_POINT('Ctrl Pts',(-49.2479958054501,36.0162343214026,
3.36123028058506));
#245934=CARTESIAN_POINT('Ctrl Pts',(-49.2479958054501,36.0162343214026,
3.23423028058506));
#245935=CARTESIAN_POINT('Ctrl Pts',(-49.2463047380073,36.1716968449942,
3.36123028058506));
#245936=CARTESIAN_POINT('Ctrl Pts',(-49.3207474263649,36.0690914679788,
3.36099641108653));
#245937=CARTESIAN_POINT('Ctrl Pts',(-49.3572244778977,36.0955935972133,
3.23423043688382));
#245938=CARTESIAN_POINT('Ctrl Pts',(-49.3152906263876,36.2215465627872,
3.4105425890531));
#245939=CARTESIAN_POINT('Ctrl Pts',(-49.3898826892439,36.1193211766501,
3.41008815825897));
#245940=CARTESIAN_POINT('Ctrl Pts',(-49.4605079583581,36.1706334382083,
3.30819867304314));
#245941=CARTESIAN_POINT('Ctrl Pts',(-49.3516463037387,36.247817802325,3.48823028058507));
#245942=CARTESIAN_POINT('Ctrl Pts',(-49.4263574835553,36.1458216659124,
3.48794691941623));
#245943=CARTESIAN_POINT('Ctrl Pts',(-49.5149391519579,36.2101800152086,
3.42473028058508));
#245944=CARTESIAN_POINT('Origin',(-49.1733470784089,36.1189794796882,3.23423028058506));
#245945=CARTESIAN_POINT('Ctrl Pts',(-47.9220530736689,35.2091516650527,
3.47153072139096));
#245946=CARTESIAN_POINT('Ctrl Pts',(-47.9968680956249,35.1070032771125,
3.47122746285101));
#245947=CARTESIAN_POINT('Ctrl Pts',(-48.0836260518489,35.1702703521464,
3.40413046676846));
#245948=CARTESIAN_POINT('Ctrl Pts',(-48.0150025575578,35.2768360036103,
3.6555381345801));
#245949=CARTESIAN_POINT('Ctrl Pts',(-48.0897575808477,35.1744910995569,
3.65520336072258));
#245950=CARTESIAN_POINT('Ctrl Pts',(-48.1580164790759,35.2243181613741,
3.55128134519869));
#245951=CARTESIAN_POINT('Ctrl Pts',(-48.1819833392252,35.3984277477531,
3.77003198860287));
#245952=CARTESIAN_POINT('Ctrl Pts',(-48.2567629686426,35.2958269999292,
3.76980209313974));
#245953=CARTESIAN_POINT('Ctrl Pts',(-48.2916555365082,35.321412620307,3.64284195387526));
#245954=CARTESIAN_POINT('Ctrl Pts',(-48.3573835402121,35.5261472678865,
3.77003198860287));
#245955=CARTESIAN_POINT('Ctrl Pts',(-48.4321440857825,35.4232482045988,
3.77003198860288));
#245956=CARTESIAN_POINT('Ctrl Pts',(-48.4320321836304,35.4234022246978,
3.64284189403891));
#245957=CARTESIAN_POINT('Origin',(-48.3573835402121,35.5261472678865,3.64303198860286));
#245958=CARTESIAN_POINT('Origin',(39.9252688514649,-28.6149541797803,3.23423028058462));
#245959=CARTESIAN_POINT('Origin',(-49.0510171431405,36.0301015792676,3.23423028058506));
#245960=CARTESIAN_POINT('Origin',(39.7707905934409,-28.5027191556737,3.64303198860243));
#245961=CARTESIAN_POINT('Origin',(-48.6820620414858,35.7621028045852,3.64299171721768));
#245962=CARTESIAN_POINT('Ctrl Pts',(-48.8727133447945,35.9012693628904,
3.48823028058505));
#245963=CARTESIAN_POINT('Ctrl Pts',(-48.9481071848799,35.7983524848935,
3.48852004212283));
#245964=CARTESIAN_POINT('Ctrl Pts',(-48.8587224664502,35.7334106856006,
3.42473028058505));
#245965=CARTESIAN_POINT('Ctrl Pts',(-48.9091935744932,35.9276271141652,
3.41028005848429));
#245966=CARTESIAN_POINT('Ctrl Pts',(-48.9843245886213,35.8246659689648,
3.4107440422049));
#245967=CARTESIAN_POINT('Ctrl Pts',(-48.9133376106124,35.7730909105076,
3.30780486244038));
#245968=CARTESIAN_POINT('Ctrl Pts',(-48.9783048775114,35.9775622448375,
3.36123028058506));
#245969=CARTESIAN_POINT('Ctrl Pts',(-49.0530211657533,35.8745769537851,
3.36146460586455));
#245970=CARTESIAN_POINT('Ctrl Pts',(-49.0168051108889,35.8482644497248,
3.23423045308401));
#245971=CARTESIAN_POINT('Ctrl Pts',(-49.0510171431405,36.0301015792676,
3.36123028058506));
#245972=CARTESIAN_POINT('Ctrl Pts',(-49.1256658701817,35.927356420982,3.36123028058506));
#245973=CARTESIAN_POINT('Ctrl Pts',(-49.1256658701817,35.927356420982,3.23423028058506));
#245974=CARTESIAN_POINT('Origin',(-48.7840737394091,35.8361558438862,3.42473028058505));
#245975=CARTESIAN_POINT('Origin',(-48.7182599907926,35.7883393569606,3.5656311352483));
#245976=CARTESIAN_POINT('Origin',(-53.3535596832588,30.4370746247569,3.56647653909402));
#245977=CARTESIAN_POINT('Origin',(-53.3918862459828,30.4591427892372,3.64299466007387));
#245978=CARTESIAN_POINT('Origin',(-53.2826856060847,30.3961554568836,3.42473028058504));
#245979=CARTESIAN_POINT('Ctrl Pts',(-53.1871522506177,30.3416565762235,
3.48823028058504));
#245980=CARTESIAN_POINT('Ctrl Pts',(-53.1243619179797,30.4513942013112,
3.4879469194162));
#245981=CARTESIAN_POINT('Ctrl Pts',(-53.2191856060847,30.5061406831642,
3.42473028058505));
#245982=CARTESIAN_POINT('Ctrl Pts',(-53.1482340195358,30.3190533624383,
3.41028005925105));
#245983=CARTESIAN_POINT('Ctrl Pts',(-53.085184983539,30.4287753876654,3.40982512231084));
#245984=CARTESIAN_POINT('Ctrl Pts',(-53.1607219582407,30.4723866803437,
3.30780486372897));
#245985=CARTESIAN_POINT('Ctrl Pts',(-53.0745038491598,30.2762311741519,
3.36123028058502));
#245986=CARTESIAN_POINT('Ctrl Pts',(-53.0110474253448,30.3859720484845,
3.36099721048431));
#245987=CARTESIAN_POINT('Ctrl Pts',(-53.0499635164575,30.4084402641651,
3.23423045308386));
#245988=CARTESIAN_POINT('Ctrl Pts',(-52.9969317578289,30.2311753956711,
3.36123028058502));
#245989=CARTESIAN_POINT('Ctrl Pts',(-52.9334317578289,30.3411606219517,
3.36123028058502));
#245990=CARTESIAN_POINT('Ctrl Pts',(-52.9334317578289,30.3411606219517,
3.23423028058502));
#245991=CARTESIAN_POINT('Origin',(-52.9969317578289,30.2311753956711,3.23423028058502));
#245992=CARTESIAN_POINT('Origin',(-0.158749999999993,-0.274963065701376,
3.64303198860262));
#245993=CARTESIAN_POINT('Origin',(-53.7394427993288,30.6598643453573,3.64303198860283));
#245994=CARTESIAN_POINT('Origin',(-0.158749999999993,-0.274963065701374,
3.23423028058481));
#245995=CARTESIAN_POINT('Origin',(-52.8659816883961,30.1555713378337,3.23423028058502));
#245996=CARTESIAN_POINT('Ctrl Pts',(-54.2060847114743,30.9286463962977,
3.47153072139093));
#245997=CARTESIAN_POINT('Ctrl Pts',(-54.1426202518671,31.0395064328256,
3.47182327902683));
#245998=CARTESIAN_POINT('Ctrl Pts',(-54.0488992551385,30.9851759176838,
3.40413028959074));
#245999=CARTESIAN_POINT('Ctrl Pts',(-54.1064496608378,30.8712564593355,
3.65553807120978));
#246000=CARTESIAN_POINT('Ctrl Pts',(-54.0429059732648,30.9819360667867,
3.65586275496898));
#246001=CARTESIAN_POINT('Ctrl Pts',(-53.9692670413545,30.9392002377691,
3.55128126837296));
#246002=CARTESIAN_POINT('Ctrl Pts',(-53.9274585619028,30.7681581606536,
3.77003198860284));
#246003=CARTESIAN_POINT('Ctrl Pts',(-53.8639133132293,30.8785940576181,
3.77025505748651));
#246004=CARTESIAN_POINT('Ctrl Pts',(-53.8262110069733,30.8566067980797,
3.64284211731175));
#246005=CARTESIAN_POINT('Ctrl Pts',(-53.7394427993288,30.6598643453573,
3.77003198860284));
#246006=CARTESIAN_POINT('Ctrl Pts',(-53.6758479332736,30.7700138844656,
3.77003198860284));
#246007=CARTESIAN_POINT('Ctrl Pts',(-53.6759428700858,30.7698494490833,
3.64284239821767));
#246008=CARTESIAN_POINT('Origin',(-54.1125387249981,30.875271378476,3.40423097483331));
#246009=CARTESIAN_POINT('Ctrl Pts',(-52.8659816883961,30.1555713378337,
3.36123028058502));
#246010=CARTESIAN_POINT('Ctrl Pts',(-52.8024816883961,30.2655565641143,
3.36123028058501));
#246011=CARTESIAN_POINT('Ctrl Pts',(-52.8024816883961,30.2655565641143,
3.23423028058502));
#246012=CARTESIAN_POINT('Ctrl Pts',(-52.7881477055081,30.1103627734739,
3.36123028058502));
#246013=CARTESIAN_POINT('Ctrl Pts',(-52.7244553345228,30.2205080277008,
3.36146538610177));
#246014=CARTESIAN_POINT('Ctrl Pts',(-52.6855560684232,30.1980495259478,
3.234230436884));
#246015=CARTESIAN_POINT('Ctrl Pts',(-52.7145506960111,30.0676130472592,
3.41054258693121));
#246016=CARTESIAN_POINT('Ctrl Pts',(-52.6510500011257,30.1781274387056,
3.41100608859674));
#246017=CARTESIAN_POINT('Ctrl Pts',(-52.5749945583554,30.1342168083481,
3.3081986697083));
#246018=CARTESIAN_POINT('Ctrl Pts',(-52.6757649139397,30.0450834959835,
3.48823028058501));
#246019=CARTESIAN_POINT('Ctrl Pts',(-52.6124111049558,30.1558192616,3.48852004212279));
#246020=CARTESIAN_POINT('Ctrl Pts',(-52.5167277788843,30.1005764675357,
3.42473028058501));
#246021=CARTESIAN_POINT('Origin',(-52.5802277788843,29.9905912412551,3.42473028058501));
#246022=CARTESIAN_POINT('Origin',(-54.2668203812018,30.9643459342447,3.11913648178522));
#246023=CARTESIAN_POINT('Origin',(-54.421102037244,31.0534204898633,2.83404198860282));
#246024=CARTESIAN_POINT('Origin',(-52.5097763801594,29.949916107244,3.56563113460861));
#246025=CARTESIAN_POINT('Origin',(-52.4710850656385,29.9275190026057,3.64299171721761));
#246026=CARTESIAN_POINT('Ctrl Pts',(-54.5275217339721,31.4638515574739,
2.59908173516044));
#246027=CARTESIAN_POINT('Ctrl Pts',(-54.4952102564867,31.4452069629852,
2.65878198860283));
#246028=CARTESIAN_POINT('Ctrl Pts',(-54.4342359163065,31.410023123206,2.65878198860283));
#246029=CARTESIAN_POINT('Ctrl Pts',(-54.5715608148709,31.3875306471678,
2.59908193475695));
#246030=CARTESIAN_POINT('Ctrl Pts',(-54.5272862282516,31.3896121658904,
2.6587871532535));
#246031=CARTESIAN_POINT('Ctrl Pts',(-54.4597196360178,31.3658411130327,
2.65878198860283));
#246032=CARTESIAN_POINT('Ctrl Pts',(-54.5905300051366,31.3046029601557,
2.63878778849901));
#246033=CARTESIAN_POINT('Ctrl Pts',(-54.5367961153115,31.3268524737457,
2.69564460180151));
#246034=CARTESIAN_POINT('Ctrl Pts',(-54.4615686025421,31.3125672934291,
2.68180481624904));
#246035=CARTESIAN_POINT('Ctrl Pts',(-54.5809273110397,31.175901474604,2.75443238878657));
#246036=CARTESIAN_POINT('Ctrl Pts',(-54.515857994007,31.2415992967183,2.79268340777087));
#246037=CARTESIAN_POINT('Ctrl Pts',(-54.4295063924931,31.222768219186,2.74885926835632));
#246038=CARTESIAN_POINT('Ctrl Pts',(-54.5540292360081,31.1295364123886,
2.82856655361696));
#246039=CARTESIAN_POINT('Ctrl Pts',(-54.4847364330947,31.2191033458789,
2.85384197230791));
#246040=CARTESIAN_POINT('Ctrl Pts',(-54.396983511837,31.1861426211012,2.79184624278568));
#246041=CARTESIAN_POINT('Ctrl Pts',(-54.514646476914,31.1067982185534,2.90134173516044));
#246042=CARTESIAN_POINT('Ctrl Pts',(-54.4512761425984,31.2174884860864,
2.90163218716412));
#246043=CARTESIAN_POINT('Ctrl Pts',(-54.357602037244,31.1634057161439,2.83404198860283));
#246044=CARTESIAN_POINT('Origin',(-54.4342359163065,31.410023123206,2.53178198860283));
#246045=CARTESIAN_POINT('Origin',(-0.158749999999993,-0.274963065701376,
3.64303198860262));
#246046=CARTESIAN_POINT('Origin',(-52.1234703131948,29.7268821954848,3.64303198860283));
#246047=CARTESIAN_POINT('Origin',(1.12590909550281E-16,1.91494989949198E-13,
2.53178198860262));
#246048=CARTESIAN_POINT('Origin',(-54.4189959163065,31.4364195775134,2.53178198860283));
#246049=CARTESIAN_POINT('Ctrl Pts',(-52.1234703131948,29.7268821954848,
3.77003198860283));
#246050=CARTESIAN_POINT('Ctrl Pts',(-52.0598751873274,29.8370321846009,
3.77003198860283));
#246051=CARTESIAN_POINT('Ctrl Pts',(-52.0599703843396,29.8368672985391,
3.64284187937076));
#246052=CARTESIAN_POINT('Ctrl Pts',(-51.9354481180168,29.6185926664424,
3.77003198860283));
#246053=CARTESIAN_POINT('Ctrl Pts',(-51.8721332876009,29.7286387544935,
3.76980208962903));
#246054=CARTESIAN_POINT('Ctrl Pts',(-51.9096995898738,29.7501084151998,
3.64284193928298));
#246055=CARTESIAN_POINT('Ctrl Pts',(-51.7564527430635,29.5155047636222,
3.65553535416608));
#246056=CARTESIAN_POINT('Ctrl Pts',(-51.6933616226613,29.6254243098818,
3.65520057834604));
#246057=CARTESIAN_POINT('Ctrl Pts',(-51.7666446199951,29.6675155901171,
3.5512791096425));
#246058=CARTESIAN_POINT('Ctrl Pts',(-51.6568155675429,29.4581217525673,
3.47153072139092));
#246059=CARTESIAN_POINT('Ctrl Pts',(-51.5939283753697,29.5680161811089,
3.47122746281603));
#246060=CARTESIAN_POINT('Ctrl Pts',(-51.6870133822662,29.6215404737379,
3.40413045901299));
#246061=CARTESIAN_POINT('Origin',(-51.7503740054945,29.5114749418004,3.4042309748333));
#246062=CARTESIAN_POINT('Ctrl Pts',(-54.1966007261209,31.6576696180583,
2.90134173516045));
#246063=CARTESIAN_POINT('Ctrl Pts',(-54.2607761425984,31.5474441649282,
2.90163218716412));
#246064=CARTESIAN_POINT('Ctrl Pts',(-54.167102037244,31.4933613949858,2.83404198860283));
#246065=CARTESIAN_POINT('Ctrl Pts',(-54.2360018544265,31.6804173066008,
2.82853349835366));
#246066=CARTESIAN_POINT('Ctrl Pts',(-54.2789150989575,31.5756301844106,
2.85381483162275));
#246067=CARTESIAN_POINT('Ctrl Pts',(-54.2065014563932,31.5161086602375,
2.79182701594199));
#246068=CARTESIAN_POINT('Ctrl Pts',(-54.2894509908545,31.6804328064624,
2.75468822073677));
#246069=CARTESIAN_POINT('Ctrl Pts',(-54.3138841827106,31.5911964272961,
2.79286913083857));
#246070=CARTESIAN_POINT('Ctrl Pts',(-54.2543268901841,31.5258675551966,
2.7490076329792));
#246071=CARTESIAN_POINT('Ctrl Pts',(-54.4049648787501,31.6250591602189,
2.639544506404));
#246072=CARTESIAN_POINT('Ctrl Pts',(-54.3976088886511,31.5671393481783,
2.6962768402888));
#246073=CARTESIAN_POINT('Ctrl Pts',(-54.3475791360315,31.5090508246494,
2.68224356036526));
#246074=CARTESIAN_POINT('Ctrl Pts',(-54.4680334478295,31.5668453499338,
2.59908178706341));
#246075=CARTESIAN_POINT('Ctrl Pts',(-54.4477213412886,31.5274226111428,
2.65878704321531));
#246076=CARTESIAN_POINT('Ctrl Pts',(-54.393390646533,31.480726337235,2.65878198860283));
#246077=CARTESIAN_POINT('Ctrl Pts',(-54.5122556166612,31.4902932482907,
2.59908173516044));
#246078=CARTESIAN_POINT('Ctrl Pts',(-54.4799531854481,31.4716329851988,
2.65878198860282));
#246079=CARTESIAN_POINT('Ctrl Pts',(-54.4189959163065,31.4364195775134,
2.65878198860283));
#246080=CARTESIAN_POINT('Origin',(-54.103602037244,31.6033466212664,2.83404198860283));
#246081=CARTESIAN_POINT('Origin',(-51.5960921371858,29.4224002636375,3.11913648167122));
#246082=CARTESIAN_POINT('Origin',(-51.4418102687787,29.3333255853454,2.83404198860282));
#246083=CARTESIAN_POINT('Origin',(-53.9493203812135,31.5142720655985,3.11913648177612));
#246084=CARTESIAN_POINT('Origin',(-53.7950387249981,31.4251975098792,3.40423097483331));
#246085=CARTESIAN_POINT('Ctrl Pts',(-51.3482501200167,29.2799753962461,
2.90134173516043));
#246086=CARTESIAN_POINT('Ctrl Pts',(-51.2854610232003,29.3897042746973,
2.90103711553249));
#246087=CARTESIAN_POINT('Ctrl Pts',(-51.3783102687786,29.443310811626,2.83404198860281));
#246088=CARTESIAN_POINT('Ctrl Pts',(-51.3089010921302,29.2572578385501,
2.8286299174797));
#246089=CARTESIAN_POINT('Ctrl Pts',(-51.2670685993223,29.3615397594617,
2.85314045886478));
#246090=CARTESIAN_POINT('Ctrl Pts',(-51.3389598763136,29.4205918519436,
2.79187960999942));
#246091=CARTESIAN_POINT('Ctrl Pts',(-51.255740761606,29.2572680623748,2.75470625793364));
#246092=CARTESIAN_POINT('Ctrl Pts',(-51.2319924817693,29.3461554108688,
2.79224250381917));
#246093=CARTESIAN_POINT('Ctrl Pts',(-51.2913733902319,29.4109522357566,
2.7490180910829));
#246094=CARTESIAN_POINT('Ctrl Pts',(-51.1410333861056,29.3127910737014,
2.639478683117));
#246095=CARTESIAN_POINT('Ctrl Pts',(-51.1485922293422,29.3705286780144,
2.69595066767927));
#246096=CARTESIAN_POINT('Ctrl Pts',(-51.1987619028145,29.4282055900902,
2.68220539436071));
#246097=CARTESIAN_POINT('Ctrl Pts',(-51.0785202710261,29.3710651187646,
2.59908178585132));
#246098=CARTESIAN_POINT('Ctrl Pts',(-51.0989122516721,29.4103605382571,
2.65877670944931));
#246099=CARTESIAN_POINT('Ctrl Pts',(-51.1533747228768,29.4568175306709,
2.65878198860281));
#246100=CARTESIAN_POINT('Ctrl Pts',(-51.0345602039888,29.4472515437734,
2.59908173516043));
#246101=CARTESIAN_POINT('Ctrl Pts',(-51.0668719738979,29.4658956314766,
2.65878198860281));
#246102=CARTESIAN_POINT('Ctrl Pts',(-51.1278468659049,29.501078514911,2.65878198860281));
#246103=CARTESIAN_POINT('Origin',(-51.1278468659049,29.501078514911,2.53178198860281));
#246104=CARTESIAN_POINT('Ctrl Pts',(-53.4219427993288,31.2097904767605,
3.77003198860284));
#246105=CARTESIAN_POINT('Ctrl Pts',(-53.485537670863,31.0996409281624,3.77003198860284));
#246106=CARTESIAN_POINT('Ctrl Pts',(-53.4854427285637,31.0998053730486,
3.6428423872761));
#246107=CARTESIAN_POINT('Ctrl Pts',(-53.6097387976567,31.3184716867865,
3.77003198860284));
#246108=CARTESIAN_POINT('Ctrl Pts',(-53.6736064794794,31.2082219299895,
3.77025506105862));
#246109=CARTESIAN_POINT('Ctrl Pts',(-53.6357132000306,31.1865640704877,
3.64284210641857));
#246110=CARTESIAN_POINT('Ctrl Pts',(-53.7885186806134,31.4219325588464,
3.65553527987851));
#246111=CARTESIAN_POINT('Ctrl Pts',(-53.8525981958195,31.3115622968595,
3.65585996533086));
#246112=CARTESIAN_POINT('Ctrl Pts',(-53.7787681009843,31.2691568563319,
3.55127902710232));
#246113=CARTESIAN_POINT('Ctrl Pts',(-53.8880358395972,31.4795232016788,
3.47153072139091));
#246114=CARTESIAN_POINT('Ctrl Pts',(-53.9523112232409,31.3691313396262,
3.47182327905207));
#246115=CARTESIAN_POINT('Ctrl Pts',(-53.8583991049521,31.3151318380582,
3.40413028378002));
#246116=CARTESIAN_POINT('Origin',(-53.4219427993288,31.2097904767605,3.64303198860284));
#246117=CARTESIAN_POINT('Origin',(3.61170357355341E-16,1.91606763369042E-13,
2.53178198860262));
#246118=CARTESIAN_POINT('Origin',(-51.1126068659049,29.5274749692184,2.53178198860281));
#246119=CARTESIAN_POINT('Origin',(46.8255917980726,-26.6681506086448,3.64303198860244));
#246120=CARTESIAN_POINT('Origin',(-53.0743345559677,31.009158450368,3.64299466007833));
#246121=CARTESIAN_POINT('Ctrl Pts',(-51.0193480105329,29.4735998357337,
2.59908173516043));
#246122=CARTESIAN_POINT('Ctrl Pts',(-51.0516501490688,29.4922606054645,
2.65878198860282));
#246123=CARTESIAN_POINT('Ctrl Pts',(-51.1126068659049,29.5274749692184,
2.65878198860281));
#246124=CARTESIAN_POINT('Ctrl Pts',(-50.9754987628538,29.549503942697,2.59908193199938));
#246125=CARTESIAN_POINT('Ctrl Pts',(-51.0197013834523,29.5475581014579,
2.65877685806621));
#246126=CARTESIAN_POINT('Ctrl Pts',(-51.0871269269763,29.5715624158005,
2.65878198860281));
#246127=CARTESIAN_POINT('Ctrl Pts',(-50.956202990229,29.6319914129672,2.63872492669836));
#246128=CARTESIAN_POINT('Ctrl Pts',(-51.0098791271091,29.610003803853,2.69532212015288));
#246129=CARTESIAN_POINT('Ctrl Pts',(-51.0848223701588,29.6246193648996,
2.68176836726668));
#246130=CARTESIAN_POINT('Ctrl Pts',(-50.9652607924605,29.760039537519,2.75442176402251));
#246131=CARTESIAN_POINT('Ctrl Pts',(-51.0303675504159,29.6951164119092,
2.79203179920169));
#246132=CARTESIAN_POINT('Ctrl Pts',(-51.1161687394135,29.714061004223,2.74885310748181));
#246133=CARTESIAN_POINT('Ctrl Pts',(-50.9919958361067,29.8061925581053,
2.82866089558436));
#246134=CARTESIAN_POINT('Ctrl Pts',(-51.0613912713661,29.7178148857784,
2.85316563119081));
#246135=CARTESIAN_POINT('Ctrl Pts',(-51.1484765898567,29.7505571803541,
2.79189751796605));
#246136=CARTESIAN_POINT('Ctrl Pts',(-51.031327575341,29.8289013456885,2.90134173516043));
#246137=CARTESIAN_POINT('Ctrl Pts',(-51.0949610232003,29.7196599535392,
2.90103711553249));
#246138=CARTESIAN_POINT('Ctrl Pts',(-51.1878102687787,29.7732664904679,
2.83404198860282));
#246139=CARTESIAN_POINT('Origin',(-51.1243102687787,29.8832517167485,2.83404198860282));
#246140=CARTESIAN_POINT('Origin',(-53.0360596824721,30.9870007553611,3.56647653971802));
#246141=CARTESIAN_POINT('Origin',(-52.9651856060848,30.9460815882867,3.42473028058505));
#246142=CARTESIAN_POINT('Origin',(-51.2785921372026,29.9723263949818,3.11913648168053));
#246143=CARTESIAN_POINT('Origin',(-51.4328740054945,30.0614010732035,3.40423097483331));
#246144=CARTESIAN_POINT('Ctrl Pts',(-52.6794317578289,30.7811015270742,
3.36123028058502));
#246145=CARTESIAN_POINT('Ctrl Pts',(-52.7429317578289,30.6711163007936,
3.36123028058502));
#246146=CARTESIAN_POINT('Ctrl Pts',(-52.7429317578289,30.6711163007936,
3.23423028058502));
#246147=CARTESIAN_POINT('Ctrl Pts',(-52.7575002129176,30.8259039490951,
3.36123028058502));
#246148=CARTESIAN_POINT('Ctrl Pts',(-52.8208099140592,30.7160792752582,
3.36099641108606));
#246149=CARTESIAN_POINT('Ctrl Pts',(-52.8598573673268,30.7386233329124,
3.23423043688387));
#246150=CARTESIAN_POINT('Ctrl Pts',(-52.8313189037795,30.868269596017,3.41054258905305));
#246151=CARTESIAN_POINT('Ctrl Pts',(-52.8948168809878,30.7588072175349,
3.41008815826047));
#246152=CARTESIAN_POINT('Ctrl Pts',(-52.9704188493371,30.802456034313,3.30819867304317));
#246153=CARTESIAN_POINT('Ctrl Pts',(-52.8702215132218,30.8905967158735,
3.48823028058505));
#246154=CARTESIAN_POINT('Ctrl Pts',(-52.9338619179797,30.7813498801531,
3.48794691941621));
#246155=CARTESIAN_POINT('Ctrl Pts',(-53.0286856060847,30.8360963620061,
3.42473028058507));
#246156=CARTESIAN_POINT('Origin',(-52.6794317578289,30.7811015270742,3.23423028058502));
#246157=CARTESIAN_POINT('Ctrl Pts',(-51.3398895692699,30.0070536838157,
3.47153072139093));
#246158=CARTESIAN_POINT('Ctrl Pts',(-51.4036173326911,29.8976445761579,
3.47122746285098));
#246159=CARTESIAN_POINT('Ctrl Pts',(-51.496513229882,29.951496391695,3.40413046676832));
#246160=CARTESIAN_POINT('Ctrl Pts',(-51.4394048060573,30.0646513737723,
3.65553813458008));
#246161=CARTESIAN_POINT('Ctrl Pts',(-51.5030523579633,29.9550530981051,
3.65520336072249));
#246162=CARTESIAN_POINT('Ctrl Pts',(-51.576145673005,29.9974722043279,3.5512813451994));
#246163=CARTESIAN_POINT('Ctrl Pts',(-51.6181806476919,30.1681227811164,
3.77003198860284));
#246164=CARTESIAN_POINT('Ctrl Pts',(-51.6818259279757,30.0582674911775,
3.76980209314012));
#246165=CARTESIAN_POINT('Ctrl Pts',(-51.7192017762845,30.0800656843511,
3.64284195387447));
#246166=CARTESIAN_POINT('Ctrl Pts',(-51.8059703131948,30.276808326888,3.77003198860284));
#246167=CARTESIAN_POINT('Ctrl Pts',(-51.8695654317172,30.1666583504938,
3.77003198860284));
#246168=CARTESIAN_POINT('Ctrl Pts',(-51.869470242061,30.1668232238147,3.64284189403868));
#246169=CARTESIAN_POINT('Origin',(-51.8059703131948,30.276808326888,3.64303198860283));
#246170=CARTESIAN_POINT('Origin',(45.6951875000003,-26.0155113828597,3.23423028058464));
#246171=CARTESIAN_POINT('Origin',(-52.5484816883961,30.7054974692368,3.23423028058502));
#246172=CARTESIAN_POINT('Origin',(45.5181711678734,-25.9133109558552,3.64303198860245));
#246173=CARTESIAN_POINT('Origin',(-52.1535342613176,30.4775331296739,3.64299171721775));
#246174=CARTESIAN_POINT('Ctrl Pts',(-52.3576880233164,30.5960088312567,
3.48823028058501));
#246175=CARTESIAN_POINT('Ctrl Pts',(-52.4219111049558,30.4857749404419,
3.48852004212278));
#246176=CARTESIAN_POINT('Ctrl Pts',(-52.3262277788843,30.4305321463775,
3.424730280585));
#246177=CARTESIAN_POINT('Ctrl Pts',(-52.3967235457371,30.6184089696597,
3.4102800584843));
#246178=CARTESIAN_POINT('Ctrl Pts',(-52.4606806140212,30.5081585269373,
3.41074404220383));
#246179=CARTESIAN_POINT('Ctrl Pts',(-52.384691448504,30.4642861617703,3.30780486244033));
#246180=CARTESIAN_POINT('Ctrl Pts',(-52.4706758922786,30.6608464521622,
3.36123028058502));
#246181=CARTESIAN_POINT('Ctrl Pts',(-52.5342179826647,30.5506153465184,
3.3614646058652));
#246182=CARTESIAN_POINT('Ctrl Pts',(-52.4954499175206,30.5282325936721,
3.23423045308406));
#246183=CARTESIAN_POINT('Ctrl Pts',(-52.5484816883961,30.7054974692368,
3.36123028058502));
#246184=CARTESIAN_POINT('Ctrl Pts',(-52.6119816883961,30.5955122429562,
3.36123028058501));
#246185=CARTESIAN_POINT('Ctrl Pts',(-52.6119816883961,30.5955122429562,
3.23423028058502));
#246186=CARTESIAN_POINT('Origin',(-52.2627277788843,30.5405173726582,3.42473028058501));
#246187=CARTESIAN_POINT('Origin',(-52.1922763809702,30.4998422394563,3.56563113524767));
#246188=CARTESIAN_POINT('Origin',(-56.2428239377265,24.6933715417287,3.56647653909453));
#246189=CARTESIAN_POINT('Origin',(-56.2832472948504,24.7113125977908,3.64299466007575));
#246190=CARTESIAN_POINT('Origin',(-56.1680608984279,24.660084891711,3.424730280585));
#246191=CARTESIAN_POINT('Ctrl Pts',(-56.0673542004327,24.6158705164592,
3.488230280585));
#246192=CARTESIAN_POINT('Ctrl Pts',(-56.0163785451199,24.7315703643334,
3.48794691941616));
#246193=CARTESIAN_POINT('Ctrl Pts',(-56.1164053447573,24.7761051648316,
3.42473028058502));
#246194=CARTESIAN_POINT('Ctrl Pts',(-56.0262864882911,24.597459188332,3.41028005925102));
#246195=CARTESIAN_POINT('Ctrl Pts',(-55.9750519161937,24.7131705636677,
3.40982512230903));
#246196=CARTESIAN_POINT('Ctrl Pts',(-56.0547337128495,24.7486471852365,
3.30780486372868));
#246197=CARTESIAN_POINT('Ctrl Pts',(-55.9484840819677,24.562578485879,3.36123028058498));
#246198=CARTESIAN_POINT('Ctrl Pts',(-55.8968463240337,24.6783511906859,
3.36099721048674));
#246199=CARTESIAN_POINT('Ctrl Pts',(-55.9378977967844,24.69662848393,3.23423045308409));
#246200=CARTESIAN_POINT('Ctrl Pts',(-55.8666273273834,24.525878019167,3.36123028058498));
#246201=CARTESIAN_POINT('Ctrl Pts',(-55.8149717737128,24.6418982922876,
3.36123028058497));
#246202=CARTESIAN_POINT('Ctrl Pts',(-55.8149717737128,24.6418982922876,
3.23423028058498));
#246203=CARTESIAN_POINT('Origin',(-55.8666273273834,24.525878019167,3.23423028058497));
#246204=CARTESIAN_POINT('Origin',(-0.129138884176559,-0.290050682801343,
3.64303198860262));
#246205=CARTESIAN_POINT('Origin',(-56.6498810128383,24.8746050278051,3.64303198860279));
#246206=CARTESIAN_POINT('Origin',(-0.129138884176559,-0.29005068280134,
3.23423028058481));
#246207=CARTESIAN_POINT('Origin',(-55.7284918401499,24.4643761377916,3.23423028058498));
#246208=CARTESIAN_POINT('Ctrl Pts',(-57.1420619865023,25.0931373005744,
3.47153072139088));
#246209=CARTESIAN_POINT('Ctrl Pts',(-57.0905332211012,25.2100238766579,
3.47182327902679));
#246210=CARTESIAN_POINT('Ctrl Pts',(-56.9916465525424,25.1657875015263,
3.40413028959055));
#246211=CARTESIAN_POINT('Ctrl Pts',(-57.0369738651803,25.0464764504226,
3.65553807120975));
#246212=CARTESIAN_POINT('Ctrl Pts',(-56.9853474458572,25.1631918674186,
3.65586275496955));
#246213=CARTESIAN_POINT('Ctrl Pts',(-56.907644805189,25.1283875141304,3.55128126837268));
#246214=CARTESIAN_POINT('Ctrl Pts',(-56.8481865914867,24.9626525995186,
3.7700319886028));
#246215=CARTESIAN_POINT('Ctrl Pts',(-56.7965331449335,25.0791258042764,
3.7702550574856));
#246216=CARTESIAN_POINT('Ctrl Pts',(-56.7567390814047,25.0611999573801,
3.64284211731171));
#246217=CARTESIAN_POINT('Ctrl Pts',(-56.6498810128383,24.8746050278051,
3.7700319886028));
#246218=CARTESIAN_POINT('Ctrl Pts',(-56.5981482881659,24.9907986298337,
3.7700319886028));
#246219=CARTESIAN_POINT('Ctrl Pts',(-56.5982255167266,24.9906251716463,
3.64284239821737));
#246220=CARTESIAN_POINT('Origin',(-57.043449246138,25.0498328948963,3.40423097483326));
#246221=CARTESIAN_POINT('Ctrl Pts',(-55.7284918401499,24.4643761377916,
3.36123028058498));
#246222=CARTESIAN_POINT('Ctrl Pts',(-55.6768362864793,24.5803964109122,
3.36123028058498));
#246223=CARTESIAN_POINT('Ctrl Pts',(-55.6768362864793,24.5803964109122,
3.23423028058498));
#246224=CARTESIAN_POINT('Ctrl Pts',(-55.6463586582055,24.427551097298,3.36123028058498));
#246225=CARTESIAN_POINT('Ctrl Pts',(-55.5945285148498,24.5437506299587,
3.36146538610153));
#246226=CARTESIAN_POINT('Ctrl Pts',(-55.553494790327,24.5254812387363,3.23423043688422));
#246227=CARTESIAN_POINT('Ctrl Pts',(-55.5686962576411,24.3927285408595,
3.41054258693117));
#246228=CARTESIAN_POINT('Ctrl Pts',(-55.5170953257178,24.5092751529588,
3.41100608859789));
#246229=CARTESIAN_POINT('Ctrl Pts',(-55.4368666119039,24.473555028187,3.3081986697083));
#246230=CARTESIAN_POINT('Ctrl Pts',(-55.5277679687684,24.3743766270213,
3.48823028058497));
#246231=CARTESIAN_POINT('Ctrl Pts',(-55.4763362579876,24.4911280468225,
3.48852004212275));
#246232=CARTESIAN_POINT('Ctrl Pts',(-55.3754026508176,24.4461895095988,
3.42473028058497));
#246233=CARTESIAN_POINT('Origin',(-55.4270582044882,24.3301692364781,3.42473028058497));
#246234=CARTESIAN_POINT('Origin',(-57.2061965577146,25.1222926664932,3.11913648178331));
#246235=CARTESIAN_POINT('Origin',(-57.3689438691197,25.1947524379615,2.83404198860278));
#246236=CARTESIAN_POINT('Origin',(-55.3527410366462,24.2970811015512,3.56563113460896));
#246237=CARTESIAN_POINT('Origin',(-55.3119205422646,24.2788510342445,3.64299171721806));
#246238=CARTESIAN_POINT('Ctrl Pts',(-57.517682316389,25.5918112338793,2.5990817351604));
#246239=CARTESIAN_POINT('Ctrl Pts',(-57.4835989537479,25.5766462455175,
2.65878198860279));
#246240=CARTESIAN_POINT('Ctrl Pts',(-57.419280924679,25.5480287005717,2.65878198860279));
#246241=CARTESIAN_POINT('Ctrl Pts',(-57.5535024391259,25.5113050800556,
2.5990819347557));
#246242=CARTESIAN_POINT('Ctrl Pts',(-57.5096879712795,25.518003150502,2.6587871532529));
#246243=CARTESIAN_POINT('Ctrl Pts',(-57.4400067642825,25.5014249500143,
2.65878198860279));
#246244=CARTESIAN_POINT('Ctrl Pts',(-57.5636994104961,25.4268488592817,
2.63878778849897));
#246245=CARTESIAN_POINT('Ctrl Pts',(-57.5125855880052,25.4545932086376,
2.69564460180146));
#246246=CARTESIAN_POINT('Ctrl Pts',(-57.4362769714766,25.4482497003383,
2.68180481624888));
#246247=CARTESIAN_POINT('Ctrl Pts',(-57.5406963524572,25.2998561687912,
2.75443238878654));
#246248=CARTESIAN_POINT('Ctrl Pts',(-57.4828507843378,25.3719956870766,
2.79268340777082));
#246249=CARTESIAN_POINT('Ctrl Pts',(-57.3950038423353,25.3622939683647,
2.7488592683564));
#246250=CARTESIAN_POINT('Ctrl Pts',(-57.5090991591923,25.2565567136861,
2.82856655361693));
#246251=CARTESIAN_POINT('Ctrl Pts',(-57.4495482434205,25.3528760603489,
2.85384197230783));
#246252=CARTESIAN_POINT('Ctrl Pts',(-57.3588307079376,25.3292685758743,
2.79184624278451));
#246253=CARTESIAN_POINT('Ctrl Pts',(-57.4675553545142,25.2380597013429,
2.90134173516042));
#246254=CARTESIAN_POINT('Ctrl Pts',(-57.4161024530845,25.3547675996714,
2.90163218716409));
#246255=CARTESIAN_POINT('Ctrl Pts',(-57.3172883154491,25.3107727110821,
2.83404198860279));
#246256=CARTESIAN_POINT('Origin',(-57.419280924679,25.5480287005717,2.53178198860278));
#246257=CARTESIAN_POINT('Origin',(-0.129138884176559,-0.290050682801343,
3.64303198860262));
#246258=CARTESIAN_POINT('Origin',(-54.945237802683,24.1156489724276,3.64303198860279));
#246259=CARTESIAN_POINT('Origin',(1.20426471881346E-16,1.91510368106146E-13,
2.53178198860262));
#246260=CARTESIAN_POINT('Origin',(-57.4068835917981,25.5758735661207,2.53178198860279));
#246261=CARTESIAN_POINT('Ctrl Pts',(-54.945237802683,24.1156489724276,3.7700319886028));
#246262=CARTESIAN_POINT('Ctrl Pts',(-54.8935048666604,24.2318430491564,
3.7700319886028));
#246263=CARTESIAN_POINT('Ctrl Pts',(-54.8935823068867,24.2316691155602,
3.64284187937053));
#246264=CARTESIAN_POINT('Ctrl Pts',(-54.7469262747044,24.0276063358781,
3.77003198860279));
#246265=CARTESIAN_POINT('Ctrl Pts',(-54.6954612380262,24.143667781871,3.76980208962941));
#246266=CARTESIAN_POINT('Ctrl Pts',(-54.7350659388072,24.1610930816817,
3.64284193928226));
#246267=CARTESIAN_POINT('Ctrl Pts',(-54.5581358350812,23.9437932708499,
3.65553535416599));
#246268=CARTESIAN_POINT('Ctrl Pts',(-54.5068800556916,24.0597054841956,
3.65520057834569));
#246269=CARTESIAN_POINT('Ctrl Pts',(-54.5841613379359,24.0939060248995,
3.55127910964314));
#246270=CARTESIAN_POINT('Ctrl Pts',(-54.4530463244694,23.8971395307767,
3.47153072139089));
#246271=CARTESIAN_POINT('Ctrl Pts',(-54.401990730652,24.0130054476976,3.47122746281599));
#246272=CARTESIAN_POINT('Ctrl Pts',(-54.5001606201972,24.056506495927,3.40413045901284));
#246273=CARTESIAN_POINT('Origin',(-54.5516691663896,23.940420925912,3.40423097483326));
#246274=CARTESIAN_POINT('Ctrl Pts',(-57.20883363247,25.8191582032619,2.90134173516041));
#246275=CARTESIAN_POINT('Ctrl Pts',(-57.2611357920726,25.7028284190332,
2.90163218716408));
#246276=CARTESIAN_POINT('Ctrl Pts',(-57.1623216544372,25.658833530444,2.83404198860279));
#246277=CARTESIAN_POINT('Ctrl Pts',(-57.2503966981986,25.837662738193,2.82853349835371));
#246278=CARTESIAN_POINT('Ctrl Pts',(-57.2821216226326,25.7289639953178,
2.85381483162252));
#246279=CARTESIAN_POINT('Ctrl Pts',(-57.203882976126,25.6773378230591,2.79182701594196));
#246280=CARTESIAN_POINT('Ctrl Pts',(-57.3035546548414,25.8320911970514,
2.75468822073663));
#246281=CARTESIAN_POINT('Ctrl Pts',(-57.3185262575346,25.74078970011,2.79286913083853));
#246282=CARTESIAN_POINT('Ctrl Pts',(-57.2524664994803,25.6820441386716,
2.74900763297921));
#246283=CARTESIAN_POINT('Ctrl Pts',(-57.4126476234251,25.7649464042484,
2.63954450640406));
#246284=CARTESIAN_POINT('Ctrl Pts',(-57.3992776612638,25.7081127933389,
2.69627684028873));
#246285=CARTESIAN_POINT('Ctrl Pts',(-57.3434500727659,25.6555720179788,
2.68224356036517));
#246286=CARTESIAN_POINT('Ctrl Pts',(-57.4692856961543,25.7004590347004,
2.59908178706325));
#246287=CARTESIAN_POINT('Ctrl Pts',(-57.4449640631538,25.6633754510796,
2.65878704321563));
#246288=CARTESIAN_POINT('Ctrl Pts',(-57.3860499078785,25.622614088278,2.65878198860279));
#246289=CARTESIAN_POINT('Ctrl Pts',(-57.5052637377733,25.6197038181296,
2.5990817351604));
#246290=CARTESIAN_POINT('Ctrl Pts',(-57.471187734033,25.604522301406,2.65878198860278));
#246291=CARTESIAN_POINT('Ctrl Pts',(-57.4068835917981,25.5758735661207,
2.65878198860279));
#246292=CARTESIAN_POINT('Origin',(-57.1106661007666,25.7748538035646,2.83404198860279));
#246293=CARTESIAN_POINT('Origin',(-54.3889216310782,23.8679610547562,3.11913648166977));
#246294=CARTESIAN_POINT('Origin',(-54.2261740956467,23.7955011834907,2.83404198860278));
#246295=CARTESIAN_POINT('Origin',(-56.9479187893697,25.7023940320473,3.11913648177554));
#246296=CARTESIAN_POINT('Origin',(-56.7851714777849,25.6299342604994,3.40423097483327));
#246297=CARTESIAN_POINT('Ctrl Pts',(-54.1275498658875,23.7522229508827,
2.90134173516039));
#246298=CARTESIAN_POINT('Ctrl Pts',(-54.0765745253537,23.8679139708567,
2.90103711553245));
#246299=CARTESIAN_POINT('Ctrl Pts',(-54.1745185419761,23.9115214566113,
2.83404198860278));
#246300=CARTESIAN_POINT('Ctrl Pts',(-54.0860417646975,23.7337429357612,
2.8286299174797));
#246301=CARTESIAN_POINT('Ctrl Pts',(-54.0553388636011,23.8418262755866,
2.85314045886488));
#246302=CARTESIAN_POINT('Ctrl Pts',(-54.1330089371355,23.8930401898205,
2.79187960999932));
#246303=CARTESIAN_POINT('Ctrl Pts',(-54.033173720707,23.7393098712348,2.75470625793354));
#246304=CARTESIAN_POINT('Ctrl Pts',(-54.0188467943743,23.8301926567297,
2.79224250381919));
#246305=CARTESIAN_POINT('Ctrl Pts',(-54.0846755205375,23.8884275227223,
2.74901809108279));
#246306=CARTESIAN_POINT('Ctrl Pts',(-53.9248984592617,23.8065189073823,
2.63947868311703));
#246307=CARTESIAN_POINT('Ctrl Pts',(-53.9384511174157,23.8631501047901,
2.69595066767925));
#246308=CARTESIAN_POINT('Ctrl Pts',(-53.9943748351524,23.9152668978359,
2.68220539436073));
#246309=CARTESIAN_POINT('Ctrl Pts',(-53.8688190939458,23.8710081209824,
2.59908178585034));
#246310=CARTESIAN_POINT('Ctrl Pts',(-53.8932068550001,23.9079567336549,
2.65877670944961));
#246311=CARTESIAN_POINT('Ctrl Pts',(-53.9522270531151,23.9484663513832,
2.65878198860278));
#246312=CARTESIAN_POINT('Ctrl Pts',(-53.8330634946839,23.9513722670364,
2.59908173516039));
#246313=CARTESIAN_POINT('Ctrl Pts',(-53.8671470951732,23.9665367208223,
2.65878198860277));
#246314=CARTESIAN_POINT('Ctrl Pts',(-53.9314655730806,23.9951532569806,
2.65878198860278));
#246315=CARTESIAN_POINT('Origin',(-53.9314655730806,23.9951532569806,2.53178198860278));
#246316=CARTESIAN_POINT('Ctrl Pts',(-56.3916032444852,25.4547063934082,
3.7700319886028));
#246317=CARTESIAN_POINT('Ctrl Pts',(-56.4433359736143,25.3385127813696,
3.7700319886028));
#246318=CARTESIAN_POINT('Ctrl Pts',(-56.4432587405903,25.3386862495819,
3.64284238727646));
#246319=CARTESIAN_POINT('Ctrl Pts',(-56.5897307565553,25.5431622092801,
3.7700319886028));
#246320=CARTESIAN_POINT('Ctrl Pts',(-56.6417243268817,25.4268404215571,
3.77025506105722));
#246321=CARTESIAN_POINT('Ctrl Pts',(-56.6017747680111,25.4092621323422,
3.64284210641916));
#246322=CARTESIAN_POINT('Ctrl Pts',(-56.7783458705719,25.627368725429,3.65553527987848));
#246323=CARTESIAN_POINT('Ctrl Pts',(-56.83053751761,25.5109049500325,3.65585996533094));
#246324=CARTESIAN_POINT('Ctrl Pts',(-56.752679296228,25.4764491573031,3.55127902710191));
#246325=CARTESIAN_POINT('Ctrl Pts',(-56.8833377255396,25.6742415049979,
3.47153072139089));
#246326=CARTESIAN_POINT('Ctrl Pts',(-56.9357219102086,25.5577357740382,
3.47182327905205));
#246327=CARTESIAN_POINT('Ctrl Pts',(-56.8366797674144,25.5138485767966,
3.40413028378021));
#246328=CARTESIAN_POINT('Origin',(-56.3916032444852,25.4547063934082,3.6430319886028));
#246329=CARTESIAN_POINT('Origin',(3.58382961824622E-16,1.91601292797291E-13,
2.53178198860262));
#246330=CARTESIAN_POINT('Origin',(-53.9190682401996,24.0229981225296,2.53178198860278));
#246331=CARTESIAN_POINT('Origin',(52.0578415156897,-22.8300973196044,3.64303198860247));
#246332=CARTESIAN_POINT('Origin',(-56.0249274780513,25.2915084057492,3.64299466007644));
#246333=CARTESIAN_POINT('Ctrl Pts',(-53.8206887816837,23.9791663275012,
2.59908173516039));
#246334=CARTESIAN_POINT('Ctrl Pts',(-53.8547645473082,23.9943483786816,
2.65878198860278));
#246335=CARTESIAN_POINT('Ctrl Pts',(-53.9190682401996,24.0229981225296,
2.65878198860278));
#246336=CARTESIAN_POINT('Ctrl Pts',(-53.7850138844278,24.0592381183001,
2.59908193199912));
#246337=CARTESIAN_POINT('Ctrl Pts',(-53.8287709626499,24.052682504579,2.65877685806659));
#246338=CARTESIAN_POINT('Ctrl Pts',(-53.8983362760843,24.0695074323274,
2.65878198860278));
#246339=CARTESIAN_POINT('Ctrl Pts',(-53.7744461045708,24.143290671037,2.63872492669814));
#246340=CARTESIAN_POINT('Ctrl Pts',(-53.8255298669648,24.1158128282435,
2.69532212015291));
#246341=CARTESIAN_POINT('Ctrl Pts',(-53.9015903052238,24.1225146216896,
2.68176836726646));
#246342=CARTESIAN_POINT('Ctrl Pts',(-53.7968389608977,24.2696905364172,
2.75442176402266));
#246343=CARTESIAN_POINT('Ctrl Pts',(-53.8548027426705,24.1983175571256,
2.79203179920153));
#246344=CARTESIAN_POINT('Ctrl Pts',(-53.9421141528989,24.2081897025477,
2.74885310748195));
#246345=CARTESIAN_POINT('Ctrl Pts',(-53.8282518514941,24.3127961529002,
2.82866089558418));
#246346=CARTESIAN_POINT('Ctrl Pts',(-53.8880291490212,24.2176488245029,
2.85316563119191));
#246347=CARTESIAN_POINT('Ctrl Pts',(-53.9780599067629,24.2411088588486,
2.79189751796559));
#246348=CARTESIAN_POINT('Ctrl Pts',(-53.8697418420146,24.3312692531087,
2.9013417351604));
#246349=CARTESIAN_POINT('Ctrl Pts',(-53.9216078643418,24.2159747902186,
2.90103711553245));
#246350=CARTESIAN_POINT('Ctrl Pts',(-54.0195518809642,24.2595822759732,
2.83404198860278));
#246351=CARTESIAN_POINT('Origin',(-53.9678963272936,24.3756025490938,2.83404198860278));
#246352=CARTESIAN_POINT('Origin',(-55.9845461685076,25.2734729066172,3.56647653971902));
#246353=CARTESIAN_POINT('Origin',(-55.9097831300748,25.240186257314,3.42473028058502));
#246354=CARTESIAN_POINT('Origin',(-54.1306438627318,24.4480624203028,3.11913648168032));
#246355=CARTESIAN_POINT('Origin',(-54.2933913980365,24.520522291515,3.40423097483327));
#246356=CARTESIAN_POINT('Ctrl Pts',(-55.6083495590303,25.10597938477,3.36123028058498));
#246357=CARTESIAN_POINT('Ctrl Pts',(-55.6600051127009,24.9899591116494,
3.36123028058499));
#246358=CARTESIAN_POINT('Ctrl Pts',(-55.6600051127009,24.9899591116494,
3.23423028058498));
#246359=CARTESIAN_POINT('Ctrl Pts',(-55.6906734752783,25.1423759987947,
3.36123028058498));
#246360=CARTESIAN_POINT('Ctrl Pts',(-55.7421565548659,25.0265352902406,
3.36099641108368));
#246361=CARTESIAN_POINT('Ctrl Pts',(-55.7833465978035,25.0448742789056,
3.23423043688348));
#246362=CARTESIAN_POINT('Ctrl Pts',(-55.768516195595,25.1767934079559,3.410542589053));
#246363=CARTESIAN_POINT('Ctrl Pts',(-55.820224390035,25.061293329859,3.41008815826136));
#246364=CARTESIAN_POINT('Ctrl Pts',(-55.8999747466295,25.0968004762774,
3.30819867304359));
#246365=CARTESIAN_POINT('Ctrl Pts',(-55.8095395120008,25.19493178753,3.488230280585));
#246366=CARTESIAN_POINT('Ctrl Pts',(-55.861411884108,25.0796311836952,3.48794691941616));
#246367=CARTESIAN_POINT('Ctrl Pts',(-55.9614386837454,25.1241659841934,
3.42473028058501));
#246368=CARTESIAN_POINT('Origin',(-55.6083495590303,25.10597938477,3.23423028058498));
#246369=CARTESIAN_POINT('Ctrl Pts',(-54.1952354911873,24.4761921430391,
3.47153072139088));
#246370=CARTESIAN_POINT('Ctrl Pts',(-54.2471777813618,24.3607210247425,
3.47122746285093));
#246371=CARTESIAN_POINT('Ctrl Pts',(-54.3451938326304,24.4045675690227,
3.40413046676807));
#246372=CARTESIAN_POINT('Ctrl Pts',(-54.3002261711157,24.5230721320469,
3.65553813458001));
#246373=CARTESIAN_POINT('Ctrl Pts',(-54.3520689157403,24.4074212664128,
3.65520336072174));
#246374=CARTESIAN_POINT('Ctrl Pts',(-54.4291958219382,24.4419676644368,
3.55128134519984));
#246375=CARTESIAN_POINT('Ctrl Pts',(-54.4888383671851,24.6072895482019,
3.7700319886028));
#246376=CARTESIAN_POINT('Ctrl Pts',(-54.5406519873247,24.491383313692,3.76980209314061));
#246377=CARTESIAN_POINT('Ctrl Pts',(-54.5801016184612,24.5091552540989,
3.64284195387371));
#246378=CARTESIAN_POINT('Ctrl Pts',(-54.6869600343299,24.6957503380306,
3.7700319886028));
#246379=CARTESIAN_POINT('Ctrl Pts',(-54.7386929643777,24.5795562747215,
3.7700319886028));
#246380=CARTESIAN_POINT('Ctrl Pts',(-54.7386155301351,24.5797301948779,
3.64284189403826));
#246381=CARTESIAN_POINT('Origin',(-54.6869600343299,24.6957503380306,3.64303198860279));
#246382=CARTESIAN_POINT('Origin',(50.7999799080417,-22.2700612497312,3.23423028058466));
#246383=CARTESIAN_POINT('Origin',(-55.4702140717968,25.0444775033946,3.23423028058498));
#246384=CARTESIAN_POINT('Origin',(50.603004322856,-22.1823620689011,3.64303198860248));
#246385=CARTESIAN_POINT('Origin',(-55.0536014459535,24.8590452239602,3.64299171721763));
#246386=CARTESIAN_POINT('Ctrl Pts',(-55.2690209153042,24.9555320242414,
3.48823028058497));
#246387=CARTESIAN_POINT('Ctrl Pts',(-55.3213695969757,24.8391888661843,
3.48852004212275));
#246388=CARTESIAN_POINT('Ctrl Pts',(-55.2204359898058,24.7942503289606,
3.42473028058497));
#246389=CARTESIAN_POINT('Ctrl Pts',(-55.3101840490931,24.9737291291706,
3.41028005848422));
#246390=CARTESIAN_POINT('Ctrl Pts',(-55.3622664445104,24.8573973158465,
3.4107440422034));
#246391=CARTESIAN_POINT('Ctrl Pts',(-55.2821076446828,24.8217083187823,
3.30780486244012));
#246392=CARTESIAN_POINT('Ctrl Pts',(-55.3881672017731,25.0082040095652,
3.36123028058498));
#246393=CARTESIAN_POINT('Ctrl Pts',(-55.4398389138642,24.8919348043908,
3.36146460586493));
#246394=CARTESIAN_POINT('Ctrl Pts',(-55.3989435894779,24.8737270328802,
3.23423045308367));
#246395=CARTESIAN_POINT('Ctrl Pts',(-55.4702140717968,25.0444775033946,
3.36123028058498));
#246396=CARTESIAN_POINT('Ctrl Pts',(-55.5218696254674,24.928457230274,3.36123028058498));
#246397=CARTESIAN_POINT('Ctrl Pts',(-55.5218696254674,24.928457230274,3.23423028058498));
#246398=CARTESIAN_POINT('Origin',(-55.1687804361351,24.9102706020812,3.42473028058497));
#246399=CARTESIAN_POINT('Origin',(-55.0944632691843,24.8771824678739,3.56563113524807));
#246400=CARTESIAN_POINT('Origin',(-58.515880043567,18.6791227126687,3.56647653909402));
#246401=CARTESIAN_POINT('Origin',(-58.5579573083296,18.6927400943494,3.64299466007494));
#246402=CARTESIAN_POINT('Origin',(-58.4380471616456,18.6538332760103,3.42473028058495));
#246403=CARTESIAN_POINT('Ctrl Pts',(-58.3332704847797,18.6203878281146,
3.48823028058495));
#246404=CARTESIAN_POINT('Ctrl Pts',(-58.2946680067389,18.7407822670301,
3.48794691941612));
#246405=CARTESIAN_POINT('Ctrl Pts',(-58.3988020033599,18.7746174535798,
3.42473028058497));
#246406=CARTESIAN_POINT('Ctrl Pts',(-58.2905032380262,18.6063701040096,
3.41028005925101));
#246407=CARTESIAN_POINT('Ctrl Pts',(-58.2516444665222,18.7268030714108,
3.40982512231007));
#246408=CARTESIAN_POINT('Ctrl Pts',(-58.3345980746907,18.7537563325796,
3.30780486372936));
#246409=CARTESIAN_POINT('Ctrl Pts',(-58.2094810152003,18.5798130476651,
3.36123028058494));
#246410=CARTESIAN_POINT('Ctrl Pts',(-58.1702276772291,18.7003491529649,
3.36099721048529));
#246411=CARTESIAN_POINT('Ctrl Pts',(-58.2129647630938,18.7142352739237,
3.23423045308396));
#246412=CARTESIAN_POINT('Ctrl Pts',(-58.1242364370958,18.5518699907149,
3.36123028058493));
#246413=CARTESIAN_POINT('Ctrl Pts',(-58.0849912788101,18.6726541682844,
3.36123028058493));
#246414=CARTESIAN_POINT('Ctrl Pts',(-58.0849912788101,18.6726541682844,
3.23423028058494));
#246415=CARTESIAN_POINT('Origin',(-58.1242364370958,18.5518699907149,3.23423028058493));
#246416=CARTESIAN_POINT('Origin',(-0.0981128957140385,-0.301960443923528,
3.64303198860262));
#246417=CARTESIAN_POINT('Origin',(-58.9396512752214,18.8168143322225,3.64303198860275));
#246418=CARTESIAN_POINT('Origin',(-0.0981128957140384,-0.301960443923525,
3.23423028058481));
#246419=CARTESIAN_POINT('Origin',(-57.9804289733665,18.505144113284,3.23423028058494));
#246420=CARTESIAN_POINT('Ctrl Pts',(-59.4519788726609,18.9827025415095,
3.47153072139084));
#246421=CARTESIAN_POINT('Ctrl Pts',(-59.4129503614028,19.1043350233604,
3.47182327902675));
#246422=CARTESIAN_POINT('Ctrl Pts',(-59.3099814440482,19.0706774512227,
3.40413028959061));
#246423=CARTESIAN_POINT('Ctrl Pts',(-59.3425890481021,18.9472820042059,
3.6555380712097));
#246424=CARTESIAN_POINT('Ctrl Pts',(-59.3034455268834,19.068754472209,3.65586275497007));
#246425=CARTESIAN_POINT('Ctrl Pts',(-59.2225305038472,19.0422629184336,
3.55128126837305));
#246426=CARTESIAN_POINT('Ctrl Pts',(-59.1460739925265,18.8836509927323,
3.77003198860275));
#246427=CARTESIAN_POINT('Ctrl Pts',(-59.1068782740642,19.0048854004787,
3.77025505748436));
#246428=CARTESIAN_POINT('Ctrl Pts',(-59.0654284453496,18.9912173655546,
3.64284211731149));
#246429=CARTESIAN_POINT('Ctrl Pts',(-58.9396512752214,18.8168143322225,
3.77003198860276));
#246430=CARTESIAN_POINT('Ctrl Pts',(-58.9003474864893,18.9377789557521,
3.77003198860276));
#246431=CARTESIAN_POINT('Ctrl Pts',(-58.900406160666,18.9375983752043,3.64284239821752));
#246432=CARTESIAN_POINT('Origin',(-59.3493798002281,18.9499432001056,3.40423097483323));
#246433=CARTESIAN_POINT('Ctrl Pts',(-57.9804289733665,18.505144113284,3.36123028058493));
#246434=CARTESIAN_POINT('Ctrl Pts',(-57.9411838150808,18.6259282908535,
3.36123028058494));
#246435=CARTESIAN_POINT('Ctrl Pts',(-57.9411838150808,18.6259282908535,
3.23423028058494));
#246436=CARTESIAN_POINT('Ctrl Pts',(-57.8948964606932,18.4771060595091,
3.36123028058493));
#246437=CARTESIAN_POINT('Ctrl Pts',(-57.8554964068695,18.5980867642079,
3.36146538610022));
#246438=CARTESIAN_POINT('Ctrl Pts',(-57.8127777979929,18.5842066467868,
3.23423043688421));
#246439=CARTESIAN_POINT('Ctrl Pts',(-57.8140195545743,18.4505921960606,
3.41054258693111));
#246440=CARTESIAN_POINT('Ctrl Pts',(-57.774883736214,18.5718941197416,3.41100608859805));
#246441=CARTESIAN_POINT('Ctrl Pts',(-57.6913607539405,18.5447558577158,
3.30819866970792));
#246442=CARTESIAN_POINT('Ctrl Pts',(-57.7713971777988,18.4366189870671,
3.48823028058494));
#246443=CARTESIAN_POINT('Ctrl Pts',(-57.7324510618071,18.5581069080659,
3.48852004212272));
#246444=CARTESIAN_POINT('Ctrl Pts',(-57.6273730232606,18.5239649837006,
3.42473028058494));
#246445=CARTESIAN_POINT('Origin',(-57.6666181815462,18.4031808061312,3.42473028058492));
#246446=CARTESIAN_POINT('Origin',(-59.5188096735787,19.0049943031105,3.11913648178394));
#246447=CARTESIAN_POINT('Origin',(-59.6882395467421,19.0600454060085,2.83404198860275));
#246448=CARTESIAN_POINT('Origin',(-57.5892494790288,18.3780421908176,3.56563113460855));
#246449=CARTESIAN_POINT('Origin',(-57.5467470426661,18.3641788932749,3.64299171721772));
#246450=CARTESIAN_POINT('Ctrl Pts',(-59.8776671349986,19.4393816709755,
2.59908173516036));
#246451=CARTESIAN_POINT('Ctrl Pts',(-59.8421853116553,19.4278624395265,
2.65878198860274));
#246452=CARTESIAN_POINT('Ctrl Pts',(-59.7752282754838,19.4061247292252,
2.65878198860274));
#246453=CARTESIAN_POINT('Ctrl Pts',(-59.9048758468121,19.3555723159024,
2.59908193475616));
#246454=CARTESIAN_POINT('Ctrl Pts',(-59.8620015382112,19.3668135526098,
2.65878715325449));
#246455=CARTESIAN_POINT('Ctrl Pts',(-59.790969158339,19.3576098387254,2.65878198860274));
#246456=CARTESIAN_POINT('Ctrl Pts',(-59.9061888791359,19.2705128813948,
2.63878778849885));
#246457=CARTESIAN_POINT('Ctrl Pts',(-59.8582551377161,19.3034480936186,
2.69564460180143));
#246458=CARTESIAN_POINT('Ctrl Pts',(-59.7817014705988,19.3051157581418,
2.6818048162491));
#246459=CARTESIAN_POINT('Ctrl Pts',(-59.8700374834723,19.1466203444582,
2.75443238878656));
#246460=CARTESIAN_POINT('Ctrl Pts',(-59.8200494324138,19.2244111832569,
2.79268340777083));
#246461=CARTESIAN_POINT('Ctrl Pts',(-59.7316696194034,19.223945117425,2.74885926835608));
#246462=CARTESIAN_POINT('Ctrl Pts',(-59.834087357436,19.1068608943533,2.82856655361682));
#246463=CARTESIAN_POINT('Ctrl Pts',(-59.7849307811037,19.2088773592683,
2.85384197230915));
#246464=CARTESIAN_POINT('Ctrl Pts',(-59.6922425516974,19.1948817636409,
2.79184624278575));
#246465=CARTESIAN_POINT('Ctrl Pts',(-59.7908376697913,19.092807720641,2.90134173516036));
#246466=CARTESIAN_POINT('Ctrl Pts',(-59.7518659300027,19.2142545736082,
2.90163218716404));
#246467=CARTESIAN_POINT('Ctrl Pts',(-59.6489943884565,19.180829583578,2.83404198860275));
#246468=CARTESIAN_POINT('Origin',(-59.7752282754838,19.4061247292252,2.53178198860274));
#246469=CARTESIAN_POINT('Origin',(-0.0981128957140385,-0.301960443923528,
3.64303198860262));
#246470=CARTESIAN_POINT('Origin',(-57.1650137687748,18.2401996527044,3.64303198860275));
#246471=CARTESIAN_POINT('Origin',(1.26611655068502E-16,1.9152648105923E-13,
2.53178198860262));
#246472=CARTESIAN_POINT('Origin',(-59.7658094374952,19.4351129318419,2.53178198860275));
#246473=CARTESIAN_POINT('Ctrl Pts',(-57.1650137687748,18.2401996527044,
3.77003198860275));
#246474=CARTESIAN_POINT('Ctrl Pts',(-57.1257098194699,18.3611647704261,
3.77003198860276));
#246475=CARTESIAN_POINT('Ctrl Pts',(-57.1257686544591,18.3609836949485,
3.64284187937046));
#246476=CARTESIAN_POINT('Ctrl Pts',(-56.9585856505954,18.1733685221988,
3.77003198860275));
#246477=CARTESIAN_POINT('Ctrl Pts',(-56.9195342693643,18.294173732641,3.76980208962824));
#246478=CARTESIAN_POINT('Ctrl Pts',(-56.960743451265,18.3073637563262,3.64284193928231));
#246479=CARTESIAN_POINT('Ctrl Pts',(-56.7620685738644,18.1097485684446,
3.65553535416594));
#246480=CARTESIAN_POINT('Ctrl Pts',(-56.7232097045379,18.2303834904073,
3.65520057834524));
#246481=CARTESIAN_POINT('Ctrl Pts',(-56.8036425617896,18.2563185833,3.55127910964302));
#246482=CARTESIAN_POINT('Ctrl Pts',(-56.6526781108325,18.074335247489,3.47153072139085));
#246483=CARTESIAN_POINT('Ctrl Pts',(-56.6140134911408,18.1949032015568,
3.47122746281596));
#246484=CARTESIAN_POINT('Ctrl Pts',(-56.7161926934815,18.227904398799,3.4041304590128));
#246485=CARTESIAN_POINT('Origin',(-56.7552848242271,18.1070706485041,3.40423097483322));
#246486=CARTESIAN_POINT('Ctrl Pts',(-59.5942745858237,19.6977666881844,
2.90134173516036));
#246487=CARTESIAN_POINT('Ctrl Pts',(-59.6341304551458,19.5766071063167,
2.90163218716403));
#246488=CARTESIAN_POINT('Ctrl Pts',(-59.5312589135996,19.5431821162865,
2.83404198860274));
#246489=CARTESIAN_POINT('Ctrl Pts',(-59.6375442153294,19.7118253299471,
2.82853349835361));
#246490=CARTESIAN_POINT('Ctrl Pts',(-59.6577332347577,19.6004058925602,
2.85381483162321));
#246491=CARTESIAN_POINT('Ctrl Pts',(-59.5745267832912,19.5572406993633,
2.79182701594235));
#246492=CARTESIAN_POINT('Ctrl Pts',(-59.6898285824899,19.7007277907733,
2.75468822073662));
#246493=CARTESIAN_POINT('Ctrl Pts',(-59.6951745640078,19.6083614943631,
2.79286913083837));
#246494=CARTESIAN_POINT('Ctrl Pts',(-59.6233361049588,19.5568428722498,
2.74900763297926));
#246495=CARTESIAN_POINT('Ctrl Pts',(-59.7913053863691,19.622547503811,2.63954450640398));
#246496=CARTESIAN_POINT('Ctrl Pts',(-59.7720679362491,19.5674227749672,
2.69627684028876));
#246497=CARTESIAN_POINT('Ctrl Pts',(-59.7110541706153,19.5210053955059,
2.68224356036503));
#246498=CARTESIAN_POINT('Ctrl Pts',(-59.8408924241701,19.5524931121162,
2.59908178706402));
#246499=CARTESIAN_POINT('Ctrl Pts',(-59.8128277376111,19.5181549791681,
2.65878704321515));
#246500=CARTESIAN_POINT('Ctrl Pts',(-59.7499755976262,19.4837751174916,
2.65878198860274));
#246501=CARTESIAN_POINT('Ctrl Pts',(-59.8682321556243,19.4684195516695,
2.59908173516036));
#246502=CARTESIAN_POINT('Ctrl Pts',(-59.8327559231847,19.4568831131882,
2.65878198860274));
#246503=CARTESIAN_POINT('Ctrl Pts',(-59.7658094374952,19.4351129318419,
2.65878198860274));
#246504=CARTESIAN_POINT('Origin',(-59.492013755314,19.663966293856,2.83404198860274));
#246505=CARTESIAN_POINT('Origin',(-56.5858547179581,18.0520194698739,3.11913648167164));
#246506=CARTESIAN_POINT('Origin',(-56.4164246115664,17.996968291141,2.83404198860274));
#246507=CARTESIAN_POINT('Origin',(-59.3225838821509,19.6089151909108,3.119136481775));
#246508=CARTESIAN_POINT('Origin',(-59.1531540088,19.5538640879531,3.40423097483322));
#246509=CARTESIAN_POINT('Ctrl Pts',(-56.3138168485096,17.9642361803971,
2.90134173516035));
#246510=CARTESIAN_POINT('Ctrl Pts',(-56.2752137607567,18.0846218068693,
2.90103711553241));
#246511=CARTESIAN_POINT('Ctrl Pts',(-56.3771794532808,18.1177524687105,
2.83404198860273));
#246512=CARTESIAN_POINT('Ctrl Pts',(-56.2706044454592,17.9501961787628,
2.82862991747976));
#246513=CARTESIAN_POINT('Ctrl Pts',(-56.2513675234854,18.0608967538129,
2.85314045886472));
#246514=CARTESIAN_POINT('Ctrl Pts',(-56.3339654239818,18.1037113794377,
2.79187960999963));
#246515=CARTESIAN_POINT('Ctrl Pts',(-56.2186079213554,17.9612588333756,
2.75470625793333));
#246516=CARTESIAN_POINT('Ctrl Pts',(-56.2138593173287,18.0531413250551,
2.79224250381896));
#246517=CARTESIAN_POINT('Ctrl Pts',(-56.2854146278934,18.1041761987738,
2.74901809108272));
#246518=CARTESIAN_POINT('Ctrl Pts',(-56.1179510603878,18.0394175380795,
2.63947868311715));
#246519=CARTESIAN_POINT('Ctrl Pts',(-56.1373490477009,18.0943218653327,
2.69595066767932));
#246520=CARTESIAN_POINT('Ctrl Pts',(-56.1984140977478,18.1403075368578,
2.68220539436072));
#246521=CARTESIAN_POINT('Ctrl Pts',(-56.0689198620979,18.1094153628977,
2.59908178585092));
#246522=CARTESIAN_POINT('Ctrl Pts',(-56.0970362061497,18.1436123520191,
2.65877670944927));
#246523=CARTESIAN_POINT('Ctrl Pts',(-56.1599674935319,18.1777307632118,
2.65878198860274));
#246524=CARTESIAN_POINT('Ctrl Pts',(-56.0417604764384,18.1930767435948,
2.59908173516036));
#246525=CARTESIAN_POINT('Ctrl Pts',(-56.0772424804485,18.2045954185344,
2.65878198860274));
#246526=CARTESIAN_POINT('Ctrl Pts',(-56.1441998575528,18.2263320786581,
2.65878198860274));
#246527=CARTESIAN_POINT('Origin',(-56.1441998575528,18.2263320786581,2.53178198860275));
#246528=CARTESIAN_POINT('Ctrl Pts',(-58.7434254837933,19.4207352200699,
3.77003198860276));
#246529=CARTESIAN_POINT('Ctrl Pts',(-58.7827292759115,19.2997705861193,
3.77003198860276));
#246530=CARTESIAN_POINT('Ctrl Pts',(-58.7826705983437,19.2999511771037,
3.64284238727657));
#246531=CARTESIAN_POINT('Ctrl Pts',(-58.9497137831219,19.4879965013601,
3.77003198860276));
#246532=CARTESIAN_POINT('Ctrl Pts',(-58.9892635895159,19.3668771285532,
3.77025506105737));
#246533=CARTESIAN_POINT('Ctrl Pts',(-58.9476954469502,19.3535710010446,
3.64284210641904));
#246534=CARTESIAN_POINT('Ctrl Pts',(-59.1460976215386,19.5520260773866,
3.65553527987843));
#246535=CARTESIAN_POINT('Ctrl Pts',(-59.1858295778038,19.4307447900779,
3.6558599653305));
#246536=CARTESIAN_POINT('Ctrl Pts',(-59.1047962608408,19.4046161500175,
3.55127902710187));
#246537=CARTESIAN_POINT('Ctrl Pts',(-59.2554138597572,19.5876674457077,
3.47153072139085));
#246538=CARTESIAN_POINT('Ctrl Pts',(-59.2953329133625,19.4663243070095,
3.47182327905201));
#246539=CARTESIAN_POINT('Ctrl Pts',(-59.1922458725048,19.4330302514113,
3.40413028378025));
#246540=CARTESIAN_POINT('Origin',(-58.7434254837933,19.4207352200699,3.64303198860276));
#246541=CARTESIAN_POINT('Origin',(3.56182666396657E-16,1.91595560831732E-13,
2.53178198860262));
#246542=CARTESIAN_POINT('Origin',(-56.1347810195643,18.2553202812748,2.53178198860275));
#246543=CARTESIAN_POINT('Origin',(56.3788528200609,-17.9847604760577,3.64303198860251));
#246544=CARTESIAN_POINT('Origin',(-58.3616995707159,19.2967593024454,3.64299466007577));
#246545=CARTESIAN_POINT('Ctrl Pts',(-56.0323588238392,18.2220120550216,
2.59908173516036));
#246546=CARTESIAN_POINT('Ctrl Pts',(-56.0678348753334,18.2335490499217,
2.65878198860274));
#246547=CARTESIAN_POINT('Ctrl Pts',(-56.1347810195643,18.2553202812748,
2.65878198860274));
#246548=CARTESIAN_POINT('Ctrl Pts',(-56.0052491386462,18.3053742463597,
2.5990819319987));
#246549=CARTESIAN_POINT('Ctrl Pts',(-56.0480812627873,18.2942806848323,
2.65877685806566));
#246550=CARTESIAN_POINT('Ctrl Pts',(-56.119024173998,18.3037418885564,2.65878198860274));
#246551=CARTESIAN_POINT('Ctrl Pts',(-56.0035251343646,18.3900709842069,
2.63872492669813));
#246552=CARTESIAN_POINT('Ctrl Pts',(-56.0514568378816,18.3574039607309,
2.69532212015273));
#246553=CARTESIAN_POINT('Ctrl Pts',(-56.1278011372716,18.3561185603239,
2.68176836726657));
#246554=CARTESIAN_POINT('Ctrl Pts',(-56.0390077039669,18.513437727039,2.75442176402259));
#246555=CARTESIAN_POINT('Ctrl Pts',(-56.0891934462348,18.4363968713614,
2.79203179920177));
#246556=CARTESIAN_POINT('Ctrl Pts',(-56.1770584756123,18.4370884086015,
2.74885310748176));
#246557=CARTESIAN_POINT('Ctrl Pts',(-56.0747542753112,18.5530236652633,
2.82866089558416));
#246558=CARTESIAN_POINT('Ctrl Pts',(-56.1242585025269,18.4521491348384,
2.85316563119105));
#246559=CARTESIAN_POINT('Ctrl Pts',(-56.2162483036943,18.4660698759072,
2.79189751796651));
#246560=CARTESIAN_POINT('Ctrl Pts',(-56.1179479440989,18.5670586829464,
2.90134173516037));
#246561=CARTESIAN_POINT('Ctrl Pts',(-56.1574782858998,18.4469743395778,
2.90103711553242));
#246562=CARTESIAN_POINT('Ctrl Pts',(-56.259443978424,18.4801050014189,2.83404198860274));
#246563=CARTESIAN_POINT('Origin',(-56.2201988201384,18.6008891789884,2.83404198860274));
#246564=CARTESIAN_POINT('Origin',(-58.3196542512031,19.2830435998995,3.56647653971794));
#246565=CARTESIAN_POINT('Origin',(-58.2418213702175,19.2577541638577,3.42473028058497));
#246566=CARTESIAN_POINT('Origin',(-56.3896289265335,18.6559403576611,3.1191364816812));
#246567=CARTESIAN_POINT('Origin',(-56.559059032799,18.7109915363515,3.40423097483323));
#246568=CARTESIAN_POINT('Ctrl Pts',(-57.9280106456677,19.1557908785623,
3.36123028058494));
#246569=CARTESIAN_POINT('Ctrl Pts',(-57.9672558039533,19.0350067009929,
3.36123028058494));
#246570=CARTESIAN_POINT('Ctrl Pts',(-57.9672558039533,19.0350067009929,
3.23423028058494));
#246571=CARTESIAN_POINT('Ctrl Pts',(-58.0136880650209,19.1833829156716,
3.36123028058494));
#246572=CARTESIAN_POINT('Ctrl Pts',(-58.0527804636619,19.0627953474459,
3.36099641108439));
#246573=CARTESIAN_POINT('Ctrl Pts',(-58.0956618095386,19.0767283413221,
3.23423043688335));
#246574=CARTESIAN_POINT('Ctrl Pts',(-58.0947019536603,19.2094750027326,
3.41054258905298));
#246575=CARTESIAN_POINT('Ctrl Pts',(-58.1340538395309,19.0892026680465,
3.41008815826044));
#246576=CARTESIAN_POINT('Ctrl Pts',(-58.2170788227766,19.1161791203809,
3.30819867304366));
#246577=CARTESIAN_POINT('Ctrl Pts',(-58.1373965169895,19.2232259141438,
3.48823028058497));
#246578=CARTESIAN_POINT('Ctrl Pts',(-58.1769325318821,19.1031347997386,
3.48794691941613));
#246579=CARTESIAN_POINT('Ctrl Pts',(-58.2810665285031,19.1369699862882,
3.42473028058499));
#246580=CARTESIAN_POINT('Origin',(-57.9280106456677,19.1557908785624,3.23423028058494));
#246581=CARTESIAN_POINT('Ctrl Pts',(-56.4568070719812,18.6771643191708,
3.47153072139085));
#246582=CARTESIAN_POINT('Ctrl Pts',(-56.496394798308,18.5568963159714,3.47122746285089));
#246583=CARTESIAN_POINT('Ctrl Pts',(-56.5984571192857,18.5902571970801,
3.40413046676783));
#246584=CARTESIAN_POINT('Ctrl Pts',(-56.5661228951882,18.7128129802646,
3.65553813458));
#246585=CARTESIAN_POINT('Ctrl Pts',(-56.6055928325701,18.5923766197431,
3.6552033607218));
#246586=CARTESIAN_POINT('Ctrl Pts',(-56.6859083114038,18.6186718120036,
3.55128134520018));
#246587=CARTESIAN_POINT('Ctrl Pts',(-56.7625049710034,18.7768537015941,
3.77003198860276));
#246588=CARTESIAN_POINT('Ctrl Pts',(-56.8019192501371,18.6561664154749,
3.76980209314185));
#246589=CARTESIAN_POINT('Ctrl Pts',(-56.8430104456864,18.6697173900123,
3.64284195387339));
#246590=CARTESIAN_POINT('Ctrl Pts',(-56.9687879773467,18.8441205405518,
3.77003198860276));
#246591=CARTESIAN_POINT('Ctrl Pts',(-57.0080919221124,18.7231554368004,
3.77003198860276));
#246592=CARTESIAN_POINT('Ctrl Pts',(-57.0080330916692,18.7233364982868,
3.64284189403783));
#246593=CARTESIAN_POINT('Origin',(-56.9687879773467,18.8441205405518,3.64303198860275));
#246594=CARTESIAN_POINT('Origin',(55.0155724295761,-17.5418038257011,3.2342302805847));
#246595=CARTESIAN_POINT('Origin',(-57.7842031819384,19.1090650011314,3.23423028058494));
#246596=CARTESIAN_POINT('Origin',(54.8020887275097,-17.472438766075,3.64303198860251));
#246597=CARTESIAN_POINT('Origin',(-57.3504898524405,18.9681964166837,3.64299171721716));
#246598=CARTESIAN_POINT('Ctrl Pts',(-57.5748148483577,19.0416371860876,
3.48823028058493));
#246599=CARTESIAN_POINT('Ctrl Pts',(-57.6147155869503,18.9204594407744,
3.48852004212271));
#246600=CARTESIAN_POINT('Ctrl Pts',(-57.5096375484038,18.8863175164091,
3.42473028058493));
#246601=CARTESIAN_POINT('Ctrl Pts',(-57.6176546016069,19.055431886254,3.41028005848419));
#246602=CARTESIAN_POINT('Ctrl Pts',(-57.6572916985355,18.9342932580161,
3.41074404220455));
#246603=CARTESIAN_POINT('Ctrl Pts',(-57.5738415009814,18.9071786451776,
3.30780486243969));
#246604=CARTESIAN_POINT('Ctrl Pts',(-57.6988141606862,19.0815664505357,
3.36123028058494));
#246605=CARTESIAN_POINT('Ctrl Pts',(-57.7380493683907,18.960533015575,3.36146460586262));
#246606=CARTESIAN_POINT('Ctrl Pts',(-57.695474842495,18.946699713554,3.23423045308351));
#246607=CARTESIAN_POINT('Ctrl Pts',(-57.7842031819384,19.1090650011314,
3.36123028058494));
#246608=CARTESIAN_POINT('Ctrl Pts',(-57.823448340224,18.9882808235619,3.36123028058494));
#246609=CARTESIAN_POINT('Ctrl Pts',(-57.823448340224,18.9882808235619,3.23423028058494));
#246610=CARTESIAN_POINT('Origin',(-57.4703923901182,19.0071016939786,3.42473028058494));
#246611=CARTESIAN_POINT('Origin',(-57.393023688561,18.9819630792892,3.56563113524718));
#246612=CARTESIAN_POINT('Origin',(-60.1478239224122,12.4602215063118,3.56647653909494));
#246613=CARTESIAN_POINT('Origin',(-60.1910940874972,12.4693660187259,3.64299466007661));
#246614=CARTESIAN_POINT('Origin',(-60.0677739512127,12.443206359372,3.42473028058491));
#246615=CARTESIAN_POINT('Ctrl Pts',(-59.9600752506738,12.4208962741585,
3.48823028058492));
#246616=CARTESIAN_POINT('Ctrl Pts',(-59.9342688867326,12.5446662374485,
3.48794691941608));
#246617=CARTESIAN_POINT('Ctrl Pts',(-60.0413691664788,12.5674311046652,
3.42473028058493));
#246618=CARTESIAN_POINT('Ctrl Pts',(-59.9160770362135,12.4114257351943,
3.41028005925095));
#246619=CARTESIAN_POINT('Ctrl Pts',(-59.8900198101354,12.5352608058721,
3.40982512231051));
#246620=CARTESIAN_POINT('Ctrl Pts',(-59.9753363727317,12.5533954010689,
3.30780486372868));
#246621=CARTESIAN_POINT('Ctrl Pts',(-59.832722693313,12.3934832896268,3.36123028058489));
#246622=CARTESIAN_POINT('Ctrl Pts',(-59.8062838430887,12.5174621766264,
3.36099721048421));
#246623=CARTESIAN_POINT('Ctrl Pts',(-59.8502383056086,12.5268049860496,
3.23423045308356));
#246624=CARTESIAN_POINT('Ctrl Pts',(-59.7450242491248,12.3746037924162,
3.36123028058489));
#246625=CARTESIAN_POINT('Ctrl Pts',(-59.718619464391,12.4988285377094,3.36123028058489));
#246626=CARTESIAN_POINT('Ctrl Pts',(-59.718619464391,12.4988285377094,3.23423028058489));
#246627=CARTESIAN_POINT('Origin',(-59.7450242491248,12.3746037924162,3.23423028058489));
#246628=CARTESIAN_POINT('Origin',(-0.0660119618346311,-0.3105618632328,
3.64303198860262));
#246629=CARTESIAN_POINT('Origin',(-60.5836663843182,12.5528626811445,3.64303198860271));
#246630=CARTESIAN_POINT('Origin',(-0.0660119618346311,-0.310561863232797,
3.23423028058481));
#246631=CARTESIAN_POINT('Origin',(-59.597120393566,12.3431658574209,3.23423028058489));
#246632=CARTESIAN_POINT('Ctrl Pts',(-61.1105274371642,12.6642893210139,
3.47153072139079));
#246633=CARTESIAN_POINT('Ctrl Pts',(-61.0844267845857,12.7893350777085,
3.4718232790267));
#246634=CARTESIAN_POINT('Ctrl Pts',(-60.9785037674409,12.7666250679675,
3.40413028959035));
#246635=CARTESIAN_POINT('Ctrl Pts',(-60.9980344071773,12.6404971713792,
3.65553807120965));
#246636=CARTESIAN_POINT('Ctrl Pts',(-60.9718026486737,12.7653958126131,
3.65586275496998));
#246637=CARTESIAN_POINT('Ctrl Pts',(-60.8885617651964,12.7475073053532,
3.55128126837319));
#246638=CARTESIAN_POINT('Ctrl Pts',(-60.7959446297927,12.597756154011,3.77003198860271));
#246639=CARTESIAN_POINT('Ctrl Pts',(-60.7696360759136,12.7224234952047,
3.77025505748454));
#246640=CARTESIAN_POINT('Ctrl Pts',(-60.7269846150095,12.7131630221038,
3.64284211731139));
#246641=CARTESIAN_POINT('Ctrl Pts',(-60.5836663843182,12.5528626811445,
3.77003198860271));
#246642=CARTESIAN_POINT('Ctrl Pts',(-60.5572221520604,12.6772730124468,
3.77003198860271));
#246643=CARTESIAN_POINT('Ctrl Pts',(-60.5572616290068,12.6770872880162,
3.64284239821708));
#246644=CARTESIAN_POINT('Origin',(-61.0050661295707,12.642433962084,3.40423097483317));
#246645=CARTESIAN_POINT('Ctrl Pts',(-59.597120393566,12.3431658574209,3.36123028058489));
#246646=CARTESIAN_POINT('Ctrl Pts',(-59.5707156088321,12.4673906027141,
3.36123028058489));
#246647=CARTESIAN_POINT('Ctrl Pts',(-59.5707156088321,12.4673906027141,
3.23423028058489));
#246648=CARTESIAN_POINT('Ctrl Pts',(-59.5091256622726,12.3242219811465,
3.36123028058489));
#246649=CARTESIAN_POINT('Ctrl Pts',(-59.4825873732106,12.448658367964,3.36146538610087));
#246650=CARTESIAN_POINT('Ctrl Pts',(-59.4386519140004,12.4393195978192,
3.23423043688379));
#246651=CARTESIAN_POINT('Ctrl Pts',(-59.4259203549057,12.3063073021292,
3.41054258693107));
#246652=CARTESIAN_POINT('Ctrl Pts',(-59.3996784303307,12.431035528135,3.41100608859863));
#246653=CARTESIAN_POINT('Ctrl Pts',(-59.3137762748665,12.4127764613286,
3.30819866970867));
#246654=CARTESIAN_POINT('Ctrl Pts',(-59.3820708699071,12.2968658913801,
3.48823028058489));
#246655=CARTESIAN_POINT('Ctrl Pts',(-59.3560370505014,12.421759266491,3.48852004212267));
#246656=CARTESIAN_POINT('Ctrl Pts',(-59.2479658375577,12.3987880210522,
3.42473028058489));
#246657=CARTESIAN_POINT('Origin',(-59.2743706222916,12.274563275759,3.42473028058489));
#246658=CARTESIAN_POINT('Origin',(-61.1793222555445,12.6794732450926,3.11913648178304));
#246659=CARTESIAN_POINT('Origin',(-61.3535783813233,12.7165125280164,2.83404198860269));
#246660=CARTESIAN_POINT('Origin',(-59.194798052794,12.2576496039905,3.56563113460843));
#246661=CARTESIAN_POINT('Origin',(-59.1510793400372,12.2483049653999,3.64299171721795));
#246662=CARTESIAN_POINT('Ctrl Pts',(-61.5816197022698,13.0739701745323,
2.59908173516032));
#246663=CARTESIAN_POINT('Ctrl Pts',(-61.545128164506,13.0662229071065,2.6587819886027));
#246664=CARTESIAN_POINT('Ctrl Pts',(-61.4762657165316,13.0516031943527,
2.6587819886027));
#246665=CARTESIAN_POINT('Ctrl Pts',(-61.5999188988198,12.9877758510418,
2.59908193475642));
#246666=CARTESIAN_POINT('Ctrl Pts',(-61.5584544893681,13.0034370926708,
2.65878715325387));
#246667=CARTESIAN_POINT('Ctrl Pts',(-61.4868491822337,13.0017087032038,
2.6587819886027));
#246668=CARTESIAN_POINT('Ctrl Pts',(-61.5923336062397,12.9030451317659,
2.63878778849879));
#246669=CARTESIAN_POINT('Ctrl Pts',(-61.5481051179917,12.94081036178,2.69564460180113));
#246670=CARTESIAN_POINT('Ctrl Pts',(-61.4721451382825,12.9504709278438,
2.68180481624893));
#246671=CARTESIAN_POINT('Ctrl Pts',(-61.5434299552079,12.7836101409429,
2.75443238878653));
#246672=CARTESIAN_POINT('Ctrl Pts',(-61.5018471007596,12.8662000075464,
2.79268340777113));
#246673=CARTESIAN_POINT('Ctrl Pts',(-61.4139027244671,12.8749747009097,
2.74885926835616));
#246674=CARTESIAN_POINT('Ctrl Pts',(-61.5035207735036,12.7478263086953,
2.82856655361677));
#246675=CARTESIAN_POINT('Ctrl Pts',(-61.4652971063431,12.8544221781235,
2.85384197230771));
#246676=CARTESIAN_POINT('Ctrl Pts',(-61.3716536946531,12.8501918100168,
2.79184624278451));
#246677=CARTESIAN_POINT('Ctrl Pts',(-61.4590390555209,12.7383709431249,
2.9013417351603));
#246678=CARTESIAN_POINT('Ctrl Pts',(-61.43297545991,12.8632261535953,2.90163218716398));
#246679=CARTESIAN_POINT('Ctrl Pts',(-61.3271735965894,12.8407372733096,
2.83404198860269));
#246680=CARTESIAN_POINT('Origin',(-61.4762657165316,13.0516031943527,2.53178198860269));
#246681=CARTESIAN_POINT('Origin',(-0.0660119618346311,-0.3105618632328,
3.64303198860262));
#246682=CARTESIAN_POINT('Origin',(-58.7584778814677,12.164906888579,3.64303198860271));
#246683=CARTESIAN_POINT('Origin',(1.31078692950416E-16,1.91543152271565E-13,
2.53178198860262));
#246684=CARTESIAN_POINT('Origin',(-61.4699285681955,13.081417133223,2.5317819886027));
#246685=CARTESIAN_POINT('Ctrl Pts',(-58.7584778814677,12.164906888579,3.77003198860271));
#246686=CARTESIAN_POINT('Ctrl Pts',(-58.732033541174,12.2893177281502,3.77003198860271));
#246687=CARTESIAN_POINT('Ctrl Pts',(-58.7320731263175,12.289131494692,3.64284187937051));
#246688=CARTESIAN_POINT('Ctrl Pts',(-58.5461948427482,12.1200194799681,
3.77003198860271));
#246689=CARTESIAN_POINT('Ctrl Pts',(-58.5199849720728,12.2442448876967,
3.76980208962782));
#246690=CARTESIAN_POINT('Ctrl Pts',(-58.5623471386682,12.253055122594,3.64284193928217));
#246691=CARTESIAN_POINT('Ctrl Pts',(-58.3441042111264,12.0772896710143,
3.65553535416591));
#246692=CARTESIAN_POINT('Ctrl Pts',(-58.3180679977595,12.2013256001486,
3.65520057834582));
#246693=CARTESIAN_POINT('Ctrl Pts',(-58.4007711908105,12.2187110949217,
3.55127910964302));
#246694=CARTESIAN_POINT('Ctrl Pts',(-58.2316113004782,12.053504764932,3.47153072139081));
#246695=CARTESIAN_POINT('Ctrl Pts',(-58.2057612725768,12.1774537884112,
3.47122746281592));
#246696=CARTESIAN_POINT('Ctrl Pts',(-58.3108302909894,12.1995935666435,
3.4041304590128));
#246697=CARTESIAN_POINT('Origin',(-58.3370777047235,12.0753355159231,3.40423097483318));
#246698=CARTESIAN_POINT('Ctrl Pts',(-61.3267881959114,13.3605623192485,
2.90134173516031));
#246699=CARTESIAN_POINT('Ctrl Pts',(-61.3537611057084,13.2359003894749,
2.90163218716398));
#246700=CARTESIAN_POINT('Ctrl Pts',(-61.2479592423879,13.2134115091892,
2.8340419886027));
#246701=CARTESIAN_POINT('Ctrl Pts',(-61.3712903180781,13.3700210384231,
2.82853349835361));
#246702=CARTESIAN_POINT('Ctrl Pts',(-61.3797222373789,13.2571016411954,
2.85381483162365));
#246703=CARTESIAN_POINT('Ctrl Pts',(-61.2924596082466,13.2228703539492,
2.79182701594243));
#246704=CARTESIAN_POINT('Ctrl Pts',(-61.422128257289,13.353519088177,2.75468822073652));
#246705=CARTESIAN_POINT('Ctrl Pts',(-61.4177900459394,13.2610999767702,
2.79286913083864));
#246706=CARTESIAN_POINT('Ctrl Pts',(-61.3409599630868,13.2173727427873,
2.74900763297921));
#246707=CARTESIAN_POINT('Ctrl Pts',(-61.5148770953649,13.2651598666399,
2.639544506404));
#246708=CARTESIAN_POINT('Ctrl Pts',(-61.4899829268154,13.2123479779268,
2.69627684028851));
#246709=CARTESIAN_POINT('Ctrl Pts',(-61.4244514636294,13.1725625528867,
2.68224356036499));
#246710=CARTESIAN_POINT('Ctrl Pts',(-61.5568698122752,13.1903059833734,
2.59908178706443));
#246711=CARTESIAN_POINT('Ctrl Pts',(-61.525369554737,13.1590895168685,2.65878704321593));
#246712=CARTESIAN_POINT('Ctrl Pts',(-61.4592680512443,13.1314678292776,
2.65878198860269));
#246713=CARTESIAN_POINT('Ctrl Pts',(-61.5752716937452,13.1038352065726,
2.59908173516031));
#246714=CARTESIAN_POINT('Ctrl Pts',(-61.5387839176329,13.0960702419678,
2.65878198860269));
#246715=CARTESIAN_POINT('Ctrl Pts',(-61.4699285681955,13.081417133223,2.65878198860269));
#246716=CARTESIAN_POINT('Origin',(-61.221554457654,13.3376362544824,2.8340419886027));
#246717=CARTESIAN_POINT('Origin',(-58.1628213392034,12.0382961820491,3.11913648167021));
#246718=CARTESIAN_POINT('Origin',(-57.988564973546,12.0012568480858,2.8340419886027));
#246719=CARTESIAN_POINT('Origin',(-61.047298331873,13.3005969715131,3.11913648177578));
#246720=CARTESIAN_POINT('Origin',(-60.8730422059014,13.26355768855,3.40423097483318));
#246721=CARTESIAN_POINT('Ctrl Pts',(-57.8830978693156,11.979429479061,2.90134173516031));
#246722=CARTESIAN_POINT('Ctrl Pts',(-57.8572899778512,12.1031907419155,
2.90103711553237));
#246723=CARTESIAN_POINT('Ctrl Pts',(-57.9621601888121,12.125481593379,2.83404198860269));
#246724=CARTESIAN_POINT('Ctrl Pts',(-57.8386546085357,11.9699833161087,
2.82862991747971));
#246725=CARTESIAN_POINT('Ctrl Pts',(-57.8310944294261,12.0820882677183,
2.85314045886447));
#246726=CARTESIAN_POINT('Ctrl Pts',(-57.9177151970033,12.1160345187366,
2.79187960999925));
#246727=CARTESIAN_POINT('Ctrl Pts',(-57.7880992891175,11.9864204851029,
2.75470625793335));
#246728=CARTESIAN_POINT('Ctrl Pts',(-57.7929810340972,12.0782959991609,
2.79224250381911));
#246729=CARTESIAN_POINT('Ctrl Pts',(-57.8694789541063,12.1215717318493,
2.74901809108265));
#246730=CARTESIAN_POINT('Ctrl Pts',(-57.6961636462598,12.0746725352387,
2.63947868311705));
#246731=CARTESIAN_POINT('Ctrl Pts',(-57.7211944343233,12.127248449038,2.69595066767917));
#246732=CARTESIAN_POINT('Ctrl Pts',(-57.7867317752136,12.1665991704024,
2.68220539436071));
#246733=CARTESIAN_POINT('Ctrl Pts',(-57.6547178110645,12.149412060458,2.59908178585055));
#246734=CARTESIAN_POINT('Ctrl Pts',(-57.6862546895618,12.1804827566583,
2.65877670944877));
#246735=CARTESIAN_POINT('Ctrl Pts',(-57.7524075778586,12.2078361528631,
2.6587819886027));
#246736=CARTESIAN_POINT('Ctrl Pts',(-57.6364522029208,12.2354540642043,
2.59908173516031));
#246737=CARTESIAN_POINT('Ctrl Pts',(-57.6729438621907,12.2432007592845,
2.6587819886027));
#246738=CARTESIAN_POINT('Ctrl Pts',(-57.7418065394566,12.2578193919766,
2.6587819886027));
#246739=CARTESIAN_POINT('Origin',(-57.7418065394566,12.2578193919766,2.5317819886027));
#246740=CARTESIAN_POINT('Ctrl Pts',(-60.451642460649,13.1739864076105,3.77003198860272));
#246741=CARTESIAN_POINT('Ctrl Pts',(-60.478086695185,13.0495760655902,3.77003198860272));
#246742=CARTESIAN_POINT('Ctrl Pts',(-60.478047215957,13.0497618007548,3.64284238727605));
#246743=CARTESIAN_POINT('Ctrl Pts',(-60.6638314094603,13.2193162256446,
3.77003198860272));
#246744=CARTESIAN_POINT('Ctrl Pts',(-60.6905041359628,13.094726276951,3.77025506105687));
#246745=CARTESIAN_POINT('Ctrl Pts',(-60.6477728389709,13.0858380958634,
3.64284210641796));
#246746=CARTESIAN_POINT('Ctrl Pts',(-60.865832349848,13.2624673401135,3.65553527987841));
#246747=CARTESIAN_POINT('Ctrl Pts',(-60.8926693037172,13.1376973240556,
3.65585996533169));
#246748=CARTESIAN_POINT('Ctrl Pts',(-60.8093487091495,13.1201821075163,
3.55127902710262));
#246749=CARTESIAN_POINT('Ctrl Pts',(-60.9782752797349,13.2864868028994,
3.4715307213908));
#246750=CARTESIAN_POINT('Ctrl Pts',(-61.0052918407716,13.1616357172824,
3.47182327905196));
#246751=CARTESIAN_POINT('Ctrl Pts',(-60.8992893450418,13.1392995799685,
3.40413028377995));
#246752=CARTESIAN_POINT('Origin',(-60.451642460649,13.1739864076105,3.64303198860272));
#246753=CARTESIAN_POINT('Origin',(3.54593577968597E-16,1.91589630272981E-13,
2.53178198860262));
#246754=CARTESIAN_POINT('Origin',(-57.7354693911205,12.2876333308469,2.5317819886027));
#246755=CARTESIAN_POINT('Origin',(59.5987607253196,-12.3435145206981,3.64303198860255));
#246756=CARTESIAN_POINT('Origin',(-60.0590486699121,13.0905908661183,3.64299466007645));
#246757=CARTESIAN_POINT('Ctrl Pts',(-57.6301266171958,12.2652136052659,
2.59908173516031));
#246758=CARTESIAN_POINT('Ctrl Pts',(-57.6666142715156,12.2729791421553,
2.6587819886027));
#246759=CARTESIAN_POINT('Ctrl Pts',(-57.7354693911205,12.2876333308469,
2.6587819886027));
#246760=CARTESIAN_POINT('Ctrl Pts',(-57.6118791634502,12.3509528635303,
2.59908193199883));
#246761=CARTESIAN_POINT('Ctrl Pts',(-57.6533170557967,12.3354428975795,
2.65877685806624));
#246762=CARTESIAN_POINT('Ctrl Pts',(-57.7248602994014,12.3374367183506,
2.6587819886027));
#246763=CARTESIAN_POINT('Ctrl Pts',(-57.619017823295,12.4353658313042,2.63872492669789));
#246764=CARTESIAN_POINT('Ctrl Pts',(-57.6632723181621,12.3978675338897,
2.6953221201529));
#246765=CARTESIAN_POINT('Ctrl Pts',(-57.7390640345625,12.3886090227466,
2.68176836726647));
#246766=CARTESIAN_POINT('Ctrl Pts',(-57.6672013517154,12.5543478197373,
2.75442176402273));
#246767=CARTESIAN_POINT('Ctrl Pts',(-57.7090592089825,12.4724831634112,
2.79203179920132));
#246768=CARTESIAN_POINT('Ctrl Pts',(-57.7965151898611,12.463986515842,2.74885310748178));
#246769=CARTESIAN_POINT('Ctrl Pts',(-57.7068899568908,12.5899803678813,
2.82866089558396));
#246770=CARTESIAN_POINT('Ctrl Pts',(-57.7455787351221,12.4844838378936,
2.85316563119178));
#246771=CARTESIAN_POINT('Ctrl Pts',(-57.8385197202049,12.4887127671321,
2.79189751796692));
#246772=CARTESIAN_POINT('Ctrl Pts',(-57.7513140650721,12.599423532447,2.90134173516031));
#246773=CARTESIAN_POINT('Ctrl Pts',(-57.7780756236496,12.4758649777951,
2.90103711553237));
#246774=CARTESIAN_POINT('Ctrl Pts',(-57.8829458346106,12.4981558292586,
2.83404198860269));
#246775=CARTESIAN_POINT('Origin',(-57.8565410498767,12.6223805745517,2.83404198860269));
#246776=CARTESIAN_POINT('Origin',(-60.0157999977489,13.08134523226,3.56647653971844));
#246777=CARTESIAN_POINT('Origin',(-59.9357500275434,13.064330085838,3.42473028058494));
#246778=CARTESIAN_POINT('Origin',(-58.0307974155282,12.6594199084519,3.11913648168203));
#246779=CARTESIAN_POINT('Origin',(-58.2050537810542,12.6964592423891,3.40423097483318));
#246780=CARTESIAN_POINT('Ctrl Pts',(-59.6130003254556,12.9957275188822,
3.3612302805849));
#246781=CARTESIAN_POINT('Ctrl Pts',(-59.6394051101894,12.871502773589,3.36123028058489));
#246782=CARTESIAN_POINT('Ctrl Pts',(-59.6394051101894,12.871502773589,3.2342302805849));
#246783=CARTESIAN_POINT('Ctrl Pts',(-59.7010925481785,13.0142126749435,
3.3612302805849));
#246784=CARTESIAN_POINT('Ctrl Pts',(-59.7273659613738,12.8901994296778,
3.36099641108629));
#246785=CARTESIAN_POINT('Ctrl Pts',(-59.7714687931894,12.899573775969,3.23423043688377));
#246786=CARTESIAN_POINT('Ctrl Pts',(-59.7843900000233,13.031693569538,3.41054258905291));
#246787=CARTESIAN_POINT('Ctrl Pts',(-59.8109544298277,12.9079667071257,
3.41008815825905));
#246788=CARTESIAN_POINT('Ctrl Pts',(-59.8963444006345,12.9261169057239,
3.30819867304326));
#246789=CARTESIAN_POINT('Ctrl Pts',(-59.8282880397056,13.0409063549237,
3.48823028058492));
#246790=CARTESIAN_POINT('Ctrl Pts',(-59.855054532531,12.9173404733281,3.48794691941607));
#246791=CARTESIAN_POINT('Ctrl Pts',(-59.9621548122772,12.9401053405448,
3.42473028058493));
#246792=CARTESIAN_POINT('Origin',(-59.6130003254556,12.9957275188822,3.2342302805849));
#246793=CARTESIAN_POINT('Ctrl Pts',(-58.0998260601481,12.6735055745739,
3.4715307213908));
#246794=CARTESIAN_POINT('Ctrl Pts',(-58.1266254912132,12.5497583678826,
3.47122746285085));
#246795=CARTESIAN_POINT('Ctrl Pts',(-58.2316158657531,12.5722680770246,
3.40413046676782));
#246796=CARTESIAN_POINT('Ctrl Pts',(-58.212269339599,12.6975323335629,3.65553813457996));
#246797=CARTESIAN_POINT('Ctrl Pts',(-58.2389340288442,12.5736300041249,
3.65520336072351));
#246798=CARTESIAN_POINT('Ctrl Pts',(-58.3215581271232,12.5913858949916,
3.55128134520024));
#246799=CARTESIAN_POINT('Ctrl Pts',(-58.4142696920426,12.7406947165204,
3.77003198860271));
#246800=CARTESIAN_POINT('Ctrl Pts',(-58.4408527990795,12.616548653954,3.7698020931406));
#246801=CARTESIAN_POINT('Ctrl Pts',(-58.4831353553017,12.6257301953102,
3.6428419538732));
#246802=CARTESIAN_POINT('Ctrl Pts',(-58.6264539577984,12.7860306150449,
3.77003198860272));
#246803=CARTESIAN_POINT('Ctrl Pts',(-58.6528982950381,12.6616197898421,
3.77003198860271));
#246804=CARTESIAN_POINT('Ctrl Pts',(-58.6528587129532,12.6618060089104,
3.64284189403786));
#246805=CARTESIAN_POINT('Origin',(-58.6264539577984,12.7860306150449,3.64303198860271));
#246806=CARTESIAN_POINT('Origin',(58.1567073854023,-12.0369966210205,3.23423028058474));
#246807=CARTESIAN_POINT('Origin',(-59.4650964698967,12.9642895838869,3.2342302805849));
#246808=CARTESIAN_POINT('Origin',(57.9308881865556,-11.9889972685545,3.64303198860255));
#246809=CARTESIAN_POINT('Origin',(-59.0190342907429,12.8695280801151,3.64299171721718));
#246810=CARTESIAN_POINT('Ctrl Pts',(-59.249807061628,12.9191181862044,3.48823028058489));
#246811=CARTESIAN_POINT('Ctrl Pts',(-59.2768226962999,12.7944335023706,
3.48852004212266));
#246812=CARTESIAN_POINT('Ctrl Pts',(-59.1687514833561,12.7714622569318,
3.42473028058488));
#246813=CARTESIAN_POINT('Ctrl Pts',(-59.2938540730359,12.9283593439868,
3.41028005848414));
#246814=CARTESIAN_POINT('Ctrl Pts',(-59.3206115991486,12.8037411209987,
3.410744042203));
#246815=CARTESIAN_POINT('Ctrl Pts',(-59.2347843016971,12.7854979657557,
3.30780486243963));
#246816=CARTESIAN_POINT('Ctrl Pts',(-59.3773008374015,12.9458672563999,
3.3612302805849));
#246817=CARTESIAN_POINT('Ctrl Pts',(-59.4036696715723,12.8213956592928,
3.36146460586466));
#246818=CARTESIAN_POINT('Ctrl Pts',(-59.3598823995813,12.8120883873135,
3.23423045308393));
#246819=CARTESIAN_POINT('Ctrl Pts',(-59.4650964698967,12.9642895838869,
3.3612302805849));
#246820=CARTESIAN_POINT('Ctrl Pts',(-59.4915012546306,12.8400648385937,
3.36123028058489));
#246821=CARTESIAN_POINT('Ctrl Pts',(-59.4915012546306,12.8400648385937,
3.2342302805849));
#246822=CARTESIAN_POINT('Origin',(-59.1423466986223,12.895687002225,3.42473028058489));
#246823=CARTESIAN_POINT('Origin',(-59.0627741301468,12.8787733309741,3.5656311352478));
#246824=CARTESIAN_POINT('Origin',(-61.1207756556248,6.10480350566248,3.56647653909434));
#246825=CARTESIAN_POINT('Origin',(-61.1647646440477,6.10937495961987,3.64299466007599));
#246826=CARTESIAN_POINT('Origin',(-61.0393856393804,6.09624906995217,3.42473028058487));
#246827=CARTESIAN_POINT('Ctrl Pts',(-60.9299448846691,6.08531878138299,
3.48823028058487));
#246828=CARTESIAN_POINT('Ctrl Pts',(-60.9172173747511,6.21110821942913,
3.48794691941604));
#246829=CARTESIAN_POINT('Ctrl Pts',(-61.0261105245455,6.22255335066394,
3.42473028058489));
#246830=CARTESIAN_POINT('Ctrl Pts',(-60.885197756147,6.08049918876632,3.4102800592509));
#246831=CARTESIAN_POINT('Ctrl Pts',(-60.8722275639178,6.20637959976664,
3.40982512230967));
#246832=CARTESIAN_POINT('Ctrl Pts',(-60.9589723348236,6.21549684257611,
3.30780486372855));
#246833=CARTESIAN_POINT('Ctrl Pts',(-60.800424540796,6.07136793516325,3.36123028058485));
#246834=CARTESIAN_POINT('Ctrl Pts',(-60.7870898478943,6.19743126523199,
3.36099721048481));
#246835=CARTESIAN_POINT('Ctrl Pts',(-60.8317801127822,6.20212840134671,
3.23423045308369));
#246836=CARTESIAN_POINT('Ctrl Pts',(-60.7112330730304,6.06175884541548,
3.36123028058485));
#246837=CARTESIAN_POINT('Ctrl Pts',(-60.6979579581954,6.18806312612726,
3.36123028058485));
#246838=CARTESIAN_POINT('Ctrl Pts',(-60.6979579581954,6.18806312612726,
3.23423028058485));
#246839=CARTESIAN_POINT('Origin',(-60.7112330730304,6.06175884541549,3.23423028058484));
#246840=CARTESIAN_POINT('Origin',(-0.0331877870874725,-0.315760701779243,
3.64303198860262));
#246841=CARTESIAN_POINT('Origin',(-61.5639141665612,6.15137923967653,3.64303198860266));
#246842=CARTESIAN_POINT('Origin',(-0.0331877870874724,-0.31576070177924,
3.23423028058481));
#246843=CARTESIAN_POINT('Origin',(-60.5608532912344,6.04595329345039,3.23423028058485));
#246844=CARTESIAN_POINT('Ctrl Pts',(-62.0995362748659,6.20712349654441,
3.47153072139075));
#246845=CARTESIAN_POINT('Ctrl Pts',(-62.0866494451786,6.33421250060425,
3.47182327902666));
#246846=CARTESIAN_POINT('Ctrl Pts',(-61.9789328429858,6.32269886887975,
3.40413028959034));
#246847=CARTESIAN_POINT('Ctrl Pts',(-61.9851725366286,6.19522040634676,
3.65553807120959));
#246848=CARTESIAN_POINT('Ctrl Pts',(-61.9721399414742,6.32217680516095,
3.6558627549699));
#246849=CARTESIAN_POINT('Ctrl Pts',(-61.887485202092,6.31308733464707,3.55128126837344));
#246850=CARTESIAN_POINT('Ctrl Pts',(-61.7797221753254,6.17383766261707,
3.77003198860267));
#246851=CARTESIAN_POINT('Ctrl Pts',(-61.7665890280525,6.30057205577847,
3.7702550574842));
#246852=CARTESIAN_POINT('Ctrl Pts',(-61.7232032332917,6.29582060418326,
3.64284211731065));
#246853=CARTESIAN_POINT('Ctrl Pts',(-61.5639141665612,6.15137923967653,
3.77003198860267));
#246854=CARTESIAN_POINT('Ctrl Pts',(-61.5506192193202,6.27787221312685,
3.77003198860267));
#246855=CARTESIAN_POINT('Ctrl Pts',(-61.5506390665185,6.27768337964962,
3.6428423982171));
#246856=CARTESIAN_POINT('Origin',(-61.9923681882669,6.19641157197441,3.40423097483313));
#246857=CARTESIAN_POINT('Ctrl Pts',(-60.5608532912344,6.04595329345039,
3.36123028058485));
#246858=CARTESIAN_POINT('Ctrl Pts',(-60.5475781763994,6.17225757416217,
3.36123028058485));
#246859=CARTESIAN_POINT('Ctrl Pts',(-60.5475781763994,6.17225757416217,
3.23423028058485));
#246860=CARTESIAN_POINT('Ctrl Pts',(-60.4713604300108,6.03631114775018,
3.36123028058485));
#246861=CARTESIAN_POINT('Ctrl Pts',(-60.457974664764,6.16283986559477,3.36146538610095));
#246862=CARTESIAN_POINT('Ctrl Pts',(-60.4133037213016,6.1581447602434,3.23423043688392));
#246863=CARTESIAN_POINT('Ctrl Pts',(-60.3867383361559,6.02719193013363,
3.41054258693102));
#246864=CARTESIAN_POINT('Ctrl Pts',(-60.3736778173768,6.1539799099147,3.41100608859762));
#246865=CARTESIAN_POINT('Ctrl Pts',(-60.286337650718,6.14480008849002,3.30819866970862));
#246866=CARTESIAN_POINT('Ctrl Pts',(-60.3421421670675,6.02238575970255,
3.48823028058484));
#246867=CARTESIAN_POINT('Ctrl Pts',(-60.3293058762212,6.14931623097225,
3.48852004212262));
#246868=CARTESIAN_POINT('Ctrl Pts',(-60.2194255397045,6.13776734223194,
3.42473028058484));
#246869=CARTESIAN_POINT('Origin',(-60.2327006545395,6.01146306152017,3.42473028058484));
#246870=CARTESIAN_POINT('Origin',(-62.1695413802837,6.21503322485355,3.11913648178332));
#246871=CARTESIAN_POINT('Origin',(-62.3467145720969,6.23365487766603,2.83404198860265));
#246872=CARTESIAN_POINT('Origin',(-60.151796031785,6.00295964302194,3.56563113460813));
#246873=CARTESIAN_POINT('Origin',(-60.1073400339998,5.998236045201,3.64299171721792));
#246874=CARTESIAN_POINT('Ctrl Pts',(-62.6108711573006,6.5653175249528,2.59908173516027));
#246875=CARTESIAN_POINT('Ctrl Pts',(-62.5737697140402,6.5614271022333,2.65878198860266));
#246876=CARTESIAN_POINT('Ctrl Pts',(-62.5037563256535,6.55408556365924,
2.65878198860265));
#246877=CARTESIAN_POINT('Ctrl Pts',(-62.6200603487601,6.47768259609059,
2.59908193475661));
#246878=CARTESIAN_POINT('Ctrl Pts',(-62.5804601312005,6.49759225479933,
2.65878715325419));
#246879=CARTESIAN_POINT('Ctrl Pts',(-62.5090664195363,6.50335812634736,
2.65878198860265));
#246880=CARTESIAN_POINT('Ctrl Pts',(-62.6036598373291,6.39420891953742,
2.63878778849883));
#246881=CARTESIAN_POINT('Ctrl Pts',(-62.5636211788254,6.4363904035792,2.69564460180115));
#246882=CARTESIAN_POINT('Ctrl Pts',(-62.4890871199581,6.45393802800009,
2.68180481624886));
#246883=CARTESIAN_POINT('Ctrl Pts',(-62.5425397295635,6.28054002958117,
2.7544323887864));
#246884=CARTESIAN_POINT('Ctrl Pts',(-62.5098176621807,6.36702405212765,
2.792683407771));
#246885=CARTESIAN_POINT('Ctrl Pts',(-62.423272259596,6.38494336730957,2.74885926835614));
#246886=CARTESIAN_POINT('Ctrl Pts',(-62.4991087455376,6.24912387034458,
2.82856655361681));
#246887=CARTESIAN_POINT('Ctrl Pts',(-62.4722367740483,6.35913125763809,
2.85384197230793));
#246888=CARTESIAN_POINT('Ctrl Pts',(-62.3786641568872,6.36471246584703,
2.79184624278445));
#246889=CARTESIAN_POINT('Ctrl Pts',(-62.4538823482276,6.24436990788037,
2.90134173516025));
#246890=CARTESIAN_POINT('Ctrl Pts',(-62.4410124550019,6.37126553604047,
2.90163218716393));
#246891=CARTESIAN_POINT('Ctrl Pts',(-62.3334394572619,6.3599591583778,2.83404198860264));
#246892=CARTESIAN_POINT('Origin',(-62.5037563256535,6.55408556365924,2.53178198860265));
#246893=CARTESIAN_POINT('Origin',(-0.0331877870874725,-0.315760701779243,
3.64303198860262));
#246894=CARTESIAN_POINT('Origin',(-59.7081718144893,5.95633285891189,3.64303198860266));
#246895=CARTESIAN_POINT('Origin',(1.33778643725276E-16,1.91560199089859E-13,
2.53178198860262));
#246896=CARTESIAN_POINT('Origin',(-62.5005702980931,6.58439859103007,2.53178198860265));
#246897=CARTESIAN_POINT('Ctrl Pts',(-59.7081718144893,5.95633285891189,
3.77003198860267));
#246898=CARTESIAN_POINT('Ctrl Pts',(-59.6948768129328,6.08282634913945,
3.77003198860267));
#246899=CARTESIAN_POINT('Ctrl Pts',(-59.6948967145276,6.08263699811361,
3.64284187937066));
#246900=CARTESIAN_POINT('Ctrl Pts',(-59.4923596726254,5.9338809680367,3.77003198860267));
#246901=CARTESIAN_POINT('Ctrl Pts',(-59.4792784733315,6.06016553348737,
3.76980208962841));
#246902=CARTESIAN_POINT('Ctrl Pts',(-59.5223294958604,6.06449945282216,
3.64284193928277));
#246903=CARTESIAN_POINT('Ctrl Pts',(-59.2869096333629,5.91250946061126,
3.65553535416586));
#246904=CARTESIAN_POINT('Ctrl Pts',(-59.2739813341607,6.03858743332211,
3.65520057834496));
#246905=CARTESIAN_POINT('Ctrl Pts',(-59.3580487495188,6.04723285085777,
3.55127910964236));
#246906=CARTESIAN_POINT('Ctrl Pts',(-59.1725467709678,5.90061356181236,
3.47153072139075));
#246907=CARTESIAN_POINT('Ctrl Pts',(-59.1597945531718,6.02658564326377,
3.47122746281586));
#246908=CARTESIAN_POINT('Ctrl Pts',(-59.2666022295036,6.03762143444283,
3.40413045901285));
#246909=CARTESIAN_POINT('Origin',(-59.2797173540686,5.91130048050322,3.40423097483314));
#246910=CARTESIAN_POINT('Ctrl Pts',(-62.3873926810692,6.87697683366542,
2.90134173516027));
#246911=CARTESIAN_POINT('Ctrl Pts',(-62.4011871104969,6.75017837817579,
2.90163218716395));
#246912=CARTESIAN_POINT('Ctrl Pts',(-62.293614112757,6.73887200051311,2.83404198860265));
#246913=CARTESIAN_POINT('Ctrl Pts',(-62.4326397213342,6.88173199854474,
2.8285334983535));
#246914=CARTESIAN_POINT('Ctrl Pts',(-62.4292221586318,6.76854981002497,
2.8538148316231));
#246915=CARTESIAN_POINT('Ctrl Pts',(-62.3388594194628,6.74362747387379,
2.79182701594245));
#246916=CARTESIAN_POINT('Ctrl Pts',(-62.4814742414946,6.86000643604713,
2.75468822073656));
#246917=CARTESIAN_POINT('Ctrl Pts',(-62.4674993676282,6.76854707276811,
2.79286913083876));
#246918=CARTESIAN_POINT('Ctrl Pts',(-62.3865194274374,6.73309031164165,
2.74900763297921));
#246919=CARTESIAN_POINT('Ctrl Pts',(-62.5644789380884,6.76243636205672,
2.63954450640386));
#246920=CARTESIAN_POINT('Ctrl Pts',(-62.5342007968299,6.71251593157883,
2.69627684028836));
#246921=CARTESIAN_POINT('Ctrl Pts',(-62.4648696125158,6.67979835840227,
2.6822435603649));
#246922=CARTESIAN_POINT('Ctrl Pts',(-62.5984172531145,6.68360310202791,
2.59908178706377));
#246923=CARTESIAN_POINT('Ctrl Pts',(-62.5638265480135,6.65585031610604,
2.65878704321558));
#246924=CARTESIAN_POINT('Ctrl Pts',(-62.4951999029147,6.63528943158945,
2.65878198860265));
#246925=CARTESIAN_POINT('Ctrl Pts',(-62.6076796697355,6.59568250079864,
2.59908173516026));
#246926=CARTESIAN_POINT('Ctrl Pts',(-62.570580117661,6.59177408464752,2.65878198860265));
#246927=CARTESIAN_POINT('Ctrl Pts',(-62.5005702980931,6.58439859103007,
2.65878198860265));
#246928=CARTESIAN_POINT('Origin',(-62.280338997922,6.86517628122488,2.83404198860265));
#246929=CARTESIAN_POINT('Origin',(-59.1025439185019,5.89267880207498,3.11913648166995));
#246930=CARTESIAN_POINT('Origin',(-58.925370482788,5.87405712357849,2.83404198860266));
#246931=CARTESIAN_POINT('Origin',(-62.1031658061019,6.84655462836655,3.11913648177607));
#246932=CARTESIAN_POINT('Origin',(-61.925992614092,6.82793297553327,3.40423097483314));
#246933=CARTESIAN_POINT('Ctrl Pts',(-58.8181995570485,5.8633736414956,2.90134173516027));
#246934=CARTESIAN_POINT('Ctrl Pts',(-58.8054696185321,5.98915458643774,
2.90103711553232));
#246935=CARTESIAN_POINT('Ctrl Pts',(-58.912095367953,6.00036140429026,2.83404198860265));
#246936=CARTESIAN_POINT('Ctrl Pts',(-58.773012368204,5.85862481136443,2.8286299174796));
#246937=CARTESIAN_POINT('Ctrl Pts',(-58.777211762863,5.97090589422323,2.85314045886469));
#246938=CARTESIAN_POINT('Ctrl Pts',(-58.8669063622641,5.99561184840491,
2.79187960999987));
#246939=CARTESIAN_POINT('Ctrl Pts',(-58.7244521481309,5.88025640567561,
2.75470625793339));
#246940=CARTESIAN_POINT('Ctrl Pts',(-58.7389107566976,5.97111833475351,
2.7922425038187));
#246941=CARTESIAN_POINT('Ctrl Pts',(-58.8195131589313,6.00616078842875,
2.74901809108258));
#246942=CARTESIAN_POINT('Ctrl Pts',(-58.6422449895249,5.97763489331422,
2.63947868311692));
#246943=CARTESIAN_POINT('Ctrl Pts',(-58.6726343357863,6.02730636094616,
2.69595066767936));
#246944=CARTESIAN_POINT('Ctrl Pts',(-58.7419259266988,6.05959099741143,
2.68220539436069));
#246945=CARTESIAN_POINT('Ctrl Pts',(-58.6088386066677,6.05629725705607,
2.59908178585));
#246946=CARTESIAN_POINT('Ctrl Pts',(-58.6434504949716,6.08390124328586,
2.65877670944815));
#246947=CARTESIAN_POINT('Ctrl Pts',(-58.7121001992953,6.10418993497001,
2.65878198860265));
#246948=CARTESIAN_POINT('Ctrl Pts',(-58.5996668978649,6.14377718965303,
2.59908173516027));
#246949=CARTESIAN_POINT('Ctrl Pts',(-58.6367684021393,6.14766703046151,
2.65878198860265));
#246950=CARTESIAN_POINT('Ctrl Pts',(-58.7067819056643,6.15500747092296,
2.65878198860265));
#246951=CARTESIAN_POINT('Origin',(-58.7067819056643,6.15500747092296,2.53178198860265));
#246952=CARTESIAN_POINT('Ctrl Pts',(-61.4975385923863,6.78290064323539,
3.77003198860267));
#246953=CARTESIAN_POINT('Ctrl Pts',(-61.5108335407726,6.65640765888754,
3.77003198860267));
#246954=CARTESIAN_POINT('Ctrl Pts',(-61.5108136924273,6.65659650327855,
3.64284238727592));
#246955=CARTESIAN_POINT('Ctrl Pts',(-61.7133034041535,6.80580235504213,
3.77003198860267));
#246956=CARTESIAN_POINT('Ctrl Pts',(-61.7268068187931,6.6791068640109,3.77025506105739));
#246957=CARTESIAN_POINT('Ctrl Pts',(-61.6833805404074,6.67473401011705,
3.64284210641797));
#246958=CARTESIAN_POINT('Ctrl Pts',(-61.9187082819379,6.82760223531323,
3.65553527987831));
#246959=CARTESIAN_POINT('Ctrl Pts',(-61.9323562021263,6.70071049691211,
3.6558599653315));
#246960=CARTESIAN_POINT('Ctrl Pts',(-61.8476612078244,6.69200060426976,
3.55127902710253));
#246961=CARTESIAN_POINT('Ctrl Pts',(-62.0330459552233,6.83973663030238,
3.47153072139074));
#246962=CARTESIAN_POINT('Ctrl Pts',(-62.046864024595,6.71274549238783,3.47182327905191));
#246963=CARTESIAN_POINT('Ctrl Pts',(-61.9391074595191,6.70161199275237,
3.40413028377984));
#246964=CARTESIAN_POINT('Origin',(-61.4975385923863,6.78290064323539,3.64303198860267));
#246965=CARTESIAN_POINT('Origin',(3.53633106925806E-16,1.9158356609748E-13,
2.53178198860262));
#246966=CARTESIAN_POINT('Origin',(-58.7035958781039,6.18532049829379,2.53178198860266));
#246967=CARTESIAN_POINT('Origin',(61.5757885448748,-6.15262728712807,3.64303198860259));
#246968=CARTESIAN_POINT('Origin',(-61.0983782637171,6.74099917687887,3.6429946600764));
#246969=CARTESIAN_POINT('Ctrl Pts',(-58.5964866834551,6.17403490859001,
2.59908173516027));
#246970=CARTESIAN_POINT('Ctrl Pts',(-58.6335861742242,6.17794390662152,
2.65878198860266));
#246971=CARTESIAN_POINT('Ctrl Pts',(-58.7035958781039,6.18532049829379,
2.65878198860265));
#246972=CARTESIAN_POINT('Ctrl Pts',(-58.5873013840785,6.26121185652523,
2.59908193199888));
#246973=CARTESIAN_POINT('Ctrl Pts',(-58.6268910424078,6.24145541658251,
2.65877685806582));
#246974=CARTESIAN_POINT('Ctrl Pts',(-58.6982507756608,6.2359600096838,2.65878198860266));
#246975=CARTESIAN_POINT('Ctrl Pts',(-58.603224495399,6.34441620808584,2.63872492669796));
#246976=CARTESIAN_POINT('Ctrl Pts',(-58.6433169201089,6.3024974759271,2.69532212015277));
#246977=CARTESIAN_POINT('Ctrl Pts',(-58.7177256636152,6.285367292233,2.68176836726637));
#246978=CARTESIAN_POINT('Ctrl Pts',(-58.6635810738165,6.45770985055656,
2.75442176402258));
#246979=CARTESIAN_POINT('Ctrl Pts',(-58.6966524426403,6.3719183198876,2.79203179920138));
#246980=CARTESIAN_POINT('Ctrl Pts',(-58.7827411889911,6.35432657855795,
2.74885310748179));
#246981=CARTESIAN_POINT('Ctrl Pts',(-58.70677687616,6.48899861096533,2.82866089558398));
#246982=CARTESIAN_POINT('Ctrl Pts',(-58.7342263230558,6.38003592347143,
2.85316563119172));
#246983=CARTESIAN_POINT('Ctrl Pts',(-58.8271002111739,6.37452670784941,
2.7918975179661));
#246984=CARTESIAN_POINT('Ctrl Pts',(-58.7519447039089,6.49374646112721,
2.90134173516027));
#246985=CARTESIAN_POINT('Ctrl Pts',(-58.7656442740271,6.36806742857306,
2.90103711553233));
#246986=CARTESIAN_POINT('Ctrl Pts',(-58.8722700234481,6.37927424642558,
2.83404198860265));
#246987=CARTESIAN_POINT('Origin',(-58.8589949086131,6.50557852713735,2.83404198860265));
#246988=CARTESIAN_POINT('Origin',(-61.0544000804056,6.7363249088106,3.56647653971873));
#246989=CARTESIAN_POINT('Origin',(-60.9730100652055,6.72777047351102,3.42473028058489));
#246990=CARTESIAN_POINT('Origin',(-59.0361683443159,6.52420020557762,3.11913648168046));
#246991=CARTESIAN_POINT('Origin',(-59.2133417798937,6.54282188406207,3.40423097483314));
#246992=CARTESIAN_POINT('Ctrl Pts',(-60.6448574988555,6.69328024897434,
3.36123028058485));
#246993=CARTESIAN_POINT('Ctrl Pts',(-60.6581326136904,6.56697596826257,
3.36123028058485));
#246994=CARTESIAN_POINT('Ctrl Pts',(-60.6581326136904,6.56697596826257,
3.23423028058485));
#246995=CARTESIAN_POINT('Ctrl Pts',(-60.7343993681214,6.70245599674945,
3.36123028058485));
#246996=CARTESIAN_POINT('Ctrl Pts',(-60.7475659388568,6.57637578951112,
3.36099641108469));
#246997=CARTESIAN_POINT('Ctrl Pts',(-60.7924070567573,6.58108878091684,
3.23423043688388));
#246998=CARTESIAN_POINT('Ctrl Pts',(-60.819067758858,6.71113417453917,3.41054258905289));
#246999=CARTESIAN_POINT('Ctrl Pts',(-60.8325536871445,6.58530836180369,
3.41008815825983));
#247000=CARTESIAN_POINT('Ctrl Pts',(-60.9193730951243,6.59443344928411,
3.30819867304282));
#247001=CARTESIAN_POINT('Ctrl Pts',(-60.8636883187845,6.71570789669389,
3.48823028058487));
#247002=CARTESIAN_POINT('Ctrl Pts',(-60.8773920302461,6.59002106156445,
3.48794691941603));
#247003=CARTESIAN_POINT('Ctrl Pts',(-60.9862851800405,6.60146619279925,
3.42473028058488));
#247004=CARTESIAN_POINT('Origin',(-60.6448574988555,6.69328024897434,3.23423028058485));
#247005=CARTESIAN_POINT('Ctrl Pts',(-59.1062911958297,6.53099325080035,
3.47153072139076));
#247006=CARTESIAN_POINT('Ctrl Pts',(-59.1200087114583,6.40512264090967,
3.4712274628508));
#247007=CARTESIAN_POINT('Ctrl Pts',(-59.2267768430462,6.41653455700106,
3.40413046676784));
#247008=CARTESIAN_POINT('Ctrl Pts',(-59.2206299794252,6.543134865483,3.6555381345799));
#247009=CARTESIAN_POINT('Ctrl Pts',(-59.2341972766254,6.41712406698062,
3.65520336072206));
#247010=CARTESIAN_POINT('Ctrl Pts',(-59.318224747432,6.42614611919712,3.55128134519965));
#247011=CARTESIAN_POINT('Ctrl Pts',(-59.4260354503639,6.5649460139706,3.77003198860267));
#247012=CARTESIAN_POINT('Ctrl Pts',(-59.4394961352151,6.43870134519708,
3.76980209314093));
#247013=CARTESIAN_POINT('Ctrl Pts',(-59.4825067955808,6.44341285848436,
3.64284195387372));
#247014=CARTESIAN_POINT('Ctrl Pts',(-59.6417962403143,6.58785426247075,
3.77003198860267));
#247015=CARTESIAN_POINT('Ctrl Pts',(-59.6550912403353,6.461360786852,3.77003198860267));
#247016=CARTESIAN_POINT('Ctrl Pts',(-59.6550713402783,6.4615501232472,3.64284189403793));
#247017=CARTESIAN_POINT('Origin',(-59.6417962403143,6.58785426247075,3.64303198860266));
#247018=CARTESIAN_POINT('Origin',(60.0850508448142,-5.99594444118149,3.23423028058478));
#247019=CARTESIAN_POINT('Origin',(-60.4944777170594,6.67747469700925,3.23423028058485));
#247020=CARTESIAN_POINT('Origin',(59.8516078896891,-5.97140859790491,3.64303198860259));
#247021=CARTESIAN_POINT('Origin',(-60.04095383883,6.62985850077774,3.64299171721822));
#247022=CARTESIAN_POINT('Ctrl Pts',(-60.2756459899119,6.65505462397374,
3.48823028058484));
#247023=CARTESIAN_POINT('Ctrl Pts',(-60.2894805317162,6.52822907310757,
3.48852004212262));
#247024=CARTESIAN_POINT('Ctrl Pts',(-60.1796001951996,6.51668018436725,
3.42473028058484));
#247025=CARTESIAN_POINT('Ctrl Pts',(-60.3204176712045,6.65964099131241,
3.41028005848409));
#247026=CARTESIAN_POINT('Ctrl Pts',(-60.3340024654463,6.53290851690435,
3.41074404220402));
#247027=CARTESIAN_POINT('Ctrl Pts',(-60.2467384099271,6.5237366950833,3.30780486243953));
#247028=CARTESIAN_POINT('Ctrl Pts',(-60.4052373806432,6.66833043150632,
3.36123028058485));
#247029=CARTESIAN_POINT('Ctrl Pts',(-60.4184509388145,6.5417844091174,3.36146460586362));
#247030=CARTESIAN_POINT('Ctrl Pts',(-60.3739306632443,6.53710513959992,
3.23423045308403));
#247031=CARTESIAN_POINT('Ctrl Pts',(-60.4944777170594,6.67747469700925,
3.36123028058485));
#247032=CARTESIAN_POINT('Ctrl Pts',(-60.5077528318944,6.55117041629748,
3.36123028058485));
#247033=CARTESIAN_POINT('Ctrl Pts',(-60.5077528318944,6.55117041629748,
3.23423028058485));
#247034=CARTESIAN_POINT('Origin',(-60.1663250803646,6.64298446507902,3.42473028058484));
#247035=CARTESIAN_POINT('Origin',(-60.0854204586811,6.63448104699066,3.56563113524784));
#247036=CARTESIAN_POINT('Origin',(-61.4240753804095,-0.317499999706852,
3.56647653909397));
#247037=CARTESIAN_POINT('Origin',(-61.4683012396086,-0.317551690014747,
3.64299466007431));
#247038=CARTESIAN_POINT('Origin',(-61.3422370451705,-0.317499999999815,
3.42473028058483));
#247039=CARTESIAN_POINT('Ctrl Pts',(-61.2322532920972,-0.316930737395729,
3.48823028058483));
#247040=CARTESIAN_POINT('Ctrl Pts',(-61.2327440814645,-0.190499999999815,
3.48794691941599));
#247041=CARTESIAN_POINT('Ctrl Pts',(-61.3422370451705,-0.190499999999815,
3.42473028058484));
#247042=CARTESIAN_POINT('Ctrl Pts',(-61.1872475084174,-0.317046579199451,
3.41028005925088));
#247043=CARTESIAN_POINT('Ctrl Pts',(-61.187506454176,-0.190499999998209,
3.4098251223097));
#247044=CARTESIAN_POINT('Ctrl Pts',(-61.274729039531,-0.190499999999814,
3.30780486372827));
#247045=CARTESIAN_POINT('Ctrl Pts',(-61.1019842137032,-0.317266596913308,
3.3612302805848));
#247046=CARTESIAN_POINT('Ctrl Pts',(-61.1018997758106,-0.190499999999807,
3.36099721048453));
#247047=CARTESIAN_POINT('Ctrl Pts',(-61.1468362071711,-0.190499999999813,
3.23423045308374));
#247048=CARTESIAN_POINT('Ctrl Pts',(-61.0122769227456,-0.317499999999814,
3.3612302805848));
#247049=CARTESIAN_POINT('Ctrl Pts',(-61.0122769227456,-0.190499999999814,
3.3612302805848));
#247050=CARTESIAN_POINT('Ctrl Pts',(-61.0122769227456,-0.190499999999813,
3.2342302805848));
#247051=CARTESIAN_POINT('Origin',(-61.0122769227456,-0.317499999999813,
3.2342302805848));
#247052=CARTESIAN_POINT('Origin',(5.50819412990574E-15,-0.317499999999816,
3.64303198860262));
#247053=CARTESIAN_POINT('Origin',(-61.8696548221181,-0.317499999999816,
3.64303198860261));
#247054=CARTESIAN_POINT('Origin',(5.56576032196012E-15,-0.317499999999813,
3.23423028058481));
#247055=CARTESIAN_POINT('Origin',(-60.8610688070707,-0.317499999999813,
3.2342302805848));
#247056=CARTESIAN_POINT('Ctrl Pts',(-62.4081695979768,-0.318048871876944,
3.4715307213907));
#247057=CARTESIAN_POINT('Ctrl Pts',(-62.4086377819835,-0.190309034175174,
3.47182327902661));
#247058=CARTESIAN_POINT('Ctrl Pts',(-62.3003077603771,-0.190500142124869,
3.40413028959024));
#247059=CARTESIAN_POINT('Ctrl Pts',(-62.2931881445371,-0.317932489889758,
3.65553807120955));
#247060=CARTESIAN_POINT('Ctrl Pts',(-62.2934975005736,-0.190309294367597,
3.65586275496964));
#247061=CARTESIAN_POINT('Ctrl Pts',(-62.208356400327,-0.190500141995283,
3.55128126837315));
#247062=CARTESIAN_POINT('Ctrl Pts',(-62.0866281564673,-0.317722686167228,
3.77003198860262));
#247063=CARTESIAN_POINT('Ctrl Pts',(-62.0868143053089,-0.190309769569541,
3.77025505748483));
#247064=CARTESIAN_POINT('Ctrl Pts',(-62.0431695205374,-0.190500141761682,
3.64284211731126));
#247065=CARTESIAN_POINT('Ctrl Pts',(-61.8696548221181,-0.317499999999817,
3.77003198860262));
#247066=CARTESIAN_POINT('Ctrl Pts',(-61.8696548221181,-0.190310267888814,
3.77003198860262));
#247067=CARTESIAN_POINT('Ctrl Pts',(-61.8696548221181,-0.190500141513731,
3.64284239821695));
#247068=CARTESIAN_POINT('Origin',(-62.3004688883554,-0.317499999999815,
3.40423097483308));
#247069=CARTESIAN_POINT('Ctrl Pts',(-60.8610688070707,-0.317499999999814,
3.3612302805848));
#247070=CARTESIAN_POINT('Ctrl Pts',(-60.8610688070707,-0.190499999999814,
3.3612302805848));
#247071=CARTESIAN_POINT('Ctrl Pts',(-60.8610688070707,-0.190499999999813,
3.2342302805848));
#247072=CARTESIAN_POINT('Ctrl Pts',(-60.7710583184321,-0.317734773760083,
3.3612302805848));
#247073=CARTESIAN_POINT('Ctrl Pts',(-60.7709717342411,-0.190499999999814,
3.36146538610122));
#247074=CARTESIAN_POINT('Ctrl Pts',(-60.7260547307361,-0.190499999999813,
3.23423043688408));
#247075=CARTESIAN_POINT('Ctrl Pts',(-60.6859465754578,-0.317958617918848,
3.41054258693099));
#247076=CARTESIAN_POINT('Ctrl Pts',(-60.6862105562575,-0.190499999999749,
3.41100608859814));
#247077=CARTESIAN_POINT('Ctrl Pts',(-60.5983892955404,-0.190499999999814,
3.3081986697084));
#247078=CARTESIAN_POINT('Ctrl Pts',(-60.6410923272405,-0.318076890623181,
3.48823028058479));
#247079=CARTESIAN_POINT('Ctrl Pts',(-60.6415942020421,-0.190499999999815,
3.48852004212257));
#247080=CARTESIAN_POINT('Ctrl Pts',(-60.5311086139135,-0.190499999999815,
3.42473028058479));
#247081=CARTESIAN_POINT('Origin',(-60.5311086139134,-0.317499999999815,
3.42473028058479));
#247082=CARTESIAN_POINT('Origin',(-62.4786179998484,-0.317499999977906,
3.11913648178393));
#247083=CARTESIAN_POINT('Origin',(-62.6567671111299,-0.31749999999981,2.8340419886026));
#247084=CARTESIAN_POINT('Origin',(-60.4497583458792,-0.317499999992805,
3.56563113460798));
#247085=CARTESIAN_POINT('Origin',(-60.4050521322801,-0.317550804320556,
3.64299171721764));
#247086=CARTESIAN_POINT('Ctrl Pts',(-62.9541448057648,-0.0152661173106757,
2.59908173516023));
#247087=CARTESIAN_POINT('Ctrl Pts',(-62.9168399481843,-0.0152570710384434,
2.65878198860261));
#247088=CARTESIAN_POINT('Ctrl Pts',(-62.8464427007196,-0.0152399999998093,
2.65878198860261));
#247089=CARTESIAN_POINT('Ctrl Pts',(-62.9541233134298,-0.103381504925207,
2.59908193475622));
#247090=CARTESIAN_POINT('Ctrl Pts',(-62.9168211560341,-0.0794415635235094,
2.65878715325368));
#247091=CARTESIAN_POINT('Ctrl Pts',(-62.8464212442881,-0.0662446030558591,
2.65878198860261));
#247092=CARTESIAN_POINT('Ctrl Pts',(-62.9290872705828,-0.184683583687337,
2.63878778849871));
#247093=CARTESIAN_POINT('Ctrl Pts',(-62.8936771137448,-0.138547994783951,
2.69564460180094));
#247094=CARTESIAN_POINT('Ctrl Pts',(-62.8213855864655,-0.113305567451219,
2.68180481624873));
#247095=CARTESIAN_POINT('Ctrl Pts',(-62.8564203507741,-0.291340992631772,
2.75443238878643));
#247096=CARTESIAN_POINT('Ctrl Pts',(-62.8329175802742,-0.201910351191337,
2.79268340777113));
#247097=CARTESIAN_POINT('Ctrl Pts',(-62.7487193609389,-0.175042741957798,
2.74885926835618));
#247098=CARTESIAN_POINT('Ctrl Pts',(-62.8099434033762,-0.318045276842425,
2.82856655361668));
#247099=CARTESIAN_POINT('Ctrl Pts',(-62.7947175425039,-0.205831635642229,
2.8538419723101));
#247100=CARTESIAN_POINT('Ctrl Pts',(-62.7022409210457,-0.190499999999808,
2.79184624278614));
#247101=CARTESIAN_POINT('Ctrl Pts',(-62.7644678366119,-0.318045750792856,
2.90134173516021));
#247102=CARTESIAN_POINT('Ctrl Pts',(-62.7649326510149,-0.190499999999814,
2.90163218716389));
#247103=CARTESIAN_POINT('Ctrl Pts',(-62.6567671111299,-0.190499999999811,
2.8340419886026));
#247104=CARTESIAN_POINT('Origin',(5.50819412990574E-15,-0.317499999999816,
3.64303198860262));
#247105=CARTESIAN_POINT('Origin',(-60.003690522373,-0.317499999999816,3.64303198860261));
#247106=CARTESIAN_POINT('Ctrl Pts',(-60.003690522373,-0.317499999999817,
3.77003198860262));
#247107=CARTESIAN_POINT('Ctrl Pts',(-60.003690522373,-0.190309748265136,
3.77003198860262));
#247108=CARTESIAN_POINT('Ctrl Pts',(-60.003690522373,-0.190500142289345,
3.64284187937063));
#247109=CARTESIAN_POINT('Ctrl Pts',(-59.7867137603524,-0.317270385524247,
3.77003198860262));
#247110=CARTESIAN_POINT('Ctrl Pts',(-59.7869045527985,-0.19031026247621,
3.76980208962919));
#247111=CARTESIAN_POINT('Ctrl Pts',(-59.8301727552496,-0.190500142032278,
3.64284193928308));
#247112=CARTESIAN_POINT('Ctrl Pts',(-59.5801552670728,-0.317049440713426,
3.65553535416585));
#247113=CARTESIAN_POINT('Ctrl Pts',(-59.5804765271849,-0.19031076108168,
3.65520057834448));
#247114=CARTESIAN_POINT('Ctrl Pts',(-59.6649871046547,-0.190500141784922,
3.55127910964229));
#247115=CARTESIAN_POINT('Ctrl Pts',(-59.4651754363832,-0.316925998272862,
3.47153072139072));
#247116=CARTESIAN_POINT('Ctrl Pts',(-59.4656607446594,-0.190311035334875,
3.47122746281582));
#247117=CARTESIAN_POINT('Ctrl Pts',(-59.5730368716575,-0.190500141646717,
3.40413045901282));
#247118=CARTESIAN_POINT('Origin',(-59.5728760150042,-0.317499999999815,
3.40423097483309));
#247119=CARTESIAN_POINT('Ctrl Pts',(-62.7644678366119,0.318045750793234,
2.90134173516022));
#247120=CARTESIAN_POINT('Ctrl Pts',(-62.7649326510149,0.190500000000189,
2.9016321871639));
#247121=CARTESIAN_POINT('Ctrl Pts',(-62.6567671111299,0.190500000000189,
2.83404198860261));
#247122=CARTESIAN_POINT('Ctrl Pts',(-62.8099640589334,0.318045262795371,
2.8285334983536));
#247123=CARTESIAN_POINT('Ctrl Pts',(-62.7947344577641,0.205840330723214,
2.85381483162463));
#247124=CARTESIAN_POINT('Ctrl Pts',(-62.7022616416344,0.19050000000019,
2.7918270159431));
#247125=CARTESIAN_POINT('Ctrl Pts',(-62.8562601188215,0.291334117855617,
2.75468822073633));
#247126=CARTESIAN_POINT('Ctrl Pts',(-62.8328016940824,0.201836550627952,
2.79286913083856));
#247127=CARTESIAN_POINT('Ctrl Pts',(-62.7485591297232,0.175038734052367,
2.74900763297916));
#247128=CARTESIAN_POINT('Ctrl Pts',(-62.928611257107,0.185622189560568,
2.63954450640401));
#247129=CARTESIAN_POINT('Ctrl Pts',(-62.8932808767899,0.139140156000274,
2.69627684028842));
#247130=CARTESIAN_POINT('Ctrl Pts',(-62.8209095783125,0.113848895265888,
2.68224356036486));
#247131=CARTESIAN_POINT('Ctrl Pts',(-62.9541233349672,0.103673266463023,
2.59908178706383));
#247132=CARTESIAN_POINT('Ctrl Pts',(-62.9168211653022,0.0796882264538794,
2.65878704321555));
#247133=CARTESIAN_POINT('Ctrl Pts',(-62.8464212664863,0.0664134143653284,
2.6587819886026));
#247134=CARTESIAN_POINT('Ctrl Pts',(-62.9541448057648,0.0152661173110572,
2.59908173516022));
#247135=CARTESIAN_POINT('Ctrl Pts',(-62.9168399481843,0.0152570710388243,
2.6587819886026));
#247136=CARTESIAN_POINT('Ctrl Pts',(-62.8464427007196,0.0152400000001903,
2.6587819886026));
#247137=CARTESIAN_POINT('Origin',(-62.6567671111299,0.317500000000189,2.83404198860261));
#247138=CARTESIAN_POINT('Origin',(-59.3947266586247,-0.317499999970537,
3.11913648167064));
#247139=CARTESIAN_POINT('Origin',(-59.2165773020941,-0.31749999999981,2.83404198860261));
#247140=CARTESIAN_POINT('Origin',(-62.4786179998343,0.317499999978364,3.11913648177509));
#247141=CARTESIAN_POINT('Origin',(-62.3004688883554,0.317500000000185,3.40423097483309));
#247142=CARTESIAN_POINT('Ctrl Pts',(-59.1088767419348,-0.3169225446755,
2.90134173516022));
#247143=CARTESIAN_POINT('Ctrl Pts',(-59.1093642282366,-0.190499999999805,
2.90103711553229));
#247144=CARTESIAN_POINT('Ctrl Pts',(-59.2165773020941,-0.190499999999811,
2.83404198860261));
#247145=CARTESIAN_POINT('Ctrl Pts',(-59.0634407053229,-0.316922012808971,
2.82862991747963));
#247146=CARTESIAN_POINT('Ctrl Pts',(-59.0793536643041,-0.205694973741207,
2.85314045886453));
#247147=CARTESIAN_POINT('Ctrl Pts',(-59.1711393827293,-0.19049999999981,
2.79187960999928));
#247148=CARTESIAN_POINT('Ctrl Pts',(-59.0174076205275,-0.290332993454825,
2.75470625793324));
#247149=CARTESIAN_POINT('Ctrl Pts',(-59.0412846811395,-0.201480151665693,
2.79224250381906));
#247150=CARTESIAN_POINT('Ctrl Pts',(-59.1251084688121,-0.175054909459551,
2.74901809108263));
#247151=CARTESIAN_POINT('Ctrl Pts',(-58.9458296250063,-0.184894967401365,
2.63947868311699));
#247152=CARTESIAN_POINT('Ctrl Pts',(-58.9812445774292,-0.138672156931012,
2.69595066767904));
#247153=CARTESIAN_POINT('Ctrl Pts',(-59.0535312451933,-0.113807322597554,
2.68220539436056));
#247154=CARTESIAN_POINT('Ctrl Pts',(-58.9208287018092,-0.103171606455547,
2.59908178585108));
#247155=CARTESIAN_POINT('Ctrl Pts',(-58.9581363848291,-0.0793367652456228,
2.65877670944851));
#247156=CARTESIAN_POINT('Ctrl Pts',(-59.0285307646525,-0.0663350652341827,
2.65878198860261));
#247157=CARTESIAN_POINT('Ctrl Pts',(-58.9208513795073,-0.0152121934557294,
2.59908173516023));
#247158=CARTESIAN_POINT('Ctrl Pts',(-58.9581562369413,-0.0152218248289167,
2.65878198860261));
#247159=CARTESIAN_POINT('Ctrl Pts',(-59.0285534841296,-0.0152399999998097,
2.65878198860261));
#247160=CARTESIAN_POINT('Ctrl Pts',(-61.8696548221181,0.317500000000183,
3.77003198860263));
#247161=CARTESIAN_POINT('Ctrl Pts',(-61.8696548221181,0.19031025693173,
3.77003198860263));
#247162=CARTESIAN_POINT('Ctrl Pts',(-61.8696548221181,0.190500141530432,
3.64284238727587));
#247163=CARTESIAN_POINT('Ctrl Pts',(-62.086631532412,0.317722689632413,
3.77003198860263));
#247164=CARTESIAN_POINT('Ctrl Pts',(-62.0868176889521,0.190309758575909,
3.77025506105731));
#247165=CARTESIAN_POINT('Ctrl Pts',(-62.0431722165663,0.190500141778416,
3.64284210641793));
#247166=CARTESIAN_POINT('Ctrl Pts',(-62.2931898887681,0.317932491655863,
3.65553527987828));
#247167=CARTESIAN_POINT('Ctrl Pts',(-62.2934992458064,0.190309283350215,
3.65585996533176));
#247168=CARTESIAN_POINT('Ctrl Pts',(-62.2083577878509,0.190500142012043,
3.55127902710248));
#247169=CARTESIAN_POINT('Ctrl Pts',(-62.4081695979768,0.318048871877314,
3.47153072139072));
#247170=CARTESIAN_POINT('Ctrl Pts',(-62.4086377820239,0.190309023146808,
3.47182327905188));
#247171=CARTESIAN_POINT('Ctrl Pts',(-62.3003077510786,0.190500142141644,
3.40413028377981));
#247172=CARTESIAN_POINT('Origin',(-61.8696548221181,0.317500000000184,3.64303198860263));
#247173=CARTESIAN_POINT('Origin',(62.2224557307631,0.317500000000184,3.64303198860263));
#247174=CARTESIAN_POINT('Origin',(-61.4683012396086,0.317551690015293,3.64299466007411));
#247175=CARTESIAN_POINT('Ctrl Pts',(-58.9208513795073,0.015212193456111,
2.59908173516023));
#247176=CARTESIAN_POINT('Ctrl Pts',(-58.9581562369413,0.0152218248292975,
2.65878198860261));
#247177=CARTESIAN_POINT('Ctrl Pts',(-59.0285534841296,0.0152400000001907,
2.65878198860261));
#247178=CARTESIAN_POINT('Ctrl Pts',(-58.9208288705614,0.102871702177517,
2.59908193199826));
#247179=CARTESIAN_POINT('Ctrl Pts',(-58.9581365422946,0.0790852439334556,
2.65877685806665));
#247180=CARTESIAN_POINT('Ctrl Pts',(-59.0285309330208,0.0661608181926717,
2.65878198860261));
#247181=CARTESIAN_POINT('Ctrl Pts',(-58.9453619764183,0.183955833237801,
2.63872492669805));
#247182=CARTESIAN_POINT('Ctrl Pts',(-58.9808530699758,0.138075936736365,
2.69532212015272));
#247183=CARTESIAN_POINT('Ctrl Pts',(-59.0530636028226,0.113261762368398,
2.6817683672664));
#247184=CARTESIAN_POINT('Ctrl Pts',(-59.0172303255293,0.290319860890742,
2.7544217640224));
#247185=CARTESIAN_POINT('Ctrl Pts',(-59.0411528690725,0.201541405841922,
2.79203179920141));
#247186=CARTESIAN_POINT('Ctrl Pts',(-59.1249311745757,0.175047309551329,
2.74885310748167));
#247187=CARTESIAN_POINT('Ctrl Pts',(-59.0634600627912,0.316922027357541,
2.82866089558407));
#247188=CARTESIAN_POINT('Ctrl Pts',(-59.0793694364673,0.205687000366578,
2.85316563119202));
#247189=CARTESIAN_POINT('Ctrl Pts',(-59.1711586818655,0.190500000000188,
2.79189751796659));
#247190=CARTESIAN_POINT('Ctrl Pts',(-59.1088767419348,0.316922544675878,
2.90134173516021));
#247191=CARTESIAN_POINT('Ctrl Pts',(-59.1093642282366,0.190500000000191,
2.90103711553228));
#247192=CARTESIAN_POINT('Ctrl Pts',(-59.2165773020941,0.190500000000189,
2.8340419886026));
#247193=CARTESIAN_POINT('Origin',(-59.2165773020941,0.317500000000189,2.83404198860261));
#247194=CARTESIAN_POINT('Origin',(-61.4240753793289,0.317499999995613,3.56647653971782));
#247195=CARTESIAN_POINT('Origin',(-61.3422370451705,0.317500000000185,3.42473028058485));
#247196=CARTESIAN_POINT('Origin',(-59.3947266586075,0.317499999970762,3.11913648168139));
#247197=CARTESIAN_POINT('Origin',(-59.5728760150042,0.317500000000185,3.4042309748331));
#247198=CARTESIAN_POINT('Ctrl Pts',(-61.0122769227456,0.317500000000186,
3.36123028058481));
#247199=CARTESIAN_POINT('Ctrl Pts',(-61.0122769227456,0.190500000000186,
3.36123028058481));
#247200=CARTESIAN_POINT('Ctrl Pts',(-61.0122769227456,0.190500000000187,
3.23423028058481));
#247201=CARTESIAN_POINT('Ctrl Pts',(-61.1022873990971,0.317265808076579,
3.36123028058481));
#247202=CARTESIAN_POINT('Ctrl Pts',(-61.1022028716701,0.190500000000177,
3.36099641108414));
#247203=CARTESIAN_POINT('Ctrl Pts',(-61.1472909869831,0.190500000000187,
3.23423043688322));
#247204=CARTESIAN_POINT('Ctrl Pts',(-61.1873990841185,0.317046189129288,
3.41054258905284));
#247205=CARTESIAN_POINT('Ctrl Pts',(-61.1876587562329,0.190500000000658,
3.41008815826044));
#247206=CARTESIAN_POINT('Ctrl Pts',(-61.2749563897845,0.190500000000186,
3.30819867304323));
#247207=CARTESIAN_POINT('Ctrl Pts',(-61.2322532920972,0.316930737396099,
3.48823028058483));
#247208=CARTESIAN_POINT('Ctrl Pts',(-61.2327440814645,0.190500000000185,
3.48794691941599));
#247209=CARTESIAN_POINT('Ctrl Pts',(-61.3422370451705,0.190500000000185,
3.42473028058484));
#247210=CARTESIAN_POINT('Origin',(-61.0122769227456,0.317500000000187,3.23423028058481));
#247211=CARTESIAN_POINT('Ctrl Pts',(-59.4651754363832,0.316925998273232,
3.47153072139073));
#247212=CARTESIAN_POINT('Ctrl Pts',(-59.4656607446034,0.190311049925318,
3.47122746285077));
#247213=CARTESIAN_POINT('Ctrl Pts',(-59.573036859247,0.190500141625231,
3.40413046676793));
#247214=CARTESIAN_POINT('Ctrl Pts',(-59.5801570044831,0.317049442579369,
3.65553813457986));
#247215=CARTESIAN_POINT('Ctrl Pts',(-59.580478263487,0.190310775687526,
3.65520336072214));
#247216=CARTESIAN_POINT('Ctrl Pts',(-59.6649884842716,0.190500141763417,
3.55128134519983));
#247217=CARTESIAN_POINT('Ctrl Pts',(-59.7867171285936,0.317270389089027,
3.77003198860263));
#247218=CARTESIAN_POINT('Ctrl Pts',(-59.7869079131821,0.190310277118411,
3.76980209314073));
#247219=CARTESIAN_POINT('Ctrl Pts',(-59.8301754438925,0.190500142010734,
3.64284195387335));
#247220=CARTESIAN_POINT('Ctrl Pts',(-60.003690522373,0.317500000000183,
3.77003198860263));
#247221=CARTESIAN_POINT('Ctrl Pts',(-60.003690522373,0.190309762955,3.77003198860263));
#247222=CARTESIAN_POINT('Ctrl Pts',(-60.003690522373,0.190500142267757,
3.64284189403812));
#247223=CARTESIAN_POINT('Origin',(-60.0036905223731,0.317500000000184,3.64303198860262));
#247224=CARTESIAN_POINT('Origin',(60.71525,0.317500000000187,3.23423028058482));
#247225=CARTESIAN_POINT('Origin',(-60.8610688070707,0.317500000000187,3.23423028058481));
#247226=CARTESIAN_POINT('Origin',(60.4792282238308,0.317500000000184,3.64303198860263));
#247227=CARTESIAN_POINT('Origin',(-60.4050521322799,0.317550804321294,3.64299171721729));
#247228=CARTESIAN_POINT('Ctrl Pts',(-60.6410923272405,0.318076890623551,
3.4882302805848));
#247229=CARTESIAN_POINT('Ctrl Pts',(-60.6415942020421,0.190500000000185,
3.48852004212258));
#247230=CARTESIAN_POINT('Ctrl Pts',(-60.5311086139134,0.190500000000185,
3.4247302805848));
#247231=CARTESIAN_POINT('Ctrl Pts',(-60.6860981505083,0.317958218318944,
3.41028005848407));
#247232=CARTESIAN_POINT('Ctrl Pts',(-60.68636137503,0.19049999999811,3.41074404220421));
#247233=CARTESIAN_POINT('Ctrl Pts',(-60.5986166446967,0.190500000000186,
3.30780486243976));
#247234=CARTESIAN_POINT('Ctrl Pts',(-60.771361502534,0.317733982967741,
3.36123028058481));
#247235=CARTESIAN_POINT('Ctrl Pts',(-60.7712750141981,0.190500000000186,
3.36146460586327));
#247236=CARTESIAN_POINT('Ctrl Pts',(-60.7265095085042,0.190500000000187,
3.2342304530835));
#247237=CARTESIAN_POINT('Ctrl Pts',(-60.8610688070707,0.317500000000186,
3.36123028058481));
#247238=CARTESIAN_POINT('Ctrl Pts',(-60.8610688070707,0.190500000000186,
3.36123028058481));
#247239=CARTESIAN_POINT('Ctrl Pts',(-60.8610688070707,0.190500000000187,
3.23423028058481));
#247240=CARTESIAN_POINT('Origin',(-60.5311086139135,0.317500000000185,3.4247302805848));
#247241=CARTESIAN_POINT('Origin',(-60.4497583469882,0.317500000300915,3.56563113524826));
#247242=CARTESIAN_POINT('Origin',(-61.0544000815108,-6.73632490863893,3.56647653909441));
#247243=CARTESIAN_POINT('Origin',(-61.0983782637178,-6.74099917688073,3.64299466007533));
#247244=CARTESIAN_POINT('Origin',(-60.9730100652054,-6.72777047351147,3.42473028058479));
#247245=CARTESIAN_POINT('Ctrl Pts',(-60.8636883187844,-6.71570789669434,
3.48823028058478));
#247246=CARTESIAN_POINT('Ctrl Pts',(-60.877392030246,-6.59002106156489,
3.48794691941594));
#247247=CARTESIAN_POINT('Ctrl Pts',(-60.9862851800404,-6.60146619279971,
3.42473028058479));
#247248=CARTESIAN_POINT('Ctrl Pts',(-60.8189169727308,-6.71111871849892,
3.41028005925082));
#247249=CARTESIAN_POINT('Ctrl Pts',(-60.8324022194101,-6.58529244190266,
3.40982512231079));
#247250=CARTESIAN_POINT('Ctrl Pts',(-60.9191469903169,-6.5944096847117,
3.30780486372924));
#247251=CARTESIAN_POINT('Ctrl Pts',(-60.7340977611528,-6.70242508976285,
3.36123028058476));
#247252=CARTESIAN_POINT('Ctrl Pts',(-60.7472645033911,-6.57634410736815,
3.36099721048396));
#247253=CARTESIAN_POINT('Ctrl Pts',(-60.7919547682784,-6.58104124348259,
3.23423045308317));
#247254=CARTESIAN_POINT('Ctrl Pts',(-60.6448574988554,-6.69328024897479,
3.36123028058476));
#247255=CARTESIAN_POINT('Ctrl Pts',(-60.6581326136904,-6.56697596826302,
3.36123028058476));
#247256=CARTESIAN_POINT('Ctrl Pts',(-60.6581326136904,-6.56697596826301,
3.23423028058476));
#247257=CARTESIAN_POINT('Origin',(-60.6448574988554,-6.69328024897478,3.23423028058476));
#247258=CARTESIAN_POINT('Origin',(0.0331877870874877,-0.315760701779243,
3.64303198860262));
#247259=CARTESIAN_POINT('Origin',(-61.4975385923862,-6.78290064323585,3.64303198860257));
#247260=CARTESIAN_POINT('Origin',(0.0331877870874878,-0.31576070177924,
3.23423028058481));
#247261=CARTESIAN_POINT('Origin',(-60.4944777170593,-6.67747469700969,3.23423028058476));
#247262=CARTESIAN_POINT('Ctrl Pts',(-62.0330459552232,-6.83973663030285,
3.47153072139065));
#247263=CARTESIAN_POINT('Ctrl Pts',(-62.0468640234019,-6.71274550335289,
3.47182327902656));
#247264=CARTESIAN_POINT('Ctrl Pts',(-61.9391074687688,-6.70161199370852,
3.40413028959046));
#247265=CARTESIAN_POINT('Ctrl Pts',(-61.9187065474464,-6.82760205123647,
3.65553807120948));
#247266=CARTESIAN_POINT('Ctrl Pts',(-61.9323544653005,-6.70071032544166,
3.65586275496829));
#247267=CARTESIAN_POINT('Ctrl Pts',(-61.8476598278987,-6.69200045921773,
3.55128126837219));
#247268=CARTESIAN_POINT('Ctrl Pts',(-61.7133000470646,-6.80580199871468,
3.77003198860258));
#247269=CARTESIAN_POINT('Ctrl Pts',(-61.7268034525382,-6.67910652125862,
3.77025505748531));
#247270=CARTESIAN_POINT('Ctrl Pts',(-61.683377859153,-6.67473372828988,
3.6428421173117));
#247271=CARTESIAN_POINT('Ctrl Pts',(-61.4975385923862,-6.78290064323585,
3.77003198860258));
#247272=CARTESIAN_POINT('Ctrl Pts',(-61.5108335396271,-6.65640766978592,
3.77003198860258));
#247273=CARTESIAN_POINT('Ctrl Pts',(-61.5108136924289,-6.65659650326277,
3.64284239821739));
#247274=CARTESIAN_POINT('Origin',(-61.9259926140919,-6.82793297553373,3.40423097483304));
#247275=CARTESIAN_POINT('Ctrl Pts',(-60.4944777170593,-6.67747469700969,
3.36123028058476));
#247276=CARTESIAN_POINT('Ctrl Pts',(-60.5077528318943,-6.55117041629792,
3.36123028058476));
#247277=CARTESIAN_POINT('Ctrl Pts',(-60.5077528318943,-6.55117041629792,
3.23423028058476));
#247278=CARTESIAN_POINT('Ctrl Pts',(-60.404935774755,-6.6682995265994,3.36123028058476));
#247279=CARTESIAN_POINT('Ctrl Pts',(-60.4181493202581,-6.54175270773036,
3.36146538610052));
#247280=CARTESIAN_POINT('Ctrl Pts',(-60.3734783767987,-6.53705760237938,
3.23423043688339));
#247281=CARTESIAN_POINT('Ctrl Pts',(-60.3202668847282,-6.65962554481726,
3.41054258693096));
#247282=CARTESIAN_POINT('Ctrl Pts',(-60.333852472873,-6.53289275204893,
3.41100608859807));
#247283=CARTESIAN_POINT('Ctrl Pts',(-60.2465123062101,-6.52371293062548,
3.30819866970814));
#247284=CARTESIAN_POINT('Ctrl Pts',(-60.2756459899118,-6.65505462397419,
3.48823028058475));
#247285=CARTESIAN_POINT('Ctrl Pts',(-60.2894805317161,-6.52822907310801,
3.48852004212253));
#247286=CARTESIAN_POINT('Ctrl Pts',(-60.1796001951995,-6.51668018436769,
3.42473028058475));
#247287=CARTESIAN_POINT('Origin',(-60.1663250803645,-6.64298446507947,3.42473028058476));
#247288=CARTESIAN_POINT('Origin',(-62.1031658061158,-6.84655462836542,3.11913648178459));
#247289=CARTESIAN_POINT('Origin',(-62.2803389979219,-6.86517628122534,2.83404198860255));
#247290=CARTESIAN_POINT('Origin',(-60.0854204576107,-6.63448104656949,3.56563113460775));
#247291=CARTESIAN_POINT('Origin',(-60.0409538388298,-6.62985850077836,3.642991717218));
#247292=CARTESIAN_POINT('Ctrl Pts',(-62.6076796697354,-6.5956825007991,
2.59908173516018));
#247293=CARTESIAN_POINT('Ctrl Pts',(-62.5705801176609,-6.59177408464798,
2.65878198860256));
#247294=CARTESIAN_POINT('Ctrl Pts',(-62.500570298093,-6.58439859103053,
2.65878198860256));
#247295=CARTESIAN_POINT('Ctrl Pts',(-62.5984477290795,-6.68331293653973,
2.59908193475685));
#247296=CARTESIAN_POINT('Ctrl Pts',(-62.5638523220891,-6.65560500345264,
2.65878715325316));
#247297=CARTESIAN_POINT('Ctrl Pts',(-62.495217526425,-6.63512154272647,
2.65878198860256));
#247298=CARTESIAN_POINT('Ctrl Pts',(-62.5650504549418,-6.76155265492275,
2.63878778849855));
#247299=CARTESIAN_POINT('Ctrl Pts',(-62.5346567608586,-6.71196843232427,
2.69564460180106));
#247300=CARTESIAN_POINT('Ctrl Pts',(-62.4653998062675,-6.67930776339584,
2.68180481624875));
#247301=CARTESIAN_POINT('Ctrl Pts',(-62.4816328770699,-6.86003002196304,
2.75443238878649));
#247302=CARTESIAN_POINT('Ctrl Pts',(-62.4676069047243,-6.76863258245081,
2.79268340777087));
#247303=CARTESIAN_POINT('Ctrl Pts',(-62.3866783619495,-6.73311104631488,
2.74885926835607));
#247304=CARTESIAN_POINT('Ctrl Pts',(-62.4326191774618,-6.88172985342201,
2.82856655361655));
#247305=CARTESIAN_POINT('Ctrl Pts',(-62.4292062449166,-6.7685393944507,
2.85384197230759));
#247306=CARTESIAN_POINT('Ctrl Pts',(-62.3388388123826,-6.74362530798286,
2.79184624278463));
#247307=CARTESIAN_POINT('Ctrl Pts',(-62.3873926810691,-6.87697683366589,
2.90134173516017));
#247308=CARTESIAN_POINT('Ctrl Pts',(-62.4011871104968,-6.75017837817627,
2.90163218716385));
#247309=CARTESIAN_POINT('Ctrl Pts',(-62.2936141127569,-6.73887200051357,
2.83404198860256));
#247310=CARTESIAN_POINT('Origin',(-62.500570298093,-6.58439859103053,2.53178198860256));
#247311=CARTESIAN_POINT('Origin',(0.0331877870874877,-0.315760701779243,
3.64303198860262));
#247312=CARTESIAN_POINT('Origin',(-59.6417962403142,-6.58785426247119,3.64303198860257));
#247313=CARTESIAN_POINT('Origin',(1.33778643725275E-16,1.9159467040135E-13,
2.53178198860262));
#247314=CARTESIAN_POINT('Origin',(-62.5037563256534,-6.5540855636597,2.53178198860256));
#247315=CARTESIAN_POINT('Ctrl Pts',(-59.6417962403142,-6.58785426247119,
3.77003198860258));
#247316=CARTESIAN_POINT('Ctrl Pts',(-59.6550912418707,-6.46136077224357,
3.77003198860258));
#247317=CARTESIAN_POINT('Ctrl Pts',(-59.6550713402759,-6.46155012326947,
3.64284187937051));
#247318=CARTESIAN_POINT('Ctrl Pts',(-59.4260321009468,-6.56494565834898,
3.77003198860258));
#247319=CARTESIAN_POINT('Ctrl Pts',(-59.4394927947708,-6.43870097938016,
3.76980208962867));
#247320=CARTESIAN_POINT('Ctrl Pts',(-59.4825041216629,-6.44341257746673,
3.6428419392824));
#247321=CARTESIAN_POINT('Ctrl Pts',(-59.2206282517276,-6.54313468201961,
3.65553535416582));
#247322=CARTESIAN_POINT('Ctrl Pts',(-59.2341955513614,-6.41712387095958,
3.65520057834495));
#247323=CARTESIAN_POINT('Ctrl Pts',(-59.3182233753721,-6.42614597501026,
3.55127910964254));
#247324=CARTESIAN_POINT('Ctrl Pts',(-59.1062911958296,-6.53099325080078,
3.47153072139067));
#247325=CARTESIAN_POINT('Ctrl Pts',(-59.1200087130388,-6.40512262640595,
3.47122746281577));
#247326=CARTESIAN_POINT('Ctrl Pts',(-59.2267768553863,-6.41653455832047,
3.40413045901273));
#247327=CARTESIAN_POINT('Origin',(-59.2133417798936,-6.5428218840625,3.40423097483305));
#247328=CARTESIAN_POINT('Ctrl Pts',(-62.4538823482275,-6.24436990788084,
2.90134173516018));
#247329=CARTESIAN_POINT('Ctrl Pts',(-62.4410124550018,-6.37126553604095,
2.90163218716386));
#247330=CARTESIAN_POINT('Ctrl Pts',(-62.3334394572618,-6.35995915837826,
2.83404198860256));
#247331=CARTESIAN_POINT('Ctrl Pts',(-62.4991292864732,-6.2491260434095,
2.82853349835336));
#247332=CARTESIAN_POINT('Ctrl Pts',(-62.4722545055301,-6.3591243783159,
2.853814831623));
#247333=CARTESIAN_POINT('Ctrl Pts',(-62.378684763968,-6.36471463173897,
2.79182701594267));
#247334=CARTESIAN_POINT('Ctrl Pts',(-62.5423796567682,-6.28053011789769,
2.75468822073656));
#247335=CARTESIAN_POINT('Ctrl Pts',(-62.5096946965644,-6.3670853349991,
2.79286913083837));
#247336=CARTESIAN_POINT('Ctrl Pts',(-62.4231124872028,-6.38493060453731,
2.74900763297902));
#247337=CARTESIAN_POINT('Ctrl Pts',(-62.6032845425346,-6.39322569848907,
2.63954450640367));
#247338=CARTESIAN_POINT('Ctrl Pts',(-62.5632890102013,-6.43576006824488,
2.69627684028849));
#247339=CARTESIAN_POINT('Ctrl Pts',(-62.4886705126495,-6.45334792019221,
2.6822435603649));
#247340=CARTESIAN_POINT('Ctrl Pts',(-62.6200908675648,-6.47739243510518,
2.59908178706394));
#247341=CARTESIAN_POINT('Ctrl Pts',(-62.5804859237136,-6.4973469440839,
2.65878704321556));
#247342=CARTESIAN_POINT('Ctrl Pts',(-62.5090840872032,-6.50319024212545,
2.65878198860256));
#247343=CARTESIAN_POINT('Ctrl Pts',(-62.6108711573005,-6.56531752495327,
2.59908173516017));
#247344=CARTESIAN_POINT('Ctrl Pts',(-62.5737697140402,-6.56142710223376,
2.65878198860256));
#247345=CARTESIAN_POINT('Ctrl Pts',(-62.5037563256534,-6.55408556365971,
2.65878198860256));
#247346=CARTESIAN_POINT('Origin',(-62.3467145720969,-6.23365487766649,2.83404198860256));
#247347=CARTESIAN_POINT('Origin',(-59.0361683443312,-6.52420020558021,3.1191364816707));
#247348=CARTESIAN_POINT('Origin',(-58.858994908613,-6.50557852713776,2.83404198860257));
#247349=CARTESIAN_POINT('Origin',(-62.1695413802711,-6.21503322485295,3.11913648177538));
#247350=CARTESIAN_POINT('Origin',(-61.9923681882668,-6.19641157197488,3.40423097483306));
#247351=CARTESIAN_POINT('Ctrl Pts',(-58.7519447039088,-6.49374646112762,
2.90134173516018));
#247352=CARTESIAN_POINT('Ctrl Pts',(-58.765644274027,-6.36806742857347,
2.90103711553224));
#247353=CARTESIAN_POINT('Ctrl Pts',(-58.872270023448,-6.37927424642599,
2.83404198860256));
#247354=CARTESIAN_POINT('Ctrl Pts',(-58.7067576262547,-6.48899657309071,
2.82862991747961));
#247355=CARTESIAN_POINT('Ctrl Pts',(-58.7342098038486,-6.38004220452862,
2.85314045886468));
#247356=CARTESIAN_POINT('Ctrl Pts',(-58.8270810177594,-6.37452469054068,
2.79187960999949));
#247357=CARTESIAN_POINT('Ctrl Pts',(-58.6637560248472,-6.45774144355344,
2.75470625793313));
#247358=CARTESIAN_POINT('Ctrl Pts',(-58.6967899354322,-6.37187117938152,
2.79224250381903));
#247359=CARTESIAN_POINT('Ctrl Pts',(-58.7829167175845,-6.35435266912788,
2.74901809108255));
#247360=CARTESIAN_POINT('Ctrl Pts',(-58.6035914159081,-6.34539908016337,
2.63947868311702));
#247361=CARTESIAN_POINT('Ctrl Pts',(-58.6436439608623,-6.30313135363866,
2.69595066767901));
#247362=CARTESIAN_POINT('Ctrl Pts',(-58.7181337176194,-6.28595874576537,
2.68220539436055));
#247363=CARTESIAN_POINT('Ctrl Pts',(-58.587269867717,-6.2615101002575,2.59908178585113));
#247364=CARTESIAN_POINT('Ctrl Pts',(-58.626864594668,-6.24170554357555,
2.65877670944858));
#247365=CARTESIAN_POINT('Ctrl Pts',(-58.6982323944353,-6.23613328458285,
2.65878198860256));
#247366=CARTESIAN_POINT('Ctrl Pts',(-58.596486683455,-6.17403490859042,
2.59908173516018));
#247367=CARTESIAN_POINT('Ctrl Pts',(-58.6335861742241,-6.17794390662193,
2.65878198860256));
#247368=CARTESIAN_POINT('Ctrl Pts',(-58.7035958781038,-6.1853204982942,
2.65878198860256));
#247369=CARTESIAN_POINT('Origin',(-58.7035958781038,-6.1853204982942,2.53178198860256));
#247370=CARTESIAN_POINT('Ctrl Pts',(-61.5639141665611,-6.151379239677,3.77003198860258));
#247371=CARTESIAN_POINT('Ctrl Pts',(-61.5506192181748,-6.27787222402455,
3.77003198860258));
#247372=CARTESIAN_POINT('Ctrl Pts',(-61.5506390665201,-6.27768337963384,
3.64284238727612));
#247373=CARTESIAN_POINT('Ctrl Pts',(-61.7797255331385,-6.17383801205345,
3.77003198860258));
#247374=CARTESIAN_POINT('Ctrl Pts',(-61.7665923920122,-6.30057242039938,
3.7702550610584));
#247375=CARTESIAN_POINT('Ctrl Pts',(-61.7232059145542,-6.29582088597933,
3.64284210641908));
#247376=CARTESIAN_POINT('Ctrl Pts',(-61.985174271489,-6.19522058691269,
3.65553527987829));
#247377=CARTESIAN_POINT('Ctrl Pts',(-61.9721416759926,-6.32217699854317,
3.65585996532999));
#247378=CARTESIAN_POINT('Ctrl Pts',(-61.8874865820152,-6.31308747966684,
3.55127902710126));
#247379=CARTESIAN_POINT('Ctrl Pts',(-62.0995362748658,-6.20712349654488,
3.47153072139067));
#247380=CARTESIAN_POINT('Ctrl Pts',(-62.0866494440659,-6.33421251157708,
3.47182327905183));
#247381=CARTESIAN_POINT('Ctrl Pts',(-61.97893283374,-6.32269886789197,3.40413028377992));
#247382=CARTESIAN_POINT('Origin',(-61.5639141665611,-6.151379239677,3.64303198860258));
#247383=CARTESIAN_POINT('Origin',(3.53633106925806E-16,1.91571303393729E-13,
2.53178198860262));
#247384=CARTESIAN_POINT('Origin',(-58.7067819056642,-6.15500747092338,2.53178198860257));
#247385=CARTESIAN_POINT('Origin',(61.5094129706996,6.78414869068811,3.64303198860268));
#247386=CARTESIAN_POINT('Origin',(-61.1647646440478,-6.10937495961993,3.64299466007541));
#247387=CARTESIAN_POINT('Ctrl Pts',(-58.5996668978648,-6.14377718965343,
2.59908173516018));
#247388=CARTESIAN_POINT('Ctrl Pts',(-58.6367684021392,-6.14766703046192,
2.65878198860256));
#247389=CARTESIAN_POINT('Ctrl Pts',(-58.7067819056642,-6.15500747092338,
2.65878198860256));
#247390=CARTESIAN_POINT('Ctrl Pts',(-58.6088074259633,-6.05659553606725,
2.59908193199915));
#247391=CARTESIAN_POINT('Ctrl Pts',(-58.6434243604382,-6.08415140319828,
2.65877685806559));
#247392=CARTESIAN_POINT('Ctrl Pts',(-58.7120821529692,-6.10436324506838,
2.65878198860257));
#247393=CARTESIAN_POINT('Ctrl Pts',(-58.6416817365139,-5.97852000021539,
2.638724926698));
#247394=CARTESIAN_POINT('Ctrl Pts',(-58.672182651072,-6.02785839131278,
2.69532212015275));
#247395=CARTESIAN_POINT('Ctrl Pts',(-58.7414038195498,-6.06008468706717,
2.6817683672663));
#247396=CARTESIAN_POINT('Ctrl Pts',(-58.7242744516463,-5.88025093392494,
2.75442176402237));
#247397=CARTESIAN_POINT('Ctrl Pts',(-58.7387860695143,-5.97104363802175,
2.79203179920121));
#247398=CARTESIAN_POINT('Ctrl Pts',(-58.819336041524,-6.00614981441041,
2.74885310748169));
#247399=CARTESIAN_POINT('Ctrl Pts',(-58.7730316211507,-5.85862682030298,
2.82866089558398));
#247400=CARTESIAN_POINT('Ctrl Pts',(-58.7772266151798,-5.97091547255899,
2.85316563119286));
#247401=CARTESIAN_POINT('Ctrl Pts',(-58.8669255556784,-5.99561386571448,
2.79189751796636));
#247402=CARTESIAN_POINT('Ctrl Pts',(-58.8181995570484,-5.86337364149602,
2.90134173516017));
#247403=CARTESIAN_POINT('Ctrl Pts',(-58.805469618532,-5.98915458643816,
2.90103711553223));
#247404=CARTESIAN_POINT('Ctrl Pts',(-58.9120953679529,-6.00036140429068,
2.83404198860256));
#247405=CARTESIAN_POINT('Origin',(-58.925370482788,-5.87405712357891,2.83404198860256));
#247406=CARTESIAN_POINT('Origin',(-61.1207756545814,-6.1048035052631,3.56647653971749));
#247407=CARTESIAN_POINT('Origin',(-61.0393856393803,-6.09624906995262,3.4247302805848));
#247408=CARTESIAN_POINT('Origin',(-59.1025439184828,-5.89267880207806,3.1191364816815));
#247409=CARTESIAN_POINT('Origin',(-59.2797173540685,-5.91130048050365,3.40423097483305));
#247410=CARTESIAN_POINT('Ctrl Pts',(-60.7112330730303,-6.06175884541593,
3.36123028058477));
#247411=CARTESIAN_POINT('Ctrl Pts',(-60.6979579581953,-6.1880631261277,
3.36123028058476));
#247412=CARTESIAN_POINT('Ctrl Pts',(-60.6979579581953,-6.1880631261277,
3.23423028058476));
#247413=CARTESIAN_POINT('Ctrl Pts',(-60.8007259828525,-6.07140041118295,
3.36123028058477));
#247414=CARTESIAN_POINT('Ctrl Pts',(-60.7873912833613,-6.19746294737669,
3.36099641108453));
#247415=CARTESIAN_POINT('Ctrl Pts',(-60.8322324012612,-6.20217593878186,
3.23423043688326));
#247416=CARTESIAN_POINT('Ctrl Pts',(-60.8853484607269,-6.08051542067575,
3.41054258905279));
#247417=CARTESIAN_POINT('Ctrl Pts',(-60.8723790316499,-6.20639551966844,
3.41008815825962));
#247418=CARTESIAN_POINT('Ctrl Pts',(-60.9591984396306,-6.21552060714939,
3.30819867304277));
#247419=CARTESIAN_POINT('Ctrl Pts',(-60.929944884669,-6.08531878138344,
3.48823028058478));
#247420=CARTESIAN_POINT('Ctrl Pts',(-60.917217374751,-6.21110821942958,
3.48794691941594));
#247421=CARTESIAN_POINT('Ctrl Pts',(-61.0261105245453,-6.22255335066439,
3.42473028058479));
#247422=CARTESIAN_POINT('Origin',(-60.7112330730303,-6.06175884541593,3.23423028058476));
#247423=CARTESIAN_POINT('Ctrl Pts',(-59.1725467709677,-5.90061356181279,
3.47153072139067));
#247424=CARTESIAN_POINT('Ctrl Pts',(-59.1597945546412,-6.02658562874829,
3.47122746285072));
#247425=CARTESIAN_POINT('Ctrl Pts',(-59.2666022171587,-6.03762143316774,
3.40413046676782));
#247426=CARTESIAN_POINT('Ctrl Pts',(-59.2869113614504,-5.91250964036502,
3.65553813457981));
#247427=CARTESIAN_POINT('Ctrl Pts',(-59.2739830624761,-6.03858760028889,
3.65520336072254));
#247428=CARTESIAN_POINT('Ctrl Pts',(-59.3580501215732,-6.04723299508893,
3.55128134519992));
#247429=CARTESIAN_POINT('Ctrl Pts',(-59.4923630227874,-5.9338813165696,
3.77003198860258));
#247430=CARTESIAN_POINT('Ctrl Pts',(-59.4792818168382,-6.06016587018229,
3.76980209314047));
#247431=CARTESIAN_POINT('Ctrl Pts',(-59.522332169774,-6.06449973388429,
3.64284195387353));
#247432=CARTESIAN_POINT('Ctrl Pts',(-59.7081718144892,-5.95633285891234,
3.77003198860258));
#247433=CARTESIAN_POINT('Ctrl Pts',(-59.6948768144682,-6.08282633453096,
3.77003198860258));
#247434=CARTESIAN_POINT('Ctrl Pts',(-59.6948967145252,-6.08263699813589,
3.64284189403797));
#247435=CARTESIAN_POINT('Origin',(-59.7081718144892,-5.95633285891233,3.64303198860258));
#247436=CARTESIAN_POINT('Origin',(60.0186752706391,6.62746584474152,3.23423028058487));
#247437=CARTESIAN_POINT('Origin',(-60.5608532912343,-6.04595329345084,3.23423028058476));
#247438=CARTESIAN_POINT('Origin',(59.785232315514,6.60293000146494,3.64303198860268));
#247439=CARTESIAN_POINT('Origin',(-60.1073400339995,-5.99823604520077,3.64299171721722));
#247440=CARTESIAN_POINT('Ctrl Pts',(-60.3421421670674,-6.02238575970299,
3.48823028058475));
#247441=CARTESIAN_POINT('Ctrl Pts',(-60.3293058762211,-6.1493162309727,
3.48852004212253));
#247442=CARTESIAN_POINT('Ctrl Pts',(-60.2194255397044,-6.13776734223238,
3.42473028058475));
#247443=CARTESIAN_POINT('Ctrl Pts',(-60.3868890390927,-6.02720817145267,
3.41028005848404));
#247444=CARTESIAN_POINT('Ctrl Pts',(-60.373827809955,-6.15399567476977,
3.41074404220476));
#247445=CARTESIAN_POINT('Ctrl Pts',(-60.2865637544338,-6.14482385294861,
3.30780486244026));
#247446=CARTESIAN_POINT('Ctrl Pts',(-60.4716618705781,-6.03634362557944,
3.36123028058477));
#247447=CARTESIAN_POINT('Ctrl Pts',(-60.4582762833165,-6.16287156698251,
3.3614646058637));
#247448=CARTESIAN_POINT('Ctrl Pts',(-60.4137560077479,-6.1581922974649,
3.23423045308351));
#247449=CARTESIAN_POINT('Ctrl Pts',(-60.5608532912343,-6.04595329345084,
3.36123028058477));
#247450=CARTESIAN_POINT('Ctrl Pts',(-60.5475781763993,-6.17225757416261,
3.36123028058476));
#247451=CARTESIAN_POINT('Ctrl Pts',(-60.5475781763993,-6.17225757416261,
3.23423028058476));
#247452=CARTESIAN_POINT('Origin',(-60.2327006545395,-6.01146306152061,3.42473028058475));
#247453=CARTESIAN_POINT('Origin',(-60.1517960329186,-6.00295964283186,3.56563113524748));
#247454=CARTESIAN_POINT('Origin',(-60.0157999988654,-13.0813452322047,3.56647653909434));
#247455=CARTESIAN_POINT('Origin',(-60.0590486699119,-13.0905908661191,3.64299466007557));
#247456=CARTESIAN_POINT('Origin',(-59.9357500275432,-13.0643300858384,3.42473028058474));
#247457=CARTESIAN_POINT('Ctrl Pts',(-59.8282880397054,-13.0409063549241,
3.48823028058474));
#247458=CARTESIAN_POINT('Ctrl Pts',(-59.8550545325308,-12.9173404733285,
3.4879469194159));
#247459=CARTESIAN_POINT('Ctrl Pts',(-59.9621548122771,-12.9401053405452,
3.42473028058475));
#247460=CARTESIAN_POINT('Ctrl Pts',(-59.7842416555145,-13.0316624367252,
3.41028005925074));
#247461=CARTESIAN_POINT('Ctrl Pts',(-59.8108054559345,-12.9079350417482,
3.40982512231036));
#247462=CARTESIAN_POINT('Ctrl Pts',(-59.8961220185277,-12.9260696369484,
3.30780486372917));
#247463=CARTESIAN_POINT('Ctrl Pts',(-59.7007958241042,-13.0141504107553,
3.36123028058472));
#247464=CARTESIAN_POINT('Ctrl Pts',(-59.727069488887,-12.8901364125062,
3.360997210484));
#247465=CARTESIAN_POINT('Ctrl Pts',(-59.7710239514086,-12.89947922193,3.23423045308327));
#247466=CARTESIAN_POINT('Ctrl Pts',(-59.6130003254554,-12.9957275188826,
3.36123028058472));
#247467=CARTESIAN_POINT('Ctrl Pts',(-59.6394051101893,-12.8715027735894,
3.36123028058472));
#247468=CARTESIAN_POINT('Ctrl Pts',(-59.6394051101892,-12.8715027735894,
3.23423028058472));
#247469=CARTESIAN_POINT('Origin',(-59.6130003254554,-12.9957275188826,3.23423028058471));
#247470=CARTESIAN_POINT('Origin',(0.0660119618346463,-0.310561863232799,
3.64303198860262));
#247471=CARTESIAN_POINT('Origin',(-60.4516424606488,-13.1739864076109,3.64303198860252));
#247472=CARTESIAN_POINT('Origin',(0.0660119618346464,-0.310561863232796,
3.23423028058481));
#247473=CARTESIAN_POINT('Origin',(-59.4650964698965,-12.9642895838873,3.23423028058472));
#247474=CARTESIAN_POINT('Ctrl Pts',(-60.9782752797347,-13.2864868028998,
3.47153072139062));
#247475=CARTESIAN_POINT('Ctrl Pts',(-61.0052918384388,-13.1616357280624,
3.47182327902652));
#247476=CARTESIAN_POINT('Ctrl Pts',(-60.8992893541404,-13.1392995818861,
3.40413028959028));
#247477=CARTESIAN_POINT('Ctrl Pts',(-60.8658306440995,-13.2624669757411,
3.65553807120949));
#247478=CARTESIAN_POINT('Ctrl Pts',(-60.8926675943329,-13.1376969719828,
3.65586275496964));
#247479=CARTESIAN_POINT('Ctrl Pts',(-60.8093473519473,-13.1201818190178,
3.55128126837224));
#247480=CARTESIAN_POINT('Ctrl Pts',(-60.663828108008,-13.2193155203586,
3.77003198860253));
#247481=CARTESIAN_POINT('Ctrl Pts',(-60.6905008239722,-13.0947255842065,
3.77025505748485));
#247482=CARTESIAN_POINT('Ctrl Pts',(-60.6477702018618,-13.0858375353123,
3.64284211731165));
#247483=CARTESIAN_POINT('Ctrl Pts',(-60.4516424606488,-13.1739864076109,
3.77003198860253));
#247484=CARTESIAN_POINT('Ctrl Pts',(-60.4780866929066,-13.0495760763088,
3.77003198860253));
#247485=CARTESIAN_POINT('Ctrl Pts',(-60.4780472159603,-13.0497618007392,
3.64284239821708));
#247486=CARTESIAN_POINT('Origin',(-60.8730422059013,-13.2635576885504,3.404230974833));
#247487=CARTESIAN_POINT('Ctrl Pts',(-59.4650964698965,-12.9642895838873,
3.36123028058472));
#247488=CARTESIAN_POINT('Ctrl Pts',(-59.4915012546304,-12.8400648385941,
3.36123028058472));
#247489=CARTESIAN_POINT('Ctrl Pts',(-59.4915012546304,-12.8400648385941,
3.23423028058472));
#247490=CARTESIAN_POINT('Ctrl Pts',(-59.3770041141842,-12.9458049943938,
3.36123028058472));
#247491=CARTESIAN_POINT('Ctrl Pts',(-59.4033730190084,-12.8213326038442,
3.36146538610113));
#247492=CARTESIAN_POINT('Ctrl Pts',(-59.3594375597972,-12.8119938336989,
3.23423043688373));
#247493=CARTESIAN_POINT('Ctrl Pts',(-59.2937057271822,-12.9283282206302,
3.4105425869309));
#247494=CARTESIAN_POINT('Ctrl Pts',(-59.3204640761297,-12.8037097640144,
3.41100608859826));
#247495=CARTESIAN_POINT('Ctrl Pts',(-59.2345619206667,-12.785450697209,
3.30819866970894));
#247496=CARTESIAN_POINT('Ctrl Pts',(-59.2498070616278,-12.9191181862048,
3.48823028058471));
#247497=CARTESIAN_POINT('Ctrl Pts',(-59.2768226962997,-12.794433502371,
3.48852004212249));
#247498=CARTESIAN_POINT('Ctrl Pts',(-59.168751483356,-12.7714622569322,
3.42473028058471));
#247499=CARTESIAN_POINT('Origin',(-59.1423466986221,-12.8956870022254,3.42473028058471));
#247500=CARTESIAN_POINT('Origin',(-61.047298331887,-13.3005969715144,3.11913648178439));
#247501=CARTESIAN_POINT('Origin',(-61.2215544576538,-13.3376362544828,2.8340419886025));
#247502=CARTESIAN_POINT('Origin',(-59.0627741291267,-12.8787733304439,3.56563113460793));
#247503=CARTESIAN_POINT('Origin',(-59.0190342907434,-12.8695280801149,3.64299171721761));
#247504=CARTESIAN_POINT('Ctrl Pts',(-61.575271693745,-13.103835206573,2.59908173516014));
#247505=CARTESIAN_POINT('Ctrl Pts',(-61.5387839176327,-13.0960702419683,
2.65878198860252));
#247506=CARTESIAN_POINT('Ctrl Pts',(-61.4699285681953,-13.0814171332235,
2.65878198860252));
#247507=CARTESIAN_POINT('Ctrl Pts',(-61.5569304518435,-13.1900205930481,
2.59908193475538));
#247508=CARTESIAN_POINT('Ctrl Pts',(-61.5254208297816,-13.1588482421894,
2.65878715325286));
#247509=CARTESIAN_POINT('Ctrl Pts',(-61.4593031273767,-13.1313027022859,
2.65878198860252));
#247510=CARTESIAN_POINT('Ctrl Pts',(-61.5155378539379,-13.2643407403246,
2.63878778849859));
#247511=CARTESIAN_POINT('Ctrl Pts',(-61.4904936222817,-13.2118511391502,
2.69564460180109));
#247512=CARTESIAN_POINT('Ctrl Pts',(-61.4250300340668,-13.1721300657494,
2.68180481624885));
#247513=CARTESIAN_POINT('Ctrl Pts',(-61.4222835584425,-13.3535591268196,
2.75443238878635));
#247514=CARTESIAN_POINT('Ctrl Pts',(-61.4178880557396,-13.2611962587088,
2.79268340777075));
#247515=CARTESIAN_POINT('Ctrl Pts',(-61.341115859575,-13.2174099770539,
2.74885926835587));
#247516=CARTESIAN_POINT('Ctrl Pts',(-61.3712701109735,-13.3700167576324,
2.82856655361658));
#247517=CARTESIAN_POINT('Ctrl Pts',(-61.3797074995628,-13.257089619245,
2.85384197230779));
#247518=CARTESIAN_POINT('Ctrl Pts',(-61.292439340452,-13.2228660458969,
2.79184624278483));
#247519=CARTESIAN_POINT('Ctrl Pts',(-61.3267881959112,-13.3605623192489,
2.90134173516012));
#247520=CARTESIAN_POINT('Ctrl Pts',(-61.3537611057082,-13.2359003894753,
2.9016321871638));
#247521=CARTESIAN_POINT('Ctrl Pts',(-61.2479592423877,-13.2134115091896,
2.83404198860251));
#247522=CARTESIAN_POINT('Origin',(-61.4699285681953,-13.0814171332235,2.53178198860251));
#247523=CARTESIAN_POINT('Origin',(0.0660119618346463,-0.310561863232799,
3.64303198860262));
#247524=CARTESIAN_POINT('Origin',(-58.6264539577983,-12.7860306150454,3.64303198860253));
#247525=CARTESIAN_POINT('Origin',(1.31078692950418E-16,1.91611717219644E-13,
2.53178198860262));
#247526=CARTESIAN_POINT('Origin',(-61.4762657165315,-13.0516031943531,2.53178198860252));
#247527=CARTESIAN_POINT('Ctrl Pts',(-58.6264539577983,-12.7860306150454,
3.77003198860253));
#247528=CARTESIAN_POINT('Ctrl Pts',(-58.652898298092,-12.6616197754743,
3.77003198860253));
#247529=CARTESIAN_POINT('Ctrl Pts',(-58.6528587129485,-12.6618060089323,
3.64284187937045));
#247530=CARTESIAN_POINT('Ctrl Pts',(-58.4142663981464,-12.7406940127381,
3.77003198860254));
#247531=CARTESIAN_POINT('Ctrl Pts',(-58.4408495151697,-12.6165479409694,
3.76980208962975));
#247532=CARTESIAN_POINT('Ctrl Pts',(-58.4831327254059,-12.6257296363314,
3.64284193928275));
#247533=CARTESIAN_POINT('Ctrl Pts',(-58.2122676405432,-12.6975319705099,
3.65553535416578));
#247534=CARTESIAN_POINT('Ctrl Pts',(-58.2389323335244,-12.5736296288428,
3.65520057834408));
#247535=CARTESIAN_POINT('Ctrl Pts',(-58.3215567776512,-12.5913856081752,
3.55127910964244));
#247536=CARTESIAN_POINT('Ctrl Pts',(-58.0998260601479,-12.6735055745743,
3.47153072139062));
#247537=CARTESIAN_POINT('Ctrl Pts',(-58.1266254943011,-12.5497583536237,
3.47122746281572));
#247538=CARTESIAN_POINT('Ctrl Pts',(-58.2316158778875,-12.5722680796267,
3.40413045901267));
#247539=CARTESIAN_POINT('Origin',(-58.2050537810541,-12.6964592423895,3.40423097483301));
#247540=CARTESIAN_POINT('Ctrl Pts',(-61.4590390555208,-12.7383709431253,
2.90134173516013));
#247541=CARTESIAN_POINT('Ctrl Pts',(-61.4329754599098,-12.8632261535958,
2.90163218716381));
#247542=CARTESIAN_POINT('Ctrl Pts',(-61.3271735965892,-12.8407372733101,
2.83404198860251));
#247543=CARTESIAN_POINT('Ctrl Pts',(-61.5035409747665,-12.7478306169679,
2.82853349835352));
#247544=CARTESIAN_POINT('Ctrl Pts',(-61.465315459776,-12.8544171899346,
2.8538148316239));
#247545=CARTESIAN_POINT('Ctrl Pts',(-61.3716739624486,-12.8501961180702,
2.79182701594278));
#247546=CARTESIAN_POINT('Ctrl Pts',(-61.5432717953614,-12.7835835513932,
2.75468822073622));
#247547=CARTESIAN_POINT('Ctrl Pts',(-61.5017184029595,-12.8662481012967,
2.79286913083806));
#247548=CARTESIAN_POINT('Ctrl Pts',(-61.4137451613973,-12.8749453072906,
2.749007632979));
#247549=CARTESIAN_POINT('Ctrl Pts',(-61.5920631419343,-12.9020280679173,
2.63954450640393));
#247550=CARTESIAN_POINT('Ctrl Pts',(-61.547840657004,-12.940148758413,2.69627684028861));
#247551=CARTESIAN_POINT('Ctrl Pts',(-61.4717924962541,-12.9498405053864,
2.68224356036484));
#247552=CARTESIAN_POINT('Ctrl Pts',(-61.5999795805209,-12.9874904696722,
2.59908178706399));
#247553=CARTESIAN_POINT('Ctrl Pts',(-61.5585057825381,-13.0031958218442,
2.65878704321563));
#247554=CARTESIAN_POINT('Ctrl Pts',(-61.4868843017912,-13.0015435854425,
2.65878198860251));
#247555=CARTESIAN_POINT('Ctrl Pts',(-61.5816197022697,-13.0739701745327,
2.59908173516013));
#247556=CARTESIAN_POINT('Ctrl Pts',(-61.5451281645058,-13.0662229071069,
2.65878198860251));
#247557=CARTESIAN_POINT('Ctrl Pts',(-61.4762657165315,-13.0516031943531,
2.65878198860251));
#247558=CARTESIAN_POINT('Origin',(-61.3535783813231,-12.7165125280169,2.83404198860251));
#247559=CARTESIAN_POINT('Origin',(-58.0307974155439,-12.6594199084572,3.11913648167152));
#247560=CARTESIAN_POINT('Origin',(-57.8565410498766,-12.6223805745522,2.83404198860253));
#247561=CARTESIAN_POINT('Origin',(-61.1793222555325,-12.6794732450918,3.11913648177545));
#247562=CARTESIAN_POINT('Origin',(-61.0050661295705,-12.6424339620845,3.40423097483301));
#247563=CARTESIAN_POINT('Ctrl Pts',(-57.7513140650719,-12.5994235324474,
2.90134173516015));
#247564=CARTESIAN_POINT('Ctrl Pts',(-57.7780756236494,-12.4758649777955,
2.9010371155322));
#247565=CARTESIAN_POINT('Ctrl Pts',(-57.8829458346104,-12.498155829259,
2.83404198860253));
#247566=CARTESIAN_POINT('Ctrl Pts',(-57.7068710254543,-12.5899763290076,
2.82862991747951));
#247567=CARTESIAN_POINT('Ctrl Pts',(-57.7455616498587,-12.4844883578129,
2.85314045886467));
#247568=CARTESIAN_POINT('Ctrl Pts',(-57.8385008428013,-12.4887087546166,
2.79187960999924));
#247569=CARTESIAN_POINT('Ctrl Pts',(-57.6673720419785,-12.5543975270269,
2.75470625793316));
#247570=CARTESIAN_POINT('Ctrl Pts',(-57.7092008760996,-12.472450653056,
2.79224250381896));
#247571=CARTESIAN_POINT('Ctrl Pts',(-57.7966870296828,-12.4640308112191,
2.7490180910825));
#247572=CARTESIAN_POINT('Ctrl Pts',(-57.6192799956673,-12.4363816727425,
2.63947868311689));
#247573=CARTESIAN_POINT('Ctrl Pts',(-57.6635313090886,-12.3985321242202,
2.69595066767898));
#247574=CARTESIAN_POINT('Ctrl Pts',(-57.7394080294758,-12.3892398894927,
2.68220539436051));
#247575=CARTESIAN_POINT('Ctrl Pts',(-57.6118166447789,-12.3512461790953,
2.59908178584993));
#247576=CARTESIAN_POINT('Ctrl Pts',(-57.6532646075496,-12.3356888898089,
2.6587767094484));
#247577=CARTESIAN_POINT('Ctrl Pts',(-57.7248239067111,-12.3376071226704,
2.65878198860252));
#247578=CARTESIAN_POINT('Ctrl Pts',(-57.6301266171956,-12.2652136052663,
2.59908173516014));
#247579=CARTESIAN_POINT('Ctrl Pts',(-57.6666142715154,-12.2729791421557,
2.65878198860252));
#247580=CARTESIAN_POINT('Ctrl Pts',(-57.7354693911204,-12.2876333308473,
2.65878198860252));
#247581=CARTESIAN_POINT('Origin',(-57.7354693911203,-12.2876333308473,2.53178198860252));
#247582=CARTESIAN_POINT('Ctrl Pts',(-60.5836663843181,-12.552862681145,
3.77003198860254));
#247583=CARTESIAN_POINT('Ctrl Pts',(-60.5572221497821,-12.6772730231647,
3.77003198860254));
#247584=CARTESIAN_POINT('Ctrl Pts',(-60.55726162901,-12.6770872880007,3.6428423872764));
#247585=CARTESIAN_POINT('Ctrl Pts',(-60.7959479326851,-12.5977568525212,
3.77003198860254));
#247586=CARTESIAN_POINT('Ctrl Pts',(-60.7696393833362,-12.7224242094577,
3.77025506105595));
#247587=CARTESIAN_POINT('Ctrl Pts',(-60.7269872521295,-12.7131635826248,
3.64284210641857));
#247588=CARTESIAN_POINT('Ctrl Pts',(-60.99803611366,-12.6404975322969,3.65553527987824));
#247589=CARTESIAN_POINT('Ctrl Pts',(-60.9718043534706,-12.7653961862418,
3.65585996533041));
#247590=CARTESIAN_POINT('Ctrl Pts',(-60.8885631224,-12.7475075938194,3.55127902710186));
#247591=CARTESIAN_POINT('Ctrl Pts',(-61.110527437164,-12.6642893210144,
3.47153072139063));
#247592=CARTESIAN_POINT('Ctrl Pts',(-61.0844267823321,-12.7893350885045,
3.47182327905179));
#247593=CARTESIAN_POINT('Ctrl Pts',(-60.9785037583493,-12.7666250660188,
3.40413028378005));
#247594=CARTESIAN_POINT('Origin',(-60.5836663843181,-12.552862681145,3.64303198860254));
#247595=CARTESIAN_POINT('Origin',(3.545935779686E-16,1.91565239218228E-13,
2.53178198860262));
#247596=CARTESIAN_POINT('Origin',(-57.7418065394565,-12.257819391977,2.53178198860253));
#247597=CARTESIAN_POINT('Origin',(59.4667368016499,12.9646382471652,3.64303198860272));
#247598=CARTESIAN_POINT('Origin',(-60.1910940874975,-12.469366018727,3.64299466007616));
#247599=CARTESIAN_POINT('Ctrl Pts',(-57.6364522029206,-12.2354540642047,
2.59908173516014));
#247600=CARTESIAN_POINT('Ctrl Pts',(-57.6729438621905,-12.2432007592849,
2.65878198860252));
#247601=CARTESIAN_POINT('Ctrl Pts',(-57.7418065394565,-12.257819391977,
2.65878198860252));
#247602=CARTESIAN_POINT('Ctrl Pts',(-57.6546556225242,-12.1497054461945,
2.59908193199905));
#247603=CARTESIAN_POINT('Ctrl Pts',(-57.6862025493678,-12.1807288143665,
2.65877685806624));
#247604=CARTESIAN_POINT('Ctrl Pts',(-57.7523715145536,-12.2080066271958,
2.65878198860252));
#247605=CARTESIAN_POINT('Ctrl Pts',(-57.6955109599434,-12.0754939174599,
2.63872492669794));
#247606=CARTESIAN_POINT('Ctrl Pts',(-57.7206875210979,-12.1277502414152,
2.69532212015257));
#247607=CARTESIAN_POINT('Ctrl Pts',(-57.7861609236006,-12.1670355805165,
2.68176836726627));
#247608=CARTESIAN_POINT('Ctrl Pts',(-57.7879231380265,-11.9863964689867,
2.75442176402234));
#247609=CARTESIAN_POINT('Ctrl Pts',(-57.7928648378994,-12.0782086782662,
2.79203179920141));
#247610=CARTESIAN_POINT('Ctrl Pts',(-57.8693039540644,-12.1215423041375,
2.74885310748163));
#247611=CARTESIAN_POINT('Ctrl Pts',(-57.8386735460213,-11.969987326523,
2.82866089558395));
#247612=CARTESIAN_POINT('Ctrl Pts',(-57.8311081991717,-12.0820993460742,
2.85316563119138));
#247613=CARTESIAN_POINT('Ctrl Pts',(-57.9177340744069,-12.1160385312531,
2.79189751796634));
#247614=CARTESIAN_POINT('Ctrl Pts',(-57.8830978693155,-11.9794294790614,
2.90134173516013));
#247615=CARTESIAN_POINT('Ctrl Pts',(-57.857289977851,-12.1031907419159,
2.90103711553219));
#247616=CARTESIAN_POINT('Ctrl Pts',(-57.962160188812,-12.1254815933794,
2.83404198860251));
#247617=CARTESIAN_POINT('Origin',(-57.9885649735458,-12.0012568480862,2.83404198860252));
#247618=CARTESIAN_POINT('Origin',(-60.1478239214165,-12.4602215058061,3.56647653971771));
#247619=CARTESIAN_POINT('Origin',(-60.0677739512125,-12.4432063593725,3.42473028058475));
#247620=CARTESIAN_POINT('Origin',(-58.1628213391876,-12.0382961820437,3.11913648168035));
#247621=CARTESIAN_POINT('Origin',(-58.3370777047234,-12.0753355159235,3.40423097483301));
#247622=CARTESIAN_POINT('Ctrl Pts',(-59.7450242491247,-12.3746037924167,
3.36123028058472));
#247623=CARTESIAN_POINT('Ctrl Pts',(-59.7186194643908,-12.4988285377098,
3.36123028058472));
#247624=CARTESIAN_POINT('Ctrl Pts',(-59.7186194643908,-12.4988285377098,
3.23423028058472));
#247625=CARTESIAN_POINT('Ctrl Pts',(-59.8330190893699,-12.3935470970144,
3.36123028058472));
#247626=CARTESIAN_POINT('Ctrl Pts',(-59.8065803155762,-12.5175251937998,
3.36099641108486));
#247627=CARTESIAN_POINT('Ctrl Pts',(-59.8506831473911,-12.5268995400899,
3.23423043688348));
#247628=CARTESIAN_POINT('Ctrl Pts',(-59.9162252185214,-12.4114576311019,
3.41054258905275));
#247629=CARTESIAN_POINT('Ctrl Pts',(-59.8901687840271,-12.5352924712482,
3.41008815826019));
#247630=CARTESIAN_POINT('Ctrl Pts',(-59.9755587548356,-12.5534426698447,
3.30819867304325));
#247631=CARTESIAN_POINT('Ctrl Pts',(-59.9600752506736,-12.4208962741589,
3.48823028058475));
#247632=CARTESIAN_POINT('Ctrl Pts',(-59.9342688867324,-12.5446662374489,
3.48794691941591));
#247633=CARTESIAN_POINT('Ctrl Pts',(-60.0413691664786,-12.5674311046657,
3.42473028058476));
#247634=CARTESIAN_POINT('Origin',(-59.7450242491247,-12.3746037924167,3.23423028058472));
#247635=CARTESIAN_POINT('Ctrl Pts',(-58.231611300478,-12.0535047649324,
3.47153072139064));
#247636=CARTESIAN_POINT('Ctrl Pts',(-58.2057612755554,-12.1774537741286,
3.47122746285068));
#247637=CARTESIAN_POINT('Ctrl Pts',(-58.3108302788452,-12.199593564085,
3.40413046676783));
#247638=CARTESIAN_POINT('Ctrl Pts',(-58.344105910958,-12.077290030417,3.65553813457981));
#247639=CARTESIAN_POINT('Ctrl Pts',(-58.3180696991555,-12.2013259468605,
3.65520336072148));
#247640=CARTESIAN_POINT('Ctrl Pts',(-58.4007725402744,-12.2187113817819,
3.55128134519937));
#247641=CARTESIAN_POINT('Ctrl Pts',(-58.546198138126,-12.1200201767791,
3.77003198860254));
#247642=CARTESIAN_POINT('Ctrl Pts',(-58.5199882620682,-12.244245572038,
3.7698020931417));
#247643=CARTESIAN_POINT('Ctrl Pts',(-58.5623497685532,-12.2530556816162,
3.64284195387403));
#247644=CARTESIAN_POINT('Ctrl Pts',(-58.7584778814675,-12.1649068885794,
3.77003198860254));
#247645=CARTESIAN_POINT('Ctrl Pts',(-58.732033544228,-12.2893177137819,
3.77003198860254));
#247646=CARTESIAN_POINT('Ctrl Pts',(-58.7320731263128,-12.2891314947139,
3.64284189403801));
#247647=CARTESIAN_POINT('Origin',(-58.7584778814675,-12.1649068885794,3.64303198860253));
#247648=CARTESIAN_POINT('Origin',(58.0246834617327,12.6581203474876,3.23423028058491));
#247649=CARTESIAN_POINT('Origin',(-59.5971203935658,-12.3431658574213,3.23423028058472));
#247650=CARTESIAN_POINT('Origin',(57.798864262886,12.6101209950216,3.64303198860272));
#247651=CARTESIAN_POINT('Origin',(-59.1510793400371,-12.2483049654003,3.64299171721781));
#247652=CARTESIAN_POINT('Ctrl Pts',(-59.382070869907,-12.2968658913806,
3.48823028058472));
#247653=CARTESIAN_POINT('Ctrl Pts',(-59.3560370505013,-12.4217592664915,
3.48852004212249));
#247654=CARTESIAN_POINT('Ctrl Pts',(-59.2479658375575,-12.3987880210526,
3.42473028058472));
#247655=CARTESIAN_POINT('Ctrl Pts',(-59.4260685345959,-12.3063392072229,
3.41028005848397));
#247656=CARTESIAN_POINT('Ctrl Pts',(-59.3998259533508,-12.4310668851207,
3.41074404220355));
#247657=CARTESIAN_POINT('Ctrl Pts',(-59.3139986558987,-12.4128237298766,
3.30780486243951));
#247658=CARTESIAN_POINT('Ctrl Pts',(-59.5094220566594,-12.324285790178,
3.36123028058472));
#247659=CARTESIAN_POINT('Ctrl Pts',(-59.4828840257729,-12.4487214234133,
3.36146460586388));
#247660=CARTESIAN_POINT('Ctrl Pts',(-59.4390967537825,-12.4394141514343,
3.23423045308373));
#247661=CARTESIAN_POINT('Ctrl Pts',(-59.5971203935658,-12.3431658574213,
3.36123028058472));
#247662=CARTESIAN_POINT('Ctrl Pts',(-59.570715608832,-12.4673906027145,
3.36123028058472));
#247663=CARTESIAN_POINT('Ctrl Pts',(-59.570715608832,-12.4673906027145,
3.23423028058472));
#247664=CARTESIAN_POINT('Origin',(-59.2743706222914,-12.2745632757594,3.42473028058471));
#247665=CARTESIAN_POINT('Origin',(-59.1947980539411,-12.2576496039197,3.56563113524763));
#247666=CARTESIAN_POINT('Origin',(-58.3196542523182,-19.283043599958,3.56647653909482));
#247667=CARTESIAN_POINT('Origin',(-58.3616995707146,-19.2967593024447,3.64299466007676));
#247668=CARTESIAN_POINT('Origin',(-58.2418213702172,-19.2577541638581,3.4247302805847));
#247669=CARTESIAN_POINT('Ctrl Pts',(-58.1373965169892,-19.2232259141442,
3.48823028058469));
#247670=CARTESIAN_POINT('Ctrl Pts',(-58.1769325318818,-19.103134799739,
3.48794691941586));
#247671=CARTESIAN_POINT('Ctrl Pts',(-58.2810665285028,-19.1369699862886,
3.4247302805847));
#247672=CARTESIAN_POINT('Ctrl Pts',(-58.0945576760629,-19.2094285342461,
3.41028005925071));
#247673=CARTESIAN_POINT('Ctrl Pts',(-58.1339089916623,-19.089155604121,
3.40982512231007));
#247674=CARTESIAN_POINT('Ctrl Pts',(-58.2168625998339,-19.1161088652885,
3.30780486372894));
#247675=CARTESIAN_POINT('Ctrl Pts',(-58.0133994748117,-19.1832899764629,
3.36123028058467));
#247676=CARTESIAN_POINT('Ctrl Pts',(-58.0524922023731,-19.062701685676,
3.36099721048547));
#247677=CARTESIAN_POINT('Ctrl Pts',(-58.0952292882365,-19.0765878066325,
3.23423045308378));
#247678=CARTESIAN_POINT('Ctrl Pts',(-57.9280106456674,-19.1557908785628,
3.36123028058467));
#247679=CARTESIAN_POINT('Ctrl Pts',(-57.967255803953,-19.0350067009933,
3.36123028058467));
#247680=CARTESIAN_POINT('Ctrl Pts',(-57.967255803953,-19.0350067009933,
3.23423028058467));
#247681=CARTESIAN_POINT('Origin',(-57.9280106456674,-19.1557908785628,3.23423028058466));
#247682=CARTESIAN_POINT('Origin',(0.0981128957140535,-0.301960443923527,
3.64303198860262));
#247683=CARTESIAN_POINT('Origin',(-58.7434254837931,-19.4207352200704,3.64303198860248));
#247684=CARTESIAN_POINT('Origin',(0.0981128957140536,-0.301960443923524,
3.23423028058481));
#247685=CARTESIAN_POINT('Origin',(-57.7842031819381,-19.1090650011318,3.23423028058467));
#247686=CARTESIAN_POINT('Ctrl Pts',(-59.255413859757,-19.5876674457081,
3.47153072139057));
#247687=CARTESIAN_POINT('Ctrl Pts',(-59.295332909916,-19.4663243174857,
3.47182327902648));
#247688=CARTESIAN_POINT('Ctrl Pts',(-59.1922458813524,-19.4330302542694,
3.40413028959002));
#247689=CARTESIAN_POINT('Ctrl Pts',(-59.1460959632219,-19.5520255367103,
3.65553807120939));
#247690=CARTESIAN_POINT('Ctrl Pts',(-59.1858279145902,-19.4307442612507,
3.65586275497065));
#247691=CARTESIAN_POINT('Ctrl Pts',(-59.1047949412349,-19.4046157212348,
3.5512812683731));
#247692=CARTESIAN_POINT('Ctrl Pts',(-58.9497105734781,-19.4879954548406,
3.77003198860249));
#247693=CARTESIAN_POINT('Ctrl Pts',(-58.989260368078,-19.3668760934051,
3.77025505748352));
#247694=CARTESIAN_POINT('Ctrl Pts',(-58.9476928828763,-19.3535701679098,
3.64284211731077));
#247695=CARTESIAN_POINT('Ctrl Pts',(-58.7434254837931,-19.4207352200704,
3.77003198860249));
#247696=CARTESIAN_POINT('Ctrl Pts',(-58.7827292725254,-19.2997705965402,
3.77003198860249));
#247697=CARTESIAN_POINT('Ctrl Pts',(-58.7826705983485,-19.2999511770886,
3.64284239821665));
#247698=CARTESIAN_POINT('Origin',(-59.1531540087997,-19.5538640879535,3.40423097483296));
#247699=CARTESIAN_POINT('Ctrl Pts',(-57.7842031819381,-19.1090650011318,
3.36123028058467));
#247700=CARTESIAN_POINT('Ctrl Pts',(-57.8234483402237,-18.9882808235623,
3.36123028058467));
#247701=CARTESIAN_POINT('Ctrl Pts',(-57.8234483402237,-18.9882808235623,
3.23423028058467));
#247702=CARTESIAN_POINT('Ctrl Pts',(-57.6985255711015,-19.0814735135855,
3.36123028058467));
#247703=CARTESIAN_POINT('Ctrl Pts',(-57.7377609320117,-18.9604392969161,
3.36146538610164));
#247704=CARTESIAN_POINT('Ctrl Pts',(-57.6950423231347,-18.9465591794953,
3.23423043688409));
#247705=CARTESIAN_POINT('Ctrl Pts',(-57.6175103216832,-19.0553854270321,
3.41054258693084));
#247706=CARTESIAN_POINT('Ctrl Pts',(-57.6571482613567,-18.934246652455,
3.41100608859688));
#247707=CARTESIAN_POINT('Ctrl Pts',(-57.5736252790849,-18.9071083904251,
3.30819866970798));
#247708=CARTESIAN_POINT('Ctrl Pts',(-57.5748148483574,-19.041637186088,
3.48823028058467));
#247709=CARTESIAN_POINT('Ctrl Pts',(-57.61471558695,-18.9204594407748,3.48852004212245));
#247710=CARTESIAN_POINT('Ctrl Pts',(-57.5096375484035,-18.8863175164095,
3.42473028058467));
#247711=CARTESIAN_POINT('Origin',(-57.4703923901179,-19.007101693979,3.42473028058467));
#247712=CARTESIAN_POINT('Origin',(-59.3225838821635,-19.6089151909163,3.11913648178334));
#247713=CARTESIAN_POINT('Origin',(-59.4920137553138,-19.6639662938564,2.83404198860248));
#247714=CARTESIAN_POINT('Origin',(-57.3930236876031,-18.981963078654,3.56563113460772));
#247715=CARTESIAN_POINT('Origin',(-57.3504898524409,-18.9681964166834,3.64299171721756));
#247716=CARTESIAN_POINT('Ctrl Pts',(-59.868232155624,-19.4684195516699,
2.59908173516009));
#247717=CARTESIAN_POINT('Ctrl Pts',(-59.8327559231845,-19.4568831131887,
2.65878198860247));
#247718=CARTESIAN_POINT('Ctrl Pts',(-59.765809437495,-19.4351129318423,
2.65878198860247));
#247719=CARTESIAN_POINT('Ctrl Pts',(-59.8409825629599,-19.5522156237497,
2.59908193475607));
#247720=CARTESIAN_POINT('Ctrl Pts',(-59.812903951835,-19.517920385918,2.65878715325408));
#247721=CARTESIAN_POINT('Ctrl Pts',(-59.750027742079,-19.4836145615373,
2.65878198860247));
#247722=CARTESIAN_POINT('Ctrl Pts',(-59.7920481472524,-19.6218019328335,
2.63878778849849));
#247723=CARTESIAN_POINT('Ctrl Pts',(-59.7726277678657,-19.5669820401374,
2.69564460180101));
#247724=CARTESIAN_POINT('Ctrl Pts',(-59.7116747787984,-19.5206357546567,
2.68180481624872));
#247725=CARTESIAN_POINT('Ctrl Pts',(-59.6899788477095,-19.700783843471,
2.75443238878638));
#247726=CARTESIAN_POINT('Ctrl Pts',(-59.6952619726973,-19.6084674936732,
2.79268340777071));
#247727=CARTESIAN_POINT('Ctrl Pts',(-59.6234872553897,-19.5568961981639,
2.74885926835593));
#247728=CARTESIAN_POINT('Ctrl Pts',(-59.6375245663856,-19.7118189603901,
2.8285665536165));
#247729=CARTESIAN_POINT('Ctrl Pts',(-59.6577198343148,-19.6003923959454,
2.85384197230792));
#247730=CARTESIAN_POINT('Ctrl Pts',(-59.5745070768389,-19.5572342963493,
2.79184624278432));
#247731=CARTESIAN_POINT('Ctrl Pts',(-59.5942745858234,-19.6977666881848,
2.90134173516009));
#247732=CARTESIAN_POINT('Ctrl Pts',(-59.6341304551456,-19.5766071063171,
2.90163218716376));
#247733=CARTESIAN_POINT('Ctrl Pts',(-59.5312589135994,-19.5431821162869,
2.83404198860247));
#247734=CARTESIAN_POINT('Origin',(-59.765809437495,-19.4351129318423,2.53178198860247));
#247735=CARTESIAN_POINT('Origin',(0.0981128957140535,-0.301960443923527,
3.64303198860262));
#247736=CARTESIAN_POINT('Origin',(-56.9687879773464,-18.8441205405522,3.64303198860249));
#247737=CARTESIAN_POINT('Origin',(1.26611655068499E-16,1.91628388431979E-13,
2.53178198860262));
#247738=CARTESIAN_POINT('Origin',(-59.7752282754835,-19.4061247292256,2.53178198860247));
#247739=CARTESIAN_POINT('Ctrl Pts',(-56.9687879773464,-18.8441205405522,
3.77003198860249));
#247740=CARTESIAN_POINT('Ctrl Pts',(-57.0080919266514,-18.7231554228304,
3.77003198860249));
#247741=CARTESIAN_POINT('Ctrl Pts',(-57.0080330916622,-18.7233364983081,
3.64284187937016));
#247742=CARTESIAN_POINT('Ctrl Pts',(-56.7625017687168,-18.7768526573614,
3.77003198860249));
#247743=CARTESIAN_POINT('Ctrl Pts',(-56.8019160587471,-18.6561653631346,
3.76980208962846));
#247744=CARTESIAN_POINT('Ctrl Pts',(-56.843007888628,-18.6697165591971,
3.64284193928235));
#247745=CARTESIAN_POINT('Ctrl Pts',(-56.5661212433886,-18.7128124416032,
3.65553535416569));
#247746=CARTESIAN_POINT('Ctrl Pts',(-56.6055911857604,-18.5923760693085,
3.65520057834524));
#247747=CARTESIAN_POINT('Ctrl Pts',(-56.6859069993033,-18.6186713856998,
3.55127910964282));
#247748=CARTESIAN_POINT('Ctrl Pts',(-56.456807071981,-18.6771643191712,
3.47153072139058));
#247749=CARTESIAN_POINT('Ctrl Pts',(-56.4963948028695,-18.5568963021131,
3.47122746281569));
#247750=CARTESIAN_POINT('Ctrl Pts',(-56.5984571310818,-18.5902572009363,
3.4041304590125));
#247751=CARTESIAN_POINT('Origin',(-56.5590590327988,-18.7109915363519,3.40423097483296));
#247752=CARTESIAN_POINT('Ctrl Pts',(-59.790837669791,-19.0928077206414,
2.9013417351601));
#247753=CARTESIAN_POINT('Ctrl Pts',(-59.7518659300024,-19.2142545736086,
2.90163218716377));
#247754=CARTESIAN_POINT('Ctrl Pts',(-59.6489943884562,-19.1808295835784,
2.83404198860248));
#247755=CARTESIAN_POINT('Ctrl Pts',(-59.8341069976971,-19.1068672906322,
2.82853349835337));
#247756=CARTESIAN_POINT('Ctrl Pts',(-59.7849495554008,-19.2088743168621,
2.85381483162398));
#247757=CARTESIAN_POINT('Ctrl Pts',(-59.6922622581484,-19.1948881666554,
2.79182701594271));
#247758=CARTESIAN_POINT('Ctrl Pts',(-59.8698829694067,-19.1465773683629,
2.75468822073635));
#247759=CARTESIAN_POINT('Ctrl Pts',(-59.8199164124675,-19.2244455609612,
2.7928691308379));
#247760=CARTESIAN_POINT('Ctrl Pts',(-59.7315159919506,-19.2238994150015,
2.74900763297901));
#247761=CARTESIAN_POINT('Ctrl Pts',(-59.9060262085834,-19.2694731179105,
2.63954450640372));
#247762=CARTESIAN_POINT('Ctrl Pts',(-59.8580612818569,-19.3027624708835,
2.69627684028866));
#247763=CARTESIAN_POINT('Ctrl Pts',(-59.7814166574708,-19.3044519280754,
2.68224356036474));
#247764=CARTESIAN_POINT('Ctrl Pts',(-59.904966026569,-19.3552948408466,
2.59908178706307));
#247765=CARTESIAN_POINT('Ctrl Pts',(-59.8620777700639,-19.3665789650873,
2.65878704321424));
#247766=CARTESIAN_POINT('Ctrl Pts',(-59.7910213450151,-19.3574492964902,
2.65878198860247));
#247767=CARTESIAN_POINT('Ctrl Pts',(-59.8776671349984,-19.4393816709759,
2.59908173516009));
#247768=CARTESIAN_POINT('Ctrl Pts',(-59.8421853116551,-19.4278624395269,
2.65878198860247));
#247769=CARTESIAN_POINT('Ctrl Pts',(-59.7752282754835,-19.4061247292257,
2.65878198860247));
#247770=CARTESIAN_POINT('Origin',(-59.6882395467419,-19.060045406009,2.83404198860248));
#247771=CARTESIAN_POINT('Origin',(-56.3896289265483,-18.6559403576673,3.11913648167084));
#247772=CARTESIAN_POINT('Origin',(-56.2201988201381,-18.6008891789888,2.83404198860249));
#247773=CARTESIAN_POINT('Origin',(-59.5188096735656,-19.0049943031088,3.11913648177563));
#247774=CARTESIAN_POINT('Origin',(-59.3493798002278,-18.9499432001061,3.40423097483296));
#247775=CARTESIAN_POINT('Ctrl Pts',(-56.1179479440987,-18.5670586829468,
2.9013417351601));
#247776=CARTESIAN_POINT('Ctrl Pts',(-56.1574782858995,-18.4469743395782,
2.90103711553216));
#247777=CARTESIAN_POINT('Ctrl Pts',(-56.2594439784237,-18.4801050014193,
2.83404198860248));
#247778=CARTESIAN_POINT('Ctrl Pts',(-56.0747358697601,-18.5530176696411,
2.82862991747934));
#247779=CARTESIAN_POINT('Ctrl Pts',(-56.1242410384002,-18.4521518441032,
2.85314045886312));
#247780=CARTESIAN_POINT('Ctrl Pts',(-56.2162299491247,-18.4660639121465,
2.79187960999912));
#247781=CARTESIAN_POINT('Ctrl Pts',(-56.0391722633446,-18.5135050040176,
2.75470625793334));
#247782=CARTESIAN_POINT('Ctrl Pts',(-56.0893377355413,-18.4363793473478,
2.79224250381873));
#247783=CARTESIAN_POINT('Ctrl Pts',(-56.1772247439499,-18.4371504234765,
2.74901809108246));
#247784=CARTESIAN_POINT('Ctrl Pts',(-56.0036796861843,-18.3911086652349,
2.63947868311664));
#247785=CARTESIAN_POINT('Ctrl Pts',(-56.0516449414232,-18.3580919822889,
2.69595066767906));
#247786=CARTESIAN_POINT('Ctrl Pts',(-56.1280773042131,-18.3567819283755,
2.68220539436048));
#247787=CARTESIAN_POINT('Ctrl Pts',(-56.0051563026341,-18.3056594201307,
2.59908178585071));
#247788=CARTESIAN_POINT('Ctrl Pts',(-56.0480033886679,-18.2945198471564,
2.65877670944857));
#247789=CARTESIAN_POINT('Ctrl Pts',(-56.1189701685705,-18.303907555312,
2.65878198860248));
#247790=CARTESIAN_POINT('Ctrl Pts',(-56.032358823839,-18.2220120550219,
2.5990817351601));
#247791=CARTESIAN_POINT('Ctrl Pts',(-56.0678348753331,-18.233549049922,
2.65878198860248));
#247792=CARTESIAN_POINT('Ctrl Pts',(-56.134781019564,-18.2553202812751,
2.65878198860248));
#247793=CARTESIAN_POINT('Origin',(-56.1347810195641,-18.2553202812751,2.53178198860248));
#247794=CARTESIAN_POINT('Ctrl Pts',(-58.9396512752212,-18.8168143322229,
3.77003198860249));
#247795=CARTESIAN_POINT('Ctrl Pts',(-58.9003474831029,-18.9377789661738,
3.77003198860249));
#247796=CARTESIAN_POINT('Ctrl Pts',(-58.9004061606708,-18.9375983751892,
3.64284238727605));
#247797=CARTESIAN_POINT('Ctrl Pts',(-59.1460772043116,-18.8836520326607,
3.77003198860249));
#247798=CARTESIAN_POINT('Ctrl Pts',(-59.1068814887054,-19.0048864565374,
3.77025506105755));
#247799=CARTESIAN_POINT('Ctrl Pts',(-59.065431009429,-18.9912181986578,
3.64284210641866));
#247800=CARTESIAN_POINT('Ctrl Pts',(-59.3425907075088,-18.9472825415269,
3.6555352798782));
#247801=CARTESIAN_POINT('Ctrl Pts',(-59.3034471832889,-19.068755021998,
3.65585996533024));
#247802=CARTESIAN_POINT('Ctrl Pts',(-59.2225318234672,-19.0422633471874,
3.55127902710179));
#247803=CARTESIAN_POINT('Ctrl Pts',(-59.4519788726606,-18.9827025415099,
3.47153072139058));
#247804=CARTESIAN_POINT('Ctrl Pts',(-59.4129503580329,-19.1043350338624,
3.47182327905174));
#247805=CARTESIAN_POINT('Ctrl Pts',(-59.3099814352094,-19.0706774483341,
3.40413028377984));
#247806=CARTESIAN_POINT('Origin',(-58.9396512752212,-18.8168143322229,3.64303198860249));
#247807=CARTESIAN_POINT('Origin',(3.56182666396656E-16,1.91559308659476E-13,
2.53178198860262));
#247808=CARTESIAN_POINT('Origin',(-56.1441998575526,-18.2263320786585,2.53178198860249));
#247809=CARTESIAN_POINT('Origin',(56.1826270286323,18.5886813639062,3.64303198860276));
#247810=CARTESIAN_POINT('Origin',(-58.5579573083294,-18.6927400943493,3.64299466007528));
#247811=CARTESIAN_POINT('Ctrl Pts',(-56.0417604764382,-18.1930767435951,
2.5990817351601));
#247812=CARTESIAN_POINT('Ctrl Pts',(-56.0772424804483,-18.2045954185348,
2.65878198860249));
#247813=CARTESIAN_POINT('Ctrl Pts',(-56.1441998575526,-18.2263320786585,
2.65878198860248));
#247814=CARTESIAN_POINT('Ctrl Pts',(-56.0688273470724,-18.1097006409635,
2.59908193199874));
#247815=CARTESIAN_POINT('Ctrl Pts',(-56.0969586315473,-18.1438516116617,
2.65877685806618));
#247816=CARTESIAN_POINT('Ctrl Pts',(-56.159913808364,-18.1778965340259,
2.65878198860248));
#247817=CARTESIAN_POINT('Ctrl Pts',(-56.1172160917339,-18.0401661963854,
2.6387249266979));
#247818=CARTESIAN_POINT('Ctrl Pts',(-56.1367924598133,-18.0947679219786,
2.69532212015264));
#247819=CARTESIAN_POINT('Ctrl Pts',(-56.1978007560412,-18.1406818860299,
2.68176836726611));
#247820=CARTESIAN_POINT('Ctrl Pts',(-56.2184352456063,-17.9612165360192,
2.75442176402231));
#247821=CARTESIAN_POINT('Ctrl Pts',(-56.2137528851846,-18.0530423367032,
2.79203179920121));
#247822=CARTESIAN_POINT('Ctrl Pts',(-56.2852436625533,-18.1041286397845,
2.74885310748172));
#247823=CARTESIAN_POINT('Ctrl Pts',(-56.270622860001,-17.9502021467133,
2.8286608955839));
#247824=CARTESIAN_POINT('Ctrl Pts',(-56.2513800597986,-18.060909210809,
2.85316563119087));
#247825=CARTESIAN_POINT('Ctrl Pts',(-56.333983778552,-18.1037173431995,
2.79189751796545));
#247826=CARTESIAN_POINT('Ctrl Pts',(-56.3138168485093,-17.9642361803975,
2.9013417351601));
#247827=CARTESIAN_POINT('Ctrl Pts',(-56.2752137607564,-18.0846218068697,
2.90103711553217));
#247828=CARTESIAN_POINT('Ctrl Pts',(-56.3771794532806,-18.1177524687109,
2.83404198860248));
#247829=CARTESIAN_POINT('Origin',(-56.4164246115662,-17.9969682911414,2.83404198860249));
#247830=CARTESIAN_POINT('Origin',(-58.5158800426277,-18.6791227120619,3.56647653971777));
#247831=CARTESIAN_POINT('Origin',(-58.4380471616453,-18.6538332760107,3.42473028058471));
#247832=CARTESIAN_POINT('Origin',(-56.5858547179447,-18.0520194698677,3.11913648168048));
#247833=CARTESIAN_POINT('Origin',(-56.7552848242269,-18.1070706485045,3.40423097483297));
#247834=CARTESIAN_POINT('Ctrl Pts',(-58.1242364370955,-18.5518699907153,
3.36123028058468));
#247835=CARTESIAN_POINT('Ctrl Pts',(-58.0849912788099,-18.6726541682848,
3.36123028058468));
#247836=CARTESIAN_POINT('Ctrl Pts',(-58.0849912788099,-18.6726541682848,
3.23423028058468));
#247837=CARTESIAN_POINT('Ctrl Pts',(-58.2097691178804,-18.5799074873338,
3.36123028058468));
#247838=CARTESIAN_POINT('Ctrl Pts',(-58.1705159385191,-18.7004428147373,
3.36099641108398));
#247839=CARTESIAN_POINT('Ctrl Pts',(-58.2133972843951,-18.714375808614,
3.23423043688317));
#247840=CARTESIAN_POINT('Ctrl Pts',(-58.2906472745454,-18.6064173144575,
3.4105425890527));
#247841=CARTESIAN_POINT('Ctrl Pts',(-58.2517893143873,-18.7268501353373,
3.41008815826044));
#247842=CARTESIAN_POINT('Ctrl Pts',(-58.3348142976333,-18.7538265876729,
3.30819867304329));
#247843=CARTESIAN_POINT('Ctrl Pts',(-58.3332704847794,-18.620387828115,
3.48823028058469));
#247844=CARTESIAN_POINT('Ctrl Pts',(-58.2946680067386,-18.7407822670305,
3.48794691941585));
#247845=CARTESIAN_POINT('Ctrl Pts',(-58.3988020033597,-18.7746174535802,
3.42473028058469));
#247846=CARTESIAN_POINT('Origin',(-58.1242364370955,-18.5518699907153,3.23423028058468));
#247847=CARTESIAN_POINT('Ctrl Pts',(-56.6526781108322,-18.0743352474894,
3.47153072139058));
#247848=CARTESIAN_POINT('Ctrl Pts',(-56.614013495596,-18.1949031876638,
3.47122746285063));
#247849=CARTESIAN_POINT('Ctrl Pts',(-56.7161926816712,-18.2279043949851,
3.40413046676769));
#247850=CARTESIAN_POINT('Ctrl Pts',(-56.7620702268155,-18.1097491035617,
3.65553813457973));
#247851=CARTESIAN_POINT('Ctrl Pts',(-56.7232113603666,-18.2303840130672,
3.65520336072325));
#247852=CARTESIAN_POINT('Ctrl Pts',(-56.8036438738754,-18.256319009646,
3.55128134519965));
#247853=CARTESIAN_POINT('Ctrl Pts',(-56.958588855084,-18.1733695596539,
3.7700319886025));
#247854=CARTESIAN_POINT('Ctrl Pts',(-56.9195374698063,-18.2941747571338,
3.76980209314045));
#247855=CARTESIAN_POINT('Ctrl Pts',(-56.9607460083098,-18.3073645871839,
3.6428419538737));
#247856=CARTESIAN_POINT('Ctrl Pts',(-57.1650137687746,-18.2401996527048,
3.7700319886025));
#247857=CARTESIAN_POINT('Ctrl Pts',(-57.125709824009,-18.3611647564559,
3.7700319886025));
#247858=CARTESIAN_POINT('Ctrl Pts',(-57.125768654452,-18.3609836949698,
3.6428418940378));
#247859=CARTESIAN_POINT('Origin',(-57.1650137687745,-18.2401996527048,3.64303198860249));
#247860=CARTESIAN_POINT('Origin',(54.8193466381475,18.1457247135496,3.23423028058495));
#247861=CARTESIAN_POINT('Origin',(-57.9804289733662,-18.5051441132844,3.23423028058468));
#247862=CARTESIAN_POINT('Origin',(54.6058629360811,18.0763596539235,3.64303198860276));
#247863=CARTESIAN_POINT('Origin',(-57.5467470426659,-18.3641788932753,3.64299171721742));
#247864=CARTESIAN_POINT('Ctrl Pts',(-57.7713971777985,-18.4366189870675,
3.48823028058468));
#247865=CARTESIAN_POINT('Ctrl Pts',(-57.7324510618069,-18.5581069080663,
3.48852004212245));
#247866=CARTESIAN_POINT('Ctrl Pts',(-57.6273730232604,-18.523964983701,
3.42473028058467));
#247867=CARTESIAN_POINT('Ctrl Pts',(-57.8141635875296,-18.4506394153724,
3.41028005848391));
#247868=CARTESIAN_POINT('Ctrl Pts',(-57.7750271733929,-18.5719407253121,
3.41074404220449));
#247869=CARTESIAN_POINT('Ctrl Pts',(-57.6915769758397,-18.5448261124701,
3.30780486243967));
#247870=CARTESIAN_POINT('Ctrl Pts',(-57.8951845615404,-18.4772005006378,
3.36123028058468));
#247871=CARTESIAN_POINT('Ctrl Pts',(-57.8557848432456,-18.5981804828674,
3.36146460586278));
#247872=CARTESIAN_POINT('Ctrl Pts',(-57.8132103173503,-18.5843471808455,
3.23423045308354));
#247873=CARTESIAN_POINT('Ctrl Pts',(-57.9804289733662,-18.5051441132844,
3.36123028058468));
#247874=CARTESIAN_POINT('Ctrl Pts',(-57.9411838150806,-18.6259282908539,
3.36123028058468));
#247875=CARTESIAN_POINT('Ctrl Pts',(-57.9411838150806,-18.6259282908539,
3.23423028058468));
#247876=CARTESIAN_POINT('Origin',(-57.666618181546,-18.4031808061316,3.42473028058467));
#247877=CARTESIAN_POINT('Origin',(-57.5892494801773,-18.3780421908695,3.56563113524827));
#247878=CARTESIAN_POINT('Origin',(-55.9845461696115,-25.2734729067952,3.56647653909449));
#247879=CARTESIAN_POINT('Origin',(-56.0249274780511,-25.2915084057487,3.64299466007633));
#247880=CARTESIAN_POINT('Origin',(-55.9097831300745,-25.2401862573144,3.42473028058465));
#247881=CARTESIAN_POINT('Ctrl Pts',(-55.8095395120005,-25.1949317875303,
3.48823028058466));
#247882=CARTESIAN_POINT('Ctrl Pts',(-55.8614118841077,-25.0796311836956,
3.48794691941582));
#247883=CARTESIAN_POINT('Ctrl Pts',(-55.9614386837451,-25.1241659841938,
3.42473028058467));
#247884=CARTESIAN_POINT('Ctrl Pts',(-55.7683775656455,-25.1767321129116,
3.41028005925067));
#247885=CARTESIAN_POINT('Ctrl Pts',(-55.8200852551846,-25.0612313830326,
3.40982512230957));
#247886=CARTESIAN_POINT('Ctrl Pts',(-55.8997670518381,-25.096708004599,
3.30780486372802));
#247887=CARTESIAN_POINT('Ctrl Pts',(-55.690396180789,-25.1422534028259,
3.36123028058463));
#247888=CARTESIAN_POINT('Ctrl Pts',(-55.7418796630183,-25.026412010048,
3.36099721048382));
#247889=CARTESIAN_POINT('Ctrl Pts',(-55.7829311357716,-25.0446893032919,
3.23423045308383));
#247890=CARTESIAN_POINT('Ctrl Pts',(-55.6083495590299,-25.1059793847704,
3.36123028058463));
#247891=CARTESIAN_POINT('Ctrl Pts',(-55.6600051127006,-24.9899591116498,
3.36123028058464));
#247892=CARTESIAN_POINT('Ctrl Pts',(-55.6600051127006,-24.9899591116498,
3.23423028058463));
#247893=CARTESIAN_POINT('Origin',(-55.6083495590299,-25.1059793847704,3.23423028058462));
#247894=CARTESIAN_POINT('Origin',(0.129138884176574,-0.290050682801341,
3.64303198860262));
#247895=CARTESIAN_POINT('Origin',(-56.3916032444848,-25.4547063934086,3.64303198860244));
#247896=CARTESIAN_POINT('Origin',(0.129138884176574,-0.290050682801338,
3.23423028058481));
#247897=CARTESIAN_POINT('Origin',(-55.4702140717965,-25.044477503395,3.23423028058463));
#247898=CARTESIAN_POINT('Ctrl Pts',(-56.8833377255392,-25.6742415049982,
3.47153072139053));
#247899=CARTESIAN_POINT('Ctrl Pts',(-56.9357219056855,-25.5577357840975,
3.47182327902644));
#247900=CARTESIAN_POINT('Ctrl Pts',(-56.8366797759155,-25.5138485805641,
3.40413028959036));
#247901=CARTESIAN_POINT('Ctrl Pts',(-56.7783442778551,-25.6273680143744,
3.65553807120938));
#247902=CARTESIAN_POINT('Ctrl Pts',(-56.8305359187788,-25.5109042502505,
3.65586275496827));
#247903=CARTESIAN_POINT('Ctrl Pts',(-56.7526780286657,-25.4764485929306,
3.55128126837231));
#247904=CARTESIAN_POINT('Ctrl Pts',(-56.589727673884,-25.5431608329973,
3.77003198860245));
#247905=CARTESIAN_POINT('Ctrl Pts',(-56.6417212312968,-25.4268390553501,
3.77025505748496));
#247906=CARTESIAN_POINT('Ctrl Pts',(-56.6017723050744,-25.4092610357548,
3.64284211731128));
#247907=CARTESIAN_POINT('Ctrl Pts',(-56.3916032444848,-25.4547063934086,
3.77003198860245));
#247908=CARTESIAN_POINT('Ctrl Pts',(-56.4433359691572,-25.3385127913803,
3.77003198860245));
#247909=CARTESIAN_POINT('Ctrl Pts',(-56.4432587405966,-25.3386862495674,
3.64284239821732));
#247910=CARTESIAN_POINT('Origin',(-56.7851714777845,-25.6299342604998,3.40423097483292));
#247911=CARTESIAN_POINT('Ctrl Pts',(-55.4702140717965,-25.044477503395,
3.36123028058463));
#247912=CARTESIAN_POINT('Ctrl Pts',(-55.5218696254671,-24.9284572302744,
3.36123028058463));
#247913=CARTESIAN_POINT('Ctrl Pts',(-55.5218696254671,-24.9284572302744,
3.23423028058463));
#247914=CARTESIAN_POINT('Ctrl Pts',(-55.3878899076689,-25.0080814159077,
3.36123028058463));
#247915=CARTESIAN_POINT('Ctrl Pts',(-55.4395618538395,-24.891811449323,
3.36146538609948));
#247916=CARTESIAN_POINT('Ctrl Pts',(-55.3985281293145,-24.8735420580984,
3.23423043688414));
#247917=CARTESIAN_POINT('Ctrl Pts',(-55.3100454158615,-24.9736678430974,
3.41054258693083));
#247918=CARTESIAN_POINT('Ctrl Pts',(-55.3621286647007,-24.8573359723233,
3.41100608859791));
#247919=CARTESIAN_POINT('Ctrl Pts',(-55.281899950892,-24.8216158475494,
3.30819866970784));
#247920=CARTESIAN_POINT('Ctrl Pts',(-55.2690209153038,-24.9555320242418,
3.48823028058463));
#247921=CARTESIAN_POINT('Ctrl Pts',(-55.3213695969754,-24.8391888661847,
3.48852004212241));
#247922=CARTESIAN_POINT('Ctrl Pts',(-55.2204359898054,-24.794250328961,
3.42473028058463));
#247923=CARTESIAN_POINT('Origin',(-55.1687804361348,-24.9102706020816,3.42473028058462));
#247924=CARTESIAN_POINT('Origin',(-56.9479187893834,-25.7023940320541,3.11913648178483));
#247925=CARTESIAN_POINT('Origin',(-57.1106661007663,-25.774853803565,2.83404198860243));
#247926=CARTESIAN_POINT('Origin',(-55.0944632682977,-24.8771824671427,3.56563113460843));
#247927=CARTESIAN_POINT('Origin',(-55.0536014459533,-24.8590452239606,3.64299171721736));
#247928=CARTESIAN_POINT('Ctrl Pts',(-57.505263737773,-25.61970381813,2.59908173516005));
#247929=CARTESIAN_POINT('Ctrl Pts',(-57.4711877340327,-25.6045223014064,
2.65878198860243));
#247930=CARTESIAN_POINT('Ctrl Pts',(-57.4068835917977,-25.5758735661211,
2.65878198860243));
#247931=CARTESIAN_POINT('Ctrl Pts',(-57.4694043465864,-25.7001924885133,
2.59908193475593));
#247932=CARTESIAN_POINT('Ctrl Pts',(-57.4450643815381,-25.6631501095106,
2.65878715325272));
#247933=CARTESIAN_POINT('Ctrl Pts',(-57.3861185493435,-25.6224598624446,
2.65878198860243));
#247934=CARTESIAN_POINT('Ctrl Pts',(-57.413464248775,-25.7642825572403,
2.63878778849862));
#247935=CARTESIAN_POINT('Ctrl Pts',(-57.3998804953982,-25.7077329912391,
2.695644601801));
#247936=CARTESIAN_POINT('Ctrl Pts',(-57.3441059191826,-25.6552692732806,
2.6818048162487));
#247937=CARTESIAN_POINT('Ctrl Pts',(-57.3036982377901,-25.8321626496792,
2.75443238878616));
#247938=CARTESIAN_POINT('Ctrl Pts',(-57.3186021074456,-25.7409042554409,
2.79268340777062));
#247939=CARTESIAN_POINT('Ctrl Pts',(-57.2526112478171,-25.6821129719829,
2.74885926835585));
#247940=CARTESIAN_POINT('Ctrl Pts',(-57.2503778226939,-25.8376543496546,
2.82856655361658));
#247941=CARTESIAN_POINT('Ctrl Pts',(-57.2821097063791,-25.7289491719107,
2.85384197230723));
#247942=CARTESIAN_POINT('Ctrl Pts',(-57.2038640469253,-25.6773293952365,
2.79184624278389));
#247943=CARTESIAN_POINT('Ctrl Pts',(-57.2088336324697,-25.8191582032623,
2.90134173516005));
#247944=CARTESIAN_POINT('Ctrl Pts',(-57.2611357920723,-25.7028284190336,
2.90163218716373));
#247945=CARTESIAN_POINT('Ctrl Pts',(-57.1623216544369,-25.6588335304443,
2.83404198860243));
#247946=CARTESIAN_POINT('Origin',(-57.4068835917977,-25.5758735661211,2.53178198860243));
#247947=CARTESIAN_POINT('Origin',(0.129138884176574,-0.290050682801341,
3.64303198860262));
#247948=CARTESIAN_POINT('Origin',(-54.6869600343295,-24.695750338031,3.64303198860244));
#247949=CARTESIAN_POINT('Origin',(1.20426471881346E-16,1.91644501385063E-13,
2.53178198860262));
#247950=CARTESIAN_POINT('Origin',(-57.4192809246787,-25.5480287005721,2.53178198860243));
#247951=CARTESIAN_POINT('Ctrl Pts',(-54.6869600343295,-24.695750338031,
3.77003198860245));
#247952=CARTESIAN_POINT('Ctrl Pts',(-54.7386929703522,-24.5795562613021,
3.77003198860245));
#247953=CARTESIAN_POINT('Ctrl Pts',(-54.7386155301258,-24.5797301948983,
3.64284187937016));
#247954=CARTESIAN_POINT('Ctrl Pts',(-54.4888352915928,-24.6072881749595,
3.77003198860245));
#247955=CARTESIAN_POINT('Ctrl Pts',(-54.5406489234192,-24.4913819335271,
3.76980208962808));
#247956=CARTESIAN_POINT('Ctrl Pts',(-54.5800991622554,-24.5091541605501,
3.64284193928258));
#247957=CARTESIAN_POINT('Ctrl Pts',(-54.3002245846692,-24.5230714236785,
3.65553535416566));
#247958=CARTESIAN_POINT('Ctrl Pts',(-54.3520673354853,-24.4074205468523,
3.65520057834542));
#247959=CARTESIAN_POINT('Ctrl Pts',(-54.4291945615855,-24.4419671033161,
3.55127910964222));
#247960=CARTESIAN_POINT('Ctrl Pts',(-54.195235491187,-24.4761921430394,
3.47153072139054));
#247961=CARTESIAN_POINT('Ctrl Pts',(-54.2471777873469,-24.3607210114367,
3.47122746281565));
#247962=CARTESIAN_POINT('Ctrl Pts',(-54.3451938439591,-24.404567574091,
3.40413045901249));
#247963=CARTESIAN_POINT('Origin',(-54.2933913980362,-24.5205222915154,3.40423097483292));
#247964=CARTESIAN_POINT('Ctrl Pts',(-57.4675553545138,-25.2380597013433,
2.90134173516005));
#247965=CARTESIAN_POINT('Ctrl Pts',(-57.4161024530841,-25.3547675996718,
2.90163218716372));
#247966=CARTESIAN_POINT('Ctrl Pts',(-57.3172883154488,-25.3107727110825,
2.83404198860243));
#247967=CARTESIAN_POINT('Ctrl Pts',(-57.5091180232691,-25.2565651278911,
2.82853349835322));
#247968=CARTESIAN_POINT('Ctrl Pts',(-57.4495672328898,-25.3528749970538,
2.85381483162274));
#247969=CARTESIAN_POINT('Ctrl Pts',(-57.3588496371379,-25.3292770036978,
2.79182701594154));
#247970=CARTESIAN_POINT('Ctrl Pts',(-57.5405471770606,-25.2997972770061,
2.75468822073643));
#247971=CARTESIAN_POINT('Ctrl Pts',(-57.482714899638,-25.3720159720864,
2.79286913083823));
#247972=CARTESIAN_POINT('Ctrl Pts',(-57.3948558336728,-25.3622324578622,
2.74900763297892));
#247973=CARTESIAN_POINT('Ctrl Pts',(-57.5636463159494,-25.4257977880272,
2.63954450640355));
#247974=CARTESIAN_POINT('Ctrl Pts',(-57.5124644612013,-25.4538910783598,
2.69627684028832));
#247975=CARTESIAN_POINT('Ctrl Pts',(-57.4360631077225,-25.447559735724,
2.68224356036474));
#247976=CARTESIAN_POINT('Ctrl Pts',(-57.553621128909,-25.5110385513889,
2.59908178706347));
#247977=CARTESIAN_POINT('Ctrl Pts',(-57.5097883065914,-25.5177778164706,
2.65878704321553));
#247978=CARTESIAN_POINT('Ctrl Pts',(-57.4400754463034,-25.5012707422377,
2.65878198860243));
#247979=CARTESIAN_POINT('Ctrl Pts',(-57.5176823163886,-25.5918112338797,
2.59908173516005));
#247980=CARTESIAN_POINT('Ctrl Pts',(-57.4835989537475,-25.5766462455179,
2.65878198860242));
#247981=CARTESIAN_POINT('Ctrl Pts',(-57.4192809246787,-25.5480287005721,
2.65878198860243));
#247982=CARTESIAN_POINT('Origin',(-57.3689438691194,-25.1947524379619,2.83404198860243));
#247983=CARTESIAN_POINT('Origin',(-54.1306438627469,-24.4480624203116,3.119136481669));
#247984=CARTESIAN_POINT('Origin',(-53.9678963272933,-24.3756025490941,2.83404198860245));
#247985=CARTESIAN_POINT('Origin',(-57.2061965577021,-25.122292666487,3.1191364817743));
#247986=CARTESIAN_POINT('Origin',(-57.0434492461377,-25.0498328948967,3.40423097483292));
#247987=CARTESIAN_POINT('Ctrl Pts',(-53.8697418420143,-24.331269253109,
2.90134173516006));
#247988=CARTESIAN_POINT('Ctrl Pts',(-53.9216078643415,-24.2159747902189,
2.90103711553211));
#247989=CARTESIAN_POINT('Ctrl Pts',(-54.0195518809639,-24.2595822759735,
2.83404198860244));
#247990=CARTESIAN_POINT('Ctrl Pts',(-53.8282341734841,-24.312788266218,
2.82862991747947));
#247991=CARTESIAN_POINT('Ctrl Pts',(-53.8880114973696,-24.2176496934278,
2.85314045886338));
#247992=CARTESIAN_POINT('Ctrl Pts',(-53.9780422761238,-24.2411010091829,
2.79187960999867));
#247993=CARTESIAN_POINT('Ctrl Pts',(-53.7969955864425,-24.2697746459844,
2.75470625793306));
#247994=CARTESIAN_POINT('Ctrl Pts',(-53.8549480733037,-24.198315211449,
2.79224250381917));
#247995=CARTESIAN_POINT('Ctrl Pts',(-53.9422730280817,-24.2082687574724,
2.74901809108243));
#247996=CARTESIAN_POINT('Ctrl Pts',(-53.7744913425365,-24.144338822604,
2.63947868311684));
#247997=CARTESIAN_POINT('Ctrl Pts',(-53.8256450222191,-24.1165167429226,
2.6959506676787));
#247998=CARTESIAN_POINT('Ctrl Pts',(-53.9017956184507,-24.1232032230477,
2.68220539436042));
#247999=CARTESIAN_POINT('Ctrl Pts',(-53.7848917482046,-24.0595120258536,
2.59908178585046));
#248000=CARTESIAN_POINT('Ctrl Pts',(-53.8286685158642,-24.0529122166849,
2.65877670944823));
#248001=CARTESIAN_POINT('Ctrl Pts',(-53.8982652496121,-24.0696665464385,
2.65878198860244));
#248002=CARTESIAN_POINT('Ctrl Pts',(-53.8206887816834,-23.9791663275016,
2.59908173516006));
#248003=CARTESIAN_POINT('Ctrl Pts',(-53.8547645473079,-23.9943483786819,
2.65878198860244));
#248004=CARTESIAN_POINT('Ctrl Pts',(-53.9190682401993,-24.0229981225299,
2.65878198860244));
#248005=CARTESIAN_POINT('Origin',(-53.9190682401993,-24.0229981225299,2.53178198860244));
#248006=CARTESIAN_POINT('Ctrl Pts',(-56.649881012838,-24.8746050278055,
3.77003198860245));
#248007=CARTESIAN_POINT('Ctrl Pts',(-56.5981482837086,-24.9907986398445,
3.77003198860245));
#248008=CARTESIAN_POINT('Ctrl Pts',(-56.5982255167329,-24.9906251716318,
3.64284238727567));
#248009=CARTESIAN_POINT('Ctrl Pts',(-56.8481896769752,-24.9626539694732,
3.77003198860245));
#248010=CARTESIAN_POINT('Ctrl Pts',(-56.7965362315762,-25.0791271905735,
3.77025506105898));
#248011=CARTESIAN_POINT('Ctrl Pts',(-56.756741544354,-25.0612010539384,
3.64284210641817));
#248012=CARTESIAN_POINT('Ctrl Pts',(-57.0369754593333,-25.0464771582507,
3.65553527987811));
#248013=CARTESIAN_POINT('Ctrl Pts',(-56.9853490357224,-25.1631925873298,
3.65585996532915));
#248014=CARTESIAN_POINT('Ctrl Pts',(-56.9076460727639,-25.1283880784738,
3.55127902710193));
#248015=CARTESIAN_POINT('Ctrl Pts',(-57.1420619865019,-25.0931373005748,
3.47153072139054));
#248016=CARTESIAN_POINT('Ctrl Pts',(-57.0905332166518,-25.2100238867502,
3.47182327905171));
#248017=CARTESIAN_POINT('Ctrl Pts',(-56.9916465440539,-25.1657874977296,
3.40413028377963));
#248018=CARTESIAN_POINT('Origin',(-56.649881012838,-24.8746050278055,3.64303198860245));
#248019=CARTESIAN_POINT('Origin',(3.58382961824623E-16,1.91553576693918E-13,
2.53178198860262));
#248020=CARTESIAN_POINT('Origin',(-53.9314655730802,-23.995153256981,2.53178198860244));
#248021=CARTESIAN_POINT('Origin',(51.799563747336,23.4101986852084,3.64303198860279));
#248022=CARTESIAN_POINT('Origin',(-56.2832472948498,-24.7113125977909,3.64299466007597));
#248023=CARTESIAN_POINT('Ctrl Pts',(-53.8330634946836,-23.9513722670367,
2.59908173516006));
#248024=CARTESIAN_POINT('Ctrl Pts',(-53.8671470951729,-23.9665367208226,
2.65878198860245));
#248025=CARTESIAN_POINT('Ctrl Pts',(-53.9314655730802,-23.995153256981,
2.65878198860244));
#248026=CARTESIAN_POINT('Ctrl Pts',(-53.8686972660494,-23.8712821658119,
2.59908193199817));
#248027=CARTESIAN_POINT('Ctrl Pts',(-53.8931046959169,-23.9081865738546,
2.65877685806513));
#248028=CARTESIAN_POINT('Ctrl Pts',(-53.9521563342717,-23.9486256024595,
2.65878198860244));
#248029=CARTESIAN_POINT('Ctrl Pts',(-53.9240892607409,-23.8071866393156,
2.63872492669793));
#248030=CARTESIAN_POINT('Ctrl Pts',(-53.9378509529598,-23.8635355386145,
2.69532212015263));
#248031=CARTESIAN_POINT('Ctrl Pts',(-53.9937257232526,-23.915575084618,
2.68176836726614));
#248032=CARTESIAN_POINT('Ctrl Pts',(-54.0330064121712,-23.7392497560572,
2.75442176402219));
#248033=CARTESIAN_POINT('Ctrl Pts',(-54.0187512923758,-23.8300830854579,
2.7920317992011));
#248034=CARTESIAN_POINT('Ctrl Pts',(-54.0845104630311,-23.8883623535217,
2.7488531074816));
#248035=CARTESIAN_POINT('Ctrl Pts',(-54.086059454542,-23.7337507958622,
2.82866089558392));
#248036=CARTESIAN_POINT('Ctrl Pts',(-54.0553500291286,-23.8418399747428,
2.85316563119167));
#248037=CARTESIAN_POINT('Ctrl Pts',(-54.1330265677737,-23.8930480394869,
2.79189751796623));
#248038=CARTESIAN_POINT('Ctrl Pts',(-54.1275498658872,-23.752222950883,
2.90134173516006));
#248039=CARTESIAN_POINT('Ctrl Pts',(-54.0765745253534,-23.8679139708571,
2.90103711553212));
#248040=CARTESIAN_POINT('Ctrl Pts',(-54.1745185419758,-23.9115214566117,
2.83404198860244));
#248041=CARTESIAN_POINT('Origin',(-54.2261740956464,-23.7955011834911,2.83404198860245));
#248042=CARTESIAN_POINT('Origin',(-56.242823936856,-24.6933715410275,3.56647653971793));
#248043=CARTESIAN_POINT('Origin',(-56.1680608984276,-24.6600848917114,3.42473028058466));
#248044=CARTESIAN_POINT('Origin',(-54.3889216310586,-23.8679610547533,3.11913648168129));
#248045=CARTESIAN_POINT('Origin',(-54.5516691663893,-23.9404209259123,3.40423097483293));
#248046=CARTESIAN_POINT('Ctrl Pts',(-55.8666273273831,-24.5258780191674,
3.36123028058464));
#248047=CARTESIAN_POINT('Ctrl Pts',(-55.8149717737125,-24.641898292288,
3.36123028058463));
#248048=CARTESIAN_POINT('Ctrl Pts',(-55.8149717737125,-24.641898292288,
3.23423028058464));
#248049=CARTESIAN_POINT('Ctrl Pts',(-55.9487607347574,-24.5627025231282,
3.36123028058464));
#248050=CARTESIAN_POINT('Ctrl Pts',(-55.897123215877,-24.678474470879,3.36099641108452));
#248051=CARTESIAN_POINT('Ctrl Pts',(-55.9383132588146,-24.696813459544,
3.23423043688322));
#248052=CARTESIAN_POINT('Ctrl Pts',(-56.0264248009273,-24.5975211960728,
3.41054258905264));
#248053=CARTESIAN_POINT('Ctrl Pts',(-55.9751910510473,-24.7132325104972,
3.41008815825997));
#248054=CARTESIAN_POINT('Ctrl Pts',(-56.0549414076416,-24.7487396569162,
3.30819867304297));
#248055=CARTESIAN_POINT('Ctrl Pts',(-56.0673542004324,-24.6158705164596,
3.48823028058465));
#248056=CARTESIAN_POINT('Ctrl Pts',(-56.0163785451196,-24.7315703643338,
3.48794691941581));
#248057=CARTESIAN_POINT('Ctrl Pts',(-56.116405344757,-24.776105164832,3.42473028058466));
#248058=CARTESIAN_POINT('Origin',(-55.8666273273831,-24.5258780191674,3.23423028058464));
#248059=CARTESIAN_POINT('Ctrl Pts',(-54.4530463244691,-23.8971395307771,
3.47153072139055));
#248060=CARTESIAN_POINT('Ctrl Pts',(-54.401990736535,-24.0130054343462,
3.4712274628506));
#248061=CARTESIAN_POINT('Ctrl Pts',(-54.50016060885,-24.0565064908994,3.40413046676784));
#248062=CARTESIAN_POINT('Ctrl Pts',(-54.5581374230422,-23.9437939758161,
3.65553813457969));
#248063=CARTESIAN_POINT('Ctrl Pts',(-54.5068816478285,-24.0597061770699,
3.65520336072201));
#248064=CARTESIAN_POINT('Ctrl Pts',(-54.5841625982709,-24.0939065860612,
3.55128134519895));
#248065=CARTESIAN_POINT('Ctrl Pts',(-54.7469293531953,-24.0276077026094,
3.77003198860246));
#248066=CARTESIAN_POINT('Ctrl Pts',(-54.6954643138418,-24.1436691352835,
3.76980209314012));
#248067=CARTESIAN_POINT('Ctrl Pts',(-54.7350683949941,-24.161094175271,
3.64284195387423));
#248068=CARTESIAN_POINT('Ctrl Pts',(-54.9452378026827,-24.1156489724279,
3.77003198860246));
#248069=CARTESIAN_POINT('Ctrl Pts',(-54.8935048726349,-24.2318430357369,
3.77003198860246));
#248070=CARTESIAN_POINT('Ctrl Pts',(-54.8935823068775,-24.2316691155806,
3.64284189403811));
#248071=CARTESIAN_POINT('Origin',(-54.9452378026827,-24.1156489724279,3.64303198860245));
#248072=CARTESIAN_POINT('Origin',(50.541702139688,22.8501626153352,3.23423028058498));
#248073=CARTESIAN_POINT('Origin',(-55.7284918401496,-24.4643761377919,3.23423028058464));
#248074=CARTESIAN_POINT('Origin',(50.3447265545023,22.7624634345051,3.64303198860279));
#248075=CARTESIAN_POINT('Origin',(-55.3119205422643,-24.2788510342452,3.642991717218));
#248076=CARTESIAN_POINT('Ctrl Pts',(-55.5277679687681,-24.3743766270216,
3.48823028058463));
#248077=CARTESIAN_POINT('Ctrl Pts',(-55.4763362579872,-24.4911280468229,
3.48852004212241));
#248078=CARTESIAN_POINT('Ctrl Pts',(-55.3754026508173,-24.4461895095991,
3.42473028058463));
#248079=CARTESIAN_POINT('Ctrl Pts',(-55.5688345658074,-24.3927905570406,
3.41028005848388));
#248080=CARTESIAN_POINT('Ctrl Pts',(-55.5172331055236,-24.5093364964831,
3.41074404220487));
#248081=CARTESIAN_POINT('Ctrl Pts',(-55.4370743056943,-24.4736474994208,
3.30780486243963));
#248082=CARTESIAN_POINT('Ctrl Pts',(-55.6466353090192,-24.4276751358089,
3.36123028058464));
#248083=CARTESIAN_POINT('Ctrl Pts',(-55.5948055748745,-24.5438739850307,
3.36146460586237));
#248084=CARTESIAN_POINT('Ctrl Pts',(-55.5539102504896,-24.5256662135188,
3.23423045308347));
#248085=CARTESIAN_POINT('Ctrl Pts',(-55.7284918401496,-24.4643761377919,
3.36123028058464));
#248086=CARTESIAN_POINT('Ctrl Pts',(-55.676836286479,-24.5803964109126,
3.36123028058464));
#248087=CARTESIAN_POINT('Ctrl Pts',(-55.676836286479,-24.5803964109126,
3.23423028058464));
#248088=CARTESIAN_POINT('Origin',(-55.4270582044879,-24.3301692364785,3.42473028058463));
#248089=CARTESIAN_POINT('Origin',(-55.3527410377819,-24.2970811017172,3.56563113524668));
#248090=CARTESIAN_POINT('Origin',(-53.0360596835501,-30.9870007556522,3.56647653909445));
#248091=CARTESIAN_POINT('Origin',(-53.0743345559668,-31.0091584503696,3.64299466007742));
#248092=CARTESIAN_POINT('Origin',(-52.9651856060843,-30.9460815882871,3.42473028058462));
#248093=CARTESIAN_POINT('Ctrl Pts',(-52.8702215132213,-30.8905967158739,
3.48823028058461));
#248094=CARTESIAN_POINT('Ctrl Pts',(-52.9338619179793,-30.7813498801535,
3.48794691941577));
#248095=CARTESIAN_POINT('Ctrl Pts',(-53.0286856060843,-30.8360963620065,
3.42473028058462));
#248096=CARTESIAN_POINT('Ctrl Pts',(-52.8311874403352,-30.8681941459794,
3.41028005925063));
#248097=CARTESIAN_POINT('Ctrl Pts',(-52.8946849835383,-30.7587310665098,
3.40982512230992));
#248098=CARTESIAN_POINT('Ctrl Pts',(-52.9702219582405,-30.802342359186,
3.30780486372843));
#248099=CARTESIAN_POINT('Ctrl Pts',(-52.7572372522459,-30.8257530395509,
3.36123028058459));
#248100=CARTESIAN_POINT('Ctrl Pts',(-52.8205474253439,-30.7159277273265,
3.36099721048426));
#248101=CARTESIAN_POINT('Ctrl Pts',(-52.8594635164569,-30.7383959430072,
3.23423045308352));
#248102=CARTESIAN_POINT('Ctrl Pts',(-52.6794317578285,-30.7811015270746,
3.36123028058459));
#248103=CARTESIAN_POINT('Ctrl Pts',(-52.7429317578285,-30.671116300794,
3.36123028058459));
#248104=CARTESIAN_POINT('Ctrl Pts',(-52.7429317578285,-30.671116300794,
3.23423028058459));
#248105=CARTESIAN_POINT('Origin',(-52.6794317578285,-30.7811015270746,3.23423028058459));
#248106=CARTESIAN_POINT('Origin',(0.158750000000008,-0.274963065701374,
3.64303198860262));
#248107=CARTESIAN_POINT('Origin',(-53.4219427993284,-31.2097904767609,3.6430319886024));
#248108=CARTESIAN_POINT('Origin',(0.158750000000008,-0.274963065701371,
3.23423028058481));
#248109=CARTESIAN_POINT('Origin',(-52.5484816883957,-30.7054974692372,3.23423028058459));
#248110=CARTESIAN_POINT('Ctrl Pts',(-53.8880358395968,-31.4795232016792,
3.47153072139049));
#248111=CARTESIAN_POINT('Ctrl Pts',(-53.9523112176908,-31.369131349158,
3.4718232790264));
#248112=CARTESIAN_POINT('Ctrl Pts',(-53.858399113013,-31.3151318426939,
3.40413028959031));
#248113=CARTESIAN_POINT('Ctrl Pts',(-53.7885171709483,-31.4219316852007,
3.65553807120931));
#248114=CARTESIAN_POINT('Ctrl Pts',(-53.8525966788936,-31.3115614337838,
3.655862754969));
#248115=CARTESIAN_POINT('Ctrl Pts',(-53.7787668993573,-31.269156162554,
3.55128126837173));
#248116=CARTESIAN_POINT('Ctrl Pts',(-53.6097358757349,-31.3184699958134,
3.7700319886024));
#248117=CARTESIAN_POINT('Ctrl Pts',(-53.6736035436603,-31.2082202476924,
3.77025505748431));
#248118=CARTESIAN_POINT('Ctrl Pts',(-53.6357108652121,-31.1865627224613,
3.64284211731183));
#248119=CARTESIAN_POINT('Ctrl Pts',(-53.4219427993284,-31.2097904767609,
3.77003198860241));
#248120=CARTESIAN_POINT('Ctrl Pts',(-53.4855376653836,-31.0996409376526,
3.77003198860241));
#248121=CARTESIAN_POINT('Ctrl Pts',(-53.4854427285714,-31.0998053730349,
3.64284239821726));
#248122=CARTESIAN_POINT('Origin',(-53.7950387249976,-31.4251975098795,3.40423097483288));
#248123=CARTESIAN_POINT('Ctrl Pts',(-52.5484816883957,-30.7054974692372,
3.36123028058459));
#248124=CARTESIAN_POINT('Ctrl Pts',(-52.6119816883957,-30.5955122429565,
3.36123028058459));
#248125=CARTESIAN_POINT('Ctrl Pts',(-52.6119816883957,-30.5955122429565,
3.23423028058459));
#248126=CARTESIAN_POINT('Ctrl Pts',(-52.4704129317469,-30.6606955449592,
3.36123028058459));
#248127=CARTESIAN_POINT('Ctrl Pts',(-52.5339553345213,-30.5504637065434,
3.36146538610071));
#248128=CARTESIAN_POINT('Ctrl Pts',(-52.4950560684224,-30.5280052047898,
3.23423043688392));
#248129=CARTESIAN_POINT('Ctrl Pts',(-52.3965920780926,-30.6183335281981,
3.41054258693078));
#248130=CARTESIAN_POINT('Ctrl Pts',(-52.4605500011258,-30.5080831175488,
3.41100608859706));
#248131=CARTESIAN_POINT('Ctrl Pts',(-52.3844945583554,-30.4641724871906,
3.30819866970773));
#248132=CARTESIAN_POINT('Ctrl Pts',(-52.357688023316,-30.5960088312571,
3.48823028058459));
#248133=CARTESIAN_POINT('Ctrl Pts',(-52.4219111049554,-30.4857749404422,
3.48852004212237));
#248134=CARTESIAN_POINT('Ctrl Pts',(-52.3262277788839,-30.4305321463779,
3.42473028058459));
#248135=CARTESIAN_POINT('Origin',(-52.2627277788839,-30.5405173726585,3.42473028058459));
#248136=CARTESIAN_POINT('Origin',(-53.9493203812227,-31.5142720656061,3.1191364817832));
#248137=CARTESIAN_POINT('Origin',(-54.1036020372436,-31.6033466212668,2.83404198860239));
#248138=CARTESIAN_POINT('Origin',(-52.1922763801639,-30.4998422386361,3.56563113460743));
#248139=CARTESIAN_POINT('Origin',(-52.1535342613171,-30.4775331296743,3.64299171721718));
#248140=CARTESIAN_POINT('Ctrl Pts',(-54.5122556166608,-31.490293248291,
2.59908173516001));
#248141=CARTESIAN_POINT('Ctrl Pts',(-54.4799531854477,-31.4716329851992,
2.65878198860239));
#248142=CARTESIAN_POINT('Ctrl Pts',(-54.4189959163061,-31.4364195775138,
2.65878198860239));
#248143=CARTESIAN_POINT('Ctrl Pts',(-54.4681793099457,-31.5665926662618,
2.59908193475578));
#248144=CARTESIAN_POINT('Ctrl Pts',(-54.447844664727,-31.5272089901454,
2.65878715325339));
#248145=CARTESIAN_POINT('Ctrl Pts',(-54.3934750329619,-31.4805801312535,
2.65878198860239));
#248146=CARTESIAN_POINT('Ctrl Pts',(-54.4058464214485,-31.6244843104274,
2.63878778849827));
#248147=CARTESIAN_POINT('Ctrl Pts',(-54.3982481205271,-31.5668246399999,
2.69564460180128));
#248148=CARTESIAN_POINT('Ctrl Pts',(-54.3482630350909,-31.5088182930364,
2.68180481624867));
#248149=CARTESIAN_POINT('Ctrl Pts',(-54.2895863184074,-31.6805188761699,
2.75443238878644));
#248150=CARTESIAN_POINT('Ctrl Pts',(-54.313947642815,-31.5913182835554,
2.79268340777014));
#248151=CARTESIAN_POINT('Ctrl Pts',(-54.254463650534,-31.5259511417531,
2.7488592683558));
#248152=CARTESIAN_POINT('Ctrl Pts',(-54.2359839591649,-31.6804069909882,
2.82856655361631));
#248153=CARTESIAN_POINT('Ctrl Pts',(-54.2789047974503,-31.5756141966208,
2.85384197230784));
#248154=CARTESIAN_POINT('Ctrl Pts',(-54.2064835118363,-31.5160982999434,
2.79184624278431));
#248155=CARTESIAN_POINT('Ctrl Pts',(-54.1966007261205,-31.6576696180587,
2.90134173516001));
#248156=CARTESIAN_POINT('Ctrl Pts',(-54.260776142598,-31.5474441649286,
2.90163218716368));
#248157=CARTESIAN_POINT('Ctrl Pts',(-54.1671020372436,-31.4933613949861,
2.83404198860239));
#248158=CARTESIAN_POINT('Origin',(-54.4189959163061,-31.4364195775138,2.53178198860238));
#248159=CARTESIAN_POINT('Origin',(0.158750000000008,-0.274963065701374,
3.64303198860262));
#248160=CARTESIAN_POINT('Origin',(-51.8059703131944,-30.2768083268883,3.64303198860241));
#248161=CARTESIAN_POINT('Origin',(1.12590909550281E-16,1.9165987954201E-13,
2.53178198860262));
#248162=CARTESIAN_POINT('Origin',(-54.4342359163061,-31.4100231232064,2.53178198860239));
#248163=CARTESIAN_POINT('Ctrl Pts',(-51.8059703131944,-30.2768083268883,
3.77003198860241));
#248164=CARTESIAN_POINT('Ctrl Pts',(-51.8695654390618,-30.1666583377722,
3.77003198860241));
#248165=CARTESIAN_POINT('Ctrl Pts',(-51.8694702420496,-30.166823223834,
3.64284187937022));
#248166=CARTESIAN_POINT('Ctrl Pts',(-51.6181777324909,-30.1681210939099,
3.77003198860241));
#248167=CARTESIAN_POINT('Ctrl Pts',(-51.6818230251198,-30.0582657983055,
3.7698020896317));
#248168=CARTESIAN_POINT('Ctrl Pts',(-51.7191994478415,-30.0800643400498,
3.64284193928267));
#248169=CARTESIAN_POINT('Ctrl Pts',(-51.439403302349,-30.0646505034507,
3.65553535416564));
#248170=CARTESIAN_POINT('Ctrl Pts',(-51.5030508615839,-29.9550522173035,
3.65520057834208));
#248171=CARTESIAN_POINT('Ctrl Pts',(-51.576144478209,-29.997471514538,3.55127910964202));
#248172=CARTESIAN_POINT('Ctrl Pts',(-51.3398895692694,-30.007053683816,
3.47153072139049));
#248173=CARTESIAN_POINT('Ctrl Pts',(-51.4036173400344,-29.8976445635504,
3.47122746281559));
#248174=CARTESIAN_POINT('Ctrl Pts',(-51.4965132406189,-29.9514963979198,
3.40413045901249));
#248175=CARTESIAN_POINT('Origin',(-51.432874005494,-30.0614010732039,3.40423097483288));
#248176=CARTESIAN_POINT('Ctrl Pts',(-54.5146464769135,-31.1067982185537,
2.90134173516001));
#248177=CARTESIAN_POINT('Ctrl Pts',(-54.451276142598,-31.2174884860868,
2.90163218716369));
#248178=CARTESIAN_POINT('Ctrl Pts',(-54.3576020372436,-31.1634057161443,
2.83404198860239));
#248179=CARTESIAN_POINT('Ctrl Pts',(-54.5540471172212,-31.1295467523333,
2.82853349835327));
#248180=CARTESIAN_POINT('Ctrl Pts',(-54.4847554296815,-31.2191042733508,
2.85381483162341));
#248181=CARTESIAN_POINT('Ctrl Pts',(-54.3970014563935,-31.1861529813964,
2.79182701594247));
#248182=CARTESIAN_POINT('Ctrl Pts',(-54.5807851087094,-31.1758273123591,
2.75468822073627));
#248183=CARTESIAN_POINT('Ctrl Pts',(-54.5157207333386,-31.241605266785,
2.79286913083788));
#248184=CARTESIAN_POINT('Ctrl Pts',(-54.4293656242358,-31.2226915745263,
2.74900763297888));
#248185=CARTESIAN_POINT('Ctrl Pts',(-54.5905870683101,-31.3035520968884,
2.63954450640362));
#248186=CARTESIAN_POINT('Ctrl Pts',(-54.5367490446502,-31.3261415286133,
2.69627684028853));
#248187=CARTESIAN_POINT('Ctrl Pts',(-54.4614280312967,-31.3118587536637,
2.6822435603647));
#248188=CARTESIAN_POINT('Ctrl Pts',(-54.571706714292,-31.3872779850341,
2.59908178706265));
#248189=CARTESIAN_POINT('Ctrl Pts',(-54.5274095677421,-31.3893985541604,
2.658787043214));
#248190=CARTESIAN_POINT('Ctrl Pts',(-54.4598040608989,-31.3656949292516,
2.65878198860239));
#248191=CARTESIAN_POINT('Ctrl Pts',(-54.5275217339717,-31.4638515574743,
2.59908173516001));
#248192=CARTESIAN_POINT('Ctrl Pts',(-54.4952102564863,-31.4452069629856,
2.65878198860239));
#248193=CARTESIAN_POINT('Ctrl Pts',(-54.4342359163061,-31.4100231232064,
2.65878198860239));
#248194=CARTESIAN_POINT('Origin',(-54.4211020372436,-31.0534204898637,2.83404198860239));
#248195=CARTESIAN_POINT('Origin',(-51.2785921372155,-29.9723263949887,3.11913648167081));
#248196=CARTESIAN_POINT('Origin',(-51.1243102687782,-29.8832517167488,2.83404198860241));
#248197=CARTESIAN_POINT('Origin',(-54.2668203811882,-30.9643459342369,3.1191364817751));
#248198=CARTESIAN_POINT('Origin',(-54.1125387249976,-30.8752713784764,3.40423097483288));
#248199=CARTESIAN_POINT('Ctrl Pts',(-51.0313275753406,-29.8289013456888,
2.90134173516002));
#248200=CARTESIAN_POINT('Ctrl Pts',(-51.0949610231999,-29.7196599535395,
2.90103711553208));
#248201=CARTESIAN_POINT('Ctrl Pts',(-51.1878102687782,-29.7732664904682,
2.8340419886024));
#248202=CARTESIAN_POINT('Ctrl Pts',(-50.9919790793208,-29.8061828667728,
2.82862991747939));
#248203=CARTESIAN_POINT('Ctrl Pts',(-51.0613736255811,-29.7178139048422,
2.85314045886485));
#248204=CARTESIAN_POINT('Ctrl Pts',(-51.1484598763123,-29.7505475307853,
2.7918796100002));
#248205=CARTESIAN_POINT('Ctrl Pts',(-50.9654077681504,-29.7601395581529,
2.75470625793304));
#248206=CARTESIAN_POINT('Ctrl Pts',(-51.0305123301025,-29.6951292702709,
2.7922425038188));
#248207=CARTESIAN_POINT('Ctrl Pts',(-51.1163184807715,-29.7141562330556,
2.74901809108243));
#248208=CARTESIAN_POINT('Ctrl Pts',(-50.9561384187038,-29.6330385513049,
2.63947868311676));
#248209=CARTESIAN_POINT('Ctrl Pts',(-51.0099200724111,-29.6107158994149,
2.69595066767886));
#248210=CARTESIAN_POINT('Ctrl Pts',(-51.0849545802165,-29.6253256551033,
2.68220539436034));
#248211=CARTESIAN_POINT('Ctrl Pts',(-50.9753486645696,-29.5497635830446,
2.59908178585031));
#248212=CARTESIAN_POINT('Ctrl Pts',(-51.0195754864256,-29.5477758465712,
2.6587767094479));
#248213=CARTESIAN_POINT('Ctrl Pts',(-51.0870396576419,-29.5717132339806,
2.6587819886024));
#248214=CARTESIAN_POINT('Ctrl Pts',(-51.0193480105325,-29.473599835734,
2.59908173516002));
#248215=CARTESIAN_POINT('Ctrl Pts',(-51.0516501490683,-29.4922606054649,
2.65878198860241));
#248216=CARTESIAN_POINT('Ctrl Pts',(-51.1126068659044,-29.5274749692187,
2.65878198860241));
#248217=CARTESIAN_POINT('Origin',(-51.1126068659044,-29.5274749692187,2.5317819886024));
#248218=CARTESIAN_POINT('Ctrl Pts',(-53.7394427993284,-30.6598643453577,
3.77003198860241));
#248219=CARTESIAN_POINT('Ctrl Pts',(-53.6758479277942,-30.7700138939557,
3.77003198860241));
#248220=CARTESIAN_POINT('Ctrl Pts',(-53.6759428700935,-30.7698494490696,
3.64284238727575));
#248221=CARTESIAN_POINT('Ctrl Pts',(-53.9274614872879,-30.7681598456274,
3.77003198860241));
#248222=CARTESIAN_POINT('Ctrl Pts',(-53.8639162380511,-30.8785957589619,
3.77025506105773));
#248223=CARTESIAN_POINT('Ctrl Pts',(-53.8262133418081,-30.8566081460789,
3.64284210641871));
#248224=CARTESIAN_POINT('Ctrl Pts',(-54.1064511722692,-30.8712573299212,
3.6555352798781));
#248225=CARTESIAN_POINT('Ctrl Pts',(-54.0429074791724,-30.9819369489465,
3.65585996533168));
#248226=CARTESIAN_POINT('Ctrl Pts',(-53.9692682429961,-30.9392009315189,
3.55127902710165));
#248227=CARTESIAN_POINT('Ctrl Pts',(-54.2060847114739,-30.9286463962981,
3.4715307213905));
#248228=CARTESIAN_POINT('Ctrl Pts',(-54.1426202463871,-31.0395064423978,
3.47182327905166));
#248229=CARTESIAN_POINT('Ctrl Pts',(-54.0488992470932,-30.9851759130206,
3.40413028377964));
#248230=CARTESIAN_POINT('Origin',(-53.7394427993284,-30.6598643453577,3.64303198860241));
#248231=CARTESIAN_POINT('Origin',(3.61170357355341E-16,1.91548106122166E-13,
2.53178198860262));
#248232=CARTESIAN_POINT('Origin',(-51.1278468659044,-29.5010785149114,2.53178198860241));
#248233=CARTESIAN_POINT('Origin',(46.5080917980719,27.2180767400487,3.64303198860282));
#248234=CARTESIAN_POINT('Origin',(-53.3918862459814,-30.4591427892374,3.64299466007567));
#248235=CARTESIAN_POINT('Ctrl Pts',(-51.0345602039884,-29.4472515437738,
2.59908173516002));
#248236=CARTESIAN_POINT('Ctrl Pts',(-51.0668719738975,-29.465895631477,
2.65878198860241));
#248237=CARTESIAN_POINT('Ctrl Pts',(-51.1278468659044,-29.5010785149114,
2.65878198860241));
#248238=CARTESIAN_POINT('Ctrl Pts',(-51.0783704650301,-29.3713249278647,
2.59908193199787));
#248239=CARTESIAN_POINT('Ctrl Pts',(-51.0987866273839,-29.410578440836,
2.65877685806612));
#248240=CARTESIAN_POINT('Ctrl Pts',(-51.1532877451685,-29.4569685172213,
2.6587819886024));
#248241=CARTESIAN_POINT('Ctrl Pts',(-51.140158823466,-29.3133705634514,
2.63872492669767));
#248242=CARTESIAN_POINT('Ctrl Pts',(-51.1479550638444,-29.3708492661236,
2.69532212015257));
#248243=CARTESIAN_POINT('Ctrl Pts',(-51.1980841325264,-29.4284442379233,
2.68176836726614));
#248244=CARTESIAN_POINT('Ctrl Pts',(-51.2555806533509,-29.2571907880104,
2.75442176402237));
#248245=CARTESIAN_POINT('Ctrl Pts',(-51.2319089562576,-29.3460364571628,
2.79203179920106));
#248246=CARTESIAN_POINT('Ctrl Pts',(-51.2912160489644,-29.4108701703526,
2.74885310748152));
#248247=CARTESIAN_POINT('Ctrl Pts',(-51.3089178634634,-29.2572675046851,
2.82866089558372));
#248248=CARTESIAN_POINT('Ctrl Pts',(-51.2670782717316,-29.361554550688,
2.85316563119145));
#248249=CARTESIAN_POINT('Ctrl Pts',(-51.3389765898555,-29.4206015015121,
2.79189751796623));
#248250=CARTESIAN_POINT('Ctrl Pts',(-51.3482501200163,-29.2799753962465,
2.90134173516001));
#248251=CARTESIAN_POINT('Ctrl Pts',(-51.2854610231999,-29.3897042746976,
2.90103711553208));
#248252=CARTESIAN_POINT('Ctrl Pts',(-51.3783102687782,-29.4433108116264,
2.8340419886024));
#248253=CARTESIAN_POINT('Origin',(-51.4418102687782,-29.3333255853457,2.8340419886024));
#248254=CARTESIAN_POINT('Origin',(-53.3535596824664,-30.4370746239676,3.56647653971759));
#248255=CARTESIAN_POINT('Origin',(-53.2826856060843,-30.396155456884,3.42473028058463));
#248256=CARTESIAN_POINT('Origin',(-51.5960921371733,-29.4224002636277,3.11913648168053));
#248257=CARTESIAN_POINT('Origin',(-51.750374005494,-29.5114749418008,3.4042309748329));
#248258=CARTESIAN_POINT('Ctrl Pts',(-52.9969317578285,-30.2311753956715,
3.3612302805846));
#248259=CARTESIAN_POINT('Ctrl Pts',(-52.9334317578285,-30.3411606219521,
3.3612302805846));
#248260=CARTESIAN_POINT('Ctrl Pts',(-52.9334317578285,-30.3411606219521,
3.23423028058459));
#248261=CARTESIAN_POINT('Ctrl Pts',(-53.0747660209934,-30.276383450003,
3.36123028058459));
#248262=CARTESIAN_POINT('Ctrl Pts',(-53.0113099140563,-30.3861235964148,
3.36099641108464));
#248263=CARTESIAN_POINT('Ctrl Pts',(-53.0503573673265,-30.4086676540709,
3.23423043688365));
#248264=CARTESIAN_POINT('Ctrl Pts',(-53.1483650929069,-30.3191294881018,
3.41054258905263));
#248265=CARTESIAN_POINT('Ctrl Pts',(-53.0853168809897,-30.4288515386974,
3.41008815825976));
#248266=CARTESIAN_POINT('Ctrl Pts',(-53.1609188493365,-30.4725003554714,
3.30819867304261));
#248267=CARTESIAN_POINT('Ctrl Pts',(-53.1871522506172,-30.3416565762239,
3.48823028058462));
#248268=CARTESIAN_POINT('Ctrl Pts',(-53.1243619179793,-30.4513942013116,
3.48794691941578));
#248269=CARTESIAN_POINT('Ctrl Pts',(-53.2191856060843,-30.5061406831646,
3.42473028058463));
#248270=CARTESIAN_POINT('Origin',(-52.9969317578285,-30.2311753956715,3.2342302805846));
#248271=CARTESIAN_POINT('Ctrl Pts',(-51.6568155675425,-29.4581217525676,
3.47153072139052));
#248272=CARTESIAN_POINT('Ctrl Pts',(-51.5939283826159,-29.5680161684459,
3.47122746285056));
#248273=CARTESIAN_POINT('Ctrl Pts',(-51.6870133715069,-29.6215404675519,
3.4041304667677));
#248274=CARTESIAN_POINT('Ctrl Pts',(-51.7564542486362,-29.5155056307139,
3.65553813457966));
#248275=CARTESIAN_POINT('Ctrl Pts',(-51.6933631336501,-29.6254251653841,
3.65520336072067));
#248276=CARTESIAN_POINT('Ctrl Pts',(-51.7666458147667,-29.6675162799447,
3.55128134519894));
#248277=CARTESIAN_POINT('Ctrl Pts',(-51.9354510367809,-29.6185943474766,
3.77003198860242));
#248278=CARTESIAN_POINT('Ctrl Pts',(-51.8721362050963,-29.7286404220041,
3.76980209314217));
#248279=CARTESIAN_POINT('Ctrl Pts',(-51.9097019182957,-29.7501097595407,
3.64284195387388));
#248280=CARTESIAN_POINT('Ctrl Pts',(-52.1234703131944,-29.7268821954852,
3.77003198860242));
#248281=CARTESIAN_POINT('Ctrl Pts',(-52.0598751946718,-29.8370321718797,
3.77003198860241));
#248282=CARTESIAN_POINT('Ctrl Pts',(-52.0599703843282,-29.8368672985585,
3.64284189403787));
#248283=CARTESIAN_POINT('Origin',(-52.1234703131944,-29.7268821954852,3.64303198860241));
#248284=CARTESIAN_POINT('Origin',(45.3776874999996,26.5654375142636,3.234230280585));
#248285=CARTESIAN_POINT('Origin',(-52.8659816883957,-30.155571337834,3.2342302805846));
#248286=CARTESIAN_POINT('Origin',(45.2006711678726,26.4632370872591,3.64303198860282));
#248287=CARTESIAN_POINT('Origin',(-52.4710850656381,-29.9275190026066,3.64299171721771));
#248288=CARTESIAN_POINT('Ctrl Pts',(-52.6757649139393,-30.0450834959839,
3.4882302805846));
#248289=CARTESIAN_POINT('Ctrl Pts',(-52.6124111049554,-30.1558192616004,
3.48852004212237));
#248290=CARTESIAN_POINT('Ctrl Pts',(-52.5167277788839,-30.100576467536,
3.42473028058459));
#248291=CARTESIAN_POINT('Ctrl Pts',(-52.7146817640548,-30.067689180849,
3.41028005848386));
#248292=CARTESIAN_POINT('Ctrl Pts',(-52.6511806140149,-30.1782028480951,
3.41074404220263));
#248293=CARTESIAN_POINT('Ctrl Pts',(-52.575191448499,-30.1343304829261,
3.30780486243823));
#248294=CARTESIAN_POINT('Ctrl Pts',(-52.7884098752459,-30.1105150503713,
3.36123028058459));
#248295=CARTESIAN_POINT('Ctrl Pts',(-52.7247179826676,-30.2206596676793,
3.36146460586396));
#248296=CARTESIAN_POINT('Ctrl Pts',(-52.6859499175236,-30.1982769148326,
3.23423045308398));
#248297=CARTESIAN_POINT('Ctrl Pts',(-52.8659816883957,-30.155571337834,
3.3612302805846));
#248298=CARTESIAN_POINT('Ctrl Pts',(-52.8024816883957,-30.2655565641147,
3.3612302805846));
#248299=CARTESIAN_POINT('Ctrl Pts',(-52.8024816883957,-30.2655565641147,
3.23423028058459));
#248300=CARTESIAN_POINT('Origin',(-52.5802277788839,-29.9905912412554,3.42473028058459));
#248301=CARTESIAN_POINT('Origin',(-52.5097763812716,-29.949916107531,3.5656311352473));
#248302=CARTESIAN_POINT('Origin',(-49.5064990290868,-36.3610285397831,3.56647653909432));
#248303=CARTESIAN_POINT('Origin',(-49.5422481179701,-36.3870656659254,3.64299466007706));
#248304=CARTESIAN_POINT('Origin',(-49.4402904249163,-36.3129251734945,3.42473028058458));
#248305=CARTESIAN_POINT('Ctrl Pts',(-49.3516463037382,-36.2478178023253,
3.48823028058457));
#248306=CARTESIAN_POINT('Ctrl Pts',(-49.4263574835548,-36.1458216659127,
3.48794691941574));
#248307=CARTESIAN_POINT('Ctrl Pts',(-49.5149391519574,-36.2101800152089,
3.42473028058459));
#248308=CARTESIAN_POINT('Ctrl Pts',(-49.3151677697923,-36.2214577843982,
3.4102800592506));
#248309=CARTESIAN_POINT('Ctrl Pts',(-49.3897594742869,-36.1192316557419,
3.40982512231162));
#248310=CARTESIAN_POINT('Ctrl Pts',(-49.4603240281359,-36.1704998050803,
3.30780486372868));
#248311=CARTESIAN_POINT('Ctrl Pts',(-49.2460589922059,-36.1715192752712,
3.36123028058456));
#248312=CARTESIAN_POINT('Ctrl Pts',(-49.3205022166689,-36.0689133127038,
3.36099721048352));
#248313=CARTESIAN_POINT('Ctrl Pts',(-49.3568565533029,-36.0953262843488,
3.23423045308384));
#248314=CARTESIAN_POINT('Ctrl Pts',(-49.1733470784084,-36.1189794796885,
3.36123028058455));
#248315=CARTESIAN_POINT('Ctrl Pts',(-49.2479958054496,-36.0162343214029,
3.36123028058456));
#248316=CARTESIAN_POINT('Ctrl Pts',(-49.2479958054496,-36.0162343214029,
3.23423028058455));
#248317=CARTESIAN_POINT('Origin',(-49.1733470784084,-36.1189794796885,3.23423028058455));
#248318=CARTESIAN_POINT('Origin',(0.186621817602868,-0.25686289571386,3.64303198860262));
#248319=CARTESIAN_POINT('Origin',(-49.8669803696023,-36.6229335645812,3.64303198860236));
#248320=CARTESIAN_POINT('Origin',(0.186621817602868,-0.256862895713858,
3.23423028058481));
#248321=CARTESIAN_POINT('Origin',(-49.05101714314,-36.0301015792679,3.23423028058455));
#248322=CARTESIAN_POINT('Ctrl Pts',(-50.3023253561992,-36.9399086546489,
3.47153072139045));
#248323=CARTESIAN_POINT('Ctrl Pts',(-50.3777877177481,-36.8368401467444,
3.47182327902636));
#248324=CARTESIAN_POINT('Ctrl Pts',(-50.2900345588339,-36.7733199672426,
3.40413028959031));
#248325=CARTESIAN_POINT('Ctrl Pts',(-50.2093718139428,-36.8722300970264,
3.65553807120931));
#248326=CARTESIAN_POINT('Ctrl Pts',(-50.2846371204117,-36.7691625978869,
3.6558627549694));
#248327=CARTESIAN_POINT('Ctrl Pts',(-50.2156443459698,-36.7192723137692,
3.55128126837172));
#248328=CARTESIAN_POINT('Ctrl Pts',(-50.0423845927721,-36.7506474475458,
3.77003198860237));
#248329=CARTESIAN_POINT('Ctrl Pts',(-50.1174266236762,-36.6476776482608,
3.77025505748412));
#248330=CARTESIAN_POINT('Ctrl Pts',(-50.0820053531159,-36.6221779017723,
3.64284211731208));
#248331=CARTESIAN_POINT('Ctrl Pts',(-49.8669803696023,-36.6229335645812,
3.77003198860237));
#248332=CARTESIAN_POINT('Ctrl Pts',(-49.9417406183798,-36.5200349097938,
3.77003198860237));
#248333=CARTESIAN_POINT('Ctrl Pts',(-49.9416290134636,-36.5201885207827,
3.64284239821728));
#248334=CARTESIAN_POINT('Origin',(-50.2155162706041,-36.8761597191957,3.40423097483284));
#248335=CARTESIAN_POINT('Ctrl Pts',(-49.05101714314,-36.0301015792679,3.36123028058455));
#248336=CARTESIAN_POINT('Ctrl Pts',(-49.1256658701812,-35.9273564209823,
3.36123028058456));
#248337=CARTESIAN_POINT('Ctrl Pts',(-49.1256658701812,-35.9273564209823,
3.23423028058455));
#248338=CARTESIAN_POINT('Ctrl Pts',(-48.9780591316062,-35.9773846774553,
3.36123028058455));
#248339=CARTESIAN_POINT('Ctrl Pts',(-49.0527758071231,-35.8743986902983,
3.36146538610146));
#248340=CARTESIAN_POINT('Ctrl Pts',(-49.0164371879478,-35.8479971380617,
3.23423043688415));
#248341=CARTESIAN_POINT('Ctrl Pts',(-48.9090707128238,-35.9275383438667,
3.41054258693074));
#248342=CARTESIAN_POINT('Ctrl Pts',(-48.9842025736633,-35.824577319909,
3.41100608859626));
#248343=CARTESIAN_POINT('Ctrl Pts',(-48.9131536812776,-35.7729572780243,
3.30819866970743));
#248344=CARTESIAN_POINT('Ctrl Pts',(-48.872713344794,-35.9012693628907,
3.48823028058455));
#248345=CARTESIAN_POINT('Ctrl Pts',(-48.9481071848794,-35.7983524848938,
3.48852004212234));
#248346=CARTESIAN_POINT('Ctrl Pts',(-48.8587224664497,-35.7334106856009,
3.42473028058455));
#248347=CARTESIAN_POINT('Origin',(-48.7840737394086,-35.8361558438865,3.42473028058455));
#248348=CARTESIAN_POINT('Origin',(-50.3596419293477,-36.9808731396205,3.11913648178297));
#248349=CARTESIAN_POINT('Origin',(-50.5037675878942,-37.0855865599605,2.83404198860235));
#248350=CARTESIAN_POINT('Origin',(-48.7182599900757,-35.7883393560614,3.56563113460791));
#248351=CARTESIAN_POINT('Origin',(-48.682062041486,-35.7621028045853,3.64299171721765));
#248352=CARTESIAN_POINT('Ctrl Pts',(-50.9219998155897,-37.0158684358562,
2.59908173515997));
#248353=CARTESIAN_POINT('Ctrl Pts',(-50.8918248690997,-36.9939338721435,
2.65878198860235));
#248354=CARTESIAN_POINT('Ctrl Pts',(-50.8348823336483,-36.9525415975214,
2.65878198860235));
#248355=CARTESIAN_POINT('Ctrl Pts',(-50.870189502586,-37.0871426490245,
2.5990819347554));
#248356=CARTESIAN_POINT('Ctrl Pts',(-50.8540829678243,-37.0458491715915,
2.65878715325316));
#248357=CARTESIAN_POINT('Ctrl Pts',(-50.8048852215546,-36.9937925764105,
2.65878198860235));
#248358=CARTESIAN_POINT('Ctrl Pts',(-50.8021467555728,-37.1382015956605,
2.63878778849862));
#248359=CARTESIAN_POINT('Ctrl Pts',(-50.8006171556812,-37.0800635522218,
2.69564460180089));
#248360=CARTESIAN_POINT('Ctrl Pts',(-50.7569692080808,-37.0171501059292,
2.68180481624872));
#248361=CARTESIAN_POINT('Ctrl Pts',(-50.6806663304944,-37.1817767082786,
2.754432388786));
#248362=CARTESIAN_POINT('Ctrl Pts',(-50.7142182018863,-37.0956112176472,
2.79268340777063));
#248363=CARTESIAN_POINT('Ctrl Pts',(-50.66189279602,-37.0243843935852,2.74885926835567));
#248364=CARTESIAN_POINT('Ctrl Pts',(-50.6273693057702,-37.1760624637761,
2.82856655361656));
#248365=CARTESIAN_POINT('Ctrl Pts',(-50.6810088489707,-37.0763301845679,
2.8538419723071));
#248366=CARTESIAN_POINT('Ctrl Pts',(-50.6152053999547,-37.0095702365079,
2.79184624278423));
#248367=CARTESIAN_POINT('Ctrl Pts',(-50.5905785208481,-37.1493329797263,
2.90134173515997));
#248368=CARTESIAN_POINT('Ctrl Pts',(-50.665924074908,-37.0464195108255,
2.90163218716364));
#248369=CARTESIAN_POINT('Ctrl Pts',(-50.5784163149354,-36.9828414016749,
2.83404198860235));
#248370=CARTESIAN_POINT('Origin',(-50.8348823336483,-36.9525415975214,2.53178198860235));
#248371=CARTESIAN_POINT('Origin',(0.186621817602868,-0.25686289571386,3.64303198860262));
#248372=CARTESIAN_POINT('Origin',(-48.3573835402116,-35.5261472678868,3.64303198860237));
#248373=CARTESIAN_POINT('Origin',(1.03190816135906E-16,1.91674354416515E-13,
2.53178198860262));
#248374=CARTESIAN_POINT('Origin',(-50.8527980281382,-36.9278827595329,2.53178198860235));
#248375=CARTESIAN_POINT('Ctrl Pts',(-48.3573835402116,-35.5261472678868,
3.77003198860238));
#248376=CARTESIAN_POINT('Ctrl Pts',(-48.4321440944168,-35.4232481927144,
3.77003198860238));
#248377=CARTESIAN_POINT('Ctrl Pts',(-48.4320321836171,-35.4234022247158,
3.64284187937009));
#248378=CARTESIAN_POINT('Ctrl Pts',(-48.1819806163558,-35.3984257650668,
3.77003198860238));
#248379=CARTESIAN_POINT('Ctrl Pts',(-48.2567602586449,-35.2958250128988,
3.76980208962771));
#248380=CARTESIAN_POINT('Ctrl Pts',(-48.2916533613408,-35.3214110399831,
3.64284193928205));
#248381=CARTESIAN_POINT('Ctrl Pts',(-48.0150011530604,-35.2768349808759,
3.65553535416558));
#248382=CARTESIAN_POINT('Ctrl Pts',(-48.0897561847331,-35.1744900671645,
3.65520057834544));
#248383=CARTESIAN_POINT('Ctrl Pts',(-48.1580153629248,-35.2243173504706,
3.55127910964284));
#248384=CARTESIAN_POINT('Ctrl Pts',(-47.9220530736684,-35.209151665053,
3.47153072139047));
#248385=CARTESIAN_POINT('Ctrl Pts',(-47.996868104246,-35.1070032653413,
3.47122746281558));
#248386=CARTESIAN_POINT('Ctrl Pts',(-48.0836260618765,-35.1702703594596,
3.40413045901242));
#248387=CARTESIAN_POINT('Origin',(-48.0088472823269,-35.2729208539817,3.40423097483285));
#248388=CARTESIAN_POINT('Ctrl Pts',(-50.964463724589,-36.6347241449657,
2.90134173515998));
#248389=CARTESIAN_POINT('Ctrl Pts',(-50.8898702560315,-36.7381840359687,
2.90163218716365));
#248390=CARTESIAN_POINT('Ctrl Pts',(-50.8023624960588,-36.674605926818,
2.83404198860236));
#248391=CARTESIAN_POINT('Ctrl Pts',(-51.001270654789,-36.6614665482798,
2.82853349835328));
#248392=CARTESIAN_POINT('Ctrl Pts',(-50.9229972443165,-36.7432905102097,
2.85381483162211));
#248393=CARTESIAN_POINT('Ctrl Pts',(-50.8391683443876,-36.7013469409082,
2.79182701594226));
#248394=CARTESIAN_POINT('Ctrl Pts',(-51.0230245369434,-36.7102884597169,
2.75468822073616));
#248395=CARTESIAN_POINT('Ctrl Pts',(-50.9514409225354,-36.768904996455,
2.79286913083798));
#248396=CARTESIAN_POINT('Ctrl Pts',(-50.8675358949429,-36.7410683485316,
2.74900763297898));
#248397=CARTESIAN_POINT('Ctrl Pts',(-51.0194219249358,-36.8383381382863,
2.63954450640366));
#248398=CARTESIAN_POINT('Ctrl Pts',(-50.9635175930187,-36.8551762168621,
2.69627684028837));
#248399=CARTESIAN_POINT('Ctrl Pts',(-50.8901021525733,-36.8330984946705,
2.68224356036453));
#248400=CARTESIAN_POINT('Ctrl Pts',(-50.9918932610483,-36.9196318328647,
2.59908178706376));
#248401=CARTESIAN_POINT('Ctrl Pts',(-50.9476171190685,-36.9171104726345,
2.65878704321395));
#248402=CARTESIAN_POINT('Ctrl Pts',(-50.8828596657519,-36.8864699989246,
2.65878198860235));
#248403=CARTESIAN_POINT('Ctrl Pts',(-50.9399462128199,-36.991167339171,
2.59908173515997));
#248404=CARTESIAN_POINT('Ctrl Pts',(-50.9097606317991,-36.9692474126343,
2.65878198860235));
#248405=CARTESIAN_POINT('Ctrl Pts',(-50.8527980281382,-36.9278827595329,
2.65878198860235));
#248406=CARTESIAN_POINT('Origin',(-50.8770112230999,-36.5718607685324,2.83404198860236));
#248407=CARTESIAN_POINT('Origin',(-47.8647214254959,-35.1682072895723,3.11913648167072));
#248408=CARTESIAN_POINT('Origin',(-47.7205955685088,-35.0634937251224,2.83404198860236));
#248409=CARTESIAN_POINT('Origin',(-50.7328855645158,-36.4671473482183,3.11913648177345));
#248410=CARTESIAN_POINT('Origin',(-50.5887599058098,-36.3624339277676,3.40423097483284));
#248411=CARTESIAN_POINT('Ctrl Pts',(-47.6338034047597,-34.9997217530262,
2.90134173515998));
#248412=CARTESIAN_POINT('Ctrl Pts',(-47.7085070967801,-34.8977303031704,
2.90103711553204));
#248413=CARTESIAN_POINT('Ctrl Pts',(-47.7952442955499,-34.9607485668368,
2.83404198860236));
#248414=CARTESIAN_POINT('Ctrl Pts',(-47.5970451916072,-34.9730146904937,
2.82862991747933));
#248415=CARTESIAN_POINT('Ctrl Pts',(-47.6752966590729,-34.8923835282615,
2.85314045886504));
#248416=CARTESIAN_POINT('Ctrl Pts',(-47.7584842465943,-34.9340408279389,
2.7918796099996));
#248417=CARTESIAN_POINT('Ctrl Pts',(-47.5754322771533,-34.9244461536125,
2.75470625793305));
#248418=CARTESIAN_POINT('Ctrl Pts',(-47.6469756149924,-34.8665972787024,
2.79224250381856));
#248419=CARTESIAN_POINT('Ctrl Pts',(-47.7303228514092,-34.8944891948624,
2.74901809108221));
#248420=CARTESIAN_POINT('Ctrl Pts',(-47.5794993790982,-34.797072508526,
2.63947868311669));
#248421=CARTESIAN_POINT('Ctrl Pts',(-47.635319763777,-34.7804938560724,
2.69595066767899));
#248422=CARTESIAN_POINT('Ctrl Pts',(-47.708416089387,-34.8028668197835,
2.68220539436048));
#248423=CARTESIAN_POINT('Ctrl Pts',(-47.6073089936882,-34.716261746734,
2.59908178585007));
#248424=CARTESIAN_POINT('Ctrl Pts',(-47.6515013114247,-34.7189078610122,
2.65877670944894));
#248425=CARTESIAN_POINT('Ctrl Pts',(-47.7160937685324,-34.7497660430522,
2.65878198860237));
#248426=CARTESIAN_POINT('Ctrl Pts',(-47.6590285860933,-34.6451144164188,
2.59908173515998));
#248427=CARTESIAN_POINT('Ctrl Pts',(-47.689203188551,-34.667049453402,2.65878198860237));
#248428=CARTESIAN_POINT('Ctrl Pts',(-47.7461450747862,-34.7084426211234,
2.65878198860237));
#248429=CARTESIAN_POINT('Origin',(-47.7461450747862,-34.7084426211234,2.53178198860237));
#248430=CARTESIAN_POINT('Ctrl Pts',(-50.240224004808,-36.1092077731531,
3.77003198860237));
#248431=CARTESIAN_POINT('Ctrl Pts',(-50.1654637495897,-36.2121064368053,
3.77003198860237));
#248432=CARTESIAN_POINT('Ctrl Pts',(-50.1655753609562,-36.2119528169383,
3.64284238727604));
#248433=CARTESIAN_POINT('Ctrl Pts',(-50.4158927445031,-36.2365633238551,
3.77003198860237));
#248434=CARTESIAN_POINT('Ctrl Pts',(-50.3411519064815,-36.3397519704547,
3.77025506105981));
#248435=CARTESIAN_POINT('Ctrl Pts',(-50.3059538820319,-36.3139437822118,
3.64284210641911));
#248436=CARTESIAN_POINT('Ctrl Pts',(-50.5831252836602,-36.357805546057,
3.65553527987808));
#248437=CARTESIAN_POINT('Ctrl Pts',(-50.5083605190661,-36.4612367259577,
3.65585996532878));
#248438=CARTESIAN_POINT('Ctrl Pts',(-50.4395918165605,-36.4110374247129,
3.55127902710112));
#248439=CARTESIAN_POINT('Ctrl Pts',(-50.6762142289945,-36.4252947698681,
3.47153072139046));
#248440=CARTESIAN_POINT('Ctrl Pts',(-50.6015093986315,-36.5289136700279,
3.47182327905162));
#248441=CARTESIAN_POINT('Ctrl Pts',(-50.5139808995222,-36.4650842569436,
3.40413028377978));
#248442=CARTESIAN_POINT('Origin',(-50.240224004808,-36.1092077731531,3.64303198860237));
#248443=CARTESIAN_POINT('Origin',(3.64514313700083E-16,1.9154295688095E-13,
2.53178198860262));
#248444=CARTESIAN_POINT('Origin',(-47.764060769276,-34.6837837831348,2.53178198860237));
#248445=CARTESIAN_POINT('Origin',(40.5385041740525,29.8453988870289,3.64303198860284));
#248446=CARTESIAN_POINT('Origin',(-49.9155525184304,-35.873256238299,3.64299466007745));
#248447=CARTESIAN_POINT('Ctrl Pts',(-47.6769115920301,-34.6205005703637,
2.59908173515998));
#248448=CARTESIAN_POINT('Ctrl Pts',(-47.7070975168461,-34.6424200234577,
2.65878198860237));
#248449=CARTESIAN_POINT('Ctrl Pts',(-47.764060769276,-34.6837837831348,
2.65878198860237));
#248450=CARTESIAN_POINT('Ctrl Pts',(-47.7284183483604,-34.5495693076632,
2.59908193199868));
#248451=CARTESIAN_POINT('Ctrl Pts',(-47.7446195594529,-34.5907418558606,
2.65877685806676));
#248452=CARTESIAN_POINT('Ctrl Pts',(-47.7939730310152,-34.6425747206414,
2.65878198860237));
#248453=CARTESIAN_POINT('Ctrl Pts',(-47.7959261043552,-34.4983910654769,
2.63872492669783));
#248454=CARTESIAN_POINT('Ctrl Pts',(-47.7976714756521,-34.5563698228278,
2.69532212015247));
#248455=CARTESIAN_POINT('Ctrl Pts',(-47.8415056181565,-34.61888919786,2.6817683672662));
#248456=CARTESIAN_POINT('Ctrl Pts',(-47.9165880269726,-34.4545839152293,
2.75442176402215));
#248457=CARTESIAN_POINT('Ctrl Pts',(-47.8837591046484,-34.5404685123898,
2.79203179920117));
#248458=CARTESIAN_POINT('Ctrl Pts',(-47.9359643384883,-34.6111463389769,
2.7488531074814));
#248459=CARTESIAN_POINT('Ctrl Pts',(-47.9696250311914,-34.4602354682501,
2.82866089558383));
#248460=CARTESIAN_POINT('Ctrl Pts',(-47.9171136764632,-34.5595777906765,
2.85316563119103));
#248461=CARTESIAN_POINT('Ctrl Pts',(-47.982446041048,-34.6258166968305,
2.79189751796547));
#248462=CARTESIAN_POINT('Ctrl Pts',(-48.0063682005184,-34.4869303039399,
2.90134173515999));
#248463=CARTESIAN_POINT('Ctrl Pts',(-47.9324532779035,-34.5894948283136,
2.90103711553205));
#248464=CARTESIAN_POINT('Ctrl Pts',(-48.0191904766733,-34.6525130919799,
2.83404198860237));
#248465=CARTESIAN_POINT('Origin',(-48.0938392037145,-34.5497679336943,2.83404198860238));
#248466=CARTESIAN_POINT('Origin',(-49.8797426632452,-35.8473027479617,3.56647653971698));
#248467=CARTESIAN_POINT('Origin',(-49.813534060122,-35.7991993820664,3.4247302805846));
#248468=CARTESIAN_POINT('Origin',(-48.2379650606552,-34.6544814981795,3.11913648168121));
#248469=CARTESIAN_POINT('Origin',(-48.3820909175326,-34.7591950625536,3.40423097483285));
#248470=CARTESIAN_POINT('Ctrl Pts',(-49.5465907136142,-35.6052536882604,
3.36123028058456));
#248471=CARTESIAN_POINT('Ctrl Pts',(-49.471941986573,-35.7079988465461,
3.36123028058455));
#248472=CARTESIAN_POINT('Ctrl Pts',(-49.471941986573,-35.7079988465461,
3.23423028058456));
#248473=CARTESIAN_POINT('Ctrl Pts',(-49.6192730640972,-35.6583499840553,
3.36123028058456));
#248474=CARTESIAN_POINT('Ctrl Pts',(-49.5446936074932,-35.7608559931208,
3.36099641108516));
#248475=CARTESIAN_POINT('Ctrl Pts',(-49.5811706590218,-35.7873581223577,
3.23423043688376));
#248476=CARTESIAN_POINT('Ctrl Pts',(-49.688000774921,-35.7085550527694,
3.41054258905262));
#248477=CARTESIAN_POINT('Ctrl Pts',(-49.6138288703661,-35.8110857017866,
3.41008815826032));
#248478=CARTESIAN_POINT('Ctrl Pts',(-49.6844541394795,-35.8623979633506,
3.30819867304285));
#248479=CARTESIAN_POINT('Ctrl Pts',(-49.7242207306172,-35.7350130971392,
3.48823028058459));
#248480=CARTESIAN_POINT('Ctrl Pts',(-49.6503036646782,-35.8375861910559,
3.48794691941575));
#248481=CARTESIAN_POINT('Ctrl Pts',(-49.7388853330808,-35.9019445403521,
3.4247302805846));
#248482=CARTESIAN_POINT('Origin',(-49.5465907136142,-35.6052536882604,3.23423028058456));
#248483=CARTESIAN_POINT('Ctrl Pts',(-48.2946219293743,-34.6963546279287,
3.47153072139047));
#248484=CARTESIAN_POINT('Ctrl Pts',(-48.2205921526131,-34.7990735298991,
3.47122746285052));
#248485=CARTESIAN_POINT('Ctrl Pts',(-48.3075723994628,-34.8620346481362,
3.40413046676745));
#248486=CARTESIAN_POINT('Ctrl Pts',(-48.38771653075,-34.7638392294014,3.6555381345796));
#248487=CARTESIAN_POINT('Ctrl Pts',(-48.313481315449,-34.866561796061,3.65520336072181));
#248488=CARTESIAN_POINT('Ctrl Pts',(-48.3819628268463,-34.9160824571361,
3.55128134519942));
#248489=CARTESIAN_POINT('Ctrl Pts',(-48.5549570506162,-34.8850734745832,
3.77003198860238));
#248490=CARTESIAN_POINT('Ctrl Pts',(-48.480486117148,-34.9878985031425,
3.76980209314177));
#248491=CARTESIAN_POINT('Ctrl Pts',(-48.5156018845791,-35.0131769156757,
3.64284195387375));
#248492=CARTESIAN_POINT('Ctrl Pts',(-48.7306271754173,-35.0124214764587,
3.77003198860238));
#248493=CARTESIAN_POINT('Ctrl Pts',(-48.6558666298463,-35.1153205397472,
3.77003198860238));
#248494=CARTESIAN_POINT('Ctrl Pts',(-48.655978531999,-35.1151665196474,
3.64284189403744));
#248495=CARTESIAN_POINT('Origin',(-48.7306271754173,-35.0124214764587,3.64303198860238));
#248496=CARTESIAN_POINT('Origin',(39.5520252162584,29.1286799712091,3.23423028058503));
#248497=CARTESIAN_POINT('Origin',(-49.4242607783458,-35.5163757878398,3.23423028058456));
#248498=CARTESIAN_POINT('Origin',(39.3975469582344,29.0164449471024,3.64303198860284));
#248499=CARTESIAN_POINT('Origin',(-49.0553654007524,-35.248294810039,3.64299171721698));
#248500=CARTESIAN_POINT('Ctrl Pts',(-49.246635155601,-35.3866101428262,
3.48823028058456));
#248501=CARTESIAN_POINT('Ctrl Pts',(-49.1720533660028,-35.4901170100369,
3.48852004212234));
#248502=CARTESIAN_POINT('Ctrl Pts',(-49.0826686475732,-35.425175210744,
3.42473028058456));
#248503=CARTESIAN_POINT('Ctrl Pts',(-49.2829758776408,-35.4131599099204,
3.41028005848381));
#248504=CARTESIAN_POINT('Ctrl Pts',(-49.2082707697412,-35.5164304941026,
3.41074404220296));
#248505=CARTESIAN_POINT('Ctrl Pts',(-49.1372837917322,-35.4648554356487,
3.30780486243887));
#248506=CARTESIAN_POINT('Ctrl Pts',(-49.3518235761955,-35.4634578610105,
3.36123028058456));
#248507=CARTESIAN_POINT('Ctrl Pts',(-49.2769673468835,-35.5663414789258,
3.36146460586393));
#248508=CARTESIAN_POINT('Ctrl Pts',(-49.2407512920142,-35.54002897487,3.23423045308351));
#248509=CARTESIAN_POINT('Ctrl Pts',(-49.4242607783458,-35.5163757878398,
3.36123028058456));
#248510=CARTESIAN_POINT('Ctrl Pts',(-49.3496120513046,-35.6191209461254,
3.36123028058456));
#248511=CARTESIAN_POINT('Ctrl Pts',(-49.3496120513046,-35.6191209461254,
3.23423028058456));
#248512=CARTESIAN_POINT('Origin',(-49.1573173746143,-35.3224300524584,3.42473028058456));
#248513=CARTESIAN_POINT('Origin',(-49.0915036263505,-35.2746135650452,3.56563113524708));
#248514=CARTESIAN_POINT('Origin',(-45.4345348113615,-41.336677286195,3.56647653909452));
#248515=CARTESIAN_POINT('Origin',(-45.4673664422113,-41.3663085755598,3.64299466007842));
#248516=CARTESIAN_POINT('Origin',(-45.3737170758069,-41.281916751533,3.42473028058454));
#248517=CARTESIAN_POINT('Ctrl Pts',(-45.2923641298554,-41.2079002115909,
3.48823028058455));
#248518=CARTESIAN_POINT('Ctrl Pts',(-45.3773275334102,-41.1142722655008,
3.48794691941571));
#248519=CARTESIAN_POINT('Ctrl Pts',(-45.4586966628145,-41.1875373586974,
3.42473028058456));
#248520=CARTESIAN_POINT('Ctrl Pts',(-45.2588408013024,-41.1778715515028,
3.41028005925058));
#248521=CARTESIAN_POINT('Ctrl Pts',(-45.3437094247774,-41.0840023845226,
3.40982512230884));
#248522=CARTESIAN_POINT('Ctrl Pts',(-45.4085284377449,-41.1423656859495,
3.30780486372779));
#248523=CARTESIAN_POINT('Ctrl Pts',(-45.1953306044449,-41.1209827764374,
3.36123028058452));
#248524=CARTESIAN_POINT('Ctrl Pts',(-45.2800912647189,-41.0267203359189,
3.36099721048419));
#248525=CARTESIAN_POINT('Ctrl Pts',(-45.3134855411615,-41.056788677484,
3.23423045308386));
#248526=CARTESIAN_POINT('Ctrl Pts',(-45.1285089182129,-41.0611303347406,
3.36123028058452));
#248527=CARTESIAN_POINT('Ctrl Pts',(-45.2134885052205,-40.966750941905,
3.36123028058452));
#248528=CARTESIAN_POINT('Ctrl Pts',(-45.2134885052205,-40.966750941905,
3.23423028058452));
#248529=CARTESIAN_POINT('Origin',(-45.1285089182129,-41.0611303347406,3.23423028058452));
#248530=CARTESIAN_POINT('Origin',(0.212448967518945,-0.235948482088887,
3.64303198860262));
#248531=CARTESIAN_POINT('Origin',(-45.7656648676103,-41.6348281284264,3.64303198860233));
#248532=CARTESIAN_POINT('Origin',(0.212448967518945,-0.235948482088884,
3.23423028058481));
#248533=CARTESIAN_POINT('Origin',(-45.016139389479,-40.9599523566127,3.23423028058452));
#248534=CARTESIAN_POINT('Ctrl Pts',(-46.1654920697608,-41.9955727382253,
3.47153072139041));
#248535=CARTESIAN_POINT('Ctrl Pts',(-46.2513146333399,-41.9009568150787,
3.47182327902632));
#248536=CARTESIAN_POINT('Ctrl Pts',(-46.1706818621619,-41.8286119029182,
3.40413028959029));
#248537=CARTESIAN_POINT('Ctrl Pts',(-46.0801220723621,-41.9185486398924,
3.65553807120923));
#248538=CARTESIAN_POINT('Ctrl Pts',(-46.1657485549025,-41.8239131221215,
3.65586275496807));
#248539=CARTESIAN_POINT('Ctrl Pts',(-46.102348684828,-41.7670844335126,
3.55128126837167));
#248540=CARTESIAN_POINT('Ctrl Pts',(-45.9267584721685,-41.7801771152759,
3.77003198860233));
#248541=CARTESIAN_POINT('Ctrl Pts',(-46.0121526898594,-41.685615423495,
3.77025505748548));
#248542=CARTESIAN_POINT('Ctrl Pts',(-45.9795909100381,-41.6565528363085,
3.64284211731204));
#248543=CARTESIAN_POINT('Ctrl Pts',(-45.7656648676103,-41.6348281284264,
3.77003198860233));
#248544=CARTESIAN_POINT('Ctrl Pts',(-45.8507714101799,-41.5403077371547,
3.77003198860233));
#248545=CARTESIAN_POINT('Ctrl Pts',(-45.8506443599266,-41.5404488407561,
3.64284239821729));
#248546=CARTESIAN_POINT('Origin',(-46.0858221116775,-41.9230990057957,3.4042309748328));
#248547=CARTESIAN_POINT('Ctrl Pts',(-45.016139389479,-40.9599523566127,
3.36123028058452));
#248548=CARTESIAN_POINT('Ctrl Pts',(-45.1011189764865,-40.865572963777,
3.36123028058452));
#248549=CARTESIAN_POINT('Ctrl Pts',(-45.1011189764865,-40.865572963777,
3.23423028058452));
#248550=CARTESIAN_POINT('Ctrl Pts',(-44.9490914663004,-40.8998980546758,
3.36123028058452));
#248551=CARTESIAN_POINT('Ctrl Pts',(-45.0341638030252,-40.8052862548027,
3.36146538610245));
#248552=CARTESIAN_POINT('Ctrl Pts',(-45.000783964292,-40.7752309130124,
3.23423043688429));
#248553=CARTESIAN_POINT('Ctrl Pts',(-44.8856913339429,-40.8431135311207,
3.41054258693071));
#248554=CARTESIAN_POINT('Ctrl Pts',(-44.9711739721998,-40.7485699563836,
3.41100608859617));
#248555=CARTESIAN_POINT('Ctrl Pts',(-44.9059100567337,-40.6898060629486,
3.3081986697077));
#248556=CARTESIAN_POINT('Ctrl Pts',(-44.8522789915938,-40.8131880745608,
3.48823028058452));
#248557=CARTESIAN_POINT('Ctrl Pts',(-44.9380175594359,-40.7187157882339,
3.48852004212231));
#248558=CARTESIAN_POINT('Ctrl Pts',(-44.8559107663282,-40.6447864996554,
3.42473028058453));
#248559=CARTESIAN_POINT('Origin',(-44.7709311793206,-40.7391658924911,3.42473028058452));
#248560=CARTESIAN_POINT('Origin',(-46.2182127020609,-42.0423040287734,3.11913648178265));
#248561=CARTESIAN_POINT('Origin',(-46.3506032922591,-42.1615090516454,2.83404198860231));
#248562=CARTESIAN_POINT('Origin',(-44.7104761485856,-40.6847319383086,3.56563113460817));
#248563=CARTESIAN_POINT('Origin',(-44.677218962551,-40.6548553974684,3.64299171721742));
#248564=CARTESIAN_POINT('Ctrl Pts',(-46.7738319284254,-42.1358900227697,
2.59908173515993));
#248565=CARTESIAN_POINT('Ctrl Pts',(-46.7461150696869,-42.1109214781063,
2.65878198860232));
#248566=CARTESIAN_POINT('Ctrl Pts',(-46.6938111422601,-42.0638038389702,
2.65878198860231));
#248567=CARTESIAN_POINT('Ctrl Pts',(-46.7148552537641,-42.2013581359414,
2.59908193475522));
#248568=CARTESIAN_POINT('Ctrl Pts',(-46.7031532960248,-42.1586072771714,
2.65878715325297));
#248569=CARTESIAN_POINT('Ctrl Pts',(-46.6596664560544,-42.1016932886521,
2.65878198860231));
#248570=CARTESIAN_POINT('Ctrl Pts',(-46.6418481388112,-42.2450249725429,
2.63878778849834));
#248571=CARTESIAN_POINT('Ctrl Pts',(-46.6464039985654,-42.1870455286632,
2.69564460180072));
#248572=CARTESIAN_POINT('Ctrl Pts',(-46.6095714048488,-42.1199142759248,
2.68180481624859));
#248573=CARTESIAN_POINT('Ctrl Pts',(-46.5164783566524,-42.2756632139847,
2.75443238878623));
#248574=CARTESIAN_POINT('Ctrl Pts',(-46.5588531737051,-42.1934768724829,
2.79268340777076));
#248575=CARTESIAN_POINT('Ctrl Pts',(-46.5142596423497,-42.1171707421505,
2.74885926835574));
#248576=CARTESIAN_POINT('Ctrl Pts',(-46.4640705998029,-42.2644092166206,
2.82856655361634));
#248577=CARTESIAN_POINT('Ctrl Pts',(-46.5278411618559,-42.1708301402943,
2.85384197230709));
#248578=CARTESIAN_POINT('Ctrl Pts',(-46.4693765057988,-42.0975575768108,
2.79184624278386));
#248579=CARTESIAN_POINT('Ctrl Pts',(-46.4302753505421,-42.2339804752703,
2.90134173515994));
#248580=CARTESIAN_POINT('Ctrl Pts',(-46.5159655405271,-42.1395065321001,
2.90163218716362));
#248581=CARTESIAN_POINT('Ctrl Pts',(-46.4355828792667,-42.0671296588098,
2.83404198860232));
#248582=CARTESIAN_POINT('Origin',(-46.6938111422601,-42.0638038389702,2.53178198860231));
#248583=CARTESIAN_POINT('Origin',(0.212448967518945,-0.235948482088887,
3.64303198860262));
#248584=CARTESIAN_POINT('Origin',(-44.3789831537292,-40.386254305094,3.64303198860234));
#248585=CARTESIAN_POINT('Origin',(9.23291810287646E-17,1.91687767418825E-13,
2.53178198860262));
#248586=CARTESIAN_POINT('Origin',(-46.7142062431419,-42.0411527846897,2.53178198860231));
#248587=CARTESIAN_POINT('Ctrl Pts',(-44.3789831537292,-40.386254305094,
3.77003198860234));
#248588=CARTESIAN_POINT('Ctrl Pts',(-44.4640900439955,-40.2917335276661,
3.77003198860234));
#248589=CARTESIAN_POINT('Ctrl Pts',(-44.4639626455265,-40.2918750180001,
3.64284187937013));
#248590=CARTESIAN_POINT('Ctrl Pts',(-44.2178916378589,-40.2408978759471,
3.77003198860235));
#248591=CARTESIAN_POINT('Ctrl Pts',(-44.3029863283988,-40.1466757825268,
3.76980208963012));
#248592=CARTESIAN_POINT('Ctrl Pts',(-44.3350138149328,-40.1757689690801,
3.64284193928242));
#248593=CARTESIAN_POINT('Ctrl Pts',(-44.0645366033553,-40.1025190720971,
3.65553535416554));
#248594=CARTESIAN_POINT('Ctrl Pts',(-44.1495800756938,-40.0085488431143,
3.65520057834386));
#248595=CARTESIAN_POINT('Ctrl Pts',(-44.2122569536148,-40.0652381943513,
3.55127910964213));
#248596=CARTESIAN_POINT('Ctrl Pts',(-43.9791725362579,-40.025490812659,
3.47153072139044));
#248597=CARTESIAN_POINT('Ctrl Pts',(-44.0642551375171,-39.9317222927446,
3.47122746281554));
#248598=CARTESIAN_POINT('Ctrl Pts',(-44.1439246138545,-40.0037114790888,
3.40413045901242));
#248599=CARTESIAN_POINT('Origin',(-44.0588255818374,-40.0979831325501,3.40423097483281));
#248600=CARTESIAN_POINT('Ctrl Pts',(-46.8559036426982,-41.7612723673365,
2.90134173515993));
#248601=CARTESIAN_POINT('Ctrl Pts',(-46.7709043015499,-41.8563683535932,
2.90163218716361));
#248602=CARTESIAN_POINT('Ctrl Pts',(-46.6905216402894,-41.7839914803029,
2.83404198860232));
#248603=CARTESIAN_POINT('Ctrl Pts',(-46.88971359836,-41.7917156448197,2.82853349835316));
#248604=CARTESIAN_POINT('Ctrl Pts',(-46.8033160448221,-41.8649095672151,
2.85381483162259));
#248605=CARTESIAN_POINT('Ctrl Pts',(-46.7243306652208,-41.8144332630849,
2.79182701594156));
#248606=CARTESIAN_POINT('Ctrl Pts',(-46.9062450310964,-41.8425440045881,
2.75468822073627));
#248607=CARTESIAN_POINT('Ctrl Pts',(-46.8289264627106,-41.8933569085959,
2.79286913083846));
#248608=CARTESIAN_POINT('Ctrl Pts',(-46.7483907976678,-41.8569022891471,
2.74900763297884));
#248609=CARTESIAN_POINT('Ctrl Pts',(-46.8892773184516,-41.9695156381235,
2.63954450640348));
#248610=CARTESIAN_POINT('Ctrl Pts',(-46.8319191778362,-41.9804178820373,
2.69627684028798));
#248611=CARTESIAN_POINT('Ctrl Pts',(-46.7612136652288,-41.9507871007489,
2.6822435603646));
#248612=CARTESIAN_POINT('Ctrl Pts',(-46.8534019544977,-42.0474864684051,
2.59908178706348));
#248613=CARTESIAN_POINT('Ctrl Pts',(-46.8096319157674,-42.0403508033706,
2.65878704321515));
#248614=CARTESIAN_POINT('Ctrl Pts',(-46.7484320121849,-42.0031091842998,
2.65878198860231));
#248615=CARTESIAN_POINT('Ctrl Pts',(-46.7942619810913,-42.1132001506003,
2.59908173515993));
#248616=CARTESIAN_POINT('Ctrl Pts',(-46.7665330160776,-42.0882450513177,
2.65878198860232));
#248617=CARTESIAN_POINT('Ctrl Pts',(-46.7142062431419,-42.0411527846897,
2.65878198860231));
#248618=CARTESIAN_POINT('Origin',(-46.7755012272969,-41.6896120874673,2.83404198860232));
#248619=CARTESIAN_POINT('Origin',(-43.9264348094997,-39.9787779456716,3.11913648167122));
#248620=CARTESIAN_POINT('Origin',(-43.7940440370141,-39.8595727587357,2.83404198860234));
#248621=CARTESIAN_POINT('Origin',(-46.6431106370605,-41.5704070646241,3.11913648177693));
#248622=CARTESIAN_POINT('Origin',(-46.5107200467153,-41.4512020416176,3.40423097483281));
#248623=CARTESIAN_POINT('Ctrl Pts',(-43.714393316062,-39.7870778846749,
2.90134173515995));
#248624=CARTESIAN_POINT('Ctrl Pts',(-43.799348782961,-39.6934538167802,
2.90103711553201));
#248625=CARTESIAN_POINT('Ctrl Pts',(-43.8790236240217,-39.7651933659001,
2.83404198860233));
#248626=CARTESIAN_POINT('Ctrl Pts',(-43.6806281164518,-39.7566748466924,
2.82862991747931));
#248627=CARTESIAN_POINT('Ctrl Pts',(-43.7668791656725,-39.6846648960484,
2.8531404588637));
#248628=CARTESIAN_POINT('Ctrl Pts',(-43.8452566693654,-39.7347894633639,
2.79187960999875));
#248629=CARTESIAN_POINT('Ctrl Pts',(-43.6642103943283,-39.7061132086032,
2.75470625793302));
#248630=CARTESIAN_POINT('Ctrl Pts',(-43.7414086642727,-39.6560595510441,
2.79224250381861));
#248631=CARTESIAN_POINT('Ctrl Pts',(-43.8213838166742,-39.6925108309091,
2.74901809108232));
#248632=CARTESIAN_POINT('Ctrl Pts',(-43.681569387645,-39.5798624575878,
2.63947868311666));
#248633=CARTESIAN_POINT('Ctrl Pts',(-43.7388169234803,-39.5692094437565,
2.6959506676789));
#248634=CARTESIAN_POINT('Ctrl Pts',(-43.8091742082548,-39.5991004926181,
2.68220539436031));
#248635=CARTESIAN_POINT('Ctrl Pts',(-43.7176736830019,-39.5024012818816,
2.59908178584979));
#248636=CARTESIAN_POINT('Ctrl Pts',(-43.7613473163388,-39.5096522555304,
2.65877670944783));
#248637=CARTESIAN_POINT('Ctrl Pts',(-43.8223603708607,-39.5470931435008,
2.65878198860234));
#248638=CARTESIAN_POINT('Ctrl Pts',(-43.7765468711719,-39.437049873601,
2.59908173515995));
#248639=CARTESIAN_POINT('Ctrl Pts',(-43.8042633382926,-39.4620188529811,
2.65878198860233));
#248640=CARTESIAN_POINT('Ctrl Pts',(-43.8565665267053,-39.5091373124624,
2.65878198860234));
#248641=CARTESIAN_POINT('Origin',(-43.8565665267053,-39.5091373124624,2.53178198860234));
#248642=CARTESIAN_POINT('Ctrl Pts',(-46.1905628026481,-41.1629311642483,
3.77003198860234));
#248643=CARTESIAN_POINT('Ctrl Pts',(-46.1054562527463,-41.2574515636632,
3.77003198860234));
#248644=CARTESIAN_POINT('Ctrl Pts',(-46.1055833103428,-41.2573104519064,
3.64284238727582));
#248645=CARTESIAN_POINT('Ctrl Pts',(-46.3519569305998,-41.3079514313262,
3.77003198860233));
#248646=CARTESIAN_POINT('Ctrl Pts',(-46.2668393800555,-41.4027622547786,
3.77025506105675));
#248647=CARTESIAN_POINT('Ctrl Pts',(-46.2345318643239,-41.3734162510837,
3.64284210641889));
#248648=CARTESIAN_POINT('Ctrl Pts',(-46.5056000892412,-41.446010036274,
3.65553527987799));
#248649=CARTESIAN_POINT('Ctrl Pts',(-46.4204333915659,-41.5410595633948,
3.65585996533104));
#248650=CARTESIAN_POINT('Ctrl Pts',(-46.3572886670225,-41.4839469723842,
3.55127902710129));
#248651=CARTESIAN_POINT('Ctrl Pts',(-46.5911245387426,-41.5228599914565,
3.47153072139041));
#248652=CARTESIAN_POINT('Ctrl Pts',(-46.5059978248575,-41.618102475323,
3.47182327905158));
#248653=CARTESIAN_POINT('Ctrl Pts',(-46.4256208064856,-41.5454735069379,
3.40413028377964));
#248654=CARTESIAN_POINT('Origin',(-46.1905628026481,-41.1629311642483,3.64303198860234));
#248655=CARTESIAN_POINT('Origin',(3.68378193773366E-16,1.91538185386435E-13,
2.53178198860262));
#248656=CARTESIAN_POINT('Origin',(-43.8769616275871,-39.4864862581819,2.53178198860234));
#248657=CARTESIAN_POINT('Origin',(34.1507877370002,31.1767457860028,3.64303198860284));
#248658=CARTESIAN_POINT('Origin',(-45.8923335519908,-40.8943347850523,3.64299466007333));
#248659=CARTESIAN_POINT('Ctrl Pts',(-43.7969047596343,-39.4144401478991,
2.59908173515995));
#248660=CARTESIAN_POINT('Ctrl Pts',(-43.8246341160482,-39.439394812269,
2.65878198860234));
#248661=CARTESIAN_POINT('Ctrl Pts',(-43.8769616275871,-39.4864862581818,
2.65878198860234));
#248662=CARTESIAN_POINT('Ctrl Pts',(-43.8555436924519,-39.3492813761644,
2.59908193199843));
#248663=CARTESIAN_POINT('Ctrl Pts',(-43.867352448422,-39.3919218645326,
2.6587768580655));
#248664=CARTESIAN_POINT('Ctrl Pts',(-43.9110175468015,-39.4486296259964,
2.65878198860234));
#248665=CARTESIAN_POINT('Ctrl Pts',(-43.9280312169042,-39.3054399757366,
2.63872492669765));
#248666=CARTESIAN_POINT('Ctrl Pts',(-43.9237065964666,-39.3632835603679,
2.69532212015234));
#248667=CARTESIAN_POINT('Ctrl Pts',(-43.9607655567554,-39.430042363277,
2.68176836726587));
#248668=CARTESIAN_POINT('Ctrl Pts',(-44.0526112349803,-39.2744854109877,
2.75442176402225));
#248669=CARTESIAN_POINT('Ctrl Pts',(-44.0109847679678,-39.3564679665374,
2.79203179920121));
#248670=CARTESIAN_POINT('Ctrl Pts',(-44.0555161714741,-39.4322155454628,
2.74885310748166));
#248671=CARTESIAN_POINT('Ctrl Pts',(-44.1047669487885,-39.2856498807566,
2.82866089558368));
#248672=CARTESIAN_POINT('Ctrl Pts',(-44.0421591564523,-39.3789590643314,
2.8531656311927));
#248673=CARTESIAN_POINT('Ctrl Pts',(-44.1002097724412,-39.4516641984997,
2.79189751796617));
#248674=CARTESIAN_POINT('Ctrl Pts',(-44.1385184650372,-39.3160391863692,
2.90134173515995));
#248675=CARTESIAN_POINT('Ctrl Pts',(-44.0542875439837,-39.4103156382733,
2.90103711553201));
#248676=CARTESIAN_POINT('Ctrl Pts',(-44.1339623850444,-39.4820551873932,
2.83404198860233));
#248677=CARTESIAN_POINT('Origin',(-44.218941972052,-39.3876757945576,2.83404198860233));
#248678=CARTESIAN_POINT('Origin',(-45.8594327453962,-40.864780321517,3.56647653971802));
#248679=CARTESIAN_POINT('Origin',(-45.7986150108448,-40.8100197873549,3.42473028058455));
#248680=CARTESIAN_POINT('Origin',(-44.3513327444876,-39.5068809815272,3.1191364816803));
#248681=CARTESIAN_POINT('Origin',(-44.4837235168753,-39.6260861683719,3.40423097483282));
#248682=CARTESIAN_POINT('Ctrl Pts',(-45.5534068532508,-40.5892333705625,
3.36123028058452));
#248683=CARTESIAN_POINT('Ctrl Pts',(-45.4684272662432,-40.6836127633981,
3.36123028058452));
#248684=CARTESIAN_POINT('Ctrl Pts',(-45.4684272662432,-40.6836127633981,
3.23423028058452));
#248685=CARTESIAN_POINT('Ctrl Pts',(-45.6201409680082,-40.6496361736963,
3.36123028058452));
#248686=CARTESIAN_POINT('Ctrl Pts',(-45.535255269862,-40.7437849681278,
3.36099641108599));
#248687=CARTESIAN_POINT('Ctrl Pts',(-45.5687622694476,-40.7739548060679,
3.23423043688381));
#248688=CARTESIAN_POINT('Ctrl Pts',(-45.6832443225589,-40.7067502157885,
3.41054258905255));
#248689=CARTESIAN_POINT('Ctrl Pts',(-45.5987613682843,-40.8009661159843,
3.41008815825802));
#248690=CARTESIAN_POINT('Ctrl Pts',(-45.6636361529328,-40.8593796344563,
3.30819867304212));
#248691=CARTESIAN_POINT('Ctrl Pts',(-45.7165002428303,-40.7368493365299,
3.48823028058454));
#248692=CARTESIAN_POINT('Ctrl Pts',(-45.6322662944329,-40.8311340869939,
3.4879469194157));
#248693=CARTESIAN_POINT('Ctrl Pts',(-45.7136354238372,-40.9043991801905,
3.42473028058455));
#248694=CARTESIAN_POINT('Origin',(-45.5534068532508,-40.5892333705625,3.23423028058452));
#248695=CARTESIAN_POINT('Ctrl Pts',(-44.4033023070486,-39.5544469813073,
3.47153072139044));
#248696=CARTESIAN_POINT('Ctrl Pts',(-44.3189410241786,-39.6488649595844,
3.47122746285048));
#248697=CARTESIAN_POINT('Ctrl Pts',(-44.3988635552007,-39.7205730817658,
3.40413046676722));
#248698=CARTESIAN_POINT('Ctrl Pts',(-44.4888328647701,-39.6312929306934,
3.65553813457959));
#248699=CARTESIAN_POINT('Ctrl Pts',(-44.404266885707,-39.7256930794079,
3.65520336072389));
#248700=CARTESIAN_POINT('Ctrl Pts',(-44.4671969296202,-39.7821007282677,
3.55128134520005));
#248701=CARTESIAN_POINT('Ctrl Pts',(-44.642484794226,-39.7693444365323,
3.77003198860235));
#248702=CARTESIAN_POINT('Ctrl Pts',(-44.5576736781029,-39.8638218465962,
3.76980209314011));
#248703=CARTESIAN_POINT('Ctrl Pts',(-44.5899547640713,-39.892632378544,
3.64284195387283));
#248704=CARTESIAN_POINT('Ctrl Pts',(-44.8038810887671,-39.9143573409159,
3.77003198860235));
#248705=CARTESIAN_POINT('Ctrl Pts',(-44.7187742083296,-40.0088781074279,
3.77003198860235));
#248706=CARTESIAN_POINT('Ctrl Pts',(-44.7189015969551,-40.0087366280261,
3.64284189403704));
#248707=CARTESIAN_POINT('Origin',(-44.8038810887671,-39.9143573409159,3.64303198860235));
#248708=CARTESIAN_POINT('Origin',(33.3184119221863,30.4272712359686,3.23423028058503));
#248709=CARTESIAN_POINT('Origin',(-45.4410373245168,-40.4880553924345,3.23423028058452));
#248710=CARTESIAN_POINT('Origin',(33.1880655373213,30.3099068238766,3.64303198860284));
#248711=CARTESIAN_POINT('Origin',(-45.1021848870407,-40.1828829233542,3.64299171721751));
#248712=CARTESIAN_POINT('Ctrl Pts',(-45.2779489569769,-40.3404336838194,
3.48823028058452));
#248713=CARTESIAN_POINT('Ctrl Pts',(-45.1929563204586,-40.435577609727,
3.4885200421223));
#248714=CARTESIAN_POINT('Ctrl Pts',(-45.1108495273509,-40.3616483211486,
3.42473028058452));
#248715=CARTESIAN_POINT('Ctrl Pts',(-45.3113153943823,-40.3706366483428,
3.41028005848378));
#248716=CARTESIAN_POINT('Ctrl Pts',(-45.2262248134149,-40.4655326953357,
3.41074404220353));
#248717=CARTESIAN_POINT('Ctrl Pts',(-45.1610177711069,-40.4068200107218,
3.30780486243963));
#248718=CARTESIAN_POINT('Ctrl Pts',(-45.374528370508,-40.4278556061233,
3.36123028058453));
#248719=CARTESIAN_POINT('Ctrl Pts',(-45.2893279449758,-40.5223510101973,
3.36146460586381));
#248720=CARTESIAN_POINT('Ctrl Pts',(-45.2560606910588,-40.4923970402283,
3.23423045308356));
#248721=CARTESIAN_POINT('Ctrl Pts',(-45.4410373245168,-40.4880553924345,
3.36123028058453));
#248722=CARTESIAN_POINT('Ctrl Pts',(-45.3560577375092,-40.5824347852702,
3.36123028058453));
#248723=CARTESIAN_POINT('Ctrl Pts',(-45.3560577375093,-40.5824347852702,
3.23423028058453));
#248724=CARTESIAN_POINT('Origin',(-45.1958291143585,-40.2672689283129,3.42473028058452));
#248725=CARTESIAN_POINT('Origin',(-45.1353740846429,-40.2128349746541,3.56563113524785));
#248726=CARTESIAN_POINT('Origin',(-40.8647803224533,-45.8594327460074,3.56647653909403));
#248727=CARTESIAN_POINT('Origin',(-40.8943347850521,-45.8923335519892,3.64299466007529));
#248728=CARTESIAN_POINT('Origin',(-40.8100197873543,-45.7986150108453,3.42473028058451));
#248729=CARTESIAN_POINT('Ctrl Pts',(-40.7368493365293,-45.7165002428309,
3.48823028058451));
#248730=CARTESIAN_POINT('Ctrl Pts',(-40.8311340869933,-45.6322662944334,
3.48794691941567));
#248731=CARTESIAN_POINT('Ctrl Pts',(-40.9043991801899,-45.7136354238377,
3.42473028058452));
#248732=CARTESIAN_POINT('Ctrl Pts',(-40.7066485019706,-45.6831319408675,
3.41028005925053));
#248733=CARTESIAN_POINT('Ctrl Pts',(-40.800864206014,-45.5986481857962,
3.40982512230997));
#248734=CARTESIAN_POINT('Ctrl Pts',(-40.8592275074395,-45.6634671987653,
3.30780486372868));
#248735=CARTESIAN_POINT('Ctrl Pts',(-40.649432716852,-45.6199161851844,
3.36123028058449));
#248736=CARTESIAN_POINT('Ctrl Pts',(-40.743582157414,-45.535030025744,3.36099721048404));
#248737=CARTESIAN_POINT('Ctrl Pts',(-40.7736504989785,-45.5684243021869,
3.23423045308392));
#248738=CARTESIAN_POINT('Ctrl Pts',(-40.5892333705618,-45.5534068532513,
3.36123028058449));
#248739=CARTESIAN_POINT('Ctrl Pts',(-40.6836127633975,-45.4684272662438,
3.36123028058449));
#248740=CARTESIAN_POINT('Ctrl Pts',(-40.6836127633975,-45.4684272662438,
3.23423028058449));
#248741=CARTESIAN_POINT('Origin',(-40.5892333705618,-45.5534068532513,3.23423028058449));
#248742=CARTESIAN_POINT('Origin',(0.23594848208908,-0.212448967518752,3.64303198860262));
#248743=CARTESIAN_POINT('Origin',(-41.1629311642476,-46.1905628026487,3.6430319886023));
#248744=CARTESIAN_POINT('Origin',(0.23594848208908,-0.212448967518749,3.23423028058481));
#248745=CARTESIAN_POINT('Origin',(-40.4880553924339,-45.4410373245173,3.23423028058449));
#248746=CARTESIAN_POINT('Ctrl Pts',(-41.5228599914559,-46.5911245387432,
3.47153072139039));
#248747=CARTESIAN_POINT('Ctrl Pts',(-41.6181024670993,-46.5059978322077,
3.47182327902629));
#248748=CARTESIAN_POINT('Ctrl Pts',(-41.5454735131715,-46.4256208133854,
3.40413028959007));
#248749=CARTESIAN_POINT('Ctrl Pts',(-41.4460088704661,-46.505598791845,
3.65553807120923));
#248750=CARTESIAN_POINT('Ctrl Pts',(-41.5410583874213,-46.4204321019767,
3.65586275496799));
#248751=CARTESIAN_POINT('Ctrl Pts',(-41.4839460439596,-46.3572876358792,
3.5512812683718));
#248752=CARTESIAN_POINT('Ctrl Pts',(-41.3079491749513,-46.3519544194672,
3.7700319886023));
#248753=CARTESIAN_POINT('Ctrl Pts',(-41.4027599825085,-46.2668368728742,
3.77025505748597));
#248754=CARTESIAN_POINT('Ctrl Pts',(-41.3734144471009,-46.2345298607748,
3.64284211731165));
#248755=CARTESIAN_POINT('Ctrl Pts',(-41.1629311642476,-46.1905628026487,
3.7700319886023));
#248756=CARTESIAN_POINT('Ctrl Pts',(-41.2574515555196,-46.1054562600788,
3.7700319886023));
#248757=CARTESIAN_POINT('Ctrl Pts',(-41.2573104519179,-46.1055833103324,
3.64284239821689));
#248758=CARTESIAN_POINT('Origin',(-41.451202041617,-46.5107200467159,3.40423097483277));
#248759=CARTESIAN_POINT('Ctrl Pts',(-40.4880553924339,-45.4410373245173,
3.36123028058449));
#248760=CARTESIAN_POINT('Ctrl Pts',(-40.5824347852696,-45.3560577375098,
3.36123028058449));
#248761=CARTESIAN_POINT('Ctrl Pts',(-40.5824347852696,-45.3560577375098,
3.23423028058449));
#248762=CARTESIAN_POINT('Ctrl Pts',(-40.4276521486877,-45.3743035899551,
3.36123028058449));
#248763=CARTESIAN_POINT('Ctrl Pts',(-40.5221480762965,-45.2891025640463,
3.36146538610272));
#248764=CARTESIAN_POINT('Ctrl Pts',(-40.4920927345057,-45.255722725316,
3.23423043688376));
#248765=CARTESIAN_POINT('Ctrl Pts',(-40.3705349278737,-45.3112030195552,
3.41054258693066));
#248766=CARTESIAN_POINT('Ctrl Pts',(-40.4654317778761,-45.2261127332245,
3.41100608859622));
#248767=CARTESIAN_POINT('Ctrl Pts',(-40.4066678844402,-45.1608488177559,
3.30819866970767));
#248768=CARTESIAN_POINT('Ctrl Pts',(-40.3404336838189,-45.2779489569774,
3.48823028058449));
#248769=CARTESIAN_POINT('Ctrl Pts',(-40.4355776097265,-45.1929563204591,
3.48852004212226));
#248770=CARTESIAN_POINT('Ctrl Pts',(-40.361648321148,-45.1108495273514,
3.42473028058448));
#248771=CARTESIAN_POINT('Origin',(-40.2672689283123,-45.195829114359,3.42473028058447));
#248772=CARTESIAN_POINT('Origin',(-41.5704070646284,-46.6431106370687,3.1191364817825));
#248773=CARTESIAN_POINT('Origin',(-41.6896120874666,-46.7755012272975,2.83404198860228));
#248774=CARTESIAN_POINT('Origin',(-40.2128349741381,-45.1353740836141,3.56563113460706));
#248775=CARTESIAN_POINT('Origin',(-40.1828829233539,-45.1021848870412,3.64299171721761));
#248776=CARTESIAN_POINT('Ctrl Pts',(-42.1132001505997,-46.7942619810919,
2.5990817351599));
#248777=CARTESIAN_POINT('Ctrl Pts',(-42.0882450513171,-46.7665330160781,
2.65878198860228));
#248778=CARTESIAN_POINT('Ctrl Pts',(-42.0411527846891,-46.7142062431424,
2.65878198860228));
#248779=CARTESIAN_POINT('Ctrl Pts',(-42.0477032750703,-46.853206711919,
2.59908193475449));
#248780=CARTESIAN_POINT('Ctrl Pts',(-42.0405341034508,-46.8094668591673,
2.65878715325307));
#248781=CARTESIAN_POINT('Ctrl Pts',(-42.0032346206989,-46.748319038878,
2.65878198860228));
#248782=CARTESIAN_POINT('Ctrl Pts',(-41.9705316734061,-46.8890030154864,
2.63878778849854));
#248783=CARTESIAN_POINT('Ctrl Pts',(-41.9811230778539,-46.8318174060855,
2.69564460180075));
#248784=CARTESIAN_POINT('Ctrl Pts',(-41.9515093836253,-46.7612038509546,
2.6818048162485));
#248785=CARTESIAN_POINT('Ctrl Pts',(-41.8426461117364,-46.906368706767,
2.75443238878597));
#248786=CARTESIAN_POINT('Ctrl Pts',(-41.8933796070862,-46.8290619651513,
2.79268340777068));
#248787=CARTESIAN_POINT('Ctrl Pts',(-41.8570065263032,-46.7485125544803,
2.74885926835577));
#248788=CARTESIAN_POINT('Ctrl Pts',(-41.7917018131134,-46.8896982576902,
2.82856655361648));
#248789=CARTESIAN_POINT('Ctrl Pts',(-41.8649047103987,-46.8032976561885,
2.8538419723072));
#248790=CARTESIAN_POINT('Ctrl Pts',(-41.8144193983033,-46.724315266822,
2.79184624278382));
#248791=CARTESIAN_POINT('Ctrl Pts',(-41.7612723673359,-46.8559036426987,
2.90134173515991));
#248792=CARTESIAN_POINT('Ctrl Pts',(-41.8563683535926,-46.7709043015504,
2.90163218716358));
#248793=CARTESIAN_POINT('Ctrl Pts',(-41.7839914803023,-46.6905216402899,
2.83404198860229));
#248794=CARTESIAN_POINT('Origin',(-42.0411527846891,-46.7142062431424,2.53178198860228));
#248795=CARTESIAN_POINT('Origin',(0.23594848208908,-0.212448967518752,3.64303198860262));
#248796=CARTESIAN_POINT('Origin',(-39.9143573409153,-44.8038810887676,3.64303198860231));
#248797=CARTESIAN_POINT('Origin',(8.0125006576031E-17,1.91699971593277E-13,
2.53178198860262));
#248798=CARTESIAN_POINT('Origin',(-42.0638038389696,-46.6938111422606,2.53178198860228));
#248799=CARTESIAN_POINT('Ctrl Pts',(-39.9143573409153,-44.8038810887676,
3.77003198860231));
#248800=CARTESIAN_POINT('Ctrl Pts',(-40.0088781183433,-44.7187741985013,
3.77003198860231));
#248801=CARTESIAN_POINT('Ctrl Pts',(-40.0087366280092,-44.7189015969703,
3.64284187937008));
#248802=CARTESIAN_POINT('Ctrl Pts',(-39.7693421853875,-44.6424822887503,
3.77003198860232));
#248803=CARTESIAN_POINT('Ctrl Pts',(-39.8638196089375,-44.5576711710521,
3.76980208962971));
#248804=CARTESIAN_POINT('Ctrl Pts',(-39.8926305794713,-44.5899527660326,
3.64284193928275));
#248805=CARTESIAN_POINT('Ctrl Pts',(-39.6312917695244,-44.4888315723753,
3.65553535416554));
#248806=CARTESIAN_POINT('Ctrl Pts',(-39.7256919284553,-44.4042655856119,
3.6552005783438));
#248807=CARTESIAN_POINT('Ctrl Pts',(-39.7820998051101,-44.4671959043835,
3.55127910964178));
#248808=CARTESIAN_POINT('Ctrl Pts',(-39.5544469813067,-44.4033023070491,
3.47153072139042));
#248809=CARTESIAN_POINT('Ctrl Pts',(-39.6488649704634,-44.3189410144583,
3.47122746281552));
#248810=CARTESIAN_POINT('Ctrl Pts',(-39.720573090053,-44.3988635644383,
3.40413045901239));
#248811=CARTESIAN_POINT('Origin',(-39.6260861683714,-44.4837235168758,3.40423097483279));
#248812=CARTESIAN_POINT('Ctrl Pts',(-42.2339804752697,-46.4302753505427,
2.90134173515991));
#248813=CARTESIAN_POINT('Ctrl Pts',(-42.1395065320995,-46.5159655405277,
2.90163218716358));
#248814=CARTESIAN_POINT('Ctrl Pts',(-42.0671296588092,-46.4355828792672,
2.83404198860229));
#248815=CARTESIAN_POINT('Ctrl Pts',(-42.2644230274465,-46.4640859592732,
2.8285334983533));
#248816=CARTESIAN_POINT('Ctrl Pts',(-42.1708479205188,-46.5278479142023,
2.85381483162399));
#248817=CARTESIAN_POINT('Ctrl Pts',(-42.0975714415919,-46.4693919041993,
2.79182701594314));
#248818=CARTESIAN_POINT('Ctrl Pts',(-42.2755508889259,-46.5163638812299,
2.754688220736));
#248819=CARTESIAN_POINT('Ctrl Pts',(-42.1933444849776,-46.5588164356978,
2.79286913083808));
#248820=CARTESIAN_POINT('Ctrl Pts',(-42.1170605480848,-46.5141432491637,
2.74900763297869));
#248821=CARTESIAN_POINT('Ctrl Pts',(-42.2454039774542,-46.6408663419435,
2.63954450640368));
#248822=CARTESIAN_POINT('Ctrl Pts',(-42.187220455932,-46.6457133039298,
2.69627684028821));
#248823=CARTESIAN_POINT('Ctrl Pts',(-42.119999535554,-46.6088541045839,
2.68224356036468));
#248824=CARTESIAN_POINT('Ctrl Pts',(-42.201574971429,-46.7146600431956,
2.5990817870629));
#248825=CARTESIAN_POINT('Ctrl Pts',(-42.1587905896506,-46.7029882531948,
2.65878704321527));
#248826=CARTESIAN_POINT('Ctrl Pts',(-42.1018187547554,-46.6595535157374,
2.65878198860228));
#248827=CARTESIAN_POINT('Ctrl Pts',(-42.1358900227691,-46.7738319284259,
2.5990817351599));
#248828=CARTESIAN_POINT('Ctrl Pts',(-42.1109214781057,-46.7461150696874,
2.65878198860228));
#248829=CARTESIAN_POINT('Ctrl Pts',(-42.0638038389696,-46.6938111422606,
2.65878198860228));
#248830=CARTESIAN_POINT('Origin',(-42.1615090516448,-46.3506032922596,2.83404198860229));
#248831=CARTESIAN_POINT('Origin',(-39.506880981537,-44.3513327445029,3.11913648166909));
#248832=CARTESIAN_POINT('Origin',(-39.387675794557,-44.2189419720524,2.8340419886023));
#248833=CARTESIAN_POINT('Origin',(-42.0423040287658,-46.2182127020492,3.11913648177404));
#248834=CARTESIAN_POINT('Origin',(-41.9230990057951,-46.085822111678,3.40423097483277));
#248835=CARTESIAN_POINT('Ctrl Pts',(-39.3160391863686,-44.1385184650377,
2.90134173515992));
#248836=CARTESIAN_POINT('Ctrl Pts',(-39.4103156382728,-44.0542875439842,
2.90103711553198));
#248837=CARTESIAN_POINT('Ctrl Pts',(-39.4820551873926,-44.1339623850449,
2.8340419886023));
#248838=CARTESIAN_POINT('Ctrl Pts',(-39.2856369388931,-44.1047525536517,
2.82862991747916));
#248839=CARTESIAN_POINT('Ctrl Pts',(-39.3789425853224,-44.0421527706803,
2.85314045886441));
#248840=CARTESIAN_POINT('Ctrl Pts',(-39.4516512848559,-44.1001954303879,
2.79187960999956));
#248841=CARTESIAN_POINT('Ctrl Pts',(-39.2745942850996,-44.0527517782421,
2.75470625793312));
#248842=CARTESIAN_POINT('Ctrl Pts',(-39.3566016867493,-44.0110417363802,
2.79224250381888));
#248843=CARTESIAN_POINT('Ctrl Pts',(-39.4323285306297,-44.0556530121005,
2.74901809108238));
#248844=CARTESIAN_POINT('Ctrl Pts',(-39.3050549810248,-43.9290071509455,
2.63947868311649));
#248845=CARTESIAN_POINT('Ctrl Pts',(-39.3631024520339,-43.9243964923857,
2.69595066767864));
#248846=CARTESIAN_POINT('Ctrl Pts',(-39.4299498468376,-43.961478133811,
2.68220539436019));
#248847=CARTESIAN_POINT('Ctrl Pts',(-39.3490583909334,-43.8557442421761,
2.59908178584995));
#248848=CARTESIAN_POINT('Ctrl Pts',(-39.3917348424044,-43.8675206320103,
2.65877670944855));
#248849=CARTESIAN_POINT('Ctrl Pts',(-39.4485000225466,-43.9111340157071,
2.6587819886023));
#248850=CARTESIAN_POINT('Ctrl Pts',(-39.4144401478986,-43.7969047596348,
2.59908173515992));
#248851=CARTESIAN_POINT('Ctrl Pts',(-39.4393948122684,-43.8246341160487,
2.6587819886023));
#248852=CARTESIAN_POINT('Ctrl Pts',(-39.4864862581813,-43.8769616275876,
2.6587819886023));
#248853=CARTESIAN_POINT('Origin',(-39.4864862581813,-43.8769616275876,2.5317819886023));
#248854=CARTESIAN_POINT('Ctrl Pts',(-41.6348281284258,-45.7656648676108,
3.77003198860231));
#248855=CARTESIAN_POINT('Ctrl Pts',(-41.5403077290109,-45.8507714175126,
3.77003198860231));
#248856=CARTESIAN_POINT('Ctrl Pts',(-41.5404488407676,-45.8506443599161,
3.64284238727582));
#248857=CARTESIAN_POINT('Ctrl Pts',(-41.7801793767998,-45.926760978665,
3.7700319886023));
#248858=CARTESIAN_POINT('Ctrl Pts',(-41.6856176794272,-46.0121552117509,
3.77025506105692));
#248859=CARTESIAN_POINT('Ctrl Pts',(-41.6565546403142,-45.9795929135662,
3.64284210641874));
#248860=CARTESIAN_POINT('Ctrl Pts',(-41.9185498083229,-46.0801233673968,
3.65553527987801));
#248861=CARTESIAN_POINT('Ctrl Pts',(-41.8239142817198,-46.1657498592366,
3.65585996533074));
#248862=CARTESIAN_POINT('Ctrl Pts',(-41.7670853619603,-46.1023497159504,
3.55127902710108));
#248863=CARTESIAN_POINT('Ctrl Pts',(-41.9955727382247,-46.1654920697614,
3.47153072139039));
#248864=CARTESIAN_POINT('Ctrl Pts',(-41.9009568069089,-46.2513146407504,
3.47182327905155));
#248865=CARTESIAN_POINT('Ctrl Pts',(-41.8286118967076,-46.1706818552411,
3.40413028377963));
#248866=CARTESIAN_POINT('Origin',(-41.6348281284258,-45.7656648676108,3.64303198860231));
#248867=CARTESIAN_POINT('Origin',(3.72719664096538E-16,1.91533843916112E-13,
2.53178198860262));
#248868=CARTESIAN_POINT('Origin',(-39.5091373124618,-43.8565665267058,2.53178198860231));
#248869=CARTESIAN_POINT('Origin',(27.6232705441538,31.1532462714326,3.64303198860284));
#248870=CARTESIAN_POINT('Origin',(-41.3663085755616,-45.4673664422114,3.64299466007618));
#248871=CARTESIAN_POINT('Ctrl Pts',(-39.4370498736004,-43.7765468711724,
2.59908173515992));
#248872=CARTESIAN_POINT('Ctrl Pts',(-39.4620188529806,-43.8042633382931,
2.65878198860231));
#248873=CARTESIAN_POINT('Ctrl Pts',(-39.5091373124618,-43.8565665267058,
2.6587819886023));
#248874=CARTESIAN_POINT('Ctrl Pts',(-39.502178522486,-43.7178744835419,
2.599081931998));
#248875=CARTESIAN_POINT('Ctrl Pts',(-39.5094654441324,-43.7615157339664,
2.65877685806551));
#248876=CARTESIAN_POINT('Ctrl Pts',(-39.5469637653732,-43.8224770900121,
2.6587819886023));
#248877=CARTESIAN_POINT('Ctrl Pts',(-39.5788516269098,-43.6818502604298,
2.63872492669776));
#248878=CARTESIAN_POINT('Ctrl Pts',(-39.5685043961835,-43.7389249259238,
2.69532212015268));
#248879=CARTESIAN_POINT('Ctrl Pts',(-39.5983821485328,-43.8091917332945,
2.68176836726603));
#248880=CARTESIAN_POINT('Ctrl Pts',(-39.7059848156955,-43.6640874258691,
2.75442176402208));
#248881=CARTESIAN_POINT('Ctrl Pts',(-39.656016872279,-43.7412697217733,
2.79203179920073));
#248882=CARTESIAN_POINT('Ctrl Pts',(-39.692386550076,-43.8212571467117,
2.74885310748143));
#248883=CARTESIAN_POINT('Ctrl Pts',(-39.7566878101782,-43.6806424921196,
2.82866089558376));
#248884=CARTESIAN_POINT('Ctrl Pts',(-39.684669524313,-43.7668962219026,
2.85316563119219));
#248885=CARTESIAN_POINT('Ctrl Pts',(-39.7348023770063,-43.8452710114193,
2.79189751796567));
#248886=CARTESIAN_POINT('Ctrl Pts',(-39.7870778846743,-43.7143933160625,
2.90134173515992));
#248887=CARTESIAN_POINT('Ctrl Pts',(-39.6934538167797,-43.7993487829614,
2.90103711553198));
#248888=CARTESIAN_POINT('Ctrl Pts',(-39.7651933658995,-43.8790236240221,
2.8340419886023));
#248889=CARTESIAN_POINT('Origin',(-39.8595727587351,-43.7940440370146,2.83404198860231));
#248890=CARTESIAN_POINT('Origin',(-41.3366772856885,-45.4345348103665,3.56647653971706));
#248891=CARTESIAN_POINT('Origin',(-41.2819167515325,-45.3737170758074,3.42473028058453));
#248892=CARTESIAN_POINT('Origin',(-39.9787779456587,-43.9264348094898,3.11913648168119));
#248893=CARTESIAN_POINT('Origin',(-40.0979831325495,-44.0588255818379,3.40423097483279));
#248894=CARTESIAN_POINT('Ctrl Pts',(-41.06113033474,-45.1285089182134,3.36123028058449));
#248895=CARTESIAN_POINT('Ctrl Pts',(-40.9667509419044,-45.213488505221,
3.36123028058449));
#248896=CARTESIAN_POINT('Ctrl Pts',(-40.9667509419044,-45.213488505221,
3.23423028058449));
#248897=CARTESIAN_POINT('Ctrl Pts',(-41.1211850608429,-45.1955564429372,
3.36123028058449));
#248898=CARTESIAN_POINT('Ctrl Pts',(-41.0269231466364,-45.2803165088395,
3.36099641108397));
#248899=CARTESIAN_POINT('Ctrl Pts',(-41.0570929845757,-45.313823508427,
3.23423043688387));
#248900=CARTESIAN_POINT('Ctrl Pts',(-41.1779726855657,-45.2589537050075,
3.41054258905252));
#248901=CARTESIAN_POINT('Ctrl Pts',(-41.0841042944903,-45.34382260726,3.41008815825996));
#248902=CARTESIAN_POINT('Ctrl Pts',(-41.1425178129606,-45.4086973919085,
3.3081986730428));
#248903=CARTESIAN_POINT('Ctrl Pts',(-41.2079002115903,-45.2923641298559,
3.48823028058451));
#248904=CARTESIAN_POINT('Ctrl Pts',(-41.1142722655002,-45.3773275334107,
3.48794691941567));
#248905=CARTESIAN_POINT('Ctrl Pts',(-41.1875373586968,-45.458696662815,
3.42473028058452));
#248906=CARTESIAN_POINT('Origin',(-41.06113033474,-45.1285089182134,3.23423028058449));
#248907=CARTESIAN_POINT('Ctrl Pts',(-40.0254908126584,-43.9791725362584,
3.47153072139041));
#248908=CARTESIAN_POINT('Ctrl Pts',(-39.9317223035493,-44.0642551277132,
3.47122746285046));
#248909=CARTESIAN_POINT('Ctrl Pts',(-40.0037114707675,-44.1439246046466,
3.40413046676764));
#248910=CARTESIAN_POINT('Ctrl Pts',(-40.1025202360401,-44.0645378932523,
3.65553813457955));
#248911=CARTESIAN_POINT('Ctrl Pts',(-40.0085500157875,-44.1495813562431,
3.65520336072111));
#248912=CARTESIAN_POINT('Ctrl Pts',(-40.0652391174783,-44.2122579788851,
3.5512813451992));
#248913=CARTESIAN_POINT('Ctrl Pts',(-40.2409001323891,-44.2178941385649,
3.77003198860231));
#248914=CARTESIAN_POINT('Ctrl Pts',(-40.1466780419446,-44.3029888158489,
3.76980209314098));
#248915=CARTESIAN_POINT('Ctrl Pts',(-40.1757707681163,-44.3350158129988,
3.64284195387372));
#248916=CARTESIAN_POINT('Ctrl Pts',(-40.3862543050934,-44.3789831537297,
3.77003198860232));
#248917=CARTESIAN_POINT('Ctrl Pts',(-40.2917335385821,-44.4640900341667,
3.77003198860231));
#248918=CARTESIAN_POINT('Ctrl Pts',(-40.2918750179832,-44.4639626455417,
3.64284189403786));
#248919=CARTESIAN_POINT('Origin',(-40.3862543050934,-44.3789831537297,3.64303198860232));
#248920=CARTESIAN_POINT('Origin',(26.9484406282047,30.4037717213984,3.23423028058503));
#248921=CARTESIAN_POINT('Origin',(-40.9599523566121,-45.0161393894795,3.23423028058449));
#248922=CARTESIAN_POINT('Origin',(26.8427652369004,30.2864073093063,3.64303198860284));
#248923=CARTESIAN_POINT('Origin',(-40.6548553974682,-44.6772189625504,3.64299171721637));
#248924=CARTESIAN_POINT('Ctrl Pts',(-40.8131880745603,-44.8522789915943,
3.48823028058449));
#248925=CARTESIAN_POINT('Ctrl Pts',(-40.7187157882333,-44.9380175594364,
3.48852004212228));
#248926=CARTESIAN_POINT('Ctrl Pts',(-40.6447864996549,-44.8559107663287,
3.42473028058449));
#248927=CARTESIAN_POINT('Ctrl Pts',(-40.8432146576644,-44.8858042435429,
3.41028005848375));
#248928=CARTESIAN_POINT('Ctrl Pts',(-40.748670873839,-44.9712860523923,
3.41074404220453));
#248929=CARTESIAN_POINT('Ctrl Pts',(-40.6899581892261,-44.9060790100825,
3.30780486243839));
#248930=CARTESIAN_POINT('Ctrl Pts',(-40.900100336765,-44.9493173051398,
3.36123028058449));
#248931=CARTESIAN_POINT('Ctrl Pts',(-40.8054891887065,-45.0343891839532,
3.36146460586165));
#248932=CARTESIAN_POINT('Ctrl Pts',(-40.7755352187361,-45.0011219300382,
3.2342304530842));
#248933=CARTESIAN_POINT('Ctrl Pts',(-40.9599523566121,-45.0161393894795,
3.36123028058449));
#248934=CARTESIAN_POINT('Ctrl Pts',(-40.8655729637765,-45.101118976487,
3.3612302805845));
#248935=CARTESIAN_POINT('Ctrl Pts',(-40.8655729637765,-45.1011189764871,
3.23423028058449));
#248936=CARTESIAN_POINT('Origin',(-40.7391658924905,-44.7709311793211,3.42473028058448));
#248937=CARTESIAN_POINT('Origin',(-40.6847319392787,-44.7104761492006,3.56563113524681));
#248938=CARTESIAN_POINT('Origin',(-35.8473027488272,-49.8797426639491,3.5664765390944));
#248939=CARTESIAN_POINT('Origin',(-35.8732562382983,-49.9155525184326,3.64299466007498));
#248940=CARTESIAN_POINT('Origin',(-35.7991993820658,-49.8135340601224,3.42473028058448));
#248941=CARTESIAN_POINT('Ctrl Pts',(-35.7350130971385,-49.7242207306176,
3.48823028058448));
#248942=CARTESIAN_POINT('Ctrl Pts',(-35.8375861910552,-49.6503036646787,
3.48794691941564));
#248943=CARTESIAN_POINT('Ctrl Pts',(-35.9019445403514,-49.7388853330813,
3.42473028058449));
#248944=CARTESIAN_POINT('Ctrl Pts',(-35.7084656432366,-49.6878783768787,
3.41028005925051));
#248945=CARTESIAN_POINT('Ctrl Pts',(-35.8109961808822,-49.6137056554105,
3.40982512230884));
#248946=CARTESIAN_POINT('Ctrl Pts',(-35.8622643302221,-49.6842702092588,
3.30780486372859));
#248947=CARTESIAN_POINT('Ctrl Pts',(-35.6581711379697,-49.6190282456277,
3.36123028058446));
#248948=CARTESIAN_POINT('Ctrl Pts',(-35.7606778378488,-49.5444483977922,
3.36099721048756));
#248949=CARTESIAN_POINT('Ctrl Pts',(-35.7870908094917,-49.5808027344274,
3.23423045308409));
#248950=CARTESIAN_POINT('Ctrl Pts',(-35.6052536882598,-49.5465907136146,
3.36123028058446));
#248951=CARTESIAN_POINT('Ctrl Pts',(-35.7079988465454,-49.4719419865735,
3.36123028058446));
#248952=CARTESIAN_POINT('Ctrl Pts',(-35.7079988465454,-49.4719419865735,
3.23423028058446));
#248953=CARTESIAN_POINT('Origin',(-35.6052536882598,-49.5465907136146,3.23423028058446));
#248954=CARTESIAN_POINT('Origin',(0.256862895714053,-0.186621817602674,
3.64303198860262));
#248955=CARTESIAN_POINT('Origin',(-36.1092077731524,-50.2402240048084,3.64303198860227));
#248956=CARTESIAN_POINT('Origin',(0.256862895714053,-0.186621817602671,
3.23423028058481));
#248957=CARTESIAN_POINT('Origin',(-35.5163757878391,-49.4242607783462,3.23423028058446));
#248958=CARTESIAN_POINT('Ctrl Pts',(-36.4252947698674,-50.676214228995,
3.47153072139035));
#248959=CARTESIAN_POINT('Ctrl Pts',(-36.5289136610807,-50.601509405082,
3.47182327902626));
#248960=CARTESIAN_POINT('Ctrl Pts',(-36.4650842624219,-50.5139809070359,
3.4041302895903));
#248961=CARTESIAN_POINT('Ctrl Pts',(-36.357804522255,-50.5831238715078,
3.6555380712092));
#248962=CARTESIAN_POINT('Ctrl Pts',(-36.461235691223,-50.5083591136197,
3.65586275496875));
#248963=CARTESIAN_POINT('Ctrl Pts',(-36.4110366091574,-50.4395906940183,
3.5512812683713));
#248964=CARTESIAN_POINT('Ctrl Pts',(-36.2365613423289,-50.4158900112688,
3.77003198860227));
#248965=CARTESIAN_POINT('Ctrl Pts',(-36.3397499727028,-50.3411491755192,
3.77025505748459));
#248966=CARTESIAN_POINT('Ctrl Pts',(-36.3139421975399,-50.3059517008918,
3.64284211731228));
#248967=CARTESIAN_POINT('Ctrl Pts',(-36.1092077731524,-50.2402240048084,
3.77003198860227));
#248968=CARTESIAN_POINT('Ctrl Pts',(-36.2121064279396,-50.165463756031,
3.77003198860227));
#248969=CARTESIAN_POINT('Ctrl Pts',(-36.2119528169509,-50.1655753609471,
3.64284239821737));
#248970=CARTESIAN_POINT('Origin',(-36.3624339277669,-50.5887599058102,3.40423097483274));
#248971=CARTESIAN_POINT('Ctrl Pts',(-35.5163757878391,-49.4242607783462,
3.36123028058446));
#248972=CARTESIAN_POINT('Ctrl Pts',(-35.6191209461248,-49.3496120513051,
3.36123028058446));
#248973=CARTESIAN_POINT('Ctrl Pts',(-35.6191209461248,-49.3496120513051,
3.23423028058446));
#248974=CARTESIAN_POINT('Ctrl Pts',(-35.4632790141045,-49.351578759919,
3.36123028058446));
#248975=CARTESIAN_POINT('Ctrl Pts',(-35.5661632154437,-49.276721988246,
3.36146538609945));
#248976=CARTESIAN_POINT('Ctrl Pts',(-35.5397616632048,-49.2403833690725,
3.23423043688379));
#248977=CARTESIAN_POINT('Ctrl Pts',(-35.4130704930567,-49.2828534857288,
3.41054258693064));
#248978=CARTESIAN_POINT('Ctrl Pts',(-35.51634184505,-49.2081487547866,3.41100608859729));
#248979=CARTESIAN_POINT('Ctrl Pts',(-35.464721803166,-49.1370998624003,
3.30819866970716));
#248980=CARTESIAN_POINT('Ctrl Pts',(-35.3866101428255,-49.2466351556014,
3.48823028058446));
#248981=CARTESIAN_POINT('Ctrl Pts',(-35.4901170100363,-49.1720533660032,
3.48852004212224));
#248982=CARTESIAN_POINT('Ctrl Pts',(-35.4251752107434,-49.0826686475736,
3.42473028058446));
#248983=CARTESIAN_POINT('Origin',(-35.3224300524577,-49.1573173746147,3.42473028058445));
#248984=CARTESIAN_POINT('Origin',(-36.4671473482312,-50.7328855645266,3.1191364817836));
#248985=CARTESIAN_POINT('Origin',(-36.5718607685317,-50.8770112231004,2.83404198860225));
#248986=CARTESIAN_POINT('Origin',(-35.2746135646431,-49.0915036252753,3.56563113460834));
#248987=CARTESIAN_POINT('Origin',(-35.2482948100394,-49.0553654007527,3.64299171721764));
#248988=CARTESIAN_POINT('Ctrl Pts',(-36.9911673391703,-50.9399462128203,
2.59908173515987));
#248989=CARTESIAN_POINT('Ctrl Pts',(-36.9692474126336,-50.9097606317995,
2.65878198860225));
#248990=CARTESIAN_POINT('Ctrl Pts',(-36.9278827595322,-50.8527980281386,
2.65878198860226));
#248991=CARTESIAN_POINT('Ctrl Pts',(-36.9198678602467,-50.9917217504956,
2.59908193475606));
#248992=CARTESIAN_POINT('Ctrl Pts',(-36.9173100216886,-50.947472126738,
2.65878715325367));
#248993=CARTESIAN_POINT('Ctrl Pts',(-36.886606557094,-50.8827604229954,
2.65878198860226));
#248994=CARTESIAN_POINT('Ctrl Pts',(-36.8393772800886,-51.0192553292379,
2.63878778849838));
#248995=CARTESIAN_POINT('Ctrl Pts',(-36.8558881875863,-50.9634900918198,
2.6956446018007));
#248996=CARTESIAN_POINT('Ctrl Pts',(-36.8338178466772,-50.8901678911825,
2.6818048162485));
#248997=CARTESIAN_POINT('Ctrl Pts',(-36.7103770798839,-51.0231582082089,
2.75443238878605));
#248998=CARTESIAN_POINT('Ctrl Pts',(-36.7689134067392,-50.9515780553173,
2.79268340777063));
#248999=CARTESIAN_POINT('Ctrl Pts',(-36.7411592876128,-50.8676678805078,
2.74885926835571));
#249000=CARTESIAN_POINT('Ctrl Pts',(-36.6614543958819,-51.0012539523501,
2.82856655361637));
#249001=CARTESIAN_POINT('Ctrl Pts',(-36.7432876021361,-50.9229784487439,
2.8538419723075));
#249002=CARTESIAN_POINT('Ctrl Pts',(-36.7013347616504,-50.8391515810786,
2.79184624278418));
#249003=CARTESIAN_POINT('Ctrl Pts',(-36.634724144965,-50.9644637245894,
2.90134173515988));
#249004=CARTESIAN_POINT('Ctrl Pts',(-36.738184035968,-50.8898702560319,
2.90163218716355));
#249005=CARTESIAN_POINT('Ctrl Pts',(-36.6746059268174,-50.8023624960592,
2.83404198860226));
#249006=CARTESIAN_POINT('Origin',(-36.9278827595322,-50.8527980281386,2.53178198860225));
#249007=CARTESIAN_POINT('Origin',(0.256862895714053,-0.186621817602674,
3.64303198860262));
#249008=CARTESIAN_POINT('Origin',(-35.0124214764581,-48.7306271754178,3.64303198860228));
#249009=CARTESIAN_POINT('Origin',(6.67120042669018E-17,1.91710833228385E-13,
2.53178198860262));
#249010=CARTESIAN_POINT('Origin',(-36.9525415975208,-50.8348823336487,2.53178198860226));
#249011=CARTESIAN_POINT('Ctrl Pts',(-35.0124214764581,-48.7306271754178,
3.77003198860228));
#249012=CARTESIAN_POINT('Ctrl Pts',(-35.1153205516304,-48.6558666212126,
3.77003198860228));
#249013=CARTESIAN_POINT('Ctrl Pts',(-35.115166519629,-48.6559785320123,
3.64284187937004));
#249014=CARTESIAN_POINT('Ctrl Pts',(-34.8850714976646,-48.5549543235565,
3.77003198860229));
#249015=CARTESIAN_POINT('Ctrl Pts',(-34.9878965398059,-48.4804833899309,
3.7698020896304));
#249016=CARTESIAN_POINT('Ctrl Pts',(-35.0131753353115,-48.5155997094328,
3.6428419392829));
#249017=CARTESIAN_POINT('Ctrl Pts',(-34.7638382096868,-48.3877151240588,
3.65553535416552));
#249018=CARTESIAN_POINT('Ctrl Pts',(-34.8665607873097,-48.3134799021651,
3.65520057834337));
#249019=CARTESIAN_POINT('Ctrl Pts',(-34.916081646201,-48.3819617107285,
3.5512791096416));
#249020=CARTESIAN_POINT('Ctrl Pts',(-34.6963546279281,-48.2946219293748,
3.47153072139038));
#249021=CARTESIAN_POINT('Ctrl Pts',(-34.7990735417348,-48.220592144083,
3.47122746281549));
#249022=CARTESIAN_POINT('Ctrl Pts',(-34.8620346554126,-48.3075724095163,
3.40413045901235));
#249023=CARTESIAN_POINT('Origin',(-34.759195062553,-48.3820909175331,3.40423097483276));
#249024=CARTESIAN_POINT('Ctrl Pts',(-37.1493329797256,-50.5905785208486,
2.90134173515987));
#249025=CARTESIAN_POINT('Ctrl Pts',(-37.0464195108248,-50.6659240749085,
2.90163218716355));
#249026=CARTESIAN_POINT('Ctrl Pts',(-36.9828414016742,-50.5784163149358,
2.83404198860226));
#249027=CARTESIAN_POINT('Ctrl Pts',(-37.1760745934433,-50.627386024724,
2.82853349835321));
#249028=CARTESIAN_POINT('Ctrl Pts',(-37.0763471615781,-50.6810174228632,
2.85381483162248));
#249029=CARTESIAN_POINT('Ctrl Pts',(-37.0095824157651,-50.6152221632656,
2.79182701594302));
#249030=CARTESIAN_POINT('Ctrl Pts',(-37.1816769644888,-50.6805407410137,
2.75468822073603));
#249031=CARTESIAN_POINT('Ctrl Pts',(-37.0954833955417,-50.7141678268703,
2.79286913083843));
#249032=CARTESIAN_POINT('Ctrl Pts',(-37.0242869695748,-50.6617655220312,
2.74900763297875));
#249033=CARTESIAN_POINT('Ctrl Pts',(-37.1386811500604,-50.8012099538927,
2.63954450640359));
#249034=CARTESIAN_POINT('Ctrl Pts',(-37.0803097184697,-50.7999485296222,
2.69627684028798));
#249035=CARTESIAN_POINT('Ctrl Pts',(-37.0173098767917,-50.7562647493203,
2.68224356036455));
#249036=CARTESIAN_POINT('Ctrl Pts',(-37.087378701726,-50.8700180268815,
2.59908178706274));
#249037=CARTESIAN_POINT('Ctrl Pts',(-37.0460487315398,-50.8539379904884,
2.6587870432159));
#249038=CARTESIAN_POINT('Ctrl Pts',(-36.9939291606759,-50.8047860147162,
2.65878198860226));
#249039=CARTESIAN_POINT('Ctrl Pts',(-37.0158684358555,-50.9219998155901,
2.59908173515987));
#249040=CARTESIAN_POINT('Ctrl Pts',(-36.9939338721428,-50.8918248691002,
2.65878198860226));
#249041=CARTESIAN_POINT('Ctrl Pts',(-36.9525415975208,-50.8348823336487,
2.65878198860226));
#249042=CARTESIAN_POINT('Origin',(-37.0855865599598,-50.5037675878947,2.83404198860224));
#249043=CARTESIAN_POINT('Origin',(-34.6544814981908,-48.2379650606661,3.11913648167141));
#249044=CARTESIAN_POINT('Origin',(-34.5497679336937,-48.0938392037149,2.83404198860227));
#249045=CARTESIAN_POINT('Origin',(-36.980873139615,-50.3596419293362,3.11913648177507));
#249046=CARTESIAN_POINT('Origin',(-36.876159719195,-50.2155162706045,3.40423097483274));
#249047=CARTESIAN_POINT('Ctrl Pts',(-34.4869303039392,-48.0063682005188,
2.9013417351599));
#249048=CARTESIAN_POINT('Ctrl Pts',(-34.5894948283129,-47.9324532779039,
2.90103711553196));
#249049=CARTESIAN_POINT('Ctrl Pts',(-34.6525130919793,-48.0191904766737,
2.83404198860228));
#249050=CARTESIAN_POINT('Ctrl Pts',(-34.4602241019853,-47.9696093621193,
2.82862991747919));
#249051=CARTESIAN_POINT('Ctrl Pts',(-34.5595620694338,-47.917105603145,
2.85314045886478));
#249052=CARTESIAN_POINT('Ctrl Pts',(-34.6258053530815,-47.9824304277182,
2.79187960999922));
#249053=CARTESIAN_POINT('Ctrl Pts',(-34.4546775021463,-47.9167391807672,
2.75470625793305));
#249054=CARTESIAN_POINT('Ctrl Pts',(-34.5405955452481,-47.8838297385507,
2.79224250381847));
#249055=CARTESIAN_POINT('Ctrl Pts',(-34.6112444014586,-47.9361122396533,
2.74901809108231));
#249056=CARTESIAN_POINT('Ctrl Pts',(-34.4979061669206,-47.7968564492221,
2.63947868311651));
#249057=CARTESIAN_POINT('Ctrl Pts',(-34.5561175928638,-47.7983386612727,
2.69595066767887));
#249058=CARTESIAN_POINT('Ctrl Pts',(-34.618722703651,-47.8422046210391,
2.68220539436021));
#249059=CARTESIAN_POINT('Ctrl Pts',(-34.5493265808144,-47.7285944911487,
2.59908178585036));
#249060=CARTESIAN_POINT('Ctrl Pts',(-34.5905382782873,-47.7447672725785,
2.65877670944848));
#249061=CARTESIAN_POINT('Ctrl Pts',(-34.6424336528567,-47.7940753146422,
2.65878198860228));
#249062=CARTESIAN_POINT('Ctrl Pts',(-34.620500570363,-47.6769115920305,
2.59908173515989));
#249063=CARTESIAN_POINT('Ctrl Pts',(-34.642420023457,-47.7070975168465,
2.65878198860227));
#249064=CARTESIAN_POINT('Ctrl Pts',(-34.6837837831342,-47.7640607692764,
2.65878198860228));
#249065=CARTESIAN_POINT('Origin',(-34.6837837831342,-47.7640607692764,2.53178198860228));
#249066=CARTESIAN_POINT('Ctrl Pts',(-36.6229335645805,-49.8669803696027,
3.77003198860228));
#249067=CARTESIAN_POINT('Ctrl Pts',(-36.5200349009281,-49.9417406248211,
3.77003198860228));
#249068=CARTESIAN_POINT('Ctrl Pts',(-36.5201885207953,-49.9416290134545,
3.64284238727569));
#249069=CARTESIAN_POINT('Ctrl Pts',(-36.7506494346799,-50.0423873219319,
3.77003198860228));
#249070=CARTESIAN_POINT('Ctrl Pts',(-36.6476796282246,-50.1174293675627,
3.77025506105825));
#249071=CARTESIAN_POINT('Ctrl Pts',(-36.6221794864696,-50.0820075342381,
3.64284210641864));
#249072=CARTESIAN_POINT('Ctrl Pts',(-36.8722311236871,-50.2093732240182,
3.65553527987796));
#249073=CARTESIAN_POINT('Ctrl Pts',(-36.7691636147942,-50.2846385388097,
3.65585996532967));
#249074=CARTESIAN_POINT('Ctrl Pts',(-36.7192731293494,-50.215645468493,
3.55127902710114));
#249075=CARTESIAN_POINT('Ctrl Pts',(-36.9399086546482,-50.3023253561997,
3.47153072139036));
#249076=CARTESIAN_POINT('Ctrl Pts',(-36.8368401378447,-50.3777877242641,
3.47182327905152));
#249077=CARTESIAN_POINT('Ctrl Pts',(-36.7733199617894,-50.2900345513018,
3.40413028377955));
#249078=CARTESIAN_POINT('Origin',(-36.6229335645805,-49.8669803696027,3.64303198860228));
#249079=CARTESIAN_POINT('Origin',(3.77491158612227E-16,1.91529980036038E-13,
2.53178198860262));
#249080=CARTESIAN_POINT('Origin',(-34.7084426211227,-47.7461450747866,2.53178198860228));
#249081=CARTESIAN_POINT('Origin',(21.2404668433927,29.7751578089173,3.64303198860283));
#249082=CARTESIAN_POINT('Origin',(-36.3870656659267,-49.5422481179708,3.6429946600742));
#249083=CARTESIAN_POINT('Ctrl Pts',(-34.6451144164181,-47.6590285860937,
2.59908173515989));
#249084=CARTESIAN_POINT('Ctrl Pts',(-34.6670494534013,-47.6892031885514,
2.65878198860228));
#249085=CARTESIAN_POINT('Ctrl Pts',(-34.7084426211227,-47.7461450747866,
2.65878198860228));
#249086=CARTESIAN_POINT('Ctrl Pts',(-34.7160192182659,-47.6074854095243,
2.59908193199792));
#249087=CARTESIAN_POINT('Ctrl Pts',(-34.7187044685505,-47.651649279334,
2.65877685806575));
#249088=CARTESIAN_POINT('Ctrl Pts',(-34.7496251731986,-47.7161963245879,
2.65878198860228));
#249089=CARTESIAN_POINT('Ctrl Pts',(-34.7960378560834,-47.5796730526552,
2.63872492669777));
#249090=CARTESIAN_POINT('Ctrl Pts',(-34.7797813814944,-47.6353534770325,
2.69532212015245));
#249091=CARTESIAN_POINT('Ctrl Pts',(-34.8021505789967,-47.7083584310193,
2.68176836726607));
#249092=CARTESIAN_POINT('Ctrl Pts',(-34.9243313177589,-47.5752965616147,
2.75442176402202));
#249093=CARTESIAN_POINT('Ctrl Pts',(-34.866569357182,-47.6468329724886,
2.79203179920103));
#249094=CARTESIAN_POINT('Ctrl Pts',(-34.8943788354693,-47.7301838844736,
2.74885310748134));
#249095=CARTESIAN_POINT('Ctrl Pts',(-34.9730260802976,-47.5970608435769,
2.82866089558375));
#249096=CARTESIAN_POINT('Ctrl Pts',(-34.8923863483133,-47.6753141056557,
2.85316563119084));
#249097=CARTESIAN_POINT('Ctrl Pts',(-34.9340521716866,-47.7584998599248,
2.79189751796537));
#249098=CARTESIAN_POINT('Ctrl Pts',(-34.9997217530256,-47.6338034047601,
2.9013417351599));
#249099=CARTESIAN_POINT('Ctrl Pts',(-34.8977303031698,-47.7085070967804,
2.90103711553195));
#249100=CARTESIAN_POINT('Ctrl Pts',(-34.9607485668361,-47.7952442955503,
2.83404198860228));
#249101=CARTESIAN_POINT('Origin',(-35.0634937251217,-47.7205955685092,2.83404198860228));
#249102=CARTESIAN_POINT('Origin',(-36.3610285393798,-49.5064990280447,3.56647653971786));
#249103=CARTESIAN_POINT('Origin',(-36.3129251734939,-49.4402904249167,3.42473028058449));
#249104=CARTESIAN_POINT('Origin',(-35.1682072895631,-47.8647214254838,3.11913648168009));
#249105=CARTESIAN_POINT('Origin',(-35.2729208539811,-48.0088472823273,3.40423097483276));
#249106=CARTESIAN_POINT('Ctrl Pts',(-36.1189794796879,-49.1733470784089,
3.36123028058446));
#249107=CARTESIAN_POINT('Ctrl Pts',(-36.0162343214022,-49.24799580545,3.36123028058446));
#249108=CARTESIAN_POINT('Ctrl Pts',(-36.0162343214022,-49.24799580545,3.23423028058446));
#249109=CARTESIAN_POINT('Ctrl Pts',(-36.1716968449929,-49.2463047380079,
3.36123028058446));
#249110=CARTESIAN_POINT('Ctrl Pts',(-36.0690914679796,-49.3207474263659,
3.36099641108385));
#249111=CARTESIAN_POINT('Ctrl Pts',(-36.0955935972142,-49.3572244778993,
3.23423043688384));
#249112=CARTESIAN_POINT('Ctrl Pts',(-36.2215465627843,-49.3152906263895,
3.41054258905249));
#249113=CARTESIAN_POINT('Ctrl Pts',(-36.1193211766459,-49.389882689244,
3.41008815826051));
#249114=CARTESIAN_POINT('Ctrl Pts',(-36.1706334382063,-49.4605079583558,
3.30819867304284));
#249115=CARTESIAN_POINT('Ctrl Pts',(-36.2478178023246,-49.3516463037386,
3.48823028058448));
#249116=CARTESIAN_POINT('Ctrl Pts',(-36.1458216659121,-49.4263574835552,
3.48794691941564));
#249117=CARTESIAN_POINT('Ctrl Pts',(-36.2101800152082,-49.5149391519578,
3.42473028058449));
#249118=CARTESIAN_POINT('Origin',(-36.1189794796879,-49.1733470784089,3.23423028058446));
#249119=CARTESIAN_POINT('Ctrl Pts',(-35.2091516650524,-47.9220530736688,
3.47153072139038));
#249120=CARTESIAN_POINT('Ctrl Pts',(-35.1070032771115,-47.9968680956253,
3.47122746285042));
#249121=CARTESIAN_POINT('Ctrl Pts',(-35.1702703521465,-48.0836260518494,
3.40413046676746));
#249122=CARTESIAN_POINT('Ctrl Pts',(-35.2768360036062,-48.0150025575606,
3.65553813457951));
#249123=CARTESIAN_POINT('Ctrl Pts',(-35.1744910995522,-48.0897575808483,
3.65520336072128));
#249124=CARTESIAN_POINT('Ctrl Pts',(-35.2243181613713,-48.1580164790724,
3.55128134519897));
#249125=CARTESIAN_POINT('Ctrl Pts',(-35.3984277477544,-48.1819833392239,
3.77003198860228));
#249126=CARTESIAN_POINT('Ctrl Pts',(-35.295826999928,-48.256762968645,3.76980209314088));
#249127=CARTESIAN_POINT('Ctrl Pts',(-35.3214126203088,-48.2916555365112,
3.64284195387367));
#249128=CARTESIAN_POINT('Ctrl Pts',(-35.5261472678861,-48.357383540212,
3.77003198860229));
#249129=CARTESIAN_POINT('Ctrl Pts',(-35.4232482045978,-48.4321440857829,
3.77003198860229));
#249130=CARTESIAN_POINT('Ctrl Pts',(-35.4234022246974,-48.4320321836304,
3.64284189403754));
#249131=CARTESIAN_POINT('Origin',(-35.5261472678861,-48.357383540212,3.64303198860229));
#249132=CARTESIAN_POINT('Origin',(20.7197400704237,29.0584388930976,3.23423028058502));
#249133=CARTESIAN_POINT('Origin',(-36.0301015792672,-49.0510171431405,3.23423028058446));
#249134=CARTESIAN_POINT('Origin',(20.6381965522785,28.9462038689909,3.64303198860283));
#249135=CARTESIAN_POINT('Origin',(-35.7621028045849,-48.6820620414858,3.64299171721696));
#249136=CARTESIAN_POINT('Ctrl Pts',(-35.90126936289,-48.8727133447945,3.48823028058447));
#249137=CARTESIAN_POINT('Ctrl Pts',(-35.7983524848931,-48.9481071848798,
3.48852004212224));
#249138=CARTESIAN_POINT('Ctrl Pts',(-35.7334106856002,-48.8587224664502,
3.42473028058446));
#249139=CARTESIAN_POINT('Ctrl Pts',(-35.9276271141657,-48.9091935744924,
3.41028005848374));
#249140=CARTESIAN_POINT('Ctrl Pts',(-35.8246659689643,-48.9843245886148,
3.41074404220222));
#249141=CARTESIAN_POINT('Ctrl Pts',(-35.7730909105047,-48.913337610609,
3.30780486243807));
#249142=CARTESIAN_POINT('Ctrl Pts',(-35.9775622448362,-48.9783048775121,
3.36123028058446));
#249143=CARTESIAN_POINT('Ctrl Pts',(-35.874576953785,-49.053021165758,3.36146460586494));
#249144=CARTESIAN_POINT('Ctrl Pts',(-35.8482644497263,-49.0168051108914,
3.23423045308429));
#249145=CARTESIAN_POINT('Ctrl Pts',(-36.0301015792672,-49.0510171431405,
3.36123028058446));
#249146=CARTESIAN_POINT('Ctrl Pts',(-35.9273564209816,-49.1256658701816,
3.36123028058446));
#249147=CARTESIAN_POINT('Ctrl Pts',(-35.9273564209816,-49.1256658701816,
3.23423028058446));
#249148=CARTESIAN_POINT('Origin',(-35.8361558438858,-48.784073739409,3.42473028058446));
#249149=CARTESIAN_POINT('Origin',(-35.7883393569603,-48.7182599907927,3.56563113524784));
#249150=CARTESIAN_POINT('Origin',(-30.4370746247564,-53.3535596832574,3.56647653909417));
#249151=CARTESIAN_POINT('Origin',(-30.4591427892363,-53.3918862459817,3.64299466007604));
#249152=CARTESIAN_POINT('Origin',(-30.3961554568832,-53.2826856060847,3.42473028058446));
#249153=CARTESIAN_POINT('Ctrl Pts',(-30.3416565762231,-53.1871522506176,
3.48823028058445));
#249154=CARTESIAN_POINT('Ctrl Pts',(-30.4513942013108,-53.1243619179796,
3.48794691941561));
#249155=CARTESIAN_POINT('Ctrl Pts',(-30.5061406831638,-53.2191856060847,
3.42473028058447));
#249156=CARTESIAN_POINT('Ctrl Pts',(-30.3190533624379,-53.1482340195357,
3.41028005925049));
#249157=CARTESIAN_POINT('Ctrl Pts',(-30.4287753876662,-53.0851849835423,
3.40982512230914));
#249158=CARTESIAN_POINT('Ctrl Pts',(-30.4723866803434,-53.1607219582409,
3.30780486372757));
#249159=CARTESIAN_POINT('Ctrl Pts',(-30.2762311741516,-53.0745038491597,
3.36123028058444));
#249160=CARTESIAN_POINT('Ctrl Pts',(-30.385972048483,-53.0110474253425,
3.36099721048402));
#249161=CARTESIAN_POINT('Ctrl Pts',(-30.4084402641646,-53.0499635164572,
3.23423045308424));
#249162=CARTESIAN_POINT('Ctrl Pts',(-30.2311753956707,-52.9969317578288,
3.36123028058444));
#249163=CARTESIAN_POINT('Ctrl Pts',(-30.3411606219514,-52.9334317578288,
3.36123028058444));
#249164=CARTESIAN_POINT('Ctrl Pts',(-30.3411606219514,-52.9334317578288,
3.23423028058444));
#249165=CARTESIAN_POINT('Origin',(-30.2311753956707,-52.9969317578288,3.23423028058444));
#249166=CARTESIAN_POINT('Origin',(0.274963065701566,-0.158749999999814,
3.64303198860263));
#249167=CARTESIAN_POINT('Origin',(-30.659864345357,-53.7394427993287,3.64303198860224));
#249168=CARTESIAN_POINT('Origin',(0.274963065701566,-0.158749999999811,
3.23423028058481));
#249169=CARTESIAN_POINT('Origin',(-30.1555713378333,-52.865981688396,3.23423028058444));
#249170=CARTESIAN_POINT('Ctrl Pts',(-30.9286463962973,-54.2060847114743,
3.47153072139033));
#249171=CARTESIAN_POINT('Ctrl Pts',(-31.0395064328255,-54.1426202518669,
3.47182327902624));
#249172=CARTESIAN_POINT('Ctrl Pts',(-30.9851759176833,-54.0488992551382,
3.40413028958997));
#249173=CARTESIAN_POINT('Ctrl Pts',(-30.8712564593353,-54.1064496608376,
3.65553807120916));
#249174=CARTESIAN_POINT('Ctrl Pts',(-30.981936066786,-54.0429059732603,
3.65586275496826));
#249175=CARTESIAN_POINT('Ctrl Pts',(-30.939200237769,-53.9692670413548,
3.55128126837159));
#249176=CARTESIAN_POINT('Ctrl Pts',(-30.7681581606549,-53.9274585619019,
3.77003198860224));
#249177=CARTESIAN_POINT('Ctrl Pts',(-30.8785940576193,-53.8639133132318,
3.77025505748453));
#249178=CARTESIAN_POINT('Ctrl Pts',(-30.856606798079,-53.8262110069728,
3.64284211731175));
#249179=CARTESIAN_POINT('Ctrl Pts',(-30.659864345357,-53.7394427993288,
3.77003198860225));
#249180=CARTESIAN_POINT('Ctrl Pts',(-30.7700138844655,-53.6758479332734,
3.77003198860225));
#249181=CARTESIAN_POINT('Ctrl Pts',(-30.769849449083,-53.6759428700857,
3.64284239821677));
#249182=CARTESIAN_POINT('Origin',(-30.8752713784757,-54.112538724998,3.40423097483272));
#249183=CARTESIAN_POINT('Ctrl Pts',(-30.1555713378333,-52.865981688396,
3.36123028058444));
#249184=CARTESIAN_POINT('Ctrl Pts',(-30.2655565641139,-52.802481688396,
3.36123028058444));
#249185=CARTESIAN_POINT('Ctrl Pts',(-30.2655565641139,-52.802481688396,
3.23423028058444));
#249186=CARTESIAN_POINT('Ctrl Pts',(-30.1103627734743,-52.7881477055076,
3.36123028058443));
#249187=CARTESIAN_POINT('Ctrl Pts',(-30.2205080277004,-52.7244553345187,
3.36146538610102));
#249188=CARTESIAN_POINT('Ctrl Pts',(-30.1980495259463,-52.6855560684212,
3.23423043688476));
#249189=CARTESIAN_POINT('Ctrl Pts',(-30.067613047258,-52.7145506960115,
3.41054258693063));
#249190=CARTESIAN_POINT('Ctrl Pts',(-30.1781274387062,-52.6510500011304,
3.4110060885975));
#249191=CARTESIAN_POINT('Ctrl Pts',(-30.1342168083493,-52.5749945583579,
3.30819866970748));
#249192=CARTESIAN_POINT('Ctrl Pts',(-30.0450834959832,-52.6757649139397,
3.48823028058443));
#249193=CARTESIAN_POINT('Ctrl Pts',(-30.1558192615997,-52.6124111049557,
3.48852004212222));
#249194=CARTESIAN_POINT('Ctrl Pts',(-30.1005764675353,-52.5167277788842,
3.42473028058443));
#249195=CARTESIAN_POINT('Origin',(-29.9905912412547,-52.5802277788842,3.42473028058442));
#249196=CARTESIAN_POINT('Origin',(-30.9643459342445,-54.266820381201,3.1191364817843));
#249197=CARTESIAN_POINT('Origin',(-31.0534204898629,-54.4211020372439,2.83404198860223));
#249198=CARTESIAN_POINT('Origin',(-29.9499161072439,-52.5097763801598,3.56563113460837));
#249199=CARTESIAN_POINT('Origin',(-29.927519002606,-52.4710850656384,3.64299171721757));
#249200=CARTESIAN_POINT('Ctrl Pts',(-31.4638515574735,-54.527521733972,
2.59908173515985));
#249201=CARTESIAN_POINT('Ctrl Pts',(-31.4452069629848,-54.4952102564866,
2.65878198860223));
#249202=CARTESIAN_POINT('Ctrl Pts',(-31.4100231232056,-54.4342359163064,
2.65878198860223));
#249203=CARTESIAN_POINT('Ctrl Pts',(-31.387530647168,-54.5715608148715,
2.59908193475496));
#249204=CARTESIAN_POINT('Ctrl Pts',(-31.3896121658904,-54.5272862282526,
2.65878715325321));
#249205=CARTESIAN_POINT('Ctrl Pts',(-31.365841113034,-54.4597196360206,
2.65878198860223));
#249206=CARTESIAN_POINT('Ctrl Pts',(-31.3046029601553,-54.5905300051367,
2.63878778849819));
#249207=CARTESIAN_POINT('Ctrl Pts',(-31.3268524737459,-54.536796115312,
2.69564460180095));
#249208=CARTESIAN_POINT('Ctrl Pts',(-31.3125672934291,-54.4615686025426,
2.68180481624847));
#249209=CARTESIAN_POINT('Ctrl Pts',(-31.1759014746037,-54.5809273110394,
2.7544323887862));
#249210=CARTESIAN_POINT('Ctrl Pts',(-31.2415992967173,-54.5158579940063,
2.79268340777024));
#249211=CARTESIAN_POINT('Ctrl Pts',(-31.2227682191853,-54.4295063924925,
2.74885926835569));
#249212=CARTESIAN_POINT('Ctrl Pts',(-31.129536412388,-54.5540292360083,
2.82856655361619));
#249213=CARTESIAN_POINT('Ctrl Pts',(-31.219103345881,-54.4847364330974,
2.85384197230905));
#249214=CARTESIAN_POINT('Ctrl Pts',(-31.1861426211013,-54.3969835118377,
2.79184624278558));
#249215=CARTESIAN_POINT('Ctrl Pts',(-31.106798218553,-54.5146464769139,
2.90134173515985));
#249216=CARTESIAN_POINT('Ctrl Pts',(-31.217488486086,-54.4512761425984,
2.90163218716352));
#249217=CARTESIAN_POINT('Ctrl Pts',(-31.1634057161435,-54.3576020372439,
2.83404198860223));
#249218=CARTESIAN_POINT('Origin',(-31.4100231232056,-54.4342359163064,2.53178198860222));
#249219=CARTESIAN_POINT('Origin',(0.274963065701566,-0.158749999999814,
3.64303198860263));
#249220=CARTESIAN_POINT('Origin',(-29.7268821954845,-52.1234703131947,3.64303198860225));
#249221=CARTESIAN_POINT('Origin',(5.22371297615222E-17,1.91720233321799E-13,
2.53178198860262));
#249222=CARTESIAN_POINT('Origin',(-31.436419577513,-54.4189959163064,2.53178198860223));
#249223=CARTESIAN_POINT('Ctrl Pts',(-29.7268821954845,-52.1234703131947,
3.77003198860226));
#249224=CARTESIAN_POINT('Ctrl Pts',(-29.8370321846009,-52.0598751873271,
3.77003198860226));
#249225=CARTESIAN_POINT('Ctrl Pts',(-29.8368672985388,-52.0599703843395,
3.64284187936975));
#249226=CARTESIAN_POINT('Ctrl Pts',(-29.6185926664433,-51.935448118016,
3.77003198860226));
#249227=CARTESIAN_POINT('Ctrl Pts',(-29.7286387544941,-51.8721332875992,
3.76980208963075));
#249228=CARTESIAN_POINT('Ctrl Pts',(-29.7501084152009,-51.9096995898763,
3.64284193928295));
#249229=CARTESIAN_POINT('Ctrl Pts',(-29.5155047636237,-51.7564527430624,
3.65553535416548));
#249230=CARTESIAN_POINT('Ctrl Pts',(-29.6254243098809,-51.693361622663,
3.65520057834344));
#249231=CARTESIAN_POINT('Ctrl Pts',(-29.667515590115,-51.7666446199922,
3.55127910964187));
#249232=CARTESIAN_POINT('Ctrl Pts',(-29.4581217525669,-51.6568155675428,
3.47153072139035));
#249233=CARTESIAN_POINT('Ctrl Pts',(-29.568016181109,-51.5939283753694,
3.47122746281545));
#249234=CARTESIAN_POINT('Ctrl Pts',(-29.6215404737378,-51.6870133822664,
3.40413045901218));
#249235=CARTESIAN_POINT('Origin',(-29.5114749418,-51.7503740054944,3.40423097483273));
#249236=CARTESIAN_POINT('Ctrl Pts',(-31.6576696180579,-54.1966007261208,
2.90134173515985));
#249237=CARTESIAN_POINT('Ctrl Pts',(-31.5474441649278,-54.2607761425984,
2.90163218716353));
#249238=CARTESIAN_POINT('Ctrl Pts',(-31.4933613949854,-54.1671020372439,
2.83404198860223));
#249239=CARTESIAN_POINT('Ctrl Pts',(-31.6804173065999,-54.2360018544267,
2.82853349835301));
#249240=CARTESIAN_POINT('Ctrl Pts',(-31.5756301844116,-54.2789150989582,
2.85381483162341));
#249241=CARTESIAN_POINT('Ctrl Pts',(-31.5161086602377,-54.2065014563942,
2.7918270159426));
#249242=CARTESIAN_POINT('Ctrl Pts',(-31.680432806462,-54.2894509908544,
2.75468822073627));
#249243=CARTESIAN_POINT('Ctrl Pts',(-31.591196427296,-54.3138841827109,
2.79286913083811));
#249244=CARTESIAN_POINT('Ctrl Pts',(-31.5258675551964,-54.254326890184,
2.7490076329788));
#249245=CARTESIAN_POINT('Ctrl Pts',(-31.6250591602186,-54.4049648787501,
2.63954450640331));
#249246=CARTESIAN_POINT('Ctrl Pts',(-31.5671393481776,-54.3976088886508,
2.69627684028808));
#249247=CARTESIAN_POINT('Ctrl Pts',(-31.5090508246488,-54.3475791360313,
2.68224356036447));
#249248=CARTESIAN_POINT('Ctrl Pts',(-31.5668453499334,-54.4680334478294,
2.59908178706285));
#249249=CARTESIAN_POINT('Ctrl Pts',(-31.5274226111427,-54.4477213412889,
2.6587870432146));
#249250=CARTESIAN_POINT('Ctrl Pts',(-31.4807263372346,-54.3933906465327,
2.65878198860223));
#249251=CARTESIAN_POINT('Ctrl Pts',(-31.4902932482903,-54.5122556166612,
2.59908173515985));
#249252=CARTESIAN_POINT('Ctrl Pts',(-31.4716329851984,-54.479953185448,
2.65878198860223));
#249253=CARTESIAN_POINT('Ctrl Pts',(-31.436419577513,-54.4189959163064,
2.65878198860223));
#249254=CARTESIAN_POINT('Origin',(-31.603346621266,-54.1036020372439,2.83404198860223));
#249255=CARTESIAN_POINT('Origin',(-29.4224002636363,-51.5960921371862,3.11913648167068));
#249256=CARTESIAN_POINT('Origin',(-29.333325585345,-51.4418102687786,2.83404198860225));
#249257=CARTESIAN_POINT('Origin',(-31.5142720655983,-53.9493203812114,3.11913648177452));
#249258=CARTESIAN_POINT('Origin',(-31.4251975098788,-53.795038724998,3.40423097483272));
#249259=CARTESIAN_POINT('Ctrl Pts',(-29.2799753962458,-51.3482501200166,
2.90134173515987));
#249260=CARTESIAN_POINT('Ctrl Pts',(-29.3897042746969,-51.2854610232002,
2.90103711553193));
#249261=CARTESIAN_POINT('Ctrl Pts',(-29.4433108116256,-51.3783102687786,
2.83404198860225));
#249262=CARTESIAN_POINT('Ctrl Pts',(-29.2572578385499,-51.3089010921301,
2.82862991747923));
#249263=CARTESIAN_POINT('Ctrl Pts',(-29.3615397594608,-51.2670685993225,
2.85314045886427));
#249264=CARTESIAN_POINT('Ctrl Pts',(-29.4205918519427,-51.3389598763126,
2.79187960999989));
#249265=CARTESIAN_POINT('Ctrl Pts',(-29.2572680623745,-51.2557407616057,
2.7547062579329));
#249266=CARTESIAN_POINT('Ctrl Pts',(-29.3461554108687,-51.2319924817692,
2.7922425038188));
#249267=CARTESIAN_POINT('Ctrl Pts',(-29.4109522357565,-51.2913733902318,
2.74901809108211));
#249268=CARTESIAN_POINT('Ctrl Pts',(-29.3127910737009,-51.1410333861057,
2.63947868311662));
#249269=CARTESIAN_POINT('Ctrl Pts',(-29.3705286780137,-51.1485922293422,
2.69595066767867));
#249270=CARTESIAN_POINT('Ctrl Pts',(-29.4282055900896,-51.1987619028143,
2.68220539436036));
#249271=CARTESIAN_POINT('Ctrl Pts',(-29.3710651187642,-51.078520271026,
2.59908178585069));
#249272=CARTESIAN_POINT('Ctrl Pts',(-29.4103605382565,-51.0989122516714,
2.65877670944823));
#249273=CARTESIAN_POINT('Ctrl Pts',(-29.4568175306708,-51.1533747228769,
2.65878198860225));
#249274=CARTESIAN_POINT('Ctrl Pts',(-29.4472515437731,-51.0345602039887,
2.59908173515987));
#249275=CARTESIAN_POINT('Ctrl Pts',(-29.4658956314762,-51.0668719738978,
2.65878198860225));
#249276=CARTESIAN_POINT('Ctrl Pts',(-29.5010785149107,-51.1278468659048,
2.65878198860225));
#249277=CARTESIAN_POINT('Origin',(-29.5010785149107,-51.1278468659048,2.53178198860225));
#249278=CARTESIAN_POINT('Ctrl Pts',(-31.2097904767601,-53.4219427993288,
3.77003198860225));
#249279=CARTESIAN_POINT('Ctrl Pts',(-31.099640928162,-53.485537670863,3.77003198860225));
#249280=CARTESIAN_POINT('Ctrl Pts',(-31.0998053730483,-53.4854427285636,
3.64284238727554));
#249281=CARTESIAN_POINT('Ctrl Pts',(-31.318471686786,-53.6097387976566,
3.77003198860225));
#249282=CARTESIAN_POINT('Ctrl Pts',(-31.2082219299925,-53.6736064794804,
3.77025506105671));
#249283=CARTESIAN_POINT('Ctrl Pts',(-31.1865640704875,-53.6357132000308,
3.64284210641846));
#249284=CARTESIAN_POINT('Ctrl Pts',(-31.4219325588451,-53.7885186806138,
3.65553527987794));
#249285=CARTESIAN_POINT('Ctrl Pts',(-31.3115622968593,-53.8525981958153,
3.65585996533033));
#249286=CARTESIAN_POINT('Ctrl Pts',(-31.2691568563313,-53.7787681009838,
3.55127902710127));
#249287=CARTESIAN_POINT('Ctrl Pts',(-31.4795232016785,-53.8880358395971,
3.47153072139033));
#249288=CARTESIAN_POINT('Ctrl Pts',(-31.3691313396259,-53.9523112232408,
3.47182327905149));
#249289=CARTESIAN_POINT('Ctrl Pts',(-31.3151318380579,-53.8583991049521,
3.40413028377945));
#249290=CARTESIAN_POINT('Origin',(-31.2097904767601,-53.4219427993288,3.64303198860225));
#249291=CARTESIAN_POINT('Origin',(3.82640399828021E-16,1.91526636079694E-13,
2.53178198860262));
#249292=CARTESIAN_POINT('Origin',(-29.527474969218,-51.1126068659048,2.53178198860225));
#249293=CARTESIAN_POINT('Origin',(15.2806508669887,27.1018636743466,3.64303198860282));
#249294=CARTESIAN_POINT('Origin',(-31.0091584503713,-53.0743345559678,3.64299466007412));
#249295=CARTESIAN_POINT('Ctrl Pts',(-29.4735998357333,-51.0193480105328,
2.59908173515987));
#249296=CARTESIAN_POINT('Ctrl Pts',(-29.4922606054642,-51.0516501490687,
2.65878198860225));
#249297=CARTESIAN_POINT('Ctrl Pts',(-29.527474969218,-51.1126068659048,
2.65878198860225));
#249298=CARTESIAN_POINT('Ctrl Pts',(-29.5495039426967,-50.9754987628538,
2.59908193199895));
#249299=CARTESIAN_POINT('Ctrl Pts',(-29.5475581014577,-51.0197013834522,
2.65877685806689));
#249300=CARTESIAN_POINT('Ctrl Pts',(-29.5715624158009,-51.0871269269774,
2.65878198860225));
#249301=CARTESIAN_POINT('Ctrl Pts',(-29.6319914129668,-50.9562029902289,
2.63872492669762));
#249302=CARTESIAN_POINT('Ctrl Pts',(-29.6100038038521,-51.0098791271087,
2.69532212015239));
#249303=CARTESIAN_POINT('Ctrl Pts',(-29.6246193648992,-51.0848223701587,
2.68176836726606));
#249304=CARTESIAN_POINT('Ctrl Pts',(-29.7600395375186,-50.9652607924606,
2.75442176402213));
#249305=CARTESIAN_POINT('Ctrl Pts',(-29.6951164119093,-51.0303675504162,
2.792031799201));
#249306=CARTESIAN_POINT('Ctrl Pts',(-29.7140610042227,-51.1161687394135,
2.74885310748131));
#249307=CARTESIAN_POINT('Ctrl Pts',(-29.8061925581062,-50.9919958361057,
2.82866089558362));
#249308=CARTESIAN_POINT('Ctrl Pts',(-29.7178148857801,-51.0613912713637,
2.85316563119169));
#249309=CARTESIAN_POINT('Ctrl Pts',(-29.7505571803534,-51.1484765898561,
2.7918975179659));
#249310=CARTESIAN_POINT('Ctrl Pts',(-29.8289013456881,-51.031327575341,
2.90134173515987));
#249311=CARTESIAN_POINT('Ctrl Pts',(-29.7196599535388,-51.0949610232002,
2.90103711553193));
#249312=CARTESIAN_POINT('Ctrl Pts',(-29.7732664904675,-51.1878102687786,
2.83404198860225));
#249313=CARTESIAN_POINT('Origin',(-29.8832517167481,-51.1243102687786,2.83404198860226));
#249314=CARTESIAN_POINT('Origin',(-30.9870007553597,-53.0360596824716,3.56647653971798));
#249315=CARTESIAN_POINT('Origin',(-30.9460815882863,-52.9651856060847,3.42473028058447));
#249316=CARTESIAN_POINT('Origin',(-29.9723263949767,-51.2785921372,3.1191364816828));
#249317=CARTESIAN_POINT('Origin',(-30.0614010732032,-51.4328740054944,3.40423097483274));
#249318=CARTESIAN_POINT('Ctrl Pts',(-30.7811015270739,-52.6794317578288,
3.36123028058444));
#249319=CARTESIAN_POINT('Ctrl Pts',(-30.6711163007932,-52.7429317578288,
3.36123028058444));
#249320=CARTESIAN_POINT('Ctrl Pts',(-30.6711163007932,-52.7429317578288,
3.23423028058444));
#249321=CARTESIAN_POINT('Ctrl Pts',(-30.8259039490958,-52.7575002129169,
3.36123028058444));
#249322=CARTESIAN_POINT('Ctrl Pts',(-30.7160792752587,-52.820809914056,
3.36099641108435));
#249323=CARTESIAN_POINT('Ctrl Pts',(-30.738623332913,-52.8598573673285,
3.2342304368839));
#249324=CARTESIAN_POINT('Ctrl Pts',(-30.8682695960177,-52.8313189037788,
3.41054258905248));
#249325=CARTESIAN_POINT('Ctrl Pts',(-30.7588072175379,-52.8948168809893,
3.41008815825996));
#249326=CARTESIAN_POINT('Ctrl Pts',(-30.8024560343113,-52.9704188493347,
3.3081986730428));
#249327=CARTESIAN_POINT('Ctrl Pts',(-30.8905967158731,-52.8702215132217,
3.48823028058445));
#249328=CARTESIAN_POINT('Ctrl Pts',(-30.7813498801527,-52.9338619179796,
3.48794691941561));
#249329=CARTESIAN_POINT('Ctrl Pts',(-30.8360963620057,-53.0286856060847,
3.42473028058446));
#249330=CARTESIAN_POINT('Origin',(-30.7811015270739,-52.6794317578288,3.23423028058444));
#249331=CARTESIAN_POINT('Ctrl Pts',(-30.0070536838153,-51.3398895692698,
3.47153072139036));
#249332=CARTESIAN_POINT('Ctrl Pts',(-29.8976445761569,-51.4036173326914,
3.4712274628504));
#249333=CARTESIAN_POINT('Ctrl Pts',(-29.951496391695,-51.4965132298825,
3.40413046676735));
#249334=CARTESIAN_POINT('Ctrl Pts',(-30.0646513737701,-51.4394048060584,
3.65553813457952));
#249335=CARTESIAN_POINT('Ctrl Pts',(-29.9550530981038,-51.5030523579586,
3.65520336072241));
#249336=CARTESIAN_POINT('Ctrl Pts',(-29.9974722043253,-51.5761456730011,
3.55128134519924));
#249337=CARTESIAN_POINT('Ctrl Pts',(-30.1681227811166,-51.6181806476914,
3.77003198860227));
#249338=CARTESIAN_POINT('Ctrl Pts',(-30.058267491178,-51.6818259279789,
3.7698020931406));
#249339=CARTESIAN_POINT('Ctrl Pts',(-30.0800656843527,-51.7192017762878,
3.64284195387371));
#249340=CARTESIAN_POINT('Ctrl Pts',(-30.2768083268876,-51.8059703131947,
3.77003198860226));
#249341=CARTESIAN_POINT('Ctrl Pts',(-30.1666583504928,-51.8695654317175,
3.77003198860226));
#249342=CARTESIAN_POINT('Ctrl Pts',(-30.1668232238143,-51.8694702420609,
3.64284189403736));
#249343=CARTESIAN_POINT('Origin',(-30.2768083268876,-51.8059703131947,3.64303198860226));
#249344=CARTESIAN_POINT('Origin',(14.903849434298,26.4492244485615,3.234230280585));
#249345=CARTESIAN_POINT('Origin',(-30.7054974692364,-52.548481688396,3.23423028058444));
#249346=CARTESIAN_POINT('Origin',(14.8448439902557,26.347024021557,3.64303198860281));
#249347=CARTESIAN_POINT('Origin',(-30.4775331296734,-52.1535342613179,3.64299171721737));
#249348=CARTESIAN_POINT('Ctrl Pts',(-30.5960088312564,-52.3576880233163,
3.48823028058444));
#249349=CARTESIAN_POINT('Ctrl Pts',(-30.4857749404415,-52.4219111049557,
3.48852004212222));
#249350=CARTESIAN_POINT('Ctrl Pts',(-30.4305321463772,-52.3262277788842,
3.42473028058444));
#249351=CARTESIAN_POINT('Ctrl Pts',(-30.6184089696598,-52.3967235457368,
3.41028005848368));
#249352=CARTESIAN_POINT('Ctrl Pts',(-30.5081585269343,-52.4606806140151,
3.41074404220138));
#249353=CARTESIAN_POINT('Ctrl Pts',(-30.4642861617676,-52.3846914484999,
3.30780486243784));
#249354=CARTESIAN_POINT('Ctrl Pts',(-30.6608464521623,-52.4706758922782,
3.36123028058443));
#249355=CARTESIAN_POINT('Ctrl Pts',(-30.5506153465215,-52.5342179826684,
3.36146460586488));
#249356=CARTESIAN_POINT('Ctrl Pts',(-30.5282325936734,-52.4954499175236,
3.23423045308435));
#249357=CARTESIAN_POINT('Ctrl Pts',(-30.7054974692364,-52.548481688396,
3.36123028058444));
#249358=CARTESIAN_POINT('Ctrl Pts',(-30.5955122429558,-52.611981688396,
3.36123028058444));
#249359=CARTESIAN_POINT('Ctrl Pts',(-30.5955122429558,-52.611981688396,
3.23423028058444));
#249360=CARTESIAN_POINT('Origin',(-30.5405173726578,-52.2627277788842,3.42473028058445));
#249361=CARTESIAN_POINT('Origin',(-30.4998422394557,-52.1922763809715,3.56563113524769));
#249362=CARTESIAN_POINT('Origin',(-24.6933715417282,-56.2428239377255,3.5664765390945));
#249363=CARTESIAN_POINT('Origin',(-24.7113125977909,-56.2832472948495,3.6429946600762));
#249364=CARTESIAN_POINT('Origin',(-24.6600848917106,-56.1680608984278,3.42473028058445));
#249365=CARTESIAN_POINT('Ctrl Pts',(-24.6158705164589,-56.0673542004326,
3.48823028058444));
#249366=CARTESIAN_POINT('Ctrl Pts',(-24.731570364333,-56.0163785451198,
3.4879469194156));
#249367=CARTESIAN_POINT('Ctrl Pts',(-24.7761051648312,-56.1164053447572,
3.42473028058445));
#249368=CARTESIAN_POINT('Ctrl Pts',(-24.5974591883325,-56.0262864882906,
3.41028005925047));
#249369=CARTESIAN_POINT('Ctrl Pts',(-24.7131705636669,-55.9750519161889,
3.40982512230921));
#249370=CARTESIAN_POINT('Ctrl Pts',(-24.7486471852345,-56.0547337128459,
3.30780486372833));
#249371=CARTESIAN_POINT('Ctrl Pts',(-24.5625784858793,-55.9484840819673,
3.36123028058441));
#249372=CARTESIAN_POINT('Ctrl Pts',(-24.6783511906883,-55.896846324036,
3.36099721048678));
#249373=CARTESIAN_POINT('Ctrl Pts',(-24.6966284839307,-55.9378977967869,
3.23423045308457));
#249374=CARTESIAN_POINT('Ctrl Pts',(-24.5258780191666,-55.8666273273833,
3.36123028058441));
#249375=CARTESIAN_POINT('Ctrl Pts',(-24.6418982922872,-55.8149717737127,
3.36123028058442));
#249376=CARTESIAN_POINT('Ctrl Pts',(-24.6418982922872,-55.8149717737127,
3.23423028058442));
#249377=CARTESIAN_POINT('Origin',(-24.5258780191666,-55.8666273273833,3.23423028058441));
#249378=CARTESIAN_POINT('Origin',(0.290050682801532,-0.12913888417638,3.64303198860263));
#249379=CARTESIAN_POINT('Origin',(-24.8746050278048,-56.6498810128382,3.64303198860222));
#249380=CARTESIAN_POINT('Origin',(0.290050682801533,-0.129138884176377,
3.23423028058481));
#249381=CARTESIAN_POINT('Origin',(-24.4643761377912,-55.7284918401498,3.23423028058442));
#249382=CARTESIAN_POINT('Ctrl Pts',(-25.0931373005741,-57.1420619865022,
3.47153072139031));
#249383=CARTESIAN_POINT('Ctrl Pts',(-25.2100238766575,-57.0905332211011,
3.47182327902622));
#249384=CARTESIAN_POINT('Ctrl Pts',(-25.165787501526,-56.9916465525423,
3.40413028959));
#249385=CARTESIAN_POINT('Ctrl Pts',(-25.0464764504208,-57.0369738651809,
3.65553807120914));
#249386=CARTESIAN_POINT('Ctrl Pts',(-25.1631918674157,-56.9853474458577,
3.65586275496877));
#249387=CARTESIAN_POINT('Ctrl Pts',(-25.1283875141298,-56.9076448051882,
3.55128126837116));
#249388=CARTESIAN_POINT('Ctrl Pts',(-24.9626525995183,-56.8481865914866,
3.77003198860223));
#249389=CARTESIAN_POINT('Ctrl Pts',(-25.0791258042765,-56.7965331449336,
3.77025505748508));
#249390=CARTESIAN_POINT('Ctrl Pts',(-25.06119995738,-56.7567390814052,3.64284211731215));
#249391=CARTESIAN_POINT('Ctrl Pts',(-24.8746050278048,-56.6498810128382,
3.77003198860223));
#249392=CARTESIAN_POINT('Ctrl Pts',(-24.9907986298333,-56.5981482881658,
3.77003198860223));
#249393=CARTESIAN_POINT('Ctrl Pts',(-24.990625171646,-56.5982255167265,
3.64284239821683));
#249394=CARTESIAN_POINT('Origin',(-25.049832894896,-57.0434492461379,3.40423097483269));
#249395=CARTESIAN_POINT('Ctrl Pts',(-24.4643761377912,-55.7284918401498,
3.36123028058442));
#249396=CARTESIAN_POINT('Ctrl Pts',(-24.5803964109118,-55.6768362864792,
3.36123028058442));
#249397=CARTESIAN_POINT('Ctrl Pts',(-24.5803964109118,-55.6768362864792,
3.23423028058442));
#249398=CARTESIAN_POINT('Ctrl Pts',(-24.4275510972983,-55.646358658205,
3.36123028058442));
#249399=CARTESIAN_POINT('Ctrl Pts',(-24.5437506299586,-55.5945285148511,
3.36146538610141));
#249400=CARTESIAN_POINT('Ctrl Pts',(-24.5254812387364,-55.553494790328,
3.23423043688428));
#249401=CARTESIAN_POINT('Ctrl Pts',(-24.3927285408595,-55.5686962576408,
3.41054258693061));
#249402=CARTESIAN_POINT('Ctrl Pts',(-24.5092751529597,-55.5170953257151,
3.41100608859654));
#249403=CARTESIAN_POINT('Ctrl Pts',(-24.473555028186,-55.4368666119022,
3.3081986697068));
#249404=CARTESIAN_POINT('Ctrl Pts',(-24.3743766270209,-55.5277679687683,
3.48823028058443));
#249405=CARTESIAN_POINT('Ctrl Pts',(-24.4911280468221,-55.4763362579875,
3.48852004212221));
#249406=CARTESIAN_POINT('Ctrl Pts',(-24.4461895095984,-55.3754026508175,
3.42473028058443));
#249407=CARTESIAN_POINT('Origin',(-24.3301692364778,-55.4270582044881,3.42473028058442));
#249408=CARTESIAN_POINT('Origin',(-25.1222926664907,-57.2061965577157,3.11913648178284));
#249409=CARTESIAN_POINT('Origin',(-25.1947524379611,-57.3689438691196,2.83404198860221));
#249410=CARTESIAN_POINT('Origin',(-24.2970811015497,-55.3527410366453,3.56563113460771));
#249411=CARTESIAN_POINT('Origin',(-24.2788510342437,-55.3119205422645,3.64299171721722));
#249412=CARTESIAN_POINT('Ctrl Pts',(-25.5918112338789,-57.5176823163889,
2.59908173515983));
#249413=CARTESIAN_POINT('Ctrl Pts',(-25.5766462455171,-57.4835989537478,
2.65878198860221));
#249414=CARTESIAN_POINT('Ctrl Pts',(-25.5480287005713,-57.4192809246789,
2.65878198860221));
#249415=CARTESIAN_POINT('Ctrl Pts',(-25.5113050800554,-57.5535024391256,
2.5990819347554));
#249416=CARTESIAN_POINT('Ctrl Pts',(-25.5180031505012,-57.5096879712772,
2.6587871532528));
#249417=CARTESIAN_POINT('Ctrl Pts',(-25.5014249500136,-57.4400067642813,
2.65878198860221));
#249418=CARTESIAN_POINT('Ctrl Pts',(-25.4268488592811,-57.5636994104961,
2.6387877884984));
#249419=CARTESIAN_POINT('Ctrl Pts',(-25.4545932086367,-57.5125855880056,
2.69564460180084));
#249420=CARTESIAN_POINT('Ctrl Pts',(-25.4482497003378,-57.4362769714768,
2.68180481624847));
#249421=CARTESIAN_POINT('Ctrl Pts',(-25.2998561687911,-57.540696352457,
2.75443238878594));
#249422=CARTESIAN_POINT('Ctrl Pts',(-25.3719956870767,-57.4828507843371,
2.79268340777035));
#249423=CARTESIAN_POINT('Ctrl Pts',(-25.3622939683644,-57.395003842335,
2.74885926835564));
#249424=CARTESIAN_POINT('Ctrl Pts',(-25.2565567136853,-57.5090991591924,
2.82856655361635));
#249425=CARTESIAN_POINT('Ctrl Pts',(-25.3528760603488,-57.4495482434215,
2.85384197230768));
#249426=CARTESIAN_POINT('Ctrl Pts',(-25.3292685758742,-57.3588307079379,
2.79184624278448));
#249427=CARTESIAN_POINT('Ctrl Pts',(-25.2380597013425,-57.4675553545141,
2.90134173515982));
#249428=CARTESIAN_POINT('Ctrl Pts',(-25.354767599671,-57.4161024530844,
2.9016321871635));
#249429=CARTESIAN_POINT('Ctrl Pts',(-25.3107727110817,-57.317288315449,
2.83404198860221));
#249430=CARTESIAN_POINT('Origin',(-25.5480287005713,-57.4192809246789,2.5317819886022));
#249431=CARTESIAN_POINT('Origin',(0.290050682801532,-0.12913888417638,3.64303198860263));
#249432=CARTESIAN_POINT('Origin',(-24.1156489724272,-54.9452378026829,3.64303198860223));
#249433=CARTESIAN_POINT('Origin',(3.68589728140376E-17,1.9172806888413E-13,
2.53178198860262));
#249434=CARTESIAN_POINT('Origin',(-25.5758735661203,-57.406883591798,2.53178198860221));
#249435=CARTESIAN_POINT('Ctrl Pts',(-24.1156489724272,-54.9452378026829,
3.77003198860224));
#249436=CARTESIAN_POINT('Ctrl Pts',(-24.2318430491567,-54.89350486666,3.77003198860224));
#249437=CARTESIAN_POINT('Ctrl Pts',(-24.2316691155599,-54.8935823068866,
3.64284187936935));
#249438=CARTESIAN_POINT('Ctrl Pts',(-24.0276063358797,-54.7469262747035,
3.77003198860224));
#249439=CARTESIAN_POINT('Ctrl Pts',(-24.1436677818743,-54.6954612380258,
3.7698020896313));
#249440=CARTESIAN_POINT('Ctrl Pts',(-24.1610930816824,-54.7350659388095,
3.64284193928315));
#249441=CARTESIAN_POINT('Ctrl Pts',(-23.9437932708537,-54.5581358350793,
3.65553535416546));
#249442=CARTESIAN_POINT('Ctrl Pts',(-24.059705484196,-54.5068800556895,
3.65520057834371));
#249443=CARTESIAN_POINT('Ctrl Pts',(-24.093906024898,-54.5841613379333,
3.55127910964144));
#249444=CARTESIAN_POINT('Ctrl Pts',(-23.8971395307763,-54.4530463244693,
3.47153072139034));
#249445=CARTESIAN_POINT('Ctrl Pts',(-24.0130054476979,-54.4019907306516,
3.47122746281544));
#249446=CARTESIAN_POINT('Ctrl Pts',(-24.0565064959269,-54.5001606201976,
3.40413045901197));
#249447=CARTESIAN_POINT('Origin',(-23.9404209259116,-54.5516691663895,3.40423097483271));
#249448=CARTESIAN_POINT('Ctrl Pts',(-25.8191582032616,-57.2088336324699,
2.90134173515983));
#249449=CARTESIAN_POINT('Ctrl Pts',(-25.7028284190329,-57.2611357920725,
2.90163218716351));
#249450=CARTESIAN_POINT('Ctrl Pts',(-25.6588335304436,-57.1623216544371,
2.83404198860221));
#249451=CARTESIAN_POINT('Ctrl Pts',(-25.8376627381934,-57.250396698198,
2.82853349835328));
#249452=CARTESIAN_POINT('Ctrl Pts',(-25.7289639953181,-57.2821216226324,
2.85381483162255));
#249453=CARTESIAN_POINT('Ctrl Pts',(-25.6773378230589,-57.2038829761261,
2.7918270159416));
#249454=CARTESIAN_POINT('Ctrl Pts',(-25.8320911970514,-57.3035546548413,
2.75468822073581));
#249455=CARTESIAN_POINT('Ctrl Pts',(-25.7407897001103,-57.3185262575348,
2.7928691308381));
#249456=CARTESIAN_POINT('Ctrl Pts',(-25.6820441386713,-57.2524664994803,
2.74900763297875));
#249457=CARTESIAN_POINT('Ctrl Pts',(-25.7649464042477,-57.4126476234249,
2.63954450640372));
#249458=CARTESIAN_POINT('Ctrl Pts',(-25.708112793338,-57.3992776612634,
2.69627684028807));
#249459=CARTESIAN_POINT('Ctrl Pts',(-25.6555720179783,-57.3434500727657,
2.68224356036447));
#249460=CARTESIAN_POINT('Ctrl Pts',(-25.7004590347002,-57.469285696154,
2.59908178706275));
#249461=CARTESIAN_POINT('Ctrl Pts',(-25.66337545108,-57.4449640631546,2.65878704321414));
#249462=CARTESIAN_POINT('Ctrl Pts',(-25.6226140882778,-57.3860499078787,
2.65878198860221));
#249463=CARTESIAN_POINT('Ctrl Pts',(-25.6197038181293,-57.5052637377732,
2.59908173515983));
#249464=CARTESIAN_POINT('Ctrl Pts',(-25.6045223014057,-57.4711877340329,
2.65878198860221));
#249465=CARTESIAN_POINT('Ctrl Pts',(-25.5758735661203,-57.406883591798,
2.65878198860221));
#249466=CARTESIAN_POINT('Origin',(-25.7748538035642,-57.1106661007665,2.83404198860221));
#249467=CARTESIAN_POINT('Origin',(-23.8679610547591,-54.3889216310751,3.11913648167016));
#249468=CARTESIAN_POINT('Origin',(-23.7955011834904,-54.2261740956466,2.83404198860223));
#249469=CARTESIAN_POINT('Origin',(-25.7023940320488,-56.9479187893697,3.11913648177552));
#249470=CARTESIAN_POINT('Origin',(-25.629934260499,-56.7851714777848,3.4042309748327));
#249471=CARTESIAN_POINT('Ctrl Pts',(-23.7522229508823,-54.1275498658874,
2.90134173515985));
#249472=CARTESIAN_POINT('Ctrl Pts',(-23.8679139708563,-54.0765745253536,
2.90103711553191));
#249473=CARTESIAN_POINT('Ctrl Pts',(-23.911521456611,-54.174518541976,2.83404198860223));
#249474=CARTESIAN_POINT('Ctrl Pts',(-23.73374293576,-54.0860417646979,2.82862991747925));
#249475=CARTESIAN_POINT('Ctrl Pts',(-23.8418262755854,-54.0553388636017,
2.85314045886441));
#249476=CARTESIAN_POINT('Ctrl Pts',(-23.8930401898202,-54.1330089371356,
2.79187960999867));
#249477=CARTESIAN_POINT('Ctrl Pts',(-23.7393098712345,-54.0331737207068,
2.75470625793287));
#249478=CARTESIAN_POINT('Ctrl Pts',(-23.8301926567295,-54.0188467943739,
2.79224250381887));
#249479=CARTESIAN_POINT('Ctrl Pts',(-23.8884275227218,-54.0846755205371,
2.7490180910822));
#249480=CARTESIAN_POINT('Ctrl Pts',(-23.8065189073819,-53.9248984592617,
2.63947868311661));
#249481=CARTESIAN_POINT('Ctrl Pts',(-23.8631501047896,-53.9384511174159,
2.69595066767855));
#249482=CARTESIAN_POINT('Ctrl Pts',(-23.9152668978356,-53.9943748351526,
2.68220539436023));
#249483=CARTESIAN_POINT('Ctrl Pts',(-23.8710081209823,-53.8688190939459,
2.59908178585036));
#249484=CARTESIAN_POINT('Ctrl Pts',(-23.9079567336557,-53.8932068550021,
2.6587767094497));
#249485=CARTESIAN_POINT('Ctrl Pts',(-23.9484663513835,-53.9522270531161,
2.65878198860223));
#249486=CARTESIAN_POINT('Ctrl Pts',(-23.951372267036,-53.8330634946838,
2.59908173515985));
#249487=CARTESIAN_POINT('Ctrl Pts',(-23.9665367208219,-53.8671470951731,
2.65878198860223));
#249488=CARTESIAN_POINT('Ctrl Pts',(-23.9951532569802,-53.9314655730804,
2.65878198860223));
#249489=CARTESIAN_POINT('Origin',(-23.9951532569802,-53.9314655730804,2.53178198860223));
#249490=CARTESIAN_POINT('Ctrl Pts',(-25.4547063934078,-56.3916032444851,
3.77003198860223));
#249491=CARTESIAN_POINT('Ctrl Pts',(-25.3385127813687,-56.4433359736145,
3.77003198860223));
#249492=CARTESIAN_POINT('Ctrl Pts',(-25.3386862495815,-56.4432587405902,
3.64284238727522));
#249493=CARTESIAN_POINT('Ctrl Pts',(-25.5431622092807,-56.5897307565548,
3.77003198860223));
#249494=CARTESIAN_POINT('Ctrl Pts',(-25.4268404215552,-56.6417243268781,
3.77025506105786));
#249495=CARTESIAN_POINT('Ctrl Pts',(-25.4092621323408,-56.6017747680085,
3.64284210641837));
#249496=CARTESIAN_POINT('Ctrl Pts',(-25.6273687254301,-56.7783458705711,
3.6555352798779));
#249497=CARTESIAN_POINT('Ctrl Pts',(-25.510904950036,-56.830537517614,3.65585996533093));
#249498=CARTESIAN_POINT('Ctrl Pts',(-25.4764491573039,-56.7526792962306,
3.55127902710141));
#249499=CARTESIAN_POINT('Ctrl Pts',(-25.6742415049975,-56.8833377255395,
3.4715307213903));
#249500=CARTESIAN_POINT('Ctrl Pts',(-25.5577357740372,-56.9357219102088,
3.47182327905146));
#249501=CARTESIAN_POINT('Ctrl Pts',(-25.513848576796,-56.8366797674138,
3.40413028377926));
#249502=CARTESIAN_POINT('Origin',(-25.4547063934078,-56.3916032444851,3.64303198860223));
#249503=CARTESIAN_POINT('Origin',(3.88110971579612E-16,1.91523848684163E-13,
2.53178198860262));
#249504=CARTESIAN_POINT('Origin',(-24.0229981225292,-53.9190682401995,2.53178198860224));
#249505=CARTESIAN_POINT('Origin',(10.0037024164483,23.2492868865828,3.64303198860279));
#249506=CARTESIAN_POINT('Origin',(-25.2915084057487,-56.0249274780514,3.64299466007511));
#249507=CARTESIAN_POINT('Ctrl Pts',(-23.9791663275009,-53.8206887816836,
2.59908173515985));
#249508=CARTESIAN_POINT('Ctrl Pts',(-23.9943483786813,-53.8547645473081,
2.65878198860223));
#249509=CARTESIAN_POINT('Ctrl Pts',(-24.0229981225292,-53.9190682401995,
2.65878198860223));
#249510=CARTESIAN_POINT('Ctrl Pts',(-24.0592381182998,-53.7850138844282,
2.59908193199934));
#249511=CARTESIAN_POINT('Ctrl Pts',(-24.0526825045791,-53.8287709626517,
2.65877685806671));
#249512=CARTESIAN_POINT('Ctrl Pts',(-24.0695074323269,-53.8983362760839,
2.65878198860223));
#249513=CARTESIAN_POINT('Ctrl Pts',(-24.1432906710369,-53.7744461045705,
2.63872492669742));
#249514=CARTESIAN_POINT('Ctrl Pts',(-24.1158128282434,-53.8255298669644,
2.69532212015236));
#249515=CARTESIAN_POINT('Ctrl Pts',(-24.1225146216894,-53.9015903052238,
2.68176836726598));
#249516=CARTESIAN_POINT('Ctrl Pts',(-24.2696905364167,-53.7968389608978,
2.75442176402227));
#249517=CARTESIAN_POINT('Ctrl Pts',(-24.1983175571249,-53.8548027426707,
2.7920317992009));
#249518=CARTESIAN_POINT('Ctrl Pts',(-24.2081897025472,-53.9421141528987,
2.74885310748134));
#249519=CARTESIAN_POINT('Ctrl Pts',(-24.3127961529001,-53.8282518514938,
2.82866089558347));
#249520=CARTESIAN_POINT('Ctrl Pts',(-24.2176488245043,-53.8880291490203,
2.85316563119182));
#249521=CARTESIAN_POINT('Ctrl Pts',(-24.2411088588481,-53.9780599067624,
2.79189751796557));
#249522=CARTESIAN_POINT('Ctrl Pts',(-24.3312692531083,-53.8697418420145,
2.90134173515984));
#249523=CARTESIAN_POINT('Ctrl Pts',(-24.2159747902182,-53.9216078643417,
2.90103711553191));
#249524=CARTESIAN_POINT('Ctrl Pts',(-24.2595822759728,-54.0195518809641,
2.83404198860223));
#249525=CARTESIAN_POINT('Origin',(-24.3756025490934,-53.9678963272935,2.83404198860223));
#249526=CARTESIAN_POINT('Origin',(-25.2734729066191,-55.9845461685084,3.56647653971746));
#249527=CARTESIAN_POINT('Origin',(-25.2401862573137,-55.9097831300747,3.42473028058445));
#249528=CARTESIAN_POINT('Origin',(-24.4480624203037,-54.1306438627319,3.11913648167933));
#249529=CARTESIAN_POINT('Origin',(-24.5205222915147,-54.2933913980364,3.40423097483272));
#249530=CARTESIAN_POINT('Ctrl Pts',(-25.1059793847697,-55.6083495590302,
3.36123028058442));
#249531=CARTESIAN_POINT('Ctrl Pts',(-24.9899591116491,-55.6600051127008,
3.36123028058442));
#249532=CARTESIAN_POINT('Ctrl Pts',(-24.9899591116491,-55.6600051127008,
3.23423028058442));
#249533=CARTESIAN_POINT('Ctrl Pts',(-25.142375998794,-55.6906734752784,
3.36123028058442));
#249534=CARTESIAN_POINT('Ctrl Pts',(-25.0265352902408,-55.7421565548675,
3.36099641108454));
#249535=CARTESIAN_POINT('Ctrl Pts',(-25.0448742789057,-55.7833465978043,
3.23423043688414));
#249536=CARTESIAN_POINT('Ctrl Pts',(-25.1767934079555,-55.7685161955949,
3.41054258905245));
#249537=CARTESIAN_POINT('Ctrl Pts',(-25.0612933298577,-55.8202243900326,
3.4100881582604));
#249538=CARTESIAN_POINT('Ctrl Pts',(-25.0968004762765,-55.8999747466282,
3.30819867304245));
#249539=CARTESIAN_POINT('Ctrl Pts',(-25.1949317875296,-55.8095395120007,
3.48823028058443));
#249540=CARTESIAN_POINT('Ctrl Pts',(-25.0796311836949,-55.8614118841079,
3.48794691941559));
#249541=CARTESIAN_POINT('Ctrl Pts',(-25.1241659841931,-55.9614386837453,
3.42473028058444));
#249542=CARTESIAN_POINT('Origin',(-25.1059793847697,-55.6083495590302,3.23423028058442));
#249543=CARTESIAN_POINT('Ctrl Pts',(-24.4761921430387,-54.1952354911872,
3.47153072139034));
#249544=CARTESIAN_POINT('Ctrl Pts',(-24.3607210247419,-54.2471777813618,
3.47122746285039));
#249545=CARTESIAN_POINT('Ctrl Pts',(-24.4045675690225,-54.3451938326306,
3.40413046676736));
#249546=CARTESIAN_POINT('Ctrl Pts',(-24.5230721320493,-54.3002261711145,
3.6555381345795));
#249547=CARTESIAN_POINT('Ctrl Pts',(-24.4074212664117,-54.3520689157374,
3.65520336072156));
#249548=CARTESIAN_POINT('Ctrl Pts',(-24.4419676644359,-54.4291958219368,
3.55128134519859));
#249549=CARTESIAN_POINT('Ctrl Pts',(-24.6072895482028,-54.4888383671844,
3.77003198860224));
#249550=CARTESIAN_POINT('Ctrl Pts',(-24.491383313694,-54.5406519873259,
3.76980209314076));
#249551=CARTESIAN_POINT('Ctrl Pts',(-24.5091552540991,-54.5801016184624,
3.64284195387403));
#249552=CARTESIAN_POINT('Ctrl Pts',(-24.6957503380303,-54.6869600343298,
3.77003198860224));
#249553=CARTESIAN_POINT('Ctrl Pts',(-24.5795562747208,-54.7386929643777,
3.77003198860224));
#249554=CARTESIAN_POINT('Ctrl Pts',(-24.5797301948775,-54.738615530135,
3.64284189403738));
#249555=CARTESIAN_POINT('Origin',(-24.6957503380303,-54.6869600343298,3.64303198860224));
#249556=CARTESIAN_POINT('Origin',(9.75435829333325,22.6892508167096,3.23423028058497));
#249557=CARTESIAN_POINT('Origin',(-25.0444775033943,-55.4702140717967,3.23423028058442));
#249558=CARTESIAN_POINT('Origin',(9.71531210234964,22.6015516358795,3.64303198860278));
#249559=CARTESIAN_POINT('Origin',(-24.8590452239598,-55.0536014459536,3.64299171721715));
#249560=CARTESIAN_POINT('Ctrl Pts',(-24.955532024241,-55.2690209153041,
3.48823028058442));
#249561=CARTESIAN_POINT('Ctrl Pts',(-24.839188866184,-55.3213695969756,
3.4885200421222));
#249562=CARTESIAN_POINT('Ctrl Pts',(-24.7942503289602,-55.2204359898057,
3.42473028058442));
#249563=CARTESIAN_POINT('Ctrl Pts',(-24.9737291291726,-55.3101840490919,
3.4102800584837));
#249564=CARTESIAN_POINT('Ctrl Pts',(-24.8573973158458,-55.3622664445036,
3.41074404220123));
#249565=CARTESIAN_POINT('Ctrl Pts',(-24.8217083187803,-55.2821076446789,
3.30780486243738));
#249566=CARTESIAN_POINT('Ctrl Pts',(-25.0082040095655,-55.3881672017728,
3.36123028058442));
#249567=CARTESIAN_POINT('Ctrl Pts',(-24.8919348043947,-55.4398389138674,
3.36146460586436));
#249568=CARTESIAN_POINT('Ctrl Pts',(-24.8737270328811,-55.3989435894807,
3.23423045308459));
#249569=CARTESIAN_POINT('Ctrl Pts',(-25.0444775033943,-55.4702140717967,
3.36123028058442));
#249570=CARTESIAN_POINT('Ctrl Pts',(-24.9284572302736,-55.5218696254673,
3.36123028058442));
#249571=CARTESIAN_POINT('Ctrl Pts',(-24.9284572302736,-55.5218696254673,
3.23423028058442));
#249572=CARTESIAN_POINT('Origin',(-24.9102706020808,-55.168780436135,3.42473028058442));
#249573=CARTESIAN_POINT('Origin',(-24.8771824678731,-55.0944632691829,3.56563113524668));
#249574=CARTESIAN_POINT('Origin',(-18.6791227126679,-58.515880043567,3.56647653909354));
#249575=CARTESIAN_POINT('Origin',(-18.6927400943479,-58.5579573083303,3.64299466007364));
#249576=CARTESIAN_POINT('Origin',(-18.6538332760099,-58.4380471616454,3.42473028058443));
#249577=CARTESIAN_POINT('Ctrl Pts',(-18.6203878281142,-58.3332704847796,
3.48823028058443));
#249578=CARTESIAN_POINT('Ctrl Pts',(-18.7407822670297,-58.2946680067388,
3.48794691941559));
#249579=CARTESIAN_POINT('Ctrl Pts',(-18.7746174535794,-58.3988020033598,
3.42473028058444));
#249580=CARTESIAN_POINT('Ctrl Pts',(-18.6063701040098,-58.2905032380258,
3.41028005925046));
#249581=CARTESIAN_POINT('Ctrl Pts',(-18.7268030714104,-58.2516444665209,
3.40982512231077));
#249582=CARTESIAN_POINT('Ctrl Pts',(-18.7537563325793,-58.3345980746911,
3.30780486372911));
#249583=CARTESIAN_POINT('Ctrl Pts',(-18.5798130476659,-58.2094810151999,
3.36123028058441));
#249584=CARTESIAN_POINT('Ctrl Pts',(-18.7003491529659,-58.1702276772295,
3.3609972104835));
#249585=CARTESIAN_POINT('Ctrl Pts',(-18.7142352739232,-58.2129647630934,
3.2342304530829));
#249586=CARTESIAN_POINT('Ctrl Pts',(-18.5518699907145,-58.1242364370956,
3.36123028058441));
#249587=CARTESIAN_POINT('Ctrl Pts',(-18.672654168284,-58.08499127881,3.36123028058441));
#249588=CARTESIAN_POINT('Ctrl Pts',(-18.672654168284,-58.08499127881,3.23423028058441));
#249589=CARTESIAN_POINT('Origin',(-18.5518699907145,-58.1242364370956,3.2342302805844));
#249590=CARTESIAN_POINT('Origin',(0.301960443923718,-0.0981128957138591,
3.64303198860263));
#249591=CARTESIAN_POINT('Origin',(-18.8168143322221,-58.9396512752213,3.64303198860221));
#249592=CARTESIAN_POINT('Origin',(0.301960443923718,-0.0981128957138562,
3.23423028058481));
#249593=CARTESIAN_POINT('Origin',(-18.5051441132836,-57.9804289733664,3.2342302805844));
#249594=CARTESIAN_POINT('Ctrl Pts',(-18.9827025415091,-59.4519788726608,
3.4715307213903));
#249595=CARTESIAN_POINT('Ctrl Pts',(-19.1043350233605,-59.4129503614026,
3.4718232790262));
#249596=CARTESIAN_POINT('Ctrl Pts',(-19.0706774512222,-59.3099814440477,
3.4041302895898));
#249597=CARTESIAN_POINT('Ctrl Pts',(-18.9472820042061,-59.3425890481018,
3.65553807120915));
#249598=CARTESIAN_POINT('Ctrl Pts',(-19.0687544722125,-59.3034455268842,
3.65586275496877));
#249599=CARTESIAN_POINT('Ctrl Pts',(-19.0422629184335,-59.2225305038481,
3.55128126837106));
#249600=CARTESIAN_POINT('Ctrl Pts',(-18.8836509927323,-59.1460739925262,
3.77003198860221));
#249601=CARTESIAN_POINT('Ctrl Pts',(-19.0048854004781,-59.1068782740624,
3.77025505748552));
#249602=CARTESIAN_POINT('Ctrl Pts',(-18.9912173655538,-59.0654284453484,
3.64284211731235));
#249603=CARTESIAN_POINT('Ctrl Pts',(-18.8168143322221,-58.9396512752213,
3.77003198860221));
#249604=CARTESIAN_POINT('Ctrl Pts',(-18.9377789557522,-58.900347486489,
3.77003198860221));
#249605=CARTESIAN_POINT('Ctrl Pts',(-18.9375983752039,-58.9004061606659,
3.64284239821646));
#249606=CARTESIAN_POINT('Origin',(-18.9499432001052,-59.349379800228,3.40423097483268));
#249607=CARTESIAN_POINT('Ctrl Pts',(-18.5051441132836,-57.9804289733663,
3.36123028058441));
#249608=CARTESIAN_POINT('Ctrl Pts',(-18.6259282908531,-57.9411838150807,
3.36123028058441));
#249609=CARTESIAN_POINT('Ctrl Pts',(-18.6259282908531,-57.9411838150807,
3.23423028058441));
#249610=CARTESIAN_POINT('Ctrl Pts',(-18.4771060595073,-57.8948964606935,
3.3612302805844));
#249611=CARTESIAN_POINT('Ctrl Pts',(-18.5980867642066,-57.8554964068691,
3.36146538610072));
#249612=CARTESIAN_POINT('Ctrl Pts',(-18.5842066467866,-57.8127777979935,
3.23423043688339));
#249613=CARTESIAN_POINT('Ctrl Pts',(-18.4505921960623,-57.8140195545735,
3.41054258693058));
#249614=CARTESIAN_POINT('Ctrl Pts',(-18.5718941197427,-57.7748837362142,
3.41100608859698));
#249615=CARTESIAN_POINT('Ctrl Pts',(-18.5447558577151,-57.6913607539395,
3.30819866970735));
#249616=CARTESIAN_POINT('Ctrl Pts',(-18.4366189870667,-57.7713971777987,
3.48823028058441));
#249617=CARTESIAN_POINT('Ctrl Pts',(-18.5581069080655,-57.732451061807,
3.48852004212219));
#249618=CARTESIAN_POINT('Ctrl Pts',(-18.5239649837002,-57.6273730232605,
3.42473028058441));
#249619=CARTESIAN_POINT('Origin',(-18.4031808061308,-57.6666181815461,3.4247302805844));
#249620=CARTESIAN_POINT('Origin',(-19.0049943031114,-59.5188096735787,3.11913648178371));
#249621=CARTESIAN_POINT('Origin',(-19.0600454060081,-59.688239546742,2.83404198860219));
#249622=CARTESIAN_POINT('Origin',(-18.3780421908164,-57.5892494790284,3.56563113460774));
#249623=CARTESIAN_POINT('Origin',(-18.3641788932745,-57.546747042666,3.64299171721713));
#249624=CARTESIAN_POINT('Ctrl Pts',(-19.4393816709751,-59.8776671349985,
2.59908173515981));
#249625=CARTESIAN_POINT('Ctrl Pts',(-19.4278624395261,-59.8421853116552,
2.65878198860219));
#249626=CARTESIAN_POINT('Ctrl Pts',(-19.4061247292248,-59.7752282754837,
2.65878198860219));
#249627=CARTESIAN_POINT('Ctrl Pts',(-19.3555723159018,-59.904875846812,
2.59908193475578));
#249628=CARTESIAN_POINT('Ctrl Pts',(-19.3668135526093,-59.8620015382112,
2.65878715325416));
#249629=CARTESIAN_POINT('Ctrl Pts',(-19.3576098387249,-59.7909691583389,
2.65878198860219));
#249630=CARTESIAN_POINT('Ctrl Pts',(-19.2705128813947,-59.9061888791358,
2.63878778849821));
#249631=CARTESIAN_POINT('Ctrl Pts',(-19.3034480936183,-59.8582551377157,
2.69564460180079));
#249632=CARTESIAN_POINT('Ctrl Pts',(-19.3051157581414,-59.7817014705981,
2.68180481624832));
#249633=CARTESIAN_POINT('Ctrl Pts',(-19.1466203444576,-59.8700374834722,
2.7544323887861));
#249634=CARTESIAN_POINT('Ctrl Pts',(-19.2244111832563,-59.820049432414,
2.79268340777034));
#249635=CARTESIAN_POINT('Ctrl Pts',(-19.2239451174245,-59.7316696194039,
2.74885926835576));
#249636=CARTESIAN_POINT('Ctrl Pts',(-19.1068608943535,-59.8340873574358,
2.82856655361622));
#249637=CARTESIAN_POINT('Ctrl Pts',(-19.2088773592695,-59.7849307811032,
2.85384197230818));
#249638=CARTESIAN_POINT('Ctrl Pts',(-19.1948817636402,-59.6922425516965,
2.79184624278462));
#249639=CARTESIAN_POINT('Ctrl Pts',(-19.0928077206406,-59.7908376697911,
2.90134173515981));
#249640=CARTESIAN_POINT('Ctrl Pts',(-19.2142545736078,-59.7518659300026,
2.90163218716348));
#249641=CARTESIAN_POINT('Ctrl Pts',(-19.1808295835776,-59.6489943884564,
2.83404198860219));
#249642=CARTESIAN_POINT('Origin',(-19.4061247292248,-59.7752282754837,2.53178198860219));
#249643=CARTESIAN_POINT('Origin',(0.301960443923718,-0.0981128957138591,
3.64303198860263));
#249644=CARTESIAN_POINT('Origin',(-18.240199652704,-57.1650137687747,3.64303198860222));
#249645=CARTESIAN_POINT('Origin',(2.07460197300492E-17,1.91734254067317E-13,
2.53178198860262));
#249646=CARTESIAN_POINT('Origin',(-19.4351129318415,-59.7658094374951,2.53178198860219));
#249647=CARTESIAN_POINT('Ctrl Pts',(-18.240199652704,-57.1650137687747,
3.77003198860223));
#249648=CARTESIAN_POINT('Ctrl Pts',(-18.3611647704261,-57.1257098194697,
3.77003198860223));
#249649=CARTESIAN_POINT('Ctrl Pts',(-18.3609836949481,-57.125768654459,
3.64284187936962));
#249650=CARTESIAN_POINT('Ctrl Pts',(-18.1733685221984,-56.9585856505952,
3.77003198860223));
#249651=CARTESIAN_POINT('Ctrl Pts',(-18.2941737326415,-56.919534269366,
3.76980208962944));
#249652=CARTESIAN_POINT('Ctrl Pts',(-18.3073637563264,-56.9607434512666,
3.6428419392832));
#249653=CARTESIAN_POINT('Ctrl Pts',(-18.1097485684455,-56.7620685738639,
3.65553535416544));
#249654=CARTESIAN_POINT('Ctrl Pts',(-18.2303834904097,-56.7232097045342,
3.65520057834419));
#249655=CARTESIAN_POINT('Ctrl Pts',(-18.256318583299,-56.8036425617875,
3.5512791096416));
#249656=CARTESIAN_POINT('Ctrl Pts',(-18.0743352474886,-56.6526781108323,
3.47153072139033));
#249657=CARTESIAN_POINT('Ctrl Pts',(-18.1949032015567,-56.6140134911406,
3.47122746281543));
#249658=CARTESIAN_POINT('Ctrl Pts',(-18.2279043987987,-56.7161926934816,
3.4041304590121));
#249659=CARTESIAN_POINT('Origin',(-18.1070706485037,-56.755284824227,3.40423097483271));
#249660=CARTESIAN_POINT('Ctrl Pts',(-19.697766688184,-59.5942745858236,
2.90134173515982));
#249661=CARTESIAN_POINT('Ctrl Pts',(-19.5766071063163,-59.6341304551457,
2.90163218716349));
#249662=CARTESIAN_POINT('Ctrl Pts',(-19.5431821162861,-59.5312589135995,
2.8340419886022));
#249663=CARTESIAN_POINT('Ctrl Pts',(-19.7118253299473,-59.637544215329,
2.82853349835315));
#249664=CARTESIAN_POINT('Ctrl Pts',(-19.6004058925606,-59.6577332347569,
2.85381483162282));
#249665=CARTESIAN_POINT('Ctrl Pts',(-19.5572406993628,-59.5745267832909,
2.79182701594181));
#249666=CARTESIAN_POINT('Ctrl Pts',(-19.7007277907732,-59.6898285824897,
2.754688220736));
#249667=CARTESIAN_POINT('Ctrl Pts',(-19.6083614943627,-59.695174564008,
2.79286913083796));
#249668=CARTESIAN_POINT('Ctrl Pts',(-19.5568428722495,-59.623336104959,
2.74900763297877));
#249669=CARTESIAN_POINT('Ctrl Pts',(-19.6225475038103,-59.791305386369,
2.63954450640351));
#249670=CARTESIAN_POINT('Ctrl Pts',(-19.5674227749668,-59.7720679362487,
2.69627684028815));
#249671=CARTESIAN_POINT('Ctrl Pts',(-19.5210053955053,-59.7110541706149,
2.68224356036443));
#249672=CARTESIAN_POINT('Ctrl Pts',(-19.5524931121159,-59.8408924241697,
2.59908178706384));
#249673=CARTESIAN_POINT('Ctrl Pts',(-19.5181549791675,-59.8128277376105,
2.6587870432151));
#249674=CARTESIAN_POINT('Ctrl Pts',(-19.4837751174913,-59.7499755976261,
2.65878198860219));
#249675=CARTESIAN_POINT('Ctrl Pts',(-19.4684195516691,-59.8682321556242,
2.59908173515981));
#249676=CARTESIAN_POINT('Ctrl Pts',(-19.4568831131878,-59.8327559231846,
2.65878198860219));
#249677=CARTESIAN_POINT('Ctrl Pts',(-19.4351129318415,-59.7658094374951,
2.65878198860219));
#249678=CARTESIAN_POINT('Origin',(-19.6639662938556,-59.4920137553139,2.83404198860219));
#249679=CARTESIAN_POINT('Origin',(-18.0520194698746,-56.585854717958,3.1191364816709));
#249680=CARTESIAN_POINT('Origin',(-17.9969682911406,-56.4164246115663,2.83404198860222));
#249681=CARTESIAN_POINT('Origin',(-19.6089151909114,-59.3225838821508,3.11913648177464));
#249682=CARTESIAN_POINT('Origin',(-19.5538640879527,-59.1531540087999,3.40423097483268));
#249683=CARTESIAN_POINT('Ctrl Pts',(-17.9642361803967,-56.3138168485095,
2.90134173515983));
#249684=CARTESIAN_POINT('Ctrl Pts',(-18.084621806869,-56.2752137607566,
2.9010371155319));
#249685=CARTESIAN_POINT('Ctrl Pts',(-18.1177524687101,-56.3771794532807,
2.83404198860222));
#249686=CARTESIAN_POINT('Ctrl Pts',(-17.9501961787623,-56.2706044454591,
2.82862991747923));
#249687=CARTESIAN_POINT('Ctrl Pts',(-18.0608967538119,-56.2513675234857,
2.85314045886425));
#249688=CARTESIAN_POINT('Ctrl Pts',(-18.1037113794371,-56.3339654239813,
2.79187960999962));
#249689=CARTESIAN_POINT('Ctrl Pts',(-17.9612588333752,-56.2186079213553,
2.75470625793283));
#249690=CARTESIAN_POINT('Ctrl Pts',(-18.0531413250547,-56.2138593173286,
2.79224250381846));
#249691=CARTESIAN_POINT('Ctrl Pts',(-18.1041761987734,-56.2854146278933,
2.74901809108221));
#249692=CARTESIAN_POINT('Ctrl Pts',(-18.0394175380791,-56.1179510603876,
2.63947868311662));
#249693=CARTESIAN_POINT('Ctrl Pts',(-18.0943218653323,-56.1373490477008,
2.69595066767879));
#249694=CARTESIAN_POINT('Ctrl Pts',(-18.1403075368575,-56.1984140977476,
2.68220539436019));
#249695=CARTESIAN_POINT('Ctrl Pts',(-18.1094153628973,-56.0689198620977,
2.59908178585038));
#249696=CARTESIAN_POINT('Ctrl Pts',(-18.1436123520185,-56.097036206149,
2.65877670944869));
#249697=CARTESIAN_POINT('Ctrl Pts',(-18.1777307632111,-56.1599674935309,
2.65878198860222));
#249698=CARTESIAN_POINT('Ctrl Pts',(-18.1930767435944,-56.0417604764383,
2.59908173515984));
#249699=CARTESIAN_POINT('Ctrl Pts',(-18.204595418534,-56.0772424804484,
2.65878198860222));
#249700=CARTESIAN_POINT('Ctrl Pts',(-18.2263320786577,-56.1441998575527,
2.65878198860222));
#249701=CARTESIAN_POINT('Origin',(-18.2263320786577,-56.1441998575527,2.53178198860222));
#249702=CARTESIAN_POINT('Ctrl Pts',(-19.4207352200695,-58.7434254837932,
3.77003198860222));
#249703=CARTESIAN_POINT('Ctrl Pts',(-19.2997705861185,-58.7827292759115,
3.77003198860222));
#249704=CARTESIAN_POINT('Ctrl Pts',(-19.2999511771033,-58.7826705983436,
3.6428423872756));
#249705=CARTESIAN_POINT('Ctrl Pts',(-19.4879965013596,-58.9497137831218,
3.77003198860221));
#249706=CARTESIAN_POINT('Ctrl Pts',(-19.3668771285525,-58.9892635895145,
3.77025506105811));
#249707=CARTESIAN_POINT('Ctrl Pts',(-19.3535710010437,-58.9476954469487,
3.6428421064192));
#249708=CARTESIAN_POINT('Ctrl Pts',(-19.5520260773863,-59.1460976215385,
3.65553527987787));
#249709=CARTESIAN_POINT('Ctrl Pts',(-19.4307447900758,-59.1858295778062,
3.65585996532951));
#249710=CARTESIAN_POINT('Ctrl Pts',(-19.4046161500175,-59.1047962608419,
3.55127902710053));
#249711=CARTESIAN_POINT('Ctrl Pts',(-19.5876674457073,-59.2554138597571,
3.47153072139031));
#249712=CARTESIAN_POINT('Ctrl Pts',(-19.4663243070087,-59.2953329133625,
3.47182327905147));
#249713=CARTESIAN_POINT('Ctrl Pts',(-19.4330302514108,-59.1922458725044,
3.40413028377948));
#249714=CARTESIAN_POINT('Origin',(-19.4207352200695,-58.7434254837932,3.64303198860222));
#249715=CARTESIAN_POINT('Origin',(3.93842937138094E-16,1.91521648388735E-13,
2.53178198860262));
#249716=CARTESIAN_POINT('Origin',(-18.2553202812744,-56.1347810195642,2.53178198860222));
#249717=CARTESIAN_POINT('Origin',(5.6397553624924,18.3848338156956,3.64303198860275));
#249718=CARTESIAN_POINT('Origin',(-19.296759302444,-58.361699570715,3.64299466007636));
#249719=CARTESIAN_POINT('Ctrl Pts',(-18.2220120550212,-56.0323588238391,
2.59908173515984));
#249720=CARTESIAN_POINT('Ctrl Pts',(-18.2335490499213,-56.0678348753332,
2.65878198860222));
#249721=CARTESIAN_POINT('Ctrl Pts',(-18.2553202812744,-56.1347810195642,
2.65878198860222));
#249722=CARTESIAN_POINT('Ctrl Pts',(-18.3053742463593,-56.0052491386464,
2.59908193199861));
#249723=CARTESIAN_POINT('Ctrl Pts',(-18.294280684832,-56.0480812627868,
2.65877685806598));
#249724=CARTESIAN_POINT('Ctrl Pts',(-18.3037418885556,-56.1190241739963,
2.65878198860222));
#249725=CARTESIAN_POINT('Ctrl Pts',(-18.3900709842066,-56.0035251343644,
2.63872492669767));
#249726=CARTESIAN_POINT('Ctrl Pts',(-18.3574039607303,-56.0514568378823,
2.69532212015237));
#249727=CARTESIAN_POINT('Ctrl Pts',(-18.3561185603237,-56.1278011372721,
2.68176836726598));
#249728=CARTESIAN_POINT('Ctrl Pts',(-18.5134377270385,-56.0390077039668,
2.75442176402201));
#249729=CARTESIAN_POINT('Ctrl Pts',(-18.4363968713611,-56.0891934462338,
2.79203179920095));
#249730=CARTESIAN_POINT('Ctrl Pts',(-18.437088408601,-56.1770584756116,
2.74885310748131));
#249731=CARTESIAN_POINT('Ctrl Pts',(-18.5530236652639,-56.0747542753108,
2.82866089558367));
#249732=CARTESIAN_POINT('Ctrl Pts',(-18.4521491348405,-56.1242585025262,
2.85316563119173));
#249733=CARTESIAN_POINT('Ctrl Pts',(-18.466069875907,-56.2162483036947,
2.79189751796582));
#249734=CARTESIAN_POINT('Ctrl Pts',(-18.567058682946,-56.1179479440988,
2.90134173515983));
#249735=CARTESIAN_POINT('Ctrl Pts',(-18.4469743395774,-56.1574782858997,
2.90103711553189));
#249736=CARTESIAN_POINT('Ctrl Pts',(-18.4801050014185,-56.2594439784239,
2.83404198860221));
#249737=CARTESIAN_POINT('Origin',(-18.600889178988,-56.2201988201382,2.83404198860222));
#249738=CARTESIAN_POINT('Origin',(-19.2830435998987,-58.3196542512035,3.56647653971717));
#249739=CARTESIAN_POINT('Origin',(-19.2577541638573,-58.2418213702174,3.42473028058445));
#249740=CARTESIAN_POINT('Origin',(-18.6559403576599,-56.389628926534,3.11913648168046));
#249741=CARTESIAN_POINT('Origin',(-18.7109915363512,-56.5590590327989,3.40423097483271));
#249742=CARTESIAN_POINT('Ctrl Pts',(-19.155790878562,-57.9280106456676,
3.36123028058441));
#249743=CARTESIAN_POINT('Ctrl Pts',(-19.0350067009925,-57.9672558039532,
3.36123028058441));
#249744=CARTESIAN_POINT('Ctrl Pts',(-19.0350067009925,-57.9672558039532,
3.23423028058441));
#249745=CARTESIAN_POINT('Ctrl Pts',(-19.1833829156714,-58.0136880650208,
3.36123028058441));
#249746=CARTESIAN_POINT('Ctrl Pts',(-19.0627953474467,-58.0527804636634,
3.36099641108351));
#249747=CARTESIAN_POINT('Ctrl Pts',(-19.0767283413222,-58.0956618095401,
3.23423043688317));
#249748=CARTESIAN_POINT('Ctrl Pts',(-19.209475002731,-58.0947019536606,
3.41054258905243));
#249749=CARTESIAN_POINT('Ctrl Pts',(-19.0892026680443,-58.1340538395287,
3.41008815826083));
#249750=CARTESIAN_POINT('Ctrl Pts',(-19.1161791203798,-58.2170788227743,
3.30819867304341));
#249751=CARTESIAN_POINT('Ctrl Pts',(-19.2232259141434,-58.1373965169893,
3.48823028058443));
#249752=CARTESIAN_POINT('Ctrl Pts',(-19.1031347997382,-58.1769325318819,
3.48794691941559));
#249753=CARTESIAN_POINT('Ctrl Pts',(-19.1369699862878,-58.281066528503,
3.42473028058444));
#249754=CARTESIAN_POINT('Origin',(-19.155790878562,-57.9280106456676,3.23423028058441));
#249755=CARTESIAN_POINT('Ctrl Pts',(-18.6771643191705,-56.4568070719811,
3.47153072139033));
#249756=CARTESIAN_POINT('Ctrl Pts',(-18.5568963159709,-56.496394798308,
3.47122746285037));
#249757=CARTESIAN_POINT('Ctrl Pts',(-18.5902571970797,-56.5984571192857,
3.40413046676725));
#249758=CARTESIAN_POINT('Ctrl Pts',(-18.7128129802646,-56.566122895188,
3.65553813457947));
#249759=CARTESIAN_POINT('Ctrl Pts',(-18.5923766197452,-56.6055928325687,
3.65520336072065));
#249760=CARTESIAN_POINT('Ctrl Pts',(-18.6186718120033,-56.6859083114039,
3.55128134519815));
#249761=CARTESIAN_POINT('Ctrl Pts',(-18.7768537015919,-56.7625049710039,
3.77003198860223));
#249762=CARTESIAN_POINT('Ctrl Pts',(-18.6561664154738,-56.8019192501375,
3.76980209314237));
#249763=CARTESIAN_POINT('Ctrl Pts',(-18.6697173900119,-56.8430104456862,
3.64284195387455));
#249764=CARTESIAN_POINT('Ctrl Pts',(-18.8441205405514,-56.9687879773466,
3.77003198860223));
#249765=CARTESIAN_POINT('Ctrl Pts',(-18.7231554367999,-57.0080919221123,
3.77003198860222));
#249766=CARTESIAN_POINT('Ctrl Pts',(-18.7233364982864,-57.0080330916691,
3.64284189403718));
#249767=CARTESIAN_POINT('Origin',(-18.8441205405514,-56.9687879773466,3.64303198860223));
#249768=CARTESIAN_POINT('Origin',(5.49583002221419,17.9418771653391,3.23423028058494));
#249769=CARTESIAN_POINT('Origin',(-19.109065001131,-57.7842031819383,3.23423028058441));
#249770=CARTESIAN_POINT('Origin',(5.4732919481113,17.872512105713,3.64303198860275));
#249771=CARTESIAN_POINT('Origin',(-18.968196416682,-57.3504898524417,3.64299171721817));
#249772=CARTESIAN_POINT('Ctrl Pts',(-19.0416371860872,-57.5748148483576,
3.4882302805844));
#249773=CARTESIAN_POINT('Ctrl Pts',(-18.920459440774,-57.6147155869502,
3.48852004212219));
#249774=CARTESIAN_POINT('Ctrl Pts',(-18.8863175164087,-57.5096375484037,
3.4247302805844));
#249775=CARTESIAN_POINT('Ctrl Pts',(-19.0554318862552,-57.6176546016062,
3.41028005848365));
#249776=CARTESIAN_POINT('Ctrl Pts',(-18.9342932580178,-57.6572916985361,
3.41074404220394));
#249777=CARTESIAN_POINT('Ctrl Pts',(-18.9071786451771,-57.5738415009809,
3.30780486243911));
#249778=CARTESIAN_POINT('Ctrl Pts',(-19.0815664505355,-57.698814160686,
3.36123028058441));
#249779=CARTESIAN_POINT('Ctrl Pts',(-18.9605330155747,-57.7380493683895,
3.36146460586264));
#249780=CARTESIAN_POINT('Ctrl Pts',(-18.9466997135536,-57.6954748424952,
3.23423045308292));
#249781=CARTESIAN_POINT('Ctrl Pts',(-19.109065001131,-57.7842031819383,
3.36123028058441));
#249782=CARTESIAN_POINT('Ctrl Pts',(-18.9882808235615,-57.8234483402239,
3.36123028058441));
#249783=CARTESIAN_POINT('Ctrl Pts',(-18.9882808235615,-57.8234483402239,
3.23423028058441));
#249784=CARTESIAN_POINT('Origin',(-19.0071016939782,-57.4703923901181,3.4247302805844));
#249785=CARTESIAN_POINT('Origin',(-18.9819630792877,-57.393023688563,3.56563113524764));
#249786=CARTESIAN_POINT('Origin',(-12.4602215063104,-60.147823922414,3.56647653909347));
#249787=CARTESIAN_POINT('Origin',(-12.4693660187251,-60.1910940874988,3.64299466007341));
#249788=CARTESIAN_POINT('Origin',(-12.4432063593716,-60.0677739512125,3.42473028058441));
#249789=CARTESIAN_POINT('Ctrl Pts',(-12.420896274158,-59.9600752506736,
3.48823028058442));
#249790=CARTESIAN_POINT('Ctrl Pts',(-12.544666237448,-59.9342688867324,
3.48794691941558));
#249791=CARTESIAN_POINT('Ctrl Pts',(-12.5674311046648,-60.0413691664787,
3.42473028058443));
#249792=CARTESIAN_POINT('Ctrl Pts',(-12.411425735194,-59.9160770362134,
3.41028005925045));
#249793=CARTESIAN_POINT('Ctrl Pts',(-12.5352608058697,-59.8900198101355,
3.40982512230985));
#249794=CARTESIAN_POINT('Ctrl Pts',(-12.5533954010684,-59.9753363727311,
3.30780486372844));
#249795=CARTESIAN_POINT('Ctrl Pts',(-12.3934832896268,-59.8327226933128,
3.36123028058439));
#249796=CARTESIAN_POINT('Ctrl Pts',(-12.5174621766265,-59.8062838430886,
3.36099721048398));
#249797=CARTESIAN_POINT('Ctrl Pts',(-12.5268049860493,-59.8502383056088,
3.23423045308289));
#249798=CARTESIAN_POINT('Ctrl Pts',(-12.3746037924158,-59.7450242491247,
3.3612302805844));
#249799=CARTESIAN_POINT('Ctrl Pts',(-12.498828537709,-59.7186194643909,
3.3612302805844));
#249800=CARTESIAN_POINT('Ctrl Pts',(-12.498828537709,-59.7186194643908,
3.2342302805844));
#249801=CARTESIAN_POINT('Origin',(-12.3746037924158,-59.7450242491247,3.23423028058439));
#249802=CARTESIAN_POINT('Origin',(0.31056186323299,-0.0660119618344516,
3.64303198860263));
#249803=CARTESIAN_POINT('Origin',(-12.5528626811441,-60.5836663843181,3.6430319886022));
#249804=CARTESIAN_POINT('Origin',(0.31056186323299,-0.0660119618344487,
3.23423028058481));
#249805=CARTESIAN_POINT('Origin',(-12.3431658574205,-59.5971203935659,3.2342302805844));
#249806=CARTESIAN_POINT('Ctrl Pts',(-12.6642893210135,-61.1105274371641,
3.47153072139029));
#249807=CARTESIAN_POINT('Ctrl Pts',(-12.7893350777076,-61.0844267845856,
3.4718232790262));
#249808=CARTESIAN_POINT('Ctrl Pts',(-12.7666250679672,-60.9785037674412,
3.4041302895901));
#249809=CARTESIAN_POINT('Ctrl Pts',(-12.6404971713776,-60.9980344071774,
3.65553807120914));
#249810=CARTESIAN_POINT('Ctrl Pts',(-12.7653958126107,-60.9718026486701,
3.65586275496848));
#249811=CARTESIAN_POINT('Ctrl Pts',(-12.7475073053521,-60.8885617651934,
3.55128126837233));
#249812=CARTESIAN_POINT('Ctrl Pts',(-12.5977561540113,-60.7959446297924,
3.77003198860221));
#249813=CARTESIAN_POINT('Ctrl Pts',(-12.7224234952042,-60.7696360759163,
3.77025505748393));
#249814=CARTESIAN_POINT('Ctrl Pts',(-12.713163022104,-60.7269846150119,
3.64284211731113));
#249815=CARTESIAN_POINT('Ctrl Pts',(-12.5528626811441,-60.5836663843181,
3.77003198860221));
#249816=CARTESIAN_POINT('Ctrl Pts',(-12.6772730124459,-60.5572221520603,
3.77003198860221));
#249817=CARTESIAN_POINT('Ctrl Pts',(-12.6770872880158,-60.5572616290067,
3.64284239821705));
#249818=CARTESIAN_POINT('Origin',(-12.6424339620836,-61.0050661295706,3.40423097483267));
#249819=CARTESIAN_POINT('Ctrl Pts',(-12.3431658574205,-59.5971203935659,
3.3612302805844));
#249820=CARTESIAN_POINT('Ctrl Pts',(-12.4673906027137,-59.570715608832,
3.3612302805844));
#249821=CARTESIAN_POINT('Ctrl Pts',(-12.4673906027137,-59.570715608832,
3.2342302805844));
#249822=CARTESIAN_POINT('Ctrl Pts',(-12.324221981146,-59.5091256622725,
3.3612302805844));
#249823=CARTESIAN_POINT('Ctrl Pts',(-12.448658367964,-59.4825873732123,
3.36146538610033));
#249824=CARTESIAN_POINT('Ctrl Pts',(-12.4393195978191,-59.4386519140016,
3.23423043688338));
#249825=CARTESIAN_POINT('Ctrl Pts',(-12.3063073021285,-59.4259203549056,
3.41054258693058));
#249826=CARTESIAN_POINT('Ctrl Pts',(-12.4310355281328,-59.3996784303283,
3.41100608859746));
#249827=CARTESIAN_POINT('Ctrl Pts',(-12.4127764613278,-59.3137762748647,
3.30819866970766));
#249828=CARTESIAN_POINT('Ctrl Pts',(-12.2968658913797,-59.382070869907,
3.4882302805844));
#249829=CARTESIAN_POINT('Ctrl Pts',(-12.4217592664906,-59.3560370505013,
3.48852004212218));
#249830=CARTESIAN_POINT('Ctrl Pts',(-12.3987880210518,-59.2479658375576,
3.4247302805844));
#249831=CARTESIAN_POINT('Origin',(-12.2745632757586,-59.2743706222914,3.4247302805844));
#249832=CARTESIAN_POINT('Origin',(-12.6794732450934,-61.1793222555458,3.11913648178362));
#249833=CARTESIAN_POINT('Origin',(-12.716512528016,-61.3535783813231,2.83404198860219));
#249834=CARTESIAN_POINT('Origin',(-12.2576496039901,-59.1947980527941,3.56563113460808));
#249835=CARTESIAN_POINT('Origin',(-12.2483049653994,-59.1510793400372,3.64299171721742));
#249836=CARTESIAN_POINT('Ctrl Pts',(-13.0739701745318,-61.5816197022697,
2.59908173515981));
#249837=CARTESIAN_POINT('Ctrl Pts',(-13.066222907106,-61.5451281645059,
2.65878198860219));
#249838=CARTESIAN_POINT('Ctrl Pts',(-13.0516031943522,-61.4762657165315,
2.65878198860219));
#249839=CARTESIAN_POINT('Ctrl Pts',(-12.9877758510414,-61.5999188988202,
2.599081934755));
#249840=CARTESIAN_POINT('Ctrl Pts',(-13.0034370926704,-61.5584544893689,
2.65878715325401));
#249841=CARTESIAN_POINT('Ctrl Pts',(-13.0017087032037,-61.4868491822356,
2.65878198860219));
#249842=CARTESIAN_POINT('Ctrl Pts',(-12.9030451317656,-61.5923336062394,
2.63878778849841));
#249843=CARTESIAN_POINT('Ctrl Pts',(-12.9408103617796,-61.5481051179913,
2.69564460180071));
#249844=CARTESIAN_POINT('Ctrl Pts',(-12.9504709278433,-61.4721451382821,
2.68180481624841));
#249845=CARTESIAN_POINT('Ctrl Pts',(-12.7836101409423,-61.5434299552079,
2.7544323887859));
#249846=CARTESIAN_POINT('Ctrl Pts',(-12.8662000075459,-61.5018471007598,
2.79268340777052));
#249847=CARTESIAN_POINT('Ctrl Pts',(-12.8749747009093,-61.4139027244673,
2.74885926835568));
#249848=CARTESIAN_POINT('Ctrl Pts',(-12.7478263086951,-61.5035207735034,
2.82856655361638));
#249849=CARTESIAN_POINT('Ctrl Pts',(-12.8544221781245,-61.4652971063435,
2.85384197230746));
#249850=CARTESIAN_POINT('Ctrl Pts',(-12.8501918100164,-61.3716536946534,
2.79184624278466));
#249851=CARTESIAN_POINT('Ctrl Pts',(-12.7383709431244,-61.4590390555208,
2.9013417351598));
#249852=CARTESIAN_POINT('Ctrl Pts',(-12.8632261535949,-61.4329754599098,
2.90163218716348));
#249853=CARTESIAN_POINT('Ctrl Pts',(-12.8407372733092,-61.3271735965893,
2.83404198860219));
#249854=CARTESIAN_POINT('Origin',(-13.0516031943522,-61.4762657165315,2.53178198860219));
#249855=CARTESIAN_POINT('Origin',(0.31056186323299,-0.0660119618344516,
3.64303198860263));
#249856=CARTESIAN_POINT('Origin',(-12.1649068885786,-58.7584778814676,3.64303198860222));
#249857=CARTESIAN_POINT('Origin',(4.07480739539809E-18,1.91738721105199E-13,
2.53178198860262));
#249858=CARTESIAN_POINT('Origin',(-13.0814171332226,-61.4699285681954,2.53178198860219));
#249859=CARTESIAN_POINT('Ctrl Pts',(-12.1649068885786,-58.7584778814676,
3.77003198860222));
#249860=CARTESIAN_POINT('Ctrl Pts',(-12.2893177281503,-58.7320335411737,
3.77003198860222));
#249861=CARTESIAN_POINT('Ctrl Pts',(-12.2891314946916,-58.7320731263174,
3.64284187936946));
#249862=CARTESIAN_POINT('Ctrl Pts',(-12.1200194799674,-58.5461948427481,
3.77003198860222));
#249863=CARTESIAN_POINT('Ctrl Pts',(-12.2442448876971,-58.519984972077,
3.76980208962876));
#249864=CARTESIAN_POINT('Ctrl Pts',(-12.2530551225943,-58.5623471386713,
3.64284193928119));
#249865=CARTESIAN_POINT('Ctrl Pts',(-12.0772896710141,-58.3441042111263,
3.65553535416544));
#249866=CARTESIAN_POINT('Ctrl Pts',(-12.2013256001494,-58.3180679977531,
3.65520057834594));
#249867=CARTESIAN_POINT('Ctrl Pts',(-12.2187110949205,-58.4007711908067,
3.55127910964318));
#249868=CARTESIAN_POINT('Ctrl Pts',(-12.0535047649316,-58.2316113004781,
3.47153072139032));
#249869=CARTESIAN_POINT('Ctrl Pts',(-12.1774537884114,-58.2057612725766,
3.47122746281542));
#249870=CARTESIAN_POINT('Ctrl Pts',(-12.1995935666432,-58.3108302909898,
3.40413045901201));
#249871=CARTESIAN_POINT('Origin',(-12.0753355159227,-58.3370777047234,3.40423097483269));
#249872=CARTESIAN_POINT('Ctrl Pts',(-13.360562319248,-61.3267881959112,
2.9013417351598));
#249873=CARTESIAN_POINT('Ctrl Pts',(-13.2359003894744,-61.3537611057082,
2.90163218716348));
#249874=CARTESIAN_POINT('Ctrl Pts',(-13.2134115091888,-61.2479592423877,
2.83404198860219));
#249875=CARTESIAN_POINT('Ctrl Pts',(-13.3700210384231,-61.3712903180778,
2.82853349835321));
#249876=CARTESIAN_POINT('Ctrl Pts',(-13.2571016411964,-61.3797222373777,
2.85381483162357));
#249877=CARTESIAN_POINT('Ctrl Pts',(-13.2228703539488,-61.2924596082469,
2.79182701594243));
#249878=CARTESIAN_POINT('Ctrl Pts',(-13.3535190881765,-61.422128257289,
2.75468822073589));
#249879=CARTESIAN_POINT('Ctrl Pts',(-13.2610999767698,-61.4177900459396,
2.79286913083762));
#249880=CARTESIAN_POINT('Ctrl Pts',(-13.2173727427868,-61.3409599630867,
2.74900763297863));
#249881=CARTESIAN_POINT('Ctrl Pts',(-13.2651598666396,-61.5148770953647,
2.6395445064036));
#249882=CARTESIAN_POINT('Ctrl Pts',(-13.2123479779263,-61.489982926815,
2.69627684028835));
#249883=CARTESIAN_POINT('Ctrl Pts',(-13.1725625528863,-61.4244514636292,
2.68224356036456));
#249884=CARTESIAN_POINT('Ctrl Pts',(-13.1903059833729,-61.5568698122753,
2.59908178706352));
#249885=CARTESIAN_POINT('Ctrl Pts',(-13.1590895168687,-61.5253695547398,
2.65878704321494));
#249886=CARTESIAN_POINT('Ctrl Pts',(-13.1314678292773,-61.4592680512454,
2.65878198860219));
#249887=CARTESIAN_POINT('Ctrl Pts',(-13.1038352065721,-61.5752716937451,
2.5990817351598));
#249888=CARTESIAN_POINT('Ctrl Pts',(-13.0960702419674,-61.5387839176327,
2.65878198860219));
#249889=CARTESIAN_POINT('Ctrl Pts',(-13.0814171332226,-61.4699285681954,
2.65878198860219));
#249890=CARTESIAN_POINT('Origin',(-13.3376362544819,-61.2215544576539,2.83404198860219));
#249891=CARTESIAN_POINT('Origin',(-12.0382961820466,-58.1628213392038,3.11913648166968));
#249892=CARTESIAN_POINT('Origin',(-12.0012568480854,-57.9885649735459,2.83404198860222));
#249893=CARTESIAN_POINT('Origin',(-13.3005969715109,-61.0472983318743,3.11913648177593));
#249894=CARTESIAN_POINT('Origin',(-13.2635576885496,-60.8730422059013,3.40423097483267));
#249895=CARTESIAN_POINT('Ctrl Pts',(-11.9794294790606,-57.8830978693155,
2.90134173515983));
#249896=CARTESIAN_POINT('Ctrl Pts',(-12.1031907419151,-57.8572899778511,
2.90103711553189));
#249897=CARTESIAN_POINT('Ctrl Pts',(-12.1254815933786,-57.962160188812,
2.83404198860222));
#249898=CARTESIAN_POINT('Ctrl Pts',(-11.9699833161087,-57.8386546085354,
2.82862991747918));
#249899=CARTESIAN_POINT('Ctrl Pts',(-12.0820882677177,-57.8310944294256,
2.85314045886411));
#249900=CARTESIAN_POINT('Ctrl Pts',(-12.1160345187361,-57.9177151970025,
2.79187960999948));
#249901=CARTESIAN_POINT('Ctrl Pts',(-11.9864204851024,-57.7880992891174,
2.75470625793289));
#249902=CARTESIAN_POINT('Ctrl Pts',(-12.0782959991606,-57.7929810340974,
2.79224250381867));
#249903=CARTESIAN_POINT('Ctrl Pts',(-12.1215717318489,-57.8694789541062,
2.74901809108219));
#249904=CARTESIAN_POINT('Ctrl Pts',(-12.0746725352384,-57.6961636462596,
2.63947868311656));
#249905=CARTESIAN_POINT('Ctrl Pts',(-12.1272484490374,-57.7211944343228,
2.69595066767865));
#249906=CARTESIAN_POINT('Ctrl Pts',(-12.166599170402,-57.7867317752134,
2.68220539436021));
#249907=CARTESIAN_POINT('Ctrl Pts',(-12.1494120604575,-57.6547178110644,
2.59908178585008));
#249908=CARTESIAN_POINT('Ctrl Pts',(-12.1804827566579,-57.6862546895615,
2.658776709448));
#249909=CARTESIAN_POINT('Ctrl Pts',(-12.2078361528628,-57.7524075778592,
2.65878198860222));
#249910=CARTESIAN_POINT('Ctrl Pts',(-12.2354540642039,-57.6364522029206,
2.59908173515984));
#249911=CARTESIAN_POINT('Ctrl Pts',(-12.2432007592841,-57.6729438621905,
2.65878198860222));
#249912=CARTESIAN_POINT('Ctrl Pts',(-12.2578193919762,-57.7418065394565,
2.65878198860222));
#249913=CARTESIAN_POINT('Origin',(-12.2578193919762,-57.7418065394565,2.53178198860222));
#249914=CARTESIAN_POINT('Ctrl Pts',(-13.1739864076101,-60.4516424606488,
3.77003198860221));
#249915=CARTESIAN_POINT('Ctrl Pts',(-13.04957606559,-60.4780866951848,3.77003198860221));
#249916=CARTESIAN_POINT('Ctrl Pts',(-13.0497618007544,-60.4780472159569,
3.64284238727576));
#249917=CARTESIAN_POINT('Ctrl Pts',(-13.2193162256439,-60.6638314094602,
3.77003198860221));
#249918=CARTESIAN_POINT('Ctrl Pts',(-13.0947262769508,-60.6905041359643,
3.77025506105674));
#249919=CARTESIAN_POINT('Ctrl Pts',(-13.0858380958633,-60.6477728389722,
3.64284210641834));
#249920=CARTESIAN_POINT('Ctrl Pts',(-13.2624673401146,-60.8658323498475,
3.65553527987789));
#249921=CARTESIAN_POINT('Ctrl Pts',(-13.1376973240572,-60.8926693037143,
3.65585996533023));
#249922=CARTESIAN_POINT('Ctrl Pts',(-13.1201821075155,-60.8093487091476,
3.55127902710125));
#249923=CARTESIAN_POINT('Ctrl Pts',(-13.2864868028989,-60.9782752797347,
3.47153072139028));
#249924=CARTESIAN_POINT('Ctrl Pts',(-13.1616357172822,-61.0052918407714,
3.47182327905145));
#249925=CARTESIAN_POINT('Ctrl Pts',(-13.1392995799681,-60.8992893450418,
3.40413028377954));
#249926=CARTESIAN_POINT('Origin',(-13.1739864076101,-60.4516424606488,3.64303198860221));
#249927=CARTESIAN_POINT('Origin',(3.9977349588932E-16,1.91520059300307E-13,
2.53178198860262));
#249928=CARTESIAN_POINT('Origin',(-12.2876333308465,-57.7354693911204,2.53178198860221));
#249929=CARTESIAN_POINT('Origin',(2.37914510404509,12.7200883457658,3.64303198860271));
#249930=CARTESIAN_POINT('Origin',(-13.090590866118,-60.0590486699122,3.64299466007532));
#249931=CARTESIAN_POINT('Ctrl Pts',(-12.2652136052655,-57.6301266171957,
2.59908173515984));
#249932=CARTESIAN_POINT('Ctrl Pts',(-12.2729791421549,-57.6666142715154,
2.65878198860222));
#249933=CARTESIAN_POINT('Ctrl Pts',(-12.2876333308465,-57.7354693911204,
2.65878198860222));
#249934=CARTESIAN_POINT('Ctrl Pts',(-12.3509528635299,-57.6118791634495,
2.59908193199748));
#249935=CARTESIAN_POINT('Ctrl Pts',(-12.3354428975789,-57.653317055794,
2.65877685806514));
#249936=CARTESIAN_POINT('Ctrl Pts',(-12.3374367183498,-57.7248602993992,
2.65878198860222));
#249937=CARTESIAN_POINT('Ctrl Pts',(-12.4353658313036,-57.6190178232951,
2.63872492669765));
#249938=CARTESIAN_POINT('Ctrl Pts',(-12.3978675338889,-57.6632723181626,
2.69532212015252));
#249939=CARTESIAN_POINT('Ctrl Pts',(-12.3886090227463,-57.739064034563,
2.68176836726592));
#249940=CARTESIAN_POINT('Ctrl Pts',(-12.554347819737,-57.6672013517151,
2.75442176402202));
#249941=CARTESIAN_POINT('Ctrl Pts',(-12.4724831634112,-57.7090592089818,
2.79203179920068));
#249942=CARTESIAN_POINT('Ctrl Pts',(-12.4639865158415,-57.7965151898604,
2.74885310748137));
#249943=CARTESIAN_POINT('Ctrl Pts',(-12.589980367881,-57.7068899568908,
2.82866089558366));
#249944=CARTESIAN_POINT('Ctrl Pts',(-12.484483837892,-57.7455787351216,
2.85316563119178));
#249945=CARTESIAN_POINT('Ctrl Pts',(-12.4887127671318,-57.838519720205,
2.79189751796654));
#249946=CARTESIAN_POINT('Ctrl Pts',(-12.5994235324466,-57.7513140650719,
2.90134173515982));
#249947=CARTESIAN_POINT('Ctrl Pts',(-12.4758649777947,-57.7780756236495,
2.90103711553188));
#249948=CARTESIAN_POINT('Ctrl Pts',(-12.4981558292581,-57.8829458346105,
2.83404198860221));
#249949=CARTESIAN_POINT('Origin',(-12.6223805745513,-57.8565410498766,2.83404198860222));
#249950=CARTESIAN_POINT('Origin',(-13.0813452322602,-60.0157999977489,3.56647653971779));
#249951=CARTESIAN_POINT('Origin',(-13.0643300858376,-59.9357500275433,3.42473028058443));
#249952=CARTESIAN_POINT('Origin',(-12.6594199084529,-58.0307974155289,3.11913648168081));
#249953=CARTESIAN_POINT('Origin',(-12.6964592423886,-58.2050537810541,3.4042309748327));
#249954=CARTESIAN_POINT('Ctrl Pts',(-12.9957275188818,-59.6130003254554,
3.3612302805844));
#249955=CARTESIAN_POINT('Ctrl Pts',(-12.8715027735886,-59.6394051101893,
3.3612302805844));
#249956=CARTESIAN_POINT('Ctrl Pts',(-12.8715027735886,-59.6394051101893,
3.2342302805844));
#249957=CARTESIAN_POINT('Ctrl Pts',(-13.0142126749438,-59.7010925481782,
3.3612302805844));
#249958=CARTESIAN_POINT('Ctrl Pts',(-12.8901994296792,-59.7273659613761,
3.36099641108416));
#249959=CARTESIAN_POINT('Ctrl Pts',(-12.8995737759689,-59.771468793191,
3.23423043688307));
#249960=CARTESIAN_POINT('Ctrl Pts',(-13.0316935695386,-59.784390000023,
3.41054258905243));
#249961=CARTESIAN_POINT('Ctrl Pts',(-12.9079667071275,-59.8109544298234,
3.41008815826071));
#249962=CARTESIAN_POINT('Ctrl Pts',(-12.926116905723,-59.8963444006322,
3.3081986730435));
#249963=CARTESIAN_POINT('Ctrl Pts',(-13.0409063549232,-59.8282880397054,
3.48823028058442));
#249964=CARTESIAN_POINT('Ctrl Pts',(-12.9173404733276,-59.8550545325309,
3.48794691941558));
#249965=CARTESIAN_POINT('Ctrl Pts',(-12.9401053405444,-59.9621548122771,
3.42473028058443));
#249966=CARTESIAN_POINT('Origin',(-12.9957275188818,-59.6130003254554,3.2342302805844));
#249967=CARTESIAN_POINT('Ctrl Pts',(-12.6735055745735,-58.0998260601479,
3.47153072139031));
#249968=CARTESIAN_POINT('Ctrl Pts',(-12.5497583678824,-58.126625491213,
3.47122746285036));
#249969=CARTESIAN_POINT('Ctrl Pts',(-12.5722680770241,-58.2316158657528,
3.40413046676745));
#249970=CARTESIAN_POINT('Ctrl Pts',(-12.6975323335627,-58.2122693395989,
3.65553813457946));
#249971=CARTESIAN_POINT('Ctrl Pts',(-12.573630004124,-58.2389340288467,
3.65520336072208));
#249972=CARTESIAN_POINT('Ctrl Pts',(-12.5913858949914,-58.3215581271244,
3.55128134519942));
#249973=CARTESIAN_POINT('Ctrl Pts',(-12.7406947165199,-58.4142696920425,
3.77003198860223));
#249974=CARTESIAN_POINT('Ctrl Pts',(-12.6165486539538,-58.4408527990774,
3.7698020931406));
#249975=CARTESIAN_POINT('Ctrl Pts',(-12.6257301953095,-58.4831353553004,
3.64284195387302));
#249976=CARTESIAN_POINT('Ctrl Pts',(-12.7860306150445,-58.6264539577983,
3.77003198860222));
#249977=CARTESIAN_POINT('Ctrl Pts',(-12.6616197898419,-58.6528982950379,
3.77003198860222));
#249978=CARTESIAN_POINT('Ctrl Pts',(-12.66180600891,-58.6528587129531,3.64284189403758));
#249979=CARTESIAN_POINT('Origin',(-12.7860306150445,-58.6264539577983,3.64303198860222));
#249980=CARTESIAN_POINT('Origin',(2.31399271319931,12.4135704460883,3.2342302805849));
#249981=CARTESIAN_POINT('Origin',(-12.9642895838864,-59.4650964698966,3.2342302805844));
#249982=CARTESIAN_POINT('Origin',(2.30379013587677,12.3655710936223,3.64303198860271));
#249983=CARTESIAN_POINT('Origin',(-12.8695280801138,-59.0190342907437,3.64299171721762));
#249984=CARTESIAN_POINT('Ctrl Pts',(-12.9191181862039,-59.2498070616279,
3.48823028058439));
#249985=CARTESIAN_POINT('Ctrl Pts',(-12.7944335023702,-59.2768226962998,
3.48852004212217));
#249986=CARTESIAN_POINT('Ctrl Pts',(-12.7714622569314,-59.168751483356,
3.42473028058439));
#249987=CARTESIAN_POINT('Ctrl Pts',(-12.9283593439864,-59.2938540730358,
3.41028005848365));
#249988=CARTESIAN_POINT('Ctrl Pts',(-12.8037411209987,-59.320611599147,
3.41074404220263));
#249989=CARTESIAN_POINT('Ctrl Pts',(-12.785497965755,-59.2347843016954,
3.30780486243861));
#249990=CARTESIAN_POINT('Ctrl Pts',(-12.9458672564,-59.3773008374012,3.3612302805844));
#249991=CARTESIAN_POINT('Ctrl Pts',(-12.8213956592928,-59.4036696715731,
3.36146460586352));
#249992=CARTESIAN_POINT('Ctrl Pts',(-12.8120883873133,-59.3598823995823,
3.23423045308352));
#249993=CARTESIAN_POINT('Ctrl Pts',(-12.9642895838864,-59.4650964698966,
3.3612302805844));
#249994=CARTESIAN_POINT('Ctrl Pts',(-12.8400648385932,-59.4915012546304,
3.3612302805844));
#249995=CARTESIAN_POINT('Ctrl Pts',(-12.8400648385932,-59.4915012546304,
3.2342302805844));
#249996=CARTESIAN_POINT('Origin',(-12.8956870022246,-59.1423466986221,3.42473028058439));
#249997=CARTESIAN_POINT('Origin',(-12.878773330973,-59.0627741301476,3.56563113524774));
#249998=CARTESIAN_POINT('Origin',(-6.10480350566428,-61.1207756556235,3.56647653909442));
#249999=CARTESIAN_POINT('Origin',(-6.1093749596214,-61.164764644046,3.64299466007773));
#250000=CARTESIAN_POINT('Origin',(-6.09624906995176,-61.0393856393803,3.42473028058441));
#250001=CARTESIAN_POINT('Ctrl Pts',(-6.08531878138258,-60.9299448846689,
3.48823028058441));
#250002=CARTESIAN_POINT('Ctrl Pts',(-6.21110821942873,-60.9172173747509,
3.48794691941557));
#250003=CARTESIAN_POINT('Ctrl Pts',(-6.22255335066354,-61.0261105245453,
3.42473028058442));
#250004=CARTESIAN_POINT('Ctrl Pts',(-6.08049918876651,-60.8851977561468,
3.41028005925044));
#250005=CARTESIAN_POINT('Ctrl Pts',(-6.20637959976652,-60.8722275639157,
3.40982512230997));
#250006=CARTESIAN_POINT('Ctrl Pts',(-6.21549684257552,-60.9589723348217,
3.30780486372864));
#250007=CARTESIAN_POINT('Ctrl Pts',(-6.0713679351627,-60.8004245407958,
3.36123028058439));
#250008=CARTESIAN_POINT('Ctrl Pts',(-6.19743126523164,-60.7870898478956,
3.36099721048403));
#250009=CARTESIAN_POINT('Ctrl Pts',(-6.20212840134644,-60.8317801127834,
3.23423045308315));
#250010=CARTESIAN_POINT('Ctrl Pts',(-6.06175884541508,-60.7112330730303,
3.36123028058439));
#250011=CARTESIAN_POINT('Ctrl Pts',(-6.18806312612685,-60.6979579581953,
3.36123028058439));
#250012=CARTESIAN_POINT('Ctrl Pts',(-6.18806312612685,-60.6979579581953,
3.23423028058439));
#250013=CARTESIAN_POINT('Origin',(-6.06175884541508,-60.7112330730303,3.23423028058438));
#250014=CARTESIAN_POINT('Origin',(0.315760701779433,-0.033187787087293,
3.64303198860263));
#250015=CARTESIAN_POINT('Origin',(-6.15137923967613,-61.5639141665611,3.64303198860219));
#250016=CARTESIAN_POINT('Origin',(0.315760701779433,-0.0331877870872902,
3.23423028058481));
#250017=CARTESIAN_POINT('Origin',(-6.04595329344999,-60.5608532912342,3.23423028058439));
#250018=CARTESIAN_POINT('Ctrl Pts',(-6.207123496544,-62.0995362748658,3.47153072139028));
#250019=CARTESIAN_POINT('Ctrl Pts',(-6.33421250060393,-62.0866494451784,
3.47182327902618));
#250020=CARTESIAN_POINT('Ctrl Pts',(-6.32269886887934,-61.9789328429855,
3.40413028958983));
#250021=CARTESIAN_POINT('Ctrl Pts',(-6.1952204063465,-61.9851725366284,
3.65553807120912));
#250022=CARTESIAN_POINT('Ctrl Pts',(-6.32217680516108,-61.9721399414743,
3.65586275496892));
#250023=CARTESIAN_POINT('Ctrl Pts',(-6.31308733464666,-61.8874852020919,
3.55128126837237));
#250024=CARTESIAN_POINT('Ctrl Pts',(-6.17383766261641,-61.7797221753252,
3.7700319886022));
#250025=CARTESIAN_POINT('Ctrl Pts',(-6.30057205577816,-61.7665890280522,
3.77025505748452));
#250026=CARTESIAN_POINT('Ctrl Pts',(-6.29582060418285,-61.7232032332915,
3.64284211731086));
#250027=CARTESIAN_POINT('Ctrl Pts',(-6.15137923967613,-61.5639141665611,
3.7700319886022));
#250028=CARTESIAN_POINT('Ctrl Pts',(-6.27787221312652,-61.5506192193201,
3.7700319886022));
#250029=CARTESIAN_POINT('Ctrl Pts',(-6.27768337964921,-61.5506390665183,
3.64284239821655));
#250030=CARTESIAN_POINT('Origin',(-6.19641157197401,-61.9923681882668,3.40423097483266));
#250031=CARTESIAN_POINT('Ctrl Pts',(-6.04595329344999,-60.5608532912342,
3.36123028058439));
#250032=CARTESIAN_POINT('Ctrl Pts',(-6.17225757416176,-60.5475781763992,
3.36123028058439));
#250033=CARTESIAN_POINT('Ctrl Pts',(-6.17225757416176,-60.5475781763992,
3.23423028058439));
#250034=CARTESIAN_POINT('Ctrl Pts',(-6.03631114774991,-60.4713604300107,
3.36123028058439));
#250035=CARTESIAN_POINT('Ctrl Pts',(-6.16283986559452,-60.4579746647647,
3.36146538610082));
#250036=CARTESIAN_POINT('Ctrl Pts',(-6.15814476024311,-60.4133037213026,
3.23423043688355));
#250037=CARTESIAN_POINT('Ctrl Pts',(-6.02719193013319,-60.3867383361557,
3.4105425869306));
#250038=CARTESIAN_POINT('Ctrl Pts',(-6.15397990991512,-60.3736778173753,
3.4110060885966));
#250039=CARTESIAN_POINT('Ctrl Pts',(-6.14480008848946,-60.2863376507164,
3.30819866970773));
#250040=CARTESIAN_POINT('Ctrl Pts',(-6.02238575970214,-60.3421421670674,
3.48823028058439));
#250041=CARTESIAN_POINT('Ctrl Pts',(-6.14931623097185,-60.329305876221,
3.48852004212216));
#250042=CARTESIAN_POINT('Ctrl Pts',(-6.13776734223154,-60.2194255397044,
3.42473028058438));
#250043=CARTESIAN_POINT('Origin',(-6.01146306151977,-60.2327006545394,3.42473028058439));
#250044=CARTESIAN_POINT('Origin',(-6.21503322485571,-62.1695413802865,3.11913648178484));
#250045=CARTESIAN_POINT('Origin',(-6.23365487766561,-62.3467145720968,2.83404198860218));
#250046=CARTESIAN_POINT('Origin',(-6.00295964302102,-60.1517960317838,3.56563113460705));
#250047=CARTESIAN_POINT('Origin',(-5.99823604520072,-60.1073400339997,3.64299171721757));
#250048=CARTESIAN_POINT('Ctrl Pts',(-6.56531752495238,-62.6108711573004,
2.5990817351598));
#250049=CARTESIAN_POINT('Ctrl Pts',(-6.56142710223288,-62.5737697140401,
2.65878198860218));
#250050=CARTESIAN_POINT('Ctrl Pts',(-6.55408556365882,-62.5037563256533,
2.65878198860218));
#250051=CARTESIAN_POINT('Ctrl Pts',(-6.4776825960902,-62.6200603487605,
2.59908193475532));
#250052=CARTESIAN_POINT('Ctrl Pts',(-6.49759225479898,-62.5804601312021,
2.65878715325233));
#250053=CARTESIAN_POINT('Ctrl Pts',(-6.50335812634735,-62.5090664195404,
2.65878198860218));
#250054=CARTESIAN_POINT('Ctrl Pts',(-6.39420891953701,-62.6036598373287,
2.63878778849862));
#250055=CARTESIAN_POINT('Ctrl Pts',(-6.43639040357881,-62.5636211788246,
2.69564460180056));
#250056=CARTESIAN_POINT('Ctrl Pts',(-6.45393802799965,-62.4890871199576,
2.68180481624838));
#250057=CARTESIAN_POINT('Ctrl Pts',(-6.28054002958074,-62.5425397295635,
2.75443238878567));
#250058=CARTESIAN_POINT('Ctrl Pts',(-6.36702405212719,-62.5098176621811,
2.79268340777068));
#250059=CARTESIAN_POINT('Ctrl Pts',(-6.38494336730917,-62.4232722595961,
2.74885926835567));
#250060=CARTESIAN_POINT('Ctrl Pts',(-6.24912387034406,-62.4991087455373,
2.82856655361656));
#250061=CARTESIAN_POINT('Ctrl Pts',(-6.35913125763714,-62.4722367740483,
2.85384197230787));
#250062=CARTESIAN_POINT('Ctrl Pts',(-6.36471246584659,-62.3786641568868,
2.79184624278385));
#250063=CARTESIAN_POINT('Ctrl Pts',(-6.24436990787996,-62.4538823482274,
2.90134173515979));
#250064=CARTESIAN_POINT('Ctrl Pts',(-6.37126553604007,-62.4410124550017,
2.90163218716347));
#250065=CARTESIAN_POINT('Ctrl Pts',(-6.35995915837738,-62.3334394572618,
2.83404198860218));
#250066=CARTESIAN_POINT('Origin',(-6.55408556365882,-62.5037563256533,2.53178198860217));
#250067=CARTESIAN_POINT('Origin',(0.315760701779433,-0.033187787087293,
3.64303198860263));
#250068=CARTESIAN_POINT('Origin',(-5.9563328589115,-59.7081718144891,3.64303198860221));
#250069=CARTESIAN_POINT('Origin',(-1.29720108988958E-17,1.91741421055974E-13,
2.53178198860262));
#250070=CARTESIAN_POINT('Origin',(-6.58439859102965,-62.5005702980929,2.53178198860218));
#250071=CARTESIAN_POINT('Ctrl Pts',(-5.9563328589115,-59.7081718144891,
3.77003198860222));
#250072=CARTESIAN_POINT('Ctrl Pts',(-6.08282634913932,-59.6948768129326,
3.77003198860221));
#250073=CARTESIAN_POINT('Ctrl Pts',(-6.08263699811322,-59.6948967145274,
3.64284187936994));
#250074=CARTESIAN_POINT('Ctrl Pts',(-5.9338809680361,-59.4923596726252,
3.77003198860222));
#250075=CARTESIAN_POINT('Ctrl Pts',(-6.06016553348731,-59.4792784733341,
3.76980208962856));
#250076=CARTESIAN_POINT('Ctrl Pts',(-6.06449945282193,-59.5223294958618,
3.64284193928205));
#250077=CARTESIAN_POINT('Ctrl Pts',(-5.91250946061122,-59.2869096333628,
3.65553535416543));
#250078=CARTESIAN_POINT('Ctrl Pts',(-6.03858743332082,-59.2739813341569,
3.6552005783451));
#250079=CARTESIAN_POINT('Ctrl Pts',(-6.04723285085718,-59.3580487495168,
3.55127910964222));
#250080=CARTESIAN_POINT('Ctrl Pts',(-5.90061356181196,-59.1725467709676,
3.47153072139032));
#250081=CARTESIAN_POINT('Ctrl Pts',(-6.02658564326364,-59.1597945531716,
3.47122746281542));
#250082=CARTESIAN_POINT('Ctrl Pts',(-6.03762143444245,-59.2666022295036,
3.40413045901226));
#250083=CARTESIAN_POINT('Origin',(-5.91130048050282,-59.2797173540685,3.40423097483269));
#250084=CARTESIAN_POINT('Ctrl Pts',(-6.87697683366501,-62.387392681069,
2.9013417351598));
#250085=CARTESIAN_POINT('Ctrl Pts',(-6.75017837817539,-62.4011871104967,
2.90163218716347));
#250086=CARTESIAN_POINT('Ctrl Pts',(-6.7388720005127,-62.2936141127568,
2.83404198860218));
#250087=CARTESIAN_POINT('Ctrl Pts',(-6.88173199854423,-62.432639721334,
2.82853349835313));
#250088=CARTESIAN_POINT('Ctrl Pts',(-6.76854981002423,-62.4292221586326,
2.85381483162327));
#250089=CARTESIAN_POINT('Ctrl Pts',(-6.74362747387351,-62.3388594194639,
2.79182701594337));
#250090=CARTESIAN_POINT('Ctrl Pts',(-6.86000643604651,-62.4814742414945,
2.75468822073597));
#250091=CARTESIAN_POINT('Ctrl Pts',(-6.76854707276773,-62.467499367628,
2.79286913083797));
#250092=CARTESIAN_POINT('Ctrl Pts',(-6.73309031164111,-62.3865194274372,
2.74900763297861));
#250093=CARTESIAN_POINT('Ctrl Pts',(-6.76243636205652,-62.5644789380881,
2.63954450640351));
#250094=CARTESIAN_POINT('Ctrl Pts',(-6.71251593157837,-62.5342007968298,
2.69627684028813));
#250095=CARTESIAN_POINT('Ctrl Pts',(-6.67979835840198,-62.4648696125157,
2.68224356036455));
#250096=CARTESIAN_POINT('Ctrl Pts',(-6.68360310202745,-62.5984172531152,
2.59908178706191));
#250097=CARTESIAN_POINT('Ctrl Pts',(-6.6558503161057,-62.5638265480139,
2.65878704321527));
#250098=CARTESIAN_POINT('Ctrl Pts',(-6.63528943158894,-62.4951999029145,
2.65878198860218));
#250099=CARTESIAN_POINT('Ctrl Pts',(-6.59568250079822,-62.6076796697353,
2.5990817351598));
#250100=CARTESIAN_POINT('Ctrl Pts',(-6.5917740846471,-62.5705801176608,
2.65878198860217));
#250101=CARTESIAN_POINT('Ctrl Pts',(-6.58439859102965,-62.500570298093,
2.65878198860218));
#250102=CARTESIAN_POINT('Origin',(-6.86517628122447,-62.2803389979218,2.83404198860218));
#250103=CARTESIAN_POINT('Origin',(-5.89267880207724,-59.102543918501,3.11913648166976));
#250104=CARTESIAN_POINT('Origin',(-5.87405712357809,-58.9253704827879,2.83404198860221));
#250105=CARTESIAN_POINT('Origin',(-6.84655462836752,-62.1031658060995,3.11913648177431));
#250106=CARTESIAN_POINT('Origin',(-6.82793297553286,-61.9259926140918,3.40423097483267));
#250107=CARTESIAN_POINT('Ctrl Pts',(-5.8633736414952,-58.8181995570483,
2.90134173515982));
#250108=CARTESIAN_POINT('Ctrl Pts',(-5.98915458643734,-58.8054696185319,
2.90103711553188));
#250109=CARTESIAN_POINT('Ctrl Pts',(-6.00036140428986,-58.9120953679529,
2.8340419886022));
#250110=CARTESIAN_POINT('Ctrl Pts',(-5.85862481136399,-58.7730123682038,
2.82862991747912));
#250111=CARTESIAN_POINT('Ctrl Pts',(-5.97090589422232,-58.7772117628634,
2.85314045886394));
#250112=CARTESIAN_POINT('Ctrl Pts',(-5.99561184840453,-58.8669063622641,
2.79187960999894));
#250113=CARTESIAN_POINT('Ctrl Pts',(-5.8802564056751,-58.7244521481308,
2.75470625793301));
#250114=CARTESIAN_POINT('Ctrl Pts',(-5.9711183347532,-58.7389107566975,
2.79224250381853));
#250115=CARTESIAN_POINT('Ctrl Pts',(-6.00616078842832,-58.8195131589315,
2.7490180910822));
#250116=CARTESIAN_POINT('Ctrl Pts',(-5.97763489331392,-58.6422449895247,
2.63947868311641));
#250117=CARTESIAN_POINT('Ctrl Pts',(-6.02730636094564,-58.6726343357861,
2.69595066767874));
#250118=CARTESIAN_POINT('Ctrl Pts',(-6.05959099741106,-58.7419259266983,
2.68220539436018));
#250119=CARTESIAN_POINT('Ctrl Pts',(-6.05629725705559,-58.6088386066676,
2.59908178584968));
#250120=CARTESIAN_POINT('Ctrl Pts',(-6.0839012432855,-58.6434504949714,
2.65877670944779));
#250121=CARTESIAN_POINT('Ctrl Pts',(-6.10418993496956,-58.7121001992951,
2.65878198860221));
#250122=CARTESIAN_POINT('Ctrl Pts',(-6.14377718965262,-58.5996668978647,
2.59908173515982));
#250123=CARTESIAN_POINT('Ctrl Pts',(-6.14766703046111,-58.6367684021391,
2.6587819886022));
#250124=CARTESIAN_POINT('Ctrl Pts',(-6.15500747092256,-58.7067819056642,
2.65878198860221));
#250125=CARTESIAN_POINT('Origin',(-6.15500747092256,-58.7067819056642,2.53178198860221));
#250126=CARTESIAN_POINT('Ctrl Pts',(-6.78290064323498,-61.4975385923861,
3.7700319886022));
#250127=CARTESIAN_POINT('Ctrl Pts',(-6.65640765888756,-61.5108335407724,
3.7700319886022));
#250128=CARTESIAN_POINT('Ctrl Pts',(-6.65659650327814,-61.5108136924271,
3.64284238727587));
#250129=CARTESIAN_POINT('Ctrl Pts',(-6.80580235504166,-61.7133034041534,
3.7700319886022));
#250130=CARTESIAN_POINT('Ctrl Pts',(-6.6791068640111,-61.7268068187958,
3.77025506105741));
#250131=CARTESIAN_POINT('Ctrl Pts',(-6.67473401011684,-61.6833805404091,
3.64284210641856));
#250132=CARTESIAN_POINT('Ctrl Pts',(-6.82760223531332,-61.9187082819377,
3.65553527987789));
#250133=CARTESIAN_POINT('Ctrl Pts',(-6.70071049690984,-61.9323562021225,
3.65585996532953));
#250134=CARTESIAN_POINT('Ctrl Pts',(-6.69200060426915,-61.8476612078223,
3.55127902710129));
#250135=CARTESIAN_POINT('Ctrl Pts',(-6.83973663030197,-62.0330459552231,
3.47153072139028));
#250136=CARTESIAN_POINT('Ctrl Pts',(-6.71274549238784,-62.0468640245948,
3.47182327905145));
#250137=CARTESIAN_POINT('Ctrl Pts',(-6.701611992752,-61.9391074595194,3.40413028377961));
#250138=CARTESIAN_POINT('Origin',(-6.78290064323498,-61.4975385923861,3.6430319886022));
#250139=CARTESIAN_POINT('Origin',(4.0583767139057E-16,1.91519098829264E-13,
2.53178198860262));
#250140=CARTESIAN_POINT('Origin',(-6.18532049829339,-58.7035958781038,2.53178198860221));
#250141=CARTESIAN_POINT('Origin',(0.364094271196318,6.50157577599512,3.64303198860267));
#250142=CARTESIAN_POINT('Origin',(-6.74099917687787,-61.0983782637168,3.64299466007654));
#250143=CARTESIAN_POINT('Ctrl Pts',(-6.17403490858961,-58.5964866834549,
2.59908173515982));
#250144=CARTESIAN_POINT('Ctrl Pts',(-6.17794390662112,-58.633586174224,
2.65878198860221));
#250145=CARTESIAN_POINT('Ctrl Pts',(-6.18532049829339,-58.7035958781038,
2.65878198860221));
#250146=CARTESIAN_POINT('Ctrl Pts',(-6.26121185652487,-58.5873013840782,
2.59908193199824));
#250147=CARTESIAN_POINT('Ctrl Pts',(-6.24145541658238,-58.6268910424079,
2.65877685806558));
#250148=CARTESIAN_POINT('Ctrl Pts',(-6.23596000968332,-58.6982507756597,
2.65878198860221));
#250149=CARTESIAN_POINT('Ctrl Pts',(-6.34441620808539,-58.603224495399,
2.63872492669768));
#250150=CARTESIAN_POINT('Ctrl Pts',(-6.30249747592639,-58.6433169201092,
2.69532212015256));
#250151=CARTESIAN_POINT('Ctrl Pts',(-6.28536729223259,-58.7177256636151,
2.68176836726592));
#250152=CARTESIAN_POINT('Ctrl Pts',(-6.45770985055622,-58.6635810738162,
2.75442176402197));
#250153=CARTESIAN_POINT('Ctrl Pts',(-6.37191831988748,-58.6966524426395,
2.79203179920061));
#250154=CARTESIAN_POINT('Ctrl Pts',(-6.35432657855756,-58.7827411889909,
2.74885310748135));
#250155=CARTESIAN_POINT('Ctrl Pts',(-6.48899861096488,-58.7067768761599,
2.82866089558365));
#250156=CARTESIAN_POINT('Ctrl Pts',(-6.38003592347285,-58.7342263230564,
2.85316563119164));
#250157=CARTESIAN_POINT('Ctrl Pts',(-6.37452670784893,-58.827100211173,
2.79189751796643));
#250158=CARTESIAN_POINT('Ctrl Pts',(-6.49374646112681,-58.7519447039087,
2.90134173515981));
#250159=CARTESIAN_POINT('Ctrl Pts',(-6.36806742857265,-58.7656442740269,
2.90103711553188));
#250160=CARTESIAN_POINT('Ctrl Pts',(-6.37927424642518,-58.8722700234479,
2.8340419886022));
#250161=CARTESIAN_POINT('Origin',(-6.50557852713695,-58.8589949086129,2.8340419886022));
#250162=CARTESIAN_POINT('Origin',(-6.73632490881102,-61.0544000804069,3.56647653971742));
#250163=CARTESIAN_POINT('Origin',(-6.72777047351062,-60.9730100652053,3.42473028058442));
#250164=CARTESIAN_POINT('Origin',(-6.52420020557653,-59.036168344315,3.1191364816805));
#250165=CARTESIAN_POINT('Origin',(-6.54282188406168,-59.2133417798935,3.40423097483269));
#250166=CARTESIAN_POINT('Ctrl Pts',(-6.69328024897394,-60.6448574988553,
3.36123028058439));
#250167=CARTESIAN_POINT('Ctrl Pts',(-6.56697596826216,-60.6581326136903,
3.36123028058439));
#250168=CARTESIAN_POINT('Ctrl Pts',(-6.56697596826216,-60.6581326136903,
3.23423028058439));
#250169=CARTESIAN_POINT('Ctrl Pts',(-6.70245599674927,-60.7343993681212,
3.36123028058439));
#250170=CARTESIAN_POINT('Ctrl Pts',(-6.57637578951115,-60.7475659388581,
3.36099641108384));
#250171=CARTESIAN_POINT('Ctrl Pts',(-6.58108878091658,-60.7924070567586,
3.23423043688315));
#250172=CARTESIAN_POINT('Ctrl Pts',(-6.71113417453891,-60.8190677588578,
3.41054258905242));
#250173=CARTESIAN_POINT('Ctrl Pts',(-6.58530836180298,-60.8325536871424,
3.41008815826015));
#250174=CARTESIAN_POINT('Ctrl Pts',(-6.5944334492835,-60.9193730951222,
3.30819867304306));
#250175=CARTESIAN_POINT('Ctrl Pts',(-6.71570789669348,-60.8636883187843,
3.48823028058441));
#250176=CARTESIAN_POINT('Ctrl Pts',(-6.59002106156404,-60.8773920302459,
3.48794691941557));
#250177=CARTESIAN_POINT('Ctrl Pts',(-6.60146619279885,-60.9862851800403,
3.42473028058442));
#250178=CARTESIAN_POINT('Origin',(-6.69328024897394,-60.6448574988553,3.23423028058439));
#250179=CARTESIAN_POINT('Ctrl Pts',(-6.53099325079995,-59.1062911958295,
3.47153072139031));
#250180=CARTESIAN_POINT('Ctrl Pts',(-6.4051226409094,-59.1200087114581,
3.47122746285036));
#250181=CARTESIAN_POINT('Ctrl Pts',(-6.41653455700065,-59.2267768430459,
3.40413046676746));
#250182=CARTESIAN_POINT('Ctrl Pts',(-6.54313486548254,-59.2206299794251,
3.65553813457947));
#250183=CARTESIAN_POINT('Ctrl Pts',(-6.4171240669808,-59.234197276625,3.65520336072176));
#250184=CARTESIAN_POINT('Ctrl Pts',(-6.42614611919671,-59.3182247474317,
3.55128134519943));
#250185=CARTESIAN_POINT('Ctrl Pts',(-6.56494601396971,-59.4260354503638,
3.77003198860222));
#250186=CARTESIAN_POINT('Ctrl Pts',(-6.43870134519636,-59.4394961352151,
3.76980209314032));
#250187=CARTESIAN_POINT('Ctrl Pts',(-6.44341285848396,-59.4825067955806,
3.64284195387329));
#250188=CARTESIAN_POINT('Ctrl Pts',(-6.58785426247035,-59.6417962403142,
3.77003198860222));
#250189=CARTESIAN_POINT('Ctrl Pts',(-6.46136078685173,-59.6550912403352,
3.77003198860222));
#250190=CARTESIAN_POINT('Ctrl Pts',(-6.46155012324679,-59.6550713402781,
3.64284189403761));
#250191=CARTESIAN_POINT('Origin',(-6.58785426247035,-59.6417962403142,3.64303198860221));
#250192=CARTESIAN_POINT('Origin',(0.347626240493858,6.34489293004856,3.23423028058486));
#250193=CARTESIAN_POINT('Origin',(-6.67747469700884,-60.4944777170593,3.23423028058439));
#250194=CARTESIAN_POINT('Origin',(0.345047419449677,6.32035708677198,3.64303198860267));
#250195=CARTESIAN_POINT('Origin',(-6.62985850077779,-60.0409538388296,3.6429917172174));
#250196=CARTESIAN_POINT('Ctrl Pts',(-6.65505462397334,-60.2756459899118,
3.48823028058439));
#250197=CARTESIAN_POINT('Ctrl Pts',(-6.52822907310716,-60.2894805317161,
3.48852004212217));
#250198=CARTESIAN_POINT('Ctrl Pts',(-6.51668018436685,-60.1796001951994,
3.42473028058438));
#250199=CARTESIAN_POINT('Ctrl Pts',(-6.65964099131231,-60.3204176712043,
3.41028005848362));
#250200=CARTESIAN_POINT('Ctrl Pts',(-6.53290851690239,-60.3340024654432,
3.4107440422026));
#250201=CARTESIAN_POINT('Ctrl Pts',(-6.52373669508263,-60.2467384099245,
3.30780486243842));
#250202=CARTESIAN_POINT('Ctrl Pts',(-6.66833043150598,-60.405237380643,
3.36123028058439));
#250203=CARTESIAN_POINT('Ctrl Pts',(-6.54178440911728,-60.4184509388167,
3.36146460586334));
#250204=CARTESIAN_POINT('Ctrl Pts',(-6.53710513959971,-60.373930663246,
3.23423045308357));
#250205=CARTESIAN_POINT('Ctrl Pts',(-6.67747469700884,-60.4944777170593,
3.36123028058439));
#250206=CARTESIAN_POINT('Ctrl Pts',(-6.55117041629707,-60.5077528318942,
3.36123028058439));
#250207=CARTESIAN_POINT('Ctrl Pts',(-6.55117041629707,-60.5077528318942,
3.23423028058439));
#250208=CARTESIAN_POINT('Origin',(-6.64298446507862,-60.1663250803644,3.42473028058439));
#250209=CARTESIAN_POINT('Origin',(-6.63448104699066,-60.0854204586806,3.56563113524721));
#250210=CARTESIAN_POINT('Origin',(0.317499999706111,-61.4240753804082,3.5664765390942));
#250211=CARTESIAN_POINT('Origin',(0.317551690013291,-61.4683012396067,3.64299466007677));
#250212=CARTESIAN_POINT('Origin',(0.317500000000648,-61.3422370451704,3.42473028058441));
#250213=CARTESIAN_POINT('Ctrl Pts',(0.316930737396561,-61.2322532920971,
3.48823028058441));
#250214=CARTESIAN_POINT('Ctrl Pts',(0.190500000000648,-61.2327440814644,
3.48794691941557));
#250215=CARTESIAN_POINT('Ctrl Pts',(0.190500000000648,-61.3422370451704,
3.42473028058442));
#250216=CARTESIAN_POINT('Ctrl Pts',(0.317046579200287,-61.1872475084172,
3.41028005925046));
#250217=CARTESIAN_POINT('Ctrl Pts',(0.190500000000573,-61.1875064541747,
3.40982512230936));
#250218=CARTESIAN_POINT('Ctrl Pts',(0.190500000000647,-61.2747290395307,
3.30780486372771));
#250219=CARTESIAN_POINT('Ctrl Pts',(0.31726659691415,-61.101984213703,3.36123028058439));
#250220=CARTESIAN_POINT('Ctrl Pts',(0.190500000000765,-61.1018997758113,
3.36099721048437));
#250221=CARTESIAN_POINT('Ctrl Pts',(0.190500000000646,-61.146836207171,
3.23423045308358));
#250222=CARTESIAN_POINT('Ctrl Pts',(0.317500000000645,-61.0122769227454,
3.36123028058439));
#250223=CARTESIAN_POINT('Ctrl Pts',(0.190500000000645,-61.0122769227454,
3.36123028058439));
#250224=CARTESIAN_POINT('Ctrl Pts',(0.190500000000645,-61.0122769227454,
3.23423028058439));
#250225=CARTESIAN_POINT('Origin',(0.317500000000645,-61.0122769227454,3.23423028058439));
#250226=CARTESIAN_POINT('Origin',(0.317500000000006,1.87143253445273E-13,
3.64303198860263));
#250227=CARTESIAN_POINT('Origin',(0.317500000000654,-61.8696548221179,3.64303198860219));
#250228=CARTESIAN_POINT('Origin',(0.317500000000006,1.89997900514936E-13,
3.23423028058481));
#250229=CARTESIAN_POINT('Origin',(0.317500000000643,-60.8610688070705,3.23423028058439));
#250230=CARTESIAN_POINT('Ctrl Pts',(0.318048871877788,-62.4081695979766,
3.47153072139028));
#250231=CARTESIAN_POINT('Ctrl Pts',(0.190309034176441,-62.4086377819833,
3.47182327902618));
#250232=CARTESIAN_POINT('Ctrl Pts',(0.190500142125711,-62.3003077603773,
3.40413028959004));
#250233=CARTESIAN_POINT('Ctrl Pts',(0.317932489890643,-62.2931881445369,
3.65553807120917));
#250234=CARTESIAN_POINT('Ctrl Pts',(0.190309294367224,-62.293497500569,
3.65586275496757));
#250235=CARTESIAN_POINT('Ctrl Pts',(0.190500141996126,-62.2083564003226,
3.55128126837138));
#250236=CARTESIAN_POINT('Ctrl Pts',(0.317722686168063,-62.0866281564671,
3.7700319886022));
#250237=CARTESIAN_POINT('Ctrl Pts',(0.190309769570757,-62.086814305312,
3.77025505748501));
#250238=CARTESIAN_POINT('Ctrl Pts',(0.190500141762521,-62.0431695205407,
3.64284211731181));
#250239=CARTESIAN_POINT('Ctrl Pts',(0.317500000000654,-61.8696548221179,
3.7700319886022));
#250240=CARTESIAN_POINT('Ctrl Pts',(0.190310267890066,-61.8696548221179,
3.7700319886022));
#250241=CARTESIAN_POINT('Ctrl Pts',(0.190500141514568,-61.8696548221179,
3.64284239821694));
#250242=CARTESIAN_POINT('Origin',(0.317500000000658,-62.3004688883553,3.40423097483266));
#250243=CARTESIAN_POINT('Ctrl Pts',(0.317500000000643,-60.8610688070705,
3.36123028058439));
#250244=CARTESIAN_POINT('Ctrl Pts',(0.190500000000643,-60.8610688070705,
3.36123028058439));
#250245=CARTESIAN_POINT('Ctrl Pts',(0.190500000000643,-60.8610688070705,
3.23423028058439));
#250246=CARTESIAN_POINT('Ctrl Pts',(0.31773477376092,-60.7710583184318,
3.36123028058438));
#250247=CARTESIAN_POINT('Ctrl Pts',(0.190500000000766,-60.7709717342426,
3.36146538610139));
#250248=CARTESIAN_POINT('Ctrl Pts',(0.190500000000642,-60.7260547307369,
3.2342304368841));
#250249=CARTESIAN_POINT('Ctrl Pts',(0.317958617919681,-60.6859465754576,
3.41054258693055));
#250250=CARTESIAN_POINT('Ctrl Pts',(0.190500000000172,-60.686210556255,
3.41100608859671));
#250251=CARTESIAN_POINT('Ctrl Pts',(0.19050000000064,-60.598389295539,3.30819866970735));
#250252=CARTESIAN_POINT('Ctrl Pts',(0.318076890624007,-60.6410923272403,
3.48823028058439));
#250253=CARTESIAN_POINT('Ctrl Pts',(0.190500000000634,-60.641594202042,
3.48852004212217));
#250254=CARTESIAN_POINT('Ctrl Pts',(0.19050000000064,-60.5311086139133,
3.42473028058439));
#250255=CARTESIAN_POINT('Origin',(0.317500000000639,-60.5311086139133,3.42473028058439));
#250256=CARTESIAN_POINT('Origin',(0.317499999979056,-62.4786179998463,3.11913648178229));
#250257=CARTESIAN_POINT('Origin',(0.317500000000662,-62.6567671111297,2.83404198860217));
#250258=CARTESIAN_POINT('Origin',(0.317499999994423,-60.4497583458796,3.56563113460789));
#250259=CARTESIAN_POINT('Origin',(0.31755080432116,-60.4050521322801,3.64299171721745));
#250260=CARTESIAN_POINT('Ctrl Pts',(0.0152661173115319,-62.9541448057646,
2.59908173515979));
#250261=CARTESIAN_POINT('Ctrl Pts',(0.0152570710392988,-62.9168399481841,
2.65878198860218));
#250262=CARTESIAN_POINT('Ctrl Pts',(0.0152400000006639,-62.8464427007194,
2.65878198860218));
#250263=CARTESIAN_POINT('Ctrl Pts',(0.10338150492588,-62.9541233134301,
2.59908193475501));
#250264=CARTESIAN_POINT('Ctrl Pts',(0.0794415635241914,-62.9168211560388,
2.65878715325371));
#250265=CARTESIAN_POINT('Ctrl Pts',(0.0662446030566008,-62.8464212442879,
2.65878198860218));
#250266=CARTESIAN_POINT('Ctrl Pts',(0.184683583688456,-62.9290872705826,
2.63878778849821));
#250267=CARTESIAN_POINT('Ctrl Pts',(0.138547994785007,-62.8936771137452,
2.69564460180082));
#250268=CARTESIAN_POINT('Ctrl Pts',(0.113305567452228,-62.8213855864653,
2.68180481624846));
#250269=CARTESIAN_POINT('Ctrl Pts',(0.291340992632371,-62.8564203507738,
2.75443238878607));
#250270=CARTESIAN_POINT('Ctrl Pts',(0.201910351191927,-62.8329175802734,
2.7926834077703));
#250271=CARTESIAN_POINT('Ctrl Pts',(0.1750427419585,-62.7487193609387,2.74885926835559));
#250272=CARTESIAN_POINT('Ctrl Pts',(0.318045276843287,-62.8099434033761,
2.82856655361622));
#250273=CARTESIAN_POINT('Ctrl Pts',(0.205831635643734,-62.7947175424999,
2.85384197230742));
#250274=CARTESIAN_POINT('Ctrl Pts',(0.190500000000664,-62.7022409210439,
2.79184624278408));
#250275=CARTESIAN_POINT('Ctrl Pts',(0.318045750793708,-62.7644678366117,
2.90134173515981));
#250276=CARTESIAN_POINT('Ctrl Pts',(0.190500000000659,-62.7649326510147,
2.90163218716348));
#250277=CARTESIAN_POINT('Ctrl Pts',(0.190500000000662,-62.6567671111297,
2.83404198860219));
#250278=CARTESIAN_POINT('Origin',(0.317500000000006,1.87143253445273E-13,
3.64303198860263));
#250279=CARTESIAN_POINT('Origin',(0.317500000000634,-60.0036905223729,3.64303198860221));
#250280=CARTESIAN_POINT('Ctrl Pts',(0.317500000000634,-60.0036905223729,
3.77003198860221));
#250281=CARTESIAN_POINT('Ctrl Pts',(0.190309748265596,-60.0036905223729,
3.77003198860221));
#250282=CARTESIAN_POINT('Ctrl Pts',(0.190500142290163,-60.0036905223729,
3.64284187936986));
#250283=CARTESIAN_POINT('Ctrl Pts',(0.31727038552505,-59.7867137603522,
3.77003198860222));
#250284=CARTESIAN_POINT('Ctrl Pts',(0.190310262476818,-59.7869045527981,
3.76980208962897));
#250285=CARTESIAN_POINT('Ctrl Pts',(0.190500142033094,-59.8301727552505,
3.6428419392825));
#250286=CARTESIAN_POINT('Ctrl Pts',(0.317049440714242,-59.5801552670726,
3.65553535416542));
#250287=CARTESIAN_POINT('Ctrl Pts',(0.190310761082648,-59.580476527185,
3.65520057834388));
#250288=CARTESIAN_POINT('Ctrl Pts',(0.190500141785736,-59.6649871046535,
3.55127910964184));
#250289=CARTESIAN_POINT('Ctrl Pts',(0.316925998273675,-59.465175436383,
3.4715307213903));
#250290=CARTESIAN_POINT('Ctrl Pts',(0.190311035335334,-59.4656607446592,
3.47122746281541));
#250291=CARTESIAN_POINT('Ctrl Pts',(0.190500141647532,-59.5730368716577,
3.40413045901222));
#250292=CARTESIAN_POINT('Origin',(0.31750000000063,-59.572876015004,3.40423097483268));
#250293=CARTESIAN_POINT('Ctrl Pts',(-0.318045750792382,-62.7644678366118,
2.9013417351598));
#250294=CARTESIAN_POINT('Ctrl Pts',(-0.190499999999336,-62.7649326510147,
2.90163218716347));
#250295=CARTESIAN_POINT('Ctrl Pts',(-0.190499999999338,-62.6567671111297,
2.83404198860218));
#250296=CARTESIAN_POINT('Ctrl Pts',(-0.318045262794514,-62.8099640589333,
2.82853349835311));
#250297=CARTESIAN_POINT('Ctrl Pts',(-0.205840330723024,-62.7947344577603,
2.85381483162217));
#250298=CARTESIAN_POINT('Ctrl Pts',(-0.190499999999339,-62.7022616416329,
2.79182701594121));
#250299=CARTESIAN_POINT('Ctrl Pts',(-0.291334117854884,-62.8562601188212,
2.75468822073599));
#250300=CARTESIAN_POINT('Ctrl Pts',(-0.201836550627177,-62.8328016940823,
2.79286913083821));
#250301=CARTESIAN_POINT('Ctrl Pts',(-0.175038734051574,-62.748559129723,
2.7490076329788));
#250302=CARTESIAN_POINT('Ctrl Pts',(-0.185622189559593,-62.9286112571069,
2.63954450640348));
#250303=CARTESIAN_POINT('Ctrl Pts',(-0.139140155999356,-62.8932808767897,
2.69627684028793));
#250304=CARTESIAN_POINT('Ctrl Pts',(-0.113848895264975,-62.8209095783123,
2.68224356036436));
#250305=CARTESIAN_POINT('Ctrl Pts',(-0.103673266462265,-62.9541233349672,
2.59908178706312));
#250306=CARTESIAN_POINT('Ctrl Pts',(-0.0796882264530914,-62.916821165302,
2.65878704321472));
#250307=CARTESIAN_POINT('Ctrl Pts',(-0.0664134143645206,-62.8464212664861,
2.65878198860218));
#250308=CARTESIAN_POINT('Ctrl Pts',(-0.0152661173102017,-62.9541448057646,
2.59908173515979));
#250309=CARTESIAN_POINT('Ctrl Pts',(-0.0152570710379694,-62.9168399481841,
2.65878198860218));
#250310=CARTESIAN_POINT('Ctrl Pts',(-0.015239999999336,-62.8464427007194,
2.65878198860218));
#250311=CARTESIAN_POINT('Origin',(-0.317499999999338,-62.6567671111297,
2.83404198860218));
#250312=CARTESIAN_POINT('Origin',(0.317499999972213,-59.3947266586248,3.11913648167007));
#250313=CARTESIAN_POINT('Origin',(0.317500000000626,-59.2165773020939,2.83404198860221));
#250314=CARTESIAN_POINT('Origin',(-0.317499999976278,-62.4786179998357,
3.11913648177568));
#250315=CARTESIAN_POINT('Origin',(-0.317499999999342,-62.3004688883553,
3.40423097483267));
#250316=CARTESIAN_POINT('Ctrl Pts',(0.316922544676314,-59.1088767419346,
2.90134173515982));
#250317=CARTESIAN_POINT('Ctrl Pts',(0.190500000000626,-59.1093642282365,
2.90103711553188));
#250318=CARTESIAN_POINT('Ctrl Pts',(0.190500000000626,-59.2165773020939,
2.8340419886022));
#250319=CARTESIAN_POINT('Ctrl Pts',(0.316922012809783,-59.0634407053228,
2.82862991747926));
#250320=CARTESIAN_POINT('Ctrl Pts',(0.205694973741507,-59.0793536643042,
2.85314045886381));
#250321=CARTESIAN_POINT('Ctrl Pts',(0.190500000000625,-59.171139382729,
2.79187960999897));
#250322=CARTESIAN_POINT('Ctrl Pts',(0.290332993455545,-59.0174076205273,
2.75470625793277));
#250323=CARTESIAN_POINT('Ctrl Pts',(0.201480151666442,-59.0412846811393,
2.79224250381859));
#250324=CARTESIAN_POINT('Ctrl Pts',(0.175054909460322,-59.1251084688119,
2.74901809108218));
#250325=CARTESIAN_POINT('Ctrl Pts',(0.184894967402272,-58.9458296250061,
2.63947868311665));
#250326=CARTESIAN_POINT('Ctrl Pts',(0.138672156931882,-58.981244577429,
2.69595066767869));
#250327=CARTESIAN_POINT('Ctrl Pts',(0.113807322598413,-59.0535312451932,
2.6822053943602));
#250328=CARTESIAN_POINT('Ctrl Pts',(0.1031716064563,-58.9208287018089,2.59908178585043));
#250329=CARTESIAN_POINT('Ctrl Pts',(0.0793367652463939,-58.958136384828,
2.65877670944839));
#250330=CARTESIAN_POINT('Ctrl Pts',(0.066335065234977,-59.0285307646514,
2.6587819886022));
#250331=CARTESIAN_POINT('Ctrl Pts',(0.015212193456543,-58.9208513795071,
2.59908173515982));
#250332=CARTESIAN_POINT('Ctrl Pts',(0.0152218248297303,-58.9581562369412,
2.65878198860221));
#250333=CARTESIAN_POINT('Ctrl Pts',(0.0152400000006241,-59.0285534841294,
2.6587819886022));
#250334=CARTESIAN_POINT('Ctrl Pts',(-0.317499999999346,-61.8696548221179,
3.7700319886022));
#250335=CARTESIAN_POINT('Ctrl Pts',(-0.190310256930768,-61.8696548221179,
3.7700319886022));
#250336=CARTESIAN_POINT('Ctrl Pts',(-0.190500141529595,-61.8696548221179,
3.64284238727532));
#250337=CARTESIAN_POINT('Ctrl Pts',(-0.317722689631596,-62.0866315324119,
3.7700319886022));
#250338=CARTESIAN_POINT('Ctrl Pts',(-0.190309758574985,-62.0868176889516,
3.77025506105797));
#250339=CARTESIAN_POINT('Ctrl Pts',(-0.190500141777577,-62.0431722165658,
3.64284210641847));
#250340=CARTESIAN_POINT('Ctrl Pts',(-0.317932491655028,-62.2931898887679,
3.6555352798779));
#250341=CARTESIAN_POINT('Ctrl Pts',(-0.190309283349165,-62.2934992458067,
3.65585996533061));
#250342=CARTESIAN_POINT('Ctrl Pts',(-0.190500142011202,-62.208357787851,
3.55127902710123));
#250343=CARTESIAN_POINT('Ctrl Pts',(-0.31804887187647,-62.4081695979766,
3.47153072139028));
#250344=CARTESIAN_POINT('Ctrl Pts',(-0.190309023145839,-62.4086377820237,
3.47182327905144));
#250345=CARTESIAN_POINT('Ctrl Pts',(-0.1905001421408,-62.3003077510783,
3.40413028377931));
#250346=CARTESIAN_POINT('Origin',(-0.317499999999346,-61.8696548221179,
3.6430319886022));
#250347=CARTESIAN_POINT('Origin',(-0.317499999999998,-4.7125364762808E-13,
3.64303198860263));
#250348=CARTESIAN_POINT('Origin',(-0.317551690011254,-61.4683012396059,
3.64299466007809));
#250349=CARTESIAN_POINT('Ctrl Pts',(-0.015212193455297,-58.9208513795071,
2.59908173515982));
#250350=CARTESIAN_POINT('Ctrl Pts',(-0.0152218248284836,-58.9581562369412,
2.6587819886022));
#250351=CARTESIAN_POINT('Ctrl Pts',(-0.0152399999993761,-59.0285534841294,
2.6587819886022));
#250352=CARTESIAN_POINT('Ctrl Pts',(-0.102871702176794,-58.9208288705613,
2.59908193199802));
#250353=CARTESIAN_POINT('Ctrl Pts',(-0.0790852439328077,-58.9581365422923,
2.65877685806533));
#250354=CARTESIAN_POINT('Ctrl Pts',(-0.0661608181919111,-59.0285309330207,
2.6587819886022));
#250355=CARTESIAN_POINT('Ctrl Pts',(-0.183955833236869,-58.9453619764181,
2.63872492669755));
#250356=CARTESIAN_POINT('Ctrl Pts',(-0.138075936735338,-58.9808530699759,
2.69532212015228));
#250357=CARTESIAN_POINT('Ctrl Pts',(-0.113261762367514,-59.0530636028224,
2.68176836726592));
#250358=CARTESIAN_POINT('Ctrl Pts',(-0.290319860890052,-59.0172303255292,
2.75442176402209));
#250359=CARTESIAN_POINT('Ctrl Pts',(-0.201541405841324,-59.041152869072,
2.79203179920101));
#250360=CARTESIAN_POINT('Ctrl Pts',(-0.175047309550586,-59.1249311745755,
2.74885310748134));
#250361=CARTESIAN_POINT('Ctrl Pts',(-0.316922027356719,-59.063460062791,
2.82866089558356));
#250362=CARTESIAN_POINT('Ctrl Pts',(-0.20568700036596,-59.0793694364685,
2.85316563119101));
#250363=CARTESIAN_POINT('Ctrl Pts',(-0.190499999999374,-59.1711586818657,
2.79189751796571));
#250364=CARTESIAN_POINT('Ctrl Pts',(-0.316922544675064,-59.1088767419346,
2.90134173515982));
#250365=CARTESIAN_POINT('Ctrl Pts',(-0.190499999999374,-59.1093642282365,
2.90103711553188));
#250366=CARTESIAN_POINT('Ctrl Pts',(-0.190499999999374,-59.2165773020939,
2.8340419886022));
#250367=CARTESIAN_POINT('Origin',(-0.317499999999374,-59.2165773020939,
2.8340419886022));
#250368=CARTESIAN_POINT('Origin',(-0.317499999993643,-61.4240753793289,
3.56647653971734));
#250369=CARTESIAN_POINT('Origin',(-0.317499999999352,-61.3422370451704,
3.42473028058442));
#250370=CARTESIAN_POINT('Origin',(-0.317499999969443,-59.3947266586082,
3.11913648168042));
#250371=CARTESIAN_POINT('Origin',(-0.31749999999937,-59.572876015004,3.40423097483268));
#250372=CARTESIAN_POINT('Ctrl Pts',(-0.317499999999355,-61.0122769227454,
3.36123028058439));
#250373=CARTESIAN_POINT('Ctrl Pts',(-0.190499999999355,-61.0122769227454,
3.36123028058439));
#250374=CARTESIAN_POINT('Ctrl Pts',(-0.190499999999355,-61.0122769227454,
3.23423028058439));
#250375=CARTESIAN_POINT('Ctrl Pts',(-0.317265808075734,-61.1022873990969,
3.36123028058439));
#250376=CARTESIAN_POINT('Ctrl Pts',(-0.190499999999337,-61.1022028716725,
3.36099641108441));
#250377=CARTESIAN_POINT('Ctrl Pts',(-0.190499999999354,-61.1472909869853,
3.2342304368835));
#250378=CARTESIAN_POINT('Ctrl Pts',(-0.317046189128469,-61.1873990841183,
3.41054258905241));
#250379=CARTESIAN_POINT('Ctrl Pts',(-0.190499999999407,-61.1876587562293,
3.41008815826042));
#250380=CARTESIAN_POINT('Ctrl Pts',(-0.190499999999353,-61.274956389781,
3.30819867304318));
#250381=CARTESIAN_POINT('Ctrl Pts',(-0.316930737395267,-61.2322532920971,
3.48823028058441));
#250382=CARTESIAN_POINT('Ctrl Pts',(-0.190499999999352,-61.2327440814644,
3.48794691941557));
#250383=CARTESIAN_POINT('Ctrl Pts',(-0.190499999999352,-61.3422370451704,
3.42473028058442));
#250384=CARTESIAN_POINT('Origin',(-0.317499999999355,-61.0122769227454,
3.23423028058439));
#250385=CARTESIAN_POINT('Ctrl Pts',(-0.316925998272419,-59.465175436383,
3.47153072139031));
#250386=CARTESIAN_POINT('Ctrl Pts',(-0.19031104992418,-59.4656607446032,
3.47122746285036));
#250387=CARTESIAN_POINT('Ctrl Pts',(-0.190500141624417,-59.5730368592471,
3.40413046676735));
#250388=CARTESIAN_POINT('Ctrl Pts',(-0.317049442578568,-59.5801570044829,
3.65553813457941));
#250389=CARTESIAN_POINT('Ctrl Pts',(-0.190310775687915,-59.5804782634818,
3.65520336072243));
#250390=CARTESIAN_POINT('Ctrl Pts',(-0.190500141762601,-59.6649884842686,
3.5512813451993));
#250391=CARTESIAN_POINT('Ctrl Pts',(-0.317270389088207,-59.7867171285934,
3.77003198860222));
#250392=CARTESIAN_POINT('Ctrl Pts',(-0.190310277117269,-59.7869079131857,
3.76980209314134));
#250393=CARTESIAN_POINT('Ctrl Pts',(-0.190500142009918,-59.8301754438947,
3.64284195387351));
#250394=CARTESIAN_POINT('Ctrl Pts',(-0.317499999999366,-60.0036905223729,
3.77003198860221));
#250395=CARTESIAN_POINT('Ctrl Pts',(-0.190309762953857,-60.0036905223729,
3.77003198860221));
#250396=CARTESIAN_POINT('Ctrl Pts',(-0.19050014226694,-60.0036905223729,
3.64284189403738));
#250397=CARTESIAN_POINT('Origin',(-0.317499999999366,-60.0036905223729,
3.64303198860221));
#250398=CARTESIAN_POINT('Origin',(-0.317499999999991,-4.52611858510147E-13,
3.23423028058481));
#250399=CARTESIAN_POINT('Origin',(-0.317499999999357,-60.8610688070705,
3.23423028058439));
#250400=CARTESIAN_POINT('Origin',(-0.317499999999991,-4.52994308698643E-13,
3.64303198860263));
#250401=CARTESIAN_POINT('Origin',(-0.317550804320116,-60.4050521322799,
3.64299171721719));
#250402=CARTESIAN_POINT('Ctrl Pts',(-0.318076890622726,-60.6410923272403,
3.48823028058439));
#250403=CARTESIAN_POINT('Ctrl Pts',(-0.19049999999936,-60.641594202042,
3.48852004212217));
#250404=CARTESIAN_POINT('Ctrl Pts',(-0.19049999999936,-60.5311086139133,
3.42473028058439));
#250405=CARTESIAN_POINT('Ctrl Pts',(-0.317958218318119,-60.6860981505082,
3.41028005848366));
#250406=CARTESIAN_POINT('Ctrl Pts',(-0.190499999999408,-60.6863613750271,
3.41074404220247));
#250407=CARTESIAN_POINT('Ctrl Pts',(-0.19049999999936,-60.5986166446941,
3.30780486243807));
#250408=CARTESIAN_POINT('Ctrl Pts',(-0.317733982966898,-60.7713615025338,
3.36123028058439));
#250409=CARTESIAN_POINT('Ctrl Pts',(-0.190499999999476,-60.7712750141999,
3.36146460586369));
#250410=CARTESIAN_POINT('Ctrl Pts',(-0.190499999999358,-60.7265095085059,
3.23423045308392));
#250411=CARTESIAN_POINT('Ctrl Pts',(-0.317499999999357,-60.8610688070705,
3.36123028058439));
#250412=CARTESIAN_POINT('Ctrl Pts',(-0.190499999999357,-60.8610688070705,
3.36123028058439));
#250413=CARTESIAN_POINT('Ctrl Pts',(-0.190499999999357,-60.8610688070705,
3.23423028058439));
#250414=CARTESIAN_POINT('Origin',(-0.31749999999936,-60.5311086139133,3.42473028058439));
#250415=CARTESIAN_POINT('Origin',(-0.317500000300995,-60.4497583469871,
3.5656311352473));
#250416=CARTESIAN_POINT('Origin',(6.7363249086388,-61.0544000815102,3.56647653909427));
#250417=CARTESIAN_POINT('Origin',(6.74099917687956,-61.098378263717,3.64299466007584));
#250418=CARTESIAN_POINT('Origin',(6.72777047351185,-60.9730100652052,3.42473028058441));
#250419=CARTESIAN_POINT('Ctrl Pts',(6.71570789669471,-60.8636883187842,
3.48823028058441));
#250420=CARTESIAN_POINT('Ctrl Pts',(6.59002106156527,-60.8773920302458,
3.48794691941557));
#250421=CARTESIAN_POINT('Ctrl Pts',(6.60146619280008,-60.9862851800402,
3.42473028058442));
#250422=CARTESIAN_POINT('Ctrl Pts',(6.71111871849912,-60.8189169727306,
3.41028005925045));
#250423=CARTESIAN_POINT('Ctrl Pts',(6.58529244190302,-60.8324022194098,
3.40982512231001));
#250424=CARTESIAN_POINT('Ctrl Pts',(6.59440968471205,-60.9191469903165,
3.30780486372833));
#250425=CARTESIAN_POINT('Ctrl Pts',(6.70242508976298,-60.7340977611526,
3.36123028058439));
#250426=CARTESIAN_POINT('Ctrl Pts',(6.57634410736829,-60.7472645033911,
3.36099721048417));
#250427=CARTESIAN_POINT('Ctrl Pts',(6.58104124348299,-60.7919547682783,
3.23423045308359));
#250428=CARTESIAN_POINT('Ctrl Pts',(6.69328024897516,-60.6448574988552,
3.36123028058439));
#250429=CARTESIAN_POINT('Ctrl Pts',(6.56697596826339,-60.6581326136902,
3.36123028058439));
#250430=CARTESIAN_POINT('Ctrl Pts',(6.56697596826339,-60.6581326136902,
3.23423028058439));
#250431=CARTESIAN_POINT('Origin',(6.69328024897516,-60.6448574988552,3.23423028058439));
#250432=CARTESIAN_POINT('Origin',(0.315760701779432,0.033187787087667,3.64303198860263));
#250433=CARTESIAN_POINT('Origin',(6.78290064323623,-61.497538592386,3.64303198860219));
#250434=CARTESIAN_POINT('Origin',(0.315760701779432,0.0331877870876699,
3.23423028058481));
#250435=CARTESIAN_POINT('Origin',(6.67747469701007,-60.4944777170591,3.23423028058439));
#250436=CARTESIAN_POINT('Ctrl Pts',(6.83973663030323,-62.033045955223,3.47153072139027));
#250437=CARTESIAN_POINT('Ctrl Pts',(6.71274550335325,-62.0468640234017,
3.47182327902618));
#250438=CARTESIAN_POINT('Ctrl Pts',(6.7016119937089,-61.9391074687686,3.40413028959007));
#250439=CARTESIAN_POINT('Ctrl Pts',(6.827602051236,-61.9187065474463,3.6555380712091));
#250440=CARTESIAN_POINT('Ctrl Pts',(6.70071032544549,-61.9323544652987,
3.65586275496805));
#250441=CARTESIAN_POINT('Ctrl Pts',(6.69200045921809,-61.8476598278984,
3.55128126837131));
#250442=CARTESIAN_POINT('Ctrl Pts',(6.80580199871532,-61.7133000470643,
3.7700319886022));
#250443=CARTESIAN_POINT('Ctrl Pts',(6.67910652125957,-61.7268034525388,
3.77025505748433));
#250444=CARTESIAN_POINT('Ctrl Pts',(6.67473372829026,-61.6833778591529,
3.64284211731188));
#250445=CARTESIAN_POINT('Ctrl Pts',(6.78290064323623,-61.497538592386,3.7700319886022));
#250446=CARTESIAN_POINT('Ctrl Pts',(6.65640766978628,-61.5108335396269,
3.7700319886022));
#250447=CARTESIAN_POINT('Ctrl Pts',(6.65659650326314,-61.5108136924287,
3.64284239821701));
#250448=CARTESIAN_POINT('Origin',(6.82793297553411,-61.9259926140917,3.40423097483266));
#250449=CARTESIAN_POINT('Ctrl Pts',(6.67747469701007,-60.4944777170591,
3.36123028058439));
#250450=CARTESIAN_POINT('Ctrl Pts',(6.5511704162983,-60.5077528318941,3.36123028058439));
#250451=CARTESIAN_POINT('Ctrl Pts',(6.5511704162983,-60.5077528318941,3.23423028058439));
#250452=CARTESIAN_POINT('Ctrl Pts',(6.66829952659989,-60.4049357747548,
3.36123028058439));
#250453=CARTESIAN_POINT('Ctrl Pts',(6.54175270773107,-60.4181493202578,
3.36146538610129));
#250454=CARTESIAN_POINT('Ctrl Pts',(6.5370576023796,-60.373478376797,3.2342304368841));
#250455=CARTESIAN_POINT('Ctrl Pts',(6.65962554481757,-60.320266884728,3.41054258693058));
#250456=CARTESIAN_POINT('Ctrl Pts',(6.53289275205065,-60.3338524728728,
3.41100608859687));
#250457=CARTESIAN_POINT('Ctrl Pts',(6.52371293062606,-60.2465123062119,
3.30819866970745));
#250458=CARTESIAN_POINT('Ctrl Pts',(6.65505462397456,-60.2756459899116,
3.48823028058439));
#250459=CARTESIAN_POINT('Ctrl Pts',(6.52822907310839,-60.2894805317159,
3.48852004212217));
#250460=CARTESIAN_POINT('Ctrl Pts',(6.51668018436807,-60.1796001951993,
3.42473028058438));
#250461=CARTESIAN_POINT('Origin',(6.64298446507984,-60.1663250803643,3.42473028058439));
#250462=CARTESIAN_POINT('Origin',(6.84655462836866,-62.1031658061142,3.11913648178355));
#250463=CARTESIAN_POINT('Origin',(6.86517628122572,-62.2803389979217,2.83404198860218));
#250464=CARTESIAN_POINT('Origin',(6.63448104656917,-60.0854204576119,3.56563113460814));
#250465=CARTESIAN_POINT('Origin',(6.62985850077906,-60.0409538388293,3.64299171721731));
#250466=CARTESIAN_POINT('Ctrl Pts',(6.59568250079948,-62.6076796697352,
2.5990817351598));
#250467=CARTESIAN_POINT('Ctrl Pts',(6.59177408464837,-62.5705801176607,
2.65878198860218));
#250468=CARTESIAN_POINT('Ctrl Pts',(6.58439859103091,-62.5005702980928,
2.65878198860218));
#250469=CARTESIAN_POINT('Ctrl Pts',(6.68331293653995,-62.5984477290791,
2.59908193475685));
#250470=CARTESIAN_POINT('Ctrl Pts',(6.65560500345326,-62.5638523220913,
2.65878715325371));
#250471=CARTESIAN_POINT('Ctrl Pts',(6.63512154272684,-62.4952175264254,
2.65878198860218));
#250472=CARTESIAN_POINT('Ctrl Pts',(6.76155265492332,-62.5650504549415,
2.63878778849831));
#250473=CARTESIAN_POINT('Ctrl Pts',(6.71196843232464,-62.5346567608584,
2.69564460180095));
#250474=CARTESIAN_POINT('Ctrl Pts',(6.67930776339634,-62.4653998062673,
2.68180481624849));
#250475=CARTESIAN_POINT('Ctrl Pts',(6.86003002196326,-62.4816328770698,
2.754432388786));
#250476=CARTESIAN_POINT('Ctrl Pts',(6.76863258245117,-62.4676069047241,
2.79268340777016));
#250477=CARTESIAN_POINT('Ctrl Pts',(6.73311104631516,-62.3866783619493,
2.74885926835558));
#250478=CARTESIAN_POINT('Ctrl Pts',(6.88172985342223,-62.4326191774616,
2.82856655361629));
#250479=CARTESIAN_POINT('Ctrl Pts',(6.76853939445093,-62.4292062449167,
2.85384197230755));
#250480=CARTESIAN_POINT('Ctrl Pts',(6.74362530798327,-62.3388388123827,
2.79184624278459));
#250481=CARTESIAN_POINT('Ctrl Pts',(6.87697683366627,-62.3873926810689,
2.90134173515981));
#250482=CARTESIAN_POINT('Ctrl Pts',(6.75017837817664,-62.4011871104966,
2.90163218716348));
#250483=CARTESIAN_POINT('Ctrl Pts',(6.73887200051396,-62.2936141127567,
2.83404198860219));
#250484=CARTESIAN_POINT('Origin',(6.58439859103091,-62.5005702980928,2.53178198860218));
#250485=CARTESIAN_POINT('Origin',(0.315760701779432,0.033187787087667,3.64303198860263));
#250486=CARTESIAN_POINT('Origin',(6.58785426247156,-59.641796240314,3.64303198860221));
#250487=CARTESIAN_POINT('Origin',(5.64744126194171E-15,1.86046536471642E-13,
2.53178198860262));
#250488=CARTESIAN_POINT('Origin',(6.55408556366009,-62.5037563256532,2.53178198860218));
#250489=CARTESIAN_POINT('Ctrl Pts',(6.58785426247156,-59.641796240314,3.77003198860222));
#250490=CARTESIAN_POINT('Ctrl Pts',(6.46136077224366,-59.6550912418705,
3.77003198860221));
#250491=CARTESIAN_POINT('Ctrl Pts',(6.46155012326984,-59.6550713402757,
3.64284187936987));
#250492=CARTESIAN_POINT('Ctrl Pts',(6.56494565834935,-59.4260321009466,
3.77003198860222));
#250493=CARTESIAN_POINT('Ctrl Pts',(6.43870097938032,-59.4394927947704,
3.76980208962893));
#250494=CARTESIAN_POINT('Ctrl Pts',(6.44341257746724,-59.482504121664,3.64284193928254));
#250495=CARTESIAN_POINT('Ctrl Pts',(6.54313468201992,-59.2206282517274,
3.65553535416544));
#250496=CARTESIAN_POINT('Ctrl Pts',(6.41712387096409,-59.2341955513611,
3.65520057834401));
#250497=CARTESIAN_POINT('Ctrl Pts',(6.42614597501047,-59.3182233753705,
3.55127910964182));
#250498=CARTESIAN_POINT('Ctrl Pts',(6.53099325080115,-59.1062911958294,
3.47153072139032));
#250499=CARTESIAN_POINT('Ctrl Pts',(6.40512262640605,-59.1200087130387,
3.47122746281542));
#250500=CARTESIAN_POINT('Ctrl Pts',(6.41653455832087,-59.2267768553863,
3.40413045901223));
#250501=CARTESIAN_POINT('Origin',(6.54282188406287,-59.2133417798934,3.40423097483269));
#250502=CARTESIAN_POINT('Ctrl Pts',(6.24436990788122,-62.4538823482273,
2.90134173515981));
#250503=CARTESIAN_POINT('Ctrl Pts',(6.37126553604134,-62.4410124550016,
2.90163218716348));
#250504=CARTESIAN_POINT('Ctrl Pts',(6.35995915837864,-62.3334394572616,
2.83404198860219));
#250505=CARTESIAN_POINT('Ctrl Pts',(6.24912604340991,-62.4991292864729,
2.82853349835311));
#250506=CARTESIAN_POINT('Ctrl Pts',(6.3591243783167,-62.4722545055298,2.853814831623));
#250507=CARTESIAN_POINT('Ctrl Pts',(6.36471463173932,-62.3786847639674,
2.79182701594183));
#250508=CARTESIAN_POINT('Ctrl Pts',(6.28053011789794,-62.5423796567681,
2.75468822073602));
#250509=CARTESIAN_POINT('Ctrl Pts',(6.36708533499931,-62.5096946965654,
2.79286913083812));
#250510=CARTESIAN_POINT('Ctrl Pts',(6.38493060453764,-62.4231124872026,
2.74900763297871));
#250511=CARTESIAN_POINT('Ctrl Pts',(6.39322569848958,-62.6032845425343,
2.63954450640347));
#250512=CARTESIAN_POINT('Ctrl Pts',(6.4357600682454,-62.5632890101999,2.69627684028802));
#250513=CARTESIAN_POINT('Ctrl Pts',(6.45334792019265,-62.4886705126493,
2.68224356036447));
#250514=CARTESIAN_POINT('Ctrl Pts',(6.47739243510548,-62.6200908675648,
2.59908178706328));
#250515=CARTESIAN_POINT('Ctrl Pts',(6.49734694408407,-62.5804859237133,
2.65878704321479));
#250516=CARTESIAN_POINT('Ctrl Pts',(6.50319024212579,-62.509084087203,2.65878198860219));
#250517=CARTESIAN_POINT('Ctrl Pts',(6.56531752495365,-62.6108711573003,
2.5990817351598));
#250518=CARTESIAN_POINT('Ctrl Pts',(6.56142710223415,-62.5737697140399,
2.65878198860219));
#250519=CARTESIAN_POINT('Ctrl Pts',(6.55408556366009,-62.5037563256532,
2.65878198860219));
#250520=CARTESIAN_POINT('Origin',(6.23365487766687,-62.3467145720966,2.83404198860219));
#250521=CARTESIAN_POINT('Origin',(6.52420020557853,-59.0361683443313,3.11913648167029));
#250522=CARTESIAN_POINT('Origin',(6.50557852713814,-58.8589949086128,2.83404198860221));
#250523=CARTESIAN_POINT('Origin',(6.21503322485436,-62.1695413802703,3.11913648177471));
#250524=CARTESIAN_POINT('Origin',(6.19641157197526,-61.9923681882667,3.40423097483267));
#250525=CARTESIAN_POINT('Ctrl Pts',(6.493746461128,-58.7519447039086,2.90134173515983));
#250526=CARTESIAN_POINT('Ctrl Pts',(6.36806742857384,-58.7656442740268,
2.90103711553189));
#250527=CARTESIAN_POINT('Ctrl Pts',(6.37927424642637,-58.8722700234478,
2.83404198860221));
#250528=CARTESIAN_POINT('Ctrl Pts',(6.48899657309107,-58.7067576262544,
2.82862991747911));
#250529=CARTESIAN_POINT('Ctrl Pts',(6.38004220453002,-58.7342098038494,
2.853140458864));
#250530=CARTESIAN_POINT('Ctrl Pts',(6.37452469054107,-58.8270810177594,
2.7918796099985));
#250531=CARTESIAN_POINT('Ctrl Pts',(6.45774144355372,-58.6637560248471,
2.75470625793298));
#250532=CARTESIAN_POINT('Ctrl Pts',(6.37187117938199,-58.696789935432,2.79224250381849));
#250533=CARTESIAN_POINT('Ctrl Pts',(6.35435266912825,-58.7829167175849,
2.74901809108212));
#250534=CARTESIAN_POINT('Ctrl Pts',(6.34539908016383,-58.6035914159078,
2.63947868311645));
#250535=CARTESIAN_POINT('Ctrl Pts',(6.30313135363891,-58.6436439608621,
2.69595066767878));
#250536=CARTESIAN_POINT('Ctrl Pts',(6.28595874576574,-58.7181337176186,
2.68220539436026));
#250537=CARTESIAN_POINT('Ctrl Pts',(6.26151010025776,-58.5872698677163,
2.59908178584991));
#250538=CARTESIAN_POINT('Ctrl Pts',(6.2417055435759,-58.6268645946668,2.65877670944829));
#250539=CARTESIAN_POINT('Ctrl Pts',(6.23613328458309,-58.6982323944341,
2.65878198860221));
#250540=CARTESIAN_POINT('Ctrl Pts',(6.17403490859079,-58.5964866834548,
2.59908173515983));
#250541=CARTESIAN_POINT('Ctrl Pts',(6.17794390662231,-58.6335861742239,
2.65878198860221));
#250542=CARTESIAN_POINT('Ctrl Pts',(6.18532049829458,-58.7035958781036,
2.65878198860221));
#250543=CARTESIAN_POINT('Origin',(6.18532049829458,-58.7035958781036,2.53178198860221));
#250544=CARTESIAN_POINT('Ctrl Pts',(6.15137923967737,-61.5639141665609,
3.7700319886022));
#250545=CARTESIAN_POINT('Ctrl Pts',(6.2778722240253,-61.5506192181746,3.7700319886022));
#250546=CARTESIAN_POINT('Ctrl Pts',(6.27768337963421,-61.5506390665199,
3.64284238727536));
#250547=CARTESIAN_POINT('Ctrl Pts',(6.17383801205427,-61.7797255331383,
3.7700319886022));
#250548=CARTESIAN_POINT('Ctrl Pts',(6.30057242040001,-61.7665923920107,
3.77025506105787));
#250549=CARTESIAN_POINT('Ctrl Pts',(6.29582088597947,-61.7232059145518,
3.64284210641839));
#250550=CARTESIAN_POINT('Ctrl Pts',(6.19522058691298,-61.9851742714888,
3.65553527987788));
#250551=CARTESIAN_POINT('Ctrl Pts',(6.32217699854598,-61.9721416759939,
3.6558599653302));
#250552=CARTESIAN_POINT('Ctrl Pts',(6.31308747966748,-61.8874865820176,
3.55127902710128));
#250553=CARTESIAN_POINT('Ctrl Pts',(6.20712349654526,-62.0995362748656,
3.47153072139027));
#250554=CARTESIAN_POINT('Ctrl Pts',(6.33421251157784,-62.0866494440657,
3.47182327905144));
#250555=CARTESIAN_POINT('Ctrl Pts',(6.32269886789231,-61.9789328337394,
3.40413028377933));
#250556=CARTESIAN_POINT('Origin',(6.15137923967737,-61.5639141665609,3.6430319886022));
#250557=CARTESIAN_POINT('Origin',(5.67080826956262E-15,1.86266390934843E-13,
2.53178198860262));
#250558=CARTESIAN_POINT('Origin',(6.15500747092375,-58.706781905664,2.53178198860221));
#250559=CARTESIAN_POINT('Origin',(0.364094271196581,-6.50157577599598,3.64303198860258));
#250560=CARTESIAN_POINT('Origin',(6.10937495962149,-61.1647646440466,3.64299466007637));
#250561=CARTESIAN_POINT('Ctrl Pts',(6.14377718965381,-58.5996668978646,
2.59908173515983));
#250562=CARTESIAN_POINT('Ctrl Pts',(6.1476670304623,-58.636768402139,2.65878198860221));
#250563=CARTESIAN_POINT('Ctrl Pts',(6.15500747092375,-58.706781905664,2.65878198860221));
#250564=CARTESIAN_POINT('Ctrl Pts',(6.05659553606754,-58.6088074259624,
2.59908193199769));
#250565=CARTESIAN_POINT('Ctrl Pts',(6.08415140319859,-58.6434243604371,
2.65877685806616));
#250566=CARTESIAN_POINT('Ctrl Pts',(6.10436324506852,-58.7120821529669,
2.65878198860221));
#250567=CARTESIAN_POINT('Ctrl Pts',(5.97852000021575,-58.6416817365137,
2.63872492669757));
#250568=CARTESIAN_POINT('Ctrl Pts',(6.027858391313,-58.672182651071,2.69532212015236));
#250569=CARTESIAN_POINT('Ctrl Pts',(6.0600846870675,-58.7414038195493,2.68176836726596));
#250570=CARTESIAN_POINT('Ctrl Pts',(5.88025093392532,-58.7242744516461,
2.7544217640221));
#250571=CARTESIAN_POINT('Ctrl Pts',(5.97104363802227,-58.7387860695151,
2.79203179920094));
#250572=CARTESIAN_POINT('Ctrl Pts',(6.00614981441083,-58.8193360415242,
2.74885310748132));
#250573=CARTESIAN_POINT('Ctrl Pts',(5.85862682030309,-58.7730316211505,
2.82866089558359));
#250574=CARTESIAN_POINT('Ctrl Pts',(5.97091547255976,-58.7772266151811,
2.85316563119105));
#250575=CARTESIAN_POINT('Ctrl Pts',(5.99561386571486,-58.8669255556784,
2.79189751796562));
#250576=CARTESIAN_POINT('Ctrl Pts',(5.86337364149639,-58.8181995570482,
2.90134173515983));
#250577=CARTESIAN_POINT('Ctrl Pts',(5.98915458643853,-58.8054696185318,
2.90103711553189));
#250578=CARTESIAN_POINT('Ctrl Pts',(6.00036140429106,-58.9120953679528,
2.83404198860221));
#250579=CARTESIAN_POINT('Origin',(5.87405712357929,-58.9253704827878,2.83404198860221));
#250580=CARTESIAN_POINT('Origin',(6.10480350526334,-61.1207756545813,3.56647653971707));
#250581=CARTESIAN_POINT('Origin',(6.096249069953,-61.0393856393802,3.42473028058442));
#250582=CARTESIAN_POINT('Origin',(5.89267880207835,-59.102543918482,3.11913648168151));
#250583=CARTESIAN_POINT('Origin',(5.91130048050402,-59.2797173540683,3.40423097483269));
#250584=CARTESIAN_POINT('Ctrl Pts',(6.06175884541631,-60.7112330730301,
3.36123028058439));
#250585=CARTESIAN_POINT('Ctrl Pts',(6.18806312612808,-60.6979579581951,
3.36123028058439));
#250586=CARTESIAN_POINT('Ctrl Pts',(6.18806312612808,-60.6979579581951,
3.23423028058439));
#250587=CARTESIAN_POINT('Ctrl Pts',(6.07140041118294,-60.8007259828523,
3.36123028058439));
#250588=CARTESIAN_POINT('Ctrl Pts',(6.19746294737698,-60.7873912833617,
3.36099641108445));
#250589=CARTESIAN_POINT('Ctrl Pts',(6.20217593878228,-60.8322324012614,
3.23423043688341));
#250590=CARTESIAN_POINT('Ctrl Pts',(6.08051542067653,-60.8853484607267,
3.41054258905241));
#250591=CARTESIAN_POINT('Ctrl Pts',(6.20639551966795,-60.872379031649,3.41008815825926));
#250592=CARTESIAN_POINT('Ctrl Pts',(6.21552060714972,-60.9591984396299,
3.30819867304214));
#250593=CARTESIAN_POINT('Ctrl Pts',(6.08531878138382,-60.9299448846688,
3.48823028058441));
#250594=CARTESIAN_POINT('Ctrl Pts',(6.21110821942996,-60.9172173747508,
3.48794691941557));
#250595=CARTESIAN_POINT('Ctrl Pts',(6.22255335066477,-61.0261105245452,
3.42473028058442));
#250596=CARTESIAN_POINT('Origin',(6.06175884541631,-60.7112330730302,3.23423028058439));
#250597=CARTESIAN_POINT('Ctrl Pts',(5.90061356181316,-59.1725467709675,
3.47153072139031));
#250598=CARTESIAN_POINT('Ctrl Pts',(6.02658562874884,-59.159794554641,3.47122746285035));
#250599=CARTESIAN_POINT('Ctrl Pts',(6.03762143316813,-59.2666022171586,
3.40413046676737));
#250600=CARTESIAN_POINT('Ctrl Pts',(5.91250964036529,-59.2869113614503,
3.65553813457948));
#250601=CARTESIAN_POINT('Ctrl Pts',(6.03858760028519,-59.2739830624735,
3.65520336072233));
#250602=CARTESIAN_POINT('Ctrl Pts',(6.04723299508931,-59.358050121573,3.55128134519909));
#250603=CARTESIAN_POINT('Ctrl Pts',(5.93388131656964,-59.4923630227872,
3.77003198860222));
#250604=CARTESIAN_POINT('Ctrl Pts',(6.06016587018304,-59.4792818168401,
3.769802093141));
#250605=CARTESIAN_POINT('Ctrl Pts',(6.06449973388468,-59.5223321697741,
3.64284195387344));
#250606=CARTESIAN_POINT('Ctrl Pts',(5.95633285891271,-59.708171814489,3.77003198860222));
#250607=CARTESIAN_POINT('Ctrl Pts',(6.0828263345315,-59.694876814468,3.77003198860222));
#250608=CARTESIAN_POINT('Ctrl Pts',(6.08263699813626,-59.694896714525,3.64284189403743));
#250609=CARTESIAN_POINT('Origin',(5.95633285891271,-59.708171814489,3.64303198860222));
#250610=CARTESIAN_POINT('Origin',(0.347626240494121,-6.34489293004938,3.23423028058477));
#250611=CARTESIAN_POINT('Origin',(6.04595329345122,-60.5608532912341,3.23423028058439));
#250612=CARTESIAN_POINT('Origin',(0.345047419449927,-6.3203570867728,3.64303198860258));
#250613=CARTESIAN_POINT('Origin',(5.99823604520151,-60.1073400339994,3.64299171721718));
#250614=CARTESIAN_POINT('Ctrl Pts',(6.02238575970336,-60.3421421670673,
3.48823028058439));
#250615=CARTESIAN_POINT('Ctrl Pts',(6.14931623097308,-60.3293058762209,
3.48852004212217));
#250616=CARTESIAN_POINT('Ctrl Pts',(6.13776734223276,-60.2194255397043,
3.42473028058438));
#250617=CARTESIAN_POINT('Ctrl Pts',(6.02720817145293,-60.3868890390925,
3.41028005848367));
#250618=CARTESIAN_POINT('Ctrl Pts',(6.15399567477074,-60.3738278099493,
3.41074404220253));
#250619=CARTESIAN_POINT('Ctrl Pts',(6.14482385294855,-60.2865637544295,
3.30780486243826));
#250620=CARTESIAN_POINT('Ctrl Pts',(6.03634362557981,-60.4716618705779,
3.36123028058439));
#250621=CARTESIAN_POINT('Ctrl Pts',(6.16287156698331,-60.4582762833204,
3.36146460586393));
#250622=CARTESIAN_POINT('Ctrl Pts',(6.15819229746561,-60.4137560077508,
3.23423045308384));
#250623=CARTESIAN_POINT('Ctrl Pts',(6.04595329345122,-60.5608532912341,
3.36123028058439));
#250624=CARTESIAN_POINT('Ctrl Pts',(6.17225757416299,-60.5475781763991,
3.36123028058439));
#250625=CARTESIAN_POINT('Ctrl Pts',(6.17225757416299,-60.5475781763991,
3.23423028058439));
#250626=CARTESIAN_POINT('Origin',(6.01146306152099,-60.2327006545393,3.42473028058439));
#250627=CARTESIAN_POINT('Origin',(6.00295964283261,-60.1517960329186,3.56563113524724));
#250628=CARTESIAN_POINT('Origin',(13.0813452322063,-60.015799998865,3.56647653909396));
#250629=CARTESIAN_POINT('Origin',(13.0905908661208,-60.059048669912,3.64299466007403));
#250630=CARTESIAN_POINT('Origin',(13.0643300858388,-59.935750027543,3.42473028058442));
#250631=CARTESIAN_POINT('Ctrl Pts',(13.0409063549245,-59.8282880397052,
3.48823028058442));
#250632=CARTESIAN_POINT('Ctrl Pts',(12.9173404733289,-59.8550545325306,
3.48794691941558));
#250633=CARTESIAN_POINT('Ctrl Pts',(12.9401053405456,-59.9621548122768,
3.42473028058443));
#250634=CARTESIAN_POINT('Ctrl Pts',(13.0316624367257,-59.7842416555143,
3.41028005925046));
#250635=CARTESIAN_POINT('Ctrl Pts',(12.9079350417485,-59.8108054559342,
3.4098251223098));
#250636=CARTESIAN_POINT('Ctrl Pts',(12.9260696369487,-59.8961220185272,
3.30780486372835));
#250637=CARTESIAN_POINT('Ctrl Pts',(13.0141504107558,-59.700795824104,3.36123028058439));
#250638=CARTESIAN_POINT('Ctrl Pts',(12.8901364125068,-59.7270694888868,
3.36099721048401));
#250639=CARTESIAN_POINT('Ctrl Pts',(12.8994792219305,-59.7710239514086,
3.23423045308377));
#250640=CARTESIAN_POINT('Ctrl Pts',(12.995727518883,-59.6130003254552,3.3612302805844));
#250641=CARTESIAN_POINT('Ctrl Pts',(12.8715027735898,-59.639405110189,3.3612302805844));
#250642=CARTESIAN_POINT('Ctrl Pts',(12.8715027735898,-59.639405110189,3.2342302805844));
#250643=CARTESIAN_POINT('Origin',(12.995727518883,-59.6130003254552,3.2342302805844));
#250644=CARTESIAN_POINT('Origin',(0.310561863232988,0.0660119618348257,
3.64303198860263));
#250645=CARTESIAN_POINT('Origin',(13.1739864076113,-60.4516424606486,3.6430319886022));
#250646=CARTESIAN_POINT('Origin',(0.310561863232988,0.0660119618348286,
3.23423028058481));
#250647=CARTESIAN_POINT('Origin',(12.9642895838877,-59.4650964698963,3.2342302805844));
#250648=CARTESIAN_POINT('Ctrl Pts',(13.2864868029002,-60.9782752797345,
3.47153072139028));
#250649=CARTESIAN_POINT('Ctrl Pts',(13.1616357280628,-61.0052918384386,
3.47182327902619));
#250650=CARTESIAN_POINT('Ctrl Pts',(13.1392995818866,-60.8992893541402,
3.40413028958995));
#250651=CARTESIAN_POINT('Ctrl Pts',(13.2624669757416,-60.8658306440993,
3.65553807120913));
#250652=CARTESIAN_POINT('Ctrl Pts',(13.1376969719827,-60.8926675943312,
3.65586275496889));
#250653=CARTESIAN_POINT('Ctrl Pts',(13.1201818190183,-60.8093473519476,
3.5512812683716));
#250654=CARTESIAN_POINT('Ctrl Pts',(13.219315520358,-60.663828108008,3.77003198860221));
#250655=CARTESIAN_POINT('Ctrl Pts',(13.0947255842068,-60.6905008239732,
3.77025505748452));
#250656=CARTESIAN_POINT('Ctrl Pts',(13.0858375353127,-60.6477702018612,
3.64284211731198));
#250657=CARTESIAN_POINT('Ctrl Pts',(13.1739864076113,-60.4516424606486,
3.77003198860221));
#250658=CARTESIAN_POINT('Ctrl Pts',(13.0495760763092,-60.4780866929064,
3.77003198860221));
#250659=CARTESIAN_POINT('Ctrl Pts',(13.0497618007396,-60.47804721596,3.64284239821677));
#250660=CARTESIAN_POINT('Origin',(13.2635576885508,-60.873042205901,3.40423097483267));
#250661=CARTESIAN_POINT('Ctrl Pts',(12.9642895838877,-59.4650964698963,
3.3612302805844));
#250662=CARTESIAN_POINT('Ctrl Pts',(12.8400648385945,-59.4915012546302,
3.3612302805844));
#250663=CARTESIAN_POINT('Ctrl Pts',(12.8400648385945,-59.4915012546302,
3.2342302805844));
#250664=CARTESIAN_POINT('Ctrl Pts',(12.9458049943944,-59.3770041141839,
3.3612302805844));
#250665=CARTESIAN_POINT('Ctrl Pts',(12.8213326038456,-59.4033730190122,
3.3614653861013));
#250666=CARTESIAN_POINT('Ctrl Pts',(12.8119938336999,-59.3594375597997,
3.23423043688426));
#250667=CARTESIAN_POINT('Ctrl Pts',(12.9283282206303,-59.2937057271821,
3.41054258693058));
#250668=CARTESIAN_POINT('Ctrl Pts',(12.8037097640131,-59.3204640761242,
3.41100608859616));
#250669=CARTESIAN_POINT('Ctrl Pts',(12.7854506972086,-59.2345619206629,
3.30819866970701));
#250670=CARTESIAN_POINT('Ctrl Pts',(12.9191181862052,-59.2498070616276,
3.4882302805844));
#250671=CARTESIAN_POINT('Ctrl Pts',(12.7944335023715,-59.2768226962995,
3.48852004212218));
#250672=CARTESIAN_POINT('Ctrl Pts',(12.7714622569326,-59.1687514833557,
3.4247302805844));
#250673=CARTESIAN_POINT('Origin',(12.8956870022258,-59.1423466986219,3.4247302805844));
#250674=CARTESIAN_POINT('Origin',(13.3005969715165,-61.0472983318859,3.11913648178374));
#250675=CARTESIAN_POINT('Origin',(13.3376362544832,-61.2215544576536,2.8340419886022));
#250676=CARTESIAN_POINT('Origin',(12.878773330444,-59.0627741291263,3.56563113460749));
#250677=CARTESIAN_POINT('Origin',(12.8695280801147,-59.0190342907436,3.64299171721792));
#250678=CARTESIAN_POINT('Ctrl Pts',(13.1038352065734,-61.5752716937448,
2.5990817351598));
#250679=CARTESIAN_POINT('Ctrl Pts',(13.0960702419687,-61.5387839176324,
2.65878198860219));
#250680=CARTESIAN_POINT('Ctrl Pts',(13.0814171332239,-61.4699285681951,
2.65878198860219));
#250681=CARTESIAN_POINT('Ctrl Pts',(13.1900205930485,-61.556930451843,2.59908193475553));
#250682=CARTESIAN_POINT('Ctrl Pts',(13.15884824219,-61.5254208297822,2.65878715325412));
#250683=CARTESIAN_POINT('Ctrl Pts',(13.1313027022866,-61.4593031273778,
2.65878198860219));
#250684=CARTESIAN_POINT('Ctrl Pts',(13.264340740325,-61.5155378539377,2.63878778849826));
#250685=CARTESIAN_POINT('Ctrl Pts',(13.2118511391505,-61.4904936222812,
2.69564460180084));
#250686=CARTESIAN_POINT('Ctrl Pts',(13.1721300657497,-61.4250300340663,
2.68180481624848));
#250687=CARTESIAN_POINT('Ctrl Pts',(13.35355912682,-61.4222835584423,2.75443238878605));
#250688=CARTESIAN_POINT('Ctrl Pts',(13.2611962587093,-61.4178880557397,
2.79268340777032));
#250689=CARTESIAN_POINT('Ctrl Pts',(13.2174099770545,-61.3411158595751,
2.7488592683556));
#250690=CARTESIAN_POINT('Ctrl Pts',(13.3700167576327,-61.3712701109733,
2.82856655361625));
#250691=CARTESIAN_POINT('Ctrl Pts',(13.2570896192444,-61.3797074995629,
2.85384197230744));
#250692=CARTESIAN_POINT('Ctrl Pts',(13.2228660458972,-61.2924393404513,
2.79184624278419));
#250693=CARTESIAN_POINT('Ctrl Pts',(13.3605623192493,-61.326788195911,2.90134173515982));
#250694=CARTESIAN_POINT('Ctrl Pts',(13.2359003894758,-61.353761105708,2.90163218716349));
#250695=CARTESIAN_POINT('Ctrl Pts',(13.21341150919,-61.2479592423874,2.8340419886022));
#250696=CARTESIAN_POINT('Origin',(13.0814171332239,-61.4699285681951,2.53178198860219));
#250697=CARTESIAN_POINT('Origin',(0.310561863232988,0.0660119618348257,
3.64303198860263));
#250698=CARTESIAN_POINT('Origin',(12.7860306150458,-58.626453957798,3.64303198860222));
#250699=CARTESIAN_POINT('Origin',(5.63039444364742E-15,1.86043836520868E-13,
2.53178198860262));
#250700=CARTESIAN_POINT('Origin',(13.0516031943535,-61.4762657165312,2.53178198860219));
#250701=CARTESIAN_POINT('Ctrl Pts',(12.7860306150458,-58.626453957798,3.77003198860222));
#250702=CARTESIAN_POINT('Ctrl Pts',(12.6616197754744,-58.6528982980918,
3.77003198860222));
#250703=CARTESIAN_POINT('Ctrl Pts',(12.6618060089327,-58.6528587129482,
3.64284187936988));
#250704=CARTESIAN_POINT('Ctrl Pts',(12.7406940127384,-58.4142663981462,
3.77003198860222));
#250705=CARTESIAN_POINT('Ctrl Pts',(12.6165479409694,-58.4408495151693,
3.76980208962966));
#250706=CARTESIAN_POINT('Ctrl Pts',(12.6257296363319,-58.4831327254061,
3.64284193928274));
#250707=CARTESIAN_POINT('Ctrl Pts',(12.6975319705104,-58.212267640543,3.65553535416545));
#250708=CARTESIAN_POINT('Ctrl Pts',(12.5736296288425,-58.2389323335247,
3.65520057834348));
#250709=CARTESIAN_POINT('Ctrl Pts',(12.5913856081756,-58.3215567776507,
3.55127910964162));
#250710=CARTESIAN_POINT('Ctrl Pts',(12.6735055745747,-58.0998260601477,
3.47153072139032));
#250711=CARTESIAN_POINT('Ctrl Pts',(12.5497583536238,-58.126625494301,3.47122746281542));
#250712=CARTESIAN_POINT('Ctrl Pts',(12.5722680796271,-58.2316158778875,
3.40413045901224));
#250713=CARTESIAN_POINT('Origin',(12.6964592423899,-58.2050537810539,3.40423097483269));
#250714=CARTESIAN_POINT('Ctrl Pts',(12.7383709431257,-61.4590390555205,
2.90134173515981));
#250715=CARTESIAN_POINT('Ctrl Pts',(12.8632261535962,-61.4329754599095,
2.90163218716349));
#250716=CARTESIAN_POINT('Ctrl Pts',(12.8407372733105,-61.327173596589,2.8340419886022));
#250717=CARTESIAN_POINT('Ctrl Pts',(12.7478306169683,-61.5035409747664,
2.82853349835311));
#250718=CARTESIAN_POINT('Ctrl Pts',(12.8544171899349,-61.465315459776,2.85381483162333));
#250719=CARTESIAN_POINT('Ctrl Pts',(12.8501961180705,-61.3716739624481,
2.79182701594231));
#250720=CARTESIAN_POINT('Ctrl Pts',(12.7835835513937,-61.543271795361,2.75468822073602));
#250721=CARTESIAN_POINT('Ctrl Pts',(12.8662481012973,-61.5017184029583,
2.79286913083775));
#250722=CARTESIAN_POINT('Ctrl Pts',(12.874945307291,-61.4137451613971,2.74900763297864));
#250723=CARTESIAN_POINT('Ctrl Pts',(12.9020280679177,-61.5920631419341,
2.63954450640349));
#250724=CARTESIAN_POINT('Ctrl Pts',(12.9401487584132,-61.5478406570046,
2.69627684028829));
#250725=CARTESIAN_POINT('Ctrl Pts',(12.9498405053868,-61.4717924962539,
2.68224356036456));
#250726=CARTESIAN_POINT('Ctrl Pts',(12.9874904696728,-61.5999795805211,
2.599081787063));
#250727=CARTESIAN_POINT('Ctrl Pts',(13.0031958218449,-61.5585057825381,
2.65878704321566));
#250728=CARTESIAN_POINT('Ctrl Pts',(13.0015435854433,-61.4868843017927,
2.65878198860219));
#250729=CARTESIAN_POINT('Ctrl Pts',(13.0739701745332,-61.5816197022694,
2.59908173515981));
#250730=CARTESIAN_POINT('Ctrl Pts',(13.0662229071073,-61.5451281645056,
2.65878198860219));
#250731=CARTESIAN_POINT('Ctrl Pts',(13.0516031943535,-61.4762657165312,
2.65878198860219));
#250732=CARTESIAN_POINT('Origin',(12.7165125280173,-61.3535783813229,2.8340419886022));
#250733=CARTESIAN_POINT('Origin',(12.6594199084589,-58.0307974155454,3.11913648166996));
#250734=CARTESIAN_POINT('Origin',(12.6223805745526,-57.8565410498763,2.83404198860222));
#250735=CARTESIAN_POINT('Origin',(12.6794732450928,-61.179322255532,3.11913648177509));
#250736=CARTESIAN_POINT('Origin',(12.6424339620849,-61.0050661295703,3.40423097483267));
#250737=CARTESIAN_POINT('Ctrl Pts',(12.5994235324478,-57.7513140650717,
2.90134173515983));
#250738=CARTESIAN_POINT('Ctrl Pts',(12.4758649777959,-57.7780756236492,
2.90103711553189));
#250739=CARTESIAN_POINT('Ctrl Pts',(12.4981558292594,-57.8829458346102,
2.83404198860222));
#250740=CARTESIAN_POINT('Ctrl Pts',(12.5899763290081,-57.7068710254541,
2.82862991747923));
#250741=CARTESIAN_POINT('Ctrl Pts',(12.4844883578133,-57.7455616498585,
2.85314045886428));
#250742=CARTESIAN_POINT('Ctrl Pts',(12.488708754617,-57.8385008428011,2.79187960999885));
#250743=CARTESIAN_POINT('Ctrl Pts',(12.5543975270272,-57.6673720419783,
2.75470625793286));
#250744=CARTESIAN_POINT('Ctrl Pts',(12.4724506530564,-57.7092008760993,
2.79224250381865));
#250745=CARTESIAN_POINT('Ctrl Pts',(12.4640308112195,-57.7966870296826,
2.74901809108221));
#250746=CARTESIAN_POINT('Ctrl Pts',(12.4363816727429,-57.619279995667,2.63947868311658));
#250747=CARTESIAN_POINT('Ctrl Pts',(12.3985321242206,-57.6635313090884,
2.69595066767867));
#250748=CARTESIAN_POINT('Ctrl Pts',(12.3892398894931,-57.7394080294756,
2.68220539436019));
#250749=CARTESIAN_POINT('Ctrl Pts',(12.3512461790957,-57.611816644779,2.59908178585008));
#250750=CARTESIAN_POINT('Ctrl Pts',(12.3356888898096,-57.6532646075507,
2.65877670944881));
#250751=CARTESIAN_POINT('Ctrl Pts',(12.337607122671,-57.724823906712,2.65878198860222));
#250752=CARTESIAN_POINT('Ctrl Pts',(12.2652136052667,-57.6301266171954,
2.59908173515984));
#250753=CARTESIAN_POINT('Ctrl Pts',(12.2729791421561,-57.6666142715152,
2.65878198860222));
#250754=CARTESIAN_POINT('Ctrl Pts',(12.2876333308477,-57.7354693911201,
2.65878198860222));
#250755=CARTESIAN_POINT('Origin',(12.2876333308477,-57.7354693911201,2.53178198860222));
#250756=CARTESIAN_POINT('Ctrl Pts',(12.5528626811454,-60.5836663843179,
3.77003198860221));
#250757=CARTESIAN_POINT('Ctrl Pts',(12.6772730231654,-60.5572221497819,
3.77003198860221));
#250758=CARTESIAN_POINT('Ctrl Pts',(12.6770872880011,-60.5572616290098,
3.64284238727576));
#250759=CARTESIAN_POINT('Ctrl Pts',(12.5977568525211,-60.795947932685,3.77003198860221));
#250760=CARTESIAN_POINT('Ctrl Pts',(12.7224242094588,-60.7696393833344,
3.77025506105822));
#250761=CARTESIAN_POINT('Ctrl Pts',(12.7131635826249,-60.7269872521279,
3.64284210641902));
#250762=CARTESIAN_POINT('Ctrl Pts',(12.6404975322993,-60.9980361136593,
3.65553527987791));
#250763=CARTESIAN_POINT('Ctrl Pts',(12.7653961862437,-60.971804353472,3.65585996532863));
#250764=CARTESIAN_POINT('Ctrl Pts',(12.7475075938202,-60.8885631224013,
3.55127902710092));
#250765=CARTESIAN_POINT('Ctrl Pts',(12.6642893210148,-61.1105274371638,
3.47153072139028));
#250766=CARTESIAN_POINT('Ctrl Pts',(12.7893350885052,-61.0844267823319,
3.47182327905145));
#250767=CARTESIAN_POINT('Ctrl Pts',(12.7666250660191,-60.9785037583489,
3.40413028377955));
#250768=CARTESIAN_POINT('Origin',(12.5528626811454,-60.5836663843179,3.64303198860221));
#250769=CARTESIAN_POINT('Origin',(5.67687244506386E-15,1.86267351405886E-13,
2.53178198860262));
#250770=CARTESIAN_POINT('Origin',(12.2578193919774,-57.7418065394563,2.53178198860222));
#250771=CARTESIAN_POINT('Origin',(2.3791451040456,-12.7200883457667,3.64303198860254));
#250772=CARTESIAN_POINT('Origin',(12.4693660187269,-60.1910940874967,3.64299466007605));
#250773=CARTESIAN_POINT('Ctrl Pts',(12.2354540642051,-57.6364522029204,
2.59908173515984));
#250774=CARTESIAN_POINT('Ctrl Pts',(12.2432007592853,-57.6729438621903,
2.65878198860222));
#250775=CARTESIAN_POINT('Ctrl Pts',(12.2578193919774,-57.7418065394563,
2.65878198860222));
#250776=CARTESIAN_POINT('Ctrl Pts',(12.1497054461947,-57.6546556225238,
2.59908193199844));
#250777=CARTESIAN_POINT('Ctrl Pts',(12.1807288143665,-57.6862025493664,
2.65877685806609));
#250778=CARTESIAN_POINT('Ctrl Pts',(12.208006627196,-57.7523715145525,2.65878198860222));
#250779=CARTESIAN_POINT('Ctrl Pts',(12.0754939174604,-57.6955109599431,
2.63872492669758));
#250780=CARTESIAN_POINT('Ctrl Pts',(12.1277502414159,-57.720687521098,2.69532212015226));
#250781=CARTESIAN_POINT('Ctrl Pts',(12.1670355805169,-57.7861609236004,
2.68176836726595));
#250782=CARTESIAN_POINT('Ctrl Pts',(11.9863964689869,-57.7879231380264,
2.7544217640221));
#250783=CARTESIAN_POINT('Ctrl Pts',(12.0782086782663,-57.7928648378988,
2.7920317992011));
#250784=CARTESIAN_POINT('Ctrl Pts',(12.1215423041379,-57.8693039540642,
2.74885310748135));
#250785=CARTESIAN_POINT('Ctrl Pts',(11.9699873265234,-57.8386735460211,
2.82866089558358));
#250786=CARTESIAN_POINT('Ctrl Pts',(12.0820993460737,-57.8311081991714,
2.85316563119168));
#250787=CARTESIAN_POINT('Ctrl Pts',(12.1160385312535,-57.9177340744066,
2.79189751796608));
#250788=CARTESIAN_POINT('Ctrl Pts',(11.9794294790618,-57.8830978693153,
2.90134173515983));
#250789=CARTESIAN_POINT('Ctrl Pts',(12.1031907419163,-57.8572899778508,
2.90103711553189));
#250790=CARTESIAN_POINT('Ctrl Pts',(12.1254815933798,-57.9621601888118,
2.83404198860222));
#250791=CARTESIAN_POINT('Origin',(12.0012568480866,-57.9885649735456,2.83404198860222));
#250792=CARTESIAN_POINT('Origin',(12.4602215058074,-60.1478239214154,3.56647653971778));
#250793=CARTESIAN_POINT('Origin',(12.4432063593729,-60.0677739512123,3.42473028058443));
#250794=CARTESIAN_POINT('Origin',(12.038296182044,-58.1628213391881,3.11913648167957));
#250795=CARTESIAN_POINT('Origin',(12.0753355159239,-58.3370777047231,3.40423097483269));
#250796=CARTESIAN_POINT('Ctrl Pts',(12.3746037924171,-59.7450242491244,
3.3612302805844));
#250797=CARTESIAN_POINT('Ctrl Pts',(12.4988285377103,-59.7186194643906,
3.3612302805844));
#250798=CARTESIAN_POINT('Ctrl Pts',(12.4988285377102,-59.7186194643906,
3.2342302805844));
#250799=CARTESIAN_POINT('Ctrl Pts',(12.3935470970153,-59.8330190893696,
3.3612302805844));
#250800=CARTESIAN_POINT('Ctrl Pts',(12.5175251937999,-59.8065803155745,
3.36099641108498));
#250801=CARTESIAN_POINT('Ctrl Pts',(12.5268995400903,-59.8506831473911,
3.2342304368836));
#250802=CARTESIAN_POINT('Ctrl Pts',(12.411457631102,-59.9162252185213,3.41054258905242));
#250803=CARTESIAN_POINT('Ctrl Pts',(12.5352924712508,-59.8901687840285,
3.41008815825911));
#250804=CARTESIAN_POINT('Ctrl Pts',(12.5534426698451,-59.9755587548351,
3.30819867304268));
#250805=CARTESIAN_POINT('Ctrl Pts',(12.4208962741593,-59.9600752506734,
3.48823028058442));
#250806=CARTESIAN_POINT('Ctrl Pts',(12.5446662374493,-59.9342688867322,
3.48794691941558));
#250807=CARTESIAN_POINT('Ctrl Pts',(12.5674311046661,-60.0413691664784,
3.42473028058443));
#250808=CARTESIAN_POINT('Origin',(12.3746037924171,-59.7450242491244,3.2342302805844));
#250809=CARTESIAN_POINT('Ctrl Pts',(12.0535047649328,-58.2316113004778,
3.47153072139032));
#250810=CARTESIAN_POINT('Ctrl Pts',(12.1774537741291,-58.2057612755552,
3.47122746285037));
#250811=CARTESIAN_POINT('Ctrl Pts',(12.1995935640854,-58.310830278845,3.40413046676749));
#250812=CARTESIAN_POINT('Ctrl Pts',(12.0772900304182,-58.3441059109576,
3.65553813457945));
#250813=CARTESIAN_POINT('Ctrl Pts',(12.201325946859,-58.3180696991554,3.65520336072166));
#250814=CARTESIAN_POINT('Ctrl Pts',(12.2187113817825,-58.4007725402752,
3.5512813451987));
#250815=CARTESIAN_POINT('Ctrl Pts',(12.120020176778,-58.5461981381262,3.77003198860223));
#250816=CARTESIAN_POINT('Ctrl Pts',(12.2442455720369,-58.5199882620684,
3.76980209314081));
#250817=CARTESIAN_POINT('Ctrl Pts',(12.2530556816164,-58.5623497685522,
3.64284195387377));
#250818=CARTESIAN_POINT('Ctrl Pts',(12.1649068885798,-58.7584778814673,
3.77003198860222));
#250819=CARTESIAN_POINT('Ctrl Pts',(12.2893177137824,-58.7320335442277,
3.77003198860222));
#250820=CARTESIAN_POINT('Ctrl Pts',(12.2891314947143,-58.7320731263126,
3.64284189403764));
#250821=CARTESIAN_POINT('Origin',(12.1649068885798,-58.7584778814673,3.64303198860222));
#250822=CARTESIAN_POINT('Origin',(2.31399271319982,-12.413570446089,3.23423028058473));
#250823=CARTESIAN_POINT('Origin',(12.3431658574217,-59.5971203935656,3.2342302805844));
#250824=CARTESIAN_POINT('Origin',(2.30379013587727,-12.3655710936231,3.64303198860254));
#250825=CARTESIAN_POINT('Origin',(12.2483049654011,-59.1510793400371,3.64299171721781));
#250826=CARTESIAN_POINT('Ctrl Pts',(12.296865891381,-59.3820708699068,3.4882302805844));
#250827=CARTESIAN_POINT('Ctrl Pts',(12.4217592664919,-59.3560370505011,
3.48852004212218));
#250828=CARTESIAN_POINT('Ctrl Pts',(12.398788021053,-59.2479658375573,3.4247302805844));
#250829=CARTESIAN_POINT('Ctrl Pts',(12.3063392072239,-59.4260685345956,
3.41028005848365));
#250830=CARTESIAN_POINT('Ctrl Pts',(12.4310668851223,-59.3998259533497,
3.41074404220255));
#250831=CARTESIAN_POINT('Ctrl Pts',(12.4128237298763,-59.3139986558953,
3.30780486243784));
#250832=CARTESIAN_POINT('Ctrl Pts',(12.3242857901785,-59.5094220566591,
3.36123028058439));
#250833=CARTESIAN_POINT('Ctrl Pts',(12.4487214234139,-59.4828840257732,
3.36146460586428));
#250834=CARTESIAN_POINT('Ctrl Pts',(12.4394141514352,-59.4390967537847,
3.23423045308405));
#250835=CARTESIAN_POINT('Ctrl Pts',(12.3431658574217,-59.5971203935656,
3.3612302805844));
#250836=CARTESIAN_POINT('Ctrl Pts',(12.4673906027149,-59.5707156088318,
3.3612302805844));
#250837=CARTESIAN_POINT('Ctrl Pts',(12.4673906027149,-59.5707156088318,
3.2342302805844));
#250838=CARTESIAN_POINT('Origin',(12.2745632757598,-59.2743706222912,3.4247302805844));
#250839=CARTESIAN_POINT('Origin',(12.2576496039196,-59.194798053941,3.56563113524728));
#250840=CARTESIAN_POINT('Origin',(19.2830435999592,-58.3196542523186,3.56647653909411));
#250841=CARTESIAN_POINT('Origin',(19.2967593024467,-58.3616995707152,3.64299466007486));
#250842=CARTESIAN_POINT('Origin',(19.2577541638585,-58.241821370217,3.42473028058443));
#250843=CARTESIAN_POINT('Ctrl Pts',(19.2232259141446,-58.137396516989,3.48823028058443));
#250844=CARTESIAN_POINT('Ctrl Pts',(19.1031347997394,-58.1769325318816,
3.48794691941559));
#250845=CARTESIAN_POINT('Ctrl Pts',(19.136969986289,-58.2810665285026,3.42473028058444));
#250846=CARTESIAN_POINT('Ctrl Pts',(19.2094285342441,-58.0945576760634,
3.41028005925047));
#250847=CARTESIAN_POINT('Ctrl Pts',(19.0891556041198,-58.1339089916623,
3.40982512230991));
#250848=CARTESIAN_POINT('Ctrl Pts',(19.116108865289,-58.2168625998338,3.30780486372806));
#250849=CARTESIAN_POINT('Ctrl Pts',(19.1832899764622,-58.0133994748118,
3.36123028058441));
#250850=CARTESIAN_POINT('Ctrl Pts',(19.0627016856762,-58.0524922023731,
3.36099721048509));
#250851=CARTESIAN_POINT('Ctrl Pts',(19.0765878066329,-58.0952292882361,
3.2342304530843));
#250852=CARTESIAN_POINT('Ctrl Pts',(19.1557908785631,-57.9280106456672,
3.36123028058441));
#250853=CARTESIAN_POINT('Ctrl Pts',(19.0350067009936,-57.9672558039528,
3.36123028058441));
#250854=CARTESIAN_POINT('Ctrl Pts',(19.0350067009936,-57.9672558039528,
3.23423028058441));
#250855=CARTESIAN_POINT('Origin',(19.1557908785631,-57.9280106456672,3.23423028058441));
#250856=CARTESIAN_POINT('Origin',(0.301960443923716,0.0981128957142328,
3.64303198860263));
#250857=CARTESIAN_POINT('Origin',(19.4207352200707,-58.7434254837928,3.64303198860222));
#250858=CARTESIAN_POINT('Origin',(0.301960443923716,0.0981128957142356,
3.23423028058481));
#250859=CARTESIAN_POINT('Origin',(19.1090650011322,-57.7842031819379,3.23423028058441));
#250860=CARTESIAN_POINT('Ctrl Pts',(19.5876674457085,-59.2554138597567,
3.4715307213903));
#250861=CARTESIAN_POINT('Ctrl Pts',(19.4663243174868,-59.2953329099155,
3.47182327902621));
#250862=CARTESIAN_POINT('Ctrl Pts',(19.4330302542699,-59.1922458813528,
3.40413028959015));
#250863=CARTESIAN_POINT('Ctrl Pts',(19.5520255367122,-59.1460959632211,
3.65553807120917));
#250864=CARTESIAN_POINT('Ctrl Pts',(19.4307442612537,-59.1858279145837,
3.65586275496688));
#250865=CARTESIAN_POINT('Ctrl Pts',(19.4046157212338,-59.1047949412303,
3.55128126837138));
#250866=CARTESIAN_POINT('Ctrl Pts',(19.4879954548421,-58.9497105734776,
3.77003198860222));
#250867=CARTESIAN_POINT('Ctrl Pts',(19.366876093408,-58.989260368081,3.77025505748598));
#250868=CARTESIAN_POINT('Ctrl Pts',(19.3535701679114,-58.9476928828799,
3.64284211731211));
#250869=CARTESIAN_POINT('Ctrl Pts',(19.4207352200707,-58.7434254837929,
3.77003198860222));
#250870=CARTESIAN_POINT('Ctrl Pts',(19.2997705965413,-58.782729272525,3.77003198860222));
#250871=CARTESIAN_POINT('Ctrl Pts',(19.299951177089,-58.7826705983483,3.64284239821712));
#250872=CARTESIAN_POINT('Origin',(19.5538640879539,-59.1531540087995,3.40423097483269));
#250873=CARTESIAN_POINT('Ctrl Pts',(19.1090650011322,-57.7842031819379,
3.36123028058441));
#250874=CARTESIAN_POINT('Ctrl Pts',(18.9882808235627,-57.8234483402235,
3.36123028058441));
#250875=CARTESIAN_POINT('Ctrl Pts',(18.9882808235627,-57.8234483402235,
3.23423028058441));
#250876=CARTESIAN_POINT('Ctrl Pts',(19.0814735135864,-57.6985255711011,
3.36123028058441));
#250877=CARTESIAN_POINT('Ctrl Pts',(18.960439296918,-57.7377609320114,3.36146538610076));
#250878=CARTESIAN_POINT('Ctrl Pts',(18.9465591794957,-57.6950423231348,
3.234230436884));
#250879=CARTESIAN_POINT('Ctrl Pts',(19.0553854270324,-57.617510321683,3.41054258693058));
#250880=CARTESIAN_POINT('Ctrl Pts',(18.9342466524541,-57.6571482613564,
3.41100608859694));
#250881=CARTESIAN_POINT('Ctrl Pts',(18.9071083904254,-57.5736252790843,
3.30819866970748));
#250882=CARTESIAN_POINT('Ctrl Pts',(19.0416371860884,-57.5748148483572,
3.4882302805844));
#250883=CARTESIAN_POINT('Ctrl Pts',(18.9204594407751,-57.6147155869498,
3.48852004212217));
#250884=CARTESIAN_POINT('Ctrl Pts',(18.8863175164099,-57.5096375484033,
3.42473028058439));
#250885=CARTESIAN_POINT('Origin',(19.0071016939793,-57.4703923901177,3.42473028058439));
#250886=CARTESIAN_POINT('Origin',(19.6089151909164,-59.3225838821625,3.11913648178257));
#250887=CARTESIAN_POINT('Origin',(19.6639662938568,-59.4920137553135,2.83404198860221));
#250888=CARTESIAN_POINT('Origin',(18.9819630786536,-57.3930236876037,3.56563113460773));
#250889=CARTESIAN_POINT('Origin',(18.9681964166838,-57.3504898524406,3.6429917172174));
#250890=CARTESIAN_POINT('Ctrl Pts',(19.4684195516703,-59.8682321556238,
2.59908173515982));
#250891=CARTESIAN_POINT('Ctrl Pts',(19.456883113189,-59.8327559231842,2.6587819886022));
#250892=CARTESIAN_POINT('Ctrl Pts',(19.4351129318427,-59.7658094374947,
2.6587819886022));
#250893=CARTESIAN_POINT('Ctrl Pts',(19.5522156237501,-59.8409825629596,
2.59908193475582));
#250894=CARTESIAN_POINT('Ctrl Pts',(19.5179203859187,-59.8129039518359,
2.6587871532548));
#250895=CARTESIAN_POINT('Ctrl Pts',(19.4836145615382,-59.7500277420804,
2.6587819886022));
#250896=CARTESIAN_POINT('Ctrl Pts',(19.6218019328337,-59.792048147252,2.63878778849858));
#250897=CARTESIAN_POINT('Ctrl Pts',(19.5669820401377,-59.7726277678648,
2.69564460180074));
#250898=CARTESIAN_POINT('Ctrl Pts',(19.5206357546569,-59.7116747787975,
2.68180481624849));
#250899=CARTESIAN_POINT('Ctrl Pts',(19.7007838434716,-59.6899788477095,
2.75443238878576));
#250900=CARTESIAN_POINT('Ctrl Pts',(19.6084674936738,-59.6952619726976,
2.79268340777048));
#250901=CARTESIAN_POINT('Ctrl Pts',(19.5568961981644,-59.6234872553901,
2.74885926835562));
#250902=CARTESIAN_POINT('Ctrl Pts',(19.7118189603907,-59.6375245663852,
2.82856655361648));
#250903=CARTESIAN_POINT('Ctrl Pts',(19.6003923959456,-59.6577198343142,
2.85384197230767));
#250904=CARTESIAN_POINT('Ctrl Pts',(19.5572342963498,-59.5745070768389,
2.79184624278477));
#250905=CARTESIAN_POINT('Ctrl Pts',(19.6977666881852,-59.5942745858232,
2.90134173515983));
#250906=CARTESIAN_POINT('Ctrl Pts',(19.5766071063175,-59.6341304551453,
2.9016321871635));
#250907=CARTESIAN_POINT('Ctrl Pts',(19.5431821162873,-59.5312589135992,
2.83404198860221));
#250908=CARTESIAN_POINT('Origin',(19.4351129318427,-59.7658094374947,2.5317819886022));
#250909=CARTESIAN_POINT('Origin',(0.301960443923716,0.0981128957142328,
3.64303198860263));
#250910=CARTESIAN_POINT('Origin',(18.8441205405526,-56.9687879773462,3.64303198860223));
#250911=CARTESIAN_POINT('Origin',(5.61372323131277E-15,1.86039369482986E-13,
2.53178198860262));
#250912=CARTESIAN_POINT('Origin',(19.406124729226,-59.7752282754833,2.5317819886022));
#250913=CARTESIAN_POINT('Ctrl Pts',(18.8441205405526,-56.9687879773462,
3.77003198860223));
#250914=CARTESIAN_POINT('Ctrl Pts',(18.7231554228308,-57.0080919266512,
3.77003198860223));
#250915=CARTESIAN_POINT('Ctrl Pts',(18.7233364983084,-57.008033091662,3.64284187936999));
#250916=CARTESIAN_POINT('Ctrl Pts',(18.7768526573602,-56.7625017687171,
3.77003198860224));
#250917=CARTESIAN_POINT('Ctrl Pts',(18.6561653631336,-56.8019160587494,
3.7698020896296));
#250918=CARTESIAN_POINT('Ctrl Pts',(18.6697165591971,-56.8430078886266,
3.64284193928345));
#250919=CARTESIAN_POINT('Ctrl Pts',(18.7128124416033,-56.5661212433884,
3.65553535416544));
#250920=CARTESIAN_POINT('Ctrl Pts',(18.5923760693075,-56.6055911857578,
3.6552005783447));
#250921=CARTESIAN_POINT('Ctrl Pts',(18.6186713857005,-56.6859069993044,
3.55127910964129));
#250922=CARTESIAN_POINT('Ctrl Pts',(18.6771643191716,-56.4568070719807,
3.47153072139033));
#250923=CARTESIAN_POINT('Ctrl Pts',(18.5568963021136,-56.4963948028693,
3.47122746281543));
#250924=CARTESIAN_POINT('Ctrl Pts',(18.5902572009366,-56.5984571310815,
3.4041304590123));
#250925=CARTESIAN_POINT('Origin',(18.7109915363523,-56.5590590327986,3.40423097483271));
#250926=CARTESIAN_POINT('Ctrl Pts',(19.0928077206418,-59.7908376697907,
2.90134173515982));
#250927=CARTESIAN_POINT('Ctrl Pts',(19.214254573609,-59.7518659300022,2.9016321871635));
#250928=CARTESIAN_POINT('Ctrl Pts',(19.1808295835788,-59.648994388456,2.83404198860221));
#250929=CARTESIAN_POINT('Ctrl Pts',(19.1068672906319,-59.834106997697,2.82853349835317));
#250930=CARTESIAN_POINT('Ctrl Pts',(19.2088743168603,-59.7849495553994,
2.85381483162279));
#250931=CARTESIAN_POINT('Ctrl Pts',(19.1948881666555,-59.6922622581471,
2.79182701594138));
#250932=CARTESIAN_POINT('Ctrl Pts',(19.1465773683633,-59.8698829694065,
2.75468822073595));
#250933=CARTESIAN_POINT('Ctrl Pts',(19.224445560962,-59.8199164124669,2.79286913083809));
#250934=CARTESIAN_POINT('Ctrl Pts',(19.223899415002,-59.7315159919503,2.74900763297869));
#250935=CARTESIAN_POINT('Ctrl Pts',(19.2694731179109,-59.9060262085831,
2.63954450640357));
#250936=CARTESIAN_POINT('Ctrl Pts',(19.3027624708834,-59.8580612818569,
2.6962768402881));
#250937=CARTESIAN_POINT('Ctrl Pts',(19.3044519280757,-59.7814166574705,
2.68224356036452));
#250938=CARTESIAN_POINT('Ctrl Pts',(19.355294840847,-59.9049660265686,2.59908178706304));
#250939=CARTESIAN_POINT('Ctrl Pts',(19.3665789650884,-59.8620777700647,
2.65878704321362));
#250940=CARTESIAN_POINT('Ctrl Pts',(19.3574492964907,-59.791021345015,2.65878198860221));
#250941=CARTESIAN_POINT('Ctrl Pts',(19.4393816709763,-59.8776671349981,
2.59908173515982));
#250942=CARTESIAN_POINT('Ctrl Pts',(19.4278624395273,-59.8421853116549,
2.65878198860221));
#250943=CARTESIAN_POINT('Ctrl Pts',(19.406124729226,-59.7752282754833,2.65878198860221));
#250944=CARTESIAN_POINT('Origin',(19.0600454060093,-59.6882395467416,2.83404198860221));
#250945=CARTESIAN_POINT('Origin',(18.6559403576674,-56.3896289265479,3.11913648167074));
#250946=CARTESIAN_POINT('Origin',(18.6008891789892,-56.2201988201379,2.83404198860223));
#250947=CARTESIAN_POINT('Origin',(19.0049943031093,-59.5188096735662,3.11913648177587));
#250948=CARTESIAN_POINT('Origin',(18.9499432001064,-59.3493798002276,3.40423097483269));
#250949=CARTESIAN_POINT('Ctrl Pts',(18.5670586829472,-56.1179479440984,
2.90134173515985));
#250950=CARTESIAN_POINT('Ctrl Pts',(18.4469743395785,-56.1574782858993,
2.90103711553191));
#250951=CARTESIAN_POINT('Ctrl Pts',(18.4801050014197,-56.2594439784235,
2.83404198860223));
#250952=CARTESIAN_POINT('Ctrl Pts',(18.553017669642,-56.0747358697598,2.82862991747918));
#250953=CARTESIAN_POINT('Ctrl Pts',(18.4521518441045,-56.124241038398,2.85314045886448));
#250954=CARTESIAN_POINT('Ctrl Pts',(18.4660639121469,-56.2162299491246,
2.79187960999894));
#250955=CARTESIAN_POINT('Ctrl Pts',(18.513505004018,-56.0391722633443,2.7547062579329));
#250956=CARTESIAN_POINT('Ctrl Pts',(18.4363793473478,-56.0893377355405,
2.79224250381869));
#250957=CARTESIAN_POINT('Ctrl Pts',(18.4371504234768,-56.1772247439493,
2.74901809108223));
#250958=CARTESIAN_POINT('Ctrl Pts',(18.3911086652352,-56.0036796861842,
2.63947868311657));
#250959=CARTESIAN_POINT('Ctrl Pts',(18.3580919822896,-56.0516449414235,
2.69595066767864));
#250960=CARTESIAN_POINT('Ctrl Pts',(18.356781928376,-56.1280773042132,2.6822053943602));
#250961=CARTESIAN_POINT('Ctrl Pts',(18.305659420131,-56.0051563026337,2.59908178585011));
#250962=CARTESIAN_POINT('Ctrl Pts',(18.2945198471568,-56.048003388668,2.658776709449));
#250963=CARTESIAN_POINT('Ctrl Pts',(18.3039075553122,-56.1189701685695,
2.65878198860223));
#250964=CARTESIAN_POINT('Ctrl Pts',(18.2220120550223,-56.0323588238387,
2.59908173515985));
#250965=CARTESIAN_POINT('Ctrl Pts',(18.2335490499224,-56.0678348753329,
2.65878198860223));
#250966=CARTESIAN_POINT('Ctrl Pts',(18.2553202812755,-56.1347810195638,
2.65878198860223));
#250967=CARTESIAN_POINT('Origin',(18.2553202812755,-56.1347810195638,2.53178198860223));
#250968=CARTESIAN_POINT('Ctrl Pts',(18.8168143322233,-58.9396512752209,
3.77003198860222));
#250969=CARTESIAN_POINT('Ctrl Pts',(18.9377789661745,-58.9003474831026,
3.77003198860222));
#250970=CARTESIAN_POINT('Ctrl Pts',(18.9375983751895,-58.9004061606706,
3.64284238727543));
#250971=CARTESIAN_POINT('Ctrl Pts',(18.8836520326624,-59.146077204311,3.77003198860222));
#250972=CARTESIAN_POINT('Ctrl Pts',(19.0048864565391,-59.1068814887043,
3.77025506105808));
#250973=CARTESIAN_POINT('Ctrl Pts',(18.9912181986578,-59.0654310094276,
3.6428421064193));
#250974=CARTESIAN_POINT('Ctrl Pts',(18.9472825415249,-59.3425907075094,
3.6555352798779));
#250975=CARTESIAN_POINT('Ctrl Pts',(19.0687550219954,-59.3034471832903,
3.65585996532954));
#250976=CARTESIAN_POINT('Ctrl Pts',(19.0422633471882,-59.2225318234682,
3.55127902710076));
#250977=CARTESIAN_POINT('Ctrl Pts',(18.9827025415103,-59.4519788726604,
3.47153072139031));
#250978=CARTESIAN_POINT('Ctrl Pts',(19.1043350338631,-59.4129503580326,
3.47182327905148));
#250979=CARTESIAN_POINT('Ctrl Pts',(19.0706774483344,-59.3099814352089,
3.4041302837794));
#250980=CARTESIAN_POINT('Origin',(18.8168143322233,-58.9396512752209,3.64303198860222));
#250981=CARTESIAN_POINT('Origin',(5.68280300381509E-15,1.86268940494314E-13,
2.53178198860262));
#250982=CARTESIAN_POINT('Origin',(18.2263320786588,-56.1441998575524,2.53178198860223));
#250983=CARTESIAN_POINT('Origin',(5.63975536249314,-18.3848338156963,3.6430319886025));
#250984=CARTESIAN_POINT('Origin',(18.6927400943504,-58.5579573083282,3.64299466007569));
#250985=CARTESIAN_POINT('Ctrl Pts',(18.1930767435955,-56.0417604764379,
2.59908173515985));
#250986=CARTESIAN_POINT('Ctrl Pts',(18.2045954185351,-56.077242480448,2.65878198860223));
#250987=CARTESIAN_POINT('Ctrl Pts',(18.2263320786588,-56.1441998575524,
2.65878198860223));
#250988=CARTESIAN_POINT('Ctrl Pts',(18.1097006409639,-56.0688273470718,
2.59908193199789));
#250989=CARTESIAN_POINT('Ctrl Pts',(18.1438516116622,-56.0969586315467,
2.6587768580669));
#250990=CARTESIAN_POINT('Ctrl Pts',(18.1778965340258,-56.159913808362,2.65878198860223));
#250991=CARTESIAN_POINT('Ctrl Pts',(18.0401661963857,-56.1172160917337,
2.6387249266977));
#250992=CARTESIAN_POINT('Ctrl Pts',(18.0947679219786,-56.136792459813,2.69532212015243));
#250993=CARTESIAN_POINT('Ctrl Pts',(18.1406818860302,-56.197800756041,2.68176836726596));
#250994=CARTESIAN_POINT('Ctrl Pts',(17.9612165360197,-56.218435245606,2.75442176402201));
#250995=CARTESIAN_POINT('Ctrl Pts',(18.0530423367039,-56.2137528851844,
2.7920317992009));
#250996=CARTESIAN_POINT('Ctrl Pts',(18.104128639785,-56.2852436625531,2.74885310748136));
#250997=CARTESIAN_POINT('Ctrl Pts',(17.9502021467132,-56.270622860001,2.82866089558369));
#250998=CARTESIAN_POINT('Ctrl Pts',(18.0609092108095,-56.2513800597957,
2.85316563119182));
#250999=CARTESIAN_POINT('Ctrl Pts',(18.1037173431996,-56.3339837785512,
2.79189751796588));
#251000=CARTESIAN_POINT('Ctrl Pts',(17.9642361803979,-56.3138168485091,
2.90134173515985));
#251001=CARTESIAN_POINT('Ctrl Pts',(18.0846218068701,-56.2752137607562,
2.90103711553191));
#251002=CARTESIAN_POINT('Ctrl Pts',(18.1177524687112,-56.3771794532803,
2.83404198860223));
#251003=CARTESIAN_POINT('Origin',(17.9969682911417,-56.416424611566,2.83404198860223));
#251004=CARTESIAN_POINT('Origin',(18.6791227120631,-58.5158800426264,3.56647653971792));
#251005=CARTESIAN_POINT('Origin',(18.6538332760111,-58.4380471616451,3.42473028058444));
#251006=CARTESIAN_POINT('Origin',(18.0520194698712,-56.5858547179415,3.1191364816814));
#251007=CARTESIAN_POINT('Origin',(18.1070706485049,-56.7552848242267,3.40423097483271));
#251008=CARTESIAN_POINT('Ctrl Pts',(18.5518699907157,-58.1242364370953,
3.36123028058441));
#251009=CARTESIAN_POINT('Ctrl Pts',(18.6726541682852,-58.0849912788096,
3.36123028058441));
#251010=CARTESIAN_POINT('Ctrl Pts',(18.6726541682852,-58.0849912788097,
3.23423028058441));
#251011=CARTESIAN_POINT('Ctrl Pts',(18.5799074873355,-58.2097691178797,
3.36123028058441));
#251012=CARTESIAN_POINT('Ctrl Pts',(18.7004428147392,-58.1705159385204,
3.36099641108505));
#251013=CARTESIAN_POINT('Ctrl Pts',(18.714375808615,-58.2133972843966,3.23423043688396));
#251014=CARTESIAN_POINT('Ctrl Pts',(18.6064173144584,-58.2906472745451,
3.41054258905244));
#251015=CARTESIAN_POINT('Ctrl Pts',(18.7268501353368,-58.2517893143846,
3.41008815825988));
#251016=CARTESIAN_POINT('Ctrl Pts',(18.7538265876725,-58.3348142976307,
3.30819867304288));
#251017=CARTESIAN_POINT('Ctrl Pts',(18.6203878281154,-58.3332704847792,
3.48823028058442));
#251018=CARTESIAN_POINT('Ctrl Pts',(18.7407822670309,-58.2946680067384,
3.48794691941558));
#251019=CARTESIAN_POINT('Ctrl Pts',(18.7746174535806,-58.3988020033595,
3.42473028058443));
#251020=CARTESIAN_POINT('Origin',(18.5518699907157,-58.1242364370953,3.23423028058441));
#251021=CARTESIAN_POINT('Ctrl Pts',(18.0743352474898,-56.652678110832,3.47153072139033));
#251022=CARTESIAN_POINT('Ctrl Pts',(18.1949031876642,-56.6140134955958,
3.47122746285038));
#251023=CARTESIAN_POINT('Ctrl Pts',(18.2279043949855,-56.716192681671,3.4041304667674));
#251024=CARTESIAN_POINT('Ctrl Pts',(18.1097491035614,-56.7620702268155,
3.6555381345795));
#251025=CARTESIAN_POINT('Ctrl Pts',(18.2303840130647,-56.723211360369,3.65520336072128));
#251026=CARTESIAN_POINT('Ctrl Pts',(18.2563190096467,-56.8036438738762,
3.55128134519865));
#251027=CARTESIAN_POINT('Ctrl Pts',(18.1733695596544,-56.9585888550836,
3.77003198860224));
#251028=CARTESIAN_POINT('Ctrl Pts',(18.2941747571344,-56.9195374698047,
3.76980209314177));
#251029=CARTESIAN_POINT('Ctrl Pts',(18.307364587184,-56.9607460083088,3.64284195387389));
#251030=CARTESIAN_POINT('Ctrl Pts',(18.2401996527051,-57.1650137687743,
3.77003198860223));
#251031=CARTESIAN_POINT('Ctrl Pts',(18.3611647564563,-57.1257098240087,
3.77003198860223));
#251032=CARTESIAN_POINT('Ctrl Pts',(18.3609836949701,-57.1257686544518,
3.64284189403747));
#251033=CARTESIAN_POINT('Origin',(18.2401996527051,-57.1650137687743,3.64303198860223));
#251034=CARTESIAN_POINT('Origin',(5.49583002221492,-17.9418771653397,3.23423028058469));
#251035=CARTESIAN_POINT('Origin',(18.5051441132848,-57.980428973366,3.23423028058441));
#251036=CARTESIAN_POINT('Origin',(5.47329194811203,-17.8725121057136,3.6430319886025));
#251037=CARTESIAN_POINT('Origin',(18.3641788932763,-57.5467470426658,3.64299171721758));
#251038=CARTESIAN_POINT('Ctrl Pts',(18.4366189870679,-57.7713971777983,
3.48823028058441));
#251039=CARTESIAN_POINT('Ctrl Pts',(18.5581069080667,-57.7324510618066,
3.48852004212219));
#251040=CARTESIAN_POINT('Ctrl Pts',(18.5239649837014,-57.6273730232601,
3.42473028058441));
#251041=CARTESIAN_POINT('Ctrl Pts',(18.4506394153723,-57.8141635875295,
3.41028005848366));
#251042=CARTESIAN_POINT('Ctrl Pts',(18.57194072531,-57.7750271733914,3.41074404220208));
#251043=CARTESIAN_POINT('Ctrl Pts',(18.5448261124699,-57.6915769758378,
3.30780486243811));
#251044=CARTESIAN_POINT('Ctrl Pts',(18.477200500637,-57.8951845615406,3.36123028058441));
#251045=CARTESIAN_POINT('Ctrl Pts',(18.5981804828674,-57.8557848432471,
3.36146460586471));
#251046=CARTESIAN_POINT('Ctrl Pts',(18.5843471808463,-57.8132103173514,
3.23423045308441));
#251047=CARTESIAN_POINT('Ctrl Pts',(18.5051441132848,-57.980428973366,3.36123028058441));
#251048=CARTESIAN_POINT('Ctrl Pts',(18.6259282908542,-57.9411838150804,
3.36123028058441));
#251049=CARTESIAN_POINT('Ctrl Pts',(18.6259282908542,-57.9411838150804,
3.23423028058441));
#251050=CARTESIAN_POINT('Origin',(18.4031808061319,-57.6666181815458,3.4247302805844));
#251051=CARTESIAN_POINT('Origin',(18.3780421908689,-57.5892494801764,3.56563113524746));
#251052=CARTESIAN_POINT('Origin',(25.2734729067949,-55.9845461696113,3.56647653909447));
#251053=CARTESIAN_POINT('Origin',(25.2915084057465,-56.0249274780504,3.64299466007821));
#251054=CARTESIAN_POINT('Origin',(25.2401862573148,-55.9097831300742,3.42473028058445));
#251055=CARTESIAN_POINT('Ctrl Pts',(25.1949317875307,-55.8095395120002,
3.48823028058445));
#251056=CARTESIAN_POINT('Ctrl Pts',(25.079631183696,-55.8614118841074,3.48794691941561));
#251057=CARTESIAN_POINT('Ctrl Pts',(25.1241659841942,-55.9614386837448,
3.42473028058446));
#251058=CARTESIAN_POINT('Ctrl Pts',(25.176732112911,-55.7683775656457,3.41028005925051));
#251059=CARTESIAN_POINT('Ctrl Pts',(25.0612313830316,-55.8200852551801,
3.40982512230935));
#251060=CARTESIAN_POINT('Ctrl Pts',(25.0967080045986,-55.899767051836,3.30780486372789));
#251061=CARTESIAN_POINT('Ctrl Pts',(25.1422534028254,-55.690396180789,3.36123028058443));
#251062=CARTESIAN_POINT('Ctrl Pts',(25.0264120100495,-55.7418796630212,
3.36099721048522));
#251063=CARTESIAN_POINT('Ctrl Pts',(25.0446893032929,-55.7829311357726,
3.23423045308423));
#251064=CARTESIAN_POINT('Ctrl Pts',(25.1059793847708,-55.6083495590297,
3.36123028058442));
#251065=CARTESIAN_POINT('Ctrl Pts',(24.9899591116502,-55.6600051127003,
3.36123028058442));
#251066=CARTESIAN_POINT('Ctrl Pts',(24.9899591116502,-55.6600051127003,
3.23423028058442));
#251067=CARTESIAN_POINT('Origin',(25.1059793847708,-55.6083495590297,3.23423028058442));
#251068=CARTESIAN_POINT('Origin',(0.29005068280153,0.129138884176754,3.64303198860263));
#251069=CARTESIAN_POINT('Origin',(25.454706393409,-56.3916032444846,3.64303198860224));
#251070=CARTESIAN_POINT('Origin',(0.29005068280153,0.129138884176756,3.23423028058481));
#251071=CARTESIAN_POINT('Origin',(25.0444775033954,-55.4702140717962,3.23423028058442));
#251072=CARTESIAN_POINT('Ctrl Pts',(25.6742415049986,-56.883337725539,3.47153072139032));
#251073=CARTESIAN_POINT('Ctrl Pts',(25.5577357840975,-56.9357219056855,
3.47182327902622));
#251074=CARTESIAN_POINT('Ctrl Pts',(25.5138485805643,-56.8366797759148,
3.40413028958989));
#251075=CARTESIAN_POINT('Ctrl Pts',(25.6273680143751,-56.7783442778547,
3.65553807120917));
#251076=CARTESIAN_POINT('Ctrl Pts',(25.5109042502509,-56.8305359187808,
3.65586275497006));
#251077=CARTESIAN_POINT('Ctrl Pts',(25.476448592932,-56.7526780286678,3.55128126837173));
#251078=CARTESIAN_POINT('Ctrl Pts',(25.5431608329964,-56.5897276738843,
3.77003198860224));
#251079=CARTESIAN_POINT('Ctrl Pts',(25.4268390553482,-56.6417212312958,
3.7702550574829));
#251080=CARTESIAN_POINT('Ctrl Pts',(25.4092610357543,-56.6017723050721,
3.64284211731164));
#251081=CARTESIAN_POINT('Ctrl Pts',(25.454706393409,-56.3916032444846,3.77003198860224));
#251082=CARTESIAN_POINT('Ctrl Pts',(25.3385127913802,-56.4433359691571,
3.77003198860224));
#251083=CARTESIAN_POINT('Ctrl Pts',(25.3386862495677,-56.4432587405963,
3.64284239821661));
#251084=CARTESIAN_POINT('Origin',(25.6299342605002,-56.7851714777843,3.40423097483271));
#251085=CARTESIAN_POINT('Ctrl Pts',(25.0444775033954,-55.4702140717962,
3.36123028058442));
#251086=CARTESIAN_POINT('Ctrl Pts',(24.9284572302748,-55.5218696254668,
3.36123028058442));
#251087=CARTESIAN_POINT('Ctrl Pts',(24.9284572302748,-55.5218696254668,
3.23423028058442));
#251088=CARTESIAN_POINT('Ctrl Pts',(25.0080814159075,-55.3878899076689,
3.36123028058442));
#251089=CARTESIAN_POINT('Ctrl Pts',(24.891811449322,-55.4395618538377,3.36146538610203));
#251090=CARTESIAN_POINT('Ctrl Pts',(24.8735420580991,-55.3985281293151,
3.23423043688475));
#251091=CARTESIAN_POINT('Ctrl Pts',(24.9736678430987,-55.3100454158608,
3.41054258693061));
#251092=CARTESIAN_POINT('Ctrl Pts',(24.8573359723247,-55.362128664703,3.41100608859636));
#251093=CARTESIAN_POINT('Ctrl Pts',(24.8216158475492,-55.2818999508905,
3.30819866970666));
#251094=CARTESIAN_POINT('Ctrl Pts',(24.9555320242421,-55.2690209153036,
3.48823028058443));
#251095=CARTESIAN_POINT('Ctrl Pts',(24.8391888661851,-55.3213695969751,
3.48852004212221));
#251096=CARTESIAN_POINT('Ctrl Pts',(24.7942503289613,-55.2204359898052,
3.42473028058442));
#251097=CARTESIAN_POINT('Origin',(24.910270602082,-55.1687804361345,3.42473028058442));
#251098=CARTESIAN_POINT('Origin',(25.7023940320527,-56.9479187893833,3.11913648178429));
#251099=CARTESIAN_POINT('Origin',(25.7748538035653,-57.110666100766,2.83404198860222));
#251100=CARTESIAN_POINT('Origin',(24.8771824671431,-55.0944632682972,3.56563113460811));
#251101=CARTESIAN_POINT('Origin',(24.859045223961,-55.053601445953,3.64299171721715));
#251102=CARTESIAN_POINT('Ctrl Pts',(25.6197038181304,-57.5052637377727,
2.59908173515983));
#251103=CARTESIAN_POINT('Ctrl Pts',(25.6045223014068,-57.4711877340324,
2.65878198860222));
#251104=CARTESIAN_POINT('Ctrl Pts',(25.5758735661215,-57.4068835917975,
2.65878198860222));
#251105=CARTESIAN_POINT('Ctrl Pts',(25.7001924885135,-57.4694043465856,
2.59908193475659));
#251106=CARTESIAN_POINT('Ctrl Pts',(25.6631501095112,-57.4450643815374,
2.65878715325396));
#251107=CARTESIAN_POINT('Ctrl Pts',(25.622459862445,-57.3861185493431,2.65878198860222));
#251108=CARTESIAN_POINT('Ctrl Pts',(25.7642825572407,-57.413464248775,2.63878778849814));
#251109=CARTESIAN_POINT('Ctrl Pts',(25.7077329912393,-57.3998804953988,
2.69564460180077));
#251110=CARTESIAN_POINT('Ctrl Pts',(25.6552692732812,-57.3441059191827,
2.68180481624851));
#251111=CARTESIAN_POINT('Ctrl Pts',(25.8321626496797,-57.3036982377896,
2.75443238878623));
#251112=CARTESIAN_POINT('Ctrl Pts',(25.7409042554415,-57.3186021074444,
2.79268340777047));
#251113=CARTESIAN_POINT('Ctrl Pts',(25.6821129719831,-57.2526112478166,
2.74885926835563));
#251114=CARTESIAN_POINT('Ctrl Pts',(25.8376543496551,-57.2503778226938,
2.82856655361616));
#251115=CARTESIAN_POINT('Ctrl Pts',(25.7289491719118,-57.2821097063799,
2.85384197230757));
#251116=CARTESIAN_POINT('Ctrl Pts',(25.6773293952372,-57.2038640469257,
2.79184624278425));
#251117=CARTESIAN_POINT('Ctrl Pts',(25.8191582032627,-57.2088336324694,
2.90134173515984));
#251118=CARTESIAN_POINT('Ctrl Pts',(25.702828419034,-57.261135792072,2.90163218716352));
#251119=CARTESIAN_POINT('Ctrl Pts',(25.6588335304447,-57.1623216544366,
2.83404198860222));
#251120=CARTESIAN_POINT('Origin',(25.5758735661215,-57.4068835917975,2.53178198860222));
#251121=CARTESIAN_POINT('Origin',(0.29005068280153,0.129138884176754,3.64303198860263));
#251122=CARTESIAN_POINT('Origin',(24.6957503380314,-54.6869600343293,3.64303198860224));
#251123=CARTESIAN_POINT('Origin',(5.59761027822878E-15,1.86033184299798E-13,
2.53178198860262));
#251124=CARTESIAN_POINT('Origin',(25.5480287005725,-57.4192809246784,2.53178198860222));
#251125=CARTESIAN_POINT('Ctrl Pts',(24.6957503380314,-54.6869600343293,
3.77003198860225));
#251126=CARTESIAN_POINT('Ctrl Pts',(24.5795562613022,-54.738692970352,3.77003198860225));
#251127=CARTESIAN_POINT('Ctrl Pts',(24.5797301948987,-54.7386155301255,
3.64284187936967));
#251128=CARTESIAN_POINT('Ctrl Pts',(24.60728817496,-54.4888352915925,3.77003198860225));
#251129=CARTESIAN_POINT('Ctrl Pts',(24.491381933528,-54.5406489234203,3.76980208962834));
#251130=CARTESIAN_POINT('Ctrl Pts',(24.5091541605509,-54.5800991622562,
3.64284193928303));
#251131=CARTESIAN_POINT('Ctrl Pts',(24.5230714236772,-54.3002245846698,
3.65553535416549));
#251132=CARTESIAN_POINT('Ctrl Pts',(24.4074205468504,-54.352067335484,3.65520057834545));
#251133=CARTESIAN_POINT('Ctrl Pts',(24.4419671033159,-54.4291945615841,
3.55127910964149));
#251134=CARTESIAN_POINT('Ctrl Pts',(24.4761921430398,-54.1952354911867,
3.47153072139034));
#251135=CARTESIAN_POINT('Ctrl Pts',(24.3607210114368,-54.2471777873468,
3.47122746281544));
#251136=CARTESIAN_POINT('Ctrl Pts',(24.4045675740915,-54.345193843959,3.40413045901214));
#251137=CARTESIAN_POINT('Origin',(24.5205222915158,-54.2933913980359,3.40423097483272));
#251138=CARTESIAN_POINT('Ctrl Pts',(25.2380597013437,-57.4675553545136,
2.90134173515984));
#251139=CARTESIAN_POINT('Ctrl Pts',(25.3547675996722,-57.4161024530839,
2.90163218716352));
#251140=CARTESIAN_POINT('Ctrl Pts',(25.3107727110829,-57.3172883154485,
2.83404198860222));
#251141=CARTESIAN_POINT('Ctrl Pts',(25.2565651278916,-57.5091180232687,
2.82853349835314));
#251142=CARTESIAN_POINT('Ctrl Pts',(25.3528749970549,-57.449567232889,2.85381483162242));
#251143=CARTESIAN_POINT('Ctrl Pts',(25.3292770036983,-57.3588496371378,
2.79182701594165));
#251144=CARTESIAN_POINT('Ctrl Pts',(25.2997972770064,-57.5405471770605,
2.75468822073607));
#251145=CARTESIAN_POINT('Ctrl Pts',(25.3720159720866,-57.4827148996383,
2.79286913083821));
#251146=CARTESIAN_POINT('Ctrl Pts',(25.3622324578626,-57.3948558336725,
2.7490076329787));
#251147=CARTESIAN_POINT('Ctrl Pts',(25.4257977880276,-57.563646315949,2.63954450640349));
#251148=CARTESIAN_POINT('Ctrl Pts',(25.4538910783603,-57.5124644612005,
2.69627684028803));
#251149=CARTESIAN_POINT('Ctrl Pts',(25.4475597357244,-57.4360631077222,
2.68224356036454));
#251150=CARTESIAN_POINT('Ctrl Pts',(25.511038551389,-57.5536211289084,2.59908178706398));
#251151=CARTESIAN_POINT('Ctrl Pts',(25.5177778164713,-57.5097883065927,
2.65878704321368));
#251152=CARTESIAN_POINT('Ctrl Pts',(25.5012707422386,-57.4400754463043,
2.65878198860223));
#251153=CARTESIAN_POINT('Ctrl Pts',(25.5918112338801,-57.5176823163884,
2.59908173515984));
#251154=CARTESIAN_POINT('Ctrl Pts',(25.5766462455183,-57.4835989537473,
2.65878198860223));
#251155=CARTESIAN_POINT('Ctrl Pts',(25.5480287005725,-57.4192809246784,
2.65878198860223));
#251156=CARTESIAN_POINT('Origin',(25.1947524379623,-57.3689438691191,2.83404198860222));
#251157=CARTESIAN_POINT('Origin',(24.4480624203097,-54.1306438627461,3.11913648166974));
#251158=CARTESIAN_POINT('Origin',(24.3756025490945,-53.967896327293,2.83404198860224));
#251159=CARTESIAN_POINT('Origin',(25.122292666488,-57.2061965577009,3.11913648177378));
#251160=CARTESIAN_POINT('Origin',(25.0498328948971,-57.0434492461374,3.4042309748327));
#251161=CARTESIAN_POINT('Ctrl Pts',(24.3312692531094,-53.869741842014,2.90134173515986));
#251162=CARTESIAN_POINT('Ctrl Pts',(24.2159747902193,-53.9216078643412,
2.90103711553192));
#251163=CARTESIAN_POINT('Ctrl Pts',(24.2595822759739,-54.0195518809636,
2.83404198860224));
#251164=CARTESIAN_POINT('Ctrl Pts',(24.3127882662185,-53.8282341734838,
2.82862991747925));
#251165=CARTESIAN_POINT('Ctrl Pts',(24.2176496934273,-53.8880114973697,
2.8531404588629));
#251166=CARTESIAN_POINT('Ctrl Pts',(24.2411010091831,-53.9780422761232,
2.79187960999868));
#251167=CARTESIAN_POINT('Ctrl Pts',(24.2697746459847,-53.7969955864423,
2.7547062579329));
#251168=CARTESIAN_POINT('Ctrl Pts',(24.1983152114494,-53.8549480733037,
2.79224250381878));
#251169=CARTESIAN_POINT('Ctrl Pts',(24.2082687574728,-53.9422730280817,
2.74901809108215));
#251170=CARTESIAN_POINT('Ctrl Pts',(24.1443388226044,-53.7744913425361,
2.63947868311661));
#251171=CARTESIAN_POINT('Ctrl Pts',(24.116516742923,-53.8256450222186,2.69595066767865));
#251172=CARTESIAN_POINT('Ctrl Pts',(24.123203223048,-53.9017956184501,2.68220539436032));
#251173=CARTESIAN_POINT('Ctrl Pts',(24.0595120258539,-53.7848917482044,
2.59908178585034));
#251174=CARTESIAN_POINT('Ctrl Pts',(24.0529122166844,-53.8286685158623,
2.65877670944859));
#251175=CARTESIAN_POINT('Ctrl Pts',(24.0696665464389,-53.8982652496122,
2.65878198860225));
#251176=CARTESIAN_POINT('Ctrl Pts',(23.979166327502,-53.8206887816831,2.59908173515986));
#251177=CARTESIAN_POINT('Ctrl Pts',(23.9943483786823,-53.8547645473076,
2.65878198860225));
#251178=CARTESIAN_POINT('Ctrl Pts',(24.0229981225303,-53.919068240199,2.65878198860225));
#251179=CARTESIAN_POINT('Origin',(24.0229981225303,-53.919068240199,2.53178198860225));
#251180=CARTESIAN_POINT('Ctrl Pts',(24.8746050278059,-56.6498810128377,
3.77003198860224));
#251181=CARTESIAN_POINT('Ctrl Pts',(24.9907986398452,-56.5981482837082,
3.77003198860224));
#251182=CARTESIAN_POINT('Ctrl Pts',(24.9906251716322,-56.5982255167326,
3.64284238727508));
#251183=CARTESIAN_POINT('Ctrl Pts',(24.962653969475,-56.8481896769742,3.77003198860223));
#251184=CARTESIAN_POINT('Ctrl Pts',(25.079127190573,-56.7965362315712,3.77025506105937));
#251185=CARTESIAN_POINT('Ctrl Pts',(25.0612010539381,-56.7567415443521,
3.64284210641882));
#251186=CARTESIAN_POINT('Ctrl Pts',(25.0464771582534,-57.036975459332,3.65553527987793));
#251187=CARTESIAN_POINT('Ctrl Pts',(25.163192587334,-56.9853490357273,3.65585996533029));
#251188=CARTESIAN_POINT('Ctrl Pts',(25.1283880784749,-56.9076460727654,
3.55127902710107));
#251189=CARTESIAN_POINT('Ctrl Pts',(25.0931373005752,-57.1420619865017,
3.47153072139031));
#251190=CARTESIAN_POINT('Ctrl Pts',(25.210023886751,-57.0905332166514,3.47182327905148));
#251191=CARTESIAN_POINT('Ctrl Pts',(25.1657874977299,-56.9916465440533,
3.4041302837792));
#251192=CARTESIAN_POINT('Origin',(24.8746050278059,-56.6498810128377,3.64303198860224));
#251193=CARTESIAN_POINT('Origin',(5.68853496937358E-15,1.86271140789742E-13,
2.53178198860262));
#251194=CARTESIAN_POINT('Origin',(23.9951532569813,-53.93146557308,2.53178198860225));
#251195=CARTESIAN_POINT('Origin',(10.0037024164492,-23.2492868865832,3.64303198860246));
#251196=CARTESIAN_POINT('Origin',(24.7113125977916,-56.2832472948501,3.64299466007465));
#251197=CARTESIAN_POINT('Ctrl Pts',(23.9513722670371,-53.8330634946833,
2.59908173515986));
#251198=CARTESIAN_POINT('Ctrl Pts',(23.966536720823,-53.8671470951726,2.65878198860225));
#251199=CARTESIAN_POINT('Ctrl Pts',(23.9951532569813,-53.93146557308,2.65878198860225));
#251200=CARTESIAN_POINT('Ctrl Pts',(23.8712821658127,-53.8686972660496,
2.59908193199887));
#251201=CARTESIAN_POINT('Ctrl Pts',(23.9081865738555,-53.8931046959176,
2.6587768580666));
#251202=CARTESIAN_POINT('Ctrl Pts',(23.9486256024606,-53.9521563342727,
2.65878198860225));
#251203=CARTESIAN_POINT('Ctrl Pts',(23.8071866393159,-53.9240892607408,
2.63872492669778));
#251204=CARTESIAN_POINT('Ctrl Pts',(23.8635355386147,-53.9378509529596,
2.69532212015233));
#251205=CARTESIAN_POINT('Ctrl Pts',(23.9155750846182,-53.9937257232522,
2.68176836726611));
#251206=CARTESIAN_POINT('Ctrl Pts',(23.7392497560577,-54.0330064121708,
2.75442176402196));
#251207=CARTESIAN_POINT('Ctrl Pts',(23.8300830854584,-54.0187512923756,
2.7920317992011));
#251208=CARTESIAN_POINT('Ctrl Pts',(23.8883623535223,-54.0845104630309,
2.74885310748125));
#251209=CARTESIAN_POINT('Ctrl Pts',(23.7337507958623,-54.0860594545419,
2.82866089558375));
#251210=CARTESIAN_POINT('Ctrl Pts',(23.8418399747441,-54.055350029128,2.85316563119103));
#251211=CARTESIAN_POINT('Ctrl Pts',(23.8930480394875,-54.133026567774,2.79189751796542));
#251212=CARTESIAN_POINT('Ctrl Pts',(23.7522229508834,-54.1275498658869,
2.90134173515987));
#251213=CARTESIAN_POINT('Ctrl Pts',(23.8679139708575,-54.0765745253531,
2.90103711553193));
#251214=CARTESIAN_POINT('Ctrl Pts',(23.9115214566121,-54.1745185419755,
2.83404198860225));
#251215=CARTESIAN_POINT('Origin',(23.7955011834915,-54.2261740956461,2.83404198860224));
#251216=CARTESIAN_POINT('Origin',(24.6933715410278,-56.2428239368551,3.56647653971807));
#251217=CARTESIAN_POINT('Origin',(24.6600848917118,-56.1680608984273,3.42473028058445));
#251218=CARTESIAN_POINT('Origin',(23.8679610547535,-54.388921631058,3.11913648168137));
#251219=CARTESIAN_POINT('Origin',(23.9404209259127,-54.551669166389,3.40423097483273));
#251220=CARTESIAN_POINT('Ctrl Pts',(24.5258780191677,-55.8666273273828,
3.36123028058442));
#251221=CARTESIAN_POINT('Ctrl Pts',(24.6418982922884,-55.8149717737122,
3.36123028058442));
#251222=CARTESIAN_POINT('Ctrl Pts',(24.6418982922884,-55.8149717737122,
3.23423028058442));
#251223=CARTESIAN_POINT('Ctrl Pts',(24.5627025231306,-55.9487607347562,
3.36123028058442));
#251224=CARTESIAN_POINT('Ctrl Pts',(24.678474470882,-55.8971232158784,3.36099641108666));
#251225=CARTESIAN_POINT('Ctrl Pts',(24.6968134595452,-55.9383132588163,
3.2342304368845));
#251226=CARTESIAN_POINT('Ctrl Pts',(24.5975211960739,-56.0264248009268,
3.41054258905248));
#251227=CARTESIAN_POINT('Ctrl Pts',(24.7132325104969,-55.9751910510436,
3.41008815825889));
#251228=CARTESIAN_POINT('Ctrl Pts',(24.7487396569155,-56.0549414076388,
3.30819867304241));
#251229=CARTESIAN_POINT('Ctrl Pts',(24.61587051646,-56.0673542004321,3.48823028058444));
#251230=CARTESIAN_POINT('Ctrl Pts',(24.7315703643342,-56.0163785451193,
3.48794691941561));
#251231=CARTESIAN_POINT('Ctrl Pts',(24.7761051648324,-56.1164053447567,
3.42473028058445));
#251232=CARTESIAN_POINT('Origin',(24.5258780191677,-55.8666273273828,3.23423028058442));
#251233=CARTESIAN_POINT('Ctrl Pts',(23.8971395307774,-54.4530463244688,
3.47153072139034));
#251234=CARTESIAN_POINT('Ctrl Pts',(24.0130054343472,-54.4019907365345,
3.47122746285038));
#251235=CARTESIAN_POINT('Ctrl Pts',(24.0565064909,-54.5001606088503,3.40413046676726));
#251236=CARTESIAN_POINT('Ctrl Pts',(23.9437939758159,-54.5581374230422,
3.6555381345795));
#251237=CARTESIAN_POINT('Ctrl Pts',(24.0597061770684,-54.5068816478246,
3.65520336072068));
#251238=CARTESIAN_POINT('Ctrl Pts',(24.0939065860604,-54.5841625982679,
3.55128134519838));
#251239=CARTESIAN_POINT('Ctrl Pts',(24.0276077026114,-54.7469293531943,
3.77003198860224));
#251240=CARTESIAN_POINT('Ctrl Pts',(24.1436691352879,-54.6954643138432,
3.76980209314288));
#251241=CARTESIAN_POINT('Ctrl Pts',(24.1610941752726,-54.7350683949964,
3.64284195387434));
#251242=CARTESIAN_POINT('Ctrl Pts',(24.1156489724283,-54.9452378026824,
3.77003198860225));
#251243=CARTESIAN_POINT('Ctrl Pts',(24.2318430357379,-54.8935048726344,
3.77003198860225));
#251244=CARTESIAN_POINT('Ctrl Pts',(24.231669115581,-54.8935823068772,3.6428418940372));
#251245=CARTESIAN_POINT('Origin',(24.1156489724283,-54.9452378026824,3.64303198860225));
#251246=CARTESIAN_POINT('Origin',(9.75435829333415,-22.68925081671,3.23423028058465));
#251247=CARTESIAN_POINT('Origin',(24.4643761377923,-55.7284918401493,3.23423028058442));
#251248=CARTESIAN_POINT('Origin',(9.71531210235053,-22.6015516358799,3.64303198860247));
#251249=CARTESIAN_POINT('Origin',(24.2788510342453,-55.311920542264,3.64299171721759));
#251250=CARTESIAN_POINT('Ctrl Pts',(24.374376627022,-55.5277679687678,3.48823028058443));
#251251=CARTESIAN_POINT('Ctrl Pts',(24.4911280468232,-55.476336257987,3.48852004212221));
#251252=CARTESIAN_POINT('Ctrl Pts',(24.4461895095995,-55.375402650817,3.42473028058442));
#251253=CARTESIAN_POINT('Ctrl Pts',(24.3927905570419,-55.5688345658067,
3.41028005848369));
#251254=CARTESIAN_POINT('Ctrl Pts',(24.5093364964853,-55.5172331055173,
3.41074404220213));
#251255=CARTESIAN_POINT('Ctrl Pts',(24.47364749942,-55.4370743056914,3.30780486243795));
#251256=CARTESIAN_POINT('Ctrl Pts',(24.4276751358093,-55.6466353090189,
3.36123028058442));
#251257=CARTESIAN_POINT('Ctrl Pts',(24.5438739850335,-55.5948055748771,
3.36146460586399));
#251258=CARTESIAN_POINT('Ctrl Pts',(24.5256662135201,-55.5539102504913,
3.23423045308425));
#251259=CARTESIAN_POINT('Ctrl Pts',(24.4643761377923,-55.7284918401493,
3.36123028058442));
#251260=CARTESIAN_POINT('Ctrl Pts',(24.5803964109129,-55.6768362864787,
3.36123028058442));
#251261=CARTESIAN_POINT('Ctrl Pts',(24.5803964109129,-55.6768362864787,
3.23423028058443));
#251262=CARTESIAN_POINT('Origin',(24.3301692364789,-55.4270582044877,3.42473028058442));
#251263=CARTESIAN_POINT('Origin',(24.2970811017196,-55.3527410377814,3.56563113524687));
#251264=CARTESIAN_POINT('Origin',(30.9870007556499,-53.036059683551,3.56647653909447));
#251265=CARTESIAN_POINT('Origin',(31.009158450368,-53.074334555967,3.64299466007827));
#251266=CARTESIAN_POINT('Origin',(30.9460815882875,-52.965185606084,3.42473028058447));
#251267=CARTESIAN_POINT('Ctrl Pts',(30.8905967158742,-52.870221513221,3.48823028058448));
#251268=CARTESIAN_POINT('Ctrl Pts',(30.7813498801538,-52.933861917979,3.48794691941564));
#251269=CARTESIAN_POINT('Ctrl Pts',(30.8360963620068,-53.028685606084,3.42473028058449));
#251270=CARTESIAN_POINT('Ctrl Pts',(30.8681941459792,-52.8311874403352,
3.41028005925052));
#251271=CARTESIAN_POINT('Ctrl Pts',(30.7587310665085,-52.8946849835364,
3.40982512230918));
#251272=CARTESIAN_POINT('Ctrl Pts',(30.8023423591864,-52.9702219582401,
3.30780486372862));
#251273=CARTESIAN_POINT('Ctrl Pts',(30.8257530395519,-52.7572372522452,
3.36123028058445));
#251274=CARTESIAN_POINT('Ctrl Pts',(30.7159277273276,-52.8205474253451,
3.36099721048575));
#251275=CARTESIAN_POINT('Ctrl Pts',(30.7383959430076,-52.8594635164567,
3.23423045308295));
#251276=CARTESIAN_POINT('Ctrl Pts',(30.781101527075,-52.6794317578282,3.36123028058445));
#251277=CARTESIAN_POINT('Ctrl Pts',(30.6711163007943,-52.7429317578282,
3.36123028058445));
#251278=CARTESIAN_POINT('Ctrl Pts',(30.6711163007943,-52.7429317578282,
3.23423028058445));
#251279=CARTESIAN_POINT('Origin',(30.781101527075,-52.6794317578282,3.23423028058445));
#251280=CARTESIAN_POINT('Origin',(0.274963065701563,0.158750000000187,3.64303198860263));
#251281=CARTESIAN_POINT('Origin',(31.2097904767612,-53.4219427993281,3.64303198860226));
#251282=CARTESIAN_POINT('Origin',(0.274963065701563,0.15875000000019,3.23423028058481));
#251283=CARTESIAN_POINT('Origin',(30.7054974692375,-52.5484816883954,3.23423028058445));
#251284=CARTESIAN_POINT('Ctrl Pts',(31.4795232016796,-53.8880358395965,
3.47153072139034));
#251285=CARTESIAN_POINT('Ctrl Pts',(31.3691313491582,-53.9523112176906,
3.47182327902625));
#251286=CARTESIAN_POINT('Ctrl Pts',(31.3151318426942,-53.8583991130125,
3.40413028959004));
#251287=CARTESIAN_POINT('Ctrl Pts',(31.4219316852033,-53.7885171709467,
3.65553807120918));
#251288=CARTESIAN_POINT('Ctrl Pts',(31.3115614337847,-53.8525966788944,
3.65586275496689));
#251289=CARTESIAN_POINT('Ctrl Pts',(31.2691561625549,-53.778766899358,3.55128126837125));
#251290=CARTESIAN_POINT('Ctrl Pts',(31.3184699958148,-53.609735875734,3.77003198860225));
#251291=CARTESIAN_POINT('Ctrl Pts',(31.2082202476924,-53.6736035436592,
3.77025505748722));
#251292=CARTESIAN_POINT('Ctrl Pts',(31.1865627224611,-53.6357108652109,
3.64284211731213));
#251293=CARTESIAN_POINT('Ctrl Pts',(31.2097904767612,-53.4219427993281,
3.77003198860226));
#251294=CARTESIAN_POINT('Ctrl Pts',(31.0996409376528,-53.4855376653835,
3.77003198860226));
#251295=CARTESIAN_POINT('Ctrl Pts',(31.0998053730353,-53.4854427285712,
3.64284239821688));
#251296=CARTESIAN_POINT('Origin',(31.4251975098799,-53.7950387249973,3.40423097483273));
#251297=CARTESIAN_POINT('Ctrl Pts',(30.7054974692375,-52.5484816883954,
3.36123028058445));
#251298=CARTESIAN_POINT('Ctrl Pts',(30.5955122429569,-52.6119816883954,
3.36123028058445));
#251299=CARTESIAN_POINT('Ctrl Pts',(30.5955122429569,-52.6119816883954,
3.23423028058445));
#251300=CARTESIAN_POINT('Ctrl Pts',(30.6606955449581,-52.4704129317475,
3.36123028058446));
#251301=CARTESIAN_POINT('Ctrl Pts',(30.5504637065427,-52.5339553345204,
3.36146538610016));
#251302=CARTESIAN_POINT('Ctrl Pts',(30.5280052047897,-52.4950560684212,
3.23423043688334));
#251303=CARTESIAN_POINT('Ctrl Pts',(30.6183335281992,-52.3965920780919,
3.41054258693063));
#251304=CARTESIAN_POINT('Ctrl Pts',(30.5080831175497,-52.4605500011269,
3.41100608859759));
#251305=CARTESIAN_POINT('Ctrl Pts',(30.4641724871917,-52.3844945583564,
3.30819866970833));
#251306=CARTESIAN_POINT('Ctrl Pts',(30.5960088312575,-52.3576880233157,
3.48823028058444));
#251307=CARTESIAN_POINT('Ctrl Pts',(30.4857749404426,-52.4219111049551,
3.48852004212222));
#251308=CARTESIAN_POINT('Ctrl Pts',(30.4305321463783,-52.3262277788836,
3.42473028058444));
#251309=CARTESIAN_POINT('Origin',(30.5405173726589,-52.2627277788836,3.42473028058445));
#251310=CARTESIAN_POINT('Origin',(31.5142720656055,-53.9493203812242,3.11913648178368));
#251311=CARTESIAN_POINT('Origin',(31.6033466212672,-54.1036020372433,2.83404198860224));
#251312=CARTESIAN_POINT('Origin',(30.4998422386366,-52.1922763801639,3.56563113460745));
#251313=CARTESIAN_POINT('Origin',(30.4775331296742,-52.1535342613178,3.64299171721798));
#251314=CARTESIAN_POINT('Ctrl Pts',(31.4902932482914,-54.5122556166605,
2.59908173515985));
#251315=CARTESIAN_POINT('Ctrl Pts',(31.4716329851996,-54.4799531854473,
2.65878198860224));
#251316=CARTESIAN_POINT('Ctrl Pts',(31.4364195775141,-54.4189959163058,
2.65878198860224));
#251317=CARTESIAN_POINT('Ctrl Pts',(31.566592666262,-54.4681793099452,2.59908193475597));
#251318=CARTESIAN_POINT('Ctrl Pts',(31.5272089901453,-54.4478446647263,
2.65878715325333));
#251319=CARTESIAN_POINT('Ctrl Pts',(31.4805801312541,-54.393475032962,2.65878198860224));
#251320=CARTESIAN_POINT('Ctrl Pts',(31.6244843104278,-54.4058464214479,
2.63878778849855));
#251321=CARTESIAN_POINT('Ctrl Pts',(31.5668246400003,-54.3982481205262,
2.69564460180097));
#251322=CARTESIAN_POINT('Ctrl Pts',(31.5088182930364,-54.3482630350898,
2.68180481624859));
#251323=CARTESIAN_POINT('Ctrl Pts',(31.6805188761703,-54.2895863184074,
2.75443238878586));
#251324=CARTESIAN_POINT('Ctrl Pts',(31.5913182835558,-54.3139476428153,
2.79268340777021));
#251325=CARTESIAN_POINT('Ctrl Pts',(31.5259511417539,-54.2544636505346,
2.74885926835559));
#251326=CARTESIAN_POINT('Ctrl Pts',(31.6804069909882,-54.2359839591646,
2.82856655361648));
#251327=CARTESIAN_POINT('Ctrl Pts',(31.5756141966219,-54.2789047974527,
2.85384197230916));
#251328=CARTESIAN_POINT('Ctrl Pts',(31.5160982999442,-54.2064835118368,
2.7918462427859));
#251329=CARTESIAN_POINT('Ctrl Pts',(31.6576696180591,-54.1966007261202,
2.90134173515986));
#251330=CARTESIAN_POINT('Ctrl Pts',(31.547444164929,-54.2607761425977,2.90163218716353));
#251331=CARTESIAN_POINT('Ctrl Pts',(31.4933613949865,-54.1671020372433,
2.83404198860224));
#251332=CARTESIAN_POINT('Origin',(31.4364195775141,-54.4189959163058,2.53178198860223));
#251333=CARTESIAN_POINT('Origin',(0.274963065701563,0.158750000000187,3.64303198860263));
#251334=CARTESIAN_POINT('Origin',(30.2768083268887,-51.8059703131941,3.64303198860226));
#251335=CARTESIAN_POINT('Origin',(5.58223212128129E-15,1.86025348737467E-13,
2.53178198860262));
#251336=CARTESIAN_POINT('Origin',(31.4100231232068,-54.4342359163058,2.53178198860224));
#251337=CARTESIAN_POINT('Ctrl Pts',(30.2768083268887,-51.8059703131941,
3.77003198860227));
#251338=CARTESIAN_POINT('Ctrl Pts',(30.1666583377722,-51.8695654390617,
3.77003198860227));
#251339=CARTESIAN_POINT('Ctrl Pts',(30.1668232238344,-51.8694702420493,
3.64284187936972));
#251340=CARTESIAN_POINT('Ctrl Pts',(30.1681210939109,-51.6181777324902,
3.77003198860227));
#251341=CARTESIAN_POINT('Ctrl Pts',(30.0582657983058,-51.6818230251218,
3.76980208963099));
#251342=CARTESIAN_POINT('Ctrl Pts',(30.080064340051,-51.7191994478426,3.64284193928307));
#251343=CARTESIAN_POINT('Ctrl Pts',(30.0646505034496,-51.4394033023496,
3.65553535416551));
#251344=CARTESIAN_POINT('Ctrl Pts',(29.9550522173029,-51.5030508615811,
3.6552005783431));
#251345=CARTESIAN_POINT('Ctrl Pts',(29.9974715145375,-51.5761444782072,
3.55127910964149));
#251346=CARTESIAN_POINT('Ctrl Pts',(30.0070536838164,-51.3398895692692,
3.47153072139037));
#251347=CARTESIAN_POINT('Ctrl Pts',(29.8976445635505,-51.4036173400343,
3.47122746281548));
#251348=CARTESIAN_POINT('Ctrl Pts',(29.9514963979204,-51.4965132406189,
3.40413045901218));
#251349=CARTESIAN_POINT('Origin',(30.0614010732043,-51.4328740054938,3.40423097483275));
#251350=CARTESIAN_POINT('Ctrl Pts',(31.1067982185541,-54.5146464769132,
2.90134173515986));
#251351=CARTESIAN_POINT('Ctrl Pts',(31.2174884860871,-54.4512761425977,
2.90163218716353));
#251352=CARTESIAN_POINT('Ctrl Pts',(31.1634057161447,-54.3576020372433,
2.83404198860224));
#251353=CARTESIAN_POINT('Ctrl Pts',(31.1295467523329,-54.5540471172212,
2.82853349835322));
#251354=CARTESIAN_POINT('Ctrl Pts',(31.2191042733523,-54.4847554296808,
2.85381483162266));
#251355=CARTESIAN_POINT('Ctrl Pts',(31.1861529813967,-54.397001456393,2.79182701594234));
#251356=CARTESIAN_POINT('Ctrl Pts',(31.1758273123594,-54.5807851087093,
2.75468822073598));
#251357=CARTESIAN_POINT('Ctrl Pts',(31.241605266786,-54.515720733338,2.792869130838));
#251358=CARTESIAN_POINT('Ctrl Pts',(31.2226915745269,-54.4293656242359,
2.74900763297872));
#251359=CARTESIAN_POINT('Ctrl Pts',(31.3035520968889,-54.5905870683097,
2.63954450640362));
#251360=CARTESIAN_POINT('Ctrl Pts',(31.326141528613,-54.5367490446502,2.69627684028817));
#251361=CARTESIAN_POINT('Ctrl Pts',(31.3118587536639,-54.4614280312961,
2.68224356036457));
#251362=CARTESIAN_POINT('Ctrl Pts',(31.3872779850338,-54.5717067142908,
2.59908178706425));
#251363=CARTESIAN_POINT('Ctrl Pts',(31.3893985541607,-54.5274095677407,
2.6587870432139));
#251364=CARTESIAN_POINT('Ctrl Pts',(31.3656949292504,-54.4598040608957,
2.65878198860224));
#251365=CARTESIAN_POINT('Ctrl Pts',(31.4638515574747,-54.5275217339714,
2.59908173515985));
#251366=CARTESIAN_POINT('Ctrl Pts',(31.445206962986,-54.495210256486,2.65878198860224));
#251367=CARTESIAN_POINT('Ctrl Pts',(31.4100231232068,-54.4342359163058,
2.65878198860224));
#251368=CARTESIAN_POINT('Origin',(31.053420489864,-54.4211020372433,2.83404198860224));
#251369=CARTESIAN_POINT('Origin',(29.9723263949905,-51.2785921372162,3.11913648166973));
#251370=CARTESIAN_POINT('Origin',(29.8832517167492,-51.1243102687779,2.83404198860226));
#251371=CARTESIAN_POINT('Origin',(30.9643459342406,-54.2668203811894,3.1191364817768));
#251372=CARTESIAN_POINT('Origin',(30.8752713784768,-54.1125387249973,3.40423097483274));
#251373=CARTESIAN_POINT('Ctrl Pts',(29.8289013456892,-51.0313275753403,
2.90134173515988));
#251374=CARTESIAN_POINT('Ctrl Pts',(29.7196599535399,-51.0949610231996,
2.90103711553193));
#251375=CARTESIAN_POINT('Ctrl Pts',(29.7732664904686,-51.1878102687779,
2.83404198860226));
#251376=CARTESIAN_POINT('Ctrl Pts',(29.8061828667731,-50.9919790793205,
2.82862991747924));
#251377=CARTESIAN_POINT('Ctrl Pts',(29.7178139048437,-51.0613736255825,
2.85314045886342));
#251378=CARTESIAN_POINT('Ctrl Pts',(29.7505475307862,-51.1484598763129,
2.79187960999871));
#251379=CARTESIAN_POINT('Ctrl Pts',(29.760139558153,-50.9654077681503,2.75470625793292));
#251380=CARTESIAN_POINT('Ctrl Pts',(29.6951292702716,-51.0305123301026,
2.79224250381854));
#251381=CARTESIAN_POINT('Ctrl Pts',(29.7141562330561,-51.1163184807715,
2.74901809108226));
#251382=CARTESIAN_POINT('Ctrl Pts',(29.6330385513056,-50.9561384187033,
2.63947868311661));
#251383=CARTESIAN_POINT('Ctrl Pts',(29.610715899415,-51.0099200724105,2.69595066767883));
#251384=CARTESIAN_POINT('Ctrl Pts',(29.6253256551035,-51.0849545802159,
2.68220539436023));
#251385=CARTESIAN_POINT('Ctrl Pts',(29.5497635830447,-50.9753486645692,
2.59908178584971));
#251386=CARTESIAN_POINT('Ctrl Pts',(29.5477758465698,-51.019575486422,2.65877670944804));
#251387=CARTESIAN_POINT('Ctrl Pts',(29.5717132339802,-51.0870396576403,
2.65878198860226));
#251388=CARTESIAN_POINT('Ctrl Pts',(29.4735998357344,-51.0193480105322,
2.59908173515988));
#251389=CARTESIAN_POINT('Ctrl Pts',(29.4922606054652,-51.0516501490681,
2.65878198860226));
#251390=CARTESIAN_POINT('Ctrl Pts',(29.5274749692191,-51.1126068659042,
2.65878198860226));
#251391=CARTESIAN_POINT('Origin',(29.5274749692191,-51.1126068659042,2.53178198860226));
#251392=CARTESIAN_POINT('Ctrl Pts',(30.6598643453581,-53.7394427993281,
3.77003198860226));
#251393=CARTESIAN_POINT('Ctrl Pts',(30.7700138939561,-53.6758479277939,
3.77003198860225));
#251394=CARTESIAN_POINT('Ctrl Pts',(30.7698494490699,-53.6759428700932,
3.64284238727559));
#251395=CARTESIAN_POINT('Ctrl Pts',(30.7681598456276,-53.9274614872877,
3.77003198860225));
#251396=CARTESIAN_POINT('Ctrl Pts',(30.878595758964,-53.8639162380547,3.77025506105976));
#251397=CARTESIAN_POINT('Ctrl Pts',(30.8566081460799,-53.8262133418089,
3.6428421064193));
#251398=CARTESIAN_POINT('Ctrl Pts',(30.8712573299226,-54.1064511722683,
3.65553527987797));
#251399=CARTESIAN_POINT('Ctrl Pts',(30.9819369489464,-54.0429074791658,
3.65585996532834));
#251400=CARTESIAN_POINT('Ctrl Pts',(30.9392009315185,-53.9692682429945,
3.55127902710052));
#251401=CARTESIAN_POINT('Ctrl Pts',(30.9286463962985,-54.2060847114736,
3.47153072139035));
#251402=CARTESIAN_POINT('Ctrl Pts',(31.0395064423981,-54.1426202463868,
3.47182327905151));
#251403=CARTESIAN_POINT('Ctrl Pts',(30.9851759130209,-54.0488992470929,
3.4041302837795));
#251404=CARTESIAN_POINT('Origin',(30.6598643453581,-53.7394427993281,3.64303198860226));
#251405=CARTESIAN_POINT('Origin',(5.69400554112517E-15,1.86273928185272E-13,
2.53178198860262));
#251406=CARTESIAN_POINT('Origin',(29.5010785149117,-51.1278468659042,2.53178198860227));
#251407=CARTESIAN_POINT('Origin',(15.2806508669898,-27.1018636743469,3.64303198860243));
#251408=CARTESIAN_POINT('Origin',(30.4591427892377,-53.3918862459826,3.64299466007281));
#251409=CARTESIAN_POINT('Ctrl Pts',(29.4472515437741,-51.0345602039881,
2.59908173515988));
#251410=CARTESIAN_POINT('Ctrl Pts',(29.4658956314773,-51.0668719738972,
2.65878198860226));
#251411=CARTESIAN_POINT('Ctrl Pts',(29.5010785149117,-51.1278468659042,
2.65878198860226));
#251412=CARTESIAN_POINT('Ctrl Pts',(29.3713249278652,-51.0783704650302,
2.59908193199828));
#251413=CARTESIAN_POINT('Ctrl Pts',(29.4105784408362,-51.0987866273834,
2.65877685806608));
#251414=CARTESIAN_POINT('Ctrl Pts',(29.4569685172211,-51.1532877451673,
2.65878198860226));
#251415=CARTESIAN_POINT('Ctrl Pts',(29.3133705634518,-51.1401588234658,
2.63872492669764));
#251416=CARTESIAN_POINT('Ctrl Pts',(29.3708492661241,-51.1479550638445,
2.69532212015224));
#251417=CARTESIAN_POINT('Ctrl Pts',(29.4284442379237,-51.1980841325261,
2.68176836726597));
#251418=CARTESIAN_POINT('Ctrl Pts',(29.2571907880108,-51.2555806533506,
2.75442176402212));
#251419=CARTESIAN_POINT('Ctrl Pts',(29.346036457163,-51.2319089562571,2.79203179920123));
#251420=CARTESIAN_POINT('Ctrl Pts',(29.410870170353,-51.2912160489642,2.74885310748141));
#251421=CARTESIAN_POINT('Ctrl Pts',(29.2572675046856,-51.308917863463,2.82866089558365));
#251422=CARTESIAN_POINT('Ctrl Pts',(29.3615545506894,-51.2670782717299,
2.85316563119133));
#251423=CARTESIAN_POINT('Ctrl Pts',(29.420601501513,-51.3389765898561,2.79189751796506));
#251424=CARTESIAN_POINT('Ctrl Pts',(29.2799753962468,-51.348250120016,2.90134173515988));
#251425=CARTESIAN_POINT('Ctrl Pts',(29.389704274698,-51.2854610231996,2.90103711553194));
#251426=CARTESIAN_POINT('Ctrl Pts',(29.4433108116267,-51.3783102687779,
2.83404198860226));
#251427=CARTESIAN_POINT('Origin',(29.3333255853461,-51.441810268778,2.83404198860226));
#251428=CARTESIAN_POINT('Origin',(30.4370746239673,-53.3535596824661,3.56647653971762));
#251429=CARTESIAN_POINT('Origin',(30.3961554568843,-53.282685606084,3.42473028058449));
#251430=CARTESIAN_POINT('Origin',(29.4224002636298,-51.5960921371717,3.11913648168056));
#251431=CARTESIAN_POINT('Origin',(29.5114749418011,-51.7503740054938,3.40423097483275));
#251432=CARTESIAN_POINT('Ctrl Pts',(30.2311753956719,-52.9969317578282,
3.36123028058445));
#251433=CARTESIAN_POINT('Ctrl Pts',(30.3411606219525,-52.9334317578282,
3.36123028058445));
#251434=CARTESIAN_POINT('Ctrl Pts',(30.3411606219525,-52.9334317578282,
3.23423028058445));
#251435=CARTESIAN_POINT('Ctrl Pts',(30.2763834500047,-53.0747660209923,
3.36123028058445));
#251436=CARTESIAN_POINT('Ctrl Pts',(30.3861235964177,-53.0113099140571,
3.36099641108313));
#251437=CARTESIAN_POINT('Ctrl Pts',(30.4086676540725,-53.0503573673283,
3.23423043688312));
#251438=CARTESIAN_POINT('Ctrl Pts',(30.3191294881016,-53.148365092907,3.41054258905248));
#251439=CARTESIAN_POINT('Ctrl Pts',(30.4288515386959,-53.0853168809873,
3.41008815826136));
#251440=CARTESIAN_POINT('Ctrl Pts',(30.4725003554702,-53.1609188493334,
3.30819867304359));
#251441=CARTESIAN_POINT('Ctrl Pts',(30.3416565762243,-53.187152250617,3.48823028058447));
#251442=CARTESIAN_POINT('Ctrl Pts',(30.451394201312,-53.124361917979,3.48794691941563));
#251443=CARTESIAN_POINT('Ctrl Pts',(30.506140683165,-53.219185606084,3.42473028058448));
#251444=CARTESIAN_POINT('Origin',(30.2311753956718,-52.9969317578282,3.23423028058445));
#251445=CARTESIAN_POINT('Ctrl Pts',(29.458121752568,-51.6568155675422,3.47153072139037));
#251446=CARTESIAN_POINT('Ctrl Pts',(29.5680161684463,-51.5939283826156,
3.47122746285042));
#251447=CARTESIAN_POINT('Ctrl Pts',(29.6215404675523,-51.6870133715067,
3.40413046676754));
#251448=CARTESIAN_POINT('Ctrl Pts',(29.5155056307128,-51.7564542486368,
3.65553813457951));
#251449=CARTESIAN_POINT('Ctrl Pts',(29.6254251653831,-51.6933631336489,
3.65520336072092));
#251450=CARTESIAN_POINT('Ctrl Pts',(29.6675162799448,-51.766645814766,3.55128134519813));
#251451=CARTESIAN_POINT('Ctrl Pts',(29.6185943474811,-51.9354510367783,
3.77003198860227));
#251452=CARTESIAN_POINT('Ctrl Pts',(29.728640422008,-51.8721362050952,3.76980209314207));
#251453=CARTESIAN_POINT('Ctrl Pts',(29.7501097595413,-51.9097019182958,
3.64284195387483));
#251454=CARTESIAN_POINT('Ctrl Pts',(29.7268821954856,-52.1234703131941,
3.77003198860227));
#251455=CARTESIAN_POINT('Ctrl Pts',(29.8370321718801,-52.0598751946715,
3.77003198860227));
#251456=CARTESIAN_POINT('Ctrl Pts',(29.8368672985589,-52.0599703843279,
3.64284189403769));
#251457=CARTESIAN_POINT('Origin',(29.7268821954856,-52.1234703131941,3.64303198860227));
#251458=CARTESIAN_POINT('Origin',(14.9038494342991,-26.4492244485618,3.23423028058463));
#251459=CARTESIAN_POINT('Origin',(30.1555713378344,-52.8659816883954,3.23423028058444));
#251460=CARTESIAN_POINT('Origin',(14.8448439902567,-26.3470240215573,3.64303198860244));
#251461=CARTESIAN_POINT('Origin',(29.9275190026069,-52.4710850656378,3.64299171721745));
#251462=CARTESIAN_POINT('Ctrl Pts',(30.0450834959843,-52.675764913939,3.48823028058445));
#251463=CARTESIAN_POINT('Ctrl Pts',(30.1558192616008,-52.6124111049551,
3.48852004212223));
#251464=CARTESIAN_POINT('Ctrl Pts',(30.1005764675364,-52.5167277788836,
3.42473028058445));
#251465=CARTESIAN_POINT('Ctrl Pts',(30.0676891808495,-52.7146817640545,
3.41028005848372));
#251466=CARTESIAN_POINT('Ctrl Pts',(30.1782028480957,-52.6511806140151,
3.41074404220182));
#251467=CARTESIAN_POINT('Ctrl Pts',(30.1343304829266,-52.5751914484988,
3.3078048624383));
#251468=CARTESIAN_POINT('Ctrl Pts',(30.1105150503728,-52.7884098752449,
3.36123028058445));
#251469=CARTESIAN_POINT('Ctrl Pts',(30.2206596676797,-52.7247179826669,
3.36146460586487));
#251470=CARTESIAN_POINT('Ctrl Pts',(30.1982769148329,-52.6859499175233,
3.23423045308358));
#251471=CARTESIAN_POINT('Ctrl Pts',(30.1555713378344,-52.8659816883954,
3.36123028058445));
#251472=CARTESIAN_POINT('Ctrl Pts',(30.265556564115,-52.8024816883954,3.36123028058445));
#251473=CARTESIAN_POINT('Ctrl Pts',(30.265556564115,-52.8024816883954,3.23423028058445));
#251474=CARTESIAN_POINT('Origin',(29.9905912412558,-52.5802277788836,3.42473028058445));
#251475=CARTESIAN_POINT('Origin',(29.9499161075317,-52.5097763812719,3.56563113524751));
#251476=CARTESIAN_POINT('Origin',(36.3610285397826,-49.5064990290875,3.56647653909407));
#251477=CARTESIAN_POINT('Origin',(36.3870656659267,-49.5422481179701,3.64299466007515));
#251478=CARTESIAN_POINT('Origin',(36.3129251734949,-49.440290424916,3.4247302805845));
#251479=CARTESIAN_POINT('Ctrl Pts',(36.2478178023256,-49.3516463037379,
3.4882302805845));
#251480=CARTESIAN_POINT('Ctrl Pts',(36.1458216659131,-49.4263574835545,
3.48794691941566));
#251481=CARTESIAN_POINT('Ctrl Pts',(36.2101800152093,-49.5149391519571,
3.42473028058451));
#251482=CARTESIAN_POINT('Ctrl Pts',(36.2214577844001,-49.3151677697908,
3.41028005925053));
#251483=CARTESIAN_POINT('Ctrl Pts',(36.1192316557429,-49.389759474289,3.4098251223104));
#251484=CARTESIAN_POINT('Ctrl Pts',(36.1704998050817,-49.460324028137,3.30780486372858));
#251485=CARTESIAN_POINT('Ctrl Pts',(36.1715192752725,-49.2460589922049,
3.36123028058448));
#251486=CARTESIAN_POINT('Ctrl Pts',(36.0689133127053,-49.3205022166655,
3.36099721048417));
#251487=CARTESIAN_POINT('Ctrl Pts',(36.0953262843484,-49.3568565533015,
3.23423045308315));
#251488=CARTESIAN_POINT('Ctrl Pts',(36.1189794796889,-49.1733470784082,
3.36123028058448));
#251489=CARTESIAN_POINT('Ctrl Pts',(36.0162343214032,-49.2479958054493,
3.36123028058448));
#251490=CARTESIAN_POINT('Ctrl Pts',(36.0162343214032,-49.2479958054493,
3.23423028058448));
#251491=CARTESIAN_POINT('Origin',(36.1189794796889,-49.1733470784082,3.23423028058447));
#251492=CARTESIAN_POINT('Origin',(0.256862895714049,0.186621817603047,3.64303198860263));
#251493=CARTESIAN_POINT('Origin',(36.6229335645815,-49.866980369602,3.64303198860229));
#251494=CARTESIAN_POINT('Origin',(0.256862895714049,0.18662181760305,3.23423028058482));
#251495=CARTESIAN_POINT('Origin',(36.0301015792682,-49.0510171431398,3.23423028058447));
#251496=CARTESIAN_POINT('Ctrl Pts',(36.9399086546492,-50.3023253561989,
3.47153072139037));
#251497=CARTESIAN_POINT('Ctrl Pts',(36.8368401467443,-50.3777877177481,
3.47182327902627));
#251498=CARTESIAN_POINT('Ctrl Pts',(36.7733199672426,-50.2900345588333,
3.40413028958994));
#251499=CARTESIAN_POINT('Ctrl Pts',(36.8722300970264,-50.2093718139428,
3.65553807120923));
#251500=CARTESIAN_POINT('Ctrl Pts',(36.7691625978881,-50.2846371204149,
3.65586275497175));
#251501=CARTESIAN_POINT('Ctrl Pts',(36.7192723137713,-50.2156443459719,
3.5512812683729));
#251502=CARTESIAN_POINT('Ctrl Pts',(36.7506474475462,-50.0423845927719,
3.7700319886023));
#251503=CARTESIAN_POINT('Ctrl Pts',(36.6476776482602,-50.1174266236734,
3.77025505748201));
#251504=CARTESIAN_POINT('Ctrl Pts',(36.6221779017711,-50.0820053531135,
3.64284211731047));
#251505=CARTESIAN_POINT('Ctrl Pts',(36.6229335645815,-49.866980369602,3.77003198860229));
#251506=CARTESIAN_POINT('Ctrl Pts',(36.5200349097938,-49.9417406183798,
3.7700319886023));
#251507=CARTESIAN_POINT('Ctrl Pts',(36.5201885207831,-49.9416290134633,
3.64284239821669));
#251508=CARTESIAN_POINT('Origin',(36.876159719196,-50.2155162706038,3.40423097483275));
#251509=CARTESIAN_POINT('Ctrl Pts',(36.0301015792682,-49.0510171431398,
3.36123028058448));
#251510=CARTESIAN_POINT('Ctrl Pts',(35.9273564209826,-49.1256658701809,
3.36123028058448));
#251511=CARTESIAN_POINT('Ctrl Pts',(35.9273564209826,-49.1256658701809,
3.23423028058448));
#251512=CARTESIAN_POINT('Ctrl Pts',(35.9773846774571,-48.9780591316049,
3.36123028058447));
#251513=CARTESIAN_POINT('Ctrl Pts',(35.874398690302,-49.052775807121,3.36146538610047));
#251514=CARTESIAN_POINT('Ctrl Pts',(35.8479971380629,-49.0164371879487,
3.23423043688354));
#251515=CARTESIAN_POINT('Ctrl Pts',(35.9275383438695,-48.9090707128217,
3.41054258693067));
#251516=CARTESIAN_POINT('Ctrl Pts',(35.8245773199107,-48.9842025736611,
3.4110060885967));
#251517=CARTESIAN_POINT('Ctrl Pts',(35.7729572780235,-48.9131536812757,
3.30819866970723));
#251518=CARTESIAN_POINT('Ctrl Pts',(35.901269362891,-48.8727133447938,3.48823028058448));
#251519=CARTESIAN_POINT('Ctrl Pts',(35.7983524848941,-48.9481071848791,
3.48852004212226));
#251520=CARTESIAN_POINT('Ctrl Pts',(35.7334106856012,-48.8587224664495,
3.42473028058448));
#251521=CARTESIAN_POINT('Origin',(35.8361558438868,-48.7840737394083,3.42473028058447));
#251522=CARTESIAN_POINT('Origin',(36.9808731396208,-50.3596419293476,3.11913648178302));
#251523=CARTESIAN_POINT('Origin',(37.0855865599608,-50.5037675878939,2.83404198860227));
#251524=CARTESIAN_POINT('Origin',(35.7883393560615,-48.7182599900757,3.5656311346079));
#251525=CARTESIAN_POINT('Origin',(35.7621028045857,-48.6820620414853,3.64299171721735));
#251526=CARTESIAN_POINT('Ctrl Pts',(37.0158684358566,-50.9219998155894,
2.59908173515989));
#251527=CARTESIAN_POINT('Ctrl Pts',(36.9939338721439,-50.8918248690994,
2.65878198860227));
#251528=CARTESIAN_POINT('Ctrl Pts',(36.9525415975218,-50.834882333648,2.65878198860227));
#251529=CARTESIAN_POINT('Ctrl Pts',(37.087142649025,-50.8701895025855,2.59908193475562));
#251530=CARTESIAN_POINT('Ctrl Pts',(37.0458491715916,-50.8540829678232,
2.65878715325282));
#251531=CARTESIAN_POINT('Ctrl Pts',(36.993792576411,-50.8048852215544,2.65878198860227));
#251532=CARTESIAN_POINT('Ctrl Pts',(37.1382015956606,-50.8021467555728,
2.63878778849844));
#251533=CARTESIAN_POINT('Ctrl Pts',(37.0800635522222,-50.8006171556816,
2.69564460180099));
#251534=CARTESIAN_POINT('Ctrl Pts',(37.0171501059297,-50.756969208081,2.68180481624857));
#251535=CARTESIAN_POINT('Ctrl Pts',(37.1817767082792,-50.6806663304938,
2.75443238878602));
#251536=CARTESIAN_POINT('Ctrl Pts',(37.0956112176475,-50.7142182018854,
2.79268340777035));
#251537=CARTESIAN_POINT('Ctrl Pts',(37.0243843935853,-50.6618927960193,
2.74885926835567));
#251538=CARTESIAN_POINT('Ctrl Pts',(37.1760624637765,-50.6273693057699,
2.8285665536164));
#251539=CARTESIAN_POINT('Ctrl Pts',(37.0763301845694,-50.681008848973,2.8538419723086));
#251540=CARTESIAN_POINT('Ctrl Pts',(37.0095702365092,-50.6152053999558,
2.79184624278548));
#251541=CARTESIAN_POINT('Ctrl Pts',(37.1493329797266,-50.5905785208478,
2.90134173515986));
#251542=CARTESIAN_POINT('Ctrl Pts',(37.0464195108259,-50.6659240749077,
2.90163218716354));
#251543=CARTESIAN_POINT('Ctrl Pts',(36.9828414016752,-50.5784163149351,
2.83404198860226));
#251544=CARTESIAN_POINT('Origin',(36.9525415975218,-50.834882333648,2.53178198860226));
#251545=CARTESIAN_POINT('Origin',(0.256862895714049,0.186621817603047,3.64303198860263));
#251546=CARTESIAN_POINT('Origin',(35.5261472678871,-48.3573835402113,3.64303198860229));
#251547=CARTESIAN_POINT('Origin',(5.56775724677591E-15,1.86015948644053E-13,
2.53178198860263));
#251548=CARTESIAN_POINT('Origin',(36.9278827595332,-50.8527980281379,2.53178198860227));
#251549=CARTESIAN_POINT('Ctrl Pts',(35.5261472678871,-48.3573835402113,
3.7700319886023));
#251550=CARTESIAN_POINT('Ctrl Pts',(35.4232481927143,-48.4321440944168,
3.7700319886023));
#251551=CARTESIAN_POINT('Ctrl Pts',(35.4234022247162,-48.4320321836168,
3.64284187936949));
#251552=CARTESIAN_POINT('Ctrl Pts',(35.3984257650692,-48.181980616354,3.7700319886023));
#251553=CARTESIAN_POINT('Ctrl Pts',(35.2958250129008,-48.2567602586468,
3.76980208963083));
#251554=CARTESIAN_POINT('Ctrl Pts',(35.3214110399847,-48.2916533613424,
3.64284193928292));
#251555=CARTESIAN_POINT('Ctrl Pts',(35.2768349808773,-48.0150011530595,
3.65553535416552));
#251556=CARTESIAN_POINT('Ctrl Pts',(35.1744900671632,-48.0897561847294,
3.65520057834393));
#251557=CARTESIAN_POINT('Ctrl Pts',(35.2243173504695,-48.1580153629225,
3.55127910964204));
#251558=CARTESIAN_POINT('Ctrl Pts',(35.2091516650533,-47.9220530736681,
3.47153072139038));
#251559=CARTESIAN_POINT('Ctrl Pts',(35.1070032653413,-47.996868104246,3.47122746281548));
#251560=CARTESIAN_POINT('Ctrl Pts',(35.1702703594602,-48.0836260618766,
3.40413045901206));
#251561=CARTESIAN_POINT('Origin',(35.272920853982,-48.0088472823266,3.40423097483277));
#251562=CARTESIAN_POINT('Ctrl Pts',(36.634724144966,-50.9644637245887,2.90134173515988));
#251563=CARTESIAN_POINT('Ctrl Pts',(36.738184035969,-50.8898702560312,2.90163218716356));
#251564=CARTESIAN_POINT('Ctrl Pts',(36.6746059268184,-50.8023624960585,
2.83404198860226));
#251565=CARTESIAN_POINT('Ctrl Pts',(36.6614665482797,-51.0012706547892,
2.82853349835304));
#251566=CARTESIAN_POINT('Ctrl Pts',(36.7432905102111,-50.9229972443175,
2.85381483162273));
#251567=CARTESIAN_POINT('Ctrl Pts',(36.7013469409089,-50.8391683443877,
2.79182701594243));
#251568=CARTESIAN_POINT('Ctrl Pts',(36.7102884597173,-51.023024536943,2.75468822073628));
#251569=CARTESIAN_POINT('Ctrl Pts',(36.7689049964556,-50.9514409225348,
2.79286913083826));
#251570=CARTESIAN_POINT('Ctrl Pts',(36.7410683485318,-50.8675358949422,
2.74900763297879));
#251571=CARTESIAN_POINT('Ctrl Pts',(36.8383381382866,-51.0194219249358,
2.63954450640335));
#251572=CARTESIAN_POINT('Ctrl Pts',(36.8551762168621,-50.9635175930187,
2.69627684028801));
#251573=CARTESIAN_POINT('Ctrl Pts',(36.8330984946711,-50.8901021525735,
2.68224356036454));
#251574=CARTESIAN_POINT('Ctrl Pts',(36.9196318328649,-50.9918932610477,
2.5990817870642));
#251575=CARTESIAN_POINT('Ctrl Pts',(36.9171104726345,-50.9476171190672,
2.65878704321513));
#251576=CARTESIAN_POINT('Ctrl Pts',(36.8864699989244,-50.8828596657507,
2.65878198860226));
#251577=CARTESIAN_POINT('Ctrl Pts',(36.9911673391713,-50.9399462128196,
2.59908173515988));
#251578=CARTESIAN_POINT('Ctrl Pts',(36.9692474126346,-50.9097606317988,
2.65878198860226));
#251579=CARTESIAN_POINT('Ctrl Pts',(36.9278827595333,-50.8527980281379,
2.65878198860226));
#251580=CARTESIAN_POINT('Origin',(36.5718607685328,-50.8770112230996,2.83404198860226));
#251581=CARTESIAN_POINT('Origin',(35.1682072895751,-47.864721425496,3.11913648166955));
#251582=CARTESIAN_POINT('Origin',(35.0634937251227,-47.7205955685085,2.8340419886023));
#251583=CARTESIAN_POINT('Origin',(36.4671473482233,-50.7328855645155,3.11913648177506));
#251584=CARTESIAN_POINT('Origin',(36.3624339277679,-50.5887599058095,3.40423097483275));
#251585=CARTESIAN_POINT('Ctrl Pts',(34.9997217530266,-47.6338034047594,
2.90134173515991));
#251586=CARTESIAN_POINT('Ctrl Pts',(34.8977303031707,-47.7085070967798,
2.90103711553197));
#251587=CARTESIAN_POINT('Ctrl Pts',(34.9607485668371,-47.7952442955496,
2.83404198860229));
#251588=CARTESIAN_POINT('Ctrl Pts',(34.9730146904946,-47.5970451916065,
2.82862991747929));
#251589=CARTESIAN_POINT('Ctrl Pts',(34.8923835282618,-47.6752966590726,
2.85314045886503));
#251590=CARTESIAN_POINT('Ctrl Pts',(34.9340408279393,-47.758484246594,2.79187960999928));
#251591=CARTESIAN_POINT('Ctrl Pts',(34.924446153613,-47.5754322771529,2.75470625793294));
#251592=CARTESIAN_POINT('Ctrl Pts',(34.8665972787031,-47.6469756149918,
2.79224250381878));
#251593=CARTESIAN_POINT('Ctrl Pts',(34.894489194863,-47.730322851409,2.74901809108229));
#251594=CARTESIAN_POINT('Ctrl Pts',(34.7970725085262,-47.579499379098,2.63947868311666));
#251595=CARTESIAN_POINT('Ctrl Pts',(34.7804938560725,-47.635319763777,2.69595066767873));
#251596=CARTESIAN_POINT('Ctrl Pts',(34.8028668197836,-47.7084160893866,
2.68220539436026));
#251597=CARTESIAN_POINT('Ctrl Pts',(34.7162617467346,-47.6073089936879,
2.59908178585027));
#251598=CARTESIAN_POINT('Ctrl Pts',(34.7189078610127,-47.651501311424,2.65877670944819));
#251599=CARTESIAN_POINT('Ctrl Pts',(34.7497660430528,-47.7160937685323,
2.65878198860229));
#251600=CARTESIAN_POINT('Ctrl Pts',(34.6451144164191,-47.659028586093,2.59908173515991));
#251601=CARTESIAN_POINT('Ctrl Pts',(34.6670494534023,-47.6892031885508,
2.65878198860229));
#251602=CARTESIAN_POINT('Ctrl Pts',(34.7084426211237,-47.7461450747859,
2.65878198860229));
#251603=CARTESIAN_POINT('Origin',(34.7084426211237,-47.7461450747859,2.53178198860229));
#251604=CARTESIAN_POINT('Ctrl Pts',(36.1092077731534,-50.2402240048077,
3.77003198860229));
#251605=CARTESIAN_POINT('Ctrl Pts',(36.212106436806,-50.1654637495892,3.77003198860229));
#251606=CARTESIAN_POINT('Ctrl Pts',(36.2119528169387,-50.165575360956,3.64284238727548));
#251607=CARTESIAN_POINT('Ctrl Pts',(36.2365633238593,-50.4158927445,3.77003198860229));
#251608=CARTESIAN_POINT('Ctrl Pts',(36.3397519704552,-50.3411519064793,
3.77025506105769));
#251609=CARTESIAN_POINT('Ctrl Pts',(36.3139437822108,-50.3059538820299,
3.64284210641761));
#251610=CARTESIAN_POINT('Ctrl Pts',(36.3578055460617,-50.5831252836568,
3.65553527987796));
#251611=CARTESIAN_POINT('Ctrl Pts',(36.4612367259639,-50.508360519064,3.65585996533066));
#251612=CARTESIAN_POINT('Ctrl Pts',(36.4110374247146,-50.4395918165622,
3.5512790271021));
#251613=CARTESIAN_POINT('Ctrl Pts',(36.4252947698684,-50.6762142289942,
3.47153072139036));
#251614=CARTESIAN_POINT('Ctrl Pts',(36.5289136700286,-50.6015093986309,
3.47182327905153));
#251615=CARTESIAN_POINT('Ctrl Pts',(36.4650842569437,-50.5139808995216,
3.40413028377944));
#251616=CARTESIAN_POINT('Origin',(36.1092077731534,-50.2402240048077,3.64303198860229));
#251617=CARTESIAN_POINT('Origin',(5.69915478234096E-15,1.86277272141617E-13,
2.53178198860262));
#251618=CARTESIAN_POINT('Origin',(34.6837837831351,-47.7640607692757,2.53178198860229));
#251619=CARTESIAN_POINT('Origin',(21.2404668433939,-29.7751578089174,3.64303198860242));
#251620=CARTESIAN_POINT('Origin',(35.8732562382986,-49.9155525184321,3.64299466007537));
#251621=CARTESIAN_POINT('Ctrl Pts',(34.620500570364,-47.6769115920298,2.59908173515991));
#251622=CARTESIAN_POINT('Ctrl Pts',(34.642420023458,-47.7070975168458,2.6587819886023));
#251623=CARTESIAN_POINT('Ctrl Pts',(34.6837837831352,-47.7640607692757,
2.65878198860229));
#251624=CARTESIAN_POINT('Ctrl Pts',(34.5495693076631,-47.7284183483594,
2.59908193199727));
#251625=CARTESIAN_POINT('Ctrl Pts',(34.590741855859,-47.74461955945,2.65877685806571));
#251626=CARTESIAN_POINT('Ctrl Pts',(34.6425747206412,-47.7939730310143,
2.65878198860229));
#251627=CARTESIAN_POINT('Ctrl Pts',(34.4983910654773,-47.795926104355,2.63872492669799));
#251628=CARTESIAN_POINT('Ctrl Pts',(34.5563698228284,-47.7976714756521,
2.69532212015248));
#251629=CARTESIAN_POINT('Ctrl Pts',(34.6188891978605,-47.8415056181566,
2.68176836726613));
#251630=CARTESIAN_POINT('Ctrl Pts',(34.4545839152295,-47.9165880269722,
2.7544217640218));
#251631=CARTESIAN_POINT('Ctrl Pts',(34.5404685123898,-47.8837591046478,
2.79203179920099));
#251632=CARTESIAN_POINT('Ctrl Pts',(34.611146338977,-47.9359643384876,2.74885310748129));
#251633=CARTESIAN_POINT('Ctrl Pts',(34.4602354682506,-47.9696250311911,
2.82866089558392));
#251634=CARTESIAN_POINT('Ctrl Pts',(34.5595777906771,-47.9171136764618,
2.85316563119149));
#251635=CARTESIAN_POINT('Ctrl Pts',(34.6258166968309,-47.9824460410477,
2.79189751796571));
#251636=CARTESIAN_POINT('Ctrl Pts',(34.4869303039402,-48.0063682005181,
2.90134173515989));
#251637=CARTESIAN_POINT('Ctrl Pts',(34.5894948283139,-47.9324532779032,
2.90103711553195));
#251638=CARTESIAN_POINT('Ctrl Pts',(34.6525130919802,-48.0191904766731,
2.83404198860228));
#251639=CARTESIAN_POINT('Origin',(34.5497679336946,-48.0938392037142,2.83404198860228));
#251640=CARTESIAN_POINT('Origin',(35.8473027479624,-49.8797426632419,3.56647653971822));
#251641=CARTESIAN_POINT('Origin',(35.7991993820668,-49.8135340601217,3.42473028058451));
#251642=CARTESIAN_POINT('Origin',(34.6544814981831,-48.2379650606531,3.1191364816809));
#251643=CARTESIAN_POINT('Origin',(34.759195062554,-48.3820909175324,3.40423097483277));
#251644=CARTESIAN_POINT('Ctrl Pts',(35.6052536882608,-49.5465907136139,
3.36123028058447));
#251645=CARTESIAN_POINT('Ctrl Pts',(35.7079988465464,-49.4719419865727,
3.36123028058447));
#251646=CARTESIAN_POINT('Ctrl Pts',(35.7079988465464,-49.4719419865727,
3.23423028058447));
#251647=CARTESIAN_POINT('Ctrl Pts',(35.6583499840581,-49.6192730640951,
3.36123028058448));
#251648=CARTESIAN_POINT('Ctrl Pts',(35.7608559931245,-49.5446936074928,
3.36099641108458));
#251649=CARTESIAN_POINT('Ctrl Pts',(35.7873581223586,-49.5811706590224,
3.23423043688335));
#251650=CARTESIAN_POINT('Ctrl Pts',(35.7085550527735,-49.688000774918,3.41054258905246));
#251651=CARTESIAN_POINT('Ctrl Pts',(35.8110857017877,-49.6138288703623,
3.41008815826126));
#251652=CARTESIAN_POINT('Ctrl Pts',(35.86239796335,-49.684454139478,3.30819867304337));
#251653=CARTESIAN_POINT('Ctrl Pts',(35.7350130971395,-49.7242207306169,
3.4882302805845));
#251654=CARTESIAN_POINT('Ctrl Pts',(35.8375861910562,-49.6503036646779,
3.48794691941566));
#251655=CARTESIAN_POINT('Ctrl Pts',(35.9019445403524,-49.7388853330806,
3.42473028058451));
#251656=CARTESIAN_POINT('Origin',(35.6052536882608,-49.5465907136139,3.23423028058447));
#251657=CARTESIAN_POINT('Ctrl Pts',(34.6963546279291,-48.2946219293741,
3.4715307213904));
#251658=CARTESIAN_POINT('Ctrl Pts',(34.7990735298992,-48.220592152613,3.47122746285045));
#251659=CARTESIAN_POINT('Ctrl Pts',(34.8620346481364,-48.3075723994623,
3.40413046676756));
#251660=CARTESIAN_POINT('Ctrl Pts',(34.7638392294046,-48.3877165307476,
3.65553813457952));
#251661=CARTESIAN_POINT('Ctrl Pts',(34.866561796066,-48.3134813154519,3.6552033607186));
#251662=CARTESIAN_POINT('Ctrl Pts',(34.9160824571381,-48.3819628268483,
3.55128134519815));
#251663=CARTESIAN_POINT('Ctrl Pts',(34.8850734745852,-48.5549570506147,
3.77003198860229));
#251664=CARTESIAN_POINT('Ctrl Pts',(34.9878985031443,-48.4804861171417,
3.7698020931439));
#251665=CARTESIAN_POINT('Ctrl Pts',(35.0131769156747,-48.5156018845769,
3.64284195387484));
#251666=CARTESIAN_POINT('Ctrl Pts',(35.012421476459,-48.7306271754171,3.77003198860229));
#251667=CARTESIAN_POINT('Ctrl Pts',(35.1153205397472,-48.6558666298463,
3.77003198860229));
#251668=CARTESIAN_POINT('Ctrl Pts',(35.1151665196478,-48.6559785319987,
3.6428418940377));
#251669=CARTESIAN_POINT('Origin',(35.012421476459,-48.7306271754171,3.64303198860229));
#251670=CARTESIAN_POINT('Origin',(20.7197400704249,-29.0584388930976,3.23423028058461));
#251671=CARTESIAN_POINT('Origin',(35.5163757878401,-49.4242607783455,3.23423028058447));
#251672=CARTESIAN_POINT('Origin',(20.6381965522797,-28.9462038689909,3.64303198860242));
#251673=CARTESIAN_POINT('Origin',(35.2482948100404,-49.055365400752,3.64299171721771));
#251674=CARTESIAN_POINT('Ctrl Pts',(35.3866101428265,-49.2466351556007,
3.48823028058447));
#251675=CARTESIAN_POINT('Ctrl Pts',(35.4901170100372,-49.1720533660025,
3.48852004212225));
#251676=CARTESIAN_POINT('Ctrl Pts',(35.4251752107443,-49.0826686475729,
3.42473028058447));
#251677=CARTESIAN_POINT('Ctrl Pts',(35.4131599099223,-49.2829758776394,
3.41028005848372));
#251678=CARTESIAN_POINT('Ctrl Pts',(35.5164304941053,-49.2082707697372,
3.41074404220328));
#251679=CARTESIAN_POINT('Ctrl Pts',(35.4648554356498,-49.137283791733,3.30780486243949));
#251680=CARTESIAN_POINT('Ctrl Pts',(35.4634578610136,-49.3518235761932,
3.36123028058447));
#251681=CARTESIAN_POINT('Ctrl Pts',(35.5663414789302,-49.2769673468818,
3.36146460586282));
#251682=CARTESIAN_POINT('Ctrl Pts',(35.5400289748697,-49.2407512920131,
3.23423045308296));
#251683=CARTESIAN_POINT('Ctrl Pts',(35.5163757878401,-49.4242607783455,
3.36123028058448));
#251684=CARTESIAN_POINT('Ctrl Pts',(35.6191209461258,-49.3496120513043,
3.36123028058447));
#251685=CARTESIAN_POINT('Ctrl Pts',(35.6191209461258,-49.3496120513043,
3.23423028058448));
#251686=CARTESIAN_POINT('Origin',(35.3224300524587,-49.157317374614,3.42473028058447));
#251687=CARTESIAN_POINT('Origin',(35.2746135650482,-49.0915036263505,3.56563113524804));
#251688=CARTESIAN_POINT('Origin',(41.3366772861966,-45.4345348113606,3.56647653909422));
#251689=CARTESIAN_POINT('Origin',(41.3663085755626,-45.4673664422105,3.64299466007593));
#251690=CARTESIAN_POINT('Origin',(41.2819167515334,-45.3737170758066,3.42473028058452));
#251691=CARTESIAN_POINT('Ctrl Pts',(41.2079002115913,-45.292364129855,3.48823028058452));
#251692=CARTESIAN_POINT('Ctrl Pts',(41.1142722655012,-45.3773275334099,
3.48794691941568));
#251693=CARTESIAN_POINT('Ctrl Pts',(41.1875373586978,-45.4586966628142,
3.42473028058454));
#251694=CARTESIAN_POINT('Ctrl Pts',(41.1778715515046,-45.2588408013008,
3.41028005925054));
#251695=CARTESIAN_POINT('Ctrl Pts',(41.0840023845213,-45.3437094247702,
3.40982512231053));
#251696=CARTESIAN_POINT('Ctrl Pts',(41.1423656859475,-45.408528437742,3.30780486372896));
#251697=CARTESIAN_POINT('Ctrl Pts',(41.1209827764392,-45.1953306044433,
3.36123028058451));
#251698=CARTESIAN_POINT('Ctrl Pts',(41.0267203359238,-45.2800912647208,
3.36099721048405));
#251699=CARTESIAN_POINT('Ctrl Pts',(41.0567886774861,-45.3134855411631,
3.23423045308344));
#251700=CARTESIAN_POINT('Ctrl Pts',(41.0611303347409,-45.1285089182126,
3.3612302805845));
#251701=CARTESIAN_POINT('Ctrl Pts',(40.9667509419053,-45.2134885052202,
3.3612302805845));
#251702=CARTESIAN_POINT('Ctrl Pts',(40.9667509419053,-45.2134885052202,
3.2342302805845));
#251703=CARTESIAN_POINT('Origin',(41.0611303347409,-45.1285089182126,3.2342302805845));
#251704=CARTESIAN_POINT('Origin',(0.235948482089076,0.212448967519124,3.64303198860263));
#251705=CARTESIAN_POINT('Origin',(41.6348281284267,-45.7656648676099,3.64303198860231));
#251706=CARTESIAN_POINT('Origin',(0.235948482089076,0.212448967519127,3.23423028058482));
#251707=CARTESIAN_POINT('Origin',(40.959952356613,-45.0161393894786,3.2342302805845));
#251708=CARTESIAN_POINT('Ctrl Pts',(41.9955727382256,-46.1654920697605,
3.4715307213904));
#251709=CARTESIAN_POINT('Ctrl Pts',(41.900956815079,-46.2513146333396,3.47182327902631));
#251710=CARTESIAN_POINT('Ctrl Pts',(41.8286119029185,-46.1706818621616,
3.40413028959028));
#251711=CARTESIAN_POINT('Ctrl Pts',(41.9185486398946,-46.0801220723601,
3.65553807120925));
#251712=CARTESIAN_POINT('Ctrl Pts',(41.82391312212,-46.1657485548994,3.65586275496646));
#251713=CARTESIAN_POINT('Ctrl Pts',(41.7670844335132,-46.1023486848279,
3.55128126837224));
#251714=CARTESIAN_POINT('Ctrl Pts',(41.7801771152784,-45.9267584721662,
3.77003198860231));
#251715=CARTESIAN_POINT('Ctrl Pts',(41.6856154235002,-46.0121526898581,
3.77025505748641));
#251716=CARTESIAN_POINT('Ctrl Pts',(41.6565528363087,-45.9795909100377,
3.64284211731136));
#251717=CARTESIAN_POINT('Ctrl Pts',(41.6348281284267,-45.76566486761,3.77003198860232));
#251718=CARTESIAN_POINT('Ctrl Pts',(41.5403077371551,-45.8507714101796,
3.77003198860231));
#251719=CARTESIAN_POINT('Ctrl Pts',(41.5404488407565,-45.8506443599262,
3.64284239821728));
#251720=CARTESIAN_POINT('Origin',(41.9230990057961,-46.0858221116771,3.40423097483278));
#251721=CARTESIAN_POINT('Ctrl Pts',(40.959952356613,-45.0161393894786,3.3612302805845));
#251722=CARTESIAN_POINT('Ctrl Pts',(40.8655729637774,-45.1011189764862,
3.3612302805845));
#251723=CARTESIAN_POINT('Ctrl Pts',(40.8655729637774,-45.1011189764862,
3.2342302805845));
#251724=CARTESIAN_POINT('Ctrl Pts',(40.8998980546775,-44.9490914662989,
3.3612302805845));
#251725=CARTESIAN_POINT('Ctrl Pts',(40.8052862548063,-45.0341638030259,
3.36146538610179));
#251726=CARTESIAN_POINT('Ctrl Pts',(40.7752309130136,-45.0007839642926,
3.23423043688384));
#251727=CARTESIAN_POINT('Ctrl Pts',(40.8431135311204,-44.8856913339431,
3.41054258693068));
#251728=CARTESIAN_POINT('Ctrl Pts',(40.7485699563807,-44.9711739721972,
3.41100608859567));
#251729=CARTESIAN_POINT('Ctrl Pts',(40.6898060629479,-44.9059100567322,
3.30819866970758));
#251730=CARTESIAN_POINT('Ctrl Pts',(40.8131880745612,-44.8522789915935,
3.48823028058449));
#251731=CARTESIAN_POINT('Ctrl Pts',(40.7187157882343,-44.9380175594356,
3.48852004212228));
#251732=CARTESIAN_POINT('Ctrl Pts',(40.6447864996558,-44.8559107663279,
3.42473028058449));
#251733=CARTESIAN_POINT('Origin',(40.7391658924914,-44.7709311793203,3.4247302805845));
#251734=CARTESIAN_POINT('Origin',(42.0423040287741,-46.2182127020635,3.11913648178416));
#251735=CARTESIAN_POINT('Origin',(42.1615090516458,-46.3506032922587,2.8340419886023));
#251736=CARTESIAN_POINT('Origin',(40.6847319383109,-44.7104761485832,3.56563113460798));
#251737=CARTESIAN_POINT('Origin',(40.6548553974687,-44.6772189625509,3.64299171721763));
#251738=CARTESIAN_POINT('Ctrl Pts',(42.1358900227701,-46.773831928425,2.59908173515991));
#251739=CARTESIAN_POINT('Ctrl Pts',(42.1109214781067,-46.7461150696865,
2.6587819886023));
#251740=CARTESIAN_POINT('Ctrl Pts',(42.0638038389706,-46.6938111422597,
2.6587819886023));
#251741=CARTESIAN_POINT('Ctrl Pts',(42.2013581359414,-46.7148552537627,
2.59908193475685));
#251742=CARTESIAN_POINT('Ctrl Pts',(42.1586072771697,-46.7031532960215,
2.65878715325369));
#251743=CARTESIAN_POINT('Ctrl Pts',(42.1016932886505,-46.6596664560516,
2.6587819886023));
#251744=CARTESIAN_POINT('Ctrl Pts',(42.2450249725429,-46.6418481388113,
2.63878778849814));
#251745=CARTESIAN_POINT('Ctrl Pts',(42.1870455286633,-46.6464039985657,
2.69564460180075));
#251746=CARTESIAN_POINT('Ctrl Pts',(42.1199142759252,-46.609571404849,2.68180481624819));
#251747=CARTESIAN_POINT('Ctrl Pts',(42.2756632139855,-46.5164783566515,
2.7544323887864));
#251748=CARTESIAN_POINT('Ctrl Pts',(42.1934768724835,-46.5588531737041,
2.79268340777068));
#251749=CARTESIAN_POINT('Ctrl Pts',(42.1171707421508,-46.5142596423488,
2.74885926835611));
#251750=CARTESIAN_POINT('Ctrl Pts',(42.2644092166197,-46.4640705998039,
2.82856655361619));
#251751=CARTESIAN_POINT('Ctrl Pts',(42.1708301402948,-46.5278411618555,
2.85384197230716));
#251752=CARTESIAN_POINT('Ctrl Pts',(42.097557576812,-46.4693765057994,2.79184624278455));
#251753=CARTESIAN_POINT('Ctrl Pts',(42.2339804752707,-46.4302753505418,
2.90134173515992));
#251754=CARTESIAN_POINT('Ctrl Pts',(42.1395065321005,-46.5159655405268,
2.9016321871636));
#251755=CARTESIAN_POINT('Ctrl Pts',(42.0671296588101,-46.4355828792663,
2.8340419886023));
#251756=CARTESIAN_POINT('Origin',(42.0638038389706,-46.6938111422597,2.53178198860229));
#251757=CARTESIAN_POINT('Origin',(0.235948482089076,0.212448967519124,3.64303198860263));
#251758=CARTESIAN_POINT('Origin',(40.3862543050944,-44.3789831537289,3.64303198860232));
#251759=CARTESIAN_POINT('Origin',(5.55434424446678E-15,1.86005087008946E-13,
2.53178198860262));
#251760=CARTESIAN_POINT('Origin',(42.0411527846901,-46.7142062431416,2.5317819886023));
#251761=CARTESIAN_POINT('Ctrl Pts',(40.3862543050944,-44.3789831537289,
3.77003198860233));
#251762=CARTESIAN_POINT('Ctrl Pts',(40.2917335276661,-44.4640900439955,
3.77003198860233));
#251763=CARTESIAN_POINT('Ctrl Pts',(40.2918750180005,-44.4639626455262,
3.64284187936968));
#251764=CARTESIAN_POINT('Ctrl Pts',(40.2408978759506,-44.2178916378556,
3.77003198860233));
#251765=CARTESIAN_POINT('Ctrl Pts',(40.1466757825319,-44.3029863283953,
3.76980208962652));
#251766=CARTESIAN_POINT('Ctrl Pts',(40.1757689690827,-44.335013814935,3.64284193928157));
#251767=CARTESIAN_POINT('Ctrl Pts',(40.1025190720993,-44.0645366033533,
3.65553535416555));
#251768=CARTESIAN_POINT('Ctrl Pts',(40.0085488431155,-44.1495800756913,
3.65520057834686));
#251769=CARTESIAN_POINT('Ctrl Pts',(40.0652381943489,-44.2122569536115,
3.55127910964328));
#251770=CARTESIAN_POINT('Ctrl Pts',(40.0254908126594,-43.9791725362576,
3.47153072139041));
#251771=CARTESIAN_POINT('Ctrl Pts',(39.9317222927446,-44.0642551375171,
3.47122746281551));
#251772=CARTESIAN_POINT('Ctrl Pts',(40.0037114790894,-44.1439246138544,
3.40413045901217));
#251773=CARTESIAN_POINT('Origin',(40.0979831325504,-44.0588255818371,3.4042309748328));
#251774=CARTESIAN_POINT('Ctrl Pts',(41.7612723673368,-46.8559036426978,
2.90134173515992));
#251775=CARTESIAN_POINT('Ctrl Pts',(41.8563683535936,-46.7709043015495,
2.90163218716359));
#251776=CARTESIAN_POINT('Ctrl Pts',(41.7839914803032,-46.690521640289,2.8340419886023));
#251777=CARTESIAN_POINT('Ctrl Pts',(41.7917156448195,-46.88971359836,2.82853349835323));
#251778=CARTESIAN_POINT('Ctrl Pts',(41.8649095672158,-46.8033160448216,
2.85381483162249));
#251779=CARTESIAN_POINT('Ctrl Pts',(41.814433263085,-46.7243306652201,2.79182701594126));
#251780=CARTESIAN_POINT('Ctrl Pts',(41.8425440045886,-46.906245031096,2.75468822073613));
#251781=CARTESIAN_POINT('Ctrl Pts',(41.8933569085963,-46.8289264627099,
2.79286913083832));
#251782=CARTESIAN_POINT('Ctrl Pts',(41.8569022891478,-46.7483907976675,
2.74900763297862));
#251783=CARTESIAN_POINT('Ctrl Pts',(41.9695156381237,-46.8892773184513,
2.63954450640359));
#251784=CARTESIAN_POINT('Ctrl Pts',(41.9804178820376,-46.8319191778361,
2.6962768402881));
#251785=CARTESIAN_POINT('Ctrl Pts',(41.950787100749,-46.7612136652285,2.68224356036478));
#251786=CARTESIAN_POINT('Ctrl Pts',(42.0474864684055,-46.8534019544972,
2.59908178706358));
#251787=CARTESIAN_POINT('Ctrl Pts',(42.0403508033704,-46.8096319157664,
2.65878704321398));
#251788=CARTESIAN_POINT('Ctrl Pts',(42.0031091843002,-46.7484320121843,
2.6587819886023));
#251789=CARTESIAN_POINT('Ctrl Pts',(42.1132001506006,-46.794261981091,2.59908173515991));
#251790=CARTESIAN_POINT('Ctrl Pts',(42.0882450513181,-46.7665330160772,
2.6587819886023));
#251791=CARTESIAN_POINT('Ctrl Pts',(42.0411527846901,-46.7142062431416,
2.6587819886023));
#251792=CARTESIAN_POINT('Origin',(41.6896120874676,-46.7755012272966,2.8340419886023));
#251793=CARTESIAN_POINT('Origin',(39.9787779456782,-43.9264348094998,3.11913648166838));
#251794=CARTESIAN_POINT('Origin',(39.859572758736,-43.7940440370138,2.83404198860232));
#251795=CARTESIAN_POINT('Origin',(41.5704070646248,-46.6431106370586,3.11913648177637));
#251796=CARTESIAN_POINT('Origin',(41.451202041618,-46.510720046715,3.40423097483279));
#251797=CARTESIAN_POINT('Ctrl Pts',(39.7870778846752,-43.7143933160617,
2.90134173515993));
#251798=CARTESIAN_POINT('Ctrl Pts',(39.6934538167806,-43.7993487829606,
2.90103711553199));
#251799=CARTESIAN_POINT('Ctrl Pts',(39.7651933659004,-43.8790236240213,
2.83404198860232));
#251800=CARTESIAN_POINT('Ctrl Pts',(39.7566748466929,-43.6806281164514,
2.82862991747937));
#251801=CARTESIAN_POINT('Ctrl Pts',(39.6846648960488,-43.766879165672,2.85314045886381));
#251802=CARTESIAN_POINT('Ctrl Pts',(39.7347894633642,-43.845256669365,2.79187960999885));
#251803=CARTESIAN_POINT('Ctrl Pts',(39.7061132086036,-43.6642103943278,
2.75470625793291));
#251804=CARTESIAN_POINT('Ctrl Pts',(39.6560595510445,-43.7414086642724,
2.79224250381877));
#251805=CARTESIAN_POINT('Ctrl Pts',(39.6925108309095,-43.8213838166739,
2.74901809108231));
#251806=CARTESIAN_POINT('Ctrl Pts',(39.579862457588,-43.6815693876449,2.63947868311675));
#251807=CARTESIAN_POINT('Ctrl Pts',(39.5692094437569,-43.73881692348,2.69595066767879));
#251808=CARTESIAN_POINT('Ctrl Pts',(39.5991004926185,-43.8091742082544,
2.68220539436029));
#251809=CARTESIAN_POINT('Ctrl Pts',(39.5024012818823,-43.7176736830018,
2.59908178585043));
#251810=CARTESIAN_POINT('Ctrl Pts',(39.5096522555313,-43.7613473163391,
2.65877670944801));
#251811=CARTESIAN_POINT('Ctrl Pts',(39.5470931435013,-43.8223603708606,
2.65878198860232));
#251812=CARTESIAN_POINT('Ctrl Pts',(39.4370498736014,-43.7765468711716,
2.59908173515994));
#251813=CARTESIAN_POINT('Ctrl Pts',(39.4620188529815,-43.8042633382923,
2.65878198860232));
#251814=CARTESIAN_POINT('Ctrl Pts',(39.5091373124628,-43.856566526705,2.65878198860232));
#251815=CARTESIAN_POINT('Origin',(39.5091373124628,-43.856566526705,2.53178198860232));
#251816=CARTESIAN_POINT('Ctrl Pts',(41.1629311642486,-46.1905628026478,
3.77003198860232));
#251817=CARTESIAN_POINT('Ctrl Pts',(41.2574515636633,-46.1054562527462,
3.77003198860232));
#251818=CARTESIAN_POINT('Ctrl Pts',(41.2573104519068,-46.1055833103425,
3.64284238727614));
#251819=CARTESIAN_POINT('Ctrl Pts',(41.307951431325,-46.351956930601,3.77003198860231));
#251820=CARTESIAN_POINT('Ctrl Pts',(41.4027622547794,-46.2668393800552,
3.770255061059));
#251821=CARTESIAN_POINT('Ctrl Pts',(41.3734162510852,-46.2345318643249,
3.64284210641861));
#251822=CARTESIAN_POINT('Ctrl Pts',(41.4460100362753,-46.5056000892401,
3.65553527987802));
#251823=CARTESIAN_POINT('Ctrl Pts',(41.541059563395,-46.4204333915652,3.65585996532922));
#251824=CARTESIAN_POINT('Ctrl Pts',(41.4839469723832,-46.3572886670207,
3.55127902710143));
#251825=CARTESIAN_POINT('Ctrl Pts',(41.5228599914568,-46.5911245387423,
3.4715307213904));
#251826=CARTESIAN_POINT('Ctrl Pts',(41.6181024753231,-46.5059978248575,
3.47182327905157));
#251827=CARTESIAN_POINT('Ctrl Pts',(41.5454735069385,-46.4256208064855,
3.40413028377981));
#251828=CARTESIAN_POINT('Origin',(41.1629311642486,-46.1905628026478,3.64303198860232));
#251829=CARTESIAN_POINT('Origin',(5.70392627685665E-15,1.86281136021691E-13,
2.53178198860262));
#251830=CARTESIAN_POINT('Origin',(39.4864862581822,-43.8769616275868,2.53178198860232));
#251831=CARTESIAN_POINT('Origin',(27.6232705441551,-31.1532462714323,3.64303198860241));
#251832=CARTESIAN_POINT('Origin',(40.8943347850531,-45.8923335519892,3.64299466007435));
#251833=CARTESIAN_POINT('Ctrl Pts',(39.4144401478995,-43.796904759634,2.59908173515994));
#251834=CARTESIAN_POINT('Ctrl Pts',(39.4393948122693,-43.8246341160479,
2.65878198860232));
#251835=CARTESIAN_POINT('Ctrl Pts',(39.4864862581822,-43.8769616275868,
2.65878198860232));
#251836=CARTESIAN_POINT('Ctrl Pts',(39.3492813761644,-43.8555436924512,
2.5990819319977));
#251837=CARTESIAN_POINT('Ctrl Pts',(39.391921864532,-43.8673524484207,2.65877685806562));
#251838=CARTESIAN_POINT('Ctrl Pts',(39.4486296259959,-43.9110175468,2.65878198860232));
#251839=CARTESIAN_POINT('Ctrl Pts',(39.305439975737,-43.9280312169039,2.63872492669775));
#251840=CARTESIAN_POINT('Ctrl Pts',(39.3632835603683,-43.9237065964663,
2.69532212015237));
#251841=CARTESIAN_POINT('Ctrl Pts',(39.4300423632771,-43.9607655567551,
2.68176836726605));
#251842=CARTESIAN_POINT('Ctrl Pts',(39.274485410988,-44.0526112349799,2.75442176402213));
#251843=CARTESIAN_POINT('Ctrl Pts',(39.3564679665378,-44.0109847679675,
2.79203179920121));
#251844=CARTESIAN_POINT('Ctrl Pts',(39.4322155454634,-44.0555161714738,
2.74885310748144));
#251845=CARTESIAN_POINT('Ctrl Pts',(39.2856498807585,-44.1047669487868,
2.82866089558373));
#251846=CARTESIAN_POINT('Ctrl Pts',(39.3789590643336,-44.0421591564527,
2.85316563119135));
#251847=CARTESIAN_POINT('Ctrl Pts',(39.4516641985005,-44.1002097724414,
2.79189751796553));
#251848=CARTESIAN_POINT('Ctrl Pts',(39.3160391863695,-44.1385184650369,
2.90134173515994));
#251849=CARTESIAN_POINT('Ctrl Pts',(39.4103156382737,-44.0542875439834,
2.901037115532));
#251850=CARTESIAN_POINT('Ctrl Pts',(39.4820551873935,-44.1339623850441,
2.83404198860232));
#251851=CARTESIAN_POINT('Origin',(39.3876757945579,-44.2189419720517,2.83404198860232));
#251852=CARTESIAN_POINT('Origin',(40.8647803215176,-45.8594327453962,3.56647653971777));
#251853=CARTESIAN_POINT('Origin',(40.8100197873553,-45.7986150108445,3.42473028058453));
#251854=CARTESIAN_POINT('Origin',(39.5068809815269,-44.3513327444847,3.11913648168179));
#251855=CARTESIAN_POINT('Origin',(39.6260861683723,-44.483723516875,3.40423097483281));
#251856=CARTESIAN_POINT('Ctrl Pts',(40.5892333705628,-45.5534068532505,
3.3612302805845));
#251857=CARTESIAN_POINT('Ctrl Pts',(40.6836127633984,-45.4684272662429,
3.3612302805845));
#251858=CARTESIAN_POINT('Ctrl Pts',(40.6836127633984,-45.4684272662429,
3.2342302805845));
#251859=CARTESIAN_POINT('Ctrl Pts',(40.6496361736987,-45.620140968006,3.3612302805845));
#251860=CARTESIAN_POINT('Ctrl Pts',(40.7437849681316,-45.5352552698632,
3.36099641108314));
#251861=CARTESIAN_POINT('Ctrl Pts',(40.7739548060703,-45.5687622694495,
3.23423043688344));
#251862=CARTESIAN_POINT('Ctrl Pts',(40.7067502157884,-45.683244322559,3.41054258905254));
#251863=CARTESIAN_POINT('Ctrl Pts',(40.8009661159811,-45.5987613682809,
3.41008815826137));
#251864=CARTESIAN_POINT('Ctrl Pts',(40.8593796344539,-45.6636361529295,
3.30819867304344));
#251865=CARTESIAN_POINT('Ctrl Pts',(40.7368493365303,-45.71650024283,3.48823028058452));
#251866=CARTESIAN_POINT('Ctrl Pts',(40.8311340869943,-45.6322662944326,
3.48794691941568));
#251867=CARTESIAN_POINT('Ctrl Pts',(40.9043991801909,-45.7136354238369,
3.42473028058453));
#251868=CARTESIAN_POINT('Origin',(40.5892333705628,-45.5534068532505,3.2342302805845));
#251869=CARTESIAN_POINT('Ctrl Pts',(39.5544469813076,-44.4033023070483,
3.47153072139043));
#251870=CARTESIAN_POINT('Ctrl Pts',(39.648864959584,-44.3189410241789,3.47122746285048));
#251871=CARTESIAN_POINT('Ctrl Pts',(39.7205730817656,-44.3988635551997,
3.40413046676773));
#251872=CARTESIAN_POINT('Ctrl Pts',(39.6312929306927,-44.4888328647708,
3.65553813457958));
#251873=CARTESIAN_POINT('Ctrl Pts',(39.7256930794106,-44.404266885713,3.65520336072251));
#251874=CARTESIAN_POINT('Ctrl Pts',(39.7821007282716,-44.4671969296237,
3.55128134519942));
#251875=CARTESIAN_POINT('Ctrl Pts',(39.7693444365344,-44.6424847942241,
3.77003198860233));
#251876=CARTESIAN_POINT('Ctrl Pts',(39.8638218465944,-44.5576736780981,
3.7698020931396));
#251877=CARTESIAN_POINT('Ctrl Pts',(39.8926323785411,-44.5899547640674,
3.64284195387346));
#251878=CARTESIAN_POINT('Ctrl Pts',(39.9143573409162,-44.8038810887668,
3.77003198860233));
#251879=CARTESIAN_POINT('Ctrl Pts',(40.0088781074275,-44.7187742083299,
3.77003198860233));
#251880=CARTESIAN_POINT('Ctrl Pts',(40.0087366280265,-44.7189015969548,
3.64284189403801));
#251881=CARTESIAN_POINT('Origin',(39.9143573409162,-44.8038810887668,3.64303198860232));
#251882=CARTESIAN_POINT('Origin',(26.948440628206,-30.4037717213981,3.2342302805846));
#251883=CARTESIAN_POINT('Origin',(40.4880553924349,-45.4410373245165,3.2342302805845));
#251884=CARTESIAN_POINT('Origin',(26.8427652369017,-30.2864073093061,3.64303198860241));
#251885=CARTESIAN_POINT('Origin',(40.1828829233546,-45.1021848870404,3.64299171721753));
#251886=CARTESIAN_POINT('Ctrl Pts',(40.3404336838198,-45.2779489569766,
3.4882302805845));
#251887=CARTESIAN_POINT('Ctrl Pts',(40.4355776097274,-45.1929563204583,
3.48852004212227));
#251888=CARTESIAN_POINT('Ctrl Pts',(40.3616483211489,-45.1108495273506,
3.42473028058449));
#251889=CARTESIAN_POINT('Ctrl Pts',(40.3706366483421,-45.311315394383,3.41028005848376));
#251890=CARTESIAN_POINT('Ctrl Pts',(40.4655326953337,-45.2262248134145,
3.410744042204));
#251891=CARTESIAN_POINT('Ctrl Pts',(40.4068200107205,-45.1610177711048,
3.30780486243926));
#251892=CARTESIAN_POINT('Ctrl Pts',(40.4278556061251,-45.3745283705064,
3.3612302805845));
#251893=CARTESIAN_POINT('Ctrl Pts',(40.5223510102001,-45.2893279449748,
3.36146460586259));
#251894=CARTESIAN_POINT('Ctrl Pts',(40.4923970402299,-45.2560606910598,
3.23423045308319));
#251895=CARTESIAN_POINT('Ctrl Pts',(40.4880553924349,-45.4410373245165,
3.3612302805845));
#251896=CARTESIAN_POINT('Ctrl Pts',(40.5824347852705,-45.3560577375089,
3.3612302805845));
#251897=CARTESIAN_POINT('Ctrl Pts',(40.5824347852705,-45.3560577375089,
3.23423028058451));
#251898=CARTESIAN_POINT('Origin',(40.2672689283133,-45.1958291143582,3.4247302805845));
#251899=CARTESIAN_POINT('Origin',(40.2128349746532,-45.1353740846434,3.56563113524767));
#251900=CARTESIAN_POINT('Origin',(45.8594327460075,-40.8647803224525,3.56647653909432));
#251901=CARTESIAN_POINT('Origin',(45.8923335519901,-40.8943347850511,3.64299466007529));
#251902=CARTESIAN_POINT('Origin',(45.7986150108456,-40.810019787354,3.42473028058456));
#251903=CARTESIAN_POINT('Ctrl Pts',(45.7165002428312,-40.736849336529,3.48823028058456));
#251904=CARTESIAN_POINT('Ctrl Pts',(45.6322662944337,-40.831134086993,3.48794691941572));
#251905=CARTESIAN_POINT('Ctrl Pts',(45.7136354238381,-40.9043991801896,
3.42473028058457));
#251906=CARTESIAN_POINT('Ctrl Pts',(45.6831319408685,-40.7066485019696,
3.41028005925058));
#251907=CARTESIAN_POINT('Ctrl Pts',(45.5986481857988,-40.8008642060155,
3.4098251223095));
#251908=CARTESIAN_POINT('Ctrl Pts',(45.6634671987668,-40.8592275074402,
3.30780486372854));
#251909=CARTESIAN_POINT('Ctrl Pts',(45.6199161851861,-40.6494327168502,
3.36123028058454));
#251910=CARTESIAN_POINT('Ctrl Pts',(45.535030025744,-40.7435821574108,3.36099721048374));
#251911=CARTESIAN_POINT('Ctrl Pts',(45.5684243021863,-40.7736504989773,
3.23423045308361));
#251912=CARTESIAN_POINT('Ctrl Pts',(45.5534068532516,-40.5892333705615,
3.36123028058454));
#251913=CARTESIAN_POINT('Ctrl Pts',(45.468427266244,-40.6836127633972,3.36123028058454));
#251914=CARTESIAN_POINT('Ctrl Pts',(45.4684272662441,-40.6836127633972,
3.23423028058454));
#251915=CARTESIAN_POINT('Origin',(45.5534068532516,-40.5892333705615,3.23423028058454));
#251916=CARTESIAN_POINT('Origin',(0.21244896751894,0.235948482089259,3.64303198860263));
#251917=CARTESIAN_POINT('Origin',(46.190562802649,-41.1629311642473,3.64303198860234));
#251918=CARTESIAN_POINT('Origin',(0.21244896751894,0.235948482089262,3.23423028058482));
#251919=CARTESIAN_POINT('Origin',(45.4410373245177,-40.4880553924336,3.23423028058454));
#251920=CARTESIAN_POINT('Ctrl Pts',(46.5911245387435,-41.5228599914555,
3.47153072139043));
#251921=CARTESIAN_POINT('Ctrl Pts',(46.5059978322082,-41.6181024670989,
3.47182327902633));
#251922=CARTESIAN_POINT('Ctrl Pts',(46.4256208133858,-41.5454735131712,
3.40413028959021));
#251923=CARTESIAN_POINT('Ctrl Pts',(46.5055987918451,-41.4460088704661,
3.65553807120927));
#251924=CARTESIAN_POINT('Ctrl Pts',(46.4204321019755,-41.5410583874223,
3.65586275497085));
#251925=CARTESIAN_POINT('Ctrl Pts',(46.3572876358795,-41.4839460439592,
3.55128126837205));
#251926=CARTESIAN_POINT('Ctrl Pts',(46.3519544194676,-41.3079491749508,
3.77003198860234));
#251927=CARTESIAN_POINT('Ctrl Pts',(46.2668368728761,-41.4027599825067,
3.77025505748214));
#251928=CARTESIAN_POINT('Ctrl Pts',(46.2345298607754,-41.3734144471008,
3.6428421173117));
#251929=CARTESIAN_POINT('Ctrl Pts',(46.190562802649,-41.1629311642473,3.77003198860235));
#251930=CARTESIAN_POINT('Ctrl Pts',(46.1054562600792,-41.2574515555191,
3.77003198860235));
#251931=CARTESIAN_POINT('Ctrl Pts',(46.1055833103327,-41.2573104519176,
3.64284239821712));
#251932=CARTESIAN_POINT('Origin',(46.5107200467162,-41.4512020416167,3.40423097483282));
#251933=CARTESIAN_POINT('Ctrl Pts',(45.4410373245177,-40.4880553924336,
3.36123028058454));
#251934=CARTESIAN_POINT('Ctrl Pts',(45.3560577375101,-40.5824347852693,
3.36123028058454));
#251935=CARTESIAN_POINT('Ctrl Pts',(45.3560577375101,-40.5824347852693,
3.23423028058454));
#251936=CARTESIAN_POINT('Ctrl Pts',(45.3743035899565,-40.4276521486862,
3.36123028058454));
#251937=CARTESIAN_POINT('Ctrl Pts',(45.289102564049,-40.5221480762958,3.36146538610066));
#251938=CARTESIAN_POINT('Ctrl Pts',(45.2557227253168,-40.4920927345057,
3.23423043688334));
#251939=CARTESIAN_POINT('Ctrl Pts',(45.3112030195546,-40.3705349278744,
3.4105425869307));
#251940=CARTESIAN_POINT('Ctrl Pts',(45.226112733224,-40.4654317778737,3.4110060885973));
#251941=CARTESIAN_POINT('Ctrl Pts',(45.1608488177557,-40.4066678844394,
3.30819866970787));
#251942=CARTESIAN_POINT('Ctrl Pts',(45.2779489569777,-40.3404336838185,
3.48823028058454));
#251943=CARTESIAN_POINT('Ctrl Pts',(45.1929563204594,-40.4355776097261,
3.48852004212231));
#251944=CARTESIAN_POINT('Ctrl Pts',(45.1108495273517,-40.3616483211477,
3.42473028058453));
#251945=CARTESIAN_POINT('Origin',(45.1958291143593,-40.267268928312,3.42473028058454));
#251946=CARTESIAN_POINT('Origin',(46.6431106370702,-41.5704070646301,3.11913648178396));
#251947=CARTESIAN_POINT('Origin',(46.7755012272978,-41.6896120874663,2.83404198860233));
#251948=CARTESIAN_POINT('Origin',(45.1353740836147,-40.2128349741379,3.56563113460728));
#251949=CARTESIAN_POINT('Origin',(45.1021848870414,-40.1828829233538,3.64299171721789));
#251950=CARTESIAN_POINT('Ctrl Pts',(46.7942619810922,-42.1132001505994,
2.59908173515994));
#251951=CARTESIAN_POINT('Ctrl Pts',(46.7665330160784,-42.0882450513168,
2.65878198860233));
#251952=CARTESIAN_POINT('Ctrl Pts',(46.7142062431428,-42.0411527846888,
2.65878198860233));
#251953=CARTESIAN_POINT('Ctrl Pts',(46.8532067119187,-42.0477032750696,
2.59908193475573));
#251954=CARTESIAN_POINT('Ctrl Pts',(46.8094668591649,-42.0405341034483,
2.65878715325369));
#251955=CARTESIAN_POINT('Ctrl Pts',(46.7483190388757,-42.0032346206964,
2.65878198860233));
#251956=CARTESIAN_POINT('Ctrl Pts',(46.8890030154869,-41.9705316734057,
2.63878778849843));
#251957=CARTESIAN_POINT('Ctrl Pts',(46.8318174060861,-41.9811230778535,
2.69564460180073));
#251958=CARTESIAN_POINT('Ctrl Pts',(46.7612038509551,-41.9515093836251,
2.6818048162486));
#251959=CARTESIAN_POINT('Ctrl Pts',(46.9063687067671,-41.8426461117362,
2.75443238878615));
#251960=CARTESIAN_POINT('Ctrl Pts',(46.8290619651513,-41.8933796070859,
2.79268340777078));
#251961=CARTESIAN_POINT('Ctrl Pts',(46.7485125544804,-41.8570065263028,
2.74885926835575));
#251962=CARTESIAN_POINT('Ctrl Pts',(46.8896982576905,-41.7917018131132,
2.82856655361643));
#251963=CARTESIAN_POINT('Ctrl Pts',(46.8032976561896,-41.8649047103977,
2.85384197230743));
#251964=CARTESIAN_POINT('Ctrl Pts',(46.7243152668226,-41.8144193983031,
2.7918462427841));
#251965=CARTESIAN_POINT('Ctrl Pts',(46.855903642699,-41.7612723673355,2.90134173515995));
#251966=CARTESIAN_POINT('Ctrl Pts',(46.7709043015507,-41.8563683535923,
2.90163218716363));
#251967=CARTESIAN_POINT('Ctrl Pts',(46.6905216402902,-41.7839914803019,
2.83404198860233));
#251968=CARTESIAN_POINT('Origin',(46.7142062431428,-42.0411527846888,2.53178198860233));
#251969=CARTESIAN_POINT('Origin',(0.21244896751894,0.235948482089259,3.64303198860263));
#251970=CARTESIAN_POINT('Origin',(44.8038810887679,-39.914357340915,3.64303198860235));
#251971=CARTESIAN_POINT('Origin',(5.54214007001405E-15,1.85992882834493E-13,
2.53178198860262));
#251972=CARTESIAN_POINT('Origin',(46.6938111422609,-42.0638038389693,2.53178198860233));
#251973=CARTESIAN_POINT('Ctrl Pts',(44.8038810887679,-39.914357340915,3.77003198860236));
#251974=CARTESIAN_POINT('Ctrl Pts',(44.7187741985015,-40.0088781183431,
3.77003198860237));
#251975=CARTESIAN_POINT('Ctrl Pts',(44.7189015969706,-40.0087366280089,
3.64284187936997));
#251976=CARTESIAN_POINT('Ctrl Pts',(44.6424822887504,-39.7693421853875,
3.77003198860237));
#251977=CARTESIAN_POINT('Ctrl Pts',(44.5576711710536,-39.8638196089392,
3.76980208962785));
#251978=CARTESIAN_POINT('Ctrl Pts',(44.5899527660337,-39.8926305794717,
3.64284193928197));
#251979=CARTESIAN_POINT('Ctrl Pts',(44.4888315723767,-39.6312917695228,
3.65553535416558));
#251980=CARTESIAN_POINT('Ctrl Pts',(44.4042655856122,-39.7256919284505,
3.65520057834616));
#251981=CARTESIAN_POINT('Ctrl Pts',(44.4671959043829,-39.7820998051089,
3.55127910964262));
#251982=CARTESIAN_POINT('Ctrl Pts',(44.4033023070494,-39.5544469813064,
3.47153072139045));
#251983=CARTESIAN_POINT('Ctrl Pts',(44.3189410144585,-39.6488649704632,
3.47122746281555));
#251984=CARTESIAN_POINT('Ctrl Pts',(44.3988635644387,-39.7205730900528,
3.40413045901234));
#251985=CARTESIAN_POINT('Origin',(44.4837235168761,-39.6260861683711,3.40423097483283));
#251986=CARTESIAN_POINT('Ctrl Pts',(46.430275350543,-42.2339804752694,2.90134173515995));
#251987=CARTESIAN_POINT('Ctrl Pts',(46.515965540528,-42.1395065320992,2.90163218716363));
#251988=CARTESIAN_POINT('Ctrl Pts',(46.4355828792675,-42.0671296588088,
2.83404198860233));
#251989=CARTESIAN_POINT('Ctrl Pts',(46.464085959275,-42.2644230274446,2.82853349835333));
#251990=CARTESIAN_POINT('Ctrl Pts',(46.5278479142045,-42.1708479205175,
2.85381483162383));
#251991=CARTESIAN_POINT('Ctrl Pts',(46.4693919041987,-42.0975714415906,
2.79182701594139));
#251992=CARTESIAN_POINT('Ctrl Pts',(46.5163638812304,-42.2755508889254,
2.75468822073606));
#251993=CARTESIAN_POINT('Ctrl Pts',(46.5588164356978,-42.193344484977,2.79286913083796));
#251994=CARTESIAN_POINT('Ctrl Pts',(46.5141432491637,-42.1170605480842,
2.74900763297871));
#251995=CARTESIAN_POINT('Ctrl Pts',(46.6408663419436,-42.245403977454,2.63954450640372));
#251996=CARTESIAN_POINT('Ctrl Pts',(46.6457133039304,-42.187220455932,2.69627684028839));
#251997=CARTESIAN_POINT('Ctrl Pts',(46.6088541045845,-42.119999535554,2.68224356036476));
#251998=CARTESIAN_POINT('Ctrl Pts',(46.714660043196,-42.2015749714284,2.59908178706311));
#251999=CARTESIAN_POINT('Ctrl Pts',(46.7029882531952,-42.1587905896503,
2.65878704321522));
#252000=CARTESIAN_POINT('Ctrl Pts',(46.6595535157378,-42.1018187547551,
2.65878198860233));
#252001=CARTESIAN_POINT('Ctrl Pts',(46.7738319284262,-42.1358900227688,
2.59908173515994));
#252002=CARTESIAN_POINT('Ctrl Pts',(46.7461150696877,-42.1109214781054,
2.65878198860233));
#252003=CARTESIAN_POINT('Ctrl Pts',(46.6938111422609,-42.0638038389693,
2.65878198860233));
#252004=CARTESIAN_POINT('Origin',(46.3506032922599,-42.1615090516445,2.83404198860233));
#252005=CARTESIAN_POINT('Origin',(44.3513327445038,-39.5068809815363,3.11913648166901));
#252006=CARTESIAN_POINT('Origin',(44.2189419720528,-39.3876757945567,2.83404198860235));
#252007=CARTESIAN_POINT('Origin',(46.2182127020562,-42.0423040287639,3.11913648177653));
#252008=CARTESIAN_POINT('Origin',(46.0858221116783,-41.9230990057948,3.4042309748328));
#252009=CARTESIAN_POINT('Ctrl Pts',(44.1385184650381,-39.3160391863683,
2.90134173515997));
#252010=CARTESIAN_POINT('Ctrl Pts',(44.0542875439845,-39.4103156382725,
2.90103711553202));
#252011=CARTESIAN_POINT('Ctrl Pts',(44.1339623850452,-39.4820551873923,
2.83404198860235));
#252012=CARTESIAN_POINT('Ctrl Pts',(44.1047525536511,-39.285636938894,2.82862991747939));
#252013=CARTESIAN_POINT('Ctrl Pts',(44.0421527706791,-39.3789425853225,
2.85314045886471));
#252014=CARTESIAN_POINT('Ctrl Pts',(44.1001954303881,-39.4516512848555,
2.79187960999985));
#252015=CARTESIAN_POINT('Ctrl Pts',(44.0527517782421,-39.2745942850993,
2.75470625793293));
#252016=CARTESIAN_POINT('Ctrl Pts',(44.0110417363805,-39.356601686749,2.79224250381871));
#252017=CARTESIAN_POINT('Ctrl Pts',(44.0556530121008,-39.4323285306294,
2.74901809108237));
#252018=CARTESIAN_POINT('Ctrl Pts',(43.9290071509461,-39.3050549810244,
2.63947868311676));
#252019=CARTESIAN_POINT('Ctrl Pts',(43.924396492386,-39.3631024520336,2.69595066767885));
#252020=CARTESIAN_POINT('Ctrl Pts',(43.9614781338114,-39.4299498468373,
2.68220539436029));
#252021=CARTESIAN_POINT('Ctrl Pts',(43.8557442421761,-39.3490583909331,
2.5990817858497));
#252022=CARTESIAN_POINT('Ctrl Pts',(43.8675206320095,-39.3917348424031,
2.65877670944714));
#252023=CARTESIAN_POINT('Ctrl Pts',(43.9111340157069,-39.4485000225459,
2.65878198860235));
#252024=CARTESIAN_POINT('Ctrl Pts',(43.7969047596351,-39.4144401478983,
2.59908173515997));
#252025=CARTESIAN_POINT('Ctrl Pts',(43.824634116049,-39.4393948122681,2.65878198860235));
#252026=CARTESIAN_POINT('Ctrl Pts',(43.8769616275879,-39.486486258181,2.65878198860235));
#252027=CARTESIAN_POINT('Origin',(43.8769616275879,-39.486486258181,2.53178198860235));
#252028=CARTESIAN_POINT('Ctrl Pts',(45.7656648676111,-41.6348281284255,
3.77003198860235));
#252029=CARTESIAN_POINT('Ctrl Pts',(45.8507714175131,-41.5403077290104,
3.77003198860235));
#252030=CARTESIAN_POINT('Ctrl Pts',(45.8506443599165,-41.5404488407673,
3.64284238727559));
#252031=CARTESIAN_POINT('Ctrl Pts',(45.9267609786678,-41.7801793767969,
3.77003198860235));
#252032=CARTESIAN_POINT('Ctrl Pts',(46.0121552117538,-41.6856176794247,
3.77025506105598));
#252033=CARTESIAN_POINT('Ctrl Pts',(45.9795929135651,-41.6565546403126,
3.6428421064184));
#252034=CARTESIAN_POINT('Ctrl Pts',(46.0801233673988,-41.9185498083207,
3.65553527987807));
#252035=CARTESIAN_POINT('Ctrl Pts',(46.1657498592337,-41.823914281722,3.65585996533128));
#252036=CARTESIAN_POINT('Ctrl Pts',(46.1023497159522,-41.7670853619614,
3.55127902710157));
#252037=CARTESIAN_POINT('Ctrl Pts',(46.1654920697617,-41.9955727382244,
3.47153072139041));
#252038=CARTESIAN_POINT('Ctrl Pts',(46.2513146407509,-41.9009568069084,
3.47182327905159));
#252039=CARTESIAN_POINT('Ctrl Pts',(46.1706818552412,-41.8286118967071,
3.40413028377952));
#252040=CARTESIAN_POINT('Origin',(45.7656648676111,-41.6348281284255,3.64303198860235));
#252041=CARTESIAN_POINT('Origin',(5.70826774717982E-15,1.86285477492014E-13,
2.53178198860262));
#252042=CARTESIAN_POINT('Origin',(43.8565665267061,-39.5091373124615,2.53178198860235));
#252043=CARTESIAN_POINT('Origin',(34.1507877370015,-31.1767457860023,3.64303198860241));
#252044=CARTESIAN_POINT('Origin',(45.4673664422113,-41.3663085755614,3.64299466007682));
#252045=CARTESIAN_POINT('Ctrl Pts',(43.7765468711727,-39.4370498736001,
2.59908173515997));
#252046=CARTESIAN_POINT('Ctrl Pts',(43.8042633382934,-39.4620188529802,
2.65878198860235));
#252047=CARTESIAN_POINT('Ctrl Pts',(43.8565665267061,-39.5091373124615,
2.65878198860235));
#252048=CARTESIAN_POINT('Ctrl Pts',(43.7178744835421,-39.5021785224855,
2.59908193199766));
#252049=CARTESIAN_POINT('Ctrl Pts',(43.7615157339677,-39.5094654441323,
2.65877685806628));
#252050=CARTESIAN_POINT('Ctrl Pts',(43.8224770900131,-39.5469637653733,
2.65878198860235));
#252051=CARTESIAN_POINT('Ctrl Pts',(43.6818502604301,-39.5788516269094,
2.63872492669768));
#252052=CARTESIAN_POINT('Ctrl Pts',(43.7389249259235,-39.5685043961835,
2.69532212015245));
#252053=CARTESIAN_POINT('Ctrl Pts',(43.8091917332947,-39.5983821485326,
2.68176836726621));
#252054=CARTESIAN_POINT('Ctrl Pts',(43.6640874258695,-39.7059848156952,
2.75442176402224));
#252055=CARTESIAN_POINT('Ctrl Pts',(43.7412697217743,-39.6560168722784,
2.79203179920111));
#252056=CARTESIAN_POINT('Ctrl Pts',(43.8212571467122,-39.6923865500756,
2.74885310748133));
#252057=CARTESIAN_POINT('Ctrl Pts',(43.6806424921203,-39.7566878101774,
2.82866089558371));
#252058=CARTESIAN_POINT('Ctrl Pts',(43.7668962219034,-39.6846695243133,
2.85316563119134));
#252059=CARTESIAN_POINT('Ctrl Pts',(43.8452710114196,-39.734802377006,2.79189751796581));
#252060=CARTESIAN_POINT('Ctrl Pts',(43.7143933160628,-39.787077884674,2.90134173515996));
#252061=CARTESIAN_POINT('Ctrl Pts',(43.7993487829618,-39.6934538167793,
2.90103711553202));
#252062=CARTESIAN_POINT('Ctrl Pts',(43.8790236240225,-39.7651933658992,
2.83404198860234));
#252063=CARTESIAN_POINT('Origin',(43.7940440370149,-39.8595727587348,2.83404198860235));
#252064=CARTESIAN_POINT('Origin',(45.434534810367,-41.3366772856856,3.56647653971801));
#252065=CARTESIAN_POINT('Origin',(45.3737170758078,-41.2819167515321,3.42473028058456));
#252066=CARTESIAN_POINT('Origin',(43.9264348094903,-39.9787779456548,3.11913648168266));
#252067=CARTESIAN_POINT('Origin',(44.0588255818383,-40.0979831325492,3.40423097483283));
#252068=CARTESIAN_POINT('Ctrl Pts',(45.1285089182138,-41.0611303347397,
3.36123028058453));
#252069=CARTESIAN_POINT('Ctrl Pts',(45.2134885052213,-40.9667509419041,
3.36123028058454));
#252070=CARTESIAN_POINT('Ctrl Pts',(45.2134885052213,-40.9667509419041,
3.23423028058453));
#252071=CARTESIAN_POINT('Ctrl Pts',(45.195556442937,-41.1211850608431,3.36123028058453));
#252072=CARTESIAN_POINT('Ctrl Pts',(45.2803165088406,-41.0269231466347,
3.36099641108291));
#252073=CARTESIAN_POINT('Ctrl Pts',(45.3138235084273,-41.0570929845754,
3.23423043688364));
#252074=CARTESIAN_POINT('Ctrl Pts',(45.2589537050094,-41.1779726855636,
3.41054258905254));
#252075=CARTESIAN_POINT('Ctrl Pts',(45.3438226072621,-41.0841042944886,
3.41008815826071));
#252076=CARTESIAN_POINT('Ctrl Pts',(45.4086973919088,-41.1425178129604,
3.308198673043));
#252077=CARTESIAN_POINT('Ctrl Pts',(45.2923641298562,-41.20790021159,3.48823028058455));
#252078=CARTESIAN_POINT('Ctrl Pts',(45.377327533411,-41.1142722654999,3.48794691941571));
#252079=CARTESIAN_POINT('Ctrl Pts',(45.4586966628153,-41.1875373586965,
3.42473028058456));
#252080=CARTESIAN_POINT('Origin',(45.1285089182138,-41.0611303347397,3.23423028058453));
#252081=CARTESIAN_POINT('Ctrl Pts',(43.9791725362587,-40.0254908126581,
3.47153072139045));
#252082=CARTESIAN_POINT('Ctrl Pts',(44.0642551277136,-39.9317223035489,
3.4712274628505));
#252083=CARTESIAN_POINT('Ctrl Pts',(44.143924604647,-40.0037114707673,3.4041304667676));
#252084=CARTESIAN_POINT('Ctrl Pts',(44.0645378932532,-40.1025202360392,
3.65553813457958));
#252085=CARTESIAN_POINT('Ctrl Pts',(44.1495813562435,-40.008550015784,3.65520336072267));
#252086=CARTESIAN_POINT('Ctrl Pts',(44.2122579788845,-40.0652391174772,
3.55128134519978));
#252087=CARTESIAN_POINT('Ctrl Pts',(44.217894138565,-40.240900132389,3.77003198860236));
#252088=CARTESIAN_POINT('Ctrl Pts',(44.3029888158522,-40.1466780419433,
3.76980209313978));
#252089=CARTESIAN_POINT('Ctrl Pts',(44.3350158129998,-40.1757707681167,
3.6428419538732));
#252090=CARTESIAN_POINT('Ctrl Pts',(44.37898315373,-40.3862543050931,3.77003198860236));
#252091=CARTESIAN_POINT('Ctrl Pts',(44.4640900341671,-40.2917335385817,
3.77003198860236));
#252092=CARTESIAN_POINT('Ctrl Pts',(44.463962645542,-40.2918750179829,3.64284189403775));
#252093=CARTESIAN_POINT('Origin',(44.37898315373,-40.3862543050931,3.64303198860235));
#252094=CARTESIAN_POINT('Origin',(33.3184119221875,-30.4272712359681,3.2342302805846));
#252095=CARTESIAN_POINT('Origin',(45.0161393894798,-40.9599523566118,3.23423028058453));
#252096=CARTESIAN_POINT('Origin',(33.1880655373225,-30.3099068238761,3.64303198860241));
#252097=CARTESIAN_POINT('Origin',(44.677218962552,-40.6548553974674,3.6429917172175));
#252098=CARTESIAN_POINT('Ctrl Pts',(44.8522789915946,-40.8131880745599,
3.48823028058453));
#252099=CARTESIAN_POINT('Ctrl Pts',(44.9380175594367,-40.718715788233,3.48852004212231));
#252100=CARTESIAN_POINT('Ctrl Pts',(44.855910766329,-40.6447864996546,3.42473028058453));
#252101=CARTESIAN_POINT('Ctrl Pts',(44.8858042435448,-40.8432146576624,
3.4102800584838));
#252102=CARTESIAN_POINT('Ctrl Pts',(44.9712860523949,-40.7486708738375,
3.41074404220322));
#252103=CARTESIAN_POINT('Ctrl Pts',(44.9060790100844,-40.6899581892272,
3.30780486243906));
#252104=CARTESIAN_POINT('Ctrl Pts',(44.9493173051415,-40.9001003367632,
3.36123028058453));
#252105=CARTESIAN_POINT('Ctrl Pts',(45.0343891839554,-40.8054891887032,
3.36146460586378));
#252106=CARTESIAN_POINT('Ctrl Pts',(45.0011219300373,-40.7755352187347,
3.2342304530841));
#252107=CARTESIAN_POINT('Ctrl Pts',(45.0161393894798,-40.9599523566118,
3.36123028058453));
#252108=CARTESIAN_POINT('Ctrl Pts',(45.1011189764874,-40.8655729637762,
3.36123028058453));
#252109=CARTESIAN_POINT('Ctrl Pts',(45.1011189764874,-40.8655729637762,
3.23423028058453));
#252110=CARTESIAN_POINT('Origin',(44.7709311793215,-40.7391658924902,3.42473028058453));
#252111=CARTESIAN_POINT('Origin',(44.7104761492018,-40.6847319392787,3.56563113524736));
#252112=CARTESIAN_POINT('Origin',(49.8797426639505,-35.8473027488283,3.56647653909349));
#252113=CARTESIAN_POINT('Origin',(49.9155525184332,-35.8732562382981,3.64299466007415));
#252114=CARTESIAN_POINT('Origin',(49.8135340601227,-35.7991993820654,3.42473028058459));
#252115=CARTESIAN_POINT('Ctrl Pts',(49.7242207306179,-35.7350130971381,
3.4882302805846));
#252116=CARTESIAN_POINT('Ctrl Pts',(49.650303664679,-35.8375861910549,3.48794691941576));
#252117=CARTESIAN_POINT('Ctrl Pts',(49.7388853330816,-35.9019445403511,
3.42473028058461));
#252118=CARTESIAN_POINT('Ctrl Pts',(49.6878783768803,-35.7084656432344,
3.41028005925061));
#252119=CARTESIAN_POINT('Ctrl Pts',(49.6137056554155,-35.8109961808836,
3.40982512231138));
#252120=CARTESIAN_POINT('Ctrl Pts',(49.6842702092623,-35.862264330224,3.307804863728));
#252121=CARTESIAN_POINT('Ctrl Pts',(49.6190282456271,-35.6581711379706,
3.36123028058457));
#252122=CARTESIAN_POINT('Ctrl Pts',(49.5444483977905,-35.7606778378451,
3.3609972104828));
#252123=CARTESIAN_POINT('Ctrl Pts',(49.5808027344254,-35.7870908094897,
3.23423045308385));
#252124=CARTESIAN_POINT('Ctrl Pts',(49.5465907136149,-35.6052536882594,
3.36123028058457));
#252125=CARTESIAN_POINT('Ctrl Pts',(49.4719419865738,-35.707998846545,3.36123028058457));
#252126=CARTESIAN_POINT('Ctrl Pts',(49.4719419865738,-35.707998846545,3.23423028058457));
#252127=CARTESIAN_POINT('Origin',(49.5465907136149,-35.6052536882594,3.23423028058457));
#252128=CARTESIAN_POINT('Origin',(0.186621817602863,0.256862895714232,3.64303198860263));
#252129=CARTESIAN_POINT('Origin',(50.2402240048087,-36.1092077731521,3.64303198860238));
#252130=CARTESIAN_POINT('Origin',(0.186621817602863,0.256862895714235,3.23423028058482));
#252131=CARTESIAN_POINT('Origin',(49.4242607783465,-35.5163757878388,3.23423028058457));
#252132=CARTESIAN_POINT('Ctrl Pts',(50.6762142289952,-36.4252947698671,
3.47153072139047));
#252133=CARTESIAN_POINT('Ctrl Pts',(50.6015094050819,-36.5289136610809,
3.47182327902638));
#252134=CARTESIAN_POINT('Ctrl Pts',(50.5139809070358,-36.4650842624213,
3.40413028959007));
#252135=CARTESIAN_POINT('Ctrl Pts',(50.583123871509,-36.3578045222534,3.65553807120933));
#252136=CARTESIAN_POINT('Ctrl Pts',(50.5083591136191,-36.4612356912204,
3.65586275496775));
#252137=CARTESIAN_POINT('Ctrl Pts',(50.4395906940212,-36.411036609159,3.55128126837191));
#252138=CARTESIAN_POINT('Ctrl Pts',(50.4158900112693,-36.2365613423283,
3.77003198860238));
#252139=CARTESIAN_POINT('Ctrl Pts',(50.3411491755206,-36.3397499727037,
3.77025505748543));
#252140=CARTESIAN_POINT('Ctrl Pts',(50.3059517008897,-36.3139421975378,
3.64284211731174));
#252141=CARTESIAN_POINT('Ctrl Pts',(50.2402240048087,-36.1092077731521,
3.77003198860239));
#252142=CARTESIAN_POINT('Ctrl Pts',(50.1654637560309,-36.2121064279398,
3.77003198860239));
#252143=CARTESIAN_POINT('Ctrl Pts',(50.1655753609474,-36.2119528169505,
3.64284239821683));
#252144=CARTESIAN_POINT('Origin',(50.5887599058106,-36.3624339277665,3.40423097483285));
#252145=CARTESIAN_POINT('Ctrl Pts',(49.4242607783465,-35.5163757878388,
3.36123028058457));
#252146=CARTESIAN_POINT('Ctrl Pts',(49.3496120513053,-35.6191209461244,
3.36123028058457));
#252147=CARTESIAN_POINT('Ctrl Pts',(49.3496120513054,-35.6191209461244,
3.23423028058457));
#252148=CARTESIAN_POINT('Ctrl Pts',(49.3515787599213,-35.4632790141014,
3.36123028058457));
#252149=CARTESIAN_POINT('Ctrl Pts',(49.2767219882466,-35.5661632154394,
3.36146538610215));
#252150=CARTESIAN_POINT('Ctrl Pts',(49.2403833690726,-35.5397616632044,
3.23423043688358));
#252151=CARTESIAN_POINT('Ctrl Pts',(49.2828534857282,-35.4130704930576,
3.41054258693075));
#252152=CARTESIAN_POINT('Ctrl Pts',(49.2081487547888,-35.5163418450519,
3.41100608859616));
#252153=CARTESIAN_POINT('Ctrl Pts',(49.1370998624009,-35.4647218031658,
3.30819866970762));
#252154=CARTESIAN_POINT('Ctrl Pts',(49.2466351556017,-35.3866101428252,
3.48823028058457));
#252155=CARTESIAN_POINT('Ctrl Pts',(49.1720533660035,-35.4901170100359,
3.48852004212235));
#252156=CARTESIAN_POINT('Ctrl Pts',(49.0826686475739,-35.425175210743,3.42473028058457));
#252157=CARTESIAN_POINT('Origin',(49.1573173746151,-35.3224300524574,3.42473028058457));
#252158=CARTESIAN_POINT('Origin',(50.7328855645279,-36.4671473482298,3.11913648178386));
#252159=CARTESIAN_POINT('Origin',(50.8770112231007,-36.5718607685314,2.83404198860237));
#252160=CARTESIAN_POINT('Origin',(49.0915036252748,-35.2746135646418,3.56563113460774));
#252161=CARTESIAN_POINT('Origin',(49.0553654007531,-35.2482948100387,3.64299171721751));
#252162=CARTESIAN_POINT('Ctrl Pts',(50.9399462128206,-36.99116733917,2.59908173515998));
#252163=CARTESIAN_POINT('Ctrl Pts',(50.9097606317998,-36.9692474126332,
2.65878198860237));
#252164=CARTESIAN_POINT('Ctrl Pts',(50.8527980281389,-36.9278827595319,
2.65878198860237));
#252165=CARTESIAN_POINT('Ctrl Pts',(50.9917217504968,-36.9198678602466,
2.59908193475485));
#252166=CARTESIAN_POINT('Ctrl Pts',(50.9474721267433,-36.9173100216915,
2.6587871532533));
#252167=CARTESIAN_POINT('Ctrl Pts',(50.8827604229973,-36.8866065570947,
2.65878198860237));
#252168=CARTESIAN_POINT('Ctrl Pts',(51.019255329238,-36.8393772800886,2.63878778849845));
#252169=CARTESIAN_POINT('Ctrl Pts',(50.9634900918198,-36.8558881875862,
2.69564460180069));
#252170=CARTESIAN_POINT('Ctrl Pts',(50.8901678911829,-36.833817846677,2.68180481624849));
#252171=CARTESIAN_POINT('Ctrl Pts',(51.0231582082094,-36.7103770798832,
2.7544323887862));
#252172=CARTESIAN_POINT('Ctrl Pts',(50.951578055318,-36.7689134067385,2.79268340777093));
#252173=CARTESIAN_POINT('Ctrl Pts',(50.8676678805081,-36.7411592876123,
2.74885926835594));
#252174=CARTESIAN_POINT('Ctrl Pts',(51.0012539523504,-36.6614543958815,
2.82856655361644));
#252175=CARTESIAN_POINT('Ctrl Pts',(50.9229784487449,-36.7432876021357,
2.85384197230816));
#252176=CARTESIAN_POINT('Ctrl Pts',(50.8391515810791,-36.7013347616501,
2.79184624278423));
#252177=CARTESIAN_POINT('Ctrl Pts',(50.9644637245897,-36.6347241449646,
2.90134173515999));
#252178=CARTESIAN_POINT('Ctrl Pts',(50.8898702560322,-36.7381840359676,
2.90163218716366));
#252179=CARTESIAN_POINT('Ctrl Pts',(50.8023624960595,-36.674605926817,2.83404198860237));
#252180=CARTESIAN_POINT('Origin',(50.8527980281389,-36.9278827595319,2.53178198860236));
#252181=CARTESIAN_POINT('Origin',(0.186621817602863,0.256862895714232,3.64303198860263));
#252182=CARTESIAN_POINT('Origin',(48.7306271754181,-35.0124214764577,3.64303198860239));
#252183=CARTESIAN_POINT('Origin',(5.53127843490691E-15,1.85979469832184E-13,
2.53178198860262));
#252184=CARTESIAN_POINT('Origin',(50.8348823336491,-36.9525415975204,2.53178198860237));
#252185=CARTESIAN_POINT('Ctrl Pts',(48.7306271754181,-35.0124214764577,
3.77003198860239));
#252186=CARTESIAN_POINT('Ctrl Pts',(48.6558666212128,-35.1153205516302,
3.77003198860239));
#252187=CARTESIAN_POINT('Ctrl Pts',(48.6559785320126,-35.1151665196287,
3.64284187937003));
#252188=CARTESIAN_POINT('Ctrl Pts',(48.5549543235587,-34.8850714976616,
3.77003198860239));
#252189=CARTESIAN_POINT('Ctrl Pts',(48.4804833899324,-34.9878965398032,
3.76980208963104));
#252190=CARTESIAN_POINT('Ctrl Pts',(48.5155997094336,-35.0131753353115,
3.64284193928289));
#252191=CARTESIAN_POINT('Ctrl Pts',(48.3877151240604,-34.7638382096847,
3.65553535416562));
#252192=CARTESIAN_POINT('Ctrl Pts',(48.3134799021691,-34.8665607873053,
3.65520057834284));
#252193=CARTESIAN_POINT('Ctrl Pts',(48.3819617107282,-34.9160816462002,
3.55127910964184));
#252194=CARTESIAN_POINT('Ctrl Pts',(48.2946219293751,-34.6963546279277,
3.47153072139048));
#252195=CARTESIAN_POINT('Ctrl Pts',(48.2205921440833,-34.7990735417346,
3.47122746281559));
#252196=CARTESIAN_POINT('Ctrl Pts',(48.3075724095167,-34.8620346554123,
3.40413045901239));
#252197=CARTESIAN_POINT('Origin',(48.3820909175334,-34.7591950625526,3.40423097483286));
#252198=CARTESIAN_POINT('Ctrl Pts',(50.5905785208489,-37.1493329797253,
2.90134173515998));
#252199=CARTESIAN_POINT('Ctrl Pts',(50.6659240749088,-37.0464195108245,
2.90163218716366));
#252200=CARTESIAN_POINT('Ctrl Pts',(50.5784163149361,-36.9828414016739,
2.83404198860236));
#252201=CARTESIAN_POINT('Ctrl Pts',(50.6273860247248,-37.1760745934425,
2.82853349835314));
#252202=CARTESIAN_POINT('Ctrl Pts',(50.6810174228652,-37.0763471615757,
2.85381483162217));
#252203=CARTESIAN_POINT('Ctrl Pts',(50.6152221632645,-37.0095824157637,
2.79182701594132));
#252204=CARTESIAN_POINT('Ctrl Pts',(50.680540741014,-37.1816769644883,2.75468822073637));
#252205=CARTESIAN_POINT('Ctrl Pts',(50.7141678268704,-37.095483395542,2.79286913083809));
#252206=CARTESIAN_POINT('Ctrl Pts',(50.6617655220316,-37.0242869695744,
2.74900763297886));
#252207=CARTESIAN_POINT('Ctrl Pts',(50.8012099538931,-37.1386811500602,
2.63954450640347));
#252208=CARTESIAN_POINT('Ctrl Pts',(50.7999485296229,-37.0803097184688,
2.69627684028837));
#252209=CARTESIAN_POINT('Ctrl Pts',(50.7562647493206,-37.0173098767914,
2.68224356036466));
#252210=CARTESIAN_POINT('Ctrl Pts',(50.8700180268814,-37.0873787017253,
2.59908178706366));
#252211=CARTESIAN_POINT('Ctrl Pts',(50.8539379904877,-37.0460487315392,
2.65878704321445));
#252212=CARTESIAN_POINT('Ctrl Pts',(50.8047860147157,-36.9939291606749,
2.65878198860237));
#252213=CARTESIAN_POINT('Ctrl Pts',(50.9219998155904,-37.0158684358552,
2.59908173515998));
#252214=CARTESIAN_POINT('Ctrl Pts',(50.8918248691005,-36.9939338721425,
2.65878198860237));
#252215=CARTESIAN_POINT('Ctrl Pts',(50.8348823336491,-36.9525415975204,
2.65878198860237));
#252216=CARTESIAN_POINT('Origin',(50.503767587895,-37.0855865599595,2.83404198860236));
#252217=CARTESIAN_POINT('Origin',(48.2379650606707,-34.6544814981893,3.11913648166982));
#252218=CARTESIAN_POINT('Origin',(48.0938392037152,-34.5497679336933,2.83404198860239));
#252219=CARTESIAN_POINT('Origin',(50.3596419293386,-36.9808731396133,3.11913648177573));
#252220=CARTESIAN_POINT('Origin',(50.2155162706049,-36.8761597191946,3.40423097483285));
#252221=CARTESIAN_POINT('Ctrl Pts',(48.0063682005191,-34.4869303039389,
2.90134173516));
#252222=CARTESIAN_POINT('Ctrl Pts',(47.9324532779042,-34.5894948283126,
2.90103711553205));
#252223=CARTESIAN_POINT('Ctrl Pts',(48.019190476674,-34.6525130919789,2.83404198860238));
#252224=CARTESIAN_POINT('Ctrl Pts',(47.9696093621204,-34.4602241019842,
2.82862991747951));
#252225=CARTESIAN_POINT('Ctrl Pts',(47.9171056031461,-34.5595620694339,
2.85314045886484));
#252226=CARTESIAN_POINT('Ctrl Pts',(47.9824304277188,-34.6258053530814,
2.79187960999931));
#252227=CARTESIAN_POINT('Ctrl Pts',(47.9167391807674,-34.4546775021458,
2.75470625793289));
#252228=CARTESIAN_POINT('Ctrl Pts',(47.88382973855,-34.5405955452474,2.79224250381846));
#252229=CARTESIAN_POINT('Ctrl Pts',(47.9361122396532,-34.611244401458,2.74901809108239));
#252230=CARTESIAN_POINT('Ctrl Pts',(47.7968564492225,-34.4979061669204,
2.63947868311689));
#252231=CARTESIAN_POINT('Ctrl Pts',(47.7983386612738,-34.5561175928637,
2.69595066767908));
#252232=CARTESIAN_POINT('Ctrl Pts',(47.8422046210398,-34.6187227036509,
2.68220539436033));
#252233=CARTESIAN_POINT('Ctrl Pts',(47.728594491149,-34.5493265808139,2.59908178585035));
#252234=CARTESIAN_POINT('Ctrl Pts',(47.7447672725775,-34.5905382782863,
2.65877670944851));
#252235=CARTESIAN_POINT('Ctrl Pts',(47.7940753146426,-34.6424336528564,
2.65878198860238));
#252236=CARTESIAN_POINT('Ctrl Pts',(47.6769115920308,-34.6205005703627,
2.59908173516));
#252237=CARTESIAN_POINT('Ctrl Pts',(47.7070975168468,-34.6424200234567,
2.65878198860238));
#252238=CARTESIAN_POINT('Ctrl Pts',(47.7640607692767,-34.6837837831338,
2.65878198860238));
#252239=CARTESIAN_POINT('Origin',(47.7640607692768,-34.6837837831338,2.53178198860238));
#252240=CARTESIAN_POINT('Ctrl Pts',(49.866980369603,-36.6229335645802,3.77003198860238));
#252241=CARTESIAN_POINT('Ctrl Pts',(49.9417406248217,-36.5200349009273,
3.77003198860239));
#252242=CARTESIAN_POINT('Ctrl Pts',(49.9416290134548,-36.5201885207949,
3.64284238727527));
#252243=CARTESIAN_POINT('Ctrl Pts',(50.0423873219322,-36.7506494346797,
3.77003198860238));
#252244=CARTESIAN_POINT('Ctrl Pts',(50.1174293675628,-36.6476796282212,
3.77025506105767));
#252245=CARTESIAN_POINT('Ctrl Pts',(50.082007534236,-36.6221794864674,3.6428421064183));
#252246=CARTESIAN_POINT('Ctrl Pts',(50.20937322402,-36.8722311236847,3.65553527987809));
#252247=CARTESIAN_POINT('Ctrl Pts',(50.2846385388137,-36.7691636147932,
3.655859965331));
#252248=CARTESIAN_POINT('Ctrl Pts',(50.2156454684962,-36.719273129351,3.55127902710179));
#252249=CARTESIAN_POINT('Ctrl Pts',(50.3023253562,-36.9399086546478,3.47153072139046));
#252250=CARTESIAN_POINT('Ctrl Pts',(50.3777877242647,-36.8368401378439,
3.47182327905163));
#252251=CARTESIAN_POINT('Ctrl Pts',(50.2900345513017,-36.7733199617888,
3.40413028377937));
#252252=CARTESIAN_POINT('Origin',(49.866980369603,-36.6229335645802,3.64303198860238));
#252253=CARTESIAN_POINT('Origin',(5.7121316272531E-15,1.86290248986529E-13,
2.53178198860262));
#252254=CARTESIAN_POINT('Origin',(47.7461450747869,-34.7084426211224,2.53178198860239));
#252255=CARTESIAN_POINT('Origin',(40.5385041740537,-29.8453988870281,3.64303198860242));
#252256=CARTESIAN_POINT('Origin',(49.5422481179707,-36.3870656659206,3.64299466008053));
#252257=CARTESIAN_POINT('Ctrl Pts',(47.659028586094,-34.6451144164178,2.59908173516));
#252258=CARTESIAN_POINT('Ctrl Pts',(47.6892031885518,-34.667049453401,2.65878198860238));
#252259=CARTESIAN_POINT('Ctrl Pts',(47.7461450747869,-34.7084426211224,
2.65878198860238));
#252260=CARTESIAN_POINT('Ctrl Pts',(47.6074854095242,-34.7160192182654,
2.59908193199744));
#252261=CARTESIAN_POINT('Ctrl Pts',(47.6516492793336,-34.7187044685494,
2.65877685806567));
#252262=CARTESIAN_POINT('Ctrl Pts',(47.7161963245873,-34.7496251731977,
2.65878198860238));
#252263=CARTESIAN_POINT('Ctrl Pts',(47.5796730526556,-34.796037856083,2.63872492669789));
#252264=CARTESIAN_POINT('Ctrl Pts',(47.6353534770334,-34.7797813814947,
2.69532212015227));
#252265=CARTESIAN_POINT('Ctrl Pts',(47.7083584310204,-34.8021505789967,
2.68176836726608));
#252266=CARTESIAN_POINT('Ctrl Pts',(47.575296561615,-34.9243313177586,2.75442176402211));
#252267=CARTESIAN_POINT('Ctrl Pts',(47.6468329724883,-34.866569357181,2.79203179920141));
#252268=CARTESIAN_POINT('Ctrl Pts',(47.7301838844732,-34.8943788354686,
2.74885310748154));
#252269=CARTESIAN_POINT('Ctrl Pts',(47.5970608435775,-34.9730260802968,
2.82866089558384));
#252270=CARTESIAN_POINT('Ctrl Pts',(47.6753141056553,-34.8923863483122,
2.85316563119167));
#252271=CARTESIAN_POINT('Ctrl Pts',(47.7584998599249,-34.9340521716862,
2.79189751796622));
#252272=CARTESIAN_POINT('Ctrl Pts',(47.6338034047604,-34.9997217530253,
2.90134173515999));
#252273=CARTESIAN_POINT('Ctrl Pts',(47.7085070967808,-34.8977303031694,
2.90103711553205));
#252274=CARTESIAN_POINT('Ctrl Pts',(47.7952442955506,-34.9607485668358,
2.83404198860238));
#252275=CARTESIAN_POINT('Origin',(47.7205955685095,-35.0634937251214,2.83404198860238));
#252276=CARTESIAN_POINT('Origin',(49.5064990280468,-36.3610285393803,3.56647653971683));
#252277=CARTESIAN_POINT('Origin',(49.440290424917,-36.3129251734935,3.42473028058461));
#252278=CARTESIAN_POINT('Origin',(47.8647214254841,-35.1682072895556,3.11913648168284));
#252279=CARTESIAN_POINT('Origin',(48.0088472823277,-35.2729208539807,3.40423097483287));
#252280=CARTESIAN_POINT('Ctrl Pts',(49.1733470784092,-36.1189794796875,
3.36123028058457));
#252281=CARTESIAN_POINT('Ctrl Pts',(49.2479958054503,-36.0162343214019,
3.36123028058457));
#252282=CARTESIAN_POINT('Ctrl Pts',(49.2479958054503,-36.0162343214019,
3.23423028058457));
#252283=CARTESIAN_POINT('Ctrl Pts',(49.2463047380091,-36.1716968449913,
3.36123028058457));
#252284=CARTESIAN_POINT('Ctrl Pts',(49.3207474263657,-36.0690914679756,
3.36099641108531));
#252285=CARTESIAN_POINT('Ctrl Pts',(49.3572244778989,-36.0955935972133,
3.23423043688377));
#252286=CARTESIAN_POINT('Ctrl Pts',(49.3152906263894,-36.2215465627845,
3.4105425890526));
#252287=CARTESIAN_POINT('Ctrl Pts',(49.3898826892475,-36.1193211766471,
3.41008815825869));
#252288=CARTESIAN_POINT('Ctrl Pts',(49.4605079583572,-36.1706334382067,
3.30819867304271));
#252289=CARTESIAN_POINT('Ctrl Pts',(49.3516463037389,-36.2478178023243,
3.48823028058459));
#252290=CARTESIAN_POINT('Ctrl Pts',(49.4263574835555,-36.1458216659117,
3.48794691941576));
#252291=CARTESIAN_POINT('Ctrl Pts',(49.5149391519582,-36.2101800152079,
3.42473028058461));
#252292=CARTESIAN_POINT('Origin',(49.1733470784092,-36.1189794796875,3.23423028058457));
#252293=CARTESIAN_POINT('Ctrl Pts',(47.9220530736691,-35.209151665052,3.47153072139048));
#252294=CARTESIAN_POINT('Ctrl Pts',(47.9968680956257,-35.1070032771111,
3.47122746285053));
#252295=CARTESIAN_POINT('Ctrl Pts',(48.0836260518497,-35.1702703521461,
3.40413046676755));
#252296=CARTESIAN_POINT('Ctrl Pts',(48.0150025575607,-35.2768360036061,
3.65553813457965));
#252297=CARTESIAN_POINT('Ctrl Pts',(48.0897575808475,-35.1744910995543,
3.65520336072245));
#252298=CARTESIAN_POINT('Ctrl Pts',(48.1580164790723,-35.2243181613706,
3.55128134519974));
#252299=CARTESIAN_POINT('Ctrl Pts',(48.1819833392254,-35.3984277477525,
3.7700319886024));
#252300=CARTESIAN_POINT('Ctrl Pts',(48.256762968645,-35.2958269999273,3.76980209313948));
#252301=CARTESIAN_POINT('Ctrl Pts',(48.2916555365119,-35.3214126203087,
3.64284195387307));
#252302=CARTESIAN_POINT('Ctrl Pts',(48.3573835402124,-35.5261472678858,
3.77003198860239));
#252303=CARTESIAN_POINT('Ctrl Pts',(48.4321440857833,-35.4232482045974,
3.77003198860239));
#252304=CARTESIAN_POINT('Ctrl Pts',(48.4320321836307,-35.4234022246971,
3.64284189403762));
#252305=CARTESIAN_POINT('Origin',(48.3573835402124,-35.5261472678858,3.64303198860239));
#252306=CARTESIAN_POINT('Origin',(39.5520252162596,-29.1286799712083,3.23423028058462));
#252307=CARTESIAN_POINT('Origin',(49.0510171431408,-36.0301015792669,3.23423028058457));
#252308=CARTESIAN_POINT('Origin',(39.3975469582356,-29.0164449471017,3.64303198860243));
#252309=CARTESIAN_POINT('Origin',(48.6820620414868,-35.7621028045843,3.64299171721786));
#252310=CARTESIAN_POINT('Ctrl Pts',(48.8727133447948,-35.9012693628897,
3.48823028058456));
#252311=CARTESIAN_POINT('Ctrl Pts',(48.9481071848801,-35.7983524848928,
3.48852004212234));
#252312=CARTESIAN_POINT('Ctrl Pts',(48.8587224664505,-35.7334106855999,
3.42473028058456));
#252313=CARTESIAN_POINT('Ctrl Pts',(48.9091935744948,-35.9276271141626,
3.41028005848382));
#252314=CARTESIAN_POINT('Ctrl Pts',(48.9843245886205,-35.8246659689611,
3.41074404220299));
#252315=CARTESIAN_POINT('Ctrl Pts',(48.9133376106103,-35.7730909105051,
3.3078048624387));
#252316=CARTESIAN_POINT('Ctrl Pts',(48.9783048775129,-35.9775622448352,
3.36123028058457));
#252317=CARTESIAN_POINT('Ctrl Pts',(49.0530211657563,-35.8745769537839,
3.36146460586502));
#252318=CARTESIAN_POINT('Ctrl Pts',(49.0168051108909,-35.8482644497254,
3.2342304530841));
#252319=CARTESIAN_POINT('Ctrl Pts',(49.0510171431408,-36.0301015792669,
3.36123028058457));
#252320=CARTESIAN_POINT('Ctrl Pts',(49.1256658701819,-35.9273564209813,
3.36123028058457));
#252321=CARTESIAN_POINT('Ctrl Pts',(49.1256658701819,-35.9273564209813,
3.23423028058457));
#252322=CARTESIAN_POINT('Origin',(48.7840737394093,-35.8361558438855,3.42473028058457));
#252323=CARTESIAN_POINT('Origin',(48.7182599907917,-35.7883393569593,3.56563113524709));
#252324=CARTESIAN_POINT('Origin',(53.3535596832581,-30.4370746247553,3.56647653909434));
#252325=CARTESIAN_POINT('Origin',(53.3918862459827,-30.4591427892358,3.64299466007485));
#252326=CARTESIAN_POINT('Origin',(53.282685606085,-30.3961554568828,3.42473028058463));
#252327=CARTESIAN_POINT('Ctrl Pts',(53.1871522506179,-30.3416565762228,
3.48823028058463));
#252328=CARTESIAN_POINT('Ctrl Pts',(53.1243619179799,-30.4513942013105,
3.48794691941579));
#252329=CARTESIAN_POINT('Ctrl Pts',(53.219185606085,-30.5061406831635,3.42473028058464));
#252330=CARTESIAN_POINT('Ctrl Pts',(53.1482340195355,-30.3190533624386,
3.41028005925068));
#252331=CARTESIAN_POINT('Ctrl Pts',(53.0851849835374,-30.4287753876651,
3.40982512231055));
#252332=CARTESIAN_POINT('Ctrl Pts',(53.1607219582391,-30.4723866803419,
3.30780486372884));
#252333=CARTESIAN_POINT('Ctrl Pts',(53.0745038491597,-30.2762311741517,
3.36123028058461));
#252334=CARTESIAN_POINT('Ctrl Pts',(53.0110474253457,-30.3859720484848,
3.36099721048422));
#252335=CARTESIAN_POINT('Ctrl Pts',(53.0499635164591,-30.4084402641652,
3.23423045308377));
#252336=CARTESIAN_POINT('Ctrl Pts',(52.9969317578291,-30.2311753956704,
3.36123028058461));
#252337=CARTESIAN_POINT('Ctrl Pts',(52.9334317578291,-30.341160621951,3.36123028058461));
#252338=CARTESIAN_POINT('Ctrl Pts',(52.9334317578291,-30.341160621951,3.23423028058461));
#252339=CARTESIAN_POINT('Origin',(52.9969317578291,-30.2311753956704,3.23423028058461));
#252340=CARTESIAN_POINT('Origin',(0.158750000000002,0.274963065701745,3.64303198860263));
#252341=CARTESIAN_POINT('Origin',(53.739442799329,-30.6598643453566,3.64303198860242));
#252342=CARTESIAN_POINT('Origin',(0.158750000000002,0.274963065701748,3.23423028058482));
#252343=CARTESIAN_POINT('Origin',(52.8659816883963,-30.1555713378329,3.23423028058461));
#252344=CARTESIAN_POINT('Ctrl Pts',(54.2060847114746,-30.9286463962969,
3.47153072139051));
#252345=CARTESIAN_POINT('Ctrl Pts',(54.1426202518673,-31.0395064328251,
3.47182327902642));
#252346=CARTESIAN_POINT('Ctrl Pts',(54.0488992551386,-30.985175917683,3.4041302895902));
#252347=CARTESIAN_POINT('Ctrl Pts',(54.1064496608375,-30.8712564593356,
3.65553807120937));
#252348=CARTESIAN_POINT('Ctrl Pts',(54.042905973262,-30.9819360667859,3.65586275496656));
#252349=CARTESIAN_POINT('Ctrl Pts',(53.9692670413556,-30.9392002377689,
3.55128126837208));
#252350=CARTESIAN_POINT('Ctrl Pts',(53.9274585619027,-30.7681581606536,
3.77003198860242));
#252351=CARTESIAN_POINT('Ctrl Pts',(53.8639133132313,-30.8785940576183,
3.77025505748772));
#252352=CARTESIAN_POINT('Ctrl Pts',(53.8262110069728,-30.8566067980785,
3.64284211731191));
#252353=CARTESIAN_POINT('Ctrl Pts',(53.7394427993291,-30.6598643453566,
3.77003198860242));
#252354=CARTESIAN_POINT('Ctrl Pts',(53.6758479332737,-30.770013884465,3.77003198860242));
#252355=CARTESIAN_POINT('Ctrl Pts',(53.675942870086,-30.7698494490826,3.64284239821704));
#252356=CARTESIAN_POINT('Origin',(54.1125387249983,-30.8752713784753,3.40423097483289));
#252357=CARTESIAN_POINT('Ctrl Pts',(52.8659816883963,-30.1555713378329,
3.36123028058461));
#252358=CARTESIAN_POINT('Ctrl Pts',(52.8024816883963,-30.2655565641136,
3.36123028058461));
#252359=CARTESIAN_POINT('Ctrl Pts',(52.8024816883963,-30.2655565641135,
3.23423028058461));
#252360=CARTESIAN_POINT('Ctrl Pts',(52.788147705508,-30.1103627734736,3.36123028058462));
#252361=CARTESIAN_POINT('Ctrl Pts',(52.7244553345199,-30.2205080276993,
3.36146538610119));
#252362=CARTESIAN_POINT('Ctrl Pts',(52.6855560684225,-30.1980495259465,
3.2342304368842));
#252363=CARTESIAN_POINT('Ctrl Pts',(52.7145506960115,-30.0676130472582,
3.4105425869308));
#252364=CARTESIAN_POINT('Ctrl Pts',(52.6510500011306,-30.1781274387051,
3.41100608859755));
#252365=CARTESIAN_POINT('Ctrl Pts',(52.5749945583568,-30.1342168083481,
3.30819866970778));
#252366=CARTESIAN_POINT('Ctrl Pts',(52.67576491394,-30.0450834959828,3.4882302805846));
#252367=CARTESIAN_POINT('Ctrl Pts',(52.612411104956,-30.1558192615993,3.48852004212238));
#252368=CARTESIAN_POINT('Ctrl Pts',(52.5167277788845,-30.1005764675349,
3.4247302805846));
#252369=CARTESIAN_POINT('Origin',(52.5802277788845,-29.9905912412543,3.42473028058461));
#252370=CARTESIAN_POINT('Origin',(54.2668203812008,-30.9643459342411,3.11913648178328));
#252371=CARTESIAN_POINT('Origin',(54.4211020372442,-31.0534204898625,2.8340419886024));
#252372=CARTESIAN_POINT('Origin',(52.5097763801598,-29.9499161072436,3.56563113460845));
#252373=CARTESIAN_POINT('Origin',(52.4710850656387,-29.927519002605,3.64299171721728));
#252374=CARTESIAN_POINT('Ctrl Pts',(54.5275217339724,-31.4638515574732,
2.59908173516002));
#252375=CARTESIAN_POINT('Ctrl Pts',(54.4952102564869,-31.4452069629845,
2.65878198860241));
#252376=CARTESIAN_POINT('Ctrl Pts',(54.4342359163067,-31.4100231232053,
2.65878198860241));
#252377=CARTESIAN_POINT('Ctrl Pts',(54.5715608148713,-31.3875306471672,
2.59908193475617));
#252378=CARTESIAN_POINT('Ctrl Pts',(54.5272862282495,-31.389612165888,2.65878715325355));
#252379=CARTESIAN_POINT('Ctrl Pts',(54.4597196360186,-31.3658411130322,
2.65878198860241));
#252380=CARTESIAN_POINT('Ctrl Pts',(54.5905300051368,-31.304602960155,2.63878778849852));
#252381=CARTESIAN_POINT('Ctrl Pts',(54.5367961153114,-31.3268524737452,
2.69564460180104));
#252382=CARTESIAN_POINT('Ctrl Pts',(54.4615686025424,-31.3125672934286,
2.68180481624844));
#252383=CARTESIAN_POINT('Ctrl Pts',(54.5809273110399,-31.1759014746032,
2.75443238878622));
#252384=CARTESIAN_POINT('Ctrl Pts',(54.5158579940075,-31.2415992967173,
2.79268340777048));
#252385=CARTESIAN_POINT('Ctrl Pts',(54.4295063924933,-31.222768219185,2.74885926835607));
#252386=CARTESIAN_POINT('Ctrl Pts',(54.5540292360083,-31.129536412388,2.82856655361651));
#252387=CARTESIAN_POINT('Ctrl Pts',(54.4847364330952,-31.2191033458799,
2.8538419723079));
#252388=CARTESIAN_POINT('Ctrl Pts',(54.3969835118378,-31.1861426211008,
2.79184624278575));
#252389=CARTESIAN_POINT('Ctrl Pts',(54.5146464769142,-31.1067982185526,
2.90134173516003));
#252390=CARTESIAN_POINT('Ctrl Pts',(54.4512761425986,-31.2174884860856,
2.9016321871637));
#252391=CARTESIAN_POINT('Ctrl Pts',(54.3576020372442,-31.1634057161431,
2.83404198860241));
#252392=CARTESIAN_POINT('Origin',(54.4342359163067,-31.4100231232053,2.5317819886024));
#252393=CARTESIAN_POINT('Origin',(0.158750000000002,0.274963065701745,3.64303198860263));
#252394=CARTESIAN_POINT('Origin',(52.123470313195,-29.7268821954841,3.64303198860242));
#252395=CARTESIAN_POINT('Origin',(5.52187834149254E-15,1.85964994957679E-13,
2.53178198860262));
#252396=CARTESIAN_POINT('Origin',(54.4189959163067,-31.4364195775126,2.5317819886024));
#252397=CARTESIAN_POINT('Ctrl Pts',(52.123470313195,-29.7268821954841,3.77003198860243));
#252398=CARTESIAN_POINT('Ctrl Pts',(52.0598751873275,-29.8370321846005,
3.77003198860243));
#252399=CARTESIAN_POINT('Ctrl Pts',(52.0599703843398,-29.8368672985384,
3.64284187937001));
#252400=CARTESIAN_POINT('Ctrl Pts',(51.9354481180157,-29.6185926664438,
3.77003198860243));
#252401=CARTESIAN_POINT('Ctrl Pts',(51.8721332876,-29.7286387544935,3.7698020896278));
#252402=CARTESIAN_POINT('Ctrl Pts',(51.9096995898758,-29.7501084152001,
3.64284193928265));
#252403=CARTESIAN_POINT('Ctrl Pts',(51.7564527430631,-29.5155047636227,
3.65553535416569));
#252404=CARTESIAN_POINT('Ctrl Pts',(51.6933616226623,-29.6254243098814,
3.65520057834603));
#252405=CARTESIAN_POINT('Ctrl Pts',(51.7666446199934,-29.6675155901152,
3.55127910964215));
#252406=CARTESIAN_POINT('Ctrl Pts',(51.6568155675431,-29.4581217525665,
3.47153072139052));
#252407=CARTESIAN_POINT('Ctrl Pts',(51.5939283753698,-29.5680161811085,
3.47122746281562));
#252408=CARTESIAN_POINT('Ctrl Pts',(51.6870133822666,-29.6215404737374,
3.4041304590124));
#252409=CARTESIAN_POINT('Origin',(51.7503740054947,-29.5114749417997,3.4042309748329));
#252410=CARTESIAN_POINT('Ctrl Pts',(54.1966007261211,-31.6576696180576,
2.90134173516003));
#252411=CARTESIAN_POINT('Ctrl Pts',(54.2607761425987,-31.5474441649275,
2.9016321871637));
#252412=CARTESIAN_POINT('Ctrl Pts',(54.1671020372442,-31.493361394985,2.83404198860241));
#252413=CARTESIAN_POINT('Ctrl Pts',(54.2360018544271,-31.6804173065994,
2.82853349835321));
#252414=CARTESIAN_POINT('Ctrl Pts',(54.2789150989581,-31.5756301844087,
2.8538148316222));
#252415=CARTESIAN_POINT('Ctrl Pts',(54.2065014563936,-31.5161086602368,
2.79182701594168));
#252416=CARTESIAN_POINT('Ctrl Pts',(54.2894509908547,-31.6804328064616,
2.75468822073639));
#252417=CARTESIAN_POINT('Ctrl Pts',(54.3138841827112,-31.5911964272959,
2.79286913083789));
#252418=CARTESIAN_POINT('Ctrl Pts',(54.2543268901844,-31.525867555196,2.74900763297894));
#252419=CARTESIAN_POINT('Ctrl Pts',(54.4049648787504,-31.6250591602182,
2.63954450640354));
#252420=CARTESIAN_POINT('Ctrl Pts',(54.3976088886511,-31.5671393481769,
2.69627684028851));
#252421=CARTESIAN_POINT('Ctrl Pts',(54.3475791360316,-31.5090508246484,
2.68224356036467));
#252422=CARTESIAN_POINT('Ctrl Pts',(54.4680334478301,-31.5668453499332,
2.59908178706226));
#252423=CARTESIAN_POINT('Ctrl Pts',(54.4477213412894,-31.5274226111426,
2.65878704321479));
#252424=CARTESIAN_POINT('Ctrl Pts',(54.3933906465336,-31.4807263372346,
2.6587819886024));
#252425=CARTESIAN_POINT('Ctrl Pts',(54.5122556166615,-31.4902932482899,
2.59908173516002));
#252426=CARTESIAN_POINT('Ctrl Pts',(54.4799531854483,-31.4716329851981,
2.6587819886024));
#252427=CARTESIAN_POINT('Ctrl Pts',(54.4189959163067,-31.4364195775126,
2.65878198860241));
#252428=CARTESIAN_POINT('Origin',(54.1036020372442,-31.6033466212656,2.8340419886024));
#252429=CARTESIAN_POINT('Origin',(51.5960921371869,-29.4224002636341,3.1191364816712));
#252430=CARTESIAN_POINT('Origin',(51.4418102687789,-29.3333255853447,2.83404198860242));
#252431=CARTESIAN_POINT('Origin',(53.9493203812085,-31.5142720655992,3.11913648177336));
#252432=CARTESIAN_POINT('Origin',(53.7950387249983,-31.4251975098784,3.40423097483289));
#252433=CARTESIAN_POINT('Ctrl Pts',(51.3482501200169,-29.2799753962454,
2.90134173516004));
#252434=CARTESIAN_POINT('Ctrl Pts',(51.2854610232005,-29.3897042746966,
2.90103711553209));
#252435=CARTESIAN_POINT('Ctrl Pts',(51.3783102687789,-29.4433108116253,
2.83404198860242));
#252436=CARTESIAN_POINT('Ctrl Pts',(51.3089010921307,-29.257257838549,2.82862991747938));
#252437=CARTESIAN_POINT('Ctrl Pts',(51.2670685993222,-29.36153975946,2.85314045886519));
#252438=CARTESIAN_POINT('Ctrl Pts',(51.3389598763133,-29.4205918519426,
2.79187960999965));
#252439=CARTESIAN_POINT('Ctrl Pts',(51.2557407616061,-29.2572680623741,
2.7547062579331));
#252440=CARTESIAN_POINT('Ctrl Pts',(51.2319924817695,-29.3461554108679,
2.7922425038186));
#252441=CARTESIAN_POINT('Ctrl Pts',(51.2913733902321,-29.4109522357559,
2.74901809108242));
#252442=CARTESIAN_POINT('Ctrl Pts',(51.1410333861059,-29.3127910737007,
2.63947868311675));
#252443=CARTESIAN_POINT('Ctrl Pts',(51.1485922293425,-29.3705286780138,
2.69595066767904));
#252444=CARTESIAN_POINT('Ctrl Pts',(51.1987619028147,-29.4282055900894,
2.68220539436038));
#252445=CARTESIAN_POINT('Ctrl Pts',(51.0785202710263,-29.3710651187638,
2.59908178585086));
#252446=CARTESIAN_POINT('Ctrl Pts',(51.0989122516733,-29.4103605382568,
2.65877670944826));
#252447=CARTESIAN_POINT('Ctrl Pts',(51.1533747228781,-29.4568175306709,
2.65878198860242));
#252448=CARTESIAN_POINT('Ctrl Pts',(51.0345602039891,-29.4472515437727,
2.59908173516004));
#252449=CARTESIAN_POINT('Ctrl Pts',(51.0668719738981,-29.4658956314759,
2.65878198860242));
#252450=CARTESIAN_POINT('Ctrl Pts',(51.1278468659051,-29.5010785149103,
2.65878198860242));
#252451=CARTESIAN_POINT('Origin',(51.1278468659051,-29.5010785149103,2.53178198860242));
#252452=CARTESIAN_POINT('Ctrl Pts',(53.421942799329,-31.2097904767597,3.77003198860242));
#252453=CARTESIAN_POINT('Ctrl Pts',(53.4855376708633,-31.0996409281616,
3.77003198860242));
#252454=CARTESIAN_POINT('Ctrl Pts',(53.4854427285639,-31.0998053730479,
3.64284238727567));
#252455=CARTESIAN_POINT('Ctrl Pts',(53.6097387976563,-31.3184716867866,
3.77003198860243));
#252456=CARTESIAN_POINT('Ctrl Pts',(53.6736064794785,-31.2082219299917,
3.77025506105756));
#252457=CARTESIAN_POINT('Ctrl Pts',(53.6357132000301,-31.1865640704865,
3.6428421064187));
#252458=CARTESIAN_POINT('Ctrl Pts',(53.7885186806147,-31.4219325588438,
3.65553527987807));
#252459=CARTESIAN_POINT('Ctrl Pts',(53.8525981958198,-31.3115622968576,
3.65585996533081));
#252460=CARTESIAN_POINT('Ctrl Pts',(53.7787681009854,-31.2691568563317,
3.55127902710171));
#252461=CARTESIAN_POINT('Ctrl Pts',(53.8880358395974,-31.4795232016781,
3.47153072139051));
#252462=CARTESIAN_POINT('Ctrl Pts',(53.9523112232411,-31.3691313396255,
3.47182327905167));
#252463=CARTESIAN_POINT('Ctrl Pts',(53.8583991049523,-31.3151318380575,
3.40413028377961));
#252464=CARTESIAN_POINT('Origin',(53.421942799329,-31.2097904767597,3.64303198860242));
#252465=CARTESIAN_POINT('Origin',(5.71547558359784E-15,1.86295398227745E-13,
2.53178198860262));
#252466=CARTESIAN_POINT('Origin',(51.1126068659051,-29.5274749692176,2.53178198860242));
#252467=CARTESIAN_POINT('Origin',(46.508091798073,-27.2180767400477,3.64303198860244));
#252468=CARTESIAN_POINT('Origin',(53.074334555967,-31.0091584503641,3.6429946600813));
#252469=CARTESIAN_POINT('Ctrl Pts',(51.0193480105331,-29.4735998357329,
2.59908173516004));
#252470=CARTESIAN_POINT('Ctrl Pts',(51.051650149069,-29.4922606054638,2.65878198860242));
#252471=CARTESIAN_POINT('Ctrl Pts',(51.1126068659051,-29.5274749692176,
2.65878198860242));
#252472=CARTESIAN_POINT('Ctrl Pts',(50.9754987628539,-29.5495039426962,
2.59908193199881));
#252473=CARTESIAN_POINT('Ctrl Pts',(51.0197013834523,-29.5475581014572,
2.6587768580658));
#252474=CARTESIAN_POINT('Ctrl Pts',(51.0871269269774,-29.5715624158004,
2.65878198860242));
#252475=CARTESIAN_POINT('Ctrl Pts',(50.9562029902293,-29.6319914129664,
2.63872492669796));
#252476=CARTESIAN_POINT('Ctrl Pts',(51.0098791271093,-29.6100038038521,
2.69532212015255));
#252477=CARTESIAN_POINT('Ctrl Pts',(51.084822370159,-29.6246193648988,2.68176836726625));
#252478=CARTESIAN_POINT('Ctrl Pts',(50.9652607924608,-29.7600395375182,
2.75442176402211));
#252479=CARTESIAN_POINT('Ctrl Pts',(51.0303675504162,-29.6951164119086,
2.7920317992012));
#252480=CARTESIAN_POINT('Ctrl Pts',(51.1161687394138,-29.7140610042223,
2.74885310748144));
#252481=CARTESIAN_POINT('Ctrl Pts',(50.9919958361066,-29.806192558105,2.82866089558394));
#252482=CARTESIAN_POINT('Ctrl Pts',(51.0613912713634,-29.7178148857786,
2.85316563119245));
#252483=CARTESIAN_POINT('Ctrl Pts',(51.1484765898563,-29.750557180353,2.79189751796625));
#252484=CARTESIAN_POINT('Ctrl Pts',(51.0313275753413,-29.8289013456877,
2.90134173516004));
#252485=CARTESIAN_POINT('Ctrl Pts',(51.0949610232005,-29.7196599535384,
2.9010371155321));
#252486=CARTESIAN_POINT('Ctrl Pts',(51.1878102687789,-29.7732664904672,
2.83404198860242));
#252487=CARTESIAN_POINT('Origin',(51.1243102687789,-29.8832517167478,2.83404198860241));
#252488=CARTESIAN_POINT('Origin',(53.0360596824734,-30.9870007553613,3.56647653971681));
#252489=CARTESIAN_POINT('Origin',(52.965185606085,-30.946081588286,3.42473028058464));
#252490=CARTESIAN_POINT('Origin',(51.2785921372034,-29.9723263949827,3.11913648167932));
#252491=CARTESIAN_POINT('Origin',(51.4328740054947,-30.0614010732028,3.4042309748329));
#252492=CARTESIAN_POINT('Ctrl Pts',(52.6794317578291,-30.7811015270735,
3.36123028058461));
#252493=CARTESIAN_POINT('Ctrl Pts',(52.7429317578291,-30.6711163007929,
3.3612302805846));
#252494=CARTESIAN_POINT('Ctrl Pts',(52.7429317578291,-30.6711163007929,
3.23423028058461));
#252495=CARTESIAN_POINT('Ctrl Pts',(52.757500212918,-30.8259039490941,3.3612302805846));
#252496=CARTESIAN_POINT('Ctrl Pts',(52.8208099140591,-30.7160792752576,
3.36099641108556));
#252497=CARTESIAN_POINT('Ctrl Pts',(52.8598573673284,-30.7386233329124,
3.23423043688372));
#252498=CARTESIAN_POINT('Ctrl Pts',(52.8313189037791,-30.8682695960174,
3.41054258905263));
#252499=CARTESIAN_POINT('Ctrl Pts',(52.8948168809884,-30.7588072175341,
3.41008815826004));
#252500=CARTESIAN_POINT('Ctrl Pts',(52.9704188493355,-30.8024560343112,
3.30819867304305));
#252501=CARTESIAN_POINT('Ctrl Pts',(52.870221513222,-30.8905967158728,3.48823028058462));
#252502=CARTESIAN_POINT('Ctrl Pts',(52.93386191798,-30.7813498801524,3.48794691941578));
#252503=CARTESIAN_POINT('Ctrl Pts',(53.028685606085,-30.8360963620053,3.42473028058463));
#252504=CARTESIAN_POINT('Origin',(52.6794317578291,-30.7811015270735,3.23423028058461));
#252505=CARTESIAN_POINT('Ctrl Pts',(51.3398895692701,-30.007053683815,3.47153072139051));
#252506=CARTESIAN_POINT('Ctrl Pts',(51.4036173326914,-29.897644576157,3.47122746285057));
#252507=CARTESIAN_POINT('Ctrl Pts',(51.4965132298824,-29.9514963916944,
3.40413046676775));
#252508=CARTESIAN_POINT('Ctrl Pts',(51.4394048060587,-30.0646513737697,
3.65553813457968));
#252509=CARTESIAN_POINT('Ctrl Pts',(51.5030523579664,-29.9550530981058,
3.65520336072045));
#252510=CARTESIAN_POINT('Ctrl Pts',(51.5761456730037,-29.9974722043263,
3.55128134519916));
#252511=CARTESIAN_POINT('Ctrl Pts',(51.6181806476918,-30.1681227811162,
3.77003198860243));
#252512=CARTESIAN_POINT('Ctrl Pts',(51.6818259279743,-30.0582674911749,
3.76980209314072));
#252513=CARTESIAN_POINT('Ctrl Pts',(51.7192017762861,-30.0800656843512,
3.64284195387399));
#252514=CARTESIAN_POINT('Ctrl Pts',(51.805970313195,-30.2768083268872,3.77003198860243));
#252515=CARTESIAN_POINT('Ctrl Pts',(51.8695654317176,-30.1666583504928,
3.77003198860243));
#252516=CARTESIAN_POINT('Ctrl Pts',(51.8694702420612,-30.166823223814,3.64284189403797));
#252517=CARTESIAN_POINT('Origin',(51.805970313195,-30.2768083268872,3.64303198860243));
#252518=CARTESIAN_POINT('Origin',(45.3776875000007,-26.5654375142626,3.23423028058464));
#252519=CARTESIAN_POINT('Origin',(52.5484816883963,-30.7054974692361,3.23423028058461));
#252520=CARTESIAN_POINT('Origin',(45.2006711678738,-26.4632370872581,3.64303198860245));
#252521=CARTESIAN_POINT('Origin',(52.1535342613181,-30.4775331296731,3.64299171721757));
#252522=CARTESIAN_POINT('Ctrl Pts',(52.3576880233166,-30.596008831256,3.48823028058461));
#252523=CARTESIAN_POINT('Ctrl Pts',(52.421911104956,-30.4857749404412,3.48852004212238));
#252524=CARTESIAN_POINT('Ctrl Pts',(52.3262277788845,-30.4305321463768,
3.42473028058461));
#252525=CARTESIAN_POINT('Ctrl Pts',(52.3967235457363,-30.6184089696608,
3.41028005848386));
#252526=CARTESIAN_POINT('Ctrl Pts',(52.4606806140205,-30.5081585269362,
3.41074404220357));
#252527=CARTESIAN_POINT('Ctrl Pts',(52.3846914485018,-30.4642861617681,
3.30780486243881));
#252528=CARTESIAN_POINT('Ctrl Pts',(52.4706758922786,-30.6608464521619,
3.3612302805846));
#252529=CARTESIAN_POINT('Ctrl Pts',(52.5342179826651,-30.5506153465188,
3.36146460586421));
#252530=CARTESIAN_POINT('Ctrl Pts',(52.4954499175227,-30.5282325936724,
3.23423045308408));
#252531=CARTESIAN_POINT('Ctrl Pts',(52.5484816883963,-30.7054974692361,
3.36123028058461));
#252532=CARTESIAN_POINT('Ctrl Pts',(52.6119816883963,-30.5955122429554,
3.36123028058461));
#252533=CARTESIAN_POINT('Ctrl Pts',(52.6119816883963,-30.5955122429554,
3.23423028058461));
#252534=CARTESIAN_POINT('Origin',(52.2627277788845,-30.5405173726574,3.42473028058461));
#252535=CARTESIAN_POINT('Origin',(52.1922763809705,-30.499842239456,3.56563113524742));
#252536=CARTESIAN_POINT('Origin',(56.2428239377254,-24.6933715417288,3.56647653909471));
#252537=CARTESIAN_POINT('Origin',(56.2832472948485,-24.7113125977914,3.64299466007753));
#252538=CARTESIAN_POINT('Origin',(56.1680608984281,-24.6600848917102,3.42473028058467));
#252539=CARTESIAN_POINT('Ctrl Pts',(56.0673542004329,-24.6158705164585,
3.48823028058467));
#252540=CARTESIAN_POINT('Ctrl Pts',(56.0163785451201,-24.7315703643327,
3.48794691941584));
#252541=CARTESIAN_POINT('Ctrl Pts',(56.1164053447575,-24.7761051648309,
3.42473028058468));
#252542=CARTESIAN_POINT('Ctrl Pts',(56.0262864882909,-24.5974591883322,
3.41028005925072));
#252543=CARTESIAN_POINT('Ctrl Pts',(55.9750519161938,-24.7131705636673,
3.40982512231105));
#252544=CARTESIAN_POINT('Ctrl Pts',(56.0547337128485,-24.7486471852352,
3.30780486372883));
#252545=CARTESIAN_POINT('Ctrl Pts',(55.948484081967,-24.5625784858803,3.36123028058465));
#252546=CARTESIAN_POINT('Ctrl Pts',(55.8968463240332,-24.6783511906867,
3.36099721048324));
#252547=CARTESIAN_POINT('Ctrl Pts',(55.9378977967854,-24.6966284839296,
3.23423045308358));
#252548=CARTESIAN_POINT('Ctrl Pts',(55.8666273273836,-24.5258780191662,
3.36123028058465));
#252549=CARTESIAN_POINT('Ctrl Pts',(55.814971773713,-24.6418982922869,3.36123028058465));
#252550=CARTESIAN_POINT('Ctrl Pts',(55.814971773713,-24.6418982922869,3.23423028058465));
#252551=CARTESIAN_POINT('Origin',(55.8666273273836,-24.5258780191662,3.23423028058465));
#252552=CARTESIAN_POINT('Origin',(0.129138884176568,0.290050682801711,3.64303198860263));
#252553=CARTESIAN_POINT('Origin',(56.6498810128385,-24.8746050278044,3.64303198860246));
#252554=CARTESIAN_POINT('Origin',(0.129138884176569,0.290050682801714,3.23423028058482));
#252555=CARTESIAN_POINT('Origin',(55.7284918401501,-24.4643761377908,3.23423028058465));
#252556=CARTESIAN_POINT('Ctrl Pts',(57.1420619865024,-25.0931373005737,
3.47153072139055));
#252557=CARTESIAN_POINT('Ctrl Pts',(57.0905332211013,-25.2100238766573,
3.47182327902645));
#252558=CARTESIAN_POINT('Ctrl Pts',(56.9916465525425,-25.1657875015256,
3.40413028959015));
#252559=CARTESIAN_POINT('Ctrl Pts',(57.0369738651809,-25.0464764504209,
3.6555380712094));
#252560=CARTESIAN_POINT('Ctrl Pts',(56.9853474458565,-25.1631918674164,
3.65586275496893));
#252561=CARTESIAN_POINT('Ctrl Pts',(56.9076448051899,-25.12838751413,3.55128126837223));
#252562=CARTESIAN_POINT('Ctrl Pts',(56.8481865914866,-24.9626525995187,
3.77003198860246));
#252563=CARTESIAN_POINT('Ctrl Pts',(56.7965331449348,-25.0791258042758,
3.77025505748516));
#252564=CARTESIAN_POINT('Ctrl Pts',(56.7567390814043,-25.0611999573791,
3.64284211731155));
#252565=CARTESIAN_POINT('Ctrl Pts',(56.6498810128385,-24.8746050278044,
3.77003198860247));
#252566=CARTESIAN_POINT('Ctrl Pts',(56.598148288166,-24.9907986298331,3.77003198860246));
#252567=CARTESIAN_POINT('Ctrl Pts',(56.5982255167268,-24.9906251716456,
3.64284239821691));
#252568=CARTESIAN_POINT('Origin',(57.0434492461382,-25.0498328948956,3.40423097483293));
#252569=CARTESIAN_POINT('Ctrl Pts',(55.7284918401501,-24.4643761377908,
3.36123028058465));
#252570=CARTESIAN_POINT('Ctrl Pts',(55.6768362864795,-24.5803964109114,
3.36123028058465));
#252571=CARTESIAN_POINT('Ctrl Pts',(55.6768362864795,-24.5803964109114,
3.23423028058465));
#252572=CARTESIAN_POINT('Ctrl Pts',(55.6463586582049,-24.427551097299,3.36123028058465));
#252573=CARTESIAN_POINT('Ctrl Pts',(55.5945285148506,-24.5437506299597,
3.3614653861003));
#252574=CARTESIAN_POINT('Ctrl Pts',(55.5534947903272,-24.5254812387356,
3.23423043688401));
#252575=CARTESIAN_POINT('Ctrl Pts',(55.5686962576401,-24.3927285408613,
3.41054258693087));
#252576=CARTESIAN_POINT('Ctrl Pts',(55.5170953257145,-24.5092751529617,
3.41100608859777));
#252577=CARTESIAN_POINT('Ctrl Pts',(55.4368666119039,-24.4735550281863,
3.30819866970782));
#252578=CARTESIAN_POINT('Ctrl Pts',(55.5277679687686,-24.3743766270205,
3.48823028058464));
#252579=CARTESIAN_POINT('Ctrl Pts',(55.4763362579878,-24.4911280468217,
3.48852004212242));
#252580=CARTESIAN_POINT('Ctrl Pts',(55.3754026508178,-24.446189509598,3.42473028058464));
#252581=CARTESIAN_POINT('Origin',(55.4270582044884,-24.3301692364774,3.42473028058465));
#252582=CARTESIAN_POINT('Origin',(57.2061965577156,-25.1222926664934,3.11913648178368));
#252583=CARTESIAN_POINT('Origin',(57.3689438691199,-25.1947524379607,2.83404198860245));
#252584=CARTESIAN_POINT('Origin',(55.3527410366456,-24.2970811015507,3.56563113460828));
#252585=CARTESIAN_POINT('Origin',(55.3119205422648,-24.2788510342438,3.64299171721779));
#252586=CARTESIAN_POINT('Ctrl Pts',(57.5176823163891,-25.5918112338785,
2.59908173516006));
#252587=CARTESIAN_POINT('Ctrl Pts',(57.4835989537481,-25.5766462455167,
2.65878198860245));
#252588=CARTESIAN_POINT('Ctrl Pts',(57.4192809246792,-25.548028700571,2.65878198860245));
#252589=CARTESIAN_POINT('Ctrl Pts',(57.5535024391265,-25.5113050800553,
2.59908193475448));
#252590=CARTESIAN_POINT('Ctrl Pts',(57.5096879712795,-25.5180031505018,
2.65878715325302));
#252591=CARTESIAN_POINT('Ctrl Pts',(57.4400067642838,-25.5014249500142,
2.65878198860245));
#252592=CARTESIAN_POINT('Ctrl Pts',(57.5636994104965,-25.4268488592806,
2.63878778849858));
#252593=CARTESIAN_POINT('Ctrl Pts',(57.5125855880062,-25.4545932086363,
2.69564460180114));
#252594=CARTESIAN_POINT('Ctrl Pts',(57.4362769714773,-25.4482497003375,
2.68180481624879));
#252595=CARTESIAN_POINT('Ctrl Pts',(57.5406963524572,-25.2998561687908,
2.75443238878624));
#252596=CARTESIAN_POINT('Ctrl Pts',(57.4828507843371,-25.3719956870763,
2.79268340777054));
#252597=CARTESIAN_POINT('Ctrl Pts',(57.395003842335,-25.362293968364,2.7488592683558));
#252598=CARTESIAN_POINT('Ctrl Pts',(57.5090991591925,-25.2565567136854,
2.82856655361656));
#252599=CARTESIAN_POINT('Ctrl Pts',(57.449548243422,-25.3528760603466,2.85384197230804));
#252600=CARTESIAN_POINT('Ctrl Pts',(57.3588307079382,-25.3292685758738,
2.79184624278452));
#252601=CARTESIAN_POINT('Ctrl Pts',(57.4675553545144,-25.2380597013421,
2.90134173516007));
#252602=CARTESIAN_POINT('Ctrl Pts',(57.4161024530847,-25.3547675996707,
2.90163218716375));
#252603=CARTESIAN_POINT('Ctrl Pts',(57.3172883154493,-25.3107727110814,
2.83404198860245));
#252604=CARTESIAN_POINT('Origin',(57.4192809246792,-25.548028700571,2.53178198860245));
#252605=CARTESIAN_POINT('Origin',(0.129138884176568,0.290050682801711,3.64303198860263));
#252606=CARTESIAN_POINT('Origin',(54.9452378026832,-24.1156489724268,3.64303198860246));
#252607=CARTESIAN_POINT('Origin',(5.51404277916147E-15,1.85949616800731E-13,
2.53178198860262));
#252608=CARTESIAN_POINT('Origin',(57.4068835917983,-25.5758735661199,2.53178198860245));
#252609=CARTESIAN_POINT('Ctrl Pts',(54.9452378026832,-24.1156489724268,
3.77003198860247));
#252610=CARTESIAN_POINT('Ctrl Pts',(54.8935048666605,-24.2318430491558,
3.77003198860247));
#252611=CARTESIAN_POINT('Ctrl Pts',(54.8935823068869,-24.2316691155595,
3.64284187937011));
#252612=CARTESIAN_POINT('Ctrl Pts',(54.7469262747042,-24.0276063358784,
3.77003198860247));
#252613=CARTESIAN_POINT('Ctrl Pts',(54.6954612380244,-24.1436677818705,
3.76980208962837));
#252614=CARTESIAN_POINT('Ctrl Pts',(54.7350659388075,-24.161093081681,3.64284193928309));
#252615=CARTESIAN_POINT('Ctrl Pts',(54.5581358350803,-23.9437932708517,
3.65553535416566));
#252616=CARTESIAN_POINT('Ctrl Pts',(54.5068800556933,-24.0597054841975,
3.65520057834521));
#252617=CARTESIAN_POINT('Ctrl Pts',(54.5841613379362,-24.0939060248988,
3.5512791096418));
#252618=CARTESIAN_POINT('Ctrl Pts',(54.4530463244696,-23.897139530776,3.47153072139058));
#252619=CARTESIAN_POINT('Ctrl Pts',(54.4019907306521,-24.013005447697,3.47122746281568));
#252620=CARTESIAN_POINT('Ctrl Pts',(54.5001606201974,-24.0565064959263,
3.40413045901248));
#252621=CARTESIAN_POINT('Origin',(54.5516691663898,-23.9404209259113,3.40423097483294));
#252622=CARTESIAN_POINT('Ctrl Pts',(57.2088336324702,-25.8191582032612,
2.90134173516006));
#252623=CARTESIAN_POINT('Ctrl Pts',(57.2611357920728,-25.7028284190325,
2.90163218716374));
#252624=CARTESIAN_POINT('Ctrl Pts',(57.1623216544374,-25.6588335304432,
2.83404198860244));
#252625=CARTESIAN_POINT('Ctrl Pts',(57.2503966981986,-25.8376627381925,
2.82853349835341));
#252626=CARTESIAN_POINT('Ctrl Pts',(57.2821216226329,-25.7289639953169,
2.85381483162237));
#252627=CARTESIAN_POINT('Ctrl Pts',(57.2038829761265,-25.6773378230585,
2.79182701594191));
#252628=CARTESIAN_POINT('Ctrl Pts',(57.3035546548416,-25.8320911970508,
2.75468822073622));
#252629=CARTESIAN_POINT('Ctrl Pts',(57.3185262575352,-25.7407897001096,
2.79286913083823));
#252630=CARTESIAN_POINT('Ctrl Pts',(57.2524664994805,-25.6820441386708,
2.74900763297889));
#252631=CARTESIAN_POINT('Ctrl Pts',(57.4126476234253,-25.7649464042475,
2.63954450640378));
#252632=CARTESIAN_POINT('Ctrl Pts',(57.3992776612637,-25.7081127933379,
2.69627684028836));
#252633=CARTESIAN_POINT('Ctrl Pts',(57.3434500727661,-25.655572017978,2.6822435603648));
#252634=CARTESIAN_POINT('Ctrl Pts',(57.4692856961539,-25.7004590346995,
2.59908178706388));
#252635=CARTESIAN_POINT('Ctrl Pts',(57.4449640631521,-25.6633754510781,
2.65878704321472));
#252636=CARTESIAN_POINT('Ctrl Pts',(57.3860499078766,-25.6226140882763,
2.65878198860245));
#252637=CARTESIAN_POINT('Ctrl Pts',(57.5052637377735,-25.6197038181289,
2.59908173516006));
#252638=CARTESIAN_POINT('Ctrl Pts',(57.4711877340332,-25.6045223014053,
2.65878198860245));
#252639=CARTESIAN_POINT('Ctrl Pts',(57.4068835917983,-25.5758735661199,
2.65878198860245));
#252640=CARTESIAN_POINT('Origin',(57.1106661007668,-25.7748538035638,2.83404198860243));
#252641=CARTESIAN_POINT('Origin',(54.3889216310736,-23.8679610547589,3.11913648167135));
#252642=CARTESIAN_POINT('Origin',(54.2261740956469,-23.79550118349,2.83404198860246));
#252643=CARTESIAN_POINT('Origin',(56.9479187893679,-25.7023940320471,3.11913648177421));
#252644=CARTESIAN_POINT('Origin',(56.7851714777851,-25.6299342604987,3.40423097483294));
#252645=CARTESIAN_POINT('Ctrl Pts',(54.1275498658877,-23.7522229508819,
2.90134173516007));
#252646=CARTESIAN_POINT('Ctrl Pts',(54.0765745253539,-23.867913970856,2.90103711553213));
#252647=CARTESIAN_POINT('Ctrl Pts',(54.1745185419763,-23.9115214566106,
2.83404198860246));
#252648=CARTESIAN_POINT('Ctrl Pts',(54.0860417646978,-23.7337429357604,
2.82862991747948));
#252649=CARTESIAN_POINT('Ctrl Pts',(54.0553388636012,-23.8418262755861,
2.85314045886458));
#252650=CARTESIAN_POINT('Ctrl Pts',(54.1330089371354,-23.8930401898196,
2.79187960999956));
#252651=CARTESIAN_POINT('Ctrl Pts',(54.0331737207071,-23.7393098712341,
2.75470625793307));
#252652=CARTESIAN_POINT('Ctrl Pts',(54.0188467943739,-23.8301926567292,
2.79224250381902));
#252653=CARTESIAN_POINT('Ctrl Pts',(54.0846755205374,-23.8884275227215,
2.74901809108241));
#252654=CARTESIAN_POINT('Ctrl Pts',(53.924898459262,-23.8065189073815,2.63947868311686));
#252655=CARTESIAN_POINT('Ctrl Pts',(53.9384511174164,-23.8631501047892,
2.69595066767885));
#252656=CARTESIAN_POINT('Ctrl Pts',(53.9943748351528,-23.9152668978352,
2.68220539436047));
#252657=CARTESIAN_POINT('Ctrl Pts',(53.8688190939462,-23.8710081209819,
2.59908178585057));
#252658=CARTESIAN_POINT('Ctrl Pts',(53.8932068550021,-23.9079567336553,
2.65877670944882));
#252659=CARTESIAN_POINT('Ctrl Pts',(53.9522270531172,-23.9484663513835,
2.65878198860246));
#252660=CARTESIAN_POINT('Ctrl Pts',(53.8330634946841,-23.9513722670356,
2.59908173516008));
#252661=CARTESIAN_POINT('Ctrl Pts',(53.8671470951733,-23.9665367208216,
2.65878198860246));
#252662=CARTESIAN_POINT('Ctrl Pts',(53.9314655730807,-23.9951532569799,
2.65878198860246));
#252663=CARTESIAN_POINT('Origin',(53.9314655730807,-23.9951532569799,2.53178198860246));
#252664=CARTESIAN_POINT('Ctrl Pts',(56.3916032444854,-25.4547063934074,
3.77003198860246));
#252665=CARTESIAN_POINT('Ctrl Pts',(56.4433359736148,-25.3385127813683,
3.77003198860246));
#252666=CARTESIAN_POINT('Ctrl Pts',(56.4432587405904,-25.3386862495811,
3.64284238727551));
#252667=CARTESIAN_POINT('Ctrl Pts',(56.5897307565554,-25.5431622092796,
3.77003198860246));
#252668=CARTESIAN_POINT('Ctrl Pts',(56.6417243268775,-25.4268404215536,
3.77025506105722));
#252669=CARTESIAN_POINT('Ctrl Pts',(56.6017747680082,-25.4092621323401,
3.64284210641832));
#252670=CARTESIAN_POINT('Ctrl Pts',(56.7783458705709,-25.6273687254308,
3.65553527987814));
#252671=CARTESIAN_POINT('Ctrl Pts',(56.8305375176153,-25.5109049500375,
3.65585996533227));
#252672=CARTESIAN_POINT('Ctrl Pts',(56.7526792962317,-25.4764491573039,
3.55127902710219));
#252673=CARTESIAN_POINT('Ctrl Pts',(56.8833377255397,-25.6742415049971,
3.47153072139053));
#252674=CARTESIAN_POINT('Ctrl Pts',(56.9357219102091,-25.5577357740369,
3.4718232790517));
#252675=CARTESIAN_POINT('Ctrl Pts',(56.8366797674141,-25.5138485767956,
3.40413028377953));
#252676=CARTESIAN_POINT('Origin',(56.3916032444854,-25.4547063934074,3.64303198860246));
#252677=CARTESIAN_POINT('Origin',(5.71826297912856E-15,1.86300868799497E-13,
2.53178198860262));
#252678=CARTESIAN_POINT('Origin',(53.9190682401998,-24.0229981225288,2.53178198860246));
#252679=CARTESIAN_POINT('Origin',(51.7995637473369,-23.4101986852072,3.64303198860247));
#252680=CARTESIAN_POINT('Origin',(56.0249274780508,-25.2915084057469,3.64299466007761));
#252681=CARTESIAN_POINT('Ctrl Pts',(53.8206887816839,-23.9791663275005,
2.59908173516008));
#252682=CARTESIAN_POINT('Ctrl Pts',(53.8547645473084,-23.9943483786809,
2.65878198860246));
#252683=CARTESIAN_POINT('Ctrl Pts',(53.9190682401998,-24.0229981225288,
2.65878198860246));
#252684=CARTESIAN_POINT('Ctrl Pts',(53.7850138844277,-24.0592381182992,
2.59908193199829));
#252685=CARTESIAN_POINT('Ctrl Pts',(53.828770962649,-24.0526825045776,2.65877685806568));
#252686=CARTESIAN_POINT('Ctrl Pts',(53.8983362760826,-24.0695074323258,
2.65878198860246));
#252687=CARTESIAN_POINT('Ctrl Pts',(53.7744461045709,-24.1432906710364,
2.63872492669783));
#252688=CARTESIAN_POINT('Ctrl Pts',(53.8255298669653,-24.115812828243,2.69532212015263));
#252689=CARTESIAN_POINT('Ctrl Pts',(53.901590305224,-24.1225146216889,2.6817683672662));
#252690=CARTESIAN_POINT('Ctrl Pts',(53.7968389608979,-24.2696905364164,
2.75442176402232));
#252691=CARTESIAN_POINT('Ctrl Pts',(53.8548027426704,-24.1983175571245,
2.79203179920113));
#252692=CARTESIAN_POINT('Ctrl Pts',(53.9421141528991,-24.2081897025468,
2.74885310748157));
#252693=CARTESIAN_POINT('Ctrl Pts',(53.8282518514941,-24.3127961528999,
2.82866089558383));
#252694=CARTESIAN_POINT('Ctrl Pts',(53.88802914902,-24.2176488245055,2.85316563119282));
#252695=CARTESIAN_POINT('Ctrl Pts',(53.9780599067619,-24.2411088588474,
2.79189751796672));
#252696=CARTESIAN_POINT('Ctrl Pts',(53.8697418420148,-24.331269253108,2.90134173516007));
#252697=CARTESIAN_POINT('Ctrl Pts',(53.921607864342,-24.2159747902178,2.90103711553213));
#252698=CARTESIAN_POINT('Ctrl Pts',(54.0195518809644,-24.2595822759724,
2.83404198860245));
#252699=CARTESIAN_POINT('Origin',(53.9678963272938,-24.3756025490931,2.83404198860246));
#252700=CARTESIAN_POINT('Origin',(55.9845461685093,-25.2734729066188,3.56647653971734));
#252701=CARTESIAN_POINT('Origin',(55.909783130075,-25.2401862573133,3.42473028058468));
#252702=CARTESIAN_POINT('Origin',(54.1306438627319,-24.4480624203046,3.11913648167937));
#252703=CARTESIAN_POINT('Origin',(54.2933913980367,-24.5205222915143,3.40423097483294));
#252704=CARTESIAN_POINT('Ctrl Pts',(55.6083495590305,-25.1059793847693,
3.36123028058464));
#252705=CARTESIAN_POINT('Ctrl Pts',(55.6600051127011,-24.9899591116487,
3.36123028058465));
#252706=CARTESIAN_POINT('Ctrl Pts',(55.6600051127011,-24.9899591116487,
3.23423028058464));
#252707=CARTESIAN_POINT('Ctrl Pts',(55.6906734752784,-25.1423759987942,
3.36123028058464));
#252708=CARTESIAN_POINT('Ctrl Pts',(55.7421565548644,-25.0265352902396,
3.36099641108402));
#252709=CARTESIAN_POINT('Ctrl Pts',(55.783346597804,-25.044874278905,3.23423043688411));
#252710=CARTESIAN_POINT('Ctrl Pts',(55.7685161955956,-25.1767934079542,
3.41054258905266));
#252711=CARTESIAN_POINT('Ctrl Pts',(55.8202243900373,-25.0612933298588,
3.41008815825996));
#252712=CARTESIAN_POINT('Ctrl Pts',(55.8999747466293,-25.0968004762765,
3.3081986730426));
#252713=CARTESIAN_POINT('Ctrl Pts',(55.809539512001,-25.1949317875292,3.48823028058467));
#252714=CARTESIAN_POINT('Ctrl Pts',(55.8614118841082,-25.0796311836945,
3.48794691941583));
#252715=CARTESIAN_POINT('Ctrl Pts',(55.9614386837456,-25.1241659841927,
3.42473028058468));
#252716=CARTESIAN_POINT('Origin',(55.6083495590305,-25.1059793847693,3.23423028058464));
#252717=CARTESIAN_POINT('Ctrl Pts',(54.1952354911875,-24.4761921430384,
3.47153072139056));
#252718=CARTESIAN_POINT('Ctrl Pts',(54.247177781362,-24.3607210247417,3.4712274628506));
#252719=CARTESIAN_POINT('Ctrl Pts',(54.3451938326307,-24.404567569022,3.40413046676767));
#252720=CARTESIAN_POINT('Ctrl Pts',(54.3002261711144,-24.5230721320496,
3.6555381345797));
#252721=CARTESIAN_POINT('Ctrl Pts',(54.3520689157398,-24.4074212664147,
3.65520336071996));
#252722=CARTESIAN_POINT('Ctrl Pts',(54.429195821938,-24.4419676644359,3.55128134519888));
#252723=CARTESIAN_POINT('Ctrl Pts',(54.4888383671849,-24.607289548202,3.77003198860246));
#252724=CARTESIAN_POINT('Ctrl Pts',(54.5406519873245,-24.4913833136915,
3.76980209314211));
#252725=CARTESIAN_POINT('Ctrl Pts',(54.5801016184618,-24.5091552540984,
3.64284195387413));
#252726=CARTESIAN_POINT('Ctrl Pts',(54.68696003433,-24.6957503380299,3.77003198860247));
#252727=CARTESIAN_POINT('Ctrl Pts',(54.7386929643779,-24.5795562747206,
3.77003198860246));
#252728=CARTESIAN_POINT('Ctrl Pts',(54.7386155301352,-24.5797301948772,
3.64284189403778));
#252729=CARTESIAN_POINT('Origin',(54.68696003433,-24.6957503380299,3.64303198860247));
#252730=CARTESIAN_POINT('Origin',(50.5417021396889,-22.850162615334,3.23423028058466));
#252731=CARTESIAN_POINT('Origin',(55.470214071797,-25.0444775033939,3.23423028058464));
#252732=CARTESIAN_POINT('Origin',(50.3447265545032,-22.7624634345039,3.64303198860247));
#252733=CARTESIAN_POINT('Origin',(55.0536014459536,-24.8590452239597,3.64299171721713));
#252734=CARTESIAN_POINT('Ctrl Pts',(55.2690209153043,-24.9555320242407,
3.48823028058464));
#252735=CARTESIAN_POINT('Ctrl Pts',(55.3213695969759,-24.8391888661836,
3.48852004212242));
#252736=CARTESIAN_POINT('Ctrl Pts',(55.2204359898059,-24.7942503289599,
3.42473028058464));
#252737=CARTESIAN_POINT('Ctrl Pts',(55.3101840490924,-24.9737291291718,
3.41028005848391));
#252738=CARTESIAN_POINT('Ctrl Pts',(55.3622664445107,-24.8573973158451,
3.41074404220333));
#252739=CARTESIAN_POINT('Ctrl Pts',(55.2821076446827,-24.8217083187814,
3.30780486243885));
#252740=CARTESIAN_POINT('Ctrl Pts',(55.3881672017731,-25.0082040095651,
3.36123028058464));
#252741=CARTESIAN_POINT('Ctrl Pts',(55.4398389138644,-24.8919348043903,
3.36146460586422));
#252742=CARTESIAN_POINT('Ctrl Pts',(55.3989435894784,-24.8737270328796,
3.23423045308444));
#252743=CARTESIAN_POINT('Ctrl Pts',(55.470214071797,-25.0444775033939,3.36123028058464));
#252744=CARTESIAN_POINT('Ctrl Pts',(55.5218696254676,-24.9284572302733,
3.36123028058465));
#252745=CARTESIAN_POINT('Ctrl Pts',(55.5218696254676,-24.9284572302733,
3.23423028058464));
#252746=CARTESIAN_POINT('Origin',(55.1687804361353,-24.9102706020805,3.42473028058464));
#252747=CARTESIAN_POINT('Origin',(55.0944632691836,-24.8771824678734,3.56563113524731));
#252748=CARTESIAN_POINT('Origin',(58.5158800435648,-18.6791227126686,3.56647653909498));
#252749=CARTESIAN_POINT('Origin',(58.5579573083276,-18.6927400943491,3.64299466007739));
#252750=CARTESIAN_POINT('Origin',(58.4380471616457,-18.6538332760095,3.42473028058472));
#252751=CARTESIAN_POINT('Ctrl Pts',(58.3332704847798,-18.6203878281138,
3.48823028058472));
#252752=CARTESIAN_POINT('Ctrl Pts',(58.2946680067391,-18.7407822670293,
3.48794691941588));
#252753=CARTESIAN_POINT('Ctrl Pts',(58.3988020033601,-18.774617453579,3.42473028058473));
#252754=CARTESIAN_POINT('Ctrl Pts',(58.2905032380258,-18.6063701040103,
3.41028005925071));
#252755=CARTESIAN_POINT('Ctrl Pts',(58.2516444665228,-18.7268030714126,
3.40982512231002));
#252756=CARTESIAN_POINT('Ctrl Pts',(58.3345980746932,-18.7537563325796,
3.30780486372849));
#252757=CARTESIAN_POINT('Ctrl Pts',(58.2094810151999,-18.5798130476665,
3.36123028058469));
#252758=CARTESIAN_POINT('Ctrl Pts',(58.170227677228,-18.7003491529652,3.36099721048435));
#252759=CARTESIAN_POINT('Ctrl Pts',(58.2129647630923,-18.7142352739224,
3.23423045308368));
#252760=CARTESIAN_POINT('Ctrl Pts',(58.1242364370959,-18.5518699907141,
3.36123028058469));
#252761=CARTESIAN_POINT('Ctrl Pts',(58.0849912788103,-18.6726541682836,
3.36123028058469));
#252762=CARTESIAN_POINT('Ctrl Pts',(58.0849912788103,-18.6726541682836,
3.23423028058469));
#252763=CARTESIAN_POINT('Origin',(58.1242364370959,-18.5518699907141,3.23423028058469));
#252764=CARTESIAN_POINT('Origin',(0.0981128957140474,0.301960443923896,
3.64303198860263));
#252765=CARTESIAN_POINT('Origin',(58.9396512752216,-18.8168143322217,3.6430319886025));
#252766=CARTESIAN_POINT('Origin',(0.0981128957140474,0.301960443923899,
3.23423028058482));
#252767=CARTESIAN_POINT('Origin',(57.9804289733666,-18.5051441132832,3.23423028058469));
#252768=CARTESIAN_POINT('Ctrl Pts',(59.451978872661,-18.9827025415087,3.47153072139059));
#252769=CARTESIAN_POINT('Ctrl Pts',(59.4129503614029,-19.1043350233598,
3.47182327902649));
#252770=CARTESIAN_POINT('Ctrl Pts',(59.3099814440481,-19.0706774512219,
3.40413028959026));
#252771=CARTESIAN_POINT('Ctrl Pts',(59.3425890481019,-18.9472820042064,
3.65553807120945));
#252772=CARTESIAN_POINT('Ctrl Pts',(59.3034455268839,-19.068754472212,3.65586275496921));
#252773=CARTESIAN_POINT('Ctrl Pts',(59.2225305038479,-19.042262918433,3.55128126837209));
#252774=CARTESIAN_POINT('Ctrl Pts',(59.1460739925266,-18.8836509927319,
3.77003198860251));
#252775=CARTESIAN_POINT('Ctrl Pts',(59.1068782740635,-19.0048854004768,
3.77025505748546));
#252776=CARTESIAN_POINT('Ctrl Pts',(59.0654284453493,-18.9912173655537,
3.64284211731207));
#252777=CARTESIAN_POINT('Ctrl Pts',(58.9396512752216,-18.8168143322217,
3.77003198860251));
#252778=CARTESIAN_POINT('Ctrl Pts',(58.9003474864893,-18.9377789557515,
3.7700319886025));
#252779=CARTESIAN_POINT('Ctrl Pts',(58.9004061606662,-18.9375983752035,
3.64284239821709));
#252780=CARTESIAN_POINT('Origin',(59.3493798002282,-18.9499432001048,3.40423097483297));
#252781=CARTESIAN_POINT('Ctrl Pts',(57.9804289733666,-18.5051441132832,
3.36123028058469));
#252782=CARTESIAN_POINT('Ctrl Pts',(57.941183815081,-18.6259282908527,3.36123028058469));
#252783=CARTESIAN_POINT('Ctrl Pts',(57.941183815081,-18.6259282908527,3.23423028058469));
#252784=CARTESIAN_POINT('Ctrl Pts',(57.8948964606934,-18.477106059508,3.36123028058469));
#252785=CARTESIAN_POINT('Ctrl Pts',(57.8554964068672,-18.5980867642055,
3.36146538610131));
#252786=CARTESIAN_POINT('Ctrl Pts',(57.8127777979909,-18.5842066467853,
3.23423043688402));
#252787=CARTESIAN_POINT('Ctrl Pts',(57.8140195545736,-18.4505921960624,
3.41054258693088));
#252788=CARTESIAN_POINT('Ctrl Pts',(57.7748837362169,-18.5718941197448,
3.41100608859783));
#252789=CARTESIAN_POINT('Ctrl Pts',(57.6913607539435,-18.5447558577159,
3.30819866970838));
#252790=CARTESIAN_POINT('Ctrl Pts',(57.7713971777989,-18.4366189870663,
3.48823028058468));
#252791=CARTESIAN_POINT('Ctrl Pts',(57.7324510618073,-18.5581069080651,
3.48852004212246));
#252792=CARTESIAN_POINT('Ctrl Pts',(57.6273730232608,-18.5239649836999,
3.42473028058468));
#252793=CARTESIAN_POINT('Origin',(57.6666181815464,-18.4031808061304,3.42473028058467));
#252794=CARTESIAN_POINT('Origin',(59.5188096735783,-19.0049943031106,3.11913648178355));
#252795=CARTESIAN_POINT('Origin',(59.6882395467423,-19.0600454060077,2.83404198860249));
#252796=CARTESIAN_POINT('Origin',(57.5892494790284,-18.3780421908168,3.565631134608));
#252797=CARTESIAN_POINT('Origin',(57.5467470426663,-18.3641788932745,3.64299171721775));
#252798=CARTESIAN_POINT('Ctrl Pts',(59.8776671349988,-19.4393816709747,
2.5990817351601));
#252799=CARTESIAN_POINT('Ctrl Pts',(59.8421853116555,-19.4278624395257,
2.65878198860249));
#252800=CARTESIAN_POINT('Ctrl Pts',(59.7752282754839,-19.4061247292244,
2.65878198860249));
#252801=CARTESIAN_POINT('Ctrl Pts',(59.9048758468124,-19.3555723159015,
2.59908193475575));
#252802=CARTESIAN_POINT('Ctrl Pts',(59.8620015382143,-19.3668135526099,
2.65878715325339));
#252803=CARTESIAN_POINT('Ctrl Pts',(59.79096915834,-19.3576098387249,2.65878198860249));
#252804=CARTESIAN_POINT('Ctrl Pts',(59.9061888791359,-19.2705128813942,
2.63878778849882));
#252805=CARTESIAN_POINT('Ctrl Pts',(59.858255137716,-19.3034480936178,2.69564460180118));
#252806=CARTESIAN_POINT('Ctrl Pts',(59.7817014705984,-19.3051157581409,
2.68180481624877));
#252807=CARTESIAN_POINT('Ctrl Pts',(59.8700374834726,-19.1466203444573,
2.75443238878609));
#252808=CARTESIAN_POINT('Ctrl Pts',(59.8200494324143,-19.2244111832561,
2.79268340777058));
#252809=CARTESIAN_POINT('Ctrl Pts',(59.7316696194041,-19.2239451174243,
2.7488592683559));
#252810=CARTESIAN_POINT('Ctrl Pts',(59.834087357436,-19.1068608943528,2.82856655361674));
#252811=CARTESIAN_POINT('Ctrl Pts',(59.7849307811011,-19.2088773592685,
2.85384197230705));
#252812=CARTESIAN_POINT('Ctrl Pts',(59.692242551696,-19.1948817636396,2.79184624278417));
#252813=CARTESIAN_POINT('Ctrl Pts',(59.7908376697914,-19.0928077206402,
2.90134173516011));
#252814=CARTESIAN_POINT('Ctrl Pts',(59.7518659300028,-19.2142545736074,
2.90163218716379));
#252815=CARTESIAN_POINT('Ctrl Pts',(59.6489943884567,-19.1808295835772,
2.83404198860249));
#252816=CARTESIAN_POINT('Origin',(59.7752282754839,-19.4061247292244,2.53178198860248));
#252817=CARTESIAN_POINT('Origin',(0.0981128957140474,0.301960443923896,
3.64303198860263));
#252818=CARTESIAN_POINT('Origin',(57.1650137687749,-18.2401996527036,3.6430319886025));
#252819=CARTESIAN_POINT('Origin',(5.50785759597432E-15,1.85933503847647E-13,
2.53178198860262));
#252820=CARTESIAN_POINT('Origin',(59.7658094374954,-19.4351129318411,2.53178198860249));
#252821=CARTESIAN_POINT('Ctrl Pts',(57.1650137687749,-18.2401996527036,
3.77003198860251));
#252822=CARTESIAN_POINT('Ctrl Pts',(57.1257098194699,-18.3611647704256,
3.77003198860251));
#252823=CARTESIAN_POINT('Ctrl Pts',(57.1257686544592,-18.3609836949477,
3.64284187936996));
#252824=CARTESIAN_POINT('Ctrl Pts',(56.9585856505954,-18.1733685221983,
3.77003198860251));
#252825=CARTESIAN_POINT('Ctrl Pts',(56.9195342693675,-18.2941737326421,
3.76980208962942));
#252826=CARTESIAN_POINT('Ctrl Pts',(56.9607434512668,-18.307363756326,3.64284193928297));
#252827=CARTESIAN_POINT('Ctrl Pts',(56.7620685738644,-18.1097485684444,
3.65553535416572));
#252828=CARTESIAN_POINT('Ctrl Pts',(56.723209704532,-18.2303834904104,3.65520057834524));
#252829=CARTESIAN_POINT('Ctrl Pts',(56.8036425617878,-18.2563185832986,
3.55127910964233));
#252830=CARTESIAN_POINT('Ctrl Pts',(56.6526781108326,-18.0743352474882,
3.4715307213906));
#252831=CARTESIAN_POINT('Ctrl Pts',(56.6140134911409,-18.1949032015562,
3.4712274628157));
#252832=CARTESIAN_POINT('Ctrl Pts',(56.7161926934818,-18.2279043987983,
3.40413045901241));
#252833=CARTESIAN_POINT('Origin',(56.7552848242273,-18.1070706485033,3.40423097483298));
#252834=CARTESIAN_POINT('Ctrl Pts',(59.5942745858238,-19.6977666881836,
2.90134173516011));
#252835=CARTESIAN_POINT('Ctrl Pts',(59.634130455146,-19.5766071063159,2.90163218716378));
#252836=CARTESIAN_POINT('Ctrl Pts',(59.5312589135998,-19.5431821162857,
2.83404198860249));
#252837=CARTESIAN_POINT('Ctrl Pts',(59.6375442153293,-19.7118253299472,
2.82853349835334));
#252838=CARTESIAN_POINT('Ctrl Pts',(59.6577332347555,-19.6004058925603,
2.8538148316221));
#252839=CARTESIAN_POINT('Ctrl Pts',(59.5745267832902,-19.5572406993621,
2.79182701594097));
#252840=CARTESIAN_POINT('Ctrl Pts',(59.6898285824899,-19.7007277907727,
2.75468822073638));
#252841=CARTESIAN_POINT('Ctrl Pts',(59.6951745640079,-19.6083614943623,
2.79286913083837));
#252842=CARTESIAN_POINT('Ctrl Pts',(59.6233361049592,-19.5568428722491,
2.74900763297906));
#252843=CARTESIAN_POINT('Ctrl Pts',(59.7913053863693,-19.62254750381,2.63954450640372));
#252844=CARTESIAN_POINT('Ctrl Pts',(59.7720679362492,-19.5674227749664,
2.69627684028835));
#252845=CARTESIAN_POINT('Ctrl Pts',(59.7110541706152,-19.521005395505,2.68224356036472));
#252846=CARTESIAN_POINT('Ctrl Pts',(59.8408924241701,-19.5524931121154,
2.59908178706399));
#252847=CARTESIAN_POINT('Ctrl Pts',(59.8128277376106,-19.5181549791671,
2.65878704321576));
#252848=CARTESIAN_POINT('Ctrl Pts',(59.7499755976266,-19.4837751174909,
2.65878198860249));
#252849=CARTESIAN_POINT('Ctrl Pts',(59.8682321556244,-19.4684195516687,
2.5990817351601));
#252850=CARTESIAN_POINT('Ctrl Pts',(59.8327559231849,-19.4568831131874,
2.65878198860249));
#252851=CARTESIAN_POINT('Ctrl Pts',(59.7658094374954,-19.4351129318411,
2.65878198860249));
#252852=CARTESIAN_POINT('Origin',(59.4920137553142,-19.6639662938552,2.83404198860249));
#252853=CARTESIAN_POINT('Origin',(56.5858547179611,-18.0520194698708,3.11913648167016));
#252854=CARTESIAN_POINT('Origin',(56.4164246115666,-17.9969682911402,2.8340419886025));
#252855=CARTESIAN_POINT('Origin',(59.3225838821516,-19.6089151909087,3.11913648177479));
#252856=CARTESIAN_POINT('Origin',(59.1531540088002,-19.5538640879523,3.40423097483297));
#252857=CARTESIAN_POINT('Ctrl Pts',(56.3138168485097,-17.9642361803963,
2.90134173516011));
#252858=CARTESIAN_POINT('Ctrl Pts',(56.2752137607568,-18.0846218068686,
2.90103711553218));
#252859=CARTESIAN_POINT('Ctrl Pts',(56.377179453281,-18.1177524687097,2.8340419886025));
#252860=CARTESIAN_POINT('Ctrl Pts',(56.2706044454597,-17.9501961787611,
2.82862991747954));
#252861=CARTESIAN_POINT('Ctrl Pts',(56.2513675234866,-18.0608967538108,
2.85314045886436));
#252862=CARTESIAN_POINT('Ctrl Pts',(56.3339654239813,-18.1037113794367,
2.79187961000014));
#252863=CARTESIAN_POINT('Ctrl Pts',(56.2186079213555,-17.961258833375,2.75470625793309));
#252864=CARTESIAN_POINT('Ctrl Pts',(56.2138593173292,-18.0531413250546,
2.79224250381889));
#252865=CARTESIAN_POINT('Ctrl Pts',(56.2854146278936,-18.1041761987731,
2.74901809108242));
#252866=CARTESIAN_POINT('Ctrl Pts',(56.1179510603879,-18.0394175380786,
2.63947868311692));
#252867=CARTESIAN_POINT('Ctrl Pts',(56.1373490477008,-18.0943218653316,
2.69595066767899));
#252868=CARTESIAN_POINT('Ctrl Pts',(56.1984140977479,-18.140307536857,2.68220539436054));
#252869=CARTESIAN_POINT('Ctrl Pts',(56.0689198620976,-18.1094153628969,
2.59908178585011));
#252870=CARTESIAN_POINT('Ctrl Pts',(56.0970362061477,-18.1436123520177,
2.65877670944876));
#252871=CARTESIAN_POINT('Ctrl Pts',(56.1599674935302,-18.1777307632104,
2.6587819886025));
#252872=CARTESIAN_POINT('Ctrl Pts',(56.0417604764386,-18.193076743594,2.59908173516011));
#252873=CARTESIAN_POINT('Ctrl Pts',(56.0772424804487,-18.2045954185336,
2.65878198860249));
#252874=CARTESIAN_POINT('Ctrl Pts',(56.144199857553,-18.2263320786573,2.6587819886025));
#252875=CARTESIAN_POINT('Origin',(56.144199857553,-18.2263320786573,2.5317819886025));
#252876=CARTESIAN_POINT('Ctrl Pts',(58.7434254837935,-19.4207352200692,
3.7700319886025));
#252877=CARTESIAN_POINT('Ctrl Pts',(58.7827292759118,-19.2997705861182,
3.7700319886025));
#252878=CARTESIAN_POINT('Ctrl Pts',(58.7826705983438,-19.2999511771029,
3.64284238727591));
#252879=CARTESIAN_POINT('Ctrl Pts',(58.9497137831223,-19.4879965013582,
3.7700319886025));
#252880=CARTESIAN_POINT('Ctrl Pts',(58.9892635895157,-19.3668771285514,
3.77025506105836));
#252881=CARTESIAN_POINT('Ctrl Pts',(58.9476954469482,-19.3535710010431,
3.64284210641898));
#252882=CARTESIAN_POINT('Ctrl Pts',(59.1460976215392,-19.5520260773845,
3.65553527987819));
#252883=CARTESIAN_POINT('Ctrl Pts',(59.1858295778045,-19.4307447900781,
3.65585996532955));
#252884=CARTESIAN_POINT('Ctrl Pts',(59.1047962608433,-19.4046161500175,
3.55127902710157));
#252885=CARTESIAN_POINT('Ctrl Pts',(59.2554138597574,-19.5876674457069,
3.47153072139058));
#252886=CARTESIAN_POINT('Ctrl Pts',(59.2953329133628,-19.4663243070084,
3.47182327905175));
#252887=CARTESIAN_POINT('Ctrl Pts',(59.1922458725046,-19.4330302514104,
3.40413028377977));
#252888=CARTESIAN_POINT('Origin',(58.7434254837935,-19.4207352200692,3.6430319886025));
#252889=CARTESIAN_POINT('Origin',(5.72046327455653E-15,1.86306600765055E-13,
2.53178198860262));
#252890=CARTESIAN_POINT('Origin',(56.1347810195644,-18.255320281274,2.5317819886025));
#252891=CARTESIAN_POINT('Origin',(56.182627028633,-18.5886813639048,3.6430319886025));
#252892=CARTESIAN_POINT('Origin',(58.3616995707162,-19.2967593024467,3.64299466007407));
#252893=CARTESIAN_POINT('Ctrl Pts',(56.0323588238394,-18.2220120550208,
2.59908173516011));
#252894=CARTESIAN_POINT('Ctrl Pts',(56.0678348753335,-18.2335490499209,
2.6587819886025));
#252895=CARTESIAN_POINT('Ctrl Pts',(56.1347810195644,-18.255320281274,2.6587819886025));
#252896=CARTESIAN_POINT('Ctrl Pts',(56.0052491386467,-18.3053742463591,
2.59908193199903));
#252897=CARTESIAN_POINT('Ctrl Pts',(56.0480812627891,-18.2942806848325,
2.6587768580666));
#252898=CARTESIAN_POINT('Ctrl Pts',(56.1190241739986,-18.3037418885559,
2.6587819886025));
#252899=CARTESIAN_POINT('Ctrl Pts',(56.0035251343647,-18.3900709842061,
2.63872492669787));
#252900=CARTESIAN_POINT('Ctrl Pts',(56.0514568378825,-18.3574039607296,
2.69532212015265));
#252901=CARTESIAN_POINT('Ctrl Pts',(56.1278011372723,-18.3561185603232,
2.68176836726616));
#252902=CARTESIAN_POINT('Ctrl Pts',(56.0390077039671,-18.5134377270383,
2.75442176402236));
#252903=CARTESIAN_POINT('Ctrl Pts',(56.089193446234,-18.436396871361,2.79203179920119));
#252904=CARTESIAN_POINT('Ctrl Pts',(56.1770584756119,-18.4370884086007,
2.74885310748169));
#252905=CARTESIAN_POINT('Ctrl Pts',(56.0747542753112,-18.5530236652629,
2.82866089558387));
#252906=CARTESIAN_POINT('Ctrl Pts',(56.1242585025264,-18.4521491348405,
2.85316563119207));
#252907=CARTESIAN_POINT('Ctrl Pts',(56.2162483036943,-18.4660698759064,
2.79189751796673));
#252908=CARTESIAN_POINT('Ctrl Pts',(56.1179479440991,-18.5670586829457,
2.90134173516011));
#252909=CARTESIAN_POINT('Ctrl Pts',(56.1574782859,-18.446974339577,2.90103711553218));
#252910=CARTESIAN_POINT('Ctrl Pts',(56.2594439784241,-18.4801050014182,
2.83404198860249));
#252911=CARTESIAN_POINT('Origin',(56.2201988201385,-18.6008891789876,2.83404198860249));
#252912=CARTESIAN_POINT('Origin',(58.319654251203,-19.2830435998979,3.56647653971795));
#252913=CARTESIAN_POINT('Origin',(58.2418213702176,-19.2577541638569,3.42473028058473));
#252914=CARTESIAN_POINT('Origin',(56.3896289265337,-18.6559403576597,3.11913648168106));
#252915=CARTESIAN_POINT('Origin',(56.5590590327992,-18.7109915363508,3.40423097483298));
#252916=CARTESIAN_POINT('Ctrl Pts',(57.9280106456678,-19.1557908785616,
3.36123028058469));
#252917=CARTESIAN_POINT('Ctrl Pts',(57.9672558039534,-19.0350067009921,
3.36123028058469));
#252918=CARTESIAN_POINT('Ctrl Pts',(57.9672558039534,-19.0350067009921,
3.23423028058469));
#252919=CARTESIAN_POINT('Ctrl Pts',(58.0136880650216,-19.1833829156693,
3.36123028058469));
#252920=CARTESIAN_POINT('Ctrl Pts',(58.0527804636641,-19.0627953474444,
3.36099641108448));
#252921=CARTESIAN_POINT('Ctrl Pts',(58.0956618095406,-19.0767283413219,
3.23423043688424));
#252922=CARTESIAN_POINT('Ctrl Pts',(58.0947019536606,-19.2094750027314,
3.4105425890527));
#252923=CARTESIAN_POINT('Ctrl Pts',(58.1340538395294,-19.0892026680431,
3.41008815826056));
#252924=CARTESIAN_POINT('Ctrl Pts',(58.2170788227743,-19.1161791203793,
3.30819867304324));
#252925=CARTESIAN_POINT('Ctrl Pts',(58.1373965169896,-19.223225914143,3.4882302805847));
#252926=CARTESIAN_POINT('Ctrl Pts',(58.1769325318822,-19.1031347997378,
3.48794691941587));
#252927=CARTESIAN_POINT('Ctrl Pts',(58.2810665285032,-19.1369699862874,
3.42473028058472));
#252928=CARTESIAN_POINT('Origin',(57.9280106456678,-19.1557908785616,3.23423028058468));
#252929=CARTESIAN_POINT('Ctrl Pts',(56.4568070719814,-18.6771643191701,
3.4715307213906));
#252930=CARTESIAN_POINT('Ctrl Pts',(56.496394798308,-18.556896315971,3.47122746285065));
#252931=CARTESIAN_POINT('Ctrl Pts',(56.5984571192855,-18.5902571970792,
3.4041304667678));
#252932=CARTESIAN_POINT('Ctrl Pts',(56.5661228951883,-18.712812980264,3.65553813457972));
#252933=CARTESIAN_POINT('Ctrl Pts',(56.605592832572,-18.5923766197432,3.65520336071961));
#252934=CARTESIAN_POINT('Ctrl Pts',(56.6859083114068,-18.6186718120037,
3.55128134519882));
#252935=CARTESIAN_POINT('Ctrl Pts',(56.7625049710036,-18.7768537015936,
3.77003198860251));
#252936=CARTESIAN_POINT('Ctrl Pts',(56.8019192501362,-18.6561664154725,
3.76980209314348));
#252937=CARTESIAN_POINT('Ctrl Pts',(56.8430104456841,-18.6697173900107,
3.64284195387422));
#252938=CARTESIAN_POINT('Ctrl Pts',(56.9687879773469,-18.844120540551,3.77003198860251));
#252939=CARTESIAN_POINT('Ctrl Pts',(57.0080919221124,-18.7231554368001,
3.77003198860251));
#252940=CARTESIAN_POINT('Ctrl Pts',(57.0080330916694,-18.723336498286,3.64284189403798));
#252941=CARTESIAN_POINT('Origin',(56.9687879773468,-18.844120540551,3.64303198860251));
#252942=CARTESIAN_POINT('Origin',(54.8193466381482,-18.1457247135482,3.23423028058469));
#252943=CARTESIAN_POINT('Origin',(57.7842031819385,-19.1090650011306,3.23423028058468));
#252944=CARTESIAN_POINT('Origin',(54.6058629360818,-18.0763596539221,3.6430319886025));
#252945=CARTESIAN_POINT('Origin',(57.3504898524411,-18.9681964166824,3.64299171721744));
#252946=CARTESIAN_POINT('Ctrl Pts',(57.5748148483578,-19.0416371860869,
3.48823028058469));
#252947=CARTESIAN_POINT('Ctrl Pts',(57.6147155869504,-18.9204594407736,
3.48852004212247));
#252948=CARTESIAN_POINT('Ctrl Pts',(57.5096375484039,-18.8863175164083,
3.42473028058469));
#252949=CARTESIAN_POINT('Ctrl Pts',(57.617654601607,-19.0554318862532,3.41028005848393));
#252950=CARTESIAN_POINT('Ctrl Pts',(57.6572916985368,-18.9342932580147,
3.41074404220321));
#252951=CARTESIAN_POINT('Ctrl Pts',(57.5738415009809,-18.9071786451766,
3.30780486243826));
#252952=CARTESIAN_POINT('Ctrl Pts',(57.6988141606862,-19.0815664505351,
3.36123028058469));
#252953=CARTESIAN_POINT('Ctrl Pts',(57.7380493683904,-18.9605330155737,
3.36146460586412));
#252954=CARTESIAN_POINT('Ctrl Pts',(57.6954748424956,-18.9466997135533,
3.2342304530846));
#252955=CARTESIAN_POINT('Ctrl Pts',(57.7842031819385,-19.1090650011306,
3.36123028058469));
#252956=CARTESIAN_POINT('Ctrl Pts',(57.8234483402241,-18.9882808235611,
3.36123028058469));
#252957=CARTESIAN_POINT('Ctrl Pts',(57.8234483402241,-18.9882808235611,
3.23423028058469));
#252958=CARTESIAN_POINT('Origin',(57.4703923901183,-19.0071016939778,3.42473028058468));
#252959=CARTESIAN_POINT('Origin',(57.393023688562,-18.9819630792874,3.56563113524724));
#252960=CARTESIAN_POINT('Origin',(60.1478239224126,-12.4602215063111,3.56647653909461));
#252961=CARTESIAN_POINT('Origin',(60.1910940874961,-12.4693660187264,3.64299466007801));
#252962=CARTESIAN_POINT('Origin',(60.0677739512127,-12.4432063593713,3.42473028058476));
#252963=CARTESIAN_POINT('Ctrl Pts',(59.9600752506739,-12.4208962741577,
3.48823028058476));
#252964=CARTESIAN_POINT('Ctrl Pts',(59.9342688867327,-12.5446662374477,
3.48794691941592));
#252965=CARTESIAN_POINT('Ctrl Pts',(60.0413691664789,-12.5674311046645,
3.42473028058477));
#252966=CARTESIAN_POINT('Ctrl Pts',(59.9160770362136,-12.4114257351938,
3.4102800592508));
#252967=CARTESIAN_POINT('Ctrl Pts',(59.8900198101331,-12.5352608058688,
3.4098251223104));
#252968=CARTESIAN_POINT('Ctrl Pts',(59.9753363727289,-12.5533954010675,
3.30780486372877));
#252969=CARTESIAN_POINT('Ctrl Pts',(59.832722693313,-12.3934832896264,3.36123028058473));
#252970=CARTESIAN_POINT('Ctrl Pts',(59.8062838430907,-12.5174621766265,
3.36099721048495));
#252971=CARTESIAN_POINT('Ctrl Pts',(59.8502383056108,-12.5268049860493,
3.2342304530841));
#252972=CARTESIAN_POINT('Ctrl Pts',(59.7450242491249,-12.3746037924155,
3.36123028058473));
#252973=CARTESIAN_POINT('Ctrl Pts',(59.7186194643911,-12.4988285377087,
3.36123028058473));
#252974=CARTESIAN_POINT('Ctrl Pts',(59.7186194643911,-12.4988285377087,
3.23423028058473));
#252975=CARTESIAN_POINT('Origin',(59.7450242491249,-12.3746037924155,3.23423028058473));
#252976=CARTESIAN_POINT('Origin',(0.0660119618346401,0.310561863233168,
3.64303198860263));
#252977=CARTESIAN_POINT('Origin',(60.5836663843183,-12.5528626811438,3.64303198860255));
#252978=CARTESIAN_POINT('Origin',(0.0660119618346402,0.310561863233171,
3.23423028058482));
#252979=CARTESIAN_POINT('Origin',(59.5971203935661,-12.3431658574201,3.23423028058473));
#252980=CARTESIAN_POINT('Ctrl Pts',(61.1105274371643,-12.6642893210132,
3.47153072139064));
#252981=CARTESIAN_POINT('Ctrl Pts',(61.0844267845858,-12.7893350777074,
3.47182327902655));
#252982=CARTESIAN_POINT('Ctrl Pts',(60.9785037674413,-12.7666250679668,
3.40413028959037));
#252983=CARTESIAN_POINT('Ctrl Pts',(60.9980344071775,-12.6404971713779,
3.65553807120949));
#252984=CARTESIAN_POINT('Ctrl Pts',(60.9718026486699,-12.7653958126134,
3.65586275496802));
#252985=CARTESIAN_POINT('Ctrl Pts',(60.8885617651942,-12.7475073053519,
3.55128126837234));
#252986=CARTESIAN_POINT('Ctrl Pts',(60.7959446297928,-12.5977561540099,
3.77003198860255));
#252987=CARTESIAN_POINT('Ctrl Pts',(60.7696360759166,-12.7224234952028,
3.77025505748547));
#252988=CARTESIAN_POINT('Ctrl Pts',(60.7269846150115,-12.7131630221035,
3.64284211731188));
#252989=CARTESIAN_POINT('Ctrl Pts',(60.5836663843183,-12.5528626811438,
3.77003198860255));
#252990=CARTESIAN_POINT('Ctrl Pts',(60.5572221520605,-12.6772730124458,
3.77003198860255));
#252991=CARTESIAN_POINT('Ctrl Pts',(60.5572616290069,-12.6770872880155,
3.64284239821724));
#252992=CARTESIAN_POINT('Origin',(61.0050661295708,-12.6424339620832,3.40423097483302));
#252993=CARTESIAN_POINT('Ctrl Pts',(59.5971203935661,-12.3431658574201,
3.36123028058473));
#252994=CARTESIAN_POINT('Ctrl Pts',(59.5707156088322,-12.4673906027133,
3.36123028058473));
#252995=CARTESIAN_POINT('Ctrl Pts',(59.5707156088322,-12.4673906027133,
3.23423028058473));
#252996=CARTESIAN_POINT('Ctrl Pts',(59.5091256622726,-12.3242219811463,
3.36123028058473));
#252997=CARTESIAN_POINT('Ctrl Pts',(59.4825873732129,-12.4486583679648,
3.36146538610098));
#252998=CARTESIAN_POINT('Ctrl Pts',(59.4386519140007,-12.4393195978185,
3.23423043688441));
#252999=CARTESIAN_POINT('Ctrl Pts',(59.4259203549056,-12.3063073021292,
3.41054258693093));
#253000=CARTESIAN_POINT('Ctrl Pts',(59.3996784303277,-12.4310355281323,
3.41100608859737));
#253001=CARTESIAN_POINT('Ctrl Pts',(59.3137762748664,-12.4127764613278,
3.30819866970788));
#253002=CARTESIAN_POINT('Ctrl Pts',(59.3820708699072,-12.2968658913794,
3.48823028058473));
#253003=CARTESIAN_POINT('Ctrl Pts',(59.3560370505015,-12.4217592664903,
3.48852004212251));
#253004=CARTESIAN_POINT('Ctrl Pts',(59.2479658375578,-12.3987880210515,
3.42473028058472));
#253005=CARTESIAN_POINT('Origin',(59.2743706222916,-12.2745632757583,3.42473028058472));
#253006=CARTESIAN_POINT('Origin',(61.1793222555443,-12.6794732450919,3.11913648178272));
#253007=CARTESIAN_POINT('Origin',(61.3535783813234,-12.7165125280156,2.83404198860254));
#253008=CARTESIAN_POINT('Origin',(59.1947980527949,-12.2576496039896,3.5656311346087));
#253009=CARTESIAN_POINT('Origin',(59.1510793400374,-12.2483049653993,3.64299171721794));
#253010=CARTESIAN_POINT('Ctrl Pts',(61.5816197022699,-13.0739701745315,
2.59908173516015));
#253011=CARTESIAN_POINT('Ctrl Pts',(61.5451281645061,-13.0662229071057,
2.65878198860253));
#253012=CARTESIAN_POINT('Ctrl Pts',(61.4762657165317,-13.0516031943519,
2.65878198860253));
#253013=CARTESIAN_POINT('Ctrl Pts',(61.5999188988205,-12.9877758510411,
2.59908193475527));
#253014=CARTESIAN_POINT('Ctrl Pts',(61.5584544893694,-13.0034370926701,
2.6587871532546));
#253015=CARTESIAN_POINT('Ctrl Pts',(61.4868491822362,-13.0017087032035,
2.65878198860253));
#253016=CARTESIAN_POINT('Ctrl Pts',(61.5923336062396,-12.9030451317651,
2.63878778849883));
#253017=CARTESIAN_POINT('Ctrl Pts',(61.5481051179915,-12.9408103617793,
2.6956446018011));
#253018=CARTESIAN_POINT('Ctrl Pts',(61.4721451382823,-12.9504709278429,
2.68180481624881));
#253019=CARTESIAN_POINT('Ctrl Pts',(61.5434299552081,-12.7836101409421,
2.75443238878618));
#253020=CARTESIAN_POINT('Ctrl Pts',(61.50184710076,-12.8662000075455,2.7926834077708));
#253021=CARTESIAN_POINT('Ctrl Pts',(61.4139027244675,-12.874974700909,2.74885926835596));
#253022=CARTESIAN_POINT('Ctrl Pts',(61.5035207735037,-12.7478263086944,
2.82856655361677));
#253023=CARTESIAN_POINT('Ctrl Pts',(61.4652971063428,-12.8544221781242,
2.85384197230719));
#253024=CARTESIAN_POINT('Ctrl Pts',(61.371653694653,-12.850191810016,2.79184624278435));
#253025=CARTESIAN_POINT('Ctrl Pts',(61.459039055521,-12.7383709431241,2.90134173516017));
#253026=CARTESIAN_POINT('Ctrl Pts',(61.43297545991,-12.8632261535945,2.90163218716384));
#253027=CARTESIAN_POINT('Ctrl Pts',(61.3271735965895,-12.8407372733088,
2.83404198860254));
#253028=CARTESIAN_POINT('Origin',(61.4762657165317,-13.0516031943519,2.53178198860253));
#253029=CARTESIAN_POINT('Origin',(0.0660119618346401,0.310561863233168,
3.64303198860263));
#253030=CARTESIAN_POINT('Origin',(58.7584778814678,-12.1649068885782,3.64303198860255));
#253031=CARTESIAN_POINT('Origin',(5.5033905580924E-15,1.85916832635312E-13,
2.53178198860262));
#253032=CARTESIAN_POINT('Origin',(61.4699285681956,-13.0814171332223,2.53178198860253));
#253033=CARTESIAN_POINT('Ctrl Pts',(58.7584778814678,-12.1649068885782,
3.77003198860255));
#253034=CARTESIAN_POINT('Ctrl Pts',(58.7320335411741,-12.289317728149,3.77003198860255));
#253035=CARTESIAN_POINT('Ctrl Pts',(58.7320731263176,-12.2891314946913,
3.64284187937075));
#253036=CARTESIAN_POINT('Ctrl Pts',(58.5461948427484,-12.120019479967,3.77003198860255));
#253037=CARTESIAN_POINT('Ctrl Pts',(58.519984972071,-12.2442448876948,3.76980208963029));
#253038=CARTESIAN_POINT('Ctrl Pts',(58.5623471386662,-12.2530551225928,
3.64284193928396));
#253039=CARTESIAN_POINT('Ctrl Pts',(58.3441042111266,-12.0772896710132,
3.6555353541658));
#253040=CARTESIAN_POINT('Ctrl Pts',(58.3180679977625,-12.2013256001478,
3.65520057834298));
#253041=CARTESIAN_POINT('Ctrl Pts',(58.4007711908129,-12.2187110949215,
3.55127910964131));
#253042=CARTESIAN_POINT('Ctrl Pts',(58.2316113004783,-12.0535047649312,
3.47153072139065));
#253043=CARTESIAN_POINT('Ctrl Pts',(58.205761272577,-12.1774537884101,3.47122746281575));
#253044=CARTESIAN_POINT('Ctrl Pts',(58.3108302909892,-12.1995935666427,
3.40413045901286));
#253045=CARTESIAN_POINT('Origin',(58.3370777047236,-12.0753355159223,3.40423097483302));
#253046=CARTESIAN_POINT('Ctrl Pts',(61.3267881959115,-13.3605623192477,
2.90134173516014));
#253047=CARTESIAN_POINT('Ctrl Pts',(61.3537611057085,-13.2359003894741,
2.90163218716382));
#253048=CARTESIAN_POINT('Ctrl Pts',(61.2479592423879,-13.2134115091884,
2.83404198860253));
#253049=CARTESIAN_POINT('Ctrl Pts',(61.3712903180781,-13.3700210384226,
2.82853349835354));
#253050=CARTESIAN_POINT('Ctrl Pts',(61.3797222373783,-13.2571016411963,
2.85381483162401));
#253051=CARTESIAN_POINT('Ctrl Pts',(61.2924596082476,-13.2228703539486,
2.79182701594302));
#253052=CARTESIAN_POINT('Ctrl Pts',(61.4221282572892,-13.3535190881762,
2.75468822073622));
#253053=CARTESIAN_POINT('Ctrl Pts',(61.4177900459398,-13.2610999767694,
2.79286913083837));
#253054=CARTESIAN_POINT('Ctrl Pts',(61.3409599630866,-13.2173727427864,
2.74900763297898));
#253055=CARTESIAN_POINT('Ctrl Pts',(61.5148770953649,-13.2651598666392,
2.63954450640396));
#253056=CARTESIAN_POINT('Ctrl Pts',(61.4899829268152,-13.2123479779261,
2.69627684028846));
#253057=CARTESIAN_POINT('Ctrl Pts',(61.4244514636298,-13.172562552886,2.68224356036489));
#253058=CARTESIAN_POINT('Ctrl Pts',(61.5568698122757,-13.1903059833726,
2.59908178706355));
#253059=CARTESIAN_POINT('Ctrl Pts',(61.5253695547391,-13.1590895168681,
2.65878704321485));
#253060=CARTESIAN_POINT('Ctrl Pts',(61.4592680512448,-13.1314678292768,
2.65878198860253));
#253061=CARTESIAN_POINT('Ctrl Pts',(61.5752716937453,-13.1038352065718,
2.59908173516015));
#253062=CARTESIAN_POINT('Ctrl Pts',(61.5387839176329,-13.096070241967,2.65878198860254));
#253063=CARTESIAN_POINT('Ctrl Pts',(61.4699285681956,-13.0814171332223,
2.65878198860253));
#253064=CARTESIAN_POINT('Origin',(61.2215544576541,-13.3376362544816,2.83404198860253));
#253065=CARTESIAN_POINT('Origin',(58.1628213392036,-12.038296182048,3.11913648167005));
#253066=CARTESIAN_POINT('Origin',(57.9885649735461,-12.001256848085,2.83404198860254));
#253067=CARTESIAN_POINT('Origin',(61.0472983318751,-13.3005969715094,3.11913648177645));
#253068=CARTESIAN_POINT('Origin',(60.8730422059015,-13.2635576885492,3.40423097483301));
#253069=CARTESIAN_POINT('Ctrl Pts',(57.8830978693157,-11.9794294790603,
2.90134173516016));
#253070=CARTESIAN_POINT('Ctrl Pts',(57.8572899778513,-12.1031907419147,
2.90103711553221));
#253071=CARTESIAN_POINT('Ctrl Pts',(57.9621601888122,-12.1254815933782,
2.83404198860254));
#253072=CARTESIAN_POINT('Ctrl Pts',(57.8386546085358,-11.9699833161078,
2.82862991747953));
#253073=CARTESIAN_POINT('Ctrl Pts',(57.8310944294269,-12.0820882677168,
2.85314045886447));
#253074=CARTESIAN_POINT('Ctrl Pts',(57.9177151970033,-12.1160345187358,
2.79187960999923));
#253075=CARTESIAN_POINT('Ctrl Pts',(57.7880992891176,-11.9864204851021,
2.75470625793319));
#253076=CARTESIAN_POINT('Ctrl Pts',(57.7929810340972,-12.07829599916,2.79224250381855));
#253077=CARTESIAN_POINT('Ctrl Pts',(57.8694789541064,-12.1215717318486,
2.74901809108248));
#253078=CARTESIAN_POINT('Ctrl Pts',(57.6961636462599,-12.074672535238,2.6394786831169));
#253079=CARTESIAN_POINT('Ctrl Pts',(57.7211944343233,-12.1272484490374,
2.69595066767926));
#253080=CARTESIAN_POINT('Ctrl Pts',(57.7867317752137,-12.1665991704016,
2.68220539436057));
#253081=CARTESIAN_POINT('Ctrl Pts',(57.6547178110648,-12.1494120604573,
2.5990817858507));
#253082=CARTESIAN_POINT('Ctrl Pts',(57.6862546895616,-12.1804827566574,
2.65877670944855));
#253083=CARTESIAN_POINT('Ctrl Pts',(57.7524075778583,-12.2078361528622,
2.65878198860254));
#253084=CARTESIAN_POINT('Ctrl Pts',(57.6364522029208,-12.2354540642035,
2.59908173516015));
#253085=CARTESIAN_POINT('Ctrl Pts',(57.6729438621908,-12.2432007592838,
2.65878198860254));
#253086=CARTESIAN_POINT('Ctrl Pts',(57.7418065394567,-12.2578193919758,
2.65878198860254));
#253087=CARTESIAN_POINT('Origin',(57.7418065394567,-12.2578193919758,2.53178198860254));
#253088=CARTESIAN_POINT('Ctrl Pts',(60.4516424606491,-13.1739864076097,
3.77003198860255));
#253089=CARTESIAN_POINT('Ctrl Pts',(60.4780866951851,-13.0495760655895,
3.77003198860255));
#253090=CARTESIAN_POINT('Ctrl Pts',(60.4780472159571,-13.049761800754,3.64284238727587));
#253091=CARTESIAN_POINT('Ctrl Pts',(60.6638314094604,-13.219316225644,3.77003198860254));
#253092=CARTESIAN_POINT('Ctrl Pts',(60.6905041359622,-13.0947262769503,
3.77025506105806));
#253093=CARTESIAN_POINT('Ctrl Pts',(60.6477728389708,-13.0858380958626,
3.64284210641946));
#253094=CARTESIAN_POINT('Ctrl Pts',(60.8658323498483,-13.2624673401118,
3.65553527987824));
#253095=CARTESIAN_POINT('Ctrl Pts',(60.8926693037177,-13.137697324057,3.65585996533074));
#253096=CARTESIAN_POINT('Ctrl Pts',(60.8093487091498,-13.1201821075156,
3.55127902710124));
#253097=CARTESIAN_POINT('Ctrl Pts',(60.978275279735,-13.2864868028986,3.47153072139063));
#253098=CARTESIAN_POINT('Ctrl Pts',(61.0052918407717,-13.1616357172817,
3.4718232790518));
#253099=CARTESIAN_POINT('Ctrl Pts',(60.8992893450419,-13.1392995799677,
3.40413028377977));
#253100=CARTESIAN_POINT('Origin',(60.4516424606491,-13.1739864076097,3.64303198860255));
#253101=CARTESIAN_POINT('Origin',(5.72205236298458E-15,1.86312531323806E-13,
2.53178198860262));
#253102=CARTESIAN_POINT('Origin',(57.7354693911206,-12.2876333308462,2.53178198860254));
#253103=CARTESIAN_POINT('Origin',(59.4667368016504,-12.9646382471637,3.64303198860254));
#253104=CARTESIAN_POINT('Origin',(60.0590486699125,-13.090590866118,3.64299466007516));
#253105=CARTESIAN_POINT('Ctrl Pts',(57.6301266171959,-12.2652136052652,
2.59908173516015));
#253106=CARTESIAN_POINT('Ctrl Pts',(57.6666142715157,-12.2729791421546,
2.65878198860254));
#253107=CARTESIAN_POINT('Ctrl Pts',(57.7354693911206,-12.2876333308462,
2.65878198860254));
#253108=CARTESIAN_POINT('Ctrl Pts',(57.6118791634504,-12.3509528635296,
2.59908193199891));
#253109=CARTESIAN_POINT('Ctrl Pts',(57.653317055794,-12.3354428975783,2.65877685806589));
#253110=CARTESIAN_POINT('Ctrl Pts',(57.7248602994012,-12.3374367183498,
2.65878198860254));
#253111=CARTESIAN_POINT('Ctrl Pts',(57.6190178232952,-12.4353658313034,
2.63872492669782));
#253112=CARTESIAN_POINT('Ctrl Pts',(57.6632723181622,-12.3978675338889,
2.69532212015261));
#253113=CARTESIAN_POINT('Ctrl Pts',(57.7390640345626,-12.3886090227458,
2.68176836726626));
#253114=CARTESIAN_POINT('Ctrl Pts',(57.6672013517154,-12.5543478197365,
2.75442176402249));
#253115=CARTESIAN_POINT('Ctrl Pts',(57.7090592089827,-12.4724831634106,
2.79203179920134));
#253116=CARTESIAN_POINT('Ctrl Pts',(57.7965151898612,-12.4639865158412,
2.74885310748168));
#253117=CARTESIAN_POINT('Ctrl Pts',(57.706889956891,-12.5899803678805,2.82866089558387));
#253118=CARTESIAN_POINT('Ctrl Pts',(57.7455787351224,-12.4844838378922,
2.85316563119125));
#253119=CARTESIAN_POINT('Ctrl Pts',(57.8385197202051,-12.4887127671314,
2.79189751796652));
#253120=CARTESIAN_POINT('Ctrl Pts',(57.7513140650722,-12.5994235324462,
2.90134173516015));
#253121=CARTESIAN_POINT('Ctrl Pts',(57.7780756236497,-12.4758649777943,
2.90103711553221));
#253122=CARTESIAN_POINT('Ctrl Pts',(57.8829458346107,-12.4981558292578,
2.83404198860253));
#253123=CARTESIAN_POINT('Origin',(57.8565410498768,-12.622380574551,2.83404198860254));
#253124=CARTESIAN_POINT('Origin',(60.0157999977487,-13.0813452322597,3.56647653971841));
#253125=CARTESIAN_POINT('Origin',(59.9357500275435,-13.0643300858372,3.42473028058477));
#253126=CARTESIAN_POINT('Origin',(58.0307974155295,-12.6594199084515,3.11913648168104));
#253127=CARTESIAN_POINT('Origin',(58.2050537810543,-12.6964592423883,3.40423097483303));
#253128=CARTESIAN_POINT('Ctrl Pts',(59.6130003254557,-12.9957275188814,
3.36123028058473));
#253129=CARTESIAN_POINT('Ctrl Pts',(59.6394051101895,-12.8715027735882,
3.36123028058473));
#253130=CARTESIAN_POINT('Ctrl Pts',(59.6394051101895,-12.8715027735882,
3.23423028058473));
#253131=CARTESIAN_POINT('Ctrl Pts',(59.7010925481785,-13.0142126749434,
3.36123028058473));
#253132=CARTESIAN_POINT('Ctrl Pts',(59.7273659613752,-12.8901994296784,
3.36099641108421));
#253133=CARTESIAN_POINT('Ctrl Pts',(59.7714687931899,-12.8995737759683,
3.23423043688393));
#253134=CARTESIAN_POINT('Ctrl Pts',(59.7843900000233,-13.0316935695379,
3.41054258905273));
#253135=CARTESIAN_POINT('Ctrl Pts',(59.8109544298256,-12.9079667071259,
3.41008815826081));
#253136=CARTESIAN_POINT('Ctrl Pts',(59.8963444006342,-12.9261169057231,
3.30819867304296));
#253137=CARTESIAN_POINT('Ctrl Pts',(59.8282880397057,-13.0409063549229,
3.48823028058476));
#253138=CARTESIAN_POINT('Ctrl Pts',(59.8550545325311,-12.9173404733273,
3.48794691941592));
#253139=CARTESIAN_POINT('Ctrl Pts',(59.9621548122773,-12.940105340544,3.42473028058477));
#253140=CARTESIAN_POINT('Origin',(59.6130003254557,-12.9957275188814,3.23423028058473));
#253141=CARTESIAN_POINT('Ctrl Pts',(58.0998260601482,-12.6735055745731,
3.47153072139064));
#253142=CARTESIAN_POINT('Ctrl Pts',(58.1266254912132,-12.5497583678821,
3.47122746285069));
#253143=CARTESIAN_POINT('Ctrl Pts',(58.2316158657529,-12.5722680770238,
3.4041304667678));
#253144=CARTESIAN_POINT('Ctrl Pts',(58.2122693395992,-12.6975323335619,
3.65553813457982));
#253145=CARTESIAN_POINT('Ctrl Pts',(58.238934028847,-12.5736300041233,3.65520336072198));
#253146=CARTESIAN_POINT('Ctrl Pts',(58.3215581271246,-12.5913858949911,
3.55128134519905));
#253147=CARTESIAN_POINT('Ctrl Pts',(58.4142696920429,-12.7406947165187,
3.77003198860255));
#253148=CARTESIAN_POINT('Ctrl Pts',(58.4408527990778,-12.6165486539527,
3.76980209314141));
#253149=CARTESIAN_POINT('Ctrl Pts',(58.4831353553006,-12.6257301953092,
3.64284195387441));
#253150=CARTESIAN_POINT('Ctrl Pts',(58.6264539577985,-12.7860306150442,
3.77003198860255));
#253151=CARTESIAN_POINT('Ctrl Pts',(58.6528982950381,-12.6616197898416,
3.77003198860255));
#253152=CARTESIAN_POINT('Ctrl Pts',(58.6528587129533,-12.6618060089097,
3.64284189403795));
#253153=CARTESIAN_POINT('Origin',(58.6264539577985,-12.7860306150442,3.64303198860255));
#253154=CARTESIAN_POINT('Origin',(58.0246834617332,-12.6581203474861,3.23423028058473));
#253155=CARTESIAN_POINT('Origin',(59.4650964698968,-12.9642895838861,3.23423028058473));
#253156=CARTESIAN_POINT('Origin',(57.7988642628865,-12.6101209950202,3.64303198860255));
#253157=CARTESIAN_POINT('Origin',(59.0190342907436,-12.8695280801137,3.64299171721763));
#253158=CARTESIAN_POINT('Ctrl Pts',(59.2498070616281,-12.9191181862036,
3.48823028058473));
#253159=CARTESIAN_POINT('Ctrl Pts',(59.2768226963,-12.7944335023699,3.48852004212251));
#253160=CARTESIAN_POINT('Ctrl Pts',(59.1687514833562,-12.771462256931,3.42473028058473));
#253161=CARTESIAN_POINT('Ctrl Pts',(59.2938540730361,-12.9283593439856,
3.41028005848398));
#253162=CARTESIAN_POINT('Ctrl Pts',(59.3206115991478,-12.8037411209985,
3.4107440422032));
#253163=CARTESIAN_POINT('Ctrl Pts',(59.2347843016956,-12.7854979657546,
3.30780486243868));
#253164=CARTESIAN_POINT('Ctrl Pts',(59.3773008374014,-12.9458672564,3.36123028058473));
#253165=CARTESIAN_POINT('Ctrl Pts',(59.4036696715728,-12.8213956592925,
3.36146460586378));
#253166=CARTESIAN_POINT('Ctrl Pts',(59.3598823995826,-12.812088387313,3.23423045308421));
#253167=CARTESIAN_POINT('Ctrl Pts',(59.4650964698968,-12.9642895838861,
3.36123028058473));
#253168=CARTESIAN_POINT('Ctrl Pts',(59.4915012546307,-12.8400648385929,
3.36123028058473));
#253169=CARTESIAN_POINT('Ctrl Pts',(59.4915012546306,-12.8400648385929,
3.23423028058473));
#253170=CARTESIAN_POINT('Origin',(59.1423466986224,-12.8956870022242,3.42473028058473));
#253171=CARTESIAN_POINT('Origin',(59.062774130148,-12.8787733309731,3.56563113524819));
#253172=CARTESIAN_POINT('Origin',(61.1207756556244,-6.10480350566308,3.56647653909447));
#253173=CARTESIAN_POINT('Origin',(61.1647646440465,-6.10937495962015,3.64299466007748));
#253174=CARTESIAN_POINT('Origin',(61.0393856393805,-6.09624906995137,3.4247302805848));
#253175=CARTESIAN_POINT('Ctrl Pts',(60.9299448846691,-6.08531878138219,
3.48823028058481));
#253176=CARTESIAN_POINT('Ctrl Pts',(60.9172173747511,-6.21110821942835,
3.48794691941597));
#253177=CARTESIAN_POINT('Ctrl Pts',(61.0261105245455,-6.22255335066314,
3.42473028058482));
#253178=CARTESIAN_POINT('Ctrl Pts',(60.8851977561471,-6.0804991887655,3.41028005925085));
#253179=CARTESIAN_POINT('Ctrl Pts',(60.8722275639199,-6.2063795997648,3.40982512230922));
#253180=CARTESIAN_POINT('Ctrl Pts',(60.9589723348255,-6.2154968425755,3.30780486372776));
#253181=CARTESIAN_POINT('Ctrl Pts',(60.800424540796,-6.07136793516245,3.36123028058478));
#253182=CARTESIAN_POINT('Ctrl Pts',(60.787089847893,-6.19743126523058,3.36099721048457));
#253183=CARTESIAN_POINT('Ctrl Pts',(60.8317801127809,-6.20212840134576,
3.23423045308397));
#253184=CARTESIAN_POINT('Ctrl Pts',(60.7112330730305,-6.06175884541469,
3.36123028058478));
#253185=CARTESIAN_POINT('Ctrl Pts',(60.6979579581955,-6.18806312612646,
3.36123028058478));
#253186=CARTESIAN_POINT('Ctrl Pts',(60.6979579581955,-6.18806312612646,
3.23423028058478));
#253187=CARTESIAN_POINT('Origin',(60.7112330730305,-6.06175884541469,3.23423028058478));
#253188=CARTESIAN_POINT('Origin',(0.0331877870874813,0.315760701779611,
3.64303198860263));
#253189=CARTESIAN_POINT('Origin',(61.5639141665613,-6.15137923967573,3.64303198860259));
#253190=CARTESIAN_POINT('Origin',(0.0331877870874813,0.315760701779614,
3.23423028058482));
#253191=CARTESIAN_POINT('Origin',(60.5608532912344,-6.0459532934496,3.23423028058478));
#253192=CARTESIAN_POINT('Ctrl Pts',(62.099536274866,-6.20712349654361,3.47153072139067));
#253193=CARTESIAN_POINT('Ctrl Pts',(62.0866494451786,-6.33421250060399,
3.47182327902658));
#253194=CARTESIAN_POINT('Ctrl Pts',(61.9789328429853,-6.3226988688789,3.40413028958998));
#253195=CARTESIAN_POINT('Ctrl Pts',(61.9851725366286,-6.195220406346,3.65553807120954));
#253196=CARTESIAN_POINT('Ctrl Pts',(61.9721399414771,-6.32217680516124,
3.65586275496904));
#253197=CARTESIAN_POINT('Ctrl Pts',(61.8874852020944,-6.31308733464651,
3.55128126837217));
#253198=CARTESIAN_POINT('Ctrl Pts',(61.7797221753255,-6.17383766261601,
3.7700319886026));
#253199=CARTESIAN_POINT('Ctrl Pts',(61.7665890280504,-6.3005720557779,3.77025505748631));
#253200=CARTESIAN_POINT('Ctrl Pts',(61.7232032332896,-6.29582060418223,
3.64284211731207));
#253201=CARTESIAN_POINT('Ctrl Pts',(61.5639141665613,-6.15137923967573,
3.77003198860259));
#253202=CARTESIAN_POINT('Ctrl Pts',(61.5506192193202,-6.27787221312659,
3.77003198860259));
#253203=CARTESIAN_POINT('Ctrl Pts',(61.5506390665185,-6.27768337964882,
3.64284239821648));
#253204=CARTESIAN_POINT('Origin',(61.992368188267,-6.19641157197361,3.40423097483306));
#253205=CARTESIAN_POINT('Ctrl Pts',(60.5608532912344,-6.0459532934496,3.36123028058478));
#253206=CARTESIAN_POINT('Ctrl Pts',(60.5475781763994,-6.17225757416137,
3.36123028058478));
#253207=CARTESIAN_POINT('Ctrl Pts',(60.5475781763994,-6.17225757416137,
3.23423028058478));
#253208=CARTESIAN_POINT('Ctrl Pts',(60.4713604300109,-6.03631114774924,
3.36123028058478));
#253209=CARTESIAN_POINT('Ctrl Pts',(60.457974664764,-6.162839865594,3.36146538610174));
#253210=CARTESIAN_POINT('Ctrl Pts',(60.4133037213019,-6.15814476024263,
3.23423043688428));
#253211=CARTESIAN_POINT('Ctrl Pts',(60.386738336156,-6.02719193013285,3.41054258693097));
#253212=CARTESIAN_POINT('Ctrl Pts',(60.3736778173769,-6.15397990991393,
3.41100608859692));
#253213=CARTESIAN_POINT('Ctrl Pts',(60.2863376507178,-6.1448000884892,3.30819866970818));
#253214=CARTESIAN_POINT('Ctrl Pts',(60.3421421670676,-6.02238575970175,
3.48823028058478));
#253215=CARTESIAN_POINT('Ctrl Pts',(60.3293058762212,-6.14931623097146,
3.48852004212255));
#253216=CARTESIAN_POINT('Ctrl Pts',(60.2194255397046,-6.13776734223115,
3.42473028058477));
#253217=CARTESIAN_POINT('Origin',(60.2327006545396,-6.01146306151938,3.42473028058478));
#253218=CARTESIAN_POINT('Origin',(62.1695413802842,-6.21503322485375,3.11913648178356));
#253219=CARTESIAN_POINT('Origin',(62.346714572097,-6.23365487766521,2.83404198860258));
#253220=CARTESIAN_POINT('Origin',(60.1517960317847,-6.00295964302144,3.56563113460787));
#253221=CARTESIAN_POINT('Origin',(60.1073400339999,-5.99823604520041,3.64299171721801));
#253222=CARTESIAN_POINT('Ctrl Pts',(62.6108711573006,-6.56531752495198,
2.59908173516019));
#253223=CARTESIAN_POINT('Ctrl Pts',(62.5737697140403,-6.56142710223248,
2.65878198860258));
#253224=CARTESIAN_POINT('Ctrl Pts',(62.5037563256536,-6.55408556365842,
2.65878198860258));
#253225=CARTESIAN_POINT('Ctrl Pts',(62.6200603487599,-6.47768259608977,
2.59908193475699));
#253226=CARTESIAN_POINT('Ctrl Pts',(62.5804601311999,-6.49759225479858,
2.65878715325436));
#253227=CARTESIAN_POINT('Ctrl Pts',(62.5090664195357,-6.50335812634647,
2.65878198860258));
#253228=CARTESIAN_POINT('Ctrl Pts',(62.6036598373291,-6.39420891953656,
2.63878778849873));
#253229=CARTESIAN_POINT('Ctrl Pts',(62.563621178826,-6.43639040357826,2.69564460180097));
#253230=CARTESIAN_POINT('Ctrl Pts',(62.4890871199578,-6.45393802799926,
2.68180481624877));
#253231=CARTESIAN_POINT('Ctrl Pts',(62.5425397295636,-6.28054002958038,
2.75443238878635));
#253232=CARTESIAN_POINT('Ctrl Pts',(62.5098176621801,-6.36702405212695,
2.79268340777105));
#253233=CARTESIAN_POINT('Ctrl Pts',(62.4232722595963,-6.38494336730876,
2.74885926835608));
#253234=CARTESIAN_POINT('Ctrl Pts',(62.4991087455377,-6.24912387034354,
2.82856655361668));
#253235=CARTESIAN_POINT('Ctrl Pts',(62.472236774049,-6.35913125763664,2.85384197230803));
#253236=CARTESIAN_POINT('Ctrl Pts',(62.378664156887,-6.36471246584618,2.79184624278429));
#253237=CARTESIAN_POINT('Ctrl Pts',(62.4538823482276,-6.24436990787956,
2.9013417351602));
#253238=CARTESIAN_POINT('Ctrl Pts',(62.4410124550019,-6.37126553603967,
2.90163218716387));
#253239=CARTESIAN_POINT('Ctrl Pts',(62.333439457262,-6.35995915837698,2.83404198860258));
#253240=CARTESIAN_POINT('Origin',(62.5037563256536,-6.55408556365842,2.53178198860258));
#253241=CARTESIAN_POINT('Origin',(0.0331877870874813,0.315760701779611,
3.64303198860263));
#253242=CARTESIAN_POINT('Origin',(59.7081718144893,-5.95633285891111,3.64303198860259));
#253243=CARTESIAN_POINT('Origin',(5.50069060731754E-15,1.85899785817018E-13,
2.53178198860262));
#253244=CARTESIAN_POINT('Origin',(62.5005702980932,-6.58439859102924,2.53178198860258));
#253245=CARTESIAN_POINT('Ctrl Pts',(59.7081718144893,-5.95633285891111,
3.7700319886026));
#253246=CARTESIAN_POINT('Ctrl Pts',(59.6948768129328,-6.08282634913903,
3.7700319886026));
#253247=CARTESIAN_POINT('Ctrl Pts',(59.6948967145276,-6.08263699811283,
3.64284187937022));
#253248=CARTESIAN_POINT('Ctrl Pts',(59.4923596726254,-5.93388096803621,
3.77003198860259));
#253249=CARTESIAN_POINT('Ctrl Pts',(59.4792784733334,-6.06016553348737,
3.76980208962883));
#253250=CARTESIAN_POINT('Ctrl Pts',(59.5223294958632,-6.06449945282166,
3.64284193928313));
#253251=CARTESIAN_POINT('Ctrl Pts',(59.286909633363,-5.91250946061063,3.65553535416583));
#253252=CARTESIAN_POINT('Ctrl Pts',(59.2739813341584,-6.03858743331987,
3.65520057834522));
#253253=CARTESIAN_POINT('Ctrl Pts',(59.3580487495157,-6.04723285085665,
3.55127910964232));
#253254=CARTESIAN_POINT('Ctrl Pts',(59.1725467709678,-5.90061356181158,
3.47153072139069));
#253255=CARTESIAN_POINT('Ctrl Pts',(59.1597945531718,-6.02658564326334,
3.47122746281579));
#253256=CARTESIAN_POINT('Ctrl Pts',(59.266602229504,-6.03762143444208,3.4041304590126));
#253257=CARTESIAN_POINT('Origin',(59.2797173540687,-5.91130048050243,3.40423097483307));
#253258=CARTESIAN_POINT('Ctrl Pts',(62.3873926810692,-6.87697683366461,
2.9013417351602));
#253259=CARTESIAN_POINT('Ctrl Pts',(62.4011871104969,-6.75017837817499,
2.90163218716387));
#253260=CARTESIAN_POINT('Ctrl Pts',(62.293614112757,-6.73887200051229,2.83404198860258));
#253261=CARTESIAN_POINT('Ctrl Pts',(62.4326397213342,-6.88173199854405,
2.82853349835343));
#253262=CARTESIAN_POINT('Ctrl Pts',(62.4292221586327,-6.76854981002352,
2.85381483162388));
#253263=CARTESIAN_POINT('Ctrl Pts',(62.3388594194629,-6.74362747387298,
2.79182701594246));
#253264=CARTESIAN_POINT('Ctrl Pts',(62.4814742414947,-6.86000643604628,
2.7546882207365));
#253265=CARTESIAN_POINT('Ctrl Pts',(62.4674993676295,-6.7685470727674,2.79286913083857));
#253266=CARTESIAN_POINT('Ctrl Pts',(62.3865194274374,-6.73309031164083,
2.74900763297913));
#253267=CARTESIAN_POINT('Ctrl Pts',(62.5644789380884,-6.76243636205594,
2.63954450640377));
#253268=CARTESIAN_POINT('Ctrl Pts',(62.5342007968288,-6.7125159315779,2.69627684028836));
#253269=CARTESIAN_POINT('Ctrl Pts',(62.4648696125159,-6.67979835840146,
2.68224356036483));
#253270=CARTESIAN_POINT('Ctrl Pts',(62.5984172531148,-6.6836031020271,2.59908178706326));
#253271=CARTESIAN_POINT('Ctrl Pts',(62.5638265480141,-6.65585031610526,
2.65878704321495));
#253272=CARTESIAN_POINT('Ctrl Pts',(62.4951999029147,-6.63528943158862,
2.65878198860258));
#253273=CARTESIAN_POINT('Ctrl Pts',(62.6076796697355,-6.59568250079781,
2.59908173516019));
#253274=CARTESIAN_POINT('Ctrl Pts',(62.570580117661,-6.5917740846467,2.65878198860258));
#253275=CARTESIAN_POINT('Ctrl Pts',(62.5005702980932,-6.58439859102924,
2.65878198860258));
#253276=CARTESIAN_POINT('Origin',(62.280338997922,-6.86517628122406,2.83404198860256));
#253277=CARTESIAN_POINT('Origin',(59.1025439185018,-5.89267880207648,3.11913648166983));
#253278=CARTESIAN_POINT('Origin',(58.9253704827881,-5.8740571235777,2.83404198860258));
#253279=CARTESIAN_POINT('Origin',(62.1031658061017,-6.84655462836415,3.11913648177572));
#253280=CARTESIAN_POINT('Origin',(61.925992614092,-6.82793297553246,3.40423097483306));
#253281=CARTESIAN_POINT('Ctrl Pts',(58.8181995570486,-5.86337364149481,
2.9013417351602));
#253282=CARTESIAN_POINT('Ctrl Pts',(58.8054696185321,-5.98915458643695,
2.90103711553225));
#253283=CARTESIAN_POINT('Ctrl Pts',(58.9120953679531,-6.00036140428947,
2.83404198860258));
#253284=CARTESIAN_POINT('Ctrl Pts',(58.7730123682041,-5.85862481136359,
2.82862991747957));
#253285=CARTESIAN_POINT('Ctrl Pts',(58.7772117628632,-5.97090589422296,
2.8531404588642));
#253286=CARTESIAN_POINT('Ctrl Pts',(58.8669063622646,-5.99561184840417,
2.79187960999922));
#253287=CARTESIAN_POINT('Ctrl Pts',(58.7244521481308,-5.88025640567477,
2.75470625793323));
#253288=CARTESIAN_POINT('Ctrl Pts',(58.7389107566974,-5.97111833475291,
2.79224250381903));
#253289=CARTESIAN_POINT('Ctrl Pts',(58.8195131589314,-6.00616078842793,
2.74901809108255));
#253290=CARTESIAN_POINT('Ctrl Pts',(58.642244989525,-5.97763489331347,2.63947868311695));
#253291=CARTESIAN_POINT('Ctrl Pts',(58.6726343357866,-6.02730636094513,
2.69595066767902));
#253292=CARTESIAN_POINT('Ctrl Pts',(58.7419259266988,-6.05959099741067,
2.68220539436058));
#253293=CARTESIAN_POINT('Ctrl Pts',(58.6088386066682,-6.05629725705532,
2.59908178585078));
#253294=CARTESIAN_POINT('Ctrl Pts',(58.6434504949713,-6.08390124328518,
2.65877670944852));
#253295=CARTESIAN_POINT('Ctrl Pts',(58.712100199296,-6.10418993496927,2.65878198860258));
#253296=CARTESIAN_POINT('Ctrl Pts',(58.5996668978649,-6.14377718965223,
2.5990817351602));
#253297=CARTESIAN_POINT('Ctrl Pts',(58.6367684021393,-6.14766703046072,
2.65878198860258));
#253298=CARTESIAN_POINT('Ctrl Pts',(58.7067819056644,-6.15500747092217,
2.65878198860258));
#253299=CARTESIAN_POINT('Origin',(58.7067819056644,-6.15500747092217,2.53178198860258));
#253300=CARTESIAN_POINT('Ctrl Pts',(61.4975385923863,-6.78290064323459,
3.77003198860259));
#253301=CARTESIAN_POINT('Ctrl Pts',(61.5108335407727,-6.65640765888671,
3.77003198860259));
#253302=CARTESIAN_POINT('Ctrl Pts',(61.5108136924274,-6.65659650327775,
3.6428423872758));
#253303=CARTESIAN_POINT('Ctrl Pts',(61.7133034041536,-6.80580235504162,
3.77003198860259));
#253304=CARTESIAN_POINT('Ctrl Pts',(61.7268068187927,-6.67910686401023,
3.7702550610589));
#253305=CARTESIAN_POINT('Ctrl Pts',(61.683380540407,-6.6747340101162,3.64284210641928));
#253306=CARTESIAN_POINT('Ctrl Pts',(61.9187082819379,-6.82760223531246,
3.65553527987827));
#253307=CARTESIAN_POINT('Ctrl Pts',(61.932356202127,-6.70071049691164,3.6558599653304));
#253308=CARTESIAN_POINT('Ctrl Pts',(61.847661207825,-6.69200060426902,3.55127902710152));
#253309=CARTESIAN_POINT('Ctrl Pts',(62.0330459552233,-6.83973663030157,
3.47153072139068));
#253310=CARTESIAN_POINT('Ctrl Pts',(62.0468640245951,-6.71274549238699,
3.47182327905184));
#253311=CARTESIAN_POINT('Ctrl Pts',(61.9391074595192,-6.70161199275156,
3.40413028377976));
#253312=CARTESIAN_POINT('Origin',(61.4975385923863,-6.78290064323459,3.64303198860259));
#253313=CARTESIAN_POINT('Origin',(5.72301283402738E-15,1.86318595499308E-13,
2.53178198860262));
#253314=CARTESIAN_POINT('Origin',(58.703595878104,-6.185320498293,2.53178198860258));
#253315=CARTESIAN_POINT('Origin',(61.5094129706999,-6.78414869068649,3.64303198860258));
#253316=CARTESIAN_POINT('Origin',(61.0983782637173,-6.74099917687762,3.64299466007604));
#253317=CARTESIAN_POINT('Ctrl Pts',(58.5964866834552,-6.17403490858921,
2.5990817351602));
#253318=CARTESIAN_POINT('Ctrl Pts',(58.6335861742243,-6.17794390662073,
2.65878198860258));
#253319=CARTESIAN_POINT('Ctrl Pts',(58.703595878104,-6.185320498293,2.65878198860258));
#253320=CARTESIAN_POINT('Ctrl Pts',(58.5873013840787,-6.26121185652445,
2.5990819319991));
#253321=CARTESIAN_POINT('Ctrl Pts',(58.626891042407,-6.24145541658163,2.65877685806647));
#253322=CARTESIAN_POINT('Ctrl Pts',(58.6982507756596,-6.23596000968288,
2.65878198860258));
#253323=CARTESIAN_POINT('Ctrl Pts',(58.6032244953991,-6.34441620808506,
2.63872492669791));
#253324=CARTESIAN_POINT('Ctrl Pts',(58.6433169201089,-6.30249747592631,
2.69532212015275));
#253325=CARTESIAN_POINT('Ctrl Pts',(58.7177256636153,-6.28536729223223,
2.68176836726633));
#253326=CARTESIAN_POINT('Ctrl Pts',(58.6635810738165,-6.45770985055576,
2.75442176402249));
#253327=CARTESIAN_POINT('Ctrl Pts',(58.6966524426404,-6.37191831988681,
2.79203179920125));
#253328=CARTESIAN_POINT('Ctrl Pts',(58.7827411889911,-6.35432657855714,
2.74885310748169));
#253329=CARTESIAN_POINT('Ctrl Pts',(58.7067768761601,-6.48899861096465,
2.82866089558393));
#253330=CARTESIAN_POINT('Ctrl Pts',(58.7342263230553,-6.38003592347135,
2.85316563119217));
#253331=CARTESIAN_POINT('Ctrl Pts',(58.8271002111739,-6.37452670784861,
2.79189751796605));
#253332=CARTESIAN_POINT('Ctrl Pts',(58.7519447039089,-6.49374646112642,
2.90134173516019));
#253333=CARTESIAN_POINT('Ctrl Pts',(58.7656442740272,-6.36806742857227,
2.90103711553225));
#253334=CARTESIAN_POINT('Ctrl Pts',(58.8722700234481,-6.37927424642479,
2.83404198860258));
#253335=CARTESIAN_POINT('Origin',(58.8589949086131,-6.50557852713656,2.83404198860258));
#253336=CARTESIAN_POINT('Origin',(61.0544000804071,-6.73632490881137,3.56647653971777));
#253337=CARTESIAN_POINT('Origin',(60.9730100652055,-6.72777047351023,3.42473028058482));
#253338=CARTESIAN_POINT('Origin',(59.0361683443145,-6.52420020557606,3.11913648168137));
#253339=CARTESIAN_POINT('Origin',(59.2133417798937,-6.54282188406129,3.40423097483307));
#253340=CARTESIAN_POINT('Ctrl Pts',(60.6448574988555,-6.69328024897354,
3.36123028058478));
#253341=CARTESIAN_POINT('Ctrl Pts',(60.6581326136905,-6.56697596826177,
3.36123028058478));
#253342=CARTESIAN_POINT('Ctrl Pts',(60.6581326136905,-6.56697596826177,
3.23423028058478));
#253343=CARTESIAN_POINT('Ctrl Pts',(60.7343993681214,-6.70245599674913,
3.36123028058477));
#253344=CARTESIAN_POINT('Ctrl Pts',(60.7475659388593,-6.57637578951109,
3.36099641108468));
#253345=CARTESIAN_POINT('Ctrl Pts',(60.7924070567585,-6.58108878091615,
3.23423043688383));
#253346=CARTESIAN_POINT('Ctrl Pts',(60.819067758858,-6.71113417453868,3.41054258905281));
#253347=CARTESIAN_POINT('Ctrl Pts',(60.8325536871411,-6.5853083618035,3.41008815826054));
#253348=CARTESIAN_POINT('Ctrl Pts',(60.9193730951228,-6.59443344928315,
3.30819867304313));
#253349=CARTESIAN_POINT('Ctrl Pts',(60.8636883187846,-6.71570789669309,
3.4882302805848));
#253350=CARTESIAN_POINT('Ctrl Pts',(60.8773920302461,-6.59002106156365,
3.48794691941596));
#253351=CARTESIAN_POINT('Ctrl Pts',(60.9862851800405,-6.60146619279846,
3.42473028058481));
#253352=CARTESIAN_POINT('Origin',(60.6448574988555,-6.69328024897354,3.23423028058478));
#253353=CARTESIAN_POINT('Ctrl Pts',(59.1062911958297,-6.53099325079956,
3.47153072139068));
#253354=CARTESIAN_POINT('Ctrl Pts',(59.1200087114583,-6.40512264090918,
3.47122746285073));
#253355=CARTESIAN_POINT('Ctrl Pts',(59.226776843046,-6.41653455700024,3.40413046676793));
#253356=CARTESIAN_POINT('Ctrl Pts',(59.2206299794252,-6.54313486548251,
3.65553813457982));
#253357=CARTESIAN_POINT('Ctrl Pts',(59.2341972766252,-6.41712406698003,
3.65520336072103));
#253358=CARTESIAN_POINT('Ctrl Pts',(59.3182247474342,-6.42614611919656,
3.55128134519899));
#253359=CARTESIAN_POINT('Ctrl Pts',(59.4260354503639,-6.56494601397015,
3.77003198860259));
#253360=CARTESIAN_POINT('Ctrl Pts',(59.4394961352153,-6.43870134519669,
3.7698020931422));
#253361=CARTESIAN_POINT('Ctrl Pts',(59.482506795579,-6.44341285848338,3.64284195387417));
#253362=CARTESIAN_POINT('Ctrl Pts',(59.6417962403144,-6.58785426246996,
3.77003198860259));
#253363=CARTESIAN_POINT('Ctrl Pts',(59.6550912403353,-6.46136078685152,
3.77003198860259));
#253364=CARTESIAN_POINT('Ctrl Pts',(59.6550713402783,-6.46155012324641,
3.64284189403816));
#253365=CARTESIAN_POINT('Origin',(59.6417962403144,-6.58785426246996,3.64303198860259));
#253366=CARTESIAN_POINT('Origin',(60.0186752706393,-6.62746584473993,3.23423028058478));
#253367=CARTESIAN_POINT('Origin',(60.4944777170595,-6.67747469700845,3.23423028058478));
#253368=CARTESIAN_POINT('Origin',(59.7852323155142,-6.60293000146335,3.64303198860259));
#253369=CARTESIAN_POINT('Origin',(60.04095383883,-6.62985850077703,3.6429917172181));
#253370=CARTESIAN_POINT('Ctrl Pts',(60.275645989912,-6.65505462397295,3.48823028058477));
#253371=CARTESIAN_POINT('Ctrl Pts',(60.2894805317163,-6.52822907310677,
3.48852004212255));
#253372=CARTESIAN_POINT('Ctrl Pts',(60.1796001951996,-6.51668018436646,
3.42473028058477));
#253373=CARTESIAN_POINT('Ctrl Pts',(60.3204176712045,-6.65964099131217,
3.41028005848403));
#253374=CARTESIAN_POINT('Ctrl Pts',(60.3340024654448,-6.53290851690499,
3.41074404220316));
#253375=CARTESIAN_POINT('Ctrl Pts',(60.2467384099257,-6.52373669508235,
3.307804862439));
#253376=CARTESIAN_POINT('Ctrl Pts',(60.4052373806432,-6.66833043150578,
3.36123028058477));
#253377=CARTESIAN_POINT('Ctrl Pts',(60.4184509388157,-6.54178440911694,
3.36146460586406));
#253378=CARTESIAN_POINT('Ctrl Pts',(60.3739306632455,-6.53710513959924,
3.23423045308408));
#253379=CARTESIAN_POINT('Ctrl Pts',(60.4944777170595,-6.67747469700845,
3.36123028058478));
#253380=CARTESIAN_POINT('Ctrl Pts',(60.5077528318945,-6.55117041629668,
3.36123028058478));
#253381=CARTESIAN_POINT('Ctrl Pts',(60.5077528318945,-6.55117041629668,
3.23423028058478));
#253382=CARTESIAN_POINT('Origin',(60.1663250803646,-6.64298446507823,3.42473028058476));
#253383=CARTESIAN_POINT('Origin',(60.0854204586802,-6.63448104699067,3.5656311352473));
#253384=CARTESIAN_POINT('Origin',(0.,0.,41.0845));
#253385=CARTESIAN_POINT('',(-65.254,-7.99131022315614E-15,41.0845));
#253386=CARTESIAN_POINT('Origin',(0.,0.,41.0845));
#253387=CARTESIAN_POINT('',(-65.381,-8.00686323750531E-15,41.2115));
#253388=CARTESIAN_POINT('Origin',(-65.381,-8.00686323750531E-15,41.0845));
#253389=CARTESIAN_POINT('Origin',(0.,0.,41.2115));
#253390=CARTESIAN_POINT('Origin',(-1.38777878078145E-14,-1.38777878078145E-14,
41.3385));
#253391=CARTESIAN_POINT('',(-68.623,-2.22816815376033E-14,41.2115));
#253392=CARTESIAN_POINT('Origin',(-1.38777878078145E-14,-1.38777878078145E-14,
41.2115));
#253393=CARTESIAN_POINT('',(-68.75,-2.22972345519525E-14,41.3385));
#253394=CARTESIAN_POINT('Origin',(-68.623,-2.22816815376033E-14,41.3385));
#253395=CARTESIAN_POINT('Origin',(-1.38777878078145E-14,-1.38777878078145E-14,
41.3385));
#253396=CARTESIAN_POINT('Origin',(-1.38777878078145E-14,-1.38777878078145E-14,
42.3545));
#253397=CARTESIAN_POINT('',(68.877,-2.23127875663017E-14,42.4815));
#253398=CARTESIAN_POINT('Origin',(-1.38777878078145E-14,-1.38777878078145E-14,
42.4815));
#253399=CARTESIAN_POINT('',(68.75,-2.22972345519525E-14,42.3545));
#253400=CARTESIAN_POINT('Origin',(68.877,-2.23127875663017E-14,42.3545));
#253401=CARTESIAN_POINT('',(-68.75,-5.4583410636764E-15,42.3545));
#253402=CARTESIAN_POINT('Origin',(-1.38777878078145E-14,-1.38777878078145E-14,
42.3545));
#253403=CARTESIAN_POINT('Origin',(-1.38777878078145E-14,-1.38777878078145E-14,
42.3545));
#253404=CARTESIAN_POINT('Origin',(0.,0.,17.4625));
#253405=CARTESIAN_POINT('',(-65.254,-7.99131022315614E-15,17.4625));
#253406=CARTESIAN_POINT('Origin',(0.,0.,17.4625));
#253407=CARTESIAN_POINT('',(-65.254,-7.99131022315614E-15,17.4625));
#253408=CARTESIAN_POINT('Origin',(-1.38777878078145E-14,-1.38777878078145E-14,
41.2115));
#253409=CARTESIAN_POINT('',(-68.75,-2.22972345519525E-14,41.2115));
#253410=CARTESIAN_POINT('Origin',(-1.38777878078145E-14,-1.38777878078145E-14,
17.4625));
#253411=CARTESIAN_POINT('',(-72.5300000000001,-2.27601510420302E-14,42.4815));
#253412=CARTESIAN_POINT('Origin',(-1.38777878078145E-14,-1.38777878078145E-14,
42.4815));
#253413=CARTESIAN_POINT('',(-72.5300000000001,-2.27601510420302E-14,17.4625));
#253414=CARTESIAN_POINT('',(-72.5300000000001,-2.27601510420302E-14,17.4625));
#253415=CARTESIAN_POINT('Origin',(-1.38777878078145E-14,-1.38777878078145E-14,
17.4625));
#253416=CARTESIAN_POINT('Origin',(-1.38777878078145E-14,-1.38777878078145E-14,
17.4625));
#253417=CARTESIAN_POINT('Origin',(-1.38777878078145E-14,-1.38777878078145E-14,
42.4815));
#253418=CARTESIAN_POINT('Origin',(-1.38777878078145E-14,-1.38777878078145E-14,
41.2115));
#253419=CARTESIAN_POINT('Origin',(0.,0.,41.1353));
#253420=CARTESIAN_POINT('',(-65.,-7.9602041944578E-15,41.1353));
#253421=CARTESIAN_POINT('Origin',(0.,0.,41.1353));
#253422=CARTESIAN_POINT('',(-65.0762,-7.9695360030673E-15,41.2115));
#253423=CARTESIAN_POINT('Origin',(-65.0762,-7.9695360030673E-15,41.1353));
#253424=CARTESIAN_POINT('Origin',(0.,0.,41.2115));
#253425=CARTESIAN_POINT('Origin',(0.,0.,41.1353));
#253426=CARTESIAN_POINT('',(-65.1778,-7.98197841454664E-15,41.2115));
#253427=CARTESIAN_POINT('Origin',(0.,0.,41.2115));
#253428=CARTESIAN_POINT('',(-65.254,-7.99131022315614E-15,41.1353));
#253429=CARTESIAN_POINT('Origin',(-65.1778,-7.98197841454664E-15,41.1353));
#253430=CARTESIAN_POINT('Origin',(0.,0.,41.1353));
#253431=CARTESIAN_POINT('Origin',(0.,0.,17.4625));
#253432=CARTESIAN_POINT('',(-65.,-7.9602041944578E-15,17.4625));
#253433=CARTESIAN_POINT('Origin',(0.,0.,17.4625));
#253434=CARTESIAN_POINT('',(-65.,-7.9602041944578E-15,17.4625));
#253435=CARTESIAN_POINT('Origin',(0.,0.,17.4625));
#253436=CARTESIAN_POINT('',(-65.254,-7.99131022315614E-15,17.4625));
#253437=CARTESIAN_POINT('',(-65.254,-7.99131022315614E-15,17.4625));
#253438=CARTESIAN_POINT('Origin',(0.,0.,17.4625));
#253439=CARTESIAN_POINT('Origin',(0.,0.,17.4625));
#253440=CARTESIAN_POINT('Origin',(0.,0.,41.2115));
#253441=CARTESIAN_POINT('Origin',(-1.38777878078145E-14,-1.38777878078145E-14,
42.037));
#253442=CARTESIAN_POINT('',(-70.625,-2.25268558267926E-14,42.4815));
#253443=CARTESIAN_POINT('Origin',(0.,0.,42.4815));
#253444=CARTESIAN_POINT('',(-71.3206076480316,-2.26120431947551E-14,42.8625));
#253445=CARTESIAN_POINT('Origin',(-71.3206076480316,-2.26120431947551E-14,
42.037));
#253446=CARTESIAN_POINT('Origin',(-1.38777878078145E-14,-1.38777878078145E-14,
42.8625));
#253447=CARTESIAN_POINT('Origin',(0.,0.,40.3225));
#253448=CARTESIAN_POINT('',(10.8580391950581,76.3872907109282,40.6320481322491));
#253449=CARTESIAN_POINT('',(-10.8580391950582,76.3872907109282,40.6320481322491));
#253450=CARTESIAN_POINT('Origin',(0.,0.,40.6320481322491));
#253451=CARTESIAN_POINT('',(10.5032495111116,73.8913131000538,42.8625));
#253452=CARTESIAN_POINT('Origin',(10.5032495111116,73.8913131000538,40.3225));
#253453=CARTESIAN_POINT('',(-10.5032495111116,73.8913131000538,42.8625));
#253454=CARTESIAN_POINT('Origin',(0.,0.,42.8625));
#253455=CARTESIAN_POINT('Origin',(-10.5032495111116,73.8913131000538,40.3225));
#253456=CARTESIAN_POINT('Origin',(90.,-90.,16.1925));
#253457=CARTESIAN_POINT('',(110.478801107225,-75.6605890912239,16.1925));
#253458=CARTESIAN_POINT('',(75.6605890912239,-110.478801107225,16.1925));
#253459=CARTESIAN_POINT('Origin',(90.,-90.,16.1925));
#253460=CARTESIAN_POINT('',(109.438478010978,-76.3890311653897,17.4625));
#253461=CARTESIAN_POINT('Origin',(109.438478010978,-76.3890311653897,16.1925));
#253462=CARTESIAN_POINT('',(76.3890311653897,-109.438478010978,17.4625));
#253463=CARTESIAN_POINT('Origin',(90.,-90.,17.4625));
#253464=CARTESIAN_POINT('Origin',(76.3890311653897,-109.438478010978,16.1925));
#253465=CARTESIAN_POINT('Origin',(90.,90.,16.1925));
#253466=CARTESIAN_POINT('',(75.6605890912238,110.478801107225,16.1925));
#253467=CARTESIAN_POINT('',(110.478801107225,75.6605890912239,16.1925));
#253468=CARTESIAN_POINT('Origin',(90.,90.,16.1925));
#253469=CARTESIAN_POINT('',(76.3890311653897,109.438478010978,17.4625));
#253470=CARTESIAN_POINT('Origin',(76.3890311653897,109.438478010978,16.1925));
#253471=CARTESIAN_POINT('',(109.438478010978,76.3890311653897,17.4625));
#253472=CARTESIAN_POINT('Origin',(90.,90.,17.4625));
#253473=CARTESIAN_POINT('Origin',(109.438478010978,76.3890311653897,16.1925));
#253474=CARTESIAN_POINT('Ctrl Pts',(-77.8839876917858,25.347849735742,12.3825));
#253475=CARTESIAN_POINT('Ctrl Pts',(-77.7859473914177,25.6490890766241,
12.3825));
#253476=CARTESIAN_POINT('Ctrl Pts',(-77.9676516999077,25.9085897226106,
12.3825));
#253477=CARTESIAN_POINT('Ctrl Pts',(-76.0725110230494,24.758292886385,12.3825));
#253478=CARTESIAN_POINT('Ctrl Pts',(-75.6803498215769,25.9632502499131,
12.3825));
#253479=CARTESIAN_POINT('Ctrl Pts',(-76.4071670555372,27.0012528338594,
12.3825));
#253480=CARTESIAN_POINT('Ctrl Pts',(-76.0725110230494,24.758292886385,14.2875));
#253481=CARTESIAN_POINT('Ctrl Pts',(-75.6803498215769,25.9632502499131,
14.2875));
#253482=CARTESIAN_POINT('Ctrl Pts',(-76.4071670555372,27.0012528338594,
14.2875));
#253483=CARTESIAN_POINT('',(-77.8839876917858,25.347849735742,12.3825));
#253484=CARTESIAN_POINT('',(-77.9676516999077,25.9085897226106,12.3825));
#253485=CARTESIAN_POINT('Origin',(-78.4878132480312,25.5443686855277,12.3825));
#253486=CARTESIAN_POINT('',(-76.0725110230494,24.758292886385,14.2875));
#253487=CARTESIAN_POINT('Origin',(-77.8839876917858,25.347849735742,14.2875));
#253488=CARTESIAN_POINT('',(-76.4071670555372,27.0012528338594,14.2875));
#253489=CARTESIAN_POINT('Origin',(-78.4878132480312,25.5443686855277,14.2875));
#253490=CARTESIAN_POINT('Origin',(-77.9676516999077,25.9085897226106,14.2875));
#253491=CARTESIAN_POINT('Ctrl Pts',(-77.9676516999077,-25.9085897226106,
12.3825));
#253492=CARTESIAN_POINT('Ctrl Pts',(-77.7859473914177,-25.6490890766241,
12.3825));
#253493=CARTESIAN_POINT('Ctrl Pts',(-77.8839876917858,-25.347849735742,
12.3825));
#253494=CARTESIAN_POINT('Ctrl Pts',(-76.4071670555372,-27.0012528338594,
12.3825));
#253495=CARTESIAN_POINT('Ctrl Pts',(-75.6803498215769,-25.9632502499131,
12.3825));
#253496=CARTESIAN_POINT('Ctrl Pts',(-76.0725110230494,-24.758292886385,
12.3825));
#253497=CARTESIAN_POINT('Ctrl Pts',(-76.4071670555372,-27.0012528338594,
14.2875));
#253498=CARTESIAN_POINT('Ctrl Pts',(-75.6803498215769,-25.9632502499131,
14.2875));
#253499=CARTESIAN_POINT('Ctrl Pts',(-76.0725110230494,-24.758292886385,
14.2875));
#253500=CARTESIAN_POINT('',(-77.9676516999077,-25.9085897226106,12.3825));
#253501=CARTESIAN_POINT('',(-77.8839876917858,-25.347849735742,12.3825));
#253502=CARTESIAN_POINT('Origin',(-78.4878132480312,-25.5443686855277,12.3825));
#253503=CARTESIAN_POINT('',(-76.4071670555372,-27.0012528338594,14.2875));
#253504=CARTESIAN_POINT('Origin',(-77.9676516999077,-25.9085897226106,14.2875));
#253505=CARTESIAN_POINT('',(-76.0725110230494,-24.758292886385,14.2875));
#253506=CARTESIAN_POINT('Origin',(-78.4878132480312,-25.5443686855277,14.2875));
#253507=CARTESIAN_POINT('Origin',(-77.8839876917858,-25.347849735742,14.2875));
#253508=CARTESIAN_POINT('Ctrl Pts',(77.8839876917858,-25.3478497357421,
12.3825));
#253509=CARTESIAN_POINT('Ctrl Pts',(77.7859473914177,-25.6490890766241,
12.3825));
#253510=CARTESIAN_POINT('Ctrl Pts',(77.9676516999078,-25.9085897226106,
12.3825));
#253511=CARTESIAN_POINT('Ctrl Pts',(76.0725110230494,-24.758292886385,12.3825));
#253512=CARTESIAN_POINT('Ctrl Pts',(75.6803498215769,-25.9632502499131,
12.3825));
#253513=CARTESIAN_POINT('Ctrl Pts',(76.4071670555372,-27.0012528338594,
12.3825));
#253514=CARTESIAN_POINT('Ctrl Pts',(76.0725110230494,-24.758292886385,14.2875));
#253515=CARTESIAN_POINT('Ctrl Pts',(75.6803498215769,-25.9632502499131,
14.2875));
#253516=CARTESIAN_POINT('Ctrl Pts',(76.4071670555372,-27.0012528338594,
14.2875));
#253517=CARTESIAN_POINT('',(77.8839876917858,-25.3478497357421,12.3825));
#253518=CARTESIAN_POINT('',(77.9676516999077,-25.9085897226107,12.3825));
#253519=CARTESIAN_POINT('Origin',(78.4878132480313,-25.5443686855277,12.3825));
#253520=CARTESIAN_POINT('',(76.0725110230494,-24.758292886385,14.2875));
#253521=CARTESIAN_POINT('Origin',(77.8839876917858,-25.3478497357421,14.2875));
#253522=CARTESIAN_POINT('',(76.4071670555372,-27.0012528338594,14.2875));
#253523=CARTESIAN_POINT('Origin',(78.4878132480313,-25.5443686855277,14.2875));
#253524=CARTESIAN_POINT('Origin',(77.9676516999077,-25.9085897226107,14.2875));
#253525=CARTESIAN_POINT('Origin',(0.,0.,14.2875));
#253526=CARTESIAN_POINT('',(76.0725110230494,24.758292886385,14.2875));
#253527=CARTESIAN_POINT('Origin',(0.,0.,14.2875));
#253528=CARTESIAN_POINT('',(77.8839876917858,25.3478497357421,12.3825));
#253529=CARTESIAN_POINT('Origin',(0.,0.,12.3825));
#253530=CARTESIAN_POINT('Origin',(77.8839876917858,25.3478497357421,14.2875));
#253531=CARTESIAN_POINT('Ctrl Pts',(77.9676516999078,25.9085897226107,12.3825));
#253532=CARTESIAN_POINT('Ctrl Pts',(77.7859473914177,25.6490890766241,12.3825));
#253533=CARTESIAN_POINT('Ctrl Pts',(77.8839876917858,25.3478497357421,12.3825));
#253534=CARTESIAN_POINT('Ctrl Pts',(76.4071670555372,27.0012528338594,12.3825));
#253535=CARTESIAN_POINT('Ctrl Pts',(75.6803498215769,25.9632502499131,12.3825));
#253536=CARTESIAN_POINT('Ctrl Pts',(76.0725110230494,24.758292886385,12.3825));
#253537=CARTESIAN_POINT('Ctrl Pts',(76.4071670555372,27.0012528338594,14.2875));
#253538=CARTESIAN_POINT('Ctrl Pts',(75.6803498215769,25.9632502499131,14.2875));
#253539=CARTESIAN_POINT('Ctrl Pts',(76.0725110230494,24.758292886385,14.2875));
#253540=CARTESIAN_POINT('',(77.9676516999077,25.9085897226107,12.3825));
#253541=CARTESIAN_POINT('Origin',(78.4878132480313,25.5443686855277,12.3825));
#253542=CARTESIAN_POINT('',(76.4071670555372,27.0012528338594,14.2875));
#253543=CARTESIAN_POINT('Origin',(77.9676516999077,25.9085897226107,14.2875));
#253544=CARTESIAN_POINT('Origin',(78.4878132480313,25.5443686855277,14.2875));
#253545=CARTESIAN_POINT('Origin',(-78.4878132480312,25.5443686855277,12.3825));
#253546=CARTESIAN_POINT('',(-76.0725110230494,24.758292886385,17.0741173620445));
#253547=CARTESIAN_POINT('',(-76.0725110230494,24.758292886385,12.3825));
#253548=CARTESIAN_POINT('',(-75.9797434607283,25.1428889948603,17.0741173620445));
#253549=CARTESIAN_POINT('Origin',(-78.4878132480312,25.5443686855277,17.0741173620445));
#253550=CARTESIAN_POINT('',(-75.9478132480312,25.544368685519,16.7790882779809));
#253551=CARTESIAN_POINT('Ctrl Pts',(-75.9797434607283,25.1428889948603,
17.0741173620445));
#253552=CARTESIAN_POINT('Ctrl Pts',(-75.9600903294859,25.2656633862951,
16.9588689369795));
#253553=CARTESIAN_POINT('Ctrl Pts',(-75.9478132480309,25.4015417700709,
16.8637563773694));
#253554=CARTESIAN_POINT('Ctrl Pts',(-75.9478132480312,25.544368685519,16.7790882779809));
#253555=CARTESIAN_POINT('',(-76.4071703643125,27.0012572613409,16.0836464440003));
#253556=CARTESIAN_POINT('Ctrl Pts',(-75.9478132480312,25.544368685519,16.7790882779809));
#253557=CARTESIAN_POINT('Ctrl Pts',(-75.9478132480303,25.6765921306316,
16.7007059383813));
#253558=CARTESIAN_POINT('Ctrl Pts',(-75.9584171366964,25.816334343438,16.6310264783953));
#253559=CARTESIAN_POINT('Ctrl Pts',(-76.0045629689351,26.0968884213634,
16.5063573484839));
#253560=CARTESIAN_POINT('Ctrl Pts',(-76.0396368564122,26.2368139673711,
16.4516393979191));
#253561=CARTESIAN_POINT('Ctrl Pts',(-76.1354463408314,26.5136044910669,
16.3525814751901));
#253562=CARTESIAN_POINT('Ctrl Pts',(-76.1966925113156,26.6511815359268,
16.308172958015));
#253563=CARTESIAN_POINT('Ctrl Pts',(-76.306792867175,26.8483691944594,16.2492604516738));
#253564=CARTESIAN_POINT('Ctrl Pts',(-76.3466590420083,26.9128851528656,
16.2309506379062));
#253565=CARTESIAN_POINT('Ctrl Pts',(-76.4002047884601,26.9913835733178,
16.2087984367714));
#253566=CARTESIAN_POINT('Ctrl Pts',(-76.4110986052641,27.0069745617798,
16.2044315143317));
#253567=CARTESIAN_POINT('Ctrl Pts',(-76.4276519058228,27.0301092948723,
16.1975104106263));
#253568=CARTESIAN_POINT('Ctrl Pts',(-76.4332238412039,27.0378039510364,
16.1952643836651));
#253569=CARTESIAN_POINT('Ctrl Pts',(-76.4442170623447,27.0528119734108,
16.1893033167685));
#253570=CARTESIAN_POINT('Ctrl Pts',(-76.4506141578954,27.0614120539566,
16.1833338857357));
#253571=CARTESIAN_POINT('Ctrl Pts',(-76.4496048710994,27.0600557662765,
16.1636449186976));
#253572=CARTESIAN_POINT('Ctrl Pts',(-76.445847589196,27.0550011412656,16.1552610170204));
#253573=CARTESIAN_POINT('Ctrl Pts',(-76.4389163531081,27.0455867516878,
16.1396560112813));
#253574=CARTESIAN_POINT('Ctrl Pts',(-76.4350958850463,27.0403618512071,
16.1323196149044));
#253575=CARTESIAN_POINT('Ctrl Pts',(-76.4234011422968,27.0242265009732,
16.1108031014866));
#253576=CARTESIAN_POINT('Ctrl Pts',(-76.4152687037725,27.0128231866378,
16.0971732455228));
#253577=CARTESIAN_POINT('Ctrl Pts',(-76.4071670555372,27.0012528338594,
16.0836603564333));
#253578=CARTESIAN_POINT('',(-76.4071670555372,27.0012528338594,17.0741173620445));
#253579=CARTESIAN_POINT('Origin',(-78.4878132480312,-25.5443686855277,12.3825));
#253580=CARTESIAN_POINT('',(-76.4071670555372,-27.0012528338594,16.0836576823356));
#253581=CARTESIAN_POINT('',(-76.4071670555372,-27.0012528338594,12.3825));
#253582=CARTESIAN_POINT('',(-75.9478282514034,-25.544368692031,16.7790882775718));
#253583=CARTESIAN_POINT('Ctrl Pts',(-76.4071670555372,-27.0012528338594,
16.0836576823356));
#253584=CARTESIAN_POINT('Ctrl Pts',(-76.4152523939033,-27.0127999068814,
16.0971460288751));
#253585=CARTESIAN_POINT('Ctrl Pts',(-76.4233804349652,-27.0241972663232,
16.1107708588669));
#253586=CARTESIAN_POINT('Ctrl Pts',(-76.4350405965502,-27.0402858986055,
16.1322149894862));
#253587=CARTESIAN_POINT('Ctrl Pts',(-76.4388439109148,-27.0454878961872,
16.1395118886607));
#253588=CARTESIAN_POINT('Ctrl Pts',(-76.4457808819976,-27.0549109871946,
16.1550922359403));
#253589=CARTESIAN_POINT('Ctrl Pts',(-76.4495262827364,-27.0599501461243,
16.1634279843414));
#253590=CARTESIAN_POINT('Ctrl Pts',(-76.4506693829202,-27.0614862780154,
16.1831233908523));
#253591=CARTESIAN_POINT('Ctrl Pts',(-76.4443470115083,-27.0529879564382,
16.1892139275835));
#253592=CARTESIAN_POINT('Ctrl Pts',(-76.4333625249832,-27.0379946731629,
16.1952076519701));
#253593=CARTESIAN_POINT('Ctrl Pts',(-76.4277817362483,-27.0302892875527,
16.1974549295803));
#253594=CARTESIAN_POINT('Ctrl Pts',(-76.4112309135534,-27.0071623375438,
16.2043785477607));
#253595=CARTESIAN_POINT('Ctrl Pts',(-76.4003361866038,-26.9915731287254,
16.2087447794625));
#253596=CARTESIAN_POINT('Ctrl Pts',(-76.3467821072315,-26.9130777753189,
16.230896934636));
#253597=CARTESIAN_POINT('Ctrl Pts',(-76.3069514286797,-26.8486340830899,
16.2491835660637));
#253598=CARTESIAN_POINT('Ctrl Pts',(-76.1968338030491,-26.6514726518305,
16.3080814902354));
#253599=CARTESIAN_POINT('Ctrl Pts',(-76.1355975399761,-26.5139532715615,
16.3524675745753));
#253600=CARTESIAN_POINT('Ctrl Pts',(-76.0398121713394,-26.2374081758968,
16.4514158583587));
#253601=CARTESIAN_POINT('Ctrl Pts',(-76.0046988236937,-26.0975162379414,
16.5060990022633));
#253602=CARTESIAN_POINT('Ctrl Pts',(-75.9584674534131,-25.816837601813,
16.6307822945995));
#253603=CARTESIAN_POINT('Ctrl Pts',(-75.9478132480311,-25.6771355556999,
16.700383794839));
#253604=CARTESIAN_POINT('Ctrl Pts',(-75.9478132480312,-25.5443686855242,
16.7790882779778));
#253605=CARTESIAN_POINT('',(-75.9797434607283,-25.1428889948604,17.0741173620445));
#253606=CARTESIAN_POINT('Ctrl Pts',(-75.9478432547756,-25.5443686985378,
16.7790882771658));
#253607=CARTESIAN_POINT('Ctrl Pts',(-75.9478592799661,-25.5087358023417,
16.8002117896876));
#253608=CARTESIAN_POINT('Ctrl Pts',(-75.9486271497168,-25.4734339822992,
16.8220725722267));
#253609=CARTESIAN_POINT('Ctrl Pts',(-75.950085661309,-25.4386219982237,
16.8447668373521));
#253610=CARTESIAN_POINT('Ctrl Pts',(-75.950632603156,-25.4255675041953,
16.8532771867742));
#253611=CARTESIAN_POINT('Ctrl Pts',(-75.9512765391559,-25.4125819305939,
16.8619047448722));
#253612=CARTESIAN_POINT('Ctrl Pts',(-75.9520137796523,-25.399673751837,
16.8706545860217));
#253613=CARTESIAN_POINT('Ctrl Pts',(-75.9526588650866,-25.3883790954247,
16.8783106970275));
#253614=CARTESIAN_POINT('Ctrl Pts',(-75.9533753830629,-25.3771436956814,
16.8860604310073));
#253615=CARTESIAN_POINT('Ctrl Pts',(-75.9541607010869,-25.3659732454842,
16.8939071875044));
#253616=CARTESIAN_POINT('Ctrl Pts',(-75.9564237260398,-25.3337837289305,
16.916518925948));
#253617=CARTESIAN_POINT('Ctrl Pts',(-75.9592588897836,-25.3021331439168,
16.939934354713));
#253618=CARTESIAN_POINT('Ctrl Pts',(-75.962596000696,-25.2711588719201,
16.9642401976005));
#253619=CARTESIAN_POINT('Ctrl Pts',(-75.9633120606089,-25.2645125736434,
16.9694556190224));
#253620=CARTESIAN_POINT('Ctrl Pts',(-75.9640511964207,-25.2578973684702,
16.9747118561142));
#253621=CARTESIAN_POINT('Ctrl Pts',(-75.9648126596724,-25.2513145358426,
16.980009460251));
#253622=CARTESIAN_POINT('Ctrl Pts',(-75.9669677451484,-25.2326838705344,
16.9950026850816));
#253623=CARTESIAN_POINT('Ctrl Pts',(-75.9693017197781,-25.2143130480956,
17.0103294780056));
#253624=CARTESIAN_POINT('Ctrl Pts',(-75.9717964668484,-25.1962321628045,
17.0260080558434));
#253625=CARTESIAN_POINT('Ctrl Pts',(-75.9742912139187,-25.1781512775134,
17.0416866336811));
#253626=CARTESIAN_POINT('Ctrl Pts',(-75.9769467318632,-25.1603603423111,
17.0577170011241));
#253627=CARTESIAN_POINT('Ctrl Pts',(-75.9797434607283,-25.1428889948604,
17.0741173620445));
#253628=CARTESIAN_POINT('',(-76.0725110230494,-24.758292886385,17.0741173620445));
#253629=CARTESIAN_POINT('Origin',(-78.4878132480312,-25.5443686855277,17.0741173620445));
#253630=CARTESIAN_POINT('',(-76.0725110230494,-24.758292886385,12.3825));
#253631=CARTESIAN_POINT('Origin',(0.,0.,17.0741173620445));
#253632=CARTESIAN_POINT('',(-76.0424582863717,24.6976449920627,17.8479876922247));
#253633=CARTESIAN_POINT('',(-76.0424582863716,-24.6976449920628,17.847987692225));
#253634=CARTESIAN_POINT('Origin',(0.,0.,17.8479876926672));
#253635=CARTESIAN_POINT('Ctrl Pts',(-76.0424582865173,24.6976449914385,
17.8479876926672));
#253636=CARTESIAN_POINT('Ctrl Pts',(-76.0624207920021,24.737936883604,17.5919904624029));
#253637=CARTESIAN_POINT('Ctrl Pts',(-76.0725110230494,24.758292886385,17.3340474816323));
#253638=CARTESIAN_POINT('Ctrl Pts',(-76.0725110230494,24.758292886385,17.0741173620445));
#253639=CARTESIAN_POINT('Origin',(0.,0.,17.0741173620445));
#253640=CARTESIAN_POINT('Ctrl Pts',(-76.0725110230494,-24.758292886385,
17.0741173620445));
#253641=CARTESIAN_POINT('Ctrl Pts',(-76.0725110230494,-24.758292886385,
17.3340474816323));
#253642=CARTESIAN_POINT('Ctrl Pts',(-76.0624207920021,-24.737936883604,
17.5919904624035));
#253643=CARTESIAN_POINT('Ctrl Pts',(-76.0424582865173,-24.6976449914384,
17.8479876926672));
#253644=CARTESIAN_POINT('Origin',(0.,0.,248.008319357841));
#253645=CARTESIAN_POINT('',(72.53,-8.88236323421576E-15,42.4815));
#253646=CARTESIAN_POINT('Origin',(0.,0.,42.4815));
#253647=CARTESIAN_POINT('',(72.53,-8.88236323421576E-15,8.25499999999998));
#253648=CARTESIAN_POINT('',(72.53,-8.88236323421576E-15,248.008319357841));
#253649=CARTESIAN_POINT('Origin',(0.,0.,8.25499999999998));
#253650=CARTESIAN_POINT('Origin',(-90.,-90.,63.5));
#253651=CARTESIAN_POINT('',(-81.5545,-90.,17.4625));
#253652=CARTESIAN_POINT('Origin',(-90.,-90.,17.4625));
#253653=CARTESIAN_POINT('',(-81.5545,-90.,8.255));
#253654=CARTESIAN_POINT('',(-81.5545,-90.,63.5));
#253655=CARTESIAN_POINT('Origin',(-90.,-90.,8.255));
#253656=CARTESIAN_POINT('Origin',(-90.,90.,63.5));
#253657=CARTESIAN_POINT('',(-81.5545,90.,17.4625));
#253658=CARTESIAN_POINT('Origin',(-90.,90.,17.4625));
#253659=CARTESIAN_POINT('',(-81.5545,90.,8.255));
#253660=CARTESIAN_POINT('',(-81.5545,90.,63.5));
#253661=CARTESIAN_POINT('Origin',(-90.,90.,8.255));
#253662=CARTESIAN_POINT('Origin',(90.,90.,63.5));
#253663=CARTESIAN_POINT('',(98.4455,90.,17.4625));
#253664=CARTESIAN_POINT('Origin',(90.,90.,17.4625));
#253665=CARTESIAN_POINT('',(98.4455,90.,8.255));
#253666=CARTESIAN_POINT('',(98.4455,90.,63.5));
#253667=CARTESIAN_POINT('Origin',(90.,90.,8.255));
#253668=CARTESIAN_POINT('Origin',(90.,-90.,63.5));
#253669=CARTESIAN_POINT('',(98.4455,-90.,17.4625));
#253670=CARTESIAN_POINT('Origin',(90.,-90.,17.4625));
#253671=CARTESIAN_POINT('',(98.4455,-90.,8.255));
#253672=CARTESIAN_POINT('',(98.4455,-90.,63.5));
#253673=CARTESIAN_POINT('Origin',(90.,-90.,8.255));
#253674=CARTESIAN_POINT('Origin',(0.,0.,12.3825));
#253675=CARTESIAN_POINT('',(76.0725110230494,24.758292886385,17.0741173620445));
#253676=CARTESIAN_POINT('',(76.0725110230494,24.758292886385,12.3825));
#253677=CARTESIAN_POINT('',(76.0725110230494,-24.758292886385,17.0741173620445));
#253678=CARTESIAN_POINT('Origin',(0.,0.,17.0741173620445));
#253679=CARTESIAN_POINT('',(76.0725110230494,-24.758292886385,12.3825));
#253680=CARTESIAN_POINT('Origin',(0.,0.,17.4625));
#253681=CARTESIAN_POINT('',(-10.8641498708349,79.2111064053766,17.8479876926672));
#253682=CARTESIAN_POINT('Ctrl Pts',(-10.8580391950582,76.3872907109282,
40.6320481322491));
#253683=CARTESIAN_POINT('Ctrl Pts',(-10.8580660689152,76.3992856302614,
40.5352987690743));
#253684=CARTESIAN_POINT('Ctrl Pts',(-10.8580929305605,76.4112804979204,
40.4385493994896));
#253685=CARTESIAN_POINT('Ctrl Pts',(-10.8581197800107,76.423275313976,40.3418000235038));
#253686=CARTESIAN_POINT('Ctrl Pts',(-10.8590524915919,76.8399581047936,
36.9808647820832));
#253687=CARTESIAN_POINT('Ctrl Pts',(-10.8599704900686,77.256578637456,33.6199218173622));
#253688=CARTESIAN_POINT('Ctrl Pts',(-10.8608744504877,77.6731397785624,
30.2589714884058));
#253689=CARTESIAN_POINT('Ctrl Pts',(-10.861987132648,78.1858836339049,26.1219878400834));
#253690=CARTESIAN_POINT('Ctrl Pts',(-10.8630785478348,78.6985375142473,
21.9849930334727));
#253691=CARTESIAN_POINT('Ctrl Pts',(-10.8641498708349,79.2111064053766,
17.8479876926672));
#253692=CARTESIAN_POINT('',(-24.6976449920629,76.0424582863716,17.847987692225));
#253693=CARTESIAN_POINT('Origin',(0.,0.,17.8479876926672));
#253694=CARTESIAN_POINT('',(-25.1183523255102,75.961488153786,17.4075632995852));
#253695=CARTESIAN_POINT('Ctrl Pts',(-24.6976449919804,76.0424582864102,
17.8479876921334));
#253696=CARTESIAN_POINT('Ctrl Pts',(-24.8421318546264,76.0139038233433,
17.7056692315415));
#253697=CARTESIAN_POINT('Ctrl Pts',(-24.9826881607289,75.9867559935942,
17.5590635300787));
#253698=CARTESIAN_POINT('Ctrl Pts',(-25.1183452685109,75.9614890268762,
17.4075745924918));
#253699=CARTESIAN_POINT('',(-28.7459974181805,74.3634602878983,19.6929518677509));
#253700=CARTESIAN_POINT('Ctrl Pts',(-25.1183716157479,75.9614818429678,
17.4075624145231));
#253701=CARTESIAN_POINT('Ctrl Pts',(-25.1663807403387,75.9292306004122,
17.5341891960434));
#253702=CARTESIAN_POINT('Ctrl Pts',(-25.2225896116214,75.8946388507543,
17.6574709249722));
#253703=CARTESIAN_POINT('Ctrl Pts',(-25.285623436093,75.8583098126767,17.7758260768801));
#253704=CARTESIAN_POINT('Ctrl Pts',(-25.3144603202055,75.8416899063051,
17.8299715111495));
#253705=CARTESIAN_POINT('Ctrl Pts',(-25.3447263486284,75.824706154463,17.8830859081177));
#253706=CARTESIAN_POINT('Ctrl Pts',(-25.3762932265105,75.8074152517247,
17.9350176026268));
#253707=CARTESIAN_POINT('Ctrl Pts',(-25.3987704081996,75.7951032719378,
17.9719955431525));
#253708=CARTESIAN_POINT('Ctrl Pts',(-25.4219292775774,75.7826225663754,
18.0084169806869));
#253709=CARTESIAN_POINT('Ctrl Pts',(-25.4457245653072,75.7699942838142,
18.0442185658015));
#253710=CARTESIAN_POINT('Ctrl Pts',(-25.5176575567036,75.7318190723546,
18.1524465117406));
#253711=CARTESIAN_POINT('Ctrl Pts',(-25.5954180175484,75.6922139916061,
18.2556268052651));
#253712=CARTESIAN_POINT('Ctrl Pts',(-25.6787085180146,75.6512007481018,
18.3538912523495));
#253713=CARTESIAN_POINT('Ctrl Pts',(-25.6911412019917,75.6450787450822,
18.3685590813329));
#253714=CARTESIAN_POINT('Ctrl Pts',(-25.7036970322645,75.6389253810112,
18.383117441432));
#253715=CARTESIAN_POINT('Ctrl Pts',(-25.7163749474321,75.6327407433448,
18.3975668354582));
#253716=CARTESIAN_POINT('Ctrl Pts',(-25.790822604906,75.5964231169445,18.4824170275406));
#253717=CARTESIAN_POINT('Ctrl Pts',(-25.8695946626573,75.5589722614061,
18.5636320093352));
#253718=CARTESIAN_POINT('Ctrl Pts',(-25.9524451451234,75.5204260075582,
18.6412309225863));
#253719=CARTESIAN_POINT('Ctrl Pts',(-26.0094901709642,75.4938857632365,
18.6946600865436));
#253720=CARTESIAN_POINT('Ctrl Pts',(-26.0681509448603,75.4669777563056,
18.746035575097));
#253721=CARTESIAN_POINT('Ctrl Pts',(-26.1282299623944,75.4397648602322,
18.7953196528862));
#253722=CARTESIAN_POINT('Ctrl Pts',(-26.1997874751994,75.4073527596494,
18.8540197810214));
#253723=CARTESIAN_POINT('Ctrl Pts',(-26.2732030109633,75.374575465988,18.909646548187));
#253724=CARTESIAN_POINT('Ctrl Pts',(-26.3483201939313,75.341453311566,18.962331304316));
#253725=CARTESIAN_POINT('Ctrl Pts',(-26.4206512997561,75.3095596493973,
19.0130619962875));
#253726=CARTESIAN_POINT('Ctrl Pts',(-26.4945609623652,75.2773460198525,
19.0610645954997));
#253727=CARTESIAN_POINT('Ctrl Pts',(-26.5699313482712,75.2448262662941,
19.1064165126252));
#253728=CARTESIAN_POINT('Ctrl Pts',(-26.5774516031997,75.2415815325166,
19.1109416052617));
#253729=CARTESIAN_POINT('Ctrl Pts',(-26.5849903403349,75.238332090922,19.1154422462802));
#253730=CARTESIAN_POINT('Ctrl Pts',(-26.5925473515409,75.2350780060009,
19.1199184134199));
#253731=CARTESIAN_POINT('Ctrl Pts',(-26.7154431586983,75.1821584876839,
19.1927120296535));
#253732=CARTESIAN_POINT('Ctrl Pts',(-26.8429293003596,75.1281185031954,
19.2588649121235));
#253733=CARTESIAN_POINT('Ctrl Pts',(-26.9733752019168,75.0735400782349,
19.3179719516907));
#253734=CARTESIAN_POINT('Ctrl Pts',(-27.0676510755531,75.0340951540677,
19.3606897966114));
#253735=CARTESIAN_POINT('Ctrl Pts',(-27.1634716618128,74.9943693681411,
19.3997280200329));
#253736=CARTESIAN_POINT('Ctrl Pts',(-27.2602089524345,74.9545859173702,
19.4349442290443));
#253737=CARTESIAN_POINT('Ctrl Pts',(-27.3823989937776,74.9043349597176,
19.4794262484123));
#253738=CARTESIAN_POINT('Ctrl Pts',(-27.5061040086162,74.85395915675,19.517975099683));
#253739=CARTESIAN_POINT('Ctrl Pts',(-27.6312030307085,74.8034579087233,
19.5507626191466));
#253740=CARTESIAN_POINT('Ctrl Pts',(-27.7301373583959,74.7635190911585,
19.5766925676019));
#253741=CARTESIAN_POINT('Ctrl Pts',(-27.829805833627,74.7235572548823,19.5989868615588));
#253742=CARTESIAN_POINT('Ctrl Pts',(-27.9303548227061,74.6834885518219,
19.61779172406));
#253743=CARTESIAN_POINT('Ctrl Pts',(-27.9505099136077,74.6754567619463,
19.621561167359));
#253744=CARTESIAN_POINT('Ctrl Pts',(-27.9707004214913,74.6674206749929,
19.6251902405012));
#253745=CARTESIAN_POINT('Ctrl Pts',(-27.9909275808283,74.6593796105368,
19.6286798784687));
#253746=CARTESIAN_POINT('Ctrl Pts',(-28.0921856244414,74.6191256904572,
19.6461491586393));
#253747=CARTESIAN_POINT('Ctrl Pts',(-28.1946046459662,74.578657249514,19.6600683967018));
#253748=CARTESIAN_POINT('Ctrl Pts',(-28.2976765638612,74.5381640664798,
19.6704349274694));
#253749=CARTESIAN_POINT('Ctrl Pts',(-28.3951370915022,74.4998753932411,
19.6802370887083));
#253750=CARTESIAN_POINT('Ctrl Pts',(-28.4931826135307,74.4615641517711,
19.6868624470815));
#253751=CARTESIAN_POINT('Ctrl Pts',(-28.5913692277015,74.4233988532873,
19.6902666744795));
#253752=CARTESIAN_POINT('Ctrl Pts',(-28.6428959768779,74.4033703211006,
19.6920531580318));
#253753=CARTESIAN_POINT('Ctrl Pts',(-28.6944612286795,74.3833821576526,
19.6929518677509));
#253754=CARTESIAN_POINT('Ctrl Pts',(-28.7459974181805,74.3634602878983,
19.6929518677509));
#253755=CARTESIAN_POINT('',(-74.3634602878982,28.7459974181806,19.6929518677509));
#253756=CARTESIAN_POINT('Origin',(0.,0.,19.6929518677509));
#253757=CARTESIAN_POINT('',(-75.9614881812303,25.1183521036896,17.4075636545403));
#253758=CARTESIAN_POINT('Ctrl Pts',(-74.3634602878982,28.7459974181806,
19.6929518677509));
#253759=CARTESIAN_POINT('Ctrl Pts',(-74.4304701497097,28.5726485820852,
19.6929518674577));
#253760=CARTESIAN_POINT('Ctrl Pts',(-74.4974864004038,28.4008490217909,
19.6830632277882));
#253761=CARTESIAN_POINT('Ctrl Pts',(-74.5645845522744,28.230491093491,19.6632610083017));
#253762=CARTESIAN_POINT('Ctrl Pts',(-74.5954989334108,28.1520014514031,
19.6541374580476));
#253763=CARTESIAN_POINT('Ctrl Pts',(-74.6264307043179,28.0738178940494,
19.6429087822487));
#253764=CARTESIAN_POINT('Ctrl Pts',(-74.6573872842513,27.9959302213503,
19.6295688156876));
#253765=CARTESIAN_POINT('Ctrl Pts',(-74.7058182219457,27.8740765465654,
19.6086987101799));
#253766=CARTESIAN_POINT('Ctrl Pts',(-74.7545517359242,27.7523615725077,
19.5824195541812));
#253767=CARTESIAN_POINT('Ctrl Pts',(-74.8031494822237,27.6319739934802,
19.5508884666966));
#253768=CARTESIAN_POINT('Ctrl Pts',(-74.8536551827056,27.5068599815951,
19.5181194643944));
#253769=CARTESIAN_POINT('Ctrl Pts',(-74.9040895744662,27.3829937092191,
19.4796267591557));
#253770=CARTESIAN_POINT('Ctrl Pts',(-74.9539558516285,27.2617318168035,
19.4355274341624));
#253771=CARTESIAN_POINT('Ctrl Pts',(-75.0221597822451,27.0958774926508,
19.3752111748938));
#253772=CARTESIAN_POINT('Ctrl Pts',(-75.0893730482371,26.934659238125,19.3046526921904));
#253773=CARTESIAN_POINT('Ctrl Pts',(-75.1556896641871,26.7783260032606,
19.223220896943));
#253774=CARTESIAN_POINT('Ctrl Pts',(-75.1820881660236,26.7160947942557,
19.1908055306641));
#253775=CARTESIAN_POINT('Ctrl Pts',(-75.2083445589399,26.6546378725531,
19.1566666832221));
#253776=CARTESIAN_POINT('Ctrl Pts',(-75.2344646706147,26.5939718531098,
19.120762400072));
#253777=CARTESIAN_POINT('Ctrl Pts',(-75.2368117983606,26.5885204638033,
19.1175360762251));
#253778=CARTESIAN_POINT('Ctrl Pts',(-75.2391574108363,26.5830764322048,
19.1142960456888));
#253779=CARTESIAN_POINT('Ctrl Pts',(-75.2415015097605,26.5776397722412,
19.1110422978748));
#253780=CARTESIAN_POINT('Ctrl Pts',(-75.2885743789447,26.4684638408701,
19.04570237402));
#253781=CARTESIAN_POINT('Ctrl Pts',(-75.3350350763048,26.3622811063522,
18.9747887273505));
#253782=CARTESIAN_POINT('Ctrl Pts',(-75.3808870959315,26.2593455383137,
18.8979255800988));
#253783=CARTESIAN_POINT('Ctrl Pts',(-75.4159393644213,26.1806548896268,
18.839166387017));
#253784=CARTESIAN_POINT('Ctrl Pts',(-75.4508169508407,26.1034760636233,
18.7765523191411));
#253785=CARTESIAN_POINT('Ctrl Pts',(-75.4849716254452,26.0291438153088,
18.7109347212577));
#253786=CARTESIAN_POINT('Ctrl Pts',(-75.4957791231815,26.0056230055015,
18.6901714714594));
#253787=CARTESIAN_POINT('Ctrl Pts',(-75.5065143688567,25.9823868773644,
18.6691073534833));
#253788=CARTESIAN_POINT('Ctrl Pts',(-75.5171603678616,25.959476755343,18.6477689489594));
#253789=CARTESIAN_POINT('Ctrl Pts',(-75.5571222432613,25.8734790541222,
18.5676710020756));
#253790=CARTESIAN_POINT('Ctrl Pts',(-75.5958350863705,25.7920071322344,
18.4838572390432));
#253791=CARTESIAN_POINT('Ctrl Pts',(-75.6333036881582,25.7152212809698,
18.3962512683447));
#253792=CARTESIAN_POINT('Ctrl Pts',(-75.6638282493733,25.6526661199667,
18.3248812761963));
#253793=CARTESIAN_POINT('Ctrl Pts',(-75.6936006486774,25.5930696741659,
18.2508225083577));
#253794=CARTESIAN_POINT('Ctrl Pts',(-75.7225799270827,25.5366139960004,
18.1741082109009));
#253795=CARTESIAN_POINT('Ctrl Pts',(-75.7376547710952,25.5072460962874,
18.1342019008987));
#253796=CARTESIAN_POINT('Ctrl Pts',(-75.7525151457545,25.4787274775003,
18.0935775396257));
#253797=CARTESIAN_POINT('Ctrl Pts',(-75.7671562637947,25.4510796000904,
18.0522434478428));
#253798=CARTESIAN_POINT('Ctrl Pts',(-75.7807604869782,25.4253897658985,
18.0138366671474));
#253799=CARTESIAN_POINT('Ctrl Pts',(-75.7942007247961,25.4004235947553,
17.9746913116853));
#253800=CARTESIAN_POINT('Ctrl Pts',(-75.807444674672,25.3762475819474,17.9349066213656));
#253801=CARTESIAN_POINT('Ctrl Pts',(-75.8430230238117,25.3113015022245,
17.8280296235003));
#253802=CARTESIAN_POINT('Ctrl Pts',(-75.8774043151913,25.2516721229845,
17.7158399467672));
#253803=CARTESIAN_POINT('Ctrl Pts',(-75.9100163344796,25.198659621202,17.5997892951994));
#253804=CARTESIAN_POINT('Ctrl Pts',(-75.9277247353295,25.1698737118314,
17.5367735267276));
#253805=CARTESIAN_POINT('Ctrl Pts',(-75.944911203035,25.1430395031978,17.4726196431217));
#253806=CARTESIAN_POINT('Ctrl Pts',(-75.961482015185,25.1183707693644,17.4075627905746));
#253807=CARTESIAN_POINT('Ctrl Pts',(-75.9614890268773,25.1183452685092,
17.4075745924872));
#253808=CARTESIAN_POINT('Ctrl Pts',(-75.9867559935951,24.9826881607244,
17.5590635300833));
#253809=CARTESIAN_POINT('Ctrl Pts',(-76.0139038233425,24.8421318546272,
17.7056692315459));
#253810=CARTESIAN_POINT('Ctrl Pts',(-76.0424582864102,24.6976449919804,
17.8479876921334));
#253811=CARTESIAN_POINT('',(-75.961488153786,-25.11835232551,17.4075632995853));
#253812=CARTESIAN_POINT('Ctrl Pts',(-76.0424582864102,-24.6976449919803,
17.8479876921334));
#253813=CARTESIAN_POINT('Ctrl Pts',(-76.0139038233691,-24.8421318545712,
17.7056692314804));
#253814=CARTESIAN_POINT('Ctrl Pts',(-75.9867559935943,-24.9826881607289,
17.5590635300785));
#253815=CARTESIAN_POINT('Ctrl Pts',(-75.9614890268762,-25.118345268511,
17.4075745924919));
#253816=CARTESIAN_POINT('',(-74.3634602878982,-28.7459974181806,19.6929518677509));
#253817=CARTESIAN_POINT('Ctrl Pts',(-75.9614818429679,-25.1183716157475,
17.4075624145233));
#253818=CARTESIAN_POINT('Ctrl Pts',(-75.929230600401,-25.166380740355,17.5341891960889));
#253819=CARTESIAN_POINT('Ctrl Pts',(-75.8946388507298,-25.2225896116613,
17.6574709250598));
#253820=CARTESIAN_POINT('Ctrl Pts',(-75.8583098126379,-25.2856234361605,
17.7758260770059));
#253821=CARTESIAN_POINT('Ctrl Pts',(-75.8416899062786,-25.314460320253,
17.8299715112316));
#253822=CARTESIAN_POINT('Ctrl Pts',(-75.8247061544494,-25.3447263486535,
17.8830859081576));
#253823=CARTESIAN_POINT('Ctrl Pts',(-75.8074152517245,-25.376293226511,
17.9350176026265));
#253824=CARTESIAN_POINT('Ctrl Pts',(-75.7951032719375,-25.3987704082004,
17.9719955431528));
#253825=CARTESIAN_POINT('Ctrl Pts',(-75.782622566375,-25.4219292775783,
18.0084169806878));
#253826=CARTESIAN_POINT('Ctrl Pts',(-75.7699942838137,-25.4457245653082,
18.0442185658031));
#253827=CARTESIAN_POINT('Ctrl Pts',(-75.7318190723905,-25.5176575566357,
18.1524465116398));
#253828=CARTESIAN_POINT('Ctrl Pts',(-75.6922139916809,-25.5954180174015,
18.2556268050704));
#253829=CARTESIAN_POINT('Ctrl Pts',(-75.6512007482183,-25.6787085177782,
18.3538912520706));
#253830=CARTESIAN_POINT('Ctrl Pts',(-75.6450787451602,-25.6911412018325,
18.3685590811484));
#253831=CARTESIAN_POINT('Ctrl Pts',(-75.6389253810504,-25.7036970321842,
18.3831174413404));
#253832=CARTESIAN_POINT('Ctrl Pts',(-75.6327407433448,-25.7163749474321,
18.3975668354582));
#253833=CARTESIAN_POINT('Ctrl Pts',(-75.5964231169443,-25.7908226049064,
18.482417027541));
#253834=CARTESIAN_POINT('Ctrl Pts',(-75.5589722614058,-25.8695946626581,
18.5636320093358));
#253835=CARTESIAN_POINT('Ctrl Pts',(-75.5204260075577,-25.9524451451245,
18.6412309225872));
#253836=CARTESIAN_POINT('Ctrl Pts',(-75.4938857632362,-26.009490170965,
18.6946600865442));
#253837=CARTESIAN_POINT('Ctrl Pts',(-75.4669777563054,-26.0681509448607,
18.7460355750973));
#253838=CARTESIAN_POINT('Ctrl Pts',(-75.4397648602322,-26.1282299623944,
18.7953196528863));
#253839=CARTESIAN_POINT('Ctrl Pts',(-75.4073527596456,-26.1997874752078,
18.8540197810283));
#253840=CARTESIAN_POINT('Ctrl Pts',(-75.3745754659803,-26.2732030109805,
18.9096465482));
#253841=CARTESIAN_POINT('Ctrl Pts',(-75.3414533115544,-26.3483201939576,
18.9623313043344));
#253842=CARTESIAN_POINT('Ctrl Pts',(-75.3095596493893,-26.4206512997743,
19.0130619962993));
#253843=CARTESIAN_POINT('Ctrl Pts',(-75.2773460198483,-26.4945609623749,
19.0610645955056));
#253844=CARTESIAN_POINT('Ctrl Pts',(-75.2448262662937,-26.5699313482721,
19.1064165126258));
#253845=CARTESIAN_POINT('Ctrl Pts',(-75.2415815325164,-26.5774516032003,
19.1109416052622));
#253846=CARTESIAN_POINT('Ctrl Pts',(-75.2383320909218,-26.5849903403352,
19.1154422462805));
#253847=CARTESIAN_POINT('Ctrl Pts',(-75.2350780060008,-26.5925473515409,
19.11991841342));
#253848=CARTESIAN_POINT('Ctrl Pts',(-75.1821584877111,-26.715443158635,
19.1927120296162));
#253849=CARTESIAN_POINT('Ctrl Pts',(-75.1281185032508,-26.8429293002287,
19.2588649120556));
#253850=CARTESIAN_POINT('Ctrl Pts',(-75.073540078319,-26.9733752017158,
19.3179719515996));
#253851=CARTESIAN_POINT('Ctrl Pts',(-75.0340951541239,-27.0676510754174,
19.360689796556));
#253852=CARTESIAN_POINT('Ctrl Pts',(-74.994369368169,-27.1634716617447,
19.3997280200081));
#253853=CARTESIAN_POINT('Ctrl Pts',(-74.9545859173699,-27.2602089524353,
19.4349442290446));
#253854=CARTESIAN_POINT('Ctrl Pts',(-74.9043349597174,-27.3823989937779,
19.4794262484125));
#253855=CARTESIAN_POINT('Ctrl Pts',(-74.8539591567499,-27.5061040086164,
19.517975099683));
#253856=CARTESIAN_POINT('Ctrl Pts',(-74.8034579087233,-27.6312030307086,
19.5507626191466));
#253857=CARTESIAN_POINT('Ctrl Pts',(-74.7635190911554,-27.7301373584036,
19.5766925676039));
#253858=CARTESIAN_POINT('Ctrl Pts',(-74.723557254876,-27.8298058336428,
19.5989868615623));
#253859=CARTESIAN_POINT('Ctrl Pts',(-74.6834885518123,-27.9303548227301,
19.6177917240647));
#253860=CARTESIAN_POINT('Ctrl Pts',(-74.6754567619398,-27.9505099136238,
19.6215611673621));
#253861=CARTESIAN_POINT('Ctrl Pts',(-74.6674206749895,-27.9707004214996,
19.6251902405029));
#253862=CARTESIAN_POINT('Ctrl Pts',(-74.6593796105366,-27.9909275808286,
19.6286798784691));
#253863=CARTESIAN_POINT('Ctrl Pts',(-74.6191256904534,-28.0921856244508,
19.6461491586415));
#253864=CARTESIAN_POINT('Ctrl Pts',(-74.5786572495067,-28.1946046459843,
19.6600683967049));
#253865=CARTESIAN_POINT('Ctrl Pts',(-74.5381640664692,-28.2976765638881,
19.6704349274727));
#253866=CARTESIAN_POINT('Ctrl Pts',(-74.4998753932249,-28.3951370915433,
19.6802370887123));
#253867=CARTESIAN_POINT('Ctrl Pts',(-74.4615641517495,-28.4931826135859,
19.6868624470852));
#253868=CARTESIAN_POINT('Ctrl Pts',(-74.4233988532603,-28.5913692277709,
19.690266674482));
#253869=CARTESIAN_POINT('Ctrl Pts',(-74.4033703210826,-28.6428959769242,
19.6920531580326));
#253870=CARTESIAN_POINT('Ctrl Pts',(-74.3833821576437,-28.6944612287026,
19.6929518677509));
#253871=CARTESIAN_POINT('Ctrl Pts',(-74.3634602878982,-28.7459974181806,
19.6929518677509));
#253872=CARTESIAN_POINT('',(-28.7459974181806,-74.3634602878982,19.6929518677509));
#253873=CARTESIAN_POINT('Origin',(0.,0.,19.6929518677509));
#253874=CARTESIAN_POINT('',(-25.1183521036895,-75.9614881812303,17.4075636545405));
#253875=CARTESIAN_POINT('Ctrl Pts',(-28.7459974181806,-74.3634602878982,
19.6929518677509));
#253876=CARTESIAN_POINT('Ctrl Pts',(-28.572648582161,-74.4304701496804,
19.6929518674578));
#253877=CARTESIAN_POINT('Ctrl Pts',(-28.4008490219403,-74.4974864003456,
19.6830632277964));
#253878=CARTESIAN_POINT('Ctrl Pts',(-28.2304910937134,-74.5645845521869,
19.6632610083272));
#253879=CARTESIAN_POINT('Ctrl Pts',(-28.1520014515506,-74.5954989333525,
19.6541374580684));
#253880=CARTESIAN_POINT('Ctrl Pts',(-28.0738178941228,-74.6264307042887,
19.642908782261));
#253881=CARTESIAN_POINT('Ctrl Pts',(-27.9959302213503,-74.6573872842512,
19.6295688156876));
#253882=CARTESIAN_POINT('Ctrl Pts',(-27.8740765465656,-74.7058182219456,
19.6086987101803));
#253883=CARTESIAN_POINT('Ctrl Pts',(-27.752361572508,-74.7545517359241,
19.5824195541813));
#253884=CARTESIAN_POINT('Ctrl Pts',(-27.6319739934803,-74.8031494822237,
19.5508884666964));
#253885=CARTESIAN_POINT('Ctrl Pts',(-27.5068599815953,-74.8536551827056,
19.518119464394));
#253886=CARTESIAN_POINT('Ctrl Pts',(-27.3829937092195,-74.9040895744661,
19.4796267591552));
#253887=CARTESIAN_POINT('Ctrl Pts',(-27.2617318168035,-74.9539558516285,
19.4355274341625));
#253888=CARTESIAN_POINT('Ctrl Pts',(-27.0958774930693,-75.0221597820729,
19.375211175047));
#253889=CARTESIAN_POINT('Ctrl Pts',(-26.9346592389393,-75.0893730478975,
19.3046526925474));
#253890=CARTESIAN_POINT('Ctrl Pts',(-26.7783260044453,-75.1556896636845,
19.2232208975604));
#253891=CARTESIAN_POINT('Ctrl Pts',(-26.7160947950356,-75.1820881656904,
19.1908055310976));
#253892=CARTESIAN_POINT('Ctrl Pts',(-26.654637872938,-75.2083445587741,
19.15666668345));
#253893=CARTESIAN_POINT('Ctrl Pts',(-26.5939718531098,-75.2344646706147,
19.1207624000721));
#253894=CARTESIAN_POINT('Ctrl Pts',(-26.5885204638033,-75.2368117983606,
19.1175360762252));
#253895=CARTESIAN_POINT('Ctrl Pts',(-26.5830764322048,-75.2391574108363,
19.114296045689));
#253896=CARTESIAN_POINT('Ctrl Pts',(-26.5776397722412,-75.2415015097604,
19.1110422978749));
#253897=CARTESIAN_POINT('Ctrl Pts',(-26.4684638408705,-75.2885743789445,
19.0457023740205));
#253898=CARTESIAN_POINT('Ctrl Pts',(-26.3622811063516,-75.3350350763051,
18.9747887273497));
#253899=CARTESIAN_POINT('Ctrl Pts',(-26.2593455383138,-75.3808870959315,
18.8979255800989));
#253900=CARTESIAN_POINT('Ctrl Pts',(-26.1806548896459,-75.4159393644128,
18.8391663870316));
#253901=CARTESIAN_POINT('Ctrl Pts',(-26.1034760636602,-75.450816950824,
18.7765523191711));
#253902=CARTESIAN_POINT('Ctrl Pts',(-26.0291438153621,-75.4849716254206,
18.7109347213048));
#253903=CARTESIAN_POINT('Ctrl Pts',(-26.0056230055367,-75.4957791231653,
18.6901714714912));
#253904=CARTESIAN_POINT('Ctrl Pts',(-25.9823868773818,-75.5065143688487,
18.6691073534994));
#253905=CARTESIAN_POINT('Ctrl Pts',(-25.9594767553431,-75.5171603678615,
18.6477689489594));
#253906=CARTESIAN_POINT('Ctrl Pts',(-25.8734790541225,-75.5571222432612,
18.5676710020758));
#253907=CARTESIAN_POINT('Ctrl Pts',(-25.7920071322347,-75.5958350863704,
18.4838572390434));
#253908=CARTESIAN_POINT('Ctrl Pts',(-25.7152212809698,-75.6333036881581,
18.3962512683447));
#253909=CARTESIAN_POINT('Ctrl Pts',(-25.6526661199683,-75.6638282493725,
18.3248812761982));
#253910=CARTESIAN_POINT('Ctrl Pts',(-25.5930696741688,-75.6936006486759,
18.2508225083616));
#253911=CARTESIAN_POINT('Ctrl Pts',(-25.5366139960046,-75.7225799270805,
18.174108210907));
#253912=CARTESIAN_POINT('Ctrl Pts',(-25.5072460962901,-75.7376547710937,
18.1342019009029));
#253913=CARTESIAN_POINT('Ctrl Pts',(-25.4787274775015,-75.7525151457539,
18.0935775396279));
#253914=CARTESIAN_POINT('Ctrl Pts',(-25.4510796000903,-75.7671562637947,
18.052243447843));
#253915=CARTESIAN_POINT('Ctrl Pts',(-25.4253897658985,-75.7807604869782,
18.0138366671475));
#253916=CARTESIAN_POINT('Ctrl Pts',(-25.4004235947553,-75.7942007247961,
17.9746913116854));
#253917=CARTESIAN_POINT('Ctrl Pts',(-25.3762475819473,-75.807444674672,
17.9349066213656));
#253918=CARTESIAN_POINT('Ctrl Pts',(-25.3113015022286,-75.8430230238094,
17.8280296235075));
#253919=CARTESIAN_POINT('Ctrl Pts',(-25.2516721229916,-75.877404315187,
17.7158399467825));
#253920=CARTESIAN_POINT('Ctrl Pts',(-25.1986596212116,-75.9100163344733,
17.599789295223));
#253921=CARTESIAN_POINT('Ctrl Pts',(-25.1698737118368,-75.9277247353256,
17.5367735267439));
#253922=CARTESIAN_POINT('Ctrl Pts',(-25.1430395031998,-75.9449112030332,
17.4726196431301));
#253923=CARTESIAN_POINT('Ctrl Pts',(-25.1183707693638,-75.9614820151852,
17.4075627905749));
#253924=CARTESIAN_POINT('',(-24.6976449920628,-76.0424582863717,17.8479876922246));
#253925=CARTESIAN_POINT('Ctrl Pts',(-25.1183452685093,-75.9614890268773,
17.4075745924872));
#253926=CARTESIAN_POINT('Ctrl Pts',(-24.9826881607245,-75.9867559935951,
17.5590635300832));
#253927=CARTESIAN_POINT('Ctrl Pts',(-24.8421318546858,-76.0139038233151,
17.7056692316105));
#253928=CARTESIAN_POINT('Ctrl Pts',(-24.6976449919805,-76.0424582864102,
17.8479876921332));
#253929=CARTESIAN_POINT('',(24.6976449920629,-76.0424582863716,17.8479876922249));
#253930=CARTESIAN_POINT('Origin',(0.,0.,17.8479876926671));
#253931=CARTESIAN_POINT('',(25.1183523255102,-75.961488153786,17.4075632995852));
#253932=CARTESIAN_POINT('Ctrl Pts',(24.6976449919804,-76.0424582864102,
17.8479876921333));
#253933=CARTESIAN_POINT('Ctrl Pts',(24.8421318545421,-76.0139038233827,
17.705669231448));
#253934=CARTESIAN_POINT('Ctrl Pts',(24.982688160729,-75.9867559935942,17.5590635300786));
#253935=CARTESIAN_POINT('Ctrl Pts',(25.118345268511,-75.9614890268762,17.4075745924918));
#253936=CARTESIAN_POINT('',(28.7459974181806,-74.3634602878982,19.6929518677509));
#253937=CARTESIAN_POINT('Ctrl Pts',(25.1183716157476,-75.9614818429679,
17.4075624145231));
#253938=CARTESIAN_POINT('Ctrl Pts',(25.1663807403153,-75.9292306004278,
17.5341891959829));
#253939=CARTESIAN_POINT('Ctrl Pts',(25.2225896115677,-75.8946388507875,
17.6574709248538));
#253940=CARTESIAN_POINT('Ctrl Pts',(25.2856234360028,-75.8583098127289,
17.7758260767094));
#253941=CARTESIAN_POINT('Ctrl Pts',(25.3144603201426,-75.8416899063406,
17.8299715110377));
#253942=CARTESIAN_POINT('Ctrl Pts',(25.3447263485959,-75.8247061544809,
17.8830859080628));
#253943=CARTESIAN_POINT('Ctrl Pts',(25.376293226511,-75.8074152517246,17.9350176026264));
#253944=CARTESIAN_POINT('Ctrl Pts',(25.3987704082003,-75.7951032719376,
17.9719955431527));
#253945=CARTESIAN_POINT('Ctrl Pts',(25.4219292775783,-75.7826225663751,
18.0084169806877));
#253946=CARTESIAN_POINT('Ctrl Pts',(25.4457245653082,-75.7699942838137,
18.0442185658029));
#253947=CARTESIAN_POINT('Ctrl Pts',(25.5176575565964,-75.7318190724114,
18.1524465115804));
#253948=CARTESIAN_POINT('Ctrl Pts',(25.5954180173166,-75.6922139917242,
18.2556268049576));
#253949=CARTESIAN_POINT('Ctrl Pts',(25.6787085176417,-75.6512007482855,
18.3538912519095));
#253950=CARTESIAN_POINT('Ctrl Pts',(25.6911412017406,-75.6450787452052,
18.3685590810418));
#253951=CARTESIAN_POINT('Ctrl Pts',(25.7036970321378,-75.638925381073,18.3831174412875));
#253952=CARTESIAN_POINT('Ctrl Pts',(25.7163749474321,-75.6327407433448,
18.3975668354581));
#253953=CARTESIAN_POINT('Ctrl Pts',(25.7908226049063,-75.5964231169443,
18.4824170275409));
#253954=CARTESIAN_POINT('Ctrl Pts',(25.8695946626579,-75.5589722614059,
18.5636320093358));
#253955=CARTESIAN_POINT('Ctrl Pts',(25.9524451451245,-75.5204260075577,
18.6412309225871));
#253956=CARTESIAN_POINT('Ctrl Pts',(26.009490170965,-75.4938857632362,18.6946600865441));
#253957=CARTESIAN_POINT('Ctrl Pts',(26.0681509448606,-75.4669777563054,
18.7460355750972));
#253958=CARTESIAN_POINT('Ctrl Pts',(26.1282299623944,-75.4397648602322,
18.7953196528862));
#253959=CARTESIAN_POINT('Ctrl Pts',(26.1997874752161,-75.4073527596418,
18.8540197810352));
#253960=CARTESIAN_POINT('Ctrl Pts',(26.2732030109977,-75.3745754659727,
18.9096465482131));
#253961=CARTESIAN_POINT('Ctrl Pts',(26.3483201939841,-75.3414533115427,
18.962331304353));
#253962=CARTESIAN_POINT('Ctrl Pts',(26.4206512997923,-75.3095596493815,
19.013061996311));
#253963=CARTESIAN_POINT('Ctrl Pts',(26.4945609623841,-75.2773460198444,
19.061064595511));
#253964=CARTESIAN_POINT('Ctrl Pts',(26.5699313482722,-75.2448262662937,
19.1064165126255));
#253965=CARTESIAN_POINT('Ctrl Pts',(26.5774516032003,-75.2415815325164,
19.1109416052619));
#253966=CARTESIAN_POINT('Ctrl Pts',(26.5849903403353,-75.2383320909218,
19.1154422462802));
#253967=CARTESIAN_POINT('Ctrl Pts',(26.592547351541,-75.2350780060008,19.1199184134197));
#253968=CARTESIAN_POINT('Ctrl Pts',(26.7154431586624,-75.1821584876994,
19.1927120296318));
#253969=CARTESIAN_POINT('Ctrl Pts',(26.8429293002847,-75.1281185032271,
19.2588649120843));
#253970=CARTESIAN_POINT('Ctrl Pts',(26.9733752018017,-75.073540078283,19.3179719516384));
#253971=CARTESIAN_POINT('Ctrl Pts',(27.0676510754753,-75.0340951540999,
19.3606897965796));
#253972=CARTESIAN_POINT('Ctrl Pts',(27.1634716617737,-74.9943693681571,
19.3997280200187));
#253973=CARTESIAN_POINT('Ctrl Pts',(27.2602089524352,-74.9545859173699,
19.4349442290445));
#253974=CARTESIAN_POINT('Ctrl Pts',(27.3823989937782,-74.9043349597173,
19.4794262484125));
#253975=CARTESIAN_POINT('Ctrl Pts',(27.5061040086165,-74.8539591567499,
19.517975099683));
#253976=CARTESIAN_POINT('Ctrl Pts',(27.6312030307086,-74.8034579087233,
19.5507626191466));
#253977=CARTESIAN_POINT('Ctrl Pts',(27.7301373584037,-74.7635190911554,
19.5766925676039));
#253978=CARTESIAN_POINT('Ctrl Pts',(27.829805833643,-74.7235572548759,19.5989868615624));
#253979=CARTESIAN_POINT('Ctrl Pts',(27.9303548227305,-74.6834885518121,
19.6177917240647));
#253980=CARTESIAN_POINT('Ctrl Pts',(27.9505099136241,-74.6754567619397,
19.6215611673621));
#253981=CARTESIAN_POINT('Ctrl Pts',(27.9707004214997,-74.6674206749895,
19.6251902405028));
#253982=CARTESIAN_POINT('Ctrl Pts',(27.9909275808286,-74.6593796105366,
19.628679878469));
#253983=CARTESIAN_POINT('Ctrl Pts',(28.0921856244513,-74.6191256904532,
19.6461491586415));
#253984=CARTESIAN_POINT('Ctrl Pts',(28.1946046459851,-74.5786572495064,
19.6600683967049));
#253985=CARTESIAN_POINT('Ctrl Pts',(28.297676563889,-74.5381640664688,19.6704349274727));
#253986=CARTESIAN_POINT('Ctrl Pts',(28.3951370915476,-74.4998753932232,
19.6802370887127));
#253987=CARTESIAN_POINT('Ctrl Pts',(28.4931826135935,-74.4615641517465,
19.6868624470857));
#253988=CARTESIAN_POINT('Ctrl Pts',(28.5913692277819,-74.423398853256,19.6902666744824));
#253989=CARTESIAN_POINT('Ctrl Pts',(28.6428959769315,-74.4033703210798,
19.6920531580327));
#253990=CARTESIAN_POINT('Ctrl Pts',(28.6944612287063,-74.3833821576423,
19.6929518677509));
#253991=CARTESIAN_POINT('Ctrl Pts',(28.7459974181806,-74.3634602878982,
19.6929518677509));
#253992=CARTESIAN_POINT('',(74.3634602878983,-28.7459974181805,19.6929518677509));
#253993=CARTESIAN_POINT('Origin',(0.,0.,19.6929518677509));
#253994=CARTESIAN_POINT('',(75.9614881812303,-25.1183521036895,17.4075636545405));
#253995=CARTESIAN_POINT('Ctrl Pts',(74.3634602878983,-28.7459974181805,
19.6929518677509));
#253996=CARTESIAN_POINT('Ctrl Pts',(74.4304701497267,-28.5726485820409,
19.6929518674584));
#253997=CARTESIAN_POINT('Ctrl Pts',(74.4974864004376,-28.4008490217041,
19.6830632277838));
#253998=CARTESIAN_POINT('Ctrl Pts',(74.5645845523253,-28.2304910933617,
19.663261008287));
#253999=CARTESIAN_POINT('Ctrl Pts',(74.5954989334447,-28.1520014513173,
19.6541374580355));
#254000=CARTESIAN_POINT('Ctrl Pts',(74.6264307043348,-28.0738178940067,
19.6429087822414));
#254001=CARTESIAN_POINT('Ctrl Pts',(74.6573872842514,-27.9959302213499,
19.6295688156875));
#254002=CARTESIAN_POINT('Ctrl Pts',(74.705818221946,-27.8740765465647,19.6086987101797));
#254003=CARTESIAN_POINT('Ctrl Pts',(74.7545517359244,-27.7523615725074,
19.5824195541808));
#254004=CARTESIAN_POINT('Ctrl Pts',(74.8031494822237,-27.6319739934803,
19.5508884666962));
#254005=CARTESIAN_POINT('Ctrl Pts',(74.8536551827057,-27.5068599815951,
19.5181194643939));
#254006=CARTESIAN_POINT('Ctrl Pts',(74.9040895744663,-27.3829937092191,
19.479626759155));
#254007=CARTESIAN_POINT('Ctrl Pts',(74.9539558516288,-27.2617318168029,
19.4355274341618));
#254008=CARTESIAN_POINT('Ctrl Pts',(75.0221597822634,-27.0958774926063,
19.3752111748775));
#254009=CARTESIAN_POINT('Ctrl Pts',(75.0893730482725,-26.93465923804,19.3046526921532));
#254010=CARTESIAN_POINT('Ctrl Pts',(75.1556896642392,-26.7783260031378,
19.2232208968787));
#254011=CARTESIAN_POINT('Ctrl Pts',(75.1820881660582,-26.7160947941749,
19.1908055306188));
#254012=CARTESIAN_POINT('Ctrl Pts',(75.208344558957,-26.6546378725134,19.156666683198));
#254013=CARTESIAN_POINT('Ctrl Pts',(75.2344646706146,-26.5939718531102,
19.1207624000714));
#254014=CARTESIAN_POINT('Ctrl Pts',(75.2368117983607,-26.5885204638034,
19.1175360762244));
#254015=CARTESIAN_POINT('Ctrl Pts',(75.2391574108366,-26.5830764322045,
19.1142960456879));
#254016=CARTESIAN_POINT('Ctrl Pts',(75.2415015097608,-26.5776397722406,
19.1110422978736));
#254017=CARTESIAN_POINT('Ctrl Pts',(75.2885743789452,-26.4684638408694,
19.0457023740184));
#254018=CARTESIAN_POINT('Ctrl Pts',(75.3350350763051,-26.3622811063518,
18.9747887273492));
#254019=CARTESIAN_POINT('Ctrl Pts',(75.3808870959319,-26.2593455383128,
18.8979255800978));
#254020=CARTESIAN_POINT('Ctrl Pts',(75.415939364422,-26.1806548896252,18.839166387016));
#254021=CARTESIAN_POINT('Ctrl Pts',(75.4508169508416,-26.1034760636214,
18.7765523191393));
#254022=CARTESIAN_POINT('Ctrl Pts',(75.4849716254462,-26.0291438153065,
18.7109347212553));
#254023=CARTESIAN_POINT('Ctrl Pts',(75.4957791231824,-26.0056230054997,
18.6901714714573));
#254024=CARTESIAN_POINT('Ctrl Pts',(75.5065143688574,-25.9823868773631,
18.6691073534816));
#254025=CARTESIAN_POINT('Ctrl Pts',(75.517160367862,-25.9594767553421,18.6477689489581));
#254026=CARTESIAN_POINT('Ctrl Pts',(75.5571222432616,-25.8734790541217,
18.5676710020748));
#254027=CARTESIAN_POINT('Ctrl Pts',(75.5958350863706,-25.7920071322341,
18.4838572390429));
#254028=CARTESIAN_POINT('Ctrl Pts',(75.6333036881581,-25.7152212809698,
18.3962512683448));
#254029=CARTESIAN_POINT('Ctrl Pts',(75.6638282493716,-25.6526661199703,
18.3248812762004));
#254030=CARTESIAN_POINT('Ctrl Pts',(75.693600648674,-25.5930696741725,18.2508225083663));
#254031=CARTESIAN_POINT('Ctrl Pts',(75.7225799270778,-25.5366139960098,
18.1741082109142));
#254032=CARTESIAN_POINT('Ctrl Pts',(75.7376547710921,-25.5072460962931,
18.1342019009073));
#254033=CARTESIAN_POINT('Ctrl Pts',(75.7525151457534,-25.4787274775024,
18.0935775396293));
#254034=CARTESIAN_POINT('Ctrl Pts',(75.7671562637952,-25.4510796000893,
18.0522434478413));
#254035=CARTESIAN_POINT('Ctrl Pts',(75.7807604869785,-25.4253897658979,
18.0138366671463));
#254036=CARTESIAN_POINT('Ctrl Pts',(75.7942007247962,-25.4004235947552,
17.9746913116847));
#254037=CARTESIAN_POINT('Ctrl Pts',(75.8074446746719,-25.3762475819477,
17.9349066213655));
#254038=CARTESIAN_POINT('Ctrl Pts',(75.8430230238029,-25.3113015022408,
17.8280296235264));
#254039=CARTESIAN_POINT('Ctrl Pts',(75.8774043151745,-25.2516721230136,
17.7158399468224));
#254040=CARTESIAN_POINT('Ctrl Pts',(75.9100163344557,-25.1986596212405,
17.599789295285));
#254041=CARTESIAN_POINT('Ctrl Pts',(75.9277247353141,-25.169873711855,17.536773526786));
#254042=CARTESIAN_POINT('Ctrl Pts',(75.9449112030276,-25.1430395032083,
17.4726196431515));
#254043=CARTESIAN_POINT('Ctrl Pts',(75.9614820151851,-25.118370769364,17.4075627905749));
#254044=CARTESIAN_POINT('',(76.0424582863717,-24.6976449920627,17.8479876922247));
#254045=CARTESIAN_POINT('Ctrl Pts',(75.9614890268773,-25.1183452685093,
17.4075745924873));
#254046=CARTESIAN_POINT('Ctrl Pts',(75.9867559935951,-24.9826881607245,
17.5590635300833));
#254047=CARTESIAN_POINT('Ctrl Pts',(76.0139038233338,-24.8421318546458,
17.7056692315664));
#254048=CARTESIAN_POINT('Ctrl Pts',(76.0424582864102,-24.6976449919804,
17.8479876921334));
#254049=CARTESIAN_POINT('',(76.0424582863716,24.6976449920628,17.847987692225));
#254050=CARTESIAN_POINT('Origin',(0.,0.,17.8479876926672));
#254051=CARTESIAN_POINT('',(75.9614886121312,25.1183470986529,17.4075730861852));
#254052=CARTESIAN_POINT('Ctrl Pts',(76.0424582864102,24.6976449919803,17.8479876921334));
#254053=CARTESIAN_POINT('Ctrl Pts',(76.0139038233584,24.842131854594,17.7056692315056));
#254054=CARTESIAN_POINT('Ctrl Pts',(75.9867559935943,24.9826881607288,17.5590635300786));
#254055=CARTESIAN_POINT('Ctrl Pts',(75.9614890268762,25.118345268511,17.4075745924918));
#254056=CARTESIAN_POINT('',(74.3634602878983,28.7459974181805,19.6929518677509));
#254057=CARTESIAN_POINT('Ctrl Pts',(75.9614877926984,25.1183497610148,17.4075725136416));
#254058=CARTESIAN_POINT('Ctrl Pts',(75.9334021721091,25.1601393821171,17.5178916380196));
#254059=CARTESIAN_POINT('Ctrl Pts',(75.9035242097614,25.2082110521886,17.6256433855426));
#254060=CARTESIAN_POINT('Ctrl Pts',(75.8722717148825,25.2615872269752,17.729813441149));
#254061=CARTESIAN_POINT('Ctrl Pts',(75.8512336859029,25.2975181027767,17.7999368875218));
#254062=CARTESIAN_POINT('Ctrl Pts',(75.82957235286,25.3358539579438,17.8684375808773));
#254063=CARTESIAN_POINT('Ctrl Pts',(75.8074111030368,25.376308989996,17.9350062768217));
#254064=CARTESIAN_POINT('Ctrl Pts',(75.7908062731773,25.4066208600191,17.9848844145148));
#254065=CARTESIAN_POINT('Ctrl Pts',(75.7738886212226,25.4381799817096,18.0337776331664));
#254066=CARTESIAN_POINT('Ctrl Pts',(75.7567136591966,25.4708669570284,18.0815237295059));
#254067=CARTESIAN_POINT('Ctrl Pts',(75.7220283060228,25.5368792883161,18.1779484093214));
#254068=CARTESIAN_POINT('Ctrl Pts',(75.6861745408806,25.6076061824442,18.2703348362656));
#254069=CARTESIAN_POINT('Ctrl Pts',(75.6491774008247,25.6828197666451,18.3587322169221));
#254070=CARTESIAN_POINT('Ctrl Pts',(75.6437233302642,25.6939076559987,18.3717636445064));
#254071=CARTESIAN_POINT('Ctrl Pts',(75.6382444253436,25.7050929860443,18.3847084446968));
#254072=CARTESIAN_POINT('Ctrl Pts',(75.6327407805507,25.716374960082,18.3975668402832));
#254073=CARTESIAN_POINT('Ctrl Pts',(75.5926129031196,25.7986334793732,18.4913192791613));
#254074=CARTESIAN_POINT('Ctrl Pts',(75.5511297118698,25.8861084238851,18.5805817736278));
#254075=CARTESIAN_POINT('Ctrl Pts',(75.5083052747818,25.9785568613914,18.6654318615666));
#254076=CARTESIAN_POINT('Ctrl Pts',(75.4856855815722,26.0273877494613,18.7102493323495));
#254077=CARTESIAN_POINT('Ctrl Pts',(75.4628315387299,26.0773070493268,18.7535439863377));
#254078=CARTESIAN_POINT('Ctrl Pts',(75.4397654989299,26.1282310684057,18.7953186220858));
#254079=CARTESIAN_POINT('Ctrl Pts',(75.4062658488513,26.2021898768762,18.855989447761));
#254080=CARTESIAN_POINT('Ctrl Pts',(75.3723921489013,26.2780930526712,18.9133588584959));
#254081=CARTESIAN_POINT('Ctrl Pts',(75.3381414872632,26.355831091728,18.9675999514268));
#254082=CARTESIAN_POINT('Ctrl Pts',(75.304189114822,26.4328921097836,19.021368658387));
#254083=CARTESIAN_POINT('Ctrl Pts',(75.2698661738243,26.5117567910974,19.0720630469863));
#254084=CARTESIAN_POINT('Ctrl Pts',(75.2351662644524,26.5923393889176,19.1198058720703));
#254085=CARTESIAN_POINT('Ctrl Pts',(75.2351370428123,26.5924072494889,19.1198460774678));
#254086=CARTESIAN_POINT('Ctrl Pts',(75.2351078207906,26.5924751115546,19.1198862808855));
#254087=CARTESIAN_POINT('Ctrl Pts',(75.2350785983874,26.5925429751146,19.1199264823231));
#254088=CARTESIAN_POINT('Ctrl Pts',(75.183303568785,26.7127807873402,19.191153705159));
#254089=CARTESIAN_POINT('Ctrl Pts',(75.1304366076855,26.8374586955589,19.2560332970306));
#254090=CARTESIAN_POINT('Ctrl Pts',(75.0770544694664,26.9649752993357,19.3141613796794));
#254091=CARTESIAN_POINT('Ctrl Pts',(75.0342358129132,27.0672583821063,19.3607868332499));
#254092=CARTESIAN_POINT('Ctrl Pts',(74.9910861388835,27.1713664534818,19.4030689498303));
#254093=CARTESIAN_POINT('Ctrl Pts',(74.9479077551293,27.2764562548044,19.4408157537664));
#254094=CARTESIAN_POINT('Ctrl Pts',(74.8999079936204,27.3932805766512,19.4827774352636));
#254095=CARTESIAN_POINT('Ctrl Pts',(74.8517145421664,27.511651646086,19.5194081094312));
#254096=CARTESIAN_POINT('Ctrl Pts',(74.8034459183259,27.631202345934,19.5507462995563));
#254097=CARTESIAN_POINT('Ctrl Pts',(74.7565343276745,27.7473919748717,19.5812034418972));
#254098=CARTESIAN_POINT('Ctrl Pts',(74.7093890816425,27.865081171539,19.6068157552163));
#254099=CARTESIAN_POINT('Ctrl Pts',(74.6621501920651,27.9838718582653,19.6275204329004));
#254100=CARTESIAN_POINT('Ctrl Pts',(74.6123504464618,28.1091022781997,19.6493475268624));
#254101=CARTESIAN_POINT('Ctrl Pts',(74.562446729845,28.2355565734727,19.6657199755857));
#254102=CARTESIAN_POINT('Ctrl Pts',(74.5126081501712,28.3627441365293,19.6766210584599));
#254103=CARTESIAN_POINT('Ctrl Pts',(74.4627695704973,28.4899316995859,19.6875221413342));
#254104=CARTESIAN_POINT('Ctrl Pts',(74.412996284741,28.617851990473,19.6929518677509));
#254105=CARTESIAN_POINT('Ctrl Pts',(74.3634602878983,28.7459974181805,19.6929518677509));
#254106=CARTESIAN_POINT('',(28.7459974181806,74.3634602878982,19.6929518677509));
#254107=CARTESIAN_POINT('Origin',(0.,0.,19.6929518677508));
#254108=CARTESIAN_POINT('',(25.1183521036895,75.9614881812303,17.4075636545405));
#254109=CARTESIAN_POINT('Ctrl Pts',(28.7459974181806,74.3634602878982,19.6929518677509));
#254110=CARTESIAN_POINT('Ctrl Pts',(28.5726485821451,74.4304701496865,19.6929518674579));
#254111=CARTESIAN_POINT('Ctrl Pts',(28.4008490219087,74.4974864003579,19.6830632277949));
#254112=CARTESIAN_POINT('Ctrl Pts',(28.2304910936664,74.5645845522053,19.663261008322));
#254113=CARTESIAN_POINT('Ctrl Pts',(28.1520014515195,74.5954989333648,19.6541374580642));
#254114=CARTESIAN_POINT('Ctrl Pts',(28.0738178941073,74.6264307042949,19.6429087822585));
#254115=CARTESIAN_POINT('Ctrl Pts',(27.9959302213504,74.6573872842512,19.6295688156876));
#254116=CARTESIAN_POINT('Ctrl Pts',(27.8740765465657,74.7058182219455,19.6086987101801));
#254117=CARTESIAN_POINT('Ctrl Pts',(27.752361572508,74.7545517359241,19.5824195541812));
#254118=CARTESIAN_POINT('Ctrl Pts',(27.6319739934803,74.8031494822237,19.5508884666963));
#254119=CARTESIAN_POINT('Ctrl Pts',(27.5068599815954,74.8536551827056,19.5181194643941));
#254120=CARTESIAN_POINT('Ctrl Pts',(27.3829937092194,74.9040895744662,19.4796267591551));
#254121=CARTESIAN_POINT('Ctrl Pts',(27.2617318168037,74.9539558516285,19.435527434162));
#254122=CARTESIAN_POINT('Ctrl Pts',(27.0958774928492,75.0221597821636,19.3752111749656));
#254123=CARTESIAN_POINT('Ctrl Pts',(26.9346592385107,75.0893730480763,19.3046526923589));
#254124=CARTESIAN_POINT('Ctrl Pts',(26.7783260038218,75.1556896639491,19.2232208972347));
#254125=CARTESIAN_POINT('Ctrl Pts',(26.7160947946252,75.1820881658658,19.1908055308687));
#254126=CARTESIAN_POINT('Ctrl Pts',(26.6546378727357,75.2083445588614,19.1566666833293));
#254127=CARTESIAN_POINT('Ctrl Pts',(26.5939718531103,75.2344646706146,19.1207624000712));
#254128=CARTESIAN_POINT('Ctrl Pts',(26.5885204638038,75.2368117983605,19.1175360762244));
#254129=CARTESIAN_POINT('Ctrl Pts',(26.5830764322053,75.2391574108362,19.1142960456881));
#254130=CARTESIAN_POINT('Ctrl Pts',(26.5776397722417,75.2415015097603,19.111042297874));
#254131=CARTESIAN_POINT('Ctrl Pts',(26.4684638408709,75.2885743789445,19.045702374019));
#254132=CARTESIAN_POINT('Ctrl Pts',(26.3622811063523,75.3350350763049,18.9747887273491));
#254133=CARTESIAN_POINT('Ctrl Pts',(26.2593455383141,75.3808870959314,18.8979255800986));
#254134=CARTESIAN_POINT('Ctrl Pts',(26.1806548896519,75.4159393644101,18.8391663870361));
#254135=CARTESIAN_POINT('Ctrl Pts',(26.1034760636718,75.4508169508188,18.7765523191803));
#254136=CARTESIAN_POINT('Ctrl Pts',(26.0291438153788,75.484971625413,18.7109347213192));
#254137=CARTESIAN_POINT('Ctrl Pts',(26.0056230055477,75.4957791231602,18.6901714715009));
#254138=CARTESIAN_POINT('Ctrl Pts',(25.9823868773873,75.5065143688461,18.6691073535043));
#254139=CARTESIAN_POINT('Ctrl Pts',(25.9594767553432,75.5171603678615,18.6477689489594));
#254140=CARTESIAN_POINT('Ctrl Pts',(25.8734790541225,75.5571222432611,18.567671002076));
#254141=CARTESIAN_POINT('Ctrl Pts',(25.7920071322346,75.5958350863704,18.4838572390433));
#254142=CARTESIAN_POINT('Ctrl Pts',(25.7152212809698,75.6333036881581,18.3962512683447));
#254143=CARTESIAN_POINT('Ctrl Pts',(25.6526661199698,75.6638282493718,18.3248812761999));
#254144=CARTESIAN_POINT('Ctrl Pts',(25.5930696741718,75.6936006486744,18.2508225083648));
#254145=CARTESIAN_POINT('Ctrl Pts',(25.5366139960088,75.7225799270784,18.1741082109121));
#254146=CARTESIAN_POINT('Ctrl Pts',(25.5072460962929,75.7376547710924,18.1342019009063));
#254147=CARTESIAN_POINT('Ctrl Pts',(25.4787274775029,75.7525151457532,18.0935775396296));
#254148=CARTESIAN_POINT('Ctrl Pts',(25.4510796000904,75.7671562637946,18.052243447843));
#254149=CARTESIAN_POINT('Ctrl Pts',(25.4253897658984,75.7807604869782,18.0138366671477));
#254150=CARTESIAN_POINT('Ctrl Pts',(25.4004235947551,75.7942007247962,17.9746913116857));
#254151=CARTESIAN_POINT('Ctrl Pts',(25.376247581947,75.8074446746721,17.9349066213659));
#254152=CARTESIAN_POINT('Ctrl Pts',(25.3113015022871,75.8430230237772,17.8280296236051));
#254153=CARTESIAN_POINT('Ctrl Pts',(25.2516721230997,75.8774043151245,17.7158399469868));
#254154=CARTESIAN_POINT('Ctrl Pts',(25.198659621356,75.9100163343844,17.5997892955397));
#254155=CARTESIAN_POINT('Ctrl Pts',(25.1698737119266,75.9277247352681,17.5367735269588));
#254156=CARTESIAN_POINT('Ctrl Pts',(25.1430395032411,75.9449112030055,17.472619643239));
#254157=CARTESIAN_POINT('Ctrl Pts',(25.1183707693638,75.9614820151852,17.4075627905749));
#254158=CARTESIAN_POINT('',(24.6976449920628,76.0424582863717,17.8479876922246));
#254159=CARTESIAN_POINT('Ctrl Pts',(25.1183452685093,75.9614890268773,17.4075745924872));
#254160=CARTESIAN_POINT('Ctrl Pts',(24.9826881607244,75.9867559935951,17.5590635300832));
#254161=CARTESIAN_POINT('Ctrl Pts',(24.8421318546464,76.0139038233335,17.7056692315669));
#254162=CARTESIAN_POINT('Ctrl Pts',(24.6976449919804,76.0424582864102,17.8479876921332));
#254163=CARTESIAN_POINT('',(10.8641498708349,79.2111064053766,17.8479876926671));
#254164=CARTESIAN_POINT('Origin',(0.,0.,17.8479876926671));
#254165=CARTESIAN_POINT('Ctrl Pts',(10.8641498708349,79.2111064053766,17.8479876926671));
#254166=CARTESIAN_POINT('Ctrl Pts',(10.8639322809376,79.1070016560343,18.6882296805948));
#254167=CARTESIAN_POINT('Ctrl Pts',(10.8637138619226,79.0028933995443,19.5284712337854));
#254168=CARTESIAN_POINT('Ctrl Pts',(10.8634946042403,78.8987815953885,20.3687123471684));
#254169=CARTESIAN_POINT('Ctrl Pts',(10.8626175735112,78.4823343787045,23.7296768011912));
#254170=CARTESIAN_POINT('Ctrl Pts',(10.8617271271499,78.0658304123124,27.0906342205866));
#254171=CARTESIAN_POINT('Ctrl Pts',(10.8608226300202,77.6492670005164,30.451584267896));
#254172=CARTESIAN_POINT('Ctrl Pts',(10.8599093742504,77.2286698235283,33.845079860324));
#254173=CARTESIAN_POINT('Ctrl Pts',(10.8589817945603,76.8080120453849,37.2385679384961));
#254174=CARTESIAN_POINT('Ctrl Pts',(10.8580391950581,76.3872907109282,40.6320481322491));
#254175=CARTESIAN_POINT('Origin',(-90.,90.,17.4625));
#254176=CARTESIAN_POINT('',(-110.478801107225,75.6605890912239,16.1925));
#254177=CARTESIAN_POINT('',(-75.6605890912239,110.478801107225,16.1925));
#254178=CARTESIAN_POINT('Origin',(-90.,90.,16.1925));
#254179=CARTESIAN_POINT('',(-75.6605890912239,110.478801107225,12.3825));
#254180=CARTESIAN_POINT('',(-75.6605890912239,110.478801107225,12.3825));
#254181=CARTESIAN_POINT('',(-80.428115389329,113.095,12.3825));
#254182=CARTESIAN_POINT('Origin',(-90.,90.,12.3825));
#254183=CARTESIAN_POINT('',(-90.,115.,10.4775));
#254184=CARTESIAN_POINT('Ctrl Pts',(-80.428115389329,113.095,12.3825));
#254185=CARTESIAN_POINT('Ctrl Pts',(-81.8924546881425,113.701905685175,
12.3825));
#254186=CARTESIAN_POINT('Ctrl Pts',(-83.5138272817594,114.202094699092,
12.1039861530196));
#254187=CARTESIAN_POINT('Ctrl Pts',(-86.8039448109204,114.851492965438,
11.3641723788953));
#254188=CARTESIAN_POINT('Ctrl Pts',(-88.4720214203075,115.,10.8992885166146));
#254189=CARTESIAN_POINT('Ctrl Pts',(-90.,115.,10.4775));
#254190=CARTESIAN_POINT('',(-90.,115.,0.0380999999999992));
#254191=CARTESIAN_POINT('',(-90.,115.,17.4625));
#254192=CARTESIAN_POINT('',(-115.,90.,0.0381));
#254193=CARTESIAN_POINT('Origin',(-90.,90.,0.0381));
#254194=CARTESIAN_POINT('',(-115.,90.,10.4775));
#254195=CARTESIAN_POINT('',(-115.,90.,17.4625));
#254196=CARTESIAN_POINT('',(-111.45976584278,77.1750847966528,14.2875));
#254197=CARTESIAN_POINT('Ctrl Pts',(-115.,90.,10.4775));
#254198=CARTESIAN_POINT('Ctrl Pts',(-115.,89.5656046367595,10.6534234416246));
#254199=CARTESIAN_POINT('Ctrl Pts',(-114.988625660063,89.1307534409601,
10.82954637956));
#254200=CARTESIAN_POINT('Ctrl Pts',(-114.965914947157,88.6961589330913,
11.0044622013578));
#254201=CARTESIAN_POINT('Ctrl Pts',(-114.943409594944,88.2654942282673,
11.1777963539982));
#254202=CARTESIAN_POINT('Ctrl Pts',(-114.909771870929,87.835080885952,11.3499462246594));
#254203=CARTESIAN_POINT('Ctrl Pts',(-114.864988738924,87.4056111020781,
11.5195411430327));
#254204=CARTESIAN_POINT('Ctrl Pts',(-114.841493243082,87.1802895341208,
11.608519214041));
#254205=CARTESIAN_POINT('Ctrl Pts',(-114.814929056248,86.9552277330983,
11.6967938816802));
#254206=CARTESIAN_POINT('Ctrl Pts',(-114.785288831497,86.7305265176408,
11.7841654473661));
#254207=CARTESIAN_POINT('Ctrl Pts',(-114.78477355285,86.726620213312,11.785684352925));
#254208=CARTESIAN_POINT('Ctrl Pts',(-114.784257346139,86.7227140306222,
11.7872029805012));
#254209=CARTESIAN_POINT('Ctrl Pts',(-114.783740211354,86.7188079702431,
11.7887213289904));
#254210=CARTESIAN_POINT('Ctrl Pts',(-114.707687724482,86.1443627503486,
12.0120174245779));
#254211=CARTESIAN_POINT('Ctrl Pts',(-114.611788003437,85.5722301476407,
12.2295806327357));
#254212=CARTESIAN_POINT('Ctrl Pts',(-114.495317720437,85.0015050763843,
12.4383933645731));
#254213=CARTESIAN_POINT('Ctrl Pts',(-114.392569776158,84.4980219018838,
12.6226041210241));
#254214=CARTESIAN_POINT('Ctrl Pts',(-114.273812458388,83.9956342995033,
12.8000049442964));
#254215=CARTESIAN_POINT('Ctrl Pts',(-114.138523507008,83.4937195188485,
12.9685020775533));
#254216=CARTESIAN_POINT('Ctrl Pts',(-114.136898423986,83.4876905476702,
12.9705260553264));
#254217=CARTESIAN_POINT('Ctrl Pts',(-114.135270955025,83.4816616434102,
12.9725487471968));
#254218=CARTESIAN_POINT('Ctrl Pts',(-114.133641099172,83.4756328049009,
12.9745701495385));
#254219=CARTESIAN_POINT('Ctrl Pts',(-114.007805694041,83.0101675093264,
13.1306354740579));
#254220=CARTESIAN_POINT('Ctrl Pts',(-113.867666657712,82.5450867340379,
13.2789353415663));
#254221=CARTESIAN_POINT('Ctrl Pts',(-113.712210319662,82.0796977881564,
13.4168816899579));
#254222=CARTESIAN_POINT('Ctrl Pts',(-113.690214571606,82.0138492153038,
13.436399923582));
#254223=CARTESIAN_POINT('Ctrl Pts',(-113.667912115099,81.9479944649698,
13.4557108194421));
#254224=CARTESIAN_POINT('Ctrl Pts',(-113.645300019736,81.8821315660405,
13.4748069823197));
#254225=CARTESIAN_POINT('Ctrl Pts',(-113.643270339836,81.8762196591617,
13.4765210692868));
#254226=CARTESIAN_POINT('Ctrl Pts',(-113.641238170047,81.8703077008491,
13.4782334211549));
#254227=CARTESIAN_POINT('Ctrl Pts',(-113.639203508438,81.8643956901358,
13.4799440324456));
#254228=CARTESIAN_POINT('Ctrl Pts',(-113.456290898634,81.332916006182,13.6337250711184));
#254229=CARTESIAN_POINT('Ctrl Pts',(-113.254273359621,80.8043691708234,
13.7724010417179));
#254230=CARTESIAN_POINT('Ctrl Pts',(-113.034078437782,80.2824267541528,
13.8900543869064));
#254231=CARTESIAN_POINT('Ctrl Pts',(-113.032069517046,80.2776648780162,
13.8911277824362));
#254232=CARTESIAN_POINT('Ctrl Pts',(-113.030059078579,80.2729035395786,
13.8921994304486));
#254233=CARTESIAN_POINT('Ctrl Pts',(-113.028047123005,80.2681427414561,
13.8932693264694));
#254234=CARTESIAN_POINT('Ctrl Pts',(-112.841564750851,79.8268780640705,
13.9924349096997));
#254235=CARTESIAN_POINT('Ctrl Pts',(-112.641760412556,79.389376763279,14.0768952568082));
#254236=CARTESIAN_POINT('Ctrl Pts',(-112.427972083071,78.9552639490499,
14.1422627631443));
#254237=CARTESIAN_POINT('Ctrl Pts',(-112.388436056326,78.8749831597535,
14.1543512222522));
#254238=CARTESIAN_POINT('Ctrl Pts',(-112.348421741625,78.7948182514345,
14.1657865821597));
#254239=CARTESIAN_POINT('Ctrl Pts',(-112.307924890089,78.7147668473371,
14.1765409023449));
#254240=CARTESIAN_POINT('Ctrl Pts',(-112.306476768944,78.7119043005831,
14.1769254645483));
#254241=CARTESIAN_POINT('Ctrl Pts',(-112.305028031036,78.7090418994725,
14.1773091556142));
#254242=CARTESIAN_POINT('Ctrl Pts',(-112.303578676147,78.7061796438514,
14.1776919742689));
#254243=CARTESIAN_POINT('Ctrl Pts',(-112.146482129816,78.3959378416688,
14.2191859444306));
#254244=CARTESIAN_POINT('Ctrl Pts',(-111.982145145801,78.0874036287513,
14.2505477198143));
#254245=CARTESIAN_POINT('Ctrl Pts',(-111.810091167185,77.7803237269415,
14.2689228991092));
#254246=CARTESIAN_POINT('Ctrl Pts',(-111.696714227447,77.577969908667,14.281031433956));
#254247=CARTESIAN_POINT('Ctrl Pts',(-111.579986000179,77.3762476415099,
14.2874999986824));
#254248=CARTESIAN_POINT('Ctrl Pts',(-111.45976584278,77.1750847966528,14.2875));
#254249=CARTESIAN_POINT('',(-110.478801107225,75.6605890912239,14.2875));
#254250=CARTESIAN_POINT('Origin',(-90.,90.,14.2875));
#254251=CARTESIAN_POINT('',(-110.478801107225,75.6605890912239,12.3825));
#254252=CARTESIAN_POINT('Origin',(-90.,-90.,17.4625));
#254253=CARTESIAN_POINT('',(-75.6605890912239,-110.478801107225,16.1925));
#254254=CARTESIAN_POINT('',(-110.478801107225,-75.6605890912239,16.1925));
#254255=CARTESIAN_POINT('Origin',(-90.,-90.,16.1925));
#254256=CARTESIAN_POINT('',(-110.478801107225,-75.6605890912239,14.2875));
#254257=CARTESIAN_POINT('',(-110.478801107225,-75.6605890912239,12.3825));
#254258=CARTESIAN_POINT('',(-111.45976584278,-77.1750847966528,14.2875));
#254259=CARTESIAN_POINT('Origin',(-90.,-90.,14.2875));
#254260=CARTESIAN_POINT('',(-115.,-90.,10.4775));
#254261=CARTESIAN_POINT('Ctrl Pts',(-111.45976584278,-77.1750847966528,
14.2875));
#254262=CARTESIAN_POINT('Ctrl Pts',(-111.642205354545,-77.4803584878129,
14.2874999980005));
#254263=CARTESIAN_POINT('Ctrl Pts',(-111.816604025059,-77.7869204404192,
14.2726057755963));
#254264=CARTESIAN_POINT('Ctrl Pts',(-111.983450207187,-78.0950229353511,
14.2457040093625));
#254265=CARTESIAN_POINT('Ctrl Pts',(-112.093394377508,-78.2980486968468,
14.2279769488387));
#254266=CARTESIAN_POINT('Ctrl Pts',(-112.200058693817,-78.5017434125774,
14.2050347428326));
#254267=CARTESIAN_POINT('Ctrl Pts',(-112.303578675868,-78.7061796433008,
14.1776919687023));
#254268=CARTESIAN_POINT('Ctrl Pts',(-112.305032747302,-78.7090512133806,
14.1773079042348));
#254269=CARTESIAN_POINT('Ctrl Pts',(-112.306486197733,-78.7119229298981,
14.1769229616686));
#254270=CARTESIAN_POINT('Ctrl Pts',(-112.30793902738,-78.7147947930089,
14.1765371422901));
#254271=CARTESIAN_POINT('Ctrl Pts',(-112.526985593222,-79.1477923942053,
14.1183662410473));
#254272=CARTESIAN_POINT('Ctrl Pts',(-112.731915857196,-79.5841110072465,
14.0402742394713));
#254273=CARTESIAN_POINT('Ctrl Pts',(-112.923395334248,-80.0241259119978,
13.9466617191921));
#254274=CARTESIAN_POINT('Ctrl Pts',(-112.958736133735,-80.1053381586554,
13.9293839338147));
#254275=CARTESIAN_POINT('Ctrl Pts',(-112.993618688072,-80.1866763161992,
13.9115773060313));
#254276=CARTESIAN_POINT('Ctrl Pts',(-113.028047122842,-80.2681427410701,
13.8932693242905));
#254277=CARTESIAN_POINT('Ctrl Pts',(-113.030067104617,-80.2729225312233,
13.8921951601673));
#254278=CARTESIAN_POINT('Ctrl Pts',(-113.03208555715,-80.2777028659974,
13.8911192300483));
#254279=CARTESIAN_POINT('Ctrl Pts',(-113.034102479811,-80.2824837427445,
13.8900415384618));
#254280=CARTESIAN_POINT('Ctrl Pts',(-113.254288025274,-80.8044075501685,
13.7723909639359));
#254281=CARTESIAN_POINT('Ctrl Pts',(-113.45629755985,-81.3329353614433,
13.6337194701883));
#254282=CARTESIAN_POINT('Ctrl Pts',(-113.639203507904,-81.8643956885853,
13.4799440259955));
#254283=CARTESIAN_POINT('Ctrl Pts',(-113.641248155289,-81.8703367144489,
13.4782250192428));
#254284=CARTESIAN_POINT('Ctrl Pts',(-113.64329028633,-81.876277687381,13.4765042547891));
#254285=CARTESIAN_POINT('Ctrl Pts',(-113.645329902986,-81.8822186083625,
13.4747817381938));
#254286=CARTESIAN_POINT('Ctrl Pts',(-113.805159040923,-82.3477630899785,
13.3398013036916));
#254287=CARTESIAN_POINT('Ctrl Pts',(-113.949521015142,-82.8129009512596,
13.1940957680642));
#254288=CARTESIAN_POINT('Ctrl Pts',(-114.079434896297,-83.2783257874079,
13.0402593946707));
#254289=CARTESIAN_POINT('Ctrl Pts',(-114.09779119816,-83.3440884196296,
13.0185229421652));
#254290=CARTESIAN_POINT('Ctrl Pts',(-114.115858992445,-83.409856773525,
12.9966241002323));
#254291=CARTESIAN_POINT('Ctrl Pts',(-114.133641097615,-83.4756327991407,
12.974570129698));
#254292=CARTESIAN_POINT('Ctrl Pts',(-114.135281411444,-83.4817003217099,
12.9725357567984));
#254293=CARTESIAN_POINT('Ctrl Pts',(-114.136919307652,-83.4877679108745,
12.9705000777652));
#254294=CARTESIAN_POINT('Ctrl Pts',(-114.138554787209,-83.493835567825,
12.9684630962949));
#254295=CARTESIAN_POINT('Ctrl Pts',(-114.291921052846,-84.0628270195057,
12.7774461925192));
#254296=CARTESIAN_POINT('Ctrl Pts',(-114.424042625778,-84.6324262924149,
12.5749877226474));
#254297=CARTESIAN_POINT('Ctrl Pts',(-114.535677960622,-85.2035403844976,
12.3641357736727));
#254298=CARTESIAN_POINT('Ctrl Pts',(-114.634136703081,-85.7072444794929,
12.178171197402));
#254299=CARTESIAN_POINT('Ctrl Pts',(-114.716659190074,-86.2121266771173,
11.9856765646618));
#254300=CARTESIAN_POINT('Ctrl Pts',(-114.783740215493,-86.7188080015107,
11.7887214170753));
#254301=CARTESIAN_POINT('Ctrl Pts',(-114.784265106949,-86.722772650178,
11.7871802946265));
#254302=CARTESIAN_POINT('Ctrl Pts',(-114.784789042279,-86.7267374248492,
11.7856388846567));
#254303=CARTESIAN_POINT('Ctrl Pts',(-114.785312021496,-86.7307023248219,
11.7840971883205));
#254304=CARTESIAN_POINT('Ctrl Pts',(-114.829106259593,-87.0627227336102,
11.6549956595777));
#254305=CARTESIAN_POINT('Ctrl Pts',(-114.866221289693,-87.3958478252276,
11.5237902415043));
#254306=CARTESIAN_POINT('Ctrl Pts',(-114.896617394504,-87.7293197437528,
11.3913030896523));
#254307=CARTESIAN_POINT('Ctrl Pts',(-114.915895932174,-87.9408222038048,
11.3072739496097));
#254308=CARTESIAN_POINT('Ctrl Pts',(-114.932472713487,-88.1524639646833,
11.222729399464));
#254309=CARTESIAN_POINT('Ctrl Pts',(-114.946348419948,-88.3640506336912,
11.137879105755));
#254310=CARTESIAN_POINT('Ctrl Pts',(-114.964225054821,-88.6366463127898,
11.0285630342664));
#254311=CARTESIAN_POINT('Ctrl Pts',(-114.977628511886,-88.9092317828258,
10.9187075038446));
#254312=CARTESIAN_POINT('Ctrl Pts',(-114.986572967953,-89.1819023106261,
10.8085488142425));
#254313=CARTESIAN_POINT('Ctrl Pts',(-114.991045195986,-89.3182375745263,
10.7534694694415));
#254314=CARTESIAN_POINT('Ctrl Pts',(-114.994415138866,-89.4551356267363,
10.6980951474548));
#254315=CARTESIAN_POINT('Ctrl Pts',(-114.996653833646,-89.5917627923241,
10.6427966362161));
#254316=CARTESIAN_POINT('Ctrl Pts',(-114.998892528426,-89.7283899579119,
10.5874981249774));
#254317=CARTESIAN_POINT('Ctrl Pts',(-115.,-89.8647460047638,10.5322757880193));
#254318=CARTESIAN_POINT('Ctrl Pts',(-115.,-90.,10.4775));
#254319=CARTESIAN_POINT('',(-115.,-90.,0.0381));
#254320=CARTESIAN_POINT('',(-115.,-90.,17.4625));
#254321=CARTESIAN_POINT('',(-90.,-115.,0.0381));
#254322=CARTESIAN_POINT('Origin',(-90.,-90.,0.0381));
#254323=CARTESIAN_POINT('',(-90.,-115.,10.4775));
#254324=CARTESIAN_POINT('',(-90.,-115.,17.4625));
#254325=CARTESIAN_POINT('',(-77.1750847966528,-111.45976584278,14.2875));
#254326=CARTESIAN_POINT('Ctrl Pts',(-90.,-115.,10.4775));
#254327=CARTESIAN_POINT('Ctrl Pts',(-89.5656046344881,-115.,10.653423442612));
#254328=CARTESIAN_POINT('Ctrl Pts',(-89.1307534363923,-114.988625659943,
10.8295463814862));
#254329=CARTESIAN_POINT('Ctrl Pts',(-88.6961589262272,-114.965914946797,
11.0044622041873));
#254330=CARTESIAN_POINT('Ctrl Pts',(-88.265494227172,-114.943409594766,
11.177796354485));
#254331=CARTESIAN_POINT('Ctrl Pts',(-87.8350808906164,-114.909771871233,
11.3499462228129));
#254332=CARTESIAN_POINT('Ctrl Pts',(-87.405611112475,-114.864988740008,
11.5195411389418));
#254333=CARTESIAN_POINT('Ctrl Pts',(-87.1802895410429,-114.841493243899,
11.6085192113325));
#254334=CARTESIAN_POINT('Ctrl Pts',(-86.9552277365531,-114.814929056704,
11.696793880338));
#254335=CARTESIAN_POINT('Ctrl Pts',(-86.7305265176413,-114.785288831497,
11.7841654473675));
#254336=CARTESIAN_POINT('Ctrl Pts',(-86.7266202133125,-114.78477355285,
11.7856843529263));
#254337=CARTESIAN_POINT('Ctrl Pts',(-86.7227140306227,-114.784257346139,
11.7872029805025));
#254338=CARTESIAN_POINT('Ctrl Pts',(-86.7188079702436,-114.783740211354,
11.7887213289917));
#254339=CARTESIAN_POINT('Ctrl Pts',(-86.1443627509354,-114.70768772456,
12.0120174243529));
#254340=CARTESIAN_POINT('Ctrl Pts',(-85.5722301488083,-114.611788003633,
12.2295806322944));
#254341=CARTESIAN_POINT('Ctrl Pts',(-85.0015050781307,-114.495317720793,
12.4383933639359));
#254342=CARTESIAN_POINT('Ctrl Pts',(-84.4980219030455,-114.392569776432,
12.6226041206147));
#254343=CARTESIAN_POINT('Ctrl Pts',(-83.9956343000833,-114.273812458544,
12.8000049441012));
#254344=CARTESIAN_POINT('Ctrl Pts',(-83.4937195188483,-114.138523507008,
12.9685020775523));
#254345=CARTESIAN_POINT('Ctrl Pts',(-83.4876905476699,-114.136898423986,
12.9705260553254));
#254346=CARTESIAN_POINT('Ctrl Pts',(-83.48166164341,-114.135270955025,12.9725487471959));
#254347=CARTESIAN_POINT('Ctrl Pts',(-83.4756328049006,-114.133641099172,
12.9745701495376));
#254348=CARTESIAN_POINT('Ctrl Pts',(-83.0101675029287,-114.007805692311,
13.1306354762013));
#254349=CARTESIAN_POINT('Ctrl Pts',(-82.5450867212538,-113.86766665386,
13.2789353456426));
#254350=CARTESIAN_POINT('Ctrl Pts',(-82.0796977689676,-113.712210313252,
13.4168816956454));
#254351=CARTESIAN_POINT('Ctrl Pts',(-82.0138492025101,-113.690214567274,
13.4363999273334));
#254352=CARTESIAN_POINT('Ctrl Pts',(-81.9479944585721,-113.667912112902,
13.4557108212968));
#254353=CARTESIAN_POINT('Ctrl Pts',(-81.8821315660405,-113.645300019736,
13.4748069823194));
#254354=CARTESIAN_POINT('Ctrl Pts',(-81.8762196591616,-113.643270339836,
13.4765210692866));
#254355=CARTESIAN_POINT('Ctrl Pts',(-81.870307700849,-113.641238170047,
13.4782334211547));
#254356=CARTESIAN_POINT('Ctrl Pts',(-81.8643956901357,-113.639203508438,
13.4799440324454));
#254357=CARTESIAN_POINT('Ctrl Pts',(-81.3329160061816,-113.456290898634,
13.633725071118));
#254358=CARTESIAN_POINT('Ctrl Pts',(-80.8043691708234,-113.254273359621,
13.7724010417179));
#254359=CARTESIAN_POINT('Ctrl Pts',(-80.2824267541528,-113.034078437782,
13.8900543869066));
#254360=CARTESIAN_POINT('Ctrl Pts',(-80.2776648780163,-113.032069517046,
13.8911277824363));
#254361=CARTESIAN_POINT('Ctrl Pts',(-80.2729035395786,-113.030059078579,
13.8921994304488));
#254362=CARTESIAN_POINT('Ctrl Pts',(-80.2681427414562,-113.028047123005,
13.8932693264696));
#254363=CARTESIAN_POINT('Ctrl Pts',(-79.826878070857,-112.84156475372,13.9924349081749));
#254364=CARTESIAN_POINT('Ctrl Pts',(-79.3893767767358,-112.641760418702,
14.0768952542102));
#254365=CARTESIAN_POINT('Ctrl Pts',(-78.9552639690786,-112.427972092934,
14.1422627601284));
#254366=CARTESIAN_POINT('Ctrl Pts',(-78.8749831730867,-112.388436062981,
14.1543512203501));
#254367=CARTESIAN_POINT('Ctrl Pts',(-78.7948182580917,-112.348421744993,
14.1657865812652));
#254368=CARTESIAN_POINT('Ctrl Pts',(-78.7147668473371,-112.307924890089,
14.1765409023448));
#254369=CARTESIAN_POINT('Ctrl Pts',(-78.711904300583,-112.306476768944,
14.1769254645481));
#254370=CARTESIAN_POINT('Ctrl Pts',(-78.7090418994725,-112.305028031036,
14.1773091556141));
#254371=CARTESIAN_POINT('Ctrl Pts',(-78.7061796438514,-112.303578676147,
14.1776919742687));
#254372=CARTESIAN_POINT('Ctrl Pts',(-78.3959378426708,-112.146482130324,
14.2191859442963));
#254373=CARTESIAN_POINT('Ctrl Pts',(-78.0874036307441,-111.982145146862,
14.2505477196114));
#254374=CARTESIAN_POINT('Ctrl Pts',(-77.7803237299166,-111.810091168852,
14.2689228989311));
#254375=CARTESIAN_POINT('Ctrl Pts',(-77.5779699106442,-111.696714228591,
14.2810314338925));
#254376=CARTESIAN_POINT('Ctrl Pts',(-77.3762476424957,-111.579986000768,
14.2874999986824));
#254377=CARTESIAN_POINT('Ctrl Pts',(-77.1750847966528,-111.45976584278,
14.2875));
#254378=CARTESIAN_POINT('',(-75.6605890912239,-110.478801107225,14.2875));
#254379=CARTESIAN_POINT('Origin',(-90.,-90.,14.2875));
#254380=CARTESIAN_POINT('',(-75.6605890912239,-110.478801107225,12.3825));
#254381=CARTESIAN_POINT('Origin',(-90.,-115.,17.4625));
#254382=CARTESIAN_POINT('',(90.,-115.,10.4775));
#254383=CARTESIAN_POINT('',(90.,-115.,0.0381));
#254384=CARTESIAN_POINT('',(90.,-115.,17.4625));
#254385=CARTESIAN_POINT('',(-90.,-115.,10.4775));
#254386=CARTESIAN_POINT('',(90.,-115.,0.0381));
#254387=CARTESIAN_POINT('Origin',(-115.,90.,17.4625));
#254388=CARTESIAN_POINT('',(-115.,90.,10.4775));
#254389=CARTESIAN_POINT('',(-115.,-90.,0.0381));
#254390=CARTESIAN_POINT('Origin',(115.,90.,17.4625));
#254391=CARTESIAN_POINT('',(115.,90.,10.4775));
#254392=CARTESIAN_POINT('',(115.,90.,0.0381));
#254393=CARTESIAN_POINT('',(115.,90.,17.4625));
#254394=CARTESIAN_POINT('',(115.,-90.,10.4775));
#254395=CARTESIAN_POINT('',(115.,-90.,10.4775));
#254396=CARTESIAN_POINT('',(115.,-90.,0.0381));
#254397=CARTESIAN_POINT('',(115.,-90.,17.4625));
#254398=CARTESIAN_POINT('',(115.,90.,0.0381));
#254399=CARTESIAN_POINT('Origin',(90.,-90.,17.4625));
#254400=CARTESIAN_POINT('',(110.478801107225,-75.6605890912239,14.2875));
#254401=CARTESIAN_POINT('',(110.478801107225,-75.6605890912239,12.3825));
#254402=CARTESIAN_POINT('',(75.6605890912239,-110.478801107225,14.2875));
#254403=CARTESIAN_POINT('',(75.6605890912239,-110.478801107225,12.3825));
#254404=CARTESIAN_POINT('',(77.1750847966528,-111.45976584278,14.2875));
#254405=CARTESIAN_POINT('Origin',(90.,-90.,14.2875));
#254406=CARTESIAN_POINT('Ctrl Pts',(77.1750847966528,-111.45976584278,14.2875));
#254407=CARTESIAN_POINT('Ctrl Pts',(77.4803584868234,-111.642205353954,
14.2874999980005));
#254408=CARTESIAN_POINT('Ctrl Pts',(77.786920438432,-111.816604023928,14.2726057756926));
#254409=CARTESIAN_POINT('Ctrl Pts',(78.0950229323553,-111.983450205564,
14.2457040096238));
#254410=CARTESIAN_POINT('Ctrl Pts',(78.298048694843,-112.093394376459,14.2279769490641));
#254411=CARTESIAN_POINT('Ctrl Pts',(78.5017434115719,-112.200058693308,
14.2050347429669));
#254412=CARTESIAN_POINT('Ctrl Pts',(78.7061796433008,-112.303578675868,
14.1776919687022));
#254413=CARTESIAN_POINT('Ctrl Pts',(78.7090512133806,-112.305032747302,
14.1773079042347));
#254414=CARTESIAN_POINT('Ctrl Pts',(78.7119229298981,-112.306486197733,
14.1769229616685));
#254415=CARTESIAN_POINT('Ctrl Pts',(78.7147947930089,-112.30793902738,14.1765371422899));
#254416=CARTESIAN_POINT('Ctrl Pts',(79.1477923875285,-112.526985589844,
14.1183662419443));
#254417=CARTESIAN_POINT('Ctrl Pts',(79.5841109937906,-112.731915850876,
14.0402742418796));
#254418=CARTESIAN_POINT('Ctrl Pts',(80.0241258916428,-112.92339532539,13.9466617235228));
#254419=CARTESIAN_POINT('Ctrl Pts',(80.1053381450643,-112.958736127907,
13.9293839367902));
#254420=CARTESIAN_POINT('Ctrl Pts',(80.186676309393,-112.993618685196,13.911577307561));
#254421=CARTESIAN_POINT('Ctrl Pts',(80.2681427410701,-113.028047122842,
13.8932693242907));
#254422=CARTESIAN_POINT('Ctrl Pts',(80.2729225312233,-113.030067104617,
13.8921951601674));
#254423=CARTESIAN_POINT('Ctrl Pts',(80.2777028659974,-113.03208555715,13.8911192300484));
#254424=CARTESIAN_POINT('Ctrl Pts',(80.2824837427445,-113.034102479811,
13.890041538462));
#254425=CARTESIAN_POINT('Ctrl Pts',(80.8044075501684,-113.254288025274,
13.7723909639359));
#254426=CARTESIAN_POINT('Ctrl Pts',(81.3329353614429,-113.45629755985,13.6337194701879));
#254427=CARTESIAN_POINT('Ctrl Pts',(81.8643956885852,-113.639203507904,
13.4799440259953));
#254428=CARTESIAN_POINT('Ctrl Pts',(81.8703367144488,-113.641248155289,
13.4782250192426));
#254429=CARTESIAN_POINT('Ctrl Pts',(81.876277687381,-113.64329028633,13.4765042547889));
#254430=CARTESIAN_POINT('Ctrl Pts',(81.8822186083625,-113.645329902986,
13.4747817381936));
#254431=CARTESIAN_POINT('Ctrl Pts',(82.3477630963775,-113.80515904312,13.3398013018362));
#254432=CARTESIAN_POINT('Ctrl Pts',(82.8129009640461,-113.94952101911,13.1940957640577));
#254433=CARTESIAN_POINT('Ctrl Pts',(83.2783258065996,-114.079434901654,
13.040259388326));
#254434=CARTESIAN_POINT('Ctrl Pts',(83.3440884324251,-114.097791201675,
13.0185229379035));
#254435=CARTESIAN_POINT('Ctrl Pts',(83.4098567799233,-114.115858994174,
12.9966240980859));
#254436=CARTESIAN_POINT('Ctrl Pts',(83.4756327991404,-114.133641097615,
12.974570129697));
#254437=CARTESIAN_POINT('Ctrl Pts',(83.4817003217096,-114.135281411444,
12.9725357567974));
#254438=CARTESIAN_POINT('Ctrl Pts',(83.4877679108742,-114.136919307652,
12.9705000777643));
#254439=CARTESIAN_POINT('Ctrl Pts',(83.4938355678247,-114.138554787209,
12.968463096294));
#254440=CARTESIAN_POINT('Ctrl Pts',(84.0628270192128,-114.291921052767,
12.7774461926172));
#254441=CARTESIAN_POINT('Ctrl Pts',(84.632426291829,-114.424042625642,12.5749877228569));
#254442=CARTESIAN_POINT('Ctrl Pts',(85.2035403836165,-114.53567796045,12.3641357739999));
#254443=CARTESIAN_POINT('Ctrl Pts',(85.7072444789046,-114.634136702985,
12.1781711976289));
#254444=CARTESIAN_POINT('Ctrl Pts',(86.2121266768225,-114.716659190035,
11.9856765647789));
#254445=CARTESIAN_POINT('Ctrl Pts',(86.718808001511,-114.783740215493,11.7887214170762));
#254446=CARTESIAN_POINT('Ctrl Pts',(86.7227726501783,-114.784265106949,
11.7871802946274));
#254447=CARTESIAN_POINT('Ctrl Pts',(86.7267374248495,-114.784789042279,
11.7856388846576));
#254448=CARTESIAN_POINT('Ctrl Pts',(86.7307023248221,-114.785312021496,
11.7840971883214));
#254449=CARTESIAN_POINT('Ctrl Pts',(87.0627227347716,-114.829106259746,
11.6549956591265));
#254450=CARTESIAN_POINT('Ctrl Pts',(87.395847827558,-114.866221289952,11.5237902405866));
#254451=CARTESIAN_POINT('Ctrl Pts',(87.729319747252,-114.896617394822,11.3913030882621));
#254452=CARTESIAN_POINT('Ctrl Pts',(87.9408222061392,-114.915895932356,
11.3072739486773));
#254453=CARTESIAN_POINT('Ctrl Pts',(88.1524639658503,-114.932472713562,
11.2227293989961));
#254454=CARTESIAN_POINT('Ctrl Pts',(88.3640506336914,-114.946348419947,
11.1378791057551));
#254455=CARTESIAN_POINT('Ctrl Pts',(88.6366463127899,-114.964225054819,
11.0285630342665));
#254456=CARTESIAN_POINT('Ctrl Pts',(88.9092317828258,-114.977628511885,
10.9187075038447));
#254457=CARTESIAN_POINT('Ctrl Pts',(89.1819023106262,-114.986572967952,
10.8085488142427));
#254458=CARTESIAN_POINT('Ctrl Pts',(89.3182375745263,-114.991045195985,
10.7534694694417));
#254459=CARTESIAN_POINT('Ctrl Pts',(89.4551356267436,-114.994415138866,
10.6980951474732));
#254460=CARTESIAN_POINT('Ctrl Pts',(89.5917627923341,-114.996653833646,
10.6427966362411));
#254461=CARTESIAN_POINT('Ctrl Pts',(89.7283899579245,-114.998892528426,
10.5874981250089));
#254462=CARTESIAN_POINT('Ctrl Pts',(89.8647460047744,-115.,10.5322757880455));
#254463=CARTESIAN_POINT('Ctrl Pts',(90.,-115.,10.4775));
#254464=CARTESIAN_POINT('Origin',(90.,-90.,0.0381));
#254465=CARTESIAN_POINT('',(111.45976584278,-77.1750847966528,14.2875));
#254466=CARTESIAN_POINT('Ctrl Pts',(115.,-90.,10.4775));
#254467=CARTESIAN_POINT('Ctrl Pts',(115.,-89.5656046355683,10.6534234421179));
#254468=CARTESIAN_POINT('Ctrl Pts',(114.98862566,-89.1307534385709,10.8295463805372));
#254469=CARTESIAN_POINT('Ctrl Pts',(114.96591494697,-88.6961589295072,11.0044622028075));
#254470=CARTESIAN_POINT('Ctrl Pts',(114.943409594942,-88.265494229423,11.1777963535319));
#254471=CARTESIAN_POINT('Ctrl Pts',(114.909771871358,-87.8350808918436,
11.3499462222986));
#254472=CARTESIAN_POINT('Ctrl Pts',(114.86498874003,-87.4056111126796,11.5195411388467));
#254473=CARTESIAN_POINT('Ctrl Pts',(114.841493243915,-87.1802895411801,
11.608519211272));
#254474=CARTESIAN_POINT('Ctrl Pts',(114.814929056713,-86.9552277366222,
11.6967938803096));
#254475=CARTESIAN_POINT('Ctrl Pts',(114.785288831497,-86.7305265176406,
11.7841654473657));
#254476=CARTESIAN_POINT('Ctrl Pts',(114.78477355285,-86.7266202133119,11.7856843529246));
#254477=CARTESIAN_POINT('Ctrl Pts',(114.784257346139,-86.7227140306221,
11.7872029805007));
#254478=CARTESIAN_POINT('Ctrl Pts',(114.783740211354,-86.718807970243,11.7887213289899));
#254479=CARTESIAN_POINT('Ctrl Pts',(114.707687724832,-86.1443627529916,
12.0120174235497));
#254480=CARTESIAN_POINT('Ctrl Pts',(114.611788004319,-85.5722301529056,
12.2295806307328));
#254481=CARTESIAN_POINT('Ctrl Pts',(114.495317722044,-85.0015050842623,
12.4383933616903));
#254482=CARTESIAN_POINT('Ctrl Pts',(114.392569777396,-84.4980219071244,
12.6226041191732));
#254483=CARTESIAN_POINT('Ctrl Pts',(114.273812459093,-83.995634302121,12.8000049434176));
#254484=CARTESIAN_POINT('Ctrl Pts',(114.138523507008,-83.4937195188485,
12.9685020775533));
#254485=CARTESIAN_POINT('Ctrl Pts',(114.136898423986,-83.4876905476702,
12.9705260553264));
#254486=CARTESIAN_POINT('Ctrl Pts',(114.135270955025,-83.4816616434103,
12.9725487471968));
#254487=CARTESIAN_POINT('Ctrl Pts',(114.133641099172,-83.4756328049009,
12.9745701495385));
#254488=CARTESIAN_POINT('Ctrl Pts',(114.007805692247,-83.0101675026927,
13.1306354762821));
#254489=CARTESIAN_POINT('Ctrl Pts',(113.867666653718,-82.5450867207814,
13.2789353457935));
#254490=CARTESIAN_POINT('Ctrl Pts',(113.712210313015,-82.0796977682585,
13.4168816958559));
#254491=CARTESIAN_POINT('Ctrl Pts',(113.690214567113,-82.0138492020373,
13.4363999274722));
#254492=CARTESIAN_POINT('Ctrl Pts',(113.667912112821,-81.9479944583357,
13.4557108213656));
#254493=CARTESIAN_POINT('Ctrl Pts',(113.645300019736,-81.8821315660405,
13.4748069823197));
#254494=CARTESIAN_POINT('Ctrl Pts',(113.643270339836,-81.8762196591617,
13.4765210692869));
#254495=CARTESIAN_POINT('Ctrl Pts',(113.641238170047,-81.8703077008491,
13.478233421155));
#254496=CARTESIAN_POINT('Ctrl Pts',(113.639203508438,-81.8643956901358,
13.4799440324457));
#254497=CARTESIAN_POINT('Ctrl Pts',(113.456290898634,-81.3329160061815,
13.6337250711187));
#254498=CARTESIAN_POINT('Ctrl Pts',(113.254273359621,-80.8043691708234,
13.7724010417179));
#254499=CARTESIAN_POINT('Ctrl Pts',(113.034078437782,-80.2824267541528,
13.8900543869065));
#254500=CARTESIAN_POINT('Ctrl Pts',(113.032069517046,-80.2776648780163,
13.8911277824363));
#254501=CARTESIAN_POINT('Ctrl Pts',(113.030059078579,-80.2729035395786,
13.8921994304487));
#254502=CARTESIAN_POINT('Ctrl Pts',(113.028047123005,-80.2681427414561,
13.8932693264695));
#254503=CARTESIAN_POINT('Ctrl Pts',(112.841564748611,-79.8268780587689,
13.9924349108913));
#254504=CARTESIAN_POINT('Ctrl Pts',(112.641760407755,-79.3893767527665,
14.0768952588379));
#254505=CARTESIAN_POINT('Ctrl Pts',(112.427972075365,-78.9552639334033,
14.1422627655002));
#254506=CARTESIAN_POINT('Ctrl Pts',(112.388436051127,-78.8749831493374,
14.1543512237378));
#254507=CARTESIAN_POINT('Ctrl Pts',(112.348421738994,-78.7948182462339,
14.165786582858));
#254508=CARTESIAN_POINT('Ctrl Pts',(112.307924890089,-78.7147668473371,
14.1765409023446));
#254509=CARTESIAN_POINT('Ctrl Pts',(112.306476768944,-78.711904300583,14.1769254645479));
#254510=CARTESIAN_POINT('Ctrl Pts',(112.305028031036,-78.7090418994725,
14.1773091556138));
#254511=CARTESIAN_POINT('Ctrl Pts',(112.303578676147,-78.7061796438514,
14.1776919742685));
#254512=CARTESIAN_POINT('Ctrl Pts',(112.146482129285,-78.3959378406196,
14.2191859445703));
#254513=CARTESIAN_POINT('Ctrl Pts',(111.98214514469,-78.0874036266646,14.2505477200261));
#254514=CARTESIAN_POINT('Ctrl Pts',(111.81009116544,-77.7803237238264,14.2689228992955));
#254515=CARTESIAN_POINT('Ctrl Pts',(111.696714226249,-77.5779699065967,
14.2810314340224));
#254516=CARTESIAN_POINT('Ctrl Pts',(111.579985999562,-77.3762476404776,
14.2874999986824));
#254517=CARTESIAN_POINT('Ctrl Pts',(111.45976584278,-77.1750847966528,14.2875));
#254518=CARTESIAN_POINT('Origin',(90.,-90.,14.2875));
#254519=CARTESIAN_POINT('Origin',(90.,90.,17.4625));
#254520=CARTESIAN_POINT('',(75.6605890912238,110.478801107225,12.3825));
#254521=CARTESIAN_POINT('',(75.6605890912238,110.478801107225,12.3825));
#254522=CARTESIAN_POINT('',(110.478801107225,75.6605890912239,14.2875));
#254523=CARTESIAN_POINT('',(110.478801107225,75.6605890912239,12.3825));
#254524=CARTESIAN_POINT('',(111.45976584278,77.1750847966528,14.2875));
#254525=CARTESIAN_POINT('Origin',(90.,90.,14.2875));
#254526=CARTESIAN_POINT('Ctrl Pts',(111.45976584278,77.1750847966528,14.2875));
#254527=CARTESIAN_POINT('Ctrl Pts',(111.642205355166,77.4803584888519,14.2874999980005));
#254528=CARTESIAN_POINT('Ctrl Pts',(111.816604026246,77.7869204425061,14.2726057754947));
#254529=CARTESIAN_POINT('Ctrl Pts',(111.98345020889,78.0950229384971,14.2457040090874));
#254530=CARTESIAN_POINT('Ctrl Pts',(112.09339437861,78.298048698951,14.2279769486012));
#254531=CARTESIAN_POINT('Ctrl Pts',(112.200058694352,78.5017434136333,14.2050347426909));
#254532=CARTESIAN_POINT('Ctrl Pts',(112.303578675868,78.7061796433008,14.1776919687019));
#254533=CARTESIAN_POINT('Ctrl Pts',(112.305032747302,78.7090512133806,14.1773079042344));
#254534=CARTESIAN_POINT('Ctrl Pts',(112.306486197733,78.7119229298981,14.1769229616682));
#254535=CARTESIAN_POINT('Ctrl Pts',(112.307939027379,78.7147947930089,14.1765371422897));
#254536=CARTESIAN_POINT('Ctrl Pts',(112.526985595836,79.1477923993722,14.1183662403531));
#254537=CARTESIAN_POINT('Ctrl Pts',(112.731915862087,79.5841110176595,14.0402742376079));
#254538=CARTESIAN_POINT('Ctrl Pts',(112.923395341103,80.0241259277498,13.946661715841));
#254539=CARTESIAN_POINT('Ctrl Pts',(112.958736138246,80.105338169173,13.9293839315123));
#254540=CARTESIAN_POINT('Ctrl Pts',(112.993618690298,80.1866763214663,13.9115773048477));
#254541=CARTESIAN_POINT('Ctrl Pts',(113.028047122842,80.2681427410701,13.8932693242906));
#254542=CARTESIAN_POINT('Ctrl Pts',(113.030067104617,80.2729225312233,13.8921951601673));
#254543=CARTESIAN_POINT('Ctrl Pts',(113.03208555715,80.2777028659974,13.8911192300484));
#254544=CARTESIAN_POINT('Ctrl Pts',(113.034102479811,80.2824837427445,13.8900415384619));
#254545=CARTESIAN_POINT('Ctrl Pts',(113.254288025274,80.8044075501685,13.7723909639359));
#254546=CARTESIAN_POINT('Ctrl Pts',(113.45629755985,81.3329353614428,13.6337194701886));
#254547=CARTESIAN_POINT('Ctrl Pts',(113.639203507904,81.8643956885853,13.4799440259956));
#254548=CARTESIAN_POINT('Ctrl Pts',(113.641248155289,81.8703367144489,13.4782250192429));
#254549=CARTESIAN_POINT('Ctrl Pts',(113.64329028633,81.876277687381,13.4765042547891));
#254550=CARTESIAN_POINT('Ctrl Pts',(113.645329902986,81.8822186083625,13.4747817381939));
#254551=CARTESIAN_POINT('Ctrl Pts',(113.805159043221,82.3477630966713,13.3398013017511));
#254552=CARTESIAN_POINT('Ctrl Pts',(113.949521019293,82.8129009646335,13.1940957638749));
#254553=CARTESIAN_POINT('Ctrl Pts',(114.0794349019,83.2783258074811,13.0402593880359));
#254554=CARTESIAN_POINT('Ctrl Pts',(114.097791201837,83.344088433013,13.0185229377089));
#254555=CARTESIAN_POINT('Ctrl Pts',(114.115858994254,83.4098567802174,12.9966240979884));
#254556=CARTESIAN_POINT('Ctrl Pts',(114.133641097615,83.4756327991407,12.974570129698));
#254557=CARTESIAN_POINT('Ctrl Pts',(114.135281411444,83.4817003217099,12.9725357567984));
#254558=CARTESIAN_POINT('Ctrl Pts',(114.136919307652,83.4877679108745,12.9705000777652));
#254559=CARTESIAN_POINT('Ctrl Pts',(114.138554787209,83.493835567825,12.9684630962949));
#254560=CARTESIAN_POINT('Ctrl Pts',(114.291921052112,84.0628270167828,12.7774461934334));
#254561=CARTESIAN_POINT('Ctrl Pts',(114.424042624513,84.6324262869634,12.5749877245847));
#254562=CARTESIAN_POINT('Ctrl Pts',(114.535677959019,85.2035403762984,12.3641357766992));
#254563=CARTESIAN_POINT('Ctrl Pts',(114.634136702185,85.707244474014,12.1781711994903));
#254564=CARTESIAN_POINT('Ctrl Pts',(114.71665918971,86.212126674368,11.9856765657298));
#254565=CARTESIAN_POINT('Ctrl Pts',(114.783740215493,86.7188080015106,11.7887214170749));
#254566=CARTESIAN_POINT('Ctrl Pts',(114.784265106949,86.7227726501778,11.7871802946262));
#254567=CARTESIAN_POINT('Ctrl Pts',(114.784789042279,86.7267374248491,11.7856388846564));
#254568=CARTESIAN_POINT('Ctrl Pts',(114.785312021496,86.7307023248217,11.7840971883202));
#254569=CARTESIAN_POINT('Ctrl Pts',(114.829106259638,87.0627227339489,11.6549956594459));
#254570=CARTESIAN_POINT('Ctrl Pts',(114.866221289769,87.3958478259074,11.5237902412365));
#254571=CARTESIAN_POINT('Ctrl Pts',(114.896617394597,87.7293197447736,11.3913030892467));
#254572=CARTESIAN_POINT('Ctrl Pts',(114.915895932227,87.9408222044859,11.3072739493377));
#254573=CARTESIAN_POINT('Ctrl Pts',(114.932472713509,88.1524639650238,11.2227293993275));
#254574=CARTESIAN_POINT('Ctrl Pts',(114.946348419948,88.3640506336913,11.137879105755));
#254575=CARTESIAN_POINT('Ctrl Pts',(114.96422505482,88.6366463127898,11.0285630342664));
#254576=CARTESIAN_POINT('Ctrl Pts',(114.977628511886,88.9092317828257,10.9187075038446));
#254577=CARTESIAN_POINT('Ctrl Pts',(114.986572967952,89.1819023106261,10.8085488142425));
#254578=CARTESIAN_POINT('Ctrl Pts',(114.991045195986,89.3182375745263,10.7534694694415));
#254579=CARTESIAN_POINT('Ctrl Pts',(114.994415138866,89.4551356267369,10.6980951474562));
#254580=CARTESIAN_POINT('Ctrl Pts',(114.996653833646,89.5917627923248,10.6427966362178));
#254581=CARTESIAN_POINT('Ctrl Pts',(114.998892528426,89.7283899579127,10.5874981249794));
#254582=CARTESIAN_POINT('Ctrl Pts',(115.,89.8647460047642,10.5322757880204));
#254583=CARTESIAN_POINT('Ctrl Pts',(115.,90.,10.4775));
#254584=CARTESIAN_POINT('',(90.,115.,0.0381));
#254585=CARTESIAN_POINT('Origin',(90.,90.,0.0381));
#254586=CARTESIAN_POINT('',(90.,115.,10.4775));
#254587=CARTESIAN_POINT('',(90.,115.,17.4625));
#254588=CARTESIAN_POINT('',(80.428115389329,113.095,12.3825));
#254589=CARTESIAN_POINT('Ctrl Pts',(90.,115.,10.4775));
#254590=CARTESIAN_POINT('Ctrl Pts',(88.4720214203075,115.,10.8992885166146));
#254591=CARTESIAN_POINT('Ctrl Pts',(86.8039448109204,114.851492965438,11.3641723788953));
#254592=CARTESIAN_POINT('Ctrl Pts',(83.5138272817594,114.202094699092,12.1039861530196));
#254593=CARTESIAN_POINT('Ctrl Pts',(81.8924546881425,113.701905685175,12.3825));
#254594=CARTESIAN_POINT('Ctrl Pts',(80.428115389329,113.095,12.3825));
#254595=CARTESIAN_POINT('Origin',(90.,90.0000000000001,12.3825));
#254596=CARTESIAN_POINT('Origin',(-90.,115.,17.4625));
#254597=CARTESIAN_POINT('',(-20.3338370957105,115.,10.4775));
#254598=CARTESIAN_POINT('',(20.3338370957106,115.,10.4775));
#254599=CARTESIAN_POINT('Ctrl Pts',(-20.3338370957105,115.,10.4775));
#254600=CARTESIAN_POINT('Ctrl Pts',(-19.9267590414958,115.,10.3125994708202));
#254601=CARTESIAN_POINT('Ctrl Pts',(-19.5174840291917,115.,10.1525816988894));
#254602=CARTESIAN_POINT('Ctrl Pts',(-19.106739643588,115.,9.99771295049682));
#254603=CARTESIAN_POINT('Ctrl Pts',(-18.6959952579844,115.,9.84284420210422));
#254604=CARTESIAN_POINT('Ctrl Pts',(-18.2837818084517,115.,9.69312450300941));
#254605=CARTESIAN_POINT('Ctrl Pts',(-17.8708421763035,115.,9.54876232402957));
#254606=CARTESIAN_POINT('Ctrl Pts',(-17.3189441652074,115.,9.35582080605997));
#254607=CARTESIAN_POINT('Ctrl Pts',(-16.7653329534949,115.,9.17228988049683));
#254608=CARTESIAN_POINT('Ctrl Pts',(-16.210031043884,115.,8.99805419968946));
#254609=CARTESIAN_POINT('Ctrl Pts',(-15.936948059999,115.,8.91236964001012));
#254610=CARTESIAN_POINT('Ctrl Pts',(-15.6634560177655,115.,8.82893383759967));
#254611=CARTESIAN_POINT('Ctrl Pts',(-15.3895567777554,115.,8.74773761914341));
#254612=CARTESIAN_POINT('Ctrl Pts',(-15.3869609596534,115.,8.74696810034636));
#254613=CARTESIAN_POINT('Ctrl Pts',(-15.3843650995479,115.,8.74619878028833));
#254614=CARTESIAN_POINT('Ctrl Pts',(-15.3817691974006,115.,8.74542965895521));
#254615=CARTESIAN_POINT('Ctrl Pts',(-13.7198971151702,115.,8.25304543225375));
#254616=CARTESIAN_POINT('Ctrl Pts',(-12.0430776052023,115.000000000003,
7.84278200114024));
#254617=CARTESIAN_POINT('Ctrl Pts',(-10.3515597238144,114.999999999997,
7.51327366480546));
#254618=CARTESIAN_POINT('Ctrl Pts',(-10.3463733638648,114.999999999997,
7.51226335988499));
#254619=CARTESIAN_POINT('Ctrl Pts',(-10.3411868667297,114.999999999997,
7.51125380869066));
#254620=CARTESIAN_POINT('Ctrl Pts',(-10.3360002323986,114.999999999997,
7.51024501128054));
#254621=CARTESIAN_POINT('Ctrl Pts',(-8.23229812819579,114.999999999991,
7.10107615554567));
#254622=CARTESIAN_POINT('Ctrl Pts',(-6.10608444318685,114.999999999993,
6.81590866941424));
#254623=CARTESIAN_POINT('Ctrl Pts',(-3.95654770808245,114.999999999993,
6.65860083511691));
#254624=CARTESIAN_POINT('Ctrl Pts',(-2.64905735818768,114.999999999993,
6.56291581054969));
#254625=CARTESIAN_POINT('Ctrl Pts',(-1.3329376678419,114.999999999994,6.51453825908851));
#254626=CARTESIAN_POINT('Ctrl Pts',(-0.00800503439004147,114.999999999976,
6.51434590949666));
#254627=CARTESIAN_POINT('Ctrl Pts',(0.00263410608483974,114.999999999976,
6.51434436493939));
#254628=CARTESIAN_POINT('Ctrl Pts',(0.0132727023277519,114.999999999976,
6.51434592797752));
#254629=CARTESIAN_POINT('Ctrl Pts',(0.0239107544103369,114.999999999976,
6.51435059818956));
#254630=CARTESIAN_POINT('Ctrl Pts',(1.77562218690493,114.999999999951,6.51511961715718));
#254631=CARTESIAN_POINT('Ctrl Pts',(3.51091746734952,114.999999999965,6.60012007887875));
#254632=CARTESIAN_POINT('Ctrl Pts',(5.23024969626955,114.99999999998,6.76702375956156));
#254633=CARTESIAN_POINT('Ctrl Pts',(6.94958192518957,114.999999999995,6.93392744024437));
#254634=CARTESIAN_POINT('Ctrl Pts',(8.65295106909785,115.,7.18273455731824));
#254635=CARTESIAN_POINT('Ctrl Pts',(10.3407978197663,114.999999999999,7.51117731045924));
#254636=CARTESIAN_POINT('Ctrl Pts',(10.3504347739428,114.999999999999,7.51305259194459));
#254637=CARTESIAN_POINT('Ctrl Pts',(10.3600712202459,114.999999999999,7.51493048841781));
#254638=CARTESIAN_POINT('Ctrl Pts',(10.3697071586587,114.999999999999,7.51681100008705));
#254639=CARTESIAN_POINT('Ctrl Pts',(11.0233231057247,114.999999999998,7.64436810589384));
#254640=CARTESIAN_POINT('Ctrl Pts',(11.6740697898699,114.999999999998,7.78384849352191));
#254641=CARTESIAN_POINT('Ctrl Pts',(12.3222929011397,114.999999999998,7.93535062636677));
#254642=CARTESIAN_POINT('Ctrl Pts',(12.9676692556127,114.999999999998,8.08618741772824));
#254643=CARTESIAN_POINT('Ctrl Pts',(13.6105441559796,114.999999999998,8.24894058328078));
#254644=CARTESIAN_POINT('Ctrl Pts',(14.2512497473851,114.999999999999,8.42375809780361));
#254645=CARTESIAN_POINT('Ctrl Pts',(14.6298031864933,114.999999999999,8.52704699090316));
#254646=CARTESIAN_POINT('Ctrl Pts',(15.0075991707994,114.999999999999,8.63454839025221));
#254647=CARTESIAN_POINT('Ctrl Pts',(15.3847047117197,114.999999999999,8.74630124832653));
#254648=CARTESIAN_POINT('Ctrl Pts',(16.0185779527073,114.999999999999,8.93414560130087));
#254649=CARTESIAN_POINT('Ctrl Pts',(16.6510152471715,115.,9.13423879107251));
#254650=CARTESIAN_POINT('Ctrl Pts',(17.2813626508644,115.,9.34652047011719));
#254651=CARTESIAN_POINT('Ctrl Pts',(17.9026823885883,115.,9.55576190805272));
#254652=CARTESIAN_POINT('Ctrl Pts',(18.5219722813344,115.,9.77684545107347));
#254653=CARTESIAN_POINT('Ctrl Pts',(19.13858688252,115.,10.0097596336116));
#254654=CARTESIAN_POINT('Ctrl Pts',(19.5381882300233,115.,10.1607012769264));
#254655=CARTESIAN_POINT('Ctrl Pts',(19.936665603688,115.,10.3166124539101));
#254656=CARTESIAN_POINT('Ctrl Pts',(20.3338370957106,115.,10.4775));
#254657=CARTESIAN_POINT('',(90.,115.,10.4775));
#254658=CARTESIAN_POINT('',(-90.,115.,0.0381));
#254659=CARTESIAN_POINT('',(-20.509804815317,115.,10.4775));
#254660=CARTESIAN_POINT('Origin',(-90.,-90.,0.));
#254661=CARTESIAN_POINT('',(-90.,-114.492,0.0381));
#254662=CARTESIAN_POINT('',(-90.,-114.492,8.255));
#254663=CARTESIAN_POINT('',(-90.,-114.492,0.));
#254664=CARTESIAN_POINT('',(-114.492,-90.,0.0381));
#254665=CARTESIAN_POINT('Origin',(-90.,-90.,0.0381));
#254666=CARTESIAN_POINT('',(-114.492,-90.,8.255));
#254667=CARTESIAN_POINT('',(-114.492,-90.,0.));
#254668=CARTESIAN_POINT('Origin',(-90.,-90.,8.255));
#254669=CARTESIAN_POINT('Origin',(-114.492,-90.,0.));
#254670=CARTESIAN_POINT('',(-114.492,90.,0.0381));
#254671=CARTESIAN_POINT('',(-114.492,-90.,0.0381));
#254672=CARTESIAN_POINT('',(-114.492,90.,8.255));
#254673=CARTESIAN_POINT('',(-114.492,90.,0.));
#254674=CARTESIAN_POINT('',(-114.492,-90.,8.255));
#254675=CARTESIAN_POINT('Origin',(-90.,90.,0.));
#254676=CARTESIAN_POINT('',(-90.,114.492,0.0381));
#254677=CARTESIAN_POINT('Origin',(-90.,90.,0.0381));
#254678=CARTESIAN_POINT('',(-90.,114.492,8.255));
#254679=CARTESIAN_POINT('',(-90.,114.492,0.));
#254680=CARTESIAN_POINT('Origin',(-90.,90.,8.255));
#254681=CARTESIAN_POINT('Origin',(-9.33180860950279E-17,114.492,0.));
#254682=CARTESIAN_POINT('',(90.,114.492,0.0381));
#254683=CARTESIAN_POINT('',(-9.33180860950279E-17,114.492,0.0381));
#254684=CARTESIAN_POINT('',(90.,114.492,8.255));
#254685=CARTESIAN_POINT('',(90.,114.492,0.));
#254686=CARTESIAN_POINT('',(-9.33180860950279E-17,114.492,8.255));
#254687=CARTESIAN_POINT('Origin',(90.,90.,0.));
#254688=CARTESIAN_POINT('',(114.492,90.,0.0381));
#254689=CARTESIAN_POINT('Origin',(90.,90.,0.0381));
#254690=CARTESIAN_POINT('',(114.492,90.,8.255));
#254691=CARTESIAN_POINT('',(114.492,90.,0.));
#254692=CARTESIAN_POINT('Origin',(90.,90.,8.255));
#254693=CARTESIAN_POINT('Origin',(114.492,90.,0.));
#254694=CARTESIAN_POINT('',(114.492,-90.,0.0381));
#254695=CARTESIAN_POINT('',(114.492,90.,0.0381));
#254696=CARTESIAN_POINT('',(114.492,-90.,8.255));
#254697=CARTESIAN_POINT('',(114.492,-90.,0.));
#254698=CARTESIAN_POINT('',(114.492,90.,8.255));
#254699=CARTESIAN_POINT('Origin',(90.,-90.,0.));
#254700=CARTESIAN_POINT('',(90.,-114.492,0.0381));
#254701=CARTESIAN_POINT('Origin',(90.,-90.,0.0381));
#254702=CARTESIAN_POINT('',(90.,-114.492,8.255));
#254703=CARTESIAN_POINT('',(90.,-114.492,0.));
#254704=CARTESIAN_POINT('Origin',(90.,-90.,8.255));
#254705=CARTESIAN_POINT('Origin',(90.,-114.492,0.));
#254706=CARTESIAN_POINT('',(90.,-114.492,0.0381));
#254707=CARTESIAN_POINT('',(90.,-114.492,8.255));
#254708=CARTESIAN_POINT('Origin',(0.,0.,42.8625));
#254709=CARTESIAN_POINT('',(7.22543403703139,77.6928637726221,42.8625));
#254710=CARTESIAN_POINT('Ctrl Pts',(10.5032495111116,73.8913131000538,42.8625));
#254711=CARTESIAN_POINT('Ctrl Pts',(10.426573623364,73.9022121619655,42.8625));
#254712=CARTESIAN_POINT('Ctrl Pts',(10.350249684026,73.9154545309663,42.8625000002269));
#254713=CARTESIAN_POINT('Ctrl Pts',(10.2745222083119,73.931001476869,42.8624999983791));
#254714=CARTESIAN_POINT('Ctrl Pts',(10.1981874108863,73.946673106682,42.8624999965164));
#254715=CARTESIAN_POINT('Ctrl Pts',(10.1224588082033,73.9646863653303,42.8624999919999));
#254716=CARTESIAN_POINT('Ctrl Pts',(10.047564266732,73.9849532592727,42.8624999868104));
#254717=CARTESIAN_POINT('Ctrl Pts',(9.97591704949705,74.0043414085884,42.862499981846));
#254718=CARTESIAN_POINT('Ctrl Pts',(9.90503303994923,74.0257915565748,42.862499976793));
#254719=CARTESIAN_POINT('Ctrl Pts',(9.83509125233263,74.0491869849564,42.8624999769173));
#254720=CARTESIAN_POINT('Ctrl Pts',(9.72723746351632,74.0852639237641,42.8624999771091));
#254721=CARTESIAN_POINT('Ctrl Pts',(9.62130801394438,74.1260630720874,42.8624999885811));
#254722=CARTESIAN_POINT('Ctrl Pts',(9.51729215731884,74.1715977877844,42.8624999942969));
#254723=CARTESIAN_POINT('Ctrl Pts',(9.41339573292933,74.2170802199826,42.8625000000061));
#254724=CARTESIAN_POINT('Ctrl Pts',(9.31140854462795,74.2672878903899,42.8625));
#254725=CARTESIAN_POINT('Ctrl Pts',(9.21136369896946,74.3222619325388,42.8625));
#254726=CARTESIAN_POINT('Ctrl Pts',(9.01115900292839,74.4322732112421,42.8625));
#254727=CARTESIAN_POINT('Ctrl Pts',(8.81948930735858,74.5614957426143,42.8625));
#254728=CARTESIAN_POINT('Ctrl Pts',(8.64328937573657,74.7047213557556,42.8625));
#254729=CARTESIAN_POINT('Ctrl Pts',(8.46708944411456,74.8479469688968,42.8625));
#254730=CARTESIAN_POINT('Ctrl Pts',(8.30424197097439,75.0062320561475,42.8625));
#254731=CARTESIAN_POINT('Ctrl Pts',(8.15502818007546,75.1798937933935,42.8625));
#254732=CARTESIAN_POINT('Ctrl Pts',(8.00581438917653,75.3535555306395,42.8625));
#254733=CARTESIAN_POINT('Ctrl Pts',(7.87211185550338,75.5409911145111,42.8625));
#254734=CARTESIAN_POINT('Ctrl Pts',(7.75712923570172,75.7366472018307,42.8625));
#254735=CARTESIAN_POINT('Ctrl Pts',(7.64214661590005,75.9323032891504,42.8625));
#254736=CARTESIAN_POINT('Ctrl Pts',(7.54459734451585,76.1376228594692,42.8625));
#254737=CARTESIAN_POINT('Ctrl Pts',(7.46502587018254,76.3529077059775,42.8625));
#254738=CARTESIAN_POINT('Ctrl Pts',(7.43032647871625,76.4467887510171,42.8625));
#254739=CARTESIAN_POINT('Ctrl Pts',(7.39936062409065,76.5417780825022,42.8625000000769));
#254740=CARTESIAN_POINT('Ctrl Pts',(7.37217896131494,76.6375793109204,42.8624999987634));
#254741=CARTESIAN_POINT('Ctrl Pts',(7.34479976166629,76.7340767541082,42.8624999974405));
#254742=CARTESIAN_POINT('Ctrl Pts',(7.32125992945122,76.8313976035036,42.8624999944439));
#254743=CARTESIAN_POINT('Ctrl Pts',(7.30155838910551,76.9292381964642,42.8624999930524));
#254744=CARTESIAN_POINT('Ctrl Pts',(7.29596637731268,76.9570089057617,42.8624999926574));
#254745=CARTESIAN_POINT('Ctrl Pts',(7.29068326752703,76.9848214996602,42.8624999924193));
#254746=CARTESIAN_POINT('Ctrl Pts',(7.28570827437986,77.0126690806324,42.8624999924233));
#254747=CARTESIAN_POINT('Ctrl Pts',(7.26767335427593,77.1136197519324,42.8624999924377));
#254748=CARTESIAN_POINT('Ctrl Pts',(7.25364515271356,77.2152466870781,42.8624999955794));
#254749=CARTESIAN_POINT('Ctrl Pts',(7.2436697699919,77.3175670299304,42.8624999975182));
#254750=CARTESIAN_POINT('Ctrl Pts',(7.23366552760738,77.4201833945677,42.8624999994626));
#254751=CARTESIAN_POINT('Ctrl Pts',(7.22773765182402,77.5234975299984,42.8624999999651));
#254752=CARTESIAN_POINT('Ctrl Pts',(7.2259844893479,77.6275198622504,42.8624999999951));
#254753=CARTESIAN_POINT('Ctrl Pts',(7.22561791497349,77.6492702258872,42.8625000000014));
#254754=CARTESIAN_POINT('Ctrl Pts',(7.22543403727889,77.6710515175201,42.8625));
#254755=CARTESIAN_POINT('Ctrl Pts',(7.2254340370314,77.6928637726221,42.8625));
#254756=CARTESIAN_POINT('',(7.22543403703139,78.3977423334149,42.8625));
#254757=CARTESIAN_POINT('',(7.22543403703139,0.,42.8625));
#254758=CARTESIAN_POINT('',(-7.22543403703142,78.3977423334149,42.8625));
#254759=CARTESIAN_POINT('Origin',(-2.7565840235444E-14,7.21644966006352E-13,
42.8625));
#254760=CARTESIAN_POINT('',(-7.22543403703142,77.692863772622,42.8625));
#254761=CARTESIAN_POINT('',(-7.22543403703142,77.3778479789282,42.8625));
#254762=CARTESIAN_POINT('Ctrl Pts',(-7.22543403703142,77.692863772622,42.8625));
#254763=CARTESIAN_POINT('Ctrl Pts',(-7.22543403725474,77.6143782234018,
42.8625));
#254764=CARTESIAN_POINT('Ctrl Pts',(-7.22781601838741,77.535875429433,42.8625000001524));
#254765=CARTESIAN_POINT('Ctrl Pts',(-7.23257896759688,77.4576191255712,
42.8624999988625));
#254766=CARTESIAN_POINT('Ctrl Pts',(-7.2373752547902,77.3788150712969,42.8624999975636));
#254767=CARTESIAN_POINT('Ctrl Pts',(-7.24458590971855,77.3002611368071,
42.8624999944325));
#254768=CARTESIAN_POINT('Ctrl Pts',(-7.25415854935673,77.2222128388911,
42.8624999909559));
#254769=CARTESIAN_POINT('Ctrl Pts',(-7.26294887859024,77.1505429274844,
42.8624999877634));
#254770=CARTESIAN_POINT('Ctrl Pts',(-7.27373024842269,77.0792993096169,
42.8624999846283));
#254771=CARTESIAN_POINT('Ctrl Pts',(-7.28642524295417,77.0086679922574,
42.8624999847095));
#254772=CARTESIAN_POINT('Ctrl Pts',(-7.30654950086703,76.896702379059,42.8624999848383));
#254773=CARTESIAN_POINT('Ctrl Pts',(-7.33152154531227,76.7859978222717,
42.8624999924738));
#254774=CARTESIAN_POINT('Ctrl Pts',(-7.36134046899601,76.6765419257663,
42.862499996246));
#254775=CARTESIAN_POINT('Ctrl Pts',(-7.39115939267974,76.5670860292609,
42.8625000000181));
#254776=CARTESIAN_POINT('Ctrl Pts',(-7.42582567269418,76.4588786827971,
42.8625));
#254777=CARTESIAN_POINT('Ctrl Pts',(-7.46538237873601,76.3519435477325,
42.8625));
#254778=CARTESIAN_POINT('Ctrl Pts',(-7.54449579081965,76.1380732776034,
42.8625));
#254779=CARTESIAN_POINT('Ctrl Pts',(-7.64384406930363,75.928944977058,42.8625));
#254780=CARTESIAN_POINT('Ctrl Pts',(-7.7591908761306,75.733143325879,42.8625));
#254781=CARTESIAN_POINT('Ctrl Pts',(-7.87453768295757,75.5373416747,42.8625));
#254782=CARTESIAN_POINT('Ctrl Pts',(-8.00653344510973,75.3526470960584,
42.8625));
#254783=CARTESIAN_POINT('Ctrl Pts',(-8.15553849975887,75.1792999831171,
42.8625));
#254784=CARTESIAN_POINT('Ctrl Pts',(-8.30454355440801,75.0059528701759,
42.8625));
#254785=CARTESIAN_POINT('Ctrl Pts',(-8.4701285640905,74.8451674277897,42.8625));
#254786=CARTESIAN_POINT('Ctrl Pts',(-8.64644770717183,74.7021568742844,
42.8625));
#254787=CARTESIAN_POINT('Ctrl Pts',(-8.82276685025317,74.5591463207792,
42.8625));
#254788=CARTESIAN_POINT('Ctrl Pts',(-9.01121135579652,74.4321791961687,
42.8625));
#254789=CARTESIAN_POINT('Ctrl Pts',(-9.21219622436481,74.3218046004446,
42.8625));
#254790=CARTESIAN_POINT('Ctrl Pts',(-9.29461898157906,74.2765406033547,
42.8625));
#254791=CARTESIAN_POINT('Ctrl Pts',(-9.3786096001277,74.234394079442,42.8625000000289));
#254792=CARTESIAN_POINT('Ctrl Pts',(-9.46387041307998,74.1954908710541,
42.862499999644));
#254793=CARTESIAN_POINT('Ctrl Pts',(-9.54941687963667,74.156457323284,42.8624999992578));
#254794=CARTESIAN_POINT('Ctrl Pts',(-9.63624170706638,74.120688949303,42.8624999983669));
#254795=CARTESIAN_POINT('Ctrl Pts',(-9.72402969290818,74.0882624434769,
42.8624999977847));
#254796=CARTESIAN_POINT('Ctrl Pts',(-9.76209983406389,74.0742003637726,
42.8624999975322));
#254797=CARTESIAN_POINT('Ctrl Pts',(-9.80035095542473,74.0607661112639,
42.8624999973601));
#254798=CARTESIAN_POINT('Ctrl Pts',(-9.83875676785274,74.0479629529335,
42.8624999973602));
#254799=CARTESIAN_POINT('Ctrl Pts',(-9.93044982501336,74.0173956857827,
42.8624999973604));
#254800=CARTESIAN_POINT('Ctrl Pts',(-10.0232647089801,73.9903401118788,
42.8624999983476));
#254801=CARTESIAN_POINT('Ctrl Pts',(-10.117219177538,73.9668292728909,42.8624999990185));
#254802=CARTESIAN_POINT('Ctrl Pts',(-10.2108353927062,73.9434030772532,
42.8624999996869));
#254803=CARTESIAN_POINT('Ctrl Pts',(-10.3055833706996,73.9234960907884,
42.8624999999561));
#254804=CARTESIAN_POINT('Ctrl Pts',(-10.4014866529399,73.9071922766141,
42.8624999999904));
#254805=CARTESIAN_POINT('Ctrl Pts',(-10.4352639087986,73.9014500528864,
42.8625000000025));
#254806=CARTESIAN_POINT('Ctrl Pts',(-10.4691845033362,73.8961552566244,
42.8625));
#254807=CARTESIAN_POINT('Ctrl Pts',(-10.5032495111116,73.8913131000538,
42.8625));
#254808=CARTESIAN_POINT('Origin',(-9.76543403703142,0.,-7.78106734735282));
#254809=CARTESIAN_POINT('',(-9.76543403703142,80.4599485582789,18.0027617587917));
#254810=CARTESIAN_POINT('',(-9.76543403703142,77.6928637726221,40.3225000000001));
#254811=CARTESIAN_POINT('Ctrl Pts',(-9.76543403703142,80.4599485582789,
18.0027617587917));
#254812=CARTESIAN_POINT('Ctrl Pts',(-9.76543403703142,79.5378854526247,
25.4427115049615));
#254813=CARTESIAN_POINT('Ctrl Pts',(-9.76543403703142,78.6155344836223,
32.882625582014));
#254814=CARTESIAN_POINT('Ctrl Pts',(-9.76543403703142,77.6928637726221,
40.3225000000001));
#254815=CARTESIAN_POINT('',(-9.76543403703142,80.6811576396149,40.3225));
#254816=CARTESIAN_POINT('',(-9.76543403703142,80.6811576396149,40.3225));
#254817=CARTESIAN_POINT('',(-9.76543404548309,80.681157776892,12.5890686048436));
#254818=CARTESIAN_POINT('',(-9.76543403703142,80.6811576396149,-7.78106734735282));
#254819=CARTESIAN_POINT('',(-9.76543403703142,80.9266905754733,12.3233805729971));
#254820=CARTESIAN_POINT('Ctrl Pts',(-9.76543403703143,80.6811579176687,
12.5890686048431));
#254821=CARTESIAN_POINT('Ctrl Pts',(-9.76543403703143,80.6811578105629,
12.5570686364181));
#254822=CARTESIAN_POINT('Ctrl Pts',(-9.76543403703142,80.6869824098219,
12.5253022376631));
#254823=CARTESIAN_POINT('Ctrl Pts',(-9.76543403703142,80.7103539169444,
12.463082263983));
#254824=CARTESIAN_POINT('Ctrl Pts',(-9.76543403703142,80.7285809497644,
12.4334024804021));
#254825=CARTESIAN_POINT('Ctrl Pts',(-9.76543403703142,80.7750888892602,
12.3827419313172));
#254826=CARTESIAN_POINT('Ctrl Pts',(-9.76543403703142,80.8029593811073,
12.3621289066386));
#254827=CARTESIAN_POINT('Ctrl Pts',(-9.76543403703142,80.8631242630206,
12.3337462130289));
#254828=CARTESIAN_POINT('Ctrl Pts',(-9.76543403703142,80.8945537377669,
12.3255084948528));
#254829=CARTESIAN_POINT('Ctrl Pts',(-9.76543403703142,80.9266905754733,
12.3233805729971));
#254830=CARTESIAN_POINT('',(-9.76543403703143,80.665181319947,12.34051373381));
#254831=CARTESIAN_POINT('Ctrl Pts',(-9.76543403703143,80.926690388265,12.3233777475718));
#254832=CARTESIAN_POINT('Ctrl Pts',(-9.76543403703143,80.8448494085605,
12.3287937059475));
#254833=CARTESIAN_POINT('Ctrl Pts',(-9.7654340370323,80.7630051677245,12.3341606246062));
#254834=CARTESIAN_POINT('Ctrl Pts',(-9.76543403703142,80.6811576390292,
12.3394767046348));
#254835=CARTESIAN_POINT('Ctrl Pts',(-9.76543403703137,80.6758322137124,
12.3398225964122));
#254836=CARTESIAN_POINT('Ctrl Pts',(-9.76543403703143,80.6705067738252,
12.340168272985));
#254837=CARTESIAN_POINT('Ctrl Pts',(-9.76543403703143,80.665181319947,12.34051373381));
#254838=CARTESIAN_POINT('',(-9.76543403703142,80.5172782442711,12.3495568918955));
#254839=CARTESIAN_POINT('Ctrl Pts',(-9.76543403703142,80.6651826441481,
12.3405342165937));
#254840=CARTESIAN_POINT('Ctrl Pts',(-9.76543403703142,80.6405620413662,
12.3421295047908));
#254841=CARTESIAN_POINT('Ctrl Pts',(-9.76543403703209,80.6159377423552,
12.3436782076836));
#254842=CARTESIAN_POINT('Ctrl Pts',(-9.76543403703209,80.5666366040391,
12.3466857490819));
#254843=CARTESIAN_POINT('Ctrl Pts',(-9.76543403703142,80.5419584195077,
12.3481444872065));
#254844=CARTESIAN_POINT('Ctrl Pts',(-9.76543403703143,80.5172782442762,
12.3495568919838));
#254845=CARTESIAN_POINT('',(-9.76543403703142,80.5172782427122,17.0741173620445));
#254846=CARTESIAN_POINT('',(-9.76543403703142,80.5172782427122,-7.78106734735282));
#254847=CARTESIAN_POINT('Origin',(-9.76543403703113,72.9739056302811,17.0745205117662));
#254848=CARTESIAN_POINT('Origin',(9.7654340370314,0.,-7.78106734735282));
#254849=CARTESIAN_POINT('',(9.76543403927482,80.6811576732767,12.5890686048444));
#254850=CARTESIAN_POINT('',(9.7654340370314,80.6811576396149,40.3225));
#254851=CARTESIAN_POINT('',(9.7654340370314,80.6811576396149,-7.78106734735282));
#254852=CARTESIAN_POINT('',(9.7654340370314,77.6928637726221,40.3225));
#254853=CARTESIAN_POINT('',(9.7654340370314,0.,40.3225));
#254854=CARTESIAN_POINT('',(9.7654340370314,80.4599485582789,18.0027617587916));
#254855=CARTESIAN_POINT('Ctrl Pts',(9.7654340370314,77.6928637726221,40.3225));
#254856=CARTESIAN_POINT('Ctrl Pts',(9.7654340370314,78.6155344836223,32.8826255820139));
#254857=CARTESIAN_POINT('Ctrl Pts',(9.7654340370314,79.5378854526247,25.4427115049614));
#254858=CARTESIAN_POINT('Ctrl Pts',(9.7654340370314,80.4599485582789,18.0027617587916));
#254859=CARTESIAN_POINT('',(9.7654340370314,80.5172782427122,17.0741173620444));
#254860=CARTESIAN_POINT('Origin',(9.76543403703169,72.973905630281,17.0745205117664));
#254861=CARTESIAN_POINT('',(9.7654340370314,80.5172782442711,12.3495568918922));
#254862=CARTESIAN_POINT('',(9.7654340370314,80.5172782427122,12.3825));
#254863=CARTESIAN_POINT('',(9.76543420245325,80.6651818783829,12.3405137312319));
#254864=CARTESIAN_POINT('Ctrl Pts',(9.76543403703139,80.5172782442762,12.3495568919806));
#254865=CARTESIAN_POINT('Ctrl Pts',(9.76543403703139,80.5419584195096,12.3481444872035));
#254866=CARTESIAN_POINT('Ctrl Pts',(9.76543403703206,80.5666366040432,12.3466857490791));
#254867=CARTESIAN_POINT('Ctrl Pts',(9.76543403703206,80.6159377423668,12.3436782076814));
#254868=CARTESIAN_POINT('Ctrl Pts',(9.7654340370314,80.6405620413825,12.3421295047889));
#254869=CARTESIAN_POINT('Ctrl Pts',(9.7654340370314,80.6651826441691,12.3405342165921));
#254870=CARTESIAN_POINT('',(9.76543402142917,80.9266904157755,12.3233781631543));
#254871=CARTESIAN_POINT('Ctrl Pts',(9.76543403703141,80.6651813199679,12.3405137338087));
#254872=CARTESIAN_POINT('Ctrl Pts',(9.76543403703141,80.6705067738392,12.340168272984));
#254873=CARTESIAN_POINT('Ctrl Pts',(9.76543403703134,80.6758322137194,12.3398225964117));
#254874=CARTESIAN_POINT('Ctrl Pts',(9.7654340370314,80.6811576390292,12.3394767046348));
#254875=CARTESIAN_POINT('Ctrl Pts',(9.76543403703227,80.7630051677206,12.3341606246064));
#254876=CARTESIAN_POINT('Ctrl Pts',(9.7654340370314,80.8448494085526,12.328793705948));
#254877=CARTESIAN_POINT('Ctrl Pts',(9.76543403703287,80.9266903882648,12.3233777475721));
#254878=CARTESIAN_POINT('Ctrl Pts',(9.76543403703139,80.9266904439379,12.3233785886619));
#254879=CARTESIAN_POINT('Ctrl Pts',(9.76543403703139,80.8945868905325,12.3255033793116));
#254880=CARTESIAN_POINT('Ctrl Pts',(9.7654340370314,80.8631886795284,12.3337259175107));
#254881=CARTESIAN_POINT('Ctrl Pts',(9.7654340370314,80.8030451610623,12.3620704955522));
#254882=CARTESIAN_POINT('Ctrl Pts',(9.7654340370314,80.775168642564,12.3826717602365));
#254883=CARTESIAN_POINT('Ctrl Pts',(9.7654340370314,80.7286417308444,12.4333137812977));
#254884=CARTESIAN_POINT('Ctrl Pts',(9.76543403703139,80.7104027846362,12.4629878785952));
#254885=CARTESIAN_POINT('Ctrl Pts',(9.76543403703139,80.6869950181105,12.5252327683005));
#254886=CARTESIAN_POINT('Ctrl Pts',(9.7654340370314,80.6811576872882,12.5570338786658));
#254887=CARTESIAN_POINT('Ctrl Pts',(9.7654340370314,80.6811577086292,12.5890686048444));
#254888=CARTESIAN_POINT('Origin',(-2.7565840235444E-14,7.21644966006352E-13,
-7.78106734735282));
#254889=CARTESIAN_POINT('Origin',(-2.7565840235444E-14,7.21644966006352E-13,
40.3225));
#254890=CARTESIAN_POINT('Ctrl Pts',(9.76543403530562,80.6811576398238,12.5890686044732));
#254891=CARTESIAN_POINT('Ctrl Pts',(8.642707260293,80.8170495206766,12.3475861026818));
#254892=CARTESIAN_POINT('Ctrl Pts',(7.51318753972854,80.929982574631,12.1455679037829));
#254893=CARTESIAN_POINT('Ctrl Pts',(6.37776783703217,81.0193617440728,11.9852102203789));
#254894=CARTESIAN_POINT('Ctrl Pts',(5.89168688638967,81.0576255786238,11.9165599979046));
#254895=CARTESIAN_POINT('Ctrl Pts',(5.40452517458145,81.0915728838979,11.8555451261434));
#254896=CARTESIAN_POINT('Ctrl Pts',(4.91635528551654,81.1211584650181,11.8023379231986));
#254897=CARTESIAN_POINT('Ctrl Pts',(4.10212074979073,81.1705052241018,11.7135918879401));
#254898=CARTESIAN_POINT('Ctrl Pts',(3.28481153395651,81.2077378726861,11.6464808182021));
#254899=CARTESIAN_POINT('Ctrl Pts',(2.46434966086494,81.2326281782696,11.6015974754808));
#254900=CARTESIAN_POINT('Ctrl Pts',(1.98330333770676,81.2472216534522,11.5752818504709));
#254901=CARTESIAN_POINT('Ctrl Pts',(1.50074701423457,81.2575796604344,11.5566086492317));
#254902=CARTESIAN_POINT('Ctrl Pts',(1.01746939332227,81.2636305860971,11.5456857536254));
#254903=CARTESIAN_POINT('Ctrl Pts',(0.676479489490327,81.267899984204,11.5379788022559));
#254904=CARTESIAN_POINT('Ctrl Pts',(0.335130586181492,81.2700262217726,
11.534130262006));
#254905=CARTESIAN_POINT('Ctrl Pts',(-0.00629963612498389,81.2699997558422,
11.5341780279657));
#254906=CARTESIAN_POINT('Ctrl Pts',(-0.861676302009446,81.2699334514031,
11.5342976948395));
#254907=CARTESIAN_POINT('Ctrl Pts',(-1.71371687815596,81.2563671514032,
11.5588752590179));
#254908=CARTESIAN_POINT('Ctrl Pts',(-2.56248731492883,81.2295916446761,
11.6072244931474));
#254909=CARTESIAN_POINT('Ctrl Pts',(-3.41597307225165,81.2026673873663,
11.6558423301021));
#254910=CARTESIAN_POINT('Ctrl Pts',(-4.26615255418888,81.1623867763625,
11.7284966963816));
#254911=CARTESIAN_POINT('Ctrl Pts',(-5.11310836102155,81.1089947101334,
11.8244898640261));
#254912=CARTESIAN_POINT('Ctrl Pts',(-5.9665546510357,81.055193484058,11.9212186568769));
#254913=CARTESIAN_POINT('Ctrl Pts',(-6.81672796889863,80.9880791154851,
12.0416453265388));
#254914=CARTESIAN_POINT('Ctrl Pts',(-7.6637240426148,80.9078502606431,12.1850559811004));
#254915=CARTESIAN_POINT('Ctrl Pts',(-8.36646147164548,80.8412858208124,
12.3040412253177));
#254916=CARTESIAN_POINT('Ctrl Pts',(-9.06701205871129,80.7656927894985,
12.4388480077385));
#254917=CARTESIAN_POINT('Ctrl Pts',(-9.76543402933603,80.6811576405463,
12.5890686031893));
#254918=CARTESIAN_POINT('Ctrl Pts',(-20.509804815317,115.,12.3825));
#254919=CARTESIAN_POINT('Ctrl Pts',(-9.76543403703142,80.,12.3825));
#254920=CARTESIAN_POINT('Ctrl Pts',(-7.2108267586496,115.,6.80385564663691));
#254921=CARTESIAN_POINT('Ctrl Pts',(-3.29772532864429,80.,11.0907130840649));
#254922=CARTESIAN_POINT('Ctrl Pts',(7.21082675864964,115.,6.80385564663692));
#254923=CARTESIAN_POINT('Ctrl Pts',(3.29772532864426,80.,11.0907130840649));
#254924=CARTESIAN_POINT('Ctrl Pts',(20.509804815317,115.,12.3825));
#254925=CARTESIAN_POINT('Ctrl Pts',(9.76543403703139,80.,12.3825));
#254926=CARTESIAN_POINT('Ctrl Pts',(-9.76543348183844,80.9266905678574,
12.3233804598558));
#254927=CARTESIAN_POINT('Ctrl Pts',(-9.21901381841984,80.9911564147534,
12.2072621082779));
#254928=CARTESIAN_POINT('Ctrl Pts',(-8.67068521395711,81.0503803664516,
12.1003581949099));
#254929=CARTESIAN_POINT('Ctrl Pts',(-8.12078457076909,81.1042435940398,
12.0029639875845));
#254930=CARTESIAN_POINT('Ctrl Pts',(-7.57790689040143,81.1574189165503,
11.9068136338632));
#254931=CARTESIAN_POINT('Ctrl Pts',(-7.03349709193297,81.2053695632012,
11.8199316855308));
#254932=CARTESIAN_POINT('Ctrl Pts',(-6.48788508382262,81.2480057885138,
11.7425585631889));
#254933=CARTESIAN_POINT('Ctrl Pts',(-5.96432468672382,81.2889188159466,
11.6683125750949));
#254934=CARTESIAN_POINT('Ctrl Pts',(-5.43965733257562,81.3249384348352,
11.6028221508719));
#254935=CARTESIAN_POINT('Ctrl Pts',(-4.91417937346711,81.3560071311834,
11.5462604754853));
#254936=CARTESIAN_POINT('Ctrl Pts',(-3.90861272828337,81.4154608993492,
11.438022759367));
#254937=CARTESIAN_POINT('Ctrl Pts',(-2.89900702900751,81.4568548427787,
11.3623506147986));
#254938=CARTESIAN_POINT('Ctrl Pts',(-1.88524103826131,81.4798101320474,
11.3203203829979));
#254939=CARTESIAN_POINT('Ctrl Pts',(-1.25840892529359,81.49400385388,11.2943322365729));
#254940=CARTESIAN_POINT('Ctrl Pts',(-0.629986214081505,81.5011476552561,
11.2812069510319));
#254941=CARTESIAN_POINT('Ctrl Pts',(5.60440135014445E-5,81.5011472661906,
11.2812077224205));
#254942=CARTESIAN_POINT('Ctrl Pts',(0.000515968424032919,81.5011472659066,
11.2812077229836));
#254943=CARTESIAN_POINT('Ctrl Pts',(0.000975892644772834,81.5011472617952,
11.2812077305293));
#254944=CARTESIAN_POINT('Ctrl Pts',(0.0014358166751247,81.5011472538564,
11.2812077450575));
#254945=CARTESIAN_POINT('Ctrl Pts',(0.826165080880329,81.5011330182027,
11.2812337967929));
#254946=CARTESIAN_POINT('Ctrl Pts',(1.65023405465531,81.4888253830682,11.3037129450655));
#254947=CARTESIAN_POINT('Ctrl Pts',(2.47001199742806,81.4644891219574,11.3481105561519));
#254948=CARTESIAN_POINT('Ctrl Pts',(2.48653380514781,81.4639986488601,11.3490053457715));
#254949=CARTESIAN_POINT('Ctrl Pts',(2.50305394112712,81.4635032893928,11.3499090412207));
#254950=CARTESIAN_POINT('Ctrl Pts',(2.51957237562734,81.4630030456335,11.3508216382509));
#254951=CARTESIAN_POINT('Ctrl Pts',(3.32266451172049,81.4386822282343,11.3951902192021));
#254952=CARTESIAN_POINT('Ctrl Pts',(4.12282671528089,81.4028175892564,11.4605982502462));
#254953=CARTESIAN_POINT('Ctrl Pts',(4.92000987776074,81.3556286372825,11.5464932122947));
#254954=CARTESIAN_POINT('Ctrl Pts',(4.95329825353372,81.3536581446283,11.550079971158));
#254955=CARTESIAN_POINT('Ctrl Pts',(4.98658143225163,81.351667909035,11.5537024490998));
#254956=CARTESIAN_POINT('Ctrl Pts',(5.01985942551591,81.3496579463146,11.5573606066733));
#254957=CARTESIAN_POINT('Ctrl Pts',(6.01122202727515,81.289780481464,11.6663383500398));
#254958=CARTESIAN_POINT('Ctrl Pts',(6.99804347270548,81.2124024895723,11.8070343424507));
#254959=CARTESIAN_POINT('Ctrl Pts',(7.98047918803816,81.1178563623326,11.9781794191987));
#254960=CARTESIAN_POINT('Ctrl Pts',(8.57707028891758,81.0604425516847,12.082108488708));
#254961=CARTESIAN_POINT('Ctrl Pts',(9.17204397683082,80.9966972889915,12.1972669259026));
#254962=CARTESIAN_POINT('Ctrl Pts',(9.76543387174275,80.9266904417031,12.3233785549721));
#254963=CARTESIAN_POINT('',(19.6234043038483,113.315263490685,12.231294241899));
#254964=CARTESIAN_POINT('Ctrl Pts',(9.76543420245325,80.6651818783829,12.3405137312319));
#254965=CARTESIAN_POINT('Ctrl Pts',(11.3799678060561,86.1153669381273,12.3153647150579));
#254966=CARTESIAN_POINT('Ctrl Pts',(13.0205007967692,91.5578166430438,12.2930000217267));
#254967=CARTESIAN_POINT('Ctrl Pts',(16.313066495143,102.439221084592,12.2572978841659));
#254968=CARTESIAN_POINT('Ctrl Pts',(17.9668525537566,107.877661915077,12.243175008079));
#254969=CARTESIAN_POINT('Ctrl Pts',(19.6234043038483,113.315263490685,12.231294241899));
#254970=CARTESIAN_POINT('',(-19.6234043038483,113.315263490685,12.231294241899));
#254971=CARTESIAN_POINT('Ctrl Pts',(19.6234043038483,113.315263490685,12.231294241899));
#254972=CARTESIAN_POINT('Ctrl Pts',(18.8409284740723,113.311274371647,11.9148273395859));
#254973=CARTESIAN_POINT('Ctrl Pts',(18.0498151499385,113.307504020477,11.6169295778476));
#254974=CARTESIAN_POINT('Ctrl Pts',(16.459706385983,113.300453260057,11.0615401298248));
#254975=CARTESIAN_POINT('Ctrl Pts',(15.6610703781754,113.297173414208,10.804088311671));
#254976=CARTESIAN_POINT('Ctrl Pts',(13.2546236809651,113.288070000624,10.0912959618231));
#254977=CARTESIAN_POINT('Ctrl Pts',(11.6362978866301,113.282981629452,9.69538531766471));
#254978=CARTESIAN_POINT('Ctrl Pts',(6.73998365714194,113.270687155678,8.74128236982949));
#254979=CARTESIAN_POINT('Ctrl Pts',(3.42104711494492,113.266433067362,8.41452184068842));
#254980=CARTESIAN_POINT('Ctrl Pts',(-3.33143264129344,113.266357991278,
8.40873611349764));
#254981=CARTESIAN_POINT('Ctrl Pts',(-6.66356650895994,113.270541327779,
8.73001511549867));
#254982=CARTESIAN_POINT('Ctrl Pts',(-11.5933138606595,113.282851235877,
9.68524203411009));
#254983=CARTESIAN_POINT('Ctrl Pts',(-13.2269544959225,113.287971157042,
10.0835711394783));
#254984=CARTESIAN_POINT('Ctrl Pts',(-16.4641399389958,113.300205589209,
11.041491514323));
#254985=CARTESIAN_POINT('Ctrl Pts',(-18.0583770680721,113.307284867316,
11.5983298709949));
#254986=CARTESIAN_POINT('Ctrl Pts',(-19.6234043038483,113.315263490685,
12.231294241899));
#254987=CARTESIAN_POINT('Ctrl Pts',(-19.6234043038483,113.315263490685,
12.231294241899));
#254988=CARTESIAN_POINT('Ctrl Pts',(-17.9668525537554,107.877661915073,
12.243175008079));
#254989=CARTESIAN_POINT('Ctrl Pts',(-16.3130664951407,102.439221084584,
12.2572978841659));
#254990=CARTESIAN_POINT('Ctrl Pts',(-13.0205007967646,91.5578166430286,
12.2930000217267));
#254991=CARTESIAN_POINT('Ctrl Pts',(-11.379967806051,86.11536693811,12.3153647150579));
#254992=CARTESIAN_POINT('Ctrl Pts',(-9.76543420245328,80.6651818783619,
12.3405137312333));
#254993=CARTESIAN_POINT('Origin',(0.,0.,12.3825));
#254994=CARTESIAN_POINT('',(24.758292886385,76.0725110230494,12.3825));
#254995=CARTESIAN_POINT('',(10.8629841634368,79.2590409673554,12.3825));
#254996=CARTESIAN_POINT('Origin',(0.,0.,12.3825));
#254997=CARTESIAN_POINT('',(10.8629841634368,79.2590409673554,17.0741173620444));
#254998=CARTESIAN_POINT('',(10.8629841634368,79.2590409673554,12.3825));
#254999=CARTESIAN_POINT('',(24.758292886385,76.0725110230494,17.0741173620444));
#255000=CARTESIAN_POINT('Origin',(0.,0.,17.0741173620444));
#255001=CARTESIAN_POINT('',(24.758292886385,76.0725110230494,12.3825));
#255002=CARTESIAN_POINT('Origin',(0.,0.,12.3825));
#255003=CARTESIAN_POINT('',(20.3338370957106,113.095,12.3825));
#255004=CARTESIAN_POINT('',(20.509804815317,113.095,12.3825));
#255005=CARTESIAN_POINT('',(9.93397247946587,79.8850738159598,12.3825));
#255006=CARTESIAN_POINT('Ctrl Pts',(20.3338370957106,113.095,12.3825));
#255007=CARTESIAN_POINT('Ctrl Pts',(18.6162390952454,107.555098952883,12.3825));
#255008=CARTESIAN_POINT('Ctrl Pts',(16.8951673474018,102.01627317443,12.3824999999886));
#255009=CARTESIAN_POINT('Ctrl Pts',(15.1653526441753,96.4801751438902,12.3824999999964));
#255010=CARTESIAN_POINT('Ctrl Pts',(15.1549732951004,96.446957080785,12.3824999999964));
#255011=CARTESIAN_POINT('Ctrl Pts',(15.1445936258827,96.4137391176421,12.3824999999965));
#255012=CARTESIAN_POINT('Ctrl Pts',(15.1342136354895,96.3805212547838,12.3824999999965));
#255013=CARTESIAN_POINT('Ctrl Pts',(14.2708587200199,93.6176280252437,12.3824999999987));
#255014=CARTESIAN_POINT('Ctrl Pts',(13.4057207197965,90.8552856382803,12.3824999997191));
#255015=CARTESIAN_POINT('Ctrl Pts',(12.5362227209559,88.0943201478487,12.3824999994597));
#255016=CARTESIAN_POINT('Ctrl Pts',(11.7595790473135,85.6282001750045,12.382499999228));
#255017=CARTESIAN_POINT('Ctrl Pts',(10.9794584946655,83.1631782350712,12.3824999997221));
#255018=CARTESIAN_POINT('Ctrl Pts',(10.1939933986301,80.6998523967545,12.3824999999539));
#255019=CARTESIAN_POINT('Ctrl Pts',(10.1073856377522,80.4282386277326,12.3824999999794));
#255020=CARTESIAN_POINT('Ctrl Pts',(10.020712846965,80.1566454956651,12.3824999999961));
#255021=CARTESIAN_POINT('Ctrl Pts',(9.93397247946587,79.8850738159598,12.3824999999994));
#255022=CARTESIAN_POINT('Origin',(11.0354340370314,80.5172782427122,12.3825));
#255023=CARTESIAN_POINT('',(27.0012528338594,76.4071670555372,12.3825));
#255024=CARTESIAN_POINT('Origin',(25.5443686855278,78.4878132480313,12.3825));
#255025=CARTESIAN_POINT('',(75.6605890912238,110.478801107225,12.3825));
#255026=CARTESIAN_POINT('Origin',(0.,0.,12.3825));
#255027=CARTESIAN_POINT('',(-10.8629841634369,79.2590409673554,12.3825));
#255028=CARTESIAN_POINT('',(-9.93397247946588,79.8850738159598,12.3825));
#255029=CARTESIAN_POINT('Origin',(-11.0354340370314,80.5172782427122,12.3825));
#255030=CARTESIAN_POINT('',(-20.3338370957106,113.095,12.3825));
#255031=CARTESIAN_POINT('Ctrl Pts',(-9.93397247946588,79.8850738159598,
12.3824999999994));
#255032=CARTESIAN_POINT('Ctrl Pts',(-10.7214025854466,82.3504048111719,
12.3824999999692));
#255033=CARTESIAN_POINT('Ctrl Pts',(-11.5032683361806,84.8175022341616,
12.3824999992383));
#255034=CARTESIAN_POINT('Ctrl Pts',(-12.281448300187,87.2857645884932,12.3824999993952));
#255035=CARTESIAN_POINT('Ctrl Pts',(-13.2367907647368,90.3159580524864,
12.3824999995878));
#255036=CARTESIAN_POINT('Ctrl Pts',(-14.1865759945479,93.3479079281245,
12.3824999999989));
#255037=CARTESIAN_POINT('Ctrl Pts',(-15.1342136355012,96.3805212547678,
12.3824999999965));
#255038=CARTESIAN_POINT('Ctrl Pts',(-15.1445936258955,96.4137391176299,
12.3824999999965));
#255039=CARTESIAN_POINT('Ctrl Pts',(-15.1549732951142,96.4469570807766,
12.3824999999964));
#255040=CARTESIAN_POINT('Ctrl Pts',(-15.1653526441902,96.4801751438856,
12.3824999999964));
#255041=CARTESIAN_POINT('Ctrl Pts',(-16.8951673474031,102.016273174429,
12.3824999999886));
#255042=CARTESIAN_POINT('Ctrl Pts',(-18.6162390953258,107.555098952858,
12.3825));
#255043=CARTESIAN_POINT('Ctrl Pts',(-20.3338370957106,113.095,12.3825));
#255044=CARTESIAN_POINT('',(-90.,113.095,12.3825));
#255045=CARTESIAN_POINT('',(-27.0012528338594,76.4071670555372,12.3825));
#255046=CARTESIAN_POINT('',(-75.6605890912239,110.478801107225,12.3825));
#255047=CARTESIAN_POINT('',(-24.758292886385,76.0725110230494,12.3825));
#255048=CARTESIAN_POINT('Origin',(-25.5443686855278,78.4878132480313,12.3825));
#255049=CARTESIAN_POINT('Origin',(0.,0.,12.3825));
#255050=CARTESIAN_POINT('Origin',(0.,0.,12.3825));
#255051=CARTESIAN_POINT('',(-24.758292886385,76.0725110230494,17.0741173620445));
#255052=CARTESIAN_POINT('',(-10.8629841634369,79.2590409673554,17.0741173620445));
#255053=CARTESIAN_POINT('Origin',(0.,0.,17.0741173620445));
#255054=CARTESIAN_POINT('',(-10.8629841634369,79.2590409673554,12.3825));
#255055=CARTESIAN_POINT('',(-24.758292886385,76.0725110230494,12.3825));
#255056=CARTESIAN_POINT('Origin',(-90.,-90.,17.4625));
#255057=CARTESIAN_POINT('',(-109.438478010978,76.3890311653897,17.4625));
#255058=CARTESIAN_POINT('',(-76.7149512087496,29.6549915892152,17.4625));
#255059=CARTESIAN_POINT('',(-24.8661421402461,-44.3927817339206,17.4625));
#255060=CARTESIAN_POINT('',(-29.6549915892152,76.7149512087496,17.4625));
#255061=CARTESIAN_POINT('Origin',(0.,0.,17.4625));
#255062=CARTESIAN_POINT('',(-76.3890311653897,109.438478010978,17.4625));
#255063=CARTESIAN_POINT('',(8.18330470534212,50.220290910288,17.4625));
#255064=CARTESIAN_POINT('Origin',(-90.,90.,17.4625));
#255065=CARTESIAN_POINT('Origin',(0.,0.,12.3825));
#255066=CARTESIAN_POINT('Origin',(0.,0.,14.2875));
#255067=CARTESIAN_POINT('Origin',(-90.,-90.,17.4625));
#255068=CARTESIAN_POINT('',(-76.3890311653897,-109.438478010978,17.4625));
#255069=CARTESIAN_POINT('',(-29.6549915892153,-76.7149512087495,17.4625));
#255070=CARTESIAN_POINT('',(-76.3890311653897,-109.438478010978,17.4625));
#255071=CARTESIAN_POINT('',(-76.7149512087496,-29.6549915892152,17.4625));
#255072=CARTESIAN_POINT('Origin',(0.,0.,17.4625));
#255073=CARTESIAN_POINT('',(-109.438478010978,-76.3890311653897,17.4625));
#255074=CARTESIAN_POINT('',(-109.438478010978,-76.3890311653897,17.4625));
#255075=CARTESIAN_POINT('Origin',(-90.,-90.,17.4625));
#255076=CARTESIAN_POINT('Origin',(0.,0.,12.3825));
#255077=CARTESIAN_POINT('',(-24.7582928863851,-76.0725110230494,17.0741173620444));
#255078=CARTESIAN_POINT('',(-24.7582928863851,-76.0725110230494,14.2875));
#255079=CARTESIAN_POINT('',(-24.7582928863851,-76.0725110230494,12.3825));
#255080=CARTESIAN_POINT('',(24.758292886385,-76.0725110230494,14.2875));
#255081=CARTESIAN_POINT('Origin',(0.,0.,14.2875));
#255082=CARTESIAN_POINT('',(24.758292886385,-76.0725110230494,17.0741173620444));
#255083=CARTESIAN_POINT('',(24.758292886385,-76.0725110230494,12.3825));
#255084=CARTESIAN_POINT('Origin',(0.,0.,17.0741173620444));
#255085=CARTESIAN_POINT('Origin',(-90.,-90.,17.4625));
#255086=CARTESIAN_POINT('',(76.7149512087496,-29.6549915892152,17.4625));
#255087=CARTESIAN_POINT('',(50.220290910288,8.18330470534212,17.4625));
#255088=CARTESIAN_POINT('',(29.6549915892152,-76.7149512087496,17.4625));
#255089=CARTESIAN_POINT('Origin',(0.,0.,17.4625));
#255090=CARTESIAN_POINT('',(-44.3927817339206,-24.8661421402461,17.4625));
#255091=CARTESIAN_POINT('Origin',(-90.,-90.,17.4625));
#255092=CARTESIAN_POINT('',(29.6549915892153,76.7149512087496,17.4625));
#255093=CARTESIAN_POINT('',(-128.965117604652,-34.3520449604438,17.4625));
#255094=CARTESIAN_POINT('',(76.7149512087496,29.6549915892152,17.4625));
#255095=CARTESIAN_POINT('Origin',(0.,0.,17.4625));
#255096=CARTESIAN_POINT('',(-34.3520449604435,-128.965117604652,17.4625));
#255097=CARTESIAN_POINT('Origin',(75.6605890912238,110.478801107225,12.3825));
#255098=CARTESIAN_POINT('',(27.0012528338594,76.4071670555372,16.0836603564334));
#255099=CARTESIAN_POINT('',(27.0012528338594,76.4071670555372,17.0741173620444));
#255100=CARTESIAN_POINT('',(27.1270025958466,76.4952184082712,16.1248510148135));
#255101=CARTESIAN_POINT('Ctrl Pts',(27.0012661163029,76.4071769818623,16.0836344441067));
#255102=CARTESIAN_POINT('Ctrl Pts',(27.004737787447,76.4096082525859,16.0839286114052));
#255103=CARTESIAN_POINT('Ctrl Pts',(27.0082239404906,76.4120499969458,16.0841797723559));
#255104=CARTESIAN_POINT('Ctrl Pts',(27.011708212666,76.4144904864622,16.0844643090931));
#255105=CARTESIAN_POINT('Ctrl Pts',(27.0164654915444,76.4178226283401,16.0848528036027));
#255106=CARTESIAN_POINT('Ctrl Pts',(27.0212167836978,76.4211512987678,16.0853190683137));
#255107=CARTESIAN_POINT('Ctrl Pts',(27.0259665551538,76.4244788255243,16.0858213410311));
#255108=CARTESIAN_POINT('Ctrl Pts',(27.0307534510001,76.4278323603537,16.0863275395306));
#255109=CARTESIAN_POINT('Ctrl Pts',(27.0355388328709,76.4311845627265,16.0868702293972));
#255110=CARTESIAN_POINT('Ctrl Pts',(27.0403202016754,76.4345322490831,16.0874595949022));
#255111=CARTESIAN_POINT('Ctrl Pts',(27.0456455283622,76.4382607888011,16.0881160102469));
#255112=CARTESIAN_POINT('Ctrl Pts',(27.0509659278642,76.4419833123646,16.088830242588));
#255113=CARTESIAN_POINT('Ctrl Pts',(27.056268164441,76.4456927956767,16.0896862961657));
#255114=CARTESIAN_POINT('Ctrl Pts',(27.058858523868,76.447505029991,16.0901045133507));
#255115=CARTESIAN_POINT('Ctrl Pts',(27.0614444000977,76.4493141547801,16.0905576105986));
#255116=CARTESIAN_POINT('Ctrl Pts',(27.0640236135651,76.4511197912151,16.0910594910215));
#255117=CARTESIAN_POINT('Ctrl Pts',(27.0646233142434,76.4515396251716,16.0911761847477));
#255118=CARTESIAN_POINT('Ctrl Pts',(27.0652224173107,76.4519590933765,16.0912956547431));
#255119=CARTESIAN_POINT('Ctrl Pts',(27.0658207705618,76.4523781037608,16.0914185979664));
#255120=CARTESIAN_POINT('Ctrl Pts',(27.0694252453324,76.4549022186638,16.092159206872));
#255121=CARTESIAN_POINT('Ctrl Pts',(27.0730526643751,76.4574399975648,16.0929214221552));
#255122=CARTESIAN_POINT('Ctrl Pts',(27.0766494404437,76.4599565375944,16.0938416360863));
#255123=CARTESIAN_POINT('Ctrl Pts',(27.0794164248046,76.4618925010164,16.094549552706));
#255124=CARTESIAN_POINT('Ctrl Pts',(27.0821652338675,76.4638159874324,16.0953521030018));
#255125=CARTESIAN_POINT('Ctrl Pts',(27.0848806691381,76.4657181558853,16.096278407548));
#255126=CARTESIAN_POINT('Ctrl Pts',(27.0856950017747,76.4662885977103,16.0965561972754));
#255127=CARTESIAN_POINT('Ctrl Pts',(27.0865064098576,76.4668571749595,16.0968447965766));
#255128=CARTESIAN_POINT('Ctrl Pts',(27.0873147048412,76.4674237928792,16.0971440360155));
#255129=CARTESIAN_POINT('Ctrl Pts',(27.0892964622733,76.4688130125285,16.0978777037902));
#255130=CARTESIAN_POINT('Ctrl Pts',(27.0912759868229,76.4702047210398,16.0986102840898));
#255131=CARTESIAN_POINT('Ctrl Pts',(27.0932317934192,76.4715818077005,16.0994143656071));
#255132=CARTESIAN_POINT('Ctrl Pts',(27.0950567908676,76.4728667914237,16.100164668178));
#255133=CARTESIAN_POINT('Ctrl Pts',(27.0968611735725,76.4741390840017,16.1009779446282));
#255134=CARTESIAN_POINT('Ctrl Pts',(27.0986398464197,76.4753926606387,16.1018707649377));
#255135=CARTESIAN_POINT('Ctrl Pts',(27.1003347056929,76.4765871669759,16.1027215142946));
#255136=CARTESIAN_POINT('Ctrl Pts',(27.102006284354,76.477764742482,16.103644760763));
#255137=CARTESIAN_POINT('Ctrl Pts',(27.1036611183332,76.4789268718445,16.1046080215383));
#255138=CARTESIAN_POINT('Ctrl Pts',(27.1040884349236,76.4792269606528,16.1048567578559));
#255139=CARTESIAN_POINT('Ctrl Pts',(27.1045146909912,76.4795260526583,16.1051079007521));
#255140=CARTESIAN_POINT('Ctrl Pts',(27.1049401152197,76.4798242409135,16.1053603339431));
#255141=CARTESIAN_POINT('Ctrl Pts',(27.107191856298,76.4814025307667,16.1066964454));
#255142=CARTESIAN_POINT('Ctrl Pts',(27.1094086966922,76.4829517841693,16.108156698499));
#255143=CARTESIAN_POINT('Ctrl Pts',(27.1115676990795,76.4844580502449,16.1097553365817));
#255144=CARTESIAN_POINT('Ctrl Pts',(27.1144415930954,76.4864630730678,16.1118833177486));
#255145=CARTESIAN_POINT('Ctrl Pts',(27.1172143946526,76.4883927334345,16.114251591047));
#255146=CARTESIAN_POINT('Ctrl Pts',(27.1198385003592,76.4902196926299,16.1168182560618));
#255147=CARTESIAN_POINT('Ctrl Pts',(27.1220343788846,76.4917485107921,16.1189660676282));
#255148=CARTESIAN_POINT('Ctrl Pts',(27.1241266280253,76.4932057033932,16.1212487745088));
#255149=CARTESIAN_POINT('Ctrl Pts',(27.1260772883368,76.4945703804111,16.1236712941908));
#255150=CARTESIAN_POINT('Ctrl Pts',(27.1263896838621,76.49478893153,16.1240592573354));
#255151=CARTESIAN_POINT('Ctrl Pts',(27.1266982100994,76.4950049324791,16.1244524123603));
#255152=CARTESIAN_POINT('Ctrl Pts',(27.127002665508,76.4952182372903,16.1248510388561));
#255153=CARTESIAN_POINT('',(27.1805645602856,76.5327357173562,16.1924969468891));
#255154=CARTESIAN_POINT('Ctrl Pts',(27.1270024565239,76.4952187502329,16.1248509667283));
#255155=CARTESIAN_POINT('Ctrl Pts',(27.1424765597207,76.506055562166,16.1451084955576));
#255156=CARTESIAN_POINT('Ctrl Pts',(27.1582694740498,76.5171175291545,16.1650670183879));
#255157=CARTESIAN_POINT('Ctrl Pts',(27.1742368508763,76.5283030898323,16.1847307983824));
#255158=CARTESIAN_POINT('Ctrl Pts',(27.1763430720179,76.5297785522477,16.1873246038395));
#255159=CARTESIAN_POINT('Ctrl Pts',(27.1784523977366,76.531256170399,16.1899133083194));
#255160=CARTESIAN_POINT('Ctrl Pts',(27.1805645602855,76.5327357173562,16.1924969468891));
#255161=CARTESIAN_POINT('',(75.6605890912238,110.478801107225,16.1925));
#255162=CARTESIAN_POINT('Origin',(-75.6605890912239,110.478801107225,12.3825));
#255163=CARTESIAN_POINT('',(-27.1805647392023,76.5327354732306,16.1924983103147));
#255164=CARTESIAN_POINT('',(-75.6605890912239,110.478801107225,16.1925));
#255165=CARTESIAN_POINT('',(-27.1270026766374,76.4952184105125,16.124850980315));
#255166=CARTESIAN_POINT('Ctrl Pts',(-27.180565219782,76.5327358093755,16.1924970380416));
#255167=CARTESIAN_POINT('Ctrl Pts',(-27.1645460760463,76.5215147101881,
16.172902641616));
#255168=CARTESIAN_POINT('Ctrl Pts',(-27.1486864769872,76.5104044317336,
16.1530153195235));
#255169=CARTESIAN_POINT('Ctrl Pts',(-27.1331242506465,76.4995059128408,
16.1328282540153));
#255170=CARTESIAN_POINT('Ctrl Pts',(-27.1310783227674,76.4980731111866,
16.1301743098291));
#255171=CARTESIAN_POINT('Ctrl Pts',(-27.1290376031219,76.496643974394,16.1275152114758));
#255172=CARTESIAN_POINT('Ctrl Pts',(-27.1270024664547,76.4952187349082,
16.1248509673414));
#255173=CARTESIAN_POINT('',(-27.0012528338594,76.4071670555372,16.0836576911637));
#255174=CARTESIAN_POINT('Ctrl Pts',(-27.1270027817058,76.4952182482985,
16.1248509867716));
#255175=CARTESIAN_POINT('Ctrl Pts',(-27.1240985616495,76.4931858448222,
16.1210498254195));
#255176=CARTESIAN_POINT('Ctrl Pts',(-27.1208691627931,76.4909301698259,
16.1175138337718));
#255177=CARTESIAN_POINT('Ctrl Pts',(-27.1174141814671,76.488512642972,16.1144000397266));
#255178=CARTESIAN_POINT('Ctrl Pts',(-27.1156443145459,76.4872742279399,
16.1128049511979));
#255179=CARTESIAN_POINT('Ctrl Pts',(-27.1138145057317,76.4859930227779,
16.1113222644235));
#255180=CARTESIAN_POINT('Ctrl Pts',(-27.1119395463074,76.4846791613504,
16.1099492036558));
#255181=CARTESIAN_POINT('Ctrl Pts',(-27.1101543718988,76.4834282159878,
16.1086418937951));
#255182=CARTESIAN_POINT('Ctrl Pts',(-27.1083279413725,76.4821474488426,
16.1074352882173));
#255183=CARTESIAN_POINT('Ctrl Pts',(-27.1064797666433,76.4808505836342,
16.1062837053202));
#255184=CARTESIAN_POINT('Ctrl Pts',(-27.1054282961436,76.4801127662151,
16.1056285424586));
#255185=CARTESIAN_POINT('Ctrl Pts',(-27.104370813704,76.4793697022192,16.1049758084275));
#255186=CARTESIAN_POINT('Ctrl Pts',(-27.1033071953436,76.4786223827172,
16.1043249532128));
#255187=CARTESIAN_POINT('Ctrl Pts',(-27.1014285386934,76.4773024010352,
16.1031753552716));
#255188=CARTESIAN_POINT('Ctrl Pts',(-27.0995243697347,76.4759644037322,
16.1020872230215));
#255189=CARTESIAN_POINT('Ctrl Pts',(-27.0975893413305,76.4746063119939,
16.1011009878118));
#255190=CARTESIAN_POINT('Ctrl Pts',(-27.0955329405811,76.4731630355737,
16.1000528921767));
#255191=CARTESIAN_POINT('Ctrl Pts',(-27.0934416537043,76.4716969840383,
16.0991197195565));
#255192=CARTESIAN_POINT('Ctrl Pts',(-27.0913213037529,76.4702124719296,
16.0982908776209));
#255193=CARTESIAN_POINT('Ctrl Pts',(-27.0902216751327,76.4694425933533,
16.0978610342767));
#255194=CARTESIAN_POINT('Ctrl Pts',(-27.0891144287658,76.4686678667903,
16.0974583211211));
#255195=CARTESIAN_POINT('Ctrl Pts',(-27.0880015580308,76.4678896257693,
16.097076081408));
#255196=CARTESIAN_POINT('Ctrl Pts',(-27.0853331024396,76.4660235495589,
16.0961595421663));
#255197=CARTESIAN_POINT('Ctrl Pts',(-27.0826307460464,76.4641359871599,
16.0953640053502));
#255198=CARTESIAN_POINT('Ctrl Pts',(-27.0799117554863,76.462236335893,16.0946554141566));
#255199=CARTESIAN_POINT('Ctrl Pts',(-27.0767300191218,76.4600133824172,
16.0938262276189));
#255200=CARTESIAN_POINT('Ctrl Pts',(-27.0735255691118,76.4577737617538,
16.0931150483633));
#255201=CARTESIAN_POINT('Ctrl Pts',(-27.0703421185465,76.4555446329423,
16.0923997928668));
#255202=CARTESIAN_POINT('Ctrl Pts',(-27.0701694407379,76.455423719779,16.0923609957349));
#255203=CARTESIAN_POINT('Ctrl Pts',(-27.0699968278378,76.4553028401788,
16.0923221754269));
#255204=CARTESIAN_POINT('Ctrl Pts',(-27.0698242878259,76.4551819993629,
16.0922833090418));
#255205=CARTESIAN_POINT('Ctrl Pts',(-27.0679952382887,76.4539009988822,
16.0918712971096));
#255206=CARTESIAN_POINT('Ctrl Pts',(-27.0661576675468,76.4526148397304,
16.0915037642175));
#255207=CARTESIAN_POINT('Ctrl Pts',(-27.0643159032437,76.4513260707313,
16.0911596237272));
#255208=CARTESIAN_POINT('Ctrl Pts',(-27.0591307079062,76.4476977459811,
16.0901907507488));
#255209=CARTESIAN_POINT('Ctrl Pts',(-27.0539254560322,76.4440580085204,
16.0893896618873));
#255210=CARTESIAN_POINT('Ctrl Pts',(-27.0487135067179,76.4404106076753,
16.0886634815155));
#255211=CARTESIAN_POINT('Ctrl Pts',(-27.0439334748512,76.4370654691831,
16.087997480158));
#255212=CARTESIAN_POINT('Ctrl Pts',(-27.0391479476081,76.4337143857031,
16.0873933983776));
#255213=CARTESIAN_POINT('Ctrl Pts',(-27.0343616852157,76.4303615098117,
16.0868217458837));
#255214=CARTESIAN_POINT('Ctrl Pts',(-27.0296521096837,76.4270623546536,
16.0862592525689));
#255215=CARTESIAN_POINT('Ctrl Pts',(-27.0249418477206,76.4237617060353,
16.0857279855821));
#255216=CARTESIAN_POINT('Ctrl Pts',(-27.0202287452912,76.4204596636729,
16.0852507551713));
#255217=CARTESIAN_POINT('Ctrl Pts',(-27.0173943327058,76.418473848476,16.0849637535831));
#255218=CARTESIAN_POINT('Ctrl Pts',(-27.0145587580626,76.4164874330431,
16.0846973118287));
#255219=CARTESIAN_POINT('Ctrl Pts',(-27.0117203818392,76.4144993121772,
16.0844653135676));
#255220=CARTESIAN_POINT('Ctrl Pts',(-27.008223903867,76.4120502285228,16.0841795245298));
#255221=CARTESIAN_POINT('Ctrl Pts',(-27.004737697993,76.4096083908123,16.0839285965694));
#255222=CARTESIAN_POINT('Ctrl Pts',(-27.0012653012945,76.4071765600896,
16.0836332011111));
#255223=CARTESIAN_POINT('',(-27.0012528338594,76.4071670555372,12.3825));
#255224=CARTESIAN_POINT('Origin',(-110.478801107225,75.6605890912239,12.3825));
#255225=CARTESIAN_POINT('',(-76.4952184082714,27.1270025958469,16.1248510148134));
#255226=CARTESIAN_POINT('Ctrl Pts',(-76.407176981863,27.0012661163039,16.0836344441047));
#255227=CARTESIAN_POINT('Ctrl Pts',(-76.4096082525859,27.0047377874469,
16.0839286114047));
#255228=CARTESIAN_POINT('Ctrl Pts',(-76.4120499969459,27.0082239404907,
16.0841797723545));
#255229=CARTESIAN_POINT('Ctrl Pts',(-76.4144904864623,27.0117082126661,
16.084464309092));
#255230=CARTESIAN_POINT('Ctrl Pts',(-76.4178226283415,27.0164654915462,
16.0848528036021));
#255231=CARTESIAN_POINT('Ctrl Pts',(-76.4211512987705,27.0212167837015,
16.0853190683136));
#255232=CARTESIAN_POINT('Ctrl Pts',(-76.4244788255282,27.0259665551592,
16.0858213410313));
#255233=CARTESIAN_POINT('Ctrl Pts',(-76.4278323603589,27.0307534510073,
16.0863275395312));
#255234=CARTESIAN_POINT('Ctrl Pts',(-76.4311845627328,27.0355388328798,
16.0868702293981));
#255235=CARTESIAN_POINT('Ctrl Pts',(-76.4345322490906,27.0403202016861,
16.0874595949035));
#255236=CARTESIAN_POINT('Ctrl Pts',(-76.4382607888103,27.0456455283754,
16.0881160102486));
#255237=CARTESIAN_POINT('Ctrl Pts',(-76.4419833123755,27.0509659278798,
16.0888302425902));
#255238=CARTESIAN_POINT('Ctrl Pts',(-76.4456927956894,27.0562681644591,
16.0896862961685));
#255239=CARTESIAN_POINT('Ctrl Pts',(-76.4475050299992,27.0588585238798,
16.0901045133526));
#255240=CARTESIAN_POINT('Ctrl Pts',(-76.4493141547839,27.0614444001031,
16.0905576105995));
#255241=CARTESIAN_POINT('Ctrl Pts',(-76.4511197912145,27.0640236135643,
16.0910594910211));
#255242=CARTESIAN_POINT('Ctrl Pts',(-76.4515396251712,27.0646233142428,
16.0911761847473));
#255243=CARTESIAN_POINT('Ctrl Pts',(-76.4519590933763,27.0652224173104,
16.0912956547428));
#255244=CARTESIAN_POINT('Ctrl Pts',(-76.4523781037608,27.0658207705619,
16.0914185979661));
#255245=CARTESIAN_POINT('Ctrl Pts',(-76.4549022186636,27.0694252453321,
16.0921592068717));
#255246=CARTESIAN_POINT('Ctrl Pts',(-76.4574399975644,27.0730526643745,
16.0929214221549));
#255247=CARTESIAN_POINT('Ctrl Pts',(-76.4599565375938,27.0766494404427,
16.0938416360861));
#255248=CARTESIAN_POINT('Ctrl Pts',(-76.4618925010159,27.0794164248039,
16.094549552706));
#255249=CARTESIAN_POINT('Ctrl Pts',(-76.463815987432,27.082165233867,16.0953521030019));
#255250=CARTESIAN_POINT('Ctrl Pts',(-76.4657181558851,27.0848806691378,
16.0962784075483));
#255251=CARTESIAN_POINT('Ctrl Pts',(-76.4662885977097,27.0856950017738,
16.0965561972754));
#255252=CARTESIAN_POINT('Ctrl Pts',(-76.4668571749586,27.0865064098562,
16.0968447965765));
#255253=CARTESIAN_POINT('Ctrl Pts',(-76.467423792878,27.0873147048393,16.0971440360151));
#255254=CARTESIAN_POINT('Ctrl Pts',(-76.4688130125272,27.0892964622714,
16.0978777037898));
#255255=CARTESIAN_POINT('Ctrl Pts',(-76.4702047210385,27.091275986821,16.0986102840892));
#255256=CARTESIAN_POINT('Ctrl Pts',(-76.4715818076992,27.0932317934172,
16.0994143656064));
#255257=CARTESIAN_POINT('Ctrl Pts',(-76.4728667914224,27.0950567908655,
16.1001646681772));
#255258=CARTESIAN_POINT('Ctrl Pts',(-76.4741390840003,27.0968611735704,
16.1009779446272));
#255259=CARTESIAN_POINT('Ctrl Pts',(-76.4753926606373,27.0986398464175,
16.1018707649366));
#255260=CARTESIAN_POINT('Ctrl Pts',(-76.4765871669744,27.1003347056906,
16.1027215142933));
#255261=CARTESIAN_POINT('Ctrl Pts',(-76.4777647424805,27.1020062843517,
16.1036447607616));
#255262=CARTESIAN_POINT('Ctrl Pts',(-76.4789268718429,27.1036611183308,
16.1046080215368));
#255263=CARTESIAN_POINT('Ctrl Pts',(-76.4792269606518,27.1040884349221,
16.1048567578548));
#255264=CARTESIAN_POINT('Ctrl Pts',(-76.4795260526579,27.1045146909905,
16.1051079007516));
#255265=CARTESIAN_POINT('Ctrl Pts',(-76.4798242409137,27.1049401152199,
16.1053603339431));
#255266=CARTESIAN_POINT('Ctrl Pts',(-76.4814025307668,27.107191856298,16.1066964453999));
#255267=CARTESIAN_POINT('Ctrl Pts',(-76.4829517841693,27.1094086966921,
16.1081566984987));
#255268=CARTESIAN_POINT('Ctrl Pts',(-76.4844580502449,27.1115676990793,
16.1097553365814));
#255269=CARTESIAN_POINT('Ctrl Pts',(-76.4864630730681,27.1144415930957,
16.1118833177486));
#255270=CARTESIAN_POINT('Ctrl Pts',(-76.4883927334351,27.1172143946534,
16.1142515910474));
#255271=CARTESIAN_POINT('Ctrl Pts',(-76.4902196926308,27.1198385003604,
16.1168182560628));
#255272=CARTESIAN_POINT('Ctrl Pts',(-76.4917485107915,27.1220343788836,
16.118966067627));
#255273=CARTESIAN_POINT('Ctrl Pts',(-76.4932057033912,27.1241266280223,
16.1212487745052));
#255274=CARTESIAN_POINT('Ctrl Pts',(-76.4945703804079,27.1260772883321,
16.1236712941847));
#255275=CARTESIAN_POINT('Ctrl Pts',(-76.494788931528,27.126389683859,16.1240592573312));
#255276=CARTESIAN_POINT('Ctrl Pts',(-76.4950049324782,27.126698210098,16.1244524123581));
#255277=CARTESIAN_POINT('Ctrl Pts',(-76.4952182372905,27.1270026655082,
16.124851038856));
#255278=CARTESIAN_POINT('',(-76.5327357173542,27.1805645602828,16.1924969468886));
#255279=CARTESIAN_POINT('Ctrl Pts',(-76.4952187502333,27.1270024565244,
16.124850966728));
#255280=CARTESIAN_POINT('Ctrl Pts',(-76.506055561861,27.1424765592851,16.1451084949868));
#255281=CARTESIAN_POINT('Ctrl Pts',(-76.5171175285349,27.1582694731656,
16.1650670172575));
#255282=CARTESIAN_POINT('Ctrl Pts',(-76.528303088887,27.1742368495269,16.1847307967182));
#255283=CARTESIAN_POINT('Ctrl Pts',(-76.529778551616,27.1763430711163,16.1873246027319));
#255284=CARTESIAN_POINT('Ctrl Pts',(-76.5312561700818,27.1784523972839,
16.1899133077663));
#255285=CARTESIAN_POINT('Ctrl Pts',(-76.5327357173542,27.1805645602828,
16.1924969468886));
#255286=CARTESIAN_POINT('',(-110.478801107225,75.6605890912239,16.1925));
#255287=CARTESIAN_POINT('',(-76.4071670555372,27.0012528338594,14.2875));
#255288=CARTESIAN_POINT('Origin',(0.,0.,12.3825));
#255289=CARTESIAN_POINT('',(-112.039285751595,74.5679259799751,12.3825));
#255290=CARTESIAN_POINT('',(-113.095,76.1978262581577,12.3825));
#255291=CARTESIAN_POINT('Origin',(-90.,90.,12.3825));
#255292=CARTESIAN_POINT('',(-113.095,-76.1978262581577,12.3825));
#255293=CARTESIAN_POINT('',(-113.095,-90.,12.3825));
#255294=CARTESIAN_POINT('',(-112.039285751595,-74.5679259799751,12.3825));
#255295=CARTESIAN_POINT('Origin',(-90.,-90.,12.3825));
#255296=CARTESIAN_POINT('',(-77.9676516999077,-25.9085897226107,12.3825));
#255297=CARTESIAN_POINT('Origin',(0.,0.,12.3825));
#255298=CARTESIAN_POINT('',(-112.039285751595,74.5679259799751,12.3825));
#255299=CARTESIAN_POINT('Origin',(-110.478801107225,-75.6605890912239,12.3825));
#255300=CARTESIAN_POINT('',(-76.5327354732302,-27.1805647392017,16.1924983103146));
#255301=CARTESIAN_POINT('',(-110.478801107225,-75.6605890912239,16.1925));
#255302=CARTESIAN_POINT('',(-76.4952184105099,-27.1270026766394,16.1248509803166));
#255303=CARTESIAN_POINT('Ctrl Pts',(-76.532735809375,-27.1805652197814,
16.1924970380414));
#255304=CARTESIAN_POINT('Ctrl Pts',(-76.5215147093823,-27.1645460748958,
16.1729026402457));
#255305=CARTESIAN_POINT('Ctrl Pts',(-76.5104044301563,-27.1486864747344,
16.1530153167097));
#255306=CARTESIAN_POINT('Ctrl Pts',(-76.4995059105232,-27.1331242473368,
16.132828249725));
#255307=CARTESIAN_POINT('Ctrl Pts',(-76.4980731096455,-27.1310783205666,
16.1301743069634));
#255308=CARTESIAN_POINT('Ctrl Pts',(-76.4966439736256,-27.1290376020245,
16.1275152100406));
#255309=CARTESIAN_POINT('Ctrl Pts',(-76.4952187349081,-27.1270024664543,
16.1248509673423));
#255310=CARTESIAN_POINT('Ctrl Pts',(-76.4952182482945,-27.1270027817086,
16.1248509867732));
#255311=CARTESIAN_POINT('Ctrl Pts',(-76.4931858448006,-27.1240985616638,
16.121049825422));
#255312=CARTESIAN_POINT('Ctrl Pts',(-76.4909301697861,-27.1208691627763,
16.1175138339431));
#255313=CARTESIAN_POINT('Ctrl Pts',(-76.4885126429384,-27.1174141814444,
16.1144000399021));
#255314=CARTESIAN_POINT('Ctrl Pts',(-76.4872742275686,-27.1156443140332,
16.1128049509365));
#255315=CARTESIAN_POINT('Ctrl Pts',(-76.4859930220507,-27.1138145047011,
16.1113222637541));
#255316=CARTESIAN_POINT('Ctrl Pts',(-76.4846791602534,-27.1119395447418,
16.1099492026215));
#255317=CARTESIAN_POINT('Ctrl Pts',(-76.4834282152446,-27.1101543708312,
16.1086418931511));
#255318=CARTESIAN_POINT('Ctrl Pts',(-76.4821474484747,-27.1083279408346,
16.1074352878857));
#255319=CARTESIAN_POINT('Ctrl Pts',(-76.4808505836411,-27.1064797666398,
16.1062837053213));
#255320=CARTESIAN_POINT('Ctrl Pts',(-76.4801127643227,-27.1054282934335,
16.1056285407733));
#255321=CARTESIAN_POINT('Ctrl Pts',(-76.4793696983962,-27.1043708082513,
16.1049758051017));
#255322=CARTESIAN_POINT('Ctrl Pts',(-76.4786223769383,-27.1033071871103,
16.1043249482959));
#255323=CARTESIAN_POINT('Ctrl Pts',(-76.4773023951153,-27.1014285302648,
16.1031753504303));
#255324=CARTESIAN_POINT('Ctrl Pts',(-76.475964397667,-27.0995243610965,
16.1020872183569));
#255325=CARTESIAN_POINT('Ctrl Pts',(-76.4746063057845,-27.0975893324811,
16.1011009833628));
#255326=CARTESIAN_POINT('Ctrl Pts',(-76.4731630291583,-27.0955329314322,
16.1000528879186));
#255327=CARTESIAN_POINT('Ctrl Pts',(-76.4716969774167,-27.0934416442518,
16.0991197155412));
#255328=CARTESIAN_POINT('Ctrl Pts',(-76.4702124651068,-27.0913212940051,
16.0982908738278));
#255329=CARTESIAN_POINT('Ctrl Pts',(-76.4694425873394,-27.0902216665361,
16.0978610311087));
#255330=CARTESIAN_POINT('Ctrl Pts',(-76.4686678615982,-27.0891144213408,
16.0974583185077));
#255331=CARTESIAN_POINT('Ctrl Pts',(-76.4678896214075,-27.0880015517915,
16.0970760792947));
#255332=CARTESIAN_POINT('Ctrl Pts',(-76.4660235449902,-27.0853330959005,
16.0961595401724));
#255333=CARTESIAN_POINT('Ctrl Pts',(-76.4641359823881,-27.0826307392147,
16.0953640034684));
#255334=CARTESIAN_POINT('Ctrl Pts',(-76.4622363309284,-27.0799117483802,
16.0946554123439));
#255335=CARTESIAN_POINT('Ctrl Pts',(-76.4600133772259,-27.0767300116927,
16.0938262258867));
#255336=CARTESIAN_POINT('Ctrl Pts',(-76.4577737563502,-27.0735255613849,
16.0931150466518));
#255337=CARTESIAN_POINT('Ctrl Pts',(-76.4555446273526,-27.070342110563,
16.092399791074));
#255338=CARTESIAN_POINT('Ctrl Pts',(-76.4554237160546,-27.0701694354188,
16.0923609945394));
#255339=CARTESIAN_POINT('Ctrl Pts',(-76.4553028383187,-27.0699968251812,
16.0923221748292));
#255340=CARTESIAN_POINT('Ctrl Pts',(-76.455181999366,-27.0698242878295,
16.0922833090433));
#255341=CARTESIAN_POINT('Ctrl Pts',(-76.4539009977357,-27.0679952366507,
16.0918712967414));
#255342=CARTESIAN_POINT('Ctrl Pts',(-76.4526148374245,-27.0661576642512,
16.0915037635639));
#255343=CARTESIAN_POINT('Ctrl Pts',(-76.4513260672622,-27.0643158982848,
16.0911596228214));
#255344=CARTESIAN_POINT('Ctrl Pts',(-76.4476977425727,-27.0591307030318,
16.0901907500241));
#255345=CARTESIAN_POINT('Ctrl Pts',(-76.4440580051801,-27.053925451258,
16.0893896612632));
#255346=CARTESIAN_POINT('Ctrl Pts',(-76.4404106044097,-27.048713502053,
16.0886634809515));
#255347=CARTESIAN_POINT('Ctrl Pts',(-76.4370654658784,-27.0439334701325,
16.0879974796278));
#255348=CARTESIAN_POINT('Ctrl Pts',(-76.4337143823643,-27.0391479428428,
16.0873933978516));
#255349=CARTESIAN_POINT('Ctrl Pts',(-76.4303615064407,-27.0343616804054,
16.0868217453606));
#255350=CARTESIAN_POINT('Ctrl Pts',(-76.4270623512098,-27.0296521047703,
16.0862592520419));
#255351=CARTESIAN_POINT('Ctrl Pts',(-76.4237617025205,-27.0249418427056,
16.0857279850509));
#255352=CARTESIAN_POINT('Ctrl Pts',(-76.4204596600846,-27.0202287401702,
16.0852507546629));
#255353=CARTESIAN_POINT('Ctrl Pts',(-76.4184738460836,-27.0173943292914,
16.0849637532678));
#255354=CARTESIAN_POINT('Ctrl Pts',(-76.4164874318464,-27.0145587563545,
16.0846973116911));
#255355=CARTESIAN_POINT('Ctrl Pts',(-76.414499312177,-27.0117203818391,
16.0844653135703));
#255356=CARTESIAN_POINT('Ctrl Pts',(-76.4120502285228,-27.0082239038667,
16.0841795245333));
#255357=CARTESIAN_POINT('Ctrl Pts',(-76.4096083908209,-27.0047376980153,
16.083928596514));
#255358=CARTESIAN_POINT('Ctrl Pts',(-76.4071765580783,-27.0012652984223,
16.0836331977649));
#255359=CARTESIAN_POINT('',(-110.478801107225,-75.6605890912239,14.2875));
#255360=CARTESIAN_POINT('Origin',(-75.6605890912239,-110.478801107225,12.3825));
#255361=CARTESIAN_POINT('',(-27.0012528338594,-76.4071670555372,14.2875));
#255362=CARTESIAN_POINT('',(-27.0012528338594,-76.4071670555372,16.0836603564332));
#255363=CARTESIAN_POINT('',(-27.0012528338594,-76.4071670555372,17.0741173620444));
#255364=CARTESIAN_POINT('',(-27.127002595847,-76.4952184082715,16.1248510148133));
#255365=CARTESIAN_POINT('Ctrl Pts',(-27.0012661163037,-76.4071769818629,
16.0836344441051));
#255366=CARTESIAN_POINT('Ctrl Pts',(-27.0047377874469,-76.4096082525859,
16.0839286114036));
#255367=CARTESIAN_POINT('Ctrl Pts',(-27.0082239404904,-76.4120499969456,
16.0841797723569));
#255368=CARTESIAN_POINT('Ctrl Pts',(-27.0117082126658,-76.4144904864621,
16.0844643090938));
#255369=CARTESIAN_POINT('Ctrl Pts',(-27.0164654915443,-76.4178226283401,
16.0848528036029));
#255370=CARTESIAN_POINT('Ctrl Pts',(-27.0212167836978,-76.4211512987679,
16.0853190683137));
#255371=CARTESIAN_POINT('Ctrl Pts',(-27.0259665551539,-76.4244788255244,
16.0858213410309));
#255372=CARTESIAN_POINT('Ctrl Pts',(-27.0307534510004,-76.427832360354,
16.0863275395304));
#255373=CARTESIAN_POINT('Ctrl Pts',(-27.0355388328714,-76.4311845627269,
16.086870229397));
#255374=CARTESIAN_POINT('Ctrl Pts',(-27.0403202016761,-76.4345322490837,
16.0874595949021));
#255375=CARTESIAN_POINT('Ctrl Pts',(-27.0456455283646,-76.4382607888028,
16.0881160102471));
#255376=CARTESIAN_POINT('Ctrl Pts',(-27.0509659278681,-76.4419833123674,
16.0888302425885));
#255377=CARTESIAN_POINT('Ctrl Pts',(-27.0562681644465,-76.4456927956806,
16.0896862961667));
#255378=CARTESIAN_POINT('Ctrl Pts',(-27.0588585238712,-76.4475050299932,
16.0901045133513));
#255379=CARTESIAN_POINT('Ctrl Pts',(-27.0614444000984,-76.4493141547807,
16.0905576105989));
#255380=CARTESIAN_POINT('Ctrl Pts',(-27.0640236135634,-76.4511197912139,
16.0910594910214));
#255381=CARTESIAN_POINT('Ctrl Pts',(-27.064623314242,-76.4515396251707,
16.0911761847476));
#255382=CARTESIAN_POINT('Ctrl Pts',(-27.0652224173098,-76.4519590933759,
16.0912956547432));
#255383=CARTESIAN_POINT('Ctrl Pts',(-27.0658207705614,-76.4523781037604,
16.0914185979665));
#255384=CARTESIAN_POINT('Ctrl Pts',(-27.0694252453316,-76.4549022186632,
16.092159206872));
#255385=CARTESIAN_POINT('Ctrl Pts',(-27.0730526643741,-76.4574399975641,
16.0929214221551));
#255386=CARTESIAN_POINT('Ctrl Pts',(-27.0766494404423,-76.4599565375935,
16.0938416360861));
#255387=CARTESIAN_POINT('Ctrl Pts',(-27.0794164248033,-76.4618925010154,
16.0945495527057));
#255388=CARTESIAN_POINT('Ctrl Pts',(-27.0821652338662,-76.4638159874314,
16.0953521030014));
#255389=CARTESIAN_POINT('Ctrl Pts',(-27.0848806691367,-76.4657181558843,
16.0962784075474));
#255390=CARTESIAN_POINT('Ctrl Pts',(-27.085695001773,-76.4662885977091,
16.0965561972746));
#255391=CARTESIAN_POINT('Ctrl Pts',(-27.0865064098557,-76.4668571749581,
16.0968447965757));
#255392=CARTESIAN_POINT('Ctrl Pts',(-27.087314704839,-76.4674237928777,
16.0971440360144));
#255393=CARTESIAN_POINT('Ctrl Pts',(-27.0892964622713,-76.4688130125271,
16.097877703789));
#255394=CARTESIAN_POINT('Ctrl Pts',(-27.091275986821,-76.4702047210384,
16.0986102840886));
#255395=CARTESIAN_POINT('Ctrl Pts',(-27.0932317934173,-76.4715818076992,
16.0994143656059));
#255396=CARTESIAN_POINT('Ctrl Pts',(-27.0950567908658,-76.4728667914225,
16.1001646681769));
#255397=CARTESIAN_POINT('Ctrl Pts',(-27.0968611735707,-76.4741390840004,
16.1009779446271));
#255398=CARTESIAN_POINT('Ctrl Pts',(-27.0986398464179,-76.4753926606374,
16.1018707649367));
#255399=CARTESIAN_POINT('Ctrl Pts',(-27.1003347056911,-76.4765871669746,
16.1027215142937));
#255400=CARTESIAN_POINT('Ctrl Pts',(-27.1020062843522,-76.4777647424807,
16.1036447607621));
#255401=CARTESIAN_POINT('Ctrl Pts',(-27.1036611183315,-76.4789268718433,
16.1046080215375));
#255402=CARTESIAN_POINT('Ctrl Pts',(-27.1040884349225,-76.479226960652,
16.1048567578554));
#255403=CARTESIAN_POINT('Ctrl Pts',(-27.1045146909907,-76.4795260526579,
16.105107900752));
#255404=CARTESIAN_POINT('Ctrl Pts',(-27.1049401152198,-76.4798242409135,
16.1053603339433));
#255405=CARTESIAN_POINT('Ctrl Pts',(-27.1071918562982,-76.4814025307668,
16.1066964454002));
#255406=CARTESIAN_POINT('Ctrl Pts',(-27.1094086966924,-76.4829517841694,
16.1081566984993));
#255407=CARTESIAN_POINT('Ctrl Pts',(-27.1115676990799,-76.4844580502452,
16.1097553365821));
#255408=CARTESIAN_POINT('Ctrl Pts',(-27.1144415930974,-76.4864630730692,
16.1118833177503));
#255409=CARTESIAN_POINT('Ctrl Pts',(-27.1172143946562,-76.488392733437,
16.1142515910502));
#255410=CARTESIAN_POINT('Ctrl Pts',(-27.1198385003641,-76.4902196926333,
16.1168182560667));
#255411=CARTESIAN_POINT('Ctrl Pts',(-27.1220343788854,-76.4917485107927,
16.1189660676294));
#255412=CARTESIAN_POINT('Ctrl Pts',(-27.1241266280224,-76.4932057033912,
16.1212487745057));
#255413=CARTESIAN_POINT('Ctrl Pts',(-27.1260772883308,-76.4945703804069,
16.1236712941829));
#255414=CARTESIAN_POINT('Ctrl Pts',(-27.1263896838582,-76.4947889315274,
16.12405925733));
#255415=CARTESIAN_POINT('Ctrl Pts',(-27.1266982100976,-76.4950049324779,
16.1244524123575));
#255416=CARTESIAN_POINT('Ctrl Pts',(-27.1270026655083,-76.4952182372905,
16.124851038856));
#255417=CARTESIAN_POINT('',(-27.1805645602868,-76.5327357173571,16.1924969468894));
#255418=CARTESIAN_POINT('Ctrl Pts',(-27.1270024565245,-76.4952187502334,
16.124850966728));
#255419=CARTESIAN_POINT('Ctrl Pts',(-27.1424765592086,-76.5060555618075,
16.1451084948867));
#255420=CARTESIAN_POINT('Ctrl Pts',(-27.1582694730108,-76.5171175284266,
16.1650670170587));
#255421=CARTESIAN_POINT('Ctrl Pts',(-27.1742368492934,-76.5283030887235,
16.1847307964267));
#255422=CARTESIAN_POINT('Ctrl Pts',(-27.1763430709617,-76.5297785515079,
16.1873246025381));
#255423=CARTESIAN_POINT('Ctrl Pts',(-27.1784523972085,-76.5312561700291,
16.1899133076699));
#255424=CARTESIAN_POINT('Ctrl Pts',(-27.1805645602868,-76.5327357173571,
16.1924969468894));
#255425=CARTESIAN_POINT('',(-75.6605890912239,-110.478801107225,16.1925));
#255426=CARTESIAN_POINT('',(-27.0012528338595,-76.4071670555372,14.2875));
#255427=CARTESIAN_POINT('Origin',(0.,0.,12.3825));
#255428=CARTESIAN_POINT('',(-74.5679259799751,-112.039285751595,12.3825));
#255429=CARTESIAN_POINT('',(-76.1978262581577,-113.095,12.3825));
#255430=CARTESIAN_POINT('Origin',(-90.,-90.,12.3825));
#255431=CARTESIAN_POINT('',(76.1978262581577,-113.095,12.3825));
#255432=CARTESIAN_POINT('',(90.,-113.095,12.3825));
#255433=CARTESIAN_POINT('',(74.5679259799751,-112.039285751595,12.3825));
#255434=CARTESIAN_POINT('Origin',(90.,-90.,12.3825));
#255435=CARTESIAN_POINT('',(25.9085897226107,-77.9676516999077,12.3825));
#255436=CARTESIAN_POINT('',(25.9085897226107,-77.9676516999077,12.3825));
#255437=CARTESIAN_POINT('',(25.3478497357421,-77.8839876917858,12.3825));
#255438=CARTESIAN_POINT('Origin',(25.5443686855278,-78.4878132480313,12.3825));
#255439=CARTESIAN_POINT('',(-25.3478497357421,-77.8839876917858,12.3825));
#255440=CARTESIAN_POINT('Origin',(0.,0.,12.3825));
#255441=CARTESIAN_POINT('',(-25.9085897226107,-77.9676516999077,12.3825));
#255442=CARTESIAN_POINT('Origin',(-25.5443686855278,-78.4878132480312,12.3825));
#255443=CARTESIAN_POINT('',(-74.5679259799751,-112.039285751595,12.3825));
#255444=CARTESIAN_POINT('Origin',(75.6605890912239,-110.478801107225,12.3825));
#255445=CARTESIAN_POINT('',(27.1805647391996,-76.5327354732286,16.1924983103144));
#255446=CARTESIAN_POINT('',(75.6605890912239,-110.478801107225,16.1925));
#255447=CARTESIAN_POINT('',(27.1270026766432,-76.4952184105121,16.1248509803218));
#255448=CARTESIAN_POINT('Ctrl Pts',(27.1805652197793,-76.5327358093735,
16.192497038041));
#255449=CARTESIAN_POINT('Ctrl Pts',(27.1645460748553,-76.5215147093538,
16.1729026401982));
#255450=CARTESIAN_POINT('Ctrl Pts',(27.1486864746558,-76.5104044301012,
16.153015316612));
#255451=CARTESIAN_POINT('Ctrl Pts',(27.1331242472215,-76.4995059104423,
16.1328282495759));
#255452=CARTESIAN_POINT('Ctrl Pts',(27.1310783204899,-76.4980731095918,
16.1301743068639));
#255453=CARTESIAN_POINT('Ctrl Pts',(27.1290376019863,-76.4966439735989,
16.127515209991));
#255454=CARTESIAN_POINT('Ctrl Pts',(27.1270024664544,-76.4952187349081,
16.1248509673428));
#255455=CARTESIAN_POINT('',(27.0012528338594,-76.4071670555372,16.0836576814802));
#255456=CARTESIAN_POINT('Ctrl Pts',(27.1270027817125,-76.4952182482966,
16.1248509867785));
#255457=CARTESIAN_POINT('Ctrl Pts',(27.1240985616685,-76.4931858448008,
16.1210498254261));
#255458=CARTESIAN_POINT('Ctrl Pts',(27.1208691627774,-76.4909301697841,
16.1175138339627));
#255459=CARTESIAN_POINT('Ctrl Pts',(27.1174141814443,-76.4885126429366,
16.1144000399211));
#255460=CARTESIAN_POINT('Ctrl Pts',(27.1156443139851,-76.4872742275337,
16.1128049509126));
#255461=CARTESIAN_POINT('Ctrl Pts',(27.1138145046022,-76.485993021981,16.1113222636901));
#255462=CARTESIAN_POINT('Ctrl Pts',(27.1119395445906,-76.4846791601475,
16.1099492025217));
#255463=CARTESIAN_POINT('Ctrl Pts',(27.110154370728,-76.4834282151728,16.1086418930888));
#255464=CARTESIAN_POINT('Ctrl Pts',(27.1083279407825,-76.4821474484391,
16.1074352878535));
#255465=CARTESIAN_POINT('Ctrl Pts',(27.1064797666391,-76.4808505836416,
16.1062837053212));
#255466=CARTESIAN_POINT('Ctrl Pts',(27.1054282931702,-76.4801127641388,
16.1056285406094));
#255467=CARTESIAN_POINT('Ctrl Pts',(27.1043708077217,-76.4793696980249,
16.1049758047786));
#255468=CARTESIAN_POINT('Ctrl Pts',(27.1033071863107,-76.4786223763771,
16.1043249478184));
#255469=CARTESIAN_POINT('Ctrl Pts',(27.1014285294456,-76.47730239454,16.1031753499598));
#255470=CARTESIAN_POINT('Ctrl Pts',(27.0995243602564,-76.4759643970771,
16.1020872179032));
#255471=CARTESIAN_POINT('Ctrl Pts',(27.0975893316198,-76.4746063051802,
16.1011009829297));
#255472=CARTESIAN_POINT('Ctrl Pts',(27.0955329305412,-76.4731630285335,
16.1000528875037));
#255473=CARTESIAN_POINT('Ctrl Pts',(27.0934416433306,-76.4716969767713,
16.0991197151495));
#255474=CARTESIAN_POINT('Ctrl Pts',(27.0913212930545,-76.4702124644414,
16.0982908734576));
#255475=CARTESIAN_POINT('Ctrl Pts',(27.0902216656986,-76.4694425867535,
16.0978610307999));
#255476=CARTESIAN_POINT('Ctrl Pts',(27.0891144206185,-76.4686678610931,
16.0974583182533));
#255477=CARTESIAN_POINT('Ctrl Pts',(27.0880015511858,-76.467889620984,16.0970760790894));
#255478=CARTESIAN_POINT('Ctrl Pts',(27.0853330952647,-76.466023544546,16.0961595399788));
#255479=CARTESIAN_POINT('Ctrl Pts',(27.0826307385496,-76.4641359819234,
16.0953640032855));
#255480=CARTESIAN_POINT('Ctrl Pts',(27.0799117476875,-76.4622363304444,
16.0946554121674));
#255481=CARTESIAN_POINT('Ctrl Pts',(27.0767300109675,-76.460013376719,16.0938262257177));
#255482=CARTESIAN_POINT('Ctrl Pts',(27.0735255606295,-76.4577737558219,
16.0931150464844));
#255483=CARTESIAN_POINT('Ctrl Pts',(27.0703421097814,-76.4555446268054,
16.0923997908983));
#255484=CARTESIAN_POINT('Ctrl Pts',(27.0701694348977,-76.4554237156897,
16.0923609944221));
#255485=CARTESIAN_POINT('Ctrl Pts',(27.0699968249205,-76.4553028381361,
16.0923221747704));
#255486=CARTESIAN_POINT('Ctrl Pts',(27.0698242878289,-76.4551819993657,
16.0922833090431));
#255487=CARTESIAN_POINT('Ctrl Pts',(27.0679952364911,-76.453900997624,16.0918712967054));
#255488=CARTESIAN_POINT('Ctrl Pts',(27.066157663931,-76.4526148372005,16.0915037635003));
#255489=CARTESIAN_POINT('Ctrl Pts',(27.0643158978034,-76.4513260669254,
16.0911596227336));
#255490=CARTESIAN_POINT('Ctrl Pts',(27.0591307025578,-76.4476977422412,
16.0901907499542));
#255491=CARTESIAN_POINT('Ctrl Pts',(27.053925450793,-76.4440580048548,16.0893896612033));
#255492=CARTESIAN_POINT('Ctrl Pts',(27.0487135015978,-76.4404106040911,
16.0886634808975));
#255493=CARTESIAN_POINT('Ctrl Pts',(27.0439334696713,-76.4370654655554,
16.087997479577));
#255494=CARTESIAN_POINT('Ctrl Pts',(27.0391479423763,-76.4337143820375,
16.087393397801));
#255495=CARTESIAN_POINT('Ctrl Pts',(27.0343616799338,-76.4303615061103,
16.0868217453101));
#255496=CARTESIAN_POINT('Ctrl Pts',(27.0296521042877,-76.4270623508715,
16.0862592519905));
#255497=CARTESIAN_POINT('Ctrl Pts',(27.0249418422122,-76.4237617021747,
16.0857279849987));
#255498=CARTESIAN_POINT('Ctrl Pts',(27.0202287396655,-76.4204596597309,
16.0852507546123));
#255499=CARTESIAN_POINT('Ctrl Pts',(27.017394328955,-76.4184738458479,16.0849637532358));
#255500=CARTESIAN_POINT('Ctrl Pts',(27.0145587561863,-76.4164874317286,
16.0846973116763));
#255501=CARTESIAN_POINT('Ctrl Pts',(27.0117203818393,-76.4144993121772,
16.0844653135687));
#255502=CARTESIAN_POINT('Ctrl Pts',(27.0082239038669,-76.4120502285229,
16.0841795245312));
#255503=CARTESIAN_POINT('Ctrl Pts',(27.0047376980176,-76.4096083908218,
16.0839285965081));
#255504=CARTESIAN_POINT('Ctrl Pts',(27.0012652981443,-76.4071765578836,
16.0836331974402));
#255505=CARTESIAN_POINT('',(27.0012528338594,-76.4071670555372,14.2875));
#255506=CARTESIAN_POINT('',(27.0012528338594,-76.4071670555372,12.3825));
#255507=CARTESIAN_POINT('',(75.6605890912239,-110.478801107225,14.2875));
#255508=CARTESIAN_POINT('Origin',(110.478801107225,-75.6605890912239,12.3825));
#255509=CARTESIAN_POINT('',(76.4071670555372,-27.0012528338594,16.0836603564331));
#255510=CARTESIAN_POINT('',(76.4071670555372,-27.0012528338594,17.0741173620445));
#255511=CARTESIAN_POINT('',(76.4952184082716,-27.1270025958472,16.1248510148123));
#255512=CARTESIAN_POINT('Ctrl Pts',(76.4071769818628,-27.0012661163035,
16.0836344441052));
#255513=CARTESIAN_POINT('Ctrl Pts',(76.4096082525859,-27.0047377874469,
16.0839286114014));
#255514=CARTESIAN_POINT('Ctrl Pts',(76.4120499969459,-27.0082239404908,
16.0841797723485));
#255515=CARTESIAN_POINT('Ctrl Pts',(76.4144904864623,-27.0117082126661,
16.0844643090874));
#255516=CARTESIAN_POINT('Ctrl Pts',(76.4178226283408,-27.0164654915454,
16.0848528035995));
#255517=CARTESIAN_POINT('Ctrl Pts',(76.4211512987692,-27.0212167836998,
16.0853190683122));
#255518=CARTESIAN_POINT('Ctrl Pts',(76.4244788255264,-27.0259665551567,
16.0858213410305));
#255519=CARTESIAN_POINT('Ctrl Pts',(76.4278323603563,-27.0307534510038,
16.0863275395311));
#255520=CARTESIAN_POINT('Ctrl Pts',(76.4311845627297,-27.0355388328754,
16.0868702293981));
#255521=CARTESIAN_POINT('Ctrl Pts',(76.4345322490869,-27.0403202016807,
16.0874595949032));
#255522=CARTESIAN_POINT('Ctrl Pts',(76.4382607888044,-27.0456455283668,
16.0881160102479));
#255523=CARTESIAN_POINT('Ctrl Pts',(76.4419833123674,-27.050965927868,16.0888302425885));
#255524=CARTESIAN_POINT('Ctrl Pts',(76.445692795679,-27.0562681644442,16.0896862961658));
#255525=CARTESIAN_POINT('Ctrl Pts',(76.4475050299921,-27.0588585238695,
16.0901045133504));
#255526=CARTESIAN_POINT('Ctrl Pts',(76.4493141547799,-27.0614444000973,
16.0905576105978));
#255527=CARTESIAN_POINT('Ctrl Pts',(76.4511197912136,-27.064023613563,16.0910594910203));
#255528=CARTESIAN_POINT('Ctrl Pts',(76.4515396251699,-27.0646233142409,
16.0911761847463));
#255529=CARTESIAN_POINT('Ctrl Pts',(76.4519590933746,-27.0652224173079,
16.0912956547417));
#255530=CARTESIAN_POINT('Ctrl Pts',(76.4523781037586,-27.0658207705587,
16.0914185979649));
#255531=CARTESIAN_POINT('Ctrl Pts',(76.4549022186616,-27.0694252453293,
16.0921592068704));
#255532=CARTESIAN_POINT('Ctrl Pts',(76.4574399975625,-27.0730526643718,
16.0929214221539));
#255533=CARTESIAN_POINT('Ctrl Pts',(76.459956537592,-27.0766494404402,16.0938416360852));
#255534=CARTESIAN_POINT('Ctrl Pts',(76.4618925010147,-27.0794164248023,
16.0945495527052));
#255535=CARTESIAN_POINT('Ctrl Pts',(76.4638159874315,-27.0821652338663,
16.0953521030014));
#255536=CARTESIAN_POINT('Ctrl Pts',(76.4657181558853,-27.0848806691381,
16.0962784075478));
#255537=CARTESIAN_POINT('Ctrl Pts',(76.4662885977095,-27.0856950017735,
16.0965561972746));
#255538=CARTESIAN_POINT('Ctrl Pts',(76.4668571749578,-27.0865064098552,
16.0968447965753));
#255539=CARTESIAN_POINT('Ctrl Pts',(76.4674237928768,-27.0873147048377,
16.0971440360135));
#255540=CARTESIAN_POINT('Ctrl Pts',(76.4688130125264,-27.0892964622702,
16.097877703788));
#255541=CARTESIAN_POINT('Ctrl Pts',(76.4702047210379,-27.0912759868201,
16.0986102840874));
#255542=CARTESIAN_POINT('Ctrl Pts',(76.4715818076988,-27.0932317934166,
16.0994143656047));
#255543=CARTESIAN_POINT('Ctrl Pts',(76.4728667914221,-27.0950567908652,
16.1001646681756));
#255544=CARTESIAN_POINT('Ctrl Pts',(76.4741390840002,-27.0968611735703,
16.1009779446259));
#255545=CARTESIAN_POINT('Ctrl Pts',(76.4753926606373,-27.0986398464177,
16.1018707649355));
#255546=CARTESIAN_POINT('Ctrl Pts',(76.4765871669746,-27.100334705691,16.1027215142925));
#255547=CARTESIAN_POINT('Ctrl Pts',(76.4777647424808,-27.1020062843523,
16.103644760761));
#255548=CARTESIAN_POINT('Ctrl Pts',(76.4789268718434,-27.1036611183317,
16.1046080215364));
#255549=CARTESIAN_POINT('Ctrl Pts',(76.479226960652,-27.1040884349225,16.1048567578542));
#255550=CARTESIAN_POINT('Ctrl Pts',(76.4795260526579,-27.1045146909906,
16.1051079007507));
#255551=CARTESIAN_POINT('Ctrl Pts',(76.4798242409133,-27.1049401152196,
16.105360333942));
#255552=CARTESIAN_POINT('Ctrl Pts',(76.4814025307667,-27.1071918562981,
16.106696445399));
#255553=CARTESIAN_POINT('Ctrl Pts',(76.4829517841694,-27.1094086966924,
16.1081566984981));
#255554=CARTESIAN_POINT('Ctrl Pts',(76.4844580502452,-27.11156769908,16.109755336581));
#255555=CARTESIAN_POINT('Ctrl Pts',(76.4864630730699,-27.1144415930985,
16.1118833177498));
#255556=CARTESIAN_POINT('Ctrl Pts',(76.4883927334383,-27.1172143946581,
16.1142515910506));
#255557=CARTESIAN_POINT('Ctrl Pts',(76.4902196926352,-27.1198385003668,
16.116818256068));
#255558=CARTESIAN_POINT('Ctrl Pts',(76.4917485107928,-27.1220343788856,
16.1189660676284));
#255559=CARTESIAN_POINT('Ctrl Pts',(76.4932057033898,-27.1241266280203,
16.1212487745022));
#255560=CARTESIAN_POINT('Ctrl Pts',(76.4945703804041,-27.1260772883268,
16.1236712941765));
#255561=CARTESIAN_POINT('Ctrl Pts',(76.4947889315256,-27.1263896838556,
16.1240592573253));
#255562=CARTESIAN_POINT('Ctrl Pts',(76.4950049324771,-27.1266982100965,
16.1244524123546));
#255563=CARTESIAN_POINT('Ctrl Pts',(76.4952182372907,-27.1270026655085,
16.1248510388549));
#255564=CARTESIAN_POINT('',(76.5327357173579,-27.1805645602878,16.1924969468896));
#255565=CARTESIAN_POINT('Ctrl Pts',(76.4952187502335,-27.1270024565246,
16.124850966727));
#255566=CARTESIAN_POINT('Ctrl Pts',(76.5060555611233,-27.1424765582316,
16.145108493606));
#255567=CARTESIAN_POINT('Ctrl Pts',(76.5171175270378,-27.1582694710288,
16.1650670145225));
#255568=CARTESIAN_POINT('Ctrl Pts',(76.5283030866075,-27.1742368462728,
16.1847307926956));
#255569=CARTESIAN_POINT('Ctrl Pts',(76.5297785500957,-27.1763430689457,
16.1873246000552));
#255570=CARTESIAN_POINT('Ctrl Pts',(76.5312561693226,-27.1784523961998,
16.1899133064308));
#255571=CARTESIAN_POINT('Ctrl Pts',(76.5327357173579,-27.1805645602878,
16.1924969468896));
#255572=CARTESIAN_POINT('',(110.478801107225,-75.6605890912239,16.1925));
#255573=CARTESIAN_POINT('',(76.4071670555372,-27.0012528338594,14.2875));
#255574=CARTESIAN_POINT('Origin',(0.,0.,12.3825));
#255575=CARTESIAN_POINT('',(112.039285751595,-74.5679259799751,12.3825));
#255576=CARTESIAN_POINT('',(113.095,-76.1978262581577,12.3825));
#255577=CARTESIAN_POINT('Origin',(90.,-90.,12.3825));
#255578=CARTESIAN_POINT('',(113.095,76.1978262581577,12.3825));
#255579=CARTESIAN_POINT('',(113.095,90.,12.3825));
#255580=CARTESIAN_POINT('',(112.039285751595,74.5679259799752,12.3825));
#255581=CARTESIAN_POINT('Origin',(90.,90.,12.3825));
#255582=CARTESIAN_POINT('',(77.9676516999077,25.9085897226107,12.3825));
#255583=CARTESIAN_POINT('',(112.039285751595,-74.5679259799751,12.3825));
#255584=CARTESIAN_POINT('Origin',(110.478801107225,75.6605890912239,12.3825));
#255585=CARTESIAN_POINT('',(76.532736336798,27.1805822708749,16.1924981569221));
#255586=CARTESIAN_POINT('',(110.478801107225,75.6605890912239,16.1925));
#255587=CARTESIAN_POINT('',(76.4071670555372,27.0012528338594,15.6374346123617));
#255588=CARTESIAN_POINT('Origin',(83.0120747021563,36.4340385244726,14.6668526149847));
#255589=CARTESIAN_POINT('',(76.4071670555372,27.0012528338594,12.3825));
#255590=CARTESIAN_POINT('',(110.478801107225,75.6605890912239,14.2875));
#255591=CARTESIAN_POINT('Origin',(-90.,-90.,8.255));
#255592=CARTESIAN_POINT('Origin',(0.,0.,42.4815));
#255593=CARTESIAN_POINT('Origin',(-90.,-90.,0.0381));
#255594=CARTESIAN_POINT('Origin',(0.,0.,17.0741173620444));
#255595=CARTESIAN_POINT('Origin',(11.0165705888139,72.9917616471425,17.0741029655967));
#255596=CARTESIAN_POINT('Ctrl Pts',(24.6976449914385,76.0424582865173,17.8479876926671));
#255597=CARTESIAN_POINT('Ctrl Pts',(24.7379368836041,76.0624207920021,17.5919904624028));
#255598=CARTESIAN_POINT('Ctrl Pts',(24.758292886385,76.0725110230494,17.3340474816321));
#255599=CARTESIAN_POINT('Ctrl Pts',(24.758292886385,76.0725110230494,17.0741173620444));
#255600=CARTESIAN_POINT('Origin',(0.,0.,17.0741173620445));
#255601=CARTESIAN_POINT('Origin',(-11.016570588808,72.9917616471582,17.0741029655978));
#255602=CARTESIAN_POINT('Ctrl Pts',(-24.758292886385,76.0725110230494,17.0741173620445));
#255603=CARTESIAN_POINT('Ctrl Pts',(-24.758292886385,76.0725110230494,17.3340474816322));
#255604=CARTESIAN_POINT('Ctrl Pts',(-24.7379368836041,76.0624207920021,
17.5919904624029));
#255605=CARTESIAN_POINT('Ctrl Pts',(-24.6976449914385,76.0424582865173,
17.8479876926672));
#255606=CARTESIAN_POINT('Origin',(0.,0.,17.0741173620444));
#255607=CARTESIAN_POINT('Ctrl Pts',(-24.6976449914385,-76.0424582865173,
17.8479876926671));
#255608=CARTESIAN_POINT('Ctrl Pts',(-24.7379368836041,-76.0624207920021,
17.5919904624028));
#255609=CARTESIAN_POINT('Ctrl Pts',(-24.7582928863851,-76.0725110230494,
17.3340474816322));
#255610=CARTESIAN_POINT('Ctrl Pts',(-24.7582928863851,-76.0725110230494,
17.0741173620444));
#255611=CARTESIAN_POINT('Ctrl Pts',(24.758292886385,-76.0725110230494,17.0741173620444));
#255612=CARTESIAN_POINT('Ctrl Pts',(24.758292886385,-76.0725110230494,17.3340474816322));
#255613=CARTESIAN_POINT('Ctrl Pts',(24.7379368836041,-76.0624207920021,
17.5919904624028));
#255614=CARTESIAN_POINT('Ctrl Pts',(24.6976449914385,-76.0424582865173,
17.8479876926671));
#255615=CARTESIAN_POINT('Origin',(0.,0.,17.0741173620445));
#255616=CARTESIAN_POINT('Ctrl Pts',(76.0424582865173,-24.6976449914385,
17.8479876926672));
#255617=CARTESIAN_POINT('Ctrl Pts',(76.0624207920021,-24.7379368836041,
17.5919904624029));
#255618=CARTESIAN_POINT('Ctrl Pts',(76.0725110230494,-24.758292886385,17.3340474816323));
#255619=CARTESIAN_POINT('Ctrl Pts',(76.0725110230494,-24.758292886385,17.0741173620445));
#255620=CARTESIAN_POINT('Ctrl Pts',(76.0725110230494,24.758292886385,17.0741173620445));
#255621=CARTESIAN_POINT('Ctrl Pts',(76.0725110230494,24.758292886385,17.3340474816323));
#255622=CARTESIAN_POINT('Ctrl Pts',(76.0624207920021,24.737936883604,17.5919904624035));
#255623=CARTESIAN_POINT('Ctrl Pts',(76.0424582865173,24.6976449914384,17.8479876926672));
#255624=CARTESIAN_POINT('Origin',(-25.5443686855278,-78.4878132480312,12.3825));
#255625=CARTESIAN_POINT('',(-25.1428889948603,-75.9797434607283,17.0741173620444));
#255626=CARTESIAN_POINT('Origin',(-25.5443686855278,-78.4878132480312,17.0741173620444));
#255627=CARTESIAN_POINT('Ctrl Pts',(-25.1428889948603,-75.9797434607284,
17.0741173620444));
#255628=CARTESIAN_POINT('Ctrl Pts',(-25.1890962633323,-75.9723468244997,
17.0307425600543));
#255629=CARTESIAN_POINT('Ctrl Pts',(-25.2371152677862,-75.965973253375,
16.9901866401575));
#255630=CARTESIAN_POINT('Ctrl Pts',(-25.2866741011431,-75.9609192056981,
16.9519675478226));
#255631=CARTESIAN_POINT('Ctrl Pts',(-25.3351466800543,-75.9559759350792,
16.9145861600128));
#255632=CARTESIAN_POINT('Ctrl Pts',(-25.385092021647,-75.9522954968805,
16.8794402829931));
#255633=CARTESIAN_POINT('Ctrl Pts',(-25.4362249260052,-75.9501164719612,
16.8460788702544));
#255634=CARTESIAN_POINT('Ctrl Pts',(-25.4862159183351,-75.9479861095381,
16.8134624924197));
#255635=CARTESIAN_POINT('Ctrl Pts',(-25.5373416156511,-75.947291198436,
16.7825517666789));
#255636=CARTESIAN_POINT('Ctrl Pts',(-25.5893110141088,-75.9482108801197,
16.7529251953267));
#255637=CARTESIAN_POINT('Ctrl Pts',(-25.5996216874803,-75.9483933439875,
16.7470473150857));
#255638=CARTESIAN_POINT('Ctrl Pts',(-25.6099655036174,-75.9486392118567,
16.7412199819069));
#255639=CARTESIAN_POINT('Ctrl Pts',(-25.620340095261,-75.948949654826,16.7354399041433));
#255640=CARTESIAN_POINT('Ctrl Pts',(-25.6678229409188,-75.9503705026149,
16.7089854132328));
#255641=CARTESIAN_POINT('Ctrl Pts',(-25.7161033957531,-75.9531525557282,
16.6835468572545));
#255642=CARTESIAN_POINT('Ctrl Pts',(-25.7648841738475,-75.9574036133256,
16.6590804688497));
#255643=CARTESIAN_POINT('Ctrl Pts',(-25.8132372046341,-75.9616173943867,
16.6348286205195));
#255644=CARTESIAN_POINT('Ctrl Pts',(-25.8620813654555,-75.9672746984588,
16.6115319650909));
#255645=CARTESIAN_POINT('Ctrl Pts',(-25.9111193560843,-75.9744302796704,
16.5891478764961));
#255646=CARTESIAN_POINT('Ctrl Pts',(-25.9597789956168,-75.981530652217,
16.5669364916428));
#255647=CARTESIAN_POINT('Ctrl Pts',(-26.0086290088543,-75.9901063190922,
16.5456236461848));
#255648=CARTESIAN_POINT('Ctrl Pts',(-26.0573782086223,-76.0001594881172,
16.5251676931017));
#255649=CARTESIAN_POINT('Ctrl Pts',(-26.0882583186412,-76.0065276534822,
16.5122098992352));
#255650=CARTESIAN_POINT('Ctrl Pts',(-26.1190979844471,-76.0134876389456,
16.499595939491));
#255651=CARTESIAN_POINT('Ctrl Pts',(-26.1498243779419,-76.0210292273835,
16.4873152282082));
#255652=CARTESIAN_POINT('Ctrl Pts',(-26.2179462859377,-76.0377492955487,
16.4600882943257));
#255653=CARTESIAN_POINT('Ctrl Pts',(-26.2860317992692,-76.0574561602205,
16.4342868904806));
#255654=CARTESIAN_POINT('Ctrl Pts',(-26.3537219308309,-76.0802112617558,
16.4098106473489));
#255655=CARTESIAN_POINT('Ctrl Pts',(-26.4210710446893,-76.1028517248309,
16.3854577136573));
#255656=CARTESIAN_POINT('Ctrl Pts',(-26.4880282443266,-76.1285099018948,
16.3624166221961));
#255657=CARTESIAN_POINT('Ctrl Pts',(-26.5542307553397,-76.1571956045824,
16.3405885129707));
#255658=CARTESIAN_POINT('Ctrl Pts',(-26.594797053722,-76.1747730764444,
16.327213105023));
#255659=CARTESIAN_POINT('Ctrl Pts',(-26.6350798348181,-76.1934863070453,
16.314293142431));
#255660=CARTESIAN_POINT('Ctrl Pts',(-26.6749951887979,-76.2133278754462,
16.3018058798072));
#255661=CARTESIAN_POINT('Ctrl Pts',(-26.7414052730145,-76.2463397392307,
16.2810299106675));
#255662=CARTESIAN_POINT('Ctrl Pts',(-26.8065749011848,-76.282357702662,
16.2615818620403));
#255663=CARTESIAN_POINT('Ctrl Pts',(-26.870393440276,-76.3214203128057,
16.2431559979634));
#255664=CARTESIAN_POINT('Ctrl Pts',(-26.8885104503037,-76.3325095309195,
16.2379252050151));
#255665=CARTESIAN_POINT('Ctrl Pts',(-26.9065183420908,-76.3438443339879,
16.2327767895739));
#255666=CARTESIAN_POINT('Ctrl Pts',(-26.9244139858109,-76.3554260952922,
16.2277037569974));
#255667=CARTESIAN_POINT('Ctrl Pts',(-26.9473795640672,-76.3702890334318,
16.2211935063209));
#255668=CARTESIAN_POINT('Ctrl Pts',(-26.9702988091961,-76.3856535929665,
16.2155241412993));
#255669=CARTESIAN_POINT('Ctrl Pts',(-26.9928245401834,-76.4012908692599,
16.2092079610165));
#255670=CARTESIAN_POINT('Ctrl Pts',(-27.0099909644426,-76.4132077353212,
16.2043945220878));
#255671=CARTESIAN_POINT('Ctrl Pts',(-27.0269293937101,-76.4252820333718,
16.1992054342301));
#255672=CARTESIAN_POINT('Ctrl Pts',(-27.0434980077865,-76.4373959063312,
16.1929822540025));
#255673=CARTESIAN_POINT('Ctrl Pts',(-27.0482867453259,-76.4408971139712,
16.1911836016449));
#255674=CARTESIAN_POINT('Ctrl Pts',(-27.0532391486278,-76.4445482450871,
16.1893664854189));
#255675=CARTESIAN_POINT('Ctrl Pts',(-27.0570025619875,-76.44733811812,16.1852582407542));
#255676=CARTESIAN_POINT('Ctrl Pts',(-27.0603326521686,-76.4498067623811,
16.1816230234896));
#255677=CARTESIAN_POINT('Ctrl Pts',(-27.0611677349716,-76.450432092947,
16.1755676007548));
#255678=CARTESIAN_POINT('Ctrl Pts',(-27.0602432495845,-76.4497444793078,
16.1701033997377));
#255679=CARTESIAN_POINT('Ctrl Pts',(-27.0601229522577,-76.4496550045753,
16.1693923784665));
#255680=CARTESIAN_POINT('Ctrl Pts',(-27.0599728200255,-76.449543354985,
16.1686913678441));
#255681=CARTESIAN_POINT('Ctrl Pts',(-27.059794441605,-76.4494107416999,
16.1680070028586));
#255682=CARTESIAN_POINT('Ctrl Pts',(-27.057267811496,-76.4475323490217,
16.1583133573314));
#255683=CARTESIAN_POINT('Ctrl Pts',(-27.0523400392582,-76.4438795871955,
16.1500702655799));
#255684=CARTESIAN_POINT('Ctrl Pts',(-27.0470895061924,-76.4400266050576,
16.1422372666814));
#255685=CARTESIAN_POINT('Ctrl Pts',(-27.0459012525003,-76.4391546325944,
16.140464572415));
#255686=CARTESIAN_POINT('Ctrl Pts',(-27.0446965952314,-76.4382722357617,
16.1387128817492));
#255687=CARTESIAN_POINT('Ctrl Pts',(-27.0434998998452,-76.4373972896805,
16.1369701348008));
#255688=CARTESIAN_POINT('Ctrl Pts',(-27.0334981288328,-76.4300846431602,
16.1224045602098));
#255689=CARTESIAN_POINT('Ctrl Pts',(-27.0225381835934,-76.4221888169319,
16.1088060042605));
#255690=CARTESIAN_POINT('Ctrl Pts',(-27.0113044494425,-76.414241579497,
16.0954740612667));
#255691=CARTESIAN_POINT('Ctrl Pts',(-27.007971666701,-76.4118838224582,
16.091518789678));
#255692=CARTESIAN_POINT('Ctrl Pts',(-27.0046149921548,-76.4095212641203,
16.0875869845165));
#255693=CARTESIAN_POINT('Ctrl Pts',(-27.0012528338594,-76.4071670555372,
16.0836603564332));
#255694=CARTESIAN_POINT('Origin',(-25.5443686855278,-78.4878132480312,14.2875));
#255695=CARTESIAN_POINT('Ctrl Pts',(-25.1452786192767,-75.9793621085789,
17.0741173620444));
#255696=CARTESIAN_POINT('Ctrl Pts',(-24.9481252017973,-76.0107288628306,
17.0741173620444));
#255697=CARTESIAN_POINT('Ctrl Pts',(-24.7582928863851,-76.0725110230494,
17.0741173620444));
#255698=CARTESIAN_POINT('Ctrl Pts',(-25.1452785074244,-75.9793621491339,
17.3508457847221));
#255699=CARTESIAN_POINT('Ctrl Pts',(-24.9481251187334,-76.0107288897049,
17.343404115285));
#255700=CARTESIAN_POINT('Ctrl Pts',(-24.7582928856604,-76.0725110232853,
17.337178022204));
#255701=CARTESIAN_POINT('Ctrl Pts',(-25.1240988983272,-75.9676381104172,
17.623822449221));
#255702=CARTESIAN_POINT('Ctrl Pts',(-24.927113661929,-75.9996785825189,
17.6090181824143));
#255703=CARTESIAN_POINT('Ctrl Pts',(-24.7374486679108,-76.0621788292388,
17.5966189870095));
#255704=CARTESIAN_POINT('Ctrl Pts',(-25.0829574281539,-75.9448790163861,
17.8928559119209));
#255705=CARTESIAN_POINT('Ctrl Pts',(-24.8862836604199,-75.9782191703494,
17.8708938349951));
#255706=CARTESIAN_POINT('Ctrl Pts',(-24.6969219387962,-76.0421000528014,
17.8525678740453));
#255707=CARTESIAN_POINT('',(-24.994844812995,-76.0045572676648,17.2916572676617));
#255708=CARTESIAN_POINT('Ctrl Pts',(-24.6976449917882,-76.0424582864821,
17.8479876920601));
#255709=CARTESIAN_POINT('Ctrl Pts',(-24.7503755173217,-76.0371538019006,
17.756416129007));
#255710=CARTESIAN_POINT('Ctrl Pts',(-24.8016570938352,-76.0312759441799,
17.6640492729856));
#255711=CARTESIAN_POINT('Ctrl Pts',(-24.8514227931199,-76.0249016926983,
17.5708849989251));
#255712=CARTESIAN_POINT('Ctrl Pts',(-24.9007299287131,-76.0185861764566,
17.4785791826788));
#255713=CARTESIAN_POINT('Ctrl Pts',(-24.9485484285534,-76.0117822407742,
17.3854910071203));
#255714=CARTESIAN_POINT('Ctrl Pts',(-24.9948448130088,-76.0045572676613,
17.2916572676744));
#255715=CARTESIAN_POINT('Ctrl Pts',(-24.9948448130088,-76.0045572676613,
17.2916572676744));
#255716=CARTESIAN_POINT('Ctrl Pts',(-25.0341234730694,-75.9984274744393,
17.2120470870499));
#255717=CARTESIAN_POINT('Ctrl Pts',(-25.0842002511862,-75.9891380711875,
17.1401458391912));
#255718=CARTESIAN_POINT('Ctrl Pts',(-25.1428889948603,-75.9797434607283,
17.0741173620444));
#255719=CARTESIAN_POINT('Origin',(25.5443686855278,-78.4878132480313,12.3825));
#255720=CARTESIAN_POINT('',(25.1428889948603,-75.9797434607284,17.0741173620444));
#255721=CARTESIAN_POINT('Ctrl Pts',(27.0012528338594,-76.4071670555372,
16.0836576814802));
#255722=CARTESIAN_POINT('Ctrl Pts',(27.0125669096155,-76.4150892566695,
16.0968733108111));
#255723=CARTESIAN_POINT('Ctrl Pts',(27.0238163261266,-76.4231092878419,
16.1101516546325));
#255724=CARTESIAN_POINT('Ctrl Pts',(27.0343062667017,-76.4307070270972,
16.124170648169));
#255725=CARTESIAN_POINT('Ctrl Pts',(27.0373959399464,-76.4329448406986,
16.1282997572844));
#255726=CARTESIAN_POINT('Ctrl Pts',(27.0404199372171,-76.4351457336101,
16.1324931191775));
#255727=CARTESIAN_POINT('Ctrl Pts',(27.0433610058765,-76.4372957466342,
16.1367680561971));
#255728=CARTESIAN_POINT('Ctrl Pts',(27.0486625218437,-76.4411713203446,
16.1444739785989));
#255729=CARTESIAN_POINT('Ctrl Pts',(27.0541110981828,-76.4451930160954,
16.1523581093346));
#255730=CARTESIAN_POINT('Ctrl Pts',(27.0576635438242,-76.4478282794951,
16.1614817309479));
#255731=CARTESIAN_POINT('Ctrl Pts',(27.0584419906684,-76.4484057443416,
16.1634809886902));
#255732=CARTESIAN_POINT('Ctrl Pts',(27.0591295221735,-76.448916457713,16.1655397641649));
#255733=CARTESIAN_POINT('Ctrl Pts',(27.0597047898622,-76.4493440942542,
16.1676692243483));
#255734=CARTESIAN_POINT('Ctrl Pts',(27.061128686084,-76.4504025754923,16.1729400406464));
#255735=CARTESIAN_POINT('Ctrl Pts',(27.0609586584413,-76.4502741704977,
16.1792319783503));
#255736=CARTESIAN_POINT('Ctrl Pts',(27.05833972207,-76.4483300535648,16.1834945076105));
#255737=CARTESIAN_POINT('Ctrl Pts',(27.0580153550188,-76.4480892659368,
16.1840224410349));
#255738=CARTESIAN_POINT('Ctrl Pts',(27.0576533814908,-76.4478206797893,
16.184519243462));
#255739=CARTESIAN_POINT('Ctrl Pts',(27.0572521366115,-76.4475231550697,
16.1849791191285));
#255740=CARTESIAN_POINT('Ctrl Pts',(27.0536112445358,-76.4448234187001,
16.1891520263895));
#255741=CARTESIAN_POINT('Ctrl Pts',(27.0486162668499,-76.441139274083,16.1910424108882));
#255742=CARTESIAN_POINT('Ctrl Pts',(27.0438314274414,-76.4376397222992,
16.1928564397759));
#255743=CARTESIAN_POINT('Ctrl Pts',(27.0219957335603,-76.4216694597787,
16.2011347906466));
#255744=CARTESIAN_POINT('Ctrl Pts',(26.9995297758924,-76.4057789951842,
16.2075349627597));
#255745=CARTESIAN_POINT('Ctrl Pts',(26.9767570400582,-76.3902280645868,
16.2136304689842));
#255746=CARTESIAN_POINT('Ctrl Pts',(26.9596083941578,-76.3785176840609,
16.2182205928317));
#255747=CARTESIAN_POINT('Ctrl Pts',(26.9422864764177,-76.3669990447857,
16.2226379527468));
#255748=CARTESIAN_POINT('Ctrl Pts',(26.9249406691735,-76.3557670482568,
16.2275544634756));
#255749=CARTESIAN_POINT('Ctrl Pts',(26.8616514023731,-76.3147851086444,
16.2454932284381));
#255750=CARTESIAN_POINT('Ctrl Pts',(26.7969330658208,-76.2768724921605,
16.2643805415009));
#255751=CARTESIAN_POINT('Ctrl Pts',(26.7309055253999,-76.2419881596448,
16.2845312318663));
#255752=CARTESIAN_POINT('Ctrl Pts',(26.7126781403842,-76.2323580847438,
16.2900939771887));
#255753=CARTESIAN_POINT('Ctrl Pts',(26.6943507540625,-76.222958992946,16.2957530015098));
#255754=CARTESIAN_POINT('Ctrl Pts',(26.675925399516,-76.2137905122108,16.3015149281042));
#255755=CARTESIAN_POINT('Ctrl Pts',(26.6064313477857,-76.1792101803703,
16.3232469183247));
#255756=CARTESIAN_POINT('Ctrl Pts',(26.5358861365389,-76.1480850328896,
16.3462666758162));
#255757=CARTESIAN_POINT('Ctrl Pts',(26.4646896591077,-76.1204076415521,
16.3707095301105));
#255758=CARTESIAN_POINT('Ctrl Pts',(26.3929595634036,-76.0925228079044,
16.3953355838293));
#255759=CARTESIAN_POINT('Ctrl Pts',(26.3205688608561,-76.0681374467385,
16.4214061465416));
#255760=CARTESIAN_POINT('Ctrl Pts',(26.2479119389207,-76.0471930623806,
16.4490596135311));
#255761=CARTESIAN_POINT('Ctrl Pts',(26.2159174362015,-76.0379701949037,
16.4612368280514));
#255762=CARTESIAN_POINT('Ctrl Pts',(26.1838710809961,-76.0294139168384,
16.4737209810889));
#255763=CARTESIAN_POINT('Ctrl Pts',(26.1518053240938,-76.0215162808905,
16.4865238898931));
#255764=CARTESIAN_POINT('Ctrl Pts',(26.1024355298056,-76.009356746865,16.5062357892841));
#255765=CARTESIAN_POINT('Ctrl Pts',(26.052778843371,-75.9987033871209,16.5268004120897));
#255766=CARTESIAN_POINT('Ctrl Pts',(26.0031235829827,-75.9895850871018,
16.5482718578781));
#255767=CARTESIAN_POINT('Ctrl Pts',(25.9532562285115,-75.9804278397996,
16.5698350153315));
#255768=CARTESIAN_POINT('Ctrl Pts',(25.9033908081985,-75.9728187929612,
16.5923127589954));
#255769=CARTESIAN_POINT('Ctrl Pts',(25.8538229261267,-75.966734496192,16.615759884635));
#255770=CARTESIAN_POINT('Ctrl Pts',(25.8036709954625,-75.9605785093523,
16.6394832831383));
#255771=CARTESIAN_POINT('Ctrl Pts',(25.7538241560404,-75.9559833526325,
16.6641990422746));
#255772=CARTESIAN_POINT('Ctrl Pts',(25.7045846567395,-75.9528712679124,
16.6899639176645));
#255773=CARTESIAN_POINT('Ctrl Pts',(25.6770558349516,-75.951131363428,16.7043685455154));
#255774=CARTESIAN_POINT('Ctrl Pts',(25.6497167346353,-75.9498540709319,
16.719101096162));
#255775=CARTESIAN_POINT('Ctrl Pts',(25.6226187918313,-75.9490188646943,
16.7341714877587));
#255776=CARTESIAN_POINT('Ctrl Pts',(25.5764663692891,-75.9475963658918,
16.7598389373462));
#255777=CARTESIAN_POINT('Ctrl Pts',(25.5307625072541,-75.9474517866683,
16.7865659943229));
#255778=CARTESIAN_POINT('Ctrl Pts',(25.4858135567854,-75.948488279285,16.8145610357063));
#255779=CARTESIAN_POINT('Ctrl Pts',(25.440208013082,-75.9495399125009,16.842965015554));
#255780=CARTESIAN_POINT('Ctrl Pts',(25.3953800373707,-75.951807126726,16.8726742946166));
#255781=CARTESIAN_POINT('Ctrl Pts',(25.3516355174112,-75.9551360230561,
16.9039065155736));
#255782=CARTESIAN_POINT('Ctrl Pts',(25.3063675036794,-75.9585808551156,
16.9362264634999));
#255783=CARTESIAN_POINT('Ctrl Pts',(25.2622601849893,-75.9631623243896,
16.9701772797651));
#255784=CARTESIAN_POINT('Ctrl Pts',(25.2196304529756,-75.9686576195877,
17.0060001477704));
#255785=CARTESIAN_POINT('Ctrl Pts',(25.1934712691005,-75.9720297364354,
17.0279823875551));
#255786=CARTESIAN_POINT('Ctrl Pts',(25.1678679994915,-75.9757449423844,
17.0506695492733));
#255787=CARTESIAN_POINT('Ctrl Pts',(25.1428889948603,-75.9797434607284,
17.0741173620444));
#255788=CARTESIAN_POINT('Origin',(25.5443686855278,-78.4878132480313,17.0741173620444));
#255789=CARTESIAN_POINT('Origin',(25.5443686855278,-78.4878132480313,14.2875));
#255790=CARTESIAN_POINT('Ctrl Pts',(24.758292886385,-76.0725110230494,17.0741173620444));
#255791=CARTESIAN_POINT('Ctrl Pts',(24.9481252017973,-76.0107288628306,
17.0741173620444));
#255792=CARTESIAN_POINT('Ctrl Pts',(25.1452786192766,-75.9793621085789,
17.0741173620444));
#255793=CARTESIAN_POINT('Ctrl Pts',(24.7582928856599,-76.0725110232854,
17.3371780222037));
#255794=CARTESIAN_POINT('Ctrl Pts',(24.9481251187328,-76.0107288897046,
17.3434041152845));
#255795=CARTESIAN_POINT('Ctrl Pts',(25.1452785074237,-75.9793621491333,
17.3508457847214));
#255796=CARTESIAN_POINT('Ctrl Pts',(24.7374486679123,-76.0621788292383,
17.5966189870099));
#255797=CARTESIAN_POINT('Ctrl Pts',(24.9271136619309,-75.9996785825196,
17.6090181824149));
#255798=CARTESIAN_POINT('Ctrl Pts',(25.1240988983294,-75.9676381104188,
17.6238224492219));
#255799=CARTESIAN_POINT('Ctrl Pts',(24.6969219387962,-76.0421000528014,
17.8525678740453));
#255800=CARTESIAN_POINT('Ctrl Pts',(24.8862836604198,-75.9782191703494,
17.8708938349951));
#255801=CARTESIAN_POINT('Ctrl Pts',(25.0829574281538,-75.9448790163861,
17.8928559119209));
#255802=CARTESIAN_POINT('',(24.9948448129998,-76.004557267664,17.2916572676518));
#255803=CARTESIAN_POINT('Ctrl Pts',(25.1428889948603,-75.9797434607284,
17.0741173620444));
#255804=CARTESIAN_POINT('Ctrl Pts',(25.0842002511886,-75.9891380711871,
17.1401458391885));
#255805=CARTESIAN_POINT('Ctrl Pts',(25.0341234730735,-75.9984274744386,
17.2120470870438));
#255806=CARTESIAN_POINT('Ctrl Pts',(24.9948448130136,-76.0045572676606,
17.2916572676645));
#255807=CARTESIAN_POINT('Ctrl Pts',(24.9948448130136,-76.0045572676606,
17.2916572676645));
#255808=CARTESIAN_POINT('Ctrl Pts',(24.9481178557882,-76.0118494355815,
17.386363694133));
#255809=CARTESIAN_POINT('Ctrl Pts',(24.8998402835406,-76.0187126993903,
17.4803105665639));
#255810=CARTESIAN_POINT('Ctrl Pts',(24.8500466861399,-76.0250777755062,
17.5734602270335));
#255811=CARTESIAN_POINT('Ctrl Pts',(24.8007119296855,-76.0313841983473,
17.6657515265775));
#255812=CARTESIAN_POINT('Ctrl Pts',(24.7498896236257,-76.0372026809097,
17.7572599295026));
#255813=CARTESIAN_POINT('Ctrl Pts',(24.697644991789,-76.0424582864817,17.8479876920608));
#255814=CARTESIAN_POINT('Origin',(78.4878132480313,-25.5443686855277,12.3825));
#255815=CARTESIAN_POINT('',(75.9797434607283,-25.1428889948603,17.0741173620445));
#255816=CARTESIAN_POINT('Origin',(78.4878132480312,-25.5443686855278,17.0741173620445));
#255817=CARTESIAN_POINT('Ctrl Pts',(75.9797434607284,-25.1428889948603,
17.0741173620445));
#255818=CARTESIAN_POINT('Ctrl Pts',(75.9723468244997,-25.1890962633322,
17.0307425600544));
#255819=CARTESIAN_POINT('Ctrl Pts',(75.965973253375,-25.2371152677861,16.9901866401576));
#255820=CARTESIAN_POINT('Ctrl Pts',(75.9609192056981,-25.286674101143,16.9519675478227));
#255821=CARTESIAN_POINT('Ctrl Pts',(75.9559759350792,-25.3351466800541,
16.914586160013));
#255822=CARTESIAN_POINT('Ctrl Pts',(75.9522954968805,-25.3850920216466,
16.8794402829934));
#255823=CARTESIAN_POINT('Ctrl Pts',(75.9501164719612,-25.4362249260047,
16.8460788702548));
#255824=CARTESIAN_POINT('Ctrl Pts',(75.9479861095382,-25.4862159183344,
16.8134624924202));
#255825=CARTESIAN_POINT('Ctrl Pts',(75.9472911984361,-25.5373416156502,
16.7825517666794));
#255826=CARTESIAN_POINT('Ctrl Pts',(75.9482108801197,-25.5893110141078,
16.7529251953273));
#255827=CARTESIAN_POINT('Ctrl Pts',(75.9483933439875,-25.5996216874797,
16.7470473150861));
#255828=CARTESIAN_POINT('Ctrl Pts',(75.9486392118567,-25.6099655036172,
16.741219981907));
#255829=CARTESIAN_POINT('Ctrl Pts',(75.948949654826,-25.6203400952611,16.7354399041433));
#255830=CARTESIAN_POINT('Ctrl Pts',(75.9503705026149,-25.667822940919,16.7089854132327));
#255831=CARTESIAN_POINT('Ctrl Pts',(75.9531525557283,-25.7161033957533,
16.6835468572544));
#255832=CARTESIAN_POINT('Ctrl Pts',(75.9574036133257,-25.7648841738477,
16.6590804688496));
#255833=CARTESIAN_POINT('Ctrl Pts',(75.9616173943868,-25.8132372046344,
16.6348286205194));
#255834=CARTESIAN_POINT('Ctrl Pts',(75.9672746984589,-25.8620813654559,
16.6115319650908));
#255835=CARTESIAN_POINT('Ctrl Pts',(75.9744302796705,-25.9111193560848,
16.5891478764959));
#255836=CARTESIAN_POINT('Ctrl Pts',(75.9815306522171,-25.9597789956173,
16.5669364916427));
#255837=CARTESIAN_POINT('Ctrl Pts',(75.9901063190923,-26.0086290088549,
16.5456236461847));
#255838=CARTESIAN_POINT('Ctrl Pts',(76.0001594881174,-26.0573782086229,
16.5251676931015));
#255839=CARTESIAN_POINT('Ctrl Pts',(76.0065276534823,-26.0882583186417,
16.5122098992351));
#255840=CARTESIAN_POINT('Ctrl Pts',(76.0134876389457,-26.1190979844475,
16.4995959394909));
#255841=CARTESIAN_POINT('Ctrl Pts',(76.0210292273836,-26.1498243779423,
16.4873152282081));
#255842=CARTESIAN_POINT('Ctrl Pts',(76.0377492955488,-26.2179462859379,
16.4600882943257));
#255843=CARTESIAN_POINT('Ctrl Pts',(76.0574561602205,-26.2860317992692,
16.4342868904806));
#255844=CARTESIAN_POINT('Ctrl Pts',(76.0802112617558,-26.3537219308308,
16.409810647349));
#255845=CARTESIAN_POINT('Ctrl Pts',(76.1028517248309,-26.4210710446892,
16.3854577136574));
#255846=CARTESIAN_POINT('Ctrl Pts',(76.1285099018948,-26.4880282443265,
16.3624166221961));
#255847=CARTESIAN_POINT('Ctrl Pts',(76.1571956045824,-26.5542307553397,
16.3405885129707));
#255848=CARTESIAN_POINT('Ctrl Pts',(76.1747730764445,-26.5947970537221,
16.327213105023));
#255849=CARTESIAN_POINT('Ctrl Pts',(76.1934863070455,-26.6350798348184,
16.3142931424309));
#255850=CARTESIAN_POINT('Ctrl Pts',(76.2133278754465,-26.6749951887984,
16.3018058798071));
#255851=CARTESIAN_POINT('Ctrl Pts',(76.2463397392302,-26.7414052730132,
16.281029910668));
#255852=CARTESIAN_POINT('Ctrl Pts',(76.2823577026604,-26.8065749011818,
16.2615818620412));
#255853=CARTESIAN_POINT('Ctrl Pts',(76.321420312803,-26.8703934402714,16.2431559979648));
#255854=CARTESIAN_POINT('Ctrl Pts',(76.3325095309177,-26.8885104503009,
16.2379252050159));
#255855=CARTESIAN_POINT('Ctrl Pts',(76.3438443339872,-26.9065183420897,
16.2327767895743));
#255856=CARTESIAN_POINT('Ctrl Pts',(76.3554260952926,-26.9244139858114,
16.2277037569972));
#255857=CARTESIAN_POINT('Ctrl Pts',(76.3702890334322,-26.9473795640677,
16.2211935063208));
#255858=CARTESIAN_POINT('Ctrl Pts',(76.3856535929669,-26.9702988091965,
16.2155241412992));
#255859=CARTESIAN_POINT('Ctrl Pts',(76.4012908692602,-26.9928245401838,
16.2092079610165));
#255860=CARTESIAN_POINT('Ctrl Pts',(76.4132077353215,-27.0099909644431,
16.2043945220878));
#255861=CARTESIAN_POINT('Ctrl Pts',(76.4252820333722,-27.0269293937106,
16.19920543423));
#255862=CARTESIAN_POINT('Ctrl Pts',(76.4373959063317,-27.043498007787,16.1929822540023));
#255863=CARTESIAN_POINT('Ctrl Pts',(76.4408971139716,-27.0482867453264,
16.1911836016447));
#255864=CARTESIAN_POINT('Ctrl Pts',(76.4445482450876,-27.0532391486283,
16.1893664854187));
#255865=CARTESIAN_POINT('Ctrl Pts',(76.4473381181204,-27.057002561988,16.1852582407538));
#255866=CARTESIAN_POINT('Ctrl Pts',(76.4498067623814,-27.0603326521689,
16.1816230234891));
#255867=CARTESIAN_POINT('Ctrl Pts',(76.4504320929472,-27.0611677349717,
16.1755676007542));
#255868=CARTESIAN_POINT('Ctrl Pts',(76.4497444793079,-27.0602432495845,
16.1701033997371));
#255869=CARTESIAN_POINT('Ctrl Pts',(76.4496550045754,-27.0601229522577,
16.1693923784658));
#255870=CARTESIAN_POINT('Ctrl Pts',(76.4495433549851,-27.0599728200255,
16.1686913678435));
#255871=CARTESIAN_POINT('Ctrl Pts',(76.4494107417,-27.059794441605,16.1680070028581));
#255872=CARTESIAN_POINT('Ctrl Pts',(76.4475323490217,-27.0572678114959,
16.158313357331));
#255873=CARTESIAN_POINT('Ctrl Pts',(76.4438795871955,-27.0523400392581,
16.1500702655797));
#255874=CARTESIAN_POINT('Ctrl Pts',(76.4400266050576,-27.0470895061923,
16.1422372666812));
#255875=CARTESIAN_POINT('Ctrl Pts',(76.4391546325943,-27.0459012525002,
16.1404645724148));
#255876=CARTESIAN_POINT('Ctrl Pts',(76.4382722357616,-27.0446965952312,
16.138712881749));
#255877=CARTESIAN_POINT('Ctrl Pts',(76.4373972896805,-27.043499899845,16.1369701348005));
#255878=CARTESIAN_POINT('Ctrl Pts',(76.4300846431601,-27.0334981288326,
16.1224045602096));
#255879=CARTESIAN_POINT('Ctrl Pts',(76.4221888169319,-27.0225381835933,
16.1088060042603));
#255880=CARTESIAN_POINT('Ctrl Pts',(76.414241579497,-27.0113044494424,16.0954740612665));
#255881=CARTESIAN_POINT('Ctrl Pts',(76.4118838224582,-27.0079716667009,
16.0915187896778));
#255882=CARTESIAN_POINT('Ctrl Pts',(76.4095212641203,-27.0046149921547,
16.0875869845164));
#255883=CARTESIAN_POINT('Ctrl Pts',(76.4071670555372,-27.0012528338594,
16.0836603564331));
#255884=CARTESIAN_POINT('Ctrl Pts',(75.9793621085789,-25.1452786192766,
17.0741173620445));
#255885=CARTESIAN_POINT('Ctrl Pts',(76.0107288628305,-24.9481252017973,
17.0741173620445));
#255886=CARTESIAN_POINT('Ctrl Pts',(76.0725110230494,-24.758292886385,17.0741173620445));
#255887=CARTESIAN_POINT('Ctrl Pts',(75.9793621491347,-25.1452785074261,
17.3508457847218));
#255888=CARTESIAN_POINT('Ctrl Pts',(76.010728889705,-24.9481251187354,17.343404115285));
#255889=CARTESIAN_POINT('Ctrl Pts',(76.0725110232845,-24.7582928856628,
17.3371780222044));
#255890=CARTESIAN_POINT('Ctrl Pts',(75.9676381104205,-25.124098898325,17.6238224492217));
#255891=CARTESIAN_POINT('Ctrl Pts',(75.9996785825213,-24.9271136619264,
17.6090181824145));
#255892=CARTESIAN_POINT('Ctrl Pts',(76.0621788292398,-24.7374486679078,
17.5966189870093));
#255893=CARTESIAN_POINT('Ctrl Pts',(75.9448790163861,-25.0829574281538,
17.892855911921));
#255894=CARTESIAN_POINT('Ctrl Pts',(75.9782191703494,-24.8862836604198,
17.8708938349952));
#255895=CARTESIAN_POINT('Ctrl Pts',(76.0421000528014,-24.6969219387962,
17.8525678740454));
#255896=CARTESIAN_POINT('',(76.0045572676648,-24.994844812995,17.2916572676618));
#255897=CARTESIAN_POINT('Ctrl Pts',(76.0424582864821,-24.6976449917882,
17.8479876920602));
#255898=CARTESIAN_POINT('Ctrl Pts',(76.0371538031763,-24.7503755046464,
17.7564161510145));
#255899=CARTESIAN_POINT('Ctrl Pts',(76.0312759470027,-24.8016570691911,
17.6640493173926));
#255900=CARTESIAN_POINT('Ctrl Pts',(76.0249016972925,-24.8514227572423,
17.5708850661044));
#255901=CARTESIAN_POINT('Ctrl Pts',(76.018586179756,-24.9007299055169,17.4785792278443));
#255902=CARTESIAN_POINT('Ctrl Pts',(76.0117822425276,-24.9485484173197,
17.3854910298794));
#255903=CARTESIAN_POINT('Ctrl Pts',(76.0045572676613,-24.9948448130087,
17.2916572676745));
#255904=CARTESIAN_POINT('Ctrl Pts',(76.0045572676613,-24.9948448130087,
17.2916572676745));
#255905=CARTESIAN_POINT('Ctrl Pts',(75.9984274744393,-25.0341234730694,
17.21204708705));
#255906=CARTESIAN_POINT('Ctrl Pts',(75.9891380711875,-25.0842002511861,
17.1401458391913));
#255907=CARTESIAN_POINT('Ctrl Pts',(75.9797434607283,-25.1428889948603,
17.0741173620445));
#255908=CARTESIAN_POINT('Origin',(78.4878132480313,25.5443686855277,12.3825));
#255909=CARTESIAN_POINT('',(76.4499922109615,27.0605762639536,16.1719291773585));
#255910=CARTESIAN_POINT('Ctrl Pts',(76.4071670555372,27.0012528338594,15.6374346123617));
#255911=CARTESIAN_POINT('Ctrl Pts',(76.4079750319809,27.0024067438069,15.6501237643143));
#255912=CARTESIAN_POINT('Ctrl Pts',(76.4087695213968,27.0035394221128,15.6628157309684));
#255913=CARTESIAN_POINT('Ctrl Pts',(76.4095938645954,27.0047125471957,15.675502067928));
#255914=CARTESIAN_POINT('Ctrl Pts',(76.4127017511593,27.0091353891497,15.7233312927615));
#255915=CARTESIAN_POINT('Ctrl Pts',(76.4160289816171,27.0138404705195,15.7711214832916));
#255916=CARTESIAN_POINT('Ctrl Pts',(76.4195777514373,27.0188183898679,15.8188607686969));
#255917=CARTESIAN_POINT('Ctrl Pts',(76.4283481319464,27.0311207506973,15.936842976462));
#255918=CARTESIAN_POINT('Ctrl Pts',(76.4384768596614,27.04509934281,16.0545629245959));
#255919=CARTESIAN_POINT('Ctrl Pts',(76.4499922109615,27.0605762639536,16.1719291773585));
#255920=CARTESIAN_POINT('',(75.9797434607283,25.1428889948603,17.0741173620445));
#255921=CARTESIAN_POINT('Ctrl Pts',(76.4499922109615,27.0605762639536,16.1719291773585));
#255922=CARTESIAN_POINT('Ctrl Pts',(76.4505698705024,27.0613526528738,16.1778167732404));
#255923=CARTESIAN_POINT('Ctrl Pts',(76.4488056783259,27.0589883665235,16.1839366447756));
#255924=CARTESIAN_POINT('Ctrl Pts',(76.4429004146046,27.0510060510084,16.1903007364945));
#255925=CARTESIAN_POINT('Ctrl Pts',(76.4394649837984,27.0463345060122,16.1919741158575));
#255926=CARTESIAN_POINT('Ctrl Pts',(76.4294701394813,27.032639963703,16.1969037700759));
#255927=CARTESIAN_POINT('Ctrl Pts',(76.4227640571818,27.0233220902657,16.1995753950398));
#255928=CARTESIAN_POINT('Ctrl Pts',(76.4028721167673,26.9952807487557,16.2077603480722));
#255929=CARTESIAN_POINT('Ctrl Pts',(76.3898418244125,26.9763750260929,16.2130348003402));
#255930=CARTESIAN_POINT('Ctrl Pts',(76.3515584858927,26.919185257365,16.2291569518415));
#255931=CARTESIAN_POINT('Ctrl Pts',(76.3271240812196,26.8804489710049,16.2401625701034));
#255932=CARTESIAN_POINT('Ctrl Pts',(76.2571329511827,26.7625715555466,16.2745485616773));
#255933=CARTESIAN_POINT('Ctrl Pts',(76.2151700755523,26.6822350597522,16.2990788049764));
#255934=CARTESIAN_POINT('Ctrl Pts',(76.1032564488141,26.4374959840272,16.3781741196505));
#255935=CARTESIAN_POINT('Ctrl Pts',(76.046615195867,26.2669884699004,16.4389027562941));
#255936=CARTESIAN_POINT('Ctrl Pts',(75.9710934258864,25.9287495116366,16.5778273625233));
#255937=CARTESIAN_POINT('Ctrl Pts',(75.9519151365713,25.7614405136926,16.6554073942778));
#255938=CARTESIAN_POINT('Ctrl Pts',(75.9448997961066,25.4371745331233,16.8391041287272));
#255939=CARTESIAN_POINT('Ctrl Pts',(75.9578405366692,25.2797179886133,16.945675869898));
#255940=CARTESIAN_POINT('Ctrl Pts',(75.9797434607283,25.1428889948603,17.0741173620445));
#255941=CARTESIAN_POINT('Origin',(78.4878132480312,25.5443686855277,17.0741173620445));
#255942=CARTESIAN_POINT('Ctrl Pts',(76.0725110230494,24.758292886385,17.0741173620445));
#255943=CARTESIAN_POINT('Ctrl Pts',(76.0107288628306,24.9481252017973,17.0741173620445));
#255944=CARTESIAN_POINT('Ctrl Pts',(75.9793621085789,25.1452786192766,17.0741173620445));
#255945=CARTESIAN_POINT('Ctrl Pts',(76.072511023285,24.7582928856611,17.3371780222032));
#255946=CARTESIAN_POINT('Ctrl Pts',(76.0107288897042,24.948125118734,17.3434041152839));
#255947=CARTESIAN_POINT('Ctrl Pts',(75.9793621491331,25.1452785074248,17.3508457847207));
#255948=CARTESIAN_POINT('Ctrl Pts',(76.0621788292375,24.7374486679144,17.5966189870109));
#255949=CARTESIAN_POINT('Ctrl Pts',(75.9996785825189,24.9271136619333,17.609018182416));
#255950=CARTESIAN_POINT('Ctrl Pts',(75.9676381104182,25.124098898332,17.6238224492231));
#255951=CARTESIAN_POINT('Ctrl Pts',(76.0421000528014,24.6969219387962,17.8525678740454));
#255952=CARTESIAN_POINT('Ctrl Pts',(75.9782191703494,24.8862836604198,17.8708938349953));
#255953=CARTESIAN_POINT('Ctrl Pts',(75.9448790163862,25.0829574281538,17.892855911921));
#255954=CARTESIAN_POINT('',(76.004557267664,24.9948448129998,17.2916572676519));
#255955=CARTESIAN_POINT('Ctrl Pts',(75.9797434607283,25.1428889948603,17.0741173620445));
#255956=CARTESIAN_POINT('Ctrl Pts',(75.9891380711871,25.0842002511886,17.1401458391886));
#255957=CARTESIAN_POINT('Ctrl Pts',(75.9984274744386,25.0341234730735,17.2120470870439));
#255958=CARTESIAN_POINT('Ctrl Pts',(76.0045572676606,24.9948448130136,17.2916572676646));
#255959=CARTESIAN_POINT('Ctrl Pts',(76.0045572676606,24.9948448130136,17.2916572676646));
#255960=CARTESIAN_POINT('Ctrl Pts',(76.0118494335674,24.9481178686905,17.3863636679988));
#255961=CARTESIAN_POINT('Ctrl Pts',(76.0187126955952,24.8998403102119,17.480310514724));
#255962=CARTESIAN_POINT('Ctrl Pts',(76.0250777702285,24.8500467273903,17.5734601499223));
#255963=CARTESIAN_POINT('Ctrl Pts',(76.0313841950981,24.8007119580207,17.6657514756104));
#255964=CARTESIAN_POINT('Ctrl Pts',(76.0372026794419,24.7498896381886,17.757259904234));
#255965=CARTESIAN_POINT('Ctrl Pts',(76.0424582864818,24.697644991789,17.8479876920609));
#255966=CARTESIAN_POINT('Origin',(25.5443686855278,78.4878132480313,12.3825));
#255967=CARTESIAN_POINT('',(25.1428889948602,75.9797434607284,17.0741173620444));
#255968=CARTESIAN_POINT('Origin',(25.5443686855278,78.4878132480313,17.0741173620444));
#255969=CARTESIAN_POINT('Ctrl Pts',(25.1428889948602,75.9797434607284,17.0741173620444));
#255970=CARTESIAN_POINT('Ctrl Pts',(25.1890962633322,75.9723468244998,17.0307425600543));
#255971=CARTESIAN_POINT('Ctrl Pts',(25.237115267786,75.9659732533751,16.9901866401575));
#255972=CARTESIAN_POINT('Ctrl Pts',(25.2866741011429,75.9609192056981,16.9519675478227));
#255973=CARTESIAN_POINT('Ctrl Pts',(25.3351466800541,75.9559759350792,16.9145861600129));
#255974=CARTESIAN_POINT('Ctrl Pts',(25.3850920216467,75.9522954968805,16.8794402829932));
#255975=CARTESIAN_POINT('Ctrl Pts',(25.4362249260049,75.9501164719612,16.8460788702546));
#255976=CARTESIAN_POINT('Ctrl Pts',(25.4862159183347,75.9479861095382,16.8134624924199));
#255977=CARTESIAN_POINT('Ctrl Pts',(25.5373416156507,75.9472911984361,16.782551766679));
#255978=CARTESIAN_POINT('Ctrl Pts',(25.5893110141084,75.9482108801197,16.7529251953268));
#255979=CARTESIAN_POINT('Ctrl Pts',(25.5996216874799,75.9483933439875,16.7470473150859));
#255980=CARTESIAN_POINT('Ctrl Pts',(25.6099655036169,75.9486392118567,16.741219981907));
#255981=CARTESIAN_POINT('Ctrl Pts',(25.6203400952605,75.948949654826,16.7354399041435));
#255982=CARTESIAN_POINT('Ctrl Pts',(25.6678229409182,75.9503705026149,16.7089854132329));
#255983=CARTESIAN_POINT('Ctrl Pts',(25.7161033957525,75.9531525557282,16.6835468572547));
#255984=CARTESIAN_POINT('Ctrl Pts',(25.7648841738468,75.9574036133256,16.6590804688499));
#255985=CARTESIAN_POINT('Ctrl Pts',(25.8132372046333,75.9616173943867,16.6348286205197));
#255986=CARTESIAN_POINT('Ctrl Pts',(25.8620813654547,75.9672746984588,16.6115319650911));
#255987=CARTESIAN_POINT('Ctrl Pts',(25.9111193560836,75.9744302796703,16.5891478764963));
#255988=CARTESIAN_POINT('Ctrl Pts',(25.959778995616,75.9815306522169,16.5669364916431));
#255989=CARTESIAN_POINT('Ctrl Pts',(26.0086290088535,75.990106319092,16.5456236461851));
#255990=CARTESIAN_POINT('Ctrl Pts',(26.0573782086215,76.0001594881171,16.5251676931019));
#255991=CARTESIAN_POINT('Ctrl Pts',(26.0882583186404,76.006527653482,16.5122098992355));
#255992=CARTESIAN_POINT('Ctrl Pts',(26.1190979844463,76.0134876389454,16.4995959394913));
#255993=CARTESIAN_POINT('Ctrl Pts',(26.1498243779411,76.0210292273833,16.4873152282084));
#255994=CARTESIAN_POINT('Ctrl Pts',(26.2179462859366,76.0377492955484,16.460088294326));
#255995=CARTESIAN_POINT('Ctrl Pts',(26.2860317992677,76.05745616022,16.434286890481));
#255996=CARTESIAN_POINT('Ctrl Pts',(26.3537219308291,76.0802112617552,16.4098106473495));
#255997=CARTESIAN_POINT('Ctrl Pts',(26.4210710446877,76.1028517248303,16.3854577136577));
#255998=CARTESIAN_POINT('Ctrl Pts',(26.4880282443252,76.1285099018942,16.3624166221964));
#255999=CARTESIAN_POINT('Ctrl Pts',(26.5542307553386,76.1571956045819,16.3405885129709));
#256000=CARTESIAN_POINT('Ctrl Pts',(26.5947970537208,76.1747730764439,16.3272131050233));
#256001=CARTESIAN_POINT('Ctrl Pts',(26.635079834817,76.1934863070448,16.3142931424312));
#256002=CARTESIAN_POINT('Ctrl Pts',(26.6749951887968,76.2133278754457,16.3018058798074));
#256003=CARTESIAN_POINT('Ctrl Pts',(26.7414052730119,76.2463397392294,16.2810299106682));
#256004=CARTESIAN_POINT('Ctrl Pts',(26.8065749011807,76.2823577026598,16.2615818620414));
#256005=CARTESIAN_POINT('Ctrl Pts',(26.8703934402706,76.3214203128024,16.2431559979649));
#256006=CARTESIAN_POINT('Ctrl Pts',(26.8885104502997,76.332509530917,16.2379252050161));
#256007=CARTESIAN_POINT('Ctrl Pts',(26.9065183420882,76.3438443339862,16.2327767895745));
#256008=CARTESIAN_POINT('Ctrl Pts',(26.9244139858097,76.3554260952914,16.2277037569976));
#256009=CARTESIAN_POINT('Ctrl Pts',(26.9473795640663,76.3702890334313,16.221193506321));
#256010=CARTESIAN_POINT('Ctrl Pts',(26.9702988091955,76.3856535929662,16.2155241412993));
#256011=CARTESIAN_POINT('Ctrl Pts',(26.9928245401832,76.4012908692597,16.2092079610164));
#256012=CARTESIAN_POINT('Ctrl Pts',(27.0099909644421,76.4132077353208,16.2043945220878));
#256013=CARTESIAN_POINT('Ctrl Pts',(27.0269293937092,76.4252820333712,16.1992054342301));
#256014=CARTESIAN_POINT('Ctrl Pts',(27.0434980077852,76.4373959063303,16.1929822540028));
#256015=CARTESIAN_POINT('Ctrl Pts',(27.0482867453246,76.4408971139703,16.1911836016452));
#256016=CARTESIAN_POINT('Ctrl Pts',(27.0532391486265,76.4445482450862,16.1893664854193));
#256017=CARTESIAN_POINT('Ctrl Pts',(27.0570025619865,76.4473381181192,16.1852582407548));
#256018=CARTESIAN_POINT('Ctrl Pts',(27.0603326521677,76.4498067623805,16.1816230234904));
#256019=CARTESIAN_POINT('Ctrl Pts',(27.0611677349713,76.4504320929469,16.1755676007557));
#256020=CARTESIAN_POINT('Ctrl Pts',(27.0602432495844,76.4497444793078,16.1701033997385));
#256021=CARTESIAN_POINT('Ctrl Pts',(27.0601229522577,76.4496550045754,16.1693923784672));
#256022=CARTESIAN_POINT('Ctrl Pts',(27.0599728200255,76.4495433549851,16.1686913678449));
#256023=CARTESIAN_POINT('Ctrl Pts',(27.0597944416051,76.4494107417,16.1680070028595));
#256024=CARTESIAN_POINT('Ctrl Pts',(27.0572678114964,76.447532349022,16.1583133573325));
#256025=CARTESIAN_POINT('Ctrl Pts',(27.0523400392588,76.443879587196,16.1500702655813));
#256026=CARTESIAN_POINT('Ctrl Pts',(27.0470895061932,76.4400266050583,16.142237266683));
#256027=CARTESIAN_POINT('Ctrl Pts',(27.0459012525009,76.4391546325948,16.1404645724163));
#256028=CARTESIAN_POINT('Ctrl Pts',(27.0446965952318,76.438272235762,16.1387128817501));
#256029=CARTESIAN_POINT('Ctrl Pts',(27.0434998998453,76.4373972896807,16.1369701348014));
#256030=CARTESIAN_POINT('Ctrl Pts',(27.0334981288334,76.4300846431606,16.1224045602109));
#256031=CARTESIAN_POINT('Ctrl Pts',(27.0225381835945,76.4221888169328,16.1088060042622));
#256032=CARTESIAN_POINT('Ctrl Pts',(27.0113044494441,76.4142415794981,16.0954740612688));
#256033=CARTESIAN_POINT('Ctrl Pts',(27.007971666702,76.4118838224589,16.0915187896795));
#256034=CARTESIAN_POINT('Ctrl Pts',(27.0046149921553,76.4095212641207,16.0875869845174));
#256035=CARTESIAN_POINT('Ctrl Pts',(27.0012528338594,76.4071670555372,16.0836603564334));
#256036=CARTESIAN_POINT('Ctrl Pts',(25.1452786192766,75.979362108579,17.0741173620444));
#256037=CARTESIAN_POINT('Ctrl Pts',(24.9481252017973,76.0107288628306,17.0741173620444));
#256038=CARTESIAN_POINT('Ctrl Pts',(24.758292886385,76.0725110230494,17.0741173620444));
#256039=CARTESIAN_POINT('Ctrl Pts',(25.1452785074235,75.9793621491333,17.3508457847216));
#256040=CARTESIAN_POINT('Ctrl Pts',(24.9481251187328,76.0107288897045,17.3434041152847));
#256041=CARTESIAN_POINT('Ctrl Pts',(24.7582928856604,76.0725110232853,17.3371780222039));
#256042=CARTESIAN_POINT('Ctrl Pts',(25.1240988983279,75.9676381104205,17.6238224492216));
#256043=CARTESIAN_POINT('Ctrl Pts',(24.9271136619295,75.9996785825208,17.6090181824146));
#256044=CARTESIAN_POINT('Ctrl Pts',(24.737448667911,76.0621788292387,17.5966189870096));
#256045=CARTESIAN_POINT('Ctrl Pts',(25.0829574281538,75.9448790163861,17.8928559119209));
#256046=CARTESIAN_POINT('Ctrl Pts',(24.8862836604198,75.9782191703494,17.8708938349951));
#256047=CARTESIAN_POINT('Ctrl Pts',(24.6969219387962,76.0421000528014,17.8525678740453));
#256048=CARTESIAN_POINT('',(24.994844812995,76.0045572676648,17.2916572676617));
#256049=CARTESIAN_POINT('Ctrl Pts',(24.6976449917882,76.0424582864821,17.8479876920601));
#256050=CARTESIAN_POINT('Ctrl Pts',(24.7503755555246,76.0371537980617,17.7564160626317));
#256051=CARTESIAN_POINT('Ctrl Pts',(24.8016571681256,76.0312759356771,17.6640491390589));
#256052=CARTESIAN_POINT('Ctrl Pts',(24.8514229012875,76.0249016788522,17.5708847963288));
#256053=CARTESIAN_POINT('Ctrl Pts',(24.9007299986423,76.0185861665134,17.478579046466));
#256054=CARTESIAN_POINT('Ctrl Pts',(24.9485484624186,76.0117822354893,17.3854909384809));
#256055=CARTESIAN_POINT('Ctrl Pts',(24.9948448130087,76.0045572676614,17.2916572676743));
#256056=CARTESIAN_POINT('Ctrl Pts',(24.9948448130087,76.0045572676614,17.2916572676743));
#256057=CARTESIAN_POINT('Ctrl Pts',(25.0341234730694,75.9984274744394,17.2120470870498));
#256058=CARTESIAN_POINT('Ctrl Pts',(25.0842002511861,75.9891380711875,17.1401458391912));
#256059=CARTESIAN_POINT('Ctrl Pts',(25.1428889948602,75.9797434607284,17.0741173620444));
#256060=CARTESIAN_POINT('Origin',(-25.5443686855278,78.4878132480313,12.3825));
#256061=CARTESIAN_POINT('',(-25.1428889948604,75.9797434607283,17.0741173620445));
#256062=CARTESIAN_POINT('Ctrl Pts',(-27.0012528338594,76.4071670555372,
16.0836576911637));
#256063=CARTESIAN_POINT('Ctrl Pts',(-27.0125669200987,76.4150892640099,
16.0968733253419));
#256064=CARTESIAN_POINT('Ctrl Pts',(-27.0238163445857,76.4231093010226,
16.1101516770522));
#256065=CARTESIAN_POINT('Ctrl Pts',(-27.0343062910082,76.4307070447021,
16.1241706807122));
#256066=CARTESIAN_POINT('Ctrl Pts',(-27.037395957053,76.4329448531444,16.1282997808854));
#256067=CARTESIAN_POINT('Ctrl Pts',(-27.0404199473186,76.4351457409871,
16.1324931336593));
#256068=CARTESIAN_POINT('Ctrl Pts',(-27.0433610093266,76.4372957491563,
16.1367680612116));
#256069=CARTESIAN_POINT('Ctrl Pts',(-27.0486625246032,76.4411713223755,
16.1444739829716));
#256070=CARTESIAN_POINT('Ctrl Pts',(-27.0541111004947,76.4451930178066,
16.1523581129506));
#256071=CARTESIAN_POINT('Ctrl Pts',(-27.0576635452245,76.4478282805339,
16.1614817339872));
#256072=CARTESIAN_POINT('Ctrl Pts',(-27.0584419922995,76.4484057455524,
16.1634809927086));
#256073=CARTESIAN_POINT('Ctrl Pts',(-27.0591295239125,76.448916459005,16.1655397692371));
#256074=CARTESIAN_POINT('Ctrl Pts',(-27.0597047915435,76.449344095504,16.1676692305701));
#256075=CARTESIAN_POINT('Ctrl Pts',(-27.0611286869983,76.4504025761738,
16.172940047404));
#256076=CARTESIAN_POINT('Ctrl Pts',(-27.0609586565846,76.4502741691125,
16.1792319847823));
#256077=CARTESIAN_POINT('Ctrl Pts',(-27.0583397186354,76.4483300510152,
16.1834945126965));
#256078=CARTESIAN_POINT('Ctrl Pts',(-27.0580153514339,76.4480892632764,
16.1840224458809));
#256079=CARTESIAN_POINT('Ctrl Pts',(-27.0576533777842,76.4478206770397,
16.184519248061));
#256080=CARTESIAN_POINT('Ctrl Pts',(-27.0572521328189,76.4475231522575,
16.1849791234756));
#256081=CARTESIAN_POINT('Ctrl Pts',(-27.0536112395122,76.4448234149856,
16.1891520289663));
#256082=CARTESIAN_POINT('Ctrl Pts',(-27.0486162619737,76.4411392704989,
16.1910424129933));
#256083=CARTESIAN_POINT('Ctrl Pts',(-27.0438314224983,76.4376397186838,
16.1928564416501));
#256084=CARTESIAN_POINT('Ctrl Pts',(-27.0219957234643,76.4216694524754,
16.2011347933047));
#256085=CARTESIAN_POINT('Ctrl Pts',(-26.9995297607086,76.4057789844929,
16.207534966411));
#256086=CARTESIAN_POINT('Ctrl Pts',(-26.9767570197927,76.3902280507481,
16.2136304740377));
#256087=CARTESIAN_POINT('Ctrl Pts',(-26.9596083789282,76.3785176739039,
16.2182205965689));
#256088=CARTESIAN_POINT('Ctrl Pts',(-26.9422864664073,76.3669990382474,
16.2226379555783));
#256089=CARTESIAN_POINT('Ctrl Pts',(-26.924940664306,76.355767045105,16.2275544648554));
#256090=CARTESIAN_POINT('Ctrl Pts',(-26.8616513977226,76.3147851058381,
16.2454932297784));
#256091=CARTESIAN_POINT('Ctrl Pts',(-26.7969330614058,76.2768724896713,
16.264380542811));
#256092=CARTESIAN_POINT('Ctrl Pts',(-26.7309055212341,76.2419881574438,
16.2845312331379));
#256093=CARTESIAN_POINT('Ctrl Pts',(-26.7126781361404,76.2323580825449,
16.2900939784944));
#256094=CARTESIAN_POINT('Ctrl Pts',(-26.6943507497403,76.2229589907508,
16.2957530028506));
#256095=CARTESIAN_POINT('Ctrl Pts',(-26.6759253951148,76.2137905100208,
16.3015149294807));
#256096=CARTESIAN_POINT('Ctrl Pts',(-26.6064313423364,76.1792101778265,
16.3232469200705));
#256097=CARTESIAN_POINT('Ctrl Pts',(-26.5358861300337,76.1480850300989,
16.3462666779649));
#256098=CARTESIAN_POINT('Ctrl Pts',(-26.4646896515466,76.1204076386128,
16.3707095327059));
#256099=CARTESIAN_POINT('Ctrl Pts',(-26.3929595547121,76.0925228047893,
16.3953355868976));
#256100=CARTESIAN_POINT('Ctrl Pts',(-26.320568851033,76.0681374435539,16.42140615013));
#256101=CARTESIAN_POINT('Ctrl Pts',(-26.2479119279717,76.0471930592244,
16.4490596176973));
#256102=CARTESIAN_POINT('Ctrl Pts',(-26.2159174278757,76.0379701926591,
16.4612368312849));
#256103=CARTESIAN_POINT('Ctrl Pts',(-26.1838710753048,76.0294139153945,
16.4737209833412));
#256104=CARTESIAN_POINT('Ctrl Pts',(-26.151805321039,76.0215162801381,16.4865238911129));
#256105=CARTESIAN_POINT('Ctrl Pts',(-26.1024355268121,76.0093567461925,
16.5062357905105));
#256106=CARTESIAN_POINT('Ctrl Pts',(-26.0527788404423,75.9987033865243,
16.5268004133223));
#256107=CARTESIAN_POINT('Ctrl Pts',(-26.0031235801223,75.9895850865765,
16.548271859116));
#256108=CARTESIAN_POINT('Ctrl Pts',(-25.9532562257184,75.9804278393458,
16.5698350165754));
#256109=CARTESIAN_POINT('Ctrl Pts',(-25.9033908054762,75.9728187925742,
16.5923127602445));
#256110=CARTESIAN_POINT('Ctrl Pts',(-25.8538229234789,75.966734495867,16.6157598858881));
#256111=CARTESIAN_POINT('Ctrl Pts',(-25.8036709928875,75.9605785090897,
16.6394832843966));
#256112=CARTESIAN_POINT('Ctrl Pts',(-25.753824153542,75.9559833524274,16.664199043537));
#256113=CARTESIAN_POINT('Ctrl Pts',(-25.7045846543213,75.9528712677596,
16.6899639189295));
#256114=CARTESIAN_POINT('Ctrl Pts',(-25.6770558328495,75.9511313633215,
16.70436854664));
#256115=CARTESIAN_POINT('Ctrl Pts',(-25.6497167328468,75.949854070861,16.7191010971392));
#256116=CARTESIAN_POINT('Ctrl Pts',(-25.6226187903523,75.9490188646487,
16.7341714885812));
#256117=CARTESIAN_POINT('Ctrl Pts',(-25.5764663678453,75.9475963658742,
16.7598389381788));
#256118=CARTESIAN_POINT('Ctrl Pts',(-25.5307625058469,75.9474517866765,
16.7865659951667));
#256119=CARTESIAN_POINT('Ctrl Pts',(-25.4858135554159,75.9484882793166,
16.8145610365622));
#256120=CARTESIAN_POINT('Ctrl Pts',(-25.4402080117497,75.9495399125562,
16.842965016423));
#256121=CARTESIAN_POINT('Ctrl Pts',(-25.3953800360767,75.9518071268027,
16.8726742954997));
#256122=CARTESIAN_POINT('Ctrl Pts',(-25.351635516157,75.9551360231516,16.9039065164716));
#256123=CARTESIAN_POINT('Ctrl Pts',(-25.3063675024672,75.9585808552304,
16.936226464413));
#256124=CARTESIAN_POINT('Ctrl Pts',(-25.2622601838204,75.9631623245209,
16.970177280694));
#256125=CARTESIAN_POINT('Ctrl Pts',(-25.2196304518514,75.9686576197326,
17.0060001487159));
#256126=CARTESIAN_POINT('Ctrl Pts',(-25.193471268367,75.9720297365418,17.0279823882055));
#256127=CARTESIAN_POINT('Ctrl Pts',(-25.1678679991337,75.9757449424417,
17.0506695496094));
#256128=CARTESIAN_POINT('Ctrl Pts',(-25.1428889948604,75.9797434607283,
17.0741173620445));
#256129=CARTESIAN_POINT('Origin',(-25.5443686855278,78.4878132480312,17.0741173620445));
#256130=CARTESIAN_POINT('Ctrl Pts',(-24.758292886385,76.0725110230494,17.0741173620445));
#256131=CARTESIAN_POINT('Ctrl Pts',(-24.9481252017973,76.0107288628305,
17.0741173620445));
#256132=CARTESIAN_POINT('Ctrl Pts',(-25.1452786192768,75.9793621085789,
17.0741173620445));
#256133=CARTESIAN_POINT('Ctrl Pts',(-24.7582928856577,76.0725110232862,
17.3371780222047));
#256134=CARTESIAN_POINT('Ctrl Pts',(-24.9481251187305,76.0107288897052,
17.3434041152857));
#256135=CARTESIAN_POINT('Ctrl Pts',(-25.1452785074214,75.9793621491338,
17.3508457847227));
#256136=CARTESIAN_POINT('Ctrl Pts',(-24.7374486679099,76.0621788292392,
17.5966189870087));
#256137=CARTESIAN_POINT('Ctrl Pts',(-24.9271136619281,75.9996785825204,
17.6090181824136));
#256138=CARTESIAN_POINT('Ctrl Pts',(-25.1240988983264,75.9676381104195,
17.6238224492204));
#256139=CARTESIAN_POINT('Ctrl Pts',(-24.6969219387962,76.0421000528014,
17.8525678740454));
#256140=CARTESIAN_POINT('Ctrl Pts',(-24.8862836604199,75.9782191703494,
17.8708938349952));
#256141=CARTESIAN_POINT('Ctrl Pts',(-25.0829574281539,75.9448790163861,
17.892855911921));
#256142=CARTESIAN_POINT('',(-24.9948448129999,76.004557267664,17.2916572676519));
#256143=CARTESIAN_POINT('Ctrl Pts',(-25.1428889948604,75.9797434607283,
17.0741173620445));
#256144=CARTESIAN_POINT('Ctrl Pts',(-25.0842002511887,75.9891380711871,
17.1401458391885));
#256145=CARTESIAN_POINT('Ctrl Pts',(-25.0341234730736,75.9984274744386,
17.2120470870439));
#256146=CARTESIAN_POINT('Ctrl Pts',(-24.9948448130136,76.0045572676606,
17.2916572676646));
#256147=CARTESIAN_POINT('Ctrl Pts',(-24.9948448130136,76.0045572676606,
17.2916572676646));
#256148=CARTESIAN_POINT('Ctrl Pts',(-24.94811785539,76.0118494356433,17.3863636949506));
#256149=CARTESIAN_POINT('Ctrl Pts',(-24.8998402827123,76.018712699508,17.4803105681817));
#256150=CARTESIAN_POINT('Ctrl Pts',(-24.850046684856,76.0250777756705,17.5734602294373));
#256151=CARTESIAN_POINT('Ctrl Pts',(-24.8007119288024,76.0313841984489,
17.6657515281657));
#256152=CARTESIAN_POINT('Ctrl Pts',(-24.7498896231699,76.0372026809562,
17.7572599302886));
#256153=CARTESIAN_POINT('Ctrl Pts',(-24.697644991789,76.0424582864817,17.8479876920609));
#256154=CARTESIAN_POINT('Ctrl Pts',(-76.0725110230494,-24.758292886385,
17.0741173620445));
#256155=CARTESIAN_POINT('Ctrl Pts',(-76.0107288628305,-24.9481252017973,
17.0741173620445));
#256156=CARTESIAN_POINT('Ctrl Pts',(-75.9793621085789,-25.1452786192767,
17.0741173620445));
#256157=CARTESIAN_POINT('Ctrl Pts',(-76.0725110232863,-24.7582928856572,
17.3371780222034));
#256158=CARTESIAN_POINT('Ctrl Pts',(-76.0107288897045,-24.9481251187298,
17.3434041152839));
#256159=CARTESIAN_POINT('Ctrl Pts',(-75.9793621491325,-25.1452785074205,
17.3508457847206));
#256160=CARTESIAN_POINT('Ctrl Pts',(-76.0621788292369,-24.7374486679163,
17.5966189870106));
#256161=CARTESIAN_POINT('Ctrl Pts',(-75.99967858252,-24.9271136619357,17.609018182416));
#256162=CARTESIAN_POINT('Ctrl Pts',(-75.9676381104206,-25.124098898335,
17.6238224492233));
#256163=CARTESIAN_POINT('Ctrl Pts',(-76.0421000528014,-24.6969219387961,
17.8525678740454));
#256164=CARTESIAN_POINT('Ctrl Pts',(-75.9782191703494,-24.8862836604199,
17.8708938349953));
#256165=CARTESIAN_POINT('Ctrl Pts',(-75.9448790163861,-25.0829574281539,
17.892855911921));
#256166=CARTESIAN_POINT('',(-76.004557267664,-24.9948448129999,17.2916572676518));
#256167=CARTESIAN_POINT('Ctrl Pts',(-75.9797434607283,-25.1428889948604,
17.0741173620445));
#256168=CARTESIAN_POINT('Ctrl Pts',(-75.989138071187,-25.0842002511887,
17.1401458391886));
#256169=CARTESIAN_POINT('Ctrl Pts',(-75.9984274744386,-25.0341234730736,
17.2120470870439));
#256170=CARTESIAN_POINT('Ctrl Pts',(-76.0045572676606,-24.9948448130136,
17.2916572676645));
#256171=CARTESIAN_POINT('Ctrl Pts',(-76.0045572676606,-24.9948448130136,
17.2916572676645));
#256172=CARTESIAN_POINT('Ctrl Pts',(-76.0118494398941,-24.9481178281451,
17.3863637502011));
#256173=CARTESIAN_POINT('Ctrl Pts',(-76.0187127075221,-24.8998402263703,
17.4803106777579));
#256174=CARTESIAN_POINT('Ctrl Pts',(-76.0250777868188,-24.8500465976989,
17.5734603924151));
#256175=CARTESIAN_POINT('Ctrl Pts',(-76.0313842053114,-24.8007118689344,
17.6657516358879));
#256176=CARTESIAN_POINT('Ctrl Pts',(-76.0372026840567,-24.7498895923968,
17.7572599836914));
#256177=CARTESIAN_POINT('Ctrl Pts',(-76.0424582864817,-24.697644991789,
17.8479876920609));
#256178=CARTESIAN_POINT('Ctrl Pts',(-75.9793621085789,25.1452786192766,
17.0741173620445));
#256179=CARTESIAN_POINT('Ctrl Pts',(-76.0107288628305,24.9481252017972,
17.0741173620445));
#256180=CARTESIAN_POINT('Ctrl Pts',(-76.0725110230494,24.758292886385,17.0741173620445));
#256181=CARTESIAN_POINT('Ctrl Pts',(-75.9793621491325,25.1452785074204,
17.3508457847207));
#256182=CARTESIAN_POINT('Ctrl Pts',(-76.0107288897045,24.9481251187298,
17.3434041152841));
#256183=CARTESIAN_POINT('Ctrl Pts',(-76.0725110232863,24.7582928856572,
17.3371780222036));
#256184=CARTESIAN_POINT('Ctrl Pts',(-75.9676381104235,25.1240988983324,
17.6238224492231));
#256185=CARTESIAN_POINT('Ctrl Pts',(-75.9996785825219,24.9271136619338,
17.6090181824158));
#256186=CARTESIAN_POINT('Ctrl Pts',(-76.0621788292373,24.7374486679152,
17.5966189870103));
#256187=CARTESIAN_POINT('Ctrl Pts',(-75.9448790163861,25.0829574281538,
17.892855911921));
#256188=CARTESIAN_POINT('Ctrl Pts',(-75.9782191703494,24.8862836604198,
17.8708938349952));
#256189=CARTESIAN_POINT('Ctrl Pts',(-76.0421000528014,24.6969219387961,
17.8525678740454));
#256190=CARTESIAN_POINT('',(-76.0045572676648,24.9948448129949,17.2916572676618));
#256191=CARTESIAN_POINT('Ctrl Pts',(-76.0424582864821,24.6976449917881,
17.8479876920602));
#256192=CARTESIAN_POINT('Ctrl Pts',(-76.0371538035502,24.7503755009267,
17.7564161574767));
#256193=CARTESIAN_POINT('Ctrl Pts',(-76.031275947831,24.8016570619565,17.6640493304302));
#256194=CARTESIAN_POINT('Ctrl Pts',(-76.0249016986412,24.8514227467087,
17.5708850858271));
#256195=CARTESIAN_POINT('Ctrl Pts',(-76.0185861807249,24.9007298987056,
17.4785792411033));
#256196=CARTESIAN_POINT('Ctrl Pts',(-76.0117822430429,24.9485484140197,
17.3854910365594));
#256197=CARTESIAN_POINT('Ctrl Pts',(-76.0045572676614,24.9948448130087,
17.2916572676745));
#256198=CARTESIAN_POINT('Ctrl Pts',(-76.0045572676613,24.9948448130087,
17.2916572676745));
#256199=CARTESIAN_POINT('Ctrl Pts',(-75.9984274744394,25.0341234730694,
17.21204708705));
#256200=CARTESIAN_POINT('Ctrl Pts',(-75.9891380711875,25.084200251186,17.1401458391913));
#256201=CARTESIAN_POINT('Ctrl Pts',(-75.9797434607283,25.1428889948603,
17.0741173620445));
#256202=CARTESIAN_POINT('Ctrl Pts',(25.9085897226107,-77.9676516999078,
12.3825));
#256203=CARTESIAN_POINT('Ctrl Pts',(25.6490890766241,-77.7859473914177,
12.3825));
#256204=CARTESIAN_POINT('Ctrl Pts',(25.3478497357421,-77.8839876917858,
12.3825));
#256205=CARTESIAN_POINT('Ctrl Pts',(27.0012528338594,-76.4071670555372,
12.3825));
#256206=CARTESIAN_POINT('Ctrl Pts',(25.9632502499131,-75.6803498215769,
12.3825));
#256207=CARTESIAN_POINT('Ctrl Pts',(24.758292886385,-76.0725110230494,12.3825));
#256208=CARTESIAN_POINT('Ctrl Pts',(27.0012528338594,-76.4071670555372,
14.2875));
#256209=CARTESIAN_POINT('Ctrl Pts',(25.9632502499131,-75.6803498215769,
14.2875));
#256210=CARTESIAN_POINT('Ctrl Pts',(24.758292886385,-76.0725110230494,14.2875));
#256211=CARTESIAN_POINT('Origin',(25.3478497357421,-77.8839876917858,14.2875));
#256212=CARTESIAN_POINT('Origin',(25.9085897226107,-77.9676516999077,14.2875));
#256213=CARTESIAN_POINT('Origin',(74.5679259799751,-112.039285751595,14.2875));
#256214=CARTESIAN_POINT('Origin',(74.5679259799751,-112.039285751595,14.2875));
#256215=CARTESIAN_POINT('Origin',(0.,0.,14.2875));
#256216=CARTESIAN_POINT('Origin',(-25.3478497357421,-77.8839876917858,14.2875));
#256217=CARTESIAN_POINT('Origin',(90.,-90.,14.2875));
#256218=CARTESIAN_POINT('Origin',(76.1978262581577,-113.095,14.2875));
#256219=CARTESIAN_POINT('Ctrl Pts',(-25.3478497357421,-77.8839876917858,
12.3825));
#256220=CARTESIAN_POINT('Ctrl Pts',(-25.6490890766241,-77.7859473914177,
12.3825));
#256221=CARTESIAN_POINT('Ctrl Pts',(-25.9085897226107,-77.9676516999077,
12.3825));
#256222=CARTESIAN_POINT('Ctrl Pts',(-24.7582928863851,-76.0725110230494,
12.3825));
#256223=CARTESIAN_POINT('Ctrl Pts',(-25.9632502499132,-75.6803498215769,
12.3825));
#256224=CARTESIAN_POINT('Ctrl Pts',(-27.0012528338595,-76.4071670555372,
12.3825));
#256225=CARTESIAN_POINT('Ctrl Pts',(-24.7582928863851,-76.0725110230494,
14.2875));
#256226=CARTESIAN_POINT('Ctrl Pts',(-25.9632502499132,-75.6803498215769,
14.2875));
#256227=CARTESIAN_POINT('Ctrl Pts',(-27.0012528338595,-76.4071670555372,
14.2875));
#256228=CARTESIAN_POINT('Origin',(-25.9085897226107,-77.9676516999077,14.2875));
#256229=CARTESIAN_POINT('Ctrl Pts',(77.1750847966528,-111.45976584278,14.2875));
#256230=CARTESIAN_POINT('Ctrl Pts',(77.1750847966528,-111.45976584278,12.3825));
#256231=CARTESIAN_POINT('Ctrl Pts',(76.1978262581577,-113.095,12.3825));
#256232=CARTESIAN_POINT('Ctrl Pts',(77.6808356682961,-111.762015741049,
14.2874999966875));
#256233=CARTESIAN_POINT('Ctrl Pts',(77.5941846099562,-111.71023081209,12.5172751948194));
#256234=CARTESIAN_POINT('Ctrl Pts',(76.7421246518763,-113.257643450726,
12.3825));
#256235=CARTESIAN_POINT('Ctrl Pts',(78.1909142917095,-112.04266475307,14.2466073426296));
#256236=CARTESIAN_POINT('Ctrl Pts',(78.0590963418289,-111.971409284925,
12.6053517687442));
#256237=CARTESIAN_POINT('Ctrl Pts',(77.2910619607791,-113.408657903693,
12.3620536717506));
#256238=CARTESIAN_POINT('Ctrl Pts',(79.2214453413673,-112.564492774109,
14.108780097621));
#256239=CARTESIAN_POINT('Ctrl Pts',(79.0242905953313,-112.468920289919,
12.6961322557778));
#256240=CARTESIAN_POINT('Ctrl Pts',(78.4001194763382,-113.689453561681,
12.2931400483747));
#256241=CARTESIAN_POINT('Ctrl Pts',(79.7419020126347,-112.805653119423,
14.0115316944756));
#256242=CARTESIAN_POINT('Ctrl Pts',(79.526944890976,-112.708892347893,12.703865475829));
#256243=CARTESIAN_POINT('Ctrl Pts',(78.9602349460145,-113.819221943657,
12.244515847471));
#256244=CARTESIAN_POINT('Ctrl Pts',(80.7943836707349,-113.250441211302,
13.7750080898747));
#256245=CARTESIAN_POINT('Ctrl Pts',(80.5569292865739,-113.155754679235,
12.6577917414232));
#256246=CARTESIAN_POINT('Ctrl Pts',(80.0929157064278,-114.058562415705,
12.1262540447041));
#256247=CARTESIAN_POINT('Ctrl Pts',(81.3276580610674,-113.45448134688,13.6352465336299));
#256248=CARTESIAN_POINT('Ctrl Pts',(81.0885336408363,-113.366292203084,
12.6062543646742));
#256249=CARTESIAN_POINT('Ctrl Pts',(80.666825605363,-114.168356412835,12.0563732669971));
#256250=CARTESIAN_POINT('Ctrl Pts',(82.4011339813139,-113.823925897865,
13.3246442856472));
#256251=CARTESIAN_POINT('Ctrl Pts',(82.1657264091691,-113.748604057329,
12.4584071352196));
#256252=CARTESIAN_POINT('Ctrl Pts',(81.8221003906478,-114.367154525562,
11.9010721426414));
#256253=CARTESIAN_POINT('Ctrl Pts',(82.9379109315738,-113.98827163761,13.1548625963702));
#256254=CARTESIAN_POINT('Ctrl Pts',(82.7112571397903,-113.921920427821,
12.3636877604077));
#256255=CARTESIAN_POINT('Ctrl Pts',(82.3997797445818,-114.455588968268,
11.8161812982783));
#256256=CARTESIAN_POINT('Ctrl Pts',(84.5510793506422,-114.424380779002,
12.6139948970955));
#256257=CARTESIAN_POINT('Ctrl Pts',(84.3341564328195,-114.375512716331,
12.0384183635703));
#256258=CARTESIAN_POINT('Ctrl Pts',(84.1358715971169,-114.690259297042,
11.5457474483613));
#256259=CARTESIAN_POINT('Ctrl Pts',(85.6303497382816,-114.639636039159,
12.2118226911433));
#256260=CARTESIAN_POINT('Ctrl Pts',(85.4594058856995,-114.611553326324,
11.7583160303656));
#256261=CARTESIAN_POINT('Ctrl Pts',(85.2973823883387,-114.806088152743,
11.3446613455991));
#256262=CARTESIAN_POINT('Ctrl Pts',(87.8072663979372,-114.927844409462,
11.3656205182415));
#256263=CARTESIAN_POINT('Ctrl Pts',(87.7104675830927,-114.920352198467,
11.1472581448906));
#256264=CARTESIAN_POINT('Ctrl Pts',(87.6401800974599,-114.96117307666,10.9215602590933));
#256265=CARTESIAN_POINT('Ctrl Pts',(88.9061071730694,-115.,10.9205098031028));
#256266=CARTESIAN_POINT('Ctrl Pts',(88.8644746746685,-115.,10.8097442389035));
#256267=CARTESIAN_POINT('Ctrl Pts',(88.8227423399098,-115.,10.6990068206853));
#256268=CARTESIAN_POINT('Ctrl Pts',(90.,-115.,10.4775));
#256269=CARTESIAN_POINT('Ctrl Pts',(90.,-115.,10.4775));
#256270=CARTESIAN_POINT('Ctrl Pts',(90.,-115.,10.4775));
#256271=CARTESIAN_POINT('Ctrl Pts',(90.,-115.,10.4775));
#256272=CARTESIAN_POINT('Ctrl Pts',(89.583543836463,-115.,10.5558582760742));
#256273=CARTESIAN_POINT('Ctrl Pts',(89.16698283296,-114.995145444742,10.6342451251674));
#256274=CARTESIAN_POINT('Ctrl Pts',(88.7504746564855,-114.985453756063,
10.7122315109298));
#256275=CARTESIAN_POINT('Ctrl Pts',(88.3493129355897,-114.976119162583,
10.7873444486486));
#256276=CARTESIAN_POINT('Ctrl Pts',(87.9481990723853,-114.962297205616,
10.8620867505664));
#256277=CARTESIAN_POINT('Ctrl Pts',(87.5472762325185,-114.943957243982,
10.9360757308279));
#256278=CARTESIAN_POINT('Ctrl Pts',(87.2069586549715,-114.928389631727,
10.9988802109521));
#256279=CARTESIAN_POINT('Ctrl Pts',(86.8667783863514,-114.909565993822,
11.0611422131555));
#256280=CARTESIAN_POINT('Ctrl Pts',(86.5268333104866,-114.887440575962,
11.1226211406014));
#256281=CARTESIAN_POINT('Ctrl Pts',(86.5074818406287,-114.886181080275,
11.1261208459827));
#256282=CARTESIAN_POINT('Ctrl Pts',(86.4881313431668,-114.884910894891,
11.1296179650593));
#256283=CARTESIAN_POINT('Ctrl Pts',(86.4687819131639,-114.883630015072,
11.1331124382524));
#256284=CARTESIAN_POINT('Ctrl Pts',(85.900400763887,-114.846004723596,11.2357610790286));
#256285=CARTESIAN_POINT('Ctrl Pts',(85.3326432827616,-114.799248326424,
11.3362547894292));
#256286=CARTESIAN_POINT('Ctrl Pts',(84.7653562148502,-114.742990120853,
11.4332724000528));
#256287=CARTESIAN_POINT('Ctrl Pts',(84.1980691469388,-114.686731915282,
11.5302900106764));
#256288=CARTESIAN_POINT('Ctrl Pts',(83.6312517469126,-114.62097164889,11.6238302836077));
#256289=CARTESIAN_POINT('Ctrl Pts',(83.0647232345981,-114.545392304676,
11.7125671552065));
#256290=CARTESIAN_POINT('Ctrl Pts',(83.0359704727094,-114.541556460864,
11.7170707769738));
#256291=CARTESIAN_POINT('Ctrl Pts',(83.0072223038157,-114.537695858892,
11.7215614148314));
#256292=CARTESIAN_POINT('Ctrl Pts',(82.978478279317,-114.533810424182,11.7260389714724));
#256293=CARTESIAN_POINT('Ctrl Pts',(82.6542583520787,-114.489984433187,
11.7765438368714));
#256294=CARTESIAN_POINT('Ctrl Pts',(82.330561948864,-114.442984724948,11.8253691505401));
#256295=CARTESIAN_POINT('Ctrl Pts',(82.0067026925525,-114.392600666908,
11.8722415248233));
#256296=CARTESIAN_POINT('Ctrl Pts',(81.7528333341015,-114.353105212505,
11.9089842127547));
#256297=CARTESIAN_POINT('Ctrl Pts',(81.4988640709653,-114.311529402532,
11.9445266216304));
#256298=CARTESIAN_POINT('Ctrl Pts',(81.2444644384059,-114.267752870079,
11.9787247352563));
#256299=CARTESIAN_POINT('Ctrl Pts',(80.9597456260951,-114.218759079476,
12.016998557419));
#256300=CARTESIAN_POINT('Ctrl Pts',(80.6753810400077,-114.167147236487,
12.0534610877611));
#256301=CARTESIAN_POINT('Ctrl Pts',(80.3915054834947,-114.112878627138,
12.0877657414697));
#256302=CARTESIAN_POINT('Ctrl Pts',(80.1315884873099,-114.063190185828,
12.1191751472552));
#256303=CARTESIAN_POINT('Ctrl Pts',(79.8720812258998,-114.011274194815,
12.1487756059618));
#256304=CARTESIAN_POINT('Ctrl Pts',(79.6131099264372,-113.957084553584,
12.1762747511384));
#256305=CARTESIAN_POINT('Ctrl Pts',(79.5842583911621,-113.951047381324,
12.1793383823544));
#256306=CARTESIAN_POINT('Ctrl Pts',(79.5554139374348,-113.944982071645,
12.1823758526507));
#256307=CARTESIAN_POINT('Ctrl Pts',(79.5265771857676,-113.938888643004,
12.1853866936196));
#256308=CARTESIAN_POINT('Ctrl Pts',(79.1552547066283,-113.860425331486,
12.2241564186487));
#256309=CARTESIAN_POINT('Ctrl Pts',(78.7846328269209,-113.777204059966,
12.2586195275686));
#256310=CARTESIAN_POINT('Ctrl Pts',(78.4147483858496,-113.688967055657,
12.2875599189643));
#256311=CARTESIAN_POINT('Ctrl Pts',(78.2248346050177,-113.6436625734,12.3024190980441));
#256312=CARTESIAN_POINT('Ctrl Pts',(78.03511493423,-113.5970358706,12.3158215393074));
#256313=CARTESIAN_POINT('Ctrl Pts',(77.8455925411284,-113.549052337868,
12.3275976932325));
#256314=CARTESIAN_POINT('Ctrl Pts',(77.5177312889421,-113.466043987941,
12.3479696635768));
#256315=CARTESIAN_POINT('Ctrl Pts',(77.1904629065562,-113.378979813794,
12.3635332048009));
#256316=CARTESIAN_POINT('Ctrl Pts',(76.8637289612717,-113.287580782422,
12.3728032157562));
#256317=CARTESIAN_POINT('Ctrl Pts',(76.6415217694246,-113.225421577993,
12.3791076207086));
#256318=CARTESIAN_POINT('Ctrl Pts',(76.4195614759289,-113.161257371659,
12.3825));
#256319=CARTESIAN_POINT('Ctrl Pts',(76.1978262581578,-113.095,12.3825));
#256320=CARTESIAN_POINT('Origin',(-74.5679259799751,-112.039285751595,14.2875));
#256321=CARTESIAN_POINT('Origin',(-74.5679259799751,-112.039285751595,14.2875));
#256322=CARTESIAN_POINT('Origin',(0.,-113.095,10.4775));
#256323=CARTESIAN_POINT('Ctrl Pts',(-90.,-115.,10.4775));
#256324=CARTESIAN_POINT('Ctrl Pts',(-89.5835438364623,-115.,10.5558582760744));
#256325=CARTESIAN_POINT('Ctrl Pts',(-89.1669828329586,-114.995145444742,
10.6342451251677));
#256326=CARTESIAN_POINT('Ctrl Pts',(-88.7504746564834,-114.985453756063,
10.7122315109302));
#256327=CARTESIAN_POINT('Ctrl Pts',(-88.3493129355877,-114.976119162583,
10.787344448649));
#256328=CARTESIAN_POINT('Ctrl Pts',(-87.9481990723833,-114.962297205616,
10.8620867505668));
#256329=CARTESIAN_POINT('Ctrl Pts',(-87.5472762325166,-114.943957243982,
10.9360757308282));
#256330=CARTESIAN_POINT('Ctrl Pts',(-87.2069586549702,-114.928389631727,
10.9988802109523));
#256331=CARTESIAN_POINT('Ctrl Pts',(-86.8667783863508,-114.909565993822,
11.0611422131556));
#256332=CARTESIAN_POINT('Ctrl Pts',(-86.5268333104866,-114.887440575962,
11.1226211406014));
#256333=CARTESIAN_POINT('Ctrl Pts',(-86.5074818406287,-114.886181080275,
11.1261208459827));
#256334=CARTESIAN_POINT('Ctrl Pts',(-86.4881313431668,-114.884910894891,
11.1296179650593));
#256335=CARTESIAN_POINT('Ctrl Pts',(-86.4687819131639,-114.883630015072,
11.1331124382524));
#256336=CARTESIAN_POINT('Ctrl Pts',(-85.900400763887,-114.846004723596,
11.2357610790286));
#256337=CARTESIAN_POINT('Ctrl Pts',(-85.3326432827616,-114.799248326424,
11.3362547894291));
#256338=CARTESIAN_POINT('Ctrl Pts',(-84.7653562148502,-114.742990120853,
11.4332724000528));
#256339=CARTESIAN_POINT('Ctrl Pts',(-84.1980691469388,-114.686731915282,
11.5302900106764));
#256340=CARTESIAN_POINT('Ctrl Pts',(-83.6312517469126,-114.62097164889,
11.6238302836077));
#256341=CARTESIAN_POINT('Ctrl Pts',(-83.0647232345982,-114.545392304676,
11.7125671552065));
#256342=CARTESIAN_POINT('Ctrl Pts',(-83.0359704727094,-114.541556460864,
11.7170707769738));
#256343=CARTESIAN_POINT('Ctrl Pts',(-83.0072223038157,-114.537695858892,
11.7215614148314));
#256344=CARTESIAN_POINT('Ctrl Pts',(-82.978478279317,-114.533810424182,
11.7260389714724));
#256345=CARTESIAN_POINT('Ctrl Pts',(-82.6542583520783,-114.489984433187,
11.7765438368714));
#256346=CARTESIAN_POINT('Ctrl Pts',(-82.3305619488634,-114.442984724948,
11.8253691505402));
#256347=CARTESIAN_POINT('Ctrl Pts',(-82.0067026925516,-114.392600666908,
11.8722415248234));
#256348=CARTESIAN_POINT('Ctrl Pts',(-81.7528333341009,-114.353105212505,
11.9089842127548));
#256349=CARTESIAN_POINT('Ctrl Pts',(-81.498864070965,-114.311529402532,
11.9445266216304));
#256350=CARTESIAN_POINT('Ctrl Pts',(-81.2444644384059,-114.267752870079,
11.9787247352563));
#256351=CARTESIAN_POINT('Ctrl Pts',(-80.9597456260961,-114.218759079476,
12.0169985574188));
#256352=CARTESIAN_POINT('Ctrl Pts',(-80.6753810400096,-114.167147236488,
12.0534610877609));
#256353=CARTESIAN_POINT('Ctrl Pts',(-80.3915054834976,-114.112878627139,
12.0877657414694));
#256354=CARTESIAN_POINT('Ctrl Pts',(-80.1315884873118,-114.063190185829,
12.119175147255));
#256355=CARTESIAN_POINT('Ctrl Pts',(-79.8720812259008,-114.011274194815,
12.1487756059617));
#256356=CARTESIAN_POINT('Ctrl Pts',(-79.6131099264372,-113.957084553584,
12.1762747511384));
#256357=CARTESIAN_POINT('Ctrl Pts',(-79.5842583911621,-113.951047381324,
12.1793383823544));
#256358=CARTESIAN_POINT('Ctrl Pts',(-79.5554139374348,-113.944982071645,
12.1823758526507));
#256359=CARTESIAN_POINT('Ctrl Pts',(-79.5265771857676,-113.938888643004,
12.1853866936196));
#256360=CARTESIAN_POINT('Ctrl Pts',(-79.1552547066275,-113.860425331486,
12.2241564186488));
#256361=CARTESIAN_POINT('Ctrl Pts',(-78.7846328269193,-113.777204059965,
12.2586195275687));
#256362=CARTESIAN_POINT('Ctrl Pts',(-78.4147483858471,-113.688967055656,
12.2875599189645));
#256363=CARTESIAN_POINT('Ctrl Pts',(-78.2248346050161,-113.643662573399,
12.3024190980442));
#256364=CARTESIAN_POINT('Ctrl Pts',(-78.0351149342292,-113.597035870599,
12.3158215393074));
#256365=CARTESIAN_POINT('Ctrl Pts',(-77.8455925411284,-113.549052337868,
12.3275976932325));
#256366=CARTESIAN_POINT('Ctrl Pts',(-77.5177312889423,-113.466043987941,
12.3479696635768));
#256367=CARTESIAN_POINT('Ctrl Pts',(-77.1904629065567,-113.378979813794,
12.3635332048009));
#256368=CARTESIAN_POINT('Ctrl Pts',(-76.8637289612724,-113.287580782422,
12.3728032157562));
#256369=CARTESIAN_POINT('Ctrl Pts',(-76.6415217694251,-113.225421577994,
12.3791076207086));
#256370=CARTESIAN_POINT('Ctrl Pts',(-76.4195614759291,-113.161257371659,
12.3825));
#256371=CARTESIAN_POINT('Ctrl Pts',(-76.1978262581577,-113.095,12.3825));
#256372=CARTESIAN_POINT('Origin',(-90.,-90.,14.2875));
#256373=CARTESIAN_POINT('Origin',(-76.1978262581577,-113.095,14.2875));
#256374=CARTESIAN_POINT('Ctrl Pts',(-76.1978262581577,-113.095,12.3825));
#256375=CARTESIAN_POINT('Ctrl Pts',(-77.1750847966528,-111.45976584278,
12.3825));
#256376=CARTESIAN_POINT('Ctrl Pts',(-77.1750847966528,-111.45976584278,
14.2875));
#256377=CARTESIAN_POINT('Ctrl Pts',(-76.7421246518763,-113.257643450726,
12.3825));
#256378=CARTESIAN_POINT('Ctrl Pts',(-77.5941846099562,-111.71023081209,
12.5172751948194));
#256379=CARTESIAN_POINT('Ctrl Pts',(-77.6808356682961,-111.762015741049,
14.2874999966875));
#256380=CARTESIAN_POINT('Ctrl Pts',(-77.2910619607791,-113.408657903693,
12.3620536717506));
#256381=CARTESIAN_POINT('Ctrl Pts',(-78.0590963418289,-111.971409284925,
12.6053517687442));
#256382=CARTESIAN_POINT('Ctrl Pts',(-78.1909142917095,-112.04266475307,
14.2466073426296));
#256383=CARTESIAN_POINT('Ctrl Pts',(-78.4001194763382,-113.689453561681,
12.2931400483747));
#256384=CARTESIAN_POINT('Ctrl Pts',(-79.0242905953313,-112.468920289919,
12.6961322557778));
#256385=CARTESIAN_POINT('Ctrl Pts',(-79.2214453413673,-112.564492774109,
14.108780097621));
#256386=CARTESIAN_POINT('Ctrl Pts',(-78.9602349460145,-113.819221943657,
12.244515847471));
#256387=CARTESIAN_POINT('Ctrl Pts',(-79.526944890976,-112.708892347893,
12.703865475829));
#256388=CARTESIAN_POINT('Ctrl Pts',(-79.7419020126347,-112.805653119423,
14.0115316944756));
#256389=CARTESIAN_POINT('Ctrl Pts',(-80.0929157064278,-114.058562415705,
12.1262540447041));
#256390=CARTESIAN_POINT('Ctrl Pts',(-80.5569292865739,-113.155754679235,
12.6577917414232));
#256391=CARTESIAN_POINT('Ctrl Pts',(-80.7943836707349,-113.250441211302,
13.7750080898747));
#256392=CARTESIAN_POINT('Ctrl Pts',(-80.666825605363,-114.168356412835,
12.0563732669971));
#256393=CARTESIAN_POINT('Ctrl Pts',(-81.0885336408363,-113.366292203084,
12.6062543646742));
#256394=CARTESIAN_POINT('Ctrl Pts',(-81.3276580610674,-113.45448134688,
13.6352465336299));
#256395=CARTESIAN_POINT('Ctrl Pts',(-81.8221003906478,-114.367154525562,
11.9010721426414));
#256396=CARTESIAN_POINT('Ctrl Pts',(-82.1657264091691,-113.748604057329,
12.4584071352196));
#256397=CARTESIAN_POINT('Ctrl Pts',(-82.4011339813139,-113.823925897865,
13.3246442856472));
#256398=CARTESIAN_POINT('Ctrl Pts',(-82.3997797445818,-114.455588968268,
11.8161812982783));
#256399=CARTESIAN_POINT('Ctrl Pts',(-82.7112571397903,-113.921920427821,
12.3636877604077));
#256400=CARTESIAN_POINT('Ctrl Pts',(-82.9379109315738,-113.98827163761,
13.1548625963702));
#256401=CARTESIAN_POINT('Ctrl Pts',(-84.1358715971169,-114.690259297042,
11.5457474483613));
#256402=CARTESIAN_POINT('Ctrl Pts',(-84.3341564328195,-114.375512716331,
12.0384183635703));
#256403=CARTESIAN_POINT('Ctrl Pts',(-84.5510793506422,-114.424380779002,
12.6139948970955));
#256404=CARTESIAN_POINT('Ctrl Pts',(-85.2973823883387,-114.806088152743,
11.3446613455991));
#256405=CARTESIAN_POINT('Ctrl Pts',(-85.4594058856995,-114.611553326324,
11.7583160303656));
#256406=CARTESIAN_POINT('Ctrl Pts',(-85.6303497382816,-114.639636039159,
12.2118226911433));
#256407=CARTESIAN_POINT('Ctrl Pts',(-87.6401800974599,-114.96117307666,
10.9215602590933));
#256408=CARTESIAN_POINT('Ctrl Pts',(-87.7104675830927,-114.920352198467,
11.1472581448906));
#256409=CARTESIAN_POINT('Ctrl Pts',(-87.8072663979372,-114.927844409462,
11.3656205182415));
#256410=CARTESIAN_POINT('Ctrl Pts',(-88.8227423399098,-115.,10.6990068206853));
#256411=CARTESIAN_POINT('Ctrl Pts',(-88.8644746746686,-115.,10.8097442389035));
#256412=CARTESIAN_POINT('Ctrl Pts',(-88.9061071730694,-115.,10.9205098031028));
#256413=CARTESIAN_POINT('Ctrl Pts',(-90.,-115.,10.4775));
#256414=CARTESIAN_POINT('Ctrl Pts',(-90.,-115.,10.4775));
#256415=CARTESIAN_POINT('Ctrl Pts',(-90.,-115.,10.4775));
#256416=CARTESIAN_POINT('Origin',(112.039285751595,74.5679259799752,14.2875));
#256417=CARTESIAN_POINT('Origin',(112.039285751595,74.5679259799752,14.2875));
#256418=CARTESIAN_POINT('Origin',(90.,90.,14.2875));
#256419=CARTESIAN_POINT('Origin',(113.095,76.1978262581577,14.2875));
#256420=CARTESIAN_POINT('Ctrl Pts',(111.45976584278,77.1750847966528,14.2875));
#256421=CARTESIAN_POINT('Ctrl Pts',(111.45976584278,77.1750847966528,12.3825));
#256422=CARTESIAN_POINT('Ctrl Pts',(113.095,76.1978262581577,12.3825));
#256423=CARTESIAN_POINT('Ctrl Pts',(111.76201574105,77.6808356682986,14.2874999966875));
#256424=CARTESIAN_POINT('Ctrl Pts',(111.710230812097,77.5941846099538,12.5172751948261));
#256425=CARTESIAN_POINT('Ctrl Pts',(113.257643450739,76.7421246518766,12.3825));
#256426=CARTESIAN_POINT('Ctrl Pts',(112.042664753068,78.1909142917061,14.2466073426296));
#256427=CARTESIAN_POINT('Ctrl Pts',(111.97140928493,78.0590963418208,12.6053517687504));
#256428=CARTESIAN_POINT('Ctrl Pts',(113.408657903689,77.2910619607747,12.3620536717516));
#256429=CARTESIAN_POINT('Ctrl Pts',(112.564492774111,79.2214453413707,14.108780097621));
#256430=CARTESIAN_POINT('Ctrl Pts',(112.468920289915,79.0242905953405,12.696132255772));
#256431=CARTESIAN_POINT('Ctrl Pts',(113.689453561686,78.4001194763425,12.2931400483737));
#256432=CARTESIAN_POINT('Ctrl Pts',(112.805653119421,79.7419020126294,14.0115316944767));
#256433=CARTESIAN_POINT('Ctrl Pts',(112.708892347889,79.5269448909711,12.7038654758262));
#256434=CARTESIAN_POINT('Ctrl Pts',(113.819221943654,78.9602349460102,12.2445158474727));
#256435=CARTESIAN_POINT('Ctrl Pts',(113.250441211304,80.7943836707402,13.7750080898736));
#256436=CARTESIAN_POINT('Ctrl Pts',(113.15575467924,80.5569292865777,12.6577917414259));
#256437=CARTESIAN_POINT('Ctrl Pts',(114.058562415709,80.0929157064321,12.1262540447024));
#256438=CARTESIAN_POINT('Ctrl Pts',(113.454481346879,81.327658061066,13.635246533631));
#256439=CARTESIAN_POINT('Ctrl Pts',(113.366292203071,81.0885336408355,12.6062543646726));
#256440=CARTESIAN_POINT('Ctrl Pts',(114.168356412835,80.666825605363,12.0563732669973));
#256441=CARTESIAN_POINT('Ctrl Pts',(113.823925897865,82.4011339813153,13.3246442856461));
#256442=CARTESIAN_POINT('Ctrl Pts',(113.748604057341,82.1657264091684,12.4584071352213));
#256443=CARTESIAN_POINT('Ctrl Pts',(114.367154525562,81.8221003906478,11.9010721426412));
#256444=CARTESIAN_POINT('Ctrl Pts',(113.98827163761,82.9379109315738,13.1548625963718));
#256445=CARTESIAN_POINT('Ctrl Pts',(113.921920427826,82.7112571397905,12.3636877604088));
#256446=CARTESIAN_POINT('Ctrl Pts',(114.455588968267,82.3997797445818,11.816181298279));
#256447=CARTESIAN_POINT('Ctrl Pts',(114.424380779002,84.5510793506422,12.6139948970922));
#256448=CARTESIAN_POINT('Ctrl Pts',(114.375512716323,84.3341564328201,12.038418363568));
#256449=CARTESIAN_POINT('Ctrl Pts',(114.690259297043,84.1358715971169,11.54574744836));
#256450=CARTESIAN_POINT('Ctrl Pts',(114.639636039159,85.6303497382827,12.2118226911378));
#256451=CARTESIAN_POINT('Ctrl Pts',(114.611553326333,85.4594058856995,11.7583160303623));
#256452=CARTESIAN_POINT('Ctrl Pts',(114.806088152744,85.2973823883387,11.3446613455943));
#256453=CARTESIAN_POINT('Ctrl Pts',(114.927844409462,87.807266397936,11.3656205182469));
#256454=CARTESIAN_POINT('Ctrl Pts',(114.920352198458,87.7104675830927,11.1472581448938));
#256455=CARTESIAN_POINT('Ctrl Pts',(114.961173076658,87.6401800974599,10.921560259098));
#256456=CARTESIAN_POINT('Ctrl Pts',(115.,88.9061071730244,10.9205098029853));
#256457=CARTESIAN_POINT('Ctrl Pts',(115.,88.8644746746419,10.8097442388102));
#256458=CARTESIAN_POINT('Ctrl Pts',(115.,88.8227423398972,10.6990068206156));
#256459=CARTESIAN_POINT('Ctrl Pts',(115.,90.,10.4775));
#256460=CARTESIAN_POINT('Ctrl Pts',(115.,90.,10.4775));
#256461=CARTESIAN_POINT('Ctrl Pts',(115.,90.,10.4775));
#256462=CARTESIAN_POINT('Ctrl Pts',(115.,90.,10.4775));
#256463=CARTESIAN_POINT('Ctrl Pts',(115.,89.5835438336671,10.5558582765748));
#256464=CARTESIAN_POINT('Ctrl Pts',(114.995145444676,89.1669828273719,10.6342451261915));
#256465=CARTESIAN_POINT('Ctrl Pts',(114.985453755867,88.7504746481075,10.7122315124746));
#256466=CARTESIAN_POINT('Ctrl Pts',(114.976119162444,88.3493129324001,10.7873444492202));
#256467=CARTESIAN_POINT('Ctrl Pts',(114.962297205651,87.9481990743845,10.862086750177));
#256468=CARTESIAN_POINT('Ctrl Pts',(114.943957244309,87.5472762396997,10.9360757294963));
#256469=CARTESIAN_POINT('Ctrl Pts',(114.92838963199,87.2069586597576,10.9988802100746));
#256470=CARTESIAN_POINT('Ctrl Pts',(114.909565993977,86.866778388743,11.0611422127244));
#256471=CARTESIAN_POINT('Ctrl Pts',(114.887440575962,86.526833310487,11.1226211406026));
#256472=CARTESIAN_POINT('Ctrl Pts',(114.886181080275,86.5074818406292,11.1261208459839));
#256473=CARTESIAN_POINT('Ctrl Pts',(114.88491089489,86.4881313431673,11.1296179650604));
#256474=CARTESIAN_POINT('Ctrl Pts',(114.883630015071,86.4687819131644,11.1331124382534));
#256475=CARTESIAN_POINT('Ctrl Pts',(114.846004723596,85.9004007638871,11.2357610790281));
#256476=CARTESIAN_POINT('Ctrl Pts',(114.799248326424,85.3326432827615,11.3362547894283));
#256477=CARTESIAN_POINT('Ctrl Pts',(114.742990120853,84.76535621485,11.4332724000518));
#256478=CARTESIAN_POINT('Ctrl Pts',(114.686731915282,84.1980691469384,11.5302900106753));
#256479=CARTESIAN_POINT('Ctrl Pts',(114.620971648891,83.6312517469121,11.6238302836067));
#256480=CARTESIAN_POINT('Ctrl Pts',(114.545392304676,83.0647232345978,11.7125671552059));
#256481=CARTESIAN_POINT('Ctrl Pts',(114.541556460865,83.0359704727091,11.7170707769731));
#256482=CARTESIAN_POINT('Ctrl Pts',(114.537695858892,83.0072223038154,11.7215614148308));
#256483=CARTESIAN_POINT('Ctrl Pts',(114.533810424182,82.9784782793166,11.7260389714718));
#256484=CARTESIAN_POINT('Ctrl Pts',(114.489984433162,82.6542583518944,11.7765438368996));
#256485=CARTESIAN_POINT('Ctrl Pts',(114.442984724895,82.3305619484957,11.8253691505951));
#256486=CARTESIAN_POINT('Ctrl Pts',(114.392600666823,82.0067026919993,11.8722415249027));
#256487=CARTESIAN_POINT('Ctrl Pts',(114.353105212445,81.7528333337324,11.9089842128056));
#256488=CARTESIAN_POINT('Ctrl Pts',(114.311529402501,81.4988640707801,11.9445266216545));
#256489=CARTESIAN_POINT('Ctrl Pts',(114.26775287008,81.2444644384055,11.9787247352557));
#256490=CARTESIAN_POINT('Ctrl Pts',(114.21875907944,80.9597456258849,12.0169985574467));
#256491=CARTESIAN_POINT('Ctrl Pts',(114.167147236413,80.6753810395896,12.053461087814));
#256492=CARTESIAN_POINT('Ctrl Pts',(114.112878627021,80.3915054828696,12.0877657415443));
#256493=CARTESIAN_POINT('Ctrl Pts',(114.063190185747,80.1315884868937,12.1191751473015));
#256494=CARTESIAN_POINT('Ctrl Pts',(114.011274194774,79.872081225692,12.1487756059824));
#256495=CARTESIAN_POINT('Ctrl Pts',(113.957084553587,79.6131099264361,12.1762747511373));
#256496=CARTESIAN_POINT('Ctrl Pts',(113.951047381326,79.5842583911611,12.1793383823534));
#256497=CARTESIAN_POINT('Ctrl Pts',(113.944982071647,79.5554139374339,12.1823758526497));
#256498=CARTESIAN_POINT('Ctrl Pts',(113.938888643006,79.5265771857666,12.1853866936187));
#256499=CARTESIAN_POINT('Ctrl Pts',(113.86042533142,79.155254706309,12.2241564186816));
#256500=CARTESIAN_POINT('Ctrl Pts',(113.777204059827,78.7846328262872,12.2586195276268));
#256501=CARTESIAN_POINT('Ctrl Pts',(113.688967055434,78.4147483849003,12.2875599190377));
#256502=CARTESIAN_POINT('Ctrl Pts',(113.643662573248,78.2248346043861,12.3024190980878));
#256503=CARTESIAN_POINT('Ctrl Pts',(113.597035870523,78.0351149339147,12.3158215393261));
#256504=CARTESIAN_POINT('Ctrl Pts',(113.54905233787,77.8455925411273,12.3275976932321));
#256505=CARTESIAN_POINT('Ctrl Pts',(113.466043987764,77.5177312882442,12.3479696636203));
#256506=CARTESIAN_POINT('Ctrl Pts',(113.378979813428,77.1904629051675,12.3635332048672));
#256507=CARTESIAN_POINT('Ctrl Pts',(113.287580781847,76.8637289591964,12.3728032158153));
#256508=CARTESIAN_POINT('Ctrl Pts',(113.2254215776,76.6415217680418,12.3791076207299));
#256509=CARTESIAN_POINT('Ctrl Pts',(113.161257371457,76.4195614752379,12.3825));
#256510=CARTESIAN_POINT('Ctrl Pts',(113.095,76.1978262581577,12.3825));
#256511=CARTESIAN_POINT('Origin',(112.039285751595,-74.5679259799751,14.2875));
#256512=CARTESIAN_POINT('Origin',(112.039285751595,-74.5679259799751,14.2875));
#256513=CARTESIAN_POINT('Origin',(113.095,0.,10.4775));
#256514=CARTESIAN_POINT('Ctrl Pts',(115.,-90.,10.4775));
#256515=CARTESIAN_POINT('Ctrl Pts',(115.,-89.5835438336648,10.5558582765753));
#256516=CARTESIAN_POINT('Ctrl Pts',(114.995145444676,-89.1669828273673,
10.6342451261923));
#256517=CARTESIAN_POINT('Ctrl Pts',(114.985453755867,-88.7504746481007,
10.7122315124758));
#256518=CARTESIAN_POINT('Ctrl Pts',(114.976119162444,-88.3493129323938,
10.7873444492214));
#256519=CARTESIAN_POINT('Ctrl Pts',(114.962297205651,-87.9481990743787,
10.862086750178));
#256520=CARTESIAN_POINT('Ctrl Pts',(114.943957244309,-87.5472762396945,
10.9360757294973));
#256521=CARTESIAN_POINT('Ctrl Pts',(114.92838963199,-87.2069586597541,10.9988802100753));
#256522=CARTESIAN_POINT('Ctrl Pts',(114.909565993977,-86.8667783887413,
11.0611422127247));
#256523=CARTESIAN_POINT('Ctrl Pts',(114.887440575962,-86.5268333104871,
11.1226211406026));
#256524=CARTESIAN_POINT('Ctrl Pts',(114.886181080275,-86.5074818406292,
11.1261208459839));
#256525=CARTESIAN_POINT('Ctrl Pts',(114.88491089489,-86.4881313431673,11.1296179650604));
#256526=CARTESIAN_POINT('Ctrl Pts',(114.883630015071,-86.4687819131644,
11.1331124382534));
#256527=CARTESIAN_POINT('Ctrl Pts',(114.846004723596,-85.9004007638872,
11.2357610790281));
#256528=CARTESIAN_POINT('Ctrl Pts',(114.799248326424,-85.3326432827615,
11.3362547894283));
#256529=CARTESIAN_POINT('Ctrl Pts',(114.742990120853,-84.76535621485,11.4332724000518));
#256530=CARTESIAN_POINT('Ctrl Pts',(114.686731915282,-84.1980691469384,
11.5302900106753));
#256531=CARTESIAN_POINT('Ctrl Pts',(114.620971648891,-83.631251746912,11.6238302836067));
#256532=CARTESIAN_POINT('Ctrl Pts',(114.545392304676,-83.0647232345978,
11.7125671552059));
#256533=CARTESIAN_POINT('Ctrl Pts',(114.541556460865,-83.035970472709,11.7170707769731));
#256534=CARTESIAN_POINT('Ctrl Pts',(114.537695858892,-83.0072223038154,
11.7215614148308));
#256535=CARTESIAN_POINT('Ctrl Pts',(114.533810424182,-82.9784782793166,
11.7260389714718));
#256536=CARTESIAN_POINT('Ctrl Pts',(114.489984433162,-82.6542583518949,
11.7765438368996));
#256537=CARTESIAN_POINT('Ctrl Pts',(114.442984724895,-82.3305619484966,
11.825369150595));
#256538=CARTESIAN_POINT('Ctrl Pts',(114.392600666823,-82.0067026920007,
11.8722415249025));
#256539=CARTESIAN_POINT('Ctrl Pts',(114.353105212445,-81.7528333337334,
11.9089842128055));
#256540=CARTESIAN_POINT('Ctrl Pts',(114.311529402501,-81.4988640707806,
11.9445266216544));
#256541=CARTESIAN_POINT('Ctrl Pts',(114.26775287008,-81.2444644384055,11.9787247352557));
#256542=CARTESIAN_POINT('Ctrl Pts',(114.21875907944,-80.959745625885,12.0169985574467));
#256543=CARTESIAN_POINT('Ctrl Pts',(114.167147236413,-80.6753810395898,
12.053461087814));
#256544=CARTESIAN_POINT('Ctrl Pts',(114.112878627021,-80.39150548287,12.0877657415442));
#256545=CARTESIAN_POINT('Ctrl Pts',(114.063190185747,-80.1315884868939,
12.1191751473015));
#256546=CARTESIAN_POINT('Ctrl Pts',(114.011274194774,-79.8720812256921,
12.1487756059824));
#256547=CARTESIAN_POINT('Ctrl Pts',(113.957084553586,-79.6131099264361,
12.1762747511373));
#256548=CARTESIAN_POINT('Ctrl Pts',(113.951047381325,-79.584258391161,12.1793383823534));
#256549=CARTESIAN_POINT('Ctrl Pts',(113.944982071647,-79.5554139374338,
12.1823758526497));
#256550=CARTESIAN_POINT('Ctrl Pts',(113.938888643006,-79.5265771857666,
12.1853866936187));
#256551=CARTESIAN_POINT('Ctrl Pts',(113.86042533142,-79.1552547063091,12.2241564186816));
#256552=CARTESIAN_POINT('Ctrl Pts',(113.777204059827,-78.7846328262874,
12.2586195276268));
#256553=CARTESIAN_POINT('Ctrl Pts',(113.688967055434,-78.4147483849006,
12.2875599190377));
#256554=CARTESIAN_POINT('Ctrl Pts',(113.643662573248,-78.2248346043863,
12.3024190980878));
#256555=CARTESIAN_POINT('Ctrl Pts',(113.597035870523,-78.0351149339149,
12.3158215393261));
#256556=CARTESIAN_POINT('Ctrl Pts',(113.54905233787,-77.8455925411274,12.3275976932321));
#256557=CARTESIAN_POINT('Ctrl Pts',(113.466043987764,-77.5177312882447,
12.3479696636203));
#256558=CARTESIAN_POINT('Ctrl Pts',(113.378979813428,-77.1904629051685,
12.3635332048671));
#256559=CARTESIAN_POINT('Ctrl Pts',(113.287580781847,-76.8637289591979,
12.3728032158152));
#256560=CARTESIAN_POINT('Ctrl Pts',(113.2254215776,-76.6415217680428,12.3791076207298));
#256561=CARTESIAN_POINT('Ctrl Pts',(113.161257371458,-76.4195614752384,
12.3825));
#256562=CARTESIAN_POINT('Ctrl Pts',(113.095,-76.1978262581577,12.3825));
#256563=CARTESIAN_POINT('Origin',(90.,-90.,14.2875));
#256564=CARTESIAN_POINT('Origin',(113.095,-76.1978262581577,14.2875));
#256565=CARTESIAN_POINT('Ctrl Pts',(113.095,-76.1978262581577,12.3825));
#256566=CARTESIAN_POINT('Ctrl Pts',(111.45976584278,-77.1750847966528,12.3825));
#256567=CARTESIAN_POINT('Ctrl Pts',(111.45976584278,-77.1750847966528,14.2875));
#256568=CARTESIAN_POINT('Ctrl Pts',(113.257643450739,-76.7421246518766,
12.3825));
#256569=CARTESIAN_POINT('Ctrl Pts',(111.710230812097,-77.5941846099538,
12.5172751948261));
#256570=CARTESIAN_POINT('Ctrl Pts',(111.76201574105,-77.6808356682986,14.2874999966875));
#256571=CARTESIAN_POINT('Ctrl Pts',(113.408657903689,-77.2910619607747,
12.3620536717516));
#256572=CARTESIAN_POINT('Ctrl Pts',(111.97140928493,-78.0590963418208,12.6053517687504));
#256573=CARTESIAN_POINT('Ctrl Pts',(112.042664753068,-78.1909142917061,
14.2466073426296));
#256574=CARTESIAN_POINT('Ctrl Pts',(113.689453561686,-78.4001194763425,
12.2931400483737));
#256575=CARTESIAN_POINT('Ctrl Pts',(112.468920289915,-79.0242905953405,
12.696132255772));
#256576=CARTESIAN_POINT('Ctrl Pts',(112.564492774111,-79.2214453413707,
14.108780097621));
#256577=CARTESIAN_POINT('Ctrl Pts',(113.819221943654,-78.9602349460102,
12.2445158474727));
#256578=CARTESIAN_POINT('Ctrl Pts',(112.708892347889,-79.5269448909711,
12.7038654758262));
#256579=CARTESIAN_POINT('Ctrl Pts',(112.805653119421,-79.7419020126294,
14.0115316944767));
#256580=CARTESIAN_POINT('Ctrl Pts',(114.058562415709,-80.0929157064321,
12.1262540447024));
#256581=CARTESIAN_POINT('Ctrl Pts',(113.15575467924,-80.5569292865777,12.6577917414259));
#256582=CARTESIAN_POINT('Ctrl Pts',(113.250441211304,-80.7943836707402,
13.7750080898736));
#256583=CARTESIAN_POINT('Ctrl Pts',(114.168356412835,-80.666825605363,12.0563732669973));
#256584=CARTESIAN_POINT('Ctrl Pts',(113.366292203071,-81.0885336408355,
12.6062543646726));
#256585=CARTESIAN_POINT('Ctrl Pts',(113.454481346879,-81.327658061066,13.635246533631));
#256586=CARTESIAN_POINT('Ctrl Pts',(114.367154525562,-81.8221003906478,
11.9010721426412));
#256587=CARTESIAN_POINT('Ctrl Pts',(113.748604057341,-82.1657264091684,
12.4584071352213));
#256588=CARTESIAN_POINT('Ctrl Pts',(113.823925897865,-82.4011339813153,
13.3246442856461));
#256589=CARTESIAN_POINT('Ctrl Pts',(114.455588968267,-82.3997797445818,
11.816181298279));
#256590=CARTESIAN_POINT('Ctrl Pts',(113.921920427826,-82.7112571397905,
12.3636877604088));
#256591=CARTESIAN_POINT('Ctrl Pts',(113.98827163761,-82.9379109315738,13.1548625963718));
#256592=CARTESIAN_POINT('Ctrl Pts',(114.690259297043,-84.1358715971169,
11.54574744836));
#256593=CARTESIAN_POINT('Ctrl Pts',(114.375512716323,-84.3341564328201,
12.038418363568));
#256594=CARTESIAN_POINT('Ctrl Pts',(114.424380779002,-84.5510793506422,
12.6139948970922));
#256595=CARTESIAN_POINT('Ctrl Pts',(114.806088152744,-85.2973823883387,
11.3446613455943));
#256596=CARTESIAN_POINT('Ctrl Pts',(114.611553326333,-85.4594058856995,
11.7583160303623));
#256597=CARTESIAN_POINT('Ctrl Pts',(114.639636039159,-85.6303497382827,
12.2118226911378));
#256598=CARTESIAN_POINT('Ctrl Pts',(114.961173076658,-87.6401800974599,
10.921560259098));
#256599=CARTESIAN_POINT('Ctrl Pts',(114.920352198458,-87.7104675830927,
11.1472581448938));
#256600=CARTESIAN_POINT('Ctrl Pts',(114.927844409462,-87.807266397936,11.3656205182469));
#256601=CARTESIAN_POINT('Ctrl Pts',(115.,-88.8227423398972,10.6990068206156));
#256602=CARTESIAN_POINT('Ctrl Pts',(115.,-88.8644746746419,10.8097442388102));
#256603=CARTESIAN_POINT('Ctrl Pts',(115.,-88.9061071730244,10.9205098029853));
#256604=CARTESIAN_POINT('Ctrl Pts',(115.,-90.,10.4775));
#256605=CARTESIAN_POINT('Ctrl Pts',(115.,-90.,10.4775));
#256606=CARTESIAN_POINT('Ctrl Pts',(115.,-90.,10.4775));
#256607=CARTESIAN_POINT('Origin',(-112.039285751595,-74.5679259799751,14.2875));
#256608=CARTESIAN_POINT('Origin',(-112.039285751595,-74.5679259799751,14.2875));
#256609=CARTESIAN_POINT('Origin',(0.,0.,14.2875));
#256610=CARTESIAN_POINT('Origin',(-90.,-90.,14.2875));
#256611=CARTESIAN_POINT('Origin',(-113.095,-76.1978262581577,14.2875));
#256612=CARTESIAN_POINT('Ctrl Pts',(-111.45976584278,-77.1750847966528,
14.2875));
#256613=CARTESIAN_POINT('Ctrl Pts',(-111.45976584278,-77.1750847966528,
12.3825));
#256614=CARTESIAN_POINT('Ctrl Pts',(-113.095,-76.1978262581577,12.3825));
#256615=CARTESIAN_POINT('Ctrl Pts',(-111.762015741049,-77.6808356682973,
14.2874999966875));
#256616=CARTESIAN_POINT('Ctrl Pts',(-111.710230812091,-77.5941846099565,
12.5172751948228));
#256617=CARTESIAN_POINT('Ctrl Pts',(-113.257643450735,-76.7421246518768,
12.3825));
#256618=CARTESIAN_POINT('Ctrl Pts',(-112.042664753069,-78.1909142917078,
14.2466073426301));
#256619=CARTESIAN_POINT('Ctrl Pts',(-111.971409284934,-78.0590963418208,
12.605351768751));
#256620=CARTESIAN_POINT('Ctrl Pts',(-113.408657903693,-77.2910619607747,
12.3620536717506));
#256621=CARTESIAN_POINT('Ctrl Pts',(-112.56449277411,-79.221445341369,14.1087800976205));
#256622=CARTESIAN_POINT('Ctrl Pts',(-112.468920289911,-79.0242905953405,
12.6961322557715));
#256623=CARTESIAN_POINT('Ctrl Pts',(-113.689453561682,-78.4001194763425,
12.2931400483747));
#256624=CARTESIAN_POINT('Ctrl Pts',(-112.805653119421,-79.741902012631,
14.0115316944761));
#256625=CARTESIAN_POINT('Ctrl Pts',(-112.708892347893,-79.5269448909712,
12.7038654758279));
#256626=CARTESIAN_POINT('Ctrl Pts',(-113.819221943657,-78.9602349460102,
12.2445158474711));
#256627=CARTESIAN_POINT('Ctrl Pts',(-113.250441211303,-80.7943836707386,
13.7750080898741));
#256628=CARTESIAN_POINT('Ctrl Pts',(-113.155754679235,-80.5569292865778,
12.6577917414243));
#256629=CARTESIAN_POINT('Ctrl Pts',(-114.058562415706,-80.0929157064321,
12.126254044704));
#256630=CARTESIAN_POINT('Ctrl Pts',(-113.454481346881,-81.3276580610713,
13.6352465336294));
#256631=CARTESIAN_POINT('Ctrl Pts',(-113.36629220308,-81.0885336408403,
12.6062543646709));
#256632=CARTESIAN_POINT('Ctrl Pts',(-114.168356412835,-80.6668256053674,
12.0563732669971));
#256633=CARTESIAN_POINT('Ctrl Pts',(-113.823925897864,-82.40113398131,13.3246442856477));
#256634=CARTESIAN_POINT('Ctrl Pts',(-113.748604057333,-82.1657264091644,
12.4584071352229));
#256635=CARTESIAN_POINT('Ctrl Pts',(-114.367154525562,-81.8221003906434,
11.9010721426414));
#256636=CARTESIAN_POINT('Ctrl Pts',(-113.98827163761,-82.9379109315738,
13.1548625963718));
#256637=CARTESIAN_POINT('Ctrl Pts',(-113.921920427826,-82.7112571397905,
12.3636877604088));
#256638=CARTESIAN_POINT('Ctrl Pts',(-114.455588968267,-82.3997797445818,
11.816181298279));
#256639=CARTESIAN_POINT('Ctrl Pts',(-114.424380779002,-84.5510793506422,
12.6139948970922));
#256640=CARTESIAN_POINT('Ctrl Pts',(-114.375512716323,-84.3341564328201,
12.038418363568));
#256641=CARTESIAN_POINT('Ctrl Pts',(-114.690259297043,-84.1358715971169,
11.54574744836));
#256642=CARTESIAN_POINT('Ctrl Pts',(-114.639636039158,-85.6303497382741,
12.2118226911422));
#256643=CARTESIAN_POINT('Ctrl Pts',(-114.611553326324,-85.4594058856993,
11.7583160303668));
#256644=CARTESIAN_POINT('Ctrl Pts',(-114.806088152744,-85.29738238833,11.3446613455963));
#256645=CARTESIAN_POINT('Ctrl Pts',(-114.927844409463,-87.8072663979446,
11.3656205182426));
#256646=CARTESIAN_POINT('Ctrl Pts',(-114.920352198467,-87.7104675830925,
11.1472581448895));
#256647=CARTESIAN_POINT('Ctrl Pts',(-114.961173076659,-87.6401800974686,
10.9215602590961));
#256648=CARTESIAN_POINT('Ctrl Pts',(-115.,-88.9061071730177,10.920509802988));
#256649=CARTESIAN_POINT('Ctrl Pts',(-115.,-88.8644746746409,10.8097442388105));
#256650=CARTESIAN_POINT('Ctrl Pts',(-115.,-88.8227423398907,10.6990068206168));
#256651=CARTESIAN_POINT('Ctrl Pts',(-115.,-90.,10.4775));
#256652=CARTESIAN_POINT('Ctrl Pts',(-115.,-90.,10.4775));
#256653=CARTESIAN_POINT('Ctrl Pts',(-115.,-90.,10.4775));
#256654=CARTESIAN_POINT('Ctrl Pts',(-115.,-90.,10.4775));
#256655=CARTESIAN_POINT('Ctrl Pts',(-115.,-89.5835438332465,10.555858276654));
#256656=CARTESIAN_POINT('Ctrl Pts',(-114.995145444666,-89.1669828265304,
10.6342451263498));
#256657=CARTESIAN_POINT('Ctrl Pts',(-114.985453755838,-88.7504746468455,
10.7122315127108));
#256658=CARTESIAN_POINT('Ctrl Pts',(-114.976119162398,-88.3493129308016,
10.7873444495187));
#256659=CARTESIAN_POINT('Ctrl Pts',(-114.96229720558,-87.9481990724496,
10.8620867505366));
#256660=CARTESIAN_POINT('Ctrl Pts',(-114.943957244205,-87.5472762374291,
10.9360757299152));
#256661=CARTESIAN_POINT('Ctrl Pts',(-114.928389631906,-87.2069586582444,
10.9988802103514));
#256662=CARTESIAN_POINT('Ctrl Pts',(-114.909565993928,-86.866778387987,
11.0611422128609));
#256663=CARTESIAN_POINT('Ctrl Pts',(-114.887440575962,-86.526833310487,
11.1226211406024));
#256664=CARTESIAN_POINT('Ctrl Pts',(-114.886181080275,-86.5074818406292,
11.1261208459838));
#256665=CARTESIAN_POINT('Ctrl Pts',(-114.884910894891,-86.4881313431672,
11.1296179650603));
#256666=CARTESIAN_POINT('Ctrl Pts',(-114.883630015071,-86.4687819131643,
11.1331124382533));
#256667=CARTESIAN_POINT('Ctrl Pts',(-114.846004723596,-85.9004007638864,
11.2357610790281));
#256668=CARTESIAN_POINT('Ctrl Pts',(-114.799248326424,-85.3326432827608,
11.3362547894284));
#256669=CARTESIAN_POINT('Ctrl Pts',(-114.742990120853,-84.7653562148494,
11.4332724000518));
#256670=CARTESIAN_POINT('Ctrl Pts',(-114.686731915283,-84.198069146938,
11.5302900106753));
#256671=CARTESIAN_POINT('Ctrl Pts',(-114.620971648891,-83.631251746912,
11.6238302836068));
#256672=CARTESIAN_POINT('Ctrl Pts',(-114.545392304676,-83.0647232345978,
11.7125671552059));
#256673=CARTESIAN_POINT('Ctrl Pts',(-114.541556460865,-83.035970472709,
11.7170707769731));
#256674=CARTESIAN_POINT('Ctrl Pts',(-114.537695858892,-83.0072223038153,
11.7215614148308));
#256675=CARTESIAN_POINT('Ctrl Pts',(-114.533810424182,-82.9784782793166,
11.7260389714718));
#256676=CARTESIAN_POINT('Ctrl Pts',(-114.489984433171,-82.6542583519608,
11.7765438368893));
#256677=CARTESIAN_POINT('Ctrl Pts',(-114.442984724914,-82.3305619486271,
11.8253691505752));
#256678=CARTESIAN_POINT('Ctrl Pts',(-114.392600666854,-82.006702692197,
11.872241524874));
#256679=CARTESIAN_POINT('Ctrl Pts',(-114.353105212467,-81.7528333338633,
11.9089842127871));
#256680=CARTESIAN_POINT('Ctrl Pts',(-114.311529402513,-81.4988640708449,
11.9445266216457));
#256681=CARTESIAN_POINT('Ctrl Pts',(-114.26775287008,-81.2444644384056,
11.9787247352559));
#256682=CARTESIAN_POINT('Ctrl Pts',(-114.218759079456,-80.9597456259818,
12.0169985574342));
#256683=CARTESIAN_POINT('Ctrl Pts',(-114.167147236446,-80.6753810397809,
12.0534610877905));
#256684=CARTESIAN_POINT('Ctrl Pts',(-114.112878627073,-80.3915054831543,
12.0877657415112));
#256685=CARTESIAN_POINT('Ctrl Pts',(-114.063190185782,-80.1315884870837,
12.1191751472815));
#256686=CARTESIAN_POINT('Ctrl Pts',(-114.01127419479,-79.8720812257873,
12.1487756059742));
#256687=CARTESIAN_POINT('Ctrl Pts',(-113.957084553584,-79.6131099264375,
12.1762747511387));
#256688=CARTESIAN_POINT('Ctrl Pts',(-113.951047381323,-79.5842583911624,
12.1793383823547));
#256689=CARTESIAN_POINT('Ctrl Pts',(-113.944982071644,-79.5554139374352,
12.182375852651));
#256690=CARTESIAN_POINT('Ctrl Pts',(-113.938888643004,-79.5265771857679,
12.1853866936199));
#256691=CARTESIAN_POINT('Ctrl Pts',(-113.860425331499,-79.1552547066897,
12.2241564186424));
#256692=CARTESIAN_POINT('Ctrl Pts',(-113.777204059993,-78.7846328270462,
12.2586195275573));
#256693=CARTESIAN_POINT('Ctrl Pts',(-113.6889670557,-78.414748386036,12.28755991895));
#256694=CARTESIAN_POINT('Ctrl Pts',(-113.643662573429,-78.224834605143,
12.3024190980355));
#256695=CARTESIAN_POINT('Ctrl Pts',(-113.597035870615,-78.0351149342934,
12.3158215393037));
#256696=CARTESIAN_POINT('Ctrl Pts',(-113.549052337867,-77.8455925411286,
12.3275976932327));
#256697=CARTESIAN_POINT('Ctrl Pts',(-113.46604398788,-77.5177312887046,
12.3479696635915));
#256698=CARTESIAN_POINT('Ctrl Pts',(-113.378979813672,-77.1904629060852,
12.3635332048232));
#256699=CARTESIAN_POINT('Ctrl Pts',(-113.28758078223,-76.8637289605696,
12.3728032157761));
#256700=CARTESIAN_POINT('Ctrl Pts',(-113.225421577863,-76.6415217689565,
12.3791076207157));
#256701=CARTESIAN_POINT('Ctrl Pts',(-113.161257371592,-76.4195614756949,
12.3825));
#256702=CARTESIAN_POINT('Ctrl Pts',(-113.095,-76.1978262581577,12.3825));
#256703=CARTESIAN_POINT('Origin',(-112.039285751595,74.5679259799751,14.2875));
#256704=CARTESIAN_POINT('Origin',(-112.039285751595,74.5679259799751,14.2875));
#256705=CARTESIAN_POINT('Origin',(-113.095,0.,10.4775));
#256706=CARTESIAN_POINT('Ctrl Pts',(-115.,90.,10.4775));
#256707=CARTESIAN_POINT('Ctrl Pts',(-115.,89.5835438332466,10.555858276654));
#256708=CARTESIAN_POINT('Ctrl Pts',(-114.995145444666,89.1669828265306,
10.6342451263498));
#256709=CARTESIAN_POINT('Ctrl Pts',(-114.985453755838,88.7504746468457,
10.7122315127108));
#256710=CARTESIAN_POINT('Ctrl Pts',(-114.976119162398,88.3493129308021,
10.7873444495186));
#256711=CARTESIAN_POINT('Ctrl Pts',(-114.96229720558,87.9481990724504,10.8620867505365));
#256712=CARTESIAN_POINT('Ctrl Pts',(-114.943957244205,87.5472762374302,
10.936075729915));
#256713=CARTESIAN_POINT('Ctrl Pts',(-114.928389631906,87.2069586582452,
10.9988802103513));
#256714=CARTESIAN_POINT('Ctrl Pts',(-114.909565993928,86.8667783879873,
11.0611422128609));
#256715=CARTESIAN_POINT('Ctrl Pts',(-114.887440575962,86.526833310487,11.1226211406024));
#256716=CARTESIAN_POINT('Ctrl Pts',(-114.886181080275,86.5074818406292,
11.1261208459838));
#256717=CARTESIAN_POINT('Ctrl Pts',(-114.884910894891,86.4881313431672,
11.1296179650603));
#256718=CARTESIAN_POINT('Ctrl Pts',(-114.883630015071,86.4687819131643,
11.1331124382533));
#256719=CARTESIAN_POINT('Ctrl Pts',(-114.846004723596,85.9004007638865,
11.2357610790281));
#256720=CARTESIAN_POINT('Ctrl Pts',(-114.799248326424,85.3326432827608,
11.3362547894284));
#256721=CARTESIAN_POINT('Ctrl Pts',(-114.742990120853,84.7653562148494,
11.4332724000518));
#256722=CARTESIAN_POINT('Ctrl Pts',(-114.686731915283,84.198069146938,11.5302900106753));
#256723=CARTESIAN_POINT('Ctrl Pts',(-114.620971648891,83.631251746912,11.6238302836068));
#256724=CARTESIAN_POINT('Ctrl Pts',(-114.545392304676,83.0647232345978,
11.7125671552059));
#256725=CARTESIAN_POINT('Ctrl Pts',(-114.541556460865,83.0359704727091,
11.7170707769731));
#256726=CARTESIAN_POINT('Ctrl Pts',(-114.537695858892,83.0072223038154,
11.7215614148308));
#256727=CARTESIAN_POINT('Ctrl Pts',(-114.533810424182,82.9784782793166,
11.7260389714718));
#256728=CARTESIAN_POINT('Ctrl Pts',(-114.489984433171,82.6542583519613,
11.7765438368892));
#256729=CARTESIAN_POINT('Ctrl Pts',(-114.442984724914,82.3305619486281,
11.825369150575));
#256730=CARTESIAN_POINT('Ctrl Pts',(-114.392600666854,82.0067026921985,
11.8722415248737));
#256731=CARTESIAN_POINT('Ctrl Pts',(-114.353105212467,81.7528333338643,
11.908984212787));
#256732=CARTESIAN_POINT('Ctrl Pts',(-114.311529402513,81.4988640708454,
11.9445266216456));
#256733=CARTESIAN_POINT('Ctrl Pts',(-114.26775287008,81.2444644384056,11.9787247352559));
#256734=CARTESIAN_POINT('Ctrl Pts',(-114.218759079456,80.9597456259804,
12.0169985574344));
#256735=CARTESIAN_POINT('Ctrl Pts',(-114.167147236445,80.6753810397781,
12.0534610877908));
#256736=CARTESIAN_POINT('Ctrl Pts',(-114.112878627072,80.3915054831501,
12.0877657415118));
#256737=CARTESIAN_POINT('Ctrl Pts',(-114.063190185782,80.131588487081,12.1191751472818));
#256738=CARTESIAN_POINT('Ctrl Pts',(-114.01127419479,79.8720812257858,12.1487756059743));
#256739=CARTESIAN_POINT('Ctrl Pts',(-113.957084553584,79.6131099264375,
12.1762747511387));
#256740=CARTESIAN_POINT('Ctrl Pts',(-113.951047381323,79.5842583911624,
12.1793383823547));
#256741=CARTESIAN_POINT('Ctrl Pts',(-113.944982071644,79.5554139374352,
12.182375852651));
#256742=CARTESIAN_POINT('Ctrl Pts',(-113.938888643004,79.5265771857679,
12.1853866936199));
#256743=CARTESIAN_POINT('Ctrl Pts',(-113.860425331499,79.1552547066895,
12.2241564186425));
#256744=CARTESIAN_POINT('Ctrl Pts',(-113.777204059993,78.7846328270459,
12.2586195275573));
#256745=CARTESIAN_POINT('Ctrl Pts',(-113.6889670557,78.4147483860356,12.2875599189501));
#256746=CARTESIAN_POINT('Ctrl Pts',(-113.643662573429,78.2248346051427,
12.3024190980356));
#256747=CARTESIAN_POINT('Ctrl Pts',(-113.597035870615,78.0351149342933,
12.3158215393037));
#256748=CARTESIAN_POINT('Ctrl Pts',(-113.549052337867,77.8455925411286,
12.3275976932327));
#256749=CARTESIAN_POINT('Ctrl Pts',(-113.466043987881,77.5177312887054,
12.3479696635914));
#256750=CARTESIAN_POINT('Ctrl Pts',(-113.378979813672,77.1904629060869,
12.3635332048232));
#256751=CARTESIAN_POINT('Ctrl Pts',(-113.28758078223,76.8637289605722,12.372803215776));
#256752=CARTESIAN_POINT('Ctrl Pts',(-113.225421577863,76.6415217689582,
12.3791076207157));
#256753=CARTESIAN_POINT('Ctrl Pts',(-113.161257371593,76.4195614756958,
12.3825));
#256754=CARTESIAN_POINT('Ctrl Pts',(-113.095,76.1978262581577,12.3825));
#256755=CARTESIAN_POINT('Origin',(-90.,90.,14.2875));
#256756=CARTESIAN_POINT('Origin',(-113.095,76.1978262581577,14.2875));
#256757=CARTESIAN_POINT('Ctrl Pts',(-113.095,76.1978262581577,12.3825));
#256758=CARTESIAN_POINT('Ctrl Pts',(-111.45976584278,77.1750847966528,12.3825));
#256759=CARTESIAN_POINT('Ctrl Pts',(-111.45976584278,77.1750847966528,14.2875));
#256760=CARTESIAN_POINT('Ctrl Pts',(-113.257643450735,76.7421246518768,
12.3825));
#256761=CARTESIAN_POINT('Ctrl Pts',(-111.710230812091,77.5941846099565,
12.5172751948228));
#256762=CARTESIAN_POINT('Ctrl Pts',(-111.762015741049,77.6808356682973,
14.2874999966875));
#256763=CARTESIAN_POINT('Ctrl Pts',(-113.408657903693,77.2910619607747,
12.3620536717506));
#256764=CARTESIAN_POINT('Ctrl Pts',(-111.971409284934,78.0590963418208,
12.605351768751));
#256765=CARTESIAN_POINT('Ctrl Pts',(-112.042664753069,78.1909142917078,
14.2466073426301));
#256766=CARTESIAN_POINT('Ctrl Pts',(-113.689453561682,78.4001194763425,
12.2931400483747));
#256767=CARTESIAN_POINT('Ctrl Pts',(-112.468920289911,79.0242905953405,
12.6961322557715));
#256768=CARTESIAN_POINT('Ctrl Pts',(-112.56449277411,79.221445341369,14.1087800976205));
#256769=CARTESIAN_POINT('Ctrl Pts',(-113.819221943657,78.9602349460102,
12.2445158474711));
#256770=CARTESIAN_POINT('Ctrl Pts',(-112.708892347893,79.5269448909712,
12.7038654758279));
#256771=CARTESIAN_POINT('Ctrl Pts',(-112.805653119421,79.741902012631,14.0115316944761));
#256772=CARTESIAN_POINT('Ctrl Pts',(-114.058562415706,80.0929157064321,
12.126254044704));
#256773=CARTESIAN_POINT('Ctrl Pts',(-113.155754679235,80.5569292865778,
12.6577917414243));
#256774=CARTESIAN_POINT('Ctrl Pts',(-113.250441211303,80.7943836707386,
13.7750080898741));
#256775=CARTESIAN_POINT('Ctrl Pts',(-114.168356412835,80.6668256053674,
12.0563732669971));
#256776=CARTESIAN_POINT('Ctrl Pts',(-113.36629220308,81.0885336408403,12.6062543646709));
#256777=CARTESIAN_POINT('Ctrl Pts',(-113.454481346881,81.3276580610713,
13.6352465336294));
#256778=CARTESIAN_POINT('Ctrl Pts',(-114.367154525562,81.8221003906434,
11.9010721426414));
#256779=CARTESIAN_POINT('Ctrl Pts',(-113.748604057333,82.1657264091644,
12.4584071352229));
#256780=CARTESIAN_POINT('Ctrl Pts',(-113.823925897864,82.40113398131,13.3246442856477));
#256781=CARTESIAN_POINT('Ctrl Pts',(-114.455588968267,82.3997797445818,
11.816181298279));
#256782=CARTESIAN_POINT('Ctrl Pts',(-113.921920427826,82.7112571397905,
12.3636877604088));
#256783=CARTESIAN_POINT('Ctrl Pts',(-113.98827163761,82.9379109315738,13.1548625963718));
#256784=CARTESIAN_POINT('Ctrl Pts',(-114.690259297043,84.1358715971169,
11.54574744836));
#256785=CARTESIAN_POINT('Ctrl Pts',(-114.375512716323,84.3341564328201,
12.038418363568));
#256786=CARTESIAN_POINT('Ctrl Pts',(-114.424380779002,84.5510793506422,
12.6139948970922));
#256787=CARTESIAN_POINT('Ctrl Pts',(-114.806088152744,85.29738238833,11.3446613455963));
#256788=CARTESIAN_POINT('Ctrl Pts',(-114.611553326324,85.4594058856993,
11.7583160303668));
#256789=CARTESIAN_POINT('Ctrl Pts',(-114.639636039158,85.6303497382741,
12.2118226911422));
#256790=CARTESIAN_POINT('Ctrl Pts',(-114.961173076659,87.6401800974686,
10.9215602590961));
#256791=CARTESIAN_POINT('Ctrl Pts',(-114.920352198467,87.7104675830925,
11.1472581448895));
#256792=CARTESIAN_POINT('Ctrl Pts',(-114.927844409463,87.8072663979446,
11.3656205182426));
#256793=CARTESIAN_POINT('Ctrl Pts',(-115.,88.8227423398907,10.6990068206168));
#256794=CARTESIAN_POINT('Ctrl Pts',(-115.,88.8644746746409,10.8097442388105));
#256795=CARTESIAN_POINT('Ctrl Pts',(-115.,88.9061071730177,10.920509802988));
#256796=CARTESIAN_POINT('Ctrl Pts',(-115.,90.,10.4775));
#256797=CARTESIAN_POINT('Ctrl Pts',(-115.,90.,10.4775));
#256798=CARTESIAN_POINT('Ctrl Pts',(-115.,90.,10.4775));
#256799=CARTESIAN_POINT('Origin',(0.,113.095,10.4775));
#256800=CARTESIAN_POINT('Origin',(-20.3338370957106,113.095,10.4775));
#256801=CARTESIAN_POINT('Ctrl Pts',(20.3391723768471,115.,10.4796615646013));
#256802=CARTESIAN_POINT('Ctrl Pts',(19.7022063230879,115.000000000001,12.0516141103967));
#256803=CARTESIAN_POINT('Ctrl Pts',(19.6285538888407,113.315275283147,12.2333790914428));
#256804=CARTESIAN_POINT('Ctrl Pts',(18.7107034466881,115.,9.81979377118478));
#256805=CARTESIAN_POINT('Ctrl Pts',(18.1189784011792,114.999999999841,11.4178986609794));
#256806=CARTESIAN_POINT('Ctrl Pts',(18.0565711864358,113.307258836677,11.5974068452245));
#256807=CARTESIAN_POINT('Ctrl Pts',(17.0532658471793,115.,9.2407677403993));
#256808=CARTESIAN_POINT('Ctrl Pts',(16.5123043069177,115.,10.8637355452915));
#256809=CARTESIAN_POINT('Ctrl Pts',(16.4567953379409,113.300163656376,11.0393495768014));
#256810=CARTESIAN_POINT('Ctrl Pts',(13.7179668220018,115.,8.25237113478313));
#256811=CARTESIAN_POINT('Ctrl Pts',(13.2794521568153,115.,9.91725072790728));
#256812=CARTESIAN_POINT('Ctrl Pts',(13.2377636482649,113.287997034874,10.0867415205811));
#256813=CARTESIAN_POINT('Ctrl Pts',(12.0365764000009,115.,7.84116032508707));
#256814=CARTESIAN_POINT('Ctrl Pts',(11.6512268683337,114.999999999988,9.52405173421115));
#256815=CARTESIAN_POINT('Ctrl Pts',(11.615100586185,113.282903110437,9.69041736234001));
#256816=CARTESIAN_POINT('Ctrl Pts',(6.94924188488841,115.,6.85120498294647));
#256817=CARTESIAN_POINT('Ctrl Pts',(6.71934777368302,115.000000000024,8.57583528434052));
#256818=CARTESIAN_POINT('Ctrl Pts',(6.70566817137969,113.270607871211,8.73629459979534));
#256819=CARTESIAN_POINT('Ctrl Pts',(3.50035936666375,115.,6.51381753263502));
#256820=CARTESIAN_POINT('Ctrl Pts',(3.38780290821946,115.000000000024,8.25451794933572));
#256821=CARTESIAN_POINT('Ctrl Pts',(3.37767114516811,113.266374083612,8.411111618798));
#256822=CARTESIAN_POINT('Ctrl Pts',(-3.51636943826656,115.,6.51485519904957));
#256823=CARTESIAN_POINT('Ctrl Pts',(-3.4032875294127,114.999999999976,8.25551029227645));
#256824=CARTESIAN_POINT('Ctrl Pts',(-3.39312006098893,113.266387061329,
8.41211174275344));
#256825=CARTESIAN_POINT('Ctrl Pts',(-6.96324106057752,115.,6.85321820905684));
#256826=CARTESIAN_POINT('Ctrl Pts',(-6.73290677808119,115.000000000168,
8.57776066608256));
#256827=CARTESIAN_POINT('Ctrl Pts',(-6.71917720241139,113.270632997186,
8.73823497354488));
#256828=CARTESIAN_POINT('Ctrl Pts',(-12.0457199621,115.,7.84329673838536));
#256829=CARTESIAN_POINT('Ctrl Pts',(-11.6600859933304,114.999999999916,
9.52609638746069));
#256830=CARTESIAN_POINT('Ctrl Pts',(-11.6239247024908,113.282929583528,
9.69247643632406));
#256831=CARTESIAN_POINT('Ctrl Pts',(-13.7251356712098,115.,8.25432671895952));
#256832=CARTESIAN_POINT('Ctrl Pts',(-13.2864050182398,114.999999999988,
9.91912443645021));
#256833=CARTESIAN_POINT('Ctrl Pts',(-13.2446823703184,113.288021171429,
10.0886263004162));
#256834=CARTESIAN_POINT('Ctrl Pts',(-17.0557976392124,115.,9.24168756304256));
#256835=CARTESIAN_POINT('Ctrl Pts',(-16.5147655959056,115.000000000012,
10.864618206466));
#256836=CARTESIAN_POINT('Ctrl Pts',(-16.4592390970313,113.300174914246,
11.0402360890187));
#256837=CARTESIAN_POINT('Ctrl Pts',(-18.7092469771287,115.,9.81920401156003));
#256838=CARTESIAN_POINT('Ctrl Pts',(-18.1175604673055,114.999999999804,
11.4173315039314));
#256839=CARTESIAN_POINT('Ctrl Pts',(-18.0551653037824,113.307251671963,
11.596838469021));
#256840=CARTESIAN_POINT('Ctrl Pts',(-20.3391771446538,115.,10.4796634955796));
#256841=CARTESIAN_POINT('Ctrl Pts',(-19.7022109484218,115.000000000001,
12.051615960838));
#256842=CARTESIAN_POINT('Ctrl Pts',(-19.6285584910498,113.315275306605,
12.2333809524079));
#256843=CARTESIAN_POINT('Origin',(20.3338370957106,113.095,10.4775));
#256844=CARTESIAN_POINT('Origin',(-20.3338370957106,113.095,10.4775));
#256845=CARTESIAN_POINT('Origin',(0.,113.095,10.4775));
#256846=CARTESIAN_POINT('Origin',(20.3338370957106,113.095,10.4775));
#256847=CARTESIAN_POINT('Origin',(-24.8661421402461,-44.3927817339206,16.1925));
#256848=CARTESIAN_POINT('Ctrl Pts',(-76.5327353708727,27.1805640649084,
16.1924982582712));
#256849=CARTESIAN_POINT('Ctrl Pts',(-76.5254460991276,27.1701424112581,
16.2200871281663));
#256850=CARTESIAN_POINT('Ctrl Pts',(-76.5184672980905,27.1617293806218,
16.248101336645));
#256851=CARTESIAN_POINT('Ctrl Pts',(-76.5118328073709,27.1555532163276,
16.2765966498027));
#256852=CARTESIAN_POINT('Ctrl Pts',(-76.505358241223,27.1495259286347,16.3044050826943));
#256853=CARTESIAN_POINT('Ctrl Pts',(-76.4992115671826,27.1456288662165,
16.3326717167532));
#256854=CARTESIAN_POINT('Ctrl Pts',(-76.4934339939447,27.144123077721,16.3614476210689));
#256855=CARTESIAN_POINT('Ctrl Pts',(-76.4921585023819,27.1437906508625,
16.3678003615113));
#256856=CARTESIAN_POINT('Ctrl Pts',(-76.4909010391257,27.1435749657779,
16.3741779191892));
#256857=CARTESIAN_POINT('Ctrl Pts',(-76.4896621154026,27.1434791718108,
16.3805808375412));
#256858=CARTESIAN_POINT('Ctrl Pts',(-76.4880193305114,27.1433521511727,
16.3890709627458));
#256859=CARTESIAN_POINT('Ctrl Pts',(-76.486416003788,27.1434370002347,16.3975719419884));
#256860=CARTESIAN_POINT('Ctrl Pts',(-76.4848537692335,27.1437355673519,
16.406076948393));
#256861=CARTESIAN_POINT('Ctrl Pts',(-76.48098548299,27.1444748565121,16.4271363976165));
#256862=CARTESIAN_POINT('Ctrl Pts',(-76.4773696370517,27.1465703673368,
16.4482618838781));
#256863=CARTESIAN_POINT('Ctrl Pts',(-76.4740424808271,27.1499697741393,
16.4691998962322));
#256864=CARTESIAN_POINT('Ctrl Pts',(-76.4707094654665,27.1533751673113,
16.4901747805127));
#256865=CARTESIAN_POINT('Ctrl Pts',(-76.4676662855572,27.15808878871,16.5109605599982));
#256866=CARTESIAN_POINT('Ctrl Pts',(-76.4649378361877,27.1640086579224,
16.5313130815541));
#256867=CARTESIAN_POINT('Ctrl Pts',(-76.4643858787519,27.1652062303853,
16.5354303379478));
#256868=CARTESIAN_POINT('Ctrl Pts',(-76.4638467601764,27.166453014181,16.5395299258882));
#256869=CARTESIAN_POINT('Ctrl Pts',(-76.4633206224266,27.1677479362274,
16.5436099312145));
#256870=CARTESIAN_POINT('Ctrl Pts',(-76.4620493955122,27.1708766601363,
16.5534678298028));
#256871=CARTESIAN_POINT('Ctrl Pts',(-76.4608504005183,27.1742844116283,
16.563227977684));
#256872=CARTESIAN_POINT('Ctrl Pts',(-76.4597221364489,27.1779555862456,
16.5728808843466));
#256873=CARTESIAN_POINT('Ctrl Pts',(-76.4555634683354,27.1914871674015,
16.608460529423));
#256874=CARTESIAN_POINT('Ctrl Pts',(-76.452368326429,27.2085635842065,16.6425190954535));
#256875=CARTESIAN_POINT('Ctrl Pts',(-76.4499894515855,27.2285145118714,
16.6751163767836));
#256876=CARTESIAN_POINT('Ctrl Pts',(-76.4481516192738,27.243927874037,16.7002998525192));
#256877=CARTESIAN_POINT('Ctrl Pts',(-76.4468125093688,27.2611648250175,
16.7246580015644));
#256878=CARTESIAN_POINT('Ctrl Pts',(-76.4459011083305,27.2797726036834,
16.7480930589391));
#256879=CARTESIAN_POINT('Ctrl Pts',(-76.4449881378312,27.2984124255237,
16.7715684722125));
#256880=CARTESIAN_POINT('Ctrl Pts',(-76.4445043286356,27.3184277738337,
16.7941176720264));
#256881=CARTESIAN_POINT('Ctrl Pts',(-76.4443826625376,27.3394063743963,
16.8156722156884));
#256882=CARTESIAN_POINT('Ctrl Pts',(-76.444260240081,27.3605153920852,16.8373607569274));
#256883=CARTESIAN_POINT('Ctrl Pts',(-76.4445044610444,27.3825996603613,
16.8580423102826));
#256884=CARTESIAN_POINT('Ctrl Pts',(-76.4450517552706,27.4052828608609,
16.8776763500028));
#256885=CARTESIAN_POINT('Ctrl Pts',(-76.4451275701148,27.4084250889914,
16.8803961880577));
#256886=CARTESIAN_POINT('Ctrl Pts',(-76.4452092083633,27.4115788786109,
16.8830959690985));
#256887=CARTESIAN_POINT('Ctrl Pts',(-76.4452965083212,27.4147432949496,
16.8857756277876));
#256888=CARTESIAN_POINT('Ctrl Pts',(-76.4456285567621,27.4267792630846,
16.895967803261));
#256889=CARTESIAN_POINT('Ctrl Pts',(-76.4460413746577,27.4390220462592,
16.9059171754194));
#256890=CARTESIAN_POINT('Ctrl Pts',(-76.4465283265827,27.4514363729673,
16.9156217934255));
#256891=CARTESIAN_POINT('Ctrl Pts',(-76.4477740792785,27.4831955265336,
16.9404487905557));
#256892=CARTESIAN_POINT('Ctrl Pts',(-76.4494849825234,27.516130412427,16.9638340074607));
#256893=CARTESIAN_POINT('Ctrl Pts',(-76.4515669382231,27.5499276827806,
16.985939396366));
#256894=CARTESIAN_POINT('Ctrl Pts',(-76.4537247726033,27.5849567239553,
17.0088504353357));
#256895=CARTESIAN_POINT('Ctrl Pts',(-76.4562812377419,27.6209122535191,
17.0303866179463));
#256896=CARTESIAN_POINT('Ctrl Pts',(-76.4591476533543,27.6574962538653,
17.0507077973838));
#256897=CARTESIAN_POINT('Ctrl Pts',(-76.4614800345039,27.6872643839364,
17.0672429905549));
#256898=CARTESIAN_POINT('Ctrl Pts',(-76.464017965945,27.7174496690713,17.0829733141292));
#256899=CARTESIAN_POINT('Ctrl Pts',(-76.466720752886,27.7479141287996,17.0979758062082));
#256900=CARTESIAN_POINT('Ctrl Pts',(-76.4677059340771,27.7590185974006,
17.1034442997812));
#256901=CARTESIAN_POINT('Ctrl Pts',(-76.4687146852109,27.7701762979155,
17.1088237343903));
#256902=CARTESIAN_POINT('Ctrl Pts',(-76.4697457322936,27.7813854912832,
17.1141186859287));
#256903=CARTESIAN_POINT('Ctrl Pts',(-76.4724297283712,27.8105649841858,
17.1279023718521));
#256904=CARTESIAN_POINT('Ctrl Pts',(-76.475268656545,27.8401032155328,17.1410999474322));
#256905=CARTESIAN_POINT('Ctrl Pts',(-76.4782264005115,27.8698177823024,
17.1537242053269));
#256906=CARTESIAN_POINT('Ctrl Pts',(-76.4814236442207,27.9019384502015,
17.1673706972462));
#256907=CARTESIAN_POINT('Ctrl Pts',(-76.4847597640874,27.9342655910912,
17.1803475370963));
#256908=CARTESIAN_POINT('Ctrl Pts',(-76.4881996908383,27.9666279531715,
17.1926699656454));
#256909=CARTESIAN_POINT('Ctrl Pts',(-76.4886519862316,27.9708830865932,
17.1942901680715));
#256910=CARTESIAN_POINT('Ctrl Pts',(-76.489106089515,27.9751389006332,17.1958990522149));
#256911=CARTESIAN_POINT('Ctrl Pts',(-76.4895619325382,27.979395067814,17.1974966476084));
#256912=CARTESIAN_POINT('Ctrl Pts',(-76.493897565698,28.019876502485,17.2126917634966));
#256913=CARTESIAN_POINT('Ctrl Pts',(-76.4984031419556,28.0605401920071,
17.2269450615766));
#256914=CARTESIAN_POINT('Ctrl Pts',(-76.5030665766358,28.1015001037827,
17.240414641407));
#256915=CARTESIAN_POINT('Ctrl Pts',(-76.5035084491037,28.1053811611021,
17.2416909188482));
#256916=CARTESIAN_POINT('Ctrl Pts',(-76.5039517474129,28.1092649053718,
17.2429601347068));
#256917=CARTESIAN_POINT('Ctrl Pts',(-76.5043964665195,28.1131514503917,
17.2442224078976));
#256918=CARTESIAN_POINT('Ctrl Pts',(-76.5073626095466,28.1390735397254,
17.2526413914031));
#256919=CARTESIAN_POINT('Ctrl Pts',(-76.5103875491063,28.1650771837688,
17.2607374323177));
#256920=CARTESIAN_POINT('Ctrl Pts',(-76.5134649041893,28.1911518975641,
17.2685330721676));
#256921=CARTESIAN_POINT('Ctrl Pts',(-76.5205941289253,28.2515584770983,
17.2865930187622));
#256922=CARTESIAN_POINT('Ctrl Pts',(-76.5280003771988,28.3123340561993,
17.3030517999703));
#256923=CARTESIAN_POINT('Ctrl Pts',(-76.5356394395758,28.3734477221374,
17.3181020342891));
#256924=CARTESIAN_POINT('Ctrl Pts',(-76.5435634587841,28.4368410862557,
17.3337136813665));
#256925=CARTESIAN_POINT('Ctrl Pts',(-76.5517380600726,28.5005983551872,
17.3478096641772));
#256926=CARTESIAN_POINT('Ctrl Pts',(-76.5601276442959,28.5647256403924,
17.3605684034646));
#256927=CARTESIAN_POINT('Ctrl Pts',(-76.5638310436267,28.5930332345229,
17.3662004711906));
#256928=CARTESIAN_POINT('Ctrl Pts',(-76.5675765027121,28.6214134362392,
17.3715715053251));
#256929=CARTESIAN_POINT('Ctrl Pts',(-76.5713617072229,28.6498690551227,
17.3766947662572));
#256930=CARTESIAN_POINT('Ctrl Pts',(-76.57901301,28.7073884190481,17.3870507775338));
#256931=CARTESIAN_POINT('Ctrl Pts',(-76.586835094676,28.7652559669882,17.396373658365));
#256932=CARTESIAN_POINT('Ctrl Pts',(-76.5947786108432,28.8232282288209,
17.4047210505559));
#256933=CARTESIAN_POINT('Ctrl Pts',(-76.5971621660813,28.8406235592321,
17.4072257940426));
#256934=CARTESIAN_POINT('Ctrl Pts',(-76.5995567234879,28.8580286627605,
17.4096426038263));
#256935=CARTESIAN_POINT('Ctrl Pts',(-76.6019611150693,28.8754377812504,
17.4119727726841));
#256936=CARTESIAN_POINT('Ctrl Pts',(-76.6127354792386,28.9534501083324,
17.4224145360162));
#256937=CARTESIAN_POINT('Ctrl Pts',(-76.6237599571578,29.0319245446931,
17.4311687491798));
#256938=CARTESIAN_POINT('Ctrl Pts',(-76.6349137015724,29.1101764698682,
17.4382612976214));
#256939=CARTESIAN_POINT('Ctrl Pts',(-76.6366048959584,29.122041473371,17.4393367102955));
#256940=CARTESIAN_POINT('Ctrl Pts',(-76.6382990798901,29.1339014546392,
17.4403739004344));
#256941=CARTESIAN_POINT('Ctrl Pts',(-76.639995850247,29.1457541224831,17.441372936404));
#256942=CARTESIAN_POINT('Ctrl Pts',(-76.6556847858336,29.2553480587374,
17.4506103744062));
#256943=CARTESIAN_POINT('Ctrl Pts',(-76.6716864104207,29.3650148910396,
17.4567325787359));
#256944=CARTESIAN_POINT('Ctrl Pts',(-76.6879909658038,29.4748980638179,
17.4599100505192));
#256945=CARTESIAN_POINT('Ctrl Pts',(-76.6968876072708,29.5348562269499,
17.4616438498508));
#256946=CARTESIAN_POINT('Ctrl Pts',(-76.7058745787282,29.5948790592221,
17.4625));
#256947=CARTESIAN_POINT('Ctrl Pts',(-76.7149512087496,29.6549915892152,
17.4625));
#256948=CARTESIAN_POINT('Origin',(-109.438478010978,76.3890311653897,16.1925));
#256949=CARTESIAN_POINT('Origin',(-90.,90.,16.1925));
#256950=CARTESIAN_POINT('Origin',(-76.3890311653897,109.438478010978,16.1925));
#256951=CARTESIAN_POINT('Origin',(8.18330470534211,50.220290910288,16.1925));
#256952=CARTESIAN_POINT('Ctrl Pts',(-29.6549915892152,76.7149512087496,
17.4625));
#256953=CARTESIAN_POINT('Ctrl Pts',(-29.5784809832296,76.7033985679885,
17.4625));
#256954=CARTESIAN_POINT('Ctrl Pts',(-29.5017645218694,76.691941913157,17.4610789773399));
#256955=CARTESIAN_POINT('Ctrl Pts',(-29.4251260133419,76.6806292437895,
17.4582328812589));
#256956=CARTESIAN_POINT('Ctrl Pts',(-29.3550776153572,76.6702893457232,
17.4556315196873));
#256957=CARTESIAN_POINT('Ctrl Pts',(-29.285091738834,76.6600693732902,17.451839079296));
#256958=CARTESIAN_POINT('Ctrl Pts',(-29.2153959726543,76.6500111634965,
17.4468147853482));
#256959=CARTESIAN_POINT('Ctrl Pts',(-29.1910127660868,76.6464922781962,
17.4450570258185));
#256960=CARTESIAN_POINT('Ctrl Pts',(-29.166665340607,76.6429932651686,17.4431481665627));
#256961=CARTESIAN_POINT('Ctrl Pts',(-29.1423646235815,76.6395162005647,
17.4410854028152));
#256962=CARTESIAN_POINT('Ctrl Pts',(-29.0717236083887,76.6294085410561,
17.4350890478487));
#256963=CARTESIAN_POINT('Ctrl Pts',(-29.0013000923889,76.619457001758,17.427816532758));
#256964=CARTESIAN_POINT('Ctrl Pts',(-28.9308900430927,76.6096539020088,
17.4191389458403));
#256965=CARTESIAN_POINT('Ctrl Pts',(-28.9125941999739,76.6071065955251,
17.4168841005379));
#256966=CARTESIAN_POINT('Ctrl Pts',(-28.894299397661,76.6045693606064,17.4145341520301));
#256967=CARTESIAN_POINT('Ctrl Pts',(-28.8760023419532,76.6020421698847,
17.4120863380179));
#256968=CARTESIAN_POINT('Ctrl Pts',(-28.8096307852525,76.5928749254407,
17.4032070281935));
#256969=CARTESIAN_POINT('Ctrl Pts',(-28.7435548276785,76.5838841660449,
17.3930871840631));
#256970=CARTESIAN_POINT('Ctrl Pts',(-28.6775616925957,76.5750605976978,
17.3815966638215));
#256971=CARTESIAN_POINT('Ctrl Pts',(-28.6679863743367,76.5737803361221,
17.3799294390694));
#256972=CARTESIAN_POINT('Ctrl Pts',(-28.6584128434657,76.5725036108741,
17.378233281295));
#256973=CARTESIAN_POINT('Ctrl Pts',(-28.6488404954756,76.5712304108411,
17.3765077138037));
#256974=CARTESIAN_POINT('Ctrl Pts',(-28.593919594324,76.5639254848986,17.3666073506202));
#256975=CARTESIAN_POINT('Ctrl Pts',(-28.5390197213121,76.5567364098792,
17.3557157603928));
#256976=CARTESIAN_POINT('Ctrl Pts',(-28.4842809217466,76.5497009035207,
17.3437734778876));
#256977=CARTESIAN_POINT('Ctrl Pts',(-28.4340312118297,76.5432423739871,
17.3328105733957));
#256978=CARTESIAN_POINT('Ctrl Pts',(-28.3839169544335,76.5369132259073,
17.3209620182621));
#256979=CARTESIAN_POINT('Ctrl Pts',(-28.3340851368407,76.5307511868738,
17.3081680846677));
#256980=CARTESIAN_POINT('Ctrl Pts',(-28.2843811713795,76.5246049576154,
17.2954069761187));
#256981=CARTESIAN_POINT('Ctrl Pts',(-28.2349573707625,76.5186248279345,
17.2817053136026));
#256982=CARTESIAN_POINT('Ctrl Pts',(-28.1860085131815,76.5128586176739,
17.2669910566473));
#256983=CARTESIAN_POINT('Ctrl Pts',(-28.1614764636036,76.5099687247739,
17.2596166070898));
#256984=CARTESIAN_POINT('Ctrl Pts',(-28.1370017452464,76.5071248960929,
17.2519719554797));
#256985=CARTESIAN_POINT('Ctrl Pts',(-28.1126036317571,76.5043336151744,
17.2440428740804));
#256986=CARTESIAN_POINT('Ctrl Pts',(-28.0701844846433,76.4994806270133,
17.2302571823916));
#256987=CARTESIAN_POINT('Ctrl Pts',(-28.0279824912822,76.4947829028992,
17.2156101298164));
#256988=CARTESIAN_POINT('Ctrl Pts',(-27.9860694428053,76.4902767919903,
17.1999930540297));
#256989=CARTESIAN_POINT('Ctrl Pts',(-27.9466341480602,76.4860370666946,
17.1852992054769));
#256990=CARTESIAN_POINT('Ctrl Pts',(-27.9074544475538,76.4819669295096,
17.1697465428278));
#256991=CARTESIAN_POINT('Ctrl Pts',(-27.8686308801042,76.4781067108578,
17.1532283189415));
#256992=CARTESIAN_POINT('Ctrl Pts',(-27.8377621230887,76.4750374372332,
17.1400946201867));
#256993=CARTESIAN_POINT('Ctrl Pts',(-27.8071191438753,76.4721010301325,
17.1263502154765));
#256994=CARTESIAN_POINT('Ctrl Pts',(-27.7767742650347,76.4693230827018,
17.1119338317452));
#256995=CARTESIAN_POINT('Ctrl Pts',(-27.7671845095149,76.468445180475,17.1073778868627));
#256996=CARTESIAN_POINT('Ctrl Pts',(-27.7576382281078,76.4675842490496,
17.1027621986441));
#256997=CARTESIAN_POINT('Ctrl Pts',(-27.7481373827153,76.4667411216781,
17.09808459864));
#256998=CARTESIAN_POINT('Ctrl Pts',(-27.7165349284568,76.4639366455401,
17.0825256000386));
#256999=CARTESIAN_POINT('Ctrl Pts',(-27.6854146210792,76.4613252274428,
17.0662758428328));
#257000=CARTESIAN_POINT('Ctrl Pts',(-27.6548074136641,76.4589379212242,
17.0492104485405));
#257001=CARTESIAN_POINT('Ctrl Pts',(-27.625042367409,76.4566163020363,17.0326146107177));
#257002=CARTESIAN_POINT('Ctrl Pts',(-27.5957623497434,76.454506551362,17.0152474880124));
#257003=CARTESIAN_POINT('Ctrl Pts',(-27.5670390174753,76.452649048605,16.9969759720338));
#257004=CARTESIAN_POINT('Ctrl Pts',(-27.5394891827037,76.4508674344954,
16.9794509425025));
#257005=CARTESIAN_POINT('Ctrl Pts',(-27.5124513532677,76.4493178278093,
16.9610939515221));
#257006=CARTESIAN_POINT('Ctrl Pts',(-27.4860313730106,76.448047775168,16.9417696634665));
#257007=CARTESIAN_POINT('Ctrl Pts',(-27.4732138949936,76.4474316175612,
16.9323946134121));
#257008=CARTESIAN_POINT('Ctrl Pts',(-27.4605425003863,76.4468814440248,
16.9227916184912));
#257009=CARTESIAN_POINT('Ctrl Pts',(-27.4480332789737,76.4464038210197,
16.9129435541772));
#257010=CARTESIAN_POINT('Ctrl Pts',(-27.4380190788527,76.4460214621024,
16.9050597312283));
#257011=CARTESIAN_POINT('Ctrl Pts',(-27.4281096389904,76.4456876024437,
16.8970089022855));
#257012=CARTESIAN_POINT('Ctrl Pts',(-27.4183213434193,76.4454060812474,
16.8887879984481));
#257013=CARTESIAN_POINT('Ctrl Pts',(-27.3952254081718,76.4447418189892,
16.8693903963502));
#257014=CARTESIAN_POINT('Ctrl Pts',(-27.3726021898248,76.4443701445099,
16.8488671319362));
#257015=CARTESIAN_POINT('Ctrl Pts',(-27.3508659753904,76.4443625463772,
16.8272552303239));
#257016=CARTESIAN_POINT('Ctrl Pts',(-27.3290708073427,76.4443549276367,
16.8055847122633));
#257017=CARTESIAN_POINT('Ctrl Pts',(-27.3081675781444,76.444713403402,16.7828195227726));
#257018=CARTESIAN_POINT('Ctrl Pts',(-27.2886142275261,76.4455134941472,
16.7590305375609));
#257019=CARTESIAN_POINT('Ctrl Pts',(-27.2688420650392,76.4463225383119,
16.7349753415904));
#257020=CARTESIAN_POINT('Ctrl Pts',(-27.2504503195707,76.4475831876966,
16.7098732026395));
#257021=CARTESIAN_POINT('Ctrl Pts',(-27.2339516170994,76.4493763637578,
16.6838334537733));
#257022=CARTESIAN_POINT('Ctrl Pts',(-27.2316065629565,76.4496312380401,
16.680132276601));
#257023=CARTESIAN_POINT('Ctrl Pts',(-27.2292998143515,76.4498968745499,
16.676412217469));
#257024=CARTESIAN_POINT('Ctrl Pts',(-27.2270329030597,76.4501735092113,
16.6726736500796));
#257025=CARTESIAN_POINT('Ctrl Pts',(-27.2082942415873,76.4524602168075,
16.6417700373291));
#257026=CARTESIAN_POINT('Ctrl Pts',(-27.1920956821034,76.4554866376469,
16.6094802657883));
#257027=CARTESIAN_POINT('Ctrl Pts',(-27.1790613975837,76.4593868180785,
16.5757650534976));
#257028=CARTESIAN_POINT('Ctrl Pts',(-27.1746643707654,76.4607025172968,
16.5643914570105));
#257029=CARTESIAN_POINT('Ctrl Pts',(-27.1706359107513,76.4621156292997,
16.5528759158128));
#257030=CARTESIAN_POINT('Ctrl Pts',(-27.1669986019352,76.4636289044872,
16.541229334737));
#257031=CARTESIAN_POINT('Ctrl Pts',(-27.1600415068138,76.4665233519912,
16.5189528725284));
#257032=CARTESIAN_POINT('Ctrl Pts',(-27.1545628735558,76.4697851638502,
16.4962407115116));
#257033=CARTESIAN_POINT('Ctrl Pts',(-27.1506549153929,76.4733862268998,
16.4733464731264));
#257034=CARTESIAN_POINT('Ctrl Pts',(-27.14674695723,76.4769872899494,16.4504522347412));
#257035=CARTESIAN_POINT('Ctrl Pts',(-27.1444098150616,76.4809274578027,
16.4273768616861));
#257036=CARTESIAN_POINT('Ctrl Pts',(-27.1436800109183,76.4851658906467,
16.4043845876077));
#257037=CARTESIAN_POINT('Ctrl Pts',(-27.1434551581826,76.4864717522655,
16.3973006654712));
#257038=CARTESIAN_POINT('Ctrl Pts',(-27.1433783458384,76.4878067469539,
16.3902160073495));
#257039=CARTESIAN_POINT('Ctrl Pts',(-27.1434490350608,76.4891701961808,
16.383133694799));
#257040=CARTESIAN_POINT('Ctrl Pts',(-27.1436556805572,76.4931559613735,
16.3624300013355));
#257041=CARTESIAN_POINT('Ctrl Pts',(-27.1451242300419,76.4973805033892,
16.3417644841304));
#257042=CARTESIAN_POINT('Ctrl Pts',(-27.1478012243608,76.501812217759,16.3212481482302));
#257043=CARTESIAN_POINT('Ctrl Pts',(-27.1505058861726,76.5062897351494,
16.3005197702));
#257044=CARTESIAN_POINT('Ctrl Pts',(-27.1544440119295,76.5109787082553,
16.2799436844039));
#257045=CARTESIAN_POINT('Ctrl Pts',(-27.1595080210178,76.5158361677242,
16.2596351519614));
#257046=CARTESIAN_POINT('Ctrl Pts',(-27.1646853029013,76.520802279844,16.2388723540944));
#257047=CARTESIAN_POINT('Ctrl Pts',(-27.1710392955917,76.525944475937,16.2183892248481));
#257048=CARTESIAN_POINT('Ctrl Pts',(-27.1784017958212,76.531206361274,16.1983095665849));
#257049=CARTESIAN_POINT('Ctrl Pts',(-27.179113452549,76.5317149732923,16.1963686737562));
#257050=CARTESIAN_POINT('Ctrl Pts',(-27.1798344925881,76.5322246958768,
16.194431550985));
#257051=CARTESIAN_POINT('Ctrl Pts',(-27.1805647392023,76.5327354732306,
16.1924983103147));
#257052=CARTESIAN_POINT('Origin',(-128.965117604652,-34.3520449604438,16.1925));
#257053=CARTESIAN_POINT('Ctrl Pts',(27.1805640649112,76.5327353708748,16.1924982582715));
#257054=CARTESIAN_POINT('Ctrl Pts',(27.1701424112491,76.5254460991215,16.2200871281998));
#257055=CARTESIAN_POINT('Ctrl Pts',(27.1617293806052,76.5184672980764,16.2481013367124));
#257056=CARTESIAN_POINT('Ctrl Pts',(27.1555532163089,76.5118328073496,16.2765966499054));
#257057=CARTESIAN_POINT('Ctrl Pts',(27.1495259286137,76.5053582411945,16.3044050828319));
#257058=CARTESIAN_POINT('Ctrl Pts',(27.1456288661985,76.4992115671475,16.3326717169268));
#257059=CARTESIAN_POINT('Ctrl Pts',(27.1441230777122,76.4934339939039,16.36144762128));
#257060=CARTESIAN_POINT('Ctrl Pts',(27.1437906508598,76.4921585023555,16.3678003616526));
#257061=CARTESIAN_POINT('Ctrl Pts',(27.1435749657788,76.4909010391133,16.3741779192602));
#257062=CARTESIAN_POINT('Ctrl Pts',(27.1434791718126,76.4896621154038,16.3805808375413));
#257063=CARTESIAN_POINT('Ctrl Pts',(27.1433521511743,76.4880193305124,16.3890709627459));
#257064=CARTESIAN_POINT('Ctrl Pts',(27.143437000236,76.4864160037888,16.3975719419885));
#257065=CARTESIAN_POINT('Ctrl Pts',(27.1437355673528,76.4848537692341,16.4060769483931));
#257066=CARTESIAN_POINT('Ctrl Pts',(27.1444748565122,76.4809854829899,16.4271363976175));
#257067=CARTESIAN_POINT('Ctrl Pts',(27.1465703673372,76.4773696370516,16.4482618838798));
#257068=CARTESIAN_POINT('Ctrl Pts',(27.1499697741402,76.474042480827,16.4691998962345));
#257069=CARTESIAN_POINT('Ctrl Pts',(27.1533751673143,76.470709465465,16.4901747805256));
#257070=CARTESIAN_POINT('Ctrl Pts',(27.1580887887164,76.4676662855546,16.5109605600215));
#257071=CARTESIAN_POINT('Ctrl Pts',(27.1640086579329,76.4649378361838,16.5313130815873));
#257072=CARTESIAN_POINT('Ctrl Pts',(27.1652062303928,76.4643858787494,16.5354303379699));
#257073=CARTESIAN_POINT('Ctrl Pts',(27.1664530141852,76.4638467601754,16.5395299258992));
#257074=CARTESIAN_POINT('Ctrl Pts',(27.167747936228,76.4633206224269,16.5436099312145));
#257075=CARTESIAN_POINT('Ctrl Pts',(27.1708766601367,76.4620493955123,16.5534678298028));
#257076=CARTESIAN_POINT('Ctrl Pts',(27.1742844116285,76.4608504005184,16.563227977684));
#257077=CARTESIAN_POINT('Ctrl Pts',(27.1779555862458,76.4597221364491,16.5728808843466));
#257078=CARTESIAN_POINT('Ctrl Pts',(27.1914871674018,76.4555634683356,16.6084605294229));
#257079=CARTESIAN_POINT('Ctrl Pts',(27.2085635842082,76.4523683264303,16.6425190954533));
#257080=CARTESIAN_POINT('Ctrl Pts',(27.2285145118719,76.4499894515858,16.6751163767836));
#257081=CARTESIAN_POINT('Ctrl Pts',(27.2439278740326,76.4481516192739,16.7002998525128));
#257082=CARTESIAN_POINT('Ctrl Pts',(27.2611648250078,76.4468125093689,16.724658001552));
#257083=CARTESIAN_POINT('Ctrl Pts',(27.2797726036682,76.4459011083305,16.7480930589212));
#257084=CARTESIAN_POINT('Ctrl Pts',(27.2984124255032,76.4449881378312,16.7715684721892));
#257085=CARTESIAN_POINT('Ctrl Pts',(27.3184277738075,76.4445043286356,16.7941176719983));
#257086=CARTESIAN_POINT('Ctrl Pts',(27.3394063743642,76.4443826625374,16.8156722156559));
#257087=CARTESIAN_POINT('Ctrl Pts',(27.3605153920477,76.4442602400808,16.8373607568908));
#257088=CARTESIAN_POINT('Ctrl Pts',(27.382599660318,76.444504461044,16.8580423102425));
#257089=CARTESIAN_POINT('Ctrl Pts',(27.4052828608116,76.4450517552697,16.8776763499597));
#257090=CARTESIAN_POINT('Ctrl Pts',(27.4084250889586,76.4451275701143,16.8803961880292));
#257091=CARTESIAN_POINT('Ctrl Pts',(27.4115788785947,76.4452092083632,16.8830959690843));
#257092=CARTESIAN_POINT('Ctrl Pts',(27.41474329495,76.4452965083216,16.8857756277874));
#257093=CARTESIAN_POINT('Ctrl Pts',(27.4267792630851,76.4456285567625,16.8959678032609));
#257094=CARTESIAN_POINT('Ctrl Pts',(27.4390220462597,76.4460413746582,16.9059171754193));
#257095=CARTESIAN_POINT('Ctrl Pts',(27.451436372968,76.4465283265831,16.9156217934254));
#257096=CARTESIAN_POINT('Ctrl Pts',(27.4831955265518,76.4477740792797,16.9404487905693));
#257097=CARTESIAN_POINT('Ctrl Pts',(27.5161304124639,76.4494849825256,16.9638340074865));
#257098=CARTESIAN_POINT('Ctrl Pts',(27.549927682837,76.4515669382265,16.9859393964028));
#257099=CARTESIAN_POINT('Ctrl Pts',(27.5849567240302,76.453724772608,17.0088504353828));
#257100=CARTESIAN_POINT('Ctrl Pts',(27.6209122536133,76.4562812377481,17.0303866180024));
#257101=CARTESIAN_POINT('Ctrl Pts',(27.6574962539793,76.4591476533624,17.0507077974477));
#257102=CARTESIAN_POINT('Ctrl Pts',(27.6872643840131,76.4614800345095,17.0672429905956));
#257103=CARTESIAN_POINT('Ctrl Pts',(27.7174496691097,76.4640179659475,17.0829733141488));
#257104=CARTESIAN_POINT('Ctrl Pts',(27.747914128799,76.4667207528852,17.0979758062085));
#257105=CARTESIAN_POINT('Ctrl Pts',(27.7590185974001,76.4677059340764,17.1034442997815));
#257106=CARTESIAN_POINT('Ctrl Pts',(27.7701762979151,76.4687146852103,17.1088237343905));
#257107=CARTESIAN_POINT('Ctrl Pts',(27.7813854912829,76.4697457322932,17.1141186859289));
#257108=CARTESIAN_POINT('Ctrl Pts',(27.8105649841802,76.4724297283706,17.1279023718495));
#257109=CARTESIAN_POINT('Ctrl Pts',(27.8401032155219,76.4752686565441,17.1410999474272));
#257110=CARTESIAN_POINT('Ctrl Pts',(27.8698177822859,76.47822640051,17.1537242053197));
#257111=CARTESIAN_POINT('Ctrl Pts',(27.9019384501796,76.4814236442187,17.167370697237));
#257112=CARTESIAN_POINT('Ctrl Pts',(27.9342655910636,76.4847597640845,17.1803475370853));
#257113=CARTESIAN_POINT('Ctrl Pts',(27.9666279531374,76.4881996908344,17.1926699656325));
#257114=CARTESIAN_POINT('Ctrl Pts',(27.9708830865704,76.4886519862289,17.194290168063));
#257115=CARTESIAN_POINT('Ctrl Pts',(27.9751389006218,76.4891060895135,17.1958990522108));
#257116=CARTESIAN_POINT('Ctrl Pts',(27.9793950678139,76.4895619325379,17.1974966476085));
#257117=CARTESIAN_POINT('Ctrl Pts',(28.019876502463,76.4938975656951,17.2126917634887));
#257118=CARTESIAN_POINT('Ctrl Pts',(28.0605401919643,76.4984031419506,17.2269450615618));
#257119=CARTESIAN_POINT('Ctrl Pts',(28.1015001037186,76.5030665766283,17.2404146413861));
#257120=CARTESIAN_POINT('Ctrl Pts',(28.1053811610594,76.5035084490985,17.2416909188343));
#257121=CARTESIAN_POINT('Ctrl Pts',(28.1092649053504,76.5039517474101,17.2429601346999));
#257122=CARTESIAN_POINT('Ctrl Pts',(28.1131514503916,76.5043964665192,17.2442224078977));
#257123=CARTESIAN_POINT('Ctrl Pts',(28.1390735397253,76.5073626095463,17.2526413914032));
#257124=CARTESIAN_POINT('Ctrl Pts',(28.1650771837687,76.510387549106,17.2607374323178));
#257125=CARTESIAN_POINT('Ctrl Pts',(28.191151897564,76.5134649041889,17.2685330721678));
#257126=CARTESIAN_POINT('Ctrl Pts',(28.2515584771483,76.5205941289305,17.2865930187776));
#257127=CARTESIAN_POINT('Ctrl Pts',(28.3123340562986,76.5280003772098,17.3030517999978));
#257128=CARTESIAN_POINT('Ctrl Pts',(28.3734477222867,76.5356394395931,17.3181020343265));
#257129=CARTESIAN_POINT('Ctrl Pts',(28.4368410864441,76.5435634588064,17.3337136814111));
#257130=CARTESIAN_POINT('Ctrl Pts',(28.5005983554152,76.5517380601004,17.3478096642272));
#257131=CARTESIAN_POINT('Ctrl Pts',(28.5647256406625,76.5601276443299,17.3605684035188));
#257132=CARTESIAN_POINT('Ctrl Pts',(28.5930332347029,76.5638310436492,17.3662004712251));
#257133=CARTESIAN_POINT('Ctrl Pts',(28.6214134363291,76.567576502723,17.3715715053416));
#257134=CARTESIAN_POINT('Ctrl Pts',(28.6498690551224,76.5713617072221,17.3766947662574));
#257135=CARTESIAN_POINT('Ctrl Pts',(28.7073884190851,76.5790130100047,17.3870507775405));
#257136=CARTESIAN_POINT('Ctrl Pts',(28.7652559670614,76.5868350946858,17.3963736583769));
#257137=CARTESIAN_POINT('Ctrl Pts',(28.8232282289298,76.5947786108581,17.4047210505717));
#257138=CARTESIAN_POINT('Ctrl Pts',(28.8406235593049,76.5971621660914,17.4072257940528));
#257139=CARTESIAN_POINT('Ctrl Pts',(28.8580286627969,76.599556723493,17.4096426038313));
#257140=CARTESIAN_POINT('Ctrl Pts',(28.8754377812505,76.6019611150693,17.4119727726842));
#257141=CARTESIAN_POINT('Ctrl Pts',(28.953450108308,76.6127354792352,17.422414536013));
#257142=CARTESIAN_POINT('Ctrl Pts',(29.0319245446426,76.6237599571516,17.431168749174));
#257143=CARTESIAN_POINT('Ctrl Pts',(29.110176469793,76.6349137015637,17.4382612976143));
#257144=CARTESIAN_POINT('Ctrl Pts',(29.1220414733213,76.6366048959535,17.4393367102908));
#257145=CARTESIAN_POINT('Ctrl Pts',(29.133901454615,76.638299079889,17.440373900432));
#257146=CARTESIAN_POINT('Ctrl Pts',(29.1457541224843,76.6399958502497,17.4413729364037));
#257147=CARTESIAN_POINT('Ctrl Pts',(29.2553480580749,76.655684785743,17.4506103743498));
#257148=CARTESIAN_POINT('Ctrl Pts',(29.3650148897119,76.6716864102272,17.4567325786613));
#257149=CARTESIAN_POINT('Ctrl Pts',(29.4748980618221,76.6879909655065,17.4599100504612));
#257150=CARTESIAN_POINT('Ctrl Pts',(29.5348562256177,76.6968876070693,17.4616438498317));
#257151=CARTESIAN_POINT('Ctrl Pts',(29.5948790585548,76.7058745786255,17.4625));
#257152=CARTESIAN_POINT('Ctrl Pts',(29.6549915892153,76.7149512087495,17.4625));
#257153=CARTESIAN_POINT('Origin',(-34.3520449604435,-128.965117604652,16.1925));
#257154=CARTESIAN_POINT('Ctrl Pts',(76.7149512087496,29.6549915892152,17.4625));
#257155=CARTESIAN_POINT('Ctrl Pts',(76.7007359098135,29.5608467821401,17.4625));
#257156=CARTESIAN_POINT('Ctrl Pts',(76.6867030088941,29.4667125209745,17.4604072289322));
#257157=CARTESIAN_POINT('Ctrl Pts',(76.6728916244736,29.3726870671455,17.4561240814492));
#257158=CARTESIAN_POINT('Ctrl Pts',(76.6599282024501,29.2844343908147,17.452103901667));
#257159=CARTESIAN_POINT('Ctrl Pts',(76.6471598475859,29.196277078863,17.4461538204625));
#257160=CARTESIAN_POINT('Ctrl Pts',(76.6346271711136,29.1083236389632,17.4381590482525));
#257161=CARTESIAN_POINT('Ctrl Pts',(76.623564612772,29.0306873844582,17.4311020852649));
#257162=CARTESIAN_POINT('Ctrl Pts',(76.612685722018,28.9532100090808,17.4224515902637));
#257163=CARTESIAN_POINT('Ctrl Pts',(76.6020251850533,28.8759903503099,17.4121058896821));
#257164=CARTESIAN_POINT('Ctrl Pts',(76.5929919275611,28.8105578994449,17.4033394103198));
#257165=CARTESIAN_POINT('Ctrl Pts',(76.5841246883598,28.7453752922117,17.3933663288476));
#257166=CARTESIAN_POINT('Ctrl Pts',(76.5754248746701,28.6803389123986,17.3820812128369));
#257167=CARTESIAN_POINT('Ctrl Pts',(76.5745077284505,28.6734826885746,17.380891520522));
#257168=CARTESIAN_POINT('Ctrl Pts',(76.5735924520281,28.6666281209666,17.3796872111787));
#257169=CARTESIAN_POINT('Ctrl Pts',(76.5726790536845,28.6597751110934,17.3784681359426));
#257170=CARTESIAN_POINT('Ctrl Pts',(76.5653610465084,28.6048698490276,17.3687010924751));
#257171=CARTESIAN_POINT('Ctrl Pts',(76.5581535830946,28.5499526452457,17.3579431897578));
#257172=CARTESIAN_POINT('Ctrl Pts',(76.551095713263,28.4951749625612,17.3461368886708));
#257173=CARTESIAN_POINT('Ctrl Pts',(76.5446169987028,28.4448922315325,17.3352993900234));
#257174=CARTESIAN_POINT('Ctrl Pts',(76.5382643026121,28.3947267788196,17.3235782727003));
#257175=CARTESIAN_POINT('Ctrl Pts',(76.5320763362567,28.3448347290616,17.3109158794063));
#257176=CARTESIAN_POINT('Ctrl Pts',(76.5260889614222,28.2965599993677,17.2986639551717));
#257177=CARTESIAN_POINT('Ctrl Pts',(76.5202557206435,28.2485407157557,17.2855307133555));
#257178=CARTESIAN_POINT('Ctrl Pts',(76.5146209503256,28.2009625196928,17.2714529746984));
#257179=CARTESIAN_POINT('Ctrl Pts',(76.5111206177552,28.1714068324292,17.262707850344));
#257180=CARTESIAN_POINT('Ctrl Pts',(76.5076867892711,28.1419437054236,17.2535816880451));
#257181=CARTESIAN_POINT('Ctrl Pts',(76.5043299432579,28.1125994901801,17.2440469306636));
#257182=CARTESIAN_POINT('Ctrl Pts',(76.4994099378461,28.0695907560184,17.2300721883809));
#257183=CARTESIAN_POINT('Ctrl Pts',(76.4946524666836,28.0268356967203,17.215222656587));
#257184=CARTESIAN_POINT('Ctrl Pts',(76.4900921572824,27.9843757811643,17.1993722202065));
#257185=CARTESIAN_POINT('Ctrl Pts',(76.4857772770164,27.9442009957251,17.1843748309661));
#257186=CARTESIAN_POINT('Ctrl Pts',(76.4816388565531,27.9042902389518,17.1684813247625));
#257187=CARTESIAN_POINT('Ctrl Pts',(76.4777167689223,27.8647187422006,17.1515646848084));
#257188=CARTESIAN_POINT('Ctrl Pts',(76.4753652742226,27.8409935800865,17.1414222828705));
#257189=CARTESIAN_POINT('Ctrl Pts',(76.4730917485966,27.817391151853,17.1309117177248));
#257190=CARTESIAN_POINT('Ctrl Pts',(76.4709068974261,27.7939357204578,17.1200019028265));
#257191=CARTESIAN_POINT('Ctrl Pts',(76.4694744690635,27.7785579109112,17.112849228767));
#257192=CARTESIAN_POINT('Ctrl Pts',(76.4680842075485,27.763288324096,17.1055472028756));
#257193=CARTESIAN_POINT('Ctrl Pts',(76.4667393807873,27.7481342818727,17.0980870415728));
#257194=CARTESIAN_POINT('Ctrl Pts',(76.4639004848743,27.7161444748761,17.0823388262306));
#257195=CARTESIAN_POINT('Ctrl Pts',(76.4612595947587,27.6846459211437,17.0658786658155));
#257196=CARTESIAN_POINT('Ctrl Pts',(76.4588488257704,27.6536746993957,17.0485804548605));
#257197=CARTESIAN_POINT('Ctrl Pts',(76.4565032661768,27.6235412247035,17.031750146832));
#257198=CARTESIAN_POINT('Ctrl Pts',(76.4543754667986,27.5939067174985,17.0141265974772));
#257199=CARTESIAN_POINT('Ctrl Pts',(76.4525070385105,27.5648480032216,16.9955752187322));
#257200=CARTESIAN_POINT('Ctrl Pts',(76.4507095662163,27.5368928314082,16.9777283527198));
#257201=CARTESIAN_POINT('Ctrl Pts',(76.4491520836248,27.5094704097394,16.9590228414135));
#257202=CARTESIAN_POINT('Ctrl Pts',(76.4478838668815,27.4826925239471,16.9393206257464));
#257203=CARTESIAN_POINT('Ctrl Pts',(76.4475882262302,27.4764501906585,16.9347277390013));
#257204=CARTESIAN_POINT('Ctrl Pts',(76.4473083613942,27.4702430809547,16.9300806058261));
#257205=CARTESIAN_POINT('Ctrl Pts',(76.4470450027163,27.4640729822085,16.9253773219914));
#257206=CARTESIAN_POINT('Ctrl Pts',(76.4463836380683,27.4485782006516,16.9135661081653));
#257207=CARTESIAN_POINT('Ctrl Pts',(76.445830245995,27.4333087681932,16.9013716940896));
#257208=CARTESIAN_POINT('Ctrl Pts',(76.4453983713746,27.4183233468248,16.8887840336497));
#257209=CARTESIAN_POINT('Ctrl Pts',(76.4447393676207,27.3954568747781,16.8695763398181));
#257210=CARTESIAN_POINT('Ctrl Pts',(76.4443666032736,27.3730391298257,16.8492614774149));
#257211=CARTESIAN_POINT('Ctrl Pts',(76.4443504330611,27.3514856269793,16.8278798165427));
#257212=CARTESIAN_POINT('Ctrl Pts',(76.4443340891035,27.3297005370019,16.8062684149396));
#257213=CARTESIAN_POINT('Ctrl Pts',(76.4446820842408,27.3087984600255,16.7835670140578));
#257214=CARTESIAN_POINT('Ctrl Pts',(76.4454707611388,27.2892498936118,16.7598514785006));
#257215=CARTESIAN_POINT('Ctrl Pts',(76.4462155696294,27.2707886729506,16.7374550671345));
#257216=CARTESIAN_POINT('Ctrl Pts',(76.4473534742746,27.2535351094313,16.7141544688201));
#257217=CARTESIAN_POINT('Ctrl Pts',(76.4489511499897,27.237916905714,16.6900423941731));
#257218=CARTESIAN_POINT('Ctrl Pts',(76.4513448875845,27.2145167369268,16.653916177179));
#257219=CARTESIAN_POINT('Ctrl Pts',(76.4547511876201,27.1945566457996,16.6158401525527));
#257220=CARTESIAN_POINT('Ctrl Pts',(76.4593869302476,27.1790626912129,16.5757647539218));
#257221=CARTESIAN_POINT('Ctrl Pts',(76.4599500333952,27.1771806422517,16.5708967996533));
#257222=CARTESIAN_POINT('Ctrl Pts',(76.4605309464294,27.1753659415636,16.5660028743095));
#257223=CARTESIAN_POINT('Ctrl Pts',(76.4611298941881,27.1736203958826,16.5610838271793));
#257224=CARTESIAN_POINT('Ctrl Pts',(76.4637830304577,27.1658882180939,16.5392941098575));
#257225=CARTESIAN_POINT('Ctrl Pts',(76.4668030340722,27.1595395614895,16.5169703441688));
#257226=CARTESIAN_POINT('Ctrl Pts',(76.4701643665394,27.1547079235266,16.4943951487428));
#257227=CARTESIAN_POINT('Ctrl Pts',(76.4735256990065,27.1498762855636,16.4718199533169));
#257228=CARTESIAN_POINT('Ctrl Pts',(76.4772282140789,27.1465619921089,16.4489944614982));
#257229=CARTESIAN_POINT('Ctrl Pts',(76.4812333698756,27.1448472169224,16.4262179830525));
#257230=CARTESIAN_POINT('Ctrl Pts',(76.4837575042377,27.1437665291311,16.4118637619405));
#257231=CARTESIAN_POINT('Ctrl Pts',(76.4864043794184,27.1432984744763,16.3974938691297));
#257232=CARTESIAN_POINT('Ctrl Pts',(76.4891686128859,27.1434396622859,16.383133975236));
#257233=CARTESIAN_POINT('Ctrl Pts',(76.4931572620936,27.1436433891605,16.3624133740009));
#257234=CARTESIAN_POINT('Ctrl Pts',(76.4973856936385,27.1451158165625,16.3417311587632));
#257235=CARTESIAN_POINT('Ctrl Pts',(76.5018218230375,27.1478003503532,16.3211985325368));
#257236=CARTESIAN_POINT('Ctrl Pts',(76.5063090129379,27.1505157835224,16.3004295727647));
#257237=CARTESIAN_POINT('Ctrl Pts',(76.5110086870996,27.1544712854893,16.2798136765402));
#257238=CARTESIAN_POINT('Ctrl Pts',(76.5158772286368,27.1595556991521,16.2594666987899));
#257239=CARTESIAN_POINT('Ctrl Pts',(76.5208630385112,27.1647625808542,16.2386296243171));
#257240=CARTESIAN_POINT('Ctrl Pts',(76.5260259237948,27.1711532997666,16.2180745910999));
#257241=CARTESIAN_POINT('Ctrl Pts',(76.531308508193,27.1785550950825,16.1979266545698));
#257242=CARTESIAN_POINT('Ctrl Pts',(76.5317837688064,27.1792210156845,16.1961139962283));
#257243=CARTESIAN_POINT('Ctrl Pts',(76.5322599915831,27.1798950860555,16.1943046333203));
#257244=CARTESIAN_POINT('Ctrl Pts',(76.5327371308321,27.1805771605214,16.1924986571));
#257245=CARTESIAN_POINT('Origin',(50.220290910288,8.18330470534212,16.1925));
#257246=CARTESIAN_POINT('Ctrl Pts',(76.5327353708766,-27.1805640649136,
16.1924982582718));
#257247=CARTESIAN_POINT('Ctrl Pts',(76.5254460991286,-27.170142411259,16.2200871281807));
#257248=CARTESIAN_POINT('Ctrl Pts',(76.5184672980879,-27.1617293806191,
16.2481013366734));
#257249=CARTESIAN_POINT('Ctrl Pts',(76.5118328073647,-27.1555532163233,
16.2765966498456));
#257250=CARTESIAN_POINT('Ctrl Pts',(76.5053582412141,-27.1495259286294,
16.304405082748));
#257251=CARTESIAN_POINT('Ctrl Pts',(76.4992115671709,-27.1456288662117,
16.3326717168179));
#257252=CARTESIAN_POINT('Ctrl Pts',(76.4934339939309,-27.144123077719,16.3614476211452));
#257253=CARTESIAN_POINT('Ctrl Pts',(76.4921585023732,-27.1437906508625,
16.3678003615623));
#257254=CARTESIAN_POINT('Ctrl Pts',(76.4909010391219,-27.1435749657791,
16.3741779192149));
#257255=CARTESIAN_POINT('Ctrl Pts',(76.4896621154036,-27.1434791718122,
16.3805808375412));
#257256=CARTESIAN_POINT('Ctrl Pts',(76.4880193305124,-27.143352151174,16.3890709627455));
#257257=CARTESIAN_POINT('Ctrl Pts',(76.4864160037888,-27.1434370002358,
16.3975719419878));
#257258=CARTESIAN_POINT('Ctrl Pts',(76.4848537692343,-27.1437355673527,
16.4060769483921));
#257259=CARTESIAN_POINT('Ctrl Pts',(76.4809854829898,-27.1444748565126,
16.4271363976198));
#257260=CARTESIAN_POINT('Ctrl Pts',(76.4773696370509,-27.1465703673381,
16.4482618838856));
#257261=CARTESIAN_POINT('Ctrl Pts',(76.4740424808257,-27.1499697741418,
16.4691998962437));
#257262=CARTESIAN_POINT('Ctrl Pts',(76.4707094654638,-27.1533751673159,
16.4901747805338));
#257263=CARTESIAN_POINT('Ctrl Pts',(76.4676662855534,-27.1580887887179,
16.5109605600287));
#257264=CARTESIAN_POINT('Ctrl Pts',(76.4649378361828,-27.1640086579344,
16.5313130815935));
#257265=CARTESIAN_POINT('Ctrl Pts',(76.4643858787488,-27.1652062303936,
16.5354303379737));
#257266=CARTESIAN_POINT('Ctrl Pts',(76.4638467601751,-27.1664530141853,
16.5395299259007));
#257267=CARTESIAN_POINT('Ctrl Pts',(76.4633206224269,-27.1677479362274,
16.5436099312137));
#257268=CARTESIAN_POINT('Ctrl Pts',(76.4620493955123,-27.1708766601362,
16.5534678298022));
#257269=CARTESIAN_POINT('Ctrl Pts',(76.4608504005183,-27.1742844116281,
16.5632279776837));
#257270=CARTESIAN_POINT('Ctrl Pts',(76.4597221364489,-27.1779555862455,
16.5728808843466));
#257271=CARTESIAN_POINT('Ctrl Pts',(76.4555634683355,-27.1914871674013,
16.6084605294227));
#257272=CARTESIAN_POINT('Ctrl Pts',(76.4523683264295,-27.2085635842067,
16.6425190954528));
#257273=CARTESIAN_POINT('Ctrl Pts',(76.4499894515854,-27.2285145118707,
16.6751163767829));
#257274=CARTESIAN_POINT('Ctrl Pts',(76.4481516192734,-27.2439278740341,
16.7002998525161));
#257275=CARTESIAN_POINT('Ctrl Pts',(76.4468125093684,-27.2611648250125,
16.7246580015589));
#257276=CARTESIAN_POINT('Ctrl Pts',(76.4459011083301,-27.2797726036762,
16.7480930589315));
#257277=CARTESIAN_POINT('Ctrl Pts',(76.4449881378309,-27.298412425514,16.7715684722023));
#257278=CARTESIAN_POINT('Ctrl Pts',(76.4445043286353,-27.3184277738214,
16.7941176720138));
#257279=CARTESIAN_POINT('Ctrl Pts',(76.4443826625373,-27.3394063743812,
16.8156722156737));
#257280=CARTESIAN_POINT('Ctrl Pts',(76.4442602400807,-27.360515392067,16.8373607569101));
#257281=CARTESIAN_POINT('Ctrl Pts',(76.444504461044,-27.3825996603397,16.858042310263));
#257282=CARTESIAN_POINT('Ctrl Pts',(76.4450517552698,-27.4052828608358,
16.8776763499813));
#257283=CARTESIAN_POINT('Ctrl Pts',(76.4451275701142,-27.4084250889746,
16.8803961880435));
#257284=CARTESIAN_POINT('Ctrl Pts',(76.445209208363,-27.4115788786024,16.8830959690915));
#257285=CARTESIAN_POINT('Ctrl Pts',(76.4452965083211,-27.4147432949493,
16.8857756277876));
#257286=CARTESIAN_POINT('Ctrl Pts',(76.4456285567619,-27.4267792630841,
16.8959678032609));
#257287=CARTESIAN_POINT('Ctrl Pts',(76.4460413746574,-27.4390220462584,
16.9059171754191));
#257288=CARTESIAN_POINT('Ctrl Pts',(76.4465283265822,-27.4514363729662,
16.9156217934251));
#257289=CARTESIAN_POINT('Ctrl Pts',(76.4477740792775,-27.4831955265325,
16.940448790556));
#257290=CARTESIAN_POINT('Ctrl Pts',(76.4494849825224,-27.5161304124262,
16.9638340074613));
#257291=CARTESIAN_POINT('Ctrl Pts',(76.4515669382221,-27.5499276827804,
16.9859393963669));
#257292=CARTESIAN_POINT('Ctrl Pts',(76.4537247726024,-27.5849567239552,
17.0088504353368));
#257293=CARTESIAN_POINT('Ctrl Pts',(76.4562812377412,-27.6209122535195,
17.0303866179473));
#257294=CARTESIAN_POINT('Ctrl Pts',(76.4591476533537,-27.657496253866,17.0507077973849));
#257295=CARTESIAN_POINT('Ctrl Pts',(76.4614800345035,-27.6872643839368,
17.0672429905556));
#257296=CARTESIAN_POINT('Ctrl Pts',(76.4640179659447,-27.7174496690714,
17.0829733141296));
#257297=CARTESIAN_POINT('Ctrl Pts',(76.4667207528857,-27.7479141287993,
17.0979758062083));
#257298=CARTESIAN_POINT('Ctrl Pts',(76.4677059340768,-27.7590185974001,
17.1034442997812));
#257299=CARTESIAN_POINT('Ctrl Pts',(76.4687146852106,-27.7701762979147,
17.1088237343901));
#257300=CARTESIAN_POINT('Ctrl Pts',(76.4697457322933,-27.7813854912822,
17.1141186859284));
#257301=CARTESIAN_POINT('Ctrl Pts',(76.472429728371,-27.8105649841859,17.1279023718524));
#257302=CARTESIAN_POINT('Ctrl Pts',(76.4752686565451,-27.840103215534,17.1410999474328));
#257303=CARTESIAN_POINT('Ctrl Pts',(76.4782264005117,-27.8698177823045,
17.1537242053278));
#257304=CARTESIAN_POINT('Ctrl Pts',(76.4814236442212,-27.9019384502044,
17.1673706972473));
#257305=CARTESIAN_POINT('Ctrl Pts',(76.4847597640879,-27.9342655910949,
17.1803475370977));
#257306=CARTESIAN_POINT('Ctrl Pts',(76.4881996908386,-27.9666279531757,
17.1926699656471));
#257307=CARTESIAN_POINT('Ctrl Pts',(76.4886519862318,-27.9708830865957,
17.1942901680725));
#257308=CARTESIAN_POINT('Ctrl Pts',(76.489106089515,-27.9751389006341,17.1958990522154));
#257309=CARTESIAN_POINT('Ctrl Pts',(76.4895619325379,-27.9793950678132,
17.1974966476082));
#257310=CARTESIAN_POINT('Ctrl Pts',(76.4938975656961,-28.0198765024714,
17.2126917634919));
#257311=CARTESIAN_POINT('Ctrl Pts',(76.4984031419524,-28.060540191981,17.2269450615677));
#257312=CARTESIAN_POINT('Ctrl Pts',(76.5030665766311,-28.1015001037439,
17.2404146413945));
#257313=CARTESIAN_POINT('Ctrl Pts',(76.5035084491004,-28.1053811610762,
17.2416909188399));
#257314=CARTESIAN_POINT('Ctrl Pts',(76.5039517474111,-28.1092649053587,
17.2429601347027));
#257315=CARTESIAN_POINT('Ctrl Pts',(76.5043964665192,-28.1131514503915,
17.2442224078977));
#257316=CARTESIAN_POINT('Ctrl Pts',(76.5073626095462,-28.139073539725,17.2526413914031));
#257317=CARTESIAN_POINT('Ctrl Pts',(76.5103875491059,-28.1650771837681,
17.2607374323177));
#257318=CARTESIAN_POINT('Ctrl Pts',(76.5134649041888,-28.1911518975632,
17.2685330721676));
#257319=CARTESIAN_POINT('Ctrl Pts',(76.5205941289288,-28.2515584771341,
17.2865930187733));
#257320=CARTESIAN_POINT('Ctrl Pts',(76.5280003772061,-28.3123340562714,
17.3030517999906));
#257321=CARTESIAN_POINT('Ctrl Pts',(76.5356394395873,-28.3734477222465,
17.3181020343168));
#257322=CARTESIAN_POINT('Ctrl Pts',(76.543563458799,-28.4368410863943,17.3337136813998));
#257323=CARTESIAN_POINT('Ctrl Pts',(76.5517380600912,-28.5005983553558,
17.3478096642148));
#257324=CARTESIAN_POINT('Ctrl Pts',(76.5601276443193,-28.5647256405924,
17.3605684035053));
#257325=CARTESIAN_POINT('Ctrl Pts',(76.5638310436417,-28.5930332346559,
17.3662004712166));
#257326=CARTESIAN_POINT('Ctrl Pts',(76.5675765027187,-28.6214134363051,
17.3715715053376));
#257327=CARTESIAN_POINT('Ctrl Pts',(76.5713617072211,-28.6498690551213,
17.3766947662575));
#257328=CARTESIAN_POINT('Ctrl Pts',(76.5790130100033,-28.7073884190766,
17.3870507775391));
#257329=CARTESIAN_POINT('Ctrl Pts',(76.5868350946836,-28.7652559670459,
17.3963736583744));
#257330=CARTESIAN_POINT('Ctrl Pts',(76.5947786108551,-28.8232282289076,
17.4047210505685));
#257331=CARTESIAN_POINT('Ctrl Pts',(76.5971621660893,-28.84062355929,17.4072257940507));
#257332=CARTESIAN_POINT('Ctrl Pts',(76.5995567234919,-28.8580286627894,
17.4096426038302));
#257333=CARTESIAN_POINT('Ctrl Pts',(76.6019611150693,-28.8754377812504,
17.4119727726841));
#257334=CARTESIAN_POINT('Ctrl Pts',(76.6127354792351,-28.9534501083073,
17.4224145360128));
#257335=CARTESIAN_POINT('Ctrl Pts',(76.6237599571512,-29.0319245446418,
17.431168749174));
#257336=CARTESIAN_POINT('Ctrl Pts',(76.6349137015633,-29.1101764697921,
17.4382612976142));
#257337=CARTESIAN_POINT('Ctrl Pts',(76.6366048959531,-29.1220414733205,
17.4393367102908));
#257338=CARTESIAN_POINT('Ctrl Pts',(76.6382990798886,-29.1339014546143,
17.440373900432));
#257339=CARTESIAN_POINT('Ctrl Pts',(76.6399958502493,-29.1457541224838,
17.4413729364037));
#257340=CARTESIAN_POINT('Ctrl Pts',(76.6556847857491,-29.2553480581192,
17.4506103743536));
#257341=CARTESIAN_POINT('Ctrl Pts',(76.6716864102403,-29.3650148897999,
17.4567325786662));
#257342=CARTESIAN_POINT('Ctrl Pts',(76.6879909655265,-29.4748980619541,
17.459910050465));
#257343=CARTESIAN_POINT('Ctrl Pts',(76.696887607083,-29.5348562257057,17.461643849833));
#257344=CARTESIAN_POINT('Ctrl Pts',(76.7058745786326,-29.5948790585987,
17.4625));
#257345=CARTESIAN_POINT('Ctrl Pts',(76.7149512087496,-29.6549915892152,
17.4625));
#257346=CARTESIAN_POINT('Origin',(-44.3927817339206,-24.8661421402461,16.1925));
#257347=CARTESIAN_POINT('Ctrl Pts',(29.6549915892152,-76.7149512087496,
17.4625));
#257348=CARTESIAN_POINT('Ctrl Pts',(29.5784809832681,-76.7033985679909,
17.4625));
#257349=CARTESIAN_POINT('Ctrl Pts',(29.5017645219472,-76.6919419131645,
17.4610789773413));
#257350=CARTESIAN_POINT('Ctrl Pts',(29.4251260134592,-76.6806292438031,
17.4582328812633));
#257351=CARTESIAN_POINT('Ctrl Pts',(29.3550776154898,-76.6702893457392,
17.4556315196937));
#257352=CARTESIAN_POINT('Ctrl Pts',(29.285091738982,-76.6600693733096,17.4518390793048));
#257353=CARTESIAN_POINT('Ctrl Pts',(29.215395972818,-76.6500111635191,17.4468147853601));
#257354=CARTESIAN_POINT('Ctrl Pts',(29.1910127661958,-76.6464922782112,
17.4450570258271));
#257355=CARTESIAN_POINT('Ctrl Pts',(29.1666653406614,-76.6429932651761,
17.4431481665674));
#257356=CARTESIAN_POINT('Ctrl Pts',(29.1423646235818,-76.6395162005647,
17.4410854028152));
#257357=CARTESIAN_POINT('Ctrl Pts',(29.0717236084288,-76.6294085410626,
17.4350890478519));
#257358=CARTESIAN_POINT('Ctrl Pts',(29.0013000924683,-76.6194570017698,
17.4278165327662));
#257359=CARTESIAN_POINT('Ctrl Pts',(28.930890043211,-76.6096539020255,17.4191389458549));
#257360=CARTESIAN_POINT('Ctrl Pts',(28.9125942000528,-76.6071065955362,
17.4168841005481));
#257361=CARTESIAN_POINT('Ctrl Pts',(28.8942993977004,-76.6045693606119,
17.4145341520355));
#257362=CARTESIAN_POINT('Ctrl Pts',(28.8760023419532,-76.6020421698846,
17.412086338018));
#257363=CARTESIAN_POINT('Ctrl Pts',(28.8096307852661,-76.5928749254421,
17.4032070281956));
#257364=CARTESIAN_POINT('Ctrl Pts',(28.7435548277056,-76.5838841660478,
17.3930871840675));
#257365=CARTESIAN_POINT('Ctrl Pts',(28.6775616926366,-76.5750605977029,
17.3815966638287));
#257366=CARTESIAN_POINT('Ctrl Pts',(28.6679863743641,-76.5737803361255,
17.3799294390744));
#257367=CARTESIAN_POINT('Ctrl Pts',(28.6584128434796,-76.5725036108758,
17.3782332812975));
#257368=CARTESIAN_POINT('Ctrl Pts',(28.648840495476,-76.571230410841,17.3765077138038));
#257369=CARTESIAN_POINT('Ctrl Pts',(28.5939195943272,-76.5639254848995,
17.3666073506207));
#257370=CARTESIAN_POINT('Ctrl Pts',(28.539019721318,-76.5567364098806,17.3557157603938));
#257371=CARTESIAN_POINT('Ctrl Pts',(28.4842809217551,-76.5497009035225,
17.3437734778892));
#257372=CARTESIAN_POINT('Ctrl Pts',(28.4340312118414,-76.5432423739892,
17.3328105733981));
#257373=CARTESIAN_POINT('Ctrl Pts',(28.3839169544482,-76.5369132259095,
17.3209620182655));
#257374=CARTESIAN_POINT('Ctrl Pts',(28.3340851368585,-76.5307511868761,
17.3081680846722));
#257375=CARTESIAN_POINT('Ctrl Pts',(28.2843811713914,-76.5246049576167,
17.2954069761221));
#257376=CARTESIAN_POINT('Ctrl Pts',(28.2349573707686,-76.518624827935,17.2817053136045));
#257377=CARTESIAN_POINT('Ctrl Pts',(28.186008513182,-76.5128586176738,17.2669910566475));
#257378=CARTESIAN_POINT('Ctrl Pts',(28.1614764636039,-76.5099687247737,
17.25961660709));
#257379=CARTESIAN_POINT('Ctrl Pts',(28.1370017452465,-76.5071248960927,
17.2519719554798));
#257380=CARTESIAN_POINT('Ctrl Pts',(28.112603631757,-76.5043336151742,17.2440428740805));
#257381=CARTESIAN_POINT('Ctrl Pts',(28.0701844846509,-76.4994806270139,
17.2302571823942));
#257382=CARTESIAN_POINT('Ctrl Pts',(28.0279824912973,-76.4947829029006,
17.2156101298218));
#257383=CARTESIAN_POINT('Ctrl Pts',(27.9860694428279,-76.4902767919924,
17.1999930540383));
#257384=CARTESIAN_POINT('Ctrl Pts',(27.9466341480905,-76.4860370666975,
17.1852992054887));
#257385=CARTESIAN_POINT('Ctrl Pts',(27.9074544475917,-76.4819669295132,
17.1697465428432));
#257386=CARTESIAN_POINT('Ctrl Pts',(27.8686308801497,-76.4781067108621,
17.153228318961));
#257387=CARTESIAN_POINT('Ctrl Pts',(27.837762123119,-76.4750374372359,17.1400946202003));
#257388=CARTESIAN_POINT('Ctrl Pts',(27.8071191438906,-76.4721010301339,
17.1263502154837));
#257389=CARTESIAN_POINT('Ctrl Pts',(27.7767742650356,-76.4693230827021,
17.1119338317454));
#257390=CARTESIAN_POINT('Ctrl Pts',(27.7671845095157,-76.4684451804754,
17.1073778868628));
#257391=CARTESIAN_POINT('Ctrl Pts',(27.7576382281084,-76.46758424905,17.1027621986441));
#257392=CARTESIAN_POINT('Ctrl Pts',(27.7481373827157,-76.4667411216785,
17.0980845986398));
#257393=CARTESIAN_POINT('Ctrl Pts',(27.7165349284677,-76.4639366455415,
17.0825256000436));
#257394=CARTESIAN_POINT('Ctrl Pts',(27.6854146211002,-76.461325227445,17.0662758428433));
#257395=CARTESIAN_POINT('Ctrl Pts',(27.6548074136947,-76.4589379212268,
17.0492104485573));
#257396=CARTESIAN_POINT('Ctrl Pts',(27.6250423674505,-76.4566163020395,
17.0326146107414));
#257397=CARTESIAN_POINT('Ctrl Pts',(27.5957623497953,-76.4545065513655,
17.0152474880437));
#257398=CARTESIAN_POINT('Ctrl Pts',(27.5670390175372,-76.4526490486086,
16.9969759720735));
#257399=CARTESIAN_POINT('Ctrl Pts',(27.5394891827774,-76.4508674344993,
16.9794509425515));
#257400=CARTESIAN_POINT('Ctrl Pts',(27.5124513533527,-76.4493178278133,
16.9610939515815));
#257401=CARTESIAN_POINT('Ctrl Pts',(27.4860313731063,-76.448047775172,16.9417696635372));
#257402=CARTESIAN_POINT('Ctrl Pts',(27.4732138950567,-76.4474316175633,
16.9323946134606));
#257403=CARTESIAN_POINT('Ctrl Pts',(27.4605425004175,-76.4468814440254,
16.9227916185164));
#257404=CARTESIAN_POINT('Ctrl Pts',(27.4480332789739,-76.4464038210192,
16.9129435541778));
#257405=CARTESIAN_POINT('Ctrl Pts',(27.4380190788529,-76.446021462102,16.9050597312288));
#257406=CARTESIAN_POINT('Ctrl Pts',(27.4281096389904,-76.4456876024434,
16.8970089022858));
#257407=CARTESIAN_POINT('Ctrl Pts',(27.4183213434191,-76.4454060812472,
16.8887879984482));
#257408=CARTESIAN_POINT('Ctrl Pts',(27.3952254081782,-76.4447418189891,
16.8693903963557));
#257409=CARTESIAN_POINT('Ctrl Pts',(27.3726021898373,-76.4443701445099,
16.8488671319478));
#257410=CARTESIAN_POINT('Ctrl Pts',(27.3508659754084,-76.4443625463769,
16.8272552303422));
#257411=CARTESIAN_POINT('Ctrl Pts',(27.3290708073661,-76.4443549276361,
16.8055847122883));
#257412=CARTESIAN_POINT('Ctrl Pts',(27.3081675781727,-76.4447134034009,
16.7828195228048));
#257413=CARTESIAN_POINT('Ctrl Pts',(27.2886142275583,-76.4455134941453,
16.7590305376009));
#257414=CARTESIAN_POINT('Ctrl Pts',(27.2688420650758,-76.4463225383092,
16.7349753416389));
#257415=CARTESIAN_POINT('Ctrl Pts',(27.2504503196107,-76.4475831876929,
16.7098732026971));
#257416=CARTESIAN_POINT('Ctrl Pts',(27.2339516171415,-76.4493763637529,
16.6838334538405));
#257417=CARTESIAN_POINT('Ctrl Pts',(27.2316065629842,-76.4496312380366,
16.6801322766463));
#257418=CARTESIAN_POINT('Ctrl Pts',(27.2292998143652,-76.449896874548,16.6764122174921));
#257419=CARTESIAN_POINT('Ctrl Pts',(27.22703290306,-76.4501735092111,16.6726736500803));
#257420=CARTESIAN_POINT('Ctrl Pts',(27.208294241588,-76.4524602168078,16.6417700373296));
#257421=CARTESIAN_POINT('Ctrl Pts',(27.1920956821037,-76.4554866376469,
16.6094802657885));
#257422=CARTESIAN_POINT('Ctrl Pts',(27.1790613975838,-76.4593868180786,
16.5757650534976));
#257423=CARTESIAN_POINT('Ctrl Pts',(27.1746643707656,-76.4607025172968,
16.5643914570107));
#257424=CARTESIAN_POINT('Ctrl Pts',(27.1706359107516,-76.4621156292997,
16.5528759158133));
#257425=CARTESIAN_POINT('Ctrl Pts',(27.1669986019356,-76.4636289044872,
16.5412293347377));
#257426=CARTESIAN_POINT('Ctrl Pts',(27.1600415068142,-76.4665233519912,
16.5189528725292));
#257427=CARTESIAN_POINT('Ctrl Pts',(27.1545628735561,-76.4697851638502,
16.4962407115125));
#257428=CARTESIAN_POINT('Ctrl Pts',(27.1506549153931,-76.4733862268997,
16.4733464731272));
#257429=CARTESIAN_POINT('Ctrl Pts',(27.14674695723,-76.4769872899492,16.450452234742));
#257430=CARTESIAN_POINT('Ctrl Pts',(27.1444098150615,-76.4809274578023,
16.4273768616869));
#257431=CARTESIAN_POINT('Ctrl Pts',(27.1436800109181,-76.4851658906463,
16.4043845876085));
#257432=CARTESIAN_POINT('Ctrl Pts',(27.1434551581823,-76.4864717522652,
16.3973006654718));
#257433=CARTESIAN_POINT('Ctrl Pts',(27.143378345838,-76.4878067469535,16.3902160073498));
#257434=CARTESIAN_POINT('Ctrl Pts',(27.1434490350604,-76.4891701961805,
16.383133694799));
#257435=CARTESIAN_POINT('Ctrl Pts',(27.1436556805567,-76.4931559613736,
16.3624300013325));
#257436=CARTESIAN_POINT('Ctrl Pts',(27.1451242300415,-76.4973805033897,
16.3417644841244));
#257437=CARTESIAN_POINT('Ctrl Pts',(27.1478012243607,-76.5018122177599,
16.3212481482212));
#257438=CARTESIAN_POINT('Ctrl Pts',(27.1505058861726,-76.5062897351503,
16.3005197701895));
#257439=CARTESIAN_POINT('Ctrl Pts',(27.1544440119297,-76.5109787082563,
16.279943684392));
#257440=CARTESIAN_POINT('Ctrl Pts',(27.1595080210185,-76.5158361677253,
16.2596351519481));
#257441=CARTESIAN_POINT('Ctrl Pts',(27.164685302902,-76.5208022798447,16.2388723540821));
#257442=CARTESIAN_POINT('Ctrl Pts',(27.1710392955923,-76.5259444759375,
16.2183892248369));
#257443=CARTESIAN_POINT('Ctrl Pts',(27.178401795822,-76.5312063612745,16.1983095665747));
#257444=CARTESIAN_POINT('Ctrl Pts',(27.1791134525487,-76.5317149732919,
16.1963686737493));
#257445=CARTESIAN_POINT('Ctrl Pts',(27.1798344925866,-76.5322246958756,
16.1944315509814));
#257446=CARTESIAN_POINT('Ctrl Pts',(27.1805647391996,-76.5327354732286,
16.1924983103144));
#257447=CARTESIAN_POINT('Origin',(-76.3890311653897,-109.438478010978,16.1925));
#257448=CARTESIAN_POINT('Ctrl Pts',(-27.1805640649125,-76.5327353708757,
16.1924982582717));
#257449=CARTESIAN_POINT('Ctrl Pts',(-27.1701424112585,-76.525446099128,
16.2200871281786));
#257450=CARTESIAN_POINT('Ctrl Pts',(-27.1617293806189,-76.5184672980878,
16.2481013366692));
#257451=CARTESIAN_POINT('Ctrl Pts',(-27.1555532163233,-76.5118328073651,
16.2765966498393));
#257452=CARTESIAN_POINT('Ctrl Pts',(-27.1495259286296,-76.5053582412149,
16.3044050827398));
#257453=CARTESIAN_POINT('Ctrl Pts',(-27.1456288662118,-76.4992115671722,
16.3326717168078));
#257454=CARTESIAN_POINT('Ctrl Pts',(-27.1441230777188,-76.4934339939327,
16.3614476211331));
#257455=CARTESIAN_POINT('Ctrl Pts',(-27.1437906508621,-76.4921585023742,
16.3678003615543));
#257456=CARTESIAN_POINT('Ctrl Pts',(-27.1435749657785,-76.4909010391221,
16.3741779192108));
#257457=CARTESIAN_POINT('Ctrl Pts',(-27.1434791718117,-76.4896621154032,
16.3805808375412));
#257458=CARTESIAN_POINT('Ctrl Pts',(-27.1433521511735,-76.4880193305119,
16.3890709627458));
#257459=CARTESIAN_POINT('Ctrl Pts',(-27.1434370002354,-76.4864160037884,
16.3975719419884));
#257460=CARTESIAN_POINT('Ctrl Pts',(-27.1437355673525,-76.4848537692339,
16.406076948393));
#257461=CARTESIAN_POINT('Ctrl Pts',(-27.1444748565128,-76.4809854829898,
16.4271363976198));
#257462=CARTESIAN_POINT('Ctrl Pts',(-27.1465703673381,-76.4773696370511,
16.4482618838846));
#257463=CARTESIAN_POINT('Ctrl Pts',(-27.1499697741416,-76.474042480826,
16.4691998962417));
#257464=CARTESIAN_POINT('Ctrl Pts',(-27.1533751673149,-76.4707094654647,
16.4901747805278));
#257465=CARTESIAN_POINT('Ctrl Pts',(-27.1580887887156,-76.4676662855547,
16.5109605600187));
#257466=CARTESIAN_POINT('Ctrl Pts',(-27.1640086579305,-76.4649378361846,
16.5313130815798));
#257467=CARTESIAN_POINT('Ctrl Pts',(-27.165206230391,-76.4643858787499,
16.5354303379649));
#257468=CARTESIAN_POINT('Ctrl Pts',(-27.1664530141842,-76.4638467601756,
16.5395299258967));
#257469=CARTESIAN_POINT('Ctrl Pts',(-27.1677479362278,-76.4633206224268,
16.5436099312145));
#257470=CARTESIAN_POINT('Ctrl Pts',(-27.1708766601366,-76.4620493955123,
16.5534678298028));
#257471=CARTESIAN_POINT('Ctrl Pts',(-27.1742844116285,-76.4608504005184,
16.563227977684));
#257472=CARTESIAN_POINT('Ctrl Pts',(-27.1779555862458,-76.4597221364491,
16.5728808843466));
#257473=CARTESIAN_POINT('Ctrl Pts',(-27.1914871674019,-76.4555634683357,
16.6084605294229));
#257474=CARTESIAN_POINT('Ctrl Pts',(-27.2085635842075,-76.4523683264298,
16.6425190954533));
#257475=CARTESIAN_POINT('Ctrl Pts',(-27.2285145118716,-76.4499894515856,
16.6751163767836));
#257476=CARTESIAN_POINT('Ctrl Pts',(-27.243927874034,-76.4481516192736,
16.7002998525154));
#257477=CARTESIAN_POINT('Ctrl Pts',(-27.2611648250113,-76.4468125093686,
16.7246580015568));
#257478=CARTESIAN_POINT('Ctrl Pts',(-27.2797726036738,-76.4459011083303,
16.7480930589281));
#257479=CARTESIAN_POINT('Ctrl Pts',(-27.2984124255103,-76.4449881378311,
16.7715684721976));
#257480=CARTESIAN_POINT('Ctrl Pts',(-27.3184277738163,-76.4445043286355,
16.794117672008));
#257481=CARTESIAN_POINT('Ctrl Pts',(-27.3394063743747,-76.4443826625374,
16.8156722156667));
#257482=CARTESIAN_POINT('Ctrl Pts',(-27.3605153920599,-76.4442602400808,
16.8373607569029));
#257483=CARTESIAN_POINT('Ctrl Pts',(-27.382599660332,-76.444504461044,16.8580423102556));
#257484=CARTESIAN_POINT('Ctrl Pts',(-27.4052828608275,-76.4450517552699,
16.8776763499738));
#257485=CARTESIAN_POINT('Ctrl Pts',(-27.4084250889692,-76.4451275701144,
16.8803961880385));
#257486=CARTESIAN_POINT('Ctrl Pts',(-27.4115788785998,-76.4452092083632,
16.8830959690889));
#257487=CARTESIAN_POINT('Ctrl Pts',(-27.4147432949497,-76.4452965083214,
16.8857756277875));
#257488=CARTESIAN_POINT('Ctrl Pts',(-27.4267792630848,-76.4456285567623,
16.895967803261));
#257489=CARTESIAN_POINT('Ctrl Pts',(-27.4390220462594,-76.4460413746579,
16.9059171754193));
#257490=CARTESIAN_POINT('Ctrl Pts',(-27.4514363729675,-76.4465283265827,
16.9156217934255));
#257491=CARTESIAN_POINT('Ctrl Pts',(-27.4831955265322,-76.4477740792784,
16.9404487905547));
#257492=CARTESIAN_POINT('Ctrl Pts',(-27.5161304124239,-76.4494849825232,
16.9638340074586));
#257493=CARTESIAN_POINT('Ctrl Pts',(-27.549927682776,-76.4515669382227,
16.985939396363));
#257494=CARTESIAN_POINT('Ctrl Pts',(-27.5849567239488,-76.4537247726028,
17.0088504353318));
#257495=CARTESIAN_POINT('Ctrl Pts',(-27.6209122535109,-76.4562812377412,
17.0303866179415));
#257496=CARTESIAN_POINT('Ctrl Pts',(-27.6574962538552,-76.4591476533534,
17.0507077973783));
#257497=CARTESIAN_POINT('Ctrl Pts',(-27.6872643839296,-76.4614800345033,
17.0672429905514));
#257498=CARTESIAN_POINT('Ctrl Pts',(-27.7174496690679,-76.4640179659447,
17.0829733141275));
#257499=CARTESIAN_POINT('Ctrl Pts',(-27.7479141287996,-76.466720752886,
17.0979758062082));
#257500=CARTESIAN_POINT('Ctrl Pts',(-27.7590185974006,-76.4677059340771,
17.1034442997812));
#257501=CARTESIAN_POINT('Ctrl Pts',(-27.7701762979155,-76.4687146852109,
17.1088237343903));
#257502=CARTESIAN_POINT('Ctrl Pts',(-27.7813854912832,-76.4697457322936,
17.1141186859287));
#257503=CARTESIAN_POINT('Ctrl Pts',(-27.8105649841822,-76.4724297283708,
17.1279023718504));
#257504=CARTESIAN_POINT('Ctrl Pts',(-27.8401032155254,-76.4752686565444,
17.1410999474288));
#257505=CARTESIAN_POINT('Ctrl Pts',(-27.8698177822912,-76.4782264005106,
17.153724205322));
#257506=CARTESIAN_POINT('Ctrl Pts',(-27.9019384501864,-76.4814236442195,
17.1673706972397));
#257507=CARTESIAN_POINT('Ctrl Pts',(-27.9342655910722,-76.4847597640857,
17.1803475370885));
#257508=CARTESIAN_POINT('Ctrl Pts',(-27.9666279531484,-76.4881996908359,
17.1926699656366));
#257509=CARTESIAN_POINT('Ctrl Pts',(-27.9708830865778,-76.48865198623,17.1942901680656));
#257510=CARTESIAN_POINT('Ctrl Pts',(-27.9751389006255,-76.4891060895142,
17.1958990522121));
#257511=CARTESIAN_POINT('Ctrl Pts',(-27.979395067814,-76.4895619325381,
17.1974966476085));
#257512=CARTESIAN_POINT('Ctrl Pts',(-28.0198765024774,-76.4938975656967,
17.2126917634941));
#257513=CARTESIAN_POINT('Ctrl Pts',(-28.0605401919919,-76.4984031419535,
17.2269450615715));
#257514=CARTESIAN_POINT('Ctrl Pts',(-28.10150010376,-76.5030665766328,17.2404146413998));
#257515=CARTESIAN_POINT('Ctrl Pts',(-28.1053811610869,-76.5035084491015,
17.2416909188434));
#257516=CARTESIAN_POINT('Ctrl Pts',(-28.1092649053641,-76.5039517474116,
17.2429601347045));
#257517=CARTESIAN_POINT('Ctrl Pts',(-28.1131514503915,-76.5043964665191,
17.2442224078978));
#257518=CARTESIAN_POINT('Ctrl Pts',(-28.1390735397251,-76.5073626095461,
17.2526413914032));
#257519=CARTESIAN_POINT('Ctrl Pts',(-28.1650771837685,-76.5103875491059,
17.2607374323178));
#257520=CARTESIAN_POINT('Ctrl Pts',(-28.191151897564,-76.5134649041889,
17.2685330721677));
#257521=CARTESIAN_POINT('Ctrl Pts',(-28.2515584771378,-76.5205941289295,
17.2865930187743));
#257522=CARTESIAN_POINT('Ctrl Pts',(-28.3123340562775,-76.5280003772075,
17.303051799992));
#257523=CARTESIAN_POINT('Ctrl Pts',(-28.3734477222549,-76.5356394395893,
17.3181020343185));
#257524=CARTESIAN_POINT('Ctrl Pts',(-28.4368410864034,-76.5435634588014,
17.3337136814015));
#257525=CARTESIAN_POINT('Ctrl Pts',(-28.5005983553654,-76.5517380600939,
17.3478096642164));
#257526=CARTESIAN_POINT('Ctrl Pts',(-28.5647256406029,-76.560127644322,
17.3605684035069));
#257527=CARTESIAN_POINT('Ctrl Pts',(-28.5930332346632,-76.5638310436439,
17.3662004712176));
#257528=CARTESIAN_POINT('Ctrl Pts',(-28.6214134363092,-76.5675765027203,
17.371571505338));
#257529=CARTESIAN_POINT('Ctrl Pts',(-28.6498690551224,-76.5713617072221,
17.3766947662573));
#257530=CARTESIAN_POINT('Ctrl Pts',(-28.7073884190778,-76.5790130100039,
17.3870507775391));
#257531=CARTESIAN_POINT('Ctrl Pts',(-28.7652559670471,-76.5868350946839,
17.3963736583745));
#257532=CARTESIAN_POINT('Ctrl Pts',(-28.8232282289088,-76.5947786108553,
17.4047210505686));
#257533=CARTESIAN_POINT('Ctrl Pts',(-28.8406235592908,-76.5971621660894,
17.4072257940508));
#257534=CARTESIAN_POINT('Ctrl Pts',(-28.8580286627899,-76.599556723492,
17.4096426038302));
#257535=CARTESIAN_POINT('Ctrl Pts',(-28.8754377812505,-76.6019611150693,
17.4119727726841));
#257536=CARTESIAN_POINT('Ctrl Pts',(-28.9534501083453,-76.6127354792404,
17.4224145360179));
#257537=CARTESIAN_POINT('Ctrl Pts',(-29.0319245447185,-76.6237599571619,
17.4311687491825));
#257538=CARTESIAN_POINT('Ctrl Pts',(-29.1101764699068,-76.6349137015798,
17.4382612976246));
#257539=CARTESIAN_POINT('Ctrl Pts',(-29.1220414733971,-76.6366048959643,
17.4393367102974));
#257540=CARTESIAN_POINT('Ctrl Pts',(-29.1339014546529,-76.6382990798944,
17.4403739004352));
#257541=CARTESIAN_POINT('Ctrl Pts',(-29.1457541224843,-76.6399958502497,
17.4413729364037));
#257542=CARTESIAN_POINT('Ctrl Pts',(-29.2553480584429,-76.6556847857963,
17.4506103743807));
#257543=CARTESIAN_POINT('Ctrl Pts',(-29.3650148904473,-76.6716864103373,
17.4567325787024));
#257544=CARTESIAN_POINT('Ctrl Pts',(-29.4748980629263,-76.687990965673,
17.4599100504931));
#257545=CARTESIAN_POINT('Ctrl Pts',(-29.5348562263547,-76.6968876071823,
17.4616438498422));
#257546=CARTESIAN_POINT('Ctrl Pts',(-29.5948790589239,-76.7058745786832,
17.4625));
#257547=CARTESIAN_POINT('Ctrl Pts',(-29.6549915892153,-76.7149512087495,
17.4625));
#257548=CARTESIAN_POINT('Origin',(-76.3890311653897,-109.438478010978,16.1925));
#257549=CARTESIAN_POINT('Origin',(-90.,-90.,16.1925));
#257550=CARTESIAN_POINT('Origin',(-109.438478010978,-76.3890311653897,16.1925));
#257551=CARTESIAN_POINT('Origin',(-109.438478010978,-76.3890311653897,16.1925));
#257552=CARTESIAN_POINT('Ctrl Pts',(-76.7149512087495,-29.6549915892152,
17.4625));
#257553=CARTESIAN_POINT('Ctrl Pts',(-76.7033985679887,-29.5784809832302,
17.4625));
#257554=CARTESIAN_POINT('Ctrl Pts',(-76.6919419131574,-29.5017645218705,
17.4610789773399));
#257555=CARTESIAN_POINT('Ctrl Pts',(-76.6806292437899,-29.4251260133434,
17.4582328812589));
#257556=CARTESIAN_POINT('Ctrl Pts',(-76.6702893457237,-29.3550776153601,
17.4556315196874));
#257557=CARTESIAN_POINT('Ctrl Pts',(-76.6600693732909,-29.2850917388382,
17.4518390792962));
#257558=CARTESIAN_POINT('Ctrl Pts',(-76.6500111634973,-29.21539597266,17.4468147853486));
#257559=CARTESIAN_POINT('Ctrl Pts',(-76.6464922781968,-29.1910127660907,
17.4450570258188));
#257560=CARTESIAN_POINT('Ctrl Pts',(-76.6429932651689,-29.166665340609,
17.4431481665629));
#257561=CARTESIAN_POINT('Ctrl Pts',(-76.6395162005647,-29.1423646235818,
17.4410854028152));
#257562=CARTESIAN_POINT('Ctrl Pts',(-76.6294085410564,-29.0717236083913,
17.4350890478489));
#257563=CARTESIAN_POINT('Ctrl Pts',(-76.6194570017585,-29.0013000923935,
17.4278165327585));
#257564=CARTESIAN_POINT('Ctrl Pts',(-76.6096539020096,-28.9308900430995,
17.4191389458411));
#257565=CARTESIAN_POINT('Ctrl Pts',(-76.6071065955256,-28.9125941999784,
17.4168841005385));
#257566=CARTESIAN_POINT('Ctrl Pts',(-76.6045693606066,-28.8942993976632,
17.4145341520304));
#257567=CARTESIAN_POINT('Ctrl Pts',(-76.6020421698846,-28.8760023419532,
17.4120863380179));
#257568=CARTESIAN_POINT('Ctrl Pts',(-76.5928749254408,-28.8096307852544,
17.4032070281938));
#257569=CARTESIAN_POINT('Ctrl Pts',(-76.5838841660453,-28.7435548276822,
17.3930871840637));
#257570=CARTESIAN_POINT('Ctrl Pts',(-76.5750605976985,-28.6775616926014,
17.3815966638225));
#257571=CARTESIAN_POINT('Ctrl Pts',(-76.5737803361226,-28.6679863743407,
17.3799294390701));
#257572=CARTESIAN_POINT('Ctrl Pts',(-76.5725036108744,-28.6584128434679,
17.3782332812954));
#257573=CARTESIAN_POINT('Ctrl Pts',(-76.5712304108411,-28.6488404954761,
17.3765077138038));
#257574=CARTESIAN_POINT('Ctrl Pts',(-76.563925484898,-28.5939195943194,
17.3666073506194));
#257575=CARTESIAN_POINT('Ctrl Pts',(-76.5567364098782,-28.5390197213025,
17.3557157603908));
#257576=CARTESIAN_POINT('Ctrl Pts',(-76.5497009035193,-28.484280921732,
17.3437734778842));
#257577=CARTESIAN_POINT('Ctrl Pts',(-76.5432423739851,-28.4340312118097,
17.3328105733909));
#257578=CARTESIAN_POINT('Ctrl Pts',(-76.5369132259047,-28.3839169544081,
17.3209620182557));
#257579=CARTESIAN_POINT('Ctrl Pts',(-76.5307511868706,-28.3340851368099,
17.3081680846594));
#257580=CARTESIAN_POINT('Ctrl Pts',(-76.5246049576135,-28.2843811713595,
17.2954069761129));
#257581=CARTESIAN_POINT('Ctrl Pts',(-76.5186248279338,-28.234957370753,
17.2817053135994));
#257582=CARTESIAN_POINT('Ctrl Pts',(-76.512858617674,-28.1860085131821,
17.2669910566475));
#257583=CARTESIAN_POINT('Ctrl Pts',(-76.5099687247737,-28.1614764636039,
17.25961660709));
#257584=CARTESIAN_POINT('Ctrl Pts',(-76.5071248960926,-28.1370017452464,
17.2519719554799));
#257585=CARTESIAN_POINT('Ctrl Pts',(-76.504333615174,-28.1126036317569,
17.2440428740805));
#257586=CARTESIAN_POINT('Ctrl Pts',(-76.499480627012,-28.0701844846356,
17.2302571823893));
#257587=CARTESIAN_POINT('Ctrl Pts',(-76.4947829028971,-28.0279824912673,
17.2156101298114));
#257588=CARTESIAN_POINT('Ctrl Pts',(-76.4902767919876,-27.9860694427833,
17.1999930540216));
#257589=CARTESIAN_POINT('Ctrl Pts',(-76.4860370666911,-27.9466341480291,
17.185299205465));
#257590=CARTESIAN_POINT('Ctrl Pts',(-76.4819669295053,-27.9074544475136,
17.1697465428116));
#257591=CARTESIAN_POINT('Ctrl Pts',(-76.4781067108528,-27.8686308800552,
17.1532283189207));
#257592=CARTESIAN_POINT('Ctrl Pts',(-76.4750374372299,-27.8377621230565,
17.1400946201722));
#257593=CARTESIAN_POINT('Ctrl Pts',(-76.4721010301308,-27.8071191438596,
17.1263502154691));
#257594=CARTESIAN_POINT('Ctrl Pts',(-76.4693230827014,-27.7767742650351,
17.1119338317457));
#257595=CARTESIAN_POINT('Ctrl Pts',(-76.4684451804744,-27.7671845095149,
17.1073778868631));
#257596=CARTESIAN_POINT('Ctrl Pts',(-76.467584249049,-27.7576382281075,
17.1027621986445));
#257597=CARTESIAN_POINT('Ctrl Pts',(-76.4667411216774,-27.7481373827148,
17.0980845986402));
#257598=CARTESIAN_POINT('Ctrl Pts',(-76.4639366455395,-27.7165349284599,
17.0825256000408));
#257599=CARTESIAN_POINT('Ctrl Pts',(-76.4613252274425,-27.685414621086,
17.066275842837));
#257600=CARTESIAN_POINT('Ctrl Pts',(-76.458937921224,-27.6548074136743,
17.049210448547));
#257601=CARTESIAN_POINT('Ctrl Pts',(-76.4566163020363,-27.6250423674227,
17.0326146107265));
#257602=CARTESIAN_POINT('Ctrl Pts',(-76.4545065513622,-27.5957623497606,
17.0152474880236));
#257603=CARTESIAN_POINT('Ctrl Pts',(-76.4526490486054,-27.5670390174958,
16.9969759720477));
#257604=CARTESIAN_POINT('Ctrl Pts',(-76.4508674344959,-27.5394891827278,
16.9794509425192));
#257605=CARTESIAN_POINT('Ctrl Pts',(-76.44931782781,-27.5124513532953,16.9610939515419));
#257606=CARTESIAN_POINT('Ctrl Pts',(-76.4480477751689,-27.4860313730415,
16.9417696634897));
#257607=CARTESIAN_POINT('Ctrl Pts',(-76.4474316175615,-27.4732138950141,
16.9323946134282));
#257608=CARTESIAN_POINT('Ctrl Pts',(-76.4468814440248,-27.4605425003966,
16.9227916184998));
#257609=CARTESIAN_POINT('Ctrl Pts',(-76.4464038210194,-27.4480332789741,
16.9129435541778));
#257610=CARTESIAN_POINT('Ctrl Pts',(-76.4460214621022,-27.438019078853,
16.9050597312288));
#257611=CARTESIAN_POINT('Ctrl Pts',(-76.4456876024435,-27.4281096389905,
16.8970089022858));
#257612=CARTESIAN_POINT('Ctrl Pts',(-76.4454060812472,-27.4183213434192,
16.8887879984481));
#257613=CARTESIAN_POINT('Ctrl Pts',(-76.4447418189892,-27.3952254081783,
16.8693903963557));
#257614=CARTESIAN_POINT('Ctrl Pts',(-76.4443701445099,-27.3726021898374,
16.8488671319479));
#257615=CARTESIAN_POINT('Ctrl Pts',(-76.444362546377,-27.3508659754085,
16.8272552303423));
#257616=CARTESIAN_POINT('Ctrl Pts',(-76.4443549276361,-27.3290708073665,
16.8055847122886));
#257617=CARTESIAN_POINT('Ctrl Pts',(-76.4447134034008,-27.3081675781732,
16.7828195228054));
#257618=CARTESIAN_POINT('Ctrl Pts',(-76.4455134941452,-27.288614227559,
16.7590305376019));
#257619=CARTESIAN_POINT('Ctrl Pts',(-76.4463225383091,-27.2688420650766,
16.73497534164));
#257620=CARTESIAN_POINT('Ctrl Pts',(-76.4475831876929,-27.2504503196115,
16.7098732026983));
#257621=CARTESIAN_POINT('Ctrl Pts',(-76.4493763637529,-27.2339516171425,
16.6838334538418));
#257622=CARTESIAN_POINT('Ctrl Pts',(-76.4496312380366,-27.2316065629849,
16.6801322766471));
#257623=CARTESIAN_POINT('Ctrl Pts',(-76.4498968745481,-27.2292998143657,
16.6764122174925));
#257624=CARTESIAN_POINT('Ctrl Pts',(-76.4501735092112,-27.2270329030601,
16.6726736500804));
#257625=CARTESIAN_POINT('Ctrl Pts',(-76.4524602168079,-27.2082942415882,
16.6417700373295));
#257626=CARTESIAN_POINT('Ctrl Pts',(-76.4554866376467,-27.1920956821034,
16.6094802657886));
#257627=CARTESIAN_POINT('Ctrl Pts',(-76.4593868180784,-27.1790613975836,
16.5757650534976));
#257628=CARTESIAN_POINT('Ctrl Pts',(-76.4607025172967,-27.1746643707655,
16.5643914570108));
#257629=CARTESIAN_POINT('Ctrl Pts',(-76.4621156292997,-27.1706359107516,
16.5528759158133));
#257630=CARTESIAN_POINT('Ctrl Pts',(-76.4636289044873,-27.1669986019358,
16.5412293347378));
#257631=CARTESIAN_POINT('Ctrl Pts',(-76.4665233519918,-27.160041506815,
16.5189528725291));
#257632=CARTESIAN_POINT('Ctrl Pts',(-76.4697851638507,-27.1545628735568,
16.4962407115123));
#257633=CARTESIAN_POINT('Ctrl Pts',(-76.4733862269001,-27.1506549153936,
16.4733464731271));
#257634=CARTESIAN_POINT('Ctrl Pts',(-76.4769872899495,-27.1467469572304,
16.4504522347419));
#257635=CARTESIAN_POINT('Ctrl Pts',(-76.4809274578024,-27.1444098150617,
16.427376861687));
#257636=CARTESIAN_POINT('Ctrl Pts',(-76.4851658906466,-27.1436800109185,
16.4043845876086));
#257637=CARTESIAN_POINT('Ctrl Pts',(-76.4864717522655,-27.1434551581829,
16.3973006654719));
#257638=CARTESIAN_POINT('Ctrl Pts',(-76.4878067469539,-27.1433783458386,
16.3902160073499));
#257639=CARTESIAN_POINT('Ctrl Pts',(-76.489170196181,-27.1434490350611,
16.3831336947991));
#257640=CARTESIAN_POINT('Ctrl Pts',(-76.4931559613738,-27.1436556805576,
16.3624300013349));
#257641=CARTESIAN_POINT('Ctrl Pts',(-76.4973805033897,-27.1451242300423,
16.3417644841291));
#257642=CARTESIAN_POINT('Ctrl Pts',(-76.5018122177595,-27.1478012243613,
16.3212481482282));
#257643=CARTESIAN_POINT('Ctrl Pts',(-76.5062897351498,-27.150505886173,
16.3005197701981));
#257644=CARTESIAN_POINT('Ctrl Pts',(-76.5109787082556,-27.1544440119297,
16.279943684402));
#257645=CARTESIAN_POINT('Ctrl Pts',(-76.5158361677243,-27.1595080210179,
16.2596351519595));
#257646=CARTESIAN_POINT('Ctrl Pts',(-76.5208022798437,-27.1646853029011,
16.2388723540938));
#257647=CARTESIAN_POINT('Ctrl Pts',(-76.5259444759364,-27.1710392955909,
16.2183892248486));
#257648=CARTESIAN_POINT('Ctrl Pts',(-76.5312063612731,-27.1784017958199,
16.1983095665865));
#257649=CARTESIAN_POINT('Ctrl Pts',(-76.5317149732915,-27.179113452548,
16.1963686737572));
#257650=CARTESIAN_POINT('Ctrl Pts',(-76.5322246958761,-27.1798344925873,
16.1944315509855));
#257651=CARTESIAN_POINT('Ctrl Pts',(-76.5327354732302,-27.1805647392017,
16.1924983103146));
#257652=CARTESIAN_POINT('Ctrl Pts',(-28.7459974181807,-74.3634602878982,
19.6929518677509));
#257653=CARTESIAN_POINT('Ctrl Pts',(-28.8447420032202,-74.6189041648808,
17.4625));
#257654=CARTESIAN_POINT('Ctrl Pts',(-29.6549915892153,-76.7149512087496,
17.4625));
#257655=CARTESIAN_POINT('Ctrl Pts',(-28.493917791474,-74.4609043857738,
19.6929518673246));
#257656=CARTESIAN_POINT('Ctrl Pts',(-28.6971725259749,-74.6660793405533,
17.5374731486204));
#257657=CARTESIAN_POINT('Ctrl Pts',(-29.4834701335364,-76.6890525018752,
17.4625));
#257658=CARTESIAN_POINT('Ctrl Pts',(-28.243859153104,-74.5588475342798,
19.6720320649342));
#257659=CARTESIAN_POINT('Ctrl Pts',(-28.5391636116372,-74.7189440966798,
17.5981072780266));
#257660=CARTESIAN_POINT('Ctrl Pts',(-29.3136797628437,-76.6640386379049,
17.4555267321202));
#257661=CARTESIAN_POINT('Ctrl Pts',(-27.7480012895967,-74.7559270342226,
19.587105566441));
#257662=CARTESIAN_POINT('Ctrl Pts',(-28.2117119618043,-74.8327386313741,
17.6836912763777));
#257663=CARTESIAN_POINT('Ctrl Pts',(-28.9778332725227,-76.6159646173257,
17.4272178998376));
#257664=CARTESIAN_POINT('Ctrl Pts',(-27.4997703917942,-74.8560677628261,
19.5220948206211));
#257665=CARTESIAN_POINT('Ctrl Pts',(-28.0404430900693,-74.8942448729349,
17.7096321218675));
#257666=CARTESIAN_POINT('Ctrl Pts',(-28.8101355628285,-76.5926880471497,
17.4055476509051));
#257667=CARTESIAN_POINT('Ctrl Pts',(-27.0236898937073,-75.0518439197728,
19.3489695261652));
#257668=CARTESIAN_POINT('Ctrl Pts',(-27.7022510777803,-75.019660969593,
17.7211023712237));
#257669=CARTESIAN_POINT('Ctrl Pts',(-28.4896086814942,-76.5500480485612,
17.3478392195234));
#257670=CARTESIAN_POINT('Ctrl Pts',(-26.7953551633964,-75.1476280619459,
19.2413577159483));
#257671=CARTESIAN_POINT('Ctrl Pts',(-27.5347169152644,-75.0836522525197,
17.7080778869111));
#257672=CARTESIAN_POINT('Ctrl Pts',(-28.3364379275085,-76.5306138623674,
17.311968615636));
#257673=CARTESIAN_POINT('Ctrl Pts',(-26.4687756770164,-75.2884389844459,
19.0458961827328));
#257674=CARTESIAN_POINT('Ctrl Pts',(-27.2898012152199,-75.1803896028198,
17.6578979817808));
#257675=CARTESIAN_POINT('Ctrl Pts',(-28.11850995103,-76.5048922024804,17.2468147718755));
#257676=CARTESIAN_POINT('Ctrl Pts',(-26.3625884843543,-75.3348967090535,
18.9750294801157));
#257677=CARTESIAN_POINT('Ctrl Pts',(-27.2097290601215,-75.2125498005336,
17.6363116935578));
#257678=CARTESIAN_POINT('Ctrl Pts',(-28.0478532106475,-76.4968949507143,
17.2231925371373));
#257679=CARTESIAN_POINT('Ctrl Pts',(-26.1560856941728,-75.4268801209917,
18.8208466626393));
#257680=CARTESIAN_POINT('Ctrl Pts',(-27.0529295129821,-75.2767579129773,
17.5825320214165));
#257681=CARTESIAN_POINT('Ctrl Pts',(-27.9109420608558,-76.482236449377,
17.1717982652804));
#257682=CARTESIAN_POINT('Ctrl Pts',(-26.055101076053,-75.4727198166016,
18.7368743964311));
#257683=CARTESIAN_POINT('Ctrl Pts',(-26.9755857935384,-75.3090585336027,
17.5501254447864));
#257684=CARTESIAN_POINT('Ctrl Pts',(-27.8442489434606,-76.4755364557142,
17.1438075095173));
#257685=CARTESIAN_POINT('Ctrl Pts',(-25.7681502580856,-75.606056054722,
18.4696518487116));
#257686=CARTESIAN_POINT('Ctrl Pts',(-26.7557364160525,-75.403048816879,
17.4386060175096));
#257687=CARTESIAN_POINT('Ctrl Pts',(-27.6556756091751,-76.4581861338663,
17.0547333270725));
#257688=CARTESIAN_POINT('Ctrl Pts',(-25.5978466210038,-75.6894118596661,
18.2718409363078));
#257689=CARTESIAN_POINT('Ctrl Pts',(-26.6226482272591,-75.4628679834562,
17.3449978161574));
#257690=CARTESIAN_POINT('Ctrl Pts',(-27.5450423948282,-76.4502012574512,
16.9887963557574));
#257691=CARTESIAN_POINT('Ctrl Pts',(-25.3042070746277,-75.8449254994659,
17.8327278472479));
#257692=CARTESIAN_POINT('Ctrl Pts',(-26.394507090712,-75.573296435284,17.1202191600563));
#257693=CARTESIAN_POINT('Ctrl Pts',(-27.3578956810273,-76.4429196593766,
16.8424253269272));
#257694=CARTESIAN_POINT('Ctrl Pts',(-25.1799509742016,-75.9179115378172,
17.5873106315629));
#257695=CARTESIAN_POINT('Ctrl Pts',(-26.2977761963299,-75.6248510373193,
16.9864091667276));
#257696=CARTESIAN_POINT('Ctrl Pts',(-27.2809002299559,-76.4437878571368,
16.7606195878723));
#257697=CARTESIAN_POINT('Ctrl Pts',(-25.0456540278885,-76.0120135407793,
17.2025309630922));
#257698=CARTESIAN_POINT('Ctrl Pts',(-26.1964580005434,-75.6888631781807,
16.7690050915921));
#257699=CARTESIAN_POINT('Ctrl Pts',(-27.2023521345511,-76.4531141362207,
16.6323596984796));
#257700=CARTESIAN_POINT('Ctrl Pts',(-25.0090870943377,-76.0410349984124,
17.0710669460344));
#257701=CARTESIAN_POINT('Ctrl Pts',(-26.1695156242371,-75.7081633852743,
16.6936245453249));
#257702=CARTESIAN_POINT('Ctrl Pts',(-27.1820075724725,-76.4575269782808,
16.5885383593541));
#257703=CARTESIAN_POINT('Ctrl Pts',(-24.9530103267672,-76.0942893550639,
16.8014952531461));
#257704=CARTESIAN_POINT('Ctrl Pts',(-26.1301341325902,-75.7423750031977,
16.5376305767303));
#257705=CARTESIAN_POINT('Ctrl Pts',(-27.1534935975724,-76.4691181075122,
16.4986811285387));
#257706=CARTESIAN_POINT('Ctrl Pts',(-24.9335061597325,-76.1186539510276,
16.662354041917));
#257707=CARTESIAN_POINT('Ctrl Pts',(-26.1176802211135,-75.7573877351405,
16.4562866616969));
#257708=CARTESIAN_POINT('Ctrl Pts',(-27.1453691430058,-76.4763708127826,
16.4523007247637));
#257709=CARTESIAN_POINT('Ctrl Pts',(-24.9029553648527,-76.1824010629028,
16.246342504105));
#257710=CARTESIAN_POINT('Ctrl Pts',(-26.1038934519079,-75.7942282194349,
16.2122544249952));
#257711=CARTESIAN_POINT('Ctrl Pts',(-27.1404954668515,-76.501838453202,
16.3136302120348));
#257712=CARTESIAN_POINT('Ctrl Pts',(-24.9185412707841,-76.21319040096,15.9685880799942));
#257713=CARTESIAN_POINT('Ctrl Pts',(-26.1252772492182,-75.8084359405768,
16.0475610164003));
#257714=CARTESIAN_POINT('Ctrl Pts',(-27.1624313528542,-76.5237673449983,
16.2210111173695));
#257715=CARTESIAN_POINT('Ctrl Pts',(-24.9689556265491,-76.2326069140441,
15.6905058513849));
#257716=CARTESIAN_POINT('Ctrl Pts',(-26.1756393943756,-75.8121214408373,
15.8859547915794));
#257717=CARTESIAN_POINT('Ctrl Pts',(-27.2087011009323,-76.55044485681,16.128351327878));
#257718=CARTESIAN_POINT('',(-25.2552738567447,-75.9418613629793,17.263393070432));
#257719=CARTESIAN_POINT('Ctrl Pts',(-27.1270026655083,-76.4952182372905,
16.124851038856));
#257720=CARTESIAN_POINT('Ctrl Pts',(-27.1261035938166,-76.4949835330535,
16.1335301302474));
#257721=CARTESIAN_POINT('Ctrl Pts',(-27.1250175086501,-76.4945938617305,
16.1433840167284));
#257722=CARTESIAN_POINT('Ctrl Pts',(-27.1236651982618,-76.4938946426406,
16.155016623084));
#257723=CARTESIAN_POINT('Ctrl Pts',(-27.1234107356413,-76.4937630714248,
16.1572055166414));
#257724=CARTESIAN_POINT('Ctrl Pts',(-27.1231468673316,-76.4936205663266,
16.1594572469012));
#257725=CARTESIAN_POINT('Ctrl Pts',(-27.1228730977808,-76.4934661405628,
16.1617756124861));
#257726=CARTESIAN_POINT('Ctrl Pts',(-27.1215904130528,-76.4927426139022,
16.1726377851477));
#257727=CARTESIAN_POINT('Ctrl Pts',(-27.1200357216283,-76.4916920130626,
16.1853170892738));
#257728=CARTESIAN_POINT('Ctrl Pts',(-27.1184437830652,-76.4903847974138,
16.1985845365603));
#257729=CARTESIAN_POINT('Ctrl Pts',(-27.1177371697055,-76.4898045639408,
16.2044735549672));
#257730=CARTESIAN_POINT('Ctrl Pts',(-27.1170231040098,-76.4891738033059,
16.2104789373705));
#257731=CARTESIAN_POINT('Ctrl Pts',(-27.1163213320445,-76.4884987572074,
16.216496794303));
#257732=CARTESIAN_POINT('Ctrl Pts',(-27.1144314500968,-76.4866808484018,
16.2327029691598));
#257733=CARTESIAN_POINT('Ctrl Pts',(-27.1126943705564,-76.4846005967063,
16.2486914456382));
#257734=CARTESIAN_POINT('Ctrl Pts',(-27.1111721910325,-76.4824017849017,
16.2640972093694));
#257735=CARTESIAN_POINT('Ctrl Pts',(-27.1106324721765,-76.481622152688,
16.2695596275976));
#257736=CARTESIAN_POINT('Ctrl Pts',(-27.1101196624094,-76.4808275267717,
16.2749492144025));
#257737=CARTESIAN_POINT('Ctrl Pts',(-27.1096361423663,-76.4800239584191,
16.2802512670944));
#257738=CARTESIAN_POINT('Ctrl Pts',(-27.1088775098617,-76.4787631770293,
16.2885700732554));
#257739=CARTESIAN_POINT('Ctrl Pts',(-27.1081924682407,-76.4774861247357,
16.2966391164394));
#257740=CARTESIAN_POINT('Ctrl Pts',(-27.1075731179889,-76.4761760059692,
16.304634384641));
#257741=CARTESIAN_POINT('Ctrl Pts',(-27.1070239809322,-76.4750144099882,
16.3117232621132));
#257742=CARTESIAN_POINT('Ctrl Pts',(-27.1065264227133,-76.4738263115719,
16.3187548885459));
#257743=CARTESIAN_POINT('Ctrl Pts',(-27.1060881023893,-76.4726008566098,
16.3258128070649));
#257744=CARTESIAN_POINT('Ctrl Pts',(-27.1060320583288,-76.4724441687532,
16.3267152393526));
#257745=CARTESIAN_POINT('Ctrl Pts',(-27.1059770032837,-76.472286877024,
16.3276180342305));
#257746=CARTESIAN_POINT('Ctrl Pts',(-27.1059229723693,-76.4721289660915,
16.3285213027645));
#257747=CARTESIAN_POINT('Ctrl Pts',(-27.1055132758134,-76.4709315855559,
16.335370455917));
#257748=CARTESIAN_POINT('Ctrl Pts',(-27.1051480063898,-76.4696860988077,
16.3423105850798));
#257749=CARTESIAN_POINT('Ctrl Pts',(-27.1048249982606,-76.4683756379704,
16.3494047007319));
#257750=CARTESIAN_POINT('Ctrl Pts',(-27.1045238256026,-76.4671537647793,
16.3560192514934));
#257751=CARTESIAN_POINT('Ctrl Pts',(-27.104259651115,-76.4658752319067,
16.3627681883308));
#257752=CARTESIAN_POINT('Ctrl Pts',(-27.1040326825549,-76.4645307210503,
16.369662327317));
#257753=CARTESIAN_POINT('Ctrl Pts',(-27.1038205223624,-76.4632739316433,
16.3761066641606));
#257754=CARTESIAN_POINT('Ctrl Pts',(-27.1036411260686,-76.4619593190139,
16.3826784026693));
#257755=CARTESIAN_POINT('Ctrl Pts',(-27.103492920931,-76.4605856089551,
16.3893426844127));
#257756=CARTESIAN_POINT('Ctrl Pts',(-27.1033578602488,-76.4593337345553,
16.3954159046341));
#257757=CARTESIAN_POINT('Ctrl Pts',(-27.1032489151466,-76.4580326598464,
16.4015662355561));
#257758=CARTESIAN_POINT('Ctrl Pts',(-27.103160260747,-76.4566888072085,
16.4077247899917));
#257759=CARTESIAN_POINT('Ctrl Pts',(-27.103122501072,-76.4561164335965,
16.4103478410223));
#257760=CARTESIAN_POINT('Ctrl Pts',(-27.1030883438962,-76.4555364067352,
16.4129718046004));
#257761=CARTESIAN_POINT('Ctrl Pts',(-27.1030568879021,-76.4549497809972,
16.4155884735489));
#257762=CARTESIAN_POINT('Ctrl Pts',(-27.102943208167,-76.4528297571273,
16.4250449298059));
#257763=CARTESIAN_POINT('Ctrl Pts',(-27.1028516325168,-76.4506276154508,
16.4344055618678));
#257764=CARTESIAN_POINT('Ctrl Pts',(-27.1027493830597,-76.448361853147,
16.4434727015495));
#257765=CARTESIAN_POINT('Ctrl Pts',(-27.1027301154649,-76.4479348993889,
16.4451812873779));
#257766=CARTESIAN_POINT('Ctrl Pts',(-27.10271035294,-76.4475057389403,16.4468793703382));
#257767=CARTESIAN_POINT('Ctrl Pts',(-27.1026896905074,-76.4470745680892,
16.448565588462));
#257768=CARTESIAN_POINT('Ctrl Pts',(-27.1026199427361,-76.445619114783,
16.454257558912));
#257769=CARTESIAN_POINT('Ctrl Pts',(-27.1025406532752,-76.4441322040595,
16.45984731347));
#257770=CARTESIAN_POINT('Ctrl Pts',(-27.1024250918521,-76.4426004684731,
16.4653566991217));
#257771=CARTESIAN_POINT('Ctrl Pts',(-27.1023811860637,-76.4420185090536,
16.4674499056151));
#257772=CARTESIAN_POINT('Ctrl Pts',(-27.1023318496948,-76.441430218622,
16.4695309610855));
#257773=CARTESIAN_POINT('Ctrl Pts',(-27.1022746925434,-76.4408353908715,
16.4715995364392));
#257774=CARTESIAN_POINT('Ctrl Pts',(-27.1020976108827,-76.43899252286,16.4780083015744));
#257775=CARTESIAN_POINT('Ctrl Pts',(-27.1018561048159,-76.4370710585175,
16.484391780117));
#257776=CARTESIAN_POINT('Ctrl Pts',(-27.1015158539173,-76.4350620986711,
16.4906542061241));
#257777=CARTESIAN_POINT('Ctrl Pts',(-27.1012261996223,-76.4333518788001,
16.4959853855483));
#257778=CARTESIAN_POINT('Ctrl Pts',(-27.1008647151594,-76.431579044118,
16.5012232667718));
#257779=CARTESIAN_POINT('Ctrl Pts',(-27.1004038747174,-76.4297403585954,
16.5063087804242));
#257780=CARTESIAN_POINT('Ctrl Pts',(-27.1000801964386,-76.4284489299119,
16.5098806681233));
#257781=CARTESIAN_POINT('Ctrl Pts',(-27.0997073598881,-76.427125151566,
16.5133767163714));
#257782=CARTESIAN_POINT('Ctrl Pts',(-27.0992746306615,-76.4257650872446,
16.5168023194477));
#257783=CARTESIAN_POINT('Ctrl Pts',(-27.0988720744437,-76.4244998564365,
16.5199890647216));
#257784=CARTESIAN_POINT('Ctrl Pts',(-27.0984176364798,-76.423203394355,
16.5231136244692));
#257785=CARTESIAN_POINT('Ctrl Pts',(-27.0979025055483,-76.4218676567963,
16.5262197343028));
#257786=CARTESIAN_POINT('Ctrl Pts',(-27.0978682970963,-76.4217789540774,
16.5264260026568));
#257787=CARTESIAN_POINT('Ctrl Pts',(-27.0978338210952,-76.4216900756695,
16.5266322092065));
#257788=CARTESIAN_POINT('Ctrl Pts',(-27.0977990750253,-76.4216010180799,
16.5268383756647));
#257789=CARTESIAN_POINT('Ctrl Pts',(-27.0976706878971,-76.4212719492622,
16.5276001630984));
#257790=CARTESIAN_POINT('Ctrl Pts',(-27.0975386143434,-76.4209404362575,
16.5283613866211));
#257791=CARTESIAN_POINT('Ctrl Pts',(-27.0974027448553,-76.4206063221419,
16.5291232095991));
#257792=CARTESIAN_POINT('Ctrl Pts',(-27.0966347185483,-76.4187176830226,
16.5334295486934));
#257793=CARTESIAN_POINT('Ctrl Pts',(-27.0957491893763,-76.4167566024487,
16.5376614540029));
#257794=CARTESIAN_POINT('Ctrl Pts',(-27.0947257635357,-76.4147290835802,
16.5417599888112));
#257795=CARTESIAN_POINT('Ctrl Pts',(-27.0938722704104,-76.413038220064,
16.5451779905302));
#257796=CARTESIAN_POINT('Ctrl Pts',(-27.0929228022848,-76.4113012291759,
16.5485028098222));
#257797=CARTESIAN_POINT('Ctrl Pts',(-27.0918686181416,-76.4095163162293,
16.5517348366204));
#257798=CARTESIAN_POINT('Ctrl Pts',(-27.0910057467585,-76.4080553283051,
16.5543803169683));
#257799=CARTESIAN_POINT('Ctrl Pts',(-27.0900727245973,-76.4065622115663,
16.5569638004546));
#257800=CARTESIAN_POINT('Ctrl Pts',(-27.0890672853603,-76.4050319318842,
16.559511402245));
#257801=CARTESIAN_POINT('Ctrl Pts',(-27.0873467993633,-76.4024133502058,
16.5638708036344));
#257802=CARTESIAN_POINT('Ctrl Pts',(-27.0854160305322,-76.3996858222803,
16.5681213015841));
#257803=CARTESIAN_POINT('Ctrl Pts',(-27.0832453437817,-76.3968549739068,
16.572200145343));
#257804=CARTESIAN_POINT('Ctrl Pts',(-27.0814237924472,-76.3944794420013,
16.5756229438146));
#257805=CARTESIAN_POINT('Ctrl Pts',(-27.0794332007604,-76.3920312477964,
16.5789244111528));
#257806=CARTESIAN_POINT('Ctrl Pts',(-27.0772609129534,-76.3895078513793,
16.5821034643336));
#257807=CARTESIAN_POINT('Ctrl Pts',(-27.0758841940305,-76.3879086122794,
16.5841182354228));
#257808=CARTESIAN_POINT('Ctrl Pts',(-27.0744345916957,-76.3862790519604,
16.5860845447352));
#257809=CARTESIAN_POINT('Ctrl Pts',(-27.0729104400651,-76.3846166914257,
16.5880130337724));
#257810=CARTESIAN_POINT('Ctrl Pts',(-27.0711860864447,-76.3827359747379,
16.5901948357575));
#257811=CARTESIAN_POINT('Ctrl Pts',(-27.0694154757843,-76.3808666413311,
16.5922669270643));
#257812=CARTESIAN_POINT('Ctrl Pts',(-27.0676055223506,-76.3790011612995,
16.5942742310318));
#257813=CARTESIAN_POINT('Ctrl Pts',(-27.0627975216184,-76.3740456584721,
16.5996064781305));
#257814=CARTESIAN_POINT('Ctrl Pts',(-27.0577058759434,-76.369127427657,
16.6044118919298));
#257815=CARTESIAN_POINT('Ctrl Pts',(-27.0523503507039,-76.3642377230746,
16.6087783050424));
#257816=CARTESIAN_POINT('Ctrl Pts',(-27.0469199087843,-76.3592796180242,
16.6132057984709));
#257817=CARTESIAN_POINT('Ctrl Pts',(-27.0412180804736,-76.354350908571,
16.6171815871679));
#257818=CARTESIAN_POINT('Ctrl Pts',(-27.0352768340224,-76.3494322419925,
16.6208506593388));
#257819=CARTESIAN_POINT('Ctrl Pts',(-27.0293355875713,-76.3445135754139,
16.6245197315096));
#257820=CARTESIAN_POINT('Ctrl Pts',(-27.0231548844627,-76.3396049868145,
16.6278819111733));
#257821=CARTESIAN_POINT('Ctrl Pts',(-27.0167787754265,-76.3346762337747,
16.6311389170592));
#257822=CARTESIAN_POINT('Ctrl Pts',(-27.0069163699867,-76.3270525622668,
16.6361767720244));
#257823=CARTESIAN_POINT('Ctrl Pts',(-26.9965742763337,-76.3193994276104,
16.6408622418843));
#257824=CARTESIAN_POINT('Ctrl Pts',(-26.9857761531998,-76.3117344496374,
16.6452464533241));
#257825=CARTESIAN_POINT('Ctrl Pts',(-26.979721736166,-76.3074367608049,
16.6477046438904));
#257826=CARTESIAN_POINT('Ctrl Pts',(-26.9735241809127,-76.3031351576549,
16.6500689942483));
#257827=CARTESIAN_POINT('Ctrl Pts',(-26.9671894394037,-76.2988312337081,
16.6523553297695));
#257828=CARTESIAN_POINT('Ctrl Pts',(-26.9465400268533,-76.2848016950067,
16.6598081177547));
#257829=CARTESIAN_POINT('Ctrl Pts',(-26.9253146403781,-76.271342038953,
16.6661261478315));
#257830=CARTESIAN_POINT('Ctrl Pts',(-26.9037854166562,-76.2582666976204,
16.6722817468521));
#257831=CARTESIAN_POINT('Ctrl Pts',(-26.8683021506932,-76.2367166491816,
16.6824270618915));
#257832=CARTESIAN_POINT('Ctrl Pts',(-26.8318654947868,-76.2163231724478,
16.6915805494727));
#257833=CARTESIAN_POINT('Ctrl Pts',(-26.7948177267223,-76.1969868424102,
16.7005093018093));
#257834=CARTESIAN_POINT('Ctrl Pts',(-26.7912042243465,-76.1951008482416,
16.7013801793133));
#257835=CARTESIAN_POINT('Ctrl Pts',(-26.7875849267696,-76.1932248857237,
16.7022489427311));
#257836=CARTESIAN_POINT('Ctrl Pts',(-26.7839601625935,-76.1913588468482,
16.7031163158079));
#257837=CARTESIAN_POINT('Ctrl Pts',(-26.7552291255581,-76.1765680275182,
16.709991391477));
#257838=CARTESIAN_POINT('Ctrl Pts',(-26.7262008738672,-76.1624139946391,
16.7168106960666));
#257839=CARTESIAN_POINT('Ctrl Pts',(-26.6969732854461,-76.1489165164748,
16.7235973395646));
#257840=CARTESIAN_POINT('Ctrl Pts',(-26.6422867919235,-76.1236619610331,
16.7362955386204));
#257841=CARTESIAN_POINT('Ctrl Pts',(-26.5866819738149,-76.1005180681777,
16.7491519989614));
#257842=CARTESIAN_POINT('Ctrl Pts',(-26.5302810836782,-76.0794074083704,
16.7625435720886));
#257843=CARTESIAN_POINT('Ctrl Pts',(-26.4900870715832,-76.0643629274487,
16.772087057146));
#257844=CARTESIAN_POINT('Ctrl Pts',(-26.4494883805146,-76.0503521064273,
16.7819023270102));
#257845=CARTESIAN_POINT('Ctrl Pts',(-26.4085292238121,-76.0373611942068,
16.7921336012861));
#257846=CARTESIAN_POINT('Ctrl Pts',(-26.3637920322324,-76.0231720122119,
16.8033085988748));
#257847=CARTESIAN_POINT('Ctrl Pts',(-26.319031000209,-76.0103384192578,
16.8148454077151));
#257848=CARTESIAN_POINT('Ctrl Pts',(-26.2743222514898,-75.9987850456328,
16.826926246749));
#257849=CARTESIAN_POINT('Ctrl Pts',(-26.2161351891259,-75.9837486849451,
16.8426490874549));
#257850=CARTESIAN_POINT('Ctrl Pts',(-26.1575989600142,-75.9708594776026,
16.8592311068001));
#257851=CARTESIAN_POINT('Ctrl Pts',(-26.0990044705762,-75.9600230530921,
16.876896595295));
#257852=CARTESIAN_POINT('Ctrl Pts',(-26.0404710851734,-75.9491979291198,
16.8945436617054));
#257853=CARTESIAN_POINT('Ctrl Pts',(-25.9818779784963,-75.9404214117235,
16.9132712882849));
#257854=CARTESIAN_POINT('Ctrl Pts',(-25.9235033740091,-75.9336439589002,
16.9333228296532));
#257855=CARTESIAN_POINT('Ctrl Pts',(-25.8876307737036,-75.9294790509174,
16.9456449847295));
#257856=CARTESIAN_POINT('Ctrl Pts',(-25.8518405543476,-75.9260699331757,
16.9584675280532));
#257857=CARTESIAN_POINT('Ctrl Pts',(-25.8161989867007,-75.9234132458685,
16.9718522765889));
#257858=CARTESIAN_POINT('Ctrl Pts',(-25.7935358469314,-75.9217239577776,
16.9803631375546));
#257859=CARTESIAN_POINT('Ctrl Pts',(-25.770890405978,-75.9203357066719,
16.9891192993506));
#257860=CARTESIAN_POINT('Ctrl Pts',(-25.7483106633375,-75.9192531417283,
16.9981274246417));
#257861=CARTESIAN_POINT('Ctrl Pts',(-25.701936632811,-75.9170297815891,
17.016628214659));
#257862=CARTESIAN_POINT('Ctrl Pts',(-25.6557154305365,-75.9160908879052,
17.0360687208423));
#257863=CARTESIAN_POINT('Ctrl Pts',(-25.6100335199459,-75.9163356254781,
17.0568346693642));
#257864=CARTESIAN_POINT('Ctrl Pts',(-25.5677572969033,-75.9165621173232,
17.0760524704599));
#257865=CARTESIAN_POINT('Ctrl Pts',(-25.5259435982419,-75.9178014945593,
17.0964068028276));
#257866=CARTESIAN_POINT('Ctrl Pts',(-25.4848871407941,-75.9199460216256,
17.1181763511646));
#257867=CARTESIAN_POINT('Ctrl Pts',(-25.4448430530074,-75.9220376689679,
17.1394091062262));
#257868=CARTESIAN_POINT('Ctrl Pts',(-25.4055198689379,-75.9249898990271,
17.1619892996639));
#257869=CARTESIAN_POINT('Ctrl Pts',(-25.367171006334,-75.9286842189027,
17.1861307294231));
#257870=CARTESIAN_POINT('Ctrl Pts',(-25.3326536302604,-75.9320094343022,
17.2078601564093));
#257871=CARTESIAN_POINT('Ctrl Pts',(-25.298925636162,-75.9359354286521,
17.2308544603259));
#257872=CARTESIAN_POINT('Ctrl Pts',(-25.2661521622731,-75.9403670675906,
17.255226251548));
#257873=CARTESIAN_POINT('Ctrl Pts',(-25.2625142518049,-75.9408589869318,
17.2579315611748));
#257874=CARTESIAN_POINT('Ctrl Pts',(-25.2588880803564,-75.9413571303143,
17.2606537951814));
#257875=CARTESIAN_POINT('Ctrl Pts',(-25.2552738568381,-75.9418613633423,
17.2633930704885));
#257876=CARTESIAN_POINT('Ctrl Pts',(-25.2552738568381,-75.9418613633423,
17.2633930704885));
#257877=CARTESIAN_POINT('Ctrl Pts',(-25.2383250955278,-75.944225947726,
17.2762387760169));
#257878=CARTESIAN_POINT('Ctrl Pts',(-25.2219501075692,-75.9466297979537,
17.2896217177115));
#257879=CARTESIAN_POINT('Ctrl Pts',(-25.2063620808095,-75.9489416166775,
17.3037656233412));
#257880=CARTESIAN_POINT('Ctrl Pts',(-25.1906119974262,-75.9512774695875,
17.3180565721873));
#257881=CARTESIAN_POINT('Ctrl Pts',(-25.1756652586958,-75.9535194008974,
17.3331243158819));
#257882=CARTESIAN_POINT('Ctrl Pts',(-25.1617083519771,-75.955550118673,
17.3491621103599));
#257883=CARTESIAN_POINT('Ctrl Pts',(-25.1475411609446,-75.9576114326331,
17.3654415412317));
#257884=CARTESIAN_POINT('Ctrl Pts',(-25.1343938076753,-75.9594551437225,
17.3827204211343));
#257885=CARTESIAN_POINT('Ctrl Pts',(-25.1224278838339,-75.9609767648616,
17.4011633328253));
#257886=CARTESIAN_POINT('Ctrl Pts',(-25.1210536712436,-75.9611515136695,
17.4032813875434));
#257887=CARTESIAN_POINT('Ctrl Pts',(-25.1196950053566,-75.9613220336047,
17.4054147552051));
#257888=CARTESIAN_POINT('Ctrl Pts',(-25.1183521036895,-75.9614881812303,
17.4075636545405));
#257889=CARTESIAN_POINT('Origin',(-29.6549915892153,-76.7149512087495,20.0025));
#257890=CARTESIAN_POINT('Origin',(0.,0.,20.0025));
#257891=CARTESIAN_POINT('Origin',(-76.7149512087496,-29.6549915892152,20.0025));
#257892=CARTESIAN_POINT('Ctrl Pts',(-76.2325975651779,-24.9689313575498,
15.6906397325508));
#257893=CARTESIAN_POINT('Ctrl Pts',(-75.8121196590786,-26.1756150602386,
15.8860328844659));
#257894=CARTESIAN_POINT('Ctrl Pts',(-76.5504320086843,-27.2086788182716,
16.1283959549333));
#257895=CARTESIAN_POINT('Ctrl Pts',(-76.2132400197751,-24.9186909562154,
15.9678244963475));
#257896=CARTESIAN_POINT('Ctrl Pts',(-75.808442527959,-26.1254229642324,
16.0471243598414));
#257897=CARTESIAN_POINT('Ctrl Pts',(-76.5238417787853,-27.1625656651766,
16.2207578908871));
#257898=CARTESIAN_POINT('Ctrl Pts',(-76.1826381079972,-24.9032159272864,
16.2438456162091));
#257899=CARTESIAN_POINT('Ctrl Pts',(-75.7943214248689,-26.1041848761176,
16.2107725763333));
#257900=CARTESIAN_POINT('Ctrl Pts',(-76.5020517602985,-27.1407766635666,
16.3127979160875));
#257901=CARTESIAN_POINT('Ctrl Pts',(-76.1197004175053,-24.9328226963043,
16.6559867599157));
#257902=CARTESIAN_POINT('Ctrl Pts',(-75.7580138780931,-26.1172873190749,
16.4525591935377));
#257903=CARTESIAN_POINT('Ctrl Pts',(-76.4767312134554,-27.1451435881163,
16.4501782974209));
#257904=CARTESIAN_POINT('Ctrl Pts',(-76.0956371509854,-24.9518097701924,
16.7941104173068));
#257905=CARTESIAN_POINT('Ctrl Pts',(-75.7432179427285,-26.1293351405288,
16.5333292440503));
#257906=CARTESIAN_POINT('Ctrl Pts',(-76.4694807636038,-27.1529468723198,
16.4962195166114));
#257907=CARTESIAN_POINT('Ctrl Pts',(-76.0425032131365,-25.007333665712,
17.0641682497331));
#257908=CARTESIAN_POINT('Ctrl Pts',(-75.7091288541233,-26.1682415554308,
16.6896570718777));
#257909=CARTESIAN_POINT('Ctrl Pts',(-76.4577808154574,-27.1810555370838,
16.5862387939012));
#257910=CARTESIAN_POINT('Ctrl Pts',(-76.0135981896351,-25.0435822919597,
17.1955505586787));
#257911=CARTESIAN_POINT('Ctrl Pts',(-75.6899232799147,-26.1949210471997,
16.765020182014));
#257912=CARTESIAN_POINT('Ctrl Pts',(-76.4533313045579,-27.2011812093656,
16.6300328970334));
#257913=CARTESIAN_POINT('Ctrl Pts',(-75.920106096032,-25.1764553135866,
17.5792969885106));
#257914=CARTESIAN_POINT('Ctrl Pts',(-75.6263767700417,-26.2950899509087,
16.9819673365851));
#257915=CARTESIAN_POINT('Ctrl Pts',(-76.4438901441625,-27.2787774842959,
16.7579483734717));
#257916=CARTESIAN_POINT('Ctrl Pts',(-75.847668483287,-25.2993526607363,
17.8240388353672));
#257917=CARTESIAN_POINT('Ctrl Pts',(-75.5752351470897,-26.3907356809332,
17.1155820316983));
#257918=CARTESIAN_POINT('Ctrl Pts',(-76.4428939284363,-27.3548544480353,
16.8395289896477));
#257919=CARTESIAN_POINT('Ctrl Pts',(-75.692343203007,-25.5919984567925,
18.2644739211062));
#257920=CARTESIAN_POINT('Ctrl Pts',(-75.4649619696469,-26.6180940171699,
17.3414092350346));
#257921=CARTESIAN_POINT('Ctrl Pts',(-76.4499649794122,-27.5412643883023,
16.9863406840095));
#257922=CARTESIAN_POINT('Ctrl Pts',(-75.6091210995778,-25.7617839502732,
18.4627331486827));
#257923=CARTESIAN_POINT('Ctrl Pts',(-75.4052371346463,-26.7507911294736,
17.4354381030785));
#257924=CARTESIAN_POINT('Ctrl Pts',(-76.4578597275968,-27.6515244073506,
17.0524270937456));
#257925=CARTESIAN_POINT('Ctrl Pts',(-75.4317357552702,-26.1430805994651,
18.8197595498718));
#257926=CARTESIAN_POINT('Ctrl Pts',(-75.2796463045429,-27.0442130694172,
17.5855829975131));
#257927=CARTESIAN_POINT('Ctrl Pts',(-76.480799671864,-27.9020344677421,
17.1714358939387));
#257928=CARTESIAN_POINT('Ctrl Pts',(-75.3392616135105,-26.3510560884165,
18.9747290102614));
#257929=CARTESIAN_POINT('Ctrl Pts',(-75.2146749685608,-27.203130220885,
17.6396375078348));
#257930=CARTESIAN_POINT('Ctrl Pts',(-76.4956562029921,-28.0399748698363,
17.2230923811499));
#257931=CARTESIAN_POINT('Ctrl Pts',(-75.1503919246079,-26.7887981118754,
19.2381193325709));
#257932=CARTESIAN_POINT('Ctrl Pts',(-75.085497318848,-27.5299162784617,
17.7075896666724));
#257933=CARTESIAN_POINT('Ctrl Pts',(-76.5300629685869,-28.3320433237824,
17.3108891546269));
#257934=CARTESIAN_POINT('Ctrl Pts',(-75.052591949809,-27.021891012889,19.3482083029788));
#257935=CARTESIAN_POINT('Ctrl Pts',(-75.0201494871657,-27.7009559314819,
17.7210643477395));
#257936=CARTESIAN_POINT('Ctrl Pts',(-76.5498913973924,-28.4884000162543,
17.3475854788264));
#257937=CARTESIAN_POINT('Ctrl Pts',(-74.856579759635,-27.4985053196498,
19.521741160188));
#257938=CARTESIAN_POINT('Ctrl Pts',(-74.8945599897644,-28.0395707962217,
17.709745105584));
#257939=CARTESIAN_POINT('Ctrl Pts',(-76.5925703049492,-28.8092814008565,
17.4054297637286));
#257940=CARTESIAN_POINT('Ctrl Pts',(-74.7582415292722,-27.7422284005858,
19.5858151824391));
#257941=CARTESIAN_POINT('Ctrl Pts',(-74.8341192521338,-28.2078168588121,
17.6844550416321));
#257942=CARTESIAN_POINT('Ctrl Pts',(-76.6154156279985,-28.9739291008627,
17.4267877716098));
#257943=CARTESIAN_POINT('Ctrl Pts',(-74.5605143304925,-28.23961600078,19.6716009699542));
#257944=CARTESIAN_POINT('Ctrl Pts',(-74.7198525855419,-28.5364711009162,
17.5990670510742));
#257945=CARTESIAN_POINT('Ctrl Pts',(-76.663616773131,-29.3108001463009,
17.4553830340207));
#257946=CARTESIAN_POINT('Ctrl Pts',(-74.4605859662119,-28.4947415154361,
19.6929518687096));
#257947=CARTESIAN_POINT('Ctrl Pts',(-74.6659231009745,-28.6976612611827,
17.5372248464359));
#257948=CARTESIAN_POINT('Ctrl Pts',(-76.6891359364477,-29.4840227026748,
17.4625));
#257949=CARTESIAN_POINT('Ctrl Pts',(-74.3634602878982,-28.7459974181806,
19.6929518677509));
#257950=CARTESIAN_POINT('Ctrl Pts',(-74.6189041648808,-28.8447420032201,
17.4625));
#257951=CARTESIAN_POINT('Ctrl Pts',(-76.7149512087496,-29.6549915892153,
17.4625));
#257952=CARTESIAN_POINT('',(-75.9418613633423,-25.2552738568382,17.2633930704886));
#257953=CARTESIAN_POINT('Ctrl Pts',(-75.961488153786,-25.11835232551,17.4075632995853));
#257954=CARTESIAN_POINT('Ctrl Pts',(-75.9600460003609,-25.1300086288942,
17.3889110252656));
#257955=CARTESIAN_POINT('Ctrl Pts',(-75.95827300491,-25.1428552490709,17.3714318668807));
#257956=CARTESIAN_POINT('Ctrl Pts',(-75.9562706193827,-25.1567358844424,
17.354967018413));
#257957=CARTESIAN_POINT('Ctrl Pts',(-75.9542900252234,-25.1704654609745,
17.3386813520096));
#257958=CARTESIAN_POINT('Ctrl Pts',(-75.9520849723632,-25.185206735533,
17.3233881142745));
#257959=CARTESIAN_POINT('Ctrl Pts',(-75.949770932865,-25.2007766447904,
17.308897933323));
#257960=CARTESIAN_POINT('Ctrl Pts',(-75.9474896654476,-25.2161260485969,
17.2946129664053));
#257961=CARTESIAN_POINT('Ctrl Pts',(-75.9451024554286,-25.2322808242905,
17.2811085191579));
#257962=CARTESIAN_POINT('Ctrl Pts',(-75.9427372332863,-25.2490337245244,
17.2681673909986));
#257963=CARTESIAN_POINT('Ctrl Pts',(-75.9424448314779,-25.2511048104648,
17.2665675373488));
#257964=CARTESIAN_POINT('Ctrl Pts',(-75.9421527879415,-25.2531849967398,
17.2649762470519));
#257965=CARTESIAN_POINT('Ctrl Pts',(-75.9418613633423,-25.2552738568382,
17.2633930704886));
#257966=CARTESIAN_POINT('Ctrl Pts',(-75.9418613633423,-25.2552738568382,
17.2633930704886));
#257967=CARTESIAN_POINT('Ctrl Pts',(-75.9348768553987,-25.3053371638262,
17.2254493240849));
#257968=CARTESIAN_POINT('Ctrl Pts',(-75.9291204561945,-25.3572644305849,
17.1911044096247));
#257969=CARTESIAN_POINT('Ctrl Pts',(-75.9248495157407,-25.4106833635671,
17.1596330730564));
#257970=CARTESIAN_POINT('Ctrl Pts',(-75.9203244072783,-25.4672813115609,
17.1262888452528));
#257971=CARTESIAN_POINT('Ctrl Pts',(-75.917466983464,-25.5255536813971,
17.096170306839));
#257972=CARTESIAN_POINT('Ctrl Pts',(-75.9165875721914,-25.5850313991953,
17.0683598417424));
#257973=CARTESIAN_POINT('Ctrl Pts',(-75.9157960130219,-25.638567366227,
17.0433276078627));
#257974=CARTESIAN_POINT('Ctrl Pts',(-75.9166071705069,-25.6930793577886,
17.0201642486696));
#257975=CARTESIAN_POINT('Ctrl Pts',(-75.9192482119006,-25.7482100068409,
16.9981680565884));
#257976=CARTESIAN_POINT('Ctrl Pts',(-75.9203084088562,-25.7703411807131,
16.9893380943108));
#257977=CARTESIAN_POINT('Ctrl Pts',(-75.9216656968683,-25.7926041372848,
16.9807230184995));
#257978=CARTESIAN_POINT('Ctrl Pts',(-75.9233227318004,-25.8149722052004,
16.9723142805678));
#257979=CARTESIAN_POINT('Ctrl Pts',(-75.9279208772768,-25.8770418866012,
16.9489806745375));
#257980=CARTESIAN_POINT('Ctrl Pts',(-75.9347968299595,-25.9395105598234,
16.9273736682912));
#257981=CARTESIAN_POINT('Ctrl Pts',(-75.9439477443067,-26.0019469535969,
16.907190121791));
#257982=CARTESIAN_POINT('Ctrl Pts',(-75.9536417898974,-26.0680891143477,
16.8858086278184));
#257983=CARTESIAN_POINT('Ctrl Pts',(-75.9658884088744,-26.134196625868,
16.8660249929661));
#257984=CARTESIAN_POINT('Ctrl Pts',(-75.9807279241721,-26.1997753181405,
16.8475110455355));
#257985=CARTESIAN_POINT('Ctrl Pts',(-75.9863597062774,-26.224663254048,
16.8404847703678));
#257986=CARTESIAN_POINT('Ctrl Pts',(-75.9923654083886,-26.2494750768498,
16.8336416501196));
#257987=CARTESIAN_POINT('Ctrl Pts',(-75.9987489547818,-26.2741836418867,
16.8269646518771));
#257988=CARTESIAN_POINT('Ctrl Pts',(-76.0104251100451,-26.3193781190517,
16.8147517433512));
#257989=CARTESIAN_POINT('Ctrl Pts',(-76.0233691012878,-26.36448065778,16.803132555762));
#257990=CARTESIAN_POINT('Ctrl Pts',(-76.0376323915296,-26.4094030264448,
16.7919150704375));
#257991=CARTESIAN_POINT('Ctrl Pts',(-76.0576095561462,-26.4723212969538,
16.7762038602531));
#257992=CARTESIAN_POINT('Ctrl Pts',(-76.0801913923979,-26.5349890927284,
16.7613285554429));
#257993=CARTESIAN_POINT('Ctrl Pts',(-76.1054321158541,-26.5968842689899,
16.7468658576575));
#257994=CARTESIAN_POINT('Ctrl Pts',(-76.1193622332291,-26.6310436333906,
16.7388840310644));
#257995=CARTESIAN_POINT('Ctrl Pts',(-76.1341013589714,-26.6649677056329,
16.7310274121387));
#257996=CARTESIAN_POINT('Ctrl Pts',(-76.1496523368462,-26.6985700833486,
16.723222678138));
#257997=CARTESIAN_POINT('Ctrl Pts',(-76.1628884630048,-26.7271705555669,
16.7165797232898));
#257998=CARTESIAN_POINT('Ctrl Pts',(-76.1767336953015,-26.7555332799854,
16.7099108265046));
#257999=CARTESIAN_POINT('Ctrl Pts',(-76.1911702998078,-26.7835861605021,
16.7031950108476));
#258000=CARTESIAN_POINT('Ctrl Pts',(-76.2098835997088,-26.8199494179402,
16.694489703972));
#258001=CARTESIAN_POINT('Ctrl Pts',(-76.2295605860698,-26.8556888249402,
16.6856585992521));
#258002=CARTESIAN_POINT('Ctrl Pts',(-76.2502978093625,-26.8905185779364,
16.6759949656899));
#258003=CARTESIAN_POINT('Ctrl Pts',(-76.2528710428106,-26.8948405203745,
16.6747958280445));
#258004=CARTESIAN_POINT('Ctrl Pts',(-76.2554605684613,-26.8991484844249,
16.6735839226241));
#258005=CARTESIAN_POINT('Ctrl Pts',(-76.258066542157,-26.9034419491172,
16.6723579473272));
#258006=CARTESIAN_POINT('Ctrl Pts',(-76.2717835028191,-26.9260412893887,
16.665904829651));
#258007=CARTESIAN_POINT('Ctrl Pts',(-76.2859122483631,-26.9482892129603,
16.6592804200412));
#258008=CARTESIAN_POINT('Ctrl Pts',(-76.300666357626,-26.9698831287184,
16.6513762614161));
#258009=CARTESIAN_POINT('Ctrl Pts',(-76.3062184665341,-26.9780091205966,
16.6484018528137));
#258010=CARTESIAN_POINT('Ctrl Pts',(-76.3119191069635,-26.986126275202,
16.6452107769913));
#258011=CARTESIAN_POINT('Ctrl Pts',(-76.3176690330962,-26.9940602891098,
16.6418055153042));
#258012=CARTESIAN_POINT('Ctrl Pts',(-76.3232350607987,-27.0017405514616,
16.6385091632385));
#258013=CARTESIAN_POINT('Ctrl Pts',(-76.3288474189586,-27.0092489790102,
16.6350110759825));
#258014=CARTESIAN_POINT('Ctrl Pts',(-76.334399446806,-27.0164426883129,
16.6313545907255));
#258015=CARTESIAN_POINT('Ctrl Pts',(-76.3384193031335,-27.0216511776528,
16.628707171476));
#258016=CARTESIAN_POINT('Ctrl Pts',(-76.342403163236,-27.0266992744414,
16.6260035905202));
#258017=CARTESIAN_POINT('Ctrl Pts',(-76.3463237494151,-27.031517147781,
16.6231740162485));
#258018=CARTESIAN_POINT('Ctrl Pts',(-76.3499412952933,-27.0359626253308,
16.620563152904));
#258019=CARTESIAN_POINT('Ctrl Pts',(-76.3535049415088,-27.0402121121311,
16.6178449684742));
#258020=CARTESIAN_POINT('Ctrl Pts',(-76.356983025863,-27.0442217723951,
16.6150107800993));
#258021=CARTESIAN_POINT('Ctrl Pts',(-76.3604504000898,-27.0482190856404,
16.6121853190914));
#258022=CARTESIAN_POINT('Ctrl Pts',(-76.3638327372829,-27.051978040091,
16.609244457524));
#258023=CARTESIAN_POINT('Ctrl Pts',(-76.3670881331192,-27.0554667046297,
16.6062292700873));
#258024=CARTESIAN_POINT('Ctrl Pts',(-76.3704697167254,-27.0590905990513,
16.6030972059948));
#258025=CARTESIAN_POINT('Ctrl Pts',(-76.3737142822046,-27.0624228841696,
16.599885043991));
#258026=CARTESIAN_POINT('Ctrl Pts',(-76.3767636735503,-27.0654401116738,
16.5966933386584));
#258027=CARTESIAN_POINT('Ctrl Pts',(-76.3774080376897,-27.0660776793009,
16.5960189022785));
#258028=CARTESIAN_POINT('Ctrl Pts',(-76.3780436509134,-27.0667012192002,
16.5953455588284));
#258029=CARTESIAN_POINT('Ctrl Pts',(-76.3786699099352,-27.0673105708824,
16.5946745306125));
#258030=CARTESIAN_POINT('Ctrl Pts',(-76.3804986138508,-27.0690899046221,
16.5927150986791));
#258031=CARTESIAN_POINT('Ctrl Pts',(-76.3822466735199,-27.0707485693709,
16.5907819642457));
#258032=CARTESIAN_POINT('Ctrl Pts',(-76.383903674753,-27.0722790207879,
16.5888786971058));
#258033=CARTESIAN_POINT('Ctrl Pts',(-76.386590118736,-27.0747602935343,
16.5857929899537));
#258034=CARTESIAN_POINT('Ctrl Pts',(-76.3892195788868,-27.0770747169505,
16.5825794796198));
#258035=CARTESIAN_POINT('Ctrl Pts',(-76.3918035037155,-27.0792241299055,
16.5791834616252));
#258036=CARTESIAN_POINT('Ctrl Pts',(-76.394700966583,-27.0816343564549,
16.5753753647613));
#258037=CARTESIAN_POINT('Ctrl Pts',(-76.397541081989,-27.083837183862,16.5713382502742));
#258038=CARTESIAN_POINT('Ctrl Pts',(-76.4003286349106,-27.0858449594434,
16.5670618114176));
#258039=CARTESIAN_POINT('Ctrl Pts',(-76.4017815005684,-27.0868914070886,
16.5648329421093));
#258040=CARTESIAN_POINT('Ctrl Pts',(-76.4032199206492,-27.0878850122277,
16.5625400515829));
#258041=CARTESIAN_POINT('Ctrl Pts',(-76.4046437010114,-27.0888282604215,
16.5601869010573));
#258042=CARTESIAN_POINT('Ctrl Pts',(-76.4066000201685,-27.0901243132119,
16.5569535979618));
#258043=CARTESIAN_POINT('Ctrl Pts',(-76.4085291383743,-27.0913240246214,
16.5536060908145));
#258044=CARTESIAN_POINT('Ctrl Pts',(-76.4104440985978,-27.0924256407899,
16.5500691174275));
#258045=CARTESIAN_POINT('Ctrl Pts',(-76.4125548612432,-27.0936398959108,
16.5461704926879));
#258046=CARTESIAN_POINT('Ctrl Pts',(-76.4146483556021,-27.0947350221951,
16.5420420631183));
#258047=CARTESIAN_POINT('Ctrl Pts',(-76.4167317428694,-27.0957153880271,
16.5376476095181));
#258048=CARTESIAN_POINT('Ctrl Pts',(-76.4178724629974,-27.0962521691886,
16.5352415078049));
#258049=CARTESIAN_POINT('Ctrl Pts',(-76.4190099865444,-27.0967546539353,
16.5327567014452));
#258050=CARTESIAN_POINT('Ctrl Pts',(-76.4201444974393,-27.0972241915704,
16.5301935105711));
#258051=CARTESIAN_POINT('Ctrl Pts',(-76.4216120382861,-27.0978315596105,
16.526877907942));
#258052=CARTESIAN_POINT('Ctrl Pts',(-76.4230689252893,-27.0983817195864,
16.5234805955633));
#258053=CARTESIAN_POINT('Ctrl Pts',(-76.4245289971094,-27.0988766739753,
16.5198985636382));
#258054=CARTESIAN_POINT('Ctrl Pts',(-76.4261225061527,-27.0994168626729,
16.5159891667252));
#258055=CARTESIAN_POINT('Ctrl Pts',(-76.4277197747631,-27.0998913111345,
16.5118599671146));
#258056=CARTESIAN_POINT('Ctrl Pts',(-76.4293303340741,-27.1003044176607,
16.5074394223229));
#258057=CARTESIAN_POINT('Ctrl Pts',(-76.4311269682898,-27.1007652521762,
16.5025081528127));
#258058=CARTESIAN_POINT('Ctrl Pts',(-76.4329400958886,-27.1011497779037,
16.4972146199272));
#258059=CARTESIAN_POINT('Ctrl Pts',(-76.4347734732722,-27.1014658926888,
16.4915299793151));
#258060=CARTESIAN_POINT('Ctrl Pts',(-76.436559162974,-27.1017737850635,
16.4859932009684));
#258061=CARTESIAN_POINT('Ctrl Pts',(-76.4383638554399,-27.1020168312817,
16.4800869015256));
#258062=CARTESIAN_POINT('Ctrl Pts',(-76.4401848092304,-27.1022032686856,
16.4738312960571));
#258063=CARTESIAN_POINT('Ctrl Pts',(-76.4402891062215,-27.1022139470786,
16.4734729998546));
#258064=CARTESIAN_POINT('Ctrl Pts',(-76.4403934995095,-27.1022244071686,
16.4731133073643));
#258065=CARTESIAN_POINT('Ctrl Pts',(-76.4404979871102,-27.1022346589781,
16.4727522097065));
#258066=CARTESIAN_POINT('Ctrl Pts',(-76.4422544935175,-27.1024069987472,
16.466681916723));
#258067=CARTESIAN_POINT('Ctrl Pts',(-76.4439950495004,-27.1025185267252,
16.4603561173103));
#258068=CARTESIAN_POINT('Ctrl Pts',(-76.4457036742994,-27.1026104632737,
16.4538373749437));
#258069=CARTESIAN_POINT('Ctrl Pts',(-76.4480632278896,-27.1027374245665,
16.4448352101831));
#258070=CARTESIAN_POINT('Ctrl Pts',(-76.4503610777997,-27.1028277926528,
16.4354693324923));
#258071=CARTESIAN_POINT('Ctrl Pts',(-76.4525659494223,-27.102929293285,
16.425993471235));
#258072=CARTESIAN_POINT('Ctrl Pts',(-76.4530853029501,-27.1029532015756,
16.4237614492331));
#258073=CARTESIAN_POINT('Ctrl Pts',(-76.453599565861,-27.1029775126962,
16.4215234003336));
#258074=CARTESIAN_POINT('Ctrl Pts',(-76.4541084608796,-27.103002507394,
16.4192825790669));
#258075=CARTESIAN_POINT('Ctrl Pts',(-76.4554445776905,-27.1030681316087,
16.4133992458547));
#258076=CARTESIAN_POINT('Ctrl Pts',(-76.4567431175969,-27.1031446841178,
16.4074886487793));
#258077=CARTESIAN_POINT('Ctrl Pts',(-76.4579907926765,-27.1032413604333,
16.4016557351671));
#258078=CARTESIAN_POINT('Ctrl Pts',(-76.4593798496605,-27.1033489917496,
16.395161857456));
#258079=CARTESIAN_POINT('Ctrl Pts',(-76.4607059920239,-27.1034813065929,
16.3887640860712));
#258080=CARTESIAN_POINT('Ctrl Pts',(-76.4619636638711,-27.1036407247952,
16.3825411928141));
#258081=CARTESIAN_POINT('Ctrl Pts',(-76.4633071546945,-27.1038110211188,
16.3758936718375));
#258082=CARTESIAN_POINT('Ctrl Pts',(-76.4645727491349,-27.1040119033633,
16.3694449721487));
#258083=CARTESIAN_POINT('Ctrl Pts',(-76.4657643117174,-27.1042403346288,
16.3632278962589));
#258084=CARTESIAN_POINT('Ctrl Pts',(-76.467089712906,-27.1044944237345,
16.3563125064213));
#258085=CARTESIAN_POINT('Ctrl Pts',(-76.468323724667,-27.1047822481845,
16.3496832154432));
#258086=CARTESIAN_POINT('Ctrl Pts',(-76.4694807350521,-27.1050982652682,
16.3433192109917));
#258087=CARTESIAN_POINT('Ctrl Pts',(-76.4700834269585,-27.1052628799864,
16.3400041724888));
#258088=CARTESIAN_POINT('Ctrl Pts',(-76.4706653444495,-27.1054351607889,
16.3367601398851));
#258089=CARTESIAN_POINT('Ctrl Pts',(-76.4712290846745,-27.1056146245867,
16.3335788333485));
#258090=CARTESIAN_POINT('Ctrl Pts',(-76.4724339017896,-27.1059981719114,
16.3267797929504));
#258091=CARTESIAN_POINT('Ctrl Pts',(-76.4735621797735,-27.1064227170056,
16.3202525650356));
#258092=CARTESIAN_POINT('Ctrl Pts',(-76.4746356788947,-27.1068761140877,
16.313884056441));
#258093=CARTESIAN_POINT('Ctrl Pts',(-76.4758416115454,-27.1073854450543,
16.3067298890093));
#258094=CARTESIAN_POINT('Ctrl Pts',(-76.4769789420409,-27.1079312851641,
16.2997754253287));
#258095=CARTESIAN_POINT('Ctrl Pts',(-76.4780834779718,-27.1085192021475,
16.2927957484855));
#258096=CARTESIAN_POINT('Ctrl Pts',(-76.4787839960327,-27.1088920704749,
16.2883691023696));
#258097=CARTESIAN_POINT('Ctrl Pts',(-76.4794713875341,-27.1092822985717,
16.2839311002524));
#258098=CARTESIAN_POINT('Ctrl Pts',(-76.4801541956933,-27.1096950708922,
16.279414560734));
#258099=CARTESIAN_POINT('Ctrl Pts',(-76.4826886889078,-27.1112272269326,
16.2626497658071));
#258100=CARTESIAN_POINT('Ctrl Pts',(-76.4851267393195,-27.1130539333954,
16.2450093206269));
#258101=CARTESIAN_POINT('Ctrl Pts',(-76.4873049753993,-27.1151298324938,
16.2267576156093));
#258102=CARTESIAN_POINT('Ctrl Pts',(-76.4874570353428,-27.1152747484203,
16.2254834868503));
#258103=CARTESIAN_POINT('Ctrl Pts',(-76.4876078243834,-27.1154208730034,
16.2242063984921));
#258104=CARTESIAN_POINT('Ctrl Pts',(-76.4877572850422,-27.1155681883144,
16.2229264487818));
#258105=CARTESIAN_POINT('Ctrl Pts',(-76.4892866792013,-27.1170756296572,
16.2098290382184));
#258106=CARTESIAN_POINT('Ctrl Pts',(-76.490635746912,-27.1186810477747,
16.1965813411996));
#258107=CARTESIAN_POINT('Ctrl Pts',(-76.4917129528964,-27.1201639637659,
16.1843381520657));
#258108=CARTESIAN_POINT('Ctrl Pts',(-76.4922558078605,-27.120911275161,
16.1781682309056));
#258109=CARTESIAN_POINT('Ctrl Pts',(-76.4927295913191,-27.1216272537546,
16.1722544699356));
#258110=CARTESIAN_POINT('Ctrl Pts',(-76.4931225596015,-27.1222827001223,
16.1667491534086));
#258111=CARTESIAN_POINT('Ctrl Pts',(-76.4940369016729,-27.1238077651632,
16.153939614461));
#258112=CARTESIAN_POINT('Ctrl Pts',(-76.4945873628664,-27.1250450109583,
16.1431163916086));
#258113=CARTESIAN_POINT('Ctrl Pts',(-76.4949373712459,-27.1260738033928,
16.133614386551));
#258114=CARTESIAN_POINT('Ctrl Pts',(-76.4950321308202,-27.1263523336762,
16.1310418597004));
#258115=CARTESIAN_POINT('Ctrl Pts',(-76.4951122559592,-27.126615626805,
16.1285658709055));
#258116=CARTESIAN_POINT('Ctrl Pts',(-76.495181094013,-27.1268653381253,
16.1261726524986));
#258117=CARTESIAN_POINT('Ctrl Pts',(-76.4951938464005,-27.1269115976483,
16.1257293039885));
#258118=CARTESIAN_POINT('Ctrl Pts',(-76.4952062292888,-27.1269574102518,
16.1252887619536));
#258119=CARTESIAN_POINT('Ctrl Pts',(-76.4952182483243,-27.1270027817512,
16.124850986829));
#258120=CARTESIAN_POINT('Ctrl Pts',(74.3634602878983,-28.7459974181805,
19.6929518677509));
#258121=CARTESIAN_POINT('Ctrl Pts',(74.6189041648809,-28.8447420032201,
17.4625));
#258122=CARTESIAN_POINT('Ctrl Pts',(76.7149512087496,-29.6549915892152,
17.4625));
#258123=CARTESIAN_POINT('Ctrl Pts',(74.4609043857744,-28.4939177914721,
19.6929518673255));
#258124=CARTESIAN_POINT('Ctrl Pts',(74.6660793405452,-28.697172525973,17.537473148621));
#258125=CARTESIAN_POINT('Ctrl Pts',(76.6890525018684,-29.4834701335371,
17.4625));
#258126=CARTESIAN_POINT('Ctrl Pts',(74.558847534279,-28.2438591531057,19.6720320649355));
#258127=CARTESIAN_POINT('Ctrl Pts',(74.7189440966799,-28.539163611637,17.5981072780281));
#258128=CARTESIAN_POINT('Ctrl Pts',(76.6640386379029,-29.313679762844,17.4555267321206));
#258129=CARTESIAN_POINT('Ctrl Pts',(74.7559270342238,-27.7480012895941,
19.5871055664396));
#258130=CARTESIAN_POINT('Ctrl Pts',(74.8327386313742,-28.2117119618038,
17.6836912763764));
#258131=CARTESIAN_POINT('Ctrl Pts',(76.6159646173277,-28.9778332725218,
17.4272178998372));
#258132=CARTESIAN_POINT('Ctrl Pts',(74.8560677628267,-27.4997703917927,
19.5220948206209));
#258133=CARTESIAN_POINT('Ctrl Pts',(74.894244872939,-28.0404430900669,17.7096321218676));
#258134=CARTESIAN_POINT('Ctrl Pts',(76.5926880471512,-28.8101355628273,
17.4055476509043));
#258135=CARTESIAN_POINT('Ctrl Pts',(75.0518439197728,-27.0236898937072,
19.3489695261648));
#258136=CARTESIAN_POINT('Ctrl Pts',(75.0196609695894,-27.7022510777816,
17.7211023712238));
#258137=CARTESIAN_POINT('Ctrl Pts',(76.5500480485596,-28.4896086814942,
17.3478392195239));
#258138=CARTESIAN_POINT('Ctrl Pts',(75.1476280619454,-26.7953551633972,
19.2413577159504));
#258139=CARTESIAN_POINT('Ctrl Pts',(75.0836522525161,-27.5347169152613,
17.7080778869124));
#258140=CARTESIAN_POINT('Ctrl Pts',(76.5306138623669,-28.3364379275068,
17.3119686156358));
#258141=CARTESIAN_POINT('Ctrl Pts',(75.2884389844469,-26.4687756770145,
19.0458961827309));
#258142=CARTESIAN_POINT('Ctrl Pts',(75.180389602822,-27.2898012152202,17.6578979817799));
#258143=CARTESIAN_POINT('Ctrl Pts',(76.5048922024806,-28.1185099510298,
17.2468147718753));
#258144=CARTESIAN_POINT('Ctrl Pts',(75.3348967090537,-26.3625884843539,
18.9750294801152));
#258145=CARTESIAN_POINT('Ctrl Pts',(75.212549800534,-27.2097290601206,17.6363116935575));
#258146=CARTESIAN_POINT('Ctrl Pts',(76.4968949507143,-28.0478532106465,
17.2231925371369));
#258147=CARTESIAN_POINT('Ctrl Pts',(75.4268801209925,-26.1560856941709,
18.8208466626381));
#258148=CARTESIAN_POINT('Ctrl Pts',(75.2767579129776,-27.0529295129812,
17.5825320214162));
#258149=CARTESIAN_POINT('Ctrl Pts',(76.4822364493769,-27.9109420608553,
17.1717982652803));
#258150=CARTESIAN_POINT('Ctrl Pts',(75.472719816602,-26.0551010760521,18.7368743964301));
#258151=CARTESIAN_POINT('Ctrl Pts',(75.309058533602,-26.9755857935382,17.5501254447855));
#258152=CARTESIAN_POINT('Ctrl Pts',(76.4755364557143,-27.8442489434604,
17.1438075095172));
#258153=CARTESIAN_POINT('Ctrl Pts',(75.6060560547227,-25.7681502580839,
18.4696518487105));
#258154=CARTESIAN_POINT('Ctrl Pts',(75.4030488168813,-26.7557364160501,
17.4386060175101));
#258155=CARTESIAN_POINT('Ctrl Pts',(76.4581861338659,-27.655675609173,17.0547333270717));
#258156=CARTESIAN_POINT('Ctrl Pts',(75.6894118596666,-25.5978466210022,
18.2718409363073));
#258157=CARTESIAN_POINT('Ctrl Pts',(75.4628679834547,-26.6226482272572,
17.3449978161576));
#258158=CARTESIAN_POINT('Ctrl Pts',(76.4502012574496,-27.5450423948262,
16.9887963557577));
#258159=CARTESIAN_POINT('Ctrl Pts',(75.8449254994665,-25.304207074627,17.8327278472453));
#258160=CARTESIAN_POINT('Ctrl Pts',(75.5732964352864,-26.394507090712,17.1202191600544));
#258161=CARTESIAN_POINT('Ctrl Pts',(76.4429196593781,-27.3578956810278,
16.8424253269258));
#258162=CARTESIAN_POINT('Ctrl Pts',(75.9179115378177,-25.1799509742013,
17.5873106315597));
#258163=CARTESIAN_POINT('Ctrl Pts',(75.6248510373197,-26.2977761963307,
16.9864091667254));
#258164=CARTESIAN_POINT('Ctrl Pts',(76.4437878571375,-27.280900229956,16.7606195878714));
#258165=CARTESIAN_POINT('Ctrl Pts',(76.0120135407799,-25.0456540278874,
17.2025309630903));
#258166=CARTESIAN_POINT('Ctrl Pts',(75.6888631781811,-26.196458000542,16.7690050915913));
#258167=CARTESIAN_POINT('Ctrl Pts',(76.4531141362205,-27.2023521345503,
16.6323596984789));
#258168=CARTESIAN_POINT('Ctrl Pts',(76.0410349984129,-25.0090870943372,
17.0710669460319));
#258169=CARTESIAN_POINT('Ctrl Pts',(75.7081633852747,-26.1695156242359,
16.6936245453235));
#258170=CARTESIAN_POINT('Ctrl Pts',(76.4575269782807,-27.1820075724719,
16.5885383593535));
#258171=CARTESIAN_POINT('Ctrl Pts',(76.0942893550644,-24.9530103267666,
16.8014952531435));
#258172=CARTESIAN_POINT('Ctrl Pts',(75.7423750031981,-26.1301341325905,
16.5376305767288));
#258173=CARTESIAN_POINT('Ctrl Pts',(76.4691181075126,-27.1534935975724,
16.4986811285377));
#258174=CARTESIAN_POINT('Ctrl Pts',(76.1186539510285,-24.9335061597308,
16.6623540419143));
#258175=CARTESIAN_POINT('Ctrl Pts',(75.7573877351407,-26.1176802211109,
16.456286661695));
#258176=CARTESIAN_POINT('Ctrl Pts',(76.4763708127823,-27.1453691430048,
16.4523007247624));
#258177=CARTESIAN_POINT('Ctrl Pts',(76.1824010629023,-24.9029553648553,
16.2463425041019));
#258178=CARTESIAN_POINT('Ctrl Pts',(75.7942282194352,-26.1038934519126,
16.212254424994));
#258179=CARTESIAN_POINT('Ctrl Pts',(76.5018384532032,-27.1404954668531,
16.3136302120345));
#258180=CARTESIAN_POINT('Ctrl Pts',(76.2131904009602,-24.9185412707845,
15.9685880799916));
#258181=CARTESIAN_POINT('Ctrl Pts',(75.8084359405788,-26.1252772492229,
16.0475610164007));
#258182=CARTESIAN_POINT('Ctrl Pts',(76.5237673449999,-27.1624313528561,
16.22101111737));
#258183=CARTESIAN_POINT('Ctrl Pts',(76.2326069140444,-24.9689556265496,
15.6905058513816));
#258184=CARTESIAN_POINT('Ctrl Pts',(75.8121214408374,-26.1756393943761,
15.8859547915775));
#258185=CARTESIAN_POINT('Ctrl Pts',(76.5504448568103,-27.2087011009328,
16.1283513278769));
#258186=CARTESIAN_POINT('',(75.9418613629793,-25.2552738567447,17.263393070432));
#258187=CARTESIAN_POINT('Ctrl Pts',(76.4952182372907,-27.1270026655085,
16.1248510388549));
#258188=CARTESIAN_POINT('Ctrl Pts',(76.4949835330537,-27.1261035938169,
16.1335301302457));
#258189=CARTESIAN_POINT('Ctrl Pts',(76.4945938617307,-27.1250175086505,
16.1433840167261));
#258190=CARTESIAN_POINT('Ctrl Pts',(76.4938946426409,-27.1236651982622,
16.155016623081));
#258191=CARTESIAN_POINT('Ctrl Pts',(76.4937630714253,-27.1234107356421,
16.1572055166349));
#258192=CARTESIAN_POINT('Ctrl Pts',(76.4936205663272,-27.1231468673327,
16.159457246891));
#258193=CARTESIAN_POINT('Ctrl Pts',(76.4934661405637,-27.1228730977824,
16.161775612472));
#258194=CARTESIAN_POINT('Ctrl Pts',(76.4927426139031,-27.121590413054,16.1726377851365));
#258195=CARTESIAN_POINT('Ctrl Pts',(76.4916920130633,-27.1200357216291,
16.1853170892665));
#258196=CARTESIAN_POINT('Ctrl Pts',(76.4903847974142,-27.1184437830655,
16.1985845365573));
#258197=CARTESIAN_POINT('Ctrl Pts',(76.4898045639417,-27.1177371697065,
16.2044735549591));
#258198=CARTESIAN_POINT('Ctrl Pts',(76.4891738033074,-27.1170231040115,
16.210478937357));
#258199=CARTESIAN_POINT('Ctrl Pts',(76.4884987572096,-27.1163213320467,
16.2164967942844));
#258200=CARTESIAN_POINT('Ctrl Pts',(76.4866808484048,-27.1144314500996,
16.2327029691354));
#258201=CARTESIAN_POINT('Ctrl Pts',(76.4846005967103,-27.1126943705596,
16.248691445609));
#258202=CARTESIAN_POINT('Ctrl Pts',(76.4824017849066,-27.1111721910359,
16.2640972093359));
#258203=CARTESIAN_POINT('Ctrl Pts',(76.4816221526914,-27.1106324721787,
16.2695596275751));
#258204=CARTESIAN_POINT('Ctrl Pts',(76.4808275267735,-27.1101196624105,
16.2749492143909));
#258205=CARTESIAN_POINT('Ctrl Pts',(76.4800239584194,-27.1096361423665,
16.2802512670932));
#258206=CARTESIAN_POINT('Ctrl Pts',(76.4787631770299,-27.1088775098621,
16.2885700732516));
#258207=CARTESIAN_POINT('Ctrl Pts',(76.4774861247368,-27.1081924682413,
16.2966391164333));
#258208=CARTESIAN_POINT('Ctrl Pts',(76.4761760059707,-27.1075731179896,
16.3046343846325));
#258209=CARTESIAN_POINT('Ctrl Pts',(76.47501440999,-27.107023980933,16.3117232621031));
#258210=CARTESIAN_POINT('Ctrl Pts',(76.473826311574,-27.1065264227142,16.3187548885341));
#258211=CARTESIAN_POINT('Ctrl Pts',(76.4726008566123,-27.1060881023903,
16.3258128070512));
#258212=CARTESIAN_POINT('Ctrl Pts',(76.4724441687559,-27.1060320583298,
16.326715239338));
#258213=CARTESIAN_POINT('Ctrl Pts',(76.4722868770268,-27.1059770032847,
16.327618034215));
#258214=CARTESIAN_POINT('Ctrl Pts',(76.4721289660945,-27.1059229723704,
16.328521302748));
#258215=CARTESIAN_POINT('Ctrl Pts',(76.4709315855592,-27.1055132758145,
16.3353704558992));
#258216=CARTESIAN_POINT('Ctrl Pts',(76.4696860988113,-27.1051480063909,
16.3423105850608));
#258217=CARTESIAN_POINT('Ctrl Pts',(76.4683756379742,-27.1048249982617,
16.3494047007118));
#258218=CARTESIAN_POINT('Ctrl Pts',(76.4671537647836,-27.1045238256037,
16.3560192514715));
#258219=CARTESIAN_POINT('Ctrl Pts',(76.4658752319113,-27.1042596511161,
16.3627681883072));
#258220=CARTESIAN_POINT('Ctrl Pts',(76.4645307210554,-27.104032682556,16.3696623272918));
#258221=CARTESIAN_POINT('Ctrl Pts',(76.463273931649,-27.1038205223635,16.3761066641332));
#258222=CARTESIAN_POINT('Ctrl Pts',(76.4619593190201,-27.1036411260697,
16.3826784026398));
#258223=CARTESIAN_POINT('Ctrl Pts',(76.4605856089619,-27.103492920932,16.3893426843809));
#258224=CARTESIAN_POINT('Ctrl Pts',(76.4593337345628,-27.1033578602498,
16.3954159045997));
#258225=CARTESIAN_POINT('Ctrl Pts',(76.4580326598547,-27.1032489151476,
16.401566235519));
#258226=CARTESIAN_POINT('Ctrl Pts',(76.4566888072176,-27.103160260748,16.4077247899517));
#258227=CARTESIAN_POINT('Ctrl Pts',(76.4561164336035,-27.1031225010727,
16.410347840992));
#258228=CARTESIAN_POINT('Ctrl Pts',(76.45553640674,-27.1030883438968,16.4129718045799));
#258229=CARTESIAN_POINT('Ctrl Pts',(76.4549497809999,-27.1030568879025,
16.415588473538));
#258230=CARTESIAN_POINT('Ctrl Pts',(76.4528297571347,-27.1029432081676,
16.425044929774));
#258231=CARTESIAN_POINT('Ctrl Pts',(76.4506276154633,-27.1028516325175,
16.434405561816));
#258232=CARTESIAN_POINT('Ctrl Pts',(76.4483618531647,-27.1027493830608,
16.4434727014798));
#258233=CARTESIAN_POINT('Ctrl Pts',(76.4479348994007,-27.1027301154657,
16.4451812873319));
#258234=CARTESIAN_POINT('Ctrl Pts',(76.4475057389463,-27.1027103529406,
16.4468793703157));
#258235=CARTESIAN_POINT('Ctrl Pts',(76.4470745680893,-27.1026896905077,
16.4485655884626));
#258236=CARTESIAN_POINT('Ctrl Pts',(76.4456191147856,-27.1026199427365,
16.454257558903));
#258237=CARTESIAN_POINT('Ctrl Pts',(76.4441322040646,-27.1025406532758,
16.4598473134519));
#258238=CARTESIAN_POINT('Ctrl Pts',(76.442600468481,-27.1024250918531,16.4653566990946));
#258239=CARTESIAN_POINT('Ctrl Pts',(76.4420185090595,-27.1023811860645,
16.4674499055955));
#258240=CARTESIAN_POINT('Ctrl Pts',(76.4414302186258,-27.1023318496955,
16.4695309610732));
#258241=CARTESIAN_POINT('Ctrl Pts',(76.4408353908733,-27.102274692544,16.471599536434));
#258242=CARTESIAN_POINT('Ctrl Pts',(76.4389925228598,-27.1020976108831,
16.4780083015764));
#258243=CARTESIAN_POINT('Ctrl Pts',(76.4370710585152,-27.1018561048159,
16.484391780126));
#258244=CARTESIAN_POINT('Ctrl Pts',(76.4350620986664,-27.1015158539167,
16.4906542061397));
#258245=CARTESIAN_POINT('Ctrl Pts',(76.4333518787977,-27.101226199622,16.4959853855563));
#258246=CARTESIAN_POINT('Ctrl Pts',(76.4315790441179,-27.1008647151594,
16.5012232667724));
#258247=CARTESIAN_POINT('Ctrl Pts',(76.4297403585978,-27.1004038747182,
16.506308780418));
#258248=CARTESIAN_POINT('Ctrl Pts',(76.428448929915,-27.1000801964396,16.5098806681154));
#258249=CARTESIAN_POINT('Ctrl Pts',(76.4271251515698,-27.0997073598893,
16.5133767163619));
#258250=CARTESIAN_POINT('Ctrl Pts',(76.4257650872491,-27.099274630663,16.5168023194369));
#258251=CARTESIAN_POINT('Ctrl Pts',(76.4244998564415,-27.0988720744456,
16.5199890647099));
#258252=CARTESIAN_POINT('Ctrl Pts',(76.4232033943605,-27.098417636482,16.5231136244567));
#258253=CARTESIAN_POINT('Ctrl Pts',(76.4218676568024,-27.0979025055511,
16.5262197342897));
#258254=CARTESIAN_POINT('Ctrl Pts',(76.4217789540814,-27.0978682970983,
16.5264260026484));
#258255=CARTESIAN_POINT('Ctrl Pts',(76.4216900756716,-27.0978338210965,
16.5266322092027));
#258256=CARTESIAN_POINT('Ctrl Pts',(76.42160101808,-27.0977990750257,16.5268383756656));
#258257=CARTESIAN_POINT('Ctrl Pts',(76.4212719492627,-27.0976706878978,
16.5276001630985));
#258258=CARTESIAN_POINT('Ctrl Pts',(76.4209404362583,-27.0975386143442,
16.5283613866205));
#258259=CARTESIAN_POINT('Ctrl Pts',(76.420606322143,-27.0974027448563,16.5291232095979));
#258260=CARTESIAN_POINT('Ctrl Pts',(76.4187176830274,-27.0966347185512,
16.5334295486848));
#258261=CARTESIAN_POINT('Ctrl Pts',(76.4167566024575,-27.0957491893814,
16.5376614539863));
#258262=CARTESIAN_POINT('Ctrl Pts',(76.4147290835934,-27.0947257635434,
16.5417599887868));
#258263=CARTESIAN_POINT('Ctrl Pts',(76.4130382200801,-27.0938722704199,
16.5451779905008));
#258264=CARTESIAN_POINT('Ctrl Pts',(76.4113012291952,-27.0929228022964,
16.5485028097877));
#258265=CARTESIAN_POINT('Ctrl Pts',(76.4095163162519,-27.0918686181557,
16.5517348365811));
#258266=CARTESIAN_POINT('Ctrl Pts',(76.4080553283209,-27.0910057467689,
16.5543803169423));
#258267=CARTESIAN_POINT('Ctrl Pts',(76.4065622115749,-27.0900727246033,
16.5569638004413));
#258268=CARTESIAN_POINT('Ctrl Pts',(76.4050319318852,-27.0890672853614,
16.5595114022443));
#258269=CARTESIAN_POINT('Ctrl Pts',(76.4024133502064,-27.0873467993641,
16.5638708036345));
#258270=CARTESIAN_POINT('Ctrl Pts',(76.3996858222803,-27.0854160305327,
16.5681213015851));
#258271=CARTESIAN_POINT('Ctrl Pts',(76.3968549739062,-27.0832453437817,
16.5722001453448));
#258272=CARTESIAN_POINT('Ctrl Pts',(76.3944794420004,-27.0814237924469,
16.5756229438169));
#258273=CARTESIAN_POINT('Ctrl Pts',(76.3920312477951,-27.0794332007598,
16.5789244111556));
#258274=CARTESIAN_POINT('Ctrl Pts',(76.3895078513776,-27.0772609129525,
16.5821034643369));
#258275=CARTESIAN_POINT('Ctrl Pts',(76.3879086122783,-27.0758841940301,
16.5841182354253));
#258276=CARTESIAN_POINT('Ctrl Pts',(76.3862790519598,-27.0744345916958,
16.5860845447371));
#258277=CARTESIAN_POINT('Ctrl Pts',(76.3846166914258,-27.0729104400659,
16.5880130337735));
#258278=CARTESIAN_POINT('Ctrl Pts',(76.3827359747383,-27.0711860864457,
16.5901948357585));
#258279=CARTESIAN_POINT('Ctrl Pts',(76.3808666413316,-27.0694154757855,
16.5922669270651));
#258280=CARTESIAN_POINT('Ctrl Pts',(76.3790011613002,-27.067605522352,16.5942742310325));
#258281=CARTESIAN_POINT('Ctrl Pts',(76.3740456584696,-27.0627975216168,
16.5996064781347));
#258282=CARTESIAN_POINT('Ctrl Pts',(76.3691274276512,-27.0577058759386,
16.6044118919374));
#258283=CARTESIAN_POINT('Ctrl Pts',(76.3642377230657,-27.0523503506956,
16.608778305053));
#258284=CARTESIAN_POINT('Ctrl Pts',(76.3592796180166,-27.0469199087776,
16.6132057984803));
#258285=CARTESIAN_POINT('Ctrl Pts',(76.3543509085649,-27.0412180804687,
16.6171815871766));
#258286=CARTESIAN_POINT('Ctrl Pts',(76.3494322419877,-27.0352768340194,
16.6208506593465));
#258287=CARTESIAN_POINT('Ctrl Pts',(76.3445135754106,-27.0293355875702,
16.6245197315165));
#258288=CARTESIAN_POINT('Ctrl Pts',(76.3396049868128,-27.0231548844634,
16.627881911179));
#258289=CARTESIAN_POINT('Ctrl Pts',(76.3346762337748,-27.0167787754288,
16.6311389170626));
#258290=CARTESIAN_POINT('Ctrl Pts',(76.3270525622607,-27.0069163699799,
16.6361767720303));
#258291=CARTESIAN_POINT('Ctrl Pts',(76.3193994275977,-26.9965742763171,
16.6408622418929));
#258292=CARTESIAN_POINT('Ctrl Pts',(76.3117344496181,-26.9857761531729,
16.6452464533356));
#258293=CARTESIAN_POINT('Ctrl Pts',(76.3074367607922,-26.9797217361478,
16.6477046438977));
#258294=CARTESIAN_POINT('Ctrl Pts',(76.3031351576487,-26.9735241809036,
16.6500689942518));
#258295=CARTESIAN_POINT('Ctrl Pts',(76.2988312337083,-26.9671894394041,
16.6523553297696));
#258296=CARTESIAN_POINT('Ctrl Pts',(76.284801695007,-26.946540026854,16.6598081177547));
#258297=CARTESIAN_POINT('Ctrl Pts',(76.2713420389531,-26.9253146403795,
16.6661261478332));
#258298=CARTESIAN_POINT('Ctrl Pts',(76.2582666976207,-26.9037854166578,
16.6722817468538));
#258299=CARTESIAN_POINT('Ctrl Pts',(76.2367166491782,-26.8683021506889,
16.6824270618949));
#258300=CARTESIAN_POINT('Ctrl Pts',(76.2163231724411,-26.8318654947762,
16.6915805494775));
#258301=CARTESIAN_POINT('Ctrl Pts',(76.1969868424008,-26.7948177267048,
16.7005093018145));
#258302=CARTESIAN_POINT('Ctrl Pts',(76.1951008482355,-26.7912042243353,
16.7013801793169));
#258303=CARTESIAN_POINT('Ctrl Pts',(76.1932248857209,-26.7875849267645,
16.702248942733));
#258304=CARTESIAN_POINT('Ctrl Pts',(76.1913588468486,-26.7839601625947,
16.7031163158082));
#258305=CARTESIAN_POINT('Ctrl Pts',(76.1765680275187,-26.7552291255587,
16.7099913914764));
#258306=CARTESIAN_POINT('Ctrl Pts',(76.1624139946396,-26.7262008738675,
16.7168106960657));
#258307=CARTESIAN_POINT('Ctrl Pts',(76.148916516475,-26.6969732854462,16.723597339564));
#258308=CARTESIAN_POINT('Ctrl Pts',(76.1236619610203,-26.6422867918957,
16.7362955386267));
#258309=CARTESIAN_POINT('Ctrl Pts',(76.1005180681542,-26.5866819737582,
16.7491519989745));
#258310=CARTESIAN_POINT('Ctrl Pts',(76.079407408338,-26.5302810835918,16.7625435721094));
#258311=CARTESIAN_POINT('Ctrl Pts',(76.0643629274286,-26.4900870715251,
16.7720870571605));
#258312=CARTESIAN_POINT('Ctrl Pts',(76.0503521064178,-26.4494883804854,
16.7819023270183));
#258313=CARTESIAN_POINT('Ctrl Pts',(76.0373611942065,-26.4085292238124,
16.7921336012873));
#258314=CARTESIAN_POINT('Ctrl Pts',(76.0231720122117,-26.363792032233,16.8033085988763));
#258315=CARTESIAN_POINT('Ctrl Pts',(76.0103384192577,-26.3190310002098,
16.8148454077162));
#258316=CARTESIAN_POINT('Ctrl Pts',(75.9987850456331,-26.2743222514904,
16.8269262467483));
#258317=CARTESIAN_POINT('Ctrl Pts',(75.9837486849486,-26.2161351891359,
16.8426490874492));
#258318=CARTESIAN_POINT('Ctrl Pts',(75.9708594776084,-26.1575989600339,
16.8592311067897));
#258319=CARTESIAN_POINT('Ctrl Pts',(75.9600230530993,-26.0990044706059,
16.87689659528));
#258320=CARTESIAN_POINT('Ctrl Pts',(75.9491979291291,-26.0404710852166,
16.8945436616849));
#258321=CARTESIAN_POINT('Ctrl Pts',(75.9404214117338,-25.9818779785533,
16.9132712882588));
#258322=CARTESIAN_POINT('Ctrl Pts',(75.9336439589103,-25.9235033740798,
16.9333228296216));
#258323=CARTESIAN_POINT('Ctrl Pts',(75.9294790509236,-25.8876307737501,
16.9456449847059));
#258324=CARTESIAN_POINT('Ctrl Pts',(75.9260699331789,-25.8518405543699,
16.9584675280385));
#258325=CARTESIAN_POINT('Ctrl Pts',(75.9234132458697,-25.8161989866991,
16.9718522765842));
#258326=CARTESIAN_POINT('Ctrl Pts',(75.9217239577786,-25.79353584693,16.9803631375505));
#258327=CARTESIAN_POINT('Ctrl Pts',(75.9203357066725,-25.7708904059774,
16.9891192993483));
#258328=CARTESIAN_POINT('Ctrl Pts',(75.9192531417283,-25.7483106633381,
16.9981274246421));
#258329=CARTESIAN_POINT('Ctrl Pts',(75.9170297815808,-25.7019366326703,
17.0166282147223));
#258330=CARTESIAN_POINT('Ctrl Pts',(75.9160908878973,-25.655715430254,17.0360687209725));
#258331=CARTESIAN_POINT('Ctrl Pts',(75.9163356254781,-25.6100335195254,
17.0568346695685));
#258332=CARTESIAN_POINT('Ctrl Pts',(75.9165621173305,-25.5677572963717,
17.0760524707252));
#258333=CARTESIAN_POINT('Ctrl Pts',(75.9178014945793,-25.525943597602,17.0964068031593));
#258334=CARTESIAN_POINT('Ctrl Pts',(75.9199460216627,-25.4848871400518,
17.1181763515707));
#258335=CARTESIAN_POINT('Ctrl Pts',(75.9220376690096,-25.4448430523975,
17.1394091065817));
#258336=CARTESIAN_POINT('Ctrl Pts',(75.9249898990674,-25.4055198684575,
17.1619892999607));
#258337=CARTESIAN_POINT('Ctrl Pts',(75.9286842189365,-25.367171005978,17.1861307296523));
#258338=CARTESIAN_POINT('Ctrl Pts',(75.9320094343453,-25.3326536298594,
17.2078601566765));
#258339=CARTESIAN_POINT('Ctrl Pts',(75.9359354287058,-25.2989256357191,
17.2308544606354));
#258340=CARTESIAN_POINT('Ctrl Pts',(75.9403670676557,-25.2661521617921,
17.2552262519058));
#258341=CARTESIAN_POINT('Ctrl Pts',(75.9408589869758,-25.2625142514853,
17.2579315614148));
#258342=CARTESIAN_POINT('Ctrl Pts',(75.9413571303365,-25.2588880801971,
17.2606537953022));
#258343=CARTESIAN_POINT('Ctrl Pts',(75.9418613633423,-25.2552738568382,
17.2633930704885));
#258344=CARTESIAN_POINT('Ctrl Pts',(75.9418613633423,-25.2552738568381,
17.2633930704885));
#258345=CARTESIAN_POINT('Ctrl Pts',(75.9442259477234,-25.2383250955474,
17.2762387760005));
#258346=CARTESIAN_POINT('Ctrl Pts',(75.9466297979483,-25.2219501076077,
17.2896217176776));
#258347=CARTESIAN_POINT('Ctrl Pts',(75.9489416166696,-25.2063620808647,
17.3037656232882));
#258348=CARTESIAN_POINT('Ctrl Pts',(75.9512774695743,-25.1906119975164,
17.3180565720987));
#258349=CARTESIAN_POINT('Ctrl Pts',(75.9535194008795,-25.1756652588171,
17.3331243157543));
#258350=CARTESIAN_POINT('Ctrl Pts',(75.9555501186517,-25.1617083521244,
17.3491621101886));
#258351=CARTESIAN_POINT('Ctrl Pts',(75.9576114326053,-25.1475411611397,
17.3654415409911));
#258352=CARTESIAN_POINT('Ctrl Pts',(75.9594551436902,-25.1343938079096,
17.3827204208166));
#258353=CARTESIAN_POINT('Ctrl Pts',(75.9609767648281,-25.1224278840972,
17.4011633324196));
#258354=CARTESIAN_POINT('Ctrl Pts',(75.9611515136477,-25.1210536714171,
17.403281387271));
#258355=CARTESIAN_POINT('Ctrl Pts',(75.9613220335941,-25.1196950054424,
17.405414755068));
#258356=CARTESIAN_POINT('Ctrl Pts',(75.9614881812303,-25.1183521036895,
17.4075636545405));
#258357=CARTESIAN_POINT('Origin',(76.7149512087496,-29.6549915892152,20.0025));
#258358=CARTESIAN_POINT('Origin',(0.,0.,20.0025));
#258359=CARTESIAN_POINT('Origin',(29.6549915892152,-76.7149512087496,20.0025));
#258360=CARTESIAN_POINT('Ctrl Pts',(24.9689313575499,-76.2325975651779,
15.6906397325506));
#258361=CARTESIAN_POINT('Ctrl Pts',(26.1756150602387,-75.8121196590786,
15.8860328844658));
#258362=CARTESIAN_POINT('Ctrl Pts',(27.2086788182716,-76.5504320086843,
16.1283959549332));
#258363=CARTESIAN_POINT('Ctrl Pts',(24.9186909562146,-76.2132400197753,
15.967824496348));
#258364=CARTESIAN_POINT('Ctrl Pts',(26.1254229642367,-75.8084425279589,
16.0471243598434));
#258365=CARTESIAN_POINT('Ctrl Pts',(27.1625656651728,-76.5238417787825,
16.2207578908838));
#258366=CARTESIAN_POINT('Ctrl Pts',(24.9032159272874,-76.1826381079971,
16.2438456162079));
#258367=CARTESIAN_POINT('Ctrl Pts',(26.1041848761176,-75.7943214248689,
16.2107725763322));
#258368=CARTESIAN_POINT('Ctrl Pts',(27.1407766635653,-76.5020517602977,
16.3127979160872));
#258369=CARTESIAN_POINT('Ctrl Pts',(24.9328226963038,-76.1197004175054,
16.655986759916));
#258370=CARTESIAN_POINT('Ctrl Pts',(26.1172873190749,-75.7580138780931,
16.4525591935381));
#258371=CARTESIAN_POINT('Ctrl Pts',(27.1451435881169,-76.4767312134558,
16.4501782974209));
#258372=CARTESIAN_POINT('Ctrl Pts',(24.9518097701927,-76.0956371509853,
16.7941104173067));
#258373=CARTESIAN_POINT('Ctrl Pts',(26.1293351405296,-75.7432179427276,
16.53332924405));
#258374=CARTESIAN_POINT('Ctrl Pts',(27.1529468723189,-76.469480763603,16.4962195166118));
#258375=CARTESIAN_POINT('Ctrl Pts',(25.0073336657117,-76.0425032131366,
17.0641682497328));
#258376=CARTESIAN_POINT('Ctrl Pts',(26.1682415554301,-75.7091288541243,
16.6896570718779));
#258377=CARTESIAN_POINT('Ctrl Pts',(27.1810555370846,-76.4577808154581,
16.5862387939007));
#258378=CARTESIAN_POINT('Ctrl Pts',(25.0435822919594,-76.0135981896352,
17.1955505586789));
#258379=CARTESIAN_POINT('Ctrl Pts',(26.1949210472009,-75.6899232799157,
16.7650201820139));
#258380=CARTESIAN_POINT('Ctrl Pts',(27.2011812093655,-76.4533313045578,
16.6300328970335));
#258381=CARTESIAN_POINT('Ctrl Pts',(25.1764553135872,-75.9201060960319,
17.5792969885097));
#258382=CARTESIAN_POINT('Ctrl Pts',(26.2950899509062,-75.6263767700398,
16.9819673365851));
#258383=CARTESIAN_POINT('Ctrl Pts',(27.2787774842961,-76.4438901441629,
16.7579483734713));
#258384=CARTESIAN_POINT('Ctrl Pts',(25.2993526607364,-75.8476684832869,
17.8240388353678));
#258385=CARTESIAN_POINT('Ctrl Pts',(26.3907356809326,-75.5752351470898,
17.1155820316982));
#258386=CARTESIAN_POINT('Ctrl Pts',(27.3548544480355,-76.4428939284366,
16.8395289896475));
#258387=CARTESIAN_POINT('Ctrl Pts',(25.5919984567923,-75.6923432030072,
18.2644739211054));
#258388=CARTESIAN_POINT('Ctrl Pts',(26.6180940171703,-75.4649619696469,
17.3414092350345));
#258389=CARTESIAN_POINT('Ctrl Pts',(27.5412643883021,-76.4499649794119,
16.9863406840096));
#258390=CARTESIAN_POINT('Ctrl Pts',(25.7617839502726,-75.6091210995781,
18.4627331486824));
#258391=CARTESIAN_POINT('Ctrl Pts',(26.750791129475,-75.4052371346464,17.4354381030784));
#258392=CARTESIAN_POINT('Ctrl Pts',(27.6515244073534,-76.4578597275994,
17.052427093745));
#258393=CARTESIAN_POINT('Ctrl Pts',(26.1430805994656,-75.43173575527,18.819759549872));
#258394=CARTESIAN_POINT('Ctrl Pts',(27.0442130694157,-75.2796463045429,
17.585582997513));
#258395=CARTESIAN_POINT('Ctrl Pts',(27.9020344677393,-76.4807996718613,
17.1714358939392));
#258396=CARTESIAN_POINT('Ctrl Pts',(26.351056088416,-75.3392616135106,18.9747290102619));
#258397=CARTESIAN_POINT('Ctrl Pts',(27.2031302208849,-75.2146749685589,
17.6396375078353));
#258398=CARTESIAN_POINT('Ctrl Pts',(28.0399748698375,-76.4956562029936,
17.2230923811496));
#258399=CARTESIAN_POINT('Ctrl Pts',(26.7887981118758,-75.1503919246078,
19.2381193325703));
#258400=CARTESIAN_POINT('Ctrl Pts',(27.5299162784616,-75.08549731885,17.7075896666719));
#258401=CARTESIAN_POINT('Ctrl Pts',(28.3320433237811,-76.5300629685854,
17.3108891546272));
#258402=CARTESIAN_POINT('Ctrl Pts',(27.0218910128879,-75.0525919498094,
19.3482083029786));
#258403=CARTESIAN_POINT('Ctrl Pts',(27.7009559314819,-75.0201494871695,
17.7210643477395));
#258404=CARTESIAN_POINT('Ctrl Pts',(28.4884000162545,-76.5498913973941,
17.3475854788259));
#258405=CARTESIAN_POINT('Ctrl Pts',(27.4985053196508,-74.8565797596346,
19.5217411601882));
#258406=CARTESIAN_POINT('Ctrl Pts',(28.0395707962217,-74.8945599897605,
17.709745105584));
#258407=CARTESIAN_POINT('Ctrl Pts',(28.8092814008563,-76.5925703049476,
17.4054297637291));
#258408=CARTESIAN_POINT('Ctrl Pts',(27.7422284005853,-74.7582415292723,
19.5858151824391));
#258409=CARTESIAN_POINT('Ctrl Pts',(28.2078168588111,-74.8341192521319,
17.6844550416302));
#258410=CARTESIAN_POINT('Ctrl Pts',(28.9739291008626,-76.6154156280005,
17.4267877716095));
#258411=CARTESIAN_POINT('Ctrl Pts',(28.2396160007804,-74.5605143304923,
19.6716009699542));
#258412=CARTESIAN_POINT('Ctrl Pts',(28.5364711009172,-74.7198525855438,
17.5990670510762));
#258413=CARTESIAN_POINT('Ctrl Pts',(29.3108001463009,-76.663616773129,17.455383034021));
#258414=CARTESIAN_POINT('Ctrl Pts',(28.4947415154358,-74.460585966212,19.6929518687096));
#258415=CARTESIAN_POINT('Ctrl Pts',(28.6976612611857,-74.6659231009672,
17.5372248464455));
#258416=CARTESIAN_POINT('Ctrl Pts',(29.4840227026762,-76.68913593644,17.4625));
#258417=CARTESIAN_POINT('Ctrl Pts',(28.7459974181806,-74.3634602878982,
19.6929518677509));
#258418=CARTESIAN_POINT('Ctrl Pts',(28.8447420032201,-74.6189041648808,
17.4625));
#258419=CARTESIAN_POINT('Ctrl Pts',(29.6549915892153,-76.7149512087496,
17.4625));
#258420=CARTESIAN_POINT('',(25.255273856838,-75.9418613633423,17.2633930704885));
#258421=CARTESIAN_POINT('Ctrl Pts',(25.1183523255102,-75.961488153786,17.4075632995852));
#258422=CARTESIAN_POINT('Ctrl Pts',(25.1300086289488,-75.9600460003542,
17.3889110251782));
#258423=CARTESIAN_POINT('Ctrl Pts',(25.1428552491918,-75.9582730048931,
17.3714318667196));
#258424=CARTESIAN_POINT('Ctrl Pts',(25.1567358846387,-75.9562706193538,
17.3549670181865));
#258425=CARTESIAN_POINT('Ctrl Pts',(25.1704654612226,-75.9542900251859,
17.3386813517454));
#258426=CARTESIAN_POINT('Ctrl Pts',(25.1852067358384,-75.9520849723162,
17.3233881139774));
#258427=CARTESIAN_POINT('Ctrl Pts',(25.2007766451559,-75.9497709328093,
17.3088979329943));
#258428=CARTESIAN_POINT('Ctrl Pts',(25.2161260489864,-75.9474896653885,
17.2946129660782));
#258429=CARTESIAN_POINT('Ctrl Pts',(25.232280824703,-75.9451024553672,17.2811085188303));
#258430=CARTESIAN_POINT('Ctrl Pts',(25.2490337249568,-75.9427372332249,
17.2681673906668));
#258431=CARTESIAN_POINT('Ctrl Pts',(25.2511048107543,-75.942444831437,17.2665675371288));
#258432=CARTESIAN_POINT('Ctrl Pts',(25.2531849968851,-75.9421527879211,
17.2649762469424));
#258433=CARTESIAN_POINT('Ctrl Pts',(25.2552738568381,-75.9418613633423,
17.2633930704885));
#258434=CARTESIAN_POINT('Ctrl Pts',(25.2552738568381,-75.9418613633423,
17.2633930704885));
#258435=CARTESIAN_POINT('Ctrl Pts',(25.3053371640301,-75.9348768553703,
17.2254493239301));
#258436=CARTESIAN_POINT('Ctrl Pts',(25.3572644310084,-75.9291204561474,
17.1911044093464));
#258437=CARTESIAN_POINT('Ctrl Pts',(25.4106833642209,-75.924849515688,17.1596330726746));
#258438=CARTESIAN_POINT('Ctrl Pts',(25.4672813124795,-75.920324407218,17.126288844749));
#258439=CARTESIAN_POINT('Ctrl Pts',(25.5255536825938,-75.9174669834122,
17.0961703062381));
#258440=CARTESIAN_POINT('Ctrl Pts',(25.5850314006763,-75.9165875721685,
17.0683598410554));
#258441=CARTESIAN_POINT('Ctrl Pts',(25.6385673672631,-75.9157960130354,
17.0433276074261));
#258442=CARTESIAN_POINT('Ctrl Pts',(25.6930793583591,-75.9166071705315,
17.0201642484432));
#258443=CARTESIAN_POINT('Ctrl Pts',(25.7482100069341,-75.9192482119053,
16.9981680565501));
#258444=CARTESIAN_POINT('Ctrl Pts',(25.7703411807749,-75.9203084088606,
16.989338094284));
#258445=CARTESIAN_POINT('Ctrl Pts',(25.7926041373149,-75.9216656968715,
16.9807230184841));
#258446=CARTESIAN_POINT('Ctrl Pts',(25.8149722051989,-75.9233227318013,
16.9723142805638));
#258447=CARTESIAN_POINT('Ctrl Pts',(25.8770418865906,-75.9279208772774,
16.9489806745353));
#258448=CARTESIAN_POINT('Ctrl Pts',(25.9395105598039,-75.9347968299589,
16.9273736682915));
#258449=CARTESIAN_POINT('Ctrl Pts',(26.0019469535689,-75.9439477443041,
16.9071901217942));
#258450=CARTESIAN_POINT('Ctrl Pts',(26.0680891143166,-75.9536417898937,
16.8858086278227));
#258451=CARTESIAN_POINT('Ctrl Pts',(26.1341966258341,-75.965888408869,16.8660249929721));
#258452=CARTESIAN_POINT('Ctrl Pts',(26.1997753181043,-75.9807279241647,
16.8475110455431));
#258453=CARTESIAN_POINT('Ctrl Pts',(26.2246632540871,-75.9863597062865,
16.8404847703544));
#258454=CARTESIAN_POINT('Ctrl Pts',(26.2494750769638,-75.9923654084165,
16.8336416500865));
#258455=CARTESIAN_POINT('Ctrl Pts',(26.274183642075,-75.9987489548308,16.8269646518251));
#258456=CARTESIAN_POINT('Ctrl Pts',(26.3193781191767,-76.0104251100811,
16.8147517433184));
#258457=CARTESIAN_POINT('Ctrl Pts',(26.3644806578422,-76.0233691013076,
16.8031325557463));
#258458=CARTESIAN_POINT('Ctrl Pts',(26.4094030264447,-76.0376323915297,
16.7919150704374));
#258459=CARTESIAN_POINT('Ctrl Pts',(26.4723212970277,-76.0576095561699,
16.7762038602346));
#258460=CARTESIAN_POINT('Ctrl Pts',(26.5349890928756,-76.0801913924513,
16.761328555408));
#258461=CARTESIAN_POINT('Ctrl Pts',(26.5968842692081,-76.1054321159433,
16.7468658576066));
#258462=CARTESIAN_POINT('Ctrl Pts',(26.6310436335351,-76.1193622332921,
16.7388840310311));
#258463=CARTESIAN_POINT('Ctrl Pts',(26.6649677057044,-76.1341013590046,
16.7310274121222));
#258464=CARTESIAN_POINT('Ctrl Pts',(26.6985700833486,-76.1496523368463,
16.7232226781382));
#258465=CARTESIAN_POINT('Ctrl Pts',(26.7271705556572,-76.1628884630466,
16.7165797232691));
#258466=CARTESIAN_POINT('Ctrl Pts',(26.7555332801645,-76.1767336953889,
16.7099108264627));
#258467=CARTESIAN_POINT('Ctrl Pts',(26.7835861607673,-76.1911702999443,
16.703195010784));
#258468=CARTESIAN_POINT('Ctrl Pts',(26.8199494181624,-76.2098835998295,
16.6944897039172));
#258469=CARTESIAN_POINT('Ctrl Pts',(26.8556888251213,-76.2295605861727,
16.6856585992062));
#258470=CARTESIAN_POINT('Ctrl Pts',(26.8905185780769,-76.2502978094459,
16.6759949656516));
#258471=CARTESIAN_POINT('Ctrl Pts',(26.8948405205601,-76.2528710429215,
16.6747958279932));
#258472=CARTESIAN_POINT('Ctrl Pts',(26.8991484846555,-76.2554605686,16.6735839225594));
#258473=CARTESIAN_POINT('Ctrl Pts',(26.9034419493924,-76.258066542324,16.6723579472489));
#258474=CARTESIAN_POINT('Ctrl Pts',(26.9260412895686,-76.2717835029343,
16.6659048295947));
#258475=CARTESIAN_POINT('Ctrl Pts',(26.9482892130479,-76.285912248423,16.6592804200091));
#258476=CARTESIAN_POINT('Ctrl Pts',(26.9698831287183,-76.3006663576261,
16.6513762614162));
#258477=CARTESIAN_POINT('Ctrl Pts',(26.9780091205859,-76.3062184665269,
16.6484018528176));
#258478=CARTESIAN_POINT('Ctrl Pts',(26.986126275181,-76.3119191069485,16.6452107770005));
#258479=CARTESIAN_POINT('Ctrl Pts',(26.9940602890789,-76.3176690330733,
16.641805515319));
#258480=CARTESIAN_POINT('Ctrl Pts',(27.0017405515385,-76.3232350608532,
16.6385091632085));
#258481=CARTESIAN_POINT('Ctrl Pts',(27.0092489791902,-76.3288474190919,
16.6350110759018));
#258482=CARTESIAN_POINT('Ctrl Pts',(27.0164426885853,-76.3343994470152,
16.6313545905897));
#258483=CARTESIAN_POINT('Ctrl Pts',(27.0216511779323,-76.3384193033514,
16.6287071713309));
#258484=CARTESIAN_POINT('Ctrl Pts',(27.0266992747262,-76.3424031634616,
16.6260035903663));
#258485=CARTESIAN_POINT('Ctrl Pts',(27.031517148069,-76.3463237496473,16.623174016085));
#258486=CARTESIAN_POINT('Ctrl Pts',(27.0359626255992,-76.3499412955132,
16.620563152745));
#258487=CARTESIAN_POINT('Ctrl Pts',(27.0402121123801,-76.3535049417161,
16.61784496832));
#258488=CARTESIAN_POINT('Ctrl Pts',(27.0442217726251,-76.3569830260576,
16.6150107799504));
#258489=CARTESIAN_POINT('Ctrl Pts',(27.0482190858534,-76.3604504002732,
16.6121853189465));
#258490=CARTESIAN_POINT('Ctrl Pts',(27.0519780402871,-76.363832737455,16.6092444573834));
#258491=CARTESIAN_POINT('Ctrl Pts',(27.0554667048094,-76.36708813328,16.6062292699511));
#258492=CARTESIAN_POINT('Ctrl Pts',(27.0590905992174,-76.3704697168776,
16.6030972058604));
#258493=CARTESIAN_POINT('Ctrl Pts',(27.062422884322,-76.373714282348,16.5998850438583));
#258494=CARTESIAN_POINT('Ctrl Pts',(27.0654401118128,-76.3767636736847,
16.5966933385278));
#258495=CARTESIAN_POINT('Ctrl Pts',(27.0660776794783,-76.3774080378641,
16.5960189021046));
#258496=CARTESIAN_POINT('Ctrl Pts',(27.0667012194144,-76.3780436511264,
16.5953455586113));
#258497=CARTESIAN_POINT('Ctrl Pts',(27.0673105711314,-76.3786699101857,
16.5946745303528));
#258498=CARTESIAN_POINT('Ctrl Pts',(27.0690899047773,-76.3804986140098,
16.5927150985099));
#258499=CARTESIAN_POINT('Ctrl Pts',(27.0707485694433,-76.3822466735942,
16.5907819641661));
#258500=CARTESIAN_POINT('Ctrl Pts',(27.0722790207895,-76.3839036747509,
16.5888786971137));
#258501=CARTESIAN_POINT('Ctrl Pts',(27.0747602935228,-76.3865901187202,
16.585792989977));
#258502=CARTESIAN_POINT('Ctrl Pts',(27.077074716928,-76.3892195788573,16.5825794796621));
#258503=CARTESIAN_POINT('Ctrl Pts',(27.0792241298737,-76.391803503673,16.579183461688));
#258504=CARTESIAN_POINT('Ctrl Pts',(27.0816343564139,-76.3947009665273,
16.5753753648454));
#258505=CARTESIAN_POINT('Ctrl Pts',(27.0838371838135,-76.3975410819206,
16.5713382503816));
#258506=CARTESIAN_POINT('Ctrl Pts',(27.0858449593888,-76.4003286348304,
16.5670618115476));
#258507=CARTESIAN_POINT('Ctrl Pts',(27.0868914071294,-76.4017815006189,
16.5648329420413));
#258508=CARTESIAN_POINT('Ctrl Pts',(27.0878850123543,-76.4032199208278,
16.5625400513047));
#258509=CARTESIAN_POINT('Ctrl Pts',(27.0888282606249,-76.4046437013157,
16.5601869005576));
#258510=CARTESIAN_POINT('Ctrl Pts',(27.0901243133997,-76.4066000204624,
16.5569535974602));
#258511=CARTESIAN_POINT('Ctrl Pts',(27.0913240247944,-76.4085291386582,
16.5536060903116));
#258512=CARTESIAN_POINT('Ctrl Pts',(27.0924256409491,-76.4104440988722,
16.5500691169233));
#258513=CARTESIAN_POINT('Ctrl Pts',(27.0936398960553,-76.4125548615076,
16.5461704921812));
#258514=CARTESIAN_POINT('Ctrl Pts',(27.0947350223258,-76.4146483558569,
16.5420420626088));
#258515=CARTESIAN_POINT('Ctrl Pts',(27.095715388145,-76.4167317431154,16.5376476090047));
#258516=CARTESIAN_POINT('Ctrl Pts',(27.0962521693207,-76.4178724632835,
16.5352415071946));
#258517=CARTESIAN_POINT('Ctrl Pts',(27.0967546540791,-76.4190099868706,
16.5327567007312));
#258518=CARTESIAN_POINT('Ctrl Pts',(27.0972241917238,-76.4201444978056,
16.530193509747));
#258519=CARTESIAN_POINT('Ctrl Pts',(27.097831559752,-76.4216120386457,16.5268779071077));
#258520=CARTESIAN_POINT('Ctrl Pts',(27.0983817197162,-76.4230689256427,
16.5234805947187));
#258521=CARTESIAN_POINT('Ctrl Pts',(27.0988766740941,-76.4245289974568,
16.5198985627827));
#258522=CARTESIAN_POINT('Ctrl Pts',(27.0994168627798,-76.426122506494,16.5159891658567));
#258523=CARTESIAN_POINT('Ctrl Pts',(27.0998913112301,-76.4277197750987,
16.5118599662324));
#258524=CARTESIAN_POINT('Ctrl Pts',(27.1003044177461,-76.4293303344044,
16.5074394214254));
#258525=CARTESIAN_POINT('Ctrl Pts',(27.1007652522506,-76.4311269686156,
16.5025081518939));
#258526=CARTESIAN_POINT('Ctrl Pts',(27.1011497779682,-76.4329400962105,
16.4972146189847));
#258527=CARTESIAN_POINT('Ctrl Pts',(27.1014658927446,-76.4347734735907,
16.4915299783456));
#258528=CARTESIAN_POINT('Ctrl Pts',(27.1017737851231,-76.4365591633602,
16.4859931997521));
#258529=CARTESIAN_POINT('Ctrl Pts',(27.1020168313413,-76.4383638558958,
16.4800869000299));
#258530=CARTESIAN_POINT('Ctrl Pts',(27.1022032687421,-76.4401848097576,
16.4738312942521));
#258531=CARTESIAN_POINT('Ctrl Pts',(27.1022139471165,-76.4402891065731,
16.4734729986491));
#258532=CARTESIAN_POINT('Ctrl Pts',(27.1022244071887,-76.4403934996852,
16.4731133067631));
#258533=CARTESIAN_POINT('Ctrl Pts',(27.102234658981,-76.4404979871097,16.4727522097143));
#258534=CARTESIAN_POINT('Ctrl Pts',(27.1024069987553,-76.4422544935438,
16.4666819166367));
#258535=CARTESIAN_POINT('Ctrl Pts',(27.1025185267331,-76.4439950495549,
16.4603561171173));
#258536=CARTESIAN_POINT('Ctrl Pts',(27.1026104632814,-76.4457036743809,
16.4538373746393));
#258537=CARTESIAN_POINT('Ctrl Pts',(27.102737424572,-76.4480632279764,16.4448352098468));
#258538=CARTESIAN_POINT('Ctrl Pts',(27.102827792657,-76.4503610778911,16.4354693321256));
#258539=CARTESIAN_POINT('Ctrl Pts',(27.1029292932916,-76.4525659495159,
16.4259934708457));
#258540=CARTESIAN_POINT('Ctrl Pts',(27.1029532015921,-76.4530853032462,
16.4237614479703));
#258541=CARTESIAN_POINT('Ctrl Pts',(27.1029775127231,-76.4535995663555,
16.421523398193));
#258542=CARTESIAN_POINT('Ctrl Pts',(27.1030025074321,-76.4541084615682,
16.4192825760479));
#258543=CARTESIAN_POINT('Ctrl Pts',(27.1030681316507,-76.4554445783686,
16.4133992428192));
#258544=CARTESIAN_POINT('Ctrl Pts',(27.1031446841667,-76.4567431182623,
16.4074886457421));
#258545=CARTESIAN_POINT('Ctrl Pts',(27.1032413604899,-76.4579907933282,
16.4016557321397));
#258546=CARTESIAN_POINT('Ctrl Pts',(27.1033489918153,-76.4593798503026,
16.3951618544127));
#258547=CARTESIAN_POINT('Ctrl Pts',(27.1034813066692,-76.4607059926544,
16.388764083027));
#258548=CARTESIAN_POINT('Ctrl Pts',(27.1036407248819,-76.461963664489,16.3825411897797));
#258549=CARTESIAN_POINT('Ctrl Pts',(27.1038110212171,-76.4633071553021,
16.375893668798));
#258550=CARTESIAN_POINT('Ctrl Pts',(27.1040119034733,-76.4645727497306,
16.3694449691171));
#258551=CARTESIAN_POINT('Ctrl Pts',(27.1042403347499,-76.4657643123006,
16.3632278932428));
#258552=CARTESIAN_POINT('Ctrl Pts',(27.1044944238694,-76.4670897134834,
16.3563125033811));
#258553=CARTESIAN_POINT('Ctrl Pts',(27.1047822483331,-76.4683237252368,
16.3496832123915));
#258554=CARTESIAN_POINT('Ctrl Pts',(27.1050982654298,-76.4694807356141,
16.343319207933));
#258555=CARTESIAN_POINT('Ctrl Pts',(27.105262880177,-76.4700834275971,16.3400041689821));
#258556=CARTESIAN_POINT('Ctrl Pts',(27.1054351610104,-76.4706653451591,
16.3367601359508));
#258557=CARTESIAN_POINT('Ctrl Pts',(27.1056146248408,-76.4712290854507,
16.333578829002));
#258558=CARTESIAN_POINT('Ctrl Pts',(27.1059981721683,-76.4724339024974,
16.326779788912));
#258559=CARTESIAN_POINT('Ctrl Pts',(27.1064227172635,-76.4735621804249,
16.3202525612503));
#258560=CARTESIAN_POINT('Ctrl Pts',(27.1068761143464,-76.4746356794987,
16.3138840528669));
#258561=CARTESIAN_POINT('Ctrl Pts',(27.1073854453231,-76.475841612118,16.3067298855434));
#258562=CARTESIAN_POINT('Ctrl Pts',(27.107931285444,-76.476978942591,16.2997754219255));
#258563=CARTESIAN_POINT('Ctrl Pts',(27.1085192024402,-76.4780834785054,
16.2927957451074));
#258564=CARTESIAN_POINT('Ctrl Pts',(27.1088920706866,-76.4787839963881,
16.2883691000673));
#258565=CARTESIAN_POINT('Ctrl Pts',(27.1092822986947,-76.47947138772,16.283931099016));
#258566=CARTESIAN_POINT('Ctrl Pts',(27.1096950709151,-76.4801541957116,
16.2794145606048));
#258567=CARTESIAN_POINT('Ctrl Pts',(27.1112272268462,-76.4826886887379,
16.2626497669182));
#258568=CARTESIAN_POINT('Ctrl Pts',(27.1130539331532,-76.4851267389767,
16.2450093231248));
#258569=CARTESIAN_POINT('Ctrl Pts',(27.1151298320358,-76.4873049749148,
16.226757619706));
#258570=CARTESIAN_POINT('Ctrl Pts',(27.1152747483161,-76.4874570352355,
16.225483487815));
#258571=CARTESIAN_POINT('Ctrl Pts',(27.1154208732589,-76.4876078246471,
16.2242063963108));
#258572=CARTESIAN_POINT('Ctrl Pts',(27.1155681889353,-76.48775728567,16.2229264434411));
#258573=CARTESIAN_POINT('Ctrl Pts',(27.1170756303587,-76.4892866798432,
16.2098290323389));
#258574=CARTESIAN_POINT('Ctrl Pts',(27.1186810485305,-76.4906357475266,
16.1965813349553));
#258575=CARTESIAN_POINT('Ctrl Pts',(27.1201639645387,-76.4917129534571,
16.1843381456719));
#258576=CARTESIAN_POINT('Ctrl Pts',(27.1209112758457,-76.4922558083237,
16.1781682252344));
#258577=CARTESIAN_POINT('Ctrl Pts',(27.1216272543498,-76.492729591696,16.1722544649754));
#258578=CARTESIAN_POINT('Ctrl Pts',(27.1222827006365,-76.4931225599098,
16.1667491490938));
#258579=CARTESIAN_POINT('Ctrl Pts',(27.1238077656216,-76.4940369019011,
16.153939610534));
#258580=CARTESIAN_POINT('Ctrl Pts',(27.1250450113581,-76.4945873630332,
16.1431163880602));
#258581=CARTESIAN_POINT('Ctrl Pts',(27.1260738037428,-76.4949373713663,
16.1336143833205));
#258582=CARTESIAN_POINT('Ctrl Pts',(27.1263523340118,-76.4950321309278,
16.131041856564));
#258583=CARTESIAN_POINT('Ctrl Pts',(27.1266156271271,-76.4951122560551,
16.1285658678582));
#258584=CARTESIAN_POINT('Ctrl Pts',(27.1268653384347,-76.4951810940983,
16.1261726495344));
#258585=CARTESIAN_POINT('Ctrl Pts',(27.1269115978525,-76.4951938464555,
16.125729302025));
#258586=CARTESIAN_POINT('Ctrl Pts',(27.1269574103529,-76.4952062293152,
16.1252887609781));
#258587=CARTESIAN_POINT('Ctrl Pts',(27.1270027817512,-76.4952182483237,
16.1248509868291));
#258588=CARTESIAN_POINT('Ctrl Pts',(28.7459974181806,74.3634602878982,19.6929518677509));
#258589=CARTESIAN_POINT('Ctrl Pts',(28.8447420032201,74.6189041648808,17.4625));
#258590=CARTESIAN_POINT('Ctrl Pts',(29.6549915892153,76.7149512087496,17.4625));
#258591=CARTESIAN_POINT('Ctrl Pts',(28.493917791474,74.4609043857737,19.6929518673248));
#258592=CARTESIAN_POINT('Ctrl Pts',(28.6971725259776,74.6660793405484,17.5374731486251));
#258593=CARTESIAN_POINT('Ctrl Pts',(29.4834701335382,76.6890525018674,17.4625));
#258594=CARTESIAN_POINT('Ctrl Pts',(28.2438591531039,74.5588475342798,19.6720320649347));
#258595=CARTESIAN_POINT('Ctrl Pts',(28.5391636116362,74.7189440966818,17.5981072780286));
#258596=CARTESIAN_POINT('Ctrl Pts',(29.3136797628433,76.6640386379029,17.4555267321205));
#258597=CARTESIAN_POINT('Ctrl Pts',(27.7480012895968,74.7559270342227,19.5871055664405));
#258598=CARTESIAN_POINT('Ctrl Pts',(28.2117119618052,74.8327386313722,17.6836912763758));
#258599=CARTESIAN_POINT('Ctrl Pts',(28.9778332725232,76.6159646173277,17.4272178998373));
#258600=CARTESIAN_POINT('Ctrl Pts',(27.4997703917934,74.8560677628264,19.5220948206211));
#258601=CARTESIAN_POINT('Ctrl Pts',(28.0404430900709,74.8942448729348,17.709632121867));
#258602=CARTESIAN_POINT('Ctrl Pts',(28.8101355628305,76.5926880471497,17.4055476509055));
#258603=CARTESIAN_POINT('Ctrl Pts',(27.0236898937082,75.0518439197725,19.3489695261652));
#258604=CARTESIAN_POINT('Ctrl Pts',(27.7022510777789,75.019660969593,17.7211023712242));
#258605=CARTESIAN_POINT('Ctrl Pts',(28.4896086814922,76.5500480485612,17.347839219523));
#258606=CARTESIAN_POINT('Ctrl Pts',(26.795355163397,75.1476280619454,19.2413577159505));
#258607=CARTESIAN_POINT('Ctrl Pts',(27.5347169152635,75.0836522525177,17.708077886913));
#258608=CARTESIAN_POINT('Ctrl Pts',(28.3364379275085,76.5306138623668,17.3119686156363));
#258609=CARTESIAN_POINT('Ctrl Pts',(26.4687756770162,75.2884389844461,19.0458961827317));
#258610=CARTESIAN_POINT('Ctrl Pts',(27.2898012152204,75.1803896028207,17.6578979817798));
#258611=CARTESIAN_POINT('Ctrl Pts',(28.1185099510301,76.5048922024807,17.2468147718754));
#258612=CARTESIAN_POINT('Ctrl Pts',(26.3625884843545,75.3348967090535,18.9750294801153));
#258613=CARTESIAN_POINT('Ctrl Pts',(27.209729060121,75.2125498005356,17.6363116935578));
#258614=CARTESIAN_POINT('Ctrl Pts',(28.0478532106456,76.4968949507142,17.2231925371365));
#258615=CARTESIAN_POINT('Ctrl Pts',(26.1560856941727,75.4268801209916,18.8208466626397));
#258616=CARTESIAN_POINT('Ctrl Pts',(27.0529295129826,75.2767579129753,17.5825320214165));
#258617=CARTESIAN_POINT('Ctrl Pts',(27.9109420608577,76.4822364493771,17.1717982652812));
#258618=CARTESIAN_POINT('Ctrl Pts',(26.055101076053,75.4727198166016,18.7368743964309));
#258619=CARTESIAN_POINT('Ctrl Pts',(26.9755857935394,75.3090585336016,17.5501254447857));
#258620=CARTESIAN_POINT('Ctrl Pts',(27.8442489434616,76.4755364557152,17.1438075095171));
#258621=CARTESIAN_POINT('Ctrl Pts',(25.7681502580856,75.6060560547219,18.4696518487122));
#258622=CARTESIAN_POINT('Ctrl Pts',(26.7557364160507,75.4030488168808,17.4386060175111));
#258623=CARTESIAN_POINT('Ctrl Pts',(27.6556756091732,76.4581861338644,17.054733327073));
#258624=CARTESIAN_POINT('Ctrl Pts',(25.5978466210046,75.689411859666,18.2718409363062));
#258625=CARTESIAN_POINT('Ctrl Pts',(26.6226482272615,75.4628679834582,17.3449978161555));
#258626=CARTESIAN_POINT('Ctrl Pts',(27.545042394829,76.4502012574522,16.9887963557568));
#258627=CARTESIAN_POINT('Ctrl Pts',(25.304207074627,75.8449254994659,17.8327278472497));
#258628=CARTESIAN_POINT('Ctrl Pts',(26.3945070907096,75.5732964352821,17.1202191600582));
#258629=CARTESIAN_POINT('Ctrl Pts',(27.3578956810266,76.4429196593756,16.8424253269279));
#258630=CARTESIAN_POINT('Ctrl Pts',(25.1799509742014,75.9179115378174,17.5873106315618));
#258631=CARTESIAN_POINT('Ctrl Pts',(26.2977761963289,75.6248510373174,16.9864091667271));
#258632=CARTESIAN_POINT('Ctrl Pts',(27.2809002299547,76.443787857136,16.7606195878724));
#258633=CARTESIAN_POINT('Ctrl Pts',(25.0456540278887,76.0120135407792,17.2025309630928));
#258634=CARTESIAN_POINT('Ctrl Pts',(26.1964580005439,75.6888631781817,16.7690050915924));
#258635=CARTESIAN_POINT('Ctrl Pts',(27.2023521345518,76.4531141362212,16.6323596984796));
#258636=CARTESIAN_POINT('Ctrl Pts',(25.0090870943394,76.0410349984119,17.0710669460338));
#258637=CARTESIAN_POINT('Ctrl Pts',(26.1695156242376,75.7081633852743,16.6936245453245));
#258638=CARTESIAN_POINT('Ctrl Pts',(27.182007572472,76.4575269782804,16.5885383593542));
#258639=CARTESIAN_POINT('Ctrl Pts',(24.9530103267656,76.0942893550643,16.8014952531469));
#258640=CARTESIAN_POINT('Ctrl Pts',(26.1301341325897,75.7423750031978,16.5376305767308));
#258641=CARTESIAN_POINT('Ctrl Pts',(27.153493597573,76.4691181075126,16.4986811285387));
#258642=CARTESIAN_POINT('Ctrl Pts',(24.9335061597312,76.118653951028,16.6623540419173));
#258643=CARTESIAN_POINT('Ctrl Pts',(26.1176802211114,75.7573877351394,16.4562866616969));
#258644=CARTESIAN_POINT('Ctrl Pts',(27.145369143004,76.4763708127814,16.4523007247639));
#258645=CARTESIAN_POINT('Ctrl Pts',(24.9029553648553,76.1824010629019,16.2463425041047));
#258646=CARTESIAN_POINT('Ctrl Pts',(26.1038934519123,75.7942282194368,16.2122544249953));
#258647=CARTESIAN_POINT('Ctrl Pts',(27.140495466855,76.5018384532045,16.3136302120344));
#258648=CARTESIAN_POINT('Ctrl Pts',(24.9185412707801,76.2131904009613,15.9685880799943));
#258649=CARTESIAN_POINT('Ctrl Pts',(26.1252772492172,75.8084359405689,16.047561016401));
#258650=CARTESIAN_POINT('Ctrl Pts',(27.16243135285,76.5237673449954,16.2210111173688));
#258651=CARTESIAN_POINT('Ctrl Pts',(24.968955626549,76.2326069140441,15.690505851385));
#258652=CARTESIAN_POINT('Ctrl Pts',(26.1756393943756,75.8121214408373,15.8859547915794));
#258653=CARTESIAN_POINT('Ctrl Pts',(27.2087011009323,76.55044485681,16.128351327878));
#258654=CARTESIAN_POINT('',(25.2552738567446,75.9418613629793,17.263393070432));
#258655=CARTESIAN_POINT('Ctrl Pts',(27.127002665508,76.4952182372903,16.1248510388561));
#258656=CARTESIAN_POINT('Ctrl Pts',(27.1261035938164,76.4949835330533,16.1335301302458));
#258657=CARTESIAN_POINT('Ctrl Pts',(27.1250175086501,76.4945938617303,16.1433840167243));
#258658=CARTESIAN_POINT('Ctrl Pts',(27.123665198262,76.4938946426406,16.1550166230771));
#258659=CARTESIAN_POINT('Ctrl Pts',(27.1234107356406,76.4937630714244,16.1572055166426));
#258660=CARTESIAN_POINT('Ctrl Pts',(27.1231468673298,76.4936205663255,16.1594572469111));
#258661=CARTESIAN_POINT('Ctrl Pts',(27.1228730977779,76.4934661405611,16.1617756125053));
#258662=CARTESIAN_POINT('Ctrl Pts',(27.1215904130496,76.4927426139001,16.1726377851693));
#258663=CARTESIAN_POINT('Ctrl Pts',(27.1200357216248,76.4916920130601,16.1853170892971));
#258664=CARTESIAN_POINT('Ctrl Pts',(27.1184437830616,76.490384797411,16.1985845365846));
#258665=CARTESIAN_POINT('Ctrl Pts',(27.117737169702,76.4898045639378,16.2044735549916));
#258666=CARTESIAN_POINT('Ctrl Pts',(27.1170231040063,76.4891738033028,16.2104789373948));
#258667=CARTESIAN_POINT('Ctrl Pts',(27.116321332041,76.4884987572042,16.2164967943271));
#258668=CARTESIAN_POINT('Ctrl Pts',(27.1144314500939,76.4866808483987,16.2327029691798));
#258669=CARTESIAN_POINT('Ctrl Pts',(27.1126943705541,76.4846005967037,16.2486914456544));
#258670=CARTESIAN_POINT('Ctrl Pts',(27.1111721910307,76.4824017848996,16.2640972093815));
#258671=CARTESIAN_POINT('Ctrl Pts',(27.1106324721751,76.4816221526864,16.2695596276057));
#258672=CARTESIAN_POINT('Ctrl Pts',(27.1101196624085,76.4808275267706,16.2749492144068));
#258673=CARTESIAN_POINT('Ctrl Pts',(27.1096361423658,76.4800239584187,16.2802512670947));
#258674=CARTESIAN_POINT('Ctrl Pts',(27.1088775098608,76.4787631770283,16.2885700732594));
#258675=CARTESIAN_POINT('Ctrl Pts',(27.1081924682396,76.4774861247342,16.2966391164468));
#258676=CARTESIAN_POINT('Ctrl Pts',(27.1075731179875,76.4761760059671,16.3046343846518));
#258677=CARTESIAN_POINT('Ctrl Pts',(27.1070239809311,76.4750144099865,16.3117232621208));
#258678=CARTESIAN_POINT('Ctrl Pts',(27.1065264227125,76.4738263115708,16.3187548885504));
#258679=CARTESIAN_POINT('Ctrl Pts',(27.1060881023887,76.4726008566093,16.3258128070659));
#258680=CARTESIAN_POINT('Ctrl Pts',(27.1060320583278,76.4724441687516,16.32671523936));
#258681=CARTESIAN_POINT('Ctrl Pts',(27.1059770032823,76.4722868770211,16.3276180342443));
#258682=CARTESIAN_POINT('Ctrl Pts',(27.1059229723675,76.4721289660875,16.3285213027847));
#258683=CARTESIAN_POINT('Ctrl Pts',(27.1055132758118,76.4709315855521,16.3353704559359));
#258684=CARTESIAN_POINT('Ctrl Pts',(27.1051480063883,76.469686098804,16.3423105850976));
#258685=CARTESIAN_POINT('Ctrl Pts',(27.1048249982592,76.4683756379668,16.3494047007489));
#258686=CARTESIAN_POINT('Ctrl Pts',(27.1045238256014,76.4671537647759,16.356019251509));
#258687=CARTESIAN_POINT('Ctrl Pts',(27.1042596511139,76.4658752319034,16.3627681883452));
#258688=CARTESIAN_POINT('Ctrl Pts',(27.1040326825539,76.4645307210473,16.3696623273304));
#258689=CARTESIAN_POINT('Ctrl Pts',(27.1038205223615,76.4632739316405,16.3761066641726));
#258690=CARTESIAN_POINT('Ctrl Pts',(27.1036411260678,76.4619593190114,16.3826784026799));
#258691=CARTESIAN_POINT('Ctrl Pts',(27.1034929209303,76.4605856089528,16.3893426844219));
#258692=CARTESIAN_POINT('Ctrl Pts',(27.1033578602482,76.4593337345533,16.3954159046419));
#258693=CARTESIAN_POINT('Ctrl Pts',(27.1032489151461,76.4580326598448,16.4015662355624));
#258694=CARTESIAN_POINT('Ctrl Pts',(27.1031602607466,76.4566888072072,16.4077247899965));
#258695=CARTESIAN_POINT('Ctrl Pts',(27.1031225010715,76.4561164335946,16.4103478410299));
#258696=CARTESIAN_POINT('Ctrl Pts',(27.1030883438957,76.4555364067326,16.4129718046109));
#258697=CARTESIAN_POINT('Ctrl Pts',(27.1030568879016,76.4549497809939,16.4155884735622));
#258698=CARTESIAN_POINT('Ctrl Pts',(27.1029432081665,76.4528297571237,16.4250449298201));
#258699=CARTESIAN_POINT('Ctrl Pts',(27.1028516325163,76.450627615447,16.4344055618827));
#258700=CARTESIAN_POINT('Ctrl Pts',(27.1027493830592,76.448361853143,16.4434727015646));
#258701=CARTESIAN_POINT('Ctrl Pts',(27.1027301154644,76.4479348993861,16.4451812873881));
#258702=CARTESIAN_POINT('Ctrl Pts',(27.1027103529397,76.4475057389387,16.4468793703434));
#258703=CARTESIAN_POINT('Ctrl Pts',(27.1026896905071,76.4470745680889,16.4485655884623));
#258704=CARTESIAN_POINT('Ctrl Pts',(27.1026199427357,76.4456191147826,16.4542575589124));
#258705=CARTESIAN_POINT('Ctrl Pts',(27.1025406532748,76.4441322040591,16.4598473134706));
#258706=CARTESIAN_POINT('Ctrl Pts',(27.1024250918518,76.4426004684727,16.4653566991224));
#258707=CARTESIAN_POINT('Ctrl Pts',(27.1023811860632,76.4420185090524,16.4674499056184));
#258708=CARTESIAN_POINT('Ctrl Pts',(27.1023318496943,76.4414302186201,16.4695309610912));
#258709=CARTESIAN_POINT('Ctrl Pts',(27.1022746925428,76.4408353908689,16.4715995364473));
#258710=CARTESIAN_POINT('Ctrl Pts',(27.1020976108819,76.4389925228555,16.4780083015884));
#258711=CARTESIAN_POINT('Ctrl Pts',(27.1018561048147,76.4370710585111,16.4843917801369));
#258712=CARTESIAN_POINT('Ctrl Pts',(27.1015158539155,76.4350620986625,16.4906542061495));
#258713=CARTESIAN_POINT('Ctrl Pts',(27.1012261996205,76.4333518787932,16.4959853855679));
#258714=CARTESIAN_POINT('Ctrl Pts',(27.1008647151577,76.4315790441127,16.5012232667857));
#258715=CARTESIAN_POINT('Ctrl Pts',(27.1004038747161,76.4297403585919,16.5063087804329));
#258716=CARTESIAN_POINT('Ctrl Pts',(27.1000801964374,76.4284489299087,16.509880668131));
#258717=CARTESIAN_POINT('Ctrl Pts',(27.0997073598869,76.4271251515631,16.5133767163781));
#258718=CARTESIAN_POINT('Ctrl Pts',(27.0992746306603,76.425765087242,16.5168023194537));
#258719=CARTESIAN_POINT('Ctrl Pts',(27.0988720744426,76.4244998564341,16.519989064727));
#258720=CARTESIAN_POINT('Ctrl Pts',(27.0984176364788,76.4232033943528,16.5231136244741));
#258721=CARTESIAN_POINT('Ctrl Pts',(27.0979025055475,76.4218676567943,16.5262197343075));
#258722=CARTESIAN_POINT('Ctrl Pts',(27.0978682970957,76.4217789540758,16.5264260026604));
#258723=CARTESIAN_POINT('Ctrl Pts',(27.0978338210948,76.4216900756685,16.526632209209));
#258724=CARTESIAN_POINT('Ctrl Pts',(27.097799075025,76.4216010180793,16.526838375666));
#258725=CARTESIAN_POINT('Ctrl Pts',(27.0976706878967,76.4212719492612,16.5276001631009));
#258726=CARTESIAN_POINT('Ctrl Pts',(27.0975386143428,76.4209404362559,16.5283613866249));
#258727=CARTESIAN_POINT('Ctrl Pts',(27.0974027448545,76.4206063221397,16.5291232096043));
#258728=CARTESIAN_POINT('Ctrl Pts',(27.0966347185492,76.4187176830239,16.5334295486912));
#258729=CARTESIAN_POINT('Ctrl Pts',(27.0957491893792,76.4167566024538,16.5376614539927));
#258730=CARTESIAN_POINT('Ctrl Pts',(27.0947257635409,76.4147290835896,16.5417599887933));
#258731=CARTESIAN_POINT('Ctrl Pts',(27.0938722704172,76.413038220076,16.5451779905074));
#258732=CARTESIAN_POINT('Ctrl Pts',(27.0929228022934,76.4113012291909,16.5485028097945));
#258733=CARTESIAN_POINT('Ctrl Pts',(27.0918686181525,76.4095163162474,16.5517348365881));
#258734=CARTESIAN_POINT('Ctrl Pts',(27.091005746766,76.4080553283169,16.5543803169481));
#258735=CARTESIAN_POINT('Ctrl Pts',(27.0900727246007,76.4065622115715,16.556963800446));
#258736=CARTESIAN_POINT('Ctrl Pts',(27.0890672853592,76.4050319318825,16.559511402248));
#258737=CARTESIAN_POINT('Ctrl Pts',(27.0873467993626,76.4024133502048,16.5638708036362));
#258738=CARTESIAN_POINT('Ctrl Pts',(27.0854160305322,76.3996858222801,16.5681213015847));
#258739=CARTESIAN_POINT('Ctrl Pts',(27.0832453437824,76.3968549739074,16.5722001453423));
#258740=CARTESIAN_POINT('Ctrl Pts',(27.0814237924483,76.3944794420026,16.5756229438131));
#258741=CARTESIAN_POINT('Ctrl Pts',(27.079433200762,76.3920312477983,16.5789244111505));
#258742=CARTESIAN_POINT('Ctrl Pts',(27.0772609129556,76.3895078513819,16.5821034643305));
#258743=CARTESIAN_POINT('Ctrl Pts',(27.0758841940319,76.387908612281,16.5841182354208));
#258744=CARTESIAN_POINT('Ctrl Pts',(27.0744345916962,76.386279051961,16.5860845447345));
#258745=CARTESIAN_POINT('Ctrl Pts',(27.0729104400646,76.3846166914253,16.5880130337727));
#258746=CARTESIAN_POINT('Ctrl Pts',(27.0711860864439,76.3827359747372,16.5901948357581));
#258747=CARTESIAN_POINT('Ctrl Pts',(27.0694154757831,76.3808666413301,16.5922669270651));
#258748=CARTESIAN_POINT('Ctrl Pts',(27.0676055223491,76.3790011612981,16.594274231033));
#258749=CARTESIAN_POINT('Ctrl Pts',(27.0627975216168,76.3740456584708,16.5996064781316));
#258750=CARTESIAN_POINT('Ctrl Pts',(27.0577058759418,76.3691274276556,16.6044118919307));
#258751=CARTESIAN_POINT('Ctrl Pts',(27.0523503507023,76.3642377230734,16.6087783050431));
#258752=CARTESIAN_POINT('Ctrl Pts',(27.0469199087826,76.3592796180229,16.6132057984716));
#258753=CARTESIAN_POINT('Ctrl Pts',(27.0412180804719,76.3543509085699,16.6171815871685));
#258754=CARTESIAN_POINT('Ctrl Pts',(27.0352768340208,76.3494322419913,16.6208506593392));
#258755=CARTESIAN_POINT('Ctrl Pts',(27.0293355875697,76.3445135754128,16.62451973151));
#258756=CARTESIAN_POINT('Ctrl Pts',(27.023154884461,76.3396049868135,16.6278819111735));
#258757=CARTESIAN_POINT('Ctrl Pts',(27.0167787754247,76.3346762337737,16.6311389170594));
#258758=CARTESIAN_POINT('Ctrl Pts',(27.0069163699815,76.3270525622631,16.6361767720262));
#258759=CARTESIAN_POINT('Ctrl Pts',(26.9965742763248,76.3193994276041,16.6408622418876));
#258760=CARTESIAN_POINT('Ctrl Pts',(26.9857761531869,76.3117344496284,16.6452464533288));
#258761=CARTESIAN_POINT('Ctrl Pts',(26.9797217361569,76.3074367607988,16.6477046438934));
#258762=CARTESIAN_POINT('Ctrl Pts',(26.9735241809076,76.3031351576516,16.6500689942496));
#258763=CARTESIAN_POINT('Ctrl Pts',(26.9671894394028,76.2988312337076,16.6523553297694));
#258764=CARTESIAN_POINT('Ctrl Pts',(26.9465400268522,76.284801695006,16.6598081177547));
#258765=CARTESIAN_POINT('Ctrl Pts',(26.9253146403767,76.2713420389522,16.6661261478315));
#258766=CARTESIAN_POINT('Ctrl Pts',(26.903785416654,76.2582666976198,16.6722817468509));
#258767=CARTESIAN_POINT('Ctrl Pts',(26.8683021506494,76.2367166491567,16.6824270618998));
#258768=CARTESIAN_POINT('Ctrl Pts',(26.8318654947013,76.2163231723991,16.6915805494964));
#258769=CARTESIAN_POINT('Ctrl Pts',(26.7948177265923,76.1969868423419,16.7005093018421));
#258770=CARTESIAN_POINT('Ctrl Pts',(26.7912042242594,76.1951008481959,16.7013801793356));
#258771=CARTESIAN_POINT('Ctrl Pts',(26.7875849267253,76.1932248857004,16.7022489427428));
#258772=CARTESIAN_POINT('Ctrl Pts',(26.7839601625922,76.1913588468472,16.7031163158091));
#258773=CARTESIAN_POINT('Ctrl Pts',(26.7552291255565,76.1765680275177,16.7099913914764));
#258774=CARTESIAN_POINT('Ctrl Pts',(26.7262008738658,76.162413994639,16.7168106960652));
#258775=CARTESIAN_POINT('Ctrl Pts',(26.696973285445,76.1489165164747,16.7235973395635));
#258776=CARTESIAN_POINT('Ctrl Pts',(26.6422867919015,76.1236619610232,16.7362955386249));
#258777=CARTESIAN_POINT('Ctrl Pts',(26.5866819737713,76.1005180681597,16.7491519989711));
#258778=CARTESIAN_POINT('Ctrl Pts',(26.5302810836122,76.0794074083457,16.7625435721042));
#258779=CARTESIAN_POINT('Ctrl Pts',(26.4900870715386,76.0643629274333,16.7720870571569));
#258780=CARTESIAN_POINT('Ctrl Pts',(26.449488380492,76.05035210642,16.7819023270163));
#258781=CARTESIAN_POINT('Ctrl Pts',(26.4085292238118,76.0373611942064,16.792133601287));
#258782=CARTESIAN_POINT('Ctrl Pts',(26.363792032232,76.0231720122115,16.8033085988761));
#258783=CARTESIAN_POINT('Ctrl Pts',(26.3190310002086,76.0103384192572,16.814845407717));
#258784=CARTESIAN_POINT('Ctrl Pts',(26.2743222514893,75.998785045632,16.826926246751));
#258785=CARTESIAN_POINT('Ctrl Pts',(26.216135189131,75.9837486849458,16.8426490874556));
#258786=CARTESIAN_POINT('Ctrl Pts',(26.1575989600244,75.9708594776047,16.859231106798));
#258787=CARTESIAN_POINT('Ctrl Pts',(26.0990044705915,75.9600230530952,16.8768965952897));
#258788=CARTESIAN_POINT('Ctrl Pts',(26.0404710852013,75.9491979291252,16.8945436616947));
#258789=CARTESIAN_POINT('Ctrl Pts',(25.9818779785369,75.9404214117304,16.9132712882681));
#258790=CARTESIAN_POINT('Ctrl Pts',(25.9235033740623,75.9336439589075,16.9333228296305));
#258791=CARTESIAN_POINT('Ctrl Pts',(25.8876307737383,75.9294790509219,16.9456449847123));
#258792=CARTESIAN_POINT('Ctrl Pts',(25.851840554364,75.9260699331781,16.9584675280423));
#258793=CARTESIAN_POINT('Ctrl Pts',(25.8161989866991,75.9234132458693,16.9718522765856));
#258794=CARTESIAN_POINT('Ctrl Pts',(25.7935358469298,75.9217239577783,16.9803631375517));
#258795=CARTESIAN_POINT('Ctrl Pts',(25.7708904059767,75.9203357066724,16.9891192993487));
#258796=CARTESIAN_POINT('Ctrl Pts',(25.7483106633367,75.9192531417285,16.9981274246413));
#258797=CARTESIAN_POINT('Ctrl Pts',(25.7019366327795,75.917029781587,17.0166282146742));
#258798=CARTESIAN_POINT('Ctrl Pts',(25.6557154304738,75.916090887903,17.0360687208733));
#258799=CARTESIAN_POINT('Ctrl Pts',(25.6100335198526,75.9163356254776,17.056834669412));
#258800=CARTESIAN_POINT('Ctrl Pts',(25.5677572967879,75.9165621173243,17.0760524705204));
#258801=CARTESIAN_POINT('Ctrl Pts',(25.5259435981048,75.9178014945631,17.0964068029014));
#258802=CARTESIAN_POINT('Ctrl Pts',(25.4848871406365,75.9199460216331,17.1181763512532));
#258803=CARTESIAN_POINT('Ctrl Pts',(25.4448430528779,75.9220376689764,17.1394091063037));
#258804=CARTESIAN_POINT('Ctrl Pts',(25.4055198688358,75.9249898990354,17.1619892997284));
#258805=CARTESIAN_POINT('Ctrl Pts',(25.3671710062583,75.9286842189098,17.1861307294728));
#258806=CARTESIAN_POINT('Ctrl Pts',(25.3326536301789,75.932009434311,17.2078601564642));
#258807=CARTESIAN_POINT('Ctrl Pts',(25.2989256360752,75.9359354286627,17.2308544603867));
#258808=CARTESIAN_POINT('Ctrl Pts',(25.2661521621818,75.9403670676029,17.2552262516159));
#258809=CARTESIAN_POINT('Ctrl Pts',(25.2625142517442,75.9408589869402,17.2579315612203));
#258810=CARTESIAN_POINT('Ctrl Pts',(25.2588880803261,75.9413571303185,17.2606537952043));
#258811=CARTESIAN_POINT('Ctrl Pts',(25.2552738568381,75.9418613633423,17.2633930704885));
#258812=CARTESIAN_POINT('Ctrl Pts',(25.2552738568381,75.9418613633423,17.2633930704885));
#258813=CARTESIAN_POINT('Ctrl Pts',(25.2383250955439,75.9442259477243,17.2762387760009));
#258814=CARTESIAN_POINT('Ctrl Pts',(25.2219501076014,75.9466297979497,17.2896217176795));
#258815=CARTESIAN_POINT('Ctrl Pts',(25.2063620808563,75.9489416166713,17.3037656232924));
#258816=CARTESIAN_POINT('Ctrl Pts',(25.1906119975066,75.9512774695763,17.3180565721045));
#258817=CARTESIAN_POINT('Ctrl Pts',(25.1756652588064,75.9535194008814,17.3331243157626));
#258818=CARTESIAN_POINT('Ctrl Pts',(25.1617083521129,75.9555501186536,17.3491621101996));
#258819=CARTESIAN_POINT('Ctrl Pts',(25.1475411611284,75.9576114326071,17.3654415410039));
#258820=CARTESIAN_POINT('Ctrl Pts',(25.1343938078986,75.9594551436918,17.3827204208315));
#258821=CARTESIAN_POINT('Ctrl Pts',(25.1224278840864,75.9609767648295,17.4011633324362));
#258822=CARTESIAN_POINT('Ctrl Pts',(25.12105367141,75.9611515136486,17.4032813872821));
#258823=CARTESIAN_POINT('Ctrl Pts',(25.1196950054388,75.9613220335946,17.4054147550736));
#258824=CARTESIAN_POINT('Ctrl Pts',(25.1183521036895,75.9614881812303,17.4075636545405));
#258825=CARTESIAN_POINT('Origin',(29.6549915892153,76.7149512087495,20.0025));
#258826=CARTESIAN_POINT('Origin',(0.,0.,20.0025));
#258827=CARTESIAN_POINT('Origin',(76.7149512087496,29.6549915892152,20.0025));
#258828=CARTESIAN_POINT('Ctrl Pts',(76.2270397428134,24.9561066903835,15.7661615844266));
#258829=CARTESIAN_POINT('Ctrl Pts',(75.8108535386762,26.1626160164788,15.9301351099137));
#258830=CARTESIAN_POINT('Ctrl Pts',(76.5433020278671,27.1967142373006,16.1535699055586));
#258831=CARTESIAN_POINT('Ctrl Pts',(76.2058614110631,24.9127382418325,16.0399812791097));
#258832=CARTESIAN_POINT('Ctrl Pts',(75.8053384807186,26.1182670027238,16.0896762568481));
#258833=CARTESIAN_POINT('Ctrl Pts',(76.517885002826,27.1555364032829,16.2448123919216));
#258834=CARTESIAN_POINT('Ctrl Pts',(76.1737533047141,24.9032085414216,16.3126628275193));
#258835=CARTESIAN_POINT('Ctrl Pts',(75.7896805171524,26.1022033001563,16.2513677269997));
#258836=CARTESIAN_POINT('Ctrl Pts',(76.4971501245561,27.1380437449529,16.3357369865075));
#258837=CARTESIAN_POINT('Ctrl Pts',(76.1088055482311,24.9409015162127,16.7198279320328));
#258838=CARTESIAN_POINT('Ctrl Pts',(75.751382754071,26.1222593418385,16.4898842731734));
#258839=CARTESIAN_POINT('Ctrl Pts',(76.4732843611527,27.1482624002493,16.4714586881349));
#258840=CARTESIAN_POINT('Ctrl Pts',(76.0840986821809,24.9625025815324,16.8562699832887));
#258841=CARTESIAN_POINT('Ctrl Pts',(75.7359563155035,26.1365526017809,16.5694930915592));
#258842=CARTESIAN_POINT('Ctrl Pts',(76.4665075541088,27.1579592507432,16.5169393719347));
#258843=CARTESIAN_POINT('Ctrl Pts',(76.0302035557089,25.0223408867823,17.1211357027625));
#258844=CARTESIAN_POINT('Ctrl Pts',(75.7010090395948,26.1792011664334,16.7223674157641));
#258845=CARTESIAN_POINT('Ctrl Pts',(76.4557551903463,27.189285584288,16.6052279449151));
#258846=CARTESIAN_POINT('Ctrl Pts',(76.0009882041842,25.0604718640614,17.2500386492964));
#258847=CARTESIAN_POINT('Ctrl Pts',(75.6814529502716,26.2075059010005,16.7960334331997));
#258848=CARTESIAN_POINT('Ctrl Pts',(76.4517310112362,27.2108217423656,16.6481955938982));
#258849=CARTESIAN_POINT('Ctrl Pts',(75.9067264066431,25.198342960339,17.6266213749776));
#258850=CARTESIAN_POINT('Ctrl Pts',(75.617033261059,26.3119626202797,17.0080082070259));
#258851=CARTESIAN_POINT('Ctrl Pts',(76.4434487742633,27.2921796118939,16.7737231689762));
#258852=CARTESIAN_POINT('Ctrl Pts',(75.8341334517195,25.3235144045994,17.8663209238626));
#258853=CARTESIAN_POINT('Ctrl Pts',(75.5656656095422,26.4095014785168,17.138034603396));
#258854=CARTESIAN_POINT('Ctrl Pts',(76.443086689911,27.3700274901018,16.8536230191253));
#258855=CARTESIAN_POINT('Ctrl Pts',(75.6793115466567,25.6181437847437,18.2967865872453));
#258856=CARTESIAN_POINT('Ctrl Pts',(75.4556558389512,26.6384413152297,17.3570330067414));
#258857=CARTESIAN_POINT('Ctrl Pts',(76.4510616926957,27.5581771453565,16.9971115727434));
#258858=CARTESIAN_POINT('Ctrl Pts',(75.5964910133644,25.7881636116429,18.4907575655788));
#258859=CARTESIAN_POINT('Ctrl Pts',(75.3962436041948,26.7712230598584,17.4481057023255));
#258860=CARTESIAN_POINT('Ctrl Pts',(76.4592507908039,27.6687468882713,17.0617685660245));
#258861=CARTESIAN_POINT('Ctrl Pts',(75.4201247071596,26.1689222277689,18.8401402132359));
#258862=CARTESIAN_POINT('Ctrl Pts',(75.2714903396935,27.063945082347,17.5930975378977));
#258863=CARTESIAN_POINT('Ctrl Pts',(76.482579458453,27.9191372577337,17.1782294484131));
#258864=CARTESIAN_POINT('Ctrl Pts',(75.3287012831505,26.3751256473571,18.9911133259122));
#258865=CARTESIAN_POINT('Ctrl Pts',(75.2073607607574,27.2212827369394,17.6447564223772));
#258866=CARTESIAN_POINT('Ctrl Pts',(76.4974527826309,28.0559817658927,17.2285538196831));
#258867=CARTESIAN_POINT('Ctrl Pts',(75.1416312561383,26.8095530404412,19.2484985828626));
#258868=CARTESIAN_POINT('Ctrl Pts',(75.0796306617783,27.5451541663913,17.709236776907));
#258869=CARTESIAN_POINT('Ctrl Pts',(76.5318000250945,28.3459497946491,17.3143489047412));
#258870=CARTESIAN_POINT('Ctrl Pts',(75.0448154219373,27.0405974954697,19.3560977072767));
#258871=CARTESIAN_POINT('Ctrl Pts',(75.0150709808039,27.7144253322462,17.7214394194467));
#258872=CARTESIAN_POINT('Ctrl Pts',(76.551521599115,28.5009695287673,17.3502152802456));
#258873=CARTESIAN_POINT('Ctrl Pts',(74.7540920556819,27.7481365991003,19.6103581821464));
#258874=CARTESIAN_POINT('Ctrl Pts',(74.8268871764671,28.2225181462175,17.7018269936053));
#258875=CARTESIAN_POINT('Ctrl Pts',(76.6150183791995,28.9773980402713,17.4349687706577));
#258876=CARTESIAN_POINT('Ctrl Pts',(74.5573270579655,28.2444805055458,19.6929518696644));
#258877=CARTESIAN_POINT('Ctrl Pts',(74.7114471924104,28.5552565684103,17.6095740109439));
#258878=CARTESIAN_POINT('Ctrl Pts',(76.6634338736826,29.3138035781366,17.4625));
#258879=CARTESIAN_POINT('Ctrl Pts',(74.3634602878982,28.7459974181806,19.6929518677509));
#258880=CARTESIAN_POINT('Ctrl Pts',(74.6189041648808,28.8447420032201,17.4625));
#258881=CARTESIAN_POINT('Ctrl Pts',(76.7149512087496,29.6549915892152,17.4625));
#258882=CARTESIAN_POINT('',(75.9418613907131,25.2552738638853,17.2633930747485));
#258883=CARTESIAN_POINT('Ctrl Pts',(75.9614888783998,25.1183464686498,17.4075726719158));
#258884=CARTESIAN_POINT('Ctrl Pts',(75.9600468328487,25.1300023941469,17.3889199736803));
#258885=CARTESIAN_POINT('Ctrl Pts',(75.9582739286019,25.1428486640187,17.3714404189718));
#258886=CARTESIAN_POINT('Ctrl Pts',(75.956271615219,25.1567289812122,17.3549752069932));
#258887=CARTESIAN_POINT('Ctrl Pts',(75.9542910924864,25.1704582425619,17.3386891815889));
#258888=CARTESIAN_POINT('Ctrl Pts',(75.952086092421,25.1851992333012,17.3233956168879));
#258889=CARTESIAN_POINT('Ctrl Pts',(75.9497720847174,25.2007688946097,17.3089051461458));
#258890=CARTESIAN_POINT('Ctrl Pts',(75.9474908499987,25.2161180448657,17.2946199020231));
#258891=CARTESIAN_POINT('Ctrl Pts',(75.945103652396,25.2322726009112,17.2811152127705));
#258892=CARTESIAN_POINT('Ctrl Pts',(75.9427384198447,25.2490253201792,17.2681738831956));
#258893=CARTESIAN_POINT('Ctrl Pts',(75.9424456215465,25.251099182933,17.2665718422994));
#258894=CARTESIAN_POINT('Ctrl Pts',(75.9421531821386,25.2531821712323,17.2649783885439));
#258895=CARTESIAN_POINT('Ctrl Pts',(75.9418613633423,25.2552738568381,17.2633930704886));
#258896=CARTESIAN_POINT('',(76.4940243385606,27.123919681122,16.1529193687788));
#258897=CARTESIAN_POINT('Ctrl Pts',(75.9418614454548,25.2552738779798,17.2633930832684));
#258898=CARTESIAN_POINT('Ctrl Pts',(75.9365384120977,25.2934285134618,17.2344751189325));
#258899=CARTESIAN_POINT('Ctrl Pts',(75.9319214636048,25.332694849713,17.2076986349233));
#258900=CARTESIAN_POINT('Ctrl Pts',(75.9281351401283,25.3728650680937,17.1826763946697));
#258901=CARTESIAN_POINT('Ctrl Pts',(75.9242738575013,25.4138305501284,17.1571587805044));
#258902=CARTESIAN_POINT('Ctrl Pts',(75.921276377852,25.4557366826118,17.1334650775218));
#258903=CARTESIAN_POINT('Ctrl Pts',(75.919265820559,25.4983989473329,17.1112236978224));
#258904=CARTESIAN_POINT('Ctrl Pts',(75.9172478169732,25.5412192158649,17.0888999450288));
#258905=CARTESIAN_POINT('Ctrl Pts',(75.9162240339414,25.5848018402272,17.0680389986439));
#258906=CARTESIAN_POINT('Ctrl Pts',(75.9163105407607,25.6289865102456,17.0483098578789));
#258907=CARTESIAN_POINT('Ctrl Pts',(75.9163971000492,25.6731979796606,17.0285687507676));
#258908=CARTESIAN_POINT('Ctrl Pts',(75.9175953146014,25.7180127240943,17.009960645641));
#258909=CARTESIAN_POINT('Ctrl Pts',(75.9200131196572,25.7632880277473,16.9922021492894));
#258910=CARTESIAN_POINT('Ctrl Pts',(75.9208133176951,25.7782723661501,16.9863247879602));
#258911=CARTESIAN_POINT('Ctrl Pts',(75.9217470339365,25.7933072658459,16.9805408907029));
#258912=CARTESIAN_POINT('Ctrl Pts',(75.92281796933,25.8083878526028,16.9748413874889));
#258913=CARTESIAN_POINT('Ctrl Pts',(75.9266539103138,25.8624044078057,16.9544265631223));
#258914=CARTESIAN_POINT('Ctrl Pts',(75.9321927734631,25.9166410369771,16.9353703453911));
#258915=CARTESIAN_POINT('Ctrl Pts',(75.939475260865,25.970905038449,16.9174202920556));
#258916=CARTESIAN_POINT('Ctrl Pts',(75.9468216077909,26.0256448764201,16.8993128362008));
#258917=CARTESIAN_POINT('Ctrl Pts',(75.9559423034969,26.0804129308954,16.8823309775028));
#258918=CARTESIAN_POINT('Ctrl Pts',(75.966865448933,26.1350308076104,16.8662635483136));
#258919=CARTESIAN_POINT('Ctrl Pts',(75.9779822941092,26.1906172211435,16.849911195988));
#258920=CARTESIAN_POINT('Ctrl Pts',(75.990966169439,26.2460483691195,16.8345059849871));
#258921=CARTESIAN_POINT('Ctrl Pts',(76.0058318119529,26.3011513056163,16.8198753596885));
#258922=CARTESIAN_POINT('Ctrl Pts',(76.0144317203761,26.3330288519297,16.8114114108466));
#258923=CARTESIAN_POINT('Ctrl Pts',(76.0236611245447,26.3647968075541,16.8032076252318));
#258924=CARTESIAN_POINT('Ctrl Pts',(76.0335204515053,26.3964234203472,16.7952379320009));
#258925=CARTESIAN_POINT('Ctrl Pts',(76.0465904882018,26.4383493034671,16.7846728920742));
#258926=CARTESIAN_POINT('Ctrl Pts',(76.0607989879201,26.4801552170103,16.7745161348116));
#258927=CARTESIAN_POINT('Ctrl Pts',(76.076181153933,26.5217114878631,16.7646135070096));
#258928=CARTESIAN_POINT('Ctrl Pts',(76.0919178815735,26.564225638056,16.754482621898));
#258929=CARTESIAN_POINT('Ctrl Pts',(76.1088831745402,26.6064784254766,16.744617907061));
#258930=CARTESIAN_POINT('Ctrl Pts',(76.1270927055454,26.6483386168421,16.7349036639692));
#258931=CARTESIAN_POINT('Ctrl Pts',(76.1321077576901,26.6598672521718,16.7322282828385));
#258932=CARTESIAN_POINT('Ctrl Pts',(76.1372170507315,26.6713661579223,16.7295645869382));
#258933=CARTESIAN_POINT('Ctrl Pts',(76.1424206041304,26.6828327105675,16.7269107591349));
#258934=CARTESIAN_POINT('Ctrl Pts',(76.1535835707417,26.7074314288879,16.7212176127617));
#258935=CARTESIAN_POINT('Ctrl Pts',(76.1651211245957,26.7318858270285,16.7157439161817));
#258936=CARTESIAN_POINT('Ctrl Pts',(76.1770916036276,26.7560986664057,16.710212104333));
#258937=CARTESIAN_POINT('Ctrl Pts',(76.1892078939106,26.7806064400448,16.7046129100175));
#258938=CARTESIAN_POINT('Ctrl Pts',(76.2017677451098,26.8048664435746,16.6989544081906));
#258939=CARTESIAN_POINT('Ctrl Pts',(76.2148157305206,26.8287898949487,16.692999142927));
#258940=CARTESIAN_POINT('Ctrl Pts',(76.2278918585853,26.8527649458142,16.687031033001));
#258941=CARTESIAN_POINT('Ctrl Pts',(76.2414581212042,26.8764013225654,16.6807652464606));
#258942=CARTESIAN_POINT('Ctrl Pts',(76.2555440512879,26.8996289161678,16.6740083767523));
#258943=CARTESIAN_POINT('Ctrl Pts',(76.2664668899232,26.9176405955741,16.6687688081142));
#258944=CARTESIAN_POINT('Ctrl Pts',(76.2777018328891,26.9354066661027,16.6632349103941));
#258945=CARTESIAN_POINT('Ctrl Pts',(76.2892574542475,26.9529072015636,16.6573331470885));
#258946=CARTESIAN_POINT('Ctrl Pts',(76.2970453605966,26.9647016803719,16.6533556560915));
#258947=CARTESIAN_POINT('Ctrl Pts',(76.3050296927762,26.9765199249428,16.6492837031864));
#258948=CARTESIAN_POINT('Ctrl Pts',(76.3131571939983,26.9880307645767,16.6447775694554));
#258949=CARTESIAN_POINT('Ctrl Pts',(76.3209361875772,26.9990480188537,16.6404646589554));
#258950=CARTESIAN_POINT('Ctrl Pts',(76.3288457889269,27.0097828635244,16.6357546796883));
#258951=CARTESIAN_POINT('Ctrl Pts',(76.3368225865422,27.019982665784,16.6303684690638));
#258952=CARTESIAN_POINT('Ctrl Pts',(76.3439369962744,27.0290797465877,16.6255645726716));
#258953=CARTESIAN_POINT('Ctrl Pts',(76.3511042487789,27.0377508834012,16.6202234204512));
#258954=CARTESIAN_POINT('Ctrl Pts',(76.3582739443018,27.0458546401499,16.6141527467482));
#258955=CARTESIAN_POINT('Ctrl Pts',(76.3648732839341,27.0533137355762,16.6085650007364));
#258956=CARTESIAN_POINT('Ctrl Pts',(76.3714742611997,27.0602917480244,16.6023596051119));
#258957=CARTESIAN_POINT('Ctrl Pts',(76.3780396076468,27.0667174263885,16.5953847330164));
#258958=CARTESIAN_POINT('Ctrl Pts',(76.3848383240895,27.0733715101451,16.5881619340393));
#258959=CARTESIAN_POINT('Ctrl Pts',(76.3914209742982,27.0790454161737,16.5799443021262));
#258960=CARTESIAN_POINT('Ctrl Pts',(76.3975982251587,27.0837210218629,16.5709392072));
#258961=CARTESIAN_POINT('Ctrl Pts',(76.3980209336111,27.0840409729365,16.5703229897554));
#258962=CARTESIAN_POINT('Ctrl Pts',(76.3984417507368,27.0843562498919,16.5697030660327));
#258963=CARTESIAN_POINT('Ctrl Pts',(76.3988606189191,27.0846668466571,16.5690794942353));
#258964=CARTESIAN_POINT('Ctrl Pts',(76.4054137841379,27.0895261126631,16.5593237543952));
#258965=CARTESIAN_POINT('Ctrl Pts',(76.4114901846566,27.093245410726,16.5486722305523));
#258966=CARTESIAN_POINT('Ctrl Pts',(76.416877640854,27.0957927187002,16.5373328835886));
#258967=CARTESIAN_POINT('Ctrl Pts',(76.4172351860215,27.095961773932,16.5365803338581));
#258968=CARTESIAN_POINT('Ctrl Pts',(76.4175897023702,27.0961256557399,16.5358247401331));
#258969=CARTESIAN_POINT('Ctrl Pts',(76.4179411301446,27.0962843493429,16.5350661571352));
#258970=CARTESIAN_POINT('Ctrl Pts',(76.4231203592808,27.0986231244543,16.5238864057029));
#258971=CARTESIAN_POINT('Ctrl Pts',(76.4276313558999,27.1000270257133,16.5124226895554));
#258972=CARTESIAN_POINT('Ctrl Pts',(76.4316784850439,27.1009185160801,16.5007540438377));
#258973=CARTESIAN_POINT('Ctrl Pts',(76.4357092910718,27.1018064108362,16.4891324607791));
#258974=CARTESIAN_POINT('Ctrl Pts',(76.4392804564639,27.1021859277025,16.4773075420962));
#258975=CARTESIAN_POINT('Ctrl Pts',(76.4425873543179,27.1024353107015,16.4653907080849));
#258976=CARTESIAN_POINT('Ctrl Pts',(76.4429680133926,27.102464017334,16.4640189538887));
#258977=CARTESIAN_POINT('Ctrl Pts',(76.4433451597764,27.1024909575151,16.4626460183039));
#258978=CARTESIAN_POINT('Ctrl Pts',(76.4437190824838,27.1025166752918,16.4612720996402));
#258979=CARTESIAN_POINT('Ctrl Pts',(76.4469339796244,27.1027377905252,16.4494594787538));
#258980=CARTESIAN_POINT('Ctrl Pts',(76.4499306971237,27.1029008537886,16.4375780171924));
#258981=CARTESIAN_POINT('Ctrl Pts',(76.4527422098279,27.1030868022619,16.4256727165939));
#258982=CARTESIAN_POINT('Ctrl Pts',(76.4559507900088,27.1032990120752,16.4120860408196));
#258983=CARTESIAN_POINT('Ctrl Pts',(76.4589211030455,27.1035230776377,16.3984375728355));
#258984=CARTESIAN_POINT('Ctrl Pts',(76.4617002467785,27.1038478560124,16.3847624646941));
#258985=CARTESIAN_POINT('Ctrl Pts',(76.4623520422173,27.1039240266187,16.3815552275135));
#258986=CARTESIAN_POINT('Ctrl Pts',(76.462993426712,27.1040058139871,16.3783464458544));
#258987=CARTESIAN_POINT('Ctrl Pts',(76.4636250782641,27.1040943433334,16.3751364513276));
#258988=CARTESIAN_POINT('Ctrl Pts',(76.4641777733722,27.1041718065114,16.3723277061167));
#258989=CARTESIAN_POINT('Ctrl Pts',(76.4647230169086,27.1042544313724,16.369518032365));
#258990=CARTESIAN_POINT('Ctrl Pts',(76.4652612709139,27.1043429664181,16.3667076535841));
#258991=CARTESIAN_POINT('Ctrl Pts',(76.4686617029972,27.1049022886096,16.3489530208693));
#258992=CARTESIAN_POINT('Ctrl Pts',(76.4717819392994,27.1056974920644,16.3311709383671));
#258993=CARTESIAN_POINT('Ctrl Pts',(76.4747456942296,27.1069148091889,16.3134161472461));
#258994=CARTESIAN_POINT('Ctrl Pts',(76.4750658663008,27.1070463149829,16.311498111382));
#258995=CARTESIAN_POINT('Ctrl Pts',(76.4753841981967,27.1071827142443,16.3095804292481));
#258996=CARTESIAN_POINT('Ctrl Pts',(76.4757008361693,27.1073242180731,16.3076631955713));
#258997=CARTESIAN_POINT('Ctrl Pts',(76.4793038165454,27.1089343708732,16.2858472546199));
#258998=CARTESIAN_POINT('Ctrl Pts',(76.4826051109754,27.1110715810776,16.2640219361389));
#258999=CARTESIAN_POINT('Ctrl Pts',(76.4854470365061,27.1134723701869,16.2421547185838));
#259000=CARTESIAN_POINT('Ctrl Pts',(76.488337228718,27.1159139338068,16.2199161126836));
#259001=CARTESIAN_POINT('Ctrl Pts',(76.4907521576887,27.1186282162397,16.1976339393734));
#259002=CARTESIAN_POINT('Ctrl Pts',(76.4925052054321,27.1212940444935,16.1752508035511));
#259003=CARTESIAN_POINT('Ctrl Pts',(76.4930872524614,27.1221791529691,16.1678191532948));
#259004=CARTESIAN_POINT('Ctrl Pts',(76.4935961816787,27.1230585570135,16.1603762016909));
#259005=CARTESIAN_POINT('Ctrl Pts',(76.4940247511736,27.1239194136308,16.1529193631625));
#259006=CARTESIAN_POINT('Origin',(77.4800206767709,27.1771821124719,15.1653884328171));
#259007=CARTESIAN_POINT('Ctrl Pts',(-24.9689313575503,76.2325975651782,
15.6906397325477));
#259008=CARTESIAN_POINT('Ctrl Pts',(-26.1756150602392,75.8121196590787,
15.8860328844641));
#259009=CARTESIAN_POINT('Ctrl Pts',(-27.2086788182721,76.5504320086846,
16.1283959549323));
#259010=CARTESIAN_POINT('Ctrl Pts',(-24.9186909562191,76.2132400197742,
15.9678244963451));
#259011=CARTESIAN_POINT('Ctrl Pts',(-26.1254229642346,75.8084425279472,
16.0471243598401));
#259012=CARTESIAN_POINT('Ctrl Pts',(-27.1625656651785,76.5238417787868,
16.2207578908869));
#259013=CARTESIAN_POINT('Ctrl Pts',(-24.9032159272866,76.1826381079975,
16.2438456162063));
#259014=CARTESIAN_POINT('Ctrl Pts',(-26.104184876118,75.7943214248672,16.2107725763316));
#259015=CARTESIAN_POINT('Ctrl Pts',(-27.1407766635656,76.5020517602981,
16.3127979160863));
#259016=CARTESIAN_POINT('Ctrl Pts',(-24.9328226963039,76.1197004175058,
16.6559867599131));
#259017=CARTESIAN_POINT('Ctrl Pts',(-26.1172873190745,75.7580138780943,
16.4525591935362));
#259018=CARTESIAN_POINT('Ctrl Pts',(-27.1451435881167,76.4767312134559,
16.4501782974201));
#259019=CARTESIAN_POINT('Ctrl Pts',(-24.9518097701917,76.0956371509859,
16.794110417305));
#259020=CARTESIAN_POINT('Ctrl Pts',(-26.1293351405267,75.7432179427279,
16.5333292440492));
#259021=CARTESIAN_POINT('Ctrl Pts',(-27.1529468723184,76.469480763603,16.4962195166108));
#259022=CARTESIAN_POINT('Ctrl Pts',(-25.0073336657117,76.042503213137,17.0641682497299));
#259023=CARTESIAN_POINT('Ctrl Pts',(-26.1682415554322,75.7091288541245,
16.689657071876));
#259024=CARTESIAN_POINT('Ctrl Pts',(-27.1810555370846,76.4577808154583,
16.5862387939002));
#259025=CARTESIAN_POINT('Ctrl Pts',(-25.043582291958,76.0135981896359,17.195550558677));
#259026=CARTESIAN_POINT('Ctrl Pts',(-26.1949210471983,75.6899232799161,
16.765020182013));
#259027=CARTESIAN_POINT('Ctrl Pts',(-27.2011812093646,76.4533313045575,
16.6300328970328));
#259028=CARTESIAN_POINT('Ctrl Pts',(-25.1764553135876,75.9201060960321,
17.5792969885075));
#259029=CARTESIAN_POINT('Ctrl Pts',(-26.2950899509095,75.6263767700401,
16.9819673365835));
#259030=CARTESIAN_POINT('Ctrl Pts',(-27.2787774842966,76.4438901441637,
16.7579483734706));
#259031=CARTESIAN_POINT('Ctrl Pts',(-25.2993526607335,75.8476684832879,
17.8240388353673));
#259032=CARTESIAN_POINT('Ctrl Pts',(-26.3907356809289,75.5752351470883,
17.1155820316989));
#259033=CARTESIAN_POINT('Ctrl Pts',(-27.3548544480324,76.4428939284352,
16.8395289896467));
#259034=CARTESIAN_POINT('Ctrl Pts',(-25.5919984567931,75.6923432030072,
18.264473921103));
#259035=CARTESIAN_POINT('Ctrl Pts',(-26.6180940171725,75.4649619696492,
17.3414092350324));
#259036=CARTESIAN_POINT('Ctrl Pts',(-27.5412643883038,76.4499649794134,
16.9863406840095));
#259037=CARTESIAN_POINT('Ctrl Pts',(-25.7617839502725,75.6091210995783,
18.4627331486811));
#259038=CARTESIAN_POINT('Ctrl Pts',(-26.7507911294727,75.4052371346467,
17.435438103078));
#259039=CARTESIAN_POINT('Ctrl Pts',(-27.6515244073507,76.4578597275981,
17.0524270937445));
#259040=CARTESIAN_POINT('Ctrl Pts',(-26.1430805994636,75.4317357552708,
18.8197595498714));
#259041=CARTESIAN_POINT('Ctrl Pts',(-27.0442130694164,75.2796463045432,
17.5855829975127));
#259042=CARTESIAN_POINT('Ctrl Pts',(-27.9020344677406,76.4807996718625,
17.171435893939));
#259043=CARTESIAN_POINT('Ctrl Pts',(-26.3510560884158,75.3392616135107,
18.9747290102613));
#259044=CARTESIAN_POINT('Ctrl Pts',(-27.2031302208847,75.2146749685611,
17.6396375078347));
#259045=CARTESIAN_POINT('Ctrl Pts',(-28.0399748698368,76.4956562029936,
17.2230923811494));
#259046=CARTESIAN_POINT('Ctrl Pts',(-26.7887981118742,75.1503919246085,
19.2381193325699));
#259047=CARTESIAN_POINT('Ctrl Pts',(-27.5299162784606,75.0854973188483,
17.7075896666723));
#259048=CARTESIAN_POINT('Ctrl Pts',(-28.3320433237805,76.5300629685854,
17.3108891546271));
#259049=CARTESIAN_POINT('Ctrl Pts',(-27.0218910128871,75.0525919498098,
19.3482083029783));
#259050=CARTESIAN_POINT('Ctrl Pts',(-27.7009559314809,75.0201494871697,
17.7210643477414));
#259051=CARTESIAN_POINT('Ctrl Pts',(-28.4884000162535,76.5498913973921,
17.3475854788263));
#259052=CARTESIAN_POINT('Ctrl Pts',(-27.4985053196503,74.8565797596348,
19.521741160188));
#259053=CARTESIAN_POINT('Ctrl Pts',(-28.0395707962218,74.8945599897606,
17.7097451055821));
#259054=CARTESIAN_POINT('Ctrl Pts',(-28.8092814008564,76.5925703049495,
17.4054297637285));
#259055=CARTESIAN_POINT('Ctrl Pts',(-27.7422284005861,74.758241529272,19.5858151824399));
#259056=CARTESIAN_POINT('Ctrl Pts',(-28.2078168588108,74.8341192521282,
17.6844550416307));
#259057=CARTESIAN_POINT('Ctrl Pts',(-28.9739291008619,76.6154156279985,
17.4267877716097));
#259058=CARTESIAN_POINT('Ctrl Pts',(-28.2396160007789,74.560514330493,19.6716009699532));
#259059=CARTESIAN_POINT('Ctrl Pts',(-28.536471100917,74.7198525855479,17.5990670510758));
#259060=CARTESIAN_POINT('Ctrl Pts',(-29.3108001463012,76.6636167731309,
17.4553830340207));
#259061=CARTESIAN_POINT('Ctrl Pts',(-28.4947415154366,74.4605859662117,
19.6929518687095));
#259062=CARTESIAN_POINT('Ctrl Pts',(-28.697661261183,74.6659231009684,17.5372248464383));
#259063=CARTESIAN_POINT('Ctrl Pts',(-29.4840227026744,76.6891359364473,
17.4625));
#259064=CARTESIAN_POINT('Ctrl Pts',(-28.7459974181806,74.3634602878982,
19.6929518677509));
#259065=CARTESIAN_POINT('Ctrl Pts',(-28.8447420032201,74.6189041648809,
17.4625));
#259066=CARTESIAN_POINT('Ctrl Pts',(-29.6549915892152,76.7149512087496,
17.4625));
#259067=CARTESIAN_POINT('',(-25.2552738568382,75.9418613633423,17.2633930704884));
#259068=CARTESIAN_POINT('Ctrl Pts',(-25.1183523255102,75.961488153786,17.4075632995852));
#259069=CARTESIAN_POINT('Ctrl Pts',(-25.1300086289606,75.9600460003527,
17.3889110251594));
#259070=CARTESIAN_POINT('Ctrl Pts',(-25.1428552492175,75.9582730048897,
17.3714318666836));
#259071=CARTESIAN_POINT('Ctrl Pts',(-25.1567358846801,75.9562706193481,
17.354967018135));
#259072=CARTESIAN_POINT('Ctrl Pts',(-25.1704654612766,75.9542900251785,
17.3386813516821));
#259073=CARTESIAN_POINT('Ctrl Pts',(-25.1852067359063,75.9520849723068,
17.3233881139037));
#259074=CARTESIAN_POINT('Ctrl Pts',(-25.2007766452391,75.9497709327977,
17.3088979329118));
#259075=CARTESIAN_POINT('Ctrl Pts',(-25.2161260490804,75.9474896653754,
17.294612965991));
#259076=CARTESIAN_POINT('Ctrl Pts',(-25.2322808248086,75.9451024553525,
17.2811085187395));
#259077=CARTESIAN_POINT('Ctrl Pts',(-25.2490337250752,75.9427372332084,
17.2681673905741));
#259078=CARTESIAN_POINT('Ctrl Pts',(-25.2511048108336,75.942444831426,17.2665675370673));
#259079=CARTESIAN_POINT('Ctrl Pts',(-25.253184996925,75.9421527879157,17.2649762469118));
#259080=CARTESIAN_POINT('Ctrl Pts',(-25.2552738568382,75.9418613633423,
17.2633930704885));
#259081=CARTESIAN_POINT('Ctrl Pts',(-25.2552738568382,75.9418613633423,
17.2633930704885));
#259082=CARTESIAN_POINT('Ctrl Pts',(-25.3053371640352,75.9348768553696,
17.2254493239264));
#259083=CARTESIAN_POINT('Ctrl Pts',(-25.35726443102,75.9291204561457,17.1911044093421));
#259084=CARTESIAN_POINT('Ctrl Pts',(-25.4106833642394,75.9248495156856,
17.1596330726701));
#259085=CARTESIAN_POINT('Ctrl Pts',(-25.4672813125568,75.9203244072107,
17.126288844714));
#259086=CARTESIAN_POINT('Ctrl Pts',(-25.5255536827334,75.9174669834034,
17.096170306179));
#259087=CARTESIAN_POINT('Ctrl Pts',(-25.5850314008785,75.9165875721633,
17.068359840973));
#259088=CARTESIAN_POINT('Ctrl Pts',(-25.6385673670598,75.9157960130403,
17.0433276075386));
#259089=CARTESIAN_POINT('Ctrl Pts',(-25.6930793577338,75.9166071705228,
17.0201642487191));
#259090=CARTESIAN_POINT('Ctrl Pts',(-25.748210005877,75.9192482118546,16.9981680569719));
#259091=CARTESIAN_POINT('Ctrl Pts',(-25.7703411800655,75.9203084088181,
16.9893380945566));
#259092=CARTESIAN_POINT('Ctrl Pts',(-25.7926041369582,75.9216656968463,
16.9807230186151));
#259093=CARTESIAN_POINT('Ctrl Pts',(-25.8149722051984,75.9233227318027,
16.9723142805604));
#259094=CARTESIAN_POINT('Ctrl Pts',(-25.8770418865484,75.9279208772763,
16.9489806745464));
#259095=CARTESIAN_POINT('Ctrl Pts',(-25.9395105597218,75.9347968299509,
16.9273736683177));
#259096=CARTESIAN_POINT('Ctrl Pts',(-26.0019469534467,75.943947744286,16.9071901218341));
#259097=CARTESIAN_POINT('Ctrl Pts',(-26.0680891141755,75.9536417898683,
16.8858086278695));
#259098=CARTESIAN_POINT('Ctrl Pts',(-26.134196625674,75.9658884088346,16.8660249930255));
#259099=CARTESIAN_POINT('Ctrl Pts',(-26.1997753179222,75.980727924121,16.8475110455998));
#259100=CARTESIAN_POINT('Ctrl Pts',(-26.2246632532517,75.9863597060933,
16.8404847705945));
#259101=CARTESIAN_POINT('Ctrl Pts',(-26.2494750754786,75.9923654080542,
16.8336416505));
#259102=CARTESIAN_POINT('Ctrl Pts',(-26.2741836399454,75.9987489542799,
16.8269646524032));
#259103=CARTESIAN_POINT('Ctrl Pts',(-26.3193781177628,76.0104251096745,
16.8147517436859));
#259104=CARTESIAN_POINT('Ctrl Pts',(-26.3644806571394,76.0233691010834,
16.8031325559241));
#259105=CARTESIAN_POINT('Ctrl Pts',(-26.4094030264466,76.037632391529,16.7919150704385));
#259106=CARTESIAN_POINT('Ctrl Pts',(-26.4723212964722,76.0576095559919,
16.7762038603737));
#259107=CARTESIAN_POINT('Ctrl Pts',(-26.5349890917676,76.0801913920499,
16.7613285556708));
#259108=CARTESIAN_POINT('Ctrl Pts',(-26.5968842675656,76.1054321152718,
16.7468658579898));
#259109=CARTESIAN_POINT('Ctrl Pts',(-26.6310436324481,76.1193622328184,
16.738884031282));
#259110=CARTESIAN_POINT('Ctrl Pts',(-26.6649677051668,76.1341013587548,
16.731027412246));
#259111=CARTESIAN_POINT('Ctrl Pts',(-26.6985700833499,76.1496523368464,
16.7232226781364));
#259112=CARTESIAN_POINT('Ctrl Pts',(-26.7271705546382,76.1628884625751,
16.7165797235039));
#259113=CARTESIAN_POINT('Ctrl Pts',(-26.7555332781428,76.1767336944032,
16.7099108269339));
#259114=CARTESIAN_POINT('Ctrl Pts',(-26.7835861577699,76.1911702984035,
16.7031950114971));
#259115=CARTESIAN_POINT('Ctrl Pts',(-26.8199494155057,76.2098835983951,
16.6944897045596));
#259116=CARTESIAN_POINT('Ctrl Pts',(-26.8556888227993,76.2295605848596,
16.6856585997866));
#259117=CARTESIAN_POINT('Ctrl Pts',(-26.8905185760864,76.250297808266,16.6759949661901));
#259118=CARTESIAN_POINT('Ctrl Pts',(-26.8948405181937,76.2528710415097,
16.6747958286422));
#259119=CARTESIAN_POINT('Ctrl Pts',(-26.8991484819158,76.2554605669536,
16.6735839233218));
#259120=CARTESIAN_POINT('Ctrl Pts',(-26.9034419462822,76.2580665404398,
16.6723579481277));
#259121=CARTESIAN_POINT('Ctrl Pts',(-26.9260412875341,76.2717835016351,
16.6659048302225));
#259122=CARTESIAN_POINT('Ctrl Pts',(-26.9482892120592,76.2859122477468,
16.6592804203713));
#259123=CARTESIAN_POINT('Ctrl Pts',(-26.9698831287204,76.3006663576261,
16.6513762614156));
#259124=CARTESIAN_POINT('Ctrl Pts',(-26.9780091206901,76.3062184665964,
16.6484018527796));
#259125=CARTESIAN_POINT('Ctrl Pts',(-26.9861262753852,76.3119191070937,
16.6452107769111));
#259126=CARTESIAN_POINT('Ctrl Pts',(-26.9940602893765,76.3176690332947,
16.6418055151727));
#259127=CARTESIAN_POINT('Ctrl Pts',(-27.0017405506363,76.3232350602132,
16.6385091635609));
#259128=CARTESIAN_POINT('Ctrl Pts',(-27.0092489771401,76.3288474175746,
16.6350110768171));
#259129=CARTESIAN_POINT('Ctrl Pts',(-27.0164426855061,76.3343994446543,
16.6313545921147));
#259130=CARTESIAN_POINT('Ctrl Pts',(-27.021651174773,76.338419300893,16.6287071729592));
#259131=CARTESIAN_POINT('Ctrl Pts',(-27.0266992715061,76.3424031609164,
16.6260035920946));
#259132=CARTESIAN_POINT('Ctrl Pts',(-27.0315171448137,76.3463237470274,
16.6231740179233));
#259133=CARTESIAN_POINT('Ctrl Pts',(-27.0359626225497,76.3499412930184,
16.6205631545447));
#259134=CARTESIAN_POINT('Ctrl Pts',(-27.0402121095371,76.3535049393509,
16.6178449700777));
#259135=CARTESIAN_POINT('Ctrl Pts',(-27.0442217699856,76.3569830238244,
16.6150107816619));
#259136=CARTESIAN_POINT('Ctrl Pts',(-27.0482190833947,76.3604503981526,
16.6121853206275));
#259137=CARTESIAN_POINT('Ctrl Pts',(-27.0519780380087,76.3638327354503,
16.6092444590309));
#259138=CARTESIAN_POINT('Ctrl Pts',(-27.0554667027077,76.3670881313929,
16.6062292715612));
#259139=CARTESIAN_POINT('Ctrl Pts',(-27.0590905972579,76.370469715074,16.6030972074673));
#259140=CARTESIAN_POINT('Ctrl Pts',(-27.0624228825075,76.3737142806329,
16.5998850454597));
#259141=CARTESIAN_POINT('Ctrl Pts',(-27.0654401101436,76.3767636720628,
16.5966933401164));
#259142=CARTESIAN_POINT('Ctrl Pts',(-27.0660776774096,76.377408035827,16.5960189041457));
#259143=CARTESIAN_POINT('Ctrl Pts',(-27.0667012169651,76.3780436486863,
16.595345561103));
#259144=CARTESIAN_POINT('Ctrl Pts',(-27.0673105683208,76.3786699073557,
16.5946745332907));
#259145=CARTESIAN_POINT('Ctrl Pts',(-27.0690899030251,76.3804986122136,
16.5927151004236));
#259146=CARTESIAN_POINT('Ctrl Pts',(-27.0707485686258,76.382246672755,16.5907819650672));
#259147=CARTESIAN_POINT('Ctrl Pts',(-27.0722790207717,76.383903674775,16.5888786970253));
#259148=CARTESIAN_POINT('Ctrl Pts',(-27.0747602936418,76.3865901188883,
16.5857929897265));
#259149=CARTESIAN_POINT('Ctrl Pts',(-27.0770747171622,76.3892195791676,
16.5825794792118));
#259150=CARTESIAN_POINT('Ctrl Pts',(-27.0792241302057,76.3918035041202,
16.579183461021));
#259151=CARTESIAN_POINT('Ctrl Pts',(-27.0816343568413,76.3947009671108,
16.5753753639578));
#259152=CARTESIAN_POINT('Ctrl Pts',(-27.083837184317,76.3975410826346,16.5713382492547));
#259153=CARTESIAN_POINT('Ctrl Pts',(-27.0858449599544,76.4003286356654,
16.5670618101874));
#259154=CARTESIAN_POINT('Ctrl Pts',(-27.0868914066365,76.4017815000024,
16.5648329428828));
#259155=CARTESIAN_POINT('Ctrl Pts',(-27.0878850109093,76.4032199187874,
16.5625400544833));
#259156=CARTESIAN_POINT('Ctrl Pts',(-27.088828258327,76.4046436978792,16.5601869061983));
#259157=CARTESIAN_POINT('Ctrl Pts',(-27.0901243112776,76.4066000171422,
16.5569536031214));
#259158=CARTESIAN_POINT('Ctrl Pts',(-27.0913240228374,76.4085291354499,
16.5536060959882));
#259159=CARTESIAN_POINT('Ctrl Pts',(-27.0924256391468,76.4104440957709,
16.5500691226174));
#259160=CARTESIAN_POINT('Ctrl Pts',(-27.0936398944198,76.4125548585178,
16.5461704979064));
#259161=CARTESIAN_POINT('Ctrl Pts',(-27.0947350208453,76.4146483529728,
16.5420420683693));
#259162=CARTESIAN_POINT('Ctrl Pts',(-27.0957153868087,76.41673174033,16.5376476148134));
#259163=CARTESIAN_POINT('Ctrl Pts',(-27.0962521678256,76.4178724600469,
16.5352415140951));
#259164=CARTESIAN_POINT('Ctrl Pts',(-27.0967546524525,76.4190099831835,
16.5327567087975));
#259165=CARTESIAN_POINT('Ctrl Pts',(-27.097224189991,76.4201444936685,16.5301935190525));
#259166=CARTESIAN_POINT('Ctrl Pts',(-27.0978315581571,76.4216120345913,
16.5268779165143));
#259167=CARTESIAN_POINT('Ctrl Pts',(-27.0983817182553,76.4230689216671,
16.5234806042216));
#259168=CARTESIAN_POINT('Ctrl Pts',(-27.0988766727596,76.4245289935568,
16.519898572385));
#259169=CARTESIAN_POINT('Ctrl Pts',(-27.0994168615817,76.4261225026722,
16.5159891755784));
#259170=CARTESIAN_POINT('Ctrl Pts',(-27.0998913101598,76.427719771351,16.5118599760785));
#259171=CARTESIAN_POINT('Ctrl Pts',(-27.1003044167921,76.4293303307267,
16.5074394314103));
#259172=CARTESIAN_POINT('Ctrl Pts',(-27.100765251422,76.4311269649994,16.5025081620798));
#259173=CARTESIAN_POINT('Ctrl Pts',(-27.1011497772522,76.4329400926505,
16.4972146293963));
#259174=CARTESIAN_POINT('Ctrl Pts',(-27.1014658921266,76.4347734700811,
16.4915299890183));
#259175=CARTESIAN_POINT('Ctrl Pts',(-27.1017737844554,76.4365591590576,
16.4859932132902));
#259176=CARTESIAN_POINT('Ctrl Pts',(-27.1020168306712,76.4383638507765,
16.4800869168181));
#259177=CARTESIAN_POINT('Ctrl Pts',(-27.1022032681051,76.4401848038024,
16.4738313146433));
#259178=CARTESIAN_POINT('Ctrl Pts',(-27.1022139466895,76.4402891026013,
16.4734730122689));
#259179=CARTESIAN_POINT('Ctrl Pts',(-27.1022244069632,76.4403934977004,
16.4731133135585));
#259180=CARTESIAN_POINT('Ctrl Pts',(-27.1022346589492,76.4404979871153,
16.4727522096321));
#259181=CARTESIAN_POINT('Ctrl Pts',(-27.1024069986673,76.4422544932462,
16.4666819176221));
#259182=CARTESIAN_POINT('Ctrl Pts',(-27.1025185266476,76.4439950489396,
16.4603561193072));
#259183=CARTESIAN_POINT('Ctrl Pts',(-27.1026104631992,76.4457036734619,
16.4538373780825));
#259184=CARTESIAN_POINT('Ctrl Pts',(-27.1027374245136,76.4480632269946,
16.4448352136609));
#259185=CARTESIAN_POINT('Ctrl Pts',(-27.1028277926133,76.4503610768553,
16.435469336288));
#259186=CARTESIAN_POINT('Ctrl Pts',(-27.1029292932191,76.4525659484553,
16.4259934752636));
#259187=CARTESIAN_POINT('Ctrl Pts',(-27.1029532014078,76.4530852998992,
16.4237614622497));
#259188=CARTESIAN_POINT('Ctrl Pts',(-27.1029775124212,76.4535995607684,
16.4215234223818));
#259189=CARTESIAN_POINT('Ctrl Pts',(-27.1030025070032,76.4541084537907,
16.4192826101514));
#259190=CARTESIAN_POINT('Ctrl Pts',(-27.103068131177,76.4554445707162,16.4133992770811));
#259191=CARTESIAN_POINT('Ctrl Pts',(-27.1031446836156,76.4567431107572,
16.407488679998));
#259192=CARTESIAN_POINT('Ctrl Pts',(-27.1032413598512,76.457990785983,16.4016557662627));
#259193=CARTESIAN_POINT('Ctrl Pts',(-27.1033489910739,76.4593798430705,
16.3951618886918));
#259194=CARTESIAN_POINT('Ctrl Pts',(-27.1034813058099,76.4607059855568,
16.3887641172962));
#259195=CARTESIAN_POINT('Ctrl Pts',(-27.1036407239054,76.4619636575372,
16.38254122392));
#259196=CARTESIAN_POINT('Ctrl Pts',(-27.1038110201107,76.4633071484696,
16.3758937029806));
#259197=CARTESIAN_POINT('Ctrl Pts',(-27.1040119022358,76.4645727430344,
16.3694450031958));
#259198=CARTESIAN_POINT('Ctrl Pts',(-27.1042403333882,76.4657643057464,
16.3632279271333));
#259199=CARTESIAN_POINT('Ctrl Pts',(-27.1044944223521,76.4670897069963,
16.3563125375353));
#259200=CARTESIAN_POINT('Ctrl Pts',(-27.1047822466638,76.4683237188364,
16.3496832466663));
#259201=CARTESIAN_POINT('Ctrl Pts',(-27.1050982636136,76.4694807293036,
16.3433192422796));
#259202=CARTESIAN_POINT('Ctrl Pts',(-27.1052628780315,76.4700834204082,
16.3400042084553));
#259203=CARTESIAN_POINT('Ctrl Pts',(-27.1054351585133,76.4706653371565,
16.3367601803189));
#259204=CARTESIAN_POINT('Ctrl Pts',(-27.1056146219711,76.4712290766849,
16.3335788780875));
#259205=CARTESIAN_POINT('Ctrl Pts',(-27.1059981692671,76.4724338945032,
16.3267798345215));
#259206=CARTESIAN_POINT('Ctrl Pts',(-27.10642271435,76.4735621730668,16.3202526040048));
#259207=CARTESIAN_POINT('Ctrl Pts',(-27.1068761114234,76.4746356726752,
16.3138840932371));
#259208=CARTESIAN_POINT('Ctrl Pts',(-27.1073854422856,76.4758416056492,
16.306729924693));
#259209=CARTESIAN_POINT('Ctrl Pts',(-27.1079312822812,76.476978936377,16.2997754603678));
#259210=CARTESIAN_POINT('Ctrl Pts',(-27.1085191991319,76.478083472477,16.292795783268));
#259211=CARTESIAN_POINT('Ctrl Pts',(-27.1088920682948,76.4787839923727,
16.2883691260731));
#259212=CARTESIAN_POINT('Ctrl Pts',(-27.1092822973043,76.4794713856191,
16.28393111298));
#259213=CARTESIAN_POINT('Ctrl Pts',(-27.1096950706557,76.4801541955039,
16.27941456206));
#259214=CARTESIAN_POINT('Ctrl Pts',(-27.1112272278191,76.4826886906515,
16.2626497543951));
#259215=CARTESIAN_POINT('Ctrl Pts',(-27.1130539358815,76.4851267428394,
16.245009294971));
#259216=CARTESIAN_POINT('Ctrl Pts',(-27.1151298371978,76.4873049803749,
16.2267575735314));
#259217=CARTESIAN_POINT('Ctrl Pts',(-27.1152747494852,76.487457036439,16.2254834769829));
#259218=CARTESIAN_POINT('Ctrl Pts',(-27.1154208703689,76.4876078216653,
16.2242064209797));
#259219=CARTESIAN_POINT('Ctrl Pts',(-27.1155681819217,76.4877572785791,
16.2229265037606));
#259220=CARTESIAN_POINT('Ctrl Pts',(-27.1170756224333,76.489286672591,16.2098290987628));
#259221=CARTESIAN_POINT('Ctrl Pts',(-27.118681039989,76.490635740581,16.1965814055142));
#259222=CARTESIAN_POINT('Ctrl Pts',(-27.120163955804,76.4917129471206,16.1843382179293));
#259223=CARTESIAN_POINT('Ctrl Pts',(-27.1209112681079,76.4922558030891,
16.1781682893142));
#259224=CARTESIAN_POINT('Ctrl Pts',(-27.1216272476248,76.4927295874375,
16.1722545210085));
#259225=CARTESIAN_POINT('Ctrl Pts',(-27.1222826948279,76.4931225564269,
16.1667491978235));
#259226=CARTESIAN_POINT('Ctrl Pts',(-27.123807760442,76.4940368993218,16.1539396548969));
#259227=CARTESIAN_POINT('Ctrl Pts',(-27.1250450068388,76.4945873611468,
16.1431164281593));
#259228=CARTESIAN_POINT('Ctrl Pts',(-27.1260737997838,76.4949373700034,
16.1336144198422));
#259229=CARTESIAN_POINT('Ctrl Pts',(-27.126352330216,76.4950321297104,16.1310418920111));
#259230=CARTESIAN_POINT('Ctrl Pts',(-27.1266156234859,76.4951122549698,
16.1285659022891));
#259231=CARTESIAN_POINT('Ctrl Pts',(-27.1268653349371,76.4951810931326,
16.1261726830171));
#259232=CARTESIAN_POINT('Ctrl Pts',(-27.1269115955426,76.4951938458321,
16.1257293242043));
#259233=CARTESIAN_POINT('Ctrl Pts',(-27.1269574092079,76.4952062290152,
16.1252887719971));
#259234=CARTESIAN_POINT('Ctrl Pts',(-27.1270027817488,76.4952182483286,
16.1248509868279));
#259235=CARTESIAN_POINT('Origin',(-29.6549915892152,76.7149512087496,20.0025));
#259236=CARTESIAN_POINT('Origin',(0.,0.,20.0025));
#259237=CARTESIAN_POINT('Origin',(-76.7149512087496,29.6549915892152,20.0025));
#259238=CARTESIAN_POINT('Ctrl Pts',(-74.3634602878982,28.7459974181806,
19.6929518677509));
#259239=CARTESIAN_POINT('Ctrl Pts',(-74.6189041648808,28.8447420032201,
17.4625));
#259240=CARTESIAN_POINT('Ctrl Pts',(-76.7149512087496,29.6549915892152,
17.4625));
#259241=CARTESIAN_POINT('Ctrl Pts',(-74.460904385774,28.4939177914733,19.6929518673245));
#259242=CARTESIAN_POINT('Ctrl Pts',(-74.6660793405586,28.6971725259743,
17.5374731486144));
#259243=CARTESIAN_POINT('Ctrl Pts',(-76.6890525018813,29.4834701335368,
17.4625));
#259244=CARTESIAN_POINT('Ctrl Pts',(-74.5588475342795,28.2438591531047,
19.6720320649351));
#259245=CARTESIAN_POINT('Ctrl Pts',(-74.7189440966779,28.5391636116357,
17.5981072780271));
#259246=CARTESIAN_POINT('Ctrl Pts',(-76.664038637903,29.3136797628422,17.4555267321203));
#259247=CARTESIAN_POINT('Ctrl Pts',(-74.7559270342231,27.7480012895958,
19.5871055664401));
#259248=CARTESIAN_POINT('Ctrl Pts',(-74.832738631376,28.2117119618056,17.6836912763772));
#259249=CARTESIAN_POINT('Ctrl Pts',(-76.6159646173276,28.9778332725242,
17.4272178998374));
#259250=CARTESIAN_POINT('Ctrl Pts',(-74.8560677628266,27.4997703917926,
19.5220948206219));
#259251=CARTESIAN_POINT('Ctrl Pts',(-74.8942448729349,28.0404430900653,
17.709632121869));
#259252=CARTESIAN_POINT('Ctrl Pts',(-76.5926880471475,28.8101355628242,
17.4055476509048));
#259253=CARTESIAN_POINT('Ctrl Pts',(-75.0518439197724,27.0236898937087,
19.3489695261644));
#259254=CARTESIAN_POINT('Ctrl Pts',(-75.019660969593,27.7022510777841,17.7211023712223));
#259255=CARTESIAN_POINT('Ctrl Pts',(-76.5500480485634,28.4896086814983,
17.3478392195236));
#259256=CARTESIAN_POINT('Ctrl Pts',(-75.1476280619453,26.7953551633978,
19.2413577159494));
#259257=CARTESIAN_POINT('Ctrl Pts',(-75.0836522525197,27.5347169152634,
17.7080778869115));
#259258=CARTESIAN_POINT('Ctrl Pts',(-76.5306138623673,28.3364379275071,
17.3119686156356));
#259259=CARTESIAN_POINT('Ctrl Pts',(-75.2884389844463,26.4687756770156,
19.0458961827322));
#259260=CARTESIAN_POINT('Ctrl Pts',(-75.1803896028198,27.2898012152202,
17.6578979817805));
#259261=CARTESIAN_POINT('Ctrl Pts',(-76.5048922024805,28.1185099510306,
17.2468147718757));
#259262=CARTESIAN_POINT('Ctrl Pts',(-75.3348967090533,26.3625884843546,
18.9750294801163));
#259263=CARTESIAN_POINT('Ctrl Pts',(-75.2125498005327,27.2097290601216,
17.636311693557));
#259264=CARTESIAN_POINT('Ctrl Pts',(-76.496894950715,28.0478532106478,17.223192537137));
#259265=CARTESIAN_POINT('Ctrl Pts',(-75.4268801209919,26.1560856941723,
18.8208466626385));
#259266=CARTESIAN_POINT('Ctrl Pts',(-75.2767579129783,27.0529295129818,
17.5825320214172));
#259267=CARTESIAN_POINT('Ctrl Pts',(-76.4822364493763,27.9109420608553,
17.1717982652807));
#259268=CARTESIAN_POINT('Ctrl Pts',(-75.4727198166015,26.0551010760532,
18.7368743964314));
#259269=CARTESIAN_POINT('Ctrl Pts',(-75.3090585336007,26.9755857935383,
17.5501254447862));
#259270=CARTESIAN_POINT('Ctrl Pts',(-76.4755364557142,27.8442489434605,
17.1438075095173));
#259271=CARTESIAN_POINT('Ctrl Pts',(-75.6060560547223,25.768150258085,18.4696518487109));
#259272=CARTESIAN_POINT('Ctrl Pts',(-75.4030488168829,26.7557364160525,
17.43860601751));
#259273=CARTESIAN_POINT('Ctrl Pts',(-76.4581861338663,27.655675609175,17.0547333270725));
#259274=CARTESIAN_POINT('Ctrl Pts',(-75.6894118596661,25.597846621004,18.271840936307));
#259275=CARTESIAN_POINT('Ctrl Pts',(-75.4628679834562,26.6226482272605,
17.3449978161568));
#259276=CARTESIAN_POINT('Ctrl Pts',(-76.4502012574515,27.5450423948284,
16.9887963557572));
#259277=CARTESIAN_POINT('Ctrl Pts',(-75.8449254994659,25.3042070746273,
17.8327278472486));
#259278=CARTESIAN_POINT('Ctrl Pts',(-75.5732964352841,26.3945070907105,
17.1202191600567));
#259279=CARTESIAN_POINT('Ctrl Pts',(-76.4429196593763,27.357895681027,16.8424253269274));
#259280=CARTESIAN_POINT('Ctrl Pts',(-75.9179115378165,25.1799509742042,
17.5873106315617));
#259281=CARTESIAN_POINT('Ctrl Pts',(-75.6248510373213,26.2977761963332,
16.986409166726));
#259282=CARTESIAN_POINT('Ctrl Pts',(-76.4437878571387,27.280900229958,16.7606195878717));
#259283=CARTESIAN_POINT('Ctrl Pts',(-76.0120135407797,25.0456540278871,
17.2025309630926));
#259284=CARTESIAN_POINT('Ctrl Pts',(-75.6888631781798,26.1964580005417,
16.7690050915928));
#259285=CARTESIAN_POINT('Ctrl Pts',(-76.4531141362198,27.20235213455,16.6323596984798));
#259286=CARTESIAN_POINT('Ctrl Pts',(-76.0410349984125,25.0090870943374,
17.0710669460341));
#259287=CARTESIAN_POINT('Ctrl Pts',(-75.7081633852753,26.1695156242373,
16.6936245453246));
#259288=CARTESIAN_POINT('Ctrl Pts',(-76.4575269782811,27.1820075724729,
16.5885383593541));
#259289=CARTESIAN_POINT('Ctrl Pts',(-76.0942893550638,24.9530103267675,
16.8014952531461));
#259290=CARTESIAN_POINT('Ctrl Pts',(-75.7423750031968,26.1301341325899,
16.5376305767305));
#259291=CARTESIAN_POINT('Ctrl Pts',(-76.4691181075119,27.1534935975719,
16.4986811285387));
#259292=CARTESIAN_POINT('Ctrl Pts',(-76.1186539510279,24.9335061597315,
16.6623540419172));
#259293=CARTESIAN_POINT('Ctrl Pts',(-75.7573877351404,26.1176802211128,
16.4562866616968));
#259294=CARTESIAN_POINT('Ctrl Pts',(-76.4763708127829,27.145369143006,16.4523007247637));
#259295=CARTESIAN_POINT('Ctrl Pts',(-76.1824010629023,24.9029553648545,
16.2463425041043));
#259296=CARTESIAN_POINT('Ctrl Pts',(-75.7942282194349,26.1038934519093,
16.2122544249952));
#259297=CARTESIAN_POINT('Ctrl Pts',(-76.5018384532016,27.1404954668508,
16.3136302120345));
#259298=CARTESIAN_POINT('Ctrl Pts',(-76.2131904009612,24.9185412707804,
15.9685880799941));
#259299=CARTESIAN_POINT('Ctrl Pts',(-75.8084359405768,26.1252772492191,
16.0475610164009));
#259300=CARTESIAN_POINT('Ctrl Pts',(-76.5237673449924,27.1624313528461,
16.2210111173636));
#259301=CARTESIAN_POINT('Ctrl Pts',(-76.2326069140442,24.9689556265491,
15.6905058513847));
#259302=CARTESIAN_POINT('Ctrl Pts',(-75.8121214408373,26.1756393943756,
15.8859547915793));
#259303=CARTESIAN_POINT('Ctrl Pts',(-76.55044485681,27.2087011009323,16.1283513278779));
#259304=CARTESIAN_POINT('',(-75.9418613629793,25.2552738567446,17.2633930704321));
#259305=CARTESIAN_POINT('Ctrl Pts',(-76.4952182372905,27.1270026655082,
16.124851038856));
#259306=CARTESIAN_POINT('Ctrl Pts',(-76.4949835330535,27.1261035938165,
16.1335301302463));
#259307=CARTESIAN_POINT('Ctrl Pts',(-76.4945938617306,27.1250175086504,
16.1433840167245));
#259308=CARTESIAN_POINT('Ctrl Pts',(-76.493894642641,27.1236651982624,16.1550166230773));
#259309=CARTESIAN_POINT('Ctrl Pts',(-76.493763071425,27.1234107356416,16.157205516638));
#259310=CARTESIAN_POINT('Ctrl Pts',(-76.4936205663265,27.1231468673314,
16.1594572469015));
#259311=CARTESIAN_POINT('Ctrl Pts',(-76.4934661405624,27.1228730977802,
16.1617756124903));
#259312=CARTESIAN_POINT('Ctrl Pts',(-76.4927426139016,27.1215904130517,
16.172637785155));
#259313=CARTESIAN_POINT('Ctrl Pts',(-76.4916920130616,27.1200357216268,
16.1853170892844));
#259314=CARTESIAN_POINT('Ctrl Pts',(-76.4903847974124,27.1184437830634,
16.1985845365741));
#259315=CARTESIAN_POINT('Ctrl Pts',(-76.4898045639396,27.1177371697041,
16.2044735549782));
#259316=CARTESIAN_POINT('Ctrl Pts',(-76.489173803305,27.1170231040088,16.2104789373784));
#259317=CARTESIAN_POINT('Ctrl Pts',(-76.4884987572068,27.1163213320438,
16.2164967943079));
#259318=CARTESIAN_POINT('Ctrl Pts',(-76.4866808484003,27.1144314500953,
16.2327029691722));
#259319=CARTESIAN_POINT('Ctrl Pts',(-76.4846005967038,27.1126943705542,
16.2486914456572));
#259320=CARTESIAN_POINT('Ctrl Pts',(-76.4824017848981,27.1111721910298,
16.2640972093943));
#259321=CARTESIAN_POINT('Ctrl Pts',(-76.4816221526855,27.1106324721747,
16.2695596276141));
#259322=CARTESIAN_POINT('Ctrl Pts',(-76.4808275267704,27.1101196624084,
16.2749492144108));
#259323=CARTESIAN_POINT('Ctrl Pts',(-76.480023958419,27.1096361423661,16.2802512670947));
#259324=CARTESIAN_POINT('Ctrl Pts',(-76.4787631770291,27.1088775098614,
16.288570073256));
#259325=CARTESIAN_POINT('Ctrl Pts',(-76.4774861247355,27.1081924682404,
16.2966391164402));
#259326=CARTESIAN_POINT('Ctrl Pts',(-76.4761760059689,27.1075731179885,
16.3046343846423));
#259327=CARTESIAN_POINT('Ctrl Pts',(-76.4750144099875,27.1070239809317,
16.3117232621168));
#259328=CARTESIAN_POINT('Ctrl Pts',(-76.4738263115708,27.1065264227128,
16.3187548885519));
#259329=CARTESIAN_POINT('Ctrl Pts',(-76.4726008566083,27.1060881023887,
16.3258128070736));
#259330=CARTESIAN_POINT('Ctrl Pts',(-76.472444168752,27.1060320583283,16.3267152393595));
#259331=CARTESIAN_POINT('Ctrl Pts',(-76.4722868770231,27.1059770032833,
16.3276180342357));
#259332=CARTESIAN_POINT('Ctrl Pts',(-76.4721289660909,27.1059229723691,
16.3285213027679));
#259333=CARTESIAN_POINT('Ctrl Pts',(-76.4709315855552,27.1055132758132,
16.3353704559211));
#259334=CARTESIAN_POINT('Ctrl Pts',(-76.469686098807,27.1051480063896,16.3423105850843));
#259335=CARTESIAN_POINT('Ctrl Pts',(-76.4683756379696,27.1048249982604,
16.3494047007367));
#259336=CARTESIAN_POINT('Ctrl Pts',(-76.4671537647784,27.1045238256025,
16.3560192514989));
#259337=CARTESIAN_POINT('Ctrl Pts',(-76.4658752319056,27.1042596511149,
16.3627681883368));
#259338=CARTESIAN_POINT('Ctrl Pts',(-76.4645307210492,27.1040326825547,
16.3696623273235));
#259339=CARTESIAN_POINT('Ctrl Pts',(-76.4632739316421,27.1038205223623,
16.3761066641678));
#259340=CARTESIAN_POINT('Ctrl Pts',(-76.4619593190125,27.1036411260684,
16.3826784026771));
#259341=CARTESIAN_POINT('Ctrl Pts',(-76.4605856089535,27.1034929209309,
16.3893426844209));
#259342=CARTESIAN_POINT('Ctrl Pts',(-76.4593337345535,27.1033578602487,
16.3954159046432));
#259343=CARTESIAN_POINT('Ctrl Pts',(-76.4580326598444,27.1032489151465,
16.4015662355659));
#259344=CARTESIAN_POINT('Ctrl Pts',(-76.4566888072063,27.1031602607469,
16.4077247900022));
#259345=CARTESIAN_POINT('Ctrl Pts',(-76.4561164335948,27.1031225010719,
16.4103478410302));
#259346=CARTESIAN_POINT('Ctrl Pts',(-76.455536406734,27.1030883438962,16.4129718046058));
#259347=CARTESIAN_POINT('Ctrl Pts',(-76.4549497809965,27.103056887902,16.4155884735518));
#259348=CARTESIAN_POINT('Ctrl Pts',(-76.4528297571289,27.102943208167,16.4250449297984));
#259349=CARTESIAN_POINT('Ctrl Pts',(-76.4506276154548,27.1028516325169,
16.4344055618506));
#259350=CARTESIAN_POINT('Ctrl Pts',(-76.4483618531535,27.1027493830599,
16.4434727015235));
#259351=CARTESIAN_POINT('Ctrl Pts',(-76.4479348993932,27.102730115465,16.4451812873606));
#259352=CARTESIAN_POINT('Ctrl Pts',(-76.4475057389425,27.1027103529401,
16.4468793703295));
#259353=CARTESIAN_POINT('Ctrl Pts',(-76.4470745680892,27.1026896905073,
16.4485655884618));
#259354=CARTESIAN_POINT('Ctrl Pts',(-76.4456191147842,27.102619942736,16.4542575589071));
#259355=CARTESIAN_POINT('Ctrl Pts',(-76.444132204062,27.1025406532752,16.4598473134608));
#259356=CARTESIAN_POINT('Ctrl Pts',(-76.4426004684769,27.1024250918524,
16.4653566991082));
#259357=CARTESIAN_POINT('Ctrl Pts',(-76.442018509056,27.1023811860638,16.4674499056068));
#259358=CARTESIAN_POINT('Ctrl Pts',(-76.4414302186229,27.1023318496948,
16.4695309610823));
#259359=CARTESIAN_POINT('Ctrl Pts',(-76.440835390871,27.1022746925433,16.4715995364411));
#259360=CARTESIAN_POINT('Ctrl Pts',(-76.4389925228595,27.1020976108826,
16.4780083015759));
#259361=CARTESIAN_POINT('Ctrl Pts',(-76.4370710585172,27.1018561048158,
16.4843917801182));
#259362=CARTESIAN_POINT('Ctrl Pts',(-76.4350620986708,27.1015158539172,
16.490654206125));
#259363=CARTESIAN_POINT('Ctrl Pts',(-76.4333518787998,27.1012261996222,
16.4959853855495));
#259364=CARTESIAN_POINT('Ctrl Pts',(-76.4315790441175,27.1008647151592,
16.5012232667733));
#259365=CARTESIAN_POINT('Ctrl Pts',(-76.4297403585947,27.1004038747172,
16.506308780426));
#259366=CARTESIAN_POINT('Ctrl Pts',(-76.4284489299112,27.1000801964384,
16.5098806681252));
#259367=CARTESIAN_POINT('Ctrl Pts',(-76.4271251515653,27.0997073598879,
16.5133767163734));
#259368=CARTESIAN_POINT('Ctrl Pts',(-76.4257650872438,27.0992746306612,
16.5168023194498));
#259369=CARTESIAN_POINT('Ctrl Pts',(-76.4244998564356,27.0988720744434,
16.5199890647238));
#259370=CARTESIAN_POINT('Ctrl Pts',(-76.4232033943541,27.0984176364795,
16.5231136244715));
#259371=CARTESIAN_POINT('Ctrl Pts',(-76.4218676567953,27.0979025055479,
16.5262197343051));
#259372=CARTESIAN_POINT('Ctrl Pts',(-76.4217789540767,27.097868297096,16.5264260026584));
#259373=CARTESIAN_POINT('Ctrl Pts',(-76.4216900756692,27.0978338210951,
16.5266322092073));
#259374=CARTESIAN_POINT('Ctrl Pts',(-76.4216010180799,27.0977990750252,
16.5268383756647));
#259375=CARTESIAN_POINT('Ctrl Pts',(-76.4212719492621,27.097670687897,16.5276001630987));
#259376=CARTESIAN_POINT('Ctrl Pts',(-76.4209404362573,27.0975386143432,
16.5283613866217));
#259377=CARTESIAN_POINT('Ctrl Pts',(-76.4206063221415,27.097402744855,16.5291232096001));
#259378=CARTESIAN_POINT('Ctrl Pts',(-76.4187176830246,27.096634718549,16.5334295486889));
#259379=CARTESIAN_POINT('Ctrl Pts',(-76.4167566024533,27.0957491893783,
16.5376614539927));
#259380=CARTESIAN_POINT('Ctrl Pts',(-76.4147290835877,27.0947257635391,
16.5417599887957));
#259381=CARTESIAN_POINT('Ctrl Pts',(-76.4130382200732,27.0938722704149,
16.5451779905115));
#259382=CARTESIAN_POINT('Ctrl Pts',(-76.411301229187,27.0929228022905,16.5485028098004));
#259383=CARTESIAN_POINT('Ctrl Pts',(-76.4095163162424,27.0918686181488,
16.551734836596));
#259384=CARTESIAN_POINT('Ctrl Pts',(-76.408055328314,27.0910057467635,16.5543803169521));
#259385=CARTESIAN_POINT('Ctrl Pts',(-76.4065622115707,27.0900727245997,
16.5569638004465));
#259386=CARTESIAN_POINT('Ctrl Pts',(-76.405031931884,27.0890672853599,16.5595114022451));
#259387=CARTESIAN_POINT('Ctrl Pts',(-76.4024133502076,27.0873467993646,
16.5638708036317));
#259388=CARTESIAN_POINT('Ctrl Pts',(-76.3996858222844,27.0854160305355,
16.5681213015784));
#259389=CARTESIAN_POINT('Ctrl Pts',(-76.3968549739135,27.0832453437873,
16.5722001453341));
#259390=CARTESIAN_POINT('Ctrl Pts',(-76.3944794420099,27.0814237924544,
16.5756229438037));
#259391=CARTESIAN_POINT('Ctrl Pts',(-76.3920312478068,27.0794332007694,
16.5789244111398));
#259392=CARTESIAN_POINT('Ctrl Pts',(-76.3895078513918,27.0772609129644,
16.5821034643185));
#259393=CARTESIAN_POINT('Ctrl Pts',(-76.3879086122879,27.0758841940382,
16.584118235413));
#259394=CARTESIAN_POINT('Ctrl Pts',(-76.3862790519647,27.0744345916997,
16.5860845447305));
#259395=CARTESIAN_POINT('Ctrl Pts',(-76.3846166914258,27.072910440065,16.5880130337724));
#259396=CARTESIAN_POINT('Ctrl Pts',(-76.3827359747379,27.0711860864444,
16.5901948357573));
#259397=CARTESIAN_POINT('Ctrl Pts',(-76.3808666413311,27.0694154757839,
16.5922669270639));
#259398=CARTESIAN_POINT('Ctrl Pts',(-76.3790011612993,27.06760552235,16.5942742310314));
#259399=CARTESIAN_POINT('Ctrl Pts',(-76.3740456584702,27.0627975216158,
16.5996064781317));
#259400=CARTESIAN_POINT('Ctrl Pts',(-76.3691274276531,27.0577058759388,
16.6044118919327));
#259401=CARTESIAN_POINT('Ctrl Pts',(-76.3642377230688,27.052350350697,16.6087783050469));
#259402=CARTESIAN_POINT('Ctrl Pts',(-76.3592796180193,27.0469199087783,
16.6132057984744));
#259403=CARTESIAN_POINT('Ctrl Pts',(-76.354350908567,27.0412180804687,16.6171815871709));
#259404=CARTESIAN_POINT('Ctrl Pts',(-76.3494322419893,27.0352768340187,
16.6208506593413));
#259405=CARTESIAN_POINT('Ctrl Pts',(-76.3445135754116,27.0293355875688,
16.6245197315117));
#259406=CARTESIAN_POINT('Ctrl Pts',(-76.3396049868132,27.0231548844613,
16.6278819111749));
#259407=CARTESIAN_POINT('Ctrl Pts',(-76.3346762337744,27.0167787754263,
16.63113891706));
#259408=CARTESIAN_POINT('Ctrl Pts',(-76.3270525622666,27.0069163699866,
16.6361767720248));
#259409=CARTESIAN_POINT('Ctrl Pts',(-76.3193994276104,26.9965742763337,
16.6408622418844));
#259410=CARTESIAN_POINT('Ctrl Pts',(-76.3117344496374,26.9857761531999,
16.6452464533241));
#259411=CARTESIAN_POINT('Ctrl Pts',(-76.307436760805,26.9797217361661,16.6477046438903));
#259412=CARTESIAN_POINT('Ctrl Pts',(-76.303135157655,26.9735241809127,16.6500689942482));
#259413=CARTESIAN_POINT('Ctrl Pts',(-76.2988312337081,26.9671894394036,
16.6523553297695));
#259414=CARTESIAN_POINT('Ctrl Pts',(-76.2848016950066,26.9465400268532,
16.6598081177547));
#259415=CARTESIAN_POINT('Ctrl Pts',(-76.2713420389528,26.925314640378,16.6661261478319));
#259416=CARTESIAN_POINT('Ctrl Pts',(-76.2582666976199,26.9037854166563,
16.6722817468537));
#259417=CARTESIAN_POINT('Ctrl Pts',(-76.236716649198,26.8683021507223,16.6824270618866));
#259418=CARTESIAN_POINT('Ctrl Pts',(-76.2163231724805,26.8318654948446,
16.6915805494573));
#259419=CARTESIAN_POINT('Ctrl Pts',(-76.1969868424568,26.7948177268109,
16.7005093017872));
#259420=CARTESIAN_POINT('Ctrl Pts',(-76.1951008482725,26.7912042244055,
16.7013801792984));
#259421=CARTESIAN_POINT('Ctrl Pts',(-76.1932248857391,26.7875849267988,
16.7022489427234));
#259422=CARTESIAN_POINT('Ctrl Pts',(-76.1913588468482,26.7839601625929,
16.7031163158074));
#259423=CARTESIAN_POINT('Ctrl Pts',(-76.176568027518,26.7552291255579,16.7099913914772));
#259424=CARTESIAN_POINT('Ctrl Pts',(-76.162413994639,26.7262008738672,16.716810696067));
#259425=CARTESIAN_POINT('Ctrl Pts',(-76.1489165164747,26.6969732854461,
16.7235973395649));
#259426=CARTESIAN_POINT('Ctrl Pts',(-76.1236619610359,26.6422867919294,
16.7362955386192));
#259427=CARTESIAN_POINT('Ctrl Pts',(-76.1005180681828,26.5866819738269,
16.7491519989587));
#259428=CARTESIAN_POINT('Ctrl Pts',(-76.0794074083773,26.5302810836964,
16.7625435720843));
#259429=CARTESIAN_POINT('Ctrl Pts',(-76.064362927453,26.4900870715955,16.7720870571431));
#259430=CARTESIAN_POINT('Ctrl Pts',(-76.0503521064293,26.4494883805208,
16.7819023270087));
#259431=CARTESIAN_POINT('Ctrl Pts',(-76.0373611942068,26.4085292238121,
16.7921336012861));
#259432=CARTESIAN_POINT('Ctrl Pts',(-76.023172012212,26.3637920322323,16.8033085988748));
#259433=CARTESIAN_POINT('Ctrl Pts',(-76.010338419258,26.3190310002086,16.8148454077145));
#259434=CARTESIAN_POINT('Ctrl Pts',(-75.9987850456331,26.2743222514891,
16.8269262467475));
#259435=CARTESIAN_POINT('Ctrl Pts',(-75.9837486849446,26.2161351891203,
16.8426490874534));
#259436=CARTESIAN_POINT('Ctrl Pts',(-75.9708594776013,26.157598960004,16.8592311067997));
#259437=CARTESIAN_POINT('Ctrl Pts',(-75.9600230530903,26.0990044705617,
16.8768965952961));
#259438=CARTESIAN_POINT('Ctrl Pts',(-75.9491979291169,26.0404710851514,
16.8945436617091));
#259439=CARTESIAN_POINT('Ctrl Pts',(-75.94042141172,25.9818779784671,16.9132712882918));
#259440=CARTESIAN_POINT('Ctrl Pts',(-75.9336439588965,25.9235033739726,
16.9333228296636));
#259441=CARTESIAN_POINT('Ctrl Pts',(-75.9294790509155,25.8876307736792,
16.9456449847365));
#259442=CARTESIAN_POINT('Ctrl Pts',(-75.9260699331751,25.8518405543353,
16.9584675280565));
#259443=CARTESIAN_POINT('Ctrl Pts',(-75.9234132458688,25.8161989867003,
16.971852276588));
#259444=CARTESIAN_POINT('Ctrl Pts',(-75.9217239577779,25.793535846931,16.9803631375538));
#259445=CARTESIAN_POINT('Ctrl Pts',(-75.9203357066719,25.7708904059779,
16.9891192993509));
#259446=CARTESIAN_POINT('Ctrl Pts',(-75.9192531417279,25.748310663338,16.9981274246436));
#259447=CARTESIAN_POINT('Ctrl Pts',(-75.9170297815819,25.7019366326876,
17.016628214714));
#259448=CARTESIAN_POINT('Ctrl Pts',(-75.9160908878986,25.6557154302892,
17.0360687209549));
#259449=CARTESIAN_POINT('Ctrl Pts',(-75.9163356254785,25.6100335195781,
17.056834669541));
#259450=CARTESIAN_POINT('Ctrl Pts',(-75.91656211733,25.567757296436,17.0760524706907));
#259451=CARTESIAN_POINT('Ctrl Pts',(-75.9178014945773,25.5259435976778,
17.0964068031176));
#259452=CARTESIAN_POINT('Ctrl Pts',(-75.9199460216587,25.4848871401385,
17.1181763515212));
#259453=CARTESIAN_POINT('Ctrl Pts',(-75.922037669005,25.4448430524687,17.1394091065384));
#259454=CARTESIAN_POINT('Ctrl Pts',(-75.9249898990629,25.4055198685136,
17.1619892999248));
#259455=CARTESIAN_POINT('Ctrl Pts',(-75.9286842189327,25.3671710060197,
17.1861307296247));
#259456=CARTESIAN_POINT('Ctrl Pts',(-75.9320094343406,25.3326536299033,
17.2078601566467));
#259457=CARTESIAN_POINT('Ctrl Pts',(-75.9359354287002,25.298925635765,17.2308544606032));
#259458=CARTESIAN_POINT('Ctrl Pts',(-75.9403670676492,25.2661521618397,
17.2552262518704));
#259459=CARTESIAN_POINT('Ctrl Pts',(-75.9408589869714,25.2625142515169,
17.2579315613911));
#259460=CARTESIAN_POINT('Ctrl Pts',(-75.9413571303343,25.2588880802128,
17.2606537952903));
#259461=CARTESIAN_POINT('Ctrl Pts',(-75.9418613633423,25.2552738568381,
17.2633930704886));
#259462=CARTESIAN_POINT('Ctrl Pts',(-75.9418613633423,25.2552738568381,
17.2633930704886));
#259463=CARTESIAN_POINT('Ctrl Pts',(-75.9442259477114,25.2383250956303,
17.2762387759409));
#259464=CARTESIAN_POINT('Ctrl Pts',(-75.9466297979243,25.221950107767,17.2896217175501));
#259465=CARTESIAN_POINT('Ctrl Pts',(-75.9489416166353,25.2063620810916,
17.3037656230845));
#259466=CARTESIAN_POINT('Ctrl Pts',(-75.9512774695206,25.1906119978725,
17.3180565717624));
#259467=CARTESIAN_POINT('Ctrl Pts',(-75.9535194008088,25.1756652592871,
17.3331243152708));
#259468=CARTESIAN_POINT('Ctrl Pts',(-75.9555501185693,25.1617083526887,
17.3491621095395));
#259469=CARTESIAN_POINT('Ctrl Pts',(-75.9576114325003,25.147541161873,17.36544154009));
#259470=CARTESIAN_POINT('Ctrl Pts',(-75.9594551435701,25.1343938087813,
17.3827204196343));
#259471=CARTESIAN_POINT('Ctrl Pts',(-75.9609767647043,25.1224278850708,
17.401163330919));
#259472=CARTESIAN_POINT('Ctrl Pts',(-75.9611515135672,25.1210536720588,
17.4032813862633));
#259473=CARTESIAN_POINT('Ctrl Pts',(-75.9613220335549,25.1196950057595,
17.4054147545603));
#259474=CARTESIAN_POINT('Ctrl Pts',(-75.9614881812303,25.1183521036896,
17.4075636545403));
#259475=CARTESIAN_POINT('Ctrl Pts',(10.8641498708349,79.2111064053766,17.847987692667));
#259476=CARTESIAN_POINT('Ctrl Pts',(9.7654340370314,79.359520501561,17.8663812527205));
#259477=CARTESIAN_POINT('Ctrl Pts',(9.7654340370314,80.4599485582789,18.0027617587916));
#259478=CARTESIAN_POINT('Ctrl Pts',(10.8621713328006,78.2644852096539,25.4882815344998));
#259479=CARTESIAN_POINT('Ctrl Pts',(9.76543403703139,78.415025968742,25.5016215881557));
#259480=CARTESIAN_POINT('Ctrl Pts',(9.7654340370314,79.5130559971843,25.6430556014337));
#259481=CARTESIAN_POINT('Ctrl Pts',(10.8601243292931,77.317574634656,33.1285376594865));
#259482=CARTESIAN_POINT('Ctrl Pts',(9.76543403703139,77.4696829514656,33.1417037687789));
#259483=CARTESIAN_POINT('Ctrl Pts',(9.7654340370314,78.5658598958838,33.2833117264721));
#259484=CARTESIAN_POINT('Ctrl Pts',(10.858001215061,76.370342253395,40.7687517688986));
#259485=CARTESIAN_POINT('Ctrl Pts',(9.7654340370314,76.5233256693937,40.7877246696809));
#259486=CARTESIAN_POINT('Ctrl Pts',(9.7654340370314,77.6183256595919,40.9235258350231));
#259487=CARTESIAN_POINT('Ctrl Pts',(9.7654340370314,77.6928637726221,40.3225));
#259488=CARTESIAN_POINT('Ctrl Pts',(9.7654340370314,77.6406907450683,40.3348699258231));
#259489=CARTESIAN_POINT('Ctrl Pts',(9.7683743292685,77.5889301320358,40.347142091233));
#259490=CARTESIAN_POINT('Ctrl Pts',(9.77421593702744,77.5376245532549,40.3593064230311));
#259491=CARTESIAN_POINT('Ctrl Pts',(9.7800356824703,77.4865109864726,40.3714252296113));
#259492=CARTESIAN_POINT('Ctrl Pts',(9.78873516574705,77.4358485949097,40.3834371171633));
#259493=CARTESIAN_POINT('Ctrl Pts',(9.80032672757758,77.3856866947242,40.3953304235289));
#259494=CARTESIAN_POINT('Ctrl Pts',(9.81145263908703,77.3375398728577,40.4067459580457));
#259495=CARTESIAN_POINT('Ctrl Pts',(9.82524326664853,77.2898538147198,40.4180523240903));
#259496=CARTESIAN_POINT('Ctrl Pts',(9.84175291335836,77.2426843219429,40.4292363172717));
#259497=CARTESIAN_POINT('Ctrl Pts',(9.84292121245742,77.2393463900729,40.4300277484506));
#259498=CARTESIAN_POINT('Ctrl Pts',(9.84410288781287,77.236011786251,40.4308183913332));
#259499=CARTESIAN_POINT('Ctrl Pts',(9.84529794460256,77.2326805409166,40.4316082386352));
#259500=CARTESIAN_POINT('Ctrl Pts',(9.86516996289905,77.1772868819652,40.4447422253815));
#259501=CARTESIAN_POINT('Ctrl Pts',(9.88842098537268,77.1237590602342,40.4574340218528));
#259502=CARTESIAN_POINT('Ctrl Pts',(9.91505186507416,77.0719801851636,40.4697110373831));
#259503=CARTESIAN_POINT('Ctrl Pts',(9.92388396091018,77.0548077901083,40.4737826932563));
#259504=CARTESIAN_POINT('Ctrl Pts',(9.93308817911335,77.0378279739812,40.4778086771577));
#259505=CARTESIAN_POINT('Ctrl Pts',(9.94266563537454,77.0210370924819,40.4817898423615));
#259506=CARTESIAN_POINT('Ctrl Pts',(9.96873208562553,76.9753382487247,40.4926251666788));
#259507=CARTESIAN_POINT('Ctrl Pts',(9.99776047110971,76.9308062595847,40.50318366357));
#259508=CARTESIAN_POINT('Ctrl Pts',(10.0295120097993,76.8880200231596,40.5133278667756));
#259509=CARTESIAN_POINT('Ctrl Pts',(10.0411035752289,76.8724000097847,40.5170312210079));
#259510=CARTESIAN_POINT('Ctrl Pts',(10.0530582321017,76.8570131032765,40.5206792556205));
#259511=CARTESIAN_POINT('Ctrl Pts',(10.0653648162887,76.8418891614267,40.5242648814378));
#259512=CARTESIAN_POINT('Ctrl Pts',(10.068651836502,76.8378496406458,40.525222582158));
#259513=CARTESIAN_POINT('Ctrl Pts',(10.0719632027711,76.8338298192818,40.5261756223058));
#259514=CARTESIAN_POINT('Ctrl Pts',(10.0752986447752,76.8298302814747,40.5271238626224));
#259515=CARTESIAN_POINT('Ctrl Pts',(10.1248353857937,76.7704306371993,40.541206774251));
#259516=CARTESIAN_POINT('Ctrl Pts',(10.1790585260117,76.7160472771173,40.5541023854872));
#259517=CARTESIAN_POINT('Ctrl Pts',(10.2380522716906,76.6666407817785,40.5658176329226));
#259518=CARTESIAN_POINT('Ctrl Pts',(10.2796785900014,76.6317792811579,40.574083977316));
#259519=CARTESIAN_POINT('Ctrl Pts',(10.3240382810484,76.5992118758775,40.5818062215632));
#259520=CARTESIAN_POINT('Ctrl Pts',(10.3703731787742,76.5696242835505,40.5888209763611));
#259521=CARTESIAN_POINT('Ctrl Pts',(10.3857677071117,76.5597939601685,40.5911515920918));
#259522=CARTESIAN_POINT('Ctrl Pts',(10.4013800550833,76.5502929101763,40.5934040296095));
#259523=CARTESIAN_POINT('Ctrl Pts',(10.4171817032987,76.5411473570588,40.5955720423396));
#259524=CARTESIAN_POINT('Ctrl Pts',(10.4205823443447,76.5391791609,40.5960386160146));
#259525=CARTESIAN_POINT('Ctrl Pts',(10.4239920323319,76.5372272679841,40.5965013264119));
#259526=CARTESIAN_POINT('Ctrl Pts',(10.427410423321,76.5352919854596,40.596960100647));
#259527=CARTESIAN_POINT('Ctrl Pts',(10.4699717833534,76.5111963637033,40.6026721609271));
#259528=CARTESIAN_POINT('Ctrl Pts',(10.5138127373806,76.4895921179992,40.6077938499824));
#259529=CARTESIAN_POINT('Ctrl Pts',(10.5587950181376,76.4706502604835,40.6122845088192));
#259530=CARTESIAN_POINT('Ctrl Pts',(10.603385198479,76.4518735148759,40.6167360235937));
#259531=CARTESIAN_POINT('Ctrl Pts',(10.649096703806,76.4357131151363,40.6205674210037));
#259532=CARTESIAN_POINT('Ctrl Pts',(10.6957749766315,76.4222898455887,40.6237499580585));
#259533=CARTESIAN_POINT('Ctrl Pts',(10.741990927449,76.4089995259674,40.6269009738759));
#259534=CARTESIAN_POINT('Ctrl Pts',(10.7891543927876,76.3983925009905,40.6294158916108));
#259535=CARTESIAN_POINT('Ctrl Pts',(10.8370986845467,76.3905388100093,40.6312780057494));
#259536=CARTESIAN_POINT('Ctrl Pts',(10.8440625860396,76.3893980625222,40.6315484775606));
#259537=CARTESIAN_POINT('Ctrl Pts',(10.8510429350674,76.3883153199295,40.6318051966655));
#259538=CARTESIAN_POINT('Ctrl Pts',(10.8580391950581,76.3872907109282,40.6320481322491));
#259539=CARTESIAN_POINT('Origin',(11.0354340370314,80.4599485582789,18.0027617587916));
#259540=CARTESIAN_POINT('Ctrl Pts',(10.8629841634368,79.2590409673554,17.0741173620444));
#259541=CARTESIAN_POINT('Ctrl Pts',(9.76543403703139,79.4094675874129,17.0741173620444));
#259542=CARTESIAN_POINT('Ctrl Pts',(9.7654340370314,80.5172782427122,17.0741173620444));
#259543=CARTESIAN_POINT('Ctrl Pts',(10.8629841634028,79.2590409673601,17.3330517996227));
#259544=CARTESIAN_POINT('Ctrl Pts',(9.7654340370314,79.4094675877083,17.3392431182821));
#259545=CARTESIAN_POINT('Ctrl Pts',(9.7654340370314,80.5172782429666,17.3848387320851));
#259546=CARTESIAN_POINT('Ctrl Pts',(10.8633722599807,79.2430601863238,17.5910193441541));
#259547=CARTESIAN_POINT('Ctrl Pts',(9.7654340370314,79.392803294839,17.6034496884161));
#259548=CARTESIAN_POINT('Ctrl Pts',(9.7654340370314,80.4981651198115,17.6943996807311));
#259549=CARTESIAN_POINT('Ctrl Pts',(10.8641498708349,79.2111064053766,17.847987692667));
#259550=CARTESIAN_POINT('Ctrl Pts',(9.7654340370314,79.359520501561,17.8663812527205));
#259551=CARTESIAN_POINT('Ctrl Pts',(9.7654340370314,80.4599485582789,18.0027617587916));
#259552=CARTESIAN_POINT('Origin',(11.0354340370314,80.5172782427122,17.0741173620444));
#259553=CARTESIAN_POINT('Origin',(11.0354340370314,80.5172782427122,12.3825));
#259554=CARTESIAN_POINT('Ctrl Pts',(9.93397247946587,79.8850738159598,12.3824999999994));
#259555=CARTESIAN_POINT('Ctrl Pts',(9.87891393978383,79.9809998523955,12.3824999342017));
#259556=CARTESIAN_POINT('Ctrl Pts',(9.83665735537327,80.0836518503505,12.3772814134038));
#259557=CARTESIAN_POINT('Ctrl Pts',(9.77984203925996,80.2969364364516,12.3639187544469));
#259558=CARTESIAN_POINT('Ctrl Pts',(9.76543403689542,80.4068623726219,12.3558758059475));
#259559=CARTESIAN_POINT('Ctrl Pts',(9.76543403703139,80.5172782442762,12.3495568919806));
#259560=CARTESIAN_POINT('Ctrl Pts',(-9.76543403703141,80.4599485582789,
18.0027617587917));
#259561=CARTESIAN_POINT('Ctrl Pts',(-9.76543403703142,79.359520501561,17.8663812527206));
#259562=CARTESIAN_POINT('Ctrl Pts',(-10.8641498708349,79.2111064053766,
17.8479876926672));
#259563=CARTESIAN_POINT('Ctrl Pts',(-9.76543403703141,79.5130559971301,
25.6430556014271));
#259564=CARTESIAN_POINT('Ctrl Pts',(-9.76543403713151,78.4150259686878,
25.5016215881491));
#259565=CARTESIAN_POINT('Ctrl Pts',(-10.86217133288,78.2644852096432,25.4882815344986));
#259566=CARTESIAN_POINT('Ctrl Pts',(-9.76543403703142,78.5658598956831,
33.2833117264472));
#259567=CARTESIAN_POINT('Ctrl Pts',(-9.76543403703142,77.4696829512648,
33.1417037687541));
#259568=CARTESIAN_POINT('Ctrl Pts',(-10.8601243293212,77.3175746346521,
33.1285376594861));
#259569=CARTESIAN_POINT('Ctrl Pts',(-9.76543403703142,77.6183256595919,
40.9235258350231));
#259570=CARTESIAN_POINT('Ctrl Pts',(-9.76543403703142,76.5233256693937,
40.7877246696809));
#259571=CARTESIAN_POINT('Ctrl Pts',(-10.8580012150611,76.370342253395,40.7687517688986));
#259572=CARTESIAN_POINT('Ctrl Pts',(-10.8580391950582,76.3872907109282,
40.6320481322491));
#259573=CARTESIAN_POINT('Ctrl Pts',(-10.8038338229833,76.3952291394678,
40.6301659271477));
#259574=CARTESIAN_POINT('Ctrl Pts',(-10.7506894857011,76.4066910151546,
40.6274486565634));
#259575=CARTESIAN_POINT('Ctrl Pts',(-10.6987376202637,76.421510168725,40.6239354244084));
#259576=CARTESIAN_POINT('Ctrl Pts',(-10.6458391128062,76.4365993498172,
40.620358175819));
#259577=CARTESIAN_POINT('Ctrl Pts',(-10.594176367347,76.4551693794646,40.6159556693214));
#259578=CARTESIAN_POINT('Ctrl Pts',(-10.5438898994474,76.4770976611215,
40.6107566553931));
#259579=CARTESIAN_POINT('Ctrl Pts',(-10.5042776831975,76.4943712512395,
40.6066612302695));
#259580=CARTESIAN_POINT('Ctrl Pts',(-10.4655194169616,76.5137297868398,
40.6020712995237));
#259581=CARTESIAN_POINT('Ctrl Pts',(-10.4276880145587,76.5351350735785,
40.5969957588345));
#259582=CARTESIAN_POINT('Ctrl Pts',(-10.4242613480823,76.5370739067654,
40.5965360300371));
#259583=CARTESIAN_POINT('Ctrl Pts',(-10.4208458708561,76.5390275045006,
40.5960727978901));
#259584=CARTESIAN_POINT('Ctrl Pts',(-10.417441529947,76.5409958524294,40.5956060656757));
#259585=CARTESIAN_POINT('Ctrl Pts',(-10.3539733392929,76.5776923775294,
40.5869046312546));
#259586=CARTESIAN_POINT('Ctrl Pts',(-10.2946065930604,76.6193798556825,
40.5770207119274));
#259587=CARTESIAN_POINT('Ctrl Pts',(-10.2391051819928,76.6657602207944,
40.5660242594495));
#259588=CARTESIAN_POINT('Ctrl Pts',(-10.1944993133031,76.7030356059813,
40.5571865325189));
#259589=CARTESIAN_POINT('Ctrl Pts',(-10.1521266719203,76.7436824784756,
40.5475495232825));
#259590=CARTESIAN_POINT('Ctrl Pts',(-10.112768827324,76.7868622699144,40.5373116645919));
#259591=CARTESIAN_POINT('Ctrl Pts',(-10.1000103154398,76.8008597305954,
40.5339928893106));
#259592=CARTESIAN_POINT('Ctrl Pts',(-10.0875683378583,76.8151236613885,
40.5306109028825));
#259593=CARTESIAN_POINT('Ctrl Pts',(-10.0754687483719,76.8296263455661,
40.5271722631609));
#259594=CARTESIAN_POINT('Ctrl Pts',(-10.0721400686965,76.8336161329977,
40.5262262698968));
#259595=CARTESIAN_POINT('Ctrl Pts',(-10.0688379426855,76.8376221197981,
40.5252764323596));
#259596=CARTESIAN_POINT('Ctrl Pts',(-10.0655622810809,76.8416442509437,
40.5243227633055));
#259597=CARTESIAN_POINT('Ctrl Pts',(-10.0197772889645,76.8978628916408,
40.5109930194578));
#259598=CARTESIAN_POINT('Ctrl Pts',(-9.97910469542405,76.9573064495693,
40.4968987634144));
#259599=CARTESIAN_POINT('Ctrl Pts',(-9.94335294128108,77.0198338045965,
40.4820734444561));
#259600=CARTESIAN_POINT('Ctrl Pts',(-9.91378625397024,77.0715439038288,
40.4698129112198));
#259601=CARTESIAN_POINT('Ctrl Pts',(-9.88745885424494,77.1258101444836,
40.4569463905791));
#259602=CARTESIAN_POINT('Ctrl Pts',(-9.8649496492485,77.1812643278188,40.4437982715083));
#259603=CARTESIAN_POINT('Ctrl Pts',(-9.85807764537128,77.1981943510226,
40.4397841837052));
#259604=CARTESIAN_POINT('Ctrl Pts',(-9.85156135507736,77.2152354151264,
40.4357437739529));
#259605=CARTESIAN_POINT('Ctrl Pts',(-9.84541680798104,77.2323494285094,
40.431686073453));
#259606=CARTESIAN_POINT('Ctrl Pts',(-9.81300496672525,77.3226240535266,
40.4102821290442));
#259607=CARTESIAN_POINT('Ctrl Pts',(-9.79038099604269,77.4153316528972,
40.3883014811186));
#259608=CARTESIAN_POINT('Ctrl Pts',(-9.7776621016632,77.5097070805337,40.3659254999368));
#259609=CARTESIAN_POINT('Ctrl Pts',(-9.7695177379922,77.5701390474441,40.3515973576626));
#259610=CARTESIAN_POINT('Ctrl Pts',(-9.76543403703142,77.6312555924454,
40.3371069464355));
#259611=CARTESIAN_POINT('Ctrl Pts',(-9.76543403703142,77.6928637726221,
40.3225000000001));
#259612=CARTESIAN_POINT('Origin',(-11.0354340370314,80.4599485582789,18.0027617587917));
#259613=CARTESIAN_POINT('Ctrl Pts',(-9.76543403703142,80.5172782427122,
17.0741173620445));
#259614=CARTESIAN_POINT('Ctrl Pts',(-9.76543403703142,79.4094675874129,
17.0741173620445));
#259615=CARTESIAN_POINT('Ctrl Pts',(-10.8629841634369,79.2590409673554,
17.0741173620445));
#259616=CARTESIAN_POINT('Ctrl Pts',(-9.76543403703142,80.5172782429666,
17.3848387320852));
#259617=CARTESIAN_POINT('Ctrl Pts',(-9.76543403703142,79.4094675877083,
17.3392431182822));
#259618=CARTESIAN_POINT('Ctrl Pts',(-10.8629841634031,79.25904096736,17.3330517996228));
#259619=CARTESIAN_POINT('Ctrl Pts',(-9.76543403703142,80.4981651198115,
17.6943996807312));
#259620=CARTESIAN_POINT('Ctrl Pts',(-9.76543403703142,79.392803294839,17.6034496884162));
#259621=CARTESIAN_POINT('Ctrl Pts',(-10.8633722599797,79.2430601863239,
17.5910193441543));
#259622=CARTESIAN_POINT('Ctrl Pts',(-9.76543403703142,80.4599485582789,
18.0027617587917));
#259623=CARTESIAN_POINT('Ctrl Pts',(-9.76543403703142,79.359520501561,17.8663812527206));
#259624=CARTESIAN_POINT('Ctrl Pts',(-10.8641498708349,79.2111064053766,
17.8479876926671));
#259625=CARTESIAN_POINT('Origin',(-11.0354340370314,80.5172782427121,17.0741173620445));
#259626=CARTESIAN_POINT('Origin',(-11.0354340370314,80.5172782427122,12.3825));
#259627=CARTESIAN_POINT('Ctrl Pts',(-9.76543403703142,80.5172782442762,
12.3495568919838));
#259628=CARTESIAN_POINT('Ctrl Pts',(-9.76543403689582,80.407164861761,12.3558584950094));
#259629=CARTESIAN_POINT('Ctrl Pts',(-9.77976311228818,80.2975378399709,
12.363874307156));
#259630=CARTESIAN_POINT('Ctrl Pts',(-9.83642681214443,80.0842125738188,
12.3772530427028));
#259631=CARTESIAN_POINT('Ctrl Pts',(-9.87876331331359,79.9812622821722,
12.3824999340235));
#259632=CARTESIAN_POINT('Ctrl Pts',(-9.93397247946588,79.8850738159598,
12.3824999999994));
#259633=CARTESIAN_POINT('Ctrl Pts',(19.6282160049318,113.33109747126,12.2312547539759));
#259634=CARTESIAN_POINT('Ctrl Pts',(19.968791267623,113.225505581264,12.3825000000002));
#259635=CARTESIAN_POINT('Ctrl Pts',(20.3387380182653,113.110807356014,12.3825));
#259636=CARTESIAN_POINT('Ctrl Pts',(17.9262673743939,107.744499663662,12.2434569899102));
#259637=CARTESIAN_POINT('Ctrl Pts',(18.257711262191,107.651751796601,12.3824999999443));
#259638=CARTESIAN_POINT('Ctrl Pts',(18.6092072977809,107.532395334702,12.3825));
#259639=CARTESIAN_POINT('Ctrl Pts',(16.2272244965966,102.15710346924,12.2580230532609));
#259640=CARTESIAN_POINT('Ctrl Pts',(16.5451782447696,102.073466334938,12.3824999999848));
#259641=CARTESIAN_POINT('Ctrl Pts',(16.8761662824142,101.955067506485,12.3825));
#259642=CARTESIAN_POINT('Ctrl Pts',(12.847024800685,90.9828768181336,12.2950955201719));
#259643=CARTESIAN_POINT('Ctrl Pts',(13.1184592484314,90.9129457862284,12.3825000000151));
#259644=CARTESIAN_POINT('Ctrl Pts',(13.3939133181762,90.811238296817,12.3825));
#259645=CARTESIAN_POINT('Ctrl Pts',(11.1637373488142,85.3967648634315,12.3186057573121));
#259646=CARTESIAN_POINT('Ctrl Pts',(11.4074622813581,85.3412573398049,12.382499999807));
#259647=CARTESIAN_POINT('Ctrl Pts',(11.6464930192604,85.2441534264155,12.3825));
#259648=CARTESIAN_POINT('Ctrl Pts',(9.50982386430973,79.8014081751007,12.3445056966244));
#259649=CARTESIAN_POINT('Ctrl Pts',(9.68831043192349,79.7443724057398,12.3825));
#259650=CARTESIAN_POINT('Ctrl Pts',(9.87042927168866,79.6861759359438,12.3825));
#259651=CARTESIAN_POINT('Origin',(20.3338370957105,113.095,10.4775));
#259652=CARTESIAN_POINT('Origin',(20.3338370957106,113.095,10.4775));
#259653=CARTESIAN_POINT('Ctrl Pts',(-20.338738022895,113.110807370947,12.3825));
#259654=CARTESIAN_POINT('Ctrl Pts',(-19.968791272205,113.225505596211,12.3824999999999));
#259655=CARTESIAN_POINT('Ctrl Pts',(-19.6282160094772,113.331097486218,
12.2312547539385));
#259656=CARTESIAN_POINT('Ctrl Pts',(-18.6092073009371,107.532395344573,
12.3825));
#259657=CARTESIAN_POINT('Ctrl Pts',(-18.2577112653127,107.6517518065,12.3825000000253));
#259658=CARTESIAN_POINT('Ctrl Pts',(-17.9262673774906,107.744499673551,
12.2434569899207));
#259659=CARTESIAN_POINT('Ctrl Pts',(-16.8761662839561,101.955067511533,
12.3825));
#259660=CARTESIAN_POINT('Ctrl Pts',(-16.5451782462744,102.073466340022,
12.3824999999898));
#259661=CARTESIAN_POINT('Ctrl Pts',(-16.2272244980822,102.157103474302,
12.2580230532285));
#259662=CARTESIAN_POINT('Ctrl Pts',(-13.3939133181817,90.8112382967211,
12.3825));
#259663=CARTESIAN_POINT('Ctrl Pts',(-13.1184592484483,90.912945786136,12.3825000000101));
#259664=CARTESIAN_POINT('Ctrl Pts',(-12.8470248006833,90.9828768180411,
12.2950955201813));
#259665=CARTESIAN_POINT('Ctrl Pts',(-11.6464930191708,85.2441534264819,
12.3825));
#259666=CARTESIAN_POINT('Ctrl Pts',(-11.4074622811763,85.3412573398973,
12.3824999999188));
#259667=CARTESIAN_POINT('Ctrl Pts',(-11.1637373486809,85.3967648635073,
12.3186057572813));
#259668=CARTESIAN_POINT('Ctrl Pts',(-9.87042927168149,79.6861759359214,
12.3825));
#259669=CARTESIAN_POINT('Ctrl Pts',(-9.68831043191372,79.7443724057182,
12.3825));
#259670=CARTESIAN_POINT('Ctrl Pts',(-9.5098238642975,79.8014081750798,12.3445056966233));
#259671=CARTESIAN_POINT('Origin',(-20.3338370957106,113.095,10.4775));
#259672=CARTESIAN_POINT('Origin',(-20.3338370957106,113.095,10.4775));
#259673=CARTESIAN_POINT('Ctrl Pts',(9.97906670428255,80.6550131021071,12.6355897418272));
#259674=CARTESIAN_POINT('Ctrl Pts',(10.0306565474884,80.6485542978432,12.3963818596608));
#259675=CARTESIAN_POINT('Ctrl Pts',(10.0626130773097,80.8910903102766,12.3874807730462));
#259676=CARTESIAN_POINT('Ctrl Pts',(8.32489473089131,80.8596741618412,12.2721732806416));
#259677=CARTESIAN_POINT('Ctrl Pts',(8.38220322552675,80.853588835157,12.0386865759819));
#259678=CARTESIAN_POINT('Ctrl Pts',(8.39484377214235,81.0939065240695,12.0224470193747));
#259679=CARTESIAN_POINT('Ctrl Pts',(6.65782497351594,81.0143136970555,11.9945489971187));
#259680=CARTESIAN_POINT('Ctrl Pts',(6.69895405423401,81.0111835475032,11.7604293808636));
#259681=CARTESIAN_POINT('Ctrl Pts',(6.71387712855119,81.2473407845731,11.7435792721713));
#259682=CARTESIAN_POINT('Ctrl Pts',(4.1545853934931,81.167929206631,11.7183089462413));
#259683=CARTESIAN_POINT('Ctrl Pts',(4.17758614754292,81.1667081501201,11.4852779313552));
#259684=CARTESIAN_POINT('Ctrl Pts',(4.18963063148697,81.3998032104587,11.4660958435514));
#259685=CARTESIAN_POINT('Ctrl Pts',(3.32813735528307,81.2060674095149,11.649567866613));
#259686=CARTESIAN_POINT('Ctrl Pts',(3.34606415307882,81.2053149583786,11.4167992749039));
#259687=CARTESIAN_POINT('Ctrl Pts',(3.35622483782533,81.4376673268027,11.3970442061328));
#259688=CARTESIAN_POINT('Ctrl Pts',(1.66882448528439,81.2571037391673,11.5575387285848));
#259689=CARTESIAN_POINT('Ctrl Pts',(1.67821450599537,81.256876957723,11.3252958333052));
#259690=CARTESIAN_POINT('Ctrl Pts',(1.68291996832573,81.4883403078153,11.3045989360452));
#259691=CARTESIAN_POINT('Ctrl Pts',(0.834784835272045,81.2699994403931,
11.5342541227382));
#259692=CARTESIAN_POINT('Ctrl Pts',(0.839074610794663,81.2699304222547,
11.3020962817064));
#259693=CARTESIAN_POINT('Ctrl Pts',(0.841835610486893,81.5011467291217,
11.2812087546069));
#259694=CARTESIAN_POINT('Ctrl Pts',(-3.37266473870902,81.2700023175606,
11.5342489298588));
#259695=CARTESIAN_POINT('Ctrl Pts',(-3.38999574980634,81.2699333290047,
11.3020911179797));
#259696=CARTESIAN_POINT('Ctrl Pts',(-3.40115100228494,81.5011495862201,
11.2812035383244));
#259697=CARTESIAN_POINT('Ctrl Pts',(-6.69953756680781,81.0607706805708,
11.9150344302535));
#259698=CARTESIAN_POINT('Ctrl Pts',(-6.78961021185513,81.0517495349953,
11.6929294186456));
#259699=CARTESIAN_POINT('Ctrl Pts',(-6.75613034542886,81.2931923541874,
11.6637198264307));
#259700=CARTESIAN_POINT('Ctrl Pts',(-9.97933244163048,80.6549803814545,
12.6356486412316));
#259701=CARTESIAN_POINT('Ctrl Pts',(-10.0309242199162,80.6485200313328,
12.3964424789898));
#259702=CARTESIAN_POINT('Ctrl Pts',(-10.0628811435792,80.8910578280727,
12.3875399644105));
#259703=CARTESIAN_POINT('Ctrl Pts',(76.532738233499,27.1805870613698,16.1925));
#259704=CARTESIAN_POINT('Ctrl Pts',(76.532738233499,27.1805870613698,16.1925));
#259705=CARTESIAN_POINT('Ctrl Pts',(76.532738233499,27.1805870613698,16.1925));
#259706=CARTESIAN_POINT('Ctrl Pts',(76.4822360033882,27.108462402101,16.0119303091303));
#259707=CARTESIAN_POINT('Ctrl Pts',(76.4461624483558,27.0569440263853,16.0425775126009));
#259708=CARTESIAN_POINT('Ctrl Pts',(76.4100103023385,27.0053134111113,16.0732804919947));
#259709=CARTESIAN_POINT('Ctrl Pts',(76.4397549856158,27.0477932212451,15.8256195009857));
#259710=CARTESIAN_POINT('Ctrl Pts',(76.3671168872244,26.9440552658148,15.8737167831498));
#259711=CARTESIAN_POINT('Ctrl Pts',(76.3145038880894,26.8290932950587,15.9238883805606));
#259712=CARTESIAN_POINT('Ctrl Pts',(76.4065721949852,27.0004032849478,15.6340057707333));
#259713=CARTESIAN_POINT('Ctrl Pts',(76.2985554613104,26.8461394020553,15.6908641824603));
#259714=CARTESIAN_POINT('Ctrl Pts',(76.2443511862693,26.664968902009,15.7450581469137));
#259715=CARTESIAN_POINT('Ctrl Pts',(76.4071670555573,27.0012528338882,15.6374346124286));
#259716=CARTESIAN_POINT('Ctrl Pts',(76.4176851262999,27.016274195654,15.7161206159306));
#259717=CARTESIAN_POINT('Ctrl Pts',(76.4293098622517,27.0328195014371,15.7940085055158));
#259718=CARTESIAN_POINT('Ctrl Pts',(76.44205216039,27.0508562735771,15.8712754089344));
#259719=CARTESIAN_POINT('Ctrl Pts',(76.4549544984364,27.069119582824,15.949512764307));
#259720=CARTESIAN_POINT('Ctrl Pts',(76.469002736108,27.0889124184517,16.0271138595694));
#259721=CARTESIAN_POINT('Ctrl Pts',(76.4842364901892,27.1102366114595,16.1042351543385));
#259722=CARTESIAN_POINT('Ctrl Pts',(76.4874461624915,27.1147295073867,16.120484207751));
#259723=CARTESIAN_POINT('Ctrl Pts',(76.4907085588544,27.1192904969234,16.1367118525517));
#259724=CARTESIAN_POINT('Ctrl Pts',(76.4940242019312,27.1239197716699,16.1529193708669));
#259725=CARTESIAN_POINT('Ctrl Pts',(76.4496012596383,27.0600511154422,16.1720905903401));
#259726=CARTESIAN_POINT('Ctrl Pts',(76.4728494185474,27.091261572645,16.1624955941075));
#259727=CARTESIAN_POINT('Ctrl Pts',(76.4940242023748,27.1239197722893,16.1529193730355));
#259728=CARTESIAN_POINT('Ctrl Pts',(76.4324251716318,27.0369532490963,15.9953515848464));
#259729=CARTESIAN_POINT('Ctrl Pts',(76.4463480572545,27.0564032612897,15.9905628215355));
#259730=CARTESIAN_POINT('Ctrl Pts',(76.4598027159916,27.0761400025693,15.9856379879077));
#259731=CARTESIAN_POINT('Ctrl Pts',(76.4184454096962,27.0173599928704,15.8170364535711));
#259732=CARTESIAN_POINT('Ctrl Pts',(76.4245770423424,27.0261168718125,15.8152865503265));
#259733=CARTESIAN_POINT('Ctrl Pts',(76.4307073155649,27.0348718092963,15.8135400053977));
#259734=CARTESIAN_POINT('Ctrl Pts',(76.4071670555573,27.0012528338882,15.6374346124286));
#259735=CARTESIAN_POINT('Ctrl Pts',(76.4071670555573,27.0012528338882,15.6374346124286));
#259736=CARTESIAN_POINT('Ctrl Pts',(76.4071670555573,27.0012528338882,15.6374346124286));
#259737=CARTESIAN_POINT('Origin',(75.4310816924321,27.8186800531739,16.171929177394));
#259738=CARTESIAN_POINT('Ctrl Pts',(76.0135189288796,24.9743362449089,17.2567539685303));
#259739=CARTESIAN_POINT('Ctrl Pts',(75.9991603762543,25.0368598246417,17.3329617590086));
#259740=CARTESIAN_POINT('Ctrl Pts',(75.9698282088072,25.0952662902613,17.4081821724392));
#259741=CARTESIAN_POINT('Ctrl Pts',(75.9684245146036,25.1582927283603,17.0243415107349));
#259742=CARTESIAN_POINT('Ctrl Pts',(75.9600761821103,25.2156521066941,17.1240992078125));
#259743=CARTESIAN_POINT('Ctrl Pts',(75.9323827028628,25.2682007021653,17.2228395557702));
#259744=CARTESIAN_POINT('Ctrl Pts',(75.9418437641948,25.3910520091979,16.862700351237));
#259745=CARTESIAN_POINT('Ctrl Pts',(75.9388483528643,25.445796768841,16.9834260323936));
#259746=CARTESIAN_POINT('Ctrl Pts',(75.9089806068547,25.4963947971894,17.1020365608016));
#259747=CARTESIAN_POINT('Ctrl Pts',(75.9541657983329,25.7887320240513,16.6415771202465));
#259748=CARTESIAN_POINT('Ctrl Pts',(75.9591105110421,25.8384885908314,16.7940129727795));
#259749=CARTESIAN_POINT('Ctrl Pts',(75.9243559941834,25.8898093808734,16.9419191856935));
#259750=CARTESIAN_POINT('Ctrl Pts',(75.9755313586025,25.9560410312404,16.5655243592805));
#259751=CARTESIAN_POINT('Ctrl Pts',(75.9835274011649,26.0037786517969,16.730097613125));
#259752=CARTESIAN_POINT('Ctrl Pts',(75.9462476067507,26.0563925183529,16.888987323054));
#259753=CARTESIAN_POINT('Ctrl Pts',(76.0537110495859,26.2901439472438,16.430093768641));
#259754=CARTESIAN_POINT('Ctrl Pts',(76.0669818398559,26.3329365721293,16.617385587321));
#259755=CARTESIAN_POINT('Ctrl Pts',(76.0249595721014,26.3897550778952,16.7964776672641));
#259756=CARTESIAN_POINT('Ctrl Pts',(76.1106254906956,26.4559143405794,16.3716494180751));
#259757=CARTESIAN_POINT('Ctrl Pts',(76.1261665775814,26.4957943220995,16.5698206523398));
#259758=CARTESIAN_POINT('Ctrl Pts',(76.0817008086393,26.5557571967131,16.7582736038159));
#259759=CARTESIAN_POINT('Ctrl Pts',(76.2206362259214,26.6928863098607,16.2954976206041));
#259760=CARTESIAN_POINT('Ctrl Pts',(76.2382520010556,26.7274552575817,16.5052911886963));
#259761=CARTESIAN_POINT('Ctrl Pts',(76.1926335678084,26.7915039216042,16.7036134975717));
#259762=CARTESIAN_POINT('Ctrl Pts',(76.2615893549122,26.7704586218702,16.2719030686384));
#259763=CARTESIAN_POINT('Ctrl Pts',(76.2797058737871,26.8031110554089,16.4852296809776));
#259764=CARTESIAN_POINT('Ctrl Pts',(76.2339253041331,26.8686071917093,16.6865119483355));
#259765=CARTESIAN_POINT('Ctrl Pts',(76.3293506348445,26.8839886375728,16.2388534884045));
#259766=CARTESIAN_POINT('Ctrl Pts',(76.3475815823904,26.9132368525625,16.4509817168048));
#259767=CARTESIAN_POINT('Ctrl Pts',(76.3047198064137,26.9781622528333,16.6513143014549));
#259768=CARTESIAN_POINT('Ctrl Pts',(76.352936031986,26.9212671030173,16.2282720121333));
#259769=CARTESIAN_POINT('Ctrl Pts',(76.3710861233276,26.949270802543,16.439505830876));
#259770=CARTESIAN_POINT('Ctrl Pts',(76.3295234781731,27.0137899593914,16.639113518033));
#259771=CARTESIAN_POINT('Ctrl Pts',(76.3897977681848,26.9762969849698,16.2127741097789));
#259772=CARTESIAN_POINT('Ctrl Pts',(76.4073792368665,27.0019658578953,16.4134596674917));
#259773=CARTESIAN_POINT('Ctrl Pts',(76.3718135183751,27.0620819877444,16.6041529821789));
#259774=CARTESIAN_POINT('Ctrl Pts',(76.4023273523985,26.9944844920511,16.2076984546917));
#259775=CARTESIAN_POINT('Ctrl Pts',(76.4196215779418,27.0192636816435,16.4043770534771));
#259776=CARTESIAN_POINT('Ctrl Pts',(76.3864139085197,27.0775694765284,16.591707715843));
#259777=CARTESIAN_POINT('Ctrl Pts',(76.4182736725831,27.0169978024882,16.2011700710385));
#259778=CARTESIAN_POINT('Ctrl Pts',(76.4349444211234,27.0403624632552,16.381098623647));
#259779=CARTESIAN_POINT('Ctrl Pts',(76.4092245675447,27.0924838923546,16.5537833743782));
#259780=CARTESIAN_POINT('Ctrl Pts',(76.4214772237873,27.0214895124959,16.1998527480328));
#259781=CARTESIAN_POINT('Ctrl Pts',(76.4380023011771,27.0445457602702,16.3757607500836));
#259782=CARTESIAN_POINT('Ctrl Pts',(76.4140487138282,27.0952122751629,16.5448980557904));
#259783=CARTESIAN_POINT('Ctrl Pts',(76.4279076878214,27.0304439095153,16.197147126751));
#259784=CARTESIAN_POINT('Ctrl Pts',(76.4441127500533,27.0528532380362,16.3617442626138));
#259785=CARTESIAN_POINT('Ctrl Pts',(76.4248418621342,27.0997179766929,16.5207709779264));
#259786=CARTESIAN_POINT('Ctrl Pts',(76.4311355139959,27.0349078309285,16.1957692072802));
#259787=CARTESIAN_POINT('Ctrl Pts',(76.4471475072276,27.0569532640503,16.353378507755));
#259788=CARTESIAN_POINT('Ctrl Pts',(76.4307401571975,27.1014806667834,16.5061220168225));
#259789=CARTESIAN_POINT('Ctrl Pts',(76.4375990464852,27.0437858881523,16.1927492164626));
#259790=CARTESIAN_POINT('Ctrl Pts',(76.4533656745128,27.0653090310172,16.3262439284466));
#259791=CARTESIAN_POINT('Ctrl Pts',(76.4456774700282,27.1032717188634,16.4567548936541));
#259792=CARTESIAN_POINT('Ctrl Pts',(76.4408619220711,27.0482365818426,16.1912703300228));
#259793=CARTESIAN_POINT('Ctrl Pts',(76.4564740580196,27.0694680856207,16.3056985101718));
#259794=CARTESIAN_POINT('Ctrl Pts',(76.455545261251,27.1023654406524,16.4183837546514));
#259795=CARTESIAN_POINT('Ctrl Pts',(76.4456024830061,27.0546608085524,16.1874122722788));
#259796=CARTESIAN_POINT('Ctrl Pts',(76.4626691372742,27.0777286074699,16.2584144265338));
#259797=CARTESIAN_POINT('Ctrl Pts',(76.4724831553652,27.105919574582,16.3289405788401));
#259798=CARTESIAN_POINT('Ctrl Pts',(76.4471920450455,27.0568070233922,16.1858770660613));
#259799=CARTESIAN_POINT('Ctrl Pts',(76.4650242491595,27.0808620750697,16.2408811596319));
#259800=CARTESIAN_POINT('Ctrl Pts',(76.4782041251027,27.1082005910335,16.2956491527569));
#259801=CARTESIAN_POINT('Ctrl Pts',(76.4824975375383,27.1043580483931,16.1112477802486));
#259802=CARTESIAN_POINT('Ctrl Pts',(76.5324864042392,27.1705424338065,15.6967037653767));
#259803=CARTESIAN_POINT('Ctrl Pts',(76.6206938565971,27.2122852390614,15.2747264778709));
#259804=CARTESIAN_POINT('Ctrl Pts',(76.0596473272883,26.5325612269295,14.9152913818395));
#259805=CARTESIAN_POINT('Ctrl Pts',(76.5169321639722,27.1543749835465,12.0112890458989));
#259806=CARTESIAN_POINT('Ctrl Pts',(76.0362901547838,28.43850005779,10.812760927815));
#259807=CARTESIAN_POINT('Ctrl Pts',(67.4282061989127,15.0466061792269,43.6759546261335));
#259808=CARTESIAN_POINT('Ctrl Pts',(66.2614595719668,13.6559904578472,92.6380204617887));
#259809=CARTESIAN_POINT('Ctrl Pts',(44.6874817572436,-42.6649830590962,
383.024483305851));
#259810=CARTESIAN_POINT('Origin',(74.7257085670769,24.9421491495265,17.0741173620445));
#259811=CARTESIAN_POINT('Ctrl Pts',(75.9397262748,25.2708374178295,17.2518520136118));
#259812=CARTESIAN_POINT('Ctrl Pts',(75.9685632596794,25.216936348383,17.1547259853702));
#259813=CARTESIAN_POINT('Ctrl Pts',(75.9772090303541,25.1589733721721,17.0560474933639));
#259814=CARTESIAN_POINT('Ctrl Pts',(75.9481612403383,25.2082186978402,17.2973276044734));
#259815=CARTESIAN_POINT('Ctrl Pts',(75.9759984326351,25.1530396512954,17.2125718697421));
#259816=CARTESIAN_POINT('Ctrl Pts',(75.987289897294,25.0938856962963,17.126659867066));
#259817=CARTESIAN_POINT('Ctrl Pts',(75.9580441980768,25.1496292036213,17.3506767479875));
#259818=CARTESIAN_POINT('Ctrl Pts',(75.9851307385962,25.0926862211882,17.2798459584166));
#259819=CARTESIAN_POINT('Ctrl Pts',(75.9990697411205,25.0322694075925,17.2080611432674));
#259820=CARTESIAN_POINT('Ctrl Pts',(75.9627753173077,25.1074704497584,17.4259425795047));
#259821=CARTESIAN_POINT('Ctrl Pts',(75.9901905947633,25.0462350072204,17.3727027235267));
#259822=CARTESIAN_POINT('Ctrl Pts',(76.0065414441445,24.9819025616069,17.318579611819));
#259823=CARTESIAN_POINT('Origin',(74.7646897896784,24.7225971487503,17.2528005263547));
#259824=CARTESIAN_POINT('Ctrl Pts',(75.961489026876,25.1183452685166,17.4075745924791));
#259825=CARTESIAN_POINT('Ctrl Pts',(75.9888185880884,25.0581838218694,17.3500764673617));
#259826=CARTESIAN_POINT('Ctrl Pts',(76.0045572676606,24.9948448130137,17.2916572676644));
#259827=CARTESIAN_POINT('Ctrl Pts',(75.9867440840342,24.9827521037965,17.5589921227903));
#259828=CARTESIAN_POINT('Ctrl Pts',(76.0047941374301,24.9436535528168,17.5184791523472));
#259829=CARTESIAN_POINT('Ctrl Pts',(76.0189046879114,24.9029090128953,17.4779931990458));
#259830=CARTESIAN_POINT('Ctrl Pts',(76.0138748889673,24.8422792694551,17.7055224896847));
#259831=CARTESIAN_POINT('Ctrl Pts',(76.0228272111373,24.8230534553229,17.6845460983331));
#259832=CARTESIAN_POINT('Ctrl Pts',(76.0317753893963,24.8038409415364,17.6635683446408));
#259833=CARTESIAN_POINT('Ctrl Pts',(76.042458286517,24.6976449914381,17.8479876926701));
#259834=CARTESIAN_POINT('Ctrl Pts',(76.042458286517,24.6976449914381,17.8479876926701));
#259835=CARTESIAN_POINT('Ctrl Pts',(76.042458286517,24.6976449914381,17.8479876926701));
#259836=CARTESIAN_POINT('Ctrl Pts',(25.0804618860237,75.9725615368778,17.42016687813));
#259837=CARTESIAN_POINT('Ctrl Pts',(25.0218849779072,76.0018311057243,17.3465486623464));
#259838=CARTESIAN_POINT('Ctrl Pts',(24.9591222047285,76.01654431203,17.2720397183974));
#259839=CARTESIAN_POINT('Ctrl Pts',(25.2741629194071,75.9311692985981,17.2143925574792));
#259840=CARTESIAN_POINT('Ctrl Pts',(25.2217620983607,75.958681184656,17.1148633560418));
#259841=CARTESIAN_POINT('Ctrl Pts',(25.1645554520732,75.9667333080871,17.0143457047747));
#259842=CARTESIAN_POINT('Ctrl Pts',(25.5065028345103,75.9076483674903,17.0946463742361));
#259843=CARTESIAN_POINT('Ctrl Pts',(25.4560812233288,75.9374572719628,16.9750964736288));
#259844=CARTESIAN_POINT('Ctrl Pts',(25.4014568018248,75.9400754392651,16.8534468191218));
#259845=CARTESIAN_POINT('Ctrl Pts',(25.9210527955236,75.9275280255501,16.929244875955));
#259846=CARTESIAN_POINT('Ctrl Pts',(25.8696322348271,75.9625142169106,16.7791814037363));
#259847=CARTESIAN_POINT('Ctrl Pts',(25.8202904741259,75.9568105611576,16.6244542312898));
#259848=CARTESIAN_POINT('Ctrl Pts',(26.1003508790249,75.9538339499108,16.8739158934014));
#259849=CARTESIAN_POINT('Ctrl Pts',(26.0473908953034,75.9915498547677,16.7122017332863));
#259850=CARTESIAN_POINT('Ctrl Pts',(26.0002790025707,75.9825893385705,16.5445597191504));
#259851=CARTESIAN_POINT('Ctrl Pts',(26.4483576685963,76.0436899102596,16.7801350408625));
#259852=CARTESIAN_POINT('Ctrl Pts',(26.3907212263412,76.0862364212148,16.5977546210469));
#259853=CARTESIAN_POINT('Ctrl Pts',(26.3489939258796,76.0719119444782,16.4067913625631));
#259854=CARTESIAN_POINT('Ctrl Pts',(26.6209880248573,76.1074179294988,16.7422284473565));
#259855=CARTESIAN_POINT('Ctrl Pts',(26.5597476890913,76.1525248745944,16.5501048951609));
#259856=CARTESIAN_POINT('Ctrl Pts',(26.5212227642717,76.1359425371639,16.3477329791976));
#259857=CARTESIAN_POINT('Ctrl Pts',(26.8247483133823,76.2123121583579,16.6934782675247));
#259858=CARTESIAN_POINT('Ctrl Pts',(26.7604265541748,76.2574262010901,16.4943208592323));
#259859=CARTESIAN_POINT('Ctrl Pts',(26.7269236186754,76.2394155534515,16.2836305889901));
#259860=CARTESIAN_POINT('Ctrl Pts',(26.8648052287377,76.2345275940671,16.6835961109164));
#259861=CARTESIAN_POINT('Ctrl Pts',(26.7999815868847,76.2794711085834,16.4833268552169));
#259862=CARTESIAN_POINT('Ctrl Pts',(26.7675182843409,76.2612367837886,16.2713262631411));
#259863=CARTESIAN_POINT('Ctrl Pts',(26.9428805656769,76.2819273824504,16.6613225028936));
#259864=CARTESIAN_POINT('Ctrl Pts',(26.877812280624,76.325608218886,16.460395029503));
#259865=CARTESIAN_POINT('Ctrl Pts',(26.8475982558576,76.307141242556,16.2476495576019));
#259866=CARTESIAN_POINT('Ctrl Pts',(26.9810543502164,76.3069759166512,16.6496028712586));
#259867=CARTESIAN_POINT('Ctrl Pts',(26.9160778594133,76.3496981928984,16.4488297968031));
#259868=CARTESIAN_POINT('Ctrl Pts',(26.8870847364683,76.3312252545636,16.236284876982));
#259869=CARTESIAN_POINT('Ctrl Pts',(27.0347146146409,76.348479787188,16.6221367327716));
#259870=CARTESIAN_POINT('Ctrl Pts',(26.9722866202233,76.3871914756644,16.4263729310828));
#259871=CARTESIAN_POINT('Ctrl Pts',(26.9454540778621,76.3690625317951,16.2198040383442));
#259872=CARTESIAN_POINT('Ctrl Pts',(27.0520461010348,76.3629033141244,16.6116902389514));
#259873=CARTESIAN_POINT('Ctrl Pts',(26.9907978709005,76.3998985070121,16.4182354344391));
#259874=CARTESIAN_POINT('Ctrl Pts',(26.9647604072736,76.381956422089,16.2144102296118));
#259875=CARTESIAN_POINT('Ctrl Pts',(27.0754324956893,76.3870229007004,16.5857176723783));
#259876=CARTESIAN_POINT('Ctrl Pts',(27.0180627224541,76.4191298939433,16.4005487707549));
#259877=CARTESIAN_POINT('Ctrl Pts',(26.993440890971,76.4016850635576,16.2063864536409));
#259878=CARTESIAN_POINT('Ctrl Pts',(27.0828077996879,76.3954507470087,16.5755244414192));
#259879=CARTESIAN_POINT('Ctrl Pts',(27.0270559839662,76.4255606544124,16.3938428354607));
#259880=CARTESIAN_POINT('Ctrl Pts',(27.0029569073645,76.4083274633204,16.2037237985546));
#259881=CARTESIAN_POINT('Ctrl Pts',(27.0922320376545,76.4098047654343,16.5516204721261));
#259882=CARTESIAN_POINT('Ctrl Pts',(27.0403670147032,76.4351975383171,16.379224441304));
#259883=CARTESIAN_POINT('Ctrl Pts',(27.0171572804521,76.4183850872755,16.1996869095685));
#259884=CARTESIAN_POINT('Ctrl Pts',(27.0950953264234,76.4148733708239,16.5422413732297));
#259885=CARTESIAN_POINT('Ctrl Pts',(27.0447678397126,76.4384035784988,16.3736104964544));
#259886=CARTESIAN_POINT('Ctrl Pts',(27.0218787739723,76.4217535244975,16.1983342860912));
#259887=CARTESIAN_POINT('Ctrl Pts',(27.0997431526784,76.4263249193079,16.5161165141993));
#259888=CARTESIAN_POINT('Ctrl Pts',(27.0535116464061,76.4448069459393,16.3585277802149));
#259889=CARTESIAN_POINT('Ctrl Pts',(27.0312909576619,76.42851717559,16.1955743904641));
#259890=CARTESIAN_POINT('Ctrl Pts',(27.1014904674051,76.4326137594198,16.500204580009));
#259891=CARTESIAN_POINT('Ctrl Pts',(27.0578166604433,76.4479765311902,16.3494953976019));
#259892=CARTESIAN_POINT('Ctrl Pts',(27.035983172867,76.4319135317257,16.1941800679768));
#259893=CARTESIAN_POINT('Ctrl Pts',(27.1026704184044,76.444945265315,16.4573094494972));
#259894=CARTESIAN_POINT('Ctrl Pts',(27.0644828819285,76.4528969605584,16.3261248042041));
#259895=CARTESIAN_POINT('Ctrl Pts',(27.0429752642404,76.4370110131298,16.1919016822556));
#259896=CARTESIAN_POINT('Ctrl Pts',(27.1027728684423,76.4496135704595,16.4393960541736));
#259897=CARTESIAN_POINT('Ctrl Pts',(27.0667393944962,76.4545638835509,16.3164891117538));
#259898=CARTESIAN_POINT('Ctrl Pts',(27.0453014012289,76.4387129855077,16.191114532674));
#259899=CARTESIAN_POINT('Ctrl Pts',(27.103348843805,76.4602856539461,16.3918070921655));
#259900=CARTESIAN_POINT('Ctrl Pts',(27.0716717101299,76.4582133271172,16.2912288897505));
#259901=CARTESIAN_POINT('Ctrl Pts',(27.0498984940075,76.4420884316598,16.1893010704596));
#259902=CARTESIAN_POINT('Ctrl Pts',(27.103921956882,76.4662567117721,16.3621450323075));
#259903=CARTESIAN_POINT('Ctrl Pts',(27.0743744435426,76.4602162047732,16.2756512778861));
#259904=CARTESIAN_POINT('Ctrl Pts',(27.0521738675702,76.4437652233597,16.1883092099684));
#259905=CARTESIAN_POINT('Ctrl Pts',(27.1079500471734,76.4780100141054,16.294962253566));
#259906=CARTESIAN_POINT('Ctrl Pts',(27.0805869451208,76.4648464736715,16.2402396311017));
#259907=CARTESIAN_POINT('Ctrl Pts',(27.0565399426139,76.44699327834,16.1852909757062));
#259908=CARTESIAN_POINT('Ctrl Pts',(27.1117437396561,76.4840868539103,16.2559882667085));
#259909=CARTESIAN_POINT('Ctrl Pts',(27.0843760577268,76.4676882621526,16.2196371037558));
#259910=CARTESIAN_POINT('Ctrl Pts',(27.0588362934594,76.4486982192428,16.1831963663287));
#259911=CARTESIAN_POINT('Ctrl Pts',(27.1186429162632,76.4907257277754,16.1967720341455));
#259912=CARTESIAN_POINT('Ctrl Pts',(27.088970607914,76.4711321232317,16.1872136925927));
#259913=CARTESIAN_POINT('Ctrl Pts',(27.0604496119645,76.449897797078,16.1776432448508));
#259914=CARTESIAN_POINT('Ctrl Pts',(27.1210505518365,76.4924398017442,16.1773616860778));
#259915=CARTESIAN_POINT('Ctrl Pts',(27.0902380459636,76.4720805095757,16.1763774272393));
#259916=CARTESIAN_POINT('Ctrl Pts',(27.0606161752026,76.4500218115713,16.1753910477049));
#259917=CARTESIAN_POINT('Ctrl Pts',(27.124723692261,76.4945108031749,16.1461844913816));
#259918=CARTESIAN_POINT('Ctrl Pts',(27.0917434440934,76.4731956267604,16.1586478057256));
#259919=CARTESIAN_POINT('Ctrl Pts',(27.0602497730199,76.4497492188553,16.171136001378));
#259920=CARTESIAN_POINT('Ctrl Pts',(27.1261031628968,76.4950020357299,16.133681728625));
#259921=CARTESIAN_POINT('Ctrl Pts',(27.0920805335392,76.4734376571502,16.1513715711389));
#259922=CARTESIAN_POINT('Ctrl Pts',(27.0597799419463,76.4493997295785,16.1691026721927));
#259923=CARTESIAN_POINT('Ctrl Pts',(27.13156819983,76.4963255984209,16.0800932837589));
#259924=CARTESIAN_POINT('Ctrl Pts',(27.0928134511323,76.4739251360543,16.1197927836122));
#259925=CARTESIAN_POINT('Ctrl Pts',(27.0569687226394,76.4473109346435,16.1596448232299));
#259926=CARTESIAN_POINT('Ctrl Pts',(27.1323195784948,76.49451130004,16.0589082957883));
#259927=CARTESIAN_POINT('Ctrl Pts',(27.09092096414,76.4724331002845,16.1061418174196));
#259928=CARTESIAN_POINT('Ctrl Pts',(27.0534134152984,76.4446774540829,16.1536294662393));
#259929=CARTESIAN_POINT('Ctrl Pts',(27.1329837771627,76.4909539904125,16.0195114651259));
#259930=CARTESIAN_POINT('Ctrl Pts',(27.0869366765608,76.4693129058743,16.0806139918041));
#259931=CARTESIAN_POINT('Ctrl Pts',(27.0464009528429,76.4395165697625,16.1421882796318));
#259932=CARTESIAN_POINT('Ctrl Pts',(27.1324755596785,76.4887423766883,16.0040405252725));
#259933=CARTESIAN_POINT('Ctrl Pts',(27.0844779770551,76.4674056396185,16.0701604569275));
#259934=CARTESIAN_POINT('Ctrl Pts',(27.0426984150638,76.436805864295,16.1368608677846));
#259935=CARTESIAN_POINT('Ctrl Pts',(27.1176445692947,76.4487554850658,15.7668594205244));
#259936=CARTESIAN_POINT('Ctrl Pts',(27.0392647575274,76.4325632146525,15.9058934996621));
#259937=CARTESIAN_POINT('Ctrl Pts',(26.978304049824,76.3899445519393,16.0485446134497));
#259938=CARTESIAN_POINT('Ctrl Pts',(27.0267181002176,76.3890441685062,15.9290103439652));
#259939=CARTESIAN_POINT('Ctrl Pts',(26.9607754137162,76.3752347443015,15.9631551147917));
#259940=CARTESIAN_POINT('Ctrl Pts',(26.9028259695809,76.3392599186689,16.0018551686532));
#259941=CARTESIAN_POINT('Ctrl Pts',(27.0702645564447,76.3535975697862,14.8756002301201));
#259942=CARTESIAN_POINT('Ctrl Pts',(26.9358287323369,76.3662706710394,15.3627392753264));
#259943=CARTESIAN_POINT('Ctrl Pts',(26.8612497825162,76.3194480577275,15.8395311951992));
#259944=CARTESIAN_POINT('Origin',(24.9421491495265,74.7257085670769,17.0741173620444));
#259945=CARTESIAN_POINT('Ctrl Pts',(25.1074704499368,75.962775317243,17.4259425795535));
#259946=CARTESIAN_POINT('Ctrl Pts',(25.0462350073064,75.9901905947506,17.3727027235419));
#259947=CARTESIAN_POINT('Ctrl Pts',(24.9819025616059,76.0065414441456,17.3185796118044));
#259948=CARTESIAN_POINT('Ctrl Pts',(25.1496292029159,75.958044198321,17.3506767478669));
#259949=CARTESIAN_POINT('Ctrl Pts',(25.0926862207362,75.9851307386925,17.2798459583226));
#259950=CARTESIAN_POINT('Ctrl Pts',(25.0322694073611,75.9990697411724,17.2080611431853));
#259951=CARTESIAN_POINT('Ctrl Pts',(25.2082186982409,75.94816124025,17.2973276043272));
#259952=CARTESIAN_POINT('Ctrl Pts',(25.1530396514998,75.9759984326018,17.2125718696368));
#259953=CARTESIAN_POINT('Ctrl Pts',(25.0938856963519,75.9872898972842,17.1266598669887));
#259954=CARTESIAN_POINT('Ctrl Pts',(25.2708374177375,75.9397262748181,17.2518520136545));
#259955=CARTESIAN_POINT('Ctrl Pts',(25.216936348314,75.968563259699,17.154725985359));
#259956=CARTESIAN_POINT('Ctrl Pts',(25.1589733721109,75.9772090303638,17.0560474933022));
#259957=CARTESIAN_POINT('Origin',(24.7225971487432,74.7646897896797,17.2528005263626));
#259958=CARTESIAN_POINT('Ctrl Pts',(24.9948448130087,76.0045572676614,17.2916572676743));
#259959=CARTESIAN_POINT('Ctrl Pts',(25.0581838218632,75.9888185880893,17.3500764673706));
#259960=CARTESIAN_POINT('Ctrl Pts',(25.1183452685093,75.9614890268773,17.4075745924872));
#259961=CARTESIAN_POINT('Ctrl Pts',(24.9029090128636,76.0189046879184,17.4779931990423));
#259962=CARTESIAN_POINT('Ctrl Pts',(24.9436535528443,76.0047941374266,17.5184791523504));
#259963=CARTESIAN_POINT('Ctrl Pts',(24.9827521037621,75.9867440840482,17.55899212277));
#259964=CARTESIAN_POINT('Ctrl Pts',(24.803840941519,76.0317753894034,17.6635683446283));
#259965=CARTESIAN_POINT('Ctrl Pts',(24.8230534553019,76.0228272111432,17.6845460983396));
#259966=CARTESIAN_POINT('Ctrl Pts',(24.8422792694592,76.0138748889657,17.7055224896865));
#259967=CARTESIAN_POINT('Ctrl Pts',(24.6976449914385,76.0424582865173,17.8479876926674));
#259968=CARTESIAN_POINT('Ctrl Pts',(24.6976449914385,76.0424582865173,17.8479876926674));
#259969=CARTESIAN_POINT('Ctrl Pts',(24.6976449914385,76.0424582865173,17.8479876926674));
#259970=CARTESIAN_POINT('Ctrl Pts',(-24.9589179253363,76.01659273472,17.271923598526));
#259971=CARTESIAN_POINT('Ctrl Pts',(-25.0217593831366,76.0018779351851,
17.3465144252831));
#259972=CARTESIAN_POINT('Ctrl Pts',(-25.0804061471587,75.9725739124909,
17.4202136823926));
#259973=CARTESIAN_POINT('Ctrl Pts',(-25.1644631759507,75.9667363952496,
17.0140601850114));
#259974=CARTESIAN_POINT('Ctrl Pts',(-25.2217418913752,75.9586992553381,
17.1147005696024));
#259975=CARTESIAN_POINT('Ctrl Pts',(-25.27420346249,75.9311549697297,17.2143522966372));
#259976=CARTESIAN_POINT('Ctrl Pts',(-25.4013568067359,75.9400924589015,
16.8531572347146));
#259977=CARTESIAN_POINT('Ctrl Pts',(-25.4560486787868,75.9375037638146,
16.9749518252951));
#259978=CARTESIAN_POINT('Ctrl Pts',(-25.5065310406966,75.9076590514475,
17.0946441542763));
#259979=CARTESIAN_POINT('Ctrl Pts',(-25.8199808098823,75.9567824207016,
16.6241920453249));
#259980=CARTESIAN_POINT('Ctrl Pts',(-25.8693789122518,75.9625371920841,
16.7790876761471));
#259981=CARTESIAN_POINT('Ctrl Pts',(-25.9208598320779,75.9275121101251,
16.9293154168732));
#259982=CARTESIAN_POINT('Ctrl Pts',(-26.0000535557612,75.9825492872224,
16.5442194952226));
#259983=CARTESIAN_POINT('Ctrl Pts',(-26.0472138461683,75.9915734867984,
16.7120520477243));
#259984=CARTESIAN_POINT('Ctrl Pts',(-26.1002356612948,75.9538145397959,
16.8739507932185));
#259985=CARTESIAN_POINT('Ctrl Pts',(-26.348734118025,76.0718263565562,16.4064067143953));
#259986=CARTESIAN_POINT('Ctrl Pts',(-26.3904925511526,76.0862325753191,
16.5975865850527));
#259987=CARTESIAN_POINT('Ctrl Pts',(-26.4481950399281,76.0436375882038,
16.7801750181481));
#259988=CARTESIAN_POINT('Ctrl Pts',(-26.5206773054617,76.1357086392241,
16.3474135480229));
#259989=CARTESIAN_POINT('Ctrl Pts',(-26.5592282331617,76.1523784609536,
16.5499987072448));
#259990=CARTESIAN_POINT('Ctrl Pts',(-26.6205318943627,76.1072227609038,
16.7423277269629));
#259991=CARTESIAN_POINT('Ctrl Pts',(-26.7264920249991,76.2391872025004,
16.2832499587999));
#259992=CARTESIAN_POINT('Ctrl Pts',(-26.7600048034107,76.2572914161368,
16.4941794865568));
#259993=CARTESIAN_POINT('Ctrl Pts',(-26.824398868812,76.2121224123054,16.6935643217025));
#259994=CARTESIAN_POINT('Ctrl Pts',(-26.7670983623262,76.2610052221557,
16.2709381057852));
#259995=CARTESIAN_POINT('Ctrl Pts',(-26.7995686636006,76.2793339264537,
16.4831824942709));
#259996=CARTESIAN_POINT('Ctrl Pts',(-26.8644662376051,76.2343342569761,
16.6836830243191));
#259997=CARTESIAN_POINT('Ctrl Pts',(-26.8471814943334,76.3068912734128,
16.2472568170159));
#259998=CARTESIAN_POINT('Ctrl Pts',(-26.8773983376708,76.3254529676178,
16.4602585575014));
#259999=CARTESIAN_POINT('Ctrl Pts',(-26.9425455013332,76.2817116055851,
16.6614278018637));
#260000=CARTESIAN_POINT('Ctrl Pts',(-26.8866594659865,76.3309600827125,
16.2358941826432));
#260001=CARTESIAN_POINT('Ctrl Pts',(-26.9156538041466,76.3495273607928,
16.4486994615681));
#260002=CARTESIAN_POINT('Ctrl Pts',(-26.9807109662172,76.3067428814873,
16.6497176791804));
#260003=CARTESIAN_POINT('Ctrl Pts',(-26.9450028183287,76.3687633480519,
16.2194335079569));
#260004=CARTESIAN_POINT('Ctrl Pts',(-26.9718386918007,76.3869839753116,
16.4263030318194));
#260005=CARTESIAN_POINT('Ctrl Pts',(-27.0343640337368,76.3481925870805,
16.6223462099112));
#260006=CARTESIAN_POINT('Ctrl Pts',(-26.9643135712108,76.381654087884,16.2140445092996));
#260007=CARTESIAN_POINT('Ctrl Pts',(-26.9903552533354,76.3996866408693,
16.418184305942));
#260008=CARTESIAN_POINT('Ctrl Pts',(-27.0517070202451,76.3626055712697,
16.6119303438144));
#260009=CARTESIAN_POINT('Ctrl Pts',(-26.9930030958707,76.401380124159,16.2060411922581));
#260010=CARTESIAN_POINT('Ctrl Pts',(-27.0176339860631,76.4189117637762,
16.4005910944646));
#260011=CARTESIAN_POINT('Ctrl Pts',(-27.0751338525107,76.3866896894671,
16.5861155304994));
#260012=CARTESIAN_POINT('Ctrl Pts',(-27.0025216597485,76.4080213751607,
16.203387528453));
#260013=CARTESIAN_POINT('Ctrl Pts',(-27.026632165822,76.4253400029413,16.3939233817012));
#260014=CARTESIAN_POINT('Ctrl Pts',(-27.0825251253766,76.3951028705659,
16.5759864041684));
#260015=CARTESIAN_POINT('Ctrl Pts',(-27.0167251805518,76.4180768548563,
16.1993760622623));
#260016=CARTESIAN_POINT('Ctrl Pts',(-27.0399520663499,76.4349711944826,
16.3794519172504));
#260017=CARTESIAN_POINT('Ctrl Pts',(-27.0919957484794,76.4094060117648,
16.5523397019094));
#260018=CARTESIAN_POINT('Ctrl Pts',(-27.0214474035482,76.4214443578374,
16.1980339064543));
#260019=CARTESIAN_POINT('Ctrl Pts',(-27.0443560687477,76.4381750002681,
16.3739005940378));
#260020=CARTESIAN_POINT('Ctrl Pts',(-27.0948782490049,76.4144529107837,
16.5430709433479));
#260021=CARTESIAN_POINT('Ctrl Pts',(-27.0308618441442,76.4282067437578,
16.19530514003));
#260022=CARTESIAN_POINT('Ctrl Pts',(-27.053106800039,76.444572163028,16.3590502469535));
#260023=CARTESIAN_POINT('Ctrl Pts',(-27.0995848854146,76.4258296167095,
16.5173659130853));
#260024=CARTESIAN_POINT('Ctrl Pts',(-27.0355558280438,76.4316029371517,
16.1939295287546));
#260025=CARTESIAN_POINT('Ctrl Pts',(-27.0574185499143,76.4477400974505,
16.3501709551169));
#260026=CARTESIAN_POINT('Ctrl Pts',(-27.1013790741377,76.4320671394762,
16.5017321290356));
#260027=CARTESIAN_POINT('Ctrl Pts',(-27.0425542463667,76.4367029519925,
16.1917093206043));
#260028=CARTESIAN_POINT('Ctrl Pts',(-27.0640786984513,76.4526420016968,
16.3273830388961));
#260029=CARTESIAN_POINT('Ctrl Pts',(-27.102629006752,76.4442399758458,16.4599278648171));
#260030=CARTESIAN_POINT('Ctrl Pts',(-27.0448820844151,76.4384054861842,
16.1909469831181));
#260031=CARTESIAN_POINT('Ctrl Pts',(-27.0663285798975,76.454298592053,16.3180252537668));
#260032=CARTESIAN_POINT('Ctrl Pts',(-27.1027558329562,76.4488339487676,
16.4425406392177));
#260033=CARTESIAN_POINT('Ctrl Pts',(-27.0494862895922,76.4417848360543,
16.1892131480628));
#260034=CARTESIAN_POINT('Ctrl Pts',(-27.0712224151044,76.4579068033435,
16.2933864311227));
#260035=CARTESIAN_POINT('Ctrl Pts',(-27.1032790984671,76.4593812159613,
16.3961238758005));
#260036=CARTESIAN_POINT('Ctrl Pts',(-27.0517726556214,76.4434690777321,
16.1882712263809));
#260037=CARTESIAN_POINT('Ctrl Pts',(-27.0738999783668,76.4598835948997,
16.2780430539621));
#260038=CARTESIAN_POINT('Ctrl Pts',(-27.1037600523946,76.4653396358795,
16.3668982051164));
#260039=CARTESIAN_POINT('Ctrl Pts',(-27.0561659022714,76.4467160440046,
16.1854342155749));
#260040=CARTESIAN_POINT('Ctrl Pts',(-27.0800526954001,76.4644564134043,
16.2430395007726));
#260041=CARTESIAN_POINT('Ctrl Pts',(-27.1075193430059,76.4771343839088,
16.3003874919345));
#260042=CARTESIAN_POINT('Ctrl Pts',(-27.058446159053,76.4484083289748,16.1835540069008));
#260043=CARTESIAN_POINT('Ctrl Pts',(-27.0837265632002,76.4672060746151,
16.2231638663765));
#260044=CARTESIAN_POINT('Ctrl Pts',(-27.1110283194281,76.4831388147606,
16.2626673994512));
#260045=CARTESIAN_POINT('Ctrl Pts',(-27.0602641873015,76.4497597899656,
16.1782706332977));
#260046=CARTESIAN_POINT('Ctrl Pts',(-27.0884790761337,76.4707669780906,
16.1906859326517));
#260047=CARTESIAN_POINT('Ctrl Pts',(-27.1178762326902,76.4900906769913,
16.2030845287967));
#260048=CARTESIAN_POINT('Ctrl Pts',(-27.0605327252718,76.4499596839005,
16.1760791918826));
#260049=CARTESIAN_POINT('Ctrl Pts',(-27.0898596110057,76.4718011937839,
16.1795821117081));
#260050=CARTESIAN_POINT('Ctrl Pts',(-27.120358948079,76.4919704112056,16.1830789607914));
#260051=CARTESIAN_POINT('Ctrl Pts',(-27.0602871265233,76.4497769572404,
16.1718015139879));
#260052=CARTESIAN_POINT('Ctrl Pts',(-27.0915502375945,76.473057377783,16.1610984554029));
#260053=CARTESIAN_POINT('Ctrl Pts',(-27.1242386851068,76.494295831555,16.150415767633));
#260054=CARTESIAN_POINT('Ctrl Pts',(-27.0598504162012,76.4494520710877,
16.1697479358136));
#260055=CARTESIAN_POINT('Ctrl Pts',(-27.0919480009677,76.4733461094145,
16.1535475368814));
#260056=CARTESIAN_POINT('Ctrl Pts',(-27.1257019179669,76.4948627285816,
16.137383211141));
#260057=CARTESIAN_POINT('Ctrl Pts',(-27.0582086402039,76.4482320673373,
16.1639666862077));
#260058=CARTESIAN_POINT('Ctrl Pts',(-27.0925161435607,76.4737375074722,
16.1338103699281));
#260059=CARTESIAN_POINT('Ctrl Pts',(-27.1291949135698,76.4958195376337,
16.1037499831074));
#260060=CARTESIAN_POINT('Ctrl Pts',(-27.0567042052342,76.4471157252128,
16.1606292110335));
#260061=CARTESIAN_POINT('Ctrl Pts',(-27.0921025230806,76.4733973732767,
16.1245076433474));
#260062=CARTESIAN_POINT('Ctrl Pts',(-27.1303768997729,76.495511080392,16.0885277310218));
#260063=CARTESIAN_POINT('Ctrl Pts',(-27.0534903168296,76.4447377920072,
16.1542190781187));
#260064=CARTESIAN_POINT('Ctrl Pts',(-27.0908610714654,76.4724034604763,
16.1076940433688));
#260065=CARTESIAN_POINT('Ctrl Pts',(-27.1320488746758,76.4944955999903,
16.0614128323374));
#260066=CARTESIAN_POINT('Ctrl Pts',(-27.0517739692635,76.4434708941462,
16.151235327988));
#260067=CARTESIAN_POINT('Ctrl Pts',(-27.089983151407,76.4717122955942,16.1006285062877));
#260068=CARTESIAN_POINT('Ctrl Pts',(-27.1324478121814,76.4937176499756,
16.0503186646554));
#260069=CARTESIAN_POINT('Ctrl Pts',(-27.0464903416048,76.4395819036986,
16.1426043113602));
#260070=CARTESIAN_POINT('Ctrl Pts',(-27.0870015822935,76.4693799219042,
16.0812344084128));
#260071=CARTESIAN_POINT('Ctrl Pts',(-27.1330005797391,76.4910613333798,
16.0203313765123));
#260072=CARTESIAN_POINT('Ctrl Pts',(-27.0427755268835,76.4368619767283,
16.1372659298901));
#260073=CARTESIAN_POINT('Ctrl Pts',(-27.0845393340012,76.4674716671333,
16.0707205771816));
#260074=CARTESIAN_POINT('Ctrl Pts',(-27.1325040255392,76.4888476730249,
16.0047512272665));
#260075=CARTESIAN_POINT('Ctrl Pts',(-26.9782305736964,76.38988746594,16.0488344459415));
#260076=CARTESIAN_POINT('Ctrl Pts',(-27.0392919375054,76.4326304782598,
15.9056407248496));
#260077=CARTESIAN_POINT('Ctrl Pts',(-27.1178463029269,76.4488518511461,
15.7660809748921));
#260078=CARTESIAN_POINT('Ctrl Pts',(-26.9009713153748,76.3379547637161,
16.0003561832371));
#260079=CARTESIAN_POINT('Ctrl Pts',(-26.9591175339555,76.3740242720092,
15.9620876053608));
#260080=CARTESIAN_POINT('Ctrl Pts',(-27.0253527090181,76.3877008594034,
15.9284160632215));
#260081=CARTESIAN_POINT('Ctrl Pts',(-26.8672868551547,76.3238925583658,
15.8466387166555));
#260082=CARTESIAN_POINT('Ctrl Pts',(-26.9411427646962,76.3705353343011,
15.3686915139899));
#260083=CARTESIAN_POINT('Ctrl Pts',(-27.0744152689117,76.3583349950857,
14.8796637100114));
#260084=CARTESIAN_POINT('Origin',(-24.9421491495268,74.7257085670769,17.0741173620444));
#260085=CARTESIAN_POINT('Ctrl Pts',(-25.2708374177665,75.9397262748117,
17.251852013646));
#260086=CARTESIAN_POINT('Ctrl Pts',(-25.2169363483573,75.9685632596837,
17.1547259853851));
#260087=CARTESIAN_POINT('Ctrl Pts',(-25.1589733721729,75.977209030354,17.0560474933636));
#260088=CARTESIAN_POINT('Ctrl Pts',(-25.2082186981158,75.9481612402803,
17.2973276043548));
#260089=CARTESIAN_POINT('Ctrl Pts',(-25.1530396514114,75.9759984326147,
17.2125718696916));
#260090=CARTESIAN_POINT('Ctrl Pts',(-25.0938856962957,75.9872898972941,
17.1266598670703));
#260091=CARTESIAN_POINT('Ctrl Pts',(-25.1496292031321,75.9580441982454,
17.3506767479114));
#260092=CARTESIAN_POINT('Ctrl Pts',(-25.0926862209603,75.9851307386431,
17.2798459583833));
#260093=CARTESIAN_POINT('Ctrl Pts',(-25.0322694075985,75.9990697411192,
17.2080611432671));
#260094=CARTESIAN_POINT('Ctrl Pts',(-25.1074704498864,75.9627753172623,
17.4259425795317));
#260095=CARTESIAN_POINT('Ctrl Pts',(-25.0462350072807,75.9901905947506,
17.3727027235389));
#260096=CARTESIAN_POINT('Ctrl Pts',(-24.9819025616059,76.0065414441447,
17.3185796118194));
#260097=CARTESIAN_POINT('Origin',(-24.7225971487503,74.7646897896784,17.2528005263547));
#260098=CARTESIAN_POINT('Ctrl Pts',(-25.1183452685167,75.961489026876,17.4075745924791));
#260099=CARTESIAN_POINT('Ctrl Pts',(-25.0581838218695,75.9888185880884,
17.3500764673617));
#260100=CARTESIAN_POINT('Ctrl Pts',(-24.9948448130137,76.0045572676605,
17.2916572676644));
#260101=CARTESIAN_POINT('Ctrl Pts',(-24.9827521037895,75.9867440840366,
17.55899212279));
#260102=CARTESIAN_POINT('Ctrl Pts',(-24.9436535528084,76.0047941374264,
17.5184791523466));
#260103=CARTESIAN_POINT('Ctrl Pts',(-24.9029090128894,76.0189046879127,
17.4779931990465));
#260104=CARTESIAN_POINT('Ctrl Pts',(-24.8422792694326,76.0138748889786,
17.7055224896539));
#260105=CARTESIAN_POINT('Ctrl Pts',(-24.8230534553004,76.0228272111476,
17.6845460983103));
#260106=CARTESIAN_POINT('Ctrl Pts',(-24.8038409415144,76.0317753894055,
17.6635683446243));
#260107=CARTESIAN_POINT('Ctrl Pts',(-24.6976449914381,76.042458286517,17.8479876926703));
#260108=CARTESIAN_POINT('Ctrl Pts',(-24.6976449914381,76.042458286517,17.8479876926703));
#260109=CARTESIAN_POINT('Ctrl Pts',(-24.6976449914381,76.042458286517,17.8479876926703));
#260110=CARTESIAN_POINT('Ctrl Pts',(-75.9418613633423,25.2552738568381,
17.2633930704886));
#260111=CARTESIAN_POINT('Ctrl Pts',(-75.9705307448155,25.2008887299308,
17.1691547678158));
#260112=CARTESIAN_POINT('Ctrl Pts',(-75.9798097533928,25.1424732627575,
17.073436084435));
#260113=CARTESIAN_POINT('Ctrl Pts',(-75.9205954929399,25.4077025358094,
17.1478651038322));
#260114=CARTESIAN_POINT('Ctrl Pts',(-75.9494543541835,25.3561156594532,
17.0372776844065));
#260115=CARTESIAN_POINT('Ctrl Pts',(-75.954463116562,25.3006469547484,16.9248602113907));
#260116=CARTESIAN_POINT('Ctrl Pts',(-75.9109616438354,25.5755944946747,
17.0670794578486));
#260117=CARTESIAN_POINT('Ctrl Pts',(-75.9415927766753,25.5249041770603,
16.942644169398));
#260118=CARTESIAN_POINT('Ctrl Pts',(-75.9428621479078,25.4713720494591,
16.8155375287585));
#260119=CARTESIAN_POINT('Ctrl Pts',(-75.9275280255483,25.9210527955289,
16.9292448759623));
#260120=CARTESIAN_POINT('Ctrl Pts',(-75.9624784012936,25.8696848744371,
16.7793350248215));
#260121=CARTESIAN_POINT('Ctrl Pts',(-75.9568220105354,25.8203898867078,
16.6247659603065));
#260122=CARTESIAN_POINT('Ctrl Pts',(-75.9538339499128,26.1003508790234,
16.8739158933932));
#260123=CARTESIAN_POINT('Ctrl Pts',(-75.9915111973655,26.0474451773173,
16.71236748428));
#260124=CARTESIAN_POINT('Ctrl Pts',(-75.9826073212052,26.0003738093527,
16.5448970501221));
#260125=CARTESIAN_POINT('Ctrl Pts',(-76.043689910258,26.4483576685996,16.7801350408706));
#260126=CARTESIAN_POINT('Ctrl Pts',(-76.0861927069939,26.3907804446495,
16.5979420070057));
#260127=CARTESIAN_POINT('Ctrl Pts',(-76.0719406400684,26.3490777035775,
16.4071746837876));
#260128=CARTESIAN_POINT('Ctrl Pts',(-76.1074179294937,26.620988024866,16.7422284473806));
#260129=CARTESIAN_POINT('Ctrl Pts',(-76.1524784685812,26.5598106931415,
16.5503025518547));
#260130=CARTESIAN_POINT('Ctrl Pts',(-76.1359757159749,26.5213000181803,
16.3481386613362));
#260131=CARTESIAN_POINT('Ctrl Pts',(-76.2123121583599,26.8247483133817,
16.6934782675186));
#260132=CARTESIAN_POINT('Ctrl Pts',(-76.2573797435207,26.7604927914798,
16.4945259476778));
#260133=CARTESIAN_POINT('Ctrl Pts',(-76.2394515594669,26.7269907489909,
16.2840525403652));
#260134=CARTESIAN_POINT('Ctrl Pts',(-76.2345275940666,26.8648052287403,
16.683596110921));
#260135=CARTESIAN_POINT('Ctrl Pts',(-76.2794248197493,26.8000483509318,
16.4835331192511));
#260136=CARTESIAN_POINT('Ctrl Pts',(-76.2612732322625,26.7675833243841,
16.271750775101));
#260137=CARTESIAN_POINT('Ctrl Pts',(-76.2819273824524,26.9428805656769,
16.6613225028887));
#260138=CARTESIAN_POINT('Ctrl Pts',(-76.3255632280466,26.8778793003309,
16.4606019828592));
#260139=CARTESIAN_POINT('Ctrl Pts',(-76.3071781559159,26.8476587910104,
16.2480755374178));
#260140=CARTESIAN_POINT('Ctrl Pts',(-76.3069759166525,26.9810543502174,
16.6496028712566));
#260141=CARTESIAN_POINT('Ctrl Pts',(-76.3496541916651,26.9161447810771,
16.4490365803292));
#260142=CARTESIAN_POINT('Ctrl Pts',(-76.3312621827901,26.887142831161,16.2367104776612));
#260143=CARTESIAN_POINT('Ctrl Pts',(-76.3484797871886,27.0347146146424,
16.6221367327725));
#260144=CARTESIAN_POINT('Ctrl Pts',(-76.3871516364481,26.9723508665169,
16.4265743967641));
#260145=CARTESIAN_POINT('Ctrl Pts',(-76.3690988044595,26.9455078882792,
16.2202180012282));
#260146=CARTESIAN_POINT('Ctrl Pts',(-76.362903314126,27.0520461010359,16.6116902389491));
#260147=CARTESIAN_POINT('Ctrl Pts',(-76.399860448142,26.9908608801288,16.4184344514163));
#260148=CARTESIAN_POINT('Ctrl Pts',(-76.3819923354247,26.964812643049,16.2148188442204));
#260149=CARTESIAN_POINT('Ctrl Pts',(-76.3870229007013,27.0754324956906,
16.5857176723783));
#260150=CARTESIAN_POINT('Ctrl Pts',(-76.4190969025662,27.0181216724747,
16.4007390401198));
#260151=CARTESIAN_POINT('Ctrl Pts',(-76.4017200269266,26.9934903445586,
16.2067761581036));
#260152=CARTESIAN_POINT('Ctrl Pts',(-76.3954507470092,27.0828077996898,
16.5755244414213));
#260153=CARTESIAN_POINT('Ctrl Pts',(-76.4255297302771,27.0271132434182,
16.3940294300836));
#260154=CARTESIAN_POINT('Ctrl Pts',(-76.4083620212357,27.0030053344321,
16.2041055763287));
#260155=CARTESIAN_POINT('Ctrl Pts',(-76.4098047654361,27.0922320376552,
16.5516204721224));
#260156=CARTESIAN_POINT('Ctrl Pts',(-76.4351714897886,27.0404202191174,
16.3794012893797));
#260157=CARTESIAN_POINT('Ctrl Pts',(-76.4184188459322,27.0172039742048,
16.2000478703811));
#260158=CARTESIAN_POINT('Ctrl Pts',(-76.4148733708259,27.0950953264236,
16.542241373224));
#260159=CARTESIAN_POINT('Ctrl Pts',(-76.4383794519954,27.0448194425868,
16.3737834007286));
#260160=CARTESIAN_POINT('Ctrl Pts',(-76.4217869746101,27.0219248435745,
16.1986868469487));
#260161=CARTESIAN_POINT('Ctrl Pts',(-76.4263249193091,27.0997431526797,
16.5161165141982));
#260162=CARTESIAN_POINT('Ctrl Pts',(-76.4447880196842,27.0535589891232,
16.3586891567135));
#260163=CARTESIAN_POINT('Ctrl Pts',(-76.4285499486556,27.0313357366994,
16.1959025863163));
#260164=CARTESIAN_POINT('Ctrl Pts',(-76.4326137594215,27.1014904674059,
16.5002045800054));
#260165=CARTESIAN_POINT('Ctrl Pts',(-76.4479608116379,27.0578613485225,
16.3496496068196));
#260166=CARTESIAN_POINT('Ctrl Pts',(-76.4319458773626,27.036027204956,16.194493130941));
#260167=CARTESIAN_POINT('Ctrl Pts',(-76.4449452653173,27.1026704184048,
16.4573094494898));
#260168=CARTESIAN_POINT('Ctrl Pts',(-76.4528888389789,27.0645218853297,
16.3262587915595));
#260169=CARTESIAN_POINT('Ctrl Pts',(-76.4370430684111,27.0430187136298,
16.1921727274436));
#260170=CARTESIAN_POINT('Ctrl Pts',(-76.4496135704622,27.1027728684425,
16.4393960541631));
#260171=CARTESIAN_POINT('Ctrl Pts',(-76.4545588311619,27.0667761709923,
16.3166145530677));
#260172=CARTESIAN_POINT('Ctrl Pts',(-76.4387449966536,27.045344739669,16.1913678957922));
#260173=CARTESIAN_POINT('Ctrl Pts',(-76.4602856539487,27.1033488438057,
16.3918070921552));
#260174=CARTESIAN_POINT('Ctrl Pts',(-76.458215438751,27.0717039880843,16.2913313756112));
#260175=CARTESIAN_POINT('Ctrl Pts',(-76.4421210567288,27.0499425769547,
16.1895073884942));
#260176=CARTESIAN_POINT('Ctrl Pts',(-76.4662567117745,27.1039219568828,
16.3621450322986));
#260177=CARTESIAN_POINT('Ctrl Pts',(-76.4602223544582,27.0744045251034,
16.2757393349363));
#260178=CARTESIAN_POINT('Ctrl Pts',(-76.4437985416506,27.0522188526216,
16.188486160607));
#260179=CARTESIAN_POINT('Ctrl Pts',(-76.4780100141095,27.1079500471749,
16.2949622535397));
#260180=CARTESIAN_POINT('Ctrl Pts',(-76.464859856734,27.080614764543,16.2402952662867));
#260181=CARTESIAN_POINT('Ctrl Pts',(-76.4470294934426,27.0565887317523,
16.1854024533813));
#260182=CARTESIAN_POINT('Ctrl Pts',(-76.4840868539133,27.1117437396586,
16.2559882666882));
#260183=CARTESIAN_POINT('Ctrl Pts',(-76.467704925846,27.0844038678372,16.2196740425616));
#260184=CARTESIAN_POINT('Ctrl Pts',(-76.4487367623946,27.0588881357365,
16.1832703333258));
#260185=CARTESIAN_POINT('Ctrl Pts',(-76.4907257277775,27.1186429162657,
16.1967720341265));
#260186=CARTESIAN_POINT('Ctrl Pts',(-76.4711520289686,27.0890007529114,
16.1872234031905));
#260187=CARTESIAN_POINT('Ctrl Pts',(-76.4499409067105,27.0605075183523,
16.1776626753881));
#260188=CARTESIAN_POINT('Ctrl Pts',(-76.4924398017457,27.1210505518387,
16.1773616860606));
#260189=CARTESIAN_POINT('Ctrl Pts',(-76.4721011935177,27.0902693498065,
16.1763784271835));
#260190=CARTESIAN_POINT('Ctrl Pts',(-76.4500665941387,27.0606763157615,
16.1753930502819));
#260191=CARTESIAN_POINT('Ctrl Pts',(-76.4945108031758,27.1247236922628,
16.1461844913689));
#260192=CARTESIAN_POINT('Ctrl Pts',(-76.4732172840265,27.0917769536449,
16.1586351423791));
#260193=CARTESIAN_POINT('Ctrl Pts',(-76.4497968134883,27.060313707542,16.1711106500328));
#260194=CARTESIAN_POINT('Ctrl Pts',(-76.4950020357304,27.126103162898,16.1336817286145));
#260195=CARTESIAN_POINT('Ctrl Pts',(-76.4734595694155,27.0921151050378,
16.1513535959096));
#260196=CARTESIAN_POINT('Ctrl Pts',(-76.4494485206262,27.0598455093621,
16.1690666806019));
#260197=CARTESIAN_POINT('Ctrl Pts',(-76.4963255984212,27.1315681998314,
16.0800932837505));
#260198=CARTESIAN_POINT('Ctrl Pts',(-76.4739479072672,27.0928528473111,
16.1197524270407));
#260199=CARTESIAN_POINT('Ctrl Pts',(-76.4473649309662,27.0570414552056,
16.1595639629175));
#260200=CARTESIAN_POINT('Ctrl Pts',(-76.4945113000399,27.1323195784954,
16.0589082957826));
#260201=CARTESIAN_POINT('Ctrl Pts',(-76.4724555516724,27.0909630625156,
16.1060937855057));
#260202=CARTESIAN_POINT('Ctrl Pts',(-76.4447337452728,27.0534894962345,
16.1535331468431));
#260203=CARTESIAN_POINT('Ctrl Pts',(-76.4909539904122,27.1329837771628,
16.019511465123));
#260204=CARTESIAN_POINT('Ctrl Pts',(-76.4693349255398,27.0869835291923,
16.0805518203704));
#260205=CARTESIAN_POINT('Ctrl Pts',(-76.4395769622165,27.0464831294603,
16.1420634614074));
#260206=CARTESIAN_POINT('Ctrl Pts',(-76.4887423766881,27.1324755596788,
16.0040405252692));
#260207=CARTESIAN_POINT('Ctrl Pts',(-76.4674273552134,27.0845268268888,
16.0700931629596));
#260208=CARTESIAN_POINT('Ctrl Pts',(-76.4368678681646,27.0427830918246,
16.1367256935079));
#260209=CARTESIAN_POINT('Ctrl Pts',(-76.4487554850644,27.1176445692895,
15.7668594205398));
#260210=CARTESIAN_POINT('Ctrl Pts',(-76.432579761112,27.0393448518373,15.9057514243235));
#260211=CARTESIAN_POINT('Ctrl Pts',(-76.3900305449946,26.9784271091622,
16.0482566941911));
#260212=CARTESIAN_POINT('Ctrl Pts',(-76.3890441685912,27.0267181004289,
15.9290103437534));
#260213=CARTESIAN_POINT('Ctrl Pts',(-76.3752488344031,26.960842696207,15.9631202761283));
#260214=CARTESIAN_POINT('Ctrl Pts',(-76.3393326181439,26.9029431213673,
16.0017769419879));
#260215=CARTESIAN_POINT('Ctrl Pts',(-76.353597569064,27.0702645546813,14.8756002316582));
#260216=CARTESIAN_POINT('Ctrl Pts',(-76.3662576106953,26.9359672642415,
15.3622372916713));
#260217=CARTESIAN_POINT('Ctrl Pts',(-76.3195417069851,26.8613991063355,
15.838576931848));
#260218=CARTESIAN_POINT('Origin',(-74.7257085670769,24.9421491495265,17.0741173620445));
#260219=CARTESIAN_POINT('Ctrl Pts',(-75.9627753172452,25.1074704499294,
17.4259425795553));
#260220=CARTESIAN_POINT('Ctrl Pts',(-75.9901905947509,25.0462350073013,
17.3727027235441));
#260221=CARTESIAN_POINT('Ctrl Pts',(-76.0065414441465,24.9819025616011,
17.3185796118072));
#260222=CARTESIAN_POINT('Ctrl Pts',(-75.9580441983129,25.1496292029441,
17.3506767478586));
#260223=CARTESIAN_POINT('Ctrl Pts',(-75.9851307386898,25.0926862207585,
17.2798459583165));
#260224=CARTESIAN_POINT('Ctrl Pts',(-75.9990697411671,25.0322694073851,
17.2080611431797));
#260225=CARTESIAN_POINT('Ctrl Pts',(-75.9481612402487,25.2082186982314,
17.2973276043539));
#260226=CARTESIAN_POINT('Ctrl Pts',(-75.9759984326013,25.1530396514968,
17.212571869659));
#260227=CARTESIAN_POINT('Ctrl Pts',(-75.9872898972843,25.0938856963526,
17.1266598670131));
#260228=CARTESIAN_POINT('Ctrl Pts',(-75.9397262748186,25.2708374177395,
17.2518520136476));
#260229=CARTESIAN_POINT('Ctrl Pts',(-75.9685632596988,25.2169363483151,
17.1547259853546));
#260230=CARTESIAN_POINT('Ctrl Pts',(-75.9772090303636,25.1589733721118,
17.0560474932984));
#260231=CARTESIAN_POINT('Origin',(-74.7646897896797,24.7225971487431,17.2528005263626));
#260232=CARTESIAN_POINT('Ctrl Pts',(-76.0045572676614,24.9948448130087,
17.2916572676744));
#260233=CARTESIAN_POINT('Ctrl Pts',(-75.9888185880893,25.0581838218632,
17.3500764673707));
#260234=CARTESIAN_POINT('Ctrl Pts',(-75.9614890268774,25.1183452685092,
17.4075745924872));
#260235=CARTESIAN_POINT('Ctrl Pts',(-76.0189046879213,24.9029090128515,
17.4779931990339));
#260236=CARTESIAN_POINT('Ctrl Pts',(-76.0047941374461,24.9436535527978,
17.5184791523175));
#260237=CARTESIAN_POINT('Ctrl Pts',(-75.9867440840532,24.9827521037523,
17.5589921227563));
#260238=CARTESIAN_POINT('Ctrl Pts',(-76.0317753893929,24.8038409415446,
17.6635683446451));
#260239=CARTESIAN_POINT('Ctrl Pts',(-76.0228272111303,24.8230534553329,
17.6845460983615));
#260240=CARTESIAN_POINT('Ctrl Pts',(-76.0138748889535,24.8422792694848,
17.7055224897174));
#260241=CARTESIAN_POINT('Ctrl Pts',(-76.0424582865173,24.6976449914384,
17.8479876926675));
#260242=CARTESIAN_POINT('Ctrl Pts',(-76.0424582865173,24.6976449914384,
17.8479876926675));
#260243=CARTESIAN_POINT('Ctrl Pts',(-76.0424582865173,24.6976449914384,
17.8479876926675));
#260244=CARTESIAN_POINT('Ctrl Pts',(-75.9797580906608,-25.1427975233705,
17.073967452658));
#260245=CARTESIAN_POINT('Ctrl Pts',(-75.9704505449959,-25.2010408670593,
17.1694183903461));
#260246=CARTESIAN_POINT('Ctrl Pts',(-75.9418613633423,-25.2552738568381,
17.2633930704886));
#260247=CARTESIAN_POINT('Ctrl Pts',(-75.9544312451061,-25.3009789767176,
16.9254608534837));
#260248=CARTESIAN_POINT('Ctrl Pts',(-75.9493702728614,-25.3562842637719,
17.0375667811434));
#260249=CARTESIAN_POINT('Ctrl Pts',(-75.9205921485561,-25.4077265047638,
17.1478469399056));
#260250=CARTESIAN_POINT('Ctrl Pts',(-75.9428615286961,-25.4716594454445,
16.8162542379909));
#260251=CARTESIAN_POINT('Ctrl Pts',(-75.9415132164522,-25.5250369424895,
16.9430041875803));
#260252=CARTESIAN_POINT('Ctrl Pts',(-75.9109678945307,-25.5755858398725,
17.0670893643824));
#260253=CARTESIAN_POINT('Ctrl Pts',(-75.956838159693,-25.8204679631934,
16.6257193108577));
#260254=CARTESIAN_POINT('Ctrl Pts',(-75.962361720977,-25.869636826486,16.7798402976816));
#260255=CARTESIAN_POINT('Ctrl Pts',(-75.9275121102471,-25.9208598333928,
16.929315416431));
#260256=CARTESIAN_POINT('Ctrl Pts',(-75.9826370080728,-26.0005181671523,
16.5458722711726));
#260257=CARTESIAN_POINT('Ctrl Pts',(-75.991384088087,-26.0474798054162,
16.7128641318258));
#260258=CARTESIAN_POINT('Ctrl Pts',(-75.9538145400774,-26.1002356629363,
16.8739507927146));
#260259=CARTESIAN_POINT('Ctrl Pts',(-76.0719664887017,-26.3491447856912,
16.408284820677));
#260260=CARTESIAN_POINT('Ctrl Pts',(-76.0860184034591,-26.3907826882672,
16.5985046605215));
#260261=CARTESIAN_POINT('Ctrl Pts',(-76.043637588925,-26.4481950421709,
16.7801750176051));
#260262=CARTESIAN_POINT('Ctrl Pts',(-76.1358706771697,-26.5210561310895,
16.349401056146));
#260263=CARTESIAN_POINT('Ctrl Pts',(-76.152151115887,-26.5595368821915,
16.550967028566));
#260264=CARTESIAN_POINT('Ctrl Pts',(-76.1072227619321,-26.6205318969174,
16.7423277264094));
#260265=CARTESIAN_POINT('Ctrl Pts',(-76.2393631100495,-26.7268213040049,
16.2853173372501));
#260266=CARTESIAN_POINT('Ctrl Pts',(-76.257063787892,-26.7603293208145,
16.495184288063));
#260267=CARTESIAN_POINT('Ctrl Pts',(-76.2121224138048,-26.8243988715869,
16.6935643210242));
#260268=CARTESIAN_POINT('Ctrl Pts',(-76.2611833023277,-26.7674174132351,
16.2730180591461));
#260269=CARTESIAN_POINT('Ctrl Pts',(-76.2791071179994,-26.7998957670328,
16.4841930682975));
#260270=CARTESIAN_POINT('Ctrl Pts',(-76.2343342585777,-26.8644662404173,
16.6836830236006));
#260271=CARTESIAN_POINT('Ctrl Pts',(-76.3070716523925,-26.8474785038813,
16.2493440730816));
#260272=CARTESIAN_POINT('Ctrl Pts',(-76.3252324890958,-26.8777267177194,
16.4612725591729));
#260273=CARTESIAN_POINT('Ctrl Pts',(-76.2817116074213,-26.9425455041864,
16.6614278009669));
#260274=CARTESIAN_POINT('Ctrl Pts',(-76.3311405493927,-26.8869445368854,
16.2379796218529));
#260275=CARTESIAN_POINT('Ctrl Pts',(-76.3493117166703,-26.9159817137041,
16.4497126498075));
#260276=CARTESIAN_POINT('Ctrl Pts',(-76.3067428834464,-26.980710969085,
16.6497176781945));
#260277=CARTESIAN_POINT('Ctrl Pts',(-76.3689406638797,-26.945266929949,
16.2214623761187));
#260278=CARTESIAN_POINT('Ctrl Pts',(-76.3867886098726,-26.972153594934,
16.4272903747554));
#260279=CARTESIAN_POINT('Ctrl Pts',(-76.34819258934,-27.0343640364953,16.6223462082648));
#260280=CARTESIAN_POINT('Ctrl Pts',(-76.3818296697896,-26.9645699757353,
16.2160473363937));
#260281=CARTESIAN_POINT('Ctrl Pts',(-76.3994999566085,-26.9906641344935,
16.4191597276068));
#260282=CARTESIAN_POINT('Ctrl Pts',(-76.3626055736382,-27.0517070229519,
16.6119303419184));
#260283=CARTESIAN_POINT('Ctrl Pts',(-76.4015511235838,-26.9932458782157,
16.2079521753699));
#260284=CARTESIAN_POINT('Ctrl Pts',(-76.4187497306501,-27.0179231387113,
16.4015240394823));
#260285=CARTESIAN_POINT('Ctrl Pts',(-76.3866896921813,-27.075133854949,
16.586115527268));
#260286=CARTESIAN_POINT('Ctrl Pts',(-76.4081904188892,-27.0027594180855,
16.2052600005569));
#260287=CARTESIAN_POINT('Ctrl Pts',(-76.4251880251479,-27.0269131016926,
16.394838476637));
#260288=CARTESIAN_POINT('Ctrl Pts',(-76.3951028734164,-27.0825251276998,
16.5759864003958));
#260289=CARTESIAN_POINT('Ctrl Pts',(-76.4182420489946,-27.0169544485405,
16.2011478343014));
#260290=CARTESIAN_POINT('Ctrl Pts',(-76.4348428493639,-27.0402133489551,
16.3803198781631));
#260291=CARTESIAN_POINT('Ctrl Pts',(-76.4094060150498,-27.0919957504364,
16.5523396960077));
#260292=CARTESIAN_POINT('Ctrl Pts',(-76.4216080672702,-27.0216736152669,
16.199765076445));
#260293=CARTESIAN_POINT('Ctrl Pts',(-76.4380559634305,-27.044609595188,
16.3747494976438));
#260294=CARTESIAN_POINT('Ctrl Pts',(-76.4144529142496,-27.0948782508066,
16.5430709365392));
#260295=CARTESIAN_POINT('Ctrl Pts',(-76.4283671919628,-27.0310817132732,
16.1969190323981));
#260296=CARTESIAN_POINT('Ctrl Pts',(-76.4444782315775,-27.0533397410452,
16.3598436849778));
#260297=CARTESIAN_POINT('Ctrl Pts',(-76.4258296207998,-27.0995848867389,
16.5173659028209));
#260298=CARTESIAN_POINT('Ctrl Pts',(-76.4317613407867,-27.0357720446273,
16.1954706757853));
#260299=CARTESIAN_POINT('Ctrl Pts',(-76.447661611145,-27.0576387022135,
16.3509299496292));
#260300=CARTESIAN_POINT('Ctrl Pts',(-76.4320671439904,-27.1013790750866,
16.5017321165198));
#260301=CARTESIAN_POINT('Ctrl Pts',(-76.436859866445,-27.0427673796964,
16.1930500015502));
#260302=CARTESIAN_POINT('Ctrl Pts',(-76.4526000023644,-27.0642714137363,
16.3280456162467));
#260303=CARTESIAN_POINT('Ctrl Pts',(-76.4442399817405,-27.1026290071146,
16.45992784308));
#260304=CARTESIAN_POINT('Ctrl Pts',(-76.4385621324104,-27.045094548124,
16.1922036321779));
#260305=CARTESIAN_POINT('Ctrl Pts',(-76.4542712961586,-27.0665105524591,
16.3186472465446));
#260306=CARTESIAN_POINT('Ctrl Pts',(-76.4488339552935,-27.1027558331057,
16.4425406130888));
#260307=CARTESIAN_POINT('Ctrl Pts',(-76.4419441675585,-27.0497018479052,
16.1902449666111));
#260308=CARTESIAN_POINT('Ctrl Pts',(-76.4579141594516,-27.0713822986317,
16.2938988063911));
#260309=CARTESIAN_POINT('Ctrl Pts',(-76.4593812236218,-27.1032790990182,
16.3961238394874));
#260310=CARTESIAN_POINT('Ctrl Pts',(-76.4436315420317,-27.0519922188866,
16.1891611954603));
#260311=CARTESIAN_POINT('Ctrl Pts',(-76.4599107853122,-27.0740487753853,
16.2784857984419));
#260312=CARTESIAN_POINT('Ctrl Pts',(-76.4653396439829,-27.1037600537445,
16.3668981633898));
#260313=CARTESIAN_POINT('Ctrl Pts',(-76.4468920465821,-27.0564031404483,
16.1860061090073));
#260314=CARTESIAN_POINT('Ctrl Pts',(-76.4645195023081,-27.0801893738403,
16.2433248387421));
#260315=CARTESIAN_POINT('Ctrl Pts',(-76.4771343917457,-27.1075193467349,
16.300387443764));
#260316=CARTESIAN_POINT('Ctrl Pts',(-76.4485949814437,-27.0586973262713,
16.183947451681));
#260317=CARTESIAN_POINT('Ctrl Pts',(-76.4672853182553,-27.0838623506706,
16.2233603028531));
#260318=CARTESIAN_POINT('Ctrl Pts',(-76.4831388228296,-27.1110283253036,
16.2626673435081));
#260319=CARTESIAN_POINT('Ctrl Pts',(-76.4499684765458,-27.0605445606376,
16.1783939855022));
#260320=CARTESIAN_POINT('Ctrl Pts',(-76.4708630581003,-27.0886252421466,
16.1907475480153));
#260321=CARTESIAN_POINT('Ctrl Pts',(-76.4900906826273,-27.1178762392995,
16.2030844742334));
#260322=CARTESIAN_POINT('Ctrl Pts',(-76.4501766603085,-27.060824146804,
16.1761139907089));
#260323=CARTESIAN_POINT('Ctrl Pts',(-76.4719014767742,-27.0900112557936,
16.1795994700338));
#260324=CARTESIAN_POINT('Ctrl Pts',(-76.4919704154291,-27.120358954105,
16.1830789111177));
#260325=CARTESIAN_POINT('Ctrl Pts',(-76.4500082006625,-27.0605977646083,
16.171695172017));
#260326=CARTESIAN_POINT('Ctrl Pts',(-76.4731629849128,-27.0917127790436,
16.1610453142631));
#260327=CARTESIAN_POINT('Ctrl Pts',(-76.4942958336546,-27.1242386896308,
16.1504157284619));
#260328=CARTESIAN_POINT('Ctrl Pts',(-76.4496893833318,-27.0601693247177,
16.1695869905218));
#260329=CARTESIAN_POINT('Ctrl Pts',(-76.4734531078006,-27.0921158531867,
16.1534671350758));
#260330=CARTESIAN_POINT('Ctrl Pts',(-76.4948627299487,-27.1257019217084,
16.1373831769476));
#260331=CARTESIAN_POINT('Ctrl Pts',(-76.4484852990103,-27.0585494357892,
16.1636671740135));
#260332=CARTESIAN_POINT('Ctrl Pts',(-76.4738473436354,-27.0926985841542,
16.1336608349858));
#260333=CARTESIAN_POINT('Ctrl Pts',(-76.495819537497,-27.1291949155818,
16.1037499599793));
#260334=CARTESIAN_POINT('Ctrl Pts',(-76.4473766016455,-27.0570557850954,
16.1602705170287));
#260335=CARTESIAN_POINT('Ctrl Pts',(-76.4735073861303,-27.0922929334494,
16.1243286343765));
#260336=CARTESIAN_POINT('Ctrl Pts',(-76.4955110799672,-27.1303769013237,
16.0885277102575));
#260337=CARTESIAN_POINT('Ctrl Pts',(-76.4450122863737,-27.0538613837634,
16.1537572314779));
#260338=CARTESIAN_POINT('Ctrl Pts',(-76.4725134018884,-27.0910660428777,
16.1074637130129));
#260339=CARTESIAN_POINT('Ctrl Pts',(-76.4944955990249,-27.1320488754092,
16.0614128160212));
#260340=CARTESIAN_POINT('Ctrl Pts',(-76.4437510438076,-27.0521533110402,
16.1507330414467));
#260341=CARTESIAN_POINT('Ctrl Pts',(-76.4718218219973,-27.0901945097804,
16.100378089317));
#260342=CARTESIAN_POINT('Ctrl Pts',(-76.4937176488737,-27.132447812647,
16.0503186498413));
#260343=CARTESIAN_POINT('Ctrl Pts',(-76.4398773268223,-27.0468923857308,
16.1419954697044));
#260344=CARTESIAN_POINT('Ctrl Pts',(-76.4694878830294,-27.0872306322465,
16.0809311346633));
#260345=CARTESIAN_POINT('Ctrl Pts',(-76.4910613319352,-27.1330005795651,
16.0203313649665));
#260346=CARTESIAN_POINT('Ctrl Pts',(-76.4371653460925,-27.043189907853,
16.1366059166316));
#260347=CARTESIAN_POINT('Ctrl Pts',(-76.4675781349584,-27.0847782338116,
16.0703919912701));
#260348=CARTESIAN_POINT('Ctrl Pts',(-76.4888476714809,-27.132504025135,
16.0047512167351));
#260349=CARTESIAN_POINT('Ctrl Pts',(-76.3903090358906,-26.9788341835779,
16.047420025793));
#260350=CARTESIAN_POINT('Ctrl Pts',(-76.4327115984196,-27.0396847828042,
15.9049427900151));
#260351=CARTESIAN_POINT('Ctrl Pts',(-76.4488518482171,-27.1178462992563,
15.7660809785745));
#260352=CARTESIAN_POINT('Ctrl Pts',(-76.3383110453087,-26.9015467539818,
15.9999776993634));
#260353=CARTESIAN_POINT('Ctrl Pts',(-76.3740925666315,-26.9594482821516,
15.9619194428568));
#260354=CARTESIAN_POINT('Ctrl Pts',(-76.3877008591798,-27.0253527112511,
15.9284160251555));
#260355=CARTESIAN_POINT('Ctrl Pts',(-76.324348131815,-26.8680119970124,
15.8419552498495));
#260356=CARTESIAN_POINT('Ctrl Pts',(-76.3704738204621,-26.9418146644021,
15.3662261076973));
#260357=CARTESIAN_POINT('Ctrl Pts',(-76.3583349938827,-27.0744152558263,
14.8796638553843));
#260358=CARTESIAN_POINT('Origin',(-74.7257085670769,-24.9421491495267,17.0741173620445));
#260359=CARTESIAN_POINT('Ctrl Pts',(-75.9397262748104,-25.2708374177706,
17.2518520136472));
#260360=CARTESIAN_POINT('Ctrl Pts',(-75.9685632596807,-25.2169363483673,
17.1547259853961));
#260361=CARTESIAN_POINT('Ctrl Pts',(-75.9772090303525,-25.1589733721825,
17.0560474933749));
#260362=CARTESIAN_POINT('Ctrl Pts',(-75.9481612402858,-25.2082186980985,
17.2973276043494));
#260363=CARTESIAN_POINT('Ctrl Pts',(-75.9759984326193,-25.1530396513852,
17.2125718696724));
#260364=CARTESIAN_POINT('Ctrl Pts',(-75.9872898972957,-25.0938856962862,
17.1266598670748));
#260365=CARTESIAN_POINT('Ctrl Pts',(-75.9580441982361,-25.1496292031562,
17.3506767479224));
#260366=CARTESIAN_POINT('Ctrl Pts',(-75.9851307386312,-25.0926862209931,
17.2798459584101));
#260367=CARTESIAN_POINT('Ctrl Pts',(-75.9990697411128,-25.0322694076272,
17.2080611432832));
#260368=CARTESIAN_POINT('Ctrl Pts',(-75.9627753172647,-25.1074704498802,
17.4259425795287));
#260369=CARTESIAN_POINT('Ctrl Pts',(-75.990190594752,-25.0462350072764,
17.3727027235357));
#260370=CARTESIAN_POINT('Ctrl Pts',(-76.0065414441443,-24.9819025616068,
17.3185796118225));
#260371=CARTESIAN_POINT('Origin',(-74.7646897896784,-24.7225971487503,17.2528005263547));
#260372=CARTESIAN_POINT('Ctrl Pts',(-75.961489026876,-25.1183452685166,
17.4075745924789));
#260373=CARTESIAN_POINT('Ctrl Pts',(-75.9888185880884,-25.0581838218695,
17.3500764673615));
#260374=CARTESIAN_POINT('Ctrl Pts',(-76.0045572676606,-24.9948448130137,
17.2916572676642));
#260375=CARTESIAN_POINT('Ctrl Pts',(-75.9867440840261,-24.9827521038113,
17.5589921228149));
#260376=CARTESIAN_POINT('Ctrl Pts',(-76.0047941374114,-24.9436535528488,
17.5184791523768));
#260377=CARTESIAN_POINT('Ctrl Pts',(-76.0189046879073,-24.9029090129121,
17.4779931990604));
#260378=CARTESIAN_POINT('Ctrl Pts',(-76.0138748889937,-24.8422792694005,
17.7055224896176));
#260379=CARTESIAN_POINT('Ctrl Pts',(-76.022827211163,-24.823053455264,17.6845460982823));
#260380=CARTESIAN_POINT('Ctrl Pts',(-76.0317753894186,-24.803840941482,
17.6635683446042));
#260381=CARTESIAN_POINT('Ctrl Pts',(-76.042458286517,-24.6976449914381,
17.8479876926702));
#260382=CARTESIAN_POINT('Ctrl Pts',(-76.042458286517,-24.6976449914381,
17.8479876926702));
#260383=CARTESIAN_POINT('Ctrl Pts',(-76.042458286517,-24.6976449914381,
17.8479876926702));
#260384=CARTESIAN_POINT('Ctrl Pts',(-25.0804618860071,-75.9725615368863,
17.4201668781018));
#260385=CARTESIAN_POINT('Ctrl Pts',(-25.0218849778562,-76.0018311057342,
17.3465486622735));
#260386=CARTESIAN_POINT('Ctrl Pts',(-24.9591222046954,-76.0165443120349,
17.2720397183493));
#260387=CARTESIAN_POINT('Ctrl Pts',(-25.2741629194232,-75.9311692985899,
17.2143925575073));
#260388=CARTESIAN_POINT('Ctrl Pts',(-25.2217620984046,-75.958681184649,
17.1148633561065));
#260389=CARTESIAN_POINT('Ctrl Pts',(-25.164555452101,-75.9667333080832,
17.0143457048175));
#260390=CARTESIAN_POINT('Ctrl Pts',(-25.5065028345047,-75.9076483674931,
17.0946463742245));
#260391=CARTESIAN_POINT('Ctrl Pts',(-25.4560812233242,-75.9374572719603,
16.975096473616));
#260392=CARTESIAN_POINT('Ctrl Pts',(-25.4014568018213,-75.940075439265,
16.8534468191097));
#260393=CARTESIAN_POINT('Ctrl Pts',(-25.9210527955286,-75.9275280255481,
16.9292448759631));
#260394=CARTESIAN_POINT('Ctrl Pts',(-25.869632234831,-75.9625142169128,
16.779181403744));
#260395=CARTESIAN_POINT('Ctrl Pts',(-25.8202904741286,-75.9568105611577,
16.6244542312956));
#260396=CARTESIAN_POINT('Ctrl Pts',(-26.1003508790253,-75.9538339499116,
16.8739158933986));
#260397=CARTESIAN_POINT('Ctrl Pts',(-26.0473908953036,-75.9915498547682,
16.712201733282));
#260398=CARTESIAN_POINT('Ctrl Pts',(-26.0002790025707,-75.9825893385704,
16.5445597191471));
#260399=CARTESIAN_POINT('Ctrl Pts',(-26.4483576685983,-76.0436899102593,
16.780135040865));
#260400=CARTESIAN_POINT('Ctrl Pts',(-26.3907212263427,-76.0862364212154,
16.5977546210492));
#260401=CARTESIAN_POINT('Ctrl Pts',(-26.348993925881,-76.0719119444786,
16.4067913625623));
#260402=CARTESIAN_POINT('Ctrl Pts',(-26.6209880248636,-76.1074179294954,
16.7422284473727));
#260403=CARTESIAN_POINT('Ctrl Pts',(-26.5597476890932,-76.1525248745973,
16.5501048951729));
#260404=CARTESIAN_POINT('Ctrl Pts',(-26.5212227642732,-76.1359425371645,
16.347732979202));
#260405=CARTESIAN_POINT('Ctrl Pts',(-26.8247483133827,-76.2123121583597,
16.6934782675206));
#260406=CARTESIAN_POINT('Ctrl Pts',(-26.7604265541758,-76.2574262010907,
16.4943208592278));
#260407=CARTESIAN_POINT('Ctrl Pts',(-26.7269236186766,-76.2394155534521,
16.2836305889859));
#260408=CARTESIAN_POINT('Ctrl Pts',(-26.86480522874,-76.2345275940673,16.6835961109188));
#260409=CARTESIAN_POINT('Ctrl Pts',(-26.7999815868866,-76.279471108584,
16.4833268552187));
#260410=CARTESIAN_POINT('Ctrl Pts',(-26.7675182843423,-76.2612367837894,
16.2713262631396));
#260411=CARTESIAN_POINT('Ctrl Pts',(-26.9428805656779,-76.2819273824521,
16.6613225028908));
#260412=CARTESIAN_POINT('Ctrl Pts',(-26.8778122806246,-76.3256082188876,
16.4603950294985));
#260413=CARTESIAN_POINT('Ctrl Pts',(-26.8475982558589,-76.3071412425567,
16.2476495575985));
#260414=CARTESIAN_POINT('Ctrl Pts',(-26.9810543502183,-76.3069759166523,
16.6496028712585));
#260415=CARTESIAN_POINT('Ctrl Pts',(-26.9160778594147,-76.3496981928992,
16.448829796802));
#260416=CARTESIAN_POINT('Ctrl Pts',(-26.8870847364698,-76.3312252545645,
16.2362848769795));
#260417=CARTESIAN_POINT('Ctrl Pts',(-27.0347146146425,-76.3484797871891,
16.6221367327712));
#260418=CARTESIAN_POINT('Ctrl Pts',(-26.9722866202247,-76.387191475666,
16.4263729310814));
#260419=CARTESIAN_POINT('Ctrl Pts',(-26.9454540778636,-76.369062531796,
16.2198040383418));
#260420=CARTESIAN_POINT('Ctrl Pts',(-27.0520461010368,-76.362903314126,
16.6116902389505));
#260421=CARTESIAN_POINT('Ctrl Pts',(-26.990797870902,-76.3998985070137,
16.4182354344378));
#260422=CARTESIAN_POINT('Ctrl Pts',(-26.9647604072753,-76.3819564220901,
16.2144102296094));
#260423=CARTESIAN_POINT('Ctrl Pts',(-27.0754324956906,-76.3870229007017,
16.5857176723771));
#260424=CARTESIAN_POINT('Ctrl Pts',(-27.0180627224554,-76.4191298939445,
16.4005487707529));
#260425=CARTESIAN_POINT('Ctrl Pts',(-26.9934408909725,-76.4016850635586,
16.2063864536385));
#260426=CARTESIAN_POINT('Ctrl Pts',(-27.082807799689,-76.3954507470103,
16.5755244414166));
#260427=CARTESIAN_POINT('Ctrl Pts',(-27.0270559839675,-76.4255606544136,
16.3938428354582));
#260428=CARTESIAN_POINT('Ctrl Pts',(-27.002956907366,-76.4083274633214,
16.2037237985522));
#260429=CARTESIAN_POINT('Ctrl Pts',(-27.0922320376559,-76.4098047654361,
16.5516204721235));
#260430=CARTESIAN_POINT('Ctrl Pts',(-27.0403670147046,-76.4351975383185,
16.3792244413015));
#260431=CARTESIAN_POINT('Ctrl Pts',(-27.0171572804536,-76.4183850872766,
16.1996869095663));
#260432=CARTESIAN_POINT('Ctrl Pts',(-27.0950953264238,-76.4148733708263,
16.542241373223));
#260433=CARTESIAN_POINT('Ctrl Pts',(-27.0447678397139,-76.4384035785,16.3736104964499));
#260434=CARTESIAN_POINT('Ctrl Pts',(-27.0218787739739,-76.4217535244985,
16.1983342860888));
#260435=CARTESIAN_POINT('Ctrl Pts',(-27.09974315268,-76.4263249193095,16.5161165141971));
#260436=CARTESIAN_POINT('Ctrl Pts',(-27.0535116464076,-76.4448069459407,
16.3585277802127));
#260437=CARTESIAN_POINT('Ctrl Pts',(-27.0312909576635,-76.4285171755911,
16.1955743904622));
#260438=CARTESIAN_POINT('Ctrl Pts',(-27.1014904674061,-76.4326137594219,
16.5002045800044));
#260439=CARTESIAN_POINT('Ctrl Pts',(-27.0578166604448,-76.4479765311915,
16.3494953975989));
#260440=CARTESIAN_POINT('Ctrl Pts',(-27.0359831728686,-76.4319135317268,
16.1941800679749));
#260441=CARTESIAN_POINT('Ctrl Pts',(-27.1026704184049,-76.4449452653179,
16.4573094494877));
#260442=CARTESIAN_POINT('Ctrl Pts',(-27.06448288193,-76.4528969605597,16.3261248041982));
#260443=CARTESIAN_POINT('Ctrl Pts',(-27.042975264242,-76.4370110131309,
16.1919016822539));
#260444=CARTESIAN_POINT('Ctrl Pts',(-27.1027728684428,-76.4496135704626,
16.4393960541623));
#260445=CARTESIAN_POINT('Ctrl Pts',(-27.0667393944978,-76.4545638835523,
16.3164891117473));
#260446=CARTESIAN_POINT('Ctrl Pts',(-27.0453014012305,-76.4387129855089,
16.1911145326723));
#260447=CARTESIAN_POINT('Ctrl Pts',(-27.1033488438058,-76.4602856539495,
16.3918070921512));
#260448=CARTESIAN_POINT('Ctrl Pts',(-27.0716717101316,-76.4582133271186,
16.2912288897422));
#260449=CARTESIAN_POINT('Ctrl Pts',(-27.0498984940091,-76.4420884316609,
16.1893010704581));
#260450=CARTESIAN_POINT('Ctrl Pts',(-27.103921956883,-76.4662567117755,
16.3621450322927));
#260451=CARTESIAN_POINT('Ctrl Pts',(-27.0743744435445,-76.4602162047745,
16.2756512778778));
#260452=CARTESIAN_POINT('Ctrl Pts',(-27.0521738675717,-76.4437652233608,
16.1883092099671));
#260453=CARTESIAN_POINT('Ctrl Pts',(-27.1079500471755,-76.4780100141098,
16.2949622535392));
#260454=CARTESIAN_POINT('Ctrl Pts',(-27.0805869451232,-76.4648464736733,
16.2402396310873));
#260455=CARTESIAN_POINT('Ctrl Pts',(-27.0565399426152,-76.446993278341,
16.1852909757043));
#260456=CARTESIAN_POINT('Ctrl Pts',(-27.1117437396593,-76.4840868539141,
16.2559882666832));
#260457=CARTESIAN_POINT('Ctrl Pts',(-27.0843760577293,-76.4676882621546,
16.2196371037421));
#260458=CARTESIAN_POINT('Ctrl Pts',(-27.0588362934608,-76.4486982192438,
16.1831963663266));
#260459=CARTESIAN_POINT('Ctrl Pts',(-27.1186429162664,-76.490725727778,
16.1967720341217));
#260460=CARTESIAN_POINT('Ctrl Pts',(-27.0889706079157,-76.4711321232331,
16.1872136925794));
#260461=CARTESIAN_POINT('Ctrl Pts',(-27.060449611965,-76.4498977970784,
16.1776432448482));
#260462=CARTESIAN_POINT('Ctrl Pts',(-27.1210505518396,-76.4924398017463,
16.1773616860554));
#260463=CARTESIAN_POINT('Ctrl Pts',(-27.0902380459652,-76.472080509577,
16.1763774272268));
#260464=CARTESIAN_POINT('Ctrl Pts',(-27.0606161752027,-76.4500218115713,
16.1753910477022));
#260465=CARTESIAN_POINT('Ctrl Pts',(-27.1247236922632,-76.4945108031759,
16.1461844913658));
#260466=CARTESIAN_POINT('Ctrl Pts',(-27.0917434440942,-76.4731956267612,
16.1586478057165));
#260467=CARTESIAN_POINT('Ctrl Pts',(-27.0602497730195,-76.4497492188549,
16.1711360013758));
#260468=CARTESIAN_POINT('Ctrl Pts',(-27.1261031628986,-76.4950020357306,
16.1336817286105));
#260469=CARTESIAN_POINT('Ctrl Pts',(-27.0920805335398,-76.4734376571505,
16.1513715711306));
#260470=CARTESIAN_POINT('Ctrl Pts',(-27.0597799419457,-76.4493997295781,
16.1691026721905));
#260471=CARTESIAN_POINT('Ctrl Pts',(-27.1315681998307,-76.4963255984206,
16.0800932837524));
#260472=CARTESIAN_POINT('Ctrl Pts',(-27.0928134511318,-76.4739251360541,
16.1197927836083));
#260473=CARTESIAN_POINT('Ctrl Pts',(-27.0569687226382,-76.4473109346426,
16.1596448232286));
#260474=CARTESIAN_POINT('Ctrl Pts',(-27.1323195784959,-76.4945113000399,
16.0589082957796));
#260475=CARTESIAN_POINT('Ctrl Pts',(-27.0909209641397,-76.4724331002842,
16.1061418174148));
#260476=CARTESIAN_POINT('Ctrl Pts',(-27.0534134152975,-76.4446774540823,
16.1536294662377));
#260477=CARTESIAN_POINT('Ctrl Pts',(-27.1329837771626,-76.490953990412,
16.0195114651226));
#260478=CARTESIAN_POINT('Ctrl Pts',(-27.0869366765604,-76.469312905874,
16.0806139918018));
#260479=CARTESIAN_POINT('Ctrl Pts',(-27.0464009528417,-76.4395165697616,
16.1421882796313));
#260480=CARTESIAN_POINT('Ctrl Pts',(-27.132475559678,-76.4887423766877,
16.0040405252701));
#260481=CARTESIAN_POINT('Ctrl Pts',(-27.0844779770543,-76.4674056396179,
16.0701604569259));
#260482=CARTESIAN_POINT('Ctrl Pts',(-27.0426984150624,-76.436805864294,
16.1368608677843));
#260483=CARTESIAN_POINT('Ctrl Pts',(-27.1176445693019,-76.4487554850671,
15.7668594205044));
#260484=CARTESIAN_POINT('Ctrl Pts',(-27.0392647575279,-76.432563214653,
15.9058934996543));
#260485=CARTESIAN_POINT('Ctrl Pts',(-26.9783040498254,-76.3899445519403,
16.0485446134454));
#260486=CARTESIAN_POINT('Ctrl Pts',(-27.0267181003067,-76.3890441685664,
15.9290103440671));
#260487=CARTESIAN_POINT('Ctrl Pts',(-26.9607754137872,-76.3752347443676,
15.9631551147876));
#260488=CARTESIAN_POINT('Ctrl Pts',(-26.9028259696071,-76.3392599186865,
16.0018551686374));
#260489=CARTESIAN_POINT('Ctrl Pts',(-27.0702645554341,-76.3535975691974,
14.8756002297544));
#260490=CARTESIAN_POINT('Ctrl Pts',(-26.9358287316524,-76.3662706704139,
15.3627392755869));
#260491=CARTESIAN_POINT('Ctrl Pts',(-26.8612497822103,-76.3194480575193,
15.8395311954951));
#260492=CARTESIAN_POINT('Origin',(-24.9421491495266,-74.7257085670769,17.0741173620444));
#260493=CARTESIAN_POINT('Ctrl Pts',(-25.1074704499414,-75.9627753172411,
17.4259425795563));
#260494=CARTESIAN_POINT('Ctrl Pts',(-25.046235007313,-75.9901905947504,
17.3727027235404));
#260495=CARTESIAN_POINT('Ctrl Pts',(-24.981902561604,-76.0065414441461,
17.3185796118018));
#260496=CARTESIAN_POINT('Ctrl Pts',(-25.1496292028979,-75.9580441983283,
17.3506767478559));
#260497=CARTESIAN_POINT('Ctrl Pts',(-25.0926862206973,-75.9851307386982,
17.2798459583171));
#260498=CARTESIAN_POINT('Ctrl Pts',(-25.032269407339,-75.9990697411774,
17.2080611431692));
#260499=CARTESIAN_POINT('Ctrl Pts',(-25.2082186982554,-75.9481612402448,
17.2973276043357));
#260500=CARTESIAN_POINT('Ctrl Pts',(-25.1530396515149,-75.9759984326107,
17.2125718696202));
#260501=CARTESIAN_POINT('Ctrl Pts',(-25.0938856963612,-75.9872898972827,
17.1266598669893));
#260502=CARTESIAN_POINT('Ctrl Pts',(-25.2708374177341,-75.9397262748193,
17.2518520136524));
#260503=CARTESIAN_POINT('Ctrl Pts',(-25.2169363483077,-75.9685632596981,
17.1547259853579));
#260504=CARTESIAN_POINT('Ctrl Pts',(-25.1589733721019,-75.9772090303652,
17.0560474932908));
#260505=CARTESIAN_POINT('Origin',(-24.7225971487431,-74.7646897896797,17.2528005263626));
#260506=CARTESIAN_POINT('Ctrl Pts',(-24.9948448130087,-76.0045572676613,
17.2916572676744));
#260507=CARTESIAN_POINT('Ctrl Pts',(-25.0581838218632,-75.9888185880893,
17.3500764673707));
#260508=CARTESIAN_POINT('Ctrl Pts',(-25.1183452685093,-75.9614890268773,
17.4075745924872));
#260509=CARTESIAN_POINT('Ctrl Pts',(-24.9029090128662,-76.0189046879179,
17.4779931990395));
#260510=CARTESIAN_POINT('Ctrl Pts',(-24.9436535528188,-76.0047941374338,
17.5184791523303));
#260511=CARTESIAN_POINT('Ctrl Pts',(-24.9827521037685,-75.9867440840462,
17.5589921227692));
#260512=CARTESIAN_POINT('Ctrl Pts',(-24.8038409415453,-76.0317753893924,
17.6635683446476));
#260513=CARTESIAN_POINT('Ctrl Pts',(-24.8230534553307,-76.0228272111309,
17.6845460983631));
#260514=CARTESIAN_POINT('Ctrl Pts',(-24.842279269484,-76.0138748889534,
17.7055224897201));
#260515=CARTESIAN_POINT('Ctrl Pts',(-24.6976449914385,-76.0424582865173,
17.8479876926674));
#260516=CARTESIAN_POINT('Ctrl Pts',(-24.6976449914385,-76.0424582865173,
17.8479876926674));
#260517=CARTESIAN_POINT('Ctrl Pts',(-24.6976449914385,-76.0424582865173,
17.8479876926674));
#260518=CARTESIAN_POINT('Ctrl Pts',(25.1183452685168,-75.9614890268759,
17.4075745924789));
#260519=CARTESIAN_POINT('Ctrl Pts',(25.0581838218696,-75.9888185880884,
17.3500764673614));
#260520=CARTESIAN_POINT('Ctrl Pts',(24.9948448130138,-76.0045572676605,
17.2916572676642));
#260521=CARTESIAN_POINT('Ctrl Pts',(24.9827521037791,-75.9867440840413,
17.5589921227799));
#260522=CARTESIAN_POINT('Ctrl Pts',(24.9436535528272,-76.0047941374361,
17.5184791523559));
#260523=CARTESIAN_POINT('Ctrl Pts',(24.9029090128812,-76.0189046879146,
17.4779931990425));
#260524=CARTESIAN_POINT('Ctrl Pts',(24.8422792694397,-76.0138748889755,
17.7055224896604));
#260525=CARTESIAN_POINT('Ctrl Pts',(24.8230534553045,-76.0228272111454,
17.6845460983164));
#260526=CARTESIAN_POINT('Ctrl Pts',(24.8038409415197,-76.0317753894035,
17.6635683446265));
#260527=CARTESIAN_POINT('Ctrl Pts',(24.6976449914381,-76.042458286517,17.8479876926702));
#260528=CARTESIAN_POINT('Ctrl Pts',(24.6976449914381,-76.042458286517,17.8479876926702));
#260529=CARTESIAN_POINT('Ctrl Pts',(24.6976449914381,-76.042458286517,17.8479876926702));
#260530=CARTESIAN_POINT('Origin',(24.7225971487503,-74.7646897896784,17.2528005263546));
#260531=CARTESIAN_POINT('Ctrl Pts',(25.2708374177646,-75.9397262748126,
17.2518520136429));
#260532=CARTESIAN_POINT('Ctrl Pts',(25.216936348354,-75.9685632596854,17.1547259853771));
#260533=CARTESIAN_POINT('Ctrl Pts',(25.1589733721664,-75.977209030355,17.0560474933546));
#260534=CARTESIAN_POINT('Ctrl Pts',(25.2082186981224,-75.9481612402767,
17.2973276043667));
#260535=CARTESIAN_POINT('Ctrl Pts',(25.1530396514148,-75.9759984326127,
17.2125718697077));
#260536=CARTESIAN_POINT('Ctrl Pts',(25.0938856963024,-75.9872898972931,
17.1266598670757));
#260537=CARTESIAN_POINT('Ctrl Pts',(25.1496292031279,-75.9580441982479,
17.3506767479025));
#260538=CARTESIAN_POINT('Ctrl Pts',(25.092686220964,-75.9851307386456,17.279845958371));
#260539=CARTESIAN_POINT('Ctrl Pts',(25.0322694075872,-75.9990697411219,
17.2080611432543));
#260540=CARTESIAN_POINT('Ctrl Pts',(25.1074704498875,-75.9627753172617,
17.4259425795336));
#260541=CARTESIAN_POINT('Ctrl Pts',(25.0462350072772,-75.9901905947512,
17.3727027235393));
#260542=CARTESIAN_POINT('Ctrl Pts',(24.9819025616038,-76.0065414441453,
17.3185796118177));
#260543=CARTESIAN_POINT('Origin',(24.9421491495265,-74.7257085670769,17.0741173620444));
#260544=CARTESIAN_POINT('Ctrl Pts',(24.9589179244775,-76.0165927349248,
17.2719235983584));
#260545=CARTESIAN_POINT('Ctrl Pts',(25.0217593825187,-76.0018779353611,
17.3465144253549));
#260546=CARTESIAN_POINT('Ctrl Pts',(25.080406146805,-75.9725739125722,17.4202136827156));
#260547=CARTESIAN_POINT('Ctrl Pts',(25.1644631755165,-75.9667363952717,
17.0140601840459));
#260548=CARTESIAN_POINT('Ctrl Pts',(25.221741891211,-75.958699255426,17.1147005690572));
#260549=CARTESIAN_POINT('Ctrl Pts',(25.2742034625189,-75.9311549696869,
17.2143522965184));
#260550=CARTESIAN_POINT('Ctrl Pts',(25.4013568068367,-75.9400924588407,
16.8531572333247));
#260551=CARTESIAN_POINT('Ctrl Pts',(25.4560486791227,-75.9375037638634,
16.9749518244653));
#260552=CARTESIAN_POINT('Ctrl Pts',(25.5065310412202,-75.9076590513784,
17.0946441539564));
#260553=CARTESIAN_POINT('Ctrl Pts',(25.8199808109355,-75.9567824207869,
16.6241920433869));
#260554=CARTESIAN_POINT('Ctrl Pts',(25.8693789134686,-75.9625371923871,
16.7790876749283));
#260555=CARTESIAN_POINT('Ctrl Pts',(25.9208598335162,-75.9275121102613,
16.9293154163786));
#260556=CARTESIAN_POINT('Ctrl Pts',(26.000053557193,-75.982549287452,16.5442194930891));
#260557=CARTESIAN_POINT('Ctrl Pts',(26.0472138477371,-75.9915734872872,
16.7120520463995));
#260558=CARTESIAN_POINT('Ctrl Pts',(26.1002356630946,-75.9538145401055,
16.8739507926621));
#260559=CARTESIAN_POINT('Ctrl Pts',(26.3487341201567,-76.0718263572337,
16.4064067119874));
#260560=CARTESIAN_POINT('Ctrl Pts',(26.3904925533402,-76.0862325763166,
16.5975865835765));
#260561=CARTESIAN_POINT('Ctrl Pts',(26.4481950423898,-76.0436375889943,
16.7801750175556));
#260562=CARTESIAN_POINT('Ctrl Pts',(26.5206773079536,-76.1357086402236,
16.3474135454721));
#260563=CARTESIAN_POINT('Ctrl Pts',(26.5592282356561,-76.1523784623028,
16.5499987057077));
#260564=CARTESIAN_POINT('Ctrl Pts',(26.6205318971682,-76.1072227620321,
16.7423277263585));
#260565=CARTESIAN_POINT('Ctrl Pts',(26.7264920278152,-76.2391872039751,
16.2832499561865));
#260566=CARTESIAN_POINT('Ctrl Pts',(26.7600048061527,-76.2572914179578,
16.4941794849072));
#260567=CARTESIAN_POINT('Ctrl Pts',(26.8243988718558,-76.2121224139505,
16.6935643209576));
#260568=CARTESIAN_POINT('Ctrl Pts',(26.7670983652051,-76.2610052237305,
16.2709381031613));
#260569=CARTESIAN_POINT('Ctrl Pts',(26.7995686663897,-76.2793339283727,
16.483182492595));
#260570=CARTESIAN_POINT('Ctrl Pts',(26.8644662406905,-76.2343342587333,
16.6836830235308));
#260571=CARTESIAN_POINT('Ctrl Pts',(26.8471814973332,-76.3068912751988,
16.2472568143868));
#260572=CARTESIAN_POINT('Ctrl Pts',(26.877398340547,-76.3254529697315,16.4602585557158));
#260573=CARTESIAN_POINT('Ctrl Pts',(26.9425455044634,-76.2817116075996,
16.6614278008798));
#260574=CARTESIAN_POINT('Ctrl Pts',(26.8866594690452,-76.3309600846097,
16.2358941800171));
#260575=CARTESIAN_POINT('Ctrl Pts',(26.9156538070631,-76.3495273630062,
16.4486994597328));
#260576=CARTESIAN_POINT('Ctrl Pts',(26.9807109693644,-76.306742883636,16.6497176781018));
#260577=CARTESIAN_POINT('Ctrl Pts',(26.9450028214736,-76.3687633501263,
16.2194335053764));
#260578=CARTESIAN_POINT('Ctrl Pts',(26.97183869477,-76.3869839776596,16.42630302961));
#260579=CARTESIAN_POINT('Ctrl Pts',(27.0343640367628,-76.3481925895598,
16.6223462081032));
#260580=CARTESIAN_POINT('Ctrl Pts',(26.9643135743833,-76.3816540900187,
16.2140445067397));
#260581=CARTESIAN_POINT('Ctrl Pts',(26.9903552563186,-76.3996866432579,
16.4181843035957));
#260582=CARTESIAN_POINT('Ctrl Pts',(27.0517070232152,-76.3626055738679,
16.6119303417357));
#260583=CARTESIAN_POINT('Ctrl Pts',(26.9930030990806,-76.4013801263841,
16.2060411897629));
#260584=CARTESIAN_POINT('Ctrl Pts',(27.0176339890546,-76.4189117662005,
16.4005910913664));
#260585=CARTESIAN_POINT('Ctrl Pts',(27.0751338551856,-76.3866896924452,
16.586115526953));
#260586=CARTESIAN_POINT('Ctrl Pts',(27.0025216629709,-76.4080213774166,
16.2033875259851));
#260587=CARTESIAN_POINT('Ctrl Pts',(27.0266321688135,-76.4253400053729,
16.3939233783011));
#260588=CARTESIAN_POINT('Ctrl Pts',(27.0825251279255,-76.3951028736931,
16.5759864000299));
#260589=CARTESIAN_POINT('Ctrl Pts',(27.0167251837918,-76.4180768571583,
16.1993760598583));
#260590=CARTESIAN_POINT('Ctrl Pts',(27.0399520693394,-76.4349711969098,
16.3794519126528));
#260591=CARTESIAN_POINT('Ctrl Pts',(27.0919957506263,-76.4094060153691,
16.5523396954336));
#260592=CARTESIAN_POINT('Ctrl Pts',(27.021447406794,-76.4214443601548,16.1980339040756));
#260593=CARTESIAN_POINT('Ctrl Pts',(27.0443560717347,-76.4381750026904,
16.3739005889315));
#260594=CARTESIAN_POINT('Ctrl Pts',(27.0948782509814,-76.4144529145863,
16.5430709358771));
#260595=CARTESIAN_POINT('Ctrl Pts',(27.0308618473994,-76.4282067461047,
16.1953051377168));
#260596=CARTESIAN_POINT('Ctrl Pts',(27.0531068030348,-76.4445721654389,
16.3590502399129));
#260597=CARTESIAN_POINT('Ctrl Pts',(27.0995848868676,-76.4258296211971,
16.5173659018241));
#260598=CARTESIAN_POINT('Ctrl Pts',(27.0355558313041,-76.431602939514,16.1939295264868));
#260599=CARTESIAN_POINT('Ctrl Pts',(27.0574185528962,-76.4477400998369,
16.3501709468135));
#260600=CARTESIAN_POINT('Ctrl Pts',(27.1013790751781,-76.4320671444298,
16.5017321152991));
#260601=CARTESIAN_POINT('Ctrl Pts',(27.0425542496203,-76.4367029543674,
16.1917093184004));
#260602=CARTESIAN_POINT('Ctrl Pts',(27.0640787016057,-76.4526420041684,
16.3273830254781));
#260603=CARTESIAN_POINT('Ctrl Pts',(27.1026290071501,-76.4442399823126,
16.4599278409708));
#260604=CARTESIAN_POINT('Ctrl Pts',(27.044882087663,-76.4384054885609,16.1909469809412));
#260605=CARTESIAN_POINT('Ctrl Pts',(27.0663285831481,-76.454298594577,16.3180252379247));
#260606=CARTESIAN_POINT('Ctrl Pts',(27.1027558331205,-76.448833955927,16.4425406105531));
#260607=CARTESIAN_POINT('Ctrl Pts',(27.0494862927941,-76.4417848384089,
16.189213145832));
#260608=CARTESIAN_POINT('Ctrl Pts',(27.0712224187978,-76.457906806159,16.2933864096896));
#260609=CARTESIAN_POINT('Ctrl Pts',(27.1032790990715,-76.4593812243663,
16.3961238359575));
#260610=CARTESIAN_POINT('Ctrl Pts',(27.0517726588334,-76.4434690801001,
16.1882712240633));
#260611=CARTESIAN_POINT('Ctrl Pts',(27.0738999824816,-76.4598835980122,
16.2780430295813));
#260612=CARTESIAN_POINT('Ctrl Pts',(27.1037600538756,-76.4653396447702,
16.3668981593358));
#260613=CARTESIAN_POINT('Ctrl Pts',(27.056165905205,-76.4467160461775,16.1854342125082));
#260614=CARTESIAN_POINT('Ctrl Pts',(27.0800527001779,-76.4644564169994,
16.2430394726561));
#260615=CARTESIAN_POINT('Ctrl Pts',(27.1075193470971,-76.477134392507,16.3003874390844));
#260616=CARTESIAN_POINT('Ctrl Pts',(27.058446161956,-76.448408331131,16.183554002614));
#260617=CARTESIAN_POINT('Ctrl Pts',(27.0837265687902,-76.4672060788238,
16.2231638334608));
#260618=CARTESIAN_POINT('Ctrl Pts',(27.1110283258744,-76.4831388236134,
16.2626673380729));
#260619=CARTESIAN_POINT('Ctrl Pts',(27.0602641883352,-76.4497597907345,
16.178270627192));
#260620=CARTESIAN_POINT('Ctrl Pts',(27.0884790804448,-76.4707669813323,
16.1906858996445));
#260621=CARTESIAN_POINT('Ctrl Pts',(27.1178762399416,-76.4900906831748,
16.2030844689337));
#260622=CARTESIAN_POINT('Ctrl Pts',(27.0605327253119,-76.4499596839301,
16.1760791854255));
#260623=CARTESIAN_POINT('Ctrl Pts',(27.0898596142588,-76.4718011962243,
16.1795820812116));
#260624=CARTESIAN_POINT('Ctrl Pts',(27.1203589546904,-76.4919704158393,
16.1830789062925));
#260625=CARTESIAN_POINT('Ctrl Pts',(27.0602871252534,-76.4497769562955,
16.1718015077251));
#260626=CARTESIAN_POINT('Ctrl Pts',(27.091550239126,-76.4730573789198,16.161098430761));
#260627=CARTESIAN_POINT('Ctrl Pts',(27.1242386900703,-76.4942958338587,
16.150415724656));
#260628=CARTESIAN_POINT('Ctrl Pts',(27.0598504145463,-76.4494520698569,
16.1697479299107));
#260629=CARTESIAN_POINT('Ctrl Pts',(27.0919480018444,-76.4733461100563,
16.1535475151469));
#260630=CARTESIAN_POINT('Ctrl Pts',(27.1257019220719,-76.4948627300815,
16.1373831736257));
#260631=CARTESIAN_POINT('Ctrl Pts',(27.0582086378074,-76.4482320655577,
16.1639666812434));
#260632=CARTESIAN_POINT('Ctrl Pts',(27.0925161430721,-76.4737375070857,
16.1338103547262));
#260633=CARTESIAN_POINT('Ctrl Pts',(27.1291949157768,-76.4958195374835,
16.1037499577342));
#260634=CARTESIAN_POINT('Ctrl Pts',(27.0567042026752,-76.4471157233158,
16.1606292063217));
#260635=CARTESIAN_POINT('Ctrl Pts',(27.0921025222746,-76.4733973726533,
16.1245076295647));
#260636=CARTESIAN_POINT('Ctrl Pts',(27.1303769014743,-76.495511079926,16.088527708241));
#260637=CARTESIAN_POINT('Ctrl Pts',(27.0534903139798,-76.4447377899016,
16.154219073874));
#260638=CARTESIAN_POINT('Ctrl Pts',(27.0908610700863,-76.4724034594285,
16.1076940322559));
#260639=CARTESIAN_POINT('Ctrl Pts',(27.1320488754804,-76.4944955989311,
16.0614128144368));
#260640=CARTESIAN_POINT('Ctrl Pts',(27.0517739663595,-76.4434708920043,
16.1512353239512));
#260641=CARTESIAN_POINT('Ctrl Pts',(27.0899831498703,-76.4717122944326,
16.1006284961015));
#260642=CARTESIAN_POINT('Ctrl Pts',(27.1324478126924,-76.4937176487667,
16.050318648402));
#260643=CARTESIAN_POINT('Ctrl Pts',(27.0464903385136,-76.4395819014306,
16.1426043077347));
#260644=CARTESIAN_POINT('Ctrl Pts',(27.087001580347,-76.4693799204485,16.0812344002251));
#260645=CARTESIAN_POINT('Ctrl Pts',(27.1330005795476,-76.4910613317947,
16.0203313638476));
#260646=CARTESIAN_POINT('Ctrl Pts',(27.0427755237225,-76.436861974418,16.1372659264035));
#260647=CARTESIAN_POINT('Ctrl Pts',(27.0845393319118,-76.4674716655807,
16.0707205696176));
#260648=CARTESIAN_POINT('Ctrl Pts',(27.1325040250962,-76.4888476713311,
16.0047512157116));
#260649=CARTESIAN_POINT('Ctrl Pts',(26.9782305695083,-76.3898874630358,
16.0488344443928));
#260650=CARTESIAN_POINT('Ctrl Pts',(27.0392919333536,-76.4326304753448,
15.9056407261267));
#260651=CARTESIAN_POINT('Ctrl Pts',(27.1178462988928,-76.4488518479317,
15.7660809789566));
#260652=CARTESIAN_POINT('Ctrl Pts',(26.9009713129947,-76.3379547623971,
16.0003561766751));
#260653=CARTESIAN_POINT('Ctrl Pts',(26.959117533273,-76.3740242719226,15.9620875813222));
#260654=CARTESIAN_POINT('Ctrl Pts',(27.0253527115695,-76.387700859183,15.9284160212411));
#260655=CARTESIAN_POINT('Ctrl Pts',(26.8672868453189,-76.323892551556,15.8466387280156));
#260656=CARTESIAN_POINT('Ctrl Pts',(26.9411427564858,-76.3705353286247,
15.3686915983964));
#260657=CARTESIAN_POINT('Ctrl Pts',(27.0744152538546,-76.3583349935937,
14.8796638708869));
#260658=CARTESIAN_POINT('Ctrl Pts',(75.9725615368492,-25.0804618860833,
17.4201668782156));
#260659=CARTESIAN_POINT('Ctrl Pts',(76.0018311057085,-25.0218849780074,
17.3465486624662));
#260660=CARTESIAN_POINT('Ctrl Pts',(76.0165443120274,-24.9591222047477,
17.2720397184167));
#260661=CARTESIAN_POINT('Ctrl Pts',(75.931169298622,-25.2741629193577,17.2143925574082));
#260662=CARTESIAN_POINT('Ctrl Pts',(75.958681184672,-25.2217620982712,17.114863355933));
#260663=CARTESIAN_POINT('Ctrl Pts',(75.9667333080915,-25.1645554520448,
17.0143457047411));
#260664=CARTESIAN_POINT('Ctrl Pts',(75.9076483674902,-25.50650283451,17.0946463742361));
#260665=CARTESIAN_POINT('Ctrl Pts',(75.9374572719645,-25.4560812233272,
16.9750964736227));
#260666=CARTESIAN_POINT('Ctrl Pts',(75.9400754392653,-25.4014568018194,
16.8534468191075));
#260667=CARTESIAN_POINT('Ctrl Pts',(75.9275280255502,-25.9210527955254,
16.9292448759546));
#260668=CARTESIAN_POINT('Ctrl Pts',(75.9625142169127,-25.869632234825,16.7791814037269));
#260669=CARTESIAN_POINT('Ctrl Pts',(75.9568105611571,-25.8202904741216,
16.6244542312725));
#260670=CARTESIAN_POINT('Ctrl Pts',(75.9538339499134,-26.1003508790237,
16.8739158933912));
#260671=CARTESIAN_POINT('Ctrl Pts',(75.9915498547703,-26.0473908953001,
16.7122017332653));
#260672=CARTESIAN_POINT('Ctrl Pts',(75.9825893385697,-26.0002790025666,
16.5445597191247));
#260673=CARTESIAN_POINT('Ctrl Pts',(76.043689910258,-26.4483576686014,16.7801350408721));
#260674=CARTESIAN_POINT('Ctrl Pts',(76.0862364212178,-26.3907212263421,
16.5977546210478));
#260675=CARTESIAN_POINT('Ctrl Pts',(76.0719119444774,-26.3489939258776,
16.4067913625481));
#260676=CARTESIAN_POINT('Ctrl Pts',(76.1074179294968,-26.6209880248623,
16.7422284473672));
#260677=CARTESIAN_POINT('Ctrl Pts',(76.1525248745982,-26.559747689091,16.5501048951559));
#260678=CARTESIAN_POINT('Ctrl Pts',(76.1359425371629,-26.5212227642695,
16.3477329791785));
#260679=CARTESIAN_POINT('Ctrl Pts',(76.21231215836,-26.8247483133844,16.6934782675217));
#260680=CARTESIAN_POINT('Ctrl Pts',(76.2574262010941,-26.7604265541735,
16.494320859219));
#260681=CARTESIAN_POINT('Ctrl Pts',(76.239415553451,-26.7269236186745,16.2836305889652));
#260682=CARTESIAN_POINT('Ctrl Pts',(76.2345275940678,-26.8648052287415,
16.6835961109194));
#260683=CARTESIAN_POINT('Ctrl Pts',(76.2794711085875,-26.7999815868845,
16.483326855209));
#260684=CARTESIAN_POINT('Ctrl Pts',(76.2612367837882,-26.7675182843401,
16.2713262631183));
#260685=CARTESIAN_POINT('Ctrl Pts',(76.2819273824529,-26.9428805656787,
16.6613225028898));
#260686=CARTESIAN_POINT('Ctrl Pts',(76.3256082188901,-26.8778122806222,
16.4603950294871));
#260687=CARTESIAN_POINT('Ctrl Pts',(76.3071412425556,-26.847598255857,16.2476495575766));
#260688=CARTESIAN_POINT('Ctrl Pts',(76.3069759166547,-26.981054350217,16.6496028712503));
#260689=CARTESIAN_POINT('Ctrl Pts',(76.3496981929022,-26.916077859412,16.4488297967862));
#260690=CARTESIAN_POINT('Ctrl Pts',(76.3312252545631,-26.8870847364676,
16.2362848769561));
#260691=CARTESIAN_POINT('Ctrl Pts',(76.3484797871891,-27.0347146146448,
16.622136732775));
#260692=CARTESIAN_POINT('Ctrl Pts',(76.3871914756689,-26.9722866202228,
16.4263729310736));
#260693=CARTESIAN_POINT('Ctrl Pts',(76.3690625317952,-26.9454540778622,
16.2198040383217));
#260694=CARTESIAN_POINT('Ctrl Pts',(76.3629033141268,-27.0520461010375,
16.6116902389496));
#260695=CARTESIAN_POINT('Ctrl Pts',(76.3998985070162,-26.9907978709001,
16.418235434428));
#260696=CARTESIAN_POINT('Ctrl Pts',(76.381956422089,-26.9647604072736,16.2144102295885));
#260697=CARTESIAN_POINT('Ctrl Pts',(76.3870229007027,-27.0754324956918,
16.5857176723765));
#260698=CARTESIAN_POINT('Ctrl Pts',(76.4191298939471,-27.0180627224535,
16.4005487707426));
#260699=CARTESIAN_POINT('Ctrl Pts',(76.4016850635578,-26.9934408909713,
16.2063864536189));
#260700=CARTESIAN_POINT('Ctrl Pts',(76.3954507470115,-27.08280779969,16.5755244414153));
#260701=CARTESIAN_POINT('Ctrl Pts',(76.4255606544161,-27.0270559839657,
16.393842835448));
#260702=CARTESIAN_POINT('Ctrl Pts',(76.4083274633205,-27.0029569073648,
16.2037237985328));
#260703=CARTESIAN_POINT('Ctrl Pts',(76.4098047654372,-27.0922320376568,
16.5516204721222));
#260704=CARTESIAN_POINT('Ctrl Pts',(76.4351975383206,-27.0403670147031,
16.3792244412919));
#260705=CARTESIAN_POINT('Ctrl Pts',(76.4183850872758,-27.0171572804525,
16.199686909548));
#260706=CARTESIAN_POINT('Ctrl Pts',(76.4148733708268,-27.0950953264254,
16.5422413732253));
#260707=CARTESIAN_POINT('Ctrl Pts',(76.4384035785022,-27.0447678397125,
16.3736104964424));
#260708=CARTESIAN_POINT('Ctrl Pts',(76.4217535244978,-27.0218787739728,
16.1983342860712));
#260709=CARTESIAN_POINT('Ctrl Pts',(76.4263249193116,-27.0997431526799,
16.5161165141907));
#260710=CARTESIAN_POINT('Ctrl Pts',(76.4448069459424,-27.0535116464063,
16.3585277802011));
#260711=CARTESIAN_POINT('Ctrl Pts',(76.4285171755903,-27.0312909576624,
16.1955743904452));
#260712=CARTESIAN_POINT('Ctrl Pts',(76.4326137594236,-27.1014904674066,
16.5002045800003));
#260713=CARTESIAN_POINT('Ctrl Pts',(76.4479765311931,-27.0578166604438,
16.3494953975893));
#260714=CARTESIAN_POINT('Ctrl Pts',(76.431913531726,-27.0359831728675,16.1941800679589));
#260715=CARTESIAN_POINT('Ctrl Pts',(76.4449452653199,-27.1026704184053,
16.4573094494813));
#260716=CARTESIAN_POINT('Ctrl Pts',(76.452896960561,-27.0644828819291,16.3261248041879));
#260717=CARTESIAN_POINT('Ctrl Pts',(76.4370110131303,-27.042975264241,16.19190168224));
#260718=CARTESIAN_POINT('Ctrl Pts',(76.4496135704653,-27.1027728684427,
16.4393960541509));
#260719=CARTESIAN_POINT('Ctrl Pts',(76.4545638835533,-27.0667393944972,
16.316489111735));
#260720=CARTESIAN_POINT('Ctrl Pts',(76.4387129855081,-27.0453014012295,
16.1911145326591));
#260721=CARTESIAN_POINT('Ctrl Pts',(76.4602856539522,-27.1033488438061,
16.3918070921387));
#260722=CARTESIAN_POINT('Ctrl Pts',(76.4582133271196,-27.0716717101313,
16.2912288897306));
#260723=CARTESIAN_POINT('Ctrl Pts',(76.4420884316602,-27.0498984940081,
16.1893010704474));
#260724=CARTESIAN_POINT('Ctrl Pts',(76.4662567117788,-27.1039219568836,
16.362145032275));
#260725=CARTESIAN_POINT('Ctrl Pts',(76.4602162047754,-27.0743744435445,
16.2756512778644));
#260726=CARTESIAN_POINT('Ctrl Pts',(76.44376522336,-27.0521738675706,16.1883092099575));
#260727=CARTESIAN_POINT('Ctrl Pts',(76.4780100141125,-27.107950047177,16.2949622535236));
#260728=CARTESIAN_POINT('Ctrl Pts',(76.4648464736739,-27.0805869451234,
16.2402396310762));
#260729=CARTESIAN_POINT('Ctrl Pts',(76.4469932783401,-27.0565399426139,
16.1852909756979));
#260730=CARTESIAN_POINT('Ctrl Pts',(76.4840868539169,-27.1117437396614,
16.255988266664));
#260731=CARTESIAN_POINT('Ctrl Pts',(76.4676882621551,-27.0843760577297,
16.2196371037299));
#260732=CARTESIAN_POINT('Ctrl Pts',(76.4486982192426,-27.0588362934592,
16.1831963663216));
#260733=CARTESIAN_POINT('Ctrl Pts',(76.4907257277799,-27.1186429162688,
16.1967720341036));
#260734=CARTESIAN_POINT('Ctrl Pts',(76.4711321232332,-27.0889706079157,
16.1872136925689));
#260735=CARTESIAN_POINT('Ctrl Pts',(76.4498977970766,-27.0604496119625,
16.1776432448454));
#260736=CARTESIAN_POINT('Ctrl Pts',(76.4924398017475,-27.1210505518414,
16.1773616860397));
#260737=CARTESIAN_POINT('Ctrl Pts',(76.4720805095765,-27.0902380459647,
16.1763774272179));
#260738=CARTESIAN_POINT('Ctrl Pts',(76.4500218115691,-27.0606161751996,
16.1753910477002));
#260739=CARTESIAN_POINT('Ctrl Pts',(76.4945108031767,-27.1247236922648,
16.1461844913533));
#260740=CARTESIAN_POINT('Ctrl Pts',(76.4731956267605,-27.091743444093,16.15864780571));
#260741=CARTESIAN_POINT('Ctrl Pts',(76.4497492188525,-27.0602497730161,
16.1711360013752));
#260742=CARTESIAN_POINT('Ctrl Pts',(76.4950020357312,-27.1261031628999,
16.1336817285995));
#260743=CARTESIAN_POINT('Ctrl Pts',(76.4734376571497,-27.0920805335384,
16.1513715711251));
#260744=CARTESIAN_POINT('Ctrl Pts',(76.4493997295754,-27.0597799419421,
16.1691026721906));
#260745=CARTESIAN_POINT('Ctrl Pts',(76.4963255984204,-27.131568199831,16.0800932837475));
#260746=CARTESIAN_POINT('Ctrl Pts',(76.4739251360527,-27.0928134511296,
16.1197927836073));
#260747=CARTESIAN_POINT('Ctrl Pts',(76.4473109346395,-27.056968722634,16.1596448232313));
#260748=CARTESIAN_POINT('Ctrl Pts',(76.4945113000399,-27.1323195784967,
16.0589082957738));
#260749=CARTESIAN_POINT('Ctrl Pts',(76.4724331002834,-27.0909209641377,
16.1061418174134));
#260750=CARTESIAN_POINT('Ctrl Pts',(76.4446774540792,-27.0534134152933,
16.1536294662411));
#260751=CARTESIAN_POINT('Ctrl Pts',(76.4909539904116,-27.1329837771621,
16.0195114651211));
#260752=CARTESIAN_POINT('Ctrl Pts',(76.4693129058723,-27.0869366765573,
16.0806139918042));
#260753=CARTESIAN_POINT('Ctrl Pts',(76.4395165697581,-27.0464009528369,
16.1421882796369));
#260754=CARTESIAN_POINT('Ctrl Pts',(76.4887423766876,-27.1324755596786,
16.0040405252658));
#260755=CARTESIAN_POINT('Ctrl Pts',(76.4674056396168,-27.0844779770519,
16.0701604569266));
#260756=CARTESIAN_POINT('Ctrl Pts',(76.4368058642907,-27.0426984150579,
16.1368608677898));
#260757=CARTESIAN_POINT('Ctrl Pts',(76.448755485065,-27.1176445692923,15.7668594205343));
#260758=CARTESIAN_POINT('Ctrl Pts',(76.4325632146506,-27.0392647575183,
15.905893499679));
#260759=CARTESIAN_POINT('Ctrl Pts',(76.3899445519341,-26.9783040498165,
16.0485446134662));
#260760=CARTESIAN_POINT('Ctrl Pts',(76.3890441685523,-27.0267181003279,
15.9290103438536));
#260761=CARTESIAN_POINT('Ctrl Pts',(76.3752347443254,-26.9607754137721,
15.9631551147061));
#260762=CARTESIAN_POINT('Ctrl Pts',(76.3392599186918,-26.9028259696125,
16.0018551686097));
#260763=CARTESIAN_POINT('Ctrl Pts',(76.353597569397,-27.0702645555105,14.8756002309254));
#260764=CARTESIAN_POINT('Ctrl Pts',(76.3662706708498,-26.9358287319212,
15.3627392759442));
#260765=CARTESIAN_POINT('Ctrl Pts',(76.3194480575026,-26.8612497821939,
15.8395311956764));
#260766=CARTESIAN_POINT('Origin',(74.7257085670769,-24.9421491495266,17.0741173620444));
#260767=CARTESIAN_POINT('Ctrl Pts',(75.9627753172425,-25.1074704499379,
17.425942579555));
#260768=CARTESIAN_POINT('Ctrl Pts',(75.9901905947506,-25.0462350073073,
17.3727027235416));
#260769=CARTESIAN_POINT('Ctrl Pts',(76.006541444146,-24.981902561604,17.3185796118039));
#260770=CARTESIAN_POINT('Ctrl Pts',(75.9580441983231,-25.1496292029117,
17.3506767478614));
#260771=CARTESIAN_POINT('Ctrl Pts',(75.9851307386948,-25.0926862207269,
17.2798459583192));
#260772=CARTESIAN_POINT('Ctrl Pts',(75.9990697411736,-25.0322694073559,
17.2080611431766));
#260773=CARTESIAN_POINT('Ctrl Pts',(75.9481612402476,-25.2082186982459,
17.2973276043341));
#260774=CARTESIAN_POINT('Ctrl Pts',(75.9759984326039,-25.1530396515039,
17.212571869635));
#260775=CARTESIAN_POINT('Ctrl Pts',(75.9872898972835,-25.0938856963563,
17.1266598669944));
#260776=CARTESIAN_POINT('Ctrl Pts',(75.9397262748187,-25.2708374177363,
17.2518520136529));
#260777=CARTESIAN_POINT('Ctrl Pts',(75.9685632596991,-25.2169363483118,
17.1547259853573));
#260778=CARTESIAN_POINT('Ctrl Pts',(75.9772090303644,-25.1589733721069,
17.0560474932961));
#260779=CARTESIAN_POINT('Origin',(74.7646897896797,-24.7225971487432,17.2528005263628));
#260780=CARTESIAN_POINT('Ctrl Pts',(76.0045572676613,-24.9948448130087,
17.2916572676745));
#260781=CARTESIAN_POINT('Ctrl Pts',(75.9888185880893,-25.0581838218632,
17.3500764673708));
#260782=CARTESIAN_POINT('Ctrl Pts',(75.9614890268773,-25.1183452685093,
17.4075745924873));
#260783=CARTESIAN_POINT('Ctrl Pts',(76.0189046879197,-24.9029090128582,
17.4779931990371));
#260784=CARTESIAN_POINT('Ctrl Pts',(76.004794137431,-24.9436535528328,17.5184791523393));
#260785=CARTESIAN_POINT('Ctrl Pts',(75.9867440840503,-24.9827521037588,
17.5589921227622));
#260786=CARTESIAN_POINT('Ctrl Pts',(76.0317753893939,-24.8038409415422,
17.663568344644));
#260787=CARTESIAN_POINT('Ctrl Pts',(76.0228272111318,-24.823053455328,17.6845460983626));
#260788=CARTESIAN_POINT('Ctrl Pts',(76.013874888955,-24.8422792694812,17.7055224897144));
#260789=CARTESIAN_POINT('Ctrl Pts',(76.0424582865173,-24.6976449914384,
17.8479876926675));
#260790=CARTESIAN_POINT('Ctrl Pts',(76.0424582865173,-24.6976449914384,
17.8479876926675));
#260791=CARTESIAN_POINT('Ctrl Pts',(76.0424582865173,-24.6976449914384,
17.8479876926675));
#260792=CARTESIAN_POINT('Ctrl Pts',(-10.5032495111116,73.8913131000538,
42.8625));
#260793=CARTESIAN_POINT('Ctrl Pts',(-10.8194981777074,76.1161511576644,
42.8625));
#260794=CARTESIAN_POINT('Ctrl Pts',(-10.8580391950582,76.3872907109282,
40.6320481322491));
#260795=CARTESIAN_POINT('Ctrl Pts',(-10.0498719735697,73.9557582643349,
42.8625));
#260796=CARTESIAN_POINT('Ctrl Pts',(-10.6359163209588,76.1470117154128,
42.8625));
#260797=CARTESIAN_POINT('Ctrl Pts',(-10.7069125966304,76.4094233456861,
40.6268004742471));
#260798=CARTESIAN_POINT('Ctrl Pts',(-9.61416596216602,74.1010554093231,
42.8625));
#260799=CARTESIAN_POINT('Ctrl Pts',(-10.4617751497477,76.2168938632405,
42.8625));
#260800=CARTESIAN_POINT('Ctrl Pts',(-10.5616780116939,76.4593229171357,
40.6149692390278));
#260801=CARTESIAN_POINT('Ctrl Pts',(-9.01121135502815,74.4321791952113,
42.8625));
#260802=CARTESIAN_POINT('Ctrl Pts',(-10.2324603050541,76.3707063913054,
42.8625));
#260803=CARTESIAN_POINT('Ctrl Pts',(-10.3606931432216,76.5730413834782,
40.5880065872607));
#260804=CARTESIAN_POINT('Ctrl Pts',(-8.82276685013128,74.5591463206078,
42.8625));
#260805=CARTESIAN_POINT('Ctrl Pts',(-10.1626132722428,76.429280000154,42.8624999999992));
#260806=CARTESIAN_POINT('Ctrl Pts',(-10.2978783081087,76.6166459400673,
40.5776679558998));
#260807=CARTESIAN_POINT('Ctrl Pts',(-8.47012856407996,74.8451674277979,
42.8625));
#260808=CARTESIAN_POINT('Ctrl Pts',(-10.0366590959459,76.5589310255573,
42.8625000000008));
#260809=CARTESIAN_POINT('Ctrl Pts',(-10.1803322126703,76.7148746948338,
40.5543779788271));
#260810=CARTESIAN_POINT('Ctrl Pts',(-8.30454355451,75.0059528700596,42.8625));
#260811=CARTESIAN_POINT('Ctrl Pts',(-9.98011487798406,76.6308815760035,
42.8625));
#260812=CARTESIAN_POINT('Ctrl Pts',(-10.1251372092705,76.7700935312232,
40.5412856450937));
#260813=CARTESIAN_POINT('Ctrl Pts',(-8.00653344424111,75.3526470955157,
42.8625));
#260814=CARTESIAN_POINT('Ctrl Pts',(-9.88423732636679,76.7826313398306,
42.8625));
#260815=CARTESIAN_POINT('Ctrl Pts',(-10.0258005063557,76.889159348055,40.5130553109125));
#260816=CARTESIAN_POINT('Ctrl Pts',(-7.87453768264795,75.537341674481,42.8625));
#260817=CARTESIAN_POINT('Ctrl Pts',(-9.84501292103885,76.862025038882,42.8625));
#260818=CARTESIAN_POINT('Ctrl Pts',(-9.98180191901158,76.9525893314949,
40.4980161791992));
#260819=CARTESIAN_POINT('Ctrl Pts',(-7.64384406928706,75.9289449770848,
42.8625));
#260820=CARTESIAN_POINT('Ctrl Pts',(-9.7832976556328,77.026013436169,42.8625));
#260821=CARTESIAN_POINT('Ctrl Pts',(-9.90490404767533,77.087078327256,40.4661291586505));
#260822=CARTESIAN_POINT('Ctrl Pts',(-7.54449579085874,76.138073277502,42.8625));
#260823=CARTESIAN_POINT('Ctrl Pts',(-9.76082396850354,77.1115552436014,
42.8625));
#260824=CARTESIAN_POINT('Ctrl Pts',(-9.87178795472008,77.1588996123912,
40.4491005377577));
#260825=CARTESIAN_POINT('Ctrl Pts',(-7.30715555334537,76.77968408777,42.8625));
#260826=CARTESIAN_POINT('Ctrl Pts',(-9.72005612520358,77.3667579800968,
42.8625));
#260827=CARTESIAN_POINT('Ctrl Pts',(-9.79267454297696,77.3792490712788,
40.3968564392364));
#260828=CARTESIAN_POINT('Ctrl Pts',(-7.22543403834982,77.2295173162425,
42.8625));
#260829=CARTESIAN_POINT('Ctrl Pts',(-9.72799316153702,77.5349482149457,
42.8625000000016));
#260830=CARTESIAN_POINT('Ctrl Pts',(-9.76543403703142,77.53373600667,40.360228281325));
#260831=CARTESIAN_POINT('Ctrl Pts',(-7.22543403703142,77.692863772622,42.8625));
#260832=CARTESIAN_POINT('Ctrl Pts',(-9.76543403703142,77.6928637726221,
42.8625));
#260833=CARTESIAN_POINT('Ctrl Pts',(-9.76543403703142,77.6928637726221,
40.3225));
#260834=CARTESIAN_POINT('Origin',(-7.22543403703142,77.692863772622,40.3225000000001));
#260835=CARTESIAN_POINT('Origin',(-7.22543403703142,0.,40.3225));
#260836=CARTESIAN_POINT('Ctrl Pts',(-9.76543403703143,80.6811576396149,
40.3225));
#260837=CARTESIAN_POINT('Ctrl Pts',(-9.76543403703143,80.6811576396149,
40.5734833092634));
#260838=CARTESIAN_POINT('Ctrl Pts',(-9.72826133827436,80.6482300667132,
40.8191813005851));
#260839=CARTESIAN_POINT('Ctrl Pts',(-9.57979077264777,80.5164913076875,
41.3141267879751));
#260840=CARTESIAN_POINT('Ctrl Pts',(-9.46269022074881,80.4125005677019,
41.5513261178172));
#260841=CARTESIAN_POINT('Ctrl Pts',(-9.13655730339021,80.1220365304268,
42.0266708314762));
#260842=CARTESIAN_POINT('Ctrl Pts',(-8.91315643821528,79.9225400586233,
42.243196993227));
#260843=CARTESIAN_POINT('Ctrl Pts',(-8.4557159958063,79.5121708037282,42.5602310880019));
#260844=CARTESIAN_POINT('Ctrl Pts',(-8.22361432068508,79.3032203173786,
42.6713019811039));
#260845=CARTESIAN_POINT('Ctrl Pts',(-7.73973487957791,78.8657441556769,
42.8233283921749));
#260846=CARTESIAN_POINT('Ctrl Pts',(-7.48535212294286,78.6347875624617,
42.8617809540987));
#260847=CARTESIAN_POINT('Ctrl Pts',(-7.23018356331462,78.4020741645152,
42.8624966696506));
#260848=CARTESIAN_POINT('Ctrl Pts',(-7.22780877734985,78.3999082730286,
42.8625));
#260849=CARTESIAN_POINT('Ctrl Pts',(-7.22543403703142,78.3977423334149,
42.8625));
#260850=CARTESIAN_POINT('Ctrl Pts',(7.2254340370314,77.6928637726221,42.8625));
#260851=CARTESIAN_POINT('Ctrl Pts',(9.7654340370314,77.6928637726221,42.8625));
#260852=CARTESIAN_POINT('Ctrl Pts',(9.7654340370314,77.6928637726221,40.3225));
#260853=CARTESIAN_POINT('Ctrl Pts',(7.22543404223311,77.2344170949798,42.8625));
#260854=CARTESIAN_POINT('Ctrl Pts',(9.72839370096131,77.5366375762832,42.8625));
#260855=CARTESIAN_POINT('Ctrl Pts',(9.76543403703139,77.5354187456466,40.3598293135595));
#260856=CARTESIAN_POINT('Ctrl Pts',(7.30588292190357,76.7834773995825,42.8625));
#260857=CARTESIAN_POINT('Ctrl Pts',(9.71986880761174,77.3682612423042,42.8625));
#260858=CARTESIAN_POINT('Ctrl Pts',(9.79225033127547,77.3805518141073,40.3965475634802));
#260859=CARTESIAN_POINT('Ctrl Pts',(7.54459734351766,76.1376228588779,42.8625));
#260860=CARTESIAN_POINT('Ctrl Pts',(9.76082461763374,77.1113880289587,42.8625));
#260861=CARTESIAN_POINT('Ctrl Pts',(9.87182180621682,77.1587449246315,40.4491372136505));
#260862=CARTESIAN_POINT('Ctrl Pts',(7.6421466156822,75.9323032890386,42.8625));
#260863=CARTESIAN_POINT('Ctrl Pts',(9.78289158219672,77.0273950913578,42.8625));
#260864=CARTESIAN_POINT('Ctrl Pts',(9.9043382299849,77.0882316781324,40.4658557023577));
#260865=CARTESIAN_POINT('Ctrl Pts',(7.87211185551081,75.5409911144992,42.8625));
#260866=CARTESIAN_POINT('Ctrl Pts',(9.84431775555056,76.8635766939471,42.8625));
#260867=CARTESIAN_POINT('Ctrl Pts',(9.98099330978796,76.9538426649305,40.4977190163966));
#260868=CARTESIAN_POINT('Ctrl Pts',(8.00581438906634,75.3535555307654,42.8625));
#260869=CARTESIAN_POINT('Ctrl Pts',(9.88401297106729,76.7830262232379,42.8624999999992));
#260870=CARTESIAN_POINT('Ctrl Pts',(10.0255608207902,76.8894713331461,40.5129813396039));
#260871=CARTESIAN_POINT('Ctrl Pts',(8.30424197032195,75.0062320553663,42.8625));
#260872=CARTESIAN_POINT('Ctrl Pts',(9.9800101345932,76.6310079116545,42.8625000000008));
#260873=CARTESIAN_POINT('Ctrl Pts',(10.1250366817144,76.7701894127781,40.5412629118058));
#260874=CARTESIAN_POINT('Ctrl Pts',(8.46708944384426,74.8479469686107,42.8625));
#260875=CARTESIAN_POINT('Ctrl Pts',(10.0356040736642,76.5601795029381,42.8625));
#260876=CARTESIAN_POINT('Ctrl Pts',(10.1793191727176,76.7158292777585,40.5541516480795));
#260877=CARTESIAN_POINT('Ctrl Pts',(8.81948930738161,74.5614957425962,42.8625));
#260878=CARTESIAN_POINT('Ctrl Pts',(10.1614125709453,76.43035700652,42.8625));
#260879=CARTESIAN_POINT('Ctrl Pts',(10.296785793733,76.6174528062696,40.5774766481521));
#260880=CARTESIAN_POINT('Ctrl Pts',(9.01115900281434,74.4322732113038,42.8625));
#260881=CARTESIAN_POINT('Ctrl Pts',(10.2324466057663,76.3707480311754,42.8625));
#260882=CARTESIAN_POINT('Ctrl Pts',(10.3606756921529,76.573073670993,40.5879989317086));
#260883=CARTESIAN_POINT('Ctrl Pts',(9.61177309064578,74.1022393738552,42.8625));
#260884=CARTESIAN_POINT('Ctrl Pts',(10.4608564764661,76.2174456694345,42.8625));
#260885=CARTESIAN_POINT('Ctrl Pts',(10.5608803885151,76.459729529522,40.6148728315803));
#260886=CARTESIAN_POINT('Ctrl Pts',(10.0442301749684,73.9565602111107,42.8625));
#260887=CARTESIAN_POINT('Ctrl Pts',(10.6336336926735,76.1473954357262,42.8625));
#260888=CARTESIAN_POINT('Ctrl Pts',(10.7050285749523,76.4096992633537,40.6267350470548));
#260889=CARTESIAN_POINT('Ctrl Pts',(10.5032495111116,73.8913131000538,42.8625));
#260890=CARTESIAN_POINT('Ctrl Pts',(10.8194981777074,76.1161511576644,42.8625));
#260891=CARTESIAN_POINT('Ctrl Pts',(10.8580391950581,76.3872907109282,40.6320481322491));
#260892=CARTESIAN_POINT('Origin',(7.22543403703139,77.6928637726221,40.3225));
#260893=CARTESIAN_POINT('Origin',(-2.7565840235444E-14,7.21644966006352E-13,
40.3225));
#260894=CARTESIAN_POINT('Ctrl Pts',(9.76543403703141,80.6811576396149,40.3225));
#260895=CARTESIAN_POINT('Ctrl Pts',(9.76543403703141,80.6811576396149,40.5734833092633));
#260896=CARTESIAN_POINT('Ctrl Pts',(9.72826133827443,80.6482300667132,40.819181300585));
#260897=CARTESIAN_POINT('Ctrl Pts',(9.57979077264777,80.5164913076875,41.3141267879752));
#260898=CARTESIAN_POINT('Ctrl Pts',(9.46269022074867,80.4125005677018,41.5513261178174));
#260899=CARTESIAN_POINT('Ctrl Pts',(9.13655730339017,80.1220365304269,42.0266708314761));
#260900=CARTESIAN_POINT('Ctrl Pts',(8.91315643821524,79.9225400586233,42.243196993227));
#260901=CARTESIAN_POINT('Ctrl Pts',(8.45571599580626,79.5121708037282,42.5602310880019));
#260902=CARTESIAN_POINT('Ctrl Pts',(8.22361432068505,79.3032203173786,42.6713019811039));
#260903=CARTESIAN_POINT('Ctrl Pts',(7.73973487957849,78.8657441556775,42.8233283921747));
#260904=CARTESIAN_POINT('Ctrl Pts',(7.4853521229467,78.6347875624646,42.8617809540987));
#260905=CARTESIAN_POINT('Ctrl Pts',(7.23018356331449,78.4020741645151,42.8624966696506));
#260906=CARTESIAN_POINT('Ctrl Pts',(7.2278087773499,78.3999082730286,42.8625));
#260907=CARTESIAN_POINT('Ctrl Pts',(7.22543403703139,78.3977423334149,42.8625));
#260908=CARTESIAN_POINT('Origin',(7.22543403703139,0.,40.3225));
#260909=CARTESIAN_POINT('Origin',(0.,92.7,30.1625));
#260910=CARTESIAN_POINT('',(-0.952500000000001,92.7,30.1625));
#260911=CARTESIAN_POINT('',(0.952500000000001,92.7,30.1625));
#260912=CARTESIAN_POINT('Origin',(0.,92.7,30.1625));
#260913=CARTESIAN_POINT('Origin',(-5.80244527768194,66.322253007815,4.445));
#260914=CARTESIAN_POINT('',(-7.70019617754672,66.1562213178808,4.445));
#260915=CARTESIAN_POINT('',(-5.80244527768194,66.322253007815,6.35));
#260916=CARTESIAN_POINT('Origin',(-5.80244527768194,66.322253007815,4.445));
#260917=CARTESIAN_POINT('',(-7.67883747572177,66.2094701536372,4.445));
#260918=CARTESIAN_POINT('Origin',(-7.63693781421789,66.1617557075452,4.445));
#260919=CARTESIAN_POINT('Origin',(-5.80690631599121,66.3732429090145,4.445));
#260920=CARTESIAN_POINT('Origin',(-5.80244527768194,66.322253007815,4.445));
#260921=CARTESIAN_POINT('Origin',(-5.79969559744267,66.2908240188643,4.445));
#260922=CARTESIAN_POINT('',(-3.9019446975779,66.4568557087986,4.445));
#260923=CARTESIAN_POINT('',(-5.79969559744267,66.2908240188643,6.35));
#260924=CARTESIAN_POINT('Origin',(-5.79969559744267,66.2908240188643,4.445));
#260925=CARTESIAN_POINT('',(-3.95966867124224,66.3880629558053,4.445));
#260926=CARTESIAN_POINT('Origin',(-3.96520306090672,66.4513213191341,4.445));
#260927=CARTESIAN_POINT('Origin',(-5.79416120777819,66.2275656555355,4.445));
#260928=CARTESIAN_POINT('Origin',(-5.79969559744267,66.2908240188643,4.445));
#260929=CARTESIAN_POINT('Ctrl Pts',(-5.62465651441568,65.8691607435455,
5.70752129153081));
#260930=CARTESIAN_POINT('Ctrl Pts',(-5.63790471104907,65.7947780994363,
5.5263494271517));
#260931=CARTESIAN_POINT('Ctrl Pts',(-5.65892533799205,65.793128368605,5.33119064940291));
#260932=CARTESIAN_POINT('Ctrl Pts',(-5.78778340659959,65.8551936059547,
5.72536825578739));
#260933=CARTESIAN_POINT('Ctrl Pts',(-5.77764549719958,65.7827958377032,
5.5416830532429));
#260934=CARTESIAN_POINT('Ctrl Pts',(-5.77361112064157,65.7832641425467,
5.34381854412852));
#260935=CARTESIAN_POINT('Ctrl Pts',(-5.95339386843844,65.8404505247366,
5.71116838370947));
#260936=CARTESIAN_POINT('Ctrl Pts',(-5.91972549086594,65.7701600468525,
5.52945686894868));
#260937=CARTESIAN_POINT('Ctrl Pts',(-5.89048374747282,65.7728957801126,
5.33371655958433));
#260938=CARTESIAN_POINT('Ctrl Pts',(-6.19051191645161,65.8185545400719,
5.64266439295642));
#260939=CARTESIAN_POINT('Ctrl Pts',(-6.12280879673811,65.7514893855043,
5.47063103361691));
#260940=CARTESIAN_POINT('Ctrl Pts',(-6.05710404049759,65.7576898743807,
5.28531446245343));
#260941=CARTESIAN_POINT('Ctrl Pts',(-6.26635324587272,65.8114233229095,
5.61246633480641));
#260942=CARTESIAN_POINT('Ctrl Pts',(-6.18780235406067,65.745412351332,5.44468251173949));
#260943=CARTESIAN_POINT('Ctrl Pts',(-6.11047600283212,65.7527482825607,
5.2639426202062));
#260944=CARTESIAN_POINT('Ctrl Pts',(-6.41227161791133,65.7974900401404,
5.5372277684103));
#260945=CARTESIAN_POINT('Ctrl Pts',(-6.31273591873296,65.7335644293773,
5.38009364421865));
#260946=CARTESIAN_POINT('Ctrl Pts',(-6.21292662446779,65.7431469168115,
5.2108238923688));
#260947=CARTESIAN_POINT('Ctrl Pts',(-6.48267530224625,65.7906533823261,
5.49171207331871));
#260948=CARTESIAN_POINT('Ctrl Pts',(-6.37301403184221,65.7277587397228,
5.34101748828414));
#260949=CARTESIAN_POINT('Ctrl Pts',(-6.26235611220587,65.7384524764899,
5.17868364459097));
#260950=CARTESIAN_POINT('Ctrl Pts',(-6.67625832145065,65.771609690581,5.3375639439796));
#260951=CARTESIAN_POINT('Ctrl Pts',(-6.53859812806969,65.7116183426713,
5.20882050652558));
#260952=CARTESIAN_POINT('Ctrl Pts',(-6.39793957073026,65.7254424976304,
5.0701310476513));
#260953=CARTESIAN_POINT('Ctrl Pts',(-6.78626175412378,65.7604319347151,
5.20765442851689));
#260954=CARTESIAN_POINT('Ctrl Pts',(-6.63260327913571,65.7021800114779,
5.09750267265541));
#260955=CARTESIAN_POINT('Ctrl Pts',(-6.47480199997683,65.7178765272223,
4.97884055097215));
#260956=CARTESIAN_POINT('Ctrl Pts',(-6.94711837759049,65.7439022860098,
4.91695248025269));
#260957=CARTESIAN_POINT('Ctrl Pts',(-6.76998082727741,65.6882320874307,
4.84858322570707));
#260958=CARTESIAN_POINT('Ctrl Pts',(-6.58701829346881,65.7067237529874,
4.7749299918791));
#260959=CARTESIAN_POINT('Ctrl Pts',(-6.99956413262688,65.7383832850395,
4.75269553806659));
#260960=CARTESIAN_POINT('Ctrl Pts',(-6.81469918225909,65.6835983754984,
4.70817642224148));
#260961=CARTESIAN_POINT('Ctrl Pts',(-6.62345593201658,65.7030378048493,
4.66021655474088));
#260962=CARTESIAN_POINT('Ctrl Pts',(-7.03663553754223,65.7344992036835,
4.42043150549321));
#260963=CARTESIAN_POINT('Ctrl Pts',(-6.84632924814695,65.680326321646,4.42392531515964));
#260964=CARTESIAN_POINT('Ctrl Pts',(-6.64925400403071,65.7004320115443,
4.42768942481514));
#260965=CARTESIAN_POINT('Ctrl Pts',(-7.02175067111833,65.7360778057269,
4.2482238053988));
#260966=CARTESIAN_POINT('Ctrl Pts',(-6.83369078626271,65.6816453095259,
4.27696682318786));
#260967=CARTESIAN_POINT('Ctrl Pts',(-6.63902317906353,65.7014735525984,
4.30793133907197));
#260968=CARTESIAN_POINT('Ctrl Pts',(-6.95157881920653,65.7433920557505,
4.00755588597506));
#260969=CARTESIAN_POINT('Ctrl Pts',(-6.77373147910964,65.687815467461,4.07078461642782));
#260970=CARTESIAN_POINT('Ctrl Pts',(-6.59000859522952,65.7064017694204,
4.13890003156499));
#260971=CARTESIAN_POINT('Ctrl Pts',(-6.91964686688078,65.7467134097066,
3.92826718530274));
#260972=CARTESIAN_POINT('Ctrl Pts',(-6.74651699790575,65.6906072261033,
4.00306354599665));
#260973=CARTESIAN_POINT('Ctrl Pts',(-6.56784982525329,65.7086239030736,
4.08364051696471));
#260974=CARTESIAN_POINT('Ctrl Pts',(-6.84256578106127,65.7546542138477,
3.78073711455572));
#260975=CARTESIAN_POINT('Ctrl Pts',(-6.68069740936757,65.6973018864277,
3.87676636256858));
#260976=CARTESIAN_POINT('Ctrl Pts',(-6.51409836326281,65.7139743814014,
3.98021640596179));
#260977=CARTESIAN_POINT('Ctrl Pts',(-6.79735138508887,65.7592837801704,
3.71148839023358));
#260978=CARTESIAN_POINT('Ctrl Pts',(-6.6419854773461,65.701216650196,3.81734832354759));
#260979=CARTESIAN_POINT('Ctrl Pts',(-6.48235366389942,65.7171182506776,
3.93138820287611));
#260980=CARTESIAN_POINT('Ctrl Pts',(-6.63878879347099,65.775312120901,3.51465375123548));
#260981=CARTESIAN_POINT('Ctrl Pts',(-6.50675035368678,65.7147367021846,
3.64903407158234));
#260982=CARTESIAN_POINT('Ctrl Pts',(-6.37211727164478,65.7279297649216,
3.79379510141207));
#260983=CARTESIAN_POINT('Ctrl Pts',(-6.51075654656604,65.7880289020976,
3.40837559058612));
#260984=CARTESIAN_POINT('Ctrl Pts',(-6.3970094597364,65.7255268760605,3.55761353944892));
#260985=CARTESIAN_POINT('Ctrl Pts',(-6.28197311160879,65.7366443924548,
3.71837851255275));
#260986=CARTESIAN_POINT('Ctrl Pts',(-6.22090193659141,65.8158107296672,
3.25007929659638));
#260987=CARTESIAN_POINT('Ctrl Pts',(-6.1489336050582,65.7491363445969,3.42177380399819));
#260988=CARTESIAN_POINT('Ctrl Pts',(-6.07865960801857,65.7557563971943,
3.60672526232144));
#260989=CARTESIAN_POINT('Ctrl Pts',(-6.063764387523,65.830429565192,3.20051147934914));
#260990=CARTESIAN_POINT('Ctrl Pts',(-6.01420487377899,65.7616099376474,
3.37914354468415));
#260991=CARTESIAN_POINT('Ctrl Pts',(-5.96793753428448,65.7659218676103,
3.57156666118844));
#260992=CARTESIAN_POINT('Ctrl Pts',(-5.89874125546025,65.8451815059264,
3.18246633414093));
#260993=CARTESIAN_POINT('Ctrl Pts',(-5.8728108939582,65.7742266046314,3.36364162741095));
#260994=CARTESIAN_POINT('Ctrl Pts',(-5.85185860383796,65.7762489610748,
3.55880407300439));
#260995=CARTESIAN_POINT('',(-5.89874124598147,65.8451814395652,3.18246636753802));
#260996=CARTESIAN_POINT('',(-5.76176670013149,65.8572952859405,5.715));
#260997=CARTESIAN_POINT('Ctrl Pts',(-5.89874124128049,65.8451813460936,
3.18246633411965));
#260998=CARTESIAN_POINT('Ctrl Pts',(-5.91453706816504,65.8437693867186,
3.18419359570151));
#260999=CARTESIAN_POINT('Ctrl Pts',(-5.93059885152208,65.8423280911914,
3.18625668216982));
#261000=CARTESIAN_POINT('Ctrl Pts',(-5.94657746690739,65.8408892064149,
3.18862589385767));
#261001=CARTESIAN_POINT('Ctrl Pts',(-5.96270790642316,65.839436649776,3.19101761710211));
#261002=CARTESIAN_POINT('Ctrl Pts',(-5.97875324884626,65.8379865797637,
3.1937213007479));
#261003=CARTESIAN_POINT('Ctrl Pts',(-5.99436250455736,65.8365709410658,
3.19665315116031));
#261004=CARTESIAN_POINT('Ctrl Pts',(-6.0021360594916,65.8358659397904,3.19811324001154));
#261005=CARTESIAN_POINT('Ctrl Pts',(-6.00980161978126,65.835169463883,3.19962909119738));
#261006=CARTESIAN_POINT('Ctrl Pts',(-6.01731694016751,65.8344853621198,
3.2011857013321));
#261007=CARTESIAN_POINT('Ctrl Pts',(-6.05487166684455,65.8310668445558,
3.20896422109546));
#261008=CARTESIAN_POINT('Ctrl Pts',(-6.092920386141,65.8275735275046,3.21863403952643));
#261009=CARTESIAN_POINT('Ctrl Pts',(-6.13123923038697,65.8240249968494,
3.23038727980661));
#261010=CARTESIAN_POINT('Ctrl Pts',(-6.15039865250996,65.8222507315218,
3.2362638999467));
#261011=CARTESIAN_POINT('Ctrl Pts',(-6.16962494894135,65.8204627202671,
3.24266113654303));
#261012=CARTESIAN_POINT('Ctrl Pts',(-6.18888612199635,65.8186637625198,
3.24960122559044));
#261013=CARTESIAN_POINT('Ctrl Pts',(-6.19851670852385,65.8177642836462,
3.25307127011415));
#261014=CARTESIAN_POINT('Ctrl Pts',(-6.20815601600891,65.8168620679918,
3.25667702289134));
#261015=CARTESIAN_POINT('Ctrl Pts',(-6.21779972592886,65.8159574933785,
3.26042110097521));
#261016=CARTESIAN_POINT('Ctrl Pts',(-6.22354858670786,65.8154182534429,
3.26265304115472));
#261017=CARTESIAN_POINT('Ctrl Pts',(-6.22977209879967,65.8148336278359,
3.26512271208716));
#261018=CARTESIAN_POINT('Ctrl Pts',(-6.23562008984126,65.8142836562234,
3.26749611071574));
#261019=CARTESIAN_POINT('Ctrl Pts',(-6.2395820996655,65.8139110508422,3.26910408662001));
#261020=CARTESIAN_POINT('Ctrl Pts',(-6.2433722047729,65.8135543114577,3.27066665087196));
#261021=CARTESIAN_POINT('Ctrl Pts',(-6.24673118035708,65.8132378771829,
3.2720673182109));
#261022=CARTESIAN_POINT('Ctrl Pts',(-6.27496153960131,65.8105784195504,
3.28383916387304));
#261023=CARTESIAN_POINT('Ctrl Pts',(-6.30403799522795,65.8078219476894,
3.29716815336018));
#261024=CARTESIAN_POINT('Ctrl Pts',(-6.33374660499682,65.8049871791206,
3.31230056833604));
#261025=CARTESIAN_POINT('Ctrl Pts',(-6.36243141784723,65.8022501003242,
3.32691150082109));
#261026=CARTESIAN_POINT('Ctrl Pts',(-6.39170562294076,65.7994400232553,
3.34320429251119));
#261027=CARTESIAN_POINT('Ctrl Pts',(-6.42132866158343,65.7965779940722,
3.36139467404666));
#261028=CARTESIAN_POINT('Ctrl Pts',(-6.43333454817107,65.7954180456213,
3.36876703244429));
#261029=CARTESIAN_POINT('Ctrl Pts',(-6.44539716698001,65.7942496131585,
3.3764509684881));
#261030=CARTESIAN_POINT('Ctrl Pts',(-6.45749812305003,65.7930743060343,
3.38446019757032));
#261031=CARTESIAN_POINT('Ctrl Pts',(-6.46235449067882,65.7926026306196,
3.38767446928749));
#261032=CARTESIAN_POINT('Ctrl Pts',(-6.46605024896355,65.7922432868207,
3.39016318463709));
#261033=CARTESIAN_POINT('Ctrl Pts',(-6.46935097253908,65.7919220986225,
3.39240185996761));
#261034=CARTESIAN_POINT('Ctrl Pts',(-6.47224219126605,65.7916407586945,
3.39436279365113));
#261035=CARTESIAN_POINT('Ctrl Pts',(-6.47482951628492,65.7913887639756,
3.39613316459923));
#261036=CARTESIAN_POINT('Ctrl Pts',(-6.47761348995547,65.7911174858446,
3.39805375361407));
#261037=CARTESIAN_POINT('Ctrl Pts',(-6.48357575222877,65.7905365064398,
3.40216695897476));
#261038=CARTESIAN_POINT('Ctrl Pts',(-6.48983134525266,65.7899261058292,
3.40655799551078));
#261039=CARTESIAN_POINT('Ctrl Pts',(-6.49636717968699,65.7892874291817,
3.41124422202922));
#261040=CARTESIAN_POINT('Ctrl Pts',(-6.50943884855564,65.7880100758867,
3.42061667506608));
#261041=CARTESIAN_POINT('Ctrl Pts',(-6.52363273791384,65.7866195086591,
3.43116809080685));
#261042=CARTESIAN_POINT('Ctrl Pts',(-6.53881665568116,65.7851272928074,
3.4430505988898));
#261043=CARTESIAN_POINT('Ctrl Pts',(-6.55465485172031,65.7835707770548,
3.45544512679351));
#261044=CARTESIAN_POINT('Ctrl Pts',(-6.57157096016989,65.7819036004173,
3.46928829748607));
#261045=CARTESIAN_POINT('Ctrl Pts',(-6.58937129934023,65.780142707847,3.48477057689116));
#261046=CARTESIAN_POINT('Ctrl Pts',(-6.60570096910835,65.7785273007531,
3.49897370569244));
#261047=CARTESIAN_POINT('Ctrl Pts',(-6.6227745709665,65.776833043257,3.51455688881379));
#261048=CARTESIAN_POINT('Ctrl Pts',(-6.64040473228574,65.7750763283395,
3.53167436232706));
#261049=CARTESIAN_POINT('Ctrl Pts',(-6.6496167612483,65.7741584179241,3.54061850406887));
#261050=CARTESIAN_POINT('Ctrl Pts',(-6.65892885831413,65.7732286293093,
3.54993916518537));
#261051=CARTESIAN_POINT('Ctrl Pts',(-6.66798038885463,65.7723231835145,
3.55928633621133));
#261052=CARTESIAN_POINT('Ctrl Pts',(-6.67703191939512,65.7714177377196,
3.5686335072373));
#261053=CARTESIAN_POINT('Ctrl Pts',(-6.68582285772196,65.7705366369923,
3.5780067897777));
#261054=CARTESIAN_POINT('Ctrl Pts',(-6.69403626419771,65.7697122795355,
3.58701472554693));
#261055=CARTESIAN_POINT('Ctrl Pts',(-6.71046307714923,65.7680635646218,
3.6050305970854));
#261056=CARTESIAN_POINT('Ctrl Pts',(-6.72530111653888,65.7665688417378,
3.62234411642252));
#261057=CARTESIAN_POINT('Ctrl Pts',(-6.73872275617943,65.765213030129,3.63876109479846));
#261058=CARTESIAN_POINT('Ctrl Pts',(-6.7531238721136,65.7637582749212,3.65637614148517));
#261059=CARTESIAN_POINT('Ctrl Pts',(-6.7658950958259,65.7624633772103,3.67295891113754));
#261060=CARTESIAN_POINT('Ctrl Pts',(-6.7772346714358,65.7613109928834,3.68832137747729));
#261061=CARTESIAN_POINT('Ctrl Pts',(-6.78703174915314,65.7603153648987,
3.70159412081779));
#261062=CARTESIAN_POINT('Ctrl Pts',(-6.795760119052,65.7594261207258,3.71395700901375));
#261063=CARTESIAN_POINT('Ctrl Pts',(-6.80353339829515,65.7586333201509,
3.72531661708647));
#261064=CARTESIAN_POINT('Ctrl Pts',(-6.80855589015674,65.7581210737346,
3.73265631727112));
#261065=CARTESIAN_POINT('Ctrl Pts',(-6.8143994459443,65.7575251087004,3.74136671501387));
#261066=CARTESIAN_POINT('Ctrl Pts',(-6.8206226487531,65.7568895371171,3.7509519120683));
#261067=CARTESIAN_POINT('Ctrl Pts',(-6.82637393849287,65.7563021617031,
3.75981025192424));
#261068=CARTESIAN_POINT('Ctrl Pts',(-6.83244860633706,65.755681035264,3.7694160965401));
#261069=CARTESIAN_POINT('Ctrl Pts',(-6.8385324498745,65.7550579827651,3.77935205384102));
#261070=CARTESIAN_POINT('Ctrl Pts',(-6.84448373672446,65.7544485055291,
3.78907152339391));
#261071=CARTESIAN_POINT('Ctrl Pts',(-6.85044347056101,65.7538372144028,
3.79910681273385));
#261072=CARTESIAN_POINT('Ctrl Pts',(-6.8561602580791,65.7532501619865,3.80903947240748));
#261073=CARTESIAN_POINT('Ctrl Pts',(-6.85939077234152,65.7529184230165,
3.81465234478341));
#261074=CARTESIAN_POINT('Ctrl Pts',(-6.86254453502902,65.7525943517106,
3.82023193151967));
#261075=CARTESIAN_POINT('Ctrl Pts',(-6.8655825571821,65.752282091527,3.82569909457176));
#261076=CARTESIAN_POINT('Ctrl Pts',(-6.88237538588129,65.7505560567885,
3.8559191285209));
#261077=CARTESIAN_POINT('Ctrl Pts',(-6.89728625413067,65.7490172503012,
3.88565223467586));
#261078=CARTESIAN_POINT('Ctrl Pts',(-6.91054998657791,65.7476451275704,
3.91466340603655));
#261079=CARTESIAN_POINT('Ctrl Pts',(-6.91297014379172,65.7473947642026,
3.91995690814306));
#261080=CARTESIAN_POINT('Ctrl Pts',(-6.91533547889627,65.7471499488435,
3.92522651374083));
#261081=CARTESIAN_POINT('Ctrl Pts',(-6.91764743439568,65.7469105552903,
3.93047097789414));
#261082=CARTESIAN_POINT('Ctrl Pts',(-6.92242338991714,65.7464160245944,
3.94130480559387));
#261083=CARTESIAN_POINT('Ctrl Pts',(-6.92710067411788,65.745931219565,3.95231420713329));
#261084=CARTESIAN_POINT('Ctrl Pts',(-6.93181538577873,65.7454422461516,
3.96389252435494));
#261085=CARTESIAN_POINT('Ctrl Pts',(-6.93449595269714,65.7451642384918,
3.97047541984203));
#261086=CARTESIAN_POINT('Ctrl Pts',(-6.93718782216788,65.7448849530287,
3.97724254552527));
#261087=CARTESIAN_POINT('Ctrl Pts',(-6.93990887240687,65.7446024604459,
3.98426875594416));
#261088=CARTESIAN_POINT('Ctrl Pts',(-6.94741583834282,65.7438231061489,
4.00365300747972));
#261089=CARTESIAN_POINT('Ctrl Pts',(-6.95437281189231,65.7430997577542,
4.02302622213965));
#261090=CARTESIAN_POINT('Ctrl Pts',(-6.96080003035281,65.7424306447279,
4.04235399436845));
#261091=CARTESIAN_POINT('Ctrl Pts',(-6.97365446727381,65.7410924186753,
4.08100953882604));
#261092=CARTESIAN_POINT('Ctrl Pts',(-6.98438972241911,65.7399711482183,
4.11948337297493));
#261093=CARTESIAN_POINT('Ctrl Pts',(-6.99318642138732,65.7390510306648,
4.1575395955445));
#261094=CARTESIAN_POINT('Ctrl Pts',(-6.99854013800823,65.738491042349,4.1807008099996));
#261095=CARTESIAN_POINT('Ctrl Pts',(-7.00333302368036,65.7379893808958,
4.20440502108826));
#261096=CARTESIAN_POINT('Ctrl Pts',(-7.00746546267396,65.7375564545666,
4.22840798423732));
#261097=CARTESIAN_POINT('Ctrl Pts',(-7.01012303973934,65.7372780390631,
4.24384432206707));
#261098=CARTESIAN_POINT('Ctrl Pts',(-7.01250843221597,65.7370279667777,
4.25940385023512));
#261099=CARTESIAN_POINT('Ctrl Pts',(-7.01460617258545,65.7368080412401,
4.27501873030309));
#261100=CARTESIAN_POINT('Ctrl Pts',(-7.01912623074679,65.7363341617097,
4.30866453657961));
#261101=CARTESIAN_POINT('Ctrl Pts',(-7.02226976618557,65.7360039022401,
4.34220383776488));
#261102=CARTESIAN_POINT('Ctrl Pts',(-7.02409087870873,65.7358125713606,
4.37571237378465));
#261103=CARTESIAN_POINT('Ctrl Pts',(-7.02592092947349,65.735620301406,4.40938537377183));
#261104=CARTESIAN_POINT('Ctrl Pts',(-7.0264156011419,65.7355683221668,4.44302806162844));
#261105=CARTESIAN_POINT('Ctrl Pts',(-7.02557811473608,65.7356563941057,
4.47672408041568));
#261106=CARTESIAN_POINT('Ctrl Pts',(-7.02527260074477,65.7356885226386,
4.48901634584167));
#261107=CARTESIAN_POINT('Ctrl Pts',(-7.02478930660299,65.7357393325811,
4.50131571716726));
#261108=CARTESIAN_POINT('Ctrl Pts',(-7.02412666816216,65.7358089628303,
4.51362617421114));
#261109=CARTESIAN_POINT('Ctrl Pts',(-7.02261121110448,65.7359682075194,
4.54178024415509));
#261110=CARTESIAN_POINT('Ctrl Pts',(-7.02014930390684,65.7362272864016,
4.57006165151967));
#261111=CARTESIAN_POINT('Ctrl Pts',(-7.01674425656352,65.7365846781431,
4.59822734515461));
#261112=CARTESIAN_POINT('Ctrl Pts',(-7.01332971002708,65.7369430669143,
4.62647161372138));
#261113=CARTESIAN_POINT('Ctrl Pts',(-7.00896679749447,65.7374003140195,
4.65459896476515));
#261114=CARTESIAN_POINT('Ctrl Pts',(-7.00371091900996,65.7379503304987,
4.68237068653922));
#261115=CARTESIAN_POINT('Ctrl Pts',(-6.99938248507902,65.7384032918824,
4.70524185131249));
#261116=CARTESIAN_POINT('Ctrl Pts',(-6.99444945044594,65.7389190814976,
4.72787181270826));
#261117=CARTESIAN_POINT('Ctrl Pts',(-6.98896824514582,65.7394920685988,
4.75013438165693));
#261118=CARTESIAN_POINT('Ctrl Pts',(-6.98417733347399,65.7399928946836,
4.76959324071821));
#261119=CARTESIAN_POINT('Ctrl Pts',(-6.97882431758015,65.7405527989667,
4.78934227036311));
#261120=CARTESIAN_POINT('Ctrl Pts',(-6.97294530311642,65.7411665604242,
4.80909223502358));
#261121=CARTESIAN_POINT('Ctrl Pts',(-6.96708556129561,65.7417783098428,
4.82877745515604));
#261122=CARTESIAN_POINT('Ctrl Pts',(-6.96070327729375,65.7424435627342,
4.848463179883));
#261123=CARTESIAN_POINT('Ctrl Pts',(-6.95388408904521,65.7431527847758,
4.86787579382654));
#261124=CARTESIAN_POINT('Ctrl Pts',(-6.94695897889933,65.7438730231058,
4.88758994232613));
#261125=CARTESIAN_POINT('Ctrl Pts',(-6.93958340157387,65.7446385970478,
4.90702200599908));
#261126=CARTESIAN_POINT('Ctrl Pts',(-6.93189785267586,65.7454350762153,
4.92590519949645));
#261127=CARTESIAN_POINT('Ctrl Pts',(-6.92499028020138,65.746150931081,4.94287692518106));
#261128=CARTESIAN_POINT('Ctrl Pts',(-6.91783323848293,65.7468916701725,
4.95940543329911));
#261129=CARTESIAN_POINT('Ctrl Pts',(-6.91056037343467,65.7476440483002,
4.97531387376239));
#261130=CARTESIAN_POINT('Ctrl Pts',(-6.89741820969321,65.7490036055702,
5.00406063697777));
#261131=CARTESIAN_POINT('Ctrl Pts',(-6.88265306472704,65.7505274323005,
5.03352893815075));
#261132=CARTESIAN_POINT('Ctrl Pts',(-6.86603348701363,65.7522357778755,
5.06348872824643));
#261133=CARTESIAN_POINT('Ctrl Pts',(-6.86284470051636,65.75256355692,5.06923709175876));
#261134=CARTESIAN_POINT('Ctrl Pts',(-6.85958766659747,65.7528981269418,
5.07500339655698));
#261135=CARTESIAN_POINT('Ctrl Pts',(-6.856260788359,65.7532396276514,5.08078579696316));
#261136=CARTESIAN_POINT('Ctrl Pts',(-6.8459277014796,65.7543003086407,5.09874559034469));
#261137=CARTESIAN_POINT('Ctrl Pts',(-6.83492067751536,65.7554278628972,
5.11686118101104));
#261138=CARTESIAN_POINT('Ctrl Pts',(-6.82319313264974,65.7566263659764,
5.135072656704));
#261139=CARTESIAN_POINT('Ctrl Pts',(-6.82026124643334,65.7569259917462,
5.13962552562724));
#261140=CARTESIAN_POINT('Ctrl Pts',(-6.81728431941741,65.7572300525387,
5.14418438193023));
#261141=CARTESIAN_POINT('Ctrl Pts',(-6.81426168033028,65.7575386070824,
5.14874816890694));
#261142=CARTESIAN_POINT('Ctrl Pts',(-6.81206183096614,65.757763170286,5.15206965175335));
#261143=CARTESIAN_POINT('Ctrl Pts',(-6.81081436432581,65.7578904337753,
5.15392926336868));
#261144=CARTESIAN_POINT('Ctrl Pts',(-6.80954130507221,65.7580203548224,
5.1558237372768));
#261145=CARTESIAN_POINT('Ctrl Pts',(-6.80906515425585,65.7580689480144,
5.15653231018524));
#261146=CARTESIAN_POINT('Ctrl Pts',(-6.80858497267273,65.7581179523965,
5.15724545910831));
#261147=CARTESIAN_POINT('Ctrl Pts',(-6.80804822984616,65.7581727169983,
5.15804058038008));
#261148=CARTESIAN_POINT('Ctrl Pts',(-6.80410462238006,65.7585750886402,
5.16388257030264));
#261149=CARTESIAN_POINT('Ctrl Pts',(-6.79988716877684,65.7590052079178,
5.17002569950334));
#261150=CARTESIAN_POINT('Ctrl Pts',(-6.79537903268354,65.7594645478209,
5.17645687223928));
#261151=CARTESIAN_POINT('Ctrl Pts',(-6.78580277267813,65.7604402855208,
5.19011807966171));
#261152=CARTESIAN_POINT('Ctrl Pts',(-6.77491644358952,65.761547737429,5.20508192788034));
#261153=CARTESIAN_POINT('Ctrl Pts',(-6.76253880448289,65.7628027600726,
5.22119211573532));
#261154=CARTESIAN_POINT('Ctrl Pts',(-6.75160877166964,65.7639110036203,
5.23541816323643));
#261155=CARTESIAN_POINT('Ctrl Pts',(-6.73951519499464,65.7651343766085,
5.25053774026995));
#261156=CARTESIAN_POINT('Ctrl Pts',(-6.72611969221624,65.7664849859145,
5.26641222989509));
#261157=CARTESIAN_POINT('Ctrl Pts',(-6.71183711917666,65.7679250345921,
5.28333795200408));
#261158=CARTESIAN_POINT('Ctrl Pts',(-6.69607408882078,65.7695097633137,
5.30112266565437));
#261159=CARTESIAN_POINT('Ctrl Pts',(-6.67865372552338,65.7712546466914,
5.31955642099153));
#261160=CARTESIAN_POINT('Ctrl Pts',(-6.67055762604082,65.7720655798028,
5.32812349358921));
#261161=CARTESIAN_POINT('Ctrl Pts',(-6.6620509552059,65.7729164113109,5.33687924790332));
#261162=CARTESIAN_POINT('Ctrl Pts',(-6.65344510022094,65.7737755720605,
5.34548002799559));
#261163=CARTESIAN_POINT('Ctrl Pts',(-6.64477621580735,65.774641025318,5.3541438003479));
#261164=CARTESIAN_POINT('Ctrl Pts',(-6.63600686527661,65.7755149148551,
5.36265013683573));
#261165=CARTESIAN_POINT('Ctrl Pts',(-6.62749295825142,65.7763616805538,
5.37068603553));
#261166=CARTESIAN_POINT('Ctrl Pts',(-6.62627270638101,65.7764830428643,
5.37183777707275));
#261167=CARTESIAN_POINT('Ctrl Pts',(-6.62505776031649,65.7766038428803,
5.37297991970546));
#261168=CARTESIAN_POINT('Ctrl Pts',(-6.62384922451688,65.7767239709552,
5.37411160598602));
#261169=CARTESIAN_POINT('Ctrl Pts',(-6.60481950617975,65.7786155189177,
5.39193124457015));
#261170=CARTESIAN_POINT('Ctrl Pts',(-6.58652892184038,65.7804258306708,
5.40795995874192));
#261171=CARTESIAN_POINT('Ctrl Pts',(-6.56920790676337,65.782134745741,5.42239957587053));
#261172=CARTESIAN_POINT('Ctrl Pts',(-6.5537403803089,65.7836607930853,5.435294037248));
#261173=CARTESIAN_POINT('Ctrl Pts',(-6.53904502063578,65.785106070809,5.44692155865749));
#261174=CARTESIAN_POINT('Ctrl Pts',(-6.5252520515588,65.7864591858047,5.45741722333808));
#261175=CARTESIAN_POINT('Ctrl Pts',(-6.51063267008387,65.7878933733383,
5.46854174083263));
#261176=CARTESIAN_POINT('Ctrl Pts',(-6.49702705057888,65.7892240235553,
5.47839520486671));
#261177=CARTESIAN_POINT('Ctrl Pts',(-6.48455627972228,65.7904405427442,
5.48712222544258));
#261178=CARTESIAN_POINT('Ctrl Pts',(-6.47832089429397,65.7910488023387,
5.49148573573051));
#261179=CARTESIAN_POINT('Ctrl Pts',(-6.47236870678754,65.7916285741663,
5.49556733942024));
#261180=CARTESIAN_POINT('Ctrl Pts',(-6.46671197311601,65.7921787859736,
5.49938314995723));
#261181=CARTESIAN_POINT('Ctrl Pts',(-6.46384655950873,65.7924574952944,
5.5013160455239));
#261182=CARTESIAN_POINT('Ctrl Pts',(-6.45959513205277,65.7928706896663,
5.5041638149449));
#261183=CARTESIAN_POINT('Ctrl Pts',(-6.45490906743274,65.7933256517398,
5.5072488405822));
#261184=CARTESIAN_POINT('Ctrl Pts',(-6.45034417454503,65.7937688494551,
5.51025409397327));
#261185=CARTESIAN_POINT('Ctrl Pts',(-6.44536610427237,65.7942517463725,
5.51348319963084));
#261186=CARTESIAN_POINT('Ctrl Pts',(-6.44088172190684,65.794686236133,5.51635105564596));
#261187=CARTESIAN_POINT('Ctrl Pts',(-6.41092000451291,65.7975892132554,
5.5355121985744));
#261188=CARTESIAN_POINT('Ctrl Pts',(-6.38123637199579,65.8004462364061,
5.552713371747));
#261189=CARTESIAN_POINT('Ctrl Pts',(-6.35208534056764,65.8032350383018,
5.56816839001326));
#261190=CARTESIAN_POINT('Ctrl Pts',(-6.34586874315358,65.8038297636959,
5.57146424686228));
#261191=CARTESIAN_POINT('Ctrl Pts',(-6.33967618401766,65.8044214025736,
5.57468073798643));
#261192=CARTESIAN_POINT('Ctrl Pts',(-6.33350983849427,65.8050097646177,
5.57781999967329));
#261193=CARTESIAN_POINT('Ctrl Pts',(-6.3220951691016,65.8060988956422,5.58363116191788));
#261194=CARTESIAN_POINT('Ctrl Pts',(-6.3110960380657,65.8071462001763,5.58901693396477));
#261195=CARTESIAN_POINT('Ctrl Pts',(-6.3001362097979,65.8081871579159,5.59419568021758));
#261196=CARTESIAN_POINT('Ctrl Pts',(-6.2887742088532,65.8092663137686,5.59956446140456));
#261197=CARTESIAN_POINT('Ctrl Pts',(-6.27745426307281,65.8103386646702,
5.60471100753469));
#261198=CARTESIAN_POINT('Ctrl Pts',(-6.2657318630546,65.81144595617,5.60982619698701));
#261199=CARTESIAN_POINT('Ctrl Pts',(-6.25472797486926,65.8124853774348,
5.61462785643327));
#261200=CARTESIAN_POINT('Ctrl Pts',(-6.24336918957263,65.8135556106234,
5.61940187932597));
#261201=CARTESIAN_POINT('Ctrl Pts',(-6.23126962222113,65.8146927786727,
5.62426010254449));
#261202=CARTESIAN_POINT('Ctrl Pts',(-6.23047956672726,65.8147670313992,
5.62457732594866));
#261203=CARTESIAN_POINT('Ctrl Pts',(-6.22968634671726,65.8148415700443,
5.6248948907272));
#261204=CARTESIAN_POINT('Ctrl Pts',(-6.22888985219174,65.8149164048895,
5.62521282041139));
#261205=CARTESIAN_POINT('Ctrl Pts',(-6.19036579175731,65.8185359427609,
5.64059012932621));
#261206=CARTESIAN_POINT('Ctrl Pts',(-6.15186901093432,65.8221216693507,
5.65375153185709));
#261207=CARTESIAN_POINT('Ctrl Pts',(-6.11365657603432,65.825651094271,5.66486594522758));
#261208=CARTESIAN_POINT('Ctrl Pts',(-6.09861523048941,65.8270403619254,
5.66924084916845));
#261209=CARTESIAN_POINT('Ctrl Pts',(-6.08388431537106,65.8283967393513,
5.67322584538408));
#261210=CARTESIAN_POINT('Ctrl Pts',(-6.06913706391957,65.8297499270775,
5.67693553666014));
#261211=CARTESIAN_POINT('Ctrl Pts',(-6.054426279115,65.8310997686738,5.68063605470129));
#261212=CARTESIAN_POINT('Ctrl Pts',(-6.039698919231,65.8324464642731,5.6840626287897));
#261213=CARTESIAN_POINT('Ctrl Pts',(-6.02461786668289,65.8338206117543,
5.6872795401997));
#261214=CARTESIAN_POINT('Ctrl Pts',(-6.01640907093671,65.8345685765241,
5.6890305432291));
#261215=CARTESIAN_POINT('Ctrl Pts',(-6.00809529157055,65.8353246915127,
5.69071857742997));
#261216=CARTESIAN_POINT('Ctrl Pts',(-5.99962103174957,65.8360939900876,
5.69234758469808));
#261217=CARTESIAN_POINT('Ctrl Pts',(-5.94977634842706,65.8406189214277,
5.70192922995375));
#261218=CARTESIAN_POINT('Ctrl Pts',(-5.89974030855588,65.8451090257662,
5.7084207146655));
#261219=CARTESIAN_POINT('Ctrl Pts',(-5.84988722567234,65.8495315549123,
5.71191535187211));
#261220=CARTESIAN_POINT('Ctrl Pts',(-5.82042620503947,65.8521450787885,
5.71398053165424));
#261221=CARTESIAN_POINT('Ctrl Pts',(-5.79102856600027,65.8547350482164,
5.71500000109184));
#261222=CARTESIAN_POINT('Ctrl Pts',(-5.76176668704775,65.8572951308982,
5.715));
#261223=CARTESIAN_POINT('',(-5.85194569933787,65.7762408833968,3.55799308010885));
#261224=CARTESIAN_POINT('Origin',(-5.94198106391481,66.7882436665578,3.557992738206));
#261225=CARTESIAN_POINT('',(-5.75542126790783,65.7847570433117,5.33729874159373));
#261226=CARTESIAN_POINT('Ctrl Pts',(-5.7554212679173,65.7847570433109,5.33729874159373));
#261227=CARTESIAN_POINT('Ctrl Pts',(-5.84313044680229,65.7770834834129,
5.33729913870664));
#261228=CARTESIAN_POINT('Ctrl Pts',(-5.93046744301797,65.7692612122682,
5.32362871093108));
#261229=CARTESIAN_POINT('Ctrl Pts',(-6.01397172210868,65.7616246556023,
5.29784699382705));
#261230=CARTESIAN_POINT('Ctrl Pts',(-6.10597963581641,65.7532104323506,
5.2694398028618));
#261231=CARTESIAN_POINT('Ctrl Pts',(-6.19333444614957,65.7450218153952,
5.22632902530969));
#261232=CARTESIAN_POINT('Ctrl Pts',(-6.27141366972007,65.7375729990231,
5.17060080687608));
#261233=CARTESIAN_POINT('Ctrl Pts',(-6.30478895463498,65.7343889718603,
5.14677955093925));
#261234=CARTESIAN_POINT('Ctrl Pts',(-6.3364695108738,65.7313408750752,5.12065287386765));
#261235=CARTESIAN_POINT('Ctrl Pts',(-6.36609460015343,65.7284715535097,
5.09238371018883));
#261236=CARTESIAN_POINT('Ctrl Pts',(-6.44701031459408,65.7206345069363,
5.01517146775067));
#261237=CARTESIAN_POINT('Ctrl Pts',(-6.51382295507419,65.7140126737621,
4.92157085026347));
#261238=CARTESIAN_POINT('Ctrl Pts',(-6.56068516324688,65.7093337617069,
4.81963336896564));
#261239=CARTESIAN_POINT('Ctrl Pts',(-6.60024843912357,65.7053836045193,
4.7335729622537));
#261240=CARTESIAN_POINT('Ctrl Pts',(-6.62613370765204,65.7027670840136,
4.64058810563573));
#261241=CARTESIAN_POINT('Ctrl Pts',(-6.63690428983301,65.7016790855929,
4.54620310203547));
#261242=CARTESIAN_POINT('Ctrl Pts',(-6.63889132827675,65.7014783634172,
4.52879024286822));
#261243=CARTESIAN_POINT('Ctrl Pts',(-6.64036391441504,65.7013295239355,
4.51132972877378));
#261244=CARTESIAN_POINT('Ctrl Pts',(-6.64131300674474,65.7012335863269,
4.49385624771197));
#261245=CARTESIAN_POINT('Ctrl Pts',(-6.64633202250417,65.7007262464669,
4.40145251197823));
#261246=CARTESIAN_POINT('Ctrl Pts',(-6.63637949906751,65.7017363710718,
4.30822438948042));
#261247=CARTESIAN_POINT('Ctrl Pts',(-6.61279609273244,65.7041099251378,
4.21848944197469));
#261248=CARTESIAN_POINT('Ctrl Pts',(-6.58652533303231,65.7067539481265,
4.11852910506948));
#261249=CARTESIAN_POINT('Ctrl Pts',(-6.54334010983073,65.711089321915,4.02290340321605));
#261250=CARTESIAN_POINT('Ctrl Pts',(-6.48508720106723,65.7168378515978,
3.93758044687316));
#261251=CARTESIAN_POINT('Ctrl Pts',(-6.46865421195338,65.7184594963826,
3.9135110700385));
#261252=CARTESIAN_POINT('Ctrl Pts',(-6.45102212258308,65.7201932683606,
3.89026157430445));
#261253=CARTESIAN_POINT('Ctrl Pts',(-6.43223233013131,65.7220322302183,
3.86796593773786));
#261254=CARTESIAN_POINT('Ctrl Pts',(-6.35963673813889,65.7291371796241,
3.78182528772519));
#261255=CARTESIAN_POINT('Ctrl Pts',(-6.27057697962562,65.7377278929563,
3.71049475514339));
#261256=CARTESIAN_POINT('Ctrl Pts',(-6.1716590922992,65.747013295412,3.65761804421069));
#261257=CARTESIAN_POINT('Ctrl Pts',(-6.09089475947035,65.7545946273091,
3.61444534414512));
#261258=CARTESIAN_POINT('Ctrl Pts',(-6.00355863234323,65.7626386207393,
3.58357464837312));
#261259=CARTESIAN_POINT('Ctrl Pts',(-5.91325097800447,65.7707579102581,
3.56698920682791));
#261260=CARTESIAN_POINT('Ctrl Pts',(-5.89295235276776,65.7725828985864,
3.5632612652179));
#261261=CARTESIAN_POINT('Ctrl Pts',(-5.87250361938545,65.7744118972737,
3.56025504919194));
#261262=CARTESIAN_POINT('Ctrl Pts',(-5.85194569928665,65.7762408834014,
3.55799308057809));
#261263=CARTESIAN_POINT('',(-5.6588379396032,65.7931355567733,5.33200232567716));
#261264=CARTESIAN_POINT('Origin',(-5.75437963344684,65.7728758969229,4.44759572280564));
#261265=CARTESIAN_POINT('',(-5.62465650879763,65.8691606621927,5.70752127913496));
#261266=CARTESIAN_POINT('Origin',(-5.74590223951866,66.8053982735026,5.33200196893336));
#261267=CARTESIAN_POINT('Ctrl Pts',(-5.76176671321524,65.8572954409828,
5.715));
#261268=CARTESIAN_POINT('Ctrl Pts',(-5.73889644435691,65.8592959118043,
5.71499999912934));
#261269=CARTESIAN_POINT('Ctrl Pts',(-5.71600351087933,65.8612858392142,
5.71437328350013));
#261270=CARTESIAN_POINT('Ctrl Pts',(-5.670326752844,65.8652384015502,5.71188182802081));
#261271=CARTESIAN_POINT('Ctrl Pts',(-5.64757588348546,65.8671983519392,
5.71002878127821));
#261272=CARTESIAN_POINT('Ctrl Pts',(-5.62465651442489,65.8691607435447,
5.70752129153182));
#261273=CARTESIAN_POINT('Origin',(-3.98912952672225E-15,8.70861844988177E-14,
17.4625000000011));
#261274=CARTESIAN_POINT('',(-5.75542048012727,65.7847571122336,3.55270126407068));
#261275=CARTESIAN_POINT('Ctrl Pts',(-5.75542048012727,65.7847571122336,
3.55270126407068));
#261276=CARTESIAN_POINT('Ctrl Pts',(-5.74247305973189,65.7858898647401,
3.55270083404508));
#261277=CARTESIAN_POINT('Ctrl Pts',(-5.72728301852202,65.7872142683301,
3.55303663437051));
#261278=CARTESIAN_POINT('Ctrl Pts',(-5.71323826307051,65.7884339513264,
3.5537085593055));
#261279=CARTESIAN_POINT('Ctrl Pts',(-5.69919350761899,65.7896536343226,
3.55438048424048));
#261280=CARTESIAN_POINT('Ctrl Pts',(-5.68515719669277,65.790868052569,3.55538858394171));
#261281=CARTESIAN_POINT('Ctrl Pts',(-5.67112933463474,65.7920772227818,
3.55673285840919));
#261282=CARTESIAN_POINT('Ctrl Pts',(-5.64307361051867,65.7944955632075,
3.55942140734414));
#261283=CARTESIAN_POINT('Ctrl Pts',(-5.61564345930465,65.7968421930535,
3.56338271048258));
#261284=CARTESIAN_POINT('Ctrl Pts',(-5.58815941470242,65.7991763441953,
3.56868087970656));
#261285=CARTESIAN_POINT('Ctrl Pts',(-5.53319132549797,65.8038446464791,
3.57927721815451));
#261286=CARTESIAN_POINT('Ctrl Pts',(-5.47901133019916,65.8083759215683,
3.59514139742869));
#261287=CARTESIAN_POINT('Ctrl Pts',(-5.42652662461076,65.812703500244,3.61617550274095));
#261288=CARTESIAN_POINT('Ctrl Pts',(-5.32155721343395,65.8213586575955,
3.65824371336546));
#261289=CARTESIAN_POINT('Ctrl Pts',(-5.22615715431841,65.828968679653,3.71966185501488));
#261290=CARTESIAN_POINT('Ctrl Pts',(-5.14453528743527,65.8353468122936,
3.79734567088282));
#261291=CARTESIAN_POINT('Ctrl Pts',(-5.06291342055214,65.8417249449342,
3.87502948675077));
#261292=CARTESIAN_POINT('Ctrl Pts',(-4.99635722470383,65.846774948607,3.96823454036102));
#261293=CARTESIAN_POINT('Ctrl Pts',(-4.94933658123897,65.850309039702,4.07025885888143));
#261294=CARTESIAN_POINT('Ctrl Pts',(-4.90963743741027,65.8532928438429,
4.15639715467043));
#261295=CARTESIAN_POINT('Ctrl Pts',(-4.88363346483278,65.855215237196,4.2509570946994));
#261296=CARTESIAN_POINT('Ctrl Pts',(-4.87286763711114,65.8560118304308,
4.34458329058431));
#261297=CARTESIAN_POINT('Ctrl Pts',(-4.87088215339171,65.8561587418378,
4.36185026646838));
#261298=CARTESIAN_POINT('Ctrl Pts',(-4.86941494537251,65.8562672203297,
4.37908548343429));
#261299=CARTESIAN_POINT('Ctrl Pts',(-4.86847567621377,65.8563366564582,
4.39623025764058));
#261300=CARTESIAN_POINT('Ctrl Pts',(-4.8635283934026,65.8567023877948,4.48653456066477));
#261301=CARTESIAN_POINT('Ctrl Pts',(-4.87299393225409,65.8560065907437,
4.58113033271353));
#261302=CARTESIAN_POINT('Ctrl Pts',(-4.8961834270689,65.8542824808466,4.67087033143761));
#261303=CARTESIAN_POINT('Ctrl Pts',(-4.90126896622311,65.8539043773795,
4.69055063412873));
#261304=CARTESIAN_POINT('Ctrl Pts',(-4.90701453125571,65.8534766187393,
4.70999740297233));
#261305=CARTESIAN_POINT('Ctrl Pts',(-4.91341283206931,65.852999229802,4.72911416018214));
#261306=CARTESIAN_POINT('Ctrl Pts',(-4.94898667534586,65.8503450002287,
4.83540121118988));
#261307=CARTESIAN_POINT('Ctrl Pts',(-5.00523480399401,65.8461241794492,
4.93580822988598));
#261308=CARTESIAN_POINT('Ctrl Pts',(-5.07790028461974,65.840519909233,5.02192061733624));
#261309=CARTESIAN_POINT('Ctrl Pts',(-5.15056576524547,65.8349156390167,
5.1080330047865));
#261310=CARTESIAN_POINT('Ctrl Pts',(-5.23976344718343,65.8279111585203,
5.17939248795535));
#261311=CARTESIAN_POINT('Ctrl Pts',(-5.33881247999378,65.8198770473032,
5.23230434621982));
#261312=CARTESIAN_POINT('Ctrl Pts',(-5.41955366575217,65.8133279306911,
5.27543617755364));
#261313=CARTESIAN_POINT('Ctrl Pts',(-5.5068409177372,65.8060942041597,5.30630970940009));
#261314=CARTESIAN_POINT('Ctrl Pts',(-5.59705836360422,65.7984199726183,
5.32292362304353));
#261315=CARTESIAN_POINT('Ctrl Pts',(-5.61751492718868,65.7966798612243,
5.32669078334792));
#261316=CARTESIAN_POINT('Ctrl Pts',(-5.63812216055857,65.7949173115934,
5.32972479472675));
#261317=CARTESIAN_POINT('Ctrl Pts',(-5.6588379396032,65.7931355567733,5.33200232567716));
#261318=CARTESIAN_POINT('Ctrl Pts',(-5.85194569898496,65.7762408834282,
3.5579930805449));
#261319=CARTESIAN_POINT('Ctrl Pts',(-5.83593933394768,65.7776649292109,
3.5562322864657));
#261320=CARTESIAN_POINT('Ctrl Pts',(-5.81987010370942,65.77908866856,3.5549075948924));
#261321=CARTESIAN_POINT('Ctrl Pts',(-5.78769205961313,65.7819277211714,
3.553143174725));
#261322=CARTESIAN_POINT('Ctrl Pts',(-5.77021143863637,65.7834630710414,
3.5527017560376));
#261323=CARTESIAN_POINT('Ctrl Pts',(-5.75542048012727,65.7847571122336,
3.55270126407068));
#261324=CARTESIAN_POINT('Origin',(10.0340663510524,-114.689903201906,4.445));
#261325=CARTESIAN_POINT('',(-5.7941612077782,66.2275656555355,3.175));
#261326=CARTESIAN_POINT('Origin',(-5.7941612077782,66.2275656555355,4.445));
#261327=CARTESIAN_POINT('',(-5.7617667341226,65.8572951273169,3.175));
#261328=CARTESIAN_POINT('',(10.0340663510524,-114.689903201906,3.175));
#261329=CARTESIAN_POINT('Origin',(-5.76074896190133,65.8337676350829,4.43574689648524));
#261330=CARTESIAN_POINT('Ctrl Pts',(-5.62465649482951,65.8691605147753,
5.70752129157735));
#261331=CARTESIAN_POINT('Ctrl Pts',(-5.58478094862187,65.8725733428444,
5.70315872721441));
#261332=CARTESIAN_POINT('Ctrl Pts',(-5.54304491598344,65.8761096064448,
5.69646988868971));
#261333=CARTESIAN_POINT('Ctrl Pts',(-5.46821395219,65.8823912144796,5.68094793183612));
#261334=CARTESIAN_POINT('Ctrl Pts',(-5.43031265137476,65.8855432879058,
5.67131322823348));
#261335=CARTESIAN_POINT('Ctrl Pts',(-5.37306241680832,65.8902593919637,
5.6537697159104));
#261336=CARTESIAN_POINT('Ctrl Pts',(-5.3443386854768,65.8926143587643,5.64422545064104));
#261337=CARTESIAN_POINT('Ctrl Pts',(-5.31553775508236,65.8949585103482,
5.63347370408195));
#261338=CARTESIAN_POINT('Ctrl Pts',(-5.29632845038175,65.8965181335808,
5.6260324645471));
#261339=CARTESIAN_POINT('Ctrl Pts',(-5.28553065111783,65.8973924062449,
5.62168005422912));
#261340=CARTESIAN_POINT('Ctrl Pts',(-5.24381167530971,65.9007628197157,
5.60433180876094));
#261341=CARTESIAN_POINT('Ctrl Pts',(-5.20925335774763,65.9035306522036,
5.58828560454417));
#261342=CARTESIAN_POINT('Ctrl Pts',(-5.13848808894195,65.9091465352246,
5.55105091210214));
#261343=CARTESIAN_POINT('Ctrl Pts',(-5.10228029053816,65.9119946598744,
5.52986074877017));
#261344=CARTESIAN_POINT('Ctrl Pts',(-5.05657131457127,65.9155541063456,
5.49967414867441));
#261345=CARTESIAN_POINT('Ctrl Pts',(-5.05164098672593,65.9159368425922,
5.49630764637292));
#261346=CARTESIAN_POINT('Ctrl Pts',(-5.03965557645362,65.9168663885211,
5.48805933378198));
#261347=CARTESIAN_POINT('Ctrl Pts',(-5.02080250933399,65.9183260383822,
5.47485591449452));
#261348=CARTESIAN_POINT('Ctrl Pts',(-4.99943768814662,65.9199717860853,
5.45901019489878));
#261349=CARTESIAN_POINT('Ctrl Pts',(-4.95375363345269,65.9234768895244,
5.42334213938015));
#261350=CARTESIAN_POINT('Ctrl Pts',(-4.91931462043666,65.9261022643759,
5.39426828545766));
#261351=CARTESIAN_POINT('Ctrl Pts',(-4.86396112783238,65.9302738558047,
5.3406626551402));
#261352=CARTESIAN_POINT('Ctrl Pts',(-4.84517703641354,65.9316813708319,
5.32127488448207));
#261353=CARTESIAN_POINT('Ctrl Pts',(-4.81231674059695,65.9341341565153,
5.28534110579567));
#261354=CARTESIAN_POINT('Ctrl Pts',(-4.79747782267421,65.9352363376361,
5.26808062242643));
#261355=CARTESIAN_POINT('Ctrl Pts',(-4.75721778545189,65.9382154751491,
5.21900018510425));
#261356=CARTESIAN_POINT('Ctrl Pts',(-4.73603395996656,65.9397667249603,
5.18991521556927));
#261357=CARTESIAN_POINT('Ctrl Pts',(-4.70254379818341,65.9422125678302,
5.14118315439145));
#261358=CARTESIAN_POINT('Ctrl Pts',(-4.67680062679918,65.9440855394807,
5.10072222188373));
#261359=CARTESIAN_POINT('Ctrl Pts',(-4.63677165145856,65.9469771382894,
5.02895983248803));
#261360=CARTESIAN_POINT('Ctrl Pts',(-4.61942342781782,65.9482215759738,
4.99377678011774));
#261361=CARTESIAN_POINT('Ctrl Pts',(-4.59680525672921,65.9498382659438,
4.94262996607723));
#261362=CARTESIAN_POINT('Ctrl Pts',(-4.58952137463054,65.9503579328167,
4.92520576511086));
#261363=CARTESIAN_POINT('Ctrl Pts',(-4.57454093443883,65.9514246648816,
4.88665216134801));
#261364=CARTESIAN_POINT('Ctrl Pts',(-4.55370826475622,65.9529048689791,
4.82885958216214));
#261365=CARTESIAN_POINT('Ctrl Pts',(-4.53760876604915,65.9540412091005,
4.77148576378849));
#261366=CARTESIAN_POINT('Ctrl Pts',(-4.5199909193678,65.9552820905794,4.69582490828914));
#261367=CARTESIAN_POINT('Ctrl Pts',(-4.51262962933517,65.9557993403288,
4.65619031440224));
#261368=CARTESIAN_POINT('Ctrl Pts',(-4.49633146802346,65.9569433440707,
4.53608031601762));
#261369=CARTESIAN_POINT('Ctrl Pts',(-4.4932116366907,65.9571603038214,4.45655263790621));
#261370=CARTESIAN_POINT('Ctrl Pts',(-4.5016784398326,65.9565681203517,4.29783458701837));
#261371=CARTESIAN_POINT('Ctrl Pts',(-4.51367679322992,65.9557276352643,
4.21750115465559));
#261372=CARTESIAN_POINT('Ctrl Pts',(-4.55112069875617,65.9530883852659,
4.06510551948798));
#261373=CARTESIAN_POINT('Ctrl Pts',(-4.57940219984027,65.95108461875,3.98465833433704));
#261374=CARTESIAN_POINT('Ctrl Pts',(-4.62647759117148,65.9477157319952,
3.88166400755938));
#261375=CARTESIAN_POINT('Ctrl Pts',(-4.64448938506461,65.9464216405874,
3.8462930296191));
#261376=CARTESIAN_POINT('Ctrl Pts',(-4.67557881765161,65.9441720386244,
3.7922777912675));
#261377=CARTESIAN_POINT('Ctrl Pts',(-4.68938079462409,65.94317046133,3.76957373396999));
#261378=CARTESIAN_POINT('Ctrl Pts',(-4.70431639697893,65.9420821438308,
3.74671681689983));
#261379=CARTESIAN_POINT('Ctrl Pts',(-4.7103827143969,65.9416397563165,3.73756396983769));
#261380=CARTESIAN_POINT('Ctrl Pts',(-4.71175591745022,65.94153953322,3.73552823755546));
#261381=CARTESIAN_POINT('Ctrl Pts',(-4.71766631767027,65.9411082008532,
3.72678303218439));
#261382=CARTESIAN_POINT('Ctrl Pts',(-4.72187699968702,65.9408007204284,
3.72065685633667));
#261383=CARTESIAN_POINT('Ctrl Pts',(-4.74436504471929,65.9391564677656,
3.68860998466841));
#261384=CARTESIAN_POINT('Ctrl Pts',(-4.76692523567626,65.9375009879014,
3.65839689018539));
#261385=CARTESIAN_POINT('Ctrl Pts',(-4.80949049683516,65.9343440177535,
3.60794709652002));
#261386=CARTESIAN_POINT('Ctrl Pts',(-4.82513750608849,65.9331790153847,
3.59028425850477));
#261387=CARTESIAN_POINT('Ctrl Pts',(-4.85969448029927,65.9305934010222,
3.55367536178758));
#261388=CARTESIAN_POINT('Ctrl Pts',(-4.87913743792476,65.9291324474435,
3.53430983686811));
#261389=CARTESIAN_POINT('Ctrl Pts',(-4.93368078409887,65.9250099373155,
3.48317767954649));
#261390=CARTESIAN_POINT('Ctrl Pts',(-4.96731044415668,65.922440365982,3.45561193051492));
#261391=CARTESIAN_POINT('Ctrl Pts',(-5.01148882032945,65.9190437725999,
3.42200008030123));
#261392=CARTESIAN_POINT('Ctrl Pts',(-5.02518131852106,65.9179869304159,
3.41208793767203));
#261393=CARTESIAN_POINT('Ctrl Pts',(-5.04398394922112,65.9165309450815,
3.3989357969476));
#261394=CARTESIAN_POINT('Ctrl Pts',(-5.04996267078607,65.9160671165245,
3.39483806869276));
#261395=CARTESIAN_POINT('Ctrl Pts',(-5.06131746615798,65.9151846467314,
3.38718237834165));
#261396=CARTESIAN_POINT('Ctrl Pts',(-5.07200690120929,65.9143524134979,
3.38010441024829));
#261397=CARTESIAN_POINT('Ctrl Pts',(-5.11727986407102,65.9108170937777,
3.3511367059735));
#261398=CARTESIAN_POINT('Ctrl Pts',(-5.15308340275494,65.9079936118378,
3.33082419418418));
#261399=CARTESIAN_POINT('Ctrl Pts',(-5.20550653408049,65.9038232860139,
3.30407887907678));
#261400=CARTESIAN_POINT('Ctrl Pts',(-5.22276891828361,65.9024438445753,
3.29578390756948));
#261401=CARTESIAN_POINT('Ctrl Pts',(-5.25677913901012,65.8997142191736,
3.28033613906633));
#261402=CARTESIAN_POINT('Ctrl Pts',(-5.27289349468372,65.8984158432432,
3.27339763828448));
#261403=CARTESIAN_POINT('Ctrl Pts',(-5.33096559013756,65.8937120368811,
3.25012126608546));
#261404=CARTESIAN_POINT('Ctrl Pts',(-5.36965444985258,65.8905467713476,
3.23683858823736));
#261405=CARTESIAN_POINT('Ctrl Pts',(-5.44645936542805,65.884203038107,3.21440327730483));
#261406=CARTESIAN_POINT('Ctrl Pts',(-5.48272834473528,65.8811802522662,
3.20559401919178));
#261407=CARTESIAN_POINT('Ctrl Pts',(-5.60232583337562,65.8711124237307,
3.18249177319905));
#261408=CARTESIAN_POINT('Ctrl Pts',(-5.6825483361046,65.8642257654837,3.17499999999995));
#261409=CARTESIAN_POINT('Ctrl Pts',(-5.7617667341226,65.8572951273169,3.175));
#261410=CARTESIAN_POINT('Origin',(-5.80522998710715,66.3540823821931,4.445));
#261411=CARTESIAN_POINT('',(-5.80522998710715,66.3540823821931,6.35));
#261412=CARTESIAN_POINT('Origin',(-5.5838544005281,63.8237478490401,4.445));
#261413=CARTESIAN_POINT('',(-5.86057388375191,66.9866660154814,4.445));
#261414=CARTESIAN_POINT('Origin',(-5.5838544005281,63.8237478490401,4.445));
#261415=CARTESIAN_POINT('Origin',(-5.7941612077782,66.2275656555355,4.445));
#261416=CARTESIAN_POINT('Ctrl Pts',(-6.15431105802085,65.8219579492574,
3.2376058358314));
#261417=CARTESIAN_POINT('Ctrl Pts',(-6.09196446923405,65.7542552094537,
3.41112704653794));
#261418=CARTESIAN_POINT('Ctrl Pts',(-6.03200067711174,65.7599158653485,
3.59808142686584));
#261419=CARTESIAN_POINT('Ctrl Pts',(-5.74917274455676,65.8600210538758,
3.10349479056237));
#261420=CARTESIAN_POINT('Ctrl Pts',(-5.74441843420203,65.7867232581855,
3.29579590096035));
#261421=CARTESIAN_POINT('Ctrl Pts',(-5.74615976170068,65.7863610329078,
3.50297858761136));
#261422=CARTESIAN_POINT('Ctrl Pts',(-5.30414356229518,65.8968204131924,
3.18782913062388));
#261423=CARTESIAN_POINT('Ctrl Pts',(-5.36319861850554,65.8183839519767,
3.36843862041187));
#261424=CARTESIAN_POINT('Ctrl Pts',(-5.43332317502891,65.8125499436892,
3.56303021908321));
#261425=CARTESIAN_POINT('Ctrl Pts',(-4.84458288585805,65.9320186944127,
3.55329062024494));
#261426=CARTESIAN_POINT('Ctrl Pts',(-4.96994589552014,65.8488657795094,
3.68202484868787));
#261427=CARTESIAN_POINT('Ctrl Pts',(-5.11113200152783,65.8380126734016,
3.82073050102231));
#261428=CARTESIAN_POINT('Ctrl Pts',(-4.73576546676296,65.9400109632291,
3.68162295226985));
#261429=CARTESIAN_POINT('Ctrl Pts',(-4.87703402958295,65.8557944238857,
3.79197796828375));
#261430=CARTESIAN_POINT('Ctrl Pts',(-5.03527059122988,65.8438185211497,
3.91088264279539));
#261431=CARTESIAN_POINT('Ctrl Pts',(-4.61386911108362,65.9488102407144,
3.90174828639309));
#261432=CARTESIAN_POINT('Ctrl Pts',(-4.77298912823442,65.8634389748918,
3.9803875182256));
#261433=CARTESIAN_POINT('Ctrl Pts',(-4.95036141413464,65.8502383625224,
4.06512039686388));
#261434=CARTESIAN_POINT('Ctrl Pts',(-4.58087640128896,65.9511594036629,
3.978277556413));
#261435=CARTESIAN_POINT('Ctrl Pts',(-4.74483475405062,65.8654819452878,
4.04588200245608));
#261436=CARTESIAN_POINT('Ctrl Pts',(-4.92739373892393,65.8519572258984,
4.11872530044206));
#261437=CARTESIAN_POINT('Ctrl Pts',(-4.52999467176735,65.954763888308,4.13775932520177));
#261438=CARTESIAN_POINT('Ctrl Pts',(-4.70143575750546,65.8686166166315,
4.18229018094601));
#261439=CARTESIAN_POINT('Ctrl Pts',(-4.89201655455833,65.8545947797837,
4.23027211590684));
#261440=CARTESIAN_POINT('Ctrl Pts',(-4.51219216318015,65.9560125449433,
4.22135767615932));
#261441=CARTESIAN_POINT('Ctrl Pts',(-4.6862523681243,65.8697037316857,4.25379868918615));
#261442=CARTESIAN_POINT('Ctrl Pts',(-4.87964094281487,65.8555108601014,
4.28875393216471));
#261443=CARTESIAN_POINT('Ctrl Pts',(-4.48446767193232,65.9579557151991,
4.47154323956553));
#261444=CARTESIAN_POINT('Ctrl Pts',(-4.6626169462531,65.8713953445337,4.46767570477302));
#261445=CARTESIAN_POINT('Ctrl Pts',(-4.86038908992741,65.8569354625126,
4.46350834785649));
#261446=CARTESIAN_POINT('Ctrl Pts',(-4.49975936877847,65.9568960291476,
4.64353769016378));
#261447=CARTESIAN_POINT('Ctrl Pts',(-4.67561628585122,65.8704766362668,
4.61463767040416));
#261448=CARTESIAN_POINT('Ctrl Pts',(-4.87092992967729,65.8561635955122,
4.58349799088226));
#261449=CARTESIAN_POINT('Ctrl Pts',(-4.59372963797714,65.9502572949783,
4.96366679064011));
#261450=CARTESIAN_POINT('Ctrl Pts',(-4.75582205540001,65.8646924066107,
4.88862271283806));
#261451=CARTESIAN_POINT('Ctrl Pts',(-4.9363817116022,65.8512898691079,4.80776315422202));
#261452=CARTESIAN_POINT('Ctrl Pts',(-4.67383602477745,65.9445549388601,
5.11609535395164));
#261453=CARTESIAN_POINT('Ctrl Pts',(-4.82406048883673,65.8597427462409,
5.01890497900004));
#261454=CARTESIAN_POINT('Ctrl Pts',(-4.99189710122369,65.8471371293895,
4.91418421673991));
#261455=CARTESIAN_POINT('Ctrl Pts',(-4.8299491643489,65.9330162944123,5.30924877121673));
#261456=CARTESIAN_POINT('Ctrl Pts',(-4.95757441530503,65.8497260824747,
5.18455891300591));
#261457=CARTESIAN_POINT('Ctrl Pts',(-5.10118680227484,65.8387301893256,
5.05021018314642));
#261458=CARTESIAN_POINT('Ctrl Pts',(-4.88942536164016,65.928563662165,5.36959095245021));
#261459=CARTESIAN_POINT('Ctrl Pts',(-5.00835572047755,65.8458708401228,
5.23621810911562));
#261460=CARTESIAN_POINT('Ctrl Pts',(-5.14264821972077,65.8355096208282,
5.09251447827068));
#261461=CARTESIAN_POINT('Ctrl Pts',(-5.01651316953247,65.9188654923848,
5.47539810873861));
#261462=CARTESIAN_POINT('Ctrl Pts',(-5.11706482667001,65.8374748101095,
5.3269745251348));
#261463=CARTESIAN_POINT('Ctrl Pts',(-5.23165922815084,65.8284961046547,
5.16705626289246));
#261464=CARTESIAN_POINT('Ctrl Pts',(-5.08472188597174,65.91357826105,5.5217149024354));
#261465=CARTESIAN_POINT('Ctrl Pts',(-5.1753714150773,65.832906099351,5.3666841446406));
#261466=CARTESIAN_POINT('Ctrl Pts',(-5.27935318699374,65.8246929385831,
5.19964768151785));
#261467=CARTESIAN_POINT('Ctrl Pts',(-5.41751533989557,65.8872370343221,
5.70319668970765));
#261468=CARTESIAN_POINT('Ctrl Pts',(-5.46050286975101,65.8101487534843,
5.52260955944026));
#261469=CARTESIAN_POINT('Ctrl Pts',(-5.51340877289195,65.8057388144173,
5.32804540784423));
#261470=CARTESIAN_POINT('Ctrl Pts',(-5.72854262822302,65.8611654382057,
5.75192877312679));
#261471=CARTESIAN_POINT('Ctrl Pts',(-5.72623641199483,65.7877711381099,
5.56425071252817));
#261472=CARTESIAN_POINT('Ctrl Pts',(-5.73060092143395,65.7873412035761,
5.36203962651343));
#261473=CARTESIAN_POINT('Ctrl Pts',(-6.01225604074569,65.8349011493704,
5.68677934832659));
#261474=CARTESIAN_POINT('Ctrl Pts',(-5.9714165725876,65.7652479247564,5.50875528664603));
#261475=CARTESIAN_POINT('Ctrl Pts',(-5.93450867162861,65.7687601808892,
5.31696209593943));
#261476=CARTESIAN_POINT('Origin',(-1.11575217567831E-14,1.92862511296078E-13,
2.30953198860262));
#261477=CARTESIAN_POINT('',(-1.92523812794069E-14,-66.0995441972306,2.30953198860216));
#261478=CARTESIAN_POINT('',(5.7609548697913,-65.8480154755621,2.30953198860216));
#261479=CARTESIAN_POINT('Origin',(-1.11575217567831E-14,1.92862511296078E-13,
2.30953198860262));
#261480=CARTESIAN_POINT('',(-1.93280139964607E-14,-66.2265441972306,2.18253198860216));
#261481=CARTESIAN_POINT('Origin',(-1.92679342937561E-14,-66.2265441972306,
2.30953198860216));
#261482=CARTESIAN_POINT('Origin',(-1.12176014594878E-14,1.93749043458829E-13,
2.18253198860262));
#261483=CARTESIAN_POINT('Origin',(-1.11575217567831E-14,1.92862511296078E-13,
2.30953198860262));
#261484=CARTESIAN_POINT('Origin',(-1.11575217567831E-14,1.92862511296078E-13,
2.30953198860262));
#261485=CARTESIAN_POINT('',(-1.93435670108099E-14,-66.3535441972306,2.18253198860216));
#261486=CARTESIAN_POINT('Origin',(-1.12176014594878E-14,1.93749043458829E-13,
2.18253198860262));
#261487=CARTESIAN_POINT('',(-1.92990403224544E-14,-66.4805441972306,2.30953198860216));
#261488=CARTESIAN_POINT('Origin',(-1.92834873081052E-14,-66.3535441972306,
2.30953198860216));
#261489=CARTESIAN_POINT('',(5.79416120777816,-66.2275656555351,2.30953198860216));
#261490=CARTESIAN_POINT('Origin',(-1.11575217567831E-14,1.92862511296078E-13,
2.30953198860262));
#261491=CARTESIAN_POINT('Origin',(-1.11575217567831E-14,1.92862511296078E-13,
2.30953198860262));
#261492=CARTESIAN_POINT('Origin',(10.0229975717235,-114.563386475249,4.445));
#261493=CARTESIAN_POINT('',(-5.76095486979065,65.8480154755627,3.17499999999344));
#261494=CARTESIAN_POINT('Ctrl Pts',(-4.49472415811104,65.9465480356947,
4.445));
#261495=CARTESIAN_POINT('Ctrl Pts',(-4.49472415811104,65.9465480356947,
4.28553175692096));
#261496=CARTESIAN_POINT('Ctrl Pts',(-4.52652892656956,65.9444044626199,
4.11543688631087));
#261497=CARTESIAN_POINT('Ctrl Pts',(-4.65584563900152,65.9354005480955,
3.80253630366508));
#261498=CARTESIAN_POINT('Ctrl Pts',(-4.75335449032797,65.9285073424601,
3.65973026004741));
#261499=CARTESIAN_POINT('Ctrl Pts',(-4.97827514565221,65.9119051150063,
3.43421851625708));
#261500=CARTESIAN_POINT('Ctrl Pts',(-5.12067995098529,65.9010838904671,
3.33647993284444));
#261501=CARTESIAN_POINT('Ctrl Pts',(-5.43259037593922,65.8761047945766,
3.20687056606523));
#261502=CARTESIAN_POINT('Ctrl Pts',(-5.60209345225226,65.8619140486688,
3.175));
#261503=CARTESIAN_POINT('Ctrl Pts',(-5.91981628733042,65.8341169024562,
3.175));
#261504=CARTESIAN_POINT('Ctrl Pts',(-6.08920842820953,65.8186581587365,
3.20687056606523));
#261505=CARTESIAN_POINT('Ctrl Pts',(-6.40071780743065,65.7890950891441,
3.33647993284444));
#261506=CARTESIAN_POINT('Ctrl Pts',(-6.54283824971022,65.7750235800303,
3.43421851625708));
#261507=CARTESIAN_POINT('Ctrl Pts',(-6.76722480142868,65.7523165204273,
3.65973026004741));
#261508=CARTESIAN_POINT('Ctrl Pts',(-6.86444926679916,65.742172768441,3.80253630366508));
#261509=CARTESIAN_POINT('Ctrl Pts',(-6.99336488114522,65.7285842818164,
4.11543688631087));
#261510=CARTESIAN_POINT('Ctrl Pts',(-7.02505869126407,65.7251724491156,
4.28553175692096));
#261511=CARTESIAN_POINT('Ctrl Pts',(-7.02505869126407,65.7251724491156,
4.60446824307904));
#261512=CARTESIAN_POINT('Ctrl Pts',(-6.99336488114522,65.7285842818164,
4.77456311368913));
#261513=CARTESIAN_POINT('Ctrl Pts',(-6.86444926679916,65.742172768441,5.08746369633492));
#261514=CARTESIAN_POINT('Ctrl Pts',(-6.76722480142868,65.7523165204273,
5.23026973995259));
#261515=CARTESIAN_POINT('Ctrl Pts',(-6.54283824971022,65.7750235800303,
5.45578148374292));
#261516=CARTESIAN_POINT('Ctrl Pts',(-6.40071780743066,65.7890950891441,
5.55352006715556));
#261517=CARTESIAN_POINT('Ctrl Pts',(-6.08920842820953,65.8186581587365,
5.68312943393477));
#261518=CARTESIAN_POINT('Ctrl Pts',(-5.91981628733042,65.8341169024562,
5.715));
#261519=CARTESIAN_POINT('Ctrl Pts',(-5.60209345225226,65.8619140486688,
5.715));
#261520=CARTESIAN_POINT('Ctrl Pts',(-5.43259037593922,65.8761047945766,
5.68312943393477));
#261521=CARTESIAN_POINT('Ctrl Pts',(-5.12067995098529,65.9010838904671,
5.55352006715557));
#261522=CARTESIAN_POINT('Ctrl Pts',(-4.97827514565221,65.9119051150063,
5.45578148374292));
#261523=CARTESIAN_POINT('Ctrl Pts',(-4.75335449032797,65.9285073424601,
5.23026973995259));
#261524=CARTESIAN_POINT('Ctrl Pts',(-4.65584563900152,65.9354005480955,
5.08746369633493));
#261525=CARTESIAN_POINT('Ctrl Pts',(-4.52652892656956,65.9444044626199,
4.77456311368913));
#261526=CARTESIAN_POINT('Ctrl Pts',(-4.49472415811104,65.9465480356947,
4.60446824307904));
#261527=CARTESIAN_POINT('Ctrl Pts',(-4.49472415811104,65.9465480356947,
4.445));
#261528=CARTESIAN_POINT('',(-5.7941612077782,66.2275656555355,3.175));
#261529=CARTESIAN_POINT('',(10.0229975717235,-114.563386475249,3.175));
#261530=CARTESIAN_POINT('',(-5.79416120777819,66.2275656555354,5.715));
#261531=CARTESIAN_POINT('Ctrl Pts',(-5.7941612077782,66.2275656555355,3.175));
#261532=CARTESIAN_POINT('Ctrl Pts',(-5.9530225774129,66.2136670866202,3.175));
#261533=CARTESIAN_POINT('Ctrl Pts',(-6.12241501552111,66.1982119784345,
3.20687054727211));
#261534=CARTESIAN_POINT('Ctrl Pts',(-6.43392555716451,66.1686620439684,
3.33647990006866));
#261535=CARTESIAN_POINT('Ctrl Pts',(-6.57604684440547,66.1545998466684,
3.43421849077535));
#261536=CARTESIAN_POINT('Ctrl Pts',(-6.80043497757575,66.1319102785373,
3.65973028551737));
#261537=CARTESIAN_POINT('Ctrl Pts',(-6.89766026532391,66.1217758425954,
3.80253635930903));
#261538=CARTESIAN_POINT('Ctrl Pts',(-7.0265770154737,66.1082004985806,4.11543695516789));
#261539=CARTESIAN_POINT('Ctrl Pts',(-7.05827112497043,66.1047923034812,
4.28553180502499));
#261540=CARTESIAN_POINT('Ctrl Pts',(-7.05827112497043,66.1047923034812,
4.60446819497501));
#261541=CARTESIAN_POINT('Ctrl Pts',(-7.0265770154737,66.1082004985806,4.77456304483211));
#261542=CARTESIAN_POINT('Ctrl Pts',(-6.89766026532391,66.1217758425954,
5.08746364069097));
#261543=CARTESIAN_POINT('Ctrl Pts',(-6.80043497757575,66.1319102785373,
5.23026971448264));
#261544=CARTESIAN_POINT('Ctrl Pts',(-6.57604684440547,66.1545998466684,
5.45578150922466));
#261545=CARTESIAN_POINT('Ctrl Pts',(-6.43392555716451,66.1686620439684,
5.55352009993134));
#261546=CARTESIAN_POINT('Ctrl Pts',(-6.12241501552111,66.1982119784344,
5.68312945272789));
#261547=CARTESIAN_POINT('Ctrl Pts',(-5.9530225774129,66.2136670866202,5.715));
#261548=CARTESIAN_POINT('Ctrl Pts',(-5.7941612077782,66.2275656555355,5.715));
#261549=CARTESIAN_POINT('Ctrl Pts',(-5.7941612077782,66.2275656555355,5.715));
#261550=CARTESIAN_POINT('Ctrl Pts',(-5.6352998381435,66.2414642244507,5.715));
#261551=CARTESIAN_POINT('Ctrl Pts',(-5.46579710042078,66.2556586022737,
5.6831294527279));
#261552=CARTESIAN_POINT('Ctrl Pts',(-5.15388781159512,66.280650835591,5.55352009993135));
#261553=CARTESIAN_POINT('Ctrl Pts',(-5.011483791117,66.2914813772026,5.45578150922466));
#261554=CARTESIAN_POINT('Ctrl Pts',(-4.78656461572897,66.3081011050097,
5.23026971448264));
#261555=CARTESIAN_POINT('Ctrl Pts',(-4.68905657223274,66.3150036279624,
5.08746364069097));
#261556=CARTESIAN_POINT('Ctrl Pts',(-4.55974102344273,66.3240206826611,
4.77456304483211));
#261557=CARTESIAN_POINT('Ctrl Pts',(-4.52793659181739,66.3261678900603,
4.60446819497501));
#261558=CARTESIAN_POINT('Ctrl Pts',(-4.52793659181739,66.3261678900603,
4.445));
#261559=CARTESIAN_POINT('Ctrl Pts',(-4.52793659181739,66.3261678900603,
4.28553180502499));
#261560=CARTESIAN_POINT('Ctrl Pts',(-4.55974102344273,66.3240206826611,
4.11543695516789));
#261561=CARTESIAN_POINT('Ctrl Pts',(-4.68905657223274,66.3150036279624,
3.80253635930903));
#261562=CARTESIAN_POINT('Ctrl Pts',(-4.78656461572897,66.3081011050097,
3.65973028551737));
#261563=CARTESIAN_POINT('Ctrl Pts',(-5.011483791117,66.2914813772026,3.43421849077535));
#261564=CARTESIAN_POINT('Ctrl Pts',(-5.15388781159512,66.280650835591,3.33647990006866));
#261565=CARTESIAN_POINT('Ctrl Pts',(-5.46579710042078,66.2556586022738,
3.20687054727211));
#261566=CARTESIAN_POINT('Ctrl Pts',(-5.6352998381435,66.2414642244507,3.175));
#261567=CARTESIAN_POINT('Ctrl Pts',(-5.7941612077782,66.2275656555355,3.175));
#261568=CARTESIAN_POINT('Origin',(-3.98912952672225E-15,8.70861844988177E-14,
17.4625000000011));
#261569=CARTESIAN_POINT('',(5.76095486979131,-65.8480154755622,17.4625000000006));
#261570=CARTESIAN_POINT('Origin',(-3.98912952672225E-15,8.70861844988177E-14,
17.4625000000011));
#261571=CARTESIAN_POINT('',(5.76095486979131,-65.8480154755622,17.4625000000006));
#261572=CARTESIAN_POINT('Origin',(-3.98912952672225E-15,8.70861844988177E-14,
17.4625000000011));
#261573=CARTESIAN_POINT('',(5.79416120777817,-66.2275656555352,17.4625000000006));
#261574=CARTESIAN_POINT('',(5.79416120777817,-66.2275656555352,17.4625000000006));
#261575=CARTESIAN_POINT('Origin',(-3.98912952672225E-15,8.70861844988177E-14,
17.4625000000011));
#261576=CARTESIAN_POINT('Origin',(-3.98912952672225E-15,8.70861844988177E-14,
17.4625000000011));
#261577=CARTESIAN_POINT('Origin',(-1.12176014594878E-14,1.93749043458829E-13,
2.18253198860262));
#261578=CARTESIAN_POINT('Origin',(5.70044441203719E-15,0.,40.48125));
#261579=CARTESIAN_POINT('',(-56.0881943187058,-6.86882276423578E-15,40.10025));
#261580=CARTESIAN_POINT('Origin',(5.64679317051213E-15,0.,40.10025));
#261581=CARTESIAN_POINT('',(-56.4113006433413,-6.9083918768607E-15,40.2793507603272));
#261582=CARTESIAN_POINT('Origin',(-56.0881943187058,-6.86882276423578E-15,
40.48125));
#261583=CARTESIAN_POINT('Origin',(5.67201358560304E-15,0.,40.2793507603272));
#261584=CARTESIAN_POINT('Origin',(0.,0.,42.1005));
#261585=CARTESIAN_POINT('',(-50.889,-6.23210509618097E-15,42.4815));
#261586=CARTESIAN_POINT('Origin',(0.,0.,42.4815));
#261587=CARTESIAN_POINT('',(-51.27,-6.27876413922848E-15,42.1005));
#261588=CARTESIAN_POINT('Origin',(-50.889,-6.23210509618097E-15,42.1005));
#261589=CARTESIAN_POINT('',(51.27,6.27876413922848E-15,42.1005));
#261590=CARTESIAN_POINT('Origin',(0.,0.,42.1005));
#261591=CARTESIAN_POINT('Origin',(0.,0.,42.1005));
#261592=CARTESIAN_POINT('Origin',(-1.38777878078145E-14,-1.38777878078145E-14,
42.1005));
#261593=CARTESIAN_POINT('',(50.,-7.75455381207769E-15,42.1005));
#261594=CARTESIAN_POINT('',(-50.,-2.00010218035512E-14,42.1005));
#261595=CARTESIAN_POINT('Origin',(-1.38777878078145E-14,-1.38777878078145E-14,
42.1005));
#261596=CARTESIAN_POINT('Origin',(-1.38777878078145E-14,-1.38777878078145E-14,
42.1005));
#261597=CARTESIAN_POINT('',(-50.381,-2.00476808465987E-14,42.4815));
#261598=CARTESIAN_POINT('Origin',(-50.381,-2.00476808465987E-14,42.1005));
#261599=CARTESIAN_POINT('Origin',(-1.38777878078145E-14,-1.38777878078145E-14,
42.4815));
#261600=CARTESIAN_POINT('Origin',(5.67808972806842E-15,0.,40.3225));
#261601=CARTESIAN_POINT('',(-56.5223703788014,-6.92199399646203E-15,40.4570994931153));
#261602=CARTESIAN_POINT('Origin',(5.69704361235785E-15,0.,40.4570994931153));
#261603=CARTESIAN_POINT('',(-56.7377745952251,-6.94837340487864E-15,40.5765));
#261604=CARTESIAN_POINT('Origin',(-56.7377745952251,-6.94837340487864E-15,
40.3225));
#261605=CARTESIAN_POINT('Origin',(5.71385722241845E-15,0.,40.5765));
#261606=CARTESIAN_POINT('Origin',(5.67808972806842E-15,0.,40.3225));
#261607=CARTESIAN_POINT('',(-57.4087519663171,-7.03054443385946E-15,40.5765));
#261608=CARTESIAN_POINT('Origin',(5.71385722241845E-15,0.,40.5765));
#261609=CARTESIAN_POINT('',(-57.6241561827409,-7.05692384227608E-15,40.1879005068848));
#261610=CARTESIAN_POINT('Origin',(-57.4087519663171,-7.03054443385946E-15,
40.3225));
#261611=CARTESIAN_POINT('Origin',(5.65913584377898E-15,0.,40.1879005068848));
#261612=CARTESIAN_POINT('Origin',(6.93889390390723E-15,0.,49.276));
#261613=CARTESIAN_POINT('',(-56.875,-6.96517867015057E-15,38.989));
#261614=CARTESIAN_POINT('Origin',(5.49031038273072E-15,0.,38.989));
#261615=CARTESIAN_POINT('',(-56.875,-6.96517867015057E-15,38.6715));
#261616=CARTESIAN_POINT('',(-56.875,-6.96517867015057E-15,49.276));
#261617=CARTESIAN_POINT('Origin',(5.44560101479317E-15,0.,38.6715));
#261618=CARTESIAN_POINT('Origin',(5.64679317051213E-15,0.,40.10025));
#261619=CARTESIAN_POINT('',(-56.2993860673093,-6.89468629412914E-15,40.10025));
#261620=CARTESIAN_POINT('Origin',(5.71385722241845E-15,0.,40.5765));
#261621=CARTESIAN_POINT('',(-57.8669800961561,-7.08666119510811E-15,40.5765));
#261622=CARTESIAN_POINT('Origin',(0.,0.,42.4815));
#261623=CARTESIAN_POINT('',(51.27,-6.27876413922848E-15,40.10025));
#261624=CARTESIAN_POINT('Origin',(5.64679317051213E-15,0.,40.10025));
#261625=CARTESIAN_POINT('',(51.27,-6.27876413922848E-15,42.4815));
#261626=CARTESIAN_POINT('Origin',(-1.38777878078145E-14,-1.38777878078145E-14,
225.059263108502));
#261627=CARTESIAN_POINT('',(50.,-2.00010218035512E-14,17.4625));
#261628=CARTESIAN_POINT('',(50.,-2.00010218035512E-14,225.059263108502));
#261629=CARTESIAN_POINT('Origin',(-1.38777878078145E-14,-1.38777878078145E-14,
17.4625));
#261630=CARTESIAN_POINT('Origin',(-1.38777878078145E-14,-1.38777878078145E-14,
225.059263108502));
#261631=CARTESIAN_POINT('',(65.,-2.18379920022723E-14,17.4625));
#261632=CARTESIAN_POINT('Origin',(-1.38777878078145E-14,-1.38777878078145E-14,
17.4625));
#261633=CARTESIAN_POINT('',(65.,-2.18379920022723E-14,38.6715));
#261634=CARTESIAN_POINT('',(65.,-2.18379920022723E-14,225.059263108502));
#261635=CARTESIAN_POINT('Origin',(-1.38777878078145E-14,-1.38777878078145E-14,
38.6715));
#261636=CARTESIAN_POINT('Origin',(-1.38777878078145E-14,-1.38777878078145E-14,
38.6715));
#261637=CARTESIAN_POINT('Origin',(-1.38777878078145E-14,-1.38777878078145E-14,
17.4625));
#261638=CARTESIAN_POINT('Origin',(0.,0.,42.4815));
#261639=CARTESIAN_POINT('Origin',(57.8669800961561,0.,40.5765));
#261640=CARTESIAN_POINT('Origin',(56.2993860673093,0.,40.10025));
#261641=CARTESIAN_POINT('Origin',(40.4567708333334,-1.14908083048704E-13,
48.26));
#261642=CARTESIAN_POINT('',(48.3916666666642,-4.72273670613199,48.26));
#261643=CARTESIAN_POINT('',(48.3968749999976,-4.72273670613199,48.26));
#261644=CARTESIAN_POINT('',(40.4567708333334,-4.72273670613191,48.26));
#261645=CARTESIAN_POINT('',(49.2650632938682,-2.14259623628835,52.4687436799701));
#261646=CARTESIAN_POINT('Ctrl Pts',(48.3916666666642,-4.72273670613199,
48.26));
#261647=CARTESIAN_POINT('Ctrl Pts',(48.4578124999975,-4.722736706132,46.303778404803));
#261648=CARTESIAN_POINT('Ctrl Pts',(48.5239583333308,-3.3394791506646,44.9205208493356));
#261649=CARTESIAN_POINT('Ctrl Pts',(48.5901041666641,-1.95622159519721,
43.5372632938682));
#261650=CARTESIAN_POINT('Ctrl Pts',(48.6562499999974,-1.70749941551634E-13,
43.5372632938682));
#261651=CARTESIAN_POINT('Ctrl Pts',(48.7223958333307,1.95622159519687,43.5372632938682));
#261652=CARTESIAN_POINT('Ctrl Pts',(48.7885416666641,3.33947915066426,44.9205208493356));
#261653=CARTESIAN_POINT('Ctrl Pts',(48.8546874999974,4.72273670613166,46.303778404803));
#261654=CARTESIAN_POINT('Ctrl Pts',(48.9208333333307,4.72273670613165,48.26));
#261655=CARTESIAN_POINT('Ctrl Pts',(48.986979166664,4.72273670613166,50.216221595197));
#261656=CARTESIAN_POINT('Ctrl Pts',(49.0531249999973,3.33947915066426,51.5994791506644));
#261657=CARTESIAN_POINT('Ctrl Pts',(49.1192708333306,1.95622159519687,52.9827367061318));
#261658=CARTESIAN_POINT('Ctrl Pts',(49.1854166666639,-1.71440780215362E-13,
52.9827367061318));
#261659=CARTESIAN_POINT('Ctrl Pts',(49.2237251595434,-1.13294968517034,
52.9827367061318));
#261660=CARTESIAN_POINT('Ctrl Pts',(49.2650632938682,-2.14259623628835,
52.4687436799701));
#261661=CARTESIAN_POINT('',(49.2650632938682,-2.01456111142428,52.5315085770466));
#261662=CARTESIAN_POINT('Origin',(49.2650632939072,4.32918355108836E-6,
48.2599912028394));
#261663=CARTESIAN_POINT('Ctrl Pts',(48.3968749999976,-4.72273670613199,
48.26));
#261664=CARTESIAN_POINT('Ctrl Pts',(48.4630208333309,-4.722736706132,46.303778404803));
#261665=CARTESIAN_POINT('Ctrl Pts',(48.5291666666642,-3.3394791506646,44.9205208493356));
#261666=CARTESIAN_POINT('Ctrl Pts',(48.5953124999975,-1.95622159519721,
43.5372632938682));
#261667=CARTESIAN_POINT('Ctrl Pts',(48.6614583333308,-1.70768126350274E-13,
43.5372632938682));
#261668=CARTESIAN_POINT('Ctrl Pts',(48.7276041666641,1.95622159519687,43.5372632938682));
#261669=CARTESIAN_POINT('Ctrl Pts',(48.7937499999974,3.33947915066426,44.9205208493356));
#261670=CARTESIAN_POINT('Ctrl Pts',(48.8598958333308,4.72273670613166,46.303778404803));
#261671=CARTESIAN_POINT('Ctrl Pts',(48.9260416666641,4.72273670613165,48.26));
#261672=CARTESIAN_POINT('Ctrl Pts',(48.9921874999974,4.72273670613166,50.216221595197));
#261673=CARTESIAN_POINT('Ctrl Pts',(49.0583333333307,3.33947915066426,51.5994791506644));
#261674=CARTESIAN_POINT('Ctrl Pts',(49.124479166664,1.95622159519687,52.9827367061318));
#261675=CARTESIAN_POINT('Ctrl Pts',(49.1906249999973,-1.71458965014002E-13,
52.9827367061318));
#261676=CARTESIAN_POINT('Ctrl Pts',(49.2263929373901,-1.05781434774344,
52.9827367061318));
#261677=CARTESIAN_POINT('Ctrl Pts',(49.2650632938682,-2.01456111142428,
52.5315085770466));
#261678=CARTESIAN_POINT('Origin',(40.4567708333334,-1.14908083048704E-13,
48.26));
#261679=CARTESIAN_POINT('',(47.3333333333312,-4.72273670613199,48.26));
#261680=CARTESIAN_POINT('',(47.3385416666645,-4.72273670613199,48.26));
#261681=CARTESIAN_POINT('',(40.4567708333334,-4.72273670613191,48.26));
#261682=CARTESIAN_POINT('Ctrl Pts',(47.3333333333312,-4.72273670613199,
48.26));
#261683=CARTESIAN_POINT('Ctrl Pts',(47.3994791666645,-4.72273670613199,
46.303778404803));
#261684=CARTESIAN_POINT('Ctrl Pts',(47.4656249999978,-3.3394791506646,44.9205208493356));
#261685=CARTESIAN_POINT('Ctrl Pts',(47.5317708333311,-1.95622159519721,
43.5372632938682));
#261686=CARTESIAN_POINT('Ctrl Pts',(47.5979166666644,-1.67054790468026E-13,
43.5372632938682));
#261687=CARTESIAN_POINT('Ctrl Pts',(47.6640624999977,1.95622159519688,43.5372632938682));
#261688=CARTESIAN_POINT('Ctrl Pts',(47.7302083333311,3.33947915066426,44.9205208493356));
#261689=CARTESIAN_POINT('Ctrl Pts',(47.7963541666644,4.72273670613166,46.303778404803));
#261690=CARTESIAN_POINT('Ctrl Pts',(47.8624999999977,4.72273670613166,48.26));
#261691=CARTESIAN_POINT('Ctrl Pts',(47.928645833331,4.72273670613166,50.216221595197));
#261692=CARTESIAN_POINT('Ctrl Pts',(47.9947916666643,3.33947915066427,51.5994791506644));
#261693=CARTESIAN_POINT('Ctrl Pts',(48.0609374999976,1.95622159519687,52.9827367061318));
#261694=CARTESIAN_POINT('Ctrl Pts',(48.1270833333309,-1.67745629131754E-13,
52.9827367061318));
#261695=CARTESIAN_POINT('Ctrl Pts',(48.1932291666642,-1.95622159519721,
52.9827367061318));
#261696=CARTESIAN_POINT('Ctrl Pts',(48.2593749999975,-3.3394791506646,51.5994791506644));
#261697=CARTESIAN_POINT('Ctrl Pts',(48.3255208333308,-4.722736706132,50.216221595197));
#261698=CARTESIAN_POINT('Ctrl Pts',(48.3916666666642,-4.72273670613199,
48.26));
#261699=CARTESIAN_POINT('Ctrl Pts',(47.3385416666645,-4.72273670613199,
48.26));
#261700=CARTESIAN_POINT('Ctrl Pts',(47.4046874999979,-4.72273670613199,
46.303778404803));
#261701=CARTESIAN_POINT('Ctrl Pts',(47.4708333333312,-3.3394791506646,44.9205208493356));
#261702=CARTESIAN_POINT('Ctrl Pts',(47.5369791666645,-1.95622159519721,
43.5372632938682));
#261703=CARTESIAN_POINT('Ctrl Pts',(47.6031249999978,-1.67072975266666E-13,
43.5372632938682));
#261704=CARTESIAN_POINT('Ctrl Pts',(47.6692708333311,1.95622159519688,43.5372632938682));
#261705=CARTESIAN_POINT('Ctrl Pts',(47.7354166666644,3.33947915066426,44.9205208493356));
#261706=CARTESIAN_POINT('Ctrl Pts',(47.8015624999978,4.72273670613166,46.303778404803));
#261707=CARTESIAN_POINT('Ctrl Pts',(47.8677083333311,4.72273670613166,48.26));
#261708=CARTESIAN_POINT('Ctrl Pts',(47.9338541666644,4.72273670613166,50.216221595197));
#261709=CARTESIAN_POINT('Ctrl Pts',(47.9999999999977,3.33947915066427,51.5994791506644));
#261710=CARTESIAN_POINT('Ctrl Pts',(48.066145833331,1.95622159519687,52.9827367061318));
#261711=CARTESIAN_POINT('Ctrl Pts',(48.1322916666643,-1.67763813930394E-13,
52.9827367061318));
#261712=CARTESIAN_POINT('Ctrl Pts',(48.1984374999976,-1.95622159519721,
52.9827367061318));
#261713=CARTESIAN_POINT('Ctrl Pts',(48.2645833333309,-3.3394791506646,51.5994791506644));
#261714=CARTESIAN_POINT('Ctrl Pts',(48.3307291666642,-4.722736706132,50.216221595197));
#261715=CARTESIAN_POINT('Ctrl Pts',(48.3968749999976,-4.72273670613199,
48.26));
#261716=CARTESIAN_POINT('Origin',(40.4567708333334,-1.14908083048704E-13,
48.26));
#261717=CARTESIAN_POINT('',(46.2749999999982,-4.72273670613199,48.26));
#261718=CARTESIAN_POINT('',(46.2802083333315,-4.72273670613199,48.26));
#261719=CARTESIAN_POINT('',(40.4567708333334,-4.72273670613191,48.26));
#261720=CARTESIAN_POINT('Ctrl Pts',(46.2749999999982,-4.72273670613199,
48.26));
#261721=CARTESIAN_POINT('Ctrl Pts',(46.3411458333315,-4.72273670613199,
46.303778404803));
#261722=CARTESIAN_POINT('Ctrl Pts',(46.4072916666648,-3.3394791506646,44.9205208493356));
#261723=CARTESIAN_POINT('Ctrl Pts',(46.4734374999981,-1.95622159519721,
43.5372632938682));
#261724=CARTESIAN_POINT('Ctrl Pts',(46.5395833333314,-1.63359639384419E-13,
43.5372632938682));
#261725=CARTESIAN_POINT('Ctrl Pts',(46.6057291666648,1.95622159519688,43.5372632938682));
#261726=CARTESIAN_POINT('Ctrl Pts',(46.6718749999981,3.33947915066427,44.9205208493356));
#261727=CARTESIAN_POINT('Ctrl Pts',(46.7380208333314,4.72273670613166,46.303778404803));
#261728=CARTESIAN_POINT('Ctrl Pts',(46.8041666666647,4.72273670613166,48.26));
#261729=CARTESIAN_POINT('Ctrl Pts',(46.870312499998,4.72273670613166,50.216221595197));
#261730=CARTESIAN_POINT('Ctrl Pts',(46.9364583333313,3.33947915066427,51.5994791506644));
#261731=CARTESIAN_POINT('Ctrl Pts',(47.0026041666646,1.95622159519688,52.9827367061318));
#261732=CARTESIAN_POINT('Ctrl Pts',(47.0687499999979,-1.64050478048146E-13,
52.9827367061318));
#261733=CARTESIAN_POINT('Ctrl Pts',(47.1348958333312,-1.95622159519721,
52.9827367061318));
#261734=CARTESIAN_POINT('Ctrl Pts',(47.2010416666646,-3.3394791506646,51.5994791506644));
#261735=CARTESIAN_POINT('Ctrl Pts',(47.2671874999979,-4.72273670613199,
50.216221595197));
#261736=CARTESIAN_POINT('Ctrl Pts',(47.3333333333312,-4.72273670613199,
48.26));
#261737=CARTESIAN_POINT('Ctrl Pts',(46.2802083333315,-4.72273670613199,
48.26));
#261738=CARTESIAN_POINT('Ctrl Pts',(46.3463541666649,-4.72273670613199,
46.303778404803));
#261739=CARTESIAN_POINT('Ctrl Pts',(46.4124999999982,-3.3394791506646,44.9205208493356));
#261740=CARTESIAN_POINT('Ctrl Pts',(46.4786458333315,-1.95622159519721,
43.5372632938682));
#261741=CARTESIAN_POINT('Ctrl Pts',(46.5447916666648,-1.63377824183059E-13,
43.5372632938682));
#261742=CARTESIAN_POINT('Ctrl Pts',(46.6109374999981,1.95622159519688,43.5372632938682));
#261743=CARTESIAN_POINT('Ctrl Pts',(46.6770833333314,3.33947915066427,44.9205208493356));
#261744=CARTESIAN_POINT('Ctrl Pts',(46.7432291666648,4.72273670613166,46.303778404803));
#261745=CARTESIAN_POINT('Ctrl Pts',(46.8093749999981,4.72273670613166,48.26));
#261746=CARTESIAN_POINT('Ctrl Pts',(46.8755208333314,4.72273670613166,50.216221595197));
#261747=CARTESIAN_POINT('Ctrl Pts',(46.9416666666647,3.33947915066427,51.5994791506644));
#261748=CARTESIAN_POINT('Ctrl Pts',(47.007812499998,1.95622159519688,52.9827367061318));
#261749=CARTESIAN_POINT('Ctrl Pts',(47.0739583333313,-1.64068662846786E-13,
52.9827367061318));
#261750=CARTESIAN_POINT('Ctrl Pts',(47.1401041666646,-1.95622159519721,
52.9827367061318));
#261751=CARTESIAN_POINT('Ctrl Pts',(47.2062499999979,-3.3394791506646,51.5994791506644));
#261752=CARTESIAN_POINT('Ctrl Pts',(47.2723958333312,-4.72273670613199,
50.216221595197));
#261753=CARTESIAN_POINT('Ctrl Pts',(47.3385416666645,-4.72273670613199,
48.26));
#261754=CARTESIAN_POINT('Origin',(40.4567708333334,-1.14908083048704E-13,
48.26));
#261755=CARTESIAN_POINT('',(45.2166666666652,-4.72273670613198,48.26));
#261756=CARTESIAN_POINT('',(45.2218749999985,-4.72273670613198,48.26));
#261757=CARTESIAN_POINT('',(40.4567708333334,-4.72273670613191,48.26));
#261758=CARTESIAN_POINT('Ctrl Pts',(45.2166666666652,-4.72273670613198,
48.26));
#261759=CARTESIAN_POINT('Ctrl Pts',(45.2828124999985,-4.72273670613199,
46.303778404803));
#261760=CARTESIAN_POINT('Ctrl Pts',(45.3489583333318,-3.33947915066459,
44.9205208493356));
#261761=CARTESIAN_POINT('Ctrl Pts',(45.4151041666651,-1.9562215951972,43.5372632938682));
#261762=CARTESIAN_POINT('Ctrl Pts',(45.4812499999984,-1.59664488300811E-13,
43.5372632938682));
#261763=CARTESIAN_POINT('Ctrl Pts',(45.5473958333317,1.95622159519688,43.5372632938682));
#261764=CARTESIAN_POINT('Ctrl Pts',(45.6135416666651,3.33947915066427,44.9205208493356));
#261765=CARTESIAN_POINT('Ctrl Pts',(45.6796874999984,4.72273670613167,46.303778404803));
#261766=CARTESIAN_POINT('Ctrl Pts',(45.7458333333317,4.72273670613167,48.26));
#261767=CARTESIAN_POINT('Ctrl Pts',(45.811979166665,4.72273670613167,50.216221595197));
#261768=CARTESIAN_POINT('Ctrl Pts',(45.8781249999983,3.33947915066427,51.5994791506644));
#261769=CARTESIAN_POINT('Ctrl Pts',(45.9442708333316,1.95622159519688,52.9827367061318));
#261770=CARTESIAN_POINT('Ctrl Pts',(46.0104166666649,-1.60355326964539E-13,
52.9827367061318));
#261771=CARTESIAN_POINT('Ctrl Pts',(46.0765624999982,-1.9562215951972,52.9827367061318));
#261772=CARTESIAN_POINT('Ctrl Pts',(46.1427083333315,-3.33947915066459,
51.5994791506644));
#261773=CARTESIAN_POINT('Ctrl Pts',(46.2088541666648,-4.72273670613199,
50.216221595197));
#261774=CARTESIAN_POINT('Ctrl Pts',(46.2749999999982,-4.72273670613199,
48.26));
#261775=CARTESIAN_POINT('Ctrl Pts',(45.2218749999985,-4.72273670613198,
48.26));
#261776=CARTESIAN_POINT('Ctrl Pts',(45.2880208333319,-4.72273670613199,
46.303778404803));
#261777=CARTESIAN_POINT('Ctrl Pts',(45.3541666666652,-3.33947915066459,
44.9205208493356));
#261778=CARTESIAN_POINT('Ctrl Pts',(45.4203124999985,-1.9562215951972,43.5372632938682));
#261779=CARTESIAN_POINT('Ctrl Pts',(45.4864583333318,-1.59682673099451E-13,
43.5372632938682));
#261780=CARTESIAN_POINT('Ctrl Pts',(45.5526041666651,1.95622159519688,43.5372632938682));
#261781=CARTESIAN_POINT('Ctrl Pts',(45.6187499999984,3.33947915066427,44.9205208493356));
#261782=CARTESIAN_POINT('Ctrl Pts',(45.6848958333318,4.72273670613167,46.303778404803));
#261783=CARTESIAN_POINT('Ctrl Pts',(45.7510416666651,4.72273670613167,48.26));
#261784=CARTESIAN_POINT('Ctrl Pts',(45.8171874999984,4.72273670613167,50.216221595197));
#261785=CARTESIAN_POINT('Ctrl Pts',(45.8833333333317,3.33947915066427,51.5994791506644));
#261786=CARTESIAN_POINT('Ctrl Pts',(45.949479166665,1.95622159519688,52.9827367061318));
#261787=CARTESIAN_POINT('Ctrl Pts',(46.0156249999983,-1.60373511763179E-13,
52.9827367061318));
#261788=CARTESIAN_POINT('Ctrl Pts',(46.0817708333316,-1.9562215951972,52.9827367061318));
#261789=CARTESIAN_POINT('Ctrl Pts',(46.1479166666649,-3.33947915066459,
51.5994791506644));
#261790=CARTESIAN_POINT('Ctrl Pts',(46.2140624999982,-4.72273670613199,
50.216221595197));
#261791=CARTESIAN_POINT('Ctrl Pts',(46.2802083333315,-4.72273670613199,
48.26));
#261792=CARTESIAN_POINT('Origin',(40.4567708333334,-1.14908083048704E-13,
48.26));
#261793=CARTESIAN_POINT('',(44.1583333333322,-4.72273670613198,48.26));
#261794=CARTESIAN_POINT('',(44.1635416666655,-4.72273670613198,48.26));
#261795=CARTESIAN_POINT('',(40.4567708333334,-4.72273670613191,48.26));
#261796=CARTESIAN_POINT('Ctrl Pts',(44.1583333333322,-4.72273670613198,
48.26));
#261797=CARTESIAN_POINT('Ctrl Pts',(44.2244791666655,-4.72273670613198,
46.303778404803));
#261798=CARTESIAN_POINT('Ctrl Pts',(44.2906249999988,-3.33947915066459,
44.9205208493356));
#261799=CARTESIAN_POINT('Ctrl Pts',(44.3567708333321,-1.9562215951972,43.5372632938682));
#261800=CARTESIAN_POINT('Ctrl Pts',(44.4229166666654,-1.55969337217203E-13,
43.5372632938682));
#261801=CARTESIAN_POINT('Ctrl Pts',(44.4890624999988,1.95622159519689,43.5372632938682));
#261802=CARTESIAN_POINT('Ctrl Pts',(44.5552083333321,3.33947915066428,44.9205208493356));
#261803=CARTESIAN_POINT('Ctrl Pts',(44.6213541666654,4.72273670613167,46.303778404803));
#261804=CARTESIAN_POINT('Ctrl Pts',(44.6874999999987,4.72273670613167,48.26));
#261805=CARTESIAN_POINT('Ctrl Pts',(44.753645833332,4.72273670613167,50.216221595197));
#261806=CARTESIAN_POINT('Ctrl Pts',(44.8197916666653,3.33947915066428,51.5994791506644));
#261807=CARTESIAN_POINT('Ctrl Pts',(44.8859374999986,1.95622159519688,52.9827367061318));
#261808=CARTESIAN_POINT('Ctrl Pts',(44.9520833333319,-1.56660175880931E-13,
52.9827367061318));
#261809=CARTESIAN_POINT('Ctrl Pts',(45.0182291666652,-1.9562215951972,52.9827367061318));
#261810=CARTESIAN_POINT('Ctrl Pts',(45.0843749999985,-3.33947915066459,
51.5994791506644));
#261811=CARTESIAN_POINT('Ctrl Pts',(45.1505208333318,-4.72273670613198,
50.216221595197));
#261812=CARTESIAN_POINT('Ctrl Pts',(45.2166666666652,-4.72273670613198,
48.26));
#261813=CARTESIAN_POINT('Ctrl Pts',(44.1635416666655,-4.72273670613198,
48.26));
#261814=CARTESIAN_POINT('Ctrl Pts',(44.2296874999989,-4.72273670613198,
46.303778404803));
#261815=CARTESIAN_POINT('Ctrl Pts',(44.2958333333322,-3.33947915066459,
44.9205208493356));
#261816=CARTESIAN_POINT('Ctrl Pts',(44.3619791666655,-1.9562215951972,43.5372632938682));
#261817=CARTESIAN_POINT('Ctrl Pts',(44.4281249999988,-1.55987522015843E-13,
43.5372632938682));
#261818=CARTESIAN_POINT('Ctrl Pts',(44.4942708333321,1.95622159519689,43.5372632938682));
#261819=CARTESIAN_POINT('Ctrl Pts',(44.5604166666654,3.33947915066428,44.9205208493356));
#261820=CARTESIAN_POINT('Ctrl Pts',(44.6265624999988,4.72273670613167,46.303778404803));
#261821=CARTESIAN_POINT('Ctrl Pts',(44.6927083333321,4.72273670613167,48.26));
#261822=CARTESIAN_POINT('Ctrl Pts',(44.7588541666654,4.72273670613167,50.216221595197));
#261823=CARTESIAN_POINT('Ctrl Pts',(44.8249999999987,3.33947915066428,51.5994791506644));
#261824=CARTESIAN_POINT('Ctrl Pts',(44.891145833332,1.95622159519688,52.9827367061318));
#261825=CARTESIAN_POINT('Ctrl Pts',(44.9572916666653,-1.56678360679571E-13,
52.9827367061318));
#261826=CARTESIAN_POINT('Ctrl Pts',(45.0234374999986,-1.9562215951972,52.9827367061318));
#261827=CARTESIAN_POINT('Ctrl Pts',(45.0895833333319,-3.33947915066459,
51.5994791506644));
#261828=CARTESIAN_POINT('Ctrl Pts',(45.1557291666652,-4.72273670613198,
50.216221595197));
#261829=CARTESIAN_POINT('Ctrl Pts',(45.2218749999985,-4.72273670613198,
48.26));
#261830=CARTESIAN_POINT('Origin',(40.4567708333334,-1.14908083048704E-13,
48.26));
#261831=CARTESIAN_POINT('',(43.0999999999992,-4.72273670613198,48.26));
#261832=CARTESIAN_POINT('',(43.1052083333325,-4.72273670613198,48.26));
#261833=CARTESIAN_POINT('',(40.4567708333334,-4.72273670613191,48.26));
#261834=CARTESIAN_POINT('Ctrl Pts',(43.0999999999992,-4.72273670613198,
48.26));
#261835=CARTESIAN_POINT('Ctrl Pts',(43.1661458333325,-4.72273670613198,
46.303778404803));
#261836=CARTESIAN_POINT('Ctrl Pts',(43.2322916666658,-3.33947915066458,
44.9205208493356));
#261837=CARTESIAN_POINT('Ctrl Pts',(43.2984374999991,-1.95622159519719,
43.5372632938682));
#261838=CARTESIAN_POINT('Ctrl Pts',(43.3645833333324,-1.52274186133595E-13,
43.5372632938682));
#261839=CARTESIAN_POINT('Ctrl Pts',(43.4307291666657,1.95622159519689,43.5372632938682));
#261840=CARTESIAN_POINT('Ctrl Pts',(43.4968749999991,3.33947915066428,44.9205208493356));
#261841=CARTESIAN_POINT('Ctrl Pts',(43.5630208333324,4.72273670613167,46.303778404803));
#261842=CARTESIAN_POINT('Ctrl Pts',(43.6291666666657,4.72273670613167,48.26));
#261843=CARTESIAN_POINT('Ctrl Pts',(43.695312499999,4.72273670613167,50.216221595197));
#261844=CARTESIAN_POINT('Ctrl Pts',(43.7614583333323,3.33947915066428,51.5994791506644));
#261845=CARTESIAN_POINT('Ctrl Pts',(43.8276041666656,1.95622159519689,52.9827367061318));
#261846=CARTESIAN_POINT('Ctrl Pts',(43.8937499999989,-1.52965024797323E-13,
52.9827367061318));
#261847=CARTESIAN_POINT('Ctrl Pts',(43.9598958333322,-1.95622159519719,
52.9827367061318));
#261848=CARTESIAN_POINT('Ctrl Pts',(44.0260416666655,-3.33947915066459,
51.5994791506644));
#261849=CARTESIAN_POINT('Ctrl Pts',(44.0921874999988,-4.72273670613198,
50.216221595197));
#261850=CARTESIAN_POINT('Ctrl Pts',(44.1583333333322,-4.72273670613198,
48.26));
#261851=CARTESIAN_POINT('Ctrl Pts',(43.1052083333325,-4.72273670613198,
48.26));
#261852=CARTESIAN_POINT('Ctrl Pts',(43.1713541666659,-4.72273670613198,
46.303778404803));
#261853=CARTESIAN_POINT('Ctrl Pts',(43.2374999999992,-3.33947915066458,
44.9205208493356));
#261854=CARTESIAN_POINT('Ctrl Pts',(43.3036458333325,-1.95622159519719,
43.5372632938682));
#261855=CARTESIAN_POINT('Ctrl Pts',(43.3697916666658,-1.52292370932235E-13,
43.5372632938682));
#261856=CARTESIAN_POINT('Ctrl Pts',(43.4359374999991,1.95622159519689,43.5372632938682));
#261857=CARTESIAN_POINT('Ctrl Pts',(43.5020833333324,3.33947915066428,44.9205208493356));
#261858=CARTESIAN_POINT('Ctrl Pts',(43.5682291666658,4.72273670613167,46.303778404803));
#261859=CARTESIAN_POINT('Ctrl Pts',(43.6343749999991,4.72273670613167,48.26));
#261860=CARTESIAN_POINT('Ctrl Pts',(43.7005208333324,4.72273670613167,50.216221595197));
#261861=CARTESIAN_POINT('Ctrl Pts',(43.7666666666657,3.33947915066428,51.5994791506644));
#261862=CARTESIAN_POINT('Ctrl Pts',(43.832812499999,1.95622159519689,52.9827367061318));
#261863=CARTESIAN_POINT('Ctrl Pts',(43.8989583333323,-1.52983209595963E-13,
52.9827367061318));
#261864=CARTESIAN_POINT('Ctrl Pts',(43.9651041666656,-1.95622159519719,
52.9827367061318));
#261865=CARTESIAN_POINT('Ctrl Pts',(44.0312499999989,-3.33947915066459,
51.5994791506644));
#261866=CARTESIAN_POINT('Ctrl Pts',(44.0973958333322,-4.72273670613198,
50.216221595197));
#261867=CARTESIAN_POINT('Ctrl Pts',(44.1635416666655,-4.72273670613198,
48.26));
#261868=CARTESIAN_POINT('Origin',(40.475,-1.41317707189676E-13,48.26));
#261869=CARTESIAN_POINT('',(42.2906249999995,-1.4205919993051E-13,43.5102));
#261870=CARTESIAN_POINT('',(42.09425,-1.46389605610939E-13,43.5102));
#261871=CARTESIAN_POINT('',(40.475,-1.40736024453017E-13,43.5102));
#261872=CARTESIAN_POINT('',(42.09425,-4.36624125519658,46.3900969700488));
#261873=CARTESIAN_POINT('Ctrl Pts',(42.2906249999995,-1.39957490041809E-13,
43.5102));
#261874=CARTESIAN_POINT('Ctrl Pts',(42.2803266558546,-0.306312377614008,
43.5102));
#261875=CARTESIAN_POINT('Ctrl Pts',(42.2696165070132,-0.612600594710988,
43.5398292002881));
#261876=CARTESIAN_POINT('Ctrl Pts',(42.2364131029764,-1.52596251485008,
43.7190485024123));
#261877=CARTESIAN_POINT('Ctrl Pts',(42.2135208891992,-2.1078242421188,43.9581541159291));
#261878=CARTESIAN_POINT('Ctrl Pts',(42.1749789086954,-3.00697611076851,
44.5550320160166));
#261879=CARTESIAN_POINT('Ctrl Pts',(42.15983788401,-3.34869201888137,44.8607436451311));
#261880=CARTESIAN_POINT('Ctrl Pts',(42.1278937490674,-3.93944645506941,
45.5661866234652));
#261881=CARTESIAN_POINT('Ctrl Pts',(42.1111319270672,-4.18359566378184,
45.9636177871492));
#261882=CARTESIAN_POINT('Ctrl Pts',(42.09425,-4.36624125519674,46.3900969700492));
#261883=CARTESIAN_POINT('Origin',(42.09425,-1.46971288347598E-13,48.26));
#261884=CARTESIAN_POINT('Origin',(40.475,-1.41317707189676E-13,48.26));
#261885=CARTESIAN_POINT('',(43.3489583333325,-1.209737311199E-13,43.5102));
#261886=CARTESIAN_POINT('',(42.3270833333327,-1.51906687130258E-13,43.5102));
#261887=CARTESIAN_POINT('',(40.475,-1.40736024453017E-13,43.5102));
#261888=CARTESIAN_POINT('Ctrl Pts',(43.3489583333325,-8.75688410673092E-14,
43.5102));
#261889=CARTESIAN_POINT('Ctrl Pts',(43.3350462619249,-0.413798530173326,
43.5102));
#261890=CARTESIAN_POINT('Ctrl Pts',(43.3204123302741,-0.826670368689188,
43.5642725719142));
#261891=CARTESIAN_POINT('Ctrl Pts',(43.2830916071324,-1.82594941130075,
43.8317260420044));
#261892=CARTESIAN_POINT('Ctrl Pts',(43.2603987577855,-2.38686058154388,
44.107094813422));
#261893=CARTESIAN_POINT('Ctrl Pts',(43.2169625534066,-3.3688243669304,44.8554914890222));
#261894=CARTESIAN_POINT('Ctrl Pts',(43.1966949382382,-3.78128185410704,
45.3203462387159));
#261895=CARTESIAN_POINT('Ctrl Pts',(43.1521835512767,-4.40771574233591,
46.3848087314946));
#261896=CARTESIAN_POINT('Ctrl Pts',(43.1294619675453,-4.61444584304949,
46.9750056411961));
#261897=CARTESIAN_POINT('Ctrl Pts',(43.0859479536865,-4.78902391945533,
48.1969672260124));
#261898=CARTESIAN_POINT('Ctrl Pts',(43.0657543266859,-4.75696102960577,
48.8168166627173));
#261899=CARTESIAN_POINT('Ctrl Pts',(43.0213051463692,-4.45711948033103,
50.0147078667041));
#261900=CARTESIAN_POINT('Ctrl Pts',(42.9985556170619,-4.19029907601681,
50.5808457666315));
#261901=CARTESIAN_POINT('Ctrl Pts',(42.9549633791372,-3.45765603924943,
51.57397596087));
#261902=CARTESIAN_POINT('Ctrl Pts',(42.9348366133039,-3.00063580575634,
51.992828129818));
#261903=CARTESIAN_POINT('Ctrl Pts',(42.8904524036951,-1.94712039905108,
52.6365582703688));
#261904=CARTESIAN_POINT('Ctrl Pts',(42.8676758816576,-1.35939952094611,
52.8532110500324));
#261905=CARTESIAN_POINT('Ctrl Pts',(42.824005292089,-0.140814301270381,
53.0471837815254));
#261906=CARTESIAN_POINT('Ctrl Pts',(42.803937588497,0.477998516061842,53.025340855115));
#261907=CARTESIAN_POINT('Ctrl Pts',(42.7596209950149,1.68036223673757,52.7458177117104));
#261908=CARTESIAN_POINT('Ctrl Pts',(42.7368185887115,2.25178562281226,52.4879606083973));
#261909=CARTESIAN_POINT('Ctrl Pts',(42.6930698118832,3.2563675740869,51.7717238131867));
#261910=CARTESIAN_POINT('Ctrl Pts',(42.673052782406,3.68179377358338,51.3227646567323));
#261911=CARTESIAN_POINT('Ctrl Pts',(42.6288062995307,4.34323297804011,50.2806811074282));
#261912=CARTESIAN_POINT('Ctrl Pts',(42.6059792614027,4.57008234897593,49.6956812528288));
#261913=CARTESIAN_POINT('Ctrl Pts',(42.5621527543214,4.7839982734579,48.4807191874492));
#261914=CARTESIAN_POINT('Ctrl Pts',(42.5421775196057,4.77260115723484,47.8629689153095));
#261915=CARTESIAN_POINT('Ctrl Pts',(42.4980034591323,4.51390729703929,46.6562169031062));
#261916=CARTESIAN_POINT('Ctrl Pts',(42.4751531709417,4.26532764079793,46.0795264810782));
#261917=CARTESIAN_POINT('Ctrl Pts',(42.4312496794982,3.56596209792612,45.063354420355));
#261918=CARTESIAN_POINT('Ctrl Pts',(42.4113069799741,3.12519122669073,44.6312525735299));
#261919=CARTESIAN_POINT('Ctrl Pts',(42.3672074406395,2.09489088525768,43.9519179105999));
#261920=CARTESIAN_POINT('Ctrl Pts',(42.3443353961348,1.51283444959629,43.7147306798429));
#261921=CARTESIAN_POINT('Ctrl Pts',(42.3113269822488,0.603833353132325,
43.5389852708176));
#261922=CARTESIAN_POINT('Ctrl Pts',(42.3007756214429,0.301918536111562,
43.5102));
#261923=CARTESIAN_POINT('Ctrl Pts',(42.2906249999995,-1.41414657761629E-13,
43.5102));
#261924=CARTESIAN_POINT('',(42.0942499999981,-4.66218791181221,47.3519229575834));
#261925=CARTESIAN_POINT('Origin',(42.09425,-1.46971288347598E-13,48.26));
#261926=CARTESIAN_POINT('Ctrl Pts',(42.0942499999949,-4.66218791181116,
47.3519229575838));
#261927=CARTESIAN_POINT('Ctrl Pts',(42.1068206953643,-4.59479830822025,
47.0059357994818));
#261928=CARTESIAN_POINT('Ctrl Pts',(42.1196360322443,-4.48910763171995,
46.6685368854524));
#261929=CARTESIAN_POINT('Ctrl Pts',(42.1452521950012,-4.20537339562081,
46.0241402159149));
#261930=CARTESIAN_POINT('Ctrl Pts',(42.157973999885,-4.02838111187797,45.7190573960525));
#261931=CARTESIAN_POINT('Ctrl Pts',(42.1918930242666,-3.45736524908123,
44.9466976226431));
#261932=CARTESIAN_POINT('Ctrl Pts',(42.2118479691889,-3.00461394811903,
44.531241285202));
#261933=CARTESIAN_POINT('Ctrl Pts',(42.2562007886005,-1.95293188098839,
43.885339138662));
#261934=CARTESIAN_POINT('Ctrl Pts',(42.2791600006447,-1.36067932859376,
43.666508184532));
#261935=CARTESIAN_POINT('Ctrl Pts',(42.3101114315129,-0.496745708215736,
43.529668100058));
#261936=CARTESIAN_POINT('Ctrl Pts',(42.3187355945367,-0.248293869611008,
43.5102));
#261937=CARTESIAN_POINT('Ctrl Pts',(42.3270833333327,-1.57374113740616E-13,
43.5102));
#261938=CARTESIAN_POINT('Origin',(40.475,-1.41317707189676E-13,48.26));
#261939=CARTESIAN_POINT('',(44.4072916666655,-1.14616064620334E-13,43.5102));
#261940=CARTESIAN_POINT('',(43.3854166666657,-1.47405174749987E-13,43.5102));
#261941=CARTESIAN_POINT('',(40.475,-1.40736024453017E-13,43.5102));
#261942=CARTESIAN_POINT('Ctrl Pts',(44.4072916666655,-7.68829444552921E-14,
43.5102));
#261943=CARTESIAN_POINT('Ctrl Pts',(44.390373149306,-0.503221800043606,
43.5102));
#261944=CARTESIAN_POINT('Ctrl Pts',(44.3724228202082,-1.00400848126724,
43.5901712341933));
#261945=CARTESIAN_POINT('Ctrl Pts',(44.3317689812627,-2.06827713231815,
43.9400702898141));
#261946=CARTESIAN_POINT('Ctrl Pts',(44.3093144518142,-2.61018179015523,
44.2442115659873));
#261947=CARTESIAN_POINT('Ctrl Pts',(44.2664558238078,-3.55263113629584,
45.0465299325764));
#261948=CARTESIAN_POINT('Ctrl Pts',(44.245434120635,-3.94250983519268,45.5389303845271));
#261949=CARTESIAN_POINT('Ctrl Pts',(44.2005289482455,-4.50748616977311,
46.640562123251));
#261950=CARTESIAN_POINT('Ctrl Pts',(44.1780452588232,-4.67930167148466,
47.2381452413367));
#261951=CARTESIAN_POINT('Ctrl Pts',(44.1351207318422,-4.78561759298201,
48.470848328726));
#261952=CARTESIAN_POINT('Ctrl Pts',(44.1142015396868,-4.71704371069777,
49.0943336232483));
#261953=CARTESIAN_POINT('Ctrl Pts',(44.0693356980773,-4.34523111346089,
50.274806553015));
#261954=CARTESIAN_POINT('Ctrl Pts',(44.0468223876693,-4.04739745399845,
50.8210722831369));
#261955=CARTESIAN_POINT('Ctrl Pts',(44.003829825242,-3.25703080618318,51.7724559182725));
#261956=CARTESIAN_POINT('Ctrl Pts',(43.9830123427014,-2.77083588879391,
52.1674392770573));
#261957=CARTESIAN_POINT('Ctrl Pts',(43.9381885376627,-1.67739508145053,
52.7463474425375));
#261958=CARTESIAN_POINT('Ctrl Pts',(43.9156452722035,-1.08129701659063,
52.9260262159433));
#261959=CARTESIAN_POINT('Ctrl Pts',(43.8725826769129,0.149139245221818,
53.0477291476656));
#261960=CARTESIAN_POINT('Ctrl Pts',(43.8518653644044,0.771810656405597,
52.9874638415031));
#261961=CARTESIAN_POINT('Ctrl Pts',(43.8070863850711,1.95644428853696,52.6319334746694));
#261962=CARTESIAN_POINT('Ctrl Pts',(43.7845129695506,2.5073606068132,52.3410113002896));
#261963=CARTESIAN_POINT('Ctrl Pts',(43.7413785072399,3.46835273705067,51.5636520648355));
#261964=CARTESIAN_POINT('Ctrl Pts',(43.7207590458096,3.86882423654003,51.0841452638541));
#261965=CARTESIAN_POINT('Ctrl Pts',(43.676027748612,4.46269147749009,49.9996522475672));
#261966=CARTESIAN_POINT('Ctrl Pts',(43.6534241378127,4.6508483976716,49.4052710434922));
#261967=CARTESIAN_POINT('Ctrl Pts',(43.6102161612666,4.78912928491696,48.1773773978022));
#261968=CARTESIAN_POINT('Ctrl Pts',(43.5896914222037,4.73776279420102,47.5555879400912));
#261969=CARTESIAN_POINT('Ctrl Pts',(43.5450107117975,4.39973740307766,46.3666264055932));
#261970=CARTESIAN_POINT('Ctrl Pts',(43.5223770192419,4.11631541612944,45.8108105370223));
#261971=CARTESIAN_POINT('Ctrl Pts',(43.4790940907976,3.35297349292576,44.8395962919077));
#261972=CARTESIAN_POINT('Ctrl Pts',(43.4586601181008,2.88059882280426,44.4332850148768));
#261973=CARTESIAN_POINT('Ctrl Pts',(43.4140329253292,1.80578318535348,43.8235300453172));
#261974=CARTESIAN_POINT('Ctrl Pts',(43.3913694300322,1.21336611326357,43.6263311050531));
#261975=CARTESIAN_POINT('Ctrl Pts',(43.3625984281871,0.40046982445354,43.5228482498025));
#261976=CARTESIAN_POINT('Ctrl Pts',(43.355686867337,0.200132489239812,43.5102));
#261977=CARTESIAN_POINT('Ctrl Pts',(43.3489583333325,-8.88872309090516E-14,
43.5102));
#261978=CARTESIAN_POINT('Ctrl Pts',(42.3270833333327,-1.58692503582358E-13,
43.5102));
#261979=CARTESIAN_POINT('Ctrl Pts',(42.3391268191607,0.358219605675742,
43.5102));
#261980=CARTESIAN_POINT('Ctrl Pts',(42.3517222752219,0.716072144886732,
43.5507220553516));
#261981=CARTESIAN_POINT('Ctrl Pts',(42.3870580817766,1.67550713468126,43.771834687857));
#261982=CARTESIAN_POINT('Ctrl Pts',(42.4100044194964,2.25071018064939,44.0309023121474));
#261983=CARTESIAN_POINT('Ctrl Pts',(42.4537685521365,3.25541035829208,44.7479563537824));
#261984=CARTESIAN_POINT('Ctrl Pts',(42.4736799101133,3.67877054229839,45.1942548347034));
#261985=CARTESIAN_POINT('Ctrl Pts',(42.5178973195813,4.34157757559234,46.2349070557574));
#261986=CARTESIAN_POINT('Ctrl Pts',(42.540829050309,4.56986676457151,46.8224244789149));
#261987=CARTESIAN_POINT('Ctrl Pts',(42.5846736373396,4.78365346537182,48.0379778377521));
#261988=CARTESIAN_POINT('Ctrl Pts',(42.6045767469768,4.77261296903086,48.6534449009786));
#261989=CARTESIAN_POINT('Ctrl Pts',(42.6487233031513,4.51547977408557,49.8600252782213));
#261990=CARTESIAN_POINT('Ctrl Pts',(42.671638691677,4.2665792047384,50.4385191081282));
#261991=CARTESIAN_POINT('Ctrl Pts',(42.715562820233,3.5670288607229,51.4552284488377));
#261992=CARTESIAN_POINT('Ctrl Pts',(42.7354671391831,3.12734152872271,51.8866946633223));
#261993=CARTESIAN_POINT('Ctrl Pts',(42.779541005205,2.09805709469439,52.5666383944541));
#261994=CARTESIAN_POINT('Ctrl Pts',(42.8024383362143,1.51551485277587,52.8044685584805));
#261995=CARTESIAN_POINT('Ctrl Pts',(42.8464407839502,0.303969126019783,
53.0392662005292));
#261996=CARTESIAN_POINT('Ctrl Pts',(42.8663559369636,-0.312565072840083,
53.0387117164381));
#261997=CARTESIAN_POINT('Ctrl Pts',(42.9103555026472,-1.52316486228873,
52.8018373341256));
#261998=CARTESIAN_POINT('Ctrl Pts',(42.9332331024559,-2.10481239179906,
52.5632640013233));
#261999=CARTESIAN_POINT('Ctrl Pts',(42.9773123779921,-3.13351782190955,
51.8815339846769));
#262000=CARTESIAN_POINT('Ctrl Pts',(42.9972479789687,-3.5731893320044,51.4485358354931));
#262001=CARTESIAN_POINT('Ctrl Pts',(43.0411719049501,-4.27027386260167,
50.430811146772));
#262002=CARTESIAN_POINT('Ctrl Pts',(43.0640281646247,-4.51759478199554,
49.8534217239611));
#262003=CARTESIAN_POINT('Ctrl Pts',(43.1081824830168,-4.7734775994132,48.6460925451697));
#262004=CARTESIAN_POINT('Ctrl Pts',(43.1281480926504,-4.7834671271449,48.0284855337753));
#262005=CARTESIAN_POINT('Ctrl Pts',(43.1719952818798,-4.5668549003936,46.8140251467023));
#262006=CARTESIAN_POINT('Ctrl Pts',(43.1948286809473,-4.33862772648435,
46.2294067979673));
#262007=CARTESIAN_POINT('Ctrl Pts',(43.2390560053496,-3.67480020980593,
45.1888823666758));
#262008=CARTESIAN_POINT('Ctrl Pts',(43.2590609647297,-3.24848507962646,
44.7410135082265));
#262009=CARTESIAN_POINT('Ctrl Pts',(43.3028305952225,-2.24235732064402,
44.027011163012));
#262010=CARTESIAN_POINT('Ctrl Pts',(43.3256397201589,-1.67022655307121,
43.7703793781029));
#262011=CARTESIAN_POINT('Ctrl Pts',(43.3608198337942,-0.714876476888766,
43.5505848889162));
#262012=CARTESIAN_POINT('Ctrl Pts',(43.3733935813015,-0.357612817396849,
43.5102));
#262013=CARTESIAN_POINT('Ctrl Pts',(43.3854166666658,-1.35585986882347E-13,
43.5102));
#262014=CARTESIAN_POINT('Origin',(40.475,-1.41317707189676E-13,48.26));
#262015=CARTESIAN_POINT('',(45.4656249999985,-1.50815726624334E-13,43.5102));
#262016=CARTESIAN_POINT('',(44.4437499999988,-1.09371457579084E-13,43.5102));
#262017=CARTESIAN_POINT('',(40.475,-1.40736024453017E-13,43.5102));
#262018=CARTESIAN_POINT('Ctrl Pts',(45.4656249999985,-1.42941214420489E-13,
43.5102));
#262019=CARTESIAN_POINT('Ctrl Pts',(45.4465902340685,-0.566167174768725,
43.5102));
#262020=CARTESIAN_POINT('Ctrl Pts',(45.4262808000091,-1.12831666969857,
43.611430906197));
#262021=CARTESIAN_POINT('Ctrl Pts',(45.3833509845901,-2.23435532889645,
44.023921560264));
#262022=CARTESIAN_POINT('Ctrl Pts',(45.3611023288805,-2.76208488292788,
44.3475011828492));
#262023=CARTESIAN_POINT('Ctrl Pts',(45.3186849235856,-3.67593158760918,
45.1871891138994));
#262024=CARTESIAN_POINT('Ctrl Pts',(45.2968843047985,-4.04943203210985,
45.6993730995744));
#262025=CARTESIAN_POINT('Ctrl Pts',(45.2517488041455,-4.5696569085595,46.8263923479332));
#262026=CARTESIAN_POINT('Ctrl Pts',(45.229477640157,-4.71644566319307,47.428020559987));
#262027=CARTESIAN_POINT('Ctrl Pts',(45.1870137044426,-4.7736692402272,48.6673586058746));
#262028=CARTESIAN_POINT('Ctrl Pts',(45.1653022980402,-4.67825065771647,
49.293389621709));
#262029=CARTESIAN_POINT('Ctrl Pts',(45.1201885041776,-4.25428195262979,
50.4596338382426));
#262030=CARTESIAN_POINT('Ctrl Pts',(45.097893833954,-3.93474684068756,50.9904073321236));
#262031=CARTESIAN_POINT('Ctrl Pts',(45.055380912789,-3.10290584598713,51.9103453537364));
#262032=CARTESIAN_POINT('Ctrl Pts',(45.0337617192976,-2.59492452463785,
52.2873404412951));
#262033=CARTESIAN_POINT('Ctrl Pts',(44.9886714132759,-1.47320517645412,
52.8171150725375));
#262034=CARTESIAN_POINT('Ctrl Pts',(44.9663522622886,-0.87234891209692,
52.9692133241849));
#262035=CARTESIAN_POINT('Ctrl Pts',(44.9237878756165,0.365654927904257,
53.0368711415337));
#262036=CARTESIAN_POINT('Ctrl Pts',(44.9022636356118,0.991153230745726,
52.9472027181652));
#262037=CARTESIAN_POINT('Ctrl Pts',(44.8571987189914,2.16054571570894,52.5343443824201));
#262038=CARTESIAN_POINT('Ctrl Pts',(44.8348541472401,2.69469457492858,52.2193747943591));
#262039=CARTESIAN_POINT('Ctrl Pts',(44.7922358051748,3.6214179089656,51.3963449289351));
#262040=CARTESIAN_POINT('Ctrl Pts',(44.7708089405814,4.00230089366428,50.8930517722625));
#262041=CARTESIAN_POINT('Ctrl Pts',(44.7257714374295,4.54270093040375,49.7773041716469));
#262042=CARTESIAN_POINT('Ctrl Pts',(44.7034005514389,4.7007270027171,49.1773644929559));
#262043=CARTESIAN_POINT('Ctrl Pts',(44.6607257712771,4.78002074245624,47.940896882699));
#262044=CARTESIAN_POINT('Ctrl Pts',(44.6393983237826,4.69673585831531,47.3159985829072));
#262045=CARTESIAN_POINT('Ctrl Pts',(44.5943903813102,4.29625205794682,46.1431750279315));
#262046=CARTESIAN_POINT('Ctrl Pts',(44.5719923468965,3.98640446044065,45.6053143854802));
#262047=CARTESIAN_POINT('Ctrl Pts',(44.5292586718744,3.17320321784598,44.6710894566896));
#262048=CARTESIAN_POINT('Ctrl Pts',(44.5080322394463,2.67510132706706,44.2859131457229));
#262049=CARTESIAN_POINT('Ctrl Pts',(44.463056127013,1.56603926024906,43.7337811473309));
#262050=CARTESIAN_POINT('Ctrl Pts',(44.4406301826481,0.967183012352598,
43.5691858099602));
#262051=CARTESIAN_POINT('Ctrl Pts',(44.4152792766867,0.235766499055907,
43.5145836208336));
#262052=CARTESIAN_POINT('Ctrl Pts',(44.4112527733547,0.117818553244039,
43.5102));
#262053=CARTESIAN_POINT('Ctrl Pts',(44.4072916666655,-7.47318873450808E-14,
43.5102));
#262054=CARTESIAN_POINT('Ctrl Pts',(43.3854166666658,-1.37945210809676E-13,
43.5102));
#262055=CARTESIAN_POINT('Ctrl Pts',(43.3939205687891,0.252938767799535,
43.5102));
#262056=CARTESIAN_POINT('Ctrl Pts',(43.4027110535074,0.506033130485796,
43.530403283693));
#262057=CARTESIAN_POINT('Ctrl Pts',(43.4336826313524,1.3695165685671,43.6697769184864));
#262058=CARTESIAN_POINT('Ctrl Pts',(43.4564661935627,1.95688726194218,43.8877806596037));
#262059=CARTESIAN_POINT('Ctrl Pts',(43.5008325659325,3.00889875965012,44.5338607011944));
#262060=CARTESIAN_POINT('Ctrl Pts',(43.520942739417,3.46485166643091,44.9535835508839));
#262061=CARTESIAN_POINT('Ctrl Pts',(43.5645559399502,4.19533395069807,45.9482322667419));
#262062=CARTESIAN_POINT('Ctrl Pts',(43.5873127911785,4.46097731607732,46.5150754942648));
#262063=CARTESIAN_POINT('Ctrl Pts',(43.6317448550053,4.75813933136105,47.7135674873043));
#262064=CARTESIAN_POINT('Ctrl Pts',(43.6519198657491,4.78885255595582,48.3332802923877));
#262065=CARTESIAN_POINT('Ctrl Pts',(43.6954547796803,4.61172004566973,49.5548054446156));
#262066=CARTESIAN_POINT('Ctrl Pts',(43.7181839244842,4.40368282860139,50.1446858243819));
#262067=CARTESIAN_POINT('Ctrl Pts',(43.7626789442841,3.77496669459671,51.2077161576492));
#262068=CARTESIAN_POINT('Ctrl Pts',(43.7829261062389,3.36166674266077,51.67153927919));
#262069=CARTESIAN_POINT('Ctrl Pts',(43.8263830720853,2.37823063200775,52.4178722866199));
#262070=CARTESIAN_POINT('Ctrl Pts',(43.8490836771301,1.81662634707887,52.6921246523139));
#262071=CARTESIAN_POINT('Ctrl Pts',(43.8936388223165,0.622625619815621,
53.0089677686193));
#262072=CARTESIAN_POINT('Ctrl Pts',(43.9139647275047,0.00191039525560578,
53.0496087451274));
#262073=CARTESIAN_POINT('Ctrl Pts',(43.9573443645712,-1.22275842556398,
52.8912158432986));
#262074=CARTESIAN_POINT('Ctrl Pts',(43.9800157646236,-1.81489342511969,
52.692768295012));
#262075=CARTESIAN_POINT('Ctrl Pts',(44.0246281409167,-2.88836171452507,
52.0808244812212));
#262076=CARTESIAN_POINT('Ctrl Pts',(44.0450386063447,-3.35975143565501,
51.6737076021874));
#262077=CARTESIAN_POINT('Ctrl Pts',(44.0883418029553,-4.12114558046663,
50.7010837075983));
#262078=CARTESIAN_POINT('Ctrl Pts',(44.110983503581,-4.40352124979238,50.1445962492606));
#262079=CARTESIAN_POINT('Ctrl Pts',(44.1556501829778,-4.73911767096824,
48.9550459386729));
#262080=CARTESIAN_POINT('Ctrl Pts',(44.1761502153232,-4.78925197630396,
48.3333793250293));
#262081=CARTESIAN_POINT('Ctrl Pts',(44.2193781136555,-4.64866775580551,
47.1058472006399));
#262082=CARTESIAN_POINT('Ctrl Pts',(44.2419897907381,-4.45933251113791,
46.5117141522488));
#262083=CARTESIAN_POINT('Ctrl Pts',(44.286707839491,-3.86339106873334,45.4284743580556));
#262084=CARTESIAN_POINT('Ctrl Pts',(44.3073016172268,-3.46215786932346,
44.9498969868947));
#262085=CARTESIAN_POINT('Ctrl Pts',(44.3504555952403,-2.49983219569656,
44.1743558263898));
#262086=CARTESIAN_POINT('Ctrl Pts',(44.3730370915411,-1.94827382197323,
43.8844034463062));
#262087=CARTESIAN_POINT('Ctrl Pts',(44.4120410312371,-0.915635083605541,
43.5766189918152));
#262088=CARTESIAN_POINT('Ctrl Pts',(44.428331374608,-0.458609242081003,
43.5102));
#262089=CARTESIAN_POINT('Ctrl Pts',(44.4437499999988,-5.89805981832114E-14,
43.5102));
#262090=CARTESIAN_POINT('Origin',(40.475,-1.41317707189676E-13,48.26));
#262091=CARTESIAN_POINT('',(46.5239583333315,-1.62531318710601E-13,43.5102));
#262092=CARTESIAN_POINT('',(45.5020833333317,-1.42870944908646E-13,43.5102));
#262093=CARTESIAN_POINT('',(40.475,-1.40736024453017E-13,43.5102));
#262094=CARTESIAN_POINT('Ctrl Pts',(46.5239583333315,-1.62370117351429E-13,
43.5102));
#262095=CARTESIAN_POINT('Ctrl Pts',(46.5036008374102,-0.605510253896953,
43.5102));
#262096=CARTESIAN_POINT('Ctrl Pts',(46.4818076969026,-1.20576070108166,
43.6259890631562));
#262097=CARTESIAN_POINT('Ctrl Pts',(46.4374905918229,-2.33611695352889,
44.0793903497508));
#262098=CARTESIAN_POINT('Ctrl Pts',(46.4153861300924,-2.85467272875886,
44.4147631522864));
#262099=CARTESIAN_POINT('Ctrl Pts',(46.3732591906852,-3.75030468937599,
45.2775675910213));
#262100=CARTESIAN_POINT('Ctrl Pts',(46.350867950729,-4.11332423204566,45.8022845225455));
#262101=CARTESIAN_POINT('Ctrl Pts',(46.3056097860154,-4.60492983715441,
46.9448067623493));
#262102=CARTESIAN_POINT('Ctrl Pts',(46.283490643379,-4.73591436814603,47.5484595982699));
#262103=CARTESIAN_POINT('Ctrl Pts',(46.2413346731749,-4.76199965834225,
48.7915354657041));
#262104=CARTESIAN_POINT('Ctrl Pts',(46.2190049601663,-4.64927095256036,
49.4191198129382));
#262105=CARTESIAN_POINT('Ctrl Pts',(46.1737580864563,-4.19207402121399,
50.5755587541874));
#262106=CARTESIAN_POINT('Ctrl Pts',(46.1516233565398,-3.85907637047691,
51.0959986418156));
#262107=CARTESIAN_POINT('Ctrl Pts',(46.1094364386808,-3.00095705659985,
51.9953552346118));
#262108=CARTESIAN_POINT('Ctrl Pts',(46.0871717251068,-2.47879870234449,
52.3605222090012));
#262109=CARTESIAN_POINT('Ctrl Pts',(46.0419371201451,-1.33940444906901,
52.8579876629451));
#262110=CARTESIAN_POINT('Ctrl Pts',(46.01978586708,-0.736131320341421,52.9921946738508));
#262111=CARTESIAN_POINT('Ctrl Pts',(45.9775659990635,0.506210804173913,
53.0246397502708));
#262112=CARTESIAN_POINT('Ctrl Pts',(45.9553698123262,1.13348286507559,52.9154651892213));
#262113=CARTESIAN_POINT('Ctrl Pts',(45.9101485354608,2.29197503236145,52.4650632422377));
#262114=CARTESIAN_POINT('Ctrl Pts',(45.8879797972532,2.81455697175497,52.1347948945605));
#262115=CARTESIAN_POINT('Ctrl Pts',(45.8457248934765,3.71815798027413,51.2820405739011));
#262116=CARTESIAN_POINT('Ctrl Pts',(45.8236007922176,4.08576925695497,50.7628005139269));
#262117=CARTESIAN_POINT('Ctrl Pts',(45.7783939899705,4.58990752858193,49.6269971919372));
#262118=CARTESIAN_POINT('Ctrl Pts',(45.7562067826859,4.72779263414618,49.0241781630782));
#262119=CARTESIAN_POINT('Ctrl Pts',(45.713914678184,4.76748967906392,47.782691311264));
#262120=CARTESIAN_POINT('Ctrl Pts',(45.6918662243994,4.6623560474797,47.155778630674));
#262121=CARTESIAN_POINT('Ctrl Pts',(45.6466751360762,4.21969723649481,45.9949770748332));
#262122=CARTESIAN_POINT('Ctrl Pts',(45.6244684589117,3.892553992568,45.469972224536));
#262123=CARTESIAN_POINT('Ctrl Pts',(45.5821369144204,3.04591872211625,44.5615570327062));
#262124=CARTESIAN_POINT('Ctrl Pts',(45.5601676411215,2.52999210496053,44.1911767212705));
#262125=CARTESIAN_POINT('Ctrl Pts',(45.5149936043689,1.39829579747449,43.6794760641619));
#262126=CARTESIAN_POINT('Ctrl Pts',(45.4927664456731,0.796019569018646,
43.5374116915684));
#262127=CARTESIAN_POINT('Ctrl Pts',(45.4697508383311,0.122230094171664,
43.5113786479076));
#262128=CARTESIAN_POINT('Ctrl Pts',(45.4676789441933,0.0610922028778175,
43.5102));
#262129=CARTESIAN_POINT('Ctrl Pts',(45.4656249999985,-1.43470754738992E-13,
43.5102));
#262130=CARTESIAN_POINT('Ctrl Pts',(44.4437499999988,-5.99173488602389E-14,
43.5102));
#262131=CARTESIAN_POINT('Ctrl Pts',(44.4490830245783,0.158624669738691,
43.5102));
#262132=CARTESIAN_POINT('Ctrl Pts',(44.4545328214474,0.317431308338911,
43.5181458728695));
#262133=CARTESIAN_POINT('Ctrl Pts',(44.4815761187494,1.08959979877602,43.5958913234831));
#262134=CARTESIAN_POINT('Ctrl Pts',(44.5041274378078,1.68548201395458,43.7766695169645));
#262135=CARTESIAN_POINT('Ctrl Pts',(44.5489395260635,2.77776933644252,44.3575210824724));
#262136=CARTESIAN_POINT('Ctrl Pts',(44.5697300255303,3.26309684251997,44.7532169626168));
#262137=CARTESIAN_POINT('Ctrl Pts',(44.612741135947,4.0517839323666,45.705847982011));
#262138=CARTESIAN_POINT('Ctrl Pts',(44.6352624336814,4.34872785466118,46.2527198271492));
#262139=CARTESIAN_POINT('Ctrl Pts',(44.6801172971881,4.71843598020359,47.4337379266194));
#262140=CARTESIAN_POINT('Ctrl Pts',(44.7010091685603,4.78593419842796,48.0571184351156));
#262141=CARTESIAN_POINT('Ctrl Pts',(44.743951694488,4.67763124679665,49.2895338255994));
#262142=CARTESIAN_POINT('Ctrl Pts',(44.7664432688965,4.50480069578187,49.8869310263233));
#262143=CARTESIAN_POINT('Ctrl Pts',(44.8113381781625,3.93802269070928,50.9875112239144));
#262144=CARTESIAN_POINT('Ctrl Pts',(44.832332415779,3.54748413748238,51.4791104293721));
#262145=CARTESIAN_POINT('Ctrl Pts',(44.8752084588664,2.60388019462774,52.279891895045));
#262146=CARTESIAN_POINT('Ctrl Pts',(44.8976707382443,2.06141002983677,52.5832244235893));
#262147=CARTESIAN_POINT('Ctrl Pts',(44.9420768352923,0.898155571040059,
52.9635927494964));
#262148=CARTESIAN_POINT('Ctrl Pts',(44.9627764100013,0.289169763904942,
53.039833984679));
#262149=CARTESIAN_POINT('Ctrl Pts',(45.005495989191,-0.94715505118126,52.9569785783005));
#262150=CARTESIAN_POINT('Ctrl Pts',(45.0284962665617,-1.56201031345564,
52.7897665739478));
#262151=CARTESIAN_POINT('Ctrl Pts',(45.0734758495259,-2.6701092429633,52.2350601445217));
#262152=CARTESIAN_POINT('Ctrl Pts',(45.0942529077285,-3.1566752646787,51.8608257934969));
#262153=CARTESIAN_POINT('Ctrl Pts',(45.1369115840167,-3.97741086967365,
50.9319524507001));
#262154=CARTESIAN_POINT('Ctrl Pts',(45.1599088389435,-4.29692068711041,
50.3802709072346));
#262155=CARTESIAN_POINT('Ctrl Pts',(45.2049197616781,-4.69422254308849,
49.2060407032733));
#262156=CARTESIAN_POINT('Ctrl Pts',(45.2257736105639,-4.77667886664448,
48.5976543478092));
#262157=CARTESIAN_POINT('Ctrl Pts',(45.2683740367194,-4.70627373513496,
47.3597165296944));
#262158=CARTESIAN_POINT('Ctrl Pts',(45.2913678851307,-4.54499228938495,
46.7425959716021));
#262159=CARTESIAN_POINT('Ctrl Pts',(45.3364080181532,-4.00068514395075,
45.6283885259276));
#262160=CARTESIAN_POINT('Ctrl Pts',(45.3573375096765,-3.63101697737368,
45.138057673055));
#262161=CARTESIAN_POINT('Ctrl Pts',(45.3998823651131,-2.70942297072614,
44.3079214437151));
#262162=CARTESIAN_POINT('Ctrl Pts',(45.4228725062249,-2.16022155508338,
43.982934896878));
#262163=CARTESIAN_POINT('Ctrl Pts',(45.4651887079935,-1.06039337333246,
43.5995131929409));
#262164=CARTESIAN_POINT('Ctrl Pts',(45.4842039863065,-0.531800571084733,
43.5102));
#262165=CARTESIAN_POINT('Ctrl Pts',(45.5020833333318,-1.29618538124987E-13,
43.5102));
#262166=CARTESIAN_POINT('Origin',(40.475,-1.41317707189676E-13,48.26));
#262167=CARTESIAN_POINT('',(47.5822916659101,-1.12196777507983E-8,43.5102));
#262168=CARTESIAN_POINT('',(46.5604166666648,-1.64744021012041E-13,43.5102));
#262169=CARTESIAN_POINT('',(40.475,-1.40736024453017E-13,43.5102));
#262170=CARTESIAN_POINT('Ctrl Pts',(47.5822916662868,-1.12323599033015E-8,
43.5102));
#262171=CARTESIAN_POINT('Ctrl Pts',(47.5619423247769,-0.605267720969552,
43.5102000014313));
#262172=CARTESIAN_POINT('Ctrl Pts',(47.5401645011038,-1.20510137850486,
43.625895412559));
#262173=CARTESIAN_POINT('Ctrl Pts',(47.4950292970466,-2.35644830837556,
44.0873667724118));
#262174=CARTESIAN_POINT('Ctrl Pts',(47.4721044817229,-2.89251300407696,
44.4393772525012));
#262175=CARTESIAN_POINT('Ctrl Pts',(47.4301570353803,-3.77706893480709,
45.3160325548263));
#262176=CARTESIAN_POINT('Ctrl Pts',(47.4082806115085,-4.12379833993764,
45.8253303490187));
#262177=CARTESIAN_POINT('Ctrl Pts',(47.3629657401008,-4.61505081519561,
46.9696855352567));
#262178=CARTESIAN_POINT('Ctrl Pts',(47.3400383819616,-4.7460112676243,47.5973877834964));
#262179=CARTESIAN_POINT('Ctrl Pts',(47.298073272432,-4.75328333135358,48.8425794136922));
#262180=CARTESIAN_POINT('Ctrl Pts',(47.2762280767327,-4.63917883647766,
49.4479616397681));
#262181=CARTESIAN_POINT('Ctrl Pts',(47.2309203610855,-4.17905205326832,
50.6049966699415));
#262182=CARTESIAN_POINT('Ctrl Pts',(47.207990303116,-3.82862449556926,51.1418729700229));
#262183=CARTESIAN_POINT('Ctrl Pts',(47.1660061719569,-2.95470207981842,
52.0286520470236));
#262184=CARTESIAN_POINT('Ctrl Pts',(47.144194401308,-2.44653487105249,52.3767460972433));
#262185=CARTESIAN_POINT('Ctrl Pts',(47.0988944542651,-1.30394588441433,
52.8711908667363));
#262186=CARTESIAN_POINT('Ctrl Pts',(47.0759615361057,-0.676834674480039,
53.0039774657885));
#262187=CARTESIAN_POINT('Ctrl Pts',(47.0339569365298,0.567965482807333,
53.0150303299691));
#262188=CARTESIAN_POINT('Ctrl Pts',(47.0121808943154,1.17352631992653,52.9028288165141));
#262189=CARTESIAN_POINT('Ctrl Pts',(46.9668893795248,2.33164582654647,52.4464835421591));
#262190=CARTESIAN_POINT('Ctrl Pts',(46.9439534386922,2.8694611262,52.0979004933294));
#262191=CARTESIAN_POINT('Ctrl Pts',(46.9019268325604,3.75882201964883,51.2271610910262));
#262192=CARTESIAN_POINT('Ctrl Pts',(46.8801889252566,4.10850263838954,50.7203080174567));
#262193=CARTESIAN_POINT('Ctrl Pts',(46.8349065609813,4.60665335937256,49.5797770653415));
#262194=CARTESIAN_POINT('Ctrl Pts',(46.8119674343812,4.7415598214872,48.9533592685245));
#262195=CARTESIAN_POINT('Ctrl Pts',(46.7699171895906,4.75700467169273,47.70902066711));
#262196=CARTESIAN_POINT('Ctrl Pts',(46.7482199214303,4.64701236019363,47.1032521937931));
#262197=CARTESIAN_POINT('Ctrl Pts',(46.7029474845507,4.19505684768359,45.9438818387573));
#262198=CARTESIAN_POINT('Ctrl Pts',(46.6800050103184,3.84861779247109,45.4049841394255));
#262199=CARTESIAN_POINT('Ctrl Pts',(46.6379293986921,2.98157626632718,44.5126339235632));
#262200=CARTESIAN_POINT('Ctrl Pts',(46.6162753641057,2.47624632147946,44.1611138927456));
#262201=CARTESIAN_POINT('Ctrl Pts',(46.5710136942996,1.33810750007012,43.6586740858176));
#262202=CARTESIAN_POINT('Ctrl Pts',(46.5480677140097,0.71250200241092,43.5213144103002));
#262203=CARTESIAN_POINT('Ctrl Pts',(46.5257182038233,0.0522560520112886,
43.5104155107889));
#262204=CARTESIAN_POINT('Ctrl Pts',(46.5248366067607,0.0261232309295294,
43.5102));
#262205=CARTESIAN_POINT('Ctrl Pts',(46.5239583333315,-1.6320678782792E-13,
43.5102));
#262206=CARTESIAN_POINT('Ctrl Pts',(45.5020833333317,-1.27453897717139E-13,
43.5102));
#262207=CARTESIAN_POINT('Ctrl Pts',(45.5046240043241,0.0755693305096932,
43.5102));
#262208=CARTESIAN_POINT('Ctrl Pts',(45.5071919115641,0.151201761329515,
43.5120034428537));
#262209=CARTESIAN_POINT('Ctrl Pts',(45.5314353880609,0.858292825627946,
43.5458101658758));
#262210=CARTESIAN_POINT('Ctrl Pts',(45.5544215964756,1.47739253944832,43.7017648941488));
#262211=CARTESIAN_POINT('Ctrl Pts',(45.5995141893975,2.5970258903536,44.2367397860434));
#262212=CARTESIAN_POINT('Ctrl Pts',(45.6205900058756,3.09072149426274,44.6023308982021));
#262213=CARTESIAN_POINT('Ctrl Pts',(45.663031759178,3.92921331639899,45.5173972508389));
#262214=CARTESIAN_POINT('Ctrl Pts',(45.6860138769148,4.25906430353926,46.0643451032907));
#262215=CARTESIAN_POINT('Ctrl Pts',(45.731129935053,4.67725347513067,47.2330506292525));
#262216=CARTESIAN_POINT('Ctrl Pts',(45.7522758227053,4.77024273033945,47.840428588214));
#262217=CARTESIAN_POINT('Ctrl Pts',(45.7946699987671,4.72090364611286,49.0809575774851));
#262218=CARTESIAN_POINT('Ctrl Pts',(45.8176479274089,4.56969597499951,49.7017773144619));
#262219=CARTESIAN_POINT('Ctrl Pts',(45.8627857499861,4.04303230143915,50.8261985886924));
#262220=CARTESIAN_POINT('Ctrl Pts',(45.8839993325933,3.68105632465102,51.3228801778135));
#262221=CARTESIAN_POINT('Ctrl Pts',(45.9263485235756,2.7717992805151,52.1687501962364));
#262222=CARTESIAN_POINT('Ctrl Pts',(45.9493222166804,2.22687990283323,52.5028933987062));
#262223=CARTESIAN_POINT('Ctrl Pts',(45.9944802071712,1.06053286026028,52.9297875312546));
#262224=CARTESIAN_POINT('Ctrl Pts',(46.0157589354208,0.453572105348301,
53.0271624369284));
#262225=CARTESIAN_POINT('Ctrl Pts',(46.0580656740932,-0.787983361553054,
52.9865801929745));
#262226=CARTESIAN_POINT('Ctrl Pts',(46.0810351299837,-1.41029123865711,
52.8395736212652));
#262227=CARTESIAN_POINT('Ctrl Pts',(46.126211793147,-2.53891297590829,52.3202616976962));
#262228=CARTESIAN_POINT('Ctrl Pts',(46.1475529902292,-3.03822772092515,
51.9614714595661));
#262229=CARTESIAN_POINT('Ctrl Pts',(46.1898197392216,-3.89057513217457,
51.0573495813617));
#262230=CARTESIAN_POINT('Ctrl Pts',(46.2127849942371,-4.22848369300958,
50.5142408474223));
#262231=CARTESIAN_POINT('Ctrl Pts',(46.2579789325657,-4.66303233929073,
49.3499951812442));
#262232=CARTESIAN_POINT('Ctrl Pts',(46.2793798352095,-4.76426216006541,
48.7433999159247));
#262233=CARTESIAN_POINT('Ctrl Pts',(46.32160897825,-4.73136914703602,47.5009674579309));
#262234=CARTESIAN_POINT('Ctrl Pts',(46.3445701005156,-4.58805767250563,
46.877376895531));
#262235=CARTESIAN_POINT('Ctrl Pts',(46.3897800102523,-4.0752097067891,45.7450888182613));
#262236=CARTESIAN_POINT('Ctrl Pts',(46.4112378051486,-3.71921141673633,
45.2434650441401));
#262237=CARTESIAN_POINT('Ctrl Pts',(46.4534316401483,-2.81960171713258,
44.3854600781061));
#262238=CARTESIAN_POINT('Ctrl Pts',(46.4763887238927,-2.27809729632209,
44.0442651253932));
#262239=CARTESIAN_POINT('Ctrl Pts',(46.5204002356443,-1.14689194172171,
43.6148577984356));
#262240=CARTESIAN_POINT('Ctrl Pts',(46.5410623551547,-0.575671689767508,
43.5102));
#262241=CARTESIAN_POINT('Ctrl Pts',(46.5604166666647,-1.66949787328008E-13,
43.5102));
#262242=CARTESIAN_POINT('Origin',(40.475,-1.41317707189676E-13,48.26));
#262243=CARTESIAN_POINT('',(48.640625002023,3.01226086749755E-8,43.5102));
#262244=CARTESIAN_POINT('',(47.6187499976816,-3.44458056410151E-8,43.5102));
#262245=CARTESIAN_POINT('',(40.475,-1.40736024453017E-13,43.5102));
#262246=CARTESIAN_POINT('Ctrl Pts',(48.6406250010114,3.01567474912057E-8,
43.5102));
#262247=CARTESIAN_POINT('Ctrl Pts',(48.6403402808376,-0.00846864324612915,
43.5101999999462));
#262248=CARTESIAN_POINT('Ctrl Pts',(48.6400552091581,-0.0169383903995125,
43.5102226487671));
#262249=CARTESIAN_POINT('Ctrl Pts',(48.6191798718932,-0.636478416209216,
43.5135369343409));
#262250=CARTESIAN_POINT('Ctrl Pts',(48.5971621151167,-1.24118429143203,
43.6346988877366));
#262251=CARTESIAN_POINT('Ctrl Pts',(48.5518367752532,-2.39313666806122,
44.1083618417949));
#262252=CARTESIAN_POINT('Ctrl Pts',(48.5290407974581,-2.92566350708343,
44.4647992630245));
#262253=CARTESIAN_POINT('Ctrl Pts',(48.4870990846606,-3.80266330856524,
45.349041959842));
#262254=CARTESIAN_POINT('Ctrl Pts',(48.4650895774633,-4.14518439984186,
45.8618125037741));
#262255=CARTESIAN_POINT('Ctrl Pts',(48.4197592212302,-4.62633837758331,
47.0108112029288));
#262256=CARTESIAN_POINT('Ctrl Pts',(48.3969299909334,-4.75166011105822,
47.6394713519076));
#262257=CARTESIAN_POINT('Ctrl Pts',(48.3550030935466,-4.74796833627022,
48.8850094101939));
#262258=CARTESIAN_POINT('Ctrl Pts',(48.3330012731708,-4.62830538735032,
49.4898621835297));
#262259=CARTESIAN_POINT('Ctrl Pts',(48.2876663003645,-4.15739165130443,
50.6432398443229));
#262260=CARTESIAN_POINT('Ctrl Pts',(48.2648060457194,-3.80196381608403,
51.1769600772513));
#262261=CARTESIAN_POINT('Ctrl Pts',(48.2228929205492,-2.91946417246145,
52.0561151610514));
#262262=CARTESIAN_POINT('Ctrl Pts',(48.200898257452,-2.40758203843062,52.3997151384207));
#262263=CARTESIAN_POINT('Ctrl Pts',(48.1555590355424,-1.25945421064565,
52.8836082121268));
#262264=CARTESIAN_POINT('Ctrl Pts',(48.1326698594116,-0.630673758570354,
53.0103761234247));
#262265=CARTESIAN_POINT('Ctrl Pts',(48.0907695298135,0.615133469116345,
53.0092419608279));
#262266=CARTESIAN_POINT('Ctrl Pts',(48.0687815264716,1.22010977350227,52.8908694158124));
#262267=CARTESIAN_POINT('Ctrl Pts',(48.023441724036,2.3746266275441,52.4223591295305));
#262268=CARTESIAN_POINT('Ctrl Pts',(48.0005256061278,2.90939118846583,52.0678343904391));
#262269=CARTESIAN_POINT('Ctrl Pts',(47.9586368751837,3.79040161835962,51.1868357272435));
#262270=CARTESIAN_POINT('Ctrl Pts',(47.936655342557,4.13495748899571,50.6757367096215));
#262271=CARTESIAN_POINT('Ctrl Pts',(47.8913170826427,4.62111654763343,49.5285760969697));
#262272=CARTESIAN_POINT('Ctrl Pts',(47.8683990003311,4.74916318677365,48.8999428065474));
#262273=CARTESIAN_POINT('Ctrl Pts',(47.8264972255023,4.75040751120774,47.6541382226684));
#262274=CARTESIAN_POINT('Ctrl Pts',(47.804539214751,4.6332666990795,47.0490405340912));
#262275=CARTESIAN_POINT('Ctrl Pts',(47.7592060980522,4.1671060394343,45.8937492923668));
#262276=CARTESIAN_POINT('Ctrl Pts',(47.7362859153077,3.81374001495502,45.3583838722651));
#262277=CARTESIAN_POINT('Ctrl Pts',(47.694370056637,2.93474341586611,44.4757372773047));
#262278=CARTESIAN_POINT('Ctrl Pts',(47.6724373335368,2.4244753413614,44.1301787960157));
#262279=CARTESIAN_POINT('Ctrl Pts',(47.6271098037818,1.27860763790808,43.64166888973));
#262280=CARTESIAN_POINT('Ctrl Pts',(47.6041873785707,0.650402238452378,
43.5122773754931));
#262281=CARTESIAN_POINT('Ctrl Pts',(47.5826358605589,0.0102342257254587,
43.5102082686246));
#262282=CARTESIAN_POINT('Ctrl Pts',(47.5824636994493,0.00511691691828377,
43.5101999999879));
#262283=CARTESIAN_POINT('Ctrl Pts',(47.5822916662868,-1.12323625723863E-8,
43.5102));
#262284=CARTESIAN_POINT('Ctrl Pts',(46.5604166666647,-1.63817944252533E-13,
43.5102));
#262285=CARTESIAN_POINT('Ctrl Pts',(46.5615367790316,0.0333164514072579,
43.5102));
#262286=CARTESIAN_POINT('Ctrl Pts',(46.5626622633208,0.0666474877714339,
43.5105505358004));
#262287=CARTESIAN_POINT('Ctrl Pts',(46.5852859802539,0.733745769366106,
43.5245966824768));
#262288=CARTESIAN_POINT('Ctrl Pts',(46.6082391406889,1.35843845899938,43.6646756633591));
#262289=CARTESIAN_POINT('Ctrl Pts',(46.6534774353482,2.49391246938954,44.1718703706478));
#262290=CARTESIAN_POINT('Ctrl Pts',(46.6750405296683,2.99755105650663,44.5254336623452));
#262291=CARTESIAN_POINT('Ctrl Pts',(46.7171702744803,3.86047541902424,45.4210993924374));
#262292=CARTESIAN_POINT('Ctrl Pts',(46.7401196432355,4.20452601484771,45.9611914936831));
#262293=CARTESIAN_POINT('Ctrl Pts',(46.7853705168101,4.65159836673637,47.1219431444179));
#262294=CARTESIAN_POINT('Ctrl Pts',(46.8069820603205,4.75913295039603,47.7279429848354));
#262295=CARTESIAN_POINT('Ctrl Pts',(46.8490828312042,4.73879860375925,48.97175913092));
#262296=CARTESIAN_POINT('Ctrl Pts',(46.8720285523032,4.60153407961332,49.5973963322325));
#262297=CARTESIAN_POINT('Ctrl Pts',(46.9172910317213,4.09926063963386,50.7356281460643));
#262298=CARTESIAN_POINT('Ctrl Pts',(46.9389482871538,3.74781202136899,51.241017215303));
#262299=CARTESIAN_POINT('Ctrl Pts',(46.9810220010193,2.85557778140817,52.1082024576298));
#262300=CARTESIAN_POINT('Ctrl Pts',(47.0039642273676,2.31672197870589,52.454724860202));
#262301=CARTESIAN_POINT('Ctrl Pts',(47.0492374108295,1.15740005626358,52.9068509099196));
#262302=CARTESIAN_POINT('Ctrl Pts',(47.0709377090647,0.551639655500766,
53.0169290494785));
#262303=CARTESIAN_POINT('Ctrl Pts',(47.1129861845493,-0.692717019939179,
53.0016548841548));
#262304=CARTESIAN_POINT('Ctrl Pts',(47.1359250749044,-1.31916190183093,
52.8668307754803));
#262305=CARTESIAN_POINT('Ctrl Pts',(47.1812081274254,-2.45977296165277,
52.368824030063));
#262306=CARTESIAN_POINT('Ctrl Pts',(47.2029488802598,-2.9666771221035,52.0192050967237));
#262307=CARTESIAN_POINT('Ctrl Pts',(47.2449738385226,-3.83754039304243,
51.1299445253089));
#262308=CARTESIAN_POINT('Ctrl Pts',(47.2679095549076,-4.18619523897315,
50.5921656409207));
#262309=CARTESIAN_POINT('Ctrl Pts',(47.313201703992,-4.64268762188745,49.4340882023249));
#262310=CARTESIAN_POINT('Ctrl Pts',(47.3349804140488,-4.75496316694576,
48.8285343178715));
#262311=CARTESIAN_POINT('Ctrl Pts',(47.3769834803082,-4.74405742910946,
47.5837188255888));
#262312=CARTESIAN_POINT('Ctrl Pts',(47.3999161858311,-4.61134187087903,
46.9565845142116));
#262313=CARTESIAN_POINT('Ctrl Pts',(47.4452167173044,-4.11702129093329,
45.8139267033697));
#262314=CARTESIAN_POINT('Ctrl Pts',(47.4670309854212,-3.76898036413851,
45.3057154872926));
#262315=CARTESIAN_POINT('Ctrl Pts',(47.5090136911057,-2.88228778831692,
44.4316865997071));
#262316=CARTESIAN_POINT('Ctrl Pts',(47.5319435481428,-2.34544301461709,
44.081197359138));
#262317=CARTESIAN_POINT('Ctrl Pts',(47.5769211080058,-1.19688904259089,
43.6243033168787));
#262318=CARTESIAN_POINT('Ctrl Pts',(47.5985411648686,-0.60108850816148,
43.5102000043641));
#262319=CARTESIAN_POINT('Ctrl Pts',(47.6187499988384,-3.44848784250562E-8,
43.5102));
#262320=CARTESIAN_POINT('Origin',(40.475,-1.41317707189676E-13,48.26));
#262321=CARTESIAN_POINT('',(49.238,-1.71331875425299E-13,43.5102));
#262322=CARTESIAN_POINT('',(48.6770833340043,1.00166031396858E-8,43.5102));
#262323=CARTESIAN_POINT('',(40.475,-1.40736024453017E-13,43.5102));
#262324=CARTESIAN_POINT('',(49.238,-1.86990303000829,52.6262412551721));
#262325=CARTESIAN_POINT('Origin',(49.238,-1.71913558161958E-13,48.26));
#262326=CARTESIAN_POINT('Ctrl Pts',(49.238,-1.86990303000829,52.6262412551721));
#262327=CARTESIAN_POINT('Ctrl Pts',(49.2258845683299,-1.56383729601022,
52.7573181265444));
#262328=CARTESIAN_POINT('Ctrl Pts',(49.2137876533848,-1.24484153160789,
52.8558494941654));
#262329=CARTESIAN_POINT('Ctrl Pts',(49.1902689990312,-0.598087148393598,
52.9832738225069));
#262330=CARTESIAN_POINT('Ctrl Pts',(49.1789970034025,-0.272399227164311,
53.0131869119213));
#262331=CARTESIAN_POINT('Ctrl Pts',(49.1473284546882,0.665150328710388,
53.0025766190358));
#262332=CARTESIAN_POINT('Ctrl Pts',(49.1252713731853,1.26947276028809,52.8776651208351));
#262333=CARTESIAN_POINT('Ctrl Pts',(49.0799708480804,2.41784395231669,52.3971383205351));
#262334=CARTESIAN_POINT('Ctrl Pts',(49.0573327453722,2.9473875112117,52.0381816129474));
#262335=CARTESIAN_POINT('Ctrl Pts',(49.0153198975399,3.8189835138927,51.1495847597557));
#262336=CARTESIAN_POINT('Ctrl Pts',(48.9932736680055,4.15879206820481,50.6345983826297));
#262337=CARTESIAN_POINT('Ctrl Pts',(48.9479661434789,4.63308233656798,49.4834357447573));
#262338=CARTESIAN_POINT('Ctrl Pts',(48.9252845812558,4.7547860276341,48.8550795761242));
#262339=CARTESIAN_POINT('Ctrl Pts',(48.8832914499036,4.74468294064032,47.6102271173403));
#262340=CARTESIAN_POINT('Ctrl Pts',(48.8612553675669,4.62178279031756,47.0056961541918));
#262341=CARTESIAN_POINT('Ctrl Pts',(48.8159414036286,4.1449356425251,45.8554010775775));
#262342=CARTESIAN_POINT('Ctrl Pts',(48.7932191294468,3.78732928008337,45.3242575343515));
#262343=CARTESIAN_POINT('Ctrl Pts',(48.7512443740699,2.90106707411043,44.4497605377253));
#262344=CARTESIAN_POINT('Ctrl Pts',(48.7292177706584,2.38726818569485,44.1084944446942));
#262345=CARTESIAN_POINT('Ctrl Pts',(48.6842061952532,1.24508730776226,43.6337718041888));
#262346=CARTESIAN_POINT('Ctrl Pts',(48.6616555802689,0.625530370510131,
43.5102000039716));
#262347=CARTESIAN_POINT('Ctrl Pts',(48.6406250010114,3.01567516791668E-8,
43.5102));
#262348=CARTESIAN_POINT('Ctrl Pts',(47.6187499988384,-3.44848800534558E-8,
43.5102));
#262349=CARTESIAN_POINT('Ctrl Pts',(47.6190554156344,0.00908423608770984,
43.510199999934));
#262350=CARTESIAN_POINT('Ctrl Pts',(47.6193612351469,0.0181696901690511,
43.5102260611622));
#262351=CARTESIAN_POINT('Ctrl Pts',(47.6410631179697,0.662136500170199,
43.5139214564747));
#262352=CARTESIAN_POINT('Ctrl Pts',(47.6639902866763,1.28985842539487,43.6448208016816));
#262353=CARTESIAN_POINT('Ctrl Pts',(47.7093056539373,2.43427260627935,44.1359664574964));
#262354=CARTESIAN_POINT('Ctrl Pts',(47.7311842575743,2.94360820937294,44.4826502313436));
#262355=CARTESIAN_POINT('Ctrl Pts',(47.7731304748416,3.82035481584508,45.3671317852305));
#262356=CARTESIAN_POINT('Ctrl Pts',(47.7960551119496,4.17241816830255,45.903169279661));
#262357=CARTESIAN_POINT('Ctrl Pts',(47.8413770300831,4.63590244033921,47.0592360290128));
#262358=CARTESIAN_POINT('Ctrl Pts',(47.8632846262197,4.7516964766686,47.6644598597278));
#262359=CARTESIAN_POINT('Ctrl Pts',(47.9052145427422,4.74777924465977,48.909994331287));
#262360=CARTESIAN_POINT('Ctrl Pts',(47.9281368006109,4.61844016403251,49.5382164720474));
#262361=CARTESIAN_POINT('Ctrl Pts',(47.9734647507917,4.13002191265737,50.6841346452895));
#262362=CARTESIAN_POINT('Ctrl Pts',(47.9953993673612,3.78450253960707,51.1944351295972));
#262363=CARTESIAN_POINT('Ctrl Pts',(48.037314169267,2.9019197434865,52.0735098685421));
#262364=CARTESIAN_POINT('Ctrl Pts',(48.0602341951523,2.36657772452769,52.4269211246324));
#262365=CARTESIAN_POINT('Ctrl Pts',(48.1055676989055,1.21131348071787,52.8931747566165));
#262366=CARTESIAN_POINT('Ctrl Pts',(48.1275274716682,0.606220172191773,
53.0103623527895));
#262367=CARTESIAN_POINT('Ctrl Pts',(48.1694282675115,-0.639593744248682,
53.0092108581361));
#262368=CARTESIAN_POINT('Ctrl Pts',(48.1923462030236,-1.26824126499063,
52.8812091154099));
#262369=CARTESIAN_POINT('Ctrl Pts',(48.2376816627341,-2.41536511316516,
52.395162376501));
#262370=CARTESIAN_POINT('Ctrl Pts',(48.2596639329102,-2.92650865236691,
52.0506691843566));
#262371=CARTESIAN_POINT('Ctrl Pts',(48.3015532619484,-3.80756031737948,
51.1697271236059));
#262372=CARTESIAN_POINT('Ctrl Pts',(48.3244673767911,-4.16214899822476,
50.6350159036455));
#262373=CARTESIAN_POINT('Ctrl Pts',(48.3698102209431,-4.63077827583694,
49.4804578650764));
#262374=CARTESIAN_POINT('Ctrl Pts',(48.3917987188872,-4.74919686669791,
48.8754859221348));
#262375=CARTESIAN_POINT('Ctrl Pts',(48.4336999981435,-4.75042231280389,
47.6296882588265));
#262376=CARTESIAN_POINT('Ctrl Pts',(48.4565870245828,-4.62370604511379,
47.0009120908299));
#262377=CARTESIAN_POINT('Ctrl Pts',(48.5019259324576,-4.13991074199294,
45.8527531057449));
#262378=CARTESIAN_POINT('Ctrl Pts',(48.523921127265,-3.79634923939758,45.3408392198344));
#262379=CARTESIAN_POINT('Ctrl Pts',(48.5658352748235,-2.91727107546747,
44.4582773051979));
#262380=CARTESIAN_POINT('Ctrl Pts',(48.5886932226241,-2.38359346820029,
44.1028133915142));
#262381=CARTESIAN_POINT('Ctrl Pts',(48.6340278542553,-1.23026664392626,
43.6318014243508));
#262382=CARTESIAN_POINT('Ctrl Pts',(48.6560302458644,-0.625419053718888,
43.5120849431333));
#262383=CARTESIAN_POINT('Ctrl Pts',(48.6767586264633,-0.00965498329010137,
43.510207359137));
#262384=CARTESIAN_POINT('Ctrl Pts',(48.6769210372467,-0.00482730997555823,
43.5101999999898));
#262385=CARTESIAN_POINT('Ctrl Pts',(48.6770833336679,1.00279621503562E-8,
43.5102));
#262386=CARTESIAN_POINT('Origin',(42.09425,-1.46971288347598E-13,48.26));
#262387=CARTESIAN_POINT('',(42.0671867061318,-4.66579641623079,47.5288462557477));
#262388=CARTESIAN_POINT('Origin',(42.0904940530805,0.0419539454483869,48.1587073448045));
#262389=CARTESIAN_POINT('',(42.0671867061318,-4.68628896694512,47.6743911597878));
#262390=CARTESIAN_POINT('Origin',(42.0671867060951,-1.1101650337908E-6,
48.259999841405));
#262391=CARTESIAN_POINT('Origin',(42.1434096703743,0.157122447872717,47.8795110986836));
#262392=CARTESIAN_POINT('',(40.475,-1.40934325385969E-13,45.12945));
#262393=CARTESIAN_POINT('',(42.09425,-1.46389605610939E-13,43.5102));
#262394=CARTESIAN_POINT('Origin',(40.475,-1.41317707189676E-13,48.26));
#262395=CARTESIAN_POINT('Origin',(50.,-1.74574066942157E-13,48.26));
#262396=CARTESIAN_POINT('',(49.238,-0.908077042619528,52.9221879117714));
#262397=CARTESIAN_POINT('',(49.238,-1.71331875425299E-13,53.0098));
#262398=CARTESIAN_POINT('Origin',(49.238,-1.71913558161958E-13,48.26));
#262399=CARTESIAN_POINT('Origin',(49.2622522741381,0.101290884806737,48.3019587266361));
#262400=CARTESIAN_POINT('Origin',(49.2681001647118,0.380373159827433,48.418111922516));
#262401=CARTESIAN_POINT('Origin',(49.238,-1.71913558161958E-13,48.26));
#262402=CARTESIAN_POINT('',(50.,-1.74085702291593E-13,52.2478));
#262403=CARTESIAN_POINT('',(50.,-1.74085702291593E-13,52.2478));
#262404=CARTESIAN_POINT('Origin',(50.,-1.74574066942157E-13,48.26));
#262405=CARTESIAN_POINT('Origin',(40.475,-1.41317707189676E-13,48.26));
#262406=CARTESIAN_POINT('Ctrl Pts',(48.6770833336679,1.00279587411656E-8,
43.5102));
#262407=CARTESIAN_POINT('Ctrl Pts',(48.698253182187,0.629672755148532,43.5102000013294));
#262408=CARTESIAN_POINT('Ctrl Pts',(48.7209607258464,1.25321726916315,43.6354136739498));
#262409=CARTESIAN_POINT('Ctrl Pts',(48.7661149856871,2.39779765933032,44.1145892634239));
#262410=CARTESIAN_POINT('Ctrl Pts',(48.7881251061508,2.91060499549462,44.4570655678307));
#262411=CARTESIAN_POINT('Ctrl Pts',(48.8300680020356,3.7949199110413,45.3339759730068));
#262412=CARTESIAN_POINT('Ctrl Pts',(48.852861329914,4.15139914838053,45.8664533561614));
#262413=CARTESIAN_POINT('Ctrl Pts',(48.89818626695,4.62517599058976,47.0183465771308));
#262414=CARTESIAN_POINT('Ctrl Pts',(48.9202046816237,4.74640007620399,47.6230462847423));
#262415=CARTESIAN_POINT('Ctrl Pts',(48.9621635943343,4.75318456347128,48.8682555584822));
#262416=CARTESIAN_POINT('Ctrl Pts',(48.9849211271637,4.62960939173084,49.4967694962158));
#262417=CARTESIAN_POINT('Ctrl Pts',(49.0302405779038,4.15176681390732,50.6468154508066));
#262418=CARTESIAN_POINT('Ctrl Pts',(49.0522678865187,3.81055277871214,51.1606568777459));
#262419=CARTESIAN_POINT('Ctrl Pts',(49.0942440076311,2.93615950038779,52.0470026674728));
#262420=CARTESIAN_POINT('Ctrl Pts',(49.1169632491864,2.40507322360049,52.4046573926883));
#262421=CARTESIAN_POINT('Ctrl Pts',(49.1570831197733,1.38668037730972,52.826967238459));
#262422=CARTESIAN_POINT('Ctrl Pts',(49.1740393274788,0.929744443720402,
52.9414176733626));
#262423=CARTESIAN_POINT('Ctrl Pts',(49.2063727902452,0.00555594936310154,
53.0320305704281));
#262424=CARTESIAN_POINT('Ctrl Pts',(49.2215907184063,-0.45643928208532,
53.0101555976911));
#262425=CARTESIAN_POINT('Ctrl Pts',(49.238,-0.908077042619906,52.9221879117714));
#262426=CARTESIAN_POINT('Origin',(40.475,-1.41317707189676E-13,48.26));
#262427=CARTESIAN_POINT('Origin',(50.,-1.74574066942157E-13,48.26));
#262428=CARTESIAN_POINT('',(50.,-1.77392992590619E-13,51.0096306570156));
#262429=CARTESIAN_POINT('',(50.,-2.38125000000018,49.6348153285078));
#262430=CARTESIAN_POINT('Origin',(50.,-1.74574066942157E-13,48.26));
#262431=CARTESIAN_POINT('',(50.,2.38124999999983,49.6348153285078));
#262432=CARTESIAN_POINT('Origin',(50.,-1.74574066942157E-13,48.26));
#262433=CARTESIAN_POINT('',(50.,2.38124999999983,46.8851846714922));
#262434=CARTESIAN_POINT('Origin',(50.,-1.74574066942157E-13,48.26));
#262435=CARTESIAN_POINT('',(50.,-1.77392992590619E-13,45.5103693429844));
#262436=CARTESIAN_POINT('Origin',(50.,-1.74574066942157E-13,48.26));
#262437=CARTESIAN_POINT('',(50.,-2.38125000000018,46.8851846714922));
#262438=CARTESIAN_POINT('Origin',(50.,-1.74574066942157E-13,48.26));
#262439=CARTESIAN_POINT('Origin',(50.,-1.74574066942157E-13,48.26));
#262440=CARTESIAN_POINT('Origin',(50.,-1.74574066942157E-13,48.26));
#262441=CARTESIAN_POINT('Ctrl Pts',(50.0000000000005,6.90208666923676E-13,
51.0096306570161));
#262442=CARTESIAN_POINT('Ctrl Pts',(49.3125923357457,-1.19062500000018,
50.3222229927617));
#262443=CARTESIAN_POINT('Ctrl Pts',(50.0000000000005,-2.38125000000105,
49.6348153285073));
#262444=CARTESIAN_POINT('Origin',(50.,-1.74574066942157E-13,48.26));
#262445=CARTESIAN_POINT('Ctrl Pts',(50.0000000000005,-2.38125000000017,
49.6348153285088));
#262446=CARTESIAN_POINT('Ctrl Pts',(49.3125923357457,-2.38125000000017,
48.26));
#262447=CARTESIAN_POINT('Ctrl Pts',(50.0000000000005,-2.38125000000017,
46.8851846714912));
#262448=CARTESIAN_POINT('Origin',(50.,-1.74574066942157E-13,48.26));
#262449=CARTESIAN_POINT('Ctrl Pts',(50.0000000000005,-2.38125000000103,
46.8851846714927));
#262450=CARTESIAN_POINT('Ctrl Pts',(49.3125923357457,-1.19062500000017,
46.1977770072383));
#262451=CARTESIAN_POINT('Ctrl Pts',(50.0000000000005,6.88211024554572E-13,
45.5103693429839));
#262452=CARTESIAN_POINT('Origin',(50.,-1.74574066942157E-13,48.26));
#262453=CARTESIAN_POINT('Ctrl Pts',(50.0000000000005,-1.01963383062804E-12,
45.5103693429839));
#262454=CARTESIAN_POINT('Ctrl Pts',(49.3125923357457,1.19062499999984,46.1977770072383));
#262455=CARTESIAN_POINT('Ctrl Pts',(50.0000000000005,2.3812500000007,46.8851846714927));
#262456=CARTESIAN_POINT('Origin',(50.,-1.74574066942157E-13,48.26));
#262457=CARTESIAN_POINT('Ctrl Pts',(50.0000000000005,2.38124999999983,46.8851846714912));
#262458=CARTESIAN_POINT('Ctrl Pts',(49.3125923357457,2.38124999999983,48.26));
#262459=CARTESIAN_POINT('Ctrl Pts',(50.0000000000005,2.38124999999983,49.6348153285088));
#262460=CARTESIAN_POINT('Origin',(50.,-1.74574066942157E-13,48.26));
#262461=CARTESIAN_POINT('Ctrl Pts',(50.0000000000005,2.38125000000067,49.6348153285073));
#262462=CARTESIAN_POINT('Ctrl Pts',(49.3125923357458,1.19062499999982,50.3222229927617));
#262463=CARTESIAN_POINT('Ctrl Pts',(50.0000000000005,-1.03770552554851E-12,
51.0096306570161));
#262464=CARTESIAN_POINT('Origin',(46.428125,2.38124999999984,49.6348153285078));
#262465=CARTESIAN_POINT('',(46.428125,2.38124999999984,49.6348153285078));
#262466=CARTESIAN_POINT('',(46.428125,-1.62265562360849E-13,51.0096306570156));
#262467=CARTESIAN_POINT('',(46.428125,-1.62265562360849E-13,51.0096306570156));
#262468=CARTESIAN_POINT('',(46.428125,-2.38125000000016,49.6348153285078));
#262469=CARTESIAN_POINT('',(46.428125,-2.38125000000016,49.6348153285078));
#262470=CARTESIAN_POINT('',(46.428125,-2.38125000000016,46.8851846714922));
#262471=CARTESIAN_POINT('',(46.428125,-2.38125000000016,46.8851846714922));
#262472=CARTESIAN_POINT('',(46.428125,-1.62265562360849E-13,45.5103693429844));
#262473=CARTESIAN_POINT('',(46.428125,-1.62265562360849E-13,45.5103693429844));
#262474=CARTESIAN_POINT('',(46.428125,2.38124999999984,46.8851846714922));
#262475=CARTESIAN_POINT('',(46.428125,2.38124999999984,46.8851846714922));
#262476=CARTESIAN_POINT('',(46.428125,2.38124999999984,49.6348153285078));
#262477=CARTESIAN_POINT('Origin',(46.428125,-2.38125000000016,49.6348153285078));
#262478=CARTESIAN_POINT('',(46.428125,-1.62265562360849E-13,51.0096306570156));
#262479=CARTESIAN_POINT('',(46.428125,-2.38125000000016,49.6348153285078));
#262480=CARTESIAN_POINT('Origin',(46.428125,-2.38125000000016,46.8851846714922));
#262481=CARTESIAN_POINT('',(46.428125,-2.38125000000016,46.8851846714922));
#262482=CARTESIAN_POINT('Origin',(46.428125,-1.62265562360849E-13,45.5103693429844));
#262483=CARTESIAN_POINT('',(46.428125,-1.62265562360849E-13,45.5103693429844));
#262484=CARTESIAN_POINT('Origin',(46.428125,2.38124999999984,46.8851846714922));
#262485=CARTESIAN_POINT('',(46.428125,2.38124999999984,46.8851846714922));
#262486=CARTESIAN_POINT('Origin',(46.428125,2.38124999999984,49.6348153285078));
#262487=CARTESIAN_POINT('',(46.428125,2.38124999999984,49.6348153285078));
#262488=CARTESIAN_POINT('Origin',(46.428125,-1.62265562360849E-13,51.0096306570156));
#262489=CARTESIAN_POINT('Ctrl Pts',(40.4593750000001,4.72273670613168,48.26));
#262490=CARTESIAN_POINT('Ctrl Pts',(40.5255208333334,4.72273670613168,50.216221595197));
#262491=CARTESIAN_POINT('Ctrl Pts',(40.5916666666667,3.33947915066429,51.5994791506644));
#262492=CARTESIAN_POINT('Ctrl Pts',(40.6578125,1.9562215951969,52.9827367061318));
#262493=CARTESIAN_POINT('Ctrl Pts',(40.7239583333333,-1.4189775634514E-13,
52.9827367061318));
#262494=CARTESIAN_POINT('Ctrl Pts',(40.7901041666666,-1.95622159519718,
52.9827367061318));
#262495=CARTESIAN_POINT('Ctrl Pts',(40.8562499999999,-3.33947915066458,
51.5994791506644));
#262496=CARTESIAN_POINT('Ctrl Pts',(40.9223958333332,-4.72273670613197,
50.216221595197));
#262497=CARTESIAN_POINT('Ctrl Pts',(40.9885416666665,-4.72273670613197,
48.26));
#262498=CARTESIAN_POINT('Ctrl Pts',(41.0546874999999,-4.72273670613197,
46.303778404803));
#262499=CARTESIAN_POINT('Ctrl Pts',(41.1208333333332,-3.33947915066458,
44.9205208493356));
#262500=CARTESIAN_POINT('Ctrl Pts',(41.1869791666665,-1.95622159519719,
43.5372632938682));
#262501=CARTESIAN_POINT('Ctrl Pts',(41.2531249999998,-1.44902068765019E-13,
43.5372632938682));
#262502=CARTESIAN_POINT('Ctrl Pts',(41.3192708333331,1.9562215951969,43.5372632938682));
#262503=CARTESIAN_POINT('Ctrl Pts',(41.3854166666664,3.33947915066429,44.9205208493356));
#262504=CARTESIAN_POINT('Ctrl Pts',(41.4515624999997,4.72273670613168,46.303778404803));
#262505=CARTESIAN_POINT('Ctrl Pts',(41.5177083333331,4.72273670613168,48.26));
#262506=CARTESIAN_POINT('Ctrl Pts',(41.5838541666664,4.72273670613168,50.216221595197));
#262507=CARTESIAN_POINT('Ctrl Pts',(41.6499999999997,3.33947915066429,51.5994791506644));
#262508=CARTESIAN_POINT('Ctrl Pts',(41.716145833333,1.9562215951969,52.9827367061318));
#262509=CARTESIAN_POINT('Ctrl Pts',(41.7822916666663,-1.45592907428747E-13,
52.9827367061318));
#262510=CARTESIAN_POINT('Ctrl Pts',(41.8484374999996,-1.95622159519719,
52.9827367061318));
#262511=CARTESIAN_POINT('Ctrl Pts',(41.9145833333329,-3.33947915066458,
51.5994791506644));
#262512=CARTESIAN_POINT('Ctrl Pts',(41.9807291666662,-4.72273670613197,
50.216221595197));
#262513=CARTESIAN_POINT('Ctrl Pts',(42.0468749999995,-4.72273670613197,
48.26));
#262514=CARTESIAN_POINT('Ctrl Pts',(42.1130208333329,-4.72273670613197,
46.303778404803));
#262515=CARTESIAN_POINT('Ctrl Pts',(42.1791666666662,-3.33947915066458,
44.9205208493356));
#262516=CARTESIAN_POINT('Ctrl Pts',(42.2453124999995,-1.95622159519719,
43.5372632938682));
#262517=CARTESIAN_POINT('Ctrl Pts',(42.3114583333328,-1.48597219848627E-13,
43.5372632938682));
#262518=CARTESIAN_POINT('Ctrl Pts',(42.3776041666661,1.95622159519689,43.5372632938682));
#262519=CARTESIAN_POINT('Ctrl Pts',(42.4437499999994,3.33947915066428,44.9205208493356));
#262520=CARTESIAN_POINT('Ctrl Pts',(42.5098958333328,4.72273670613168,46.303778404803));
#262521=CARTESIAN_POINT('Ctrl Pts',(42.5760416666661,4.72273670613168,48.26));
#262522=CARTESIAN_POINT('Ctrl Pts',(42.6421874999994,4.72273670613168,50.216221595197));
#262523=CARTESIAN_POINT('Ctrl Pts',(42.7083333333327,3.33947915066428,51.5994791506644));
#262524=CARTESIAN_POINT('Ctrl Pts',(42.774479166666,1.95622159519689,52.9827367061318));
#262525=CARTESIAN_POINT('Ctrl Pts',(42.8406249999993,-1.49288058512355E-13,
52.9827367061318));
#262526=CARTESIAN_POINT('Ctrl Pts',(42.9067708333326,-1.95622159519719,
52.9827367061318));
#262527=CARTESIAN_POINT('Ctrl Pts',(42.9729166666659,-3.33947915066458,
51.5994791506644));
#262528=CARTESIAN_POINT('Ctrl Pts',(43.0390624999992,-4.72273670613198,
50.216221595197));
#262529=CARTESIAN_POINT('Ctrl Pts',(43.1052083333325,-4.72273670613198,
48.26));
#262530=CARTESIAN_POINT('Ctrl Pts',(43.1713541666659,-4.72273670613198,
46.303778404803));
#262531=CARTESIAN_POINT('Ctrl Pts',(43.2374999999992,-3.33947915066458,
44.9205208493356));
#262532=CARTESIAN_POINT('Ctrl Pts',(43.3036458333325,-1.95622159519719,
43.5372632938682));
#262533=CARTESIAN_POINT('Ctrl Pts',(43.3697916666658,-1.52292370932235E-13,
43.5372632938682));
#262534=CARTESIAN_POINT('Ctrl Pts',(43.4359374999991,1.95622159519689,43.5372632938682));
#262535=CARTESIAN_POINT('Ctrl Pts',(43.5020833333324,3.33947915066428,44.9205208493356));
#262536=CARTESIAN_POINT('Ctrl Pts',(43.5682291666658,4.72273670613167,46.303778404803));
#262537=CARTESIAN_POINT('Ctrl Pts',(43.6343749999991,4.72273670613167,48.26));
#262538=CARTESIAN_POINT('Ctrl Pts',(43.7005208333324,4.72273670613167,50.216221595197));
#262539=CARTESIAN_POINT('Ctrl Pts',(43.7666666666657,3.33947915066428,51.5994791506644));
#262540=CARTESIAN_POINT('Ctrl Pts',(43.832812499999,1.95622159519689,52.9827367061318));
#262541=CARTESIAN_POINT('Ctrl Pts',(43.8989583333323,-1.52983209595963E-13,
52.9827367061318));
#262542=CARTESIAN_POINT('Ctrl Pts',(43.9651041666656,-1.95622159519719,
52.9827367061318));
#262543=CARTESIAN_POINT('Ctrl Pts',(44.0312499999989,-3.33947915066459,
51.5994791506644));
#262544=CARTESIAN_POINT('Ctrl Pts',(44.0973958333322,-4.72273670613198,
50.216221595197));
#262545=CARTESIAN_POINT('Ctrl Pts',(44.1635416666655,-4.72273670613198,
48.26));
#262546=CARTESIAN_POINT('Ctrl Pts',(44.2296874999989,-4.72273670613198,
46.303778404803));
#262547=CARTESIAN_POINT('Ctrl Pts',(44.2958333333322,-3.33947915066459,
44.9205208493356));
#262548=CARTESIAN_POINT('Ctrl Pts',(44.3619791666655,-1.9562215951972,43.5372632938682));
#262549=CARTESIAN_POINT('Ctrl Pts',(44.4281249999988,-1.55987522015843E-13,
43.5372632938682));
#262550=CARTESIAN_POINT('Ctrl Pts',(44.4942708333321,1.95622159519689,43.5372632938682));
#262551=CARTESIAN_POINT('Ctrl Pts',(44.5604166666654,3.33947915066428,44.9205208493356));
#262552=CARTESIAN_POINT('Ctrl Pts',(44.6265624999988,4.72273670613167,46.303778404803));
#262553=CARTESIAN_POINT('Ctrl Pts',(44.6927083333321,4.72273670613167,48.26));
#262554=CARTESIAN_POINT('Ctrl Pts',(44.7588541666654,4.72273670613167,50.216221595197));
#262555=CARTESIAN_POINT('Ctrl Pts',(44.8249999999987,3.33947915066428,51.5994791506644));
#262556=CARTESIAN_POINT('Ctrl Pts',(44.891145833332,1.95622159519688,52.9827367061318));
#262557=CARTESIAN_POINT('Ctrl Pts',(44.9572916666653,-1.56678360679571E-13,
52.9827367061318));
#262558=CARTESIAN_POINT('Ctrl Pts',(45.0234374999986,-1.9562215951972,52.9827367061318));
#262559=CARTESIAN_POINT('Ctrl Pts',(45.0895833333319,-3.33947915066459,
51.5994791506644));
#262560=CARTESIAN_POINT('Ctrl Pts',(45.1557291666652,-4.72273670613198,
50.216221595197));
#262561=CARTESIAN_POINT('Ctrl Pts',(45.2218749999985,-4.72273670613198,
48.26));
#262562=CARTESIAN_POINT('Ctrl Pts',(45.2880208333319,-4.72273670613199,
46.303778404803));
#262563=CARTESIAN_POINT('Ctrl Pts',(45.3541666666652,-3.33947915066459,
44.9205208493356));
#262564=CARTESIAN_POINT('Ctrl Pts',(45.4203124999985,-1.9562215951972,43.5372632938682));
#262565=CARTESIAN_POINT('Ctrl Pts',(45.4864583333318,-1.59682673099451E-13,
43.5372632938682));
#262566=CARTESIAN_POINT('Ctrl Pts',(45.5526041666651,1.95622159519688,43.5372632938682));
#262567=CARTESIAN_POINT('Ctrl Pts',(45.6187499999984,3.33947915066427,44.9205208493356));
#262568=CARTESIAN_POINT('Ctrl Pts',(45.6848958333318,4.72273670613167,46.303778404803));
#262569=CARTESIAN_POINT('Ctrl Pts',(45.7510416666651,4.72273670613167,48.26));
#262570=CARTESIAN_POINT('Ctrl Pts',(45.8171874999984,4.72273670613167,50.216221595197));
#262571=CARTESIAN_POINT('Ctrl Pts',(45.8833333333317,3.33947915066427,51.5994791506644));
#262572=CARTESIAN_POINT('Ctrl Pts',(45.949479166665,1.95622159519688,52.9827367061318));
#262573=CARTESIAN_POINT('Ctrl Pts',(46.0156249999983,-1.60373511763179E-13,
52.9827367061318));
#262574=CARTESIAN_POINT('Ctrl Pts',(46.0817708333316,-1.9562215951972,52.9827367061318));
#262575=CARTESIAN_POINT('Ctrl Pts',(46.1479166666649,-3.33947915066459,
51.5994791506644));
#262576=CARTESIAN_POINT('Ctrl Pts',(46.2140624999982,-4.72273670613199,
50.216221595197));
#262577=CARTESIAN_POINT('Ctrl Pts',(46.2802083333315,-4.72273670613199,
48.26));
#262578=CARTESIAN_POINT('Ctrl Pts',(46.3463541666649,-4.72273670613199,
46.303778404803));
#262579=CARTESIAN_POINT('Ctrl Pts',(46.4124999999982,-3.3394791506646,44.9205208493356));
#262580=CARTESIAN_POINT('Ctrl Pts',(46.4786458333315,-1.95622159519721,
43.5372632938682));
#262581=CARTESIAN_POINT('Ctrl Pts',(46.5447916666648,-1.63377824183059E-13,
43.5372632938682));
#262582=CARTESIAN_POINT('Ctrl Pts',(46.6109374999981,1.95622159519688,43.5372632938682));
#262583=CARTESIAN_POINT('Ctrl Pts',(46.6770833333314,3.33947915066427,44.9205208493356));
#262584=CARTESIAN_POINT('Ctrl Pts',(46.7432291666648,4.72273670613166,46.303778404803));
#262585=CARTESIAN_POINT('Ctrl Pts',(46.8093749999981,4.72273670613166,48.26));
#262586=CARTESIAN_POINT('Ctrl Pts',(46.8755208333314,4.72273670613166,50.216221595197));
#262587=CARTESIAN_POINT('Ctrl Pts',(46.9416666666647,3.33947915066427,51.5994791506644));
#262588=CARTESIAN_POINT('Ctrl Pts',(47.007812499998,1.95622159519688,52.9827367061318));
#262589=CARTESIAN_POINT('Ctrl Pts',(47.0739583333313,-1.64068662846786E-13,
52.9827367061318));
#262590=CARTESIAN_POINT('Ctrl Pts',(47.1401041666646,-1.95622159519721,
52.9827367061318));
#262591=CARTESIAN_POINT('Ctrl Pts',(47.2062499999979,-3.3394791506646,51.5994791506644));
#262592=CARTESIAN_POINT('Ctrl Pts',(47.2723958333312,-4.72273670613199,
50.216221595197));
#262593=CARTESIAN_POINT('Ctrl Pts',(47.3385416666645,-4.72273670613199,
48.26));
#262594=CARTESIAN_POINT('Ctrl Pts',(47.4046874999979,-4.72273670613199,
46.303778404803));
#262595=CARTESIAN_POINT('Ctrl Pts',(47.4708333333312,-3.3394791506646,44.9205208493356));
#262596=CARTESIAN_POINT('Ctrl Pts',(47.5369791666645,-1.95622159519721,
43.5372632938682));
#262597=CARTESIAN_POINT('Ctrl Pts',(47.6031249999978,-1.67072975266666E-13,
43.5372632938682));
#262598=CARTESIAN_POINT('Ctrl Pts',(47.6692708333311,1.95622159519688,43.5372632938682));
#262599=CARTESIAN_POINT('Ctrl Pts',(47.7354166666644,3.33947915066426,44.9205208493356));
#262600=CARTESIAN_POINT('Ctrl Pts',(47.8015624999978,4.72273670613166,46.303778404803));
#262601=CARTESIAN_POINT('Ctrl Pts',(47.8677083333311,4.72273670613166,48.26));
#262602=CARTESIAN_POINT('Ctrl Pts',(47.9338541666644,4.72273670613166,50.216221595197));
#262603=CARTESIAN_POINT('Ctrl Pts',(47.9999999999977,3.33947915066427,51.5994791506644));
#262604=CARTESIAN_POINT('Ctrl Pts',(48.066145833331,1.95622159519687,52.9827367061318));
#262605=CARTESIAN_POINT('Ctrl Pts',(48.1322916666643,-1.67763813930394E-13,
52.9827367061318));
#262606=CARTESIAN_POINT('Ctrl Pts',(48.1984374999976,-1.95622159519721,
52.9827367061318));
#262607=CARTESIAN_POINT('Ctrl Pts',(48.2645833333309,-3.3394791506646,51.5994791506644));
#262608=CARTESIAN_POINT('Ctrl Pts',(48.3307291666642,-4.722736706132,50.216221595197));
#262609=CARTESIAN_POINT('Ctrl Pts',(48.3968749999976,-4.72273670613199,
48.26));
#262610=CARTESIAN_POINT('Ctrl Pts',(48.4630208333309,-4.722736706132,46.303778404803));
#262611=CARTESIAN_POINT('Ctrl Pts',(48.5291666666642,-3.3394791506646,44.9205208493356));
#262612=CARTESIAN_POINT('Ctrl Pts',(48.5953124999975,-1.95622159519721,
43.5372632938682));
#262613=CARTESIAN_POINT('Ctrl Pts',(48.6614583333308,-1.70768126350274E-13,
43.5372632938682));
#262614=CARTESIAN_POINT('Ctrl Pts',(48.7276041666641,1.95622159519687,43.5372632938682));
#262615=CARTESIAN_POINT('Ctrl Pts',(48.7937499999974,3.33947915066426,44.9205208493356));
#262616=CARTESIAN_POINT('Ctrl Pts',(48.8598958333308,4.72273670613165,46.303778404803));
#262617=CARTESIAN_POINT('Ctrl Pts',(48.9260416666641,4.72273670613165,48.26));
#262618=CARTESIAN_POINT('Ctrl Pts',(48.9921874999974,4.72273670613165,50.216221595197));
#262619=CARTESIAN_POINT('Ctrl Pts',(49.0583333333307,3.33947915066426,51.5994791506644));
#262620=CARTESIAN_POINT('Ctrl Pts',(49.124479166664,1.95622159519687,52.9827367061318));
#262621=CARTESIAN_POINT('Ctrl Pts',(49.1906249999973,-1.71458965014002E-13,
52.9827367061318));
#262622=CARTESIAN_POINT('Ctrl Pts',(49.2567708333306,-1.95622159519721,
52.9827367061318));
#262623=CARTESIAN_POINT('Ctrl Pts',(49.3229166666639,-3.33947915066461,
51.5994791506644));
#262624=CARTESIAN_POINT('Ctrl Pts',(49.3890624999972,-4.722736706132,50.216221595197));
#262625=CARTESIAN_POINT('Ctrl Pts',(49.4552083333306,-4.722736706132,48.26));
#262626=CARTESIAN_POINT('Ctrl Pts',(49.5213541666639,-4.722736706132,46.303778404803));
#262627=CARTESIAN_POINT('Ctrl Pts',(49.5874999999972,-3.33947915066461,
44.9205208493356));
#262628=CARTESIAN_POINT('Ctrl Pts',(49.6536458333305,-1.95622159519722,
43.5372632938682));
#262629=CARTESIAN_POINT('Ctrl Pts',(49.7197916666638,-1.74463277433882E-13,
43.5372632938682));
#262630=CARTESIAN_POINT('Ctrl Pts',(49.7859374999971,1.95622159519687,43.5372632938682));
#262631=CARTESIAN_POINT('Ctrl Pts',(49.8520833333304,3.33947915066426,44.9205208493356));
#262632=CARTESIAN_POINT('Ctrl Pts',(49.9182291666638,4.72273670613165,46.303778404803));
#262633=CARTESIAN_POINT('Ctrl Pts',(49.9843749999971,4.72273670613165,48.26));
#262634=CARTESIAN_POINT('Ctrl Pts',(50.0505208333304,4.72273670613165,50.216221595197));
#262635=CARTESIAN_POINT('Ctrl Pts',(50.1166666666637,3.33947915066426,51.5994791506644));
#262636=CARTESIAN_POINT('Ctrl Pts',(50.182812499997,1.95622159519687,52.9827367061318));
#262637=CARTESIAN_POINT('Ctrl Pts',(50.2489583333303,-1.7515411609761E-13,
52.9827367061318));
#262638=CARTESIAN_POINT('Ctrl Pts',(50.3151041666636,-1.95622159519722,
52.9827367061318));
#262639=CARTESIAN_POINT('Ctrl Pts',(50.3812499999969,-3.33947915066461,
51.5994791506644));
#262640=CARTESIAN_POINT('Ctrl Pts',(50.4473958333302,-4.722736706132,50.216221595197));
#262641=CARTESIAN_POINT('Ctrl Pts',(50.5135416666635,-4.722736706132,48.26));
#262642=CARTESIAN_POINT('Ctrl Pts',(50.5796874999969,-4.722736706132,46.303778404803));
#262643=CARTESIAN_POINT('Ctrl Pts',(50.6458333333302,-3.33947915066461,
44.9205208493356));
#262644=CARTESIAN_POINT('Ctrl Pts',(50.7119791666635,-1.95622159519722,
43.5372632938682));
#262645=CARTESIAN_POINT('Ctrl Pts',(50.7781249999968,-1.7815842851749E-13,
43.5372632938682));
#262646=CARTESIAN_POINT('Ctrl Pts',(50.8442708333301,1.95622159519686,43.5372632938682));
#262647=CARTESIAN_POINT('Ctrl Pts',(50.9104166666634,3.33947915066425,44.9205208493356));
#262648=CARTESIAN_POINT('Ctrl Pts',(50.9765624999968,4.72273670613165,46.303778404803));
#262649=CARTESIAN_POINT('Ctrl Pts',(51.0427083333301,4.72273670613165,48.26));
#262650=CARTESIAN_POINT('Ctrl Pts',(40.4763020833334,4.7520552744889,48.26));
#262651=CARTESIAN_POINT('Ctrl Pts',(40.5424479166667,4.7520552744889,50.22836574384));
#262652=CARTESIAN_POINT('Ctrl Pts',(40.60859375,3.36021050916436,51.6202105091645));
#262653=CARTESIAN_POINT('Ctrl Pts',(40.6747395833333,1.96836574383982,53.0120552744891));
#262654=CARTESIAN_POINT('Ctrl Pts',(40.7408854166666,-1.41955061696174E-13,
53.012055274489));
#262655=CARTESIAN_POINT('Ctrl Pts',(40.8070312499999,-1.96836574384011,
53.0120552744891));
#262656=CARTESIAN_POINT('Ctrl Pts',(40.8731770833332,-3.36021050916465,
51.6202105091645));
#262657=CARTESIAN_POINT('Ctrl Pts',(40.9393229166665,-4.75205527448919,
50.22836574384));
#262658=CARTESIAN_POINT('Ctrl Pts',(41.0054687499998,-4.75205527448919,
48.26));
#262659=CARTESIAN_POINT('Ctrl Pts',(41.0716145833332,-4.75205527448919,
46.29163425616));
#262660=CARTESIAN_POINT('Ctrl Pts',(41.1377604166665,-3.36021050916465,
44.8997894908355));
#262661=CARTESIAN_POINT('Ctrl Pts',(41.2039062499998,-1.96836574384011,
43.507944725511));
#262662=CARTESIAN_POINT('Ctrl Pts',(41.2700520833331,-1.44966555094233E-13,
43.507944725511));
#262663=CARTESIAN_POINT('Ctrl Pts',(41.3361979166664,1.96836574383982,43.507944725511));
#262664=CARTESIAN_POINT('Ctrl Pts',(41.4023437499997,3.36021050916436,44.8997894908355));
#262665=CARTESIAN_POINT('Ctrl Pts',(41.468489583333,4.7520552744889,46.29163425616));
#262666=CARTESIAN_POINT('Ctrl Pts',(41.5346354166664,4.7520552744889,48.26));
#262667=CARTESIAN_POINT('Ctrl Pts',(41.6007812499997,4.7520552744889,50.22836574384));
#262668=CARTESIAN_POINT('Ctrl Pts',(41.666927083333,3.36021050916436,51.6202105091645));
#262669=CARTESIAN_POINT('Ctrl Pts',(41.7330729166663,1.96836574383982,53.0120552744891));
#262670=CARTESIAN_POINT('Ctrl Pts',(41.7992187499996,-1.45650212779782E-13,
53.012055274489));
#262671=CARTESIAN_POINT('Ctrl Pts',(41.8653645833329,-1.96836574384011,
53.0120552744891));
#262672=CARTESIAN_POINT('Ctrl Pts',(41.9315104166662,-3.36021050916465,
51.6202105091645));
#262673=CARTESIAN_POINT('Ctrl Pts',(41.9976562499995,-4.75205527448919,
50.22836574384));
#262674=CARTESIAN_POINT('Ctrl Pts',(42.0638020833328,-4.75205527448919,
48.26));
#262675=CARTESIAN_POINT('Ctrl Pts',(42.1299479166662,-4.75205527448919,
46.29163425616));
#262676=CARTESIAN_POINT('Ctrl Pts',(42.1960937499995,-3.36021050916465,
44.8997894908355));
#262677=CARTESIAN_POINT('Ctrl Pts',(42.2622395833328,-1.96836574384011,
43.507944725511));
#262678=CARTESIAN_POINT('Ctrl Pts',(42.3283854166661,-1.48661706177841E-13,
43.507944725511));
#262679=CARTESIAN_POINT('Ctrl Pts',(42.3945312499994,1.96836574383982,43.507944725511));
#262680=CARTESIAN_POINT('Ctrl Pts',(42.4606770833327,3.36021050916436,44.8997894908355));
#262681=CARTESIAN_POINT('Ctrl Pts',(42.526822916666,4.7520552744889,46.29163425616));
#262682=CARTESIAN_POINT('Ctrl Pts',(42.5929687499994,4.7520552744889,48.26));
#262683=CARTESIAN_POINT('Ctrl Pts',(42.6591145833327,4.7520552744889,50.22836574384));
#262684=CARTESIAN_POINT('Ctrl Pts',(42.725260416666,3.36021050916436,51.6202105091645));
#262685=CARTESIAN_POINT('Ctrl Pts',(42.7914062499993,1.96836574383981,53.0120552744891));
#262686=CARTESIAN_POINT('Ctrl Pts',(42.8575520833326,-1.4934536386339E-13,
53.012055274489));
#262687=CARTESIAN_POINT('Ctrl Pts',(42.9236979166659,-1.96836574384011,
53.0120552744891));
#262688=CARTESIAN_POINT('Ctrl Pts',(42.9898437499992,-3.36021050916465,
51.6202105091645));
#262689=CARTESIAN_POINT('Ctrl Pts',(43.0559895833325,-4.7520552744892,50.22836574384));
#262690=CARTESIAN_POINT('Ctrl Pts',(43.1221354166658,-4.7520552744892,48.26));
#262691=CARTESIAN_POINT('Ctrl Pts',(43.1882812499991,-4.7520552744892,46.29163425616));
#262692=CARTESIAN_POINT('Ctrl Pts',(43.2544270833325,-3.36021050916466,
44.8997894908355));
#262693=CARTESIAN_POINT('Ctrl Pts',(43.3205729166658,-1.96836574384012,
43.507944725511));
#262694=CARTESIAN_POINT('Ctrl Pts',(43.3867187499991,-1.52356857261448E-13,
43.507944725511));
#262695=CARTESIAN_POINT('Ctrl Pts',(43.4528645833324,1.96836574383981,43.507944725511));
#262696=CARTESIAN_POINT('Ctrl Pts',(43.5190104166657,3.36021050916435,44.8997894908355));
#262697=CARTESIAN_POINT('Ctrl Pts',(43.5851562499991,4.75205527448889,46.29163425616));
#262698=CARTESIAN_POINT('Ctrl Pts',(43.6513020833324,4.75205527448889,48.26));
#262699=CARTESIAN_POINT('Ctrl Pts',(43.7174479166657,4.75205527448889,50.22836574384));
#262700=CARTESIAN_POINT('Ctrl Pts',(43.783593749999,3.36021050916435,51.6202105091645));
#262701=CARTESIAN_POINT('Ctrl Pts',(43.8497395833323,1.96836574383981,53.0120552744891));
#262702=CARTESIAN_POINT('Ctrl Pts',(43.9158854166656,-1.53040514946997E-13,
53.012055274489));
#262703=CARTESIAN_POINT('Ctrl Pts',(43.9820312499989,-1.96836574384012,
53.0120552744891));
#262704=CARTESIAN_POINT('Ctrl Pts',(44.0481770833322,-3.36021050916466,
51.6202105091645));
#262705=CARTESIAN_POINT('Ctrl Pts',(44.1143229166655,-4.7520552744892,50.22836574384));
#262706=CARTESIAN_POINT('Ctrl Pts',(44.1804687499988,-4.7520552744892,48.26));
#262707=CARTESIAN_POINT('Ctrl Pts',(44.2466145833321,-4.7520552744892,46.29163425616));
#262708=CARTESIAN_POINT('Ctrl Pts',(44.3127604166655,-3.36021050916466,
44.8997894908355));
#262709=CARTESIAN_POINT('Ctrl Pts',(44.3789062499988,-1.96836574384012,
43.507944725511));
#262710=CARTESIAN_POINT('Ctrl Pts',(44.4450520833321,-1.56052008345056E-13,
43.507944725511));
#262711=CARTESIAN_POINT('Ctrl Pts',(44.5111979166654,1.96836574383981,43.507944725511));
#262712=CARTESIAN_POINT('Ctrl Pts',(44.5773437499987,3.36021050916435,44.8997894908355));
#262713=CARTESIAN_POINT('Ctrl Pts',(44.643489583332,4.75205527448889,46.29163425616));
#262714=CARTESIAN_POINT('Ctrl Pts',(44.7096354166654,4.75205527448889,48.26));
#262715=CARTESIAN_POINT('Ctrl Pts',(44.7757812499987,4.75205527448889,50.22836574384));
#262716=CARTESIAN_POINT('Ctrl Pts',(44.841927083332,3.36021050916435,51.6202105091645));
#262717=CARTESIAN_POINT('Ctrl Pts',(44.9080729166653,1.96836574383981,53.0120552744891));
#262718=CARTESIAN_POINT('Ctrl Pts',(44.9742187499986,-1.56735666030605E-13,
53.012055274489));
#262719=CARTESIAN_POINT('Ctrl Pts',(45.0403645833319,-1.96836574384012,
53.0120552744891));
#262720=CARTESIAN_POINT('Ctrl Pts',(45.1065104166652,-3.36021050916466,
51.6202105091645));
#262721=CARTESIAN_POINT('Ctrl Pts',(45.1726562499985,-4.7520552744892,50.22836574384));
#262722=CARTESIAN_POINT('Ctrl Pts',(45.2388020833318,-4.7520552744892,48.26));
#262723=CARTESIAN_POINT('Ctrl Pts',(45.3049479166651,-4.75205527448921,
46.29163425616));
#262724=CARTESIAN_POINT('Ctrl Pts',(45.3710937499985,-3.36021050916466,
44.8997894908355));
#262725=CARTESIAN_POINT('Ctrl Pts',(45.4372395833318,-1.96836574384013,
43.507944725511));
#262726=CARTESIAN_POINT('Ctrl Pts',(45.5033854166651,-1.59747159428664E-13,
43.507944725511));
#262727=CARTESIAN_POINT('Ctrl Pts',(45.5695312499984,1.96836574383981,43.507944725511));
#262728=CARTESIAN_POINT('Ctrl Pts',(45.6356770833317,3.36021050916434,44.8997894908355));
#262729=CARTESIAN_POINT('Ctrl Pts',(45.701822916665,4.75205527448889,46.29163425616));
#262730=CARTESIAN_POINT('Ctrl Pts',(45.7679687499984,4.75205527448889,48.26));
#262731=CARTESIAN_POINT('Ctrl Pts',(45.8341145833317,4.75205527448889,50.22836574384));
#262732=CARTESIAN_POINT('Ctrl Pts',(45.900260416665,3.36021050916434,51.6202105091645));
#262733=CARTESIAN_POINT('Ctrl Pts',(45.9664062499983,1.9683657438398,53.0120552744891));
#262734=CARTESIAN_POINT('Ctrl Pts',(46.0325520833316,-1.60430817114213E-13,
53.012055274489));
#262735=CARTESIAN_POINT('Ctrl Pts',(46.0986979166649,-1.96836574384012,
53.0120552744891));
#262736=CARTESIAN_POINT('Ctrl Pts',(46.1648437499982,-3.36021050916467,
51.6202105091645));
#262737=CARTESIAN_POINT('Ctrl Pts',(46.2309895833315,-4.75205527448921,
50.22836574384));
#262738=CARTESIAN_POINT('Ctrl Pts',(46.2971354166648,-4.75205527448921,
48.26));
#262739=CARTESIAN_POINT('Ctrl Pts',(46.3632812499981,-4.75205527448921,
46.29163425616));
#262740=CARTESIAN_POINT('Ctrl Pts',(46.4294270833315,-3.36021050916467,
44.8997894908355));
#262741=CARTESIAN_POINT('Ctrl Pts',(46.4955729166648,-1.96836574384013,
43.507944725511));
#262742=CARTESIAN_POINT('Ctrl Pts',(46.5617187499981,-1.63442310512272E-13,
43.507944725511));
#262743=CARTESIAN_POINT('Ctrl Pts',(46.6278645833314,1.9683657438398,43.507944725511));
#262744=CARTESIAN_POINT('Ctrl Pts',(46.6940104166647,3.36021050916434,44.8997894908355));
#262745=CARTESIAN_POINT('Ctrl Pts',(46.7601562499981,4.75205527448888,46.29163425616));
#262746=CARTESIAN_POINT('Ctrl Pts',(46.8263020833314,4.75205527448888,48.26));
#262747=CARTESIAN_POINT('Ctrl Pts',(46.8924479166647,4.75205527448888,50.22836574384));
#262748=CARTESIAN_POINT('Ctrl Pts',(46.958593749998,3.36021050916434,51.6202105091645));
#262749=CARTESIAN_POINT('Ctrl Pts',(47.0247395833313,1.9683657438398,53.0120552744891));
#262750=CARTESIAN_POINT('Ctrl Pts',(47.0908854166646,-1.64125968197821E-13,
53.012055274489));
#262751=CARTESIAN_POINT('Ctrl Pts',(47.1570312499979,-1.96836574384013,
53.0120552744891));
#262752=CARTESIAN_POINT('Ctrl Pts',(47.2231770833312,-3.36021050916467,
51.6202105091645));
#262753=CARTESIAN_POINT('Ctrl Pts',(47.2893229166645,-4.75205527448921,
50.22836574384));
#262754=CARTESIAN_POINT('Ctrl Pts',(47.3554687499978,-4.75205527448921,
48.26));
#262755=CARTESIAN_POINT('Ctrl Pts',(47.4216145833312,-4.75205527448921,
46.29163425616));
#262756=CARTESIAN_POINT('Ctrl Pts',(47.4877604166645,-3.36021050916467,
44.8997894908355));
#262757=CARTESIAN_POINT('Ctrl Pts',(47.5539062499978,-1.96836574384013,
43.507944725511));
#262758=CARTESIAN_POINT('Ctrl Pts',(47.6200520833311,-1.6713746159588E-13,
43.507944725511));
#262759=CARTESIAN_POINT('Ctrl Pts',(47.6861979166644,1.9683657438398,43.507944725511));
#262760=CARTESIAN_POINT('Ctrl Pts',(47.7523437499977,3.36021050916434,44.8997894908355));
#262761=CARTESIAN_POINT('Ctrl Pts',(47.818489583331,4.75205527448888,46.29163425616));
#262762=CARTESIAN_POINT('Ctrl Pts',(47.8846354166644,4.75205527448888,48.26));
#262763=CARTESIAN_POINT('Ctrl Pts',(47.9507812499977,4.75205527448888,50.22836574384));
#262764=CARTESIAN_POINT('Ctrl Pts',(48.016927083331,3.36021050916434,51.6202105091645));
#262765=CARTESIAN_POINT('Ctrl Pts',(48.0830729166643,1.9683657438398,53.0120552744891));
#262766=CARTESIAN_POINT('Ctrl Pts',(48.1492187499976,-1.67821119281429E-13,
53.012055274489));
#262767=CARTESIAN_POINT('Ctrl Pts',(48.2153645833309,-1.96836574384013,
53.0120552744891));
#262768=CARTESIAN_POINT('Ctrl Pts',(48.2815104166642,-3.36021050916467,
51.6202105091645));
#262769=CARTESIAN_POINT('Ctrl Pts',(48.3476562499975,-4.75205527448922,
50.22836574384));
#262770=CARTESIAN_POINT('Ctrl Pts',(48.4138020833308,-4.75205527448921,
48.26));
#262771=CARTESIAN_POINT('Ctrl Pts',(48.4799479166642,-4.75205527448922,
46.29163425616));
#262772=CARTESIAN_POINT('Ctrl Pts',(48.5460937499975,-3.36021050916468,
44.8997894908355));
#262773=CARTESIAN_POINT('Ctrl Pts',(48.6122395833308,-1.96836574384014,
43.507944725511));
#262774=CARTESIAN_POINT('Ctrl Pts',(48.6783854166641,-1.70832612679488E-13,
43.507944725511));
#262775=CARTESIAN_POINT('Ctrl Pts',(48.7445312499974,1.96836574383979,43.507944725511));
#262776=CARTESIAN_POINT('Ctrl Pts',(48.8106770833307,3.36021050916433,44.8997894908355));
#262777=CARTESIAN_POINT('Ctrl Pts',(48.876822916664,4.75205527448887,46.29163425616));
#262778=CARTESIAN_POINT('Ctrl Pts',(48.9429687499974,4.75205527448887,48.26));
#262779=CARTESIAN_POINT('Ctrl Pts',(49.0091145833307,4.75205527448887,50.22836574384));
#262780=CARTESIAN_POINT('Ctrl Pts',(49.075260416664,3.36021050916433,51.6202105091645));
#262781=CARTESIAN_POINT('Ctrl Pts',(49.1414062499973,1.96836574383979,53.0120552744891));
#262782=CARTESIAN_POINT('Ctrl Pts',(49.2075520833306,-1.71516270365037E-13,
53.012055274489));
#262783=CARTESIAN_POINT('Ctrl Pts',(49.2736979166639,-1.96836574384014,
53.0120552744891));
#262784=CARTESIAN_POINT('Ctrl Pts',(49.3398437499972,-3.36021050916468,
51.6202105091645));
#262785=CARTESIAN_POINT('Ctrl Pts',(49.4059895833305,-4.75205527448922,
50.22836574384));
#262786=CARTESIAN_POINT('Ctrl Pts',(49.4721354166638,-4.75205527448922,
48.26));
#262787=CARTESIAN_POINT('Ctrl Pts',(49.5382812499972,-4.75205527448922,
46.29163425616));
#262788=CARTESIAN_POINT('Ctrl Pts',(49.6044270833305,-3.36021050916468,
44.8997894908355));
#262789=CARTESIAN_POINT('Ctrl Pts',(49.6705729166638,-1.96836574384014,
43.507944725511));
#262790=CARTESIAN_POINT('Ctrl Pts',(49.7367187499971,-1.74527763763095E-13,
43.507944725511));
#262791=CARTESIAN_POINT('Ctrl Pts',(49.8028645833304,1.96836574383979,43.507944725511));
#262792=CARTESIAN_POINT('Ctrl Pts',(49.8690104166637,3.36021050916433,44.8997894908355));
#262793=CARTESIAN_POINT('Ctrl Pts',(49.935156249997,4.75205527448887,46.29163425616));
#262794=CARTESIAN_POINT('Ctrl Pts',(50.0013020833304,4.75205527448887,48.26));
#262795=CARTESIAN_POINT('Ctrl Pts',(50.0674479166637,4.75205527448887,50.22836574384));
#262796=CARTESIAN_POINT('Ctrl Pts',(50.133593749997,3.36021050916433,51.6202105091645));
#262797=CARTESIAN_POINT('Ctrl Pts',(50.1997395833303,1.96836574383979,53.0120552744891));
#262798=CARTESIAN_POINT('Ctrl Pts',(50.2658854166636,-1.75211421448644E-13,
53.012055274489));
#262799=CARTESIAN_POINT('Ctrl Pts',(50.3320312499969,-1.96836574384014,
53.0120552744891));
#262800=CARTESIAN_POINT('Ctrl Pts',(50.3981770833302,-3.36021050916468,
51.6202105091645));
#262801=CARTESIAN_POINT('Ctrl Pts',(50.4643229166635,-4.75205527448922,
50.22836574384));
#262802=CARTESIAN_POINT('Ctrl Pts',(50.5304687499968,-4.75205527448922,
48.26));
#262803=CARTESIAN_POINT('Ctrl Pts',(50.5966145833301,-4.75205527448922,
46.29163425616));
#262804=CARTESIAN_POINT('Ctrl Pts',(50.6627604166635,-3.36021050916468,
44.8997894908355));
#262805=CARTESIAN_POINT('Ctrl Pts',(50.7289062499968,-1.96836574384014,
43.507944725511));
#262806=CARTESIAN_POINT('Ctrl Pts',(50.7950520833301,-1.78222914846703E-13,
43.507944725511));
#262807=CARTESIAN_POINT('Ctrl Pts',(50.8611979166634,1.96836574383979,43.507944725511));
#262808=CARTESIAN_POINT('Ctrl Pts',(50.9273437499967,3.36021050916433,44.8997894908355));
#262809=CARTESIAN_POINT('Ctrl Pts',(50.99348958333,4.75205527448887,46.29163425616));
#262810=CARTESIAN_POINT('Ctrl Pts',(51.0596354166634,4.75205527448887,48.26));
#262811=CARTESIAN_POINT('Ctrl Pts',(42.0671867061318,-4.68628896694512,
47.6743911597878));
#262812=CARTESIAN_POINT('Ctrl Pts',(42.1243724082372,-4.48534984498616,
46.0663915436572));
#262813=CARTESIAN_POINT('Ctrl Pts',(42.1791666666662,-3.33947915066458,
44.9205208493356));
#262814=CARTESIAN_POINT('Ctrl Pts',(42.2453124999995,-1.95622159519719,
43.5372632938682));
#262815=CARTESIAN_POINT('Ctrl Pts',(42.3114583333328,-1.48597219848627E-13,
43.5372632938682));
#262816=CARTESIAN_POINT('Ctrl Pts',(42.3776041666661,1.95622159519689,43.5372632938682));
#262817=CARTESIAN_POINT('Ctrl Pts',(42.4437499999994,3.33947915066428,44.9205208493356));
#262818=CARTESIAN_POINT('Ctrl Pts',(42.5098958333328,4.72273670613168,46.303778404803));
#262819=CARTESIAN_POINT('Ctrl Pts',(42.5760416666661,4.72273670613168,48.26));
#262820=CARTESIAN_POINT('Ctrl Pts',(42.6421874999994,4.72273670613168,50.216221595197));
#262821=CARTESIAN_POINT('Ctrl Pts',(42.7083333333327,3.33947915066428,51.5994791506644));
#262822=CARTESIAN_POINT('Ctrl Pts',(42.774479166666,1.95622159519689,52.9827367061318));
#262823=CARTESIAN_POINT('Ctrl Pts',(42.8406249999993,-1.49288058512355E-13,
52.9827367061318));
#262824=CARTESIAN_POINT('Ctrl Pts',(42.9067708333326,-1.95622159519719,
52.9827367061318));
#262825=CARTESIAN_POINT('Ctrl Pts',(42.9729166666659,-3.33947915066458,
51.5994791506644));
#262826=CARTESIAN_POINT('Ctrl Pts',(43.0390624999992,-4.72273670613198,
50.216221595197));
#262827=CARTESIAN_POINT('Ctrl Pts',(43.1052083333325,-4.72273670613198,
48.26));
#262828=CARTESIAN_POINT('Origin',(40.4567708333334,-1.14908083048704E-13,
48.26));
#262829=CARTESIAN_POINT('Ctrl Pts',(42.0671867061318,-4.66579641623079,
47.5288462557477));
#262830=CARTESIAN_POINT('Ctrl Pts',(42.1219271548081,-4.4275676543112,46.0086093529822));
#262831=CARTESIAN_POINT('Ctrl Pts',(42.1739583333328,-3.33947915066458,
44.9205208493356));
#262832=CARTESIAN_POINT('Ctrl Pts',(42.2401041666661,-1.95622159519719,
43.5372632938682));
#262833=CARTESIAN_POINT('Ctrl Pts',(42.3062499999994,-1.48579035049987E-13,
43.5372632938682));
#262834=CARTESIAN_POINT('Ctrl Pts',(42.3723958333328,1.95622159519689,43.5372632938682));
#262835=CARTESIAN_POINT('Ctrl Pts',(42.4385416666661,3.33947915066428,44.9205208493356));
#262836=CARTESIAN_POINT('Ctrl Pts',(42.5046874999994,4.72273670613168,46.303778404803));
#262837=CARTESIAN_POINT('Ctrl Pts',(42.5708333333327,4.72273670613168,48.26));
#262838=CARTESIAN_POINT('Ctrl Pts',(42.636979166666,4.72273670613168,50.216221595197));
#262839=CARTESIAN_POINT('Ctrl Pts',(42.7031249999993,3.33947915066428,51.5994791506644));
#262840=CARTESIAN_POINT('Ctrl Pts',(42.7692708333326,1.95622159519689,52.9827367061318));
#262841=CARTESIAN_POINT('Ctrl Pts',(42.8354166666659,-1.49269873713715E-13,
52.9827367061318));
#262842=CARTESIAN_POINT('Ctrl Pts',(42.9015624999992,-1.95622159519719,
52.9827367061318));
#262843=CARTESIAN_POINT('Ctrl Pts',(42.9677083333325,-3.33947915066458,
51.5994791506644));
#262844=CARTESIAN_POINT('Ctrl Pts',(43.0338541666658,-4.72273670613198,
50.216221595197));
#262845=CARTESIAN_POINT('Ctrl Pts',(43.0999999999992,-4.72273670613198,
48.26));
#262846=CARTESIAN_POINT('Ctrl Pts',(40.4372395833334,4.75205527448891,48.26));
#262847=CARTESIAN_POINT('Ctrl Pts',(40.5033854166667,4.75205527448891,50.22836574384));
#262848=CARTESIAN_POINT('Ctrl Pts',(40.56953125,3.36021050916437,51.6202105091645));
#262849=CARTESIAN_POINT('Ctrl Pts',(40.6356770833333,1.96836574383982,53.0120552744891));
#262850=CARTESIAN_POINT('Ctrl Pts',(40.7018229166666,-1.41818675706376E-13,
53.012055274489));
#262851=CARTESIAN_POINT('Ctrl Pts',(40.7679687499999,-1.96836574384011,
53.0120552744891));
#262852=CARTESIAN_POINT('Ctrl Pts',(40.8341145833332,-3.36021050916465,
51.6202105091645));
#262853=CARTESIAN_POINT('Ctrl Pts',(40.9002604166665,-4.75205527448919,
50.22836574384));
#262854=CARTESIAN_POINT('Ctrl Pts',(40.9664062499999,-4.75205527448919,
48.26));
#262855=CARTESIAN_POINT('Ctrl Pts',(41.0325520833332,-4.75205527448919,
46.29163425616));
#262856=CARTESIAN_POINT('Ctrl Pts',(41.0986979166665,-3.36021050916465,
44.8997894908355));
#262857=CARTESIAN_POINT('Ctrl Pts',(41.1648437499998,-1.96836574384011,
43.507944725511));
#262858=CARTESIAN_POINT('Ctrl Pts',(41.2309895833331,-1.44830169104434E-13,
43.507944725511));
#262859=CARTESIAN_POINT('Ctrl Pts',(41.2971354166664,1.96836574383982,43.507944725511));
#262860=CARTESIAN_POINT('Ctrl Pts',(41.3632812499998,3.36021050916436,44.8997894908355));
#262861=CARTESIAN_POINT('Ctrl Pts',(41.4294270833331,4.7520552744889,46.29163425616));
#262862=CARTESIAN_POINT('Ctrl Pts',(41.4955729166664,4.7520552744889,48.26));
#262863=CARTESIAN_POINT('Ctrl Pts',(41.5617187499997,4.7520552744889,50.22836574384));
#262864=CARTESIAN_POINT('Ctrl Pts',(41.627864583333,3.36021050916436,51.6202105091645));
#262865=CARTESIAN_POINT('Ctrl Pts',(41.6940104166663,1.96836574383982,53.0120552744891));
#262866=CARTESIAN_POINT('Ctrl Pts',(41.7601562499996,-1.45513826789983E-13,
53.012055274489));
#262867=CARTESIAN_POINT('Ctrl Pts',(41.8263020833329,-1.96836574384011,
53.0120552744891));
#262868=CARTESIAN_POINT('Ctrl Pts',(41.8924479166662,-3.36021050916465,
51.6202105091645));
#262869=CARTESIAN_POINT('Ctrl Pts',(41.9585937499996,-4.7520552744892,50.22836574384));
#262870=CARTESIAN_POINT('Ctrl Pts',(42.0247395833329,-4.7520552744892,48.26));
#262871=CARTESIAN_POINT('Ctrl Pts',(42.0908854166662,-4.7520552744892,46.29163425616));
#262872=CARTESIAN_POINT('Ctrl Pts',(42.1570312499995,-3.36021050916466,
44.8997894908355));
#262873=CARTESIAN_POINT('Ctrl Pts',(42.2231770833328,-1.96836574384011,
43.507944725511));
#262874=CARTESIAN_POINT('Ctrl Pts',(42.2893229166661,-1.48525320188042E-13,
43.507944725511));
#262875=CARTESIAN_POINT('Ctrl Pts',(42.3554687499994,1.96836574383982,43.507944725511));
#262876=CARTESIAN_POINT('Ctrl Pts',(42.4216145833328,3.36021050916436,44.8997894908355));
#262877=CARTESIAN_POINT('Ctrl Pts',(42.4877604166661,4.7520552744889,46.29163425616));
#262878=CARTESIAN_POINT('Ctrl Pts',(42.5539062499994,4.7520552744889,48.26));
#262879=CARTESIAN_POINT('Ctrl Pts',(42.6200520833327,4.7520552744889,50.22836574384));
#262880=CARTESIAN_POINT('Ctrl Pts',(42.686197916666,3.36021050916436,51.6202105091645));
#262881=CARTESIAN_POINT('Ctrl Pts',(42.7523437499993,1.96836574383982,53.0120552744891));
#262882=CARTESIAN_POINT('Ctrl Pts',(42.8184895833326,-1.49208977873591E-13,
53.012055274489));
#262883=CARTESIAN_POINT('Ctrl Pts',(42.8846354166659,-1.96836574384011,
53.0120552744891));
#262884=CARTESIAN_POINT('Ctrl Pts',(42.9507812499992,-3.36021050916466,
51.6202105091645));
#262885=CARTESIAN_POINT('Ctrl Pts',(43.0169270833326,-4.7520552744892,50.22836574384));
#262886=CARTESIAN_POINT('Ctrl Pts',(43.0830729166659,-4.7520552744892,48.26));
#262887=CARTESIAN_POINT('Ctrl Pts',(43.1492187499992,-4.7520552744892,46.29163425616));
#262888=CARTESIAN_POINT('Ctrl Pts',(43.2153645833325,-3.36021050916466,
44.8997894908355));
#262889=CARTESIAN_POINT('Ctrl Pts',(43.2815104166658,-1.96836574384012,
43.507944725511));
#262890=CARTESIAN_POINT('Ctrl Pts',(43.3476562499991,-1.5222047127165E-13,
43.507944725511));
#262891=CARTESIAN_POINT('Ctrl Pts',(43.4138020833324,1.96836574383981,43.507944725511));
#262892=CARTESIAN_POINT('Ctrl Pts',(43.4799479166658,3.36021050916435,44.8997894908355));
#262893=CARTESIAN_POINT('Ctrl Pts',(43.5460937499991,4.7520552744889,46.29163425616));
#262894=CARTESIAN_POINT('Ctrl Pts',(43.6122395833324,4.7520552744889,48.26));
#262895=CARTESIAN_POINT('Ctrl Pts',(43.6783854166657,4.7520552744889,50.22836574384));
#262896=CARTESIAN_POINT('Ctrl Pts',(43.744531249999,3.36021050916435,51.6202105091645));
#262897=CARTESIAN_POINT('Ctrl Pts',(43.8106770833323,1.96836574383981,53.0120552744891));
#262898=CARTESIAN_POINT('Ctrl Pts',(43.8768229166656,-1.52904128957199E-13,
53.012055274489));
#262899=CARTESIAN_POINT('Ctrl Pts',(43.9429687499989,-1.96836574384012,
53.0120552744891));
#262900=CARTESIAN_POINT('Ctrl Pts',(44.0091145833323,-3.36021050916466,
51.6202105091645));
#262901=CARTESIAN_POINT('Ctrl Pts',(44.0752604166656,-4.7520552744892,50.22836574384));
#262902=CARTESIAN_POINT('Ctrl Pts',(44.1414062499989,-4.7520552744892,48.26));
#262903=CARTESIAN_POINT('Ctrl Pts',(44.2075520833322,-4.75205527448921,
46.29163425616));
#262904=CARTESIAN_POINT('Ctrl Pts',(44.2736979166655,-3.36021050916466,
44.8997894908355));
#262905=CARTESIAN_POINT('Ctrl Pts',(44.3398437499988,-1.96836574384012,
43.507944725511));
#262906=CARTESIAN_POINT('Ctrl Pts',(44.4059895833321,-1.55915622355258E-13,
43.507944725511));
#262907=CARTESIAN_POINT('Ctrl Pts',(44.4721354166655,1.96836574383981,43.507944725511));
#262908=CARTESIAN_POINT('Ctrl Pts',(44.5382812499988,3.36021050916435,44.8997894908355));
#262909=CARTESIAN_POINT('Ctrl Pts',(44.6044270833321,4.75205527448889,46.29163425616));
#262910=CARTESIAN_POINT('Ctrl Pts',(44.6705729166654,4.75205527448889,48.26));
#262911=CARTESIAN_POINT('Ctrl Pts',(44.7367187499987,4.75205527448889,50.22836574384));
#262912=CARTESIAN_POINT('Ctrl Pts',(44.802864583332,3.36021050916435,51.6202105091645));
#262913=CARTESIAN_POINT('Ctrl Pts',(44.8690104166653,1.96836574383981,53.0120552744891));
#262914=CARTESIAN_POINT('Ctrl Pts',(44.9351562499986,-1.56599280040807E-13,
53.012055274489));
#262915=CARTESIAN_POINT('Ctrl Pts',(45.001302083332,-1.96836574384012,53.0120552744891));
#262916=CARTESIAN_POINT('Ctrl Pts',(45.0674479166652,-3.36021050916466,
51.6202105091645));
#262917=CARTESIAN_POINT('Ctrl Pts',(45.1335937499986,-4.75205527448921,
50.22836574384));
#262918=CARTESIAN_POINT('Ctrl Pts',(45.1997395833319,-4.75205527448921,
48.26));
#262919=CARTESIAN_POINT('Ctrl Pts',(45.2658854166652,-4.75205527448921,
46.29163425616));
#262920=CARTESIAN_POINT('Ctrl Pts',(45.3320312499985,-3.36021050916467,
44.8997894908355));
#262921=CARTESIAN_POINT('Ctrl Pts',(45.3981770833318,-1.96836574384013,
43.507944725511));
#262922=CARTESIAN_POINT('Ctrl Pts',(45.4643229166651,-1.59610773438866E-13,
43.507944725511));
#262923=CARTESIAN_POINT('Ctrl Pts',(45.5304687499984,1.96836574383981,43.507944725511));
#262924=CARTESIAN_POINT('Ctrl Pts',(45.5966145833318,3.36021050916435,44.8997894908355));
#262925=CARTESIAN_POINT('Ctrl Pts',(45.6627604166651,4.75205527448889,46.29163425616));
#262926=CARTESIAN_POINT('Ctrl Pts',(45.7289062499984,4.75205527448889,48.26));
#262927=CARTESIAN_POINT('Ctrl Pts',(45.7950520833317,4.75205527448889,50.22836574384));
#262928=CARTESIAN_POINT('Ctrl Pts',(45.861197916665,3.36021050916435,51.6202105091645));
#262929=CARTESIAN_POINT('Ctrl Pts',(45.9273437499983,1.96836574383981,53.0120552744891));
#262930=CARTESIAN_POINT('Ctrl Pts',(45.9934895833316,-1.60294431124415E-13,
53.012055274489));
#262931=CARTESIAN_POINT('Ctrl Pts',(46.0596354166649,-1.96836574384013,
53.0120552744891));
#262932=CARTESIAN_POINT('Ctrl Pts',(46.1257812499982,-3.36021050916467,
51.6202105091645));
#262933=CARTESIAN_POINT('Ctrl Pts',(46.1919270833316,-4.75205527448921,
50.22836574384));
#262934=CARTESIAN_POINT('Ctrl Pts',(46.2580729166649,-4.75205527448921,
48.26));
#262935=CARTESIAN_POINT('Ctrl Pts',(46.3242187499982,-4.75205527448921,
46.29163425616));
#262936=CARTESIAN_POINT('Ctrl Pts',(46.3903645833315,-3.36021050916467,
44.8997894908355));
#262937=CARTESIAN_POINT('Ctrl Pts',(46.4565104166648,-1.96836574384013,
43.507944725511));
#262938=CARTESIAN_POINT('Ctrl Pts',(46.5226562499981,-1.63305924522473E-13,
43.507944725511));
#262939=CARTESIAN_POINT('Ctrl Pts',(46.5888020833314,1.9683657438398,43.507944725511));
#262940=CARTESIAN_POINT('Ctrl Pts',(46.6549479166648,3.36021050916434,44.8997894908355));
#262941=CARTESIAN_POINT('Ctrl Pts',(46.7210937499981,4.75205527448889,46.29163425616));
#262942=CARTESIAN_POINT('Ctrl Pts',(46.7872395833314,4.75205527448888,48.26));
#262943=CARTESIAN_POINT('Ctrl Pts',(46.8533854166647,4.75205527448889,50.22836574384));
#262944=CARTESIAN_POINT('Ctrl Pts',(46.919531249998,3.36021050916434,51.6202105091645));
#262945=CARTESIAN_POINT('Ctrl Pts',(46.9856770833313,1.9683657438398,53.0120552744891));
#262946=CARTESIAN_POINT('Ctrl Pts',(47.0518229166646,-1.63989582208022E-13,
53.012055274489));
#262947=CARTESIAN_POINT('Ctrl Pts',(47.1179687499979,-1.96836574384013,
53.0120552744891));
#262948=CARTESIAN_POINT('Ctrl Pts',(47.1841145833313,-3.36021050916467,
51.6202105091645));
#262949=CARTESIAN_POINT('Ctrl Pts',(47.2502604166646,-4.75205527448921,
50.22836574384));
#262950=CARTESIAN_POINT('Ctrl Pts',(47.3164062499979,-4.75205527448921,
48.26));
#262951=CARTESIAN_POINT('Ctrl Pts',(47.3825520833312,-4.75205527448922,
46.29163425616));
#262952=CARTESIAN_POINT('Ctrl Pts',(47.4486979166645,-3.36021050916467,
44.8997894908355));
#262953=CARTESIAN_POINT('Ctrl Pts',(47.5148437499978,-1.96836574384013,
43.507944725511));
#262954=CARTESIAN_POINT('Ctrl Pts',(47.5809895833311,-1.67001075606081E-13,
43.507944725511));
#262955=CARTESIAN_POINT('Ctrl Pts',(47.6471354166645,1.9683657438398,43.507944725511));
#262956=CARTESIAN_POINT('Ctrl Pts',(47.7132812499978,3.36021050916434,44.8997894908355));
#262957=CARTESIAN_POINT('Ctrl Pts',(47.7794270833311,4.75205527448888,46.29163425616));
#262958=CARTESIAN_POINT('Ctrl Pts',(47.8455729166644,4.75205527448888,48.26));
#262959=CARTESIAN_POINT('Ctrl Pts',(47.9117187499977,4.75205527448888,50.22836574384));
#262960=CARTESIAN_POINT('Ctrl Pts',(47.977864583331,3.36021050916434,51.6202105091645));
#262961=CARTESIAN_POINT('Ctrl Pts',(48.0440104166643,1.9683657438398,53.0120552744891));
#262962=CARTESIAN_POINT('Ctrl Pts',(48.1101562499976,-1.6768473329163E-13,
53.012055274489));
#262963=CARTESIAN_POINT('Ctrl Pts',(48.1763020833309,-1.96836574384013,
53.0120552744891));
#262964=CARTESIAN_POINT('Ctrl Pts',(48.2424479166642,-3.36021050916468,
51.6202105091645));
#262965=CARTESIAN_POINT('Ctrl Pts',(48.3085937499975,-4.75205527448922,
50.22836574384));
#262966=CARTESIAN_POINT('Ctrl Pts',(48.3747395833309,-4.75205527448922,
48.26));
#262967=CARTESIAN_POINT('Ctrl Pts',(48.4408854166642,-4.75205527448922,
46.29163425616));
#262968=CARTESIAN_POINT('Ctrl Pts',(48.5070312499975,-3.36021050916468,
44.8997894908355));
#262969=CARTESIAN_POINT('Ctrl Pts',(48.5731770833308,-1.96836574384014,
43.507944725511));
#262970=CARTESIAN_POINT('Ctrl Pts',(48.6393229166641,-1.70696226689689E-13,
43.507944725511));
#262971=CARTESIAN_POINT('Ctrl Pts',(48.7054687499974,1.9683657438398,43.507944725511));
#262972=CARTESIAN_POINT('Ctrl Pts',(48.7716145833308,3.36021050916434,44.8997894908355));
#262973=CARTESIAN_POINT('Ctrl Pts',(48.8377604166641,4.75205527448888,46.29163425616));
#262974=CARTESIAN_POINT('Ctrl Pts',(48.9039062499974,4.75205527448888,48.26));
#262975=CARTESIAN_POINT('Ctrl Pts',(48.9700520833307,4.75205527448888,50.22836574384));
#262976=CARTESIAN_POINT('Ctrl Pts',(49.036197916664,3.36021050916434,51.6202105091645));
#262977=CARTESIAN_POINT('Ctrl Pts',(49.1023437499973,1.96836574383979,53.0120552744891));
#262978=CARTESIAN_POINT('Ctrl Pts',(49.1684895833306,-1.71379884375238E-13,
53.012055274489));
#262979=CARTESIAN_POINT('Ctrl Pts',(49.2346354166639,-1.96836574384014,
53.0120552744891));
#262980=CARTESIAN_POINT('Ctrl Pts',(49.3007812499973,-3.36021050916468,
51.6202105091645));
#262981=CARTESIAN_POINT('Ctrl Pts',(49.3669270833306,-4.75205527448922,
50.22836574384));
#262982=CARTESIAN_POINT('Ctrl Pts',(49.4330729166639,-4.75205527448922,
48.26));
#262983=CARTESIAN_POINT('Ctrl Pts',(49.4992187499972,-4.75205527448922,
46.29163425616));
#262984=CARTESIAN_POINT('Ctrl Pts',(49.5653645833305,-3.36021050916468,
44.8997894908355));
#262985=CARTESIAN_POINT('Ctrl Pts',(49.6315104166638,-1.96836574384014,
43.507944725511));
#262986=CARTESIAN_POINT('Ctrl Pts',(49.6976562499971,-1.74391377773297E-13,
43.507944725511));
#262987=CARTESIAN_POINT('Ctrl Pts',(49.7638020833305,1.96836574383979,43.507944725511));
#262988=CARTESIAN_POINT('Ctrl Pts',(49.8299479166638,3.36021050916433,44.8997894908355));
#262989=CARTESIAN_POINT('Ctrl Pts',(49.8960937499971,4.75205527448887,46.29163425616));
#262990=CARTESIAN_POINT('Ctrl Pts',(49.9622395833304,4.75205527448887,48.26));
#262991=CARTESIAN_POINT('Ctrl Pts',(50.0283854166637,4.75205527448887,50.22836574384));
#262992=CARTESIAN_POINT('Ctrl Pts',(50.094531249997,3.36021050916433,51.6202105091645));
#262993=CARTESIAN_POINT('Ctrl Pts',(50.1606770833303,1.96836574383979,53.0120552744891));
#262994=CARTESIAN_POINT('Ctrl Pts',(50.2268229166636,-1.75075035458846E-13,
53.012055274489));
#262995=CARTESIAN_POINT('Ctrl Pts',(50.2929687499969,-1.96836574384014,
53.0120552744891));
#262996=CARTESIAN_POINT('Ctrl Pts',(50.3591145833302,-3.36021050916468,
51.6202105091645));
#262997=CARTESIAN_POINT('Ctrl Pts',(50.4252604166636,-4.75205527448922,
50.22836574384));
#262998=CARTESIAN_POINT('Ctrl Pts',(50.4914062499969,-4.75205527448922,
48.26));
#262999=CARTESIAN_POINT('Ctrl Pts',(50.5575520833302,-4.75205527448923,
46.29163425616));
#263000=CARTESIAN_POINT('Ctrl Pts',(50.6236979166635,-3.36021050916468,
44.8997894908355));
#263001=CARTESIAN_POINT('Ctrl Pts',(50.6898437499968,-1.96836574384015,
43.507944725511));
#263002=CARTESIAN_POINT('Ctrl Pts',(50.7559895833301,-1.78086528856905E-13,
43.507944725511));
#263003=CARTESIAN_POINT('Ctrl Pts',(50.8221354166634,1.96836574383979,43.507944725511));
#263004=CARTESIAN_POINT('Ctrl Pts',(50.8882812499968,3.36021050916433,44.8997894908355));
#263005=CARTESIAN_POINT('Ctrl Pts',(50.9544270833301,4.75205527448887,46.29163425616));
#263006=CARTESIAN_POINT('Ctrl Pts',(51.0205729166634,4.75205527448887,48.26));
#263007=CARTESIAN_POINT('Ctrl Pts',(40.4541666666667,4.72273670613168,48.26));
#263008=CARTESIAN_POINT('Ctrl Pts',(40.5203125,4.72273670613168,50.216221595197));
#263009=CARTESIAN_POINT('Ctrl Pts',(40.5864583333333,3.33947915066429,51.5994791506644));
#263010=CARTESIAN_POINT('Ctrl Pts',(40.6526041666666,1.9562215951969,52.9827367061318));
#263011=CARTESIAN_POINT('Ctrl Pts',(40.7187499999999,-1.418795715465E-13,
52.9827367061318));
#263012=CARTESIAN_POINT('Ctrl Pts',(40.7848958333332,-1.95622159519718,
52.9827367061318));
#263013=CARTESIAN_POINT('Ctrl Pts',(40.8510416666665,-3.33947915066458,
51.5994791506644));
#263014=CARTESIAN_POINT('Ctrl Pts',(40.9171874999998,-4.72273670613197,
50.216221595197));
#263015=CARTESIAN_POINT('Ctrl Pts',(40.9833333333332,-4.72273670613197,
48.26));
#263016=CARTESIAN_POINT('Ctrl Pts',(41.0494791666665,-4.72273670613197,
46.303778404803));
#263017=CARTESIAN_POINT('Ctrl Pts',(41.1156249999998,-3.33947915066458,
44.9205208493356));
#263018=CARTESIAN_POINT('Ctrl Pts',(41.1817708333331,-1.95622159519719,
43.5372632938682));
#263019=CARTESIAN_POINT('Ctrl Pts',(41.2479166666664,-1.44883883966379E-13,
43.5372632938682));
#263020=CARTESIAN_POINT('Ctrl Pts',(41.3140624999997,1.9562215951969,43.5372632938682));
#263021=CARTESIAN_POINT('Ctrl Pts',(41.3802083333331,3.33947915066429,44.9205208493356));
#263022=CARTESIAN_POINT('Ctrl Pts',(41.4463541666664,4.72273670613168,46.303778404803));
#263023=CARTESIAN_POINT('Ctrl Pts',(41.5124999999997,4.72273670613168,48.26));
#263024=CARTESIAN_POINT('Ctrl Pts',(41.578645833333,4.72273670613168,50.216221595197));
#263025=CARTESIAN_POINT('Ctrl Pts',(41.6447916666663,3.33947915066429,51.5994791506644));
#263026=CARTESIAN_POINT('Ctrl Pts',(41.7109374999996,1.9562215951969,52.9827367061318));
#263027=CARTESIAN_POINT('Ctrl Pts',(41.7770833333329,-1.45574722630107E-13,
52.9827367061318));
#263028=CARTESIAN_POINT('Ctrl Pts',(41.8432291666662,-1.95622159519719,
52.9827367061318));
#263029=CARTESIAN_POINT('Ctrl Pts',(41.9093749999995,-3.33947915066458,
51.5994791506644));
#263030=CARTESIAN_POINT('Ctrl Pts',(41.9755208333328,-4.72273670613197,
50.216221595197));
#263031=CARTESIAN_POINT('Ctrl Pts',(42.0416666666662,-4.72273670613197,
48.26));
#263032=CARTESIAN_POINT('Ctrl Pts',(42.1078124999995,-4.72273670613197,
46.303778404803));
#263033=CARTESIAN_POINT('Ctrl Pts',(42.1739583333328,-3.33947915066458,
44.9205208493356));
#263034=CARTESIAN_POINT('Ctrl Pts',(42.2401041666661,-1.95622159519719,
43.5372632938682));
#263035=CARTESIAN_POINT('Ctrl Pts',(42.3062499999994,-1.48579035049987E-13,
43.5372632938682));
#263036=CARTESIAN_POINT('Ctrl Pts',(42.3723958333328,1.95622159519689,43.5372632938682));
#263037=CARTESIAN_POINT('Ctrl Pts',(42.4385416666661,3.33947915066428,44.9205208493356));
#263038=CARTESIAN_POINT('Ctrl Pts',(42.5046874999994,4.72273670613168,46.303778404803));
#263039=CARTESIAN_POINT('Ctrl Pts',(42.5708333333327,4.72273670613168,48.26));
#263040=CARTESIAN_POINT('Ctrl Pts',(42.636979166666,4.72273670613168,50.216221595197));
#263041=CARTESIAN_POINT('Ctrl Pts',(42.7031249999993,3.33947915066428,51.5994791506644));
#263042=CARTESIAN_POINT('Ctrl Pts',(42.7692708333326,1.95622159519689,52.9827367061318));
#263043=CARTESIAN_POINT('Ctrl Pts',(42.8354166666659,-1.49269873713715E-13,
52.9827367061318));
#263044=CARTESIAN_POINT('Ctrl Pts',(42.9015624999992,-1.95622159519719,
52.9827367061318));
#263045=CARTESIAN_POINT('Ctrl Pts',(42.9677083333325,-3.33947915066458,
51.5994791506644));
#263046=CARTESIAN_POINT('Ctrl Pts',(43.0338541666658,-4.72273670613198,
50.216221595197));
#263047=CARTESIAN_POINT('Ctrl Pts',(43.0999999999992,-4.72273670613198,
48.26));
#263048=CARTESIAN_POINT('Ctrl Pts',(43.1661458333325,-4.72273670613198,
46.303778404803));
#263049=CARTESIAN_POINT('Ctrl Pts',(43.2322916666658,-3.33947915066458,
44.9205208493356));
#263050=CARTESIAN_POINT('Ctrl Pts',(43.2984374999991,-1.95622159519719,
43.5372632938682));
#263051=CARTESIAN_POINT('Ctrl Pts',(43.3645833333324,-1.52274186133595E-13,
43.5372632938682));
#263052=CARTESIAN_POINT('Ctrl Pts',(43.4307291666657,1.95622159519689,43.5372632938682));
#263053=CARTESIAN_POINT('Ctrl Pts',(43.4968749999991,3.33947915066428,44.9205208493356));
#263054=CARTESIAN_POINT('Ctrl Pts',(43.5630208333324,4.72273670613167,46.303778404803));
#263055=CARTESIAN_POINT('Ctrl Pts',(43.6291666666657,4.72273670613167,48.26));
#263056=CARTESIAN_POINT('Ctrl Pts',(43.695312499999,4.72273670613167,50.216221595197));
#263057=CARTESIAN_POINT('Ctrl Pts',(43.7614583333323,3.33947915066428,51.5994791506644));
#263058=CARTESIAN_POINT('Ctrl Pts',(43.8276041666656,1.95622159519689,52.9827367061318));
#263059=CARTESIAN_POINT('Ctrl Pts',(43.8937499999989,-1.52965024797323E-13,
52.9827367061318));
#263060=CARTESIAN_POINT('Ctrl Pts',(43.9598958333322,-1.95622159519719,
52.9827367061318));
#263061=CARTESIAN_POINT('Ctrl Pts',(44.0260416666655,-3.33947915066459,
51.5994791506644));
#263062=CARTESIAN_POINT('Ctrl Pts',(44.0921874999988,-4.72273670613198,
50.216221595197));
#263063=CARTESIAN_POINT('Ctrl Pts',(44.1583333333322,-4.72273670613198,
48.26));
#263064=CARTESIAN_POINT('Ctrl Pts',(44.2244791666655,-4.72273670613198,
46.303778404803));
#263065=CARTESIAN_POINT('Ctrl Pts',(44.2906249999988,-3.33947915066459,
44.9205208493356));
#263066=CARTESIAN_POINT('Ctrl Pts',(44.3567708333321,-1.9562215951972,43.5372632938682));
#263067=CARTESIAN_POINT('Ctrl Pts',(44.4229166666654,-1.55969337217203E-13,
43.5372632938682));
#263068=CARTESIAN_POINT('Ctrl Pts',(44.4890624999988,1.95622159519689,43.5372632938682));
#263069=CARTESIAN_POINT('Ctrl Pts',(44.5552083333321,3.33947915066428,44.9205208493356));
#263070=CARTESIAN_POINT('Ctrl Pts',(44.6213541666654,4.72273670613167,46.303778404803));
#263071=CARTESIAN_POINT('Ctrl Pts',(44.6874999999987,4.72273670613167,48.26));
#263072=CARTESIAN_POINT('Ctrl Pts',(44.753645833332,4.72273670613167,50.216221595197));
#263073=CARTESIAN_POINT('Ctrl Pts',(44.8197916666653,3.33947915066428,51.5994791506644));
#263074=CARTESIAN_POINT('Ctrl Pts',(44.8859374999986,1.95622159519688,52.9827367061318));
#263075=CARTESIAN_POINT('Ctrl Pts',(44.9520833333319,-1.56660175880931E-13,
52.9827367061318));
#263076=CARTESIAN_POINT('Ctrl Pts',(45.0182291666652,-1.9562215951972,52.9827367061318));
#263077=CARTESIAN_POINT('Ctrl Pts',(45.0843749999985,-3.33947915066459,
51.5994791506644));
#263078=CARTESIAN_POINT('Ctrl Pts',(45.1505208333318,-4.72273670613198,
50.216221595197));
#263079=CARTESIAN_POINT('Ctrl Pts',(45.2166666666652,-4.72273670613198,
48.26));
#263080=CARTESIAN_POINT('Ctrl Pts',(45.2828124999985,-4.72273670613199,
46.303778404803));
#263081=CARTESIAN_POINT('Ctrl Pts',(45.3489583333318,-3.33947915066459,
44.9205208493356));
#263082=CARTESIAN_POINT('Ctrl Pts',(45.4151041666651,-1.9562215951972,43.5372632938682));
#263083=CARTESIAN_POINT('Ctrl Pts',(45.4812499999984,-1.59664488300811E-13,
43.5372632938682));
#263084=CARTESIAN_POINT('Ctrl Pts',(45.5473958333317,1.95622159519688,43.5372632938682));
#263085=CARTESIAN_POINT('Ctrl Pts',(45.6135416666651,3.33947915066427,44.9205208493356));
#263086=CARTESIAN_POINT('Ctrl Pts',(45.6796874999984,4.72273670613167,46.303778404803));
#263087=CARTESIAN_POINT('Ctrl Pts',(45.7458333333317,4.72273670613167,48.26));
#263088=CARTESIAN_POINT('Ctrl Pts',(45.811979166665,4.72273670613167,50.216221595197));
#263089=CARTESIAN_POINT('Ctrl Pts',(45.8781249999983,3.33947915066427,51.5994791506644));
#263090=CARTESIAN_POINT('Ctrl Pts',(45.9442708333316,1.95622159519688,52.9827367061318));
#263091=CARTESIAN_POINT('Ctrl Pts',(46.0104166666649,-1.60355326964539E-13,
52.9827367061318));
#263092=CARTESIAN_POINT('Ctrl Pts',(46.0765624999982,-1.9562215951972,52.9827367061318));
#263093=CARTESIAN_POINT('Ctrl Pts',(46.1427083333315,-3.33947915066459,
51.5994791506644));
#263094=CARTESIAN_POINT('Ctrl Pts',(46.2088541666649,-4.72273670613199,
50.216221595197));
#263095=CARTESIAN_POINT('Ctrl Pts',(46.2749999999982,-4.72273670613199,
48.26));
#263096=CARTESIAN_POINT('Ctrl Pts',(46.3411458333315,-4.72273670613199,
46.303778404803));
#263097=CARTESIAN_POINT('Ctrl Pts',(46.4072916666648,-3.3394791506646,44.9205208493356));
#263098=CARTESIAN_POINT('Ctrl Pts',(46.4734374999981,-1.95622159519721,
43.5372632938682));
#263099=CARTESIAN_POINT('Ctrl Pts',(46.5395833333314,-1.63359639384419E-13,
43.5372632938682));
#263100=CARTESIAN_POINT('Ctrl Pts',(46.6057291666647,1.95622159519688,43.5372632938682));
#263101=CARTESIAN_POINT('Ctrl Pts',(46.6718749999981,3.33947915066427,44.9205208493356));
#263102=CARTESIAN_POINT('Ctrl Pts',(46.7380208333314,4.72273670613166,46.303778404803));
#263103=CARTESIAN_POINT('Ctrl Pts',(46.8041666666647,4.72273670613166,48.26));
#263104=CARTESIAN_POINT('Ctrl Pts',(46.870312499998,4.72273670613166,50.216221595197));
#263105=CARTESIAN_POINT('Ctrl Pts',(46.9364583333313,3.33947915066427,51.5994791506644));
#263106=CARTESIAN_POINT('Ctrl Pts',(47.0026041666646,1.95622159519688,52.9827367061318));
#263107=CARTESIAN_POINT('Ctrl Pts',(47.0687499999979,-1.64050478048146E-13,
52.9827367061318));
#263108=CARTESIAN_POINT('Ctrl Pts',(47.1348958333312,-1.95622159519721,
52.9827367061318));
#263109=CARTESIAN_POINT('Ctrl Pts',(47.2010416666646,-3.3394791506646,51.5994791506644));
#263110=CARTESIAN_POINT('Ctrl Pts',(47.2671874999979,-4.72273670613199,
50.216221595197));
#263111=CARTESIAN_POINT('Ctrl Pts',(47.3333333333312,-4.72273670613199,
48.26));
#263112=CARTESIAN_POINT('Ctrl Pts',(47.3994791666645,-4.72273670613199,
46.303778404803));
#263113=CARTESIAN_POINT('Ctrl Pts',(47.4656249999978,-3.3394791506646,44.9205208493356));
#263114=CARTESIAN_POINT('Ctrl Pts',(47.5317708333311,-1.95622159519721,
43.5372632938682));
#263115=CARTESIAN_POINT('Ctrl Pts',(47.5979166666644,-1.67054790468026E-13,
43.5372632938682));
#263116=CARTESIAN_POINT('Ctrl Pts',(47.6640624999977,1.95622159519688,43.5372632938682));
#263117=CARTESIAN_POINT('Ctrl Pts',(47.7302083333311,3.33947915066426,44.9205208493356));
#263118=CARTESIAN_POINT('Ctrl Pts',(47.7963541666644,4.72273670613166,46.303778404803));
#263119=CARTESIAN_POINT('Ctrl Pts',(47.8624999999977,4.72273670613166,48.26));
#263120=CARTESIAN_POINT('Ctrl Pts',(47.928645833331,4.72273670613166,50.216221595197));
#263121=CARTESIAN_POINT('Ctrl Pts',(47.9947916666643,3.33947915066427,51.5994791506644));
#263122=CARTESIAN_POINT('Ctrl Pts',(48.0609374999976,1.95622159519687,52.9827367061318));
#263123=CARTESIAN_POINT('Ctrl Pts',(48.1270833333309,-1.67745629131754E-13,
52.9827367061318));
#263124=CARTESIAN_POINT('Ctrl Pts',(48.1932291666642,-1.95622159519721,
52.9827367061318));
#263125=CARTESIAN_POINT('Ctrl Pts',(48.2593749999975,-3.3394791506646,51.5994791506644));
#263126=CARTESIAN_POINT('Ctrl Pts',(48.3255208333308,-4.722736706132,50.216221595197));
#263127=CARTESIAN_POINT('Ctrl Pts',(48.3916666666642,-4.72273670613199,
48.26));
#263128=CARTESIAN_POINT('Ctrl Pts',(48.4578124999975,-4.722736706132,46.303778404803));
#263129=CARTESIAN_POINT('Ctrl Pts',(48.5239583333308,-3.3394791506646,44.9205208493356));
#263130=CARTESIAN_POINT('Ctrl Pts',(48.5901041666641,-1.95622159519721,
43.5372632938682));
#263131=CARTESIAN_POINT('Ctrl Pts',(48.6562499999974,-1.70749941551634E-13,
43.5372632938682));
#263132=CARTESIAN_POINT('Ctrl Pts',(48.7223958333307,1.95622159519687,43.5372632938682));
#263133=CARTESIAN_POINT('Ctrl Pts',(48.7885416666641,3.33947915066426,44.9205208493356));
#263134=CARTESIAN_POINT('Ctrl Pts',(48.8546874999974,4.72273670613165,46.303778404803));
#263135=CARTESIAN_POINT('Ctrl Pts',(48.9208333333307,4.72273670613165,48.26));
#263136=CARTESIAN_POINT('Ctrl Pts',(48.986979166664,4.72273670613165,50.216221595197));
#263137=CARTESIAN_POINT('Ctrl Pts',(49.0531249999973,3.33947915066426,51.5994791506644));
#263138=CARTESIAN_POINT('Ctrl Pts',(49.1192708333306,1.95622159519687,52.9827367061318));
#263139=CARTESIAN_POINT('Ctrl Pts',(49.1854166666639,-1.71440780215362E-13,
52.9827367061318));
#263140=CARTESIAN_POINT('Ctrl Pts',(49.2515624999972,-1.95622159519721,
52.9827367061318));
#263141=CARTESIAN_POINT('Ctrl Pts',(49.3177083333305,-3.33947915066461,
51.5994791506644));
#263142=CARTESIAN_POINT('Ctrl Pts',(49.3838541666639,-4.722736706132,50.216221595197));
#263143=CARTESIAN_POINT('Ctrl Pts',(49.4499999999972,-4.722736706132,48.26));
#263144=CARTESIAN_POINT('Ctrl Pts',(49.5161458333305,-4.722736706132,46.303778404803));
#263145=CARTESIAN_POINT('Ctrl Pts',(49.5822916666638,-3.33947915066461,
44.9205208493356));
#263146=CARTESIAN_POINT('Ctrl Pts',(49.6484374999971,-1.95622159519722,
43.5372632938682));
#263147=CARTESIAN_POINT('Ctrl Pts',(49.7145833333304,-1.74445092635242E-13,
43.5372632938682));
#263148=CARTESIAN_POINT('Ctrl Pts',(49.7807291666637,1.95622159519687,43.5372632938682));
#263149=CARTESIAN_POINT('Ctrl Pts',(49.8468749999971,3.33947915066426,44.9205208493356));
#263150=CARTESIAN_POINT('Ctrl Pts',(49.9130208333304,4.72273670613165,46.303778404803));
#263151=CARTESIAN_POINT('Ctrl Pts',(49.9791666666637,4.72273670613165,48.26));
#263152=CARTESIAN_POINT('Ctrl Pts',(50.045312499997,4.72273670613165,50.216221595197));
#263153=CARTESIAN_POINT('Ctrl Pts',(50.1114583333303,3.33947915066426,51.5994791506644));
#263154=CARTESIAN_POINT('Ctrl Pts',(50.1776041666636,1.95622159519687,52.9827367061318));
#263155=CARTESIAN_POINT('Ctrl Pts',(50.2437499999969,-1.7513593129897E-13,
52.9827367061318));
#263156=CARTESIAN_POINT('Ctrl Pts',(50.3098958333302,-1.95622159519722,
52.9827367061318));
#263157=CARTESIAN_POINT('Ctrl Pts',(50.3760416666635,-3.33947915066461,
51.5994791506644));
#263158=CARTESIAN_POINT('Ctrl Pts',(50.4421874999969,-4.722736706132,50.216221595197));
#263159=CARTESIAN_POINT('Ctrl Pts',(50.5083333333302,-4.722736706132,48.26));
#263160=CARTESIAN_POINT('Ctrl Pts',(50.5744791666635,-4.722736706132,46.303778404803));
#263161=CARTESIAN_POINT('Ctrl Pts',(50.6406249999968,-3.33947915066461,
44.9205208493356));
#263162=CARTESIAN_POINT('Ctrl Pts',(50.7067708333301,-1.95622159519722,
43.5372632938682));
#263163=CARTESIAN_POINT('Ctrl Pts',(50.7729166666634,-1.7814024371885E-13,
43.5372632938682));
#263164=CARTESIAN_POINT('Ctrl Pts',(50.8390624999967,1.95622159519686,43.5372632938682));
#263165=CARTESIAN_POINT('Ctrl Pts',(50.9052083333301,3.33947915066425,44.9205208493356));
#263166=CARTESIAN_POINT('Ctrl Pts',(50.9713541666634,4.72273670613165,46.303778404803));
#263167=CARTESIAN_POINT('Ctrl Pts',(51.0374999999967,4.72273670613165,48.26));
#263168=CARTESIAN_POINT('Origin',(-3.05311331771918E-14,40.4567708333334,
48.26));
#263169=CARTESIAN_POINT('',(4.72273670613183,48.3916666666642,48.26));
#263170=CARTESIAN_POINT('',(4.72273670613183,48.3968749999976,48.26));
#263171=CARTESIAN_POINT('',(4.72273670613176,40.4567708333334,48.26));
#263172=CARTESIAN_POINT('',(2.14259623628819,49.2650632938682,52.4687436799701));
#263173=CARTESIAN_POINT('Ctrl Pts',(4.72273670613183,48.3916666666642,48.26));
#263174=CARTESIAN_POINT('Ctrl Pts',(4.72273670613183,48.4578124999975,46.303778404803));
#263175=CARTESIAN_POINT('Ctrl Pts',(3.33947915066444,48.5239583333308,44.9205208493356));
#263176=CARTESIAN_POINT('Ctrl Pts',(1.95622159519705,48.5901041666641,43.5372632938682));
#263177=CARTESIAN_POINT('Ctrl Pts',(6.99833541005117E-15,48.6562499999974,
43.5372632938682));
#263178=CARTESIAN_POINT('Ctrl Pts',(-1.95622159519704,48.7223958333307,
43.5372632938682));
#263179=CARTESIAN_POINT('Ctrl Pts',(-3.33947915066443,48.788541666664,44.9205208493356));
#263180=CARTESIAN_POINT('Ctrl Pts',(-4.72273670613182,48.8546874999974,
46.303778404803));
#263181=CARTESIAN_POINT('Ctrl Pts',(-4.72273670613182,48.9208333333307,
48.26));
#263182=CARTESIAN_POINT('Ctrl Pts',(-4.72273670613182,48.986979166664,50.216221595197));
#263183=CARTESIAN_POINT('Ctrl Pts',(-3.33947915066443,49.0531249999973,
51.5994791506644));
#263184=CARTESIAN_POINT('Ctrl Pts',(-1.95622159519703,49.1192708333306,
52.9827367061318));
#263185=CARTESIAN_POINT('Ctrl Pts',(7.17168088200102E-15,49.1854166666639,
52.9827367061318));
#263186=CARTESIAN_POINT('Ctrl Pts',(1.13294968517018,49.2237251595434,52.9827367061318));
#263187=CARTESIAN_POINT('Ctrl Pts',(2.14259623628819,49.2650632938682,52.4687436799701));
#263188=CARTESIAN_POINT('',(2.01456111142411,49.2650632938682,52.5315085770466));
#263189=CARTESIAN_POINT('Origin',(-4.11914963277527E-6,49.2650632939072,
48.2599916315336));
#263190=CARTESIAN_POINT('Ctrl Pts',(4.72273670613183,48.3968749999976,48.26));
#263191=CARTESIAN_POINT('Ctrl Pts',(4.72273670613183,48.4630208333309,46.303778404803));
#263192=CARTESIAN_POINT('Ctrl Pts',(3.33947915066444,48.5291666666642,44.9205208493356));
#263193=CARTESIAN_POINT('Ctrl Pts',(1.95622159519705,48.5953124999975,43.5372632938682));
#263194=CARTESIAN_POINT('Ctrl Pts',(6.99833541005117E-15,48.6614583333308,
43.5372632938682));
#263195=CARTESIAN_POINT('Ctrl Pts',(-1.95622159519704,48.7276041666641,
43.5372632938682));
#263196=CARTESIAN_POINT('Ctrl Pts',(-3.33947915066443,48.7937499999974,
44.9205208493356));
#263197=CARTESIAN_POINT('Ctrl Pts',(-4.72273670613182,48.8598958333307,
46.303778404803));
#263198=CARTESIAN_POINT('Ctrl Pts',(-4.72273670613182,48.9260416666641,
48.26));
#263199=CARTESIAN_POINT('Ctrl Pts',(-4.72273670613182,48.9921874999974,
50.216221595197));
#263200=CARTESIAN_POINT('Ctrl Pts',(-3.33947915066443,49.0583333333307,
51.5994791506644));
#263201=CARTESIAN_POINT('Ctrl Pts',(-1.95622159519703,49.124479166664,52.9827367061318));
#263202=CARTESIAN_POINT('Ctrl Pts',(7.17168088200102E-15,49.1906249999973,
52.9827367061318));
#263203=CARTESIAN_POINT('Ctrl Pts',(1.05781434774328,49.2263929373901,52.9827367061318));
#263204=CARTESIAN_POINT('Ctrl Pts',(2.01456111142411,49.2650632938682,52.5315085770466));
#263205=CARTESIAN_POINT('Origin',(-3.05311331771918E-14,40.4567708333334,
48.26));
#263206=CARTESIAN_POINT('',(4.72273670613183,47.3333333333312,48.26));
#263207=CARTESIAN_POINT('',(4.72273670613183,47.3385416666645,48.26));
#263208=CARTESIAN_POINT('',(4.72273670613176,40.4567708333334,48.26));
#263209=CARTESIAN_POINT('Ctrl Pts',(4.72273670613183,47.3333333333312,48.26));
#263210=CARTESIAN_POINT('Ctrl Pts',(4.72273670613183,47.3994791666645,46.303778404803));
#263211=CARTESIAN_POINT('Ctrl Pts',(3.33947915066444,47.4656249999978,44.9205208493356));
#263212=CARTESIAN_POINT('Ctrl Pts',(1.95622159519705,47.5317708333311,43.5372632938682));
#263213=CARTESIAN_POINT('Ctrl Pts',(6.99833541005117E-15,47.5979166666644,
43.5372632938682));
#263214=CARTESIAN_POINT('Ctrl Pts',(-1.95622159519704,47.6640624999977,
43.5372632938682));
#263215=CARTESIAN_POINT('Ctrl Pts',(-3.33947915066443,47.730208333331,44.9205208493356));
#263216=CARTESIAN_POINT('Ctrl Pts',(-4.72273670613182,47.7963541666644,
46.303778404803));
#263217=CARTESIAN_POINT('Ctrl Pts',(-4.72273670613182,47.8624999999977,
48.26));
#263218=CARTESIAN_POINT('Ctrl Pts',(-4.72273670613182,47.928645833331,50.216221595197));
#263219=CARTESIAN_POINT('Ctrl Pts',(-3.33947915066443,47.9947916666643,
51.5994791506644));
#263220=CARTESIAN_POINT('Ctrl Pts',(-1.95622159519703,48.0609374999976,
52.9827367061318));
#263221=CARTESIAN_POINT('Ctrl Pts',(7.17168088200102E-15,48.1270833333309,
52.9827367061318));
#263222=CARTESIAN_POINT('Ctrl Pts',(1.95622159519705,48.1932291666642,52.9827367061318));
#263223=CARTESIAN_POINT('Ctrl Pts',(3.33947915066444,48.2593749999975,51.5994791506644));
#263224=CARTESIAN_POINT('Ctrl Pts',(4.72273670613183,48.3255208333309,50.216221595197));
#263225=CARTESIAN_POINT('Ctrl Pts',(4.72273670613183,48.3916666666642,48.26));
#263226=CARTESIAN_POINT('Ctrl Pts',(4.72273670613183,47.3385416666645,48.26));
#263227=CARTESIAN_POINT('Ctrl Pts',(4.72273670613183,47.4046874999979,46.303778404803));
#263228=CARTESIAN_POINT('Ctrl Pts',(3.33947915066444,47.4708333333312,44.9205208493356));
#263229=CARTESIAN_POINT('Ctrl Pts',(1.95622159519705,47.5369791666645,43.5372632938682));
#263230=CARTESIAN_POINT('Ctrl Pts',(6.99833541005117E-15,47.6031249999978,
43.5372632938682));
#263231=CARTESIAN_POINT('Ctrl Pts',(-1.95622159519704,47.6692708333311,
43.5372632938682));
#263232=CARTESIAN_POINT('Ctrl Pts',(-3.33947915066443,47.7354166666644,
44.9205208493356));
#263233=CARTESIAN_POINT('Ctrl Pts',(-4.72273670613182,47.8015624999977,
46.303778404803));
#263234=CARTESIAN_POINT('Ctrl Pts',(-4.72273670613182,47.867708333331,48.26));
#263235=CARTESIAN_POINT('Ctrl Pts',(-4.72273670613182,47.9338541666644,
50.216221595197));
#263236=CARTESIAN_POINT('Ctrl Pts',(-3.33947915066443,47.9999999999977,
51.5994791506644));
#263237=CARTESIAN_POINT('Ctrl Pts',(-1.95622159519703,48.066145833331,52.9827367061318));
#263238=CARTESIAN_POINT('Ctrl Pts',(7.17168088200104E-15,48.1322916666643,
52.9827367061318));
#263239=CARTESIAN_POINT('Ctrl Pts',(1.95622159519705,48.1984374999976,52.9827367061318));
#263240=CARTESIAN_POINT('Ctrl Pts',(3.33947915066444,48.2645833333309,51.5994791506644));
#263241=CARTESIAN_POINT('Ctrl Pts',(4.72273670613183,48.3307291666642,50.216221595197));
#263242=CARTESIAN_POINT('Ctrl Pts',(4.72273670613183,48.3968749999976,48.26));
#263243=CARTESIAN_POINT('Origin',(-3.05311331771918E-14,40.4567708333334,
48.26));
#263244=CARTESIAN_POINT('',(4.72273670613183,46.2749999999982,48.26));
#263245=CARTESIAN_POINT('',(4.72273670613183,46.2802083333315,48.26));
#263246=CARTESIAN_POINT('',(4.72273670613176,40.4567708333334,48.26));
#263247=CARTESIAN_POINT('Ctrl Pts',(4.72273670613183,46.2749999999982,48.26));
#263248=CARTESIAN_POINT('Ctrl Pts',(4.72273670613183,46.3411458333315,46.303778404803));
#263249=CARTESIAN_POINT('Ctrl Pts',(3.33947915066444,46.4072916666648,44.9205208493356));
#263250=CARTESIAN_POINT('Ctrl Pts',(1.95622159519705,46.4734374999981,43.5372632938682));
#263251=CARTESIAN_POINT('Ctrl Pts',(6.99833541005117E-15,46.5395833333314,
43.5372632938682));
#263252=CARTESIAN_POINT('Ctrl Pts',(-1.95622159519704,46.6057291666647,
43.5372632938682));
#263253=CARTESIAN_POINT('Ctrl Pts',(-3.33947915066443,46.671874999998,44.9205208493356));
#263254=CARTESIAN_POINT('Ctrl Pts',(-4.72273670613182,46.7380208333314,
46.303778404803));
#263255=CARTESIAN_POINT('Ctrl Pts',(-4.72273670613182,46.8041666666647,
48.26));
#263256=CARTESIAN_POINT('Ctrl Pts',(-4.72273670613182,46.870312499998,50.216221595197));
#263257=CARTESIAN_POINT('Ctrl Pts',(-3.33947915066443,46.9364583333313,
51.5994791506644));
#263258=CARTESIAN_POINT('Ctrl Pts',(-1.95622159519703,47.0026041666646,
52.9827367061318));
#263259=CARTESIAN_POINT('Ctrl Pts',(7.17168088200104E-15,47.0687499999979,
52.9827367061318));
#263260=CARTESIAN_POINT('Ctrl Pts',(1.95622159519705,47.1348958333312,52.9827367061318));
#263261=CARTESIAN_POINT('Ctrl Pts',(3.33947915066444,47.2010416666646,51.5994791506644));
#263262=CARTESIAN_POINT('Ctrl Pts',(4.72273670613183,47.2671874999979,50.216221595197));
#263263=CARTESIAN_POINT('Ctrl Pts',(4.72273670613183,47.3333333333312,48.26));
#263264=CARTESIAN_POINT('Ctrl Pts',(4.72273670613183,46.2802083333315,48.26));
#263265=CARTESIAN_POINT('Ctrl Pts',(4.72273670613183,46.3463541666649,46.303778404803));
#263266=CARTESIAN_POINT('Ctrl Pts',(3.33947915066444,46.4124999999982,44.9205208493356));
#263267=CARTESIAN_POINT('Ctrl Pts',(1.95622159519705,46.4786458333315,43.5372632938682));
#263268=CARTESIAN_POINT('Ctrl Pts',(6.99833541005117E-15,46.5447916666648,
43.5372632938682));
#263269=CARTESIAN_POINT('Ctrl Pts',(-1.95622159519704,46.6109374999981,
43.5372632938682));
#263270=CARTESIAN_POINT('Ctrl Pts',(-3.33947915066443,46.6770833333314,
44.9205208493356));
#263271=CARTESIAN_POINT('Ctrl Pts',(-4.72273670613182,46.7432291666647,
46.303778404803));
#263272=CARTESIAN_POINT('Ctrl Pts',(-4.72273670613182,46.8093749999981,
48.26));
#263273=CARTESIAN_POINT('Ctrl Pts',(-4.72273670613182,46.8755208333314,
50.216221595197));
#263274=CARTESIAN_POINT('Ctrl Pts',(-3.33947915066443,46.9416666666647,
51.5994791506644));
#263275=CARTESIAN_POINT('Ctrl Pts',(-1.95622159519703,47.007812499998,52.9827367061318));
#263276=CARTESIAN_POINT('Ctrl Pts',(7.17168088200104E-15,47.0739583333313,
52.9827367061318));
#263277=CARTESIAN_POINT('Ctrl Pts',(1.95622159519705,47.1401041666646,52.9827367061318));
#263278=CARTESIAN_POINT('Ctrl Pts',(3.33947915066444,47.2062499999979,51.5994791506644));
#263279=CARTESIAN_POINT('Ctrl Pts',(4.72273670613183,47.2723958333312,50.216221595197));
#263280=CARTESIAN_POINT('Ctrl Pts',(4.72273670613183,47.3385416666645,48.26));
#263281=CARTESIAN_POINT('Origin',(-3.05311331771918E-14,40.4567708333334,
48.26));
#263282=CARTESIAN_POINT('',(4.72273670613183,45.2166666666652,48.26));
#263283=CARTESIAN_POINT('',(4.72273670613183,45.2218749999985,48.26));
#263284=CARTESIAN_POINT('',(4.72273670613176,40.4567708333334,48.26));
#263285=CARTESIAN_POINT('Ctrl Pts',(4.72273670613183,45.2166666666652,48.26));
#263286=CARTESIAN_POINT('Ctrl Pts',(4.72273670613183,45.2828124999985,46.303778404803));
#263287=CARTESIAN_POINT('Ctrl Pts',(3.33947915066444,45.3489583333318,44.9205208493356));
#263288=CARTESIAN_POINT('Ctrl Pts',(1.95622159519705,45.4151041666651,43.5372632938682));
#263289=CARTESIAN_POINT('Ctrl Pts',(6.99833541005117E-15,45.4812499999984,
43.5372632938682));
#263290=CARTESIAN_POINT('Ctrl Pts',(-1.95622159519704,45.5473958333317,
43.5372632938682));
#263291=CARTESIAN_POINT('Ctrl Pts',(-3.33947915066443,45.613541666665,44.9205208493356));
#263292=CARTESIAN_POINT('Ctrl Pts',(-4.72273670613182,45.6796874999984,
46.303778404803));
#263293=CARTESIAN_POINT('Ctrl Pts',(-4.72273670613182,45.7458333333317,
48.26));
#263294=CARTESIAN_POINT('Ctrl Pts',(-4.72273670613182,45.811979166665,50.216221595197));
#263295=CARTESIAN_POINT('Ctrl Pts',(-3.33947915066443,45.8781249999983,
51.5994791506644));
#263296=CARTESIAN_POINT('Ctrl Pts',(-1.95622159519703,45.9442708333316,
52.9827367061318));
#263297=CARTESIAN_POINT('Ctrl Pts',(7.17168088200104E-15,46.0104166666649,
52.9827367061318));
#263298=CARTESIAN_POINT('Ctrl Pts',(1.95622159519705,46.0765624999982,52.9827367061318));
#263299=CARTESIAN_POINT('Ctrl Pts',(3.33947915066444,46.1427083333315,51.5994791506644));
#263300=CARTESIAN_POINT('Ctrl Pts',(4.72273670613183,46.2088541666649,50.216221595197));
#263301=CARTESIAN_POINT('Ctrl Pts',(4.72273670613183,46.2749999999982,48.26));
#263302=CARTESIAN_POINT('Ctrl Pts',(4.72273670613183,45.2218749999985,48.26));
#263303=CARTESIAN_POINT('Ctrl Pts',(4.72273670613183,45.2880208333319,46.303778404803));
#263304=CARTESIAN_POINT('Ctrl Pts',(3.33947915066444,45.3541666666652,44.9205208493356));
#263305=CARTESIAN_POINT('Ctrl Pts',(1.95622159519705,45.4203124999985,43.5372632938682));
#263306=CARTESIAN_POINT('Ctrl Pts',(6.99833541005117E-15,45.4864583333318,
43.5372632938682));
#263307=CARTESIAN_POINT('Ctrl Pts',(-1.95622159519704,45.5526041666651,
43.5372632938682));
#263308=CARTESIAN_POINT('Ctrl Pts',(-3.33947915066443,45.6187499999984,
44.9205208493356));
#263309=CARTESIAN_POINT('Ctrl Pts',(-4.72273670613182,45.6848958333317,
46.303778404803));
#263310=CARTESIAN_POINT('Ctrl Pts',(-4.72273670613182,45.7510416666651,
48.26));
#263311=CARTESIAN_POINT('Ctrl Pts',(-4.72273670613182,45.8171874999984,
50.216221595197));
#263312=CARTESIAN_POINT('Ctrl Pts',(-3.33947915066443,45.8833333333317,
51.5994791506644));
#263313=CARTESIAN_POINT('Ctrl Pts',(-1.95622159519703,45.949479166665,52.9827367061318));
#263314=CARTESIAN_POINT('Ctrl Pts',(7.17168088200107E-15,46.0156249999983,
52.9827367061318));
#263315=CARTESIAN_POINT('Ctrl Pts',(1.95622159519705,46.0817708333316,52.9827367061318));
#263316=CARTESIAN_POINT('Ctrl Pts',(3.33947915066444,46.1479166666649,51.5994791506644));
#263317=CARTESIAN_POINT('Ctrl Pts',(4.72273670613183,46.2140624999982,50.216221595197));
#263318=CARTESIAN_POINT('Ctrl Pts',(4.72273670613183,46.2802083333315,48.26));
#263319=CARTESIAN_POINT('Origin',(-3.05311331771918E-14,40.4567708333334,
48.26));
#263320=CARTESIAN_POINT('',(4.72273670613183,44.1583333333322,48.26));
#263321=CARTESIAN_POINT('',(4.72273670613183,44.1635416666656,48.26));
#263322=CARTESIAN_POINT('',(4.72273670613176,40.4567708333334,48.26));
#263323=CARTESIAN_POINT('Ctrl Pts',(4.72273670613183,44.1583333333322,48.26));
#263324=CARTESIAN_POINT('Ctrl Pts',(4.72273670613183,44.2244791666655,46.303778404803));
#263325=CARTESIAN_POINT('Ctrl Pts',(3.33947915066444,44.2906249999988,44.9205208493356));
#263326=CARTESIAN_POINT('Ctrl Pts',(1.95622159519705,44.3567708333321,43.5372632938682));
#263327=CARTESIAN_POINT('Ctrl Pts',(6.99833541005117E-15,44.4229166666654,
43.5372632938682));
#263328=CARTESIAN_POINT('Ctrl Pts',(-1.95622159519704,44.4890624999987,
43.5372632938682));
#263329=CARTESIAN_POINT('Ctrl Pts',(-3.33947915066443,44.555208333332,44.9205208493356));
#263330=CARTESIAN_POINT('Ctrl Pts',(-4.72273670613182,44.6213541666654,
46.303778404803));
#263331=CARTESIAN_POINT('Ctrl Pts',(-4.72273670613182,44.6874999999987,
48.26));
#263332=CARTESIAN_POINT('Ctrl Pts',(-4.72273670613182,44.753645833332,50.216221595197));
#263333=CARTESIAN_POINT('Ctrl Pts',(-3.33947915066443,44.8197916666653,
51.5994791506644));
#263334=CARTESIAN_POINT('Ctrl Pts',(-1.95622159519703,44.8859374999986,
52.9827367061318));
#263335=CARTESIAN_POINT('Ctrl Pts',(7.17168088200107E-15,44.9520833333319,
52.9827367061318));
#263336=CARTESIAN_POINT('Ctrl Pts',(1.95622159519705,45.0182291666652,52.9827367061318));
#263337=CARTESIAN_POINT('Ctrl Pts',(3.33947915066444,45.0843749999985,51.5994791506644));
#263338=CARTESIAN_POINT('Ctrl Pts',(4.72273670613183,45.1505208333318,50.216221595197));
#263339=CARTESIAN_POINT('Ctrl Pts',(4.72273670613183,45.2166666666652,48.26));
#263340=CARTESIAN_POINT('Ctrl Pts',(4.72273670613183,44.1635416666656,48.26));
#263341=CARTESIAN_POINT('Ctrl Pts',(4.72273670613183,44.2296874999989,46.303778404803));
#263342=CARTESIAN_POINT('Ctrl Pts',(3.33947915066444,44.2958333333322,44.9205208493356));
#263343=CARTESIAN_POINT('Ctrl Pts',(1.95622159519705,44.3619791666655,43.5372632938682));
#263344=CARTESIAN_POINT('Ctrl Pts',(6.99833541005117E-15,44.4281249999988,
43.5372632938682));
#263345=CARTESIAN_POINT('Ctrl Pts',(-1.95622159519704,44.4942708333321,
43.5372632938682));
#263346=CARTESIAN_POINT('Ctrl Pts',(-3.33947915066443,44.5604166666654,
44.9205208493356));
#263347=CARTESIAN_POINT('Ctrl Pts',(-4.72273670613182,44.6265624999987,
46.303778404803));
#263348=CARTESIAN_POINT('Ctrl Pts',(-4.72273670613182,44.692708333332,48.26));
#263349=CARTESIAN_POINT('Ctrl Pts',(-4.72273670613182,44.7588541666654,
50.216221595197));
#263350=CARTESIAN_POINT('Ctrl Pts',(-3.33947915066443,44.8249999999987,
51.5994791506644));
#263351=CARTESIAN_POINT('Ctrl Pts',(-1.95622159519703,44.891145833332,52.9827367061318));
#263352=CARTESIAN_POINT('Ctrl Pts',(7.17168088200107E-15,44.9572916666653,
52.9827367061318));
#263353=CARTESIAN_POINT('Ctrl Pts',(1.95622159519705,45.0234374999986,52.9827367061318));
#263354=CARTESIAN_POINT('Ctrl Pts',(3.33947915066444,45.0895833333319,51.5994791506644));
#263355=CARTESIAN_POINT('Ctrl Pts',(4.72273670613183,45.1557291666652,50.216221595197));
#263356=CARTESIAN_POINT('Ctrl Pts',(4.72273670613183,45.2218749999985,48.26));
#263357=CARTESIAN_POINT('Origin',(-3.05311331771918E-14,40.4567708333334,
48.26));
#263358=CARTESIAN_POINT('',(4.72273670613183,43.0999999999992,48.26));
#263359=CARTESIAN_POINT('',(4.72273670613183,43.1052083333326,48.26));
#263360=CARTESIAN_POINT('',(4.72273670613176,40.4567708333334,48.26));
#263361=CARTESIAN_POINT('Ctrl Pts',(4.72273670613183,43.0999999999992,48.26));
#263362=CARTESIAN_POINT('Ctrl Pts',(4.72273670613183,43.1661458333325,46.303778404803));
#263363=CARTESIAN_POINT('Ctrl Pts',(3.33947915066444,43.2322916666658,44.9205208493356));
#263364=CARTESIAN_POINT('Ctrl Pts',(1.95622159519705,43.2984374999991,43.5372632938682));
#263365=CARTESIAN_POINT('Ctrl Pts',(6.99833541005117E-15,43.3645833333324,
43.5372632938682));
#263366=CARTESIAN_POINT('Ctrl Pts',(-1.95622159519704,43.4307291666657,
43.5372632938682));
#263367=CARTESIAN_POINT('Ctrl Pts',(-3.33947915066443,43.496874999999,44.9205208493356));
#263368=CARTESIAN_POINT('Ctrl Pts',(-4.72273670613182,43.5630208333324,
46.303778404803));
#263369=CARTESIAN_POINT('Ctrl Pts',(-4.72273670613182,43.6291666666657,
48.26));
#263370=CARTESIAN_POINT('Ctrl Pts',(-4.72273670613182,43.695312499999,50.216221595197));
#263371=CARTESIAN_POINT('Ctrl Pts',(-3.33947915066443,43.7614583333323,
51.5994791506644));
#263372=CARTESIAN_POINT('Ctrl Pts',(-1.95622159519703,43.8276041666656,
52.9827367061318));
#263373=CARTESIAN_POINT('Ctrl Pts',(7.17168088200102E-15,43.8937499999989,
52.9827367061318));
#263374=CARTESIAN_POINT('Ctrl Pts',(1.95622159519705,43.9598958333322,52.9827367061318));
#263375=CARTESIAN_POINT('Ctrl Pts',(3.33947915066444,44.0260416666656,51.5994791506644));
#263376=CARTESIAN_POINT('Ctrl Pts',(4.72273670613183,44.0921874999989,50.216221595197));
#263377=CARTESIAN_POINT('Ctrl Pts',(4.72273670613183,44.1583333333322,48.26));
#263378=CARTESIAN_POINT('Ctrl Pts',(4.72273670613183,43.1052083333326,48.26));
#263379=CARTESIAN_POINT('Ctrl Pts',(4.72273670613183,43.1713541666659,46.303778404803));
#263380=CARTESIAN_POINT('Ctrl Pts',(3.33947915066444,43.2374999999992,44.9205208493356));
#263381=CARTESIAN_POINT('Ctrl Pts',(1.95622159519705,43.3036458333325,43.5372632938682));
#263382=CARTESIAN_POINT('Ctrl Pts',(6.99833541005117E-15,43.3697916666658,
43.5372632938682));
#263383=CARTESIAN_POINT('Ctrl Pts',(-1.95622159519704,43.4359374999991,
43.5372632938682));
#263384=CARTESIAN_POINT('Ctrl Pts',(-3.33947915066443,43.5020833333324,
44.9205208493356));
#263385=CARTESIAN_POINT('Ctrl Pts',(-4.72273670613182,43.5682291666657,
46.303778404803));
#263386=CARTESIAN_POINT('Ctrl Pts',(-4.72273670613182,43.634374999999,48.26));
#263387=CARTESIAN_POINT('Ctrl Pts',(-4.72273670613182,43.7005208333324,
50.216221595197));
#263388=CARTESIAN_POINT('Ctrl Pts',(-3.33947915066443,43.7666666666657,
51.5994791506644));
#263389=CARTESIAN_POINT('Ctrl Pts',(-1.95622159519703,43.832812499999,52.9827367061318));
#263390=CARTESIAN_POINT('Ctrl Pts',(7.17168088200102E-15,43.8989583333323,
52.9827367061318));
#263391=CARTESIAN_POINT('Ctrl Pts',(1.95622159519705,43.9651041666656,52.9827367061318));
#263392=CARTESIAN_POINT('Ctrl Pts',(3.33947915066444,44.0312499999989,51.5994791506644));
#263393=CARTESIAN_POINT('Ctrl Pts',(4.72273670613183,44.0973958333322,50.216221595197));
#263394=CARTESIAN_POINT('Ctrl Pts',(4.72273670613183,44.1635416666656,48.26));
#263395=CARTESIAN_POINT('Origin',(6.7958239265071E-15,40.475,48.26));
#263396=CARTESIAN_POINT('',(4.40328459016939E-15,42.2906249999995,43.5102));
#263397=CARTESIAN_POINT('',(5.54528904550239E-15,42.09425,43.5102));
#263398=CARTESIAN_POINT('',(5.54528904550239E-15,40.475,43.5102));
#263399=CARTESIAN_POINT('',(4.36624125519644,42.09425,46.3900969700488));
#263400=CARTESIAN_POINT('Ctrl Pts',(7.7715611723761E-15,42.2906249999995,
43.5102));
#263401=CARTESIAN_POINT('Ctrl Pts',(0.306312377613604,42.2803266558546,
43.5102));
#263402=CARTESIAN_POINT('Ctrl Pts',(0.612600594710301,42.2696165070132,
43.539829200288));
#263403=CARTESIAN_POINT('Ctrl Pts',(1.5259625148491,42.2364131029764,43.719048502412));
#263404=CARTESIAN_POINT('Ctrl Pts',(2.10782424211785,42.2135208891992,43.9581541159287));
#263405=CARTESIAN_POINT('Ctrl Pts',(3.00697611076785,42.1749789086954,44.5550320160162));
#263406=CARTESIAN_POINT('Ctrl Pts',(3.34869201888086,42.15983788401,44.8607436451307));
#263407=CARTESIAN_POINT('Ctrl Pts',(3.93944645506913,42.1278937490674,45.5661866234649));
#263408=CARTESIAN_POINT('Ctrl Pts',(4.18359566378164,42.1111319270672,45.9636177871491));
#263409=CARTESIAN_POINT('Ctrl Pts',(4.36624125519659,42.09425,46.3900969700491));
#263410=CARTESIAN_POINT('Origin',(6.7958239265071E-15,42.09425,48.26));
#263411=CARTESIAN_POINT('Origin',(6.7958239265071E-15,40.475,48.26));
#263412=CARTESIAN_POINT('',(-1.95879410825898E-14,43.3489583333325,43.5102));
#263413=CARTESIAN_POINT('',(1.07523725122445E-14,42.3270833333327,43.5102));
#263414=CARTESIAN_POINT('',(5.54528904550239E-15,40.475,43.5102));
#263415=CARTESIAN_POINT('Ctrl Pts',(-4.29517532651857E-14,43.3489583333325,
43.5102));
#263416=CARTESIAN_POINT('Ctrl Pts',(0.413798530172926,43.3350462619249,
43.5102));
#263417=CARTESIAN_POINT('Ctrl Pts',(0.826670368688511,43.3204123302741,
43.5642725719141));
#263418=CARTESIAN_POINT('Ctrl Pts',(1.8259494112998,43.2830916071325,43.831726042004));
#263419=CARTESIAN_POINT('Ctrl Pts',(2.38686058154301,43.2603987577855,44.1070948134215));
#263420=CARTESIAN_POINT('Ctrl Pts',(3.36882436692966,43.2169625534067,44.8554914890216));
#263421=CARTESIAN_POINT('Ctrl Pts',(3.78128185410638,43.1966949382382,45.3203462387152));
#263422=CARTESIAN_POINT('Ctrl Pts',(4.40771574233544,43.1521835512767,46.3848087314939));
#263423=CARTESIAN_POINT('Ctrl Pts',(4.61444584304911,43.1294619675453,46.9750056411953));
#263424=CARTESIAN_POINT('Ctrl Pts',(4.78902391945517,43.0859479536866,48.1969672260116));
#263425=CARTESIAN_POINT('Ctrl Pts',(4.75696102960572,43.0657543266859,48.8168166627164));
#263426=CARTESIAN_POINT('Ctrl Pts',(4.45711948033121,43.0213051463692,50.0147078667033));
#263427=CARTESIAN_POINT('Ctrl Pts',(4.1902990760171,42.998555617062,50.5808457666307));
#263428=CARTESIAN_POINT('Ctrl Pts',(3.45765603924985,42.9549633791373,51.5739759608694));
#263429=CARTESIAN_POINT('Ctrl Pts',(3.00063580575679,42.9348366133039,51.9928281298175));
#263430=CARTESIAN_POINT('Ctrl Pts',(1.94712039905175,42.8904524036952,52.6365582703685));
#263431=CARTESIAN_POINT('Ctrl Pts',(1.35939952094681,42.8676758816576,52.8532110500321));
#263432=CARTESIAN_POINT('Ctrl Pts',(0.140814301271115,42.824005292089,53.0471837815253));
#263433=CARTESIAN_POINT('Ctrl Pts',(-0.477998516061079,42.803937588497,
53.0253408551151));
#263434=CARTESIAN_POINT('Ctrl Pts',(-1.68036223673691,42.7596209950149,
52.7458177117107));
#263435=CARTESIAN_POINT('Ctrl Pts',(-2.25178562281166,42.7368185887116,
52.4879606083977));
#263436=CARTESIAN_POINT('Ctrl Pts',(-3.25636757408644,42.6930698118832,
51.7717238131873));
#263437=CARTESIAN_POINT('Ctrl Pts',(-3.68179377358298,42.673052782406,51.3227646567329));
#263438=CARTESIAN_POINT('Ctrl Pts',(-4.3432329780399,42.6288062995307,50.280681107429));
#263439=CARTESIAN_POINT('Ctrl Pts',(-4.57008234897582,42.6059792614027,
49.6956812528296));
#263440=CARTESIAN_POINT('Ctrl Pts',(-4.783998273458,42.5621527543215,48.48071918745));
#263441=CARTESIAN_POINT('Ctrl Pts',(-4.77260115723503,42.5421775196058,
47.8629689153103));
#263442=CARTESIAN_POINT('Ctrl Pts',(-4.51390729703972,42.4980034591323,
46.656216903107));
#263443=CARTESIAN_POINT('Ctrl Pts',(-4.26532764079846,42.4751531709417,
46.079526481079));
#263444=CARTESIAN_POINT('Ctrl Pts',(-3.56596209792685,42.4312496794982,
45.0633544203556));
#263445=CARTESIAN_POINT('Ctrl Pts',(-3.1251912266916,42.4113069799741,44.6312525735305));
#263446=CARTESIAN_POINT('Ctrl Pts',(-2.09489088525855,42.3672074406395,
43.9519179106002));
#263447=CARTESIAN_POINT('Ctrl Pts',(-1.5128344495972,42.3443353961348,43.7147306798431));
#263448=CARTESIAN_POINT('Ctrl Pts',(-0.603833353133009,42.3113269822488,
43.5389852708177));
#263449=CARTESIAN_POINT('Ctrl Pts',(-0.301918536111969,42.3007756214429,
43.5102));
#263450=CARTESIAN_POINT('Ctrl Pts',(6.17561557447743E-15,42.2906249999995,
43.5102));
#263451=CARTESIAN_POINT('',(4.66218791181207,42.0942499999981,47.3519229575834));
#263452=CARTESIAN_POINT('Origin',(6.7958239265071E-15,42.09425,48.26));
#263453=CARTESIAN_POINT('Ctrl Pts',(4.66218791181102,42.0942499999949,47.3519229575838));
#263454=CARTESIAN_POINT('Ctrl Pts',(4.5947983082204,42.1068206953643,47.0059357994833));
#263455=CARTESIAN_POINT('Ctrl Pts',(4.48910763172072,42.1196360322442,46.6685368854553));
#263456=CARTESIAN_POINT('Ctrl Pts',(4.20537339562347,42.145252195001,46.0241402159205));
#263457=CARTESIAN_POINT('Ctrl Pts',(4.0283811118818,42.1579739998848,45.7190573960589));
#263458=CARTESIAN_POINT('Ctrl Pts',(3.45736524908729,42.1918930242663,44.9466976226496));
#263459=CARTESIAN_POINT('Ctrl Pts',(3.00461394812578,42.2118479691886,44.5312412852076));
#263460=CARTESIAN_POINT('Ctrl Pts',(1.95293188099643,42.2562007886002,43.8853391386656));
#263461=CARTESIAN_POINT('Ctrl Pts',(1.36067932860232,42.2791600006444,43.6665081845346));
#263462=CARTESIAN_POINT('Ctrl Pts',(0.496745708221664,42.3101114315127,
43.5296681000585));
#263463=CARTESIAN_POINT('Ctrl Pts',(0.248293869613903,42.3187355945366,
43.5102));
#263464=CARTESIAN_POINT('Ctrl Pts',(1.48492329543615E-14,42.3270833333328,
43.5102));
#263465=CARTESIAN_POINT('Origin',(6.7958239265071E-15,40.475,48.26));
#263466=CARTESIAN_POINT('',(-3.7455592885151E-14,44.4072916666655,43.5102));
#263467=CARTESIAN_POINT('',(2.32161641899723E-15,43.3854166666658,43.5102));
#263468=CARTESIAN_POINT('',(5.54528904550239E-15,40.475,43.5102));
#263469=CARTESIAN_POINT('Ctrl Pts',(-7.39686090156511E-14,44.4072916666655,
43.5102));
#263470=CARTESIAN_POINT('Ctrl Pts',(0.503221800043281,44.390373149306,43.5102));
#263471=CARTESIAN_POINT('Ctrl Pts',(1.00400848126672,44.3724228202082,43.5901712341933));
#263472=CARTESIAN_POINT('Ctrl Pts',(2.06827713231742,44.3317689812627,43.9400702898139));
#263473=CARTESIAN_POINT('Ctrl Pts',(2.61018179015456,44.3093144518143,44.2442115659869));
#263474=CARTESIAN_POINT('Ctrl Pts',(3.55263113629528,44.2664558238078,45.046529932576));
#263475=CARTESIAN_POINT('Ctrl Pts',(3.94250983519217,44.2454341206351,45.5389303845267));
#263476=CARTESIAN_POINT('Ctrl Pts',(4.50748616977274,44.2005289482455,46.6405621232504));
#263477=CARTESIAN_POINT('Ctrl Pts',(4.67930167148437,44.1780452588232,47.2381452413361));
#263478=CARTESIAN_POINT('Ctrl Pts',(4.78561759298189,44.1351207318422,48.4708483287254));
#263479=CARTESIAN_POINT('Ctrl Pts',(4.71704371069774,44.1142015396868,49.0943336232476));
#263480=CARTESIAN_POINT('Ctrl Pts',(4.34523111346103,44.0693356980773,50.2748065530144));
#263481=CARTESIAN_POINT('Ctrl Pts',(4.04739745399867,44.0468223876693,50.8210722831364));
#263482=CARTESIAN_POINT('Ctrl Pts',(3.25703080618358,44.003829825242,51.7724559182719));
#263483=CARTESIAN_POINT('Ctrl Pts',(2.77083588879443,43.9830123427014,52.1674392770568));
#263484=CARTESIAN_POINT('Ctrl Pts',(1.67739508145102,43.9381885376627,52.7463474425373));
#263485=CARTESIAN_POINT('Ctrl Pts',(1.08129701659115,43.9156452722035,52.9260262159432));
#263486=CARTESIAN_POINT('Ctrl Pts',(-0.149139245221289,43.8725826769129,
53.0477291476657));
#263487=CARTESIAN_POINT('Ctrl Pts',(-0.771810656405107,43.8518653644044,
52.9874638415032));
#263488=CARTESIAN_POINT('Ctrl Pts',(-1.95644428853647,43.8070863850711,
52.6319334746697));
#263489=CARTESIAN_POINT('Ctrl Pts',(-2.50736060681273,43.7845129695506,
52.3410113002899));
#263490=CARTESIAN_POINT('Ctrl Pts',(-3.46835273705026,43.7413785072399,
51.563652064836));
#263491=CARTESIAN_POINT('Ctrl Pts',(-3.86882423653969,43.7207590458096,
51.0841452638547));
#263492=CARTESIAN_POINT('Ctrl Pts',(-4.46269147748995,43.676027748612,49.9996522475679));
#263493=CARTESIAN_POINT('Ctrl Pts',(-4.65084839767155,43.6534241378127,
49.4052710434929));
#263494=CARTESIAN_POINT('Ctrl Pts',(-4.7891292849171,43.6102161612666,48.177377397803));
#263495=CARTESIAN_POINT('Ctrl Pts',(-4.73776279420127,43.5896914222037,
47.555587940092));
#263496=CARTESIAN_POINT('Ctrl Pts',(-4.39973740307815,43.5450107117975,
46.3666264055941));
#263497=CARTESIAN_POINT('Ctrl Pts',(-4.11631541613004,43.5223770192419,
45.810810537023));
#263498=CARTESIAN_POINT('Ctrl Pts',(-3.35297349292649,43.4790940907976,
44.8395962919083));
#263499=CARTESIAN_POINT('Ctrl Pts',(-2.88059882280507,43.4586601181008,
44.4332850148773));
#263500=CARTESIAN_POINT('Ctrl Pts',(-1.80578318535429,43.4140329253292,
43.8235300453175));
#263501=CARTESIAN_POINT('Ctrl Pts',(-1.21336611326443,43.3913694300323,
43.6263311050534));
#263502=CARTESIAN_POINT('Ctrl Pts',(-0.400469824454208,43.3625984281871,
43.5228482498025));
#263503=CARTESIAN_POINT('Ctrl Pts',(-0.200132489240207,43.355686867337,
43.5102));
#263504=CARTESIAN_POINT('Ctrl Pts',(-3.99680288865056E-14,43.3489583333325,
43.5102));
#263505=CARTESIAN_POINT('Ctrl Pts',(1.54737334057131E-14,42.3270833333327,
43.5102));
#263506=CARTESIAN_POINT('Ctrl Pts',(-0.35821960567291,42.3391268191606,
43.5102));
#263507=CARTESIAN_POINT('Ctrl Pts',(-0.71607214488095,42.3517222752217,
43.5507220553509));
#263508=CARTESIAN_POINT('Ctrl Pts',(-1.67550713467282,42.3870580817763,
43.7718346878538));
#263509=CARTESIAN_POINT('Ctrl Pts',(-2.25071018064137,42.4100044194961,
44.030902312143));
#263510=CARTESIAN_POINT('Ctrl Pts',(-3.25541035828551,42.4537685521362,
44.7479563537761));
#263511=CARTESIAN_POINT('Ctrl Pts',(-3.67877054229274,42.473679910113,45.1942548346965));
#263512=CARTESIAN_POINT('Ctrl Pts',(-4.34157757558856,42.5178973195809,
46.234907055749));
#263513=CARTESIAN_POINT('Ctrl Pts',(-4.56986676456883,42.5408290503086,
46.822424478906));
#263514=CARTESIAN_POINT('Ctrl Pts',(-4.78365346537154,42.5846736373392,
48.0379778377428));
#263515=CARTESIAN_POINT('Ctrl Pts',(-4.77261296903176,42.6045767469765,
48.6534449009694));
#263516=CARTESIAN_POINT('Ctrl Pts',(-4.51547977408878,42.648723303151,49.8600252782126));
#263517=CARTESIAN_POINT('Ctrl Pts',(-4.26657920474278,42.6716386916767,
50.4385191081198));
#263518=CARTESIAN_POINT('Ctrl Pts',(-3.56702886072932,42.7155628202327,
51.4552284488307));
#263519=CARTESIAN_POINT('Ctrl Pts',(-3.1273415287299,42.7354671391827,51.8866946633162));
#263520=CARTESIAN_POINT('Ctrl Pts',(-2.09805709470288,42.7795410052046,
52.56663839445));
#263521=CARTESIAN_POINT('Ctrl Pts',(-1.51551485278494,42.802438336214,52.8044685584775));
#263522=CARTESIAN_POINT('Ctrl Pts',(-0.303969126029313,42.8464407839499,
53.0392662005286));
#263523=CARTESIAN_POINT('Ctrl Pts',(0.312565072830679,42.8663559369633,
53.0387117164387));
#263524=CARTESIAN_POINT('Ctrl Pts',(1.52316486227975,42.9103555026468,52.8018373341285));
#263525=CARTESIAN_POINT('Ctrl Pts',(2.10481239179041,42.9332331024555,52.5632640013275));
#263526=CARTESIAN_POINT('Ctrl Pts',(3.13351782190229,42.9773123779918,51.881533984683));
#263527=CARTESIAN_POINT('Ctrl Pts',(3.57318933199809,42.9972479789684,51.4485358355));
#263528=CARTESIAN_POINT('Ctrl Pts',(4.27027386259732,43.0411719049498,50.4308111467803));
#263529=CARTESIAN_POINT('Ctrl Pts',(4.51759478199226,43.0640281646244,49.8534217239699));
#263530=CARTESIAN_POINT('Ctrl Pts',(4.77347759941231,43.1081824830165,48.646092545179));
#263531=CARTESIAN_POINT('Ctrl Pts',(4.78346712714521,43.1281480926501,48.0284855337845));
#263532=CARTESIAN_POINT('Ctrl Pts',(4.5668549003962,43.1719952818795,46.814025146711));
#263533=CARTESIAN_POINT('Ctrl Pts',(4.33862772648812,43.194828680947,46.2294067979757));
#263534=CARTESIAN_POINT('Ctrl Pts',(3.67480020981176,43.2390560053493,45.188882366683));
#263535=CARTESIAN_POINT('Ctrl Pts',(3.24848507963304,43.2590609647294,44.7410135082327));
#263536=CARTESIAN_POINT('Ctrl Pts',(2.24235732065186,43.3028305952222,44.0270111630162));
#263537=CARTESIAN_POINT('Ctrl Pts',(1.6702265530796,43.3256397201586,43.7703793781061));
#263538=CARTESIAN_POINT('Ctrl Pts',(0.714876476894768,43.360819833794,43.5505848889169));
#263539=CARTESIAN_POINT('Ctrl Pts',(0.357612817399793,43.3733935813014,
43.5102));
#263540=CARTESIAN_POINT('Ctrl Pts',(-6.45317133063372E-15,43.3854166666658,
43.5102));
#263541=CARTESIAN_POINT('Origin',(6.7958239265071E-15,40.475,48.26));
#263542=CARTESIAN_POINT('',(-9.87175814600512E-15,45.4656249999985,43.5102));
#263543=CARTESIAN_POINT('',(-3.83749963274187E-14,44.4437499999987,43.5102));
#263544=CARTESIAN_POINT('',(5.54528904550239E-15,40.475,43.5102));
#263545=CARTESIAN_POINT('Ctrl Pts',(-2.48412401759879E-14,45.4656249999985,
43.5102));
#263546=CARTESIAN_POINT('Ctrl Pts',(0.566167174768376,45.4465902340685,
43.5102));
#263547=CARTESIAN_POINT('Ctrl Pts',(1.12831666969806,45.4262808000092,43.6114309061969));
#263548=CARTESIAN_POINT('Ctrl Pts',(2.23435532889598,45.3833509845901,44.0239215602639));
#263549=CARTESIAN_POINT('Ctrl Pts',(2.76208488292739,45.3611023288806,44.3475011828489));
#263550=CARTESIAN_POINT('Ctrl Pts',(3.67593158760873,45.3186849235856,45.1871891138991));
#263551=CARTESIAN_POINT('Ctrl Pts',(4.04943203210943,45.2968843047985,45.699373099574));
#263552=CARTESIAN_POINT('Ctrl Pts',(4.5696569085592,45.2517488041455,46.8263923479328));
#263553=CARTESIAN_POINT('Ctrl Pts',(4.71644566319283,45.2294776401571,47.4280205599865));
#263554=CARTESIAN_POINT('Ctrl Pts',(4.77366924022708,45.1870137044427,48.6673586058741));
#263555=CARTESIAN_POINT('Ctrl Pts',(4.67825065771643,45.1653022980402,49.2933896217085));
#263556=CARTESIAN_POINT('Ctrl Pts',(4.25428195262986,45.1201885041776,50.4596338382421));
#263557=CARTESIAN_POINT('Ctrl Pts',(3.93474684068767,45.097893833954,50.9904073321232));
#263558=CARTESIAN_POINT('Ctrl Pts',(3.10290584598736,45.055380912789,51.9103453537361));
#263559=CARTESIAN_POINT('Ctrl Pts',(2.59492452463815,45.0337617192976,52.2873404412948));
#263560=CARTESIAN_POINT('Ctrl Pts',(1.47320517645446,44.9886714132759,52.8171150725373));
#263561=CARTESIAN_POINT('Ctrl Pts',(0.872348912097263,44.9663522622886,
52.9692133241848));
#263562=CARTESIAN_POINT('Ctrl Pts',(-0.365654927903947,44.9237878756165,
53.0368711415338));
#263563=CARTESIAN_POINT('Ctrl Pts',(-0.991153230745437,44.9022636356118,
52.9472027181653));
#263564=CARTESIAN_POINT('Ctrl Pts',(-2.16054571570856,44.8571987189914,
52.5343443824203));
#263565=CARTESIAN_POINT('Ctrl Pts',(-2.69469457492828,44.8348541472401,
52.2193747943595));
#263566=CARTESIAN_POINT('Ctrl Pts',(-3.62141790896547,44.7922358051748,
51.3963449289355));
#263567=CARTESIAN_POINT('Ctrl Pts',(-4.00230089366418,44.7708089405814,
50.8930517722628));
#263568=CARTESIAN_POINT('Ctrl Pts',(-4.5427009304037,44.7257714374295,49.7773041716474));
#263569=CARTESIAN_POINT('Ctrl Pts',(-4.70072700271712,44.7034005514389,
49.1773644929565));
#263570=CARTESIAN_POINT('Ctrl Pts',(-4.7800207424564,44.6607257712771,47.9408968826995));
#263571=CARTESIAN_POINT('Ctrl Pts',(-4.69673585831553,44.6393983237826,
47.3159985829078));
#263572=CARTESIAN_POINT('Ctrl Pts',(-4.29625205794725,44.5943903813102,
46.1431750279321));
#263573=CARTESIAN_POINT('Ctrl Pts',(-3.98640446044117,44.5719923468965,
45.6053143854807));
#263574=CARTESIAN_POINT('Ctrl Pts',(-3.17320321784656,44.5292586718744,
44.67108945669));
#263575=CARTESIAN_POINT('Ctrl Pts',(-2.67510132706769,44.5080322394464,
44.2859131457232));
#263576=CARTESIAN_POINT('Ctrl Pts',(-1.5660392602498,44.463056127013,43.7337811473311));
#263577=CARTESIAN_POINT('Ctrl Pts',(-0.967183012353343,44.4406301826481,
43.5691858099604));
#263578=CARTESIAN_POINT('Ctrl Pts',(-0.235766499056439,44.4152792766867,
43.5145836208336));
#263579=CARTESIAN_POINT('Ctrl Pts',(-0.117818553244376,44.4112527733547,
43.5102));
#263580=CARTESIAN_POINT('Ctrl Pts',(-7.35869698509362E-14,44.4072916666655,
43.5102));
#263581=CARTESIAN_POINT('Ctrl Pts',(-7.56339435525888E-15,43.3854166666658,
43.5102));
#263582=CARTESIAN_POINT('Ctrl Pts',(-0.252938767796752,43.393920568789,
43.5102));
#263583=CARTESIAN_POINT('Ctrl Pts',(-0.506033130480092,43.4027110535072,
43.5304032836925));
#263584=CARTESIAN_POINT('Ctrl Pts',(-1.36951656855858,43.433682631352,43.6697769184839));
#263585=CARTESIAN_POINT('Ctrl Pts',(-1.95688726193394,43.4564661935624,
43.8877806596));
#263586=CARTESIAN_POINT('Ctrl Pts',(-3.0088987596432,43.5008325659322,44.5338607011886));
#263587=CARTESIAN_POINT('Ctrl Pts',(-3.46485166642493,43.5209427394167,
44.9535835508775));
#263588=CARTESIAN_POINT('Ctrl Pts',(-4.19533395069392,43.5645559399498,
45.9482322667341));
#263589=CARTESIAN_POINT('Ctrl Pts',(-4.46097731607419,43.5873127911782,
46.5150754942565));
#263590=CARTESIAN_POINT('Ctrl Pts',(-4.75813933136021,43.631744855005,47.7135674872954));
#263591=CARTESIAN_POINT('Ctrl Pts',(-4.78885255595613,43.6519198657488,
48.333280292379));
#263592=CARTESIAN_POINT('Ctrl Pts',(-4.61172004567221,43.69545477968,49.5548054446073));
#263593=CARTESIAN_POINT('Ctrl Pts',(-4.40368282860499,43.7181839244839,
50.1446858243739));
#263594=CARTESIAN_POINT('Ctrl Pts',(-3.77496669460223,43.7626789442838,
51.2077161576424));
#263595=CARTESIAN_POINT('Ctrl Pts',(-3.36166674266701,43.7829261062386,
51.6715392791841));
#263596=CARTESIAN_POINT('Ctrl Pts',(-2.37823063201529,43.826383072085,52.4178722866157));
#263597=CARTESIAN_POINT('Ctrl Pts',(-1.81662634708705,43.8490836771297,
52.6921246523106));
#263598=CARTESIAN_POINT('Ctrl Pts',(-0.622625619824168,43.8936388223162,
53.0089677686183));
#263599=CARTESIAN_POINT('Ctrl Pts',(-0.00191039526407429,43.9139647275044,
53.0496087451274));
#263600=CARTESIAN_POINT('Ctrl Pts',(1.22275842555576,43.9573443645708,52.8912158433007));
#263601=CARTESIAN_POINT('Ctrl Pts',(1.81489342511168,43.9800157646233,52.6927682950152));
#263602=CARTESIAN_POINT('Ctrl Pts',(2.88836171451833,44.0246281409164,52.0808244812262));
#263603=CARTESIAN_POINT('Ctrl Pts',(3.35975143564909,44.0450386063444,51.6737076021931));
#263604=CARTESIAN_POINT('Ctrl Pts',(4.12114558046236,44.088341802955,50.7010837076052));
#263605=CARTESIAN_POINT('Ctrl Pts',(4.40352124978901,44.1109835035808,50.1445962492681));
#263606=CARTESIAN_POINT('Ctrl Pts',(4.73911767096697,44.1556501829775,48.9550459386809));
#263607=CARTESIAN_POINT('Ctrl Pts',(4.78925197630372,44.1761502153229,48.3333793250371));
#263608=CARTESIAN_POINT('Ctrl Pts',(4.64866775580724,44.2193781136552,47.1058472006474));
#263609=CARTESIAN_POINT('Ctrl Pts',(4.45933251114065,44.2419897907378,46.5117141522562));
#263610=CARTESIAN_POINT('Ctrl Pts',(3.86339106873776,44.2867078394907,45.4284743580617));
#263611=CARTESIAN_POINT('Ctrl Pts',(3.46215786932851,44.3073016172265,44.9498969869002));
#263612=CARTESIAN_POINT('Ctrl Pts',(2.49983219570281,44.35045559524,44.1743558263937));
#263613=CARTESIAN_POINT('Ctrl Pts',(1.94827382198002,44.3730370915408,43.8844034463094));
#263614=CARTESIAN_POINT('Ctrl Pts',(0.915635083610503,44.4120410312369,
43.5766189918159));
#263615=CARTESIAN_POINT('Ctrl Pts',(0.458609242083433,44.4283313746079,
43.5102));
#263616=CARTESIAN_POINT('Ctrl Pts',(-9.20097331658098E-14,44.4437499999987,
43.5102));
#263617=CARTESIAN_POINT('Origin',(6.7958239265071E-15,40.475,48.26));
#263618=CARTESIAN_POINT('',(6.38086935278296E-15,46.5239583333315,43.5102));
#263619=CARTESIAN_POINT('',(-9.87175814600512E-15,45.5020833333317,43.5102));
#263620=CARTESIAN_POINT('',(5.54528904550239E-15,40.475,43.5102));
#263621=CARTESIAN_POINT('Ctrl Pts',(6.38378239159465E-15,46.5239583333315,
43.5102));
#263622=CARTESIAN_POINT('Ctrl Pts',(0.605510253896708,46.5036008374102,
43.5102));
#263623=CARTESIAN_POINT('Ctrl Pts',(1.20576070108133,46.4818076969026,43.6259890631561));
#263624=CARTESIAN_POINT('Ctrl Pts',(2.33611695352849,46.4374905918229,44.0793903497507));
#263625=CARTESIAN_POINT('Ctrl Pts',(2.8546727287585,46.4153861300924,44.4147631522863));
#263626=CARTESIAN_POINT('Ctrl Pts',(3.75030468937568,46.3732591906852,45.277567591021));
#263627=CARTESIAN_POINT('Ctrl Pts',(4.11332423204537,46.350867950729,45.8022845225452));
#263628=CARTESIAN_POINT('Ctrl Pts',(4.60492983715419,46.3056097860154,46.944806762349));
#263629=CARTESIAN_POINT('Ctrl Pts',(4.73591436814583,46.283490643379,47.5484595982696));
#263630=CARTESIAN_POINT('Ctrl Pts',(4.76199965834213,46.2413346731749,48.7915354657038));
#263631=CARTESIAN_POINT('Ctrl Pts',(4.6492709525603,46.2190049601663,49.4191198129379));
#263632=CARTESIAN_POINT('Ctrl Pts',(4.19207402121399,46.1737580864564,50.5755587541872));
#263633=CARTESIAN_POINT('Ctrl Pts',(3.85907637047694,46.1516233565398,51.0959986418154));
#263634=CARTESIAN_POINT('Ctrl Pts',(3.00095705659992,46.1094364386808,51.9953552346117));
#263635=CARTESIAN_POINT('Ctrl Pts',(2.47879870234457,46.0871717251068,52.3605222090011));
#263636=CARTESIAN_POINT('Ctrl Pts',(1.33940444906917,46.0419371201451,52.857987662945));
#263637=CARTESIAN_POINT('Ctrl Pts',(0.736131320341591,46.01978586708,52.9921946738508));
#263638=CARTESIAN_POINT('Ctrl Pts',(-0.506210804173773,45.9775659990635,
53.0246397502708));
#263639=CARTESIAN_POINT('Ctrl Pts',(-1.13348286507548,45.9553698123262,
52.9154651892213));
#263640=CARTESIAN_POINT('Ctrl Pts',(-2.29197503236124,45.9101485354608,
52.4650632422378));
#263641=CARTESIAN_POINT('Ctrl Pts',(-2.81455697175483,45.8879797972532,
52.1347948945607));
#263642=CARTESIAN_POINT('Ctrl Pts',(-3.71815798027405,45.8457248934765,
51.2820405739014));
#263643=CARTESIAN_POINT('Ctrl Pts',(-4.08576925695492,45.8236007922176,
50.7628005139273));
#263644=CARTESIAN_POINT('Ctrl Pts',(-4.58990752858198,45.7783939899705,
49.6269971919376));
#263645=CARTESIAN_POINT('Ctrl Pts',(-4.72779263414628,45.7562067826859,
49.0241781630785));
#263646=CARTESIAN_POINT('Ctrl Pts',(-4.76748967906412,45.713914678184,47.7826913112644));
#263647=CARTESIAN_POINT('Ctrl Pts',(-4.66235604747994,45.6918662243994,
47.1557786306744));
#263648=CARTESIAN_POINT('Ctrl Pts',(-4.21969723649514,45.6466751360762,
45.9949770748335));
#263649=CARTESIAN_POINT('Ctrl Pts',(-3.89255399256836,45.6244684589117,
45.4699722245363));
#263650=CARTESIAN_POINT('Ctrl Pts',(-3.04591872211673,45.5821369144204,
44.5615570327065));
#263651=CARTESIAN_POINT('Ctrl Pts',(-2.52999210496112,45.5601676411215,
44.1911767212708));
#263652=CARTESIAN_POINT('Ctrl Pts',(-1.39829579747494,45.5149936043689,
43.6794760641619));
#263653=CARTESIAN_POINT('Ctrl Pts',(-0.796019569019148,45.4927664456731,
43.5374116915685));
#263654=CARTESIAN_POINT('Ctrl Pts',(-0.12223009417209,45.4697508383311,
43.5113786479076));
#263655=CARTESIAN_POINT('Ctrl Pts',(-0.061092202878116,45.4676789441933,
43.5102));
#263656=CARTESIAN_POINT('Ctrl Pts',(-2.52888053375127E-14,45.4656249999985,
43.5102));
#263657=CARTESIAN_POINT('Ctrl Pts',(-9.15240105925363E-14,44.4437499999988,
43.5102));
#263658=CARTESIAN_POINT('Ctrl Pts',(-0.158624669736482,44.4490830245783,
43.5102));
#263659=CARTESIAN_POINT('Ctrl Pts',(-0.317431308334336,44.4545328214472,
43.5181458728693));
#263660=CARTESIAN_POINT('Ctrl Pts',(-1.08959979876912,44.4815761187491,
43.5958913234815));
#263661=CARTESIAN_POINT('Ctrl Pts',(-1.68548201394787,44.5041274378075,
43.7766695169619));
#263662=CARTESIAN_POINT('Ctrl Pts',(-2.77776933643676,44.5489395260632,
44.3575210824682));
#263663=CARTESIAN_POINT('Ctrl Pts',(-3.26309684251495,44.56973002553,44.753216962612));
#263664=CARTESIAN_POINT('Ctrl Pts',(-4.051783932363,44.6127411359467,45.7058479820052));
#263665=CARTESIAN_POINT('Ctrl Pts',(-4.34872785465835,44.6352624336811,
46.2527198271428));
#263666=CARTESIAN_POINT('Ctrl Pts',(-4.71843598020254,44.6801172971878,
47.4337379266126));
#263667=CARTESIAN_POINT('Ctrl Pts',(-4.78593419842782,44.7010091685601,
48.0571184351088));
#263668=CARTESIAN_POINT('Ctrl Pts',(-4.6776312467982,44.7439516944877,49.2895338255929));
#263669=CARTESIAN_POINT('Ctrl Pts',(-4.50480069578428,44.7664432688962,
49.886931026317));
#263670=CARTESIAN_POINT('Ctrl Pts',(-3.93802269071322,44.8113381781622,
50.987511223909));
#263671=CARTESIAN_POINT('Ctrl Pts',(-3.54748413748688,44.8323324157788,
51.4791104293673));
#263672=CARTESIAN_POINT('Ctrl Pts',(-2.6038801946333,44.8752084588662,52.2798918950414));
#263673=CARTESIAN_POINT('Ctrl Pts',(-2.06141002984294,44.897670738244,52.5832244235865));
#263674=CARTESIAN_POINT('Ctrl Pts',(-0.898155571046601,44.942076835292,
52.9635927494952));
#263675=CARTESIAN_POINT('Ctrl Pts',(-0.289169763911568,44.9627764100011,
53.0398339846786));
#263676=CARTESIAN_POINT('Ctrl Pts',(0.947155051174923,45.0054959891908,
52.9569785783018));
#263677=CARTESIAN_POINT('Ctrl Pts',(1.56201031344966,45.0284962665614,52.7897665739497));
#263678=CARTESIAN_POINT('Ctrl Pts',(2.67010924295794,45.0734758495257,52.2350601445252));
#263679=CARTESIAN_POINT('Ctrl Pts',(3.1566752646739,45.0942529077283,51.860825793501));
#263680=CARTESIAN_POINT('Ctrl Pts',(3.97741086967013,45.1369115840165,50.9319524507052));
#263681=CARTESIAN_POINT('Ctrl Pts',(4.29692068710763,45.1599088389433,50.3802709072399));
#263682=CARTESIAN_POINT('Ctrl Pts',(4.69422254308719,45.2049197616779,49.2060407032791));
#263683=CARTESIAN_POINT('Ctrl Pts',(4.77667886664393,45.2257736105637,48.5976543478151));
#263684=CARTESIAN_POINT('Ctrl Pts',(4.7062737351359,45.2683740367192,47.3597165297));
#263685=CARTESIAN_POINT('Ctrl Pts',(4.54499228938658,45.2913678851305,46.7425959716075));
#263686=CARTESIAN_POINT('Ctrl Pts',(4.00068514395364,45.336408018153,45.6283885259323));
#263687=CARTESIAN_POINT('Ctrl Pts',(3.63101697737713,45.3573375096764,45.1380576730592));
#263688=CARTESIAN_POINT('Ctrl Pts',(2.70942297073046,45.3998823651129,44.3079214437182));
#263689=CARTESIAN_POINT('Ctrl Pts',(2.16022155508803,45.4228725062247,43.9829348968804));
#263690=CARTESIAN_POINT('Ctrl Pts',(1.06039337333579,45.4651887079934,43.5995131929415));
#263691=CARTESIAN_POINT('Ctrl Pts',(0.531800571086339,45.4842039863064,
43.5102));
#263692=CARTESIAN_POINT('Ctrl Pts',(-2.62290189567693E-14,45.5020833333317,
43.5102));
#263693=CARTESIAN_POINT('Origin',(6.7958239265071E-15,40.475,48.26));
#263694=CARTESIAN_POINT('',(1.12195103872683E-8,47.58229166591,43.5102));
#263695=CARTESIAN_POINT('',(6.10331359662667E-15,46.5604166666648,43.5102));
#263696=CARTESIAN_POINT('',(5.54528904550239E-15,40.475,43.5102));
#263697=CARTESIAN_POINT('Ctrl Pts',(1.12322018352984E-8,47.5822916662868,
43.5102));
#263698=CARTESIAN_POINT('Ctrl Pts',(0.605267720969338,47.5619423247769,
43.5102000014313));
#263699=CARTESIAN_POINT('Ctrl Pts',(1.20510137850458,47.5401645011038,43.625895412559));
#263700=CARTESIAN_POINT('Ctrl Pts',(2.35644830837524,47.4950292970466,44.0873667724117));
#263701=CARTESIAN_POINT('Ctrl Pts',(2.89251300407666,47.472104481723,44.4393772525011));
#263702=CARTESIAN_POINT('Ctrl Pts',(3.77706893480681,47.4301570353803,45.3160325548261));
#263703=CARTESIAN_POINT('Ctrl Pts',(4.12379833993738,47.4082806115086,45.8253303490186));
#263704=CARTESIAN_POINT('Ctrl Pts',(4.6150508151954,47.3629657401008,46.9696855352565));
#263705=CARTESIAN_POINT('Ctrl Pts',(4.74601126762411,47.3400383819616,47.5973877834963));
#263706=CARTESIAN_POINT('Ctrl Pts',(4.75328333135343,47.298073272432,48.842579413692));
#263707=CARTESIAN_POINT('Ctrl Pts',(4.63917883647753,47.2762280767327,49.447961639768));
#263708=CARTESIAN_POINT('Ctrl Pts',(4.17905205326823,47.2309203610855,50.6049966699414));
#263709=CARTESIAN_POINT('Ctrl Pts',(3.82862449556919,47.207990303116,51.1418729700227));
#263710=CARTESIAN_POINT('Ctrl Pts',(2.95470207981838,47.1660061719569,52.0286520470234));
#263711=CARTESIAN_POINT('Ctrl Pts',(2.44653487105245,47.144194401308,52.3767460972432));
#263712=CARTESIAN_POINT('Ctrl Pts',(1.30394588441443,47.0988944542651,52.8711908667362));
#263713=CARTESIAN_POINT('Ctrl Pts',(0.676834674480104,47.0759615361057,
53.0039774657885));
#263714=CARTESIAN_POINT('Ctrl Pts',(-0.567965482807374,47.0339569365298,
53.0150303299691));
#263715=CARTESIAN_POINT('Ctrl Pts',(-1.17352631992661,47.0121808943154,
52.9028288165141));
#263716=CARTESIAN_POINT('Ctrl Pts',(-2.33164582654648,46.9668893795248,
52.4464835421592));
#263717=CARTESIAN_POINT('Ctrl Pts',(-2.86946112620001,46.9439534386922,
52.0979004933295));
#263718=CARTESIAN_POINT('Ctrl Pts',(-3.75882201964882,46.9019268325604,
51.2271610910263));
#263719=CARTESIAN_POINT('Ctrl Pts',(-4.10850263838956,46.8801889252566,
50.7203080174569));
#263720=CARTESIAN_POINT('Ctrl Pts',(-4.60665335937267,46.8349065609813,
49.5797770653417));
#263721=CARTESIAN_POINT('Ctrl Pts',(-4.74155982148733,46.8119674343811,
48.9533592685247));
#263722=CARTESIAN_POINT('Ctrl Pts',(-4.75700467169291,46.7699171895905,
47.7090206671102));
#263723=CARTESIAN_POINT('Ctrl Pts',(-4.64701236019383,46.7482199214303,
47.1032521937933));
#263724=CARTESIAN_POINT('Ctrl Pts',(-4.19505684768385,46.7029474845507,
45.9438818387575));
#263725=CARTESIAN_POINT('Ctrl Pts',(-3.84861779247138,46.6800050103184,
45.4049841394257));
#263726=CARTESIAN_POINT('Ctrl Pts',(-2.98157626632749,46.6379293986921,
44.5126339235633));
#263727=CARTESIAN_POINT('Ctrl Pts',(-2.47624632147977,46.6162753641057,
44.1611138927457));
#263728=CARTESIAN_POINT('Ctrl Pts',(-1.33810750007046,46.5710136942996,
43.6586740858177));
#263729=CARTESIAN_POINT('Ctrl Pts',(-0.712502002411283,46.5480677140097,
43.5213144103002));
#263730=CARTESIAN_POINT('Ctrl Pts',(-0.0522560520115934,46.5257182038233,
43.5104155107889));
#263731=CARTESIAN_POINT('Ctrl Pts',(-0.0261232309297634,46.5248366067607,
43.5102));
#263732=CARTESIAN_POINT('Ctrl Pts',(7.21644966006352E-15,46.5239583333315,
43.5102));
#263733=CARTESIAN_POINT('Ctrl Pts',(-2.52888053375126E-14,45.5020833333317,
43.5102));
#263734=CARTESIAN_POINT('Ctrl Pts',(-0.0755693305081445,45.504624004324,
43.5102));
#263735=CARTESIAN_POINT('Ctrl Pts',(-0.151201761326261,45.507191911564,
43.5120034428536));
#263736=CARTESIAN_POINT('Ctrl Pts',(-0.858292825623087,45.5314353880608,
43.5458101658749));
#263737=CARTESIAN_POINT('Ctrl Pts',(-1.4773925394437,45.5544215964754,43.7017648941472));
#263738=CARTESIAN_POINT('Ctrl Pts',(-2.59702589034967,45.5995141893973,
44.2367397860407));
#263739=CARTESIAN_POINT('Ctrl Pts',(-3.09072149425917,45.6205900058754,
44.6023308981989));
#263740=CARTESIAN_POINT('Ctrl Pts',(-3.9292133163964,45.6630317591778,45.517397250835));
#263741=CARTESIAN_POINT('Ctrl Pts',(-4.25906430353724,45.6860138769146,
46.0643451032865));
#263742=CARTESIAN_POINT('Ctrl Pts',(-4.67725347512983,45.7311299350528,
47.2330506292479));
#263743=CARTESIAN_POINT('Ctrl Pts',(-4.7702427303392,45.7522758227052,47.8404285882094));
#263744=CARTESIAN_POINT('Ctrl Pts',(-4.72090364611379,45.7946699987669,
49.0809575774807));
#263745=CARTESIAN_POINT('Ctrl Pts',(-4.56969597500102,45.8176479274087,
49.7017773144576));
#263746=CARTESIAN_POINT('Ctrl Pts',(-4.04303230144165,45.862785749986,50.8261985886888));
#263747=CARTESIAN_POINT('Ctrl Pts',(-3.68105632465394,45.8839993325931,
51.3228801778102));
#263748=CARTESIAN_POINT('Ctrl Pts',(-2.7717992805187,45.9263485235755,52.168750196234));
#263749=CARTESIAN_POINT('Ctrl Pts',(-2.22687990283705,45.9493222166802,
52.5028933987043));
#263750=CARTESIAN_POINT('Ctrl Pts',(-1.06053286026439,45.994480207171,52.9297875312537));
#263751=CARTESIAN_POINT('Ctrl Pts',(-0.453572105352478,46.0157589354207,
53.027162436928));
#263752=CARTESIAN_POINT('Ctrl Pts',(0.787983361548988,46.0580656740931,
52.9865801929752));
#263753=CARTESIAN_POINT('Ctrl Pts',(1.41029123865322,46.0810351299836,52.8395736212663));
#263754=CARTESIAN_POINT('Ctrl Pts',(2.53891297590485,46.1262117931469,52.3202616976982));
#263755=CARTESIAN_POINT('Ctrl Pts',(3.03822772092204,46.147552990229,51.9614714595685));
#263756=CARTESIAN_POINT('Ctrl Pts',(3.89057513217224,46.1898197392215,51.0573495813647));
#263757=CARTESIAN_POINT('Ctrl Pts',(4.22848369300769,46.212784994237,50.5142408474255));
#263758=CARTESIAN_POINT('Ctrl Pts',(4.66303233928975,46.2579789325656,49.3499951812477));
#263759=CARTESIAN_POINT('Ctrl Pts',(4.76426216006489,46.2793798352094,48.7433999159282));
#263760=CARTESIAN_POINT('Ctrl Pts',(4.73136914703641,46.3216089782499,47.5009674579344));
#263761=CARTESIAN_POINT('Ctrl Pts',(4.58805767250648,46.3445701005154,46.8773768955343));
#263762=CARTESIAN_POINT('Ctrl Pts',(4.07520970679068,46.3897800102521,45.7450888182641));
#263763=CARTESIAN_POINT('Ctrl Pts',(3.71921141673823,46.4112378051485,45.2434650441426));
#263764=CARTESIAN_POINT('Ctrl Pts',(2.819601717135,46.4534316401482,44.385460078108));
#263765=CARTESIAN_POINT('Ctrl Pts',(2.27809729632468,46.4763887238926,44.0442651253947));
#263766=CARTESIAN_POINT('Ctrl Pts',(1.14689194172361,46.5204002356443,43.6148577984359));
#263767=CARTESIAN_POINT('Ctrl Pts',(0.575671689768406,46.5410623551547,
43.5102));
#263768=CARTESIAN_POINT('Ctrl Pts',(8.04911692853238E-15,46.5604166666648,
43.5102));
#263769=CARTESIAN_POINT('Origin',(6.7958239265071E-15,40.475,48.26));
#263770=CARTESIAN_POINT('',(-3.0122773445189E-8,48.6406250020229,43.5102));
#263771=CARTESIAN_POINT('',(3.44456304422771E-8,47.6187499976816,43.5102));
#263772=CARTESIAN_POINT('',(5.54528904550239E-15,40.475,43.5102));
#263773=CARTESIAN_POINT('Ctrl Pts',(-3.01569111920684E-8,48.6406250010114,
43.5102));
#263774=CARTESIAN_POINT('Ctrl Pts',(0.00846864324595446,48.6403402808376,
43.5101999999462));
#263775=CARTESIAN_POINT('Ctrl Pts',(0.0169383903993272,48.6400552091581,
43.5102226487671));
#263776=CARTESIAN_POINT('Ctrl Pts',(0.636478416209048,48.6191798718932,
43.5135369343409));
#263777=CARTESIAN_POINT('Ctrl Pts',(1.24118429143188,48.5971621151167,43.6346988877366));
#263778=CARTESIAN_POINT('Ctrl Pts',(2.39313666806093,48.5518367752532,44.1083618417949));
#263779=CARTESIAN_POINT('Ctrl Pts',(2.9256635070832,48.5290407974581,44.4647992630245));
#263780=CARTESIAN_POINT('Ctrl Pts',(3.80266330856505,48.4870990846606,45.349041959842));
#263781=CARTESIAN_POINT('Ctrl Pts',(4.14518439984167,48.4650895774633,45.8618125037741));
#263782=CARTESIAN_POINT('Ctrl Pts',(4.62633837758311,48.4197592212302,47.0108112029287));
#263783=CARTESIAN_POINT('Ctrl Pts',(4.75166011105805,48.3969299909334,47.6394713519075));
#263784=CARTESIAN_POINT('Ctrl Pts',(4.74796833627008,48.3550030935466,48.8850094101938));
#263785=CARTESIAN_POINT('Ctrl Pts',(4.62830538735018,48.3330012731708,49.4898621835296));
#263786=CARTESIAN_POINT('Ctrl Pts',(4.15739165130435,48.2876663003646,50.6432398443227));
#263787=CARTESIAN_POINT('Ctrl Pts',(3.80196381608398,48.2648060457194,51.1769600772512));
#263788=CARTESIAN_POINT('Ctrl Pts',(2.91946417246134,48.2228929205492,52.0561151610514));
#263789=CARTESIAN_POINT('Ctrl Pts',(2.40758203843045,48.200898257452,52.3997151384207));
#263790=CARTESIAN_POINT('Ctrl Pts',(1.25945421064558,48.1555590355424,52.8836082121267));
#263791=CARTESIAN_POINT('Ctrl Pts',(0.630673758570287,48.1326698594116,
53.0103761234246));
#263792=CARTESIAN_POINT('Ctrl Pts',(-0.615133469116459,48.0907695298135,
53.0092419608279));
#263793=CARTESIAN_POINT('Ctrl Pts',(-1.22010977350242,48.0687815264716,
52.8908694158124));
#263794=CARTESIAN_POINT('Ctrl Pts',(-2.37462662754409,48.0234417240359,
52.4223591295305));
#263795=CARTESIAN_POINT('Ctrl Pts',(-2.90939118846586,48.0005256061278,
52.0678343904392));
#263796=CARTESIAN_POINT('Ctrl Pts',(-3.7904016183597,47.9586368751837,51.1868357272436));
#263797=CARTESIAN_POINT('Ctrl Pts',(-4.13495748899581,47.9366553425569,
50.6757367096216));
#263798=CARTESIAN_POINT('Ctrl Pts',(-4.62111654763354,47.8913170826427,
49.5285760969698));
#263799=CARTESIAN_POINT('Ctrl Pts',(-4.74916318677378,47.868399000331,48.8999428065475));
#263800=CARTESIAN_POINT('Ctrl Pts',(-4.7504075112079,47.8264972255023,47.6541382226685));
#263801=CARTESIAN_POINT('Ctrl Pts',(-4.6332666990797,47.8045392147509,47.0490405340914));
#263802=CARTESIAN_POINT('Ctrl Pts',(-4.16710603943454,47.7592060980522,
45.893749292367));
#263803=CARTESIAN_POINT('Ctrl Pts',(-3.8137400149553,47.7362859153077,45.3583838722653));
#263804=CARTESIAN_POINT('Ctrl Pts',(-2.93474341586644,47.694370056637,44.4757372773048));
#263805=CARTESIAN_POINT('Ctrl Pts',(-2.42447534136177,47.6724373335368,
44.1301787960158));
#263806=CARTESIAN_POINT('Ctrl Pts',(-1.27860763790831,47.6271098037818,
43.64166888973));
#263807=CARTESIAN_POINT('Ctrl Pts',(-0.650402238452651,47.6041873785707,
43.5122773754931));
#263808=CARTESIAN_POINT('Ctrl Pts',(-0.0102342257257289,47.5826358605589,
43.5102082686246));
#263809=CARTESIAN_POINT('Ctrl Pts',(-0.0051169169184957,47.5824636994492,
43.5101999999879));
#263810=CARTESIAN_POINT('Ctrl Pts',(1.12322026959339E-8,47.5822916662868,
43.5102));
#263811=CARTESIAN_POINT('Ctrl Pts',(6.66133814775094E-15,46.5604166666648,
43.5102));
#263812=CARTESIAN_POINT('Ctrl Pts',(-0.0333164514064297,46.5615367790316,
43.5102));
#263813=CARTESIAN_POINT('Ctrl Pts',(-0.0666474877696299,46.5626622633207,
43.5105505358004));
#263814=CARTESIAN_POINT('Ctrl Pts',(-0.733745769363326,46.5852859802539,
43.5245966824763));
#263815=CARTESIAN_POINT('Ctrl Pts',(-1.35843845899671,46.6082391406888,
43.6646756633582));
#263816=CARTESIAN_POINT('Ctrl Pts',(-2.4939124693873,46.6534774353481,44.1718703706464));
#263817=CARTESIAN_POINT('Ctrl Pts',(-2.99755105650462,46.6750405296682,
44.5254336623435));
#263818=CARTESIAN_POINT('Ctrl Pts',(-3.86047541902279,46.7171702744801,
45.4210993924352));
#263819=CARTESIAN_POINT('Ctrl Pts',(-4.20452601484658,46.7401196432354,
45.9611914936807));
#263820=CARTESIAN_POINT('Ctrl Pts',(-4.65159836673592,46.7853705168099,
47.1219431444154));
#263821=CARTESIAN_POINT('Ctrl Pts',(-4.75913295039592,46.8069820603204,
47.7279429848328));
#263822=CARTESIAN_POINT('Ctrl Pts',(-4.73879860375981,46.849082831204,48.9717591309175));
#263823=CARTESIAN_POINT('Ctrl Pts',(-4.60153407961421,46.8720285523031,
49.5973963322301));
#263824=CARTESIAN_POINT('Ctrl Pts',(-4.09926063963529,46.9172910317212,
50.7356281460623));
#263825=CARTESIAN_POINT('Ctrl Pts',(-3.74781202137065,46.9389482871537,
51.2410172153012));
#263826=CARTESIAN_POINT('Ctrl Pts',(-2.85557778141026,46.9810220010192,
52.1082024576284));
#263827=CARTESIAN_POINT('Ctrl Pts',(-2.31672197870818,47.0039642273675,
52.4547248602009));
#263828=CARTESIAN_POINT('Ctrl Pts',(-1.15740005626589,47.0492374108295,
52.9068509099192));
#263829=CARTESIAN_POINT('Ctrl Pts',(-0.551639655503142,47.0709377090647,
53.0169290494783));
#263830=CARTESIAN_POINT('Ctrl Pts',(0.692717019936865,47.1129861845493,
53.0016548841551));
#263831=CARTESIAN_POINT('Ctrl Pts',(1.31916190182874,47.1359250749043,52.8668307754809));
#263832=CARTESIAN_POINT('Ctrl Pts',(2.45977296165077,47.1812081274254,52.3688240300641));
#263833=CARTESIAN_POINT('Ctrl Pts',(2.96667712210168,47.2029488802598,52.019205096725));
#263834=CARTESIAN_POINT('Ctrl Pts',(3.83754039304105,47.2449738385225,51.1299445253105));
#263835=CARTESIAN_POINT('Ctrl Pts',(4.18619523897202,47.2679095549076,50.5921656409225));
#263836=CARTESIAN_POINT('Ctrl Pts',(4.6426876218868,47.3132017039919,49.4340882023268));
#263837=CARTESIAN_POINT('Ctrl Pts',(4.75496316694537,47.3349804140488,48.8285343178734));
#263838=CARTESIAN_POINT('Ctrl Pts',(4.74405742910957,47.3769834803082,47.5837188255907));
#263839=CARTESIAN_POINT('Ctrl Pts',(4.61134187087939,47.3999161858311,46.9565845142134));
#263840=CARTESIAN_POINT('Ctrl Pts',(4.11702129093406,47.4452167173043,45.8139267033713));
#263841=CARTESIAN_POINT('Ctrl Pts',(3.76898036413946,47.4670309854212,45.305715487294));
#263842=CARTESIAN_POINT('Ctrl Pts',(2.88228778831814,47.5090136911056,44.4316865997081));
#263843=CARTESIAN_POINT('Ctrl Pts',(2.34544301461838,47.5319435481428,44.0811973591388));
#263844=CARTESIAN_POINT('Ctrl Pts',(1.19688904259188,47.5769211080058,43.6243033168789));
#263845=CARTESIAN_POINT('Ctrl Pts',(0.601088508161882,47.5985411648686,
43.5102000043641));
#263846=CARTESIAN_POINT('Ctrl Pts',(3.44846856625836E-8,47.6187499988384,
43.5102));
#263847=CARTESIAN_POINT('Origin',(6.7958239265071E-15,40.475,48.26));
#263848=CARTESIAN_POINT('',(5.54528904550239E-15,49.238,43.5102));
#263849=CARTESIAN_POINT('',(-1.00167620060974E-8,48.6770833340043,43.5102));
#263850=CARTESIAN_POINT('',(5.54528904550239E-15,40.475,43.5102));
#263851=CARTESIAN_POINT('',(1.86990303000813,49.238,52.6262412551721));
#263852=CARTESIAN_POINT('Origin',(6.7958239265071E-15,49.238,48.26));
#263853=CARTESIAN_POINT('Ctrl Pts',(1.86990303000838,49.238,52.626241255172));
#263854=CARTESIAN_POINT('Ctrl Pts',(1.56383729601047,49.2258845683299,52.7573181265442));
#263855=CARTESIAN_POINT('Ctrl Pts',(1.24484153160777,49.2137876533848,52.8558494941654));
#263856=CARTESIAN_POINT('Ctrl Pts',(0.598087148393397,49.1902689990312,
52.9832738225069));
#263857=CARTESIAN_POINT('Ctrl Pts',(0.272399227164127,49.1789970034025,
53.0131869119213));
#263858=CARTESIAN_POINT('Ctrl Pts',(-0.665150328710527,49.1473284546882,
53.0025766190358));
#263859=CARTESIAN_POINT('Ctrl Pts',(-1.26947276028821,49.1252713731853,
52.8776651208351));
#263860=CARTESIAN_POINT('Ctrl Pts',(-2.4178439523169,49.0799708480804,52.3971383205351));
#263861=CARTESIAN_POINT('Ctrl Pts',(-2.94738751121186,49.0573327453721,
52.0381816129474));
#263862=CARTESIAN_POINT('Ctrl Pts',(-3.81898351389284,49.0153198975399,
51.1495847597557));
#263863=CARTESIAN_POINT('Ctrl Pts',(-4.15879206820495,48.9932736680055,
50.6345983826297));
#263864=CARTESIAN_POINT('Ctrl Pts',(-4.63308233656813,48.9479661434788,
49.4834357447574));
#263865=CARTESIAN_POINT('Ctrl Pts',(-4.75478602763426,48.9252845812558,
48.8550795761242));
#263866=CARTESIAN_POINT('Ctrl Pts',(-4.74468294064049,48.8832914499036,
47.6102271173403));
#263867=CARTESIAN_POINT('Ctrl Pts',(-4.62178279031773,48.8612553675669,
47.0056961541918));
#263868=CARTESIAN_POINT('Ctrl Pts',(-4.14493564252529,48.8159414036286,
45.8554010775775));
#263869=CARTESIAN_POINT('Ctrl Pts',(-3.78732928008356,48.7932191294468,
45.3242575343515));
#263870=CARTESIAN_POINT('Ctrl Pts',(-2.90106707411062,48.7512443740699,
44.4497605377253));
#263871=CARTESIAN_POINT('Ctrl Pts',(-2.38726818569504,48.7292177706584,
44.1084944446942));
#263872=CARTESIAN_POINT('Ctrl Pts',(-1.24508730776246,48.6842061952532,
43.6337718041888));
#263873=CARTESIAN_POINT('Ctrl Pts',(-0.625530370510309,48.6616555802689,
43.5102000039715));
#263874=CARTESIAN_POINT('Ctrl Pts',(-3.0156908498169E-8,48.6406250010113,
43.5102));
#263875=CARTESIAN_POINT('Ctrl Pts',(3.44846877406766E-8,47.6187499988384,
43.5102));
#263876=CARTESIAN_POINT('Ctrl Pts',(-0.00908423608736038,47.6190554156343,
43.510199999934));
#263877=CARTESIAN_POINT('Ctrl Pts',(-0.0181696901681403,47.6193612351469,
43.5102260611621));
#263878=CARTESIAN_POINT('Ctrl Pts',(-0.662136500168755,47.6410631179696,
43.5139214564745));
#263879=CARTESIAN_POINT('Ctrl Pts',(-1.28985842539348,47.6639902866762,
43.6448208016811));
#263880=CARTESIAN_POINT('Ctrl Pts',(-2.43427260627819,47.7093056539372,
44.1359664574956));
#263881=CARTESIAN_POINT('Ctrl Pts',(-2.94360820937189,47.7311842575742,
44.4826502313427));
#263882=CARTESIAN_POINT('Ctrl Pts',(-3.82035481584433,47.7731304748415,
45.3671317852293));
#263883=CARTESIAN_POINT('Ctrl Pts',(-4.17241816830197,47.7960551119495,
45.9031692796597));
#263884=CARTESIAN_POINT('Ctrl Pts',(-4.63590244033901,47.841377030083,47.0592360290114));
#263885=CARTESIAN_POINT('Ctrl Pts',(-4.75169647666858,47.8632846262196,
47.6644598597264));
#263886=CARTESIAN_POINT('Ctrl Pts',(-4.74777924466011,47.9052145427421,
48.9099943312856));
#263887=CARTESIAN_POINT('Ctrl Pts',(-4.61844016403301,47.9281368006108,
49.5382164720461));
#263888=CARTESIAN_POINT('Ctrl Pts',(-4.13002191265821,47.9734647507916,
50.6841346452883));
#263889=CARTESIAN_POINT('Ctrl Pts',(-3.78450253960804,47.9953993673611,
51.1944351295961));
#263890=CARTESIAN_POINT('Ctrl Pts',(-2.90191974348767,48.037314169267,52.0735098685414));
#263891=CARTESIAN_POINT('Ctrl Pts',(-2.36657772452895,48.0602341951522,
52.4269211246317));
#263892=CARTESIAN_POINT('Ctrl Pts',(-1.21131348071913,48.1055676989055,
52.8931747566162));
#263893=CARTESIAN_POINT('Ctrl Pts',(-0.606220172193079,48.1275274716681,
53.0103623527893));
#263894=CARTESIAN_POINT('Ctrl Pts',(0.639593744247375,48.1694282675114,
53.0092108581362));
#263895=CARTESIAN_POINT('Ctrl Pts',(1.26824126498937,48.1923462030235,52.8812091154102));
#263896=CARTESIAN_POINT('Ctrl Pts',(2.41536511316397,48.237681662734,52.3951623765016));
#263897=CARTESIAN_POINT('Ctrl Pts',(2.92650865236586,48.2596639329101,52.0506691843573));
#263898=CARTESIAN_POINT('Ctrl Pts',(3.80756031737863,48.3015532619483,51.1697271236068));
#263899=CARTESIAN_POINT('Ctrl Pts',(4.16214899822401,48.3244673767911,50.6350159036465));
#263900=CARTESIAN_POINT('Ctrl Pts',(4.63077827583646,48.3698102209431,49.4804578650776));
#263901=CARTESIAN_POINT('Ctrl Pts',(4.7491968666976,48.3917987188872,48.875485922136));
#263902=CARTESIAN_POINT('Ctrl Pts',(4.75042231280387,48.4336999981435,47.6296882588277));
#263903=CARTESIAN_POINT('Ctrl Pts',(4.62370604511392,48.4565870245828,47.0009120908311));
#263904=CARTESIAN_POINT('Ctrl Pts',(4.13991074199344,48.5019259324576,45.8527531057461));
#263905=CARTESIAN_POINT('Ctrl Pts',(3.79634923939821,48.523921127265,45.3408392198354));
#263906=CARTESIAN_POINT('Ctrl Pts',(2.91727107546832,48.5658352748234,44.4582773051987));
#263907=CARTESIAN_POINT('Ctrl Pts',(2.38359346820129,48.588693222624,44.1028133915149));
#263908=CARTESIAN_POINT('Ctrl Pts',(1.23026664392749,48.6340278542552,43.6318014243512));
#263909=CARTESIAN_POINT('Ctrl Pts',(0.625419053720088,48.6560302458643,
43.5120849431335));
#263910=CARTESIAN_POINT('Ctrl Pts',(0.00965498329080251,48.6767586264632,
43.510207359137));
#263911=CARTESIAN_POINT('Ctrl Pts',(0.00482730997582324,48.6769210372467,
43.5101999999898));
#263912=CARTESIAN_POINT('Ctrl Pts',(-1.00281259683004E-8,48.6770833336679,
43.5102));
#263913=CARTESIAN_POINT('Origin',(6.7958239265071E-15,42.09425,48.26));
#263914=CARTESIAN_POINT('',(4.66579641623065,42.0671867061318,47.5288462557477));
#263915=CARTESIAN_POINT('Origin',(-0.0419539454484924,42.0904940530822,
48.1587073448045));
#263916=CARTESIAN_POINT('',(4.68628896694498,42.0671867061318,47.6743911597878));
#263917=CARTESIAN_POINT('Origin',(1.58033521102663E-6,42.0671867060952,
48.2599997745674));
#263918=CARTESIAN_POINT('Origin',(-0.157122447866724,42.1434096703623,47.879511098682));
#263919=CARTESIAN_POINT('',(5.97160775493582E-15,40.475,45.12945));
#263920=CARTESIAN_POINT('',(5.54528904550239E-15,42.09425,43.5102));
#263921=CARTESIAN_POINT('Origin',(6.7958239265071E-15,40.475,48.26));
#263922=CARTESIAN_POINT('Origin',(6.7958239265071E-15,50.,48.26));
#263923=CARTESIAN_POINT('',(0.908077042619364,49.238,52.9221879117715));
#263924=CARTESIAN_POINT('',(6.88299333419379E-15,49.238,53.0098));
#263925=CARTESIAN_POINT('Origin',(6.7958239265071E-15,49.238,48.26));
#263926=CARTESIAN_POINT('Origin',(-0.101290884807203,49.2622522741402,48.3019587266354));
#263927=CARTESIAN_POINT('Origin',(-0.380373159828188,49.2681001647224,48.4181119225168));
#263928=CARTESIAN_POINT('Origin',(6.7958239265071E-15,49.238,48.26));
#263929=CARTESIAN_POINT('',(6.86900893723871E-15,50.,52.2478));
#263930=CARTESIAN_POINT('',(6.86900893723871E-15,50.,52.2478));
#263931=CARTESIAN_POINT('Origin',(6.7958239265071E-15,50.,48.26));
#263932=CARTESIAN_POINT('Origin',(6.7958239265071E-15,40.475,48.26));
#263933=CARTESIAN_POINT('Ctrl Pts',(-1.00281261072865E-8,48.6770833336679,
43.5102));
#263934=CARTESIAN_POINT('Ctrl Pts',(-0.629672755148192,48.6982531821869,
43.5102000013294));
#263935=CARTESIAN_POINT('Ctrl Pts',(-1.25321726916232,48.7209607258464,
43.6354136739496));
#263936=CARTESIAN_POINT('Ctrl Pts',(-2.39779765932932,48.766114985687,44.1145892634232));
#263937=CARTESIAN_POINT('Ctrl Pts',(-2.91060499549369,48.7881251061508,
44.4570655678299));
#263938=CARTESIAN_POINT('Ctrl Pts',(-3.79491991104055,48.8300680020356,
45.3339759730056));
#263939=CARTESIAN_POINT('Ctrl Pts',(-4.15139914837991,48.8528613299139,
45.86645335616));
#263940=CARTESIAN_POINT('Ctrl Pts',(-4.62517599058953,48.8981862669499,
47.0183465771293));
#263941=CARTESIAN_POINT('Ctrl Pts',(-4.74640007620397,48.9202046816236,
47.6230462847408));
#263942=CARTESIAN_POINT('Ctrl Pts',(-4.75318456347165,48.9621635943342,
48.8682555584807));
#263943=CARTESIAN_POINT('Ctrl Pts',(-4.62960939173144,48.9849211271636,
49.4967694962143));
#263944=CARTESIAN_POINT('Ctrl Pts',(-4.15176681390835,49.0302405779038,
50.6468154508051));
#263945=CARTESIAN_POINT('Ctrl Pts',(-3.81055277871335,49.0522678865187,
51.1606568777446));
#263946=CARTESIAN_POINT('Ctrl Pts',(-2.93615950038935,49.094244007631,52.0470026674717));
#263947=CARTESIAN_POINT('Ctrl Pts',(-2.40507322360229,49.1169632491863,
52.4046573926874));
#263948=CARTESIAN_POINT('Ctrl Pts',(-1.38668037731136,49.1570831197733,
52.8269672384587));
#263949=CARTESIAN_POINT('Ctrl Pts',(-0.929744443721774,49.1740393274787,
52.9414176733624));
#263950=CARTESIAN_POINT('Ctrl Pts',(-0.00555594936379633,49.2063727902452,
53.0320305704281));
#263951=CARTESIAN_POINT('Ctrl Pts',(0.456439282085028,49.2215907184063,
53.0101555976912));
#263952=CARTESIAN_POINT('Ctrl Pts',(0.908077042619743,49.238,52.9221879117714));
#263953=CARTESIAN_POINT('Origin',(6.7958239265071E-15,40.475,48.26));
#263954=CARTESIAN_POINT('Origin',(6.7958239265071E-15,50.,48.26));
#263955=CARTESIAN_POINT('',(1.000194405918E-14,50.,51.0096306570156));
#263956=CARTESIAN_POINT('',(2.38125000000001,50.,49.6348153285078));
#263957=CARTESIAN_POINT('Origin',(6.7958239265071E-15,50.,48.26));
#263958=CARTESIAN_POINT('',(-2.38124999999999,50.,49.6348153285078));
#263959=CARTESIAN_POINT('Origin',(6.7958239265071E-15,50.,48.26));
#263960=CARTESIAN_POINT('',(-2.38125,50.,46.8851846714922));
#263961=CARTESIAN_POINT('Origin',(6.7958239265071E-15,50.,48.26));
#263962=CARTESIAN_POINT('',(9.22755509075881E-15,50.,45.5103693429844));
#263963=CARTESIAN_POINT('Origin',(6.7958239265071E-15,50.,48.26));
#263964=CARTESIAN_POINT('',(2.38125000000001,50.,46.8851846714922));
#263965=CARTESIAN_POINT('Origin',(6.7958239265071E-15,50.,48.26));
#263966=CARTESIAN_POINT('Origin',(6.7958239265071E-15,50.,48.26));
#263967=CARTESIAN_POINT('Origin',(6.7958239265071E-15,50.,48.26));
#263968=CARTESIAN_POINT('Ctrl Pts',(-8.35153880681623E-13,50.0000000000005,
51.0096306570161));
#263969=CARTESIAN_POINT('Ctrl Pts',(1.19062500000002,49.3125923357457,50.3222229927617));
#263970=CARTESIAN_POINT('Ctrl Pts',(2.38125000000088,50.0000000000005,49.6348153285073));
#263971=CARTESIAN_POINT('Origin',(6.7958239265071E-15,50.,48.26));
#263972=CARTESIAN_POINT('Ctrl Pts',(2.38125000000001,50.0000000000005,49.6348153285088));
#263973=CARTESIAN_POINT('Ctrl Pts',(2.38125000000001,49.3125923357457,48.26));
#263974=CARTESIAN_POINT('Ctrl Pts',(2.38125000000001,50.0000000000005,46.8851846714912));
#263975=CARTESIAN_POINT('Origin',(6.7958239265071E-15,50.,48.26));
#263976=CARTESIAN_POINT('Ctrl Pts',(2.38125000000087,50.0000000000005,46.8851846714927));
#263977=CARTESIAN_POINT('Ctrl Pts',(1.19062500000001,49.3125923357457,46.1977770072383));
#263978=CARTESIAN_POINT('Ctrl Pts',(-8.54108254788434E-13,50.0000000000005,
45.5103693429839));
#263979=CARTESIAN_POINT('Origin',(6.7958239265071E-15,50.,48.26));
#263980=CARTESIAN_POINT('Ctrl Pts',(8.99821745281327E-13,50.0000000000005,
45.5103693429839));
#263981=CARTESIAN_POINT('Ctrl Pts',(-1.19062499999999,49.3125923357457,
46.1977770072383));
#263982=CARTESIAN_POINT('Ctrl Pts',(-2.38125000000087,50.0000000000005,
46.8851846714927));
#263983=CARTESIAN_POINT('Origin',(6.7958239265071E-15,50.,48.26));
#263984=CARTESIAN_POINT('Ctrl Pts',(-2.38124999999999,50.0000000000005,
46.8851846714912));
#263985=CARTESIAN_POINT('Ctrl Pts',(-2.38124999999999,49.3125923357457,
48.26));
#263986=CARTESIAN_POINT('Ctrl Pts',(-2.38124999999999,50.0000000000005,
49.6348153285088));
#263987=CARTESIAN_POINT('Origin',(6.7958239265071E-15,50.,48.26));
#263988=CARTESIAN_POINT('Ctrl Pts',(-2.38125000000084,50.0000000000005,
49.6348153285073));
#263989=CARTESIAN_POINT('Ctrl Pts',(-1.19062499999998,49.3125923357457,
50.3222229927617));
#263990=CARTESIAN_POINT('Ctrl Pts',(8.74084678479433E-13,50.0000000000005,
51.0096306570161));
#263991=CARTESIAN_POINT('Origin',(-2.38124999999999,46.428125,49.6348153285078));
#263992=CARTESIAN_POINT('',(-2.38124999999999,46.428125,49.6348153285078));
#263993=CARTESIAN_POINT('',(7.34564873659056E-15,46.428125,51.0096306570156));
#263994=CARTESIAN_POINT('',(7.34564873659056E-15,46.428125,51.0096306570156));
#263995=CARTESIAN_POINT('',(2.38125000000001,46.428125,49.6348153285078));
#263996=CARTESIAN_POINT('',(2.38125000000001,46.428125,49.6348153285078));
#263997=CARTESIAN_POINT('',(2.38125000000001,46.428125,46.8851846714922));
#263998=CARTESIAN_POINT('',(2.38125000000001,46.428125,46.8851846714922));
#263999=CARTESIAN_POINT('',(6.57125976816934E-15,46.428125,45.5103693429844));
#264000=CARTESIAN_POINT('',(6.57125976816934E-15,46.428125,45.5103693429844));
#264001=CARTESIAN_POINT('',(-2.38124999999999,46.428125,46.8851846714922));
#264002=CARTESIAN_POINT('',(-2.38124999999999,46.428125,46.8851846714922));
#264003=CARTESIAN_POINT('',(-2.38124999999999,46.428125,49.6348153285078));
#264004=CARTESIAN_POINT('Origin',(2.38125000000001,46.428125,49.6348153285078));
#264005=CARTESIAN_POINT('',(7.34564873659056E-15,46.428125,51.0096306570156));
#264006=CARTESIAN_POINT('',(2.38125000000001,46.428125,49.6348153285078));
#264007=CARTESIAN_POINT('Origin',(2.38125000000001,46.428125,46.8851846714922));
#264008=CARTESIAN_POINT('',(2.38125000000001,46.428125,46.8851846714922));
#264009=CARTESIAN_POINT('Origin',(6.57125976816934E-15,46.428125,45.5103693429844));
#264010=CARTESIAN_POINT('',(6.57125976816934E-15,46.428125,45.5103693429844));
#264011=CARTESIAN_POINT('Origin',(-2.38124999999999,46.428125,46.8851846714922));
#264012=CARTESIAN_POINT('',(-2.38124999999999,46.428125,46.8851846714922));
#264013=CARTESIAN_POINT('Origin',(-2.38124999999999,46.428125,49.6348153285078));
#264014=CARTESIAN_POINT('',(-2.38124999999999,46.428125,49.6348153285078));
#264015=CARTESIAN_POINT('Origin',(7.34564873659056E-15,46.428125,51.0096306570156));
#264016=CARTESIAN_POINT('Ctrl Pts',(-4.72273670613182,40.459375,48.26));
#264017=CARTESIAN_POINT('Ctrl Pts',(-4.72273670613182,40.5255208333334,
50.216221595197));
#264018=CARTESIAN_POINT('Ctrl Pts',(-3.33947915066443,40.5916666666667,
51.5994791506644));
#264019=CARTESIAN_POINT('Ctrl Pts',(-1.95622159519703,40.6578125,52.9827367061318));
#264020=CARTESIAN_POINT('Ctrl Pts',(7.17168088200107E-15,40.7239583333333,
52.9827367061318));
#264021=CARTESIAN_POINT('Ctrl Pts',(1.95622159519705,40.7901041666666,52.9827367061318));
#264022=CARTESIAN_POINT('Ctrl Pts',(3.33947915066444,40.8562499999999,51.5994791506644));
#264023=CARTESIAN_POINT('Ctrl Pts',(4.72273670613183,40.9223958333332,50.216221595197));
#264024=CARTESIAN_POINT('Ctrl Pts',(4.72273670613183,40.9885416666665,48.26));
#264025=CARTESIAN_POINT('Ctrl Pts',(4.72273670613183,41.0546874999999,46.303778404803));
#264026=CARTESIAN_POINT('Ctrl Pts',(3.33947915066444,41.1208333333332,44.9205208493356));
#264027=CARTESIAN_POINT('Ctrl Pts',(1.95622159519705,41.1869791666665,43.5372632938682));
#264028=CARTESIAN_POINT('Ctrl Pts',(6.99833541005117E-15,41.2531249999998,
43.5372632938682));
#264029=CARTESIAN_POINT('Ctrl Pts',(-1.95622159519704,41.3192708333331,
43.5372632938682));
#264030=CARTESIAN_POINT('Ctrl Pts',(-3.33947915066443,41.3854166666664,
44.9205208493356));
#264031=CARTESIAN_POINT('Ctrl Pts',(-4.72273670613182,41.4515624999997,
46.303778404803));
#264032=CARTESIAN_POINT('Ctrl Pts',(-4.72273670613182,41.517708333333,48.26));
#264033=CARTESIAN_POINT('Ctrl Pts',(-4.72273670613182,41.5838541666664,
50.216221595197));
#264034=CARTESIAN_POINT('Ctrl Pts',(-3.33947915066443,41.6499999999997,
51.5994791506644));
#264035=CARTESIAN_POINT('Ctrl Pts',(-1.95622159519703,41.716145833333,52.9827367061318));
#264036=CARTESIAN_POINT('Ctrl Pts',(7.17168088200104E-15,41.7822916666663,
52.9827367061318));
#264037=CARTESIAN_POINT('Ctrl Pts',(1.95622159519705,41.8484374999996,52.9827367061318));
#264038=CARTESIAN_POINT('Ctrl Pts',(3.33947915066444,41.9145833333329,51.5994791506644));
#264039=CARTESIAN_POINT('Ctrl Pts',(4.72273670613183,41.9807291666662,50.216221595197));
#264040=CARTESIAN_POINT('Ctrl Pts',(4.72273670613183,42.0468749999996,48.26));
#264041=CARTESIAN_POINT('Ctrl Pts',(4.72273670613183,42.1130208333329,46.303778404803));
#264042=CARTESIAN_POINT('Ctrl Pts',(3.33947915066444,42.1791666666662,44.9205208493356));
#264043=CARTESIAN_POINT('Ctrl Pts',(1.95622159519705,42.2453124999995,43.5372632938682));
#264044=CARTESIAN_POINT('Ctrl Pts',(6.9983354100512E-15,42.3114583333328,
43.5372632938682));
#264045=CARTESIAN_POINT('Ctrl Pts',(-1.95622159519704,42.3776041666661,
43.5372632938682));
#264046=CARTESIAN_POINT('Ctrl Pts',(-3.33947915066443,42.4437499999994,
44.9205208493356));
#264047=CARTESIAN_POINT('Ctrl Pts',(-4.72273670613182,42.5098958333327,
46.303778404803));
#264048=CARTESIAN_POINT('Ctrl Pts',(-4.72273670613182,42.5760416666661,
48.26));
#264049=CARTESIAN_POINT('Ctrl Pts',(-4.72273670613182,42.6421874999994,
50.216221595197));
#264050=CARTESIAN_POINT('Ctrl Pts',(-3.33947915066443,42.7083333333327,
51.5994791506644));
#264051=CARTESIAN_POINT('Ctrl Pts',(-1.95622159519703,42.774479166666,52.9827367061318));
#264052=CARTESIAN_POINT('Ctrl Pts',(7.17168088200104E-15,42.8406249999993,
52.9827367061318));
#264053=CARTESIAN_POINT('Ctrl Pts',(1.95622159519705,42.9067708333326,52.9827367061318));
#264054=CARTESIAN_POINT('Ctrl Pts',(3.33947915066444,42.9729166666659,51.5994791506644));
#264055=CARTESIAN_POINT('Ctrl Pts',(4.72273670613183,43.0390624999992,50.216221595197));
#264056=CARTESIAN_POINT('Ctrl Pts',(4.72273670613183,43.1052083333326,48.26));
#264057=CARTESIAN_POINT('Ctrl Pts',(4.72273670613183,43.1713541666659,46.303778404803));
#264058=CARTESIAN_POINT('Ctrl Pts',(3.33947915066444,43.2374999999992,44.9205208493356));
#264059=CARTESIAN_POINT('Ctrl Pts',(1.95622159519705,43.3036458333325,43.5372632938682));
#264060=CARTESIAN_POINT('Ctrl Pts',(6.99833541005117E-15,43.3697916666658,
43.5372632938682));
#264061=CARTESIAN_POINT('Ctrl Pts',(-1.95622159519704,43.4359374999991,
43.5372632938682));
#264062=CARTESIAN_POINT('Ctrl Pts',(-3.33947915066443,43.5020833333324,
44.9205208493356));
#264063=CARTESIAN_POINT('Ctrl Pts',(-4.72273670613182,43.5682291666657,
46.303778404803));
#264064=CARTESIAN_POINT('Ctrl Pts',(-4.72273670613182,43.634374999999,48.26));
#264065=CARTESIAN_POINT('Ctrl Pts',(-4.72273670613182,43.7005208333324,
50.216221595197));
#264066=CARTESIAN_POINT('Ctrl Pts',(-3.33947915066443,43.7666666666657,
51.5994791506644));
#264067=CARTESIAN_POINT('Ctrl Pts',(-1.95622159519703,43.832812499999,52.9827367061318));
#264068=CARTESIAN_POINT('Ctrl Pts',(7.17168088200102E-15,43.8989583333323,
52.9827367061318));
#264069=CARTESIAN_POINT('Ctrl Pts',(1.95622159519705,43.9651041666656,52.9827367061318));
#264070=CARTESIAN_POINT('Ctrl Pts',(3.33947915066444,44.0312499999989,51.5994791506644));
#264071=CARTESIAN_POINT('Ctrl Pts',(4.72273670613183,44.0973958333322,50.216221595197));
#264072=CARTESIAN_POINT('Ctrl Pts',(4.72273670613183,44.1635416666656,48.26));
#264073=CARTESIAN_POINT('Ctrl Pts',(4.72273670613183,44.2296874999989,46.303778404803));
#264074=CARTESIAN_POINT('Ctrl Pts',(3.33947915066444,44.2958333333322,44.9205208493356));
#264075=CARTESIAN_POINT('Ctrl Pts',(1.95622159519705,44.3619791666655,43.5372632938682));
#264076=CARTESIAN_POINT('Ctrl Pts',(6.99833541005117E-15,44.4281249999988,
43.5372632938682));
#264077=CARTESIAN_POINT('Ctrl Pts',(-1.95622159519704,44.4942708333321,
43.5372632938682));
#264078=CARTESIAN_POINT('Ctrl Pts',(-3.33947915066443,44.5604166666654,
44.9205208493356));
#264079=CARTESIAN_POINT('Ctrl Pts',(-4.72273670613182,44.6265624999987,
46.303778404803));
#264080=CARTESIAN_POINT('Ctrl Pts',(-4.72273670613182,44.692708333332,48.26));
#264081=CARTESIAN_POINT('Ctrl Pts',(-4.72273670613182,44.7588541666654,
50.216221595197));
#264082=CARTESIAN_POINT('Ctrl Pts',(-3.33947915066443,44.8249999999987,
51.5994791506644));
#264083=CARTESIAN_POINT('Ctrl Pts',(-1.95622159519703,44.891145833332,52.9827367061318));
#264084=CARTESIAN_POINT('Ctrl Pts',(7.17168088200107E-15,44.9572916666653,
52.9827367061318));
#264085=CARTESIAN_POINT('Ctrl Pts',(1.95622159519705,45.0234374999986,52.9827367061318));
#264086=CARTESIAN_POINT('Ctrl Pts',(3.33947915066444,45.0895833333319,51.5994791506644));
#264087=CARTESIAN_POINT('Ctrl Pts',(4.72273670613183,45.1557291666652,50.216221595197));
#264088=CARTESIAN_POINT('Ctrl Pts',(4.72273670613183,45.2218749999985,48.26));
#264089=CARTESIAN_POINT('Ctrl Pts',(4.72273670613183,45.2880208333319,46.303778404803));
#264090=CARTESIAN_POINT('Ctrl Pts',(3.33947915066444,45.3541666666652,44.9205208493356));
#264091=CARTESIAN_POINT('Ctrl Pts',(1.95622159519705,45.4203124999985,43.5372632938682));
#264092=CARTESIAN_POINT('Ctrl Pts',(6.99833541005117E-15,45.4864583333318,
43.5372632938682));
#264093=CARTESIAN_POINT('Ctrl Pts',(-1.95622159519704,45.5526041666651,
43.5372632938682));
#264094=CARTESIAN_POINT('Ctrl Pts',(-3.33947915066443,45.6187499999984,
44.9205208493356));
#264095=CARTESIAN_POINT('Ctrl Pts',(-4.72273670613182,45.6848958333317,
46.303778404803));
#264096=CARTESIAN_POINT('Ctrl Pts',(-4.72273670613182,45.7510416666651,
48.26));
#264097=CARTESIAN_POINT('Ctrl Pts',(-4.72273670613182,45.8171874999984,
50.216221595197));
#264098=CARTESIAN_POINT('Ctrl Pts',(-3.33947915066443,45.8833333333317,
51.5994791506644));
#264099=CARTESIAN_POINT('Ctrl Pts',(-1.95622159519703,45.949479166665,52.9827367061318));
#264100=CARTESIAN_POINT('Ctrl Pts',(7.17168088200107E-15,46.0156249999983,
52.9827367061318));
#264101=CARTESIAN_POINT('Ctrl Pts',(1.95622159519705,46.0817708333316,52.9827367061318));
#264102=CARTESIAN_POINT('Ctrl Pts',(3.33947915066444,46.1479166666649,51.5994791506644));
#264103=CARTESIAN_POINT('Ctrl Pts',(4.72273670613183,46.2140624999982,50.216221595197));
#264104=CARTESIAN_POINT('Ctrl Pts',(4.72273670613183,46.2802083333315,48.26));
#264105=CARTESIAN_POINT('Ctrl Pts',(4.72273670613183,46.3463541666649,46.303778404803));
#264106=CARTESIAN_POINT('Ctrl Pts',(3.33947915066444,46.4124999999982,44.9205208493356));
#264107=CARTESIAN_POINT('Ctrl Pts',(1.95622159519705,46.4786458333315,43.5372632938682));
#264108=CARTESIAN_POINT('Ctrl Pts',(6.99833541005117E-15,46.5447916666648,
43.5372632938682));
#264109=CARTESIAN_POINT('Ctrl Pts',(-1.95622159519704,46.6109374999981,
43.5372632938682));
#264110=CARTESIAN_POINT('Ctrl Pts',(-3.33947915066443,46.6770833333314,
44.9205208493356));
#264111=CARTESIAN_POINT('Ctrl Pts',(-4.72273670613182,46.7432291666647,
46.303778404803));
#264112=CARTESIAN_POINT('Ctrl Pts',(-4.72273670613182,46.8093749999981,
48.26));
#264113=CARTESIAN_POINT('Ctrl Pts',(-4.72273670613182,46.8755208333314,
50.216221595197));
#264114=CARTESIAN_POINT('Ctrl Pts',(-3.33947915066443,46.9416666666647,
51.5994791506644));
#264115=CARTESIAN_POINT('Ctrl Pts',(-1.95622159519703,47.007812499998,52.9827367061318));
#264116=CARTESIAN_POINT('Ctrl Pts',(7.17168088200104E-15,47.0739583333313,
52.9827367061318));
#264117=CARTESIAN_POINT('Ctrl Pts',(1.95622159519705,47.1401041666646,52.9827367061318));
#264118=CARTESIAN_POINT('Ctrl Pts',(3.33947915066444,47.2062499999979,51.5994791506644));
#264119=CARTESIAN_POINT('Ctrl Pts',(4.72273670613183,47.2723958333312,50.216221595197));
#264120=CARTESIAN_POINT('Ctrl Pts',(4.72273670613183,47.3385416666645,48.26));
#264121=CARTESIAN_POINT('Ctrl Pts',(4.72273670613183,47.4046874999979,46.303778404803));
#264122=CARTESIAN_POINT('Ctrl Pts',(3.33947915066444,47.4708333333312,44.9205208493356));
#264123=CARTESIAN_POINT('Ctrl Pts',(1.95622159519705,47.5369791666645,43.5372632938682));
#264124=CARTESIAN_POINT('Ctrl Pts',(6.99833541005117E-15,47.6031249999978,
43.5372632938682));
#264125=CARTESIAN_POINT('Ctrl Pts',(-1.95622159519704,47.6692708333311,
43.5372632938682));
#264126=CARTESIAN_POINT('Ctrl Pts',(-3.33947915066443,47.7354166666644,
44.9205208493356));
#264127=CARTESIAN_POINT('Ctrl Pts',(-4.72273670613182,47.8015624999977,
46.303778404803));
#264128=CARTESIAN_POINT('Ctrl Pts',(-4.72273670613182,47.867708333331,48.26));
#264129=CARTESIAN_POINT('Ctrl Pts',(-4.72273670613182,47.9338541666644,
50.216221595197));
#264130=CARTESIAN_POINT('Ctrl Pts',(-3.33947915066443,47.9999999999977,
51.5994791506644));
#264131=CARTESIAN_POINT('Ctrl Pts',(-1.95622159519703,48.066145833331,52.9827367061318));
#264132=CARTESIAN_POINT('Ctrl Pts',(7.17168088200104E-15,48.1322916666643,
52.9827367061318));
#264133=CARTESIAN_POINT('Ctrl Pts',(1.95622159519705,48.1984374999976,52.9827367061318));
#264134=CARTESIAN_POINT('Ctrl Pts',(3.33947915066444,48.2645833333309,51.5994791506644));
#264135=CARTESIAN_POINT('Ctrl Pts',(4.72273670613183,48.3307291666642,50.216221595197));
#264136=CARTESIAN_POINT('Ctrl Pts',(4.72273670613183,48.3968749999976,48.26));
#264137=CARTESIAN_POINT('Ctrl Pts',(4.72273670613183,48.4630208333309,46.303778404803));
#264138=CARTESIAN_POINT('Ctrl Pts',(3.33947915066444,48.5291666666642,44.9205208493356));
#264139=CARTESIAN_POINT('Ctrl Pts',(1.95622159519705,48.5953124999975,43.5372632938682));
#264140=CARTESIAN_POINT('Ctrl Pts',(6.99833541005117E-15,48.6614583333308,
43.5372632938682));
#264141=CARTESIAN_POINT('Ctrl Pts',(-1.95622159519704,48.7276041666641,
43.5372632938682));
#264142=CARTESIAN_POINT('Ctrl Pts',(-3.33947915066443,48.7937499999974,
44.9205208493356));
#264143=CARTESIAN_POINT('Ctrl Pts',(-4.72273670613182,48.8598958333307,
46.303778404803));
#264144=CARTESIAN_POINT('Ctrl Pts',(-4.72273670613182,48.9260416666641,
48.26));
#264145=CARTESIAN_POINT('Ctrl Pts',(-4.72273670613182,48.9921874999974,
50.216221595197));
#264146=CARTESIAN_POINT('Ctrl Pts',(-3.33947915066443,49.0583333333307,
51.5994791506644));
#264147=CARTESIAN_POINT('Ctrl Pts',(-1.95622159519703,49.124479166664,52.9827367061318));
#264148=CARTESIAN_POINT('Ctrl Pts',(7.17168088200102E-15,49.1906249999973,
52.9827367061318));
#264149=CARTESIAN_POINT('Ctrl Pts',(1.95622159519705,49.2567708333306,52.9827367061318));
#264150=CARTESIAN_POINT('Ctrl Pts',(3.33947915066444,49.3229166666639,51.5994791506644));
#264151=CARTESIAN_POINT('Ctrl Pts',(4.72273670613183,49.3890624999972,50.216221595197));
#264152=CARTESIAN_POINT('Ctrl Pts',(4.72273670613183,49.4552083333306,48.26));
#264153=CARTESIAN_POINT('Ctrl Pts',(4.72273670613183,49.5213541666639,46.303778404803));
#264154=CARTESIAN_POINT('Ctrl Pts',(3.33947915066444,49.5874999999972,44.9205208493356));
#264155=CARTESIAN_POINT('Ctrl Pts',(1.95622159519705,49.6536458333305,43.5372632938682));
#264156=CARTESIAN_POINT('Ctrl Pts',(6.99833541005115E-15,49.7197916666638,
43.5372632938682));
#264157=CARTESIAN_POINT('Ctrl Pts',(-1.95622159519704,49.7859374999971,
43.5372632938682));
#264158=CARTESIAN_POINT('Ctrl Pts',(-3.33947915066443,49.8520833333304,
44.9205208493356));
#264159=CARTESIAN_POINT('Ctrl Pts',(-4.72273670613182,49.9182291666637,
46.303778404803));
#264160=CARTESIAN_POINT('Ctrl Pts',(-4.72273670613182,49.9843749999971,
48.26));
#264161=CARTESIAN_POINT('Ctrl Pts',(-4.72273670613182,50.0505208333304,
50.216221595197));
#264162=CARTESIAN_POINT('Ctrl Pts',(-3.33947915066443,50.1166666666637,
51.5994791506644));
#264163=CARTESIAN_POINT('Ctrl Pts',(-1.95622159519703,50.182812499997,52.9827367061318));
#264164=CARTESIAN_POINT('Ctrl Pts',(7.17168088200107E-15,50.2489583333303,
52.9827367061318));
#264165=CARTESIAN_POINT('Ctrl Pts',(1.95622159519705,50.3151041666636,52.9827367061318));
#264166=CARTESIAN_POINT('Ctrl Pts',(3.33947915066444,50.3812499999969,51.5994791506644));
#264167=CARTESIAN_POINT('Ctrl Pts',(4.72273670613183,50.4473958333302,50.216221595197));
#264168=CARTESIAN_POINT('Ctrl Pts',(4.72273670613183,50.5135416666636,48.26));
#264169=CARTESIAN_POINT('Ctrl Pts',(4.72273670613183,50.5796874999969,46.303778404803));
#264170=CARTESIAN_POINT('Ctrl Pts',(3.33947915066444,50.6458333333302,44.9205208493356));
#264171=CARTESIAN_POINT('Ctrl Pts',(1.95622159519705,50.7119791666635,43.5372632938682));
#264172=CARTESIAN_POINT('Ctrl Pts',(6.99833541005117E-15,50.7781249999968,
43.5372632938682));
#264173=CARTESIAN_POINT('Ctrl Pts',(-1.95622159519704,50.8442708333301,
43.5372632938682));
#264174=CARTESIAN_POINT('Ctrl Pts',(-3.33947915066443,50.9104166666634,
44.9205208493356));
#264175=CARTESIAN_POINT('Ctrl Pts',(-4.72273670613182,50.9765624999967,
46.303778404803));
#264176=CARTESIAN_POINT('Ctrl Pts',(-4.72273670613182,51.04270833333,48.26));
#264177=CARTESIAN_POINT('Ctrl Pts',(-4.75205527448904,40.4763020833333,
48.26));
#264178=CARTESIAN_POINT('Ctrl Pts',(-4.75205527448904,40.5424479166667,
50.22836574384));
#264179=CARTESIAN_POINT('Ctrl Pts',(-3.3602105091645,40.60859375,51.6202105091645));
#264180=CARTESIAN_POINT('Ctrl Pts',(-1.96836574383996,40.6747395833333,
53.0120552744891));
#264181=CARTESIAN_POINT('Ctrl Pts',(7.17401418756681E-15,40.7408854166666,
53.0120552744891));
#264182=CARTESIAN_POINT('Ctrl Pts',(1.96836574383997,40.8070312499999,53.0120552744891));
#264183=CARTESIAN_POINT('Ctrl Pts',(3.36021050916451,40.8731770833332,51.6202105091645));
#264184=CARTESIAN_POINT('Ctrl Pts',(4.75205527448905,40.9393229166665,50.22836574384));
#264185=CARTESIAN_POINT('Ctrl Pts',(4.75205527448905,41.0054687499998,48.26));
#264186=CARTESIAN_POINT('Ctrl Pts',(4.75205527448905,41.0716145833332,46.29163425616));
#264187=CARTESIAN_POINT('Ctrl Pts',(3.36021050916451,41.1377604166665,44.8997894908355));
#264188=CARTESIAN_POINT('Ctrl Pts',(1.96836574383997,41.2039062499998,43.507944725511));
#264189=CARTESIAN_POINT('Ctrl Pts',(6.99959259357482E-15,41.2700520833331,
43.507944725511));
#264190=CARTESIAN_POINT('Ctrl Pts',(-1.96836574383996,41.3361979166664,
43.507944725511));
#264191=CARTESIAN_POINT('Ctrl Pts',(-3.3602105091645,41.4023437499997,44.8997894908355));
#264192=CARTESIAN_POINT('Ctrl Pts',(-4.75205527448904,41.468489583333,46.29163425616));
#264193=CARTESIAN_POINT('Ctrl Pts',(-4.75205527448904,41.5346354166663,
48.26));
#264194=CARTESIAN_POINT('Ctrl Pts',(-4.75205527448904,41.6007812499997,
50.22836574384));
#264195=CARTESIAN_POINT('Ctrl Pts',(-3.3602105091645,41.666927083333,51.6202105091645));
#264196=CARTESIAN_POINT('Ctrl Pts',(-1.96836574383996,41.7330729166663,
53.0120552744891));
#264197=CARTESIAN_POINT('Ctrl Pts',(7.17401418756681E-15,41.7992187499996,
53.0120552744891));
#264198=CARTESIAN_POINT('Ctrl Pts',(1.96836574383997,41.8653645833329,53.0120552744891));
#264199=CARTESIAN_POINT('Ctrl Pts',(3.36021050916451,41.9315104166662,51.6202105091645));
#264200=CARTESIAN_POINT('Ctrl Pts',(4.75205527448905,41.9976562499995,50.22836574384));
#264201=CARTESIAN_POINT('Ctrl Pts',(4.75205527448905,42.0638020833328,48.26));
#264202=CARTESIAN_POINT('Ctrl Pts',(4.75205527448905,42.1299479166662,46.29163425616));
#264203=CARTESIAN_POINT('Ctrl Pts',(3.36021050916451,42.1960937499995,44.8997894908355));
#264204=CARTESIAN_POINT('Ctrl Pts',(1.96836574383997,42.2622395833328,43.507944725511));
#264205=CARTESIAN_POINT('Ctrl Pts',(6.99959259357482E-15,42.3283854166661,
43.507944725511));
#264206=CARTESIAN_POINT('Ctrl Pts',(-1.96836574383996,42.3945312499994,
43.507944725511));
#264207=CARTESIAN_POINT('Ctrl Pts',(-3.3602105091645,42.4606770833327,44.8997894908355));
#264208=CARTESIAN_POINT('Ctrl Pts',(-4.75205527448904,42.526822916666,46.29163425616));
#264209=CARTESIAN_POINT('Ctrl Pts',(-4.75205527448904,42.5929687499993,
48.26));
#264210=CARTESIAN_POINT('Ctrl Pts',(-4.75205527448904,42.6591145833326,
50.22836574384));
#264211=CARTESIAN_POINT('Ctrl Pts',(-3.3602105091645,42.725260416666,51.6202105091645));
#264212=CARTESIAN_POINT('Ctrl Pts',(-1.96836574383996,42.7914062499993,
53.0120552744891));
#264213=CARTESIAN_POINT('Ctrl Pts',(7.17401418756679E-15,42.8575520833326,
53.0120552744891));
#264214=CARTESIAN_POINT('Ctrl Pts',(1.96836574383997,42.9236979166659,53.0120552744891));
#264215=CARTESIAN_POINT('Ctrl Pts',(3.36021050916451,42.9898437499992,51.6202105091645));
#264216=CARTESIAN_POINT('Ctrl Pts',(4.75205527448905,43.0559895833325,50.22836574384));
#264217=CARTESIAN_POINT('Ctrl Pts',(4.75205527448905,43.1221354166658,48.26));
#264218=CARTESIAN_POINT('Ctrl Pts',(4.75205527448905,43.1882812499991,46.29163425616));
#264219=CARTESIAN_POINT('Ctrl Pts',(3.36021050916451,43.2544270833325,44.8997894908355));
#264220=CARTESIAN_POINT('Ctrl Pts',(1.96836574383997,43.3205729166658,43.507944725511));
#264221=CARTESIAN_POINT('Ctrl Pts',(6.99959259357482E-15,43.3867187499991,
43.507944725511));
#264222=CARTESIAN_POINT('Ctrl Pts',(-1.96836574383996,43.4528645833324,
43.507944725511));
#264223=CARTESIAN_POINT('Ctrl Pts',(-3.3602105091645,43.5190104166657,44.8997894908355));
#264224=CARTESIAN_POINT('Ctrl Pts',(-4.75205527448904,43.585156249999,46.29163425616));
#264225=CARTESIAN_POINT('Ctrl Pts',(-4.75205527448904,43.6513020833323,
48.26));
#264226=CARTESIAN_POINT('Ctrl Pts',(-4.75205527448904,43.7174479166656,
50.22836574384));
#264227=CARTESIAN_POINT('Ctrl Pts',(-3.3602105091645,43.783593749999,51.6202105091645));
#264228=CARTESIAN_POINT('Ctrl Pts',(-1.96836574383996,43.8497395833323,
53.0120552744891));
#264229=CARTESIAN_POINT('Ctrl Pts',(7.17401418756679E-15,43.9158854166656,
53.0120552744891));
#264230=CARTESIAN_POINT('Ctrl Pts',(1.96836574383997,43.9820312499989,53.0120552744891));
#264231=CARTESIAN_POINT('Ctrl Pts',(3.36021050916451,44.0481770833322,51.6202105091645));
#264232=CARTESIAN_POINT('Ctrl Pts',(4.75205527448905,44.1143229166655,50.22836574384));
#264233=CARTESIAN_POINT('Ctrl Pts',(4.75205527448905,44.1804687499988,48.26));
#264234=CARTESIAN_POINT('Ctrl Pts',(4.75205527448905,44.2466145833322,46.29163425616));
#264235=CARTESIAN_POINT('Ctrl Pts',(3.36021050916451,44.3127604166655,44.8997894908355));
#264236=CARTESIAN_POINT('Ctrl Pts',(1.96836574383997,44.3789062499988,43.507944725511));
#264237=CARTESIAN_POINT('Ctrl Pts',(6.99959259357479E-15,44.4450520833321,
43.507944725511));
#264238=CARTESIAN_POINT('Ctrl Pts',(-1.96836574383996,44.5111979166654,
43.507944725511));
#264239=CARTESIAN_POINT('Ctrl Pts',(-3.3602105091645,44.5773437499987,44.8997894908355));
#264240=CARTESIAN_POINT('Ctrl Pts',(-4.75205527448904,44.643489583332,46.29163425616));
#264241=CARTESIAN_POINT('Ctrl Pts',(-4.75205527448904,44.7096354166653,
48.26));
#264242=CARTESIAN_POINT('Ctrl Pts',(-4.75205527448904,44.7757812499987,
50.22836574384));
#264243=CARTESIAN_POINT('Ctrl Pts',(-3.3602105091645,44.841927083332,51.6202105091645));
#264244=CARTESIAN_POINT('Ctrl Pts',(-1.96836574383996,44.9080729166653,
53.0120552744891));
#264245=CARTESIAN_POINT('Ctrl Pts',(7.17401418756681E-15,44.9742187499986,
53.0120552744891));
#264246=CARTESIAN_POINT('Ctrl Pts',(1.96836574383997,45.0403645833319,53.0120552744891));
#264247=CARTESIAN_POINT('Ctrl Pts',(3.36021050916451,45.1065104166652,51.6202105091645));
#264248=CARTESIAN_POINT('Ctrl Pts',(4.75205527448905,45.1726562499985,50.22836574384));
#264249=CARTESIAN_POINT('Ctrl Pts',(4.75205527448905,45.2388020833318,48.26));
#264250=CARTESIAN_POINT('Ctrl Pts',(4.75205527448905,45.3049479166652,46.29163425616));
#264251=CARTESIAN_POINT('Ctrl Pts',(3.36021050916451,45.3710937499985,44.8997894908355));
#264252=CARTESIAN_POINT('Ctrl Pts',(1.96836574383997,45.4372395833318,43.507944725511));
#264253=CARTESIAN_POINT('Ctrl Pts',(6.99959259357482E-15,45.5033854166651,
43.507944725511));
#264254=CARTESIAN_POINT('Ctrl Pts',(-1.96836574383996,45.5695312499984,
43.507944725511));
#264255=CARTESIAN_POINT('Ctrl Pts',(-3.3602105091645,45.6356770833317,44.8997894908355));
#264256=CARTESIAN_POINT('Ctrl Pts',(-4.75205527448904,45.701822916665,46.29163425616));
#264257=CARTESIAN_POINT('Ctrl Pts',(-4.75205527448904,45.7679687499983,
48.26));
#264258=CARTESIAN_POINT('Ctrl Pts',(-4.75205527448904,45.8341145833317,
50.22836574384));
#264259=CARTESIAN_POINT('Ctrl Pts',(-3.3602105091645,45.900260416665,51.6202105091645));
#264260=CARTESIAN_POINT('Ctrl Pts',(-1.96836574383996,45.9664062499983,
53.0120552744891));
#264261=CARTESIAN_POINT('Ctrl Pts',(7.17401418756681E-15,46.0325520833316,
53.0120552744891));
#264262=CARTESIAN_POINT('Ctrl Pts',(1.96836574383997,46.0986979166649,53.0120552744891));
#264263=CARTESIAN_POINT('Ctrl Pts',(3.36021050916451,46.1648437499982,51.6202105091645));
#264264=CARTESIAN_POINT('Ctrl Pts',(4.75205527448905,46.2309895833315,50.22836574384));
#264265=CARTESIAN_POINT('Ctrl Pts',(4.75205527448905,46.2971354166648,48.26));
#264266=CARTESIAN_POINT('Ctrl Pts',(4.75205527448905,46.3632812499982,46.29163425616));
#264267=CARTESIAN_POINT('Ctrl Pts',(3.36021050916451,46.4294270833315,44.8997894908355));
#264268=CARTESIAN_POINT('Ctrl Pts',(1.96836574383997,46.4955729166648,43.507944725511));
#264269=CARTESIAN_POINT('Ctrl Pts',(6.99959259357482E-15,46.5617187499981,
43.507944725511));
#264270=CARTESIAN_POINT('Ctrl Pts',(-1.96836574383996,46.6278645833314,
43.507944725511));
#264271=CARTESIAN_POINT('Ctrl Pts',(-3.3602105091645,46.6940104166647,44.8997894908355));
#264272=CARTESIAN_POINT('Ctrl Pts',(-4.75205527448904,46.760156249998,46.29163425616));
#264273=CARTESIAN_POINT('Ctrl Pts',(-4.75205527448904,46.8263020833313,
48.26));
#264274=CARTESIAN_POINT('Ctrl Pts',(-4.75205527448904,46.8924479166647,
50.22836574384));
#264275=CARTESIAN_POINT('Ctrl Pts',(-3.3602105091645,46.958593749998,51.6202105091645));
#264276=CARTESIAN_POINT('Ctrl Pts',(-1.96836574383996,47.0247395833313,
53.0120552744891));
#264277=CARTESIAN_POINT('Ctrl Pts',(7.17401418756681E-15,47.0908854166646,
53.0120552744891));
#264278=CARTESIAN_POINT('Ctrl Pts',(1.96836574383997,47.1570312499979,53.0120552744891));
#264279=CARTESIAN_POINT('Ctrl Pts',(3.36021050916451,47.2231770833312,51.6202105091645));
#264280=CARTESIAN_POINT('Ctrl Pts',(4.75205527448905,47.2893229166645,50.22836574384));
#264281=CARTESIAN_POINT('Ctrl Pts',(4.75205527448905,47.3554687499978,48.26));
#264282=CARTESIAN_POINT('Ctrl Pts',(4.75205527448905,47.4216145833312,46.29163425616));
#264283=CARTESIAN_POINT('Ctrl Pts',(3.36021050916451,47.4877604166645,44.8997894908355));
#264284=CARTESIAN_POINT('Ctrl Pts',(1.96836574383997,47.5539062499978,43.507944725511));
#264285=CARTESIAN_POINT('Ctrl Pts',(6.99959259357482E-15,47.6200520833311,
43.507944725511));
#264286=CARTESIAN_POINT('Ctrl Pts',(-1.96836574383996,47.6861979166644,
43.507944725511));
#264287=CARTESIAN_POINT('Ctrl Pts',(-3.3602105091645,47.7523437499977,44.8997894908355));
#264288=CARTESIAN_POINT('Ctrl Pts',(-4.75205527448904,47.818489583331,46.29163425616));
#264289=CARTESIAN_POINT('Ctrl Pts',(-4.75205527448904,47.8846354166643,
48.26));
#264290=CARTESIAN_POINT('Ctrl Pts',(-4.75205527448904,47.9507812499977,
50.22836574384));
#264291=CARTESIAN_POINT('Ctrl Pts',(-3.3602105091645,48.016927083331,51.6202105091645));
#264292=CARTESIAN_POINT('Ctrl Pts',(-1.96836574383996,48.0830729166643,
53.0120552744891));
#264293=CARTESIAN_POINT('Ctrl Pts',(7.17401418756679E-15,48.1492187499976,
53.0120552744891));
#264294=CARTESIAN_POINT('Ctrl Pts',(1.96836574383997,48.2153645833309,53.0120552744891));
#264295=CARTESIAN_POINT('Ctrl Pts',(3.36021050916451,48.2815104166642,51.6202105091645));
#264296=CARTESIAN_POINT('Ctrl Pts',(4.75205527448905,48.3476562499975,50.22836574384));
#264297=CARTESIAN_POINT('Ctrl Pts',(4.75205527448905,48.4138020833309,48.26));
#264298=CARTESIAN_POINT('Ctrl Pts',(4.75205527448905,48.4799479166642,46.29163425616));
#264299=CARTESIAN_POINT('Ctrl Pts',(3.36021050916451,48.5460937499975,44.8997894908355));
#264300=CARTESIAN_POINT('Ctrl Pts',(1.96836574383997,48.6122395833308,43.507944725511));
#264301=CARTESIAN_POINT('Ctrl Pts',(6.99959259357482E-15,48.6783854166641,
43.507944725511));
#264302=CARTESIAN_POINT('Ctrl Pts',(-1.96836574383996,48.7445312499974,
43.507944725511));
#264303=CARTESIAN_POINT('Ctrl Pts',(-3.3602105091645,48.8106770833307,44.8997894908355));
#264304=CARTESIAN_POINT('Ctrl Pts',(-4.75205527448904,48.876822916664,46.29163425616));
#264305=CARTESIAN_POINT('Ctrl Pts',(-4.75205527448904,48.9429687499973,
48.26));
#264306=CARTESIAN_POINT('Ctrl Pts',(-4.75205527448904,49.0091145833307,
50.22836574384));
#264307=CARTESIAN_POINT('Ctrl Pts',(-3.3602105091645,49.075260416664,51.6202105091645));
#264308=CARTESIAN_POINT('Ctrl Pts',(-1.96836574383996,49.1414062499973,
53.0120552744891));
#264309=CARTESIAN_POINT('Ctrl Pts',(7.17401418756684E-15,49.2075520833306,
53.0120552744891));
#264310=CARTESIAN_POINT('Ctrl Pts',(1.96836574383997,49.2736979166639,53.0120552744891));
#264311=CARTESIAN_POINT('Ctrl Pts',(3.36021050916451,49.3398437499972,51.6202105091645));
#264312=CARTESIAN_POINT('Ctrl Pts',(4.75205527448905,49.4059895833305,50.22836574384));
#264313=CARTESIAN_POINT('Ctrl Pts',(4.75205527448905,49.4721354166639,48.26));
#264314=CARTESIAN_POINT('Ctrl Pts',(4.75205527448905,49.5382812499972,46.29163425616));
#264315=CARTESIAN_POINT('Ctrl Pts',(3.36021050916451,49.6044270833305,44.8997894908355));
#264316=CARTESIAN_POINT('Ctrl Pts',(1.96836574383997,49.6705729166638,43.507944725511));
#264317=CARTESIAN_POINT('Ctrl Pts',(6.99959259357482E-15,49.7367187499971,
43.507944725511));
#264318=CARTESIAN_POINT('Ctrl Pts',(-1.96836574383996,49.8028645833304,
43.507944725511));
#264319=CARTESIAN_POINT('Ctrl Pts',(-3.3602105091645,49.8690104166637,44.8997894908355));
#264320=CARTESIAN_POINT('Ctrl Pts',(-4.75205527448904,49.935156249997,46.29163425616));
#264321=CARTESIAN_POINT('Ctrl Pts',(-4.75205527448904,50.0013020833303,
48.26));
#264322=CARTESIAN_POINT('Ctrl Pts',(-4.75205527448904,50.0674479166637,
50.22836574384));
#264323=CARTESIAN_POINT('Ctrl Pts',(-3.3602105091645,50.133593749997,51.6202105091645));
#264324=CARTESIAN_POINT('Ctrl Pts',(-1.96836574383996,50.1997395833303,
53.0120552744891));
#264325=CARTESIAN_POINT('Ctrl Pts',(7.17401418756681E-15,50.2658854166636,
53.0120552744891));
#264326=CARTESIAN_POINT('Ctrl Pts',(1.96836574383997,50.3320312499969,53.0120552744891));
#264327=CARTESIAN_POINT('Ctrl Pts',(3.36021050916451,50.3981770833302,51.6202105091645));
#264328=CARTESIAN_POINT('Ctrl Pts',(4.75205527448905,50.4643229166635,50.22836574384));
#264329=CARTESIAN_POINT('Ctrl Pts',(4.75205527448905,50.5304687499968,48.26));
#264330=CARTESIAN_POINT('Ctrl Pts',(4.75205527448905,50.5966145833302,46.29163425616));
#264331=CARTESIAN_POINT('Ctrl Pts',(3.36021050916451,50.6627604166635,44.8997894908355));
#264332=CARTESIAN_POINT('Ctrl Pts',(1.96836574383997,50.7289062499968,43.507944725511));
#264333=CARTESIAN_POINT('Ctrl Pts',(6.99959259357482E-15,50.7950520833301,
43.507944725511));
#264334=CARTESIAN_POINT('Ctrl Pts',(-1.96836574383996,50.8611979166634,
43.507944725511));
#264335=CARTESIAN_POINT('Ctrl Pts',(-3.3602105091645,50.9273437499967,44.8997894908355));
#264336=CARTESIAN_POINT('Ctrl Pts',(-4.75205527448904,50.99348958333,46.29163425616));
#264337=CARTESIAN_POINT('Ctrl Pts',(-4.75205527448904,51.0596354166633,
48.26));
#264338=CARTESIAN_POINT('Ctrl Pts',(4.68628896694498,42.0671867061318,47.6743911597878));
#264339=CARTESIAN_POINT('Ctrl Pts',(4.48534984498601,42.1243724082372,46.0663915436572));
#264340=CARTESIAN_POINT('Ctrl Pts',(3.33947915066444,42.1791666666662,44.9205208493356));
#264341=CARTESIAN_POINT('Ctrl Pts',(1.95622159519705,42.2453124999995,43.5372632938682));
#264342=CARTESIAN_POINT('Ctrl Pts',(6.9983354100512E-15,42.3114583333328,
43.5372632938682));
#264343=CARTESIAN_POINT('Ctrl Pts',(-1.95622159519704,42.3776041666661,
43.5372632938682));
#264344=CARTESIAN_POINT('Ctrl Pts',(-3.33947915066443,42.4437499999994,
44.9205208493356));
#264345=CARTESIAN_POINT('Ctrl Pts',(-4.72273670613182,42.5098958333327,
46.303778404803));
#264346=CARTESIAN_POINT('Ctrl Pts',(-4.72273670613182,42.5760416666661,
48.26));
#264347=CARTESIAN_POINT('Ctrl Pts',(-4.72273670613182,42.6421874999994,
50.216221595197));
#264348=CARTESIAN_POINT('Ctrl Pts',(-3.33947915066443,42.7083333333327,
51.5994791506644));
#264349=CARTESIAN_POINT('Ctrl Pts',(-1.95622159519703,42.774479166666,52.9827367061318));
#264350=CARTESIAN_POINT('Ctrl Pts',(7.17168088200104E-15,42.8406249999993,
52.9827367061318));
#264351=CARTESIAN_POINT('Ctrl Pts',(1.95622159519705,42.9067708333326,52.9827367061318));
#264352=CARTESIAN_POINT('Ctrl Pts',(3.33947915066444,42.9729166666659,51.5994791506644));
#264353=CARTESIAN_POINT('Ctrl Pts',(4.72273670613183,43.0390624999992,50.216221595197));
#264354=CARTESIAN_POINT('Ctrl Pts',(4.72273670613183,43.1052083333326,48.26));
#264355=CARTESIAN_POINT('Origin',(-3.05311331771918E-14,40.4567708333334,
48.26));
#264356=CARTESIAN_POINT('Ctrl Pts',(4.66579641623065,42.0671867061318,47.5288462557477));
#264357=CARTESIAN_POINT('Ctrl Pts',(4.42756765431106,42.1219271548081,46.0086093529822));
#264358=CARTESIAN_POINT('Ctrl Pts',(3.33947915066444,42.1739583333328,44.9205208493356));
#264359=CARTESIAN_POINT('Ctrl Pts',(1.95622159519705,42.2401041666661,43.5372632938682));
#264360=CARTESIAN_POINT('Ctrl Pts',(6.99833541005117E-15,42.3062499999994,
43.5372632938682));
#264361=CARTESIAN_POINT('Ctrl Pts',(-1.95622159519704,42.3723958333327,
43.5372632938682));
#264362=CARTESIAN_POINT('Ctrl Pts',(-3.33947915066443,42.438541666666,44.9205208493356));
#264363=CARTESIAN_POINT('Ctrl Pts',(-4.72273670613182,42.5046874999994,
46.303778404803));
#264364=CARTESIAN_POINT('Ctrl Pts',(-4.72273670613182,42.5708333333327,
48.26));
#264365=CARTESIAN_POINT('Ctrl Pts',(-4.72273670613182,42.636979166666,50.216221595197));
#264366=CARTESIAN_POINT('Ctrl Pts',(-3.33947915066443,42.7031249999993,
51.5994791506644));
#264367=CARTESIAN_POINT('Ctrl Pts',(-1.95622159519703,42.7692708333326,
52.9827367061318));
#264368=CARTESIAN_POINT('Ctrl Pts',(7.17168088200104E-15,42.8354166666659,
52.9827367061318));
#264369=CARTESIAN_POINT('Ctrl Pts',(1.95622159519705,42.9015624999992,52.9827367061318));
#264370=CARTESIAN_POINT('Ctrl Pts',(3.33947915066444,42.9677083333326,51.5994791506644));
#264371=CARTESIAN_POINT('Ctrl Pts',(4.72273670613183,43.0338541666659,50.216221595197));
#264372=CARTESIAN_POINT('Ctrl Pts',(4.72273670613183,43.0999999999992,48.26));
#264373=CARTESIAN_POINT('Ctrl Pts',(-4.75205527448904,40.4372395833334,
48.26));
#264374=CARTESIAN_POINT('Ctrl Pts',(-4.75205527448904,40.5033854166667,
50.22836574384));
#264375=CARTESIAN_POINT('Ctrl Pts',(-3.3602105091645,40.56953125,51.6202105091645));
#264376=CARTESIAN_POINT('Ctrl Pts',(-1.96836574383996,40.6356770833333,
53.0120552744891));
#264377=CARTESIAN_POINT('Ctrl Pts',(7.17401418756681E-15,40.7018229166666,
53.0120552744891));
#264378=CARTESIAN_POINT('Ctrl Pts',(1.96836574383997,40.7679687499999,53.0120552744891));
#264379=CARTESIAN_POINT('Ctrl Pts',(3.36021050916451,40.8341145833332,51.6202105091645));
#264380=CARTESIAN_POINT('Ctrl Pts',(4.75205527448906,40.9002604166666,50.22836574384));
#264381=CARTESIAN_POINT('Ctrl Pts',(4.75205527448906,40.9664062499999,48.26));
#264382=CARTESIAN_POINT('Ctrl Pts',(4.75205527448906,41.0325520833332,46.29163425616));
#264383=CARTESIAN_POINT('Ctrl Pts',(3.36021050916451,41.0986979166665,44.8997894908355));
#264384=CARTESIAN_POINT('Ctrl Pts',(1.96836574383997,41.1648437499998,43.507944725511));
#264385=CARTESIAN_POINT('Ctrl Pts',(6.99959259357479E-15,41.2309895833331,
43.507944725511));
#264386=CARTESIAN_POINT('Ctrl Pts',(-1.96836574383996,41.2971354166664,
43.507944725511));
#264387=CARTESIAN_POINT('Ctrl Pts',(-3.3602105091645,41.3632812499997,44.8997894908355));
#264388=CARTESIAN_POINT('Ctrl Pts',(-4.75205527448904,41.4294270833331,
46.29163425616));
#264389=CARTESIAN_POINT('Ctrl Pts',(-4.75205527448904,41.4955729166664,
48.26));
#264390=CARTESIAN_POINT('Ctrl Pts',(-4.75205527448904,41.5617187499997,
50.22836574384));
#264391=CARTESIAN_POINT('Ctrl Pts',(-3.3602105091645,41.627864583333,51.6202105091645));
#264392=CARTESIAN_POINT('Ctrl Pts',(-1.96836574383996,41.6940104166663,
53.0120552744891));
#264393=CARTESIAN_POINT('Ctrl Pts',(7.17401418756681E-15,41.7601562499996,
53.0120552744891));
#264394=CARTESIAN_POINT('Ctrl Pts',(1.96836574383997,41.8263020833329,53.0120552744891));
#264395=CARTESIAN_POINT('Ctrl Pts',(3.36021050916451,41.8924479166662,51.6202105091645));
#264396=CARTESIAN_POINT('Ctrl Pts',(4.75205527448906,41.9585937499996,50.22836574384));
#264397=CARTESIAN_POINT('Ctrl Pts',(4.75205527448906,42.0247395833329,48.26));
#264398=CARTESIAN_POINT('Ctrl Pts',(4.75205527448906,42.0908854166662,46.29163425616));
#264399=CARTESIAN_POINT('Ctrl Pts',(3.36021050916451,42.1570312499995,44.8997894908355));
#264400=CARTESIAN_POINT('Ctrl Pts',(1.96836574383997,42.2231770833328,43.507944725511));
#264401=CARTESIAN_POINT('Ctrl Pts',(6.99959259357482E-15,42.2893229166661,
43.507944725511));
#264402=CARTESIAN_POINT('Ctrl Pts',(-1.96836574383996,42.3554687499994,
43.507944725511));
#264403=CARTESIAN_POINT('Ctrl Pts',(-3.3602105091645,42.4216145833327,44.8997894908355));
#264404=CARTESIAN_POINT('Ctrl Pts',(-4.75205527448904,42.4877604166661,
46.29163425616));
#264405=CARTESIAN_POINT('Ctrl Pts',(-4.75205527448904,42.5539062499994,
48.26));
#264406=CARTESIAN_POINT('Ctrl Pts',(-4.75205527448904,42.6200520833327,
50.22836574384));
#264407=CARTESIAN_POINT('Ctrl Pts',(-3.3602105091645,42.686197916666,51.6202105091645));
#264408=CARTESIAN_POINT('Ctrl Pts',(-1.96836574383996,42.7523437499993,
53.0120552744891));
#264409=CARTESIAN_POINT('Ctrl Pts',(7.17401418756679E-15,42.8184895833326,
53.0120552744891));
#264410=CARTESIAN_POINT('Ctrl Pts',(1.96836574383997,42.8846354166659,53.0120552744891));
#264411=CARTESIAN_POINT('Ctrl Pts',(3.36021050916451,42.9507812499993,51.6202105091645));
#264412=CARTESIAN_POINT('Ctrl Pts',(4.75205527448906,43.0169270833326,50.22836574384));
#264413=CARTESIAN_POINT('Ctrl Pts',(4.75205527448906,43.0830729166659,48.26));
#264414=CARTESIAN_POINT('Ctrl Pts',(4.75205527448906,43.1492187499992,46.29163425616));
#264415=CARTESIAN_POINT('Ctrl Pts',(3.36021050916451,43.2153645833325,44.8997894908355));
#264416=CARTESIAN_POINT('Ctrl Pts',(1.96836574383997,43.2815104166658,43.507944725511));
#264417=CARTESIAN_POINT('Ctrl Pts',(6.99959259357479E-15,43.3476562499991,
43.507944725511));
#264418=CARTESIAN_POINT('Ctrl Pts',(-1.96836574383996,43.4138020833324,
43.507944725511));
#264419=CARTESIAN_POINT('Ctrl Pts',(-3.3602105091645,43.4799479166657,44.8997894908355));
#264420=CARTESIAN_POINT('Ctrl Pts',(-4.75205527448904,43.5460937499991,
46.29163425616));
#264421=CARTESIAN_POINT('Ctrl Pts',(-4.75205527448904,43.6122395833324,
48.26));
#264422=CARTESIAN_POINT('Ctrl Pts',(-4.75205527448904,43.6783854166657,
50.22836574384));
#264423=CARTESIAN_POINT('Ctrl Pts',(-3.3602105091645,43.744531249999,51.6202105091645));
#264424=CARTESIAN_POINT('Ctrl Pts',(-1.96836574383996,43.8106770833323,
53.0120552744891));
#264425=CARTESIAN_POINT('Ctrl Pts',(7.17401418756679E-15,43.8768229166656,
53.0120552744891));
#264426=CARTESIAN_POINT('Ctrl Pts',(1.96836574383997,43.9429687499989,53.0120552744891));
#264427=CARTESIAN_POINT('Ctrl Pts',(3.36021050916451,44.0091145833323,51.6202105091645));
#264428=CARTESIAN_POINT('Ctrl Pts',(4.75205527448906,44.0752604166656,50.22836574384));
#264429=CARTESIAN_POINT('Ctrl Pts',(4.75205527448906,44.1414062499989,48.26));
#264430=CARTESIAN_POINT('Ctrl Pts',(4.75205527448906,44.2075520833322,46.29163425616));
#264431=CARTESIAN_POINT('Ctrl Pts',(3.36021050916451,44.2736979166655,44.8997894908355));
#264432=CARTESIAN_POINT('Ctrl Pts',(1.96836574383997,44.3398437499988,43.507944725511));
#264433=CARTESIAN_POINT('Ctrl Pts',(6.99959259357479E-15,44.4059895833321,
43.507944725511));
#264434=CARTESIAN_POINT('Ctrl Pts',(-1.96836574383996,44.4721354166654,
43.507944725511));
#264435=CARTESIAN_POINT('Ctrl Pts',(-3.3602105091645,44.5382812499987,44.8997894908355));
#264436=CARTESIAN_POINT('Ctrl Pts',(-4.75205527448904,44.6044270833321,
46.29163425616));
#264437=CARTESIAN_POINT('Ctrl Pts',(-4.75205527448904,44.6705729166654,
48.26));
#264438=CARTESIAN_POINT('Ctrl Pts',(-4.75205527448904,44.7367187499987,
50.22836574384));
#264439=CARTESIAN_POINT('Ctrl Pts',(-3.3602105091645,44.802864583332,51.6202105091645));
#264440=CARTESIAN_POINT('Ctrl Pts',(-1.96836574383996,44.8690104166653,
53.0120552744891));
#264441=CARTESIAN_POINT('Ctrl Pts',(7.17401418756679E-15,44.9351562499986,
53.0120552744891));
#264442=CARTESIAN_POINT('Ctrl Pts',(1.96836574383997,45.001302083332,53.0120552744891));
#264443=CARTESIAN_POINT('Ctrl Pts',(3.36021050916451,45.0674479166652,51.6202105091645));
#264444=CARTESIAN_POINT('Ctrl Pts',(4.75205527448906,45.1335937499986,50.22836574384));
#264445=CARTESIAN_POINT('Ctrl Pts',(4.75205527448906,45.1997395833319,48.26));
#264446=CARTESIAN_POINT('Ctrl Pts',(4.75205527448906,45.2658854166652,46.29163425616));
#264447=CARTESIAN_POINT('Ctrl Pts',(3.36021050916451,45.3320312499985,44.8997894908355));
#264448=CARTESIAN_POINT('Ctrl Pts',(1.96836574383997,45.3981770833318,43.507944725511));
#264449=CARTESIAN_POINT('Ctrl Pts',(6.99959259357482E-15,45.4643229166651,
43.507944725511));
#264450=CARTESIAN_POINT('Ctrl Pts',(-1.96836574383996,45.5304687499984,
43.507944725511));
#264451=CARTESIAN_POINT('Ctrl Pts',(-3.3602105091645,45.5966145833317,44.8997894908355));
#264452=CARTESIAN_POINT('Ctrl Pts',(-4.75205527448904,45.6627604166651,
46.29163425616));
#264453=CARTESIAN_POINT('Ctrl Pts',(-4.75205527448904,45.7289062499984,
48.26));
#264454=CARTESIAN_POINT('Ctrl Pts',(-4.75205527448904,45.7950520833317,
50.22836574384));
#264455=CARTESIAN_POINT('Ctrl Pts',(-3.3602105091645,45.861197916665,51.6202105091645));
#264456=CARTESIAN_POINT('Ctrl Pts',(-1.96836574383996,45.9273437499983,
53.0120552744891));
#264457=CARTESIAN_POINT('Ctrl Pts',(7.17401418756681E-15,45.9934895833316,
53.0120552744891));
#264458=CARTESIAN_POINT('Ctrl Pts',(1.96836574383997,46.0596354166649,53.0120552744891));
#264459=CARTESIAN_POINT('Ctrl Pts',(3.36021050916451,46.1257812499982,51.6202105091645));
#264460=CARTESIAN_POINT('Ctrl Pts',(4.75205527448906,46.1919270833316,50.22836574384));
#264461=CARTESIAN_POINT('Ctrl Pts',(4.75205527448906,46.2580729166649,48.26));
#264462=CARTESIAN_POINT('Ctrl Pts',(4.75205527448906,46.3242187499982,46.29163425616));
#264463=CARTESIAN_POINT('Ctrl Pts',(3.36021050916451,46.3903645833315,44.8997894908355));
#264464=CARTESIAN_POINT('Ctrl Pts',(1.96836574383997,46.4565104166648,43.507944725511));
#264465=CARTESIAN_POINT('Ctrl Pts',(6.99959259357479E-15,46.5226562499981,
43.507944725511));
#264466=CARTESIAN_POINT('Ctrl Pts',(-1.96836574383996,46.5888020833314,
43.507944725511));
#264467=CARTESIAN_POINT('Ctrl Pts',(-3.3602105091645,46.6549479166647,44.8997894908355));
#264468=CARTESIAN_POINT('Ctrl Pts',(-4.75205527448904,46.7210937499981,
46.29163425616));
#264469=CARTESIAN_POINT('Ctrl Pts',(-4.75205527448904,46.7872395833314,
48.26));
#264470=CARTESIAN_POINT('Ctrl Pts',(-4.75205527448904,46.8533854166647,
50.22836574384));
#264471=CARTESIAN_POINT('Ctrl Pts',(-3.3602105091645,46.919531249998,51.6202105091645));
#264472=CARTESIAN_POINT('Ctrl Pts',(-1.96836574383996,46.9856770833313,
53.0120552744891));
#264473=CARTESIAN_POINT('Ctrl Pts',(7.17401418756679E-15,47.0518229166646,
53.0120552744891));
#264474=CARTESIAN_POINT('Ctrl Pts',(1.96836574383997,47.1179687499979,53.0120552744891));
#264475=CARTESIAN_POINT('Ctrl Pts',(3.36021050916451,47.1841145833313,51.6202105091645));
#264476=CARTESIAN_POINT('Ctrl Pts',(4.75205527448906,47.2502604166646,50.22836574384));
#264477=CARTESIAN_POINT('Ctrl Pts',(4.75205527448906,47.3164062499979,48.26));
#264478=CARTESIAN_POINT('Ctrl Pts',(4.75205527448906,47.3825520833312,46.29163425616));
#264479=CARTESIAN_POINT('Ctrl Pts',(3.36021050916451,47.4486979166645,44.8997894908355));
#264480=CARTESIAN_POINT('Ctrl Pts',(1.96836574383997,47.5148437499978,43.507944725511));
#264481=CARTESIAN_POINT('Ctrl Pts',(6.99959259357482E-15,47.5809895833311,
43.507944725511));
#264482=CARTESIAN_POINT('Ctrl Pts',(-1.96836574383996,47.6471354166644,
43.507944725511));
#264483=CARTESIAN_POINT('Ctrl Pts',(-3.3602105091645,47.7132812499977,44.8997894908355));
#264484=CARTESIAN_POINT('Ctrl Pts',(-4.75205527448904,47.7794270833311,
46.29163425616));
#264485=CARTESIAN_POINT('Ctrl Pts',(-4.75205527448904,47.8455729166644,
48.26));
#264486=CARTESIAN_POINT('Ctrl Pts',(-4.75205527448904,47.9117187499977,
50.22836574384));
#264487=CARTESIAN_POINT('Ctrl Pts',(-3.3602105091645,47.977864583331,51.6202105091645));
#264488=CARTESIAN_POINT('Ctrl Pts',(-1.96836574383996,48.0440104166643,
53.0120552744891));
#264489=CARTESIAN_POINT('Ctrl Pts',(7.17401418756679E-15,48.1101562499976,
53.0120552744891));
#264490=CARTESIAN_POINT('Ctrl Pts',(1.96836574383997,48.1763020833309,53.0120552744891));
#264491=CARTESIAN_POINT('Ctrl Pts',(3.36021050916451,48.2424479166643,51.6202105091645));
#264492=CARTESIAN_POINT('Ctrl Pts',(4.75205527448906,48.3085937499975,50.22836574384));
#264493=CARTESIAN_POINT('Ctrl Pts',(4.75205527448906,48.3747395833309,48.26));
#264494=CARTESIAN_POINT('Ctrl Pts',(4.75205527448906,48.4408854166642,46.29163425616));
#264495=CARTESIAN_POINT('Ctrl Pts',(3.36021050916451,48.5070312499975,44.8997894908355));
#264496=CARTESIAN_POINT('Ctrl Pts',(1.96836574383997,48.5731770833308,43.507944725511));
#264497=CARTESIAN_POINT('Ctrl Pts',(6.99959259357479E-15,48.6393229166641,
43.507944725511));
#264498=CARTESIAN_POINT('Ctrl Pts',(-1.96836574383996,48.7054687499974,
43.507944725511));
#264499=CARTESIAN_POINT('Ctrl Pts',(-3.3602105091645,48.7716145833307,44.8997894908355));
#264500=CARTESIAN_POINT('Ctrl Pts',(-4.75205527448904,48.8377604166641,
46.29163425616));
#264501=CARTESIAN_POINT('Ctrl Pts',(-4.75205527448904,48.9039062499974,
48.26));
#264502=CARTESIAN_POINT('Ctrl Pts',(-4.75205527448904,48.9700520833307,
50.22836574384));
#264503=CARTESIAN_POINT('Ctrl Pts',(-3.3602105091645,49.036197916664,51.6202105091645));
#264504=CARTESIAN_POINT('Ctrl Pts',(-1.96836574383996,49.1023437499973,
53.0120552744891));
#264505=CARTESIAN_POINT('Ctrl Pts',(7.17401418756679E-15,49.1684895833306,
53.0120552744891));
#264506=CARTESIAN_POINT('Ctrl Pts',(1.96836574383997,49.2346354166639,53.0120552744891));
#264507=CARTESIAN_POINT('Ctrl Pts',(3.36021050916451,49.3007812499973,51.6202105091645));
#264508=CARTESIAN_POINT('Ctrl Pts',(4.75205527448906,49.3669270833306,50.22836574384));
#264509=CARTESIAN_POINT('Ctrl Pts',(4.75205527448906,49.4330729166639,48.26));
#264510=CARTESIAN_POINT('Ctrl Pts',(4.75205527448906,49.4992187499972,46.29163425616));
#264511=CARTESIAN_POINT('Ctrl Pts',(3.36021050916451,49.5653645833305,44.8997894908355));
#264512=CARTESIAN_POINT('Ctrl Pts',(1.96836574383997,49.6315104166638,43.507944725511));
#264513=CARTESIAN_POINT('Ctrl Pts',(6.99959259357482E-15,49.6976562499971,
43.507944725511));
#264514=CARTESIAN_POINT('Ctrl Pts',(-1.96836574383996,49.7638020833304,
43.507944725511));
#264515=CARTESIAN_POINT('Ctrl Pts',(-3.3602105091645,49.8299479166637,44.8997894908355));
#264516=CARTESIAN_POINT('Ctrl Pts',(-4.75205527448904,49.8960937499971,
46.29163425616));
#264517=CARTESIAN_POINT('Ctrl Pts',(-4.75205527448904,49.9622395833304,
48.26));
#264518=CARTESIAN_POINT('Ctrl Pts',(-4.75205527448904,50.0283854166637,
50.22836574384));
#264519=CARTESIAN_POINT('Ctrl Pts',(-3.3602105091645,50.094531249997,51.6202105091645));
#264520=CARTESIAN_POINT('Ctrl Pts',(-1.96836574383996,50.1606770833303,
53.0120552744891));
#264521=CARTESIAN_POINT('Ctrl Pts',(7.17401418756681E-15,50.2268229166636,
53.0120552744891));
#264522=CARTESIAN_POINT('Ctrl Pts',(1.96836574383997,50.2929687499969,53.0120552744891));
#264523=CARTESIAN_POINT('Ctrl Pts',(3.36021050916451,50.3591145833303,51.6202105091645));
#264524=CARTESIAN_POINT('Ctrl Pts',(4.75205527448906,50.4252604166636,50.22836574384));
#264525=CARTESIAN_POINT('Ctrl Pts',(4.75205527448906,50.4914062499969,48.26));
#264526=CARTESIAN_POINT('Ctrl Pts',(4.75205527448906,50.5575520833302,46.29163425616));
#264527=CARTESIAN_POINT('Ctrl Pts',(3.36021050916451,50.6236979166635,44.8997894908355));
#264528=CARTESIAN_POINT('Ctrl Pts',(1.96836574383997,50.6898437499968,43.507944725511));
#264529=CARTESIAN_POINT('Ctrl Pts',(6.99959259357482E-15,50.7559895833301,
43.507944725511));
#264530=CARTESIAN_POINT('Ctrl Pts',(-1.96836574383996,50.8221354166634,
43.507944725511));
#264531=CARTESIAN_POINT('Ctrl Pts',(-3.3602105091645,50.8882812499967,44.8997894908355));
#264532=CARTESIAN_POINT('Ctrl Pts',(-4.75205527448904,50.9544270833301,
46.29163425616));
#264533=CARTESIAN_POINT('Ctrl Pts',(-4.75205527448904,51.0205729166634,
48.26));
#264534=CARTESIAN_POINT('Ctrl Pts',(-4.72273670613182,40.4541666666667,
48.26));
#264535=CARTESIAN_POINT('Ctrl Pts',(-4.72273670613182,40.5203125,50.216221595197));
#264536=CARTESIAN_POINT('Ctrl Pts',(-3.33947915066443,40.5864583333333,
51.5994791506644));
#264537=CARTESIAN_POINT('Ctrl Pts',(-1.95622159519703,40.6526041666666,
52.9827367061318));
#264538=CARTESIAN_POINT('Ctrl Pts',(7.17168088200107E-15,40.7187499999999,
52.9827367061318));
#264539=CARTESIAN_POINT('Ctrl Pts',(1.95622159519705,40.7848958333332,52.9827367061318));
#264540=CARTESIAN_POINT('Ctrl Pts',(3.33947915066444,40.8510416666665,51.5994791506644));
#264541=CARTESIAN_POINT('Ctrl Pts',(4.72273670613183,40.9171874999999,50.216221595197));
#264542=CARTESIAN_POINT('Ctrl Pts',(4.72273670613183,40.9833333333332,48.26));
#264543=CARTESIAN_POINT('Ctrl Pts',(4.72273670613183,41.0494791666665,46.303778404803));
#264544=CARTESIAN_POINT('Ctrl Pts',(3.33947915066444,41.1156249999998,44.9205208493356));
#264545=CARTESIAN_POINT('Ctrl Pts',(1.95622159519705,41.1817708333331,43.5372632938682));
#264546=CARTESIAN_POINT('Ctrl Pts',(6.99833541005117E-15,41.2479166666664,
43.5372632938682));
#264547=CARTESIAN_POINT('Ctrl Pts',(-1.95622159519704,41.3140624999997,
43.5372632938682));
#264548=CARTESIAN_POINT('Ctrl Pts',(-3.33947915066443,41.380208333333,44.9205208493356));
#264549=CARTESIAN_POINT('Ctrl Pts',(-4.72273670613182,41.4463541666663,
46.303778404803));
#264550=CARTESIAN_POINT('Ctrl Pts',(-4.72273670613182,41.5124999999997,
48.26));
#264551=CARTESIAN_POINT('Ctrl Pts',(-4.72273670613182,41.578645833333,50.216221595197));
#264552=CARTESIAN_POINT('Ctrl Pts',(-3.33947915066443,41.6447916666663,
51.5994791506644));
#264553=CARTESIAN_POINT('Ctrl Pts',(-1.95622159519703,41.7109374999996,
52.9827367061318));
#264554=CARTESIAN_POINT('Ctrl Pts',(7.17168088200104E-15,41.7770833333329,
52.9827367061318));
#264555=CARTESIAN_POINT('Ctrl Pts',(1.95622159519705,41.8432291666662,52.9827367061318));
#264556=CARTESIAN_POINT('Ctrl Pts',(3.33947915066444,41.9093749999995,51.5994791506644));
#264557=CARTESIAN_POINT('Ctrl Pts',(4.72273670613183,41.9755208333329,50.216221595197));
#264558=CARTESIAN_POINT('Ctrl Pts',(4.72273670613183,42.0416666666662,48.26));
#264559=CARTESIAN_POINT('Ctrl Pts',(4.72273670613183,42.1078124999995,46.303778404803));
#264560=CARTESIAN_POINT('Ctrl Pts',(3.33947915066444,42.1739583333328,44.9205208493356));
#264561=CARTESIAN_POINT('Ctrl Pts',(1.95622159519705,42.2401041666661,43.5372632938682));
#264562=CARTESIAN_POINT('Ctrl Pts',(6.99833541005117E-15,42.3062499999994,
43.5372632938682));
#264563=CARTESIAN_POINT('Ctrl Pts',(-1.95622159519704,42.3723958333327,
43.5372632938682));
#264564=CARTESIAN_POINT('Ctrl Pts',(-3.33947915066443,42.438541666666,44.9205208493356));
#264565=CARTESIAN_POINT('Ctrl Pts',(-4.72273670613182,42.5046874999994,
46.303778404803));
#264566=CARTESIAN_POINT('Ctrl Pts',(-4.72273670613182,42.5708333333327,
48.26));
#264567=CARTESIAN_POINT('Ctrl Pts',(-4.72273670613182,42.636979166666,50.216221595197));
#264568=CARTESIAN_POINT('Ctrl Pts',(-3.33947915066443,42.7031249999993,
51.5994791506644));
#264569=CARTESIAN_POINT('Ctrl Pts',(-1.95622159519703,42.7692708333326,
52.9827367061318));
#264570=CARTESIAN_POINT('Ctrl Pts',(7.17168088200104E-15,42.8354166666659,
52.9827367061318));
#264571=CARTESIAN_POINT('Ctrl Pts',(1.95622159519705,42.9015624999992,52.9827367061318));
#264572=CARTESIAN_POINT('Ctrl Pts',(3.33947915066444,42.9677083333326,51.5994791506644));
#264573=CARTESIAN_POINT('Ctrl Pts',(4.72273670613183,43.0338541666659,50.216221595197));
#264574=CARTESIAN_POINT('Ctrl Pts',(4.72273670613183,43.0999999999992,48.26));
#264575=CARTESIAN_POINT('Ctrl Pts',(4.72273670613183,43.1661458333325,46.303778404803));
#264576=CARTESIAN_POINT('Ctrl Pts',(3.33947915066444,43.2322916666658,44.9205208493356));
#264577=CARTESIAN_POINT('Ctrl Pts',(1.95622159519705,43.2984374999991,43.5372632938682));
#264578=CARTESIAN_POINT('Ctrl Pts',(6.99833541005117E-15,43.3645833333324,
43.5372632938682));
#264579=CARTESIAN_POINT('Ctrl Pts',(-1.95622159519704,43.4307291666657,
43.5372632938682));
#264580=CARTESIAN_POINT('Ctrl Pts',(-3.33947915066443,43.496874999999,44.9205208493356));
#264581=CARTESIAN_POINT('Ctrl Pts',(-4.72273670613182,43.5630208333324,
46.303778404803));
#264582=CARTESIAN_POINT('Ctrl Pts',(-4.72273670613182,43.6291666666657,
48.26));
#264583=CARTESIAN_POINT('Ctrl Pts',(-4.72273670613182,43.695312499999,50.216221595197));
#264584=CARTESIAN_POINT('Ctrl Pts',(-3.33947915066443,43.7614583333323,
51.5994791506644));
#264585=CARTESIAN_POINT('Ctrl Pts',(-1.95622159519703,43.8276041666656,
52.9827367061318));
#264586=CARTESIAN_POINT('Ctrl Pts',(7.17168088200102E-15,43.8937499999989,
52.9827367061318));
#264587=CARTESIAN_POINT('Ctrl Pts',(1.95622159519705,43.9598958333322,52.9827367061318));
#264588=CARTESIAN_POINT('Ctrl Pts',(3.33947915066444,44.0260416666656,51.5994791506644));
#264589=CARTESIAN_POINT('Ctrl Pts',(4.72273670613183,44.0921874999989,50.216221595197));
#264590=CARTESIAN_POINT('Ctrl Pts',(4.72273670613183,44.1583333333322,48.26));
#264591=CARTESIAN_POINT('Ctrl Pts',(4.72273670613183,44.2244791666655,46.303778404803));
#264592=CARTESIAN_POINT('Ctrl Pts',(3.33947915066444,44.2906249999988,44.9205208493356));
#264593=CARTESIAN_POINT('Ctrl Pts',(1.95622159519705,44.3567708333321,43.5372632938682));
#264594=CARTESIAN_POINT('Ctrl Pts',(6.99833541005117E-15,44.4229166666654,
43.5372632938682));
#264595=CARTESIAN_POINT('Ctrl Pts',(-1.95622159519704,44.4890624999988,
43.5372632938682));
#264596=CARTESIAN_POINT('Ctrl Pts',(-3.33947915066443,44.555208333332,44.9205208493356));
#264597=CARTESIAN_POINT('Ctrl Pts',(-4.72273670613182,44.6213541666654,
46.303778404803));
#264598=CARTESIAN_POINT('Ctrl Pts',(-4.72273670613182,44.6874999999987,
48.26));
#264599=CARTESIAN_POINT('Ctrl Pts',(-4.72273670613182,44.753645833332,50.216221595197));
#264600=CARTESIAN_POINT('Ctrl Pts',(-3.33947915066443,44.8197916666653,
51.5994791506644));
#264601=CARTESIAN_POINT('Ctrl Pts',(-1.95622159519703,44.8859374999986,
52.9827367061318));
#264602=CARTESIAN_POINT('Ctrl Pts',(7.17168088200107E-15,44.9520833333319,
52.9827367061318));
#264603=CARTESIAN_POINT('Ctrl Pts',(1.95622159519705,45.0182291666652,52.9827367061318));
#264604=CARTESIAN_POINT('Ctrl Pts',(3.33947915066444,45.0843749999985,51.5994791506644));
#264605=CARTESIAN_POINT('Ctrl Pts',(4.72273670613183,45.1505208333318,50.216221595197));
#264606=CARTESIAN_POINT('Ctrl Pts',(4.72273670613183,45.2166666666652,48.26));
#264607=CARTESIAN_POINT('Ctrl Pts',(4.72273670613183,45.2828124999985,46.303778404803));
#264608=CARTESIAN_POINT('Ctrl Pts',(3.33947915066444,45.3489583333318,44.9205208493356));
#264609=CARTESIAN_POINT('Ctrl Pts',(1.95622159519705,45.4151041666651,43.5372632938682));
#264610=CARTESIAN_POINT('Ctrl Pts',(6.99833541005117E-15,45.4812499999984,
43.5372632938682));
#264611=CARTESIAN_POINT('Ctrl Pts',(-1.95622159519704,45.5473958333317,
43.5372632938682));
#264612=CARTESIAN_POINT('Ctrl Pts',(-3.33947915066443,45.613541666665,44.9205208493356));
#264613=CARTESIAN_POINT('Ctrl Pts',(-4.72273670613182,45.6796874999984,
46.303778404803));
#264614=CARTESIAN_POINT('Ctrl Pts',(-4.72273670613182,45.7458333333317,
48.26));
#264615=CARTESIAN_POINT('Ctrl Pts',(-4.72273670613182,45.811979166665,50.216221595197));
#264616=CARTESIAN_POINT('Ctrl Pts',(-3.33947915066443,45.8781249999983,
51.5994791506644));
#264617=CARTESIAN_POINT('Ctrl Pts',(-1.95622159519703,45.9442708333316,
52.9827367061318));
#264618=CARTESIAN_POINT('Ctrl Pts',(7.17168088200104E-15,46.0104166666649,
52.9827367061318));
#264619=CARTESIAN_POINT('Ctrl Pts',(1.95622159519705,46.0765624999982,52.9827367061318));
#264620=CARTESIAN_POINT('Ctrl Pts',(3.33947915066444,46.1427083333315,51.5994791506644));
#264621=CARTESIAN_POINT('Ctrl Pts',(4.72273670613183,46.2088541666649,50.216221595197));
#264622=CARTESIAN_POINT('Ctrl Pts',(4.72273670613183,46.2749999999982,48.26));
#264623=CARTESIAN_POINT('Ctrl Pts',(4.72273670613183,46.3411458333315,46.303778404803));
#264624=CARTESIAN_POINT('Ctrl Pts',(3.33947915066444,46.4072916666648,44.9205208493356));
#264625=CARTESIAN_POINT('Ctrl Pts',(1.95622159519705,46.4734374999981,43.5372632938682));
#264626=CARTESIAN_POINT('Ctrl Pts',(6.99833541005117E-15,46.5395833333314,
43.5372632938682));
#264627=CARTESIAN_POINT('Ctrl Pts',(-1.95622159519704,46.6057291666647,
43.5372632938682));
#264628=CARTESIAN_POINT('Ctrl Pts',(-3.33947915066443,46.671874999998,44.9205208493356));
#264629=CARTESIAN_POINT('Ctrl Pts',(-4.72273670613182,46.7380208333314,
46.303778404803));
#264630=CARTESIAN_POINT('Ctrl Pts',(-4.72273670613182,46.8041666666647,
48.26));
#264631=CARTESIAN_POINT('Ctrl Pts',(-4.72273670613182,46.870312499998,50.216221595197));
#264632=CARTESIAN_POINT('Ctrl Pts',(-3.33947915066443,46.9364583333313,
51.5994791506644));
#264633=CARTESIAN_POINT('Ctrl Pts',(-1.95622159519703,47.0026041666646,
52.9827367061318));
#264634=CARTESIAN_POINT('Ctrl Pts',(7.17168088200104E-15,47.0687499999979,
52.9827367061318));
#264635=CARTESIAN_POINT('Ctrl Pts',(1.95622159519705,47.1348958333312,52.9827367061318));
#264636=CARTESIAN_POINT('Ctrl Pts',(3.33947915066444,47.2010416666646,51.5994791506644));
#264637=CARTESIAN_POINT('Ctrl Pts',(4.72273670613183,47.2671874999979,50.216221595197));
#264638=CARTESIAN_POINT('Ctrl Pts',(4.72273670613183,47.3333333333312,48.26));
#264639=CARTESIAN_POINT('Ctrl Pts',(4.72273670613183,47.3994791666645,46.303778404803));
#264640=CARTESIAN_POINT('Ctrl Pts',(3.33947915066444,47.4656249999978,44.9205208493356));
#264641=CARTESIAN_POINT('Ctrl Pts',(1.95622159519705,47.5317708333311,43.5372632938682));
#264642=CARTESIAN_POINT('Ctrl Pts',(6.99833541005117E-15,47.5979166666644,
43.5372632938682));
#264643=CARTESIAN_POINT('Ctrl Pts',(-1.95622159519704,47.6640624999977,
43.5372632938682));
#264644=CARTESIAN_POINT('Ctrl Pts',(-3.33947915066443,47.730208333331,44.9205208493356));
#264645=CARTESIAN_POINT('Ctrl Pts',(-4.72273670613182,47.7963541666644,
46.303778404803));
#264646=CARTESIAN_POINT('Ctrl Pts',(-4.72273670613182,47.8624999999977,
48.26));
#264647=CARTESIAN_POINT('Ctrl Pts',(-4.72273670613182,47.928645833331,50.216221595197));
#264648=CARTESIAN_POINT('Ctrl Pts',(-3.33947915066443,47.9947916666643,
51.5994791506644));
#264649=CARTESIAN_POINT('Ctrl Pts',(-1.95622159519703,48.0609374999976,
52.9827367061318));
#264650=CARTESIAN_POINT('Ctrl Pts',(7.17168088200102E-15,48.1270833333309,
52.9827367061318));
#264651=CARTESIAN_POINT('Ctrl Pts',(1.95622159519705,48.1932291666642,52.9827367061318));
#264652=CARTESIAN_POINT('Ctrl Pts',(3.33947915066444,48.2593749999975,51.5994791506644));
#264653=CARTESIAN_POINT('Ctrl Pts',(4.72273670613183,48.3255208333309,50.216221595197));
#264654=CARTESIAN_POINT('Ctrl Pts',(4.72273670613183,48.3916666666642,48.26));
#264655=CARTESIAN_POINT('Ctrl Pts',(4.72273670613183,48.4578124999975,46.303778404803));
#264656=CARTESIAN_POINT('Ctrl Pts',(3.33947915066444,48.5239583333308,44.9205208493356));
#264657=CARTESIAN_POINT('Ctrl Pts',(1.95622159519705,48.5901041666641,43.5372632938682));
#264658=CARTESIAN_POINT('Ctrl Pts',(6.99833541005117E-15,48.6562499999974,
43.5372632938682));
#264659=CARTESIAN_POINT('Ctrl Pts',(-1.95622159519704,48.7223958333307,
43.5372632938682));
#264660=CARTESIAN_POINT('Ctrl Pts',(-3.33947915066443,48.788541666664,44.9205208493356));
#264661=CARTESIAN_POINT('Ctrl Pts',(-4.72273670613182,48.8546874999974,
46.303778404803));
#264662=CARTESIAN_POINT('Ctrl Pts',(-4.72273670613182,48.9208333333307,
48.26));
#264663=CARTESIAN_POINT('Ctrl Pts',(-4.72273670613182,48.986979166664,50.216221595197));
#264664=CARTESIAN_POINT('Ctrl Pts',(-3.33947915066443,49.0531249999973,
51.5994791506644));
#264665=CARTESIAN_POINT('Ctrl Pts',(-1.95622159519703,49.1192708333306,
52.9827367061318));
#264666=CARTESIAN_POINT('Ctrl Pts',(7.17168088200102E-15,49.1854166666639,
52.9827367061318));
#264667=CARTESIAN_POINT('Ctrl Pts',(1.95622159519705,49.2515624999972,52.9827367061318));
#264668=CARTESIAN_POINT('Ctrl Pts',(3.33947915066444,49.3177083333306,51.5994791506644));
#264669=CARTESIAN_POINT('Ctrl Pts',(4.72273670613183,49.3838541666639,50.216221595197));
#264670=CARTESIAN_POINT('Ctrl Pts',(4.72273670613183,49.4499999999972,48.26));
#264671=CARTESIAN_POINT('Ctrl Pts',(4.72273670613183,49.5161458333305,46.303778404803));
#264672=CARTESIAN_POINT('Ctrl Pts',(3.33947915066444,49.5822916666638,44.9205208493356));
#264673=CARTESIAN_POINT('Ctrl Pts',(1.95622159519705,49.6484374999971,43.5372632938682));
#264674=CARTESIAN_POINT('Ctrl Pts',(6.99833541005115E-15,49.7145833333304,
43.5372632938682));
#264675=CARTESIAN_POINT('Ctrl Pts',(-1.95622159519704,49.7807291666637,
43.5372632938682));
#264676=CARTESIAN_POINT('Ctrl Pts',(-3.33947915066443,49.846874999997,44.9205208493356));
#264677=CARTESIAN_POINT('Ctrl Pts',(-4.72273670613182,49.9130208333304,
46.303778404803));
#264678=CARTESIAN_POINT('Ctrl Pts',(-4.72273670613182,49.9791666666637,
48.26));
#264679=CARTESIAN_POINT('Ctrl Pts',(-4.72273670613182,50.045312499997,50.216221595197));
#264680=CARTESIAN_POINT('Ctrl Pts',(-3.33947915066443,50.1114583333303,
51.5994791506644));
#264681=CARTESIAN_POINT('Ctrl Pts',(-1.95622159519703,50.1776041666636,
52.9827367061318));
#264682=CARTESIAN_POINT('Ctrl Pts',(7.17168088200107E-15,50.2437499999969,
52.9827367061318));
#264683=CARTESIAN_POINT('Ctrl Pts',(1.95622159519705,50.3098958333302,52.9827367061318));
#264684=CARTESIAN_POINT('Ctrl Pts',(3.33947915066444,50.3760416666636,51.5994791506644));
#264685=CARTESIAN_POINT('Ctrl Pts',(4.72273670613183,50.4421874999969,50.216221595197));
#264686=CARTESIAN_POINT('Ctrl Pts',(4.72273670613183,50.5083333333302,48.26));
#264687=CARTESIAN_POINT('Ctrl Pts',(4.72273670613183,50.5744791666635,46.303778404803));
#264688=CARTESIAN_POINT('Ctrl Pts',(3.33947915066444,50.6406249999968,44.9205208493356));
#264689=CARTESIAN_POINT('Ctrl Pts',(1.95622159519705,50.7067708333301,43.5372632938682));
#264690=CARTESIAN_POINT('Ctrl Pts',(6.99833541005117E-15,50.7729166666634,
43.5372632938682));
#264691=CARTESIAN_POINT('Ctrl Pts',(-1.95622159519704,50.8390624999967,
43.5372632938682));
#264692=CARTESIAN_POINT('Ctrl Pts',(-3.33947915066443,50.90520833333,44.9205208493356));
#264693=CARTESIAN_POINT('Ctrl Pts',(-4.72273670613182,50.9713541666634,
46.303778404803));
#264694=CARTESIAN_POINT('Ctrl Pts',(-4.72273670613182,51.0374999999967,
48.26));
#264695=CARTESIAN_POINT('Origin',(-1.38777878078145E-14,-1.38777878078145E-14,
4.05352706259476));
#264696=CARTESIAN_POINT('',(40.,-1.87763750044039E-14,4.05352706259477));
#264697=CARTESIAN_POINT('Origin',(-1.38777878078145E-14,-1.38777878078145E-14,
4.05352706259476));
#264698=CARTESIAN_POINT('',(41.2700000000001,-1.89319051478956E-14,2.54));
#264699=CARTESIAN_POINT('',(40.,-1.87763750044039E-14,4.05352706259476));
#264700=CARTESIAN_POINT('Origin',(-1.38777878078145E-14,-1.38777878078145E-14,
2.54));
#264701=CARTESIAN_POINT('Origin',(-1.38777878078145E-14,-1.38777878078145E-14,
61.9864729374053));
#264702=CARTESIAN_POINT('',(40.,-8.97920061122505E-15,61.9864729374053));
#264703=CARTESIAN_POINT('',(-40.,-1.87763750044039E-14,61.9864729374053));
#264704=CARTESIAN_POINT('Origin',(-1.38777878078145E-14,-1.38777878078145E-14,
61.9864729374053));
#264705=CARTESIAN_POINT('Origin',(-1.38777878078145E-14,-1.38777878078145E-14,
61.9864729374053));
#264706=CARTESIAN_POINT('',(-41.2700000000001,-1.89319051478956E-14,63.5));
#264707=CARTESIAN_POINT('',(-40.,-1.87763750044039E-14,61.9864729374053));
#264708=CARTESIAN_POINT('Origin',(-1.38777878078145E-14,-1.38777878078145E-14,
63.5));
#264709=CARTESIAN_POINT('Origin',(-1.38777878078145E-14,-1.38777878078145E-14,
63.5));
#264710=CARTESIAN_POINT('',(50.,-2.00010218035512E-14,62.2300000000001));
#264711=CARTESIAN_POINT('Origin',(-1.38777878078145E-14,-1.38777878078145E-14,
62.2300000000001));
#264712=CARTESIAN_POINT('',(48.4864729374054,-1.98156681962883E-14,63.5));
#264713=CARTESIAN_POINT('',(48.4864729374054,-1.98156681962883E-14,63.5));
#264714=CARTESIAN_POINT('Origin',(-1.38777878078145E-14,-1.38777878078145E-14,
63.5));
#264715=CARTESIAN_POINT('Origin',(-1.38777878078145E-14,-1.38777878078145E-14,
2.53999999999999));
#264716=CARTESIAN_POINT('',(50.,-7.75455381207769E-15,3.80999999999998));
#264717=CARTESIAN_POINT('',(-50.,-2.00010218035512E-14,3.80999999999998));
#264718=CARTESIAN_POINT('Origin',(-1.38777878078145E-14,-1.38777878078145E-14,
3.80999999999998));
#264719=CARTESIAN_POINT('Origin',(-1.38777878078145E-14,-1.38777878078145E-14,
3.80999999999998));
#264720=CARTESIAN_POINT('',(-48.4864729374054,-1.98156681962883E-14,2.54));
#264721=CARTESIAN_POINT('',(-48.4864729374054,-1.98156681962883E-14,2.53999999999999));
#264722=CARTESIAN_POINT('Origin',(-1.38777878078145E-14,-1.38777878078145E-14,
2.54));
#264723=CARTESIAN_POINT('Origin',(-1.38777878078145E-14,-1.38777878078145E-14,
268.42135623731));
#264724=CARTESIAN_POINT('',(50.,-9.74305740910067E-14,43.4975));
#264725=CARTESIAN_POINT('',(50.,-2.00010218035512E-14,268.42135623731));
#264726=CARTESIAN_POINT('',(50.,-1.75157305013873E-13,53.0225));
#264727=CARTESIAN_POINT('Ctrl Pts',(50.,-1.7499890425654E-13,53.0225));
#264728=CARTESIAN_POINT('Ctrl Pts',(50.,-0.598378688298317,53.0225));
#264729=CARTESIAN_POINT('Ctrl Pts',(49.9881578769847,-1.23639552071279,
52.9028396534865));
#264730=CARTESIAN_POINT('Ctrl Pts',(49.9453510199711,-2.40967078999247,
52.4166958716389));
#264731=CARTESIAN_POINT('Ctrl Pts',(49.9149942232673,-2.94495962679791,
52.0502324640042));
#264732=CARTESIAN_POINT('Ctrl Pts',(49.8579338261974,-3.79023364706856,
51.2049584437335));
#264733=CARTESIAN_POINT('Ctrl Pts',(49.8275167150177,-4.15669613276604,
50.6696701266124));
#264734=CARTESIAN_POINT('Ctrl Pts',(49.7845717960014,-4.64283922274571,
49.4963965934443));
#264735=CARTESIAN_POINT('Ctrl Pts',(49.7726691443205,-4.76250000000018,
48.8583803633087));
#264736=CARTESIAN_POINT('Ctrl Pts',(49.7726691443205,-4.76250000000018,
47.6616196366914));
#264737=CARTESIAN_POINT('Ctrl Pts',(49.7845717960014,-4.64283922274571,
47.0236034065557));
#264738=CARTESIAN_POINT('Ctrl Pts',(49.8275167150177,-4.15669613276604,
45.8503298733876));
#264739=CARTESIAN_POINT('Ctrl Pts',(49.8579338261974,-3.79023364706856,
45.3150415562665));
#264740=CARTESIAN_POINT('Ctrl Pts',(49.9149942232673,-2.94495962679791,
44.4697675359959));
#264741=CARTESIAN_POINT('Ctrl Pts',(49.9453510199711,-2.40967078999247,
44.1033041283611));
#264742=CARTESIAN_POINT('Ctrl Pts',(49.9881578769847,-1.23639552071278,
43.6171603465136));
#264743=CARTESIAN_POINT('Ctrl Pts',(50.,-0.598378688298317,43.4975));
#264744=CARTESIAN_POINT('Ctrl Pts',(50.,-1.74860126378462E-13,43.4975));
#264745=CARTESIAN_POINT('',(50.,-2.00010218035512E-14,268.42135623731));
#264746=CARTESIAN_POINT('Ctrl Pts',(50.,-1.74582570622306E-13,43.4975));
#264747=CARTESIAN_POINT('Ctrl Pts',(50.,0.598378688297968,43.4975));
#264748=CARTESIAN_POINT('Ctrl Pts',(49.9881578769847,1.23639552071243,43.6171603465136));
#264749=CARTESIAN_POINT('Ctrl Pts',(49.9453510199711,2.40967078999212,44.1033041283611));
#264750=CARTESIAN_POINT('Ctrl Pts',(49.9149942232673,2.94495962679757,44.4697675359959));
#264751=CARTESIAN_POINT('Ctrl Pts',(49.8579338261974,3.79023364706821,45.3150415562665));
#264752=CARTESIAN_POINT('Ctrl Pts',(49.8275167150177,4.15669613276569,45.8503298733876));
#264753=CARTESIAN_POINT('Ctrl Pts',(49.7845717960014,4.64283922274536,47.0236034065557));
#264754=CARTESIAN_POINT('Ctrl Pts',(49.7726691443206,4.76249999999983,47.6616196366914));
#264755=CARTESIAN_POINT('Ctrl Pts',(49.7726691443206,4.76249999999983,48.26));
#264756=CARTESIAN_POINT('Ctrl Pts',(49.7726691443206,4.76249999999983,48.8583803633087));
#264757=CARTESIAN_POINT('Ctrl Pts',(49.7845717960014,4.64283922274536,49.4963965934443));
#264758=CARTESIAN_POINT('Ctrl Pts',(49.8275167150177,4.15669613276569,50.6696701266124));
#264759=CARTESIAN_POINT('Ctrl Pts',(49.8579338261974,3.79023364706821,51.2049584437335));
#264760=CARTESIAN_POINT('Ctrl Pts',(49.9149942232673,2.94495962679757,52.0502324640042));
#264761=CARTESIAN_POINT('Ctrl Pts',(49.9453510199711,2.40967078999212,52.4166958716389));
#264762=CARTESIAN_POINT('Ctrl Pts',(49.9881578769847,1.23639552071243,52.9028396534865));
#264763=CARTESIAN_POINT('Ctrl Pts',(50.,0.598378688297967,53.0225));
#264764=CARTESIAN_POINT('Ctrl Pts',(50.,-1.75276460012697E-13,53.0225));
#264765=CARTESIAN_POINT('',(1.31536147873854E-15,50.,43.4975));
#264766=CARTESIAN_POINT('',(-5.83238038093927E-16,50.,53.0225));
#264767=CARTESIAN_POINT('Ctrl Pts',(4.16333634234434E-16,50.,43.4975));
#264768=CARTESIAN_POINT('Ctrl Pts',(-0.598378688298142,50.,43.4975));
#264769=CARTESIAN_POINT('Ctrl Pts',(-1.23639552071261,49.9881578769847,
43.6171603465136));
#264770=CARTESIAN_POINT('Ctrl Pts',(-2.40967078999229,49.9453510199711,
44.1033041283611));
#264771=CARTESIAN_POINT('Ctrl Pts',(-2.94495962679774,49.9149942232673,
44.4697675359959));
#264772=CARTESIAN_POINT('Ctrl Pts',(-3.79023364706838,49.8579338261974,
45.3150415562665));
#264773=CARTESIAN_POINT('Ctrl Pts',(-4.15669613276586,49.8275167150177,
45.8503298733876));
#264774=CARTESIAN_POINT('Ctrl Pts',(-4.64283922274554,49.7845717960014,
47.0236034065557));
#264775=CARTESIAN_POINT('Ctrl Pts',(-4.7625,49.7726691443205,47.6616196366914));
#264776=CARTESIAN_POINT('Ctrl Pts',(-4.7625,49.7726691443205,48.26));
#264777=CARTESIAN_POINT('Ctrl Pts',(-4.7625,49.7726691443205,48.8583803633087));
#264778=CARTESIAN_POINT('Ctrl Pts',(-4.64283922274554,49.7845717960014,
49.4963965934443));
#264779=CARTESIAN_POINT('Ctrl Pts',(-4.15669613276586,49.8275167150177,
50.6696701266124));
#264780=CARTESIAN_POINT('Ctrl Pts',(-3.79023364706839,49.8579338261974,
51.2049584437335));
#264781=CARTESIAN_POINT('Ctrl Pts',(-2.94495962679774,49.9149942232673,
52.0502324640042));
#264782=CARTESIAN_POINT('Ctrl Pts',(-2.4096707899923,49.9453510199711,52.4166958716389));
#264783=CARTESIAN_POINT('Ctrl Pts',(-1.23639552071261,49.9881578769847,
52.9028396534865));
#264784=CARTESIAN_POINT('Ctrl Pts',(-0.598378688298142,50.,53.0225));
#264785=CARTESIAN_POINT('Ctrl Pts',(1.38777878078145E-16,50.,53.0225));
#264786=CARTESIAN_POINT('Ctrl Pts',(-5.55111512312578E-16,50.,53.0225));
#264787=CARTESIAN_POINT('Ctrl Pts',(0.598378688298142,50.,53.0225));
#264788=CARTESIAN_POINT('Ctrl Pts',(1.23639552071261,49.9881578769847,52.9028396534865));
#264789=CARTESIAN_POINT('Ctrl Pts',(2.40967078999229,49.9453510199711,52.4166958716389));
#264790=CARTESIAN_POINT('Ctrl Pts',(2.94495962679774,49.9149942232673,52.0502324640042));
#264791=CARTESIAN_POINT('Ctrl Pts',(3.79023364706838,49.8579338261974,51.2049584437335));
#264792=CARTESIAN_POINT('Ctrl Pts',(4.15669613276586,49.8275167150177,50.6696701266124));
#264793=CARTESIAN_POINT('Ctrl Pts',(4.64283922274554,49.7845717960014,49.4963965934443));
#264794=CARTESIAN_POINT('Ctrl Pts',(4.7625,49.7726691443205,48.8583803633087));
#264795=CARTESIAN_POINT('Ctrl Pts',(4.7625,49.7726691443205,47.6616196366914));
#264796=CARTESIAN_POINT('Ctrl Pts',(4.64283922274554,49.7845717960014,47.0236034065557));
#264797=CARTESIAN_POINT('Ctrl Pts',(4.15669613276586,49.8275167150177,45.8503298733876));
#264798=CARTESIAN_POINT('Ctrl Pts',(3.79023364706839,49.8579338261974,45.3150415562665));
#264799=CARTESIAN_POINT('Ctrl Pts',(2.94495962679774,49.9149942232673,44.4697675359959));
#264800=CARTESIAN_POINT('Ctrl Pts',(2.4096707899923,49.9453510199711,44.1033041283611));
#264801=CARTESIAN_POINT('Ctrl Pts',(1.23639552071261,49.9881578769847,43.6171603465136));
#264802=CARTESIAN_POINT('Ctrl Pts',(0.598378688298144,50.,43.4975));
#264803=CARTESIAN_POINT('Ctrl Pts',(1.11022302462516E-15,50.,43.4975));
#264804=CARTESIAN_POINT('Origin',(0.,115.,48.26));
#264805=CARTESIAN_POINT('',(5.83238094526905E-16,40.,53.0225));
#264806=CARTESIAN_POINT('',(-5.83238038093927E-16,115.,53.0225));
#264807=CARTESIAN_POINT('Ctrl Pts',(-4.7625,39.7154704586261,48.26));
#264808=CARTESIAN_POINT('Ctrl Pts',(-4.7625,39.7154704586261,48.8586021223598));
#264809=CARTESIAN_POINT('Ctrl Pts',(-4.64275284127331,39.7303998106907,
49.4967123644842));
#264810=CARTESIAN_POINT('Ctrl Pts',(-4.15654655972588,39.7842046972333,
50.6699237637271));
#264811=CARTESIAN_POINT('Ctrl Pts',(-3.79011828934085,39.8222902757623,
51.205073801461));
#264812=CARTESIAN_POINT('Ctrl Pts',(-2.94507670291011,39.8936877237352,
52.0501153878918));
#264813=CARTESIAN_POINT('Ctrl Pts',(-2.40992540144616,39.9316551722397,
52.416545929979));
#264814=CARTESIAN_POINT('Ctrl Pts',(-1.23670973303352,39.9851894363656,
52.9027538828458));
#264815=CARTESIAN_POINT('Ctrl Pts',(-0.598598011774796,40.,53.0225));
#264816=CARTESIAN_POINT('Ctrl Pts',(0.598598011774795,40.,53.0225));
#264817=CARTESIAN_POINT('Ctrl Pts',(1.23670973303352,39.9851894363656,52.9027538828458));
#264818=CARTESIAN_POINT('Ctrl Pts',(2.40992540144616,39.9316551722397,52.416545929979));
#264819=CARTESIAN_POINT('Ctrl Pts',(2.94507670291011,39.8936877237352,52.0501153878918));
#264820=CARTESIAN_POINT('Ctrl Pts',(3.79011828934085,39.8222902757623,51.205073801461));
#264821=CARTESIAN_POINT('Ctrl Pts',(4.15654655972588,39.7842046972333,50.6699237637271));
#264822=CARTESIAN_POINT('Ctrl Pts',(4.64275284127331,39.7303998106907,49.4967123644842));
#264823=CARTESIAN_POINT('Ctrl Pts',(4.7625,39.7154704586261,48.8586021223598));
#264824=CARTESIAN_POINT('Ctrl Pts',(4.7625,39.7154704586261,47.6613978776402));
#264825=CARTESIAN_POINT('Ctrl Pts',(4.64275284127331,39.7303998106907,47.0232876355158));
#264826=CARTESIAN_POINT('Ctrl Pts',(4.15654655972588,39.7842046972333,45.8500762362729));
#264827=CARTESIAN_POINT('Ctrl Pts',(3.79011828934085,39.8222902757623,45.314926198539));
#264828=CARTESIAN_POINT('Ctrl Pts',(2.94507670291011,39.8936877237352,44.4698846121082));
#264829=CARTESIAN_POINT('Ctrl Pts',(2.40992540144616,39.9316551722397,44.103454070021));
#264830=CARTESIAN_POINT('Ctrl Pts',(1.23670973303352,39.9851894363656,43.6172461171542));
#264831=CARTESIAN_POINT('Ctrl Pts',(0.598598011774796,40.,43.4975));
#264832=CARTESIAN_POINT('Ctrl Pts',(-0.598598011774794,40.,43.4975));
#264833=CARTESIAN_POINT('Ctrl Pts',(-1.23670973303352,39.9851894363656,
43.6172461171542));
#264834=CARTESIAN_POINT('Ctrl Pts',(-2.40992540144616,39.9316551722397,
44.103454070021));
#264835=CARTESIAN_POINT('Ctrl Pts',(-2.94507670291011,39.8936877237352,
44.4698846121082));
#264836=CARTESIAN_POINT('Ctrl Pts',(-3.79011828934085,39.8222902757623,
45.314926198539));
#264837=CARTESIAN_POINT('Ctrl Pts',(-4.15654655972588,39.7842046972333,
45.8500762362729));
#264838=CARTESIAN_POINT('Ctrl Pts',(-4.64275284127331,39.7303998106907,
47.0232876355158));
#264839=CARTESIAN_POINT('Ctrl Pts',(-4.7625,39.7154704586261,47.6613978776402));
#264840=CARTESIAN_POINT('Ctrl Pts',(-4.7625,39.7154704586261,48.26));
#264841=CARTESIAN_POINT('Origin',(115.,-4.0152035396696E-13,48.26));
#264842=CARTESIAN_POINT('',(40.,-8.97920066765691E-15,53.0225));
#264843=CARTESIAN_POINT('',(115.,-4.00937115928867E-13,53.0225));
#264844=CARTESIAN_POINT('',(40.,-7.98179606268603E-14,43.4975));
#264845=CARTESIAN_POINT('Ctrl Pts',(40.,-1.40998324127395E-13,43.4975));
#264846=CARTESIAN_POINT('Ctrl Pts',(40.,0.598598011774654,43.4975));
#264847=CARTESIAN_POINT('Ctrl Pts',(39.9851894363656,1.23670973303338,43.6172461171542));
#264848=CARTESIAN_POINT('Ctrl Pts',(39.9316551722397,2.40992540144602,44.103454070021));
#264849=CARTESIAN_POINT('Ctrl Pts',(39.8936877237352,2.94507670290997,44.4698846121082));
#264850=CARTESIAN_POINT('Ctrl Pts',(39.8222902757623,3.79011828934071,45.314926198539));
#264851=CARTESIAN_POINT('Ctrl Pts',(39.7842046972333,4.15654655972574,45.8500762362729));
#264852=CARTESIAN_POINT('Ctrl Pts',(39.7303998106907,4.64275284127317,47.0232876355158));
#264853=CARTESIAN_POINT('Ctrl Pts',(39.7154704586261,4.76249999999986,47.6613978776402));
#264854=CARTESIAN_POINT('Ctrl Pts',(39.7154704586261,4.76249999999986,48.26));
#264855=CARTESIAN_POINT('Ctrl Pts',(39.7154704586261,4.76249999999986,48.8586021223598));
#264856=CARTESIAN_POINT('Ctrl Pts',(39.7303998106907,4.64275284127317,49.4967123644842));
#264857=CARTESIAN_POINT('Ctrl Pts',(39.7842046972333,4.15654655972574,50.6699237637271));
#264858=CARTESIAN_POINT('Ctrl Pts',(39.8222902757623,3.79011828934071,51.205073801461));
#264859=CARTESIAN_POINT('Ctrl Pts',(39.8936877237352,2.94507670290997,52.0501153878918));
#264860=CARTESIAN_POINT('Ctrl Pts',(39.9316551722397,2.40992540144602,52.416545929979));
#264861=CARTESIAN_POINT('Ctrl Pts',(39.9851894363656,1.23670973303338,52.9027538828458));
#264862=CARTESIAN_POINT('Ctrl Pts',(40.,0.598598011774656,53.0225));
#264863=CARTESIAN_POINT('Ctrl Pts',(40.,-1.39471767468535E-13,53.0225));
#264864=CARTESIAN_POINT('Ctrl Pts',(40.,-1.38777878078145E-13,53.0225));
#264865=CARTESIAN_POINT('Ctrl Pts',(40.,-0.598598011774934,53.0225));
#264866=CARTESIAN_POINT('Ctrl Pts',(39.9851894363656,-1.23670973303366,
52.9027538828458));
#264867=CARTESIAN_POINT('Ctrl Pts',(39.9316551722397,-2.4099254014463,52.416545929979));
#264868=CARTESIAN_POINT('Ctrl Pts',(39.8936877237351,-2.94507670291025,
52.0501153878918));
#264869=CARTESIAN_POINT('Ctrl Pts',(39.8222902757623,-3.79011828934099,
51.205073801461));
#264870=CARTESIAN_POINT('Ctrl Pts',(39.7842046972333,-4.15654655972601,
50.6699237637271));
#264871=CARTESIAN_POINT('Ctrl Pts',(39.7303998106907,-4.64275284127345,
49.4967123644842));
#264872=CARTESIAN_POINT('Ctrl Pts',(39.715470458626,-4.76250000000014,48.8586021223598));
#264873=CARTESIAN_POINT('Ctrl Pts',(39.715470458626,-4.76250000000014,47.6613978776402));
#264874=CARTESIAN_POINT('Ctrl Pts',(39.7303998106907,-4.64275284127345,
47.0232876355158));
#264875=CARTESIAN_POINT('Ctrl Pts',(39.7842046972333,-4.15654655972602,
45.850076236273));
#264876=CARTESIAN_POINT('Ctrl Pts',(39.8222902757623,-3.79011828934099,
45.314926198539));
#264877=CARTESIAN_POINT('Ctrl Pts',(39.8936877237351,-2.94507670291025,
44.4698846121082));
#264878=CARTESIAN_POINT('Ctrl Pts',(39.9316551722397,-2.4099254014463,44.103454070021));
#264879=CARTESIAN_POINT('Ctrl Pts',(39.9851894363656,-1.23670973303366,
43.6172461171542));
#264880=CARTESIAN_POINT('Ctrl Pts',(40.,-0.598598011774937,43.4975));
#264881=CARTESIAN_POINT('Ctrl Pts',(40.,-1.41414657761629E-13,43.4975));
#264882=CARTESIAN_POINT('Origin',(-1.38777878078145E-14,-1.38777878078145E-14,
268.42135623731));
#264883=CARTESIAN_POINT('',(40.,-1.87763750044039E-14,268.42135623731));
#264884=CARTESIAN_POINT('',(40.,-1.87763750044039E-14,268.42135623731));
#264885=CARTESIAN_POINT('Origin',(-90.,-90.,63.5));
#264886=CARTESIAN_POINT('Origin',(-90.,-90.,2.54));
#264887=CARTESIAN_POINT('Origin',(0.,0.,0.));
#264888=CARTESIAN_POINT('',(65.0000000000002,-7.96020419445782E-15,4.08753198860307));
#264889=CARTESIAN_POINT('Origin',(5.7559361144865E-16,0.,4.08753198860308));
#264890=CARTESIAN_POINT('',(65.0000000000002,-7.96020419445782E-15,7.62));
#264891=CARTESIAN_POINT('',(65.0000000000002,-7.96020419445782E-15,-9.15309894784421E-15));
#264892=CARTESIAN_POINT('Origin',(8.94187358750932E-16,0.,7.62));
#264893=CARTESIAN_POINT('Origin',(0.,0.,-195.421614460986));
#264894=CARTESIAN_POINT('',(-56.875,-6.96517867015057E-15,4.08753198860303));
#264895=CARTESIAN_POINT('Origin',(5.75593611448643E-16,0.,4.08753198860302));
#264896=CARTESIAN_POINT('',(-56.875,-6.96517867015057E-15,17.4625));
#264897=CARTESIAN_POINT('',(-56.875,-6.96517867015057E-15,-195.421614460986));
#264898=CARTESIAN_POINT('Origin',(0.,0.,17.4625));
#264899=CARTESIAN_POINT('Origin',(0.,0.,0.952499999999995));
#264900=CARTESIAN_POINT('',(74.8702478255888,-9.16896093509764E-15,2.54));
#264901=CARTESIAN_POINT('Origin',(0.,0.,2.54));
#264902=CARTESIAN_POINT('',(76.4577478255888,-9.36337361446228E-15,0.952499999999995));
#264903=CARTESIAN_POINT('Origin',(74.8702478255888,-9.16896093509764E-15,
0.952499999999995));
#264904=CARTESIAN_POINT('',(-76.4577478255888,9.36337361446228E-15,0.952499999999995));
#264905=CARTESIAN_POINT('Origin',(0.,0.,0.952499999999995));
#264906=CARTESIAN_POINT('Origin',(0.,0.,0.952499999999995));
#264907=CARTESIAN_POINT('Origin',(0.,0.,-216.614378091742));
#264908=CARTESIAN_POINT('',(-76.4577478255888,-9.36337361446228E-15,0.));
#264909=CARTESIAN_POINT('Origin',(0.,0.,0.));
#264910=CARTESIAN_POINT('',(-76.4577478255888,-9.36337361446228E-15,-216.614378091742));
#264911=CARTESIAN_POINT('Origin',(0.,0.,-195.421614460986));
#264912=CARTESIAN_POINT('',(17.3379110419349,64.705964905612,2.54));
#264913=CARTESIAN_POINT('',(17.3379110419349,-64.705964905612,2.54));
#264914=CARTESIAN_POINT('Origin',(0.,0.,2.53999999999999));
#264915=CARTESIAN_POINT('',(17.3379110419349,-64.705964905612,7.62));
#264916=CARTESIAN_POINT('',(17.3379110419349,-64.705964905612,7.62));
#264917=CARTESIAN_POINT('',(17.3379110419349,64.705964905612,7.62));
#264918=CARTESIAN_POINT('Origin',(0.,0.,7.62));
#264919=CARTESIAN_POINT('',(17.3379110419349,64.705964905612,7.62));
#264920=CARTESIAN_POINT('Origin',(0.,0.,-197.2176656852));
#264921=CARTESIAN_POINT('',(-70.625,-8.64906801897818E-15,17.4625));
#264922=CARTESIAN_POINT('Origin',(0.,0.,17.4625));
#264923=CARTESIAN_POINT('',(-70.625,-8.64906801897818E-15,8.25500000000002));
#264924=CARTESIAN_POINT('',(-70.625,-8.64906801897818E-15,-197.2176656852));
#264925=CARTESIAN_POINT('Origin',(0.,0.,8.255));
#264926=CARTESIAN_POINT('Origin',(0.,0.,228.814169979695));
#264927=CARTESIAN_POINT('',(76.5847478255888,-9.37892662881146E-15,0.));
#264928=CARTESIAN_POINT('Origin',(0.,0.,0.));
#264929=CARTESIAN_POINT('',(76.5847478255888,-9.37892662881146E-15,-8.00000000000001));
#264930=CARTESIAN_POINT('',(76.5847478255888,-9.37892662881146E-15,228.814169979695));
#264931=CARTESIAN_POINT('Origin',(0.,0.,-8.));
#264932=CARTESIAN_POINT('Origin',(-90.,-90.,63.5));
#264933=CARTESIAN_POINT('',(-81.5545,-90.,8.255));
#264934=CARTESIAN_POINT('Origin',(-90.,-90.,8.255));
#264935=CARTESIAN_POINT('',(-81.5545,-90.,3.175));
#264936=CARTESIAN_POINT('',(-81.5545,-90.,63.5));
#264937=CARTESIAN_POINT('Origin',(-90.,-90.,3.175));
#264938=CARTESIAN_POINT('Origin',(-90.,90.,63.5));
#264939=CARTESIAN_POINT('',(-81.5545,90.,8.255));
#264940=CARTESIAN_POINT('Origin',(-90.,90.,8.255));
#264941=CARTESIAN_POINT('',(-81.5545,90.,3.175));
#264942=CARTESIAN_POINT('',(-81.5545,90.,63.5));
#264943=CARTESIAN_POINT('Origin',(-90.,90.,3.175));
#264944=CARTESIAN_POINT('Origin',(90.,90.,63.5));
#264945=CARTESIAN_POINT('',(98.4455,90.,8.255));
#264946=CARTESIAN_POINT('Origin',(90.,90.,8.255));
#264947=CARTESIAN_POINT('',(98.4455,90.,3.175));
#264948=CARTESIAN_POINT('',(98.4455,90.,63.5));
#264949=CARTESIAN_POINT('Origin',(90.,90.,3.175));
#264950=CARTESIAN_POINT('Origin',(90.,-90.,63.5));
#264951=CARTESIAN_POINT('',(98.4455,-90.,8.255));
#264952=CARTESIAN_POINT('Origin',(90.,-90.,8.255));
#264953=CARTESIAN_POINT('',(98.4455,-90.,3.175));
#264954=CARTESIAN_POINT('',(98.4455,-90.,63.5));
#264955=CARTESIAN_POINT('Origin',(90.,-90.,3.175));
#264956=CARTESIAN_POINT('Origin',(90.,-90.,0.));
#264957=CARTESIAN_POINT('',(82.0625,-90.,-8.));
#264958=CARTESIAN_POINT('Origin',(90.,-90.,-8.));
#264959=CARTESIAN_POINT('',(82.0625,-90.,3.175));
#264960=CARTESIAN_POINT('',(82.0625,-90.,0.));
#264961=CARTESIAN_POINT('Origin',(90.,-90.,3.175));
#264962=CARTESIAN_POINT('Origin',(90.,90.,0.));
#264963=CARTESIAN_POINT('',(82.0625,90.,-8.));
#264964=CARTESIAN_POINT('Origin',(90.,90.,-8.));
#264965=CARTESIAN_POINT('',(82.0625,90.,3.175));
#264966=CARTESIAN_POINT('',(82.0625,90.,0.));
#264967=CARTESIAN_POINT('Origin',(90.,90.,3.175));
#264968=CARTESIAN_POINT('Origin',(-90.,90.,0.));
#264969=CARTESIAN_POINT('',(-97.9375,90.,-8.));
#264970=CARTESIAN_POINT('Origin',(-90.,90.,-8.));
#264971=CARTESIAN_POINT('',(-97.9375,90.,3.175));
#264972=CARTESIAN_POINT('',(-97.9375,90.,0.));
#264973=CARTESIAN_POINT('Origin',(-90.,90.,3.175));
#264974=CARTESIAN_POINT('Origin',(-90.,-90.,0.));
#264975=CARTESIAN_POINT('',(-97.9375,-90.,-8.));
#264976=CARTESIAN_POINT('Origin',(-90.,-90.,-8.));
#264977=CARTESIAN_POINT('',(-97.9375,-90.,3.175));
#264978=CARTESIAN_POINT('',(-97.9375,-90.,0.));
#264979=CARTESIAN_POINT('Origin',(-90.,-90.,3.175));
#264980=CARTESIAN_POINT('Origin',(-90.,-90.,0.));
#264981=CARTESIAN_POINT('',(-90.,-114.492,0.0381));
#264982=CARTESIAN_POINT('',(-90.,-114.492,7.493));
#264983=CARTESIAN_POINT('',(-90.,-114.492,0.));
#264984=CARTESIAN_POINT('',(-114.492,-90.,7.493));
#264985=CARTESIAN_POINT('Origin',(-90.,-90.,7.493));
#264986=CARTESIAN_POINT('',(-114.492,-90.,0.0381));
#264987=CARTESIAN_POINT('',(-114.492,-90.,0.));
#264988=CARTESIAN_POINT('Origin',(-90.,-90.,0.0381));
#264989=CARTESIAN_POINT('Origin',(-114.492,-90.,0.));
#264990=CARTESIAN_POINT('',(-114.492,90.,7.493));
#264991=CARTESIAN_POINT('',(-114.492,-90.,7.493));
#264992=CARTESIAN_POINT('',(-114.492,90.,0.0381));
#264993=CARTESIAN_POINT('',(-114.492,90.,0.));
#264994=CARTESIAN_POINT('',(-114.492,-90.,0.0381));
#264995=CARTESIAN_POINT('Origin',(-90.,90.,0.));
#264996=CARTESIAN_POINT('',(-90.,114.492,7.493));
#264997=CARTESIAN_POINT('Origin',(-90.,90.,7.493));
#264998=CARTESIAN_POINT('',(-90.,114.492,0.0381));
#264999=CARTESIAN_POINT('',(-90.,114.492,0.));
#265000=CARTESIAN_POINT('Origin',(-90.,90.,0.0381));
#265001=CARTESIAN_POINT('Origin',(-90.,114.492,0.));
#265002=CARTESIAN_POINT('',(90.,114.492,7.493));
#265003=CARTESIAN_POINT('',(-90.,114.492,7.493));
#265004=CARTESIAN_POINT('',(90.,114.492,0.0381));
#265005=CARTESIAN_POINT('',(90.,114.492,0.));
#265006=CARTESIAN_POINT('',(-90.,114.492,0.0381));
#265007=CARTESIAN_POINT('Origin',(90.,90.,0.));
#265008=CARTESIAN_POINT('',(114.492,90.,7.493));
#265009=CARTESIAN_POINT('Origin',(90.,90.,7.493));
#265010=CARTESIAN_POINT('',(114.492,90.,0.0381));
#265011=CARTESIAN_POINT('',(114.492,90.,0.));
#265012=CARTESIAN_POINT('Origin',(90.,90.,0.0381));
#265013=CARTESIAN_POINT('Origin',(114.492,90.,0.));
#265014=CARTESIAN_POINT('',(114.492,-90.,7.493));
#265015=CARTESIAN_POINT('',(114.492,90.,7.493));
#265016=CARTESIAN_POINT('',(114.492,-90.,0.0381));
#265017=CARTESIAN_POINT('',(114.492,-90.,0.));
#265018=CARTESIAN_POINT('',(114.492,90.,0.0381));
#265019=CARTESIAN_POINT('Origin',(90.,-90.,0.));
#265020=CARTESIAN_POINT('',(90.,-114.492,7.493));
#265021=CARTESIAN_POINT('Origin',(90.,-90.,7.493));
#265022=CARTESIAN_POINT('',(90.,-114.492,0.0381));
#265023=CARTESIAN_POINT('',(90.,-114.492,0.));
#265024=CARTESIAN_POINT('Origin',(90.,-90.,0.0381));
#265025=CARTESIAN_POINT('Origin',(90.,-114.492,0.));
#265026=CARTESIAN_POINT('',(90.,-114.492,7.493));
#265027=CARTESIAN_POINT('',(90.,-114.492,0.0381));
#265028=CARTESIAN_POINT('Origin',(-90.,-90.,8.255));
#265029=CARTESIAN_POINT('',(-113.73,90.,8.255));
#265030=CARTESIAN_POINT('',(-113.73,-90.,8.255));
#265031=CARTESIAN_POINT('',(-113.73,-90.,8.255));
#265032=CARTESIAN_POINT('',(-90.,-113.73,8.255));
#265033=CARTESIAN_POINT('Origin',(-90.,-90.,8.255));
#265034=CARTESIAN_POINT('',(90.,-113.73,8.255));
#265035=CARTESIAN_POINT('',(-90.,-113.73,8.255));
#265036=CARTESIAN_POINT('',(113.73,-90.,8.255));
#265037=CARTESIAN_POINT('Origin',(90.,-90.,8.255));
#265038=CARTESIAN_POINT('',(113.73,90.,8.255));
#265039=CARTESIAN_POINT('',(113.73,-90.0000000000001,8.255));
#265040=CARTESIAN_POINT('',(90.,113.73,8.255));
#265041=CARTESIAN_POINT('Origin',(90.,90.,8.255));
#265042=CARTESIAN_POINT('',(-90.,113.73,8.255));
#265043=CARTESIAN_POINT('',(-90.,113.73,8.255));
#265044=CARTESIAN_POINT('Origin',(-90.,90.,8.255));
#265045=CARTESIAN_POINT('Origin',(90.,-90.,3.175));
#265046=CARTESIAN_POINT('Origin',(90.,90.,3.175));
#265047=CARTESIAN_POINT('Origin',(-90.,90.,3.175));
#265048=CARTESIAN_POINT('Origin',(-90.,-90.,3.175));
#265049=CARTESIAN_POINT('Origin',(90.,90.,0.0381));
#265050=CARTESIAN_POINT('',(90.,115.,0.0381));
#265051=CARTESIAN_POINT('',(115.,90.,0.0381));
#265052=CARTESIAN_POINT('Origin',(90.,90.,0.0381));
#265053=CARTESIAN_POINT('',(-90.,115.,0.0381));
#265054=CARTESIAN_POINT('',(-90.,115.,0.0381));
#265055=CARTESIAN_POINT('',(-115.,90.,0.0381));
#265056=CARTESIAN_POINT('Origin',(-90.,90.,0.0381));
#265057=CARTESIAN_POINT('',(-115.,-90.,0.0381));
#265058=CARTESIAN_POINT('',(-115.,-90.,0.0381));
#265059=CARTESIAN_POINT('',(-90.,-115.,0.0381));
#265060=CARTESIAN_POINT('Origin',(-90.,-90.,0.0381));
#265061=CARTESIAN_POINT('',(90.,-115.,0.0381));
#265062=CARTESIAN_POINT('',(90.,-115.,0.0381));
#265063=CARTESIAN_POINT('',(115.,-90.,0.0381));
#265064=CARTESIAN_POINT('Origin',(90.,-90.,0.0381));
#265065=CARTESIAN_POINT('',(115.,90.,0.0381));
#265066=CARTESIAN_POINT('Origin',(90.,90.,0.));
#265067=CARTESIAN_POINT('',(115.,90.,-8.));
#265068=CARTESIAN_POINT('',(115.,90.,0.));
#265069=CARTESIAN_POINT('',(90.,115.,-8.));
#265070=CARTESIAN_POINT('Origin',(90.,90.,-8.));
#265071=CARTESIAN_POINT('',(90.,115.,0.));
#265072=CARTESIAN_POINT('Origin',(115.,90.,0.));
#265073=CARTESIAN_POINT('',(115.,-90.,-8.));
#265074=CARTESIAN_POINT('',(115.,-90.,0.));
#265075=CARTESIAN_POINT('',(115.,90.,-8.));
#265076=CARTESIAN_POINT('Origin',(90.,-90.,0.));
#265077=CARTESIAN_POINT('',(90.,-115.,-8.));
#265078=CARTESIAN_POINT('',(90.,-115.,0.));
#265079=CARTESIAN_POINT('Origin',(90.,-90.,-8.));
#265080=CARTESIAN_POINT('Origin',(90.,-115.,0.));
#265081=CARTESIAN_POINT('',(-90.,-115.,-8.));
#265082=CARTESIAN_POINT('',(-90.,-115.,0.));
#265083=CARTESIAN_POINT('',(90.,-115.,-8.));
#265084=CARTESIAN_POINT('Origin',(-90.,-90.,0.));
#265085=CARTESIAN_POINT('',(-115.,-90.,-8.));
#265086=CARTESIAN_POINT('',(-115.,-90.,0.));
#265087=CARTESIAN_POINT('Origin',(-90.,-90.,-8.));
#265088=CARTESIAN_POINT('Origin',(-115.,-90.,0.));
#265089=CARTESIAN_POINT('',(-115.,90.,-8.));
#265090=CARTESIAN_POINT('',(-115.,90.,0.));
#265091=CARTESIAN_POINT('',(-115.,-90.,-8.));
#265092=CARTESIAN_POINT('Origin',(-90.,90.,0.));
#265093=CARTESIAN_POINT('',(-90.,115.,-8.));
#265094=CARTESIAN_POINT('',(-90.,115.,0.));
#265095=CARTESIAN_POINT('Origin',(-90.,90.,-8.));
#265096=CARTESIAN_POINT('Origin',(-90.,115.,0.));
#265097=CARTESIAN_POINT('',(-90.,115.,-8.));
#265098=CARTESIAN_POINT('Origin',(90.,90.,7.493));
#265099=CARTESIAN_POINT('Origin',(90.,113.73,7.493));
#265100=CARTESIAN_POINT('Origin',(113.73,90.,7.493));
#265101=CARTESIAN_POINT('Origin',(113.73,90.,7.493));
#265102=CARTESIAN_POINT('Origin',(113.73,-90.,7.493));
#265103=CARTESIAN_POINT('Origin',(-90.,113.73,7.493));
#265104=CARTESIAN_POINT('Origin',(-90.,113.73,7.493));
#265105=CARTESIAN_POINT('Origin',(90.,-90.,7.493));
#265106=CARTESIAN_POINT('Origin',(90.,-113.73,7.493));
#265107=CARTESIAN_POINT('Origin',(-90.,90.,7.493));
#265108=CARTESIAN_POINT('Origin',(-113.73,90.,7.493));
#265109=CARTESIAN_POINT('Origin',(90.,-113.73,7.493));
#265110=CARTESIAN_POINT('Origin',(-90.,-113.73,7.493));
#265111=CARTESIAN_POINT('Origin',(-113.73,-90.,7.493));
#265112=CARTESIAN_POINT('Origin',(-113.73,-90.,7.493));
#265113=CARTESIAN_POINT('Origin',(-90.,-90.,7.493));
#265114=CARTESIAN_POINT('Origin',(90.,90.,-8.));
#265115=CARTESIAN_POINT('Origin',(0.,0.,-195.421614460986));
#265116=CARTESIAN_POINT('',(-17.3379110419348,-64.705964905612,7.62));
#265117=CARTESIAN_POINT('',(-17.3379110419348,-64.705964905612,2.54));
#265118=CARTESIAN_POINT('',(-17.3379110419348,-64.705964905612,7.62));
#265119=CARTESIAN_POINT('',(-17.3379110419348,64.705964905612,2.54));
#265120=CARTESIAN_POINT('Origin',(0.,0.,2.53999999999999));
#265121=CARTESIAN_POINT('',(-17.3379110419348,64.705964905612,7.62));
#265122=CARTESIAN_POINT('',(-17.3379110419348,64.705964905612,7.62));
#265123=CARTESIAN_POINT('Origin',(0.,0.,7.62));
#265124=CARTESIAN_POINT('Origin',(-90.,-90.,2.54));
#265125=CARTESIAN_POINT('',(-17.3379110419348,-71.5863792036332,2.54));
#265126=CARTESIAN_POINT('',(-17.3379110419348,-71.5863792036332,2.54));
#265127=CARTESIAN_POINT('',(17.3379110419348,-71.5863792036332,2.54));
#265128=CARTESIAN_POINT('Origin',(0.,0.,2.54));
#265129=CARTESIAN_POINT('',(17.3379110419348,-71.5863792036332,2.54));
#265130=CARTESIAN_POINT('',(17.3379110419348,71.5863792036332,2.54));
#265131=CARTESIAN_POINT('',(17.3379110419348,71.5863792036332,2.54));
#265132=CARTESIAN_POINT('',(-17.3379110419348,71.5863792036332,2.54));
#265133=CARTESIAN_POINT('Origin',(0.,0.,2.54));
#265134=CARTESIAN_POINT('',(-17.3379110419348,71.5863792036332,2.54));
#265135=CARTESIAN_POINT('Origin',(0.,0.,17.4625));
#265136=CARTESIAN_POINT('Origin',(90.,90.,0.));
#265137=CARTESIAN_POINT('Origin',(5.94817889868156E-29,-2.83629507977407E-14,
4.08753198860305));
#265138=CARTESIAN_POINT('Origin',(0.,0.,7.62));
#265139=CARTESIAN_POINT('',(17.3379110419348,71.5863792036332,7.62));
#265140=CARTESIAN_POINT('',(17.3379110419348,71.5863792036332,7.62));
#265141=CARTESIAN_POINT('',(-17.3379110419348,71.5863792036332,7.62));
#265142=CARTESIAN_POINT('Origin',(0.,0.,7.62));
#265143=CARTESIAN_POINT('',(-17.3379110419348,71.5863792036332,7.62));
#265144=CARTESIAN_POINT('Origin',(-17.3379110419348,71.5863792036332,7.62));
#265145=CARTESIAN_POINT('',(-17.3379110419348,71.5863792036332,7.62));
#265146=CARTESIAN_POINT('Origin',(17.3379110419348,71.5863792036332,7.62));
#265147=CARTESIAN_POINT('',(17.3379110419348,71.5863792036332,7.62));
#265148=CARTESIAN_POINT('Origin',(0.,0.,7.62));
#265149=CARTESIAN_POINT('',(17.3379110419348,-71.5863792036332,7.62));
#265150=CARTESIAN_POINT('',(17.3379110419348,-71.5863792036332,7.62));
#265151=CARTESIAN_POINT('',(-17.3379110419348,-71.5863792036332,7.62));
#265152=CARTESIAN_POINT('Origin',(0.,0.,7.62));
#265153=CARTESIAN_POINT('',(-17.3379110419348,-71.5863792036332,7.62));
#265154=CARTESIAN_POINT('Origin',(0.,0.,7.62));
#265155=CARTESIAN_POINT('',(-17.3379110419348,-71.5863792036332,7.62));
#265156=CARTESIAN_POINT('',(17.3379110419348,-71.5863792036332,7.62));
#265157=CARTESIAN_POINT('Origin',(-17.3379110419348,-71.5863792036332,7.62));
#265158=CARTESIAN_POINT('Origin',(17.3379110419348,-71.5863792036332,7.62));
#276450=UNCERTAINTY_MEASURE_WITH_UNIT(LENGTH_MEASURE(0.01),#276463,
'DISTANCE_ACCURACY_VALUE',
'Maximum model space distance between geometric entities at asserted c
onnectivities');
#276454=UNCERTAINTY_MEASURE_WITH_UNIT(LENGTH_MEASURE(0.01),#276463,
'DISTANCE_ACCURACY_VALUE',
'Maximum model space distance between geometric entities at asserted c
onnectivities');
#276458=(
GEOMETRIC_REPRESENTATION_CONTEXT(3)
GLOBAL_UNCERTAINTY_ASSIGNED_CONTEXT((#276450))
GLOBAL_UNIT_ASSIGNED_CONTEXT((#276463,#276465,#276466))
REPRESENTATION_CONTEXT('','3D')
);
#276462=(
GEOMETRIC_REPRESENTATION_CONTEXT(3)
GLOBAL_UNCERTAINTY_ASSIGNED_CONTEXT((#276454))
GLOBAL_UNIT_ASSIGNED_CONTEXT((#276463,#276465,#276466))
REPRESENTATION_CONTEXT('','3D')
);
#276463=(
LENGTH_UNIT()
NAMED_UNIT(*)
SI_UNIT(.MILLI.,.METRE.)
);
#276465=(
NAMED_UNIT(*)
PLANE_ANGLE_UNIT()
SI_UNIT($,.RADIAN.)
);
#276466=(
NAMED_UNIT(*)
SI_UNIT($,.STERADIAN.)
SOLID_ANGLE_UNIT()
);
#276470=SHAPE_DEFINITION_REPRESENTATION(#276477,#276490);
#276477=PRODUCT_DEFINITION_SHAPE('',$,#276498);
#276490=SHAPE_REPRESENTATION('',(#98939),#276458);
#276494=PRODUCT_DEFINITION_CONTEXT('part definition',#276517,'design');
#276498=PRODUCT_DEFINITION('Quick-release clamp ring with bearing',
'Quick-release clamp ring with bearing',#276505,#276494);
#276505=PRODUCT_DEFINITION_FORMATION('',$,#276522);
#276517=APPLICATION_CONTEXT(
'Core Data for Automotive Mechanical Design Process');
#276518=PRODUCT_CONTEXT('part definition',#276517,'mechanical');
#276522=PRODUCT('Quick-release clamp ring with bearing',
'Quick-release clamp ring with bearing',$,(#276518));
#276529=PRESENTATION_STYLE_ASSIGNMENT((#276534));
#276534=SURFACE_STYLE_USAGE(.BOTH.,#276539);
#276539=SURFACE_SIDE_STYLE('',(#276544));
#276544=SURFACE_STYLE_FILL_AREA(#276549);
#276549=FILL_AREA_STYLE('Opaque(122,133,145)',(#276554));
#276554=FILL_AREA_STYLE_COLOUR('Opaque(122,133,145)',#276559);
#276559=COLOUR_RGB('Opaque(122,133,145)',0.47843137254902,0.52156862745098,
0.568627450980392);
ENDSEC;
END-ISO-10303-21;
